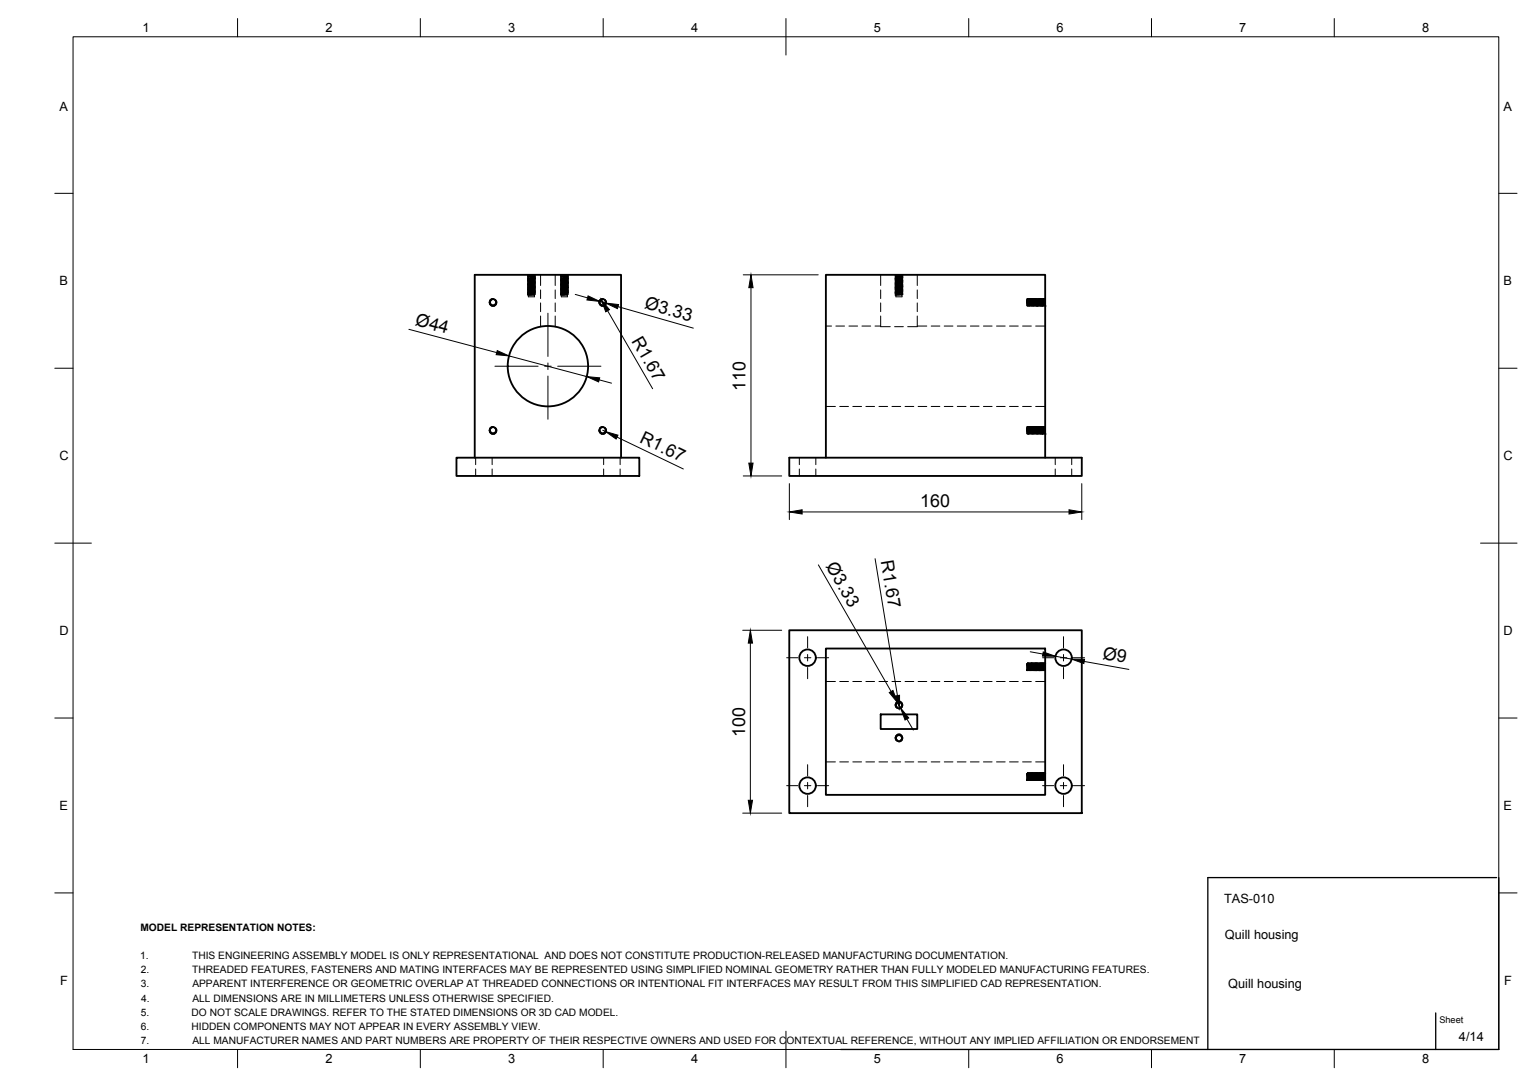
ISO-10303-21;
HEADER;
/* Generated by software containing ST-Developer
 * from STEP Tools, Inc. (www.steptools.com) 
 */

FILE_DESCRIPTION(
/* description */ (
'Independent keyed-quill tailstock, native coupled50mm slider andM16x2
 feed screw, conical dead center, bronze sleeves/thrust washers, cross
-pinned handwheel and bolted guide key. Custom center taper; no standa
rd taper compatibility, machine-bed compatibility or load rating assig
ned.'),
/* implementation_level */ '2;1');

FILE_NAME(
/* name */ 'Quill housing.step',
/* time_stamp */ '2026-11-14T07:17:36-08:00',
/* author */ (''),
/* organization */ (''),
/* preprocessor_version */ 'ST-DEVELOPER v20.2',
/* originating_system */ 'Autodesk Translation Framework v15.17.0.0',
/* authorisation */ '');

FILE_SCHEMA (('AUTOMOTIVE_DESIGN { 1 0 10303 214 3 1 1 }'));
ENDSEC;

DATA;
#10=MECHANICAL_DESIGN_GEOMETRIC_PRESENTATION_REPRESENTATION('',(#154),#289387);
#120=SHAPE_REPRESENTATION_RELATIONSHIP('SRR','None',#289455,#137);
#137=ADVANCED_BREP_SHAPE_REPRESENTATION('',(#171),#289371);
#154=STYLED_ITEM('',(#289549),#171);
#171=MANIFOLD_SOLID_BREP('Body1',#16842);
#199=FACE_BOUND('',#1414,.T.);
#200=FACE_BOUND('',#1416,.T.);
#201=FACE_BOUND('',#1417,.T.);
#202=FACE_BOUND('',#1418,.T.);
#203=FACE_BOUND('',#1419,.T.);
#204=FACE_BOUND('',#1420,.T.);
#205=FACE_BOUND('',#1426,.T.);
#206=FACE_BOUND('',#1427,.T.);
#207=FACE_BOUND('',#1428,.T.);
#208=FACE_BOUND('',#1429,.T.);
#209=FACE_BOUND('',#1432,.T.);
#210=FACE_BOUND('',#1435,.T.);
#211=FACE_BOUND('',#1436,.T.);
#212=FACE_BOUND('',#1437,.T.);
#213=FACE_BOUND('',#1438,.T.);
#214=FACE_BOUND('',#1439,.T.);
#215=FACE_BOUND('',#1441,.T.);
#216=FACE_BOUND('',#1442,.T.);
#217=FACE_BOUND('',#1443,.T.);
#281=B_SPLINE_SURFACE_WITH_KNOTS('',3,3,((#129776,#129777,#129778,#129779,
#129780,#129781,#129782,#129783,#129784,#129785,#129786,#129787,#129788,
#129789,#129790,#129791,#129792,#129793,#129794,#129795,#129796,#129797,
#129798,#129799,#129800,#129801,#129802,#129803,#129804,#129805,#129806,
#129807,#129808,#129809,#129810,#129811,#129812,#129813,#129814,#129815,
#129816,#129817,#129818,#129819,#129820,#129821,#129822,#129823,#129824,
#129825,#129826,#129827,#129828,#129829,#129830,#129831,#129832,#129833,
#129834,#129835,#129836,#129837,#129838,#129839,#129840,#129841,#129842,
#129843,#129844,#129845,#129846,#129847,#129848,#129849,#129850,#129851,
#129852,#129853,#129854,#129855,#129856,#129857,#129858,#129859,#129860,
#129861,#129862,#129863,#129864,#129865,#129866,#129867,#129868,#129869,
#129870,#129871,#129872,#129873,#129874,#129875,#129876,#129877,#129878,
#129879),(#129880,#129881,#129882,#129883,#129884,#129885,#129886,#129887,
#129888,#129889,#129890,#129891,#129892,#129893,#129894,#129895,#129896,
#129897,#129898,#129899,#129900,#129901,#129902,#129903,#129904,#129905,
#129906,#129907,#129908,#129909,#129910,#129911,#129912,#129913,#129914,
#129915,#129916,#129917,#129918,#129919,#129920,#129921,#129922,#129923,
#129924,#129925,#129926,#129927,#129928,#129929,#129930,#129931,#129932,
#129933,#129934,#129935,#129936,#129937,#129938,#129939,#129940,#129941,
#129942,#129943,#129944,#129945,#129946,#129947,#129948,#129949,#129950,
#129951,#129952,#129953,#129954,#129955,#129956,#129957,#129958,#129959,
#129960,#129961,#129962,#129963,#129964,#129965,#129966,#129967,#129968,
#129969,#129970,#129971,#129972,#129973,#129974,#129975,#129976,#129977,
#129978,#129979,#129980,#129981,#129982,#129983),(#129984,#129985,#129986,
#129987,#129988,#129989,#129990,#129991,#129992,#129993,#129994,#129995,
#129996,#129997,#129998,#129999,#130000,#130001,#130002,#130003,#130004,
#130005,#130006,#130007,#130008,#130009,#130010,#130011,#130012,#130013,
#130014,#130015,#130016,#130017,#130018,#130019,#130020,#130021,#130022,
#130023,#130024,#130025,#130026,#130027,#130028,#130029,#130030,#130031,
#130032,#130033,#130034,#130035,#130036,#130037,#130038,#130039,#130040,
#130041,#130042,#130043,#130044,#130045,#130046,#130047,#130048,#130049,
#130050,#130051,#130052,#130053,#130054,#130055,#130056,#130057,#130058,
#130059,#130060,#130061,#130062,#130063,#130064,#130065,#130066,#130067,
#130068,#130069,#130070,#130071,#130072,#130073,#130074,#130075,#130076,
#130077,#130078,#130079,#130080,#130081,#130082,#130083,#130084,#130085,
#130086,#130087),(#130088,#130089,#130090,#130091,#130092,#130093,#130094,
#130095,#130096,#130097,#130098,#130099,#130100,#130101,#130102,#130103,
#130104,#130105,#130106,#130107,#130108,#130109,#130110,#130111,#130112,
#130113,#130114,#130115,#130116,#130117,#130118,#130119,#130120,#130121,
#130122,#130123,#130124,#130125,#130126,#130127,#130128,#130129,#130130,
#130131,#130132,#130133,#130134,#130135,#130136,#130137,#130138,#130139,
#130140,#130141,#130142,#130143,#130144,#130145,#130146,#130147,#130148,
#130149,#130150,#130151,#130152,#130153,#130154,#130155,#130156,#130157,
#130158,#130159,#130160,#130161,#130162,#130163,#130164,#130165,#130166,
#130167,#130168,#130169,#130170,#130171,#130172,#130173,#130174,#130175,
#130176,#130177,#130178,#130179,#130180,#130181,#130182,#130183,#130184,
#130185,#130186,#130187,#130188,#130189,#130190,#130191)),.UNSPECIFIED.,
 .F.,.F.,.F.,(4,4),(4,1,1,1,1,1,1,1,1,1,1,1,1,1,1,1,1,1,1,1,1,1,1,1,1,1,
1,1,1,1,1,1,1,1,1,1,1,1,1,1,1,1,1,1,1,1,1,1,1,1,1,1,1,1,1,1,1,1,1,1,1,1,
1,1,1,1,1,1,1,1,1,1,1,1,1,1,1,1,1,1,1,1,1,1,1,1,1,1,1,1,1,1,1,1,1,1,1,1,
1,1,1,4),(-0.000353809570517248,0.0451882118607677),(11.8612261946863,12.8591085386934,
13.85663707313,14.8541656075666,15.8516941420032,16.8492226764398,17.8467512108764,
18.844279745313,19.8418082797496,20.8393368141862,21.8368653486228,22.8343938830594,
23.831922417496,24.8294509519326,25.8269794863692,26.8245080208058,27.8220365552424,
28.819565089679,29.8170936241156,30.8146221585522,31.8121506929888,32.8096792274254,
33.807207761862,34.8047362962986,35.8022648307352,36.7997933651718,37.7973218996084,
38.794850434045,39.7923789684816,40.7899075029182,41.7874360373548,42.7849645717913,
43.782493106228,44.7800216406646,45.7775501751012,46.7750787095378,47.7726072439743,
48.7701357784109,49.7676643128475,50.7651928472842,51.7627213817208,52.7602499161573,
53.7577784505939,54.7553069850305,55.7528355194671,56.7503640539037,57.7478925883403,
58.7454211227769,59.7429496572135,60.7404781916501,61.7380067260867,62.7355352605233,
63.7330637949599,64.7305923293965,65.7281208638331,66.7256493982697,67.7231779327063,
68.7207064671429,69.7182350015795,70.7157635360161,71.7132920704527,72.7108206048893,
73.7083491393259,74.7058776737625,75.7034062081991,76.7009347426357,77.6984632770723,
78.6959918115089,79.6935203459455,80.6910488803821,81.6885774148187,82.6861059492553,
83.6836344836919,84.6811630181285,85.6786915525651,86.6762200870017,87.6737486214383,
88.6712771558749,89.6688056903115,90.6663342247481,91.6638627591847,92.6613912936213,
93.6589198280579,94.6564483624945,95.6539768969311,96.6515054313677,97.6490339658043,
98.6465625002409,99.6440910346775,100.641619569114,101.639148103551,102.636676637987,
103.634205172424,104.631733706861,105.629262241297,106.626790775734,107.62431931017,
108.621847844607,109.619376379044,110.61690491348,111.614433447917,112.611961982353),
 .UNSPECIFIED.);
#282=B_SPLINE_SURFACE_WITH_KNOTS('',3,3,((#130274,#130275,#130276,#130277,
#130278,#130279,#130280,#130281,#130282,#130283,#130284,#130285,#130286,
#130287,#130288,#130289,#130290,#130291,#130292,#130293,#130294,#130295,
#130296,#130297,#130298,#130299,#130300,#130301,#130302,#130303,#130304,
#130305,#130306,#130307,#130308,#130309,#130310,#130311,#130312,#130313,
#130314,#130315,#130316,#130317,#130318,#130319,#130320,#130321,#130322,
#130323,#130324,#130325,#130326,#130327,#130328,#130329,#130330,#130331,
#130332,#130333,#130334,#130335,#130336,#130337,#130338,#130339,#130340,
#130341,#130342,#130343,#130344,#130345,#130346,#130347,#130348,#130349,
#130350,#130351,#130352,#130353,#130354,#130355,#130356,#130357,#130358,
#130359,#130360,#130361,#130362,#130363,#130364,#130365,#130366,#130367,
#130368,#130369,#130370,#130371,#130372,#130373,#130374,#130375,#130376,
#130377),(#130378,#130379,#130380,#130381,#130382,#130383,#130384,#130385,
#130386,#130387,#130388,#130389,#130390,#130391,#130392,#130393,#130394,
#130395,#130396,#130397,#130398,#130399,#130400,#130401,#130402,#130403,
#130404,#130405,#130406,#130407,#130408,#130409,#130410,#130411,#130412,
#130413,#130414,#130415,#130416,#130417,#130418,#130419,#130420,#130421,
#130422,#130423,#130424,#130425,#130426,#130427,#130428,#130429,#130430,
#130431,#130432,#130433,#130434,#130435,#130436,#130437,#130438,#130439,
#130440,#130441,#130442,#130443,#130444,#130445,#130446,#130447,#130448,
#130449,#130450,#130451,#130452,#130453,#130454,#130455,#130456,#130457,
#130458,#130459,#130460,#130461,#130462,#130463,#130464,#130465,#130466,
#130467,#130468,#130469,#130470,#130471,#130472,#130473,#130474,#130475,
#130476,#130477,#130478,#130479,#130480,#130481),(#130482,#130483,#130484,
#130485,#130486,#130487,#130488,#130489,#130490,#130491,#130492,#130493,
#130494,#130495,#130496,#130497,#130498,#130499,#130500,#130501,#130502,
#130503,#130504,#130505,#130506,#130507,#130508,#130509,#130510,#130511,
#130512,#130513,#130514,#130515,#130516,#130517,#130518,#130519,#130520,
#130521,#130522,#130523,#130524,#130525,#130526,#130527,#130528,#130529,
#130530,#130531,#130532,#130533,#130534,#130535,#130536,#130537,#130538,
#130539,#130540,#130541,#130542,#130543,#130544,#130545,#130546,#130547,
#130548,#130549,#130550,#130551,#130552,#130553,#130554,#130555,#130556,
#130557,#130558,#130559,#130560,#130561,#130562,#130563,#130564,#130565,
#130566,#130567,#130568,#130569,#130570,#130571,#130572,#130573,#130574,
#130575,#130576,#130577,#130578,#130579,#130580,#130581,#130582,#130583,
#130584,#130585),(#130586,#130587,#130588,#130589,#130590,#130591,#130592,
#130593,#130594,#130595,#130596,#130597,#130598,#130599,#130600,#130601,
#130602,#130603,#130604,#130605,#130606,#130607,#130608,#130609,#130610,
#130611,#130612,#130613,#130614,#130615,#130616,#130617,#130618,#130619,
#130620,#130621,#130622,#130623,#130624,#130625,#130626,#130627,#130628,
#130629,#130630,#130631,#130632,#130633,#130634,#130635,#130636,#130637,
#130638,#130639,#130640,#130641,#130642,#130643,#130644,#130645,#130646,
#130647,#130648,#130649,#130650,#130651,#130652,#130653,#130654,#130655,
#130656,#130657,#130658,#130659,#130660,#130661,#130662,#130663,#130664,
#130665,#130666,#130667,#130668,#130669,#130670,#130671,#130672,#130673,
#130674,#130675,#130676,#130677,#130678,#130679,#130680,#130681,#130682,
#130683,#130684,#130685,#130686,#130687,#130688,#130689)),.UNSPECIFIED.,
 .F.,.F.,.F.,(4,4),(4,1,1,1,1,1,1,1,1,1,1,1,1,1,1,1,1,1,1,1,1,1,1,1,1,1,
1,1,1,1,1,1,1,1,1,1,1,1,1,1,1,1,1,1,1,1,1,1,1,1,1,1,1,1,1,1,1,1,1,1,1,1,
1,1,1,1,1,1,1,1,1,1,1,1,1,1,1,1,1,1,1,1,1,1,1,1,1,1,1,1,1,1,1,1,1,1,1,1,
1,1,1,4),(-0.000311884246383574,0.0452427689821445),(14.398141012777,15.3956695472136,
16.3931980816502,17.3907266160868,18.3882551505234,19.38578368496,20.3833122193966,
21.3808407538332,22.3783692882698,23.3758978227064,24.373426357143,25.3709548915796,
26.3684834260162,27.3660119604528,28.3635404948894,29.361069029326,30.3585975637626,
31.3561260981992,32.3536546326358,33.3511831670724,34.348711701509,35.3462402359456,
36.3437687703822,37.3412973048188,38.3388258392554,39.336354373692,40.3338829081286,
41.3314114425652,42.3289399770018,43.3264685114384,44.323997045875,45.3215255803116,
46.3190541147482,47.3165826491848,48.3141111836214,49.311639718058,50.3091682524946,
51.3066967869312,52.3042253213678,53.3017538558044,54.299282390241,55.2968109246776,
56.2943394591142,57.2918679935508,58.2893965279874,59.286925062424,60.2844535968606,
61.2819821312972,62.2795106657338,63.2770392001704,64.274567734607,65.2720962690436,
66.2696248034802,67.2671533379168,68.2646818723534,69.26221040679,70.2597389412266,
71.2572674756632,72.2547960100998,73.2523245445364,74.249853078973,75.2473816134096,
76.2449101478462,77.2424386822828,78.2399672167194,79.237495751156,80.2350242855926,
81.2325528200292,82.2300813544658,83.2276098889024,84.225138423339,85.2226669577756,
86.2201954922122,87.2177240266488,88.2152525610854,89.212781095522,90.2103096299586,
91.2078381643952,92.2053666988318,93.2028952332684,94.2004237677049,95.1979523021416,
96.1954808365782,97.1930093710148,98.1905379054514,99.1880664398879,100.185594974325,
101.183123508761,102.180652043198,103.178180577634,104.175709112071,105.173237646508,
106.170766180944,107.168294715381,108.165823249817,109.163351784254,110.160880318691,
111.158408853127,112.155937387564,113.153465922,114.150994456437,115.148876776427),
 .UNSPECIFIED.);
#283=B_SPLINE_SURFACE_WITH_KNOTS('',3,3,((#130957,#130958,#130959,#130960,
#130961,#130962,#130963,#130964,#130965,#130966,#130967,#130968,#130969,
#130970,#130971,#130972,#130973,#130974,#130975,#130976,#130977,#130978,
#130979,#130980,#130981,#130982,#130983,#130984,#130985,#130986,#130987,
#130988,#130989,#130990,#130991,#130992,#130993,#130994,#130995,#130996,
#130997,#130998,#130999,#131000,#131001,#131002,#131003,#131004,#131005,
#131006,#131007,#131008,#131009,#131010,#131011,#131012,#131013,#131014,
#131015,#131016,#131017,#131018,#131019,#131020,#131021,#131022,#131023,
#131024,#131025,#131026,#131027,#131028,#131029,#131030,#131031,#131032,
#131033,#131034,#131035,#131036,#131037,#131038,#131039,#131040,#131041,
#131042,#131043,#131044,#131045,#131046,#131047,#131048,#131049,#131050,
#131051,#131052,#131053,#131054,#131055,#131056,#131057,#131058,#131059,
#131060),(#131061,#131062,#131063,#131064,#131065,#131066,#131067,#131068,
#131069,#131070,#131071,#131072,#131073,#131074,#131075,#131076,#131077,
#131078,#131079,#131080,#131081,#131082,#131083,#131084,#131085,#131086,
#131087,#131088,#131089,#131090,#131091,#131092,#131093,#131094,#131095,
#131096,#131097,#131098,#131099,#131100,#131101,#131102,#131103,#131104,
#131105,#131106,#131107,#131108,#131109,#131110,#131111,#131112,#131113,
#131114,#131115,#131116,#131117,#131118,#131119,#131120,#131121,#131122,
#131123,#131124,#131125,#131126,#131127,#131128,#131129,#131130,#131131,
#131132,#131133,#131134,#131135,#131136,#131137,#131138,#131139,#131140,
#131141,#131142,#131143,#131144,#131145,#131146,#131147,#131148,#131149,
#131150,#131151,#131152,#131153,#131154,#131155,#131156,#131157,#131158,
#131159,#131160,#131161,#131162,#131163,#131164),(#131165,#131166,#131167,
#131168,#131169,#131170,#131171,#131172,#131173,#131174,#131175,#131176,
#131177,#131178,#131179,#131180,#131181,#131182,#131183,#131184,#131185,
#131186,#131187,#131188,#131189,#131190,#131191,#131192,#131193,#131194,
#131195,#131196,#131197,#131198,#131199,#131200,#131201,#131202,#131203,
#131204,#131205,#131206,#131207,#131208,#131209,#131210,#131211,#131212,
#131213,#131214,#131215,#131216,#131217,#131218,#131219,#131220,#131221,
#131222,#131223,#131224,#131225,#131226,#131227,#131228,#131229,#131230,
#131231,#131232,#131233,#131234,#131235,#131236,#131237,#131238,#131239,
#131240,#131241,#131242,#131243,#131244,#131245,#131246,#131247,#131248,
#131249,#131250,#131251,#131252,#131253,#131254,#131255,#131256,#131257,
#131258,#131259,#131260,#131261,#131262,#131263,#131264,#131265,#131266,
#131267,#131268),(#131269,#131270,#131271,#131272,#131273,#131274,#131275,
#131276,#131277,#131278,#131279,#131280,#131281,#131282,#131283,#131284,
#131285,#131286,#131287,#131288,#131289,#131290,#131291,#131292,#131293,
#131294,#131295,#131296,#131297,#131298,#131299,#131300,#131301,#131302,
#131303,#131304,#131305,#131306,#131307,#131308,#131309,#131310,#131311,
#131312,#131313,#131314,#131315,#131316,#131317,#131318,#131319,#131320,
#131321,#131322,#131323,#131324,#131325,#131326,#131327,#131328,#131329,
#131330,#131331,#131332,#131333,#131334,#131335,#131336,#131337,#131338,
#131339,#131340,#131341,#131342,#131343,#131344,#131345,#131346,#131347,
#131348,#131349,#131350,#131351,#131352,#131353,#131354,#131355,#131356,
#131357,#131358,#131359,#131360,#131361,#131362,#131363,#131364,#131365,
#131366,#131367,#131368,#131369,#131370,#131371,#131372)),.UNSPECIFIED.,
 .F.,.F.,.F.,(4,4),(4,1,1,1,1,1,1,1,1,1,1,1,1,1,1,1,1,1,1,1,1,1,1,1,1,1,
1,1,1,1,1,1,1,1,1,1,1,1,1,1,1,1,1,1,1,1,1,1,1,1,1,1,1,1,1,1,1,1,1,1,1,1,
1,1,1,1,1,1,1,1,1,1,1,1,1,1,1,1,1,1,1,1,1,1,1,1,1,1,1,1,1,1,1,1,1,1,1,1,
1,1,1,4),(-0.000353803744797756,0.045188208347436),(11.8612262005118,12.8591085386932,
13.8566370731298,14.8541656075664,15.851694142003,16.8492226764396,17.8467512108762,
18.8442797453128,19.8418082797494,20.839336814186,21.8368653486226,22.8343938830592,
23.8319224174958,24.8294509519324,25.826979486369,26.8245080208056,27.8220365552422,
28.8195650896788,29.8170936241154,30.814622158552,31.8121506929886,32.8096792274252,
33.8072077618618,34.8047362962984,35.802264830735,36.7997933651716,37.7973218996082,
38.7948504340448,39.7923789684814,40.789907502918,41.7874360373546,42.7849645717912,
43.7824931062278,44.7800216406644,45.777550175101,46.7750787095376,47.7726072439742,
48.7701357784108,49.7676643128474,50.765192847284,51.7627213817206,52.7602499161572,
53.7577784505938,54.7553069850304,55.752835519467,56.7503640539036,57.7478925883402,
58.7454211227768,59.7429496572134,60.74047819165,61.7380067260866,62.7355352605232,
63.7330637949598,64.7305923293964,65.728120863833,66.7256493982696,67.7231779327062,
68.7207064671428,69.7182350015794,70.715763536016,71.7132920704526,72.7108206048892,
73.7083491393258,74.7058776737624,75.703406208199,76.7009347426356,77.6984632770722,
78.6959918115088,79.6935203459454,80.691048880382,81.6885774148186,82.6861059492552,
83.6836344836918,84.6811630181284,85.678691552565,86.6762200870016,87.6737486214382,
88.6712771558748,89.6688056903114,90.666334224748,91.6638627591846,92.6613912936212,
93.6589198280578,94.6564483624944,95.653976896931,96.6515054313676,97.6490339658042,
98.6465625002408,99.6440910346774,100.641619569114,101.639148103551,102.636676637987,
103.634205172424,104.63173370686,105.629262241297,106.626790775734,107.62431931017,
108.621847844607,109.619376379043,110.61690491348,111.614433447917,112.611961982353),
 .UNSPECIFIED.);
#284=B_SPLINE_SURFACE_WITH_KNOTS('',3,3,((#131455,#131456,#131457,#131458,
#131459,#131460,#131461,#131462,#131463,#131464,#131465,#131466,#131467,
#131468,#131469,#131470,#131471,#131472,#131473,#131474,#131475,#131476,
#131477,#131478,#131479,#131480,#131481,#131482,#131483,#131484,#131485,
#131486,#131487,#131488,#131489,#131490,#131491,#131492,#131493,#131494,
#131495,#131496,#131497,#131498,#131499,#131500,#131501,#131502,#131503,
#131504,#131505,#131506,#131507,#131508,#131509,#131510,#131511,#131512,
#131513,#131514,#131515,#131516,#131517,#131518,#131519,#131520,#131521,
#131522,#131523,#131524,#131525,#131526,#131527,#131528,#131529,#131530,
#131531,#131532,#131533,#131534,#131535,#131536,#131537,#131538,#131539,
#131540,#131541,#131542,#131543,#131544,#131545,#131546,#131547,#131548,
#131549,#131550,#131551,#131552,#131553,#131554,#131555,#131556,#131557,
#131558),(#131559,#131560,#131561,#131562,#131563,#131564,#131565,#131566,
#131567,#131568,#131569,#131570,#131571,#131572,#131573,#131574,#131575,
#131576,#131577,#131578,#131579,#131580,#131581,#131582,#131583,#131584,
#131585,#131586,#131587,#131588,#131589,#131590,#131591,#131592,#131593,
#131594,#131595,#131596,#131597,#131598,#131599,#131600,#131601,#131602,
#131603,#131604,#131605,#131606,#131607,#131608,#131609,#131610,#131611,
#131612,#131613,#131614,#131615,#131616,#131617,#131618,#131619,#131620,
#131621,#131622,#131623,#131624,#131625,#131626,#131627,#131628,#131629,
#131630,#131631,#131632,#131633,#131634,#131635,#131636,#131637,#131638,
#131639,#131640,#131641,#131642,#131643,#131644,#131645,#131646,#131647,
#131648,#131649,#131650,#131651,#131652,#131653,#131654,#131655,#131656,
#131657,#131658,#131659,#131660,#131661,#131662),(#131663,#131664,#131665,
#131666,#131667,#131668,#131669,#131670,#131671,#131672,#131673,#131674,
#131675,#131676,#131677,#131678,#131679,#131680,#131681,#131682,#131683,
#131684,#131685,#131686,#131687,#131688,#131689,#131690,#131691,#131692,
#131693,#131694,#131695,#131696,#131697,#131698,#131699,#131700,#131701,
#131702,#131703,#131704,#131705,#131706,#131707,#131708,#131709,#131710,
#131711,#131712,#131713,#131714,#131715,#131716,#131717,#131718,#131719,
#131720,#131721,#131722,#131723,#131724,#131725,#131726,#131727,#131728,
#131729,#131730,#131731,#131732,#131733,#131734,#131735,#131736,#131737,
#131738,#131739,#131740,#131741,#131742,#131743,#131744,#131745,#131746,
#131747,#131748,#131749,#131750,#131751,#131752,#131753,#131754,#131755,
#131756,#131757,#131758,#131759,#131760,#131761,#131762,#131763,#131764,
#131765,#131766),(#131767,#131768,#131769,#131770,#131771,#131772,#131773,
#131774,#131775,#131776,#131777,#131778,#131779,#131780,#131781,#131782,
#131783,#131784,#131785,#131786,#131787,#131788,#131789,#131790,#131791,
#131792,#131793,#131794,#131795,#131796,#131797,#131798,#131799,#131800,
#131801,#131802,#131803,#131804,#131805,#131806,#131807,#131808,#131809,
#131810,#131811,#131812,#131813,#131814,#131815,#131816,#131817,#131818,
#131819,#131820,#131821,#131822,#131823,#131824,#131825,#131826,#131827,
#131828,#131829,#131830,#131831,#131832,#131833,#131834,#131835,#131836,
#131837,#131838,#131839,#131840,#131841,#131842,#131843,#131844,#131845,
#131846,#131847,#131848,#131849,#131850,#131851,#131852,#131853,#131854,
#131855,#131856,#131857,#131858,#131859,#131860,#131861,#131862,#131863,
#131864,#131865,#131866,#131867,#131868,#131869,#131870)),.UNSPECIFIED.,
 .F.,.F.,.F.,(4,4),(4,1,1,1,1,1,1,1,1,1,1,1,1,1,1,1,1,1,1,1,1,1,1,1,1,1,
1,1,1,1,1,1,1,1,1,1,1,1,1,1,1,1,1,1,1,1,1,1,1,1,1,1,1,1,1,1,1,1,1,1,1,1,
1,1,1,1,1,1,1,1,1,1,1,1,1,1,1,1,1,1,1,1,1,1,1,1,1,1,1,1,1,1,1,1,1,1,1,1,
1,1,1,4),(-0.000311879380046352,0.0452427611100038),(14.3981410127768,15.3956695472134,
16.39319808165,17.3907266160866,18.3882551505232,19.3857836849598,20.3833122193964,
21.380840753833,22.3783692882696,23.3758978227062,24.3734263571428,25.3709548915794,
26.368483426016,27.3660119604526,28.3635404948892,29.3610690293258,30.3585975637624,
31.356126098199,32.3536546326356,33.3511831670722,34.3487117015088,35.3462402359454,
36.343768770382,37.3412973048186,38.3388258392552,39.3363543736918,40.3338829081284,
41.331411442565,42.3289399770016,43.3264685114382,44.3239970458748,45.3215255803114,
46.319054114748,47.3165826491846,48.3141111836212,49.3116397180578,50.3091682524944,
51.306696786931,52.3042253213676,53.3017538558042,54.2992823902408,55.2968109246774,
56.294339459114,57.2918679935506,58.2893965279872,59.2869250624238,60.2844535968604,
61.281982131297,62.2795106657336,63.2770392001702,64.2745677346068,65.2720962690434,
66.26962480348,67.2671533379166,68.2646818723532,69.2622104067898,70.2597389412264,
71.257267475663,72.2547960100996,73.2523245445362,74.2498530789728,75.2473816134094,
76.244910147846,77.2424386822826,78.2399672167192,79.2374957511558,80.2350242855924,
81.232552820029,82.2300813544656,83.2276098889022,84.2251384233388,85.2226669577754,
86.220195492212,87.2177240266486,88.2152525610852,89.2127810955218,90.2103096299584,
91.207838164395,92.2053666988316,93.2028952332682,94.2004237677048,95.1979523021414,
96.195480836578,97.1930093710146,98.1905379054512,99.1880664398878,100.185594974324,
101.183123508761,102.180652043198,103.178180577634,104.175709112071,105.173237646507,
106.170766180944,107.168294715381,108.165823249817,109.163351784254,110.16088031869,
111.158408853127,112.155937387564,113.153465922,114.150994456437,115.148876768553),
 .UNSPECIFIED.);
#285=B_SPLINE_SURFACE_WITH_KNOTS('',3,3,((#132011,#132012,#132013,#132014,
#132015,#132016,#132017,#132018,#132019,#132020,#132021,#132022,#132023,
#132024,#132025,#132026,#132027,#132028,#132029,#132030,#132031,#132032,
#132033,#132034,#132035,#132036,#132037,#132038,#132039,#132040,#132041,
#132042,#132043,#132044,#132045,#132046,#132047,#132048,#132049,#132050,
#132051,#132052,#132053,#132054,#132055,#132056,#132057,#132058,#132059,
#132060,#132061,#132062,#132063,#132064,#132065,#132066,#132067,#132068,
#132069,#132070,#132071,#132072,#132073,#132074,#132075,#132076,#132077,
#132078,#132079,#132080,#132081,#132082,#132083,#132084,#132085,#132086,
#132087,#132088,#132089,#132090,#132091,#132092,#132093,#132094,#132095,
#132096,#132097,#132098,#132099,#132100,#132101,#132102,#132103,#132104,
#132105),(#132106,#132107,#132108,#132109,#132110,#132111,#132112,#132113,
#132114,#132115,#132116,#132117,#132118,#132119,#132120,#132121,#132122,
#132123,#132124,#132125,#132126,#132127,#132128,#132129,#132130,#132131,
#132132,#132133,#132134,#132135,#132136,#132137,#132138,#132139,#132140,
#132141,#132142,#132143,#132144,#132145,#132146,#132147,#132148,#132149,
#132150,#132151,#132152,#132153,#132154,#132155,#132156,#132157,#132158,
#132159,#132160,#132161,#132162,#132163,#132164,#132165,#132166,#132167,
#132168,#132169,#132170,#132171,#132172,#132173,#132174,#132175,#132176,
#132177,#132178,#132179,#132180,#132181,#132182,#132183,#132184,#132185,
#132186,#132187,#132188,#132189,#132190,#132191,#132192,#132193,#132194,
#132195,#132196,#132197,#132198,#132199,#132200),(#132201,#132202,#132203,
#132204,#132205,#132206,#132207,#132208,#132209,#132210,#132211,#132212,
#132213,#132214,#132215,#132216,#132217,#132218,#132219,#132220,#132221,
#132222,#132223,#132224,#132225,#132226,#132227,#132228,#132229,#132230,
#132231,#132232,#132233,#132234,#132235,#132236,#132237,#132238,#132239,
#132240,#132241,#132242,#132243,#132244,#132245,#132246,#132247,#132248,
#132249,#132250,#132251,#132252,#132253,#132254,#132255,#132256,#132257,
#132258,#132259,#132260,#132261,#132262,#132263,#132264,#132265,#132266,
#132267,#132268,#132269,#132270,#132271,#132272,#132273,#132274,#132275,
#132276,#132277,#132278,#132279,#132280,#132281,#132282,#132283,#132284,
#132285,#132286,#132287,#132288,#132289,#132290,#132291,#132292,#132293,
#132294,#132295),(#132296,#132297,#132298,#132299,#132300,#132301,#132302,
#132303,#132304,#132305,#132306,#132307,#132308,#132309,#132310,#132311,
#132312,#132313,#132314,#132315,#132316,#132317,#132318,#132319,#132320,
#132321,#132322,#132323,#132324,#132325,#132326,#132327,#132328,#132329,
#132330,#132331,#132332,#132333,#132334,#132335,#132336,#132337,#132338,
#132339,#132340,#132341,#132342,#132343,#132344,#132345,#132346,#132347,
#132348,#132349,#132350,#132351,#132352,#132353,#132354,#132355,#132356,
#132357,#132358,#132359,#132360,#132361,#132362,#132363,#132364,#132365,
#132366,#132367,#132368,#132369,#132370,#132371,#132372,#132373,#132374,
#132375,#132376,#132377,#132378,#132379,#132380,#132381,#132382,#132383,
#132384,#132385,#132386,#132387,#132388,#132389,#132390)),.UNSPECIFIED.,
 .F.,.F.,.F.,(4,4),(4,1,1,1,1,1,1,1,1,1,1,1,1,1,1,1,1,1,1,1,1,1,1,1,1,1,
1,1,1,1,1,1,1,1,1,1,1,1,1,1,1,1,1,1,1,1,1,1,1,1,1,1,1,1,1,1,1,1,1,1,1,1,
1,1,1,1,1,1,1,1,1,1,1,1,1,1,1,1,1,1,1,1,1,1,1,1,1,1,1,1,1,1,4),(-0.000348318790885902,
0.0451835916777494),(11.8612316854658,12.8591278626027,13.8566757209488,
14.8542235792949,15.851771437641,16.8493192959871,17.8468671543332,18.8444150126793,
19.8419628710254,20.8395107293714,21.8370585877175,22.8346064460636,23.8321543044097,
24.8297021627558,25.8272500211019,26.824797879448,27.822345737794,28.8198935961401,
29.8174414544862,30.8149893128323,31.8125371711784,32.8100850295245,33.8076328878706,
34.8051807462166,35.8027286045627,36.8002764629088,37.7978243212549,38.795372179601,
39.7929200379471,40.7904678962932,41.7880157546393,42.7855636129853,43.7831114713314,
44.7806593296775,45.7782071880236,46.7757550463697,47.7733029047158,48.7708507630619,
49.768398621408,50.765946479754,51.7634943381001,52.7610421964462,53.7585900547923,
54.7561379131384,55.7536857714845,56.7512336298306,57.7487814881766,58.7463293465227,
59.7438772048688,60.7414250632149,61.738972921561,62.7365207799071,63.7340686382532,
64.7316164965993,65.7291643549453,66.7267122132914,67.7242600716375,68.7218079299836,
69.7193557883297,70.7169036466758,71.7144515050219,72.711999363368,73.709547221714,
74.7070950800601,75.7046429384062,76.7021907967523,77.6997386550984,78.6972865134445,
79.6948343717905,80.6923822301366,81.6899300884827,82.6874779468288,83.6850258051749,
84.682573663521,85.6801215218671,86.6776693802132,87.6752172385592,88.6727650969053,
89.6703129552514,90.6678608135975,91.6654086719436,92.6629565302897,93.6605043886358,
94.6580522469819,95.6556001053279,96.653147963674,97.6506958220201,98.6482436803662,
99.6457915387123,100.643339397058,101.640887255404,102.638435113751,103.635982972097),
 .UNSPECIFIED.);
#286=B_SPLINE_SURFACE_WITH_KNOTS('',3,3,((#132563,#132564,#132565,#132566,
#132567,#132568,#132569,#132570,#132571,#132572,#132573,#132574,#132575,
#132576,#132577,#132578,#132579,#132580,#132581,#132582,#132583,#132584,
#132585,#132586,#132587,#132588,#132589,#132590,#132591,#132592,#132593,
#132594,#132595,#132596,#132597,#132598,#132599,#132600,#132601,#132602,
#132603,#132604,#132605,#132606,#132607,#132608,#132609,#132610,#132611,
#132612,#132613,#132614,#132615,#132616,#132617,#132618,#132619,#132620,
#132621,#132622,#132623,#132624,#132625,#132626,#132627,#132628,#132629,
#132630,#132631,#132632,#132633,#132634,#132635,#132636,#132637,#132638,
#132639,#132640,#132641,#132642,#132643,#132644,#132645,#132646,#132647,
#132648,#132649,#132650,#132651,#132652,#132653,#132654,#132655,#132656,
#132657),(#132658,#132659,#132660,#132661,#132662,#132663,#132664,#132665,
#132666,#132667,#132668,#132669,#132670,#132671,#132672,#132673,#132674,
#132675,#132676,#132677,#132678,#132679,#132680,#132681,#132682,#132683,
#132684,#132685,#132686,#132687,#132688,#132689,#132690,#132691,#132692,
#132693,#132694,#132695,#132696,#132697,#132698,#132699,#132700,#132701,
#132702,#132703,#132704,#132705,#132706,#132707,#132708,#132709,#132710,
#132711,#132712,#132713,#132714,#132715,#132716,#132717,#132718,#132719,
#132720,#132721,#132722,#132723,#132724,#132725,#132726,#132727,#132728,
#132729,#132730,#132731,#132732,#132733,#132734,#132735,#132736,#132737,
#132738,#132739,#132740,#132741,#132742,#132743,#132744,#132745,#132746,
#132747,#132748,#132749,#132750,#132751,#132752),(#132753,#132754,#132755,
#132756,#132757,#132758,#132759,#132760,#132761,#132762,#132763,#132764,
#132765,#132766,#132767,#132768,#132769,#132770,#132771,#132772,#132773,
#132774,#132775,#132776,#132777,#132778,#132779,#132780,#132781,#132782,
#132783,#132784,#132785,#132786,#132787,#132788,#132789,#132790,#132791,
#132792,#132793,#132794,#132795,#132796,#132797,#132798,#132799,#132800,
#132801,#132802,#132803,#132804,#132805,#132806,#132807,#132808,#132809,
#132810,#132811,#132812,#132813,#132814,#132815,#132816,#132817,#132818,
#132819,#132820,#132821,#132822,#132823,#132824,#132825,#132826,#132827,
#132828,#132829,#132830,#132831,#132832,#132833,#132834,#132835,#132836,
#132837,#132838,#132839,#132840,#132841,#132842,#132843,#132844,#132845,
#132846,#132847),(#132848,#132849,#132850,#132851,#132852,#132853,#132854,
#132855,#132856,#132857,#132858,#132859,#132860,#132861,#132862,#132863,
#132864,#132865,#132866,#132867,#132868,#132869,#132870,#132871,#132872,
#132873,#132874,#132875,#132876,#132877,#132878,#132879,#132880,#132881,
#132882,#132883,#132884,#132885,#132886,#132887,#132888,#132889,#132890,
#132891,#132892,#132893,#132894,#132895,#132896,#132897,#132898,#132899,
#132900,#132901,#132902,#132903,#132904,#132905,#132906,#132907,#132908,
#132909,#132910,#132911,#132912,#132913,#132914,#132915,#132916,#132917,
#132918,#132919,#132920,#132921,#132922,#132923,#132924,#132925,#132926,
#132927,#132928,#132929,#132930,#132931,#132932,#132933,#132934,#132935,
#132936,#132937,#132938,#132939,#132940,#132941,#132942)),.UNSPECIFIED.,
 .F.,.F.,.F.,(4,4),(4,1,1,1,1,1,1,1,1,1,1,1,1,1,1,1,1,1,1,1,1,1,1,1,1,1,
1,1,1,1,1,1,1,1,1,1,1,1,1,1,1,1,1,1,1,1,1,1,1,1,1,1,1,1,1,1,1,1,1,1,1,1,
1,1,1,1,1,1,1,1,1,1,1,1,1,1,1,1,1,1,1,1,1,1,1,1,1,1,1,1,1,1,4),(-0.000309367040895943,
0.0452373400660471),(14.3981410127769,15.395688871123,16.3932367294691,
17.3907845878152,18.3883324461612,19.3858803045073,20.3834281628534,21.3809760211995,
22.3785238795456,23.3760717378917,24.3736195962378,25.3711674545839,26.3687153129299,
27.366263171276,28.3638110296221,29.3613588879682,30.3589067463143,31.3564546046604,
32.3540024630065,33.3515503213525,34.3490981796986,35.3466460380447,36.3441938963908,
37.3417417547369,38.339289613083,39.3368374714291,40.3343853297752,41.3319331881212,
42.3294810464673,43.3270289048134,44.3245767631595,45.3221246215056,46.3196724798517,
47.3172203381978,48.3147681965438,49.3123160548899,50.309863913236,51.3074117715821,
52.3049596299282,53.3025074882743,54.3000553466204,55.2976032049664,56.2951510633125,
57.2926989216586,58.2902467800047,59.2877946383508,60.2853424966969,61.282890355043,
62.2804382133891,63.2779860717351,64.2755339300812,65.2730817884273,66.2706296467734,
67.2681775051195,68.2657253634656,69.2632732218117,70.2608210801578,71.2583689385038,
72.2559167968499,73.253464655196,74.2510125135421,75.2485603718882,76.2461082302343,
77.2436560885804,78.2412039469264,79.2387518052725,80.2362996636186,81.2338475219647,
82.2313953803108,83.2289432386569,84.226491097003,85.2240389553491,86.2215868136952,
87.2191346720412,88.2166825303873,89.2142303887334,90.2117782470795,91.2093261054256,
92.2068739637717,93.2044218221178,94.2019696804638,95.1995175388099,96.197065397156,
97.1946132555021,98.1921611138482,99.1897089721943,100.18725683054,101.184804688886,
102.182352547233,103.179900405579,104.177448263925,105.174996122271,106.172892337254),
 .UNSPECIFIED.);
#287=B_SPLINE_SURFACE_WITH_KNOTS('',3,3,((#133121,#133122,#133123,#133124,
#133125,#133126,#133127,#133128,#133129,#133130,#133131,#133132,#133133,
#133134,#133135,#133136,#133137,#133138,#133139,#133140,#133141,#133142,
#133143,#133144,#133145,#133146,#133147,#133148,#133149,#133150,#133151,
#133152,#133153,#133154,#133155,#133156,#133157,#133158,#133159,#133160,
#133161,#133162,#133163,#133164,#133165,#133166,#133167,#133168,#133169,
#133170,#133171,#133172,#133173,#133174,#133175,#133176,#133177,#133178,
#133179,#133180,#133181,#133182,#133183,#133184,#133185,#133186,#133187,
#133188,#133189,#133190,#133191,#133192,#133193,#133194,#133195,#133196,
#133197,#133198,#133199,#133200,#133201,#133202,#133203,#133204,#133205,
#133206,#133207,#133208,#133209,#133210,#133211,#133212,#133213,#133214,
#133215),(#133216,#133217,#133218,#133219,#133220,#133221,#133222,#133223,
#133224,#133225,#133226,#133227,#133228,#133229,#133230,#133231,#133232,
#133233,#133234,#133235,#133236,#133237,#133238,#133239,#133240,#133241,
#133242,#133243,#133244,#133245,#133246,#133247,#133248,#133249,#133250,
#133251,#133252,#133253,#133254,#133255,#133256,#133257,#133258,#133259,
#133260,#133261,#133262,#133263,#133264,#133265,#133266,#133267,#133268,
#133269,#133270,#133271,#133272,#133273,#133274,#133275,#133276,#133277,
#133278,#133279,#133280,#133281,#133282,#133283,#133284,#133285,#133286,
#133287,#133288,#133289,#133290,#133291,#133292,#133293,#133294,#133295,
#133296,#133297,#133298,#133299,#133300,#133301,#133302,#133303,#133304,
#133305,#133306,#133307,#133308,#133309,#133310),(#133311,#133312,#133313,
#133314,#133315,#133316,#133317,#133318,#133319,#133320,#133321,#133322,
#133323,#133324,#133325,#133326,#133327,#133328,#133329,#133330,#133331,
#133332,#133333,#133334,#133335,#133336,#133337,#133338,#133339,#133340,
#133341,#133342,#133343,#133344,#133345,#133346,#133347,#133348,#133349,
#133350,#133351,#133352,#133353,#133354,#133355,#133356,#133357,#133358,
#133359,#133360,#133361,#133362,#133363,#133364,#133365,#133366,#133367,
#133368,#133369,#133370,#133371,#133372,#133373,#133374,#133375,#133376,
#133377,#133378,#133379,#133380,#133381,#133382,#133383,#133384,#133385,
#133386,#133387,#133388,#133389,#133390,#133391,#133392,#133393,#133394,
#133395,#133396,#133397,#133398,#133399,#133400,#133401,#133402,#133403,
#133404,#133405),(#133406,#133407,#133408,#133409,#133410,#133411,#133412,
#133413,#133414,#133415,#133416,#133417,#133418,#133419,#133420,#133421,
#133422,#133423,#133424,#133425,#133426,#133427,#133428,#133429,#133430,
#133431,#133432,#133433,#133434,#133435,#133436,#133437,#133438,#133439,
#133440,#133441,#133442,#133443,#133444,#133445,#133446,#133447,#133448,
#133449,#133450,#133451,#133452,#133453,#133454,#133455,#133456,#133457,
#133458,#133459,#133460,#133461,#133462,#133463,#133464,#133465,#133466,
#133467,#133468,#133469,#133470,#133471,#133472,#133473,#133474,#133475,
#133476,#133477,#133478,#133479,#133480,#133481,#133482,#133483,#133484,
#133485,#133486,#133487,#133488,#133489,#133490,#133491,#133492,#133493,
#133494,#133495,#133496,#133497,#133498,#133499,#133500)),.UNSPECIFIED.,
 .F.,.F.,.F.,(4,4),(4,1,1,1,1,1,1,1,1,1,1,1,1,1,1,1,1,1,1,1,1,1,1,1,1,1,
1,1,1,1,1,1,1,1,1,1,1,1,1,1,1,1,1,1,1,1,1,1,1,1,1,1,1,1,1,1,1,1,1,1,1,1,
1,1,1,1,1,1,1,1,1,1,1,1,1,1,1,1,1,1,1,1,1,1,1,1,1,1,1,1,1,1,4),(-0.000348309906186967,
0.0451835872598144),(11.8612316943504,12.8591278626027,13.8566757209488,
14.8542235792949,15.851771437641,16.8493192959871,17.8468671543332,18.8444150126793,
19.8419628710253,20.8395107293714,21.8370585877175,22.8346064460636,23.8321543044097,
24.8297021627558,25.8272500211019,26.8247978794479,27.822345737794,28.8198935961401,
29.8174414544862,30.8149893128323,31.8125371711784,32.8100850295245,33.8076328878706,
34.8051807462166,35.8027286045627,36.8002764629088,37.7978243212549,38.795372179601,
39.7929200379471,40.7904678962932,41.7880157546392,42.7855636129853,43.7831114713314,
44.7806593296775,45.7782071880236,46.7757550463697,47.7733029047158,48.7708507630619,
49.7683986214079,50.765946479754,51.7634943381001,52.7610421964462,53.7585900547923,
54.7561379131384,55.7536857714845,56.7512336298306,57.7487814881766,58.7463293465227,
59.7438772048688,60.7414250632149,61.738972921561,62.7365207799071,63.7340686382532,
64.7316164965992,65.7291643549453,66.7267122132914,67.7242600716375,68.7218079299836,
69.7193557883297,70.7169036466758,71.7144515050219,72.7119993633679,73.709547221714,
74.7070950800601,75.7046429384062,76.7021907967523,77.6997386550984,78.6972865134445,
79.6948343717906,80.6923822301366,81.6899300884827,82.6874779468288,83.6850258051749,
84.682573663521,85.6801215218671,86.6776693802132,87.6752172385592,88.6727650969053,
89.6703129552514,90.6678608135975,91.6654086719436,92.6629565302897,93.6605043886358,
94.6580522469818,95.6556001053279,96.653147963674,97.6506958220201,98.6482436803662,
99.6457915387123,100.643339397058,101.640887255404,102.638435113751,103.635982972097),
 .UNSPECIFIED.);
#288=B_SPLINE_SURFACE_WITH_KNOTS('',3,3,((#133673,#133674,#133675,#133676,
#133677,#133678,#133679,#133680,#133681,#133682,#133683,#133684,#133685,
#133686,#133687,#133688,#133689,#133690,#133691,#133692,#133693,#133694,
#133695,#133696,#133697,#133698,#133699,#133700,#133701,#133702,#133703,
#133704,#133705,#133706,#133707,#133708,#133709,#133710,#133711,#133712,
#133713,#133714,#133715,#133716,#133717,#133718,#133719,#133720,#133721,
#133722,#133723,#133724,#133725,#133726,#133727,#133728,#133729,#133730,
#133731,#133732,#133733,#133734,#133735,#133736,#133737,#133738,#133739,
#133740,#133741,#133742,#133743,#133744,#133745,#133746,#133747,#133748,
#133749,#133750,#133751,#133752,#133753,#133754,#133755,#133756,#133757,
#133758,#133759,#133760,#133761,#133762,#133763,#133764,#133765,#133766,
#133767),(#133768,#133769,#133770,#133771,#133772,#133773,#133774,#133775,
#133776,#133777,#133778,#133779,#133780,#133781,#133782,#133783,#133784,
#133785,#133786,#133787,#133788,#133789,#133790,#133791,#133792,#133793,
#133794,#133795,#133796,#133797,#133798,#133799,#133800,#133801,#133802,
#133803,#133804,#133805,#133806,#133807,#133808,#133809,#133810,#133811,
#133812,#133813,#133814,#133815,#133816,#133817,#133818,#133819,#133820,
#133821,#133822,#133823,#133824,#133825,#133826,#133827,#133828,#133829,
#133830,#133831,#133832,#133833,#133834,#133835,#133836,#133837,#133838,
#133839,#133840,#133841,#133842,#133843,#133844,#133845,#133846,#133847,
#133848,#133849,#133850,#133851,#133852,#133853,#133854,#133855,#133856,
#133857,#133858,#133859,#133860,#133861,#133862),(#133863,#133864,#133865,
#133866,#133867,#133868,#133869,#133870,#133871,#133872,#133873,#133874,
#133875,#133876,#133877,#133878,#133879,#133880,#133881,#133882,#133883,
#133884,#133885,#133886,#133887,#133888,#133889,#133890,#133891,#133892,
#133893,#133894,#133895,#133896,#133897,#133898,#133899,#133900,#133901,
#133902,#133903,#133904,#133905,#133906,#133907,#133908,#133909,#133910,
#133911,#133912,#133913,#133914,#133915,#133916,#133917,#133918,#133919,
#133920,#133921,#133922,#133923,#133924,#133925,#133926,#133927,#133928,
#133929,#133930,#133931,#133932,#133933,#133934,#133935,#133936,#133937,
#133938,#133939,#133940,#133941,#133942,#133943,#133944,#133945,#133946,
#133947,#133948,#133949,#133950,#133951,#133952,#133953,#133954,#133955,
#133956,#133957),(#133958,#133959,#133960,#133961,#133962,#133963,#133964,
#133965,#133966,#133967,#133968,#133969,#133970,#133971,#133972,#133973,
#133974,#133975,#133976,#133977,#133978,#133979,#133980,#133981,#133982,
#133983,#133984,#133985,#133986,#133987,#133988,#133989,#133990,#133991,
#133992,#133993,#133994,#133995,#133996,#133997,#133998,#133999,#134000,
#134001,#134002,#134003,#134004,#134005,#134006,#134007,#134008,#134009,
#134010,#134011,#134012,#134013,#134014,#134015,#134016,#134017,#134018,
#134019,#134020,#134021,#134022,#134023,#134024,#134025,#134026,#134027,
#134028,#134029,#134030,#134031,#134032,#134033,#134034,#134035,#134036,
#134037,#134038,#134039,#134040,#134041,#134042,#134043,#134044,#134045,
#134046,#134047,#134048,#134049,#134050,#134051,#134052)),.UNSPECIFIED.,
 .F.,.F.,.F.,(4,4),(4,1,1,1,1,1,1,1,1,1,1,1,1,1,1,1,1,1,1,1,1,1,1,1,1,1,
1,1,1,1,1,1,1,1,1,1,1,1,1,1,1,1,1,1,1,1,1,1,1,1,1,1,1,1,1,1,1,1,1,1,1,1,
1,1,1,1,1,1,1,1,1,1,1,1,1,1,1,1,1,1,1,1,1,1,1,1,1,1,1,1,1,1,4),(-0.000309363066806194,
0.0452373281646787),(14.3981410127769,15.395688871123,16.3932367294691,
17.3907845878152,18.3883324461612,19.3858803045073,20.3834281628534,21.3809760211995,
22.3785238795456,23.3760717378917,24.3736195962378,25.3711674545838,26.3687153129299,
27.366263171276,28.3638110296221,29.3613588879682,30.3589067463143,31.3564546046604,
32.3540024630065,33.3515503213525,34.3490981796986,35.3466460380447,36.3441938963908,
37.3417417547369,38.339289613083,39.3368374714291,40.3343853297751,41.3319331881212,
42.3294810464673,43.3270289048134,44.3245767631595,45.3221246215056,46.3196724798517,
47.3172203381977,48.3147681965438,49.3123160548899,50.309863913236,51.3074117715821,
52.3049596299282,53.3025074882743,54.3000553466204,55.2976032049664,56.2951510633125,
57.2926989216586,58.2902467800047,59.2877946383508,60.2853424966969,61.282890355043,
62.2804382133891,63.2779860717351,64.2755339300812,65.2730817884273,66.2706296467734,
67.2681775051195,68.2657253634656,69.2632732218117,70.2608210801577,71.2583689385038,
72.2559167968499,73.253464655196,74.2510125135421,75.2485603718882,76.2461082302343,
77.2436560885804,78.2412039469264,79.2387518052725,80.2362996636186,81.2338475219647,
82.2313953803108,83.2289432386569,84.226491097003,85.224038955349,86.2215868136951,
87.2191346720412,88.2166825303873,89.2142303887334,90.2117782470795,91.2093261054256,
92.2068739637717,93.2044218221177,94.2019696804638,95.1995175388099,96.197065397156,
97.1946132555021,98.1921611138482,99.1897089721943,100.18725683054,101.184804688886,
102.182352547233,103.179900405579,104.177448263925,105.174996122271,106.172892325352),
 .UNSPECIFIED.);
#289=B_SPLINE_SURFACE_WITH_KNOTS('',3,3,((#134231,#134232,#134233,#134234,
#134235,#134236,#134237,#134238,#134239,#134240,#134241,#134242,#134243,
#134244,#134245,#134246,#134247,#134248,#134249,#134250,#134251,#134252,
#134253,#134254,#134255,#134256,#134257,#134258,#134259,#134260,#134261,
#134262,#134263,#134264,#134265,#134266,#134267,#134268,#134269,#134270,
#134271,#134272,#134273,#134274,#134275,#134276,#134277,#134278,#134279,
#134280,#134281,#134282,#134283,#134284,#134285,#134286,#134287,#134288,
#134289,#134290,#134291,#134292,#134293,#134294,#134295,#134296,#134297,
#134298,#134299,#134300,#134301,#134302,#134303,#134304,#134305,#134306,
#134307,#134308,#134309,#134310,#134311,#134312,#134313,#134314,#134315,
#134316,#134317,#134318,#134319,#134320,#134321,#134322,#134323,#134324,
#134325),(#134326,#134327,#134328,#134329,#134330,#134331,#134332,#134333,
#134334,#134335,#134336,#134337,#134338,#134339,#134340,#134341,#134342,
#134343,#134344,#134345,#134346,#134347,#134348,#134349,#134350,#134351,
#134352,#134353,#134354,#134355,#134356,#134357,#134358,#134359,#134360,
#134361,#134362,#134363,#134364,#134365,#134366,#134367,#134368,#134369,
#134370,#134371,#134372,#134373,#134374,#134375,#134376,#134377,#134378,
#134379,#134380,#134381,#134382,#134383,#134384,#134385,#134386,#134387,
#134388,#134389,#134390,#134391,#134392,#134393,#134394,#134395,#134396,
#134397,#134398,#134399,#134400,#134401,#134402,#134403,#134404,#134405,
#134406,#134407,#134408,#134409,#134410,#134411,#134412,#134413,#134414,
#134415,#134416,#134417,#134418,#134419,#134420),(#134421,#134422,#134423,
#134424,#134425,#134426,#134427,#134428,#134429,#134430,#134431,#134432,
#134433,#134434,#134435,#134436,#134437,#134438,#134439,#134440,#134441,
#134442,#134443,#134444,#134445,#134446,#134447,#134448,#134449,#134450,
#134451,#134452,#134453,#134454,#134455,#134456,#134457,#134458,#134459,
#134460,#134461,#134462,#134463,#134464,#134465,#134466,#134467,#134468,
#134469,#134470,#134471,#134472,#134473,#134474,#134475,#134476,#134477,
#134478,#134479,#134480,#134481,#134482,#134483,#134484,#134485,#134486,
#134487,#134488,#134489,#134490,#134491,#134492,#134493,#134494,#134495,
#134496,#134497,#134498,#134499,#134500,#134501,#134502,#134503,#134504,
#134505,#134506,#134507,#134508,#134509,#134510,#134511,#134512,#134513,
#134514,#134515),(#134516,#134517,#134518,#134519,#134520,#134521,#134522,
#134523,#134524,#134525,#134526,#134527,#134528,#134529,#134530,#134531,
#134532,#134533,#134534,#134535,#134536,#134537,#134538,#134539,#134540,
#134541,#134542,#134543,#134544,#134545,#134546,#134547,#134548,#134549,
#134550,#134551,#134552,#134553,#134554,#134555,#134556,#134557,#134558,
#134559,#134560,#134561,#134562,#134563,#134564,#134565,#134566,#134567,
#134568,#134569,#134570,#134571,#134572,#134573,#134574,#134575,#134576,
#134577,#134578,#134579,#134580,#134581,#134582,#134583,#134584,#134585,
#134586,#134587,#134588,#134589,#134590,#134591,#134592,#134593,#134594,
#134595,#134596,#134597,#134598,#134599,#134600,#134601,#134602,#134603,
#134604,#134605,#134606,#134607,#134608,#134609,#134610)),.UNSPECIFIED.,
 .F.,.F.,.F.,(4,4),(4,1,1,1,1,1,1,1,1,1,1,1,1,1,1,1,1,1,1,1,1,1,1,1,1,1,
1,1,1,1,1,1,1,1,1,1,1,1,1,1,1,1,1,1,1,1,1,1,1,1,1,1,1,1,1,1,1,1,1,1,1,1,
1,1,1,1,1,1,1,1,1,1,1,1,1,1,1,1,1,1,1,1,1,1,1,1,1,1,1,1,1,1,4),(-0.000351924294538534,
0.0451855438310995),(11.8612280799621,12.8591278626027,13.8566757209488,
14.8542235792949,15.851771437641,16.8493192959871,17.8468671543332,18.8444150126793,
19.8419628710253,20.8395107293714,21.8370585877175,22.8346064460636,23.8321543044097,
24.8297021627558,25.8272500211019,26.8247978794479,27.822345737794,28.8198935961401,
29.8174414544862,30.8149893128323,31.8125371711784,32.8100850295245,33.8076328878706,
34.8051807462166,35.8027286045627,36.8002764629088,37.7978243212549,38.795372179601,
39.7929200379471,40.7904678962932,41.7880157546392,42.7855636129853,43.7831114713314,
44.7806593296775,45.7782071880236,46.7757550463697,47.7733029047158,48.7708507630618,
49.7683986214079,50.765946479754,51.7634943381001,52.7610421964462,53.7585900547923,
54.7561379131384,55.7536857714845,56.7512336298305,57.7487814881766,58.7463293465227,
59.7438772048688,60.7414250632149,61.738972921561,62.7365207799071,63.7340686382531,
64.7316164965992,65.7291643549453,66.7267122132914,67.7242600716375,68.7218079299836,
69.7193557883297,70.7169036466757,71.7144515050218,72.7119993633679,73.709547221714,
74.7070950800601,75.7046429384062,76.7021907967523,77.6997386550984,78.6972865134445,
79.6948343717905,80.6923822301366,81.6899300884827,82.6874779468288,83.6850258051749,
84.682573663521,85.6801215218671,86.6776693802131,87.6752172385592,88.6727650969053,
89.6703129552514,90.6678608135975,91.6654086719436,92.6629565302897,93.6605043886357,
94.6580522469818,95.6556001053279,96.653147963674,97.6506958220201,98.6482436803662,
99.6457915387123,100.643339397058,101.640887255404,102.638435113751,103.635982972097),
 .UNSPECIFIED.);
#290=B_SPLINE_SURFACE_WITH_KNOTS('',3,3,((#134783,#134784,#134785,#134786,
#134787,#134788,#134789,#134790,#134791,#134792,#134793,#134794,#134795,
#134796,#134797,#134798,#134799,#134800,#134801,#134802,#134803,#134804,
#134805,#134806,#134807,#134808,#134809,#134810,#134811,#134812,#134813,
#134814,#134815,#134816,#134817,#134818,#134819,#134820,#134821,#134822,
#134823,#134824,#134825,#134826,#134827,#134828,#134829,#134830,#134831,
#134832,#134833,#134834,#134835,#134836,#134837,#134838,#134839,#134840,
#134841,#134842,#134843,#134844,#134845,#134846,#134847,#134848,#134849,
#134850,#134851,#134852,#134853,#134854,#134855,#134856,#134857,#134858,
#134859,#134860,#134861,#134862,#134863,#134864,#134865,#134866,#134867,
#134868,#134869,#134870,#134871,#134872,#134873,#134874,#134875,#134876,
#134877),(#134878,#134879,#134880,#134881,#134882,#134883,#134884,#134885,
#134886,#134887,#134888,#134889,#134890,#134891,#134892,#134893,#134894,
#134895,#134896,#134897,#134898,#134899,#134900,#134901,#134902,#134903,
#134904,#134905,#134906,#134907,#134908,#134909,#134910,#134911,#134912,
#134913,#134914,#134915,#134916,#134917,#134918,#134919,#134920,#134921,
#134922,#134923,#134924,#134925,#134926,#134927,#134928,#134929,#134930,
#134931,#134932,#134933,#134934,#134935,#134936,#134937,#134938,#134939,
#134940,#134941,#134942,#134943,#134944,#134945,#134946,#134947,#134948,
#134949,#134950,#134951,#134952,#134953,#134954,#134955,#134956,#134957,
#134958,#134959,#134960,#134961,#134962,#134963,#134964,#134965,#134966,
#134967,#134968,#134969,#134970,#134971,#134972),(#134973,#134974,#134975,
#134976,#134977,#134978,#134979,#134980,#134981,#134982,#134983,#134984,
#134985,#134986,#134987,#134988,#134989,#134990,#134991,#134992,#134993,
#134994,#134995,#134996,#134997,#134998,#134999,#135000,#135001,#135002,
#135003,#135004,#135005,#135006,#135007,#135008,#135009,#135010,#135011,
#135012,#135013,#135014,#135015,#135016,#135017,#135018,#135019,#135020,
#135021,#135022,#135023,#135024,#135025,#135026,#135027,#135028,#135029,
#135030,#135031,#135032,#135033,#135034,#135035,#135036,#135037,#135038,
#135039,#135040,#135041,#135042,#135043,#135044,#135045,#135046,#135047,
#135048,#135049,#135050,#135051,#135052,#135053,#135054,#135055,#135056,
#135057,#135058,#135059,#135060,#135061,#135062,#135063,#135064,#135065,
#135066,#135067),(#135068,#135069,#135070,#135071,#135072,#135073,#135074,
#135075,#135076,#135077,#135078,#135079,#135080,#135081,#135082,#135083,
#135084,#135085,#135086,#135087,#135088,#135089,#135090,#135091,#135092,
#135093,#135094,#135095,#135096,#135097,#135098,#135099,#135100,#135101,
#135102,#135103,#135104,#135105,#135106,#135107,#135108,#135109,#135110,
#135111,#135112,#135113,#135114,#135115,#135116,#135117,#135118,#135119,
#135120,#135121,#135122,#135123,#135124,#135125,#135126,#135127,#135128,
#135129,#135130,#135131,#135132,#135133,#135134,#135135,#135136,#135137,
#135138,#135139,#135140,#135141,#135142,#135143,#135144,#135145,#135146,
#135147,#135148,#135149,#135150,#135151,#135152,#135153,#135154,#135155,
#135156,#135157,#135158,#135159,#135160,#135161,#135162)),.UNSPECIFIED.,
 .F.,.F.,.F.,(4,4),(4,1,1,1,1,1,1,1,1,1,1,1,1,1,1,1,1,1,1,1,1,1,1,1,1,1,
1,1,1,1,1,1,1,1,1,1,1,1,1,1,1,1,1,1,1,1,1,1,1,1,1,1,1,1,1,1,1,1,1,1,1,1,
1,1,1,1,1,1,1,1,1,1,1,1,1,1,1,1,1,1,1,1,1,1,1,1,1,1,1,1,1,1,4),(-0.000310865142038579,
0.0452409353936679),(14.3981410127769,15.395688871123,16.3932367294691,
17.3907845878152,18.3883324461612,19.3858803045073,20.3834281628534,21.3809760211995,
22.3785238795456,23.3760717378917,24.3736195962378,25.3711674545838,26.3687153129299,
27.366263171276,28.3638110296221,29.3613588879682,30.3589067463143,31.3564546046604,
32.3540024630065,33.3515503213525,34.3490981796986,35.3466460380447,36.3441938963908,
37.3417417547369,38.339289613083,39.3368374714291,40.3343853297751,41.3319331881212,
42.3294810464673,43.3270289048134,44.3245767631595,45.3221246215056,46.3196724798517,
47.3172203381978,48.3147681965438,49.3123160548899,50.309863913236,51.3074117715821,
52.3049596299282,53.3025074882743,54.3000553466204,55.2976032049664,56.2951510633125,
57.2926989216586,58.2902467800047,59.2877946383508,60.2853424966969,61.282890355043,
62.2804382133891,63.2779860717351,64.2755339300812,65.2730817884273,66.2706296467734,
67.2681775051195,68.2657253634656,69.2632732218117,70.2608210801578,71.2583689385038,
72.2559167968499,73.253464655196,74.2510125135421,75.2485603718882,76.2461082302343,
77.2436560885804,78.2412039469264,79.2387518052725,80.2362996636186,81.2338475219647,
82.2313953803108,83.2289432386569,84.226491097003,85.2240389553491,86.2215868136951,
87.2191346720412,88.2166825303873,89.2142303887334,90.2117782470795,91.2093261054256,
92.2068739637717,93.2044218221178,94.2019696804638,95.1995175388099,96.197065397156,
97.1946132555021,98.1921611138482,99.1897089721943,100.18725683054,101.184804688886,
102.182352547233,103.179900405579,104.177448263925,105.174996122271,106.172895932581),
 .UNSPECIFIED.);
#291=B_SPLINE_SURFACE_WITH_KNOTS('',3,3,((#135341,#135342,#135343,#135344,
#135345,#135346,#135347,#135348,#135349,#135350,#135351,#135352,#135353,
#135354,#135355,#135356,#135357,#135358,#135359,#135360,#135361,#135362,
#135363,#135364,#135365,#135366,#135367,#135368,#135369,#135370,#135371,
#135372,#135373,#135374,#135375,#135376,#135377,#135378,#135379,#135380,
#135381,#135382,#135383,#135384,#135385,#135386,#135387,#135388,#135389,
#135390,#135391,#135392,#135393,#135394,#135395,#135396,#135397,#135398,
#135399,#135400,#135401,#135402,#135403,#135404,#135405,#135406,#135407,
#135408,#135409,#135410,#135411,#135412,#135413,#135414,#135415,#135416,
#135417,#135418,#135419,#135420,#135421,#135422,#135423,#135424,#135425,
#135426,#135427,#135428,#135429,#135430,#135431,#135432,#135433,#135434,
#135435),(#135436,#135437,#135438,#135439,#135440,#135441,#135442,#135443,
#135444,#135445,#135446,#135447,#135448,#135449,#135450,#135451,#135452,
#135453,#135454,#135455,#135456,#135457,#135458,#135459,#135460,#135461,
#135462,#135463,#135464,#135465,#135466,#135467,#135468,#135469,#135470,
#135471,#135472,#135473,#135474,#135475,#135476,#135477,#135478,#135479,
#135480,#135481,#135482,#135483,#135484,#135485,#135486,#135487,#135488,
#135489,#135490,#135491,#135492,#135493,#135494,#135495,#135496,#135497,
#135498,#135499,#135500,#135501,#135502,#135503,#135504,#135505,#135506,
#135507,#135508,#135509,#135510,#135511,#135512,#135513,#135514,#135515,
#135516,#135517,#135518,#135519,#135520,#135521,#135522,#135523,#135524,
#135525,#135526,#135527,#135528,#135529,#135530),(#135531,#135532,#135533,
#135534,#135535,#135536,#135537,#135538,#135539,#135540,#135541,#135542,
#135543,#135544,#135545,#135546,#135547,#135548,#135549,#135550,#135551,
#135552,#135553,#135554,#135555,#135556,#135557,#135558,#135559,#135560,
#135561,#135562,#135563,#135564,#135565,#135566,#135567,#135568,#135569,
#135570,#135571,#135572,#135573,#135574,#135575,#135576,#135577,#135578,
#135579,#135580,#135581,#135582,#135583,#135584,#135585,#135586,#135587,
#135588,#135589,#135590,#135591,#135592,#135593,#135594,#135595,#135596,
#135597,#135598,#135599,#135600,#135601,#135602,#135603,#135604,#135605,
#135606,#135607,#135608,#135609,#135610,#135611,#135612,#135613,#135614,
#135615,#135616,#135617,#135618,#135619,#135620,#135621,#135622,#135623,
#135624,#135625),(#135626,#135627,#135628,#135629,#135630,#135631,#135632,
#135633,#135634,#135635,#135636,#135637,#135638,#135639,#135640,#135641,
#135642,#135643,#135644,#135645,#135646,#135647,#135648,#135649,#135650,
#135651,#135652,#135653,#135654,#135655,#135656,#135657,#135658,#135659,
#135660,#135661,#135662,#135663,#135664,#135665,#135666,#135667,#135668,
#135669,#135670,#135671,#135672,#135673,#135674,#135675,#135676,#135677,
#135678,#135679,#135680,#135681,#135682,#135683,#135684,#135685,#135686,
#135687,#135688,#135689,#135690,#135691,#135692,#135693,#135694,#135695,
#135696,#135697,#135698,#135699,#135700,#135701,#135702,#135703,#135704,
#135705,#135706,#135707,#135708,#135709,#135710,#135711,#135712,#135713,
#135714,#135715,#135716,#135717,#135718,#135719,#135720)),.UNSPECIFIED.,
 .F.,.F.,.F.,(4,4),(4,1,1,1,1,1,1,1,1,1,1,1,1,1,1,1,1,1,1,1,1,1,1,1,1,1,
1,1,1,1,1,1,1,1,1,1,1,1,1,1,1,1,1,1,1,1,1,1,1,1,1,1,1,1,1,1,1,1,1,1,1,1,
1,1,1,1,1,1,1,1,1,1,1,1,1,1,1,1,1,1,1,1,1,1,1,1,1,1,1,1,1,1,4),(-0.000351931351939438,
0.0451855479770649),(11.8612280729047,12.8591278626027,13.8566757209488,
14.8542235792949,15.851771437641,16.8493192959871,17.8468671543332,18.8444150126792,
19.8419628710253,20.8395107293714,21.8370585877175,22.8346064460636,23.8321543044097,
24.8297021627558,25.8272500211019,26.8247978794479,27.822345737794,28.8198935961401,
29.8174414544862,30.8149893128323,31.8125371711784,32.8100850295245,33.8076328878705,
34.8051807462166,35.8027286045627,36.8002764629088,37.7978243212549,38.795372179601,
39.7929200379471,40.7904678962932,41.7880157546392,42.7855636129853,43.7831114713314,
44.7806593296775,45.7782071880236,46.7757550463697,47.7733029047158,48.7708507630618,
49.7683986214079,50.765946479754,51.7634943381001,52.7610421964462,53.7585900547923,
54.7561379131384,55.7536857714844,56.7512336298305,57.7487814881766,58.7463293465227,
59.7438772048688,60.7414250632149,61.738972921561,62.7365207799071,63.7340686382531,
64.7316164965992,65.7291643549453,66.7267122132914,67.7242600716375,68.7218079299836,
69.7193557883297,70.7169036466757,71.7144515050218,72.7119993633679,73.709547221714,
74.7070950800601,75.7046429384062,76.7021907967523,77.6997386550983,78.6972865134445,
79.6948343717905,80.6923822301366,81.6899300884827,82.6874779468288,83.6850258051749,
84.682573663521,85.6801215218671,86.6776693802131,87.6752172385592,88.6727650969053,
89.6703129552514,90.6678608135975,91.6654086719436,92.6629565302896,93.6605043886357,
94.6580522469818,95.6556001053279,96.653147963674,97.6506958220201,98.6482436803662,
99.6457915387122,100.643339397058,101.640887255404,102.638435113751,103.635982972097),
 .UNSPECIFIED.);
#292=B_SPLINE_SURFACE_WITH_KNOTS('',3,3,((#135893,#135894,#135895,#135896,
#135897,#135898,#135899,#135900,#135901,#135902,#135903,#135904,#135905,
#135906,#135907,#135908,#135909,#135910,#135911,#135912,#135913,#135914,
#135915,#135916,#135917,#135918,#135919,#135920,#135921,#135922,#135923,
#135924,#135925,#135926,#135927,#135928,#135929,#135930,#135931,#135932,
#135933,#135934,#135935,#135936,#135937,#135938,#135939,#135940,#135941,
#135942,#135943,#135944,#135945,#135946,#135947,#135948,#135949,#135950,
#135951,#135952,#135953,#135954,#135955,#135956,#135957,#135958,#135959,
#135960,#135961,#135962,#135963,#135964,#135965,#135966,#135967,#135968,
#135969,#135970,#135971,#135972,#135973,#135974,#135975,#135976,#135977,
#135978,#135979,#135980,#135981,#135982,#135983,#135984,#135985,#135986,
#135987),(#135988,#135989,#135990,#135991,#135992,#135993,#135994,#135995,
#135996,#135997,#135998,#135999,#136000,#136001,#136002,#136003,#136004,
#136005,#136006,#136007,#136008,#136009,#136010,#136011,#136012,#136013,
#136014,#136015,#136016,#136017,#136018,#136019,#136020,#136021,#136022,
#136023,#136024,#136025,#136026,#136027,#136028,#136029,#136030,#136031,
#136032,#136033,#136034,#136035,#136036,#136037,#136038,#136039,#136040,
#136041,#136042,#136043,#136044,#136045,#136046,#136047,#136048,#136049,
#136050,#136051,#136052,#136053,#136054,#136055,#136056,#136057,#136058,
#136059,#136060,#136061,#136062,#136063,#136064,#136065,#136066,#136067,
#136068,#136069,#136070,#136071,#136072,#136073,#136074,#136075,#136076,
#136077,#136078,#136079,#136080,#136081,#136082),(#136083,#136084,#136085,
#136086,#136087,#136088,#136089,#136090,#136091,#136092,#136093,#136094,
#136095,#136096,#136097,#136098,#136099,#136100,#136101,#136102,#136103,
#136104,#136105,#136106,#136107,#136108,#136109,#136110,#136111,#136112,
#136113,#136114,#136115,#136116,#136117,#136118,#136119,#136120,#136121,
#136122,#136123,#136124,#136125,#136126,#136127,#136128,#136129,#136130,
#136131,#136132,#136133,#136134,#136135,#136136,#136137,#136138,#136139,
#136140,#136141,#136142,#136143,#136144,#136145,#136146,#136147,#136148,
#136149,#136150,#136151,#136152,#136153,#136154,#136155,#136156,#136157,
#136158,#136159,#136160,#136161,#136162,#136163,#136164,#136165,#136166,
#136167,#136168,#136169,#136170,#136171,#136172,#136173,#136174,#136175,
#136176,#136177),(#136178,#136179,#136180,#136181,#136182,#136183,#136184,
#136185,#136186,#136187,#136188,#136189,#136190,#136191,#136192,#136193,
#136194,#136195,#136196,#136197,#136198,#136199,#136200,#136201,#136202,
#136203,#136204,#136205,#136206,#136207,#136208,#136209,#136210,#136211,
#136212,#136213,#136214,#136215,#136216,#136217,#136218,#136219,#136220,
#136221,#136222,#136223,#136224,#136225,#136226,#136227,#136228,#136229,
#136230,#136231,#136232,#136233,#136234,#136235,#136236,#136237,#136238,
#136239,#136240,#136241,#136242,#136243,#136244,#136245,#136246,#136247,
#136248,#136249,#136250,#136251,#136252,#136253,#136254,#136255,#136256,
#136257,#136258,#136259,#136260,#136261,#136262,#136263,#136264,#136265,
#136266,#136267,#136268,#136269,#136270,#136271,#136272)),.UNSPECIFIED.,
 .F.,.F.,.F.,(4,4),(4,1,1,1,1,1,1,1,1,1,1,1,1,1,1,1,1,1,1,1,1,1,1,1,1,1,
1,1,1,1,1,1,1,1,1,1,1,1,1,1,1,1,1,1,1,1,1,1,1,1,1,1,1,1,1,1,1,1,1,1,1,1,
1,1,1,1,1,1,1,1,1,1,1,1,1,1,1,1,1,1,1,1,1,1,1,1,1,1,1,1,1,1,4),(-0.000310869945906298,
0.0452409448509825),(14.3981410127769,15.395688871123,16.3932367294691,
17.3907845878152,18.3883324461612,19.3858803045073,20.3834281628534,21.3809760211995,
22.3785238795456,23.3760717378917,24.3736195962378,25.3711674545838,26.3687153129299,
27.366263171276,28.3638110296221,29.3613588879682,30.3589067463143,31.3564546046604,
32.3540024630065,33.3515503213525,34.3490981796986,35.3466460380447,36.3441938963908,
37.3417417547369,38.339289613083,39.3368374714291,40.3343853297751,41.3319331881212,
42.3294810464673,43.3270289048134,44.3245767631595,45.3221246215056,46.3196724798517,
47.3172203381978,48.3147681965438,49.3123160548899,50.309863913236,51.3074117715821,
52.3049596299282,53.3025074882743,54.3000553466204,55.2976032049664,56.2951510633125,
57.2926989216586,58.2902467800047,59.2877946383508,60.2853424966969,61.282890355043,
62.2804382133891,63.2779860717351,64.2755339300812,65.2730817884273,66.2706296467734,
67.2681775051195,68.2657253634656,69.2632732218117,70.2608210801578,71.2583689385038,
72.2559167968499,73.253464655196,74.2510125135421,75.2485603718882,76.2461082302343,
77.2436560885804,78.2412039469264,79.2387518052725,80.2362996636186,81.2338475219647,
82.2313953803108,83.2289432386569,84.226491097003,85.2240389553491,86.2215868136951,
87.2191346720412,88.2166825303873,89.2142303887334,90.2117782470795,91.2093261054256,
92.2068739637717,93.2044218221178,94.2019696804638,95.1995175388099,96.197065397156,
97.1946132555021,98.1921611138482,99.1897089721943,100.18725683054,101.184804688886,
102.182352547233,103.179900405579,104.177448263925,105.174996122271,106.172895942038),
 .UNSPECIFIED.);
#317=PLANE('',#17399);
#318=PLANE('',#17400);
#319=PLANE('',#17401);
#320=PLANE('',#17402);
#321=PLANE('',#17403);
#322=PLANE('',#17404);
#323=PLANE('',#17406);
#324=PLANE('',#17407);
#325=PLANE('',#17421);
#326=PLANE('',#17422);
#327=PLANE('',#17423);
#328=PLANE('',#17424);
#329=PLANE('',#17428);
#330=PLANE('',#17429);
#331=PLANE('',#17430);
#332=PLANE('',#17431);
#333=PLANE('',#17432);
#334=PLANE('',#17433);
#335=PLANE('',#17434);
#336=PLANE('',#17435);
#337=PLANE('',#17436);
#338=PLANE('',#17437);
#339=PLANE('',#17438);
#537=FACE_OUTER_BOUND('',#1199,.T.);
#538=FACE_OUTER_BOUND('',#1200,.T.);
#539=FACE_OUTER_BOUND('',#1201,.T.);
#540=FACE_OUTER_BOUND('',#1202,.T.);
#541=FACE_OUTER_BOUND('',#1203,.T.);
#542=FACE_OUTER_BOUND('',#1204,.T.);
#543=FACE_OUTER_BOUND('',#1205,.T.);
#544=FACE_OUTER_BOUND('',#1206,.T.);
#545=FACE_OUTER_BOUND('',#1207,.T.);
#546=FACE_OUTER_BOUND('',#1208,.T.);
#547=FACE_OUTER_BOUND('',#1209,.T.);
#548=FACE_OUTER_BOUND('',#1210,.T.);
#549=FACE_OUTER_BOUND('',#1211,.T.);
#550=FACE_OUTER_BOUND('',#1212,.T.);
#551=FACE_OUTER_BOUND('',#1213,.T.);
#552=FACE_OUTER_BOUND('',#1214,.T.);
#553=FACE_OUTER_BOUND('',#1215,.T.);
#554=FACE_OUTER_BOUND('',#1216,.T.);
#555=FACE_OUTER_BOUND('',#1217,.T.);
#556=FACE_OUTER_BOUND('',#1218,.T.);
#557=FACE_OUTER_BOUND('',#1219,.T.);
#558=FACE_OUTER_BOUND('',#1220,.T.);
#559=FACE_OUTER_BOUND('',#1221,.T.);
#560=FACE_OUTER_BOUND('',#1222,.T.);
#561=FACE_OUTER_BOUND('',#1223,.T.);
#562=FACE_OUTER_BOUND('',#1224,.T.);
#563=FACE_OUTER_BOUND('',#1225,.T.);
#564=FACE_OUTER_BOUND('',#1226,.T.);
#565=FACE_OUTER_BOUND('',#1227,.T.);
#566=FACE_OUTER_BOUND('',#1228,.T.);
#567=FACE_OUTER_BOUND('',#1229,.T.);
#568=FACE_OUTER_BOUND('',#1230,.T.);
#569=FACE_OUTER_BOUND('',#1231,.T.);
#570=FACE_OUTER_BOUND('',#1232,.T.);
#571=FACE_OUTER_BOUND('',#1233,.T.);
#572=FACE_OUTER_BOUND('',#1234,.T.);
#573=FACE_OUTER_BOUND('',#1235,.T.);
#574=FACE_OUTER_BOUND('',#1236,.T.);
#575=FACE_OUTER_BOUND('',#1237,.T.);
#576=FACE_OUTER_BOUND('',#1238,.T.);
#577=FACE_OUTER_BOUND('',#1239,.T.);
#578=FACE_OUTER_BOUND('',#1240,.T.);
#579=FACE_OUTER_BOUND('',#1241,.T.);
#580=FACE_OUTER_BOUND('',#1242,.T.);
#581=FACE_OUTER_BOUND('',#1243,.T.);
#582=FACE_OUTER_BOUND('',#1244,.T.);
#583=FACE_OUTER_BOUND('',#1245,.T.);
#584=FACE_OUTER_BOUND('',#1246,.T.);
#585=FACE_OUTER_BOUND('',#1247,.T.);
#586=FACE_OUTER_BOUND('',#1248,.T.);
#587=FACE_OUTER_BOUND('',#1249,.T.);
#588=FACE_OUTER_BOUND('',#1250,.T.);
#589=FACE_OUTER_BOUND('',#1251,.T.);
#590=FACE_OUTER_BOUND('',#1252,.T.);
#591=FACE_OUTER_BOUND('',#1253,.T.);
#592=FACE_OUTER_BOUND('',#1254,.T.);
#593=FACE_OUTER_BOUND('',#1255,.T.);
#594=FACE_OUTER_BOUND('',#1256,.T.);
#595=FACE_OUTER_BOUND('',#1257,.T.);
#596=FACE_OUTER_BOUND('',#1258,.T.);
#597=FACE_OUTER_BOUND('',#1259,.T.);
#598=FACE_OUTER_BOUND('',#1260,.T.);
#599=FACE_OUTER_BOUND('',#1261,.T.);
#600=FACE_OUTER_BOUND('',#1262,.T.);
#601=FACE_OUTER_BOUND('',#1263,.T.);
#602=FACE_OUTER_BOUND('',#1264,.T.);
#603=FACE_OUTER_BOUND('',#1265,.T.);
#604=FACE_OUTER_BOUND('',#1266,.T.);
#605=FACE_OUTER_BOUND('',#1267,.T.);
#606=FACE_OUTER_BOUND('',#1268,.T.);
#607=FACE_OUTER_BOUND('',#1269,.T.);
#608=FACE_OUTER_BOUND('',#1270,.T.);
#609=FACE_OUTER_BOUND('',#1271,.T.);
#610=FACE_OUTER_BOUND('',#1272,.T.);
#611=FACE_OUTER_BOUND('',#1273,.T.);
#612=FACE_OUTER_BOUND('',#1274,.T.);
#613=FACE_OUTER_BOUND('',#1275,.T.);
#614=FACE_OUTER_BOUND('',#1276,.T.);
#615=FACE_OUTER_BOUND('',#1277,.T.);
#616=FACE_OUTER_BOUND('',#1278,.T.);
#617=FACE_OUTER_BOUND('',#1279,.T.);
#618=FACE_OUTER_BOUND('',#1280,.T.);
#619=FACE_OUTER_BOUND('',#1281,.T.);
#620=FACE_OUTER_BOUND('',#1282,.T.);
#621=FACE_OUTER_BOUND('',#1283,.T.);
#622=FACE_OUTER_BOUND('',#1284,.T.);
#623=FACE_OUTER_BOUND('',#1285,.T.);
#624=FACE_OUTER_BOUND('',#1286,.T.);
#625=FACE_OUTER_BOUND('',#1287,.T.);
#626=FACE_OUTER_BOUND('',#1288,.T.);
#627=FACE_OUTER_BOUND('',#1289,.T.);
#628=FACE_OUTER_BOUND('',#1290,.T.);
#629=FACE_OUTER_BOUND('',#1291,.T.);
#630=FACE_OUTER_BOUND('',#1292,.T.);
#631=FACE_OUTER_BOUND('',#1293,.T.);
#632=FACE_OUTER_BOUND('',#1294,.T.);
#633=FACE_OUTER_BOUND('',#1295,.T.);
#634=FACE_OUTER_BOUND('',#1296,.T.);
#635=FACE_OUTER_BOUND('',#1297,.T.);
#636=FACE_OUTER_BOUND('',#1298,.T.);
#637=FACE_OUTER_BOUND('',#1299,.T.);
#638=FACE_OUTER_BOUND('',#1300,.T.);
#639=FACE_OUTER_BOUND('',#1301,.T.);
#640=FACE_OUTER_BOUND('',#1302,.T.);
#641=FACE_OUTER_BOUND('',#1303,.T.);
#642=FACE_OUTER_BOUND('',#1304,.T.);
#643=FACE_OUTER_BOUND('',#1305,.T.);
#644=FACE_OUTER_BOUND('',#1306,.T.);
#645=FACE_OUTER_BOUND('',#1307,.T.);
#646=FACE_OUTER_BOUND('',#1308,.T.);
#647=FACE_OUTER_BOUND('',#1309,.T.);
#648=FACE_OUTER_BOUND('',#1310,.T.);
#649=FACE_OUTER_BOUND('',#1311,.T.);
#650=FACE_OUTER_BOUND('',#1312,.T.);
#651=FACE_OUTER_BOUND('',#1313,.T.);
#652=FACE_OUTER_BOUND('',#1314,.T.);
#653=FACE_OUTER_BOUND('',#1315,.T.);
#654=FACE_OUTER_BOUND('',#1316,.T.);
#655=FACE_OUTER_BOUND('',#1317,.T.);
#656=FACE_OUTER_BOUND('',#1318,.T.);
#657=FACE_OUTER_BOUND('',#1319,.T.);
#658=FACE_OUTER_BOUND('',#1320,.T.);
#659=FACE_OUTER_BOUND('',#1321,.T.);
#660=FACE_OUTER_BOUND('',#1322,.T.);
#661=FACE_OUTER_BOUND('',#1323,.T.);
#662=FACE_OUTER_BOUND('',#1324,.T.);
#663=FACE_OUTER_BOUND('',#1325,.T.);
#664=FACE_OUTER_BOUND('',#1326,.T.);
#665=FACE_OUTER_BOUND('',#1327,.T.);
#666=FACE_OUTER_BOUND('',#1328,.T.);
#667=FACE_OUTER_BOUND('',#1329,.T.);
#668=FACE_OUTER_BOUND('',#1330,.T.);
#669=FACE_OUTER_BOUND('',#1331,.T.);
#670=FACE_OUTER_BOUND('',#1332,.T.);
#671=FACE_OUTER_BOUND('',#1333,.T.);
#672=FACE_OUTER_BOUND('',#1334,.T.);
#673=FACE_OUTER_BOUND('',#1335,.T.);
#674=FACE_OUTER_BOUND('',#1336,.T.);
#675=FACE_OUTER_BOUND('',#1337,.T.);
#676=FACE_OUTER_BOUND('',#1338,.T.);
#677=FACE_OUTER_BOUND('',#1339,.T.);
#678=FACE_OUTER_BOUND('',#1340,.T.);
#679=FACE_OUTER_BOUND('',#1341,.T.);
#680=FACE_OUTER_BOUND('',#1342,.T.);
#681=FACE_OUTER_BOUND('',#1343,.T.);
#682=FACE_OUTER_BOUND('',#1344,.T.);
#683=FACE_OUTER_BOUND('',#1345,.T.);
#684=FACE_OUTER_BOUND('',#1346,.T.);
#685=FACE_OUTER_BOUND('',#1347,.T.);
#686=FACE_OUTER_BOUND('',#1348,.T.);
#687=FACE_OUTER_BOUND('',#1349,.T.);
#688=FACE_OUTER_BOUND('',#1350,.T.);
#689=FACE_OUTER_BOUND('',#1351,.T.);
#690=FACE_OUTER_BOUND('',#1352,.T.);
#691=FACE_OUTER_BOUND('',#1353,.T.);
#692=FACE_OUTER_BOUND('',#1354,.T.);
#693=FACE_OUTER_BOUND('',#1355,.T.);
#694=FACE_OUTER_BOUND('',#1356,.T.);
#695=FACE_OUTER_BOUND('',#1357,.T.);
#696=FACE_OUTER_BOUND('',#1358,.T.);
#697=FACE_OUTER_BOUND('',#1359,.T.);
#698=FACE_OUTER_BOUND('',#1360,.T.);
#699=FACE_OUTER_BOUND('',#1361,.T.);
#700=FACE_OUTER_BOUND('',#1362,.T.);
#701=FACE_OUTER_BOUND('',#1363,.T.);
#702=FACE_OUTER_BOUND('',#1364,.T.);
#703=FACE_OUTER_BOUND('',#1365,.T.);
#704=FACE_OUTER_BOUND('',#1366,.T.);
#705=FACE_OUTER_BOUND('',#1367,.T.);
#706=FACE_OUTER_BOUND('',#1368,.T.);
#707=FACE_OUTER_BOUND('',#1369,.T.);
#708=FACE_OUTER_BOUND('',#1370,.T.);
#709=FACE_OUTER_BOUND('',#1371,.T.);
#710=FACE_OUTER_BOUND('',#1372,.T.);
#711=FACE_OUTER_BOUND('',#1373,.T.);
#712=FACE_OUTER_BOUND('',#1374,.T.);
#713=FACE_OUTER_BOUND('',#1375,.T.);
#714=FACE_OUTER_BOUND('',#1376,.T.);
#715=FACE_OUTER_BOUND('',#1377,.T.);
#716=FACE_OUTER_BOUND('',#1378,.T.);
#717=FACE_OUTER_BOUND('',#1379,.T.);
#718=FACE_OUTER_BOUND('',#1380,.T.);
#719=FACE_OUTER_BOUND('',#1381,.T.);
#720=FACE_OUTER_BOUND('',#1382,.T.);
#721=FACE_OUTER_BOUND('',#1383,.T.);
#722=FACE_OUTER_BOUND('',#1384,.T.);
#723=FACE_OUTER_BOUND('',#1385,.T.);
#724=FACE_OUTER_BOUND('',#1386,.T.);
#725=FACE_OUTER_BOUND('',#1387,.T.);
#726=FACE_OUTER_BOUND('',#1388,.T.);
#727=FACE_OUTER_BOUND('',#1389,.T.);
#728=FACE_OUTER_BOUND('',#1390,.T.);
#729=FACE_OUTER_BOUND('',#1391,.T.);
#730=FACE_OUTER_BOUND('',#1392,.T.);
#731=FACE_OUTER_BOUND('',#1393,.T.);
#732=FACE_OUTER_BOUND('',#1394,.T.);
#733=FACE_OUTER_BOUND('',#1395,.T.);
#734=FACE_OUTER_BOUND('',#1396,.T.);
#735=FACE_OUTER_BOUND('',#1397,.T.);
#736=FACE_OUTER_BOUND('',#1398,.T.);
#737=FACE_OUTER_BOUND('',#1399,.T.);
#738=FACE_OUTER_BOUND('',#1400,.T.);
#739=FACE_OUTER_BOUND('',#1401,.T.);
#740=FACE_OUTER_BOUND('',#1402,.T.);
#741=FACE_OUTER_BOUND('',#1403,.T.);
#742=FACE_OUTER_BOUND('',#1404,.T.);
#743=FACE_OUTER_BOUND('',#1405,.T.);
#744=FACE_OUTER_BOUND('',#1406,.T.);
#745=FACE_OUTER_BOUND('',#1407,.T.);
#746=FACE_OUTER_BOUND('',#1408,.T.);
#747=FACE_OUTER_BOUND('',#1409,.T.);
#748=FACE_OUTER_BOUND('',#1410,.T.);
#749=FACE_OUTER_BOUND('',#1411,.T.);
#750=FACE_OUTER_BOUND('',#1412,.T.);
#751=FACE_OUTER_BOUND('',#1413,.T.);
#752=FACE_OUTER_BOUND('',#1415,.T.);
#753=FACE_OUTER_BOUND('',#1421,.T.);
#754=FACE_OUTER_BOUND('',#1422,.T.);
#755=FACE_OUTER_BOUND('',#1423,.T.);
#756=FACE_OUTER_BOUND('',#1424,.T.);
#757=FACE_OUTER_BOUND('',#1425,.T.);
#758=FACE_OUTER_BOUND('',#1430,.T.);
#759=FACE_OUTER_BOUND('',#1431,.T.);
#760=FACE_OUTER_BOUND('',#1433,.T.);
#761=FACE_OUTER_BOUND('',#1434,.T.);
#762=FACE_OUTER_BOUND('',#1440,.T.);
#1199=EDGE_LOOP('',(#11073,#11074,#11075,#11076));
#1200=EDGE_LOOP('',(#11077,#11078,#11079,#11080,#11081,#11082));
#1201=EDGE_LOOP('',(#11083,#11084,#11085,#11086,#11087,#11088));
#1202=EDGE_LOOP('',(#11089,#11090,#11091,#11092,#11093,#11094));
#1203=EDGE_LOOP('',(#11095,#11096,#11097,#11098,#11099,#11100));
#1204=EDGE_LOOP('',(#11101,#11102,#11103,#11104,#11105,#11106));
#1205=EDGE_LOOP('',(#11107,#11108,#11109,#11110,#11111,#11112));
#1206=EDGE_LOOP('',(#11113,#11114,#11115,#11116,#11117,#11118));
#1207=EDGE_LOOP('',(#11119,#11120,#11121,#11122,#11123,#11124));
#1208=EDGE_LOOP('',(#11125,#11126,#11127,#11128,#11129,#11130));
#1209=EDGE_LOOP('',(#11131,#11132,#11133,#11134,#11135,#11136));
#1210=EDGE_LOOP('',(#11137,#11138,#11139,#11140,#11141,#11142));
#1211=EDGE_LOOP('',(#11143,#11144,#11145,#11146,#11147,#11148));
#1212=EDGE_LOOP('',(#11149,#11150,#11151,#11152,#11153,#11154));
#1213=EDGE_LOOP('',(#11155,#11156,#11157,#11158,#11159,#11160));
#1214=EDGE_LOOP('',(#11161,#11162,#11163,#11164,#11165,#11166));
#1215=EDGE_LOOP('',(#11167,#11168,#11169,#11170,#11171,#11172,#11173,#11174));
#1216=EDGE_LOOP('',(#11175,#11176,#11177,#11178,#11179));
#1217=EDGE_LOOP('',(#11180,#11181,#11182,#11183,#11184,#11185));
#1218=EDGE_LOOP('',(#11186,#11187,#11188,#11189));
#1219=EDGE_LOOP('',(#11190,#11191,#11192,#11193,#11194,#11195));
#1220=EDGE_LOOP('',(#11196,#11197,#11198,#11199));
#1221=EDGE_LOOP('',(#11200,#11201,#11202,#11203,#11204,#11205));
#1222=EDGE_LOOP('',(#11206,#11207,#11208,#11209));
#1223=EDGE_LOOP('',(#11210,#11211,#11212,#11213,#11214,#11215));
#1224=EDGE_LOOP('',(#11216,#11217,#11218,#11219));
#1225=EDGE_LOOP('',(#11220,#11221,#11222,#11223,#11224,#11225));
#1226=EDGE_LOOP('',(#11226,#11227,#11228,#11229));
#1227=EDGE_LOOP('',(#11230,#11231,#11232,#11233,#11234,#11235));
#1228=EDGE_LOOP('',(#11236,#11237,#11238,#11239));
#1229=EDGE_LOOP('',(#11240,#11241,#11242,#11243));
#1230=EDGE_LOOP('',(#11244,#11245,#11246,#11247));
#1231=EDGE_LOOP('',(#11248,#11249,#11250,#11251,#11252,#11253));
#1232=EDGE_LOOP('',(#11254,#11255,#11256,#11257,#11258,#11259));
#1233=EDGE_LOOP('',(#11260,#11261,#11262,#11263,#11264,#11265));
#1234=EDGE_LOOP('',(#11266,#11267,#11268,#11269,#11270,#11271));
#1235=EDGE_LOOP('',(#11272,#11273,#11274,#11275,#11276,#11277));
#1236=EDGE_LOOP('',(#11278,#11279,#11280,#11281,#11282,#11283));
#1237=EDGE_LOOP('',(#11284,#11285,#11286,#11287,#11288,#11289));
#1238=EDGE_LOOP('',(#11290,#11291,#11292,#11293,#11294,#11295));
#1239=EDGE_LOOP('',(#11296,#11297,#11298,#11299,#11300,#11301));
#1240=EDGE_LOOP('',(#11302,#11303,#11304,#11305,#11306,#11307));
#1241=EDGE_LOOP('',(#11308,#11309,#11310,#11311,#11312,#11313));
#1242=EDGE_LOOP('',(#11314,#11315,#11316,#11317,#11318,#11319));
#1243=EDGE_LOOP('',(#11320,#11321,#11322,#11323,#11324,#11325));
#1244=EDGE_LOOP('',(#11326,#11327,#11328,#11329,#11330,#11331));
#1245=EDGE_LOOP('',(#11332,#11333,#11334,#11335,#11336,#11337));
#1246=EDGE_LOOP('',(#11338,#11339,#11340,#11341,#11342,#11343,#11344,#11345));
#1247=EDGE_LOOP('',(#11346,#11347,#11348,#11349,#11350));
#1248=EDGE_LOOP('',(#11351,#11352,#11353,#11354,#11355,#11356));
#1249=EDGE_LOOP('',(#11357,#11358,#11359,#11360));
#1250=EDGE_LOOP('',(#11361,#11362,#11363,#11364,#11365,#11366));
#1251=EDGE_LOOP('',(#11367,#11368,#11369,#11370));
#1252=EDGE_LOOP('',(#11371,#11372,#11373,#11374,#11375,#11376));
#1253=EDGE_LOOP('',(#11377,#11378,#11379,#11380));
#1254=EDGE_LOOP('',(#11381,#11382,#11383,#11384,#11385,#11386));
#1255=EDGE_LOOP('',(#11387,#11388,#11389,#11390));
#1256=EDGE_LOOP('',(#11391,#11392,#11393,#11394,#11395,#11396));
#1257=EDGE_LOOP('',(#11397,#11398,#11399,#11400));
#1258=EDGE_LOOP('',(#11401,#11402,#11403,#11404,#11405,#11406));
#1259=EDGE_LOOP('',(#11407,#11408,#11409,#11410));
#1260=EDGE_LOOP('',(#11411,#11412,#11413,#11414));
#1261=EDGE_LOOP('',(#11415,#11416,#11417,#11418,#11419));
#1262=EDGE_LOOP('',(#11420,#11421,#11422,#11423,#11424,#11425));
#1263=EDGE_LOOP('',(#11426,#11427,#11428,#11429,#11430,#11431));
#1264=EDGE_LOOP('',(#11432,#11433,#11434,#11435,#11436,#11437));
#1265=EDGE_LOOP('',(#11438,#11439,#11440,#11441,#11442,#11443));
#1266=EDGE_LOOP('',(#11444,#11445,#11446,#11447,#11448,#11449));
#1267=EDGE_LOOP('',(#11450,#11451,#11452,#11453,#11454,#11455));
#1268=EDGE_LOOP('',(#11456,#11457,#11458,#11459,#11460,#11461));
#1269=EDGE_LOOP('',(#11462,#11463,#11464,#11465,#11466,#11467));
#1270=EDGE_LOOP('',(#11468,#11469,#11470,#11471,#11472,#11473));
#1271=EDGE_LOOP('',(#11474,#11475,#11476,#11477,#11478,#11479));
#1272=EDGE_LOOP('',(#11480,#11481,#11482,#11483,#11484,#11485));
#1273=EDGE_LOOP('',(#11486,#11487,#11488,#11489,#11490,#11491));
#1274=EDGE_LOOP('',(#11492,#11493,#11494,#11495,#11496,#11497));
#1275=EDGE_LOOP('',(#11498,#11499,#11500,#11501,#11502));
#1276=EDGE_LOOP('',(#11503,#11504,#11505,#11506,#11507,#11508));
#1277=EDGE_LOOP('',(#11509,#11510,#11511,#11512,#11513,#11514));
#1278=EDGE_LOOP('',(#11515,#11516,#11517,#11518,#11519,#11520));
#1279=EDGE_LOOP('',(#11521,#11522,#11523,#11524,#11525,#11526));
#1280=EDGE_LOOP('',(#11527,#11528,#11529,#11530,#11531,#11532));
#1281=EDGE_LOOP('',(#11533,#11534,#11535,#11536,#11537,#11538));
#1282=EDGE_LOOP('',(#11539,#11540,#11541,#11542,#11543,#11544));
#1283=EDGE_LOOP('',(#11545,#11546,#11547,#11548,#11549,#11550));
#1284=EDGE_LOOP('',(#11551,#11552,#11553,#11554,#11555,#11556));
#1285=EDGE_LOOP('',(#11557,#11558,#11559,#11560,#11561,#11562));
#1286=EDGE_LOOP('',(#11563,#11564,#11565,#11566,#11567,#11568));
#1287=EDGE_LOOP('',(#11569,#11570,#11571,#11572,#11573,#11574));
#1288=EDGE_LOOP('',(#11575,#11576,#11577,#11578,#11579,#11580));
#1289=EDGE_LOOP('',(#11581,#11582,#11583,#11584,#11585));
#1290=EDGE_LOOP('',(#11586,#11587,#11588,#11589,#11590,#11591));
#1291=EDGE_LOOP('',(#11592,#11593,#11594,#11595,#11596,#11597));
#1292=EDGE_LOOP('',(#11598,#11599,#11600,#11601,#11602,#11603));
#1293=EDGE_LOOP('',(#11604,#11605,#11606,#11607,#11608,#11609));
#1294=EDGE_LOOP('',(#11610,#11611,#11612,#11613,#11614,#11615));
#1295=EDGE_LOOP('',(#11616,#11617,#11618,#11619,#11620,#11621));
#1296=EDGE_LOOP('',(#11622,#11623,#11624,#11625,#11626,#11627));
#1297=EDGE_LOOP('',(#11628,#11629,#11630,#11631,#11632,#11633));
#1298=EDGE_LOOP('',(#11634,#11635,#11636,#11637,#11638,#11639));
#1299=EDGE_LOOP('',(#11640,#11641,#11642,#11643,#11644,#11645));
#1300=EDGE_LOOP('',(#11646,#11647,#11648,#11649,#11650,#11651));
#1301=EDGE_LOOP('',(#11652,#11653,#11654,#11655,#11656,#11657));
#1302=EDGE_LOOP('',(#11658,#11659,#11660,#11661,#11662,#11663));
#1303=EDGE_LOOP('',(#11664,#11665,#11666,#11667,#11668));
#1304=EDGE_LOOP('',(#11669,#11670,#11671,#11672,#11673,#11674));
#1305=EDGE_LOOP('',(#11675,#11676,#11677,#11678,#11679,#11680));
#1306=EDGE_LOOP('',(#11681,#11682,#11683,#11684,#11685,#11686));
#1307=EDGE_LOOP('',(#11687,#11688,#11689,#11690,#11691,#11692));
#1308=EDGE_LOOP('',(#11693,#11694,#11695,#11696,#11697,#11698));
#1309=EDGE_LOOP('',(#11699,#11700,#11701,#11702,#11703,#11704));
#1310=EDGE_LOOP('',(#11705,#11706,#11707,#11708,#11709,#11710));
#1311=EDGE_LOOP('',(#11711,#11712,#11713,#11714,#11715,#11716));
#1312=EDGE_LOOP('',(#11717,#11718,#11719,#11720,#11721,#11722));
#1313=EDGE_LOOP('',(#11723,#11724,#11725,#11726,#11727,#11728));
#1314=EDGE_LOOP('',(#11729,#11730,#11731,#11732,#11733,#11734));
#1315=EDGE_LOOP('',(#11735,#11736,#11737,#11738,#11739,#11740));
#1316=EDGE_LOOP('',(#11741,#11742,#11743,#11744,#11745,#11746));
#1317=EDGE_LOOP('',(#11747,#11748,#11749,#11750));
#1318=EDGE_LOOP('',(#11751,#11752,#11753,#11754,#11755));
#1319=EDGE_LOOP('',(#11756,#11757,#11758,#11759,#11760));
#1320=EDGE_LOOP('',(#11761,#11762,#11763,#11764,#11765));
#1321=EDGE_LOOP('',(#11766,#11767,#11768,#11769,#11770));
#1322=EDGE_LOOP('',(#11771,#11772,#11773,#11774,#11775));
#1323=EDGE_LOOP('',(#11776,#11777,#11778,#11779,#11780));
#1324=EDGE_LOOP('',(#11781,#11782,#11783,#11784,#11785,#11786));
#1325=EDGE_LOOP('',(#11787,#11788,#11789,#11790,#11791));
#1326=EDGE_LOOP('',(#11792,#11793,#11794,#11795,#11796));
#1327=EDGE_LOOP('',(#11797,#11798,#11799,#11800,#11801));
#1328=EDGE_LOOP('',(#11802,#11803,#11804,#11805,#11806));
#1329=EDGE_LOOP('',(#11807,#11808,#11809,#11810,#11811));
#1330=EDGE_LOOP('',(#11812,#11813,#11814,#11815,#11816));
#1331=EDGE_LOOP('',(#11817,#11818,#11819,#11820));
#1332=EDGE_LOOP('',(#11821,#11822,#11823,#11824,#11825));
#1333=EDGE_LOOP('',(#11826,#11827,#11828,#11829,#11830));
#1334=EDGE_LOOP('',(#11831,#11832,#11833,#11834,#11835));
#1335=EDGE_LOOP('',(#11836,#11837,#11838,#11839,#11840));
#1336=EDGE_LOOP('',(#11841,#11842,#11843,#11844,#11845));
#1337=EDGE_LOOP('',(#11846,#11847,#11848,#11849,#11850));
#1338=EDGE_LOOP('',(#11851,#11852,#11853,#11854,#11855,#11856));
#1339=EDGE_LOOP('',(#11857,#11858,#11859,#11860,#11861));
#1340=EDGE_LOOP('',(#11862,#11863,#11864,#11865,#11866));
#1341=EDGE_LOOP('',(#11867,#11868,#11869,#11870,#11871));
#1342=EDGE_LOOP('',(#11872,#11873,#11874,#11875,#11876));
#1343=EDGE_LOOP('',(#11877,#11878,#11879,#11880,#11881));
#1344=EDGE_LOOP('',(#11882,#11883,#11884,#11885,#11886));
#1345=EDGE_LOOP('',(#11887,#11888,#11889,#11890));
#1346=EDGE_LOOP('',(#11891,#11892,#11893,#11894));
#1347=EDGE_LOOP('',(#11895,#11896,#11897,#11898,#11899));
#1348=EDGE_LOOP('',(#11900,#11901,#11902,#11903));
#1349=EDGE_LOOP('',(#11904,#11905,#11906,#11907,#11908));
#1350=EDGE_LOOP('',(#11909,#11910,#11911,#11912,#11913));
#1351=EDGE_LOOP('',(#11914,#11915,#11916,#11917,#11918));
#1352=EDGE_LOOP('',(#11919,#11920,#11921,#11922,#11923,#11924));
#1353=EDGE_LOOP('',(#11925,#11926,#11927,#11928,#11929));
#1354=EDGE_LOOP('',(#11930,#11931,#11932,#11933,#11934));
#1355=EDGE_LOOP('',(#11935,#11936,#11937,#11938,#11939));
#1356=EDGE_LOOP('',(#11940,#11941,#11942,#11943,#11944));
#1357=EDGE_LOOP('',(#11945,#11946,#11947,#11948));
#1358=EDGE_LOOP('',(#11949,#11950,#11951,#11952));
#1359=EDGE_LOOP('',(#11953,#11954,#11955,#11956));
#1360=EDGE_LOOP('',(#11957,#11958,#11959,#11960));
#1361=EDGE_LOOP('',(#11961,#11962,#11963,#11964,#11965));
#1362=EDGE_LOOP('',(#11966,#11967,#11968,#11969));
#1363=EDGE_LOOP('',(#11970,#11971,#11972,#11973,#11974));
#1364=EDGE_LOOP('',(#11975,#11976,#11977,#11978,#11979));
#1365=EDGE_LOOP('',(#11980,#11981,#11982,#11983,#11984));
#1366=EDGE_LOOP('',(#11985,#11986,#11987,#11988,#11989,#11990));
#1367=EDGE_LOOP('',(#11991,#11992,#11993,#11994,#11995));
#1368=EDGE_LOOP('',(#11996,#11997,#11998,#11999,#12000));
#1369=EDGE_LOOP('',(#12001,#12002,#12003,#12004,#12005));
#1370=EDGE_LOOP('',(#12006,#12007,#12008,#12009,#12010));
#1371=EDGE_LOOP('',(#12011,#12012,#12013,#12014));
#1372=EDGE_LOOP('',(#12015,#12016,#12017,#12018));
#1373=EDGE_LOOP('',(#12019,#12020,#12021,#12022,#12023));
#1374=EDGE_LOOP('',(#12024,#12025,#12026,#12027,#12028));
#1375=EDGE_LOOP('',(#12029,#12030,#12031,#12032,#12033));
#1376=EDGE_LOOP('',(#12034,#12035,#12036,#12037,#12038));
#1377=EDGE_LOOP('',(#12039,#12040,#12041,#12042,#12043,#12044));
#1378=EDGE_LOOP('',(#12045,#12046,#12047,#12048,#12049,#12050));
#1379=EDGE_LOOP('',(#12051,#12052,#12053,#12054,#12055,#12056));
#1380=EDGE_LOOP('',(#12057,#12058,#12059,#12060,#12061,#12062));
#1381=EDGE_LOOP('',(#12063,#12064,#12065,#12066,#12067));
#1382=EDGE_LOOP('',(#12068,#12069,#12070,#12071,#12072,#12073));
#1383=EDGE_LOOP('',(#12074,#12075,#12076,#12077,#12078));
#1384=EDGE_LOOP('',(#12079,#12080,#12081,#12082,#12083,#12084));
#1385=EDGE_LOOP('',(#12085,#12086,#12087,#12088));
#1386=EDGE_LOOP('',(#12089,#12090,#12091,#12092,#12093,#12094,#12095,#12096,
#12097,#12098,#12099,#12100,#12101,#12102,#12103,#12104,#12105,#12106,#12107,
#12108,#12109,#12110,#12111,#12112,#12113,#12114,#12115,#12116,#12117,#12118,
#12119,#12120,#12121,#12122,#12123,#12124,#12125,#12126,#12127,#12128,#12129,
#12130,#12131,#12132,#12133,#12134,#12135,#12136,#12137,#12138,#12139,#12140,
#12141,#12142,#12143,#12144,#12145,#12146,#12147));
#1387=EDGE_LOOP('',(#12148,#12149,#12150,#12151,#12152,#12153,#12154,#12155,
#12156,#12157,#12158,#12159,#12160,#12161,#12162,#12163,#12164,#12165,#12166,
#12167,#12168,#12169,#12170,#12171,#12172,#12173,#12174,#12175,#12176,#12177,
#12178,#12179,#12180,#12181,#12182,#12183,#12184,#12185,#12186,#12187,#12188,
#12189,#12190,#12191,#12192,#12193,#12194,#12195,#12196,#12197,#12198,#12199,
#12200,#12201,#12202,#12203,#12204,#12205,#12206));
#1388=EDGE_LOOP('',(#12207,#12208,#12209,#12210));
#1389=EDGE_LOOP('',(#12211,#12212,#12213,#12214,#12215,#12216,#12217,#12218,
#12219,#12220,#12221,#12222,#12223,#12224,#12225,#12226,#12227,#12228,#12229,
#12230,#12231,#12232,#12233,#12234,#12235,#12236,#12237,#12238,#12239,#12240,
#12241,#12242,#12243,#12244,#12245,#12246,#12247,#12248,#12249,#12250,#12251,
#12252,#12253,#12254,#12255,#12256,#12257,#12258,#12259,#12260,#12261,#12262,
#12263,#12264,#12265,#12266,#12267,#12268,#12269));
#1390=EDGE_LOOP('',(#12270,#12271,#12272,#12273,#12274,#12275,#12276,#12277,
#12278,#12279,#12280,#12281,#12282,#12283,#12284,#12285,#12286,#12287,#12288,
#12289,#12290,#12291,#12292,#12293,#12294,#12295,#12296,#12297,#12298,#12299,
#12300,#12301,#12302,#12303,#12304,#12305,#12306,#12307,#12308,#12309,#12310,
#12311,#12312,#12313,#12314,#12315,#12316,#12317,#12318,#12319,#12320,#12321,
#12322,#12323,#12324,#12325,#12326,#12327,#12328));
#1391=EDGE_LOOP('',(#12329));
#1392=EDGE_LOOP('',(#12330));
#1393=EDGE_LOOP('',(#12331,#12332,#12333,#12334));
#1394=EDGE_LOOP('',(#12335,#12336,#12337,#12338));
#1395=EDGE_LOOP('',(#12339,#12340,#12341,#12342));
#1396=EDGE_LOOP('',(#12343,#12344,#12345,#12346));
#1397=EDGE_LOOP('',(#12347,#12348,#12349,#12350));
#1398=EDGE_LOOP('',(#12351,#12352,#12353,#12354));
#1399=EDGE_LOOP('',(#12355,#12356,#12357,#12358));
#1400=EDGE_LOOP('',(#12359,#12360,#12361,#12362));
#1401=EDGE_LOOP('',(#12363,#12364,#12365,#12366,#12367,#12368,#12369,#12370,
#12371,#12372,#12373,#12374,#12375,#12376,#12377,#12378,#12379,#12380,#12381,
#12382,#12383,#12384,#12385,#12386,#12387,#12388,#12389,#12390,#12391,#12392,
#12393,#12394,#12395,#12396,#12397,#12398,#12399,#12400,#12401,#12402,#12403,
#12404,#12405,#12406,#12407,#12408,#12409,#12410,#12411,#12412,#12413,#12414,
#12415,#12416,#12417));
#1402=EDGE_LOOP('',(#12418,#12419,#12420,#12421,#12422,#12423,#12424,#12425,
#12426,#12427,#12428,#12429,#12430,#12431,#12432,#12433,#12434,#12435,#12436,
#12437,#12438,#12439,#12440,#12441,#12442,#12443,#12444,#12445,#12446,#12447,
#12448,#12449,#12450,#12451,#12452,#12453,#12454,#12455,#12456,#12457,#12458,
#12459,#12460,#12461,#12462,#12463,#12464,#12465,#12466,#12467,#12468,#12469,
#12470,#12471,#12472));
#1403=EDGE_LOOP('',(#12473,#12474,#12475,#12476,#12477,#12478,#12479,#12480,
#12481,#12482,#12483,#12484,#12485,#12486,#12487,#12488,#12489,#12490,#12491,
#12492,#12493,#12494,#12495,#12496,#12497,#12498,#12499,#12500,#12501,#12502,
#12503,#12504,#12505,#12506,#12507,#12508,#12509,#12510,#12511,#12512,#12513,
#12514,#12515,#12516,#12517,#12518,#12519,#12520,#12521,#12522,#12523,#12524,
#12525,#12526,#12527));
#1404=EDGE_LOOP('',(#12528,#12529,#12530,#12531,#12532,#12533,#12534,#12535,
#12536,#12537,#12538,#12539,#12540,#12541,#12542,#12543,#12544,#12545,#12546,
#12547,#12548,#12549,#12550,#12551,#12552,#12553,#12554,#12555,#12556,#12557,
#12558,#12559,#12560,#12561,#12562,#12563,#12564,#12565,#12566,#12567,#12568,
#12569,#12570,#12571,#12572,#12573,#12574,#12575,#12576,#12577,#12578,#12579,
#12580,#12581,#12582));
#1405=EDGE_LOOP('',(#12583,#12584,#12585,#12586,#12587,#12588,#12589,#12590,
#12591,#12592,#12593,#12594,#12595,#12596,#12597,#12598,#12599,#12600,#12601,
#12602,#12603,#12604,#12605,#12606,#12607,#12608,#12609,#12610,#12611,#12612,
#12613,#12614,#12615,#12616,#12617,#12618,#12619,#12620,#12621,#12622,#12623,
#12624,#12625,#12626,#12627,#12628,#12629,#12630,#12631,#12632,#12633,#12634,
#12635));
#1406=EDGE_LOOP('',(#12636,#12637,#12638,#12639,#12640,#12641,#12642,#12643,
#12644,#12645,#12646,#12647,#12648,#12649,#12650,#12651,#12652,#12653,#12654,
#12655,#12656,#12657,#12658,#12659,#12660,#12661,#12662,#12663,#12664,#12665,
#12666,#12667,#12668,#12669,#12670,#12671,#12672,#12673,#12674,#12675,#12676,
#12677,#12678,#12679,#12680,#12681,#12682,#12683,#12684,#12685,#12686,#12687,
#12688));
#1407=EDGE_LOOP('',(#12689,#12690,#12691,#12692,#12693,#12694,#12695,#12696,
#12697,#12698,#12699,#12700,#12701,#12702,#12703,#12704,#12705,#12706,#12707,
#12708,#12709,#12710,#12711,#12712,#12713,#12714,#12715,#12716,#12717,#12718,
#12719,#12720,#12721,#12722,#12723,#12724,#12725,#12726,#12727,#12728,#12729,
#12730,#12731,#12732,#12733,#12734,#12735,#12736,#12737,#12738,#12739,#12740,
#12741));
#1408=EDGE_LOOP('',(#12742,#12743,#12744,#12745,#12746,#12747,#12748,#12749,
#12750,#12751,#12752,#12753,#12754,#12755,#12756,#12757,#12758,#12759,#12760,
#12761,#12762,#12763,#12764,#12765,#12766,#12767,#12768,#12769,#12770,#12771,
#12772,#12773,#12774,#12775,#12776,#12777,#12778,#12779,#12780,#12781,#12782,
#12783,#12784,#12785,#12786,#12787,#12788,#12789,#12790,#12791,#12792,#12793,
#12794));
#1409=EDGE_LOOP('',(#12795,#12796,#12797,#12798,#12799));
#1410=EDGE_LOOP('',(#12800,#12801,#12802,#12803,#12804));
#1411=EDGE_LOOP('',(#12805,#12806,#12807,#12808,#12809));
#1412=EDGE_LOOP('',(#12810,#12811,#12812,#12813,#12814));
#1413=EDGE_LOOP('',(#12815,#12816,#12817,#12818));
#1414=EDGE_LOOP('',(#12819,#12820,#12821,#12822));
#1415=EDGE_LOOP('',(#12823,#12824,#12825,#12826));
#1416=EDGE_LOOP('',(#12827,#12828,#12829,#12830));
#1417=EDGE_LOOP('',(#12831));
#1418=EDGE_LOOP('',(#12832));
#1419=EDGE_LOOP('',(#12833));
#1420=EDGE_LOOP('',(#12834));
#1421=EDGE_LOOP('',(#12835,#12836,#12837,#12838));
#1422=EDGE_LOOP('',(#12839,#12840,#12841,#12842));
#1423=EDGE_LOOP('',(#12843,#12844,#12845,#12846));
#1424=EDGE_LOOP('',(#12847,#12848,#12849,#12850));
#1425=EDGE_LOOP('',(#12851,#12852,#12853,#12854));
#1426=EDGE_LOOP('',(#12855));
#1427=EDGE_LOOP('',(#12856));
#1428=EDGE_LOOP('',(#12857));
#1429=EDGE_LOOP('',(#12858));
#1430=EDGE_LOOP('',(#12859,#12860,#12861,#12862));
#1431=EDGE_LOOP('',(#12863,#12864,#12865,#12866));
#1432=EDGE_LOOP('',(#12867));
#1433=EDGE_LOOP('',(#12868,#12869,#12870,#12871));
#1434=EDGE_LOOP('',(#12872,#12873,#12874,#12875));
#1435=EDGE_LOOP('',(#12876,#12877,#12878,#12879,#12880));
#1436=EDGE_LOOP('',(#12881,#12882,#12883,#12884,#12885));
#1437=EDGE_LOOP('',(#12886,#12887,#12888,#12889,#12890));
#1438=EDGE_LOOP('',(#12891,#12892,#12893,#12894,#12895));
#1439=EDGE_LOOP('',(#12896));
#1440=EDGE_LOOP('',(#12897,#12898,#12899,#12900));
#1441=EDGE_LOOP('',(#12901,#12902,#12903,#12904,#12905));
#1442=EDGE_LOOP('',(#12906,#12907,#12908,#12909,#12910));
#1443=EDGE_LOOP('',(#12911,#12912,#12913,#12914));
#1841=CIRCLE('',#17188,2.05475);
#1842=CIRCLE('',#17204,2.05475);
#1843=CIRCLE('',#17206,1.666);
#1844=CIRCLE('',#17207,1.666);
#1845=CIRCLE('',#17222,1.666);
#1846=CIRCLE('',#17224,2.05475);
#1847=CIRCLE('',#17240,2.05475);
#1848=CIRCLE('',#17242,1.666);
#1849=CIRCLE('',#17243,1.666);
#1850=CIRCLE('',#17258,1.666);
#1851=CIRCLE('',#17260,2.05475);
#1852=CIRCLE('',#17274,2.05475);
#1853=CIRCLE('',#17276,2.05475);
#1854=CIRCLE('',#17290,2.05475);
#1855=CIRCLE('',#17292,2.05475);
#1856=CIRCLE('',#17306,2.05475);
#1857=CIRCLE('',#17308,2.05475);
#1858=CIRCLE('',#17322,2.05475);
#1859=CIRCLE('',#17324,1.666);
#1860=CIRCLE('',#17338,1.666);
#1861=CIRCLE('',#17340,1.666);
#1862=CIRCLE('',#17354,1.666);
#1863=CIRCLE('',#17356,1.666);
#1864=CIRCLE('',#17370,1.666);
#1865=CIRCLE('',#17372,1.666);
#1866=CIRCLE('',#17386,1.666);
#1867=CIRCLE('',#17405,22.);
#1868=CIRCLE('',#17408,22.);
#1869=CIRCLE('',#17410,4.5);
#1870=CIRCLE('',#17411,4.5);
#1871=CIRCLE('',#17413,4.5);
#1872=CIRCLE('',#17414,4.5);
#1873=CIRCLE('',#17416,4.5);
#1874=CIRCLE('',#17417,4.5);
#1875=CIRCLE('',#17419,4.5);
#1876=CIRCLE('',#17420,4.5);
#1877=CIRCLE('',#17426,22.);
#1878=CIRCLE('',#17427,22.);
#2313=B_SPLINE_CURVE_WITH_KNOTS('',3,(#59501,#59502,#59503,#59504),
 .UNSPECIFIED.,.F.,.F.,(4,4),(112.182489743597,112.611961982353),
 .UNSPECIFIED.);
#2314=B_SPLINE_CURVE_WITH_KNOTS('',3,(#59507,#59508,#59509,#59510,#59511,
#59512,#59513,#59514,#59515,#59516,#59517,#59518,#59519,#59520,#59521,#59522,
#59523,#59524,#59525,#59526,#59527,#59528,#59529,#59530,#59531,#59532,#59533,
#59534,#59535,#59536,#59537),.UNSPECIFIED.,.F.,.F.,(4,3,3,3,3,3,3,3,3,3,
4),(112.181968556931,112.285773472651,112.391790544659,112.495346156522,
112.59884907986,112.702334544286,112.810228420394,112.91385103149,113.017546973854,
113.121410915295,113.133910048719),.UNSPECIFIED.);
#2315=B_SPLINE_CURVE_WITH_KNOTS('',3,(#59543,#59544,#59545,#59546,#59547,
#59548,#59549,#59550,#59551,#59552,#59553,#59554,#59555,#59556,#59557,#59558,
#59559,#59560,#59561,#59562,#59563,#59564,#59565,#59566,#59567,#59568,#59569,
#59570,#59571,#59572,#59573,#59574,#59575,#59576,#59577,#59578,#59579,#59580,
#59581,#59582,#59583,#59584,#59585,#59586,#59587,#59588,#59589,#59590,#59591,
#59592,#59593,#59594,#59595,#59596,#59597,#59598,#59599,#59600,#59601,#59602,
#59603,#59604,#59605,#59606,#59607,#59608,#59609,#59610,#59611,#59612,#59613,
#59614,#59615,#59616,#59617,#59618,#59619,#59620,#59621,#59622,#59623,#59624,
#59625,#59626,#59627,#59628,#59629,#59630,#59631,#59632,#59633,#59634,#59635,
#59636,#59637,#59638,#59639,#59640,#59641,#59642,#59643,#59644,#59645,#59646,
#59647,#59648,#59649,#59650,#59651,#59652,#59653,#59654,#59655,#59656,#59657,
#59658,#59659,#59660,#59661,#59662,#59663),.UNSPECIFIED.,.F.,.F.,(4,3,3,
3,3,3,3,3,3,3,3,3,3,3,3,3,3,3,3,3,3,3,3,3,3,3,3,3,3,3,3,3,3,3,3,3,3,3,3,
3,4),(105.899140451686,106.003024815435,106.106864212787,106.210693366653,
106.314717718923,106.418692007997,106.522861281791,106.626790775734,106.730987263758,
106.835028766578,106.93894855402,107.042803073214,107.146627085189,107.250455307722,
107.354392349897,107.458388337965,107.562566286003,107.62431931017,107.728406127187,
107.832337435927,107.936146784475,108.039890771643,108.143604319905,108.24732230847,
108.351150224774,108.455037544721,108.55910873153,108.621847844607,108.726214065306,
108.830424643138,108.934511720786,109.038532332813,109.142520999285,109.246512195638,
109.350608540247,109.454761991411,109.559092813096,109.619376379044,109.740298293392,
109.860139275301,109.955742676499),.UNSPECIFIED.);
#2316=B_SPLINE_CURVE_WITH_KNOTS('',3,(#59664,#59665,#59666,#59667,#59668,
#59669),.UNSPECIFIED.,.F.,.F.,(4,1,1,4),(109.955742875643,110.61690491348,
111.614433447917,112.182489743597),.UNSPECIFIED.);
#2317=B_SPLINE_CURVE_WITH_KNOTS('',3,(#59671,#59672,#59673,#59674,#59675,
#59676,#59677,#59678,#59679,#59680,#59681,#59682,#59683,#59684,#59685,#59686,
#59687,#59688,#59689,#59690,#59691,#59692,#59693,#59694,#59695,#59696,#59697,
#59698,#59699,#59700,#59701,#59702,#59703,#59704,#59705,#59706,#59707,#59708,
#59709,#59710,#59711,#59712,#59713,#59714,#59715,#59716,#59717,#59718,#59719,
#59720,#59721,#59722,#59723,#59724,#59725,#59726,#59727,#59728,#59729,#59730,
#59731,#59732,#59733,#59734,#59735,#59736,#59737,#59738,#59739,#59740),
 .UNSPECIFIED.,.F.,.F.,(4,3,3,3,3,3,3,3,3,3,3,3,3,3,3,3,3,3,3,3,3,3,3,4),
(109.955742875643,110.103310972773,110.160880318691,110.264967062808,110.368898298551,
110.472707574298,110.576451488819,110.68016496469,110.783882881219,110.887710726514,
110.991597975919,111.095669093687,111.158408853127,111.262775109417,111.366985722483,
111.47107283468,111.575093480817,111.679082180912,111.783073410354,111.887169787029,
111.991323269728,112.095654121783,112.155937387564,112.181968556931),
 .UNSPECIFIED.);
#2318=B_SPLINE_CURVE_WITH_KNOTS('',3,(#59741,#59742,#59743,#59744,#59745,
#59746,#59747,#59748,#59749,#59750,#59751,#59752,#59753,#59754,#59755,#59756,
#59757,#59758,#59759,#59760,#59761,#59762,#59763,#59764,#59765,#59766,#59767,
#59768,#59769,#59770,#59771,#59772,#59773,#59774,#59775,#59776,#59777,#59778,
#59779,#59780,#59781,#59782,#59783,#59784,#59785,#59786,#59787,#59788,#59789,
#59790,#59791,#59792,#59793,#59794,#59795,#59796,#59797,#59798,#59799,#59800,
#59801,#59802,#59803,#59804,#59805,#59806,#59807,#59808,#59809,#59810,#59811,
#59812,#59813,#59814,#59815,#59816,#59817,#59818,#59819,#59820,#59821,#59822,
#59823,#59824,#59825,#59826,#59827,#59828,#59829,#59830,#59831,#59832,#59833,
#59834,#59835,#59836,#59837,#59838,#59839,#59840,#59841,#59842,#59843,#59844,
#59845,#59846,#59847,#59848,#59849,#59850,#59851,#59852,#59853,#59854,#59855,
#59856,#59857,#59858,#59859,#59860,#59861,#59862,#59863,#59864),
 .UNSPECIFIED.,.F.,.F.,(4,3,3,3,3,3,3,3,3,3,3,3,3,3,3,3,3,3,3,3,3,3,3,3,
3,3,3,3,3,3,3,3,3,3,3,3,3,3,3,3,3,4),(105.898025478301,106.00200980369,
106.106176851874,106.170766180944,106.274954662883,106.378987940918,106.482899222427,
106.586745067332,106.690560250991,106.794379505344,106.89830743079,107.002294204721,
107.106462887271,107.168294715381,107.27246889799,107.376487822855,107.480384740769,
107.584216223424,107.688017067289,107.791822025433,107.895735819492,107.999708533646,
108.10386342229,108.165823249817,108.270028204319,108.37407786237,108.478005309915,
108.581867180328,108.685698226556,108.78953315797,108.893476372029,108.997478238522,
109.101661542088,109.163351784254,109.266012649306,109.368536778223,109.470960989788,
109.57332195874,109.675698114947,109.778078147715,109.88056957456,109.955742875311),
 .UNSPECIFIED.);
#2319=B_SPLINE_CURVE_WITH_KNOTS('',3,(#59870,#59871,#59872,#59873,#59874,
#59875,#59876,#59877,#59878,#59879,#59880,#59881,#59882,#59883,#59884,#59885,
#59886,#59887,#59888,#59889,#59890,#59891,#59892,#59893,#59894,#59895,#59896,
#59897,#59898,#59899,#59900,#59901,#59902,#59903,#59904,#59905,#59906,#59907,
#59908,#59909,#59910,#59911,#59912,#59913,#59914,#59915,#59916,#59917,#59918,
#59919,#59920,#59921,#59922,#59923,#59924,#59925,#59926,#59927,#59928,#59929,
#59930,#59931,#59932,#59933,#59934,#59935,#59936,#59937,#59938,#59939,#59940,
#59941,#59942,#59943,#59944,#59945,#59946,#59947,#59948,#59949,#59950,#59951,
#59952,#59953,#59954,#59955,#59956,#59957,#59958,#59959,#59960,#59961,#59962,
#59963,#59964,#59965,#59966,#59967,#59968,#59969,#59970,#59971,#59972,#59973,
#59974,#59975,#59976,#59977,#59978,#59979,#59980,#59981,#59982,#59983,#59984,
#59985,#59986,#59987,#59988,#59989,#59990,#59991,#59992,#59993,#59994,#59995,
#59996),.UNSPECIFIED.,.F.,.F.,(4,3,3,3,3,3,3,3,3,3,3,3,3,3,3,3,3,3,3,3,
3,3,3,3,3,3,3,3,3,3,3,3,3,3,3,3,3,3,3,3,3,3,4),(99.6152316573692,99.6440910346775,
99.7482776242847,99.852308980079,99.9562183047007,100.060062172463,100.163875361819,
100.267692607789,100.371618517559,100.475603268673,100.579769939392,100.641619569114,
100.745806326648,100.849837854855,100.953747357642,101.057591407011,101.161404781119,
101.265222214687,101.369148315049,101.473133258728,101.577300122986,101.639148103551,
101.743333059736,101.847362781364,101.951270478531,102.055112723852,102.158924298124,
102.262739938717,102.366664268879,102.470647452536,102.574812591943,102.636676637987,
102.740864888504,102.8448978973,102.948808855441,103.052654343846,103.156469138697,
103.260287972727,103.36421543326,103.468201716448,103.572369873255,103.634205172424,
103.672557568463),.UNSPECIFIED.);
#2320=B_SPLINE_CURVE_WITH_KNOTS('',3,(#59997,#59998,#59999,#60000,#60001,
#60002,#60003,#60004,#60005,#60006,#60007,#60008,#60009,#60010,#60011,#60012,
#60013,#60014,#60015,#60016,#60017,#60018,#60019,#60020,#60021,#60022,#60023,
#60024,#60025,#60026,#60027,#60028,#60029,#60030,#60031,#60032,#60033,#60034,
#60035,#60036,#60037,#60038,#60039,#60040,#60041,#60042,#60043,#60044,#60045,
#60046,#60047,#60048,#60049,#60050,#60051,#60052,#60053,#60054,#60055,#60056,
#60057,#60058,#60059,#60060,#60061,#60062,#60063,#60064,#60065,#60066),
 .UNSPECIFIED.,.F.,.F.,(4,3,3,3,3,3,3,3,3,3,3,3,3,3,3,3,3,3,3,3,3,3,3,4),
(103.672557568736,103.776099131449,103.883053453376,103.986323984164,104.089534941353,
104.192721969991,104.295920677775,104.399231122839,104.502608908511,104.606156363019,
104.631733706861,104.735907902116,104.839926839642,104.943823770182,105.047655265435,
105.151456121852,105.255261092482,105.359174898845,105.463147625218,105.567302525815,
105.629262241297,105.73346168362,105.837495278037,105.899140451686),
 .UNSPECIFIED.);
#2321=B_SPLINE_CURVE_WITH_KNOTS('',3,(#60068,#60069,#60070,#60071,#60072,
#60073,#60074,#60075,#60076,#60077,#60078,#60079,#60080,#60081,#60082,#60083,
#60084,#60085,#60086,#60087,#60088,#60089,#60090,#60091,#60092,#60093,#60094,
#60095,#60096,#60097,#60098,#60099,#60100,#60101,#60102,#60103,#60104,#60105,
#60106,#60107,#60108,#60109,#60110,#60111,#60112,#60113,#60114,#60115,#60116,
#60117,#60118,#60119,#60120,#60121,#60122,#60123,#60124,#60125,#60126,#60127,
#60128,#60129,#60130,#60131,#60132,#60133,#60134),.UNSPECIFIED.,.F.,.F.,
(4,3,3,3,3,3,3,3,3,3,3,3,3,3,3,3,3,3,3,3,3,3,4),(103.672557568463,103.781092798507,
103.889920271511,103.998901190727,104.108175816525,104.175709112071,104.279894066294,
104.383923785958,104.487831481169,104.591673724538,104.695485296866,104.799300935527,
104.903225263787,105.007208445554,105.111373583115,105.173237646508,105.277400211582,
105.381419534253,105.485330617835,105.58918653948,105.69300465016,105.796876384297,
105.898025478301),.UNSPECIFIED.);
#2322=B_SPLINE_CURVE_WITH_KNOTS('',3,(#60135,#60136,#60137,#60138,#60139,
#60140,#60141,#60142,#60143,#60144,#60145,#60146,#60147,#60148,#60149,#60150,
#60151,#60152,#60153,#60154,#60155,#60156,#60157,#60158,#60159,#60160,#60161,
#60162,#60163,#60164,#60165,#60166,#60167,#60168,#60169,#60170,#60171,#60172,
#60173,#60174,#60175,#60176,#60177,#60178,#60179,#60180,#60181,#60182,#60183,
#60184,#60185,#60186,#60187,#60188,#60189,#60190,#60191,#60192,#60193,#60194,
#60195,#60196,#60197,#60198,#60199,#60200,#60201,#60202,#60203,#60204,#60205,
#60206,#60207,#60208,#60209,#60210,#60211,#60212,#60213,#60214,#60215,#60216,
#60217,#60218,#60219,#60220,#60221,#60222,#60223,#60224,#60225,#60226,#60227,
#60228,#60229,#60230,#60231,#60232,#60233,#60234,#60235,#60236,#60237,#60238,
#60239,#60240,#60241,#60242,#60243,#60244,#60245,#60246,#60247,#60248,#60249,
#60250,#60251,#60252,#60253,#60254,#60255,#60256,#60257,#60258),
 .UNSPECIFIED.,.F.,.F.,(4,3,3,3,3,3,3,3,3,3,3,3,3,3,3,3,3,3,3,3,3,3,3,3,
3,3,3,3,3,3,3,3,3,3,3,3,3,3,3,3,3,4),(99.6156110735334,99.7194228461579,
99.8232425484925,99.9271733249442,100.031166423026,100.135337924969,100.185594974325,
100.289781443786,100.393812681037,100.497721890031,100.601565644022,100.705378721615,
100.809195857982,100.913121662166,101.0171063098,101.121272881461,101.183123508761,
101.287309756554,101.391340771663,101.49524975888,101.599093291441,101.70290614827,
101.806723064866,101.910648652299,102.014633084558,102.118799445352,102.180652043198,
102.284838632953,102.388869988893,102.492779313656,102.596623181558,102.700436371051,
102.804253617154,102.908179527053,103.012164278294,103.116330949132,103.178180577634,
103.287930451885,103.397356063251,103.506584798371,103.615565394141,103.672557568099),
 .UNSPECIFIED.);
#2323=B_SPLINE_CURVE_WITH_KNOTS('',3,(#60264,#60265,#60266,#60267,#60268,
#60269,#60270,#60271,#60272,#60273,#60274,#60275,#60276,#60277,#60278,#60279,
#60280,#60281,#60282,#60283,#60284,#60285,#60286,#60287,#60288,#60289,#60290,
#60291,#60292,#60293,#60294,#60295,#60296,#60297,#60298,#60299,#60300,#60301,
#60302,#60303,#60304,#60305,#60306,#60307,#60308,#60309,#60310,#60311,#60312,
#60313,#60314,#60315,#60316,#60317,#60318,#60319,#60320,#60321,#60322,#60323,
#60324,#60325,#60326,#60327,#60328,#60329,#60330,#60331,#60332,#60333,#60334,
#60335,#60336,#60337,#60338,#60339,#60340,#60341,#60342,#60343,#60344,#60345,
#60346,#60347,#60348,#60349,#60350,#60351,#60352,#60353,#60354,#60355,#60356,
#60357,#60358,#60359,#60360,#60361,#60362,#60363,#60364,#60365,#60366,#60367,
#60368,#60369,#60370,#60371,#60372,#60373,#60374,#60375,#60376,#60377,#60378,
#60379,#60380,#60381,#60382,#60383,#60384,#60385,#60386,#60387,#60388,#60389,
#60390),.UNSPECIFIED.,.F.,.F.,(4,3,3,3,3,3,3,3,3,3,3,3,3,3,3,3,3,3,3,3,
3,3,3,3,3,3,3,3,3,3,3,3,3,3,3,3,3,3,3,3,3,3,4),(93.3317416570353,93.4356900182446,
93.5397112732845,93.6439007855695,93.6589198280579,93.7631062483201,93.867137435993,
93.9710465950891,94.0748902990129,94.1787033264439,94.2825204126295,94.3864461669513,
94.4904307648283,94.5945972874407,94.6564483624945,94.7606347887181,94.8646659824113,
94.9685751475859,95.0724188576205,95.1762318911854,95.2800489835188,95.3839747439665,
95.4879593479663,95.5921258766296,95.6539768969311,95.7581632966126,95.8621944637261,
95.9661036023919,96.069947285976,96.1737602931869,96.2775773593012,96.3815030939157,
96.4854876722607,96.589654175829,96.6515054313677,96.7545601138384,96.8574737137944,
96.960282655331,97.0675550568191,97.1702894267118,97.2730248740603,97.3758310709248,
97.3893722612835),.UNSPECIFIED.);
#2324=B_SPLINE_CURVE_WITH_KNOTS('',3,(#60391,#60392,#60393,#60394,#60395,
#60396,#60397,#60398,#60399,#60400,#60401,#60402,#60403,#60404,#60405,#60406,
#60407,#60408,#60409,#60410,#60411,#60412,#60413,#60414,#60415,#60416,#60417,
#60418,#60419,#60420,#60421,#60422,#60423,#60424,#60425,#60426,#60427,#60428,
#60429,#60430,#60431,#60432,#60433,#60434,#60435,#60436,#60437,#60438,#60439,
#60440,#60441,#60442,#60443,#60444,#60445,#60446,#60447,#60448,#60449,#60450,
#60451,#60452,#60453,#60454,#60455,#60456,#60457),.UNSPECIFIED.,.F.,.F.,
(4,3,3,3,3,3,3,3,3,3,3,3,3,3,3,3,3,3,3,3,3,3,4),(97.3893722615608,97.5221133461261,
97.6490339658043,97.7532204351495,97.8572516722844,97.961160881162,98.0650046350367,
98.1688177125131,98.2726348487633,98.3765606528317,98.4805453003508,98.5847118718985,
98.6465625002409,98.750750772808,98.8588108833781,98.9627158777204,99.0665559339843,
99.170365829249,99.274180297392,99.3780947560921,99.4820689269285,99.5862024311775,
99.6152316573692),.UNSPECIFIED.);
#2325=B_SPLINE_CURVE_WITH_KNOTS('',3,(#60459,#60460,#60461,#60462,#60463,
#60464,#60465,#60466,#60467,#60468,#60469,#60470,#60471,#60472,#60473,#60474,
#60475,#60476,#60477,#60478,#60479,#60480,#60481,#60482,#60483,#60484,#60485,
#60486,#60487,#60488,#60489,#60490,#60491,#60492,#60493,#60494,#60495,#60496,
#60497,#60498,#60499,#60500,#60501,#60502,#60503,#60504,#60505,#60506,#60507,
#60508,#60509,#60510,#60511,#60512,#60513,#60514,#60515,#60516,#60517,#60518,
#60519,#60520,#60521,#60522,#60523,#60524,#60525),.UNSPECIFIED.,.F.,.F.,
(4,3,3,3,3,3,3,3,3,3,3,3,3,3,3,3,3,3,3,3,3,3,4),(97.389372261676,97.4918503890655,
97.5942398116576,97.6965771922798,97.7988991181241,97.9013122938342,98.0037702233957,
98.1064116155926,98.1905379054514,98.2947243050946,98.3987554721697,98.5026646107974,
98.6065082943435,98.7103213015167,98.8141383675937,98.9180641021713,99.0220486804797,
99.1262151840124,99.1880664398879,99.2949525982993,99.3989655196461,99.5072882965898,
99.6156110735334),.UNSPECIFIED.);
#2326=B_SPLINE_CURVE_WITH_KNOTS('',3,(#60526,#60527,#60528,#60529,#60530,
#60531,#60532,#60533,#60534,#60535,#60536,#60537,#60538,#60539,#60540,#60541,
#60542,#60543,#60544,#60545,#60546,#60547,#60548,#60549,#60550,#60551,#60552,
#60553,#60554,#60555,#60556,#60557,#60558,#60559,#60560,#60561,#60562,#60563,
#60564,#60565,#60566,#60567,#60568,#60569,#60570,#60571,#60572,#60573,#60574,
#60575,#60576,#60577,#60578,#60579,#60580,#60581,#60582,#60583,#60584,#60585,
#60586,#60587,#60588,#60589,#60590,#60591,#60592,#60593,#60594,#60595,#60596,
#60597,#60598,#60599,#60600,#60601,#60602,#60603,#60604,#60605,#60606,#60607,
#60608,#60609,#60610,#60611,#60612,#60613,#60614,#60615,#60616,#60617,#60618,
#60619,#60620,#60621,#60622,#60623,#60624,#60625,#60626,#60627,#60628,#60629,
#60630,#60631,#60632,#60633,#60634,#60635,#60636,#60637,#60638,#60639,#60640,
#60641,#60642,#60643,#60644,#60645,#60646,#60647,#60648,#60649),
 .UNSPECIFIED.,.F.,.F.,(4,3,3,3,3,3,3,3,3,3,3,3,3,3,3,3,3,3,3,3,3,3,3,3,
3,3,3,3,3,3,3,3,3,3,3,3,3,3,3,3,3,4),(93.3327269072094,93.4411890147714,
93.545075652954,93.6489069061472,93.7527175368652,93.8565422742999,93.9604818343983,
94.0644892674887,94.1686696731495,94.2004237677049,94.3046101878998,94.40864137553,
94.5125505346197,94.6163942385596,94.7202072660287,94.8240243522744,94.9279501066888,
95.0319347046769,95.1361012274282,95.1979523021416,95.302138719216,95.4061699037234,
95.5100790597019,95.6139227605392,95.7177357849191,95.8215528680932,95.9254786194841,
96.0294632144714,96.1336297342899,96.1954808365782,96.2996672568408,96.403698444514,
96.5076076036104,96.6114513075345,96.7152643349658,96.8190814211517,96.9230071754736,
97.0269917733508,97.1311582959633,97.1930093710148,97.3433995555629,97.3893722612835),
 .UNSPECIFIED.);
#2327=B_SPLINE_CURVE_WITH_KNOTS('',3,(#60655,#60656,#60657,#60658,#60659,
#60660,#60661,#60662,#60663,#60664,#60665,#60666,#60667,#60668,#60669,#60670,
#60671,#60672,#60673,#60674,#60675,#60676,#60677,#60678,#60679,#60680,#60681,
#60682,#60683,#60684,#60685,#60686,#60687,#60688,#60689,#60690,#60691,#60692,
#60693,#60694,#60695,#60696,#60697,#60698,#60699,#60700,#60701,#60702,#60703,
#60704,#60705,#60706,#60707,#60708,#60709,#60710,#60711,#60712,#60713,#60714,
#60715,#60716,#60717,#60718,#60719,#60720,#60721,#60722,#60723,#60724,#60725,
#60726,#60727,#60728,#60729,#60730,#60731,#60732,#60733,#60734,#60735,#60736,
#60737,#60738,#60739,#60740,#60741,#60742,#60743,#60744,#60745,#60746,#60747,
#60748,#60749,#60750,#60751,#60752,#60753,#60754,#60755,#60756,#60757,#60758,
#60759,#60760,#60761,#60762,#60763,#60764,#60765,#60766,#60767,#60768,#60769,
#60770,#60771,#60772,#60773,#60774,#60775),.UNSPECIFIED.,.F.,.F.,(4,3,3,
3,3,3,3,3,3,3,3,3,3,3,3,3,3,3,3,3,3,3,3,3,3,3,3,3,3,3,3,3,3,3,3,3,3,3,3,
3,4),(87.0493885881288,87.1532100506506,87.2570212560048,87.3612030973632,
87.4651598347553,87.5694542280968,87.6737486214383,87.7779350407011,87.881966227395,
87.9858753855465,88.0897190885474,88.1935321150783,88.297349200388,88.4012749538761,
88.505259550942,88.6094260727875,88.6712771558749,88.775463575262,88.8794947620805,
88.9834039203575,89.0872476234842,89.1910606501409,89.2948777355758,89.3988034891882,
89.502788086378,89.6069546083453,89.6688056903115,89.7729921093415,89.8770232958033,
89.9809324537247,90.0847761564972,90.1885891828012,90.2924062678863,90.3963320211544,
90.5003166180026,90.6044831396363,90.6663342247481,90.7790776483305,90.8915379903017,
91.0035447872594,91.1061869538188),.UNSPECIFIED.);
#2328=B_SPLINE_CURVE_WITH_KNOTS('',3,(#60776,#60777,#60778,#60779,#60780,
#60781,#60782,#60783,#60784,#60785,#60786,#60787,#60788,#60789,#60790,#60791,
#60792,#60793,#60794,#60795,#60796,#60797,#60798,#60799,#60800,#60801,#60802,
#60803,#60804,#60805,#60806,#60807,#60808,#60809,#60810,#60811,#60812,#60813,
#60814,#60815,#60816,#60817,#60818,#60819,#60820,#60821,#60822,#60823,#60824,
#60825,#60826,#60827,#60828,#60829,#60830,#60831,#60832,#60833,#60834,#60835,
#60836,#60837,#60838,#60839,#60840,#60841,#60842,#60843,#60844,#60845),
 .UNSPECIFIED.,.F.,.F.,(4,3,3,3,3,3,3,3,3,3,3,3,3,3,3,3,3,3,3,3,3,3,3,4),
(91.106186954104,91.2126211265272,91.3191385231278,91.425852667608,91.5326811228738,
91.6397298025484,91.6638627591847,91.768049179377,91.8720803670044,91.9759895260916,
92.0798332300288,92.1836462574954,92.2874633437386,92.3913890981505,92.495373696136,
92.5995402188847,92.6613912936213,92.7655571769376,92.8695782420305,92.9734895025858,
93.0773351539117,93.1811423844798,93.28497571317,93.3317416570353),
 .UNSPECIFIED.);
#2329=B_SPLINE_CURVE_WITH_KNOTS('',3,(#60847,#60848,#60849,#60850,#60851,
#60852,#60853,#60854,#60855,#60856,#60857,#60858,#60859,#60860,#60861,#60862,
#60863,#60864,#60865,#60866,#60867,#60868,#60869,#60870,#60871,#60872,#60873,
#60874,#60875,#60876,#60877,#60878,#60879,#60880,#60881,#60882,#60883,#60884,
#60885,#60886,#60887,#60888,#60889,#60890,#60891,#60892,#60893,#60894,#60895,
#60896,#60897,#60898,#60899,#60900,#60901,#60902,#60903,#60904,#60905,#60906,
#60907,#60908,#60909,#60910,#60911,#60912,#60913,#60914,#60915,#60916),
 .UNSPECIFIED.,.F.,.F.,(4,3,3,3,3,3,3,3,3,3,3,3,3,3,3,3,3,3,3,3,3,3,3,4),
(91.106186954104,91.2078381643952,91.3120245837827,91.4160557706019,91.5199649288792,
91.6238086320062,91.7276216586632,91.8314387440987,91.9353644977115,92.0393490949017,
92.1435156168694,92.2053666988318,92.3095531178613,92.4135843043225,92.5174934622435,
92.6213371650153,92.725150191319,92.8289672764033,92.9328930296709,93.0368776265185,
93.1410441481518,93.2028952332684,93.3070788474263,93.3327269072094),
 .UNSPECIFIED.);
#2330=B_SPLINE_CURVE_WITH_KNOTS('',3,(#60917,#60918,#60919,#60920,#60921,
#60922,#60923,#60924,#60925,#60926,#60927,#60928,#60929,#60930,#60931,#60932,
#60933,#60934,#60935,#60936,#60937,#60938,#60939,#60940,#60941,#60942,#60943,
#60944,#60945,#60946,#60947,#60948,#60949,#60950,#60951,#60952,#60953,#60954,
#60955,#60956,#60957,#60958,#60959,#60960,#60961,#60962,#60963,#60964,#60965,
#60966,#60967,#60968,#60969,#60970,#60971,#60972,#60973,#60974,#60975,#60976,
#60977,#60978,#60979,#60980,#60981,#60982,#60983,#60984,#60985,#60986,#60987,
#60988,#60989,#60990,#60991,#60992,#60993,#60994,#60995,#60996,#60997,#60998,
#60999,#61000,#61001,#61002,#61003,#61004,#61005,#61006,#61007,#61008,#61009,
#61010,#61011,#61012,#61013,#61014,#61015,#61016,#61017,#61018,#61019,#61020,
#61021,#61022,#61023,#61024,#61025,#61026,#61027,#61028,#61029,#61030,#61031,
#61032,#61033,#61034,#61035,#61036,#61037,#61038,#61039,#61040),
 .UNSPECIFIED.,.F.,.F.,(4,3,3,3,3,3,3,3,3,3,3,3,3,3,3,3,3,3,3,3,3,3,3,3,
3,3,3,3,3,3,3,3,3,3,3,3,3,3,3,3,3,4),(87.0484498294534,87.1526150410913,
87.2177240266488,87.3219104459156,87.4259416326137,87.5298507907699,87.6336944937756,
87.7375075203117,87.8413246056266,87.9452503591202,88.0492349561918,88.1534014780432,
88.2152525610854,88.3194389803689,88.4234701670837,88.5273793252565,88.631223028279,
88.7350360548318,88.8388531401634,88.9427788936735,89.0467634907616,89.1509300126291,
89.212781095522,89.3169675147653,89.4209987014401,89.5249078595731,89.6287515625559,
89.7325645890692,89.8363816743616,89.9403074278333,90.0442920248832,90.1484585467135,
90.2103096299586,90.3131827203157,90.4158805807014,90.5184806860294,90.621019531032,
90.7235335248247,90.8261208448599,90.9287446854245,91.0315305435812,91.1061869536406),
 .UNSPECIFIED.);
#2331=B_SPLINE_CURVE_WITH_KNOTS('',3,(#61046,#61047,#61048,#61049,#61050,
#61051,#61052,#61053,#61054,#61055,#61056,#61057,#61058,#61059,#61060,#61061,
#61062,#61063,#61064,#61065,#61066,#61067,#61068,#61069,#61070,#61071,#61072,
#61073,#61074,#61075,#61076,#61077,#61078,#61079,#61080,#61081,#61082,#61083,
#61084,#61085,#61086,#61087,#61088,#61089,#61090,#61091,#61092,#61093,#61094,
#61095,#61096,#61097,#61098,#61099,#61100,#61101,#61102,#61103,#61104,#61105,
#61106,#61107,#61108,#61109,#61110,#61111,#61112,#61113,#61114,#61115,#61116,
#61117,#61118,#61119,#61120,#61121,#61122,#61123,#61124,#61125,#61126,#61127,
#61128,#61129,#61130,#61131,#61132,#61133,#61134,#61135,#61136,#61137,#61138,
#61139,#61140,#61141,#61142,#61143,#61144,#61145,#61146,#61147,#61148,#61149,
#61150,#61151,#61152,#61153,#61154,#61155,#61156,#61157,#61158,#61159,#61160,
#61161,#61162,#61163,#61164,#61165,#61166),.UNSPECIFIED.,.F.,.F.,(4,3,3,
3,3,3,3,3,3,3,3,3,3,3,3,3,3,3,3,3,3,3,3,3,3,3,3,3,3,3,3,3,3,3,3,3,3,3,3,
3,4),(80.7662045556485,80.8702751267713,80.9742087479646,81.0780672034999,
81.1818852904301,81.2856977526014,81.3896126700318,81.4935777329238,81.5977339187956,
81.6885774148187,81.792763834087,81.8967950207866,82.0007041789443,82.1045478819516,
82.2083609084893,82.3121779938057,82.416103747301,82.5200883443742,82.6242548662273,
82.6861059492553,82.7902923685257,82.8943235552275,82.9982327133873,83.1020764163968,
83.2058894429367,83.3097065282554,83.4136322817528,83.5176168788281,83.6217834006832,
83.6836344836919,83.787820902958,83.8918520896554,83.9957612478108,84.099604950816,
84.2034179773515,84.3072350626659,84.4111608161591,84.5151454132304,84.6193119350814,
84.6811630181285,84.8230016469244),.UNSPECIFIED.);
#2332=B_SPLINE_CURVE_WITH_KNOTS('',3,(#61167,#61168,#61169,#61170,#61171,
#61172,#61173,#61174,#61175,#61176,#61177,#61178,#61179,#61180,#61181,#61182,
#61183,#61184,#61185,#61186,#61187,#61188,#61189,#61190,#61191,#61192,#61193,
#61194,#61195,#61196,#61197,#61198,#61199,#61200,#61201,#61202,#61203,#61204,
#61205,#61206,#61207,#61208,#61209,#61210,#61211,#61212,#61213,#61214,#61215,
#61216,#61217,#61218,#61219,#61220,#61221,#61222,#61223,#61224,#61225,#61226,
#61227,#61228,#61229,#61230,#61231,#61232,#61233,#61234,#61235,#61236),
 .UNSPECIFIED.,.F.,.F.,(4,3,3,3,3,3,3,3,3,3,3,3,3,3,3,3,3,3,3,3,3,3,3,4),
(84.8230016473368,84.9299628854903,85.0323879596833,85.1347430254586,85.2370647046657,
85.3393895675522,85.4418181479453,85.544308232961,85.6469663801133,85.6786915525651,
85.7828779718485,85.8869091585633,85.9908183167361,86.0946620197585,86.1984750463114,
86.3022921316428,86.4062178851529,86.510202482241,86.6143690041085,86.6762200870017,
86.7803789666152,86.8844021488389,86.9883093146419,87.0493885881288),
 .UNSPECIFIED.);
#2333=B_SPLINE_CURVE_WITH_KNOTS('',3,(#61238,#61239,#61240,#61241,#61242,
#61243,#61244,#61245,#61246,#61247,#61248,#61249,#61250,#61251,#61252,#61253,
#61254,#61255,#61256,#61257,#61258,#61259,#61260,#61261,#61262,#61263,#61264,
#61265,#61266,#61267,#61268,#61269,#61270,#61271,#61272,#61273,#61274,#61275,
#61276,#61277,#61278,#61279,#61280,#61281,#61282,#61283,#61284,#61285,#61286,
#61287,#61288,#61289,#61290,#61291,#61292,#61293,#61294,#61295,#61296,#61297,
#61298,#61299,#61300,#61301,#61302,#61303,#61304),.UNSPECIFIED.,.F.,.F.,
(4,3,3,3,3,3,3,3,3,3,3,3,3,3,3,3,3,3,3,3,3,3,4),(84.8230016473359,84.9377580239963,
85.0529300598084,85.1686593350748,85.2226669577756,85.3268533770461,85.4308845637479,
85.5347937219076,85.6386374249172,85.742450451457,85.8462675367755,85.9501932902729,
86.0541778873482,86.1583444092033,86.2201954922122,86.3243482554789,86.4283607948039,
86.5322681022207,86.6361050469233,86.739945971975,86.8437814338426,86.947723902542,
87.0484498294534),.UNSPECIFIED.);
#2334=B_SPLINE_CURVE_WITH_KNOTS('',3,(#61305,#61306,#61307,#61308,#61309,
#61310,#61311,#61312,#61313,#61314,#61315,#61316,#61317,#61318,#61319,#61320,
#61321,#61322,#61323,#61324,#61325,#61326,#61327,#61328,#61329,#61330,#61331,
#61332,#61333,#61334,#61335,#61336,#61337,#61338,#61339,#61340,#61341,#61342,
#61343,#61344,#61345,#61346,#61347,#61348,#61349,#61350,#61351,#61352,#61353,
#61354,#61355,#61356,#61357,#61358,#61359,#61360,#61361,#61362,#61363,#61364,
#61365,#61366,#61367,#61368,#61369,#61370,#61371,#61372,#61373,#61374,#61375,
#61376,#61377,#61378,#61379,#61380,#61381,#61382,#61383,#61384,#61385,#61386,
#61387,#61388,#61389,#61390,#61391,#61392,#61393,#61394,#61395,#61396,#61397,
#61398,#61399,#61400,#61401,#61402,#61403,#61404,#61405,#61406,#61407,#61408,
#61409,#61410,#61411,#61412,#61413,#61414,#61415,#61416,#61417,#61418,#61419,
#61420,#61421,#61422,#61423,#61424,#61425,#61426,#61427,#61428),
 .UNSPECIFIED.,.F.,.F.,(4,3,3,3,3,3,3,3,3,3,3,3,3,3,3,3,3,3,3,3,3,3,3,3,
3,3,3,3,3,3,3,3,3,3,3,3,3,3,3,3,3,4),(80.76574074697,80.8695602808333,80.9734907573594,
81.0774833634171,81.1816545661312,81.2325528200292,81.3367392392979,81.4407704259977,
81.5446795841557,81.6485232871634,81.7523363137014,81.8561533990182,81.9600791525138,
82.0640637495873,82.1682302714407,82.2300813544658,82.3342677737346,82.438298960435,
82.5422081185932,82.6460518216011,82.7498648481394,82.8536819334565,82.9576076869522,
83.0615922840261,83.1657588058797,83.2276098889024,83.3317963081708,83.4358274948703,
83.539736653028,83.6435803560355,83.7473933825735,83.8512104678899,83.9551362213854,
84.0591208184588,84.1632873403121,84.225138423339,84.3308712802875,84.4364337114794,
84.5418329411289,84.6471360606506,84.7523779621414,84.8230016469245),
 .UNSPECIFIED.);
#2335=B_SPLINE_CURVE_WITH_KNOTS('',3,(#61434,#61435,#61436,#61437,#61438,
#61439,#61440,#61441,#61442,#61443,#61444,#61445,#61446,#61447,#61448,#61449,
#61450,#61451,#61452,#61453,#61454,#61455,#61456,#61457,#61458,#61459,#61460,
#61461,#61462,#61463,#61464,#61465,#61466,#61467,#61468,#61469,#61470,#61471,
#61472,#61473,#61474,#61475,#61476,#61477,#61478,#61479,#61480,#61481,#61482,
#61483,#61484,#61485,#61486,#61487,#61488,#61489,#61490,#61491,#61492,#61493,
#61494,#61495,#61496,#61497,#61498,#61499,#61500,#61501,#61502,#61503,#61504,
#61505,#61506,#61507,#61508,#61509,#61510,#61511,#61512,#61513,#61514,#61515,
#61516,#61517,#61518,#61519,#61520,#61521,#61522,#61523,#61524,#61525,#61526,
#61527,#61528,#61529,#61530,#61531,#61532,#61533,#61534,#61535,#61536,#61537,
#61538,#61539,#61540,#61541,#61542,#61543,#61544,#61545,#61546,#61547,#61548,
#61549,#61550,#61551,#61552,#61553,#61554,#61555,#61556,#61557,#61558,#61559,
#61560),.UNSPECIFIED.,.F.,.F.,(4,3,3,3,3,3,3,3,3,3,3,3,3,3,3,3,3,3,3,3,
3,3,3,3,3,3,3,3,3,3,3,3,3,3,3,3,3,3,3,3,3,3,4),(74.482061581652,74.5860823401427,
74.6902715180945,74.7058776737625,74.8100640930311,74.9140952797311,75.0180044378891,
75.1218481408968,75.2256611674348,75.3294782527516,75.4334040062472,75.5373886033208,
75.6415551251742,75.7034062081991,75.8075926274677,75.9116238141677,76.0155329723257,
76.1193766753334,76.2231897018714,76.3270067871883,76.4309325406839,76.5349171377575,
76.6390836596109,76.7009347426357,76.8051211619044,76.9091523486044,77.0130615067624,
77.1169052097702,77.2207182363082,77.3245353216251,77.4284610751208,77.5324456721944,
77.6366121940478,77.6984632770723,77.8036324098607,77.9060965907541,78.0084634414062,
78.1107696824821,78.2180313467064,78.3203753326912,78.4227592903787,78.5252692706971,
78.5398163393791),.UNSPECIFIED.);
#2336=B_SPLINE_CURVE_WITH_KNOTS('',3,(#61561,#61562,#61563,#61564,#61565,
#61566,#61567,#61568,#61569,#61570,#61571,#61572,#61573,#61574,#61575,#61576,
#61577,#61578,#61579,#61580,#61581,#61582,#61583,#61584,#61585,#61586,#61587,
#61588,#61589,#61590,#61591,#61592,#61593,#61594,#61595,#61596,#61597,#61598,
#61599,#61600,#61601,#61602,#61603,#61604,#61605,#61606,#61607,#61608,#61609,
#61610,#61611,#61612,#61613,#61614,#61615,#61616,#61617,#61618,#61619,#61620,
#61621,#61622,#61623,#61624,#61625,#61626,#61627),.UNSPECIFIED.,.F.,.F.,
(4,3,3,3,3,3,3,3,3,3,3,3,3,3,3,3,3,3,3,3,3,3,4),(78.5398163397449,78.6959918115089,
78.8001782307774,78.9042094174774,79.0081185756353,79.111962278643,79.2157753051809,
79.3195923904978,79.4235181439933,79.5275027410669,79.6316692629202,79.6935203459455,
79.7977067652144,79.9017379519145,80.0056471100728,80.1094908130807,80.2133038396189,
80.317120924936,80.4210466784318,80.5250312755056,80.6291977973592,80.6910488803821,
80.7662045556485),.UNSPECIFIED.);
#2337=B_SPLINE_CURVE_WITH_KNOTS('',3,(#61629,#61630,#61631,#61632,#61633,
#61634,#61635,#61636,#61637,#61638,#61639,#61640,#61641,#61642,#61643,#61644,
#61645,#61646,#61647,#61648,#61649,#61650,#61651,#61652,#61653,#61654,#61655,
#61656,#61657,#61658,#61659,#61660,#61661,#61662,#61663,#61664,#61665,#61666,
#61667,#61668,#61669,#61670,#61671,#61672,#61673,#61674,#61675,#61676,#61677,
#61678,#61679,#61680,#61681,#61682,#61683,#61684,#61685,#61686,#61687,#61688,
#61689,#61690,#61691,#61692,#61693,#61694,#61695),.UNSPECIFIED.,.F.,.F.,
(4,3,3,3,3,3,3,3,3,3,3,3,3,3,3,3,3,3,3,3,3,3,4),(78.5398163397448,78.6430648259428,
78.7462751676037,78.8494829022752,78.9527963206924,79.0561639752372,79.1597213368926,
79.237495751156,79.3416821704247,79.4457133571247,79.5496225152827,79.6534662182905,
79.7572792448284,79.8610963301453,79.9650220836409,80.0690066807144,80.1731732025678,
80.2350242855926,80.3392063862691,80.4458399764443,80.5497449585483,80.6577428527591,
80.76574074697),.UNSPECIFIED.);
#2338=B_SPLINE_CURVE_WITH_KNOTS('',3,(#61696,#61697,#61698,#61699,#61700,
#61701,#61702,#61703,#61704,#61705,#61706,#61707,#61708,#61709,#61710,#61711,
#61712,#61713,#61714,#61715,#61716,#61717,#61718,#61719,#61720,#61721,#61722,
#61723,#61724,#61725,#61726,#61727,#61728,#61729,#61730,#61731,#61732,#61733,
#61734,#61735,#61736,#61737,#61738,#61739,#61740,#61741,#61742,#61743,#61744,
#61745,#61746,#61747,#61748,#61749,#61750,#61751,#61752,#61753,#61754,#61755,
#61756,#61757,#61758,#61759,#61760,#61761,#61762,#61763,#61764,#61765,#61766,
#61767,#61768,#61769,#61770,#61771,#61772,#61773,#61774,#61775,#61776,#61777,
#61778,#61779,#61780,#61781,#61782,#61783,#61784,#61785,#61786,#61787,#61788,
#61789,#61790,#61791,#61792,#61793,#61794,#61795,#61796,#61797,#61798,#61799,
#61800,#61801,#61802,#61803,#61804,#61805,#61806,#61807,#61808,#61809,#61810,
#61811,#61812,#61813,#61814,#61815,#61816,#61817,#61818,#61819),
 .UNSPECIFIED.,.F.,.F.,(4,3,3,3,3,3,3,3,3,3,3,3,3,3,3,3,3,3,3,3,3,3,3,3,
3,3,3,3,3,3,3,3,3,3,3,3,3,3,3,3,3,4),(74.4832427137469,74.5871328253029,
74.6909659100892,74.7947767330557,74.898600024183,75.0025371546479,75.1065406853698,
75.2107186073821,75.2473816134096,75.3515680326783,75.4555992193782,75.5595083775362,
75.663352080544,75.7671651070821,75.8709821923987,75.9749079458944,76.0788925429681,
76.1830590648215,76.2449101478462,76.3490965671148,76.453127753815,76.557036911973,
76.6608806149807,76.7646936415184,76.8685107268352,76.9724364803309,77.0764210774044,
77.1805875992577,77.2424386822828,77.3466251015514,77.4506562882513,77.5545654464092,
77.658409149417,77.7622221759551,77.866039261272,77.9699650147675,78.0739496118412,
78.1781161336946,78.2399672167194,78.3667743014798,78.4918646575237,78.5398163394183),
 .UNSPECIFIED.);
#2339=B_SPLINE_CURVE_WITH_KNOTS('',3,(#61825,#61826,#61827,#61828,#61829,
#61830,#61831,#61832,#61833,#61834,#61835,#61836,#61837,#61838,#61839,#61840,
#61841,#61842,#61843,#61844,#61845,#61846,#61847,#61848,#61849,#61850,#61851,
#61852,#61853,#61854,#61855,#61856,#61857,#61858,#61859,#61860,#61861,#61862,
#61863,#61864,#61865,#61866,#61867,#61868,#61869,#61870,#61871,#61872,#61873,
#61874,#61875,#61876,#61877,#61878,#61879,#61880,#61881,#61882,#61883,#61884,
#61885,#61886,#61887,#61888,#61889,#61890,#61891,#61892,#61893,#61894,#61895,
#61896,#61897,#61898,#61899,#61900,#61901,#61902,#61903,#61904,#61905,#61906,
#61907,#61908,#61909,#61910,#61911,#61912,#61913,#61914,#61915,#61916,#61917,
#61918,#61919,#61920,#61921,#61922,#61923,#61924,#61925,#61926,#61927,#61928,
#61929,#61930,#61931,#61932,#61933,#61934,#61935,#61936,#61937,#61938,#61939,
#61940,#61941,#61942,#61943,#61944,#61945),.UNSPECIFIED.,.F.,.F.,(4,3,3,
3,3,3,3,3,3,3,3,3,3,3,3,3,3,3,3,3,3,3,3,3,3,3,3,3,3,3,3,3,3,3,3,3,3,3,3,
3,4),(68.1995378123589,68.303348975242,68.4076883482173,68.5116448055075,
68.6161756363252,68.7207064671429,68.8248928864116,68.9289240731113,69.0328332312694,
69.1366769342771,69.2404899608151,69.3443070461318,69.4482327996275,69.5522173967011,
69.6563839185545,69.7182350015795,69.8224214208481,69.9264526075479,70.0303617657059,
70.1342054687136,70.2380184952514,70.3418355805683,70.4457613340638,70.5497459311376,
70.653912452991,70.7157635360161,70.8199499552846,70.9239811419846,71.0278903001425,
71.1317340031501,71.2355470296882,71.339364115005,71.4432898685007,71.5472744655741,
71.6514409874275,71.7132920704527,71.8208733890792,71.9298127999507,72.0369795361949,
72.1468052843801,72.2566310325652),.UNSPECIFIED.);
#2340=B_SPLINE_CURVE_WITH_KNOTS('',3,(#61946,#61947,#61948,#61949,#61950,
#61951,#61952,#61953,#61954,#61955,#61956,#61957,#61958,#61959,#61960,#61961,
#61962,#61963,#61964,#61965,#61966,#61967,#61968,#61969,#61970,#61971,#61972,
#61973,#61974,#61975,#61976,#61977,#61978,#61979,#61980,#61981,#61982,#61983,
#61984,#61985,#61986,#61987,#61988,#61989,#61990,#61991,#61992,#61993,#61994,
#61995,#61996,#61997,#61998,#61999,#62000,#62001,#62002,#62003,#62004,#62005,
#62006,#62007,#62008,#62009,#62010,#62011,#62012),.UNSPECIFIED.,.F.,.F.,
(4,3,3,3,3,3,3,3,3,3,3,3,3,3,3,3,3,3,3,3,3,3,4),(72.2566310330111,72.3701784259807,
72.4815873942032,72.5962039995462,72.7108206048893,72.8150070241579,72.9190382108579,
73.022947369016,73.1267910720237,73.2306040985618,73.3344211838786,73.4383469373742,
73.5423315344479,73.6464980563013,73.7083491393259,73.8125058091446,73.9165206688818,
74.0204287176382,74.1242648292319,74.2280916123974,74.3319123054245,74.4358068055344,
74.482061581652),.UNSPECIFIED.);
#2341=B_SPLINE_CURVE_WITH_KNOTS('',3,(#62014,#62015,#62016,#62017,#62018,
#62019,#62020,#62021,#62022,#62023,#62024,#62025,#62026,#62027,#62028,#62029,
#62030,#62031,#62032,#62033,#62034,#62035,#62036,#62037,#62038,#62039,#62040,
#62041,#62042,#62043,#62044,#62045,#62046,#62047,#62048,#62049,#62050,#62051,
#62052,#62053,#62054,#62055,#62056,#62057,#62058,#62059,#62060,#62061,#62062,
#62063,#62064,#62065,#62066,#62067,#62068,#62069,#62070,#62071,#62072,#62073,
#62074,#62075,#62076,#62077,#62078,#62079,#62080,#62081,#62082,#62083),
 .UNSPECIFIED.,.F.,.F.,(4,3,3,3,3,3,3,3,3,3,3,3,3,3,3,3,3,3,3,3,3,3,3,4),
(72.2566310325652,72.3607828828408,72.4647795326403,72.5686542861375,72.6724637223968,
72.7762426721719,72.880025922937,72.9839179050169,73.0878690474532,73.1920015684937,
73.2523245445364,73.3565109638049,73.4605421505048,73.5644513086627,73.6682950116704,
73.7721080382084,73.8759251235251,73.9798508770207,74.0838354740943,74.1880019959476,
74.249853078973,74.3540440480012,74.4580688912286,74.4832427137469),
 .UNSPECIFIED.);
#2342=B_SPLINE_CURVE_WITH_KNOTS('',3,(#62084,#62085,#62086,#62087,#62088,
#62089,#62090,#62091,#62092,#62093,#62094,#62095,#62096,#62097,#62098,#62099,
#62100,#62101,#62102,#62103,#62104,#62105,#62106,#62107,#62108,#62109,#62110,
#62111,#62112,#62113,#62114,#62115,#62116,#62117,#62118,#62119,#62120,#62121,
#62122,#62123,#62124,#62125,#62126,#62127,#62128,#62129,#62130,#62131,#62132,
#62133,#62134,#62135,#62136,#62137,#62138,#62139,#62140,#62141,#62142,#62143,
#62144,#62145,#62146,#62147,#62148,#62149,#62150,#62151,#62152,#62153,#62154,
#62155,#62156,#62157,#62158,#62159,#62160,#62161,#62162,#62163,#62164,#62165,
#62166,#62167,#62168,#62169,#62170,#62171,#62172,#62173,#62174,#62175,#62176,
#62177,#62178,#62179,#62180,#62181,#62182,#62183,#62184,#62185,#62186,#62187,
#62188,#62189,#62190,#62191,#62192,#62193,#62194,#62195,#62196,#62197,#62198,
#62199,#62200,#62201,#62202,#62203,#62204,#62205,#62206,#62207,#62208,#62209,
#62210),.UNSPECIFIED.,.F.,.F.,(4,3,3,3,3,3,3,3,3,3,3,3,3,3,3,3,3,3,3,3,
3,3,3,3,3,3,3,3,3,3,3,3,3,3,3,3,3,3,3,3,3,3,4),(68.1991393899546,68.2646818723534,
68.368868291622,68.4728994783219,68.5768086364799,68.6806523394876,68.7844653660256,
68.8882824513424,68.992208204838,69.0961928019116,69.200359323765,69.26221040679,
69.3663968260586,69.4704280127586,69.5743371709166,69.6781808739243,69.7819939004623,
69.8858109857791,69.9897367392748,70.0937213363484,70.1978878582018,70.2597389412266,
70.3639253604953,70.4679565471953,70.5718657053533,70.675709408361,70.779522434899,
70.8833395202159,70.9872652737115,71.0912498707852,71.1954163926385,71.2572674756632,
71.3614538949318,71.4654850816318,71.5693942397898,71.6732379427976,71.7770509693356,
71.8808680546524,71.9847938081481,72.0887784052216,72.192944927075,72.2547960100998,
72.256631032138),.UNSPECIFIED.);
#2343=B_SPLINE_CURVE_WITH_KNOTS('',3,(#62216,#62217,#62218,#62219,#62220,
#62221,#62222,#62223,#62224,#62225,#62226,#62227,#62228,#62229,#62230,#62231,
#62232,#62233,#62234,#62235,#62236,#62237,#62238,#62239,#62240,#62241,#62242,
#62243,#62244,#62245,#62246,#62247,#62248,#62249,#62250,#62251,#62252,#62253,
#62254,#62255,#62256,#62257,#62258,#62259,#62260,#62261,#62262,#62263,#62264,
#62265,#62266,#62267,#62268,#62269,#62270,#62271,#62272,#62273,#62274,#62275,
#62276,#62277,#62278,#62279,#62280,#62281,#62282,#62283,#62284,#62285,#62286,
#62287,#62288,#62289,#62290,#62291,#62292,#62293,#62294,#62295,#62296,#62297,
#62298,#62299,#62300,#62301,#62302,#62303,#62304,#62305,#62306,#62307,#62308,
#62309,#62310,#62311,#62312,#62313,#62314,#62315,#62316,#62317,#62318,#62319,
#62320,#62321,#62322,#62323,#62324,#62325,#62326,#62327,#62328,#62329,#62330,
#62331,#62332,#62333,#62334,#62335,#62336),.UNSPECIFIED.,.F.,.F.,(4,3,3,
3,3,3,3,3,3,3,3,3,3,3,3,3,3,3,3,3,3,3,3,3,3,3,3,3,3,3,3,3,3,3,3,3,3,3,3,
3,4),(61.916866067234,62.0208000153523,62.1246586748948,62.2284768431646,
62.332289264134,62.436204059969,62.5401688912189,62.6443249654368,62.7355352605233,
62.8397216797919,62.9437528664919,63.0476620246499,63.1515057276576,63.2553187541956,
63.3591358395125,63.4630615930081,63.5670461900817,63.6712127119351,63.7330637949599,
63.8372502142285,63.9412814009285,64.0451905590865,64.1490342620942,64.2528472886322,
64.3566643739491,64.4605901274447,64.5645747245183,64.6687412463717,64.7305923293965,
64.8347787486651,64.9388099353651,65.0427190935231,65.1465627965308,65.2503758230689,
65.3541929083857,65.4581186618813,65.5621032589549,65.6662697808083,65.7281208638331,
65.8639211020862,65.9734457249235),.UNSPECIFIED.);
#2344=B_SPLINE_CURVE_WITH_KNOTS('',3,(#62337,#62338,#62339,#62340,#62341,
#62342,#62343,#62344,#62345,#62346,#62347,#62348,#62349,#62350,#62351,#62352,
#62353,#62354,#62355,#62356,#62357,#62358,#62359,#62360,#62361,#62362,#62363,
#62364,#62365,#62366,#62367,#62368,#62369,#62370,#62371,#62372,#62373,#62374,
#62375,#62376,#62377,#62378,#62379,#62380,#62381,#62382,#62383,#62384,#62385,
#62386,#62387,#62388,#62389,#62390,#62391,#62392,#62393,#62394,#62395,#62396,
#62397,#62398,#62399,#62400,#62401,#62402,#62403,#62404,#62405,#62406),
 .UNSPECIFIED.,.F.,.F.,(4,3,3,3,3,3,3,3,3,3,3,3,3,3,3,3,3,3,3,3,3,3,3,4),
(65.9734457253856,66.0761394376291,66.1787659097615,66.2813614741682,66.3839624163265,
66.4866699517349,66.5894404069822,66.6923813783738,66.7256493982697,66.8298358175384,
66.9338670042384,67.0377761623964,67.1416198654042,67.2454328919421,67.3492499772588,
67.4531757307544,67.557160327828,67.6613268496814,67.7231779327063,67.8273675151293,
67.9313793154479,68.0352880094723,68.1391301362491,68.1995378123589),
 .UNSPECIFIED.);
#2345=B_SPLINE_CURVE_WITH_KNOTS('',3,(#62408,#62409,#62410,#62411,#62412,
#62413,#62414,#62415,#62416,#62417,#62418,#62419,#62420,#62421,#62422,#62423,
#62424,#62425,#62426,#62427,#62428,#62429,#62430,#62431,#62432,#62433,#62434,
#62435,#62436,#62437,#62438,#62439,#62440,#62441,#62442,#62443,#62444,#62445,
#62446,#62447,#62448,#62449,#62450,#62451,#62452,#62453,#62454,#62455,#62456,
#62457,#62458,#62459,#62460,#62461,#62462,#62463,#62464,#62465,#62466,#62467,
#62468,#62469,#62470,#62471,#62472,#62473,#62474),.UNSPECIFIED.,.F.,.F.,
(4,3,3,3,3,3,3,3,3,3,3,3,3,3,3,3,3,3,3,3,3,3,4),(65.973445725698,66.0988776153497,
66.226129946551,66.2696248034802,66.3738112227488,66.4778424094487,66.5817515676067,
66.6855952706144,66.7894082971523,66.8932253824693,66.9971511359649,67.1011357330385,
67.2053022548918,67.2671533379168,67.3713444216424,67.4753543191426,67.5792620015281,
67.6831023303074,67.7869100855494,67.8907809267929,67.9946786620491,68.0987368470952,
68.1991393899546),.UNSPECIFIED.);
#2346=B_SPLINE_CURVE_WITH_KNOTS('',3,(#62475,#62476,#62477,#62478,#62479,
#62480,#62481,#62482,#62483,#62484,#62485,#62486,#62487,#62488,#62489,#62490,
#62491,#62492,#62493,#62494,#62495,#62496,#62497,#62498,#62499,#62500,#62501,
#62502,#62503,#62504,#62505,#62506,#62507,#62508,#62509,#62510,#62511,#62512,
#62513,#62514,#62515,#62516,#62517,#62518,#62519,#62520,#62521,#62522,#62523,
#62524,#62525,#62526,#62527,#62528,#62529,#62530,#62531,#62532,#62533,#62534,
#62535,#62536,#62537,#62538,#62539,#62540,#62541,#62542,#62543,#62544,#62545,
#62546,#62547,#62548,#62549,#62550,#62551,#62552,#62553,#62554,#62555,#62556,
#62557,#62558,#62559,#62560,#62561,#62562,#62563,#62564,#62565,#62566,#62567,
#62568,#62569,#62570,#62571,#62572,#62573,#62574,#62575,#62576,#62577,#62578,
#62579,#62580,#62581,#62582,#62583,#62584,#62585,#62586,#62587,#62588,#62589,
#62590,#62591,#62592,#62593,#62594,#62595,#62596,#62597,#62598),
 .UNSPECIFIED.,.F.,.F.,(4,3,3,3,3,3,3,3,3,3,3,3,3,3,3,3,3,3,3,3,3,3,3,3,
3,3,3,3,3,3,3,3,3,3,3,3,3,3,3,3,3,4),(61.9158957506032,62.0198259490519,
62.1238180900071,62.2279890148855,62.2795106657338,62.3836970850024,62.4877282717021,
62.5916374298601,62.6954811328678,62.7992941594057,62.9031112447225,63.0070369982182,
63.1110215952918,63.2151881171452,63.2770392001704,63.3812256194391,63.4852568061391,
63.5891659642971,63.6930096673048,63.7968226938427,63.9006397791598,64.0045655326555,
64.1085501297291,64.2127166515826,64.274567734607,64.3787541538756,64.4827853405758,
64.5866944987338,64.6905382017415,64.7943512282798,64.8981683135967,65.0020940670924,
65.1060786641661,65.2102451860196,65.2720962690436,65.3756018854378,65.4789620265338,
65.5822125841125,65.6854054642092,65.7885610860738,65.8917634870123,65.9734457253856),
 .UNSPECIFIED.);
#2347=B_SPLINE_CURVE_WITH_KNOTS('',3,(#62604,#62605,#62606,#62607,#62608,
#62609,#62610,#62611,#62612,#62613,#62614,#62615,#62616,#62617,#62618,#62619,
#62620,#62621,#62622,#62623,#62624,#62625,#62626,#62627,#62628,#62629,#62630,
#62631,#62632,#62633,#62634,#62635,#62636,#62637,#62638,#62639,#62640,#62641,
#62642,#62643,#62644,#62645,#62646,#62647,#62648,#62649,#62650,#62651,#62652,
#62653,#62654,#62655,#62656,#62657,#62658,#62659,#62660,#62661,#62662,#62663,
#62664,#62665,#62666,#62667,#62668,#62669,#62670,#62671,#62672,#62673,#62674,
#62675,#62676,#62677,#62678,#62679,#62680,#62681,#62682,#62683,#62684,#62685,
#62686,#62687,#62688,#62689,#62690,#62691,#62692,#62693,#62694,#62695,#62696,
#62697,#62698,#62699,#62700,#62701,#62702,#62703,#62704,#62705,#62706,#62707,
#62708,#62709,#62710,#62711,#62712,#62713,#62714,#62715,#62716,#62717,#62718,
#62719,#62720,#62721,#62722,#62723,#62724,#62725,#62726,#62727,#62728,#62729,
#62730),.UNSPECIFIED.,.F.,.F.,(4,3,3,3,3,3,3,3,3,3,3,3,3,3,3,3,3,3,3,3,
3,3,3,3,3,3,3,3,3,3,3,3,3,3,3,3,3,3,3,3,3,3,4),(55.6326012668771,55.7367901940337,
55.7528355194671,55.8570219387357,55.9610531254356,56.0649622835936,56.1688059866013,
56.2726190131393,56.3764360984561,56.4803618519517,56.5843464490253,56.6885129708787,
56.7503640539037,56.8545504731724,56.9585816598724,57.0624908180304,57.1663345210382,
57.2701475475762,57.3739646328931,57.4778903863887,57.5818749834624,57.6860415053158,
57.7478925883403,57.8520790076089,57.9561101943089,58.0600193524668,58.1638630554745,
58.2676760820125,58.3714931673293,58.4754189208249,58.5794035178985,58.6835700397519,
58.7454211227769,58.8487780338705,58.95396333187,59.0570447634803,59.160064366593,
59.2630580262836,59.3698586241792,59.4729706208884,59.5761501528113,59.679489744252,
59.6902604178662),.UNSPECIFIED.);
#2348=B_SPLINE_CURVE_WITH_KNOTS('',3,(#62731,#62732,#62733,#62734,#62735,
#62736,#62737,#62738,#62739,#62740,#62741,#62742,#62743,#62744,#62745,#62746,
#62747,#62748,#62749,#62750,#62751,#62752,#62753,#62754,#62755,#62756,#62757,
#62758,#62759,#62760,#62761,#62762,#62763,#62764,#62765,#62766,#62767,#62768,
#62769,#62770,#62771,#62772,#62773,#62774,#62775,#62776,#62777,#62778,#62779,
#62780,#62781,#62782,#62783,#62784,#62785,#62786,#62787,#62788,#62789,#62790,
#62791,#62792,#62793,#62794,#62795,#62796,#62797,#62798,#62799,#62800),
 .UNSPECIFIED.,.F.,.F.,(4,3,3,3,3,3,3,3,3,3,3,3,3,3,3,3,3,3,3,3,3,3,3,4),
(59.690260418206,59.7429496572135,59.8471360764822,59.9511672631822,60.0550764213402,
60.1589201243479,60.2627331508859,60.3665502362028,60.4704759896984,60.574460586772,
60.6786271086254,60.7404781916501,60.8446646109187,60.9486957976186,61.0526049557766,
61.1564486587843,61.2602616853224,61.3640787706392,61.4680045241348,61.5719891212084,
61.6761556430618,61.7380067260867,61.8421682999702,61.916866067234),
 .UNSPECIFIED.);
#2349=B_SPLINE_CURVE_WITH_KNOTS('',3,(#62802,#62803,#62804,#62805,#62806,
#62807,#62808,#62809,#62810,#62811,#62812,#62813,#62814,#62815,#62816,#62817,
#62818,#62819,#62820,#62821,#62822,#62823,#62824,#62825,#62826,#62827,#62828,
#62829,#62830,#62831,#62832,#62833,#62834,#62835,#62836,#62837,#62838,#62839,
#62840,#62841,#62842,#62843,#62844,#62845,#62846,#62847,#62848,#62849,#62850,
#62851,#62852,#62853,#62854,#62855,#62856,#62857,#62858,#62859,#62860,#62861,
#62862,#62863,#62864,#62865,#62866,#62867,#62868),.UNSPECIFIED.,.F.,.F.,
(4,3,3,3,3,3,3,3,3,3,3,3,3,3,3,3,3,3,3,3,3,3,4),(59.690260418206,59.7955870148004,
59.900955252961,60.0064809160437,60.1120913042759,60.2179183210518,60.2844535968606,
60.3886400161293,60.4926712028292,60.5965803609872,60.7004240639949,60.804237090533,
60.9080541758499,61.0119799293455,61.115964526419,61.2201310482724,61.2819821312972,
61.3861518308917,61.4901756511522,61.5966056760149,61.7004458108553,61.8081707807292,
61.9158957506032),.UNSPECIFIED.);
#2350=B_SPLINE_CURVE_WITH_KNOTS('',3,(#62869,#62870,#62871,#62872,#62873,
#62874,#62875,#62876,#62877,#62878,#62879,#62880,#62881,#62882,#62883,#62884,
#62885,#62886,#62887,#62888,#62889,#62890,#62891,#62892,#62893,#62894,#62895,
#62896,#62897,#62898,#62899,#62900,#62901,#62902,#62903,#62904,#62905,#62906,
#62907,#62908,#62909,#62910,#62911,#62912,#62913,#62914,#62915,#62916,#62917,
#62918,#62919,#62920,#62921,#62922,#62923,#62924,#62925,#62926,#62927,#62928,
#62929,#62930,#62931,#62932,#62933,#62934,#62935,#62936,#62937,#62938,#62939,
#62940,#62941,#62942,#62943,#62944,#62945,#62946,#62947,#62948,#62949,#62950,
#62951,#62952,#62953,#62954,#62955,#62956,#62957,#62958,#62959,#62960,#62961,
#62962,#62963,#62964,#62965,#62966,#62967,#62968,#62969,#62970,#62971,#62972,
#62973,#62974,#62975,#62976,#62977,#62978,#62979,#62980,#62981,#62982,#62983,
#62984,#62985,#62986,#62987,#62988,#62989,#62990,#62991,#62992),
 .UNSPECIFIED.,.F.,.F.,(4,3,3,3,3,3,3,3,3,3,3,3,3,3,3,3,3,3,3,3,3,3,3,3,
3,3,3,3,3,3,3,3,3,3,3,3,3,3,3,3,3,4),(55.6335465335838,55.7373798265119,
55.841190675596,55.9450138109094,56.0489506758914,56.1529537776165,56.2571314291437,
56.2943394591142,56.3985258783828,56.5025570650831,56.606466223241,56.7103099262487,
56.8141229527868,56.9179400381039,57.0218657915995,57.1258503886731,57.2300169105264,
57.2918679935508,57.3960544128195,57.5000855995193,57.6039947576773,57.7078384606851,
57.8116514872232,57.9154685725402,58.0193943260358,58.1233789231093,58.2275454449626,
58.2893965279874,58.3935829472562,58.4976141339562,58.6015232921141,58.7053669951219,
58.80918002166,58.9129971069773,59.0169228604729,59.1209074575463,59.2250739793998,
59.286925062424,59.4023023747485,59.517314278657,59.6317214277123,59.6902604178031),
 .UNSPECIFIED.);
#2351=B_SPLINE_CURVE_WITH_KNOTS('',3,(#62998,#62999,#63000,#63001,#63002,
#63003,#63004,#63005,#63006,#63007,#63008,#63009,#63010,#63011,#63012,#63013,
#63014,#63015,#63016,#63017,#63018,#63019,#63020,#63021,#63022,#63023,#63024,
#63025,#63026,#63027,#63028,#63029,#63030,#63031,#63032,#63033,#63034,#63035,
#63036,#63037,#63038,#63039,#63040,#63041,#63042,#63043,#63044,#63045,#63046,
#63047,#63048,#63049,#63050,#63051,#63052,#63053,#63054,#63055,#63056,#63057,
#63058,#63059,#63060,#63061,#63062,#63063,#63064,#63065,#63066,#63067,#63068,
#63069,#63070,#63071,#63072,#63073,#63074,#63075,#63076,#63077,#63078,#63079,
#63080,#63081,#63082,#63083,#63084,#63085,#63086,#63087,#63088,#63089,#63090,
#63091,#63092,#63093,#63094,#63095,#63096,#63097,#63098,#63099,#63100,#63101,
#63102,#63103,#63104,#63105,#63106,#63107,#63108,#63109,#63110,#63111,#63112,
#63113,#63114,#63115,#63116,#63117,#63118,#63119,#63120,#63121),
 .UNSPECIFIED.,.F.,.F.,(4,3,3,3,3,3,3,3,3,3,3,3,3,3,3,3,3,3,3,3,3,3,3,3,
3,3,3,3,3,3,3,3,3,3,3,3,3,3,3,3,3,4),(49.3496692790113,49.4541680374703,
49.5581242119948,49.6628942624211,49.7676643128475,49.8718507321162,49.975881918816,
50.079791076974,50.1836347799817,50.2874478065198,50.3912648918367,50.4951906453324,
50.5991752424061,50.7033417642595,50.7651928472842,50.8693792665528,50.9734104532528,
51.0773196114108,51.1811633144184,51.2849763409564,51.3887934262732,51.4927191797688,
51.5967037768424,51.7008702986958,51.7627213817208,51.8669078009894,51.9709389876895,
52.0748481458475,52.1786918488552,52.2825048753932,52.3863219607103,52.4902477142059,
52.5942323112796,52.6983988331331,52.7602499161573,52.8647413337414,52.9690770723351,
53.0785765820079,53.1827008676145,53.2867777522309,53.39085559745,53.4070751110264),
 .UNSPECIFIED.);
#2352=B_SPLINE_CURVE_WITH_KNOTS('',3,(#63122,#63123,#63124,#63125,#63126,
#63127,#63128,#63129,#63130,#63131,#63132,#63133,#63134,#63135,#63136,#63137,
#63138,#63139,#63140,#63141,#63142,#63143,#63144,#63145,#63146,#63147,#63148,
#63149,#63150,#63151,#63152,#63153,#63154,#63155,#63156,#63157,#63158,#63159,
#63160,#63161,#63162,#63163,#63164,#63165,#63166,#63167,#63168,#63169,#63170,
#63171,#63172,#63173,#63174,#63175,#63176,#63177,#63178,#63179,#63180,#63181,
#63182,#63183,#63184,#63185,#63186,#63187,#63188),.UNSPECIFIED.,.F.,.F.,
(4,3,3,3,3,3,3,3,3,3,3,3,3,3,3,3,3,3,3,3,3,3,4),(53.4070751114695,53.5260746317928,
53.646159585465,53.7577784505939,53.8619648698625,53.9659960565624,54.0699052147203,
54.173748917728,54.277561944266,54.3813790295827,54.4853047830783,54.5892893801519,
54.6934559020053,54.7553069850305,54.8649687702613,54.9689734123707,55.0728760912958,
55.1767116670854,55.2805149180024,55.3843665183207,55.4882460132565,55.592246094713,
55.6326012668771),.UNSPECIFIED.);
#2353=B_SPLINE_CURVE_WITH_KNOTS('',3,(#63190,#63191,#63192,#63193,#63194,
#63195,#63196,#63197,#63198,#63199,#63200,#63201,#63202,#63203,#63204,#63205,
#63206,#63207,#63208,#63209,#63210,#63211,#63212,#63213,#63214,#63215,#63216,
#63217,#63218,#63219,#63220,#63221,#63222,#63223,#63224,#63225,#63226,#63227,
#63228,#63229,#63230,#63231,#63232,#63233,#63234,#63235,#63236,#63237,#63238,
#63239,#63240,#63241,#63242,#63243,#63244,#63245,#63246,#63247,#63248,#63249,
#63250,#63251,#63252,#63253,#63254,#63255,#63256,#63257,#63258,#63259),
 .UNSPECIFIED.,.F.,.F.,(4,3,3,3,3,3,3,3,3,3,3,3,3,3,3,3,3,3,3,3,3,3,3,4),
(53.407075111485,53.5098558320716,53.6124863111895,53.7150344153237,53.8175366234483,
53.9200293486254,54.0226180274753,54.1252565130567,54.2280753277761,54.299282390241,
54.4034688095096,54.5074999962097,54.6114091543677,54.7152528573754,54.8190658839134,
54.9228829692301,55.0268087227257,55.1307933197994,55.2349598416528,55.2968109246776,
55.4009764972008,55.505005936927,55.6089152722148,55.6335465335838),
 .UNSPECIFIED.);
#2354=B_SPLINE_CURVE_WITH_KNOTS('',3,(#63260,#63261,#63262,#63263,#63264,
#63265,#63266,#63267,#63268,#63269,#63270,#63271,#63272,#63273,#63274,#63275,
#63276,#63277,#63278,#63279,#63280,#63281,#63282,#63283,#63284,#63285,#63286,
#63287,#63288,#63289,#63290,#63291,#63292,#63293,#63294,#63295,#63296,#63297,
#63298,#63299,#63300,#63301,#63302,#63303,#63304,#63305,#63306,#63307,#63308,
#63309,#63310,#63311,#63312,#63313,#63314,#63315,#63316,#63317,#63318,#63319,
#63320,#63321,#63322,#63323,#63324,#63325,#63326,#63327,#63328,#63329,#63330,
#63331,#63332,#63333,#63334,#63335,#63336,#63337,#63338,#63339,#63340,#63341,
#63342,#63343,#63344,#63345,#63346,#63347,#63348,#63349,#63350,#63351,#63352,
#63353,#63354,#63355,#63356,#63357,#63358,#63359,#63360,#63361,#63362,#63363,
#63364,#63365,#63366,#63367,#63368,#63369,#63370,#63371,#63372,#63373,#63374,
#63375,#63376,#63377,#63378,#63379,#63380,#63381,#63382,#63383),
 .UNSPECIFIED.,.F.,.F.,(4,3,3,3,3,3,3,3,3,3,3,3,3,3,3,3,3,3,3,3,3,3,3,3,
3,3,3,3,3,3,3,3,3,3,3,3,3,3,3,3,3,4),(49.350124038248,49.4542486334836,
49.56111358586,49.6649925950448,49.7688199617351,49.8726304431839,49.9817648955116,
50.0857131347655,50.1897342001324,50.2939235850304,50.3091682524946,50.4133546717632,
50.5173858584632,50.6212950166212,50.725138719629,50.828951746167,50.9327688314839,
51.0366945849795,51.1406791820532,51.2448457039066,51.3066967869312,51.4108832061998,
51.5149143928998,51.6188235510578,51.7226672540655,51.8264802806035,51.9302973659203,
52.0342231194159,52.1382077164896,52.2423742383429,52.3042253213678,52.4084117406365,
52.5124429273365,52.6163520854945,52.7201957885023,52.8240088150403,52.9278259003573,
53.0317516538529,53.1357362509266,53.23990277278,53.3017538558044,53.4070751110264),
 .UNSPECIFIED.);
#2355=B_SPLINE_CURVE_WITH_KNOTS('',3,(#63389,#63390,#63391,#63392,#63393,
#63394,#63395,#63396,#63397,#63398,#63399,#63400,#63401,#63402,#63403,#63404,
#63405,#63406,#63407,#63408,#63409,#63410,#63411,#63412,#63413,#63414,#63415,
#63416,#63417,#63418,#63419,#63420,#63421,#63422,#63423,#63424,#63425,#63426,
#63427,#63428,#63429,#63430,#63431,#63432,#63433,#63434,#63435,#63436,#63437,
#63438,#63439,#63440,#63441,#63442,#63443,#63444,#63445,#63446,#63447,#63448,
#63449,#63450,#63451,#63452,#63453,#63454,#63455,#63456,#63457,#63458,#63459,
#63460,#63461,#63462,#63463,#63464,#63465,#63466,#63467,#63468,#63469,#63470,
#63471,#63472,#63473,#63474,#63475,#63476,#63477,#63478,#63479,#63480,#63481,
#63482,#63483,#63484,#63485,#63486,#63487,#63488,#63489,#63490,#63491,#63492,
#63493,#63494,#63495,#63496,#63497,#63498,#63499,#63500,#63501,#63502,#63503,
#63504,#63505,#63506,#63507,#63508,#63509),.UNSPECIFIED.,.F.,.F.,(4,3,3,
3,3,3,3,3,3,3,3,3,3,3,3,3,3,3,3,3,3,3,3,3,3,3,3,3,3,3,3,3,3,3,3,3,3,3,3,
3,4),(43.0672711160795,43.171130047172,43.2749483241126,43.3787606910417,
43.4826753260211,43.5866398502954,43.6907957769975,43.782493106228,43.8866795254969,
43.9907107121971,44.0946198703554,44.1984635733632,44.3022765999014,44.4060936852183,
44.5100194387141,44.614004035788,44.7181705576416,44.7800216406646,44.8842080599332,
44.9882392466327,45.0921484047906,45.1959921077983,45.299805134336,45.4036222196529,
45.5075479731484,45.6115325702219,45.7156990920752,45.7775501751012,45.8817365943696,
45.9857677810696,46.0896769392276,46.1935206422352,46.2973336687731,46.4011507540897,
46.5050765075852,46.6090611046589,46.7132276265123,46.7750787095378,46.8955468165434,
47.0149579004648,47.1238898034052),.UNSPECIFIED.);
#2356=B_SPLINE_CURVE_WITH_KNOTS('',3,(#63510,#63511,#63512,#63513,#63514,
#63515,#63516,#63517,#63518,#63519,#63520,#63521,#63522,#63523,#63524,#63525,
#63526,#63527,#63528,#63529,#63530,#63531,#63532,#63533,#63534,#63535,#63536,
#63537,#63538,#63539,#63540,#63541,#63542,#63543,#63544,#63545,#63546,#63547,
#63548,#63549,#63550,#63551,#63552,#63553,#63554,#63555,#63556,#63557,#63558,
#63559,#63560,#63561,#63562,#63563,#63564,#63565,#63566,#63567,#63568,#63569,
#63570,#63571,#63572,#63573,#63574,#63575,#63576,#63577,#63578,#63579),
 .UNSPECIFIED.,.F.,.F.,(4,3,3,3,3,3,3,3,3,3,3,3,3,3,3,3,3,3,3,3,3,3,3,4),
(47.1238898038468,47.2279417400956,47.3319880830487,47.4360629830603,47.5402700680329,
47.6445565808272,47.749025499834,47.7726072439743,47.8767936632429,47.9808248499428,
48.0847340081008,48.1885777111084,48.2923907376463,48.396207822963,48.5001335764586,
48.6041181735321,48.7082846953855,48.7701357784109,48.8743117183295,48.9783401946021,
49.0822482051315,49.1860855662751,49.2899055677676,49.3496692790113),
 .UNSPECIFIED.);
#2357=B_SPLINE_CURVE_WITH_KNOTS('',3,(#63581,#63582,#63583,#63584,#63585,
#63586,#63587,#63588,#63589,#63590,#63591,#63592,#63593,#63594,#63595,#63596,
#63597,#63598,#63599,#63600,#63601,#63602,#63603,#63604,#63605,#63606,#63607,
#63608,#63609,#63610,#63611,#63612,#63613,#63614,#63615,#63616,#63617,#63618,
#63619,#63620,#63621,#63622,#63623,#63624,#63625,#63626,#63627,#63628,#63629,
#63630,#63631,#63632,#63633,#63634,#63635,#63636,#63637,#63638,#63639,#63640,
#63641,#63642,#63643,#63644,#63645,#63646,#63647,#63648,#63649,#63650),
 .UNSPECIFIED.,.F.,.F.,(4,3,3,3,3,3,3,3,3,3,3,3,3,3,3,3,3,3,3,3,3,3,3,4),
(47.1238898038468,47.2757519674211,47.3165826491848,47.4207690684534,47.5248002551535,
47.6287094133114,47.7325531163191,47.8363661428571,47.9401832281739,48.0441089816695,
48.1480935787431,48.2522601005964,48.3141111836214,48.41829760289,48.52232878959,
48.626237947748,48.7300816507557,48.8338946772937,48.9377117626105,49.0416375161061,
49.1456221131797,49.249788635033,49.311639718058,49.350124038248),
 .UNSPECIFIED.);
#2358=B_SPLINE_CURVE_WITH_KNOTS('',3,(#63651,#63652,#63653,#63654,#63655,
#63656,#63657,#63658,#63659,#63660,#63661,#63662,#63663,#63664,#63665,#63666,
#63667,#63668,#63669,#63670,#63671,#63672,#63673,#63674,#63675,#63676,#63677,
#63678,#63679,#63680,#63681,#63682,#63683,#63684,#63685,#63686,#63687,#63688,
#63689,#63690,#63691,#63692,#63693,#63694,#63695,#63696,#63697,#63698,#63699,
#63700,#63701,#63702,#63703,#63704,#63705,#63706,#63707,#63708,#63709,#63710,
#63711,#63712,#63713,#63714,#63715,#63716,#63717,#63718,#63719,#63720,#63721,
#63722,#63723,#63724,#63725,#63726,#63727,#63728,#63729,#63730,#63731,#63732,
#63733,#63734,#63735,#63736,#63737,#63738,#63739,#63740,#63741,#63742,#63743,
#63744,#63745,#63746,#63747,#63748,#63749,#63750,#63751,#63752,#63753,#63754,
#63755,#63756,#63757,#63758,#63759,#63760,#63761,#63762,#63763,#63764,#63765,
#63766,#63767,#63768,#63769,#63770,#63771,#63772,#63773,#63774),
 .UNSPECIFIED.,.F.,.F.,(4,3,3,3,3,3,3,3,3,3,3,3,3,3,3,3,3,3,3,3,3,3,3,3,
3,3,3,3,3,3,3,3,3,3,3,3,3,3,3,3,3,4),(43.0661580857027,43.1701497603984,
43.2743204074643,43.3264685114384,43.4306549307087,43.5346861174104,43.6385952755701,
43.7424389785796,43.8462520051194,43.950069090438,44.0539948439354,44.1579794410109,
44.262145962866,44.323997045875,44.4281834651433,44.5322146518429,44.6361238100006,
44.7399675130079,44.8437805395456,44.9475976248621,45.0515233783574,45.1555079754306,
45.2596744972837,45.3215255803116,45.42571199958,45.5297431862797,45.6336523444374,
45.7374960474449,45.8413090739826,45.9451261592993,46.0490519127946,46.153036509868,
46.2572030317211,46.3190541147482,46.4216814718161,46.5241724459798,46.6265638875465,
46.728892502623,46.831240038188,46.9335916782507,47.0360639088855,47.1238898034172),
 .UNSPECIFIED.);
#2359=B_SPLINE_CURVE_WITH_KNOTS('',3,(#63780,#63781,#63782,#63783,#63784,
#63785,#63786,#63787,#63788,#63789,#63790,#63791,#63792,#63793,#63794,#63795,
#63796,#63797,#63798,#63799,#63800,#63801,#63802,#63803,#63804,#63805,#63806,
#63807,#63808,#63809,#63810,#63811,#63812,#63813,#63814,#63815,#63816,#63817,
#63818,#63819,#63820,#63821,#63822,#63823,#63824,#63825,#63826,#63827,#63828,
#63829,#63830,#63831,#63832,#63833,#63834,#63835,#63836,#63837,#63838,#63839,
#63840,#63841,#63842,#63843,#63844,#63845,#63846,#63847,#63848,#63849,#63850,
#63851,#63852,#63853,#63854,#63855,#63856,#63857,#63858,#63859,#63860,#63861,
#63862,#63863,#63864,#63865,#63866,#63867,#63868,#63869,#63870,#63871,#63872,
#63873,#63874,#63875,#63876,#63877,#63878,#63879,#63880,#63881,#63882,#63883,
#63884,#63885,#63886,#63887,#63888,#63889,#63890,#63891,#63892,#63893,#63894,
#63895,#63896,#63897,#63898,#63899,#63900,#63901,#63902,#63903,#63904,#63905,
#63906),.UNSPECIFIED.,.F.,.F.,(4,3,3,3,3,3,3,3,3,3,3,3,3,3,3,3,3,3,3,3,
3,3,3,3,3,3,3,3,3,3,3,3,3,3,3,3,3,3,3,3,3,3,4),(36.78344581208,36.7997933651718,
36.9039797844176,37.0080109710943,37.1119201292284,37.2157638322118,37.3195768587253,
37.4233939440173,37.5273196974879,37.6313042945363,37.7354708163644,37.7973218996084,
37.9015083188911,38.0055395056052,38.1094486637777,38.2132923668,38.3171053933527,
38.4209224786844,38.5248482321949,38.6288328292834,38.7329993511516,38.794850434045,
38.8990368533117,39.0030680400096,39.1069771981657,39.2108209011714,39.3146339277075,
39.4184510130225,39.5223767665163,39.626361363588,39.7305278854396,39.7923789684816,
39.8965653877479,40.0005965744455,40.1045057326011,40.2083494356064,40.3121624621419,
40.4159795474563,40.5199053009494,40.6238898980205,40.7280564198712,40.7899075029182,
40.8407044966672),.UNSPECIFIED.);
#2360=B_SPLINE_CURVE_WITH_KNOTS('',3,(#63907,#63908,#63909,#63910,#63911,
#63912,#63913,#63914,#63915,#63916,#63917,#63918,#63919,#63920,#63921,#63922,
#63923,#63924,#63925,#63926,#63927,#63928,#63929,#63930,#63931,#63932,#63933,
#63934,#63935,#63936,#63937,#63938,#63939,#63940,#63941,#63942,#63943,#63944,
#63945,#63946,#63947,#63948,#63949,#63950,#63951,#63952,#63953,#63954,#63955,
#63956,#63957,#63958,#63959,#63960,#63961,#63962,#63963,#63964,#63965,#63966,
#63967,#63968,#63969,#63970,#63971,#63972,#63973,#63974,#63975,#63976),
 .UNSPECIFIED.,.F.,.F.,(4,3,3,3,3,3,3,3,3,3,3,3,3,3,3,3,3,3,3,3,3,3,3,4),
(40.8407044970057,40.9440672893056,41.0494883828117,41.152586115044,41.2556259852181,
41.3586438439567,41.4658418923063,41.5689883265361,41.672205701304,41.7755885097155,
41.7874360373548,41.8916224566231,41.9956536433224,42.09956280148,42.2034065044874,
42.3072195310251,42.4110366163415,42.5149623698368,42.61894696691,42.723113488763,
42.7849645717913,42.889142338587,42.993155286009,43.0672711160795),
 .UNSPECIFIED.);
#2361=B_SPLINE_CURVE_WITH_KNOTS('',3,(#63978,#63979,#63980,#63981,#63982,
#63983,#63984,#63985,#63986,#63987,#63988,#63989,#63990,#63991,#63992,#63993,
#63994,#63995,#63996,#63997,#63998,#63999,#64000,#64001,#64002,#64003,#64004,
#64005,#64006,#64007,#64008,#64009,#64010,#64011,#64012,#64013,#64014,#64015,
#64016,#64017,#64018,#64019,#64020,#64021,#64022,#64023,#64024,#64025,#64026,
#64027,#64028,#64029,#64030,#64031,#64032,#64033,#64034,#64035,#64036,#64037,
#64038,#64039,#64040,#64041,#64042,#64043,#64044),.UNSPECIFIED.,.F.,.F.,
(4,3,3,3,3,3,3,3,3,3,3,3,3,3,3,3,3,3,3,3,3,3,4),(40.8407044970049,40.9498036597885,
41.059225021957,41.1688181464335,41.2787131705263,41.3314114425652,41.4355978618318,
41.5396290485299,41.6435382066859,41.7473819096916,41.8511949362276,41.9550120215426,
42.0589377750363,42.162922372108,42.2670888939596,42.3289399770018,42.4330996296936,
42.537116410545,42.6410253236269,42.7473085141458,42.8511267993879,42.9586424425453,
43.0661580857027),.UNSPECIFIED.);
#2362=B_SPLINE_CURVE_WITH_KNOTS('',3,(#64045,#64046,#64047,#64048,#64049,
#64050,#64051,#64052,#64053,#64054,#64055,#64056,#64057,#64058,#64059,#64060,
#64061,#64062,#64063,#64064,#64065,#64066,#64067,#64068,#64069,#64070,#64071,
#64072,#64073,#64074,#64075,#64076,#64077,#64078,#64079,#64080,#64081,#64082,
#64083,#64084,#64085,#64086,#64087,#64088,#64089,#64090,#64091,#64092,#64093,
#64094,#64095,#64096,#64097,#64098,#64099,#64100,#64101,#64102,#64103,#64104,
#64105,#64106,#64107,#64108,#64109,#64110,#64111,#64112,#64113,#64114,#64115,
#64116,#64117,#64118,#64119,#64120,#64121,#64122,#64123,#64124,#64125,#64126,
#64127,#64128,#64129,#64130,#64131,#64132,#64133,#64134,#64135,#64136,#64137,
#64138,#64139,#64140,#64141,#64142,#64143,#64144,#64145,#64146,#64147,#64148,
#64149,#64150,#64151,#64152,#64153,#64154,#64155,#64156,#64157,#64158,#64159,
#64160,#64161,#64162,#64163,#64164,#64165,#64166,#64167,#64168),
 .UNSPECIFIED.,.F.,.F.,(4,3,3,3,3,3,3,3,3,3,3,3,3,3,3,3,3,3,3,3,3,3,3,3,
3,3,3,3,3,3,3,3,3,3,3,3,3,3,3,3,3,4),(36.7837215602892,36.8875324398736,
36.9913553996099,37.0952919646733,37.1992945812679,37.3034719274497,37.3412973048188,
37.4454837242011,37.5495149110163,37.6534240692914,37.7572677724171,37.861080799074,
37.9648978845105,38.068823638126,38.1728082353197,38.2769747572924,38.3388258392554,
38.443012258516,38.5470434452082,38.6509526033586,38.7547963063589,38.8586093328897,
38.9624264181996,39.0663521716886,39.170336768756,39.2745032906034,39.336354373692,
39.4405407929378,39.5445719796144,39.6484811377484,39.7523248407317,39.8561378672449,
39.9599549525368,40.0638807060072,40.1678653030555,40.2720318248834,40.3338829081286,
40.4430298277098,40.5518710894771,40.6605292198773,40.7689635848472,40.8407044966672),
 .UNSPECIFIED.);
#2363=B_SPLINE_CURVE_WITH_KNOTS('',3,(#64174,#64175,#64176,#64177,#64178,
#64179,#64180,#64181,#64182,#64183,#64184,#64185,#64186,#64187,#64188,#64189,
#64190,#64191,#64192,#64193,#64194,#64195,#64196,#64197,#64198,#64199,#64200,
#64201,#64202,#64203,#64204,#64205,#64206,#64207,#64208,#64209,#64210,#64211,
#64212,#64213,#64214,#64215,#64216,#64217,#64218,#64219,#64220,#64221,#64222,
#64223,#64224,#64225,#64226,#64227,#64228,#64229,#64230,#64231,#64232,#64233,
#64234,#64235,#64236,#64237,#64238,#64239,#64240,#64241,#64242,#64243,#64244,
#64245,#64246,#64247,#64248,#64249,#64250,#64251,#64252,#64253,#64254,#64255,
#64256,#64257,#64258,#64259,#64260,#64261,#64262,#64263,#64264,#64265,#64266,
#64267,#64268,#64269,#64270,#64271,#64272,#64273,#64274,#64275,#64276,#64277,
#64278,#64279,#64280,#64281,#64282,#64283,#64284,#64285,#64286,#64287,#64288,
#64289,#64290,#64291,#64292,#64293,#64294,#64295,#64296,#64297),
 .UNSPECIFIED.,.F.,.F.,(4,3,3,3,3,3,3,3,3,3,3,3,3,3,3,3,3,3,3,3,3,3,3,3,
3,3,3,3,3,3,3,3,3,3,3,3,3,3,3,3,3,4),(30.4998648058973,30.6038202387868,
30.7092211986695,30.8146221585522,30.9188085758045,31.0228397604511,31.1267489165103,
31.2305926173923,31.3344056417809,31.438222724928,31.5421484762373,31.6461330711119,
31.7502995907701,31.8121506929888,31.9163371131478,32.0203683007497,32.1242774598222,
32.2281211637518,32.3319341912178,32.4357512774668,32.5396770318953,32.6436616299036,
32.7478281526841,32.8096792274254,32.9138656467037,33.0178968334161,33.1218059915907,
33.2256496946177,33.3294627211775,33.4332798065179,33.5372055600414,33.6411901571448,
33.7453566790312,33.807207761862,33.9101447146387,34.0129417465494,34.1156354071316,
34.2182621038502,34.3208882127981,34.4235151981878,34.5262219085223,34.5575191894877),
 .UNSPECIFIED.);
#2364=B_SPLINE_CURVE_WITH_KNOTS('',3,(#64298,#64299,#64300,#64301,#64302,
#64303,#64304,#64305,#64306,#64307,#64308,#64309,#64310,#64311,#64312,#64313,
#64314,#64315,#64316,#64317,#64318,#64319,#64320,#64321,#64322,#64323,#64324,
#64325,#64326,#64327,#64328,#64329,#64330,#64331,#64332,#64333,#64334,#64335,
#64336,#64337,#64338,#64339,#64340,#64341,#64342,#64343,#64344,#64345,#64346,
#64347,#64348,#64349,#64350,#64351,#64352,#64353,#64354,#64355,#64356,#64357,
#64358,#64359,#64360,#64361,#64362,#64363,#64364),.UNSPECIFIED.,.F.,.F.,
(4,3,3,3,3,3,3,3,3,3,3,3,3,3,3,3,3,3,3,3,3,3,4),(34.5575191897626,34.6928922558157,
34.8047362962986,34.9089227156805,35.0129539024955,35.1168630607702,35.2207067638956,
35.3245197905522,35.4283368759883,35.5322626296034,35.6362472267968,35.7404137487692,
35.8022648307352,35.9064523911116,36.0104843860351,36.1143930817558,36.2182358509204,
36.3220474724968,36.4258626813829,36.5297810858963,36.6337581406846,36.7379046401028,
36.78344581208),.UNSPECIFIED.);
#2365=B_SPLINE_CURVE_WITH_KNOTS('',3,(#64366,#64367,#64368,#64369,#64370,
#64371,#64372,#64373,#64374,#64375,#64376,#64377,#64378,#64379,#64380,#64381,
#64382,#64383,#64384,#64385,#64386,#64387,#64388,#64389,#64390,#64391,#64392,
#64393,#64394,#64395,#64396,#64397,#64398,#64399,#64400,#64401,#64402,#64403,
#64404,#64405,#64406,#64407,#64408,#64409,#64410,#64411,#64412,#64413,#64414,
#64415,#64416,#64417,#64418,#64419,#64420,#64421,#64422,#64423,#64424,#64425,
#64426,#64427,#64428,#64429,#64430,#64431,#64432,#64433,#64434,#64435),
 .UNSPECIFIED.,.F.,.F.,(4,3,3,3,3,3,3,3,3,3,3,3,3,3,3,3,3,3,3,3,3,3,3,4),
(34.5575191897576,34.6600276231159,34.7624524447675,34.8648302599766,34.9671976054275,
35.0696598596247,35.1721712597452,35.2748625288751,35.3462402359456,35.4504266552239,
35.5544578419364,35.658367000111,35.7622107031378,35.8660237296973,35.9698408150383,
36.0737665685617,36.1777511656652,36.2819176875515,36.3437687703822,36.4479637300609,
36.5519784470328,36.6558896321121,36.7597264522879,36.7837215602892),
 .UNSPECIFIED.);
#2366=B_SPLINE_CURVE_WITH_KNOTS('',3,(#64436,#64437,#64438,#64439,#64440,
#64441,#64442,#64443,#64444,#64445,#64446,#64447,#64448,#64449,#64450,#64451,
#64452,#64453,#64454,#64455,#64456,#64457,#64458,#64459,#64460,#64461,#64462,
#64463,#64464,#64465,#64466,#64467,#64468,#64469,#64470,#64471,#64472,#64473,
#64474,#64475,#64476,#64477,#64478,#64479,#64480,#64481,#64482,#64483,#64484,
#64485,#64486,#64487,#64488,#64489,#64490,#64491,#64492,#64493,#64494,#64495,
#64496,#64497,#64498,#64499,#64500,#64501,#64502,#64503,#64504,#64505,#64506,
#64507,#64508,#64509,#64510,#64511,#64512,#64513,#64514,#64515,#64516,#64517,
#64518,#64519,#64520,#64521,#64522,#64523,#64524,#64525,#64526,#64527,#64528,
#64529,#64530,#64531,#64532,#64533,#64534,#64535,#64536,#64537,#64538,#64539,
#64540,#64541,#64542,#64543,#64544,#64545,#64546,#64547,#64548,#64549,#64550,
#64551,#64552,#64553,#64554,#64555,#64556,#64557,#64558,#64559),
 .UNSPECIFIED.,.F.,.F.,(4,3,3,3,3,3,3,3,3,3,3,3,3,3,3,3,3,3,3,3,3,3,3,3,
3,3,3,3,3,3,3,3,3,3,3,3,3,3,3,3,3,4),(30.5008964778001,30.60780018035,30.7116793508395,
30.8155067878367,30.9193172487462,31.0285194611095,31.1324675689032,31.2364884416467,
31.3406776902349,31.3561260981992,31.4603125242579,31.5643437178277,31.66825288294,
31.7720965929505,31.8759096265291,31.9797267189139,32.0836524794704,32.1876370836113,
32.2918036124655,32.3536546326358,32.4578410526536,32.5618722401372,32.6657813991263,
32.769625102994,32.8734381304197,32.9772552166506,33.0811809710948,33.1851655691379,
33.2893320919833,33.3511831670724,33.4553695843202,33.5594007689621,33.6633099250166,
33.7671536258938,33.8709666502777,33.9747837334197,34.078709484724,34.1826940795938,
34.2868605992471,34.348711701509,34.4945927534407,34.5575191894877),
 .UNSPECIFIED.);
#2367=B_SPLINE_CURVE_WITH_KNOTS('',3,(#64565,#64566,#64567,#64568,#64569,
#64570,#64571,#64572,#64573,#64574,#64575,#64576,#64577,#64578,#64579,#64580,
#64581,#64582,#64583,#64584,#64585,#64586,#64587,#64588,#64589,#64590,#64591,
#64592,#64593,#64594,#64595,#64596,#64597,#64598,#64599,#64600,#64601,#64602,
#64603,#64604,#64605,#64606,#64607,#64608,#64609,#64610,#64611,#64612,#64613,
#64614,#64615,#64616,#64617,#64618,#64619,#64620,#64621,#64622,#64623,#64624,
#64625,#64626,#64627,#64628,#64629,#64630,#64631,#64632,#64633,#64634,#64635,
#64636,#64637,#64638,#64639,#64640,#64641,#64642,#64643,#64644,#64645,#64646,
#64647,#64648,#64649,#64650,#64651,#64652,#64653,#64654,#64655,#64656,#64657,
#64658,#64659,#64660,#64661,#64662,#64663,#64664,#64665,#64666,#64667,#64668,
#64669,#64670,#64671,#64672,#64673,#64674,#64675,#64676,#64677,#64678,#64679,
#64680,#64681,#64682,#64683,#64684,#64685),.UNSPECIFIED.,.F.,.F.,(4,3,3,
3,3,3,3,3,3,3,3,3,3,3,3,3,3,3,3,3,3,3,3,3,3,3,3,3,3,3,3,3,3,3,3,3,3,3,3,
3,4),(24.217503635835,24.3213222059318,24.425134673036,24.5290492826193,
24.6330136077226,24.7371695283197,24.8294509519326,24.9336372114634,25.0376682357345,
25.1415772282558,25.2454207637364,25.3492336211072,25.4530505358651,25.5569761178482,
25.6609605426126,25.765126892764,25.8269794863692,25.9311659550804,26.0351971917238,
26.1391064003233,26.2429501540519,26.3467632315137,26.450580367881,26.554506172266,
26.6584908202149,26.7626573923662,26.8245080208058,26.9286944520351,27.0327256510729,
27.1366348220718,27.2404785382244,27.3442915781914,27.4481086772032,27.5520344447068,
27.6560190559863,27.7601855922066,27.8220365552424,27.935110886893,28.0468017146134,
28.1605677982292,28.274333881845),.UNSPECIFIED.);
#2368=B_SPLINE_CURVE_WITH_KNOTS('',3,(#64686,#64687,#64688,#64689,#64690,
#64691,#64692,#64693,#64694,#64695,#64696,#64697,#64698,#64699,#64700,#64701,
#64702,#64703,#64704,#64705,#64706,#64707,#64708,#64709,#64710,#64711,#64712,
#64713,#64714,#64715,#64716,#64717,#64718,#64719,#64720,#64721,#64722,#64723,
#64724,#64725,#64726,#64727,#64728,#64729,#64730,#64731,#64732,#64733,#64734,
#64735,#64736,#64737,#64738,#64739,#64740,#64741,#64742,#64743,#64744,#64745,
#64746,#64747,#64748,#64749,#64750,#64751,#64752),.UNSPECIFIED.,.F.,.F.,
(4,3,3,3,3,3,3,3,3,3,3,3,3,3,3,3,3,3,3,3,3,3,4),(28.2743338823081,28.3811973776,
28.4907893056198,28.5979678654125,28.7087664775457,28.819565089679,28.9237515157207,
29.0277827092731,29.131691874368,29.2355355843608,29.3393486179216,29.4431657102888,
29.5470914708273,29.6510760749505,29.755242603787,29.8170936241156,29.9212582775509,
30.0252784744297,30.1291892265987,30.23303658542,30.3368456659329,30.440686438367,
30.4998648058973),.UNSPECIFIED.);
#2369=B_SPLINE_CURVE_WITH_KNOTS('',3,(#64754,#64755,#64756,#64757,#64758,
#64759,#64760,#64761,#64762,#64763,#64764,#64765,#64766,#64767,#64768,#64769,
#64770,#64771,#64772,#64773,#64774,#64775,#64776,#64777,#64778,#64779,#64780,
#64781,#64782,#64783,#64784,#64785,#64786,#64787,#64788,#64789,#64790,#64791,
#64792,#64793,#64794,#64795,#64796,#64797,#64798,#64799,#64800,#64801,#64802,
#64803,#64804,#64805,#64806,#64807,#64808,#64809,#64810,#64811,#64812,#64813,
#64814,#64815,#64816,#64817,#64818,#64819,#64820,#64821,#64822,#64823),
 .UNSPECIFIED.,.F.,.F.,(4,3,3,3,3,3,3,3,3,3,3,3,3,3,3,3,3,3,3,3,3,3,3,4),
(28.2743338823081,28.3635404948894,28.4677269637131,28.5717582004703,28.6756674091851,
28.7795111630297,28.8833242406082,28.9871413770926,29.0910671815947,29.1950518296606,
29.299218401928,29.361069029326,29.4652554605646,29.5692866596124,29.6731958306218,
29.777039546785,29.8808525867634,29.9846696857866,30.0885954533024,30.1925800645945,
30.2967466008277,30.3585975637626,30.4627747459839,30.5008964778001),
 .UNSPECIFIED.);
#2370=B_SPLINE_CURVE_WITH_KNOTS('',3,(#64824,#64825,#64826,#64827,#64828,
#64829,#64830,#64831,#64832,#64833,#64834,#64835,#64836,#64837,#64838,#64839,
#64840,#64841,#64842,#64843,#64844,#64845,#64846,#64847,#64848,#64849,#64850,
#64851,#64852,#64853,#64854,#64855,#64856,#64857,#64858,#64859,#64860,#64861,
#64862,#64863,#64864,#64865,#64866,#64867,#64868,#64869,#64870,#64871,#64872,
#64873,#64874,#64875,#64876,#64877,#64878,#64879,#64880,#64881,#64882,#64883,
#64884,#64885,#64886,#64887,#64888,#64889,#64890,#64891,#64892,#64893,#64894,
#64895,#64896,#64897,#64898,#64899,#64900,#64901,#64902,#64903,#64904,#64905,
#64906,#64907,#64908,#64909,#64910,#64911,#64912,#64913,#64914,#64915,#64916,
#64917,#64918,#64919,#64920,#64921,#64922,#64923,#64924,#64925,#64926,#64927,
#64928,#64929,#64930,#64931,#64932,#64933,#64934,#64935,#64936,#64937,#64938,
#64939,#64940,#64941,#64942,#64943,#64944,#64945,#64946,#64947),
 .UNSPECIFIED.,.F.,.F.,(4,3,3,3,3,3,3,3,3,3,3,3,3,3,3,3,3,3,3,3,3,3,3,3,
3,3,3,3,3,3,3,3,3,3,3,3,3,3,3,3,3,4),(24.216610822454,24.3207830806826,
24.373426357143,24.4776114009861,24.5816411901214,24.6855489246265,24.7893911886519,
24.8932027630289,24.9970183851422,25.1009426686368,25.2049257896555,25.3090908418869,
25.3709548915796,25.4751416524088,25.5791731833385,25.683082687985,25.7869267386815,
25.8907401135825,25.9945575474114,26.0984836472173,26.2024685898807,26.3066354524068,
26.3684834260162,26.4726699929772,26.5767013312479,26.6806106460173,26.7844545086655,
26.8882676976377,26.9920849479502,27.0960108692345,27.1999956359264,27.3041623284679,
27.3660119604528,27.4689825722287,27.5717780278883,27.6744756345683,27.7771117866933,
27.8797227943392,27.9824096578291,28.0851324769858,28.1880251700446,28.2743338818544),
 .UNSPECIFIED.);
#2371=B_SPLINE_CURVE_WITH_KNOTS('',3,(#64953,#64954,#64955,#64956,#64957,
#64958,#64959,#64960,#64961,#64962,#64963,#64964,#64965,#64966,#64967,#64968,
#64969,#64970,#64971,#64972,#64973,#64974,#64975,#64976,#64977,#64978,#64979,
#64980,#64981,#64982,#64983,#64984,#64985,#64986,#64987,#64988,#64989,#64990,
#64991,#64992,#64993,#64994,#64995,#64996,#64997,#64998,#64999,#65000,#65001,
#65002,#65003,#65004,#65005,#65006,#65007,#65008,#65009,#65010,#65011,#65012,
#65013,#65014,#65015,#65016,#65017,#65018,#65019,#65020,#65021,#65022),
 .UNSPECIFIED.,.F.,.F.,(4,3,3,3,3,3,3,3,3,3,3,3,3,3,3,3,3,3,3,3,3,3,3,4),
(15.7079632679489,15.8108075207976,15.9136176294312,16.0164295592376,16.1193522355562,
16.2223337901453,16.3255055953843,16.3931980816502,16.4974234526802,16.601492102817,
16.7054363083021,16.8093135437171,16.913158532871,17.0170059545467,17.1209593297386,
17.2249700571636,17.3291600474277,17.3907266160868,17.4950704177087,17.5992688449958,
17.7033463481182,17.8073550286743,17.9113372683337,17.9338028151035),
 .UNSPECIFIED.);
#2372=B_SPLINE_CURVE_WITH_KNOTS('',3,(#65024,#65025,#65026,#65027,#65028),
 .UNSPECIFIED.,.F.,.F.,(4,1,4),(14.398141012777,15.3956695472136,15.7079548703062),
 .UNSPECIFIED.);
#2373=B_SPLINE_CURVE_WITH_KNOTS('',3,(#65032,#65033,#65034,#65035,#65036,
#65037,#65038,#65039,#65040,#65041,#65042,#65043,#65044,#65045,#65046,#65047,
#65048,#65049,#65050,#65051,#65052,#65053,#65054,#65055,#65056,#65057,#65058,
#65059,#65060,#65061,#65062,#65063,#65064,#65065,#65066,#65067,#65068,#65069,
#65070,#65071,#65072,#65073,#65074,#65075,#65076,#65077,#65078,#65079,#65080,
#65081,#65082,#65083,#65084,#65085,#65086,#65087,#65088,#65089),
 .UNSPECIFIED.,.F.,.F.,(4,3,3,3,3,3,3,3,3,3,3,3,3,3,3,3,3,3,3,4),(13.8761929464654,
13.9800533101315,14.0837576809506,14.1873395169571,14.2908561363859,14.3943427883844,
14.4978346788727,14.6014334411966,14.7050930721393,14.808926366747,14.8541656075666,
14.9608903150643,15.0635179860614,15.1660515649805,15.2685276082899,15.3709825899125,
15.4735044952598,15.5760669075167,15.6787650973359,15.7079632675479),
 .UNSPECIFIED.);
#2374=B_SPLINE_CURVE_WITH_KNOTS('',3,(#65090,#65091,#65092,#65093,#65094,
#65095,#65096,#65097,#65098,#65099,#65100,#65101,#65102,#65103,#65104,#65105,
#65106,#65107,#65108,#65109,#65110,#65111,#65112,#65113,#65114,#65115,#65116,
#65117,#65118,#65119,#65120,#65121,#65122,#65123,#65124,#65125,#65126,#65127,
#65128,#65129,#65130,#65131,#65132,#65133,#65134,#65135,#65136,#65137,#65138,
#65139,#65140,#65141,#65142,#65143,#65144,#65145,#65146,#65147,#65148,#65149,
#65150,#65151,#65152,#65153,#65154,#65155,#65156),.UNSPECIFIED.,.F.,.F.,
(4,3,3,3,3,3,3,3,3,3,3,3,3,3,3,3,3,3,3,3,3,3,4),(15.7079632679489,15.8516941420032,
15.9557858042368,16.0597208697947,16.1635323445499,16.2672774512289,16.3709911139846,
16.4747082126587,16.5785337136997,16.6824177550802,16.7864843330176,16.8492226764398,
16.9534205021522,17.0574630418792,17.1613834157788,17.2652382431943,17.3690622856147,
17.4728902609929,17.576826634821,17.6808217159442,17.7849983901856,17.8467512108764,
17.9343860548896),.UNSPECIFIED.);
#2375=B_SPLINE_CURVE_WITH_KNOTS('',3,(#65162,#65163,#65164,#65165,#65166,
#65167,#65168,#65169,#65170,#65171,#65172,#65173,#65174,#65175,#65176,#65177,
#65178,#65179,#65180,#65181,#65182,#65183,#65184,#65185,#65186,#65187,#65188,
#65189,#65190,#65191,#65192,#65193,#65194,#65195,#65196,#65197,#65198,#65199,
#65200,#65201,#65202,#65203,#65204,#65205,#65206,#65207,#65208,#65209,#65210,
#65211,#65212,#65213,#65214,#65215,#65216,#65217,#65218,#65219,#65220,#65221,
#65222,#65223,#65224,#65225,#65226,#65227,#65228,#65229,#65230,#65231,#65232,
#65233,#65234,#65235,#65236,#65237,#65238,#65239,#65240,#65241,#65242,#65243,
#65244,#65245,#65246,#65247,#65248,#65249,#65250,#65251,#65252,#65253,#65254,
#65255,#65256,#65257,#65258,#65259,#65260,#65261,#65262,#65263,#65264,#65265,
#65266,#65267,#65268,#65269,#65270,#65271,#65272,#65273,#65274,#65275,#65276,
#65277,#65278,#65279,#65280,#65281,#65282,#65283,#65284,#65285,#65286,#65287,
#65288,#65289,#65290,#65291,#65292,#65293,#65294,#65295,#65296,#65297,#65298,
#65299,#65300,#65301,#65302,#65303,#65304,#65305,#65306,#65307,#65308,#65309,
#65310,#65311,#65312,#65313,#65314,#65315,#65316,#65317,#65318,#65319,#65320,
#65321),.UNSPECIFIED.,.F.,.F.,(4,2,2,2,2,2,2,2,2,2,2,2,2,2,2,2,2,2,2,2,
2,2,2,2,2,2,2,2,2,2,2,2,2,2,2,2,2,2,2,2,2,2,2,2,2,2,2,2,2,2,2,2,2,2,2,2,
2,2,2,2,2,2,2,2,2,2,2,2,2,2,2,2,2,2,2,2,2,2,2,4),(-0.808582055129663,-0.803750614026372,
-0.763920330281699,-0.755667253465798,-0.75190245147688,-0.748972613107904,
-0.745765373766368,-0.740511450747678,-0.719053209338083,-0.69846875698509,
-0.691967490889064,-0.672374345367434,-0.668941281667516,-0.667023789605648,
-0.665537186039255,-0.663440027933879,-0.659063955571724,-0.641129598341453,
-0.609238275446381,-0.591965953341908,-0.586791614385876,-0.583578500081481,
-0.580606426328198,-0.576666530975811,-0.567786478554396,-0.555350320334861,
-0.532819209479985,-0.507841520573553,-0.503028370410831,-0.500866708614739,
-0.499194069315333,-0.497221158872559,-0.493559031526201,-0.488855239769308,
-0.477797381356973,-0.456889776921505,-0.42796240650032,-0.422295505956326,
-0.418967878059288,-0.41600699396248,-0.412244951825184,-0.404420493997271,
-0.393962716344978,-0.367392978153513,-0.342227285733235,-0.337519719142119,
-0.33535920705291,-0.333720165398493,-0.331917713334656,-0.328671763421213,
-0.310469465232343,-0.274328821835838,-0.257188434838968,-0.252160474892508,
-0.249075844823561,-0.246251013205195,-0.242552244870408,-0.234440828804303,
-0.215769155900156,-0.187732945517661,-0.171746381145023,-0.168478623810818,
-0.16662470038414,-0.164968853319369,-0.163325419308313,-0.159701628571505,
-0.154862417972763,-0.143393153682017,-0.108931284928433,-0.0861875646209558,
-0.0802886329468558,-0.0767063052521176,-0.0734367767388694,-0.0691524045541401,
-0.0595712385022908,-0.0329949355909643,-0.00749774509555919,-0.00328704030493268,
-0.00149795699922902,-5.90725362616208E-5),.UNSPECIFIED.);
#2376=B_SPLINE_CURVE_WITH_KNOTS('',3,(#65325,#65326,#65327,#65328,#65329,
#65330,#65331,#65332,#65333,#65334),.UNSPECIFIED.,.F.,.F.,(4,2,2,2,4),(-1.15749276218983,
-1.15572035722263,-1.15208331877872,-1.12811344528877,-1.10921379458959),
 .UNSPECIFIED.);
#2377=B_SPLINE_CURVE_WITH_KNOTS('',3,(#65338,#65339,#65340,#65341,#65342,
#65343,#65344,#65345,#65346,#65347,#65348,#65349,#65350,#65351,#65352,#65353,
#65354,#65355,#65356,#65357,#65358,#65359,#65360,#65361,#65362,#65363,#65364,
#65365,#65366,#65367,#65368,#65369,#65370,#65371,#65372,#65373,#65374,#65375,
#65376,#65377,#65378,#65379,#65380,#65381,#65382,#65383,#65384,#65385,#65386,
#65387,#65388,#65389,#65390,#65391,#65392,#65393,#65394,#65395,#65396,#65397,
#65398,#65399,#65400,#65401,#65402,#65403,#65404,#65405,#65406,#65407,#65408,
#65409,#65410,#65411,#65412,#65413,#65414,#65415,#65416,#65417,#65418,#65419,
#65420,#65421,#65422,#65423,#65424,#65425,#65426,#65427,#65428,#65429,#65430,
#65431,#65432,#65433,#65434,#65435,#65436,#65437,#65438,#65439,#65440,#65441,
#65442,#65443,#65444,#65445,#65446,#65447,#65448,#65449,#65450,#65451,#65452,
#65453,#65454,#65455,#65456,#65457,#65458,#65459,#65460,#65461,#65462,#65463,
#65464,#65465,#65466,#65467,#65468,#65469,#65470,#65471,#65472,#65473,#65474,
#65475,#65476,#65477,#65478,#65479,#65480,#65481,#65482,#65483,#65484,#65485,
#65486,#65487,#65488,#65489,#65490,#65491,#65492,#65493,#65494,#65495,#65496,
#65497,#65498,#65499,#65500,#65501,#65502,#65503,#65504,#65505,#65506,#65507,
#65508,#65509,#65510,#65511,#65512,#65513,#65514,#65515,#65516,#65517,#65518,
#65519,#65520,#65521,#65522,#65523,#65524,#65525,#65526,#65527,#65528,#65529,
#65530,#65531,#65532,#65533,#65534,#65535,#65536,#65537,#65538,#65539,#65540,
#65541,#65542,#65543,#65544,#65545,#65546,#65547,#65548,#65549,#65550,#65551,
#65552,#65553,#65554,#65555,#65556,#65557,#65558,#65559,#65560,#65561,#65562,
#65563,#65564,#65565,#65566,#65567,#65568,#65569,#65570,#65571,#65572,#65573,
#65574,#65575,#65576,#65577,#65578,#65579,#65580,#65581,#65582,#65583),
 .UNSPECIFIED.,.F.,.F.,(4,2,2,2,2,2,2,2,2,2,2,2,2,2,2,2,2,2,2,2,2,2,2,2,
2,2,2,2,2,2,2,2,2,2,2,2,2,2,2,2,2,2,2,2,2,2,2,2,2,2,2,2,2,2,2,2,2,2,2,2,
2,2,2,2,2,2,2,2,2,2,2,2,2,2,2,2,2,2,2,2,2,2,2,2,2,2,2,2,2,2,2,2,2,2,2,2,
2,2,2,2,2,2,2,2,2,2,2,2,2,2,2,2,2,2,2,2,2,2,2,2,2,2,4),(-1.10921379458959,
-1.1076622373938,-1.08543029392662,-1.08007660077131,-1.07681618900784,
-1.07384144573965,-1.07002200227276,-1.06362969737749,-1.03625654951167,
-1.01337557673973,-1.00413366587587,-0.998062465708908,-0.995654503029387,
-0.995584277422565,-0.995514581954951,-0.994634984079058,-0.992976116028102,
-0.990699970051695,-0.986534035181013,-0.95638691292609,-0.932673550488202,
-0.918981357511638,-0.914363492443028,-0.911268149014135,-0.908270632900765,
-0.903997613306416,-0.893720029061984,-0.856272923844288,-0.840725640414238,
-0.834891118125428,-0.830578552244249,-0.828493879803355,-0.827008934693503,
-0.825083117447351,-0.821611454849291,-0.800373373787523,-0.795878501794505,
-0.775697105914707,-0.75357378904031,-0.748280596185468,-0.745065450117817,
-0.742138744625703,-0.738392298060851,-0.732156623046581,-0.694465634680216,
-0.666738258049506,-0.663195678002921,-0.661278515404786,-0.65963265045503,
-0.657494032312746,-0.652918871567297,-0.623432265430871,-0.59912137250215,
-0.589806414114396,-0.582658273763377,-0.579044736771133,-0.576119956577928,
-0.572745584710808,-0.566772416941517,-0.53448537490031,-0.501621091196771,
-0.497196429139702,-0.49509160053332,-0.493444676853058,-0.491454876526423,
-0.487604356959964,-0.482567470634422,-0.470231421438504,-0.433118198255328,
-0.419075378204661,-0.414291071255023,-0.411172166491054,-0.408181866721782,
-0.40405128380816,-0.393914186715727,-0.378950192964909,-0.359038211076391,
-0.356823833118952,-0.333520724434363,-0.33002920063043,-0.32809416072214,
-0.32644584832746,-0.324277862816438,-0.319490470960679,-0.297575056806468,
-0.256724250613953,-0.24961066582482,-0.245962076794916,-0.243040707618046,
-0.239705129944953,-0.233893905956809,-0.226762494548428,-0.211069025012032,
-0.181557437977702,-0.16648146851152,-0.163191867885106,-0.161303248197036,
-0.159692646635295,-0.159675204713457,-0.159658113308516,-0.15964134997403,
-0.159624893753413,-0.159608725047098,-0.159592825484932,-0.159577177801894,
-0.159561765764004,-0.159546574017785,-0.159531588127396,-0.15951679434262,
-0.159502179667159,-0.159487731745921,-0.159473438765623,-0.157288660723066,
-0.154702145306918,-0.150102155419665,-0.106320137254155,-0.0867330356464405,
-0.0814335128342001,-0.0782058172347371,-0.0752616337348794,-0.0714195197704843,
-0.0630253608599946,-0.0594837367698858),.UNSPECIFIED.);
#2378=B_SPLINE_CURVE_WITH_KNOTS('',3,(#65588,#65589,#65590,#65591,#65592,
#65593,#65594,#65595,#65596,#65597,#65598,#65599,#65600,#65601,#65602,#65603,
#65604,#65605,#65606,#65607,#65608,#65609,#65610,#65611,#65612,#65613,#65614,
#65615,#65616,#65617,#65618,#65619,#65620,#65621,#65622,#65623,#65624,#65625,
#65626,#65627,#65628,#65629,#65630,#65631,#65632,#65633,#65634,#65635,#65636,
#65637,#65638,#65639,#65640,#65641,#65642,#65643,#65644,#65645,#65646,#65647,
#65648,#65649,#65650,#65651,#65652,#65653,#65654,#65655,#65656,#65657,#65658,
#65659,#65660,#65661,#65662,#65663,#65664,#65665,#65666,#65667,#65668,#65669,
#65670,#65671,#65672,#65673,#65674,#65675,#65676,#65677,#65678,#65679,#65680,
#65681,#65682,#65683,#65684,#65685,#65686,#65687,#65688,#65689,#65690,#65691,
#65692,#65693,#65694,#65695,#65696,#65697,#65698,#65699,#65700,#65701,#65702,
#65703,#65704,#65705,#65706,#65707,#65708,#65709,#65710,#65711,#65712,#65713,
#65714,#65715,#65716,#65717,#65718,#65719,#65720,#65721,#65722,#65723,#65724,
#65725,#65726,#65727,#65728,#65729,#65730,#65731,#65732,#65733,#65734,#65735,
#65736,#65737,#65738,#65739,#65740,#65741,#65742,#65743,#65744,#65745,#65746,
#65747,#65748,#65749,#65750,#65751,#65752,#65753,#65754,#65755,#65756,#65757,
#65758,#65759,#65760,#65761,#65762,#65763,#65764,#65765,#65766,#65767,#65768,
#65769,#65770,#65771,#65772,#65773,#65774,#65775,#65776,#65777,#65778,#65779,
#65780,#65781,#65782,#65783,#65784,#65785,#65786,#65787,#65788,#65789,#65790,
#65791,#65792,#65793),.UNSPECIFIED.,.F.,.F.,(4,2,2,2,2,2,2,2,2,2,2,2,2,
2,2,2,2,2,2,2,2,2,2,2,2,2,2,2,2,2,2,2,2,2,2,2,2,2,2,2,2,2,2,2,2,2,2,2,2,
2,2,2,2,2,2,2,2,2,2,2,2,2,2,2,2,2,2,2,2,2,2,2,2,2,2,2,2,2,2,2,2,2,2,2,2,
2,2,2,2,2,2,2,2,2,2,2,2,2,2,2,2,2,4),(-1.85846886095936,-1.83940746062439,
-1.83584410856664,-1.83391468281092,-1.83226448898463,-1.83012226369945,
-1.82535591730456,-1.80035676732322,-1.77297800175295,-1.76304851740448,
-1.75554658385211,-1.75259517608712,-1.74960920593114,-1.74648440515245,
-1.74166992480376,-1.72733708559932,-1.69375758835966,-1.67430341423461,
-1.6697663072851,-1.66764318548338,-1.66615436934787,-1.66425192801052,
-1.66090687750724,-1.64486336622851,-1.61437034361168,-1.59258605810712,
-1.58729403195599,-1.58406722219309,-1.58112146812251,-1.57733837612187,
-1.57101172952175,-1.53487894154682,-1.51483572827075,-1.50806052845142,
-1.50323563971223,-1.50105966179817,-1.49942416983499,-1.49749802835678,
-1.49404903860049,-1.47439651711881,-1.46756476285612,-1.44599525673569,
-1.42575798766076,-1.4205649458911,-1.41735896958992,-1.41440623622628,
-1.41057755467444,-1.40203015604819,-1.36270968135944,-1.34127876933968,
-1.33653713800039,-1.33437620702495,-1.33274284051056,-1.33080884318828,
-1.32731946098936,-1.30448740517577,-1.30173400770234,-1.28561352722048,
-1.25963283693165,-1.25413250054938,-1.25086226218927,-1.24792908125744,
-1.24417130761191,-1.23807099264858,-1.19226636828357,-1.1740287969165,
-1.1696260424052,-1.16752863401233,-1.16604278240289,-1.16412267488346,
-1.1607005570197,-1.14311944415211,-1.09804721401168,-1.08934483797966,
-1.08544687611174,-1.08249299916335,-1.07928692081737,-1.07409623560765,
-1.05598913768461,-1.02459976863163,-1.01174140477052,-1.00656771909017,
-1.00263635224312,-1.00062973789446,-0.998983142740153,-0.996896518036183,
-0.992569302577529,-0.958661620705056,-0.926714198535095,-0.921025586144166,
-0.9177109377958,-0.915071589931665,-0.911511887496554,-0.904639540027466,
-0.879761342924638,-0.862527715430148,-0.839367465758799,-0.835876498401726,
-0.833941437923539,-0.832298862120824,-0.830144346188354,-0.825392157409788,
-0.808582055129663),.UNSPECIFIED.);
#2379=B_SPLINE_CURVE_WITH_KNOTS('',3,(#65795,#65796,#65797,#65798,#65799,
#65800,#65801,#65802),.UNSPECIFIED.,.F.,.F.,(4,2,2,4),(-0.0594837367698858,
-0.0402893593164964,-0.00570478766600024,-0.000519914712907845),
 .UNSPECIFIED.);
#2380=B_SPLINE_CURVE_WITH_KNOTS('',3,(#65803,#65804,#65805,#65806,#65807,
#65808,#65809,#65810,#65811,#65812,#65813),.UNSPECIFIED.,.F.,.F.,(4,2,1,
1,1,1,1,4),(-91.8109775642064,-91.7726251681672,-90.7750966337306,-89.777568099294,
-88.7800395648573,-87.7825110304207,-86.7849824959842,-85.8810481711785),
 .UNSPECIFIED.);
#2381=B_SPLINE_CURVE_WITH_KNOTS('',3,(#65819,#65820,#65821,#65822,#65823,
#65824,#65825,#65826,#65827,#65828,#65829,#65830,#65831,#65832,#65833,#65834,
#65835,#65836,#65837,#65838,#65839,#65840,#65841,#65842,#65843,#65844,#65845,
#65846,#65847,#65848,#65849,#65850,#65851,#65852,#65853,#65854,#65855,#65856,
#65857,#65858,#65859,#65860,#65861,#65862,#65863,#65864,#65865,#65866,#65867,
#65868,#65869,#65870,#65871,#65872,#65873,#65874,#65875,#65876,#65877,#65878,
#65879,#65880,#65881,#65882,#65883,#65884,#65885,#65886,#65887,#65888,#65889,
#65890,#65891,#65892,#65893,#65894,#65895,#65896,#65897,#65898,#65899,#65900,
#65901,#65902,#65903,#65904,#65905,#65906,#65907,#65908,#65909,#65910,#65911,
#65912,#65913,#65914,#65915,#65916,#65917,#65918,#65919,#65920,#65921,#65922,
#65923,#65924,#65925,#65926,#65927,#65928,#65929,#65930,#65931,#65932,#65933,
#65934,#65935,#65936,#65937,#65938,#65939,#65940,#65941,#65942,#65943,#65944,
#65945,#65946,#65947,#65948,#65949,#65950,#65951,#65952,#65953,#65954,#65955,
#65956,#65957,#65958,#65959,#65960,#65961,#65962,#65963,#65964,#65965,#65966,
#65967,#65968,#65969,#65970,#65971,#65972,#65973,#65974,#65975,#65976,#65977,
#65978,#65979,#65980,#65981,#65982,#65983,#65984,#65985,#65986,#65987,#65988,
#65989,#65990,#65991,#65992,#65993,#65994,#65995,#65996,#65997,#65998,#65999,
#66000,#66001,#66002,#66003,#66004,#66005,#66006,#66007,#66008,#66009,#66010),
 .UNSPECIFIED.,.F.,.F.,(4,2,2,2,2,2,2,2,2,2,2,2,2,2,2,2,2,2,2,2,2,2,2,2,
2,2,2,2,2,2,2,2,2,2,2,2,2,2,2,2,2,2,2,2,2,2,2,2,2,2,2,2,2,2,2,2,2,2,2,2,
2,2,2,2,2,2,2,2,2,2,2,2,2,2,2,2,2,2,2,2,2,2,2,2,2,2,2,2,2,2,2,2,2,2,2,4),
(-0.991262637114908,-0.990030252789208,-0.964527390077046,-0.944362212569878,
-0.922374036844681,-0.918886818977652,-0.916952565365279,-0.91531878672021,
-0.913156466960908,-0.908406383444986,-0.886886962178832,-0.847304463235204,
-0.838984566926019,-0.835196135180223,-0.832249899261719,-0.829026281497939,
-0.823748072949235,-0.80217954981134,-0.781695306292921,-0.775418038969063,
-0.755652765737664,-0.752201922684275,-0.750275855961832,-0.74864097689561,
-0.746466720698178,-0.741650014618699,-0.734888983996405,-0.714919338689796,
-0.678641842268481,-0.672321416351242,-0.668540371424746,-0.665595239400699,
-0.662368125913504,-0.657073298748417,-0.635227958438309,-0.604487035879512,
-0.588763616771329,-0.585445145543287,-0.583548821242408,-0.581892680820745,
-0.579660050052783,-0.574510941017902,-0.567116707527369,-0.543611162637253,
-0.512259918175071,-0.505168607929871,-0.501522597149624,-0.498598920688561,
-0.495255888335385,-0.489418751926246,-0.454493428867502,-0.42414295424235,
-0.419520884632951,-0.417404696033666,-0.415757055510615,-0.413809412693716,
-0.410158687053075,-0.40545650268177,-0.394352189656478,-0.372833388782713,
-0.343029282271306,-0.337355579530089,-0.334047276832857,-0.331411905411525,
-0.327856286025243,-0.320987859283398,-0.296099589263666,-0.278896086712574,
-0.255762494913994,-0.252271942542737,-0.25033702846841,-0.248703473997468,
-0.246542473035566,-0.24179918967524,-0.220346644129287,-0.1809766917338,
-0.172464914557856,-0.168643181998464,-0.165692330929846,-0.162957682269341,
-0.158213118362014,-0.143229348464024,-0.115398714033831,-0.108393955572286,
-0.0890224012168137,-0.0855820925314036,-0.0836584253521946,-0.0821731792243276,
-0.0800811858767538,-0.0757086538011402,-0.0577400170824042,-0.020644334918703,
-0.00771115206037433,-0.00324887219255287,-0.00155419658315507,-0.000491736839017494),
 .UNSPECIFIED.);
#2382=B_SPLINE_CURVE_WITH_KNOTS('',3,(#66011,#66012,#66013,#66014,#66015,
#66016,#66017,#66018,#66019,#66020,#66021,#66022,#66023,#66024),
 .UNSPECIFIED.,.F.,.F.,(4,2,2,2,2,2,4),(-1.91741114141026,-1.91639157322029,
-1.91462258465228,-1.91113044186193,-1.90404850449963,-1.8694194204246,
-1.85846886095936),.UNSPECIFIED.);
#2383=B_SPLINE_CURVE_WITH_KNOTS('',3,(#66026,#66027,#66028,#66029,#66030),
 .UNSPECIFIED.,.F.,.F.,(4,1,4),(-85.8810481711785,-85.7874539615476,-85.5277944653042),
 .UNSPECIFIED.);
#2384=B_SPLINE_CURVE_WITH_KNOTS('',3,(#66031,#66032,#66033,#66034,#66035,
#66036,#66037,#66038,#66039,#66040,#66041,#66042,#66043,#66044,#66045,#66046,
#66047,#66048,#66049,#66050,#66051,#66052,#66053,#66054,#66055,#66056,#66057,
#66058,#66059,#66060,#66061,#66062,#66063,#66064,#66065,#66066,#66067,#66068,
#66069,#66070,#66071,#66072,#66073,#66074,#66075,#66076,#66077,#66078,#66079,
#66080,#66081,#66082,#66083,#66084,#66085,#66086,#66087,#66088,#66089,#66090,
#66091,#66092,#66093,#66094,#66095,#66096,#66097,#66098,#66099,#66100,#66101,
#66102,#66103,#66104,#66105,#66106,#66107,#66108,#66109,#66110,#66111,#66112,
#66113,#66114,#66115,#66116,#66117,#66118,#66119,#66120,#66121,#66122,#66123,
#66124,#66125,#66126,#66127,#66128,#66129,#66130,#66131,#66132,#66133,#66134,
#66135,#66136,#66137,#66138,#66139,#66140,#66141,#66142,#66143,#66144,#66145,
#66146,#66147,#66148,#66149,#66150,#66151,#66152,#66153,#66154,#66155,#66156,
#66157,#66158,#66159,#66160,#66161,#66162,#66163,#66164,#66165,#66166,#66167,
#66168,#66169,#66170,#66171,#66172,#66173,#66174,#66175,#66176,#66177,#66178,
#66179,#66180,#66181,#66182,#66183,#66184,#66185,#66186,#66187,#66188,#66189,
#66190,#66191,#66192,#66193,#66194,#66195,#66196,#66197,#66198,#66199,#66200,
#66201,#66202,#66203,#66204,#66205,#66206,#66207,#66208,#66209,#66210,#66211,
#66212,#66213,#66214,#66215,#66216,#66217,#66218,#66219,#66220,#66221,#66222,
#66223,#66224,#66225,#66226),.UNSPECIFIED.,.F.,.F.,(4,2,2,2,2,2,2,2,2,2,
2,2,2,2,2,2,2,2,2,2,2,2,2,2,2,2,2,2,2,2,2,2,2,2,2,2,2,2,2,2,2,2,2,2,2,2,
2,2,2,2,2,2,2,2,2,2,2,2,2,2,2,2,2,2,2,2,2,2,2,2,2,2,2,2,2,2,2,2,2,2,2,2,
2,2,2,2,2,2,2,2,2,2,2,2,2,2,2,4),(-2.10008743950006,-2.07854758539132,-2.06877862930352,
-2.06503838939257,-2.06216829021424,-2.05922429423112,-2.05599570021913,
-2.05069216043087,-2.03102510249862,-2.00168280493975,-1.98255848273885,
-1.9792220524613,-1.97728355240748,-1.97563519043276,-1.97350747600006,
-1.96898873895325,-1.93818697272705,-1.90358154539059,-1.8977555977107,
-1.89441544227115,-1.89149226372879,-1.88784424526438,-1.88074062426806,
-1.84985466702855,-1.82603089322516,-1.81858514856592,-1.81340927420629,
-1.81117240061264,-1.80951606479392,-1.80762300535485,-1.80431769066657,
-1.7888211309634,-1.75993741222275,-1.74412320851496,-1.73695564665984,
-1.73112123017635,-1.72777932196644,-1.72485640810646,-1.72121107940999,
-1.71412029633266,-1.68295169443865,-1.65933233966515,-1.65192035299934,
-1.64676189882025,-1.64452803392657,-1.64287210544079,-1.64097741210199,
-1.6376647637853,-1.62201995662916,-1.59123768309075,-1.56931402662564,
-1.56401518113037,-1.56078779532817,-1.5578438456884,-1.55406632578062,
-1.54775647857148,-1.51134486933854,-1.49148906085177,-1.48475078730921,
-1.47994609221674,-1.47777436960016,-1.47614015179838,-1.47421345641829,
-1.4707582897344,-1.45080620780897,-1.44422628400323,-1.42257348373837,
-1.40244782344601,-1.39726429089917,-1.39406159600309,-1.39111021501586,
-1.38728096677913,-1.3787223542671,-1.33942298786977,-1.31799890436937,
-1.31325885529179,-1.31109876033984,-1.30946563868309,-1.30753101246325,
-1.30404046854004,-1.2809101718976,-1.26371676454656,-1.23878206653153,
-1.2319085560276,-1.22835246299673,-1.22571764938885,-1.22241122638425,
-1.21674379980181,-1.1859481371649,-1.16109781882375,-1.15268110023202,
-1.14701778961442,-1.14470027386306,-1.14303250902419,-1.14118049436591,
-1.13797580709458,-1.12495134819297,-1.10916695937962),.UNSPECIFIED.);
#2385=B_SPLINE_CURVE_WITH_KNOTS('',3,(#66231,#66232,#66233,#66234,#66235,
#66236,#66237,#66238,#66239,#66240,#66241,#66242,#66243,#66244,#66245,#66246,
#66247,#66248,#66249,#66250,#66251,#66252,#66253,#66254,#66255,#66256,#66257,
#66258,#66259,#66260,#66261,#66262,#66263,#66264,#66265,#66266,#66267,#66268,
#66269,#66270,#66271,#66272,#66273,#66274,#66275,#66276,#66277,#66278,#66279,
#66280,#66281,#66282,#66283,#66284,#66285,#66286,#66287,#66288,#66289,#66290,
#66291,#66292,#66293,#66294,#66295,#66296,#66297,#66298,#66299,#66300,#66301,
#66302,#66303,#66304,#66305,#66306,#66307,#66308,#66309,#66310,#66311,#66312,
#66313,#66314,#66315,#66316,#66317,#66318,#66319,#66320,#66321,#66322,#66323,
#66324,#66325,#66326,#66327,#66328,#66329,#66330,#66331,#66332,#66333,#66334,
#66335,#66336,#66337,#66338,#66339,#66340,#66341,#66342,#66343,#66344,#66345,
#66346,#66347,#66348,#66349,#66350,#66351,#66352,#66353,#66354,#66355,#66356,
#66357,#66358,#66359,#66360,#66361,#66362,#66363,#66364,#66365,#66366,#66367,
#66368,#66369,#66370,#66371,#66372,#66373,#66374,#66375,#66376,#66377,#66378,
#66379,#66380,#66381,#66382,#66383,#66384,#66385,#66386,#66387,#66388,#66389,
#66390,#66391,#66392,#66393,#66394,#66395,#66396,#66397,#66398,#66399,#66400,
#66401,#66402,#66403,#66404,#66405,#66406,#66407,#66408,#66409,#66410,#66411,
#66412,#66413,#66414,#66415,#66416,#66417,#66418,#66419,#66420,#66421,#66422,
#66423,#66424,#66425,#66426,#66427,#66428,#66429,#66430,#66431,#66432,#66433,
#66434),.UNSPECIFIED.,.F.,.F.,(4,2,2,2,2,2,2,2,2,2,2,2,2,2,2,2,2,2,2,2,
2,2,2,2,2,2,2,2,2,2,2,2,2,2,2,2,2,2,2,2,2,2,2,2,2,2,2,2,2,2,2,2,2,2,2,2,
2,2,2,2,2,2,2,2,2,2,2,2,2,2,2,2,2,2,2,2,2,2,2,2,2,2,2,2,2,2,2,2,2,2,2,2,
2,2,2,2,2,2,2,2,2,4),(-2.04109563196961,-2.03715166773698,-2.01184485869293,
-2.00492313862756,-2.00135674269587,-1.99872014403853,-1.99541903998376,
-1.98977977271561,-1.9625587603051,-1.94281058529977,-1.92394171208846,
-1.91946817563695,-1.91735695221755,-1.91586952367419,-1.91395912560044,
-1.91057850924682,-1.89356466756653,-1.86496597641253,-1.84241737865986,
-1.83708119169235,-1.83384507126245,-1.8309021145354,-1.82713819870818,
-1.82087882015238,-1.78367129416691,-1.75594594539535,-1.75229721405626,
-1.75034989376827,-1.74870208936822,-1.74658510843154,-1.74195918188692,
-1.70306723415312,-1.68077297087022,-1.67238655265899,-1.66854520687439,
-1.66560053599183,-1.66237124360447,-1.65706660533259,-1.6373914453673,
-1.593689662428,-1.58911259941301,-1.5855370929312,-1.58360513725545,-1.58195527996346,
-1.57981668163954,-1.57507102486309,-1.54946079707402,-1.52714225126485,
-1.51476112371381,-1.50591628141653,-1.50199508401009,-1.49903907249871,
-1.49584558576601,-1.49070872035556,-1.47365075930622,-1.44171997951546,
-1.42375032635273,-1.41937730102091,-1.41728507992514,-1.41579964612381,
-1.41387572895629,-1.41043498620636,-1.39107237832122,-1.38403770584597,
-1.36305971324366,-1.34919519049433,-1.33959438691019,-1.33554818274283,
-1.33257256844589,-1.3294269142354,-1.32451446334915,-1.30929130373869,
-1.27648270213017,-1.25730678594088,-1.2527995987844,-1.25068199203506,
-1.24919377127372,-1.24728753521754,-1.24392567755249,-1.2274651145437,
-1.19771105536898,-1.17567014700486,-1.17036299720748,-1.16713301119125,
-1.16418825384889,-1.16041184023517,-1.15216101112613,-1.11252226898492,
-1.09098941404171,-1.08623779520677,-1.08407512288789,-1.08244121292983,
-1.08050699739299,-1.07702023269248,-1.05524045376991,-1.05036481417599,
-1.0116168663927,-1.00548338386893,-1.00171495280942,-0.998779155699581,
-0.995511802796277,-0.991262637114908),.UNSPECIFIED.);
#2386=B_SPLINE_CURVE_WITH_KNOTS('',3,(#66435,#66436,#66437,#66438,#66439,
#66440,#66441,#66442,#66443,#66444,#66445,#66446,#66447,#66448,#66449,#66450,
#66451,#66452,#66453,#66454,#66455,#66456,#66457,#66458,#66459,#66460,#66461,
#66462,#66463,#66464,#66465,#66466,#66467,#66468,#66469,#66470,#66471,#66472,
#66473,#66474,#66475,#66476,#66477,#66478,#66479,#66480,#66481,#66482,#66483,
#66484,#66485,#66486,#66487,#66488,#66489,#66490,#66491,#66492,#66493,#66494,
#66495,#66496,#66497,#66498,#66499,#66500,#66501,#66502,#66503,#66504,#66505,
#66506,#66507,#66508,#66509,#66510,#66511,#66512,#66513,#66514,#66515,#66516,
#66517,#66518,#66519,#66520,#66521,#66522,#66523,#66524,#66525,#66526,#66527,
#66528,#66529,#66530,#66531,#66532,#66533,#66534,#66535,#66536,#66537,#66538,
#66539,#66540,#66541,#66542,#66543,#66544,#66545,#66546,#66547,#66548,#66549,
#66550,#66551,#66552,#66553,#66554,#66555,#66556,#66557,#66558,#66559,#66560,
#66561,#66562,#66563,#66564,#66565,#66566,#66567,#66568,#66569,#66570,#66571,
#66572,#66573,#66574,#66575,#66576,#66577,#66578,#66579,#66580,#66581,#66582,
#66583,#66584,#66585,#66586,#66587,#66588,#66589,#66590,#66591,#66592,#66593,
#66594,#66595,#66596,#66597,#66598,#66599,#66600,#66601,#66602,#66603,#66604,
#66605,#66606,#66607,#66608,#66609,#66610,#66611,#66612,#66613,#66614,#66615,
#66616,#66617,#66618,#66619,#66620,#66621,#66622,#66623,#66624,#66625,#66626,
#66627,#66628,#66629,#66630,#66631,#66632,#66633,#66634,#66635,#66636,#66637,
#66638,#66639,#66640,#66641,#66642,#66643,#66644,#66645,#66646,#66647,#66648,
#66649,#66650,#66651,#66652,#66653,#66654,#66655,#66656,#66657,#66658,#66659,
#66660,#66661,#66662,#66663,#66664,#66665,#66666,#66667,#66668,#66669,#66670,
#66671,#66672),.UNSPECIFIED.,.F.,.F.,(4,2,2,2,2,2,2,2,2,2,2,2,2,2,2,2,2,
2,2,2,2,2,2,2,2,2,2,2,2,2,2,2,2,2,2,2,2,2,2,2,2,2,2,2,2,2,2,2,2,2,2,2,2,
2,2,2,2,2,2,2,2,2,2,2,2,2,2,2,2,2,2,2,2,2,2,2,2,2,2,2,2,2,2,2,2,2,2,2,2,
2,2,2,2,2,2,2,2,2,2,2,2,2,2,2,2,2,2,2,2,2,2,2,2,2,2,2,2,2,4),(-1.10916695937962,
-1.09785195841207,-1.07226864233564,-1.06531323034322,-1.06174092605676,
-1.05910454465279,-1.0558096438895,-1.05019595022401,-1.02083592305063,
-0.991387429212326,-0.981669540765042,-0.978749037959597,-0.97695925254149,
-0.975263122680412,-0.9727837578719,-0.966034814558207,-0.922226828297954,
-0.902675719034099,-0.897378507909132,-0.89415160224643,-0.891207758227922,
-0.887365563769124,-0.878969252877936,-0.85619628815039,-0.830091811939781,
-0.815697950286459,-0.812447122794245,-0.810566532129448,-0.808907449766328,
-0.806648381931185,-0.801340698496335,-0.79363595111145,-0.76818292718107,
-0.73937940400311,-0.732254783421282,-0.72860268913279,-0.725679490342722,
-0.722342831441816,-0.716532187548575,-0.682184275913402,-0.651090204741507,
-0.646551180600829,-0.6444281909992,-0.642783289586587,-0.640815528728321,
-0.637066012409968,-0.63219831607411,-0.620489823571801,-0.599279371849155,
-0.570182032143738,-0.564536252593569,-0.561202930568941,-0.558307094544375,
-0.554663791565358,-0.547344301304792,-0.537731571237426,-0.511962107665647,
-0.484744484464426,-0.480019022507963,-0.477884616107571,-0.476235812879305,
-0.474302546218574,-0.470718319451695,-0.442099374994455,-0.405754974018102,
-0.39943990984595,-0.395661162926829,-0.392717324841462,-0.38949114357372,
-0.384196767274576,-0.362335538446676,-0.331560175530213,-0.315888801721569,
-0.312575041309464,-0.31068023933258,-0.309024620880329,-0.306791669882353,
-0.301637556163642,-0.294232777094044,-0.270658540912069,-0.239402364645259,
-0.232311699916303,-0.228666690483956,-0.225744166606889,-0.222402851162856,
-0.216569825877009,-0.209404896987984,-0.193599036620314,-0.165317328395053,
-0.14932369071598,-0.145982141213971,-0.144081071524549,-0.142592923032059,
-0.142579128536054,-0.142565964393677,-0.142553393344733,-0.142541380979266,
-0.142529895482768,-0.142509885233177,-0.142490030749955,-0.142470325188627,
-0.14245076194988,-0.142431334553265,-0.142412036723164,-0.142392862367559,
-0.142373805566179,-0.142354860503376,-0.142336021523246,-0.142317283109273,
-0.142298639845394,-0.142280086458585,-0.140162043029368,-0.135247659671907,
-0.128141754728387,-0.106305341310492,-0.072704223676547,-0.0656632114127612,
-0.0620284846312131,-0.0595287291512849),.UNSPECIFIED.);
#2387=B_SPLINE_CURVE_WITH_KNOTS('',3,(#66678,#66679,#66680,#66681,#66682,
#66683,#66684,#66685,#66686,#66687,#66688,#66689,#66690,#66691,#66692,#66693,
#66694,#66695,#66696,#66697,#66698,#66699,#66700,#66701,#66702,#66703,#66704,
#66705,#66706,#66707,#66708,#66709,#66710,#66711,#66712,#66713,#66714,#66715,
#66716,#66717,#66718,#66719,#66720,#66721,#66722,#66723,#66724,#66725,#66726,
#66727,#66728,#66729,#66730,#66731,#66732,#66733,#66734,#66735,#66736,#66737,
#66738,#66739,#66740,#66741,#66742,#66743,#66744,#66745,#66746,#66747,#66748,
#66749,#66750,#66751,#66752,#66753,#66754,#66755,#66756,#66757,#66758,#66759,
#66760,#66761,#66762,#66763,#66764,#66765,#66766,#66767,#66768,#66769,#66770,
#66771,#66772,#66773,#66774,#66775,#66776,#66777,#66778,#66779,#66780,#66781,
#66782,#66783,#66784,#66785,#66786,#66787,#66788,#66789,#66790,#66791,#66792,
#66793,#66794,#66795,#66796,#66797,#66798,#66799,#66800,#66801,#66802,#66803,
#66804,#66805,#66806,#66807,#66808,#66809,#66810,#66811,#66812,#66813,#66814,
#66815,#66816,#66817,#66818,#66819,#66820,#66821,#66822,#66823,#66824,#66825,
#66826,#66827,#66828,#66829,#66830,#66831,#66832,#66833,#66834,#66835,#66836,
#66837,#66838,#66839,#66840,#66841,#66842,#66843,#66844,#66845,#66846,#66847,
#66848,#66849,#66850,#66851,#66852,#66853,#66854,#66855,#66856,#66857,#66858,
#66859,#66860,#66861,#66862,#66863,#66864,#66865,#66866,#66867,#66868,#66869,
#66870,#66871,#66872,#66873,#66874,#66875,#66876,#66877,#66878,#66879,#66880,
#66881,#66882,#66883,#66884,#66885,#66886,#66887,#66888,#66889,#66890,#66891,
#66892,#66893,#66894,#66895,#66896,#66897,#66898,#66899,#66900,#66901,#66902,
#66903),.UNSPECIFIED.,.F.,.F.,(4,2,2,2,2,2,2,2,2,2,2,2,2,2,2,2,2,2,2,2,
2,2,2,2,2,2,2,2,2,2,2,2,2,2,2,2,2,2,2,2,2,2,2,2,2,2,2,2,2,2,2,2,2,2,2,2,
2,2,2,2,2,2,2,2,2,2,2,2,2,2,2,2,2,2,2,2,2,2,2,2,2,2,2,2,2,2,2,2,2,2,2,2,
2,2,2,2,2,2,2,2,2,2,2,2,2,2,2,2,2,2,2,2,4),(-0.991194904658961,-0.989058491626383,
-0.985746034335273,-0.983851197030988,-0.982194965446795,-0.979960349182465,
-0.974798752808426,-0.967380016124243,-0.943724386415452,-0.912576510451123,
-0.90548403672454,-0.901838034646032,-0.89891465974563,-0.895572292867348,
-0.889737164279442,-0.882569425933697,-0.866755685093601,-0.837909878960278,
-0.822426100828139,-0.819121429452957,-0.817228355206994,-0.815571733408831,
-0.813334003219074,-0.808154192747193,-0.800700081459465,-0.77682948391001,
-0.745962654520282,-0.738867704777704,-0.735221196377737,-0.732297786767454,
-0.728955783804222,-0.72312235362758,-0.715957282228572,-0.700152639618032,
-0.671304545212078,-0.655809351069932,-0.652504140663196,-0.650610946596399,
-0.648954355676494,-0.64671684902612,-0.641538331851979,-0.634086729332441,
-0.610231397602398,-0.579344742099706,-0.57224998935752,-0.568603525612343,
-0.565680124390798,-0.562338101220941,-0.556504557299234,-0.549339303327267,
-0.533534020766918,-0.504686172267139,-0.489191833461697,-0.485886668598096,
-0.483993486958045,-0.482336897099563,-0.480099378739821,-0.47492077839181,
-0.467469009380936,-0.443612622131685,-0.412727460531904,-0.405632707781558,
-0.401986248085462,-0.399062852073509,-0.395720836993071,-0.389887312809662,
-0.382722086150404,-0.366916880819668,-0.338069072199305,-0.322574702883354,
-0.319269541326764,-0.317376362560824,-0.315719775922348,-0.313482262853182,
-0.308303678767825,-0.300851936514463,-0.27699567239423,-0.246110465049564,
-0.23901572641041,-0.235369273677834,-0.232445883108845,-0.229103874098857,
-0.223270360112144,-0.216105145760034,-0.200299966375875,-0.171802739950951,
-0.156005557003889,-0.152674181454946,-0.150775084015369,-0.149175409652698,
-0.149155773580123,-0.149136266281287,-0.149116881360587,-0.14909761257984,
-0.149078453872716,-0.149059399305514,-0.149040443054649,-0.14902157946385,
-0.14900280305385,-0.148984108405387,-0.14686707330857,-0.144354652225158,
-0.13994845932989,-0.129882787025892,-0.0914884568668121,-0.0755866350468697,
-0.07060407606162,-0.0674441109984219,-0.0644762356056652,-0.0604736220423971,
-0.0511374369443929,-0.0378016688393984,-0.000492023165766259),
 .UNSPECIFIED.);
#2388=B_SPLINE_CURVE_WITH_KNOTS('',3,(#66904,#66905,#66906,#66907,#66908,
#66909,#66910,#66911,#66912,#66913,#66914,#66915,#66916,#66917,#66918,#66919,
#66920,#66921,#66922,#66923),.UNSPECIFIED.,.F.,.F.,(4,2,2,2,2,2,2,2,2,4),
(-2.09991839469697,-2.0886857961363,-2.08627102604875,-2.08454940902833,
-2.08301335512356,-2.08147524148558,-2.07935219203929,-2.0739136789937,
-2.059231498808,-2.04109563196961),.UNSPECIFIED.);
#2389=B_SPLINE_CURVE_WITH_KNOTS('',3,(#66925,#66926,#66927,#66928,#66929,
#66930,#66931,#66932,#66933,#66934,#66935,#66936),.UNSPECIFIED.,.F.,.F.,
(4,2,2,2,2,4),(-0.0595287291512849,-0.059106780442287,-0.0557582976601512,
-0.0498913034740727,-0.016627889067852,-0.00049195452369095),
 .UNSPECIFIED.);
#2390=B_SPLINE_CURVE_WITH_KNOTS('',3,(#66937,#66938,#66939,#66940,#66941,
#66942,#66943,#66944,#66945,#66946,#66947,#66948,#66949,#66950,#66951,#66952,
#66953,#66954,#66955,#66956,#66957,#66958,#66959,#66960,#66961,#66962,#66963,
#66964,#66965,#66966,#66967,#66968,#66969,#66970,#66971,#66972,#66973,#66974,
#66975,#66976,#66977,#66978,#66979,#66980,#66981,#66982,#66983,#66984,#66985,
#66986,#66987,#66988,#66989,#66990,#66991,#66992,#66993,#66994,#66995,#66996,
#66997,#66998,#66999,#67000,#67001,#67002,#67003,#67004,#67005,#67006,#67007,
#67008,#67009,#67010,#67011,#67012,#67013,#67014,#67015,#67016,#67017,#67018,
#67019,#67020,#67021,#67022,#67023,#67024,#67025,#67026,#67027,#67028,#67029,
#67030,#67031,#67032,#67033,#67034,#67035,#67036,#67037,#67038,#67039,#67040,
#67041,#67042,#67043,#67044,#67045,#67046,#67047,#67048,#67049,#67050,#67051,
#67052,#67053,#67054,#67055,#67056,#67057,#67058,#67059,#67060,#67061,#67062,
#67063,#67064,#67065,#67066,#67067,#67068,#67069,#67070,#67071,#67072,#67073,
#67074,#67075,#67076,#67077,#67078,#67079,#67080,#67081,#67082,#67083,#67084,
#67085,#67086,#67087,#67088,#67089,#67090,#67091,#67092,#67093,#67094,#67095,
#67096,#67097,#67098,#67099,#67100,#67101,#67102,#67103,#67104,#67105,#67106,
#67107,#67108,#67109,#67110,#67111,#67112,#67113,#67114,#67115,#67116,#67117,
#67118,#67119,#67120,#67121,#67122,#67123,#67124,#67125,#67126,#67127,#67128),
 .UNSPECIFIED.,.F.,.F.,(4,2,2,2,2,2,2,2,2,2,2,2,2,2,2,2,2,2,2,2,2,2,2,2,
2,2,2,2,2,2,2,2,2,2,2,2,2,2,2,2,2,2,2,2,2,2,2,2,2,2,2,2,2,2,2,2,2,2,2,2,
2,2,2,2,2,2,2,2,2,2,2,2,2,2,2,2,2,2,2,2,2,2,2,2,2,2,2,2,2,2,2,2,2,2,2,4),
(-2.09972951695153,-2.08762494873157,-2.08160922163102,-2.07926464619698,
-2.07756995289858,-2.07588864726461,-2.07407041354946,-2.0710206138509,
-2.0599397817213,-2.04192034850692,-2.01035678597967,-1.99976485160584,
-1.99556694831247,-1.99256567514997,-1.98983237580441,-1.98544641751165,
-1.97436485107193,-1.93166229369477,-1.92046297263968,-1.91573442843177,
-1.91206766930225,-1.91011685239375,-1.90846990090058,-1.90635882692954,
-1.90176372976302,-1.86272928461758,-1.83584647360384,-1.83031075555954,
-1.82703240618409,-1.82409985914047,-1.82035378996897,-1.81429550014344,
-1.77483027179431,-1.74914995239231,-1.74540675712624,-1.74344009580529,
-1.74179479404348,-1.7396695685506,-1.73511973418902,-1.7040896211669,-1.66971564387023,
-1.66386534967124,-1.66051996650054,-1.65759726293833,-1.65395645029617,
-1.64688811049169,-1.6142995184733,-1.59174317797869,-1.58099321034783,
-1.57807440153557,-1.57628491885698,-1.57460818384061,-1.57253670508038,
-1.56841806937079,-1.53751669813052,-1.50300585905392,-1.49717290596144,
-1.49383125417834,-1.49090822736861,-1.48726231554419,-1.4801689744172,
-1.44927314347284,-1.42544383362372,-1.41799716422669,-1.41282080725194,
-1.41058384417993,-1.40892749041593,-1.4070344668602,-1.40372933182265,
-1.38823677207131,-1.35935394998613,-1.34353633706865,-1.336367767452,-1.3305327051611,
-1.32719065175309,-1.32426774116309,-1.32062258740339,-1.31353269480601,
-1.28226643076721,-1.25872134993977,-1.2513216573233,-1.24616953939659,
-1.24393675552747,-1.24228095677482,-1.24038563639913,-1.23707023673077,
-1.22138033464888,-1.19067429075411,-1.16872688871161,-1.16342661352892,
-1.16019891038352,-1.15725502804261,-1.15347808863828,-1.14717033205657,
-1.11072211711538,-1.10894444197162),.UNSPECIFIED.);
#2391=B_SPLINE_CURVE_WITH_KNOTS('',3,(#67133,#67134,#67135,#67136,#67137,
#67138,#67139,#67140,#67141,#67142,#67143,#67144,#67145,#67146,#67147,#67148,
#67149,#67150,#67151,#67152,#67153,#67154,#67155,#67156,#67157,#67158,#67159,
#67160,#67161,#67162,#67163,#67164,#67165,#67166,#67167,#67168,#67169,#67170,
#67171,#67172,#67173,#67174,#67175,#67176,#67177,#67178,#67179,#67180,#67181,
#67182,#67183,#67184,#67185,#67186,#67187,#67188,#67189,#67190,#67191,#67192,
#67193,#67194,#67195,#67196,#67197,#67198,#67199,#67200,#67201,#67202,#67203,
#67204,#67205,#67206,#67207,#67208,#67209,#67210,#67211,#67212,#67213,#67214,
#67215,#67216,#67217,#67218,#67219,#67220,#67221,#67222,#67223,#67224,#67225,
#67226,#67227,#67228,#67229,#67230,#67231,#67232,#67233,#67234,#67235,#67236,
#67237,#67238,#67239,#67240,#67241,#67242,#67243,#67244,#67245,#67246,#67247,
#67248,#67249,#67250,#67251,#67252,#67253,#67254,#67255,#67256,#67257,#67258,
#67259,#67260,#67261,#67262,#67263,#67264,#67265,#67266,#67267,#67268,#67269,
#67270,#67271,#67272,#67273,#67274,#67275,#67276,#67277,#67278,#67279,#67280,
#67281,#67282,#67283,#67284,#67285,#67286,#67287,#67288,#67289,#67290,#67291,
#67292,#67293,#67294,#67295,#67296,#67297,#67298,#67299,#67300,#67301,#67302,
#67303,#67304,#67305,#67306,#67307,#67308,#67309,#67310,#67311,#67312,#67313,
#67314,#67315,#67316,#67317,#67318,#67319,#67320,#67321,#67322,#67323,#67324,
#67325,#67326,#67327,#67328,#67329,#67330,#67331,#67332,#67333,#67334),
 .UNSPECIFIED.,.F.,.F.,(4,2,2,2,2,2,2,2,2,2,2,2,2,2,2,2,2,2,2,2,2,2,2,2,
2,2,2,2,2,2,2,2,2,2,2,2,2,2,2,2,2,2,2,2,2,2,2,2,2,2,2,2,2,2,2,2,2,2,2,2,
2,2,2,2,2,2,2,2,2,2,2,2,2,2,2,2,2,2,2,2,2,2,2,2,2,2,2,2,2,2,2,2,2,2,2,2,
2,2,2,2,4),(-2.04074305503047,-2.02176080152629,-1.99384987027655,-1.98710611557191,
-1.98462713436291,-1.98293077150667,-1.98114019282429,-1.97821731248195,
-1.96848114424382,-1.9329647641981,-1.91720136870814,-1.91004840441284,
-1.9042230673634,-1.90088266277738,-1.89795889794749,-1.89430964280617,
-1.88720188374861,-1.85636083673836,-1.83251384732456,-1.82506419838601,
-1.81988617265438,-1.81764869367751,-1.81599202616616,-1.81409867224156,
-1.81079296270405,-1.79529482930241,-1.7664215516926,-1.75060743488931,
-1.74343967161567,-1.73760494974324,-1.734262600938,-1.73133912750374,-1.72769285124944,
-1.72059932197814,-1.68974702487582,-1.66589205386159,-1.65844117369326,
-1.65326254347845,-1.65102499052903,-1.64936834343959,-1.64747509951189,
-1.64416976632013,-1.62867836833479,-1.59980717527062,-1.5839882391475,
-1.57681912105258,-1.5709835654804,-1.56764108564395,-1.56471769844216,
-1.56107179312776,-1.55397983344114,-1.5229640496197,-1.49923529656856,
-1.49180522827657,-1.48663734319411,-1.48440165718248,-1.4827452756282,
-1.48085104734367,-1.47754125304301,-1.46195639825263,-1.43191758295835,
-1.41687236308896,-1.40669916778648,-1.40256401223938,-1.39957377750021,
-1.39645793794689,-1.39168439733425,-1.37773034360203,-1.34383483598883,
-1.32426896056079,-1.31972036402197,-1.31759532801764,-1.31610652886066,
-1.31420602388915,-1.31086836948689,-1.29499934795618,-1.26456344967935,
-1.24258072683854,-1.23727798761749,-1.23404945875012,-1.23110523923404,
-1.22732842082489,-1.2210220479472,-1.18455963312416,-1.15609582848917,
-1.15250324513326,-1.15056793435959,-1.1489189499622,-1.14678618252229,
-1.14207156602555,-1.11468307184424,-1.08900037948016,-1.07466390661277,
-1.06998852261704,-1.0668931076755,-1.06392412876924,-1.05974129419506,
-1.05002072744021,-1.03548481317483,-1.00469839400656,-0.991194904658961),
 .UNSPECIFIED.);
#2392=B_SPLINE_CURVE_WITH_KNOTS('',3,(#67335,#67336,#67337,#67338,#67339,
#67340,#67341,#67342,#67343,#67344,#67345,#67346,#67347,#67348,#67349,#67350,
#67351,#67352,#67353,#67354,#67355,#67356,#67357,#67358,#67359,#67360,#67361,
#67362,#67363,#67364,#67365,#67366,#67367,#67368,#67369,#67370,#67371,#67372,
#67373,#67374,#67375,#67376,#67377,#67378,#67379,#67380,#67381,#67382,#67383,
#67384,#67385,#67386,#67387,#67388,#67389,#67390,#67391,#67392,#67393,#67394,
#67395,#67396,#67397,#67398,#67399,#67400,#67401,#67402,#67403,#67404,#67405,
#67406,#67407,#67408,#67409,#67410,#67411,#67412,#67413,#67414,#67415,#67416,
#67417,#67418,#67419,#67420,#67421,#67422,#67423,#67424,#67425,#67426,#67427,
#67428,#67429,#67430,#67431,#67432,#67433,#67434,#67435,#67436,#67437,#67438,
#67439,#67440,#67441,#67442,#67443,#67444,#67445,#67446,#67447,#67448,#67449,
#67450,#67451,#67452,#67453,#67454,#67455,#67456,#67457,#67458,#67459,#67460,
#67461,#67462,#67463,#67464,#67465,#67466,#67467,#67468,#67469,#67470,#67471,
#67472,#67473,#67474,#67475,#67476,#67477,#67478,#67479,#67480,#67481,#67482,
#67483,#67484,#67485,#67486,#67487,#67488,#67489,#67490,#67491,#67492,#67493,
#67494,#67495,#67496,#67497,#67498,#67499,#67500,#67501,#67502,#67503,#67504,
#67505,#67506,#67507,#67508,#67509,#67510,#67511,#67512,#67513,#67514,#67515,
#67516,#67517,#67518,#67519,#67520,#67521,#67522,#67523,#67524,#67525,#67526,
#67527,#67528,#67529,#67530,#67531,#67532,#67533,#67534,#67535,#67536,#67537,
#67538,#67539,#67540,#67541,#67542,#67543,#67544,#67545,#67546,#67547,#67548,
#67549,#67550,#67551,#67552,#67553,#67554,#67555,#67556,#67557,#67558,#67559,
#67560),.UNSPECIFIED.,.F.,.F.,(4,2,2,2,2,2,2,2,2,2,2,2,2,2,2,2,2,2,2,2,
2,2,2,2,2,2,2,2,2,2,2,2,2,2,2,2,2,2,2,2,2,2,2,2,2,2,2,2,2,2,2,2,2,2,2,2,
2,2,2,2,2,2,2,2,2,2,2,2,2,2,2,2,2,2,2,2,2,2,2,2,2,2,2,2,2,2,2,2,2,2,2,2,
2,2,2,2,2,2,2,2,2,2,2,2,2,2,2,2,2,2,2,2,4),(-1.10894444197162,-1.09089037655592,
-1.08415673956179,-1.07935451739902,-1.07718323275036,-1.0755490522122,
-1.07362205003105,-1.07016553621993,-1.05015894330672,-1.00482988921112,
-0.9986247928755,-0.994877149968059,-0.991937411299972,-0.988695082365399,
-0.98332570959186,-0.960135671977726,-0.928328678479021,-0.914931135687885,
-0.911703892112214,-0.909847096522318,-0.908181184114637,-0.90587463306034,
-0.900278591256796,-0.891997440140209,-0.862453253489691,-0.836016300195138,
-0.830390634826198,-0.827093385934435,-0.824457656189739,-0.82088957566476,
-0.813954305730896,-0.788529788800003,-0.761746855292337,-0.748309387119202,
-0.745079594319196,-0.743222243293156,-0.74155650652568,-0.739251122986672,
-0.733662316760718,-0.725395842303092,-0.695965248052592,-0.669394038897802,
-0.663766083718624,-0.660468342903045,-0.657832680934087,-0.654265296671087,
-0.647333552011604,-0.621937100275696,-0.595212690067308,-0.581701278464992,
-0.57846136206839,-0.576601810292879,-0.574936768258777,-0.572636000128682,
-0.56707569812071,-0.558866924475694,-0.52987746694275,-0.502782721339736,
-0.497146456614218,-0.493846937544746,-0.491211528055736,-0.487646677809804,
-0.480727720528842,-0.455432768920035,-0.428921743268478,-0.41509896592003,
-0.411845751260955,-0.409983311383686,-0.408319160044401,-0.406024373637239,
-0.400500848305203,-0.392366270165909,-0.363931998791517,-0.336176653628017,
-0.330529219537321,-0.327227312306831,-0.324592238284008,-0.321030774621129,
-0.314128881203692,-0.288968850040101,-0.262745703274513,-0.24852090429876,
-0.24524096413246,-0.243372730086959,-0.241710296067741,-0.239427261335879,
-0.233975446541185,-0.225984731803385,-0.198590728969246,-0.169517932224578,
-0.163887738783788,-0.160589509162061,-0.157732828173098,-0.157546413679192,
-0.157380327295911,-0.157228306947839,-0.157086037941978,-0.156950352757707,
-0.15681878652873,-0.156689310236186,-0.156560158753731,-0.156429711576455,
-0.152313747556579,-0.140655079980355,-0.122288555785325,-0.0959586558801422,
-0.0818862949928874,-0.0786145565632204,-0.0767481097014717,-0.075085175726414,
-0.0727986058168453,-0.0673252172130096,-0.0593761644650439),
 .UNSPECIFIED.);
#2393=B_SPLINE_CURVE_WITH_KNOTS('',3,(#67566,#67567,#67568,#67569,#67570,
#67571,#67572,#67573,#67574,#67575,#67576,#67577,#67578,#67579,#67580,#67581,
#67582,#67583,#67584,#67585,#67586,#67587,#67588,#67589,#67590,#67591,#67592,
#67593,#67594,#67595,#67596,#67597,#67598,#67599,#67600,#67601,#67602,#67603,
#67604,#67605,#67606,#67607,#67608,#67609,#67610,#67611,#67612,#67613,#67614,
#67615,#67616,#67617,#67618,#67619,#67620,#67621,#67622,#67623,#67624,#67625,
#67626,#67627,#67628,#67629,#67630,#67631,#67632,#67633,#67634,#67635,#67636,
#67637,#67638,#67639,#67640,#67641,#67642,#67643,#67644,#67645,#67646,#67647,
#67648,#67649,#67650,#67651,#67652,#67653,#67654,#67655,#67656,#67657,#67658,
#67659,#67660,#67661,#67662,#67663,#67664,#67665,#67666,#67667,#67668,#67669,
#67670,#67671,#67672,#67673,#67674,#67675,#67676,#67677,#67678,#67679,#67680,
#67681,#67682,#67683,#67684,#67685,#67686,#67687,#67688,#67689,#67690,#67691,
#67692,#67693,#67694,#67695,#67696,#67697,#67698,#67699,#67700,#67701,#67702,
#67703,#67704,#67705,#67706,#67707,#67708,#67709,#67710,#67711,#67712,#67713,
#67714,#67715,#67716,#67717,#67718,#67719,#67720,#67721,#67722,#67723,#67724,
#67725,#67726,#67727,#67728,#67729,#67730,#67731,#67732,#67733,#67734,#67735,
#67736,#67737,#67738,#67739,#67740,#67741,#67742,#67743,#67744,#67745,#67746,
#67747,#67748,#67749,#67750,#67751,#67752,#67753,#67754,#67755,#67756,#67757,
#67758,#67759,#67760,#67761,#67762,#67763,#67764,#67765,#67766,#67767,#67768,
#67769,#67770,#67771,#67772,#67773),.UNSPECIFIED.,.F.,.F.,(4,2,2,2,2,2,
2,2,2,2,2,2,2,2,2,2,2,2,2,2,2,2,2,2,2,2,2,2,2,2,2,2,2,2,2,2,2,2,2,2,2,2,
2,2,2,2,2,2,2,2,2,2,2,2,2,2,2,2,2,2,2,2,2,2,2,2,2,2,2,2,2,2,2,2,2,2,2,2,
2,2,2,2,2,2,2,2,2,2,2,2,2,2,2,2,2,2,2,2,2,2,2,2,2,4),(-0.991238213430677,
-0.976641098909451,-0.971230807864263,-0.967978531114308,-0.965039079154578,
-0.961241742758999,-0.953103229758448,-0.925083580910352,-0.891127935454698,
-0.886797858173586,-0.884713751144305,-0.883070102675632,-0.881068500737586,
-0.877156636841558,-0.872014680897714,-0.859274844728248,-0.828002733313391,
-0.809602906575744,-0.804375953569787,-0.801163009680009,-0.798213051105526,
-0.794335341475655,-0.785743700959912,-0.758090115601303,-0.72450349102752,
-0.720134861275554,-0.71804337759993,-0.716399431371068,-0.714404184847302,
-0.710523612973384,-0.705435001796337,-0.692899901914688,-0.654316896289965,
-0.641653679920653,-0.637036579568481,-0.634260816191678,-0.631290139889179,
-0.627274387086287,-0.617862219996585,-0.604377302909968,-0.582858406290926,
-0.576004895198285,-0.556406456687993,-0.552959641722108,-0.551034353252153,
-0.549399146856339,-0.54722316280081,-0.542397598994321,-0.535620209360751,
-0.51556697007537,-0.479407361604222,-0.473079687412401,-0.469296387173338,
-0.466350689785722,-0.463124164445328,-0.457833101308611,-0.436057485466618,
-0.405583031730287,-0.389553840963494,-0.386209695742535,-0.384307459223142,
-0.382818572822939,-0.380695026841,-0.376155991265821,-0.356683892684253,
-0.323061797240769,-0.308751121174757,-0.303938737272029,-0.300814288931752,
-0.297827927808991,-0.29371776307728,-0.283710276033602,-0.269014953284204,
-0.248834278459128,-0.244849051881725,-0.223158171046896,-0.219672848435838,
-0.217739029785914,-0.216105209456666,-0.213942302507689,-0.209188904993565,
-0.18763574474434,-0.147983885056826,-0.139736774480289,-0.135961189517189,
-0.133016750198675,-0.131759432379266,-0.131703476977391,-0.13157000340885,
-0.131441985762563,-0.131318625722611,-0.131199224891469,-0.13108316602606,
-0.127592372240812,-0.119051126452774,-0.107127561791166,-0.0807651978249793,
-0.0565214939093335,-0.0530212881142028,-0.0510842239026097,-0.0494352662233957,
-0.0472681091763347,-0.0424908150203636,-0.000491816551951527),
 .UNSPECIFIED.);
#2394=B_SPLINE_CURVE_WITH_KNOTS('',3,(#67774,#67775,#67776,#67777,#67778,
#67779,#67780,#67781,#67782,#67783,#67784,#67785,#67786,#67787,#67788,#67789,
#67790,#67791),.UNSPECIFIED.,.F.,.F.,(4,2,2,2,2,2,2,2,4),(-2.09980330258049,
-2.07619390304051,-2.07214372682003,-2.06916417689941,-2.06616224626754,
-2.06306409603706,-2.05837678839064,-2.04518472895466,-2.04074305503047),
 .UNSPECIFIED.);
#2395=B_SPLINE_CURVE_WITH_KNOTS('',3,(#67793,#67794,#67795,#67796,#67797,
#67798,#67799,#67800,#67801,#67802),.UNSPECIFIED.,.F.,.F.,(4,2,2,2,4),(-0.0593761644650439,
-0.0592913074490973,-0.0342070986254461,-0.00945211975966167,-0.00049169905348269),
 .UNSPECIFIED.);
#2396=B_SPLINE_CURVE_WITH_KNOTS('',3,(#67803,#67804,#67805,#67806,#67807,
#67808,#67809,#67810,#67811,#67812,#67813,#67814,#67815,#67816,#67817,#67818,
#67819,#67820,#67821,#67822,#67823,#67824,#67825,#67826,#67827,#67828,#67829,
#67830,#67831,#67832,#67833,#67834,#67835,#67836,#67837,#67838,#67839,#67840,
#67841,#67842,#67843,#67844,#67845,#67846,#67847,#67848,#67849,#67850,#67851,
#67852,#67853,#67854,#67855,#67856,#67857,#67858,#67859,#67860,#67861,#67862,
#67863,#67864,#67865,#67866,#67867,#67868,#67869,#67870,#67871,#67872,#67873,
#67874,#67875,#67876,#67877,#67878,#67879,#67880,#67881,#67882,#67883,#67884,
#67885,#67886,#67887,#67888,#67889,#67890,#67891,#67892,#67893,#67894,#67895,
#67896,#67897,#67898,#67899,#67900,#67901,#67902,#67903,#67904,#67905,#67906,
#67907,#67908,#67909,#67910,#67911,#67912,#67913,#67914,#67915,#67916,#67917,
#67918,#67919,#67920,#67921,#67922,#67923,#67924,#67925,#67926,#67927,#67928,
#67929,#67930,#67931,#67932,#67933,#67934,#67935,#67936,#67937,#67938,#67939,
#67940,#67941,#67942,#67943,#67944,#67945,#67946,#67947,#67948,#67949,#67950,
#67951,#67952,#67953,#67954,#67955,#67956,#67957,#67958,#67959,#67960,#67961,
#67962,#67963,#67964,#67965,#67966,#67967,#67968,#67969,#67970,#67971,#67972,
#67973,#67974,#67975,#67976,#67977,#67978,#67979,#67980,#67981,#67982,#67983,
#67984,#67985,#67986,#67987,#67988,#67989,#67990,#67991,#67992),
 .UNSPECIFIED.,.F.,.F.,(4,2,2,2,2,2,2,2,2,2,2,2,2,2,2,2,2,2,2,2,2,2,2,2,
2,2,2,2,2,2,2,2,2,2,2,2,2,2,2,2,2,2,2,2,2,2,2,2,2,2,2,2,2,2,2,2,2,2,2,2,
2,2,2,2,2,2,2,2,2,2,2,2,2,2,2,2,2,2,2,2,2,2,2,2,2,2,2,2,2,2,2,2,2,2,4),
(-2.10024504072334,-2.09787273841388,-2.09523860874424,-2.09246330528043,
-2.08935977733162,-2.08464641798153,-2.07112934357474,-2.04408003428377,
-2.01566772564429,-2.01200283565764,-2.01005224938009,-2.00840502045651,
-2.00629300155547,-2.00169366717601,-1.97108418808107,-1.93630774981785,
-1.93048139131627,-1.92714074190697,-1.92421698095752,-1.92056803847037,
-1.91346198160399,-1.88096440418894,-1.85837622794891,-1.84761720780912,
-1.8446972972018,-1.8429073874589,-1.84123046149147,-1.83915896107834,-1.83504093330713,
-1.80412213877854,-1.76961599056957,-1.76378213197677,-1.76043994885644,
-1.75751644997828,-1.75386993977086,-1.74677540363776,-1.71588047192911,
-1.6920428168382,-1.68459420820755,-1.67941663649243,-1.67717924779383,
-1.67552261877299,-1.67362932661174,-1.6703238203993,-1.65483216059785,
-1.62594546978692,-1.61012255769803,-1.60295202816064,-1.5971155138448,
-1.59377281327351,-1.59084944358724,-1.58720385745557,-1.58011357497684,
-1.54876799246582,-1.52527567895461,-1.51788419285912,-1.51273609566101,
-1.51050378408327,-1.50884782213758,-1.50695172217838,-1.5036336910992,
-1.48791320988004,-1.45713439125066,-1.43527278329857,-1.42997697129172,
-1.4267498888739,-1.42380521958709,-1.42002539514928,-1.41370856253163,
-1.37739504125981,-1.35746665629243,-1.35071390093406,-1.3459012665092,
-1.34372789953177,-1.34209327888696,-1.34016710917275,-1.33671515486238,
-1.31691095177069,-1.31065234924921,-1.29014526813032,-1.26856989282184,
-1.26329131237934,-1.26006788303582,-1.25712211529855,-1.25333472147441,
-1.24699120920666,-1.21118885186706,-1.18240397849715,-1.17863478312334,
-1.17666264847304,-1.17501765314872,-1.17289908874325,-1.16838552857327,
-1.13691431709602,-1.10919217566827),.UNSPECIFIED.);
#2397=B_SPLINE_CURVE_WITH_KNOTS('',3,(#67997,#67998,#67999,#68000,#68001,
#68002,#68003,#68004,#68005,#68006,#68007,#68008,#68009,#68010,#68011,#68012,
#68013,#68014,#68015,#68016,#68017,#68018,#68019,#68020,#68021,#68022,#68023,
#68024,#68025,#68026,#68027,#68028,#68029,#68030,#68031,#68032,#68033,#68034,
#68035,#68036,#68037,#68038,#68039,#68040,#68041,#68042,#68043,#68044,#68045,
#68046,#68047,#68048,#68049,#68050,#68051,#68052,#68053,#68054,#68055,#68056,
#68057,#68058,#68059,#68060,#68061,#68062,#68063,#68064,#68065,#68066,#68067,
#68068,#68069,#68070,#68071,#68072,#68073,#68074,#68075,#68076,#68077,#68078,
#68079,#68080,#68081,#68082,#68083,#68084,#68085,#68086,#68087,#68088,#68089,
#68090,#68091,#68092,#68093,#68094,#68095,#68096,#68097,#68098,#68099,#68100,
#68101,#68102,#68103,#68104,#68105,#68106,#68107,#68108,#68109,#68110,#68111,
#68112,#68113,#68114,#68115,#68116,#68117,#68118,#68119,#68120,#68121,#68122,
#68123,#68124,#68125,#68126,#68127,#68128,#68129,#68130,#68131,#68132,#68133,
#68134,#68135,#68136,#68137,#68138,#68139,#68140,#68141,#68142,#68143,#68144,
#68145,#68146,#68147,#68148,#68149,#68150,#68151,#68152,#68153,#68154,#68155,
#68156,#68157,#68158,#68159,#68160,#68161,#68162,#68163,#68164,#68165,#68166,
#68167,#68168,#68169,#68170,#68171,#68172,#68173,#68174,#68175,#68176,#68177,
#68178,#68179,#68180,#68181,#68182,#68183,#68184,#68185,#68186,#68187,#68188,
#68189,#68190,#68191,#68192),.UNSPECIFIED.,.F.,.F.,(4,2,2,2,2,2,2,2,2,2,
2,2,2,2,2,2,2,2,2,2,2,2,2,2,2,2,2,2,2,2,2,2,2,2,2,2,2,2,2,2,2,2,2,2,2,2,
2,2,2,2,2,2,2,2,2,2,2,2,2,2,2,2,2,2,2,2,2,2,2,2,2,2,2,2,2,2,2,2,2,2,2,2,
2,2,2,2,2,2,2,2,2,2,2,2,2,2,2,4),(-2.0412663643322,-2.01060717261452,-1.98828790130411,
-1.97511847098684,-1.97112742661626,-1.96803319828237,-1.96508135997042,
-1.9612574310206,-1.95273657878317,-1.91339267278809,-1.89194377310661,
-1.88720010779772,-1.8850386909596,-1.88340469790752,-1.88146914146686,
-1.87797709584422,-1.8548274488637,-1.83760928190919,-1.81269888917485,
-1.80582684315187,-1.80226992237025,-1.79963383762293,-1.79632494669173,
-1.79065101663131,-1.76084503878615,-1.73931689071548,-1.7282336780585,
-1.72353686181082,-1.71988887908675,-1.71794149996365,-1.71629336048578,
-1.71417559231816,-1.70954661352483,-1.67065837436693,-1.64367872984786,
-1.63813790037239,-1.63485759808724,-1.63192394379233,-1.62817732016164,
-1.6203166952437,-1.58023817567784,-1.5585658093168,-1.55380013103779,-1.55163477525613,
-1.55000045310844,-1.54806769301185,-1.54458801201727,-1.5234848008202,
-1.5187966136912,-1.4987575837135,-1.47655718878509,-1.47124012733842,-1.46800770745067,
-1.46506304478681,-1.46128994989667,-1.45499950750342,-1.41822384803917,
-1.39859794336622,-1.38865786258578,-1.38581134779563,-1.384037184282,-1.38234962929046,
-1.379830723386,-1.37332386187274,-1.34126769928369,-1.31543259691161,-1.3067129472373,
-1.30281286390363,-1.29985957088073,-1.29665627485738,-1.29147502602385,
-1.27349368529231,-1.24202474900111,-1.22910099098222,-1.22391134039225,
-1.21997121665099,-1.21796381967116,-1.21632029735965,-1.21424250100709,
-1.20994565330823,-1.17565638974526,-1.1487627648545,-1.14002778855009,
-1.13612517425918,-1.13317162651532,-1.12996966128824,-1.12479418140525,
-1.10689369033933,-1.06939817794942,-1.06025456089091,-1.05424110806619,
-1.05186817121142,-1.05019077942413,-1.04836130290588,-1.04526232091129,
-1.03215413643346,-0.998040183333568,-0.991238213430677),.UNSPECIFIED.);
#2398=B_SPLINE_CURVE_WITH_KNOTS('',3,(#68193,#68194,#68195,#68196,#68197,
#68198,#68199,#68200,#68201,#68202,#68203,#68204,#68205,#68206,#68207,#68208,
#68209,#68210,#68211,#68212,#68213,#68214,#68215,#68216,#68217,#68218,#68219,
#68220,#68221,#68222,#68223,#68224,#68225,#68226,#68227,#68228,#68229,#68230,
#68231,#68232,#68233,#68234,#68235,#68236,#68237,#68238,#68239,#68240,#68241,
#68242,#68243,#68244,#68245,#68246,#68247,#68248,#68249,#68250,#68251,#68252,
#68253,#68254,#68255,#68256,#68257,#68258,#68259,#68260,#68261,#68262,#68263,
#68264,#68265,#68266,#68267,#68268,#68269,#68270,#68271,#68272,#68273,#68274,
#68275,#68276,#68277,#68278,#68279,#68280,#68281,#68282,#68283,#68284,#68285,
#68286,#68287,#68288,#68289,#68290,#68291,#68292,#68293,#68294,#68295,#68296,
#68297,#68298,#68299,#68300,#68301,#68302,#68303,#68304,#68305,#68306,#68307,
#68308,#68309,#68310,#68311,#68312,#68313,#68314,#68315,#68316,#68317,#68318,
#68319,#68320,#68321,#68322,#68323,#68324,#68325,#68326,#68327,#68328,#68329,
#68330,#68331,#68332,#68333,#68334,#68335,#68336,#68337,#68338,#68339,#68340,
#68341,#68342,#68343,#68344,#68345,#68346,#68347,#68348,#68349,#68350,#68351,
#68352,#68353,#68354,#68355,#68356,#68357,#68358,#68359,#68360,#68361,#68362,
#68363,#68364,#68365,#68366,#68367,#68368,#68369,#68370,#68371,#68372,#68373,
#68374,#68375,#68376,#68377,#68378,#68379,#68380,#68381,#68382,#68383,#68384,
#68385,#68386,#68387,#68388,#68389,#68390,#68391,#68392),.UNSPECIFIED.,
 .F.,.F.,(4,2,2,2,2,2,2,2,2,2,2,2,2,2,2,2,2,2,2,2,2,2,2,2,2,2,2,2,2,2,2,
2,2,2,2,2,2,2,2,2,2,2,2,2,2,2,2,2,2,2,2,2,2,2,2,2,2,2,2,2,2,2,2,2,2,2,2,
2,2,2,2,2,2,2,2,2,2,2,2,2,2,2,2,2,2,2,2,2,2,2,2,2,2,2,2,2,2,2,2,4),(-1.10919217566827,
-1.10285109736999,-1.09703854338629,-1.09370097916952,-1.09077710882766,
-1.08712433418365,-1.0799988642058,-1.05011741528275,-1.016673667526,-1.01229135522323,
-1.01019762194584,-1.00855403458269,-1.00656186397993,-1.00269470075188,
-0.997628539458234,-0.985177693009459,-0.947242927744185,-0.933976867973413,
-0.929280727424155,-0.926181092711504,-0.923180991732553,-0.918990174932144,
-0.908446744395041,-0.892613381054371,-0.863756518159548,-0.848295087897,
-0.844991443623137,-0.84309864886408,-0.841442073412207,-0.839204199365472,
-0.834023256276718,-0.826567030450243,-0.802685929930445,-0.771815824415442,
-0.764719877234269,-0.761073243945101,-0.758149946739275,-0.75480832178638,
-0.748976269457675,-0.714573756006922,-0.683572745356013,-0.679022836427378,
-0.676897560246747,-0.675252201047247,-0.673285470285616,-0.669542102515961,
-0.642615199985557,-0.604620306015733,-0.598419830165685,-0.594632581617534,
-0.591695266433446,-0.588439619122877,-0.583010017818449,-0.558639141554511,
-0.547105513424786,-0.517020980839767,-0.512442047091056,-0.510302697376582,
-0.50865319759588,-0.506722874304056,-0.503153394592692,-0.498585490451799,
-0.454907512380181,-0.435164561979905,-0.429857209668909,-0.426628074085135,
-0.42368473772664,-0.419846870705144,-0.411475346106364,-0.389611885824379,
-0.350104274878984,-0.345668989673887,-0.343557720325191,-0.341910995435389,
-0.339960935820364,-0.336296810781593,-0.308459750706929,-0.271382650059542,
-0.265113250095761,-0.261347333872226,-0.258405141660985,-0.255172255417685,
-0.249847029937188,-0.227459982195111,-0.207626394063551,-0.183840506494559,
-0.17909860665286,-0.176961315837899,-0.175312293245642,-0.173381190221304,
-0.169806965046338,-0.14118435153848,-0.104828648157685,-0.0985146312613983,
-0.0947362774301334,-0.0917926116789703,-0.0885664833990601,-0.0832718787415284,
-0.0614035604514639,-0.0593668323253494),.UNSPECIFIED.);
#2399=B_SPLINE_CURVE_WITH_KNOTS('',3,(#68398,#68399,#68400,#68401,#68402,
#68403,#68404,#68405,#68406,#68407,#68408,#68409,#68410,#68411,#68412,#68413,
#68414,#68415,#68416,#68417,#68418,#68419,#68420,#68421,#68422,#68423,#68424,
#68425,#68426,#68427,#68428,#68429,#68430,#68431,#68432,#68433,#68434,#68435,
#68436,#68437,#68438,#68439,#68440,#68441,#68442,#68443,#68444,#68445,#68446,
#68447,#68448,#68449,#68450,#68451,#68452,#68453,#68454,#68455,#68456,#68457,
#68458,#68459,#68460,#68461,#68462,#68463,#68464,#68465,#68466,#68467,#68468,
#68469,#68470,#68471,#68472,#68473,#68474,#68475,#68476,#68477,#68478,#68479,
#68480,#68481,#68482,#68483,#68484,#68485,#68486,#68487,#68488,#68489,#68490,
#68491,#68492,#68493,#68494,#68495,#68496,#68497,#68498,#68499,#68500,#68501,
#68502,#68503,#68504,#68505,#68506,#68507,#68508,#68509,#68510,#68511,#68512,
#68513,#68514,#68515,#68516,#68517,#68518,#68519,#68520,#68521,#68522,#68523,
#68524,#68525,#68526,#68527,#68528,#68529,#68530,#68531,#68532,#68533,#68534,
#68535,#68536,#68537,#68538,#68539,#68540,#68541,#68542,#68543,#68544,#68545,
#68546,#68547,#68548,#68549,#68550,#68551,#68552,#68553,#68554,#68555,#68556,
#68557,#68558,#68559,#68560,#68561,#68562,#68563,#68564,#68565,#68566,#68567,
#68568,#68569,#68570,#68571,#68572,#68573,#68574,#68575,#68576,#68577,#68578,
#68579,#68580,#68581,#68582,#68583,#68584,#68585,#68586,#68587,#68588,#68589,
#68590,#68591,#68592,#68593,#68594,#68595),.UNSPECIFIED.,.F.,.F.,(4,2,2,
2,2,2,2,2,2,2,2,2,2,2,2,2,2,2,2,2,2,2,2,2,2,2,2,2,2,2,2,2,2,2,2,2,2,2,2,
2,2,2,2,2,2,2,2,2,2,2,2,2,2,2,2,2,2,2,2,2,2,2,2,2,2,2,2,2,2,2,2,2,2,2,2,
2,2,2,2,2,2,2,2,2,2,2,2,2,2,2,2,2,2,2,2,2,2,2,4),(-0.991317167272335,-0.971269366237599,
-0.956601880946314,-0.953336414956754,-0.951452096944215,-0.949793172520064,
-0.947538903310674,-0.942262563977142,-0.934620200965425,-0.909575086141311,
-0.8776750491207,-0.87204184857997,-0.868710676257753,-0.865813490371843,
-0.86216424209734,-0.854817562117453,-0.84515866654821,-0.81916330323871,
-0.81766818945004,-0.79230722832396,-0.787549888779139,-0.785409366960424,
-0.783759480653418,-0.781829275791654,-0.778261359027506,-0.749637794469464,
-0.713265210641895,-0.706950799053849,-0.703171613546739,-0.700226932995384,
-0.696999302507008,-0.691701278980093,-0.669796948385164,-0.639023568800072,
-0.623392855537778,-0.62008083009688,-0.618186055919584,-0.616529747807254,
-0.61429485201946,-0.609131861330975,-0.601710497585804,-0.578039612039028,
-0.546909828799278,-0.539816970239891,-0.536170823043493,-0.533247357323859,
-0.529904914376362,-0.524069726140404,-0.516901954488812,-0.501088361452861,
-0.472241543781939,-0.456756494487105,-0.453451685267782,-0.451558545332174,
-0.449901875585303,-0.44766409340259,-0.442484217105164,-0.435030056613093,
-0.411159810067018,-0.380290652944542,-0.373195502510553,-0.3695488869495,
-0.366625389483783,-0.363283283971826,-0.357449669232071,-0.350284368098833,
-0.334479201918933,-0.305630252231526,-0.290134649832783,-0.286829342649177,
-0.284936092182368,-0.283279451215878,-0.281041876037474,-0.275863196291234,
-0.268411356523578,-0.24455522826089,-0.213690410647705,-0.206581480733163,
-0.202932030775213,-0.20000831507877,-0.196668190564797,-0.190843899976307,
-0.157099963228134,-0.125363236630374,-0.120921297079108,-0.118808420797331,
-0.117161188585463,-0.11521138282097,-0.111549863208933,-0.0816363119513023,
-0.0570291304981712,-0.0427557720175263,-0.0379479202928798,-0.0348247944232061,
-0.0318385255683217,-0.028886410225576,-0.0249107123818784,-0.016294700971784,
-0.000491204019444046),.UNSPECIFIED.);
#2400=B_SPLINE_CURVE_WITH_KNOTS('',3,(#68596,#68597,#68598,#68599,#68600,
#68601,#68602,#68603,#68604,#68605,#68606,#68607,#68608,#68609,#68610,#68611,
#68612,#68613),.UNSPECIFIED.,.F.,.F.,(4,2,2,2,2,2,2,2,4),(-2.10008377485422,
-2.05932312996458,-2.05571269775278,-2.05274146765247,-2.05093995362208,
-2.04926853040962,-2.04722042808529,-2.04319839434716,-2.0412663643322),
 .UNSPECIFIED.);
#2401=B_SPLINE_CURVE_WITH_KNOTS('',3,(#68615,#68616,#68617,#68618,#68619,
#68620,#68621,#68622,#68623,#68624,#68625,#68626,#68627,#68628,#68629,#68630,
#68631,#68632),.UNSPECIFIED.,.F.,.F.,(4,2,2,2,2,2,2,2,4),(-0.0593668323253494,
-0.0244934904075403,-0.0142512542297031,-0.0112790705132887,-0.00947813354296127,
-0.00791635031254044,-0.00623769422981492,-0.00362381055065628,-0.000491106187273373),
 .UNSPECIFIED.);
#2402=B_SPLINE_CURVE_WITH_KNOTS('',3,(#68633,#68634,#68635,#68636,#68637,
#68638,#68639,#68640,#68641,#68642,#68643,#68644,#68645,#68646,#68647,#68648,
#68649,#68650,#68651,#68652,#68653,#68654,#68655,#68656,#68657,#68658,#68659,
#68660,#68661,#68662,#68663,#68664,#68665,#68666,#68667,#68668,#68669,#68670,
#68671,#68672,#68673,#68674,#68675,#68676,#68677,#68678,#68679,#68680,#68681,
#68682,#68683,#68684,#68685,#68686,#68687,#68688,#68689,#68690,#68691,#68692,
#68693,#68694,#68695,#68696,#68697,#68698,#68699,#68700,#68701,#68702,#68703,
#68704,#68705,#68706,#68707,#68708,#68709,#68710,#68711,#68712,#68713,#68714,
#68715,#68716,#68717,#68718,#68719,#68720,#68721,#68722,#68723,#68724,#68725,
#68726,#68727,#68728,#68729,#68730,#68731,#68732,#68733,#68734,#68735,#68736,
#68737,#68738,#68739,#68740,#68741,#68742,#68743,#68744,#68745,#68746,#68747,
#68748,#68749,#68750,#68751,#68752,#68753,#68754,#68755,#68756,#68757,#68758,
#68759,#68760,#68761,#68762,#68763,#68764,#68765,#68766,#68767,#68768,#68769,
#68770,#68771,#68772,#68773,#68774,#68775,#68776,#68777,#68778,#68779,#68780,
#68781,#68782,#68783,#68784,#68785,#68786,#68787,#68788,#68789,#68790,#68791,
#68792,#68793,#68794,#68795,#68796,#68797,#68798,#68799,#68800,#68801,#68802,
#68803,#68804,#68805,#68806,#68807,#68808,#68809,#68810,#68811,#68812,#68813,
#68814,#68815,#68816,#68817,#68818,#68819,#68820,#68821,#68822,#68823,#68824,
#68825,#68826,#68827,#68828,#68829,#68830,#68831,#68832,#68833,#68834,#68835,
#68836,#68837,#68838,#68839,#68840,#68841,#68842,#68843,#68844,#68845,#68846),
 .UNSPECIFIED.,.F.,.F.,(4,2,2,2,2,2,2,2,2,2,2,2,2,2,2,2,2,2,2,2,2,2,2,2,
2,2,2,2,2,2,2,2,2,2,2,2,2,2,2,2,2,2,2,2,2,2,2,2,2,2,2,2,2,2,2,2,2,2,2,2,
2,2,2,2,2,2,2,2,2,2,2,2,2,2,2,2,2,2,2,2,2,2,2,2,2,2,2,2,2,2,2,2,2,2,2,2,
2,2,2,2,2,2,2,2,2,2,4),(-2.10004855717667,-2.05968761413315,-2.03975706519315,
-2.03143220897157,-2.02760249894487,-2.0246601144664,-2.02142674536316,
-2.01610008933595,-1.99598846901806,-1.95258145943588,-1.94809650511923,
-1.9455538598408,-1.94340707952417,-1.9433868459708,-1.94336657917876,-1.94334627310399,
-1.94332592166687,-1.94330551860702,-1.94329463534735,-1.94328348333027,
-1.9432720490865,-1.94326031831007,-1.94324827571214,-1.94323590498146,
-1.94322318859647,-1.94321010778596,-1.94160157551812,-1.9397063782228,
-1.93639165246691,-1.92091182682553,-1.89202782939398,-1.87621349707516,
-1.86904587472698,-1.86321140840924,-1.85986947092063,-1.85694653106624,
-1.85330116949128,-1.84621032123755,-1.81504121816665,-1.79142177788148,
-1.78400974459386,-1.77885125434831,-1.77661737146842,-1.77496142847113,
-1.7730667168685,-1.7697540346938,-1.7541090257833,-1.72332658729998,-1.70140266668787,
-1.69610376797199,-1.69287635112243,-1.68993237403934,-1.68615482012498,
-1.67984491880162,-1.64343290472883,-1.62357696288477,-1.61683863647587,
-1.61203390181177,-1.60986215968526,-1.60822792651323,-1.60630121216711,
-1.60284600940396,-1.58289359533735,-1.57631373898952,-1.5546607004643,
-1.53453490564711,-1.52935132810845,-1.52614860385069,-1.5231971947656,
-1.51936790859076,-1.51080920467632,-1.47150948359011,-1.45008520417026,
-1.44534511109266,-1.44318499591757,-1.44155185895655,-1.43961721464028,
-1.43612663783686,-1.4129960351218,-1.39580234125571,-1.37086758946653,
-1.36399403779003,-1.36043791624384,-1.35780307860567,-1.35449662167666,
-1.34882912739601,-1.31805963838061,-1.29321564236277,-1.28477925339823,
-1.27910630227377,-1.27678723158176,-1.27511921296331,-1.27326788565249,
-1.27006640430231,-1.25709197869054,-1.22995706084433,-1.20196211208017,
-1.19638823425894,-1.19310183322284,-1.19017096081421,-1.1864392185505,
-1.18042976981119,-1.13421948993561,-1.11619276436942,-1.11181376051969,
-1.10972075181354,-1.10913504811783),.UNSPECIFIED.);
#2403=B_SPLINE_CURVE_WITH_KNOTS('',3,(#68851,#68852,#68853,#68854,#68855,
#68856,#68857,#68858,#68859,#68860,#68861,#68862,#68863,#68864,#68865,#68866,
#68867,#68868,#68869,#68870,#68871,#68872,#68873,#68874,#68875,#68876,#68877,
#68878,#68879,#68880,#68881,#68882,#68883,#68884,#68885,#68886,#68887,#68888,
#68889,#68890,#68891,#68892,#68893,#68894,#68895,#68896,#68897,#68898,#68899,
#68900,#68901,#68902,#68903,#68904,#68905,#68906,#68907,#68908,#68909,#68910,
#68911,#68912,#68913,#68914,#68915,#68916,#68917,#68918,#68919,#68920,#68921,
#68922,#68923,#68924,#68925,#68926,#68927,#68928,#68929,#68930,#68931,#68932,
#68933,#68934,#68935,#68936,#68937,#68938,#68939,#68940,#68941,#68942,#68943,
#68944,#68945,#68946,#68947,#68948,#68949,#68950,#68951,#68952,#68953,#68954,
#68955,#68956,#68957,#68958,#68959,#68960,#68961,#68962,#68963,#68964,#68965,
#68966,#68967,#68968,#68969,#68970,#68971,#68972,#68973,#68974,#68975,#68976,
#68977,#68978,#68979,#68980,#68981,#68982,#68983,#68984,#68985,#68986,#68987,
#68988,#68989,#68990,#68991,#68992,#68993,#68994,#68995,#68996,#68997,#68998,
#68999,#69000,#69001,#69002,#69003,#69004,#69005,#69006,#69007,#69008,#69009,
#69010,#69011,#69012,#69013,#69014,#69015,#69016,#69017,#69018,#69019,#69020,
#69021,#69022,#69023,#69024,#69025,#69026,#69027,#69028,#69029,#69030,#69031,
#69032,#69033,#69034,#69035,#69036,#69037,#69038,#69039,#69040,#69041,#69042,
#69043,#69044,#69045,#69046,#69047,#69048,#69049,#69050,#69051,#69052,#69053,
#69054,#69055,#69056,#69057,#69058,#69059,#69060,#69061,#69062,#69063,#69064,
#69065,#69066,#69067,#69068,#69069,#69070,#69071,#69072),.UNSPECIFIED.,
 .F.,.F.,(4,2,2,2,2,2,2,2,2,2,2,2,2,2,2,2,2,2,2,2,2,2,2,2,2,2,2,2,2,2,2,
2,2,2,2,2,2,2,2,2,2,2,2,2,2,2,2,2,2,2,2,2,2,2,2,2,2,2,2,2,2,2,2,2,2,2,2,
2,2,2,2,2,2,2,2,2,2,2,2,2,2,2,2,2,2,2,2,2,2,2,2,2,2,2,2,2,2,2,2,2,2,2,2,
2,2,2,2,2,2,2,4),(-2.04101140854792,-2.04046337870567,-2.03653625905841,
-2.03357960775552,-2.03038909176893,-2.02526514219354,-2.00834243620288,
-1.97136839202077,-1.9612482612546,-1.9568258979117,-1.95430708832056,-1.95218567019774,
-1.95216703017222,-1.95214830931894,-1.9521295023838,-1.95211060384299,
-1.95209160806915,-1.95207250935541,-1.95046480157463,-1.94859516110489,
-1.94531075704223,-1.93108870305978,-1.90488147509855,-1.87967340979029,
-1.87276446354262,-1.8692007754161,-1.8665646254764,-1.86326207227536,-1.85761525405566,
-1.82993192835102,-1.80146430773374,-1.79332570216422,-1.78779927473401,
-1.78550352819917,-1.78383873054021,-1.78197561983068,-1.77872121911457,
-1.76497882626153,-1.73366860665032,-1.71034598777799,-1.70496803706325,
-1.7017231267894,-1.69878268551681,-1.69503636317025,-1.68695308718502,
-1.64713531104907,-1.6255469237547,-1.62079014296674,-1.6186267004731,-1.6169928963441,
-1.61505963420629,-1.61157649017881,-1.59014769302804,-1.58584023140218,
-1.56599649612362,-1.54359177332018,-1.53826389971339,-1.53502964742402,
-1.53208635606883,-1.52831921112367,-1.52204815025309,-1.48501177542775,
-1.4573154741099,-1.45356216169409,-1.45159316073597,-1.44994766514024,
-1.44782439748652,-1.44328647981571,-1.4121377777625,-1.37785279325446,
-1.37201179059481,-1.36866793711337,-1.3657443598411,-1.36209954296318,
-1.35501396406215,-1.32333438623621,-1.30010544265524,-1.29275819707013,
-1.28763293603589,-1.2854044257926,-1.28374879282641,-1.28185013881087,
-1.27852129110098,-1.26271797510652,-1.23202119299304,-1.21019098936377,
-1.20489685657338,-1.2016699283642,-1.1987248198463,-1.19494360491054,-1.1886224959578,
-1.15240226435025,-1.13242106683317,-1.12565825687406,-1.12084021722084,
-1.11866575663189,-1.11703087675297,-1.11510502490475,-1.11165499438319,
-1.09192898410201,-1.08515634493058,-1.06398241637997,-1.05030761329503,
-1.04100698586047,-1.03730468635691,-1.03456653400743,-1.03156857619638,
-1.02739150479001,-1.01694276714278,-1.00131402756476,-0.991317167272335),
 .UNSPECIFIED.);
#2404=B_SPLINE_CURVE_WITH_KNOTS('',3,(#69073,#69074,#69075,#69076,#69077,
#69078,#69079,#69080,#69081,#69082,#69083,#69084,#69085,#69086,#69087,#69088,
#69089,#69090,#69091,#69092,#69093,#69094,#69095,#69096,#69097,#69098,#69099,
#69100,#69101,#69102,#69103,#69104,#69105,#69106,#69107,#69108,#69109,#69110,
#69111,#69112,#69113,#69114,#69115,#69116,#69117,#69118,#69119,#69120,#69121,
#69122,#69123,#69124,#69125,#69126,#69127,#69128,#69129,#69130,#69131,#69132,
#69133,#69134,#69135,#69136,#69137,#69138,#69139,#69140,#69141,#69142,#69143,
#69144,#69145,#69146,#69147,#69148,#69149,#69150,#69151,#69152,#69153,#69154,
#69155,#69156,#69157,#69158,#69159,#69160,#69161,#69162,#69163,#69164,#69165,
#69166,#69167,#69168,#69169,#69170,#69171,#69172,#69173,#69174,#69175,#69176,
#69177,#69178,#69179,#69180,#69181,#69182,#69183,#69184,#69185,#69186,#69187,
#69188,#69189,#69190,#69191,#69192,#69193,#69194,#69195,#69196,#69197,#69198,
#69199,#69200,#69201,#69202,#69203,#69204,#69205,#69206,#69207,#69208,#69209,
#69210,#69211,#69212,#69213,#69214,#69215,#69216,#69217,#69218,#69219,#69220,
#69221,#69222,#69223,#69224,#69225,#69226,#69227,#69228,#69229,#69230,#69231,
#69232,#69233,#69234,#69235,#69236,#69237,#69238,#69239,#69240,#69241,#69242,
#69243,#69244,#69245,#69246,#69247,#69248,#69249,#69250,#69251,#69252,#69253,
#69254,#69255,#69256,#69257,#69258,#69259,#69260,#69261,#69262,#69263,#69264,
#69265,#69266,#69267,#69268,#69269,#69270,#69271,#69272,#69273,#69274,#69275,
#69276,#69277,#69278,#69279,#69280,#69281,#69282),.UNSPECIFIED.,.F.,.F.,
(4,2,2,2,2,2,2,2,2,2,2,2,2,2,2,2,2,2,2,2,2,2,2,2,2,2,2,2,2,2,2,2,2,2,2,
2,2,2,2,2,2,2,2,2,2,2,2,2,2,2,2,2,2,2,2,2,2,2,2,2,2,2,2,2,2,2,2,2,2,2,2,
2,2,2,2,2,2,2,2,2,2,2,2,2,2,2,2,2,2,2,2,2,2,2,2,2,2,2,2,2,2,2,2,2,4),(-1.10913504811783,
-1.10823560503746,-1.10631330339019,-1.10287832932864,-1.08370403298245,
-1.05030685623411,-1.03416536900961,-1.02915549735935,-1.02598982139593,
-1.02302460379695,-1.01903794937058,-1.0097982501277,-0.996652896361306,
-0.974781043006941,-0.969710435674911,-0.948164892381695,-0.94468152465253,
-0.942748483825111,-0.941115138832031,-0.938952681783957,-0.934199661955977,
-0.912644467143313,-0.872950197330228,-0.864733254059146,-0.860963676975315,
-0.858020786486407,-0.854789336661378,-0.849471623255825,-0.827221407080959,
-0.807213264855721,-0.802961309911672,-0.781508944026267,-0.778026731674855,
-0.776094023368769,-0.774460754865315,-0.772298132842778,-0.76754373499156,
-0.74597288823947,-0.706227413696758,-0.698866794604389,-0.695167444018825,
-0.692430646405077,-0.689433383240041,-0.685255826313089,-0.674798033122222,
-0.659148240024944,-0.629313387590438,-0.614488009316962,-0.611215445706952,
-0.609329912615716,-0.607672042447271,-0.605422123259851,-0.600168787258228,
-0.592570798251011,-0.567803909265849,-0.538167540447757,-0.531018828690988,
-0.527361765927307,-0.524438140402175,-0.521104833478843,-0.515310066090627,
-0.508205327189741,-0.492604851163101,-0.462266997689265,-0.447827701524631,
-0.44453646012659,-0.442665759508467,-0.441003990244195,-0.438725754101463,
-0.433303165466993,-0.425370829025148,-0.398386656774325,-0.36888498189887,
-0.363210094915109,-0.3599022908539,-0.3572679728734,-0.353714645907345,
-0.346853825140484,-0.322016627510291,-0.304779644281041,-0.281622361172221,
-0.278132616732218,-0.27619829662491,-0.274549670659312,-0.272380386757878,
-0.267588715152776,-0.260873851115541,-0.241139611040287,-0.204522650875372,
-0.19821743862134,-0.194441404982222,-0.191497854760682,-0.188270134535489,
-0.182968924783193,-0.160995004480972,-0.130535732850021,-0.123177334826571,
-0.113800611199239,-0.110916416949167,-0.109134732495719,-0.107433892212634,
-0.104929514194292,-0.0979968478002638,-0.0868051149359963,-0.0595087853850942),
 .UNSPECIFIED.);
#2405=B_SPLINE_CURVE_WITH_KNOTS('',3,(#69288,#69289,#69290,#69291,#69292,
#69293,#69294,#69295,#69296,#69297,#69298,#69299,#69300,#69301,#69302,#69303,
#69304,#69305,#69306,#69307,#69308,#69309,#69310,#69311,#69312,#69313,#69314,
#69315,#69316,#69317,#69318,#69319,#69320,#69321,#69322,#69323,#69324,#69325,
#69326,#69327,#69328,#69329,#69330,#69331,#69332,#69333,#69334,#69335,#69336,
#69337,#69338,#69339,#69340,#69341,#69342,#69343,#69344,#69345,#69346,#69347,
#69348,#69349,#69350,#69351,#69352,#69353,#69354,#69355,#69356,#69357,#69358,
#69359,#69360,#69361,#69362,#69363,#69364,#69365,#69366,#69367,#69368,#69369,
#69370,#69371,#69372,#69373,#69374,#69375,#69376,#69377,#69378,#69379,#69380,
#69381,#69382,#69383,#69384,#69385,#69386,#69387,#69388,#69389,#69390,#69391,
#69392,#69393,#69394,#69395,#69396,#69397,#69398,#69399,#69400,#69401,#69402,
#69403,#69404,#69405,#69406,#69407,#69408,#69409,#69410,#69411,#69412,#69413,
#69414,#69415,#69416,#69417,#69418,#69419,#69420,#69421,#69422,#69423,#69424,
#69425,#69426,#69427,#69428,#69429,#69430,#69431,#69432,#69433,#69434,#69435,
#69436,#69437,#69438,#69439,#69440,#69441,#69442,#69443,#69444,#69445,#69446,
#69447,#69448,#69449,#69450,#69451,#69452,#69453,#69454,#69455,#69456,#69457,
#69458,#69459,#69460,#69461,#69462,#69463,#69464,#69465,#69466,#69467,#69468,
#69469,#69470,#69471,#69472,#69473,#69474,#69475,#69476,#69477,#69478,#69479),
 .UNSPECIFIED.,.F.,.F.,(4,2,2,2,2,2,2,2,2,2,2,2,2,2,2,2,2,2,2,2,2,2,2,2,
2,2,2,2,2,2,2,2,2,2,2,2,2,2,2,2,2,2,2,2,2,2,2,2,2,2,2,2,2,2,2,2,2,2,2,2,
2,2,2,2,2,2,2,2,2,2,2,2,2,2,2,2,2,2,2,2,2,2,2,2,2,2,2,2,2,2,2,2,2,2,2,4),
(-0.991163524485056,-0.983026878049841,-0.946840881123856,-0.940514739899372,
-0.936731902269777,-0.933786305147567,-0.930559626163103,-0.925267700523123,
-0.903476746194706,-0.872928633379073,-0.85698523250164,-0.853644440917111,
-0.851742977510495,-0.850253978123014,-0.848129332477108,-0.843584299672713,
-0.824055904383233,-0.790277106245328,-0.7761488197356,-0.771355848435598,
-0.768235512862652,-0.765246922322243,-0.761123713198903,-0.75103148423286,
-0.736159374155473,-0.716318227516734,-0.711906048239111,-0.690591657393007,
-0.687110183998657,-0.685177241068084,-0.683543325407487,-0.681379204472702,
-0.676618987639848,-0.654996410856421,-0.61508748628777,-0.607064295570715,
-0.603288286669525,-0.600351826229788,-0.597089090892841,-0.591628249201624,
-0.566591761526637,-0.545401491976722,-0.52393317807978,-0.520450148231912,
-0.518516925855081,-0.516883161525052,-0.514719745650531,-0.50996300585608,
-0.488374089218609,-0.448570204691978,-0.44045511065525,-0.43670314900139,
-0.433762050818472,-0.430520289160432,-0.425156685979125,-0.402095391058122,
-0.369991487142957,-0.356731237735257,-0.353512132287395,-0.351656734925377,
-0.349989612670611,-0.347677940578411,-0.342052879929887,-0.333713513013906,
-0.307620851035729,-0.277916229645545,-0.272241940121711,-0.268933628690639,
-0.266298428938596,-0.26274327309274,-0.255876562220893,-0.231000047624151,
-0.213789577352936,-0.190640688277787,-0.187157545067066,-0.185224344104027,
-0.183590653753023,-0.181427408603687,-0.176671321802497,-0.155087942023666,
-0.11530042288264,-0.107172335637809,-0.103418147571817,-0.100476855747706,
-0.0972364734954749,-0.0918789076298382,-0.0689263607924405,-0.0424639151764528,
-0.0276457662303507,-0.0218131531556057,-0.0194033301914297,-0.0177365551928999,
-0.0162021746202994,-0.0143991140069215,-0.0117759024763317,-0.000490981604578286),
 .UNSPECIFIED.);
#2406=B_SPLINE_CURVE_WITH_KNOTS('',3,(#69480,#69481,#69482,#69483,#69484,
#69485,#69486,#69487),.UNSPECIFIED.,.F.,.F.,(4,2,2,4),(-2.10006443375851,
-2.06179515910853,-2.04934439557115,-2.04101140854792),.UNSPECIFIED.);
#2407=B_SPLINE_CURVE_WITH_KNOTS('',3,(#69489,#69490,#69491,#69492,#69493,
#69494,#69495,#69496,#69497,#69498,#69499,#69500,#69501,#69502,#69503,#69504,
#69505,#69506,#69507,#69508),.UNSPECIFIED.,.F.,.F.,(4,2,2,2,2,2,2,2,2,4),
(-0.0595087853850942,-0.058697510888168,-0.0373425346330193,-0.0313459871363057,
-0.0276182118008791,-0.0246879939402665,-0.0219472169507867,-0.0187144205006066,
-0.0116643663455923,-0.000491076436926665),.UNSPECIFIED.);
#2408=B_SPLINE_CURVE_WITH_KNOTS('',3,(#69509,#69510,#69511,#69512,#69513,
#69514,#69515,#69516,#69517,#69518,#69519,#69520,#69521,#69522,#69523,#69524,
#69525,#69526,#69527,#69528,#69529,#69530,#69531,#69532,#69533,#69534,#69535,
#69536,#69537,#69538,#69539,#69540,#69541,#69542,#69543,#69544,#69545,#69546,
#69547,#69548,#69549,#69550,#69551,#69552,#69553,#69554,#69555,#69556,#69557,
#69558,#69559,#69560,#69561,#69562,#69563,#69564,#69565,#69566,#69567,#69568,
#69569,#69570,#69571,#69572,#69573,#69574,#69575,#69576,#69577,#69578,#69579,
#69580,#69581,#69582,#69583,#69584,#69585,#69586,#69587,#69588,#69589,#69590,
#69591,#69592,#69593,#69594,#69595,#69596,#69597,#69598,#69599,#69600,#69601,
#69602,#69603,#69604,#69605,#69606,#69607,#69608,#69609,#69610,#69611,#69612,
#69613,#69614,#69615,#69616,#69617,#69618,#69619,#69620,#69621,#69622,#69623,
#69624,#69625,#69626,#69627,#69628,#69629,#69630,#69631,#69632,#69633,#69634,
#69635,#69636,#69637,#69638,#69639,#69640,#69641,#69642,#69643,#69644,#69645,
#69646,#69647,#69648,#69649,#69650,#69651,#69652,#69653,#69654,#69655,#69656,
#69657,#69658,#69659,#69660,#69661,#69662,#69663,#69664,#69665,#69666,#69667,
#69668,#69669,#69670,#69671,#69672,#69673,#69674,#69675,#69676,#69677,#69678,
#69679,#69680,#69681,#69682,#69683,#69684,#69685,#69686,#69687,#69688,#69689,
#69690,#69691,#69692,#69693,#69694,#69695,#69696,#69697,#69698,#69699,#69700,
#69701,#69702,#69703,#69704,#69705,#69706,#69707,#69708,#69709,#69710),
 .UNSPECIFIED.,.F.,.F.,(4,2,2,2,2,2,2,2,2,2,2,2,2,2,2,2,2,2,2,2,2,2,2,2,
2,2,2,2,2,2,2,2,2,2,2,2,2,2,2,2,2,2,2,2,2,2,2,2,2,2,2,2,2,2,2,2,2,2,2,2,
2,2,2,2,2,2,2,2,2,2,2,2,2,2,2,2,2,2,2,2,2,2,2,2,2,2,2,2,2,2,2,2,2,2,2,2,
2,2,2,2,4),(-2.0999449091563,-2.07666843174284,-2.05663022798428,-2.04985598714527,
-2.04503172429198,-2.04285609986559,-2.04122106328592,-2.03929593936723,
-2.03584933571057,-2.0162658540418,-2.00970872068847,-1.98894044934525,
-1.97479736590467,-1.9681325953507,-1.96270191399168,-1.95952553435962,
-1.95660082664708,-1.95294252311187,-1.9457917166481,-1.91498654752645,
-1.89114436075095,-1.88369465537011,-1.87851638492341,-1.87627874169996,
-1.87462194326698,-1.87272847944043,-1.86942272020192,-1.85393113535256,
-1.82504191296418,-1.80921612105338,-1.80204449518046,-1.79620715621365,
-1.79286407052072,-1.78994041453539,-1.78629453759939,-1.77920390264542,
-1.74782168489845,-1.72435250645261,-1.71696452366693,-1.71181810224293,
-1.70958594355634,-1.70792986295426,-1.70603335916057,-1.70271404796654,
-1.68698096982917,-1.65632445893487,-1.63435970241686,-1.62905735206147,
-1.62582865660556,-1.62288404414013,-1.61910641025159,-1.61279804328298,
-1.57632257064629,-1.55649737904291,-1.5497642500766,-1.54496198523726,
-1.54279035075285,-1.54115576473028,-1.53922811379701,-1.53577004856255,
-1.51573153165179,-1.50922182889146,-1.48754394320841,-1.46744096082619,
-1.46225798541871,-1.4590548516825,-1.45610254825058,-1.45227136855492,
-1.44370518965421,-1.40440103426611,-1.3829730660501,-1.37823193432449,
-1.37607129600652,-1.3744377417672,-1.37250257691791,-1.36901100049347,
-1.34584796857757,-1.3286126925848,-1.30372432040562,-1.29685574863177,
-1.29330005676774,-1.29066467190686,-1.28735640231491,-1.28168294109517,
-1.2519057211615,-1.23044639716875,-1.21929854323627,-1.21458402175456,
-1.2109255560697,-1.20897628078701,-1.20732885317225,-1.20521494849235,
-1.20060545823935,-1.17008388438205,-1.1352766573348,-1.12942594440636,
-1.12608007836878,-1.12315681226014,-1.11951511480466,-1.11244446697478,
-1.10905562449139),.UNSPECIFIED.);
#2409=B_SPLINE_CURVE_WITH_KNOTS('',3,(#69715,#69716,#69717,#69718,#69719,
#69720,#69721,#69722,#69723,#69724,#69725,#69726,#69727,#69728,#69729,#69730,
#69731,#69732,#69733,#69734,#69735,#69736,#69737,#69738,#69739,#69740,#69741,
#69742,#69743,#69744,#69745,#69746,#69747,#69748,#69749,#69750,#69751,#69752,
#69753,#69754,#69755,#69756,#69757,#69758,#69759,#69760,#69761,#69762,#69763,
#69764,#69765,#69766,#69767,#69768,#69769,#69770,#69771,#69772,#69773,#69774,
#69775,#69776,#69777,#69778,#69779,#69780,#69781,#69782,#69783,#69784,#69785,
#69786,#69787,#69788,#69789,#69790,#69791,#69792,#69793,#69794,#69795,#69796,
#69797,#69798,#69799,#69800,#69801,#69802,#69803,#69804,#69805,#69806,#69807,
#69808,#69809,#69810,#69811,#69812,#69813,#69814,#69815,#69816,#69817,#69818,
#69819,#69820,#69821,#69822,#69823,#69824,#69825,#69826,#69827,#69828,#69829,
#69830,#69831,#69832,#69833,#69834,#69835,#69836,#69837,#69838,#69839,#69840,
#69841,#69842,#69843,#69844,#69845,#69846,#69847,#69848,#69849,#69850,#69851,
#69852,#69853,#69854,#69855,#69856,#69857,#69858,#69859,#69860,#69861,#69862,
#69863,#69864,#69865,#69866,#69867,#69868,#69869,#69870,#69871,#69872,#69873,
#69874,#69875,#69876,#69877,#69878,#69879,#69880,#69881,#69882,#69883,#69884,
#69885,#69886,#69887,#69888,#69889,#69890,#69891,#69892,#69893,#69894,#69895,
#69896,#69897,#69898,#69899,#69900,#69901,#69902,#69903,#69904,#69905,#69906,
#69907,#69908,#69909,#69910,#69911,#69912,#69913,#69914,#69915,#69916,#69917,
#69918,#69919,#69920,#69921,#69922),.UNSPECIFIED.,.F.,.F.,(4,2,2,2,2,2,
2,2,2,2,2,2,2,2,2,2,2,2,2,2,2,2,2,2,2,2,2,2,2,2,2,2,2,2,2,2,2,2,2,2,2,2,
2,2,2,2,2,2,2,2,2,2,2,2,2,2,2,2,2,2,2,2,2,2,2,2,2,2,2,2,2,2,2,2,2,2,2,2,
2,2,2,2,2,2,2,2,2,2,2,2,2,2,2,2,2,2,2,2,2,2,2,2,2,4),(-2.04100968074023,
-2.03439341721675,-2.02297208680151,-2.01999681466115,-2.01819454724547,
-2.01652381416569,-2.01409361028992,-2.00813160460378,-1.97558280665141,
-1.94549964499961,-1.93931383584393,-1.93648730330084,-1.93361592778463,
-1.93031666442807,-1.92468625636374,-1.89486258036765,-1.87346874408809,
-1.86226766895491,-1.85753836365978,-1.853870983418,-1.8519197458714,-1.85027236297233,
-1.84816058519643,-1.84356332864188,-1.81294426093334,-1.77816547431661,
-1.77235132864021,-1.76901303600551,-1.76608861529528,-1.76243524726692,
-1.7553088240529,-1.72544357404806,-1.70085180256665,-1.69328148741012,
-1.68804138603088,-1.68579317299043,-1.68413495334223,-1.68224716875178,
-1.67896667939265,-1.66400272486342,-1.63388848960519,-1.61069216619181,
-1.6053206322687,-1.60207697036066,-1.59913599462872,-1.59538671563614,
-1.58728770367076,-1.54748442042224,-1.52590005392727,-1.52114350990261,
-1.51898003055573,-1.51734613570246,-1.51541269050827,-1.51192904273728,
-1.49047240580192,-1.48619489444995,-1.46600864759744,-1.44390691087414,
-1.4385962932408,-1.43536561622489,-1.43242114244946,-1.42864635593185,
-1.42234871711739,-1.38571080260644,-1.36600217559981,-1.35929174677412,
-1.35450159301531,-1.35233201506896,-1.35068270295506,-1.3487470087112,
-1.34525335447357,-1.32166210329583,-1.31974023549024,-1.2997534085865,
-1.27728565163176,-1.27195389524837,-1.26871865536853,-1.26577534259461,
-1.26200937866661,-1.25574300697643,-1.21862978724824,-1.19081885319169,
-1.18717087943119,-1.18522367818891,-1.18357579699012,-1.1814584954005,
-1.17683103946109,-1.13794450673776,-1.11097149976371,-1.10543158939837,
-1.10215179506053,-1.09921857283084,-1.09547247037635,-1.08941581554992,
-1.04993129528466,-1.04347828010905,-1.02384316590393,-1.02039543059192,
-1.01846995372311,-1.0168348062201,-1.01465918681382,-1.00983554628724,
-1.00306172752569,-0.991163524485056),.UNSPECIFIED.);
#2410=B_SPLINE_CURVE_WITH_KNOTS('',3,(#69923,#69924,#69925,#69926,#69927,
#69928,#69929,#69930,#69931,#69932,#69933,#69934,#69935,#69936,#69937,#69938,
#69939,#69940,#69941,#69942,#69943,#69944,#69945,#69946,#69947,#69948,#69949,
#69950,#69951,#69952,#69953,#69954,#69955,#69956,#69957,#69958,#69959,#69960,
#69961,#69962,#69963,#69964,#69965,#69966,#69967,#69968,#69969,#69970,#69971,
#69972,#69973,#69974,#69975,#69976,#69977,#69978,#69979,#69980,#69981,#69982,
#69983,#69984,#69985,#69986,#69987,#69988,#69989,#69990,#69991,#69992,#69993,
#69994,#69995,#69996,#69997,#69998,#69999,#70000,#70001,#70002,#70003,#70004,
#70005,#70006,#70007,#70008,#70009,#70010,#70011,#70012,#70013,#70014,#70015,
#70016,#70017,#70018,#70019,#70020,#70021,#70022,#70023,#70024,#70025,#70026,
#70027,#70028,#70029,#70030,#70031,#70032,#70033,#70034,#70035,#70036,#70037,
#70038,#70039,#70040,#70041,#70042,#70043,#70044,#70045,#70046,#70047,#70048,
#70049,#70050,#70051,#70052,#70053,#70054,#70055,#70056,#70057,#70058,#70059,
#70060,#70061,#70062,#70063,#70064,#70065,#70066,#70067,#70068,#70069,#70070,
#70071,#70072,#70073,#70074,#70075,#70076,#70077,#70078,#70079,#70080,#70081,
#70082,#70083,#70084,#70085,#70086,#70087,#70088,#70089,#70090,#70091,#70092,
#70093,#70094,#70095,#70096,#70097,#70098,#70099,#70100,#70101,#70102,#70103,
#70104,#70105,#70106,#70107,#70108,#70109,#70110,#70111,#70112,#70113,#70114,
#70115,#70116,#70117,#70118,#70119,#70120,#70121,#70122),.UNSPECIFIED.,
 .F.,.F.,(4,2,2,2,2,2,2,2,2,2,2,2,2,2,2,2,2,2,2,2,2,2,2,2,2,2,2,2,2,2,2,
2,2,2,2,2,2,2,2,2,2,2,2,2,2,2,2,2,2,2,2,2,2,2,2,2,2,2,2,2,2,2,2,2,2,2,2,
2,2,2,2,2,2,2,2,2,2,2,2,2,2,2,2,2,2,2,2,2,2,2,2,2,2,2,2,2,2,2,2,4),(-1.10905562449139,
-1.07989244897315,-1.05730042595185,-1.05006129332725,-1.04499207021526,
-1.04279696482964,-1.04114070610046,-1.03924522530671,-1.03584062890829,
-1.0163425517279,-0.984420591344482,-0.967263607724238,-0.962117959284015,
-0.958922924628183,-0.955968117583588,-0.952052472653241,-0.943237867116354,
-0.930915726366584,-0.908812842023499,-0.882916425894852,-0.878169764964598,
-0.876031218996987,-0.874381621456611,-0.872450319227578,-0.868876896109351,
-0.864302653965787,-0.820600428693777,-0.800882681570439,-0.795576107638928,
-0.792346877254098,-0.789403088582272,-0.785564104439011,-0.777187939684759,
-0.755187724277675,-0.715881435606778,-0.711346817088701,-0.709224458103667,
-0.707579373329921,-0.705610585271609,-0.701856962634299,-0.69698258240651,
-0.685250360640255,-0.664060526454366,-0.634967456491648,-0.629321590846922,
-0.625987938810331,-0.623091647262524,-0.619447549811745,-0.612125676554942,
-0.602509287955301,-0.576724986844258,-0.549531944393667,-0.544796766739653,
-0.542660424558333,-0.541011212689661,-0.539078777207386,-0.535499337812354,
-0.50710062650664,-0.470489299967225,-0.464188636666517,-0.460413659685079,
-0.457469975402225,-0.454241134674979,-0.448935820559023,-0.426900089951852,
-0.39720995078659,-0.380724528236157,-0.377362509239088,-0.375456655652501,
-0.373969076554226,-0.371852839288409,-0.367350471909351,-0.348211383825908,
-0.315511320694204,-0.300136343144856,-0.295209195026829,-0.292061234930895,
-0.28908845702985,-0.285054003249958,-0.275520291811714,-0.261790984403908,
-0.240704888547187,-0.233880753958874,-0.214246581124304,-0.210799804236854,
-0.208874988957851,-0.207240509976586,-0.205065977117349,-0.200245586322434,
-0.193477133505267,-0.173466367316549,-0.137203133275546,-0.130905950455872,
-0.127132055051805,-0.124188637422674,-0.120959502684205,-0.116856108227694,
-0.10229688074443,-0.0758263288672487,-0.0592761367658359),
 .UNSPECIFIED.);
#2411=B_SPLINE_CURVE_WITH_KNOTS('',3,(#70128,#70129,#70130,#70131,#70132,
#70133,#70134,#70135,#70136,#70137,#70138,#70139,#70140,#70141,#70142,#70143,
#70144,#70145,#70146,#70147,#70148,#70149,#70150,#70151,#70152,#70153,#70154,
#70155,#70156,#70157,#70158,#70159,#70160,#70161,#70162,#70163,#70164,#70165,
#70166,#70167,#70168,#70169,#70170,#70171,#70172,#70173,#70174,#70175,#70176,
#70177,#70178,#70179,#70180,#70181,#70182,#70183,#70184,#70185,#70186,#70187,
#70188,#70189,#70190,#70191,#70192,#70193,#70194,#70195,#70196,#70197,#70198,
#70199,#70200,#70201,#70202,#70203,#70204,#70205,#70206,#70207,#70208,#70209,
#70210,#70211,#70212,#70213,#70214,#70215,#70216,#70217,#70218,#70219,#70220,
#70221,#70222,#70223,#70224,#70225,#70226,#70227,#70228,#70229,#70230,#70231,
#70232,#70233,#70234,#70235,#70236,#70237,#70238,#70239,#70240,#70241,#70242,
#70243,#70244,#70245,#70246,#70247,#70248,#70249,#70250,#70251,#70252,#70253,
#70254,#70255,#70256,#70257,#70258,#70259,#70260,#70261,#70262,#70263,#70264,
#70265,#70266,#70267,#70268,#70269,#70270,#70271,#70272,#70273,#70274,#70275,
#70276,#70277,#70278,#70279,#70280,#70281,#70282,#70283,#70284,#70285,#70286,
#70287,#70288,#70289,#70290,#70291,#70292,#70293,#70294,#70295,#70296,#70297,
#70298,#70299,#70300,#70301,#70302,#70303,#70304,#70305,#70306,#70307,#70308,
#70309,#70310,#70311,#70312,#70313,#70314,#70315,#70316,#70317,#70318,#70319,
#70320,#70321,#70322,#70323,#70324,#70325,#70326,#70327),.UNSPECIFIED.,
 .F.,.F.,(4,2,2,2,2,2,2,2,2,2,2,2,2,2,2,2,2,2,2,2,2,2,2,2,2,2,2,2,2,2,2,
2,2,2,2,2,2,2,2,2,2,2,2,2,2,2,2,2,2,2,2,2,2,2,2,2,2,2,2,2,2,2,2,2,2,2,2,
2,2,2,2,2,2,2,2,2,2,2,2,2,2,2,2,2,2,2,2,2,2,2,2,2,2,2,2,2,2,2,2,4),(-0.99120270234892,
-0.97052252555347,-0.939735350119543,-0.924083754505977,-0.920770361811558,
-0.9188751846278,-0.917218795782781,-0.914984154366355,-0.909823293709255,
-0.902406274798288,-0.878763406618566,-0.847591871469973,-0.840498787049143,
-0.836852414567577,-0.833928715320508,-0.830585947864055,-0.824750041580279,
-0.817581305133379,-0.801765125299225,-0.772916237343243,-0.757431589785655,
-0.754126589546358,-0.752233312669292,-0.75057650330905,-0.748338506059432,
-0.743158018947439,-0.735702885127382,-0.71182846794561,-0.680959680363722,
-0.673863922219174,-0.67021700265696,-0.667293265511549,-0.663950890391726,
-0.658116816619414,-0.650950957983923,-0.635144597049421,-0.606293257588039,
-0.590796265317911,-0.587490681830606,-0.585597275112588,-0.58394049885595,
-0.581702742875006,-0.576523652940169,-0.569071229829163,-0.54521331101059,
-0.514323087469682,-0.507227541313684,-0.503580669463235,-0.500656940906681,
-0.49731454335963,-0.491480345509626,-0.484314288078922,-0.468507231841814,
-0.439656154821301,-0.424160086011945,-0.420854551289094,-0.418961157710516,
-0.4173043823476,-0.415066613351608,-0.409887432561786,-0.402434828022451,
-0.378575762536819,-0.347687151906452,-0.340591604679309,-0.336944736677004,
-0.334021013336721,-0.330678624071017,-0.324844446784518,-0.317678417953824,
-0.301871443319617,-0.273020404257259,-0.257524299505362,-0.2542187678492,
-0.252325377102621,-0.250668604979746,-0.248430841390909,-0.243251677543792,
-0.235799101082807,-0.211940166784878,-0.181091284246506,-0.173971234913882,
-0.170319325609872,-0.167395208383418,-0.164646527632672,-0.159497944058016,
-0.139876590636164,-0.117778313715728,-0.112151457641064,-0.0911956300773815,
-0.0877194391207717,-0.0857877493419125,-0.0841537775195616,-0.0819881285101866,
-0.077218988696509,-0.0555040962299258,-0.0133614193897104,-0.00693652874026658,
-0.0034762226063785,-0.00170446823000911,-0.000491451950976528),
 .UNSPECIFIED.);
#2412=B_SPLINE_CURVE_WITH_KNOTS('',3,(#70328,#70329,#70330,#70331,#70332,
#70333,#70334,#70335,#70336,#70337,#70338,#70339),.UNSPECIFIED.,.F.,.F.,
(4,2,2,2,2,4),(-2.09993530652335,-2.09836798240351,-2.09573911449367,-2.0897004343036,
-2.05968687098578,-2.04100968074023),.UNSPECIFIED.);
#2413=B_SPLINE_CURVE_WITH_KNOTS('',3,(#70341,#70342,#70343,#70344,#70345,
#70346,#70347,#70348,#70349,#70350,#70351,#70352,#70353,#70354,#70355,#70356,
#70357,#70358),.UNSPECIFIED.,.F.,.F.,(4,2,2,2,2,2,2,2,4),(-0.0592761367658359,
-0.0496220222850414,-0.0448654569977602,-0.0427254520128323,-0.0410760525436666,
-0.0391465757575324,-0.0370769471246982,-0.0337915651063874,-0.000491569424012399),
 .UNSPECIFIED.);
#2414=B_SPLINE_CURVE_WITH_KNOTS('',3,(#70359,#70360,#70361,#70362,#70363,
#70364,#70365,#70366,#70367,#70368,#70369,#70370,#70371,#70372,#70373,#70374,
#70375,#70376,#70377,#70378,#70379,#70380,#70381,#70382,#70383,#70384,#70385,
#70386,#70387,#70388,#70389,#70390,#70391,#70392,#70393,#70394,#70395,#70396,
#70397,#70398,#70399,#70400,#70401,#70402,#70403,#70404,#70405,#70406,#70407,
#70408,#70409,#70410,#70411,#70412,#70413,#70414,#70415,#70416,#70417,#70418,
#70419,#70420,#70421,#70422,#70423,#70424,#70425,#70426,#70427,#70428,#70429,
#70430,#70431,#70432,#70433,#70434,#70435,#70436,#70437,#70438,#70439,#70440,
#70441,#70442,#70443,#70444,#70445,#70446,#70447,#70448,#70449,#70450,#70451,
#70452,#70453,#70454,#70455,#70456,#70457,#70458,#70459,#70460,#70461,#70462,
#70463,#70464,#70465,#70466,#70467,#70468,#70469,#70470,#70471,#70472,#70473,
#70474,#70475,#70476,#70477,#70478,#70479,#70480,#70481,#70482,#70483,#70484,
#70485,#70486,#70487,#70488,#70489,#70490,#70491,#70492,#70493,#70494,#70495,
#70496,#70497,#70498,#70499,#70500,#70501,#70502,#70503,#70504,#70505,#70506,
#70507,#70508,#70509,#70510,#70511,#70512,#70513,#70514,#70515,#70516,#70517,
#70518,#70519,#70520,#70521,#70522,#70523,#70524,#70525,#70526,#70527,#70528,
#70529,#70530,#70531,#70532,#70533,#70534,#70535,#70536,#70537,#70538,#70539,
#70540,#70541,#70542,#70543,#70544,#70545,#70546,#70547,#70548,#70549,#70550),
 .UNSPECIFIED.,.F.,.F.,(4,2,2,2,2,2,2,2,2,2,2,2,2,2,2,2,2,2,2,2,2,2,2,2,
2,2,2,2,2,2,2,2,2,2,2,2,2,2,2,2,2,2,2,2,2,2,2,2,2,2,2,2,2,2,2,2,2,2,2,2,
2,2,2,2,2,2,2,2,2,2,2,2,2,2,2,2,2,2,2,2,2,2,2,2,2,2,2,2,2,2,2,2,2,2,2,4),
(-3.79226700229728,-3.76869309243093,-3.75873057225281,-3.75503207360883,
-3.75217532363195,-3.74923690382806,-3.74598349774788,-3.7405659291042,
-3.71904230119387,-3.6861177964198,-3.67290152969814,-3.66940475781104,
-3.66743175262454,-3.66578672717982,-3.66366901637314,-3.65916039317879,
-3.62759765040527,-3.59368461298066,-3.58783286893347,-3.58448687771056,
-3.58156377063674,-3.57792262239557,-3.57085416670093,-3.54294319709848,
-3.51990632971899,-3.51017510517246,-3.50388851079092,-3.50147502727588,
-3.49979093442464,-3.4979780454196,-3.49495313928996,-3.48415790858637,
-3.45546593040333,-3.42655658270721,-3.42095409978053,-3.41766127227018,
-3.41473100106272,-3.41100867096407,-3.4032750674506,-3.36305414166583,
-3.34133723487464,-3.33656779911085,-3.33440216903122,-3.33275347136614,
-3.3308157274676,-3.32731200828443,-3.30286778409506,-3.29864108845374,
-3.28401949248064,-3.25954979435285,-3.25411463701085,-3.25085755282036,
-3.24792013742936,-3.24413443934036,-3.23794020488466,-3.19989419800612,
-3.17306207259627,-3.16930240833762,-3.16733219363184,-3.16568696971176,
-3.16356576112158,-3.15903832496542,-3.12775840538289,-3.09355822524701,
-3.08772545474756,-3.08438352009275,-3.08146002118793,-3.07781322579846,
-3.07071721640639,-3.03998361348104,-3.01602287067233,-3.00855415536765,
-3.00336625129351,-3.00112710906581,-2.99947026858237,-2.99757798606214,
-2.99427690186518,-2.9788781286353,-2.94974049468255,-2.93400996604774,
-2.92686653039648,-2.92104726342291,-2.91770824027695,-2.91478448473236,
-2.91113368530306,-2.90401799207782,-2.87398594511903,-2.8495040927997,
-2.84195134189891,-2.83672035646905,-2.83447391380086,-2.8328161651913,
-2.83092800895798,-2.82764501847077,-2.81262343738359,-2.8011229575537),
 .UNSPECIFIED.);
#2415=B_SPLINE_CURVE_WITH_KNOTS('',3,(#70555,#70556,#70557,#70558,#70559,
#70560,#70561,#70562,#70563,#70564,#70565,#70566,#70567,#70568,#70569,#70570,
#70571,#70572,#70573,#70574,#70575,#70576,#70577,#70578,#70579,#70580,#70581,
#70582,#70583,#70584,#70585,#70586,#70587,#70588,#70589,#70590,#70591,#70592,
#70593,#70594,#70595,#70596,#70597,#70598,#70599,#70600,#70601,#70602,#70603,
#70604,#70605,#70606,#70607,#70608,#70609,#70610,#70611,#70612,#70613,#70614,
#70615,#70616,#70617,#70618,#70619,#70620,#70621,#70622,#70623,#70624,#70625,
#70626,#70627,#70628,#70629,#70630,#70631,#70632,#70633,#70634,#70635,#70636,
#70637,#70638,#70639,#70640,#70641,#70642,#70643,#70644,#70645,#70646,#70647,
#70648,#70649,#70650,#70651,#70652,#70653,#70654,#70655,#70656,#70657,#70658,
#70659,#70660,#70661,#70662,#70663,#70664,#70665,#70666,#70667,#70668,#70669,
#70670,#70671,#70672,#70673,#70674,#70675,#70676,#70677,#70678,#70679,#70680,
#70681,#70682,#70683,#70684,#70685,#70686,#70687,#70688,#70689,#70690,#70691,
#70692,#70693,#70694,#70695,#70696,#70697,#70698,#70699,#70700,#70701,#70702,
#70703,#70704,#70705,#70706,#70707,#70708,#70709,#70710,#70711,#70712,#70713,
#70714,#70715,#70716,#70717,#70718,#70719,#70720,#70721,#70722,#70723,#70724,
#70725,#70726,#70727,#70728,#70729,#70730,#70731,#70732,#70733,#70734,#70735,
#70736,#70737,#70738,#70739,#70740,#70741,#70742,#70743,#70744,#70745,#70746,
#70747,#70748,#70749,#70750,#70751,#70752,#70753,#70754,#70755,#70756,#70757,
#70758,#70759,#70760,#70761,#70762),.UNSPECIFIED.,.F.,.F.,(4,2,2,2,2,2,
2,2,2,2,2,2,2,2,2,2,2,2,2,2,2,2,2,2,2,2,2,2,2,2,2,2,2,2,2,2,2,2,2,2,2,2,
2,2,2,2,2,2,2,2,2,2,2,2,2,2,2,2,2,2,2,2,2,2,2,2,2,2,2,2,2,2,2,2,2,2,2,2,
2,2,2,2,2,2,2,2,2,2,2,2,2,2,2,2,2,2,2,2,2,2,2,2,2,4),(-2.04091635741276,
-2.01188440141379,-2.00604604582115,-2.0027028119587,-1.99977925725802,
-1.99613378764944,-1.98904474763334,-1.95766446818376,-1.93421060428989,
-1.92682581712301,-1.92168118733302,-1.91944938286909,-1.91779338148413,
-1.9158967080275,-1.91257647188455,-1.8968382004011,-1.8662062219757,-1.84424795757977,
-1.83894632433521,-1.8357178542413,-1.83277329220927,-1.82899548590859,
-1.82268621963769,-1.78626073551712,-1.76641764465789,-1.75968154248347,
-1.75487781196599,-1.75270596542566,-1.75107139944688,-1.74914393610478,
-1.74568652200117,-1.72566178062299,-1.71914866046625,-1.6978608478062,
-1.67742568669057,-1.67222031391028,-1.66901245037617,-1.66606177377225,
-1.66224114435686,-1.65373551905202,-1.61438138215118,-1.592940603598,-1.58819848549181,
-1.58603771825878,-1.58440419154811,-1.58246915722536,-1.57897798674924,
-1.55580604680546,-1.53855216395096,-1.51370641022303,-1.50684367675923,
-1.50328923016203,-1.5006540324295,-1.49734502271663,-1.49166775627426,
-1.463070649468,-1.43539023864011,-1.42735975105312,-1.42188719356276,-1.41960028864593,
-1.41793681308113,-1.41606941644598,-1.41279514919074,-1.39869421968225,
-1.3723603288208,-1.3494621286389,-1.34105924791458,-1.33721511682368,-1.33427020961318,
-1.33104253967295,-1.32574493653194,-1.30619974878455,-1.26241174157648,
-1.25566851990902,-1.25318956160024,-1.25149316267505,-1.24970249091616,
-1.2467793601807,-1.2370413872218,-1.22916886224959,-1.19970539116409,-1.17765134840756,
-1.17234377523831,-1.16911388030224,-1.16616943053372,-1.16239372201584,
-1.15609238692101,-1.11952338704043,-1.09977209988514,-1.09305356543346,
-1.08825914618606,-1.08608888036663,-1.08445437127228,-1.08252561457446,
-1.07906278484435,-1.05881614755769,-1.05029467111737,-1.01396627163369,
-1.00764867838686,-1.003868430845,-1.00092340556157,-0.997695887130462,
-0.992399184576247,-0.99120270234892),.UNSPECIFIED.);
#2416=B_SPLINE_CURVE_WITH_KNOTS('',3,(#70763,#70764,#70765,#70766,#70767,
#70768,#70769,#70770,#70771,#70772,#70773,#70774,#70775,#70776,#70777,#70778,
#70779,#70780,#70781,#70782,#70783,#70784,#70785,#70786,#70787,#70788,#70789,
#70790,#70791,#70792,#70793,#70794,#70795,#70796,#70797,#70798,#70799,#70800,
#70801,#70802,#70803,#70804,#70805,#70806,#70807,#70808,#70809,#70810,#70811,
#70812,#70813,#70814,#70815,#70816,#70817,#70818,#70819,#70820,#70821,#70822,
#70823,#70824,#70825,#70826,#70827,#70828,#70829,#70830,#70831,#70832,#70833,
#70834,#70835,#70836,#70837,#70838,#70839,#70840,#70841,#70842,#70843,#70844,
#70845,#70846,#70847,#70848,#70849,#70850,#70851,#70852,#70853,#70854,#70855,
#70856,#70857,#70858,#70859,#70860,#70861,#70862,#70863,#70864,#70865,#70866,
#70867,#70868,#70869,#70870,#70871,#70872,#70873,#70874,#70875,#70876,#70877,
#70878,#70879,#70880,#70881,#70882,#70883,#70884,#70885,#70886,#70887,#70888,
#70889,#70890,#70891,#70892,#70893,#70894,#70895,#70896,#70897,#70898,#70899,
#70900,#70901,#70902,#70903,#70904,#70905,#70906,#70907,#70908,#70909,#70910,
#70911,#70912,#70913,#70914,#70915,#70916,#70917,#70918,#70919,#70920,#70921,
#70922,#70923,#70924,#70925,#70926,#70927,#70928,#70929,#70930,#70931,#70932,
#70933,#70934,#70935,#70936,#70937,#70938,#70939,#70940,#70941,#70942,#70943,
#70944,#70945,#70946,#70947,#70948,#70949,#70950,#70951,#70952,#70953,#70954,
#70955,#70956,#70957,#70958,#70959,#70960,#70961,#70962,#70963,#70964,#70965,
#70966),.UNSPECIFIED.,.F.,.F.,(4,2,2,2,2,2,2,2,2,2,2,2,2,2,2,2,2,2,2,2,
2,2,2,2,2,2,2,2,2,2,2,2,2,2,2,2,2,2,2,2,2,2,2,2,2,2,2,2,2,2,2,2,2,2,2,2,
2,2,2,2,2,2,2,2,2,2,2,2,2,2,2,2,2,2,2,2,2,2,2,2,2,2,2,2,2,2,2,2,2,2,2,2,
2,2,2,2,2,2,2,2,2,4),(-2.8011229575537,-2.78201200322399,-2.75931380357193,
-2.75396983018629,-2.7507324431721,-2.74779056166631,-2.74403110375789,
-2.73778613865376,-2.7003798056338,-2.67286380037986,-2.66918924645564,
-2.66723676339263,-2.66558993475131,-2.66348092555206,-2.65889735871189,
-2.62816051076856,-2.59350948324537,-2.58767554299368,-2.58433349504516,
-2.5814102199381,-2.57776412729436,-2.57067084939012,-2.53969193573025,
-2.5159220617994,-2.50848483988439,-2.50331322692069,-2.50107695364546,
-2.49942056148905,-2.4975268568489,-2.49421918710097,-2.47867860536094,
-2.44977528617931,-2.43399856307833,-2.42684173657609,-2.4210140261735,
-2.41767333674605,-2.41474996701798,-2.41110207207943,-2.40399985778457,
-2.37365955652556,-2.34940500599255,-2.34188894447155,-2.33667684138815,
-2.33443368952596,-2.33277645504829,-2.3308866901916,-2.32759625015505,
-2.31241645765007,-2.28346467734357,-2.26747742931689,-2.25686425335046,
-2.25266320235526,-2.24966134668931,-2.24692864066463,-2.24254611002863,
-2.23148686410769,-2.1949111663011,-2.17252573584712,-2.16904399777374,
-2.16713220022499,-2.16547953798074,-2.16331186084413,-2.15858497934311,
-2.13261461629105,-2.11057936863224,-2.09827401605867,-2.08946926238429,
-2.0855554898841,-2.08260116725428,-2.07940576609371,-2.07425752039094,
-2.05706600201563,-2.0252071235108,-2.00730754564543,-2.00294293579344,
-2.00085262050588,-1.99936767593071,-1.99744320189741,-1.99399889126439,
-1.9744865486143,-1.96754022107747,-1.94602522857578,-1.93251513734213,
-1.92309164822183,-1.91907459867671,-1.91610427769247,-1.91332981030916,
-1.90871713231743,-1.89608118171501,-1.87465946199703,-1.84057714992198,
-1.8362615595842,-1.83418062354002,-1.83253765966788,-1.83053475220116,
-1.82661407884321,-1.82145657163933,-1.80865474801016,-1.77730579185153,
-1.75902463604075,-1.75382443359162,-1.75130590682506),.UNSPECIFIED.);
#2417=B_SPLINE_CURVE_WITH_KNOTS('',3,(#70972,#70973,#70974,#70975,#70976,
#70977,#70978,#70979,#70980,#70981,#70982,#70983,#70984,#70985,#70986,#70987,
#70988,#70989,#70990,#70991,#70992,#70993,#70994,#70995,#70996,#70997,#70998,
#70999,#71000,#71001,#71002,#71003,#71004,#71005,#71006,#71007,#71008,#71009,
#71010,#71011,#71012,#71013,#71014,#71015,#71016,#71017,#71018,#71019,#71020,
#71021,#71022,#71023,#71024,#71025,#71026,#71027,#71028,#71029,#71030,#71031,
#71032,#71033,#71034,#71035,#71036,#71037,#71038,#71039,#71040,#71041,#71042,
#71043,#71044,#71045,#71046,#71047,#71048,#71049,#71050,#71051,#71052,#71053,
#71054,#71055,#71056,#71057,#71058,#71059,#71060,#71061,#71062,#71063,#71064,
#71065,#71066,#71067,#71068,#71069,#71070,#71071,#71072,#71073,#71074,#71075,
#71076,#71077,#71078,#71079,#71080,#71081,#71082,#71083,#71084,#71085,#71086,
#71087,#71088,#71089,#71090,#71091,#71092,#71093,#71094,#71095,#71096,#71097,
#71098,#71099,#71100,#71101,#71102,#71103,#71104,#71105),.UNSPECIFIED.,
 .F.,.F.,(4,2,2,2,2,2,2,2,2,2,2,2,2,2,2,2,2,2,2,2,2,2,2,2,2,2,2,2,2,2,2,
2,2,2,2,2,2,2,2,2,2,2,2,2,2,2,2,2,2,2,2,2,2,2,2,2,2,2,2,2,2,2,2,2,2,2,4),
(-0.70148998943205,-0.674345982124341,-0.669634945455482,-0.667508045624986,
-0.665860654918974,-0.66392105878315,-0.660327484968321,-0.631872921662852,
-0.595208727900692,-0.588883875984432,-0.585091036444246,-0.582131102575772,
-0.578881721765312,-0.573535203379432,-0.551080372117306,-0.522334388217699,
-0.507846378871563,-0.503479856208418,-0.501339156663809,-0.499631792915702,
-0.497824610182475,-0.494927290037092,-0.484780961145284,-0.464415855447431,
-0.43024241330435,-0.423924288357904,-0.42012594748679,-0.417154262742281,
-0.413883542885037,-0.408480900672828,-0.385371235409442,-0.353258122573531,
-0.339703210370992,-0.33650341488823,-0.334637737794428,-0.333038569022195,
-0.330913764757876,-0.325971684055829,-0.318891048670801,-0.296964711156488,
-0.260800289639285,-0.253654577622875,-0.250133257313443,-0.247329437297859,
-0.244147924441893,-0.238664866797341,-0.20809129696095,-0.176127965725983,
-0.169958056443735,-0.167532591865511,-0.165880672760035,-0.164092500729214,
-0.161545039821543,-0.153204821355754,-0.138616386182872,-0.106317607615673,
-0.0858385280892805,-0.080091366127395,-0.0765419995099983,-0.0732636428181496,
-0.0689097683989476,-0.0588996440771098,-0.0327532108786773,-0.00751310391364335,
-0.0032923198447157,-0.00149869915253042,-2.71738506628892E-6),
 .UNSPECIFIED.);
#2418=B_SPLINE_CURVE_WITH_KNOTS('',3,(#71108,#71109,#71110,#71111,#71112,
#71113,#71114,#71115,#71116,#71117,#71118,#71119,#71120,#71121,#71122,#71123,
#71124,#71125,#71126,#71127,#71128,#71129,#71130,#71131,#71132,#71133,#71134,
#71135,#71136,#71137,#71138,#71139,#71140,#71141,#71142,#71143,#71144,#71145,
#71146,#71147,#71148,#71149,#71150,#71151,#71152,#71153,#71154,#71155,#71156,
#71157,#71158,#71159,#71160,#71161,#71162,#71163,#71164,#71165,#71166,#71167,
#71168,#71169,#71170,#71171,#71172,#71173,#71174,#71175,#71176,#71177,#71178,
#71179,#71180,#71181,#71182,#71183,#71184,#71185,#71186,#71187,#71188,#71189,
#71190,#71191,#71192,#71193,#71194,#71195,#71196,#71197,#71198,#71199,#71200,
#71201,#71202,#71203,#71204,#71205,#71206,#71207,#71208,#71209,#71210,#71211,
#71212,#71213,#71214,#71215,#71216,#71217,#71218,#71219,#71220,#71221,#71222,
#71223,#71224,#71225,#71226,#71227,#71228,#71229,#71230,#71231,#71232,#71233,
#71234,#71235,#71236,#71237,#71238,#71239,#71240,#71241,#71242,#71243,#71244,
#71245,#71246,#71247,#71248,#71249,#71250,#71251,#71252,#71253,#71254,#71255,
#71256,#71257,#71258,#71259,#71260,#71261,#71262,#71263,#71264,#71265,#71266,
#71267,#71268,#71269,#71270,#71271,#71272,#71273,#71274,#71275,#71276,#71277,
#71278,#71279,#71280,#71281,#71282,#71283,#71284,#71285,#71286,#71287,#71288,
#71289,#71290,#71291,#71292,#71293,#71294,#71295,#71296,#71297,#71298,#71299,
#71300,#71301,#71302,#71303,#71304,#71305,#71306,#71307,#71308,#71309),
 .UNSPECIFIED.,.F.,.F.,(4,2,2,2,2,2,2,2,2,2,2,2,2,2,2,2,2,2,2,2,2,2,2,2,
2,2,2,2,2,2,2,2,2,2,2,2,2,2,2,2,2,2,2,2,2,2,2,2,2,2,2,2,2,2,2,2,2,2,2,2,
2,2,2,2,2,2,2,2,2,2,2,2,2,2,2,2,2,2,2,2,2,2,2,2,2,2,2,2,2,2,2,2,2,2,2,2,
2,2,2,2,4),(-1.97976470944902,-1.9789712957795,-1.97074210865653,-1.93649408360935,
-1.91058676406563,-1.90504851710588,-1.90174802558588,-1.89878194842719,
-1.89497249570069,-1.88876114646882,-1.84487804431934,-1.82653872045245,
-1.82209852679182,-1.82038768953402,-1.82033407244368,-1.82028049490831,
-1.8202261642487,-1.8201701514512,-1.82011129453788,-1.82004803697691,-1.8199781321918,
-1.8198980424709,-1.81980152783548,-1.81967551012305,-1.81957959146175,
-1.81797039159875,-1.81583786265784,-1.81107867663494,-1.78734873691932,
-1.76750359022668,-1.74521560180538,-1.73987704677321,-1.73662860265687,
-1.73366700024715,-1.72986851373612,-1.72352627521349,-1.68717785705456,
-1.65852384971955,-1.65489808386762,-1.65295131809612,-1.65130413467331,
-1.64918560379227,-1.64469069652582,-1.61372580922956,-1.57916926509896,
-1.57340079941526,-1.57008337888019,-1.56717457013396,-1.56353770564219,
-1.5564364795931,-1.52588130075209,-1.50157454603749,-1.49405384932749,
-1.48884432047777,-1.48660977662906,-1.48495885435688,-1.48307271734828,
-1.47979937055345,-1.46498187316288,-1.43913539251414,-1.41412704498556,
-1.40723837650883,-1.40367550035633,-1.40103594761735,-1.39772381672729,
-1.39204657758675,-1.36003638674829,-1.33522098697313,-1.32391346182469,
-1.32094309913931,-1.31913907659717,-1.31746480371394,-1.31541036793998,
-1.3113658157162,-1.27921958619855,-1.25664684563837,-1.24335503377768,
-1.23879707130675,-1.23572440008365,-1.23273601301409,-1.22845400895434,
-1.21805065760952,-1.18081533402403,-1.15817687343832,-1.15468855825223,
-1.15277487992886,-1.15112250965675,-1.14895719108698,-1.14424089400683,
-1.11903185060416,-1.09613103324159,-1.08387831592845,-1.0751019600958,
-1.07119397330868,-1.06824145213024,-1.06504555872083,-1.05989114519951,
-1.0423194907008,-1.01063738401214,-0.991343892686251,-0.991336294305795),
 .UNSPECIFIED.);
#2419=B_SPLINE_CURVE_WITH_KNOTS('',3,(#71315,#71316,#71317,#71318),
 .UNSPECIFIED.,.F.,.F.,(4,4),(112.182489717842,112.611961982353),
 .UNSPECIFIED.);
#2420=B_SPLINE_CURVE_WITH_KNOTS('',3,(#71321,#71322,#71323,#71324,#71325,
#71326,#71327,#71328,#71329,#71330,#71331,#71332,#71333,#71334,#71335,#71336,
#71337,#71338,#71339,#71340,#71341,#71342,#71343,#71344,#71345,#71346,#71347,
#71348,#71349,#71350,#71351),.UNSPECIFIED.,.F.,.F.,(4,3,3,3,3,3,3,3,3,3,
4),(112.181968561873,112.285773547054,112.391790609764,112.495346290868,
112.598849283204,112.70233481629,112.810228624402,112.913851302595,113.017547311481,
113.121411318193,113.133910048737),.UNSPECIFIED.);
#2421=B_SPLINE_CURVE_WITH_KNOTS('',3,(#71357,#71358,#71359,#71360,#71361,
#71362,#71363,#71364,#71365,#71366,#71367,#71368,#71369,#71370,#71371,#71372,
#71373,#71374,#71375,#71376,#71377,#71378,#71379,#71380,#71381,#71382,#71383,
#71384,#71385,#71386,#71387,#71388,#71389,#71390,#71391,#71392,#71393,#71394,
#71395,#71396,#71397,#71398,#71399,#71400,#71401,#71402,#71403,#71404,#71405,
#71406,#71407,#71408,#71409,#71410,#71411,#71412,#71413,#71414,#71415,#71416,
#71417,#71418,#71419,#71420,#71421,#71422,#71423,#71424,#71425,#71426,#71427,
#71428,#71429,#71430,#71431,#71432,#71433,#71434,#71435,#71436,#71437,#71438,
#71439,#71440,#71441,#71442,#71443,#71444,#71445,#71446,#71447,#71448,#71449,
#71450,#71451,#71452,#71453,#71454,#71455,#71456,#71457,#71458,#71459,#71460,
#71461,#71462,#71463,#71464,#71465,#71466,#71467,#71468,#71469,#71470,#71471,
#71472,#71473,#71474,#71475,#71476,#71477),.UNSPECIFIED.,.F.,.F.,(4,3,3,
3,3,3,3,3,3,3,3,3,3,3,3,3,3,3,3,3,3,3,3,3,3,3,3,3,3,3,3,3,3,3,3,3,3,3,3,
3,4),(105.89914045238,106.003024818123,106.106864217443,106.21069337325,
106.314717723871,106.4186920148,106.522861290385,106.626790775734,106.730987270237,
106.835028779578,106.938948573574,107.042803099337,107.146627117888,107.250455346994,
107.354392395691,107.458388390263,107.562566344703,107.62431931017,107.728406109515,
107.832337400558,107.936146731458,108.039890701015,108.143604231727,108.24732220283,
108.351150101919,108.455037404766,108.559108574838,108.621847844607,108.726214073937,
108.830424660313,108.934511746338,109.038532366638,109.142521041264,109.24651224564,
109.350608598025,109.454762056837,109.559092885886,109.619376379043,109.74029827114,
109.860139236864,109.955742676496),.UNSPECIFIED.);
#2422=B_SPLINE_CURVE_WITH_KNOTS('',3,(#71478,#71479,#71480,#71481,#71482,
#71483),.UNSPECIFIED.,.F.,.F.,(4,1,1,4),(109.955742875643,110.61690491348,
111.614433447917,112.182489717842),.UNSPECIFIED.);
#2423=B_SPLINE_CURVE_WITH_KNOTS('',3,(#71485,#71486,#71487,#71488,#71489,
#71490,#71491,#71492,#71493,#71494,#71495,#71496,#71497,#71498,#71499,#71500,
#71501,#71502,#71503,#71504,#71505,#71506,#71507,#71508,#71509,#71510,#71511,
#71512,#71513,#71514,#71515,#71516,#71517,#71518,#71519,#71520,#71521,#71522,
#71523,#71524,#71525,#71526,#71527,#71528,#71529,#71530,#71531,#71532,#71533,
#71534,#71535,#71536,#71537,#71538,#71539,#71540,#71541,#71542,#71543,#71544,
#71545,#71546,#71547,#71548,#71549,#71550,#71551,#71552,#71553,#71554),
 .UNSPECIFIED.,.F.,.F.,(4,3,3,3,3,3,3,3,3,3,3,3,3,3,3,3,3,3,3,3,3,3,3,4),
(109.955742875643,110.103311094288,110.16088031869,110.264967038889,110.368898250683,
110.472707502544,110.576451393231,110.680164845351,110.783882738247,110.887710560244,
110.991597786505,111.095668881621,111.158408853127,111.262775121087,111.366985745707,
111.471072869233,111.575093526554,111.679082237674,111.783073477966,111.887169865156,
111.991323358195,112.095654220209,112.155937387564,112.181968561873),
 .UNSPECIFIED.);
#2424=B_SPLINE_CURVE_WITH_KNOTS('',3,(#71555,#71556,#71557,#71558,#71559,
#71560,#71561,#71562,#71563,#71564,#71565,#71566,#71567,#71568,#71569,#71570,
#71571,#71572,#71573,#71574,#71575,#71576,#71577,#71578,#71579,#71580,#71581,
#71582,#71583,#71584,#71585,#71586,#71587,#71588,#71589,#71590,#71591,#71592,
#71593,#71594,#71595,#71596,#71597,#71598,#71599,#71600,#71601,#71602,#71603,
#71604,#71605,#71606,#71607,#71608,#71609,#71610,#71611,#71612,#71613,#71614,
#71615,#71616,#71617,#71618,#71619,#71620,#71621,#71622,#71623,#71624,#71625,
#71626,#71627,#71628,#71629,#71630,#71631,#71632,#71633,#71634,#71635,#71636,
#71637,#71638,#71639,#71640,#71641,#71642,#71643,#71644,#71645,#71646,#71647,
#71648,#71649,#71650,#71651,#71652,#71653,#71654,#71655,#71656,#71657,#71658,
#71659,#71660,#71661,#71662,#71663,#71664,#71665,#71666,#71667,#71668,#71669,
#71670,#71671,#71672,#71673,#71674,#71675,#71676,#71677,#71678),
 .UNSPECIFIED.,.F.,.F.,(4,3,3,3,3,3,3,3,3,3,3,3,3,3,3,3,3,3,3,3,3,3,3,3,
3,3,3,3,3,3,3,3,3,3,3,3,3,3,3,3,3,4),(105.898025479477,106.002009805234,
106.106176853772,106.170766180944,106.274954664328,106.378987943816,106.482899226787,
106.586745073159,106.690560258285,106.794379514107,106.89830744101,107.002294216394,
107.106462900374,107.168294715381,107.27246889384,107.37648781455,107.48038472832,
107.584216206841,107.688017046587,107.791822000632,107.895735790654,107.999708500798,
108.103863385519,108.165823249817,108.270028207098,108.374077867905,108.478005318162,
108.581867191257,108.685698240133,108.789533174159,108.893476390757,108.997478259752,
109.101661565735,109.163351784254,109.266012653708,109.368536787086,109.470961003165,
109.573321976682,109.675698137509,109.778078174934,109.88056960646,109.955742875311),
 .UNSPECIFIED.);
#2425=B_SPLINE_CURVE_WITH_KNOTS('',3,(#71684,#71685,#71686,#71687,#71688,
#71689,#71690,#71691,#71692,#71693,#71694,#71695,#71696,#71697,#71698,#71699,
#71700,#71701,#71702,#71703,#71704,#71705,#71706,#71707,#71708,#71709,#71710,
#71711,#71712,#71713,#71714,#71715,#71716,#71717,#71718,#71719,#71720,#71721,
#71722,#71723,#71724,#71725,#71726,#71727,#71728,#71729,#71730,#71731,#71732,
#71733,#71734,#71735,#71736,#71737,#71738,#71739,#71740,#71741,#71742,#71743,
#71744,#71745,#71746,#71747,#71748,#71749,#71750,#71751,#71752,#71753,#71754,
#71755,#71756,#71757,#71758,#71759,#71760,#71761,#71762,#71763,#71764,#71765,
#71766,#71767,#71768,#71769,#71770,#71771,#71772,#71773,#71774,#71775,#71776,
#71777,#71778,#71779,#71780,#71781,#71782,#71783,#71784,#71785,#71786,#71787,
#71788,#71789,#71790,#71791,#71792,#71793,#71794,#71795,#71796,#71797,#71798,
#71799,#71800,#71801,#71802,#71803,#71804,#71805,#71806,#71807,#71808,#71809,
#71810),.UNSPECIFIED.,.F.,.F.,(4,3,3,3,3,3,3,3,3,3,3,3,3,3,3,3,3,3,3,3,
3,3,3,3,3,3,3,3,3,3,3,3,3,3,3,3,3,3,3,3,3,3,4),(99.6152316583351,99.6440910346774,
99.7482776243203,99.8523089801499,99.956218304806,100.060062172602,100.163875361992,
100.267692607994,100.371618517795,100.47560326894,100.579769939687,100.641619569114,
100.745806326823,100.849837855208,100.953747358172,101.05759140772,101.161404782005,
101.265222215752,101.36914831629,101.473133260145,101.577300124576,101.639148103551,
101.743333059261,101.847362780412,101.951270477105,102.055112721953,102.158924295754,
102.262739935879,102.366664265581,102.470647448779,102.574812587739,102.636676637987,
102.740864888811,102.844897897912,102.948808856351,103.052654345051,103.156469140193,
103.260287974509,103.36421543532,103.46820171878,103.57236987585,103.634205172424,
103.672557568463),.UNSPECIFIED.);
#2426=B_SPLINE_CURVE_WITH_KNOTS('',3,(#71811,#71812,#71813,#71814,#71815,
#71816,#71817,#71818,#71819,#71820,#71821,#71822,#71823,#71824,#71825,#71826,
#71827,#71828,#71829,#71830,#71831,#71832,#71833,#71834,#71835,#71836,#71837,
#71838,#71839,#71840,#71841,#71842,#71843,#71844,#71845,#71846,#71847,#71848,
#71849,#71850,#71851,#71852,#71853,#71854,#71855,#71856,#71857,#71858,#71859,
#71860,#71861,#71862,#71863,#71864,#71865,#71866,#71867,#71868,#71869,#71870,
#71871,#71872,#71873,#71874,#71875,#71876,#71877,#71878,#71879,#71880),
 .UNSPECIFIED.,.F.,.F.,(4,3,3,3,3,3,3,3,3,3,3,3,3,3,3,3,3,3,3,3,3,3,3,4),
(103.672557568736,103.776099132589,103.883053454373,103.986323986313,104.089534944656,
104.192721974449,104.295920683386,104.399231129595,104.502608916411,104.606156372049,
104.63173370686,104.73590789905,104.839926833507,104.943823760987,105.047655253186,
105.151456106561,105.255261074165,105.359174877546,105.463147600957,105.567302498657,
105.629262241297,105.733461685671,105.837495282119,105.89914045238),
 .UNSPECIFIED.);
#2427=B_SPLINE_CURVE_WITH_KNOTS('',3,(#71882,#71883,#71884,#71885,#71886,
#71887,#71888,#71889,#71890,#71891,#71892,#71893,#71894,#71895,#71896,#71897,
#71898,#71899,#71900,#71901,#71902,#71903,#71904,#71905,#71906,#71907,#71908,
#71909,#71910,#71911,#71912,#71913,#71914,#71915,#71916,#71917,#71918,#71919,
#71920,#71921,#71922,#71923,#71924,#71925,#71926,#71927,#71928,#71929,#71930,
#71931,#71932,#71933,#71934,#71935,#71936,#71937,#71938,#71939,#71940,#71941,
#71942,#71943,#71944,#71945,#71946,#71947,#71948),.UNSPECIFIED.,.F.,.F.,
(4,3,3,3,3,3,3,3,3,3,3,3,3,3,3,3,3,3,3,3,3,3,4),(103.672557568463,103.781092799078,
103.889920272668,103.998901192476,104.108175818866,104.175709112071,104.27989406565,
104.38392378467,104.487831479238,104.591673721967,104.695485293658,104.799300931684,
104.903225259319,105.007208440466,105.111373577421,105.173237646507,105.277400211996,
105.381419535078,105.485330619066,105.589186541108,105.693004652181,105.796876386701,
105.898025479477),.UNSPECIFIED.);
#2428=B_SPLINE_CURVE_WITH_KNOTS('',3,(#71949,#71950,#71951,#71952,#71953,
#71954,#71955,#71956,#71957,#71958,#71959,#71960,#71961,#71962,#71963,#71964,
#71965,#71966,#71967,#71968,#71969,#71970,#71971,#71972,#71973,#71974,#71975,
#71976,#71977,#71978,#71979,#71980,#71981,#71982,#71983,#71984,#71985,#71986,
#71987,#71988,#71989,#71990,#71991,#71992,#71993,#71994,#71995,#71996,#71997,
#71998,#71999,#72000,#72001,#72002,#72003,#72004,#72005,#72006,#72007,#72008,
#72009,#72010,#72011,#72012,#72013,#72014,#72015,#72016,#72017,#72018,#72019,
#72020,#72021,#72022,#72023,#72024,#72025,#72026,#72027,#72028,#72029,#72030,
#72031,#72032,#72033,#72034,#72035,#72036,#72037,#72038,#72039,#72040,#72041,
#72042,#72043,#72044,#72045,#72046,#72047,#72048,#72049,#72050,#72051,#72052,
#72053,#72054,#72055,#72056,#72057,#72058,#72059,#72060,#72061,#72062,#72063,
#72064,#72065,#72066,#72067,#72068,#72069,#72070,#72071,#72072),
 .UNSPECIFIED.,.F.,.F.,(4,3,3,3,3,3,3,3,3,3,3,3,3,3,3,3,3,3,3,3,3,3,3,3,
3,3,3,3,3,3,3,3,3,3,3,3,3,3,3,3,3,4),(99.6156110745197,99.7194228471478,
99.8232425494864,99.9271733259419,100.031166424027,100.135337925974,100.185594974324,
100.289781443823,100.393812681112,100.497721890145,100.601565644175,100.705378721806,
100.809195858211,100.913121662433,101.017106310105,101.121272881802,101.183123508761,
101.287309756461,101.391340771478,101.495249758603,101.599093291071,101.70290614781,
101.806723064315,101.910648651658,102.014633083828,102.118799444536,102.180652043198,
102.284838633001,102.388869988989,102.492779313799,102.596623181746,102.700436371284,
102.804253617431,102.908179527372,103.012164278654,103.116330949532,103.178180577634,
103.287930451836,103.397356063165,103.506584798252,103.615565393999,103.672557568099),
 .UNSPECIFIED.);
#2429=B_SPLINE_CURVE_WITH_KNOTS('',3,(#72078,#72079,#72080,#72081,#72082,
#72083,#72084,#72085,#72086,#72087,#72088,#72089,#72090,#72091,#72092,#72093,
#72094,#72095,#72096,#72097,#72098,#72099,#72100,#72101,#72102,#72103,#72104,
#72105,#72106,#72107,#72108,#72109,#72110,#72111,#72112,#72113,#72114,#72115,
#72116,#72117,#72118,#72119,#72120,#72121,#72122,#72123,#72124,#72125,#72126,
#72127,#72128,#72129,#72130,#72131,#72132,#72133,#72134,#72135,#72136,#72137,
#72138,#72139,#72140,#72141,#72142,#72143,#72144,#72145,#72146,#72147,#72148,
#72149,#72150,#72151,#72152,#72153,#72154,#72155,#72156,#72157,#72158,#72159,
#72160,#72161,#72162,#72163,#72164,#72165,#72166,#72167,#72168,#72169,#72170,
#72171,#72172,#72173,#72174,#72175,#72176,#72177,#72178,#72179,#72180,#72181,
#72182,#72183,#72184,#72185,#72186,#72187,#72188,#72189,#72190,#72191,#72192,
#72193,#72194,#72195,#72196,#72197,#72198,#72199,#72200,#72201,#72202,#72203,
#72204),.UNSPECIFIED.,.F.,.F.,(4,3,3,3,3,3,3,3,3,3,3,3,3,3,3,3,3,3,3,3,
3,3,3,3,3,3,3,3,3,3,3,3,3,3,3,3,3,3,3,3,3,3,4),(93.3317416580215,93.4356900192302,
93.5397112742701,93.643900786555,93.6589198280578,93.7631062483201,93.867137435993,
93.9710465950891,94.0748902990131,94.1787033264443,94.2825204126297,94.3864461669516,
94.4904307648287,94.5945972874411,94.6564483624944,94.7606347887222,94.8646659824197,
94.9685751475987,95.0724188576377,95.1762318912073,95.2800489835447,95.3839747439967,
95.4879593480006,95.5921258766681,95.653976896931,95.7581632966032,95.862194463707,
95.9661036023635,96.0699472859383,96.1737602931401,96.2775773592453,96.3815030938508,
96.4854876721868,96.5896541757464,96.6515054313676,96.7545601138494,96.8574737138164,
96.9602826553637,97.0675550568436,97.1702894267471,97.2730248741062,97.3758310709812,
97.3893722612835),.UNSPECIFIED.);
#2430=B_SPLINE_CURVE_WITH_KNOTS('',3,(#72205,#72206,#72207,#72208,#72209,
#72210,#72211,#72212,#72213,#72214,#72215,#72216,#72217,#72218,#72219,#72220,
#72221,#72222,#72223,#72224,#72225,#72226,#72227,#72228,#72229,#72230,#72231,
#72232,#72233,#72234,#72235,#72236,#72237,#72238,#72239,#72240,#72241,#72242,
#72243,#72244,#72245,#72246,#72247,#72248,#72249,#72250,#72251,#72252,#72253,
#72254,#72255,#72256,#72257,#72258,#72259,#72260,#72261,#72262,#72263,#72264,
#72265,#72266,#72267,#72268,#72269,#72270,#72271),.UNSPECIFIED.,.F.,.F.,
(4,3,3,3,3,3,3,3,3,3,3,3,3,3,3,3,3,3,3,3,3,3,4),(97.3893722615608,97.5221133460531,
97.6490339658042,97.7532204351774,97.8572516723404,97.9611608812461,98.0650046351491,
98.1688177126537,98.2726348489321,98.3765606530284,98.4805453005753,98.5847118721504,
98.6465625002408,98.7507507727395,98.8588108834389,98.9627158777129,99.0665559339089,
99.170365829106,99.2741802971821,99.3780947558165,99.4820689265879,99.5862024307738,
99.6152316583351),.UNSPECIFIED.);
#2431=B_SPLINE_CURVE_WITH_KNOTS('',3,(#72273,#72274,#72275,#72276,#72277,
#72278,#72279,#72280,#72281,#72282,#72283,#72284,#72285,#72286,#72287,#72288,
#72289,#72290,#72291,#72292,#72293,#72294,#72295,#72296,#72297,#72298,#72299,
#72300,#72301,#72302,#72303,#72304,#72305,#72306,#72307,#72308,#72309,#72310,
#72311,#72312,#72313,#72314,#72315,#72316,#72317,#72318,#72319,#72320,#72321,
#72322,#72323,#72324,#72325,#72326,#72327,#72328,#72329,#72330,#72331,#72332,
#72333,#72334,#72335,#72336,#72337,#72338,#72339),.UNSPECIFIED.,.F.,.F.,
(4,3,3,3,3,3,3,3,3,3,3,3,3,3,3,3,3,3,3,3,3,3,4),(97.389372261676,97.4918503890726,
97.5942398116719,97.6965771923013,97.7988991181528,97.9013122938702,98.0037702234387,
98.1064116156427,98.1905379054512,98.2947243050817,98.3987554721441,98.5026646107592,
98.6065082942927,98.7103213014536,98.8141383675183,98.9180641020837,99.0220486803801,
99.1262151839011,99.1880664398878,99.2949525985458,99.3989655198962,99.507288297208,
99.6156110745197),.UNSPECIFIED.);
#2432=B_SPLINE_CURVE_WITH_KNOTS('',3,(#72340,#72341,#72342,#72343,#72344,
#72345,#72346,#72347,#72348,#72349,#72350,#72351,#72352,#72353,#72354,#72355,
#72356,#72357,#72358,#72359,#72360,#72361,#72362,#72363,#72364,#72365,#72366,
#72367,#72368,#72369,#72370,#72371,#72372,#72373,#72374,#72375,#72376,#72377,
#72378,#72379,#72380,#72381,#72382,#72383,#72384,#72385,#72386,#72387,#72388,
#72389,#72390,#72391,#72392,#72393,#72394,#72395,#72396,#72397,#72398,#72399,
#72400,#72401,#72402,#72403,#72404,#72405,#72406,#72407,#72408,#72409,#72410,
#72411,#72412,#72413,#72414,#72415,#72416,#72417,#72418,#72419,#72420,#72421,
#72422,#72423,#72424,#72425,#72426,#72427,#72428,#72429,#72430,#72431,#72432,
#72433,#72434,#72435,#72436,#72437,#72438,#72439,#72440,#72441,#72442,#72443,
#72444,#72445,#72446,#72447,#72448,#72449,#72450,#72451,#72452,#72453,#72454,
#72455,#72456,#72457,#72458,#72459,#72460,#72461,#72462,#72463),
 .UNSPECIFIED.,.F.,.F.,(4,3,3,3,3,3,3,3,3,3,3,3,3,3,3,3,3,3,3,3,3,3,3,3,
3,3,3,3,3,3,3,3,3,3,3,3,3,3,3,3,3,4),(93.3327269082001,93.4411890156382,
93.5450756538202,93.648906907013,93.7527175377309,93.8565422751658,93.9604818352646,
94.0644892683557,94.1686696740169,94.2004237677048,94.3046101879005,94.4086413755316,
94.5125505346222,94.6163942385629,94.7202072660329,94.8240243522793,94.9279501066946,
95.0319347046836,95.1361012274356,95.1979523021414,95.3021387192142,95.40616990372,
95.5100790596968,95.6139227605325,95.7177357849108,95.8215528680832,95.9254786194727,
96.0294632144584,96.1336297342753,96.195480836578,96.2996672568408,96.4036984445142,
96.5076076036108,96.6114513075351,96.7152643349665,96.8190814211525,96.9230071754745,
97.0269917733517,97.1311582959642,97.1930093710146,97.3433995555511,97.3893722612835),
 .UNSPECIFIED.);
#2433=B_SPLINE_CURVE_WITH_KNOTS('',3,(#72469,#72470,#72471,#72472,#72473,
#72474,#72475,#72476,#72477,#72478,#72479,#72480,#72481,#72482,#72483,#72484,
#72485,#72486,#72487,#72488,#72489,#72490,#72491,#72492,#72493,#72494,#72495,
#72496,#72497,#72498,#72499,#72500,#72501,#72502,#72503,#72504,#72505,#72506,
#72507,#72508,#72509,#72510,#72511,#72512,#72513,#72514,#72515,#72516,#72517,
#72518,#72519,#72520,#72521,#72522,#72523,#72524,#72525,#72526,#72527,#72528,
#72529,#72530,#72531,#72532,#72533,#72534,#72535,#72536,#72537,#72538,#72539,
#72540,#72541,#72542,#72543,#72544,#72545,#72546,#72547,#72548,#72549,#72550,
#72551,#72552,#72553,#72554,#72555,#72556,#72557,#72558,#72559,#72560,#72561,
#72562,#72563,#72564,#72565,#72566,#72567,#72568,#72569,#72570,#72571,#72572,
#72573,#72574,#72575,#72576,#72577,#72578,#72579,#72580,#72581,#72582,#72583,
#72584,#72585,#72586,#72587,#72588,#72589),.UNSPECIFIED.,.F.,.F.,(4,3,3,
3,3,3,3,3,3,3,3,3,3,3,3,3,3,3,3,3,3,3,3,3,3,3,3,3,3,3,3,3,3,3,3,3,3,3,3,
3,4),(87.0493885891151,87.1532100516366,87.2570212569905,87.3612030981024,
87.465159835495,87.5694542284666,87.6737486214382,87.777935040701,87.8819662273946,
87.985875385546,88.0897190885468,88.1935321150776,88.297349200387,88.401274953875,
88.505259550941,88.6094260727864,88.6712771558748,88.7754635752621,88.879494762081,
88.983403920358,89.0872476234846,89.1910606501414,89.2948777355764,89.3988034891889,
89.5027880863789,89.6069546083463,89.6688056903114,89.7729921093414,89.8770232958027,
89.9809324537241,90.0847761564964,90.1885891828006,90.2924062678855,90.3963320211534,
90.5003166180017,90.6044831396355,90.666334224748,90.7790776483314,90.8915379903038,
91.003544787262,91.1061869538187),.UNSPECIFIED.);
#2434=B_SPLINE_CURVE_WITH_KNOTS('',3,(#72590,#72591,#72592,#72593,#72594,
#72595,#72596,#72597,#72598,#72599,#72600,#72601,#72602,#72603,#72604,#72605,
#72606,#72607,#72608,#72609,#72610,#72611,#72612,#72613,#72614,#72615,#72616,
#72617,#72618,#72619,#72620,#72621,#72622,#72623,#72624,#72625,#72626,#72627,
#72628,#72629,#72630,#72631,#72632,#72633,#72634,#72635,#72636,#72637,#72638,
#72639,#72640,#72641,#72642,#72643,#72644,#72645,#72646,#72647,#72648,#72649,
#72650,#72651,#72652,#72653,#72654,#72655,#72656,#72657,#72658,#72659),
 .UNSPECIFIED.,.F.,.F.,(4,3,3,3,3,3,3,3,3,3,3,3,3,3,3,3,3,3,3,3,3,3,3,4),
(91.1061869541039,91.2126211265267,91.3191385231275,91.4258526676074,91.5326811228729,
91.639729802547,91.6638627591846,91.7680491793775,91.872080367006,91.9759895260938,
92.0798332300317,92.1836462574988,92.2874633437425,92.391389098155,92.4953736961413,
92.5995402188908,92.6613912936212,92.7655571769362,92.8695782420278,92.9734895025819,
93.0773351539067,93.1811423844738,93.2849757131635,93.3317416580215),
 .UNSPECIFIED.);
#2435=B_SPLINE_CURVE_WITH_KNOTS('',3,(#72661,#72662,#72663,#72664,#72665,
#72666,#72667,#72668,#72669,#72670,#72671,#72672,#72673,#72674,#72675,#72676,
#72677,#72678,#72679,#72680,#72681,#72682,#72683,#72684,#72685,#72686,#72687,
#72688,#72689,#72690,#72691,#72692,#72693,#72694,#72695,#72696,#72697,#72698,
#72699,#72700,#72701,#72702,#72703,#72704,#72705,#72706,#72707,#72708,#72709,
#72710,#72711,#72712,#72713,#72714,#72715,#72716,#72717,#72718,#72719,#72720,
#72721,#72722,#72723,#72724,#72725,#72726,#72727,#72728,#72729,#72730),
 .UNSPECIFIED.,.F.,.F.,(4,3,3,3,3,3,3,3,3,3,3,3,3,3,3,3,3,3,3,3,3,3,3,4),
(91.1061869541039,91.207838164395,91.3120245837827,91.4160557706021,91.5199649288795,
91.6238086320066,91.7276216586639,91.8314387440995,91.9353644977125,92.0393490949027,
92.1435156168706,92.2053666988316,92.3095531178609,92.4135843043219,92.5174934622426,
92.6213371650143,92.7251501913177,92.8289672764019,92.9328930296692,93.0368776265167,
93.1410441481497,93.2028952332682,93.3070788474255,93.3327269082001),
 .UNSPECIFIED.);
#2436=B_SPLINE_CURVE_WITH_KNOTS('',3,(#72731,#72732,#72733,#72734,#72735,
#72736,#72737,#72738,#72739,#72740,#72741,#72742,#72743,#72744,#72745,#72746,
#72747,#72748,#72749,#72750,#72751,#72752,#72753,#72754,#72755,#72756,#72757,
#72758,#72759,#72760,#72761,#72762,#72763,#72764,#72765,#72766,#72767,#72768,
#72769,#72770,#72771,#72772,#72773,#72774,#72775,#72776,#72777,#72778,#72779,
#72780,#72781,#72782,#72783,#72784,#72785,#72786,#72787,#72788,#72789,#72790,
#72791,#72792,#72793,#72794,#72795,#72796,#72797,#72798,#72799,#72800,#72801,
#72802,#72803,#72804,#72805,#72806,#72807,#72808,#72809,#72810,#72811,#72812,
#72813,#72814,#72815,#72816,#72817,#72818,#72819,#72820,#72821,#72822,#72823,
#72824,#72825,#72826,#72827,#72828,#72829,#72830,#72831,#72832,#72833,#72834,
#72835,#72836,#72837,#72838,#72839,#72840,#72841,#72842,#72843,#72844,#72845,
#72846,#72847,#72848,#72849,#72850,#72851,#72852,#72853,#72854),
 .UNSPECIFIED.,.F.,.F.,(4,3,3,3,3,3,3,3,3,3,3,3,3,3,3,3,3,3,3,3,3,3,3,3,
3,3,3,3,3,3,3,3,3,3,3,3,3,3,3,3,3,4),(87.048449830443,87.1526150420814,
87.2177240266486,87.3219104459154,87.4259416326135,87.5298507907696,87.6336944937754,
87.7375075203115,87.8413246056263,87.94525035912,88.0492349561916,88.153401478043,
88.2152525610852,88.3194389803687,88.4234701670835,88.5273793252564,88.631223028279,
88.7350360548318,88.8388531401634,88.9427788936735,89.0467634907616,89.1509300126291,
89.2127810955218,89.3169675147651,89.4209987014398,89.5249078595728,89.6287515625556,
89.7325645890689,89.8363816743613,89.9403074278329,90.0442920248827,90.148458546713,
90.2103096299584,90.3131827203155,90.4158805807012,90.5184806860292,90.6210195310318,
90.7235335248246,90.8261208448598,90.9287446854243,91.031530543581,91.1061869536405),
 .UNSPECIFIED.);
#2437=B_SPLINE_CURVE_WITH_KNOTS('',3,(#72860,#72861,#72862,#72863,#72864,
#72865,#72866,#72867,#72868,#72869,#72870,#72871,#72872,#72873,#72874,#72875,
#72876,#72877,#72878,#72879,#72880,#72881,#72882,#72883,#72884,#72885,#72886,
#72887,#72888,#72889,#72890,#72891,#72892,#72893,#72894,#72895,#72896,#72897,
#72898,#72899,#72900,#72901,#72902,#72903,#72904,#72905,#72906,#72907,#72908,
#72909,#72910,#72911,#72912,#72913,#72914,#72915,#72916,#72917,#72918,#72919,
#72920,#72921,#72922,#72923,#72924,#72925,#72926,#72927,#72928,#72929,#72930,
#72931,#72932,#72933,#72934,#72935,#72936,#72937,#72938,#72939,#72940,#72941,
#72942,#72943,#72944,#72945,#72946,#72947,#72948,#72949,#72950,#72951,#72952,
#72953,#72954,#72955,#72956,#72957,#72958,#72959,#72960,#72961,#72962,#72963,
#72964,#72965,#72966,#72967,#72968,#72969,#72970,#72971,#72972,#72973,#72974,
#72975,#72976,#72977,#72978,#72979,#72980),.UNSPECIFIED.,.F.,.F.,(4,3,3,
3,3,3,3,3,3,3,3,3,3,3,3,3,3,3,3,3,3,3,3,3,3,3,3,3,3,3,3,3,3,3,3,3,3,3,3,
3,4),(80.7662045566408,80.8702751277622,80.9742087489547,81.0780672044894,
81.1818852914194,81.2856977535908,81.3896126710214,81.4935777339141,81.5977339197861,
81.6885774148186,81.7927638340869,81.8967950207865,82.0007041789442,82.1045478819516,
82.2083609084892,82.3121779938057,82.416103747301,82.5200883443743,82.6242548662274,
82.6861059492552,82.7902923685257,82.8943235552275,82.9982327133873,83.1020764163968,
83.2058894429366,83.3097065282552,83.4136322817526,83.517616878828,83.6217834006831,
83.6836344836918,83.7878209029578,83.8918520896552,83.9957612478106,84.0996049508158,
84.2034179773513,84.3072350626658,84.4111608161589,84.5151454132301,84.6193119350812,
84.6811630181284,84.8230016469245),.UNSPECIFIED.);
#2438=B_SPLINE_CURVE_WITH_KNOTS('',3,(#72981,#72982,#72983,#72984,#72985,
#72986,#72987,#72988,#72989,#72990,#72991,#72992,#72993,#72994,#72995,#72996,
#72997,#72998,#72999,#73000,#73001,#73002,#73003,#73004,#73005,#73006,#73007,
#73008,#73009,#73010,#73011,#73012,#73013,#73014,#73015,#73016,#73017,#73018,
#73019,#73020,#73021,#73022,#73023,#73024,#73025,#73026,#73027,#73028,#73029,
#73030,#73031,#73032,#73033,#73034,#73035,#73036,#73037,#73038,#73039,#73040,
#73041,#73042,#73043,#73044,#73045,#73046,#73047,#73048,#73049,#73050),
 .UNSPECIFIED.,.F.,.F.,(4,3,3,3,3,3,3,3,3,3,3,3,3,3,3,3,3,3,3,3,3,3,3,4),
(84.8230016473369,84.9299628854904,85.0323879596834,85.1347430254586,85.2370647046656,
85.3393895675522,85.4418181479453,85.5443082329609,85.6469663801132,85.678691552565,
85.7828779718483,85.8869091585631,85.9908183167359,86.0946620197583,86.1984750463112,
86.3022921316428,86.4062178851529,86.5102024822409,86.6143690041083,86.6762200870016,
86.7803789666147,86.8844021488383,86.9883093146412,87.0493885891151),
 .UNSPECIFIED.);
#2439=B_SPLINE_CURVE_WITH_KNOTS('',3,(#73052,#73053,#73054,#73055,#73056,
#73057,#73058,#73059,#73060,#73061,#73062,#73063,#73064,#73065,#73066,#73067,
#73068,#73069,#73070,#73071,#73072,#73073,#73074,#73075,#73076,#73077,#73078,
#73079,#73080,#73081,#73082,#73083,#73084,#73085,#73086,#73087,#73088,#73089,
#73090,#73091,#73092,#73093,#73094,#73095,#73096,#73097,#73098,#73099,#73100,
#73101,#73102,#73103,#73104,#73105,#73106,#73107,#73108,#73109,#73110,#73111,
#73112,#73113,#73114,#73115,#73116,#73117,#73118),.UNSPECIFIED.,.F.,.F.,
(4,3,3,3,3,3,3,3,3,3,3,3,3,3,3,3,3,3,3,3,3,3,4),(84.8230016473359,84.9377580239967,
85.0529300598089,85.1686593350758,85.2226669577754,85.3268533770458,85.4308845637476,
85.5347937219074,85.6386374249169,85.7424504514566,85.8462675367751,85.9501932902725,
86.0541778873479,86.1583444092029,86.220195492212,86.3243482554787,86.4283607948036,
86.5322681022204,86.6361050469229,86.739945971975,86.8437814338429,86.9477239025433,
87.048449830443),.UNSPECIFIED.);
#2440=B_SPLINE_CURVE_WITH_KNOTS('',3,(#73119,#73120,#73121,#73122,#73123,
#73124,#73125,#73126,#73127,#73128,#73129,#73130,#73131,#73132,#73133,#73134,
#73135,#73136,#73137,#73138,#73139,#73140,#73141,#73142,#73143,#73144,#73145,
#73146,#73147,#73148,#73149,#73150,#73151,#73152,#73153,#73154,#73155,#73156,
#73157,#73158,#73159,#73160,#73161,#73162,#73163,#73164,#73165,#73166,#73167,
#73168,#73169,#73170,#73171,#73172,#73173,#73174,#73175,#73176,#73177,#73178,
#73179,#73180,#73181,#73182,#73183,#73184,#73185,#73186,#73187,#73188,#73189,
#73190,#73191,#73192,#73193,#73194,#73195,#73196,#73197,#73198,#73199,#73200,
#73201,#73202,#73203,#73204,#73205,#73206,#73207,#73208,#73209,#73210,#73211,
#73212,#73213,#73214,#73215,#73216,#73217,#73218,#73219,#73220,#73221,#73222,
#73223,#73224,#73225,#73226,#73227,#73228,#73229,#73230,#73231,#73232,#73233,
#73234,#73235,#73236,#73237,#73238,#73239,#73240,#73241,#73242),
 .UNSPECIFIED.,.F.,.F.,(4,3,3,3,3,3,3,3,3,3,3,3,3,3,3,3,3,3,3,3,3,3,3,3,
3,3,3,3,3,3,3,3,3,3,3,3,3,3,3,3,3,4),(80.7657407479557,80.8695602818193,
80.9734907583458,81.077483364404,81.1816545671184,81.232552820029,81.3367392392976,
81.4407704259972,81.5446795841552,81.6485232871629,81.7523363137008,81.8561533990176,
81.9600791525132,82.0640637495867,82.1682302714401,82.2300813544656,82.3342677737345,
82.4382989604349,82.5422081185931,82.646051821601,82.7498648481392,82.8536819334563,
82.9576076869522,83.061592284026,83.1657588058796,83.2276098889022,83.3317963081706,
83.4358274948705,83.5397366530282,83.6435803560358,83.7473933825737,83.8512104678904,
83.9551362213858,84.0591208184592,84.1632873403125,84.2251384233388,84.3308712802876,
84.43643371148,84.5418329411296,84.6471360606518,84.7523779621428,84.8230016469245),
 .UNSPECIFIED.);
#2441=B_SPLINE_CURVE_WITH_KNOTS('',3,(#73248,#73249,#73250,#73251,#73252,
#73253,#73254,#73255,#73256,#73257,#73258,#73259,#73260,#73261,#73262,#73263,
#73264,#73265,#73266,#73267,#73268,#73269,#73270,#73271,#73272,#73273,#73274,
#73275,#73276,#73277,#73278,#73279,#73280,#73281,#73282,#73283,#73284,#73285,
#73286,#73287,#73288,#73289,#73290,#73291,#73292,#73293,#73294,#73295,#73296,
#73297,#73298,#73299,#73300,#73301,#73302,#73303,#73304,#73305,#73306,#73307,
#73308,#73309,#73310,#73311,#73312,#73313,#73314,#73315,#73316,#73317,#73318,
#73319,#73320,#73321,#73322,#73323,#73324,#73325,#73326,#73327,#73328,#73329,
#73330,#73331,#73332,#73333,#73334,#73335,#73336,#73337,#73338,#73339,#73340,
#73341,#73342,#73343,#73344,#73345,#73346,#73347,#73348,#73349,#73350,#73351,
#73352,#73353,#73354,#73355,#73356,#73357,#73358,#73359,#73360,#73361,#73362,
#73363,#73364,#73365,#73366,#73367,#73368,#73369,#73370,#73371,#73372,#73373,
#73374),.UNSPECIFIED.,.F.,.F.,(4,3,3,3,3,3,3,3,3,3,3,3,3,3,3,3,3,3,3,3,
3,3,3,3,3,3,3,3,3,3,3,3,3,3,3,3,3,3,3,3,3,3,4),(74.4820615826405,74.586082341132,
74.6902715190842,74.7058776737624,74.810064093031,74.914095279731,75.018004437889,
75.1218481408967,75.2256611674347,75.3294782527516,75.4334040062472,75.5373886033208,
75.6415551251742,75.703406208199,75.8075926274676,75.9116238141675,76.0155329723255,
76.1193766753332,76.2231897018712,76.327006787188,76.4309325406836,76.5349171377572,
76.6390836596106,76.7009347426356,76.8051211619043,76.9091523486042,77.0130615067623,
77.11690520977,77.220718236308,77.3245353216249,77.4284610751206,77.5324456721942,
77.6366121940476,77.6984632770722,77.8036324098605,77.906096590754,78.008463441406,
78.1107696824819,78.2180313467062,78.320375332691,78.4227592903783,78.5252692706967,
78.539816339379),.UNSPECIFIED.);
#2442=B_SPLINE_CURVE_WITH_KNOTS('',3,(#73375,#73376,#73377,#73378,#73379,
#73380,#73381,#73382,#73383,#73384,#73385,#73386,#73387,#73388,#73389,#73390,
#73391,#73392,#73393,#73394,#73395,#73396,#73397,#73398,#73399,#73400,#73401,
#73402,#73403,#73404,#73405,#73406,#73407,#73408,#73409,#73410,#73411,#73412,
#73413,#73414,#73415,#73416,#73417,#73418,#73419,#73420,#73421,#73422,#73423,
#73424,#73425,#73426,#73427,#73428,#73429,#73430,#73431,#73432,#73433,#73434,
#73435,#73436,#73437,#73438,#73439,#73440,#73441),.UNSPECIFIED.,.F.,.F.,
(4,3,3,3,3,3,3,3,3,3,3,3,3,3,3,3,3,3,3,3,3,3,4),(78.5398163397448,78.6959918115088,
78.8001782307773,78.9042094174771,79.008118575635,79.1119622786427,79.2157753051806,
79.3195923904974,79.4235181439929,79.5275027410665,79.6316692629198,79.6935203459454,
79.7977067652143,79.9017379519144,80.0056471100727,80.1094908130806,80.2133038396189,
80.317120924936,80.4210466784319,80.5250312755058,80.6291977973594,80.691048880382,
80.7662045566408),.UNSPECIFIED.);
#2443=B_SPLINE_CURVE_WITH_KNOTS('',3,(#73443,#73444,#73445,#73446,#73447,
#73448,#73449,#73450,#73451,#73452,#73453,#73454,#73455,#73456,#73457,#73458,
#73459,#73460,#73461,#73462,#73463,#73464,#73465,#73466,#73467,#73468,#73469,
#73470,#73471,#73472,#73473,#73474,#73475,#73476,#73477,#73478,#73479,#73480,
#73481,#73482,#73483,#73484,#73485,#73486,#73487,#73488,#73489,#73490,#73491,
#73492,#73493,#73494,#73495,#73496,#73497,#73498,#73499,#73500,#73501,#73502,
#73503,#73504,#73505,#73506,#73507,#73508,#73509),.UNSPECIFIED.,.F.,.F.,
(4,3,3,3,3,3,3,3,3,3,3,3,3,3,3,3,3,3,3,3,3,3,4),(78.5398163397448,78.6430648259427,
78.7462751676035,78.849482902275,78.9527963206921,79.0561639752369,79.1597213368922,
79.2374957511558,79.3416821704245,79.4457133571245,79.5496225152826,79.6534662182904,
79.7572792448286,79.8610963301457,79.9650220836414,80.0690066807151,80.1731732025685,
80.2350242855924,80.3392063862685,80.4458399766903,80.5497449587941,80.6577428533749,
80.7657407479557),.UNSPECIFIED.);
#2444=B_SPLINE_CURVE_WITH_KNOTS('',3,(#73510,#73511,#73512,#73513,#73514,
#73515,#73516,#73517,#73518,#73519,#73520,#73521,#73522,#73523,#73524,#73525,
#73526,#73527,#73528,#73529,#73530,#73531,#73532,#73533,#73534,#73535,#73536,
#73537,#73538,#73539,#73540,#73541,#73542,#73543,#73544,#73545,#73546,#73547,
#73548,#73549,#73550,#73551,#73552,#73553,#73554,#73555,#73556,#73557,#73558,
#73559,#73560,#73561,#73562,#73563,#73564,#73565,#73566,#73567,#73568,#73569,
#73570,#73571,#73572,#73573,#73574,#73575,#73576,#73577,#73578,#73579,#73580,
#73581,#73582,#73583,#73584,#73585,#73586,#73587,#73588,#73589,#73590,#73591,
#73592,#73593,#73594,#73595,#73596,#73597,#73598,#73599,#73600,#73601,#73602,
#73603,#73604,#73605,#73606,#73607,#73608,#73609,#73610,#73611,#73612,#73613,
#73614,#73615,#73616,#73617,#73618,#73619,#73620,#73621,#73622,#73623,#73624,
#73625,#73626,#73627,#73628,#73629,#73630,#73631,#73632,#73633),
 .UNSPECIFIED.,.F.,.F.,(4,3,3,3,3,3,3,3,3,3,3,3,3,3,3,3,3,3,3,3,3,3,3,3,
3,3,3,3,3,3,3,3,3,3,3,3,3,3,3,3,3,4),(74.4832427147351,74.5871328262904,
74.6909659110764,74.7947767340429,74.8986000251703,75.0025371556357,75.1065406863584,
75.2107186083713,75.2473816134094,75.351568032678,75.4555992193779,75.5595083775359,
75.6633520805436,75.7671651070816,75.8709821923983,75.974907945894,76.0788925429675,
76.1830590648209,76.244910147846,76.3490965671146,76.4531277538149,76.5570369119729,
76.6608806149806,76.7646936415186,76.8685107268354,76.972436480331,77.0764210774045,
77.1805875992579,77.2424386822826,77.3466251015511,77.4506562882511,77.5545654464091,
77.6584091494169,77.7622221759549,77.8660392612711,77.9699650147667,78.0739496118403,
78.1781161336937,78.2399672167192,78.3667743014806,78.4918646575244,78.5398163394183),
 .UNSPECIFIED.);
#2445=B_SPLINE_CURVE_WITH_KNOTS('',3,(#73639,#73640,#73641,#73642,#73643,
#73644,#73645,#73646,#73647,#73648,#73649,#73650,#73651,#73652,#73653,#73654,
#73655,#73656,#73657,#73658,#73659,#73660,#73661,#73662,#73663,#73664,#73665,
#73666,#73667,#73668,#73669,#73670,#73671,#73672,#73673,#73674,#73675,#73676,
#73677,#73678,#73679,#73680,#73681,#73682,#73683,#73684,#73685,#73686,#73687,
#73688,#73689,#73690,#73691,#73692,#73693,#73694,#73695,#73696,#73697,#73698,
#73699,#73700,#73701,#73702,#73703,#73704,#73705,#73706,#73707,#73708,#73709,
#73710,#73711,#73712,#73713,#73714,#73715,#73716,#73717,#73718,#73719,#73720,
#73721,#73722,#73723,#73724,#73725,#73726,#73727,#73728,#73729,#73730,#73731,
#73732,#73733,#73734,#73735,#73736,#73737,#73738,#73739,#73740,#73741,#73742,
#73743,#73744,#73745,#73746,#73747,#73748,#73749,#73750,#73751,#73752,#73753,
#73754,#73755,#73756,#73757,#73758,#73759),.UNSPECIFIED.,.F.,.F.,(4,3,3,
3,3,3,3,3,3,3,3,3,3,3,3,3,3,3,3,3,3,3,3,3,3,3,3,3,3,3,3,3,3,3,3,3,3,3,3,
3,4),(68.1995378133446,68.3033489762282,68.4076883489568,68.5116448062476,
68.6161756366952,68.7207064671428,68.8248928864114,68.9289240731113,69.0328332312693,
69.1366769342769,69.240489960815,69.3443070461318,69.4482327996275,69.5522173967011,
69.6563839185545,69.7182350015794,69.822421420848,69.9264526075478,70.0303617657057,
70.1342054687134,70.2380184952513,70.341835580568,70.4457613340636,70.5497459311372,
70.6539124529906,70.715763536016,70.8199499552846,70.9239811419848,71.0278903001428,
71.1317340031507,71.2355470296887,71.3393641150054,71.4432898685011,71.5472744655748,
71.6514409874282,71.7132920704526,71.820873389079,71.9298127999506,72.0369795361944,
72.1468052843798,72.2566310325652),.UNSPECIFIED.);
#2446=B_SPLINE_CURVE_WITH_KNOTS('',3,(#73760,#73761,#73762,#73763,#73764,
#73765,#73766,#73767,#73768,#73769,#73770,#73771,#73772,#73773,#73774,#73775,
#73776,#73777,#73778,#73779,#73780,#73781,#73782,#73783,#73784,#73785,#73786,
#73787,#73788,#73789,#73790,#73791,#73792,#73793,#73794,#73795,#73796,#73797,
#73798,#73799,#73800,#73801,#73802,#73803,#73804,#73805,#73806,#73807,#73808,
#73809,#73810,#73811,#73812,#73813,#73814,#73815,#73816,#73817,#73818,#73819,
#73820,#73821,#73822,#73823,#73824,#73825,#73826),.UNSPECIFIED.,.F.,.F.,
(4,3,3,3,3,3,3,3,3,3,3,3,3,3,3,3,3,3,3,3,3,3,4),(72.2566310330111,72.3701784259806,
72.4815873942033,72.5962039995462,72.7108206048892,72.8150070241578,72.9190382108577,
73.0229473690157,73.1267910720234,73.2306040985614,73.3344211838782,73.4383469373738,
73.5423315344474,73.6464980563008,73.7083491393258,73.8125058091445,73.9165206688817,
74.020428717638,74.1242648292318,74.2280916123976,74.3319123054249,74.4358068055356,
74.4820615826405),.UNSPECIFIED.);
#2447=B_SPLINE_CURVE_WITH_KNOTS('',3,(#73828,#73829,#73830,#73831,#73832,
#73833,#73834,#73835,#73836,#73837,#73838,#73839,#73840,#73841,#73842,#73843,
#73844,#73845,#73846,#73847,#73848,#73849,#73850,#73851,#73852,#73853,#73854,
#73855,#73856,#73857,#73858,#73859,#73860,#73861,#73862,#73863,#73864,#73865,
#73866,#73867,#73868,#73869,#73870,#73871,#73872,#73873,#73874,#73875,#73876,
#73877,#73878,#73879,#73880,#73881,#73882,#73883,#73884,#73885,#73886,#73887,
#73888,#73889,#73890,#73891,#73892,#73893,#73894,#73895,#73896,#73897),
 .UNSPECIFIED.,.F.,.F.,(4,3,3,3,3,3,3,3,3,3,3,3,3,3,3,3,3,3,3,3,3,3,3,4),
(72.2566310325652,72.3607828828408,72.4647795326403,72.5686542861374,72.6724637223968,
72.7762426721719,72.880025922937,72.983917905017,73.0878690474532,73.1920015684936,
73.2523245445362,73.3565109638048,73.460542150505,73.5644513086631,73.6682950116708,
73.7721080382089,73.8759251235256,73.9798508770212,74.0838354740948,74.1880019959482,
74.2498530789728,74.3540440480005,74.4580688912275,74.4832427147351),
 .UNSPECIFIED.);
#2448=B_SPLINE_CURVE_WITH_KNOTS('',3,(#73898,#73899,#73900,#73901,#73902,
#73903,#73904,#73905,#73906,#73907,#73908,#73909,#73910,#73911,#73912,#73913,
#73914,#73915,#73916,#73917,#73918,#73919,#73920,#73921,#73922,#73923,#73924,
#73925,#73926,#73927,#73928,#73929,#73930,#73931,#73932,#73933,#73934,#73935,
#73936,#73937,#73938,#73939,#73940,#73941,#73942,#73943,#73944,#73945,#73946,
#73947,#73948,#73949,#73950,#73951,#73952,#73953,#73954,#73955,#73956,#73957,
#73958,#73959,#73960,#73961,#73962,#73963,#73964,#73965,#73966,#73967,#73968,
#73969,#73970,#73971,#73972,#73973,#73974,#73975,#73976,#73977,#73978,#73979,
#73980,#73981,#73982,#73983,#73984,#73985,#73986,#73987,#73988,#73989,#73990,
#73991,#73992,#73993,#73994,#73995,#73996,#73997,#73998,#73999,#74000,#74001,
#74002,#74003,#74004,#74005,#74006,#74007,#74008,#74009,#74010,#74011,#74012,
#74013,#74014,#74015,#74016,#74017,#74018,#74019,#74020,#74021,#74022,#74023,
#74024),.UNSPECIFIED.,.F.,.F.,(4,3,3,3,3,3,3,3,3,3,3,3,3,3,3,3,3,3,3,3,
3,3,3,3,3,3,3,3,3,3,3,3,3,3,3,3,3,3,3,3,3,3,4),(68.1991393909471,68.2646818723532,
68.3688682916219,68.4728994783218,68.5768086364799,68.6806523394876,68.7844653660257,
68.8882824513425,68.9922082048382,69.0961928019119,69.2003593237653,69.2622104067898,
69.3663968260585,69.4704280127584,69.5743371709164,69.6781808739241,69.7819939004622,
69.885810985779,69.9897367392746,70.0937213363482,70.1978878582016,70.2597389412264,
70.3639253604951,70.467956547195,70.571865705353,70.6757094083608,70.7795224348988,
70.8833395202156,70.9872652737112,71.0912498707849,71.1954163926383,71.257267475663,
71.3614538949317,71.4654850816316,71.5693942397896,71.6732379427972,71.7770509693352,
71.880868054652,71.9847938081477,72.0887784052212,72.1929449270746,72.2547960100996,
72.256631032138),.UNSPECIFIED.);
#2449=B_SPLINE_CURVE_WITH_KNOTS('',3,(#74030,#74031,#74032,#74033,#74034,
#74035,#74036,#74037,#74038,#74039,#74040,#74041,#74042,#74043,#74044,#74045,
#74046,#74047,#74048,#74049,#74050,#74051,#74052,#74053,#74054,#74055,#74056,
#74057,#74058,#74059,#74060,#74061,#74062,#74063,#74064,#74065,#74066,#74067,
#74068,#74069,#74070,#74071,#74072,#74073,#74074,#74075,#74076,#74077,#74078,
#74079,#74080,#74081,#74082,#74083,#74084,#74085,#74086,#74087,#74088,#74089,
#74090,#74091,#74092,#74093,#74094,#74095,#74096,#74097,#74098,#74099,#74100,
#74101,#74102,#74103,#74104,#74105,#74106,#74107,#74108,#74109,#74110,#74111,
#74112,#74113,#74114,#74115,#74116,#74117,#74118,#74119,#74120,#74121,#74122,
#74123,#74124,#74125,#74126,#74127,#74128,#74129,#74130,#74131,#74132,#74133,
#74134,#74135,#74136,#74137,#74138,#74139,#74140,#74141,#74142,#74143,#74144,
#74145,#74146,#74147,#74148,#74149,#74150),.UNSPECIFIED.,.F.,.F.,(4,3,3,
3,3,3,3,3,3,3,3,3,3,3,3,3,3,3,3,3,3,3,3,3,3,3,3,3,3,3,3,3,3,3,3,3,3,3,3,
3,4),(61.9168660682235,62.020800016341,62.1246586758828,62.2284768441524,
62.332289265122,62.4362040609573,62.5401688922078,62.644324966426,62.7355352605232,
62.8397216797919,62.9437528664918,63.0476620246499,63.1515057276576,63.2553187541956,
63.3591358395125,63.4630615930081,63.5670461900818,63.6712127119352,63.7330637949598,
63.8372502142284,63.9412814009284,64.0451905590864,64.149034262094,64.252847288632,
64.3566643739488,64.4605901274444,64.5645747245179,64.6687412463713,64.7305923293964,
64.8347787486651,64.9388099353651,65.0427190935232,65.1465627965309,65.250375823069,
65.354192908386,65.4581186618817,65.5621032589553,65.6662697808087,65.728120863833,
65.8639211020867,65.9734457249234),.UNSPECIFIED.);
#2450=B_SPLINE_CURVE_WITH_KNOTS('',3,(#74151,#74152,#74153,#74154,#74155,
#74156,#74157,#74158,#74159,#74160,#74161,#74162,#74163,#74164,#74165,#74166,
#74167,#74168,#74169,#74170,#74171,#74172,#74173,#74174,#74175,#74176,#74177,
#74178,#74179,#74180,#74181,#74182,#74183,#74184,#74185,#74186,#74187,#74188,
#74189,#74190,#74191,#74192,#74193,#74194,#74195,#74196,#74197,#74198,#74199,
#74200,#74201,#74202,#74203,#74204,#74205,#74206,#74207,#74208,#74209,#74210,
#74211,#74212,#74213,#74214,#74215,#74216,#74217,#74218,#74219,#74220),
 .UNSPECIFIED.,.F.,.F.,(4,3,3,3,3,3,3,3,3,3,3,3,3,3,3,3,3,3,3,3,3,3,3,4),
(65.9734457253856,66.0761394376291,66.1787659097615,66.2813614741681,66.3839624163262,
66.4866699517346,66.5894404069818,66.6923813783733,66.7256493982696,66.8298358175382,
66.9338670042381,67.0377761623961,67.1416198654038,67.2454328919417,67.3492499772587,
67.4531757307542,67.5571603278279,67.6613268496813,67.7231779327062,67.8273675151291,
67.9313793154477,68.035288009472,68.1391301362488,68.1995378133446),
 .UNSPECIFIED.);
#2451=B_SPLINE_CURVE_WITH_KNOTS('',3,(#74222,#74223,#74224,#74225,#74226,
#74227,#74228,#74229,#74230,#74231,#74232,#74233,#74234,#74235,#74236,#74237,
#74238,#74239,#74240,#74241,#74242,#74243,#74244,#74245,#74246,#74247,#74248,
#74249,#74250,#74251,#74252,#74253,#74254,#74255,#74256,#74257,#74258,#74259,
#74260,#74261,#74262,#74263,#74264,#74265,#74266,#74267,#74268,#74269,#74270,
#74271,#74272,#74273,#74274,#74275,#74276,#74277,#74278,#74279,#74280,#74281,
#74282,#74283,#74284,#74285,#74286,#74287,#74288),.UNSPECIFIED.,.F.,.F.,
(4,3,3,3,3,3,3,3,3,3,3,3,3,3,3,3,3,3,3,3,3,3,4),(65.973445725698,66.0988776153487,
66.2261299465501,66.26962480348,66.3738112227487,66.4778424094486,66.5817515676066,
66.6855952706143,66.7894082971523,66.8932253824692,66.9971511359649,67.1011357330385,
67.2053022548919,67.2671533379166,67.3713444216421,67.4753543191422,67.5792620015276,
67.683102330307,67.786910085549,67.8907809267929,67.9946786620494,68.0987368470966,
68.1991393909471),.UNSPECIFIED.);
#2452=B_SPLINE_CURVE_WITH_KNOTS('',3,(#74289,#74290,#74291,#74292,#74293,
#74294,#74295,#74296,#74297,#74298,#74299,#74300,#74301,#74302,#74303,#74304,
#74305,#74306,#74307,#74308,#74309,#74310,#74311,#74312,#74313,#74314,#74315,
#74316,#74317,#74318,#74319,#74320,#74321,#74322,#74323,#74324,#74325,#74326,
#74327,#74328,#74329,#74330,#74331,#74332,#74333,#74334,#74335,#74336,#74337,
#74338,#74339,#74340,#74341,#74342,#74343,#74344,#74345,#74346,#74347,#74348,
#74349,#74350,#74351,#74352,#74353,#74354,#74355,#74356,#74357,#74358,#74359,
#74360,#74361,#74362,#74363,#74364,#74365,#74366,#74367,#74368,#74369,#74370,
#74371,#74372,#74373,#74374,#74375,#74376,#74377,#74378,#74379,#74380,#74381,
#74382,#74383,#74384,#74385,#74386,#74387,#74388,#74389,#74390,#74391,#74392,
#74393,#74394,#74395,#74396,#74397,#74398,#74399,#74400,#74401,#74402,#74403,
#74404,#74405,#74406,#74407,#74408,#74409,#74410,#74411,#74412),
 .UNSPECIFIED.,.F.,.F.,(4,3,3,3,3,3,3,3,3,3,3,3,3,3,3,3,3,3,3,3,3,3,3,3,
3,3,3,3,3,3,3,3,3,3,3,3,3,3,3,3,3,4),(61.9158957515895,62.0198259500386,
62.1238180909945,62.2279890158734,62.2795106657336,62.3836970850022,62.4877282717022,
62.5916374298602,62.6954811328679,62.7992941594058,62.9031112447227,63.0070369982183,
63.1110215952918,63.2151881171452,63.2770392001702,63.3812256194389,63.4852568061389,
63.589165964297,63.6930096673046,63.7968226938427,63.9006397791592,64.0045655326549,
64.1085501297284,64.2127166515818,64.2745677346068,64.3787541538753,64.4827853405749,
64.5866944987329,64.6905382017405,64.7943512282787,64.8981683135958,65.0020940670913,
65.1060786641648,65.2102451860182,65.2720962690434,65.3756018854376,65.4789620265334,
65.5822125841115,65.6854054642083,65.7885610860729,65.8917634870112,65.9734457253856),
 .UNSPECIFIED.);
#2453=B_SPLINE_CURVE_WITH_KNOTS('',3,(#74418,#74419,#74420,#74421,#74422,
#74423,#74424,#74425,#74426,#74427,#74428,#74429,#74430,#74431,#74432,#74433,
#74434,#74435,#74436,#74437,#74438,#74439,#74440,#74441,#74442,#74443,#74444,
#74445,#74446,#74447,#74448,#74449,#74450,#74451,#74452,#74453,#74454,#74455,
#74456,#74457,#74458,#74459,#74460,#74461,#74462,#74463,#74464,#74465,#74466,
#74467,#74468,#74469,#74470,#74471,#74472,#74473,#74474,#74475,#74476,#74477,
#74478,#74479,#74480,#74481,#74482,#74483,#74484,#74485,#74486,#74487,#74488,
#74489,#74490,#74491,#74492,#74493,#74494,#74495,#74496,#74497,#74498,#74499,
#74500,#74501,#74502,#74503,#74504,#74505,#74506,#74507,#74508,#74509,#74510,
#74511,#74512,#74513,#74514,#74515,#74516,#74517,#74518,#74519,#74520,#74521,
#74522,#74523,#74524,#74525,#74526,#74527,#74528,#74529,#74530,#74531,#74532,
#74533,#74534,#74535,#74536,#74537,#74538,#74539,#74540,#74541,#74542,#74543,
#74544),.UNSPECIFIED.,.F.,.F.,(4,3,3,3,3,3,3,3,3,3,3,3,3,3,3,3,3,3,3,3,
3,3,3,3,3,3,3,3,3,3,3,3,3,3,3,3,3,3,3,3,3,3,4),(55.632601267868,55.7367901950251,
55.752835519467,55.8570219387357,55.9610531254356,56.0649622835936,56.1688059866013,
56.2726190131393,56.3764360984562,56.4803618519518,56.5843464490254,56.6885129708788,
56.7503640539036,56.8545504731722,56.9585816598722,57.0624908180302,57.1663345210379,
57.270147547576,57.3739646328928,57.4778903863884,57.581874983462,57.6860415053154,
57.7478925883402,57.8520790076088,57.9561101943088,58.0600193524668,58.1638630554745,
58.2676760820125,58.3714931673294,58.475418920825,58.5794035178986,58.683570039752,
58.7454211227768,58.8487780338704,58.9539633318698,59.0570447634801,59.1600643665929,
59.2630580262833,59.369858624179,59.4729706208883,59.5761501528112,59.6794897442517,
59.6902604178662),.UNSPECIFIED.);
#2454=B_SPLINE_CURVE_WITH_KNOTS('',3,(#74545,#74546,#74547,#74548,#74549,
#74550,#74551,#74552,#74553,#74554,#74555,#74556,#74557,#74558,#74559,#74560,
#74561,#74562,#74563,#74564,#74565,#74566,#74567,#74568,#74569,#74570,#74571,
#74572,#74573,#74574,#74575,#74576,#74577,#74578,#74579,#74580,#74581,#74582,
#74583,#74584,#74585,#74586,#74587,#74588,#74589,#74590,#74591,#74592,#74593,
#74594,#74595,#74596,#74597,#74598,#74599,#74600,#74601,#74602,#74603,#74604,
#74605,#74606,#74607,#74608,#74609,#74610,#74611,#74612,#74613,#74614),
 .UNSPECIFIED.,.F.,.F.,(4,3,3,3,3,3,3,3,3,3,3,3,3,3,3,3,3,3,3,3,3,3,3,4),
(59.690260418206,59.7429496572134,59.847136076482,59.9511672631821,60.0550764213401,
60.1589201243478,60.2627331508858,60.3665502362027,60.4704759896983,60.5744605867719,
60.6786271086253,60.74047819165,60.8446646109187,60.9486957976187,61.0526049557767,
61.1564486587844,61.2602616853225,61.3640787706394,61.468004524135,61.5719891212086,
61.676155643062,61.7380067260866,61.8421682999697,61.9168660682235),
 .UNSPECIFIED.);
#2455=B_SPLINE_CURVE_WITH_KNOTS('',3,(#74616,#74617,#74618,#74619,#74620,
#74621,#74622,#74623,#74624,#74625,#74626,#74627,#74628,#74629,#74630,#74631,
#74632,#74633,#74634,#74635,#74636,#74637,#74638,#74639,#74640,#74641,#74642,
#74643,#74644,#74645,#74646,#74647,#74648,#74649,#74650,#74651,#74652,#74653,
#74654,#74655,#74656,#74657,#74658,#74659,#74660,#74661,#74662,#74663,#74664,
#74665,#74666,#74667,#74668,#74669,#74670,#74671,#74672,#74673,#74674,#74675,
#74676,#74677,#74678,#74679,#74680,#74681,#74682),.UNSPECIFIED.,.F.,.F.,
(4,3,3,3,3,3,3,3,3,3,3,3,3,3,3,3,3,3,3,3,3,3,4),(59.690260418206,59.7955870148005,
59.9009552529612,60.0064809160439,60.1120913042762,60.2179183210521,60.2844535968604,
60.388640016129,60.492671202829,60.596580360987,60.7004240639947,60.8042370905327,
60.9080541758494,61.011979929345,61.1159645264186,61.220131048272,61.281982131297,
61.3861518308915,61.4901756511519,61.5966056762613,61.7004458111016,61.8081707813456,
61.9158957515895),.UNSPECIFIED.);
#2456=B_SPLINE_CURVE_WITH_KNOTS('',3,(#74683,#74684,#74685,#74686,#74687,
#74688,#74689,#74690,#74691,#74692,#74693,#74694,#74695,#74696,#74697,#74698,
#74699,#74700,#74701,#74702,#74703,#74704,#74705,#74706,#74707,#74708,#74709,
#74710,#74711,#74712,#74713,#74714,#74715,#74716,#74717,#74718,#74719,#74720,
#74721,#74722,#74723,#74724,#74725,#74726,#74727,#74728,#74729,#74730,#74731,
#74732,#74733,#74734,#74735,#74736,#74737,#74738,#74739,#74740,#74741,#74742,
#74743,#74744,#74745,#74746,#74747,#74748,#74749,#74750,#74751,#74752,#74753,
#74754,#74755,#74756,#74757,#74758,#74759,#74760,#74761,#74762,#74763,#74764,
#74765,#74766,#74767,#74768,#74769,#74770,#74771,#74772,#74773,#74774,#74775,
#74776,#74777,#74778,#74779,#74780,#74781,#74782,#74783,#74784,#74785,#74786,
#74787,#74788,#74789,#74790,#74791,#74792,#74793,#74794,#74795,#74796,#74797,
#74798,#74799,#74800,#74801,#74802,#74803,#74804,#74805,#74806),
 .UNSPECIFIED.,.F.,.F.,(4,3,3,3,3,3,3,3,3,3,3,3,3,3,3,3,3,3,3,3,3,3,3,3,
3,3,3,3,3,3,3,3,3,3,3,3,3,3,3,3,3,4),(55.6335465345705,55.7373798274981,
55.8411906765822,55.9450138118952,56.0489506768776,56.1529537786039,56.2571314301315,
56.294339459114,56.3985258783826,56.5025570650827,56.6064662232407,56.7103099262484,
56.8141229527865,56.9179400381034,57.021865791599,57.1258503886726,57.230016910526,
57.2918679935506,57.3960544128192,57.5000855995191,57.6039947576771,57.7078384606849,
57.8116514872229,57.9154685725399,58.0193943260355,58.1233789231092,58.2275454449625,
58.2893965279872,58.3935829472558,58.4976141339561,58.6015232921142,58.7053669951219,
58.8091800216597,58.9129971069763,59.0169228604719,59.1209074575456,59.2250739793991,
59.2869250624238,59.4023023747482,59.5173142786563,59.6317214277102,59.6902604178031),
 .UNSPECIFIED.);
#2457=B_SPLINE_CURVE_WITH_KNOTS('',3,(#74812,#74813,#74814,#74815,#74816,
#74817,#74818,#74819,#74820,#74821,#74822,#74823,#74824,#74825,#74826,#74827,
#74828,#74829,#74830,#74831,#74832,#74833,#74834,#74835,#74836,#74837,#74838,
#74839,#74840,#74841,#74842,#74843,#74844,#74845,#74846,#74847,#74848,#74849,
#74850,#74851,#74852,#74853,#74854,#74855,#74856,#74857,#74858,#74859,#74860,
#74861,#74862,#74863,#74864,#74865,#74866,#74867,#74868,#74869,#74870,#74871,
#74872,#74873,#74874,#74875,#74876,#74877,#74878,#74879,#74880,#74881,#74882,
#74883,#74884,#74885,#74886,#74887,#74888,#74889,#74890,#74891,#74892,#74893,
#74894,#74895,#74896,#74897,#74898,#74899,#74900,#74901,#74902,#74903,#74904,
#74905,#74906,#74907,#74908,#74909,#74910,#74911,#74912,#74913,#74914,#74915,
#74916,#74917,#74918,#74919,#74920,#74921,#74922,#74923,#74924,#74925,#74926,
#74927,#74928,#74929,#74930,#74931,#74932,#74933,#74934,#74935),
 .UNSPECIFIED.,.F.,.F.,(4,3,3,3,3,3,3,3,3,3,3,3,3,3,3,3,3,3,3,3,3,3,3,3,
3,3,3,3,3,3,3,3,3,3,3,3,3,3,3,3,3,4),(49.3496692799972,49.4541680382097,
49.5581242127346,49.662894262791,49.7676643128474,49.871850732116,49.9758819188161,
50.0797910769742,50.1836347799818,50.2874478065199,50.3912648918368,50.4951906453325,
50.5991752424062,50.7033417642596,50.765192847284,50.8693792665526,50.9734104532527,
51.0773196114107,51.1811633144184,51.2849763409564,51.3887934262736,51.4927191797692,
51.5967037768428,51.7008702986961,51.7627213817206,51.8669078009892,51.9709389876889,
52.0748481458469,52.1786918488547,52.2825048753927,52.3863219607096,52.4902477142051,
52.5942323112789,52.6983988331322,52.7602499161572,52.8647413337412,52.9690770723351,
53.0785765820079,53.1827008676143,53.2867777522301,53.3908555974491,53.4070751110264),
 .UNSPECIFIED.);
#2458=B_SPLINE_CURVE_WITH_KNOTS('',3,(#74936,#74937,#74938,#74939,#74940,
#74941,#74942,#74943,#74944,#74945,#74946,#74947,#74948,#74949,#74950,#74951,
#74952,#74953,#74954,#74955,#74956,#74957,#74958,#74959,#74960,#74961,#74962,
#74963,#74964,#74965,#74966,#74967,#74968,#74969,#74970,#74971,#74972,#74973,
#74974,#74975,#74976,#74977,#74978,#74979,#74980,#74981,#74982,#74983,#74984,
#74985,#74986,#74987,#74988,#74989,#74990,#74991,#74992,#74993,#74994,#74995,
#74996,#74997,#74998,#74999,#75000,#75001,#75002),.UNSPECIFIED.,.F.,.F.,
(4,3,3,3,3,3,3,3,3,3,3,3,3,3,3,3,3,3,3,3,3,3,4),(53.4070751114695,53.5260746317924,
53.6461595854636,53.7577784505938,53.8619648698624,53.9659960565624,54.0699052147205,
54.1737489177282,54.2775619442662,54.3813790295831,54.4853047830788,54.5892893801525,
54.6934559020058,54.7553069850304,54.8649687703851,54.9689734124943,55.0728760914193,
55.1767116672088,55.280514918126,55.3843665184446,55.4882460133807,55.5922460948382,
55.632601267868),.UNSPECIFIED.);
#2459=B_SPLINE_CURVE_WITH_KNOTS('',3,(#75004,#75005,#75006,#75007,#75008,
#75009,#75010,#75011,#75012,#75013,#75014,#75015,#75016,#75017,#75018,#75019,
#75020,#75021,#75022,#75023,#75024,#75025,#75026,#75027,#75028,#75029,#75030,
#75031,#75032,#75033,#75034,#75035,#75036,#75037,#75038,#75039,#75040,#75041,
#75042,#75043,#75044,#75045,#75046,#75047,#75048,#75049,#75050,#75051,#75052,
#75053,#75054,#75055,#75056,#75057,#75058,#75059,#75060,#75061,#75062,#75063,
#75064,#75065,#75066,#75067,#75068,#75069,#75070,#75071,#75072,#75073),
 .UNSPECIFIED.,.F.,.F.,(4,3,3,3,3,3,3,3,3,3,3,3,3,3,3,3,3,3,3,3,3,3,3,4),
(53.407075111485,53.5098558320716,53.6124863111895,53.7150344153237,53.8175366234483,
53.9200293486255,54.0226180274754,54.1252565130568,54.2280753277761,54.2992823902408,
54.4034688095096,54.5074999962094,54.6114091543675,54.7152528573751,54.8190658839131,
54.9228829692299,55.0268087227256,55.1307933197992,55.2349598416526,55.2968109246774,
55.4009764972003,55.5050059369267,55.6089152722145,55.6335465345705),
 .UNSPECIFIED.);
#2460=B_SPLINE_CURVE_WITH_KNOTS('',3,(#75074,#75075,#75076,#75077,#75078,
#75079,#75080,#75081,#75082,#75083,#75084,#75085,#75086,#75087,#75088,#75089,
#75090,#75091,#75092,#75093,#75094,#75095,#75096,#75097,#75098,#75099,#75100,
#75101,#75102,#75103,#75104,#75105,#75106,#75107,#75108,#75109,#75110,#75111,
#75112,#75113,#75114,#75115,#75116,#75117,#75118,#75119,#75120,#75121,#75122,
#75123,#75124,#75125,#75126,#75127,#75128,#75129,#75130,#75131,#75132,#75133,
#75134,#75135,#75136,#75137,#75138,#75139,#75140,#75141,#75142,#75143,#75144,
#75145,#75146,#75147,#75148,#75149,#75150,#75151,#75152,#75153,#75154,#75155,
#75156,#75157,#75158,#75159,#75160,#75161,#75162,#75163,#75164,#75165,#75166,
#75167,#75168,#75169,#75170,#75171,#75172,#75173,#75174,#75175,#75176,#75177,
#75178,#75179,#75180,#75181,#75182,#75183,#75184,#75185,#75186,#75187,#75188,
#75189,#75190,#75191,#75192,#75193,#75194,#75195,#75196,#75197),
 .UNSPECIFIED.,.F.,.F.,(4,3,3,3,3,3,3,3,3,3,3,3,3,3,3,3,3,3,3,3,3,3,3,3,
3,3,3,3,3,3,3,3,3,3,3,3,3,3,3,3,3,4),(49.3501240392415,49.4542486344756,
49.5611135867279,49.6649925959122,49.7688199626021,49.8726304440509,49.9817648961618,
50.0857131354161,50.1897342007835,50.2939235856819,50.3091682524944,50.413354671763,
50.517385858463,50.621295016621,50.7251387196287,50.8289517461667,50.9327688314835,
51.0366945849791,51.1406791820528,51.2448457039061,51.306696786931,51.4108832061996,
51.5149143928996,51.6188235510576,51.7226672540653,51.8264802806034,51.9302973659202,
52.0342231194158,52.1382077164894,52.2423742383427,52.3042253213676,52.4084117406363,
52.5124429273362,52.6163520854942,52.720195788502,52.82400881504,52.9278259003569,
53.0317516538525,53.1357362509261,53.2399027727795,53.3017538558042,53.4070751110264),
 .UNSPECIFIED.);
#2461=B_SPLINE_CURVE_WITH_KNOTS('',3,(#75203,#75204,#75205,#75206,#75207,
#75208,#75209,#75210,#75211,#75212,#75213,#75214,#75215,#75216,#75217,#75218,
#75219,#75220,#75221,#75222,#75223,#75224,#75225,#75226,#75227,#75228,#75229,
#75230,#75231,#75232,#75233,#75234,#75235,#75236,#75237,#75238,#75239,#75240,
#75241,#75242,#75243,#75244,#75245,#75246,#75247,#75248,#75249,#75250,#75251,
#75252,#75253,#75254,#75255,#75256,#75257,#75258,#75259,#75260,#75261,#75262,
#75263,#75264,#75265,#75266,#75267,#75268,#75269,#75270,#75271,#75272,#75273,
#75274,#75275,#75276,#75277,#75278,#75279,#75280,#75281,#75282,#75283,#75284,
#75285,#75286,#75287,#75288,#75289,#75290,#75291,#75292,#75293,#75294,#75295,
#75296,#75297,#75298,#75299,#75300,#75301,#75302,#75303,#75304,#75305,#75306,
#75307,#75308,#75309,#75310,#75311,#75312,#75313,#75314,#75315,#75316,#75317,
#75318,#75319,#75320,#75321,#75322,#75323),.UNSPECIFIED.,.F.,.F.,(4,3,3,
3,3,3,3,3,3,3,3,3,3,3,3,3,3,3,3,3,3,3,3,3,3,3,3,3,3,3,3,3,3,3,3,3,3,3,3,
3,4),(43.0672711170668,43.1711300481588,43.2749483250992,43.3787606920285,
43.4826753270082,43.5866398512832,43.6907957779855,43.7824931062278,43.8866795254967,
43.990710712197,44.0946198703552,44.1984635733631,44.3022765999014,44.4060936852184,
44.5100194387142,44.6140040357881,44.7181705576417,44.7800216406644,44.884208059933,
44.9882392466327,45.0921484047907,45.1959921077982,45.2998051343363,45.4036222196529,
45.5075479731485,45.6115325702221,45.7156990920753,45.777550175101,45.8817365943698,
45.9857677810699,46.0896769392279,46.1935206422355,46.2973336687735,46.4011507540907,
46.5050765075864,46.6090611046601,46.7132276265135,46.7750787095376,46.8955468165443,
47.0149579004655,47.1238898034052),.UNSPECIFIED.);
#2462=B_SPLINE_CURVE_WITH_KNOTS('',3,(#75324,#75325,#75326,#75327,#75328,
#75329,#75330,#75331,#75332,#75333,#75334,#75335,#75336,#75337,#75338,#75339,
#75340,#75341,#75342,#75343,#75344,#75345,#75346,#75347,#75348,#75349,#75350,
#75351,#75352,#75353,#75354,#75355,#75356,#75357,#75358,#75359,#75360,#75361,
#75362,#75363,#75364,#75365,#75366,#75367,#75368,#75369,#75370,#75371,#75372,
#75373,#75374,#75375,#75376,#75377,#75378,#75379,#75380,#75381,#75382,#75383,
#75384,#75385,#75386,#75387,#75388,#75389,#75390,#75391,#75392,#75393),
 .UNSPECIFIED.,.F.,.F.,(4,3,3,3,3,3,3,3,3,3,3,3,3,3,3,3,3,3,3,3,3,3,3,4),
(47.1238898038468,47.2279417400956,47.3319880830488,47.4360629830602,47.5402700680327,
47.6445565808268,47.7490254998337,47.7726072439742,47.8767936632428,47.9808248499427,
48.0847340081007,48.1885777111083,48.2923907376463,48.3962078229629,48.5001335764585,
48.6041181735321,48.7082846953854,48.7701357784108,48.8743117183293,48.9783401946018,
49.0822482051312,49.1860855662745,49.2899055677676,49.3496692799972),
 .UNSPECIFIED.);
#2463=B_SPLINE_CURVE_WITH_KNOTS('',3,(#75395,#75396,#75397,#75398,#75399,
#75400,#75401,#75402,#75403,#75404,#75405,#75406,#75407,#75408,#75409,#75410,
#75411,#75412,#75413,#75414,#75415,#75416,#75417,#75418,#75419,#75420,#75421,
#75422,#75423,#75424,#75425,#75426,#75427,#75428,#75429,#75430,#75431,#75432,
#75433,#75434,#75435,#75436,#75437,#75438,#75439,#75440,#75441,#75442,#75443,
#75444,#75445,#75446,#75447,#75448,#75449,#75450,#75451,#75452,#75453,#75454,
#75455,#75456,#75457,#75458,#75459,#75460,#75461,#75462,#75463,#75464),
 .UNSPECIFIED.,.F.,.F.,(4,3,3,3,3,3,3,3,3,3,3,3,3,3,3,3,3,3,3,3,3,3,3,4),
(47.1238898038468,47.2757519674259,47.3165826491846,47.4207690684532,47.5248002551532,
47.6287094133112,47.7325531163188,47.8363661428568,47.9401832281736,48.0441089816691,
48.1480935787427,48.252260100596,48.3141111836212,48.4182976028898,48.5223287895898,
48.6262379477478,48.7300816507555,48.8338946772934,48.9377117626103,49.0416375161059,
49.1456221131795,49.2497886350328,49.3116397180578,49.3501240392415),
 .UNSPECIFIED.);
#2464=B_SPLINE_CURVE_WITH_KNOTS('',3,(#75465,#75466,#75467,#75468,#75469,
#75470,#75471,#75472,#75473,#75474,#75475,#75476,#75477,#75478,#75479,#75480,
#75481,#75482,#75483,#75484,#75485,#75486,#75487,#75488,#75489,#75490,#75491,
#75492,#75493,#75494,#75495,#75496,#75497,#75498,#75499,#75500,#75501,#75502,
#75503,#75504,#75505,#75506,#75507,#75508,#75509,#75510,#75511,#75512,#75513,
#75514,#75515,#75516,#75517,#75518,#75519,#75520,#75521,#75522,#75523,#75524,
#75525,#75526,#75527,#75528,#75529,#75530,#75531,#75532,#75533,#75534,#75535,
#75536,#75537,#75538,#75539,#75540,#75541,#75542,#75543,#75544,#75545,#75546,
#75547,#75548,#75549,#75550,#75551,#75552,#75553,#75554,#75555,#75556,#75557,
#75558,#75559,#75560,#75561,#75562,#75563,#75564,#75565,#75566,#75567,#75568,
#75569,#75570,#75571,#75572,#75573,#75574,#75575,#75576,#75577,#75578,#75579,
#75580,#75581,#75582,#75583,#75584,#75585,#75586,#75587,#75588),
 .UNSPECIFIED.,.F.,.F.,(4,3,3,3,3,3,3,3,3,3,3,3,3,3,3,3,3,3,3,3,3,3,3,3,
3,3,3,3,3,3,3,3,3,3,3,3,3,3,3,3,3,4),(43.0661580866905,43.1701497613869,
43.2743204084533,43.3264685114382,43.4306549307085,43.5346861174102,43.63859527557,
43.7424389785794,43.8462520051192,43.9500690904379,44.0539948439353,44.1579794410107,
44.2621459628659,44.3239970458748,44.4281834651431,44.5322146518427,44.6361238100004,
44.7399675130077,44.8437805395454,44.9475976248619,45.0515233783572,45.1555079754305,
45.2596744972836,45.3215255803114,45.4257119995798,45.5297431862795,45.6336523444373,
45.7374960474447,45.8413090739825,45.9451261592991,46.0490519127945,46.1530365098678,
46.2572030317209,46.319054114748,46.4216814718159,46.5241724459795,46.6265638875462,
46.7288925026225,46.8312400381875,46.9335916782503,47.036063908885,47.1238898034172),
 .UNSPECIFIED.);
#2465=B_SPLINE_CURVE_WITH_KNOTS('',3,(#75594,#75595,#75596,#75597,#75598,
#75599,#75600,#75601,#75602,#75603,#75604,#75605,#75606,#75607,#75608,#75609,
#75610,#75611,#75612,#75613,#75614,#75615,#75616,#75617,#75618,#75619,#75620,
#75621,#75622,#75623,#75624,#75625,#75626,#75627,#75628,#75629,#75630,#75631,
#75632,#75633,#75634,#75635,#75636,#75637,#75638,#75639,#75640,#75641,#75642,
#75643,#75644,#75645,#75646,#75647,#75648,#75649,#75650,#75651,#75652,#75653,
#75654,#75655,#75656,#75657,#75658,#75659,#75660,#75661,#75662,#75663,#75664,
#75665,#75666,#75667,#75668,#75669,#75670,#75671,#75672,#75673,#75674,#75675,
#75676,#75677,#75678,#75679,#75680,#75681,#75682,#75683,#75684,#75685,#75686,
#75687,#75688,#75689,#75690,#75691,#75692,#75693,#75694,#75695,#75696,#75697,
#75698,#75699,#75700,#75701,#75702,#75703,#75704,#75705,#75706,#75707,#75708,
#75709,#75710,#75711,#75712,#75713,#75714,#75715,#75716,#75717,#75718,#75719,
#75720),.UNSPECIFIED.,.F.,.F.,(4,3,3,3,3,3,3,3,3,3,3,3,3,3,3,3,3,3,3,3,
3,3,3,3,3,3,3,3,3,3,3,3,3,3,3,3,3,3,3,3,3,3,4),(36.7834458130743,36.7997933651716,
36.9039797844174,37.008010971094,37.1119201292281,37.2157638322115,37.3195768587249,
37.4233939440169,37.5273196974874,37.6313042945357,37.7354708163638,37.7973218996082,
37.9015083188909,38.005539505605,38.1094486637775,38.2132923667998,38.3171053933525,
38.4209224786842,38.5248482321947,38.6288328292833,38.7329993511515,38.7948504340448,
38.8990368533114,39.0030680400094,39.1069771981654,39.2108209011712,39.3146339277072,
39.4184510130221,39.5223767665159,39.6263613635876,39.7305278854392,39.7923789684814,
39.8965653877477,40.0005965744453,40.1045057326009,40.2083494356062,40.3121624621417,
40.4159795474562,40.5199053009493,40.6238898980203,40.7280564198711,40.789907502918,
40.8407044966673),.UNSPECIFIED.);
#2466=B_SPLINE_CURVE_WITH_KNOTS('',3,(#75721,#75722,#75723,#75724,#75725,
#75726,#75727,#75728,#75729,#75730,#75731,#75732,#75733,#75734,#75735,#75736,
#75737,#75738,#75739,#75740,#75741,#75742,#75743,#75744,#75745,#75746,#75747,
#75748,#75749,#75750,#75751,#75752,#75753,#75754,#75755,#75756,#75757,#75758,
#75759,#75760,#75761,#75762,#75763,#75764,#75765,#75766,#75767,#75768,#75769,
#75770,#75771,#75772,#75773,#75774,#75775,#75776,#75777,#75778,#75779,#75780,
#75781,#75782,#75783,#75784,#75785,#75786,#75787,#75788,#75789,#75790),
 .UNSPECIFIED.,.F.,.F.,(4,3,3,3,3,3,3,3,3,3,3,3,3,3,3,3,3,3,3,3,3,3,3,4),
(40.8407044970058,40.9440672893056,41.0494883828118,41.1525861150441,41.2556259852182,
41.3586438439569,41.4658418923063,41.5689883265361,41.6722057013042,41.7755885097156,
41.7874360373546,41.8916224566229,41.9956536433225,42.0995628014801,42.2034065044874,
42.307219531025,42.4110366163413,42.5149623698365,42.6189469669099,42.7231134887628,
42.7849645717912,42.8891423385872,42.9931552860089,43.0672711170668),
 .UNSPECIFIED.);
#2467=B_SPLINE_CURVE_WITH_KNOTS('',3,(#75792,#75793,#75794,#75795,#75796,
#75797,#75798,#75799,#75800,#75801,#75802,#75803,#75804,#75805,#75806,#75807,
#75808,#75809,#75810,#75811,#75812,#75813,#75814,#75815,#75816,#75817,#75818,
#75819,#75820,#75821,#75822,#75823,#75824,#75825,#75826,#75827,#75828,#75829,
#75830,#75831,#75832,#75833,#75834,#75835,#75836,#75837,#75838,#75839,#75840,
#75841,#75842,#75843,#75844,#75845,#75846,#75847,#75848,#75849,#75850,#75851,
#75852,#75853,#75854,#75855,#75856,#75857,#75858),.UNSPECIFIED.,.F.,.F.,
(4,3,3,3,3,3,3,3,3,3,3,3,3,3,3,3,3,3,3,3,3,3,4),(40.8407044970049,40.9498036597887,
41.0592250219573,41.1688181464341,41.2787131705271,41.331411442565,41.4355978618316,
41.5396290485296,41.6435382066856,41.7473819096913,41.8511949362273,41.9550120215421,
42.0589377750358,42.1629223721075,42.2670888939591,42.3289399770016,42.4330996296933,
42.5371164105446,42.6410253236265,42.7473085143925,42.8511267996347,42.9586424431626,
43.0661580866905),.UNSPECIFIED.);
#2468=B_SPLINE_CURVE_WITH_KNOTS('',3,(#75859,#75860,#75861,#75862,#75863,
#75864,#75865,#75866,#75867,#75868,#75869,#75870,#75871,#75872,#75873,#75874,
#75875,#75876,#75877,#75878,#75879,#75880,#75881,#75882,#75883,#75884,#75885,
#75886,#75887,#75888,#75889,#75890,#75891,#75892,#75893,#75894,#75895,#75896,
#75897,#75898,#75899,#75900,#75901,#75902,#75903,#75904,#75905,#75906,#75907,
#75908,#75909,#75910,#75911,#75912,#75913,#75914,#75915,#75916,#75917,#75918,
#75919,#75920,#75921,#75922,#75923,#75924,#75925,#75926,#75927,#75928,#75929,
#75930,#75931,#75932,#75933,#75934,#75935,#75936,#75937,#75938,#75939,#75940,
#75941,#75942,#75943,#75944,#75945,#75946,#75947,#75948,#75949,#75950,#75951,
#75952,#75953,#75954,#75955,#75956,#75957,#75958,#75959,#75960,#75961,#75962,
#75963,#75964,#75965,#75966,#75967,#75968,#75969,#75970,#75971,#75972,#75973,
#75974,#75975,#75976,#75977,#75978,#75979,#75980,#75981,#75982),
 .UNSPECIFIED.,.F.,.F.,(4,3,3,3,3,3,3,3,3,3,3,3,3,3,3,3,3,3,3,3,3,3,3,3,
3,3,3,3,3,3,3,3,3,3,3,3,3,3,3,3,3,4),(36.783721561275,36.8875324408591,
36.991355400596,37.0952919656597,37.1992945822548,37.303471928437,37.3412973048186,
37.445483724201,37.5495149110165,37.6534240692916,37.7572677724174,37.8610807990743,
37.964897884511,38.0688236381266,38.1728082353203,38.2769747572932,38.3388258392552,
38.4430122585159,38.5470434452078,38.6509526033583,38.7547963063587,38.8586093328897,
38.9624264181998,39.0663521716889,39.1703367687562,39.2745032906037,39.3363543736918,
39.4405407929374,39.5445719796139,39.6484811377479,39.7523248407311,39.8561378672445,
39.9599549525365,40.0638807060069,40.1678653030551,40.2720318248831,40.3338829081284,
40.4430298277097,40.551871089477,40.6605292198771,40.7689635848466,40.8407044966672),
 .UNSPECIFIED.);
#2469=B_SPLINE_CURVE_WITH_KNOTS('',3,(#75988,#75989,#75990,#75991,#75992,
#75993,#75994,#75995,#75996,#75997,#75998,#75999,#76000,#76001,#76002,#76003,
#76004,#76005,#76006,#76007,#76008,#76009,#76010,#76011,#76012,#76013,#76014,
#76015,#76016,#76017,#76018,#76019,#76020,#76021,#76022,#76023,#76024,#76025,
#76026,#76027,#76028,#76029,#76030,#76031,#76032,#76033,#76034,#76035,#76036,
#76037,#76038,#76039,#76040,#76041,#76042,#76043,#76044,#76045,#76046,#76047,
#76048,#76049,#76050,#76051,#76052,#76053,#76054,#76055,#76056,#76057,#76058,
#76059,#76060,#76061,#76062,#76063,#76064,#76065,#76066,#76067,#76068,#76069,
#76070,#76071,#76072,#76073,#76074,#76075,#76076,#76077,#76078,#76079,#76080,
#76081,#76082,#76083,#76084,#76085,#76086,#76087,#76088,#76089,#76090,#76091,
#76092,#76093,#76094,#76095,#76096,#76097,#76098,#76099,#76100,#76101,#76102,
#76103,#76104,#76105,#76106,#76107,#76108,#76109,#76110,#76111),
 .UNSPECIFIED.,.F.,.F.,(4,3,3,3,3,3,3,3,3,3,3,3,3,3,3,3,3,3,3,3,3,3,3,3,
3,3,3,3,3,3,3,3,3,3,3,3,3,3,3,3,3,4),(30.4998648068842,30.6038202397747,
30.7092211991633,30.814622158552,30.9188085758033,31.0228397604486,31.1267489165067,
31.2305926173876,31.3344056417751,31.4382227249208,31.5421484762289,31.6461330711024,
31.7502995907594,31.8121506929886,31.9163371131481,32.0203683007503,32.1242774598234,
32.2281211637535,32.3319341912199,32.4357512774697,32.5396770318988,32.6436616299078,
32.747828152689,32.8096792274252,32.9138656467035,33.0178968334163,33.1218059915909,
33.2256496946177,33.3294627211775,33.4332798065188,33.5372055600422,33.6411901571455,
33.7453566790319,33.8072077618618,33.9101447146383,34.0129417465488,34.1156354071306,
34.2182621038491,34.320888212797,34.4235151981865,34.5262219085209,34.5575191894877),
 .UNSPECIFIED.);
#2470=B_SPLINE_CURVE_WITH_KNOTS('',3,(#76112,#76113,#76114,#76115,#76116,
#76117,#76118,#76119,#76120,#76121,#76122,#76123,#76124,#76125,#76126,#76127,
#76128,#76129,#76130,#76131,#76132,#76133,#76134,#76135,#76136,#76137,#76138,
#76139,#76140,#76141,#76142,#76143,#76144,#76145,#76146,#76147,#76148,#76149,
#76150,#76151,#76152,#76153,#76154,#76155,#76156,#76157,#76158,#76159,#76160,
#76161,#76162,#76163,#76164,#76165,#76166,#76167,#76168,#76169,#76170,#76171,
#76172,#76173,#76174,#76175,#76176,#76177,#76178),.UNSPECIFIED.,.F.,.F.,
(4,3,3,3,3,3,3,3,3,3,3,3,3,3,3,3,3,3,3,3,3,3,4),(34.5575191897626,34.6928922558173,
34.8047362962984,34.9089227156804,35.0129539024952,35.1168630607699,35.2207067638953,
35.324519790552,35.4283368759881,35.5322626296032,35.6362472267967,35.7404137487691,
35.802264830735,35.9064523911115,36.0104843860349,36.1143930817557,36.2182358509203,
36.3220474724968,36.4258626813831,36.529781085897,36.6337581406858,36.7379046401052,
36.7834458130743),.UNSPECIFIED.);
#2471=B_SPLINE_CURVE_WITH_KNOTS('',3,(#76180,#76181,#76182,#76183,#76184,
#76185,#76186,#76187,#76188,#76189,#76190,#76191,#76192,#76193,#76194,#76195,
#76196,#76197,#76198,#76199,#76200,#76201,#76202,#76203,#76204,#76205,#76206,
#76207,#76208,#76209,#76210,#76211,#76212,#76213,#76214,#76215,#76216,#76217,
#76218,#76219,#76220,#76221,#76222,#76223,#76224,#76225,#76226,#76227,#76228,
#76229,#76230,#76231,#76232,#76233,#76234,#76235,#76236,#76237,#76238,#76239,
#76240,#76241,#76242,#76243,#76244,#76245,#76246,#76247,#76248,#76249),
 .UNSPECIFIED.,.F.,.F.,(4,3,3,3,3,3,3,3,3,3,3,3,3,3,3,3,3,3,3,3,3,3,3,4),
(34.5575191897576,34.6600276231165,34.7624524447688,34.8648302599786,34.9671976054302,
35.0696598596281,35.1721712597493,35.2748625288798,35.3462402359454,35.4504266552236,
35.554457841936,35.6583670001104,35.7622107031371,35.8660237296966,35.9698408150375,
36.0737665685608,36.1777511656642,36.2819176875504,36.343768770382,36.4479637300599,
36.5519784470317,36.6558896321107,36.7597264522864,36.783721561275),
 .UNSPECIFIED.);
#2472=B_SPLINE_CURVE_WITH_KNOTS('',3,(#76250,#76251,#76252,#76253,#76254,
#76255,#76256,#76257,#76258,#76259,#76260,#76261,#76262,#76263,#76264,#76265,
#76266,#76267,#76268,#76269,#76270,#76271,#76272,#76273,#76274,#76275,#76276,
#76277,#76278,#76279,#76280,#76281,#76282,#76283,#76284,#76285,#76286,#76287,
#76288,#76289,#76290,#76291,#76292,#76293,#76294,#76295,#76296,#76297,#76298,
#76299,#76300,#76301,#76302,#76303,#76304,#76305,#76306,#76307,#76308,#76309,
#76310,#76311,#76312,#76313,#76314,#76315,#76316,#76317,#76318,#76319,#76320,
#76321,#76322,#76323,#76324,#76325,#76326,#76327,#76328,#76329,#76330,#76331,
#76332,#76333,#76334,#76335,#76336,#76337,#76338,#76339,#76340,#76341,#76342,
#76343,#76344,#76345,#76346,#76347,#76348,#76349,#76350,#76351,#76352,#76353,
#76354,#76355,#76356,#76357,#76358,#76359,#76360,#76361,#76362,#76363,#76364,
#76365,#76366,#76367,#76368,#76369,#76370,#76371,#76372,#76373),
 .UNSPECIFIED.,.F.,.F.,(4,3,3,3,3,3,3,3,3,3,3,3,3,3,3,3,3,3,3,3,3,3,3,3,
3,3,3,3,3,3,3,3,3,3,3,3,3,3,3,3,3,4),(30.5008964787964,30.6078001812217,
30.7116793516984,30.8155067886831,30.9193172495801,31.0285194617349,31.1324675695164,
31.2364884422478,31.3406776908237,31.356126098199,31.4603125242633,31.5643437178387,
31.6682528829569,31.7720965929731,31.8759096265576,31.9797267189483,32.0836524795105,
32.1876370836574,32.2918036125174,32.3536546326356,32.4578410526534,32.5618722401369,
32.6657813991261,32.7696251029939,32.8734381304197,32.9772552166507,33.0811809710951,
33.1851655691382,33.2893320919839,33.3511831670722,33.4553695843185,33.5594007689589,
33.6633099250119,33.7671536258876,33.8709666502698,33.9747837334102,34.0787094847129,
34.1826940795811,34.2868605992328,34.3487117015088,34.494592753444,34.5575191894877),
 .UNSPECIFIED.);
#2473=B_SPLINE_CURVE_WITH_KNOTS('',3,(#76379,#76380,#76381,#76382,#76383,
#76384,#76385,#76386,#76387,#76388,#76389,#76390,#76391,#76392,#76393,#76394,
#76395,#76396,#76397,#76398,#76399,#76400,#76401,#76402,#76403,#76404,#76405,
#76406,#76407,#76408,#76409,#76410,#76411,#76412,#76413,#76414,#76415,#76416,
#76417,#76418,#76419,#76420,#76421,#76422,#76423,#76424,#76425,#76426,#76427,
#76428,#76429,#76430,#76431,#76432,#76433,#76434,#76435,#76436,#76437,#76438,
#76439,#76440,#76441,#76442,#76443,#76444,#76445,#76446,#76447,#76448,#76449,
#76450,#76451,#76452,#76453,#76454,#76455,#76456,#76457,#76458,#76459,#76460,
#76461,#76462,#76463,#76464,#76465,#76466,#76467,#76468,#76469,#76470,#76471,
#76472,#76473,#76474,#76475,#76476,#76477,#76478,#76479,#76480,#76481,#76482,
#76483,#76484,#76485,#76486,#76487,#76488,#76489,#76490,#76491,#76492,#76493,
#76494,#76495,#76496,#76497,#76498,#76499),.UNSPECIFIED.,.F.,.F.,(4,3,3,
3,3,3,3,3,3,3,3,3,3,3,3,3,3,3,3,3,3,3,3,3,3,3,3,3,3,3,3,3,3,3,3,3,3,3,3,
3,4),(24.2175036368067,24.3213222069362,24.425134674074,24.5290492836921,
24.6330136088311,24.7371695294641,24.8294509519324,24.9336372113995,25.0376682356061,
25.1415772280614,25.2454207634752,25.3492336207785,25.4530505354683,25.556976117383,
25.6609605420786,25.7651268921614,25.826979486369,25.9311659551075,26.0351971917786,
26.1391064004061,26.2429501541627,26.346763231653,26.4505803680486,26.554506172462,
26.6584908204392,26.7626573926187,26.8245080208056,26.9286944520373,27.0327256510777,
27.1366348220792,27.2404785382343,27.3442915782043,27.448108677219,27.5520344447255,
27.6560190560083,27.7601855922317,27.8220365552422,27.9351108868929,28.0468017146056,
28.1605677982253,28.274333881845),.UNSPECIFIED.);
#2474=B_SPLINE_CURVE_WITH_KNOTS('',3,(#76500,#76501,#76502,#76503,#76504,
#76505,#76506,#76507,#76508,#76509,#76510,#76511,#76512,#76513,#76514,#76515,
#76516,#76517,#76518,#76519,#76520,#76521,#76522,#76523,#76524,#76525,#76526,
#76527,#76528,#76529,#76530,#76531,#76532,#76533,#76534,#76535,#76536,#76537,
#76538,#76539,#76540,#76541,#76542,#76543,#76544,#76545,#76546,#76547,#76548,
#76549,#76550,#76551,#76552,#76553,#76554,#76555,#76556,#76557,#76558,#76559,
#76560,#76561,#76562,#76563,#76564,#76565,#76566),.UNSPECIFIED.,.F.,.F.,
(4,3,3,3,3,3,3,3,3,3,3,3,3,3,3,3,3,3,3,3,3,3,4),(28.2743338823081,28.3811973775882,
28.4907893056108,28.5979678653913,28.7087664775351,28.8195650896788,28.9237515157247,
29.0277827092813,29.1316918743805,29.2355355843776,29.3393486179428,29.4431657103141,
29.5470914708569,29.6510760749844,29.7552426038252,29.8170936241154,29.9212582775505,
30.0252784744292,30.1291892265981,30.2330365854196,30.3368456659329,30.4406864383677,
30.4998648068842),.UNSPECIFIED.);
#2475=B_SPLINE_CURVE_WITH_KNOTS('',3,(#76568,#76569,#76570,#76571,#76572,
#76573,#76574,#76575,#76576,#76577,#76578,#76579,#76580,#76581,#76582,#76583,
#76584,#76585,#76586,#76587,#76588,#76589,#76590,#76591,#76592,#76593,#76594,
#76595,#76596,#76597,#76598,#76599,#76600,#76601,#76602,#76603,#76604,#76605,
#76606,#76607,#76608,#76609,#76610,#76611,#76612,#76613,#76614,#76615,#76616,
#76617,#76618,#76619,#76620,#76621,#76622,#76623,#76624,#76625,#76626,#76627,
#76628,#76629,#76630,#76631,#76632,#76633,#76634,#76635,#76636,#76637),
 .UNSPECIFIED.,.F.,.F.,(4,3,3,3,3,3,3,3,3,3,3,3,3,3,3,3,3,3,3,3,3,3,3,4),
(28.2743338823081,28.3635404948892,28.4677269637498,28.5717582005445,28.6756674092971,
28.7795111631798,28.8833242407966,28.9871413773194,29.0910671818599,29.1950518299642,
29.2992184022696,29.3610690293258,29.4652554605675,29.5692866596186,29.6731958306314,
29.7770395467982,29.8808525867803,29.9846696858073,30.0885954533271,30.1925800646233,
30.2967466008608,30.3585975637624,30.4627747459715,30.5008964787964),
 .UNSPECIFIED.);
#2476=B_SPLINE_CURVE_WITH_KNOTS('',3,(#76638,#76639,#76640,#76641,#76642,
#76643,#76644,#76645,#76646,#76647,#76648,#76649,#76650,#76651,#76652,#76653,
#76654,#76655,#76656,#76657,#76658,#76659,#76660,#76661,#76662,#76663,#76664,
#76665,#76666,#76667,#76668,#76669,#76670,#76671,#76672,#76673,#76674,#76675,
#76676,#76677,#76678,#76679,#76680,#76681,#76682,#76683,#76684,#76685,#76686,
#76687,#76688,#76689,#76690,#76691,#76692,#76693,#76694,#76695,#76696,#76697,
#76698,#76699,#76700,#76701,#76702,#76703,#76704,#76705,#76706,#76707,#76708,
#76709,#76710,#76711,#76712,#76713,#76714,#76715,#76716,#76717,#76718,#76719,
#76720,#76721,#76722,#76723,#76724,#76725,#76726,#76727,#76728,#76729,#76730,
#76731,#76732,#76733,#76734,#76735,#76736,#76737,#76738,#76739,#76740,#76741,
#76742,#76743,#76744,#76745,#76746,#76747,#76748,#76749,#76750,#76751,#76752,
#76753,#76754,#76755,#76756,#76757,#76758,#76759,#76760,#76761),
 .UNSPECIFIED.,.F.,.F.,(4,3,3,3,3,3,3,3,3,3,3,3,3,3,3,3,3,3,3,3,3,3,3,3,
3,3,3,3,3,3,3,3,3,3,3,3,3,3,3,3,3,4),(24.2166108235789,24.3207830822233,
24.3734263571428,24.4776114003836,24.5816411889067,24.6855489227878,24.7893911861822,
24.8932027599223,24.9970183813936,25.1009426642427,25.2049257846131,25.3090908361986,
25.3709548915794,25.4751416526421,25.5791731838078,25.683082688693,25.7869267396297,
25.890740114772,25.9945575488429,26.0984836488904,26.2024685917955,26.3066354545608,
26.368483426016,26.4726699930161,26.5767013313274,26.6806106461392,26.7844545088309,
26.8882676978477,26.9920849482059,27.0960108695371,27.1999956362766,27.3041623288664,
27.3660119604526,27.4689825721463,27.571778027722,27.6744756343169,27.7771117863559,
27.8797227939149,27.982409657317,28.0851324763853,28.1880251693553,28.2743338818544),
 .UNSPECIFIED.);
#2477=B_SPLINE_CURVE_WITH_KNOTS('',3,(#76767,#76768,#76769,#76770,#76771,
#76772,#76773,#76774,#76775,#76776,#76777,#76778,#76779,#76780,#76781,#76782,
#76783,#76784,#76785,#76786,#76787,#76788,#76789,#76790,#76791,#76792,#76793,
#76794,#76795,#76796,#76797,#76798,#76799,#76800,#76801,#76802,#76803,#76804,
#76805,#76806,#76807,#76808,#76809,#76810,#76811,#76812,#76813,#76814,#76815,
#76816,#76817,#76818,#76819,#76820,#76821,#76822,#76823,#76824,#76825,#76826,
#76827,#76828,#76829,#76830,#76831,#76832,#76833,#76834,#76835,#76836),
 .UNSPECIFIED.,.F.,.F.,(4,3,3,3,3,3,3,3,3,3,3,3,3,3,3,3,3,3,3,3,3,3,3,4),
(15.7079632679489,15.8108073354867,15.9136172573649,16.0164289991591,16.1193514864967,
16.2223328513092,16.3255044670683,16.39319808165,16.4974235198284,16.6014922383089,
16.7054365135598,16.8093138195759,16.9131588800528,17.0170063736613,17.1209598212046,
17.2249706213236,17.3291606840235,17.3907266160866,17.4950704275919,17.5992688650338,
17.7033463786647,17.8073550699353,17.9113373205562,17.9338028153519),
 .UNSPECIFIED.);
#2478=B_SPLINE_CURVE_WITH_KNOTS('',3,(#76838,#76839,#76840,#76841,#76842),
 .UNSPECIFIED.,.F.,.F.,(4,1,4),(14.3981410127768,15.3956695472134,15.7079548702164),
 .UNSPECIFIED.);
#2479=B_SPLINE_CURVE_WITH_KNOTS('',3,(#76846,#76847,#76848,#76849,#76850,
#76851,#76852,#76853,#76854,#76855,#76856,#76857,#76858,#76859,#76860,#76861,
#76862,#76863,#76864,#76865,#76866,#76867,#76868,#76869,#76870,#76871,#76872,
#76873,#76874,#76875,#76876,#76877,#76878,#76879,#76880,#76881,#76882,#76883,
#76884,#76885,#76886,#76887,#76888,#76889,#76890,#76891,#76892,#76893,#76894,
#76895,#76896,#76897,#76898,#76899,#76900,#76901,#76902,#76903),
 .UNSPECIFIED.,.F.,.F.,(4,3,3,3,3,3,3,3,3,3,3,3,3,3,3,3,3,3,3,4),(13.876192946452,
13.9800533582401,14.0837577779462,14.1873396637409,14.2908563334949,14.3943430362838,
14.4978349779569,14.6014337917251,14.7050934743387,14.808926820442,14.8541656075664,
14.9608903150641,15.0635179865448,15.1660515661335,15.2685276102982,15.3709825929619,
15.4735044996228,15.5760669133534,15.6787651048717,15.7079632675479),
 .UNSPECIFIED.);
#2480=B_SPLINE_CURVE_WITH_KNOTS('',3,(#76904,#76905,#76906,#76907,#76908,
#76909,#76910,#76911,#76912,#76913,#76914,#76915,#76916,#76917,#76918,#76919,
#76920,#76921,#76922,#76923,#76924,#76925,#76926,#76927,#76928,#76929,#76930,
#76931,#76932,#76933,#76934,#76935,#76936,#76937,#76938,#76939,#76940,#76941,
#76942,#76943,#76944,#76945,#76946,#76947,#76948,#76949,#76950,#76951,#76952,
#76953,#76954,#76955,#76956,#76957,#76958,#76959,#76960,#76961,#76962,#76963,
#76964,#76965,#76966,#76967,#76968,#76969,#76970),.UNSPECIFIED.,.F.,.F.,
(4,3,3,3,3,3,3,3,3,3,3,3,3,3,3,3,3,3,3,3,3,3,4),(15.7079632679489,15.851694142003,
15.9557857876061,16.0597208362763,16.1635322938407,16.2672773831501,16.3709910283821,
16.474708109403,16.5785335927115,16.6824176162874,16.7864841764974,16.8492226764396,
16.9534205085217,17.0574630546861,17.1613834350916,17.2652382690518,17.3690623180458,
17.4728903000167,17.5768266804211,17.6808217681209,17.7849984488684,17.8467512108762,
17.9343860550099),.UNSPECIFIED.);
#2481=B_SPLINE_CURVE_WITH_KNOTS('',3,(#76976,#76977,#76978,#76979,#76980,
#76981,#76982,#76983,#76984,#76985,#76986,#76987,#76988,#76989,#76990,#76991,
#76992,#76993,#76994,#76995,#76996,#76997,#76998,#76999,#77000,#77001,#77002,
#77003,#77004,#77005,#77006,#77007,#77008,#77009,#77010,#77011,#77012,#77013,
#77014,#77015,#77016,#77017,#77018,#77019,#77020,#77021,#77022,#77023,#77024,
#77025,#77026,#77027,#77028,#77029,#77030,#77031,#77032,#77033,#77034,#77035,
#77036,#77037,#77038,#77039,#77040,#77041,#77042,#77043,#77044,#77045,#77046,
#77047,#77048,#77049,#77050,#77051,#77052,#77053,#77054,#77055,#77056,#77057,
#77058,#77059,#77060,#77061,#77062,#77063,#77064,#77065,#77066,#77067,#77068,
#77069,#77070,#77071,#77072,#77073,#77074,#77075,#77076,#77077,#77078,#77079,
#77080,#77081,#77082,#77083,#77084,#77085,#77086,#77087,#77088,#77089,#77090,
#77091,#77092,#77093,#77094,#77095,#77096,#77097,#77098,#77099,#77100,#77101,
#77102,#77103,#77104,#77105,#77106,#77107,#77108,#77109,#77110,#77111,#77112,
#77113,#77114,#77115,#77116,#77117,#77118,#77119,#77120,#77121,#77122,#77123,
#77124,#77125,#77126,#77127,#77128,#77129,#77130,#77131,#77132,#77133,#77134,
#77135),.UNSPECIFIED.,.F.,.F.,(4,2,2,2,2,2,2,2,2,2,2,2,2,2,2,2,2,2,2,2,
2,2,2,2,2,2,2,2,2,2,2,2,2,2,2,2,2,2,2,2,2,2,2,2,2,2,2,2,2,2,2,2,2,2,2,2,
2,2,2,2,2,2,2,2,2,2,2,2,2,2,2,2,2,2,2,2,2,2,2,4),(-0.808582078280263,-0.80375073768972,
-0.763920677015728,-0.755667383612783,-0.751902546185843,-0.748972705871124,
-0.745765490437097,-0.740511666997364,-0.719054979581247,-0.698469123996048,
-0.691966489838367,-0.67237433173504,-0.668941290065012,-0.667023804346531,
-0.665537202421465,-0.663440042769142,-0.659063952645029,-0.64112942335304,
-0.609237968511569,-0.591965807738614,-0.586791483937901,-0.583578373841748,
-0.580606300588323,-0.576666400900211,-0.567786316437348,-0.555350092855608,
-0.532818709676239,-0.507841569834796,-0.503028355554244,-0.50086668124496,
-0.499194036422899,-0.497221122700889,-0.493559006971449,-0.488855239208183,
-0.477797482513651,-0.456889868740997,-0.42796259767417,-0.422295691517184,
-0.418968054825641,-0.416007159183182,-0.412245096918113,-0.404420574707277,
-0.393962693740305,-0.367392504352035,-0.342227416889973,-0.337519843331241,
-0.335359327113237,-0.333720281885442,-0.331917834124533,-0.328671895219693,
-0.310469648551046,-0.274329221166817,-0.257188758276896,-0.252160820829705,
-0.24907621421,-0.246251410997066,-0.242552690871855,-0.234441434443417,
-0.215777455632103,-0.187749031893301,-0.171748096241792,-0.168479233864655,
-0.166625078437752,-0.164969301318631,-0.163326004565586,-0.159703725776366,
-0.154866878239808,-0.143406084942028,-0.108936770040443,-0.0861876884502441,
-0.0802883743038012,-0.0767059478252727,-0.0734364140006466,-0.069152157193184,
-0.0595717908539198,-0.0329949830249145,-0.00749777013076311,-0.00328705758577433,
-0.00149796591859924,-5.90712218287499E-5),.UNSPECIFIED.);
#2482=B_SPLINE_CURVE_WITH_KNOTS('',3,(#77139,#77140,#77141,#77142,#77143,
#77144,#77145,#77146,#77147,#77148,#77149,#77150),.UNSPECIFIED.,.F.,.F.,
(4,2,2,2,2,4),(-1.15749903584995,-1.15636148542137,-1.15405073254735,-1.14499624866471,
-1.11159362809321,-1.10921304536313),.UNSPECIFIED.);
#2483=B_SPLINE_CURVE_WITH_KNOTS('',3,(#77154,#77155,#77156,#77157,#77158,
#77159,#77160,#77161,#77162,#77163,#77164,#77165,#77166,#77167,#77168,#77169,
#77170,#77171,#77172,#77173,#77174,#77175,#77176,#77177,#77178,#77179,#77180,
#77181,#77182,#77183,#77184,#77185,#77186,#77187,#77188,#77189,#77190,#77191,
#77192,#77193,#77194,#77195,#77196,#77197,#77198,#77199,#77200,#77201,#77202,
#77203,#77204,#77205,#77206,#77207,#77208,#77209,#77210,#77211,#77212,#77213,
#77214,#77215,#77216,#77217,#77218,#77219,#77220,#77221,#77222,#77223,#77224,
#77225,#77226,#77227,#77228,#77229,#77230,#77231,#77232,#77233,#77234,#77235,
#77236,#77237,#77238,#77239,#77240,#77241,#77242,#77243,#77244,#77245,#77246,
#77247,#77248,#77249,#77250,#77251,#77252,#77253,#77254,#77255,#77256,#77257,
#77258,#77259,#77260,#77261,#77262,#77263,#77264,#77265,#77266,#77267,#77268,
#77269,#77270,#77271,#77272,#77273,#77274,#77275,#77276,#77277,#77278,#77279,
#77280,#77281,#77282,#77283,#77284,#77285,#77286,#77287,#77288,#77289,#77290,
#77291,#77292,#77293,#77294,#77295,#77296,#77297,#77298,#77299,#77300,#77301,
#77302,#77303,#77304,#77305,#77306,#77307,#77308,#77309,#77310,#77311,#77312,
#77313,#77314,#77315,#77316,#77317,#77318,#77319,#77320,#77321,#77322,#77323,
#77324,#77325,#77326,#77327,#77328,#77329,#77330,#77331,#77332,#77333,#77334,
#77335,#77336,#77337,#77338,#77339,#77340,#77341,#77342,#77343,#77344,#77345,
#77346,#77347,#77348,#77349,#77350,#77351,#77352,#77353,#77354,#77355,#77356,
#77357,#77358,#77359,#77360,#77361,#77362,#77363,#77364,#77365,#77366,#77367,
#77368,#77369,#77370,#77371,#77372,#77373,#77374,#77375,#77376,#77377,#77378,
#77379,#77380,#77381,#77382,#77383,#77384,#77385,#77386,#77387,#77388,#77389,
#77390,#77391,#77392,#77393,#77394,#77395,#77396,#77397,#77398,#77399,#77400,
#77401,#77402,#77403,#77404,#77405,#77406,#77407,#77408,#77409,#77410,#77411,
#77412,#77413,#77414,#77415,#77416,#77417,#77418,#77419,#77420,#77421,#77422,
#77423,#77424,#77425,#77426,#77427,#77428,#77429,#77430,#77431,#77432,#77433,
#77434,#77435,#77436,#77437,#77438,#77439,#77440,#77441,#77442,#77443,#77444,
#77445),.UNSPECIFIED.,.F.,.F.,(4,2,2,2,2,2,2,2,2,2,2,2,2,2,2,2,2,2,2,2,
2,2,2,2,2,2,2,2,2,2,2,2,2,2,2,2,2,2,2,2,2,2,2,2,2,2,2,2,2,2,2,2,2,2,2,2,
2,2,2,2,2,2,2,2,2,2,2,2,2,2,2,2,2,2,2,2,2,2,2,2,2,2,2,2,2,2,2,2,2,2,2,2,
2,2,2,2,2,2,2,2,2,2,2,2,2,2,2,2,2,2,2,2,2,2,2,2,2,2,2,2,2,2,2,2,2,2,2,2,
2,2,2,2,2,2,2,2,2,2,2,2,2,2,2,2,2,4),(-1.10921304536313,-1.08577119322405,
-1.08023789382835,-1.07693925638659,-1.07397418658779,-1.07016513228311,
-1.06395257927994,-1.02008265239652,-1.00173885418572,-0.997298899019347,
-0.995588566735163,-0.995518644712131,-0.995448796458939,-0.995377673235652,
-0.995303608163833,-0.995224348210243,-0.995136529222863,-0.995034488957759,
-0.994906967059261,-0.994779717941947,-0.993170997624818,-0.991039059035374,
-0.986280553047312,-0.96227438564749,-0.941787766874852,-0.927527236686034,
-0.917726530430184,-0.913636099260019,-0.910640938109294,-0.907486036037498,
-0.902582190720856,-0.887581496086737,-0.851324751753463,-0.834868822453056,
-0.830557604876965,-0.828473231876027,-0.82698835841122,-0.825062426160662,
-0.821590084065918,-0.800290720371377,-0.795867224537264,-0.775684410828935,
-0.753556406652984,-0.748263067150557,-0.745047955270015,-0.742121360064723,
-0.738375163877525,-0.732140151813139,-0.694444213623796,-0.666722858872337,
-0.663180423026752,-0.661263327820058,-0.659617512803783,-0.6574789506901,
-0.652903880244482,-0.623419046990851,-0.599108331163135,-0.589793535635475,
-0.582645542039741,-0.579032101247776,-0.576107409243365,-0.572733150550537,
-0.566760214001137,-0.534475438739381,-0.501610642558943,-0.497186242311823,
-0.495081501618787,-0.49343462931103,-0.491444869845802,-0.487594369368031,
-0.482557469483099,-0.470221161640095,-0.433104684538486,-0.419066668075373,
-0.414282975853528,-0.411164265394002,-0.408174001606482,-0.404043224012585,
-0.393904338163363,-0.378936396887228,-0.359032533171688,-0.356815362649411,
-0.333515590386699,-0.330024186704325,-0.328089209449799,-0.326440947869545,
-0.324273025928824,-0.319485762091414,-0.297570820176915,-0.2567206097833,
-0.249607788516314,-0.245959424378439,-0.243038154814013,-0.239702603673773,
-0.233891197218771,-0.198245857868445,-0.168549564860159,-0.163927082024161,
-0.16181214618442,-0.160223079670209,-0.160199713943012,-0.160162681572964,
-0.160127591614206,-0.160094253908694,-0.16006250290469,-0.160032193600147,
-0.160003198416574,-0.159975404506412,-0.159948711611694,-0.159923030353875,
-0.159898280637115,-0.159874390473207,-0.159851294966483,-0.159828935373871,
-0.159807258363925,-0.159786215393173,-0.159765762141485,-0.159745858072496,
-0.159726465948691,-0.159707551462467,-0.159689083040975,-0.15967103147113,
-0.15965336966453,-0.159636072497843,-0.15961911659791,-0.159602480131411,
-0.159586142697773,-0.159570085204795,-0.159554289786106,-0.159538739575203,
-0.159523418664764,-0.159508312135062,-0.159493405771622,-0.159478686223586,
-0.15946414071833,-0.159449757148495,-0.15727084496776,-0.154692765577617,
-0.12620987529064,-0.0896910803513349,-0.0833849232407711,-0.0796082418622991,
-0.0766641226864439,-0.0734356955169596,-0.0681330712760033,-0.0594613373173496),
 .UNSPECIFIED.);
#2484=B_SPLINE_CURVE_WITH_KNOTS('',3,(#77450,#77451,#77452,#77453,#77454,
#77455,#77456,#77457,#77458,#77459,#77460,#77461,#77462,#77463,#77464,#77465,
#77466,#77467,#77468,#77469,#77470,#77471,#77472,#77473,#77474,#77475,#77476,
#77477,#77478,#77479,#77480,#77481,#77482,#77483,#77484,#77485,#77486,#77487,
#77488,#77489,#77490,#77491,#77492,#77493,#77494,#77495,#77496,#77497,#77498,
#77499,#77500,#77501,#77502,#77503,#77504,#77505,#77506,#77507,#77508,#77509,
#77510,#77511,#77512,#77513,#77514,#77515,#77516,#77517,#77518,#77519,#77520,
#77521,#77522,#77523,#77524,#77525,#77526,#77527,#77528,#77529,#77530,#77531,
#77532,#77533,#77534,#77535,#77536,#77537,#77538,#77539,#77540,#77541,#77542,
#77543,#77544,#77545,#77546,#77547,#77548,#77549,#77550,#77551,#77552,#77553,
#77554,#77555,#77556,#77557,#77558,#77559,#77560,#77561,#77562,#77563,#77564,
#77565,#77566,#77567,#77568,#77569,#77570,#77571,#77572,#77573,#77574,#77575,
#77576,#77577,#77578,#77579,#77580,#77581,#77582,#77583,#77584,#77585,#77586,
#77587,#77588,#77589,#77590,#77591,#77592,#77593,#77594,#77595,#77596,#77597,
#77598,#77599,#77600,#77601,#77602,#77603,#77604,#77605,#77606,#77607,#77608,
#77609,#77610,#77611,#77612,#77613,#77614,#77615,#77616,#77617,#77618,#77619,
#77620,#77621,#77622,#77623,#77624,#77625,#77626,#77627,#77628,#77629,#77630,
#77631,#77632,#77633,#77634,#77635,#77636,#77637,#77638,#77639,#77640,#77641,
#77642,#77643,#77644,#77645,#77646,#77647,#77648,#77649,#77650,#77651,#77652,
#77653,#77654,#77655,#77656,#77657),.UNSPECIFIED.,.F.,.F.,(4,2,2,2,2,2,
2,2,2,2,2,2,2,2,2,2,2,2,2,2,2,2,2,2,2,2,2,2,2,2,2,2,2,2,2,2,2,2,2,2,2,2,
2,2,2,2,2,2,2,2,2,2,2,2,2,2,2,2,2,2,2,2,2,2,2,2,2,2,2,2,2,2,2,2,2,2,2,2,
2,2,2,2,2,2,2,2,2,2,2,2,2,2,2,2,2,2,2,2,2,2,2,2,2,4),(-1.85845337396871,
-1.84131054128932,-1.83654050741002,-1.83437450613097,-1.83274032618178,
-1.8308085474797,-1.82733226476466,-1.80641330329208,-1.800721727262,-1.77859509583064,
-1.75897648724238,-1.75382760231245,-1.75107863399526,-1.74815434146029,
-1.74450217234471,-1.7373814774257,-1.70622943200099,-1.68262934433417,
-1.67521982763483,-1.67006229476785,-1.66782815892246,-1.66617172039623,
-1.66427600621078,-1.66096075542767,-1.64528537056015,-1.61447922017851,
-1.59259734538965,-1.58729948150606,-1.58407142410794,-1.58112602325968,
-1.57734545413148,-1.57102772809561,-1.53473165997819,-1.51479785309131,
-1.50804367998779,-1.50323002005008,-1.50105606062821,-1.49942077879233,
-1.49749331889511,-1.49403841837235,-1.47415479593914,-1.46751760455528,
-1.44626826366349,-1.42578977715592,-1.42058038169334,-1.41737090220697,
-1.41441928374303,-1.41059818004274,-1.40209463227193,-1.36272680903702,
-1.34128070722827,-1.33653756879021,-1.33437636584309,-1.33274297467705,
-1.3308091670142,-1.3273206300265,-1.30478747307554,-1.30170640644457,-1.28561597609658,
-1.25963304110213,-1.25413261511685,-1.25086235852088,-1.24792918292639,
-1.2441714462761,-1.23807125582121,-1.19226605905035,-1.17402877644563,
-1.16962605528447,-1.16752865379655,-1.16604280349328,-1.16412269273341,
-1.16070055814407,-1.14311916245153,-1.09804723870709,-1.08934485135883,
-1.08544688816033,-1.08249301169568,-1.07928693534511,-1.07409625673538,
-1.05598924312224,-1.02459983214061,-1.01174143731849,-1.006567743755,-1.00263637235194,
-1.00062975715949,-0.998983161499943,-0.996896536437269,-0.992569322989255,
-0.958661648316373,-0.926714267688992,-0.921025653446815,-0.917711004123216,
-0.915071655499159,-0.911511952038025,-0.904639602485034,-0.87976139783165,
-0.862527766013537,-0.839367510086651,-0.835876542736559,-0.83394148237466,
-0.832298907904304,-0.830144395165269,-0.825392215126631,-0.808582078280263),
 .UNSPECIFIED.);
#2485=B_SPLINE_CURVE_WITH_KNOTS('',3,(#77659,#77660,#77661,#77662,#77663,
#77664,#77665,#77666,#77667,#77668),.UNSPECIFIED.,.F.,.F.,(4,2,2,2,4),(-0.0594613373173496,
-0.0461429177535532,-0.0258669114392458,-0.00683129514723689,-0.000519912267460154),
 .UNSPECIFIED.);
#2486=B_SPLINE_CURVE_WITH_KNOTS('',3,(#77669,#77670,#77671,#77672,#77673,
#77674,#77675,#77676,#77677,#77678,#77679),.UNSPECIFIED.,.F.,.F.,(4,2,1,
1,1,1,1,4),(-91.8109775642065,-91.7726251681672,-90.7750966337306,-89.777568099294,
-88.7800395648574,-87.7825110304208,-86.7849824959842,-85.8810481731868),
 .UNSPECIFIED.);
#2487=B_SPLINE_CURVE_WITH_KNOTS('',3,(#77685,#77686,#77687,#77688,#77689,
#77690,#77691,#77692,#77693,#77694,#77695,#77696,#77697,#77698,#77699,#77700,
#77701,#77702,#77703,#77704,#77705,#77706,#77707,#77708,#77709,#77710,#77711,
#77712,#77713,#77714,#77715,#77716,#77717,#77718,#77719,#77720,#77721,#77722,
#77723,#77724,#77725,#77726,#77727,#77728,#77729,#77730,#77731,#77732,#77733,
#77734,#77735,#77736,#77737,#77738,#77739,#77740,#77741,#77742,#77743,#77744,
#77745,#77746,#77747,#77748,#77749,#77750,#77751,#77752,#77753,#77754,#77755,
#77756,#77757,#77758,#77759,#77760,#77761,#77762,#77763,#77764,#77765,#77766,
#77767,#77768,#77769,#77770,#77771,#77772,#77773,#77774,#77775,#77776,#77777,
#77778,#77779,#77780,#77781,#77782,#77783,#77784,#77785,#77786,#77787,#77788,
#77789,#77790,#77791,#77792,#77793,#77794,#77795,#77796,#77797,#77798,#77799,
#77800,#77801,#77802,#77803,#77804,#77805,#77806,#77807,#77808,#77809,#77810,
#77811,#77812,#77813,#77814,#77815,#77816,#77817,#77818,#77819,#77820,#77821,
#77822,#77823,#77824,#77825,#77826,#77827,#77828,#77829,#77830,#77831,#77832,
#77833,#77834,#77835,#77836,#77837,#77838,#77839,#77840,#77841,#77842,#77843,
#77844,#77845,#77846,#77847,#77848,#77849,#77850,#77851,#77852,#77853,#77854,
#77855,#77856,#77857,#77858,#77859,#77860,#77861,#77862,#77863,#77864,#77865,
#77866,#77867,#77868,#77869,#77870,#77871,#77872),.UNSPECIFIED.,.F.,.F.,
(4,2,2,2,2,2,2,2,2,2,2,2,2,2,2,2,2,2,2,2,2,2,2,2,2,2,2,2,2,2,2,2,2,2,2,
2,2,2,2,2,2,2,2,2,2,2,2,2,2,2,2,2,2,2,2,2,2,2,2,2,2,2,2,2,2,2,2,2,2,2,2,
2,2,2,2,2,2,2,2,2,2,2,2,2,2,2,2,2,2,2,2,2,2,4),(-0.991334733589914,-0.990102265102668,
-0.964597591785105,-0.944430702475018,-0.922441130210619,-0.918953660764064,
-0.917019267435139,-0.915385370687477,-0.913222894564673,-0.908472467431247,
-0.88695149042055,-0.847366140145738,-0.839045619107897,-0.835256909385074,
-0.832310459919263,-0.82908661118544,-0.823808030704901,-0.802238109082765,
-0.781752229472162,-0.775474297656371,-0.755707750683598,-0.752256661904654,
-0.750330456779003,-0.748695459417471,-0.746521044894084,-0.741703984253366,
-0.734942453136958,-0.714971305485189,-0.678691251199009,-0.672370362892898,
-0.668589043069049,-0.665643697933355,-0.662416351976517,-0.657121145870946,
-0.635274293929251,-0.604531306456788,-0.588806529328377,-0.58548779833751,
-0.583591332459823,-0.581935073317462,-0.579702289154817,-0.574552854601264,
-0.567158177300022,-0.543651482000971,-0.512297228346512,-0.505205411759204,
-0.501559138690346,-0.498635250985148,-0.495291976109734,-0.489454413729528,
-0.455740342694028,-0.423984861309953,-0.419542819874911,-0.417407110622622,
-0.415760662980193,-0.413800941799578,-0.410092643436106,-0.381161874569464,
-0.345381283411759,-0.339035085119007,-0.335246690997869,-0.332300445847088,
-0.329076779607281,-0.323798404474412,-0.302227641210784,-0.281744814060202,
-0.275469268701799,-0.255702403588537,-0.252251495373005,-0.250325406847744,
-0.248690516096501,-0.246516257422108,-0.241699609367859,-0.234938715713343,
-0.21497000995162,-0.178708160723568,-0.172377387379905,-0.168593392444139,
-0.165647817545095,-0.1629120783284,-0.158110450006515,-0.142566963737101,
-0.116188035330296,-0.0911116313795588,-0.086383436873767,-0.0842153247984322,
-0.0825623561530884,-0.0806501880045891,-0.0771677145706554,-0.0547810151635225,
-0.0157430710729671,-0.00643938555809663,-0.00281936615891565,-0.000491738252050606),
 .UNSPECIFIED.);
#2488=B_SPLINE_CURVE_WITH_KNOTS('',3,(#77873,#77874,#77875,#77876,#77877,
#77878,#77879,#77880,#77881,#77882,#77883,#77884,#77885,#77886),
 .UNSPECIFIED.,.F.,.F.,(4,2,2,2,2,2,4),(-1.91741621048356,-1.91647148486793,
-1.91479231205858,-1.91153539840836,-1.90506053883497,-1.8630301192281,
-1.85845337396871),.UNSPECIFIED.);
#2489=B_SPLINE_CURVE_WITH_KNOTS('',3,(#77888,#77889,#77890,#77891,#77892),
 .UNSPECIFIED.,.F.,.F.,(4,1,4),(-85.8810481731868,-85.7874539615476,-85.5277944654987),
 .UNSPECIFIED.);
#2490=B_SPLINE_CURVE_WITH_KNOTS('',3,(#77893,#77894,#77895,#77896,#77897,
#77898,#77899,#77900,#77901,#77902,#77903,#77904,#77905,#77906,#77907,#77908,
#77909,#77910,#77911,#77912,#77913,#77914,#77915,#77916,#77917,#77918,#77919,
#77920,#77921,#77922,#77923,#77924,#77925,#77926,#77927,#77928,#77929,#77930,
#77931,#77932,#77933,#77934,#77935,#77936,#77937,#77938,#77939,#77940,#77941,
#77942,#77943,#77944,#77945,#77946,#77947,#77948,#77949,#77950,#77951,#77952,
#77953,#77954,#77955,#77956,#77957,#77958,#77959,#77960,#77961,#77962,#77963,
#77964,#77965,#77966,#77967,#77968,#77969,#77970,#77971,#77972,#77973,#77974,
#77975,#77976,#77977,#77978,#77979,#77980,#77981,#77982,#77983,#77984,#77985,
#77986,#77987,#77988,#77989,#77990,#77991,#77992,#77993,#77994,#77995,#77996,
#77997,#77998,#77999,#78000,#78001,#78002,#78003,#78004,#78005,#78006,#78007,
#78008,#78009,#78010,#78011,#78012,#78013,#78014,#78015,#78016,#78017,#78018,
#78019,#78020,#78021,#78022,#78023,#78024,#78025,#78026,#78027,#78028,#78029,
#78030,#78031,#78032,#78033,#78034,#78035,#78036,#78037,#78038,#78039,#78040,
#78041,#78042,#78043,#78044,#78045,#78046,#78047,#78048,#78049,#78050,#78051,
#78052,#78053,#78054,#78055,#78056,#78057,#78058,#78059,#78060,#78061,#78062,
#78063,#78064,#78065,#78066,#78067,#78068,#78069,#78070,#78071,#78072,#78073,
#78074,#78075,#78076,#78077,#78078,#78079,#78080,#78081,#78082,#78083,#78084,
#78085,#78086,#78087,#78088,#78089,#78090),.UNSPECIFIED.,.F.,.F.,(4,2,2,
2,2,2,2,2,2,2,2,2,2,2,2,2,2,2,2,2,2,2,2,2,2,2,2,2,2,2,2,2,2,2,2,2,2,2,2,
2,2,2,2,2,2,2,2,2,2,2,2,2,2,2,2,2,2,2,2,2,2,2,2,2,2,2,2,2,2,2,2,2,2,2,2,
2,2,2,2,2,2,2,2,2,2,2,2,2,2,2,2,2,2,2,2,2,2,2,4),(-2.10003485435709,-2.07850560390307,
-2.06873850594009,-2.06499512105155,-2.06212405960105,-2.05917970464634,
-2.05595308752978,-2.0506582991449,-2.03115413057728,-2.00232285686385,
-1.98394654317753,-1.97972213189053,-1.9776034371064,-1.97611556214451,
-1.97421137067608,-1.9708566830803,-1.9545420992892,-1.92445096184892,-1.90257565119817,
-1.89727962506651,-1.89405281362857,-1.89110865072312,-1.88732983556868,
-1.88101550585438,-1.84455493658851,-1.82474049876445,-1.81801017899794,
-1.81320971901879,-1.81103873882641,-1.80940457509716,-1.80747733747423,
-1.8040198242005,-1.7839732054177,-1.77747686119903,-1.75580139364505,-1.73570783528188,
-1.73052646350142,-1.72732419823762,-1.72437261414037,-1.72054225281815,
-1.71197739413161,-1.67268402166767,-1.65126173154683,-1.64652181929395,
-1.64436172820778,-1.64272858427348,-1.64079390156835,-1.63730318445725,
-1.6141414406195,-1.59690412174929,-1.5720310402902,-1.56516535075129,-1.56161078295364,
-1.55897608281634,-1.55566847969271,-1.54999567083819,-1.52030823166117,
-1.49905667838791,-1.48772979684491,-1.48073863687029,-1.47822619213792,
-1.47652360855114,-1.47474404827802,-1.47187015349627,-1.46259104948464,
-1.45418552540459,-1.42469859942303,-1.40264392524141,-1.39733718731262,
-1.39410802915073,-1.39116441707891,-1.38739003477805,-1.38109155753135,
-1.3444838638238,-1.32475599329554,-1.31804238698899,-1.31325084264328,
-1.31108143716655,-1.30943262390914,-1.30749800166354,-1.30400746472248,
-1.28087720299464,-1.26368381722062,-1.23874917991307,-1.23187568466448,
-1.22831959923908,-1.225684791166,-1.22237837499058,-1.21671095986433,-1.18591530836976,
-1.16106502622968,-1.1526483558149,-1.14698507190639,-1.14466756337246,
-1.14299980239345,-1.14114779056651,-1.13794310521154,-1.12491860040256,
-1.10913431935646),.UNSPECIFIED.);
#2491=B_SPLINE_CURVE_WITH_KNOTS('',3,(#78095,#78096,#78097,#78098,#78099,
#78100,#78101,#78102,#78103,#78104,#78105,#78106,#78107,#78108,#78109,#78110,
#78111,#78112,#78113,#78114,#78115,#78116,#78117,#78118,#78119,#78120,#78121,
#78122,#78123,#78124,#78125,#78126,#78127,#78128,#78129,#78130,#78131,#78132,
#78133,#78134,#78135,#78136,#78137,#78138,#78139,#78140,#78141,#78142,#78143,
#78144,#78145,#78146,#78147,#78148,#78149,#78150,#78151,#78152,#78153,#78154,
#78155,#78156,#78157,#78158,#78159,#78160,#78161,#78162,#78163,#78164,#78165,
#78166,#78167,#78168,#78169,#78170,#78171,#78172,#78173,#78174,#78175,#78176,
#78177,#78178,#78179,#78180,#78181,#78182,#78183,#78184,#78185,#78186,#78187,
#78188,#78189,#78190,#78191,#78192,#78193,#78194,#78195,#78196,#78197,#78198,
#78199,#78200,#78201,#78202,#78203,#78204,#78205,#78206,#78207,#78208,#78209,
#78210,#78211,#78212,#78213,#78214,#78215,#78216,#78217,#78218,#78219,#78220,
#78221,#78222,#78223,#78224,#78225,#78226,#78227,#78228,#78229,#78230,#78231,
#78232,#78233,#78234,#78235,#78236,#78237,#78238,#78239,#78240,#78241,#78242,
#78243,#78244,#78245,#78246,#78247,#78248,#78249,#78250,#78251,#78252,#78253,
#78254,#78255,#78256,#78257,#78258,#78259,#78260,#78261,#78262,#78263,#78264,
#78265,#78266,#78267,#78268,#78269,#78270,#78271,#78272,#78273,#78274,#78275,
#78276,#78277,#78278,#78279,#78280,#78281,#78282,#78283,#78284,#78285,#78286,
#78287,#78288,#78289,#78290,#78291,#78292,#78293,#78294,#78295,#78296,#78297,
#78298,#78299,#78300,#78301,#78302,#78303,#78304),.UNSPECIFIED.,.F.,.F.,
(4,2,2,2,2,2,2,2,2,2,2,2,2,2,2,2,2,2,2,2,2,2,2,2,2,2,2,2,2,2,2,2,2,2,2,
2,2,2,2,2,2,2,2,2,2,2,2,2,2,2,2,2,2,2,2,2,2,2,2,2,2,2,2,2,2,2,2,2,2,2,2,
2,2,2,2,2,2,2,2,2,2,2,2,2,2,2,2,2,2,2,2,2,2,2,2,2,2,2,2,2,2,2,2,2,4),(-2.041194238912,
-2.03308372227273,-2.01726389886191,-2.0100937942116,-2.00425724602399,
-2.00091395364408,-1.99798971438316,-1.99434256101024,-1.98724757679346,
-1.95633935560485,-1.93251464995055,-1.92506779672676,-1.91989088397756,
-1.9176532671926,-1.91599624905273,-1.91410220792294,-1.91079468905737,
-1.89530638199369,-1.86642842142523,-1.85060179359057,-1.84342975318844,
-1.83759200180659,-1.83424849980843,-1.83132435512702,-1.82767768415656,
-1.82058481152324,-1.78944983567494,-1.76579967476789,-1.75838164414872,
-1.75321960883726,-1.75098456727759,-1.74932790299428,-1.74743247440499,
-1.74411871213512,-1.72847022164124,-1.69766006537984,-1.67575727173645,
-1.67045817199177,-1.66722984744401,-1.66428451698462,-1.66050447606793,
-1.6541886432,-1.61784983238833,-1.58922739944954,-1.58565204897448,-1.58372004111667,
-1.58207005196638,-1.57993117280608,-1.57518446704707,-1.54959169305137,
-1.52725906575456,-1.51487375200263,-1.50602654743202,-1.5021047729433,
-1.4991485047876,-1.49595491192632,-1.49081825693143,-1.47376538737418,
-1.44182880612635,-1.42385444566274,-1.41948071598479,-1.41738826965094,
-1.41590272101662,-1.41397871877751,-1.41053796856741,-1.39118285066854,
-1.38414460233122,-1.36318504073295,-1.34930407770668,-1.33969492554978,
-1.33564720283574,-1.33267117065915,-1.32952571297752,-1.32461490616774,
-1.30940992439892,-1.27658245477355,-1.25739919109829,-1.25289103087495,
-1.25077314971435,-1.24928480724988,-1.24737851483225,-1.24401677610271,
-1.22756277939691,-1.19779757004878,-1.17575557117689,-1.17044806709,-1.16721785387563,
-1.16427288196664,-1.16049618293017,-1.15224468715182,-1.11260314132832,
-1.09106874607068,-1.08631678512989,-1.08415395671605,-1.08251992867439,
-1.08058557322332,-1.07709855607751,-1.05531719734113,-1.05044120166454,
-1.01169043941936,-1.00555651234072,-1.00178780850829,-0.998851799137522,
-0.995584210270059,-0.991334733589914),.UNSPECIFIED.);
#2492=B_SPLINE_CURVE_WITH_KNOTS('',3,(#78305,#78306,#78307,#78308,#78309,
#78310,#78311,#78312,#78313,#78314,#78315,#78316,#78317,#78318,#78319,#78320,
#78321,#78322,#78323,#78324,#78325,#78326,#78327,#78328,#78329,#78330,#78331,
#78332,#78333,#78334,#78335,#78336,#78337,#78338,#78339,#78340,#78341,#78342,
#78343,#78344,#78345,#78346,#78347,#78348,#78349,#78350,#78351,#78352,#78353,
#78354,#78355,#78356,#78357,#78358,#78359,#78360,#78361,#78362,#78363,#78364,
#78365,#78366,#78367,#78368,#78369,#78370,#78371,#78372,#78373,#78374,#78375,
#78376,#78377,#78378,#78379,#78380,#78381,#78382,#78383,#78384,#78385,#78386,
#78387,#78388,#78389,#78390,#78391,#78392,#78393,#78394,#78395,#78396,#78397,
#78398,#78399,#78400,#78401,#78402,#78403,#78404,#78405,#78406,#78407,#78408,
#78409,#78410,#78411,#78412,#78413,#78414,#78415,#78416,#78417,#78418,#78419,
#78420,#78421,#78422,#78423,#78424,#78425,#78426,#78427,#78428,#78429,#78430,
#78431,#78432,#78433,#78434,#78435,#78436,#78437,#78438,#78439,#78440,#78441,
#78442,#78443,#78444,#78445,#78446,#78447,#78448,#78449,#78450,#78451,#78452,
#78453,#78454,#78455,#78456,#78457,#78458,#78459,#78460,#78461,#78462,#78463,
#78464,#78465,#78466,#78467,#78468,#78469,#78470,#78471,#78472,#78473,#78474,
#78475,#78476,#78477,#78478,#78479,#78480,#78481,#78482,#78483,#78484,#78485,
#78486,#78487,#78488,#78489,#78490,#78491,#78492,#78493,#78494,#78495,#78496,
#78497,#78498,#78499,#78500,#78501,#78502,#78503,#78504,#78505,#78506),
 .UNSPECIFIED.,.F.,.F.,(4,2,2,2,2,2,2,2,2,2,2,2,2,2,2,2,2,2,2,2,2,2,2,2,
2,2,2,2,2,2,2,2,2,2,2,2,2,2,2,2,2,2,2,2,2,2,2,2,2,2,2,2,2,2,2,2,2,2,2,2,
2,2,2,2,2,2,2,2,2,2,2,2,2,2,2,2,2,2,2,2,2,2,2,2,2,2,2,2,2,2,2,2,2,2,2,2,
2,2,2,2,4),(-1.10913431935646,-1.09781930985798,-1.07223606504576,-1.0652806695971,
-1.06170837316959,-1.05907199732737,-1.05577710322132,-1.05016342020783,
-1.02080342513179,-0.991354948502371,-0.981637127978031,-0.97871663617906,
-0.976926855580005,-0.975230728648835,-0.972751365795229,-0.966002413402223,
-0.922194469142564,-0.902643457043816,-0.897346259745326,-0.894119361422423,
-0.891175523416381,-0.887333335837165,-0.878937036052964,-0.856163927241126,
-0.830059152552783,-0.815665810777979,-0.812377000601324,-0.81050684523887,
-0.80884495821503,-0.806565742205296,-0.801137086709259,-0.793192609444553,
-0.766123429011453,-0.736730094066658,-0.731120955789178,-0.727795905742393,
-0.725163804162955,-0.721634021674743,-0.7148905967575,-0.690956391977639,
-0.677288939969948,-0.651397443677576,-0.646651577444513,-0.64451356645842,
-0.642864459728906,-0.640933826329793,-0.63736187328623,-0.608745836965906,
-0.572377866117934,-0.56606447896315,-0.562286287478029,-0.559342625252688,
-0.556116376073141,-0.550821283475333,-0.528945304044135,-0.498156258215985,
-0.482514710219044,-0.479202839900898,-0.477308512033124,-0.475652873695394,
-0.473419314974251,-0.468261334213619,-0.460848950628351,-0.43722796370488,
-0.4060355796341,-0.398944610029881,-0.395299626919058,-0.392377212841247,
-0.389036119376414,-0.383203735717486,-0.376039733824192,-0.360236687326912,
-0.331382629821045,-0.315892063539941,-0.312587772879159,-0.31069516145134,
-0.309039144172838,-0.306802556979367,-0.30162686658604,-0.294180097575663,
-0.270350460839101,-0.239430976621142,-0.232337603292078,-0.228692128934005,
-0.225769681483076,-0.222428941716038,-0.216598207433253,-0.182099864476957,
-0.151225305399553,-0.146669298363086,-0.144543254571615,-0.142898273871101,
-0.140936052663352,-0.137463837855134,-0.132881079484305,-0.122199874554399,
-0.0934396652852915,-0.0699637714697171,-0.0644321743130892,-0.0611551620833314,
-0.0595329710308153),.UNSPECIFIED.);
#2493=B_SPLINE_CURVE_WITH_KNOTS('',3,(#78512,#78513,#78514,#78515,#78516,
#78517,#78518,#78519,#78520,#78521,#78522,#78523,#78524,#78525,#78526,#78527,
#78528,#78529,#78530,#78531,#78532,#78533,#78534,#78535,#78536,#78537,#78538,
#78539,#78540,#78541,#78542,#78543,#78544,#78545,#78546,#78547,#78548,#78549,
#78550,#78551,#78552,#78553,#78554,#78555,#78556,#78557,#78558,#78559,#78560,
#78561,#78562,#78563,#78564,#78565,#78566,#78567,#78568,#78569,#78570,#78571,
#78572,#78573,#78574,#78575,#78576,#78577,#78578,#78579,#78580,#78581,#78582,
#78583,#78584,#78585,#78586,#78587,#78588,#78589,#78590,#78591,#78592,#78593,
#78594,#78595,#78596,#78597,#78598,#78599,#78600,#78601,#78602,#78603,#78604,
#78605,#78606,#78607,#78608,#78609,#78610,#78611,#78612,#78613,#78614,#78615,
#78616,#78617,#78618,#78619,#78620,#78621,#78622,#78623,#78624,#78625,#78626,
#78627,#78628,#78629,#78630,#78631,#78632,#78633,#78634,#78635,#78636,#78637,
#78638,#78639,#78640,#78641,#78642,#78643,#78644,#78645,#78646,#78647,#78648,
#78649,#78650,#78651,#78652,#78653,#78654,#78655,#78656,#78657,#78658,#78659,
#78660,#78661,#78662,#78663,#78664,#78665,#78666,#78667,#78668,#78669,#78670,
#78671,#78672,#78673,#78674,#78675,#78676,#78677,#78678,#78679,#78680,#78681,
#78682,#78683,#78684,#78685,#78686,#78687,#78688,#78689,#78690,#78691,#78692,
#78693,#78694,#78695,#78696,#78697,#78698,#78699,#78700,#78701,#78702,#78703,
#78704,#78705,#78706,#78707,#78708,#78709,#78710,#78711,#78712,#78713,#78714,
#78715,#78716,#78717,#78718,#78719,#78720,#78721,#78722,#78723,#78724,#78725,
#78726,#78727,#78728,#78729,#78730,#78731,#78732,#78733,#78734,#78735,#78736,
#78737),.UNSPECIFIED.,.F.,.F.,(4,2,2,2,2,2,2,2,2,2,2,2,2,2,2,2,2,2,2,2,
2,2,2,2,2,2,2,2,2,2,2,2,2,2,2,2,2,2,2,2,2,2,2,2,2,2,2,2,2,2,2,2,2,2,2,2,
2,2,2,2,2,2,2,2,2,2,2,2,2,2,2,2,2,2,2,2,2,2,2,2,2,2,2,2,2,2,2,2,2,2,2,2,
2,2,2,2,2,2,2,2,2,2,2,2,2,2,2,2,2,2,2,2,4),(-0.991195152289668,-0.989058737366125,
-0.985746280099643,-0.983851442811526,-0.982195211269073,-0.979960595162866,
-0.974798999678037,-0.96738026490964,-0.943724650164412,-0.912576733438614,
-0.905484258671559,-0.901838256388501,-0.898914881511217,-0.895572514883543,
-0.889737387391909,-0.882569650841099,-0.866755916923555,-0.837910091686941,
-0.822426299183513,-0.819121626992332,-0.817228552572286,-0.815571930858969,
-0.813334201167262,-0.80815439357529,-0.800700288077559,-0.776829729324303,
-0.745962828097812,-0.738867877613459,-0.73522136907014,-0.732297959487918,
-0.728955956732874,-0.72312252745063,-0.715957457528714,-0.700152820751079,
-0.671304706731191,-0.655809500323241,-0.65250428919936,-0.650611094981761,
-0.648954504142384,-0.646716997950348,-0.641538483424944,-0.634086886242263,
-0.610231590499407,-0.579344866883861,-0.572250113360556,-0.568603649466183,
-0.565680248275633,-0.562338225324299,-0.55650468233309,-0.549339429892438,
-0.533534153341871,-0.50468628527434,-0.489191933969395,-0.485886768380858,
-0.48399358658996,-0.482336996814266,-0.480099478917327,-0.474920881242815,
-0.467469117620409,-0.443612766683756,-0.412727536516204,-0.405632782987422,
-0.401986323141544,-0.399062927157852,-0.395720912291749,-0.389887389030682,
-0.382722163892274,-0.366916964541923,-0.3380691363239,-0.322574754519552,
-0.319269592236183,-0.317376413316051,-0.31571982675763,-0.313482314150901,
-0.308303732737519,-0.300851995868541,-0.276995768039286,-0.246110492151411,
-0.239015752732565,-0.235369299849701,-0.232445909308944,-0.229103900513498,
-0.223270387449267,-0.216105174617946,-0.200300001214167,-0.171802768170646,
-0.156005560667715,-0.152674183893643,-0.150775086188452,-0.149175411933742,
-0.149155775872824,-0.14913626859957,-0.149116883729205,-0.14909761504051,
-0.149078456409151,-0.149059401867339,-0.149040445661379,-0.149021582134666,
-0.149002805768776,-0.148984111130622,-0.146867077204812,-0.144354657772053,
-0.139948468617413,-0.129882808126354,-0.0914865226515943,-0.0755862809040869,
-0.070603894380746,-0.0674439666543175,-0.0644760764373484,-0.0604733657444209,
-0.0511365831183054,-0.0377996321450267,-0.000492023790732501),
 .UNSPECIFIED.);
#2494=B_SPLINE_CURVE_WITH_KNOTS('',3,(#78738,#78739,#78740,#78741,#78742,
#78743,#78744,#78745,#78746,#78747,#78748,#78749,#78750,#78751,#78752,#78753,
#78754,#78755,#78756,#78757),.UNSPECIFIED.,.F.,.F.,(4,2,2,2,2,2,2,2,2,4),
(-2.10002542706347,-2.08879172315445,-2.08637671723263,-2.08465493193565,
-2.08311872769319,-2.08158046349029,-2.07945720600073,-2.07401815885657,
-2.05933454423903,-2.041194238912),.UNSPECIFIED.);
#2495=B_SPLINE_CURVE_WITH_KNOTS('',3,(#78759,#78760,#78761,#78762,#78763,
#78764,#78765,#78766,#78767,#78768,#78769,#78770),.UNSPECIFIED.,.F.,.F.,
(4,2,2,2,2,4),(-0.0595329710308153,-0.0582231334989721,-0.0544767912751946,
-0.0466099706509627,-0.0360357102531513,-0.000491966010066645),
 .UNSPECIFIED.);
#2496=B_SPLINE_CURVE_WITH_KNOTS('',3,(#78771,#78772,#78773,#78774,#78775,
#78776,#78777,#78778,#78779,#78780,#78781,#78782,#78783,#78784,#78785,#78786,
#78787,#78788,#78789,#78790,#78791,#78792,#78793,#78794,#78795,#78796,#78797,
#78798,#78799,#78800,#78801,#78802,#78803,#78804,#78805,#78806,#78807,#78808,
#78809,#78810,#78811,#78812,#78813,#78814,#78815,#78816,#78817,#78818,#78819,
#78820,#78821,#78822,#78823,#78824,#78825,#78826,#78827,#78828,#78829,#78830,
#78831,#78832,#78833,#78834,#78835,#78836,#78837,#78838,#78839,#78840,#78841,
#78842,#78843,#78844,#78845,#78846,#78847,#78848,#78849,#78850,#78851,#78852,
#78853,#78854,#78855,#78856,#78857,#78858,#78859,#78860,#78861,#78862,#78863,
#78864,#78865,#78866,#78867,#78868,#78869,#78870,#78871,#78872,#78873,#78874,
#78875,#78876,#78877,#78878,#78879,#78880,#78881,#78882,#78883,#78884,#78885,
#78886,#78887,#78888,#78889,#78890,#78891,#78892,#78893,#78894,#78895,#78896,
#78897,#78898,#78899,#78900,#78901,#78902,#78903,#78904,#78905,#78906,#78907,
#78908,#78909,#78910,#78911,#78912,#78913,#78914,#78915,#78916,#78917,#78918,
#78919,#78920,#78921,#78922,#78923,#78924,#78925,#78926,#78927,#78928,#78929,
#78930,#78931,#78932,#78933,#78934,#78935,#78936,#78937,#78938,#78939,#78940,
#78941,#78942,#78943,#78944,#78945,#78946,#78947,#78948,#78949,#78950,#78951,
#78952,#78953,#78954,#78955,#78956,#78957,#78958,#78959,#78960,#78961,#78962,
#78963,#78964),.UNSPECIFIED.,.F.,.F.,(4,2,2,2,2,2,2,2,2,2,2,2,2,2,2,2,2,
2,2,2,2,2,2,2,2,2,2,2,2,2,2,2,2,2,2,2,2,2,2,2,2,2,2,2,2,2,2,2,2,2,2,2,2,
2,2,2,2,2,2,2,2,2,2,2,2,2,2,2,2,2,2,2,2,2,2,2,2,2,2,2,2,2,2,2,2,2,2,2,2,
2,2,2,2,2,2,2,4),(-2.10005280646433,-2.0877597629007,-2.08172244365619,
-2.07944716492984,-2.07777813107226,-2.07610982925215,-2.07425779309637,
-2.07105426528615,-2.05805651907365,-2.03137046923152,-2.00296064397461,
-1.9973726251449,-1.99408272127116,-1.99115166457165,-1.98742370918956,
-1.97966090812949,-1.93946926949472,-1.91776072920575,-1.91299190557234,
-1.91082628185997,-1.90917746883294,-1.90723944714018,-1.90373489576291,
-1.8805961089851,-1.86335972444155,-1.83847241728195,-1.83160406865398,
-1.8280484729552,-1.82541315158058,-1.82210495156465,-1.81643158399557,
-1.78665917735656,-1.76520973906637,-1.75405354523577,-1.74933674551142,
-1.74567692997824,-1.74372740094089,-1.74208004726036,-1.73996659763525,
-1.73535943661535,-1.70481855439636,-1.67003000907514,-1.66417877955591,
-1.66083285404909,-1.65790967236107,-1.65426825849505,-1.64719873351372,
-1.61460605219853,-1.59204510201406,-1.58129313707818,-1.57837383047155,
-1.57658405077925,-1.57490704437578,-1.57283523745277,-1.56871597092744,
-1.53780912361497,-1.50329298016392,-1.49745907442349,-1.49411687664774,
-1.49119337212889,-1.48754686431964,-1.48045236331481,-1.44955142963723,
-1.42571825408513,-1.41827037195165,-1.41309317112305,-1.41085584282117,
-1.40919921841139,-1.40730588533527,-1.40400020950129,-1.38850510678613,
-1.35961754925217,-1.34379735703839,-1.33662761736679,-1.33079160236652,
-1.32744900296032,-1.32452561467342,-1.32087986496728,-1.31378881264165,
-1.28251743255758,-1.25896849631792,-1.2515675927052,-1.24641463182871,
-1.24418148289032,-1.24252541351683,-1.24062978354035,-1.237313842706,-1.22162138737103,
-1.19091029750774,-1.16895930632299,-1.16365816462727,-1.16042993391906,
-1.1574855704957,-1.15370801401654,-1.14739922726299,-1.11094501937456,
-1.10916707781729),.UNSPECIFIED.);
#2497=B_SPLINE_CURVE_WITH_KNOTS('',3,(#78969,#78970,#78971,#78972,#78973,
#78974,#78975,#78976,#78977,#78978,#78979,#78980,#78981,#78982,#78983,#78984,
#78985,#78986,#78987,#78988,#78989,#78990,#78991,#78992,#78993,#78994,#78995,
#78996,#78997,#78998,#78999,#79000,#79001,#79002,#79003,#79004,#79005,#79006,
#79007,#79008,#79009,#79010,#79011,#79012,#79013,#79014,#79015,#79016,#79017,
#79018,#79019,#79020,#79021,#79022,#79023,#79024,#79025,#79026,#79027,#79028,
#79029,#79030,#79031,#79032,#79033,#79034,#79035,#79036,#79037,#79038,#79039,
#79040,#79041,#79042,#79043,#79044,#79045,#79046,#79047,#79048,#79049,#79050,
#79051,#79052,#79053,#79054,#79055,#79056,#79057,#79058,#79059,#79060,#79061,
#79062,#79063,#79064,#79065,#79066,#79067,#79068,#79069,#79070,#79071,#79072,
#79073,#79074,#79075,#79076,#79077,#79078,#79079,#79080,#79081,#79082,#79083,
#79084,#79085,#79086,#79087,#79088,#79089,#79090,#79091,#79092,#79093,#79094,
#79095,#79096,#79097,#79098,#79099,#79100,#79101,#79102,#79103,#79104,#79105,
#79106,#79107,#79108,#79109,#79110,#79111,#79112,#79113,#79114,#79115,#79116,
#79117,#79118,#79119,#79120,#79121,#79122,#79123,#79124,#79125,#79126,#79127,
#79128,#79129,#79130,#79131,#79132,#79133,#79134,#79135,#79136,#79137,#79138,
#79139,#79140,#79141,#79142,#79143,#79144,#79145,#79146,#79147,#79148,#79149,
#79150,#79151,#79152,#79153,#79154,#79155,#79156,#79157,#79158,#79159,#79160,
#79161,#79162,#79163,#79164,#79165,#79166),.UNSPECIFIED.,.F.,.F.,(4,2,2,
2,2,2,2,2,2,2,2,2,2,2,2,2,2,2,2,2,2,2,2,2,2,2,2,2,2,2,2,2,2,2,2,2,2,2,2,
2,2,2,2,2,2,2,2,2,2,2,2,2,2,2,2,2,2,2,2,2,2,2,2,2,2,2,2,2,2,2,2,2,2,2,2,
2,2,2,2,2,2,2,2,2,2,2,2,2,2,2,2,2,2,2,2,2,2,2,4),(-2.04073105386379,-2.01788573118281,
-1.99770242346565,-1.98788298098068,-1.98503652231967,-1.98326279792523,
-1.98157601515141,-1.9790587938368,-1.97255913313296,-1.93157182655116,
-1.91665091197269,-1.90653703053737,-1.90241108072283,-1.89942256326465,
-1.89630413499345,-1.8915177851908,-1.87744267553201,-1.8436541590879,-1.82412698116097,
-1.81958263756561,-1.81745845374037,-1.81596981437242,-1.81406890364664,
-1.81072921267484,-1.79480388389642,-1.76422447883087,-1.74242735628701,
-1.73713586443389,-1.73390984754384,-1.73096511971517,-1.72718376780104,
-1.72086100746439,-1.68469636504952,-1.66468520152603,-1.65791711877805,
-1.65309646339385,-1.65092174930524,-1.64928707586521,-1.64736194306839,
-1.64391427796677,-1.62426068280426,-1.61781278124661,-1.59714270782084,
-1.57576531612937,-1.57049941015663,-1.5672788397993,-1.56433249769137,
-1.56053990144258,-1.55250394374847,-1.51275489361259,-1.49118950094329,
-1.48643536924891,-1.48427259321251,-1.48263905806711,-1.48070583220232,
-1.47722210549815,-1.45569353991343,-1.45150361788558,-1.43156538227889,
-1.41673251373306,-1.40666057071851,-1.40254095316983,-1.39955343442379,
-1.39643286013491,-1.39163675686681,-1.3774714617082,-1.34375869992897,
-1.32425849193193,-1.31971692326121,-1.31759319794413,-1.31610455649027,
-1.31420319198498,-1.31086172334449,-1.29489352658803,-1.26457729768814,
-1.24258245085058,-1.23727899537566,-1.23405031296662,-1.23110613549109,
-1.22732962308369,-1.22102433277704,-1.18454356864269,-1.15609611901115,
-1.15250353815158,-1.15056822791244,-1.1489192434793,-1.14678647543737,
-1.14207185555499,-1.11468329984751,-1.08900063900744,-1.07466417491557,
-1.06998879182356,-1.06689337709286,-1.06392439812577,-1.05974156304932,
-1.05002099290182,-1.03548507247329,-1.00469863726224,-0.991195152289668),
 .UNSPECIFIED.);
#2498=B_SPLINE_CURVE_WITH_KNOTS('',3,(#79167,#79168,#79169,#79170,#79171,
#79172,#79173,#79174,#79175,#79176,#79177,#79178,#79179,#79180,#79181,#79182,
#79183,#79184,#79185,#79186,#79187,#79188,#79189,#79190,#79191,#79192,#79193,
#79194,#79195,#79196,#79197,#79198,#79199,#79200,#79201,#79202,#79203,#79204,
#79205,#79206,#79207,#79208,#79209,#79210,#79211,#79212,#79213,#79214,#79215,
#79216,#79217,#79218,#79219,#79220,#79221,#79222,#79223,#79224,#79225,#79226,
#79227,#79228,#79229,#79230,#79231,#79232,#79233,#79234,#79235,#79236,#79237,
#79238,#79239,#79240,#79241,#79242,#79243,#79244,#79245,#79246,#79247,#79248,
#79249,#79250,#79251,#79252,#79253,#79254,#79255,#79256,#79257,#79258,#79259,
#79260,#79261,#79262,#79263,#79264,#79265,#79266,#79267,#79268,#79269,#79270,
#79271,#79272,#79273,#79274,#79275,#79276,#79277,#79278,#79279,#79280,#79281,
#79282,#79283,#79284,#79285,#79286,#79287,#79288,#79289,#79290,#79291,#79292,
#79293,#79294,#79295,#79296,#79297,#79298,#79299,#79300,#79301,#79302,#79303,
#79304,#79305,#79306,#79307,#79308,#79309,#79310,#79311,#79312,#79313,#79314,
#79315,#79316,#79317,#79318,#79319,#79320,#79321,#79322,#79323,#79324,#79325,
#79326,#79327,#79328,#79329,#79330,#79331,#79332,#79333,#79334,#79335,#79336,
#79337,#79338,#79339,#79340,#79341,#79342,#79343,#79344,#79345,#79346,#79347,
#79348,#79349,#79350,#79351,#79352,#79353,#79354,#79355,#79356,#79357,#79358,
#79359,#79360,#79361,#79362,#79363,#79364,#79365,#79366,#79367,#79368,#79369,
#79370,#79371,#79372,#79373,#79374,#79375,#79376,#79377,#79378,#79379,#79380,
#79381,#79382,#79383,#79384,#79385,#79386,#79387,#79388,#79389,#79390,#79391,
#79392),.UNSPECIFIED.,.F.,.F.,(4,2,2,2,2,2,2,2,2,2,2,2,2,2,2,2,2,2,2,2,
2,2,2,2,2,2,2,2,2,2,2,2,2,2,2,2,2,2,2,2,2,2,2,2,2,2,2,2,2,2,2,2,2,2,2,2,
2,2,2,2,2,2,2,2,2,2,2,2,2,2,2,2,2,2,2,2,2,2,2,2,2,2,2,2,2,2,2,2,2,2,2,2,
2,2,2,2,2,2,2,2,2,2,2,2,2,2,2,2,2,2,2,2,4),(-1.10916707781729,-1.09111005051036,
-1.08437531519816,-1.07957230929726,-1.0774006699881,-1.07576622240333,
-1.07383890522614,-1.07038182622291,-1.05037195859777,-1.00503548555728,
-0.99882937402838,-0.995081118323409,-0.99214089918231,-0.988898040559397,
-0.983527791216712,-0.960333984789916,-0.930255836988196,-0.91528849065879,
-0.912008612459382,-0.910121261011901,-0.908463533073702,-0.906216147456696,
-0.900978895097846,-0.893412754136719,-0.868849967399443,-0.838903260267914,
-0.831779106211155,-0.828126783088954,-0.825203175430626,-0.821865805284968,
-0.816053281751308,-0.808920952252066,-0.793227918181996,-0.763827919844489,
-0.748658963323564,-0.745369347094501,-0.743479788226645,-0.741822579646835,
-0.739579198092381,-0.734365530458577,-0.726845447361443,-0.702570185551568,
-0.672223437673162,-0.665119151694647,-0.661470915525603,-0.658547631114411,
-0.655207430293604,-0.649381571504329,-0.615617569649209,-0.583892867035995,
-0.579449934977405,-0.577337011823108,-0.575689965108573,-0.573740701726336,
-0.570081090091581,-0.542248640752413,-0.505148187639104,-0.498879320270475,
-0.495113310376012,-0.492170806413761,-0.488937334145717,-0.483610574010584,
-0.461205328655347,-0.441388928167931,-0.436937911633644,-0.415658863703378,
-0.412178539154411,-0.410246206462,-0.40861280977731,-0.406449437731836,
-0.40169117591681,-0.380082259441481,-0.340217446042829,-0.33295252926446,
-0.329276223730558,-0.326544913199139,-0.323542361876597,-0.319336083541556,
-0.30868502953963,-0.292616303977421,-0.263539992876104,-0.260487630636203,
-0.248334354819878,-0.245189861020655,-0.243351038619057,-0.241678699999058,
-0.239331890452382,-0.233482786241947,-0.224681658745724,-0.190699845878194,
-0.169194737364665,-0.163766776555625,-0.160511769363704,-0.157646324101798,
-0.157475736519576,-0.157320586494377,-0.157176158205232,-0.157039043053849,
-0.156906627047732,-0.156776788899757,-0.156647708924034,-0.15651773901719,
-0.156385307023362,-0.153274062122428,-0.148877173631576,-0.115650479679955,
-0.0839169527816737,-0.0794751547393593,-0.0773626137672975,-0.0757157884155579,
-0.0737666939116656,-0.070107160882403,-0.0593894328077706),
 .UNSPECIFIED.);
#2499=B_SPLINE_CURVE_WITH_KNOTS('',3,(#79398,#79399,#79400,#79401,#79402,
#79403,#79404,#79405,#79406,#79407,#79408,#79409,#79410,#79411,#79412,#79413,
#79414,#79415,#79416,#79417,#79418,#79419,#79420,#79421,#79422,#79423,#79424,
#79425,#79426,#79427,#79428,#79429,#79430,#79431,#79432,#79433,#79434,#79435,
#79436,#79437,#79438,#79439,#79440,#79441,#79442,#79443,#79444,#79445,#79446,
#79447,#79448,#79449,#79450,#79451,#79452,#79453,#79454,#79455,#79456,#79457,
#79458,#79459,#79460,#79461,#79462,#79463,#79464,#79465,#79466,#79467,#79468,
#79469,#79470,#79471,#79472,#79473,#79474,#79475,#79476,#79477,#79478,#79479,
#79480,#79481,#79482,#79483,#79484,#79485,#79486,#79487,#79488,#79489,#79490,
#79491,#79492,#79493,#79494,#79495,#79496,#79497,#79498,#79499,#79500,#79501,
#79502,#79503,#79504,#79505,#79506,#79507,#79508,#79509,#79510,#79511,#79512,
#79513,#79514,#79515,#79516,#79517,#79518,#79519,#79520,#79521,#79522,#79523,
#79524,#79525,#79526,#79527,#79528,#79529,#79530,#79531,#79532,#79533,#79534,
#79535,#79536,#79537,#79538,#79539,#79540,#79541,#79542,#79543,#79544,#79545,
#79546,#79547,#79548,#79549,#79550,#79551,#79552,#79553,#79554,#79555,#79556,
#79557,#79558,#79559,#79560,#79561,#79562,#79563,#79564,#79565,#79566,#79567,
#79568,#79569,#79570,#79571,#79572,#79573,#79574,#79575,#79576,#79577,#79578,
#79579,#79580,#79581,#79582,#79583),.UNSPECIFIED.,.F.,.F.,(4,2,2,2,2,2,
2,2,2,2,2,2,2,2,2,2,2,2,2,2,2,2,2,2,2,2,2,2,2,2,2,2,2,2,2,2,2,2,2,2,2,2,
2,2,2,2,2,2,2,2,2,2,2,2,2,2,2,2,2,2,2,2,2,2,2,2,2,2,2,2,2,2,2,2,2,2,2,2,
2,2,2,2,2,2,2,2,2,2,2,2,2,2,4),(-0.991309629175169,-0.976712442897297,-0.971302120168656,
-0.968049826107873,-0.965110359617235,-0.961313006050606,-0.953174462853071,
-0.925021072452987,-0.891225409952512,-0.886878244931272,-0.884790856603695,
-0.883147072261764,-0.881148294324108,-0.877250383151033,-0.872132242708788,
-0.85948407060637,-0.828328745793215,-0.809705627784808,-0.80446223390786,
-0.801245753691646,-0.798296841362354,-0.794426783850327,-0.785879079445045,
-0.758917436432243,-0.724418734700649,-0.720149274913234,-0.718076841380421,
-0.716433571742665,-0.714421598709655,-0.710458417627441,-0.686991859704004,
-0.645122196010641,-0.639335331082444,-0.635668184529889,-0.632742487414995,
-0.629413253066882,-0.623642246159036,-0.58925948691401,-0.558106058843816,
-0.553570727268718,-0.551447826590666,-0.549802208635513,-0.547832592819959,
-0.54407682407163,-0.517791031746947,-0.479054908839158,-0.472920325757895,
-0.469151582002897,-0.466215756384377,-0.462948592225075,-0.457467894255967,
-0.431984730623042,-0.411714045452939,-0.389809541094334,-0.386322752234575,
-0.384388597228262,-0.38275480858553,-0.380592354762241,-0.375841519551348,
-0.354314463689881,-0.314707927377083,-0.306410089545184,-0.302625539800229,
-0.299679847136787,-0.29645431729276,-0.291167179866853,-0.26945181549805,
-0.239312824709431,-0.222912954694419,-0.219554343178574,-0.217648932795758,
-0.216160744505729,-0.214042343867601,-0.209530327769631,-0.190307154362733,
-0.157403488206974,-0.142277943590563,-0.137375828169927,-0.134232581601323,
-0.131256277672675,-0.131138659838767,-0.13102409447788,-0.127507537188148,
-0.118778756966979,-0.106504121992404,-0.0804932699024008,-0.0565150980680115,
-0.0530185413914019,-0.051082288915653,-0.0494332201491776,-0.0472648689814095,
-0.0424809567350256,-0.000491817198503198),.UNSPECIFIED.);
#2500=B_SPLINE_CURVE_WITH_KNOTS('',3,(#79584,#79585,#79586,#79587,#79588,
#79589,#79590,#79591,#79592,#79593,#79594,#79595,#79596,#79597,#79598,#79599,
#79600,#79601,#79602,#79603),.UNSPECIFIED.,.F.,.F.,(4,2,2,2,2,2,2,2,2,4),
(-2.09977849986764,-2.0844228726502,-2.07591358257984,-2.07195021108648,
-2.06900251719241,-2.06601878699063,-2.06289098508343,-2.05806093965961,
-2.04357697080365,-2.04073105386379),.UNSPECIFIED.);
#2501=B_SPLINE_CURVE_WITH_KNOTS('',3,(#79605,#79606,#79607,#79608,#79609,
#79610,#79611,#79612),.UNSPECIFIED.,.F.,.F.,(4,2,2,4),(-0.0593894328077706,
-0.0422597363646323,-0.00975713810380856,-0.000491699695232061),
 .UNSPECIFIED.);
#2502=B_SPLINE_CURVE_WITH_KNOTS('',3,(#79613,#79614,#79615,#79616,#79617,
#79618,#79619,#79620,#79621,#79622,#79623,#79624,#79625,#79626,#79627,#79628,
#79629,#79630,#79631,#79632,#79633,#79634,#79635,#79636,#79637,#79638,#79639,
#79640,#79641,#79642,#79643,#79644,#79645,#79646,#79647,#79648,#79649,#79650,
#79651,#79652,#79653,#79654,#79655,#79656,#79657,#79658,#79659,#79660,#79661,
#79662,#79663,#79664,#79665,#79666,#79667,#79668,#79669,#79670,#79671,#79672,
#79673,#79674,#79675,#79676,#79677,#79678,#79679,#79680,#79681,#79682,#79683,
#79684,#79685,#79686,#79687,#79688,#79689,#79690,#79691,#79692,#79693,#79694,
#79695,#79696,#79697,#79698,#79699,#79700,#79701,#79702,#79703,#79704,#79705,
#79706,#79707,#79708,#79709,#79710,#79711,#79712,#79713,#79714,#79715,#79716,
#79717,#79718,#79719,#79720,#79721,#79722,#79723,#79724,#79725,#79726,#79727,
#79728,#79729,#79730,#79731,#79732,#79733,#79734,#79735,#79736,#79737,#79738,
#79739,#79740,#79741,#79742,#79743,#79744,#79745,#79746,#79747,#79748,#79749,
#79750,#79751,#79752,#79753,#79754,#79755,#79756,#79757,#79758,#79759,#79760,
#79761,#79762,#79763,#79764,#79765,#79766,#79767,#79768,#79769,#79770,#79771,
#79772,#79773,#79774,#79775,#79776,#79777,#79778,#79779,#79780,#79781,#79782,
#79783,#79784,#79785,#79786,#79787,#79788,#79789,#79790,#79791,#79792,#79793,
#79794,#79795,#79796,#79797,#79798,#79799,#79800,#79801,#79802),
 .UNSPECIFIED.,.F.,.F.,(4,2,2,2,2,2,2,2,2,2,2,2,2,2,2,2,2,2,2,2,2,2,2,2,
2,2,2,2,2,2,2,2,2,2,2,2,2,2,2,2,2,2,2,2,2,2,2,2,2,2,2,2,2,2,2,2,2,2,2,2,
2,2,2,2,2,2,2,2,2,2,2,2,2,2,2,2,2,2,2,2,2,2,2,2,2,2,2,2,2,2,2,2,2,2,4),
(-2.09983941200445,-2.09746751631786,-2.0948338360985,-2.09205900815291,
-2.08895601197975,-2.08424346038491,-2.07072870422845,-2.04417007690264,
-2.01545120294433,-2.01168261622109,-2.00971072883515,-2.00806589739413,
-2.00594748975691,-2.00143407369735,-1.96997115631921,-1.93593070229513,
-1.93010550852794,-1.9267654771214,-1.92384222814522,-1.92019388666864,
-1.91308887786692,-1.88061006830047,-1.85801612226665,-1.84725646898209,
-1.84433685500827,-1.8425472129118,-1.84087060996899,-1.83879958263684,
-1.83468272029919,-1.80376504574054,-1.76926853712739,-1.76343571849032,
-1.7600941269723,-1.75717114317716,-1.75352527229697,-1.74643196998487,
-1.71554427387772,-1.69170943797669,-1.6842619151255,-1.67908513905351,
-1.67684812474515,-1.67519178522279,-1.6732988381194,-1.66999396460366,
-1.65450608953998,-1.62562470986355,-1.60980373877781,-1.60263422492724,
-1.59679858154048,-1.59345643673825,-1.59053358612691,-1.58688869062496,
-1.57979989082555,-1.54843769500868,-1.52496635054924,-1.51757896761954,
-1.51243322356617,-1.5102015535971,-1.50854591443657,-1.50665000725737,
-1.50333193524757,-1.48760685047761,-1.45683903482583,-1.4349838879438,
-1.42968916476265,-1.4264626843352,-1.42351852468058,-1.41973929942555,
-1.41342334332628,-1.37712041031413,-1.35719273061045,-1.35044062428245,
-1.34562854885656,-1.34345551289555,-1.34182117493535,-1.33989537880054,
-1.3364441858045,-1.31664949145988,-1.3103841727319,-1.28987487506093,-1.26830987181352,
-1.26303262378709,-1.25980984873576,-1.25686457570851,-1.25307767435187,
-1.24673465949466,-1.2109515999346,-1.18215998900108,-1.17839141487176,
-1.17641961891532,-1.1747749142392,-1.17265673463904,-1.16814403101848,
-1.13667735610574,-1.10896100326588),.UNSPECIFIED.);
#2503=B_SPLINE_CURVE_WITH_KNOTS('',3,(#79807,#79808,#79809,#79810,#79811,
#79812,#79813,#79814,#79815,#79816,#79817,#79818,#79819,#79820,#79821,#79822,
#79823,#79824,#79825,#79826,#79827,#79828,#79829,#79830,#79831,#79832,#79833,
#79834,#79835,#79836,#79837,#79838,#79839,#79840,#79841,#79842,#79843,#79844,
#79845,#79846,#79847,#79848,#79849,#79850,#79851,#79852,#79853,#79854,#79855,
#79856,#79857,#79858,#79859,#79860,#79861,#79862,#79863,#79864,#79865,#79866,
#79867,#79868,#79869,#79870,#79871,#79872,#79873,#79874,#79875,#79876,#79877,
#79878,#79879,#79880,#79881,#79882,#79883,#79884,#79885,#79886,#79887,#79888,
#79889,#79890,#79891,#79892,#79893,#79894,#79895,#79896,#79897,#79898,#79899,
#79900,#79901,#79902,#79903,#79904,#79905,#79906,#79907,#79908,#79909,#79910,
#79911,#79912,#79913,#79914,#79915,#79916,#79917,#79918,#79919,#79920,#79921,
#79922,#79923,#79924,#79925,#79926,#79927,#79928,#79929,#79930,#79931,#79932,
#79933,#79934,#79935,#79936,#79937,#79938,#79939,#79940,#79941,#79942,#79943,
#79944,#79945,#79946,#79947,#79948,#79949,#79950,#79951,#79952,#79953,#79954,
#79955,#79956,#79957,#79958,#79959,#79960,#79961,#79962,#79963,#79964,#79965,
#79966,#79967,#79968,#79969,#79970,#79971,#79972,#79973,#79974,#79975,#79976,
#79977,#79978,#79979,#79980,#79981,#79982,#79983,#79984,#79985,#79986,#79987,
#79988,#79989,#79990,#79991,#79992,#79993,#79994,#79995,#79996,#79997,#79998,
#79999,#80000,#80001,#80002,#80003,#80004,#80005,#80006,#80007,#80008,#80009,
#80010,#80011,#80012,#80013,#80014,#80015,#80016,#80017,#80018,#80019,#80020,
#80021,#80022,#80023,#80024),.UNSPECIFIED.,.F.,.F.,(4,2,2,2,2,2,2,2,2,2,
2,2,2,2,2,2,2,2,2,2,2,2,2,2,2,2,2,2,2,2,2,2,2,2,2,2,2,2,2,2,2,2,2,2,2,2,
2,2,2,2,2,2,2,2,2,2,2,2,2,2,2,2,2,2,2,2,2,2,2,2,2,2,2,2,2,2,2,2,2,2,2,2,
2,2,2,2,2,2,2,2,2,2,2,2,2,2,2,2,2,2,2,2,2,2,2,2,2,2,4),(-2.04129650139704,
-2.02050217143667,-1.99426655112003,-1.98221452337952,-1.97360583333227,
-1.97010352814216,-1.96998780013201,-1.9698688148636,-1.96974596659654,
-1.96961857114194,-1.96948584782904,-1.96943549110545,-1.96937038609358,
-1.9692853020307,-1.96917249655033,-1.96901997039242,-1.96638351810006,
-1.96307725609551,-1.95741566967795,-1.92990954666347,-1.90130402088819,
-1.89314571267282,-1.88760910985177,-1.88531133445469,-1.88364588390244,
-1.88178296643051,-1.87853087229507,-1.8647544620661,-1.83817666852669,
-1.81284218465127,-1.80591636255214,-1.80234879391527,-1.79971170487989,
-1.79641047388868,-1.79077221717103,-1.76366977906844,-1.73470132532085,
-1.72649480152456,-1.72093434154722,-1.71863272123562,-1.71696672914608,
-1.71510573723172,-1.71186238123998,-1.69827517011355,-1.66630217610909,
-1.64340450040082,-1.63804832203251,-1.63480758504775,-1.63186521873499,
-1.62810862968909,-1.61997095566159,-1.58020192101911,-1.55862677998297,
-1.55387068497824,-1.55170705715486,-1.55007289666676,-1.54813895240977,
-1.54465398097334,-1.52312554234726,-1.51892456839007,-1.49898714598307,
-1.47664707068934,-1.47132193213445,-1.46808777018811,-1.4651435540136,
-1.46137383687282,-1.45509536143535,-1.41813714279326,-1.39862980620633,
-1.3887247358984,-1.38588152843768,-1.38410808345957,-1.38242003202009,
-1.37989861330407,-1.37337562863872,-1.34133360627301,-1.3155059098064,
-1.30678609826977,-1.30288597496673,-1.29993266419096,-1.29672936104297,
-1.29154812806111,-1.27356731064997,-1.24209788214621,-1.22917380128435,
-1.22398405804918,-1.22004387557362,-1.21803646063817,-1.21639293036682,
-1.21431513251944,-1.21001830968317,-1.17572844148365,-1.1488350020391,
-1.14009999130656,-1.13619735900707,-1.13324379665879,-1.13004181467583,
-1.12486630568284,-1.10696568358054,-1.06947000405028,-1.06032634168688,
-1.05431285877752,-1.05193991000559,-1.05026250979406,-1.0484330241394,
-1.04533402683798,-1.03222578157483,-0.998111700818972,-0.991309629175169),
 .UNSPECIFIED.);
#2504=B_SPLINE_CURVE_WITH_KNOTS('',3,(#80025,#80026,#80027,#80028,#80029,
#80030,#80031,#80032,#80033,#80034,#80035,#80036,#80037,#80038,#80039,#80040,
#80041,#80042,#80043,#80044,#80045,#80046,#80047,#80048,#80049,#80050,#80051,
#80052,#80053,#80054,#80055,#80056,#80057,#80058,#80059,#80060,#80061,#80062,
#80063,#80064,#80065,#80066,#80067,#80068,#80069,#80070,#80071,#80072,#80073,
#80074,#80075,#80076,#80077,#80078,#80079,#80080,#80081,#80082,#80083,#80084,
#80085,#80086,#80087,#80088,#80089,#80090,#80091,#80092,#80093,#80094,#80095,
#80096,#80097,#80098,#80099,#80100,#80101,#80102,#80103,#80104,#80105,#80106,
#80107,#80108,#80109,#80110,#80111,#80112,#80113,#80114,#80115,#80116,#80117,
#80118,#80119,#80120,#80121,#80122,#80123,#80124,#80125,#80126,#80127,#80128,
#80129,#80130,#80131,#80132,#80133,#80134,#80135,#80136,#80137,#80138,#80139,
#80140,#80141,#80142,#80143,#80144,#80145,#80146,#80147,#80148,#80149,#80150,
#80151,#80152,#80153,#80154,#80155,#80156,#80157,#80158,#80159,#80160,#80161,
#80162,#80163,#80164,#80165,#80166,#80167,#80168,#80169,#80170,#80171,#80172,
#80173,#80174,#80175,#80176,#80177,#80178,#80179,#80180,#80181,#80182,#80183,
#80184,#80185,#80186,#80187,#80188,#80189,#80190,#80191,#80192,#80193,#80194,
#80195,#80196,#80197,#80198,#80199,#80200,#80201,#80202,#80203,#80204,#80205,
#80206,#80207,#80208,#80209,#80210,#80211,#80212,#80213,#80214,#80215,#80216,
#80217,#80218,#80219,#80220,#80221,#80222,#80223,#80224,#80225,#80226,#80227,
#80228,#80229,#80230),.UNSPECIFIED.,.F.,.F.,(4,2,2,2,2,2,2,2,2,2,2,2,2,
2,2,2,2,2,2,2,2,2,2,2,2,2,2,2,2,2,2,2,2,2,2,2,2,2,2,2,2,2,2,2,2,2,2,2,2,
2,2,2,2,2,2,2,2,2,2,2,2,2,2,2,2,2,2,2,2,2,2,2,2,2,2,2,2,2,2,2,2,2,2,2,2,
2,2,2,2,2,2,2,2,2,2,2,2,2,2,2,2,2,4),(-1.10896100326588,-1.10262103694887,
-1.09680950829537,-1.09347253248744,-1.09054917744227,-1.08689704633842,
-1.0797728310934,-1.04989664098759,-1.01645877921795,-1.01207723862595,
-1.00998387422742,-1.0083405765361,-1.00634875720638,-1.00248227637776,
-0.997417009453012,-0.984968363565762,-0.947040343215284,-0.933776552618257,
-0.929081231408675,-0.925982141253907,-0.922982570162637,-0.918792498268505,
-0.90825096870595,-0.892420489245415,-0.863568688361532,-0.848109848545278,
-0.844806780010933,-0.842914317368835,-0.841258034223744,-0.839020557297983,
-0.833840543231992,-0.826385662620472,-0.802508963608914,-0.771644030973076,
-0.764549335811273,-0.760903345492693,-0.757980563523399,-0.754639527340026,
-0.74880850210391,-0.714411980850648,-0.683416500478926,-0.678867385009774,
-0.676742481818722,-0.675097412500106,-0.673131029622788,-0.669388327723223,
-0.642520965989869,-0.604467894639204,-0.598274003720881,-0.594489006285154,
-0.591552398663583,-0.588296480525749,-0.582863895335284,-0.55841418540684,
-0.543849367171461,-0.542495082316909,-0.517075007846038,-0.512323397368113,
-0.510184367439247,-0.508535166710451,-0.506605256642582,-0.503036697028638,
-0.474375738926622,-0.438051858426659,-0.4317360382244,-0.427957173251727,
-0.425013434844205,-0.421787557268093,-0.416494130552386,-0.394645610858004,
-0.363891692130062,-0.348191822161565,-0.344876158178873,-0.342980980957539,
-0.341325544493112,-0.339093520889043,-0.333944436473672,-0.326549281630532,
-0.303031993480562,-0.271704051062899,-0.26461445842908,-0.260969774914935,
-0.258047403262549,-0.254706143252063,-0.248872902315979,-0.241707537936841,
-0.225899772874974,-0.197047311799649,-0.181568423389682,-0.17826133638004,
-0.176368100924025,-0.174712239129969,-0.17247680124674,-0.167307772205462,
-0.159873923085579,-0.13612272070742,-0.105101243386457,-0.0980088199640418,
-0.0943635576300295,-0.0914411464006612,-0.0881003026529644,-0.0822690040247909,
-0.0593466407402418),.UNSPECIFIED.);
#2505=B_SPLINE_CURVE_WITH_KNOTS('',3,(#80236,#80237,#80238,#80239,#80240,
#80241,#80242,#80243,#80244,#80245,#80246,#80247,#80248,#80249,#80250,#80251,
#80252,#80253,#80254,#80255,#80256,#80257,#80258,#80259,#80260,#80261,#80262,
#80263,#80264,#80265,#80266,#80267,#80268,#80269,#80270,#80271,#80272,#80273,
#80274,#80275,#80276,#80277,#80278,#80279,#80280,#80281,#80282,#80283,#80284,
#80285,#80286,#80287,#80288,#80289,#80290,#80291,#80292,#80293,#80294,#80295,
#80296,#80297,#80298,#80299,#80300,#80301,#80302,#80303,#80304,#80305,#80306,
#80307,#80308,#80309,#80310,#80311,#80312,#80313,#80314,#80315,#80316,#80317,
#80318,#80319,#80320,#80321,#80322,#80323,#80324,#80325,#80326,#80327,#80328,
#80329,#80330,#80331,#80332,#80333,#80334,#80335,#80336,#80337,#80338,#80339,
#80340,#80341,#80342,#80343,#80344,#80345,#80346,#80347,#80348,#80349,#80350,
#80351,#80352,#80353,#80354,#80355,#80356,#80357,#80358,#80359,#80360,#80361,
#80362,#80363,#80364,#80365,#80366,#80367,#80368,#80369,#80370,#80371,#80372,
#80373,#80374,#80375,#80376,#80377,#80378,#80379,#80380,#80381,#80382,#80383,
#80384,#80385,#80386,#80387,#80388,#80389,#80390,#80391,#80392,#80393,#80394,
#80395,#80396,#80397,#80398,#80399,#80400,#80401,#80402,#80403,#80404,#80405,
#80406,#80407,#80408,#80409,#80410,#80411,#80412,#80413,#80414,#80415,#80416,
#80417,#80418,#80419,#80420,#80421,#80422,#80423,#80424,#80425,#80426,#80427,
#80428,#80429,#80430,#80431),.UNSPECIFIED.,.F.,.F.,(4,2,2,2,2,2,2,2,2,2,
2,2,2,2,2,2,2,2,2,2,2,2,2,2,2,2,2,2,2,2,2,2,2,2,2,2,2,2,2,2,2,2,2,2,2,2,
2,2,2,2,2,2,2,2,2,2,2,2,2,2,2,2,2,2,2,2,2,2,2,2,2,2,2,2,2,2,2,2,2,2,2,2,
2,2,2,2,2,2,2,2,2,2,2,2,2,2,2,4),(-0.991375509315892,-0.971325647813708,
-0.956656946350987,-0.953391182320626,-0.951506689619944,-0.949847609452942,
-0.947593126047794,-0.942316274240613,-0.934673159706958,-0.909625473790717,
-0.877722768848919,-0.872089010915296,-0.868757519973074,-0.865860063663532,
-0.862210483579645,-0.854863167175326,-0.845203456380488,-0.819206108415393,
-0.813692841681796,-0.790404323367302,-0.786912860339961,-0.784977658463859,
-0.783344007246142,-0.781183064370636,-0.776440602213076,-0.754998072415802,
-0.715655928564857,-0.7071146577489,-0.703287680514103,-0.700335905265575,
-0.697130631576916,-0.691938003285569,-0.671690929813469,-0.65014110811581,
-0.643366909545774,-0.623672966677335,-0.620223945958354,-0.618298279848431,
-0.616663326782288,-0.614488430502789,-0.609668200140982,-0.602900579483171,
-0.582896724136379,-0.546670099216769,-0.540346852572707,-0.536565001517774,
-0.533619746346397,-0.530393009767133,-0.525099987881885,-0.503285136397791,
-0.47263504888351,-0.465714154600991,-0.455981719639317,-0.453059268566414,
-0.451268762047407,-0.44957232481929,-0.447092995787216,-0.440347040601106,
-0.396536034896136,-0.376986912031471,-0.371688981728305,-0.368461388271975,
-0.365516736840972,-0.361673205304913,-0.353272626051038,-0.33037475660221,
-0.304036260414623,-0.289977806463287,-0.286706271216534,-0.284839558690544,
-0.283176085859649,-0.280888303557429,-0.275409744945854,-0.267366027029317,
-0.239596839505482,-0.211024487297737,-0.205376326231097,-0.202073719706845,
-0.19943792172997,-0.195875244917472,-0.188970070985356,-0.163789678747696,
-0.137521325723465,-0.123362936621702,-0.1200860067375,-0.118218123681791,
-0.116554989982739,-0.114269556516894,-0.108805308367515,-0.0803572397899584,
-0.0564804299161656,-0.0426614192773625,-0.0379022588577338,-0.0347893747368273,
-0.0317972752601317,-0.0288347686752118,-0.0248304547526201,-0.000491209455975046),
 .UNSPECIFIED.);
#2506=B_SPLINE_CURVE_WITH_KNOTS('',3,(#80432,#80433,#80434,#80435,#80436,
#80437,#80438,#80439,#80440,#80441,#80442,#80443,#80444,#80445,#80446,#80447),
 .UNSPECIFIED.,.F.,.F.,(4,2,2,2,2,2,2,4),(-2.10011893460937,-2.05874039818313,
-2.0539606684199,-2.0517927065913,-2.0501432533371,-2.04820577425607,-2.0447051496043,
-2.04129650139704),.UNSPECIFIED.);
#2507=B_SPLINE_CURVE_WITH_KNOTS('',3,(#80449,#80450,#80451,#80452,#80453,
#80454,#80455,#80456,#80457,#80458,#80459,#80460,#80461,#80462,#80463,#80464,
#80465,#80466,#80467,#80468),.UNSPECIFIED.,.F.,.F.,(4,2,2,2,2,2,2,2,2,4),
(-0.0593466407402418,-0.0475921036961166,-0.0244934883160425,-0.0142512537367275,
-0.0112790705691864,-0.00947813397535948,-0.00791635107762846,-0.00623769541915255,
-0.00362381139487444,-0.000491106664933776),.UNSPECIFIED.);
#2508=B_SPLINE_CURVE_WITH_KNOTS('',3,(#80469,#80470,#80471,#80472,#80473,
#80474,#80475,#80476,#80477,#80478,#80479,#80480,#80481,#80482,#80483,#80484,
#80485,#80486,#80487,#80488,#80489,#80490,#80491,#80492,#80493,#80494,#80495,
#80496,#80497,#80498,#80499,#80500,#80501,#80502,#80503,#80504,#80505,#80506,
#80507,#80508,#80509,#80510,#80511,#80512,#80513,#80514,#80515,#80516,#80517,
#80518,#80519,#80520,#80521,#80522,#80523,#80524,#80525,#80526,#80527,#80528,
#80529,#80530,#80531,#80532,#80533,#80534,#80535,#80536,#80537,#80538,#80539,
#80540,#80541,#80542,#80543,#80544,#80545,#80546,#80547,#80548,#80549,#80550,
#80551,#80552,#80553,#80554,#80555,#80556,#80557,#80558,#80559,#80560,#80561,
#80562,#80563,#80564,#80565,#80566,#80567,#80568,#80569,#80570,#80571,#80572,
#80573,#80574,#80575,#80576,#80577,#80578,#80579,#80580,#80581,#80582,#80583,
#80584,#80585,#80586,#80587,#80588,#80589,#80590,#80591,#80592,#80593,#80594,
#80595,#80596,#80597,#80598,#80599,#80600,#80601,#80602,#80603,#80604,#80605,
#80606,#80607,#80608,#80609,#80610,#80611,#80612,#80613,#80614,#80615,#80616,
#80617,#80618,#80619,#80620,#80621,#80622,#80623,#80624,#80625,#80626,#80627,
#80628,#80629,#80630,#80631,#80632,#80633,#80634,#80635,#80636,#80637,#80638,
#80639,#80640,#80641,#80642,#80643,#80644,#80645,#80646,#80647,#80648,#80649,
#80650,#80651,#80652,#80653,#80654,#80655,#80656,#80657,#80658,#80659,#80660,
#80661,#80662,#80663,#80664,#80665,#80666,#80667,#80668,#80669,#80670,#80671,
#80672,#80673,#80674,#80675,#80676,#80677,#80678,#80679,#80680,#80681,#80682),
 .UNSPECIFIED.,.F.,.F.,(4,2,2,2,2,2,2,2,2,2,2,2,2,2,2,2,2,2,2,2,2,2,2,2,
2,2,2,2,2,2,2,2,2,2,2,2,2,2,2,2,2,2,2,2,2,2,2,2,2,2,2,2,2,2,2,2,2,2,2,2,
2,2,2,2,2,2,2,2,2,2,2,2,2,2,2,2,2,2,2,2,2,2,2,2,2,2,2,2,2,2,2,2,2,2,2,2,
2,2,2,2,2,2,2,2,2,2,4),(-2.10025436568081,-2.05988935967928,-2.03995709080465,
-2.03163144250381,-2.02780136713765,-2.02485870160554,-2.02162502330748,
-2.01629785714225,-1.99618429740599,-1.95277314195091,-1.94828775920848,
-1.94574487101294,-1.94359788555784,-1.94357765013498,-1.94355738141956,
-1.9435370734256,-1.94351672001049,-1.94349631496814,-1.94348543071906,
-1.94347427766195,-1.94346284237382,-1.94345111059155,-1.94343906694274,
-1.94342669509122,-1.9434139775649,-1.94340089554668,-1.94179220588074,
-1.93989682336244,-1.93658177415496,-1.92110045184647,-1.89221362083911,
-1.87639772330963,-1.86922939426582,-1.8633943536282,-1.86005208844235,
-1.85712886272789,-1.85348314564426,-1.84639160917657,-1.81521873512535,
-1.79159752295975,-1.78418485327014,-1.77902590403342,-1.77679181042879,
-1.77513570641277,-1.77324080506401,-1.76992777942584,-1.7542808926877,
-1.7234962075332,-1.70156978300996,-1.69627034437933,-1.69304260715778,
-1.69009834331992,-1.68632042906834,-1.68000994317976,-1.64359377630011,
-1.62373627241731,-1.61699735994837,-1.61219219426706,-1.61002024668369,
-1.60838585434544,-1.60645894691865,-1.6030033856196,-1.58304819400471,
-1.57646841529328,-1.55481305118713,-1.53468557648691,-1.52950151165228,
-1.52629847830387,-1.5233467791006,-1.51951710904556,-1.51095751424969,
-1.47165399466463,-1.45022763169339,-1.44548707594442,-1.44332674962259,
-1.44169345290579,-1.43975861923866,-1.43626770061208,-1.41313482149133,
-1.39593943117429,-1.37100224826789,-1.36412802496839,-1.36057155566827,
-1.35793646027117,-1.35462967976717,-1.34896163061532,-1.31818921891525,
-1.29334281292321,-1.28490552376879,-1.27923198092879,-1.27691267747497,
-1.2752444947542,-1.27339298905891,-1.27019120708184,-1.25721570791507,
-1.23007798867549,-1.20208021574403,-1.19650578957859,-1.1932190663698,
-1.19028790734917,-1.18655580114359,-1.18054576845566,-1.13433093390365,
-1.11630245151555,-1.11192301990235,-1.10982980654801,-1.1092440461416),
 .UNSPECIFIED.);
#2509=B_SPLINE_CURVE_WITH_KNOTS('',3,(#80687,#80688,#80689,#80690,#80691,
#80692,#80693,#80694,#80695,#80696,#80697,#80698,#80699,#80700,#80701,#80702,
#80703,#80704,#80705,#80706,#80707,#80708,#80709,#80710,#80711,#80712,#80713,
#80714,#80715,#80716,#80717,#80718,#80719,#80720,#80721,#80722,#80723,#80724,
#80725,#80726,#80727,#80728,#80729,#80730,#80731,#80732,#80733,#80734,#80735,
#80736,#80737,#80738,#80739,#80740,#80741,#80742,#80743,#80744,#80745,#80746,
#80747,#80748,#80749,#80750,#80751,#80752,#80753,#80754,#80755,#80756,#80757,
#80758,#80759,#80760,#80761,#80762,#80763,#80764,#80765,#80766,#80767,#80768,
#80769,#80770,#80771,#80772,#80773,#80774,#80775,#80776,#80777,#80778,#80779,
#80780,#80781,#80782,#80783,#80784,#80785,#80786,#80787,#80788,#80789,#80790,
#80791,#80792,#80793,#80794,#80795,#80796,#80797,#80798,#80799,#80800,#80801,
#80802,#80803,#80804,#80805,#80806,#80807,#80808,#80809,#80810,#80811,#80812,
#80813,#80814,#80815,#80816,#80817,#80818,#80819,#80820,#80821,#80822,#80823,
#80824,#80825,#80826,#80827,#80828,#80829,#80830,#80831,#80832,#80833,#80834,
#80835,#80836,#80837,#80838,#80839,#80840,#80841,#80842,#80843,#80844,#80845,
#80846,#80847,#80848,#80849,#80850,#80851,#80852,#80853,#80854,#80855,#80856,
#80857,#80858,#80859,#80860,#80861,#80862,#80863,#80864,#80865,#80866,#80867,
#80868,#80869,#80870,#80871,#80872,#80873,#80874,#80875,#80876,#80877,#80878,
#80879,#80880,#80881,#80882,#80883,#80884,#80885,#80886,#80887,#80888,#80889,
#80890,#80891,#80892,#80893,#80894,#80895,#80896,#80897,#80898,#80899,#80900,
#80901,#80902,#80903,#80904,#80905,#80906,#80907,#80908,#80909,#80910,#80911,
#80912,#80913,#80914,#80915,#80916,#80917,#80918),.UNSPECIFIED.,.F.,.F.,
(4,2,2,2,2,2,2,2,2,2,2,2,2,2,2,2,2,2,2,2,2,2,2,2,2,2,2,2,2,2,2,2,2,2,2,
2,2,2,2,2,2,2,2,2,2,2,2,2,2,2,2,2,2,2,2,2,2,2,2,2,2,2,2,2,2,2,2,2,2,2,2,
2,2,2,2,2,2,2,2,2,2,2,2,2,2,2,2,2,2,2,2,2,2,2,2,2,2,2,2,2,2,2,2,2,2,2,2,
2,2,2,2,2,2,2,2,4),(-2.04114771859458,-2.03955044215046,-2.0359873324451,
-2.03335094243348,-2.03004722296548,-2.02439622375842,-1.99426110152052,
-1.97146852859624,-1.96137220605286,-1.95695661231143,-1.95444032036714,
-1.95232057439764,-1.95230191979688,-1.95228318355207,-1.95226436027608,
-1.95224544449622,-1.95222643057772,-1.95220731278866,-1.95218808522726,
-1.95216874185421,-1.95214927649478,-1.95212968277069,-1.95052983024196,
-1.94863206629821,-1.94530782384571,-1.92968643462709,-1.89896211512878,
-1.87697689695211,-1.87167301735613,-1.86844372537231,-1.86549876562277,
-1.86172093631104,-1.8554127364574,-1.81894571801047,-1.79912306194497,
-1.79239043970653,-1.78758837442089,-1.78541661388233,-1.78378182562157,
-1.78185375549402,-1.77839446936323,-1.75831195675354,-1.75184651269745,
-1.73053971193123,-1.71697501531594,-1.70752370297998,-1.70350157902085,
-1.70052989019903,-1.69737570651913,-1.6924231617866,-1.67681314288446,
-1.64433457652749,-1.62527779231291,-1.62078354944626,-1.61866836142678,
-1.61718041098861,-1.61527252070741,-1.61190334846076,-1.59528796598961,
-1.56571231358035,-1.54366161884458,-1.53835386255701,-1.5351237303543,
-1.53217898328665,-1.52840278148661,-1.52210036933827,-1.48553581095097,
-1.45727936758489,-1.45360822980282,-1.45165617107427,-1.45000882202314,
-1.44789799477105,-1.44346777915029,-1.41139822010568,-1.37794745453774,
-1.37210589899874,-1.36876173115749,-1.3658378803048,-1.36219272404055,
-1.35510649089822,-1.32342317864337,-1.30019262299668,-1.29284478356411,
-1.28771909121993,-1.28549038067231,-1.28383459371998,-1.28193575719009,
-1.27860657681105,-1.26280177682535,-1.23210213589126,-1.21026988985006,
-1.20497526123325,-1.2017480308493,-1.19880264659717,-1.19502107774251,
-1.18869937743779,-1.15247571026872,-1.13249265593414,-1.12572921501757,
-1.12091072535199,-1.11873606135403,-1.11710102842371,-1.11517499620138,
-1.11172464242704,-1.09199678587012,-1.08522350290935,-1.06404758724812,
-1.05037149736466,-1.0410699957019,-1.03736734894764,-1.03462894007553,
-1.03163070170678,-1.02745323999756,-1.01700352970447,-1.00137333991101,
-0.991375509315892),.UNSPECIFIED.);
#2510=B_SPLINE_CURVE_WITH_KNOTS('',3,(#80919,#80920,#80921,#80922,#80923,
#80924,#80925,#80926,#80927,#80928,#80929,#80930,#80931,#80932,#80933,#80934,
#80935,#80936,#80937,#80938,#80939,#80940,#80941,#80942,#80943,#80944,#80945,
#80946,#80947,#80948,#80949,#80950,#80951,#80952,#80953,#80954,#80955,#80956,
#80957,#80958,#80959,#80960,#80961,#80962,#80963,#80964,#80965,#80966,#80967,
#80968,#80969,#80970,#80971,#80972,#80973,#80974,#80975,#80976,#80977,#80978,
#80979,#80980,#80981,#80982,#80983,#80984,#80985,#80986,#80987,#80988,#80989,
#80990,#80991,#80992,#80993,#80994,#80995,#80996,#80997,#80998,#80999,#81000,
#81001,#81002,#81003,#81004,#81005,#81006,#81007,#81008,#81009,#81010,#81011,
#81012,#81013,#81014,#81015,#81016,#81017,#81018,#81019,#81020,#81021,#81022,
#81023,#81024,#81025,#81026,#81027,#81028,#81029,#81030,#81031,#81032,#81033,
#81034,#81035,#81036,#81037,#81038,#81039,#81040,#81041,#81042,#81043,#81044,
#81045,#81046,#81047,#81048,#81049,#81050,#81051,#81052,#81053,#81054,#81055,
#81056,#81057,#81058,#81059,#81060,#81061,#81062,#81063,#81064,#81065,#81066,
#81067,#81068,#81069,#81070,#81071,#81072,#81073,#81074,#81075,#81076,#81077,
#81078,#81079,#81080,#81081,#81082,#81083,#81084,#81085,#81086,#81087,#81088,
#81089,#81090,#81091,#81092,#81093,#81094,#81095,#81096,#81097,#81098,#81099,
#81100,#81101,#81102,#81103,#81104,#81105,#81106,#81107,#81108,#81109,#81110,
#81111,#81112,#81113,#81114,#81115,#81116,#81117,#81118,#81119,#81120,#81121,
#81122,#81123,#81124,#81125,#81126),.UNSPECIFIED.,.F.,.F.,(4,2,2,2,2,2,
2,2,2,2,2,2,2,2,2,2,2,2,2,2,2,2,2,2,2,2,2,2,2,2,2,2,2,2,2,2,2,2,2,2,2,2,
2,2,2,2,2,2,2,2,2,2,2,2,2,2,2,2,2,2,2,2,2,2,2,2,2,2,2,2,2,2,2,2,2,2,2,2,
2,2,2,2,2,2,2,2,2,2,2,2,2,2,2,2,2,2,2,2,2,2,2,2,2,4),(-1.1092440461416,
-1.10834451449087,-1.10642202474537,-1.10298671449132,-1.08381054346351,
-1.0504100854777,-1.03426701466328,-1.02925665226071,-1.02609066645499,
-1.02312515882606,-1.01913811477839,-1.00989751419581,-0.996750879904674,
-0.974876872255874,-0.969805854640356,-0.94825810638846,-0.944774396692011,
-0.942841166484129,-0.941207661746437,-0.939044993609643,-0.934291511417377,
-0.91273423613294,-0.873036179927103,-0.864818334381091,-0.861048371066553,
-0.85810519030908,-0.854873433241854,-0.849555241083263,-0.827303569840712,
-0.807292604730401,-0.803040718692191,-0.781585822563856,-0.778103264704438,
-0.776170366235679,-0.774536938111132,-0.772374106185186,-0.767619252470507,
-0.746046390857894,-0.706297337120878,-0.698935735727955,-0.695235960067629,
-0.69249887939359,-0.689501336746625,-0.68532344758395,-0.674865143808652,
-0.659214923536852,-0.629365499275763,-0.614547677125586,-0.611275237441311,
-0.609389620513822,-0.607731563596552,-0.605481238897973,-0.600226293513572,
-0.592625416003843,-0.567842517002867,-0.53822360296346,-0.531072297611526,
-0.527414488088338,-0.524490544361041,-0.521157175903367,-0.515363088287735,
-0.508259610180924,-0.492664244006215,-0.462258486331871,-0.447867117307472,
-0.444578118847412,-0.44270778988695,-0.441045700710015,-0.438766142346748,
-0.43333637407794,-0.425390008211735,-0.398310902818856,-0.368922795369496,
-0.363246544866067,-0.359938244165254,-0.357303690848199,-0.353750254844742,
-0.346889962726889,-0.32205971132695,-0.304814407871312,-0.281650150469743,
-0.278160044115444,-0.276225529854654,-0.274592437922467,-0.272432264596464,
-0.267691676801547,-0.246261209468699,-0.206960920297067,-0.198384182370283,
-0.194551864359339,-0.191600104691203,-0.188398969347303,-0.183222381242241,
-0.163191711660756,-0.141495438283894,-0.135264345803247,-0.114955763361533,
-0.111492672353607,-0.109564250233118,-0.107930389284136,-0.105761481838837,
-0.10097214377063,-0.0942617145351005,-0.0595087977532423),
 .UNSPECIFIED.);
#2511=B_SPLINE_CURVE_WITH_KNOTS('',3,(#81132,#81133,#81134,#81135,#81136,
#81137,#81138,#81139,#81140,#81141,#81142,#81143,#81144,#81145,#81146,#81147,
#81148,#81149,#81150,#81151,#81152,#81153,#81154,#81155,#81156,#81157,#81158,
#81159,#81160,#81161,#81162,#81163,#81164,#81165,#81166,#81167,#81168,#81169,
#81170,#81171,#81172,#81173,#81174,#81175,#81176,#81177,#81178,#81179,#81180,
#81181,#81182,#81183,#81184,#81185,#81186,#81187,#81188,#81189,#81190,#81191,
#81192,#81193,#81194,#81195,#81196,#81197,#81198,#81199,#81200,#81201,#81202,
#81203,#81204,#81205,#81206,#81207,#81208,#81209,#81210,#81211,#81212,#81213,
#81214,#81215,#81216,#81217,#81218,#81219,#81220,#81221,#81222,#81223,#81224,
#81225,#81226,#81227,#81228,#81229,#81230,#81231,#81232,#81233,#81234,#81235,
#81236,#81237,#81238,#81239,#81240,#81241,#81242,#81243,#81244,#81245,#81246,
#81247,#81248,#81249,#81250,#81251,#81252,#81253,#81254,#81255,#81256,#81257,
#81258,#81259,#81260,#81261,#81262,#81263,#81264,#81265,#81266,#81267,#81268,
#81269,#81270,#81271,#81272,#81273,#81274,#81275,#81276,#81277,#81278,#81279,
#81280,#81281,#81282,#81283,#81284,#81285,#81286,#81287,#81288,#81289,#81290,
#81291,#81292,#81293,#81294,#81295,#81296,#81297,#81298,#81299,#81300,#81301,
#81302,#81303,#81304,#81305,#81306,#81307,#81308,#81309,#81310,#81311,#81312,
#81313,#81314,#81315,#81316,#81317,#81318,#81319,#81320,#81321,#81322,#81323),
 .UNSPECIFIED.,.F.,.F.,(4,2,2,2,2,2,2,2,2,2,2,2,2,2,2,2,2,2,2,2,2,2,2,2,
2,2,2,2,2,2,2,2,2,2,2,2,2,2,2,2,2,2,2,2,2,2,2,2,2,2,2,2,2,2,2,2,2,2,2,2,
2,2,2,2,2,2,2,2,2,2,2,2,2,2,2,2,2,2,2,2,2,2,2,2,2,2,2,2,2,2,2,2,2,2,2,4),
(-0.991163431562309,-0.983026812983697,-0.946840791955441,-0.940514654088063,
-0.93673181834429,-0.933786222648764,-0.930559545204441,-0.925267622091985,
-0.903476681762918,-0.872928619819918,-0.856985166116892,-0.853644373617409,
-0.851742910550934,-0.85025391199805,-0.848129268342275,-0.843584242970056,
-0.824055907907021,-0.790277275137965,-0.776148805171909,-0.771355815786866,
-0.768235477427027,-0.765246890764966,-0.761123697641,-0.751031564934833,
-0.736159654005757,-0.716318134095772,-0.711906387224396,-0.690591623746885,
-0.687110147030128,-0.685177203908985,-0.683543289207713,-0.681379171066148,
-0.676618966274426,-0.654996501094427,-0.615087927979628,-0.607064429282978,
-0.603288365301109,-0.600351899616149,-0.597089196853831,-0.591628502524685,
-0.566595277446982,-0.54540975777923,-0.523933315526696,-0.520450202276971,
-0.518516961887957,-0.516883201098184,-0.514719814405494,-0.50996323232123,
-0.488375900745767,-0.448577027546068,-0.440457420126384,-0.436704653655309,
-0.433763451149865,-0.43052211536294,-0.425160492711937,-0.402135965730442,
-0.370001367280284,-0.356732274298548,-0.353512600958904,-0.351657080526661,
-0.349989999528961,-0.347678593320234,-0.34205518155407,-0.333719168119961,
-0.307647687571344,-0.277915753685912,-0.272241716735928,-0.26893345999275,
-0.266298254058415,-0.262743025146357,-0.255875943489336,-0.230996521707243,
-0.213788097923434,-0.190640849959093,-0.187157610616563,-0.185224388704467,
-0.18359070214555,-0.181427490070131,-0.176671583085754,-0.155090014022952,
-0.115308219377761,-0.107174966849337,-0.103419858380921,-0.100478446324007,
-0.0972385481211124,-0.0918832347812257,-0.0689721053730947,-0.0424639122988463,
-0.0276457692725278,-0.0218131539447601,-0.0194033311085543,-0.0177365565132501,
-0.0162021764441248,-0.0143991166696238,-0.0117759066718596,-0.000490982254256552),
 .UNSPECIFIED.);
#2512=B_SPLINE_CURVE_WITH_KNOTS('',3,(#81324,#81325,#81326,#81327,#81328,
#81329,#81330,#81331),.UNSPECIFIED.,.F.,.F.,(4,2,2,4),(-2.10019346878139,
-2.07162495664198,-2.04645503985977,-2.04114771859458),.UNSPECIFIED.);
#2513=B_SPLINE_CURVE_WITH_KNOTS('',3,(#81333,#81334,#81335,#81336,#81337,
#81338,#81339,#81340,#81341,#81342,#81343,#81344,#81345,#81346,#81347,#81348,
#81349,#81350,#81351,#81352),.UNSPECIFIED.,.F.,.F.,(4,2,2,2,2,2,2,2,2,4),
(-0.0595087977532423,-0.0586975082944341,-0.0373425380828879,-0.0313459888537824,
-0.0276182134449585,-0.0246879961510923,-0.0219472198498188,-0.0187144246772699,
-0.0116643696517348,-0.00049107690068497),.UNSPECIFIED.);
#2514=B_SPLINE_CURVE_WITH_KNOTS('',3,(#81353,#81354,#81355,#81356,#81357,
#81358,#81359,#81360,#81361,#81362,#81363,#81364,#81365,#81366,#81367,#81368,
#81369,#81370,#81371,#81372,#81373,#81374,#81375,#81376,#81377,#81378,#81379,
#81380,#81381,#81382,#81383,#81384,#81385,#81386,#81387,#81388,#81389,#81390,
#81391,#81392,#81393,#81394,#81395,#81396,#81397,#81398,#81399,#81400,#81401,
#81402,#81403,#81404,#81405,#81406,#81407,#81408,#81409,#81410,#81411,#81412,
#81413,#81414,#81415,#81416,#81417,#81418,#81419,#81420,#81421,#81422,#81423,
#81424,#81425,#81426,#81427,#81428,#81429,#81430,#81431,#81432,#81433,#81434,
#81435,#81436,#81437,#81438,#81439,#81440,#81441,#81442,#81443,#81444,#81445,
#81446,#81447,#81448,#81449,#81450,#81451,#81452,#81453,#81454,#81455,#81456,
#81457,#81458,#81459,#81460,#81461,#81462,#81463,#81464,#81465,#81466,#81467,
#81468,#81469,#81470,#81471,#81472,#81473,#81474,#81475,#81476,#81477,#81478,
#81479,#81480,#81481,#81482,#81483,#81484,#81485,#81486,#81487,#81488,#81489,
#81490,#81491,#81492,#81493,#81494,#81495,#81496,#81497,#81498,#81499,#81500,
#81501,#81502,#81503,#81504,#81505,#81506,#81507,#81508,#81509,#81510,#81511,
#81512,#81513,#81514,#81515,#81516,#81517,#81518,#81519,#81520,#81521,#81522,
#81523,#81524,#81525,#81526,#81527,#81528,#81529,#81530,#81531,#81532,#81533,
#81534,#81535,#81536,#81537,#81538,#81539,#81540,#81541,#81542,#81543,#81544,
#81545,#81546,#81547,#81548,#81549,#81550,#81551,#81552,#81553,#81554),
 .UNSPECIFIED.,.F.,.F.,(4,2,2,2,2,2,2,2,2,2,2,2,2,2,2,2,2,2,2,2,2,2,2,2,
2,2,2,2,2,2,2,2,2,2,2,2,2,2,2,2,2,2,2,2,2,2,2,2,2,2,2,2,2,2,2,2,2,2,2,2,
2,2,2,2,2,2,2,2,2,2,2,2,2,2,2,2,2,2,2,2,2,2,2,2,2,2,2,2,2,2,2,2,2,2,2,2,
2,2,2,2,4),(-2.09985433564141,-2.07657965371477,-2.05654300630488,-2.04976929128882,
-2.04494540288815,-2.04276994739049,-2.04113503780234,-2.03921006349314,
-2.03576372793023,-2.01618178886459,-2.00962512910649,-1.98885844223598,
-1.97471647142805,-1.96805222276279,-1.962621965938,-1.95944583360317,-1.95652135298477,
-1.95286333271904,-1.94571307748359,-1.91491073286433,-1.89107005387601,
-1.88362087024361,-1.87844297263702,-1.87620549818488,-1.87454882780183,
-1.87265551391689,-1.86935002416176,-1.85385991267236,-1.82497297918086,
-1.80914819767212,-1.80197706462812,-1.7961401381916,-1.79279730349086,
-1.78987387556106,-1.78622829424746,-1.7791382704522,-1.74775279268874,
-1.72428975604382,-1.71690306601617,-1.71175741547485,-1.70952549386682,
-1.70786954981482,-1.7059731570057,-1.7026539429633,-1.68692030590257,-1.6562687506758,
-1.63430523221504,-1.62900326569337,-1.62577481493943,-1.62283043273642,
-1.61905310408836,-1.61274526921994,-1.57627188535292,-1.55644871384975,
-1.5497162003448,-1.54491435786216,-1.54274290088386,-1.54110844267879,
-1.5391809355745,-1.53572311271344,-1.51568507597026,-1.50917683223058,
-1.4875003775627,-1.46739930889587,-1.46221676020551,-1.45901388037046,
-1.45606180447947,-1.45223091089343,-1.44366533127775,-1.40436428711742,
-1.38293799933997,-1.37819723722115,-1.37603676692299,-1.37440333954468,
-1.37246832481659,-1.36897701892388,-1.34581571155995,-1.32858167438782,
-1.30369536362377,-1.29682734142661,-1.29327192886806,-1.29063674894047,
-1.28732873391396,-1.28165570246101,-1.25188183601931,-1.23042656095483,
-1.21927738019487,-1.21456261563906,-1.21090406784536,-1.20895486746383,
-1.20730757669922,-1.20519393951989,-1.20058537384566,-1.1700610192424,
-1.13526077399985,-1.12941051648516,-1.1260649105148,-1.12314187142691,
-1.11950045654299,-1.11243035665219,-1.1090417761794),.UNSPECIFIED.);
#2515=B_SPLINE_CURVE_WITH_KNOTS('',3,(#81559,#81560,#81561,#81562,#81563,
#81564,#81565,#81566,#81567,#81568,#81569,#81570,#81571,#81572,#81573,#81574,
#81575,#81576,#81577,#81578,#81579,#81580,#81581,#81582,#81583,#81584,#81585,
#81586,#81587,#81588,#81589,#81590,#81591,#81592,#81593,#81594,#81595,#81596,
#81597,#81598,#81599,#81600,#81601,#81602,#81603,#81604,#81605,#81606,#81607,
#81608,#81609,#81610,#81611,#81612,#81613,#81614,#81615,#81616,#81617,#81618,
#81619,#81620,#81621,#81622,#81623,#81624,#81625,#81626,#81627,#81628,#81629,
#81630,#81631,#81632,#81633,#81634,#81635,#81636,#81637,#81638,#81639,#81640,
#81641,#81642,#81643,#81644,#81645,#81646,#81647,#81648,#81649,#81650,#81651,
#81652,#81653,#81654,#81655,#81656,#81657,#81658,#81659,#81660,#81661,#81662,
#81663,#81664,#81665,#81666,#81667,#81668,#81669,#81670,#81671,#81672,#81673,
#81674,#81675,#81676,#81677,#81678,#81679,#81680,#81681,#81682,#81683,#81684,
#81685,#81686,#81687,#81688,#81689,#81690,#81691,#81692,#81693,#81694,#81695,
#81696,#81697,#81698,#81699,#81700,#81701,#81702,#81703,#81704,#81705,#81706,
#81707,#81708,#81709,#81710,#81711,#81712,#81713,#81714,#81715,#81716,#81717,
#81718,#81719,#81720,#81721,#81722,#81723,#81724,#81725,#81726,#81727,#81728,
#81729,#81730,#81731,#81732,#81733,#81734,#81735,#81736,#81737,#81738,#81739,
#81740,#81741,#81742,#81743,#81744,#81745,#81746,#81747,#81748,#81749,#81750,
#81751,#81752,#81753,#81754,#81755,#81756,#81757,#81758,#81759,#81760,#81761,
#81762,#81763,#81764,#81765,#81766,#81767,#81768,#81769,#81770,#81771,#81772),
 .UNSPECIFIED.,.F.,.F.,(4,2,2,2,2,2,2,2,2,2,2,2,2,2,2,2,2,2,2,2,2,2,2,2,
2,2,2,2,2,2,2,2,2,2,2,2,2,2,2,2,2,2,2,2,2,2,2,2,2,2,2,2,2,2,2,2,2,2,2,2,
2,2,2,2,2,2,2,2,2,2,2,2,2,2,2,2,2,2,2,2,2,2,2,2,2,2,2,2,2,2,2,2,2,2,2,2,
2,2,2,2,2,2,2,2,2,2,4),(-2.04098557160315,-2.03563970820405,-2.02721151915856,
-2.02154202375354,-2.01922288867902,-2.01755427494498,-2.01570162385464,
-2.01249641222889,-1.99947887565978,-1.96066340863327,-1.94321709398517,
-1.93823899648528,-1.93549755095925,-1.93273585369067,-1.92908317184212,
-1.92196074102959,-1.89115500174544,-1.86728847958394,-1.85983496990153,
-1.85465470693968,-1.85241659378497,-1.85075959027282,-1.84886600631082,
-1.84556022263514,-1.83007058311279,-1.8011943549787,-1.78536820180773,
-1.77819644395789,-1.7723589444424,-1.76901561486162,-1.76609163729158,
-1.76244519612132,-1.75535283932053,-1.72420677790114,-1.70056776856453,
-1.69315177983521,-1.68799087287038,-1.68575610094944,-1.68409954824832,
-1.68220414545671,-1.67889021088619,-1.66323617717807,-1.63246337766471,
-1.6105362474992,-1.60523592518145,-1.60200745612423,-1.59906238096588,
-1.59528320413929,-1.58897003262656,-1.55259277947306,-1.53271181706041,
-1.52596801241401,-1.52116000269857,-1.51898721050742,-1.51735235775532,
-1.51542506572358,-1.51196911578833,-1.49202070237809,-1.48543673595591,
-1.4641707523055,-1.44370011333476,-1.4384918382117,-1.43528307077011,-1.43233214484196,
-1.4285120140822,-1.42001109821947,-1.38064535966,-1.35919967996132,-1.35445672368895,
-1.3522956293284,-1.35066187982258,-1.34872661164412,-1.34523508561935,
-1.32208877616988,-1.30487302360003,-1.27996654209721,-1.27309554531736,
-1.26953915959961,-1.26690346818418,-1.26359506681647,-1.25792196573599,
-1.22812200957773,-1.20660055156191,-1.19551575715169,-1.19081873993744,
-1.18717075868413,-1.18522355643755,-1.18357567627554,-1.18145837843927,
-1.17683093982489,-1.13794433370012,-1.11097138129367,-1.10543147475197,
-1.10215168223015,-1.09921846137134,-1.09547236034357,-1.0894157072123,
-1.04993119268329,-1.0434781664719,-1.02384306614861,-1.02039533237019,
-1.01846985639277,-1.01683470969483,-1.01465909148722,-1.00983545419509,
-1.00306164058815,-0.991163431562309),.UNSPECIFIED.);
#2516=B_SPLINE_CURVE_WITH_KNOTS('',3,(#81773,#81774,#81775,#81776,#81777,
#81778,#81779,#81780,#81781,#81782,#81783,#81784,#81785,#81786,#81787,#81788,
#81789,#81790,#81791,#81792,#81793,#81794,#81795,#81796,#81797,#81798,#81799,
#81800,#81801,#81802,#81803,#81804,#81805,#81806,#81807,#81808,#81809,#81810,
#81811,#81812,#81813,#81814,#81815,#81816,#81817,#81818,#81819,#81820,#81821,
#81822,#81823,#81824,#81825,#81826,#81827,#81828,#81829,#81830,#81831,#81832,
#81833,#81834,#81835,#81836,#81837,#81838,#81839,#81840,#81841,#81842,#81843,
#81844,#81845,#81846,#81847,#81848,#81849,#81850,#81851,#81852,#81853,#81854,
#81855,#81856,#81857,#81858,#81859,#81860,#81861,#81862,#81863,#81864,#81865,
#81866,#81867,#81868,#81869,#81870,#81871,#81872,#81873,#81874,#81875,#81876,
#81877,#81878,#81879,#81880,#81881,#81882,#81883,#81884,#81885,#81886,#81887,
#81888,#81889,#81890,#81891,#81892,#81893,#81894,#81895,#81896,#81897,#81898,
#81899,#81900,#81901,#81902,#81903,#81904,#81905,#81906,#81907,#81908,#81909,
#81910,#81911,#81912,#81913,#81914,#81915,#81916,#81917,#81918,#81919,#81920,
#81921,#81922,#81923,#81924,#81925,#81926,#81927,#81928,#81929,#81930,#81931,
#81932,#81933,#81934,#81935,#81936,#81937,#81938,#81939,#81940,#81941,#81942,
#81943,#81944,#81945,#81946,#81947,#81948,#81949,#81950,#81951,#81952,#81953,
#81954,#81955,#81956,#81957,#81958,#81959,#81960,#81961,#81962,#81963,#81964,
#81965,#81966),.UNSPECIFIED.,.F.,.F.,(4,2,2,2,2,2,2,2,2,2,2,2,2,2,2,2,2,
2,2,2,2,2,2,2,2,2,2,2,2,2,2,2,2,2,2,2,2,2,2,2,2,2,2,2,2,2,2,2,2,2,2,2,2,
2,2,2,2,2,2,2,2,2,2,2,2,2,2,2,2,2,2,2,2,2,2,2,2,2,2,2,2,2,2,2,2,2,2,2,2,
2,2,2,2,2,2,2,4),(-1.1090417761794,-1.07988086625166,-1.05729058618643,
-1.05005201336957,-1.04498318261964,-1.04278824747931,-1.0411321173552,
-1.03923678396174,-1.03583245287252,-1.01633592113168,-0.984416466042156,
-0.967260749509081,-0.962115494665457,-0.958920706854573,-0.955966129746268,
-0.952050792004092,-0.943236889210629,-0.93091574040323,-0.908814707192146,
-0.882920137911538,-0.87817381196359,-0.876035426052958,-0.874385956020462,
-0.872454807990772,-0.86888168237218,-0.864307828480602,-0.820609106792188,
-0.800892714355112,-0.795586543110736,-0.792357561489918,-0.789414002000317,
-0.785575320221527,-0.777199829895772,-0.755202250859291,-0.715897573098805,
-0.711363607055685,-0.709241468934196,-0.707596515637242,-0.705627837219407,
-0.701874296690441,-0.674622394323279,-0.637038786295313,-0.630806184936431,
-0.627050603703619,-0.624109669725413,-0.620871185835822,-0.615520349037995,
-0.592678764357737,-0.560884677171424,-0.547125872121436,-0.543876284284986,
-0.542014563100982,-0.54035005960954,-0.538053428045315,-0.532519087268654,
-0.524362897063695,-0.495770183643399,-0.468199425752467,-0.462555140124699,
-0.459253781368635,-0.456618446620025,-0.453055717410229,-0.446148106701857,
-0.420944683457092,-0.394630088295682,-0.380532404007987,-0.37725912367687,
-0.375392263624808,-0.373729299752075,-0.371443149625252,-0.365972894134721,
-0.357945459765812,-0.330292062635853,-0.301627450836764,-0.295947942145964,
-0.292639065264374,-0.290004763357313,-0.286452589986169,-0.279598008689047,
-0.254810676685214,-0.216118799307858,-0.211914807871398,-0.209822563100135,
-0.208140569202345,-0.206360285111265,-0.203482890147348,-0.193199397885009,
-0.172371538738913,-0.137331708581453,-0.130962802562926,-0.127168680490406,
-0.12422246343744,-0.121003367345744,-0.116909623789973,-0.102586557738656,
-0.0768746775274151,-0.0592762986750658),.UNSPECIFIED.);
#2517=B_SPLINE_CURVE_WITH_KNOTS('',3,(#81972,#81973,#81974,#81975,#81976,
#81977,#81978,#81979,#81980,#81981,#81982,#81983,#81984,#81985,#81986,#81987,
#81988,#81989,#81990,#81991,#81992,#81993,#81994,#81995,#81996,#81997,#81998,
#81999,#82000,#82001,#82002,#82003,#82004,#82005,#82006,#82007,#82008,#82009,
#82010,#82011,#82012,#82013,#82014,#82015,#82016,#82017,#82018,#82019,#82020,
#82021,#82022,#82023,#82024,#82025,#82026,#82027,#82028,#82029,#82030,#82031,
#82032,#82033,#82034,#82035,#82036,#82037,#82038,#82039,#82040,#82041,#82042,
#82043,#82044,#82045,#82046,#82047,#82048,#82049,#82050,#82051,#82052,#82053,
#82054,#82055,#82056,#82057,#82058,#82059,#82060,#82061,#82062,#82063,#82064,
#82065,#82066,#82067,#82068,#82069,#82070,#82071,#82072,#82073,#82074,#82075,
#82076,#82077,#82078,#82079,#82080,#82081,#82082,#82083,#82084,#82085,#82086,
#82087,#82088,#82089,#82090,#82091,#82092,#82093,#82094,#82095,#82096,#82097,
#82098,#82099,#82100,#82101,#82102,#82103,#82104,#82105,#82106,#82107,#82108,
#82109,#82110,#82111,#82112,#82113,#82114,#82115,#82116,#82117,#82118,#82119,
#82120,#82121,#82122,#82123,#82124,#82125,#82126,#82127,#82128,#82129,#82130,
#82131,#82132,#82133,#82134,#82135,#82136,#82137,#82138,#82139,#82140,#82141,
#82142,#82143,#82144,#82145,#82146,#82147,#82148,#82149,#82150,#82151,#82152,
#82153,#82154,#82155,#82156,#82157,#82158,#82159,#82160,#82161,#82162,#82163,
#82164,#82165,#82166,#82167,#82168,#82169,#82170,#82171),.UNSPECIFIED.,
 .F.,.F.,(4,2,2,2,2,2,2,2,2,2,2,2,2,2,2,2,2,2,2,2,2,2,2,2,2,2,2,2,2,2,2,
2,2,2,2,2,2,2,2,2,2,2,2,2,2,2,2,2,2,2,2,2,2,2,2,2,2,2,2,2,2,2,2,2,2,2,2,
2,2,2,2,2,2,2,2,2,2,2,2,2,2,2,2,2,2,2,2,2,2,2,2,2,2,2,2,2,2,2,2,4),(-0.991202703725535,
-0.970522559222933,-0.939735394018657,-0.924083759353349,-0.920770364998682,
-0.918875187784806,-0.917218799597893,-0.914984160051106,-0.909823307970298,
-0.902406305126986,-0.878763531249245,-0.847591869623134,-0.840498787106726,
-0.836852415666169,-0.833928717311233,-0.830585950957878,-0.824750046886789,
-0.817581313403194,-0.801765141945526,-0.772916244083387,-0.757431590730897,
-0.754126590834429,-0.752233314380364,-0.750576505579371,-0.748338509404223,
-0.743158026232733,-0.735702899500169,-0.711828522715385,-0.680959679338312,
-0.673863922461446,-0.670217003808648,-0.667293267545249,-0.663950893619949,
-0.658116822490968,-0.650950967495996,-0.635144617249224,-0.606293266531227,
-0.590796266244502,-0.587490682993342,-0.585597276674732,-0.583940500982808,
-0.581702746118521,-0.576523660374982,-0.569071244836912,-0.545213369345774,
-0.514323086198759,-0.507227541336903,-0.503580670401441,-0.50065694272665,
-0.497314546370527,-0.491480351148642,-0.484314297334193,-0.468507251701242,
-0.439656163517481,-0.424160086739221,-0.420854552255572,-0.418961159077121,
-0.417304384280238,-0.415066616403597,-0.409887439804569,-0.402434842836434,
-0.378575820652435,-0.347687150498304,-0.340591604570006,-0.336944737486079,
-0.334021015030818,-0.330678626959087,-0.324844452304657,-0.317678427094565,
-0.301871463072638,-0.273020412866674,-0.257524300170147,-0.254218768756,
-0.252325378410742,-0.250668606854038,-0.248430844383581,-0.24325168472544,
-0.235799115831433,-0.211940224808054,-0.181091284162821,-0.173971235279214,
-0.170319326718561,-0.16739521036242,-0.164646530503026,-0.159497949413282,
-0.139876617129393,-0.117778325588309,-0.112151591383416,-0.0911956334541362,
-0.087719441072008,-0.0857877513251872,-0.0841537801009711,-0.0819881326914908,
-0.077218999577992,-0.0555041694092805,-0.0133613952491335,-0.00693651896192096,
-0.00347621653055332,-0.0017044654462795,-0.000491452588193953),
 .UNSPECIFIED.);
#2518=B_SPLINE_CURVE_WITH_KNOTS('',3,(#82172,#82173,#82174,#82175,#82176,
#82177,#82178,#82179,#82180,#82181),.UNSPECIFIED.,.F.,.F.,(4,2,2,2,4),(-2.09994892392206,
-2.09740773666934,-2.09305353736742,-2.08013651306197,-2.04098557160315),
 .UNSPECIFIED.);
#2519=B_SPLINE_CURVE_WITH_KNOTS('',3,(#82183,#82184,#82185,#82186,#82187,
#82188,#82189,#82190,#82191,#82192,#82193,#82194,#82195,#82196,#82197,#82198,
#82199,#82200),.UNSPECIFIED.,.F.,.F.,(4,2,2,2,2,2,2,2,4),(-0.0592762986750658,
-0.0495542205447057,-0.0448430910167832,-0.0427112328124616,-0.0410626509152269,
-0.0391275338177746,-0.0370497816162303,-0.0337442454856563,-0.000491569883824227),
 .UNSPECIFIED.);
#2520=B_SPLINE_CURVE_WITH_KNOTS('',3,(#82201,#82202,#82203,#82204,#82205,
#82206,#82207,#82208,#82209,#82210,#82211,#82212,#82213,#82214,#82215,#82216,
#82217,#82218,#82219,#82220,#82221,#82222,#82223,#82224,#82225,#82226,#82227,
#82228,#82229,#82230,#82231,#82232,#82233,#82234,#82235,#82236,#82237,#82238,
#82239,#82240,#82241,#82242,#82243,#82244,#82245,#82246,#82247,#82248,#82249,
#82250,#82251,#82252,#82253,#82254,#82255,#82256,#82257,#82258,#82259,#82260,
#82261,#82262,#82263,#82264,#82265,#82266,#82267,#82268,#82269,#82270,#82271,
#82272,#82273,#82274,#82275,#82276,#82277,#82278,#82279,#82280,#82281,#82282,
#82283,#82284,#82285,#82286,#82287,#82288,#82289,#82290,#82291,#82292,#82293,
#82294,#82295,#82296,#82297,#82298,#82299,#82300,#82301,#82302,#82303,#82304,
#82305,#82306,#82307,#82308,#82309,#82310,#82311,#82312,#82313,#82314,#82315,
#82316,#82317,#82318,#82319,#82320,#82321,#82322,#82323,#82324,#82325,#82326,
#82327,#82328,#82329,#82330,#82331,#82332,#82333,#82334,#82335,#82336,#82337,
#82338,#82339,#82340,#82341,#82342,#82343,#82344,#82345,#82346,#82347,#82348,
#82349,#82350,#82351,#82352,#82353,#82354,#82355,#82356,#82357,#82358,#82359,
#82360,#82361,#82362,#82363,#82364,#82365,#82366,#82367,#82368,#82369,#82370,
#82371,#82372,#82373,#82374,#82375,#82376,#82377,#82378,#82379,#82380,#82381,
#82382,#82383,#82384,#82385,#82386,#82387,#82388,#82389,#82390),
 .UNSPECIFIED.,.F.,.F.,(4,2,2,2,2,2,2,2,2,2,2,2,2,2,2,2,2,2,2,2,2,2,2,2,
2,2,2,2,2,2,2,2,2,2,2,2,2,2,2,2,2,2,2,2,2,2,2,2,2,2,2,2,2,2,2,2,2,2,2,2,
2,2,2,2,2,2,2,2,2,2,2,2,2,2,2,2,2,2,2,2,2,2,2,2,2,2,2,2,2,2,2,2,2,2,4),
(-3.79235008026687,-3.76879104347154,-3.75883026516241,-3.75512635641919,
-3.75226780474209,-3.74932856094105,-3.74607818361715,-3.74067505922862,
-3.71937735048599,-3.68731998843125,-3.67635882076812,-3.67058549835473,
-3.66820568956278,-3.66652741236532,-3.66470137813792,-3.66161693879173,
-3.65015300503789,-3.6219716319717,-3.5933140491505,-3.5877185302108,-3.58442701644351,
-3.58149622845065,-3.57777094090938,-3.57178518594219,-3.53165638983071,
-3.50653993698235,-3.50276659469806,-3.50079349474002,-3.4991484104026,
-3.49703064963911,-3.49252201064742,-3.46095531282508,-3.42698696341232,
-3.42116638000915,-3.4178269176096,-3.41490296122218,-3.41125215266787,
-3.40413722284319,-3.37511937734592,-3.34983534343432,-3.34215632841335,
-3.33686081537245,-3.33460336692293,-3.3329440564725,-3.33106162722549,
-3.32780427023879,-3.31330283380641,-3.28300653913868,-3.26738435055625,
-3.26027265974359,-3.25447355349318,-3.2511387167445,-3.24821432322312,
-3.24455705540249,-3.23741036201886,-3.20777528667571,-3.18301921430959,
-3.17542276176001,-3.17016937059013,-3.16791907195565,-3.16626075763165,
-3.16437457171243,-3.16110049826273,-3.14626360082182,-3.11546827062215,
-3.09275149299329,-3.0874063116763,-3.08416857478599,-3.08122661918422,
-3.07746740143087,-3.07122358693279,-3.03379680981587,-3.00627035238142,
-3.00261077882638,-3.00066136853779,-2.999014108332,-2.99690077018904,-2.99245653363706,
-2.9607122720554,-2.92693317192425,-2.9211019549393,-2.91776039548315,-2.91483692612768,
-2.91118977566164,-2.90409181244655,-2.87352577323981,-2.8494382911359,
-2.84194902811961,-2.83675059471398,-2.83450968654787,-2.83285265165939,
-2.83096142877433,-2.8276649057338,-2.81236115396795,-2.80116782631181),
 .UNSPECIFIED.);
#2521=B_SPLINE_CURVE_WITH_KNOTS('',3,(#82395,#82396,#82397,#82398,#82399,
#82400,#82401,#82402,#82403,#82404,#82405,#82406,#82407,#82408,#82409,#82410,
#82411,#82412,#82413,#82414,#82415,#82416,#82417,#82418,#82419,#82420,#82421,
#82422,#82423,#82424,#82425,#82426,#82427,#82428,#82429,#82430,#82431,#82432,
#82433,#82434,#82435,#82436,#82437,#82438,#82439,#82440,#82441,#82442,#82443,
#82444,#82445,#82446,#82447,#82448,#82449,#82450,#82451,#82452,#82453,#82454,
#82455,#82456,#82457,#82458,#82459,#82460,#82461,#82462,#82463,#82464,#82465,
#82466,#82467,#82468,#82469,#82470,#82471,#82472,#82473,#82474,#82475,#82476,
#82477,#82478,#82479,#82480,#82481,#82482,#82483,#82484,#82485,#82486,#82487,
#82488,#82489,#82490,#82491,#82492,#82493,#82494,#82495,#82496,#82497,#82498,
#82499,#82500,#82501,#82502,#82503,#82504,#82505,#82506,#82507,#82508,#82509,
#82510,#82511,#82512,#82513,#82514,#82515,#82516,#82517,#82518,#82519,#82520,
#82521,#82522,#82523,#82524,#82525,#82526,#82527,#82528,#82529,#82530,#82531,
#82532,#82533,#82534,#82535,#82536,#82537,#82538,#82539,#82540,#82541,#82542,
#82543,#82544,#82545,#82546,#82547,#82548,#82549,#82550,#82551,#82552,#82553,
#82554,#82555,#82556,#82557,#82558,#82559,#82560,#82561,#82562,#82563,#82564,
#82565,#82566,#82567,#82568,#82569,#82570,#82571,#82572,#82573,#82574,#82575,
#82576,#82577,#82578,#82579,#82580,#82581,#82582,#82583,#82584,#82585,#82586,
#82587,#82588,#82589,#82590,#82591,#82592,#82593,#82594,#82595,#82596,#82597,
#82598,#82599,#82600,#82601,#82602,#82603,#82604,#82605,#82606),
 .UNSPECIFIED.,.F.,.F.,(4,2,2,2,2,2,2,2,2,2,2,2,2,2,2,2,2,2,2,2,2,2,2,2,
2,2,2,2,2,2,2,2,2,2,2,2,2,2,2,2,2,2,2,2,2,2,2,2,2,2,2,2,2,2,2,2,2,2,2,2,
2,2,2,2,2,2,2,2,2,2,2,2,2,2,2,2,2,2,2,2,2,2,2,2,2,2,2,2,2,2,2,2,2,2,2,2,
2,2,2,2,2,2,2,2,2,4),(-2.04089325283701,-2.03488002345817,-2.01905373839352,
-2.01188227520751,-2.00604512953212,-2.00270214928738,-1.99977856191135,
-1.99613271797884,-1.98904187672968,-1.95783920246601,-1.93424999138621,
-1.92684271232618,-1.92168647215752,-1.91945267404391,-1.91779642241602,
-1.91590088077647,-1.91258565837322,-1.89694549843513,-1.86614272293891,
-1.84424133897509,-1.83894308347855,-1.83571533796038,-1.83277057751776,
-1.82899132605999,-1.82267694399171,-1.78634047600345,-1.76643820778235,
-1.75969068256678,-1.75488084600167,-1.75270790168013,-1.75107322378854,
-1.74914648520908,-1.74569231611137,-1.7257996322519,-1.7191700797636,-1.69792530801829,
-1.6774333267711,-1.67222413498434,-1.66901545280829,-1.66606503292354,
-1.66224616064027,-1.6537506877938,-1.61438555152277,-1.5929412425914,-1.58819877356428,
-1.58603794271696,-1.58440440997375,-1.58246941923715,-1.57897844440839,
-1.55585755676623,-1.53867538939302,-1.51372775712608,-1.50685199516778,
-1.50329495167688,-1.50065950146912,-1.49735235032511,-1.49168379841302,
-1.4632566528171,-1.4354259318336,-1.42737453362951,-1.42189153944527,-1.41960292161523,
-1.41793919682846,-1.41607264897645,-1.41280229794322,-1.39877347449417,
-1.37238893832772,-1.34946330208362,-1.34105963914633,-1.33721537056422,
-1.33427044600554,-1.33104284422303,-1.32574555533296,-1.30620631217469,
-1.26241419098538,-1.25566910647138,-1.25318988995585,-1.25149344190071,
-1.24970285388847,-1.24678010302129,-1.23704579310809,-1.2291690541304,
-1.1997053828338,-1.17765134794191,-1.17234377622827,-1.1691138822367,-1.16616943338814,
-1.16239372615637,-1.15609239353053,-1.1195233629592,-1.09977209401011,
-1.09305356353447,-1.08825914668566,-1.08608888168716,-1.08445437311293,
-1.08252561696834,-1.0790627881582,-1.05881616229235,-1.05029467310212,
-1.01396627191361,-1.00764867937674,-1.0038684326236,-1.00092340819177,
-0.997695890953684,-0.992399191014008,-0.991202703725535),.UNSPECIFIED.);
#2522=B_SPLINE_CURVE_WITH_KNOTS('',3,(#82607,#82608,#82609,#82610,#82611,
#82612,#82613,#82614,#82615,#82616,#82617,#82618,#82619,#82620,#82621,#82622,
#82623,#82624,#82625,#82626,#82627,#82628,#82629,#82630,#82631,#82632,#82633,
#82634,#82635,#82636,#82637,#82638,#82639,#82640,#82641,#82642,#82643,#82644,
#82645,#82646,#82647,#82648,#82649,#82650,#82651,#82652,#82653,#82654,#82655,
#82656,#82657,#82658,#82659,#82660,#82661,#82662,#82663,#82664,#82665,#82666,
#82667,#82668,#82669,#82670,#82671,#82672,#82673,#82674,#82675,#82676,#82677,
#82678,#82679,#82680,#82681,#82682,#82683,#82684,#82685,#82686,#82687,#82688,
#82689,#82690,#82691,#82692,#82693,#82694,#82695,#82696,#82697,#82698,#82699,
#82700,#82701,#82702,#82703,#82704,#82705,#82706,#82707,#82708,#82709,#82710,
#82711,#82712,#82713,#82714,#82715,#82716,#82717,#82718,#82719,#82720,#82721,
#82722,#82723,#82724,#82725,#82726,#82727,#82728,#82729,#82730,#82731,#82732,
#82733,#82734,#82735,#82736,#82737,#82738,#82739,#82740,#82741,#82742,#82743,
#82744,#82745,#82746,#82747,#82748,#82749,#82750,#82751,#82752,#82753,#82754,
#82755,#82756,#82757,#82758,#82759,#82760,#82761,#82762,#82763,#82764,#82765,
#82766,#82767,#82768,#82769,#82770,#82771,#82772,#82773,#82774,#82775,#82776,
#82777,#82778,#82779,#82780,#82781,#82782,#82783,#82784,#82785,#82786,#82787,
#82788,#82789,#82790,#82791,#82792,#82793,#82794,#82795,#82796,#82797,#82798,
#82799,#82800,#82801,#82802,#82803,#82804,#82805,#82806,#82807,#82808,#82809,
#82810,#82811,#82812,#82813,#82814,#82815,#82816),.UNSPECIFIED.,.F.,.F.,
(4,2,2,2,2,2,2,2,2,2,2,2,2,2,2,2,2,2,2,2,2,2,2,2,2,2,2,2,2,2,2,2,2,2,2,
2,2,2,2,2,2,2,2,2,2,2,2,2,2,2,2,2,2,2,2,2,2,2,2,2,2,2,2,2,2,2,2,2,2,2,2,
2,2,2,2,2,2,2,2,2,2,2,2,2,2,2,2,2,2,2,2,2,2,2,2,2,2,2,2,2,2,2,2,2,4),(-2.80116782631181,
-2.78345590479573,-2.76752029609109,-2.76031694495084,-2.75445961730744,
-2.75111257458051,-2.74818978514135,-2.74455064852746,-2.73749127432704,
-2.70985972968383,-2.68710773507315,-2.6770199676966,-2.67057130291734,
-2.66813428564755,-2.66644599107477,-2.66464174578481,-2.66165588854913,
-2.65128716642556,-2.64412803770998,-2.61526530905202,-2.60027008346914,
-2.59012040289523,-2.58598888338326,-2.58299935706053,-2.57988257312088,
-2.57510423029716,-2.56110563901031,-2.52723649010585,-2.50767777851583,
-2.50312984630463,-2.50100496403787,-2.49951622113102,-2.49761576272922,
-2.49427820286278,-2.47841408752629,-2.44776855049549,-2.42595142674195,
-2.42065845973856,-2.41743208075945,-2.41448738785635,-2.4107066097561,
-2.40438608446808,-2.36814603262279,-2.34817067278152,-2.34140901587174,
-2.33659168369742,-2.3344175340602,-2.33278290413906,-2.3308574243206,-2.32740826826218,
-2.30770686444933,-2.30131499788068,-2.2807009110262,-2.25924717837823,
-2.25397629975452,-2.25075463981858,-2.24780858690943,-2.24401817826321,
-2.23766357188359,-2.20211151093786,-2.17275056624929,-2.16918864667136,
-2.16725981503818,-2.16560993671905,-2.16346797894878,-2.15870199111724,
-2.13274418915726,-2.11067813679549,-2.09836429633697,-2.08955500120654,
-2.08564036330166,-2.08268582671481,-2.07949061657841,-2.07434362233748,
-2.05716749156462,-2.02529865620164,-2.0073898210671,-2.00302406836584,
-2.00093348852086,-1.99944847027742,-1.9975240620685,-1.99408023644856,
-1.97459008553509,-1.96762703131112,-1.94612239807934,-1.93260090140743,
-1.92317158612055,-1.91915349793937,-1.91618292336195,-1.91340858598037,
-1.90879699485854,-1.8961697534092,-1.87477223497412,-1.84064401704851,
-1.83633318782534,-1.83425312099807,-1.83261013002256,-1.83060631706391,
-1.82668138959702,-1.82151666665777,-1.80868719972153,-1.77730233395422,
-1.75908736583416,-1.75389141464338,-1.75137704512006),.UNSPECIFIED.);
#2523=B_SPLINE_CURVE_WITH_KNOTS('',3,(#82822,#82823,#82824,#82825,#82826,
#82827,#82828,#82829,#82830,#82831,#82832,#82833,#82834,#82835,#82836,#82837,
#82838,#82839,#82840,#82841,#82842,#82843,#82844,#82845,#82846,#82847,#82848,
#82849,#82850,#82851,#82852,#82853,#82854,#82855,#82856,#82857,#82858,#82859,
#82860,#82861,#82862,#82863,#82864,#82865,#82866,#82867,#82868,#82869,#82870,
#82871,#82872,#82873,#82874,#82875,#82876,#82877,#82878,#82879,#82880,#82881,
#82882,#82883,#82884,#82885,#82886,#82887,#82888,#82889,#82890,#82891,#82892,
#82893,#82894,#82895,#82896,#82897,#82898,#82899,#82900,#82901,#82902,#82903,
#82904,#82905,#82906,#82907,#82908,#82909,#82910,#82911,#82912,#82913,#82914,
#82915,#82916,#82917,#82918,#82919,#82920,#82921,#82922,#82923,#82924,#82925,
#82926,#82927,#82928,#82929,#82930,#82931,#82932,#82933,#82934,#82935,#82936,
#82937,#82938,#82939,#82940,#82941,#82942,#82943,#82944,#82945,#82946,#82947,
#82948,#82949,#82950,#82951,#82952,#82953,#82954,#82955,#82956,#82957,#82958,
#82959,#82960,#82961,#82962,#82963,#82964,#82965),.UNSPECIFIED.,.F.,.F.,
(4,2,2,2,2,2,2,2,2,2,2,2,2,2,2,2,2,2,2,2,2,2,2,2,2,2,2,2,2,2,2,2,2,2,2,
2,2,2,2,2,2,2,2,2,2,2,2,2,2,2,2,2,2,2,2,2,2,2,2,2,2,2,2,2,2,2,2,2,2,2,2,
4),(-0.701455818686197,-0.698653963592177,-0.691733645617641,-0.67233866922822,
-0.668909941523022,-0.666993636225862,-0.665507204284839,-0.663409406310534,
-0.659028751159122,-0.641051618920354,-0.609116173669334,-0.591917434080134,
-0.586750285374402,-0.58353911656745,-0.580567178226023,-0.576625002024718,
-0.567728957486467,-0.555261715585714,-0.532610357436752,-0.507747248261715,
-0.50296958310099,-0.500814510256348,-0.499142720004325,-0.497165956102399,
-0.493484291703485,-0.466294859234326,-0.430016946196202,-0.423807661692584,
-0.419999365597747,-0.417034130629177,-0.413734538725469,-0.408197743417828,
-0.382292138534256,-0.361569207108754,-0.340175889225034,-0.337002642524091,
-0.334978232915764,-0.333362195540539,-0.331436557804319,-0.327574485585619,
-0.322455936128793,-0.309597496131773,-0.269851509362339,-0.256289974976441,
-0.251669583775284,-0.248672768437047,-0.245813765045003,-0.241891739593872,
-0.232442279509338,-0.218698164151186,-0.197987678407573,-0.193654360067149,
-0.171938229712865,-0.168523693226541,-0.166637316892073,-0.164990049769026,
-0.162823727698003,-0.158373869897881,-0.152163018407613,-0.135220922452886,
-0.103808910639883,-0.0854968837232444,-0.0799212842823975,-0.0764082854379601,
-0.0731161486297614,-0.0686710206803845,-0.058080089679953,-0.0324939177520532,
-0.00750210209393403,-0.00328873696137956,-0.00149728998100912,-2.30206508348421E-6),
 .UNSPECIFIED.);
#2524=B_SPLINE_CURVE_WITH_KNOTS('',3,(#82968,#82969,#82970,#82971,#82972,
#82973,#82974,#82975,#82976,#82977,#82978,#82979,#82980,#82981,#82982,#82983,
#82984,#82985,#82986,#82987,#82988,#82989,#82990,#82991,#82992,#82993,#82994,
#82995,#82996,#82997,#82998,#82999,#83000,#83001,#83002,#83003,#83004,#83005,
#83006,#83007,#83008,#83009,#83010,#83011,#83012,#83013,#83014,#83015,#83016,
#83017,#83018,#83019,#83020,#83021,#83022,#83023,#83024,#83025,#83026,#83027,
#83028,#83029,#83030,#83031,#83032,#83033,#83034,#83035,#83036,#83037,#83038,
#83039,#83040,#83041,#83042,#83043,#83044,#83045,#83046,#83047,#83048,#83049,
#83050,#83051,#83052,#83053,#83054,#83055,#83056,#83057,#83058,#83059,#83060,
#83061,#83062,#83063,#83064,#83065,#83066,#83067,#83068,#83069,#83070,#83071,
#83072,#83073,#83074,#83075,#83076,#83077,#83078,#83079,#83080,#83081,#83082,
#83083,#83084,#83085,#83086,#83087,#83088,#83089,#83090,#83091,#83092,#83093,
#83094,#83095,#83096,#83097,#83098,#83099,#83100,#83101,#83102,#83103,#83104,
#83105,#83106,#83107,#83108,#83109,#83110,#83111,#83112,#83113,#83114,#83115,
#83116,#83117,#83118,#83119,#83120,#83121,#83122,#83123,#83124,#83125,#83126,
#83127,#83128,#83129,#83130,#83131,#83132,#83133,#83134,#83135,#83136,#83137,
#83138,#83139,#83140,#83141,#83142,#83143,#83144,#83145,#83146,#83147,#83148,
#83149,#83150,#83151,#83152,#83153,#83154,#83155,#83156,#83157,#83158,#83159,
#83160,#83161,#83162,#83163,#83164,#83165,#83166,#83167,#83168,#83169,#83170,
#83171,#83172,#83173),.UNSPECIFIED.,.F.,.F.,(4,2,2,2,2,2,2,2,2,2,2,2,2,
2,2,2,2,2,2,2,2,2,2,2,2,2,2,2,2,2,2,2,2,2,2,2,2,2,2,2,2,2,2,2,2,2,2,2,2,
2,2,2,2,2,2,2,2,2,2,2,2,2,2,2,2,2,2,2,2,2,2,2,2,2,2,2,2,2,2,2,2,2,2,2,2,
2,2,2,2,2,2,2,2,2,2,2,2,2,2,2,2,2,4),(-1.97983394230133,-1.97900451886366,
-1.97063146157784,-1.93648801128863,-1.91065213232886,-1.90511696257423,
-1.90181716899311,-1.89885101333463,-1.89504047381688,-1.88882522384161,
-1.84496296546329,-1.82661363535744,-1.82217236919534,-1.8204614449492,
-1.82040777467674,-1.82035415061966,-1.82029977953099,-1.82024373210191,
-1.82018484641563,-1.82012156651851,-1.82005164731877,-1.8199715544604,
-1.81987505596187,-1.81974909698431,-1.81965240054471,-1.81804302975405,
-1.81591017172596,-1.81114898786551,-1.78667034155205,-1.76371333245863,
-1.75116537602916,-1.7422277354903,-1.73827787479246,-1.735304195007,-1.73209500887285,
-1.72693958121286,-1.70956507108421,-1.67774153037674,-1.65983436156657,
-1.65546120451375,-1.65336455111082,-1.65187793303597,-1.64995992905371,
-1.646524764736,-1.62685214439612,-1.62043001027448,-1.59988466043694,-1.57835621247424,
-1.57309756788494,-1.56988924018687,-1.56695957608449,-1.56319662250912,
-1.55495434497435,-1.51513377921272,-1.49350021054638,-1.48874870441909,
-1.48659429026472,-1.48495168817658,-1.48301649259009,-1.47952499891444,
-1.4563828866039,-1.43917887815406,-1.4142276305881,-1.40734606897575,-1.40378450037163,
-1.40114496183966,-1.39783160731943,-1.39214911656198,-1.36018433952475,
-1.33533804670777,-1.32402299358437,-1.32105191789151,-1.31924768161973,
-1.31757339097878,-1.31551911809628,-1.31147543164471,-1.27930347712204,
-1.25674501813584,-1.24345805845707,-1.23890052791752,-1.23582783994372,
-1.23283920424316,-1.22855643497251,-1.21814946913638,-1.18091548599778,
-1.15827711380007,-1.15478865391077,-1.15287488798208,-1.15122243670024,
-1.14905700523686,-1.14434043776846,-1.11913052204263,-1.09622838271795,
-1.08397500647484,-1.07519819064596,-1.07129000843219,-1.0683373432556,
-1.06514129752539,-1.05998664636342,-1.04241427631523,-1.01073053722208,
-0.991436009503103,-0.991428410285835),.UNSPECIFIED.);
#2525=B_SPLINE_CURVE_WITH_KNOTS('',3,(#83179,#83180,#83181,#83182,#83183,
#83184,#83185,#83186),.UNSPECIFIED.,.F.,.F.,(4,1,1,1,1,4),(99.6151588638684,
99.6457915387123,100.643339397058,101.640887255404,102.638435113751,103.635982972097),
 .UNSPECIFIED.);
#2526=B_SPLINE_CURVE_WITH_KNOTS('',3,(#83190,#83191,#83192,#83193,#83194,
#83195,#83196,#83197,#83198,#83199,#83200,#83201,#83202,#83203,#83204,#83205),
 .UNSPECIFIED.,.F.,.F.,(4,3,3,3,3,4),(103.672557568922,103.780375531908,
103.888461548137,103.996693219235,104.105202005396,104.157845013106),
 .UNSPECIFIED.);
#2527=B_SPLINE_CURVE_WITH_KNOTS('',3,(#83206,#83207,#83208,#83209,#83210,
#83211,#83212,#83213,#83214,#83215,#83216,#83217,#83218,#83219,#83220,#83221,
#83222,#83223,#83224,#83225,#83226,#83227,#83228,#83229,#83230,#83231,#83232,
#83233,#83234,#83235,#83236,#83237,#83238,#83239,#83240,#83241,#83242,#83243,
#83244,#83245,#83246,#83247,#83248,#83249,#83250,#83251,#83252,#83253,#83254,
#83255,#83256,#83257,#83258,#83259,#83260,#83261,#83262,#83263,#83264,#83265,
#83266,#83267,#83268,#83269,#83270,#83271,#83272,#83273,#83274,#83275,#83276,
#83277,#83278,#83279,#83280,#83281,#83282,#83283,#83284,#83285,#83286,#83287,
#83288,#83289,#83290,#83291,#83292,#83293,#83294,#83295,#83296,#83297,#83298,
#83299,#83300,#83301,#83302,#83303,#83304,#83305,#83306,#83307,#83308,#83309,
#83310,#83311,#83312,#83313,#83314,#83315,#83316,#83317,#83318,#83319,#83320,
#83321,#83322,#83323,#83324,#83325,#83326,#83327,#83328,#83329),
 .UNSPECIFIED.,.F.,.F.,(4,3,3,3,3,3,3,3,3,3,3,3,3,3,3,3,3,3,3,3,3,3,3,3,
3,3,3,3,3,3,3,3,3,3,3,3,3,3,3,3,3,4),(99.615625602745,99.7194574215928,
99.823296387637,99.9272456323374,100.031256457386,100.135445667234,100.18725683054,
100.291460612789,100.395509455028,100.499436614079,100.603298520284,100.707129923664,
100.810965531,100.91490990262,101.018913196422,101.12309834819,101.184804688886,
101.288871403733,101.392782575209,101.496571828225,101.600295754678,101.703989304635,
101.807687384949,101.911495669506,102.01536347923,102.119415573608,102.182352547233,
102.286727524034,102.390946759316,102.495042311179,102.599071279357,102.703068173021,
102.807067456587,102.911171629233,103.015332769855,103.119670998472,103.179900405579,
103.28927700551,103.398344095977,103.507224113031,103.615874575054,103.672557568463),
 .UNSPECIFIED.);
#2528=B_SPLINE_CURVE_WITH_KNOTS('',3,(#83335,#83336,#83337,#83338,#83339,
#83340,#83341,#83342,#83343,#83344,#83345,#83346,#83347,#83348,#83349,#83350,
#83351,#83352,#83353,#83354,#83355,#83356,#83357,#83358,#83359,#83360,#83361,
#83362,#83363,#83364,#83365,#83366,#83367,#83368,#83369,#83370,#83371,#83372,
#83373,#83374,#83375,#83376,#83377,#83378,#83379,#83380,#83381,#83382,#83383,
#83384,#83385,#83386,#83387,#83388,#83389,#83390,#83391,#83392,#83393,#83394,
#83395,#83396,#83397,#83398,#83399,#83400,#83401,#83402,#83403,#83404,#83405,
#83406,#83407,#83408,#83409,#83410,#83411,#83412,#83413,#83414,#83415,#83416,
#83417,#83418,#83419,#83420,#83421,#83422,#83423,#83424,#83425,#83426,#83427,
#83428,#83429,#83430,#83431,#83432,#83433,#83434,#83435,#83436,#83437,#83438,
#83439,#83440,#83441,#83442,#83443,#83444,#83445,#83446,#83447,#83448,#83449,
#83450,#83451,#83452,#83453,#83454,#83455,#83456,#83457,#83458,#83459,#83460,
#83461),.UNSPECIFIED.,.F.,.F.,(4,3,3,3,3,3,3,3,3,3,3,3,3,3,3,3,3,3,3,3,
3,3,3,3,3,3,3,3,3,3,3,3,3,3,3,3,3,3,3,3,3,3,4),(93.3317490773308,93.4356943203675,
93.5397120063864,93.6438984303392,93.6605043886358,93.7646927373985,93.8687258349393,
93.9726368683761,94.0764824233719,94.1802972760791,94.284116159193,94.3880436609508,
94.492029977504,94.5961981698983,94.6580522469819,94.7622418063083,94.8662761651276,
94.9701885281509,95.0740354540436,95.1778517165687,95.2816720460736,95.3856010393288,
95.4895888750435,95.5937586132198,95.6556001053279,95.7597703830589,95.8637853923205,
95.967678398161,96.071505972573,96.1753029176117,96.2791039919371,96.3830139571369,
96.4869828641112,96.5911340358051,96.653147963674,96.7562487060057,96.8592080768891,
96.9620624522899,97.0688899045384,97.1716683414833,97.2744473203426,97.3772955171232,
97.3893722612836),.UNSPECIFIED.);
#2529=B_SPLINE_CURVE_WITH_KNOTS('',3,(#83462,#83463,#83464,#83465,#83466,
#83467),.UNSPECIFIED.,.F.,.F.,(4,1,1,4),(97.3893748526128,97.6506958220201,
98.6482436803662,99.6151588638684),.UNSPECIFIED.);
#2530=B_SPLINE_CURVE_WITH_KNOTS('',3,(#83469,#83470,#83471,#83472,#83473,
#83474,#83475,#83476,#83477,#83478,#83479,#83480,#83481,#83482,#83483,#83484,
#83485,#83486,#83487,#83488,#83489,#83490,#83491,#83492,#83493,#83494,#83495,
#83496,#83497,#83498,#83499,#83500,#83501,#83502,#83503,#83504,#83505,#83506,
#83507,#83508,#83509,#83510,#83511,#83512,#83513,#83514,#83515,#83516,#83517,
#83518,#83519,#83520,#83521,#83522,#83523,#83524,#83525,#83526,#83527,#83528,
#83529,#83530,#83531,#83532,#83533,#83534,#83535),.UNSPECIFIED.,.F.,.F.,
(4,3,3,3,3,3,3,3,3,3,3,3,3,3,3,3,3,3,3,3,3,3,4),(97.3893722616737,97.4918529892095,
97.5942444088535,97.6965831845408,97.7989059037925,97.9013194298888,98.0037771698216,
98.1064188388956,98.1921611138482,98.2963314227872,98.4003464633012,98.5042395003148,
98.6080671058345,98.7118640818712,98.8156651870409,98.9195751826418,99.0235441198136,
99.1276953210577,99.1897089721943,99.296188129832,99.4002221364742,99.5079238696096,
99.615625602745),.UNSPECIFIED.);
#2531=B_SPLINE_CURVE_WITH_KNOTS('',3,(#83536,#83537,#83538,#83539,#83540,
#83541,#83542,#83543,#83544,#83545,#83546,#83547,#83548,#83549,#83550,#83551,
#83552,#83553,#83554,#83555,#83556,#83557,#83558,#83559,#83560,#83561,#83562,
#83563,#83564,#83565,#83566,#83567,#83568,#83569,#83570,#83571,#83572,#83573,
#83574,#83575,#83576,#83577,#83578,#83579,#83580,#83581,#83582,#83583,#83584,
#83585,#83586,#83587,#83588,#83589,#83590,#83591,#83592,#83593,#83594,#83595,
#83596,#83597,#83598,#83599,#83600,#83601,#83602,#83603,#83604,#83605,#83606,
#83607,#83608,#83609,#83610,#83611,#83612,#83613,#83614,#83615,#83616,#83617,
#83618,#83619,#83620,#83621,#83622,#83623,#83624,#83625,#83626,#83627,#83628,
#83629,#83630,#83631,#83632,#83633,#83634,#83635,#83636,#83637,#83638,#83639,
#83640,#83641,#83642,#83643,#83644,#83645,#83646,#83647,#83648,#83649,#83650,
#83651,#83652,#83653,#83654,#83655,#83656,#83657,#83658,#83659),
 .UNSPECIFIED.,.F.,.F.,(4,3,3,3,3,3,3,3,3,3,3,3,3,3,3,3,3,3,3,3,3,3,3,3,
3,3,3,3,3,3,3,3,3,3,3,3,3,3,3,3,3,4),(93.3327290376809,93.4413841180287,
93.5452716275018,93.6491032997823,93.7529138981754,93.8567381522104,93.9606769597197,
94.0646832349844,94.1688628732916,94.2019696804638,94.3061564126513,94.4101879112232,
94.5140973791007,94.6179413899405,94.7217547219675,94.8255721099723,94.9294981655111,
95.0334830612258,95.1376498879826,95.1995175388099,95.3037016482382,95.4077305168747,
95.5116373568137,95.6154787423622,95.7192894555727,95.8231042350685,95.9270277156885,
96.0310100515411,96.135174369962,96.197065397156,96.3012537430123,96.4052868376805,
96.5091978683075,96.6130434205334,96.7168582705147,96.8206771509499,96.9246046501185,
97.0285909641294,97.1327591540816,97.1946132555021,97.3456022854055,97.3893722612836),
 .UNSPECIFIED.);
#2532=B_SPLINE_CURVE_WITH_KNOTS('',3,(#83665,#83666,#83667,#83668,#83669,
#83670,#83671,#83672,#83673,#83674,#83675,#83676,#83677,#83678,#83679,#83680,
#83681,#83682,#83683,#83684,#83685,#83686,#83687,#83688,#83689,#83690,#83691,
#83692,#83693,#83694,#83695,#83696,#83697,#83698,#83699,#83700,#83701,#83702,
#83703,#83704,#83705,#83706,#83707,#83708,#83709,#83710,#83711,#83712,#83713,
#83714,#83715,#83716,#83717,#83718,#83719,#83720,#83721,#83722,#83723,#83724,
#83725,#83726,#83727,#83728,#83729,#83730,#83731,#83732,#83733,#83734,#83735,
#83736,#83737,#83738,#83739,#83740,#83741,#83742,#83743,#83744,#83745,#83746,
#83747,#83748,#83749,#83750,#83751,#83752,#83753,#83754,#83755,#83756,#83757,
#83758,#83759,#83760,#83761,#83762,#83763,#83764,#83765,#83766,#83767,#83768,
#83769,#83770,#83771,#83772,#83773,#83774,#83775,#83776,#83777,#83778,#83779,
#83780,#83781,#83782,#83783,#83784,#83785),.UNSPECIFIED.,.F.,.F.,(4,3,3,
3,3,3,3,3,3,3,3,3,3,3,3,3,3,3,3,3,3,3,3,3,3,3,3,3,3,3,3,3,3,3,3,3,3,3,3,
3,4),(87.0493974330828,87.1532189759333,87.2570297769115,87.3615766423234,
87.4655324356433,87.5703748371013,87.6752172385592,87.7794034197749,87.8834343624418,
87.9873432698304,88.0911867176639,88.1949994850163,88.2988163075253,88.4027418002447,
88.5067261338019,88.6108924055833,88.6727650969053,88.7769513493665,88.8809823641162,
88.9848913444718,89.0887348657768,89.1925477069926,89.2963646036455,89.4002901704179,
89.5042745780882,89.6084409232665,89.6703129552514,89.7744988577207,89.8785295217727,
89.9824381520657,90.0862813238876,90.1900938167078,90.2939103665602,90.3978355913381,
90.5018196592078,90.60598567173,90.6678608135975,90.7807059010898,90.8932651225515,
91.0053652788941,91.106186953809),.UNSPECIFIED.);
#2533=B_SPLINE_CURVE_WITH_KNOTS('',3,(#83786,#83787,#83788,#83789,#83790,
#83791,#83792,#83793,#83794,#83795,#83796,#83797,#83798,#83799,#83800,#83801,
#83802,#83803,#83804,#83805,#83806,#83807,#83808,#83809,#83810,#83811,#83812,
#83813,#83814,#83815,#83816,#83817,#83818,#83819,#83820,#83821,#83822,#83823,
#83824,#83825,#83826,#83827,#83828,#83829,#83830,#83831,#83832,#83833,#83834,
#83835,#83836,#83837,#83838,#83839,#83840,#83841,#83842,#83843,#83844,#83845,
#83846,#83847,#83848,#83849,#83850,#83851,#83852,#83853,#83854,#83855),
 .UNSPECIFIED.,.F.,.F.,(4,3,3,3,3,3,3,3,3,3,3,3,3,3,3,3,3,3,3,3,3,3,3,4),
(91.106186954104,91.212569719702,91.3190337392315,91.4256926630366,91.5324645384253,
91.6394564162905,91.6654086719436,91.7695954062995,91.873626907053,91.977536377121,
92.0813803901557,92.1851937243787,92.2890111145775,92.3929371722919,92.4969220701752,
92.6010888990659,92.6629565302897,92.7671202580396,92.8711391143289,92.9750481164967,
93.0788912429734,93.1826959325472,93.2865260637055,93.3317490773308),
 .UNSPECIFIED.);
#2534=B_SPLINE_CURVE_WITH_KNOTS('',3,(#83857,#83858,#83859,#83860,#83861,
#83862,#83863,#83864,#83865,#83866,#83867,#83868,#83869,#83870,#83871,#83872,
#83873,#83874,#83875,#83876,#83877,#83878,#83879,#83880,#83881,#83882,#83883,
#83884,#83885,#83886,#83887,#83888,#83889,#83890,#83891,#83892,#83893,#83894,
#83895,#83896,#83897,#83898,#83899,#83900,#83901,#83902,#83903,#83904,#83905,
#83906,#83907,#83908,#83909,#83910,#83911,#83912,#83913,#83914,#83915,#83916,
#83917,#83918,#83919,#83920,#83921,#83922,#83923,#83924,#83925,#83926),
 .UNSPECIFIED.,.F.,.F.,(4,3,3,3,3,3,3,3,3,3,3,3,3,3,3,3,3,3,3,3,3,3,3,4),
(91.106186954104,91.2093261054256,91.3135123575092,91.4175433718793,91.5214523518541,
91.6252958727778,91.7291087136125,91.8329256098846,91.9368511762801,92.040835583575,
92.145001928384,92.2068739637717,92.3110598670734,92.4150905319584,92.5189991630805,
92.6228423357289,92.7266548293718,92.8304713800421,92.9343966056245,93.0383806742926,
93.1425466875947,93.2044218221178,93.3086062150329,93.3327290376809),
 .UNSPECIFIED.);
#2535=B_SPLINE_CURVE_WITH_KNOTS('',3,(#83927,#83928,#83929,#83930,#83931,
#83932,#83933,#83934,#83935,#83936,#83937,#83938,#83939,#83940,#83941,#83942,
#83943,#83944,#83945,#83946,#83947,#83948,#83949,#83950,#83951,#83952,#83953,
#83954,#83955,#83956,#83957,#83958,#83959,#83960,#83961,#83962,#83963,#83964,
#83965,#83966,#83967,#83968,#83969,#83970,#83971,#83972,#83973,#83974,#83975,
#83976,#83977,#83978,#83979,#83980,#83981,#83982,#83983,#83984,#83985,#83986,
#83987,#83988,#83989,#83990,#83991,#83992,#83993,#83994,#83995,#83996,#83997,
#83998,#83999,#84000,#84001,#84002,#84003,#84004,#84005,#84006,#84007,#84008,
#84009,#84010,#84011,#84012,#84013,#84014,#84015,#84016,#84017,#84018,#84019,
#84020,#84021,#84022,#84023,#84024,#84025,#84026,#84027,#84028,#84029,#84030,
#84031,#84032,#84033,#84034,#84035,#84036,#84037,#84038,#84039,#84040,#84041,
#84042,#84043,#84044,#84045,#84046,#84047,#84048,#84049,#84050),
 .UNSPECIFIED.,.F.,.F.,(4,3,3,3,3,3,3,3,3,3,3,3,3,3,3,3,3,3,3,3,3,3,3,3,
3,3,3,3,3,3,3,3,3,3,3,3,3,3,3,3,3,4),(87.0484536449252,87.1526180428666,
87.2191346720412,87.3233208365449,87.427351762735,87.5312606540702,87.6351040861194,
87.7389168379772,87.8427336453024,87.9466591234119,88.0506434426604,88.1548097007605,
88.2166825303873,88.3208687069942,88.4248996453911,88.5288085490268,88.6326519934275,
88.7364647576692,88.8402815773922,88.9442070678346,89.048191399398,89.1523576696502,
89.2142303887334,89.318416520009,89.4224474130143,89.5263562713859,89.6301996706254,
89.7340123898743,89.8378291648382,89.9417546111836,90.0457388989569,90.1499051263774,
90.2117782470795,90.3146405386459,90.4173275776686,90.519916863471,90.6224449017458,
90.7249481124086,90.8275243327546,90.9301371295155,91.0329110104793,91.1061869536468),
 .UNSPECIFIED.);
#2536=B_SPLINE_CURVE_WITH_KNOTS('',3,(#84056,#84057,#84058,#84059,#84060,
#84061,#84062,#84063,#84064,#84065,#84066,#84067,#84068,#84069,#84070,#84071,
#84072,#84073,#84074,#84075,#84076,#84077,#84078,#84079,#84080,#84081,#84082,
#84083,#84084,#84085,#84086,#84087,#84088,#84089,#84090,#84091,#84092,#84093,
#84094,#84095,#84096,#84097,#84098,#84099,#84100,#84101,#84102,#84103,#84104,
#84105,#84106,#84107,#84108,#84109,#84110,#84111,#84112,#84113,#84114,#84115,
#84116,#84117,#84118,#84119,#84120,#84121,#84122,#84123,#84124,#84125,#84126,
#84127,#84128,#84129,#84130,#84131,#84132,#84133,#84134,#84135,#84136,#84137,
#84138,#84139,#84140,#84141,#84142,#84143,#84144,#84145,#84146,#84147,#84148,
#84149,#84150,#84151,#84152,#84153,#84154,#84155,#84156,#84157,#84158,#84159,
#84160,#84161,#84162,#84163,#84164,#84165,#84166,#84167,#84168,#84169,#84170,
#84171,#84172,#84173,#84174,#84175,#84176),.UNSPECIFIED.,.F.,.F.,(4,3,3,
3,3,3,3,3,3,3,3,3,3,3,3,3,3,3,3,3,3,3,3,3,3,3,3,3,3,3,3,3,3,3,3,3,3,3,3,
3,4),(80.7662049517566,80.8702771424413,80.9742116846458,81.0780706111053,
81.1818887201993,81.2857007566465,81.3896149590624,81.4935789052622,81.5977344251198,
81.6899300884827,81.7941162519364,81.8981471771091,82.0020560674793,82.1058994985962,
82.2097122495556,82.3135290560174,82.4174545333221,82.5214388517977,82.6256051091832,
82.6874779468288,82.7916641121974,82.8956950392976,82.9996039316046,83.103447364663,
83.2072601175657,83.3110769259696,83.4150024052014,83.5189867255985,83.6231529848757,
83.6850258051749,83.7892119647545,83.8932428860618,83.997151772598,84.1009951999023,
84.2048079470758,84.3086247497839,84.4125502234095,84.5165345382425,84.6207007920821,
84.682573663521,84.8230016469244),.UNSPECIFIED.);
#2537=B_SPLINE_CURVE_WITH_KNOTS('',3,(#84177,#84178,#84179,#84180,#84181,
#84182,#84183,#84184,#84185,#84186,#84187,#84188,#84189,#84190,#84191,#84192,
#84193,#84194,#84195,#84196,#84197,#84198,#84199,#84200,#84201,#84202,#84203,
#84204,#84205,#84206,#84207,#84208,#84209,#84210,#84211,#84212,#84213,#84214,
#84215,#84216,#84217,#84218,#84219,#84220,#84221,#84222,#84223,#84224,#84225,
#84226,#84227,#84228,#84229,#84230,#84231,#84232,#84233,#84234,#84235,#84236,
#84237,#84238,#84239,#84240,#84241,#84242,#84243,#84244,#84245,#84246),
 .UNSPECIFIED.,.F.,.F.,(4,3,3,3,3,3,3,3,3,3,3,3,3,3,3,3,3,3,3,3,3,3,3,4),
(84.8230016473326,84.9301416316494,85.0325714156837,85.1349307967564,85.2372563939059,
85.3395847740871,85.4420166327826,85.5445096289189,85.647171050854,85.6801215218671,
85.7843076985368,85.8883386369968,85.9922475406958,86.0960909851597,86.1999037494645,
86.3037205692504,86.4076460597552,86.5116303913806,86.6157966616937,86.6776693802132,
86.7818282136128,86.8858513274357,86.9897581895972,87.0493974330828),
 .UNSPECIFIED.);
#2538=B_SPLINE_CURVE_WITH_KNOTS('',3,(#84248,#84249,#84250,#84251,#84252,
#84253,#84254,#84255,#84256,#84257,#84258,#84259,#84260,#84261,#84262,#84263,
#84264,#84265,#84266,#84267,#84268,#84269,#84270,#84271,#84272,#84273,#84274,
#84275,#84276,#84277,#84278,#84279,#84280,#84281,#84282,#84283,#84284,#84285,
#84286,#84287,#84288,#84289,#84290,#84291,#84292,#84293,#84294,#84295,#84296,
#84297,#84298,#84299,#84300,#84301,#84302,#84303,#84304,#84305,#84306,#84307,
#84308,#84309,#84310,#84311,#84312,#84313,#84314),.UNSPECIFIED.,.F.,.F.,
(4,3,3,3,3,3,3,3,3,3,3,3,3,3,3,3,3,3,3,3,3,3,4),(84.8230016473381,84.9376554433318,
85.0527190367478,85.1683359261974,85.2240389553491,85.3282251207077,85.4322560477978,
85.5361649400947,85.6400083731431,85.7438211260357,85.8476379344296,85.9515634136515,
86.0555477340388,86.1597139933064,86.2215868136952,86.3257394075668,86.4297517315697,
86.5336587783484,86.6374954176377,86.7413356684595,86.8451704367942,86.949111266428,
87.0484536449252),.UNSPECIFIED.);
#2539=B_SPLINE_CURVE_WITH_KNOTS('',3,(#84315,#84316,#84317,#84318,#84319,
#84320,#84321,#84322,#84323,#84324,#84325,#84326,#84327,#84328,#84329,#84330,
#84331,#84332,#84333,#84334,#84335,#84336,#84337,#84338,#84339,#84340,#84341,
#84342,#84343,#84344,#84345,#84346,#84347,#84348,#84349,#84350,#84351,#84352,
#84353,#84354,#84355,#84356,#84357,#84358,#84359,#84360,#84361,#84362,#84363,
#84364,#84365,#84366,#84367,#84368,#84369,#84370,#84371,#84372,#84373,#84374,
#84375,#84376,#84377,#84378,#84379,#84380,#84381,#84382,#84383,#84384,#84385,
#84386,#84387,#84388,#84389,#84390,#84391,#84392,#84393,#84394,#84395,#84396,
#84397,#84398,#84399,#84400,#84401,#84402,#84403,#84404,#84405,#84406,#84407,
#84408,#84409,#84410,#84411,#84412,#84413,#84414,#84415,#84416,#84417,#84418,
#84419,#84420,#84421,#84422,#84423,#84424,#84425,#84426,#84427,#84428,#84429,
#84430,#84431,#84432,#84433,#84434,#84435,#84436,#84437,#84438),
 .UNSPECIFIED.,.F.,.F.,(4,3,3,3,3,3,3,3,3,3,3,3,3,3,3,3,3,3,3,3,3,3,3,3,
3,3,3,3,3,3,3,3,3,3,3,3,3,3,3,3,3,4),(80.7657498360629,80.8695687878009,
80.9734984237827,81.0774898067219,81.1816601811464,81.2338475219647,81.3380336854277,
81.442064610614,81.5459735010043,81.6498169321452,81.7536296831326,81.8574464896258,
81.9613719669677,82.0653562854834,82.1695225429137,82.2313953803108,82.3355815440577,
82.4396124695294,82.5435213602058,82.6473647916331,82.7511775429067,82.8549943496858,
82.9589198273108,83.0629041461088,83.1670704038163,83.2289432386569,83.3331294016878,
83.4371603264439,83.541069216408,83.6449126471255,83.7487253976928,83.8525422037707,
83.9564676807057,84.060451998819,84.1646182558581,84.226491097003,84.3322636670966,
84.4378652907378,84.5433026053193,84.6486432054607,84.7539210457271,84.8230016469244),
 .UNSPECIFIED.);
#2540=B_SPLINE_CURVE_WITH_KNOTS('',3,(#84444,#84445,#84446,#84447,#84448,
#84449,#84450,#84451,#84452,#84453,#84454,#84455,#84456,#84457,#84458,#84459,
#84460,#84461,#84462,#84463,#84464,#84465,#84466,#84467,#84468,#84469,#84470,
#84471,#84472,#84473,#84474,#84475,#84476,#84477,#84478,#84479,#84480,#84481,
#84482,#84483,#84484,#84485,#84486,#84487,#84488,#84489,#84490,#84491,#84492,
#84493,#84494,#84495,#84496,#84497,#84498,#84499,#84500,#84501,#84502,#84503,
#84504,#84505,#84506,#84507,#84508,#84509,#84510,#84511,#84512,#84513,#84514,
#84515,#84516,#84517,#84518,#84519,#84520,#84521,#84522,#84523,#84524,#84525,
#84526,#84527,#84528,#84529,#84530,#84531,#84532,#84533,#84534,#84535,#84536,
#84537,#84538,#84539,#84540,#84541,#84542,#84543,#84544,#84545,#84546,#84547,
#84548,#84549,#84550,#84551,#84552,#84553,#84554,#84555,#84556,#84557,#84558,
#84559,#84560,#84561,#84562,#84563,#84564,#84565,#84566,#84567,#84568,#84569,
#84570),.UNSPECIFIED.,.F.,.F.,(4,3,3,3,3,3,3,3,3,3,3,3,3,3,3,3,3,3,3,3,
3,3,3,3,3,3,3,3,3,3,3,3,3,3,3,3,3,3,3,3,3,3,4),(74.4820670614279,74.586086530966,
74.6902747630355,74.7070950800601,74.8112812435426,74.9153121687491,75.0192210591604,
75.1230644903229,75.2268772413324,75.3306940478484,75.4346195252135,75.538603843753,
75.6427701012071,75.7046429384062,75.8088291018885,75.9128600270946,76.0167689175055,
76.1206123486675,76.2244250996763,76.3282419061915,76.4321673835557,76.5361517020942,
76.6403179595472,76.7021907967523,76.8063769602756,76.9104078855229,77.014316775975,
77.1181602071782,77.2219729582282,77.3257897647846,77.4297152421893,77.5336995607682,
77.637865818261,77.6997386550984,77.8047483656351,77.9072108121554,78.0095758369095,
78.11188016269,78.2188642068654,78.3212057259318,78.423587071241,78.5260937325055,
78.5398163393917),.UNSPECIFIED.);
#2541=B_SPLINE_CURVE_WITH_KNOTS('',3,(#84571,#84572,#84573,#84574,#84575,
#84576,#84577,#84578,#84579,#84580,#84581,#84582,#84583,#84584,#84585,#84586,
#84587,#84588,#84589,#84590,#84591,#84592,#84593,#84594,#84595,#84596,#84597,
#84598,#84599,#84600,#84601,#84602,#84603,#84604,#84605,#84606,#84607,#84608,
#84609,#84610,#84611,#84612,#84613,#84614,#84615,#84616,#84617,#84618,#84619,
#84620,#84621,#84622,#84623,#84624,#84625,#84626,#84627,#84628,#84629,#84630,
#84631,#84632,#84633,#84634,#84635,#84636,#84637),.UNSPECIFIED.,.F.,.F.,
(4,3,3,3,3,3,3,3,3,3,3,3,3,3,3,3,3,3,3,3,3,3,4),(78.5398163397448,78.6972865134445,
78.8014726769072,78.9055036020933,79.0094124924833,79.113255923624,79.217068674611,
79.3208854811044,79.4248109584459,79.5287952769616,79.6329615343917,79.6948343717905,
79.7990205355389,79.9030514610121,80.0069603516901,80.1108037831191,80.2146165343943,
80.3184333411751,80.4223588188016,80.5263431376011,80.6305093953101,80.6923822301366,
80.7662049517566),.UNSPECIFIED.);
#2542=B_SPLINE_CURVE_WITH_KNOTS('',3,(#84639,#84640,#84641,#84642,#84643,
#84644,#84645,#84646,#84647,#84648,#84649,#84650,#84651,#84652,#84653,#84654,
#84655,#84656,#84657,#84658,#84659,#84660,#84661,#84662,#84663,#84664,#84665,
#84666,#84667,#84668,#84669,#84670,#84671,#84672,#84673,#84674,#84675,#84676,
#84677,#84678,#84679,#84680,#84681,#84682,#84683,#84684,#84685,#84686,#84687,
#84688,#84689,#84690,#84691,#84692,#84693,#84694,#84695,#84696,#84697,#84698,
#84699,#84700,#84701,#84702,#84703,#84704,#84705),.UNSPECIFIED.,.F.,.F.,
(4,3,3,3,3,3,3,3,3,3,3,3,3,3,3,3,3,3,3,3,3,3,4),(78.5398163397448,78.6430480181452,
78.7462408135878,78.849430289094,78.9527248465251,79.0560730499682,79.1596112159241,
79.2387518052725,79.3429379687956,79.4469688940427,79.5508777844945,79.6547212156975,
79.7585339667471,79.8623507733033,79.9662762507078,80.0702605692864,80.174426826779,
80.2362996636186,80.3404816764164,80.446798716328,80.5507036981358,80.6582267670993,
80.7657498360629),.UNSPECIFIED.);
#2543=B_SPLINE_CURVE_WITH_KNOTS('',3,(#84706,#84707,#84708,#84709,#84710,
#84711,#84712,#84713,#84714,#84715,#84716,#84717,#84718,#84719,#84720,#84721,
#84722,#84723,#84724,#84725,#84726,#84727,#84728,#84729,#84730,#84731,#84732,
#84733,#84734,#84735,#84736,#84737,#84738,#84739,#84740,#84741,#84742,#84743,
#84744,#84745,#84746,#84747,#84748,#84749,#84750,#84751,#84752,#84753,#84754,
#84755,#84756,#84757,#84758,#84759,#84760,#84761,#84762,#84763,#84764,#84765,
#84766,#84767,#84768,#84769,#84770,#84771,#84772,#84773,#84774,#84775,#84776,
#84777,#84778,#84779,#84780,#84781,#84782,#84783,#84784,#84785,#84786,#84787,
#84788,#84789,#84790,#84791,#84792,#84793,#84794,#84795,#84796,#84797,#84798,
#84799,#84800,#84801,#84802,#84803,#84804,#84805,#84806,#84807,#84808,#84809,
#84810,#84811,#84812,#84813,#84814,#84815,#84816,#84817,#84818,#84819,#84820,
#84821,#84822,#84823,#84824,#84825,#84826,#84827,#84828,#84829),
 .UNSPECIFIED.,.F.,.F.,(4,3,3,3,3,3,3,3,3,3,3,3,3,3,3,3,3,3,3,3,3,3,3,3,
3,3,3,3,3,3,3,3,3,3,3,3,3,3,3,3,3,4),(74.4832484951464,74.5871391658907,
74.690972419831,74.7947830229148,74.8986057057301,75.0025419983178,75.1065443425921,
75.2107214275004,75.2485603718882,75.3527465353754,75.4567774605867,75.5606863510026,
75.6645297821697,75.7683425331835,75.8721593397041,75.9760848170733,76.080069135617,
76.1842353930752,76.2461082302343,76.350294393727,76.454325318944,76.5582342093655,
76.6620776405382,76.7658903915577,76.8697071980837,76.9736326754586,77.0776169940078,
77.1817832514714,77.2436560885804,77.3478422520627,77.451873177269,77.5557820676804,
77.6596254988429,77.7634382498522,77.8672550563685,77.9711805337336,78.0751648522732,
78.1793311097274,78.2412039469264,78.3682032552001,78.4934616304961,78.5398163394136),
 .UNSPECIFIED.);
#2544=B_SPLINE_CURVE_WITH_KNOTS('',3,(#84835,#84836,#84837,#84838,#84839,
#84840,#84841,#84842,#84843,#84844,#84845,#84846,#84847,#84848,#84849,#84850,
#84851,#84852,#84853,#84854,#84855,#84856,#84857,#84858,#84859,#84860,#84861,
#84862,#84863,#84864,#84865,#84866,#84867,#84868,#84869,#84870,#84871,#84872,
#84873,#84874,#84875,#84876,#84877,#84878,#84879,#84880,#84881,#84882,#84883,
#84884,#84885,#84886,#84887,#84888,#84889,#84890,#84891,#84892,#84893,#84894,
#84895,#84896,#84897,#84898,#84899,#84900,#84901,#84902,#84903,#84904,#84905,
#84906,#84907,#84908,#84909,#84910,#84911,#84912,#84913,#84914,#84915,#84916,
#84917,#84918,#84919,#84920,#84921,#84922,#84923,#84924,#84925,#84926,#84927,
#84928,#84929,#84930,#84931,#84932,#84933,#84934,#84935,#84936,#84937,#84938,
#84939,#84940,#84941,#84942,#84943,#84944,#84945,#84946,#84947,#84948,#84949,
#84950,#84951,#84952,#84953,#84954,#84955),.UNSPECIFIED.,.F.,.F.,(4,3,3,
3,3,3,3,3,3,3,3,3,3,3,3,3,3,3,3,3,3,3,3,3,3,3,3,3,3,3,3,3,3,3,3,3,3,3,3,
3,4),(68.1995463442873,68.303357160343,68.4079698527532,68.5119255604329,
68.6168667452082,68.7218079299836,68.8259940934717,68.9300250186839,69.0339339091008,
69.1377773402689,69.2415900912838,69.3454068978052,69.4493323751756,69.5533166937201,
69.6574829511793,69.7193557883297,69.8235419518176,69.9275728770298,70.0314817674466,
70.1353251986145,70.2391379496291,70.3429547561503,70.4468802335205,70.5508645520649,
70.655030809524,70.7169036466758,70.8210898101647,70.9251207353772,71.0290296257948,
71.1328730569634,71.2366858079789,71.3405026145003,71.4444280918713,71.5484124104167,
71.6525786678765,71.7144515050219,71.8220784528936,71.9307165978115,72.0379272940082,
72.1472791632867,72.2566310325652),.UNSPECIFIED.);
#2545=B_SPLINE_CURVE_WITH_KNOTS('',3,(#84956,#84957,#84958,#84959,#84960,
#84961,#84962,#84963,#84964,#84965,#84966,#84967,#84968,#84969,#84970,#84971,
#84972,#84973,#84974,#84975,#84976,#84977,#84978,#84979,#84980,#84981,#84982,
#84983,#84984,#84985,#84986,#84987,#84988,#84989,#84990,#84991,#84992,#84993,
#84994,#84995,#84996,#84997,#84998,#84999,#85000,#85001,#85002,#85003,#85004,
#85005,#85006,#85007,#85008,#85009,#85010,#85011,#85012,#85013,#85014,#85015,
#85016,#85017,#85018,#85019,#85020,#85021,#85022),.UNSPECIFIED.,.F.,.F.,
(4,3,3,3,3,3,3,3,3,3,3,3,3,3,3,3,3,3,3,3,3,3,4),(72.2566310330054,72.3704731155961,
72.4818133112498,72.5969063373089,72.711999363368,72.8161855268551,72.9202164520663,
73.0241253424822,73.1279687736492,73.231781524663,73.3355983311835,73.4395238085528,
73.5435081270964,73.6476743845545,73.709547221714,73.8137037279895,73.9177183838733,
74.021626189057,74.1254620178884,74.2292882438035,74.3331083624519,74.437001647525,
74.4820670614279),.UNSPECIFIED.);
#2546=B_SPLINE_CURVE_WITH_KNOTS('',3,(#85024,#85025,#85026,#85027,#85028,
#85029,#85030,#85031,#85032,#85033,#85034,#85035,#85036,#85037,#85038,#85039,
#85040,#85041,#85042,#85043,#85044,#85045,#85046,#85047,#85048,#85049,#85050,
#85051,#85052,#85053,#85054,#85055,#85056,#85057,#85058,#85059,#85060,#85061,
#85062,#85063,#85064,#85065,#85066,#85067,#85068,#85069,#85070,#85071,#85072,
#85073,#85074,#85075,#85076,#85077,#85078,#85079,#85080,#85081,#85082,#85083,
#85084,#85085,#85086,#85087,#85088,#85089,#85090,#85091,#85092,#85093),
 .UNSPECIFIED.,.F.,.F.,(4,3,3,3,3,3,3,3,3,3,3,3,3,3,3,3,3,3,3,3,3,3,3,4),
(72.2566310325652,72.3608036974115,72.4648211348936,72.5687165871306,72.6725466326848,
72.7763460710619,72.8801496583902,72.9840619405009,73.0880331866151,73.1921861589882,
73.253464655196,73.3576508186848,73.4616817438974,73.565590634315,73.6694340654837,
73.7732468164993,73.8770636230215,73.9809891003924,74.0849734189378,74.1891396763976,
74.2510125135421,74.3552035653643,74.4592285306948,74.4832484951464),
 .UNSPECIFIED.);
#2547=B_SPLINE_CURVE_WITH_KNOTS('',3,(#85094,#85095,#85096,#85097,#85098,
#85099,#85100,#85101,#85102,#85103,#85104,#85105,#85106,#85107,#85108,#85109,
#85110,#85111,#85112,#85113,#85114,#85115,#85116,#85117,#85118,#85119,#85120,
#85121,#85122,#85123,#85124,#85125,#85126,#85127,#85128,#85129,#85130,#85131,
#85132,#85133,#85134,#85135,#85136,#85137,#85138,#85139,#85140,#85141,#85142,
#85143,#85144,#85145,#85146,#85147,#85148,#85149,#85150,#85151,#85152,#85153,
#85154,#85155,#85156,#85157,#85158,#85159,#85160,#85161,#85162,#85163,#85164,
#85165,#85166,#85167,#85168,#85169,#85170,#85171,#85172,#85173,#85174,#85175,
#85176,#85177,#85178,#85179,#85180,#85181,#85182,#85183,#85184,#85185,#85186,
#85187,#85188,#85189,#85190,#85191,#85192,#85193,#85194,#85195,#85196,#85197,
#85198,#85199,#85200,#85201,#85202,#85203,#85204,#85205,#85206,#85207,#85208,
#85209,#85210,#85211,#85212,#85213,#85214,#85215,#85216,#85217,#85218,#85219,
#85220),.UNSPECIFIED.,.F.,.F.,(4,3,3,3,3,3,3,3,3,3,3,3,3,3,3,3,3,3,3,3,
3,3,3,3,3,3,3,3,3,3,3,3,3,3,3,3,3,3,3,3,3,3,4),(68.1991404978387,68.2657253634656,
68.3699115269538,68.473942452166,68.5778513425829,68.6816947737511,68.785507524766,
68.8893243312875,68.9932498086579,69.0972341272027,69.2014003846619,69.2632732218117,
69.3674593852998,69.4714903105119,69.5753992009289,69.6792426320969,69.7830553831118,
69.8868721896332,69.9907976670036,70.0947819855483,70.1989482430075,70.2608210801578,
70.365007243646,70.4690381688583,70.5729470592753,70.6767904904435,70.7806032414585,
70.8844200479801,70.9883455253506,71.0923298438955,71.1964961013548,71.2583689385038,
71.3625551019919,71.466586027204,71.5704949176209,71.674338348789,71.7781510998038,
71.8819679063252,71.9858933836955,72.0898777022403,72.1940439596994,72.2559167968499,
72.2566310325397),.UNSPECIFIED.);
#2548=B_SPLINE_CURVE_WITH_KNOTS('',3,(#85226,#85227,#85228,#85229,#85230,
#85231,#85232,#85233,#85234,#85235,#85236,#85237,#85238,#85239,#85240,#85241,
#85242,#85243,#85244,#85245,#85246,#85247,#85248,#85249,#85250,#85251,#85252,
#85253,#85254,#85255,#85256,#85257,#85258,#85259,#85260,#85261,#85262,#85263,
#85264,#85265,#85266,#85267,#85268,#85269,#85270,#85271,#85272,#85273,#85274,
#85275,#85276,#85277,#85278,#85279,#85280,#85281,#85282,#85283,#85284,#85285,
#85286,#85287,#85288,#85289,#85290,#85291,#85292,#85293,#85294,#85295,#85296,
#85297,#85298,#85299,#85300,#85301,#85302,#85303,#85304,#85305,#85306,#85307,
#85308,#85309,#85310,#85311,#85312,#85313,#85314,#85315,#85316,#85317,#85318,
#85319,#85320,#85321,#85322,#85323,#85324,#85325,#85326,#85327,#85328,#85329,
#85330,#85331,#85332,#85333,#85334,#85335,#85336,#85337,#85338,#85339,#85340,
#85341,#85342,#85343,#85344,#85345,#85346),.UNSPECIFIED.,.F.,.F.,(4,3,3,
3,3,3,3,3,3,3,3,3,3,3,3,3,3,3,3,3,3,3,3,3,3,3,3,3,3,3,3,3,3,3,3,3,3,3,3,
3,4),(61.9168706104259,62.0208051506025,62.1246640759619,62.2284821848811,
62.3322942220771,62.4362084258424,62.5401723742201,62.6443278953337,62.7365207799071,
62.8407069433953,62.9447378686075,63.0486467590245,63.1524901901926,63.2563029412075,
63.3601197477291,63.4640452250995,63.5680295436442,63.6721958011035,63.7340686382532,
63.8382548017414,63.9422857269535,64.0461946173705,64.1500380485386,64.2538507995536,
64.357667606075,64.4615930834454,64.5655774019902,64.6697436594494,64.7316164965993,
64.8358026600875,64.9398335852996,65.0437424757166,65.1475859068847,65.2513986578996,
65.3552154644213,65.4591409417916,65.5631252603364,65.6672915177956,65.7291643549453,
65.8652061647553,65.973445725137),.UNSPECIFIED.);
#2549=B_SPLINE_CURVE_WITH_KNOTS('',3,(#85347,#85348,#85349,#85350,#85351,
#85352,#85353,#85354,#85355,#85356,#85357,#85358,#85359,#85360,#85361,#85362,
#85363,#85364,#85365,#85366,#85367,#85368,#85369,#85370,#85371,#85372,#85373,
#85374,#85375,#85376,#85377,#85378,#85379,#85380,#85381,#85382,#85383,#85384,
#85385,#85386,#85387,#85388,#85389,#85390,#85391,#85392,#85393,#85394,#85395,
#85396,#85397,#85398,#85399,#85400,#85401,#85402,#85403,#85404,#85405,#85406,
#85407,#85408,#85409,#85410,#85411,#85412,#85413,#85414,#85415,#85416),
 .UNSPECIFIED.,.F.,.F.,(4,3,3,3,3,3,3,3,3,3,3,3,3,3,3,3,3,3,3,3,3,3,3,4),
(65.9734457253856,66.07613177282,66.1787500761625,66.2813369783484,66.3839287747715,
66.4866268116115,66.5893873525257,66.6923186639464,66.7267122132914,66.8308983767795,
66.9349293019917,67.0388381924086,67.1426816235766,67.2464943745915,67.3503111811129,
67.4542366584833,67.558220977028,67.6623872344871,67.7242600716375,67.8284495541671,
67.9324611612316,68.036369644885,68.1402112750346,68.1995463442873),
 .UNSPECIFIED.);
#2550=B_SPLINE_CURVE_WITH_KNOTS('',3,(#85418,#85419,#85420,#85421,#85422,
#85423,#85424,#85425,#85426,#85427,#85428,#85429,#85430,#85431,#85432,#85433,
#85434,#85435,#85436,#85437,#85438,#85439,#85440,#85441,#85442,#85443,#85444,
#85445,#85446,#85447,#85448,#85449,#85450,#85451,#85452,#85453,#85454,#85455,
#85456,#85457,#85458,#85459,#85460,#85461,#85462,#85463,#85464,#85465,#85466,
#85467,#85468,#85469,#85470,#85471,#85472,#85473,#85474,#85475,#85476,#85477,
#85478,#85479,#85480,#85481,#85482,#85483,#85484),.UNSPECIFIED.,.F.,.F.,
(4,3,3,3,3,3,3,3,3,3,3,3,3,3,3,3,3,3,3,3,3,3,4),(65.9734457257113,66.0987387056004,
66.225833092448,66.2706296467734,66.3748158102615,66.4788467354737,66.5827556258906,
66.6865990570587,66.7904118080736,66.8942286145952,66.9981540919656,67.1021384105103,
67.2063046679696,67.2681775051195,67.3723684093497,67.4763780578101,67.580285456456,
67.684125467286,67.7879328708108,67.8918030347045,67.995700077725,68.099756768058,
68.1991404978387),.UNSPECIFIED.);
#2551=B_SPLINE_CURVE_WITH_KNOTS('',3,(#85485,#85486,#85487,#85488,#85489,
#85490,#85491,#85492,#85493,#85494,#85495,#85496,#85497,#85498,#85499,#85500,
#85501,#85502,#85503,#85504,#85505,#85506,#85507,#85508,#85509,#85510,#85511,
#85512,#85513,#85514,#85515,#85516,#85517,#85518,#85519,#85520,#85521,#85522,
#85523,#85524,#85525,#85526,#85527,#85528,#85529,#85530,#85531,#85532,#85533,
#85534,#85535,#85536,#85537,#85538,#85539,#85540,#85541,#85542,#85543,#85544,
#85545,#85546,#85547,#85548,#85549,#85550,#85551,#85552,#85553,#85554,#85555,
#85556,#85557,#85558,#85559,#85560,#85561,#85562,#85563,#85564,#85565,#85566,
#85567,#85568,#85569,#85570,#85571,#85572,#85573,#85574,#85575,#85576,#85577,
#85578,#85579,#85580,#85581,#85582,#85583,#85584,#85585,#85586,#85587,#85588,
#85589,#85590,#85591,#85592,#85593,#85594,#85595,#85596,#85597,#85598,#85599,
#85600,#85601,#85602,#85603,#85604,#85605,#85606,#85607,#85608),
 .UNSPECIFIED.,.F.,.F.,(4,3,3,3,3,3,3,3,3,3,3,3,3,3,3,3,3,3,3,3,3,3,3,3,
3,3,3,3,3,3,3,3,3,3,3,3,3,3,3,3,3,4),(61.9159031139283,62.0198326362226,
62.1238238284354,62.2279940894635,62.2804382133891,62.3846243768772,62.4886553020894,
62.5925641925064,62.6964076236745,62.8002203746894,62.9040371812111,63.0079626585815,
63.1119469771264,63.2161132345856,63.2779860717351,63.3821722352233,63.4862031604358,
63.5901120508527,63.6939554820209,63.7977682330357,63.9015850395574,64.0055105169278,
64.1094948354724,64.2136610929316,64.2755339300812,64.3797200935694,64.4837510187815,
64.5876599091985,64.6915033403665,64.7953160913815,64.8991328979027,65.0030583752731,
65.1070426938177,65.2112089512769,65.2730817884273,65.376601737324,65.4799760620944,
65.583240636246,65.6864470474333,65.789616042058,65.8928309399417,65.9734457253856),
 .UNSPECIFIED.);
#2552=B_SPLINE_CURVE_WITH_KNOTS('',3,(#85614,#85615,#85616,#85617,#85618,
#85619,#85620,#85621,#85622,#85623,#85624,#85625,#85626,#85627,#85628,#85629,
#85630,#85631,#85632,#85633,#85634,#85635,#85636,#85637,#85638,#85639,#85640,
#85641,#85642,#85643,#85644,#85645,#85646,#85647,#85648,#85649,#85650,#85651,
#85652,#85653,#85654,#85655,#85656,#85657,#85658,#85659,#85660,#85661,#85662,
#85663,#85664,#85665,#85666,#85667,#85668,#85669,#85670,#85671,#85672,#85673,
#85674,#85675,#85676,#85677,#85678,#85679,#85680,#85681,#85682,#85683,#85684,
#85685,#85686,#85687,#85688,#85689,#85690,#85691,#85692,#85693,#85694,#85695,
#85696,#85697,#85698,#85699,#85700,#85701,#85702,#85703,#85704,#85705,#85706,
#85707,#85708,#85709,#85710,#85711,#85712,#85713,#85714,#85715,#85716,#85717,
#85718,#85719,#85720,#85721,#85722,#85723,#85724,#85725,#85726,#85727,#85728,
#85729,#85730,#85731,#85732,#85733,#85734,#85735,#85736,#85737),
 .UNSPECIFIED.,.F.,.F.,(4,3,3,3,3,3,3,3,3,3,3,3,3,3,3,3,3,3,3,3,3,3,3,3,
3,3,3,3,3,3,3,3,3,3,3,3,3,3,3,3,3,4),(55.6326045181743,55.7367927089603,
55.7536857714845,55.8578719349726,55.9619028601848,56.0658117506018,56.1696551817699,
56.2734679327848,56.3772847393064,56.4812102166767,56.5851945352215,56.6893607926807,
56.7512336298306,56.8554197933188,56.959450718531,57.0633596089479,57.1672030401161,
57.271015791131,57.3748325976526,57.478758075023,57.5827423935677,57.6869086510269,
57.7487814881766,57.8529676516647,57.9569985768769,58.0609074672939,58.1647508984619,
58.2685636494768,58.3723804559983,58.4763059333687,58.5802902519134,58.6844565093726,
58.7463293465227,58.8496743122095,58.9547475754165,59.0578171667581,59.1608249277454,
59.2638067574364,59.3704201725438,59.4735201525633,59.5818902852146,59.6902604178659),
 .UNSPECIFIED.);
#2553=B_SPLINE_CURVE_WITH_KNOTS('',3,(#85738,#85739,#85740,#85741,#85742,
#85743,#85744,#85745,#85746,#85747,#85748,#85749,#85750,#85751,#85752,#85753,
#85754,#85755,#85756,#85757,#85758,#85759,#85760,#85761,#85762,#85763,#85764,
#85765,#85766,#85767,#85768,#85769,#85770,#85771,#85772,#85773,#85774,#85775,
#85776,#85777,#85778,#85779,#85780,#85781,#85782,#85783,#85784,#85785,#85786,
#85787,#85788,#85789,#85790,#85791,#85792,#85793,#85794,#85795,#85796,#85797,
#85798,#85799,#85800,#85801,#85802,#85803,#85804,#85805,#85806,#85807),
 .UNSPECIFIED.,.F.,.F.,(4,3,3,3,3,3,3,3,3,3,3,3,3,3,3,3,3,3,3,3,3,3,3,4),
(59.690260418206,59.7438772048688,59.8480633683569,59.9520942935691,60.0560031839861,
60.1598466151541,60.2636593661691,60.3674761726906,60.471401650061,60.5753859686057,
60.679552226065,60.7414250632149,60.8456112267031,60.9496421519151,61.0535510423321,
61.1573944735002,61.2612072245151,61.3650240310367,61.468949508407,61.5729338269518,
61.677100084411,61.738972921561,61.8431345897348,61.9168706104259),
 .UNSPECIFIED.);
#2554=B_SPLINE_CURVE_WITH_KNOTS('',3,(#85809,#85810,#85811,#85812,#85813,
#85814,#85815,#85816,#85817,#85818,#85819,#85820,#85821,#85822,#85823,#85824,
#85825,#85826,#85827,#85828,#85829,#85830,#85831,#85832,#85833,#85834,#85835,
#85836,#85837,#85838,#85839,#85840,#85841,#85842,#85843,#85844,#85845,#85846,
#85847,#85848,#85849,#85850,#85851,#85852,#85853,#85854,#85855,#85856,#85857,
#85858,#85859,#85860,#85861,#85862,#85863,#85864,#85865,#85866,#85867,#85868,
#85869,#85870,#85871,#85872,#85873,#85874,#85875),.UNSPECIFIED.,.F.,.F.,
(4,3,3,3,3,3,3,3,3,3,3,3,3,3,3,3,3,3,3,3,3,3,4),(59.690260418206,59.7955628120766,
59.9009059652378,60.0064057077464,60.1119895277645,60.2177899509134,60.2853424966969,
60.3895286601851,60.4935595853974,60.5974684758143,60.7013119069825,60.8051246579974,
60.9089414645189,61.0128669418892,61.116851260434,61.2210175178932,61.282890355043,
61.3870598972607,61.4910835282165,61.5972884246445,61.701128313575,61.8085157137517,
61.9159031139283),.UNSPECIFIED.);
#2555=B_SPLINE_CURVE_WITH_KNOTS('',3,(#85876,#85877,#85878,#85879,#85880,
#85881,#85882,#85883,#85884,#85885,#85886,#85887,#85888,#85889,#85890,#85891,
#85892,#85893,#85894,#85895,#85896,#85897,#85898,#85899,#85900,#85901,#85902,
#85903,#85904,#85905,#85906,#85907,#85908,#85909,#85910,#85911,#85912,#85913,
#85914,#85915,#85916,#85917,#85918,#85919,#85920,#85921,#85922,#85923,#85924,
#85925,#85926,#85927,#85928,#85929,#85930,#85931,#85932,#85933,#85934,#85935,
#85936,#85937,#85938,#85939,#85940,#85941,#85942,#85943,#85944,#85945,#85946,
#85947,#85948,#85949,#85950,#85951,#85952,#85953,#85954,#85955,#85956,#85957,
#85958,#85959,#85960,#85961,#85962,#85963,#85964,#85965,#85966,#85967,#85968,
#85969,#85970,#85971,#85972,#85973,#85974,#85975,#85976,#85977,#85978,#85979,
#85980,#85981,#85982,#85983,#85984,#85985,#85986,#85987,#85988,#85989,#85990,
#85991,#85992,#85993,#85994,#85995,#85996,#85997,#85998,#85999),
 .UNSPECIFIED.,.F.,.F.,(4,3,3,3,3,3,3,3,3,3,3,3,3,3,3,3,3,3,3,3,3,3,3,3,
3,3,3,3,3,3,3,3,3,3,3,3,3,3,3,3,3,4),(55.6335534449754,55.7373867669536,
55.8411973790614,55.9450200119163,56.0489562189317,56.1529584246219,56.2571354224554,
56.2951510633125,56.3993372268006,56.5033681520127,56.6072770424296,56.7111204735977,
56.8149332246126,56.9187500311341,57.0226755085045,57.1266598270492,57.2308260845083,
57.2926989216586,57.3968850851468,57.5009160103587,57.6048249007757,57.7086683319439,
57.812481082959,57.9162978894803,58.0202233668508,58.1242076853956,58.2283739428548,
58.2902467800047,58.3944329434929,58.4984638687049,58.6023727591219,58.70621619029,
58.8100289413049,58.9138457478266,59.0177712251969,59.1217555437416,59.2259218012008,
59.2877946383508,59.4032420886154,59.5183215991948,59.6327919924172,59.6902604177957),
 .UNSPECIFIED.);
#2556=B_SPLINE_CURVE_WITH_KNOTS('',3,(#86005,#86006,#86007,#86008,#86009,
#86010,#86011,#86012,#86013,#86014,#86015,#86016,#86017,#86018,#86019,#86020,
#86021,#86022,#86023,#86024,#86025,#86026,#86027,#86028,#86029,#86030,#86031,
#86032,#86033,#86034,#86035,#86036,#86037,#86038,#86039,#86040,#86041,#86042,
#86043,#86044,#86045,#86046,#86047,#86048,#86049,#86050,#86051,#86052,#86053,
#86054,#86055,#86056,#86057,#86058,#86059,#86060,#86061,#86062,#86063,#86064,
#86065,#86066,#86067,#86068,#86069,#86070,#86071,#86072,#86073,#86074,#86075,
#86076,#86077,#86078,#86079,#86080,#86081,#86082,#86083,#86084,#86085,#86086,
#86087,#86088,#86089,#86090,#86091,#86092,#86093,#86094,#86095,#86096,#86097,
#86098,#86099,#86100,#86101,#86102,#86103,#86104,#86105,#86106,#86107,#86108,
#86109,#86110,#86111,#86112,#86113,#86114,#86115,#86116,#86117,#86118,#86119,
#86120,#86121,#86122,#86123,#86124,#86125,#86126,#86127,#86128),
 .UNSPECIFIED.,.F.,.F.,(4,3,3,3,3,3,3,3,3,3,3,3,3,3,3,3,3,3,3,3,3,3,3,3,
3,3,3,3,3,3,3,3,3,3,3,3,3,3,3,3,3,4),(49.3496765008647,49.4543570310005,
49.5583126187223,49.6633556200652,49.768398621408,49.8725847848962,49.9766157101085,
50.0805246005255,50.1843680316935,50.2881807827084,50.3919975892301,50.4959230666004,
50.5999073851451,50.7040736426044,50.765946479754,50.8701326432422,50.9741635684545,
51.0780724588715,51.1819158900396,51.2857286410545,51.3895454475762,51.4934709249466,
51.5974552434913,51.7016215009506,51.7634943381001,51.8676805015883,51.9717114268002,
52.0756203172172,52.1794637483851,52.2832764994002,52.3870933059214,52.4910187832919,
52.5950031018364,52.6991693592957,52.7610421964462,52.8655509126695,52.9699037514312,
53.07919659133,53.1833373805659,53.2874304651171,53.3915238347378,53.4070751110264),
 .UNSPECIFIED.);
#2557=B_SPLINE_CURVE_WITH_KNOTS('',3,(#86129,#86130,#86131,#86132,#86133,
#86134,#86135,#86136,#86137,#86138,#86139,#86140,#86141,#86142,#86143,#86144,
#86145,#86146,#86147,#86148,#86149,#86150,#86151,#86152,#86153,#86154,#86155,
#86156,#86157,#86158,#86159,#86160,#86161,#86162,#86163,#86164,#86165,#86166,
#86167,#86168,#86169,#86170,#86171,#86172,#86173,#86174,#86175,#86176,#86177,
#86178,#86179,#86180,#86181,#86182,#86183,#86184,#86185,#86186,#86187,#86188,
#86189,#86190,#86191,#86192,#86193,#86194,#86195),.UNSPECIFIED.,.F.,.F.,
(4,3,3,3,3,3,3,3,3,3,3,3,3,3,3,3,3,3,3,3,3,3,4),(53.4070751114777,53.5259953052185,
53.6459937542286,53.7585900547923,53.8627762182805,53.9668071434928,54.0707160339098,
54.1745594650779,54.2783722160929,54.3821890226143,54.4861144999848,54.5900988185296,
54.6942650759888,54.7561379131384,54.8656962387679,54.9697007565417,55.0736032474321,
55.1774385720688,55.28124150922,55.38509253526,55.4889714123817,55.5929703714219,
55.6326045181743),.UNSPECIFIED.);
#2558=B_SPLINE_CURVE_WITH_KNOTS('',3,(#86197,#86198,#86199,#86200,#86201,
#86202,#86203,#86204,#86205,#86206,#86207,#86208,#86209,#86210,#86211,#86212,
#86213,#86214,#86215,#86216,#86217,#86218,#86219,#86220,#86221,#86222,#86223,
#86224,#86225,#86226,#86227,#86228,#86229,#86230,#86231,#86232,#86233,#86234,
#86235,#86236,#86237,#86238,#86239,#86240,#86241,#86242,#86243,#86244,#86245,
#86246,#86247,#86248,#86249,#86250,#86251,#86252,#86253,#86254,#86255,#86256,
#86257,#86258,#86259,#86260,#86261,#86262,#86263,#86264,#86265,#86266),
 .UNSPECIFIED.,.F.,.F.,(4,3,3,3,3,3,3,3,3,3,3,3,3,3,3,3,3,3,3,3,3,3,3,4),
(53.4070751114785,53.5098614913148,53.6124973139475,53.7150505550742,53.8175576893134,
53.9200551251567,54.0226483900827,54.1252912590462,54.2281147116669,54.3000553466204,
54.4042415101085,54.5082724353207,54.6121813257377,54.7160247569058,54.8198375079206,
54.9236543144423,55.0275797918127,55.1315641103575,55.2357303678167,55.2976032049664,
55.401768679066,55.5057980059528,55.609707173043,55.6335534449754),
 .UNSPECIFIED.);
#2559=B_SPLINE_CURVE_WITH_KNOTS('',3,(#86267,#86268,#86269,#86270,#86271,
#86272,#86273,#86274,#86275,#86276,#86277,#86278,#86279,#86280,#86281,#86282,
#86283,#86284,#86285,#86286,#86287,#86288,#86289,#86290,#86291,#86292,#86293,
#86294,#86295,#86296,#86297,#86298,#86299,#86300,#86301,#86302,#86303,#86304,
#86305,#86306,#86307,#86308,#86309,#86310,#86311,#86312,#86313,#86314,#86315,
#86316,#86317,#86318,#86319,#86320,#86321,#86322,#86323,#86324,#86325,#86326,
#86327,#86328,#86329,#86330,#86331,#86332,#86333,#86334,#86335,#86336,#86337,
#86338,#86339,#86340,#86341,#86342,#86343,#86344,#86345,#86346,#86347,#86348,
#86349,#86350,#86351,#86352,#86353,#86354,#86355,#86356,#86357,#86358,#86359,
#86360,#86361,#86362,#86363,#86364,#86365,#86366,#86367,#86368,#86369,#86370,
#86371,#86372,#86373,#86374,#86375,#86376,#86377,#86378,#86379,#86380,#86381,
#86382,#86383,#86384,#86385,#86386,#86387,#86388,#86389,#86390),
 .UNSPECIFIED.,.F.,.F.,(4,3,3,3,3,3,3,3,3,3,3,3,3,3,3,3,3,3,3,3,3,3,3,3,
3,3,3,3,3,3,3,3,3,3,3,3,3,3,3,3,3,4),(49.3501259974606,49.4542513728051,
49.561202940359,49.6650820702675,49.7689093574742,49.8727195599115,49.9820056482427,
50.085953371695,50.1899737885933,50.2941626580275,50.309863913236,50.4140500767242,
50.5180810019363,50.6219898923532,50.7258333235213,50.8296460745363,50.9334628810578,
51.0373883584282,51.1413726769729,51.2455389344321,51.3074117715821,51.4115979350703,
51.5156288602825,51.6195377506995,51.7233811818676,51.8271939328825,51.9310107394041,
52.0349362167745,52.1389205353193,52.2430867927785,52.3049596299282,52.4091457934164,
52.5131767186286,52.6170856090455,52.7209290402137,52.8247417912286,52.9285585977501,
53.0324840751205,53.1364683936651,53.2406346511244,53.3025074882743,53.4070751110264),
 .UNSPECIFIED.);
#2560=B_SPLINE_CURVE_WITH_KNOTS('',3,(#86396,#86397,#86398,#86399,#86400,
#86401,#86402,#86403,#86404,#86405,#86406,#86407,#86408,#86409,#86410,#86411,
#86412,#86413,#86414,#86415,#86416,#86417,#86418,#86419,#86420,#86421,#86422,
#86423,#86424,#86425,#86426,#86427,#86428,#86429,#86430,#86431,#86432,#86433,
#86434,#86435,#86436,#86437,#86438,#86439,#86440,#86441,#86442,#86443,#86444,
#86445,#86446,#86447,#86448,#86449,#86450,#86451,#86452,#86453,#86454,#86455,
#86456,#86457,#86458,#86459,#86460,#86461,#86462,#86463,#86464,#86465,#86466,
#86467,#86468,#86469,#86470,#86471,#86472,#86473,#86474,#86475,#86476,#86477,
#86478,#86479,#86480,#86481,#86482,#86483,#86484,#86485,#86486,#86487,#86488,
#86489,#86490,#86491,#86492,#86493,#86494,#86495,#86496,#86497,#86498,#86499,
#86500,#86501,#86502,#86503,#86504,#86505,#86506,#86507,#86508,#86509,#86510,
#86511,#86512,#86513,#86514,#86515,#86516),.UNSPECIFIED.,.F.,.F.,(4,3,3,
3,3,3,3,3,3,3,3,3,3,3,3,3,3,3,3,3,3,3,3,3,3,3,3,3,3,3,3,3,3,3,3,3,3,3,3,
3,4),(43.0672771687041,43.171136160571,43.2749542962854,43.3787663206053,
43.482680485421,43.5866443592237,43.690799844705,43.7831114713314,43.8872976348201,
43.9913285600328,44.0952374504504,44.1990808816191,44.3028936326345,44.4067104391567,
44.5106359165277,44.614620235073,44.7187864925329,44.7806593296775,44.8848454931656,
44.9888764183777,45.0927853087945,45.1966287399624,45.3004414909772,45.4042582974987,
45.5081837748689,45.6121680934133,45.7163343508724,45.7782071880236,45.8823933515117,
45.9864242767239,46.0903331671409,46.1941765983088,46.2979893493237,46.401806155845,
46.5057316332152,46.6097159517598,46.713882209219,46.7757550463697,46.8962986192151,
47.0157785770634,47.123889803398),.UNSPECIFIED.);
#2561=B_SPLINE_CURVE_WITH_KNOTS('',3,(#86517,#86518,#86519,#86520,#86521,
#86522,#86523,#86524,#86525,#86526,#86527,#86528,#86529,#86530,#86531,#86532,
#86533,#86534,#86535,#86536,#86537,#86538,#86539,#86540,#86541,#86542,#86543,
#86544,#86545,#86546,#86547,#86548,#86549,#86550,#86551,#86552,#86553,#86554,
#86555,#86556,#86557,#86558,#86559,#86560,#86561,#86562,#86563,#86564,#86565,
#86566,#86567,#86568,#86569,#86570,#86571,#86572,#86573,#86574,#86575,#86576,
#86577,#86578,#86579,#86580,#86581,#86582,#86583,#86584,#86585,#86586),
 .UNSPECIFIED.,.F.,.F.,(4,3,3,3,3,3,3,3,3,3,3,3,3,3,3,3,3,3,3,3,3,3,3,4),
(47.1238898038468,47.2279281355325,47.3319603652862,47.4360206698574,47.5402127556636,
47.644483889522,47.7489375131547,47.7733029047158,47.877489068204,47.9815199934162,
48.0854288838331,48.1892723150013,48.2930850660162,48.3969018725376,48.500827349908,
48.6048116684528,48.7089779259121,48.7708507630619,48.8750265334989,48.9790548139493,
49.0829625287115,49.186799581749,49.2906190127585,49.3496765008647),
 .UNSPECIFIED.);
#2562=B_SPLINE_CURVE_WITH_KNOTS('',3,(#86588,#86589,#86590,#86591,#86592,
#86593,#86594,#86595,#86596,#86597,#86598,#86599,#86600,#86601,#86602,#86603,
#86604,#86605,#86606,#86607,#86608,#86609,#86610,#86611,#86612,#86613,#86614,
#86615,#86616,#86617,#86618,#86619,#86620,#86621,#86622,#86623,#86624,#86625,
#86626,#86627,#86628,#86629,#86630,#86631,#86632,#86633,#86634,#86635,#86636,
#86637,#86638,#86639,#86640,#86641,#86642,#86643,#86644,#86645,#86646,#86647,
#86648,#86649,#86650,#86651,#86652,#86653,#86654,#86655,#86656,#86657),
 .UNSPECIFIED.,.F.,.F.,(4,3,3,3,3,3,3,3,3,3,3,3,3,3,3,3,3,3,3,3,3,3,3,4),
(47.1238898038468,47.2754958859011,47.3172203381978,47.4214065016858,47.5254374268979,
47.6293463173146,47.7331897484826,47.8370024994973,47.9408193060187,48.0447447833889,
48.1487291019335,48.2528953593925,48.3147681965438,48.4189543600319,48.522985285244,
48.6268941756609,48.730737606829,48.8345503578439,48.9383671643653,49.0422926417356,
49.1462769602803,49.2504432177395,49.3123160548899,49.3501259974606),
 .UNSPECIFIED.);
#2563=B_SPLINE_CURVE_WITH_KNOTS('',3,(#86658,#86659,#86660,#86661,#86662,
#86663,#86664,#86665,#86666,#86667,#86668,#86669,#86670,#86671,#86672,#86673,
#86674,#86675,#86676,#86677,#86678,#86679,#86680,#86681,#86682,#86683,#86684,
#86685,#86686,#86687,#86688,#86689,#86690,#86691,#86692,#86693,#86694,#86695,
#86696,#86697,#86698,#86699,#86700,#86701,#86702,#86703,#86704,#86705,#86706,
#86707,#86708,#86709,#86710,#86711,#86712,#86713,#86714,#86715,#86716,#86717,
#86718,#86719,#86720,#86721,#86722,#86723,#86724,#86725,#86726,#86727,#86728,
#86729,#86730,#86731,#86732,#86733,#86734,#86735,#86736,#86737,#86738,#86739,
#86740,#86741,#86742,#86743,#86744,#86745,#86746,#86747,#86748,#86749,#86750,
#86751,#86752,#86753,#86754,#86755,#86756,#86757,#86758,#86759,#86760,#86761,
#86762,#86763,#86764,#86765,#86766,#86767,#86768,#86769,#86770,#86771,#86772,
#86773,#86774,#86775,#86776,#86777,#86778,#86779,#86780,#86781),
 .UNSPECIFIED.,.F.,.F.,(4,3,3,3,3,3,3,3,3,3,3,3,3,3,3,3,3,3,3,3,3,3,3,3,
3,3,3,3,3,3,3,3,3,3,3,3,3,3,3,3,3,4),(43.0661637600767,43.1701547594049,
43.2743249058554,43.3270289048134,43.431215068306,43.5352459935225,43.639154883944,
43.7429983151167,43.8468110661362,43.9506278726624,44.0545533500374,44.1585376685868,
44.2627039260507,44.3245767631595,44.4287629266466,44.5327938518577,44.6367027422735,
44.7405461734405,44.8443589244543,44.9481757309747,45.052101208344,45.1560855268876,
45.2602517843458,45.3221246215056,45.4263107849933,45.530341710205,45.6342506006214,
45.738094031789,45.8419067828034,45.9457235893243,46.0496490666941,46.1536333852383,
46.2577996426969,46.3196724798517,46.4223012412914,46.5247935864418,46.6271863644391,
46.729516280193,46.8318649061931,46.9342176129156,47.0366904241979,47.1238898034407),
 .UNSPECIFIED.);
#2564=B_SPLINE_CURVE_WITH_KNOTS('',3,(#86787,#86788,#86789,#86790,#86791,
#86792,#86793,#86794,#86795,#86796,#86797,#86798,#86799,#86800,#86801,#86802,
#86803,#86804,#86805,#86806,#86807,#86808,#86809,#86810,#86811,#86812,#86813,
#86814,#86815,#86816,#86817,#86818,#86819,#86820,#86821,#86822,#86823,#86824,
#86825,#86826,#86827,#86828,#86829,#86830,#86831,#86832,#86833,#86834,#86835,
#86836,#86837,#86838,#86839,#86840,#86841,#86842,#86843,#86844,#86845,#86846,
#86847,#86848,#86849,#86850,#86851,#86852,#86853,#86854,#86855,#86856,#86857,
#86858,#86859,#86860,#86861,#86862,#86863,#86864,#86865,#86866,#86867,#86868,
#86869,#86870,#86871,#86872,#86873,#86874,#86875,#86876,#86877,#86878,#86879,
#86880,#86881,#86882,#86883,#86884,#86885,#86886,#86887,#86888,#86889,#86890,
#86891,#86892,#86893,#86894,#86895,#86896,#86897,#86898,#86899,#86900,#86901,
#86902,#86903,#86904,#86905,#86906,#86907,#86908,#86909,#86910,#86911,#86912,
#86913),.UNSPECIFIED.,.F.,.F.,(4,3,3,3,3,3,3,3,3,3,3,3,3,3,3,3,3,3,3,3,
3,3,3,3,3,3,3,3,3,3,3,3,3,3,3,3,3,3,3,3,3,3,4),(36.7834483157109,36.8002764629088,
36.9044626263498,37.0084935515138,37.1124024418814,37.2162458729993,37.3200586239635,
37.4238754304336,37.527800907752,37.6317852262444,37.7359514836513,37.7978243212549,
37.9020104847763,38.0060414100222,38.1099503004735,38.2137937316762,38.3176064827261,
38.4214232892828,38.5253487666884,38.6293330852686,38.733499342763,38.795372179601,
38.899558343083,39.003589268289,39.1074981586998,39.2113415898617,39.3151543408705,
39.4189711473858,39.5228966247501,39.6268809432888,39.7310472007422,39.7929200379471,
39.8971062014302,40.0011371266371,40.1050460170487,40.2088894482114,40.3127021992209,
40.4165190057369,40.5204444831017,40.6244288016407,40.7285950590942,40.7904678962932,
40.8407044966673),.UNSPECIFIED.);
#2565=B_SPLINE_CURVE_WITH_KNOTS('',3,(#86914,#86915,#86916,#86917,#86918,
#86919,#86920,#86921,#86922,#86923,#86924,#86925,#86926,#86927,#86928,#86929,
#86930,#86931,#86932,#86933,#86934,#86935,#86936,#86937,#86938,#86939,#86940,
#86941,#86942,#86943,#86944,#86945,#86946,#86947,#86948,#86949,#86950,#86951,
#86952,#86953,#86954,#86955,#86956,#86957,#86958,#86959,#86960,#86961,#86962,
#86963,#86964,#86965,#86966,#86967,#86968,#86969,#86970,#86971,#86972,#86973,
#86974,#86975,#86976,#86977,#86978,#86979,#86980,#86981,#86982,#86983),
 .UNSPECIFIED.,.F.,.F.,(4,3,3,3,3,3,3,3,3,3,3,3,3,3,3,3,3,3,3,3,3,3,3,4),
(40.8407044969994,40.9440746115611,41.0495672544459,41.1526720053879,41.2557188072319,
41.3587435025164,41.4660615655471,41.5692147500897,41.6724388016654,41.7758284060395,
41.7880157546393,41.8922019181263,41.9962328433371,42.100141733753,42.20398516492,
42.3077979159338,42.4116147224541,42.5155401998234,42.6195245183671,42.7236907758253,
42.7855636129853,42.8897412721982,42.9937540506562,43.0672771687041),
 .UNSPECIFIED.);
#2566=B_SPLINE_CURVE_WITH_KNOTS('',3,(#86985,#86986,#86987,#86988,#86989,
#86990,#86991,#86992,#86993,#86994,#86995,#86996,#86997,#86998,#86999,#87000,
#87001,#87002,#87003,#87004,#87005,#87006,#87007,#87008,#87009,#87010,#87011,
#87012,#87013,#87014,#87015,#87016,#87017,#87018,#87019,#87020,#87021,#87022,
#87023,#87024,#87025,#87026,#87027,#87028,#87029,#87030,#87031,#87032,#87033,
#87034,#87035,#87036,#87037,#87038,#87039,#87040,#87041,#87042,#87043,#87044,
#87045,#87046,#87047,#87048,#87049,#87050,#87051),.UNSPECIFIED.,.F.,.F.,
(4,3,3,3,3,3,3,3,3,3,3,3,3,3,3,3,3,3,3,3,3,3,4),(40.8407044969871,40.9497796083699,
41.0591756422983,41.1687426604485,41.2786112447893,41.3319331881212,41.4361193516032,
41.5401502768092,41.64405916722,41.7479025983819,41.8517153493907,41.9555321559061,
42.0594576332705,42.1634419518092,42.2676082092626,42.3294810464673,42.4336404890036,
42.5376570384834,42.6415656994843,42.7477152146324,42.8515331414174,42.9588484507471,
43.0661637600767),.UNSPECIFIED.);
#2567=B_SPLINE_CURVE_WITH_KNOTS('',3,(#87052,#87053,#87054,#87055,#87056,
#87057,#87058,#87059,#87060,#87061,#87062,#87063,#87064,#87065,#87066,#87067,
#87068,#87069,#87070,#87071,#87072,#87073,#87074,#87075,#87076,#87077,#87078,
#87079,#87080,#87081,#87082,#87083,#87084,#87085,#87086,#87087,#87088,#87089,
#87090,#87091,#87092,#87093,#87094,#87095,#87096,#87097,#87098,#87099,#87100,
#87101,#87102,#87103,#87104,#87105,#87106,#87107,#87108,#87109,#87110,#87111,
#87112,#87113,#87114,#87115,#87116,#87117,#87118,#87119,#87120,#87121,#87122,
#87123,#87124,#87125,#87126,#87127,#87128,#87129,#87130,#87131,#87132,#87133,
#87134,#87135,#87136,#87137,#87138,#87139,#87140,#87141,#87142,#87143,#87144,
#87145,#87146,#87147,#87148,#87149,#87150,#87151,#87152,#87153,#87154,#87155,
#87156,#87157,#87158,#87159,#87160,#87161,#87162,#87163,#87164,#87165,#87166,
#87167,#87168,#87169,#87170,#87171,#87172,#87173,#87174,#87175),
 .UNSPECIFIED.,.F.,.F.,(4,3,3,3,3,3,3,3,3,3,3,3,3,3,3,3,3,3,3,3,3,3,3,3,
3,3,3,3,3,3,3,3,3,3,3,3,3,3,3,3,3,4),(36.7837280398568,36.8875386644498,
36.9913612263603,37.095297312041,37.1992993214154,37.3034761958223,37.3417417547369,
37.4459279184719,37.5499588439342,37.6538677346054,37.75771116603,37.8615239173034,
37.9653407240849,38.069266201716,38.1732505205219,38.2774167782407,38.339289613083,
38.4434757765423,38.5475067017258,38.6514155921144,38.7552590232545,38.8590717742416,
38.9628885807358,39.0668140580795,39.170798376598,39.2749646340317,39.3368374714291,
39.4410236348703,39.5450545600342,39.6489634504021,39.7528068815202,39.8566196324845,
39.9604364389551,40.0643619162737,40.1683462347665,40.2725124921736,40.3343853297752,
40.4435562695039,40.5524208008743,40.6611016633605,40.769557770341,40.8407044966673),
 .UNSPECIFIED.);
#2568=B_SPLINE_CURVE_WITH_KNOTS('',3,(#87181,#87182,#87183,#87184,#87185,
#87186,#87187,#87188),.UNSPECIFIED.,.F.,.F.,(4,1,1,1,1,4),(30.4995505102364,
30.8149893128323,31.8125371711784,32.8100850295245,33.8076328878706,34.5575191894876),
 .UNSPECIFIED.);
#2569=B_SPLINE_CURVE_WITH_KNOTS('',3,(#87189,#87190,#87191,#87192,#87193,
#87194,#87195,#87196,#87197,#87198,#87199,#87200,#87201,#87202,#87203,#87204,
#87205,#87206,#87207,#87208,#87209,#87210,#87211,#87212,#87213,#87214,#87215,
#87216,#87217,#87218,#87219,#87220,#87221,#87222,#87223,#87224,#87225,#87226,
#87227,#87228,#87229,#87230,#87231,#87232,#87233,#87234,#87235,#87236,#87237,
#87238,#87239,#87240,#87241,#87242,#87243,#87244,#87245,#87246,#87247,#87248,
#87249,#87250,#87251,#87252,#87253,#87254,#87255),.UNSPECIFIED.,.F.,.F.,
(4,3,3,3,3,3,3,3,3,3,3,3,3,3,3,3,3,3,3,3,3,3,4),(34.557519274484,34.6927957333214,
34.8051807462166,34.909366909953,35.0133978354169,35.1173067260896,35.2211501575158,
35.3249629087908,35.4287797155739,35.5327051932064,35.6366895120138,35.7408557697342,
35.8027286045627,35.9069159429535,36.0109477003919,36.1148561156626,36.2186985864117,
36.3225098920313,36.426324767821,36.5302426834859,36.6342192413344,36.73836490079,
36.7834483157109),.UNSPECIFIED.);
#2570=B_SPLINE_CURVE_WITH_KNOTS('',3,(#87257,#87258,#87259,#87260,#87261,
#87262,#87263,#87264,#87265,#87266,#87267,#87268,#87269,#87270,#87271,#87272,
#87273,#87274,#87275,#87276,#87277,#87278,#87279,#87280,#87281,#87282,#87283,
#87284,#87285,#87286,#87287,#87288,#87289,#87290,#87291,#87292,#87293,#87294,
#87295,#87296,#87297,#87298,#87299,#87300,#87301,#87302,#87303,#87304,#87305,
#87306,#87307,#87308,#87309,#87310,#87311,#87312,#87313,#87314,#87315,#87316,
#87317,#87318,#87319,#87320,#87321,#87322,#87323,#87324,#87325,#87326),
 .UNSPECIFIED.,.F.,.F.,(4,3,3,3,3,3,3,3,3,3,3,3,3,3,3,3,3,3,3,3,3,3,3,4),
(34.5575191897439,34.6600261058214,34.7624492437677,34.8648252112055,34.9671905469454,
35.0696506767749,35.1721598105506,35.2748489352923,35.3466460380447,35.4508322014595,
35.554863126602,35.6587720169556,35.7626154480643,35.8664281990237,35.970245005494,
36.0741704828196,36.1781548013232,36.2823210587477,36.3441938963908,36.4483886654221,
36.5524031605798,36.6563141143402,36.7601506285695,36.7837280398568),
 .UNSPECIFIED.);
#2571=B_SPLINE_CURVE_WITH_KNOTS('',3,(#87327,#87328,#87329,#87330,#87331,
#87332,#87333,#87334,#87335,#87336,#87337,#87338,#87339,#87340,#87341,#87342,
#87343,#87344,#87345,#87346,#87347,#87348,#87349,#87350,#87351,#87352,#87353,
#87354,#87355,#87356,#87357,#87358,#87359,#87360,#87361,#87362,#87363,#87364,
#87365,#87366,#87367,#87368,#87369,#87370,#87371,#87372,#87373,#87374,#87375,
#87376,#87377,#87378,#87379,#87380,#87381,#87382,#87383,#87384,#87385,#87386,
#87387,#87388,#87389,#87390,#87391,#87392,#87393,#87394,#87395,#87396,#87397,
#87398,#87399,#87400,#87401,#87402,#87403,#87404,#87405,#87406,#87407,#87408,
#87409,#87410,#87411,#87412,#87413,#87414,#87415,#87416,#87417,#87418,#87419,
#87420,#87421,#87422,#87423,#87424,#87425,#87426,#87427,#87428,#87429,#87430,
#87431,#87432,#87433,#87434,#87435,#87436,#87437,#87438,#87439,#87440,#87441,
#87442,#87443,#87444,#87445,#87446,#87447,#87448,#87449,#87450),
 .UNSPECIFIED.,.F.,.F.,(4,3,3,3,3,3,3,3,3,3,3,3,3,3,3,3,3,3,3,3,3,3,3,3,
3,3,3,3,3,3,3,3,3,3,3,3,3,3,3,3,3,4),(30.5009012256866,30.6078453980583,
30.7117244622742,30.8155517007811,30.9193618715342,31.0286350548158,31.1325827673511,
31.2366031848782,31.3407920442357,31.3564546046604,31.4606407808707,31.5646717189603,
31.6685806224221,31.7724240667314,31.8762368309641,31.9800536507603,32.0839791414007,
32.1879634732329,32.2921297438626,32.3540024630065,32.4581886271226,32.5622195530122,
32.6661284441775,32.7699718761373,32.8737846279862,32.9776014353829,33.081526913686,
33.1855112331973,33.2896774916665,33.3515503213525,33.455736481262,33.5597674028288,
33.6636762895192,33.7675197169125,33.8713324641099,33.975149266777,34.0790747402627,
34.1830590548998,34.2872253084573,34.3490981796986,34.4951131661248,34.5575191894876),
 .UNSPECIFIED.);
#2572=B_SPLINE_CURVE_WITH_KNOTS('',3,(#87456,#87457,#87458,#87459,#87460,
#87461,#87462,#87463,#87464,#87465,#87466,#87467,#87468,#87469,#87470,#87471,
#87472,#87473,#87474,#87475,#87476,#87477,#87478,#87479,#87480,#87481,#87482,
#87483,#87484,#87485,#87486,#87487,#87488,#87489,#87490,#87491,#87492,#87493,
#87494,#87495,#87496,#87497,#87498,#87499,#87500,#87501,#87502,#87503,#87504,
#87505,#87506,#87507,#87508,#87509,#87510,#87511,#87512,#87513,#87514,#87515,
#87516,#87517,#87518,#87519,#87520,#87521,#87522,#87523,#87524,#87525,#87526,
#87527,#87528,#87529,#87530,#87531,#87532,#87533,#87534,#87535,#87536,#87537,
#87538,#87539,#87540,#87541,#87542,#87543,#87544,#87545,#87546,#87547,#87548,
#87549,#87550,#87551,#87552,#87553,#87554,#87555,#87556,#87557,#87558,#87559,
#87560,#87561,#87562,#87563,#87564,#87565,#87566,#87567,#87568,#87569,#87570,
#87571,#87572,#87573,#87574,#87575,#87576),.UNSPECIFIED.,.F.,.F.,(4,3,3,
3,3,3,3,3,3,3,3,3,3,3,3,3,3,3,3,3,3,3,3,3,3,3,3,3,3,3,3,3,3,3,3,3,3,3,3,
3,4),(24.2175094594017,24.3213278434285,24.4251400466915,24.5290543466609,
24.633018292731,24.737173924033,24.8297021627558,24.9338880829223,25.0379187606929,
25.1418273987454,25.2456705746464,25.3494830678712,25.4532996144562,25.5572248303944,
25.6612088862683,25.7653748819406,25.8272500211019,25.9314362718495,26.0354672852708,
26.1393762648751,26.2432197857851,26.3470326269618,26.4508495239306,26.5547750915589,
26.6587595003909,26.7629258472006,26.824797879448,26.9289840570988,27.0330149970021,
27.1369239028275,27.2407673498393,27.3445801171099,27.4483969402773,27.5523224347774,
27.6563067707512,27.7604730459268,27.822345737794,27.9353427130054,28.0470527868882,
28.160693212764,28.2743336386397),.UNSPECIFIED.);
#2573=B_SPLINE_CURVE_WITH_KNOTS('',3,(#87577,#87578,#87579,#87580,#87581,
#87582),.UNSPECIFIED.,.F.,.F.,(4,1,1,4),(28.2743338823081,28.8198935961401,
29.8174414544862,30.4995505102364),.UNSPECIFIED.);
#2574=B_SPLINE_CURVE_WITH_KNOTS('',3,(#87584,#87585,#87586,#87587,#87588,
#87589,#87590,#87591,#87592,#87593,#87594,#87595,#87596,#87597,#87598,#87599,
#87600,#87601,#87602,#87603,#87604,#87605,#87606,#87607,#87608,#87609,#87610,
#87611,#87612,#87613,#87614,#87615,#87616,#87617,#87618,#87619,#87620,#87621,
#87622,#87623,#87624,#87625,#87626,#87627,#87628,#87629,#87630,#87631,#87632,
#87633,#87634,#87635,#87636,#87637,#87638,#87639,#87640,#87641,#87642,#87643,
#87644,#87645,#87646,#87647,#87648,#87649,#87650,#87651,#87652,#87653),
 .UNSPECIFIED.,.F.,.F.,(4,3,3,3,3,3,3,3,3,3,3,3,3,3,3,3,3,3,3,3,3,3,3,4),
(28.2743338823081,28.3638110296221,28.4679972800027,28.5720282930528,28.675937272281,
28.7797807928121,28.8835936336079,28.9874105301943,29.0913360974404,29.1953205058895,
29.29948685232,29.3613588879682,29.4655450656047,29.5695760054923,29.6734849113002,
29.7773283582932,29.881141125544,29.9849579486899,30.0888834431674,30.1928677791174,
30.2970340542683,30.3589067463143,30.4630838119772,30.5009012256866),
 .UNSPECIFIED.);
#2575=B_SPLINE_CURVE_WITH_KNOTS('',3,(#87654,#87655,#87656,#87657,#87658,
#87659,#87660,#87661,#87662,#87663,#87664,#87665,#87666,#87667,#87668,#87669,
#87670,#87671,#87672,#87673,#87674,#87675,#87676,#87677,#87678,#87679,#87680,
#87681,#87682,#87683,#87684,#87685,#87686,#87687,#87688,#87689,#87690,#87691,
#87692,#87693,#87694,#87695,#87696,#87697,#87698,#87699,#87700,#87701,#87702,
#87703,#87704,#87705,#87706,#87707,#87708,#87709,#87710,#87711,#87712,#87713,
#87714,#87715,#87716,#87717,#87718,#87719,#87720,#87721,#87722,#87723,#87724,
#87725,#87726,#87727,#87728,#87729,#87730,#87731,#87732,#87733,#87734,#87735,
#87736,#87737,#87738,#87739,#87740,#87741,#87742,#87743,#87744,#87745,#87746,
#87747,#87748,#87749,#87750,#87751,#87752,#87753,#87754,#87755,#87756,#87757,
#87758,#87759,#87760,#87761,#87762,#87763,#87764,#87765,#87766,#87767,#87768,
#87769,#87770,#87771,#87772,#87773,#87774,#87775,#87776,#87777),
 .UNSPECIFIED.,.F.,.F.,(4,3,3,3,3,3,3,3,3,3,3,3,3,3,3,3,3,3,3,3,3,3,3,3,
3,3,3,3,3,3,3,3,3,3,3,3,3,3,3,3,3,4),(24.2166158528785,24.3207881219797,
24.3736195962378,24.4778038331522,24.5818328006132,24.685739696451,24.7895811113854,
24.8933918275129,24.9972065834734,25.101130000418,25.2051122498594,25.3092764469012,
25.3711674545839,25.4753541846193,25.5793856815231,25.6832951484569,25.7871391588007,
25.8909524907785,25.9947698791806,26.0986959357944,26.2026808329677,26.3068476617735,
26.3687153129299,26.4729016564542,26.5769327668191,26.680841849117,26.7846854762195,
26.8884984269359,26.9923154366431,27.0962411211505,27.2002256493751,27.3043921182881,
27.366263171276,27.4692311191777,27.572023901783,27.6747188328349,27.7773523095505,
27.8799606447598,27.9826447839181,28.085364888699,28.1882547111826,28.27433388186),
 .UNSPECIFIED.);
#2576=B_SPLINE_CURVE_WITH_KNOTS('',3,(#87783,#87784,#87785,#87786,#87787,
#87788,#87789,#87790,#87791,#87792,#87793,#87794,#87795,#87796,#87797,#87798,
#87799,#87800,#87801,#87802,#87803,#87804,#87805,#87806,#87807,#87808,#87809,
#87810,#87811,#87812,#87813,#87814,#87815,#87816,#87817,#87818,#87819,#87820,
#87821,#87822,#87823,#87824,#87825,#87826,#87827,#87828,#87829,#87830,#87831,
#87832,#87833,#87834,#87835,#87836,#87837,#87838,#87839,#87840,#87841,#87842,
#87843,#87844,#87845,#87846,#87847,#87848,#87849,#87850,#87851,#87852),
 .UNSPECIFIED.,.F.,.F.,(4,3,3,3,3,3,3,3,3,3,3,3,3,3,3,3,3,3,3,3,3,3,3,4),
(15.7079632679489,15.8106738927763,15.9133494515527,16.0160260414383,16.1188128612619,
16.2216580789275,16.3246939332088,16.3932367294691,16.4975142314111,16.6016358337152,
16.7056339423556,16.8095656348978,16.9134655491479,17.0173682784092,17.1213771604187,
17.2254435848118,17.3296889783796,17.3907845878152,17.4951357241063,17.6048037953017,
17.7088847254726,17.8128986127177,17.9168871416275,17.9338080088879),
 .UNSPECIFIED.);
#2577=B_SPLINE_CURVE_WITH_KNOTS('',3,(#87854,#87855,#87856,#87857,#87858),
 .UNSPECIFIED.,.F.,.F.,(4,1,4),(14.3981410127769,15.395688871123,15.7079548164659),
 .UNSPECIFIED.);
#2578=B_SPLINE_CURVE_WITH_KNOTS('',3,(#87862,#87863,#87864,#87865,#87866,
#87867,#87868,#87869,#87870,#87871,#87872,#87873,#87874,#87875,#87876,#87877,
#87878,#87879,#87880,#87881,#87882,#87883,#87884,#87885,#87886,#87887,#87888,
#87889,#87890,#87891,#87892,#87893,#87894,#87895,#87896,#87897,#87898,#87899,
#87900,#87901,#87902,#87903,#87904,#87905,#87906,#87907,#87908,#87909,#87910,
#87911,#87912,#87913,#87914,#87915,#87916,#87917,#87918,#87919),
 .UNSPECIFIED.,.F.,.F.,(4,3,3,3,3,3,3,3,3,3,3,3,3,3,3,3,3,3,3,4),(13.8761929172068,
13.9801050066969,14.0838618081371,14.1874968767277,14.2910672014661,14.3946079563068,
14.4981542724688,14.6018076115749,14.7055219776147,14.8094097434174,14.8542235792949,
14.9609410403274,15.0635681569975,15.1661013730925,15.2685772460228,15.3710322508939,
15.4735544551065,15.5761173355011,15.6788162057539,15.7079632675546),
 .UNSPECIFIED.);
#2579=B_SPLINE_CURVE_WITH_KNOTS('',3,(#87920,#87921,#87922,#87923,#87924,
#87925,#87926,#87927,#87928,#87929,#87930,#87931,#87932,#87933,#87934,#87935,
#87936,#87937,#87938,#87939,#87940,#87941,#87942,#87943,#87944,#87945,#87946,
#87947,#87948,#87949,#87950,#87951,#87952,#87953,#87954,#87955,#87956,#87957,
#87958,#87959,#87960,#87961,#87962,#87963,#87964,#87965,#87966,#87967,#87968,
#87969,#87970,#87971,#87972,#87973,#87974,#87975,#87976,#87977,#87978,#87979,
#87980,#87981,#87982,#87983,#87984,#87985,#87986),.UNSPECIFIED.,.F.,.F.,
(4,3,3,3,3,3,3,3,3,3,3,3,3,3,3,3,3,3,3,3,3,3,4),(15.7079632679489,15.851771437641,
15.9558439816741,16.0597596364386,16.1635513569498,16.2672765065998,16.3709700377575,
16.4746668582794,16.5784719990463,16.6823355986529,16.7863818407608,16.8493192959871,
16.9535243585492,17.0575742080196,17.1615019650239,17.2653642163339,17.3691957122932,
17.4730311597456,17.5769749880005,17.6809775212887,17.785161578003,17.8468671543332,
17.9343899947098),.UNSPECIFIED.);
#2580=B_SPLINE_CURVE_WITH_KNOTS('',3,(#87992,#87993,#87994,#87995,#87996,
#87997,#87998,#87999),.UNSPECIFIED.,.F.,.F.,(4,1,1,1,1,4),(99.6151588600969,
99.6457915387123,100.643339397058,101.640887255404,102.638435113751,103.635982972097),
 .UNSPECIFIED.);
#2581=B_SPLINE_CURVE_WITH_KNOTS('',3,(#88003,#88004,#88005,#88006,#88007,
#88008,#88009,#88010,#88011,#88012,#88013,#88014,#88015,#88016,#88017,#88018),
 .UNSPECIFIED.,.F.,.F.,(4,3,3,3,3,4),(103.672557568922,103.78037580106,
103.888462090901,103.99669403761,104.105203098963,104.157845063177),
 .UNSPECIFIED.);
#2582=B_SPLINE_CURVE_WITH_KNOTS('',3,(#88019,#88020,#88021,#88022,#88023,
#88024,#88025,#88026,#88027,#88028,#88029,#88030,#88031,#88032,#88033,#88034,
#88035,#88036,#88037,#88038,#88039,#88040,#88041,#88042,#88043,#88044,#88045,
#88046,#88047,#88048,#88049,#88050,#88051,#88052,#88053,#88054,#88055,#88056,
#88057,#88058,#88059,#88060,#88061,#88062,#88063,#88064,#88065,#88066,#88067,
#88068,#88069,#88070,#88071,#88072,#88073,#88074,#88075,#88076,#88077,#88078,
#88079,#88080,#88081,#88082,#88083,#88084,#88085,#88086,#88087,#88088,#88089,
#88090,#88091,#88092,#88093,#88094,#88095,#88096,#88097,#88098,#88099,#88100,
#88101,#88102,#88103,#88104,#88105,#88106,#88107,#88108,#88109,#88110,#88111,
#88112,#88113,#88114,#88115,#88116,#88117,#88118,#88119,#88120,#88121,#88122,
#88123,#88124,#88125,#88126,#88127,#88128,#88129,#88130,#88131,#88132,#88133,
#88134,#88135,#88136,#88137,#88138,#88139,#88140,#88141,#88142),
 .UNSPECIFIED.,.F.,.F.,(4,3,3,3,3,3,3,3,3,3,3,3,3,3,3,3,3,3,3,3,3,3,3,3,
3,3,3,3,3,3,3,3,3,3,3,3,3,3,3,3,3,4),(99.6156256169323,99.7194574413302,
99.8232964128399,99.9272456628453,100.031256493114,100.135445708004,100.18725683054,
100.291460632875,100.395509495336,100.499436674714,100.603298601299,100.707130025082,
100.810965652815,100.914910044679,101.018913358671,101.123098530321,101.184804688886,
101.288871352726,101.392782473111,101.49657167515,101.600295550718,101.703989049953,
101.807687079777,101.911495314534,102.015363074771,102.119415120688,102.182352547233,
102.286727546173,102.39094680336,102.495042376685,102.59907136604,102.703068280569,
102.807067584658,102.911171777178,103.015332937334,103.11967118475,103.179900405579,
103.289277016351,103.398344121045,103.507224154213,103.615874635127,103.672557568463),
 .UNSPECIFIED.);
#2583=B_SPLINE_CURVE_WITH_KNOTS('',3,(#88148,#88149,#88150,#88151,#88152,
#88153,#88154,#88155,#88156,#88157,#88158,#88159,#88160,#88161,#88162,#88163,
#88164,#88165,#88166,#88167,#88168,#88169,#88170,#88171,#88172,#88173,#88174,
#88175,#88176,#88177,#88178,#88179,#88180,#88181,#88182,#88183,#88184,#88185,
#88186,#88187,#88188,#88189,#88190,#88191,#88192,#88193,#88194,#88195,#88196,
#88197,#88198,#88199,#88200,#88201,#88202,#88203,#88204,#88205,#88206,#88207,
#88208,#88209,#88210,#88211,#88212,#88213,#88214,#88215,#88216,#88217,#88218,
#88219,#88220,#88221,#88222,#88223,#88224,#88225,#88226,#88227,#88228,#88229,
#88230,#88231,#88232,#88233,#88234,#88235,#88236,#88237,#88238,#88239,#88240,
#88241,#88242,#88243,#88244,#88245,#88246,#88247,#88248,#88249,#88250,#88251,
#88252,#88253,#88254,#88255,#88256,#88257,#88258,#88259,#88260,#88261,#88262,
#88263,#88264,#88265,#88266,#88267,#88268,#88269,#88270,#88271,#88272,#88273,
#88274),.UNSPECIFIED.,.F.,.F.,(4,3,3,3,3,3,3,3,3,3,3,3,3,3,3,3,3,3,3,3,
3,3,3,3,3,3,3,3,3,3,3,3,3,3,3,3,3,3,3,3,3,3,4),(93.3317490905774,93.435694332417,
93.5397120172538,93.6438984400441,93.6605043886358,93.7646927380818,93.8687258362982,
93.9726368703958,94.0764824260428,94.180297279391,94.284116163135,94.3880436655015,
94.4920299826526,94.596198175621,94.6580522469818,94.7622418091092,94.8662761707485,
94.9701885366066,95.0740354653412,95.1778517307116,95.2816720630607,95.3856010591389,
95.489588897669,95.5937586386179,95.6556001053279,95.7597703757183,95.8637853776279,
95.9676783761358,96.0715059432305,96.1753028809778,96.2791039480478,96.3830139060965,
96.4869828059679,96.5911339707109,96.653147963674,96.7562487155586,96.8592080959374,
96.9620624807666,97.0688899258958,97.1716683720447,97.2744473600228,97.3772955657622,
97.3893722612836),.UNSPECIFIED.);
#2584=B_SPLINE_CURVE_WITH_KNOTS('',3,(#88275,#88276,#88277,#88278,#88279,
#88280),.UNSPECIFIED.,.F.,.F.,(4,1,1,4),(97.3893748528935,97.6506958220201,
98.6482436803662,99.6151588600969),.UNSPECIFIED.);
#2585=B_SPLINE_CURVE_WITH_KNOTS('',3,(#88282,#88283,#88284,#88285,#88286,
#88287,#88288,#88289,#88290,#88291,#88292,#88293,#88294,#88295,#88296,#88297,
#88298,#88299,#88300,#88301,#88302,#88303,#88304,#88305,#88306,#88307,#88308,
#88309,#88310,#88311,#88312,#88313,#88314,#88315,#88316,#88317,#88318,#88319,
#88320,#88321,#88322,#88323,#88324,#88325,#88326,#88327,#88328,#88329,#88330,
#88331,#88332,#88333,#88334,#88335,#88336,#88337,#88338,#88339,#88340,#88341,
#88342,#88343,#88344,#88345,#88346,#88347,#88348),.UNSPECIFIED.,.F.,.F.,
(4,3,3,3,3,3,3,3,3,3,3,3,3,3,3,3,3,3,3,3,3,3,4),(97.3893722616736,97.4918529942681,
97.5942444189893,97.6965831997679,97.7989059241202,97.9013194553043,98.0037772003265,
98.1064188744439,98.1921611138482,98.296331412984,98.4003464436805,98.5042394709017,
98.6080670666496,98.711864032949,98.8156651284298,98.9195751144808,99.0235440421667,
99.1276952341283,99.1897089721943,99.2961881333788,99.4002221458023,99.5079238813673,
99.6156256169323),.UNSPECIFIED.);
#2586=B_SPLINE_CURVE_WITH_KNOTS('',3,(#88349,#88350,#88351,#88352,#88353,
#88354,#88355,#88356,#88357,#88358,#88359,#88360,#88361,#88362,#88363,#88364,
#88365,#88366,#88367,#88368,#88369,#88370,#88371,#88372,#88373,#88374,#88375,
#88376,#88377,#88378,#88379,#88380,#88381,#88382,#88383,#88384,#88385,#88386,
#88387,#88388,#88389,#88390,#88391,#88392,#88393,#88394,#88395,#88396,#88397,
#88398,#88399,#88400,#88401,#88402,#88403,#88404,#88405,#88406,#88407,#88408,
#88409,#88410,#88411,#88412,#88413,#88414,#88415,#88416,#88417,#88418,#88419,
#88420,#88421,#88422,#88423,#88424,#88425,#88426,#88427,#88428,#88429,#88430,
#88431,#88432,#88433,#88434,#88435,#88436,#88437,#88438,#88439,#88440,#88441,
#88442,#88443,#88444,#88445,#88446,#88447,#88448,#88449,#88450,#88451,#88452,
#88453,#88454,#88455,#88456,#88457,#88458,#88459,#88460,#88461,#88462,#88463,
#88464,#88465,#88466,#88467,#88468,#88469,#88470,#88471,#88472),
 .UNSPECIFIED.,.F.,.F.,(4,3,3,3,3,3,3,3,3,3,3,3,3,3,3,3,3,3,3,3,3,3,3,3,
3,3,3,3,3,3,3,3,3,3,3,3,3,3,3,3,3,4),(93.3327290514497,93.4413841300764,
93.5452716396415,93.6491033120159,93.7529139105045,93.8567381646366,93.9606769722411,
94.0646832476024,94.1688628859985,94.2019696804638,94.3061564133321,94.410187912589,
94.5140973811542,94.6179413926832,94.7217547253996,94.8255721140933,94.9294981703152,
95.0334830667106,95.1376498941375,95.1995175388099,95.3037016465712,95.4077305135391,
95.5116373518152,95.615478735705,95.7192894472635,95.8231042251162,95.9270277041183,
96.0310100383646,96.1351743552147,96.197065397156,96.3012537439254,96.4052868394961,
96.509197871006,96.6130434241022,96.71685827494,96.8206771562169,96.9246046561991,
97.0285909710088,97.1327591617284,97.1946132555021,97.345602266741,97.3893722612836),
 .UNSPECIFIED.);
#2587=B_SPLINE_CURVE_WITH_KNOTS('',3,(#88478,#88479,#88480,#88481,#88482,
#88483,#88484,#88485,#88486,#88487,#88488,#88489,#88490,#88491,#88492,#88493,
#88494,#88495,#88496,#88497,#88498,#88499,#88500,#88501,#88502,#88503,#88504,
#88505,#88506,#88507,#88508,#88509,#88510,#88511,#88512,#88513,#88514,#88515,
#88516,#88517,#88518,#88519,#88520,#88521,#88522,#88523,#88524,#88525,#88526,
#88527,#88528,#88529,#88530,#88531,#88532,#88533,#88534,#88535,#88536,#88537,
#88538,#88539,#88540,#88541,#88542,#88543,#88544,#88545,#88546,#88547,#88548,
#88549,#88550,#88551,#88552,#88553,#88554,#88555,#88556,#88557,#88558,#88559,
#88560,#88561,#88562,#88563,#88564,#88565,#88566,#88567,#88568,#88569,#88570,
#88571,#88572,#88573,#88574,#88575,#88576,#88577,#88578,#88579,#88580,#88581,
#88582,#88583,#88584,#88585,#88586,#88587,#88588,#88589,#88590,#88591,#88592,
#88593,#88594,#88595,#88596,#88597,#88598),.UNSPECIFIED.,.F.,.F.,(4,3,3,
3,3,3,3,3,3,3,3,3,3,3,3,3,3,3,3,3,3,3,3,3,3,3,3,3,3,3,3,3,3,3,3,3,3,3,3,
3,4),(87.0493974468485,87.1532189896668,87.2570297906175,87.3615766526029,
87.4655324459015,87.5703748422304,87.6752172385592,87.7794034197809,87.8834343624533,
87.9873432698471,88.0911867176855,88.1949994850426,88.2988163075558,88.4027418002793,
88.5067261338403,88.6108924056251,88.6727650969053,88.7769513494554,88.8809823642944,
88.9848913447398,89.0887348661345,89.1925477074401,89.2963646041826,89.4002901710438,
89.5042745788026,89.6084409240676,89.6703129552514,89.7744988575247,89.8785295213807,
89.9824381514785,90.0862813231058,90.1900938157322,90.2939103653924,90.3978355899808,
90.5018196576624,90.6059856700009,90.6678608135975,90.7807059016893,90.8932651237372,
91.005365280633,91.106186953809),.UNSPECIFIED.);
#2588=B_SPLINE_CURVE_WITH_KNOTS('',3,(#88599,#88600,#88601,#88602,#88603,
#88604,#88605,#88606,#88607,#88608,#88609,#88610,#88611,#88612,#88613,#88614,
#88615,#88616,#88617,#88618,#88619,#88620,#88621,#88622,#88623,#88624,#88625,
#88626,#88627,#88628,#88629,#88630,#88631,#88632,#88633,#88634,#88635,#88636,
#88637,#88638,#88639,#88640,#88641,#88642,#88643,#88644,#88645,#88646,#88647,
#88648,#88649,#88650,#88651,#88652,#88653,#88654,#88655,#88656,#88657,#88658,
#88659,#88660,#88661,#88662,#88663,#88664,#88665,#88666,#88667,#88668),
 .UNSPECIFIED.,.F.,.F.,(4,3,3,3,3,3,3,3,3,3,3,3,3,3,3,3,3,3,3,3,3,3,3,4),
(91.106186954104,91.2125697194757,91.3190337387694,91.4256926623267,91.5324645374607,
91.6394564150643,91.6654086719436,91.76959540681,91.8736269080771,91.9775363786608,
92.0813803922122,92.1851937269521,92.2890111176673,92.3929371758939,92.4969220742875,
92.6010889036804,92.6629565302897,92.7671202567895,92.8711391118278,92.9750481127459,
93.078891237982,93.1826959263191,93.2865260562585,93.3317490905774),
 .UNSPECIFIED.);
#2589=B_SPLINE_CURVE_WITH_KNOTS('',3,(#88670,#88671,#88672,#88673,#88674,
#88675,#88676,#88677,#88678,#88679,#88680,#88681,#88682,#88683,#88684,#88685,
#88686,#88687,#88688,#88689,#88690,#88691,#88692,#88693,#88694,#88695,#88696,
#88697,#88698,#88699,#88700,#88701,#88702,#88703,#88704,#88705,#88706,#88707,
#88708,#88709,#88710,#88711,#88712,#88713,#88714,#88715,#88716,#88717,#88718,
#88719,#88720,#88721,#88722,#88723,#88724,#88725,#88726,#88727,#88728,#88729,
#88730,#88731,#88732,#88733,#88734,#88735,#88736,#88737,#88738,#88739),
 .UNSPECIFIED.,.F.,.F.,(4,3,3,3,3,3,3,3,3,3,3,3,3,3,3,3,3,3,3,3,3,3,3,4),
(91.106186954104,91.2093261054256,91.3135123576276,91.4175433721169,91.5214523522112,
91.6252958732545,91.7291087142088,91.8329256106003,91.9368511771141,92.0408355845268,
92.1450019294517,92.2068739637717,92.3110598668121,92.4150905314355,92.5189991622972,
92.6228423346862,92.7266548280707,92.8304713784842,92.9343966038141,93.0383806722314,
93.1425466852886,93.2044218221177,93.3086062151315,93.3327290514497),
 .UNSPECIFIED.);
#2590=B_SPLINE_CURVE_WITH_KNOTS('',3,(#88740,#88741,#88742,#88743,#88744,
#88745,#88746,#88747,#88748,#88749,#88750,#88751,#88752,#88753,#88754,#88755,
#88756,#88757,#88758,#88759,#88760,#88761,#88762,#88763,#88764,#88765,#88766,
#88767,#88768,#88769,#88770,#88771,#88772,#88773,#88774,#88775,#88776,#88777,
#88778,#88779,#88780,#88781,#88782,#88783,#88784,#88785,#88786,#88787,#88788,
#88789,#88790,#88791,#88792,#88793,#88794,#88795,#88796,#88797,#88798,#88799,
#88800,#88801,#88802,#88803,#88804,#88805,#88806,#88807,#88808,#88809,#88810,
#88811,#88812,#88813,#88814,#88815,#88816,#88817,#88818,#88819,#88820,#88821,
#88822,#88823,#88824,#88825,#88826,#88827,#88828,#88829,#88830,#88831,#88832,
#88833,#88834,#88835,#88836,#88837,#88838,#88839,#88840,#88841,#88842,#88843,
#88844,#88845,#88846,#88847,#88848,#88849,#88850,#88851,#88852,#88853,#88854,
#88855,#88856,#88857,#88858,#88859,#88860,#88861,#88862,#88863),
 .UNSPECIFIED.,.F.,.F.,(4,3,3,3,3,3,3,3,3,3,3,3,3,3,3,3,3,3,3,3,3,3,3,3,
3,3,3,3,3,3,3,3,3,3,3,3,3,3,3,3,3,4),(87.0484536587393,87.1526180566811,
87.2191346720412,87.3233208365446,87.4273517627344,87.5312606540692,87.6351040861179,
87.7389168379752,87.8427336452998,87.9466591234087,88.0506434426566,88.154809700756,
88.2166825303873,88.3208687070139,88.4248996454306,88.5288085490861,88.6326519935066,
88.7364647577682,88.840281577511,88.9442070679729,89.0481913995558,89.1523576698271,
89.2142303887334,89.3184165199705,89.4224474129372,89.5263562712705,89.6301996704719,
89.7340123896828,89.8378291646089,89.9417546109172,90.0457388986538,90.1499051260383,
90.2117782470795,90.3146405386673,90.4173275777108,90.5199168635336,90.6224449018284,
90.7249481125111,90.8275243328762,90.9301371296558,91.0329110106376,91.1061869536468),
 .UNSPECIFIED.);
#2591=B_SPLINE_CURVE_WITH_KNOTS('',3,(#88869,#88870,#88871,#88872,#88873,
#88874,#88875,#88876,#88877,#88878,#88879,#88880,#88881,#88882,#88883,#88884,
#88885,#88886,#88887,#88888,#88889,#88890,#88891,#88892,#88893,#88894,#88895,
#88896,#88897,#88898,#88899,#88900,#88901,#88902,#88903,#88904,#88905,#88906,
#88907,#88908,#88909,#88910,#88911,#88912,#88913,#88914,#88915,#88916,#88917,
#88918,#88919,#88920,#88921,#88922,#88923,#88924,#88925,#88926,#88927,#88928,
#88929,#88930,#88931,#88932,#88933,#88934,#88935,#88936,#88937,#88938,#88939,
#88940,#88941,#88942,#88943,#88944,#88945,#88946,#88947,#88948,#88949,#88950,
#88951,#88952,#88953,#88954,#88955,#88956,#88957,#88958,#88959,#88960,#88961,
#88962,#88963,#88964,#88965,#88966,#88967,#88968,#88969,#88970,#88971,#88972,
#88973,#88974,#88975,#88976,#88977,#88978,#88979,#88980,#88981,#88982,#88983,
#88984,#88985,#88986,#88987,#88988,#88989),.UNSPECIFIED.,.F.,.F.,(4,3,3,
3,3,3,3,3,3,3,3,3,3,3,3,3,3,3,3,3,3,3,3,3,3,3,3,3,3,3,3,3,3,3,3,3,3,3,3,
3,4),(80.7662049656111,80.8702771562758,80.9742116984674,81.0780706249186,
81.181888734009,81.2857007704572,81.3896149728771,81.4935789190852,81.5977344389464,
81.6899300884827,81.7941162519362,81.8981471771086,82.0020560674785,82.1058994985952,
82.2097122495543,82.3135290560159,82.4174545333203,82.5214388517957,82.6256051091809,
82.6874779468288,82.7916641121998,82.8956950393023,82.9996039316116,83.1034473646724,
83.2072601175775,83.3110769259838,83.4150024052179,83.5189867256173,83.6231529848968,
83.6850258051749,83.7892119647504,83.8932428860536,83.9971517725858,84.100995199886,
84.2048079470555,84.3086247497596,84.4125502233813,84.5165345382103,84.6207007920462,
84.682573663521,84.8230016469244),.UNSPECIFIED.);
#2592=B_SPLINE_CURVE_WITH_KNOTS('',3,(#88990,#88991,#88992,#88993,#88994,
#88995,#88996,#88997,#88998,#88999,#89000,#89001,#89002,#89003,#89004,#89005,
#89006,#89007,#89008,#89009,#89010,#89011,#89012,#89013,#89014,#89015,#89016,
#89017,#89018,#89019,#89020,#89021,#89022,#89023,#89024,#89025,#89026,#89027,
#89028,#89029,#89030,#89031,#89032,#89033,#89034,#89035,#89036,#89037,#89038,
#89039,#89040,#89041,#89042,#89043,#89044,#89045,#89046,#89047,#89048,#89049,
#89050,#89051,#89052,#89053,#89054,#89055,#89056,#89057,#89058,#89059),
 .UNSPECIFIED.,.F.,.F.,(4,3,3,3,3,3,3,3,3,3,3,3,3,3,3,3,3,3,3,3,3,3,3,4),
(84.8230016473325,84.9301416316494,85.0325714156815,85.1349307967517,85.2372563938986,
85.3395847740774,85.4420166327704,85.5445096289043,85.6471710508368,85.6801215218671,
85.7843076985516,85.8883386370265,85.9922475407404,86.0960909852193,86.1999037495391,
86.3037205693399,86.4076460598594,86.5116303914995,86.6157966618271,86.6776693802132,
86.7818282135815,86.8858513273734,86.9897581895063,87.0493974468485),
 .UNSPECIFIED.);
#2593=B_SPLINE_CURVE_WITH_KNOTS('',3,(#89061,#89062,#89063,#89064,#89065,
#89066,#89067,#89068,#89069,#89070,#89071,#89072,#89073,#89074,#89075,#89076,
#89077,#89078,#89079,#89080,#89081,#89082,#89083,#89084,#89085,#89086,#89087,
#89088,#89089,#89090,#89091,#89092,#89093,#89094,#89095,#89096,#89097,#89098,
#89099,#89100,#89101,#89102,#89103,#89104,#89105,#89106,#89107,#89108,#89109,
#89110,#89111,#89112,#89113,#89114,#89115,#89116,#89117,#89118,#89119,#89120,
#89121,#89122,#89123,#89124,#89125,#89126,#89127),.UNSPECIFIED.,.F.,.F.,
(4,3,3,3,3,3,3,3,3,3,3,3,3,3,3,3,3,3,3,3,3,3,4),(84.8230016473381,84.9376554433282,
85.0527190367408,85.1683359261865,85.224038955349,85.3282251207107,85.4322560478039,
85.536164940104,85.6400083731555,85.7438211260512,85.8476379344483,85.9515634136733,
86.0555477340635,86.1597139933341,86.2215868136951,86.3257394075604,86.4297517315574,
86.5336587783306,86.6374954176148,86.7413356684352,86.8451704367688,86.9491112664109,
87.0484536587393),.UNSPECIFIED.);
#2594=B_SPLINE_CURVE_WITH_KNOTS('',3,(#89128,#89129,#89130,#89131,#89132,
#89133,#89134,#89135,#89136,#89137,#89138,#89139,#89140,#89141,#89142,#89143,
#89144,#89145,#89146,#89147,#89148,#89149,#89150,#89151,#89152,#89153,#89154,
#89155,#89156,#89157,#89158,#89159,#89160,#89161,#89162,#89163,#89164,#89165,
#89166,#89167,#89168,#89169,#89170,#89171,#89172,#89173,#89174,#89175,#89176,
#89177,#89178,#89179,#89180,#89181,#89182,#89183,#89184,#89185,#89186,#89187,
#89188,#89189,#89190,#89191,#89192,#89193,#89194,#89195,#89196,#89197,#89198,
#89199,#89200,#89201,#89202,#89203,#89204,#89205,#89206,#89207,#89208,#89209,
#89210,#89211,#89212,#89213,#89214,#89215,#89216,#89217,#89218,#89219,#89220,
#89221,#89222,#89223,#89224,#89225,#89226,#89227,#89228,#89229,#89230,#89231,
#89232,#89233,#89234,#89235,#89236,#89237,#89238,#89239,#89240,#89241,#89242,
#89243,#89244,#89245,#89246,#89247,#89248,#89249,#89250,#89251),
 .UNSPECIFIED.,.F.,.F.,(4,3,3,3,3,3,3,3,3,3,3,3,3,3,3,3,3,3,3,3,3,3,3,3,
3,3,3,3,3,3,3,3,3,3,3,3,3,3,3,3,3,4),(80.7657498498246,80.8695688015658,
80.9734984375536,81.0774898205032,81.1816601949338,81.2338475219647,81.3380336854276,
81.4420646106138,81.545973501004,81.6498169321448,81.7536296831319,81.8574464896251,
81.9613719669668,82.0653562854825,82.1695225429127,82.2313953803108,82.3355815440582,
82.4396124695303,82.5435213602072,82.6473647916352,82.7511775429095,82.8549943496892,
82.9589198273146,83.0629041461133,83.1670704038213,83.2289432386569,83.3331294016869,
83.4371603264421,83.5410692164054,83.6449126471221,83.7487253976887,83.8525422037659,
83.9564676807001,84.0604519988128,84.1646182558513,84.226491097003,84.3322636670979,
84.4378652907398,84.5433026053224,84.6486432054657,84.7539210457329,84.8230016469244),
 .UNSPECIFIED.);
#2595=B_SPLINE_CURVE_WITH_KNOTS('',3,(#89257,#89258,#89259,#89260,#89261,
#89262,#89263,#89264,#89265,#89266,#89267,#89268,#89269,#89270,#89271,#89272,
#89273,#89274,#89275,#89276,#89277,#89278,#89279,#89280,#89281,#89282,#89283,
#89284,#89285,#89286,#89287,#89288,#89289,#89290,#89291,#89292,#89293,#89294,
#89295,#89296,#89297,#89298,#89299,#89300,#89301,#89302,#89303,#89304,#89305,
#89306,#89307,#89308,#89309,#89310,#89311,#89312,#89313,#89314,#89315,#89316,
#89317,#89318,#89319,#89320,#89321,#89322,#89323,#89324,#89325,#89326,#89327,
#89328,#89329,#89330,#89331,#89332,#89333,#89334,#89335,#89336,#89337,#89338,
#89339,#89340,#89341,#89342,#89343,#89344,#89345,#89346,#89347,#89348,#89349,
#89350,#89351,#89352,#89353,#89354,#89355,#89356,#89357,#89358,#89359,#89360,
#89361,#89362,#89363,#89364,#89365,#89366,#89367,#89368,#89369,#89370,#89371,
#89372,#89373,#89374,#89375,#89376,#89377,#89378,#89379,#89380,#89381,#89382,
#89383),.UNSPECIFIED.,.F.,.F.,(4,3,3,3,3,3,3,3,3,3,3,3,3,3,3,3,3,3,3,3,
3,3,3,3,3,3,3,3,3,3,3,3,3,3,3,3,3,3,3,3,3,3,4),(74.4820670752277,74.5860865447775,
74.6902747768549,74.7070950800601,74.8112812435426,74.9153121687491,75.0192210591604,
75.123064490323,75.2268772413324,75.3306940478485,75.4346195252135,75.538603843753,
75.6427701012072,75.7046429384062,75.8088291018885,75.9128600270946,76.0167689175055,
76.1206123486675,76.2244250996762,76.3282419061915,76.4321673835557,76.5361517020941,
76.6403179595472,76.7021907967523,76.8063769602756,76.9104078855229,77.0143167759751,
77.1181602071783,77.2219729582282,77.3257897647846,77.4297152421894,77.5336995607683,
77.6378658182611,77.6997386550984,77.8047483656351,77.9072108121553,78.0095758369094,
78.1118801626899,78.2188642068654,78.3212057259318,78.4235870712412,78.5260937325057,
78.5398163393917),.UNSPECIFIED.);
#2596=B_SPLINE_CURVE_WITH_KNOTS('',3,(#89384,#89385,#89386,#89387,#89388,
#89389,#89390,#89391,#89392,#89393,#89394,#89395,#89396,#89397,#89398,#89399,
#89400,#89401,#89402,#89403,#89404,#89405,#89406,#89407,#89408,#89409,#89410,
#89411,#89412,#89413,#89414,#89415,#89416,#89417,#89418,#89419,#89420,#89421,
#89422,#89423,#89424,#89425,#89426,#89427,#89428,#89429,#89430,#89431,#89432,
#89433,#89434,#89435,#89436,#89437,#89438,#89439,#89440,#89441,#89442,#89443,
#89444,#89445,#89446,#89447,#89448,#89449,#89450),.UNSPECIFIED.,.F.,.F.,
(4,3,3,3,3,3,3,3,3,3,3,3,3,3,3,3,3,3,3,3,3,3,4),(78.5398163397448,78.6972865134445,
78.8014726769072,78.9055036020932,79.0094124924832,79.1132559236238,79.2170686746107,
79.3208854811037,79.4248109584452,79.5287952769607,79.6329615343907,79.6948343717906,
79.7990205355393,79.9030514610129,80.0069603516911,80.1108037831204,80.214616534396,
80.3184333411772,80.4223588188041,80.5263431376039,80.6305093953132,80.6923822301366,
80.7662049656111),.UNSPECIFIED.);
#2597=B_SPLINE_CURVE_WITH_KNOTS('',3,(#89452,#89453,#89454,#89455,#89456,
#89457,#89458,#89459,#89460,#89461,#89462,#89463,#89464,#89465,#89466,#89467,
#89468,#89469,#89470,#89471,#89472,#89473,#89474,#89475,#89476,#89477,#89478,
#89479,#89480,#89481,#89482,#89483,#89484,#89485,#89486,#89487,#89488,#89489,
#89490,#89491,#89492,#89493,#89494,#89495,#89496,#89497,#89498,#89499,#89500,
#89501,#89502,#89503,#89504,#89505,#89506,#89507,#89508,#89509,#89510,#89511,
#89512,#89513,#89514,#89515,#89516,#89517,#89518),.UNSPECIFIED.,.F.,.F.,
(4,3,3,3,3,3,3,3,3,3,3,3,3,3,3,3,3,3,3,3,3,3,4),(78.5398163397448,78.6430480181452,
78.7462408135878,78.8494302890941,78.9527248465251,79.0560730499683,79.1596112159242,
79.2387518052725,79.3429379687955,79.4469688940425,79.5508777844944,79.6547212156974,
79.7585339667471,79.8623507733033,79.9662762507079,80.0702605692866,80.1744268267791,
80.2362996636186,80.3404816764144,80.4467987197669,80.5507037015718,80.6582267756982,
80.7657498498246),.UNSPECIFIED.);
#2598=B_SPLINE_CURVE_WITH_KNOTS('',3,(#89519,#89520,#89521,#89522,#89523,
#89524,#89525,#89526,#89527,#89528,#89529,#89530,#89531,#89532,#89533,#89534,
#89535,#89536,#89537,#89538,#89539,#89540,#89541,#89542,#89543,#89544,#89545,
#89546,#89547,#89548,#89549,#89550,#89551,#89552,#89553,#89554,#89555,#89556,
#89557,#89558,#89559,#89560,#89561,#89562,#89563,#89564,#89565,#89566,#89567,
#89568,#89569,#89570,#89571,#89572,#89573,#89574,#89575,#89576,#89577,#89578,
#89579,#89580,#89581,#89582,#89583,#89584,#89585,#89586,#89587,#89588,#89589,
#89590,#89591,#89592,#89593,#89594,#89595,#89596,#89597,#89598,#89599,#89600,
#89601,#89602,#89603,#89604,#89605,#89606,#89607,#89608,#89609,#89610,#89611,
#89612,#89613,#89614,#89615,#89616,#89617,#89618,#89619,#89620,#89621,#89622,
#89623,#89624,#89625,#89626,#89627,#89628,#89629,#89630,#89631,#89632,#89633,
#89634,#89635,#89636,#89637,#89638,#89639,#89640,#89641,#89642),
 .UNSPECIFIED.,.F.,.F.,(4,3,3,3,3,3,3,3,3,3,3,3,3,3,3,3,3,3,3,3,3,3,3,3,
3,3,3,3,3,3,3,3,3,3,3,3,3,3,3,3,3,4),(74.4832485089442,74.5871391796787,
74.6909724336135,74.7947830366967,74.8986057195159,75.0025420121103,75.1065443563955,
75.2107214413106,75.2485603718882,75.3527465353754,75.4567774605866,75.5606863510025,
75.6645297821696,75.7683425331833,75.8721593397041,75.9760848170734,76.0800691356172,
76.1842353930753,76.2461082302343,76.350294393727,76.4543253189437,76.5582342093654,
76.662077640538,76.7658903915576,76.8697071980835,76.9736326754583,77.0776169940075,
77.1817832514711,77.2436560885804,77.3478422520629,77.4518731772695,77.5557820676809,
77.6596254988434,77.7634382498528,77.867255056369,77.9711805337341,78.0751648522737,
78.1793311097278,78.2412039469264,78.3682032551961,78.4934616304905,78.5398163394136),
 .UNSPECIFIED.);
#2599=B_SPLINE_CURVE_WITH_KNOTS('',3,(#89648,#89649,#89650,#89651,#89652,
#89653,#89654,#89655,#89656,#89657,#89658,#89659,#89660,#89661,#89662,#89663,
#89664,#89665,#89666,#89667,#89668,#89669,#89670,#89671,#89672,#89673,#89674,
#89675,#89676,#89677,#89678,#89679,#89680,#89681,#89682,#89683,#89684,#89685,
#89686,#89687,#89688,#89689,#89690,#89691,#89692,#89693,#89694,#89695,#89696,
#89697,#89698,#89699,#89700,#89701,#89702,#89703,#89704,#89705,#89706,#89707,
#89708,#89709,#89710,#89711,#89712,#89713,#89714,#89715,#89716,#89717,#89718,
#89719,#89720,#89721,#89722,#89723,#89724,#89725,#89726,#89727,#89728,#89729,
#89730,#89731,#89732,#89733,#89734,#89735,#89736,#89737,#89738,#89739,#89740,
#89741,#89742,#89743,#89744,#89745,#89746,#89747,#89748,#89749,#89750,#89751,
#89752,#89753,#89754,#89755,#89756,#89757,#89758,#89759,#89760,#89761,#89762,
#89763,#89764,#89765,#89766,#89767,#89768),.UNSPECIFIED.,.F.,.F.,(4,3,3,
3,3,3,3,3,3,3,3,3,3,3,3,3,3,3,3,3,3,3,3,3,3,3,3,3,3,3,3,3,3,3,3,3,3,3,3,
3,4),(68.1995463580489,68.3033571741053,68.4079698630748,68.5119255707606,
68.6168667503721,68.7218079299836,68.8259940934717,68.930025018684,69.0339339091009,
69.1377773402689,69.2415900912839,69.3454068978052,69.4493323751755,69.5533166937202,
69.6574829511794,69.7193557883297,69.8235419518177,69.9275728770295,70.0314817674464,
70.1353251986144,70.239137949629,70.34295475615,70.4468802335202,70.550864552065,
70.6550308095241,70.7169036466758,70.8210898101646,70.9251207353769,71.0290296257945,
71.1328730569633,71.2366858079789,71.3405026145007,71.4444280918716,71.5484124104166,
71.6525786678764,71.7144515050219,71.8220784528937,71.9307165978116,72.0379272940085,
72.1472791632869,72.2566310325652),.UNSPECIFIED.);
#2600=B_SPLINE_CURVE_WITH_KNOTS('',3,(#89769,#89770,#89771,#89772,#89773,
#89774,#89775,#89776,#89777,#89778,#89779,#89780,#89781,#89782,#89783,#89784,
#89785,#89786,#89787,#89788,#89789,#89790,#89791,#89792,#89793,#89794,#89795,
#89796,#89797,#89798,#89799,#89800,#89801,#89802,#89803,#89804,#89805,#89806,
#89807,#89808,#89809,#89810,#89811,#89812,#89813,#89814,#89815,#89816,#89817,
#89818,#89819,#89820,#89821,#89822,#89823,#89824,#89825,#89826,#89827,#89828,
#89829,#89830,#89831,#89832,#89833,#89834,#89835),.UNSPECIFIED.,.F.,.F.,
(4,3,3,3,3,3,3,3,3,3,3,3,3,3,3,3,3,3,3,3,3,3,4),(72.2566310330055,72.3704731155961,
72.4818133112497,72.5969063373088,72.7119993633679,72.816185526855,72.9202164520661,
73.024125342482,73.127968773649,73.2317815246628,73.3355983311831,73.4395238085524,
73.543508127096,73.6476743845542,73.709547221714,73.8137037279885,73.9177183838715,
74.021626189055,74.1254620178865,74.2292882438049,74.3331083624566,74.4370016475404,
74.4820670752277),.UNSPECIFIED.);
#2601=B_SPLINE_CURVE_WITH_KNOTS('',3,(#89837,#89838,#89839,#89840,#89841,
#89842,#89843,#89844,#89845,#89846,#89847,#89848,#89849,#89850,#89851,#89852,
#89853,#89854,#89855,#89856,#89857,#89858,#89859,#89860,#89861,#89862,#89863,
#89864,#89865,#89866,#89867,#89868,#89869,#89870,#89871,#89872,#89873,#89874,
#89875,#89876,#89877,#89878,#89879,#89880,#89881,#89882,#89883,#89884,#89885,
#89886,#89887,#89888,#89889,#89890,#89891,#89892,#89893,#89894,#89895,#89896,
#89897,#89898,#89899,#89900,#89901,#89902,#89903,#89904,#89905,#89906),
 .UNSPECIFIED.,.F.,.F.,(4,3,3,3,3,3,3,3,3,3,3,3,3,3,3,3,3,3,3,3,3,3,3,4),
(72.2566310325652,72.3608036974116,72.4648211348936,72.5687165871306,72.6725466326848,
72.776346071062,72.8801496583905,72.9840619405011,73.0880331866153,73.1921861589884,
73.253464655196,73.3576508186849,73.4616817438977,73.5655906343152,73.6694340654839,
73.7732468164996,73.8770636230217,73.9809891003927,74.0849734189379,74.1891396763978,
74.2510125135421,74.3552035653614,74.459228530687,74.4832485089442),
 .UNSPECIFIED.);
#2602=B_SPLINE_CURVE_WITH_KNOTS('',3,(#89907,#89908,#89909,#89910,#89911,
#89912,#89913,#89914,#89915,#89916,#89917,#89918,#89919,#89920,#89921,#89922,
#89923,#89924,#89925,#89926,#89927,#89928,#89929,#89930,#89931,#89932,#89933,
#89934,#89935,#89936,#89937,#89938,#89939,#89940,#89941,#89942,#89943,#89944,
#89945,#89946,#89947,#89948,#89949,#89950,#89951,#89952,#89953,#89954,#89955,
#89956,#89957,#89958,#89959,#89960,#89961,#89962,#89963,#89964,#89965,#89966,
#89967,#89968,#89969,#89970,#89971,#89972,#89973,#89974,#89975,#89976,#89977,
#89978,#89979,#89980,#89981,#89982,#89983,#89984,#89985,#89986,#89987,#89988,
#89989,#89990,#89991,#89992,#89993,#89994,#89995,#89996,#89997,#89998,#89999,
#90000,#90001,#90002,#90003,#90004,#90005,#90006,#90007,#90008,#90009,#90010,
#90011,#90012,#90013,#90014,#90015,#90016,#90017,#90018,#90019,#90020,#90021,
#90022,#90023,#90024,#90025,#90026,#90027,#90028,#90029,#90030,#90031,#90032,
#90033),.UNSPECIFIED.,.F.,.F.,(4,3,3,3,3,3,3,3,3,3,3,3,3,3,3,3,3,3,3,3,
3,3,3,3,3,3,3,3,3,3,3,3,3,3,3,3,3,3,3,3,3,3,4),(68.1991405116964,68.2657253634656,
68.3699115269538,68.4739424521659,68.5778513425829,68.681694773751,68.785507524766,
68.8893243312875,68.9932498086579,69.0972341272026,69.2014003846619,69.2632732218117,
69.3674593852998,69.471490310512,69.5753992009289,69.679242632097,69.7830553831119,
69.8868721896334,69.9907976670037,70.0947819855484,70.1989482430077,70.2608210801577,
70.365007243646,70.4690381688582,70.5729470592752,70.6767904904434,70.7806032414584,
70.8844200479799,70.9883455253504,71.0923298438952,71.1964961013545,71.2583689385038,
71.3625551019919,71.4665860272041,71.570494917621,71.674338348789,71.7781510998039,
71.8819679063254,71.9858933836958,72.0898777022405,72.1940439596997,72.2559167968499,
72.2566310325397),.UNSPECIFIED.);
#2603=B_SPLINE_CURVE_WITH_KNOTS('',3,(#90039,#90040,#90041,#90042,#90043,
#90044,#90045,#90046,#90047,#90048,#90049,#90050,#90051,#90052,#90053,#90054,
#90055,#90056,#90057,#90058,#90059,#90060,#90061,#90062,#90063,#90064,#90065,
#90066,#90067,#90068,#90069,#90070,#90071,#90072,#90073,#90074,#90075,#90076,
#90077,#90078,#90079,#90080,#90081,#90082,#90083,#90084,#90085,#90086,#90087,
#90088,#90089,#90090,#90091,#90092,#90093,#90094,#90095,#90096,#90097,#90098,
#90099,#90100,#90101,#90102,#90103,#90104,#90105,#90106,#90107,#90108,#90109,
#90110,#90111,#90112,#90113,#90114,#90115,#90116,#90117,#90118,#90119,#90120,
#90121,#90122,#90123,#90124,#90125,#90126,#90127,#90128,#90129,#90130,#90131,
#90132,#90133,#90134,#90135,#90136,#90137,#90138,#90139,#90140,#90141,#90142,
#90143,#90144,#90145,#90146,#90147,#90148,#90149,#90150,#90151,#90152,#90153,
#90154,#90155,#90156,#90157,#90158,#90159),.UNSPECIFIED.,.F.,.F.,(4,3,3,
3,3,3,3,3,3,3,3,3,3,3,3,3,3,3,3,3,3,3,3,3,3,3,3,3,3,3,3,3,3,3,3,3,3,3,3,
3,4),(61.9168706242402,62.0208051644045,62.1246640897561,62.2284821986722,
62.3322942358697,62.4362084396395,62.540172388026,62.6443279091437,62.7365207799071,
62.8407069433953,62.9447378686074,63.0486467590244,63.1524901901925,63.2563029412074,
63.3601197477289,63.4640452250993,63.5680295436441,63.6721958011033,63.7340686382532,
63.8382548017414,63.9422857269536,64.0461946173705,64.1500380485386,64.2538507995535,
64.357667606075,64.4615930834454,64.5655774019901,64.6697436594494,64.7316164965992,
64.8358026600874,64.9398335852995,65.0437424757165,65.1475859068846,65.2513986578996,
65.3552154644212,65.4591409417916,65.5631252603363,65.6672915177955,65.7291643549453,
65.8652061647477,65.9734457251369),.UNSPECIFIED.);
#2604=B_SPLINE_CURVE_WITH_KNOTS('',3,(#90160,#90161,#90162,#90163,#90164,
#90165,#90166,#90167,#90168,#90169,#90170,#90171,#90172,#90173,#90174,#90175,
#90176,#90177,#90178,#90179,#90180,#90181,#90182,#90183,#90184,#90185,#90186,
#90187,#90188,#90189,#90190,#90191,#90192,#90193,#90194,#90195,#90196,#90197,
#90198,#90199,#90200,#90201,#90202,#90203,#90204,#90205,#90206,#90207,#90208,
#90209,#90210,#90211,#90212,#90213,#90214,#90215,#90216,#90217,#90218,#90219,
#90220,#90221,#90222,#90223,#90224,#90225,#90226,#90227,#90228,#90229),
 .UNSPECIFIED.,.F.,.F.,(4,3,3,3,3,3,3,3,3,3,3,3,3,3,3,3,3,3,3,3,3,3,3,4),
(65.9734457253856,66.0761317728201,66.1787500761627,66.2813369783486,66.3839287747718,
66.4866268116119,66.5893873525262,66.692318663947,66.7267122132914,66.8308983767796,
66.9349293019916,67.0388381924084,67.1426816235765,67.2464943745914,67.3503111811128,
67.4542366584832,67.5582209770279,67.6623872344871,67.7242600716375,67.8284495541652,
67.9324611612288,68.0363696448814,68.1402112750339,68.1995463580489),
 .UNSPECIFIED.);
#2605=B_SPLINE_CURVE_WITH_KNOTS('',3,(#90231,#90232,#90233,#90234,#90235,
#90236,#90237,#90238,#90239,#90240,#90241,#90242,#90243,#90244,#90245,#90246,
#90247,#90248,#90249,#90250,#90251,#90252,#90253,#90254,#90255,#90256,#90257,
#90258,#90259,#90260,#90261,#90262,#90263,#90264,#90265,#90266,#90267,#90268,
#90269,#90270,#90271,#90272,#90273,#90274,#90275,#90276,#90277,#90278,#90279,
#90280,#90281,#90282,#90283,#90284,#90285,#90286,#90287,#90288,#90289,#90290,
#90291,#90292,#90293,#90294,#90295,#90296,#90297),.UNSPECIFIED.,.F.,.F.,
(4,3,3,3,3,3,3,3,3,3,3,3,3,3,3,3,3,3,3,3,3,3,4),(65.9734457257113,66.0987387055991,
66.2258330924451,66.2706296467734,66.3748158102616,66.4788467354737,66.5827556258907,
66.6865990570588,66.7904118080738,66.8942286145953,66.9981540919657,67.1021384105105,
67.2063046679698,67.2681775051195,67.3723684093487,67.4763780578089,67.580285456455,
67.6841254672856,67.7879328708114,67.8918030347104,67.9957000777364,68.0997567680858,
68.1991405116964),.UNSPECIFIED.);
#2606=B_SPLINE_CURVE_WITH_KNOTS('',3,(#90298,#90299,#90300,#90301,#90302,
#90303,#90304,#90305,#90306,#90307,#90308,#90309,#90310,#90311,#90312,#90313,
#90314,#90315,#90316,#90317,#90318,#90319,#90320,#90321,#90322,#90323,#90324,
#90325,#90326,#90327,#90328,#90329,#90330,#90331,#90332,#90333,#90334,#90335,
#90336,#90337,#90338,#90339,#90340,#90341,#90342,#90343,#90344,#90345,#90346,
#90347,#90348,#90349,#90350,#90351,#90352,#90353,#90354,#90355,#90356,#90357,
#90358,#90359,#90360,#90361,#90362,#90363,#90364,#90365,#90366,#90367,#90368,
#90369,#90370,#90371,#90372,#90373,#90374,#90375,#90376,#90377,#90378,#90379,
#90380,#90381,#90382,#90383,#90384,#90385,#90386,#90387,#90388,#90389,#90390,
#90391,#90392,#90393,#90394,#90395,#90396,#90397,#90398,#90399,#90400,#90401,
#90402,#90403,#90404,#90405,#90406,#90407,#90408,#90409,#90410,#90411,#90412,
#90413,#90414,#90415,#90416,#90417,#90418,#90419,#90420,#90421),
 .UNSPECIFIED.,.F.,.F.,(4,3,3,3,3,3,3,3,3,3,3,3,3,3,3,3,3,3,3,3,3,3,3,3,
3,3,3,3,3,3,3,3,3,3,3,3,3,3,3,3,3,4),(61.9159031276989,62.0198326499991,
62.1238238422221,62.2279941032561,62.2804382133891,62.3846243768772,62.4886553020894,
62.5925641925064,62.6964076236745,62.8002203746894,62.9040371812107,63.0079626585811,
63.1119469771257,63.216113234585,63.2779860717351,63.3821722352232,63.4862031604353,
63.5901120508523,63.6939554820204,63.7977682330354,63.901585039557,64.0055105169275,
64.1094948354721,64.2136610929313,64.2755339300812,64.3797200935694,64.4837510187816,
64.5876599091986,64.6915033403668,64.7953160913818,64.8991328979035,65.0030583752739,
65.1070426938189,65.2112089512782,65.2730817884273,65.3766017373238,65.4799760620943,
65.5832406362457,65.6864470474328,65.7896160420576,65.8928309399411,65.9734457253856),
 .UNSPECIFIED.);
#2607=B_SPLINE_CURVE_WITH_KNOTS('',3,(#90427,#90428,#90429,#90430,#90431,
#90432,#90433,#90434,#90435,#90436,#90437,#90438,#90439,#90440,#90441,#90442,
#90443,#90444,#90445,#90446,#90447,#90448,#90449,#90450,#90451,#90452,#90453,
#90454,#90455,#90456,#90457,#90458,#90459,#90460,#90461,#90462,#90463,#90464,
#90465,#90466,#90467,#90468,#90469,#90470,#90471,#90472,#90473,#90474,#90475,
#90476,#90477,#90478,#90479,#90480,#90481,#90482,#90483,#90484,#90485,#90486,
#90487,#90488,#90489,#90490,#90491,#90492,#90493,#90494,#90495,#90496,#90497,
#90498,#90499,#90500,#90501,#90502,#90503,#90504,#90505,#90506,#90507,#90508,
#90509,#90510,#90511,#90512,#90513,#90514,#90515,#90516,#90517,#90518,#90519,
#90520,#90521,#90522,#90523,#90524,#90525,#90526,#90527,#90528,#90529,#90530,
#90531,#90532,#90533,#90534,#90535,#90536,#90537,#90538,#90539,#90540,#90541,
#90542,#90543,#90544,#90545,#90546,#90547,#90548,#90549,#90550),
 .UNSPECIFIED.,.F.,.F.,(4,3,3,3,3,3,3,3,3,3,3,3,3,3,3,3,3,3,3,3,3,3,3,3,
3,3,3,3,3,3,3,3,3,3,3,3,3,3,3,3,3,4),(55.6326045320091,55.736792722803,
55.7536857714845,55.8578719349727,55.9619028601848,56.0658117506018,56.1696551817699,
56.2734679327848,56.3772847393064,56.4812102166767,56.5851945352215,56.6893607926807,
56.7512336298306,56.8554197933188,56.959450718531,57.063359608948,57.1672030401161,
57.2710157911311,57.3748325976526,57.478758075023,57.5827423935677,57.686908651027,
57.7487814881766,57.8529676516648,57.9569985768769,58.0609074672938,58.1647508984619,
58.2685636494768,58.3723804559983,58.4763059333687,58.5802902519134,58.6844565093726,
58.7463293465227,58.8496743122095,58.9547475754165,59.0578171667581,59.1608249277454,
59.2638067574364,59.3704201725438,59.4735201525633,59.5818902852146,59.6902604178659),
 .UNSPECIFIED.);
#2608=B_SPLINE_CURVE_WITH_KNOTS('',3,(#90551,#90552,#90553,#90554,#90555,
#90556,#90557,#90558,#90559,#90560,#90561,#90562,#90563,#90564,#90565,#90566,
#90567,#90568,#90569,#90570,#90571,#90572,#90573,#90574,#90575,#90576,#90577,
#90578,#90579,#90580,#90581,#90582,#90583,#90584,#90585,#90586,#90587,#90588,
#90589,#90590,#90591,#90592,#90593,#90594,#90595,#90596,#90597,#90598,#90599,
#90600,#90601,#90602,#90603,#90604,#90605,#90606,#90607,#90608,#90609,#90610,
#90611,#90612,#90613,#90614,#90615,#90616,#90617,#90618,#90619,#90620),
 .UNSPECIFIED.,.F.,.F.,(4,3,3,3,3,3,3,3,3,3,3,3,3,3,3,3,3,3,3,3,3,3,3,4),
(59.690260418206,59.7438772048688,59.8480633683569,59.9520942935691,60.056003183986,
60.1598466151541,60.263659366169,60.3674761726906,60.4714016500609,60.5753859686056,
60.6795522260648,60.7414250632149,60.845611226703,60.9496421519152,61.0535510423322,
61.1573944735003,61.2612072245152,61.3650240310368,61.4689495084072,61.5729338269519,
61.6771000844111,61.738972921561,61.8431345897298,61.9168706242402),
 .UNSPECIFIED.);
#2609=B_SPLINE_CURVE_WITH_KNOTS('',3,(#90622,#90623,#90624,#90625,#90626,
#90627,#90628,#90629,#90630,#90631,#90632,#90633,#90634,#90635,#90636,#90637,
#90638,#90639,#90640,#90641,#90642,#90643,#90644,#90645,#90646,#90647,#90648,
#90649,#90650,#90651,#90652,#90653,#90654,#90655,#90656,#90657,#90658,#90659,
#90660,#90661,#90662,#90663,#90664,#90665,#90666,#90667,#90668,#90669,#90670,
#90671,#90672,#90673,#90674,#90675,#90676,#90677,#90678,#90679,#90680,#90681,
#90682,#90683,#90684,#90685,#90686,#90687,#90688),.UNSPECIFIED.,.F.,.F.,
(4,3,3,3,3,3,3,3,3,3,3,3,3,3,3,3,3,3,3,3,3,3,4),(59.690260418206,59.7955628120765,
59.9009059652381,60.0064057077468,60.1119895277649,60.2177899509138,60.2853424966969,
60.3895286601852,60.4935595853974,60.5974684758143,60.7013119069825,60.8051246579975,
60.9089414645191,61.0128669418895,61.1168512604342,61.2210175178934,61.282890355043,
61.3870598972592,61.4910835282141,61.5972884280853,61.7011283170153,61.8085157223571,
61.9159031276989),.UNSPECIFIED.);
#2610=B_SPLINE_CURVE_WITH_KNOTS('',3,(#90689,#90690,#90691,#90692,#90693,
#90694,#90695,#90696,#90697,#90698,#90699,#90700,#90701,#90702,#90703,#90704,
#90705,#90706,#90707,#90708,#90709,#90710,#90711,#90712,#90713,#90714,#90715,
#90716,#90717,#90718,#90719,#90720,#90721,#90722,#90723,#90724,#90725,#90726,
#90727,#90728,#90729,#90730,#90731,#90732,#90733,#90734,#90735,#90736,#90737,
#90738,#90739,#90740,#90741,#90742,#90743,#90744,#90745,#90746,#90747,#90748,
#90749,#90750,#90751,#90752,#90753,#90754,#90755,#90756,#90757,#90758,#90759,
#90760,#90761,#90762,#90763,#90764,#90765,#90766,#90767,#90768,#90769,#90770,
#90771,#90772,#90773,#90774,#90775,#90776,#90777,#90778,#90779,#90780,#90781,
#90782,#90783,#90784,#90785,#90786,#90787,#90788,#90789,#90790,#90791,#90792,
#90793,#90794,#90795,#90796,#90797,#90798,#90799,#90800,#90801,#90802,#90803,
#90804,#90805,#90806,#90807,#90808,#90809,#90810,#90811,#90812),
 .UNSPECIFIED.,.F.,.F.,(4,3,3,3,3,3,3,3,3,3,3,3,3,3,3,3,3,3,3,3,3,3,3,3,
3,3,3,3,3,3,3,3,3,3,3,3,3,3,3,3,3,4),(55.6335534587503,55.7373867807232,
55.8411973928298,55.9450200256885,56.0489562327104,56.1529584384112,56.2571354362515,
56.2951510633125,56.3993372268008,56.5033681520131,56.6072770424301,56.7111204735982,
56.8149332246131,56.9187500311349,57.0226755085053,57.12665982705,57.2308260845093,
57.2926989216586,57.3968850851468,57.5009160103588,57.6048249007758,57.7086683319439,
57.8124810829588,57.9162978894801,58.0202233668504,58.124207685395,58.2283739428542,
58.2902467800047,58.3944329434929,58.498463868705,58.6023727591219,58.7062161902901,
58.8100289413054,58.9138457478275,59.0177712251979,59.1217555437426,59.2259218012019,
59.2877946383508,59.4032420886161,59.5183215991953,59.6327919924175,59.6902604177957),
 .UNSPECIFIED.);
#2611=B_SPLINE_CURVE_WITH_KNOTS('',3,(#90818,#90819,#90820,#90821,#90822,
#90823,#90824,#90825,#90826,#90827,#90828,#90829,#90830,#90831,#90832,#90833,
#90834,#90835,#90836,#90837,#90838,#90839,#90840,#90841,#90842,#90843,#90844,
#90845,#90846,#90847,#90848,#90849,#90850,#90851,#90852,#90853,#90854,#90855,
#90856,#90857,#90858,#90859,#90860,#90861,#90862,#90863,#90864,#90865,#90866,
#90867,#90868,#90869,#90870,#90871,#90872,#90873,#90874,#90875,#90876,#90877,
#90878,#90879,#90880,#90881,#90882,#90883,#90884,#90885,#90886,#90887,#90888,
#90889,#90890,#90891,#90892,#90893,#90894,#90895,#90896,#90897,#90898,#90899,
#90900,#90901,#90902,#90903,#90904,#90905,#90906,#90907,#90908,#90909,#90910,
#90911,#90912,#90913,#90914,#90915,#90916,#90917,#90918,#90919,#90920,#90921,
#90922,#90923,#90924,#90925,#90926,#90927,#90928,#90929,#90930,#90931,#90932,
#90933,#90934,#90935,#90936,#90937,#90938,#90939,#90940,#90941),
 .UNSPECIFIED.,.F.,.F.,(4,3,3,3,3,3,3,3,3,3,3,3,3,3,3,3,3,3,3,3,3,3,3,3,
3,3,3,3,3,3,3,3,3,3,3,3,3,3,3,3,3,4),(49.3496765146293,49.4543570413239,
49.558312629052,49.6633556252299,49.7683986214079,49.872584784896,49.9766157101083,
50.0805246005252,50.1843680316934,50.2881807827085,50.3919975892302,50.4959230666005,
50.5999073851452,50.7040736426044,50.765946479754,50.8701326432422,50.9741635684541,
51.0780724588711,51.1819158900391,51.2857286410542,51.3895454475755,51.493470924946,
51.5974552434908,51.70162150095,51.7634943381001,51.8676805015882,51.9717114268003,
52.0756203172173,52.1794637483854,52.2832764994004,52.387093305922,52.4910187832924,
52.5950031018373,52.6991693592965,52.7610421964462,52.8655509126696,52.9699037514317,
53.0791965913304,53.1833373805663,53.2874304651177,53.3915238347385,53.4070751110264),
 .UNSPECIFIED.);
#2612=B_SPLINE_CURVE_WITH_KNOTS('',3,(#90942,#90943,#90944,#90945,#90946,
#90947,#90948,#90949,#90950,#90951,#90952,#90953,#90954,#90955,#90956,#90957,
#90958,#90959,#90960,#90961,#90962,#90963,#90964,#90965,#90966,#90967,#90968,
#90969,#90970,#90971,#90972,#90973,#90974,#90975,#90976,#90977,#90978,#90979,
#90980,#90981,#90982,#90983,#90984,#90985,#90986,#90987,#90988,#90989,#90990,
#90991,#90992,#90993,#90994,#90995,#90996,#90997,#90998,#90999,#91000,#91001,
#91002,#91003,#91004,#91005,#91006,#91007,#91008),.UNSPECIFIED.,.F.,.F.,
(4,3,3,3,3,3,3,3,3,3,3,3,3,3,3,3,3,3,3,3,3,3,4),(53.4070751114778,53.5259953052186,
53.6459937542289,53.7585900547923,53.8627762182805,53.9668071434927,54.0707160339097,
54.1745594650778,54.2783722160927,54.3821890226141,54.4861144999845,54.5900988185292,
54.6942650759884,54.7561379131384,54.8656962404972,54.9697007582687,55.0736032491578,
55.1774385737942,55.281241510946,55.385092536991,55.4889714141182,55.5929703731723,
55.6326045320091),.UNSPECIFIED.);
#2613=B_SPLINE_CURVE_WITH_KNOTS('',3,(#91010,#91011,#91012,#91013,#91014,
#91015,#91016,#91017,#91018,#91019,#91020,#91021,#91022,#91023,#91024,#91025,
#91026,#91027,#91028,#91029,#91030,#91031,#91032,#91033,#91034,#91035,#91036,
#91037,#91038,#91039,#91040,#91041,#91042,#91043,#91044,#91045,#91046,#91047,
#91048,#91049,#91050,#91051,#91052,#91053,#91054,#91055,#91056,#91057,#91058,
#91059,#91060,#91061,#91062,#91063,#91064,#91065,#91066,#91067,#91068,#91069,
#91070,#91071,#91072,#91073,#91074,#91075,#91076,#91077,#91078,#91079),
 .UNSPECIFIED.,.F.,.F.,(4,3,3,3,3,3,3,3,3,3,3,3,3,3,3,3,3,3,3,3,3,3,3,4),
(53.4070751114786,53.5098614913149,53.6124973139476,53.7150505550743,53.8175576893134,
53.9200551251567,54.0226483900827,54.1252912590462,54.2281147116669,54.3000553466204,
54.4042415101086,54.5082724353209,54.6121813257378,54.7160247569059,54.8198375079208,
54.9236543144422,55.0275797918125,55.1315641103571,55.2357303678164,55.2976032049664,
55.4017686790633,55.5057980059472,55.6097071730358,55.6335534587503),
 .UNSPECIFIED.);
#2614=B_SPLINE_CURVE_WITH_KNOTS('',3,(#91080,#91081,#91082,#91083,#91084,
#91085,#91086,#91087,#91088,#91089,#91090,#91091,#91092,#91093,#91094,#91095,
#91096,#91097,#91098,#91099,#91100,#91101,#91102,#91103,#91104,#91105,#91106,
#91107,#91108,#91109,#91110,#91111,#91112,#91113,#91114,#91115,#91116,#91117,
#91118,#91119,#91120,#91121,#91122,#91123,#91124,#91125,#91126,#91127,#91128,
#91129,#91130,#91131,#91132,#91133,#91134,#91135,#91136,#91137,#91138,#91139,
#91140,#91141,#91142,#91143,#91144,#91145,#91146,#91147,#91148,#91149,#91150,
#91151,#91152,#91153,#91154,#91155,#91156,#91157,#91158,#91159,#91160,#91161,
#91162,#91163,#91164,#91165,#91166,#91167,#91168,#91169,#91170,#91171,#91172,
#91173,#91174,#91175,#91176,#91177,#91178,#91179,#91180,#91181,#91182,#91183,
#91184,#91185,#91186,#91187,#91188,#91189,#91190,#91191,#91192,#91193,#91194,
#91195,#91196,#91197,#91198,#91199,#91200,#91201,#91202,#91203),
 .UNSPECIFIED.,.F.,.F.,(4,3,3,3,3,3,3,3,3,3,3,3,3,3,3,3,3,3,3,3,3,3,3,3,
3,3,3,3,3,3,3,3,3,3,3,3,3,3,3,3,3,4),(49.3501260113316,49.4542513866548,
49.5612029524774,49.6650820823779,49.7689093695806,49.872719572018,49.9820056573225,
50.0859533807799,50.1899737976859,50.2941626671254,50.309863913236,50.4140500767241,
50.5180810019363,50.6219898923532,50.7258333235213,50.8296460745361,50.9334628810576,
51.0373883584279,51.1413726769726,51.2455389344318,51.3074117715821,51.4115979350703,
51.5156288602825,51.6195377506995,51.7233811818676,51.8271939328825,51.9310107394041,
52.0349362167745,52.1389205353193,52.2430867927785,52.3049596299282,52.4091457934164,
52.5131767186285,52.6170856090454,52.7209290402135,52.8247417912284,52.92855859775,
53.0324840751203,53.136468393665,53.2406346511242,53.3025074882743,53.4070751110265),
 .UNSPECIFIED.);
#2615=B_SPLINE_CURVE_WITH_KNOTS('',3,(#91209,#91210,#91211,#91212,#91213,
#91214,#91215,#91216,#91217,#91218,#91219,#91220,#91221,#91222,#91223,#91224,
#91225,#91226,#91227,#91228,#91229,#91230,#91231,#91232,#91233,#91234,#91235,
#91236,#91237,#91238,#91239,#91240,#91241,#91242,#91243,#91244,#91245,#91246,
#91247,#91248,#91249,#91250,#91251,#91252,#91253,#91254,#91255,#91256,#91257,
#91258,#91259,#91260,#91261,#91262,#91263,#91264,#91265,#91266,#91267,#91268,
#91269,#91270,#91271,#91272,#91273,#91274,#91275,#91276,#91277,#91278,#91279,
#91280,#91281,#91282,#91283,#91284,#91285,#91286,#91287,#91288,#91289,#91290,
#91291,#91292,#91293,#91294,#91295,#91296,#91297,#91298,#91299,#91300,#91301,
#91302,#91303,#91304,#91305,#91306,#91307,#91308,#91309,#91310,#91311,#91312,
#91313,#91314,#91315,#91316,#91317,#91318,#91319,#91320,#91321,#91322,#91323,
#91324,#91325,#91326,#91327,#91328,#91329),.UNSPECIFIED.,.F.,.F.,(4,3,3,
3,3,3,3,3,3,3,3,3,3,3,3,3,3,3,3,3,3,3,3,3,3,3,3,3,3,3,3,3,3,3,3,3,3,3,3,
3,4),(43.0672771824896,43.1711361743488,43.2749543100599,43.3787663343812,
43.4826804992014,43.5866443730128,43.6907998584982,43.7831114713314,43.8872976348202,
43.991328560033,44.0952374504505,44.1990808816192,44.3028936326347,44.4067104391569,
44.5106359165279,44.6146202350732,44.718786492533,44.7806593296775,44.8848454931655,
44.9888764183773,45.0927853087942,45.1966287399621,45.3004414909768,45.4042582974981,
45.5081837748683,45.6121680934129,45.7163343508719,45.7782071880236,45.8823933515116,
45.9864242767236,46.0903331671405,46.1941765983085,46.2979893493234,46.4018061558448,
46.5057316332153,46.60971595176,46.7138822092192,46.7757550463697,46.8962986192144,
47.0157785770619,47.123889803398),.UNSPECIFIED.);
#2616=B_SPLINE_CURVE_WITH_KNOTS('',3,(#91330,#91331,#91332,#91333,#91334,
#91335,#91336,#91337,#91338,#91339,#91340,#91341,#91342,#91343,#91344,#91345,
#91346,#91347,#91348,#91349,#91350,#91351,#91352,#91353,#91354,#91355,#91356,
#91357,#91358,#91359,#91360,#91361,#91362,#91363,#91364,#91365,#91366,#91367,
#91368,#91369,#91370,#91371,#91372,#91373,#91374,#91375,#91376,#91377,#91378,
#91379,#91380,#91381,#91382,#91383,#91384,#91385,#91386,#91387,#91388,#91389,
#91390,#91391,#91392,#91393,#91394,#91395,#91396,#91397,#91398,#91399),
 .UNSPECIFIED.,.F.,.F.,(4,3,3,3,3,3,3,3,3,3,3,3,3,3,3,3,3,3,3,3,3,3,3,4),
(47.1238898038468,47.2279281355327,47.3319603652865,47.4360206698572,47.5402127556636,
47.6444838895222,47.7489375131551,47.7733029047158,47.8774890682039,47.981519993416,
48.0854288838329,48.189272315001,48.2930850660159,48.3969018725375,48.5008273499079,
48.6048116684526,48.7089779259118,48.7708507630619,48.8750265334971,48.9790548139466,
49.0829625287093,49.1867995817475,49.2906190127626,49.3496765146293),
 .UNSPECIFIED.);
#2617=B_SPLINE_CURVE_WITH_KNOTS('',3,(#91401,#91402,#91403,#91404,#91405,
#91406,#91407,#91408,#91409,#91410,#91411,#91412,#91413,#91414,#91415,#91416,
#91417,#91418,#91419,#91420,#91421,#91422,#91423,#91424,#91425,#91426,#91427,
#91428,#91429,#91430,#91431,#91432,#91433,#91434,#91435,#91436,#91437,#91438,
#91439,#91440,#91441,#91442,#91443,#91444,#91445,#91446,#91447,#91448,#91449,
#91450,#91451,#91452,#91453,#91454,#91455,#91456,#91457,#91458,#91459,#91460,
#91461,#91462,#91463,#91464,#91465,#91466,#91467,#91468,#91469,#91470),
 .UNSPECIFIED.,.F.,.F.,(4,3,3,3,3,3,3,3,3,3,3,3,3,3,3,3,3,3,3,3,3,3,3,4),
(47.1238898038469,47.2754958859209,47.3172203381977,47.4214065016857,47.5254374268976,
47.6293463173144,47.7331897484823,47.837002499497,47.9408193060184,48.0447447833886,
48.1487291019331,48.2528953593921,48.3147681965438,48.4189543600319,48.522985285244,
48.626894175661,48.730737606829,48.8345503578439,48.9383671643654,49.0422926417358,
49.1462769602805,49.2504432177397,49.3123160548899,49.3501260113316),
 .UNSPECIFIED.);
#2618=B_SPLINE_CURVE_WITH_KNOTS('',3,(#91471,#91472,#91473,#91474,#91475,
#91476,#91477,#91478,#91479,#91480,#91481,#91482,#91483,#91484,#91485,#91486,
#91487,#91488,#91489,#91490,#91491,#91492,#91493,#91494,#91495,#91496,#91497,
#91498,#91499,#91500,#91501,#91502,#91503,#91504,#91505,#91506,#91507,#91508,
#91509,#91510,#91511,#91512,#91513,#91514,#91515,#91516,#91517,#91518,#91519,
#91520,#91521,#91522,#91523,#91524,#91525,#91526,#91527,#91528,#91529,#91530,
#91531,#91532,#91533,#91534,#91535,#91536,#91537,#91538,#91539,#91540,#91541,
#91542,#91543,#91544,#91545,#91546,#91547,#91548,#91549,#91550,#91551,#91552,
#91553,#91554,#91555,#91556,#91557,#91558,#91559,#91560,#91561,#91562,#91563,
#91564,#91565,#91566,#91567,#91568,#91569,#91570,#91571,#91572,#91573,#91574,
#91575,#91576,#91577,#91578,#91579,#91580,#91581,#91582,#91583,#91584,#91585,
#91586,#91587,#91588,#91589,#91590,#91591,#91592,#91593,#91594),
 .UNSPECIFIED.,.F.,.F.,(4,3,3,3,3,3,3,3,3,3,3,3,3,3,3,3,3,3,3,3,3,3,3,3,
3,3,3,3,3,3,3,3,3,3,3,3,3,3,3,3,3,4),(43.0661637738671,43.1701547732055,
43.2743249196621,43.3270289048134,43.431215068306,43.5352459935225,43.639154883944,
43.7429983151167,43.8468110661362,43.9506278726623,44.0545533500374,44.1585376685868,
44.2627039260507,44.3245767631595,44.4287629266466,44.5327938518577,44.6367027422736,
44.7405461734406,44.8443589244544,44.9481757309749,45.0521012083441,45.1560855268878,
45.260251784346,45.3221246215056,45.4263107849932,45.5303417102049,45.6342506006213,
45.7380940317888,45.8419067828031,45.9457235893239,46.0496490666937,46.1536333852379,
46.2577996426965,46.3196724798517,46.4223012412915,46.524793586442,46.6271863644393,
46.7295162801934,46.8318649061936,46.9342176129162,47.0366904241986,47.1238898034408),
 .UNSPECIFIED.);
#2619=B_SPLINE_CURVE_WITH_KNOTS('',3,(#91600,#91601,#91602,#91603,#91604,
#91605,#91606,#91607,#91608,#91609,#91610,#91611,#91612,#91613,#91614,#91615,
#91616,#91617,#91618,#91619,#91620,#91621,#91622,#91623,#91624,#91625,#91626,
#91627,#91628,#91629,#91630,#91631,#91632,#91633,#91634,#91635,#91636,#91637,
#91638,#91639,#91640,#91641,#91642,#91643,#91644,#91645,#91646,#91647,#91648,
#91649,#91650,#91651,#91652,#91653,#91654,#91655,#91656,#91657,#91658,#91659,
#91660,#91661,#91662,#91663,#91664,#91665,#91666,#91667,#91668,#91669,#91670,
#91671,#91672,#91673,#91674,#91675,#91676,#91677,#91678,#91679,#91680,#91681,
#91682,#91683,#91684,#91685,#91686,#91687,#91688,#91689,#91690,#91691,#91692,
#91693,#91694,#91695,#91696,#91697,#91698,#91699,#91700,#91701,#91702,#91703,
#91704,#91705,#91706,#91707,#91708,#91709,#91710,#91711,#91712,#91713,#91714,
#91715,#91716,#91717,#91718,#91719,#91720,#91721,#91722,#91723,#91724,#91725,
#91726),.UNSPECIFIED.,.F.,.F.,(4,3,3,3,3,3,3,3,3,3,3,3,3,3,3,3,3,3,3,3,
3,3,3,3,3,3,3,3,3,3,3,3,3,3,3,3,3,3,3,3,3,3,4),(36.7834483295922,36.8002764629088,
36.9044626263497,37.0084935515136,37.1124024418811,37.216245872999,37.3200586239631,
37.4238754304332,37.5278009077515,37.6317852262439,37.7359514836507,37.7978243212549,
37.9020104847764,38.0060414100223,38.1099503004736,38.2137937316764,38.3176064827263,
38.4214232892831,38.5253487666888,38.629333085269,38.7334993427635,38.795372179601,
38.899558343083,39.0035892682889,39.1074981586996,39.2113415898615,39.3151543408703,
39.4189711473856,39.5228966247499,39.6268809432886,39.7310472007419,39.7929200379471,
39.8971062014302,40.0011371266371,40.1050460170488,40.2088894482115,40.3127021992209,
40.4165190057368,40.5204444831015,40.6244288016405,40.7285950590941,40.7904678962932,
40.8407044966673),.UNSPECIFIED.);
#2620=B_SPLINE_CURVE_WITH_KNOTS('',3,(#91727,#91728,#91729,#91730,#91731,
#91732,#91733,#91734,#91735,#91736,#91737,#91738,#91739,#91740,#91741,#91742,
#91743,#91744,#91745,#91746,#91747,#91748,#91749,#91750,#91751,#91752,#91753,
#91754,#91755,#91756,#91757,#91758,#91759,#91760,#91761,#91762,#91763,#91764,
#91765,#91766,#91767,#91768,#91769,#91770,#91771,#91772,#91773,#91774,#91775,
#91776,#91777,#91778,#91779,#91780,#91781,#91782,#91783,#91784,#91785,#91786,
#91787,#91788,#91789,#91790,#91791,#91792,#91793,#91794,#91795,#91796),
 .UNSPECIFIED.,.F.,.F.,(4,3,3,3,3,3,3,3,3,3,3,3,3,3,3,3,3,3,3,3,3,3,3,4),
(40.8407044969994,40.9440746115612,41.0495672544459,41.152672005388,41.2557188072321,
41.3587435025167,41.4660615655473,41.56921475009,41.6724388016659,41.7758284060399,
41.7880157546392,41.8922019181263,41.9962328433373,42.1001417337531,42.2039851649202,
42.3077979159341,42.4116147224543,42.5155401998236,42.6195245183673,42.7236907758254,
42.7855636129853,42.8897412721946,42.9937540506505,43.0672771824896),
 .UNSPECIFIED.);
#2621=B_SPLINE_CURVE_WITH_KNOTS('',3,(#91798,#91799,#91800,#91801,#91802,
#91803,#91804,#91805,#91806,#91807,#91808,#91809,#91810,#91811,#91812,#91813,
#91814,#91815,#91816,#91817,#91818,#91819,#91820,#91821,#91822,#91823,#91824,
#91825,#91826,#91827,#91828,#91829,#91830,#91831,#91832,#91833,#91834,#91835,
#91836,#91837,#91838,#91839,#91840,#91841,#91842,#91843,#91844,#91845,#91846,
#91847,#91848,#91849,#91850,#91851,#91852,#91853,#91854,#91855,#91856,#91857,
#91858,#91859,#91860,#91861,#91862,#91863,#91864),.UNSPECIFIED.,.F.,.F.,
(4,3,3,3,3,3,3,3,3,3,3,3,3,3,3,3,3,3,3,3,3,3,4),(40.8407044969871,40.9497796083695,
41.0591756422976,41.1687426604475,41.278611244788,41.3319331881212,41.4361193516033,
41.5401502768092,41.64405916722,41.747902598382,41.8517153493908,41.9555321559062,
42.0594576332706,42.1634419518094,42.2676082092628,42.3294810464673,42.4336404890024,
42.5376570384814,42.6415656994819,42.7477152180782,42.8515331448653,42.9588484593662,
43.0661637738671),.UNSPECIFIED.);
#2622=B_SPLINE_CURVE_WITH_KNOTS('',3,(#91865,#91866,#91867,#91868,#91869,
#91870,#91871,#91872,#91873,#91874,#91875,#91876,#91877,#91878,#91879,#91880,
#91881,#91882,#91883,#91884,#91885,#91886,#91887,#91888,#91889,#91890,#91891,
#91892,#91893,#91894,#91895,#91896,#91897,#91898,#91899,#91900,#91901,#91902,
#91903,#91904,#91905,#91906,#91907,#91908,#91909,#91910,#91911,#91912,#91913,
#91914,#91915,#91916,#91917,#91918,#91919,#91920,#91921,#91922,#91923,#91924,
#91925,#91926,#91927,#91928,#91929,#91930,#91931,#91932,#91933,#91934,#91935,
#91936,#91937,#91938,#91939,#91940,#91941,#91942,#91943,#91944,#91945,#91946,
#91947,#91948,#91949,#91950,#91951,#91952,#91953,#91954,#91955,#91956,#91957,
#91958,#91959,#91960,#91961,#91962,#91963,#91964,#91965,#91966,#91967,#91968,
#91969,#91970,#91971,#91972,#91973,#91974,#91975,#91976,#91977,#91978,#91979,
#91980,#91981,#91982,#91983,#91984,#91985,#91986,#91987,#91988),
 .UNSPECIFIED.,.F.,.F.,(4,3,3,3,3,3,3,3,3,3,3,3,3,3,3,3,3,3,3,3,3,3,3,3,
3,3,3,3,3,3,3,3,3,3,3,3,3,3,3,3,3,4),(36.7837280536202,36.8875386782118,
36.9913612401259,37.0952973258126,37.199299335197,37.30347620961,37.3417417547369,
37.4459279184724,37.5499588439353,37.6538677346069,37.7577111660321,37.861523917306,
37.9653407240879,38.0692662017194,38.173250520526,38.2774167782453,38.339289613083,
38.443475776542,38.547506701725,38.6514155921136,38.7552590232534,38.8590717742405,
38.9628885807346,39.0668140580781,39.1707983765966,39.2749646340303,39.3368374714291,
39.4410236348703,39.5450545600343,39.6489634504021,39.7528068815202,39.8566196324846,
39.9604364389555,40.0643619162741,40.1683462347668,40.272512492174,40.3343853297751,
40.4435562695043,40.5524208008746,40.6611016633604,40.769557770341,40.8407044966673),
 .UNSPECIFIED.);
#2623=B_SPLINE_CURVE_WITH_KNOTS('',3,(#91994,#91995,#91996,#91997,#91998,
#91999,#92000,#92001),.UNSPECIFIED.,.F.,.F.,(4,1,1,1,1,4),(30.4995505242199,
30.8149893128323,31.8125371711784,32.8100850295245,33.8076328878706,34.5575191894876),
 .UNSPECIFIED.);
#2624=B_SPLINE_CURVE_WITH_KNOTS('',3,(#92002,#92003,#92004,#92005,#92006,
#92007,#92008,#92009,#92010,#92011,#92012,#92013,#92014,#92015,#92016,#92017,
#92018,#92019,#92020,#92021,#92022,#92023,#92024,#92025,#92026,#92027,#92028,
#92029,#92030,#92031,#92032,#92033,#92034,#92035,#92036,#92037,#92038,#92039,
#92040,#92041,#92042,#92043,#92044,#92045,#92046,#92047,#92048,#92049,#92050,
#92051,#92052,#92053,#92054,#92055,#92056,#92057,#92058,#92059,#92060,#92061,
#92062,#92063,#92064,#92065,#92066,#92067,#92068),.UNSPECIFIED.,.F.,.F.,
(4,3,3,3,3,3,3,3,3,3,3,3,3,3,3,3,3,3,3,3,3,3,4),(34.5575192744995,34.6927957333311,
34.8051807462166,34.9093669099533,35.0133978354175,35.1173067260906,35.2211501575171,
35.3249629087925,35.4287797155758,35.5327051932087,35.6366895120167,35.7408557697374,
35.8027286045627,35.9069159429525,36.0109477003902,36.1148561156612,36.218698586411,
36.3225098920317,36.4263247678229,36.5302426834939,36.6342192413487,36.7383649008209,
36.7834483295922),.UNSPECIFIED.);
#2625=B_SPLINE_CURVE_WITH_KNOTS('',3,(#92070,#92071,#92072,#92073,#92074,
#92075,#92076,#92077,#92078,#92079,#92080,#92081,#92082,#92083,#92084,#92085,
#92086,#92087,#92088,#92089,#92090,#92091,#92092,#92093,#92094,#92095,#92096,
#92097,#92098,#92099,#92100,#92101,#92102,#92103,#92104,#92105,#92106,#92107,
#92108,#92109,#92110,#92111,#92112,#92113,#92114,#92115,#92116,#92117,#92118,
#92119,#92120,#92121,#92122,#92123,#92124,#92125,#92126,#92127,#92128,#92129,
#92130,#92131,#92132,#92133,#92134,#92135,#92136,#92137,#92138,#92139),
 .UNSPECIFIED.,.F.,.F.,(4,3,3,3,3,3,3,3,3,3,3,3,3,3,3,3,3,3,3,3,3,3,3,4),
(34.5575191897439,34.6600261058238,34.7624492437726,34.8648252112128,34.9671905469551,
35.0696506767871,35.1721598105652,35.2748489353093,35.3466460380447,35.4508322014592,
35.5548631266016,35.6587720169549,35.7626154480633,35.8664281990224,35.9702450054921,
36.0741704828175,36.1781548013209,36.2823210587452,36.3441938963908,36.4483886654195,
36.5524031605752,36.6563141143339,36.7601506285633,36.7837280536202),
 .UNSPECIFIED.);
#2626=B_SPLINE_CURVE_WITH_KNOTS('',3,(#92140,#92141,#92142,#92143,#92144,
#92145,#92146,#92147,#92148,#92149,#92150,#92151,#92152,#92153,#92154,#92155,
#92156,#92157,#92158,#92159,#92160,#92161,#92162,#92163,#92164,#92165,#92166,
#92167,#92168,#92169,#92170,#92171,#92172,#92173,#92174,#92175,#92176,#92177,
#92178,#92179,#92180,#92181,#92182,#92183,#92184,#92185,#92186,#92187,#92188,
#92189,#92190,#92191,#92192,#92193,#92194,#92195,#92196,#92197,#92198,#92199,
#92200,#92201,#92202,#92203,#92204,#92205,#92206,#92207,#92208,#92209,#92210,
#92211,#92212,#92213,#92214,#92215,#92216,#92217,#92218,#92219,#92220,#92221,
#92222,#92223,#92224,#92225,#92226,#92227,#92228,#92229,#92230,#92231,#92232,
#92233,#92234,#92235,#92236,#92237,#92238,#92239,#92240,#92241,#92242,#92243,
#92244,#92245,#92246,#92247,#92248,#92249,#92250,#92251,#92252,#92253,#92254,
#92255,#92256,#92257,#92258,#92259,#92260,#92261,#92262,#92263),
 .UNSPECIFIED.,.F.,.F.,(4,3,3,3,3,3,3,3,3,3,3,3,3,3,3,3,3,3,3,3,3,3,3,3,
3,3,3,3,3,3,3,3,3,3,3,3,3,3,3,3,3,4),(30.5009012395315,30.6078454101726,
30.7117244743431,30.8155517128082,30.9193618835234,31.0286350638077,31.1325827763094,
31.2366031938056,31.3407920531297,31.3564546046604,31.4606407808898,31.5646717189986,
31.6685806224799,31.7724240668089,31.8762368310614,31.9800536508775,32.0839791415378,
32.18796347339,32.2921297440395,32.3540024630065,32.4581886271218,32.5622195530108,
32.6661284441755,32.7699718761347,32.873784627983,32.9776014353793,33.0815269136819,
33.1855112331928,33.2896774916617,33.3515503213525,33.4557364812571,33.5597674028189,
33.6636762895042,33.7675197168922,33.8713324640845,33.9751492667464,34.0790747402267,
34.1830590548584,34.2872253084106,34.3490981796986,34.4951131661409,34.5575191894877),
 .UNSPECIFIED.);
#2627=B_SPLINE_CURVE_WITH_KNOTS('',3,(#92269,#92270,#92271,#92272,#92273,
#92274,#92275,#92276,#92277,#92278,#92279,#92280,#92281,#92282,#92283,#92284,
#92285,#92286,#92287,#92288,#92289,#92290,#92291,#92292,#92293,#92294,#92295,
#92296,#92297,#92298,#92299,#92300,#92301,#92302,#92303,#92304,#92305,#92306,
#92307,#92308,#92309,#92310,#92311,#92312,#92313,#92314,#92315,#92316,#92317,
#92318,#92319,#92320,#92321,#92322,#92323,#92324,#92325,#92326,#92327,#92328,
#92329,#92330,#92331,#92332,#92333,#92334,#92335,#92336,#92337,#92338,#92339,
#92340,#92341,#92342,#92343,#92344,#92345,#92346,#92347,#92348,#92349,#92350,
#92351,#92352,#92353,#92354,#92355,#92356,#92357,#92358,#92359,#92360,#92361,
#92362,#92363,#92364,#92365,#92366,#92367,#92368,#92369,#92370,#92371,#92372,
#92373,#92374,#92375,#92376,#92377,#92378,#92379,#92380,#92381,#92382,#92383,
#92384,#92385,#92386,#92387,#92388,#92389),.UNSPECIFIED.,.F.,.F.,(4,3,3,
3,3,3,3,3,3,3,3,3,3,3,3,3,3,3,3,3,3,3,3,3,3,3,3,3,3,3,3,3,3,3,3,3,3,3,3,
3,4),(24.2175094731414,24.3213278572364,24.4251400605738,24.5290543606235,
24.6330183067792,24.7371739381643,24.8297021627558,24.93388808274,25.037918760325,
25.1418273981882,25.2456705738977,25.3494830669292,25.4532996133197,25.5572248290617,
25.6612088847385,25.7653748802143,25.8272500211019,25.931436271936,26.0354672854447,
26.1393762651375,26.2432197861367,26.347032627403,26.450849524462,26.5547750921803,
26.6587595011022,26.7629258480012,26.8247978794479,26.928984057102,27.0330149970091,
27.1369239028387,27.2407673498547,27.34458011713,27.4483969403018,27.5523224348072,
27.6563067707863,27.7604730459679,27.822345737794,27.9353427130044,28.0470527868677,
28.1606932127517,28.2743336386358),.UNSPECIFIED.);
#2628=B_SPLINE_CURVE_WITH_KNOTS('',3,(#92390,#92391,#92392,#92393,#92394,
#92395),.UNSPECIFIED.,.F.,.F.,(4,1,1,4),(28.2743338823081,28.8198935961401,
29.8174414544862,30.4995505242199),.UNSPECIFIED.);
#2629=B_SPLINE_CURVE_WITH_KNOTS('',3,(#92397,#92398,#92399,#92400,#92401,
#92402,#92403,#92404,#92405,#92406,#92407,#92408,#92409,#92410,#92411,#92412,
#92413,#92414,#92415,#92416,#92417,#92418,#92419,#92420,#92421,#92422,#92423,
#92424,#92425,#92426,#92427,#92428,#92429,#92430,#92431,#92432,#92433,#92434,
#92435,#92436,#92437,#92438,#92439,#92440,#92441,#92442,#92443,#92444,#92445,
#92446,#92447,#92448,#92449,#92450,#92451,#92452,#92453,#92454,#92455,#92456,
#92457,#92458,#92459,#92460,#92461,#92462,#92463,#92464,#92465,#92466),
 .UNSPECIFIED.,.F.,.F.,(4,3,3,3,3,3,3,3,3,3,3,3,3,3,3,3,3,3,3,3,3,3,3,4),
(28.2743338823081,28.3638110296221,28.4679972801179,28.5720282932844,28.6759372726305,
28.7797807932806,28.8835936341959,28.9874105309025,29.0913360982685,29.1953205068379,
29.2994868533873,29.3613588879682,29.4655450656092,29.5695760055018,29.6734849113152,
29.7773283583141,29.8811411255711,29.9849579487237,30.0888834432082,30.1928677791657,
30.2970340543243,30.3589067463143,30.4630838119347,30.5009012395315),
 .UNSPECIFIED.);
#2630=B_SPLINE_CURVE_WITH_KNOTS('',3,(#92467,#92468,#92469,#92470,#92471,
#92472,#92473,#92474,#92475,#92476,#92477,#92478,#92479,#92480,#92481,#92482,
#92483,#92484,#92485,#92486,#92487,#92488,#92489,#92490,#92491,#92492,#92493,
#92494,#92495,#92496,#92497,#92498,#92499,#92500,#92501,#92502,#92503,#92504,
#92505,#92506,#92507,#92508,#92509,#92510,#92511,#92512,#92513,#92514,#92515,
#92516,#92517,#92518,#92519,#92520,#92521,#92522,#92523,#92524,#92525,#92526,
#92527,#92528,#92529,#92530,#92531,#92532,#92533,#92534,#92535,#92536,#92537,
#92538,#92539,#92540,#92541,#92542,#92543,#92544,#92545,#92546,#92547,#92548,
#92549,#92550,#92551,#92552,#92553,#92554,#92555,#92556,#92557,#92558,#92559,
#92560,#92561,#92562,#92563,#92564,#92565,#92566,#92567,#92568,#92569,#92570,
#92571,#92572,#92573,#92574,#92575,#92576,#92577,#92578,#92579,#92580,#92581,
#92582,#92583,#92584,#92585,#92586,#92587,#92588,#92589,#92590),
 .UNSPECIFIED.,.F.,.F.,(4,3,3,3,3,3,3,3,3,3,3,3,3,3,3,3,3,3,3,3,3,3,3,3,
3,3,3,3,3,3,3,3,3,3,3,3,3,3,3,3,3,4),(24.2166158670722,24.3207881370909,
24.3736195962378,24.4778038315917,24.5818327974666,24.6857396916881,24.7895811049884,
24.8933918194664,24.9972065737642,25.1011299890377,25.2051122368004,25.3092764321701,
25.3711674545838,25.4753541852857,25.5793856828633,25.6832951504786,25.7871391615083,
25.8909524941752,25.9947698832689,26.098695940573,26.2026808384369,26.3068476679265,
26.3687153129299,26.4729016565365,26.576932766987,26.6808418493753,26.7846854765711,
26.8884984273835,26.9923154371893,27.0962411217986,27.2002256501272,27.3043921191463,
27.366263171276,27.4692311189486,27.5720239013197,27.6747188321344,27.77735230861,
27.8799606435766,27.9826447824898,28.0853648870236,28.1882547092596,28.27433388186),
 .UNSPECIFIED.);
#2631=B_SPLINE_CURVE_WITH_KNOTS('',3,(#92596,#92597,#92598,#92599,#92600,
#92601,#92602,#92603,#92604,#92605,#92606,#92607,#92608,#92609,#92610,#92611,
#92612,#92613,#92614,#92615,#92616,#92617,#92618,#92619,#92620,#92621,#92622,
#92623,#92624,#92625,#92626,#92627,#92628,#92629,#92630,#92631,#92632,#92633,
#92634,#92635,#92636,#92637,#92638,#92639,#92640,#92641,#92642,#92643,#92644,
#92645,#92646,#92647,#92648,#92649,#92650,#92651,#92652,#92653,#92654,#92655,
#92656,#92657,#92658,#92659,#92660,#92661,#92662,#92663,#92664,#92665),
 .UNSPECIFIED.,.F.,.F.,(4,3,3,3,3,3,3,3,3,3,3,3,3,3,3,3,3,3,3,3,3,3,3,4),
(15.7079632679489,15.8106735934767,15.91334885119,16.0160251385365,16.1188116550667,
16.2216565686017,16.3246921199071,16.3932367294691,16.4975143581255,16.6016360889328,
16.7056343280856,16.8095661523013,16.9134661991799,17.0173690618201,17.1213780774191,
17.2254446357146,17.329690162223,17.3907845878152,17.495135742761,17.6048038128368,
17.7088847629099,17.8128986704477,17.916887220124,17.9338080230641),
 .UNSPECIFIED.);
#2632=B_SPLINE_CURVE_WITH_KNOTS('',3,(#92667,#92668,#92669,#92670,#92671),
 .UNSPECIFIED.,.F.,.F.,(4,1,4),(14.3981410127769,15.395688871123,15.7079548163673),
 .UNSPECIFIED.);
#2633=B_SPLINE_CURVE_WITH_KNOTS('',3,(#92675,#92676,#92677,#92678,#92679,
#92680,#92681,#92682,#92683,#92684,#92685,#92686,#92687,#92688,#92689,#92690,
#92691,#92692,#92693,#92694,#92695,#92696,#92697,#92698,#92699,#92700,#92701,
#92702,#92703,#92704,#92705,#92706,#92707,#92708,#92709,#92710,#92711,#92712,
#92713,#92714,#92715,#92716,#92717,#92718,#92719,#92720,#92721,#92722,#92723,
#92724,#92725,#92726,#92727,#92728,#92729,#92730,#92731,#92732),
 .UNSPECIFIED.,.F.,.F.,(4,3,3,3,3,3,3,3,3,3,3,3,3,3,3,3,3,3,3,4),(13.8761929171444,
13.9801050982006,14.0838619923275,14.1874971548373,14.2910675742173,14.394608424291,
14.4981548361472,14.6018082710274,14.7055227330307,14.809410594129,14.8542235792949,
14.9609410403274,15.0635681563456,15.1661013721572,15.2685772451739,15.3710322505032,
15.473554455726,15.5761173374535,15.6788162095048,15.7079632675546),
 .UNSPECIFIED.);
#2634=B_SPLINE_CURVE_WITH_KNOTS('',3,(#92733,#92734,#92735,#92736,#92737,
#92738,#92739,#92740,#92741,#92742,#92743,#92744,#92745,#92746,#92747,#92748,
#92749,#92750,#92751,#92752,#92753,#92754,#92755,#92756,#92757,#92758,#92759,
#92760,#92761,#92762,#92763,#92764,#92765,#92766,#92767,#92768,#92769,#92770,
#92771,#92772,#92773,#92774,#92775,#92776,#92777,#92778,#92779,#92780,#92781,
#92782,#92783,#92784,#92785,#92786,#92787,#92788,#92789,#92790,#92791,#92792,
#92793,#92794,#92795,#92796,#92797,#92798,#92799),.UNSPECIFIED.,.F.,.F.,
(4,3,3,3,3,3,3,3,3,3,3,3,3,3,3,3,3,3,3,3,3,3,4),(15.7079632679489,15.851771437641,
15.9558439456397,16.0597595638296,16.1635512471327,16.2672763592019,16.3709698524584,
16.4746666348114,16.5784717372559,16.6823352983937,16.7863815022145,16.8493192959871,
16.9535243733574,17.0575742377897,17.1615020099112,17.2653642764257,17.3691957876541,
17.4730312504175,17.5769750939415,17.6809776424981,17.7851617143139,17.8468671543332,
17.9343900068785),.UNSPECIFIED.);
#2635=B_SPLINE_CURVE_WITH_KNOTS('',3,(#92805,#92806,#92807,#92808,#92809,
#92810,#92811,#92812),.UNSPECIFIED.,.F.,.F.,(4,1,1,1,1,4),(99.6151611513019,
99.6457915387123,100.643339397058,101.640887255404,102.638435113751,103.635982972097),
 .UNSPECIFIED.);
#2636=B_SPLINE_CURVE_WITH_KNOTS('',3,(#92816,#92817,#92818,#92819,#92820,
#92821,#92822,#92823,#92824,#92825,#92826,#92827,#92828,#92829,#92830,#92831),
 .UNSPECIFIED.,.F.,.F.,(4,3,3,3,3,4),(103.672557568829,103.780299930425,
103.88830919533,103.996463610122,104.104895341938,104.157833394917),
 .UNSPECIFIED.);
#2637=B_SPLINE_CURVE_WITH_KNOTS('',3,(#92832,#92833,#92834,#92835,#92836,
#92837,#92838,#92839,#92840,#92841,#92842,#92843,#92844,#92845,#92846,#92847,
#92848,#92849,#92850,#92851,#92852,#92853,#92854,#92855,#92856,#92857,#92858,
#92859,#92860,#92861,#92862,#92863,#92864,#92865,#92866,#92867,#92868,#92869,
#92870,#92871,#92872,#92873,#92874,#92875,#92876,#92877,#92878,#92879,#92880,
#92881,#92882,#92883,#92884,#92885,#92886,#92887,#92888,#92889,#92890,#92891,
#92892,#92893,#92894,#92895,#92896,#92897,#92898,#92899,#92900,#92901,#92902,
#92903,#92904,#92905,#92906,#92907,#92908,#92909,#92910,#92911,#92912,#92913,
#92914,#92915,#92916,#92917,#92918,#92919,#92920,#92921,#92922,#92923,#92924,
#92925,#92926,#92927,#92928,#92929,#92930,#92931,#92932,#92933,#92934,#92935,
#92936,#92937,#92938,#92939,#92940,#92941,#92942,#92943,#92944,#92945,#92946,
#92947,#92948,#92949,#92950,#92951,#92952,#92953,#92954,#92955),
 .UNSPECIFIED.,.F.,.F.,(4,3,3,3,3,3,3,3,3,3,3,3,3,3,3,3,3,3,3,3,3,3,3,3,
3,3,3,3,3,3,3,3,3,3,3,3,3,3,3,3,3,4),(99.6156213899676,99.719451702261,
99.8232891842525,99.9272369878061,100.03124639439,100.135434233686,100.18725683054,
100.291455310788,100.395498815188,100.499420609254,100.603277136689,100.707103155531,
100.810933380572,100.914872410489,101.018870377466,101.123050283818,101.184804688886,
101.288885178202,101.392810145172,101.496613161362,101.600350824598,101.704058066099,
101.807769773832,101.911591496786,102.015472659481,102.119537827642,102.182352547233,
102.286721401994,102.390934579093,102.495024194029,102.599047303358,102.703038423928,
102.807032027915,102.911130699731,103.015286432589,103.119619455548,103.179900405579,
103.289272719893,103.398334669506,103.507209075267,103.615853248157,103.672557568463),
 .UNSPECIFIED.);
#2638=B_SPLINE_CURVE_WITH_KNOTS('',3,(#92961,#92962,#92963,#92964,#92965,
#92966,#92967,#92968,#92969,#92970,#92971,#92972,#92973,#92974,#92975,#92976,
#92977,#92978,#92979,#92980,#92981,#92982,#92983,#92984,#92985,#92986,#92987,
#92988,#92989,#92990,#92991,#92992,#92993,#92994,#92995,#92996,#92997,#92998,
#92999,#93000,#93001,#93002,#93003,#93004,#93005,#93006,#93007,#93008,#93009,
#93010,#93011,#93012,#93013,#93014,#93015,#93016,#93017,#93018,#93019,#93020,
#93021,#93022,#93023,#93024,#93025,#93026,#93027,#93028,#93029,#93030,#93031,
#93032,#93033,#93034,#93035,#93036,#93037,#93038,#93039,#93040,#93041,#93042,
#93043,#93044,#93045,#93046,#93047,#93048,#93049,#93050,#93051,#93052,#93053,
#93054,#93055,#93056,#93057,#93058,#93059,#93060,#93061,#93062,#93063,#93064,
#93065,#93066,#93067,#93068,#93069,#93070,#93071,#93072,#93073,#93074,#93075,
#93076,#93077,#93078,#93079,#93080,#93081,#93082,#93083,#93084,#93085,#93086,
#93087),.UNSPECIFIED.,.F.,.F.,(4,3,3,3,3,3,3,3,3,3,3,3,3,3,3,3,3,3,3,3,
3,3,3,3,3,3,3,3,3,3,3,3,3,3,3,3,3,3,3,3,3,3,4),(93.3317451830118,93.4356908335088,
93.539708921792,93.6438957414934,93.6605043886357,93.7646924917536,93.868725346352,
93.9726361419404,94.076481462347,94.1802960840316,94.28411474,94.3880420220064,
94.4920281226445,94.5961961074607,94.6580522469818,94.7622408524121,94.8662742508428,
94.9701856485116,95.0740316065126,95.1778469000452,95.2816662608905,95.3855942926708,
95.489581169514,95.5937499633514,95.6556001053279,95.7597729568001,95.8637905433978,
95.9676861197645,96.071516259166,96.1753157600107,96.279119377306,96.3830318486896,
96.4870032449124,96.5911568522755,96.653147963674,96.7562452951427,96.8592012753662,
96.9620522837591,97.0688822781402,97.1716574277158,97.2744331495273,97.3772781459456,
97.3893722612836),.UNSPECIFIED.);
#2639=B_SPLINE_CURVE_WITH_KNOTS('',3,(#93088,#93089,#93090,#93091,#93092,
#93093),.UNSPECIFIED.,.F.,.F.,(4,1,1,4),(97.3893747333975,97.6506958220201,
98.6482436803662,99.6151611513019),.UNSPECIFIED.);
#2640=B_SPLINE_CURVE_WITH_KNOTS('',3,(#93095,#93096,#93097,#93098,#93099,
#93100,#93101,#93102,#93103,#93104,#93105,#93106,#93107,#93108,#93109,#93110,
#93111,#93112,#93113,#93114,#93115,#93116,#93117,#93118,#93119,#93120,#93121,
#93122,#93123,#93124,#93125,#93126,#93127,#93128,#93129,#93130,#93131,#93132,
#93133,#93134,#93135,#93136,#93137,#93138,#93139,#93140,#93141,#93142,#93143,
#93144,#93145,#93146,#93147,#93148,#93149,#93150,#93151,#93152,#93153,#93154,
#93155,#93156,#93157,#93158,#93159,#93160,#93161),.UNSPECIFIED.,.F.,.F.,
(4,3,3,3,3,3,3,3,3,3,3,3,3,3,3,3,3,3,3,3,3,3,4),(97.3893722616848,97.4918516969082,
97.5942418193773,97.6965792942248,97.7989007101473,97.901312936064,98.0037693753309,
98.1064097553564,98.1921611138482,98.2963339822745,98.4003515858491,98.5042471791462,
98.6080773354404,98.7118768531167,98.8156804871574,98.9195929750428,99.0235643876549,
99.1277180110528,99.1897089721943,99.2961870766376,99.4002195153588,99.5079204526632,
99.6156213899676),.UNSPECIFIED.);
#2641=B_SPLINE_CURVE_WITH_KNOTS('',3,(#93162,#93163,#93164,#93165,#93166,
#93167,#93168,#93169,#93170,#93171,#93172,#93173,#93174,#93175,#93176,#93177,
#93178,#93179,#93180,#93181,#93182,#93183,#93184,#93185,#93186,#93187,#93188,
#93189,#93190,#93191,#93192,#93193,#93194,#93195,#93196,#93197,#93198,#93199,
#93200,#93201,#93202,#93203,#93204,#93205,#93206,#93207,#93208,#93209,#93210,
#93211,#93212,#93213,#93214,#93215,#93216,#93217,#93218,#93219,#93220,#93221,
#93222,#93223,#93224,#93225,#93226,#93227,#93228,#93229,#93230,#93231,#93232,
#93233,#93234,#93235,#93236,#93237,#93238,#93239,#93240,#93241,#93242,#93243,
#93244,#93245,#93246,#93247,#93248,#93249,#93250,#93251,#93252,#93253,#93254,
#93255,#93256,#93257,#93258,#93259,#93260,#93261,#93262,#93263,#93264,#93265,
#93266,#93267,#93268,#93269,#93270,#93271,#93272,#93273,#93274,#93275,#93276,
#93277,#93278,#93279,#93280,#93281,#93282,#93283,#93284,#93285),
 .UNSPECIFIED.,.F.,.F.,(4,3,3,3,3,3,3,3,3,3,3,3,3,3,3,3,3,3,3,3,3,3,3,3,
3,3,3,3,3,3,3,3,3,3,3,3,3,3,3,3,3,4),(93.3327249610222,93.4413805509524,
93.5452680358632,93.6490996829472,93.7529102555451,93.8567344832209,93.9606732647267,
94.0646795135131,94.1688591274354,94.2019696804638,94.3061562454964,94.4101875758906,
94.5140968748872,94.6179407165043,94.7217538792165,94.8255710980645,94.9294969858512,
95.033481714353,95.1376483765647,95.1995175388099,95.303702070536,95.4077313618506,
95.511638623033,95.6154804287179,95.7192915603578,95.8231067559746,95.9270306463741,
96.0310133890498,96.1351781052391,96.197065397156,96.3012534986124,96.4052863515668,
96.5091971455439,96.6130424643603,96.716857084478,96.8206757389046,96.9246030194181,
97.0285891185885,97.1327571019925,97.1946132555021,97.345607244739,97.3893722612836),
 .UNSPECIFIED.);
#2642=B_SPLINE_CURVE_WITH_KNOTS('',3,(#93291,#93292,#93293,#93294,#93295,
#93296,#93297,#93298,#93299,#93300,#93301,#93302,#93303,#93304,#93305,#93306,
#93307,#93308,#93309,#93310,#93311,#93312,#93313,#93314,#93315,#93316,#93317,
#93318,#93319,#93320,#93321,#93322,#93323,#93324,#93325,#93326,#93327,#93328,
#93329,#93330,#93331,#93332,#93333,#93334,#93335,#93336,#93337,#93338,#93339,
#93340,#93341,#93342,#93343,#93344,#93345,#93346,#93347,#93348,#93349,#93350,
#93351,#93352,#93353,#93354,#93355,#93356,#93357,#93358,#93359,#93360,#93361,
#93362,#93363,#93364,#93365,#93366,#93367,#93368,#93369,#93370,#93371,#93372,
#93373,#93374,#93375,#93376,#93377,#93378,#93379,#93380,#93381,#93382,#93383,
#93384,#93385,#93386,#93387,#93388,#93389,#93390,#93391,#93392,#93393,#93394,
#93395,#93396,#93397,#93398,#93399,#93400,#93401,#93402,#93403,#93404,#93405,
#93406,#93407,#93408,#93409,#93410,#93411),.UNSPECIFIED.,.F.,.F.,(4,3,3,
3,3,3,3,3,3,3,3,3,3,3,3,3,3,3,3,3,3,3,3,3,3,3,3,3,3,3,3,3,3,3,3,3,3,3,3,
3,4),(87.0493933608437,87.1532149139967,87.2570257238478,87.3615736025257,
87.4655294029247,87.5703733207419,87.6752172385592,87.7794034175018,87.8834343579763,
87.9873432633011,88.091186709151,88.194999474602,88.2988162952939,88.4027417863365,
88.5067261182931,88.6108923886106,88.6727650969053,88.7769513208729,88.8809823069786,
88.9848912586063,89.0887347511468,89.1925475636041,89.2963644315469,89.4002899698799,
89.5042743492206,89.6084406665499,89.6703129552514,89.7744989225328,89.8785296514156,
89.9824383462603,90.0862815824279,90.1900941392956,90.293910752806,90.3978360402153,
90.5018201702324,90.6059862434675,90.6678608135975,90.7807057008014,90.8932647263971,
91.0053646978595,91.1061869538111),.UNSPECIFIED.);
#2643=B_SPLINE_CURVE_WITH_KNOTS('',3,(#93412,#93413,#93414,#93415,#93416,
#93417,#93418,#93419,#93420,#93421,#93422,#93423,#93424,#93425,#93426,#93427,
#93428,#93429,#93430,#93431,#93432,#93433,#93434,#93435,#93436,#93437,#93438,
#93439,#93440,#93441,#93442,#93443,#93444,#93445,#93446,#93447,#93448,#93449,
#93450,#93451,#93452,#93453,#93454,#93455,#93456,#93457,#93458,#93459,#93460,
#93461,#93462,#93463,#93464,#93465,#93466,#93467,#93468,#93469,#93470,#93471,
#93472,#93473,#93474,#93475,#93476,#93477,#93478,#93479,#93480,#93481),
 .UNSPECIFIED.,.F.,.F.,(4,3,3,3,3,3,3,3,3,3,3,3,3,3,3,3,3,3,3,3,3,3,3,4),
(91.106186954104,91.2125697915894,91.3190338862199,91.4256928890665,91.5324648457377,
91.6394568072871,91.6654086719436,91.7695952380118,91.8736265694479,91.977535869491,
92.0813797121567,92.1851928759182,92.2890100958143,92.3929359846407,92.4969207141789,
92.6010873774105,92.6629565302897,92.7671206832539,92.8711399649714,92.9750493921735,
93.0788929406494,93.1826980509479,93.2865285969047,93.3317451830118),
 .UNSPECIFIED.);
#2644=B_SPLINE_CURVE_WITH_KNOTS('',3,(#93483,#93484,#93485,#93486,#93487,
#93488,#93489,#93490,#93491,#93492,#93493,#93494,#93495,#93496,#93497,#93498,
#93499,#93500,#93501,#93502,#93503,#93504,#93505,#93506,#93507,#93508,#93509,
#93510,#93511,#93512,#93513,#93514,#93515,#93516,#93517,#93518,#93519,#93520,
#93521,#93522,#93523,#93524,#93525,#93526,#93527,#93528,#93529,#93530,#93531,
#93532,#93533,#93534,#93535,#93536,#93537,#93538,#93539,#93540,#93541,#93542,
#93543,#93544,#93545,#93546,#93547,#93548,#93549,#93550,#93551,#93552),
 .UNSPECIFIED.,.F.,.F.,(4,3,3,3,3,3,3,3,3,3,3,3,3,3,3,3,3,3,3,3,3,3,3,4),
(91.106186954104,91.2093261054256,91.3135123292234,91.4175433151588,91.5214522666154,
91.6252957589846,91.7291085712708,91.8329254390422,91.9368509772058,92.0408353563778,
92.1450016735413,92.2068739637717,92.3110599314537,92.4150906607374,92.5189993559811,
92.6228425925464,92.7266551498102,92.830471763714,92.9343970515104,93.0383811819116,
93.1425472555219,93.2044218221178,93.3086061887592,93.3327249610222),
 .UNSPECIFIED.);
#2645=B_SPLINE_CURVE_WITH_KNOTS('',3,(#93553,#93554,#93555,#93556,#93557,
#93558,#93559,#93560,#93561,#93562,#93563,#93564,#93565,#93566,#93567,#93568,
#93569,#93570,#93571,#93572,#93573,#93574,#93575,#93576,#93577,#93578,#93579,
#93580,#93581,#93582,#93583,#93584,#93585,#93586,#93587,#93588,#93589,#93590,
#93591,#93592,#93593,#93594,#93595,#93596,#93597,#93598,#93599,#93600,#93601,
#93602,#93603,#93604,#93605,#93606,#93607,#93608,#93609,#93610,#93611,#93612,
#93613,#93614,#93615,#93616,#93617,#93618,#93619,#93620,#93621,#93622,#93623,
#93624,#93625,#93626,#93627,#93628,#93629,#93630,#93631,#93632,#93633,#93634,
#93635,#93636,#93637,#93638,#93639,#93640,#93641,#93642,#93643,#93644,#93645,
#93646,#93647,#93648,#93649,#93650,#93651,#93652,#93653,#93654,#93655,#93656,
#93657,#93658,#93659,#93660,#93661,#93662,#93663,#93664,#93665,#93666,#93667,
#93668,#93669,#93670,#93671,#93672,#93673,#93674,#93675,#93676),
 .UNSPECIFIED.,.F.,.F.,(4,3,3,3,3,3,3,3,3,3,3,3,3,3,3,3,3,3,3,3,3,3,3,3,
3,3,3,3,3,3,3,3,3,3,3,3,3,3,3,3,3,4),(87.0484495580493,87.1526139555506,
87.2191346720412,87.323320836556,87.4273517627698,87.5312606541471,87.6351040862496,
87.7389168381718,87.8427336455723,87.946659123773,88.0506434431219,88.1548097013355,
88.2166825303873,88.3208687024162,88.4248996362149,88.5288085352445,88.6326519750365,
88.736464734674,88.8402815498039,88.9442070357016,89.0481913627408,89.1523576285501,
89.2142303887334,89.3184165292485,89.4224474314894,89.5263562990473,89.6301997074378,
89.7340124357895,89.8378292197948,89.9417546750267,90.0457389716127,90.1499052076343,
90.2117782470795,90.3146405331901,90.4173275668862,90.5199168474419,90.6224448805545,
90.7249480861439,90.8275243015791,90.9301370935116,91.0329109698248,91.1061869536426),
 .UNSPECIFIED.);
#2646=B_SPLINE_CURVE_WITH_KNOTS('',3,(#93682,#93683,#93684,#93685,#93686,
#93687,#93688,#93689,#93690,#93691,#93692,#93693,#93694,#93695,#93696,#93697,
#93698,#93699,#93700,#93701,#93702,#93703,#93704,#93705,#93706,#93707,#93708,
#93709,#93710,#93711,#93712,#93713,#93714,#93715,#93716,#93717,#93718,#93719,
#93720,#93721,#93722,#93723,#93724,#93725,#93726,#93727,#93728,#93729,#93730,
#93731,#93732,#93733,#93734,#93735,#93736,#93737,#93738,#93739,#93740,#93741,
#93742,#93743,#93744,#93745,#93746,#93747,#93748,#93749,#93750,#93751,#93752,
#93753,#93754,#93755,#93756,#93757,#93758,#93759,#93760,#93761,#93762,#93763,
#93764,#93765,#93766,#93767,#93768,#93769,#93770,#93771,#93772,#93773,#93774,
#93775,#93776,#93777,#93778,#93779,#93780,#93781,#93782,#93783,#93784,#93785,
#93786,#93787,#93788,#93789,#93790,#93791,#93792,#93793,#93794,#93795,#93796,
#93797,#93798,#93799,#93800,#93801,#93802),.UNSPECIFIED.,.F.,.F.,(4,3,3,
3,3,3,3,3,3,3,3,3,3,3,3,3,3,3,3,3,3,3,3,3,3,3,3,3,3,3,3,3,3,3,3,3,3,3,3,
3,4),(80.7662008530864,80.8702730497271,80.9742075957574,81.0780665246705,
81.1818846348487,81.2856966710118,81.389610872242,81.4935748160271,81.5977303348073,
81.6899300884827,81.7941162519913,81.8981471772207,82.0020560676502,82.1058994988279,
82.2097122498495,82.3135290563748,82.4174545337446,82.5214388522863,82.6256051097386,
82.6874779468288,82.7916641114806,82.8956950378613,82.9996039294484,83.103447361787,
83.2072601139711,83.3110769216587,83.4150024001824,83.518986719875,83.6231529784611,
83.6850258051749,83.7892119660234,83.893242888598,83.9971517763933,84.1009952049509,
84.2048079533701,84.3086247573145,84.4125502321539,84.5165345481899,84.6207008032023,
84.682573663521,84.8230016469244),.UNSPECIFIED.);
#2647=B_SPLINE_CURVE_WITH_KNOTS('',3,(#93803,#93804,#93805,#93806,#93807,
#93808,#93809,#93810,#93811,#93812,#93813,#93814,#93815,#93816,#93817,#93818,
#93819,#93820,#93821,#93822,#93823,#93824,#93825,#93826,#93827,#93828,#93829,
#93830,#93831,#93832,#93833,#93834,#93835,#93836,#93837,#93838,#93839,#93840,
#93841,#93842,#93843,#93844,#93845,#93846,#93847,#93848,#93849,#93850,#93851,
#93852,#93853,#93854,#93855,#93856,#93857,#93858,#93859,#93860,#93861,#93862,
#93863,#93864,#93865,#93866,#93867,#93868,#93869,#93870,#93871,#93872),
 .UNSPECIFIED.,.F.,.F.,(4,3,3,3,3,3,3,3,3,3,3,3,3,3,3,3,3,3,3,3,3,3,3,4),
(84.8230016473375,84.9301416316537,85.0325714163376,85.1349307980759,85.2372563959065,
85.3395847767837,85.4420166361939,85.5445096330566,85.6471710557298,85.6801215218671,
85.7843076939228,85.8883386277482,85.9922475268047,86.0960909666236,86.199903726288,
86.3037205414444,86.4076460273685,86.5116303544343,86.6157966202695,86.6776693802131,
86.7818282235991,86.8858513473607,86.9897582187876,87.0493933608437),
 .UNSPECIFIED.);
#2648=B_SPLINE_CURVE_WITH_KNOTS('',3,(#93874,#93875,#93876,#93877,#93878,
#93879,#93880,#93881,#93882,#93883,#93884,#93885,#93886,#93887,#93888,#93889,
#93890,#93891,#93892,#93893,#93894,#93895,#93896,#93897,#93898,#93899,#93900,
#93901,#93902,#93903,#93904,#93905,#93906,#93907,#93908,#93909,#93910,#93911,
#93912,#93913,#93914,#93915,#93916,#93917,#93918,#93919,#93920,#93921,#93922,
#93923,#93924,#93925,#93926,#93927,#93928,#93929,#93930,#93931,#93932,#93933,
#93934,#93935,#93936,#93937,#93938,#93939,#93940),.UNSPECIFIED.,.F.,.F.,
(4,3,3,3,3,3,3,3,3,3,3,3,3,3,3,3,3,3,3,3,3,3,4),(84.8230016473347,84.9376554440836,
85.0527190382934,85.1683359285703,85.2240389553491,85.3282251199969,85.4322560463736,
85.5361649379567,85.6400083702913,85.7438211224714,85.847637930155,85.9515634086748,
86.0555477283636,86.1597139869458,86.2215868136951,86.3257394090933,86.4297517345021,
86.5336587825648,86.6374954230147,86.7413356739134,86.8451704422707,86.9491112691339,
87.0484495580493),.UNSPECIFIED.);
#2649=B_SPLINE_CURVE_WITH_KNOTS('',3,(#93941,#93942,#93943,#93944,#93945,
#93946,#93947,#93948,#93949,#93950,#93951,#93952,#93953,#93954,#93955,#93956,
#93957,#93958,#93959,#93960,#93961,#93962,#93963,#93964,#93965,#93966,#93967,
#93968,#93969,#93970,#93971,#93972,#93973,#93974,#93975,#93976,#93977,#93978,
#93979,#93980,#93981,#93982,#93983,#93984,#93985,#93986,#93987,#93988,#93989,
#93990,#93991,#93992,#93993,#93994,#93995,#93996,#93997,#93998,#93999,#94000,
#94001,#94002,#94003,#94004,#94005,#94006,#94007,#94008,#94009,#94010,#94011,
#94012,#94013,#94014,#94015,#94016,#94017,#94018,#94019,#94020,#94021,#94022,
#94023,#94024,#94025,#94026,#94027,#94028,#94029,#94030,#94031,#94032,#94033,
#94034,#94035,#94036,#94037,#94038,#94039,#94040,#94041,#94042,#94043,#94044,
#94045,#94046,#94047,#94048,#94049,#94050,#94051,#94052,#94053,#94054,#94055,
#94056,#94057,#94058,#94059,#94060,#94061,#94062,#94063,#94064),
 .UNSPECIFIED.,.F.,.F.,(4,3,3,3,3,3,3,3,3,3,3,3,3,3,3,3,3,3,3,3,3,3,3,3,
3,3,3,3,3,3,3,3,3,3,3,3,3,3,3,3,3,4),(80.7657457648301,80.8695647156208,
80.9734943498133,81.0774857297398,81.1816561023789,81.2338475219647,81.3380336854432,
81.4420646106447,81.5459735010509,81.6498169322079,81.7536296832115,81.8574464897212,
81.9613719670797,82.0653562856124,82.1695225430592,82.2313953803108,82.3355815439513,
82.4396124693163,82.5435213598861,82.6473647912069,82.7511775423742,82.8549943490479,
82.9589198265682,83.0629041452623,83.1670704028679,83.2289432386569,83.3331294018511,
83.4371603267697,83.5410692168954,83.6449126477737,83.7487253985006,83.8525422047368,
83.956467681827,84.0604520000942,84.1646182572832,84.226491097003,84.3322636668447,
84.4378652902381,84.5433026045803,84.6486432044876,84.7539210445285,84.8230016469244),
 .UNSPECIFIED.);
#2650=B_SPLINE_CURVE_WITH_KNOTS('',3,(#94070,#94071,#94072,#94073,#94074,
#94075,#94076,#94077,#94078,#94079,#94080,#94081,#94082,#94083,#94084,#94085,
#94086,#94087,#94088,#94089,#94090,#94091,#94092,#94093,#94094,#94095,#94096,
#94097,#94098,#94099,#94100,#94101,#94102,#94103,#94104,#94105,#94106,#94107,
#94108,#94109,#94110,#94111,#94112,#94113,#94114,#94115,#94116,#94117,#94118,
#94119,#94120,#94121,#94122,#94123,#94124,#94125,#94126,#94127,#94128,#94129,
#94130,#94131,#94132,#94133,#94134,#94135,#94136,#94137,#94138,#94139,#94140,
#94141,#94142,#94143,#94144,#94145,#94146,#94147,#94148,#94149,#94150,#94151,
#94152,#94153,#94154,#94155,#94156,#94157,#94158,#94159,#94160,#94161,#94162,
#94163,#94164,#94165,#94166,#94167,#94168,#94169,#94170,#94171,#94172,#94173,
#94174,#94175,#94176,#94177,#94178,#94179,#94180,#94181,#94182,#94183,#94184,
#94185,#94186,#94187,#94188,#94189,#94190,#94191,#94192,#94193,#94194,#94195,
#94196),.UNSPECIFIED.,.F.,.F.,(4,3,3,3,3,3,3,3,3,3,3,3,3,3,3,3,3,3,3,3,
3,3,3,3,3,3,3,3,3,3,3,3,3,3,3,3,3,3,3,3,3,3,4),(74.4820629789471,74.5860824450287,
74.6902706747757,74.7070950800601,74.811281243545,74.9153121687539,75.0192210591676,
75.1230644903326,75.2268772413443,75.3306940478627,75.43461952523,75.5386038437718,
75.6427701012281,75.7046429384062,75.8088291018917,75.9128600271012,76.0167689175154,
76.1206123486807,76.2244250996928,76.3282419062114,76.4321673835789,76.5361517021208,
76.6403179595772,76.7021907967523,76.80637696026,76.9104078854918,77.0143167759283,
77.1181602071159,77.2219729581504,77.3257897646913,77.4297152420809,77.5336995606446,
77.6378658181225,77.6997386550984,77.8047483656344,77.9072108121793,78.0095758369578,
78.1118801627626,78.2188642069186,78.3212057260089,78.4235870713419,78.5260937326297,
78.5398163393865),.UNSPECIFIED.);
#2651=B_SPLINE_CURVE_WITH_KNOTS('',3,(#94197,#94198,#94199,#94200,#94201,
#94202,#94203,#94204,#94205,#94206,#94207,#94208,#94209,#94210,#94211,#94212,
#94213,#94214,#94215,#94216,#94217,#94218,#94219,#94220,#94221,#94222,#94223,
#94224,#94225,#94226,#94227,#94228,#94229,#94230,#94231,#94232,#94233,#94234,
#94235,#94236,#94237,#94238,#94239,#94240,#94241,#94242,#94243,#94244,#94245,
#94246,#94247,#94248,#94249,#94250,#94251,#94252,#94253,#94254,#94255,#94256,
#94257,#94258,#94259,#94260,#94261,#94262,#94263),.UNSPECIFIED.,.F.,.F.,
(4,3,3,3,3,3,3,3,3,3,3,3,3,3,3,3,3,3,3,3,3,3,4),(78.5398163397448,78.6972865134445,
78.8014726769225,78.905503602124,79.0094124925299,79.1132559236866,79.2170686746898,
79.3208854811994,79.4248109585574,79.5287952770896,79.6329615345361,79.6948343717905,
79.7990205354316,79.9030514607972,80.0069603513676,80.1108037826891,80.2146165338571,
80.3184333405311,80.4223588180522,80.5263431367468,80.630509394353,80.6923822301366,
80.7662008530864),.UNSPECIFIED.);
#2652=B_SPLINE_CURVE_WITH_KNOTS('',3,(#94265,#94266,#94267,#94268,#94269,
#94270,#94271,#94272,#94273,#94274,#94275,#94276,#94277,#94278,#94279,#94280,
#94281,#94282,#94283,#94284,#94285,#94286,#94287,#94288,#94289,#94290,#94291,
#94292,#94293,#94294,#94295,#94296,#94297,#94298,#94299,#94300,#94301,#94302,
#94303,#94304,#94305,#94306,#94307,#94308,#94309,#94310,#94311,#94312,#94313,
#94314,#94315,#94316,#94317,#94318,#94319,#94320,#94321,#94322,#94323,#94324,
#94325,#94326,#94327,#94328,#94329,#94330,#94331),.UNSPECIFIED.,.F.,.F.,
(4,3,3,3,3,3,3,3,3,3,3,3,3,3,3,3,3,3,3,3,3,3,4),(78.5398163397448,78.6430480181522,
78.7462408136019,78.8494302891154,78.9527248465537,79.056073050004,79.159611215967,
79.2387518052725,79.3429379687801,79.4469688940118,79.5508777844482,79.6547212156358,
79.7585339666699,79.8623507732107,79.9662762506001,80.0702605691636,80.1744268266413,
80.2362996636186,80.3404816769733,80.4467976989375,80.550702681629,80.6582242232296,
80.7657457648301),.UNSPECIFIED.);
#2653=B_SPLINE_CURVE_WITH_KNOTS('',3,(#94332,#94333,#94334,#94335,#94336,
#94337,#94338,#94339,#94340,#94341,#94342,#94343,#94344,#94345,#94346,#94347,
#94348,#94349,#94350,#94351,#94352,#94353,#94354,#94355,#94356,#94357,#94358,
#94359,#94360,#94361,#94362,#94363,#94364,#94365,#94366,#94367,#94368,#94369,
#94370,#94371,#94372,#94373,#94374,#94375,#94376,#94377,#94378,#94379,#94380,
#94381,#94382,#94383,#94384,#94385,#94386,#94387,#94388,#94389,#94390,#94391,
#94392,#94393,#94394,#94395,#94396,#94397,#94398,#94399,#94400,#94401,#94402,
#94403,#94404,#94405,#94406,#94407,#94408,#94409,#94410,#94411,#94412,#94413,
#94414,#94415,#94416,#94417,#94418,#94419,#94420,#94421,#94422,#94423,#94424,
#94425,#94426,#94427,#94428,#94429,#94430,#94431,#94432,#94433,#94434,#94435,
#94436,#94437,#94438,#94439,#94440,#94441,#94442,#94443,#94444,#94445,#94446,
#94447,#94448,#94449,#94450,#94451,#94452,#94453,#94454,#94455),
 .UNSPECIFIED.,.F.,.F.,(4,3,3,3,3,3,3,3,3,3,3,3,3,3,3,3,3,3,3,3,3,3,3,3,
3,3,3,3,3,3,3,3,3,3,3,3,3,3,3,3,3,4),(74.4832444132594,74.5871350869426,
74.6909683424548,74.7947789457462,74.8986016274051,75.0025379180133,75.1065402590823,
75.210717341976,75.2485603718882,75.3527465353761,75.4567774605879,75.5606863510045,
75.6645297821723,75.7683425331867,75.8721593397079,75.9760848170779,76.0800691356223,
76.1842353930812,76.2461082302343,76.3502943937249,76.4543253189398,76.5582342093591,
76.6620776405297,76.7658903915471,76.8697071980708,76.9736326754436,77.0776169939906,
77.1817832514521,77.2436560885804,77.3478422520653,77.4518731772742,77.5557820676879,
77.6596254988527,77.7634382498646,77.8672550563835,77.9711805337506,78.0751648522923,
78.1793311097485,78.2412039469264,78.3682032551823,78.4934616304658,78.5398163394195),
 .UNSPECIFIED.);
#2654=B_SPLINE_CURVE_WITH_KNOTS('',3,(#94461,#94462,#94463,#94464,#94465,
#94466,#94467,#94468,#94469,#94470,#94471,#94472,#94473,#94474,#94475,#94476,
#94477,#94478,#94479,#94480,#94481,#94482,#94483,#94484,#94485,#94486,#94487,
#94488,#94489,#94490,#94491,#94492,#94493,#94494,#94495,#94496,#94497,#94498,
#94499,#94500,#94501,#94502,#94503,#94504,#94505,#94506,#94507,#94508,#94509,
#94510,#94511,#94512,#94513,#94514,#94515,#94516,#94517,#94518,#94519,#94520,
#94521,#94522,#94523,#94524,#94525,#94526,#94527,#94528,#94529,#94530,#94531,
#94532,#94533,#94534,#94535,#94536,#94537,#94538,#94539,#94540,#94541,#94542,
#94543,#94544,#94545,#94546,#94547,#94548,#94549,#94550,#94551,#94552,#94553,
#94554,#94555,#94556,#94557,#94558,#94559,#94560,#94561,#94562,#94563,#94564,
#94565,#94566,#94567,#94568,#94569,#94570,#94571,#94572,#94573,#94574,#94575,
#94576,#94577,#94578,#94579,#94580,#94581),.UNSPECIFIED.,.F.,.F.,(4,3,3,
3,3,3,3,3,3,3,3,3,3,3,3,3,3,3,3,3,3,3,3,3,3,3,3,3,3,3,3,3,3,3,3,3,3,3,3,
3,4),(68.199542273107,68.3033530889066,68.4079667991759,68.5119225050548,
68.6168652175192,68.7218079299836,68.8259940934717,68.9300250186838,69.0339339091007,
69.1377773402688,69.2415900912837,69.3454068978053,69.4493323751756,69.5533166937204,
69.6574829511797,69.7193557883297,69.8235419518178,69.9275728770296,70.0314817674465,
70.1353251986146,70.2391379496294,70.342954756151,70.4468802335214,70.5508645520662,
70.6550308095254,70.7169036466757,70.8210898101641,70.9251207353764,71.0290296257936,
71.1328730569619,71.2366858079772,71.340502614499,71.4444280918697,71.5484124104147,
71.6525786678742,71.7144515050218,71.8220784528947,71.9307165978123,72.0379272940099,
72.1472791632875,72.2566310325652),.UNSPECIFIED.);
#2655=B_SPLINE_CURVE_WITH_KNOTS('',3,(#94582,#94583,#94584,#94585,#94586,
#94587,#94588,#94589,#94590,#94591,#94592,#94593,#94594,#94595,#94596,#94597,
#94598,#94599,#94600,#94601,#94602,#94603,#94604,#94605,#94606,#94607,#94608,
#94609,#94610,#94611,#94612,#94613,#94614,#94615,#94616,#94617,#94618,#94619,
#94620,#94621,#94622,#94623,#94624,#94625,#94626,#94627,#94628,#94629,#94630,
#94631,#94632,#94633,#94634,#94635,#94636,#94637,#94638,#94639,#94640,#94641,
#94642,#94643,#94644,#94645,#94646,#94647,#94648),.UNSPECIFIED.,.F.,.F.,
(4,3,3,3,3,3,3,3,3,3,3,3,3,3,3,3,3,3,3,3,3,3,4),(72.2566310330023,72.3704731155937,
72.481813311248,72.5969063373079,72.7119993633679,72.8161855268555,72.920216452067,
73.0241253424834,73.127968773651,73.2317815246655,73.3355983311864,73.4395238085563,
73.5435081271006,73.6476743845593,73.709547221714,73.8137037283056,73.9177183843865,
74.0216261896493,74.125462018442,74.2292882433997,74.3331083610436,74.4370016429364,
74.4820629789471),.UNSPECIFIED.);
#2656=B_SPLINE_CURVE_WITH_KNOTS('',3,(#94650,#94651,#94652,#94653,#94654,
#94655,#94656,#94657,#94658,#94659,#94660,#94661,#94662,#94663,#94664,#94665,
#94666,#94667,#94668,#94669,#94670,#94671,#94672,#94673,#94674,#94675,#94676,
#94677,#94678,#94679,#94680,#94681,#94682,#94683,#94684,#94685,#94686,#94687,
#94688,#94689,#94690,#94691,#94692,#94693,#94694,#94695,#94696,#94697,#94698,
#94699,#94700,#94701,#94702,#94703,#94704,#94705,#94706,#94707,#94708,#94709,
#94710,#94711,#94712,#94713,#94714,#94715,#94716,#94717,#94718,#94719),
 .UNSPECIFIED.,.F.,.F.,(4,3,3,3,3,3,3,3,3,3,3,3,3,3,3,3,3,3,3,3,3,3,3,4),
(72.2566310325652,72.3608036974116,72.4648211348936,72.5687165871306,72.6725466326848,
72.7763460710619,72.8801496583902,72.9840619405008,73.088033186615,73.1921861589881,
73.253464655196,73.3576508186845,73.4616817438972,73.5655906343145,73.669434065483,
73.7732468164982,73.8770636230202,73.980989100391,74.0849734189361,74.1891396763956,
74.2510125135421,74.3552035665589,74.4592285332535,74.4832444132594),
 .UNSPECIFIED.);
#2657=B_SPLINE_CURVE_WITH_KNOTS('',3,(#94720,#94721,#94722,#94723,#94724,
#94725,#94726,#94727,#94728,#94729,#94730,#94731,#94732,#94733,#94734,#94735,
#94736,#94737,#94738,#94739,#94740,#94741,#94742,#94743,#94744,#94745,#94746,
#94747,#94748,#94749,#94750,#94751,#94752,#94753,#94754,#94755,#94756,#94757,
#94758,#94759,#94760,#94761,#94762,#94763,#94764,#94765,#94766,#94767,#94768,
#94769,#94770,#94771,#94772,#94773,#94774,#94775,#94776,#94777,#94778,#94779,
#94780,#94781,#94782,#94783,#94784,#94785,#94786,#94787,#94788,#94789,#94790,
#94791,#94792,#94793,#94794,#94795,#94796,#94797,#94798,#94799,#94800,#94801,
#94802,#94803,#94804,#94805,#94806,#94807,#94808,#94809,#94810,#94811,#94812,
#94813,#94814,#94815,#94816,#94817,#94818,#94819,#94820,#94821,#94822,#94823,
#94824,#94825,#94826,#94827,#94828,#94829,#94830,#94831,#94832,#94833,#94834,
#94835,#94836,#94837,#94838,#94839,#94840,#94841,#94842,#94843,#94844,#94845,
#94846),.UNSPECIFIED.,.F.,.F.,(4,3,3,3,3,3,3,3,3,3,3,3,3,3,3,3,3,3,3,3,
3,3,3,3,3,3,3,3,3,3,3,3,3,3,3,3,3,3,3,3,3,3,4),(68.1991363982496,68.2657253634656,
68.3699115269536,68.4739424521657,68.5778513425825,68.6816947737505,68.7855075247653,
68.8893243312867,68.993249808657,69.0972341272016,69.2014003846607,69.2632732218117,
69.3674593852999,69.4714903105121,69.5753992009292,69.6792426320973,69.7830553831123,
69.8868721896339,69.9907976670044,70.0947819855492,70.1989482430085,70.2608210801578,
70.365007243646,70.4690381688582,70.5729470592753,70.6767904904434,70.7806032414585,
70.88442004798,70.9883455253505,71.0923298438953,71.1964961013546,71.2583689385038,
71.3625551019918,71.4665860272038,71.5704949176206,71.6743383487885,71.7781510998033,
71.8819679063248,71.985893383695,72.0898777022396,72.1940439596986,72.2559167968499,
72.2566310325399),.UNSPECIFIED.);
#2658=B_SPLINE_CURVE_WITH_KNOTS('',3,(#94852,#94853,#94854,#94855,#94856,
#94857,#94858,#94859,#94860,#94861,#94862,#94863,#94864,#94865,#94866,#94867,
#94868,#94869,#94870,#94871,#94872,#94873,#94874,#94875,#94876,#94877,#94878,
#94879,#94880,#94881,#94882,#94883,#94884,#94885,#94886,#94887,#94888,#94889,
#94890,#94891,#94892,#94893,#94894,#94895,#94896,#94897,#94898,#94899,#94900,
#94901,#94902,#94903,#94904,#94905,#94906,#94907,#94908,#94909,#94910,#94911,
#94912,#94913,#94914,#94915,#94916,#94917,#94918,#94919,#94920,#94921,#94922,
#94923,#94924,#94925,#94926,#94927,#94928,#94929,#94930,#94931,#94932,#94933,
#94934,#94935,#94936,#94937,#94938,#94939,#94940,#94941,#94942,#94943,#94944,
#94945,#94946,#94947,#94948,#94949,#94950,#94951,#94952,#94953,#94954,#94955,
#94956,#94957,#94958,#94959,#94960,#94961,#94962,#94963,#94964,#94965,#94966,
#94967,#94968,#94969,#94970,#94971,#94972),.UNSPECIFIED.,.F.,.F.,(4,3,3,
3,3,3,3,3,3,3,3,3,3,3,3,3,3,3,3,3,3,3,3,3,3,3,3,3,3,3,3,3,3,3,3,3,3,3,3,
3,4),(61.9168665236723,62.0208010675058,62.1246599951528,62.2284781049933,
62.3322901417457,62.4362043441703,62.5401682899817,62.6443238098686,62.7365207799071,
62.8407069433952,62.9447378686072,63.048646759024,63.152490190192,63.2563029412068,
63.3601197477283,63.4640452250985,63.5680295436432,63.6721958011023,63.7340686382531,
63.8382548017413,63.9422857269535,64.0461946173705,64.1500380485387,64.2538507995537,
64.3576676060754,64.4615930834458,64.5655774019906,64.6697436594499,64.7316164965992,
64.8358026600872,64.9398335852992,65.043742475716,65.147585906884,65.2513986578987,
65.3552154644202,65.4591409417905,65.5631252603351,65.6672915177941,65.7291643549453,
65.8652061647349,65.9734457249408),.UNSPECIFIED.);
#2659=B_SPLINE_CURVE_WITH_KNOTS('',3,(#94973,#94974,#94975,#94976,#94977,
#94978,#94979,#94980,#94981,#94982,#94983,#94984,#94985,#94986,#94987,#94988,
#94989,#94990,#94991,#94992,#94993,#94994,#94995,#94996,#94997,#94998,#94999,
#95000,#95001,#95002,#95003,#95004,#95005,#95006,#95007,#95008,#95009,#95010,
#95011,#95012,#95013,#95014,#95015,#95016,#95017,#95018,#95019,#95020,#95021,
#95022,#95023,#95024,#95025,#95026,#95027,#95028,#95029,#95030,#95031,#95032,
#95033,#95034,#95035,#95036,#95037,#95038,#95039,#95040,#95041,#95042),
 .UNSPECIFIED.,.F.,.F.,(4,3,3,3,3,3,3,3,3,3,3,3,3,3,3,3,3,3,3,3,3,3,3,4),
(65.9734457253856,66.0761317728206,66.1787500761636,66.2813369783501,66.3839287747738,
66.4866268116144,66.5893873525292,66.6923186639505,66.7267122132914,66.8308983767795,
66.9349293019916,67.0388381924084,67.1426816235763,67.2464943745912,67.3503111811127,
67.454236658483,67.5582209770277,67.6623872344868,67.7242600716375,67.828449554753,
67.9324611620818,68.0363696459519,68.1402112752601,68.199542273107),
 .UNSPECIFIED.);
#2660=B_SPLINE_CURVE_WITH_KNOTS('',3,(#95044,#95045,#95046,#95047,#95048,
#95049,#95050,#95051,#95052,#95053,#95054,#95055,#95056,#95057,#95058,#95059,
#95060,#95061,#95062,#95063,#95064,#95065,#95066,#95067,#95068,#95069,#95070,
#95071,#95072,#95073,#95074,#95075,#95076,#95077,#95078,#95079,#95080,#95081,
#95082,#95083,#95084,#95085,#95086,#95087,#95088,#95089,#95090,#95091,#95092,
#95093,#95094,#95095,#95096,#95097,#95098,#95099,#95100,#95101,#95102,#95103,
#95104,#95105,#95106,#95107,#95108,#95109,#95110),.UNSPECIFIED.,.F.,.F.,
(4,3,3,3,3,3,3,3,3,3,3,3,3,3,3,3,3,3,3,3,3,3,4),(65.9734457257054,66.0987387056024,
66.2258330924599,66.2706296467734,66.3748158102617,66.4788467354739,66.582755625891,
66.6865990570591,66.7904118080742,66.8942286145957,66.9981540919662,67.102138410511,
67.2063046679703,67.2681775051195,67.3723684096492,67.4763780581656,67.580285456749,
67.6841254673981,67.7879328706238,67.8918030329342,67.9957000743238,68.0997567598233,
68.1991363982496),.UNSPECIFIED.);
#2661=B_SPLINE_CURVE_WITH_KNOTS('',3,(#95111,#95112,#95113,#95114,#95115,
#95116,#95117,#95118,#95119,#95120,#95121,#95122,#95123,#95124,#95125,#95126,
#95127,#95128,#95129,#95130,#95131,#95132,#95133,#95134,#95135,#95136,#95137,
#95138,#95139,#95140,#95141,#95142,#95143,#95144,#95145,#95146,#95147,#95148,
#95149,#95150,#95151,#95152,#95153,#95154,#95155,#95156,#95157,#95158,#95159,
#95160,#95161,#95162,#95163,#95164,#95165,#95166,#95167,#95168,#95169,#95170,
#95171,#95172,#95173,#95174,#95175,#95176,#95177,#95178,#95179,#95180,#95181,
#95182,#95183,#95184,#95185,#95186,#95187,#95188,#95189,#95190,#95191,#95192,
#95193,#95194,#95195,#95196,#95197,#95198,#95199,#95200,#95201,#95202,#95203,
#95204,#95205,#95206,#95207,#95208,#95209,#95210,#95211,#95212,#95213,#95214,
#95215,#95216,#95217,#95218,#95219,#95220,#95221,#95222,#95223,#95224,#95225,
#95226,#95227,#95228,#95229,#95230,#95231,#95232,#95233,#95234),
 .UNSPECIFIED.,.F.,.F.,(4,3,3,3,3,3,3,3,3,3,3,3,3,3,3,3,3,3,3,3,3,3,3,3,
3,3,3,3,3,3,3,3,3,3,3,3,3,3,3,3,3,4),(61.9158990401002,62.0198285605887,
62.1238197497715,62.2279900089989,62.2804382133891,62.3846243768772,62.4886553020892,
62.5925641925062,62.6964076236741,62.800220374689,62.9040371812104,63.0079626585807,
63.1119469771253,63.2161132345845,63.2779860717351,63.3821722352234,63.4862031604355,
63.5901120508525,63.6939554820206,63.7977682330355,63.9015850395571,64.0055105169275,
64.1094948354722,64.2136610929316,64.2755339300812,64.3797200935693,64.4837510187814,
64.5876599091983,64.6915033403663,64.795316091381,64.8991328979023,65.0030583752726,
65.107042693817,65.2112089512763,65.2730817884273,65.3766017373238,65.4799760620941,
65.5832406362455,65.6864470474328,65.7896160420574,65.892830939941,65.9734457253856),
 .UNSPECIFIED.);
#2662=B_SPLINE_CURVE_WITH_KNOTS('',3,(#95240,#95241,#95242,#95243,#95244,
#95245,#95246,#95247,#95248,#95249,#95250,#95251,#95252,#95253,#95254,#95255,
#95256,#95257,#95258,#95259,#95260,#95261,#95262,#95263,#95264,#95265,#95266,
#95267,#95268,#95269,#95270,#95271,#95272,#95273,#95274,#95275,#95276,#95277,
#95278,#95279,#95280,#95281,#95282,#95283,#95284,#95285,#95286,#95287,#95288,
#95289,#95290,#95291,#95292,#95293,#95294,#95295,#95296,#95297,#95298,#95299,
#95300,#95301,#95302,#95303,#95304,#95305,#95306,#95307,#95308,#95309,#95310,
#95311,#95312,#95313,#95314,#95315,#95316,#95317,#95318,#95319,#95320,#95321,
#95322,#95323,#95324,#95325,#95326,#95327,#95328,#95329,#95330,#95331,#95332,
#95333,#95334,#95335,#95336,#95337,#95338,#95339,#95340,#95341,#95342,#95343,
#95344,#95345,#95346,#95347,#95348,#95349,#95350,#95351,#95352,#95353,#95354,
#95355,#95356,#95357,#95358,#95359,#95360,#95361,#95362,#95363),
 .UNSPECIFIED.,.F.,.F.,(4,3,3,3,3,3,3,3,3,3,3,3,3,3,3,3,3,3,3,3,3,3,3,3,
3,3,3,3,3,3,3,3,3,3,3,3,3,3,3,3,3,4),(55.6326004253535,55.7367886138164,
55.7536857714845,55.8578719349726,55.9619028601848,56.0658117506017,56.1696551817698,
56.2734679327847,56.3772847393062,56.4812102166765,56.5851945352213,56.6893607926805,
56.7512336298305,56.8554197933186,56.9594507185307,57.0633596089476,57.1672030401157,
57.2710157911306,57.3748325976521,57.4787580750224,57.5827423935671,57.6869086510263,
57.7487814881766,57.8529676516648,57.9569985768771,58.0609074672941,58.1647508984623,
58.2685636494773,58.3723804559989,58.4763059333693,58.5802902519141,58.6844565093734,
58.7463293465227,58.8496743122095,58.9547475754163,59.057817166758,59.1608249277454,
59.2638067574365,59.3704201725432,59.4735201525628,59.5818902852131,59.6902604178635),
 .UNSPECIFIED.);
#2663=B_SPLINE_CURVE_WITH_KNOTS('',3,(#95364,#95365,#95366,#95367,#95368,
#95369,#95370,#95371,#95372,#95373,#95374,#95375,#95376,#95377,#95378,#95379,
#95380,#95381,#95382,#95383,#95384,#95385,#95386,#95387,#95388,#95389,#95390,
#95391,#95392,#95393,#95394,#95395,#95396,#95397,#95398,#95399,#95400,#95401,
#95402,#95403,#95404,#95405,#95406,#95407,#95408,#95409,#95410,#95411,#95412,
#95413,#95414,#95415,#95416,#95417,#95418,#95419,#95420,#95421,#95422,#95423,
#95424,#95425,#95426,#95427,#95428,#95429,#95430,#95431,#95432,#95433),
 .UNSPECIFIED.,.F.,.F.,(4,3,3,3,3,3,3,3,3,3,3,3,3,3,3,3,3,3,3,3,3,3,3,4),
(59.690260418206,59.7438772048688,59.8480633683568,59.9520942935688,60.0560031839856,
60.1598466151536,60.2636593661684,60.3674761726897,60.4714016500599,60.5753859686045,
60.6795522260636,60.7414250632149,60.8456112267031,60.9496421519152,61.0535510423322,
61.1573944735003,61.2612072245152,61.3650240310366,61.468949508407,61.5729338269518,
61.677100084411,61.738972921561,61.8431345912304,61.9168665236723),
 .UNSPECIFIED.);
#2664=B_SPLINE_CURVE_WITH_KNOTS('',3,(#95435,#95436,#95437,#95438,#95439,
#95440,#95441,#95442,#95443,#95444,#95445,#95446,#95447,#95448,#95449,#95450,
#95451,#95452,#95453,#95454,#95455,#95456,#95457,#95458,#95459,#95460,#95461,
#95462,#95463,#95464,#95465,#95466,#95467,#95468,#95469,#95470,#95471,#95472,
#95473,#95474,#95475,#95476,#95477,#95478,#95479,#95480,#95481,#95482,#95483,
#95484,#95485,#95486,#95487,#95488,#95489,#95490,#95491,#95492,#95493,#95494,
#95495,#95496,#95497,#95498,#95499,#95500,#95501),.UNSPECIFIED.,.F.,.F.,
(4,3,3,3,3,3,3,3,3,3,3,3,3,3,3,3,3,3,3,3,3,3,4),(59.690260418206,59.7955628120771,
59.9009059652391,60.0064057077483,60.1119895277669,60.2177899509164,60.2853424966969,
60.3895286601851,60.4935595853973,60.5974684758143,60.7013119069824,60.8051246579973,
60.9089414645188,61.0128669418892,61.116851260434,61.2210175178933,61.282890355043,
61.3870598977045,61.4910835289854,61.5972874067641,61.7011272958194,61.8085131679598,
61.9158990401002),.UNSPECIFIED.);
#2665=B_SPLINE_CURVE_WITH_KNOTS('',3,(#95502,#95503,#95504,#95505,#95506,
#95507,#95508,#95509,#95510,#95511,#95512,#95513,#95514,#95515,#95516,#95517,
#95518,#95519,#95520,#95521,#95522,#95523,#95524,#95525,#95526,#95527,#95528,
#95529,#95530,#95531,#95532,#95533,#95534,#95535,#95536,#95537,#95538,#95539,
#95540,#95541,#95542,#95543,#95544,#95545,#95546,#95547,#95548,#95549,#95550,
#95551,#95552,#95553,#95554,#95555,#95556,#95557,#95558,#95559,#95560,#95561,
#95562,#95563,#95564,#95565,#95566,#95567,#95568,#95569,#95570,#95571,#95572,
#95573,#95574,#95575,#95576,#95577,#95578,#95579,#95580,#95581,#95582,#95583,
#95584,#95585,#95586,#95587,#95588,#95589,#95590,#95591,#95592,#95593,#95594,
#95595,#95596,#95597,#95598,#95599,#95600,#95601,#95602,#95603,#95604,#95605,
#95606,#95607,#95608,#95609,#95610,#95611,#95612,#95613,#95614,#95615,#95616,
#95617,#95618,#95619,#95620,#95621,#95622,#95623,#95624,#95625),
 .UNSPECIFIED.,.F.,.F.,(4,3,3,3,3,3,3,3,3,3,3,3,3,3,3,3,3,3,3,3,3,3,3,3,
3,3,3,3,3,3,3,3,3,3,3,3,3,3,3,3,3,4),(55.6335493698586,55.7373826934096,
55.8411933057268,55.9450159374289,56.0489521424687,56.1529543449585,56.2571313407819,
56.2951510633125,56.3993372268007,56.503368152013,56.6072770424299,56.7111204735982,
56.8149332246131,56.9187500311345,57.0226755085049,57.1266598270495,57.2308260845087,
57.2926989216586,57.3968850851467,57.5009160103588,57.6048249007758,57.7086683319438,
57.8124810829587,57.9162978894804,58.0202233668507,58.1242076853955,58.2283739428547,
58.2902467800047,58.3944329434928,58.498463868705,58.602372759122,58.70621619029,
58.810028941305,58.9138457478263,59.0177712251967,59.1217555437414,59.2259218012006,
59.2877946383508,59.403242088617,59.5183215991976,59.6327919924206,59.690260417799),
 .UNSPECIFIED.);
#2666=B_SPLINE_CURVE_WITH_KNOTS('',3,(#95631,#95632,#95633,#95634,#95635,
#95636,#95637,#95638,#95639,#95640,#95641,#95642,#95643,#95644,#95645,#95646,
#95647,#95648,#95649,#95650,#95651,#95652,#95653,#95654,#95655,#95656,#95657,
#95658,#95659,#95660,#95661,#95662,#95663,#95664,#95665,#95666,#95667,#95668,
#95669,#95670,#95671,#95672,#95673,#95674,#95675,#95676,#95677,#95678,#95679,
#95680,#95681,#95682,#95683,#95684,#95685,#95686,#95687,#95688,#95689,#95690,
#95691,#95692,#95693,#95694,#95695,#95696,#95697,#95698,#95699,#95700,#95701,
#95702,#95703,#95704,#95705,#95706,#95707,#95708,#95709,#95710,#95711,#95712,
#95713,#95714,#95715,#95716,#95717,#95718,#95719,#95720,#95721,#95722,#95723,
#95724,#95725,#95726,#95727,#95728,#95729,#95730,#95731,#95732,#95733,#95734,
#95735,#95736,#95737,#95738,#95739,#95740,#95741,#95742,#95743,#95744,#95745,
#95746,#95747,#95748,#95749,#95750,#95751,#95752,#95753,#95754),
 .UNSPECIFIED.,.F.,.F.,(4,3,3,3,3,3,3,3,3,3,3,3,3,3,3,3,3,3,3,3,3,3,3,3,
3,3,3,3,3,3,3,3,3,3,3,3,3,3,3,3,3,4),(49.349672428797,49.4543539769497,
49.5583095628721,49.66335409214,49.7683986214079,49.872584784896,49.976615710108,
50.0805246005249,50.184368031693,50.2881807827079,50.3919975892296,50.4959230665999,
50.5999073851446,50.7040736426038,50.765946479754,50.8701326432423,50.9741635684547,
51.0780724588717,51.1819158900398,51.2857286410548,51.3895454475765,51.4934709249469,
51.5974552434917,51.701621500951,51.7634943381001,51.8676805015885,51.9717114268005,
52.0756203172177,52.1794637483859,52.283276499401,52.3870933059224,52.491018783293,
52.595003101838,52.6991693592974,52.7610421964462,52.8655509126688,52.9699037514302,
53.0791965913293,53.1833373805645,53.2874304651154,53.3915238347356,53.4070751110264),
 .UNSPECIFIED.);
#2667=B_SPLINE_CURVE_WITH_KNOTS('',3,(#95755,#95756,#95757,#95758,#95759,
#95760,#95761,#95762,#95763,#95764,#95765,#95766,#95767,#95768,#95769,#95770,
#95771,#95772,#95773,#95774,#95775,#95776,#95777,#95778,#95779,#95780,#95781,
#95782,#95783,#95784,#95785,#95786,#95787,#95788,#95789,#95790,#95791,#95792,
#95793,#95794,#95795,#95796,#95797,#95798,#95799,#95800,#95801,#95802,#95803,
#95804,#95805,#95806,#95807,#95808,#95809,#95810,#95811,#95812,#95813,#95814,
#95815,#95816,#95817,#95818,#95819,#95820,#95821),.UNSPECIFIED.,.F.,.F.,
(4,3,3,3,3,3,3,3,3,3,3,3,3,3,3,3,3,3,3,3,3,3,4),(53.407075111473,53.5259953052154,
53.6459937542275,53.7585900547923,53.8627762182805,53.9668071434925,54.0707160339095,
54.1745594650776,54.2783722160926,54.3821890226141,54.4861144999845,54.5900988185293,
54.6942650759886,54.7561379131384,54.8656957271653,54.9697002456262,55.0736027369136,
55.177438061658,55.2812409986278,55.3850920232226,55.4889708986981,55.5929698536114,
55.6326004253535),.UNSPECIFIED.);
#2668=B_SPLINE_CURVE_WITH_KNOTS('',3,(#95823,#95824,#95825,#95826,#95827,
#95828,#95829,#95830,#95831,#95832,#95833,#95834,#95835,#95836,#95837,#95838,
#95839,#95840,#95841,#95842,#95843,#95844,#95845,#95846,#95847,#95848,#95849,
#95850,#95851,#95852,#95853,#95854,#95855,#95856,#95857,#95858,#95859,#95860,
#95861,#95862,#95863,#95864,#95865,#95866,#95867,#95868,#95869,#95870,#95871,
#95872,#95873,#95874,#95875,#95876,#95877,#95878,#95879,#95880,#95881,#95882,
#95883,#95884,#95885,#95886,#95887,#95888,#95889,#95890,#95891,#95892),
 .UNSPECIFIED.,.F.,.F.,(4,3,3,3,3,3,3,3,3,3,3,3,3,3,3,3,3,3,3,3,3,3,3,4),
(53.4070751114826,53.5098614913189,53.6124973139516,53.7150505550782,53.8175576893174,
53.9200551251608,54.0226483900868,54.1252912590503,54.2281147116709,54.3000553466204,
54.4042415101085,54.5082724353208,54.6121813257378,54.7160247569059,54.8198375079209,
54.9236543144423,55.0275797918127,55.1315641103574,55.2357303678167,55.2976032049664,
55.4017686798836,55.5057980075389,55.6097071751473,55.6335493698586),
 .UNSPECIFIED.);
#2669=B_SPLINE_CURVE_WITH_KNOTS('',3,(#95893,#95894,#95895,#95896,#95897,
#95898,#95899,#95900,#95901,#95902,#95903,#95904,#95905,#95906,#95907,#95908,
#95909,#95910,#95911,#95912,#95913,#95914,#95915,#95916,#95917,#95918,#95919,
#95920,#95921,#95922,#95923,#95924,#95925,#95926,#95927,#95928,#95929,#95930,
#95931,#95932,#95933,#95934,#95935,#95936,#95937,#95938,#95939,#95940,#95941,
#95942,#95943,#95944,#95945,#95946,#95947,#95948,#95949,#95950,#95951,#95952,
#95953,#95954,#95955,#95956,#95957,#95958,#95959,#95960,#95961,#95962,#95963,
#95964,#95965,#95966,#95967,#95968,#95969,#95970,#95971,#95972,#95973,#95974,
#95975,#95976,#95977,#95978,#95979,#95980,#95981,#95982,#95983,#95984,#95985,
#95986,#95987,#95988,#95989,#95990,#95991,#95992,#95993,#95994,#95995,#95996,
#95997,#95998,#95999,#96000,#96001,#96002,#96003,#96004,#96005,#96006,#96007,
#96008,#96009,#96010,#96011,#96012,#96013,#96014,#96015,#96016),
 .UNSPECIFIED.,.F.,.F.,(4,3,3,3,3,3,3,3,3,3,3,3,3,3,3,3,3,3,3,3,3,3,3,3,
3,3,3,3,3,3,3,3,3,3,3,3,3,3,3,3,3,4),(49.3501218939192,49.4542472755859,
49.5611993552922,49.6650784875894,49.7689057759847,49.8727159784123,49.9820029621182,
50.0859506840952,50.1899710987106,50.2941599666065,50.309863913236,50.4140500767242,
50.5180810019365,50.6219898923535,50.7258333235217,50.8296460745367,50.9334628810583,
51.0373883584288,51.1413726769736,51.2455389344329,51.3074117715821,51.4115979350702,
51.5156288602824,51.6195377506993,51.7233811818674,51.8271939328822,51.9310107394038,
52.0349362167741,52.1389205353188,52.2430867927781,52.3049596299282,52.4091457934165,
52.5131767186288,52.6170856090459,52.7209290402142,52.8247417912293,52.928558597751,
53.0324840751215,53.1364683936664,53.2406346511258,53.3025074882743,53.4070751110264),
 .UNSPECIFIED.);
#2670=B_SPLINE_CURVE_WITH_KNOTS('',3,(#96022,#96023,#96024,#96025,#96026,
#96027,#96028,#96029,#96030,#96031,#96032,#96033,#96034,#96035,#96036,#96037,
#96038,#96039,#96040,#96041,#96042,#96043,#96044,#96045,#96046,#96047,#96048,
#96049,#96050,#96051,#96052,#96053,#96054,#96055,#96056,#96057,#96058,#96059,
#96060,#96061,#96062,#96063,#96064,#96065,#96066,#96067,#96068,#96069,#96070,
#96071,#96072,#96073,#96074,#96075,#96076,#96077,#96078,#96079,#96080,#96081,
#96082,#96083,#96084,#96085,#96086,#96087,#96088,#96089,#96090,#96091,#96092,
#96093,#96094,#96095,#96096,#96097,#96098,#96099,#96100,#96101,#96102,#96103,
#96104,#96105,#96106,#96107,#96108,#96109,#96110,#96111,#96112,#96113,#96114,
#96115,#96116,#96117,#96118,#96119,#96120,#96121,#96122,#96123,#96124,#96125,
#96126,#96127,#96128,#96129,#96130,#96131,#96132,#96133,#96134,#96135,#96136,
#96137,#96138,#96139,#96140,#96141,#96142),.UNSPECIFIED.,.F.,.F.,(4,3,3,
3,3,3,3,3,3,3,3,3,3,3,3,3,3,3,3,3,3,3,3,3,3,3,3,3,3,3,3,3,3,3,3,3,3,3,3,
3,4),(43.0672730904575,43.1711320846111,43.2749502212473,43.3787622451258,
43.482676408604,43.586640279845,43.6907957641029,43.7831114713314,43.8872976348199,
43.9913285600324,44.0952374504496,44.199080881618,44.3028936326331,44.4067104391551,
44.5106359165258,44.6146202350706,44.7187864925301,44.7806593296775,44.8848454931656,
44.9888764183775,45.0927853087944,45.1966287399624,45.3004414909772,45.4042582974986,
45.5081837748688,45.6121680934134,45.7163343508724,45.7782071880236,45.882393351512,
45.986424276724,46.090333167141,46.1941765983091,46.2979893493239,46.4018061558458,
46.5057316332163,46.6097159517613,46.7138822092206,46.7757550463697,46.8962986192127,
47.0157785770585,47.1238898034029),.UNSPECIFIED.);
#2671=B_SPLINE_CURVE_WITH_KNOTS('',3,(#96143,#96144,#96145,#96146,#96147,
#96148,#96149,#96150,#96151,#96152,#96153,#96154,#96155,#96156,#96157,#96158,
#96159,#96160,#96161,#96162,#96163,#96164,#96165,#96166,#96167,#96168,#96169,
#96170,#96171,#96172,#96173,#96174,#96175,#96176,#96177,#96178,#96179,#96180,
#96181,#96182,#96183,#96184,#96185,#96186,#96187,#96188,#96189,#96190,#96191,
#96192,#96193,#96194,#96195,#96196,#96197,#96198,#96199,#96200,#96201,#96202,
#96203,#96204,#96205,#96206,#96207,#96208,#96209,#96210,#96211,#96212),
 .UNSPECIFIED.,.F.,.F.,(4,3,3,3,3,3,3,3,3,3,3,3,3,3,3,3,3,3,3,3,3,3,3,4),
(47.1238898038468,47.227928135532,47.3319603652853,47.4360206698557,47.5402127556614,
47.6444838895193,47.7489375131514,47.7733029047158,47.8774890682039,47.981519993416,
48.0854288838329,48.189272315001,48.2930850660161,48.3969018725377,48.5008273499081,
48.6048116684528,48.7089779259121,48.7708507630618,48.8750265339913,48.9790548148158,
49.0829625294199,49.1867995822523,49.2906190115793,49.349672428797),
 .UNSPECIFIED.);
#2672=B_SPLINE_CURVE_WITH_KNOTS('',3,(#96214,#96215,#96216,#96217,#96218,
#96219,#96220,#96221,#96222,#96223,#96224,#96225,#96226,#96227,#96228,#96229,
#96230,#96231,#96232,#96233,#96234,#96235,#96236,#96237,#96238,#96239,#96240,
#96241,#96242,#96243,#96244,#96245,#96246,#96247,#96248,#96249,#96250,#96251,
#96252,#96253,#96254,#96255,#96256,#96257,#96258,#96259,#96260,#96261,#96262,
#96263,#96264,#96265,#96266,#96267,#96268,#96269,#96270,#96271,#96272,#96273,
#96274,#96275,#96276,#96277,#96278,#96279,#96280,#96281,#96282,#96283),
 .UNSPECIFIED.,.F.,.F.,(4,3,3,3,3,3,3,3,3,3,3,3,3,3,3,3,3,3,3,3,3,3,3,4),
(47.1238898038468,47.2754958859059,47.3172203381978,47.4214065016861,47.5254374268983,
47.6293463173154,47.7331897484836,47.8370024994987,47.9408193060204,48.0447447833909,
48.1487291019357,48.2528953593951,48.3147681965438,48.4189543600319,48.5229852852439,
48.6268941756608,48.7307376068289,48.8345503578437,48.9383671643652,49.0422926417355,
49.1462769602802,49.2504432177394,49.3123160548899,49.3501218939192),
 .UNSPECIFIED.);
#2673=B_SPLINE_CURVE_WITH_KNOTS('',3,(#96284,#96285,#96286,#96287,#96288,
#96289,#96290,#96291,#96292,#96293,#96294,#96295,#96296,#96297,#96298,#96299,
#96300,#96301,#96302,#96303,#96304,#96305,#96306,#96307,#96308,#96309,#96310,
#96311,#96312,#96313,#96314,#96315,#96316,#96317,#96318,#96319,#96320,#96321,
#96322,#96323,#96324,#96325,#96326,#96327,#96328,#96329,#96330,#96331,#96332,
#96333,#96334,#96335,#96336,#96337,#96338,#96339,#96340,#96341,#96342,#96343,
#96344,#96345,#96346,#96347,#96348,#96349,#96350,#96351,#96352,#96353,#96354,
#96355,#96356,#96357,#96358,#96359,#96360,#96361,#96362,#96363,#96364,#96365,
#96366,#96367,#96368,#96369,#96370,#96371,#96372,#96373,#96374,#96375,#96376,
#96377,#96378,#96379,#96380,#96381,#96382,#96383,#96384,#96385,#96386,#96387,
#96388,#96389,#96390,#96391,#96392,#96393,#96394,#96395,#96396,#96397,#96398,
#96399,#96400,#96401,#96402,#96403,#96404,#96405,#96406,#96407),
 .UNSPECIFIED.,.F.,.F.,(4,3,3,3,3,3,3,3,3,3,3,3,3,3,3,3,3,3,3,3,3,3,3,3,
3,3,3,3,3,3,3,3,3,3,3,3,3,3,3,3,3,4),(43.0661596803882,43.1701506766889,
43.274320821343,43.3270289048134,43.4312150683039,43.5352459935185,43.6391548839378,
43.7429983151084,43.8468110661257,43.9506278726497,44.0545533500226,44.1585376685698,
44.2627039260315,44.3245767631595,44.4287629266471,44.5327938518588,44.6367027422752,
44.7405461734428,44.8443589244572,44.9481757309782,45.0521012083481,45.1560855268923,
45.2602517843511,45.3221246215056,45.4263107849935,45.5303417102054,45.6342506006221,
45.7380940317899,45.8419067828045,45.9457235893257,46.0496490666958,46.1536333852403,
46.2577996426992,46.3196724798517,46.4223012412912,46.5247935864413,46.6271863644384,
46.729516280192,46.8318649061918,46.934217612914,47.0366904241961,47.1238898034296),
 .UNSPECIFIED.);
#2674=B_SPLINE_CURVE_WITH_KNOTS('',3,(#96413,#96414,#96415,#96416,#96417,
#96418,#96419,#96420,#96421,#96422,#96423,#96424,#96425,#96426,#96427,#96428,
#96429,#96430,#96431,#96432,#96433,#96434,#96435,#96436,#96437,#96438,#96439,
#96440,#96441,#96442,#96443,#96444,#96445,#96446,#96447,#96448,#96449,#96450,
#96451,#96452,#96453,#96454,#96455,#96456,#96457,#96458,#96459,#96460,#96461,
#96462,#96463,#96464,#96465,#96466,#96467,#96468,#96469,#96470,#96471,#96472,
#96473,#96474,#96475,#96476,#96477,#96478,#96479,#96480,#96481,#96482,#96483,
#96484,#96485,#96486,#96487,#96488,#96489,#96490,#96491,#96492,#96493,#96494,
#96495,#96496,#96497,#96498,#96499,#96500,#96501,#96502,#96503,#96504,#96505,
#96506,#96507,#96508,#96509,#96510,#96511,#96512,#96513,#96514,#96515,#96516,
#96517,#96518,#96519,#96520,#96521,#96522,#96523,#96524,#96525,#96526,#96527,
#96528,#96529,#96530,#96531,#96532,#96533,#96534,#96535,#96536,#96537,#96538,
#96539),.UNSPECIFIED.,.F.,.F.,(4,3,3,3,3,3,3,3,3,3,3,3,3,3,3,3,3,3,3,3,
3,3,3,3,3,3,3,3,3,3,3,3,3,3,3,3,3,3,3,3,3,3,4),(36.7834442091166,36.8002764629088,
36.904462626368,37.0084935515507,37.1124024419373,37.2162458730747,37.3200586240585,
37.4238754305486,37.5278009078871,37.6317852263998,37.735951483827,37.7978243212549,
37.9020104847617,38.0060414099927,38.1099503004289,38.2137937316164,38.3176064826509,
38.4214232891921,38.5253487665822,38.6293330851467,38.7334993426256,38.795372179601,
38.8995583430862,39.0035892682954,39.1074981587095,39.2113415898746,39.3151543408867,
39.4189711474052,39.5228966247727,39.6268809433146,39.7310472007711,39.7929200379471,
39.8971062014326,40.0011371266419,40.105046017056,40.2088894482213,40.3127021992333,
40.4165190057517,40.520444483119,40.6244288016607,40.7285950591169,40.7904678962932,
40.8407044966672),.UNSPECIFIED.);
#2675=B_SPLINE_CURVE_WITH_KNOTS('',3,(#96540,#96541,#96542,#96543,#96544,
#96545,#96546,#96547,#96548,#96549,#96550,#96551,#96552,#96553,#96554,#96555,
#96556,#96557,#96558,#96559,#96560,#96561,#96562,#96563,#96564,#96565,#96566,
#96567,#96568,#96569,#96570,#96571,#96572,#96573,#96574,#96575,#96576,#96577,
#96578,#96579,#96580,#96581,#96582,#96583,#96584,#96585,#96586,#96587,#96588,
#96589,#96590,#96591,#96592,#96593,#96594,#96595,#96596,#96597,#96598,#96599,
#96600,#96601,#96602,#96603,#96604,#96605,#96606,#96607,#96608,#96609),
 .UNSPECIFIED.,.F.,.F.,(4,3,3,3,3,3,3,3,3,3,3,3,3,3,3,3,3,3,3,3,3,3,3,4),
(40.8407044970017,40.9440746115611,41.0495672544458,41.1526720053855,41.2557188072273,
41.3587435025094,41.4660615655418,41.569214750082,41.6724388016555,41.7758284060269,
41.7880157546392,41.8922019181268,41.9962328433386,42.1001417337551,42.2039851649227,
42.3077979159372,42.4116147224583,42.5155401998282,42.6195245183725,42.7236907758313,
42.7855636129853,42.8897412732124,42.9937540523167,43.0672730904575),
 .UNSPECIFIED.);
#2676=B_SPLINE_CURVE_WITH_KNOTS('',3,(#96611,#96612,#96613,#96614,#96615,
#96616,#96617,#96618,#96619,#96620,#96621,#96622,#96623,#96624,#96625,#96626,
#96627,#96628,#96629,#96630,#96631,#96632,#96633,#96634,#96635,#96636,#96637,
#96638,#96639,#96640,#96641,#96642,#96643,#96644,#96645,#96646,#96647,#96648,
#96649,#96650,#96651,#96652,#96653,#96654,#96655,#96656,#96657,#96658,#96659,
#96660,#96661,#96662,#96663,#96664,#96665,#96666,#96667,#96668,#96669,#96670,
#96671,#96672,#96673,#96674,#96675,#96676,#96677),.UNSPECIFIED.,.F.,.F.,
(4,3,3,3,3,3,3,3,3,3,3,3,3,3,3,3,3,3,3,3,3,3,4),(40.8407044969848,40.9497796083564,
41.0591756422735,41.1687426604124,41.2786112447421,41.3319331881212,41.4361193516064,
41.5401502768156,41.6440591672297,41.7479025983948,41.8517153494069,41.9555321559254,
42.059457633293,42.1634419518348,42.2676082092913,42.3294810464673,42.4336404893563,
42.53765703907,42.6415657001868,42.7477141952371,42.851532121409,42.9588459008986,
43.0661596803882),.UNSPECIFIED.);
#2677=B_SPLINE_CURVE_WITH_KNOTS('',3,(#96678,#96679,#96680,#96681,#96682,
#96683,#96684,#96685,#96686,#96687,#96688,#96689,#96690,#96691,#96692,#96693,
#96694,#96695,#96696,#96697,#96698,#96699,#96700,#96701,#96702,#96703,#96704,
#96705,#96706,#96707,#96708,#96709,#96710,#96711,#96712,#96713,#96714,#96715,
#96716,#96717,#96718,#96719,#96720,#96721,#96722,#96723,#96724,#96725,#96726,
#96727,#96728,#96729,#96730,#96731,#96732,#96733,#96734,#96735,#96736,#96737,
#96738,#96739,#96740,#96741,#96742,#96743,#96744,#96745,#96746,#96747,#96748,
#96749,#96750,#96751,#96752,#96753,#96754,#96755,#96756,#96757,#96758,#96759,
#96760,#96761,#96762,#96763,#96764,#96765,#96766,#96767,#96768,#96769,#96770,
#96771,#96772,#96773,#96774,#96775,#96776,#96777,#96778,#96779,#96780,#96781,
#96782,#96783,#96784,#96785,#96786,#96787,#96788,#96789,#96790,#96791,#96792,
#96793,#96794,#96795,#96796,#96797,#96798,#96799,#96800,#96801),
 .UNSPECIFIED.,.F.,.F.,(4,3,3,3,3,3,3,3,3,3,3,3,3,3,3,3,3,3,3,3,3,3,3,3,
3,3,3,3,3,3,3,3,3,3,3,3,3,3,3,3,3,4),(36.783723968172,36.8875345931376,
36.9913571540606,37.0952932379323,37.1992952442744,37.3034721168394,37.3417417547369,
37.4459279183704,37.5499588437298,37.6538677342965,37.7577111656157,37.8615239167828,
37.965340723457,38.0692662009808,38.1732505196793,38.2774167772914,38.339289613083,
38.4434757765587,38.5475067017588,38.6514155921638,38.7552590233201,38.8590717743237,
38.9628885808336,39.0668140581933,39.1707983767274,39.2749646341767,39.3368374714291,
39.4410236348884,39.5450545600711,39.6489634504579,39.7528068815956,39.8566196325795,
39.9604364390695,40.0643619164082,40.168346234921,40.2725124923483,40.3343853297751,
40.443556269481,40.5524208008283,40.6611016632913,40.7695577702486,40.8407044966672),
 .UNSPECIFIED.);
#2678=B_SPLINE_CURVE_WITH_KNOTS('',3,(#96807,#96808,#96809,#96810,#96811,
#96812,#96813,#96814,#96815,#96816,#96817,#96818,#96819,#96820,#96821,#96822,
#96823,#96824,#96825,#96826,#96827,#96828,#96829,#96830,#96831,#96832,#96833,
#96834,#96835,#96836,#96837,#96838,#96839,#96840,#96841,#96842,#96843,#96844,
#96845,#96846,#96847,#96848,#96849,#96850,#96851,#96852,#96853,#96854,#96855,
#96856,#96857,#96858,#96859,#96860,#96861,#96862,#96863,#96864,#96865,#96866,
#96867,#96868,#96869,#96870,#96871,#96872,#96873,#96874,#96875,#96876,#96877,
#96878,#96879,#96880,#96881,#96882,#96883,#96884,#96885,#96886,#96887,#96888,
#96889,#96890,#96891,#96892,#96893,#96894,#96895,#96896,#96897,#96898,#96899,
#96900,#96901,#96902,#96903,#96904,#96905,#96906,#96907,#96908,#96909,#96910,
#96911,#96912,#96913,#96914,#96915,#96916,#96917,#96918,#96919,#96920,#96921,
#96922,#96923,#96924,#96925,#96926,#96927,#96928,#96929,#96930),
 .UNSPECIFIED.,.F.,.F.,(4,3,3,3,3,3,3,3,3,3,3,3,3,3,3,3,3,3,3,3,3,3,3,3,
3,3,3,3,3,3,3,3,3,3,3,3,3,3,3,3,3,4),(30.4998665259952,30.6038214794107,
30.7094053961215,30.8149893128323,30.9191754738907,31.0232063966284,31.1271152845158,
31.230958713122,31.3347714615463,31.4385882654523,31.5425137401869,31.6464980560807,
31.7506643108935,31.8125371711784,31.9167233357869,32.0207542621341,32.1246631537022,
32.2285065860308,32.3323193382138,32.4361361459094,32.5400616244546,32.6440459441764,
32.7482122028035,32.8100850295245,32.9142711930052,33.0183021182129,33.1222110086302,
33.2260544398017,33.3298671908226,33.4336839973534,33.5376094747372,33.6415937932978,
33.7457600507769,33.8076328878706,33.9105733956083,34.0133739392442,34.1160710646397,
34.2187011756055,34.3213305265982,34.4239607110243,34.5266703118432,34.5575191894876),
 .UNSPECIFIED.);
#2679=B_SPLINE_CURVE_WITH_KNOTS('',3,(#96931,#96932,#96933,#96934,#96935,
#96936,#96937,#96938,#96939,#96940,#96941,#96942,#96943,#96944,#96945,#96946,
#96947,#96948,#96949,#96950,#96951,#96952,#96953,#96954,#96955,#96956,#96957,
#96958,#96959,#96960,#96961,#96962,#96963,#96964,#96965,#96966,#96967,#96968,
#96969,#96970,#96971,#96972,#96973,#96974,#96975,#96976,#96977,#96978,#96979,
#96980,#96981,#96982,#96983,#96984,#96985,#96986,#96987,#96988,#96989,#96990,
#96991,#96992,#96993,#96994,#96995,#96996,#96997),.UNSPECIFIED.,.F.,.F.,
(4,3,3,3,3,3,3,3,3,3,3,3,3,3,3,3,3,3,3,3,3,3,4),(34.5575191897883,34.6927956482481,
34.8051807462166,34.909366909851,35.0133978352114,35.1173067257789,35.2211501570989,
35.3249629082669,35.4287797149424,35.532705192467,35.6366895111664,35.7408557687793,
35.8027286045627,35.9069159432588,36.0109477009189,36.1148561160979,36.2186985866368,
36.3225098919278,36.4263247672704,36.5302426811368,36.6342192371381,36.738364891705,
36.7834442091166),.UNSPECIFIED.);
#2680=B_SPLINE_CURVE_WITH_KNOTS('',3,(#96999,#97000,#97001,#97002,#97003,
#97004,#97005,#97006,#97007,#97008,#97009,#97010,#97011,#97012,#97013,#97014,
#97015,#97016,#97017,#97018,#97019,#97020,#97021,#97022,#97023,#97024,#97025,
#97026,#97027,#97028,#97029,#97030,#97031,#97032,#97033,#97034,#97035,#97036,
#97037,#97038,#97039,#97040,#97041,#97042,#97043,#97044,#97045,#97046,#97047,
#97048,#97049,#97050,#97051,#97052,#97053,#97054,#97055,#97056,#97057,#97058,
#97059,#97060,#97061,#97062,#97063,#97064,#97065,#97066,#97067,#97068),
 .UNSPECIFIED.,.F.,.F.,(4,3,3,3,3,3,3,3,3,3,3,3,3,3,3,3,3,3,3,3,3,3,3,4),
(34.557519189755,34.6600261052929,34.7624492426979,34.8648252095929,34.9671905447891,
35.0696506740761,35.1721598073091,35.2748489315128,35.3466460380447,35.4508322015257,
35.5548631267337,35.6587720171512,35.7626154483228,35.8664281993442,35.9702450058752,
36.0741704832593,36.1781548018204,36.2823210592997,36.3441938963908,36.4483886661888,
36.5524031618926,36.6563141161534,36.7601506302161,36.783723968172),
 .UNSPECIFIED.);
#2681=B_SPLINE_CURVE_WITH_KNOTS('',3,(#97069,#97070,#97071,#97072,#97073,
#97074,#97075,#97076,#97077,#97078,#97079,#97080,#97081,#97082,#97083,#97084,
#97085,#97086,#97087,#97088,#97089,#97090,#97091,#97092,#97093,#97094,#97095,
#97096,#97097,#97098,#97099,#97100,#97101,#97102,#97103,#97104,#97105,#97106,
#97107,#97108,#97109,#97110,#97111,#97112,#97113,#97114,#97115,#97116,#97117,
#97118,#97119,#97120,#97121,#97122,#97123,#97124,#97125,#97126,#97127,#97128,
#97129,#97130,#97131,#97132,#97133,#97134,#97135,#97136,#97137,#97138,#97139,
#97140,#97141,#97142,#97143,#97144,#97145,#97146,#97147,#97148,#97149,#97150,
#97151,#97152,#97153,#97154,#97155,#97156,#97157,#97158,#97159,#97160,#97161,
#97162,#97163,#97164,#97165,#97166,#97167,#97168,#97169,#97170,#97171,#97172,
#97173,#97174,#97175,#97176,#97177,#97178,#97179,#97180,#97181,#97182,#97183,
#97184,#97185,#97186,#97187,#97188,#97189,#97190,#97191,#97192),
 .UNSPECIFIED.,.F.,.F.,(4,3,3,3,3,3,3,3,3,3,3,3,3,3,3,3,3,3,3,3,3,3,3,3,
3,3,3,3,3,3,3,3,3,3,3,3,3,3,3,3,3,4),(30.5008971308904,30.6078418151117,
30.7117208906534,30.8155481393843,30.9193583192481,31.0286323906012,31.1325801108998,
31.2366005354176,31.3407894024993,31.3564546046604,31.4606407764529,31.5646717100683,
31.6685806089942,31.7724240487317,31.8762368083637,31.980053623537,32.0839791095526,
32.1879634367518,32.2921297027861,32.3540024630065,32.4581886272382,32.5622195532326,
32.6661284444858,32.7699718765231,32.8737846284388,32.9776014358916,33.0815269142338,
33.1855112337746,33.2896774922579,33.3515503213525,33.4557364824179,33.5597674051624,
33.663676293057,33.7675197216704,33.871332470102,33.9751492740155,34.0790747487577,
34.183059064659,34.2872253194792,34.3490981796986,34.4951131604683,34.5575191894876),
 .UNSPECIFIED.);
#2682=B_SPLINE_CURVE_WITH_KNOTS('',3,(#97198,#97199,#97200,#97201,#97202,
#97203,#97204,#97205,#97206,#97207,#97208,#97209,#97210,#97211,#97212,#97213,
#97214,#97215,#97216,#97217,#97218,#97219,#97220,#97221,#97222,#97223,#97224,
#97225,#97226,#97227,#97228,#97229,#97230,#97231,#97232,#97233,#97234,#97235,
#97236,#97237,#97238,#97239,#97240,#97241,#97242,#97243,#97244,#97245,#97246,
#97247,#97248,#97249,#97250,#97251,#97252,#97253,#97254,#97255,#97256,#97257,
#97258,#97259,#97260,#97261,#97262,#97263,#97264,#97265,#97266,#97267,#97268,
#97269,#97270,#97271,#97272,#97273,#97274,#97275,#97276,#97277,#97278,#97279,
#97280,#97281,#97282,#97283,#97284,#97285,#97286,#97287,#97288,#97289,#97290,
#97291,#97292,#97293,#97294,#97295,#97296,#97297,#97298,#97299,#97300,#97301,
#97302,#97303,#97304,#97305,#97306,#97307,#97308,#97309,#97310,#97311,#97312,
#97313,#97314,#97315,#97316,#97317,#97318),.UNSPECIFIED.,.F.,.F.,(4,3,3,
3,3,3,3,3,3,3,3,3,3,3,3,3,3,3,3,3,3,3,3,3,3,3,3,3,3,3,3,3,3,3,3,3,3,3,3,
3,4),(24.2175053970322,24.321323756092,24.4251359323839,24.5290502036337,
24.6330141192664,24.7371697208814,24.8297021627558,24.9338881432323,25.0379188823439,
25.1418275829741,25.2456708221829,25.3494833793523,25.4532999904265,25.5572252712448,
25.6612093923175,25.7653754529891,25.8272500211019,25.931436244153,26.035467229549,
26.1393761807748,26.2432196731041,26.3470324855408,26.4508493536522,26.5547748924429,
26.6587592724048,26.7629255906066,26.8247978794479,26.9289840556633,27.0330149940236,
27.1369238981528,27.2407673433741,27.3445801087626,27.4483969299582,27.5523224223632,
27.6563067561686,27.760473029083,27.822345737794,27.9353427738055,28.0470528540681,
28.1606933679541,28.27433388184),.UNSPECIFIED.);
#2683=B_SPLINE_CURVE_WITH_KNOTS('',3,(#97319,#97320,#97321,#97322,#97323,
#97324,#97325,#97326,#97327,#97328,#97329,#97330,#97331,#97332,#97333,#97334,
#97335,#97336,#97337,#97338,#97339,#97340,#97341,#97342,#97343,#97344,#97345,
#97346,#97347,#97348,#97349,#97350,#97351,#97352,#97353,#97354,#97355,#97356,
#97357,#97358,#97359,#97360,#97361,#97362,#97363,#97364,#97365,#97366,#97367,
#97368,#97369,#97370,#97371,#97372,#97373,#97374,#97375,#97376,#97377,#97378,
#97379,#97380,#97381,#97382,#97383,#97384,#97385),.UNSPECIFIED.,.F.,.F.,
(4,3,3,3,3,3,3,3,3,3,3,3,3,3,3,3,3,3,3,3,3,3,4),(28.2743338823081,28.381185874661,
28.4908628050308,28.5980291137702,28.7089613549551,28.8198935961401,28.9240797679585,
29.0281107016001,29.1320196005526,29.2358630403168,29.3396757999759,29.4434926151765,
29.5474181012193,29.6514024284455,29.7555686945067,29.8174414544862,29.9216058860559,
30.025625845333,30.1295363446483,30.2333833809726,30.3371921312322,30.4410324079646,
30.4998665259952),.UNSPECIFIED.);
#2684=B_SPLINE_CURVE_WITH_KNOTS('',3,(#97387,#97388,#97389,#97390,#97391,
#97392,#97393,#97394,#97395,#97396,#97397,#97398,#97399,#97400,#97401,#97402,
#97403,#97404,#97405,#97406,#97407,#97408,#97409,#97410,#97411,#97412,#97413,
#97414,#97415,#97416,#97417,#97418,#97419,#97420,#97421,#97422,#97423,#97424,
#97425,#97426,#97427,#97428,#97429,#97430,#97431,#97432,#97433,#97434,#97435,
#97436,#97437,#97438,#97439,#97440,#97441,#97442,#97443,#97444,#97445,#97446,
#97447,#97448,#97449,#97450,#97451,#97452,#97453,#97454,#97455,#97456),
 .UNSPECIFIED.,.F.,.F.,(4,3,3,3,3,3,3,3,3,3,3,3,3,3,3,3,3,3,3,3,3,3,3,4),
(28.2743338823081,28.3638110296221,28.4679972525077,28.5720282377358,28.6759371887921,
28.7797806809506,28.8835934932153,28.9874103611545,29.0913358997729,29.1953202795622,
29.2994865975932,29.3613588879682,29.4655450641724,29.569576002521,29.6734849066373,
29.7773283518453,29.8811411172201,29.9849579384014,30.0888834307912,30.1928677645809,
30.297034037479,30.3589067463143,30.4630838225526,30.5008971308904),
 .UNSPECIFIED.);
#2685=B_SPLINE_CURVE_WITH_KNOTS('',3,(#97457,#97458,#97459,#97460,#97461,
#97462,#97463,#97464,#97465,#97466,#97467,#97468,#97469,#97470,#97471,#97472,
#97473,#97474,#97475,#97476,#97477,#97478,#97479,#97480,#97481,#97482,#97483,
#97484,#97485,#97486,#97487,#97488,#97489,#97490,#97491,#97492,#97493,#97494,
#97495,#97496,#97497,#97498,#97499,#97500,#97501,#97502,#97503,#97504,#97505,
#97506,#97507,#97508,#97509,#97510,#97511,#97512,#97513,#97514,#97515,#97516,
#97517,#97518,#97519,#97520,#97521,#97522,#97523,#97524,#97525,#97526,#97527,
#97528,#97529,#97530,#97531,#97532,#97533,#97534,#97535,#97536,#97537,#97538,
#97539,#97540,#97541,#97542,#97543,#97544,#97545,#97546,#97547,#97548,#97549,
#97550,#97551,#97552,#97553,#97554,#97555,#97556,#97557,#97558,#97559,#97560,
#97561,#97562,#97563,#97564,#97565,#97566,#97567,#97568,#97569,#97570,#97571,
#97572,#97573,#97574,#97575,#97576,#97577,#97578,#97579,#97580),
 .UNSPECIFIED.,.F.,.F.,(4,3,3,3,3,3,3,3,3,3,3,3,3,3,3,3,3,3,3,3,3,3,3,3,
3,3,3,3,3,3,3,3,3,3,3,3,3,3,3,3,3,4),(24.2166116715314,24.3207836948893,
24.3736195962378,24.4778042283434,24.5818335974701,24.6857409026657,24.789582731488,
24.8933938654244,24.9972090425095,25.101132882772,25.2051155574088,25.3092801780267,
25.3711674545838,25.4753540209415,25.5793853523628,25.6832946519404,25.7871384938629,
25.8909516566054,25.9947688752086,26.0986947623334,26.2026794899368,26.3068461508868,
26.3687153129299,26.4729016340226,26.5769327210748,26.6808417788562,26.7846853807111,
26.8884983054843,26.9923152885876,27.096240945657,27.2002254459312,27.304391886379,
27.366263171276,27.4692311758098,27.5720240162915,27.674719005969,27.7773525419992,
27.8799609371538,27.9826451368982,28.0853653027244,28.1882551863936,28.2743338818562),
 .UNSPECIFIED.);
#2686=B_SPLINE_CURVE_WITH_KNOTS('',3,(#97586,#97587,#97588,#97589,#97590,
#97591,#97592,#97593,#97594,#97595,#97596,#97597,#97598,#97599,#97600,#97601,
#97602,#97603,#97604,#97605,#97606,#97607,#97608,#97609,#97610,#97611,#97612,
#97613,#97614,#97615,#97616,#97617,#97618,#97619,#97620,#97621,#97622,#97623,
#97624,#97625,#97626,#97627,#97628,#97629,#97630,#97631,#97632,#97633,#97634,
#97635,#97636,#97637,#97638,#97639,#97640,#97641,#97642,#97643,#97644,#97645,
#97646,#97647,#97648,#97649,#97650,#97651,#97652,#97653,#97654,#97655),
 .UNSPECIFIED.,.F.,.F.,(4,3,3,3,3,3,3,3,3,3,3,3,3,3,3,3,3,3,3,3,3,3,3,4),
(15.7079632679489,15.810762470857,15.9135271820867,16.0162934123199,16.1191701702764,
16.2221056149525,16.325231416605,16.3932367294691,16.4974784029602,16.6015636324797,
16.7055247443385,16.8094190773204,16.9132813279835,17.0171461480443,17.1211170127319,
17.2251453032834,17.3293527949952,17.3907845878152,17.495130558486,17.6047989097489,
17.7088743312222,17.8128826024111,17.9168653850884,17.9338039635375),
 .UNSPECIFIED.);
#2687=B_SPLINE_CURVE_WITH_KNOTS('',3,(#97657,#97658,#97659,#97660,#97661),
 .UNSPECIFIED.,.F.,.F.,(4,1,4),(14.3981410127769,15.395688871123,15.7079548497411),
 .UNSPECIFIED.);
#2688=B_SPLINE_CURVE_WITH_KNOTS('',3,(#97665,#97666,#97667,#97668,#97669,
#97670,#97671,#97672,#97673,#97674,#97675,#97676,#97677,#97678,#97679,#97680,
#97681,#97682,#97683,#97684,#97685,#97686,#97687,#97688,#97689,#97690,#97691,
#97692,#97693,#97694,#97695,#97696,#97697,#97698,#97699,#97700,#97701,#97702,
#97703,#97704,#97705,#97706,#97707,#97708,#97709,#97710,#97711,#97712,#97713,
#97714,#97715,#97716,#97717,#97718,#97719,#97720,#97721,#97722),
 .UNSPECIFIED.,.F.,.F.,(4,3,3,3,3,3,3,3,3,3,3,3,3,3,3,3,3,3,3,4),(13.8761929392347,
13.9800702154537,14.0837917405706,14.1873910108393,14.2909252293335,14.3944296203396,
14.4979393650901,14.6015560560448,14.7052336748237,14.809084909705,14.8542235792949,
14.9609410403269,15.0635682984915,15.1661015202186,15.2685772625233,15.3710319999417,
15.473553733857,15.5761160252208,15.6788141359347,15.7079632675506),
 .UNSPECIFIED.);
#2689=B_SPLINE_CURVE_WITH_KNOTS('',3,(#97723,#97724,#97725,#97726,#97727,
#97728,#97729,#97730,#97731,#97732,#97733,#97734,#97735,#97736,#97737,#97738,
#97739,#97740,#97741,#97742,#97743,#97744,#97745,#97746,#97747,#97748,#97749,
#97750,#97751,#97752,#97753,#97754,#97755,#97756,#97757,#97758,#97759,#97760,
#97761,#97762,#97763,#97764,#97765,#97766,#97767,#97768,#97769,#97770,#97771,
#97772,#97773,#97774,#97775,#97776,#97777,#97778,#97779,#97780,#97781,#97782,
#97783,#97784,#97785,#97786,#97787,#97788,#97789),.UNSPECIFIED.,.F.,.F.,
(4,3,3,3,3,3,3,3,3,3,3,3,3,3,3,3,3,3,3,3,3,3,4),(15.7079632679489,15.851771437641,
15.9558570373361,16.0597859454429,16.1635911514287,16.2673299233138,16.3710371942513,
16.4747478530179,16.5785668897293,16.682444439463,16.7865045674077,16.8493192959871,
16.9535191120831,17.0575636601841,17.1614860602557,17.2653429233163,17.3691690078,
17.4729990286134,17.5769374445946,17.6809345655956,17.7851132688137,17.8468671543332,
17.9343865323097),.UNSPECIFIED.);
#2690=B_SPLINE_CURVE_WITH_KNOTS('',3,(#97795,#97796,#97797,#97798,#97799,
#97800,#97801,#97802),.UNSPECIFIED.,.F.,.F.,(4,1,1,1,1,4),(99.6151611575392,
99.6457915387122,100.643339397058,101.640887255404,102.638435113751,103.635982972097),
 .UNSPECIFIED.);
#2691=B_SPLINE_CURVE_WITH_KNOTS('',3,(#97806,#97807,#97808,#97809,#97810,
#97811,#97812,#97813,#97814,#97815,#97816,#97817,#97818,#97819,#97820,#97821),
 .UNSPECIFIED.,.F.,.F.,(4,3,3,3,3,4),(103.672557568828,103.780299746495,
103.888308824944,103.996463052203,104.104894597203,104.157833373966),
 .UNSPECIFIED.);
#2692=B_SPLINE_CURVE_WITH_KNOTS('',3,(#97822,#97823,#97824,#97825,#97826,
#97827,#97828,#97829,#97830,#97831,#97832,#97833,#97834,#97835,#97836,#97837,
#97838,#97839,#97840,#97841,#97842,#97843,#97844,#97845,#97846,#97847,#97848,
#97849,#97850,#97851,#97852,#97853,#97854,#97855,#97856,#97857,#97858,#97859,
#97860,#97861,#97862,#97863,#97864,#97865,#97866,#97867,#97868,#97869,#97870,
#97871,#97872,#97873,#97874,#97875,#97876,#97877,#97878,#97879,#97880,#97881,
#97882,#97883,#97884,#97885,#97886,#97887,#97888,#97889,#97890,#97891,#97892,
#97893,#97894,#97895,#97896,#97897,#97898,#97899,#97900,#97901,#97902,#97903,
#97904,#97905,#97906,#97907,#97908,#97909,#97910,#97911,#97912,#97913,#97914,
#97915,#97916,#97917,#97918,#97919,#97920,#97921,#97922,#97923,#97924,#97925,
#97926,#97927,#97928,#97929,#97930,#97931,#97932,#97933,#97934,#97935,#97936,
#97937,#97938,#97939,#97940,#97941,#97942,#97943,#97944,#97945),
 .UNSPECIFIED.,.F.,.F.,(4,3,3,3,3,3,3,3,3,3,3,3,3,3,3,3,3,3,3,3,3,3,3,3,
3,3,3,3,3,3,3,3,3,3,3,3,3,3,3,3,3,4),(99.615621384741,99.7194516934841,
99.823289171979,99.9272369721367,100.031246375379,100.135434211443,100.18725683054,
100.291455298671,100.395498790872,100.499420572679,100.603277087823,100.707103094362,
100.810933307106,100.91487232482,101.018870279629,101.123050173999,101.184804688886,
101.28888521047,101.392810209752,101.496613258174,101.600350953578,101.704058227136,
101.807769966774,101.911591721183,102.015472915131,102.119538113885,102.182352547233,
102.286721387124,102.390934549507,102.495024150017,102.599047245106,102.703038351641,
102.807031941819,102.911130600256,103.015286319959,103.119619330251,103.179900405579,
103.289272706435,103.398334640765,103.507209030259,103.615853185506,103.672557568463),
 .UNSPECIFIED.);
#2693=B_SPLINE_CURVE_WITH_KNOTS('',3,(#97951,#97952,#97953,#97954,#97955,
#97956,#97957,#97958,#97959,#97960,#97961,#97962,#97963,#97964,#97965,#97966,
#97967,#97968,#97969,#97970,#97971,#97972,#97973,#97974,#97975,#97976,#97977,
#97978,#97979,#97980,#97981,#97982,#97983,#97984,#97985,#97986,#97987,#97988,
#97989,#97990,#97991,#97992,#97993,#97994,#97995,#97996,#97997,#97998,#97999,
#98000,#98001,#98002,#98003,#98004,#98005,#98006,#98007,#98008,#98009,#98010,
#98011,#98012,#98013,#98014,#98015,#98016,#98017,#98018,#98019,#98020,#98021,
#98022,#98023,#98024,#98025,#98026,#98027,#98028,#98029,#98030,#98031,#98032,
#98033,#98034,#98035,#98036,#98037,#98038,#98039,#98040,#98041,#98042,#98043,
#98044,#98045,#98046,#98047,#98048,#98049,#98050,#98051,#98052,#98053,#98054,
#98055,#98056,#98057,#98058,#98059,#98060,#98061,#98062,#98063,#98064,#98065,
#98066,#98067,#98068,#98069,#98070,#98071,#98072,#98073,#98074,#98075,#98076,
#98077),.UNSPECIFIED.,.F.,.F.,(4,3,3,3,3,3,3,3,3,3,3,3,3,3,3,3,3,3,3,3,
3,3,3,3,3,3,3,3,3,3,3,3,3,3,3,3,3,3,3,3,3,3,4),(93.3317451784711,93.4356908296324,
93.5397089185721,93.6438957389185,93.6605043886357,93.7646924913296,93.8687253455085,
93.9726361406856,94.0764814606864,94.1802960819711,94.2841147375458,94.388042019171,
94.4920281194343,94.5961961038901,94.6580522469818,94.7622408508587,94.8662742477253,
94.970185643822,95.0740316002466,95.1778468922007,95.2816662514685,95.3855942816827,
95.4895811569642,95.5937499492636,95.6556001053279,95.759772961128,95.8637905520596,
95.9676861327482,96.0715162764619,96.1753157816034,96.2791194031735,96.3830318787696,
96.4870032791763,96.5911568906327,96.653147963674,96.7562452892943,96.8592012637035,
96.9620522663221,97.0688822650625,97.1716574089993,97.2744331252244,97.3772781161521,
97.3893722612836),.UNSPECIFIED.);
#2694=B_SPLINE_CURVE_WITH_KNOTS('',3,(#98078,#98079,#98080,#98081,#98082,
#98083),.UNSPECIFIED.,.F.,.F.,(4,1,1,4),(97.3893747331526,97.6506958220201,
98.6482436803662,99.6151611575392),.UNSPECIFIED.);
#2695=B_SPLINE_CURVE_WITH_KNOTS('',3,(#98085,#98086,#98087,#98088,#98089,
#98090,#98091,#98092,#98093,#98094,#98095,#98096,#98097,#98098,#98099,#98100,
#98101,#98102,#98103,#98104,#98105,#98106,#98107,#98108,#98109,#98110,#98111,
#98112,#98113,#98114,#98115,#98116,#98117,#98118,#98119,#98120,#98121,#98122,
#98123,#98124,#98125,#98126,#98127,#98128,#98129,#98130,#98131,#98132,#98133,
#98134,#98135,#98136,#98137,#98138,#98139,#98140,#98141,#98142,#98143,#98144,
#98145,#98146,#98147,#98148,#98149,#98150,#98151),.UNSPECIFIED.,.F.,.F.,
(4,3,3,3,3,3,3,3,3,3,3,3,3,3,3,3,3,3,3,3,3,3,4),(97.3893722616848,97.4918516940551,
97.5942418136602,97.6965792856351,97.7989006986796,97.9013129217246,98.0037693581187,
98.1064097352967,98.1921611138482,98.2963339880605,98.400351597429,98.504247196504,
98.6080773585636,98.7118768819842,98.8156805217399,98.9195930152571,99.0235644334626,
99.1277180623331,99.1897089721943,99.296187075331,99.4002195103592,99.5079204475501,
99.615621384741),.UNSPECIFIED.);
#2696=B_SPLINE_CURVE_WITH_KNOTS('',3,(#98152,#98153,#98154,#98155,#98156,
#98157,#98158,#98159,#98160,#98161,#98162,#98163,#98164,#98165,#98166,#98167,
#98168,#98169,#98170,#98171,#98172,#98173,#98174,#98175,#98176,#98177,#98178,
#98179,#98180,#98181,#98182,#98183,#98184,#98185,#98186,#98187,#98188,#98189,
#98190,#98191,#98192,#98193,#98194,#98195,#98196,#98197,#98198,#98199,#98200,
#98201,#98202,#98203,#98204,#98205,#98206,#98207,#98208,#98209,#98210,#98211,
#98212,#98213,#98214,#98215,#98216,#98217,#98218,#98219,#98220,#98221,#98222,
#98223,#98224,#98225,#98226,#98227,#98228,#98229,#98230,#98231,#98232,#98233,
#98234,#98235,#98236,#98237,#98238,#98239,#98240,#98241,#98242,#98243,#98244,
#98245,#98246,#98247,#98248,#98249,#98250,#98251,#98252,#98253,#98254,#98255,
#98256,#98257,#98258,#98259,#98260,#98261,#98262,#98263,#98264,#98265,#98266,
#98267,#98268,#98269,#98270,#98271,#98272,#98273,#98274,#98275),
 .UNSPECIFIED.,.F.,.F.,(4,3,3,3,3,3,3,3,3,3,3,3,3,3,3,3,3,3,3,3,3,3,3,3,
3,3,3,3,3,3,3,3,3,3,3,3,3,3,3,3,3,4),(93.3327249561973,93.4413805467306,
93.5452680315814,93.6490996786052,93.7529102511427,93.8567344787581,93.960673260205,
94.0646795089325,94.1688591227995,94.2019696804638,94.3061562451431,94.4101875751818,
94.5140968738215,94.6179407150807,94.721753877435,94.8255710959254,94.9294969833574,
95.0334817115056,95.1376483733693,95.1995175388099,95.3037020714602,95.4077313636999,
95.5116386258043,95.6154804324086,95.7192915649643,95.8231067614917,95.9270306527879,
96.0310133963537,96.1351781134134,96.197065397156,96.3012534980456,96.405286350439,
96.5091971438664,96.6130424621404,96.7168570817235,96.8206757356245,96.9246030156287,
97.0285891142985,97.1327570972207,97.1946132555021,97.3456072562199,97.3893722612836),
 .UNSPECIFIED.);
#2697=B_SPLINE_CURVE_WITH_KNOTS('',3,(#98281,#98282,#98283,#98284,#98285,
#98286,#98287,#98288,#98289,#98290,#98291,#98292,#98293,#98294,#98295,#98296,
#98297,#98298,#98299,#98300,#98301,#98302,#98303,#98304,#98305,#98306,#98307,
#98308,#98309,#98310,#98311,#98312,#98313,#98314,#98315,#98316,#98317,#98318,
#98319,#98320,#98321,#98322,#98323,#98324,#98325,#98326,#98327,#98328,#98329,
#98330,#98331,#98332,#98333,#98334,#98335,#98336,#98337,#98338,#98339,#98340,
#98341,#98342,#98343,#98344,#98345,#98346,#98347,#98348,#98349,#98350,#98351,
#98352,#98353,#98354,#98355,#98356,#98357,#98358,#98359,#98360,#98361,#98362,
#98363,#98364,#98365,#98366,#98367,#98368,#98369,#98370,#98371,#98372,#98373,
#98374,#98375,#98376,#98377,#98378,#98379,#98380,#98381,#98382,#98383,#98384,
#98385,#98386,#98387,#98388,#98389,#98390,#98391,#98392,#98393,#98394,#98395,
#98396,#98397,#98398,#98399,#98400,#98401),.UNSPECIFIED.,.F.,.F.,(4,3,3,
3,3,3,3,3,3,3,3,3,3,3,3,3,3,3,3,3,3,3,3,3,3,3,3,3,3,3,3,3,3,3,3,3,3,3,3,
3,4),(87.0493933560106,87.1532149091787,87.2570257190436,87.3615735989225,
87.4655293993329,87.570373318946,87.6752172385592,87.7794034174978,87.8834343579682,
87.9873432632894,88.0911867091357,88.1949994745833,88.2988162952719,88.4027417863115,
88.5067261182652,88.6108923885799,88.6727650969053,88.7769513208292,88.8809823068916,
88.9848912584753,89.088734750972,89.1925475633854,89.2963644312838,89.4002899695733,
89.5042743488706,89.6084406661575,89.6703129552514,89.7744989226349,89.8785296516199,
89.9824383465664,90.0862815828356,90.1900941398043,90.2939107534151,90.3978360409233,
90.5018201710385,90.6059862443694,90.6678608135975,90.7807057004803,90.8932647257622,
91.0053646969276,91.1061869538112),.UNSPECIFIED.);
#2698=B_SPLINE_CURVE_WITH_KNOTS('',3,(#98402,#98403,#98404,#98405,#98406,
#98407,#98408,#98409,#98410,#98411,#98412,#98413,#98414,#98415,#98416,#98417,
#98418,#98419,#98420,#98421,#98422,#98423,#98424,#98425,#98426,#98427,#98428,
#98429,#98430,#98431,#98432,#98433,#98434,#98435,#98436,#98437,#98438,#98439,
#98440,#98441,#98442,#98443,#98444,#98445,#98446,#98447,#98448,#98449,#98450,
#98451,#98452,#98453,#98454,#98455,#98456,#98457,#98458,#98459,#98460,#98461,
#98462,#98463,#98464,#98465,#98466,#98467,#98468,#98469,#98470,#98471),
 .UNSPECIFIED.,.F.,.F.,(4,3,3,3,3,3,3,3,3,3,3,3,3,3,3,3,3,3,3,3,3,3,3,4),
(91.106186954104,91.2125697916978,91.319033886442,91.4256928894083,91.5324648462027,
91.6394568078794,91.6654086719436,91.7695952377474,91.8736265689175,91.9775358686934,
92.0813797110913,92.1851928745849,92.2890100942136,92.3929359827745,92.496920712048,
92.6010873750192,92.6629565302896,92.7671206839459,92.8711399663559,92.9750493942499,
93.078892943413,93.1826980543968,93.2865286010299,93.3317451784711),
 .UNSPECIFIED.);
#2699=B_SPLINE_CURVE_WITH_KNOTS('',3,(#98473,#98474,#98475,#98476,#98477,
#98478,#98479,#98480,#98481,#98482,#98483,#98484,#98485,#98486,#98487,#98488,
#98489,#98490,#98491,#98492,#98493,#98494,#98495,#98496,#98497,#98498,#98499,
#98500,#98501,#98502,#98503,#98504,#98505,#98506,#98507,#98508,#98509,#98510,
#98511,#98512,#98513,#98514,#98515,#98516,#98517,#98518,#98519,#98520,#98521,
#98522,#98523,#98524,#98525,#98526,#98527,#98528,#98529,#98530,#98531,#98532,
#98533,#98534,#98535,#98536,#98537,#98538,#98539,#98540,#98541,#98542),
 .UNSPECIFIED.,.F.,.F.,(4,3,3,3,3,3,3,3,3,3,3,3,3,3,3,3,3,3,3,3,3,3,3,4),
(91.106186954104,91.2093261054256,91.3135123291656,91.4175433150428,91.5214522664409,
91.6252957587517,91.7291085709795,91.8329254386925,91.9368509767983,92.0408353559126,
92.1450016730195,92.2068739637717,92.3110599315904,92.4150906610108,92.5189993563906,
92.6228425930916,92.7266551504905,92.8304717645285,92.934397052457,93.0383811829892,
93.1425472567276,93.2044218221178,93.3086061886958,93.3327249561973),
 .UNSPECIFIED.);
#2700=B_SPLINE_CURVE_WITH_KNOTS('',3,(#98543,#98544,#98545,#98546,#98547,
#98548,#98549,#98550,#98551,#98552,#98553,#98554,#98555,#98556,#98557,#98558,
#98559,#98560,#98561,#98562,#98563,#98564,#98565,#98566,#98567,#98568,#98569,
#98570,#98571,#98572,#98573,#98574,#98575,#98576,#98577,#98578,#98579,#98580,
#98581,#98582,#98583,#98584,#98585,#98586,#98587,#98588,#98589,#98590,#98591,
#98592,#98593,#98594,#98595,#98596,#98597,#98598,#98599,#98600,#98601,#98602,
#98603,#98604,#98605,#98606,#98607,#98608,#98609,#98610,#98611,#98612,#98613,
#98614,#98615,#98616,#98617,#98618,#98619,#98620,#98621,#98622,#98623,#98624,
#98625,#98626,#98627,#98628,#98629,#98630,#98631,#98632,#98633,#98634,#98635,
#98636,#98637,#98638,#98639,#98640,#98641,#98642,#98643,#98644,#98645,#98646,
#98647,#98648,#98649,#98650,#98651,#98652,#98653,#98654,#98655,#98656,#98657,
#98658,#98659,#98660,#98661,#98662,#98663,#98664,#98665,#98666),
 .UNSPECIFIED.,.F.,.F.,(4,3,3,3,3,3,3,3,3,3,3,3,3,3,3,3,3,3,3,3,3,3,3,3,
3,3,3,3,3,3,3,3,3,3,3,3,3,3,3,3,3,4),(87.0484495531988,87.1526139507006,
87.2191346720412,87.3233208365559,87.4273517627696,87.5312606541469,87.6351040862493,
87.7389168381715,87.8427336455721,87.9466591237729,88.0506434431218,88.1548097013355,
88.2166825303873,88.3208687024072,88.4248996361967,88.5288085352171,88.632651975,
88.7364647346284,88.8402815497491,88.9442070356378,89.048191362668,89.1523576284685,
89.2142303887334,89.3184165292674,89.4224474315273,89.5263562991041,89.6301997075135,
89.7340124358838,89.8378292199076,89.9417546751579,90.0457389717619,90.1499052078012,
90.2117782470795,90.3146405331782,90.4173275668627,90.519916847407,90.6224448805082,
90.7249480860865,90.8275243015109,90.9301370934329,91.0329109697359,91.1061869536426),
 .UNSPECIFIED.);
#2701=B_SPLINE_CURVE_WITH_KNOTS('',3,(#98672,#98673,#98674,#98675,#98676,
#98677,#98678,#98679,#98680,#98681,#98682,#98683,#98684,#98685,#98686,#98687,
#98688,#98689,#98690,#98691,#98692,#98693,#98694,#98695,#98696,#98697,#98698,
#98699,#98700,#98701,#98702,#98703,#98704,#98705,#98706,#98707,#98708,#98709,
#98710,#98711,#98712,#98713,#98714,#98715,#98716,#98717,#98718,#98719,#98720,
#98721,#98722,#98723,#98724,#98725,#98726,#98727,#98728,#98729,#98730,#98731,
#98732,#98733,#98734,#98735,#98736,#98737,#98738,#98739,#98740,#98741,#98742,
#98743,#98744,#98745,#98746,#98747,#98748,#98749,#98750,#98751,#98752,#98753,
#98754,#98755,#98756,#98757,#98758,#98759,#98760,#98761,#98762,#98763,#98764,
#98765,#98766,#98767,#98768,#98769,#98770,#98771,#98772,#98773,#98774,#98775,
#98776,#98777,#98778,#98779,#98780,#98781,#98782,#98783,#98784,#98785,#98786,
#98787,#98788,#98789,#98790,#98791,#98792),.UNSPECIFIED.,.F.,.F.,(4,3,3,
3,3,3,3,3,3,3,3,3,3,3,3,3,3,3,3,3,3,3,3,3,3,3,3,3,3,3,3,3,3,3,3,3,3,3,3,
3,4),(80.7662008482215,80.8702730448693,80.974207590904,81.0780665198201,
81.1818846299995,81.2856966661622,81.389610867391,81.4935748111732,81.5977303299521,
81.6899300884827,81.7941162519914,81.8981471772209,82.0020560676505,82.1058994988283,
82.2097122498501,82.3135290563755,82.4174545337454,82.5214388522872,82.6256051097397,
82.6874779468288,82.7916641114795,82.8956950378591,82.9996039294452,83.1034473617827,
83.2072601139657,83.3110769216523,83.4150024001749,83.5189867198666,83.6231529784516,
83.6850258051749,83.7892119660255,83.8932428886023,83.9971517763997,84.1009952049595,
84.2048079533809,84.3086247573275,84.412550232169,84.5165345482068,84.6207008032212,
84.682573663521,84.8230016469244),.UNSPECIFIED.);
#2702=B_SPLINE_CURVE_WITH_KNOTS('',3,(#98793,#98794,#98795,#98796,#98797,
#98798,#98799,#98800,#98801,#98802,#98803,#98804,#98805,#98806,#98807,#98808,
#98809,#98810,#98811,#98812,#98813,#98814,#98815,#98816,#98817,#98818,#98819,
#98820,#98821,#98822,#98823,#98824,#98825,#98826,#98827,#98828,#98829,#98830,
#98831,#98832,#98833,#98834,#98835,#98836,#98837,#98838,#98839,#98840,#98841,
#98842,#98843,#98844,#98845,#98846,#98847,#98848,#98849,#98850,#98851,#98852,
#98853,#98854,#98855,#98856,#98857,#98858,#98859,#98860,#98861,#98862),
 .UNSPECIFIED.,.F.,.F.,(4,3,3,3,3,3,3,3,3,3,3,3,3,3,3,3,3,3,3,3,3,3,3,4),
(84.8230016473375,84.9301416316537,85.0325714163389,85.1349307980786,85.2372563959105,
85.3395847767895,85.4420166362011,85.5445096330654,85.64717105574,85.6801215218671,
85.7843076939159,85.8883386277345,85.9922475267839,86.096090966596,86.1999037262534,
86.3037205414031,86.4076460273204,86.5116303543791,86.6157966202077,86.6776693802131,
86.7818282236142,86.8858513473907,86.9897582188318,87.0493933560106),
 .UNSPECIFIED.);
#2703=B_SPLINE_CURVE_WITH_KNOTS('',3,(#98864,#98865,#98866,#98867,#98868,
#98869,#98870,#98871,#98872,#98873,#98874,#98875,#98876,#98877,#98878,#98879,
#98880,#98881,#98882,#98883,#98884,#98885,#98886,#98887,#98888,#98889,#98890,
#98891,#98892,#98893,#98894,#98895,#98896,#98897,#98898,#98899,#98900,#98901,
#98902,#98903,#98904,#98905,#98906,#98907,#98908,#98909,#98910,#98911,#98912,
#98913,#98914,#98915,#98916,#98917,#98918,#98919,#98920,#98921,#98922,#98923,
#98924,#98925,#98926,#98927,#98928,#98929,#98930),.UNSPECIFIED.,.F.,.F.,
(4,3,3,3,3,3,3,3,3,3,3,3,3,3,3,3,3,3,3,3,3,3,4),(84.8230016473347,84.9376554440844,
85.0527190382953,85.1683359285729,85.2240389553491,85.3282251199953,85.4322560463704,
85.5361649379519,85.640008370285,85.7438211224634,85.8476379301455,85.9515634086638,
86.0555477283509,86.1597139869317,86.2215868136951,86.3257394090962,86.4297517345076,
86.5336587825729,86.6374954230253,86.741335673925,86.8451704422834,86.9491112691442,
87.0484495531988),.UNSPECIFIED.);
#2704=B_SPLINE_CURVE_WITH_KNOTS('',3,(#98931,#98932,#98933,#98934,#98935,
#98936,#98937,#98938,#98939,#98940,#98941,#98942,#98943,#98944,#98945,#98946,
#98947,#98948,#98949,#98950,#98951,#98952,#98953,#98954,#98955,#98956,#98957,
#98958,#98959,#98960,#98961,#98962,#98963,#98964,#98965,#98966,#98967,#98968,
#98969,#98970,#98971,#98972,#98973,#98974,#98975,#98976,#98977,#98978,#98979,
#98980,#98981,#98982,#98983,#98984,#98985,#98986,#98987,#98988,#98989,#98990,
#98991,#98992,#98993,#98994,#98995,#98996,#98997,#98998,#98999,#99000,#99001,
#99002,#99003,#99004,#99005,#99006,#99007,#99008,#99009,#99010,#99011,#99012,
#99013,#99014,#99015,#99016,#99017,#99018,#99019,#99020,#99021,#99022,#99023,
#99024,#99025,#99026,#99027,#99028,#99029,#99030,#99031,#99032,#99033,#99034,
#99035,#99036,#99037,#99038,#99039,#99040,#99041,#99042,#99043,#99044,#99045,
#99046,#99047,#99048,#99049,#99050,#99051,#99052,#99053,#99054),
 .UNSPECIFIED.,.F.,.F.,(4,3,3,3,3,3,3,3,3,3,3,3,3,3,3,3,3,3,3,3,3,3,3,3,
3,3,3,3,3,3,3,3,3,3,3,3,3,3,3,3,3,4),(80.7657457599978,80.8695647107879,
80.9734943449784,81.0774857249014,81.1816560975386,81.2338475219647,81.3380336854428,
81.4420646106446,81.5459735010506,81.6498169322074,81.7536296832108,81.8574464897206,
81.9613719670788,82.065356285611,82.1695225430577,82.2313953803108,82.335581543951,
82.439612469316,82.5435213598856,82.6473647912064,82.7511775423736,82.8549943490468,
82.9589198265672,83.0629041452611,83.1670704028666,83.2289432386569,83.3331294018515,
83.4371603267706,83.5410692168966,83.6449126477754,83.748725398503,83.8525422047394,
83.95646768183,84.0604520000977,84.1646182572869,84.226491097003,84.3322636668441,
84.437865290237,84.5433026045784,84.6486432044847,84.7539210445246,84.8230016469244),
 .UNSPECIFIED.);
#2705=B_SPLINE_CURVE_WITH_KNOTS('',3,(#99060,#99061,#99062,#99063,#99064,
#99065,#99066,#99067,#99068,#99069,#99070,#99071,#99072,#99073,#99074,#99075,
#99076,#99077,#99078,#99079,#99080,#99081,#99082,#99083,#99084,#99085,#99086,
#99087,#99088,#99089,#99090,#99091,#99092,#99093,#99094,#99095,#99096,#99097,
#99098,#99099,#99100,#99101,#99102,#99103,#99104,#99105,#99106,#99107,#99108,
#99109,#99110,#99111,#99112,#99113,#99114,#99115,#99116,#99117,#99118,#99119,
#99120,#99121,#99122,#99123,#99124,#99125,#99126,#99127,#99128,#99129,#99130,
#99131,#99132,#99133,#99134,#99135,#99136,#99137,#99138,#99139,#99140,#99141,
#99142,#99143,#99144,#99145,#99146,#99147,#99148,#99149,#99150,#99151,#99152,
#99153,#99154,#99155,#99156,#99157,#99158,#99159,#99160,#99161,#99162,#99163,
#99164,#99165,#99166,#99167,#99168,#99169,#99170,#99171,#99172,#99173,#99174,
#99175,#99176,#99177,#99178,#99179,#99180,#99181,#99182,#99183,#99184,#99185,
#99186),.UNSPECIFIED.,.F.,.F.,(4,3,3,3,3,3,3,3,3,3,3,3,3,3,3,3,3,3,3,3,
3,3,3,3,3,3,3,3,3,3,3,3,3,3,3,3,3,3,3,3,3,3,4),(74.4820629741015,74.5860824401791,
74.6902706699235,74.7070950800601,74.8112812435448,74.9153121687535,75.0192210591671,
75.1230644903318,75.2268772413434,75.3306940478616,75.4346195252287,75.5386038437702,
75.6427701012263,75.7046429384062,75.8088291018918,75.9128600271013,76.0167689175156,
76.120612348681,76.2244250996931,76.3282419062119,76.4321673835794,76.5361517021214,
76.6403179595778,76.7021907967523,76.8063769602599,76.9104078854914,77.0143167759279,
77.1181602071154,77.2219729581496,77.3257897646905,77.4297152420799,77.5336995606436,
77.6378658181213,77.6997386550983,77.8047483656343,77.9072108121797,78.0095758369587,
78.111880162764,78.2188642069196,78.3212057260103,78.4235870713438,78.526093732632,
78.5398163393865),.UNSPECIFIED.);
#2706=B_SPLINE_CURVE_WITH_KNOTS('',3,(#99187,#99188,#99189,#99190,#99191,
#99192,#99193,#99194,#99195,#99196,#99197,#99198,#99199,#99200,#99201,#99202,
#99203,#99204,#99205,#99206,#99207,#99208,#99209,#99210,#99211,#99212,#99213,
#99214,#99215,#99216,#99217,#99218,#99219,#99220,#99221,#99222,#99223,#99224,
#99225,#99226,#99227,#99228,#99229,#99230,#99231,#99232,#99233,#99234,#99235,
#99236,#99237,#99238,#99239,#99240,#99241,#99242,#99243,#99244,#99245,#99246,
#99247,#99248,#99249,#99250,#99251,#99252,#99253),.UNSPECIFIED.,.F.,.F.,
(4,3,3,3,3,3,3,3,3,3,3,3,3,3,3,3,3,3,3,3,3,3,4),(78.5398163397448,78.6972865134445,
78.8014726769226,78.9055036021242,79.0094124925302,79.1132559236869,79.2170686746902,
79.3208854811998,79.4248109585579,79.5287952770901,79.6329615345367,79.6948343717905,
79.7990205354315,79.9030514607969,80.0069603513672,80.1108037826886,80.2146165338564,
80.3184333405304,80.4223588180514,80.5263431367459,80.630509394352,80.6923822301366,
80.7662008482215),.UNSPECIFIED.);
#2707=B_SPLINE_CURVE_WITH_KNOTS('',3,(#99255,#99256,#99257,#99258,#99259,
#99260,#99261,#99262,#99263,#99264,#99265,#99266,#99267,#99268,#99269,#99270,
#99271,#99272,#99273,#99274,#99275,#99276,#99277,#99278,#99279,#99280,#99281,
#99282,#99283,#99284,#99285,#99286,#99287,#99288,#99289,#99290,#99291,#99292,
#99293,#99294,#99295,#99296,#99297,#99298,#99299,#99300,#99301,#99302,#99303,
#99304,#99305,#99306,#99307,#99308,#99309,#99310,#99311,#99312,#99313,#99314,
#99315,#99316,#99317,#99318,#99319,#99320,#99321),.UNSPECIFIED.,.F.,.F.,
(4,3,3,3,3,3,3,3,3,3,3,3,3,3,3,3,3,3,3,3,3,3,4),(78.5398163397448,78.6430480181532,
78.7462408136039,78.8494302891181,78.9527248465574,79.0560730500088,79.159611215973,
79.2387518052725,79.3429379687799,79.4469688940115,79.5508777844477,79.6547212156351,
79.7585339666693,79.8623507732101,79.9662762505993,80.0702605691627,80.1744268266403,
80.2362996636186,80.3404816769743,80.4467976977302,80.5507026804229,80.6582242202103,
80.7657457599978),.UNSPECIFIED.);
#2708=B_SPLINE_CURVE_WITH_KNOTS('',3,(#99322,#99323,#99324,#99325,#99326,
#99327,#99328,#99329,#99330,#99331,#99332,#99333,#99334,#99335,#99336,#99337,
#99338,#99339,#99340,#99341,#99342,#99343,#99344,#99345,#99346,#99347,#99348,
#99349,#99350,#99351,#99352,#99353,#99354,#99355,#99356,#99357,#99358,#99359,
#99360,#99361,#99362,#99363,#99364,#99365,#99366,#99367,#99368,#99369,#99370,
#99371,#99372,#99373,#99374,#99375,#99376,#99377,#99378,#99379,#99380,#99381,
#99382,#99383,#99384,#99385,#99386,#99387,#99388,#99389,#99390,#99391,#99392,
#99393,#99394,#99395,#99396,#99397,#99398,#99399,#99400,#99401,#99402,#99403,
#99404,#99405,#99406,#99407,#99408,#99409,#99410,#99411,#99412,#99413,#99414,
#99415,#99416,#99417,#99418,#99419,#99420,#99421,#99422,#99423,#99424,#99425,
#99426,#99427,#99428,#99429,#99430,#99431,#99432,#99433,#99434,#99435,#99436,
#99437,#99438,#99439,#99440,#99441,#99442,#99443,#99444,#99445),
 .UNSPECIFIED.,.F.,.F.,(4,3,3,3,3,3,3,3,3,3,3,3,3,3,3,3,3,3,3,3,3,3,3,3,
3,3,3,3,3,3,3,3,3,3,3,3,3,3,3,3,3,4),(74.4832444084144,74.5871350821012,
74.6909683376155,74.7947789409073,74.8986016225652,75.0025379131712,75.1065402542367,
75.2107173371283,75.2485603718882,75.3527465353759,75.4567774605873,75.5606863510037,
75.6645297821712,75.7683425331857,75.8721593397066,75.9760848170764,76.0800691356207,
76.1842353930795,76.2461082302343,76.3502943937249,76.4543253189395,76.5582342093588,
76.6620776405292,76.7658903915466,76.8697071980705,76.9736326754433,77.0776169939903,
77.1817832514518,77.2436560885804,77.3478422520654,77.4518731772744,77.5557820676882,
77.6596254988533,77.7634382498651,77.8672550563838,77.9711805337513,78.0751648522932,
78.1793311097497,78.2412039469264,78.3682032551631,78.4934616304309,78.5398163394195),
 .UNSPECIFIED.);
#2709=B_SPLINE_CURVE_WITH_KNOTS('',3,(#99451,#99452,#99453,#99454,#99455,
#99456,#99457,#99458,#99459,#99460,#99461,#99462,#99463,#99464,#99465,#99466,
#99467,#99468,#99469,#99470,#99471,#99472,#99473,#99474,#99475,#99476,#99477,
#99478,#99479,#99480,#99481,#99482,#99483,#99484,#99485,#99486,#99487,#99488,
#99489,#99490,#99491,#99492,#99493,#99494,#99495,#99496,#99497,#99498,#99499,
#99500,#99501,#99502,#99503,#99504,#99505,#99506,#99507,#99508,#99509,#99510,
#99511,#99512,#99513,#99514,#99515,#99516,#99517,#99518,#99519,#99520,#99521,
#99522,#99523,#99524,#99525,#99526,#99527,#99528,#99529,#99530,#99531,#99532,
#99533,#99534,#99535,#99536,#99537,#99538,#99539,#99540,#99541,#99542,#99543,
#99544,#99545,#99546,#99547,#99548,#99549,#99550,#99551,#99552,#99553,#99554,
#99555,#99556,#99557,#99558,#99559,#99560,#99561,#99562,#99563,#99564,#99565,
#99566,#99567,#99568,#99569,#99570,#99571),.UNSPECIFIED.,.F.,.F.,(4,3,3,
3,3,3,3,3,3,3,3,3,3,3,3,3,3,3,3,3,3,3,3,3,3,3,3,3,3,3,3,3,3,3,3,3,3,3,3,
3,4),(68.1995422682746,68.3033530840735,68.407966795551,68.5119225014276,
68.6168652157056,68.7218079299836,68.8259940934719,68.9300250186842,69.0339339091014,
69.1377773402697,69.2415900912848,69.3454068978068,69.4493323751773,69.5533166937223,
69.6574829511817,69.7193557883297,69.8235419518177,69.9275728770298,70.0314817674467,
70.1353251986146,70.2391379496294,70.3429547561507,70.4468802335209,70.5508645520653,
70.6550308095243,70.7169036466757,70.821089810164,70.9251207353765,71.0290296257937,
71.132873056962,71.2366858079771,71.3405026144985,71.4444280918692,71.5484124104144,
71.6525786678739,71.7144515050218,71.8220784528942,71.930716597812,72.0379272940092,
72.1472791632872,72.2566310325652),.UNSPECIFIED.);
#2710=B_SPLINE_CURVE_WITH_KNOTS('',3,(#99572,#99573,#99574,#99575,#99576,
#99577,#99578,#99579,#99580,#99581,#99582,#99583,#99584,#99585,#99586,#99587,
#99588,#99589,#99590,#99591,#99592,#99593,#99594,#99595,#99596,#99597,#99598,
#99599,#99600,#99601,#99602,#99603,#99604,#99605,#99606,#99607,#99608,#99609,
#99610,#99611,#99612,#99613,#99614,#99615,#99616,#99617,#99618,#99619,#99620,
#99621,#99622,#99623,#99624,#99625,#99626,#99627,#99628,#99629,#99630,#99631,
#99632,#99633,#99634,#99635,#99636,#99637,#99638),.UNSPECIFIED.,.F.,.F.,
(4,3,3,3,3,3,3,3,3,3,3,3,3,3,3,3,3,3,3,3,3,3,4),(72.2566310330023,72.3704731155937,
72.4818133112494,72.5969063373086,72.7119993633679,72.8161855268553,72.9202164520667,
73.0241253424829,73.1279687736503,73.2317815246645,73.3355983311853,73.439523808555,
73.5435081270989,73.6476743845574,73.709547221714,73.8137037283061,73.9177183843876,
74.0216261896506,74.1254620184434,74.2292882434002,74.3331083610432,74.4370016429324,
74.4820629741015),.UNSPECIFIED.);
#2711=B_SPLINE_CURVE_WITH_KNOTS('',3,(#99640,#99641,#99642,#99643,#99644,
#99645,#99646,#99647,#99648,#99649,#99650,#99651,#99652,#99653,#99654,#99655,
#99656,#99657,#99658,#99659,#99660,#99661,#99662,#99663,#99664,#99665,#99666,
#99667,#99668,#99669,#99670,#99671,#99672,#99673,#99674,#99675,#99676,#99677,
#99678,#99679,#99680,#99681,#99682,#99683,#99684,#99685,#99686,#99687,#99688,
#99689,#99690,#99691,#99692,#99693,#99694,#99695,#99696,#99697,#99698,#99699,
#99700,#99701,#99702,#99703,#99704,#99705,#99706,#99707,#99708,#99709),
 .UNSPECIFIED.,.F.,.F.,(4,3,3,3,3,3,3,3,3,3,3,3,3,3,3,3,3,3,3,3,3,3,3,4),
(72.256631032763,72.3608036976092,72.4648211350913,72.5687165873283,72.6725466328826,
72.7763460712598,72.8801496585883,72.9840619406992,73.0880331868138,73.1921861591871,
73.253464655196,73.3576508186844,73.4616817438966,73.5655906343139,73.6694340654822,
73.7732468164974,73.8770636230193,73.9809891003899,74.084973418935,74.1891396763946,
74.2510125135421,74.3552035665601,74.4592285332565,74.4832444084144),
 .UNSPECIFIED.);
#2712=B_SPLINE_CURVE_WITH_KNOTS('',3,(#99710,#99711,#99712,#99713,#99714,
#99715,#99716,#99717,#99718,#99719,#99720,#99721,#99722,#99723,#99724,#99725,
#99726,#99727,#99728,#99729,#99730,#99731,#99732,#99733,#99734,#99735,#99736,
#99737,#99738,#99739,#99740,#99741,#99742,#99743,#99744,#99745,#99746,#99747,
#99748,#99749,#99750,#99751,#99752,#99753,#99754,#99755,#99756,#99757,#99758,
#99759,#99760,#99761,#99762,#99763,#99764,#99765,#99766,#99767,#99768,#99769,
#99770,#99771,#99772,#99773,#99774,#99775,#99776,#99777,#99778,#99779,#99780,
#99781,#99782,#99783,#99784,#99785,#99786,#99787,#99788,#99789,#99790,#99791,
#99792,#99793,#99794,#99795,#99796,#99797,#99798,#99799,#99800,#99801,#99802,
#99803,#99804,#99805,#99806,#99807,#99808,#99809,#99810,#99811,#99812,#99813,
#99814,#99815,#99816,#99817,#99818,#99819,#99820,#99821,#99822,#99823,#99824,
#99825,#99826,#99827,#99828,#99829,#99830,#99831,#99832,#99833,#99834,#99835,
#99836),.UNSPECIFIED.,.F.,.F.,(4,3,3,3,3,3,3,3,3,3,3,3,3,3,3,3,3,3,3,3,
3,3,3,3,3,3,3,3,3,3,3,3,3,3,3,3,3,3,3,3,3,3,4),(68.1991363933835,68.2657253634656,
68.3699115269538,68.4739424521661,68.5778513425831,68.6816947737513,68.7855075247663,
68.8893243312879,68.9932498086583,69.0972341272032,69.2014003846625,69.2632732218117,
69.3674593852998,69.4714903105119,69.5753992009287,69.6792426320967,69.7830553831116,
69.886872189633,69.9907976670033,70.094781985548,70.1989482430071,70.2608210801578,
70.3650072436461,70.4690381688584,70.5729470592755,70.6767904904437,70.7806032414588,
70.8844200479804,70.988345525351,71.0923298438958,71.1964961013552,71.2583689385038,
71.3625551019916,71.4665860272034,71.57049491762,71.6743383487877,71.7781510998022,
71.8819679063233,71.9858933836933,72.0898777022377,72.1940439596966,72.2559167968499,
72.2566310325399),.UNSPECIFIED.);
#2713=B_SPLINE_CURVE_WITH_KNOTS('',3,(#99842,#99843,#99844,#99845,#99846,
#99847,#99848,#99849,#99850,#99851,#99852,#99853,#99854,#99855,#99856,#99857,
#99858,#99859,#99860,#99861,#99862,#99863,#99864,#99865,#99866,#99867,#99868,
#99869,#99870,#99871,#99872,#99873,#99874,#99875,#99876,#99877,#99878,#99879,
#99880,#99881,#99882,#99883,#99884,#99885,#99886,#99887,#99888,#99889,#99890,
#99891,#99892,#99893,#99894,#99895,#99896,#99897,#99898,#99899,#99900,#99901,
#99902,#99903,#99904,#99905,#99906,#99907,#99908,#99909,#99910,#99911,#99912,
#99913,#99914,#99915,#99916,#99917,#99918,#99919,#99920,#99921,#99922,#99923,
#99924,#99925,#99926,#99927,#99928,#99929,#99930,#99931,#99932,#99933,#99934,
#99935,#99936,#99937,#99938,#99939,#99940,#99941,#99942,#99943,#99944,#99945,
#99946,#99947,#99948,#99949,#99950,#99951,#99952,#99953,#99954,#99955,#99956,
#99957,#99958,#99959,#99960,#99961,#99962),.UNSPECIFIED.,.F.,.F.,(4,3,3,
3,3,3,3,3,3,3,3,3,3,3,3,3,3,3,3,3,3,3,3,3,3,3,3,3,3,3,3,3,3,3,3,3,3,3,3,
3,4),(61.9168665188216,62.0208010626594,62.1246599903092,62.2284781001507,
62.3322901369026,62.4362043393257,62.540168285134,62.6443238050195,62.7365207799071,
62.8407069433951,62.944737868607,63.0486467590238,63.1524901901917,63.2563029412064,
63.3601197477278,63.464045225098,63.5680295436425,63.6721958011016,63.7340686382531,
63.8382548017414,63.9422857269537,64.0461946173708,64.1500380485391,64.2538507995541,
64.3576676060758,64.4615930834463,64.5655774019912,64.6697436594505,64.7316164965992,
64.8358026600872,64.9398335852992,65.043742475716,65.147585906884,65.2513986578988,
65.3552154644202,65.4591409417905,65.5631252603351,65.6672915177942,65.7291643549453,
65.8652061647753,65.9734457249409),.UNSPECIFIED.);
#2714=B_SPLINE_CURVE_WITH_KNOTS('',3,(#99963,#99964,#99965,#99966,#99967,
#99968,#99969,#99970,#99971,#99972,#99973,#99974,#99975,#99976,#99977,#99978,
#99979,#99980,#99981,#99982,#99983,#99984,#99985,#99986,#99987,#99988,#99989,
#99990,#99991,#99992,#99993,#99994,#99995,#99996,#99997,#99998,#99999,#100000,
#100001,#100002,#100003,#100004,#100005,#100006,#100007,#100008,#100009,
#100010,#100011,#100012,#100013,#100014,#100015,#100016,#100017,#100018,
#100019,#100020,#100021,#100022,#100023,#100024,#100025,#100026,#100027,
#100028,#100029,#100030,#100031,#100032),.UNSPECIFIED.,.F.,.F.,(4,3,3,3,
3,3,3,3,3,3,3,3,3,3,3,3,3,3,3,3,3,3,3,4),(65.9734457253856,66.07613177282,
66.1787500761624,66.2813369783481,66.3839287747712,66.4866268116111,66.5893873525251,
66.6923186639457,66.7267122132914,66.8308983767795,66.9349293019917,67.0388381924087,
67.1426816235768,67.2464943745917,67.3503111811132,67.4542366584835,67.5582209770282,
67.6623872344874,67.7242600716375,67.8284495547535,67.9324611620825,68.0363696459528,
68.14021127526,68.1995422682746),.UNSPECIFIED.);
#2715=B_SPLINE_CURVE_WITH_KNOTS('',3,(#100034,#100035,#100036,#100037,#100038,
#100039,#100040,#100041,#100042,#100043,#100044,#100045,#100046,#100047,
#100048,#100049,#100050,#100051,#100052,#100053,#100054,#100055,#100056,
#100057,#100058,#100059,#100060,#100061,#100062,#100063,#100064,#100065,
#100066,#100067,#100068,#100069,#100070,#100071,#100072,#100073,#100074,
#100075,#100076,#100077,#100078,#100079,#100080,#100081,#100082,#100083,
#100084,#100085,#100086,#100087,#100088,#100089,#100090,#100091,#100092,
#100093,#100094,#100095,#100096,#100097,#100098,#100099,#100100),
 .UNSPECIFIED.,.F.,.F.,(4,3,3,3,3,3,3,3,3,3,3,3,3,3,3,3,3,3,3,3,3,3,4),
(65.9734457257054,66.0987387055914,66.2258330924359,66.2706296467734,66.3748158102617,
66.4788467354739,66.582755625891,66.6865990570592,66.7904118080743,66.8942286145959,
66.9981540919664,67.1021384105113,67.2063046679707,67.2681775051195,67.3723684096495,
67.4763780581658,67.580285456749,67.6841254673978,67.7879328706231,67.8918030329315,
67.995700074319,68.0997567598127,68.1991363933835),.UNSPECIFIED.);
#2716=B_SPLINE_CURVE_WITH_KNOTS('',3,(#100101,#100102,#100103,#100104,#100105,
#100106,#100107,#100108,#100109,#100110,#100111,#100112,#100113,#100114,
#100115,#100116,#100117,#100118,#100119,#100120,#100121,#100122,#100123,
#100124,#100125,#100126,#100127,#100128,#100129,#100130,#100131,#100132,
#100133,#100134,#100135,#100136,#100137,#100138,#100139,#100140,#100141,
#100142,#100143,#100144,#100145,#100146,#100147,#100148,#100149,#100150,
#100151,#100152,#100153,#100154,#100155,#100156,#100157,#100158,#100159,
#100160,#100161,#100162,#100163,#100164,#100165,#100166,#100167,#100168,
#100169,#100170,#100171,#100172,#100173,#100174,#100175,#100176,#100177,
#100178,#100179,#100180,#100181,#100182,#100183,#100184,#100185,#100186,
#100187,#100188,#100189,#100190,#100191,#100192,#100193,#100194,#100195,
#100196,#100197,#100198,#100199,#100200,#100201,#100202,#100203,#100204,
#100205,#100206,#100207,#100208,#100209,#100210,#100211,#100212,#100213,
#100214,#100215,#100216,#100217,#100218,#100219,#100220,#100221,#100222,
#100223,#100224),.UNSPECIFIED.,.F.,.F.,(4,3,3,3,3,3,3,3,3,3,3,3,3,3,3,3,
3,3,3,3,3,3,3,3,3,3,3,3,3,3,3,3,3,3,3,3,3,3,3,3,3,4),(61.9158990352648,
62.0198285557511,62.1238197449305,62.2279900041556,62.2804382133891,62.3846243768772,
62.4886553020892,62.5925641925061,62.6964076236741,62.8002203746889,62.9040371812104,
63.0079626585807,63.1119469771254,63.2161132345845,63.2779860717351,63.3821722352233,
63.4862031604357,63.5901120508526,63.6939554820208,63.7977682330357,63.9015850395572,
64.0055105169275,64.1094948354721,64.2136610929314,64.2755339300812,64.3797200935694,
64.4837510187817,64.5876599091986,64.6915033403668,64.7953160913816,64.899132897903,
65.0030583752734,65.1070426938181,65.2112089512772,65.2730817884273,65.3766017373241,
65.4799760620947,65.583240636247,65.6864470474344,65.7896160420592,65.8928309399432,
65.9734457253856),.UNSPECIFIED.);
#2717=B_SPLINE_CURVE_WITH_KNOTS('',3,(#100230,#100231,#100232,#100233,#100234,
#100235,#100236,#100237,#100238,#100239,#100240,#100241,#100242,#100243,
#100244,#100245,#100246,#100247,#100248,#100249,#100250,#100251,#100252,
#100253,#100254,#100255,#100256,#100257,#100258,#100259,#100260,#100261,
#100262,#100263,#100264,#100265,#100266,#100267,#100268,#100269,#100270,
#100271,#100272,#100273,#100274,#100275,#100276,#100277,#100278,#100279,
#100280,#100281,#100282,#100283,#100284,#100285,#100286,#100287,#100288,
#100289,#100290,#100291,#100292,#100293,#100294,#100295,#100296,#100297,
#100298,#100299,#100300,#100301,#100302,#100303,#100304,#100305,#100306,
#100307,#100308,#100309,#100310,#100311,#100312,#100313,#100314,#100315,
#100316,#100317,#100318,#100319,#100320,#100321,#100322,#100323,#100324,
#100325,#100326,#100327,#100328,#100329,#100330,#100331,#100332,#100333,
#100334,#100335,#100336,#100337,#100338,#100339,#100340,#100341,#100342,
#100343,#100344,#100345,#100346,#100347,#100348,#100349,#100350,#100351,
#100352,#100353),.UNSPECIFIED.,.F.,.F.,(4,3,3,3,3,3,3,3,3,3,3,3,3,3,3,3,
3,3,3,3,3,3,3,3,3,3,3,3,3,3,3,3,3,3,3,3,3,3,3,3,3,4),(55.6326004204955,
55.7367886089557,55.7536857714844,55.8578719349727,55.961902860185,56.065811750602,
56.1696551817703,56.2734679327853,56.3772847393069,56.4812102166774,56.5851945352223,
56.6893607926816,56.7512336298305,56.8554197933186,56.9594507185306,57.0633596089474,
57.1672030401154,57.2710157911302,57.3748325976516,57.4787580750219,57.5827423935665,
57.6869086510257,57.7487814881766,57.8529676516648,57.956998576877,58.060907467294,
58.1647508984621,58.2685636494771,58.3723804559986,58.4763059333691,58.5802902519139,
58.6844565093732,58.7463293465227,58.8496743122095,58.9547475754162,59.0578171667579,
59.1608249277453,59.2638067574362,59.370420172543,59.4735201525627,59.5818902852131,
59.6902604178635),.UNSPECIFIED.);
#2718=B_SPLINE_CURVE_WITH_KNOTS('',3,(#100354,#100355,#100356,#100357,#100358,
#100359,#100360,#100361,#100362,#100363,#100364,#100365,#100366,#100367,
#100368,#100369,#100370,#100371,#100372,#100373,#100374,#100375,#100376,
#100377,#100378,#100379,#100380,#100381,#100382,#100383,#100384,#100385,
#100386,#100387,#100388,#100389,#100390,#100391,#100392,#100393,#100394,
#100395,#100396,#100397,#100398,#100399,#100400,#100401,#100402,#100403,
#100404,#100405,#100406,#100407,#100408,#100409,#100410,#100411,#100412,
#100413,#100414,#100415,#100416,#100417,#100418,#100419,#100420,#100421,
#100422,#100423),.UNSPECIFIED.,.F.,.F.,(4,3,3,3,3,3,3,3,3,3,3,3,3,3,3,3,
3,3,3,3,3,3,3,4),(59.690260418206,59.7438772048688,59.8480633683569,59.952094293569,
60.0560031839859,60.1598466151539,60.2636593661687,60.36747617269,60.4714016500603,
60.5753859686049,60.6795522260641,60.7414250632149,60.8456112267031,60.9496421519152,
61.0535510423322,61.1573944735003,61.2612072245153,61.3650240310368,61.4689495084072,
61.5729338269519,61.6771000844112,61.738972921561,61.8431345912322,61.9168665188216),
 .UNSPECIFIED.);
#2719=B_SPLINE_CURVE_WITH_KNOTS('',3,(#100425,#100426,#100427,#100428,#100429,
#100430,#100431,#100432,#100433,#100434,#100435,#100436,#100437,#100438,
#100439,#100440,#100441,#100442,#100443,#100444,#100445,#100446,#100447,
#100448,#100449,#100450,#100451,#100452,#100453,#100454,#100455,#100456,
#100457,#100458,#100459,#100460,#100461,#100462,#100463,#100464,#100465,
#100466,#100467,#100468,#100469,#100470,#100471,#100472,#100473,#100474,
#100475,#100476,#100477,#100478,#100479,#100480,#100481,#100482,#100483,
#100484,#100485,#100486,#100487,#100488,#100489,#100490,#100491),
 .UNSPECIFIED.,.F.,.F.,(4,3,3,3,3,3,3,3,3,3,3,3,3,3,3,3,3,3,3,3,3,3,4),
(59.690260418206,59.7955628120765,59.9009059652381,60.0064057077467,60.1119895277649,
60.2177899509138,60.2853424966969,60.3895286601851,60.4935595853973,60.5974684758143,
60.7013119069824,60.8051246579975,60.9089414645192,61.0128669418897,61.1168512604345,
61.2210175178938,61.282890355043,61.3870598977049,61.4910835289864,61.597287405556,
61.7011272946116,61.8085131649381,61.9158990352648),.UNSPECIFIED.);
#2720=B_SPLINE_CURVE_WITH_KNOTS('',3,(#100492,#100493,#100494,#100495,#100496,
#100497,#100498,#100499,#100500,#100501,#100502,#100503,#100504,#100505,
#100506,#100507,#100508,#100509,#100510,#100511,#100512,#100513,#100514,
#100515,#100516,#100517,#100518,#100519,#100520,#100521,#100522,#100523,
#100524,#100525,#100526,#100527,#100528,#100529,#100530,#100531,#100532,
#100533,#100534,#100535,#100536,#100537,#100538,#100539,#100540,#100541,
#100542,#100543,#100544,#100545,#100546,#100547,#100548,#100549,#100550,
#100551,#100552,#100553,#100554,#100555,#100556,#100557,#100558,#100559,
#100560,#100561,#100562,#100563,#100564,#100565,#100566,#100567,#100568,
#100569,#100570,#100571,#100572,#100573,#100574,#100575,#100576,#100577,
#100578,#100579,#100580,#100581,#100582,#100583,#100584,#100585,#100586,
#100587,#100588,#100589,#100590,#100591,#100592,#100593,#100594,#100595,
#100596,#100597,#100598,#100599,#100600,#100601,#100602,#100603,#100604,
#100605,#100606,#100607,#100608,#100609,#100610,#100611,#100612,#100613,
#100614,#100615),.UNSPECIFIED.,.F.,.F.,(4,3,3,3,3,3,3,3,3,3,3,3,3,3,3,3,
3,3,3,3,3,3,3,3,3,3,3,3,3,3,3,3,3,3,3,3,3,3,3,3,3,4),(55.6335493650217,
55.7373826885747,55.8411933008923,55.945015932593,56.0489521376303,56.1529543401164,
56.2571313359375,56.2951510633125,56.3993372268005,56.5033681520124,56.6072770424293,
56.7111204735973,56.8149332246122,56.9187500311337,57.022675508504,57.1266598270485,
57.2308260845077,57.2926989216586,57.3968850851468,57.500916010359,57.604824900776,
57.7086683319441,57.812481082959,57.9162978894807,58.0202233668511,58.124207685396,
58.2283739428553,58.2902467800047,58.3944329434927,58.4984638687049,58.6023727591218,
58.7062161902899,58.8100289413047,58.9138457478264,59.0177712251967,59.1217555437412,
59.2259218012003,59.2877946383508,59.4032420886146,59.5183215991923,59.6327919924132,
59.690260417799),.UNSPECIFIED.);
#2721=B_SPLINE_CURVE_WITH_KNOTS('',3,(#100621,#100622,#100623,#100624,#100625,
#100626,#100627,#100628,#100629,#100630,#100631,#100632,#100633,#100634,
#100635,#100636,#100637,#100638,#100639,#100640,#100641,#100642,#100643,
#100644,#100645,#100646,#100647,#100648,#100649,#100650,#100651,#100652,
#100653,#100654,#100655,#100656,#100657,#100658,#100659,#100660,#100661,
#100662,#100663,#100664,#100665,#100666,#100667,#100668,#100669,#100670,
#100671,#100672,#100673,#100674,#100675,#100676,#100677,#100678,#100679,
#100680,#100681,#100682,#100683,#100684,#100685,#100686,#100687,#100688,
#100689,#100690,#100691,#100692,#100693,#100694,#100695,#100696,#100697,
#100698,#100699,#100700,#100701,#100702,#100703,#100704,#100705,#100706,
#100707,#100708,#100709,#100710,#100711,#100712,#100713,#100714,#100715,
#100716,#100717,#100718,#100719,#100720,#100721,#100722,#100723,#100724,
#100725,#100726,#100727,#100728,#100729,#100730,#100731,#100732,#100733,
#100734,#100735,#100736,#100737,#100738,#100739,#100740,#100741,#100742,
#100743,#100744),.UNSPECIFIED.,.F.,.F.,(4,3,3,3,3,3,3,3,3,3,3,3,3,3,3,3,
3,3,3,3,3,3,3,3,3,3,3,3,3,3,3,3,3,3,3,3,3,3,3,3,3,4),(49.3496724239637,
49.4543539733247,49.5583095592452,49.6633540903265,49.7683986214079,49.8725847848961,
49.9766157101083,50.0805246005253,50.1843680316935,50.2881807827085,50.3919975892302,
50.4959230666006,50.5999073851454,50.7040736426047,50.765946479754,50.8701326432421,
50.9741635684544,51.0780724588712,51.1819158900393,51.2857286410541,51.3895454475756,
51.493470924946,51.5974552434907,51.7016215009499,51.7634943381001,51.8676805015883,
51.9717114268001,52.0756203172171,52.1794637483852,52.2832764994001,52.387093305922,
52.4910187832923,52.5950031018368,52.699169359296,52.7610421964462,52.86555091267,
52.9699037514327,53.0791965913311,53.1833373805671,53.2874304651186,53.3915238347397,
53.4070751110264),.UNSPECIFIED.);
#2722=B_SPLINE_CURVE_WITH_KNOTS('',3,(#100745,#100746,#100747,#100748,#100749,
#100750,#100751,#100752,#100753,#100754,#100755,#100756,#100757,#100758,
#100759,#100760,#100761,#100762,#100763,#100764,#100765,#100766,#100767,
#100768,#100769,#100770,#100771,#100772,#100773,#100774,#100775,#100776,
#100777,#100778,#100779,#100780,#100781,#100782,#100783,#100784,#100785,
#100786,#100787,#100788,#100789,#100790,#100791,#100792,#100793,#100794,
#100795,#100796,#100797,#100798,#100799,#100800,#100801,#100802,#100803,
#100804,#100805,#100806,#100807,#100808,#100809,#100810,#100811),
 .UNSPECIFIED.,.F.,.F.,(4,3,3,3,3,3,3,3,3,3,3,3,3,3,3,3,3,3,3,3,3,3,4),
(53.407075111473,53.5259953052066,53.6459937542086,53.7585900547923,53.8627762182803,
53.9668071434923,54.070716033909,54.174559465077,54.2783722160917,54.3821890226131,
54.4861144999833,54.5900988185279,54.6942650759869,54.7561379131384,54.865695726558,
54.9697002450198,55.0736027363077,55.1774380610522,55.2812409980219,55.3850920226149,
55.4889708980885,55.5929698529969,55.6326004204955),.UNSPECIFIED.);
#2723=B_SPLINE_CURVE_WITH_KNOTS('',3,(#100813,#100814,#100815,#100816,#100817,
#100818,#100819,#100820,#100821,#100822,#100823,#100824,#100825,#100826,
#100827,#100828,#100829,#100830,#100831,#100832,#100833,#100834,#100835,
#100836,#100837,#100838,#100839,#100840,#100841,#100842,#100843,#100844,
#100845,#100846,#100847,#100848,#100849,#100850,#100851,#100852,#100853,
#100854,#100855,#100856,#100857,#100858,#100859,#100860,#100861,#100862,
#100863,#100864,#100865,#100866,#100867,#100868,#100869,#100870,#100871,
#100872,#100873,#100874,#100875,#100876,#100877,#100878,#100879,#100880,
#100881,#100882),.UNSPECIFIED.,.F.,.F.,(4,3,3,3,3,3,3,3,3,3,3,3,3,3,3,3,
3,3,3,3,3,3,3,4),(53.4070751114826,53.509861491319,53.6124973139519,53.7150505550788,
53.8175576893182,53.9200551251618,54.0226483900881,54.1252912590518,54.2281147116727,
54.3000553466204,54.4042415101085,54.5082724353208,54.6121813257378,54.7160247569059,
54.8198375079208,54.9236543144423,55.0275797918127,55.1315641103575,55.2357303678167,
55.2976032049664,55.4017686798842,55.5057980075404,55.609707175149,55.6335493650217),
 .UNSPECIFIED.);
#2724=B_SPLINE_CURVE_WITH_KNOTS('',3,(#100883,#100884,#100885,#100886,#100887,
#100888,#100889,#100890,#100891,#100892,#100893,#100894,#100895,#100896,
#100897,#100898,#100899,#100900,#100901,#100902,#100903,#100904,#100905,
#100906,#100907,#100908,#100909,#100910,#100911,#100912,#100913,#100914,
#100915,#100916,#100917,#100918,#100919,#100920,#100921,#100922,#100923,
#100924,#100925,#100926,#100927,#100928,#100929,#100930,#100931,#100932,
#100933,#100934,#100935,#100936,#100937,#100938,#100939,#100940,#100941,
#100942,#100943,#100944,#100945,#100946,#100947,#100948,#100949,#100950,
#100951,#100952,#100953,#100954,#100955,#100956,#100957,#100958,#100959,
#100960,#100961,#100962,#100963,#100964,#100965,#100966,#100967,#100968,
#100969,#100970,#100971,#100972,#100973,#100974,#100975,#100976,#100977,
#100978,#100979,#100980,#100981,#100982,#100983,#100984,#100985,#100986,
#100987,#100988,#100989,#100990,#100991,#100992,#100993,#100994,#100995,
#100996,#100997,#100998,#100999,#101000,#101001,#101002,#101003,#101004,
#101005,#101006),.UNSPECIFIED.,.F.,.F.,(4,3,3,3,3,3,3,3,3,3,3,3,3,3,3,3,
3,3,3,3,3,3,3,3,3,3,3,3,3,3,3,3,3,3,3,3,3,3,3,3,3,4),(49.3501218890484,
49.4542472707228,49.5611993510369,49.6650784833371,49.7689057717339,49.8727159741616,
49.9820029589302,50.0859506809055,50.1899710955183,50.2941599634125,50.309863913236,
50.4140500767242,50.5180810019363,50.6219898923533,50.7258333235213,50.8296460745363,
50.9334628810577,51.0373883584281,51.1413726769728,51.2455389344321,51.3074117715821,
51.4115979350702,51.5156288602823,51.6195377506992,51.7233811818673,51.8271939328822,
51.9310107394036,52.0349362167739,52.1389205353186,52.2430867927778,52.3049596299282,
52.4091457934165,52.5131767186289,52.6170856090461,52.7209290402144,52.8247417912295,
52.9285585977512,53.0324840751217,53.1364683936667,53.2406346511261,53.3025074882743,
53.4070751110264),.UNSPECIFIED.);
#2725=B_SPLINE_CURVE_WITH_KNOTS('',3,(#101012,#101013,#101014,#101015,#101016,
#101017,#101018,#101019,#101020,#101021,#101022,#101023,#101024,#101025,
#101026,#101027,#101028,#101029,#101030,#101031,#101032,#101033,#101034,
#101035,#101036,#101037,#101038,#101039,#101040,#101041,#101042,#101043,
#101044,#101045,#101046,#101047,#101048,#101049,#101050,#101051,#101052,
#101053,#101054,#101055,#101056,#101057,#101058,#101059,#101060,#101061,
#101062,#101063,#101064,#101065,#101066,#101067,#101068,#101069,#101070,
#101071,#101072,#101073,#101074,#101075,#101076,#101077,#101078,#101079,
#101080,#101081,#101082,#101083,#101084,#101085,#101086,#101087,#101088,
#101089,#101090,#101091,#101092,#101093,#101094,#101095,#101096,#101097,
#101098,#101099,#101100,#101101,#101102,#101103,#101104,#101105,#101106,
#101107,#101108,#101109,#101110,#101111,#101112,#101113,#101114,#101115,
#101116,#101117,#101118,#101119,#101120,#101121,#101122,#101123,#101124,
#101125,#101126,#101127,#101128,#101129,#101130,#101131,#101132),
 .UNSPECIFIED.,.F.,.F.,(4,3,3,3,3,3,3,3,3,3,3,3,3,3,3,3,3,3,3,3,3,3,3,3,
3,3,3,3,3,3,3,3,3,3,3,3,3,3,3,3,4),(43.0672730856169,43.1711320797731,43.2749502164102,
43.3787622402884,43.4826764037649,43.5866402750026,43.6907957592589,43.7831114713314,
43.8872976348198,43.991328560032,44.0952374504493,44.1990808816178,44.3028936326331,
44.406710439155,44.5106359165257,44.6146202350708,44.7187864925303,44.7806593296775,
44.8848454931656,44.9888764183774,45.0927853087944,45.1966287399625,45.3004414909774,
45.4042582974991,45.5081837748694,45.6121680934142,45.7163343508734,45.7782071880236,
45.8823933515121,45.9864242767244,46.0903331671415,46.1941765983097,46.2979893493246,
46.401806155846,46.5057316332165,46.6097159517615,46.7138822092208,46.7757550463697,
46.8962986192121,47.0157785770578,47.123889803403),.UNSPECIFIED.);
#2726=B_SPLINE_CURVE_WITH_KNOTS('',3,(#101133,#101134,#101135,#101136,#101137,
#101138,#101139,#101140,#101141,#101142,#101143,#101144,#101145,#101146,
#101147,#101148,#101149,#101150,#101151,#101152,#101153,#101154,#101155,
#101156,#101157,#101158,#101159,#101160,#101161,#101162,#101163,#101164,
#101165,#101166,#101167,#101168,#101169,#101170,#101171,#101172,#101173,
#101174,#101175,#101176,#101177,#101178,#101179,#101180,#101181,#101182,
#101183,#101184,#101185,#101186,#101187,#101188,#101189,#101190,#101191,
#101192,#101193,#101194,#101195,#101196,#101197,#101198,#101199,#101200,
#101201,#101202),.UNSPECIFIED.,.F.,.F.,(4,3,3,3,3,3,3,3,3,3,3,3,3,3,3,3,
3,3,3,3,3,3,3,4),(47.1238898038469,47.227928135533,47.3319603652871,47.4360206698583,
47.540212755665,47.6444838895238,47.7489375131569,47.7733029047158,47.8774890682039,
47.981519993416,48.0854288838329,48.1892723150009,48.2930850660158,48.3969018725371,
48.5008273499074,48.604811668452,48.7089779259112,48.7708507630618,48.8750265339919,
48.9790548148166,49.0829625294207,49.1867995822529,49.290619011578,49.3496724239637),
 .UNSPECIFIED.);
#2727=B_SPLINE_CURVE_WITH_KNOTS('',3,(#101204,#101205,#101206,#101207,#101208,
#101209,#101210,#101211,#101212,#101213,#101214,#101215,#101216,#101217,
#101218,#101219,#101220,#101221,#101222,#101223,#101224,#101225,#101226,
#101227,#101228,#101229,#101230,#101231,#101232,#101233,#101234,#101235,
#101236,#101237,#101238,#101239,#101240,#101241,#101242,#101243,#101244,
#101245,#101246,#101247,#101248,#101249,#101250,#101251,#101252,#101253,
#101254,#101255,#101256,#101257,#101258,#101259,#101260,#101261,#101262,
#101263,#101264,#101265,#101266,#101267,#101268,#101269,#101270,#101271,
#101272,#101273),.UNSPECIFIED.,.F.,.F.,(4,3,3,3,3,3,3,3,3,3,3,3,3,3,3,3,
3,3,3,3,3,3,3,4),(47.1238898038468,47.2754958858741,47.3172203381978,47.4214065016859,
47.5254374268981,47.629346317315,47.7331897484832,47.8370024994981,47.9408193060197,
48.0447447833901,48.1487291019349,48.2528953593942,48.3147681965438,48.4189543600319,
48.5229852852439,48.6268941756608,48.7307376068288,48.8345503578437,48.9383671643651,
49.0422926417354,49.14627696028,49.2504432177392,49.3123160548899,49.3501218890484),
 .UNSPECIFIED.);
#2728=B_SPLINE_CURVE_WITH_KNOTS('',3,(#101274,#101275,#101276,#101277,#101278,
#101279,#101280,#101281,#101282,#101283,#101284,#101285,#101286,#101287,
#101288,#101289,#101290,#101291,#101292,#101293,#101294,#101295,#101296,
#101297,#101298,#101299,#101300,#101301,#101302,#101303,#101304,#101305,
#101306,#101307,#101308,#101309,#101310,#101311,#101312,#101313,#101314,
#101315,#101316,#101317,#101318,#101319,#101320,#101321,#101322,#101323,
#101324,#101325,#101326,#101327,#101328,#101329,#101330,#101331,#101332,
#101333,#101334,#101335,#101336,#101337,#101338,#101339,#101340,#101341,
#101342,#101343,#101344,#101345,#101346,#101347,#101348,#101349,#101350,
#101351,#101352,#101353,#101354,#101355,#101356,#101357,#101358,#101359,
#101360,#101361,#101362,#101363,#101364,#101365,#101366,#101367,#101368,
#101369,#101370,#101371,#101372,#101373,#101374,#101375,#101376,#101377,
#101378,#101379,#101380,#101381,#101382,#101383,#101384,#101385,#101386,
#101387,#101388,#101389,#101390,#101391,#101392,#101393,#101394,#101395,
#101396,#101397),.UNSPECIFIED.,.F.,.F.,(4,3,3,3,3,3,3,3,3,3,3,3,3,3,3,3,
3,3,3,3,3,3,3,3,3,3,3,3,3,3,3,3,3,3,3,3,3,3,3,3,3,4),(43.0661596755458,
43.1701506718428,43.2743208164948,43.3270289048134,43.4312150683038,43.5352459935183,
43.6391548839376,43.7429983151081,43.8468110661254,43.9506278726493,44.0545533500222,
44.1585376685693,44.262703926031,44.3245767631595,44.4287629266472,44.5327938518589,
44.6367027422754,44.740546173443,44.8443589244575,44.9481757309785,45.0521012083484,
45.1560855268927,45.2602517843515,45.3221246215056,45.4263107849935,45.5303417102053,
45.6342506006219,45.7380940317896,45.8419067828042,45.9457235893253,46.0496490666953,
46.1536333852397,46.2577996426985,46.3196724798517,46.4223012412911,46.5247935864412,
46.6271863644381,46.7295162801918,46.8318649061915,46.9342176129136,47.0366904241956,
47.1238898034296),.UNSPECIFIED.);
#2729=B_SPLINE_CURVE_WITH_KNOTS('',3,(#101403,#101404,#101405,#101406,#101407,
#101408,#101409,#101410,#101411,#101412,#101413,#101414,#101415,#101416,
#101417,#101418,#101419,#101420,#101421,#101422,#101423,#101424,#101425,
#101426,#101427,#101428,#101429,#101430,#101431,#101432,#101433,#101434,
#101435,#101436,#101437,#101438,#101439,#101440,#101441,#101442,#101443,
#101444,#101445,#101446,#101447,#101448,#101449,#101450,#101451,#101452,
#101453,#101454,#101455,#101456,#101457,#101458,#101459,#101460,#101461,
#101462,#101463,#101464,#101465,#101466,#101467,#101468,#101469,#101470,
#101471,#101472,#101473,#101474,#101475,#101476,#101477,#101478,#101479,
#101480,#101481,#101482,#101483,#101484,#101485,#101486,#101487,#101488,
#101489,#101490,#101491,#101492,#101493,#101494,#101495,#101496,#101497,
#101498,#101499,#101500,#101501,#101502,#101503,#101504,#101505,#101506,
#101507,#101508,#101509,#101510,#101511,#101512,#101513,#101514,#101515,
#101516,#101517,#101518,#101519,#101520,#101521,#101522,#101523,#101524,
#101525,#101526,#101527,#101528,#101529),.UNSPECIFIED.,.F.,.F.,(4,3,3,3,
3,3,3,3,3,3,3,3,3,3,3,3,3,3,3,3,3,3,3,3,3,3,3,3,3,3,3,3,3,3,3,3,3,3,3,3,
3,3,4),(36.7834442042422,36.8002764629088,36.904462626368,37.0084935515507,
37.1124024419373,37.2162458730747,37.3200586240585,37.4238754305485,37.5278009078871,
37.6317852263998,37.735951483827,37.7978243212549,37.9020104847617,38.0060414099928,
38.1099503004289,38.2137937316164,38.317606482651,38.4214232891922,38.5253487665823,
38.6293330851469,38.7334993426258,38.795372179601,38.8995583430862,39.0035892682954,
39.1074981587095,39.2113415898747,39.3151543408867,39.4189711474052,39.5228966247728,
39.6268809433147,39.7310472007711,39.7929200379471,39.8971062014322,40.0011371266412,
40.1050460170549,40.2088894482198,40.3127021992315,40.4165190057495,40.5204444831166,
40.624428801658,40.7285950591138,40.7904678962932,40.8407044966673),
 .UNSPECIFIED.);
#2730=B_SPLINE_CURVE_WITH_KNOTS('',3,(#101530,#101531,#101532,#101533,#101534,
#101535,#101536,#101537,#101538,#101539,#101540,#101541,#101542,#101543,
#101544,#101545,#101546,#101547,#101548,#101549,#101550,#101551,#101552,
#101553,#101554,#101555,#101556,#101557,#101558,#101559,#101560,#101561,
#101562,#101563,#101564,#101565,#101566,#101567,#101568,#101569,#101570,
#101571,#101572,#101573,#101574,#101575,#101576,#101577,#101578,#101579,
#101580,#101581,#101582,#101583,#101584,#101585,#101586,#101587,#101588,
#101589,#101590,#101591,#101592,#101593,#101594,#101595,#101596,#101597,
#101598,#101599),.UNSPECIFIED.,.F.,.F.,(4,3,3,3,3,3,3,3,3,3,3,3,3,3,3,3,
3,3,3,3,3,3,3,4),(40.8407044970018,40.9440746115614,41.0495672544461,41.1526720053859,
41.2557188072278,41.3587435025102,41.4660615655424,41.5692147500828,41.6724388016563,
41.7758284060282,41.7880157546392,41.8922019181269,41.9962328433386,42.1001417337551,
42.2039851649228,42.3077979159374,42.4116147224584,42.5155401998284,42.6195245183727,
42.7236907758316,42.7855636129853,42.8897412732137,42.9937540523187,43.0672730856169),
 .UNSPECIFIED.);
#2731=B_SPLINE_CURVE_WITH_KNOTS('',3,(#101601,#101602,#101603,#101604,#101605,
#101606,#101607,#101608,#101609,#101610,#101611,#101612,#101613,#101614,
#101615,#101616,#101617,#101618,#101619,#101620,#101621,#101622,#101623,
#101624,#101625,#101626,#101627,#101628,#101629,#101630,#101631,#101632,
#101633,#101634,#101635,#101636,#101637,#101638,#101639,#101640,#101641,
#101642,#101643,#101644,#101645,#101646,#101647,#101648,#101649,#101650,
#101651,#101652,#101653,#101654,#101655,#101656,#101657,#101658,#101659,
#101660,#101661,#101662,#101663,#101664,#101665,#101666,#101667),
 .UNSPECIFIED.,.F.,.F.,(4,3,3,3,3,3,3,3,3,3,3,3,3,3,3,3,3,3,3,3,3,3,4),
(40.8407044969849,40.9497796083558,41.0591756422725,41.1687426604111,41.2786112447405,
41.3319331881212,41.4361193516065,41.5401502768156,41.6440591672296,41.7479025983948,
41.8517153494068,41.9555321559254,42.059457633293,42.1634419518349,42.2676082092914,
42.3294810464673,42.4336404893567,42.5376570390707,42.6415657001877,42.7477141940272,
42.8515321201983,42.9588458978721,43.0661596755458),.UNSPECIFIED.);
#2732=B_SPLINE_CURVE_WITH_KNOTS('',3,(#101668,#101669,#101670,#101671,#101672,
#101673,#101674,#101675,#101676,#101677,#101678,#101679,#101680,#101681,
#101682,#101683,#101684,#101685,#101686,#101687,#101688,#101689,#101690,
#101691,#101692,#101693,#101694,#101695,#101696,#101697,#101698,#101699,
#101700,#101701,#101702,#101703,#101704,#101705,#101706,#101707,#101708,
#101709,#101710,#101711,#101712,#101713,#101714,#101715,#101716,#101717,
#101718,#101719,#101720,#101721,#101722,#101723,#101724,#101725,#101726,
#101727,#101728,#101729,#101730,#101731,#101732,#101733,#101734,#101735,
#101736,#101737,#101738,#101739,#101740,#101741,#101742,#101743,#101744,
#101745,#101746,#101747,#101748,#101749,#101750,#101751,#101752,#101753,
#101754,#101755,#101756,#101757,#101758,#101759,#101760,#101761,#101762,
#101763,#101764,#101765,#101766,#101767,#101768,#101769,#101770,#101771,
#101772,#101773,#101774,#101775,#101776,#101777,#101778,#101779,#101780,
#101781,#101782,#101783,#101784,#101785,#101786,#101787,#101788,#101789,
#101790,#101791),.UNSPECIFIED.,.F.,.F.,(4,3,3,3,3,3,3,3,3,3,3,3,3,3,3,3,
3,3,3,3,3,3,3,3,3,3,3,3,3,3,3,3,3,3,3,3,3,3,3,3,3,4),(36.7837239633391,
36.8875345883055,36.9913571492279,37.0952932330975,37.1992952394363,37.3034721119993,
37.3417417547369,37.4459279183704,37.5499588437299,37.6538677342964,37.7577111656155,
37.8615239167826,37.9653407234571,38.0692662009808,38.1732505196793,38.2774167772912,
38.339289613083,38.4434757765587,38.5475067017587,38.6514155921638,38.7552590233201,
38.8590717743235,38.9628885808337,39.0668140581934,39.1707983767275,39.2749646341767,
39.3368374714291,39.4410236348886,39.5450545600716,39.6489634504586,39.7528068815964,
39.8566196325803,39.960436439071,40.0643619164099,40.1683462349231,40.2725124923507,
40.3343853297751,40.4435562694802,40.5524208008269,40.6611016632894,40.7695577702461,
40.8407044966673),.UNSPECIFIED.);
#2733=B_SPLINE_CURVE_WITH_KNOTS('',3,(#101797,#101798,#101799,#101800,#101801,
#101802,#101803,#101804,#101805,#101806,#101807,#101808,#101809,#101810,
#101811,#101812,#101813,#101814,#101815,#101816,#101817,#101818,#101819,
#101820,#101821,#101822,#101823,#101824,#101825,#101826,#101827,#101828,
#101829,#101830,#101831,#101832,#101833,#101834,#101835,#101836,#101837,
#101838,#101839,#101840,#101841,#101842,#101843,#101844,#101845,#101846,
#101847,#101848,#101849,#101850,#101851,#101852,#101853,#101854,#101855,
#101856,#101857,#101858,#101859,#101860,#101861,#101862,#101863,#101864,
#101865,#101866,#101867,#101868,#101869,#101870,#101871,#101872,#101873,
#101874,#101875,#101876,#101877,#101878,#101879,#101880,#101881,#101882,
#101883,#101884,#101885,#101886,#101887,#101888,#101889,#101890,#101891,
#101892,#101893,#101894,#101895,#101896,#101897,#101898,#101899,#101900,
#101901,#101902,#101903,#101904,#101905,#101906,#101907,#101908,#101909,
#101910,#101911,#101912,#101913,#101914,#101915,#101916,#101917,#101918,
#101919,#101920),.UNSPECIFIED.,.F.,.F.,(4,3,3,3,3,3,3,3,3,3,3,3,3,3,3,3,
3,3,3,3,3,3,3,3,3,3,3,3,3,3,3,3,3,3,3,3,3,3,3,3,3,4),(30.4998665211569,
30.6038214745698,30.7094053937011,30.8149893128323,30.9191754738923,31.0232063966314,
31.1271152845205,31.2309587131284,31.3347714615544,31.4385882654618,31.5425137401983,
31.6464980560938,31.7506643109082,31.8125371711784,31.916723335786,32.0207542621321,
32.1246631536991,32.2285065860268,32.3323193382088,32.4361361459029,32.5400616244471,
32.6440459441679,32.7482122027941,32.8100850295245,32.9142711930052,33.0183021182129,
33.1222110086303,33.2260544398016,33.3298671908228,33.4336839973533,33.5376094747372,
33.641593793298,33.7457600507772,33.8076328878705,33.9105733956088,34.0133739392451,
34.1160710646413,34.2187011756074,34.3213305266006,34.4239607110272,34.5266703118465,
34.5575191894877),.UNSPECIFIED.);
#2734=B_SPLINE_CURVE_WITH_KNOTS('',3,(#101921,#101922,#101923,#101924,#101925,
#101926,#101927,#101928,#101929,#101930,#101931,#101932,#101933,#101934,
#101935,#101936,#101937,#101938,#101939,#101940,#101941,#101942,#101943,
#101944,#101945,#101946,#101947,#101948,#101949,#101950,#101951,#101952,
#101953,#101954,#101955,#101956,#101957,#101958,#101959,#101960,#101961,
#101962,#101963,#101964,#101965,#101966,#101967,#101968,#101969,#101970,
#101971,#101972,#101973,#101974,#101975,#101976,#101977,#101978,#101979,
#101980,#101981,#101982,#101983,#101984,#101985,#101986,#101987),
 .UNSPECIFIED.,.F.,.F.,(4,3,3,3,3,3,3,3,3,3,3,3,3,3,3,3,3,3,3,3,3,3,4),
(34.5575191897883,34.6927956482503,34.8051807462166,34.9093669098508,35.0133978352109,
35.1173067257782,35.221150157098,35.3249629082657,35.4287797149408,35.5327051924652,
35.6366895111642,35.7408557687768,35.8027286045627,35.9069159432592,36.0109477009195,
36.1148561160984,36.2186985866371,36.3225098919277,36.4263247672698,36.5302426811341,
36.6342192371332,36.7383648916943,36.7834442042422),.UNSPECIFIED.);
#2735=B_SPLINE_CURVE_WITH_KNOTS('',3,(#101989,#101990,#101991,#101992,#101993,
#101994,#101995,#101996,#101997,#101998,#101999,#102000,#102001,#102002,
#102003,#102004,#102005,#102006,#102007,#102008,#102009,#102010,#102011,
#102012,#102013,#102014,#102015,#102016,#102017,#102018,#102019,#102020,
#102021,#102022,#102023,#102024,#102025,#102026,#102027,#102028,#102029,
#102030,#102031,#102032,#102033,#102034,#102035,#102036,#102037,#102038,
#102039,#102040,#102041,#102042,#102043,#102044,#102045,#102046,#102047,
#102048,#102049,#102050,#102051,#102052,#102053,#102054,#102055,#102056,
#102057,#102058),.UNSPECIFIED.,.F.,.F.,(4,3,3,3,3,3,3,3,3,3,3,3,3,3,3,3,
3,3,3,3,3,3,3,4),(34.557519189755,34.6600261052919,34.7624492426958,34.8648252095896,
34.9671905447845,35.0696506740705,35.1721598073025,35.274848931505,35.3466460380447,
35.4508322015257,35.5548631267338,35.6587720171514,35.7626154483231,35.8664281993446,
35.9702450058755,36.0741704832597,36.1781548018206,36.2823210593,36.3441938963908,
36.44838866619,36.5524031618947,36.6563141161565,36.7601506302188,36.7837239633391),
 .UNSPECIFIED.);
#2736=B_SPLINE_CURVE_WITH_KNOTS('',3,(#102059,#102060,#102061,#102062,#102063,
#102064,#102065,#102066,#102067,#102068,#102069,#102070,#102071,#102072,
#102073,#102074,#102075,#102076,#102077,#102078,#102079,#102080,#102081,
#102082,#102083,#102084,#102085,#102086,#102087,#102088,#102089,#102090,
#102091,#102092,#102093,#102094,#102095,#102096,#102097,#102098,#102099,
#102100,#102101,#102102,#102103,#102104,#102105,#102106,#102107,#102108,
#102109,#102110,#102111,#102112,#102113,#102114,#102115,#102116,#102117,
#102118,#102119,#102120,#102121,#102122,#102123,#102124,#102125,#102126,
#102127,#102128,#102129,#102130,#102131,#102132,#102133,#102134,#102135,
#102136,#102137,#102138,#102139,#102140,#102141,#102142,#102143,#102144,
#102145,#102146,#102147,#102148,#102149,#102150,#102151,#102152,#102153,
#102154,#102155,#102156,#102157,#102158,#102159,#102160,#102161,#102162,
#102163,#102164,#102165,#102166,#102167,#102168,#102169,#102170,#102171,
#102172,#102173,#102174,#102175,#102176,#102177,#102178,#102179,#102180,
#102181,#102182),.UNSPECIFIED.,.F.,.F.,(4,3,3,3,3,3,3,3,3,3,3,3,3,3,3,3,
3,3,3,3,3,3,3,3,3,3,3,3,3,3,3,3,3,3,3,3,3,3,3,3,3,4),(30.5008971260263,
30.6078418108556,30.7117208864184,30.8155481351692,30.9193583150517,31.0286323874539,
31.1325801077697,31.2366005323038,31.3407893994026,31.3564546046604,31.4606407764442,
31.5646717100508,31.6685806089678,31.7724240486963,31.8762368083192,31.9800536234836,
32.0839791094901,32.1879634366803,32.2921297027055,32.3540024630065,32.4581886272383,
32.5622195532328,32.6661284444861,32.7699718765233,32.8737846284391,32.977601435892,
33.0815269142341,33.1855112337748,33.2896774922579,33.3515503213525,33.45573648242,
33.5597674051667,33.6636762930636,33.7675197216792,33.8713324701132,33.9751492740289,
34.0790747487735,34.1830590646772,34.2872253194997,34.3490981796986,34.4951131604689,
34.5575191894876),.UNSPECIFIED.);
#2737=B_SPLINE_CURVE_WITH_KNOTS('',3,(#102188,#102189,#102190,#102191,#102192,
#102193,#102194,#102195,#102196,#102197,#102198,#102199,#102200,#102201,
#102202,#102203,#102204,#102205,#102206,#102207,#102208,#102209,#102210,
#102211,#102212,#102213,#102214,#102215,#102216,#102217,#102218,#102219,
#102220,#102221,#102222,#102223,#102224,#102225,#102226,#102227,#102228,
#102229,#102230,#102231,#102232,#102233,#102234,#102235,#102236,#102237,
#102238,#102239,#102240,#102241,#102242,#102243,#102244,#102245,#102246,
#102247,#102248,#102249,#102250,#102251,#102252,#102253,#102254,#102255,
#102256,#102257,#102258,#102259,#102260,#102261,#102262,#102263,#102264,
#102265,#102266,#102267,#102268,#102269,#102270,#102271,#102272,#102273,
#102274,#102275,#102276,#102277,#102278,#102279,#102280,#102281,#102282,
#102283,#102284,#102285,#102286,#102287,#102288,#102289,#102290,#102291,
#102292,#102293,#102294,#102295,#102296,#102297,#102298,#102299,#102300,
#102301,#102302,#102303,#102304,#102305,#102306,#102307,#102308),
 .UNSPECIFIED.,.F.,.F.,(4,3,3,3,3,3,3,3,3,3,3,3,3,3,3,3,3,3,3,3,3,3,3,3,
3,3,3,3,3,3,3,3,3,3,3,3,3,3,3,3,4),(24.2175053922168,24.3213237512326,24.4251359274773,
24.529050198678,24.6330141142592,24.7371697158236,24.8297021627558,24.9338881433276,
25.0379188825363,25.1418275832654,25.2456708225743,25.3494833798447,25.4532999910205,
25.5572252719414,25.6612093931172,25.7653754538915,25.8272500211019,25.9314362441109,
26.0354672294637,26.1393761806463,26.2432196729321,26.3470324853247,26.4508493533922,
26.5547748921389,26.6587592720567,26.762925590215,26.8247978794479,26.9289840556603,
27.0330149940174,27.1369238981433,27.2407673433612,27.3445801087465,27.4483969299387,
27.5523224223397,27.6563067561414,27.7604730290516,27.822345737794,27.9353427738055,
28.0470528540771,28.1606933679585,28.27433388184),.UNSPECIFIED.);
#2738=B_SPLINE_CURVE_WITH_KNOTS('',3,(#102309,#102310,#102311,#102312,#102313,
#102314,#102315,#102316,#102317,#102318,#102319,#102320,#102321,#102322,
#102323,#102324,#102325,#102326,#102327,#102328,#102329,#102330,#102331,
#102332,#102333,#102334,#102335,#102336,#102337,#102338,#102339,#102340,
#102341,#102342,#102343,#102344,#102345,#102346,#102347,#102348,#102349,
#102350,#102351,#102352,#102353,#102354,#102355,#102356,#102357,#102358,
#102359,#102360,#102361,#102362,#102363,#102364,#102365,#102366,#102367,
#102368,#102369,#102370,#102371,#102372,#102373,#102374,#102375),
 .UNSPECIFIED.,.F.,.F.,(4,3,3,3,3,3,3,3,3,3,3,3,3,3,3,3,3,3,3,3,3,3,4),
(28.2743338823081,28.3811858746811,28.4908628050458,28.598029113806,28.7089613549731,
28.8198935961401,28.9240797679517,29.0281107015868,29.1320196005323,29.2358630402896,
29.3396757999416,29.4434926151352,29.5474181011709,29.6514024283902,29.7555686944444,
29.8174414544862,29.9216058860566,30.0256258453343,30.1295363446499,30.2333833809737,
30.3371921312327,30.4410324079623,30.4998665211569),.UNSPECIFIED.);
#2739=B_SPLINE_CURVE_WITH_KNOTS('',3,(#102377,#102378,#102379,#102380,#102381,
#102382,#102383,#102384,#102385,#102386,#102387,#102388,#102389,#102390,
#102391,#102392,#102393,#102394,#102395,#102396,#102397,#102398,#102399,
#102400,#102401,#102402,#102403,#102404,#102405,#102406,#102407,#102408,
#102409,#102410,#102411,#102412,#102413,#102414,#102415,#102416,#102417,
#102418,#102419,#102420,#102421,#102422,#102423,#102424,#102425,#102426,
#102427,#102428,#102429,#102430,#102431,#102432,#102433,#102434,#102435,
#102436,#102437,#102438,#102439,#102440,#102441,#102442,#102443,#102444,
#102445,#102446),.UNSPECIFIED.,.F.,.F.,(4,3,3,3,3,3,3,3,3,3,3,3,3,3,3,3,
3,3,3,3,3,3,3,4),(28.2743338823081,28.3638110296221,28.4679972524518,28.5720282376233,
28.6759371886222,28.779780680723,28.8835934929296,28.9874103608106,29.0913358993708,
29.1953202791018,29.2994865970749,29.3613588879682,29.4655450641685,29.569576002513,
29.6734849066249,29.7773283518282,29.8811411171982,29.9849579383745,30.0888834307589,
30.1928677645433,30.2970340374357,30.3589067463143,30.4630838225724,30.5008971260263),
 .UNSPECIFIED.);
#2740=B_SPLINE_CURVE_WITH_KNOTS('',3,(#102447,#102448,#102449,#102450,#102451,
#102452,#102453,#102454,#102455,#102456,#102457,#102458,#102459,#102460,
#102461,#102462,#102463,#102464,#102465,#102466,#102467,#102468,#102469,
#102470,#102471,#102472,#102473,#102474,#102475,#102476,#102477,#102478,
#102479,#102480,#102481,#102482,#102483,#102484,#102485,#102486,#102487,
#102488,#102489,#102490,#102491,#102492,#102493,#102494,#102495,#102496,
#102497,#102498,#102499,#102500,#102501,#102502,#102503,#102504,#102505,
#102506,#102507,#102508,#102509,#102510,#102511,#102512,#102513,#102514,
#102515,#102516,#102517,#102518,#102519,#102520,#102521,#102522,#102523,
#102524,#102525,#102526,#102527,#102528,#102529,#102530,#102531,#102532,
#102533,#102534,#102535,#102536,#102537,#102538,#102539,#102540,#102541,
#102542,#102543,#102544,#102545,#102546,#102547,#102548,#102549,#102550,
#102551,#102552,#102553,#102554,#102555,#102556,#102557,#102558,#102559,
#102560,#102561,#102562,#102563,#102564,#102565,#102566,#102567,#102568,
#102569,#102570),.UNSPECIFIED.,.F.,.F.,(4,3,3,3,3,3,3,3,3,3,3,3,3,3,3,3,
3,3,3,3,3,3,3,3,3,3,3,3,3,3,3,3,3,3,3,3,3,3,3,3,3,4),(24.2166116664802,
24.3207836892698,24.3736195962378,24.4778042292082,24.5818335992139,24.6857409053055,
24.7895827350337,24.8933938698845,24.9972090478915,25.1011328890806,25.2051155646482,
25.3092801861933,25.3711674545838,25.4753540205954,25.5793853516668,25.6832946508906,
25.787138492457,25.8909516548417,25.994768873086,26.0986947598526,26.2026794870977,
26.3068461476929,26.3687153129299,26.4729016339696,26.5769327209669,26.6808417786907,
26.7846853804865,26.8884983051989,26.9923152882402,27.0962409452456,27.2002254454547,
27.3043918858362,27.366263171276,27.4692311759306,27.5720240165358,27.6747190063384,
27.7773525424952,27.8799609377777,27.9826451376514,28.0853653036078,28.1882551874075,
28.2743338818562),.UNSPECIFIED.);
#2741=B_SPLINE_CURVE_WITH_KNOTS('',3,(#102576,#102577,#102578,#102579,#102580,
#102581,#102582,#102583,#102584,#102585,#102586,#102587,#102588,#102589,
#102590,#102591,#102592,#102593,#102594,#102595,#102596,#102597,#102598,
#102599,#102600,#102601,#102602,#102603,#102604,#102605,#102606,#102607,
#102608,#102609,#102610,#102611,#102612,#102613,#102614,#102615,#102616,
#102617,#102618,#102619,#102620,#102621,#102622,#102623,#102624,#102625,
#102626,#102627,#102628,#102629,#102630,#102631,#102632,#102633,#102634,
#102635,#102636,#102637,#102638,#102639,#102640,#102641,#102642,#102643,
#102644,#102645),.UNSPECIFIED.,.F.,.F.,(4,3,3,3,3,3,3,3,3,3,3,3,3,3,3,3,
3,3,3,3,3,3,3,4),(15.7079632679489,15.8107626988751,15.9135276397438,16.0162941010105,
16.1191710909696,16.2221067685037,16.3252328024632,16.3932367294691,16.4974783152938,
16.601563455709,16.7055244767834,16.8094187179986,16.9132808760585,17.0171456028236,
17.1211163738189,17.2251445703169,17.3293519684345,17.3907845878152,17.4951305459153,
17.6047988992279,17.7088743073029,17.8128825648351,17.9168653335439,17.9338039591658),
 .UNSPECIFIED.);
#2742=B_SPLINE_CURVE_WITH_KNOTS('',3,(#102647,#102648,#102649,#102650,#102651),
 .UNSPECIFIED.,.F.,.F.,(4,1,4),(14.3981410127769,15.395688871123,15.7079548498383),
 .UNSPECIFIED.);
#2743=B_SPLINE_CURVE_WITH_KNOTS('',3,(#102655,#102656,#102657,#102658,#102659,
#102660,#102661,#102662,#102663,#102664,#102665,#102666,#102667,#102668,
#102669,#102670,#102671,#102672,#102673,#102674,#102675,#102676,#102677,
#102678,#102679,#102680,#102681,#102682,#102683,#102684,#102685,#102686,
#102687,#102688,#102689,#102690,#102691,#102692,#102693,#102694,#102695,
#102696,#102697,#102698,#102699,#102700,#102701,#102702,#102703,#102704,
#102705,#102706,#102707,#102708,#102709,#102710,#102711,#102712),
 .UNSPECIFIED.,.F.,.F.,(4,3,3,3,3,3,3,3,3,3,3,3,3,3,3,3,3,3,3,4),(13.8761929392676,
13.9800701520378,14.0837916127864,14.1873908176266,14.2909249700636,14.3944292944766,
14.4979389721904,14.6015555958747,14.7052331471479,14.8090843148421,14.8542235792949,
14.9609410403269,15.0635682984263,15.1661015198455,15.2685772615991,15.3710319982226,
15.473553730983,15.5761160209808,15.6788141300276,15.7079632675506),
 .UNSPECIFIED.);
#2744=B_SPLINE_CURVE_WITH_KNOTS('',3,(#102713,#102714,#102715,#102716,#102717,
#102718,#102719,#102720,#102721,#102722,#102723,#102724,#102725,#102726,
#102727,#102728,#102729,#102730,#102731,#102732,#102733,#102734,#102735,
#102736,#102737,#102738,#102739,#102740,#102741,#102742,#102743,#102744,
#102745,#102746,#102747,#102748,#102749,#102750,#102751,#102752,#102753,
#102754,#102755,#102756,#102757,#102758,#102759,#102760,#102761,#102762,
#102763,#102764,#102765,#102766,#102767,#102768,#102769,#102770,#102771,
#102772,#102773,#102774,#102775,#102776,#102777,#102778,#102779),
 .UNSPECIFIED.,.F.,.F.,(4,3,3,3,3,3,3,3,3,3,3,3,3,3,3,3,3,3,3,3,3,3,4),
(15.7079632679489,15.851771437641,15.9558570600629,16.0597859912443,16.1635912207135,
16.2673300163232,16.3710373111926,16.4747479940652,16.578567054987,16.6824446290273,
16.7865047811698,16.8493192959871,16.9535191031687,17.0575636422614,17.1614860332293,
17.2653428871325,17.3691689624188,17.4729989740083,17.5769373807894,17.6809344925897,
17.7851131867065,17.8468671543332,17.9343865285971),.UNSPECIFIED.);
#2745=B_SPLINE_CURVE_WITH_KNOTS('',3,(#102785,#102786,#102787,#102788,#102789,
#102790,#102791,#102792,#102793,#102794,#102795,#102796,#102797,#102798,
#102799,#102800,#102801,#102802,#102803,#102804,#102805,#102806,#102807,
#102808,#102809,#102810,#102811,#102812,#102813,#102814,#102815,#102816,
#102817,#102818,#102819,#102820,#102821,#102822,#102823,#102824,#102825,
#102826,#102827,#102828,#102829,#102830,#102831,#102832,#102833,#102834,
#102835,#102836,#102837,#102838,#102839,#102840,#102841,#102842,#102843,
#102844,#102845,#102846,#102847,#102848),.UNSPECIFIED.,.F.,.F.,(4,3,3,3,
3,3,3,3,3,3,3,3,3,3,3,3,3,3,3,3,3,4),(89.6265204900684,89.7423240812235,
89.7793072511478,89.8880546694006,89.9991547244123,90.1076029303331,90.2159879164032,
90.324351856268,90.4374776695745,90.5460056337737,90.6546213577008,90.7634384533039,
90.7768551094939,90.8896161868303,91.0021364331478,91.1145147206211,91.2267846088042,
91.3389795079967,91.4511679814058,91.5633431986276,91.675606607642,91.7744029678399),
 .UNSPECIFIED.);
#2746=B_SPLINE_CURVE_WITH_KNOTS('',3,(#102851,#102852,#102853,#102854,#102855,
#102856,#102857,#102858,#102859,#102860,#102861,#102862,#102863,#102864,
#102865,#102866,#102867,#102868,#102869,#102870,#102871,#102872,#102873,
#102874,#102875,#102876,#102877,#102878,#102879,#102880,#102881,#102882,
#102883,#102884,#102885,#102886,#102887,#102888,#102889,#102890,#102891,
#102892,#102893,#102894,#102895,#102896,#102897,#102898,#102899,#102900,
#102901,#102902,#102903,#102904,#102905,#102906,#102907,#102908,#102909,
#102910,#102911,#102912,#102913,#102914,#102915,#102916,#102917,#102918,
#102919,#102920,#102921,#102922,#102923,#102924,#102925,#102926,#102927,
#102928,#102929,#102930,#102931,#102932,#102933,#102934,#102935,#102936,
#102937,#102938,#102939,#102940,#102941,#102942,#102943,#102944,#102945,
#102946,#102947,#102948,#102949,#102950,#102951,#102952,#102953,#102954,
#102955,#102956,#102957,#102958,#102959,#102960,#102961,#102962,#102963,
#102964,#102965,#102966,#102967,#102968,#102969,#102970),.UNSPECIFIED.,
 .F.,.F.,(4,2,2,2,2,2,2,2,2,2,2,2,2,2,2,2,2,2,2,2,2,2,2,2,2,2,2,2,2,2,2,
2,2,2,2,2,2,2,2,2,2,2,2,2,2,2,2,2,2,2,2,2,2,2,2,2,2,2,2,4),(-1.75478141683255,
-1.75474714622055,-1.75154566303739,-1.71244934856324,-1.69483238573248,
-1.68695596995421,-1.68054846350455,-1.67685394387567,-1.67359857524207,
-1.66949553212815,-1.66293957404403,-1.62998536351094,-1.60154438751122,
-1.59714207279607,-1.59489598236586,-1.59305759514252,-1.59070389455029,
-1.58582216073164,-1.56157050494364,-1.53947860741533,-1.5267269204622,
-1.51753715024743,-1.51332270787878,-1.51007730786042,-1.50649576904019,
-1.50053816651313,-1.47409251915458,-1.44517675981777,-1.4368177153129,
-1.43108068460839,-1.42861752332292,-1.42679807750872,-1.42471145136723,
-1.42100639265604,-1.39657501271319,-1.36801382302935,-1.352634645584,-1.34759671952704,
-1.34423546772831,-1.34098617056533,-1.33635431768738,-1.32511563116455,
-1.28876527539643,-1.27368221212848,-1.26508274154723,-1.26223065867346,
-1.26035249587754,-1.25841798138827,-1.25534160276798,-1.24569846165095,
-1.21643969142406,-1.19706671198549,-1.18479961744929,-1.18011648208558,
-1.1768052418789,-1.17380872819427,-1.16903000431917,-1.15701838544427,
-1.11837736041743,-1.10915475680411),.UNSPECIFIED.);
#2747=B_SPLINE_CURVE_WITH_KNOTS('',3,(#102976,#102977,#102978,#102979,#102980,
#102981,#102982,#102983,#102984,#102985,#102986,#102987,#102988,#102989,
#102990,#102991,#102992,#102993,#102994,#102995,#102996,#102997,#102998,
#102999,#103000,#103001,#103002,#103003,#103004,#103005,#103006,#103007,
#103008,#103009,#103010,#103011,#103012,#103013,#103014,#103015,#103016,
#103017,#103018,#103019,#103020,#103021,#103022,#103023,#103024,#103025,
#103026,#103027,#103028,#103029,#103030,#103031,#103032,#103033,#103034,
#103035,#103036,#103037,#103038,#103039,#103040,#103041,#103042,#103043,
#103044,#103045,#103046,#103047,#103048,#103049,#103050,#103051,#103052,
#103053,#103054,#103055,#103056,#103057,#103058,#103059,#103060,#103061,
#103062,#103063,#103064,#103065,#103066,#103067,#103068,#103069,#103070,
#103071,#103072,#103073,#103074,#103075,#103076,#103077,#103078,#103079,
#103080,#103081,#103082,#103083,#103084,#103085,#103086,#103087,#103088,
#103089,#103090,#103091,#103092,#103093,#103094,#103095,#103096,#103097,
#103098,#103099,#103100,#103101,#103102,#103103,#103104,#103105,#103106,
#103107,#103108,#103109,#103110,#103111,#103112,#103113,#103114,#103115,
#103116,#103117,#103118,#103119,#103120,#103121,#103122,#103123,#103124,
#103125,#103126,#103127,#103128,#103129,#103130,#103131,#103132,#103133,
#103134,#103135,#103136,#103137,#103138,#103139,#103140,#103141,#103142,
#103143,#103144,#103145,#103146,#103147,#103148,#103149,#103150,#103151,
#103152,#103153,#103154,#103155,#103156,#103157,#103158,#103159,#103160,
#103161,#103162,#103163,#103164,#103165,#103166,#103167,#103168,#103169,
#103170,#103171),.UNSPECIFIED.,.F.,.F.,(4,2,2,2,2,2,2,2,2,2,2,2,2,2,2,2,
2,2,2,2,2,2,2,2,2,2,2,2,2,2,2,2,2,2,2,2,2,2,2,2,2,2,2,2,2,2,2,2,2,2,2,2,
2,2,2,2,2,2,2,2,2,2,2,2,2,2,2,2,2,2,2,2,2,2,2,2,2,2,2,2,2,2,2,2,2,2,2,2,
2,2,2,2,2,2,2,2,2,4),(-0.991222240709418,-0.988027886510137,-0.950886399888337,
-0.924345861055636,-0.91939272677848,-0.917071588897676,-0.915265403854227,
-0.913074670459631,-0.908788938176693,-0.903122234160721,-0.888766291940011,
-0.854914221798932,-0.841198188334745,-0.836187351597118,-0.833155052601022,
-0.829888975005128,-0.825426509686339,-0.81463091207118,-0.798615464231531,
-0.781977473278559,-0.777830949901933,-0.755715088919002,-0.752024837541532,
-0.749936119343352,-0.74811598639392,-0.745645412251508,-0.739842832637144,
-0.731343456422572,-0.701271273382964,-0.676328173391544,-0.670426337811458,
-0.666867761715694,-0.663636852275534,-0.659432704790222,-0.650233601775503,
-0.637457774523331,-0.61531379424856,-0.611209132472771,-0.589073143637183,
-0.585379077426616,-0.583287273735827,-0.581461429124973,-0.57897943684902,
-0.573136104128642,-0.564558346736028,-0.533822637681052,-0.509893132988251,
-0.50402697404592,-0.500472737586186,-0.497234545897751,-0.493004471675793,
-0.483676907308556,-0.43930484978909,-0.42235425926687,-0.418771555600446,
-0.416705924315107,-0.41488881339156,-0.412392684417977,-0.406370448494366,
-0.397410028659741,-0.363340767616483,-0.342468561364955,-0.336809871273662,
-0.333317967621712,-0.33009612876436,-0.325828838066538,-0.31616398715047,
-0.302460908956749,-0.281564485489673,-0.277755910692359,-0.255644113267809,
-0.251963257435088,-0.24988178959726,-0.248060682024771,-0.245587143236691,
-0.239789998047193,-0.231309788374238,-0.201479588045942,-0.176111312588489,
-0.170162170914639,-0.166582013185077,-0.163335511683964,-0.159116231810544,
-0.149901036997746,-0.137102693271951,-0.115168965334172,-0.111682021691364,
-0.0889718063890053,-0.0852573968865036,-0.0831502676931111,-0.0812886601938547,
-0.0787377028270211,-0.0726542678425233,-0.0363620134325881,-0.0113176275066724,
-0.00552567108098689,-0.00256674334763014,-0.000511608811820447),
 .UNSPECIFIED.);
#2748=B_SPLINE_CURVE_WITH_KNOTS('',3,(#103172,#103173,#103174,#103175,#103176,
#103177,#103178,#103179,#103180,#103181),.UNSPECIFIED.,.F.,.F.,(4,3,3,4),
(89.2744165561713,89.3894329271381,89.5079767086033,89.6265204900684),
 .UNSPECIFIED.);
#2749=B_SPLINE_CURVE_WITH_KNOTS('',3,(#103182,#103183,#103184,#103185,#103186,
#103187,#103188,#103189,#103190,#103191,#103192,#103193,#103194,#103195,
#103196,#103197,#103198,#103199,#103200,#103201,#103202,#103203,#103204,
#103205,#103206,#103207,#103208,#103209,#103210,#103211,#103212,#103213,
#103214,#103215,#103216,#103217,#103218,#103219,#103220,#103221,#103222,
#103223,#103224,#103225,#103226,#103227,#103228,#103229,#103230,#103231,
#103232,#103233,#103234,#103235,#103236,#103237,#103238,#103239,#103240,
#103241,#103242,#103243,#103244,#103245,#103246,#103247,#103248,#103249,
#103250,#103251,#103252,#103253,#103254,#103255,#103256,#103257,#103258,
#103259,#103260,#103261,#103262,#103263,#103264,#103265,#103266,#103267,
#103268,#103269,#103270,#103271,#103272,#103273,#103274,#103275,#103276,
#103277,#103278,#103279,#103280,#103281,#103282,#103283,#103284,#103285,
#103286,#103287,#103288,#103289,#103290,#103291,#103292,#103293,#103294,
#103295,#103296,#103297,#103298,#103299,#103300,#103301,#103302,#103303,
#103304,#103305,#103306,#103307,#103308,#103309,#103310,#103311,#103312,
#103313,#103314,#103315,#103316,#103317,#103318,#103319,#103320,#103321,
#103322,#103323,#103324,#103325,#103326,#103327,#103328,#103329,#103330,
#103331,#103332,#103333,#103334,#103335,#103336,#103337,#103338,#103339,
#103340,#103341,#103342,#103343,#103344,#103345,#103346,#103347,#103348,
#103349,#103350,#103351,#103352,#103353,#103354,#103355,#103356,#103357,
#103358,#103359,#103360,#103361,#103362,#103363,#103364,#103365,#103366,
#103367,#103368,#103369,#103370,#103371,#103372,#103373,#103374,#103375,
#103376,#103377,#103378,#103379,#103380,#103381,#103382,#103383,#103384,
#103385,#103386,#103387,#103388,#103389,#103390,#103391,#103392,#103393,
#103394,#103395,#103396,#103397,#103398,#103399),.UNSPECIFIED.,.F.,.F.,
(4,2,2,2,2,2,2,2,2,2,2,2,2,2,2,2,2,2,2,2,2,2,2,2,2,2,2,2,2,2,2,2,2,2,2,
2,2,2,2,2,2,2,2,2,2,2,2,2,2,2,2,2,2,2,2,2,2,2,2,2,2,2,2,2,2,2,2,2,2,2,2,
2,2,2,2,2,2,2,2,2,2,2,2,2,2,2,2,2,2,2,2,2,2,2,2,2,2,2,2,2,2,2,2,2,2,2,2,
2,4),(-1.10915475680411,-1.10590829758048,-1.09831161527419,-1.0955682913694,
-1.09369941402947,-1.09172085515654,-1.08844853815534,-1.07683204011244,
-1.04904897643187,-1.02093801199038,-1.01503665165844,-1.01147865015438,
-1.00824844491306,-1.00411566609876,-0.995066094606954,-0.952417953911051,
-0.939448552235861,-0.931650082640437,-0.928885238508515,-0.927016294348523,
-0.925051909309595,-0.921834195894843,-0.910795265200498,-0.878917578122148,
-0.854166835149102,-0.848276575307823,-0.844723781974713,-0.841497499285981,
-0.837298670188879,-0.828109782162662,-0.81535121284868,-0.79317009368756,
-0.789184196923743,-0.766857343376418,-0.763166659664749,-0.761078350117616,
-0.759258782181685,-0.756789566808509,-0.750993529741101,-0.742506521548799,
-0.712520275057755,-0.687505554106076,-0.681603733744546,-0.678046098167778,
-0.674816651296248,-0.670615317425667,-0.661426604830529,-0.648670055245723,
-0.626513207218797,-0.622406915862476,-0.600236593914423,-0.596544406651792,
-0.594454130792412,-0.592633539121673,-0.590162332514379,-0.584354649314002,
-0.575844183719526,-0.545670575765058,-0.520882316207129,-0.514988473781557,
-0.511433178795329,-0.50820432315119,-0.504001605406358,-0.494801135016941,
-0.482022284355135,-0.459859124408289,-0.455687901260009,-0.43359084300555,
-0.42989958696087,-0.427810164081731,-0.425990265862755,-0.423520359822213,
-0.417718389337441,-0.409218909876642,-0.379129533244734,-0.354240080201269,
-0.348343609205929,-0.34478809507672,-0.341559918258493,-0.337359357241499,
-0.328169097342547,-0.315409057612669,-0.293241579517659,-0.289168801363912,
-0.266951351589867,-0.263259953184448,-0.261170607434454,-0.259350666912133,
-0.256880707718876,-0.251079153859075,-0.242580682598317,-0.2124999395904,
-0.187582914355486,-0.181696072390992,-0.178142339924079,-0.174913216716446,
-0.170707721102072,-0.161490724083596,-0.148679746909174,-0.126536571672967,
-0.122249600366427,-0.100319329977102,-0.0966288118337607,-0.094539486612291,
-0.0927194160660713,-0.0902488910351242,-0.0844437354937957,-0.0759379299276961,
-0.0594803408397951),.UNSPECIFIED.);
#2750=B_SPLINE_CURVE_WITH_KNOTS('',3,(#103404,#103405,#103406,#103407,#103408,
#103409,#103410,#103411,#103412,#103413,#103414,#103415,#103416,#103417,
#103418,#103419,#103420,#103421,#103422,#103423,#103424,#103425,#103426,
#103427,#103428,#103429,#103430,#103431,#103432,#103433,#103434,#103435,
#103436,#103437,#103438,#103439,#103440,#103441,#103442,#103443,#103444,
#103445,#103446,#103447,#103448,#103449,#103450,#103451,#103452,#103453,
#103454,#103455,#103456,#103457,#103458,#103459,#103460,#103461,#103462,
#103463,#103464,#103465,#103466,#103467,#103468,#103469,#103470,#103471,
#103472,#103473,#103474,#103475,#103476,#103477,#103478,#103479,#103480,
#103481,#103482,#103483,#103484,#103485,#103486,#103487,#103488,#103489,
#103490,#103491,#103492,#103493,#103494,#103495,#103496,#103497,#103498,
#103499,#103500,#103501,#103502,#103503,#103504,#103505,#103506,#103507,
#103508,#103509,#103510,#103511,#103512,#103513,#103514,#103515,#103516,
#103517,#103518,#103519,#103520,#103521,#103522,#103523,#103524,#103525,
#103526,#103527,#103528,#103529,#103530,#103531,#103532,#103533,#103534,
#103535,#103536,#103537,#103538,#103539,#103540,#103541,#103542,#103543,
#103544,#103545,#103546,#103547,#103548,#103549,#103550,#103551,#103552,
#103553,#103554,#103555,#103556,#103557,#103558,#103559,#103560,#103561,
#103562,#103563,#103564,#103565,#103566,#103567,#103568,#103569,#103570,
#103571,#103572,#103573,#103574,#103575,#103576,#103577,#103578,#103579,
#103580,#103581,#103582,#103583,#103584,#103585,#103586,#103587,#103588,
#103589,#103590,#103591,#103592,#103593,#103594,#103595,#103596,#103597,
#103598,#103599,#103600,#103601,#103602,#103603,#103604,#103605,#103606,
#103607,#103608,#103609,#103610,#103611,#103612,#103613,#103614,#103615,
#103616,#103617,#103618,#103619),.UNSPECIFIED.,.F.,.F.,(4,2,2,2,2,2,2,2,
2,2,2,2,2,2,2,2,2,2,2,2,2,2,2,2,2,2,2,2,2,2,2,2,2,2,2,2,2,2,2,2,2,2,2,2,
2,2,2,2,2,2,2,2,2,2,2,2,2,2,2,2,2,2,2,2,2,2,2,2,2,2,2,2,2,2,2,2,2,2,2,2,
2,2,2,2,2,2,2,2,2,2,2,2,2,2,2,2,2,2,2,2,2,2,2,2,2,2,2,4),(-2.040887232292,
-2.03666953291386,-2.0185720126827,-2.01059751838255,-2.00414950872928,
-2.00047651251808,-1.99726744017411,-1.99326106182471,-1.98694722344255,
-1.94834691626407,-1.92309843911034,-1.91886514099533,-1.91668379939785,
-1.91487611940143,-1.91254070485979,-1.90768712736404,-1.88333166076441,
-1.86116015524922,-1.84836589844149,-1.83915786005575,-1.83495306334523,
-1.83172313944319,-1.82816717314162,-1.82227332125794,-1.79749633400461,
-1.76734066126651,-1.75883371237663,-1.75302706307418,-1.75055576875164,
-1.7487350547587,-1.74664493382882,-1.74295259629403,-1.7209534966772,-1.71668992074694,
-1.69451921602787,-1.68172257591819,-1.67251327119726,-1.66830824174573,
-1.66507827484309,-1.66152239593185,-1.65562900606932,-1.63086664042829,
-1.60069923242269,-1.59219081053239,-1.58638341468938,-1.58391196909029,
-1.58209118032001,-1.58000095951105,-1.57630853701169,-1.55430482274811,
-1.55004567236767,-1.52787603274915,-1.51508209200769,-1.50587422114435,
-1.50166935980776,-1.49843931856505,-1.49488314919549,-1.4889887699192,
-1.46419883956259,-1.43405487367914,-1.42554940409071,-1.41974347875045,
-1.41727228543911,-1.41545162873656,-1.41336166106002,-1.40966942642515,
-1.38763559713052,-1.38339728456899,-1.36122341224976,-1.34843346352139,
-1.33922783408728,-1.33502371350972,-1.33179415647721,-1.32823845050265,
-1.32234471172692,-1.2975590206639,-1.2674111639463,-1.25890541597281,-1.25309947941384,
-1.25062844768177,-1.24880788817346,-1.24671787694427,-1.24302578039765,
-1.22108241257199,-1.21677978374381,-1.19461377713962,-1.18180182076469,
-1.17258438924115,-1.16837790792402,-1.16514771916264,-1.1615924861753,
-1.15570227338321,-1.13103844638362,-1.10078946033223,-1.09227077558248,
-1.08645820359103,-1.0839857597272,-1.0821645353642,-1.08007383292645,-1.07638136684009,
-1.05448561699236,-1.05031828120701,-1.01168417378539,-1.00537323267675,
-1.0013672146156,-0.998157426840153,-0.994482483610981,-0.991222240709418),
 .UNSPECIFIED.);
#2751=B_SPLINE_CURVE_WITH_KNOTS('',3,(#103621,#103622,#103623,#103624,#103625,
#103626,#103627,#103628,#103629,#103630,#103631,#103632,#103633,#103634,
#103635,#103636),.UNSPECIFIED.,.F.,.F.,(4,2,2,2,2,2,2,4),(-0.0594803408397951,
-0.0341317359818735,-0.0193897131176647,-0.0142713275473659,-0.0108796444644127,
-0.00784109551082508,-0.0042585004903553,-0.000493910869673254),
 .UNSPECIFIED.);
#2752=B_SPLINE_CURVE_WITH_KNOTS('',3,(#103637,#103638,#103639,#103640,#103641,
#103642,#103643,#103644,#103645,#103646,#103647,#103648,#103649,#103650,
#103651,#103652,#103653,#103654,#103655,#103656,#103657,#103658,#103659,
#103660,#103661,#103662,#103663,#103664,#103665,#103666,#103667,#103668,
#103669,#103670,#103671,#103672,#103673,#103674,#103675,#103676,#103677,
#103678,#103679,#103680,#103681,#103682,#103683,#103684,#103685,#103686,
#103687,#103688,#103689,#103690,#103691,#103692,#103693,#103694,#103695,
#103696,#103697,#103698,#103699,#103700,#103701,#103702,#103703,#103704,
#103705,#103706,#103707,#103708,#103709,#103710,#103711,#103712,#103713,
#103714,#103715,#103716,#103717,#103718,#103719,#103720,#103721,#103722,
#103723,#103724,#103725,#103726,#103727,#103728,#103729,#103730,#103731,
#103732,#103733,#103734,#103735,#103736,#103737,#103738,#103739,#103740,
#103741,#103742,#103743,#103744,#103745,#103746,#103747,#103748,#103749,
#103750,#103751,#103752,#103753,#103754,#103755,#103756,#103757,#103758,
#103759,#103760,#103761,#103762,#103763,#103764,#103765,#103766,#103767,
#103768,#103769,#103770,#103771,#103772,#103773,#103774,#103775,#103776,
#103777,#103778,#103779,#103780,#103781,#103782,#103783,#103784,#103785,
#103786,#103787,#103788,#103789,#103790,#103791,#103792,#103793,#103794,
#103795,#103796,#103797,#103798,#103799,#103800,#103801,#103802,#103803,
#103804,#103805,#103806,#103807,#103808,#103809,#103810,#103811,#103812,
#103813,#103814,#103815,#103816,#103817,#103818,#103819,#103820,#103821,
#103822,#103823,#103824,#103825,#103826,#103827,#103828,#103829,#103830,
#103831,#103832),.UNSPECIFIED.,.F.,.F.,(4,2,2,2,2,2,2,2,2,2,2,2,2,2,2,2,
2,2,2,2,2,2,2,2,2,2,2,2,2,2,2,2,2,2,2,2,2,2,2,2,2,2,2,2,2,2,2,2,2,2,2,2,
2,2,2,2,2,2,2,2,2,2,2,2,2,2,2,2,2,2,2,2,2,2,2,2,2,2,2,2,2,2,2,2,2,2,2,2,
2,2,2,2,2,2,2,2,2,4),(-2.09955737348478,-2.09249363804168,-2.05186478690352,
-2.03400314306285,-2.02947537347083,-2.0272357297974,-2.02543105400486,
-2.02316384751153,-2.01849400394995,-1.9873709083723,-1.9541141692392,-1.94952711601161,
-1.9453345446043,-1.94210703370573,-1.93854676517244,-1.93262924894321,
-1.90781234846578,-1.87772525631266,-1.86922745320003,-1.86342568254911,
-1.86095566271704,-1.85913558857435,-1.85704591490962,-1.853353868358,-1.83124248110219,
-1.82705931735847,-1.80487911738487,-1.79210538553673,-1.78290858945313,
-1.77870651816563,-1.77547777925015,-1.77192223645062,-1.76602706289011,
-1.74117144173959,-1.71108225543972,-1.70258421325185,-1.69678231830782,
-1.69431226066999,-1.69249217443838,-1.69040251932229,-1.68671050682692,
-1.66460000893884,-1.66041651063186,-1.6382365892748,-1.62546275382996,
-1.61626593658586,-1.61206389636168,-1.60883519830179,-1.60527971819416,
-1.59938469322923,-1.57453249944831,-1.54444016056601,-1.53594174913135,
-1.53013968954824,-1.52766962982034,-1.52584956587825,-1.52375996058633,
-1.52006811355725,-1.49799401422789,-1.49378267950112,-1.47160508382937,
-1.45882522618436,-1.44962527419592,-1.44542270858241,-1.44219396510963,
-1.43863879273166,-1.43274512905879,-1.40793663212211,-1.37780676136823,
-1.36930365386673,-1.36349927471159,-1.36102883831851,-1.35920873596894,
-1.35711936331163,-1.35342852653399,-1.33159286973978,-1.32723609446333,
-1.30470510220014,-1.29207102500343,-1.2829475836689,-1.2787583958394,-1.27553135379609,
-1.27196945817642,-1.26604409931025,-1.23992280513,-1.21091816593292,-1.19851546132101,
-1.19528414826038,-1.19331603493944,-1.19147054838449,-1.18917264054935,
-1.18337493725435,-1.15093572219253,-1.12524601824734,-1.11623303387197,
-1.11206331586998,-1.10883870340174,-1.10882130641878),.UNSPECIFIED.);
#2753=B_SPLINE_CURVE_WITH_KNOTS('',3,(#103838,#103839,#103840,#103841,#103842,
#103843,#103844,#103845,#103846,#103847,#103848,#103849,#103850,#103851,
#103852,#103853,#103854,#103855,#103856,#103857,#103858,#103859,#103860,
#103861,#103862,#103863,#103864,#103865,#103866,#103867,#103868,#103869,
#103870,#103871,#103872,#103873,#103874,#103875,#103876,#103877,#103878,
#103879,#103880,#103881,#103882,#103883,#103884,#103885,#103886,#103887,
#103888,#103889,#103890,#103891,#103892,#103893,#103894,#103895,#103896,
#103897,#103898,#103899,#103900,#103901,#103902,#103903,#103904,#103905,
#103906,#103907,#103908,#103909,#103910,#103911,#103912,#103913,#103914,
#103915,#103916,#103917,#103918,#103919,#103920,#103921,#103922,#103923,
#103924,#103925,#103926,#103927,#103928,#103929,#103930,#103931,#103932,
#103933,#103934,#103935,#103936,#103937,#103938,#103939,#103940,#103941,
#103942,#103943,#103944,#103945,#103946,#103947,#103948,#103949,#103950,
#103951,#103952,#103953,#103954,#103955,#103956,#103957,#103958,#103959,
#103960,#103961,#103962,#103963,#103964,#103965,#103966,#103967,#103968,
#103969,#103970,#103971,#103972,#103973,#103974,#103975,#103976,#103977,
#103978,#103979,#103980,#103981,#103982,#103983,#103984,#103985,#103986,
#103987,#103988,#103989,#103990,#103991,#103992,#103993,#103994,#103995,
#103996,#103997,#103998,#103999,#104000,#104001,#104002,#104003,#104004,
#104005,#104006,#104007,#104008,#104009,#104010,#104011,#104012,#104013,
#104014,#104015,#104016,#104017,#104018,#104019,#104020,#104021,#104022,
#104023,#104024,#104025,#104026,#104027,#104028,#104029,#104030,#104031,
#104032,#104033,#104034,#104035,#104036,#104037,#104038,#104039,#104040,
#104041),.UNSPECIFIED.,.F.,.F.,(4,2,2,2,2,2,2,2,2,2,2,2,2,2,2,2,2,2,2,2,
2,2,2,2,2,2,2,2,2,2,2,2,2,2,2,2,2,2,2,2,2,2,2,2,2,2,2,2,2,2,2,2,2,2,2,2,
2,2,2,2,2,2,2,2,2,2,2,2,2,2,2,2,2,2,2,2,2,2,2,2,2,2,2,2,2,2,2,2,2,2,2,2,
2,2,2,2,2,2,2,2,2,4),(-0.991134658234024,-0.989393770439243,-0.985702139618141,
-0.983612358447809,-0.981791924665051,-0.979320930487852,-0.973514818048519,
-0.96500746119274,-0.934855935054433,-0.9100501113684,-0.90415544427592,
-0.900599670820795,-0.89737036637796,-0.89316700846563,-0.883964624168734,
-0.871182009641986,-0.849028683931204,-0.844834803383067,-0.82277855198614,
-0.819087319716109,-0.816997653907286,-0.815177242189328,-0.812706172704248,
-0.806899418659536,-0.798390701952386,-0.768227605827526,-0.743436286898861,
-0.737542171952347,-0.73398656428089,-0.73075730455012,-0.726553852890641,
-0.717350616097084,-0.704566271854376,-0.682414222128694,-0.678212664596025,
-0.656167297778629,-0.652476182179802,-0.650386569088503,-0.648566193710558,
-0.64609516089619,-0.640288437683084,-0.631779716589814,-0.601615813029859,
-0.576826631096773,-0.570932687960036,-0.567377164647168,-0.564147969337476,
-0.55994458402742,-0.550741417839805,-0.53795710810973,-0.515805619963614,
-0.511603297382461,-0.489559558032337,-0.485868523031835,-0.483778953869424,
-0.481958614062506,-0.479487626576206,-0.473680999501288,-0.465172407768735,
-0.435008749362983,-0.410220601814559,-0.40432679571375,-0.400771347344671,
-0.397542215077954,-0.393338904482458,-0.384135869830907,-0.371351715421386,
-0.34920072853768,-0.344998000516914,-0.322955350331874,-0.319264393601979,
-0.317174867834826,-0.315354568567354,-0.312883637679022,-0.307077143138314,
-0.298568747939646,-0.268405860680431,-0.243617990564167,-0.237724305658577,
-0.234168935720165,-0.230939878292876,-0.226736670573006,-0.217533886255367,
-0.204750103840634,-0.182599525294963,-0.158267438071558,-0.153413460110191,
-0.151078328699636,-0.149271108133408,-0.147179669269353,-0.143468184043144,
-0.138511203216898,-0.126878925379223,-0.105635912780473,-0.0772181914200325,
-0.0712212824659521,-0.0676440420580335,-0.0644202985524751,-0.0602596924002813,
-0.0512989624219987,-0.00636760239601622,-0.000492473137004156),
 .UNSPECIFIED.);
#2754=B_SPLINE_CURVE_WITH_KNOTS('',3,(#104042,#104043,#104044,#104045,#104046,
#104047,#104048,#104049,#104050,#104051,#104052,#104053,#104054,#104055,
#104056,#104057,#104058,#104059,#104060,#104061),.UNSPECIFIED.,.F.,.F.,
(4,2,2,2,2,2,2,2,2,4),(-2.09970265449674,-2.09186541748599,-2.08704536647685,
-2.08492637274696,-2.08321642563898,-2.08140245998211,-2.07903034634331,
-2.07385587384966,-2.057152820964,-2.040887232292),.UNSPECIFIED.);
#2755=B_SPLINE_CURVE_WITH_KNOTS('',3,(#104062,#104063,#104064,#104065,#104066,
#104067,#104068,#104069,#104070,#104071,#104072,#104073,#104074,#104075,
#104076,#104077,#104078,#104079,#104080,#104081,#104082,#104083,#104084,
#104085,#104086,#104087,#104088,#104089,#104090,#104091,#104092,#104093,
#104094,#104095,#104096,#104097,#104098,#104099,#104100,#104101,#104102,
#104103,#104104,#104105,#104106,#104107,#104108,#104109,#104110,#104111,
#104112,#104113,#104114,#104115,#104116,#104117,#104118,#104119,#104120,
#104121,#104122,#104123,#104124,#104125,#104126,#104127,#104128,#104129,
#104130,#104131,#104132,#104133,#104134,#104135,#104136,#104137,#104138,
#104139,#104140,#104141,#104142,#104143,#104144,#104145,#104146,#104147,
#104148,#104149,#104150,#104151,#104152,#104153,#104154,#104155,#104156,
#104157,#104158,#104159,#104160,#104161,#104162,#104163,#104164,#104165,
#104166,#104167,#104168,#104169,#104170,#104171,#104172,#104173,#104174,
#104175,#104176,#104177,#104178,#104179,#104180,#104181,#104182,#104183,
#104184,#104185,#104186,#104187,#104188,#104189,#104190,#104191,#104192,
#104193,#104194,#104195,#104196,#104197,#104198,#104199,#104200,#104201,
#104202,#104203,#104204,#104205,#104206,#104207,#104208,#104209,#104210,
#104211,#104212,#104213,#104214,#104215,#104216,#104217,#104218,#104219,
#104220,#104221,#104222,#104223,#104224,#104225,#104226,#104227,#104228,
#104229,#104230,#104231,#104232,#104233,#104234,#104235,#104236,#104237,
#104238,#104239,#104240,#104241,#104242,#104243,#104244,#104245,#104246,
#104247,#104248,#104249,#104250,#104251,#104252,#104253,#104254,#104255,
#104256,#104257,#104258,#104259,#104260,#104261,#104262,#104263,#104264,
#104265,#104266,#104267,#104268,#104269),.UNSPECIFIED.,.F.,.F.,(4,2,2,2,
2,2,2,2,2,2,2,2,2,2,2,2,2,2,2,2,2,2,2,2,2,2,2,2,2,2,2,2,2,2,2,2,2,2,2,2,
2,2,2,2,2,2,2,2,2,2,2,2,2,2,2,2,2,2,2,2,2,2,2,2,2,2,2,2,2,2,2,2,2,2,2,2,
2,2,2,2,2,2,2,2,2,2,2,2,2,2,2,2,2,2,2,2,2,2,2,2,2,2,2,4),(-1.10882130641878,
-1.10526679940843,-1.09929416858599,-1.07124182863778,-1.04978224507737,
-1.03261309916525,-1.02901859513812,-1.0269508692399,-1.02512549235125,
-1.02261513154994,-1.01656742080071,-1.0075668423812,-0.97311244338185,
-0.952936247658493,-0.947296301784389,-0.943795119647905,-0.940550174283224,
-0.936229606484671,-0.926332766823546,-0.912188999288603,-0.891751518712453,
-0.890602302139632,-0.866184405812538,-0.862471273019752,-0.860376962533257,
-0.858558048943376,-0.856096500177943,-0.850344966230737,-0.841946911634021,
-0.812645844209904,-0.786842140877459,-0.780922528658991,-0.777361961893787,
-0.774134797989161,-0.769943554181892,-0.760807455057905,-0.748150693251636,
-0.725521450964616,-0.721449714601169,-0.6995129487726,-0.695822543273843,
-0.69373333814469,-0.691913357886711,-0.689442999862523,-0.683638606677296,
-0.675134267439443,-0.645005466786183,-0.620165728542786,-0.614270716983036,
-0.610715424066274,-0.607487021297597,-0.603285541068394,-0.594090516808393,
-0.581321345463812,-0.559159715171629,-0.555024203999076,-0.532886515600972,
-0.52919542362308,-0.527106091103647,-0.52528618644532,-0.522816180975426,
-0.517013717335917,-0.508513200005048,-0.478413903667141,-0.453541477754723,
-0.447645590053882,-0.444090158226479,-0.440861875705518,-0.436660905531994,
-0.427468502450932,-0.414704238642015,-0.392541428554948,-0.388430977889081,
-0.366262337160064,-0.362571204701923,-0.360481888980159,-0.358662027335582,
-0.356192118217168,-0.350390048069933,-0.341890258147388,-0.311795956979986,
-0.286919007150828,-0.281023090080332,-0.277467699139969,-0.274239490806532,
-0.270038670350879,-0.260846821164539,-0.248083517011967,-0.225920921886999,
-0.201545888528755,-0.196697066266929,-0.194363217222348,-0.192556416795263,
-0.19037583703054,-0.186143204541015,-0.160916035860181,-0.122261374434154,
-0.11595196999513,-0.111947958382465,-0.108740517883322,-0.105069133520523,
-0.0986233217537091,-0.0777398511691188,-0.059270596115177),
 .UNSPECIFIED.);
#2756=B_SPLINE_CURVE_WITH_KNOTS('',3,(#104274,#104275,#104276,#104277,#104278,
#104279,#104280,#104281,#104282,#104283,#104284,#104285,#104286,#104287,
#104288,#104289,#104290,#104291,#104292,#104293,#104294,#104295,#104296,
#104297,#104298,#104299,#104300,#104301,#104302,#104303,#104304,#104305,
#104306,#104307,#104308,#104309,#104310,#104311,#104312,#104313,#104314,
#104315,#104316,#104317,#104318,#104319,#104320,#104321,#104322,#104323,
#104324,#104325,#104326,#104327,#104328,#104329,#104330,#104331,#104332,
#104333,#104334,#104335,#104336,#104337,#104338,#104339,#104340,#104341,
#104342,#104343,#104344,#104345,#104346,#104347,#104348,#104349,#104350,
#104351,#104352,#104353,#104354,#104355,#104356,#104357,#104358,#104359,
#104360,#104361,#104362,#104363,#104364,#104365,#104366,#104367,#104368,
#104369,#104370,#104371,#104372,#104373,#104374,#104375,#104376,#104377,
#104378,#104379,#104380,#104381,#104382,#104383,#104384,#104385,#104386,
#104387,#104388,#104389,#104390,#104391,#104392,#104393,#104394,#104395,
#104396,#104397,#104398,#104399,#104400,#104401,#104402,#104403,#104404,
#104405,#104406,#104407,#104408,#104409,#104410,#104411,#104412,#104413,
#104414,#104415,#104416,#104417,#104418,#104419,#104420,#104421,#104422,
#104423,#104424,#104425,#104426,#104427,#104428,#104429,#104430,#104431,
#104432,#104433,#104434,#104435,#104436,#104437,#104438,#104439,#104440,
#104441,#104442,#104443,#104444,#104445,#104446,#104447,#104448,#104449,
#104450,#104451,#104452,#104453,#104454,#104455,#104456,#104457,#104458,
#104459,#104460,#104461,#104462,#104463,#104464,#104465,#104466,#104467,
#104468,#104469,#104470,#104471,#104472,#104473),.UNSPECIFIED.,.F.,.F.,
(4,2,2,2,2,2,2,2,2,2,2,2,2,2,2,2,2,2,2,2,2,2,2,2,2,2,2,2,2,2,2,2,2,2,2,
2,2,2,2,2,2,2,2,2,2,2,2,2,2,2,2,2,2,2,2,2,2,2,2,2,2,2,2,2,2,2,2,2,2,2,2,
2,2,2,2,2,2,2,2,2,2,2,2,2,2,2,2,2,2,2,2,2,2,2,2,2,2,2,2,4),(-2.04071874618918,
-2.01961546049806,-1.99508613993201,-1.98732410099392,-1.98456387022839,
-1.98269551899839,-1.98072776909657,-1.9774994004954,-1.96635980234788,
-1.93822854429145,-1.91932946004213,-1.90726512582464,-1.9026149791725,
-1.89931415047375,-1.89592079794045,-1.89079831020504,-1.87611539979841,
-1.84315966082654,-1.82906442346955,-1.82082638711687,-1.81800560900694,
-1.81612529129228,-1.81441340890215,-1.81149639993504,-1.80316570486508,
-1.76971950645519,-1.75201166396843,-1.74045465128701,-1.73587666863379,
-1.73258894838706,-1.72917596183277,-1.72395779314342,-1.70837145446095,
-1.66922697733333,-1.65979372110739,-1.65353803863191,-1.65099419516361,
-1.64916361240751,-1.64711177126416,-1.6434964357234,-1.62670620419294,
-1.59208048384329,-1.57521728519362,-1.57000985238046,-1.56659913551912,
-1.56334728386305,-1.55878770901516,-1.5481986355223,-1.51142267142515,
-1.49626443202158,-1.48763084957389,-1.48476232305994,-1.48287230012894,
-1.48093546872148,-1.47784842443634,-1.46810946931968,-1.43894936540656,
-1.41963182371838,-1.40739501512038,-1.40272119391912,-1.39941615380399,
-1.39642515253182,-1.39241496618285,-1.38245951795514,-1.34503893597047,
-1.32970696593158,-1.32380454627599,-1.31938266977623,-1.31716371042709,
-1.31535829981061,-1.31306805182323,-1.30827846743112,-1.2782909051088,
-1.26674571982802,-1.2509211652044,-1.24021410642035,-1.23576340877781,
-1.23249747474174,-1.22945930711066,-1.22442441322099,-1.21052708360301,
-1.17090754868407,-1.16048900064823,-1.15377736382872,-1.15116374621136,
-1.14932207539876,-1.14730143844741,-1.14383046949961,-1.1296720110462,
-1.09931376619849,-1.07624189647906,-1.07056686680982,-1.06705771578794,
-1.0638145043765,-1.05958375829601,-1.04995277931304,-1.03633858779808,
-1.01533355633792,-1.01153671361318,-0.991134658234024),.UNSPECIFIED.);
#2757=B_SPLINE_CURVE_WITH_KNOTS('',3,(#104475,#104476,#104477,#104478,#104479,
#104480,#104481,#104482,#104483,#104484,#104485,#104486,#104487,#104488,
#104489,#104490,#104491,#104492,#104493,#104494),.UNSPECIFIED.,.F.,.F.,
(4,2,2,2,2,2,2,2,2,4),(-0.059270596115177,-0.0463606215788353,-0.0324747524269931,
-0.0290287076097999,-0.0270139937505328,-0.0251710223838709,-0.0233127838313809,
-0.0207405458901744,-0.0142423388580124,-0.000491547373460261),
 .UNSPECIFIED.);
#2758=B_SPLINE_CURVE_WITH_KNOTS('',3,(#104495,#104496,#104497,#104498,#104499,
#104500,#104501,#104502,#104503,#104504,#104505,#104506,#104507,#104508,
#104509,#104510,#104511,#104512,#104513,#104514,#104515,#104516,#104517,
#104518,#104519,#104520,#104521,#104522,#104523,#104524,#104525,#104526,
#104527,#104528,#104529,#104530,#104531,#104532,#104533,#104534,#104535,
#104536,#104537,#104538,#104539,#104540,#104541,#104542,#104543,#104544,
#104545,#104546,#104547,#104548,#104549,#104550,#104551,#104552,#104553,
#104554,#104555,#104556,#104557,#104558,#104559,#104560,#104561,#104562,
#104563,#104564,#104565,#104566,#104567,#104568,#104569,#104570,#104571,
#104572,#104573,#104574,#104575,#104576,#104577,#104578,#104579,#104580,
#104581,#104582,#104583,#104584,#104585,#104586,#104587,#104588,#104589,
#104590,#104591,#104592,#104593,#104594,#104595,#104596,#104597,#104598,
#104599,#104600,#104601,#104602,#104603,#104604,#104605,#104606,#104607,
#104608,#104609,#104610,#104611,#104612,#104613,#104614,#104615,#104616,
#104617,#104618,#104619,#104620,#104621,#104622,#104623,#104624,#104625,
#104626,#104627,#104628,#104629,#104630,#104631,#104632,#104633,#104634,
#104635,#104636,#104637,#104638,#104639,#104640,#104641,#104642,#104643,
#104644,#104645,#104646,#104647,#104648,#104649,#104650,#104651,#104652,
#104653,#104654,#104655,#104656,#104657,#104658,#104659,#104660,#104661,
#104662,#104663,#104664,#104665,#104666,#104667,#104668,#104669,#104670,
#104671,#104672,#104673,#104674,#104675,#104676,#104677,#104678,#104679,
#104680,#104681,#104682,#104683,#104684,#104685,#104686,#104687,#104688,
#104689,#104690,#104691,#104692,#104693,#104694,#104695,#104696,#104697,
#104698,#104699,#104700,#104701,#104702,#104703,#104704,#104705,#104706,
#104707,#104708,#104709,#104710,#104711,#104712,#104713,#104714,#104715,
#104716,#104717,#104718,#104719,#104720,#104721,#104722,#104723,#104724,
#104725,#104726,#104727,#104728,#104729,#104730,#104731,#104732,#104733,
#104734,#104735,#104736,#104737,#104738,#104739,#104740,#104741,#104742,
#104743,#104744,#104745,#104746,#104747,#104748,#104749,#104750,#104751,
#104752,#104753,#104754),.UNSPECIFIED.,.F.,.F.,(4,2,2,2,2,2,2,2,2,2,2,2,
2,2,2,2,2,2,2,2,2,2,2,2,2,2,2,2,2,2,2,2,2,2,2,2,2,2,2,2,2,2,2,2,2,2,2,2,
2,2,2,2,2,2,2,2,2,2,2,2,2,2,2,2,2,2,2,2,2,2,2,2,2,2,2,2,2,2,2,2,2,2,2,2,
2,2,2,2,2,2,2,2,2,2,2,2,2,2,2,2,2,2,2,2,2,2,2,2,2,2,2,2,2,2,2,2,2,2,2,2,
2,2,2,2,2,2,2,2,2,4),(-2.09991236431288,-2.05890814058238,-2.04942205507822,
-2.04517041685067,-2.04193540108864,-2.03840424310071,-2.03262268862309,
-2.01022431038967,-1.97796231366217,-1.96917168160048,-1.96331605603006,
-1.96094125373947,-1.96092453242584,-1.96090748382121,-1.96089009076418,
-1.96087233502679,-1.96085419725018,-1.96083565682671,-1.96081669174899,
-1.9607972786029,-1.96077739238786,-1.96075700641465,-1.96073609197738,
-1.96071461834799,-1.96069255255636,-1.96066985907439,-1.96064649965018,
-1.96062243302663,-1.96059761458855,-1.96057199603318,-1.96054552493718,
-1.96051814433738,-1.96048979225843,-1.960460401058,-1.96042989675817,-1.96039819832757,
-1.96036521684046,-1.9603308543533,-1.96029500277823,-1.96025754263415,
-1.96021834137281,-1.96017725155573,-1.95837029312953,-1.95603585834615,
-1.95118461416921,-1.92679835442126,-1.90461953487397,-1.89184728047984,
-1.88265144690322,-1.87844974116405,-1.87522125468098,-1.87166596212373,
-1.86577113961512,-1.84091474816518,-1.81082947983554,-1.80233226152457,
-1.79653089347695,-1.79406104145929,-1.79224109639157,-1.79015158736273,
-1.78645982225327,-1.76434674591972,-1.76016667379764,-1.73798804520478,
-1.72521579651358,-1.71601998411648,-1.71181830091257,-1.70858983682433,
-1.70503457400087,-1.6991398128623,-1.67428422602823,-1.64419863240782,
-1.63570140706375,-1.62990004699466,-1.62743020720255,-1.62561027461307,
-1.62352078394823,-1.61982905998773,-1.59772008498846,-1.59353698491781,
-1.57135873861843,-1.55858594727366,-1.54938986898487,-1.5451881582712,
-1.54195971016492,-1.53840450200631,-1.53250991970523,-1.50765906946368,
-1.47756972979603,-1.46907206543475,-1.46327049884719,-1.46080063550284,
-1.45898071086584,-1.4568912587972,-1.45319966646328,-1.43111947532519,
-1.4269144080036,-1.40473803983379,-1.3919605448457,-1.38276202263598,-1.37855990482942,
-1.37533142411474,-1.37177645978604,-1.36588294731705,-1.34106641469367,
-1.31094757684405,-1.30244622415752,-1.2966428378658,-1.29417268199262,
-1.29235273130574,-1.29026346994139,-1.2865726894119,-1.26469242852159,
-1.26050792417017,-1.23789272794201,-1.22523750836744,-1.21610314271166,
-1.21191224626731,-1.20868520387774,-1.20512462787616,-1.19920462500042,
-1.17333065400964,-1.14412056857565,-1.13573616760502,-1.12999101849191,
-1.12753061443486,-1.12571188575448,-1.1236170637095,-1.11990136925088,
-1.10912241679603),.UNSPECIFIED.);
#2759=B_SPLINE_CURVE_WITH_KNOTS('',3,(#104760,#104761,#104762,#104763,#104764,
#104765,#104766,#104767,#104768,#104769,#104770,#104771,#104772,#104773,
#104774,#104775,#104776,#104777,#104778,#104779,#104780,#104781,#104782,
#104783,#104784,#104785,#104786,#104787,#104788,#104789,#104790,#104791,
#104792,#104793,#104794,#104795,#104796,#104797,#104798,#104799,#104800,
#104801,#104802,#104803,#104804,#104805,#104806,#104807,#104808,#104809,
#104810,#104811,#104812,#104813,#104814,#104815,#104816,#104817,#104818,
#104819,#104820,#104821,#104822,#104823,#104824,#104825,#104826,#104827,
#104828,#104829,#104830,#104831,#104832,#104833,#104834,#104835,#104836,
#104837,#104838,#104839,#104840,#104841,#104842,#104843,#104844,#104845,
#104846,#104847,#104848,#104849,#104850,#104851,#104852,#104853,#104854,
#104855,#104856,#104857,#104858,#104859,#104860,#104861,#104862,#104863,
#104864,#104865,#104866,#104867,#104868,#104869,#104870,#104871,#104872,
#104873,#104874,#104875,#104876,#104877,#104878,#104879,#104880,#104881,
#104882,#104883,#104884,#104885,#104886,#104887,#104888,#104889,#104890,
#104891,#104892,#104893,#104894,#104895,#104896,#104897,#104898,#104899,
#104900,#104901,#104902,#104903,#104904,#104905,#104906,#104907,#104908,
#104909,#104910,#104911,#104912,#104913,#104914,#104915,#104916,#104917,
#104918,#104919,#104920,#104921,#104922,#104923,#104924,#104925,#104926,
#104927,#104928,#104929,#104930,#104931,#104932,#104933,#104934,#104935,
#104936,#104937,#104938,#104939,#104940,#104941,#104942,#104943,#104944,
#104945,#104946,#104947,#104948,#104949,#104950,#104951,#104952,#104953,
#104954,#104955,#104956,#104957,#104958,#104959,#104960,#104961,#104962,
#104963,#104964,#104965,#104966,#104967,#104968,#104969,#104970,#104971,
#104972,#104973,#104974,#104975,#104976,#104977,#104978,#104979,#104980,
#104981),.UNSPECIFIED.,.F.,.F.,(4,2,2,2,2,2,2,2,2,2,2,2,2,2,2,2,2,2,2,2,
2,2,2,2,2,2,2,2,2,2,2,2,2,2,2,2,2,2,2,2,2,2,2,2,2,2,2,2,2,2,2,2,2,2,2,2,
2,2,2,2,2,2,2,2,2,2,2,2,2,2,2,2,2,2,2,2,2,2,2,2,2,2,2,2,2,2,2,2,2,2,2,2,
2,2,2,2,2,2,2,2,2,2,2,2,2,2,2,2,2,2,4),(-0.991205554037858,-0.979929488239522,
-0.973239680348427,-0.969124100324602,-0.96590456768069,-0.962300386779387,
-0.956179932514309,-0.921052257246141,-0.891628407896895,-0.886845712937254,
-0.884556476683887,-0.882750718757385,-0.88052993113071,-0.876100275497577,
-0.870183962523765,-0.854795534377931,-0.817182797173947,-0.807377773103285,
-0.803391583271509,-0.8001073485437,-0.796741462203431,-0.791755968593157,
-0.777027038131106,-0.750739733210124,-0.725140728152079,-0.7202978832177,
-0.71796453677848,-0.716156915981696,-0.713973798356414,-0.70973188745755,
-0.704142062956238,-0.690100988823647,-0.657347521488646,-0.642394121064468,
-0.637243019677451,-0.633843521538133,-0.630546274055562,-0.625917293356997,
-0.614005991356797,-0.595475186460841,-0.568243261838846,-0.555883599898062,
-0.552541068481579,-0.550548245130541,-0.548693674369856,-0.546007268064864,
-0.538792364667649,-0.527228811182223,-0.506007000557386,-0.477461266304887,
-0.471451539889824,-0.467870895582047,-0.464646712316049,-0.460489238715048,
-0.451550443978713,-0.425068681636558,-0.391103554260244,-0.386665001386152,
-0.384442506470657,-0.38263688140735,-0.380349724468751,-0.375577694724279,
-0.355540891292406,-0.31978169523648,-0.308117911232646,-0.303394216420157,
-0.30011249911231,-0.296743747198049,-0.291743575231823,-0.276883187416715,
-0.250164442692066,-0.225260701749933,-0.220294179723399,-0.217970593637933,
-0.216163578025005,-0.213972707013279,-0.209692181873003,-0.185106378317987,
-0.145694351108715,-0.139480476804126,-0.135503536322483,-0.132296684993092,
-0.131787137618101,-0.131527804925709,-0.13132014286362,-0.131149430904764,
-0.131006168900059,-0.13088392131668,-0.130778157724808,-0.130685587416395,
-0.130603757150829,-0.130530797308936,-0.130465255932637,-0.130405986857194,
-0.130352072267633,-0.130302767846003,-0.130257463110954,-0.130215652326327,
-0.130057786506376,-0.129899898005545,-0.124976252442725,-0.10988205423827,
-0.0822694396196656,-0.0804589308759995,-0.0566193668578111,-0.0529166787477501,
-0.0508243112860018,-0.0490042430694455,-0.0465372457426665,-0.0407558851820747,
-0.000492258923205386),.UNSPECIFIED.);
#2760=B_SPLINE_CURVE_WITH_KNOTS('',3,(#104982,#104983,#104984,#104985,#104986,
#104987,#104988,#104989,#104990,#104991,#104992,#104993,#104994,#104995,
#104996,#104997,#104998,#104999),.UNSPECIFIED.,.F.,.F.,(4,2,2,2,2,2,2,2,
4),(-2.09977792447378,-2.07701759521765,-2.07253004579203,-2.06924681052091,
-2.06594529428715,-2.06295025244637,-2.05815818445511,-2.04603073547732,
-2.04071874618918),.UNSPECIFIED.);
#2761=B_SPLINE_CURVE_WITH_KNOTS('',3,(#105000,#105001,#105002,#105003,#105004,
#105005,#105006,#105007,#105008,#105009,#105010,#105011,#105012,#105013,
#105014,#105015,#105016,#105017,#105018,#105019,#105020,#105021,#105022,
#105023,#105024,#105025,#105026,#105027,#105028,#105029,#105030,#105031,
#105032,#105033,#105034,#105035,#105036,#105037,#105038,#105039,#105040,
#105041,#105042,#105043,#105044,#105045,#105046,#105047,#105048,#105049,
#105050,#105051,#105052,#105053,#105054,#105055,#105056,#105057,#105058,
#105059,#105060,#105061,#105062,#105063,#105064,#105065,#105066,#105067,
#105068,#105069,#105070,#105071,#105072,#105073,#105074,#105075,#105076,
#105077,#105078,#105079,#105080,#105081,#105082,#105083,#105084,#105085,
#105086,#105087,#105088,#105089,#105090,#105091,#105092,#105093,#105094,
#105095,#105096,#105097,#105098,#105099,#105100,#105101,#105102,#105103,
#105104,#105105,#105106,#105107,#105108,#105109,#105110,#105111,#105112,
#105113,#105114,#105115,#105116,#105117,#105118,#105119,#105120,#105121,
#105122,#105123,#105124,#105125,#105126,#105127,#105128,#105129,#105130,
#105131,#105132,#105133,#105134,#105135,#105136,#105137,#105138,#105139,
#105140,#105141,#105142,#105143,#105144,#105145,#105146,#105147,#105148,
#105149,#105150,#105151,#105152,#105153,#105154,#105155,#105156,#105157,
#105158,#105159,#105160,#105161,#105162,#105163,#105164,#105165,#105166,
#105167,#105168,#105169,#105170,#105171,#105172,#105173,#105174,#105175,
#105176,#105177,#105178,#105179,#105180,#105181,#105182,#105183,#105184,
#105185,#105186,#105187,#105188,#105189,#105190,#105191,#105192,#105193,
#105194,#105195,#105196,#105197),.UNSPECIFIED.,.F.,.F.,(4,2,2,2,2,2,2,2,
2,2,2,2,2,2,2,2,2,2,2,2,2,2,2,2,2,2,2,2,2,2,2,2,2,2,2,2,2,2,2,2,2,2,2,2,
2,2,2,2,2,2,2,2,2,2,2,2,2,2,2,2,2,2,2,2,2,2,2,2,2,2,2,2,2,2,2,2,2,2,2,2,
2,2,2,2,2,2,2,2,2,2,2,2,2,2,2,2,2,2,4),(-1.10912241679603,-1.09537616038099,
-1.07747396274481,-1.06117113868342,-1.05024299434426,-1.04620603905425,
-1.04320923530063,-1.03991167869396,-1.03527510639529,-1.02330113889305,
-1.00461877832252,-0.977009612586079,-0.965169028350568,-0.961879849746099,
-0.959899223268496,-0.958039491207421,-0.955321984160442,-0.947876355979257,
-0.935765227971143,-0.900051965429733,-0.885129537697124,-0.879983103809995,
-0.876585638973385,-0.873289611476752,-0.868661120861592,-0.856744178551556,
-0.838197160155459,-0.810923613877317,-0.798628264142535,-0.795291796493434,
-0.793300872978823,-0.791446689910993,-0.788758967192956,-0.781529311498818,
-0.769929524591374,-0.748753934919004,-0.720223032384794,-0.714216426599012,
-0.710637494906361,-0.707414793028382,-0.703259179597336,-0.694324410716642,
-0.667815224220001,-0.633886307497032,-0.629445156774992,-0.627222756755551,
-0.625418003697579,-0.623133036513319,-0.618369249228712,-0.598400130521092,
-0.562835222525317,-0.550973114514668,-0.54622232076107,-0.542936663406515,
-0.539576175286326,-0.534611778118246,-0.520054724256004,-0.494312875574829,
-0.467968686324046,-0.463123628792559,-0.46079051256424,-0.458983741420501,
-0.456802543264675,-0.452566915501582,-0.42679727919605,-0.388813513831111,
-0.38243847116907,-0.378415241075314,-0.375206226601998,-0.371547978758963,
-0.365164920259045,-0.357293913441052,-0.339569945749232,-0.30613493905344,
-0.297849302311913,-0.294938933959659,-0.293228785125839,-0.291348251526259,
-0.288523707660054,-0.280249850114902,-0.26605718374843,-0.232768512616576,
-0.218444422325762,-0.213361428469145,-0.210315254278324,-0.207056460603241,
-0.202643586668177,-0.192171767052842,-0.176846014280266,-0.146551191965447,
-0.132329082941721,-0.128859438601076,-0.126839594476986,-0.124998726569516,
-0.12238641645134,-0.11606002628771,-0.0944046175112616,-0.0678885621054014,
-0.0595555566481069),.UNSPECIFIED.);
#2762=B_SPLINE_CURVE_WITH_KNOTS('',3,(#105202,#105203,#105204,#105205,#105206,
#105207,#105208,#105209,#105210,#105211,#105212,#105213,#105214,#105215,
#105216,#105217,#105218,#105219,#105220,#105221,#105222,#105223,#105224,
#105225,#105226,#105227,#105228,#105229,#105230,#105231,#105232,#105233,
#105234,#105235,#105236,#105237,#105238,#105239,#105240,#105241,#105242,
#105243,#105244,#105245,#105246,#105247,#105248,#105249,#105250,#105251,
#105252,#105253,#105254,#105255,#105256,#105257,#105258,#105259,#105260,
#105261,#105262,#105263,#105264,#105265,#105266,#105267,#105268,#105269,
#105270,#105271,#105272,#105273,#105274,#105275,#105276,#105277,#105278,
#105279,#105280,#105281,#105282,#105283,#105284,#105285,#105286,#105287,
#105288,#105289,#105290,#105291,#105292,#105293,#105294,#105295,#105296,
#105297,#105298,#105299,#105300,#105301,#105302,#105303,#105304,#105305,
#105306,#105307,#105308,#105309,#105310,#105311,#105312,#105313,#105314,
#105315,#105316,#105317,#105318,#105319,#105320,#105321,#105322,#105323,
#105324,#105325,#105326,#105327,#105328,#105329,#105330,#105331,#105332,
#105333,#105334,#105335,#105336,#105337,#105338,#105339,#105340,#105341,
#105342,#105343,#105344,#105345,#105346,#105347,#105348,#105349,#105350,
#105351,#105352,#105353,#105354,#105355,#105356,#105357,#105358,#105359,
#105360,#105361,#105362,#105363,#105364,#105365,#105366,#105367,#105368,
#105369,#105370,#105371,#105372,#105373,#105374,#105375,#105376,#105377,
#105378,#105379,#105380,#105381,#105382,#105383,#105384,#105385,#105386,
#105387,#105388,#105389,#105390,#105391,#105392,#105393,#105394,#105395,
#105396,#105397,#105398,#105399,#105400,#105401,#105402,#105403,#105404,
#105405,#105406,#105407,#105408,#105409,#105410,#105411,#105412,#105413,
#105414,#105415,#105416,#105417,#105418,#105419,#105420,#105421,#105422,
#105423,#105424,#105425,#105426,#105427,#105428,#105429,#105430,#105431,
#105432,#105433,#105434,#105435,#105436,#105437),.UNSPECIFIED.,.F.,.F.,
(4,2,2,2,2,2,2,2,2,2,2,2,2,2,2,2,2,2,2,2,2,2,2,2,2,2,2,2,2,2,2,2,2,2,2,
2,2,2,2,2,2,2,2,2,2,2,2,2,2,2,2,2,2,2,2,2,2,2,2,2,2,2,2,2,2,2,2,2,2,2,2,
2,2,2,2,2,2,2,2,2,2,2,2,2,2,2,2,2,2,2,2,2,2,2,2,2,2,2,2,2,2,2,2,2,2,2,2,
2,2,2,2,2,2,2,2,2,2,4),(-2.04099839520778,-2.01939573360936,-2.01831944035928,
-1.9906444489668,-1.9755310051931,-1.97060527853868,-1.97044735083837,-1.97028944353156,
-1.97024760888034,-1.97020227361801,-1.97015293101081,-1.97009896938324,
-1.97003964291678,-1.96997403196382,-1.96990098801235,-1.96981905616593,
-1.96972636299089,-1.96962045018923,-1.96949802030445,-1.96935453368078,
-1.96918354181598,-1.96897552594511,-1.96871573814881,-1.96806955035828,
-1.96485695328726,-1.9608084691524,-1.9524682042581,-1.91308143183545,-1.89722023380667,
-1.88833466357603,-1.88543653049693,-1.88354015844704,-1.8816103879941,
-1.87855663265051,-1.86911353166549,-1.83634965688227,-1.81908433252053,
-1.80772124937577,-1.80317125991983,-1.79988820011862,-1.7968724903244,
-1.7919632564458,-1.7790259856766,-1.74450215625132,-1.72996454631121,-1.72425243998551,
-1.7199395222239,-1.71774215112674,-1.71593556301261,-1.71361988816888,
-1.70869584268628,-1.68530494250538,-1.66523433708602,-1.65068347229347,
-1.64058578819142,-1.63623137082558,-1.63298039200552,-1.62949100537016,
-1.62391058415889,-1.60471680059066,-1.56121982196668,-1.55440303719899,
-1.55177363457131,-1.54992907673756,-1.54791442729921,-1.54447190894558,
-1.53066901158982,-1.50442861802324,-1.48627728381298,-1.47452804242991,
-1.46992189534187,-1.46662870195648,-1.46362423583537,-1.45955919989408,
-1.44926613205415,-1.40847253598747,-1.39572105892504,-1.38801067860277,
-1.38525694464806,-1.38338963129241,-1.38141936946125,-1.37818045677944,
-1.36692740607782,-1.33516254934427,-1.31862416523762,-1.3075871883527,
-1.30308554780868,-1.29981062285941,-1.29678386394173,-1.2918139878612,
-1.27843362866053,-1.24431536573725,-1.22989107396882,-1.22420650605244,
-1.21990938860676,-1.21771508652841,-1.21590816366619,-1.21358840858768,
-1.20864304259139,-1.18220319675944,-1.16749602490232,-1.15157547130906,
-1.14082292105715,-1.13636460945623,-1.13309689095308,-1.13005973846244,
-1.12503283608603,-1.11120709438071,-1.07749135416292,-1.06318025572464,
-1.05485981693471,-1.05202857007244,-1.0501459009344,-1.04819854897539,
-1.04506450603386,-1.03384432349115,-1.01015486702639,-0.991205554037858),
 .UNSPECIFIED.);
#2763=B_SPLINE_CURVE_WITH_KNOTS('',3,(#105439,#105440,#105441,#105442,#105443,
#105444,#105445,#105446,#105447,#105448,#105449,#105450,#105451,#105452,
#105453,#105454),.UNSPECIFIED.,.F.,.F.,(4,2,2,2,2,2,2,4),(-0.0595555566481069,
-0.052158634671153,-0.0469231542530946,-0.0435074117017776,-0.0402233239291963,
-0.0369694877437875,-0.0325599867995973,-0.000491890560030468),
 .UNSPECIFIED.);
#2764=B_SPLINE_CURVE_WITH_KNOTS('',3,(#105455,#105456,#105457,#105458,#105459,
#105460,#105461,#105462,#105463,#105464,#105465,#105466,#105467,#105468,
#105469,#105470,#105471,#105472,#105473,#105474,#105475,#105476,#105477,
#105478,#105479,#105480,#105481,#105482,#105483,#105484,#105485,#105486,
#105487,#105488,#105489,#105490,#105491,#105492,#105493,#105494,#105495,
#105496,#105497,#105498,#105499,#105500,#105501,#105502,#105503,#105504,
#105505,#105506,#105507,#105508,#105509,#105510,#105511,#105512,#105513,
#105514,#105515,#105516,#105517,#105518,#105519,#105520,#105521,#105522,
#105523,#105524,#105525,#105526,#105527,#105528,#105529,#105530,#105531,
#105532,#105533,#105534,#105535,#105536,#105537,#105538,#105539,#105540,
#105541,#105542,#105543,#105544,#105545,#105546,#105547,#105548,#105549,
#105550,#105551,#105552,#105553,#105554,#105555,#105556,#105557,#105558,
#105559,#105560,#105561,#105562,#105563,#105564,#105565,#105566,#105567,
#105568,#105569,#105570,#105571,#105572,#105573,#105574,#105575,#105576,
#105577,#105578,#105579,#105580,#105581,#105582,#105583,#105584,#105585,
#105586,#105587,#105588,#105589,#105590,#105591,#105592,#105593,#105594,
#105595,#105596,#105597,#105598,#105599,#105600,#105601,#105602,#105603,
#105604,#105605,#105606,#105607,#105608,#105609,#105610,#105611,#105612,
#105613,#105614,#105615,#105616,#105617),.UNSPECIFIED.,.F.,.F.,(4,3,3,3,
3,3,3,3,3,3,3,3,3,3,3,3,3,3,3,3,3,3,3,3,3,3,3,3,3,3,3,3,3,3,3,3,3,3,3,3,
3,3,3,3,3,3,3,3,3,3,3,3,3,3,4),(-54.1118657207119,-53.968500634934,-53.8675843506887,
-53.7577897347117,-53.6468205794156,-53.5373284361958,-53.4279032844601,
-53.3185044306203,-53.2063874460508,-53.0968489113658,-52.9834427018542,
-52.8700364923426,-52.7602418763654,-52.6492727210693,-52.5397805778494,
-52.4303554261136,-52.3209565722737,-52.2088395877044,-52.0993010530191,
-51.9858948435078,-51.8724886339965,-51.7626940180194,-51.6517248627233,
-51.5422327195034,-51.4328075677676,-51.3234087139278,-51.2112917293584,
-51.1017531946732,-50.9883469851618,-50.8749407756504,-50.7651461596733,
-50.6541770043772,-50.5446848611574,-50.4352597094216,-50.3258608555818,
-50.2137438710124,-50.1042053363273,-49.9907991268158,-49.8773929173043,
-49.7675983013272,-49.6566291460311,-49.5471370028112,-49.4377118510754,
-49.3283129972355,-49.2161960126662,-49.1066574779811,-48.9932512684696,
-48.8798450589582,-48.7700749181095,-48.6604636787918,-48.5509703718656,
-48.4415394130409,-48.3321442536605,-48.2227090186297,-48.1819144221909),
 .UNSPECIFIED.);
#2765=B_SPLINE_CURVE_WITH_KNOTS('',3,(#105623,#105624,#105625,#105626,#105627,
#105628,#105629,#105630,#105631,#105632,#105633,#105634,#105635,#105636,
#105637,#105638,#105639,#105640,#105641,#105642,#105643,#105644,#105645,
#105646,#105647,#105648,#105649,#105650,#105651,#105652,#105653,#105654,
#105655,#105656,#105657,#105658,#105659,#105660,#105661,#105662,#105663,
#105664,#105665,#105666,#105667,#105668,#105669,#105670,#105671,#105672,
#105673,#105674,#105675,#105676,#105677,#105678,#105679,#105680,#105681,
#105682,#105683,#105684,#105685,#105686,#105687,#105688,#105689,#105690,
#105691,#105692,#105693,#105694,#105695,#105696,#105697,#105698,#105699,
#105700,#105701,#105702,#105703,#105704,#105705,#105706,#105707,#105708,
#105709,#105710,#105711,#105712,#105713,#105714,#105715,#105716,#105717,
#105718,#105719,#105720,#105721,#105722,#105723,#105724,#105725,#105726,
#105727,#105728,#105729,#105730,#105731,#105732,#105733,#105734,#105735,
#105736,#105737,#105738,#105739,#105740,#105741,#105742,#105743,#105744,
#105745,#105746,#105747,#105748,#105749,#105750,#105751,#105752,#105753,
#105754,#105755,#105756,#105757,#105758,#105759,#105760,#105761,#105762,
#105763,#105764,#105765,#105766,#105767,#105768,#105769,#105770,#105771,
#105772,#105773,#105774,#105775,#105776,#105777,#105778,#105779,#105780,
#105781,#105782,#105783,#105784,#105785,#105786,#105787,#105788,#105789,
#105790,#105791,#105792,#105793,#105794,#105795,#105796,#105797,#105798,
#105799,#105800,#105801,#105802,#105803,#105804,#105805,#105806,#105807,
#105808,#105809,#105810,#105811,#105812,#105813,#105814,#105815,#105816,
#105817,#105818,#105819,#105820,#105821,#105822,#105823,#105824,#105825,
#105826,#105827,#105828),.UNSPECIFIED.,.F.,.F.,(4,2,2,2,2,2,2,2,2,2,2,2,
2,2,2,2,2,2,2,2,2,2,2,2,2,2,2,2,2,2,2,2,2,2,2,2,2,2,2,2,2,2,2,2,2,2,2,2,
2,2,2,2,2,2,2,2,2,2,2,2,2,2,2,2,2,2,2,2,2,2,2,2,2,2,2,2,2,2,2,2,2,2,2,2,
2,2,2,2,2,2,2,2,2,2,2,2,2,2,2,2,2,2,4),(-0.991228980721755,-0.983399078957842,
-0.979460113584548,-0.957084565640262,-0.953391691373635,-0.951301495530232,
-0.949480907430011,-0.947009980657939,-0.941205245558575,-0.932701008487992,
-0.902578244436011,-0.877732967343426,-0.871836546988952,-0.868280152433777,
-0.865050560141928,-0.860847224092474,-0.851646576915701,-0.83886779977462,
-0.816710006188954,-0.812537405379585,-0.790450018785875,-0.786758279881265,
-0.784668364252601,-0.782847761123251,-0.780376467081482,-0.774569341318892,
-0.766060220822828,-0.735897959636949,-0.711099264715003,-0.705204368136027,
-0.701648345184216,-0.698418743869457,-0.694214898646253,-0.685011017654734,
-0.672225961689675,-0.650071244330366,-0.645871809402301,-0.623820593470023,
-0.620129065532894,-0.618039223390797,-0.616218651426804,-0.613747355708804,
-0.607940032226353,-0.599430446836377,-0.569263718166024,-0.544471384435351,
-0.538576790007748,-0.535020879171879,-0.531791335278851,-0.527587501045188,
-0.518383372429963,-0.505597743317259,-0.483443832258745,-0.479241265067081,
-0.457194845703296,-0.453503410940628,-0.451413615940351,-0.449593081035736,
-0.447121830257443,-0.441314588734614,-0.432805102066618,-0.40263837927036,
-0.377847274631405,-0.371952824777447,-0.368396992584879,-0.365167514691985,
-0.360963758579918,-0.35175976781384,-0.338974302188154,-0.316820894417893,
-0.312618024795321,-0.290572590485879,-0.286881234515208,-0.284791483440623,
-0.282970986315148,-0.280499786167051,-0.274692660752007,-0.26618334162358,
-0.236017170985046,-0.211219097846803,-0.205328748067624,-0.201773835172136,
-0.198544207948106,-0.194338843513685,-0.185125300529055,-0.172321473124871,
-0.149944659398351,-0.145934749141311,-0.123953037556204,-0.120261997744582,
-0.118172343197543,-0.116351871197342,-0.113880626212398,-0.108073047562501,
-0.0818761565133594,-0.0549676500763384,-0.0424561977089353,-0.0376077067301623,
-0.0346029870465107,-0.0313111572356573,-0.0280446275150207,-0.0236019623783744,
-0.000491634459526482),.UNSPECIFIED.);
#2766=B_SPLINE_CURVE_WITH_KNOTS('',3,(#105829,#105830,#105831,#105832,#105833,
#105834,#105835,#105836,#105837,#105838,#105839,#105840,#105841,#105842,
#105843,#105844),.UNSPECIFIED.,.F.,.F.,(4,2,2,2,2,2,2,4),(-2.09980207912905,
-2.05974703936122,-2.05399628535234,-2.05153435059402,-2.04971481350122,
-2.04761936391674,-2.04390312850233,-2.04099839520778),.UNSPECIFIED.);
#2767=B_SPLINE_CURVE_WITH_KNOTS('',3,(#105846,#105847,#105848,#105849,#105850,
#105851,#105852,#105853,#105854,#105855,#105856,#105857,#105858),
 .UNSPECIFIED.,.F.,.F.,(4,3,3,3,4),(-48.1819144221909,-48.0723535220419,
-47.9625891320687,-47.8822972006122,-47.8286804139494),.UNSPECIFIED.);
#2768=B_SPLINE_CURVE_WITH_KNOTS('',3,(#105859,#105860,#105861,#105862,#105863,
#105864,#105865,#105866,#105867),.UNSPECIFIED.,.F.,.F.,(4,1,1,1,1,1,4),
(-47.8286738934412,-46.8847493422661,-45.88720148392,-44.8896536255739,
-43.8921057672278,-42.8945579088817,-41.8982186577127),.UNSPECIFIED.);
#2769=B_SPLINE_CURVE_WITH_KNOTS('',3,(#105872,#105873,#105874,#105875,#105876,
#105877,#105878,#105879,#105880,#105881,#105882,#105883,#105884,#105885,
#105886,#105887,#105888,#105889,#105890,#105891,#105892,#105893,#105894,
#105895,#105896,#105897,#105898,#105899,#105900,#105901,#105902,#105903,
#105904,#105905,#105906,#105907,#105908,#105909,#105910,#105911,#105912,
#105913,#105914,#105915,#105916,#105917,#105918,#105919,#105920,#105921,
#105922,#105923,#105924,#105925,#105926,#105927,#105928,#105929,#105930,
#105931,#105932,#105933,#105934,#105935,#105936,#105937,#105938,#105939,
#105940,#105941,#105942,#105943,#105944,#105945,#105946,#105947,#105948,
#105949,#105950,#105951,#105952,#105953,#105954,#105955,#105956,#105957,
#105958,#105959,#105960,#105961,#105962,#105963,#105964,#105965,#105966,
#105967,#105968,#105969,#105970,#105971,#105972,#105973,#105974,#105975,
#105976,#105977,#105978,#105979,#105980,#105981,#105982,#105983,#105984,
#105985,#105986,#105987,#105988,#105989,#105990,#105991,#105992,#105993,
#105994,#105995,#105996,#105997,#105998,#105999,#106000,#106001,#106002,
#106003,#106004,#106005,#106006,#106007,#106008,#106009,#106010,#106011,
#106012,#106013,#106014,#106015,#106016,#106017,#106018,#106019,#106020,
#106021,#106022,#106023,#106024,#106025,#106026,#106027,#106028,#106029,
#106030,#106031,#106032,#106033,#106034,#106035,#106036,#106037,#106038,
#106039,#106040,#106041,#106042,#106043,#106044,#106045,#106046,#106047,
#106048,#106049,#106050,#106051,#106052,#106053,#106054,#106055,#106056,
#106057,#106058,#106059,#106060,#106061,#106062,#106063,#106064,#106065,
#106066,#106067,#106068,#106069,#106070,#106071,#106072,#106073,#106074,
#106075,#106076,#106077),.UNSPECIFIED.,.F.,.F.,(4,2,2,2,2,2,2,2,2,2,2,2,
2,2,2,2,2,2,2,2,2,2,2,2,2,2,2,2,2,2,2,2,2,2,2,2,2,2,2,2,2,2,2,2,2,2,2,2,
2,2,2,2,2,2,2,2,2,2,2,2,2,2,2,2,2,2,2,2,2,2,2,2,2,2,2,2,2,2,2,2,2,2,2,2,
2,2,2,2,2,2,2,2,2,2,2,2,2,2,2,2,2,2,4),(-2.04104007014271,-2.0387525359055,
-2.03514317100133,-2.03192444057663,-2.0278173682406,-2.02115754469679,
-1.98880506671721,-1.96672848881058,-1.95943883257924,-1.95580738612716,
-1.95292532574864,-1.95103268219419,-1.94919305726299,-1.94692052220931,
-1.94119266427461,-1.90869784896389,-1.8829003498935,-1.87389715730153,
-1.86972808226165,-1.86650235363778,-1.86292755179802,-1.85694596726494,
-1.82754916128068,-1.80533947904071,-1.79492278112375,-1.78821162585083,
-1.78559779403393,-1.7837558389576,-1.78173474119667,-1.77826268249817,
-1.76402689582707,-1.73369326423287,-1.71836584183501,-1.70789277115906,
-1.70347813427133,-1.70021760141858,-1.69716948850042,-1.69208239359735,
-1.67773598291939,-1.64145865182086,-1.62927324680306,-1.62179529747193,
-1.61907264261978,-1.617211282177,-1.6154769339966,-1.61244502578709,-1.60319029021224,
-1.57031221478931,-1.5529701490403,-1.54157292972686,-1.53701777282535,
-1.53373367625438,-1.53071885529284,-1.52581525223006,-1.51291955083575,
-1.47835452282733,-1.46380512849904,-1.45809003230311,-1.4537753371727,
-1.4515775381009,-1.44977087104003,-1.44745544311587,-1.44253312301147,
-1.41924099168559,-1.39126246543584,-1.37603081688486,-1.37098945439346,
-1.36761232917214,-1.36433695078348,-1.35964795279919,-1.34818367976645,
-1.30873945363392,-1.29614993194195,-1.28850546335625,-1.28576047473732,
-1.28389486636067,-1.28192185865187,-1.27867028479885,-1.26727401006814,
-1.23932112787998,-1.22049431678454,-1.20845948096966,-1.20381300759226,
-1.20051248893365,-1.19711749130626,-1.19198866924457,-1.17725004030893,
-1.13717557409296,-1.12766615899306,-1.12137410103298,-1.11882424158117,
-1.11699247244179,-1.11494287637059,-1.11133911737094,-1.09484515789665,
-1.05022618693345,-1.04074433881468,-1.0365382240233,-1.03329840976035,
-1.02977758489838,-1.02404866411753,-0.999989180191607,-0.991228980721755),
 .UNSPECIFIED.);
#2770=B_SPLINE_CURVE_WITH_KNOTS('',3,(#106079,#106080,#106081,#106082,#106083),
 .UNSPECIFIED.,.F.,.F.,(4,1,4),(-41.8982186577127,-41.8970100505357,-41.5455025263571),
 .UNSPECIFIED.);
#2771=B_SPLINE_CURVE_WITH_KNOTS('',3,(#106084,#106085,#106086,#106087,#106088,
#106089,#106090,#106091,#106092,#106093,#106094,#106095,#106096,#106097,
#106098,#106099,#106100,#106101,#106102,#106103,#106104,#106105,#106106,
#106107,#106108,#106109,#106110,#106111,#106112,#106113,#106114,#106115,
#106116,#106117,#106118,#106119,#106120,#106121,#106122,#106123,#106124,
#106125,#106126,#106127,#106128,#106129,#106130,#106131,#106132,#106133,
#106134,#106135,#106136,#106137,#106138,#106139,#106140,#106141,#106142,
#106143,#106144,#106145,#106146,#106147,#106148,#106149,#106150,#106151,
#106152,#106153,#106154,#106155,#106156,#106157,#106158,#106159,#106160,
#106161,#106162,#106163,#106164,#106165,#106166,#106167,#106168,#106169,
#106170,#106171,#106172,#106173,#106174,#106175,#106176,#106177,#106178,
#106179,#106180,#106181,#106182,#106183,#106184,#106185,#106186,#106187,
#106188,#106189,#106190,#106191,#106192,#106193,#106194,#106195,#106196,
#106197,#106198,#106199,#106200,#106201,#106202,#106203,#106204,#106205,
#106206,#106207,#106208,#106209,#106210,#106211,#106212,#106213,#106214,
#106215,#106216,#106217,#106218,#106219,#106220,#106221,#106222,#106223,
#106224,#106225,#106226,#106227,#106228,#106229,#106230,#106231,#106232,
#106233,#106234,#106235,#106236,#106237,#106238,#106239,#106240,#106241,
#106242,#106243,#106244,#106245,#106246,#106247,#106248,#106249,#106250,
#106251,#106252,#106253,#106254,#106255,#106256,#106257,#106258,#106259,
#106260,#106261,#106262,#106263,#106264,#106265,#106266,#106267,#106268,
#106269,#106270,#106271),.UNSPECIFIED.,.F.,.F.,(4,2,2,2,2,2,2,2,2,2,2,2,
2,2,2,2,2,2,2,2,2,2,2,2,2,2,2,2,2,2,2,2,2,2,2,2,2,2,2,2,2,2,2,2,2,2,2,2,
2,2,2,2,2,2,2,2,2,2,2,2,2,2,2,2,2,2,2,2,2,2,2,2,2,2,2,2,2,2,2,2,2,2,2,2,
2,2,2,2,2,2,2,2,2,4),(-2.0999861052273,-2.08479811344361,-2.08072130504199,
-2.07758229687025,-2.07447976083113,-2.07095046814617,-2.06517836607562,
-2.04122384415751,-2.01745915487528,-1.99960623806886,-1.99507973234757,
-1.99284046335875,-1.99103595124351,-1.98876877237535,-1.98409842203353,
-1.95299505284556,-1.91972780320091,-1.91339999589749,-1.90975309020251,
-1.90654219000092,-1.90250081158415,-1.89606440827894,-1.85879803922154,
-1.8324595733498,-1.82822129934136,-1.82603943778134,-1.8242325383008,-1.82189977284635,
-1.8170571352358,-1.79135334870695,-1.76511595349078,-1.75040359007509,
-1.74542112761741,-1.74205683803193,-1.73877385721018,-1.73478886659469,
-1.72488166282933,-1.68737042139817,-1.67201284469986,-1.66610457837662,
-1.6616795163636,-1.65946020386398,-1.65765522167537,-1.65536650363912,
-1.65058348758094,-1.6205343449857,-1.58619676800124,-1.57997261724512,
-1.57634752311013,-1.57313334449525,-1.56905744179811,-1.56250213901544,
-1.51862602993176,-1.50465899356999,-1.49647018029549,-1.49365587960851,
-1.49177716149441,-1.48982624360926,-1.48667353911659,-1.47632350257792,
-1.44407866758827,-1.42717771362486,-1.41953697949825,-1.41329945485087,
-1.40967146361122,-1.40645762206397,-1.40238608746289,-1.39584612765182,
-1.35189016674987,-1.33795594904815,-1.32977963593475,-1.32696683364986,
-1.32508837421632,-1.32313694257043,-1.31998207182596,-1.3096118970306,
-1.2773769983291,-1.2604835037349,-1.2492867578625,-1.24476216742133,-1.24148425132606,
-1.23846421036066,-1.23352724709438,-1.22038282572925,-1.18604888771317,
-1.17156359541554,-1.16317837008891,-1.16033989869803,-1.15845627809937,
-1.15651204009753,-1.15338998818168,-1.14332915741797,-1.11092203612512,
-1.1089889728157),.UNSPECIFIED.);
#2772=B_SPLINE_CURVE_WITH_KNOTS('',3,(#106277,#106278,#106279,#106280,#106281,
#106282,#106283,#106284,#106285,#106286,#106287,#106288,#106289,#106290,
#106291,#106292,#106293,#106294,#106295,#106296,#106297,#106298,#106299,
#106300,#106301,#106302,#106303,#106304,#106305,#106306,#106307,#106308,
#106309,#106310,#106311,#106312,#106313,#106314,#106315,#106316,#106317,
#106318,#106319,#106320,#106321,#106322,#106323,#106324,#106325,#106326,
#106327,#106328,#106329,#106330,#106331,#106332,#106333,#106334,#106335,
#106336,#106337,#106338,#106339,#106340,#106341,#106342,#106343,#106344,
#106345,#106346,#106347,#106348,#106349,#106350,#106351,#106352,#106353,
#106354,#106355,#106356,#106357,#106358,#106359,#106360,#106361,#106362,
#106363,#106364,#106365,#106366,#106367,#106368,#106369,#106370,#106371,
#106372,#106373,#106374,#106375,#106376,#106377,#106378,#106379,#106380,
#106381,#106382,#106383,#106384,#106385,#106386,#106387,#106388,#106389,
#106390,#106391,#106392,#106393,#106394,#106395,#106396,#106397,#106398,
#106399,#106400,#106401,#106402,#106403,#106404,#106405,#106406,#106407,
#106408,#106409,#106410,#106411,#106412,#106413,#106414,#106415,#106416,
#106417,#106418,#106419,#106420,#106421,#106422,#106423,#106424,#106425,
#106426,#106427,#106428,#106429,#106430,#106431,#106432,#106433,#106434,
#106435,#106436,#106437,#106438,#106439,#106440,#106441,#106442,#106443,
#106444,#106445,#106446,#106447,#106448,#106449,#106450,#106451,#106452,
#106453,#106454,#106455,#106456,#106457,#106458,#106459,#106460,#106461,
#106462,#106463,#106464,#106465,#106466,#106467,#106468,#106469,#106470,
#106471,#106472,#106473,#106474,#106475,#106476,#106477,#106478,#106479,
#106480),.UNSPECIFIED.,.F.,.F.,(4,2,2,2,2,2,2,2,2,2,2,2,2,2,2,2,2,2,2,2,
2,2,2,2,2,2,2,2,2,2,2,2,2,2,2,2,2,2,2,2,2,2,2,2,2,2,2,2,2,2,2,2,2,2,2,2,
2,2,2,2,2,2,2,2,2,2,2,2,2,2,2,2,2,2,2,2,2,2,2,2,2,2,2,2,2,2,2,2,2,2,2,2,
2,2,2,2,2,2,2,2,2,4),(-0.991072635368184,-0.969596543045493,-0.944678719631752,
-0.938779709992405,-0.935222573374277,-0.931992825682933,-0.927790031406633,
-0.918593737599609,-0.905823675865204,-0.883660390886621,-0.879534039801498,
-0.857384842615779,-0.853692572712348,-0.851602432914164,-0.849781689150038,
-0.847310277367632,-0.841503197222112,-0.832994434878307,-0.802838130039271,
-0.778027646791767,-0.772131961052143,-0.768575578377908,-0.765345723986346,
-0.761141655047993,-0.751937734662634,-0.739153003863647,-0.716995871741904,
-0.712801538341332,-0.690741174039202,-0.687049310762138,-0.684959288211624,
-0.683138565829683,-0.680667074960377,-0.674859332681809,-0.666349169592394,
-0.636180971994663,-0.61138537080215,-0.605490247999528,-0.601934032840117,
-0.598704221680831,-0.594500052655769,-0.58529524686925,-0.572508724189121,
-0.550352894801331,-0.546150634773762,-0.524101489984738,-0.520409744085937,
-0.518319774092841,-0.51649908756241,-0.514027632059696,-0.508219914290156,
-0.499709734140254,-0.46954062331062,-0.444747305679363,-0.438852359866513,
-0.435296230240233,-0.432066483322266,-0.427862378619087,-0.418657631417134,
-0.405871120740144,-0.383715857180284,-0.379512716851832,-0.357465336771777,
-0.353773672614241,-0.351683747207611,-0.349863098311555,-0.347391692278746,
-0.341584083637129,-0.333074056956888,-0.302905386541787,-0.278112799595176,
-0.272217983039022,-0.268661928804817,-0.265432248724814,-0.261228228676944,
-0.252023656825121,-0.239237381295077,-0.217082591459106,-0.19274122279055,
-0.187889351840766,-0.185554371677818,-0.183746838367228,-0.181565469863344,
-0.177331470787363,-0.15204128050393,-0.113463271695869,-0.107144754786843,
-0.103137247646399,-0.0999283891798736,-0.0962568557303748,-0.0898146312481536,
-0.0818500030684211,-0.0637876457998723,-0.0434746717486012,-0.0267336435729644,
-0.0214005665803968,-0.0190362204664168,-0.0172232234894831,-0.0155121948018241,
-0.0133884108843324,-0.00853636427515829,-0.000491426210657643),
 .UNSPECIFIED.);
#2773=B_SPLINE_CURVE_WITH_KNOTS('',3,(#106481,#106482,#106483,#106484,#106485,
#106486,#106487,#106488,#106489,#106490),.UNSPECIFIED.,.F.,.F.,(4,2,2,2,
4),(-2.10008367110316,-2.06877505387508,-2.05239041309396,-2.04489701650639,
-2.04104007014271),.UNSPECIFIED.);
#2774=B_SPLINE_CURVE_WITH_KNOTS('',3,(#106491,#106492,#106493,#106494,#106495,
#106496,#106497,#106498,#106499,#106500,#106501,#106502,#106503,#106504,
#106505,#106506,#106507,#106508,#106509,#106510,#106511,#106512,#106513,
#106514,#106515,#106516,#106517,#106518,#106519,#106520,#106521,#106522,
#106523,#106524,#106525,#106526,#106527,#106528,#106529,#106530,#106531,
#106532,#106533,#106534,#106535,#106536,#106537,#106538,#106539,#106540,
#106541,#106542,#106543,#106544,#106545,#106546,#106547,#106548,#106549,
#106550,#106551,#106552,#106553,#106554,#106555,#106556,#106557,#106558,
#106559,#106560,#106561,#106562,#106563,#106564,#106565,#106566,#106567,
#106568,#106569,#106570,#106571,#106572,#106573,#106574,#106575,#106576,
#106577,#106578,#106579,#106580,#106581,#106582,#106583,#106584,#106585,
#106586,#106587,#106588,#106589,#106590,#106591,#106592,#106593,#106594,
#106595,#106596,#106597,#106598,#106599,#106600,#106601,#106602,#106603,
#106604,#106605,#106606,#106607,#106608,#106609,#106610,#106611,#106612,
#106613,#106614,#106615,#106616,#106617,#106618,#106619,#106620,#106621,
#106622,#106623,#106624,#106625,#106626,#106627,#106628,#106629,#106630,
#106631,#106632,#106633,#106634,#106635,#106636,#106637,#106638,#106639,
#106640,#106641,#106642,#106643,#106644,#106645,#106646,#106647,#106648,
#106649,#106650,#106651,#106652,#106653,#106654,#106655,#106656,#106657,
#106658,#106659,#106660,#106661,#106662,#106663,#106664,#106665,#106666,
#106667,#106668,#106669,#106670,#106671,#106672,#106673,#106674,#106675,
#106676,#106677,#106678,#106679,#106680,#106681,#106682,#106683,#106684,
#106685,#106686,#106687,#106688,#106689,#106690,#106691,#106692,#106693,
#106694,#106695,#106696,#106697,#106698,#106699,#106700,#106701,#106702,
#106703,#106704,#106705,#106706),.UNSPECIFIED.,.F.,.F.,(4,2,2,2,2,2,2,2,
2,2,2,2,2,2,2,2,2,2,2,2,2,2,2,2,2,2,2,2,2,2,2,2,2,2,2,2,2,2,2,2,2,2,2,2,
2,2,2,2,2,2,2,2,2,2,2,2,2,2,2,2,2,2,2,2,2,2,2,2,2,2,2,2,2,2,2,2,2,2,2,2,
2,2,2,2,2,2,2,2,2,2,2,2,2,2,2,2,2,2,2,2,2,2,2,2,2,2,2,4),(-1.1089889728157,
-1.09390413199034,-1.08265173652397,-1.07811894729916,-1.07483967776895,
-1.07141429716938,-1.06613416749878,-1.04996520560814,-1.02124021050552,
-0.998263004278718,-0.994568306427569,-0.992478075489208,-0.990658204302517,
-0.988189336114603,-0.982394345455833,-0.973909108028063,-0.943933102140492,
-0.918914312155114,-0.913013794878952,-0.909457211950628,-0.906228921420988,
-0.902029428305775,-0.892846582087099,-0.880100909907931,-0.857930445448674,
-0.853947569498232,-0.831621684569698,-0.827929712876744,-0.825840117333333,
-0.824020151489138,-0.821550287698292,-0.815749145962188,-0.807251458413545,
-0.777176491751801,-0.752272965702892,-0.74637588459982,-0.742820078557052,
-0.739591674739637,-0.735390860198296,-0.726200131530252,-0.713439315930764,
-0.6912739573022,-0.687187080682848,-0.66498773275848,-0.661296298047347,
-0.659206848475852,-0.657386896882586,-0.654916901325263,-0.649114784964344,
-0.640615069012252,-0.610523300550814,-0.585640320492522,-0.579743953767783,
-0.576188346635443,-0.572959976771102,-0.568758996004514,-0.559567008353891,
-0.546803690778839,-0.52463971049363,-0.520536775452562,-0.498357893186431,
-0.494666607719804,-0.492577217418344,-0.490757299434606,-0.488287325375634,
-0.482485153348242,-0.473985259954077,-0.443891326351587,-0.419012054787095,
-0.41311590403831,-0.40956038996555,-0.406332081080179,-0.402131145921418,
-0.392939114469771,-0.380175615144535,-0.358012239679808,-0.35390686628024,
-0.331731579184435,-0.328040380915067,-0.325951036008301,-0.324131154733593,
-0.321661226706775,-0.31585914612673,-0.307359371626219,-0.277265617386782,
-0.252387358302804,-0.246491343327156,-0.242935905281727,-0.239707661728668,
-0.235506806278244,-0.226314926651039,-0.213551619119762,-0.191388721522952,
-0.167084329966978,-0.162128643290664,-0.159807694581368,-0.158001596142522,
-0.155810531906684,-0.151526082090662,-0.145862056975638,-0.131518121766425,
-0.0976949918441955,-0.0839718529526503,-0.0789592205958121,-0.0759258305504556,
-0.0726585305873539,-0.0681942348434812,-0.0594454739927945),
 .UNSPECIFIED.);
#2775=B_SPLINE_CURVE_WITH_KNOTS('',3,(#106711,#106712,#106713,#106714,#106715,
#106716,#106717,#106718,#106719,#106720,#106721,#106722,#106723,#106724,
#106725,#106726,#106727,#106728,#106729,#106730,#106731,#106732,#106733,
#106734,#106735,#106736,#106737,#106738,#106739,#106740,#106741,#106742,
#106743,#106744,#106745,#106746,#106747,#106748,#106749,#106750,#106751,
#106752,#106753,#106754,#106755,#106756,#106757,#106758,#106759,#106760,
#106761,#106762,#106763,#106764,#106765,#106766,#106767,#106768,#106769,
#106770,#106771,#106772,#106773,#106774,#106775,#106776,#106777,#106778,
#106779,#106780,#106781,#106782,#106783,#106784,#106785,#106786,#106787,
#106788,#106789,#106790,#106791,#106792,#106793,#106794,#106795,#106796,
#106797,#106798,#106799,#106800,#106801,#106802,#106803,#106804,#106805,
#106806,#106807,#106808,#106809,#106810,#106811,#106812,#106813,#106814,
#106815,#106816,#106817,#106818,#106819,#106820,#106821,#106822,#106823,
#106824,#106825,#106826,#106827,#106828,#106829,#106830,#106831,#106832,
#106833,#106834,#106835,#106836,#106837,#106838,#106839,#106840,#106841,
#106842,#106843,#106844,#106845,#106846,#106847,#106848,#106849,#106850,
#106851,#106852,#106853,#106854,#106855,#106856,#106857,#106858,#106859,
#106860,#106861,#106862,#106863,#106864,#106865,#106866,#106867,#106868,
#106869,#106870,#106871,#106872,#106873,#106874,#106875,#106876,#106877,
#106878,#106879,#106880,#106881,#106882,#106883,#106884,#106885,#106886,
#106887,#106888,#106889,#106890,#106891,#106892,#106893,#106894,#106895,
#106896,#106897,#106898,#106899,#106900,#106901,#106902,#106903,#106904,
#106905,#106906,#106907,#106908),.UNSPECIFIED.,.F.,.F.,(4,2,2,2,2,2,2,2,
2,2,2,2,2,2,2,2,2,2,2,2,2,2,2,2,2,2,2,2,2,2,2,2,2,2,2,2,2,2,2,2,2,2,2,2,
2,2,2,2,2,2,2,2,2,2,2,2,2,2,2,2,2,2,2,2,2,2,2,2,2,2,2,2,2,2,2,2,2,2,2,2,
2,2,2,2,2,2,2,2,2,2,2,2,2,2,2,2,2,2,4),(-2.04093771886338,-2.02934880549598,
-2.02208728420423,-2.01939460153838,-2.01753903188509,-2.01554880266114,
-2.01221744650086,-1.99999639770519,-1.97264867053721,-1.95406888501436,
-1.94596437990255,-1.93943534866577,-1.93574559522477,-1.93253853150594,
-1.92855634836747,-1.92232435336443,-1.87687277414369,-1.858814724624,-1.85426367841449,
-1.852019179815,-1.85021411053806,-1.8479507327422,-1.84330238579878,-1.8117269651815,
-1.77921103001925,-1.77270841521009,-1.76902409775747,-1.76581637920758,
-1.76182637916616,-1.75379651199526,-1.70985147132532,-1.692063355684,-1.6875437850885,
-1.68530540896126,-1.68350022696993,-1.68123038059221,-1.67654859845027,
-1.64560421939891,-1.61181826504183,-1.60569498564409,-1.60209046598481,
-1.59887144737075,-1.59475764912396,-1.58807322779605,-1.54327776624413,
-1.52537337940295,-1.52084010980807,-1.51859901171743,-1.51679381025957,
-1.51452666899179,-1.50985916867113,-1.47869032466852,-1.44518440640319,
-1.43901777186325,-1.43540400857167,-1.43218654237743,-1.42808820227649,
-1.42145778039966,-1.3879596731307,-1.36671281712231,-1.35957386728726,
-1.35447057091157,-1.35212188061865,-1.3504853011976,-1.348389114066,-1.34466952444868,
-1.32003753521421,-1.30210209767399,-1.28588654130804,-1.27499766230629,
-1.27051871073989,-1.26724780750002,-1.26380366587999,-1.25843743789684,
-1.24145938424182,-1.20379992283226,-1.18998986735269,-1.18665622691549,
-1.18466533684014,-1.18283105292315,-1.1801557120098,-1.17350603734251,
-1.14182623222866,-1.11243487352282,-1.10595171469238,-1.10227130429957,
-1.09906293989677,-1.09506685072939,-1.08878828639482,-1.04984422968113,
-1.04683086993838,-1.0240357954697,-1.0203409895536,-1.01825025635086,-1.01642959739132,
-1.01395910600654,-1.0081577327812,-0.999660533259873,-0.991072635368184),
 .UNSPECIFIED.);
#2776=B_SPLINE_CURVE_WITH_KNOTS('',3,(#106910,#106911,#106912,#106913,#106914,
#106915,#106916,#106917,#106918,#106919),.UNSPECIFIED.,.F.,.F.,(4,2,2,2,
4),(-0.0594454739927945,-0.0573927227399692,-0.0413658239800665,-0.0230003290355216,
-0.000492308750634391),.UNSPECIFIED.);
#2777=B_SPLINE_CURVE_WITH_KNOTS('',3,(#106920,#106921,#106922,#106923,#106924,
#106925,#106926,#106927,#106928,#106929,#106930,#106931,#106932,#106933,
#106934,#106935,#106936,#106937,#106938,#106939,#106940,#106941,#106942,
#106943,#106944,#106945,#106946,#106947,#106948,#106949,#106950,#106951,
#106952,#106953,#106954,#106955,#106956,#106957,#106958,#106959,#106960,
#106961,#106962,#106963,#106964,#106965,#106966,#106967,#106968,#106969,
#106970,#106971,#106972,#106973,#106974,#106975,#106976,#106977,#106978,
#106979,#106980,#106981,#106982,#106983,#106984,#106985,#106986,#106987,
#106988,#106989,#106990,#106991,#106992,#106993,#106994,#106995,#106996,
#106997,#106998,#106999,#107000,#107001,#107002,#107003,#107004,#107005,
#107006,#107007,#107008,#107009,#107010,#107011,#107012,#107013,#107014,
#107015,#107016,#107017,#107018,#107019,#107020,#107021,#107022,#107023,
#107024,#107025,#107026,#107027,#107028,#107029,#107030,#107031,#107032,
#107033,#107034,#107035,#107036,#107037,#107038,#107039,#107040,#107041,
#107042,#107043,#107044,#107045,#107046,#107047,#107048,#107049,#107050,
#107051,#107052,#107053,#107054,#107055,#107056,#107057,#107058,#107059,
#107060,#107061,#107062,#107063,#107064,#107065,#107066,#107067,#107068,
#107069,#107070,#107071,#107072,#107073,#107074,#107075,#107076,#107077,
#107078,#107079,#107080,#107081,#107082,#107083,#107084,#107085,#107086,
#107087,#107088,#107089,#107090,#107091,#107092,#107093,#107094,#107095,
#107096,#107097,#107098,#107099,#107100,#107101,#107102,#107103,#107104,
#107105,#107106,#107107,#107108,#107109,#107110,#107111,#107112,#107113,
#107114,#107115),.UNSPECIFIED.,.F.,.F.,(4,2,2,2,2,2,2,2,2,2,2,2,2,2,2,2,
2,2,2,2,2,2,2,2,2,2,2,2,2,2,2,2,2,2,2,2,2,2,2,2,2,2,2,2,2,2,2,2,2,2,2,2,
2,2,2,2,2,2,2,2,2,2,2,2,2,2,2,2,2,2,2,2,2,2,2,2,2,2,2,2,2,2,2,2,2,2,2,2,
2,2,2,2,2,2,2,2,2,4),(-2.0999332011157,-2.09739257213916,-2.09498989078277,
-2.09312545477489,-2.09142054753589,-2.08945798611463,-2.08625190489876,
-2.07532885103696,-2.05324117035067,-2.01909304476526,-2.01291996774835,
-2.00930561995666,-2.00608958104554,-2.00199576136644,-1.9953785284513,
-1.96145632974956,-1.9322235428279,-1.92791495351409,-1.92571887553611,
-1.92391285774309,-1.92159736719967,-1.91667193680883,-1.89231320551945,
-1.87013520243629,-1.8573569327959,-1.84815782576031,-1.84395542035515,
-1.84072671060947,-1.83717148603319,-1.8312775229547,-1.8064582405382,-1.77633810170779,
-1.76783624896193,-1.76203250133046,-1.75956217786685,-1.7577420982829,
-1.7556526826346,-1.75196161597438,-1.73007499878915,-1.7258976861844,-1.70327904647239,
-1.6906224535315,-1.68148718866209,-1.67729594969833,-1.67406867142039,
-1.6705078630853,-1.6645875407792,-1.63871671453179,-1.60950030599841,-1.60111475018943,
-1.59536891312331,-1.59290828673919,-1.59108942246822,-1.58899447782239,
-1.58527863890755,-1.56075626580516,-1.54281501020186,-1.52653120562676,
-1.51561153054425,-1.51112874037027,-1.5078580121975,-1.50482851831038,
-1.49983880987619,-1.48629841320236,-1.45232893461133,-1.43794613501771,
-1.43227234129906,-1.42798177683983,-1.42578931697462,-1.42398307511072,
-1.4216632082487,-1.41671428804292,-1.39165550396451,-1.36500095017407,
-1.35016065053659,-1.34516366344477,-1.34179638079056,-1.3385156210613,
-1.3345396637354,-1.32676441568341,-1.28361005229642,-1.27058873479754,
-1.26277026407991,-1.26000299063039,-1.25813353583669,-1.25641064298414,
-1.2534354337856,-1.24464497765278,-1.21148405375483,-1.19395537315626,
-1.18247674363694,-1.17791061589915,-1.17462545041544,-1.17161433286871,
-1.1667274068165,-1.15394354632791,-1.11927429955175,-1.10920668715445),
 .UNSPECIFIED.);
#2778=B_SPLINE_CURVE_WITH_KNOTS('',3,(#107121,#107122,#107123,#107124,#107125,
#107126,#107127,#107128,#107129,#107130,#107131,#107132,#107133,#107134,
#107135,#107136,#107137,#107138,#107139,#107140,#107141,#107142,#107143,
#107144,#107145,#107146,#107147,#107148,#107149,#107150,#107151,#107152,
#107153,#107154,#107155,#107156,#107157,#107158,#107159,#107160,#107161,
#107162,#107163,#107164,#107165,#107166,#107167,#107168,#107169,#107170,
#107171,#107172,#107173,#107174,#107175,#107176,#107177,#107178,#107179,
#107180,#107181,#107182,#107183,#107184,#107185,#107186,#107187,#107188,
#107189,#107190,#107191,#107192,#107193,#107194,#107195,#107196,#107197,
#107198,#107199,#107200,#107201,#107202,#107203,#107204,#107205,#107206,
#107207,#107208,#107209,#107210,#107211,#107212,#107213,#107214,#107215,
#107216,#107217,#107218,#107219,#107220,#107221,#107222,#107223,#107224,
#107225,#107226,#107227,#107228,#107229,#107230,#107231,#107232,#107233,
#107234,#107235,#107236,#107237,#107238,#107239,#107240,#107241,#107242,
#107243,#107244,#107245,#107246,#107247,#107248,#107249,#107250,#107251,
#107252,#107253,#107254,#107255,#107256,#107257,#107258,#107259,#107260,
#107261,#107262,#107263,#107264,#107265,#107266,#107267,#107268,#107269,
#107270,#107271,#107272,#107273,#107274,#107275,#107276,#107277,#107278,
#107279,#107280,#107281,#107282,#107283,#107284,#107285,#107286,#107287,
#107288,#107289,#107290,#107291,#107292,#107293,#107294,#107295,#107296,
#107297,#107298,#107299,#107300,#107301,#107302,#107303,#107304),
 .UNSPECIFIED.,.F.,.F.,(4,2,2,2,2,2,2,2,2,2,2,2,2,2,2,2,2,2,2,2,2,2,2,2,
2,2,2,2,2,2,2,2,2,2,2,2,2,2,2,2,2,2,2,2,2,2,2,2,2,2,2,2,2,2,2,2,2,2,2,2,
2,2,2,2,2,2,2,2,2,2,2,2,2,2,2,2,2,2,2,2,2,2,2,2,2,2,2,2,2,2,2,4),(-0.991330164355917,
-0.990766673158264,-0.959591636185856,-0.925979033127857,-0.921500948499669,
-0.919270680392501,-0.917465297118865,-0.915186703690311,-0.910459471075429,
-0.890836516252776,-0.856260979658556,-0.843351122288363,-0.83844554343868,
-0.835430412585874,-0.832146711864749,-0.827593431388309,-0.816208070289606,
-0.798894632841549,-0.766094469815978,-0.756774845606066,-0.753735485512362,
-0.751999734313239,-0.750139600382626,-0.747423060730761,-0.739989739037843,
-0.727909772889895,-0.692422293359357,-0.677270997051221,-0.672099599596438,
-0.66869598311718,-0.665401620099456,-0.66078822864453,-0.648986548240062,
-0.630713966697872,-0.604142184920789,-0.590846857313886,-0.587436936983213,
-0.585429456181567,-0.58358195392054,-0.580934936181083,-0.573996687579575,
-0.534763104895739,-0.511901266438737,-0.506090472113298,-0.50255235059563,
-0.499317956599565,-0.495077316434386,-0.485660193901215,-0.441152234568637,
-0.424501457388614,-0.420892603736543,-0.418841993136153,-0.417010739822306,
-0.414463475561524,-0.408187368209675,-0.39871031712467,-0.359075980765575,
-0.343908557072825,-0.33873560008038,-0.335331731704337,-0.332037698399195,
-0.327425728979654,-0.315633435910989,-0.297382590401466,-0.270867039032409,
-0.25749308392221,-0.254078082402757,-0.252069533138092,-0.250222590701594,
-0.247578545543798,-0.240660485235741,-0.196897818160312,-0.178027596320046,
-0.172473276582961,-0.168989755030561,-0.165737165851204,-0.161369754541182,
-0.151189044584545,-0.136469210954872,-0.106935850396378,-0.0910898619089166,
-0.0875346131291738,-0.0854957609543481,-0.0836610100241452,-0.0810895833329044,
-0.0746565105184794,-0.064844202217108,-0.0421401538965219,-0.0122237431867097,
-0.00636347452454314,-0.00292195652754838,-0.000491893798650521),
 .UNSPECIFIED.);
#2779=B_SPLINE_CURVE_WITH_KNOTS('',3,(#107305,#107306,#107307,#107308,#107309,
#107310,#107311,#107312,#107313,#107314,#107315,#107316),.UNSPECIFIED.,
 .F.,.F.,(4,2,2,2,2,4),(-2.09986416909328,-2.09704942948014,-2.09234257063096,
-2.07828695470315,-2.04102086288901,-2.04093771886338),.UNSPECIFIED.);
#2780=B_SPLINE_CURVE_WITH_KNOTS('',3,(#107317,#107318,#107319,#107320,#107321,
#107322,#107323,#107324,#107325,#107326,#107327,#107328,#107329,#107330,
#107331,#107332,#107333,#107334,#107335,#107336,#107337,#107338,#107339,
#107340,#107341,#107342,#107343,#107344,#107345,#107346,#107347,#107348,
#107349,#107350,#107351,#107352,#107353,#107354,#107355,#107356,#107357,
#107358,#107359,#107360,#107361,#107362,#107363,#107364,#107365,#107366,
#107367,#107368,#107369,#107370,#107371,#107372,#107373,#107374,#107375,
#107376,#107377,#107378,#107379,#107380,#107381,#107382,#107383,#107384,
#107385,#107386,#107387,#107388,#107389,#107390,#107391,#107392,#107393,
#107394,#107395,#107396,#107397,#107398,#107399,#107400,#107401,#107402,
#107403,#107404,#107405,#107406,#107407,#107408,#107409,#107410,#107411,
#107412,#107413,#107414,#107415,#107416,#107417,#107418,#107419,#107420,
#107421,#107422,#107423,#107424,#107425,#107426,#107427,#107428,#107429,
#107430,#107431,#107432,#107433,#107434,#107435,#107436,#107437,#107438,
#107439,#107440,#107441,#107442,#107443,#107444,#107445,#107446,#107447,
#107448,#107449,#107450,#107451,#107452,#107453,#107454,#107455,#107456,
#107457,#107458,#107459,#107460,#107461,#107462,#107463,#107464,#107465,
#107466,#107467,#107468,#107469,#107470,#107471,#107472,#107473,#107474,
#107475,#107476,#107477,#107478,#107479,#107480,#107481,#107482,#107483,
#107484,#107485,#107486,#107487,#107488,#107489,#107490,#107491,#107492,
#107493,#107494,#107495,#107496,#107497,#107498,#107499,#107500,#107501,
#107502,#107503,#107504,#107505,#107506,#107507,#107508,#107509,#107510,
#107511,#107512,#107513,#107514,#107515,#107516),.UNSPECIFIED.,.F.,.F.,
(4,2,2,2,2,2,2,2,2,2,2,2,2,2,2,2,2,2,2,2,2,2,2,2,2,2,2,2,2,2,2,2,2,2,2,
2,2,2,2,2,2,2,2,2,2,2,2,2,2,2,2,2,2,2,2,2,2,2,2,2,2,2,2,2,2,2,2,2,2,2,2,
2,2,2,2,2,2,2,2,2,2,2,2,2,2,2,2,2,2,2,2,2,2,2,2,2,2,2,2,4),(-1.10920668715445,
-1.0996208901351,-1.09489094482217,-1.09261228347598,-1.09080749542534,
-1.08857885286122,-1.08410677844814,-1.05041616918713,-1.02139402565753,
-1.01465732244867,-1.01052920981668,-1.00730947983556,-1.00371501157452,
-0.997635836565699,-0.963375204078934,-0.93293484609209,-0.928205233836145,
-0.925926673263352,-0.92412193484134,-0.921893316214902,-0.91742117838395,
-0.911429462598563,-0.895715643008634,-0.856865639577424,-0.848010232232837,
-0.843868615178909,-0.840647407737652,-0.837060572532154,-0.831017203768369,
-0.823681911626312,-0.807834520690982,-0.79509607326041,-0.766424290357316,
-0.761603593758634,-0.7593078388466,-0.757502742922307,-0.755289986964268,
-0.750897506396175,-0.721124777032205,-0.687884599740569,-0.681246898014919,
-0.677147393987621,-0.673931008264072,-0.670320567965648,-0.664164974236288,
-0.630349770704053,-0.599552372370897,-0.594862189026562,-0.592591300529295,
-0.590786864391447,-0.588551451550751,-0.584044123259823,-0.548497466815328,
-0.521257443239317,-0.514596958620304,-0.51049097885111,-0.507274007092641,
-0.503667582783319,-0.497530589476048,-0.463714253489563,-0.432881191133514,
-0.428194387216505,-0.425924194315586,-0.424119829481707,-0.421883907545715,
-0.417373747266782,-0.411314614179666,-0.395307361004748,-0.355298314354327,
-0.347564513551573,-0.343582449680913,-0.340376568042505,-0.336689399422382,
-0.330168327408791,-0.322076682893815,-0.303541812768545,-0.276297384622105,
-0.263964430063889,-0.260625139999804,-0.258633686713554,-0.256779967352318,
-0.254094280815001,-0.246878396123331,-0.235310453118137,-0.214100216860016,
-0.185482989472097,-0.179517064827112,-0.175946926720627,-0.172722520394608,
-0.168551098522937,-0.159526083262268,-0.114639209580094,-0.0978078882512786,
-0.0941910559951095,-0.0921392492594382,-0.0903094205536025,-0.0877676294695378,
-0.0815223303886219,-0.0721091902688607,-0.0594666017457383),
 .UNSPECIFIED.);
#2781=B_SPLINE_CURVE_WITH_KNOTS('',3,(#107521,#107522,#107523,#107524,#107525,
#107526,#107527,#107528,#107529,#107530,#107531,#107532,#107533,#107534,
#107535,#107536,#107537,#107538,#107539,#107540,#107541,#107542,#107543,
#107544,#107545,#107546,#107547,#107548,#107549,#107550,#107551,#107552,
#107553,#107554,#107555,#107556,#107557,#107558,#107559,#107560,#107561,
#107562,#107563,#107564,#107565,#107566,#107567,#107568,#107569,#107570,
#107571,#107572,#107573,#107574,#107575,#107576,#107577,#107578,#107579,
#107580,#107581,#107582,#107583,#107584,#107585,#107586,#107587,#107588,
#107589,#107590,#107591,#107592,#107593,#107594,#107595,#107596,#107597,
#107598,#107599,#107600,#107601,#107602,#107603,#107604,#107605,#107606,
#107607,#107608,#107609,#107610,#107611,#107612,#107613,#107614,#107615,
#107616,#107617,#107618,#107619,#107620,#107621,#107622,#107623,#107624,
#107625,#107626,#107627,#107628,#107629,#107630,#107631,#107632,#107633,
#107634,#107635,#107636,#107637,#107638,#107639,#107640,#107641,#107642,
#107643,#107644,#107645,#107646,#107647,#107648,#107649,#107650,#107651,
#107652,#107653,#107654,#107655,#107656,#107657,#107658,#107659,#107660,
#107661,#107662,#107663,#107664,#107665,#107666,#107667,#107668,#107669,
#107670,#107671,#107672,#107673,#107674,#107675,#107676,#107677,#107678,
#107679,#107680,#107681,#107682,#107683,#107684,#107685,#107686,#107687,
#107688,#107689,#107690,#107691,#107692,#107693,#107694,#107695,#107696,
#107697,#107698,#107699,#107700,#107701,#107702,#107703,#107704,#107705,
#107706,#107707,#107708,#107709,#107710,#107711,#107712,#107713,#107714,
#107715,#107716,#107717,#107718),.UNSPECIFIED.,.F.,.F.,(4,2,2,2,2,2,2,2,
2,2,2,2,2,2,2,2,2,2,2,2,2,2,2,2,2,2,2,2,2,2,2,2,2,2,2,2,2,2,2,2,2,2,2,2,
2,2,2,2,2,2,2,2,2,2,2,2,2,2,2,2,2,2,2,2,2,2,2,2,2,2,2,2,2,2,2,2,2,2,2,2,
2,2,2,2,2,2,2,2,2,2,2,2,2,2,2,2,2,2,4),(-2.0412420799731,-2.04034028984006,
-2.02158199735914,-2.00957594468979,-2.00493359672236,-2.00163391631721,
-1.99863650512635,-1.99460071303198,-1.98448875220065,-1.94722404217195,
-1.93193304781641,-1.9260399202716,-1.92162316274255,-1.91940498657613,
-1.91759923076491,-1.91530729835558,-1.91051003425248,-1.88146752229286,
-1.84673917232611,-1.84018223804752,-1.83648641450168,-1.83327953241321,
-1.82930464138898,-1.82309820286662,-1.77751834262795,-1.7595199556566,
-1.75497558586645,-1.75273224635372,-1.75092697206141,-1.74866191211158,
-1.74400559751323,-1.71259623433521,-1.67981225399705,-1.67336865881302,
-1.66969644353272,-1.66648706129433,-1.66247899304551,-1.65435520769229,
-1.61470143687081,-1.59878745547793,-1.59274894142858,-1.58824956964224,
-1.58601505429387,-1.5842096706824,-1.58193540040753,-1.5772311046547,-1.54652905447861,
-1.51275274146498,-1.50650813211005,-1.50287778022188,-1.49966286065376,
-1.49559129860902,-1.487127133432,-1.44786181710417,-1.43204628652902,-1.42317663268646,
-1.42028021952343,-1.41838413325667,-1.41645378952942,-1.41339772770353,
-1.40393557935066,-1.37118077950192,-1.35392191498966,-1.34256148238213,
-1.33801171939212,-1.33472855794252,-1.33171257327552,-1.32680247897091,
-1.31386029331505,-1.27933837199892,-1.26480101608667,-1.25639572777873,
-1.25355421855214,-1.25166952241778,-1.24996145219351,-1.24706530673577,
-1.23889475695405,-1.20533945783425,-1.18756518601257,-1.1796791906009,
-1.17328659578504,-1.16962515881791,-1.1664146460508,-1.16239122297399,
-1.15601930283333,-1.11801032093176,-1.09228266080915,-1.08804663163659,
-1.0858647006441,-1.08405699639688,-1.0817221501291,-1.07687173054787,-1.05042524709968,
-1.01446375046852,-1.0079305684096,-1.00386026813836,-1.000645543293,-0.997014566849272,
-0.991330164355917),.UNSPECIFIED.);
#2782=B_SPLINE_CURVE_WITH_KNOTS('',3,(#107720,#107721,#107722,#107723,#107724,
#107725,#107726,#107727,#107728,#107729,#107730,#107731,#107732,#107733,
#107734,#107735),.UNSPECIFIED.,.F.,.F.,(4,2,2,2,2,2,2,4),(-0.0594666017457383,
-0.032621887068177,-0.0172456592650443,-0.012157102551331,-0.008731466438282,
-0.0056783971083446,-0.00301214739693347,-0.000491717955116048),
 .UNSPECIFIED.);
#2783=B_SPLINE_CURVE_WITH_KNOTS('',3,(#107736,#107737,#107738,#107739,#107740,
#107741,#107742,#107743,#107744,#107745,#107746,#107747,#107748,#107749,
#107750,#107751,#107752,#107753,#107754,#107755,#107756,#107757,#107758,
#107759,#107760,#107761,#107762,#107763,#107764,#107765,#107766,#107767,
#107768,#107769,#107770,#107771,#107772,#107773,#107774,#107775,#107776,
#107777,#107778,#107779,#107780,#107781,#107782,#107783,#107784,#107785,
#107786,#107787,#107788,#107789,#107790,#107791,#107792,#107793,#107794,
#107795,#107796,#107797,#107798,#107799,#107800,#107801,#107802,#107803,
#107804,#107805,#107806,#107807,#107808,#107809,#107810,#107811,#107812,
#107813,#107814,#107815,#107816,#107817,#107818,#107819,#107820,#107821,
#107822,#107823,#107824,#107825,#107826,#107827,#107828,#107829,#107830,
#107831,#107832,#107833,#107834,#107835,#107836,#107837,#107838,#107839,
#107840,#107841,#107842,#107843,#107844,#107845,#107846,#107847,#107848,
#107849,#107850,#107851,#107852,#107853,#107854,#107855,#107856,#107857,
#107858,#107859,#107860,#107861,#107862,#107863,#107864,#107865,#107866,
#107867,#107868,#107869,#107870,#107871,#107872,#107873,#107874,#107875,
#107876,#107877,#107878,#107879,#107880,#107881,#107882,#107883,#107884,
#107885,#107886,#107887,#107888,#107889,#107890,#107891,#107892,#107893,
#107894,#107895,#107896,#107897,#107898,#107899,#107900,#107901,#107902,
#107903,#107904,#107905,#107906,#107907,#107908,#107909,#107910,#107911,
#107912,#107913,#107914,#107915,#107916,#107917,#107918,#107919,#107920,
#107921,#107922,#107923,#107924,#107925,#107926,#107927,#107928,#107929,
#107930,#107931,#107932,#107933),.UNSPECIFIED.,.F.,.F.,(4,2,2,2,2,2,2,2,
2,2,2,2,2,2,2,2,2,2,2,2,2,2,2,2,2,2,2,2,2,2,2,2,2,2,2,2,2,2,2,2,2,2,2,2,
2,2,2,2,2,2,2,2,2,2,2,2,2,2,2,2,2,2,2,2,2,2,2,2,2,2,2,2,2,2,2,2,2,2,2,2,
2,2,2,2,2,2,2,2,2,2,2,2,2,2,2,2,2,2,4),(-2.09987818931514,-2.09265685916745,
-2.04920876173439,-2.03648785482216,-2.02879046050777,-2.02603905676681,
-2.02417269259838,-2.02244616551281,-2.019452239282,-2.01050935080262,-1.9774428436789,
-1.95997517026093,-1.95217475319003,-1.94758124349242,-1.94338415960361,
-1.94015612592297,-1.9365982335642,-1.93069171455341,-1.90585709216354,
-1.87576930286984,-1.86727153065022,-1.86146980714479,-1.85899981872863,
-1.85717977494456,-1.85509014713664,-1.85139817990397,-1.82928256869064,
-1.82510347560292,-1.80292379079051,-1.79015128634646,-1.78095521137088,
-1.77675333815717,-1.77352469905287,-1.76996921381308,-1.76407401157867,
-1.73921302722891,-1.7091295051988,-1.70063230028604,-1.69483086794757,
-1.69236093685382,-1.69054092080869,-1.68845132825768,-1.68475936950186,
-1.66262952579751,-1.65846163420306,-1.63628113390123,-1.62351070725589,
-1.61431575741793,-1.61011414106341,-1.60688560092258,-1.60333012823298,
-1.59743472210822,-1.57256366448291,-1.54248915881248,-1.53399315068875,
-1.5281923400351,-1.52572254473798,-1.52390257009703,-1.52181294613885,
-1.5181208168879,-1.49594210025623,-1.49181276074532,-1.4696297562061,-1.45686643453461,
-1.44767518629898,-1.44347420405053,-1.44024573278455,-1.43668991729546,
-1.43079294299026,-1.40586805919897,-1.37584136231047,-1.36735140769438,
-1.36155358860689,-1.35908426598509,-1.35726429563889,-1.35517421925982,
-1.35148042744211,-1.32885913541171,-1.31192821630655,-1.29380910736794,
-1.2820746357516,-1.27747158899413,-1.27417983369694,-1.27117617106732,
-1.26711146923517,-1.2568150911615,-1.21602760324243,-1.20327728745127,
-1.19556800697994,-1.19281505441106,-1.19094842809758,-1.18897931324107,
-1.18574278720833,-1.17450551448091,-1.14643858817064,-1.12756418754894,
-1.11938163011068,-1.11280441351441,-1.10915669663231),.UNSPECIFIED.);
#2784=B_SPLINE_CURVE_WITH_KNOTS('',3,(#107939,#107940,#107941,#107942,#107943,
#107944,#107945,#107946,#107947,#107948,#107949,#107950,#107951,#107952,
#107953,#107954,#107955,#107956,#107957,#107958),.UNSPECIFIED.,.F.,.F.,
(4,2,2,2,2,2,2,2,2,4),(-0.0592977063510342,-0.0406565713569759,-0.0296459142995207,
-0.0264393932675981,-0.0244829701643915,-0.0227840180597207,-0.0209206230480024,
-0.0183407941751122,-0.012273668438799,-0.000511201039480913),
 .UNSPECIFIED.);
#2785=B_SPLINE_CURVE_WITH_KNOTS('',3,(#107960,#107961,#107962,#107963,#107964,
#107965,#107966,#107967,#107968,#107969,#107970,#107971,#107972,#107973,
#107974,#107975,#107976,#107977,#107978,#107979,#107980,#107981,#107982,
#107983,#107984,#107985,#107986,#107987,#107988,#107989,#107990,#107991,
#107992,#107993,#107994,#107995,#107996,#107997,#107998,#107999,#108000,
#108001,#108002,#108003,#108004,#108005,#108006,#108007,#108008,#108009,
#108010,#108011,#108012,#108013,#108014,#108015,#108016,#108017,#108018,
#108019,#108020,#108021,#108022,#108023,#108024,#108025,#108026,#108027,
#108028,#108029,#108030,#108031,#108032,#108033,#108034,#108035,#108036,
#108037,#108038,#108039,#108040,#108041,#108042,#108043,#108044,#108045,
#108046,#108047,#108048,#108049,#108050,#108051,#108052,#108053,#108054,
#108055,#108056,#108057,#108058,#108059,#108060,#108061,#108062,#108063,
#108064,#108065,#108066,#108067,#108068),.UNSPECIFIED.,.F.,.F.,(4,3,3,3,
3,3,3,3,3,3,3,3,3,3,3,3,3,3,3,3,3,3,3,3,3,3,3,3,3,3,3,3,3,3,3,3,4),(-3.84638326322104,
-3.73817304644031,-3.63008307635761,-3.52207051640325,-3.41409265085555,
-3.30603153247512,-3.19793262975346,-3.08963570929982,-2.99264357503826,
-2.88276576904152,-2.77180701249785,-2.6622259577447,-2.55271003115832,
-2.44321871026559,-2.33118796187223,-2.22155393901983,-2.108324827856,-1.99509571669217,
-1.88634917197483,-1.77524900777124,-1.66680167782881,-1.55841756692922,
-1.45005450048505,-1.33692783995031,-1.22840073648774,-1.11978586886727,
-1.01096961743765,-0.997547858346085,-0.884786118899249,-0.772265208178043,
-0.659886256614288,-0.547615706777961,-0.43542015049968,-0.323231033746395,
-0.211055181000669,-0.0987911575872374,0.),.UNSPECIFIED.);
#2786=B_SPLINE_CURVE_WITH_KNOTS('',3,(#108071,#108072,#108073,#108074,#108075,
#108076,#108077,#108078,#108079,#108080,#108081,#108082,#108083,#108084,
#108085,#108086,#108087,#108088,#108089,#108090,#108091,#108092,#108093,
#108094,#108095,#108096,#108097,#108098,#108099,#108100,#108101,#108102,
#108103,#108104,#108105,#108106,#108107,#108108,#108109,#108110,#108111,
#108112,#108113,#108114,#108115,#108116,#108117,#108118,#108119,#108120,
#108121,#108122,#108123,#108124,#108125,#108126,#108127,#108128,#108129,
#108130,#108131,#108132,#108133,#108134,#108135,#108136,#108137,#108138,
#108139,#108140,#108141,#108142,#108143,#108144,#108145,#108146,#108147,
#108148,#108149,#108150,#108151,#108152,#108153,#108154,#108155,#108156,
#108157,#108158,#108159,#108160,#108161,#108162,#108163,#108164,#108165,
#108166,#108167,#108168,#108169,#108170,#108171,#108172,#108173,#108174,
#108175,#108176,#108177,#108178,#108179,#108180,#108181,#108182,#108183,
#108184,#108185,#108186,#108187,#108188,#108189,#108190,#108191,#108192,
#108193,#108194,#108195,#108196,#108197,#108198,#108199,#108200,#108201,
#108202,#108203,#108204,#108205,#108206,#108207,#108208,#108209,#108210,
#108211,#108212,#108213,#108214,#108215,#108216,#108217,#108218,#108219,
#108220,#108221,#108222,#108223,#108224,#108225,#108226,#108227,#108228,
#108229,#108230,#108231,#108232,#108233,#108234,#108235,#108236,#108237,
#108238,#108239,#108240,#108241,#108242,#108243,#108244,#108245,#108246,
#108247,#108248,#108249,#108250),.UNSPECIFIED.,.F.,.F.,(4,2,2,2,2,2,2,2,
2,2,2,2,2,2,2,2,2,2,2,2,2,2,2,2,2,2,2,2,2,2,2,2,2,2,2,2,2,2,2,2,2,2,2,2,
2,2,2,2,2,2,2,2,2,2,2,2,2,2,2,2,2,2,2,2,2,2,2,2,2,2,2,2,2,2,2,2,2,2,2,2,
2,2,2,2,2,2,2,2,2,4),(-1.9798082478801,-1.97972857885761,-1.97636370684344,
-1.93875794853755,-1.92034230820633,-1.90842989899881,-1.90376413773363,
-1.900427415003,-1.89697415830706,-1.89171126908936,-1.8759895379423,-1.84031468570726,
-1.82499010409875,-1.82151830834034,-1.81946738308023,-1.81761159279483,
-1.8153496532383,-1.81090414679126,-1.78707124954771,-1.76439509235973,
-1.75172599216021,-1.74257924009979,-1.7383717667015,-1.73512660116134,
-1.73154013228812,-1.72556177893816,-1.69808723799443,-1.67004433406912,
-1.65781653480299,-1.65459244300484,-1.6526222427315,-1.65078120674275,
-1.64804459181953,-1.64097352945887,-1.60966033578755,-1.58067315828821,
-1.57409363647062,-1.57040718173468,-1.56722144981701,-1.56329026534161,
-1.55718906344407,-1.51650588498505,-1.49271417254024,-1.48844567288275,
-1.48626659336839,-1.48446520562592,-1.48214832529626,-1.47721925534661,
-1.45363371065508,-1.43337047940566,-1.41901690938295,-1.40901067535155,
-1.40466598470465,-1.40141121869766,-1.3979070732372,-1.39227857560915,
-1.3724240621606,-1.33789274299452,-1.32453323833562,-1.32122410181192,
-1.31923432254535,-1.31739280198788,-1.31512089888867,-1.30949427575413,
-1.27689820567008,-1.25112716224158,-1.24212609660851,-1.23795630698055,
-1.23472924745761,-1.23115214436295,-1.22516464537184,-1.19608432621958,
-1.16951459537087,-1.15761641614849,-1.15442448805689,-1.15246445640105,
-1.15061397541791,-1.1478474270415,-1.14061619101804,-1.10944393232432,
-1.08438063722298,-1.0753951491831,-1.07123121727475,-1.06800835004163,
-1.06443566654792,-1.05845531946044,-1.02913335488853,-1.00714774457551,
-0.991411872917561,-0.991403523612787),.UNSPECIFIED.);
#2787=B_SPLINE_CURVE_WITH_KNOTS('',3,(#108256,#108257,#108258,#108259,#108260,
#108261,#108262,#108263,#108264,#108265,#108266,#108267,#108268,#108269,
#108270,#108271,#108272,#108273,#108274,#108275,#108276,#108277,#108278,
#108279,#108280,#108281,#108282,#108283,#108284,#108285,#108286,#108287,
#108288,#108289,#108290,#108291,#108292,#108293,#108294,#108295,#108296,
#108297,#108298,#108299,#108300,#108301,#108302,#108303,#108304,#108305,
#108306,#108307,#108308,#108309,#108310,#108311,#108312,#108313,#108314,
#108315,#108316,#108317,#108318,#108319),.UNSPECIFIED.,.F.,.F.,(4,3,3,3,
3,3,3,3,3,3,3,3,3,3,3,3,3,3,3,3,3,4),(89.6265204120243,89.7423236955964,
89.7793072511478,89.8880549678023,89.9991549855138,90.1076034906654,90.2159887756881,
90.3243530139057,90.4374785378027,90.5460067960164,90.6546228124427,90.7634401963979,
90.7768551094939,90.8896159606061,91.0021359799181,91.1145140404942,91.2267837026141,
91.3389783773049,91.4511666309088,91.5633416309981,91.6756048300988,91.77440296784),
 .UNSPECIFIED.);
#2788=B_SPLINE_CURVE_WITH_KNOTS('',3,(#108322,#108323,#108324,#108325,#108326,
#108327,#108328,#108329,#108330,#108331,#108332,#108333,#108334,#108335,
#108336,#108337,#108338,#108339,#108340,#108341,#108342,#108343,#108344,
#108345,#108346,#108347,#108348,#108349,#108350,#108351,#108352,#108353,
#108354,#108355,#108356,#108357,#108358,#108359,#108360,#108361,#108362,
#108363,#108364,#108365,#108366,#108367,#108368,#108369,#108370,#108371,
#108372,#108373,#108374,#108375,#108376,#108377,#108378,#108379,#108380,
#108381,#108382,#108383,#108384,#108385,#108386,#108387,#108388,#108389,
#108390,#108391,#108392,#108393,#108394,#108395,#108396,#108397,#108398,
#108399,#108400,#108401,#108402,#108403,#108404,#108405,#108406,#108407,
#108408,#108409,#108410,#108411,#108412,#108413,#108414,#108415,#108416,
#108417,#108418,#108419,#108420,#108421,#108422,#108423,#108424,#108425,
#108426,#108427,#108428,#108429,#108430,#108431,#108432,#108433,#108434,
#108435,#108436,#108437,#108438,#108439),.UNSPECIFIED.,.F.,.F.,(4,2,2,2,
2,2,2,2,2,2,2,2,2,2,2,2,2,2,2,2,2,2,2,2,2,2,2,2,2,2,2,2,2,2,2,2,2,2,2,2,
2,2,2,2,2,2,2,2,2,2,2,2,2,2,2,2,2,2,4),(-1.75481728510969,-1.75477181337264,
-1.75153187178093,-1.71275849427788,-1.69497582072548,-1.683337395363,-1.67871180999002,
-1.67538295114897,-1.67191960250538,-1.66660456046912,-1.65037913960663,
-1.60504731770615,-1.59826860042396,-1.59560949386773,-1.59373031824308,
-1.59167630480205,-1.58810673052832,-1.57241518926486,-1.54292081107085,
-1.52819502118948,-1.51800868340683,-1.51362687471493,-1.51035825589616,
-1.50685212820087,-1.50124890871277,-1.48201218035526,-1.4384075977429,
-1.43151370044267,-1.42886927969711,-1.42702102419335,-1.4250209951348,
-1.42161605848922,-1.40824164098538,-1.38168743495141,-1.36341339699232,
-1.35162601713303,-1.34703193709419,-1.34375687734004,-1.34037859829957,
-1.33525779623736,-1.32041932433269,-1.28441371753311,-1.27223733355736,
-1.26477052417365,-1.26206143967995,-1.26021071906368,-1.2584793794237,
-1.25546173708441,-1.2463249096779,-1.21667700630301,-1.19715006646039,
-1.18482019530896,-1.1801284704705,-1.17681564299213,-1.17382065619317,
-1.16905081057468,-1.15709755632943,-1.11839002684626,-1.10915476758989),
 .UNSPECIFIED.);
#2789=B_SPLINE_CURVE_WITH_KNOTS('',3,(#108445,#108446,#108447,#108448,#108449,
#108450,#108451,#108452,#108453,#108454,#108455,#108456,#108457,#108458,
#108459,#108460,#108461,#108462,#108463,#108464,#108465,#108466,#108467,
#108468,#108469,#108470,#108471,#108472,#108473,#108474,#108475,#108476,
#108477,#108478,#108479,#108480,#108481,#108482,#108483,#108484,#108485,
#108486,#108487,#108488,#108489,#108490,#108491,#108492,#108493,#108494,
#108495,#108496,#108497,#108498,#108499,#108500,#108501,#108502,#108503,
#108504,#108505,#108506,#108507,#108508,#108509,#108510,#108511,#108512,
#108513,#108514,#108515,#108516,#108517,#108518,#108519,#108520,#108521,
#108522,#108523,#108524,#108525,#108526,#108527,#108528,#108529,#108530,
#108531,#108532,#108533,#108534,#108535,#108536,#108537,#108538,#108539,
#108540,#108541,#108542,#108543,#108544,#108545,#108546,#108547,#108548,
#108549,#108550,#108551,#108552,#108553,#108554,#108555,#108556,#108557,
#108558,#108559,#108560,#108561,#108562,#108563,#108564,#108565,#108566,
#108567,#108568,#108569,#108570,#108571,#108572,#108573,#108574,#108575,
#108576,#108577,#108578,#108579,#108580,#108581,#108582,#108583,#108584,
#108585,#108586,#108587,#108588,#108589,#108590,#108591,#108592,#108593,
#108594,#108595,#108596,#108597,#108598,#108599,#108600,#108601,#108602,
#108603,#108604,#108605,#108606,#108607,#108608,#108609,#108610,#108611,
#108612,#108613,#108614,#108615,#108616,#108617,#108618,#108619,#108620,
#108621,#108622,#108623,#108624,#108625,#108626,#108627,#108628),
 .UNSPECIFIED.,.F.,.F.,(4,2,2,2,2,2,2,2,2,2,2,2,2,2,2,2,2,2,2,2,2,2,2,2,
2,2,2,2,2,2,2,2,2,2,2,2,2,2,2,2,2,2,2,2,2,2,2,2,2,2,2,2,2,2,2,2,2,2,2,2,
2,2,2,2,2,2,2,2,2,2,2,2,2,2,2,2,2,2,2,2,2,2,2,2,2,2,2,2,2,2,2,4),(-0.991365966097619,
-0.988171403346623,-0.951027708418659,-0.924485213621447,-0.919532060449943,
-0.917210835975265,-0.91540454613298,-0.913213639481231,-0.908927440911297,
-0.877285678772001,-0.84577788527823,-0.839101439246275,-0.834991520611357,
-0.83177503323073,-0.828172910207905,-0.822052804129883,-0.788117655616523,
-0.757375988151864,-0.752680411982564,-0.750408822704871,-0.748604220264088,
-0.746369106028614,-0.741866430389762,-0.735821578711076,-0.71988238002869,
-0.680158740793254,-0.672049915076576,-0.668043654999549,-0.66483322181507,
-0.661157052101005,-0.654698917509413,-0.621093460965964,-0.590739757177692,
-0.585998485575938,-0.58371576167084,-0.581906308604257,-0.579668955140634,
-0.575176607633632,-0.569153334899086,-0.553314308664931,-0.513867326472703,
-0.505674317180689,-0.501648920062505,-0.498432738193541,-0.494760148481005,
-0.488334920949002,-0.480402422841681,-0.462476277896191,-0.428742094787966,
-0.42089209671108,-0.418039325772129,-0.416339634829174,-0.414459619557906,
-0.411599685015836,-0.402936981831098,-0.387679147675741,-0.350697237862635,
-0.340099791172841,-0.335556591542221,-0.332322551037855,-0.328936500753204,
-0.323780105104325,-0.307248622439695,-0.274080309521543,-0.255531550411014,
-0.251924635015031,-0.24985975941104,-0.248034397591261,-0.245530546972807,
-0.239549921144152,-0.230697456376526,-0.206475386124692,-0.1787310156925,
-0.172040192323377,-0.167912677850742,-0.164676766789898,-0.161046485613818,
-0.154860499093797,-0.14730965957079,-0.130746118999874,-0.0988550790677954,
-0.0879914983010599,-0.0847701619770891,-0.0827915461032264,-0.0808695332414206,
-0.0779944094387794,-0.0696293301742921,-0.0552214154328846,-0.0133076718806713,
-0.00643057283658562,-0.00291508547563278,-0.0005116043560236),
 .UNSPECIFIED.);
#2790=B_SPLINE_CURVE_WITH_KNOTS('',3,(#108629,#108630,#108631,#108632,#108633,
#108634,#108635,#108636,#108637,#108638),.UNSPECIFIED.,.F.,.F.,(4,3,3,4),
(89.2744165561707,89.38943262493,89.5079765184772,89.6265204120243),
 .UNSPECIFIED.);
#2791=B_SPLINE_CURVE_WITH_KNOTS('',3,(#108639,#108640,#108641,#108642,#108643,
#108644,#108645,#108646,#108647,#108648,#108649,#108650,#108651,#108652,
#108653,#108654,#108655,#108656,#108657,#108658,#108659,#108660,#108661,
#108662,#108663,#108664,#108665,#108666,#108667,#108668,#108669,#108670,
#108671,#108672,#108673,#108674,#108675,#108676,#108677,#108678,#108679,
#108680,#108681,#108682,#108683,#108684,#108685,#108686,#108687,#108688,
#108689,#108690,#108691,#108692,#108693,#108694,#108695,#108696,#108697,
#108698,#108699,#108700,#108701,#108702,#108703,#108704,#108705,#108706,
#108707,#108708,#108709,#108710,#108711,#108712,#108713,#108714,#108715,
#108716,#108717,#108718,#108719,#108720,#108721,#108722,#108723,#108724,
#108725,#108726,#108727,#108728,#108729,#108730,#108731,#108732,#108733,
#108734,#108735,#108736,#108737,#108738,#108739,#108740,#108741,#108742,
#108743,#108744,#108745,#108746,#108747,#108748,#108749,#108750,#108751,
#108752,#108753,#108754,#108755,#108756,#108757,#108758,#108759,#108760,
#108761,#108762,#108763,#108764,#108765,#108766,#108767,#108768,#108769,
#108770,#108771,#108772,#108773,#108774,#108775,#108776,#108777,#108778,
#108779,#108780,#108781,#108782,#108783,#108784,#108785,#108786,#108787,
#108788,#108789,#108790,#108791,#108792,#108793,#108794,#108795,#108796,
#108797,#108798,#108799,#108800,#108801,#108802,#108803,#108804,#108805,
#108806,#108807,#108808,#108809,#108810,#108811,#108812,#108813,#108814,
#108815,#108816,#108817,#108818,#108819,#108820,#108821,#108822,#108823,
#108824,#108825,#108826,#108827,#108828,#108829,#108830,#108831,#108832,
#108833,#108834,#108835,#108836,#108837,#108838,#108839,#108840,#108841,
#108842,#108843,#108844,#108845,#108846,#108847,#108848,#108849,#108850,
#108851,#108852,#108853,#108854,#108855,#108856),.UNSPECIFIED.,.F.,.F.,
(4,2,2,2,2,2,2,2,2,2,2,2,2,2,2,2,2,2,2,2,2,2,2,2,2,2,2,2,2,2,2,2,2,2,2,
2,2,2,2,2,2,2,2,2,2,2,2,2,2,2,2,2,2,2,2,2,2,2,2,2,2,2,2,2,2,2,2,2,2,2,2,
2,2,2,2,2,2,2,2,2,2,2,2,2,2,2,2,2,2,2,2,2,2,2,2,2,2,2,2,2,2,2,2,2,2,2,2,
2,4),(-1.10915476758989,-1.10591269887554,-1.09831262663028,-1.09556885125491,
-1.09369988839749,-1.09172147898789,-1.08844984566113,-1.07684122676752,
-1.04905253340296,-1.02093818842599,-1.01503671458796,-1.011478688229,-1.00824848794993,
-1.00411575334142,-0.995066440372814,-0.95241799962058,-0.939448567678061,
-0.931650085503435,-0.928885238733866,-0.927016293223566,-0.925051907038574,
-0.921834192030397,-0.910795257199551,-0.878917573244537,-0.854166838220865,
-0.848276576579817,-0.844723781452716,-0.841497496625485,-0.837298663939667,
-0.828109764114612,-0.815351174088964,-0.793170065098792,-0.78918399667406,
-0.76685734926639,-0.763166664998647,-0.761078354558164,-0.759258785846163,
-0.756789568927929,-0.75099352474985,-0.742506502740908,-0.712520149688132,
-0.687505557982705,-0.681603740934655,-0.678046105746995,-0.674816658201571,
-0.670615321973303,-0.661426597907566,-0.648670027263927,-0.626513181060461,
-0.622406803408179,-0.600236589277191,-0.596544402090522,-0.594454126190604,
-0.592633534159041,-0.590162326809779,-0.584354641376705,-0.57584417185639,
-0.545670536684166,-0.520882308009663,-0.514988465362761,-0.511433169593473,
-0.508204312797849,-0.504001592882966,-0.494801114593605,-0.482022249631789,
-0.459859098790976,-0.455687809651332,-0.433590842226422,-0.429899585768213,
-0.427810162328844,-0.425990263346943,-0.423520355790637,-0.41771837945405,
-0.409218889008852,-0.379129430160548,-0.354240075731908,-0.348343606438635,
-0.344788091837284,-0.341559913607819,-0.337359349303703,-0.328169075750749,
-0.315409011071738,-0.293241542476824,-0.289168613256107,-0.266951351457106,
-0.263259952931647,-0.261170606702629,-0.259350665511173,-0.256880704924071,
-0.251079145312153,-0.242580663107586,-0.212499837262792,-0.187582909402351,
-0.181696070158885,-0.178142337625143,-0.174913213247982,-0.170707714485491,
-0.161490703421122,-0.148679700319745,-0.126536537743213,-0.122249519500312,
-0.10031932867716,-0.0966288102038732,-0.0945394845739377,-0.0927194134372372,
-0.0902488872540718,-0.0844437274590148,-0.0759379139851325,-0.0594803364103627),
 .UNSPECIFIED.);
#2792=B_SPLINE_CURVE_WITH_KNOTS('',3,(#108861,#108862,#108863,#108864,#108865,
#108866,#108867,#108868,#108869,#108870,#108871,#108872,#108873,#108874,
#108875,#108876,#108877,#108878,#108879,#108880,#108881,#108882,#108883,
#108884,#108885,#108886,#108887,#108888,#108889,#108890,#108891,#108892,
#108893,#108894,#108895,#108896,#108897,#108898,#108899,#108900,#108901,
#108902,#108903,#108904,#108905,#108906,#108907,#108908,#108909,#108910,
#108911,#108912,#108913,#108914,#108915,#108916,#108917,#108918,#108919,
#108920,#108921,#108922,#108923,#108924,#108925,#108926,#108927,#108928,
#108929,#108930,#108931,#108932,#108933,#108934,#108935,#108936,#108937,
#108938,#108939,#108940,#108941,#108942,#108943,#108944,#108945,#108946,
#108947,#108948,#108949,#108950,#108951,#108952,#108953,#108954,#108955,
#108956,#108957,#108958,#108959,#108960,#108961,#108962,#108963,#108964,
#108965,#108966,#108967,#108968,#108969,#108970,#108971,#108972,#108973,
#108974,#108975,#108976,#108977,#108978,#108979,#108980,#108981,#108982,
#108983,#108984,#108985,#108986,#108987,#108988,#108989,#108990,#108991,
#108992,#108993,#108994,#108995,#108996,#108997,#108998,#108999,#109000,
#109001,#109002,#109003,#109004,#109005,#109006,#109007,#109008,#109009,
#109010,#109011,#109012,#109013,#109014,#109015,#109016,#109017,#109018,
#109019,#109020,#109021,#109022,#109023,#109024,#109025,#109026,#109027,
#109028,#109029,#109030,#109031,#109032,#109033,#109034,#109035,#109036,
#109037,#109038,#109039,#109040,#109041,#109042,#109043,#109044,#109045,
#109046,#109047,#109048,#109049,#109050,#109051,#109052,#109053,#109054,
#109055,#109056,#109057,#109058,#109059,#109060,#109061,#109062,#109063,
#109064,#109065,#109066,#109067,#109068,#109069,#109070,#109071,#109072,
#109073,#109074,#109075,#109076),.UNSPECIFIED.,.F.,.F.,(4,2,2,2,2,2,2,2,
2,2,2,2,2,2,2,2,2,2,2,2,2,2,2,2,2,2,2,2,2,2,2,2,2,2,2,2,2,2,2,2,2,2,2,2,
2,2,2,2,2,2,2,2,2,2,2,2,2,2,2,2,2,2,2,2,2,2,2,2,2,2,2,2,2,2,2,2,2,2,2,2,
2,2,2,2,2,2,2,2,2,2,2,2,2,2,2,2,2,2,2,2,2,2,2,2,2,2,2,4),(-2.04109288767521,
-2.03687409690353,-2.01877604215181,-2.01080122194488,-2.00435292186267,
-2.00067972693583,-1.99747046188616,-1.99346381783989,-1.98714950953611,
-1.94854787787447,-1.92329715138688,-1.91906359849201,-1.91688212668974,
-1.91507433937708,-1.91273878684722,-1.90788492461484,-1.88352805463694,
-1.86135525310743,-1.84856021519006,-1.83935161916744,-1.83514657090432,
-1.83191645493625,-1.82836027830888,-1.82246608040773,-1.79768773004298,
-1.76753019545428,-1.75902273361361,-1.75321573581784,-1.75074429413677,
-1.74892347192538,-1.74683322707306,-1.74314067118672,-1.72114037231852,
-1.71687648042423,-1.69470447950986,-1.68190706046456,-1.67269719927741,
-1.66849191849167,-1.66526175956431,-1.66170567024749,-1.6558119339385,
-1.63104819090398,-1.60087893266394,-1.59236999930377,-1.58656225572344,
-1.58409066292257,-1.58226976601499,-1.58017942139659,-1.57648678065388,
-1.55448186952836,-1.55022240019711,-1.52805146305322,-1.51525674181924,
-1.50604831367855,-1.50184320097003,-1.49861296781623,-1.49505658831395,
-1.4891618634075,-1.46437057717612,-1.43422474338118,-1.42571876013822,
-1.41991248598996,-1.41744114531021,-1.41562038039269,-1.41353028875066,
-1.40983783581059,-1.38780284910498,-1.38356418636957,-1.3613890194487,
-1.34859828616354,-1.33939209720686,-1.33518772461819,-1.33195797531807,
-1.32840205894175,-1.32250797435515,-1.29772093261388,-1.26757120412798,
-1.25906494186905,-1.25325865609181,-1.25078747679406,-1.2489668089471,
-1.24687667366901,-1.24318435855359,-1.22123974221259,-1.21693683767769,
-1.19476953421665,-1.18195680853648,-1.17273882568845,-1.16853209392249,
-1.16530171323064,-1.16174626935345,-1.15585570791226,-1.13119043522373,
-1.10093965540801,-1.09242046631484,-1.0866075501802,-1.08413495980609,
-1.08231362761373,-1.08022280171974,-1.07653011743228,-1.05463307154296,
-1.05046548987067,-1.01182908984538,-1.00551777533215,-1.00151152028973,
-0.998301542668516,-0.994626382112296,-0.991365966097619),.UNSPECIFIED.);
#2793=B_SPLINE_CURVE_WITH_KNOTS('',3,(#109078,#109079,#109080,#109081,#109082,
#109083,#109084,#109085,#109086,#109087,#109088,#109089,#109090,#109091,
#109092,#109093),.UNSPECIFIED.,.F.,.F.,(4,2,2,2,2,2,2,4),(-0.0594803364103627,
-0.034131742218652,-0.0193897135688908,-0.014271326393632,-0.0108796422400385,
-0.0078410923203492,-0.0042584985369012,-0.000493909690971492),
 .UNSPECIFIED.);
#2794=B_SPLINE_CURVE_WITH_KNOTS('',3,(#109094,#109095,#109096,#109097,#109098,
#109099,#109100,#109101,#109102,#109103,#109104,#109105,#109106,#109107,
#109108,#109109,#109110,#109111,#109112,#109113,#109114,#109115,#109116,
#109117,#109118,#109119,#109120,#109121,#109122,#109123,#109124,#109125,
#109126,#109127,#109128,#109129,#109130,#109131,#109132,#109133,#109134,
#109135,#109136,#109137,#109138,#109139,#109140,#109141,#109142,#109143,
#109144,#109145,#109146,#109147,#109148,#109149,#109150,#109151,#109152,
#109153,#109154,#109155,#109156,#109157,#109158,#109159,#109160,#109161,
#109162,#109163,#109164,#109165,#109166,#109167,#109168,#109169,#109170,
#109171,#109172,#109173,#109174,#109175,#109176,#109177,#109178,#109179,
#109180,#109181,#109182,#109183,#109184,#109185,#109186,#109187,#109188,
#109189,#109190,#109191,#109192,#109193,#109194,#109195,#109196,#109197,
#109198,#109199,#109200,#109201,#109202,#109203,#109204,#109205,#109206,
#109207,#109208,#109209,#109210,#109211,#109212,#109213,#109214,#109215,
#109216,#109217,#109218,#109219,#109220,#109221,#109222,#109223,#109224,
#109225,#109226,#109227,#109228,#109229,#109230,#109231,#109232,#109233,
#109234,#109235,#109236,#109237,#109238,#109239,#109240,#109241,#109242,
#109243,#109244,#109245,#109246,#109247,#109248,#109249,#109250,#109251,
#109252,#109253,#109254,#109255,#109256,#109257,#109258,#109259,#109260,
#109261,#109262,#109263,#109264,#109265,#109266,#109267,#109268,#109269,
#109270,#109271,#109272,#109273,#109274,#109275,#109276,#109277,#109278,
#109279,#109280,#109281,#109282,#109283,#109284,#109285,#109286,#109287,
#109288,#109289),.UNSPECIFIED.,.F.,.F.,(4,2,2,2,2,2,2,2,2,2,2,2,2,2,2,2,
2,2,2,2,2,2,2,2,2,2,2,2,2,2,2,2,2,2,2,2,2,2,2,2,2,2,2,2,2,2,2,2,2,2,2,2,
2,2,2,2,2,2,2,2,2,2,2,2,2,2,2,2,2,2,2,2,2,2,2,2,2,2,2,2,2,2,2,2,2,2,2,2,
2,2,2,2,2,2,2,2,2,4),(-2.0995573720879,-2.09249387521299,-2.05186434588951,
-2.03400307225783,-2.02947534543108,-2.02723570969831,-2.02543103320115,
-2.02316381682362,-2.01849392411303,-1.98737166433328,-1.95411421456467,
-1.94952714451913,-1.94533456101474,-1.94210704772032,-1.9385467834496,
-1.93262929074251,-1.9078124325039,-1.87772526984883,-1.86922745731235,
-1.86342568163711,-1.86095566050007,-1.85913558570642,-1.85704591159258,
-1.85335386477429,-1.83124259739022,-1.82705934336081,-1.80487915151732,
-1.79210539935868,-1.78290859214452,-1.77870651814824,-1.77547777804642,
-1.7719222348084,-1.76602706251188,-1.7411715190181,-1.71108226749418,-1.70258421655863,
-1.69678231693862,-1.69431225807351,-1.69249217121317,-1.69040251562105,
-1.68671050274879,-1.66460009727419,-1.66041652985141,-1.63823661501789,
-1.62546276368338,-1.61626593760668,-1.61206389505721,-1.60883519584189,
-1.60527971506497,-1.59938469034904,-1.57453254064439,-1.54444016618074,
-1.53594174974159,-1.53013968733281,-1.52766962667202,-1.52584956212675,
-1.52375995616905,-1.52006810793253,-1.49799387613972,-1.49378264450325,
-1.47160504151074,-1.45882520625341,-1.44962526546874,-1.44542270101988,
-1.44219395683686,-1.43863878204683,-1.43274511042184,-1.40793638725411,
-1.37780671616153,-1.36930363331068,-1.36349926605032,-1.36102883117992,
-1.35920872853993,-1.35711935383474,-1.35342850965987,-1.33159158669275,
-1.32723501167766,-1.30470476004276,-1.29207087331815,-1.28294753169795,
-1.2787583605621,-1.27553131974899,-1.27196941378826,-1.26604400961055,
-1.23992041729621,-1.21091772203325,-1.19851540047147,-1.19528411658948,
-1.19331600925641,-1.1914705182135,-1.18917259443,-1.18337479633972,-1.15093567368114,
-1.12524602335481,-1.11623303348141,-1.1120633137374,-1.10883870020187,
-1.10882129953008),.UNSPECIFIED.);
#2795=B_SPLINE_CURVE_WITH_KNOTS('',3,(#109295,#109296,#109297,#109298,#109299,
#109300,#109301,#109302,#109303,#109304,#109305,#109306,#109307,#109308,
#109309,#109310,#109311,#109312,#109313,#109314,#109315,#109316,#109317,
#109318,#109319,#109320,#109321,#109322,#109323,#109324,#109325,#109326,
#109327,#109328,#109329,#109330,#109331,#109332,#109333,#109334,#109335,
#109336,#109337,#109338,#109339,#109340,#109341,#109342,#109343,#109344,
#109345,#109346,#109347,#109348,#109349,#109350,#109351,#109352,#109353,
#109354,#109355,#109356,#109357,#109358,#109359,#109360,#109361,#109362,
#109363,#109364,#109365,#109366,#109367,#109368,#109369,#109370,#109371,
#109372,#109373,#109374,#109375,#109376,#109377,#109378,#109379,#109380,
#109381,#109382,#109383,#109384,#109385,#109386,#109387,#109388,#109389,
#109390,#109391,#109392,#109393,#109394,#109395,#109396,#109397,#109398,
#109399,#109400,#109401,#109402,#109403,#109404,#109405,#109406,#109407,
#109408,#109409,#109410,#109411,#109412,#109413,#109414,#109415,#109416,
#109417,#109418,#109419,#109420,#109421,#109422,#109423,#109424,#109425,
#109426,#109427,#109428,#109429,#109430,#109431,#109432,#109433,#109434,
#109435,#109436,#109437,#109438,#109439,#109440,#109441,#109442,#109443,
#109444,#109445,#109446,#109447,#109448,#109449,#109450,#109451,#109452,
#109453,#109454,#109455,#109456,#109457,#109458,#109459,#109460,#109461,
#109462,#109463,#109464,#109465,#109466,#109467,#109468,#109469,#109470,
#109471,#109472,#109473,#109474,#109475,#109476,#109477,#109478,#109479,
#109480,#109481,#109482,#109483,#109484,#109485,#109486,#109487,#109488,
#109489,#109490,#109491,#109492,#109493,#109494,#109495,#109496,#109497,
#109498),.UNSPECIFIED.,.F.,.F.,(4,2,2,2,2,2,2,2,2,2,2,2,2,2,2,2,2,2,2,2,
2,2,2,2,2,2,2,2,2,2,2,2,2,2,2,2,2,2,2,2,2,2,2,2,2,2,2,2,2,2,2,2,2,2,2,2,
2,2,2,2,2,2,2,2,2,2,2,2,2,2,2,2,2,2,2,2,2,2,2,2,2,2,2,2,2,2,2,2,2,2,2,2,
2,2,2,2,2,2,2,2,2,4),(-0.991134662338154,-0.989393772578213,-0.985702140833392,
-0.983612358980175,-0.981791924446668,-0.97932092894059,-0.973514811855033,
-0.965007446467625,-0.934855857628895,-0.910050109404556,-0.904155443320496,
-0.900599669208326,-0.897370363333034,-0.893167002313335,-0.883964605623374,
-0.871181968600566,-0.849028653124806,-0.844834692257524,-0.822778552785723,
-0.819087320069484,-0.816997653685516,-0.815177241193076,-0.812706170189455,
-0.806899410365834,-0.798390682843575,-0.768227505857458,-0.743436283209991,
-0.737542169922906,-0.733986561731969,-0.730757300532083,-0.72655384548527,
-0.717350594695106,-0.704566224891441,-0.682414186805858,-0.678212540654213,
-0.656167298020162,-0.652476182021449,-0.650386568364238,-0.648566192208087,
-0.646095157854975,-0.64028842874351,-0.631779696595099,-0.601615710259276,
-0.576826626836023,-0.5709326854297,-0.567377161612114,-0.564147964829037,
-0.559944576101074,-0.550741395741389,-0.537957060115449,-0.515805583759316,
-0.5116031716918,-0.489559557810953,-0.485868522416741,-0.483778952690514,
-0.481958612108759,-0.479487623089475,-0.473680990127681,-0.465172387358052,
-0.435008646302392,-0.410220597040677,-0.404326792668917,-0.400771343799169,
-0.397542210066243,-0.393338896067229,-0.384135847296285,-0.371351667082328,
-0.349200691987352,-0.344997875086687,-0.322955349682106,-0.319264392560079,
-0.317174866231494,-0.31535456618774,-0.312883633761692,-0.307077133325061,
-0.298568727074793,-0.268405757051954,-0.24361798544822,-0.237724302272828,
-0.23416893182949,-0.230939872928728,-0.226736661790037,-0.217533863293973,
-0.204750054967559,-0.182599488272133,-0.158267438953356,-0.153413459536601,
-0.151078327325675,-0.149271106059955,-0.14717966677521,-0.143468180324395,
-0.138511197619789,-0.126878914663252,-0.105635883196703,-0.0772181880988006,
-0.0712212799721465,-0.0676440388692883,-0.0644202939646342,-0.0602596848747935,
-0.0512989436365756,-0.00636782713373653,-0.000492472357443245),
 .UNSPECIFIED.);
#2796=B_SPLINE_CURVE_WITH_KNOTS('',3,(#109499,#109500,#109501,#109502,#109503,
#109504,#109505,#109506,#109507,#109508,#109509,#109510,#109511,#109512,
#109513,#109514,#109515,#109516,#109517,#109518),.UNSPECIFIED.,.F.,.F.,
(4,2,2,2,2,2,2,2,2,4),(-2.09991177729522,-2.09207408138876,-2.08725374609279,
-2.08513462603622,-2.08342457726091,-2.08161050394509,-2.07923825003836,
-2.07406347330844,-2.05735942596725,-2.04109288767521),.UNSPECIFIED.);
#2797=B_SPLINE_CURVE_WITH_KNOTS('',3,(#109519,#109520,#109521,#109522,#109523,
#109524,#109525,#109526,#109527,#109528,#109529,#109530,#109531,#109532,
#109533,#109534,#109535,#109536,#109537,#109538,#109539,#109540,#109541,
#109542,#109543,#109544,#109545,#109546,#109547,#109548,#109549,#109550,
#109551,#109552,#109553,#109554,#109555,#109556,#109557,#109558,#109559,
#109560,#109561,#109562,#109563,#109564,#109565,#109566,#109567,#109568,
#109569,#109570,#109571,#109572,#109573,#109574,#109575,#109576,#109577,
#109578,#109579,#109580,#109581,#109582,#109583,#109584,#109585,#109586,
#109587,#109588,#109589,#109590,#109591,#109592,#109593,#109594,#109595,
#109596,#109597,#109598,#109599,#109600,#109601,#109602,#109603,#109604,
#109605,#109606,#109607,#109608,#109609,#109610,#109611,#109612,#109613,
#109614,#109615,#109616,#109617,#109618,#109619,#109620,#109621,#109622,
#109623,#109624,#109625,#109626,#109627,#109628,#109629,#109630,#109631,
#109632,#109633,#109634,#109635,#109636,#109637,#109638,#109639,#109640,
#109641,#109642,#109643,#109644,#109645,#109646,#109647,#109648,#109649,
#109650,#109651,#109652,#109653,#109654,#109655,#109656,#109657,#109658,
#109659,#109660,#109661,#109662,#109663,#109664,#109665,#109666,#109667,
#109668,#109669,#109670,#109671,#109672,#109673,#109674,#109675,#109676,
#109677,#109678,#109679,#109680,#109681,#109682,#109683,#109684,#109685,
#109686,#109687,#109688,#109689,#109690,#109691,#109692,#109693,#109694,
#109695,#109696,#109697,#109698,#109699,#109700,#109701,#109702,#109703,
#109704,#109705,#109706,#109707,#109708,#109709,#109710,#109711,#109712,
#109713,#109714,#109715,#109716,#109717,#109718,#109719,#109720,#109721,
#109722,#109723,#109724,#109725,#109726),.UNSPECIFIED.,.F.,.F.,(4,2,2,2,
2,2,2,2,2,2,2,2,2,2,2,2,2,2,2,2,2,2,2,2,2,2,2,2,2,2,2,2,2,2,2,2,2,2,2,2,
2,2,2,2,2,2,2,2,2,2,2,2,2,2,2,2,2,2,2,2,2,2,2,2,2,2,2,2,2,2,2,2,2,2,2,2,
2,2,2,2,2,2,2,2,2,2,2,2,2,2,2,2,2,2,2,2,2,2,2,2,2,2,2,4),(-1.10882129953008,
-1.10526679528211,-1.09929416345195,-1.07124182550192,-1.04978224149019,
-1.03261309667385,-1.0290185920319,-1.02695086560713,-1.02512548808884,
-1.02261512611383,-1.01656741095832,-1.00756682415849,-0.973112349166505,
-0.952936237953287,-0.947296295079374,-0.943795112865223,-0.940550166108246,
-0.936229594429629,-0.926332736062728,-0.91218893201069,-0.891751501520659,
-0.890602460875589,-0.866184410411082,-0.86247127304989,-0.860376961154501,
-0.858558047134264,-0.856096498761252,-0.850344969839385,-0.841946925977698,
-0.812645944373628,-0.786842143338621,-0.780922527996549,-0.777361959856718,
-0.774134794994737,-0.769943550320701,-0.760807450656747,-0.748150688772646,
-0.725521448732133,-0.721449722606859,-0.699512946972071,-0.695822540733412,
-0.693733335049984,-0.691913354177291,-0.689442995058895,-0.683638598029587,
-0.675134251720369,-0.645005398979941,-0.620165723773691,-0.61427071306575,
-0.610715419617843,-0.607487015676931,-0.603285532896211,-0.594090498440146,
-0.581321308581274,-0.559159686034164,-0.555024085602284,-0.53288651341158,
-0.529195421161299,-0.527106088192019,-0.52528618289593,-0.522816176147932,
-0.517013707557131,-0.50851318092388,-0.47841381489131,-0.453541472344877,
-0.447645586081739,-0.444090153848873,-0.440861870125438,-0.43666089715462,
-0.427468482464292,-0.414704197444107,-0.392541395749679,-0.388430832861548,
-0.366262335317689,-0.362571202686006,-0.360481886536925,-0.358662024250052,
-0.356192113814487,-0.350390038484483,-0.341890238794491,-0.311795864278021,
-0.286919002007577,-0.281023086493249,-0.277467695171247,-0.274239485627579,
-0.270038662322151,-0.260846801230966,-0.248083475305109,-0.225920888704558,
-0.20154588699152,-0.196697064740808,-0.194363215280882,-0.192556414298842,
-0.190375833504921,-0.1861431979326,-0.160915595012162,-0.122261479818827,
-0.115952019129516,-0.111947990382275,-0.108740547642508,-0.105069173181969,
-0.0986234121112929,-0.0777398413434496,-0.059270592353646),
 .UNSPECIFIED.);
#2798=B_SPLINE_CURVE_WITH_KNOTS('',3,(#109731,#109732,#109733,#109734,#109735,
#109736,#109737,#109738,#109739,#109740,#109741,#109742,#109743,#109744,
#109745,#109746,#109747,#109748,#109749,#109750,#109751,#109752,#109753,
#109754,#109755,#109756,#109757,#109758,#109759,#109760,#109761,#109762,
#109763,#109764,#109765,#109766,#109767,#109768,#109769,#109770,#109771,
#109772,#109773,#109774,#109775,#109776,#109777,#109778,#109779,#109780,
#109781,#109782,#109783,#109784,#109785,#109786,#109787,#109788,#109789,
#109790,#109791,#109792,#109793,#109794,#109795,#109796,#109797,#109798,
#109799,#109800,#109801,#109802,#109803,#109804,#109805,#109806,#109807,
#109808,#109809,#109810,#109811,#109812,#109813,#109814,#109815,#109816,
#109817,#109818,#109819,#109820,#109821,#109822,#109823,#109824,#109825,
#109826,#109827,#109828,#109829,#109830,#109831,#109832,#109833,#109834,
#109835,#109836,#109837,#109838,#109839,#109840,#109841,#109842,#109843,
#109844,#109845,#109846,#109847,#109848,#109849,#109850,#109851,#109852,
#109853,#109854,#109855,#109856,#109857,#109858,#109859,#109860,#109861,
#109862,#109863,#109864,#109865,#109866,#109867,#109868,#109869,#109870,
#109871,#109872,#109873,#109874,#109875,#109876,#109877,#109878,#109879,
#109880,#109881,#109882,#109883,#109884,#109885,#109886,#109887,#109888,
#109889,#109890,#109891,#109892,#109893,#109894,#109895,#109896,#109897,
#109898,#109899,#109900,#109901,#109902,#109903,#109904,#109905,#109906,
#109907,#109908,#109909,#109910,#109911,#109912,#109913,#109914,#109915,
#109916,#109917,#109918,#109919,#109920,#109921,#109922,#109923,#109924,
#109925,#109926,#109927,#109928,#109929,#109930,#109931,#109932,#109933,
#109934,#109935,#109936,#109937,#109938),.UNSPECIFIED.,.F.,.F.,(4,2,2,2,
2,2,2,2,2,2,2,2,2,2,2,2,2,2,2,2,2,2,2,2,2,2,2,2,2,2,2,2,2,2,2,2,2,2,2,2,
2,2,2,2,2,2,2,2,2,2,2,2,2,2,2,2,2,2,2,2,2,2,2,2,2,2,2,2,2,2,2,2,2,2,2,2,
2,2,2,2,2,2,2,2,2,2,2,2,2,2,2,2,2,2,2,2,2,2,2,2,2,2,2,4),(-2.0406532363113,
-2.01879651888547,-1.99238066791252,-1.98657417046703,-1.98410307949025,
-1.98228257015237,-1.98019274581841,-1.97650105154882,-1.95454871727625,
-1.95046807602693,-1.92810477819024,-1.9152929004022,-1.90607597756734,
-1.90186996389921,-1.89864022294136,-1.89508557179966,-1.88919654334807,
-1.86441758445059,-1.8342642856284,-1.82575826484962,-1.81995228083814,
-1.81748128633533,-1.81566080012792,-1.81357094653259,-1.80987908044253,
-1.78787432395361,-1.78361778033117,-1.76144966868946,-1.74865705504362,
-1.73945022254613,-1.73524598260645,-1.7320164868859,-1.72846099132732,
-1.72256791491311,-1.69779327829074,-1.66764318319486,-1.65913759824842,
-1.65333184146872,-1.65086089519909,-1.64904042548142,-1.64695056864638,
-1.64325864911555,-1.62123294175447,-1.61699149170688,-1.59482168700347,
-1.58203367703209,-1.57282927028346,-1.56862547074867,-1.56539604996123,
-1.56184037403629,-1.5559463735015,-1.53114033476139,-1.50101796151513,
-1.49251590193294,-1.48671190598062,-1.48424126358828,-1.48242084262927,
-1.48033083784776,-1.47663821803773,-1.4544137137572,-1.45069200970983,
-1.42326105907623,-1.40818941285548,-1.40316621558188,-1.39979321671459,
-1.39651582226178,-1.39255487107151,-1.38289952391565,-1.34516178337439,
-1.3297452207056,-1.32382287957242,-1.31938965239073,-1.31716844311672,
-1.31536310200235,-1.31307534335792,-1.30829889124567,-1.27819911735721,
-1.26674243556599,-1.25091986982357,-1.24021374006788,-1.23576318522774,
-1.23249727370469,-1.22945906902001,-1.22442397663453,-1.21052500807858,
-1.17090762880138,-1.16048903259338,-1.15377737352765,-1.1511637520117,
-1.14932208000624,-1.14730144340032,-1.14383047825102,-1.12967209877461,
-1.09931381951288,-1.07624190458356,-1.07056687101835,-1.06705771829471,
-1.06381450574458,-1.05958375875845,-1.04995278007793,-1.03633859043345,
-1.0153335574178,-1.01153673043049,-0.991134662338154),.UNSPECIFIED.);
#2799=B_SPLINE_CURVE_WITH_KNOTS('',3,(#109940,#109941,#109942,#109943,#109944,
#109945,#109946,#109947,#109948,#109949,#109950,#109951,#109952,#109953,
#109954,#109955,#109956,#109957,#109958,#109959),.UNSPECIFIED.,.F.,.F.,
(4,2,2,2,2,2,2,2,2,4),(-0.059270592353646,-0.0463606160273744,-0.0324747523360294,
-0.0290287071869147,-0.0270139928621692,-0.0251710208137734,-0.023312781478327,
-0.0207405421945336,-0.0142423352689885,-0.000491546785663075),
 .UNSPECIFIED.);
#2800=B_SPLINE_CURVE_WITH_KNOTS('',3,(#109960,#109961,#109962,#109963,#109964,
#109965,#109966,#109967,#109968,#109969,#109970,#109971,#109972,#109973,
#109974,#109975,#109976,#109977,#109978,#109979,#109980,#109981,#109982,
#109983,#109984,#109985,#109986,#109987,#109988,#109989,#109990,#109991,
#109992,#109993,#109994,#109995,#109996,#109997,#109998,#109999,#110000,
#110001,#110002,#110003,#110004,#110005,#110006,#110007,#110008,#110009,
#110010,#110011,#110012,#110013,#110014,#110015,#110016,#110017,#110018,
#110019,#110020,#110021,#110022,#110023,#110024,#110025,#110026,#110027,
#110028,#110029,#110030,#110031,#110032,#110033,#110034,#110035,#110036,
#110037,#110038,#110039,#110040,#110041,#110042,#110043,#110044,#110045,
#110046,#110047,#110048,#110049,#110050,#110051,#110052,#110053,#110054,
#110055,#110056,#110057,#110058,#110059,#110060,#110061,#110062,#110063,
#110064,#110065,#110066,#110067,#110068,#110069,#110070,#110071,#110072,
#110073,#110074,#110075,#110076,#110077,#110078,#110079,#110080,#110081,
#110082,#110083,#110084,#110085,#110086,#110087,#110088,#110089,#110090,
#110091,#110092,#110093,#110094,#110095,#110096,#110097,#110098,#110099,
#110100,#110101,#110102,#110103,#110104,#110105,#110106,#110107,#110108,
#110109,#110110,#110111,#110112,#110113,#110114,#110115,#110116,#110117,
#110118,#110119,#110120,#110121,#110122,#110123,#110124,#110125,#110126,
#110127,#110128,#110129,#110130,#110131,#110132,#110133,#110134,#110135,
#110136,#110137,#110138,#110139,#110140,#110141,#110142,#110143,#110144,
#110145,#110146,#110147,#110148,#110149,#110150,#110151,#110152,#110153,
#110154,#110155,#110156,#110157,#110158,#110159,#110160,#110161,#110162,
#110163,#110164,#110165,#110166,#110167,#110168,#110169,#110170,#110171,
#110172,#110173,#110174,#110175,#110176,#110177,#110178,#110179,#110180,
#110181,#110182,#110183,#110184,#110185,#110186,#110187,#110188,#110189,
#110190,#110191,#110192,#110193,#110194,#110195,#110196,#110197,#110198,
#110199,#110200,#110201,#110202,#110203,#110204,#110205,#110206,#110207,
#110208,#110209,#110210,#110211,#110212,#110213,#110214,#110215,#110216,
#110217,#110218,#110219),.UNSPECIFIED.,.F.,.F.,(4,2,2,2,2,2,2,2,2,2,2,2,
2,2,2,2,2,2,2,2,2,2,2,2,2,2,2,2,2,2,2,2,2,2,2,2,2,2,2,2,2,2,2,2,2,2,2,2,
2,2,2,2,2,2,2,2,2,2,2,2,2,2,2,2,2,2,2,2,2,2,2,2,2,2,2,2,2,2,2,2,2,2,2,2,
2,2,2,2,2,2,2,2,2,2,2,2,2,2,2,2,2,2,2,2,2,2,2,2,2,2,2,2,2,2,2,2,2,2,2,2,
2,2,2,2,2,2,2,2,2,4),(-2.10016655421883,-2.05915717791619,-2.04966988750992,
-2.04541771109872,-2.04218228650197,-2.03865068287498,-2.03286840012186,
-2.01046722110432,-1.97820115934944,-1.96940940620449,-1.96355303580982,
-1.9611779328342,-1.96116120944313,-1.96114415872831,-1.96112676351043,
-1.96110900550471,-1.961090865398,-1.9610723226097,-1.96105335515769,-1.96103393962189,
-1.96101405095407,-1.96099366237524,-1.9609727452907,-1.96095126897391,
-1.96092920041967,-1.96090650411634,-1.96088314179674,-1.96085907218092,
-1.96083425064338,-1.96080862887707,-1.9607821544609,-1.96075477045221,
-1.96072641487644,-1.96069702003232,-1.96066651196783,-1.96063480962126,
-1.96060182401781,-1.96056745725225,-1.9605316012524,-1.96049413645845,
-1.9604549303156,-1.96041383539265,-1.95860665287326,-1.95627192877903,
-1.95142008391805,-1.92703083938438,-1.90484928473807,-1.89207542889865,
-1.8828784460171,-1.8786762176849,-1.87544733061379,-1.87189159784961,-1.86599604759875,
-1.84113666609858,-1.81104760506436,-1.80254932613724,-1.79674723539548,
-1.79427707655157,-1.79245690570709,-1.79036713775207,-1.78667491571159,
-1.76455923127716,-1.7603785457002,-1.73819718197419,-1.72542333198084,
-1.71622637035485,-1.7120241645721,-1.70879529989845,-1.70523959686264,
-1.69934410795363,-1.67448553005861,-1.64439614462895,-1.63589785878363,
-1.63009577607805,-1.62762562946949,-1.62580547110471,-1.62371572150919,
-1.6200235405967,-1.59791195105464,-1.59372824276747,-1.57154726109244,
-1.55877286929777,-1.54957564222735,-1.5453734090141,-1.54214456033358,
-1.53858891192559,-1.53269360167488,-1.50783975415642,-1.47774662810177,
-1.46924790392769,-1.46344561504617,-1.46097544494368,-1.45915529453949,
-1.45706558350824,-1.45337353408022,-1.43129068858072,-1.42708504511212,
-1.40490593989988,-1.39212684990688,-1.38292718176827,-1.3787245419601,
-1.37549566073552,-1.37194025591082,-1.3660460143265,-1.34122644492246,
-1.31110385504905,-1.30260144689542,-1.29679734046845,-1.29432687819739,
-1.29250670178993,-1.29041718126206,-1.28672594272973,-1.26484282150886,
-1.26065803570967,-1.23803998838052,-1.22538318888839,-1.21624768519038,
-1.21205626812063,-1.20882882540122,-1.20526780822604,-1.19934707303047,
-1.173469953063,-1.14425621295001,-1.13587076886993,-1.13012490576551,-1.12766419633862,
-1.12584524206693,-1.12375016027356,-1.1200340051944,-1.10925371751591),
 .UNSPECIFIED.);
#2801=B_SPLINE_CURVE_WITH_KNOTS('',3,(#110225,#110226,#110227,#110228,#110229,
#110230,#110231,#110232,#110233,#110234,#110235,#110236,#110237,#110238,
#110239,#110240,#110241,#110242,#110243,#110244,#110245,#110246,#110247,
#110248,#110249,#110250,#110251,#110252,#110253,#110254,#110255,#110256,
#110257,#110258,#110259,#110260,#110261,#110262,#110263,#110264,#110265,
#110266,#110267,#110268,#110269,#110270,#110271,#110272,#110273,#110274,
#110275,#110276,#110277,#110278,#110279,#110280,#110281,#110282,#110283,
#110284,#110285,#110286,#110287,#110288,#110289,#110290,#110291,#110292,
#110293,#110294,#110295,#110296,#110297,#110298,#110299,#110300,#110301,
#110302,#110303,#110304,#110305,#110306,#110307,#110308,#110309,#110310,
#110311,#110312,#110313,#110314,#110315,#110316,#110317,#110318,#110319,
#110320,#110321,#110322,#110323,#110324,#110325,#110326,#110327,#110328,
#110329,#110330,#110331,#110332,#110333,#110334,#110335,#110336,#110337,
#110338,#110339,#110340,#110341,#110342,#110343,#110344,#110345,#110346,
#110347,#110348,#110349,#110350,#110351,#110352,#110353,#110354,#110355,
#110356,#110357,#110358,#110359,#110360,#110361,#110362,#110363,#110364,
#110365,#110366,#110367,#110368,#110369,#110370,#110371,#110372,#110373,
#110374,#110375,#110376,#110377,#110378,#110379,#110380,#110381,#110382,
#110383,#110384,#110385,#110386,#110387,#110388,#110389,#110390,#110391,
#110392,#110393,#110394,#110395,#110396,#110397,#110398,#110399,#110400,
#110401,#110402,#110403,#110404,#110405,#110406,#110407,#110408,#110409,
#110410,#110411,#110412,#110413,#110414,#110415,#110416,#110417,#110418,
#110419,#110420,#110421,#110422,#110423,#110424,#110425,#110426,#110427,
#110428,#110429,#110430,#110431,#110432,#110433,#110434,#110435,#110436,
#110437,#110438,#110439,#110440,#110441,#110442,#110443,#110444,#110445,
#110446,#110447,#110448),.UNSPECIFIED.,.F.,.F.,(4,2,2,2,2,2,2,2,2,2,2,2,
2,2,2,2,2,2,2,2,2,2,2,2,2,2,2,2,2,2,2,2,2,2,2,2,2,2,2,2,2,2,2,2,2,2,2,2,
2,2,2,2,2,2,2,2,2,2,2,2,2,2,2,2,2,2,2,2,2,2,2,2,2,2,2,2,2,2,2,2,2,2,2,2,
2,2,2,2,2,2,2,2,2,2,2,2,2,2,2,2,2,2,2,2,2,2,2,2,2,2,2,4),(-0.991198145747101,
-0.979922139387548,-0.973232366071378,-0.969116806922089,-0.965897290328937,
-0.962293127073538,-0.9561727018672,-0.921045055981403,-0.891621506969829,
-0.886838852062437,-0.88454963029269,-0.882743881421336,-0.880523101915277,
-0.876093453497073,-0.870177143769939,-0.854788679461095,-0.817175695968832,
-0.807371148699922,-0.803385048987159,-0.800100848466217,-0.796734956829209,
-0.791749378218907,-0.777019549346137,-0.750729215994269,-0.725134844432903,
-0.720291958278169,-0.717958610530376,-0.716150997953339,-0.713967901386552,
-0.709726061906691,-0.704136351782836,-0.690095693703073,-0.657343598080886,
-0.64238888567584,-0.637237667375068,-0.633838156814175,-0.63054094544253,
-0.625912096471104,-0.614001624710468,-0.595472736993051,-0.568245519300723,
-0.555879485407219,-0.552536464519145,-0.550543540630084,-0.548689034921384,
-0.546002948478418,-0.538790272453764,-0.527231894476751,-0.506004313869084,
-0.477456941445017,-0.471447069061,-0.467866405285966,-0.46464224625417,
-0.460484862635421,-0.451546501851753,-0.425059047755777,-0.391100545075304,
-0.386661277976547,-0.384438648506088,-0.382633036795257,-0.380346051650563,
-0.37557488977765,-0.355546054752669,-0.319809736554227,-0.308122495890007,
-0.303395286082738,-0.300112929251811,-0.296745016497769,-0.291748957244756,
-0.27692509249976,-0.250326697406234,-0.22521380130329,-0.220276037671602,
-0.217957798506011,-0.216151063702564,-0.213955796125457,-0.20965339983341,
-0.184256259388925,-0.14589091042111,-0.13957251014971,-0.135564879815861,
-0.13235580040956,-0.132069740304737,-0.131797747524467,-0.131536018698235,
-0.131326680520065,-0.131154744544695,-0.13101055825957,-0.130887593749863,
-0.130781261702504,-0.130688232298338,-0.130606025406809,-0.130532752426627,
-0.130466947644139,-0.130407454724,-0.130353348164902,-0.130303877767377,
-0.130258428498361,-0.130216490986225,-0.130058621965028,-0.129900736399659,
-0.124978408329008,-0.109896163487368,-0.0823246596791248,-0.0799968337057307,
-0.0566107160938009,-0.0529128640661709,-0.0508215781362848,-0.0490012733873011,
-0.04653238028064,-0.040739670100114,-0.00049225813125148),
 .UNSPECIFIED.);
#2802=B_SPLINE_CURVE_WITH_KNOTS('',3,(#110449,#110450,#110451,#110452,#110453,
#110454,#110455,#110456,#110457,#110458,#110459,#110460,#110461,#110462,
#110463,#110464,#110465,#110466),.UNSPECIFIED.,.F.,.F.,(4,2,2,2,2,2,2,2,
4),(-2.09971007316713,-2.07686154414363,-2.07240379950036,-2.0691316260327,
-2.06583659076626,-2.06283508760716,-2.05800539344515,-2.04562339467567,
-2.0406532363113),.UNSPECIFIED.);
#2803=B_SPLINE_CURVE_WITH_KNOTS('',3,(#110467,#110468,#110469,#110470,#110471,
#110472,#110473,#110474,#110475,#110476,#110477,#110478,#110479,#110480,
#110481,#110482,#110483,#110484,#110485,#110486,#110487,#110488,#110489,
#110490,#110491,#110492,#110493,#110494,#110495,#110496,#110497,#110498,
#110499,#110500,#110501,#110502,#110503,#110504,#110505,#110506,#110507,
#110508,#110509,#110510,#110511,#110512,#110513,#110514,#110515,#110516,
#110517,#110518,#110519,#110520,#110521,#110522,#110523,#110524,#110525,
#110526,#110527,#110528,#110529,#110530,#110531,#110532,#110533,#110534,
#110535,#110536,#110537,#110538,#110539,#110540,#110541,#110542,#110543,
#110544,#110545,#110546,#110547,#110548,#110549,#110550,#110551,#110552,
#110553,#110554,#110555,#110556,#110557,#110558,#110559,#110560,#110561,
#110562,#110563,#110564,#110565,#110566,#110567,#110568,#110569,#110570,
#110571,#110572,#110573,#110574,#110575,#110576,#110577,#110578,#110579,
#110580,#110581,#110582,#110583,#110584,#110585,#110586,#110587,#110588,
#110589,#110590,#110591,#110592,#110593,#110594,#110595,#110596,#110597,
#110598,#110599,#110600,#110601,#110602,#110603,#110604,#110605,#110606,
#110607,#110608,#110609,#110610,#110611,#110612,#110613,#110614,#110615,
#110616,#110617,#110618,#110619,#110620,#110621,#110622,#110623,#110624,
#110625,#110626,#110627,#110628,#110629,#110630,#110631,#110632,#110633,
#110634,#110635,#110636,#110637,#110638,#110639,#110640,#110641,#110642,
#110643,#110644,#110645,#110646,#110647,#110648,#110649,#110650,#110651,
#110652,#110653,#110654,#110655,#110656,#110657,#110658,#110659,#110660,
#110661,#110662),.UNSPECIFIED.,.F.,.F.,(4,2,2,2,2,2,2,2,2,2,2,2,2,2,2,2,
2,2,2,2,2,2,2,2,2,2,2,2,2,2,2,2,2,2,2,2,2,2,2,2,2,2,2,2,2,2,2,2,2,2,2,2,
2,2,2,2,2,2,2,2,2,2,2,2,2,2,2,2,2,2,2,2,2,2,2,2,2,2,2,2,2,2,2,2,2,2,2,2,
2,2,2,2,2,2,2,2,2,4),(-1.10925371751591,-1.09550575347277,-1.07760134236261,
-1.06129650828734,-1.0503670145866,-1.0463295595019,-1.04333238429216,-1.04003441850288,
-1.03539726996905,-1.02342180831539,-1.00473710734787,-0.977124452427724,
-0.965282507648974,-0.961992930843178,-0.960012060857267,-0.958152096937334,
-0.955434246388055,-0.947987646926929,-0.935874901400657,-0.900156364718153,
-0.885232944651148,-0.880085961122931,-0.87668809317706,-0.873391644591205,
-0.868762512047352,-0.856843608831029,-0.838293143269312,-0.811013335325888,
-0.798720539667249,-0.795383983253299,-0.793392883780173,-0.791538434537175,
-0.788850180178022,-0.78161820620513,-0.770013652602038,-0.748839355675297,
-0.720306026606756,-0.714298783809371,-0.710719431158664,-0.707496324550867,
-0.703340153062685,-0.694404035854607,-0.66789503648395,-0.633958123959357,
-0.629516857310411,-0.62729426764726,-0.625489288238946,-0.623203943024099,
-0.618439067109707,-0.598462838181849,-0.562880173529267,-0.55103040634141,
-0.546281146697222,-0.542995478854425,-0.539634097367556,-0.534666702572268,
-0.520087043393112,-0.494275953501948,-0.468025303824664,-0.463176653256218,
-0.460842655797137,-0.459035625313025,-0.456854627929886,-0.452620800670174,
-0.427274460800672,-0.388759280375416,-0.38243442669773,-0.378425603973951,
-0.375217403096375,-0.371548509222647,-0.365116058244221,-0.357166576372186,
-0.339158256166385,-0.305244122311836,-0.297669328822782,-0.29485592966468,
-0.293163719407085,-0.291262116354979,-0.288336762155728,-0.279205017395535,
-0.262630674196795,-0.221534827622289,-0.214918434208845,-0.211172390744529,
-0.208001126639539,-0.20410778017653,-0.196572793331421,-0.186801821689084,
-0.161111208546359,-0.134697968926734,-0.129851213757669,-0.127517758502845,
-0.12571096330473,-0.123530025758696,-0.119668349808246,-0.095716333480646,
-0.0686383347465613,-0.059539451546452),.UNSPECIFIED.);
#2804=B_SPLINE_CURVE_WITH_KNOTS('',3,(#110667,#110668,#110669,#110670,#110671,
#110672,#110673,#110674,#110675,#110676,#110677,#110678,#110679,#110680,
#110681,#110682,#110683,#110684,#110685,#110686,#110687,#110688,#110689,
#110690,#110691,#110692,#110693,#110694,#110695,#110696,#110697,#110698,
#110699,#110700,#110701,#110702,#110703,#110704,#110705,#110706,#110707,
#110708,#110709,#110710,#110711,#110712,#110713,#110714,#110715,#110716,
#110717,#110718,#110719,#110720,#110721,#110722,#110723,#110724,#110725,
#110726,#110727,#110728,#110729,#110730,#110731,#110732,#110733,#110734,
#110735,#110736,#110737,#110738,#110739,#110740,#110741,#110742,#110743,
#110744,#110745,#110746,#110747,#110748,#110749,#110750,#110751,#110752,
#110753,#110754,#110755,#110756,#110757,#110758,#110759,#110760,#110761,
#110762,#110763,#110764,#110765,#110766,#110767,#110768,#110769,#110770,
#110771,#110772,#110773,#110774,#110775,#110776,#110777,#110778,#110779,
#110780,#110781,#110782,#110783,#110784,#110785,#110786,#110787,#110788,
#110789,#110790,#110791,#110792,#110793,#110794,#110795,#110796,#110797,
#110798,#110799,#110800,#110801,#110802,#110803,#110804,#110805,#110806,
#110807,#110808,#110809,#110810,#110811,#110812,#110813,#110814,#110815,
#110816,#110817,#110818,#110819,#110820,#110821,#110822,#110823,#110824,
#110825,#110826,#110827,#110828,#110829,#110830,#110831,#110832,#110833,
#110834,#110835,#110836,#110837,#110838,#110839,#110840,#110841,#110842,
#110843,#110844,#110845,#110846,#110847,#110848,#110849,#110850,#110851,
#110852,#110853,#110854,#110855,#110856,#110857,#110858,#110859,#110860,
#110861,#110862,#110863,#110864,#110865,#110866,#110867,#110868,#110869,
#110870,#110871,#110872,#110873,#110874,#110875,#110876,#110877,#110878,
#110879,#110880,#110881,#110882,#110883,#110884,#110885,#110886,#110887,
#110888,#110889,#110890,#110891,#110892,#110893,#110894,#110895,#110896,
#110897,#110898,#110899,#110900,#110901,#110902),.UNSPECIFIED.,.F.,.F.,
(4,2,2,2,2,2,2,2,2,2,2,2,2,2,2,2,2,2,2,2,2,2,2,2,2,2,2,2,2,2,2,2,2,2,2,
2,2,2,2,2,2,2,2,2,2,2,2,2,2,2,2,2,2,2,2,2,2,2,2,2,2,2,2,2,2,2,2,2,2,2,2,
2,2,2,2,2,2,2,2,2,2,2,2,2,2,2,2,2,2,2,2,2,2,2,2,2,2,2,2,2,2,2,2,2,2,2,2,
2,2,2,2,2,2,2,2,2,2,4),(-2.040918156169,-2.02175067309694,-2.01788165223792,
-1.99046735632266,-1.97542931270169,-1.97051160677594,-1.97035368350289,
-1.97019574120493,-1.97015308637871,-1.97010681483818,-1.97005639631913,
-1.9700011892782,-1.96994040937482,-1.96987308657721,-1.96979800545037,
-1.96971362041797,-1.9696179325652,-1.96950830560969,-1.96938118221942,
-1.96923162994881,-1.9659999595357,-1.96244981971617,-1.95658396976085,
-1.93175403352981,-1.90159550124659,-1.89308797260048,-1.88728095462328,
-1.88480951680331,-1.88298870270076,-1.88089847119671,-1.87720593428999,
-1.85519579285069,-1.85093948269398,-1.82876724466515,-1.81597263871272,
-1.80676431068209,-1.80255934145753,-1.79932926724188,-1.79577311653556,
-1.78987891082858,-1.76509762745267,-1.73494399884569,-1.72643712010952,
-1.72063043561765,-1.71815906373745,-1.7163382683564,-1.71424802358168,
-1.71055538841534,-1.68851223904125,-1.68427982208249,-1.6621049388479,
-1.64931735030738,-1.64011271100341,-1.63590840219731,-1.63267843107337,
-1.62912199039068,-1.62322634437522,-1.59839657334952,-1.56828554296313,
-1.55978406623875,-1.5539800742714,-1.55150916162431,-1.54968843463254,
-1.54759795403942,-1.54390422553654,-1.52155174540561,-1.51756637299942,
-1.4953777226605,-1.48263425390937,-1.47345273724259,-1.46925247885318,
-1.46602304387734,-1.46246461936437,-1.456559552413,-1.43139637668425,-1.40157465600602,
-1.39310994954888,-1.38732424137398,-1.3848563916168,-1.38303606022093,
-1.38094386444565,-1.37724242397059,-1.35355262152704,-1.35154159802529,
-1.33516457613535,-1.31862774103887,-1.31109053263891,-1.30491825651194,
-1.30130316409646,-1.29808570272378,-1.29398899693472,-1.28736469788042,
-1.25363524697903,-1.224200131285,-1.21990163021065,-1.21770705640311,-1.21590015950091,
-1.21358075658974,-1.20863724765885,-1.18219637948464,-1.16748776792177,
-1.15156724093908,-1.1408147202471,-1.13635642719867,-1.13308872434762,
-1.13005158782473,-1.12502471516559,-1.11119907948001,-1.07748349221746,
-1.06317246346268,-1.05485206601686,-1.05202083327608,-1.05013817351247,
-1.04819083116008,-1.04505680342147,-1.03383667143882,-1.01014730675737,
-0.991198145747101),.UNSPECIFIED.);
#2805=B_SPLINE_CURVE_WITH_KNOTS('',3,(#110904,#110905,#110906,#110907,#110908,
#110909,#110910,#110911,#110912,#110913,#110914,#110915,#110916,#110917,
#110918,#110919,#110920,#110921),.UNSPECIFIED.,.F.,.F.,(4,2,2,2,2,2,2,2,
4),(-0.059539451546452,-0.0522753828638611,-0.0469759703147907,-0.0435468468193094,
-0.0402703039018171,-0.0370299854246382,-0.0326579013504971,-0.0227235598706649,
-0.000491884265946706),.UNSPECIFIED.);
#2806=B_SPLINE_CURVE_WITH_KNOTS('',3,(#110922,#110923,#110924,#110925,#110926,
#110927,#110928,#110929,#110930,#110931,#110932,#110933,#110934,#110935,
#110936,#110937,#110938,#110939,#110940,#110941,#110942,#110943,#110944,
#110945,#110946,#110947,#110948,#110949,#110950,#110951,#110952,#110953,
#110954,#110955,#110956,#110957,#110958,#110959,#110960,#110961,#110962,
#110963,#110964,#110965,#110966,#110967,#110968,#110969,#110970,#110971,
#110972,#110973,#110974,#110975,#110976,#110977,#110978,#110979,#110980,
#110981,#110982,#110983,#110984,#110985,#110986,#110987,#110988,#110989,
#110990,#110991,#110992,#110993,#110994,#110995,#110996,#110997,#110998,
#110999,#111000,#111001,#111002,#111003,#111004,#111005,#111006,#111007,
#111008,#111009,#111010,#111011,#111012,#111013,#111014,#111015,#111016,
#111017,#111018,#111019,#111020,#111021,#111022,#111023,#111024,#111025,
#111026,#111027,#111028,#111029,#111030,#111031,#111032,#111033,#111034,
#111035,#111036,#111037,#111038,#111039,#111040,#111041,#111042,#111043,
#111044,#111045,#111046,#111047,#111048,#111049,#111050,#111051,#111052,
#111053,#111054,#111055,#111056,#111057,#111058,#111059,#111060,#111061,
#111062,#111063,#111064,#111065,#111066,#111067,#111068,#111069,#111070,
#111071,#111072,#111073,#111074,#111075,#111076,#111077,#111078,#111079,
#111080,#111081,#111082,#111083,#111084),.UNSPECIFIED.,.F.,.F.,(4,3,3,3,
3,3,3,3,3,3,3,3,3,3,3,3,3,3,3,3,3,3,3,3,3,3,3,3,3,3,3,3,3,3,3,3,3,3,3,3,
3,3,3,3,3,3,3,3,3,3,3,3,3,3,4),(-54.111865720712,-53.9685006349437,-53.8675843506887,
-53.7577897347117,-53.6468205794155,-53.5373284361958,-53.42790328446,-53.3185044306203,
-53.2063874460508,-53.0968489113657,-52.9834427018542,-52.8700364923426,
-52.7602418763655,-52.6492727210694,-52.5397805778495,-52.4303554261137,
-52.3209565722739,-52.2088395877045,-52.0993010530194,-51.9858948435079,
-51.8724886339965,-51.7626940180194,-51.6517248627233,-51.5422327195034,
-51.4328075677676,-51.3234087139277,-51.2112917293584,-51.1017531946732,
-50.9883469851618,-50.8749407756504,-50.7651461596733,-50.6541770043772,
-50.5446848611574,-50.4352597094216,-50.3258608555818,-50.2137438710124,
-50.1042053363273,-49.9907991268158,-49.8773929173043,-49.7675983013272,
-49.6566291460311,-49.5471370028112,-49.4377118510755,-49.3283129972356,
-49.2161960126663,-49.1066574779811,-48.9932512684697,-48.8798450589583,
-48.7700749181116,-48.6604636787953,-48.5509703718697,-48.4415394130417,
-48.3321442536577,-48.2227090186136,-48.1819144021787),.UNSPECIFIED.);
#2807=B_SPLINE_CURVE_WITH_KNOTS('',3,(#111090,#111091,#111092,#111093,#111094,
#111095,#111096,#111097,#111098,#111099,#111100,#111101,#111102,#111103,
#111104,#111105,#111106,#111107,#111108,#111109,#111110,#111111,#111112,
#111113,#111114,#111115,#111116,#111117,#111118,#111119,#111120,#111121,
#111122,#111123,#111124,#111125,#111126,#111127,#111128,#111129,#111130,
#111131,#111132,#111133,#111134,#111135,#111136,#111137,#111138,#111139,
#111140,#111141,#111142,#111143,#111144,#111145,#111146,#111147,#111148,
#111149,#111150,#111151,#111152,#111153,#111154,#111155,#111156,#111157,
#111158,#111159,#111160,#111161,#111162,#111163,#111164,#111165,#111166,
#111167,#111168,#111169,#111170,#111171,#111172,#111173,#111174,#111175,
#111176,#111177,#111178,#111179,#111180,#111181,#111182,#111183,#111184,
#111185,#111186,#111187,#111188,#111189,#111190,#111191,#111192,#111193,
#111194,#111195,#111196,#111197,#111198,#111199,#111200,#111201,#111202,
#111203,#111204,#111205,#111206,#111207,#111208,#111209,#111210,#111211,
#111212,#111213,#111214,#111215,#111216,#111217,#111218,#111219,#111220,
#111221,#111222,#111223,#111224,#111225,#111226,#111227,#111228,#111229,
#111230,#111231,#111232,#111233,#111234,#111235,#111236,#111237,#111238,
#111239,#111240,#111241,#111242,#111243,#111244,#111245,#111246,#111247,
#111248,#111249,#111250,#111251,#111252,#111253,#111254,#111255,#111256,
#111257,#111258,#111259,#111260,#111261,#111262,#111263,#111264,#111265,
#111266,#111267,#111268,#111269,#111270,#111271,#111272,#111273,#111274,
#111275,#111276,#111277,#111278,#111279,#111280,#111281,#111282,#111283,
#111284,#111285,#111286,#111287,#111288,#111289,#111290,#111291,#111292,
#111293,#111294,#111295),.UNSPECIFIED.,.F.,.F.,(4,2,2,2,2,2,2,2,2,2,2,2,
2,2,2,2,2,2,2,2,2,2,2,2,2,2,2,2,2,2,2,2,2,2,2,2,2,2,2,2,2,2,2,2,2,2,2,2,
2,2,2,2,2,2,2,2,2,2,2,2,2,2,2,2,2,2,2,2,2,2,2,2,2,2,2,2,2,2,2,2,2,2,2,2,
2,2,2,2,2,2,2,2,2,2,2,2,2,2,2,2,2,2,4),(-0.991228979995648,-0.983398525141886,
-0.979456642710194,-0.957084543893986,-0.953391681410358,-0.951301487728045,
-0.949480898246093,-0.947009965128886,-0.941205195284152,-0.932700889037199,
-0.902577581866334,-0.877732932348373,-0.871836529632574,-0.868280137956607,
-0.865050543334509,-0.860847197111809,-0.851646496958872,-0.838867619783047,
-0.816709866285661,-0.812536837742524,-0.790450015766714,-0.786758278114422,
-0.784668362291761,-0.782847758306616,-0.780376462084198,-0.774569326542554,
-0.766060187161313,-0.735897780977709,-0.711099256102759,-0.70520436345605,
-0.701648340474268,-0.698418737576984,-0.694214888018101,-0.685010987541685,
-0.67222589551464,-0.650071194126225,-0.645871628579444,-0.623820593002631,
-0.620129064887983,-0.618039222233125,-0.616218649486103,-0.613747352154976,
-0.607940022297441,-0.59943042488059,-0.569263605607128,-0.544471379517814,
-0.538576787116965,-0.535020875847633,-0.531791330477299,-0.527587492722427,
-0.518383349291159,-0.50559769303497,-0.483443794371823,-0.479241132714011,
-0.457194845616134,-0.45350341049653,-0.451413614944705,-0.449593079267466,
-0.447121826948301,-0.441314579481198,-0.432805081653765,-0.402638275129165,
-0.377847270257112,-0.371952822190027,-0.368396989513062,-0.365167510156696,
-0.360963750627403,-0.35175974563816,-0.338974254000734,-0.316820858173598,
-0.312617898578013,-0.290572590536178,-0.286881234186267,-0.28479148255478,
-0.28297098465775,-0.28049978297823,-0.274692651672097,-0.266183321492254,
-0.236017067984694,-0.21121909433528,-0.205328745936947,-0.201773832470939,
-0.198544203804684,-0.194338836121906,-0.185125279874042,-0.172321428276487,
-0.149944620177697,-0.145934869022723,-0.123953039086726,-0.120261997965209,
-0.118172342653606,-0.11635186992887,-0.113880623781306,-0.108073041451337,
-0.0818761625613097,-0.0549676433734573,-0.0424561965430678,-0.037607705320321,
-0.0346029847776142,-0.0313111534385748,-0.0280446219939228,-0.0236019538334248,
-0.000491633709745548),.UNSPECIFIED.);
#2808=B_SPLINE_CURVE_WITH_KNOTS('',3,(#111296,#111297,#111298,#111299,#111300,
#111301,#111302,#111303,#111304,#111305,#111306,#111307,#111308,#111309,
#111310,#111311),.UNSPECIFIED.,.F.,.F.,(4,2,2,2,2,2,2,4),(-2.09972660864104,
-2.05974670160645,-2.05394046144309,-2.05146911933196,-2.04964828326592,
-2.04755791888203,-2.04386491549341,-2.040918156169),.UNSPECIFIED.);
#2809=B_SPLINE_CURVE_WITH_KNOTS('',3,(#111313,#111314,#111315,#111316,#111317,
#111318,#111319,#111320,#111321,#111322,#111323,#111324,#111325),
 .UNSPECIFIED.,.F.,.F.,(4,3,3,3,4),(-48.1819144021787,-48.0723535020162,
-47.9625891120362,-47.8822972006122,-47.8286804139494),.UNSPECIFIED.);
#2810=B_SPLINE_CURVE_WITH_KNOTS('',3,(#111326,#111327,#111328,#111329,#111330,
#111331,#111332,#111333,#111334),.UNSPECIFIED.,.F.,.F.,(4,1,1,1,1,1,4),
(-47.8286738933328,-46.8847493422661,-45.88720148392,-44.8896536255739,
-43.8921057672278,-42.8945579088817,-41.8982186375431),.UNSPECIFIED.);
#2811=B_SPLINE_CURVE_WITH_KNOTS('',3,(#111339,#111340,#111341,#111342,#111343,
#111344,#111345,#111346,#111347,#111348,#111349,#111350,#111351,#111352,
#111353,#111354,#111355,#111356,#111357,#111358,#111359,#111360,#111361,
#111362,#111363,#111364,#111365,#111366,#111367,#111368,#111369,#111370,
#111371,#111372,#111373,#111374,#111375,#111376,#111377,#111378,#111379,
#111380,#111381,#111382,#111383,#111384,#111385,#111386,#111387,#111388,
#111389,#111390,#111391,#111392,#111393,#111394,#111395,#111396,#111397,
#111398,#111399,#111400,#111401,#111402,#111403,#111404,#111405,#111406,
#111407,#111408,#111409,#111410,#111411,#111412,#111413,#111414,#111415,
#111416,#111417,#111418,#111419,#111420,#111421,#111422,#111423,#111424,
#111425,#111426,#111427,#111428,#111429,#111430,#111431,#111432,#111433,
#111434,#111435,#111436,#111437,#111438,#111439,#111440,#111441,#111442,
#111443,#111444,#111445,#111446,#111447,#111448,#111449,#111450,#111451,
#111452,#111453,#111454,#111455,#111456,#111457,#111458,#111459,#111460,
#111461,#111462,#111463,#111464,#111465,#111466,#111467,#111468,#111469,
#111470,#111471,#111472,#111473,#111474,#111475,#111476,#111477,#111478,
#111479,#111480,#111481,#111482,#111483,#111484,#111485,#111486,#111487,
#111488,#111489,#111490,#111491,#111492,#111493,#111494,#111495,#111496,
#111497,#111498,#111499,#111500,#111501,#111502,#111503,#111504,#111505,
#111506,#111507,#111508,#111509,#111510,#111511,#111512,#111513,#111514,
#111515,#111516,#111517,#111518,#111519,#111520,#111521,#111522,#111523,
#111524,#111525,#111526,#111527,#111528,#111529,#111530,#111531,#111532,
#111533,#111534,#111535,#111536,#111537,#111538,#111539,#111540,#111541,
#111542,#111543,#111544),.UNSPECIFIED.,.F.,.F.,(4,2,2,2,2,2,2,2,2,2,2,2,
2,2,2,2,2,2,2,2,2,2,2,2,2,2,2,2,2,2,2,2,2,2,2,2,2,2,2,2,2,2,2,2,2,2,2,2,
2,2,2,2,2,2,2,2,2,2,2,2,2,2,2,2,2,2,2,2,2,2,2,2,2,2,2,2,2,2,2,2,2,2,2,2,
2,2,2,2,2,2,2,2,2,2,2,2,2,2,2,2,2,2,4),(-2.04103609068276,-2.04054941593494,
-2.03638930931414,-2.0331647411395,-2.02958535692507,-2.02358182574604,
-1.99511926535833,-1.97392481751964,-1.96230843101843,-1.95735522553996,
-1.95364416819374,-1.95155528640585,-1.94974748440359,-1.94741148929928,
-1.94255537899236,-1.91820227759977,-1.89602978402057,-1.88323506906757,
-1.87402665648728,-1.86982164406692,-1.86659153486022,-1.86303534382467,
-1.8571410669784,-1.83235929653687,-1.80220552606283,-1.7936985779156,-1.78789184163143,
-1.78542044466259,-1.78359962960099,-1.78150936084036,-1.77781668030054,
-1.75577195471019,-1.75154046932956,-1.72936523983956,-1.71657777544251,
-1.70737317358789,-1.7031688428402,-1.6999388394456,-1.69638234784322,-1.69048658081274,
-1.66565466455493,-1.6355449355966,-1.62704357161517,-1.62123961829485,
-1.61876869564025,-1.61694795087102,-1.6148574377532,-1.61116362569786,
-1.58879882328383,-1.58524470974868,-1.54571246651399,-1.53912333351665,
-1.53542081779393,-1.53221454242607,-1.52824867188314,-1.52207278698063,
-1.48219759365406,-1.4579488398525,-1.45372092376101,-1.4515406349014,-1.44973280232156,
-1.44739587751078,-1.44253495436364,-1.41929935626618,-1.39127773326232,
-1.37603376065766,-1.37099105646683,-1.36761365849837,-1.36433848231425,
-1.359650594565,-1.34819225379622,-1.30874080178992,-1.29615039921359,-1.28850557048288,
-1.28576053342001,-1.28389491523809,-1.28192192195282,-1.27867041630235,
-1.26727492418798,-1.23932148366182,-1.22049444413354,-1.20845951221053,
-1.20381302436367,-1.2005125021138,-1.19711750647856,-1.19198869851601,
-1.17725021657295,-1.13717559364277,-1.12766616554681,-1.12137410099424,
-1.11882423992933,-1.1169924699832,-1.11494287332612,-1.11133911386276,
-1.09484516582397,-1.05022618321615,-1.04074433564576,-1.03653821998532,
-1.03329840457556,-1.02977757796083,-1.02404865308315,-0.999989116222332,
-0.991228979995648),.UNSPECIFIED.);
#2812=B_SPLINE_CURVE_WITH_KNOTS('',3,(#111546,#111547,#111548,#111549,#111550),
 .UNSPECIFIED.,.F.,.F.,(4,1,4),(-41.8982186375431,-41.8970100505357,-41.5455025261802),
 .UNSPECIFIED.);
#2813=B_SPLINE_CURVE_WITH_KNOTS('',3,(#111551,#111552,#111553,#111554,#111555,
#111556,#111557,#111558,#111559,#111560,#111561,#111562,#111563,#111564,
#111565,#111566,#111567,#111568,#111569,#111570,#111571,#111572,#111573,
#111574,#111575,#111576,#111577,#111578,#111579,#111580,#111581,#111582,
#111583,#111584,#111585,#111586,#111587,#111588,#111589,#111590,#111591,
#111592,#111593,#111594,#111595,#111596,#111597,#111598,#111599,#111600,
#111601,#111602,#111603,#111604,#111605,#111606,#111607,#111608,#111609,
#111610,#111611,#111612,#111613,#111614,#111615,#111616,#111617,#111618,
#111619,#111620,#111621,#111622,#111623,#111624,#111625,#111626,#111627,
#111628,#111629,#111630,#111631,#111632,#111633,#111634,#111635,#111636,
#111637,#111638,#111639,#111640,#111641,#111642,#111643,#111644,#111645,
#111646,#111647,#111648,#111649,#111650,#111651,#111652,#111653,#111654,
#111655,#111656,#111657,#111658,#111659,#111660,#111661,#111662,#111663,
#111664,#111665,#111666,#111667,#111668,#111669,#111670,#111671,#111672,
#111673,#111674,#111675,#111676,#111677,#111678,#111679,#111680,#111681,
#111682,#111683,#111684,#111685,#111686,#111687,#111688,#111689,#111690,
#111691,#111692,#111693,#111694,#111695,#111696,#111697,#111698,#111699,
#111700,#111701,#111702,#111703,#111704,#111705,#111706,#111707,#111708,
#111709,#111710,#111711,#111712,#111713,#111714,#111715,#111716,#111717,
#111718,#111719,#111720,#111721,#111722,#111723,#111724,#111725,#111726,
#111727,#111728,#111729,#111730,#111731,#111732),.UNSPECIFIED.,.F.,.F.,
(4,2,2,2,2,2,2,2,2,2,2,2,2,2,2,2,2,2,2,2,2,2,2,2,2,2,2,2,2,2,2,2,2,2,2,
2,2,2,2,2,2,2,2,2,2,2,2,2,2,2,2,2,2,2,2,2,2,2,2,2,2,2,2,2,2,2,2,2,2,2,2,
2,2,2,2,2,2,2,2,2,2,2,2,2,2,2,2,2,2,2,4),(-2.10002519268564,-2.08483697761129,
-2.08076010466194,-2.07762104738156,-2.07451846365738,-2.07098911710212,
-2.06521692955025,-2.0412620342241,-2.01777849298488,-1.99968771820987,
-1.99513344827512,-1.99288873432114,-1.99108424964152,-1.98882263458331,
-1.98418126591821,-1.952465126248,-1.92007509049889,-1.91357429925143,-1.90989107678948,
-1.90668437857483,-1.90269576781476,-1.89643994721236,-1.85729541493937,
-1.8325934643758,-1.82829243893082,-1.82609788722754,-1.82429178973132,
-1.82197449252604,-1.81703932319838,-1.79232357174609,-1.76540498367543,
-1.75048509424041,-1.7454792391055,-1.74211019255397,-1.73883088408269,
-1.73411547576099,-1.72249744487282,-1.68671915254156,-1.66667894727015,
-1.66190728080995,-1.6596207041872,-1.65781576035324,-1.65559446835355,
-1.65115947511068,-1.61714294401893,-1.58677871070461,-1.58024841123671,
-1.5765590208519,-1.57335291429377,-1.56937278509163,-1.56314583015784,
-1.51766815206114,-1.49962009538053,-1.49507069463302,-1.49282688068273,
-1.49102232151892,-1.48875961312834,-1.48411283977927,-1.45250755888057,
-1.41953482703475,-1.41329846734298,-1.40967072118342,-1.40645683990408,
-1.40238490678399,-1.39584357224068,-1.35189453119925,-1.33795738379518,
-1.3297799453804,-1.32696700235239,-1.3250885142317,-1.32313712161813,-1.31998243146455,
-1.3096139964638,-1.27737813414181,-1.26048393738696,-1.24928687557285,
-1.24476223722666,-1.24148431207925,-1.23846428044022,-1.23352737292429,
-1.22038336666716,-1.18604904588521,-1.17156364698001,-1.16317838123143,
-1.160339904387,-1.15845628226542,-1.15651204482705,-1.15338999731221,-1.14332921274324,
-1.110922065625,-1.10898896929382),.UNSPECIFIED.);
#2814=B_SPLINE_CURVE_WITH_KNOTS('',3,(#111738,#111739,#111740,#111741,#111742,
#111743,#111744,#111745,#111746,#111747,#111748,#111749,#111750,#111751,
#111752,#111753,#111754,#111755,#111756,#111757,#111758,#111759,#111760,
#111761,#111762,#111763,#111764,#111765,#111766,#111767,#111768,#111769,
#111770,#111771,#111772,#111773,#111774,#111775,#111776,#111777,#111778,
#111779,#111780,#111781,#111782,#111783,#111784,#111785,#111786,#111787,
#111788,#111789,#111790,#111791,#111792,#111793,#111794,#111795,#111796,
#111797,#111798,#111799,#111800,#111801,#111802,#111803,#111804,#111805,
#111806,#111807,#111808,#111809,#111810,#111811,#111812,#111813,#111814,
#111815,#111816,#111817,#111818,#111819,#111820,#111821,#111822,#111823,
#111824,#111825,#111826,#111827,#111828,#111829,#111830,#111831,#111832,
#111833,#111834,#111835,#111836,#111837,#111838,#111839,#111840,#111841,
#111842,#111843,#111844,#111845,#111846,#111847,#111848,#111849,#111850,
#111851,#111852,#111853,#111854,#111855,#111856,#111857,#111858,#111859,
#111860,#111861,#111862,#111863,#111864,#111865,#111866,#111867,#111868,
#111869,#111870,#111871,#111872,#111873,#111874,#111875,#111876,#111877,
#111878,#111879,#111880,#111881,#111882,#111883,#111884,#111885,#111886,
#111887,#111888,#111889,#111890,#111891,#111892,#111893,#111894,#111895,
#111896,#111897,#111898,#111899,#111900,#111901,#111902,#111903,#111904,
#111905,#111906,#111907,#111908,#111909,#111910,#111911,#111912,#111913,
#111914,#111915,#111916,#111917,#111918,#111919,#111920,#111921,#111922,
#111923,#111924,#111925,#111926,#111927,#111928,#111929,#111930,#111931,
#111932,#111933,#111934,#111935,#111936,#111937,#111938,#111939,#111940,
#111941),.UNSPECIFIED.,.F.,.F.,(4,2,2,2,2,2,2,2,2,2,2,2,2,2,2,2,2,2,2,2,
2,2,2,2,2,2,2,2,2,2,2,2,2,2,2,2,2,2,2,2,2,2,2,2,2,2,2,2,2,2,2,2,2,2,2,2,
2,2,2,2,2,2,2,2,2,2,2,2,2,2,2,2,2,2,2,2,2,2,2,2,2,2,2,2,2,2,2,2,2,2,2,2,
2,2,2,2,2,2,2,2,2,4),(-0.991072633050833,-0.96959646129034,-0.944678711933136,
-0.938779703203733,-0.935222565921512,-0.931992816825189,-0.927790019527473,
-0.918593713735521,-0.905823630266165,-0.883660354338812,-0.879533898535787,
-0.857384837860035,-0.853692567617605,-0.851602427275458,-0.849781682743783,
-0.847310269425852,-0.841503183341829,-0.83299440984175,-0.802838021238123,
-0.778027638027302,-0.772131954079662,-0.768575570929295,-0.765345715084556,
-0.761141642746596,-0.751937708198761,-0.739152951492851,-0.716995831160663,
-0.712801403497338,-0.690741169910172,-0.687049306280662,-0.684959283183059,
-0.683138560034392,-0.680667067635752,-0.674859319450391,-0.66634914526616,
-0.636180864331508,-0.611385362667729,-0.605490241659954,-0.601934026026214,
-0.598704213415621,-0.594500040993152,-0.585295221045302,-0.57250867245532,
-0.550352855042596,-0.546150504741942,-0.524101486558228,-0.520409740294744,
-0.518319769752558,-0.5164990824572,-0.514027625432059,-0.50821990179108,
-0.499709710617032,-0.469540516995256,-0.444747298279119,-0.438852354245613,
-0.435296224142,-0.4320664757741,-0.427862367681426,-0.418657606361045,
-0.405871069855022,-0.383715818262087,-0.379512588450659,-0.357465334068013,
-0.353773669542994,-0.351683743586794,-0.349863093926034,-0.347391686372291,
-0.341584071870001,-0.333074034185266,-0.302905281117464,-0.2781127929516,
-0.272217978172867,-0.268661923461474,-0.265432241932784,-0.261228218498917,
-0.252023632543302,-0.239237331210165,-0.217082553343851,-0.192741218097675,
-0.187889348685176,-0.185554368323922,-0.183746834363978,-0.181565464383872,
-0.177331460424884,-0.152040531888699,-0.113463448222951,-0.107144837200523,
-0.103137301711613,-0.09992843993598,-0.0962569237434189,-0.0898147857437402,
-0.081850296451155,-0.0637884509081943,-0.0434746763101988,-0.0267336396863527,
-0.0214005651163529,-0.0190362188986482,-0.0172232213069115,-0.0155121918094399,
-0.0133884064464265,-0.0085363605493341,-0.000491425429689316),
 .UNSPECIFIED.);
#2815=B_SPLINE_CURVE_WITH_KNOTS('',3,(#111942,#111943,#111944,#111945,#111946,
#111947,#111948,#111949),.UNSPECIFIED.,.F.,.F.,(4,2,2,4),(-2.10007518485579,
-2.07578500626469,-2.04950247907538,-2.04103609068276),.UNSPECIFIED.);
#2816=B_SPLINE_CURVE_WITH_KNOTS('',3,(#111950,#111951,#111952,#111953,#111954,
#111955,#111956,#111957,#111958,#111959,#111960,#111961,#111962,#111963,
#111964,#111965,#111966,#111967,#111968,#111969,#111970,#111971,#111972,
#111973,#111974,#111975,#111976,#111977,#111978,#111979,#111980,#111981,
#111982,#111983,#111984,#111985,#111986,#111987,#111988,#111989,#111990,
#111991,#111992,#111993,#111994,#111995,#111996,#111997,#111998,#111999,
#112000,#112001,#112002,#112003,#112004,#112005,#112006,#112007,#112008,
#112009,#112010,#112011,#112012,#112013,#112014,#112015,#112016,#112017,
#112018,#112019,#112020,#112021,#112022,#112023,#112024,#112025,#112026,
#112027,#112028,#112029,#112030,#112031,#112032,#112033,#112034,#112035,
#112036,#112037,#112038,#112039,#112040,#112041,#112042,#112043,#112044,
#112045,#112046,#112047,#112048,#112049,#112050,#112051,#112052,#112053,
#112054,#112055,#112056,#112057,#112058,#112059,#112060,#112061,#112062,
#112063,#112064,#112065,#112066,#112067,#112068,#112069,#112070,#112071,
#112072,#112073,#112074,#112075,#112076,#112077,#112078,#112079,#112080,
#112081,#112082,#112083,#112084,#112085,#112086,#112087,#112088,#112089,
#112090,#112091,#112092,#112093,#112094,#112095,#112096,#112097,#112098,
#112099,#112100,#112101,#112102,#112103,#112104,#112105,#112106,#112107,
#112108,#112109,#112110,#112111,#112112,#112113,#112114,#112115,#112116,
#112117,#112118,#112119,#112120,#112121,#112122,#112123,#112124,#112125,
#112126,#112127,#112128,#112129,#112130,#112131,#112132,#112133,#112134,
#112135,#112136,#112137,#112138,#112139,#112140,#112141,#112142,#112143,
#112144,#112145,#112146,#112147,#112148,#112149,#112150,#112151,#112152,
#112153,#112154,#112155,#112156,#112157,#112158,#112159,#112160,#112161,
#112162,#112163,#112164,#112165),.UNSPECIFIED.,.F.,.F.,(4,2,2,2,2,2,2,2,
2,2,2,2,2,2,2,2,2,2,2,2,2,2,2,2,2,2,2,2,2,2,2,2,2,2,2,2,2,2,2,2,2,2,2,2,
2,2,2,2,2,2,2,2,2,2,2,2,2,2,2,2,2,2,2,2,2,2,2,2,2,2,2,2,2,2,2,2,2,2,2,2,
2,2,2,2,2,2,2,2,2,2,2,2,2,2,2,2,2,2,2,2,2,2,2,2,2,2,2,4),(-1.10898896929382,
-1.09390414405012,-1.08265174018518,-1.07811894887099,-1.07483967818805,
-1.07141429667589,-1.06613416613628,-1.04996520517984,-1.0212402150986,
-0.998263005053497,-0.994568306464459,-0.992478074967628,-0.990658203159696,
-0.988189333864909,-0.982394339314872,-0.97390909473674,-0.943933036608764,
-0.918914309952309,-0.913013793398772,-0.909457209904748,-0.906228918199669,
-0.902029422570637,-0.892846566427281,-0.88010087628242,-0.857930417791147,
-0.853947411233765,-0.831621684243135,-0.827929712412916,-0.825840116445942,
-0.824020149951253,-0.821550284817142,-0.815749137769432,-0.807251440203605,
-0.777176398388081,-0.752272961871932,-0.746375882345796,-0.742820075919541,
-0.739591670881674,-0.735390853465189,-0.726200112785101,-0.713439275221727,
-0.691273924862846,-0.687186923354377,-0.66498773247137,-0.661296297625461,
-0.659206847631488,-0.657386895388385,-0.654916898488686,-0.649114776814038,
-0.640615050839285,-0.610523207114743,-0.585640316679858,-0.579743951555371,
-0.576188344045373,-0.572959972959557,-0.568758989307938,-0.559566989587237,
-0.546803649935171,-0.524639678165284,-0.52053662343781,-0.498357892991948,
-0.494666607373074,-0.492577216645518,-0.490757298013267,-0.488287322619683,
-0.482485145323523,-0.473985241995247,-0.443891233805176,-0.419012051104974,
-0.413115901939393,-0.409560387486356,-0.406332077382064,-0.40213113934847,
-0.392939095878337,-0.380175574572132,-0.358012207634889,-0.353906715989856,
-0.331731579130073,-0.328040380704382,-0.325951035371735,-0.324131153449181,
-0.321661224087886,-0.315859138247062,-0.307359353831219,-0.27726552517987,
-0.252387354711478,-0.246491341308215,-0.242935902878609,-0.239707658104643,
-0.235506799779487,-0.226314908143842,-0.213551578653512,-0.191388689565356,
-0.167084324828378,-0.162128641449716,-0.159807692922468,-0.158001593951376,
-0.155810528171104,-0.151526072728155,-0.145862038301895,-0.131518066937979,
-0.0976948063532052,-0.0839718135821706,-0.0789591985615271,-0.0759258110012352,
-0.0726585076248189,-0.0681941961652964,-0.0594454700439993),
 .UNSPECIFIED.);
#2817=B_SPLINE_CURVE_WITH_KNOTS('',3,(#112170,#112171,#112172,#112173,#112174,
#112175,#112176,#112177,#112178,#112179,#112180,#112181,#112182,#112183,
#112184,#112185,#112186,#112187,#112188,#112189,#112190,#112191,#112192,
#112193,#112194,#112195,#112196,#112197,#112198,#112199,#112200,#112201,
#112202,#112203,#112204,#112205,#112206,#112207,#112208,#112209,#112210,
#112211,#112212,#112213,#112214,#112215,#112216,#112217,#112218,#112219,
#112220,#112221,#112222,#112223,#112224,#112225,#112226,#112227,#112228,
#112229,#112230,#112231,#112232,#112233,#112234,#112235,#112236,#112237,
#112238,#112239,#112240,#112241,#112242,#112243,#112244,#112245,#112246,
#112247,#112248,#112249,#112250,#112251,#112252,#112253,#112254,#112255,
#112256,#112257,#112258,#112259,#112260,#112261,#112262,#112263,#112264,
#112265,#112266,#112267,#112268,#112269,#112270,#112271,#112272,#112273,
#112274,#112275,#112276,#112277,#112278,#112279,#112280,#112281,#112282,
#112283,#112284,#112285,#112286,#112287,#112288,#112289,#112290,#112291,
#112292,#112293,#112294,#112295,#112296,#112297,#112298,#112299,#112300,
#112301,#112302,#112303,#112304,#112305,#112306,#112307,#112308,#112309,
#112310,#112311,#112312,#112313,#112314,#112315,#112316,#112317,#112318,
#112319,#112320,#112321,#112322,#112323,#112324,#112325,#112326,#112327,
#112328,#112329,#112330,#112331,#112332,#112333,#112334,#112335,#112336,
#112337,#112338,#112339,#112340,#112341,#112342,#112343,#112344,#112345,
#112346,#112347,#112348,#112349,#112350,#112351,#112352,#112353,#112354,
#112355,#112356,#112357,#112358,#112359,#112360,#112361,#112362,#112363,
#112364,#112365,#112366,#112367,#112368,#112369,#112370,#112371,#112372,
#112373,#112374,#112375,#112376,#112377,#112378,#112379,#112380,#112381,
#112382,#112383,#112384,#112385,#112386,#112387),.UNSPECIFIED.,.F.,.F.,
(4,2,2,2,2,2,2,2,2,2,2,2,2,2,2,2,2,2,2,2,2,2,2,2,2,2,2,2,2,2,2,2,2,2,2,
2,2,2,2,2,2,2,2,2,2,2,2,2,2,2,2,2,2,2,2,2,2,2,2,2,2,2,2,2,2,2,2,2,2,2,2,
2,2,2,2,2,2,2,2,2,2,2,2,2,2,2,2,2,2,2,2,2,2,2,2,2,2,2,2,2,2,2,2,2,2,2,2,
2,4),(-2.04074275515961,-2.03567152604733,-2.02716445779139,-2.02135773787919,
-2.01888641574544,-2.01706568248613,-2.01497553868023,-2.01128314570221,
-1.98926911488306,-1.9850164310383,-1.96284472739362,-1.95005174554692,
-1.94084437755,-1.93663968972439,-1.9334097697126,-1.92985372694521,-1.92395955310253,
-1.89918605886234,-1.86902859243381,-1.86052143735779,-1.85471468531573,
-1.85224336822928,-1.85042264604395,-1.84833252351285,-1.84464018655162,
-1.82263444372556,-1.81837603816447,-1.79620522974131,-1.78341054614093,
-1.77420230531716,-1.76999748347622,-1.76676756491554,-1.76321162793297,
-1.75731787718544,-1.73254290960076,-1.70238640492463,-1.69387940337996,
-1.68807273845119,-1.68560144623766,-1.68378073758281,-1.68169062500232,
-1.67799829360566,-1.65598740217461,-1.65173276604165,-1.62956162348202,
-1.6167681999837,-1.60756063565841,-1.60335594954367,-1.60012606690004,
-1.59657010125634,-1.59067614081617,-1.56589319683425,-1.53574400245634,
-1.52723795392019,-1.52143177291809,-1.51896057172024,-1.51713988495493,
-1.51504974491978,-1.51135725184818,-1.48929621441268,-1.48536041100123,
-1.4626987670826,-1.45003044035949,-1.4408884844046,-1.43669526989925,-1.4334668605366,
-1.42990516749844,-1.42398416471475,-1.39813346218269,-1.36890257175063,
-1.36051458655116,-1.3547671903463,-1.35230583284256,-1.35048638025678,
-1.34839062841658,-1.34467298790539,-1.32011159936551,-1.3021563694808,
-1.2859076860515,-1.27500355436319,-1.2705222754074,-1.26725098092633,-1.26380760725131,
-1.25844504228341,-1.24149757322114,-1.20380483139539,-1.18999041672601,
-1.18665648394224,-1.18466552957027,-1.18283127595654,-1.18015610877049,
-1.17350749935577,-1.14182673800396,-1.11243487519151,-1.10595171198221,
-1.10227129981328,-1.09906293422879,-1.0950668440296,-1.08878827885696,
-1.04984422365689,-1.04683088503486,-1.02403579115356,-1.02034098430461,
-1.01825025042474,-1.01642959072702,-1.01395909804104,-1.0081577202863,
-0.999660512452531,-0.991072633050833),.UNSPECIFIED.);
#2818=B_SPLINE_CURVE_WITH_KNOTS('',3,(#112389,#112390,#112391,#112392,#112393,
#112394,#112395,#112396,#112397,#112398),.UNSPECIFIED.,.F.,.F.,(4,2,2,2,
4),(-0.0594454700439993,-0.0573925871556223,-0.0413654807553726,-0.0230001708345523,
-0.000492308184977265),.UNSPECIFIED.);
#2819=B_SPLINE_CURVE_WITH_KNOTS('',3,(#112399,#112400,#112401,#112402,#112403,
#112404,#112405,#112406,#112407,#112408,#112409,#112410,#112411,#112412,
#112413,#112414,#112415,#112416,#112417,#112418,#112419,#112420,#112421,
#112422,#112423,#112424,#112425,#112426,#112427,#112428,#112429,#112430,
#112431,#112432,#112433,#112434,#112435,#112436,#112437,#112438,#112439,
#112440,#112441,#112442,#112443,#112444,#112445,#112446,#112447,#112448,
#112449,#112450,#112451,#112452,#112453,#112454,#112455,#112456,#112457,
#112458,#112459,#112460,#112461,#112462,#112463,#112464,#112465,#112466,
#112467,#112468,#112469,#112470,#112471,#112472,#112473,#112474,#112475,
#112476,#112477,#112478,#112479,#112480,#112481,#112482,#112483,#112484,
#112485,#112486,#112487,#112488,#112489,#112490,#112491,#112492,#112493,
#112494,#112495,#112496,#112497,#112498,#112499,#112500,#112501,#112502,
#112503,#112504,#112505,#112506,#112507,#112508,#112509,#112510,#112511,
#112512,#112513,#112514,#112515,#112516,#112517,#112518,#112519,#112520,
#112521,#112522,#112523,#112524,#112525,#112526,#112527,#112528,#112529,
#112530,#112531,#112532,#112533,#112534,#112535,#112536,#112537,#112538,
#112539,#112540,#112541,#112542,#112543,#112544,#112545,#112546,#112547,
#112548,#112549,#112550,#112551,#112552,#112553,#112554,#112555,#112556,
#112557,#112558,#112559,#112560,#112561,#112562,#112563,#112564,#112565,
#112566,#112567,#112568,#112569,#112570,#112571,#112572,#112573,#112574,
#112575,#112576,#112577,#112578),.UNSPECIFIED.,.F.,.F.,(4,2,2,2,2,2,2,2,
2,2,2,2,2,2,2,2,2,2,2,2,2,2,2,2,2,2,2,2,2,2,2,2,2,2,2,2,2,2,2,2,2,2,2,2,
2,2,2,2,2,2,2,2,2,2,2,2,2,2,2,2,2,2,2,2,2,2,2,2,2,2,2,2,2,2,2,2,2,2,2,2,
2,2,2,2,2,2,2,2,2,4),(-2.10013203330852,-2.09759133984381,-2.09518859571947,
-2.09332411054461,-2.09161915840831,-2.08965654530031,-2.08645037965014,
-2.0755270373007,-2.05064612886903,-2.01943176311094,-2.01318289201795,
-2.00955246284213,-2.0063389283563,-2.00227112178533,-1.99574418275092,
-1.95172132127184,-1.9329171861995,-1.92828117442073,-1.92602048956945,
-1.92421587321082,-1.9219699096027,-1.91740976479451,-1.88478270033251,
-1.85269560506489,-1.84645767066889,-1.84282950840846,-1.83961555528948,
-1.83554393342112,-1.82900394740178,-1.79321394901279,-1.7657959211102,
-1.76142857768398,-1.75922066872306,-1.75741515094544,-1.75511328725454,
-1.75026105181688,-1.72215353043311,-1.68631970579769,-1.67990532972719,
-1.67624006501671,-1.67303120972583,-1.66901651982944,-1.66267215261942,
-1.61774987856709,-1.59941743577169,-1.59483504998088,-1.59258473951846,
-1.59078012093854,-1.58852379390723,-1.58391040438392,-1.5517110974274,
-1.51966212114605,-1.51321232924929,-1.50953957456019,-1.50633146505512,
-1.50232730979013,-1.49601914469461,-1.45736350723146,-1.43223071045562,
-1.42795099687785,-1.42576062150971,-1.42395410072611,-1.42163132223635,
-1.41666728715779,-1.39171226642141,-1.36499522660805,-1.35013547676979,
-1.34513605508485,-1.34176810199038,-1.33848742013393,-1.3345124571801,
-1.32674197855803,-1.28357657343487,-1.27055340575811,-1.26273399565356,
-1.25996646627421,-1.25809685991349,-1.25637384538573,-1.25339846029372,
-1.2446077475669,-1.21144404316211,-1.19391386449296,-1.18243428876635,
-1.17786780202552,-1.17458238365523,-1.17157103797963,-1.16668374991637,
-1.15389899343611,-1.11922703591869,-1.10915862425753),.UNSPECIFIED.);
#2820=B_SPLINE_CURVE_WITH_KNOTS('',3,(#112584,#112585,#112586,#112587,#112588,
#112589,#112590,#112591,#112592,#112593,#112594,#112595,#112596,#112597,
#112598,#112599,#112600,#112601,#112602,#112603,#112604,#112605,#112606,
#112607,#112608,#112609,#112610,#112611,#112612,#112613,#112614,#112615,
#112616,#112617,#112618,#112619,#112620,#112621,#112622,#112623,#112624,
#112625,#112626,#112627,#112628,#112629,#112630,#112631,#112632,#112633,
#112634,#112635,#112636,#112637,#112638,#112639,#112640,#112641,#112642,
#112643,#112644,#112645,#112646,#112647,#112648,#112649,#112650,#112651,
#112652,#112653,#112654,#112655,#112656,#112657,#112658,#112659,#112660,
#112661,#112662,#112663,#112664,#112665,#112666,#112667,#112668,#112669,
#112670,#112671,#112672,#112673,#112674,#112675,#112676,#112677,#112678,
#112679,#112680,#112681,#112682,#112683,#112684,#112685,#112686,#112687,
#112688,#112689,#112690,#112691,#112692,#112693,#112694,#112695,#112696,
#112697,#112698,#112699,#112700,#112701,#112702,#112703,#112704,#112705,
#112706,#112707,#112708,#112709,#112710,#112711,#112712,#112713,#112714,
#112715,#112716,#112717,#112718,#112719,#112720,#112721,#112722,#112723,
#112724,#112725,#112726,#112727,#112728,#112729,#112730,#112731,#112732,
#112733,#112734,#112735,#112736,#112737,#112738,#112739,#112740,#112741,
#112742,#112743,#112744,#112745,#112746,#112747,#112748,#112749,#112750,
#112751,#112752,#112753,#112754,#112755,#112756,#112757,#112758,#112759,
#112760,#112761,#112762,#112763,#112764,#112765,#112766,#112767,#112768,
#112769),.UNSPECIFIED.,.F.,.F.,(4,2,2,2,2,2,2,2,2,2,2,2,2,2,2,2,2,2,2,2,
2,2,2,2,2,2,2,2,2,2,2,2,2,2,2,2,2,2,2,2,2,2,2,2,2,2,2,2,2,2,2,2,2,2,2,2,
2,2,2,2,2,2,2,2,2,2,2,2,2,2,2,2,2,2,2,2,2,2,2,2,2,2,2,2,2,2,2,2,2,2,2,2,
4),(-0.991436796285106,-0.990873237000083,-0.959694946413161,-0.926078997117896,
-0.921600444224151,-0.919369945546251,-0.917564377032642,-0.915285551485311,
-0.910557842618623,-0.890932952857412,-0.856354081040102,-0.843442690479383,
-0.838536579266132,-0.835521133852138,-0.832237100385693,-0.827683376769096,
-0.816297010993809,-0.79898216555433,-0.766179185054227,-0.756857710136171,
-0.753817933684952,-0.752081983920873,-0.750221674330721,-0.747504937187699,
-0.740071449256155,-0.727991669949014,-0.692510586278405,-0.677347736849901,
-0.672174775334541,-0.668770596327473,-0.665476034563454,-0.660862943687471,
-0.64906549850864,-0.630803816212285,-0.604262694454322,-0.59091843245324,
-0.587505034000453,-0.585496666053101,-0.583649279181806,-0.58100373777366,
-0.574076853981764,-0.534863724499452,-0.511962982677311,-0.506149512588472,
-0.502610585636146,-0.499375985242109,-0.495135846774915,-0.485723229113441,
-0.441218178082258,-0.424551201922221,-0.420941449638163,-0.418890514763205,
-0.417059109091292,-0.41451182058211,-0.408236580046016,-0.398761750883128,
-0.359162915599921,-0.343957269007202,-0.338779983990421,-0.335374982044542,
-0.332081120105781,-0.32747151259717,-0.315697938945907,-0.297491903760072,
-0.271096452551978,-0.257545955725953,-0.254119349432689,-0.252108144248591,
-0.250262091054276,-0.247623996452157,-0.240748029607144,-0.197089898625644,
-0.178075038189032,-0.172508447131054,-0.169022087870296,-0.165770138875317,
-0.161408622714191,-0.151266142330518,-0.136625311781776,-0.116709169310579,
-0.0933595528039877,-0.0884373357017265,-0.0861220891024877,-0.0843156172162147,
-0.0821181388438962,-0.0778042765599675,-0.0720898137195765,-0.0575422230559856,
-0.0173414858727192,-0.0084227495550825,-0.00426260359061961,-0.00206331470985932,
-0.000491892551814876),.UNSPECIFIED.);
#2821=B_SPLINE_CURVE_WITH_KNOTS('',3,(#112770,#112771,#112772,#112773,#112774,
#112775,#112776,#112777,#112778,#112779,#112780,#112781),.UNSPECIFIED.,
 .F.,.F.,(4,2,2,2,2,4),(-2.09967868133144,-2.09854857464352,-2.09658609675878,
-2.09129232863807,-2.07408596053682,-2.04074275515961),.UNSPECIFIED.);
#2822=B_SPLINE_CURVE_WITH_KNOTS('',3,(#112782,#112783,#112784,#112785,#112786,
#112787,#112788,#112789,#112790,#112791,#112792,#112793,#112794,#112795,
#112796,#112797,#112798,#112799,#112800,#112801,#112802,#112803,#112804,
#112805,#112806,#112807,#112808,#112809,#112810,#112811,#112812,#112813,
#112814,#112815,#112816,#112817,#112818,#112819,#112820,#112821,#112822,
#112823,#112824,#112825,#112826,#112827,#112828,#112829,#112830,#112831,
#112832,#112833,#112834,#112835,#112836,#112837,#112838,#112839,#112840,
#112841,#112842,#112843,#112844,#112845,#112846,#112847,#112848,#112849,
#112850,#112851,#112852,#112853,#112854,#112855,#112856,#112857,#112858,
#112859,#112860,#112861,#112862,#112863,#112864,#112865,#112866,#112867,
#112868,#112869,#112870,#112871,#112872,#112873,#112874,#112875,#112876,
#112877,#112878,#112879,#112880,#112881,#112882,#112883,#112884,#112885,
#112886,#112887,#112888,#112889,#112890,#112891,#112892,#112893,#112894,
#112895,#112896,#112897,#112898,#112899,#112900,#112901,#112902,#112903,
#112904,#112905,#112906,#112907,#112908,#112909,#112910,#112911,#112912,
#112913,#112914,#112915,#112916,#112917,#112918,#112919,#112920,#112921,
#112922,#112923,#112924,#112925,#112926,#112927,#112928,#112929,#112930,
#112931,#112932,#112933,#112934,#112935,#112936,#112937,#112938,#112939,
#112940,#112941,#112942,#112943,#112944,#112945,#112946,#112947,#112948,
#112949,#112950,#112951,#112952,#112953,#112954,#112955,#112956,#112957,
#112958,#112959,#112960,#112961,#112962,#112963,#112964,#112965,#112966,
#112967,#112968,#112969,#112970,#112971,#112972,#112973,#112974,#112975,
#112976,#112977,#112978,#112979,#112980,#112981,#112982,#112983,#112984,
#112985,#112986,#112987,#112988,#112989,#112990,#112991,#112992,#112993,
#112994,#112995),.UNSPECIFIED.,.F.,.F.,(4,2,2,2,2,2,2,2,2,2,2,2,2,2,2,2,
2,2,2,2,2,2,2,2,2,2,2,2,2,2,2,2,2,2,2,2,2,2,2,2,2,2,2,2,2,2,2,2,2,2,2,2,
2,2,2,2,2,2,2,2,2,2,2,2,2,2,2,2,2,2,2,2,2,2,2,2,2,2,2,2,2,2,2,2,2,2,2,2,
2,2,2,2,2,2,2,2,2,2,2,2,2,2,2,2,2,2,4),(-1.10915862425753,-1.09957210592967,
-1.09484179727824,-1.09256296141637,-1.09075803538217,-1.08852922264832,
-1.08405680732055,-1.05036363381549,-1.02133928243396,-1.01460206567239,
-1.01047363790624,-1.00725366183995,-1.00365891852038,-0.997579277411207,
-0.963305891606409,-0.932875775063358,-0.928144245981082,-0.925865214356625,
-0.924060331650434,-0.921831817932682,-0.91736073514768,-0.911371024271775,
-0.895666606520307,-0.856854632074688,-0.848073379039098,-0.843929396786707,
-0.840699048998021,-0.837149698070751,-0.831283659047388,-0.804123490951329,
-0.787193995873125,-0.764574926695985,-0.760881652399191,-0.758791692521814,
-0.756971675552142,-0.754502098642413,-0.748703198242827,-0.740210208396916,
-0.71017447799593,-0.685222364066652,-0.679323562997927,-0.675767258293627,
-0.672538742150467,-0.668338269719849,-0.659150365976129,-0.64639521976583,
-0.624226550142749,-0.62017969728572,-0.597929761116141,-0.594237932509529,
-0.592148321706141,-0.590328273987628,-0.587858207029735,-0.582056182221982,
-0.57355683436559,-0.543470115374455,-0.518577910446857,-0.512680972733161,
-0.509125111514382,-0.505896568002824,-0.501695443119888,-0.4925034882971,
-0.479740509337504,-0.457574892404385,-0.45347790684298,-0.431290064530191,
-0.427598538235355,-0.425509021254347,-0.423688999964353,-0.421218895037618,
-0.415416456431553,-0.406916209673484,-0.376821623946476,-0.351939660087849,
-0.346043131569558,-0.342487404384609,-0.3392589112882,-0.335057749733842,
-0.325865279395831,-0.31310121748992,-0.290936514004643,-0.286831906161462,
-0.264654111038677,-0.260962695081183,-0.258873228272477,-0.257053240419455,
-0.254583167787781,-0.248780750098684,-0.240280482221082,-0.210184964095294,
-0.185286677485233,-0.17940013856418,-0.175846579580633,-0.172617612476978,
-0.168412324610933,-0.159195857633063,-0.14638583744142,-0.124240829247567,
-0.119957852905529,-0.0980203369861578,-0.0943299017410368,-0.0922406803234062,
-0.0904206881795931,-0.0879503157389445,-0.0821458916829303,-0.0736415108296685,
-0.0594688639043352),.UNSPECIFIED.);
#2823=B_SPLINE_CURVE_WITH_KNOTS('',3,(#113000,#113001,#113002,#113003,#113004,
#113005,#113006,#113007,#113008,#113009,#113010,#113011,#113012,#113013,
#113014,#113015,#113016,#113017,#113018,#113019,#113020,#113021,#113022,
#113023,#113024,#113025,#113026,#113027,#113028,#113029,#113030,#113031,
#113032,#113033,#113034,#113035,#113036,#113037,#113038,#113039,#113040,
#113041,#113042,#113043,#113044,#113045,#113046,#113047,#113048,#113049,
#113050,#113051,#113052,#113053,#113054,#113055,#113056,#113057,#113058,
#113059,#113060,#113061,#113062,#113063,#113064,#113065,#113066,#113067,
#113068,#113069,#113070,#113071,#113072,#113073,#113074,#113075,#113076,
#113077,#113078,#113079,#113080,#113081,#113082,#113083,#113084,#113085,
#113086,#113087,#113088,#113089,#113090,#113091,#113092,#113093,#113094,
#113095,#113096,#113097,#113098,#113099,#113100,#113101,#113102,#113103,
#113104,#113105,#113106,#113107,#113108,#113109,#113110,#113111,#113112,
#113113,#113114,#113115,#113116,#113117,#113118,#113119,#113120,#113121,
#113122,#113123,#113124,#113125,#113126,#113127,#113128,#113129,#113130,
#113131,#113132,#113133,#113134,#113135,#113136,#113137,#113138,#113139,
#113140,#113141,#113142,#113143,#113144,#113145,#113146,#113147,#113148,
#113149,#113150,#113151,#113152,#113153,#113154,#113155,#113156,#113157,
#113158,#113159,#113160,#113161,#113162,#113163,#113164,#113165,#113166,
#113167,#113168,#113169,#113170,#113171,#113172,#113173,#113174,#113175,
#113176,#113177,#113178,#113179,#113180,#113181,#113182,#113183,#113184,
#113185,#113186,#113187,#113188,#113189,#113190,#113191,#113192,#113193,
#113194,#113195,#113196,#113197,#113198,#113199,#113200,#113201),
 .UNSPECIFIED.,.F.,.F.,(4,2,2,2,2,2,2,2,2,2,2,2,2,2,2,2,2,2,2,2,2,2,2,2,
2,2,2,2,2,2,2,2,2,2,2,2,2,2,2,2,2,2,2,2,2,2,2,2,2,2,2,2,2,2,2,2,2,2,2,2,
2,2,2,2,2,2,2,2,2,2,2,2,2,2,2,2,2,2,2,2,2,2,2,2,2,2,2,2,2,2,2,2,2,2,2,2,
2,2,2,2,4),(-2.04139270538101,-2.03966297411823,-2.02143180415736,-2.00964813248972,
-2.00503685889942,-2.00174255800547,-1.99873880357734,-1.99467736075789,
-1.98440851892978,-1.94730249018665,-1.93205365570485,-1.92338634940782,
-1.92051332622025,-1.91862200772741,-1.91691962021657,-1.91405434050606,
-1.90611416035622,-1.87553438979116,-1.84674360174858,-1.8402635075626,
-1.83658349869667,-1.83337472229398,-1.82937712371914,-1.8230941722876,
-1.77786825265898,-1.7596877588869,-1.75512201921192,-1.75287437799442,
-1.75106895911633,-1.74880786954449,-1.74417282306118,-1.71230093028663,
-1.67943786113303,-1.67326966219273,-1.66965522303164,-1.66643730007494,
-1.662338577063,-1.6557079612845,-1.6221760222767,-1.60094644885751,-1.59381020216466,
-1.58870815112307,-1.5863594754392,-1.58472269424159,-1.58262594992414,
-1.57890472223976,-1.55423117001562,-1.53631271472844,-1.52010697864088,
-1.51266553036367,-1.50655413693591,-1.5029517122836,-1.49973158725669,
-1.49561225750841,-1.48688771423292,-1.44790822996209,-1.4321652724848,
-1.42332094406712,-1.42042725510494,-1.4185316067398,-1.41660032053548,
-1.41354051948908,-1.40404758720192,-1.37130702441355,-1.35405837832461,
-1.3427020929498,-1.33815264483204,-1.33486928295805,-1.33185282123776,
-1.32694128349747,-1.31399101295887,-1.27947185340709,-1.26493477226171,
-1.25652928216197,-1.2536875615668,-1.25180268839609,-1.25009442727391,
-1.24719790207228,-1.23902589273424,-1.20546757144143,-1.18769173174651,
-1.17980499814139,-1.17341179203,-1.16974998873271,-1.16653914534787,-1.16251529544889,
-1.15614267358652,-1.11813033375047,-1.09239961558534,-1.08816315014852,
-1.08598099494507,-1.08417310520198,-1.08183801958286,-1.07698710341559,
-1.05053791714071,-1.01457274599916,-1.00803889506752,-1.0039681775919,
-1.00075312290307,-0.997121773519071,-0.991436796285106),.UNSPECIFIED.);
#2824=B_SPLINE_CURVE_WITH_KNOTS('',3,(#113203,#113204,#113205,#113206,#113207,
#113208,#113209,#113210,#113211,#113212,#113213,#113214,#113215,#113216,
#113217,#113218),.UNSPECIFIED.,.F.,.F.,(4,2,2,2,2,2,2,4),(-0.0594688639043352,
-0.0326218974226338,-0.0172456618715315,-0.0121571034009043,-0.00873146617640893,
-0.0056783958676778,-0.00301214665044019,-0.000491717384029574),
 .UNSPECIFIED.);
#2825=B_SPLINE_CURVE_WITH_KNOTS('',3,(#113219,#113220,#113221,#113222,#113223,
#113224,#113225,#113226,#113227,#113228,#113229,#113230,#113231,#113232,
#113233,#113234,#113235,#113236,#113237,#113238,#113239,#113240,#113241,
#113242,#113243,#113244,#113245,#113246,#113247,#113248,#113249,#113250,
#113251,#113252,#113253,#113254,#113255,#113256,#113257,#113258,#113259,
#113260,#113261,#113262,#113263,#113264,#113265,#113266,#113267,#113268,
#113269,#113270,#113271,#113272,#113273,#113274,#113275,#113276,#113277,
#113278,#113279,#113280,#113281,#113282,#113283,#113284,#113285,#113286,
#113287,#113288,#113289,#113290,#113291,#113292,#113293,#113294,#113295,
#113296,#113297,#113298,#113299,#113300,#113301,#113302,#113303,#113304,
#113305,#113306,#113307,#113308,#113309,#113310,#113311,#113312,#113313,
#113314,#113315,#113316,#113317,#113318,#113319,#113320,#113321,#113322,
#113323,#113324,#113325,#113326,#113327,#113328,#113329,#113330,#113331,
#113332,#113333,#113334,#113335,#113336,#113337,#113338,#113339,#113340,
#113341,#113342,#113343,#113344,#113345,#113346,#113347,#113348,#113349,
#113350,#113351,#113352,#113353,#113354,#113355,#113356,#113357,#113358,
#113359,#113360,#113361,#113362,#113363,#113364,#113365,#113366,#113367,
#113368,#113369,#113370,#113371,#113372,#113373,#113374,#113375,#113376,
#113377,#113378,#113379,#113380,#113381,#113382,#113383,#113384,#113385,
#113386,#113387,#113388,#113389,#113390,#113391,#113392,#113393,#113394,
#113395,#113396,#113397,#113398,#113399,#113400,#113401,#113402,#113403,
#113404,#113405,#113406,#113407,#113408,#113409,#113410,#113411,#113412,
#113413,#113414,#113415,#113416),.UNSPECIFIED.,.F.,.F.,(4,2,2,2,2,2,2,2,
2,2,2,2,2,2,2,2,2,2,2,2,2,2,2,2,2,2,2,2,2,2,2,2,2,2,2,2,2,2,2,2,2,2,2,2,
2,2,2,2,2,2,2,2,2,2,2,2,2,2,2,2,2,2,2,2,2,2,2,2,2,2,2,2,2,2,2,2,2,2,2,2,
2,2,2,2,2,2,2,2,2,2,2,2,2,2,2,2,2,2,4),(-2.09998383653095,-2.09276187432922,
-2.04931092824687,-2.03658895661001,-2.02889094500792,-2.02613933279381,
-2.02427283064363,-2.02254617878129,-2.01955204162526,-2.01060856563066,
-1.97753960942744,-1.96007063848493,-1.95226964552112,-1.94767579772682,
-1.94347840532854,-1.94025013518944,-1.93669198300295,-1.9307850344639,
-1.90594868743843,-1.8758586343696,-1.86736023334257,-1.86155808195318,
-1.8590879122204,-1.85726773514597,-1.85517795460678,-1.8514857180737,-1.82936862835452,
-1.82518912950081,-1.80300783675231,-1.79023437904749,-1.78103762161853,
-1.77683543925848,-1.77360656362741,-1.77005081890408,-1.76415518870671,
-1.73929248468774,-1.70920669243844,-1.70070885790683,-1.69490699728263,
-1.69243688480716,-1.69061673545728,-1.6885269901847,-1.6848347622449,-1.66270347852578,
-1.65853515017027,-1.63635304366883,-1.62358165866505,-1.61438602368991,
-1.61018409769296,-1.60695532093096,-1.60339958893912,-1.59750375582772,
-1.57263101302232,-1.54255420729113,-1.5340575657574,-1.52825632492363,
-1.52578634791339,-1.52396623991239,-1.52187646339001,-1.51818406568841,
-1.49600411278805,-1.49187417032022,-1.46968956732065,-1.45692526173437,
-1.44773331499792,-1.44353202078688,-1.44030331261454,-1.43674723900525,
-1.43084984323837,-1.40592346679972,-1.37589430228139,-1.36740369301914,
-1.36160543321638,-1.35913592714686,-1.35731582326821,-1.35522559545671,
-1.35153153995683,-1.3289102431425,-1.31198036598065,-1.29385744310058,
-1.28212104668599,-1.27751751088763,-1.27422548739567,-1.27122163501549,
-1.26715676047054,-1.25686043765124,-1.21606900355127,-1.20331764375839,
-1.19560775446792,-1.19285459455618,-1.19098783047074,-1.1890185731371,
-1.18578181812122,-1.174543811827,-1.14647477958792,-1.12759897919872,-1.11941581829126,
-1.11283811745965,-1.10919012835353),.UNSPECIFIED.);
#2826=B_SPLINE_CURVE_WITH_KNOTS('',3,(#113422,#113423,#113424,#113425,#113426,
#113427,#113428,#113429,#113430,#113431,#113432,#113433,#113434,#113435,
#113436,#113437,#113438,#113439,#113440,#113441),.UNSPECIFIED.,.F.,.F.,
(4,2,2,2,2,2,2,2,2,4),(-0.0593009426660634,-0.0417078351293523,-0.0297985383297815,
-0.0265125915388237,-0.0245388090859083,-0.0228313209054354,-0.020979224624226,
-0.0184296819045016,-0.0123504048007048,-0.000511197579002299),
 .UNSPECIFIED.);
#2827=B_SPLINE_CURVE_WITH_KNOTS('',3,(#113443,#113444,#113445,#113446,#113447,
#113448,#113449,#113450,#113451,#113452,#113453,#113454,#113455,#113456,
#113457,#113458,#113459,#113460,#113461,#113462,#113463,#113464,#113465,
#113466,#113467,#113468,#113469,#113470,#113471,#113472,#113473,#113474,
#113475,#113476,#113477,#113478,#113479,#113480,#113481,#113482,#113483,
#113484,#113485,#113486,#113487,#113488,#113489,#113490,#113491,#113492,
#113493,#113494,#113495,#113496,#113497,#113498,#113499,#113500,#113501,
#113502,#113503,#113504,#113505,#113506,#113507,#113508,#113509,#113510,
#113511,#113512,#113513,#113514,#113515,#113516,#113517,#113518,#113519,
#113520,#113521,#113522,#113523,#113524,#113525,#113526,#113527,#113528,
#113529,#113530,#113531,#113532,#113533,#113534,#113535,#113536,#113537,
#113538,#113539,#113540,#113541,#113542,#113543,#113544,#113545,#113546,
#113547,#113548,#113549,#113550,#113551),.UNSPECIFIED.,.F.,.F.,(4,3,3,3,
3,3,3,3,3,3,3,3,3,3,3,3,3,3,3,3,3,3,3,3,3,3,3,3,3,3,3,3,3,3,3,3,4),(-3.84638326322101,
-3.73817304815445,-3.63008307936253,-3.5220705202799,-3.41409265518859,
-3.30603153662545,-3.1979326333689,-3.08963571181038,-2.99264357503826,
-2.88276587336857,-2.77180710378402,-2.66222615391215,-2.55271033211294,
-2.44321911573495,-2.33118826597426,-2.22155434572583,-2.108325031209,-1.99509571669217,
-1.88634894910193,-1.77524881275745,-1.6668012593166,-1.55841692512387,
-1.45005363583211,-1.3369271914606,-1.22839986838443,-1.11978478227982,
-1.01096831546058,-0.997547858346086,-0.884786287810336,-0.772265546586226,
-0.659886764440191,-0.547616383400315,-0.435420994753685,-0.323232042127002,
-0.211056351513135,-0.0987924848427668,0.),.UNSPECIFIED.);
#2828=B_SPLINE_CURVE_WITH_KNOTS('',3,(#113554,#113555,#113556,#113557,#113558,
#113559,#113560,#113561,#113562,#113563,#113564,#113565,#113566,#113567,
#113568,#113569,#113570,#113571,#113572,#113573,#113574,#113575,#113576,
#113577,#113578,#113579,#113580,#113581,#113582,#113583,#113584,#113585,
#113586,#113587,#113588,#113589,#113590,#113591,#113592,#113593,#113594,
#113595,#113596,#113597,#113598,#113599,#113600,#113601,#113602,#113603,
#113604,#113605,#113606,#113607,#113608,#113609,#113610,#113611,#113612,
#113613,#113614,#113615,#113616,#113617,#113618,#113619,#113620,#113621,
#113622,#113623,#113624,#113625,#113626,#113627,#113628,#113629,#113630,
#113631,#113632,#113633,#113634,#113635,#113636,#113637,#113638,#113639,
#113640,#113641,#113642,#113643,#113644,#113645,#113646,#113647,#113648,
#113649,#113650,#113651,#113652,#113653,#113654,#113655,#113656,#113657,
#113658,#113659,#113660,#113661,#113662,#113663,#113664,#113665,#113666,
#113667,#113668,#113669,#113670,#113671,#113672,#113673,#113674,#113675,
#113676,#113677,#113678,#113679,#113680,#113681,#113682,#113683,#113684,
#113685,#113686,#113687,#113688,#113689,#113690,#113691,#113692,#113693,
#113694,#113695,#113696,#113697,#113698,#113699,#113700,#113701,#113702,
#113703,#113704,#113705,#113706,#113707,#113708,#113709,#113710,#113711,
#113712,#113713,#113714,#113715,#113716,#113717,#113718,#113719,#113720,
#113721,#113722,#113723,#113724,#113725,#113726,#113727),.UNSPECIFIED.,
 .F.,.F.,(4,2,2,2,2,2,2,2,2,2,2,2,2,2,2,2,2,2,2,2,2,2,2,2,2,2,2,2,2,2,2,
2,2,2,2,2,2,2,2,2,2,2,2,2,2,2,2,2,2,2,2,2,2,2,2,2,2,2,2,2,2,2,2,2,2,2,2,
2,2,2,2,2,2,2,2,2,2,2,2,2,2,2,2,2,2,2,4),(-1.97974873256733,-1.97958676484942,
-1.97600317519578,-1.94100267198266,-1.91218505529882,-1.90564031731873,
-1.9019167803576,-1.89866458475273,-1.8946035001476,-1.88819277658925,-1.84516230481906,
-1.8268530631516,-1.8222403185383,-1.81995237340242,-1.81811430865174,-1.81580717439324,
-1.8109982706693,-1.78203085302772,-1.74742922907714,-1.74088809205394,
-1.73718328526767,-1.73395784525245,-1.72994542773198,-1.72365032994016,
-1.67819898302672,-1.66000371616132,-1.65543013307975,-1.65317771385458,
-1.65137444696111,-1.64912511855927,-1.64451610078777,-1.61236237640466,
-1.58034694595528,-1.57386903681223,-1.57020392136783,-1.5670165564695,
-1.56305737434019,-1.55537141625159,-1.50598651336961,-1.49589568419349,
-1.48933969801489,-1.48676018964219,-1.48493100819737,-1.48290460177259,
-1.47940855239251,-1.46481199898505,-1.43463085145165,-1.41942457669491,
-1.40900371157641,-1.40459236030265,-1.40132744991803,-1.39784947166614,
-1.39234398857133,-1.37407308225253,-1.33797363397781,-1.32438480726431,
-1.32105986807721,-1.3190667047929,-1.31722705114186,-1.31496256381588,
-1.30937921898769,-1.27674225740609,-1.25095248133566,-1.24195152052659,
-1.23778188066505,-1.23455497790459,-1.23097808993293,-1.22499105122535,
-1.19589143082964,-1.1693394209813,-1.15744545711871,-1.15425398771316,
-1.15229412002961,-1.1504436913603,-1.14767706816644,-1.14044464862549,
-1.10927529676266,-1.08421404337261,-1.07522899956281,-1.07106527631507,
-1.06784257160284,-1.06427006922935,-1.058290027436,-1.02896945181402,-1.00698497526331,
-0.991250018193274,-0.991241672647406),.UNSPECIFIED.);
#2829=B_SPLINE_CURVE_WITH_KNOTS('',3,(#113733,#113734,#113735,#113736,#113737,
#113738,#113739,#113740,#113741,#113742,#113743,#113744,#113745,#113746,
#113747,#113748,#113749,#113750,#113751,#113752,#113753,#113754,#113755,
#113756,#113757,#113758,#113759,#113760,#113761,#113762,#113763,#113764,
#113765,#113766,#113767,#113768,#113769,#113770,#113771,#113772,#113773,
#113774,#113775,#113776,#113777,#113778,#113779,#113780,#113781,#113782,
#113783,#113784,#113785,#113786,#113787,#113788,#113789,#113790,#113791,
#113792,#113793,#113794,#113795,#113796,#113797,#113798,#113799,#113800,
#113801,#113802,#113803,#113804),.UNSPECIFIED.,.F.,.F.,(4,2,2,2,2,2,2,2,
2,2,2,2,2,2,2,2,2,2,2,2,2,2,2,2,2,2,2,2,2,2,2,2,2,2,2,4),(-0.358760731569834,
-0.357588714416537,-0.340406456573176,-0.336834571924863,-0.334774389493125,
-0.333018019472239,-0.330672679582775,-0.325139584554118,-0.317082275139463,
-0.290068178055794,-0.258861954651025,-0.252959280030101,-0.249499198163838,
-0.246422960364231,-0.242515505307593,-0.234373396072529,-0.201704582837242,
-0.174054602645336,-0.16974968847418,-0.167567493002712,-0.165748347082853,
-0.163743231260215,-0.160392353643154,-0.146811877258289,-0.113203671548509,
-0.086995627305843,-0.0805483037650247,-0.0766221547171091,-0.0730213521738901,
-0.0682621214379093,-0.0572868734598832,-0.0321802295361602,-0.00778597364073482,
-0.0034563959859211,-0.00158264500599872,-5.87679558657036E-5),
 .UNSPECIFIED.);
#2830=B_SPLINE_CURVE_WITH_KNOTS('',3,(#113807,#113808,#113809,#113810,#113811,
#113812,#113813,#113814,#113815,#113816,#113817,#113818,#113819,#113820,
#113821,#113822,#113823,#113824,#113825,#113826,#113827,#113828,#113829,
#113830,#113831,#113832,#113833,#113834,#113835,#113836,#113837,#113838,
#113839,#113840,#113841,#113842,#113843,#113844,#113845,#113846,#113847,
#113848,#113849,#113850,#113851,#113852,#113853,#113854,#113855,#113856,
#113857,#113858,#113859,#113860,#113861,#113862,#113863,#113864,#113865,
#113866,#113867,#113868,#113869,#113870,#113871,#113872,#113873,#113874,
#113875,#113876,#113877,#113878,#113879,#113880,#113881,#113882,#113883,
#113884,#113885,#113886,#113887,#113888,#113889,#113890,#113891,#113892,
#113893,#113894,#113895,#113896,#113897,#113898,#113899,#113900,#113901,
#113902,#113903,#113904,#113905,#113906,#113907,#113908,#113909,#113910,
#113911,#113912,#113913,#113914,#113915,#113916,#113917,#113918,#113919,
#113920,#113921,#113922,#113923,#113924,#113925,#113926),.UNSPECIFIED.,
 .F.,.F.,(4,2,2,2,2,2,2,2,2,2,2,2,2,2,2,2,2,2,2,2,2,2,2,2,2,2,2,2,2,2,2,
2,2,2,2,2,2,2,2,2,2,2,2,2,2,2,2,2,2,2,2,2,2,2,2,2,2,2,2,4),(-1.75478037324913,
-1.75157699880387,-1.72680890478214,-1.70436781523072,-1.69162498350517,
-1.68241391197646,-1.67818088615358,-1.67491705814343,-1.67131004331383,
-1.66529325591384,-1.63706718497493,-1.61632460687294,-1.60530876936184,
-1.59831925399475,-1.59563330166604,-1.59375272143998,-1.59171445466058,
-1.58821527004706,-1.57390064920759,-1.54363468613963,-1.52844718498748,
-1.51803625632712,-1.51361751510249,-1.51034227165868,-1.50684850913675,
-1.50130739417962,-1.4828116871778,-1.44660558241407,-1.43297165383395,
-1.4296425648391,-1.42764863798456,-1.42581830637429,-1.42314642011918,
-1.41647814742639,-1.38016276823827,-1.36286107158849,-1.35149411852575,
-1.34695871618315,-1.34369238877248,-1.34069673237757,-1.33583180407813,
-1.32310319370023,-1.28487643314327,-1.27240852083981,-1.26482026775864,
-1.26209371528085,-1.2602390155936,-1.25826751071241,-1.25502208329052,
-1.24369353186293,-1.21196073855142,-1.19542895810817,-1.1843900026814,
-1.17988418445069,-1.17660488891761,-1.17357302530719,-1.16859195814515,
-1.15515324807121,-1.12121414778627,-1.10916128661629),.UNSPECIFIED.);
#2831=B_SPLINE_CURVE_WITH_KNOTS('',3,(#113931,#113932,#113933,#113934,#113935,
#113936,#113937,#113938,#113939,#113940,#113941,#113942,#113943,#113944,
#113945,#113946,#113947,#113948,#113949,#113950,#113951,#113952,#113953,
#113954,#113955,#113956,#113957,#113958,#113959,#113960,#113961,#113962,
#113963,#113964,#113965,#113966,#113967,#113968,#113969,#113970,#113971,
#113972,#113973,#113974,#113975,#113976,#113977,#113978,#113979,#113980,
#113981,#113982,#113983,#113984,#113985,#113986,#113987,#113988,#113989,
#113990,#113991,#113992,#113993,#113994,#113995,#113996,#113997,#113998,
#113999,#114000,#114001,#114002,#114003,#114004,#114005,#114006,#114007,
#114008,#114009,#114010,#114011,#114012,#114013,#114014,#114015,#114016,
#114017,#114018,#114019,#114020,#114021,#114022,#114023,#114024,#114025,
#114026,#114027,#114028,#114029,#114030,#114031,#114032,#114033,#114034,
#114035,#114036,#114037,#114038,#114039,#114040,#114041,#114042,#114043,
#114044,#114045,#114046,#114047,#114048,#114049,#114050,#114051,#114052,
#114053,#114054,#114055,#114056,#114057,#114058,#114059,#114060,#114061,
#114062,#114063,#114064,#114065,#114066,#114067,#114068,#114069,#114070,
#114071,#114072,#114073,#114074,#114075,#114076,#114077,#114078,#114079,
#114080,#114081,#114082,#114083,#114084,#114085,#114086,#114087,#114088,
#114089,#114090,#114091,#114092,#114093,#114094,#114095,#114096,#114097,
#114098,#114099,#114100,#114101,#114102,#114103,#114104,#114105,#114106,
#114107,#114108,#114109,#114110,#114111,#114112,#114113,#114114,#114115,
#114116,#114117,#114118,#114119,#114120,#114121,#114122,#114123,#114124,
#114125,#114126,#114127,#114128,#114129,#114130,#114131,#114132,#114133,
#114134),.UNSPECIFIED.,.F.,.F.,(4,2,2,2,2,2,2,2,2,2,2,2,2,2,2,2,2,2,2,2,
2,2,2,2,2,2,2,2,2,2,2,2,2,2,2,2,2,2,2,2,2,2,2,2,2,2,2,2,2,2,2,2,2,2,2,2,
2,2,2,2,2,2,2,2,2,2,2,2,2,2,2,2,2,2,2,2,2,2,2,2,2,2,2,2,2,2,2,2,2,2,2,2,
2,2,2,2,2,2,2,2,2,4),(-1.40833512650497,-1.40069098176856,-1.38787474148805,
-1.36573398785996,-1.36142474486855,-1.33952291888054,-1.33583168467958,
-1.33374174701002,-1.33192195928846,-1.3294522385009,-1.32364851669501,
-1.31514499277648,-1.28502396579597,-1.26015341685752,-1.25425797890798,
-1.2507032120157,-1.24747582068171,-1.2432764626835,-1.23408973699226,-1.22133535388231,
-1.19916987032535,-1.19515532407055,-1.17287860500929,-1.1691874323788,
-1.16709828604177,-1.16527782164968,-1.16280676494455,-1.15700274439171,
-1.14850063352328,-1.11840425844881,-1.09350544645594,-1.08760505451081,
-1.08404663296064,-1.08081539307692,-1.07661012370494,-1.06740554943454,
-1.05461967175103,-1.03247886802765,-1.02833096610872,-1.00625015383823,
-1.002556444386,-1.00046480350253,-0.998639633790782,-0.996158960985884,
-0.990319553033095,-0.981749001120184,-0.951072859652514,-0.927051797544536,
-0.921182418045694,-0.917628104023132,-0.91439107207908,-0.910164325254045,
-0.900852081647703,-0.856495923805341,-0.839524843366962,-0.835941140859538,
-0.833875333054979,-0.832057501469606,-0.829560052009865,-0.82353535656955,
-0.814571150674254,-0.780470453505149,-0.759646769933166,-0.753989719912425,
-0.750496765690896,-0.747272530583065,-0.742999853831133,-0.733312013273571,
-0.719565278171568,-0.698733462106393,-0.695051892923753,-0.672835017627635,
-0.669152369497,-0.667069703583026,-0.665247106699071,-0.662770814571849,
-0.656963692222392,-0.648464165926929,-0.61847180994102,-0.593341832579235,
-0.587413589620244,-0.583837432304097,-0.580589073195544,-0.576359462345094,
-0.567087876225144,-0.554183574582817,-0.532300339159159,-0.528708008494463,
-0.506205857281313,-0.502493257712591,-0.500387207557482,-0.498530469081444,
-0.495988404157892,-0.489933486740911,-0.45408616114669,-0.428439332762879,
-0.422521926965401,-0.418935970626578,-0.415666728570026,-0.411391351813892,
-0.401935764996784,-0.358760731569834),.UNSPECIFIED.);
#2832=B_SPLINE_CURVE_WITH_KNOTS('',3,(#114135,#114136,#114137,#114138,#114139,
#114140,#114141,#114142,#114143,#114144,#114145,#114146,#114147,#114148,
#114149,#114150,#114151,#114152,#114153,#114154,#114155,#114156,#114157,
#114158,#114159,#114160,#114161,#114162,#114163,#114164,#114165,#114166,
#114167,#114168,#114169,#114170,#114171,#114172,#114173,#114174,#114175,
#114176,#114177,#114178,#114179,#114180,#114181,#114182,#114183,#114184,
#114185,#114186,#114187,#114188,#114189,#114190,#114191,#114192,#114193,
#114194,#114195,#114196,#114197,#114198,#114199,#114200,#114201,#114202,
#114203,#114204,#114205,#114206,#114207,#114208,#114209,#114210,#114211,
#114212,#114213,#114214,#114215,#114216,#114217,#114218,#114219,#114220,
#114221,#114222,#114223,#114224,#114225,#114226,#114227,#114228,#114229,
#114230,#114231,#114232,#114233,#114234,#114235,#114236,#114237,#114238,
#114239,#114240,#114241,#114242,#114243,#114244,#114245,#114246,#114247,
#114248,#114249,#114250,#114251,#114252,#114253,#114254,#114255,#114256,
#114257,#114258,#114259,#114260,#114261,#114262,#114263,#114264,#114265,
#114266,#114267,#114268,#114269,#114270,#114271,#114272,#114273,#114274,
#114275,#114276,#114277,#114278,#114279,#114280,#114281,#114282,#114283,
#114284,#114285,#114286,#114287,#114288,#114289,#114290,#114291,#114292,
#114293,#114294,#114295,#114296,#114297,#114298,#114299,#114300,#114301,
#114302,#114303,#114304,#114305,#114306,#114307,#114308,#114309,#114310,
#114311,#114312,#114313,#114314,#114315,#114316,#114317,#114318,#114319,
#114320,#114321,#114322,#114323,#114324,#114325,#114326,#114327,#114328,
#114329,#114330,#114331,#114332,#114333,#114334,#114335,#114336,#114337,
#114338,#114339,#114340,#114341,#114342,#114343,#114344,#114345,#114346,
#114347,#114348,#114349,#114350,#114351,#114352),.UNSPECIFIED.,.F.,.F.,
(4,2,2,2,2,2,2,2,2,2,2,2,2,2,2,2,2,2,2,2,2,2,2,2,2,2,2,2,2,2,2,2,2,2,2,
2,2,2,2,2,2,2,2,2,2,2,2,2,2,2,2,2,2,2,2,2,2,2,2,2,2,2,2,2,2,2,2,2,2,2,2,
2,2,2,2,2,2,2,2,2,2,2,2,2,2,2,2,2,2,2,2,2,2,2,2,2,2,2,2,2,2,2,2,2,2,2,2,
2,4),(-1.10916128661629,-1.1068588965783,-1.09852086339214,-1.09568326149892,
-1.09379611024995,-1.09208378124754,-1.08917097179547,-1.08088503629987,
-1.05059279909283,-1.02100922286385,-1.01506309006501,-1.01149527084022,
-1.00826692931509,-1.00415127566961,-0.995201602349336,-0.952436159590886,
-0.939454819477996,-0.931651380621814,-0.928885506458069,-0.927016041622359,
-0.925051224025353,-0.921832934565604,-0.910792820809623,-0.878916105003638,
-0.854168053021811,-0.848277080273857,-0.844723588494016,-0.841496478241594,
-0.837296265876073,-0.828102846067531,-0.81533632466192,-0.793159236903368,
-0.789112411061338,-0.76685967816142,-0.763168754363048,-0.761080091243742,
-0.759260204867692,-0.756790362652809,-0.750991517565072,-0.742499079037655,
-0.712471105207643,-0.68750691684465,-0.681606342784592,-0.678048810090404,
-0.674819040719495,-0.67061668530613,-0.66142315451214,-0.648657768073693,
-0.626502235929794,-0.622360398120677,-0.600235247130315,-0.596543063041667,
-0.594452738884643,-0.592631974565978,-0.590160416588509,-0.584351596258526,
-0.575839087038066,-0.54565089345244,-0.520879544049048,-0.514985742609532,
-0.511430149464382,-0.50820080629351,-0.503997126759067,-0.494793038202192,
-0.482007620330627,-0.459848371053637,-0.455649576826883,-0.433590902091073,
-0.429899478776002,-0.427809829004612,-0.425989620877812,-0.423519099229366,
-0.417714756101117,-0.409210824442457,-0.379088111536539,-0.354238613563417,
-0.348342834854102,-0.344787126252018,-0.341558371680152,-0.337356466024755,
-0.328160622381927,-0.31539037793302,-0.293226968063353,-0.289097820187359,
-0.266951706979895,-0.26326023877772,-0.261170691826645,-0.259350472016111,
-0.256879936560673,-0.251076035023471,-0.24257310800339,-0.212458684830971,
-0.187581296624008,-0.181695527966676,-0.178141746162406,-0.174912124997448,
-0.170705316048839,-0.161482509779152,-0.148660816668445,-0.126636332986425,
-0.122694017829648,-0.100322083409943,-0.0966296442692932,-0.0945397429891191,
-0.092719507624359,-0.0902491906182205,-0.0844464131731029,-0.0759456808677562,
-0.0594792545525924),.UNSPECIFIED.);
#2833=B_SPLINE_CURVE_WITH_KNOTS('',3,(#114357,#114358,#114359,#114360,#114361,
#114362,#114363,#114364,#114365,#114366,#114367,#114368,#114369,#114370,
#114371,#114372,#114373,#114374,#114375,#114376,#114377,#114378,#114379,
#114380,#114381,#114382,#114383,#114384,#114385,#114386,#114387,#114388,
#114389,#114390,#114391,#114392,#114393,#114394,#114395,#114396,#114397,
#114398,#114399,#114400,#114401,#114402,#114403,#114404,#114405,#114406,
#114407,#114408,#114409,#114410,#114411,#114412,#114413,#114414,#114415,
#114416,#114417,#114418,#114419,#114420,#114421,#114422,#114423,#114424,
#114425,#114426,#114427,#114428,#114429,#114430,#114431,#114432,#114433,
#114434,#114435,#114436,#114437,#114438,#114439,#114440,#114441,#114442,
#114443,#114444,#114445,#114446,#114447,#114448,#114449,#114450,#114451,
#114452,#114453,#114454,#114455,#114456,#114457,#114458,#114459,#114460,
#114461,#114462,#114463,#114464,#114465,#114466,#114467,#114468,#114469,
#114470,#114471,#114472,#114473,#114474,#114475,#114476,#114477,#114478,
#114479,#114480,#114481,#114482,#114483,#114484,#114485,#114486,#114487,
#114488,#114489,#114490,#114491,#114492,#114493,#114494,#114495,#114496,
#114497,#114498,#114499,#114500,#114501,#114502,#114503,#114504,#114505,
#114506,#114507,#114508,#114509,#114510,#114511,#114512,#114513,#114514,
#114515,#114516,#114517,#114518,#114519,#114520,#114521,#114522,#114523,
#114524,#114525,#114526,#114527,#114528,#114529,#114530,#114531,#114532,
#114533,#114534,#114535,#114536,#114537,#114538,#114539,#114540,#114541,
#114542,#114543,#114544,#114545,#114546,#114547,#114548,#114549,#114550,
#114551,#114552,#114553,#114554,#114555,#114556,#114557,#114558,#114559,
#114560,#114561,#114562,#114563,#114564,#114565,#114566,#114567,#114568,
#114569,#114570),.UNSPECIFIED.,.F.,.F.,(4,2,2,2,2,2,2,2,2,2,2,2,2,2,2,2,
2,2,2,2,2,2,2,2,2,2,2,2,2,2,2,2,2,2,2,2,2,2,2,2,2,2,2,2,2,2,2,2,2,2,2,2,
2,2,2,2,2,2,2,2,2,2,2,2,2,2,2,2,2,2,2,2,2,2,2,2,2,2,2,2,2,2,2,2,2,2,2,2,
2,2,2,2,2,2,2,2,2,2,2,2,2,2,2,2,2,2,4),(-2.45793897795708,-2.45615588549777,
-2.43177484350015,-2.422770787873,-2.41860144465758,-2.41537554387078,-2.4118005758735,
-2.40581874108697,-2.3757599172176,-2.35166693513045,-2.34279824546252,
-2.33681354770945,-2.33431273065983,-2.33248795396218,-2.33041355500885,
-2.32679191692295,-2.30813529131414,-2.26748366486948,-2.25705557726181,
-2.25297054985888,-2.24996125765374,-2.24667237344482,-2.24209027298485,
-2.23050772719489,-2.21274425295155,-2.17924202763386,-2.17105341531066,
-2.16815489995836,-2.16644635967471,-2.164562085245,-2.16172271163067,-2.15333558004233,
-2.13884522533033,-2.10449960657346,-2.09134549528806,-2.08640611142508,
-2.08338484027012,-2.08010577929559,-2.07557986682592,-2.06438030184675,
-2.0474837375862,-2.0152778102446,-2.00492997510858,-2.00177688807338,-1.99982539359666,
-1.99794570017531,-1.9951292220909,-1.98692889493808,-1.97293182164206,
-1.95227316982027,-1.92671054005153,-1.92079468807121,-1.91723381909934,
-1.91400471938894,-1.9098085300844,-1.90065100469766,-1.88795498508286,
-1.86517631931624,-1.86233811018274,-1.8393949897911,-1.83569957863761,
-1.83360867524846,-1.83178810163029,-1.8293179304999,-1.82351788735836,
-1.81502314868086,-1.78497591757588,-1.76004335518708,-1.7541442494569,
-1.75058722713463,-1.74735768969231,-1.74315531823811,-1.73396055598287,
-1.72119305852158,-1.69903174454589,-1.69491721654909,-1.6727573919502,
-1.66906533783053,-1.66697531287706,-1.6651545875148,-1.662683134092,-1.65687582763822,
-1.64836658292982,-1.6182055819652,-1.59340262799116,-1.58750704379221,
-1.58395055907596,-1.58072049703089,-1.57651597597271,-1.56731015486083,
-1.55452164405268,-1.53237067567287,-1.52816814108077,-1.50612815974973,
-1.50243625349907,-1.50034606538026,-1.49852471174085,-1.49605182893906,
-1.49023903029735,-1.48171913363843,-1.45146950699641,-1.42679775646766,
-1.42090631466174,-1.41735031433094,-1.41411938081594,-1.40991180845125,
-1.40833512650497),.UNSPECIFIED.);
#2834=B_SPLINE_CURVE_WITH_KNOTS('',3,(#114572,#114573,#114574,#114575,#114576,
#114577,#114578,#114579,#114580,#114581,#114582,#114583,#114584,#114585,
#114586,#114587),.UNSPECIFIED.,.F.,.F.,(4,2,2,2,2,2,2,4),(-0.0594792545525924,
-0.0341344864849067,-0.019390033663532,-0.0142709737956861,-0.010878840635614,
-0.00783988566160054,-0.00425775618985681,-0.000493435409444853),
 .UNSPECIFIED.);
#2835=B_SPLINE_CURVE_WITH_KNOTS('',3,(#114588,#114589,#114590,#114591,#114592,
#114593,#114594,#114595,#114596,#114597,#114598,#114599,#114600,#114601,
#114602,#114603,#114604,#114605,#114606,#114607,#114608,#114609,#114610,
#114611,#114612,#114613,#114614,#114615,#114616,#114617,#114618,#114619,
#114620,#114621,#114622,#114623,#114624,#114625,#114626,#114627,#114628,
#114629,#114630,#114631,#114632,#114633,#114634,#114635,#114636,#114637,
#114638,#114639,#114640,#114641,#114642,#114643,#114644,#114645,#114646,
#114647,#114648,#114649,#114650,#114651,#114652,#114653,#114654,#114655,
#114656,#114657,#114658,#114659,#114660,#114661,#114662,#114663,#114664,
#114665,#114666,#114667,#114668,#114669,#114670,#114671,#114672,#114673,
#114674,#114675,#114676,#114677,#114678,#114679,#114680,#114681,#114682,
#114683,#114684,#114685,#114686,#114687,#114688,#114689,#114690,#114691,
#114692,#114693,#114694,#114695,#114696,#114697,#114698,#114699,#114700,
#114701,#114702,#114703,#114704,#114705,#114706,#114707,#114708,#114709,
#114710,#114711,#114712,#114713,#114714,#114715,#114716,#114717,#114718,
#114719,#114720,#114721,#114722,#114723,#114724,#114725,#114726,#114727,
#114728,#114729,#114730,#114731,#114732,#114733,#114734,#114735,#114736,
#114737,#114738,#114739,#114740,#114741,#114742,#114743,#114744,#114745,
#114746,#114747,#114748,#114749,#114750,#114751,#114752,#114753,#114754,
#114755,#114756,#114757,#114758,#114759,#114760,#114761,#114762,#114763,
#114764,#114765,#114766,#114767,#114768,#114769,#114770,#114771,#114772,
#114773,#114774,#114775,#114776,#114777),.UNSPECIFIED.,.F.,.F.,(4,2,2,2,
2,2,2,2,2,2,2,2,2,2,2,2,2,2,2,2,2,2,2,2,2,2,2,2,2,2,2,2,2,2,2,2,2,2,2,2,
2,2,2,2,2,2,2,2,2,2,2,2,2,2,2,2,2,2,2,2,2,2,2,2,2,2,2,2,2,2,2,2,2,2,2,2,
2,2,2,2,2,2,2,2,2,2,2,2,2,2,2,2,2,2,4),(-2.09963543973955,-2.09246016825572,
-2.05214587400277,-2.03411221550204,-2.0295640431354,-2.02732018798611,
-2.02551524420154,-2.02325158294973,-2.01860131270733,-1.98705841801055,
-1.9541653926891,-1.94958605950917,-1.94539874969976,-1.94217144551413,
-1.93860753350505,-1.93267464846004,-1.90794177813569,-1.87780813839569,
-1.86930410252211,-1.86349904491058,-1.86102823590822,-1.85920781240094,
-1.85711798013648,-1.85342612918277,-1.83147633674116,-1.8010425187358,
-1.78514656111749,-1.78003536689141,-1.77664449778827,-1.77338010703456,
-1.76874907804524,-1.75760008563841,-1.71777425874744,-1.70513848736707,
-1.6974754699745,-1.69472835409607,-1.6928626086916,-1.69089090727048,-1.68764412572019,
-1.6762975315996,-1.64458222116772,-1.62808152417664,-1.6205551223639,-1.61438996085163,
-1.61077684469602,-1.60755984276245,-1.60346196095107,-1.59683205799805,
-1.56331925309136,-1.54207957645314,-1.53494210168959,-1.52983971505768,
-1.52749139392588,-1.52585506336916,-1.52375922601036,-1.52004037660899,
-1.4954233957183,-1.49447237304159,-1.47404277590453,-1.4598737595407,-1.4499648701824,
-1.44564178967674,-1.44239598064091,-1.43889483500637,-1.43325706269018,
-1.41312913216072,-1.37865819240984,-1.36965775011106,-1.36360937822551,
-1.36109867339561,-1.35927297595365,-1.35720482846713,-1.35360935419312,
-1.33576538698223,-1.30453320706305,-1.2919951550504,-1.28292211503648,
-1.27874144678629,-1.27551509896906,-1.2719480514783,-1.26599986233491,
-1.23868978064015,-1.21068491649701,-1.19848378036798,-1.195268059158,-1.19330318875485,
-1.19145535674275,-1.18914899894471,-1.18330057417155,-1.15091055774667,
-1.12524857048015,-1.11623326674394,-1.11206281319984,-1.10883774977028,
-1.10881952756263),.UNSPECIFIED.);
#2836=B_SPLINE_CURVE_WITH_KNOTS('',3,(#114782,#114783,#114784,#114785,#114786,
#114787,#114788,#114789,#114790,#114791,#114792,#114793,#114794,#114795,
#114796,#114797,#114798,#114799,#114800,#114801,#114802,#114803,#114804,
#114805,#114806,#114807,#114808,#114809,#114810,#114811,#114812,#114813,
#114814,#114815,#114816,#114817,#114818,#114819,#114820,#114821,#114822,
#114823,#114824,#114825,#114826,#114827,#114828,#114829,#114830,#114831,
#114832,#114833,#114834,#114835,#114836,#114837,#114838,#114839,#114840,
#114841,#114842,#114843,#114844,#114845,#114846,#114847,#114848,#114849,
#114850,#114851,#114852,#114853,#114854,#114855,#114856,#114857,#114858,
#114859,#114860,#114861,#114862,#114863,#114864,#114865,#114866,#114867,
#114868,#114869,#114870,#114871,#114872,#114873,#114874,#114875,#114876,
#114877,#114878,#114879,#114880,#114881,#114882,#114883,#114884,#114885,
#114886,#114887,#114888,#114889,#114890,#114891,#114892,#114893,#114894,
#114895,#114896,#114897,#114898,#114899,#114900,#114901,#114902,#114903,
#114904,#114905,#114906,#114907,#114908,#114909,#114910,#114911,#114912,
#114913,#114914,#114915,#114916,#114917,#114918,#114919,#114920,#114921,
#114922,#114923,#114924,#114925,#114926,#114927,#114928,#114929,#114930,
#114931,#114932,#114933,#114934,#114935,#114936,#114937,#114938,#114939,
#114940,#114941,#114942,#114943,#114944,#114945,#114946,#114947,#114948,
#114949,#114950,#114951,#114952,#114953,#114954,#114955,#114956,#114957,
#114958,#114959,#114960,#114961,#114962,#114963,#114964,#114965,#114966,
#114967,#114968,#114969,#114970,#114971,#114972,#114973,#114974,#114975,
#114976,#114977,#114978,#114979,#114980,#114981),.UNSPECIFIED.,.F.,.F.,
(4,2,2,2,2,2,2,2,2,2,2,2,2,2,2,2,2,2,2,2,2,2,2,2,2,2,2,2,2,2,2,2,2,2,2,
2,2,2,2,2,2,2,2,2,2,2,2,2,2,2,2,2,2,2,2,2,2,2,2,2,2,2,2,2,2,2,2,2,2,2,2,
2,2,2,2,2,2,2,2,2,2,2,2,2,2,2,2,2,2,2,2,2,2,2,2,2,2,2,2,4),(-3.50773961833004,
-3.50421851324702,-3.50140422409568,-3.49952512581685,-3.49781174931706,
-3.49488732096498,-3.48650041962016,-3.45309269569678,-3.43540885820288,
-3.42754817280637,-3.42117159836907,-3.41751368105993,-3.41430296631894,
-3.4102749156194,-3.4038866306081,-3.359189777365,-3.34075014175589,-3.33615510086918,
-3.33390199359663,-3.33209689304258,-3.32984205206654,-3.32523807673874,
-3.2929181834735,-3.2610020422903,-3.25454568610755,-3.25087097401481,-3.24766212901855,
-3.24365828861399,-3.23735299799631,-3.19867971531989,-3.1734976500103,
-3.16926497027186,-3.1670837683819,-3.16527607312614,-3.16294044288485,
-3.1580857852602,-3.13510956096479,-3.1077653779617,-3.091761871451,-3.08663914360522,
-3.08324551126884,-3.07998200934138,-3.07535831287171,-3.06426076892656,
-3.02795873720578,-3.01292965956498,-3.00434285530471,-3.00147959659049,
-2.99959045940212,-2.9976518215459,-2.99455738830669,-2.98475461330809,
-2.95564198409292,-2.93634341310926,-2.92411398166636,-2.91944073329676,
-2.91613541498287,-2.9131437018507,-2.90913185905408,-2.89916841868622,
-2.85339010162891,-2.84349418300337,-2.83702142701227,-2.83444358813303,
-2.83260750499024,-2.83057082863891,-2.82702687572773,-2.81144639395432,
-2.7817423009744,-2.76692582871821,-2.75669858123361,-2.75232310330469,
-2.74906874623193,-2.74558729376446,-2.74004489986829,-2.72107097154034,
-2.67738520586696,-2.67049253016324,-2.6678519606445,-2.66600540600267,
-2.66399501833808,-2.66057239144719,-2.64708876071342,-2.62062747577998,
-2.60239359734701,-2.59438178236599,-2.58791028038803,-2.58423206844143,
-2.58102308927683,-2.57702290942623,-2.57073114778078,-2.52555606454651,
-2.51212497284043,-2.50414335298965,-2.50135431986496,-2.49947999037183,
-2.49776079997681,-2.49480737267149,-2.4861971077323,-2.45793897795708),
 .UNSPECIFIED.);
#2837=B_SPLINE_CURVE_WITH_KNOTS('',3,(#114982,#114983,#114984,#114985,#114986,
#114987,#114988,#114989,#114990,#114991,#114992,#114993,#114994,#114995,
#114996,#114997,#114998,#114999,#115000,#115001,#115002,#115003,#115004,
#115005,#115006,#115007,#115008,#115009,#115010,#115011,#115012,#115013,
#115014,#115015,#115016,#115017,#115018,#115019,#115020,#115021,#115022,
#115023,#115024,#115025,#115026,#115027,#115028,#115029,#115030,#115031,
#115032,#115033,#115034,#115035,#115036,#115037,#115038,#115039,#115040,
#115041,#115042,#115043,#115044,#115045,#115046,#115047,#115048,#115049,
#115050,#115051,#115052,#115053,#115054,#115055,#115056,#115057,#115058,
#115059,#115060,#115061,#115062,#115063,#115064,#115065,#115066,#115067,
#115068,#115069,#115070,#115071,#115072,#115073,#115074,#115075,#115076,
#115077,#115078,#115079,#115080,#115081,#115082,#115083,#115084,#115085,
#115086,#115087,#115088,#115089,#115090,#115091,#115092,#115093,#115094,
#115095,#115096,#115097,#115098,#115099,#115100,#115101,#115102,#115103,
#115104,#115105,#115106,#115107,#115108,#115109,#115110,#115111,#115112,
#115113,#115114,#115115,#115116,#115117,#115118,#115119,#115120,#115121,
#115122,#115123,#115124,#115125,#115126,#115127,#115128,#115129,#115130,
#115131,#115132,#115133,#115134,#115135,#115136,#115137,#115138,#115139,
#115140,#115141,#115142,#115143,#115144,#115145,#115146,#115147,#115148,
#115149,#115150,#115151,#115152,#115153,#115154,#115155,#115156,#115157,
#115158,#115159,#115160,#115161,#115162,#115163,#115164,#115165,#115166,
#115167,#115168,#115169,#115170,#115171,#115172,#115173,#115174,#115175,
#115176,#115177,#115178,#115179,#115180,#115181,#115182,#115183,#115184,
#115185,#115186,#115187,#115188,#115189),.UNSPECIFIED.,.F.,.F.,(4,2,2,2,
2,2,2,2,2,2,2,2,2,2,2,2,2,2,2,2,2,2,2,2,2,2,2,2,2,2,2,2,2,2,2,2,2,2,2,2,
2,2,2,2,2,2,2,2,2,2,2,2,2,2,2,2,2,2,2,2,2,2,2,2,2,2,2,2,2,2,2,2,2,2,2,2,
2,2,2,2,2,2,2,2,2,2,2,2,2,2,2,2,2,2,2,2,2,2,2,2,2,2,2,4),(-1.10881952756263,
-1.10526545399088,-1.09929239582824,-1.07124087827899,-1.04978109997219,
-1.03261241192772,-1.02901764768895,-1.02694969915861,-1.02512405626675,
-1.02261320002931,-1.01656362981476,-1.00755951542083,-0.973073045011544,
-0.952932463075774,-0.94729379316776,-0.943792579956133,-0.940547045415271,
-0.936224833044692,-0.926320057601762,-0.912160792999993,-0.891744393308104,
-0.890671867433004,-0.866186808478679,-0.862471651204054,-0.860376723898788,
-0.858557632186536,-0.856096284592217,-0.850347086728083,-0.841953994196577,
-0.812692423777212,-0.786843576578137,-0.780922568284288,-0.777361404005235,
-0.774133838775332,-0.769942259306126,-0.760806110455771,-0.748149656686722,
-0.725522705128143,-0.721448598660605,-0.6995123715649,-0.695821670641751,
-0.693732235042527,-0.691911994143761,-0.689441167079172,-0.683635108764058,
-0.675127699342708,-0.644976234310481,-0.620163851146711,-0.614269224860633,
-0.610713712917142,-0.607484813396225,-0.603282244222032,-0.59408284925815,
-0.581305735078787,-0.559147509791194,-0.554976486444893,-0.532885759700978,
-0.529194545150015,-0.52710502090039,-0.52528484718224,-0.52281430474735,
-0.517009767680641,-0.50850535761216,-0.478376903370673,-0.453539325064248,
-0.447644039466366,-0.444088434989167,-0.440859644516826,-0.43665749441707,
-0.427460197067178,-0.414686990999679,-0.392527839470723,-0.38837380375174,
-0.366261674775286,-0.362570454821976,-0.360480955412108,-0.358660823271831,
-0.356190363955751,-0.350386139688619,-0.34188229407636,-0.311757544241278,
-0.286916937434843,-0.281021666409002,-0.277466112498312,-0.274237394376277,
-0.270035376372078,-0.260838529656829,-0.248066085519974,-0.225907205357697,
-0.201545621156838,-0.196696607247021,-0.194362544109177,-0.192555507068455,
-0.190374523689871,-0.186140743347986,-0.160758199549301,-0.12229858435053,
-0.11596928382334,-0.111959169966519,-0.108750866326691,-0.10508285304095,
-0.0986545714332097,-0.0777366651724035,-0.0592697367048556),
 .UNSPECIFIED.);
#2838=B_SPLINE_CURVE_WITH_KNOTS('',3,(#115194,#115195,#115196,#115197,#115198,
#115199,#115200,#115201,#115202,#115203,#115204,#115205,#115206,#115207,
#115208,#115209,#115210,#115211,#115212,#115213,#115214,#115215,#115216,
#115217,#115218,#115219,#115220,#115221,#115222,#115223,#115224,#115225,
#115226,#115227,#115228,#115229,#115230,#115231,#115232,#115233,#115234,
#115235,#115236,#115237,#115238,#115239,#115240,#115241,#115242,#115243,
#115244,#115245,#115246,#115247,#115248,#115249,#115250,#115251,#115252,
#115253,#115254,#115255,#115256,#115257,#115258,#115259,#115260,#115261,
#115262,#115263,#115264,#115265,#115266,#115267,#115268,#115269,#115270,
#115271,#115272,#115273,#115274,#115275,#115276,#115277,#115278,#115279,
#115280,#115281,#115282,#115283,#115284,#115285,#115286,#115287,#115288,
#115289,#115290,#115291,#115292,#115293,#115294,#115295,#115296,#115297,
#115298,#115299,#115300,#115301,#115302,#115303,#115304,#115305,#115306,
#115307,#115308,#115309,#115310,#115311,#115312,#115313,#115314,#115315,
#115316,#115317,#115318,#115319,#115320,#115321,#115322,#115323,#115324,
#115325,#115326,#115327,#115328,#115329,#115330,#115331,#115332,#115333,
#115334,#115335,#115336,#115337,#115338,#115339,#115340,#115341,#115342,
#115343,#115344,#115345,#115346,#115347,#115348,#115349,#115350,#115351,
#115352,#115353,#115354,#115355,#115356,#115357,#115358,#115359,#115360,
#115361,#115362,#115363,#115364,#115365,#115366,#115367,#115368,#115369,
#115370,#115371,#115372,#115373,#115374,#115375,#115376,#115377,#115378,
#115379,#115380,#115381,#115382,#115383,#115384,#115385,#115386,#115387,
#115388,#115389,#115390,#115391,#115392,#115393,#115394,#115395,#115396,
#115397),.UNSPECIFIED.,.F.,.F.,(4,2,2,2,2,2,2,2,2,2,2,2,2,2,2,2,2,2,2,2,
2,2,2,2,2,2,2,2,2,2,2,2,2,2,2,2,2,2,2,2,2,2,2,2,2,2,2,2,2,2,2,2,2,2,2,2,
2,2,2,2,2,2,2,2,2,2,2,2,2,2,2,2,2,2,2,2,2,2,2,2,2,2,2,2,2,2,2,2,2,2,2,2,
2,2,2,2,2,2,2,2,2,4),(-4.55723119340549,-4.53542832434012,-4.50896448142615,
-4.50315716589731,-4.50068590262253,-4.49886532687413,-4.49677546896773,
-4.49308377390169,-4.47111463237268,-4.46705960011841,-4.44470686225495,
-4.43188840544058,-4.4226680833791,-4.41846141968583,-4.41523151747225,
-4.41167701522777,-4.40578897923254,-4.38104299002909,-4.35086699346539,
-4.34235836236679,-4.33655110072032,-4.33407985738933,-4.33225929516264,
-4.33016945141772,-4.3264777784293,-4.30450751493001,-4.30023042820911,
-4.27806833262354,-4.26526862974408,-4.25605812824239,-4.2518531905726,
-4.24862352737678,-4.24506820457166,-4.23917623405573,-4.21443515666992,
-4.18426169514232,-4.17575341482362,-4.16994633799681,-4.1674751356603,
-4.16565458884208,-4.16356474556491,-4.15987303635166,-4.13788669860107,
-4.13362061826904,-4.11145693602026,-4.09866131259351,-4.08945296167763,
-4.08524841607183,-4.08201882134212,-4.07846334174193,-4.07257055938531,
-4.04780211202449,-4.01765287466579,-4.00914767472118,-4.00334213740832,
-4.00087120183978,-3.9990506989405,-3.99696072838722,-3.99326841192948,
-3.9711107381612,-3.96730661424229,-3.94463125680002,-3.93196069340678,
-3.92281792141579,-3.91862484134117,-3.915396720625,-3.91183552108742,-3.90591572765924,
-3.88008502814496,-3.85084962367526,-3.84246186834696,-3.83671480575467,
-3.83425366226978,-3.83243438760605,-3.83033883582133,-3.82662150615858,
-3.8020569584203,-3.78411049970614,-3.76786872080134,-3.76041756915105,
-3.75430035560356,-3.75069728500477,-3.74747826158471,-3.74336264926896,
-3.73667133881025,-3.69189773896525,-3.67399856592375,-3.66946614775791,
-3.66722531440779,-3.66542023230273,-3.66315309239069,-3.65848508199062,
-3.6273443310578,-3.59394615017214,-3.58771472518229,-3.58408743406314,
-3.58087247761976,-3.57679712967696,-3.57024583531637,-3.52635959716301,
-3.51240340853765,-3.50773961833004),.UNSPECIFIED.);
#2839=B_SPLINE_CURVE_WITH_KNOTS('',3,(#115399,#115400,#115401,#115402,#115403,
#115404,#115405,#115406,#115407,#115408,#115409,#115410,#115411,#115412,
#115413,#115414,#115415,#115416,#115417,#115418),.UNSPECIFIED.,.F.,.F.,
(4,2,2,2,2,2,2,2,2,4),(-0.0592697367048556,-0.0463583666809266,-0.0324747160269597,
-0.0290285262924044,-0.027013615035921,-0.0251703567530109,-0.0233117892002817,
-0.0207389877446909,-0.0142408263042859,-0.000491288661123149),
 .UNSPECIFIED.);
#2840=B_SPLINE_CURVE_WITH_KNOTS('',3,(#115419,#115420,#115421,#115422,#115423,
#115424,#115425,#115426,#115427,#115428,#115429,#115430,#115431,#115432,
#115433,#115434,#115435,#115436,#115437,#115438,#115439,#115440,#115441,
#115442,#115443,#115444,#115445,#115446,#115447,#115448,#115449,#115450,
#115451,#115452,#115453,#115454,#115455,#115456,#115457,#115458,#115459,
#115460,#115461,#115462,#115463,#115464,#115465,#115466,#115467,#115468,
#115469,#115470,#115471,#115472,#115473,#115474,#115475,#115476,#115477,
#115478,#115479,#115480,#115481,#115482,#115483,#115484,#115485,#115486,
#115487,#115488,#115489,#115490,#115491,#115492,#115493,#115494,#115495,
#115496,#115497,#115498,#115499,#115500,#115501,#115502,#115503,#115504,
#115505,#115506,#115507,#115508,#115509,#115510,#115511,#115512,#115513,
#115514,#115515,#115516,#115517,#115518,#115519,#115520,#115521,#115522,
#115523,#115524,#115525,#115526,#115527,#115528,#115529,#115530,#115531,
#115532,#115533,#115534,#115535,#115536,#115537,#115538,#115539,#115540,
#115541,#115542,#115543,#115544,#115545,#115546,#115547,#115548,#115549,
#115550,#115551,#115552,#115553,#115554,#115555,#115556,#115557,#115558,
#115559,#115560,#115561,#115562,#115563,#115564,#115565,#115566,#115567,
#115568,#115569,#115570,#115571,#115572,#115573,#115574,#115575,#115576,
#115577,#115578,#115579,#115580,#115581,#115582,#115583,#115584,#115585,
#115586,#115587,#115588,#115589,#115590,#115591,#115592,#115593,#115594,
#115595,#115596,#115597,#115598,#115599,#115600,#115601,#115602,#115603,
#115604,#115605,#115606,#115607,#115608,#115609,#115610,#115611,#115612,
#115613,#115614,#115615,#115616,#115617,#115618,#115619,#115620,#115621,
#115622,#115623,#115624,#115625,#115626,#115627,#115628,#115629,#115630,
#115631,#115632,#115633,#115634,#115635,#115636,#115637,#115638,#115639,
#115640,#115641,#115642,#115643,#115644,#115645,#115646,#115647,#115648,
#115649,#115650,#115651,#115652,#115653,#115654,#115655,#115656,#115657,
#115658,#115659,#115660,#115661,#115662,#115663,#115664,#115665,#115666,
#115667,#115668,#115669,#115670,#115671,#115672,#115673,#115674,#115675,
#115676,#115677,#115678),.UNSPECIFIED.,.F.,.F.,(4,2,2,2,2,2,2,2,2,2,2,2,
2,2,2,2,2,2,2,2,2,2,2,2,2,2,2,2,2,2,2,2,2,2,2,2,2,2,2,2,2,2,2,2,2,2,2,2,
2,2,2,2,2,2,2,2,2,2,2,2,2,2,2,2,2,2,2,2,2,2,2,2,2,2,2,2,2,2,2,2,2,2,2,2,
2,2,2,2,2,2,2,2,2,2,2,2,2,2,2,2,2,2,2,2,2,2,2,2,2,2,2,2,2,2,2,2,2,2,2,2,
2,2,2,2,2,2,2,2,2,4),(-2.09994048470851,-2.05894043935947,-2.04944988533331,
-2.04519702509862,-2.04196135890193,-2.03842975304143,-2.03264804227002,
-2.01025775568754,-1.97799440335339,-1.9691977268642,-1.96333889887151,
-1.96096338195135,-1.9609466439916,-1.96092957897279,-1.96091216966876,
-1.96089439783931,-1.96087624407058,-1.9608576877646,-1.96083870708189,
-1.96081927849993,-1.96079937700362,-1.9607789758323,-1.96075804639954,
-1.96073655794338,-1.96071447746922,-1.96069176947358,-1.96066839572713,
-1.96064431499208,-1.96061948256786,-1.96059385023083,-1.96056736555582,
-1.96053997163244,-1.96051160648292,-1.96048220244113,-1.96045168554925,
-1.96041997482767,-1.96038698133963,-1.96035260718332,-1.96031674436325,
-1.96027927338378,-1.96024006176422,-1.96019896214376,-1.95839169712927,
-1.95605694997279,-1.95120528464012,-1.92683135224008,-1.90465539517672,
-1.89187364807633,-1.88267253745642,-1.87846948558848,-1.87524036669506,
-1.87168476754328,-1.86579033211436,-1.84096818824147,-1.81085229888347,
-1.8023508250377,-1.79654714241649,-1.79407665569003,-1.79225637149713,
-1.79016659264472,-1.78647457203492,-1.76441056172453,-1.76019334415021,
-1.73801755634917,-1.72523586766422,-1.71603480541696,-1.71183178040185,
-1.70860268401789,-1.70504711152692,-1.69915272475734,-1.67433098467606,
-1.64421511017746,-1.6357136715291,-1.62991001760038,-1.62743954630897,
-1.62561927475397,-1.62352951188227,-1.61983752268174,-1.59777509026306,
-1.59355683706387,-1.57138130495276,-1.5585994458685,-1.54939831224275,
-1.54519529321184,-1.5419662166612,-1.53841068121885,-1.53251639205084,
-1.50769667405415,-1.47757940530244,-1.46907782412491,-1.46327411065517,
-1.46080364008518,-1.45898337930664,-1.45689364073358,-1.45320172013757,
-1.43115092236588,-1.42692413980631,-1.40474958360488,-1.39196566997983,
-1.3827634789852,-1.37856029415126,-1.37533121543923,-1.37177580261758,
-1.36588201407026,-1.34107759647615,-1.31094736749012,-1.30244418553558,
-1.29663968862182,-1.29416909808649,-1.29234883283046,-1.29025918681035,
-1.28656764000556,-1.2646097013561,-1.26053672195974,-1.23789810131862,
-1.22523632756718,-1.21609820982578,-1.21190623038655,-1.20867858948283,
-1.2051175777133,-1.19919735541953,-1.17334413446036,-1.14411561858126,
-1.13572841400601,-1.12998166527577,-1.12752074458941,-1.12570169168781,
-1.12360653326024,-1.11989028656003,-1.10911089706055),.UNSPECIFIED.);
#2841=B_SPLINE_CURVE_WITH_KNOTS('',3,(#115684,#115685,#115686,#115687,#115688,
#115689,#115690,#115691,#115692,#115693,#115694,#115695,#115696,#115697,
#115698,#115699,#115700,#115701,#115702,#115703,#115704,#115705,#115706,
#115707,#115708,#115709,#115710,#115711,#115712,#115713,#115714,#115715,
#115716,#115717,#115718,#115719,#115720,#115721,#115722,#115723,#115724,
#115725,#115726,#115727,#115728,#115729,#115730,#115731,#115732,#115733,
#115734,#115735,#115736,#115737,#115738,#115739,#115740,#115741,#115742,
#115743,#115744,#115745,#115746,#115747,#115748,#115749,#115750,#115751,
#115752,#115753,#115754,#115755,#115756,#115757,#115758,#115759,#115760,
#115761,#115762,#115763,#115764,#115765,#115766,#115767,#115768,#115769,
#115770,#115771,#115772,#115773,#115774,#115775,#115776,#115777,#115778,
#115779,#115780,#115781,#115782,#115783,#115784,#115785,#115786,#115787,
#115788,#115789,#115790,#115791,#115792,#115793,#115794,#115795,#115796,
#115797,#115798,#115799,#115800,#115801,#115802,#115803,#115804,#115805,
#115806,#115807,#115808,#115809,#115810,#115811,#115812,#115813,#115814,
#115815,#115816,#115817,#115818,#115819,#115820,#115821,#115822,#115823,
#115824,#115825,#115826,#115827,#115828,#115829,#115830,#115831,#115832,
#115833,#115834,#115835,#115836,#115837,#115838,#115839,#115840,#115841,
#115842,#115843,#115844,#115845,#115846,#115847,#115848,#115849,#115850,
#115851,#115852,#115853,#115854,#115855,#115856,#115857,#115858,#115859,
#115860,#115861,#115862,#115863,#115864,#115865,#115866,#115867,#115868,
#115869,#115870,#115871,#115872,#115873,#115874,#115875,#115876,#115877,
#115878,#115879,#115880,#115881,#115882,#115883,#115884,#115885,#115886,
#115887,#115888,#115889),.UNSPECIFIED.,.F.,.F.,(4,2,2,2,2,2,2,2,2,2,2,2,
2,2,2,2,2,2,2,2,2,2,2,2,2,2,2,2,2,2,2,2,2,2,2,2,2,2,2,2,2,2,2,2,2,2,2,2,
2,2,2,2,2,2,2,2,2,2,2,2,2,2,2,2,2,2,2,2,2,2,2,2,2,2,2,2,2,2,2,2,2,2,2,2,
2,2,2,2,2,2,2,2,2,2,2,2,2,2,2,2,2,2,4),(-0.991117350869854,-0.97984114832981,
-0.97315088018324,-0.969034875902649,-0.965814913416383,-0.96221013912214,
-0.956088364065775,-0.922212018621459,-0.89139638286004,-0.886705650402648,
-0.884433775824448,-0.882628151356282,-0.880390653797248,-0.875877129508642,
-0.869813159247332,-0.853790017647763,-0.813718357180651,-0.806027118561792,
-0.802052141548575,-0.798844714949337,-0.795147729252929,-0.788587180245253,
-0.780433524141206,-0.761672250318317,-0.733869798740763,-0.722294141832624,
-0.719026802650053,-0.717050204070622,-0.71518636533546,-0.712451356666229,
-0.704883288898493,-0.692479135787954,-0.654558944539558,-0.641728001349262,
-0.636833076423305,-0.633819537974329,-0.630533689629472,-0.625970175679782,
-0.614517540205833,-0.597052167100155,-0.564022075176314,-0.555081553385852,
-0.552087202000881,-0.550360083667683,-0.54849269948845,-0.545739031266206,
-0.538030256209511,-0.525281516417833,-0.484547396888387,-0.474186772710357,
-0.47011130745134,-0.467104206214309,-0.463813027832059,-0.459218900211225,
-0.44755411924597,-0.429601229977824,-0.395780606180549,-0.388066975755315,
-0.385233144566462,-0.383536612427477,-0.381638432420609,-0.378732291569356,
-0.369778809938577,-0.353723321308674,-0.31351842856002,-0.306607384464841,
-0.302473506591906,-0.299243524743061,-0.295686865876557,-0.289790337620561,
-0.261804282803683,-0.234243515820459,-0.222334976743252,-0.219038586989944,
-0.217055762409074,-0.215195723081021,-0.212480165594264,-0.205054796833161,
-0.192993933742022,-0.157614396084684,-0.142354688441775,-0.137171881433024,
-0.133765755930204,-0.130472649978809,-0.130401637889918,-0.130337722882927,
-0.130279824211306,-0.130227073492749,-0.130178764235331,-0.130134315424739,
-0.12997631229673,-0.12981840149605,-0.124918477348795,-0.110040017949518,
-0.0831589239800696,-0.0584362202721239,-0.0535016838739476,-0.0511839823228503,
-0.0493771883808169,-0.0471812350995658,-0.0428757301979037,-0.0371759277505071,
-0.00039473036140113),.UNSPECIFIED.);
#2842=B_SPLINE_CURVE_WITH_KNOTS('',3,(#115890,#115891,#115892,#115893,#115894,
#115895,#115896,#115897,#115898,#115899,#115900,#115901,#115902,#115903,
#115904,#115905,#115906,#115907),.UNSPECIFIED.,.F.,.F.,(4,2,2,2,2,2,2,2,
4),(-4.61628182467573,-4.59344808068452,-4.58898643506661,-4.58571278198089,
-4.58241685164426,-4.57941610975834,-4.57459111966926,-4.56224152719433,
-4.55723119340549),.UNSPECIFIED.);
#2843=B_SPLINE_CURVE_WITH_KNOTS('',3,(#115908,#115909,#115910,#115911,#115912,
#115913,#115914,#115915,#115916,#115917,#115918,#115919,#115920,#115921,
#115922,#115923,#115924,#115925,#115926,#115927,#115928,#115929,#115930,
#115931,#115932,#115933,#115934,#115935,#115936,#115937,#115938,#115939,
#115940,#115941,#115942,#115943,#115944,#115945,#115946,#115947,#115948,
#115949,#115950,#115951,#115952,#115953,#115954,#115955,#115956,#115957,
#115958,#115959,#115960,#115961,#115962,#115963,#115964,#115965,#115966,
#115967,#115968,#115969,#115970,#115971,#115972,#115973,#115974,#115975,
#115976,#115977,#115978,#115979,#115980,#115981,#115982,#115983,#115984,
#115985,#115986,#115987,#115988,#115989,#115990,#115991,#115992,#115993,
#115994,#115995,#115996,#115997,#115998,#115999,#116000,#116001,#116002,
#116003,#116004,#116005,#116006,#116007,#116008,#116009,#116010,#116011,
#116012,#116013,#116014,#116015,#116016,#116017,#116018,#116019,#116020,
#116021,#116022,#116023,#116024,#116025,#116026,#116027,#116028,#116029,
#116030,#116031,#116032,#116033,#116034,#116035,#116036,#116037,#116038,
#116039,#116040,#116041,#116042,#116043,#116044,#116045,#116046,#116047,
#116048,#116049,#116050,#116051,#116052,#116053,#116054,#116055,#116056,
#116057,#116058,#116059,#116060,#116061,#116062,#116063,#116064,#116065,
#116066,#116067,#116068,#116069,#116070,#116071,#116072,#116073,#116074,
#116075,#116076,#116077,#116078,#116079,#116080,#116081,#116082,#116083,
#116084,#116085,#116086,#116087,#116088,#116089,#116090,#116091,#116092,
#116093,#116094,#116095,#116096,#116097,#116098,#116099,#116100,#116101,
#116102,#116103,#116104,#116105,#116106,#116107),.UNSPECIFIED.,.F.,.F.,
(4,2,2,2,2,2,2,2,2,2,2,2,2,2,2,2,2,2,2,2,2,2,2,2,2,2,2,2,2,2,2,2,2,2,2,
2,2,2,2,2,2,2,2,2,2,2,2,2,2,2,2,2,2,2,2,2,2,2,2,2,2,2,2,2,2,2,2,2,2,2,2,
2,2,2,2,2,2,2,2,2,2,2,2,2,2,2,2,2,2,2,2,2,2,2,2,2,2,2,2,4),(-1.10911089706055,
-1.09536029552188,-1.07745793675764,-1.06115734615668,-1.05022985049061,
-1.04619257319148,-1.04319534546673,-1.03989713287019,-1.03525925835878,
-1.02327938236834,-1.0045839344241,-0.976942564988807,-0.965145595450497,
-0.96185992353093,-0.959879849791299,-0.958019289807807,-0.955298600738319,
-0.94783158868073,-0.935669812887117,-0.899590940595222,-0.885029401543547,
-0.879920000095205,-0.876868450620587,-0.873611642311612,-0.869215130994038,
-0.858850743905504,-0.84375085594157,-0.824247732367925,-0.801248771186571,
-0.796394867994558,-0.794059799098971,-0.792252654269116,-0.790072355452397,
-0.785842137889164,-0.761130010121192,-0.721824007066994,-0.715582876189345,
-0.711598568957438,-0.708392120598604,-0.704705650115049,-0.698189441331689,
-0.690105872516136,-0.671602084187366,-0.644435189368545,-0.631992992293171,
-0.628644872050281,-0.62665131852,-0.624798248140955,-0.622117165970806,
-0.614935723784745,-0.603448560816518,-0.582547219523575,-0.553527797774557,
-0.547543880083569,-0.543969608259826,-0.54074558535044,-0.53658046698623,
-0.527593033377261,-0.502797192499772,-0.472074461225718,-0.464339701664443,
-0.461503676613933,-0.45980727868709,-0.457910810065908,-0.455010014635448,
-0.446096154750107,-0.430150965791991,-0.390388305733253,-0.382348520519313,
-0.378357379187259,-0.375150507862693,-0.371469115056092,-0.36497695357909,
-0.333679093611474,-0.300758822563763,-0.296210472234194,-0.293966957403228,
-0.292162511143119,-0.289899751249717,-0.285252218322695,-0.266342011292558,
-0.245695073367644,-0.220114961852737,-0.21420045061068,-0.210640929160301,
-0.207413425676202,-0.203219885717632,-0.194070840020895,-0.181389305457178,
-0.158661196553583,-0.155314707243115,-0.132807718545252,-0.129115302201541,
-0.127025625334977,-0.125205695777603,-0.122735989446099,-0.11733032510801,
-0.0949096646472632,-0.0681866851383444,-0.0595548159224536),
 .UNSPECIFIED.);
#2844=B_SPLINE_CURVE_WITH_KNOTS('',3,(#116112,#116113,#116114,#116115,#116116,
#116117,#116118,#116119,#116120,#116121,#116122,#116123,#116124,#116125,
#116126,#116127,#116128,#116129,#116130,#116131,#116132,#116133,#116134,
#116135,#116136,#116137,#116138,#116139,#116140,#116141,#116142,#116143,
#116144,#116145,#116146,#116147,#116148,#116149,#116150,#116151,#116152,
#116153,#116154,#116155,#116156,#116157,#116158,#116159,#116160,#116161,
#116162,#116163,#116164,#116165,#116166,#116167,#116168,#116169,#116170,
#116171,#116172,#116173,#116174,#116175,#116176,#116177,#116178,#116179,
#116180,#116181,#116182,#116183,#116184,#116185,#116186,#116187,#116188,
#116189,#116190,#116191,#116192,#116193,#116194,#116195,#116196,#116197,
#116198,#116199,#116200,#116201,#116202,#116203,#116204,#116205,#116206,
#116207,#116208,#116209,#116210,#116211,#116212,#116213,#116214,#116215,
#116216,#116217,#116218,#116219,#116220,#116221,#116222,#116223,#116224,
#116225,#116226,#116227,#116228,#116229,#116230,#116231,#116232,#116233,
#116234,#116235,#116236,#116237,#116238,#116239,#116240,#116241,#116242,
#116243,#116244,#116245,#116246,#116247,#116248,#116249,#116250,#116251,
#116252,#116253,#116254,#116255,#116256,#116257,#116258,#116259,#116260,
#116261,#116262,#116263,#116264,#116265,#116266,#116267,#116268,#116269,
#116270,#116271,#116272,#116273,#116274,#116275,#116276,#116277,#116278,
#116279,#116280,#116281,#116282,#116283,#116284,#116285,#116286,#116287,
#116288,#116289,#116290,#116291,#116292,#116293,#116294,#116295,#116296,
#116297,#116298,#116299,#116300,#116301,#116302,#116303,#116304,#116305,
#116306,#116307,#116308,#116309,#116310,#116311,#116312,#116313,#116314,
#116315,#116316,#116317,#116318,#116319,#116320,#116321,#116322,#116323,
#116324,#116325,#116326,#116327,#116328,#116329,#116330,#116331,#116332,
#116333,#116334,#116335,#116336,#116337,#116338,#116339,#116340,#116341),
 .UNSPECIFIED.,.F.,.F.,(4,2,2,2,2,2,2,2,2,2,2,2,2,2,2,2,2,2,2,2,2,2,2,2,
2,2,2,2,2,2,2,2,2,2,2,2,2,2,2,2,2,2,2,2,2,2,2,2,2,2,2,2,2,2,2,2,2,2,2,2,
2,2,2,2,2,2,2,2,2,2,2,2,2,2,2,2,2,2,2,2,2,2,2,2,2,2,2,2,2,2,2,2,2,2,2,2,
2,2,2,2,2,2,2,2,2,2,2,2,2,2,2,2,2,2,4),(-2.04091987557192,-2.0214364672295,
-2.01795486345245,-1.99048502414608,-1.97542996731522,-1.97050981628791,
-1.97035181158444,-1.97019379604683,-1.97015105764711,-1.97010470448076,
-1.97005420664619,-1.96999892305641,-1.96993806999392,-1.96987067832227,
-1.96979553378446,-1.96971109244413,-1.96961535776459,-1.96950569690538,
-1.96937855768623,-1.96922901564825,-1.9659966455919,-1.96244616112557,
-1.95658071392048,-1.93177799622883,-1.90159286333757,-1.89308148004259,
-1.88727231358038,-1.88480024145603,-1.88297906150313,-1.8808885003324,
-1.87719554210386,-1.85520996783483,-1.85093669278227,-1.82876619989233,
-1.81596410538435,-1.80675149718162,-1.80254530794657,-1.79931456915889,
-1.79575794824884,-1.78986355531596,-1.76510057004488,-1.73492861745318,
-1.72641892425985,-1.72061060729511,-1.71813868693701,-1.71631753638898,
-1.71422691303833,-1.71053363851319,-1.68845667774375,-1.68424910428063,
-1.66207096420474,-1.64928823997298,-1.64008578306475,-1.63588137965813,
-1.63265088769092,-1.62909341550034,-1.62319494011144,-1.59829546438007,
-1.56824268921601,-1.55974806512833,-1.55394724049454,-1.5514765796572,
-1.5496555982326,-1.54756428526641,-1.54386788877696,-1.52095915663146,
-1.51804887530415,-1.4952644517905,-1.48256373641869,-1.4734042903589,-1.46920741993812,
-1.46597791203902,-1.46241671581398,-1.45650059382646,-1.43092008409314,
-1.41028446701765,-1.39138437548358,-1.38673666997502,-1.3844730986558,
-1.38266760104559,-1.38042220123916,-1.37586815433095,-1.34295204710857,
-1.31160807899895,-1.30511190262722,-1.30142839889663,-1.29821976723592,
-1.29422650381571,-1.28795872529718,-1.24890691838106,-1.22401413920869,
-1.21978223072504,-1.21760092102095,-1.21579283991067,-1.2134563302972,
-1.20859861389451,-1.18281016658834,-1.1674554137225,-1.15150727932758,
-1.14074161219738,-1.13628091436378,-1.13301245193946,-1.1299753068327,
-1.12495004358513,-1.11114100498908,-1.07740997159974,-1.06309475938427,
-1.05477253568418,-1.05194083493369,-1.05005789433015,-1.04811026978677,
-1.04497576778931,-1.03375343852834,-1.01005667358214,-0.991117350869854),
 .UNSPECIFIED.);
#2845=B_SPLINE_CURVE_WITH_KNOTS('',3,(#116343,#116344,#116345,#116346,#116347,
#116348,#116349,#116350,#116351,#116352,#116353,#116354,#116355,#116356,
#116357,#116358),.UNSPECIFIED.,.F.,.F.,(4,2,2,2,2,2,2,4),(-0.0595548159224536,
-0.0522110906588228,-0.0469503809994493,-0.0435290859888312,-0.0402475629379682,
-0.0369986128403095,-0.0326031491967441,-0.000491644909933951),
 .UNSPECIFIED.);
#2846=B_SPLINE_CURVE_WITH_KNOTS('',3,(#116359,#116360,#116361,#116362,#116363,
#116364,#116365,#116366,#116367,#116368,#116369,#116370,#116371,#116372,
#116373,#116374,#116375,#116376,#116377,#116378,#116379,#116380,#116381,
#116382,#116383,#116384,#116385,#116386,#116387,#116388,#116389,#116390,
#116391,#116392,#116393,#116394,#116395,#116396,#116397,#116398,#116399,
#116400,#116401,#116402,#116403,#116404,#116405,#116406,#116407,#116408,
#116409,#116410,#116411,#116412,#116413,#116414,#116415,#116416,#116417,
#116418,#116419,#116420,#116421,#116422,#116423,#116424,#116425,#116426,
#116427,#116428,#116429,#116430,#116431,#116432,#116433,#116434,#116435,
#116436,#116437,#116438,#116439,#116440,#116441,#116442,#116443,#116444,
#116445,#116446,#116447,#116448,#116449,#116450,#116451,#116452,#116453,
#116454,#116455,#116456,#116457,#116458,#116459,#116460,#116461,#116462,
#116463,#116464,#116465,#116466,#116467,#116468,#116469,#116470,#116471,
#116472,#116473,#116474,#116475,#116476,#116477,#116478,#116479,#116480,
#116481,#116482,#116483,#116484,#116485,#116486,#116487,#116488,#116489,
#116490,#116491,#116492,#116493,#116494,#116495,#116496,#116497,#116498,
#116499,#116500,#116501,#116502,#116503,#116504,#116505,#116506,#116507,
#116508,#116509,#116510,#116511,#116512,#116513,#116514,#116515,#116516,
#116517,#116518,#116519,#116520,#116521),.UNSPECIFIED.,.F.,.F.,(4,3,3,3,
3,3,3,3,3,3,3,3,3,3,3,3,3,3,3,3,3,3,3,3,3,3,3,3,3,3,3,3,3,3,3,3,3,3,3,3,
3,3,3,3,3,3,3,3,3,3,3,3,3,3,4),(-54.111865720756,-53.9685006350433,-53.8675843506887,
-53.7577897347099,-53.646820579414,-53.5373284361922,-53.4279032844545,
-53.3185044306127,-53.2063874460452,-53.0968489113581,-52.9834427018503,
-52.8700364923426,-52.7602418763656,-52.6492727210695,-52.5397805778498,
-52.4303554261141,-52.3209565722744,-52.208839587705,-52.0993010530199,
-51.9858948435082,-51.8724886339965,-51.76269401802,-51.6517248627238,-51.5422327195046,
-51.4328075677695,-51.3234087139303,-51.2112917293603,-51.1017531946758,
-50.9883469851631,-50.8749407756504,-50.7651461596728,-50.6541770043767,
-50.5446848611563,-50.43525970942,-50.3258608555796,-50.2137438710108,-50.1042053363251,
-49.9907991268147,-49.8773929173043,-49.7675983013272,-49.6566291460311,
-49.5471370028112,-49.4377118510754,-49.3283129972356,-49.2161960126663,
-49.1066574779811,-48.9932512684696,-48.8798450589582,-48.770074918514,
-48.6604636794697,-48.5509703726863,-48.4415394131865,-48.3321442530794,
-48.22270901535,-48.1819103663467),.UNSPECIFIED.);
#2847=B_SPLINE_CURVE_WITH_KNOTS('',3,(#116527,#116528,#116529,#116530,#116531,
#116532,#116533,#116534,#116535,#116536,#116537,#116538,#116539,#116540,
#116541,#116542,#116543,#116544,#116545,#116546,#116547,#116548,#116549,
#116550,#116551,#116552,#116553,#116554,#116555,#116556,#116557,#116558,
#116559,#116560,#116561,#116562,#116563,#116564,#116565,#116566,#116567,
#116568,#116569,#116570,#116571,#116572,#116573,#116574,#116575,#116576,
#116577,#116578,#116579,#116580,#116581,#116582,#116583,#116584,#116585,
#116586,#116587,#116588,#116589,#116590,#116591,#116592,#116593,#116594,
#116595,#116596,#116597,#116598,#116599,#116600,#116601,#116602,#116603,
#116604,#116605,#116606,#116607,#116608,#116609,#116610,#116611,#116612,
#116613,#116614,#116615,#116616,#116617,#116618,#116619,#116620,#116621,
#116622,#116623,#116624,#116625,#116626,#116627,#116628,#116629,#116630,
#116631,#116632,#116633,#116634,#116635,#116636,#116637,#116638,#116639,
#116640,#116641,#116642,#116643,#116644,#116645,#116646,#116647,#116648,
#116649,#116650,#116651,#116652,#116653,#116654,#116655,#116656,#116657,
#116658,#116659,#116660,#116661,#116662,#116663,#116664,#116665,#116666,
#116667,#116668,#116669,#116670,#116671,#116672,#116673,#116674,#116675,
#116676,#116677,#116678,#116679,#116680,#116681,#116682,#116683,#116684,
#116685,#116686,#116687,#116688,#116689,#116690,#116691,#116692,#116693,
#116694,#116695,#116696,#116697,#116698,#116699,#116700,#116701,#116702,
#116703,#116704,#116705,#116706,#116707,#116708,#116709,#116710,#116711,
#116712,#116713,#116714,#116715,#116716,#116717,#116718,#116719,#116720,
#116721,#116722,#116723,#116724,#116725,#116726,#116727,#116728,#116729,
#116730,#116731,#116732),.UNSPECIFIED.,.F.,.F.,(4,2,2,2,2,2,2,2,2,2,2,2,
2,2,2,2,2,2,2,2,2,2,2,2,2,2,2,2,2,2,2,2,2,2,2,2,2,2,2,2,2,2,2,2,2,2,2,2,
2,2,2,2,2,2,2,2,2,2,2,2,2,2,2,2,2,2,2,2,2,2,2,2,2,2,2,2,2,2,2,2,2,2,2,2,
2,2,2,2,2,2,2,2,2,2,2,2,2,2,2,2,2,2,4),(-0.991229013558196,-0.983226807241693,
-0.978905720506465,-0.957081037524643,-0.953390024519641,-0.951300091834927,
-0.949479154193232,-0.947006945545792,-0.941195589161653,-0.932678274344057,
-0.902453257244407,-0.877726437790873,-0.871833252991677,-0.868277265642927,
-0.865047054071154,-0.860841477772183,-0.851629717019773,-0.838830079244984,
-0.816681461932387,-0.8124367997064,-0.790449607248132,-0.786757969855074,
-0.784667923948854,-0.782847059550454,-0.780375180480012,-0.774565613368112,
-0.766051838499369,-0.735854191130525,-0.71109726075852,-0.705203239670551,
-0.701647122844623,-0.698417031180796,-0.694211952144567,-0.685002735411832,
-0.672207860662359,-0.650057696043303,-0.645826704446605,-0.623820542642875,
-0.620128908148945,-0.618038889331176,-0.616218066731327,-0.613746268767549,
-0.607936999666053,-0.599423758636789,-0.569229570716515,-0.544469917019493,
-0.538575918279128,-0.535019854380151,-0.53178983576337,-0.527584887688922,
-0.518376110689972,-0.505581975967506,-0.483432066825163,-0.479202667774492,
-0.457194844287983,-0.453503278898882,-0.451413301976146,-0.449592517856909,
-0.447120774783903,-0.441311646381643,-0.432798622115862,-0.402605373502923,
-0.377845884641074,-0.371951998169329,-0.368396006298207,-0.365166055822773,
-0.36096120035973,-0.351752642818699,-0.338958827043643,-0.316809358516629,
-0.312580212461516,-0.290572617361072,-0.286881128281577,-0.284791194864381,
-0.282970448863579,-0.280498757826556,-0.274689752997988,-0.266176910979542,
-0.235984327366617,-0.211217976131495,-0.205328065501688,-0.201772966766826,
-0.198542873748514,-0.194336462231084,-0.185118648564916,-0.172307031514681,
-0.149932020347275,-0.14597502588274,-0.123953541227381,-0.120262072847819,
-0.118172169834451,-0.116351463683811,-0.11387984463443,-0.108071087843485,
-0.0818781132822752,-0.0549654806149681,-0.0424558181115558,-0.0376072481790382,
-0.0346022506871433,-0.0313099267277518,-0.0280428395245619,-0.0235991964975932,
-0.000491388196465075),.UNSPECIFIED.);
#2848=B_SPLINE_CURVE_WITH_KNOTS('',3,(#116733,#116734,#116735,#116736,#116737,
#116738,#116739,#116740,#116741,#116742,#116743,#116744,#116745,#116746,
#116747,#116748),.UNSPECIFIED.,.F.,.F.,(4,2,2,2,2,2,2,4),(-2.0997315227576,
-2.05974751902068,-2.05394201031784,-2.05147051231299,-2.04964936915767,
-2.0475584005859,-2.04386375467915,-2.04091987557192),.UNSPECIFIED.);
#2849=B_SPLINE_CURVE_WITH_KNOTS('',3,(#116750,#116751,#116752,#116753,#116754,
#116755,#116756,#116757,#116758,#116759,#116760,#116761,#116762),
 .UNSPECIFIED.,.F.,.F.,(4,3,3,3,4),(-48.1819103663467,-48.072349463502,
-47.9625850721489,-47.8822972006122,-47.8286804139494),.UNSPECIFIED.);
#2850=B_SPLINE_CURVE_WITH_KNOTS('',3,(#116763,#116764,#116765,#116766,#116767,
#116768,#116769,#116770,#116771),.UNSPECIFIED.,.F.,.F.,(4,1,1,1,1,1,4),
(-47.8286738455222,-46.8847493422661,-45.88720148392,-44.8896536255739,
-43.8921057672278,-42.8945579088817,-41.8982145706828),.UNSPECIFIED.);
#2851=B_SPLINE_CURVE_WITH_KNOTS('',3,(#116776,#116777,#116778,#116779,#116780,
#116781,#116782,#116783,#116784,#116785,#116786,#116787,#116788,#116789,
#116790,#116791,#116792,#116793,#116794,#116795,#116796,#116797,#116798,
#116799,#116800,#116801,#116802,#116803,#116804,#116805,#116806,#116807,
#116808,#116809,#116810,#116811,#116812,#116813,#116814,#116815,#116816,
#116817,#116818,#116819,#116820,#116821,#116822,#116823,#116824,#116825,
#116826,#116827,#116828,#116829,#116830,#116831,#116832,#116833,#116834,
#116835,#116836,#116837,#116838,#116839,#116840,#116841,#116842,#116843,
#116844,#116845,#116846,#116847,#116848,#116849,#116850,#116851,#116852,
#116853,#116854,#116855,#116856,#116857,#116858,#116859,#116860,#116861,
#116862,#116863,#116864,#116865,#116866,#116867,#116868,#116869,#116870,
#116871,#116872,#116873,#116874,#116875,#116876,#116877,#116878,#116879,
#116880,#116881,#116882,#116883,#116884,#116885,#116886,#116887,#116888,
#116889,#116890,#116891,#116892,#116893,#116894,#116895,#116896,#116897,
#116898,#116899,#116900,#116901,#116902,#116903,#116904,#116905,#116906,
#116907,#116908,#116909,#116910,#116911,#116912,#116913,#116914,#116915,
#116916,#116917,#116918,#116919,#116920,#116921,#116922,#116923,#116924,
#116925,#116926,#116927,#116928,#116929,#116930,#116931,#116932,#116933,
#116934,#116935,#116936,#116937,#116938,#116939,#116940,#116941,#116942,
#116943,#116944,#116945,#116946,#116947,#116948,#116949,#116950,#116951,
#116952,#116953,#116954,#116955,#116956,#116957,#116958,#116959,#116960,
#116961,#116962,#116963,#116964,#116965,#116966,#116967,#116968,#116969,
#116970,#116971,#116972,#116973,#116974,#116975,#116976,#116977,#116978,
#116979,#116980,#116981,#116982,#116983,#116984,#116985,#116986,#116987),
 .UNSPECIFIED.,.F.,.F.,(4,2,2,2,2,2,2,2,2,2,2,2,2,2,2,2,2,2,2,2,2,2,2,2,
2,2,2,2,2,2,2,2,2,2,2,2,2,2,2,2,2,2,2,2,2,2,2,2,2,2,2,2,2,2,2,2,2,2,2,2,
2,2,2,2,2,2,2,2,2,2,2,2,2,2,2,2,2,2,2,2,2,2,2,2,2,2,2,2,2,2,2,2,2,2,2,2,
2,2,2,2,2,2,2,2,2,4),(-2.04102384583476,-2.03717390456845,-2.03386856318245,
-2.03087609430279,-2.02610132939005,-2.01409214424512,-1.97527843971127,
-1.96276676574619,-1.95757056645696,-1.95468374034383,-1.95229856898726,
-1.9522812677756,-1.95226367370402,-1.95224577013204,-1.9504566851066,-1.94845249689006,
-1.9450585732234,-1.93200836201607,-1.90526296711851,-1.88689799636911,
-1.87505751891548,-1.87043815277717,-1.86714234946013,-1.86414009400134,
-1.8593090550742,-1.84692258743775,-1.80853471522224,-1.79607605977328,
-1.78848507236628,-1.78574705589783,-1.78388265434416,-1.78190709148508,
-1.77864436332611,-1.76712279750479,-1.73926078485881,-1.72047168354213,
-1.70845247017219,-1.70380792676097,-1.70050752884884,-1.69711157551711,
-1.69197916848967,-1.67720862078734,-1.64136463985673,-1.62923867236717,
-1.62178538057471,-1.61906592455901,-1.61720504149698,-1.61546965723968,
-1.61243298547157,-1.60313903830861,-1.57028576242051,-1.55296054728561,
-1.54157065124103,-1.53701632864956,-1.53373214880123,-1.53071677533512,
-1.52581117415722,-1.51290293781228,-1.47835134793742,-1.46380613887436,
-1.45809196666741,-1.45377773840045,-1.45157991397355,-1.4497730646489,
-1.44745716595493,-1.44253298524169,-1.41915283243522,-1.39915608757709,
-1.37721353684339,-1.37160533272437,-1.36810973120506,-1.36486045710184,
-1.36059487808944,-1.35115454588705,-1.30919352609576,-1.29630658157641,
-1.28854134334157,-1.28578023304681,-1.28391134998825,-1.28194308352469,
-1.2787139104237,-1.26757167050972,-1.23943731070387,-1.22053611421464,
-1.20847003305595,-1.20381886605605,-1.20051718586692,-1.19712283901868,
-1.19199859608921,-1.17730755383502,-1.13718238987883,-1.12766878359463,
-1.1213746016566,-1.11882422358746,-1.11699219571001,-1.11494241266772,
-1.11133850798002,-1.09484826360241,-1.05022558244646,-1.04074392397264,
-1.03653753341718,-1.03329735228271,-1.02977596482141,-1.02404572578345,
-0.99996913194226,-0.991229013558196),.UNSPECIFIED.);
#2852=B_SPLINE_CURVE_WITH_KNOTS('',3,(#116989,#116990,#116991,#116992,#116993),
 .UNSPECIFIED.,.F.,.F.,(4,1,4),(-41.8982145706828,-41.8970100505356,-41.5455022209794),
 .UNSPECIFIED.);
#2853=B_SPLINE_CURVE_WITH_KNOTS('',3,(#116994,#116995,#116996,#116997,#116998,
#116999,#117000,#117001,#117002,#117003,#117004,#117005,#117006,#117007,
#117008,#117009,#117010,#117011,#117012,#117013,#117014,#117015,#117016,
#117017,#117018,#117019,#117020,#117021,#117022,#117023,#117024,#117025,
#117026,#117027,#117028,#117029,#117030,#117031,#117032,#117033,#117034,
#117035,#117036,#117037,#117038,#117039,#117040,#117041,#117042,#117043,
#117044,#117045,#117046,#117047,#117048,#117049,#117050,#117051,#117052,
#117053,#117054,#117055,#117056,#117057,#117058,#117059,#117060,#117061,
#117062,#117063,#117064,#117065,#117066,#117067,#117068,#117069,#117070,
#117071,#117072,#117073,#117074,#117075,#117076,#117077,#117078,#117079,
#117080,#117081,#117082,#117083,#117084,#117085,#117086,#117087,#117088,
#117089,#117090,#117091,#117092,#117093,#117094,#117095,#117096,#117097,
#117098,#117099,#117100,#117101,#117102,#117103,#117104,#117105,#117106,
#117107,#117108,#117109,#117110,#117111,#117112,#117113,#117114,#117115,
#117116,#117117,#117118,#117119,#117120,#117121,#117122,#117123,#117124,
#117125,#117126,#117127,#117128,#117129,#117130,#117131,#117132,#117133,
#117134,#117135,#117136,#117137,#117138,#117139,#117140,#117141,#117142,
#117143,#117144,#117145,#117146,#117147,#117148,#117149,#117150,#117151,
#117152,#117153,#117154,#117155,#117156,#117157,#117158,#117159,#117160,
#117161,#117162,#117163,#117164,#117165,#117166,#117167,#117168,#117169,
#117170,#117171,#117172,#117173,#117174,#117175,#117176,#117177,#117178,
#117179,#117180,#117181,#117182,#117183,#117184,#117185),.UNSPECIFIED.,
 .F.,.F.,(4,2,2,2,2,2,2,2,2,2,2,2,2,2,2,2,2,2,2,2,2,2,2,2,2,2,2,2,2,2,2,
2,2,2,2,2,2,2,2,2,2,2,2,2,2,2,2,2,2,2,2,2,2,2,2,2,2,2,2,2,2,2,2,2,2,2,2,
2,2,2,2,2,2,2,2,2,2,2,2,2,2,2,2,2,2,2,2,2,2,2,2,2,2,2,2,4),(-2.10009212962413,
-2.08490754922681,-2.08082970724367,-2.07769015352275,-2.07458743933971,
-2.07105810229777,-2.06528703791036,-2.04132892984664,-2.01676155463722,
-2.00413300982311,-1.99647320851046,-1.99372671244327,-1.99186123545881,
-1.98988964740601,-1.98664276414969,-1.97529230046428,-1.94358297681593,
-1.9270860547046,-1.91956103523844,-1.91339689896894,-1.90978424484896,
-1.90656757076755,-1.90246999196441,-1.89584033369671,-1.8617643040054,
-1.83271131688535,-1.82840298143906,-1.82620684143748,-1.82440065117089,
-1.82208475070102,-1.81715775098882,-1.79356838485433,-1.77357042685395,
-1.75909779056585,-1.7490389808044,-1.74469150256002,-1.74144219680918,
-1.7379513106206,-1.7323612416949,-1.71302518102365,-1.66963618258593,-1.66286242183498,
-1.66023972487545,-1.65839664295815,-1.65638005092924,-1.65292722128992,
-1.63894650536415,-1.63524495756845,-1.60109049047854,-1.58432538648303,
-1.57912754172571,-1.57571896554424,-1.57246620255507,-1.56790039549497,
-1.55726104784524,-1.5123446410461,-1.50249967742783,-1.49605079062568,
-1.49347696546924,-1.49164184000464,-1.48960418084608,-1.48605432980396,
-1.47033536664883,-1.44099831528898,-1.4185312217029,-1.41289174465181,
-1.4093902567661,-1.40614461851851,-1.40189702317331,-1.39216355071117,
-1.35427493631468,-1.33881700675578,-1.33007499052363,-1.3271937448826,
-1.3253011060979,-1.32336759872777,-1.32029572815181,-1.31069170443886,
-1.27802107309806,-1.26081908534582,-1.24948433851868,-1.24493894381946,
-1.24165708611289,-1.23864104407536,-1.23372802603151,-1.2207603576303,
-1.18626292302198,-1.17173212778256,-1.16332966745509,-1.16048887435627,
-1.15860460638206,-1.15666060994102,-1.15354043430082,-1.14349926014873,
-1.11108111999421,-1.10913474690605),.UNSPECIFIED.);
#2854=B_SPLINE_CURVE_WITH_KNOTS('',3,(#117191,#117192,#117193,#117194,#117195,
#117196,#117197,#117198,#117199,#117200,#117201,#117202,#117203,#117204,
#117205,#117206,#117207,#117208,#117209,#117210,#117211,#117212,#117213,
#117214,#117215,#117216,#117217,#117218,#117219,#117220,#117221,#117222,
#117223,#117224,#117225,#117226,#117227,#117228,#117229,#117230,#117231,
#117232,#117233,#117234,#117235,#117236,#117237,#117238,#117239,#117240,
#117241,#117242,#117243,#117244,#117245,#117246,#117247,#117248,#117249,
#117250,#117251,#117252,#117253,#117254,#117255,#117256,#117257,#117258,
#117259,#117260,#117261,#117262,#117263,#117264,#117265,#117266,#117267,
#117268,#117269,#117270,#117271,#117272,#117273,#117274,#117275,#117276,
#117277,#117278,#117279,#117280,#117281,#117282,#117283,#117284,#117285,
#117286,#117287,#117288,#117289,#117290,#117291,#117292,#117293,#117294,
#117295,#117296,#117297,#117298,#117299,#117300,#117301,#117302,#117303,
#117304,#117305,#117306,#117307,#117308,#117309,#117310,#117311,#117312,
#117313,#117314,#117315,#117316,#117317,#117318,#117319,#117320,#117321,
#117322,#117323,#117324,#117325,#117326,#117327,#117328,#117329,#117330,
#117331,#117332,#117333,#117334,#117335,#117336,#117337,#117338,#117339,
#117340,#117341,#117342,#117343,#117344,#117345,#117346,#117347,#117348,
#117349,#117350,#117351,#117352,#117353,#117354,#117355,#117356,#117357,
#117358,#117359,#117360,#117361,#117362,#117363,#117364,#117365,#117366,
#117367,#117368,#117369,#117370,#117371,#117372,#117373,#117374,#117375,
#117376,#117377,#117378,#117379,#117380,#117381,#117382,#117383,#117384,
#117385,#117386,#117387,#117388,#117389,#117390,#117391,#117392),
 .UNSPECIFIED.,.F.,.F.,(4,2,2,2,2,2,2,2,2,2,2,2,2,2,2,2,2,2,2,2,2,2,2,2,
2,2,2,2,2,2,2,2,2,2,2,2,2,2,2,2,2,2,2,2,2,2,2,2,2,2,2,2,2,2,2,2,2,2,2,2,
2,2,2,2,2,2,2,2,2,2,2,2,2,2,2,2,2,2,2,2,2,2,2,2,2,2,2,2,2,2,2,2,2,2,2,2,
2,2,2,2,4),(-0.991067550591075,-0.969566444920773,-0.944672893744101,-0.938774257899021,
-0.93521695335431,-0.931986793055493,-0.927783074758645,-0.918583015696578,
-0.905806073276034,-0.883646087270495,-0.879488069453632,-0.857381114331676,
-0.853688774908553,-0.851598484581849,-0.849777516680721,-0.847305643612251,
-0.841496736283739,-0.832984512122551,-0.80280177488619,-0.778023648310773,
-0.772128614964703,-0.768572123824428,-0.765341841835967,-0.761136729971568,
-0.751928357736591,-0.739135429703427,-0.716982499516558,-0.712760451921669,
-0.690739821070485,-0.687047882069024,-0.684957707740074,-0.683136761734768,
-0.680664812413146,-0.674855258847695,-0.666341665386737,-0.636147266425527,
-0.611383750563235,-0.605489277480675,-0.601932953539672,-0.598702715276033,
-0.594497505030695,-0.585288255243221,-0.572493549211428,-0.550341971535362,
-0.546113285198583,-0.524102525380969,-0.520410699398215,-0.518320576787415,
-0.516499667065637,-0.514027755253209,-0.508218238072402,-0.499704651117111,
-0.469509520453648,-0.4447480847128,-0.438853783472498,-0.435297544217477,
-0.432067370851557,-0.42786222782289,-0.418653051607689,-0.405858385644574,
-0.383707370871188,-0.379478042220937,-0.357468771112168,-0.353777026247587,
-0.351686948219359,-0.349866076378106,-0.347394214704811,-0.341584809696551,
-0.333071382001998,-0.302876733591189,-0.278115986605916,-0.272221813941492,
-0.268665650181972,-0.265435544072389,-0.261230486709362,-0.25202149004021,
-0.239227066724125,-0.21707652607314,-0.192746236712413,-0.187894860924606,
-0.185559834444997,-0.183752114101933,-0.181570306669531,-0.177334833101406,
-0.151815053196087,-0.113524426206123,-0.107177305066877,-0.103161200548965,
-0.0999513432637862,-0.0962850354621321,-0.0898689258003784,-0.0672497308052082,
-0.0434761411833771,-0.0267323817985043,-0.0214000897555977,-0.0190357103558771,
-0.0172225145287875,-0.0155112239908774,-0.0133869725079222,-0.00853515704896566,
-0.00049116967053566),.UNSPECIFIED.);
#2855=B_SPLINE_CURVE_WITH_KNOTS('',3,(#117393,#117394,#117395,#117396,#117397,
#117398,#117399,#117400,#117401,#117402),.UNSPECIFIED.,.F.,.F.,(4,2,2,2,
4),(-2.10005510352121,-2.07332448423479,-2.05406114578682,-2.04184561685977,
-2.04102384583476),.UNSPECIFIED.);
#2856=B_SPLINE_CURVE_WITH_KNOTS('',3,(#117403,#117404,#117405,#117406,#117407,
#117408,#117409,#117410,#117411,#117412,#117413,#117414,#117415,#117416,
#117417,#117418,#117419,#117420,#117421,#117422,#117423,#117424,#117425,
#117426,#117427,#117428,#117429,#117430,#117431,#117432,#117433,#117434,
#117435,#117436,#117437,#117438,#117439,#117440,#117441,#117442,#117443,
#117444,#117445,#117446,#117447,#117448,#117449,#117450,#117451,#117452,
#117453,#117454,#117455,#117456,#117457,#117458,#117459,#117460,#117461,
#117462,#117463,#117464,#117465,#117466,#117467,#117468,#117469,#117470,
#117471,#117472,#117473,#117474,#117475,#117476,#117477,#117478,#117479,
#117480,#117481,#117482,#117483,#117484,#117485,#117486,#117487,#117488,
#117489,#117490,#117491,#117492,#117493,#117494,#117495,#117496,#117497,
#117498,#117499,#117500,#117501,#117502,#117503,#117504,#117505,#117506,
#117507,#117508,#117509,#117510,#117511,#117512,#117513,#117514,#117515,
#117516,#117517,#117518,#117519,#117520,#117521,#117522,#117523,#117524,
#117525,#117526,#117527,#117528,#117529,#117530,#117531,#117532,#117533,
#117534,#117535,#117536,#117537,#117538,#117539,#117540,#117541,#117542,
#117543,#117544,#117545,#117546,#117547,#117548,#117549,#117550,#117551,
#117552,#117553,#117554,#117555,#117556,#117557,#117558,#117559,#117560,
#117561,#117562,#117563,#117564,#117565,#117566,#117567,#117568,#117569,
#117570,#117571,#117572,#117573,#117574,#117575,#117576,#117577,#117578,
#117579,#117580,#117581,#117582,#117583,#117584,#117585,#117586,#117587,
#117588,#117589,#117590,#117591,#117592,#117593,#117594,#117595,#117596,
#117597,#117598,#117599,#117600,#117601,#117602,#117603,#117604,#117605,
#117606,#117607,#117608,#117609,#117610,#117611,#117612,#117613,#117614,
#117615,#117616,#117617,#117618),.UNSPECIFIED.,.F.,.F.,(4,2,2,2,2,2,2,2,
2,2,2,2,2,2,2,2,2,2,2,2,2,2,2,2,2,2,2,2,2,2,2,2,2,2,2,2,2,2,2,2,2,2,2,2,
2,2,2,2,2,2,2,2,2,2,2,2,2,2,2,2,2,2,2,2,2,2,2,2,2,2,2,2,2,2,2,2,2,2,2,2,
2,2,2,2,2,2,2,2,2,2,2,2,2,2,2,2,2,2,2,2,2,2,2,2,2,2,2,4),(-1.10913474690605,
-1.09405577864177,-1.08279980310246,-1.07826612582831,-1.07498636782013,
-1.07156060223005,-1.06628011075756,-1.05011160751438,-1.02138896784798,
-0.998409798010556,-0.994714785429516,-0.992624317599637,-0.990804183579028,
-0.988334847959111,-0.982538217590795,-0.97404996881074,-0.944051974893915,
-0.919059796258301,-0.913159581922442,-0.909602758784431,-0.906373970703262,
-0.902173414618555,-0.892986374032505,-0.880233109938923,-0.858065249111541,
-0.854030551272188,-0.831767927548374,-0.82807588384919,-0.82598610590262,
-0.824165865359523,-0.821695438568383,-0.815892081749962,-0.807390221684309,
-0.77728397436924,-0.752417670586788,-0.746521243032921,-0.742965271631544,
-0.7397363515573,-0.735534324979346,-0.726338542003137,-0.713568487318554,
-0.691406728957578,-0.687271479146896,-0.665133878532598,-0.661442369110651,
-0.659352736718786,-0.657532510829956,-0.655061953827518,-0.649257630184002,
-0.640753756560917,-0.610630795677304,-0.585784924543672,-0.579889216925326,
-0.576333445951882,-0.573104559985799,-0.568902365546806,-0.559705311546098,
-0.546932730299792,-0.524772448679891,-0.520623351499045,-0.498503970857649,
-0.494812603522999,-0.492723028981166,-0.490902837341678,-0.488432305215404,
-0.48262794484907,-0.474123931434673,-0.443999094661869,-0.419156604762584,
-0.413261105285596,-0.409705426035708,-0.406476601970075,-0.402274457388477,
-0.393077381776438,-0.380304660344582,-0.358144985515712,-0.353994012833381,
-0.331877601814207,-0.328186319967777,-0.326096790617799,-0.324276636055914,
-0.321806151191492,-0.316001888372612,-0.307498005686736,-0.277373436276523,
-0.252531865444521,-0.246636499845286,-0.243080896543273,-0.239852138409481,
-0.235650075280472,-0.226453159398117,-0.213680644168415,-0.191521447692658,
-0.167222930703103,-0.162272064729742,-0.159951829229269,-0.158145538600874,
-0.1559532972431,-0.151663863205703,-0.14599139004664,-0.131613805531639,
-0.09767025037255,-0.0840808012901606,-0.0790847074119322,-0.0760540389961014,
-0.072784119565897,-0.0683061592401258,-0.0595903483156433),
 .UNSPECIFIED.);
#2857=B_SPLINE_CURVE_WITH_KNOTS('',3,(#117623,#117624,#117625,#117626,#117627,
#117628,#117629,#117630,#117631,#117632,#117633,#117634,#117635,#117636,
#117637,#117638,#117639,#117640,#117641,#117642,#117643,#117644,#117645,
#117646,#117647,#117648,#117649,#117650,#117651,#117652,#117653,#117654,
#117655,#117656,#117657,#117658,#117659,#117660,#117661,#117662,#117663,
#117664,#117665,#117666,#117667,#117668,#117669,#117670,#117671,#117672,
#117673,#117674,#117675,#117676,#117677,#117678,#117679,#117680,#117681,
#117682,#117683,#117684,#117685,#117686,#117687,#117688,#117689,#117690,
#117691,#117692,#117693,#117694,#117695,#117696,#117697,#117698,#117699,
#117700,#117701,#117702,#117703,#117704,#117705,#117706,#117707,#117708,
#117709,#117710,#117711,#117712,#117713,#117714,#117715,#117716,#117717,
#117718,#117719,#117720,#117721,#117722,#117723,#117724,#117725,#117726,
#117727,#117728,#117729,#117730,#117731,#117732,#117733,#117734,#117735,
#117736,#117737,#117738,#117739,#117740,#117741,#117742,#117743,#117744,
#117745,#117746,#117747,#117748,#117749,#117750,#117751,#117752,#117753,
#117754,#117755,#117756,#117757,#117758,#117759,#117760,#117761,#117762,
#117763,#117764,#117765,#117766,#117767,#117768,#117769,#117770,#117771,
#117772,#117773,#117774,#117775,#117776,#117777,#117778,#117779,#117780,
#117781,#117782,#117783,#117784,#117785,#117786,#117787,#117788,#117789,
#117790,#117791,#117792,#117793,#117794,#117795,#117796,#117797,#117798,
#117799,#117800,#117801,#117802,#117803,#117804,#117805,#117806,#117807,
#117808,#117809,#117810,#117811,#117812,#117813,#117814),.UNSPECIFIED.,
 .F.,.F.,(4,2,2,2,2,2,2,2,2,2,2,2,2,2,2,2,2,2,2,2,2,2,2,2,2,2,2,2,2,2,2,
2,2,2,2,2,2,2,2,2,2,2,2,2,2,2,2,2,2,2,2,2,2,2,2,2,2,2,2,2,2,2,2,2,2,2,2,
2,2,2,2,2,2,2,2,2,2,2,2,2,2,2,2,2,2,2,2,2,2,2,2,2,2,2,2,4),(-2.04098006789499,
-2.02522521486599,-2.02086040667168,-2.01865248161769,-2.01684618147899,
-2.01454223012355,-2.00968175907203,-1.9817750950153,-1.94576838995064,
-1.93934734843213,-1.93567977524879,-1.93246971838089,-1.92845456020461,
-1.92211144006445,-1.87718498781505,-1.85885824647768,-1.8542757962952,
-1.85202494365312,-1.85021958394375,-1.84796183626162,-1.8433438518936,
-1.81120632585006,-1.77924205456829,-1.77271612362426,-1.76902653269481,
-1.76581869982293,-1.76183436658643,-1.75559657229383,-1.71016533658795,
-1.69209394211437,-1.68754090276748,-1.6852957337116,-1.68349028122673,
-1.68122658768647,-1.67657807347583,-1.64499021822129,-1.61190735517013,
-1.60572096682812,-1.60210267046644,-1.59888538161607,-1.59479301900264,
-1.58818449594299,-1.55394305729052,-1.525010106732,-1.52070087857754,-1.51850402153859,
-1.51669706348198,-1.51437987167012,-1.50944895745569,-1.48349956513394,
-1.45746841759021,-1.44281857824617,-1.4378416429685,-1.43447722624759,
-1.43119115960431,-1.42644584581865,-1.41462968076956,-1.37903874842166,
-1.35906409526328,-1.35429846704416,-1.35201236213213,-1.35020654161012,
-1.34798251871097,-1.34353705634913,-1.30960304018494,-1.28296758976692,
-1.27409376101385,-1.26994761831544,-1.26672450789409,-1.26313716876311,
-1.25709680652037,-1.22771236752431,-1.20603640852029,-1.19020915967174,
-1.18675406011428,-1.18473657007402,-1.18289298590798,-1.18026990277285,
-1.17397661585752,-1.14198363602638,-1.11242990987644,-1.10594541898531,
-1.10226448200625,-1.09905577707768,-1.09505940613091,-1.08878065242618,
-1.04983758824488,-1.04683110841985,-1.0240300419919,-1.02033498226642,
-1.01824405716327,-1.016423183105,-1.01395230309862,-1.00814954041404,-0.999649762948563,
-0.991067550591075),.UNSPECIFIED.);
#2858=B_SPLINE_CURVE_WITH_KNOTS('',3,(#117816,#117817,#117818,#117819,#117820,
#117821,#117822,#117823,#117824,#117825),.UNSPECIFIED.,.F.,.F.,(4,2,2,2,
4),(-0.0595903483156433,-0.0574176870545041,-0.0412032104811654,-0.0229709702128129,
-0.000637632363922989),.UNSPECIFIED.);
#2859=B_SPLINE_CURVE_WITH_KNOTS('',3,(#117826,#117827,#117828,#117829,#117830,
#117831,#117832,#117833,#117834,#117835,#117836,#117837,#117838,#117839,
#117840,#117841,#117842,#117843,#117844,#117845,#117846,#117847,#117848,
#117849,#117850,#117851,#117852,#117853,#117854,#117855,#117856,#117857,
#117858,#117859,#117860,#117861,#117862,#117863,#117864,#117865,#117866,
#117867,#117868,#117869,#117870,#117871,#117872,#117873,#117874,#117875,
#117876,#117877,#117878,#117879,#117880,#117881,#117882,#117883,#117884,
#117885,#117886,#117887,#117888,#117889,#117890,#117891,#117892,#117893,
#117894,#117895,#117896,#117897,#117898,#117899,#117900,#117901,#117902,
#117903,#117904,#117905,#117906,#117907,#117908,#117909,#117910,#117911,
#117912,#117913,#117914,#117915,#117916,#117917,#117918,#117919,#117920,
#117921,#117922,#117923,#117924,#117925,#117926,#117927,#117928,#117929,
#117930,#117931,#117932,#117933,#117934,#117935,#117936,#117937,#117938,
#117939,#117940,#117941,#117942,#117943,#117944,#117945,#117946,#117947,
#117948,#117949,#117950,#117951,#117952,#117953,#117954,#117955,#117956,
#117957,#117958,#117959,#117960,#117961,#117962,#117963,#117964,#117965,
#117966,#117967,#117968,#117969,#117970,#117971,#117972,#117973,#117974,
#117975,#117976,#117977,#117978,#117979,#117980,#117981,#117982,#117983,
#117984,#117985,#117986,#117987,#117988,#117989,#117990,#117991,#117992,
#117993,#117994,#117995,#117996,#117997,#117998,#117999,#118000,#118001,
#118002,#118003,#118004,#118005,#118006,#118007,#118008,#118009,#118010,
#118011,#118012,#118013,#118014,#118015,#118016,#118017),.UNSPECIFIED.,
 .F.,.F.,(4,2,2,2,2,2,2,2,2,2,2,2,2,2,2,2,2,2,2,2,2,2,2,2,2,2,2,2,2,2,2,
2,2,2,2,2,2,2,2,2,2,2,2,2,2,2,2,2,2,2,2,2,2,2,2,2,2,2,2,2,2,2,2,2,2,2,2,
2,2,2,2,2,2,2,2,2,2,2,2,2,2,2,2,2,2,2,2,2,2,2,2,2,2,2,2,4),(-4.84271254774332,
-4.84012768829738,-4.83777417014381,-4.83590804710275,-4.83420334357131,
-4.83224168845127,-4.8290415726128,-4.81818716236885,-4.79064993423761,
-4.77113401652686,-4.76278265360574,-4.75610047150057,-4.75237866273415,
-4.7491739283282,-4.74523326551119,-4.73914256559883,-4.69853163718669,
-4.68170896766004,-4.67249140236879,-4.66955583113591,-4.66765153314793,
-4.66596008167783,-4.66315345728532,-4.65563211266913,-4.62163345122425,
-4.60359803047165,-4.59189843136318,-4.58729954245183,-4.58400782125478,
-4.58060026889897,-4.575409625978,-4.56007206107721,-4.52478866764198,-4.51274045237939,
-4.50531974472201,-4.5026049912957,-4.500745224134,-4.4987624799809,-4.4954658740778,
-4.48355459791503,-4.45596543489156,-4.43728588230758,-4.42915421528554,
-4.42260810879727,-4.41891459717433,-4.41570760574005,-4.41172985926363,
-4.40551357025942,-4.35996858521503,-4.34194556880708,-4.33739828460921,
-4.33515440472622,-4.33334919027422,-4.33108487220036,-4.3264322554881,
-4.29492302645612,-4.2616947666015,-4.25553988143409,-4.2519285365293,-4.24871055012987,
-4.24460789708212,-4.23796274221672,-4.2049774005901,-4.17498073713445,
-4.17058515702043,-4.16837120942027,-4.16656534220687,-4.16426881425934,
-4.15944717647472,-4.13071733800393,-4.11960641266917,-4.10276015417838,
-4.09513405656174,-4.08890530508023,-4.0852782862359,-4.08206283742387,
-4.0779859024176,-4.07143012023272,-4.02753425890174,-4.01356689740275,
-4.00537696017486,-4.00256179019265,-4.00068235366973,-3.9989689219708,
-3.99604494820572,-3.98766363502708,-3.95423511197276,-3.9365387416129,
-3.92867386204842,-3.92229439490861,-3.91863557603538,-3.91542453955849,
-3.91139674080356,-3.90316849788938,-3.8636243306166,-3.85165705040524),
 .UNSPECIFIED.);
#2860=B_SPLINE_CURVE_WITH_KNOTS('',3,(#118023,#118024,#118025,#118026,#118027,
#118028,#118029,#118030,#118031,#118032,#118033,#118034,#118035,#118036,
#118037,#118038,#118039,#118040,#118041,#118042,#118043,#118044,#118045,
#118046,#118047,#118048,#118049,#118050,#118051,#118052,#118053,#118054,
#118055,#118056,#118057,#118058,#118059,#118060,#118061,#118062,#118063,
#118064,#118065,#118066,#118067,#118068,#118069,#118070,#118071,#118072,
#118073,#118074,#118075,#118076,#118077,#118078,#118079,#118080,#118081,
#118082,#118083,#118084,#118085,#118086,#118087,#118088,#118089,#118090,
#118091,#118092,#118093,#118094,#118095,#118096,#118097,#118098,#118099,
#118100,#118101,#118102,#118103,#118104,#118105,#118106,#118107,#118108,
#118109,#118110,#118111,#118112,#118113,#118114,#118115,#118116,#118117,
#118118,#118119,#118120,#118121,#118122,#118123,#118124,#118125,#118126,
#118127,#118128,#118129,#118130,#118131,#118132,#118133,#118134,#118135,
#118136,#118137,#118138,#118139,#118140,#118141,#118142,#118143,#118144,
#118145,#118146,#118147,#118148,#118149,#118150,#118151,#118152,#118153,
#118154,#118155,#118156,#118157,#118158,#118159,#118160,#118161,#118162,
#118163,#118164,#118165,#118166,#118167,#118168,#118169,#118170,#118171,
#118172,#118173,#118174,#118175,#118176,#118177,#118178,#118179,#118180,
#118181,#118182,#118183,#118184,#118185,#118186,#118187,#118188,#118189,
#118190,#118191,#118192,#118193,#118194,#118195,#118196,#118197,#118198,
#118199,#118200,#118201,#118202,#118203,#118204),.UNSPECIFIED.,.F.,.F.,
(4,2,2,2,2,2,2,2,2,2,2,2,2,2,2,2,2,2,2,2,2,2,2,2,2,2,2,2,2,2,2,2,2,2,2,
2,2,2,2,2,2,2,2,2,2,2,2,2,2,2,2,2,2,2,2,2,2,2,2,2,2,2,2,2,2,2,2,2,2,2,2,
2,2,2,2,2,2,2,2,2,2,2,2,2,2,2,2,2,2,2,4),(-0.991352361073962,-0.990785819095057,
-0.959585665065777,-0.925998326718025,-0.921516348606512,-0.919284995238621,
-0.917479186863969,-0.915200597113129,-0.910475083406357,-0.890872791533548,
-0.856357510059553,-0.843377392364806,-0.838461333403668,-0.835443822219316,
-0.832160681069746,-0.827614016808728,-0.8162781471615,-0.799077934258794,
-0.766442539955367,-0.756836394738463,-0.75376361475442,-0.751829392196886,
-0.749935898574271,-0.747052981652967,-0.738303174683399,-0.722824525338107,
-0.684872011772322,-0.675173622661728,-0.67093078325403,-0.667684848926292,
-0.66417916475887,-0.658524129209144,-0.635813856385057,-0.616312219791162,
-0.593318764350412,-0.58846360436213,-0.586127622592189,-0.584319593906533,
-0.58213793803104,-0.577904195217436,-0.552813301292244,-0.513977098190511,
-0.507683421879438,-0.5036826457543,-0.500473551250248,-0.49679560475275,
-0.490325592592735,-0.460876725520823,-0.429121763263375,-0.42258002933251,
-0.419921706549396,-0.418090261206941,-0.416092750127235,-0.412729337964036,
-0.398469412503287,-0.357073354133918,-0.343504508377478,-0.338509941723328,
-0.335478742611898,-0.332207118541547,-0.327724727981747,-0.316813858900941,
-0.300552487738364,-0.28264373837956,-0.25810368914916,-0.254386489001736,
-0.252290780158785,-0.250471238260137,-0.24800950370595,-0.242260237354865,
-0.233867514389904,-0.204610844989118,-0.178869962029906,-0.172891292784176,
-0.169317285617291,-0.166091685045245,-0.161921924948362,-0.152913474476151,
-0.127226133212799,-0.0947870245274841,-0.0889866339693035,-0.0867034225230636,
-0.0848612479928007,-0.0828855227919735,-0.0796212086708388,-0.066794844031369,
-0.0427074182221363,-0.0122260965999769,-0.00636443773219676,-0.00292236187236719,
-0.000491642045001233),.UNSPECIFIED.);
#2861=B_SPLINE_CURVE_WITH_KNOTS('',3,(#118205,#118206,#118207,#118208,#118209,
#118210,#118211,#118212,#118213,#118214,#118215,#118216),.UNSPECIFIED.,
 .F.,.F.,(4,2,2,2,2,4),(-2.09991228399511,-2.0981766975392,-2.09536860074707,
-2.08896114076016,-2.05232170099698,-2.04098006789499),.UNSPECIFIED.);
#2862=B_SPLINE_CURVE_WITH_KNOTS('',3,(#118217,#118218,#118219,#118220,#118221,
#118222,#118223,#118224,#118225,#118226,#118227,#118228,#118229,#118230,
#118231,#118232,#118233,#118234,#118235,#118236,#118237,#118238,#118239,
#118240,#118241,#118242,#118243,#118244,#118245,#118246,#118247,#118248,
#118249,#118250,#118251,#118252,#118253,#118254,#118255,#118256,#118257,
#118258,#118259,#118260,#118261,#118262,#118263,#118264,#118265,#118266,
#118267,#118268,#118269,#118270,#118271,#118272,#118273,#118274,#118275,
#118276,#118277,#118278,#118279,#118280,#118281,#118282,#118283,#118284,
#118285,#118286,#118287,#118288,#118289,#118290,#118291,#118292,#118293,
#118294,#118295,#118296,#118297,#118298,#118299,#118300,#118301,#118302,
#118303,#118304,#118305,#118306,#118307,#118308,#118309,#118310,#118311,
#118312,#118313,#118314,#118315,#118316,#118317,#118318,#118319,#118320,
#118321,#118322,#118323,#118324,#118325,#118326,#118327,#118328,#118329,
#118330,#118331,#118332,#118333,#118334,#118335,#118336,#118337,#118338,
#118339,#118340,#118341,#118342,#118343,#118344,#118345,#118346,#118347,
#118348,#118349,#118350,#118351,#118352,#118353,#118354,#118355,#118356,
#118357,#118358,#118359,#118360,#118361,#118362,#118363,#118364,#118365,
#118366,#118367,#118368,#118369,#118370,#118371,#118372,#118373,#118374,
#118375,#118376,#118377,#118378,#118379,#118380,#118381,#118382,#118383,
#118384,#118385,#118386,#118387,#118388,#118389,#118390,#118391,#118392,
#118393,#118394,#118395,#118396,#118397,#118398,#118399,#118400,#118401,
#118402,#118403,#118404,#118405,#118406,#118407,#118408,#118409,#118410),
 .UNSPECIFIED.,.F.,.F.,(4,2,2,2,2,2,2,2,2,2,2,2,2,2,2,2,2,2,2,2,2,2,2,2,
2,2,2,2,2,2,2,2,2,2,2,2,2,2,2,2,2,2,2,2,2,2,2,2,2,2,2,2,2,2,2,2,2,2,2,2,
2,2,2,2,2,2,2,2,2,2,2,2,2,2,2,2,2,2,2,2,2,2,2,2,2,2,2,2,2,2,2,2,2,2,2,2,
4),(-3.85165705040524,-3.84773626708953,-3.84170348636172,-3.83720728714827,
-3.83497336099093,-3.83316793769921,-3.83089301598045,-3.82618549112559,
-3.79550069641113,-3.76200603729926,-3.75558970629686,-3.75192316520475,
-3.74871308777263,-3.74469671700828,-3.73834934471633,-3.69342273925938,
-3.67508294657127,-3.6704988670315,-3.66824772085402,-3.66644241898978,
-3.66418518826562,-3.65956975372796,-3.62737305006666,-3.59502640566234,
-3.58873073175417,-3.58508949428779,-3.5818760268942,-3.57782126255208,
-3.57134233279209,-3.52705805416671,-3.50838183381107,-3.50375932557205,
-3.50150069562743,-3.49969534882156,-3.49744548676033,-3.49286816583341,
-3.46018889526995,-3.42823556803621,-3.42195506515446,-3.41831697775172,
-3.41510297692661,-3.41104307937502,-3.4045466152527,-3.36034805304638,
-3.3416255366469,-3.33699773965129,-3.33473805978999,-3.33293267330861,
-3.33068375835262,-3.32611143923264,-3.29337438452813,-3.26191577247669,
-3.25538698090293,-3.25169674423949,-3.24848892995598,-3.24450540488065,
-3.23827053909956,-3.19889354396288,-3.17423895585541,-3.17000794674697,
-3.16782686271051,-3.16601885794631,-3.16368238497483,-3.15882464407283,
-3.13577803230431,-3.10759604463177,-3.09230455359476,-3.08725619975889,
-3.08387736472069,-3.08060255860486,-3.0759183254839,-3.06448126138436,
-3.02850150745686,-3.01355765144878,-3.00500111239543,-3.00214113029365,
-3.00025246372277,-2.99831260667428,-2.99521349854256,-2.9853718913831,
-2.95627064920763,-2.93697235825231,-2.92474164431994,-2.92006767763124,
-2.9167618460622,-2.91376968455636,-2.90899709029393,-2.89700330787531,
-2.85815267040784,-2.84563357950202,-2.83801740928312,-2.83527596055657,
-2.83341087066797,-2.83143641886148,-2.82817892831593,-2.81671901668128,
-2.80139424742162),.UNSPECIFIED.);
#2863=B_SPLINE_CURVE_WITH_KNOTS('',3,(#118415,#118416,#118417,#118418,#118419,
#118420,#118421,#118422,#118423,#118424,#118425,#118426,#118427,#118428,
#118429,#118430,#118431,#118432,#118433,#118434,#118435,#118436,#118437,
#118438,#118439,#118440,#118441,#118442,#118443,#118444,#118445,#118446,
#118447,#118448,#118449,#118450,#118451,#118452,#118453,#118454,#118455,
#118456,#118457,#118458,#118459,#118460,#118461,#118462,#118463,#118464,
#118465,#118466,#118467,#118468,#118469,#118470,#118471,#118472,#118473,
#118474,#118475,#118476,#118477,#118478,#118479,#118480,#118481,#118482,
#118483,#118484,#118485,#118486,#118487,#118488,#118489,#118490,#118491,
#118492,#118493,#118494,#118495,#118496,#118497,#118498,#118499,#118500,
#118501,#118502,#118503,#118504,#118505,#118506,#118507,#118508,#118509,
#118510,#118511,#118512,#118513,#118514,#118515,#118516,#118517,#118518,
#118519,#118520,#118521,#118522,#118523,#118524,#118525,#118526,#118527,
#118528,#118529,#118530,#118531,#118532,#118533,#118534,#118535,#118536,
#118537,#118538,#118539,#118540,#118541,#118542,#118543,#118544,#118545,
#118546,#118547,#118548,#118549,#118550,#118551,#118552,#118553,#118554,
#118555,#118556,#118557,#118558,#118559,#118560,#118561,#118562,#118563,
#118564,#118565,#118566,#118567,#118568,#118569,#118570,#118571,#118572,
#118573,#118574,#118575,#118576,#118577,#118578,#118579,#118580,#118581,
#118582,#118583,#118584,#118585,#118586,#118587,#118588,#118589,#118590,
#118591,#118592,#118593,#118594,#118595,#118596,#118597,#118598,#118599,
#118600,#118601,#118602,#118603,#118604,#118605,#118606,#118607,#118608,
#118609,#118610,#118611,#118612,#118613,#118614,#118615,#118616,#118617,
#118618,#118619,#118620,#118621,#118622),.UNSPECIFIED.,.F.,.F.,(4,2,2,2,
2,2,2,2,2,2,2,2,2,2,2,2,2,2,2,2,2,2,2,2,2,2,2,2,2,2,2,2,2,2,2,2,2,2,2,2,
2,2,2,2,2,2,2,2,2,2,2,2,2,2,2,2,2,2,2,2,2,2,2,2,2,2,2,2,2,2,2,2,2,2,2,2,
2,2,2,2,2,2,2,2,2,2,2,2,2,2,2,2,2,2,2,2,2,2,2,2,2,2,2,4),(-2.04123955694236,
-2.01327501084785,-2.00679074355191,-2.00310945529361,-1.99990017148169,
-1.99590272256132,-1.98962155099611,-1.9506852467667,-1.92569508725374,
-1.92146217165324,-1.91928049978993,-1.91747221512462,-1.91513556324801,
-1.91027792484376,-1.88593457720521,-1.86376311785202,-1.85095801790333,
-1.84174363074351,-1.83753691654822,-1.83430588785183,-1.83074906089007,
-1.82485459557057,-1.80010304267298,-1.76991672286717,-1.76140482883313,
-1.75559528866267,-1.75312304129038,-1.75130172600092,-1.74921100262007,
-1.74551774366588,-1.72352468874556,-1.71925502626877,-1.69708222718193,
-1.68428057181914,-1.67506800306226,-1.67086162494451,-1.66763065960917,
-1.66407370809877,-1.65817857445507,-1.63340415052541,-1.6032382173864,
-1.5947289241423,-1.58892068591823,-1.58644866549858,-1.5846273881578,-1.5825365565741,
-1.57884278307905,-1.55670484848467,-1.55254233311288,-1.53035892953634,
-1.51758528106422,-1.50838738289188,-1.5041835748061,-1.50095295246795,
-1.49739474956413,-1.49149366469679,-1.46651784237616,-1.43652744124927,
-1.42804036269385,-1.4222431656361,-1.41977299473349,-1.41795195925015,
-1.41586010095475,-1.41216169650971,-1.38892565404076,-1.38639127722076,
-1.36357218520573,-1.35086214106202,-1.34169761278491,-1.33749966044732,
-1.33426981455549,-1.33070874082922,-1.32479400527926,-1.29929036373455,
-1.27861601125049,-1.26460256702155,-1.25639487085693,-1.25357719866206,
-1.25169701972495,-1.24998363870439,-1.24706102653929,-1.23869241426644,
-1.20526110597922,-1.18756357370876,-1.17969819538669,-1.17331823412724,
-1.16965889852808,-1.16644724285562,-1.16241841512708,-1.15602972836495,
-1.11818667978574,-1.09231760570813,-1.08808005212805,-1.08589749888602,
-1.08408936332077,-1.08175403657471,-1.07690282671219,-1.05045357632628,
-1.0144885612206,-1.007954313239,-1.0038831925696,-1.00066771132886,-0.997035755158936,
-0.991352361073962),.UNSPECIFIED.);
#2864=B_SPLINE_CURVE_WITH_KNOTS('',3,(#118623,#118624,#118625,#118626,#118627,
#118628,#118629,#118630,#118631,#118632,#118633,#118634,#118635,#118636,
#118637,#118638,#118639,#118640,#118641,#118642,#118643,#118644,#118645,
#118646,#118647,#118648,#118649,#118650,#118651,#118652,#118653,#118654,
#118655,#118656,#118657,#118658,#118659,#118660,#118661,#118662,#118663,
#118664,#118665,#118666,#118667,#118668,#118669,#118670,#118671,#118672,
#118673,#118674,#118675,#118676,#118677,#118678,#118679,#118680,#118681,
#118682,#118683,#118684,#118685,#118686,#118687,#118688,#118689,#118690,
#118691,#118692,#118693,#118694,#118695,#118696,#118697,#118698,#118699,
#118700,#118701,#118702,#118703,#118704,#118705,#118706,#118707,#118708,
#118709,#118710,#118711,#118712,#118713,#118714,#118715,#118716,#118717,
#118718,#118719,#118720,#118721,#118722,#118723,#118724,#118725,#118726,
#118727,#118728,#118729,#118730,#118731,#118732,#118733,#118734,#118735,
#118736,#118737,#118738,#118739,#118740,#118741,#118742,#118743,#118744,
#118745,#118746,#118747,#118748,#118749,#118750,#118751,#118752,#118753,
#118754,#118755,#118756,#118757,#118758,#118759,#118760,#118761,#118762,
#118763,#118764,#118765,#118766,#118767,#118768,#118769,#118770,#118771,
#118772,#118773,#118774,#118775,#118776,#118777,#118778,#118779,#118780,
#118781,#118782,#118783,#118784,#118785,#118786,#118787,#118788,#118789,
#118790,#118791,#118792,#118793,#118794,#118795,#118796,#118797,#118798,
#118799,#118800,#118801,#118802,#118803,#118804,#118805,#118806,#118807,
#118808,#118809,#118810,#118811,#118812,#118813,#118814,#118815,#118816,
#118817,#118818,#118819,#118820,#118821,#118822,#118823,#118824,#118825,
#118826,#118827,#118828,#118829,#118830),.UNSPECIFIED.,.F.,.F.,(4,2,2,2,
2,2,2,2,2,2,2,2,2,2,2,2,2,2,2,2,2,2,2,2,2,2,2,2,2,2,2,2,2,2,2,2,2,2,2,2,
2,2,2,2,2,2,2,2,2,2,2,2,2,2,2,2,2,2,2,2,2,2,2,2,2,2,2,2,2,2,2,2,2,2,2,2,
2,2,2,2,2,2,2,2,2,2,2,2,2,2,2,2,2,2,2,2,2,2,2,2,2,2,2,4),(-2.80139424742162,
-2.78879988481108,-2.76059118451529,-2.75468573714338,-2.75112695351419,
-2.7478971404036,-2.74376640214512,-2.73472788769955,-2.69208714102528,
-2.67912025544343,-2.67132247751412,-2.66855705497056,-2.66668731004663,
-2.66496282540459,-2.66198230834239,-2.65315624447851,-2.62327143071968,
-2.59897543857137,-2.58997243766197,-2.58580315645675,-2.58257717533914,
-2.57900201601199,-2.57301969250743,-2.54358894258563,-2.52138064730654,
-2.51097123635177,-2.50426305974586,-2.5016495181741,-2.49980749003473,
-2.49778603533429,-2.49431287701566,-2.48006188648858,-2.44972465011842,
-2.42668927079624,-2.42101499953902,-2.41750539194453,-2.41426116266904,
-2.40995431598043,-2.40014826329148,-2.38618880427075,-2.36563868474424,
-2.3625331492555,-2.33981071641887,-2.33611569806529,-2.33402482029518,
-2.33220405294256,-2.32973347922363,-2.32393224533036,-2.31543573385929,
-2.28538439452081,-2.26043431254946,-2.25453367291383,-2.25097603889298,
-2.24774616505472,-2.24354369600926,-2.23435035092273,-2.22158656367306,
-2.19941354038118,-2.19533658760213,-2.17311683009265,-2.16942380250306,
-2.1673334092204,-2.16551258808853,-2.1630413201258,-2.15723576975335,-2.14873051427573,
-2.11860951176809,-2.09374024754866,-2.08784205241695,-2.08428496192231,
-2.08105499242064,-2.07685155247179,-2.06765247109752,-2.05487764317136,
-2.03270916866623,-2.02857009567257,-2.00642906012432,-2.00273635625956,
-2.00064603668727,-1.99882515297661,-1.99635364640066,-1.99054693353229,
-1.98203934201765,-1.95189874177632,-1.92705684519228,-1.92115955207053,
-1.91760263146637,-1.9143725745099,-1.91016866896318,-1.90096704712059,
-1.88818741556761,-1.86602095158355,-1.86185377720641,-1.83974773467214,
-1.83605522742889,-1.83396497793084,-1.83214430146993,-1.82967317323945,
-1.82386741517223,-1.815361459849,-1.78523282504622,-1.76037274810103,-1.75447527727419,
-1.75139041054252),.UNSPECIFIED.);
#2865=B_SPLINE_CURVE_WITH_KNOTS('',3,(#118836,#118837,#118838,#118839,#118840,
#118841,#118842,#118843,#118844,#118845,#118846,#118847,#118848,#118849,
#118850,#118851,#118852,#118853,#118854,#118855,#118856,#118857,#118858,
#118859,#118860,#118861,#118862,#118863,#118864,#118865,#118866,#118867,
#118868,#118869,#118870,#118871,#118872,#118873,#118874,#118875,#118876,
#118877,#118878,#118879,#118880,#118881,#118882,#118883,#118884,#118885,
#118886,#118887,#118888,#118889,#118890,#118891,#118892,#118893,#118894,
#118895,#118896,#118897,#118898,#118899,#118900,#118901,#118902,#118903,
#118904,#118905,#118906,#118907,#118908,#118909,#118910,#118911,#118912,
#118913,#118914,#118915,#118916,#118917,#118918,#118919,#118920,#118921,
#118922,#118923,#118924,#118925,#118926,#118927,#118928,#118929,#118930,
#118931,#118932,#118933,#118934,#118935,#118936,#118937,#118938,#118939,
#118940,#118941,#118942,#118943,#118944,#118945,#118946,#118947,#118948,
#118949,#118950,#118951,#118952,#118953,#118954,#118955,#118956,#118957,
#118958,#118959,#118960,#118961,#118962,#118963,#118964,#118965),
 .UNSPECIFIED.,.F.,.F.,(4,2,2,2,2,2,2,2,2,2,2,2,2,2,2,2,2,2,2,2,2,2,2,2,
2,2,2,2,2,2,2,2,2,2,2,2,2,2,2,2,2,2,2,2,2,2,2,2,2,2,2,2,2,2,2,2,2,2,2,2,
2,2,2,2,4),(-0.701622587363262,-0.69782520809542,-0.674829255171103,-0.669922846048609,
-0.667616398149043,-0.665811282498163,-0.663608201244988,-0.659287945074347,
-0.630959998494923,-0.595874548539514,-0.589266617774786,-0.585162989422959,
-0.581929453747833,-0.578284673240364,-0.572030341479378,-0.538732930775711,
-0.507736833265961,-0.503053466152945,-0.500771249654345,-0.498936855248173,
-0.496634187412443,-0.491925021622171,-0.47271714137948,-0.438767709036483,
-0.426269118459773,-0.421396439902457,-0.41836328394742,-0.415028341171548,
-0.410341821925662,-0.398238653475179,-0.379359681618992,-0.35152676465907,
-0.339810678256997,-0.336535629198157,-0.33456067082642,-0.332769732602333,
-0.330225049012681,-0.323393145686127,-0.286831973998349,-0.258805743436394,
-0.252937601621296,-0.249485437965486,-0.246408799842315,-0.242490682540656,
-0.234287538356714,-0.210701559508584,-0.183370211347027,-0.171493461538258,
-0.168263425178072,-0.166329600535944,-0.164466454136752,-0.161776174892017,
-0.154649964298831,-0.116968940589261,-0.0871764818775304,-0.0806335737492376,
-0.0766880313159956,-0.073094175717419,-0.068380569947616,-0.0576891236866487,
-0.0323137982564055,-0.00779173997406027,-0.00345811667600707,-0.00158327751243333,
-5.87629350645707E-5),.UNSPECIFIED.);
#2866=B_SPLINE_CURVE_WITH_KNOTS('',3,(#118968,#118969,#118970,#118971,#118972,
#118973,#118974,#118975,#118976,#118977,#118978,#118979,#118980,#118981,
#118982,#118983,#118984,#118985,#118986,#118987,#118988,#118989,#118990,
#118991,#118992,#118993,#118994,#118995,#118996,#118997,#118998,#118999,
#119000,#119001,#119002,#119003,#119004,#119005,#119006,#119007,#119008,
#119009,#119010,#119011,#119012,#119013,#119014,#119015,#119016,#119017,
#119018,#119019,#119020,#119021,#119022,#119023,#119024,#119025,#119026,
#119027,#119028,#119029,#119030,#119031,#119032,#119033,#119034,#119035,
#119036,#119037,#119038,#119039,#119040,#119041,#119042,#119043,#119044,
#119045,#119046,#119047,#119048,#119049,#119050,#119051,#119052,#119053,
#119054,#119055,#119056,#119057,#119058,#119059,#119060,#119061,#119062,
#119063,#119064,#119065,#119066,#119067,#119068,#119069,#119070,#119071,
#119072,#119073,#119074,#119075,#119076,#119077,#119078,#119079,#119080,
#119081,#119082,#119083,#119084,#119085,#119086,#119087,#119088,#119089,
#119090,#119091,#119092,#119093,#119094,#119095,#119096,#119097,#119098,
#119099,#119100,#119101,#119102,#119103,#119104,#119105,#119106,#119107,
#119108,#119109,#119110,#119111,#119112,#119113,#119114,#119115,#119116,
#119117,#119118,#119119,#119120,#119121,#119122,#119123,#119124,#119125,
#119126,#119127,#119128,#119129,#119130,#119131,#119132,#119133,#119134,
#119135,#119136,#119137,#119138,#119139,#119140,#119141,#119142,#119143,
#119144,#119145,#119146,#119147,#119148,#119149,#119150,#119151,#119152,
#119153,#119154,#119155),.UNSPECIFIED.,.F.,.F.,(4,2,2,2,2,2,2,2,2,2,2,2,
2,2,2,2,2,2,2,2,2,2,2,2,2,2,2,2,2,2,2,2,2,2,2,2,2,2,2,2,2,2,2,2,2,2,2,2,
2,2,2,2,2,2,2,2,2,2,2,2,2,2,2,2,2,2,2,2,2,2,2,2,2,2,2,2,2,2,2,2,2,2,2,2,
2,2,2,2,2,2,2,2,2,4),(-1.97963597789807,-1.97911067462062,-1.97224667709571,
-1.93765234953483,-1.91989061416732,-1.91197821045077,-1.9055506793358,
-1.9018562152793,-1.8986078498892,-1.89452319207106,-1.88801757096771,-1.85356143477461,
-1.8263655964811,-1.82198065731588,-1.81974157734617,-1.81790619020366,
-1.8155529425272,-1.81067156433301,-1.78639735018608,-1.76444854551698,
-1.75161386122014,-1.74237922748276,-1.73815580252188,-1.73490801345122,
-1.73132830795588,-1.7253841935851,-1.699589449833,-1.67019323447981,-1.66177185612889,
-1.65600305061343,-1.65353308438504,-1.65171121529384,-1.6496247175336,
-1.64592526592048,-1.62182019415646,-1.62032066973509,-1.59985864135478,
-1.58571524772036,-1.57582953022289,-1.57152386326298,-1.56829467044939,
-1.56481536620152,-1.55922304091608,-1.53963040587853,-1.49637493856359,
-1.48949938211316,-1.48687155964858,-1.48503396364113,-1.4830266243612,
-1.47961824512937,-1.46635505603671,-1.43972422161585,-1.42141361064092,
-1.40959049038942,-1.40496920547385,-1.40166911105502,-1.39866083063639,
-1.39381505113879,-1.38135377026963,-1.34650958156531,-1.3319022443993,
-1.32617103933515,-1.32184531493975,-1.31964157356574,-1.31783128421811,
-1.31551153706946,-1.31057397859131,-1.28586393467364,-1.25896291674913,
-1.24895028845789,-1.24127410510196,-1.23735060493909,-1.23414477678659,
-1.23040459988526,-1.22382601853695,-1.1824229670469,-1.16601160169481,
-1.15693324864388,-1.15401263966414,-1.15211117226386,-1.15041776427746,
-1.1475982143147,-1.13998043185423,-1.10913161968521,-1.08425772901165,
-1.07526848621783,-1.07110341817376,-1.06787988252065,-1.06430665059646,
-1.05832579086072,-1.02900642671826,-1.00699144824307,-0.991285459946718,
-0.991277804245244),.UNSPECIFIED.);
#2867=B_SPLINE_CURVE_WITH_KNOTS('',3,(#119161,#119162,#119163,#119164,#119165,
#119166,#119167,#119168,#119169,#119170,#119171,#119172,#119173,#119174,
#119175,#119176,#119177,#119178,#119179,#119180,#119181,#119182,#119183,
#119184,#119185,#119186,#119187,#119188,#119189,#119190,#119191,#119192,
#119193,#119194,#119195,#119196,#119197,#119198,#119199,#119200,#119201,
#119202,#119203,#119204,#119205,#119206,#119207,#119208,#119209,#119210,
#119211,#119212,#119213,#119214,#119215,#119216,#119217,#119218,#119219,
#119220,#119221,#119222,#119223,#119224,#119225,#119226,#119227,#119228,
#119229,#119230,#119231,#119232,#119233,#119234),.UNSPECIFIED.,.F.,.F.,
(4,2,2,2,2,2,2,2,2,2,2,2,2,2,2,2,2,2,2,2,2,2,2,2,2,2,2,2,2,2,2,2,2,2,2,
2,4),(-0.358752339019158,-0.35758003104028,-0.340398688796483,-0.336826897283715,
-0.33476676533837,-0.333010439188268,-0.330665170257151,-0.325132231676164,
-0.31707514359999,-0.290061737059928,-0.258856486316567,-0.25295401397713,
-0.249494058015947,-0.246417937613128,-0.242510640506838,-0.234368903731933,
-0.199769648266984,-0.174157594760246,-0.169316644024535,-0.167058190656923,
-0.165265662645593,-0.163073803167974,-0.158845281495978,-0.153310662188677,
-0.139694106829365,-0.103511073302855,-0.0857756328518154,-0.0799370029750358,
-0.0761379594961528,-0.0724812087849253,-0.0673685912890846,-0.0538912888095538,
-0.030966518726725,-0.00771475696196283,-0.00343253357673936,-0.00157316844153016,
-5.8766376665821E-5),.UNSPECIFIED.);
#2868=B_SPLINE_CURVE_WITH_KNOTS('',3,(#119237,#119238,#119239,#119240,#119241,
#119242,#119243,#119244,#119245,#119246,#119247,#119248,#119249,#119250,
#119251,#119252,#119253,#119254,#119255,#119256,#119257,#119258,#119259,
#119260,#119261,#119262,#119263,#119264,#119265,#119266,#119267,#119268,
#119269,#119270,#119271,#119272,#119273,#119274,#119275,#119276,#119277,
#119278,#119279,#119280,#119281,#119282,#119283,#119284,#119285,#119286,
#119287,#119288,#119289,#119290,#119291,#119292,#119293,#119294,#119295,
#119296,#119297,#119298,#119299,#119300,#119301,#119302,#119303,#119304,
#119305,#119306,#119307,#119308,#119309,#119310,#119311,#119312,#119313,
#119314,#119315,#119316,#119317,#119318,#119319,#119320,#119321,#119322,
#119323,#119324,#119325,#119326,#119327,#119328,#119329,#119330,#119331,
#119332,#119333,#119334,#119335,#119336,#119337,#119338,#119339,#119340,
#119341,#119342,#119343,#119344,#119345,#119346,#119347,#119348,#119349,
#119350,#119351,#119352,#119353,#119354,#119355,#119356,#119357,#119358),
 .UNSPECIFIED.,.F.,.F.,(4,2,2,2,2,2,2,2,2,2,2,2,2,2,2,2,2,2,2,2,2,2,2,2,
2,2,2,2,2,2,2,2,2,2,2,2,2,2,2,2,2,2,2,2,2,2,2,2,2,2,2,2,2,2,2,2,2,2,2,2,
4),(-1.75473859914493,-1.75154088040687,-1.72689079662622,-1.70467625101938,
-1.69173746421963,-1.68242362321274,-1.67817272951846,-1.67490672226881,
-1.67130890727376,-1.66533530028674,-1.63676084184676,-1.61487708686701,
-1.5998560152629,-1.59640767418699,-1.59436566649252,-1.59251150052433,
-1.59024704870894,-1.58578837015164,-1.56116797072278,-1.53901736556639,
-1.52648093052477,-1.51740303061522,-1.51320745070685,-1.50996354794196,
-1.50637047787112,-1.50036170283648,-1.47112902592979,-1.44979535915428,
-1.43862692122266,-1.43157598618139,-1.42890757062421,-1.42705372906987,
-1.42506024854931,-1.42168964849452,-1.40884212253478,-1.38191893140923,
-1.36350388087488,-1.35165518326397,-1.34705047948789,-1.34377172622376,
-1.34039291048129,-1.33527761912014,-1.32051306287125,-1.2844406463443,
-1.27225590916121,-1.26478465725884,-1.26207378716518,-1.26022197076231,
-1.25824532632989,-1.25497638312579,-1.24337961458778,-1.21178438857809,
-1.19536079393811,-1.18437122843983,-1.17987288167479,-1.1765948503032,
-1.17356125046985,-1.16857057843087,-1.15505860396329,-1.12118637585851,
-1.10916127312679),.UNSPECIFIED.);
#2869=B_SPLINE_CURVE_WITH_KNOTS('',3,(#119363,#119364,#119365,#119366,#119367,
#119368,#119369,#119370,#119371,#119372,#119373,#119374,#119375,#119376,
#119377,#119378,#119379,#119380,#119381,#119382,#119383,#119384,#119385,
#119386,#119387,#119388,#119389,#119390,#119391,#119392,#119393,#119394,
#119395,#119396,#119397,#119398,#119399,#119400,#119401,#119402,#119403,
#119404,#119405,#119406,#119407,#119408,#119409,#119410,#119411,#119412,
#119413,#119414,#119415,#119416,#119417,#119418,#119419,#119420,#119421,
#119422,#119423,#119424,#119425,#119426,#119427,#119428,#119429,#119430,
#119431,#119432,#119433,#119434,#119435,#119436,#119437,#119438,#119439,
#119440,#119441,#119442,#119443,#119444,#119445,#119446,#119447,#119448,
#119449,#119450,#119451,#119452,#119453,#119454,#119455,#119456,#119457,
#119458,#119459,#119460,#119461,#119462,#119463,#119464,#119465,#119466,
#119467,#119468,#119469,#119470,#119471,#119472,#119473,#119474,#119475,
#119476,#119477,#119478,#119479,#119480,#119481,#119482,#119483,#119484,
#119485,#119486,#119487,#119488,#119489,#119490,#119491,#119492,#119493,
#119494,#119495,#119496,#119497,#119498,#119499,#119500,#119501,#119502,
#119503,#119504,#119505,#119506,#119507,#119508,#119509,#119510,#119511,
#119512,#119513,#119514,#119515,#119516,#119517,#119518,#119519,#119520,
#119521,#119522,#119523,#119524,#119525,#119526,#119527,#119528,#119529,
#119530,#119531,#119532,#119533,#119534,#119535,#119536,#119537,#119538,
#119539,#119540,#119541,#119542,#119543,#119544,#119545,#119546,#119547,
#119548,#119549,#119550,#119551,#119552,#119553,#119554,#119555,#119556,
#119557,#119558,#119559,#119560,#119561,#119562,#119563,#119564,#119565,
#119566),.UNSPECIFIED.,.F.,.F.,(4,2,2,2,2,2,2,2,2,2,2,2,2,2,2,2,2,2,2,2,
2,2,2,2,2,2,2,2,2,2,2,2,2,2,2,2,2,2,2,2,2,2,2,2,2,2,2,2,2,2,2,2,2,2,2,2,
2,2,2,2,2,2,2,2,2,2,2,2,2,2,2,2,2,2,2,2,2,2,2,2,2,2,2,2,2,2,2,2,2,2,2,2,
2,2,2,2,2,2,2,2,2,4),(-1.4082992289097,-1.4006552888223,-1.3878393759836,
-1.36569920472157,-1.36139004195681,-1.33948882989881,-1.33579769323099,
-1.33370781087495,-1.33188807180438,-1.32941841755152,-1.32361485359034,
-1.31511156287969,-1.28499140100962,-1.26012140732392,-1.25422612287674,
-1.25067145026165,-1.24744414566674,-1.24324490224264,-1.23405843495863,
-1.22130441803123,-1.1991395030373,-1.1951252761621,-1.17284887851717,-1.16915780297844,
-1.16706871220799,-1.16524829673333,-1.162777307309,-1.15697344907893,-1.14847158070023,
-1.11837615034095,-1.09347778154855,-1.08757753858206,-1.08401920986116,
-1.08078805620498,-1.07658290187221,-1.0673785916205,-1.05459309089071,
-1.03245285482807,-1.02830520677559,-1.00622478069049,-1.00253116757083,
-1.00043958145166,-0.99861445840005,-0.996133848230994,-0.990294586525929,
-0.981724246627302,-0.951048798860375,-0.927028553861187,-0.921159335391849,
-0.917605115086725,-0.914368165997088,-0.910141523679551,-0.900829494129505,
-0.85647447470958,-0.839503876800746,-0.835920270476699,-0.833854517442367,
-0.832036735584689,-0.829539355501921,-0.823514827105592,-0.814550871432306,
-0.780451195333079,-0.759627894309259,-0.753970985735232,-0.750478125285507,
-0.747253981141342,-0.742981431706823,-0.733293912473096,-0.719547665976067,
-0.698716209736333,-0.695034411371129,-0.672818392628126,-0.66913584587516,
-0.667053237701345,-0.665230692390564,-0.662754472044112,-0.656947526264486,
-0.648448269514703,-0.618457088136563,-0.593327152240948,-0.587399045923802,
-0.583822979777057,-0.580574709162931,-0.576345221812675,-0.567073941984854,
-0.554170094308864,-0.53228738943782,-0.528695248397369,-0.506193517731935,
-0.502481013139736,-0.500375016286649,-0.498518315441251,-0.495976296299316,
-0.489921469046412,-0.454074013905421,-0.428429311324733,-0.422512079111116,
-0.418926209619868,-0.415657034357046,-0.411381726273356,-0.401926205740997,
-0.358752339019158),.UNSPECIFIED.);
#2870=B_SPLINE_CURVE_WITH_KNOTS('',3,(#119567,#119568,#119569,#119570,#119571,
#119572,#119573,#119574,#119575,#119576,#119577,#119578,#119579,#119580,
#119581,#119582,#119583,#119584,#119585,#119586,#119587,#119588,#119589,
#119590,#119591,#119592,#119593,#119594,#119595,#119596,#119597,#119598,
#119599,#119600,#119601,#119602,#119603,#119604,#119605,#119606,#119607,
#119608,#119609,#119610,#119611,#119612,#119613,#119614,#119615,#119616,
#119617,#119618,#119619,#119620,#119621,#119622,#119623,#119624,#119625,
#119626,#119627,#119628,#119629,#119630,#119631,#119632,#119633,#119634,
#119635,#119636,#119637,#119638,#119639,#119640,#119641,#119642,#119643,
#119644,#119645,#119646,#119647,#119648,#119649,#119650,#119651,#119652,
#119653,#119654,#119655,#119656,#119657,#119658,#119659,#119660,#119661,
#119662,#119663,#119664,#119665,#119666,#119667,#119668,#119669,#119670,
#119671,#119672,#119673,#119674,#119675,#119676,#119677,#119678,#119679,
#119680,#119681,#119682,#119683,#119684,#119685,#119686,#119687,#119688,
#119689,#119690,#119691,#119692,#119693,#119694,#119695,#119696,#119697,
#119698,#119699,#119700,#119701,#119702,#119703,#119704,#119705,#119706,
#119707,#119708,#119709,#119710,#119711,#119712,#119713,#119714,#119715,
#119716,#119717,#119718,#119719,#119720,#119721,#119722,#119723,#119724,
#119725,#119726,#119727,#119728,#119729,#119730,#119731,#119732,#119733,
#119734,#119735,#119736,#119737,#119738,#119739,#119740,#119741,#119742,
#119743,#119744,#119745,#119746,#119747,#119748,#119749,#119750,#119751,
#119752,#119753,#119754,#119755,#119756,#119757,#119758,#119759,#119760,
#119761,#119762,#119763,#119764,#119765,#119766,#119767,#119768,#119769,
#119770,#119771,#119772,#119773,#119774,#119775,#119776,#119777,#119778,
#119779,#119780,#119781,#119782,#119783,#119784),.UNSPECIFIED.,.F.,.F.,
(4,2,2,2,2,2,2,2,2,2,2,2,2,2,2,2,2,2,2,2,2,2,2,2,2,2,2,2,2,2,2,2,2,2,2,
2,2,2,2,2,2,2,2,2,2,2,2,2,2,2,2,2,2,2,2,2,2,2,2,2,2,2,2,2,2,2,2,2,2,2,2,
2,2,2,2,2,2,2,2,2,2,2,2,2,2,2,2,2,2,2,2,2,2,2,2,2,2,2,2,2,2,2,2,2,2,2,2,
2,4),(-1.10916127312679,-1.10684992829868,-1.09851897869292,-1.09568224371337,
-1.09379526882295,-1.09208276821439,-1.08916905046944,-1.08087619471203,
-1.05058953079179,-1.02100908595183,-1.01506303853347,-1.01149523805187,
-1.00826689314242,-1.00415120741369,-0.995201347428553,-0.952436126518047,
-0.93945480919547,-0.931651379837895,-0.928885507616449,-0.927016043747836,
-0.925051226932677,-0.921832938457102,-0.910792826002045,-0.878916108873371,
-0.854168052641419,-0.848277081248516,-0.84472359077435,-0.841496482060365,
-0.837296272257313,-0.828102860813718,-0.81533635407929,-0.793159258660976,
-0.789112536219431,-0.766859675684666,-0.763168752377515,-0.761080089928424,
-0.759260204177435,-0.756790363183674,-0.750991523428633,-0.742499095167402,
-0.71247119994093,-0.68750691652322,-0.681606340209787,-0.678048807414275,
-0.67481903875931,-0.670616685451146,-0.661423164336513,-0.64865779563753,
-0.626502259855582,-0.622360491332471,-0.60023525072509,-0.596543066681321,
-0.594452742674484,-0.592631978737739,-0.590160421532918,-0.584351603822365,
-0.575839099370099,-0.545650940385055,-0.520879550394758,-0.514985748646116,
-0.51143015604782,-0.508200813862756,-0.503997136345933,-0.494793055567726,
-0.482007651843694,-0.459848394515748,-0.455649654479213,-0.433590903204346,
-0.429899480218252,-0.42780983088922,-0.425989623366819,-0.423519102918438,
-0.417714764405128,-0.409210841403266,-0.379088193343223,-0.354238617680801,
-0.348342837619647,-0.34478712940166,-0.341558375964348,-0.337356472947442,
-0.328160640260706,-0.315390415839926,-0.293226997624212,-0.289097950171124,
-0.266951707406135,-0.263260239378087,-0.261170692832636,-0.25935047358136,
-0.256879939267643,-0.251076042327961,-0.2425731240137,-0.212458766561942,
-0.18758130092732,-0.181695530236592,-0.178141748568729,-0.174912128415632,
-0.17070532208897,-0.16148252732833,-0.148660855434975,-0.126636360293058,
-0.122694179406678,-0.100322084771383,-0.0966296456084877,-0.0945397446247031,
-0.0927195097909353,-0.0902491939164962,-0.0844464209777026,-0.0759456971816959,
-0.059479256607861),.UNSPECIFIED.);
#2871=B_SPLINE_CURVE_WITH_KNOTS('',3,(#119789,#119790,#119791,#119792,#119793,
#119794,#119795,#119796,#119797,#119798,#119799,#119800,#119801,#119802,
#119803,#119804,#119805,#119806,#119807,#119808,#119809,#119810,#119811,
#119812,#119813,#119814,#119815,#119816,#119817,#119818,#119819,#119820,
#119821,#119822,#119823,#119824,#119825,#119826,#119827,#119828,#119829,
#119830,#119831,#119832,#119833,#119834,#119835,#119836,#119837,#119838,
#119839,#119840,#119841,#119842,#119843,#119844,#119845,#119846,#119847,
#119848,#119849,#119850,#119851,#119852,#119853,#119854,#119855,#119856,
#119857,#119858,#119859,#119860,#119861,#119862,#119863,#119864,#119865,
#119866,#119867,#119868,#119869,#119870,#119871,#119872,#119873,#119874,
#119875,#119876,#119877,#119878,#119879,#119880,#119881,#119882,#119883,
#119884,#119885,#119886,#119887,#119888,#119889,#119890,#119891,#119892,
#119893,#119894,#119895,#119896,#119897,#119898,#119899,#119900,#119901,
#119902,#119903,#119904,#119905,#119906,#119907,#119908,#119909,#119910,
#119911,#119912,#119913,#119914,#119915,#119916,#119917,#119918,#119919,
#119920,#119921,#119922,#119923,#119924,#119925,#119926,#119927,#119928,
#119929,#119930,#119931,#119932,#119933,#119934,#119935,#119936,#119937,
#119938,#119939,#119940,#119941,#119942,#119943,#119944,#119945,#119946,
#119947,#119948,#119949,#119950,#119951,#119952,#119953,#119954,#119955,
#119956,#119957,#119958,#119959,#119960,#119961,#119962,#119963,#119964,
#119965,#119966,#119967,#119968,#119969,#119970,#119971,#119972,#119973,
#119974,#119975,#119976,#119977,#119978,#119979,#119980,#119981,#119982,
#119983,#119984,#119985,#119986,#119987,#119988,#119989,#119990,#119991,
#119992,#119993,#119994,#119995,#119996,#119997,#119998,#119999,#120000,
#120001,#120002),.UNSPECIFIED.,.F.,.F.,(4,2,2,2,2,2,2,2,2,2,2,2,2,2,2,2,
2,2,2,2,2,2,2,2,2,2,2,2,2,2,2,2,2,2,2,2,2,2,2,2,2,2,2,2,2,2,2,2,2,2,2,2,
2,2,2,2,2,2,2,2,2,2,2,2,2,2,2,2,2,2,2,2,2,2,2,2,2,2,2,2,2,2,2,2,2,2,2,2,
2,2,2,2,2,2,2,2,2,2,2,2,2,2,2,2,2,2,4),(-2.45787557075319,-2.4560892806585,
-2.43171211345447,-2.42270830022384,-2.41853906802341,-2.41531325268146,
-2.41173837894919,-2.40575670094468,-2.37569865246704,-2.35160629332699,
-2.34273784398871,-2.33675330716433,-2.33425255668742,-2.33242782833755,
-2.33035348416521,-2.32673194141415,-2.30807580213373,-2.26742523312263,
-2.25699742029425,-2.25291250078726,-2.24990328817644,-2.2466144910873,
-2.24203251229508,-2.23045027627985,-2.21268728113272,-2.17918595748121,
-2.17099751766033,-2.16809907310687,-2.16639057692035,-2.16450635358482,
-2.1616670611253,-2.15328020122357,-2.13879036408145,-2.10444614120628,
-2.09129183178161,-2.08635250401723,-2.08333129942591,-2.08005233564363,
-2.07552660338358,-2.06432774102652,-2.04743252989996,-2.01522869464926,
-2.00487887289385,-2.00172563327065,-1.99977413889167,-1.99789453183547,
-1.9950783105745,-1.98687966763053,-1.97288679736377,-1.95223340085464,
-1.92666144498823,-1.92074551811907,-1.91718469412539,-1.91395569200765,
-1.90975971082744,-1.90060298394815,-1.88790836033308,-1.8651344733792,
-1.8622507540964,-1.8393474606752,-1.83565233377208,-1.83356152749511,-1.83174099303775,
-1.82927081431317,-1.82347048632978,-1.81497508977261,-1.784921688362,-1.75999778692551,
-1.75409907118345,-1.75054219294227,-1.7473127287515,-1.74311037006333,
-1.73391528472747,-1.72114704352049,-1.6989866899069,-1.69486658782451,
-1.6727145166617,-1.66902258671762,-1.66693262314929,-1.66511194493657,
-1.6626405471572,-1.6568333348081,-1.64832419526621,-1.61816304597322,-1.59336181147711,
-1.58746641563755,-1.58391003210748,-1.58068005412256,-1.57647563126804,
-1.56726997763091,-1.55448165977799,-1.532331331972,-1.52812840508173,-1.50608969203846,
-1.50239788585388,-1.5003077536233,-1.49848644795217,-1.49601362949135,
-1.49020097915688,-1.48168129722469,-1.45143239026524,-1.42676137799863,
-1.42087009445924,-1.41731418862032,-1.41408334031537,-1.40987587801174,
-1.4082992289097),.UNSPECIFIED.);
#2872=B_SPLINE_CURVE_WITH_KNOTS('',3,(#120004,#120005,#120006,#120007,#120008,
#120009,#120010,#120011,#120012,#120013,#120014,#120015,#120016,#120017,
#120018,#120019),.UNSPECIFIED.,.F.,.F.,(4,2,2,2,2,2,2,4),(-0.059479256607861,
-0.0341344807334151,-0.0193900327960261,-0.0142709742838432,-0.0108788420291215,
-0.00783988787161742,-0.00425775755582772,-0.000493436327504615),
 .UNSPECIFIED.);
#2873=B_SPLINE_CURVE_WITH_KNOTS('',3,(#120020,#120021,#120022,#120023,#120024,
#120025,#120026,#120027,#120028,#120029,#120030,#120031,#120032,#120033,
#120034,#120035,#120036,#120037,#120038,#120039,#120040,#120041,#120042,
#120043,#120044,#120045,#120046,#120047,#120048,#120049,#120050,#120051,
#120052,#120053,#120054,#120055,#120056,#120057,#120058,#120059,#120060,
#120061,#120062,#120063,#120064,#120065,#120066,#120067,#120068,#120069,
#120070,#120071,#120072,#120073,#120074,#120075,#120076,#120077,#120078,
#120079,#120080,#120081,#120082,#120083,#120084,#120085,#120086,#120087,
#120088,#120089,#120090,#120091,#120092,#120093,#120094,#120095,#120096,
#120097,#120098,#120099,#120100,#120101,#120102,#120103,#120104,#120105,
#120106,#120107,#120108,#120109,#120110,#120111,#120112,#120113,#120114,
#120115,#120116,#120117,#120118,#120119,#120120,#120121,#120122,#120123,
#120124,#120125,#120126,#120127,#120128,#120129,#120130,#120131,#120132,
#120133,#120134,#120135,#120136,#120137,#120138,#120139,#120140,#120141,
#120142,#120143,#120144,#120145,#120146,#120147,#120148,#120149,#120150,
#120151,#120152,#120153,#120154,#120155,#120156,#120157,#120158,#120159,
#120160,#120161,#120162,#120163,#120164,#120165,#120166,#120167,#120168,
#120169,#120170,#120171,#120172,#120173,#120174,#120175,#120176,#120177,
#120178,#120179,#120180,#120181,#120182,#120183,#120184,#120185,#120186,
#120187,#120188,#120189,#120190,#120191,#120192,#120193,#120194,#120195,
#120196,#120197,#120198,#120199,#120200,#120201,#120202,#120203,#120204,
#120205,#120206,#120207),.UNSPECIFIED.,.F.,.F.,(4,2,2,2,2,2,2,2,2,2,2,2,
2,2,2,2,2,2,2,2,2,2,2,2,2,2,2,2,2,2,2,2,2,2,2,2,2,2,2,2,2,2,2,2,2,2,2,2,
2,2,2,2,2,2,2,2,2,2,2,2,2,2,2,2,2,2,2,2,2,2,2,2,2,2,2,2,2,2,2,2,2,2,2,2,
2,2,2,2,2,2,2,2,2,4),(-2.09996244461801,-2.08157373924918,-2.03783073252861,
-2.0309126457687,-2.02826864878956,-2.02642174480607,-2.02441331549537,
-2.02099866755253,-2.00763364657633,-1.98108316517676,-1.95595416763879,
-1.95085521205658,-1.94630520621802,-1.94302229887663,-1.94000685411733,
-1.93509836541476,-1.92216551037023,-1.8876305583691,-1.87308870326431,
-1.86737552789088,-1.86306201100004,-1.86086459686778,-1.85905813002354,
-1.85674286313071,-1.85182065890753,-1.82853418279768,-1.8271798322326,
-1.80018667625805,-1.78524312797341,-1.7802337337003,-1.77686330084659,
-1.77358338025717,-1.76886838053297,-1.75725745698622,-1.72146557792443,
-1.70657460017759,-1.69803818204913,-1.6951810089968,-1.69329320835359,
-1.69135321857799,-1.68825218632507,-1.67838899428806,-1.64931233365744,
-1.62041385138224,-1.61448801535696,-1.61092545065065,-1.60769756211002,
-1.60357663525929,-1.59459088120873,-1.55189552818646,-1.53892445554888,
-1.5311256175077,-1.52836047569698,-1.52649110442872,-1.52476712008828,
-1.52178776512585,-1.51296744161078,-1.47982063791151,-1.4623018971236,
-1.45448665277853,-1.44813857207455,-1.44448663536194,-1.44127517035593,
-1.4372382229071,-1.43081948515339,-1.39332078934756,-1.36727035981716,
-1.36296726884326,-1.36077189181912,-1.3589652331119,-1.35664733329347,
-1.35171124610737,-1.32692131061649,-1.30475451107767,-1.29221393423136,
-1.28313913358878,-1.27895770538371,-1.27573079167078,-1.27216313928785,
-1.26621399152472,-1.23890265707268,-1.21088995053926,-1.19868607597286,
-1.19546974578855,-1.19350452244951,-1.19165637504518,-1.18934964051302,
-1.18350035104981,-1.15110453375573,-1.12543798825827,-1.11642111640819,
-1.11224993677954,-1.10902431162195,-1.10900608777772),.UNSPECIFIED.);
#2874=B_SPLINE_CURVE_WITH_KNOTS('',3,(#120212,#120213,#120214,#120215,#120216,
#120217,#120218,#120219,#120220,#120221,#120222,#120223,#120224,#120225,
#120226,#120227,#120228,#120229,#120230,#120231,#120232,#120233,#120234,
#120235,#120236,#120237,#120238,#120239,#120240,#120241,#120242,#120243,
#120244,#120245,#120246,#120247,#120248,#120249,#120250,#120251,#120252,
#120253,#120254,#120255,#120256,#120257,#120258,#120259,#120260,#120261,
#120262,#120263,#120264,#120265,#120266,#120267,#120268,#120269,#120270,
#120271,#120272,#120273,#120274,#120275,#120276,#120277,#120278,#120279,
#120280,#120281,#120282,#120283,#120284,#120285,#120286,#120287,#120288,
#120289,#120290,#120291,#120292,#120293,#120294,#120295,#120296,#120297,
#120298,#120299,#120300,#120301,#120302,#120303,#120304,#120305,#120306,
#120307,#120308,#120309,#120310,#120311,#120312,#120313,#120314,#120315,
#120316,#120317,#120318,#120319,#120320,#120321,#120322,#120323,#120324,
#120325,#120326,#120327,#120328,#120329,#120330,#120331,#120332,#120333,
#120334,#120335,#120336,#120337,#120338,#120339,#120340,#120341,#120342,
#120343,#120344,#120345,#120346,#120347,#120348,#120349,#120350,#120351,
#120352,#120353,#120354,#120355,#120356,#120357,#120358,#120359,#120360,
#120361,#120362,#120363,#120364,#120365,#120366,#120367,#120368,#120369,
#120370,#120371,#120372,#120373,#120374,#120375,#120376,#120377,#120378,
#120379,#120380,#120381,#120382,#120383,#120384,#120385,#120386,#120387,
#120388,#120389,#120390,#120391,#120392,#120393,#120394,#120395,#120396,
#120397,#120398,#120399,#120400,#120401,#120402,#120403,#120404,#120405,
#120406,#120407,#120408,#120409,#120410,#120411,#120412,#120413,#120414,
#120415,#120416,#120417,#120418,#120419,#120420,#120421,#120422,#120423),
 .UNSPECIFIED.,.F.,.F.,(4,2,2,2,2,2,2,2,2,2,2,2,2,2,2,2,2,2,2,2,2,2,2,2,
2,2,2,2,2,2,2,2,2,2,2,2,2,2,2,2,2,2,2,2,2,2,2,2,2,2,2,2,2,2,2,2,2,2,2,2,
2,2,2,2,2,2,2,2,2,2,2,2,2,2,2,2,2,2,2,2,2,2,2,2,2,2,2,2,2,2,2,2,2,2,2,2,
2,2,2,2,2,2,2,2,2,4),(-3.50758932112955,-3.50326607780528,-3.50079423187189,
-3.49897322688236,-3.49688287624308,-3.49319031109068,-3.47121619820863,
-3.46693706942608,-3.44476974818732,-3.43196655138824,-3.4227536106868,
-3.4185476159197,-3.41531716311827,-3.41176099337353,-3.40586767232834,
-3.38112322683398,-3.35094010361961,-3.34242946150377,-3.3366208272391,
-3.3341489998827,-3.33232800752881,-3.33023767036684,-3.32654512618697,
-3.30457000327504,-3.30029167548298,-3.27812437271735,-3.26532155636205,
-3.25610883190379,-3.25190289283497,-3.24867246587322,-3.24511630768812,
-3.239222965705,-3.21447671298175,-3.18429551574369,-3.17578514806509,-3.16997666091744,
-3.16750486851562,-3.16568389102516,-3.16359355824415,-3.15990099480974,
-3.13791430816717,-3.1336438955831,-3.11147546561411,-3.09867564466832,
-3.08946450349017,-3.08525885760357,-3.08202848634971,-3.07847222038706,
-3.07257829774191,-3.04781217963822,-3.017648669765,-3.00914055926497,-3.00333320283615,
-3.00086160875178,-2.99904066581063,-2.99695024202945,-2.99325723855445,
-2.97114570015141,-2.96696672690247,-2.94478871182247,-2.93201385004535,
-2.9228157857984,-2.91861243426604,-2.91538237316369,-2.91182499855187,
-2.90592578776943,-2.88098154639055,-2.85097333805115,-2.84248487425747,
-2.83668728408946,-2.83421732872331,-2.8323966033404,-2.83030527815063,
-2.8266081963218,-2.80348296664562,-2.77484417510541,-2.75845207107761,
-2.75328979462628,-2.74988782298085,-2.74662925781049,-2.74203469914272,
-2.73115917144329,-2.69464288990083,-2.67955486592204,-2.6709462566399,
-2.66808024234911,-2.66619041807537,-2.66448679822252,-2.66161475329431,
-2.65362442408945,-2.62308648845793,-2.59432929986754,-2.58784992150024,
-2.58417012355828,-2.5809614076584,-2.57696371053926,-2.57068021708651,
-2.52546769247341,-2.51205237661471,-2.50407702746396,-2.50128884125485,
-2.49941471422187,-2.49769540121728,-2.49474118218841,-2.48612426776342,
-2.45787557075319),.UNSPECIFIED.);
#2875=B_SPLINE_CURVE_WITH_KNOTS('',3,(#120424,#120425,#120426,#120427,#120428,
#120429,#120430,#120431,#120432,#120433,#120434,#120435,#120436,#120437,
#120438,#120439,#120440,#120441,#120442,#120443,#120444,#120445,#120446,
#120447,#120448,#120449,#120450,#120451,#120452,#120453,#120454,#120455,
#120456,#120457,#120458,#120459,#120460,#120461,#120462,#120463,#120464,
#120465,#120466,#120467,#120468,#120469,#120470,#120471,#120472,#120473,
#120474,#120475,#120476,#120477,#120478,#120479,#120480,#120481,#120482,
#120483,#120484,#120485,#120486,#120487,#120488,#120489,#120490,#120491,
#120492,#120493,#120494,#120495,#120496,#120497,#120498,#120499,#120500,
#120501,#120502,#120503,#120504,#120505,#120506,#120507,#120508,#120509,
#120510,#120511,#120512,#120513,#120514,#120515,#120516,#120517,#120518,
#120519,#120520,#120521,#120522,#120523,#120524,#120525,#120526,#120527,
#120528,#120529,#120530,#120531,#120532,#120533,#120534,#120535,#120536,
#120537,#120538,#120539,#120540,#120541,#120542,#120543,#120544,#120545,
#120546,#120547,#120548,#120549,#120550,#120551,#120552,#120553,#120554,
#120555,#120556,#120557,#120558,#120559,#120560,#120561,#120562,#120563,
#120564,#120565,#120566,#120567,#120568,#120569,#120570,#120571,#120572,
#120573,#120574,#120575,#120576,#120577,#120578,#120579,#120580,#120581,
#120582,#120583,#120584,#120585,#120586,#120587,#120588,#120589,#120590,
#120591,#120592,#120593,#120594,#120595,#120596,#120597,#120598,#120599,
#120600,#120601,#120602,#120603,#120604,#120605,#120606,#120607,#120608,
#120609,#120610,#120611,#120612,#120613,#120614,#120615,#120616,#120617,
#120618,#120619,#120620,#120621,#120622,#120623),.UNSPECIFIED.,.F.,.F.,
(4,2,2,2,2,2,2,2,2,2,2,2,2,2,2,2,2,2,2,2,2,2,2,2,2,2,2,2,2,2,2,2,2,2,2,
2,2,2,2,2,2,2,2,2,2,2,2,2,2,2,2,2,2,2,2,2,2,2,2,2,2,2,2,2,2,2,2,2,2,2,2,
2,2,2,2,2,2,2,2,2,2,2,2,2,2,2,2,2,2,2,2,2,2,2,2,2,2,2,2,4),(-1.10900608777772,
-1.10545139341803,-1.09947729407191,-1.07142088108024,-1.04995735933683,
-1.03278567515519,-1.02914828651982,-1.02709159286259,-1.02526233148902,
-1.02272801005496,-1.01653354013363,-1.00722847017117,-0.969627029959607,
-0.952560546317377,-0.947183262997452,-0.943736907974779,-0.940467375339906,
-0.935995856459047,-0.925154559814216,-0.909044306241189,-0.891499869558333,
-0.868213455465457,-0.863292167320898,-0.860977130563375,-0.859170727773056,
-0.856973263964287,-0.852659293234556,-0.846944663378402,-0.83239676275621,
-0.797850516980509,-0.784905556412788,-0.779995426927117,-0.776979759363738,
-0.773697247989051,-0.769148938770557,-0.757795148543991,-0.740552733335049,
-0.707857661685441,-0.698356281477206,-0.695296102610414,-0.693365081899662,
-0.691470245806252,-0.688578626646476,-0.679748272137217,-0.664041823595915,
-0.625220852497486,-0.616447547972186,-0.61230472294534,-0.609074158238372,
-0.605523418072018,-0.599652329166598,-0.572369311100458,-0.546032573426438,
-0.532398526305794,-0.528967111313501,-0.526955124571645,-0.525110004392858,
-0.522475610176029,-0.515622730908919,-0.472028954160963,-0.452891447081516,
-0.447339572300788,-0.443856812389304,-0.440604427478022,-0.436236536103075,
-0.42605122199956,-0.411321761042372,-0.38175362970548,-0.365947927471022,
-0.362394686034681,-0.360356400595963,-0.35852174247136,-0.355949922001723,
-0.349513273134975,-0.339693122008154,-0.295231615598122,-0.284190392509096,
-0.279575593646994,-0.276314497194065,-0.272920078327508,-0.267789652890676,
-0.251699059252475,-0.22406652340404,-0.201534498859147,-0.196613723098055,
-0.194299124529777,-0.192493158599055,-0.190296342329874,-0.185983970152466,
-0.180271679975482,-0.16573119296879,-0.13120715471522,-0.118250598598311,
-0.113339620552802,-0.110324326612007,-0.107042918372219,-0.102497431494663,
-0.0911580184665465,-0.0666476919421411,-0.0592664597001961),
 .UNSPECIFIED.);
#2876=B_SPLINE_CURVE_WITH_KNOTS('',3,(#120628,#120629,#120630,#120631,#120632,
#120633,#120634,#120635,#120636,#120637,#120638,#120639,#120640,#120641,
#120642,#120643,#120644,#120645,#120646,#120647,#120648,#120649,#120650,
#120651,#120652,#120653,#120654,#120655,#120656,#120657,#120658,#120659,
#120660,#120661,#120662,#120663,#120664,#120665,#120666,#120667,#120668,
#120669,#120670,#120671,#120672,#120673,#120674,#120675,#120676,#120677,
#120678,#120679,#120680,#120681,#120682,#120683,#120684,#120685,#120686,
#120687,#120688,#120689,#120690,#120691,#120692,#120693,#120694,#120695,
#120696,#120697,#120698,#120699,#120700,#120701,#120702,#120703,#120704,
#120705,#120706,#120707,#120708,#120709,#120710,#120711,#120712,#120713,
#120714,#120715,#120716,#120717,#120718,#120719,#120720,#120721,#120722,
#120723,#120724,#120725,#120726,#120727,#120728,#120729,#120730,#120731,
#120732,#120733,#120734,#120735,#120736,#120737,#120738,#120739,#120740,
#120741,#120742,#120743,#120744,#120745,#120746,#120747,#120748,#120749,
#120750,#120751,#120752,#120753,#120754,#120755,#120756,#120757,#120758,
#120759,#120760,#120761,#120762,#120763,#120764,#120765,#120766,#120767,
#120768,#120769,#120770,#120771,#120772,#120773,#120774,#120775,#120776,
#120777,#120778,#120779,#120780,#120781,#120782,#120783,#120784,#120785,
#120786,#120787,#120788,#120789,#120790,#120791,#120792,#120793,#120794,
#120795,#120796,#120797,#120798,#120799,#120800,#120801,#120802,#120803,
#120804,#120805,#120806,#120807,#120808,#120809,#120810,#120811,#120812,
#120813,#120814,#120815,#120816,#120817,#120818,#120819,#120820,#120821,
#120822,#120823,#120824,#120825,#120826,#120827,#120828,#120829,#120830,
#120831,#120832,#120833,#120834,#120835,#120836,#120837,#120838,#120839),
 .UNSPECIFIED.,.F.,.F.,(4,2,2,2,2,2,2,2,2,2,2,2,2,2,2,2,2,2,2,2,2,2,2,2,
2,2,2,2,2,2,2,2,2,2,2,2,2,2,2,2,2,2,2,2,2,2,2,2,2,2,2,2,2,2,2,2,2,2,2,2,
2,2,2,2,2,2,2,2,2,2,2,2,2,2,2,2,2,2,2,2,2,2,2,2,2,2,2,2,2,2,2,2,2,2,2,2,
2,2,2,2,2,2,2,2,2,4),(-4.55725054622971,-4.53544163392311,-4.50897044576888,
-4.50316152446864,-4.50068957721346,-4.49886849734356,-4.49677806055521,
-4.49308534258128,-4.47111009193486,-4.46705396399047,-4.44469504134589,
-4.43187301532949,-4.4226501294377,-4.41844229892793,-4.4152115020168,-4.41165601637588,
-4.40576635435688,-4.38101369904171,-4.35082916311207,-4.34231815166661,
-4.33650926970097,-4.33403733996817,-4.3322162733169,-4.33012585206608,
-4.32643316231025,-4.30445841021736,-4.30017906553463,-4.2780110038721,
-4.26520734459116,-4.25599407676876,-4.25178793703333,-4.24855737462706,
-4.24500108597025,-4.23910757202739,-4.21436249943664,-4.18417816870753,
-4.1756672150268,-4.16985837247322,-4.16738645950494,-4.16556540520201,
-4.16347499812535,-4.15978233340483,-4.13780773121874,-4.13352841481556,
-4.11136050343049,-4.09855693060044,-4.08934372504939,-4.08513761379573,
-4.08190707328687,-4.07835080875626,-4.07245733484652,-4.04771243253357,
-4.01752830426367,-4.00901740800195,-4.00320860468576,-4.00073670844734,
-3.99891566647474,-3.99682527354528,-3.99313263383623,-3.97115818149917,
-3.9668788936373,-3.94471113281501,-3.93190764680303,-3.92269450371204,
-3.91848842094588,-3.91525790230331,-3.91170166182919,-3.90580822774859,
-3.88106349057684,-3.8508795691259,-3.84236873082204,-3.83655996700689,
-3.83408808753619,-3.83226705791252,-3.83017667917522,-3.82648406450324,
-3.80450975403519,-3.80023049993793,-3.77806288850072,-3.76525949086604,
-3.75604641108258,-3.7518403570185,-3.7486098603463,-3.74505364398424,-3.7391602496926,
-3.71441567341441,-3.68423196219169,-3.67572118231075,-3.66991245825377,
-3.66744059563131,-3.66561957839373,-3.66352921385181,-3.65983662421744,
-3.63786246229042,-3.63358323679476,-3.61141577488531,-3.59861246352816,
-3.58939944589447,-3.58519342029235,-3.58196294551784,-3.5784067533001,
-3.57251339911424,-3.54776899467422,-3.51758548525494,-3.50907476269372,
-3.50758932112955),.UNSPECIFIED.);
#2877=B_SPLINE_CURVE_WITH_KNOTS('',3,(#120841,#120842,#120843,#120844,#120845,
#120846,#120847,#120848,#120849,#120850,#120851,#120852,#120853,#120854,
#120855,#120856,#120857,#120858,#120859,#120860),.UNSPECIFIED.,.F.,.F.,
(4,2,2,2,2,2,2,2,2,4),(-0.0592664597001961,-0.044487464262689,-0.0322596332417712,
-0.0289284677612067,-0.0269386209323888,-0.0250836837176406,-0.0232035109203273,
-0.0205734943312831,-0.0140923816516964,-0.000491289129905891),
 .UNSPECIFIED.);
#2878=B_SPLINE_CURVE_WITH_KNOTS('',3,(#120861,#120862,#120863,#120864,#120865,
#120866,#120867,#120868,#120869,#120870,#120871,#120872,#120873,#120874,
#120875,#120876,#120877,#120878,#120879,#120880,#120881,#120882,#120883,
#120884,#120885,#120886,#120887,#120888,#120889,#120890,#120891,#120892,
#120893,#120894,#120895,#120896,#120897,#120898,#120899,#120900,#120901,
#120902,#120903,#120904,#120905,#120906,#120907,#120908,#120909,#120910,
#120911,#120912,#120913,#120914,#120915,#120916,#120917,#120918,#120919,
#120920,#120921,#120922,#120923,#120924,#120925,#120926,#120927,#120928,
#120929,#120930,#120931,#120932,#120933,#120934,#120935,#120936,#120937,
#120938,#120939,#120940,#120941,#120942,#120943,#120944,#120945,#120946,
#120947,#120948,#120949,#120950,#120951,#120952,#120953,#120954,#120955,
#120956,#120957,#120958,#120959,#120960,#120961,#120962,#120963,#120964,
#120965,#120966,#120967,#120968,#120969,#120970,#120971,#120972,#120973,
#120974,#120975,#120976,#120977,#120978,#120979,#120980,#120981,#120982,
#120983,#120984,#120985,#120986,#120987,#120988,#120989,#120990,#120991,
#120992,#120993,#120994,#120995,#120996,#120997,#120998,#120999,#121000,
#121001,#121002,#121003,#121004,#121005,#121006,#121007,#121008,#121009,
#121010,#121011,#121012,#121013,#121014,#121015,#121016,#121017,#121018,
#121019,#121020,#121021,#121022,#121023,#121024,#121025,#121026,#121027,
#121028,#121029,#121030,#121031,#121032,#121033,#121034,#121035,#121036,
#121037,#121038,#121039,#121040,#121041,#121042,#121043,#121044,#121045,
#121046,#121047,#121048,#121049,#121050,#121051,#121052,#121053,#121054,
#121055,#121056,#121057,#121058,#121059,#121060,#121061,#121062,#121063,
#121064,#121065,#121066,#121067,#121068,#121069,#121070,#121071,#121072,
#121073,#121074,#121075,#121076,#121077,#121078,#121079,#121080,#121081,
#121082,#121083,#121084,#121085,#121086,#121087,#121088,#121089,#121090,
#121091,#121092,#121093,#121094,#121095,#121096,#121097,#121098,#121099,
#121100,#121101,#121102,#121103,#121104,#121105,#121106,#121107,#121108,
#121109,#121110,#121111,#121112,#121113,#121114,#121115,#121116,#121117,
#121118,#121119,#121120),.UNSPECIFIED.,.F.,.F.,(4,2,2,2,2,2,2,2,2,2,2,2,
2,2,2,2,2,2,2,2,2,2,2,2,2,2,2,2,2,2,2,2,2,2,2,2,2,2,2,2,2,2,2,2,2,2,2,2,
2,2,2,2,2,2,2,2,2,2,2,2,2,2,2,2,2,2,2,2,2,2,2,2,2,2,2,2,2,2,2,2,2,2,2,2,
2,2,2,2,2,2,2,2,2,2,2,2,2,2,2,2,2,2,2,2,2,2,2,2,2,2,2,2,2,2,2,2,2,2,2,2,
2,2,2,2,2,2,2,2,2,4),(-2.10010132658151,-2.05909871254268,-2.04960757489194,
-2.04535445155139,-2.04211858461491,-2.03858675912585,-2.03280468762879,
-2.010412986564,-1.97814762227775,-1.96935040867242,-1.96349122128359,-1.9611155574656,
-1.96109881849124,-1.9610817523395,-1.96106434189489,-1.96104656894127,
-1.96102841406951,-1.96100985661037,-1.96099087460414,-1.96097144472476,
-1.96095154193326,-1.96093113946981,-1.96091020873649,-1.96088871894084,
-1.96086663698487,-1.96084392747736,-1.96082055216478,-1.9607964698133,
-1.96077163577537,-1.9607460017532,-1.96071951530737,-1.96069211955835,
-1.96066375252865,-1.9606343465167,-1.96060382759794,-1.9605721147809,-1.96053911910075,
-1.96050474266919,-1.9604688774505,-1.96043140393448,-1.96039218966669,
-1.96035108723155,-1.95854369721215,-1.95620878839875,-1.9513567866793,
-1.92698113559443,-1.90480363110378,-1.89202101462245,-1.88281927504242,
-1.87861593373155,-1.87538659166102,-1.87183074598661,-1.8659359000808,
-1.84111196286137,-1.81099404103307,-1.80249198472382,-1.79668790330436,
-1.79421724612741,-1.79239683609119,-1.79030691253007,-1.78661463583356,
-1.76454900029655,-1.76033155745025,-1.73815422228204,-1.72537166413491,
-1.71616997288781,-1.71196665842624,-1.70873733886666,-1.70518151986088,
-1.69928672264213,-1.67446318993796,-1.64434528239983,-1.63584326122125,
-1.63003920846295,-1.62756856671766,-1.6257481693208,-1.62365826174634,
-1.61996601647707,-1.59790196319905,-1.59368348138443,-1.57150640217843,
-1.55872367291172,-1.54952190991072,-1.54531860136918,-1.54208930163608,
-1.53853351971351,-1.53263882025434,-1.50781731482975,-1.47769800854007,
-1.46919584426651,-1.46339173168703,-1.46092109061689,-1.45910070399122,
-1.45701082074339,-1.45331864420221,-1.43126625813019,-1.42703922213361,
-1.40486312089635,-1.39207833149864,-1.38287550820517,-1.37867203335387,
-1.37544273139674,-1.37188707235244,-1.36599287471854,-1.34118670951267,
-1.31105440836896,-1.30255063895464,-1.2967457407654,-1.29427497937038,
-1.29245458822376,-1.29036479773676,-1.28667299590718,-1.26471371171253,
-1.26064020020926,-1.23800005326314,-1.22533741263083,-1.21619866728069,
-1.21200639864797,-1.20877853460267,-1.20521727619113,-1.1992966428348,
-1.17344158319503,-1.14421107271519,-1.13582329079243,-1.13007614583047,
-1.12761505512968,-1.12579587644223,-1.12370057306247,-1.11998406916987,
-1.10920393116059),.UNSPECIFIED.);
#2879=B_SPLINE_CURVE_WITH_KNOTS('',3,(#121126,#121127,#121128,#121129,#121130,
#121131,#121132,#121133,#121134,#121135,#121136,#121137,#121138,#121139,
#121140,#121141,#121142,#121143,#121144,#121145,#121146,#121147,#121148,
#121149,#121150,#121151,#121152,#121153,#121154,#121155,#121156,#121157,
#121158,#121159,#121160,#121161,#121162,#121163,#121164,#121165,#121166,
#121167,#121168,#121169,#121170,#121171,#121172,#121173,#121174,#121175,
#121176,#121177,#121178,#121179,#121180,#121181,#121182,#121183,#121184,
#121185,#121186,#121187,#121188,#121189,#121190,#121191,#121192,#121193,
#121194,#121195,#121196,#121197,#121198,#121199,#121200,#121201,#121202,
#121203,#121204,#121205,#121206,#121207,#121208,#121209,#121210,#121211,
#121212,#121213,#121214,#121215,#121216,#121217,#121218,#121219,#121220,
#121221,#121222,#121223,#121224,#121225,#121226,#121227,#121228,#121229,
#121230,#121231,#121232,#121233,#121234,#121235,#121236,#121237,#121238,
#121239,#121240,#121241,#121242,#121243,#121244,#121245,#121246,#121247,
#121248,#121249,#121250,#121251,#121252,#121253,#121254,#121255,#121256,
#121257,#121258,#121259,#121260,#121261,#121262,#121263,#121264,#121265,
#121266,#121267,#121268,#121269,#121270,#121271,#121272,#121273,#121274,
#121275,#121276,#121277,#121278,#121279,#121280,#121281,#121282,#121283,
#121284,#121285,#121286,#121287,#121288,#121289,#121290,#121291,#121292,
#121293,#121294,#121295,#121296,#121297,#121298,#121299,#121300,#121301,
#121302,#121303,#121304,#121305,#121306,#121307,#121308,#121309,#121310,
#121311,#121312,#121313,#121314,#121315,#121316,#121317,#121318,#121319,
#121320,#121321,#121322,#121323,#121324,#121325,#121326,#121327,#121328,
#121329,#121330,#121331,#121332,#121333,#121334,#121335,#121336,#121337,
#121338,#121339,#121340,#121341,#121342,#121343,#121344,#121345,#121346,
#121347,#121348,#121349,#121350,#121351,#121352,#121353,#121354,#121355),
 .UNSPECIFIED.,.F.,.F.,(4,2,2,2,2,2,2,2,2,2,2,2,2,2,2,2,2,2,2,2,2,2,2,2,
2,2,2,2,2,2,2,2,2,2,2,2,2,2,2,2,2,2,2,2,2,2,2,2,2,2,2,2,2,2,2,2,2,2,2,2,
2,2,2,2,2,2,2,2,2,2,2,2,2,2,2,2,2,2,2,2,2,2,2,2,2,2,2,2,2,2,2,2,2,2,2,2,
2,2,2,2,2,2,2,2,2,2,2,2,2,2,2,2,2,2,4),(-0.990948248867995,-0.979672455295316,
-0.9729824314885,-0.968866577885365,-0.965646733523735,-0.962042091760025,
-0.955920542585719,-0.948463977709807,-0.932206608285816,-0.914289696023135,
-0.889742600356832,-0.886024818384269,-0.883928817823629,-0.882109048395981,
-0.879647040461974,-0.873897285336823,-0.86550398302534,-0.836247344745194,
-0.810391097282374,-0.804468465538512,-0.800906067000483,-0.79767719191891,
-0.79348360323458,-0.784341535802918,-0.771675142627436,-0.749014066464878,
-0.745144139235457,-0.72305312630508,-0.719360850125708,-0.717270575387693,
-0.715449606649019,-0.712977713232605,-0.707168673574408,-0.698656179402299,
-0.668471262965041,-0.64369567950319,-0.63780073013176,-0.634244259464411,
-0.63101397699056,-0.626808837131111,-0.617600287210655,-0.604807014617657,
-0.582654254540736,-0.578431014816997,-0.556412062067877,-0.552720133122025,
-0.550629962485371,-0.548809018303582,-0.546337069682407,-0.540527510083862,
-0.532013901151589,-0.501819344713932,-0.477056053765409,-0.471161592954264,
-0.467605274252917,-0.46437503941024,-0.460169831734166,-0.450960579806937,
-0.438165864759744,-0.416014312308193,-0.411785558904403,-0.389774911020015,
-0.386083089138364,-0.383992968887352,-0.382172061286059,-0.379700152530363,
-0.373890643459777,-0.365377069540588,-0.335182007953019,-0.310420537464163,
-0.304526240420762,-0.300970004689545,-0.297739835183687,-0.293534698165558,
-0.284325539581565,-0.271530902397935,-0.249379896282433,-0.245150621965675,
-0.22314129192691,-0.219449550512143,-0.21735947469704,-0.215538605008919,
-0.213066746651598,-0.207257351302723,-0.198743939766618,-0.168549385239458,
-0.143733525969834,-0.137868207155276,-0.134318178656801,-0.131086476558862,
-0.130937166136611,-0.130810214512794,-0.130700707519312,-0.130605100312627,
-0.130520765388843,-0.130445710163882,-0.13037839377642,-0.130317604294817,
-0.130262374402493,-0.130211921922581,-0.130165606914334,-0.130122900457604,
-0.129964945395609,-0.129806999613464,-0.124889320967317,-0.10985157029812,
-0.0824337556331517,-0.0786938298884941,-0.0565031873151528,-0.0528107881770321,
-0.0507205723091913,-0.0488997467220234,-0.0464281706108214,-0.0406204185046636,
-0.000394732259851559),.UNSPECIFIED.);
#2880=B_SPLINE_CURVE_WITH_KNOTS('',3,(#121356,#121357,#121358,#121359,#121360,
#121361,#121362,#121363,#121364,#121365,#121366,#121367,#121368,#121369,
#121370,#121371,#121372,#121373),.UNSPECIFIED.,.F.,.F.,(4,2,2,2,2,2,2,2,
4),(-4.61631755219529,-4.59347746858498,-4.58901458892267,-4.58574002981368,
-4.58244318705041,-4.57944161384394,-4.57461528573861,-4.56226226150011,
-4.55725054622971),.UNSPECIFIED.);
#2881=B_SPLINE_CURVE_WITH_KNOTS('',3,(#121374,#121375,#121376,#121377,#121378,
#121379,#121380,#121381,#121382,#121383,#121384,#121385,#121386,#121387,
#121388,#121389,#121390,#121391,#121392,#121393,#121394,#121395,#121396,
#121397,#121398,#121399,#121400,#121401,#121402,#121403,#121404,#121405,
#121406,#121407,#121408,#121409,#121410,#121411,#121412,#121413,#121414,
#121415,#121416,#121417,#121418,#121419,#121420,#121421,#121422,#121423,
#121424,#121425,#121426,#121427,#121428,#121429,#121430,#121431,#121432,
#121433,#121434,#121435,#121436,#121437,#121438,#121439,#121440,#121441,
#121442,#121443,#121444,#121445,#121446,#121447,#121448,#121449,#121450,
#121451,#121452,#121453,#121454,#121455,#121456,#121457,#121458,#121459,
#121460,#121461,#121462,#121463,#121464,#121465,#121466,#121467,#121468,
#121469,#121470,#121471,#121472,#121473,#121474,#121475,#121476,#121477,
#121478,#121479,#121480,#121481,#121482,#121483,#121484,#121485,#121486,
#121487,#121488,#121489,#121490,#121491,#121492,#121493,#121494,#121495,
#121496,#121497,#121498,#121499,#121500,#121501,#121502,#121503,#121504,
#121505,#121506,#121507,#121508,#121509,#121510,#121511,#121512,#121513,
#121514,#121515,#121516,#121517,#121518,#121519,#121520,#121521,#121522,
#121523,#121524,#121525,#121526,#121527,#121528,#121529,#121530,#121531,
#121532,#121533,#121534,#121535,#121536,#121537,#121538,#121539,#121540,
#121541,#121542,#121543,#121544,#121545,#121546,#121547,#121548,#121549,
#121550,#121551,#121552,#121553,#121554,#121555,#121556,#121557,#121558,
#121559,#121560,#121561,#121562,#121563,#121564,#121565,#121566,#121567,
#121568,#121569),.UNSPECIFIED.,.F.,.F.,(4,2,2,2,2,2,2,2,2,2,2,2,2,2,2,2,
2,2,2,2,2,2,2,2,2,2,2,2,2,2,2,2,2,2,2,2,2,2,2,2,2,2,2,2,2,2,2,2,2,2,2,2,
2,2,2,2,2,2,2,2,2,2,2,2,2,2,2,2,2,2,2,2,2,2,2,2,2,2,2,2,2,2,2,2,2,2,2,2,
2,2,2,2,2,2,2,2,2,4),(-1.10920393116059,-1.09545238288575,-1.07754877998225,
-1.06124705181696,-1.05031879527491,-1.04628123799819,-1.04328380279532,
-1.03998536226846,-1.03534716801461,-1.02336647125924,-1.00466975027437,
-0.977026524576556,-0.965228646836615,-0.96194273950729,-0.959962527031071,
-0.958101839391524,-0.955380967614092,-0.94791347960185,-0.935750960576131,
-0.899670325468565,-0.88510704318887,-0.879997210234699,-0.876945435282821,
-0.873688410207201,-0.869291648473138,-0.858926882346821,-0.843826654134602,
-0.824321712371313,-0.801320453629943,-0.796466197493382,-0.794130963671087,
-0.792323693643512,-0.790143246806896,-0.785912750439751,-0.761201507267572,
-0.72188945679387,-0.715648255304336,-0.71166377864048,-0.708457116007543,
-0.704770313589069,-0.698253285582592,-0.690168566300328,-0.671661295578562,
-0.644486982967404,-0.632051739530787,-0.62870399332545,-0.626710434067188,
-0.624857169476173,-0.622175537833955,-0.614991004919582,-0.603497008081052,
-0.58260144584094,-0.553582276257446,-0.547597928525964,-0.544023406016454,
-0.540799160857263,-0.536633760867165,-0.527645742479134,-0.502845970348658,
-0.472117369601396,-0.464386583012527,-0.461550992195022,-0.459854593020427,
-0.457957850420898,-0.455056174332297,-0.446135751111089,-0.430172511085007,
-0.390339533374479,-0.382455664197478,-0.378442682477746,-0.375233945566496,
-0.371567454837926,-0.365147222348091,-0.332841176353624,-0.300920563530067,
-0.296292264495551,-0.294033125964616,-0.292228581255045,-0.289981224950562,
-0.285413647684281,-0.260909675478603,-0.222021586841373,-0.215735631499108,
-0.211738131613172,-0.208530683930541,-0.204853581918325,-0.198382343042951,
-0.170477631411324,-0.141387560819282,-0.131593262330374,-0.128500501728611,
-0.12656267104444,-0.12467417677269,-0.121811716440772,-0.113580981861986,
-0.0993097405969179,-0.0703226089993763,-0.0595389284169461),
 .UNSPECIFIED.);
#2882=B_SPLINE_CURVE_WITH_KNOTS('',3,(#121574,#121575,#121576,#121577,#121578,
#121579,#121580,#121581,#121582,#121583,#121584,#121585,#121586,#121587,
#121588,#121589,#121590,#121591,#121592,#121593,#121594,#121595,#121596,
#121597,#121598,#121599,#121600,#121601,#121602,#121603,#121604,#121605,
#121606,#121607,#121608,#121609,#121610,#121611,#121612,#121613,#121614,
#121615,#121616,#121617,#121618,#121619,#121620,#121621,#121622,#121623,
#121624,#121625,#121626,#121627,#121628,#121629,#121630,#121631,#121632,
#121633,#121634,#121635,#121636,#121637,#121638,#121639,#121640,#121641,
#121642,#121643,#121644,#121645,#121646,#121647,#121648,#121649,#121650,
#121651,#121652,#121653,#121654,#121655,#121656,#121657,#121658,#121659,
#121660,#121661,#121662,#121663,#121664,#121665,#121666,#121667,#121668,
#121669,#121670,#121671,#121672,#121673,#121674,#121675,#121676,#121677,
#121678,#121679,#121680,#121681,#121682,#121683,#121684,#121685,#121686,
#121687,#121688,#121689,#121690,#121691,#121692,#121693,#121694,#121695,
#121696,#121697,#121698,#121699,#121700,#121701,#121702,#121703,#121704,
#121705,#121706,#121707,#121708,#121709,#121710,#121711,#121712,#121713,
#121714,#121715,#121716,#121717,#121718,#121719,#121720,#121721,#121722,
#121723,#121724,#121725,#121726,#121727,#121728,#121729,#121730,#121731,
#121732,#121733,#121734,#121735,#121736,#121737,#121738,#121739,#121740,
#121741,#121742,#121743,#121744,#121745,#121746,#121747,#121748,#121749,
#121750,#121751,#121752,#121753,#121754,#121755,#121756,#121757,#121758,
#121759,#121760,#121761,#121762,#121763,#121764,#121765,#121766,#121767,
#121768,#121769,#121770,#121771,#121772,#121773,#121774,#121775,#121776,
#121777,#121778,#121779,#121780,#121781,#121782,#121783,#121784,#121785,
#121786,#121787,#121788,#121789,#121790,#121791,#121792,#121793),
 .UNSPECIFIED.,.F.,.F.,(4,2,2,2,2,2,2,2,2,2,2,2,2,2,2,2,2,2,2,2,2,2,2,2,
2,2,2,2,2,2,2,2,2,2,2,2,2,2,2,2,2,2,2,2,2,2,2,2,2,2,2,2,2,2,2,2,2,2,2,2,
2,2,2,2,2,2,2,2,2,2,2,2,2,2,2,2,2,2,2,2,2,2,2,2,2,2,2,2,2,2,2,2,2,2,2,2,
2,2,2,2,2,2,2,2,2,2,2,2,2,4),(-2.04079439360869,-2.01832232010227,-1.99049537877606,
-1.97533771893915,-1.9704067674467,-1.97024875981206,-1.97009079499496,
-1.97004916905279,-1.97000408540807,-1.96995504583547,-1.96990144953348,
-1.96984256472043,-1.9697774900404,-1.96970510125454,-1.96962397628702,
-1.96953228694736,-1.96942763891705,-1.96930682773932,-1.96916545357647,
-1.96899728677888,-1.96879316848958,-1.96778835158514,-1.9645712676515,
-1.96047979810822,-1.95387406447519,-1.91929814144932,-1.89069615561188,
-1.88638777793846,-1.8841911447973,-1.8823842508756,-1.88006698821341,-1.87513539421651,
-1.84993687316705,-1.823366335713,-1.80855054804381,-1.80355496652656,-1.80018689839258,
-1.79690402950124,-1.7921754059665,-1.78047978243619,-1.74131194830112,
-1.72875667254374,-1.72112613377165,-1.71838287379085,-1.71651749291244,
-1.71454368155929,-1.71128887113857,-1.69985734884655,-1.67193163462875,
-1.65311654936921,-1.64108655176165,-1.63644055183092,-1.6331399291254,
-1.62974443757469,-1.62461408894545,-1.60986279884279,-1.57696170163996,
-1.55793792431243,-1.55327655566788,-1.55101045008676,-1.54920505897758,
-1.54696243768545,-1.54242211451408,-1.50937094860917,-1.47822566960969,
-1.47168486444353,-1.46799220879308,-1.46478472601858,-1.46080473830769,
-1.45458159127082,-1.40908262477423,-1.39104586784176,-1.38649689377451,
-1.38425254071481,-1.38244711150284,-1.38018265392315,-1.37553006031856,
-1.34403633925316,-1.31144178087576,-1.30493780235371,-1.30125275389038,
-1.2980444103757,-1.2940536354481,-1.28779405904147,-1.24866916810283,-1.22383604239752,
-1.21960461170361,-1.21742344740542,-1.21561542766506,-1.21327892147486,
-1.20842096692003,-1.18263287407177,-1.16727981523855,-1.15133231258097,
-1.1405670616318,-1.13610653068114,-1.13283818872568,-1.12980115431093,
-1.12477607132239,-1.11096750683819,-1.07723772368443,-1.06292303788748,
-1.05460111952307,-1.05176952263733,-1.04988665111793,-1.047939098118,-1.04480471150353,
-1.03358279893802,-1.00988692766837,-0.990948248867995),.UNSPECIFIED.);
#2883=B_SPLINE_CURVE_WITH_KNOTS('',3,(#121795,#121796,#121797,#121798,#121799,
#121800,#121801,#121802,#121803,#121804,#121805,#121806,#121807,#121808,
#121809,#121810,#121811,#121812),.UNSPECIFIED.,.F.,.F.,(4,2,2,2,2,2,2,2,
4),(-0.0595389284169461,-0.0526460477562469,-0.0471652681643023,-0.0436977380443621,
-0.0404394032049224,-0.0372330969659463,-0.032957136393493,-0.0229767669222253,
-0.000491639810663164),.UNSPECIFIED.);
#2884=B_SPLINE_CURVE_WITH_KNOTS('',3,(#121813,#121814,#121815,#121816,#121817,
#121818,#121819,#121820,#121821,#121822,#121823,#121824,#121825,#121826,
#121827,#121828,#121829,#121830,#121831,#121832,#121833,#121834,#121835,
#121836,#121837,#121838,#121839,#121840,#121841,#121842,#121843,#121844,
#121845,#121846,#121847,#121848,#121849,#121850,#121851,#121852,#121853,
#121854,#121855,#121856,#121857,#121858,#121859,#121860,#121861,#121862,
#121863,#121864,#121865,#121866,#121867,#121868,#121869,#121870,#121871,
#121872,#121873,#121874,#121875,#121876,#121877,#121878,#121879,#121880,
#121881,#121882,#121883,#121884,#121885,#121886,#121887,#121888,#121889,
#121890,#121891,#121892,#121893,#121894,#121895,#121896,#121897,#121898,
#121899,#121900,#121901,#121902,#121903,#121904,#121905,#121906,#121907,
#121908,#121909,#121910,#121911,#121912,#121913,#121914,#121915,#121916,
#121917,#121918,#121919,#121920,#121921,#121922,#121923,#121924,#121925,
#121926,#121927,#121928,#121929,#121930,#121931,#121932,#121933,#121934,
#121935,#121936,#121937,#121938,#121939,#121940,#121941,#121942,#121943,
#121944,#121945,#121946,#121947,#121948,#121949,#121950,#121951,#121952,
#121953,#121954,#121955,#121956,#121957,#121958,#121959,#121960,#121961,
#121962,#121963,#121964,#121965,#121966,#121967,#121968,#121969,#121970,
#121971,#121972,#121973,#121974,#121975),.UNSPECIFIED.,.F.,.F.,(4,3,3,3,
3,3,3,3,3,3,3,3,3,3,3,3,3,3,3,3,3,3,3,3,3,3,3,3,3,3,3,3,3,3,3,3,3,3,3,3,
3,3,3,3,3,3,3,3,3,3,3,3,3,3,4),(-54.1118657207559,-53.9685006349923,-53.8675843506887,
-53.7577897347119,-53.6468205794158,-53.5373284361963,-53.4279032844608,
-53.3185044306213,-53.2063874460516,-53.0968489113668,-52.9834427018547,
-52.8700364923426,-52.7602418763654,-52.6492727210693,-52.5397805778494,
-52.4303554261136,-52.3209565722737,-52.2088395877044,-52.0993010530192,
-51.9858948435079,-51.8724886339965,-51.7626940180193,-51.6517248627232,
-51.5422327195032,-51.4328075677673,-51.3234087139274,-51.2112917293581,
-51.1017531946728,-50.9883469851616,-50.8749407756504,-50.7651461596733,
-50.6541770043772,-50.5446848611573,-50.4352597094216,-50.3258608555817,
-50.2137438710124,-50.1042053363272,-49.9907991268158,-49.8773929173043,
-49.7675983013271,-49.656629146031,-49.5471370028111,-49.4377118510753,
-49.3283129972354,-49.2161960126661,-49.1066574779808,-48.9932512684695,
-48.8798450589582,-48.7700749185132,-48.6604636794684,-48.5509703726848,
-48.4415394131861,-48.3321442530804,-48.2227090153558,-48.1819103737702),
 .UNSPECIFIED.);
#2885=B_SPLINE_CURVE_WITH_KNOTS('',3,(#121981,#121982,#121983,#121984,#121985,
#121986,#121987,#121988,#121989,#121990,#121991,#121992,#121993,#121994,
#121995,#121996,#121997,#121998,#121999,#122000,#122001,#122002,#122003,
#122004,#122005,#122006,#122007,#122008,#122009,#122010,#122011,#122012,
#122013,#122014,#122015,#122016,#122017,#122018,#122019,#122020,#122021,
#122022,#122023,#122024,#122025,#122026,#122027,#122028,#122029,#122030,
#122031,#122032,#122033,#122034,#122035,#122036,#122037,#122038,#122039,
#122040,#122041,#122042,#122043,#122044,#122045,#122046,#122047,#122048,
#122049,#122050,#122051,#122052,#122053,#122054,#122055,#122056,#122057,
#122058,#122059,#122060,#122061,#122062,#122063,#122064,#122065,#122066,
#122067,#122068,#122069,#122070,#122071,#122072,#122073,#122074,#122075,
#122076,#122077,#122078,#122079,#122080,#122081,#122082,#122083,#122084,
#122085,#122086,#122087,#122088,#122089,#122090,#122091,#122092,#122093,
#122094,#122095,#122096,#122097,#122098,#122099,#122100,#122101,#122102,
#122103,#122104,#122105,#122106,#122107,#122108,#122109,#122110,#122111,
#122112,#122113,#122114,#122115,#122116,#122117,#122118,#122119,#122120,
#122121,#122122,#122123,#122124,#122125,#122126,#122127,#122128,#122129,
#122130,#122131,#122132,#122133,#122134,#122135,#122136,#122137,#122138,
#122139,#122140,#122141,#122142,#122143,#122144,#122145,#122146,#122147,
#122148,#122149,#122150,#122151,#122152,#122153,#122154,#122155,#122156,
#122157,#122158,#122159,#122160,#122161,#122162,#122163,#122164,#122165,
#122166,#122167,#122168,#122169,#122170,#122171,#122172,#122173,#122174,
#122175,#122176,#122177,#122178,#122179,#122180,#122181,#122182,#122183,
#122184,#122185,#122186),.UNSPECIFIED.,.F.,.F.,(4,2,2,2,2,2,2,2,2,2,2,2,
2,2,2,2,2,2,2,2,2,2,2,2,2,2,2,2,2,2,2,2,2,2,2,2,2,2,2,2,2,2,2,2,2,2,2,2,
2,2,2,2,2,2,2,2,2,2,2,2,2,2,2,2,2,2,2,2,2,2,2,2,2,2,2,2,2,2,2,2,2,2,2,2,
2,2,2,2,2,2,2,2,2,2,2,2,2,2,2,2,2,2,4),(-0.99122901227168,-0.983227268753514,
-0.978906015803561,-0.957081038950441,-0.953390025194915,-0.951300092768376,
-0.949479155878613,-0.947006949049697,-0.941195600594014,-0.932678301015368,
-0.902453400744925,-0.877726444255291,-0.871833256301421,-0.868277269064003,
-0.865047058902015,-0.860841486355785,-0.851629742266183,-0.838830135286176,
-0.816681502993497,-0.812436920807133,-0.790449606973926,-0.786757969892135,
-0.784667924485216,-0.782847060789057,-0.780375183117481,-0.774565621412512,
-0.76605185669774,-0.735854285600317,-0.711097264555212,-0.705203241805246,
-0.701647125408222,-0.69841703507173,-0.694211959148986,-0.685002755409117,
-0.672207904435414,-0.650057728330045,-0.64582680367583,-0.62382054238759,
-0.620128908290396,-0.618038889988993,-0.61621806808448,-0.61374627148331,
-0.607937007578999,-0.59942377628223,-0.569229661290363,-0.544469920718849,
-0.538575920435688,-0.535019856989821,-0.531789839691983,-0.527584894676421,
-0.5183761303656,-0.505582018838782,-0.483432098484161,-0.479202765304772,
-0.457194844110276,-0.453503279123129,-0.451413302716797,-0.4495925192915,
-0.447120777577551,-0.441311654353651,-0.432798639784977,-0.402605463838678,
-0.377845888367626,-0.371952000358812,-0.368396008940593,-0.365166059781741,
-0.360961207371143,-0.351752662490332,-0.338958869860906,-0.316809390129865,
-0.312580309891305,-0.290572617179392,-0.286881128500756,-0.284791195598822,
-0.282970450291284,-0.280498760613538,-0.274689760959446,-0.266176928631103,
-0.235984417645231,-0.211217979187828,-0.205328067355939,-0.201772969145187,
-0.198542877425826,-0.19433646882046,-0.185118667016619,-0.172307071600673,
-0.149932055461014,-0.145974909398137,-0.123953539802761,-0.120262072634282,
-0.11817217031765,-0.116351464819597,-0.113879846807658,-0.108071093268383,
-0.0818781078266959,-0.0549654866670009,-0.0424558191754459,-0.0376072494629689,
-0.0346022527455657,-0.0313099301635705,-0.0280428445143505,-0.0235992042135266,
-0.000491388890533752),.UNSPECIFIED.);
#2886=B_SPLINE_CURVE_WITH_KNOTS('',3,(#122187,#122188,#122189,#122190,#122191,
#122192,#122193,#122194,#122195,#122196,#122197,#122198,#122199,#122200,
#122201,#122202,#122203,#122204),.UNSPECIFIED.,.F.,.F.,(4,2,2,2,2,2,2,2,
4),(-2.0995834550408,-2.06307905068172,-2.05736778314294,-2.05305526557987,
-2.05085783283395,-2.04905103120409,-2.04673484375579,-2.04180884207193,
-2.04079439360869),.UNSPECIFIED.);
#2887=B_SPLINE_CURVE_WITH_KNOTS('',3,(#122206,#122207,#122208,#122209,#122210,
#122211,#122212,#122213,#122214,#122215,#122216,#122217,#122218),
 .UNSPECIFIED.,.F.,.F.,(4,3,3,3,4),(-48.1819103737702,-48.0723494709303,
-47.9625850795796,-47.8822972006122,-47.8286804139494),.UNSPECIFIED.);
#2888=B_SPLINE_CURVE_WITH_KNOTS('',3,(#122219,#122220,#122221,#122222,#122223,
#122224,#122225,#122226,#122227),.UNSPECIFIED.,.F.,.F.,(4,1,1,1,1,1,4),
(-47.8286738456232,-46.8847493422661,-45.88720148392,-44.8896536255739,
-43.8921057672278,-42.8945579088817,-41.8982145781629),.UNSPECIFIED.);
#2889=B_SPLINE_CURVE_WITH_KNOTS('',3,(#122232,#122233,#122234,#122235,#122236,
#122237,#122238,#122239,#122240,#122241,#122242,#122243,#122244,#122245,
#122246,#122247,#122248,#122249,#122250,#122251,#122252,#122253,#122254,
#122255,#122256,#122257,#122258,#122259,#122260,#122261,#122262,#122263,
#122264,#122265,#122266,#122267,#122268,#122269,#122270,#122271,#122272,
#122273,#122274,#122275,#122276,#122277,#122278,#122279,#122280,#122281,
#122282,#122283,#122284,#122285,#122286,#122287,#122288,#122289,#122290,
#122291,#122292,#122293,#122294,#122295,#122296,#122297,#122298,#122299,
#122300,#122301,#122302,#122303,#122304,#122305,#122306,#122307,#122308,
#122309,#122310,#122311,#122312,#122313,#122314,#122315,#122316,#122317,
#122318,#122319,#122320,#122321,#122322,#122323,#122324,#122325,#122326,
#122327,#122328,#122329,#122330,#122331,#122332,#122333,#122334,#122335,
#122336,#122337,#122338,#122339,#122340,#122341,#122342,#122343,#122344,
#122345,#122346,#122347,#122348,#122349,#122350,#122351,#122352,#122353,
#122354,#122355,#122356,#122357,#122358,#122359,#122360,#122361,#122362,
#122363,#122364,#122365,#122366,#122367,#122368,#122369,#122370,#122371,
#122372,#122373,#122374,#122375,#122376,#122377,#122378,#122379,#122380,
#122381,#122382,#122383,#122384,#122385,#122386,#122387,#122388,#122389,
#122390,#122391,#122392,#122393,#122394,#122395,#122396,#122397,#122398,
#122399,#122400,#122401,#122402,#122403,#122404,#122405,#122406,#122407,
#122408,#122409,#122410,#122411,#122412,#122413,#122414,#122415,#122416,
#122417,#122418,#122419,#122420,#122421,#122422,#122423,#122424,#122425,
#122426,#122427,#122428,#122429,#122430,#122431,#122432,#122433,#122434,
#122435,#122436,#122437),.UNSPECIFIED.,.F.,.F.,(4,2,2,2,2,2,2,2,2,2,2,2,
2,2,2,2,2,2,2,2,2,2,2,2,2,2,2,2,2,2,2,2,2,2,2,2,2,2,2,2,2,2,2,2,2,2,2,2,
2,2,2,2,2,2,2,2,2,2,2,2,2,2,2,2,2,2,2,2,2,2,2,2,2,2,2,2,2,2,2,2,2,2,2,2,
2,2,2,2,2,2,2,2,2,2,2,2,2,2,2,2,2,2,4),(-2.04104836935547,-2.03714760643148,
-2.03384845018572,-2.03084882225062,-2.02603457887804,-2.0137649795725,
-1.97860410490939,-1.96388825609362,-1.95813225930661,-1.95503846348167,
-1.95251440409047,-1.95066795756041,-1.94895862152159,-1.94605733496182,
-1.93785136604741,-1.89539815447764,-1.88293084620018,-1.87389455395044,
-1.86971942006444,-1.86649271851588,-1.86292058366996,-1.85695249516301,
-1.82903629522694,-1.80749470991633,-1.79570851325417,-1.78839802852381,
-1.78569813276929,-1.7838408838656,-1.78185241498258,-1.77853061208035,
-1.76643333284362,-1.73899316752314,-1.72037545542265,-1.70842810153789,
-1.70379362613964,-1.70049506138052,-1.69709643016222,-1.69195099152614,
-1.67705435586687,-1.64133739110251,-1.62922903399014,-1.62178308966165,
-1.61906463265654,-1.61720393742357,-1.61546830423004,-1.61243035898823,
-1.60312554052276,-1.57027875748764,-1.55295790183522,-1.54156993263592,
-1.53701589354917,-1.53373176397268,-1.53071633122226,-1.52581039405415,
-1.51289974496388,-1.4783503978887,-1.46380581493756,-1.45809179571037,
-1.45377765578006,-1.45157984942926,-1.44977299960447,-1.44745708076006,
-1.44253279004588,-1.41914693007446,-1.39911833192168,-1.37720930719193,
-1.37160322612921,-1.36810807540033,-1.36485863475455,-1.36059198584682,
-1.35114565726767,-1.3091922065552,-1.2963061283585,-1.28854123950048,-1.28578017549339,
-1.28391130187087,-1.281943021965,-1.27871378539896,-1.26757083438192,-1.2394369833839,
-1.22053599577561,-1.20847000221757,-1.20381884834996,-1.20051717140189,
-1.19712282272305,-1.19199856697369,-1.17730739190922,-1.13718236939856,
-1.1276687747763,-1.1213745987438,-1.11882422211446,-1.11699219495391,-1.11494241242747,
-1.11133850813704,-1.09484825336649,-1.05022558243909,-1.04074392341031,
-1.03653753361252,-1.03329735349281,-1.02977596759147,-1.02404573221537,
-0.999969186069353,-0.99122901227168),.UNSPECIFIED.);
#2890=B_SPLINE_CURVE_WITH_KNOTS('',3,(#122439,#122440,#122441,#122442,#122443),
 .UNSPECIFIED.,.F.,.F.,(4,1,4),(-41.8982145781629,-41.8970100505356,-41.5455022211392),
 .UNSPECIFIED.);
#2891=B_SPLINE_CURVE_WITH_KNOTS('',3,(#122444,#122445,#122446,#122447,#122448,
#122449,#122450,#122451,#122452,#122453,#122454,#122455,#122456,#122457,
#122458,#122459,#122460,#122461,#122462,#122463,#122464,#122465,#122466,
#122467,#122468,#122469,#122470,#122471,#122472,#122473,#122474,#122475,
#122476,#122477,#122478,#122479,#122480,#122481,#122482,#122483,#122484,
#122485,#122486,#122487,#122488,#122489,#122490,#122491,#122492,#122493,
#122494,#122495,#122496,#122497,#122498,#122499,#122500,#122501,#122502,
#122503,#122504,#122505,#122506,#122507,#122508,#122509,#122510,#122511,
#122512,#122513,#122514,#122515,#122516,#122517,#122518,#122519,#122520,
#122521,#122522,#122523,#122524,#122525,#122526,#122527,#122528,#122529,
#122530,#122531,#122532,#122533,#122534,#122535,#122536,#122537,#122538,
#122539,#122540,#122541,#122542,#122543,#122544,#122545,#122546,#122547,
#122548,#122549,#122550,#122551,#122552,#122553,#122554,#122555,#122556,
#122557,#122558,#122559,#122560,#122561,#122562,#122563,#122564,#122565,
#122566,#122567,#122568,#122569,#122570,#122571,#122572,#122573,#122574,
#122575,#122576,#122577,#122578,#122579,#122580,#122581,#122582,#122583,
#122584,#122585,#122586,#122587,#122588,#122589,#122590,#122591,#122592,
#122593,#122594,#122595,#122596,#122597,#122598,#122599,#122600,#122601,
#122602,#122603,#122604,#122605,#122606,#122607,#122608,#122609,#122610,
#122611,#122612,#122613,#122614,#122615,#122616,#122617,#122618,#122619,
#122620,#122621,#122622,#122623,#122624,#122625,#122626,#122627,#122628,
#122629,#122630,#122631,#122632,#122633,#122634,#122635,#122636,#122637,
#122638,#122639,#122640,#122641,#122642,#122643),.UNSPECIFIED.,.F.,.F.,
(4,2,2,2,2,2,2,2,2,2,2,2,2,2,2,2,2,2,2,2,2,2,2,2,2,2,2,2,2,2,2,2,2,2,2,
2,2,2,2,2,2,2,2,2,2,2,2,2,2,2,2,2,2,2,2,2,2,2,2,2,2,2,2,2,2,2,2,2,2,2,2,
2,2,2,2,2,2,2,2,2,2,2,2,2,2,2,2,2,2,2,2,2,2,2,2,2,2,2,2,4),(-2.1000414668587,
-2.08485542041858,-2.08077718866876,-2.07763733435763,-2.07453432238086,
-2.07100464627802,-2.06523302522097,-2.04127262215763,-2.01005811635457,
-2.00155299813749,-1.99574737751126,-1.99327644547223,-1.99145598237474,
-1.98936617189274,-1.98567446947417,-1.96376871100479,-1.95944263777065,
-1.93728236085358,-1.92446023275039,-1.91523781786169,-1.91103086424852,
-1.90780104534508,-1.90424696669279,-1.89836049584397,-1.87352015997578,
-1.8434022656422,-1.83490018635286,-1.82909608462182,-1.82662541561,-1.82480499559872,
-1.82271505912222,-1.81902275646713,-1.79695558933515,-1.79273917895481,
-1.77056162210722,-1.75777924941491,-1.74857764109656,-1.74437432646234,
-1.7411449917458,-1.73758914105032,-1.73169425561274,-1.70686876120012,
-1.6767522709345,-1.66825040207843,-1.66244641603708,-1.6599757769634,-1.65815537142206,
-1.65606544272256,-1.65237313478429,-1.63029759444262,-1.62608763847407,
-1.60390966358946,-1.59112892038175,-1.58192818266925,-1.57772503815865,
-1.57449574428734,-1.57093984885771,-1.56504467583315,-1.54020843369436,
-1.51010166697522,-1.50160105823871,-1.49579770902668,-1.49332718678545,
-1.49150680669156,-1.48941683660854,-1.4857243035667,-1.46358018107037,
-1.4332958309038,-1.41743831176737,-1.4123311420795,-1.40894112918672,-1.40567623321714,
-1.401765487456,-1.39214405565269,-1.35426952809928,-1.33881532900511,-1.33007465122383,
-1.32719356222227,-1.32530095638157,-1.32336741030808,-1.32029536025266,
-1.31068974797531,-1.27802004463933,-1.26081869484812,-1.24948423174351,
-1.24493887957704,-1.24165702995712,-1.23864097985865,-1.2337279134282,
-1.22075989088108,-1.18626278481832,-1.1717320809302,-1.16332965516964,
-1.16048886672462,-1.15860460005043,-1.15666060313107,-1.15354042374703,
-1.14349921037197,-1.11108109221267,-1.10913474556486),.UNSPECIFIED.);
#2892=B_SPLINE_CURVE_WITH_KNOTS('',3,(#122649,#122650,#122651,#122652,#122653,
#122654,#122655,#122656,#122657,#122658,#122659,#122660,#122661,#122662,
#122663,#122664,#122665,#122666,#122667,#122668,#122669,#122670,#122671,
#122672,#122673,#122674,#122675,#122676,#122677,#122678,#122679,#122680,
#122681,#122682,#122683,#122684,#122685,#122686,#122687,#122688,#122689,
#122690,#122691,#122692,#122693,#122694,#122695,#122696,#122697,#122698,
#122699,#122700,#122701,#122702,#122703,#122704,#122705,#122706,#122707,
#122708,#122709,#122710,#122711,#122712,#122713,#122714,#122715,#122716,
#122717,#122718,#122719,#122720,#122721,#122722,#122723,#122724,#122725,
#122726,#122727,#122728,#122729,#122730,#122731,#122732,#122733,#122734,
#122735,#122736,#122737,#122738,#122739,#122740,#122741,#122742,#122743,
#122744,#122745,#122746,#122747,#122748,#122749,#122750,#122751,#122752,
#122753,#122754,#122755,#122756,#122757,#122758,#122759,#122760,#122761,
#122762,#122763,#122764,#122765,#122766,#122767,#122768,#122769,#122770,
#122771,#122772,#122773,#122774,#122775,#122776,#122777,#122778,#122779,
#122780,#122781,#122782,#122783,#122784,#122785,#122786,#122787,#122788,
#122789,#122790,#122791,#122792,#122793,#122794,#122795,#122796,#122797,
#122798,#122799,#122800,#122801,#122802,#122803,#122804,#122805,#122806,
#122807,#122808,#122809,#122810,#122811,#122812,#122813,#122814,#122815,
#122816,#122817,#122818,#122819,#122820,#122821,#122822,#122823,#122824,
#122825,#122826,#122827,#122828,#122829,#122830,#122831,#122832,#122833,
#122834,#122835,#122836,#122837,#122838,#122839,#122840,#122841,#122842,
#122843,#122844,#122845,#122846,#122847,#122848,#122849,#122850),
 .UNSPECIFIED.,.F.,.F.,(4,2,2,2,2,2,2,2,2,2,2,2,2,2,2,2,2,2,2,2,2,2,2,2,
2,2,2,2,2,2,2,2,2,2,2,2,2,2,2,2,2,2,2,2,2,2,2,2,2,2,2,2,2,2,2,2,2,2,2,2,
2,2,2,2,2,2,2,2,2,2,2,2,2,2,2,2,2,2,2,2,2,2,2,2,2,2,2,2,2,2,2,2,2,2,2,2,
2,2,2,2,4),(-0.991067510703159,-0.969566476182921,-0.944672859721234,-0.938774223388853,
-0.935216919650418,-0.931986760811124,-0.927783045495996,-0.91858299783399,
-0.905806075864837,-0.883646082544692,-0.879488147545464,-0.857381082759265,
-0.853688743904557,-0.851598454201426,-0.84977748709762,-0.847305615543153,
-0.841496713817424,-0.832984500027537,-0.802801838660546,-0.778023625108033,
-0.772128590518732,-0.768572100025024,-0.765341819538381,-0.761136710980887,
-0.751928352019178,-0.73913544802847,-0.716982507979576,-0.712760530712895,
-0.690739798845815,-0.687047860436213,-0.68495768673693,-0.683136741528078,
-0.680664793709547,-0.67485524568444,-0.666341662471877,-0.636147338465189,
-0.611383736675271,-0.605489262364102,-0.601932939070134,-0.59870270230495,
-0.594497495356017,-0.585288258792793,-0.572493576715306,-0.550341989050687,
-0.546113369480386,-0.52410251242266,-0.520410687042745,-0.518320565062926,
-0.516499656135749,-0.514027745820546,-0.508218234146404,-0.499704657372448,
-0.469509601148857,-0.444748080051911,-0.438853777598179,-0.435297538992551,
-0.432067367121868,-0.427862227380027,-0.418653064344215,-0.405858422252137,
-0.383707397496495,-0.379478134999086,-0.357468767370291,-0.353777023110643,
-0.351686945712757,-0.349866074664626,-0.347394214486147,-0.341584814974732,
-0.333071397443817,-0.302876823348433,-0.278115991124243,-0.272221817247314,
-0.26866565413597,-0.265435549521099,-0.26123049544298,-0.252021511942407,
-0.239227112477597,-0.217076561846425,-0.192746244043969,-0.187894867516914,
-0.185559841425146,-0.183752121778224,-0.181570315748068,-0.177334846557921,
-0.151815685007491,-0.113524293960377,-0.107177248464375,-0.103161166903685,
-0.0999513126258957,-0.0962849916768693,-0.0898688149715362,-0.0673539059889128,
-0.043476137094742,-0.026732385323984,-0.0214000910904637,-0.0190357117834795,
-0.0172225165109289,-0.0155112267029777,-0.0133869765241974,-0.00853516041908881,
-0.000491170393658215),.UNSPECIFIED.);
#2893=B_SPLINE_CURVE_WITH_KNOTS('',3,(#122851,#122852,#122853,#122854,#122855,
#122856,#122857,#122858,#122859,#122860),.UNSPECIFIED.,.F.,.F.,(4,2,2,2,
4),(-2.10008953608574,-2.07237373101306,-2.05373873006262,-2.04178356612171,
-2.04104836935547),.UNSPECIFIED.);
#2894=B_SPLINE_CURVE_WITH_KNOTS('',3,(#122861,#122862,#122863,#122864,#122865,
#122866,#122867,#122868,#122869,#122870,#122871,#122872,#122873,#122874,
#122875,#122876,#122877,#122878,#122879,#122880,#122881,#122882,#122883,
#122884,#122885,#122886,#122887,#122888,#122889,#122890,#122891,#122892,
#122893,#122894,#122895,#122896,#122897,#122898,#122899,#122900,#122901,
#122902,#122903,#122904,#122905,#122906,#122907,#122908,#122909,#122910,
#122911,#122912,#122913,#122914,#122915,#122916,#122917,#122918,#122919,
#122920,#122921,#122922,#122923,#122924,#122925,#122926,#122927,#122928,
#122929,#122930,#122931,#122932,#122933,#122934,#122935,#122936,#122937,
#122938,#122939,#122940,#122941,#122942,#122943,#122944,#122945,#122946,
#122947,#122948,#122949,#122950,#122951,#122952,#122953,#122954,#122955,
#122956,#122957,#122958,#122959,#122960,#122961,#122962,#122963,#122964,
#122965,#122966,#122967,#122968,#122969,#122970,#122971,#122972,#122973,
#122974,#122975,#122976,#122977,#122978,#122979,#122980,#122981,#122982,
#122983,#122984,#122985,#122986,#122987,#122988,#122989,#122990,#122991,
#122992,#122993,#122994,#122995,#122996,#122997,#122998,#122999,#123000,
#123001,#123002,#123003,#123004,#123005,#123006,#123007,#123008,#123009,
#123010,#123011,#123012,#123013,#123014,#123015,#123016,#123017,#123018,
#123019,#123020,#123021,#123022,#123023,#123024,#123025,#123026,#123027,
#123028,#123029,#123030,#123031,#123032,#123033,#123034,#123035,#123036,
#123037,#123038,#123039,#123040,#123041,#123042,#123043,#123044,#123045,
#123046,#123047,#123048,#123049,#123050,#123051,#123052,#123053,#123054,
#123055,#123056,#123057,#123058,#123059,#123060,#123061,#123062,#123063,
#123064,#123065,#123066,#123067,#123068,#123069,#123070,#123071,#123072,
#123073,#123074,#123075,#123076),.UNSPECIFIED.,.F.,.F.,(4,2,2,2,2,2,2,2,
2,2,2,2,2,2,2,2,2,2,2,2,2,2,2,2,2,2,2,2,2,2,2,2,2,2,2,2,2,2,2,2,2,2,2,2,
2,2,2,2,2,2,2,2,2,2,2,2,2,2,2,2,2,2,2,2,2,2,2,2,2,2,2,2,2,2,2,2,2,2,2,2,
2,2,2,2,2,2,2,2,2,2,2,2,2,2,2,2,2,2,2,2,2,2,2,2,2,2,2,4),(-1.10913474556486,
-1.09405576568703,-1.08279979728913,-1.07826612179371,-1.0749863647678,
-1.07156059995665,-1.06628010922902,-1.05011160521927,-1.0213889613544,
-0.998409794735737,-0.994714782785097,-0.992624315431684,-0.990804181940742,
-0.988334847264225,-0.982538220210314,-0.974049977518646,-0.944052028088183,
-0.919059795644637,-0.913159580686374,-0.909602758030787,-0.906373970953528,
-0.902173417017199,-0.892986384919195,-0.880233136193736,-0.858065269904299,
-0.854030670440583,-0.831767925363533,-0.828075881831663,-0.825986104259027,
-0.824165864269339,-0.821695438602947,-0.815892086195546,-0.807390234433797,
-0.77728404937972,-0.752417671497103,-0.746521242636705,-0.742965271570152,
-0.739736352535635,-0.735534328395455,-0.726338555578801,-0.713568519466804,
-0.691406753585429,-0.687271593018449,-0.665133876505458,-0.66144236726291,
-0.659352735245371,-0.657532509906766,-0.655061954021645,-0.649257634751549,
-0.640753769360755,-0.610630870260464,-0.585784925552515,-0.579889216621454,
-0.576333445978787,-0.573104561047988,-0.568902369041317,-0.559705325191687,
-0.546932762510047,-0.524772473165564,-0.520623460756081,-0.498503968793178,
-0.494812601649143,-0.492723027482836,-0.490902836391282,-0.488432305375315,
-0.482627949343261,-0.474123944083238,-0.443999168495455,-0.419156605698403,
-0.41326110492502,-0.409705426009209,-0.406476602977054,-0.402274460818685,
-0.393077395310913,-0.380304692356088,-0.358145009801013,-0.353994120845126,
-0.331877599673955,-0.328186318020879,-0.326096789046958,-0.324276635032258,
-0.321806151275039,-0.316001892778133,-0.307498018223077,-0.277373509828933,
-0.252531866268621,-0.246636499375252,-0.243080896407582,-0.239852139307401,
-0.235650078599824,-0.226453172809721,-0.213680676034172,-0.191521471838072,
-0.167222933306922,-0.162272064254352,-0.1599518285471,-0.158145538368494,
-0.155953298366559,-0.151663869331122,-0.14599140447005,-0.131613852291793,
-0.0976704140317422,-0.0840808351867522,-0.0790847254395175,-0.0760540547136202,
-0.0727841383799814,-0.0683061924789343,-0.0595903478899269),
 .UNSPECIFIED.);
#2895=B_SPLINE_CURVE_WITH_KNOTS('',3,(#123081,#123082,#123083,#123084,#123085,
#123086,#123087,#123088,#123089,#123090,#123091,#123092,#123093,#123094,
#123095,#123096,#123097,#123098,#123099,#123100,#123101,#123102,#123103,
#123104,#123105,#123106,#123107,#123108,#123109,#123110,#123111,#123112,
#123113,#123114,#123115,#123116,#123117,#123118,#123119,#123120,#123121,
#123122,#123123,#123124,#123125,#123126,#123127,#123128,#123129,#123130,
#123131,#123132,#123133,#123134,#123135,#123136,#123137,#123138,#123139,
#123140,#123141,#123142,#123143,#123144,#123145,#123146,#123147,#123148,
#123149,#123150,#123151,#123152,#123153,#123154,#123155,#123156,#123157,
#123158,#123159,#123160,#123161,#123162,#123163,#123164,#123165,#123166,
#123167,#123168,#123169,#123170,#123171,#123172,#123173,#123174,#123175,
#123176,#123177,#123178,#123179,#123180,#123181,#123182,#123183,#123184,
#123185,#123186,#123187,#123188,#123189,#123190,#123191,#123192,#123193,
#123194,#123195,#123196,#123197,#123198,#123199,#123200,#123201,#123202,
#123203,#123204,#123205,#123206,#123207,#123208,#123209,#123210,#123211,
#123212,#123213,#123214,#123215,#123216,#123217,#123218,#123219,#123220,
#123221,#123222,#123223,#123224,#123225,#123226,#123227,#123228,#123229,
#123230,#123231,#123232,#123233,#123234,#123235,#123236,#123237,#123238,
#123239,#123240,#123241,#123242,#123243,#123244,#123245,#123246,#123247,
#123248,#123249,#123250,#123251,#123252,#123253,#123254,#123255,#123256,
#123257,#123258,#123259,#123260,#123261,#123262,#123263,#123264,#123265,
#123266,#123267,#123268,#123269,#123270,#123271,#123272,#123273,#123274,
#123275,#123276,#123277,#123278,#123279,#123280,#123281,#123282,#123283,
#123284,#123285,#123286),.UNSPECIFIED.,.F.,.F.,(4,2,2,2,2,2,2,2,2,2,2,2,
2,2,2,2,2,2,2,2,2,2,2,2,2,2,2,2,2,2,2,2,2,2,2,2,2,2,2,2,2,2,2,2,2,2,2,2,
2,2,2,2,2,2,2,2,2,2,2,2,2,2,2,2,2,2,2,2,2,2,2,2,2,2,2,2,2,2,2,2,2,2,2,2,
2,2,2,2,2,2,2,2,2,2,2,2,2,2,2,2,2,2,4),(-2.04084412535128,-2.03783344299161,
-2.02809527437528,-2.02169589036857,-2.01912933929048,-2.01729501143891,
-2.01525320173045,-2.01168551557941,-1.99558471766472,-1.9662330821357,
-1.9515417756892,-1.94137540720377,-1.93700972669471,-1.93375687175612,
-1.93027160010572,-1.92471122137928,-1.9057732633403,-1.86208714680868,
-1.85519439216568,-1.85255380240412,-1.85070723674901,-1.84869684021687,
-1.8452742039963,-1.83179062892292,-1.80532919468405,-1.78709524173683,
-1.77908339465956,-1.77261186671085,-1.76893363887402,-1.76572464513885,
-1.76172444617817,-1.75543265269942,-1.71661397467131,-1.69153946808137,
-1.68730677657481,-1.6851253779524,-1.68331740777108,-1.68098127868356,
-1.67612512020677,-1.65311220368238,-1.63359347797964,-1.61848303859685,
-1.60811353163126,-1.60371499750885,-1.6004567341046,-1.59740385141958,
-1.59229217527738,-1.57772052372698,-1.5416740848356,-1.52952015345061,
-1.52205515309274,-1.51933406933972,-1.51747285027636,-1.51573781778083,
-1.51270307408575,-1.50342592679449,-1.47390592434904,-1.4544444405685,
-1.44214780051682,-1.43746488447436,-1.43415740784466,-1.43116683353677,
-1.42640341801443,-1.41446931791054,-1.37899245107612,-1.35905741507545,
-1.35429604918236,-1.35201075564647,-1.35020495714318,-1.34798019687965,
-1.34353099980867,-1.30962977344053,-1.28297203494131,-1.27409521596028,
-1.26994854026439,-1.26672536961805,-1.26313832552059,-1.25709934955502,
-1.22770826950123,-1.20603167292204,-1.19020868362467,-1.18675381386956,
-1.18473637427786,-1.18289277029456,-1.18026956689495,-1.17397521987442,
-1.14198312886049,-1.11242985742344,-1.10594537086438,-1.10226443570444,
-1.09905573203107,-1.09505936225061,-1.08878060967185,-1.04983754644215,
-1.04683104770034,-1.02403000017116,-1.02033494150564,-1.01824401713651,
-1.01642314385123,-1.01395226516392,-1.00814950690654,-0.999649737438738,
-0.991067510703159),.UNSPECIFIED.);
#2896=B_SPLINE_CURVE_WITH_KNOTS('',3,(#123288,#123289,#123290,#123291,#123292,
#123293,#123294,#123295,#123296,#123297),.UNSPECIFIED.,.F.,.F.,(4,2,2,2,
4),(-0.0595903478899269,-0.0574178101975677,-0.0412035277078622,-0.0229711166027303,
-0.000637630673692526),.UNSPECIFIED.);
#2897=B_SPLINE_CURVE_WITH_KNOTS('',3,(#123298,#123299,#123300,#123301,#123302,
#123303,#123304,#123305,#123306,#123307,#123308,#123309,#123310,#123311,
#123312,#123313,#123314,#123315,#123316,#123317,#123318,#123319,#123320,
#123321,#123322,#123323,#123324,#123325,#123326,#123327,#123328,#123329,
#123330,#123331,#123332,#123333,#123334,#123335,#123336,#123337,#123338,
#123339,#123340,#123341,#123342,#123343,#123344,#123345,#123346,#123347,
#123348,#123349,#123350,#123351,#123352,#123353,#123354,#123355,#123356,
#123357,#123358,#123359,#123360,#123361,#123362,#123363,#123364,#123365,
#123366,#123367,#123368,#123369,#123370,#123371,#123372,#123373,#123374,
#123375,#123376,#123377,#123378,#123379,#123380,#123381,#123382,#123383,
#123384,#123385,#123386,#123387,#123388,#123389,#123390,#123391,#123392,
#123393,#123394,#123395,#123396,#123397,#123398,#123399,#123400,#123401,
#123402,#123403,#123404,#123405,#123406,#123407,#123408,#123409,#123410,
#123411,#123412,#123413,#123414,#123415,#123416,#123417,#123418,#123419,
#123420,#123421,#123422,#123423,#123424,#123425,#123426,#123427,#123428,
#123429,#123430,#123431,#123432,#123433,#123434,#123435,#123436,#123437,
#123438,#123439,#123440,#123441,#123442,#123443,#123444,#123445,#123446,
#123447,#123448,#123449,#123450,#123451,#123452,#123453,#123454,#123455,
#123456,#123457,#123458,#123459,#123460,#123461,#123462,#123463,#123464,
#123465,#123466,#123467,#123468,#123469,#123470,#123471,#123472,#123473,
#123474,#123475,#123476,#123477,#123478,#123479,#123480,#123481,#123482,
#123483,#123484,#123485,#123486,#123487,#123488,#123489,#123490,#123491,
#123492,#123493,#123494,#123495),.UNSPECIFIED.,.F.,.F.,(4,2,2,2,2,2,2,2,
2,2,2,2,2,2,2,2,2,2,2,2,2,2,2,2,2,2,2,2,2,2,2,2,2,2,2,2,2,2,2,2,2,2,2,2,
2,2,2,2,2,2,2,2,2,2,2,2,2,2,2,2,2,2,2,2,2,2,2,2,2,2,2,2,2,2,2,2,2,2,2,2,
2,2,2,2,2,2,2,2,2,2,2,2,2,2,2,2,2,2,4),(-4.84275027886607,-4.84016473224924,
-4.83781058688713,-4.8359439682687,-4.83423881191794,-4.83227663570649,
-4.82907566964572,-4.81821837465505,-4.78590128633185,-4.76939626374703,
-4.76186754653844,-4.75570038046285,-4.75208594971086,-4.74886769319487,
-4.74476809788961,-4.7381351756049,-4.70462640946889,-4.67497749940669,
-4.67066585404631,-4.66846839615449,-4.66666133332427,-4.66434458374319,
-4.65941670883551,-4.63505226931717,-4.61286602466617,-4.60007876296943,
-4.59087361610647,-4.58666867067668,-4.58343807736947,-4.57988083516064,
-4.57398362939074,-4.54914776203764,-4.5190201234511,-4.51051501377239,
-4.50470880122425,-4.50223720464507,-4.50041608977555,-4.49832534227604,
-4.49463157816885,-4.47254312207794,-4.46833478111313,-4.44614787245157,
-4.43336290723675,-4.4241589800867,-4.41995426562249,-4.41672372095439,
-4.41316640370285,-4.40726876756833,-4.38241739881447,-4.3523036213571,
-4.34380029404838,-4.33799497763074,-4.33552354112721,-4.3337024571724,
-4.3316116438335,-4.32791754524114,-4.30573021130639,-4.3019450688493,-4.27924799478739,
-4.26656801350084,-4.25741915716489,-4.25322407723578,-4.24999477459079,
-4.24643265670455,-4.24051233517303,-4.21477341083528,-4.18542359623272,
-4.17701837068339,-4.17126189229053,-4.16879863404778,-4.16697857985096,
-4.16488311622511,-4.16116817101942,-4.13674691676291,-4.11776137357766,
-4.09412199189254,-4.08841367945736,-4.08489665642377,-4.08165455002852,
-4.0774372352923,-4.06789238573397,-4.02978623754438,-4.01426865956622,
-4.00550399190194,-4.00261936019934,-4.00072549845072,-3.99879177759986,
-3.99572125639844,-3.98613613015403,-3.95343909709813,-3.93622106346518,
-3.92487771208003,-3.92032989752612,-3.91704662057629,-3.91362310414737,
-3.90835816025227,-3.89235947550556,-3.85363058724457,-3.85161562629314),
 .UNSPECIFIED.);
#2898=B_SPLINE_CURVE_WITH_KNOTS('',3,(#123501,#123502,#123503,#123504,#123505,
#123506,#123507,#123508,#123509,#123510,#123511,#123512,#123513,#123514,
#123515,#123516,#123517,#123518,#123519,#123520,#123521,#123522,#123523,
#123524,#123525,#123526,#123527,#123528,#123529,#123530,#123531,#123532,
#123533,#123534,#123535,#123536,#123537,#123538,#123539,#123540,#123541,
#123542,#123543,#123544,#123545,#123546,#123547,#123548,#123549,#123550,
#123551,#123552,#123553,#123554,#123555,#123556,#123557,#123558,#123559,
#123560,#123561,#123562,#123563,#123564,#123565,#123566,#123567,#123568,
#123569,#123570,#123571,#123572,#123573,#123574,#123575,#123576,#123577,
#123578,#123579,#123580,#123581,#123582,#123583,#123584,#123585,#123586,
#123587,#123588,#123589,#123590,#123591,#123592,#123593,#123594,#123595,
#123596,#123597,#123598,#123599,#123600,#123601,#123602,#123603,#123604,
#123605,#123606,#123607,#123608,#123609,#123610,#123611,#123612,#123613,
#123614,#123615,#123616,#123617,#123618,#123619,#123620,#123621,#123622,
#123623,#123624,#123625,#123626,#123627,#123628,#123629,#123630,#123631,
#123632,#123633,#123634,#123635,#123636,#123637,#123638,#123639,#123640,
#123641,#123642,#123643,#123644,#123645,#123646,#123647,#123648,#123649,
#123650,#123651,#123652,#123653,#123654,#123655,#123656,#123657,#123658,
#123659,#123660,#123661,#123662,#123663,#123664,#123665,#123666,#123667,
#123668,#123669,#123670,#123671,#123672,#123673,#123674,#123675,#123676,
#123677,#123678,#123679,#123680,#123681,#123682,#123683,#123684,#123685,
#123686,#123687,#123688),.UNSPECIFIED.,.F.,.F.,(4,2,2,2,2,2,2,2,2,2,2,2,
2,2,2,2,2,2,2,2,2,2,2,2,2,2,2,2,2,2,2,2,2,2,2,2,2,2,2,2,2,2,2,2,2,2,2,2,
2,2,2,2,2,2,2,2,2,2,2,2,2,2,2,2,2,2,2,2,2,2,2,2,2,2,2,2,2,2,2,2,2,2,2,2,
2,2,2,2,2,2,2,2,2,4),(-0.991269537285924,-0.990703049540231,-0.95950551951661,
-0.925920860047596,-0.921439259655927,-0.919208091960617,-0.917402432588172,
-0.915124029349346,-0.910398897690839,-0.89079815305279,-0.856285529713042,
-0.843306669751067,-0.838391042245147,-0.835373784673303,-0.832090910761312,
-0.827544600475137,-0.816209522722367,-0.799010407219534,-0.766377237774403,
-0.756772664097815,-0.753700225855695,-0.751766182089873,-0.749872828918714,
-0.746990073976569,-0.738240338359172,-0.722761152276517,-0.684804927974626,
-0.675113854394691,-0.670872442820286,-0.667626940805385,-0.664121076440339,
-0.658464295085302,-0.635718332442822,-0.616234319537125,-0.5932677177682,
-0.588413548878501,-0.586077876644514,-0.584270004264512,-0.582088435938074,
-0.577854585990412,-0.552682616179897,-0.513954012550315,-0.507650058425638,
-0.503646446615236,-0.500437376027691,-0.496761961955253,-0.490303135060156,
-0.456188255095197,-0.426416994098503,-0.421610575446495,-0.419316885964097,
-0.417511034148025,-0.415294311147537,-0.410884957570827,-0.405004152691311,
-0.38976535247827,-0.352705900857596,-0.342377724326619,-0.338307306313728,
-0.335301571860482,-0.332009608003629,-0.327410077377925,-0.315706132234414,
-0.297661638587813,-0.280686460663491,-0.258037466083515,-0.25434354042531,
-0.252253047272971,-0.250432399530354,-0.247961626157025,-0.242158231868365,
-0.233656732839965,-0.203554561739876,-0.178684499340552,-0.172790928289895,
-0.169235024933393,-0.166005090441219,-0.161800163308476,-0.152591054755118,
-0.139796141315294,-0.117647405365759,-0.113414453814164,-0.0914124834427105,
-0.0877210490486593,-0.0856311396626544,-0.0838104096785013,-0.0813387338904072,
-0.07552973642375,-0.0670168797564971,-0.0429024945777408,-0.0122258448422594,
-0.00636431777156412,-0.00292231655515231,-0.000491642754462011),
 .UNSPECIFIED.);
#2899=B_SPLINE_CURVE_WITH_KNOTS('',3,(#123689,#123690,#123691,#123692,#123693,
#123694,#123695,#123696,#123697,#123698,#123699,#123700),.UNSPECIFIED.,
 .F.,.F.,(4,2,2,2,2,4),(-2.09975934511255,-2.09808945502736,-2.09537980374138,
-2.08928500501059,-2.06056864970726,-2.04084412535128),.UNSPECIFIED.);
#2900=B_SPLINE_CURVE_WITH_KNOTS('',3,(#123701,#123702,#123703,#123704,#123705,
#123706,#123707,#123708,#123709,#123710,#123711,#123712,#123713,#123714,
#123715,#123716,#123717,#123718,#123719,#123720,#123721,#123722,#123723,
#123724,#123725,#123726,#123727,#123728,#123729,#123730,#123731,#123732,
#123733,#123734,#123735,#123736,#123737,#123738,#123739,#123740,#123741,
#123742,#123743,#123744,#123745,#123746,#123747,#123748,#123749,#123750,
#123751,#123752,#123753,#123754,#123755,#123756,#123757,#123758,#123759,
#123760,#123761,#123762,#123763,#123764,#123765,#123766,#123767,#123768,
#123769,#123770,#123771,#123772,#123773,#123774,#123775,#123776,#123777,
#123778,#123779,#123780,#123781,#123782,#123783,#123784,#123785,#123786,
#123787,#123788,#123789,#123790,#123791,#123792,#123793,#123794,#123795,
#123796,#123797,#123798,#123799,#123800,#123801,#123802,#123803,#123804,
#123805,#123806,#123807,#123808,#123809,#123810,#123811,#123812,#123813,
#123814,#123815,#123816,#123817,#123818,#123819,#123820,#123821,#123822,
#123823,#123824,#123825,#123826,#123827,#123828,#123829,#123830,#123831,
#123832,#123833,#123834,#123835,#123836,#123837,#123838,#123839,#123840,
#123841,#123842,#123843,#123844,#123845,#123846,#123847,#123848,#123849,
#123850,#123851,#123852,#123853,#123854,#123855,#123856,#123857,#123858,
#123859,#123860,#123861,#123862,#123863,#123864,#123865,#123866,#123867,
#123868,#123869,#123870,#123871,#123872,#123873,#123874,#123875,#123876,
#123877,#123878,#123879,#123880,#123881,#123882,#123883,#123884,#123885,
#123886,#123887,#123888,#123889,#123890,#123891,#123892,#123893,#123894,
#123895,#123896,#123897,#123898,#123899,#123900,#123901,#123902),
 .UNSPECIFIED.,.F.,.F.,(4,2,2,2,2,2,2,2,2,2,2,2,2,2,2,2,2,2,2,2,2,2,2,2,
2,2,2,2,2,2,2,2,2,2,2,2,2,2,2,2,2,2,2,2,2,2,2,2,2,2,2,2,2,2,2,2,2,2,2,2,
2,2,2,2,2,2,2,2,2,2,2,2,2,2,2,2,2,2,2,2,2,2,2,2,2,2,2,2,2,2,2,2,2,2,2,2,
2,2,2,2,4),(-3.85161562629314,-3.84422898914919,-3.83798758874284,-3.83544544478692,
-3.83361461612228,-3.83156086629186,-3.82793872235395,-3.81104232570972,
-3.76661694324815,-3.75728141288532,-3.75305420445616,-3.74982106203738,
-3.74627544532569,-3.74043157114328,-3.71695604383362,-3.68562584202229,
-3.67278495216338,-3.66951931682024,-3.66754312803081,-3.66570087304714,
-3.66341793431746,-3.65762050424875,-3.6251407403044,-3.59942500517989,
-3.59041095938543,-3.58623988922321,-3.58301386561286,-3.57944001720798,
-3.5734631783833,-3.54361456492192,-3.51766322693072,-3.50590426735176,
-3.50272387945276,-3.50076633606268,-3.49891296446719,-3.49613569747234,
-3.48883454057117,-3.45771289498189,-3.4326781868821,-3.42368807467503,
-3.41952125061821,-3.41629575074859,-3.41271968558842,-3.40673235307988,
-3.37846980362368,-3.35711780516387,-3.34544249729264,-3.33817898138171,
-3.33548568813289,-3.3336297504521,-3.33163922331026,-3.32830760265149,
-3.31608955147722,-3.28872548937564,-3.27013588463974,-3.25819998694201,
-3.25356726072747,-3.25026918906866,-3.24726975266234,-3.24322596209173,
-3.23306607732978,-3.18752384558539,-3.1776393815424,-3.17117158652448,
-3.16859437418031,-3.16675829128008,-3.16472117835881,-3.16117565342831,
-3.14556988072911,-3.11584778519816,-3.10104078083207,-3.09081751466479,
-3.08644243092351,-3.08318795252335,-3.0797060088438,-3.07416210705314,
-3.05517421163516,-3.0114791587665,-3.0045824383886,-3.0019411378807,-3.00009435699782,
-2.99808410321265,-2.99466253744258,-2.98120061049044,-2.95470942306851,
-2.93646039638031,-2.92466850831725,-2.92005587535993,-2.9167612068738,
-2.91375753592395,-2.90969686342703,-2.89943386723997,-2.85858612601351,
-2.84582565906082,-2.83811110538271,-2.8353565848152,-2.83348895174086,
-2.83151862172262,-2.82828012678467,-2.81703552151411,-2.80145779137746),
 .UNSPECIFIED.);
#2901=B_SPLINE_CURVE_WITH_KNOTS('',3,(#123907,#123908,#123909,#123910,#123911,
#123912,#123913,#123914,#123915,#123916,#123917,#123918,#123919,#123920,
#123921,#123922,#123923,#123924,#123925,#123926,#123927,#123928,#123929,
#123930,#123931,#123932,#123933,#123934,#123935,#123936,#123937,#123938,
#123939,#123940,#123941,#123942,#123943,#123944,#123945,#123946,#123947,
#123948,#123949,#123950,#123951,#123952,#123953,#123954,#123955,#123956,
#123957,#123958,#123959,#123960,#123961,#123962,#123963,#123964,#123965,
#123966,#123967,#123968,#123969,#123970,#123971,#123972,#123973,#123974,
#123975,#123976,#123977,#123978,#123979,#123980,#123981,#123982,#123983,
#123984,#123985,#123986,#123987,#123988,#123989,#123990,#123991,#123992,
#123993,#123994,#123995,#123996,#123997,#123998,#123999,#124000,#124001,
#124002,#124003,#124004,#124005,#124006,#124007,#124008,#124009,#124010,
#124011,#124012,#124013,#124014,#124015,#124016,#124017,#124018,#124019,
#124020,#124021,#124022,#124023,#124024,#124025,#124026,#124027,#124028,
#124029,#124030,#124031,#124032,#124033,#124034,#124035,#124036,#124037,
#124038,#124039,#124040,#124041,#124042,#124043,#124044,#124045,#124046,
#124047,#124048,#124049,#124050,#124051,#124052,#124053,#124054,#124055,
#124056,#124057,#124058,#124059,#124060,#124061,#124062,#124063,#124064,
#124065,#124066,#124067,#124068,#124069,#124070,#124071,#124072,#124073,
#124074,#124075,#124076,#124077,#124078,#124079,#124080,#124081,#124082,
#124083,#124084,#124085,#124086,#124087,#124088,#124089,#124090,#124091,
#124092,#124093,#124094,#124095,#124096,#124097,#124098,#124099,#124100,
#124101,#124102,#124103,#124104,#124105,#124106,#124107,#124108,#124109,
#124110,#124111,#124112,#124113,#124114),.UNSPECIFIED.,.F.,.F.,(4,2,2,2,
2,2,2,2,2,2,2,2,2,2,2,2,2,2,2,2,2,2,2,2,2,2,2,2,2,2,2,2,2,2,2,2,2,2,2,2,
2,2,2,2,2,2,2,2,2,2,2,2,2,2,2,2,2,2,2,2,2,2,2,2,2,2,2,2,2,2,2,2,2,2,2,2,
2,2,2,2,2,2,2,2,2,2,2,2,2,2,2,2,2,2,2,2,2,2,2,2,2,2,2,4),(-2.04107054618519,
-2.01310847198346,-2.00662462122167,-2.00294361178816,-1.99973459518817,
-1.99573751068811,-1.98945697572702,-1.95052272761901,-1.92553552185573,
-1.92130295956127,-1.91912146844143,-1.91731333282856,-1.9149768726701,
-1.91011963004885,-1.88577824426209,-1.86360859074923,-1.85080457342558,
-1.84159095974072,-1.83738459475986,-1.83415383279138,-1.83059729799196,
-1.8247033134626,-1.79995365193905,-1.76976993096714,-1.76125875153898,
-1.75544969655322,-1.75297765404215,-1.75115648906623,-1.74906593760263,
-1.74537298107917,-1.72338130415929,-1.71911228084971,-1.69694125636454,
-1.68414075681005,-1.67492899980363,-1.67072297756311,-1.66749227980551,
-1.66393561713663,-1.65804094865667,-1.63326790790759,-1.60310501672582,
-1.59459649388533,-1.58878876853925,-1.58631695759483,-1.5844958311485,
-1.58240516886669,-1.57871168611666,-1.55657190302086,-1.55241258667971,
-1.53023080902313,-1.51745878609539,-1.50826194567617,-1.50405853636767,
-1.50082818708284,-1.4972702515797,-1.49136953088272,-1.46639150666275,
-1.43640725307171,-1.42792133953288,-1.42212485147269,-1.41965492279101,
-1.4178340423157,-1.41574233471353,-1.41204413776501,-1.38879472627267,
-1.38627809892863,-1.36345942603214,-1.3507500573391,-1.34158608909442,
-1.33738844886172,-1.33415886518938,-1.33059810271997,-1.3246839371242,
-1.29918590247435,-1.27851159046928,-1.26449794602418,-1.25629040763044,
-1.25347290339832,-1.25159286662889,-1.24987964025549,-1.24695733860765,
-1.238589950454,-1.20516104438669,-1.18746475181874,-1.17959996114186,-1.17322048769713,
-1.16956144594394,-1.16635005634423,-1.16232157327202,-1.15593345555153,
-1.11809304305186,-1.09222648107476,-1.08798927861505,-1.08580690576362,
-1.0839989194083,-1.0816637851635,-1.07681297460773,-1.05036589697884,-1.0144038356493,
-1.00787012551006,-1.00379934037544,-1.00058412445147,-0.996952468312172,
-0.991269537285924),.UNSPECIFIED.);
#2902=B_SPLINE_CURVE_WITH_KNOTS('',3,(#124115,#124116,#124117,#124118,#124119,
#124120,#124121,#124122,#124123,#124124,#124125,#124126,#124127,#124128,
#124129,#124130,#124131,#124132,#124133,#124134,#124135,#124136,#124137,
#124138,#124139,#124140,#124141,#124142,#124143,#124144,#124145,#124146,
#124147,#124148,#124149,#124150,#124151,#124152,#124153,#124154,#124155,
#124156,#124157,#124158,#124159,#124160,#124161,#124162,#124163,#124164,
#124165,#124166,#124167,#124168,#124169,#124170,#124171,#124172,#124173,
#124174,#124175,#124176,#124177,#124178,#124179,#124180,#124181,#124182,
#124183,#124184,#124185,#124186,#124187,#124188,#124189,#124190,#124191,
#124192,#124193,#124194,#124195,#124196,#124197,#124198,#124199,#124200,
#124201,#124202,#124203,#124204,#124205,#124206,#124207,#124208,#124209,
#124210,#124211,#124212,#124213,#124214,#124215,#124216,#124217,#124218,
#124219,#124220,#124221,#124222,#124223,#124224,#124225,#124226,#124227,
#124228,#124229,#124230,#124231,#124232,#124233,#124234,#124235,#124236,
#124237,#124238,#124239,#124240,#124241,#124242,#124243,#124244,#124245,
#124246,#124247,#124248,#124249,#124250,#124251,#124252,#124253,#124254,
#124255,#124256,#124257,#124258,#124259,#124260,#124261,#124262,#124263,
#124264,#124265,#124266,#124267,#124268,#124269,#124270,#124271,#124272,
#124273,#124274,#124275,#124276,#124277,#124278,#124279,#124280,#124281,
#124282,#124283,#124284,#124285,#124286,#124287,#124288,#124289,#124290,
#124291,#124292,#124293,#124294,#124295,#124296,#124297,#124298,#124299,
#124300,#124301,#124302,#124303,#124304,#124305,#124306,#124307,#124308,
#124309,#124310,#124311,#124312,#124313,#124314,#124315,#124316,#124317,
#124318,#124319,#124320,#124321,#124322),.UNSPECIFIED.,.F.,.F.,(4,2,2,2,
2,2,2,2,2,2,2,2,2,2,2,2,2,2,2,2,2,2,2,2,2,2,2,2,2,2,2,2,2,2,2,2,2,2,2,2,
2,2,2,2,2,2,2,2,2,2,2,2,2,2,2,2,2,2,2,2,2,2,2,2,2,2,2,2,2,2,2,2,2,2,2,2,
2,2,2,2,2,2,2,2,2,2,2,2,2,2,2,2,2,2,2,2,2,2,2,2,2,2,2,4),(-2.80145779137746,
-2.78896159018484,-2.76065937660977,-2.75475076405021,-2.75119125405688,
-2.74796152760446,-2.74383192612798,-2.73480028451152,-2.69214947388333,
-2.67918126361283,-2.67138289311765,-2.66861735239108,-2.66674755332195,
-2.66502304060338,-2.66204251681594,-2.65321675681465,-2.62333083237893,
-2.59903401702736,-2.59003080747544,-2.58586142906437,-2.58263537253487,
-2.57906012945557,-2.57307766544307,-2.54364620796484,-2.5214373896112,
-2.51102773651572,-2.50431940340741,-2.50170580074452,-2.49986372952664,
-2.4978422275805,-2.49436898823024,-2.48011767320355,-2.44977971349942,
-2.42674378021518,-2.42106937511479,-2.41755968518172,-2.41431538011272,
-2.41000843331411,-2.40020215529185,-2.38624237839934,-2.36569175343155,
-2.36258610885424,-2.33986316981788,-2.33616806478412,-2.33407713804524,
-2.33225632814433,-2.32978569688586,-2.32398432882326,-2.31548762194585,
-2.28543561237568,-2.26048489065247,-2.25458411090553,-2.25102639323188,
-2.24779644399342,-2.24359387765608,-2.23440032340412,-2.22163624925089,
-2.19946269564246,-2.19538573290667,-2.1731653409063,-2.16947222616816,
-2.16738178382152,-2.16556092017402,-2.16308959487641,-2.15728391154746,
-2.14877846310981,-2.11865680998143,-2.09378688310051,-2.08788854710639,
-2.08433137279343,-2.08110132792379,-2.07689779098648,-2.06769850222521,
-2.05492339079155,-2.03275438431432,-2.02861530251389,-2.00647362740441,
-2.00278083635211,-2.00069046769594,-1.99886954142242,-1.99639797741833,
-1.99059113130804,-1.98208334630553,-1.95194209120561,-1.92709953879681,
-1.92120210497237,-1.91764510054041,-1.91441496813857,-1.91021096540058,
-1.90100913527937,-1.88822921860791,-1.86606222275285,-1.86189502278057,
-1.83978835955354,-1.83609576517553,-1.8340054666012,-1.83218474764661,
-1.82971356212138,-1.82390767112326,-1.81540152283688,-1.78527223705395,
-1.7604114978068,-1.75451388622684,-1.75142894609207),.UNSPECIFIED.);
#2903=B_SPLINE_CURVE_WITH_KNOTS('',3,(#124328,#124329,#124330,#124331,#124332,
#124333,#124334,#124335,#124336,#124337,#124338,#124339,#124340,#124341,
#124342,#124343,#124344,#124345,#124346,#124347,#124348,#124349,#124350,
#124351,#124352,#124353,#124354,#124355,#124356,#124357,#124358,#124359,
#124360,#124361,#124362,#124363,#124364,#124365,#124366,#124367,#124368,
#124369,#124370,#124371,#124372,#124373,#124374,#124375,#124376,#124377,
#124378,#124379,#124380,#124381,#124382,#124383,#124384,#124385,#124386,
#124387,#124388,#124389,#124390,#124391,#124392,#124393,#124394,#124395,
#124396,#124397,#124398,#124399,#124400,#124401,#124402,#124403,#124404,
#124405,#124406,#124407,#124408,#124409,#124410,#124411,#124412,#124413,
#124414,#124415,#124416,#124417,#124418,#124419,#124420,#124421,#124422,
#124423,#124424,#124425,#124426,#124427,#124428,#124429,#124430,#124431,
#124432,#124433,#124434,#124435,#124436,#124437,#124438,#124439,#124440,
#124441,#124442,#124443,#124444,#124445,#124446,#124447,#124448,#124449,
#124450,#124451,#124452,#124453,#124454,#124455,#124456,#124457,#124458,
#124459),.UNSPECIFIED.,.F.,.F.,(4,2,2,2,2,2,2,2,2,2,2,2,2,2,2,2,2,2,2,2,
2,2,2,2,2,2,2,2,2,2,2,2,2,2,2,2,2,2,2,2,2,2,2,2,2,2,2,2,2,2,2,2,2,2,2,2,
2,2,2,2,2,2,2,2,2,4),(-0.701636287487779,-0.697839022662261,-0.674842325607004,
-0.669935798104173,-0.667629296920877,-0.665824141089188,-0.663621013114632,
-0.659300671945522,-0.630980069288784,-0.59588492751791,-0.589277207730714,
-0.585173589306852,-0.581939989173495,-0.578295060076084,-0.57204027932623,
-0.538649314979816,-0.507757634175514,-0.503066608646091,-0.500782882059722,
-0.498948465648512,-0.496647185185076,-0.491945406013739,-0.472805016475768,
-0.439048031476098,-0.426344007398241,-0.421441693617695,-0.418403301137768,
-0.415073076198448,-0.410413078920198,-0.398498664926513,-0.380066513848475,
-0.353359115340523,-0.340063944669906,-0.336658492707012,-0.334655043329414,
-0.332872377637875,-0.330400026083402,-0.324064296950665,-0.314351289671585,
-0.272080613631591,-0.257154727894049,-0.252128682248939,-0.248855833352114,
-0.245718104367162,-0.241379608577404,-0.230653790706167,-0.214561853511444,
-0.183199278226535,-0.17147019173188,-0.16825229308572,-0.166320947747948,
-0.164456275517811,-0.161758386229062,-0.154578958792954,-0.116805722640352,
-0.0871659769434536,-0.0806283029311778,-0.0766838441689992,-0.0730896597176575,
-0.0683736923888758,-0.0576675656256708,-0.0323065871038856,-0.00779140283112945,
-0.00345801209014825,-0.00158323791527608,-5.8761756664911E-5),
 .UNSPECIFIED.);
#2904=B_SPLINE_CURVE_WITH_KNOTS('',3,(#124462,#124463,#124464,#124465,#124466,
#124467,#124468,#124469,#124470,#124471,#124472,#124473,#124474,#124475,
#124476,#124477,#124478,#124479,#124480,#124481,#124482,#124483,#124484,
#124485,#124486,#124487,#124488,#124489,#124490,#124491,#124492,#124493,
#124494,#124495,#124496,#124497,#124498,#124499,#124500,#124501,#124502,
#124503,#124504,#124505,#124506,#124507,#124508,#124509,#124510,#124511,
#124512,#124513,#124514,#124515,#124516,#124517,#124518,#124519,#124520,
#124521,#124522,#124523,#124524,#124525,#124526,#124527,#124528,#124529,
#124530,#124531,#124532,#124533,#124534,#124535,#124536,#124537,#124538,
#124539,#124540,#124541,#124542,#124543,#124544,#124545,#124546,#124547,
#124548,#124549,#124550,#124551,#124552,#124553,#124554,#124555,#124556,
#124557,#124558,#124559,#124560,#124561,#124562,#124563,#124564,#124565,
#124566,#124567,#124568,#124569,#124570,#124571,#124572,#124573,#124574,
#124575,#124576,#124577,#124578,#124579,#124580,#124581,#124582,#124583,
#124584,#124585,#124586,#124587,#124588,#124589,#124590,#124591,#124592,
#124593,#124594,#124595,#124596,#124597,#124598,#124599,#124600,#124601,
#124602,#124603,#124604,#124605,#124606,#124607,#124608,#124609,#124610,
#124611,#124612,#124613,#124614,#124615,#124616,#124617,#124618,#124619,
#124620,#124621,#124622,#124623,#124624,#124625,#124626,#124627,#124628,
#124629,#124630,#124631,#124632,#124633,#124634,#124635,#124636,#124637,
#124638,#124639,#124640,#124641,#124642,#124643,#124644,#124645,#124646,
#124647,#124648,#124649),.UNSPECIFIED.,.F.,.F.,(4,2,2,2,2,2,2,2,2,2,2,2,
2,2,2,2,2,2,2,2,2,2,2,2,2,2,2,2,2,2,2,2,2,2,2,2,2,2,2,2,2,2,2,2,2,2,2,2,
2,2,2,2,2,2,2,2,2,2,2,2,2,2,2,2,2,2,2,2,2,2,2,2,2,2,2,2,2,2,2,2,2,2,2,2,
2,2,2,2,2,2,2,2,2,4),(-1.97964531136435,-1.97911906260677,-1.97225183621543,
-1.93766010376271,-1.91989896127257,-1.91198669364148,-1.90555923283692,
-1.90186475831735,-1.8986163535856,-1.89453160537323,-1.88802575250684,
-1.85357382618518,-1.82637417573715,-1.82198916105945,-1.81975004909482,
-1.81791464338252,-1.81556138103437,-1.81067997802214,-1.78640428098552,
-1.76445474780961,-1.75162112186658,-1.74238702862777,-1.73816368383357,
-1.73491589042239,-1.73133611421782,-1.72539172543349,-1.69958592330072,
-1.67019866891438,-1.66177843083949,-1.65601018612154,-1.65354030782054,
-1.65171844439193,-1.64963188226422,-1.64593216701741,-1.62181468261427,
-1.62032922398492,-1.59987229126258,-1.58572494923463,-1.57583725480986,
-1.57153125059668,-1.56830199632932,-1.56482280808428,-1.55923107601898,
-1.539648107259,-1.49638525171747,-1.48950671320994,-1.48687845082069,-1.48504077470034,
-1.48303359177249,-1.47962596458339,-1.46637430092727,-1.43973515849324,
-1.4214213025529,-1.40959677425905,-1.40497527064041,-1.40167512107569,
-1.39866685832657,-1.39382125836553,-1.38136134147017,-1.34651562821764,
-1.3319078439555,-1.32617651666678,-1.32185071527014,-1.31964694934694,
-1.31783664899341,-1.31551689909332,-1.31057937031736,-1.2858478321638,
-1.25896213776951,-1.24895244016569,-1.24127794540381,-1.23735476108039,
-1.23414893049417,-1.23040845522217,-1.22382856709703,-1.18243440748928,
-1.16601811569556,-1.15693804872218,-1.15401723704396,-1.15211571981282,
-1.15042233358238,-1.14760293755012,-1.13998630650627,-1.1091363132709,
-1.08426168631806,-1.07527240257569,-1.0711073135409,-1.06788376091033,
-1.0643105094788,-1.0583296155778,-1.02901015493119,-1.00699503835577,-0.99128888870559,
-0.991281231630979),.UNSPECIFIED.);
#2905=B_SPLINE_CURVE_WITH_KNOTS('',3,(#124652,#124653,#124654,#124655,#124656,
#124657,#124658,#124659,#124660,#124661,#124662,#124663,#124664,#124665,
#124666,#124667,#124668,#124669,#124670,#124671,#124672,#124673,#124674,
#124675,#124676,#124677,#124678,#124679,#124680,#124681,#124682,#124683,
#124684,#124685,#124686,#124687,#124688,#124689,#124690,#124691,#124692,
#124693,#124694,#124695,#124696,#124697,#124698,#124699,#124700,#124701,
#124702,#124703,#124704,#124705,#124706,#124707,#124708,#124709,#124710,
#124711,#124712,#124713,#124714,#124715,#124716,#124717,#124718,#124719,
#124720,#124721,#124722,#124723,#124724,#124725,#124726,#124727,#124728,
#124729,#124730,#124731,#124732,#124733,#124734,#124735,#124736,#124737,
#124738,#124739,#124740,#124741,#124742,#124743,#124744,#124745,#124746,
#124747,#124748,#124749,#124750,#124751,#124752,#124753,#124754,#124755,
#124756,#124757,#124758,#124759,#124760,#124761,#124762,#124763,#124764,
#124765,#124766,#124767,#124768,#124769,#124770,#124771,#124772,#124773,
#124774,#124775,#124776,#124777,#124778,#124779,#124780,#124781,#124782,
#124783,#124784,#124785,#124786,#124787,#124788,#124789,#124790,#124791,
#124792,#124793,#124794,#124795,#124796,#124797,#124798,#124799,#124800,
#124801,#124802,#124803,#124804,#124805,#124806,#124807,#124808,#124809,
#124810,#124811,#124812,#124813,#124814,#124815,#124816,#124817,#124818,
#124819,#124820,#124821,#124822,#124823,#124824,#124825,#124826,#124827,
#124828,#124829,#124830,#124831,#124832,#124833,#124834,#124835,#124836,
#124837,#124838,#124839,#124840,#124841,#124842,#124843,#124844,#124845,
#124846,#124847,#124848,#124849,#124850,#124851,#124852,#124853,#124854,
#124855,#124856,#124857,#124858,#124859,#124860,#124861,#124862,#124863,
#124864,#124865,#124866,#124867,#124868,#124869,#124870,#124871,#124872,
#124873,#124874,#124875,#124876,#124877,#124878,#124879,#124880,#124881,
#124882,#124883,#124884,#124885,#124886,#124887,#124888,#124889,#124890,
#124891,#124892,#124893,#124894,#124895,#124896,#124897,#124898,#124899,
#124900,#124901,#124902,#124903,#124904,#124905,#124906,#124907),
 .UNSPECIFIED.,.F.,.F.,(4,2,2,2,2,2,2,2,2,2,2,2,2,2,2,2,2,2,2,2,2,2,2,2,
2,2,2,2,2,2,2,2,2,2,2,2,2,2,2,2,2,2,2,2,2,2,2,2,2,2,2,2,2,2,2,2,2,2,2,2,
2,2,2,2,2,2,2,2,2,2,2,2,2,2,2,2,2,2,2,2,2,2,2,2,2,2,2,2,2,2,2,2,2,2,2,2,
2,2,2,2,2,2,2,2,2,2,2,2,2,2,2,2,2,2,2,2,2,2,2,2,2,2,2,2,2,2,2,4),(-0.991281231630979,
-0.987841854375976,-0.985827044042622,-0.983983179222014,-0.98135732077623,
-0.974566319623724,-0.931108639327705,-0.911819953225727,-0.906231241791206,
-0.902739454556782,-0.899488089452126,-0.895135911242685,-0.8850558789029,
-0.870542721323148,-0.850460109323952,-0.82708850730907,-0.822165749574291,
-0.819849781275316,-0.818042680006527,-0.815844301721315,-0.811527240667509,
-0.80580748114327,-0.791239087038924,-0.75661318667677,-0.743766727958745,
-0.738869990459187,-0.735856370801476,-0.732571241315397,-0.728010229665721,
-0.716572520714517,-0.699140392147666,-0.666165381766055,-0.657142292836879,
-0.654138218993048,-0.652409390323099,-0.650544039211167,-0.64779948203039,
-0.640156770976696,-0.627569281044651,-0.588167522956102,-0.5766552017642,
-0.571957755024135,-0.568681194006056,-0.565306807515165,-0.560277176713261,
-0.545146916752413,-0.517514277810206,-0.516002232605101,-0.491903183835174,
-0.488196457495654,-0.486103263408001,-0.484283385877947,-0.481817932880979,
-0.476046074904421,-0.467607887531038,-0.438000026011006,-0.412566265076903,
-0.406653986717998,-0.40309413949198,-0.39986525522998,-0.395668327792562,
-0.386504863542936,-0.373796875944327,-0.351624831145559,-0.347995439706742,
-0.32526916214332,-0.321575095137334,-0.319484593450501,-0.31766403004118,
-0.315193446071637,-0.309390695753284,-0.300890308539575,-0.270794594335009,
-0.245927954475505,-0.240031187576714,-0.236474752157447,-0.233245217746195,
-0.229042079835067,-0.219842298474118,-0.20706492889809,-0.184910337920613,
-0.160592686606324,-0.155661279801007,-0.153344353186599,-0.151609418164389,
-0.151583300442266,-0.151541932247801,-0.1515024327774,-0.151464648530632,
-0.151428442165346,-0.151393690519353,-0.151360282819415,-0.151328119031109,
-0.151297108611142,-0.151267169372692,-0.151238226498512,-0.151210211768088,
-0.151183062866975,-0.151156722613911,-0.151131138490097,-0.151106262085664,
-0.151082048741073,-0.151058457392603,-0.151035449836252,-0.151012990563013,
-0.15099104666073,-0.150969587475618,-0.150948584314081,-0.150928010558224,
-0.1509078410711,-0.150888052474096,-0.150868622766498,-0.150849531147258,
-0.150830758147573,-0.15081228521397,-0.150794094974534,-0.148405459333805,
-0.145516080973216,-0.140312230792917,-0.127769787531509,-0.0887276269360894,
-0.0769078943937671,-0.0721628819432224,-0.0688776120374353,-0.0655145066124617,
-0.0605404380655912,-0.0459057461101224,-0.000494228016458911),
 .UNSPECIFIED.);
#2906=B_SPLINE_CURVE_WITH_KNOTS('',3,(#124908,#124909,#124910,#124911,#124912,
#124913,#124914,#124915,#124916,#124917,#124918,#124919,#124920,#124921,
#124922,#124923,#124924,#124925,#124926,#124927),.UNSPECIFIED.,.F.,.F.,
(4,2,2,2,2,2,2,2,2,4),(-2.09990490037868,-2.09043166092189,-2.08804132421848,
-2.08624835223061,-2.08446713995306,-2.0823589812838,-2.07858689204649,
-2.0625197928987,-2.04247110725939,-2.04107054618519),.UNSPECIFIED.);
#2907=B_SPLINE_CURVE_WITH_KNOTS('',3,(#124928,#124929,#124930,#124931,#124932,
#124933,#124934,#124935,#124936,#124937,#124938,#124939,#124940,#124941,
#124942,#124943,#124944,#124945,#124946,#124947,#124948,#124949,#124950,
#124951,#124952,#124953,#124954,#124955,#124956,#124957,#124958,#124959,
#124960,#124961,#124962,#124963,#124964,#124965,#124966,#124967,#124968,
#124969,#124970,#124971,#124972,#124973,#124974,#124975,#124976,#124977,
#124978,#124979,#124980,#124981,#124982,#124983,#124984,#124985,#124986,
#124987,#124988,#124989,#124990,#124991,#124992,#124993,#124994,#124995,
#124996,#124997,#124998,#124999,#125000,#125001,#125002,#125003,#125004,
#125005,#125006,#125007,#125008,#125009,#125010,#125011,#125012,#125013,
#125014,#125015,#125016,#125017,#125018,#125019,#125020,#125021,#125022,
#125023,#125024,#125025,#125026,#125027,#125028,#125029,#125030,#125031,
#125032,#125033,#125034,#125035,#125036,#125037,#125038,#125039,#125040,
#125041,#125042,#125043,#125044,#125045,#125046,#125047,#125048,#125049,
#125050,#125051,#125052,#125053,#125054,#125055,#125056,#125057,#125058,
#125059,#125060,#125061,#125062,#125063,#125064,#125065,#125066,#125067,
#125068,#125069,#125070,#125071,#125072,#125073,#125074,#125075,#125076,
#125077,#125078,#125079,#125080,#125081,#125082,#125083,#125084,#125085,
#125086,#125087,#125088,#125089,#125090,#125091,#125092,#125093,#125094,
#125095,#125096,#125097,#125098,#125099,#125100,#125101,#125102,#125103,
#125104,#125105,#125106,#125107,#125108,#125109,#125110,#125111,#125112,
#125113,#125114,#125115,#125116,#125117,#125118,#125119,#125120,#125121,
#125122,#125123,#125124,#125125,#125126,#125127,#125128,#125129,#125130,
#125131,#125132,#125133,#125134,#125135,#125136,#125137,#125138,#125139,
#125140,#125141,#125142,#125143,#125144,#125145,#125146,#125147),
 .UNSPECIFIED.,.F.,.F.,(4,2,2,2,2,2,2,2,2,2,2,2,2,2,2,2,2,2,2,2,2,2,2,2,
2,2,2,2,2,2,2,2,2,2,2,2,2,2,2,2,2,2,2,2,2,2,2,2,2,2,2,2,2,2,2,2,2,2,2,2,
2,2,2,2,2,2,2,2,2,2,2,2,2,2,2,2,2,2,2,2,2,2,2,2,2,2,2,2,2,2,2,2,2,2,2,2,
2,2,2,2,2,2,2,2,2,2,2,2,2,4),(-1.75142894609207,-1.75095713874224,-1.74772748361246,
-1.74352446718888,-1.73432644337936,-1.72155332420707,-1.69938424111941,
-1.69525426652509,-1.67310192840444,-1.66940942498326,-1.66731927438308,
-1.66549856604467,-1.66302738794025,-1.65722197012572,-1.64871690159625,
-1.61859723219913,-1.59372423678049,-1.58782589978092,-1.58426878683924,
-1.58103883626336,-1.57683547439035,-1.56763675368805,-1.55486241908422,
-1.53269596525806,-1.52856245150482,-1.50641870843793,-1.50272593505734,
-1.50063552704098,-1.49881420938223,-1.49634176309703,-1.49053183263272,
-1.48201809215829,-1.45182576528587,-1.42706593931722,-1.42117109341108,
-1.41761432461896,-1.41438353616731,-1.41017739928,-1.40096528114554,-1.38816631177653,
-1.36600722716564,-1.36174248910034,-1.3397586580243,-1.33606662227047,
-1.33397647904982,-1.3321567252544,-1.32968741846762,-1.32388641432743,
-1.31538873480248,-1.28532212280671,-1.2603663198895,-1.25446772902036,
-1.25091224982781,-1.24768499218589,-1.24348696239449,-1.23430829110508,
-1.22156988424774,-1.19939047269532,-1.19552891957004,-1.17306010274023,
-1.16936774074632,-1.16727830310697,-1.16545789277088,-1.16298740348159,
-1.15718702352554,-1.14869261632144,-1.11866528213641,-1.09366419091909,
-1.08776016999212,-1.08420093187642,-1.0809698469739,-1.07676610057186,
-1.06757072604844,-1.05480303659534,-1.03264531143523,-1.02857602498704,
-1.00637624614241,-1.00268161094015,-1.00058973459417,-0.99876459702422,
-0.996284369391697,-0.990447932930247,-0.981883776358615,-0.951268355677309,
-0.927157000105235,-0.921283515208742,-0.917728276059511,-0.914491424142104,
-0.910266424699868,-0.90096480605169,-0.888000799238241,-0.866041260337691,
-0.861497363765283,-0.839845667046236,-0.836155330683252,-0.834065657641216,
-0.832435350289788,-0.830094796724561,-0.82498563971461,-0.817825118097722,
-0.796437579356522,-0.762792692199946,-0.756158679111235,-0.752070995436364,
-0.748870480093518,-0.745285310224462,-0.739193186305052,-0.731771727027432,
-0.715598489243652,-0.701636287487779),.UNSPECIFIED.);
#2908=B_SPLINE_CURVE_WITH_KNOTS('',3,(#125150,#125151,#125152,#125153,#125154,
#125155,#125156,#125157,#125158,#125159,#125160,#125161,#125162,#125163,
#125164,#125165,#125166,#125167,#125168,#125169,#125170,#125171,#125172,
#125173,#125174,#125175,#125176,#125177,#125178,#125179,#125180,#125181,
#125182,#125183,#125184,#125185,#125186,#125187,#125188,#125189,#125190,
#125191,#125192,#125193,#125194,#125195,#125196,#125197,#125198,#125199,
#125200,#125201,#125202,#125203,#125204,#125205,#125206,#125207,#125208,
#125209,#125210,#125211,#125212,#125213,#125214,#125215,#125216,#125217,
#125218,#125219,#125220,#125221,#125222,#125223,#125224,#125225,#125226,
#125227,#125228,#125229,#125230,#125231,#125232,#125233,#125234,#125235,
#125236,#125237,#125238,#125239,#125240,#125241,#125242,#125243,#125244,
#125245,#125246,#125247,#125248,#125249,#125250,#125251,#125252,#125253,
#125254,#125255,#125256,#125257,#125258,#125259,#125260,#125261,#125262,
#125263,#125264,#125265,#125266,#125267,#125268,#125269,#125270,#125271,
#125272,#125273,#125274,#125275,#125276,#125277,#125278,#125279,#125280,
#125281,#125282,#125283,#125284,#125285,#125286,#125287,#125288,#125289,
#125290,#125291,#125292,#125293,#125294,#125295,#125296,#125297,#125298,
#125299,#125300,#125301,#125302,#125303,#125304,#125305,#125306,#125307,
#125308,#125309,#125310,#125311,#125312,#125313,#125314,#125315,#125316,
#125317,#125318,#125319,#125320,#125321,#125322,#125323,#125324,#125325,
#125326,#125327,#125328,#125329,#125330,#125331,#125332,#125333,#125334,
#125335,#125336,#125337,#125338,#125339,#125340,#125341,#125342,#125343,
#125344,#125345,#125346,#125347,#125348,#125349,#125350,#125351,#125352,
#125353,#125354,#125355,#125356,#125357,#125358,#125359,#125360,#125361,
#125362,#125363,#125364,#125365,#125366,#125367,#125368,#125369,#125370,
#125371,#125372,#125373,#125374,#125375,#125376,#125377,#125378,#125379,
#125380,#125381,#125382,#125383,#125384,#125385,#125386,#125387,#125388,
#125389,#125390,#125391,#125392,#125393,#125394,#125395,#125396,#125397,
#125398,#125399,#125400,#125401,#125402,#125403,#125404,#125405),
 .UNSPECIFIED.,.F.,.F.,(4,2,2,2,2,2,2,2,2,2,2,2,2,2,2,2,2,2,2,2,2,2,2,2,
2,2,2,2,2,2,2,2,2,2,2,2,2,2,2,2,2,2,2,2,2,2,2,2,2,2,2,2,2,2,2,2,2,2,2,2,
2,2,2,2,2,2,2,2,2,2,2,2,2,2,2,2,2,2,2,2,2,2,2,2,2,2,2,2,2,2,2,2,2,2,2,2,
2,2,2,2,2,2,2,2,2,2,2,2,2,2,2,2,2,2,2,2,2,2,2,2,2,2,2,2,2,2,2,4),(-0.991277804245244,
-0.987838448409618,-0.985823649756141,-0.983979794703957,-0.98135394827412,
-0.974562966697378,-0.931105483638177,-0.911816991114433,-0.906228317826688,
-0.902736551807322,-0.899485204675701,-0.895133047792989,-0.885053051592897,
-0.870539933308402,-0.850457508069912,-0.827086044899166,-0.822163315600623,
-0.819847360658439,-0.81804026966992,-0.815841903638442,-0.811524866438444,
-0.805805138274295,-0.791236822040495,-0.756611094699905,-0.743764744147221,
-0.738868039097699,-0.735854437103005,-0.732569325042841,-0.728008334130301,
-0.71657065681125,-0.699138550843459,-0.666163608442,-0.657140782212213,
-0.654136750727445,-0.652407936626109,-0.650542591683229,-0.647798028158866,
-0.640155197245282,-0.627567378870247,-0.588162555419262,-0.576653032048378,
-0.571956112453222,-0.568679661538219,-0.565305172825671,-0.560274972272466,
-0.545139343808745,-0.517488068241534,-0.516247630991732,-0.491911198802518,
-0.488199484486295,-0.48610518199033,-0.484285553773042,-0.481822057758018,
-0.476061839671524,-0.467646997273333,-0.4382190656533,-0.412575153260324,
-0.406658005106013,-0.40309713426503,-0.39986852461374,-0.395673675123066,
-0.386522030649031,-0.373836535048676,-0.35109515600548,-0.347920538781888,
-0.325267942885641,-0.321574187066173,-0.319483759665895,-0.317663188142843,
-0.315192495640078,-0.30938906116643,-0.300887283669319,-0.270780418733576,
-0.245926838186652,-0.240030481959969,-0.236474142258809,-0.233244598582025,
-0.229041310507891,-0.219840611989913,-0.207061471873289,-0.184907685339927,
-0.160592809930546,-0.15566131976479,-0.153344382769017,-0.15160945433713,
-0.151583329528716,-0.151541959998941,-0.151502459357567,-0.151464673950257,
-0.151428466513842,-0.151393713866275,-0.151360305234534,-0.15132814056872,
-0.151297129297126,-0.151267189253574,-0.151238245600769,-0.151210230223545,
-0.151183080707512,-0.151156739847435,-0.151131155108219,-0.151106278201253,
-0.151082064444723,-0.151058472662611,-0.151035464570663,-0.151013004791237,
-0.15099106048062,-0.150969600899822,-0.15094859739742,-0.150928023288037,
-0.150907853609781,-0.150888064783097,-0.150868634772398,-0.150849542917034,
-0.150830769580642,-0.150812296239459,-0.150794105727963,-0.148405476337537,
-0.145516107341229,-0.140312282915775,-0.127769938121448,-0.0887285733398078,
-0.0769081481431902,-0.0721630279763587,-0.0688777371691399,-0.0655146546045517,
-0.0605407041033007,-0.0459070567405313,-0.000494226792898512),
 .UNSPECIFIED.);
#2909=B_SPLINE_CURVE_WITH_KNOTS('',3,(#125406,#125407,#125408,#125409,#125410,
#125411,#125412,#125413,#125414,#125415,#125416,#125417,#125418,#125419,
#125420,#125421,#125422,#125423,#125424,#125425),.UNSPECIFIED.,.F.,.F.,
(4,2,2,2,2,2,2,2,2,4),(-2.1000787529661,-2.09060473924815,-2.08821420497033,
-2.08642108497951,-2.08463972604253,-2.08253139390499,-2.0787589951723,
-2.0626905691525,-2.04262123048289,-2.04123955694236),.UNSPECIFIED.);
#2910=B_SPLINE_CURVE_WITH_KNOTS('',3,(#125426,#125427,#125428,#125429,#125430,
#125431,#125432,#125433,#125434,#125435,#125436,#125437,#125438,#125439,
#125440,#125441,#125442,#125443,#125444,#125445,#125446,#125447,#125448,
#125449,#125450,#125451,#125452,#125453,#125454,#125455,#125456,#125457,
#125458,#125459,#125460,#125461,#125462,#125463,#125464,#125465,#125466,
#125467,#125468,#125469,#125470,#125471,#125472,#125473,#125474,#125475,
#125476,#125477,#125478,#125479,#125480,#125481,#125482,#125483,#125484,
#125485,#125486,#125487,#125488,#125489,#125490,#125491,#125492,#125493,
#125494,#125495,#125496,#125497,#125498,#125499,#125500,#125501,#125502,
#125503,#125504,#125505,#125506,#125507,#125508,#125509,#125510,#125511,
#125512,#125513,#125514,#125515,#125516,#125517,#125518,#125519,#125520,
#125521,#125522,#125523,#125524,#125525,#125526,#125527,#125528,#125529,
#125530,#125531,#125532,#125533,#125534,#125535,#125536,#125537,#125538,
#125539,#125540,#125541,#125542,#125543,#125544,#125545,#125546,#125547,
#125548,#125549,#125550,#125551,#125552,#125553,#125554,#125555,#125556,
#125557,#125558,#125559,#125560,#125561,#125562,#125563,#125564,#125565,
#125566,#125567,#125568,#125569,#125570,#125571,#125572,#125573,#125574,
#125575,#125576,#125577,#125578,#125579,#125580,#125581,#125582,#125583,
#125584,#125585,#125586,#125587,#125588,#125589,#125590,#125591,#125592,
#125593,#125594,#125595,#125596,#125597,#125598,#125599,#125600,#125601,
#125602,#125603,#125604,#125605,#125606,#125607,#125608,#125609,#125610,
#125611,#125612,#125613,#125614,#125615,#125616,#125617,#125618,#125619,
#125620,#125621,#125622,#125623,#125624,#125625,#125626,#125627,#125628,
#125629,#125630,#125631,#125632,#125633,#125634,#125635,#125636,#125637,
#125638,#125639,#125640,#125641,#125642,#125643,#125644,#125645),
 .UNSPECIFIED.,.F.,.F.,(4,2,2,2,2,2,2,2,2,2,2,2,2,2,2,2,2,2,2,2,2,2,2,2,
2,2,2,2,2,2,2,2,2,2,2,2,2,2,2,2,2,2,2,2,2,2,2,2,2,2,2,2,2,2,2,2,2,2,2,2,
2,2,2,2,2,2,2,2,2,2,2,2,2,2,2,2,2,2,2,2,2,2,2,2,2,2,2,2,2,2,2,2,2,2,2,2,
2,2,2,2,2,2,2,2,2,2,2,2,2,4),(-1.75139041054252,-1.75091861351771,-1.74768903365539,
-1.74348611405865,-1.734288297127,-1.72151546056368,-1.69934690996806,-1.69521693622104,
-1.67306524734637,-1.6693728310676,-1.6672827294943,-1.6654620636133,-1.66299094271596,
-1.65718565731196,-1.64868078066227,-1.61856175284192,-1.5936894333588,
-1.58779123767793,-1.58423420864993,-1.58100433341346,-1.57680106832482,
-1.56760255385934,-1.55482850063813,-1.53266257892508,-1.52852906289671,
-1.50638597233275,-1.50269328624427,-1.50060292737515,-1.49878165248302,
-1.49630926403521,-1.49049946810993,-1.48198592353092,-1.45179427085578,
-1.4270350706234,-1.42114036468366,-1.41758367976233,-1.41435296711625,
-1.41014692835945,-1.400935022627,-1.38813634586288,-1.36597779158899,-1.36171313379183,
-1.33972985928813,-1.33603791052661,-1.33394781638972,-1.33212810489372,
-1.329658855026,-1.32385798305222,-1.31536049528632,-1.28529452616742,-1.26033939970604,
-1.25444094943778,-1.2508855535634,-1.24765837059915,-1.2434604365347,-1.23428196817663,
-1.22154383691827,-1.19936495812372,-1.19550325868213,-1.17303525131699,
-1.1693429767004,-1.16725358793298,-1.16543321972153,-1.16296278682649,
-1.15716253556433,-1.14866831284602,-1.11864155909669,-1.09364123173764,
-1.08773735497822,-1.08417820141472,-1.08094719174171,-1.07674354099047,
-1.06754836606575,-1.05478094569836,-1.03262375266717,-1.02855439687768,
-1.00635534843598,-1.00266080118208,-1.00056897439197,-0.99874388084189,
-0.996263713532163,-0.990427419550083,-0.981863473668625,-0.95124884871039,
-0.927137935427773,-0.921264584662462,-0.917709429289234,-0.914472655349134,
-0.91024776020222,-0.900946382214685,-0.887982719896956,-0.866023680170908,
-0.861479939346711,-0.839828679330764,-0.836138429701869,-0.834048805862784,
-0.832418535713938,-0.830078034263107,-0.82496898973213,-0.817808623856327,
-0.796421525510616,-0.762777552759297,-0.756143691609615,-0.752056100635309,
-0.748855657166228,-0.745270566959701,-0.739178575936893,-0.731757276806803,
-0.715584375973475,-0.701622587363262),.UNSPECIFIED.);
#2911=B_SPLINE_CURVE_WITH_KNOTS('',3,(#125648,#125649,#125650,#125651,#125652,
#125653,#125654,#125655,#125656,#125657,#125658,#125659,#125660,#125661,
#125662,#125663,#125664,#125665,#125666,#125667,#125668,#125669,#125670,
#125671,#125672,#125673,#125674,#125675,#125676,#125677,#125678,#125679,
#125680,#125681,#125682,#125683,#125684,#125685,#125686,#125687,#125688,
#125689,#125690,#125691,#125692,#125693,#125694,#125695,#125696,#125697,
#125698,#125699,#125700,#125701,#125702,#125703,#125704,#125705,#125706,
#125707,#125708,#125709,#125710,#125711,#125712,#125713,#125714,#125715,
#125716,#125717,#125718,#125719,#125720,#125721,#125722,#125723,#125724,
#125725,#125726,#125727,#125728,#125729,#125730,#125731,#125732,#125733,
#125734,#125735,#125736,#125737,#125738,#125739,#125740,#125741,#125742,
#125743,#125744,#125745,#125746,#125747,#125748,#125749,#125750,#125751,
#125752,#125753,#125754,#125755,#125756,#125757,#125758,#125759,#125760,
#125761,#125762,#125763,#125764,#125765,#125766,#125767,#125768,#125769,
#125770,#125771,#125772,#125773,#125774,#125775,#125776,#125777,#125778,
#125779,#125780,#125781,#125782,#125783,#125784,#125785,#125786,#125787,
#125788,#125789,#125790,#125791,#125792,#125793,#125794,#125795,#125796,
#125797,#125798,#125799,#125800,#125801,#125802,#125803,#125804,#125805,
#125806,#125807,#125808,#125809,#125810,#125811,#125812,#125813,#125814,
#125815,#125816,#125817,#125818,#125819,#125820,#125821,#125822,#125823,
#125824,#125825,#125826,#125827,#125828,#125829,#125830,#125831,#125832,
#125833,#125834,#125835,#125836,#125837,#125838,#125839,#125840,#125841),
 .UNSPECIFIED.,.F.,.F.,(4,2,2,2,2,2,2,2,2,2,2,2,2,2,2,2,2,2,2,2,2,2,2,2,
2,2,2,2,2,2,2,2,2,2,2,2,2,2,2,2,2,2,2,2,2,2,2,2,2,2,2,2,2,2,2,2,2,2,2,2,
2,2,2,2,2,2,2,2,2,2,2,2,2,2,2,2,2,2,2,2,2,2,2,2,2,2,2,2,2,2,2,2,2,2,2,2,
4),(-0.991241672647406,-0.987801969057869,-0.985787251833555,-0.983943844576314,
-0.98131941668712,-0.974536850515025,-0.931103314466294,-0.911783187657511,
-0.906192464811081,-0.902700439670065,-0.899449543974688,-0.895099050706998,
-0.885028019935898,-0.870532653808531,-0.850424789455911,-0.827053982341092,
-0.822131543385535,-0.819815705223421,-0.818008752444826,-0.815810639713148,
-0.811494104550115,-0.805775079343375,-0.791208931698783,-0.756591530319789,
-0.743737556131094,-0.738840178503933,-0.735826755702091,-0.732542311574434,
-0.727983146023538,-0.716555396200904,-0.699145320780396,-0.666205792614875,
-0.65712477184505,-0.654114006252745,-0.652384056219475,-0.650520149227365,
-0.647782007792058,-0.640185482990252,-0.62771022543606,-0.589215949700183,
-0.576908372559458,-0.572090036841543,-0.569090867154059,-0.565794660217369,
-0.56116750046865,-0.549263264734076,-0.530747045972717,-0.503549298549489,
-0.491149133524473,-0.487804077729745,-0.485811074377502,-0.483957262456012,
-0.48127350053131,-0.474075338245919,-0.462549890183645,-0.441694548303605,
-0.41269008695447,-0.406705223403245,-0.403130210426581,-0.399905387081769,
-0.395739020600716,-0.386747818274057,-0.362152876872644,-0.331764774982016,
-0.323623983186662,-0.3207320817232,-0.319024957349219,-0.317139807864442,
-0.314294952251012,-0.305859814869978,-0.291239717000893,-0.256429593668564,
-0.243779394345411,-0.238911013336089,-0.235902840794419,-0.232614223483765,
-0.228030711621876,-0.216434369678132,-0.198637853958558,-0.165082934194895,
-0.156979916535476,-0.154093190700569,-0.152387132188572,-0.150557471433941,
-0.148033041673921,-0.14494182417323,-0.139191493718343,-0.124495614464095,
-0.0894136332252241,-0.0770511115725383,-0.0722244674544098,-0.069223671106362,
-0.0659284937116466,-0.061308128069644,-0.0494535380316552,-0.0310548575729361,
-0.000494688380018427),.UNSPECIFIED.);
#2912=B_SPLINE_CURVE_WITH_KNOTS('',3,(#125842,#125843,#125844,#125845,#125846,
#125847,#125848,#125849,#125850,#125851,#125852,#125853,#125854,#125855,
#125856,#125857,#125858,#125859),.UNSPECIFIED.,.F.,.F.,(4,2,2,2,2,2,2,2,
4),(-2.1002328439837,-2.09075795692932,-2.08836800179074,-2.0865752450318,
-2.08479410976863,-2.0826860017187,-2.07891367771575,-2.06284869790601,
-2.04139270538101),.UNSPECIFIED.);
#2913=B_SPLINE_CURVE_WITH_KNOTS('',3,(#125860,#125861,#125862,#125863,#125864,
#125865,#125866,#125867,#125868,#125869,#125870,#125871,#125872,#125873,
#125874,#125875,#125876,#125877,#125878,#125879,#125880,#125881,#125882,
#125883,#125884,#125885,#125886,#125887,#125888,#125889,#125890,#125891,
#125892,#125893,#125894,#125895,#125896,#125897,#125898,#125899,#125900,
#125901,#125902,#125903,#125904,#125905,#125906,#125907,#125908,#125909,
#125910,#125911,#125912,#125913,#125914,#125915,#125916,#125917,#125918,
#125919,#125920,#125921,#125922,#125923,#125924,#125925,#125926,#125927,
#125928,#125929,#125930,#125931,#125932,#125933,#125934,#125935,#125936,
#125937,#125938,#125939,#125940,#125941,#125942,#125943,#125944,#125945,
#125946,#125947,#125948,#125949,#125950,#125951,#125952,#125953,#125954,
#125955,#125956,#125957,#125958,#125959,#125960,#125961,#125962,#125963,
#125964,#125965,#125966,#125967,#125968,#125969,#125970,#125971,#125972,
#125973,#125974,#125975,#125976,#125977,#125978,#125979,#125980,#125981,
#125982,#125983,#125984,#125985,#125986,#125987,#125988,#125989,#125990,
#125991,#125992,#125993,#125994,#125995,#125996,#125997,#125998,#125999,
#126000,#126001,#126002,#126003,#126004,#126005,#126006,#126007,#126008,
#126009,#126010,#126011,#126012,#126013,#126014,#126015,#126016,#126017,
#126018,#126019,#126020,#126021,#126022,#126023,#126024,#126025,#126026,
#126027,#126028,#126029,#126030,#126031,#126032,#126033,#126034,#126035,
#126036,#126037,#126038,#126039,#126040,#126041,#126042,#126043,#126044,
#126045,#126046,#126047,#126048,#126049,#126050,#126051,#126052,#126053,
#126054,#126055,#126056,#126057),.UNSPECIFIED.,.F.,.F.,(4,2,2,2,2,2,2,2,
2,2,2,2,2,2,2,2,2,2,2,2,2,2,2,2,2,2,2,2,2,2,2,2,2,2,2,2,2,2,2,2,2,2,2,2,
2,2,2,2,2,2,2,2,2,2,2,2,2,2,2,2,2,2,2,2,2,2,2,2,2,2,2,2,2,2,2,2,2,2,2,2,
2,2,2,2,2,2,2,2,2,2,2,2,2,2,2,2,2,2,4),(-1.10919012835353,-1.10913875417106,
-1.10593342114521,-1.10196645615564,-1.09578448318376,-1.0500864642212,
-1.03072304953975,-1.0270802212056,-1.02500150158327,-1.02317867498968,
-1.02068840394978,-1.01476547192955,-1.00602163637137,-0.981814942237135,
-0.951595900714783,-0.945614220704339,-0.942039871157921,-0.938814911385374,
-0.93464736987415,-0.925649751212604,-0.901338062431275,-0.871421105147256,
-0.862674342874921,-0.859704134962655,-0.85798190232104,-0.856110348158008,
-0.85333607858205,-0.845471552122435,-0.832335192846778,-0.788160082136583,
-0.780385814105817,-0.776394129439986,-0.773185836631225,-0.76950170701144,
-0.763001666553775,-0.730914529150247,-0.698881751937265,-0.694258618415944,
-0.692000232246089,-0.690196236265524,-0.687949721338137,-0.683381333738985,
-0.658877518901604,-0.619939582641716,-0.613655103108357,-0.609659392014902,
-0.606454040653568,-0.60278015979646,-0.59631710004486,-0.588317513035871,
-0.570121671574884,-0.543757980180209,-0.530156781362266,-0.52672900048763,
-0.524718769931408,-0.522874002160885,-0.520239705715888,-0.513387030987529,
-0.469825673898867,-0.450655181612665,-0.445075319115728,-0.441585726434461,
-0.438334197254077,-0.433978473811924,-0.423874383380412,-0.409310896292576,
-0.389308092099506,-0.365945659924148,-0.36108235132119,-0.358743999396581,
-0.356933054192068,-0.354745094212323,-0.350497797610437,-0.344901582146626,
-0.330842171519697,-0.2979484331142,-0.283332375685576,-0.278212655171611,
-0.275155343231835,-0.271892483482143,-0.267487649245627,-0.257101019259404,
-0.241966369841405,-0.211896127282767,-0.197129491172343,-0.193625802333691,
-0.191598252214357,-0.189770593270479,-0.187196905370401,-0.180675249612337,
-0.170656664963624,-0.122908095629107,-0.113977499342045,-0.109881990866413,
-0.106675228360909,-0.103137900339826,-0.0972603476961556,-0.0691137077990027,
-0.0593009426660634),.UNSPECIFIED.);
#2914=B_SPLINE_CURVE_WITH_KNOTS('',3,(#126060,#126061,#126062,#126063,#126064,
#126065,#126066,#126067,#126068,#126069,#126070,#126071,#126072,#126073,
#126074,#126075,#126076,#126077,#126078,#126079,#126080,#126081,#126082,
#126083,#126084,#126085,#126086,#126087,#126088,#126089,#126090,#126091,
#126092,#126093,#126094,#126095,#126096,#126097,#126098,#126099,#126100,
#126101,#126102,#126103,#126104,#126105,#126106,#126107,#126108,#126109,
#126110,#126111,#126112,#126113,#126114,#126115,#126116,#126117,#126118,
#126119,#126120,#126121,#126122,#126123,#126124,#126125,#126126,#126127,
#126128,#126129,#126130,#126131,#126132,#126133,#126134,#126135,#126136,
#126137,#126138,#126139,#126140,#126141,#126142,#126143,#126144,#126145,
#126146,#126147,#126148,#126149,#126150,#126151,#126152,#126153,#126154,
#126155,#126156,#126157,#126158,#126159,#126160,#126161,#126162,#126163,
#126164,#126165,#126166,#126167,#126168,#126169,#126170,#126171,#126172,
#126173,#126174,#126175,#126176,#126177,#126178,#126179,#126180,#126181,
#126182,#126183,#126184,#126185,#126186,#126187,#126188,#126189,#126190,
#126191,#126192,#126193,#126194,#126195,#126196,#126197,#126198,#126199,
#126200,#126201,#126202,#126203,#126204,#126205,#126206,#126207,#126208,
#126209,#126210,#126211,#126212,#126213,#126214,#126215,#126216,#126217,
#126218,#126219,#126220,#126221,#126222,#126223,#126224,#126225,#126226,
#126227,#126228,#126229,#126230,#126231,#126232,#126233,#126234,#126235,
#126236,#126237,#126238,#126239,#126240,#126241,#126242,#126243,#126244,
#126245,#126246,#126247),.UNSPECIFIED.,.F.,.F.,(4,2,2,2,2,2,2,2,2,2,2,2,
2,2,2,2,2,2,2,2,2,2,2,2,2,2,2,2,2,2,2,2,2,2,2,2,2,2,2,2,2,2,2,2,2,2,2,2,
2,2,2,2,2,2,2,2,2,2,2,2,2,2,2,2,2,2,2,2,2,2,2,2,2,2,2,2,2,2,2,2,2,2,2,2,
2,2,2,2,2,2,2,2,2,4),(-0.991403523612787,-0.987963642821703,-0.985948822364639,
-0.984105321973104,-0.981480764294791,-0.974697879765066,-0.931262196775588,
-0.911940967777414,-0.906349950602837,-0.902857745100171,-0.899606683850455,
-0.895255972618923,-0.885184454504479,-0.870688403025017,-0.850579423167714,
-0.827207420967211,-0.822344972442386,-0.820007291415794,-0.818199058221792,
-0.816018537885941,-0.811789534988751,-0.787448795578598,-0.747669641655126,
-0.741481014250267,-0.737511615470875,-0.734305398334489,-0.730606174008498,
-0.724031722976422,-0.68939917349318,-0.660331441517993,-0.655535125391971,
-0.653243639221105,-0.651438286732821,-0.649220721612908,-0.644805316034479,
-0.638913490495356,-0.623626330875805,-0.586388315789502,-0.576234872873496,
-0.572192897897606,-0.569194552209554,-0.565897428171752,-0.561265503200992,
-0.54932785567536,-0.530732586900761,-0.503337572388864,-0.491214431464943,
-0.487891523741086,-0.485903328305085,-0.484046987026729,-0.48134957160757,
-0.474053624903393,-0.46229902588501,-0.440810893855001,-0.412772996888117,
-0.406800605632133,-0.403228189056408,-0.400002682827013,-0.395831152665152,
-0.386811070180518,-0.374374706742553,-0.327302348459393,-0.322323206557624,
-0.319997287952923,-0.31819018476347,-0.316001311014742,-0.311730357115074,
-0.283243699264422,-0.248428409195011,-0.241840072325533,-0.237754078483996,
-0.23453812620516,-0.230917498814929,-0.224717376189783,-0.217136823783367,
-0.200448139197663,-0.168523618213428,-0.15765772047135,-0.154454553250421,
-0.152492343536114,-0.150677171307585,-0.148216037619876,-0.145218916596553,
-0.139725312086273,-0.126066129584397,-0.0814235618930086,-0.0750182323098244,
-0.0709854884195602,-0.0677747342105745,-0.0641207645063932,-0.0577615849681248,
-0.0499291798106559,-0.0323468223698187,-0.000494690693803759),
 .UNSPECIFIED.);
#2915=B_SPLINE_CURVE_WITH_KNOTS('',3,(#126248,#126249,#126250,#126251,#126252,
#126253,#126254,#126255,#126256,#126257,#126258,#126259,#126260,#126261,
#126262,#126263,#126264,#126265),.UNSPECIFIED.,.F.,.F.,(4,2,2,2,2,2,2,2,
4),(-2.10007532875945,-2.0906014191503,-2.08821171307978,-2.08641914292706,
-2.08463819261998,-2.08253030334906,-2.07875836979288,-2.06269506268221,
-2.0412420799731),.UNSPECIFIED.);
#2916=B_SPLINE_CURVE_WITH_KNOTS('',3,(#126266,#126267,#126268,#126269,#126270,
#126271,#126272,#126273,#126274,#126275,#126276,#126277,#126278,#126279,
#126280,#126281,#126282,#126283,#126284,#126285,#126286,#126287,#126288,
#126289,#126290,#126291,#126292,#126293,#126294,#126295,#126296,#126297,
#126298,#126299,#126300,#126301,#126302,#126303,#126304,#126305,#126306,
#126307,#126308,#126309,#126310,#126311,#126312,#126313,#126314,#126315,
#126316,#126317,#126318,#126319,#126320,#126321,#126322,#126323,#126324,
#126325,#126326,#126327,#126328,#126329,#126330,#126331,#126332,#126333,
#126334,#126335,#126336,#126337,#126338,#126339,#126340,#126341,#126342,
#126343,#126344,#126345,#126346,#126347,#126348,#126349,#126350,#126351,
#126352,#126353,#126354,#126355,#126356,#126357,#126358,#126359,#126360,
#126361,#126362,#126363,#126364,#126365,#126366,#126367,#126368,#126369,
#126370,#126371,#126372,#126373,#126374,#126375,#126376,#126377,#126378,
#126379,#126380,#126381,#126382,#126383,#126384,#126385,#126386,#126387,
#126388,#126389,#126390,#126391,#126392,#126393,#126394,#126395,#126396,
#126397,#126398,#126399,#126400,#126401,#126402,#126403,#126404,#126405,
#126406,#126407,#126408,#126409,#126410,#126411,#126412,#126413,#126414,
#126415,#126416,#126417,#126418,#126419,#126420,#126421,#126422,#126423,
#126424,#126425,#126426,#126427,#126428,#126429,#126430,#126431,#126432,
#126433,#126434,#126435,#126436,#126437,#126438,#126439,#126440,#126441,
#126442,#126443,#126444,#126445,#126446,#126447,#126448,#126449,#126450,
#126451,#126452,#126453,#126454,#126455,#126456,#126457,#126458,#126459),
 .UNSPECIFIED.,.F.,.F.,(4,2,2,2,2,2,2,2,2,2,2,2,2,2,2,2,2,2,2,2,2,2,2,2,
2,2,2,2,2,2,2,2,2,2,2,2,2,2,2,2,2,2,2,2,2,2,2,2,2,2,2,2,2,2,2,2,2,2,2,2,
2,2,2,2,2,2,2,2,2,2,2,2,2,2,2,2,2,2,2,2,2,2,2,2,2,2,2,2,2,2,2,2,2,2,2,2,
4),(-1.10915669663231,-1.10910532171049,-1.10590022347286,-1.10193354852953,
-1.09575202659879,-1.05005733740566,-1.03069533293189,-1.02705277091948,
-1.02497420345805,-1.02315151048225,-1.02066142234617,-1.01473892716117,
-1.00599573860429,-0.981790799667696,-0.951573944185358,-0.945592701348895,
-0.942018613321529,-0.938793889716136,-0.934626653734317,-0.925629696316969,
-0.901319497113162,-0.871404258772762,-0.862658720247753,-0.859688802304535,
-0.857966709744681,-0.856095279788858,-0.853321149648226,-0.845456710341012,
-0.832320086986627,-0.788136837005273,-0.780371288386305,-0.776381555805368,
-0.773173617037327,-0.769488561997317,-0.762983280400771,-0.754918204531033,
-0.736487450828257,-0.709514301513081,-0.696783567833986,-0.693413309283975,
-0.691414733393968,-0.689565230657145,-0.686899534787704,-0.679818508622548,
-0.668562553195977,-0.6473706194628,-0.618227667962999,-0.612245495167454,
-0.608673157429048,-0.605451537953733,-0.601290572072463,-0.59231714259212,
-0.566855992752182,-0.534969172607089,-0.528571081335433,-0.525936210195109,
-0.524110051136577,-0.522105620554195,-0.518708344248468,-0.503891324519974,
-0.456498464670831,-0.447464401826884,-0.443334614889865,-0.440105146715298,
-0.436546315642099,-0.430639634673135,-0.402327357768225,-0.374202936201015,
-0.363100614784437,-0.359874221289477,-0.357905864330772,-0.356031190392509,
-0.353257075600444,-0.345425355063952,-0.332373552100607,-0.288782401483648,
-0.280604428910652,-0.276582820453261,-0.273368099744482,-0.269695511161125,
-0.263265941294114,-0.232755830952575,-0.19928539238687,-0.194466407168421,
-0.192170852235826,-0.190371466264548,-0.18817642497511,-0.183824932519784,
-0.156777231243627,-0.120224568449024,-0.113721030701917,-0.109673133659428,
-0.106479523132496,-0.102876701450989,-0.0966903149974414,-0.0631983996702185,
-0.0592977063510342),.UNSPECIFIED.);
#2917=B_SPLINE_CURVE_WITH_KNOTS('',3,(#126462,#126463,#126464,#126465,#126466,
#126467,#126468,#126469,#126470,#126471,#126472,#126473,#126474,#126475,
#126476,#126477,#126478,#126479,#126480,#126481,#126482,#126483,#126484,
#126485,#126486,#126487,#126488,#126489,#126490,#126491,#126492,#126493,
#126494,#126495,#126496,#126497,#126498,#126499,#126500,#126501,#126502,
#126503,#126504,#126505,#126506,#126507,#126508,#126509,#126510,#126511,
#126512,#126513,#126514,#126515,#126516,#126517,#126518,#126519,#126520,
#126521,#126522,#126523,#126524,#126525,#126526,#126527,#126528,#126529,
#126530,#126531,#126532,#126533,#126534,#126535,#126536,#126537,#126538,
#126539,#126540,#126541,#126542,#126543,#126544,#126545,#126546,#126547,
#126548,#126549,#126550,#126551,#126552,#126553,#126554,#126555,#126556,
#126557,#126558,#126559,#126560,#126561,#126562,#126563,#126564,#126565,
#126566,#126567,#126568,#126569,#126570,#126571,#126572,#126573,#126574,
#126575,#126576,#126577,#126578,#126579,#126580,#126581,#126582),
 .UNSPECIFIED.,.F.,.F.,(4,3,3,3,3,3,3,3,3,3,3,3,3,3,3,3,3,3,3,3,3,3,3,3,
3,3,3,3,3,3,3,3,3,3,3,3,3,3,3,3,4),(17.9343865285971,18.0384572998024,18.1423979804763,
18.2462679090633,18.3501018475111,18.4539345090056,18.5578725321006,18.6618645536724,
18.7660437678494,18.8444150126792,18.9485886091815,19.0526067743066,19.1565026798016,
19.2603329942975,19.3641325164526,19.4679360013634,19.5718481070875,19.6758190055391,
19.7799719118523,19.8419628710253,19.9461515595277,20.0501850219937,20.1540964551946,
20.2579424311235,20.3617577250111,20.4655770686522,20.5695050565948,20.6734918745117,
20.7776605862359,20.8395107293714,20.9436986058482,21.0477312846702,21.1516419806614,
21.2554872485236,21.3593018646391,21.4631205619848,21.5670479566075,21.6710342102137,
21.7752024100578,21.8370585877175,21.9911485751285),.UNSPECIFIED.);
#2918=B_SPLINE_CURVE_WITH_KNOTS('',3,(#126583,#126584,#126585,#126586,#126587,
#126588,#126589,#126590,#126591,#126592,#126593,#126594,#126595,#126596,
#126597,#126598,#126599,#126600,#126601,#126602,#126603,#126604,#126605,
#126606,#126607,#126608,#126609,#126610,#126611,#126612,#126613,#126614,
#126615,#126616,#126617,#126618,#126619,#126620,#126621,#126622,#126623,
#126624,#126625,#126626,#126627,#126628,#126629,#126630,#126631,#126632,
#126633,#126634,#126635,#126636,#126637,#126638,#126639,#126640,#126641,
#126642,#126643,#126644,#126645,#126646,#126647,#126648,#126649,#126650,
#126651,#126652),.UNSPECIFIED.,.F.,.F.,(4,3,3,3,3,3,3,3,3,3,3,3,3,3,3,3,
3,3,3,3,3,3,3,4),(21.9911485755009,22.0965808093213,22.1989692644131,22.3012912063502,
22.4035832768669,22.505882070425,22.6082867494055,22.7107561649705,22.8133906742477,
22.8346064460636,22.9387930131769,23.0428243453621,23.1467336457121,23.2505774884119,
23.3543906519354,23.4582078713222,23.5621337592291,23.666118487615,23.7702851493394,
23.8321543044097,23.9363111118011,24.0403323654621,24.1442397578549,24.2175053922168),
 .UNSPECIFIED.);
#2919=B_SPLINE_CURVE_WITH_KNOTS('',3,(#126654,#126655,#126656,#126657,#126658,
#126659,#126660,#126661,#126662,#126663,#126664,#126665,#126666,#126667,
#126668,#126669,#126670,#126671,#126672,#126673,#126674,#126675,#126676,
#126677,#126678,#126679,#126680,#126681,#126682,#126683,#126684,#126685,
#126686,#126687,#126688,#126689,#126690,#126691,#126692,#126693,#126694,
#126695,#126696,#126697,#126698,#126699,#126700,#126701,#126702,#126703,
#126704,#126705,#126706,#126707,#126708,#126709,#126710,#126711,#126712,
#126713,#126714,#126715,#126716,#126717,#126718,#126719,#126720),
 .UNSPECIFIED.,.F.,.F.,(4,3,3,3,3,3,3,3,3,3,3,3,3,3,3,3,3,3,3,3,3,3,4),
(21.9911485755661,22.1068555809328,22.2230357332073,22.3398118814748,22.3785238795456,
22.4827125615403,22.5867460174313,22.6906574439895,22.7945034132374,22.8983187004159,
23.0021380373295,23.1060660185635,23.2100528297722,23.3142215348618,23.3760717378917,
23.4811392289653,23.5851517657021,23.6890597620316,23.7928980829185,23.8988264788089,
24.0026675510491,24.1096396087646,24.2166116664802),.UNSPECIFIED.);
#2920=B_SPLINE_CURVE_WITH_KNOTS('',3,(#126721,#126722,#126723,#126724,#126725,
#126726,#126727,#126728,#126729,#126730,#126731,#126732,#126733,#126734,
#126735,#126736,#126737,#126738,#126739,#126740,#126741,#126742,#126743,
#126744,#126745,#126746,#126747,#126748,#126749,#126750,#126751,#126752,
#126753,#126754,#126755,#126756,#126757,#126758,#126759,#126760,#126761,
#126762,#126763,#126764,#126765,#126766,#126767,#126768,#126769,#126770,
#126771,#126772,#126773,#126774,#126775,#126776,#126777,#126778,#126779,
#126780,#126781,#126782,#126783,#126784,#126785,#126786,#126787,#126788,
#126789,#126790,#126791,#126792,#126793,#126794,#126795,#126796,#126797,
#126798,#126799,#126800,#126801,#126802,#126803,#126804,#126805,#126806,
#126807,#126808,#126809,#126810,#126811,#126812,#126813,#126814,#126815,
#126816,#126817,#126818,#126819,#126820,#126821,#126822,#126823,#126824,
#126825,#126826,#126827,#126828,#126829,#126830,#126831,#126832,#126833,
#126834,#126835,#126836,#126837,#126838,#126839,#126840,#126841,#126842,
#126843,#126844),.UNSPECIFIED.,.F.,.F.,(4,3,3,3,3,3,3,3,3,3,3,3,3,3,3,3,
3,3,3,3,3,3,3,3,3,3,3,3,3,3,3,3,3,3,3,3,3,3,3,3,3,4),(17.9338039591658,
18.0378065512601,18.1419241164839,18.2461084709875,18.3504680705561,18.3883324461612,
18.4924181653028,18.5963471946834,18.7001525240931,18.8038914206691,18.9075988173882,
19.0113096028515,19.1151287668075,19.2190064442924,19.3230666994159,19.3858803045073,
19.4900800737608,19.5941245745256,19.6980469267599,19.8019037417006,19.905729777854,
20.0095597501986,20.1134981178355,20.2174951904896,20.3216738458828,20.3834281628534,
20.4876315786543,20.591680131366,20.6956071218429,20.7994689350635,20.9033003228197,
21.0071359937425,21.1110805544,21.2150841085133,21.3192696347798,21.3809760211995,
21.4863458581892,21.5915494442598,21.6965991972893,21.8015577704351,21.9064689038258,
21.9911485751285),.UNSPECIFIED.);
#2921=B_SPLINE_CURVE_WITH_KNOTS('',3,(#126847,#126848,#126849,#126850,#126851,
#126852,#126853,#126854,#126855,#126856,#126857,#126858,#126859,#126860,
#126861,#126862,#126863,#126864,#126865,#126866,#126867,#126868,#126869,
#126870,#126871,#126872,#126873,#126874,#126875,#126876,#126877,#126878,
#126879,#126880,#126881,#126882,#126883,#126884,#126885,#126886,#126887,
#126888,#126889,#126890,#126891,#126892,#126893,#126894,#126895,#126896,
#126897,#126898,#126899,#126900,#126901,#126902,#126903,#126904,#126905,
#126906,#126907,#126908,#126909,#126910,#126911,#126912,#126913,#126914,
#126915,#126916,#126917,#126918,#126919,#126920,#126921,#126922,#126923,
#126924,#126925,#126926,#126927,#126928,#126929,#126930,#126931,#126932,
#126933,#126934,#126935,#126936,#126937,#126938,#126939,#126940,#126941,
#126942,#126943,#126944,#126945,#126946,#126947,#126948,#126949,#126950,
#126951,#126952,#126953,#126954,#126955,#126956,#126957,#126958,#126959,
#126960,#126961,#126962,#126963,#126964,#126965,#126966,#126967),
 .UNSPECIFIED.,.F.,.F.,(4,3,3,3,3,3,3,3,3,3,3,3,3,3,3,3,3,3,3,3,3,3,3,3,
3,3,3,3,3,3,3,3,3,3,3,3,3,3,3,3,4),(17.9343865323097,18.0384573059669,18.1423979891803,
18.2462679203589,18.350101861447,18.4539345256267,18.5578725514576,18.6618645757981,
18.7660437927651,18.8444150126793,18.9485886051143,19.0526067661076,19.156502667395,
19.2603329776386,19.3641324955029,19.4679359760908,19.5718480774722,19.6758189715633,
19.779971873535,19.8419628710253,19.9461515610579,20.0501850250699,20.1540964598329,
20.2579424373327,20.3617577327979,20.4655770780209,20.5695050675409,20.6734918870352,
20.7776606003195,20.8395107293714,20.9436986062052,21.0477312853947,21.1516419817676,
21.2554872500202,21.359301866534,21.4631205642854,21.5670479593226,21.6710342133488,
21.7752024136171,21.8370585877175,21.9911485751285),.UNSPECIFIED.);
#2922=B_SPLINE_CURVE_WITH_KNOTS('',3,(#126968,#126969,#126970,#126971,#126972,
#126973,#126974,#126975,#126976,#126977,#126978,#126979,#126980,#126981,
#126982,#126983,#126984,#126985,#126986,#126987,#126988,#126989,#126990,
#126991,#126992,#126993,#126994,#126995,#126996,#126997,#126998,#126999,
#127000,#127001,#127002,#127003,#127004,#127005,#127006,#127007,#127008,
#127009,#127010,#127011,#127012,#127013,#127014,#127015,#127016,#127017,
#127018,#127019,#127020,#127021,#127022,#127023,#127024,#127025,#127026,
#127027,#127028,#127029,#127030,#127031,#127032,#127033,#127034,#127035,
#127036,#127037),.UNSPECIFIED.,.F.,.F.,(4,3,3,3,3,3,3,3,3,3,3,3,3,3,3,3,
3,3,3,3,3,3,3,4),(21.9911485755009,22.0965808093213,22.1989692637443,22.3012912050081,
22.4035832748472,22.5058820677243,22.6082867460218,22.7107561609016,22.8133906694953,
22.8346064460636,22.9387930134359,23.042824345883,23.1467336464979,23.250577489464,
23.3543906532553,23.4582078729108,23.5621337610859,23.66611848974,23.77028515173,
23.8321543044097,23.9363111118405,24.0403323655425,24.1442397579785,24.2175053970322),
 .UNSPECIFIED.);
#2923=B_SPLINE_CURVE_WITH_KNOTS('',3,(#127039,#127040,#127041,#127042,#127043,
#127044,#127045,#127046,#127047,#127048,#127049,#127050,#127051,#127052,
#127053,#127054,#127055,#127056,#127057,#127058,#127059,#127060,#127061,
#127062,#127063,#127064,#127065,#127066,#127067,#127068,#127069,#127070,
#127071,#127072,#127073,#127074,#127075,#127076,#127077,#127078,#127079,
#127080,#127081,#127082,#127083,#127084,#127085,#127086,#127087,#127088,
#127089,#127090,#127091,#127092,#127093,#127094,#127095,#127096,#127097,
#127098,#127099,#127100,#127101,#127102,#127103,#127104,#127105),
 .UNSPECIFIED.,.F.,.F.,(4,3,3,3,3,3,3,3,3,3,3,3,3,3,3,3,3,3,3,3,3,3,4),
(21.9911485755662,22.1068555730249,22.2230357171705,22.3398118572522,22.3785238795456,
22.4827125635847,22.5867460215413,22.6906574501864,22.7945034215332,22.8983187108193,
23.0021380498465,23.1060660331879,23.210052846504,23.3142215536779,23.3760717378917,
23.4811392295967,23.5851517668296,23.6890597636676,23.7928980850748,23.898826481689,
24.0026675544749,24.1096396130032,24.2166116715314),.UNSPECIFIED.);
#2924=B_SPLINE_CURVE_WITH_KNOTS('',3,(#127106,#127107,#127108,#127109,#127110,
#127111,#127112,#127113,#127114,#127115,#127116,#127117,#127118,#127119,
#127120,#127121,#127122,#127123,#127124,#127125,#127126,#127127,#127128,
#127129,#127130,#127131,#127132,#127133,#127134,#127135,#127136,#127137,
#127138,#127139,#127140,#127141,#127142,#127143,#127144,#127145,#127146,
#127147,#127148,#127149,#127150,#127151,#127152,#127153,#127154,#127155,
#127156,#127157,#127158,#127159,#127160,#127161,#127162,#127163,#127164,
#127165,#127166,#127167,#127168,#127169,#127170,#127171,#127172,#127173,
#127174,#127175,#127176,#127177,#127178,#127179,#127180,#127181,#127182,
#127183,#127184,#127185,#127186,#127187,#127188,#127189,#127190,#127191,
#127192,#127193,#127194,#127195,#127196,#127197,#127198,#127199,#127200,
#127201,#127202,#127203,#127204,#127205,#127206,#127207,#127208,#127209,
#127210,#127211,#127212,#127213,#127214,#127215,#127216,#127217,#127218,
#127219,#127220,#127221,#127222,#127223,#127224,#127225,#127226,#127227,
#127228,#127229),.UNSPECIFIED.,.F.,.F.,(4,3,3,3,3,3,3,3,3,3,3,3,3,3,3,3,
3,3,3,3,3,3,3,3,3,3,3,3,3,3,3,3,3,3,3,3,3,3,3,3,3,4),(17.9338039635375,
18.0378065699095,18.141924149687,18.2461085189123,18.3504681333591,18.3883324461612,
18.4924181349029,18.5963471334187,18.7001524314161,18.8038912962574,18.907598660964,
19.0113094141818,19.115128545753,19.2190061907243,19.3230664134798,19.3858803045073,
19.4900800856805,19.5941245984907,19.6980469628977,19.8019037900831,19.9057298385346,
20.0095598232127,20.1134982031513,20.2174952881079,20.3216739556707,20.3834281628534,
20.4876315818645,20.5916801378724,20.6956071317597,20.7994689484591,20.9033003397573,
21.0071360142814,21.1110805786052,21.2150841364274,21.3192696664305,21.3809760211995,
21.4863458526797,21.5915494331531,21.6965991804852,21.8015577478801,21.9064688754743,
21.9911485751285),.UNSPECIFIED.);
#2925=B_SPLINE_CURVE_WITH_KNOTS('',3,(#127232,#127233,#127234,#127235,#127236,
#127237,#127238,#127239,#127240,#127241,#127242,#127243,#127244,#127245,
#127246,#127247,#127248,#127249,#127250,#127251,#127252,#127253,#127254,
#127255,#127256,#127257,#127258,#127259,#127260,#127261,#127262,#127263,
#127264,#127265,#127266,#127267,#127268,#127269,#127270,#127271,#127272,
#127273,#127274,#127275,#127276,#127277,#127278,#127279,#127280,#127281,
#127282,#127283,#127284,#127285,#127286,#127287,#127288,#127289,#127290,
#127291,#127292,#127293,#127294,#127295,#127296,#127297,#127298,#127299,
#127300,#127301,#127302,#127303,#127304,#127305,#127306,#127307,#127308,
#127309,#127310,#127311,#127312,#127313,#127314,#127315,#127316,#127317,
#127318,#127319,#127320,#127321,#127322,#127323,#127324,#127325,#127326,
#127327,#127328,#127329,#127330,#127331,#127332,#127333,#127334,#127335,
#127336,#127337,#127338,#127339,#127340,#127341,#127342,#127343,#127344,
#127345,#127346,#127347,#127348,#127349,#127350,#127351,#127352),
 .UNSPECIFIED.,.F.,.F.,(4,3,3,3,3,3,3,3,3,3,3,3,3,3,3,3,3,3,3,3,3,3,3,3,
3,3,3,3,3,3,3,3,3,3,3,3,3,3,3,3,4),(17.9343900068785,18.0384621797793,18.1424043135119,
18.2462757259662,18.3501111769658,18.4539453776036,18.5578849698345,18.6618785800864,
18.766059395221,18.8444150126793,18.9485861780031,19.0526018736708,19.1564952646259,
19.2603230380769,19.3641199963983,19.4679208983768,19.5718304095614,19.6757987029868,
19.7799490157806,19.8419628710253,19.9461525033199,20.0501869193504,20.1540993159731,
20.2579462608792,20.361762527852,20.4655828472436,20.5695118082714,20.6734995992369,
20.7776692733765,20.8395107293714,20.9436988123426,21.0477317039952,21.1516426212559,
21.2554881154862,21.3593029627459,21.4631218956947,21.5670495311687,21.6710360289524,
21.7752044756406,21.8370585877175,21.9911485751285),.UNSPECIFIED.);
#2926=B_SPLINE_CURVE_WITH_KNOTS('',3,(#127353,#127354,#127355,#127356,#127357,
#127358,#127359,#127360,#127361,#127362,#127363,#127364,#127365,#127366,
#127367,#127368,#127369,#127370,#127371,#127372,#127373,#127374,#127375,
#127376,#127377,#127378,#127379,#127380,#127381,#127382,#127383,#127384,
#127385,#127386,#127387,#127388,#127389,#127390,#127391,#127392,#127393,
#127394,#127395,#127396,#127397,#127398,#127399,#127400,#127401,#127402,
#127403,#127404,#127405,#127406,#127407,#127408,#127409,#127410,#127411,
#127412,#127413,#127414,#127415,#127416,#127417,#127418,#127419,#127420,
#127421,#127422),.UNSPECIFIED.,.F.,.F.,(4,3,3,3,3,3,3,3,3,3,3,3,3,3,3,3,
3,3,3,3,3,3,3,4),(21.9911485754958,22.0965808093167,22.1989688491809,22.301290373003,
22.4035820228761,22.5058803936157,22.6082846484721,22.7107536385604,22.8133877234273,
22.8346064460636,22.9387931787213,23.0428246782763,23.1467341478916,23.2505781609339,
23.3543914956235,23.4582088867465,23.5621349460763,23.6661198459672,23.7702866774631,
23.8321543044097,23.9363111340917,24.0403324108138,24.1442398280771,24.2175094731414),
 .UNSPECIFIED.);
#2927=B_SPLINE_CURVE_WITH_KNOTS('',3,(#127424,#127425,#127426,#127427,#127428,
#127429,#127430,#127431,#127432,#127433,#127434,#127435,#127436,#127437,
#127438,#127439,#127440,#127441,#127442,#127443,#127444,#127445,#127446,
#127447,#127448,#127449,#127450,#127451,#127452,#127453,#127454,#127455,
#127456,#127457,#127458,#127459,#127460,#127461,#127462,#127463,#127464,
#127465,#127466,#127467,#127468,#127469,#127470,#127471,#127472,#127473,
#127474,#127475,#127476,#127477,#127478,#127479,#127480,#127481,#127482,
#127483,#127484,#127485,#127486,#127487,#127488,#127489,#127490),
 .UNSPECIFIED.,.F.,.F.,(4,3,3,3,3,3,3,3,3,3,3,3,3,3,3,3,3,3,3,3,3,3,4),
(21.99114857557,22.1068519865695,22.2230284424145,22.3398008663504,22.3785238795456,
22.4827135010409,22.5867479061601,22.6906602917587,22.7945072255769,22.8983234814147,
23.0021437896405,23.1060727395329,23.2100605193632,23.3142301824888,23.3760717378917,
23.4811397540393,23.5851525044163,23.6890607200774,23.7928992656579,23.8988284160114,
24.0026697250665,24.1096427960693,24.2166158670722),.UNSPECIFIED.);
#2928=B_SPLINE_CURVE_WITH_KNOTS('',3,(#127491,#127492,#127493,#127494,#127495,
#127496,#127497,#127498,#127499,#127500,#127501,#127502,#127503,#127504,
#127505,#127506,#127507,#127508,#127509,#127510,#127511,#127512,#127513,
#127514,#127515,#127516,#127517,#127518,#127519,#127520,#127521,#127522,
#127523,#127524,#127525,#127526,#127527,#127528,#127529,#127530,#127531,
#127532,#127533,#127534,#127535,#127536,#127537,#127538,#127539,#127540,
#127541,#127542,#127543,#127544,#127545,#127546,#127547,#127548,#127549,
#127550,#127551,#127552,#127553,#127554,#127555,#127556,#127557,#127558,
#127559,#127560,#127561,#127562,#127563,#127564,#127565,#127566,#127567,
#127568,#127569,#127570,#127571,#127572,#127573,#127574,#127575,#127576,
#127577,#127578,#127579,#127580,#127581,#127582,#127583,#127584,#127585,
#127586,#127587,#127588,#127589,#127590,#127591,#127592,#127593,#127594,
#127595,#127596,#127597,#127598,#127599,#127600,#127601,#127602,#127603,
#127604,#127605,#127606,#127607,#127608,#127609,#127610,#127611,#127612,
#127613,#127614),.UNSPECIFIED.,.F.,.F.,(4,3,3,3,3,3,3,3,3,3,3,3,3,3,3,3,
3,3,3,3,3,3,3,3,3,3,3,3,3,3,3,3,3,3,3,3,3,3,3,3,3,4),(17.9338080230641,
18.037816525777,18.1419401180095,18.2461305705873,18.3504963338971,18.3883324461612,
18.4924050953013,18.5963208567489,18.7001126857905,18.803837945059,18.9075315867694,
19.0112285186248,19.1150337711737,19.2188974829894,19.3229438367761,19.3858803045073,
19.4900853238861,19.5941351297246,19.6980628426444,19.801925049615,19.9057565010466,
20.0095919038493,20.1135356875764,20.2175381763388,20.3217221890141,20.3834281628534,
20.4876329473777,20.5916829062076,20.6956113519136,20.799474649947,20.9033075499886,
21.0071447585888,21.1110908855051,21.2150960243741,21.3192831478159,21.3809760211995,
21.4863434371408,21.5915445630699,21.6965918110537,21.8015478551884,21.9064564387841,
21.9911485751285),.UNSPECIFIED.);
#2929=B_SPLINE_CURVE_WITH_KNOTS('',3,(#127617,#127618,#127619,#127620,#127621,
#127622,#127623,#127624,#127625,#127626,#127627,#127628,#127629,#127630,
#127631,#127632,#127633,#127634,#127635,#127636,#127637,#127638,#127639,
#127640,#127641,#127642,#127643,#127644,#127645,#127646,#127647,#127648,
#127649,#127650,#127651,#127652,#127653,#127654,#127655,#127656,#127657,
#127658,#127659,#127660,#127661,#127662,#127663,#127664,#127665,#127666,
#127667,#127668,#127669,#127670,#127671,#127672,#127673,#127674,#127675,
#127676,#127677,#127678,#127679,#127680,#127681,#127682,#127683,#127684,
#127685,#127686,#127687,#127688,#127689,#127690,#127691,#127692,#127693,
#127694,#127695,#127696,#127697,#127698,#127699,#127700,#127701,#127702,
#127703,#127704,#127705,#127706,#127707,#127708,#127709,#127710,#127711,
#127712,#127713,#127714,#127715,#127716,#127717,#127718,#127719,#127720,
#127721,#127722,#127723,#127724,#127725,#127726,#127727,#127728,#127729,
#127730,#127731,#127732,#127733,#127734,#127735,#127736,#127737),
 .UNSPECIFIED.,.F.,.F.,(4,3,3,3,3,3,3,3,3,3,3,3,3,3,3,3,3,3,3,3,3,3,3,3,
3,3,3,3,3,3,3,3,3,3,3,3,3,3,3,3,4),(17.9343899947098,18.0384621637907,18.1424042935601,
18.2462757019651,18.3501111488352,18.4539453452689,18.5578849332116,18.6618785391202,
18.7660593498775,18.8444150126793,18.9485861849099,19.0526018875928,19.1564952856901,
19.2603230663583,19.3641200319611,19.4679209412748,19.5718304598269,19.6757987606494,
19.779949080807,19.8419628710254,19.9461525005616,20.050186913805,20.1540993076118,
20.2579462496858,20.3617625138143,20.4655828303539,20.5695117885374,20.6734995766586,
20.7776692479848,20.8395107293714,20.9436988117741,21.0477317028403,21.1516426194906,
21.2554881130961,21.3593029597174,21.4631218920152,21.567049526823,21.6710360239309,
21.7752044699356,21.8370585877175,21.9911485751285),.UNSPECIFIED.);
#2930=B_SPLINE_CURVE_WITH_KNOTS('',3,(#127738,#127739,#127740,#127741,#127742,
#127743,#127744,#127745,#127746,#127747,#127748,#127749,#127750,#127751,
#127752,#127753,#127754,#127755,#127756,#127757,#127758,#127759,#127760,
#127761,#127762,#127763,#127764,#127765,#127766,#127767,#127768,#127769,
#127770,#127771,#127772,#127773,#127774,#127775,#127776,#127777,#127778,
#127779,#127780,#127781,#127782,#127783,#127784,#127785,#127786,#127787,
#127788,#127789,#127790,#127791,#127792,#127793,#127794,#127795,#127796,
#127797,#127798,#127799,#127800,#127801,#127802,#127803,#127804,#127805,
#127806,#127807),.UNSPECIFIED.,.F.,.F.,(4,3,3,3,3,3,3,3,3,3,3,3,3,3,3,3,
3,3,3,3,3,3,3,4),(21.9911485754958,22.0965808093167,22.1989688504026,22.3012903754547,
22.4035820265653,22.5058803985488,22.6082846546529,22.7107536459929,22.8133877321084,
22.8346064460636,22.9387931782215,23.0428246772713,23.1467341463756,23.2505781589037,
23.3543914930764,23.458208883681,23.5621349424933,23.6661198418661,23.7702866728494,
23.8321543044097,23.9363111340315,24.0403324106909,24.1442398278863,24.2175094594017),
 .UNSPECIFIED.);
#2931=B_SPLINE_CURVE_WITH_KNOTS('',3,(#127809,#127810,#127811,#127812,#127813,
#127814,#127815,#127816,#127817,#127818,#127819,#127820,#127821,#127822,
#127823,#127824,#127825,#127826,#127827,#127828,#127829,#127830,#127831,
#127832,#127833,#127834,#127835,#127836,#127837,#127838,#127839,#127840,
#127841,#127842,#127843,#127844,#127845,#127846,#127847,#127848,#127849,
#127850,#127851,#127852,#127853,#127854,#127855,#127856,#127857,#127858,
#127859,#127860,#127861,#127862,#127863,#127864,#127865,#127866,#127867,
#127868,#127869,#127870,#127871,#127872,#127873,#127874,#127875),
 .UNSPECIFIED.,.F.,.F.,(4,3,3,3,3,3,3,3,3,3,3,3,3,3,3,3,3,3,3,3,3,3,4),
(21.99114857557,22.1068520005075,22.2230284706919,22.3398009090817,22.3785238795456,
22.4827134973594,22.5867478987589,22.6906602805993,22.7945072106377,22.8983234626795,
23.0021437670992,23.1060727131954,23.2100604892296,23.3142301486006,23.3760717378917,
23.481139752265,23.5851525018523,23.6890607167021,23.7928992614511,23.8988284093079,
24.0026697174858,24.1096427851821,24.2166158528785),.UNSPECIFIED.);
#2932=B_SPLINE_CURVE_WITH_KNOTS('',3,(#127876,#127877,#127878,#127879,#127880,
#127881,#127882,#127883,#127884,#127885,#127886,#127887,#127888,#127889,
#127890,#127891,#127892,#127893,#127894,#127895,#127896,#127897,#127898,
#127899,#127900,#127901,#127902,#127903,#127904,#127905,#127906,#127907,
#127908,#127909,#127910,#127911,#127912,#127913,#127914,#127915,#127916,
#127917,#127918,#127919,#127920,#127921,#127922,#127923,#127924,#127925,
#127926,#127927,#127928,#127929,#127930,#127931,#127932,#127933,#127934,
#127935,#127936,#127937,#127938,#127939,#127940,#127941,#127942,#127943,
#127944,#127945,#127946,#127947,#127948,#127949,#127950,#127951,#127952,
#127953,#127954,#127955,#127956,#127957,#127958,#127959,#127960,#127961,
#127962,#127963,#127964,#127965,#127966,#127967,#127968,#127969,#127970,
#127971,#127972,#127973,#127974,#127975,#127976,#127977,#127978,#127979,
#127980,#127981,#127982,#127983,#127984,#127985,#127986,#127987,#127988,
#127989,#127990,#127991,#127992,#127993,#127994,#127995,#127996,#127997,
#127998,#127999),.UNSPECIFIED.,.F.,.F.,(4,3,3,3,3,3,3,3,3,3,3,3,3,3,3,3,
3,3,3,3,3,3,3,3,3,3,3,3,3,3,3,3,3,3,3,3,3,3,3,3,3,4),(17.9338080088879,
18.0378164903648,18.1419400609392,18.2461304916012,18.3504962327555,18.3883324461612,
18.4924051434582,18.5963209537852,18.7001128325525,18.8038381420455,18.9075318344083,
19.0112288172744,19.115034121039,19.2188978842661,19.3229442892214,19.3858803045073,
19.4900853041056,19.5941350899583,19.6980627826847,19.8019249693451,19.9057564003801,
20.0095917827304,20.113535546061,20.2175380144279,20.3217220069307,20.3834281628534,
20.4876329423721,20.5916828960584,20.6956113364386,20.7994746290363,20.9033075235404,
21.0071447265092,21.1110908476868,21.2150959807482,21.3192830983351,21.3809760211995,
21.4863434462503,21.5915445814378,21.6965918388519,21.8015478925087,21.9064564857074,
21.9911485751285),.UNSPECIFIED.);
#2933=B_SPLINE_CURVE_WITH_KNOTS('',3,(#128002,#128003,#128004,#128005,#128006,
#128007,#128008,#128009,#128010,#128011,#128012,#128013,#128014,#128015,
#128016,#128017,#128018,#128019,#128020,#128021,#128022,#128023,#128024,
#128025,#128026,#128027,#128028,#128029,#128030,#128031,#128032,#128033,
#128034,#128035,#128036,#128037,#128038,#128039,#128040,#128041,#128042,
#128043,#128044,#128045,#128046,#128047,#128048,#128049,#128050,#128051,
#128052,#128053,#128054,#128055,#128056,#128057,#128058,#128059,#128060,
#128061,#128062,#128063,#128064,#128065,#128066,#128067,#128068,#128069,
#128070,#128071,#128072,#128073,#128074,#128075,#128076,#128077,#128078,
#128079,#128080,#128081,#128082,#128083,#128084,#128085,#128086,#128087,
#128088,#128089,#128090,#128091,#128092,#128093,#128094,#128095,#128096,
#128097,#128098,#128099,#128100,#128101,#128102,#128103,#128104,#128105,
#128106,#128107,#128108,#128109,#128110,#128111,#128112,#128113,#128114,
#128115,#128116,#128117,#128118,#128119,#128120,#128121,#128122,#128123,
#128124,#128125,#128126,#128127,#128128,#128129,#128130,#128131,#128132,
#128133,#128134,#128135,#128136,#128137,#128138,#128139,#128140,#128141,
#128142,#128143,#128144,#128145,#128146,#128147,#128148,#128149,#128150,
#128151,#128152,#128153,#128154,#128155,#128156,#128157,#128158,#128159,
#128160,#128161,#128162,#128163,#128164,#128165,#128166,#128167,#128168,
#128169,#128170,#128171,#128172,#128173,#128174,#128175,#128176,#128177,
#128178,#128179,#128180,#128181,#128182,#128183,#128184,#128185,#128186,
#128187,#128188,#128189,#128190,#128191,#128192,#128193),.UNSPECIFIED.,
 .F.,.F.,(4,2,2,2,2,2,2,2,2,2,2,2,2,2,2,2,2,2,2,2,2,2,2,2,2,2,2,2,2,2,2,
2,2,2,2,2,2,2,2,2,2,2,2,2,2,2,2,2,2,2,2,2,2,2,2,2,2,2,2,2,2,2,2,2,2,2,2,
2,2,2,2,2,2,2,2,2,2,2,2,2,2,2,2,2,2,2,2,2,2,2,2,2,2,2,2,4),(-0.991428410285835,
-0.988079051914102,-0.986174702512279,-0.984686720637925,-0.982568327636504,
-0.978057342726682,-0.958846858953674,-0.925949063822915,-0.910796371618096,
-0.905890468462402,-0.90274575578572,-0.89976872626918,-0.895716929755394,
-0.886083974166438,-0.872156372916892,-0.851296795768739,-0.844281720716043,
-0.824951803310466,-0.821511726513893,-0.819587581485021,-0.818101821779044,
-0.816008744738817,-0.811631822475302,-0.793628448958833,-0.761621483382622,
-0.744632225717325,-0.739501522247694,-0.736309326998721,-0.733352816301539,
-0.729428417369128,-0.720564804316846,-0.708149564548891,-0.675417687548301,
-0.658218517705773,-0.654819631418646,-0.652905103656635,-0.65141838021344,
-0.649313192190328,-0.644871404736423,-0.626288555738524,-0.581124760367325,
-0.574882839187131,-0.571124120715254,-0.568182147552947,-0.56494395926655,
-0.559596962681835,-0.536841489904728,-0.505575230366341,-0.491254572171557,
-0.487968880243975,-0.48609905153233,-0.484436286563665,-0.482154321579273,
-0.476712199079443,-0.468741731538051,-0.441496748860293,-0.412387717576688,
-0.406739585552727,-0.403404967233731,-0.400508038898117,-0.396863382055824,
-0.389541116597339,-0.379924474232353,-0.354139622884094,-0.326964804441683,
-0.322224587258243,-0.320087043524696,-0.318437380115702,-0.316504946503874,
-0.312926655053968,-0.308344436582049,-0.26461115235902,-0.244951083691612,
-0.239647439108722,-0.236418664904477,-0.233474418659642,-0.229633554968816,
-0.221247768178535,-0.198872379938102,-0.160140751580241,-0.1559475005551,
-0.153857693129254,-0.152176139033525,-0.150430206099431,-0.14781516987963,
-0.144570044779037,-0.138158827217404,-0.119941501135129,-0.0808892449979691,
-0.0747875341691031,-0.0710287905266305,-0.068094704374682,-0.0648232573106013,
-0.0593202236501849,-0.0332727463327188,-0.000493937522251609),
 .UNSPECIFIED.);
#2934=B_SPLINE_CURVE_WITH_KNOTS('',3,(#128194,#128195,#128196,#128197,#128198,
#128199,#128200,#128201,#128202,#128203,#128204,#128205,#128206,#128207,
#128208,#128209,#128210,#128211,#128212,#128213),.UNSPECIFIED.,.F.,.F.,
(4,2,2,2,2,2,2,2,2,4),(-2.09972702821217,-2.09332876904563,-2.08914070274811,
-2.08717690472677,-2.08561029790526,-2.08408096225861,-2.08202773782795,
-2.07785554176778,-2.06362842930142,-2.04089325283701),.UNSPECIFIED.);
#2935=B_SPLINE_CURVE_WITH_KNOTS('',3,(#128214,#128215,#128216,#128217,#128218,
#128219,#128220,#128221,#128222,#128223,#128224,#128225,#128226,#128227,
#128228,#128229,#128230,#128231,#128232,#128233,#128234,#128235,#128236,
#128237,#128238,#128239,#128240,#128241,#128242,#128243,#128244,#128245,
#128246,#128247,#128248,#128249,#128250,#128251,#128252,#128253,#128254,
#128255,#128256,#128257,#128258,#128259,#128260,#128261,#128262,#128263,
#128264,#128265,#128266,#128267,#128268,#128269,#128270,#128271,#128272,
#128273,#128274,#128275,#128276,#128277,#128278,#128279,#128280,#128281,
#128282,#128283,#128284,#128285,#128286,#128287,#128288,#128289,#128290,
#128291,#128292,#128293,#128294,#128295,#128296,#128297,#128298,#128299,
#128300,#128301,#128302,#128303,#128304,#128305,#128306,#128307,#128308,
#128309,#128310,#128311,#128312,#128313,#128314,#128315,#128316,#128317,
#128318,#128319,#128320,#128321,#128322,#128323,#128324,#128325,#128326,
#128327,#128328,#128329,#128330,#128331,#128332,#128333,#128334,#128335,
#128336,#128337,#128338,#128339,#128340,#128341,#128342,#128343,#128344,
#128345,#128346,#128347,#128348,#128349,#128350,#128351,#128352,#128353,
#128354,#128355,#128356,#128357,#128358,#128359,#128360,#128361,#128362,
#128363,#128364,#128365,#128366,#128367,#128368,#128369,#128370,#128371,
#128372,#128373,#128374,#128375,#128376,#128377,#128378,#128379,#128380,
#128381,#128382,#128383,#128384,#128385,#128386,#128387,#128388,#128389,
#128390,#128391,#128392,#128393,#128394,#128395,#128396,#128397,#128398,
#128399,#128400,#128401,#128402,#128403,#128404,#128405,#128406,#128407,
#128408,#128409,#128410,#128411,#128412,#128413),.UNSPECIFIED.,.F.,.F.,
(4,2,2,2,2,2,2,2,2,2,2,2,2,2,2,2,2,2,2,2,2,2,2,2,2,2,2,2,2,2,2,2,2,2,2,
2,2,2,2,2,2,2,2,2,2,2,2,2,2,2,2,2,2,2,2,2,2,2,2,2,2,2,2,2,2,2,2,2,2,2,2,
2,2,2,2,2,2,2,2,2,2,2,2,2,2,2,2,2,2,2,2,2,2,2,2,2,2,2,2,4),(-1.75137704512006,
-1.75068586141549,-1.74773502972146,-1.74384492978998,-1.73517717150812,
-1.70756333847727,-1.67406144166101,-1.6696848637827,-1.66759229681557,
-1.6659488161001,-1.66395579085683,-1.66008441585536,-1.65501110865308,
-1.64253315520674,-1.60439630157427,-1.59131627393385,-1.58664387665479,
-1.58385831735353,-1.58089453160312,-1.5769185418947,-1.56774476698758,
-1.52303114913358,-1.50580683490755,-1.50240662273871,-1.50049185289282,
-1.4990049665169,-1.49689969713169,-1.49245905629593,-1.47388979843424,
-1.42871407639495,-1.42247706030726,-1.41871950393603,-1.41577738265347,
-1.41253793923695,-1.40718629000793,-1.38435578994611,-1.352638704996,-1.33878463943771,
-1.33552894718525,-1.33366566185352,-1.33200215173781,-1.32970942554851,
-1.32419459703652,-1.31607697962534,-1.28777223434872,-1.25982060941732,
-1.25416928215468,-1.25086734937448,-1.24823352273214,-1.24467544776299,
-1.23778643396667,-1.21272093777518,-1.18670930496516,-1.17216906670648,
-1.16891123022386,-1.16702936965349,-1.16537041375951,-1.16311396155721,
-1.15782516983446,-1.15015885150216,-1.12496725237433,-1.09577693192094,
-1.08865718470918,-1.08500453074326,-1.08207938288981,-1.0787388427316,
-1.07291697071022,-1.03935143486294,-1.00742403873065,-1.00298861170436,
-1.0008532998799,-0.999204598484219,-0.997238008388753,-0.993510036178509,
-0.988681208620626,-0.977124402256908,-0.955825141315264,-0.926759379615489,
-0.921110912166493,-0.917773525313023,-0.914872458758619,-0.911220183221169,
-0.903873501595287,-0.894219283714354,-0.868273613820256,-0.841255103291184,
-0.836525628966603,-0.834390221870311,-0.832744582165012,-0.830824946150585,
-0.827271074801043,-0.798463059903333,-0.761980772425169,-0.755661402129203,
-0.751891185075146,-0.748961058139669,-0.745757486285535,-0.740518802882096,
-0.719296593176995,-0.701455818686197),.UNSPECIFIED.);
#2936=B_SPLINE_CURVE_WITH_KNOTS('',3,(#128416,#128417,#128418,#128419,#128420,
#128421,#128422,#128423,#128424,#128425,#128426,#128427,#128428,#128429,
#128430,#128431,#128432,#128433,#128434,#128435,#128436,#128437,#128438,
#128439,#128440,#128441,#128442,#128443,#128444,#128445,#128446,#128447,
#128448,#128449,#128450,#128451,#128452,#128453,#128454,#128455,#128456,
#128457,#128458,#128459,#128460,#128461,#128462,#128463,#128464,#128465,
#128466,#128467,#128468,#128469,#128470,#128471,#128472,#128473,#128474,
#128475,#128476,#128477,#128478,#128479,#128480,#128481,#128482,#128483,
#128484,#128485,#128486,#128487,#128488,#128489,#128490,#128491,#128492,
#128493,#128494,#128495,#128496,#128497,#128498,#128499,#128500,#128501,
#128502,#128503,#128504,#128505,#128506,#128507,#128508,#128509,#128510,
#128511,#128512,#128513,#128514,#128515,#128516,#128517,#128518,#128519,
#128520,#128521,#128522,#128523,#128524,#128525,#128526,#128527,#128528,
#128529,#128530,#128531,#128532,#128533,#128534,#128535,#128536),
 .UNSPECIFIED.,.F.,.F.,(4,3,3,3,3,3,3,3,3,3,3,3,3,3,3,3,3,3,3,3,3,3,3,3,
3,3,3,3,3,3,3,3,3,3,3,3,3,3,3,3,4),(17.9343860550099,18.0384563012467,18.1423965009774,
18.2462659783595,18.3500994957989,18.4539317669694,18.5578694092301,18.6618610789189,
18.7660398843486,18.8442797453128,18.9484546129248,19.0524740709654,19.1563712946165,
19.2602029425331,19.3640038114039,19.4678086543699,19.5717221204532,19.675694386121,
19.779848640803,19.8418082797494,19.9459968485137,20.0500301930795,20.1539415107437,
20.2577873730439,20.3616025553732,20.46542178969,20.5693496667369,20.6733363761974,
20.7775049695994,20.839336814186,20.9435248555288,21.0475577022467,21.1514685688393,
21.2553140092606,21.3591287996192,21.4629476726207,21.5668752380743,21.6708616635392,
21.7750300200673,21.8368653486226,21.9911485751285),.UNSPECIFIED.);
#2937=B_SPLINE_CURVE_WITH_KNOTS('',3,(#128537,#128538,#128539,#128540,#128541,
#128542,#128543,#128544,#128545,#128546,#128547,#128548,#128549,#128550,
#128551,#128552,#128553,#128554,#128555,#128556,#128557,#128558,#128559,
#128560,#128561,#128562,#128563,#128564,#128565,#128566,#128567,#128568,
#128569,#128570,#128571,#128572,#128573,#128574,#128575,#128576,#128577,
#128578,#128579,#128580,#128581,#128582,#128583,#128584,#128585,#128586,
#128587,#128588,#128589,#128590,#128591,#128592,#128593,#128594,#128595,
#128596,#128597,#128598,#128599,#128600,#128601,#128602,#128603,#128604,
#128605,#128606),.UNSPECIFIED.,.F.,.F.,(4,3,3,3,3,3,3,3,3,3,3,3,3,3,3,3,
3,3,3,3,3,3,3,4),(21.9911485755033,22.0965542389478,22.1989427477135,22.3012648047145,
22.4035570514261,22.5058560821305,22.6082610316386,22.7107307725331,22.8133655493976,
22.8343938830592,22.9385806433496,23.0426121737347,23.1465216778305,23.2503657279729,
23.3541791023172,23.4579965355874,23.5619226348359,23.6659075769415,23.7700744389157,
23.8319224174958,23.9360794349529,24.0401009061163,24.1440085667296,24.2175036368067),
 .UNSPECIFIED.);
#2938=B_SPLINE_CURVE_WITH_KNOTS('',3,(#128608,#128609,#128610,#128611,#128612,
#128613,#128614,#128615,#128616,#128617,#128618,#128619,#128620,#128621,
#128622,#128623,#128624,#128625,#128626,#128627,#128628,#128629,#128630,
#128631,#128632,#128633,#128634,#128635,#128636,#128637,#128638,#128639,
#128640,#128641,#128642,#128643,#128644,#128645,#128646,#128647,#128648,
#128649,#128650,#128651,#128652,#128653,#128654,#128655,#128656,#128657,
#128658,#128659,#128660,#128661,#128662,#128663,#128664,#128665,#128666,
#128667,#128668,#128669,#128670,#128671,#128672,#128673,#128674),
 .UNSPECIFIED.,.F.,.F.,(4,3,3,3,3,3,3,3,3,3,3,3,3,3,3,3,3,3,3,3,3,3,4),
(21.9911485755641,22.1068686936971,22.2230626932475,22.3398531219692,22.3783692882696,
22.4825578617427,22.5865912110659,22.6905025335363,22.7943484006702,22.8981635878534,
23.0019828270372,23.1059107089372,23.2098974232505,23.3140660214517,23.3758978227062,
23.4809869478153,23.5849996243381,23.6889077755763,23.7927462661774,23.8987124055277,
24.0025537182315,24.1095822709052,24.2166108235789),.UNSPECIFIED.);
#2939=B_SPLINE_CURVE_WITH_KNOTS('',3,(#128675,#128676,#128677,#128678,#128679,
#128680,#128681,#128682,#128683,#128684,#128685,#128686,#128687,#128688,
#128689,#128690,#128691,#128692,#128693,#128694,#128695,#128696,#128697,
#128698,#128699,#128700,#128701,#128702,#128703,#128704,#128705,#128706,
#128707,#128708,#128709,#128710,#128711,#128712,#128713,#128714,#128715,
#128716,#128717,#128718,#128719,#128720,#128721,#128722,#128723,#128724,
#128725,#128726,#128727,#128728,#128729,#128730,#128731,#128732,#128733,
#128734,#128735,#128736,#128737,#128738,#128739,#128740,#128741,#128742,
#128743,#128744,#128745,#128746,#128747,#128748,#128749,#128750,#128751,
#128752,#128753,#128754,#128755,#128756,#128757,#128758,#128759,#128760,
#128761,#128762,#128763,#128764,#128765,#128766,#128767,#128768,#128769,
#128770,#128771,#128772,#128773,#128774,#128775,#128776,#128777,#128778,
#128779,#128780,#128781,#128782,#128783,#128784,#128785,#128786,#128787,
#128788,#128789,#128790,#128791,#128792,#128793,#128794,#128795,#128796,
#128797,#128798),.UNSPECIFIED.,.F.,.F.,(4,3,3,3,3,3,3,3,3,3,3,3,3,3,3,3,
3,3,3,3,3,3,3,3,3,3,3,3,3,3,3,3,3,3,3,3,3,3,3,3,3,4),(17.9338028153519,
18.037802986915,18.1419180880466,18.2460999659707,18.3504570297057,18.3882551505232,
18.4923467216465,18.5962816946849,18.7000930752598,18.8038380867795,18.9075516535319,
19.0112686554929,19.1150940593869,19.2189780032249,19.3230444840438,19.3857836849598,
19.4899815455746,19.5940241205743,19.6979445301226,19.8017993933992,19.905623471839,
20.0094514833414,20.113387893203,20.2173830103628,20.3215597202534,20.3833122193964,
20.4875152949366,20.5915634971424,20.6954901224722,20.7993515620656,20.9031825682167,
21.0070178500512,21.1109620069549,21.2149651519192,21.319150249886,21.380840753833,
21.4862078208751,21.5914087085921,21.6964558994253,21.8014119807972,21.9063207971622,
21.9911485751285),.UNSPECIFIED.);
#2940=B_SPLINE_CURVE_WITH_KNOTS('',3,(#128801,#128802,#128803,#128804,#128805,
#128806,#128807,#128808,#128809,#128810,#128811,#128812,#128813,#128814,
#128815,#128816,#128817,#128818,#128819,#128820,#128821,#128822,#128823,
#128824,#128825,#128826,#128827,#128828,#128829,#128830,#128831,#128832,
#128833,#128834,#128835,#128836,#128837,#128838,#128839,#128840,#128841,
#128842,#128843,#128844,#128845,#128846,#128847,#128848,#128849,#128850,
#128851,#128852,#128853,#128854,#128855,#128856,#128857,#128858,#128859,
#128860,#128861,#128862,#128863,#128864,#128865,#128866,#128867,#128868,
#128869,#128870,#128871,#128872,#128873,#128874,#128875,#128876,#128877,
#128878,#128879,#128880,#128881,#128882,#128883,#128884,#128885,#128886,
#128887,#128888,#128889,#128890,#128891,#128892,#128893,#128894,#128895,
#128896,#128897,#128898,#128899,#128900,#128901,#128902,#128903,#128904,
#128905,#128906,#128907,#128908,#128909,#128910,#128911,#128912,#128913,
#128914,#128915,#128916,#128917,#128918,#128919,#128920,#128921,#128922,
#128923,#128924,#128925,#128926,#128927,#128928,#128929,#128930,#128931,
#128932,#128933,#128934,#128935,#128936,#128937,#128938,#128939,#128940,
#128941,#128942,#128943,#128944,#128945,#128946,#128947,#128948,#128949,
#128950,#128951,#128952,#128953,#128954,#128955,#128956,#128957,#128958,
#128959,#128960,#128961,#128962,#128963,#128964,#128965,#128966,#128967,
#128968,#128969,#128970,#128971,#128972,#128973,#128974,#128975,#128976,
#128977,#128978,#128979,#128980,#128981,#128982,#128983,#128984,#128985,
#128986,#128987,#128988,#128989,#128990,#128991,#128992),.UNSPECIFIED.,
 .F.,.F.,(4,2,2,2,2,2,2,2,2,2,2,2,2,2,2,2,2,2,2,2,2,2,2,2,2,2,2,2,2,2,2,
2,2,2,2,2,2,2,2,2,2,2,2,2,2,2,2,2,2,2,2,2,2,2,2,2,2,2,2,2,2,2,2,2,2,2,2,
2,2,2,2,2,2,2,2,2,2,2,2,2,2,2,2,2,2,2,2,2,2,2,2,2,2,2,2,4),(-0.991336294305795,
-0.987987101398143,-0.986082845117753,-0.984594935419473,-0.982476644211697,
-0.97796587170094,-0.958756254912108,-0.925859865691171,-0.910708157934416,
-0.905802519572545,-0.902657965632366,-0.899681078608121,-0.895629463748385,
-0.885996878357646,-0.872069755009444,-0.851211466103253,-0.844196737899769,
-0.824867832965056,-0.821427925970876,-0.819503875272155,-0.818018187896217,
-0.815925212111296,-0.811548499507635,-0.793545971044919,-0.761540534867801,
-0.744552177334396,-0.739421730477923,-0.736229692036535,-0.733273324640428,
-0.729349113007491,-0.720485909664926,-0.708071232202234,-0.67534783706546,
-0.658143341132571,-0.654744275577906,-0.652829763641028,-0.651343124631843,
-0.649238149828613,-0.644797164492093,-0.626220490021437,-0.581048922266406,
-0.57480940999282,-0.571051471845711,-0.568109721197564,-0.56487138004869,
-0.559523195959956,-0.536742575705524,-0.505289792168805,-0.491167620015925,
-0.487892604346136,-0.486025143280338,-0.484361799559493,-0.482075384822308,
-0.476605830689058,-0.468580378857207,-0.440944363429201,-0.412262885621592,
-0.406581292007913,-0.403271345951693,-0.400636251064664,-0.397083063475046,
-0.390226616239235,-0.365430809386113,-0.348165274326103,-0.324988850227267,
-0.321498237784412,-0.31956331640413,-0.317929805578128,-0.315768895589642,
-0.311025822745156,-0.289574163504058,-0.250200258349139,-0.241694054567859,
-0.237873414071076,-0.234922852552908,-0.231715236094792,-0.226510522016004,
-0.206078785196696,-0.184811426749428,-0.160274311105911,-0.155528860473532,
-0.153390586163907,-0.151808624763331,-0.1499682351261,-0.146859212096279,
-0.142857193929927,-0.134136398320465,-0.100900011079064,-0.0785973214288766,
-0.0731311387372958,-0.0698675843457679,-0.0669318734674677,-0.0631589053512889,
-0.0551502767508302,-0.019766497034221,-0.000493928755314768),
 .UNSPECIFIED.);
#2941=B_SPLINE_CURVE_WITH_KNOTS('',3,(#128993,#128994,#128995,#128996,#128997,
#128998,#128999,#129000,#129001,#129002,#129003,#129004,#129005,#129006,
#129007,#129008,#129009,#129010,#129011,#129012,#129013,#129014),
 .UNSPECIFIED.,.F.,.F.,(4,2,2,2,2,2,2,2,2,2,4),(-2.09974145399818,-2.09334315366096,
-2.08915505855463,-2.0871912462299,-2.08562462813712,-2.08409528173233,
-2.08204204294441,-2.0778698186273,-2.06364260288612,-2.04644554779855,
-2.04091635741276),.UNSPECIFIED.);
#2942=B_SPLINE_CURVE_WITH_KNOTS('',3,(#129015,#129016,#129017,#129018,#129019,
#129020,#129021,#129022,#129023,#129024,#129025,#129026,#129027,#129028,
#129029,#129030,#129031,#129032,#129033,#129034,#129035,#129036,#129037,
#129038,#129039,#129040,#129041,#129042,#129043,#129044,#129045,#129046,
#129047,#129048,#129049,#129050,#129051,#129052,#129053,#129054,#129055,
#129056,#129057,#129058,#129059,#129060,#129061,#129062,#129063,#129064,
#129065,#129066,#129067,#129068,#129069,#129070,#129071,#129072,#129073,
#129074,#129075,#129076,#129077,#129078,#129079,#129080,#129081,#129082,
#129083,#129084,#129085,#129086,#129087,#129088,#129089,#129090,#129091,
#129092,#129093,#129094,#129095,#129096,#129097,#129098,#129099,#129100,
#129101,#129102,#129103,#129104,#129105,#129106,#129107,#129108,#129109,
#129110,#129111,#129112,#129113,#129114,#129115,#129116,#129117,#129118,
#129119,#129120,#129121,#129122,#129123,#129124,#129125,#129126,#129127,
#129128,#129129,#129130,#129131,#129132,#129133,#129134,#129135,#129136,
#129137,#129138,#129139,#129140,#129141,#129142,#129143,#129144,#129145,
#129146,#129147,#129148,#129149,#129150,#129151,#129152,#129153,#129154,
#129155,#129156,#129157,#129158,#129159,#129160,#129161,#129162,#129163,
#129164,#129165,#129166,#129167,#129168,#129169,#129170,#129171,#129172,
#129173,#129174,#129175,#129176,#129177,#129178,#129179,#129180,#129181,
#129182,#129183,#129184,#129185,#129186,#129187,#129188,#129189,#129190,
#129191,#129192,#129193,#129194,#129195,#129196,#129197,#129198,#129199,
#129200,#129201,#129202,#129203,#129204,#129205,#129206,#129207,#129208,
#129209,#129210,#129211,#129212,#129213,#129214,#129215,#129216),
 .UNSPECIFIED.,.F.,.F.,(4,2,2,2,2,2,2,2,2,2,2,2,2,2,2,2,2,2,2,2,2,2,2,2,
2,2,2,2,2,2,2,2,2,2,2,2,2,2,2,2,2,2,2,2,2,2,2,2,2,2,2,2,2,2,2,2,2,2,2,2,
2,2,2,2,2,2,2,2,2,2,2,2,2,2,2,2,2,2,2,2,2,2,2,2,2,2,2,2,2,2,2,2,2,2,2,2,
2,2,2,2,4),(-1.75130590682506,-1.75061804629367,-1.74766762561627,-1.74377980457627,
-1.73512470195656,-1.70734178850423,-1.67401985750049,-1.66962622496779,
-1.66753045685401,-1.66588688574552,-1.66389669415773,-1.66003900346778,
-1.65498889582004,-1.64259896704644,-1.60511275082854,-1.59141072418469,
-1.5866644495711,-1.58355435656397,-1.58056081662683,-1.5764066612657,-1.56610809015788,
-1.5507999490363,-1.51866019675941,-1.50539963831284,-1.50218052644649,
-1.50032516243598,-1.49865779364918,-1.49634566606401,-1.49071948012675,
-1.48237815950512,-1.45627308193678,-1.42659499878978,-1.42092049689232,
-1.41761197985444,-1.41497656647377,-1.41142105868874,-1.40455345080713,
-1.37967351499626,-1.36245840759542,-1.33931437673376,-1.33582399778277,
-1.3338892891024,-1.33224112786826,-1.33007316787738,-1.32528507609731,
-1.30336304724814,-1.26250389254157,-1.255379422689,-1.25172840870059,-1.24880663367437,
-1.24547225710487,-1.23966746663796,-1.20514407131681,-1.17423617344591,
-1.17012218360522,-1.16805239224227,-1.16637654611349,-1.16458659938468,
-1.16166646043304,-1.15090593393718,-1.12831455185246,-1.0957114459424,
-1.08863811929518,-1.0849952741147,-1.08207118331994,-1.07872445072472,
-1.07287227130779,-1.03970996496604,-1.00741513181906,-1.00337939226342,
-1.0013274128128,-0.999654052427862,-0.997849692926993,-0.99487632835588,
-0.983526600014533,-0.958531015489666,-0.926759634757129,-0.921055737384536,
-0.917738503173626,-0.915100499254351,-0.911547044420506,-0.904702531898288,
-0.880033831251204,-0.841083278609066,-0.836470880983687,-0.834356776632777,
-0.832713508390733,-0.830779098882874,-0.827154299592165,-0.822488474943991,
-0.811491760080047,-0.789736134853379,-0.759698371655822,-0.754103557698703,
-0.750792344359605,-0.747911395839402,-0.744281645528209,-0.736973319207148,
-0.727366827344797,-0.701574795806025,-0.70148998943205),.UNSPECIFIED.);
#2943=B_SPLINE_CURVE_WITH_KNOTS('',3,(#129219,#129220,#129221,#129222,#129223,
#129224,#129225,#129226,#129227,#129228,#129229,#129230,#129231,#129232,
#129233,#129234,#129235,#129236,#129237,#129238,#129239,#129240,#129241,
#129242,#129243,#129244,#129245,#129246,#129247,#129248,#129249,#129250,
#129251,#129252,#129253,#129254,#129255,#129256,#129257,#129258,#129259,
#129260,#129261,#129262,#129263,#129264,#129265,#129266,#129267,#129268,
#129269,#129270,#129271,#129272,#129273,#129274,#129275,#129276,#129277,
#129278,#129279,#129280,#129281,#129282,#129283,#129284,#129285,#129286,
#129287,#129288,#129289,#129290,#129291,#129292,#129293,#129294,#129295,
#129296,#129297,#129298,#129299,#129300,#129301,#129302,#129303,#129304,
#129305,#129306,#129307,#129308,#129309,#129310,#129311,#129312,#129313,
#129314,#129315,#129316,#129317,#129318,#129319,#129320,#129321,#129322,
#129323,#129324,#129325,#129326,#129327,#129328,#129329,#129330,#129331,
#129332,#129333,#129334,#129335,#129336,#129337,#129338,#129339),
 .UNSPECIFIED.,.F.,.F.,(4,3,3,3,3,3,3,3,3,3,3,3,3,3,3,3,3,3,3,3,3,3,3,3,
3,3,3,3,3,3,3,3,3,3,3,3,3,3,3,3,4),(17.9343860548896,18.0384562993147,18.1423964971713,
18.2462659726421,18.3500994881357,18.4539317573288,18.5578693975759,18.6618610652281,
18.7660398686056,18.844279745313,18.9484546158039,19.0524740767691,19.1563713033989,
19.2602029543261,19.3640038262347,19.4678086722615,19.5717221414199,19.6756944101755,
19.7798486679322,19.8418082797496,19.945996847463,20.0500301909672,20.1539415075587,
20.2577873687803,20.3616025500263,20.465421783257,20.5693496592209,20.6733363675984,
20.7775049599295,20.8393368141862,20.9435248552688,21.0475577017188,21.1514685680337,
21.255314008171,21.3591287982401,21.4629476709467,21.5668752360994,21.6708616612596,
21.7750300174801,21.8368653486228,21.9911485751285),.UNSPECIFIED.);
#2944=B_SPLINE_CURVE_WITH_KNOTS('',3,(#129340,#129341,#129342,#129343,#129344,
#129345,#129346,#129347,#129348,#129349,#129350,#129351,#129352,#129353,
#129354,#129355,#129356,#129357,#129358,#129359,#129360,#129361,#129362,
#129363,#129364,#129365,#129366,#129367,#129368,#129369,#129370,#129371,
#129372,#129373,#129374,#129375,#129376,#129377,#129378,#129379,#129380,
#129381,#129382,#129383,#129384,#129385,#129386,#129387,#129388,#129389,
#129390,#129391,#129392,#129393,#129394,#129395,#129396,#129397,#129398,
#129399,#129400,#129401,#129402,#129403,#129404,#129405,#129406,#129407,
#129408,#129409),.UNSPECIFIED.,.F.,.F.,(4,3,3,3,3,3,3,3,3,3,3,3,3,3,3,3,
3,3,3,3,3,3,3,4),(21.9911485755033,22.0965542389478,22.1989427481708,22.3012648056322,
22.4035570528071,22.5058560839769,22.6082610339522,22.7107307753153,22.8133655526472,
22.8343938830594,22.9385806431776,23.0426121733884,23.1465216773082,23.2503657272733,
23.3541791014396,23.4579965345313,23.5619226336016,23.6659075755289,23.7700744373266,
23.831922417496,23.9360794349241,24.0401009060572,24.1440085666394,24.217503635835),
 .UNSPECIFIED.);
#2945=B_SPLINE_CURVE_WITH_KNOTS('',3,(#129411,#129412,#129413,#129414,#129415,
#129416,#129417,#129418,#129419,#129420,#129421,#129422,#129423,#129424,
#129425,#129426,#129427,#129428,#129429,#129430,#129431,#129432,#129433,
#129434,#129435,#129436,#129437,#129438,#129439,#129440,#129441,#129442,
#129443,#129444,#129445,#129446,#129447,#129448,#129449,#129450,#129451,
#129452,#129453,#129454,#129455,#129456,#129457,#129458,#129459,#129460,
#129461,#129462,#129463,#129464,#129465,#129466,#129467,#129468,#129469,
#129470,#129471,#129472,#129473,#129474,#129475,#129476,#129477),
 .UNSPECIFIED.,.F.,.F.,(4,3,3,3,3,3,3,3,3,3,3,3,3,3,3,3,3,3,3,3,3,3,4),
(21.9911485755641,22.1068686992636,22.2230627045344,22.3398531390132,22.3783692882698,
22.4825578603194,22.5865912082046,22.6905025292221,22.7943483948948,22.8981635806107,
23.0019828183231,23.1059106987561,23.2098974116023,23.3140660083528,23.3758978227064,
23.4809869476749,23.5849996238318,23.6889077746951,23.7927462649133,23.8987124042985,
24.0025537166019,24.109582269528,24.216610822454),.UNSPECIFIED.);
#2946=B_SPLINE_CURVE_WITH_KNOTS('',3,(#129478,#129479,#129480,#129481,#129482,
#129483,#129484,#129485,#129486,#129487,#129488,#129489,#129490,#129491,
#129492,#129493,#129494,#129495,#129496,#129497,#129498,#129499,#129500,
#129501,#129502,#129503,#129504,#129505,#129506,#129507,#129508,#129509,
#129510,#129511,#129512,#129513,#129514,#129515,#129516,#129517,#129518,
#129519,#129520,#129521,#129522,#129523,#129524,#129525,#129526,#129527,
#129528,#129529,#129530,#129531,#129532,#129533,#129534,#129535,#129536,
#129537,#129538,#129539,#129540,#129541,#129542,#129543,#129544,#129545,
#129546,#129547,#129548,#129549,#129550,#129551,#129552,#129553,#129554,
#129555,#129556,#129557,#129558,#129559,#129560,#129561,#129562,#129563,
#129564,#129565,#129566,#129567,#129568,#129569,#129570,#129571,#129572,
#129573,#129574,#129575,#129576,#129577,#129578,#129579,#129580,#129581,
#129582,#129583,#129584,#129585,#129586,#129587,#129588,#129589,#129590,
#129591,#129592,#129593,#129594,#129595,#129596,#129597,#129598,#129599,
#129600,#129601),.UNSPECIFIED.,.F.,.F.,(4,3,3,3,3,3,3,3,3,3,3,3,3,3,3,3,
3,3,3,3,3,3,3,3,3,3,3,3,3,3,3,3,3,3,3,3,3,3,3,3,3,4),(17.9338028151035,
18.0378029754529,18.1419180651585,18.2460999315279,18.350456983587,18.3882551505234,
18.4923467441545,18.5962817400488,18.70009314389,18.8038381789175,18.9075517693863,
19.0112687952391,19.115094223132,19.2189781910668,19.3230446958775,19.38578368496,
19.4899815369513,19.5940241032359,19.6979445039763,19.8017993583924,19.9056234279328,
20.00945143051,20.1133878314687,20.2173829397245,20.321559640807,20.3833122193966,
20.4875152925416,20.5915634922881,20.695490115075,20.7993515520751,20.903182555586,
21.0070178347373,21.1109619889101,21.2149651311122,21.3191502262971,21.3808407538332,
21.4862078248736,21.5914087166519,21.6964559116178,21.8014119971609,21.9063208177285,
21.9911485751285),.UNSPECIFIED.);
#2947=B_SPLINE_CURVE_WITH_KNOTS('',3,(#129603,#129604,#129605,#129606,#129607,
#129608,#129609,#129610,#129611,#129612,#129613,#129614,#129615,#129616,
#129617,#129618,#129619,#129620,#129621,#129622,#129623,#129624,#129625,
#129626,#129627,#129628,#129629,#129630,#129631,#129632,#129633,#129634,
#129635,#129636,#129637,#129638,#129639,#129640,#129641,#129642,#129643,
#129644,#129645,#129646,#129647,#129648,#129649,#129650,#129651,#129652,
#129653,#129654,#129655,#129656,#129657,#129658,#129659,#129660,#129661,
#129662,#129663,#129664,#129665,#129666,#129667,#129668,#129669,#129670,
#129671,#129672,#129673,#129674,#129675,#129676,#129677,#129678,#129679,
#129680,#129681,#129682,#129683,#129684,#129685,#129686,#129687,#129688,
#129689,#129690),.UNSPECIFIED.,.F.,.F.,(4,3,3,3,3,3,3,3,3,3,3,3,3,3,3,3,
3,3,3,3,3,3,3,3,3,3,3,3,3,4),(-0.378621596831377,-0.359800574898229,-0.347867415310614,
-0.339791008828829,-0.335413943756389,-0.315538205554487,-0.301206604784367,
-0.297325827080498,-0.293234930684288,-0.272788407631258,-0.252085100561485,
-0.239312075104769,-0.228816208612987,-0.224508526527948,-0.203203874900672,
-0.200837552551317,-0.179573256408454,-0.15830896026559,-0.154318299386255,
-0.150807254524542,-0.129197322625765,-0.107587390726988,-0.0856207534556525,
-0.0801950788551404,-0.0759413631771757,-0.0534076236452386,-0.0309843347957576,
-0.00876238345449811,-0.0040342792039191,-4.65033222477994E-5),
 .UNSPECIFIED.);
#2948=B_SPLINE_CURVE_WITH_KNOTS('',3,(#129691,#129692,#129693,#129694,#129695,
#129696,#129697,#129698,#129699,#129700,#129701,#129702,#129703,#129704,
#129705,#129706,#129707,#129708,#129709,#129710,#129711,#129712,#129713,
#129714,#129715,#129716,#129717,#129718,#129719,#129720,#129721,#129722,
#129723,#129724,#129725,#129726,#129727,#129728,#129729,#129730,#129731,
#129732,#129733,#129734,#129735,#129736,#129737,#129738,#129739,#129740,
#129741,#129742,#129743,#129744,#129745,#129746,#129747,#129748,#129749,
#129750,#129751,#129752,#129753,#129754,#129755,#129756,#129757,#129758,
#129759,#129760,#129761,#129762,#129763,#129764,#129765,#129766,#129767,
#129768,#129769,#129770,#129771,#129772,#129773,#129774,#129775),
 .UNSPECIFIED.,.F.,.F.,(4,3,3,3,3,3,3,3,3,3,3,3,3,3,3,3,3,3,3,3,3,3,3,3,
3,3,3,3,4),(-0.376940817211572,-0.354434745142103,-0.332914589324204,-0.328066558023255,
-0.30581833788643,-0.290198565614503,-0.28426487902006,-0.278600185330508,
-0.256937232807856,-0.235771146027844,-0.214945582624746,-0.208198463847886,
-0.20440189481038,-0.183824971878735,-0.180862865680233,-0.159776402420874,
-0.140305786244226,-0.136020080940874,-0.132586895718958,-0.112127717435514,
-0.0917629328401109,-0.071833700248866,-0.0676158682049212,-0.0636581831340513,
-0.0440997736349179,-0.0251751445195747,-0.0063477261176011,-0.00328482218945227,
0.),.UNSPECIFIED.);
#2949=B_SPLINE_CURVE_WITH_KNOTS('',3,(#130192,#130193,#130194,#130195,#130196,
#130197,#130198,#130199,#130200,#130201,#130202,#130203,#130204,#130205,
#130206,#130207,#130208,#130209,#130210,#130211,#130212,#130213,#130214,
#130215,#130216,#130217,#130218,#130219,#130220,#130221,#130222,#130223,
#130224,#130225,#130226,#130227,#130228,#130229,#130230,#130231,#130232,
#130233,#130234,#130235,#130236,#130237,#130238,#130239,#130240,#130241,
#130242,#130243,#130244,#130245,#130246,#130247,#130248,#130249,#130250,
#130251,#130252,#130253,#130254,#130255,#130256,#130257,#130258,#130259,
#130260,#130261,#130262,#130263,#130264,#130265,#130266,#130267,#130268,
#130269,#130270,#130271,#130272,#130273),.UNSPECIFIED.,.F.,.F.,(4,3,3,3,
3,3,3,3,3,3,3,3,3,3,3,3,3,3,3,3,3,3,3,3,3,3,3,4),(0.,0.0185942586373532,
0.0384196304941899,0.055766830868922,0.0644671558767212,0.0684494988071322,
0.0886798835323776,0.108910268257623,0.129281600569207,0.133842973757118,
0.137281880988472,0.158357027632817,0.177197233492047,0.197726581113147,
0.205650448408311,0.209125900862407,0.230376280882011,0.251626660901614,
0.273336565247494,0.278315660173636,0.284045110735794,0.306314217788196,
0.322966455755941,0.328173582351109,0.333184502846979,0.355705889915315,
0.372923169659177,0.376894494387216),.UNSPECIFIED.);
#2950=B_SPLINE_CURVE_WITH_KNOTS('',3,(#130691,#130692,#130693,#130694),
 .UNSPECIFIED.,.F.,.F.,(4,4),(-0.015320457083931,0.),.UNSPECIFIED.);
#2951=B_SPLINE_CURVE_WITH_KNOTS('',3,(#130695,#130696,#130697,#130698,#130699,
#130700,#130701,#130702,#130703,#130704,#130705,#130706,#130707,#130708,
#130709,#130710,#130711,#130712,#130713,#130714,#130715,#130716,#130717,
#130718,#130719,#130720,#130721,#130722,#130723,#130724,#130725,#130726,
#130727,#130728,#130729,#130730,#130731,#130732,#130733,#130734,#130735,
#130736,#130737,#130738,#130739,#130740,#130741,#130742,#130743,#130744,
#130745,#130746,#130747,#130748,#130749,#130750,#130751,#130752,#130753,
#130754,#130755,#130756,#130757,#130758,#130759,#130760,#130761,#130762,
#130763,#130764,#130765,#130766,#130767,#130768,#130769,#130770,#130771,
#130772,#130773,#130774,#130775,#130776,#130777,#130778,#130779,#130780,
#130781,#130782),.UNSPECIFIED.,.F.,.F.,(4,3,3,3,3,3,3,3,3,3,3,3,3,3,3,3,
3,3,3,3,3,3,3,3,3,3,3,3,3,4),(0.,0.022076465099833,0.0446500161040329,0.0636175020481042,
0.0720961742632357,0.0767527781954435,0.0810480993262889,0.102995208587912,
0.12460210360104,0.142867742472728,0.150422572110747,0.153916820895177,
0.157566347805364,0.178337891460959,0.197155519647459,0.219426672701599,
0.224328424195588,0.229401239967913,0.250066209825086,0.270727085266657,
0.285675668497039,0.294182634390874,0.299799559450732,0.300624251727421,
0.320446372412837,0.334305514499652,0.338771695116765,0.357798190520139,
0.375324744080579,0.378621596831434),.UNSPECIFIED.);
#2952=B_SPLINE_CURVE_WITH_KNOTS('',3,(#130784,#130785,#130786,#130787,#130788,
#130789,#130790,#130791,#130792,#130793,#130794,#130795,#130796,#130797,
#130798,#130799,#130800,#130801,#130802,#130803,#130804,#130805,#130806,
#130807,#130808,#130809,#130810,#130811,#130812,#130813,#130814,#130815,
#130816,#130817,#130818,#130819,#130820,#130821,#130822,#130823,#130824,
#130825,#130826,#130827,#130828,#130829,#130830,#130831,#130832,#130833,
#130834,#130835,#130836,#130837,#130838,#130839,#130840,#130841,#130842,
#130843,#130844,#130845,#130846,#130847,#130848,#130849,#130850,#130851,
#130852,#130853,#130854,#130855,#130856,#130857,#130858,#130859,#130860,
#130861,#130862,#130863,#130864,#130865,#130866,#130867,#130868,#130869,
#130870,#130871),.UNSPECIFIED.,.F.,.F.,(4,3,3,3,3,3,3,3,3,3,3,3,3,3,3,3,
3,3,3,3,3,3,3,3,3,3,3,3,3,4),(-0.37862159683151,-0.359800569631031,-0.347867401893819,
-0.33979089123365,-0.335413899311082,-0.315538156337577,-0.301206561819263,
-0.297325731230975,-0.293234920420453,-0.272730298566073,-0.252027833031437,
-0.231534606194204,-0.22881619359477,-0.224508521722788,-0.203203870189045,
-0.200837552551386,-0.17957325789842,-0.158308963245454,-0.154318319294633,
-0.15080725817,-0.129484179150672,-0.107552470160347,-0.0856207611700218,
-0.0801950922726167,-0.075941367905241,-0.0534076290690578,-0.0309843400776861,
-0.0087623891159908,-0.0040342792039104,-4.65028613182856E-5),
 .UNSPECIFIED.);
#2953=B_SPLINE_CURVE_WITH_KNOTS('',3,(#130872,#130873,#130874,#130875,#130876,
#130877,#130878,#130879,#130880,#130881,#130882,#130883,#130884,#130885,
#130886,#130887,#130888,#130889,#130890,#130891,#130892,#130893,#130894,
#130895,#130896,#130897,#130898,#130899,#130900,#130901,#130902,#130903,
#130904,#130905,#130906,#130907,#130908,#130909,#130910,#130911,#130912,
#130913,#130914,#130915,#130916,#130917,#130918,#130919,#130920,#130921,
#130922,#130923,#130924,#130925,#130926,#130927,#130928,#130929,#130930,
#130931,#130932,#130933,#130934,#130935,#130936,#130937,#130938,#130939,
#130940,#130941,#130942,#130943,#130944,#130945,#130946,#130947,#130948,
#130949,#130950,#130951,#130952,#130953,#130954,#130955,#130956),
 .UNSPECIFIED.,.F.,.F.,(4,3,3,3,3,3,3,3,3,3,3,3,3,3,3,3,3,3,3,3,3,3,3,3,
3,3,3,3,4),(-0.37694081721158,-0.354434743621784,-0.332914587130445,-0.328066555497701,
-0.305817948776869,-0.290198563389788,-0.284264874081428,-0.278600185634699,
-0.256937233660704,-0.235771147852844,-0.214945584943483,-0.208198462262405,
-0.204401894988106,-0.183824973032507,-0.180862865680225,-0.159776402234228,
-0.14030578623386,-0.136020082340253,-0.132586896844658,-0.11213480581913,
-0.0918985800495415,-0.0718337025226597,-0.0676158747446753,-0.0636581853937461,
-0.0440844999903763,-0.0251601150180132,-0.00634773272082092,-0.00328482218946405,
0.),.UNSPECIFIED.);
#2954=B_SPLINE_CURVE_WITH_KNOTS('',3,(#131373,#131374,#131375,#131376,#131377,
#131378,#131379,#131380,#131381,#131382,#131383,#131384,#131385,#131386,
#131387,#131388,#131389,#131390,#131391,#131392,#131393,#131394,#131395,
#131396,#131397,#131398,#131399,#131400,#131401,#131402,#131403,#131404,
#131405,#131406,#131407,#131408,#131409,#131410,#131411,#131412,#131413,
#131414,#131415,#131416,#131417,#131418,#131419,#131420,#131421,#131422,
#131423,#131424,#131425,#131426,#131427,#131428,#131429,#131430,#131431,
#131432,#131433,#131434,#131435,#131436,#131437,#131438,#131439,#131440,
#131441,#131442,#131443,#131444,#131445,#131446,#131447,#131448,#131449,
#131450,#131451,#131452,#131453,#131454),.UNSPECIFIED.,.F.,.F.,(4,3,3,3,
3,3,3,3,3,3,3,3,3,3,3,3,3,3,3,3,3,3,3,3,3,3,3,4),(0.,0.0185942627018445,
0.0384196340506189,0.0557668339807965,0.0644671612702412,0.0684495001941655,
0.0885013648033302,0.108965744896479,0.125982013797114,0.1338429804339,
0.137281884411352,0.158357030774089,0.17719723349204,0.197726579166287,
0.205650447451187,0.20912590019485,0.230033568486251,0.25139264958201,0.273102086639384,
0.278315662662554,0.284045110154865,0.30631421705641,0.322966455207104,
0.328173581206648,0.33318450226615,0.355705889383306,0.372923169659185,
0.376894494728837),.UNSPECIFIED.);
#2955=B_SPLINE_CURVE_WITH_KNOTS('',3,(#131872,#131873,#131874,#131875),
 .UNSPECIFIED.,.F.,.F.,(4,4),(-0.0153203085855325,0.),.UNSPECIFIED.);
#2956=B_SPLINE_CURVE_WITH_KNOTS('',3,(#131876,#131877,#131878,#131879,#131880,
#131881,#131882,#131883,#131884,#131885,#131886,#131887,#131888,#131889,
#131890,#131891,#131892,#131893,#131894,#131895,#131896,#131897,#131898,
#131899,#131900,#131901,#131902,#131903,#131904,#131905,#131906,#131907,
#131908,#131909,#131910,#131911,#131912,#131913,#131914,#131915,#131916,
#131917,#131918,#131919,#131920,#131921,#131922,#131923,#131924,#131925,
#131926,#131927,#131928,#131929,#131930,#131931,#131932,#131933,#131934,
#131935,#131936,#131937,#131938,#131939,#131940,#131941,#131942,#131943,
#131944,#131945,#131946,#131947,#131948,#131949,#131950,#131951,#131952,
#131953,#131954,#131955,#131956,#131957,#131958,#131959,#131960),
 .UNSPECIFIED.,.F.,.F.,(4,3,3,3,3,3,3,3,3,3,3,3,3,3,3,3,3,3,3,3,3,3,3,3,
3,3,3,3,4),(0.,0.0220764692885148,0.0446500209087305,0.0636175065071147,
0.0720961755907872,0.0767527810215644,0.0810481000867341,0.102973125105672,
0.124771816179149,0.142867742046223,0.150422572478512,0.153916822796493,
0.157566348353921,0.178337890695287,0.197155519647444,0.21942667270158,
0.224328423930133,0.229401239955034,0.25009123940773,0.270727085421763,
0.285678464935528,0.296896068115054,0.300624249977848,0.320446369477332,
0.334305509215125,0.338771690168848,0.357798183302138,0.375324744080529,
0.378621596831382),.UNSPECIFIED.);
#2957=B_SPLINE_CURVE_WITH_KNOTS('',3,(#132392,#132393,#132394,#132395,#132396,
#132397,#132398,#132399,#132400,#132401,#132402,#132403,#132404,#132405,
#132406,#132407,#132408,#132409,#132410,#132411,#132412,#132413,#132414,
#132415,#132416,#132417,#132418,#132419,#132420,#132421,#132422,#132423,
#132424,#132425,#132426,#132427,#132428,#132429,#132430,#132431,#132432,
#132433,#132434,#132435,#132436,#132437,#132438,#132439,#132440,#132441,
#132442,#132443,#132444,#132445,#132446,#132447,#132448,#132449,#132450,
#132451,#132452,#132453,#132454,#132455,#132456,#132457,#132458,#132459,
#132460,#132461,#132462,#132463,#132464,#132465,#132466,#132467,#132468,
#132469,#132470,#132471,#132472,#132473,#132474,#132475,#132476),
 .UNSPECIFIED.,.F.,.F.,(4,3,3,3,3,3,3,3,3,3,3,3,3,3,3,3,3,3,3,3,3,3,3,3,
3,3,3,3,4),(-0.37694081721164,-0.354433306894873,-0.332912068438051,-0.328063707750488,
-0.305815531960939,-0.290195622062823,-0.284258173761416,-0.278600680525688,
-0.256917565609304,-0.235752667545141,-0.214948063833036,-0.208200328709319,
-0.204401454487156,-0.183825513702696,-0.180859240376696,-0.159772587659609,
-0.140301766015443,-0.136001540232934,-0.132615023040107,-0.112155832609778,
-0.0919195811109376,-0.0718621010890796,-0.0660721542666673,-0.0628432174816503,
-0.0432905316599473,-0.0240214811309868,-0.0047524306020263,-0.00327832057784897,
0.),.UNSPECIFIED.);
#2958=B_SPLINE_CURVE_WITH_KNOTS('',3,(#132477,#132478,#132479,#132480,#132481,
#132482,#132483,#132484,#132485,#132486,#132487,#132488,#132489,#132490,
#132491,#132492,#132493,#132494,#132495,#132496,#132497,#132498,#132499,
#132500,#132501,#132502,#132503,#132504,#132505,#132506,#132507,#132508,
#132509,#132510,#132511,#132512,#132513,#132514,#132515,#132516,#132517,
#132518,#132519,#132520,#132521,#132522,#132523,#132524,#132525,#132526,
#132527,#132528,#132529,#132530,#132531,#132532,#132533,#132534,#132535,
#132536,#132537,#132538,#132539,#132540,#132541,#132542,#132543,#132544,
#132545,#132546,#132547,#132548,#132549,#132550,#132551,#132552,#132553,
#132554,#132555,#132556,#132557,#132558),.UNSPECIFIED.,.F.,.F.,(4,3,3,3,
3,3,3,3,3,3,3,3,3,3,3,3,3,3,3,3,3,3,3,3,3,3,3,4),(0.,0.0186893861989584,
0.0380628975178282,0.0557706344050115,0.0644740455004294,0.0684512583734907,
0.0885273404451008,0.108992143028824,0.125987244216384,0.133851910987726,
0.138086378825073,0.158361294974393,0.177200852458616,0.197728340288859,
0.205651029746871,0.209126190448893,0.229948761197729,0.251461698426111,
0.268072642545509,0.278312078768208,0.284045428971702,0.306303003925287,
0.32296858048919,0.328170230546098,0.333183543693291,0.355704946189745,
0.372931104637556,0.376894629385132),.UNSPECIFIED.);
#2959=B_SPLINE_CURVE_WITH_KNOTS('',3,(#132559,#132560,#132561,#132562),
 .UNSPECIFIED.,.F.,.F.,(4,4),(0.,0.0152331259156648),.UNSPECIFIED.);
#2960=B_SPLINE_CURVE_WITH_KNOTS('',3,(#132943,#132944,#132945,#132946,#132947,
#132948,#132949,#132950,#132951,#132952,#132953,#132954,#132955,#132956,
#132957,#132958,#132959,#132960,#132961,#132962,#132963,#132964,#132965,
#132966,#132967,#132968,#132969,#132970,#132971,#132972,#132973,#132974,
#132975,#132976,#132977,#132978,#132979,#132980,#132981,#132982,#132983,
#132984,#132985,#132986,#132987,#132988,#132989,#132990,#132991,#132992,
#132993,#132994,#132995,#132996,#132997,#132998,#132999,#133000,#133001,
#133002,#133003,#133004,#133005,#133006,#133007,#133008,#133009,#133010,
#133011,#133012,#133013,#133014,#133015,#133016,#133017,#133018,#133019,
#133020,#133021,#133022,#133023,#133024,#133025,#133026,#133027,#133028,
#133029,#133030),.UNSPECIFIED.,.F.,.F.,(4,3,3,3,3,3,3,3,3,3,3,3,3,3,3,3,
3,3,3,3,3,3,3,3,3,3,3,3,3,4),(-0.378621596831385,-0.359796914683931,-0.347856916184549,
-0.339696030242093,-0.335370733333621,-0.315491445945434,-0.301165295210856,
-0.29723257379588,-0.293223461848749,-0.272774488137517,-0.252071366520374,
-0.239300846331472,-0.228798122014357,-0.224502765173222,-0.203198222803892,
-0.200833918205808,-0.180346956049432,-0.158306875253142,-0.154304247957037,
-0.150804929022692,-0.129421873498757,-0.107501185980079,-0.0856211676534625,
-0.079697906231664,-0.0759421505311957,-0.0534088813988902,-0.0309855250275342,
-0.00876395290387212,-0.00402630967910949,-3.65615898988344E-5),
 .UNSPECIFIED.);
#2961=B_SPLINE_CURVE_WITH_KNOTS('',3,(#133032,#133033,#133034,#133035),
 .UNSPECIFIED.,.F.,.F.,(4,4),(-0.0152759716381044,0.),.UNSPECIFIED.);
#2962=B_SPLINE_CURVE_WITH_KNOTS('',3,(#133036,#133037,#133038,#133039,#133040,
#133041,#133042,#133043,#133044,#133045,#133046,#133047,#133048,#133049,
#133050,#133051,#133052,#133053,#133054,#133055,#133056,#133057,#133058,
#133059,#133060,#133061,#133062,#133063,#133064,#133065,#133066,#133067,
#133068,#133069,#133070,#133071,#133072,#133073,#133074,#133075,#133076,
#133077,#133078,#133079,#133080,#133081,#133082,#133083,#133084,#133085,
#133086,#133087,#133088,#133089,#133090,#133091,#133092,#133093,#133094,
#133095,#133096,#133097,#133098,#133099,#133100,#133101,#133102,#133103,
#133104,#133105,#133106,#133107,#133108,#133109,#133110,#133111,#133112,
#133113,#133114,#133115,#133116,#133117,#133118,#133119,#133120),
 .UNSPECIFIED.,.F.,.F.,(4,3,3,3,3,3,3,3,3,3,3,3,3,3,3,3,3,3,3,3,3,3,3,3,
3,3,3,3,4),(0.,0.0220793683187804,0.0446533402441453,0.0636210331214285,
0.0720970319424637,0.0767544326890563,0.0810485639074834,0.102973109377672,
0.124771319639633,0.142868280227078,0.150423140460159,0.153919004023562,
0.157566869486277,0.17833745054201,0.197159161989412,0.21943067529714,0.224333068719436,
0.229400005005982,0.250090151731939,0.270725926661941,0.285677006128735,
0.29689344012605,0.300623371473114,0.320444582327625,0.334304749326293,
0.338770888038792,0.357795589733676,0.375331268451236,0.378621596831424),
 .UNSPECIFIED.);
#2963=B_SPLINE_CURVE_WITH_KNOTS('',3,(#133502,#133503,#133504,#133505,#133506,
#133507,#133508,#133509,#133510,#133511,#133512,#133513,#133514,#133515,
#133516,#133517,#133518,#133519,#133520,#133521,#133522,#133523,#133524,
#133525,#133526,#133527,#133528,#133529,#133530,#133531,#133532,#133533,
#133534,#133535,#133536,#133537,#133538,#133539,#133540,#133541,#133542,
#133543,#133544,#133545,#133546,#133547,#133548,#133549,#133550,#133551,
#133552,#133553,#133554,#133555,#133556,#133557,#133558,#133559,#133560,
#133561,#133562,#133563,#133564,#133565,#133566,#133567,#133568,#133569,
#133570,#133571,#133572,#133573,#133574,#133575,#133576,#133577,#133578,
#133579,#133580,#133581,#133582,#133583,#133584,#133585,#133586),
 .UNSPECIFIED.,.F.,.F.,(4,3,3,3,3,3,3,3,3,3,3,3,3,3,3,3,3,3,3,3,3,3,3,3,
3,3,3,3,4),(-0.376940817211642,-0.35463389721075,-0.332912065106493,-0.328063703915442,
-0.305815101391439,-0.290195618764596,-0.284258166436133,-0.278600681034138,
-0.256938276420847,-0.235773098280606,-0.214948067698175,-0.208200326246104,
-0.204401454712377,-0.183825515521996,-0.180859240376695,-0.159772587429043,
-0.140301766028677,-0.136001542949448,-0.132615024954702,-0.112162993959112,
-0.0919266612212684,-0.0718621053887858,-0.066072166338472,-0.0628432204529464,
-0.0432905357930386,-0.0240214863956556,-0.00475243699827259,-0.00327832057784904,
0.),.UNSPECIFIED.);
#2964=B_SPLINE_CURVE_WITH_KNOTS('',3,(#133587,#133588,#133589,#133590,#133591,
#133592,#133593,#133594,#133595,#133596,#133597,#133598,#133599,#133600,
#133601,#133602,#133603,#133604,#133605,#133606,#133607,#133608,#133609,
#133610,#133611,#133612,#133613,#133614,#133615,#133616,#133617,#133618,
#133619,#133620,#133621,#133622,#133623,#133624,#133625,#133626,#133627,
#133628,#133629,#133630,#133631,#133632,#133633,#133634,#133635,#133636,
#133637,#133638,#133639,#133640,#133641,#133642,#133643,#133644,#133645,
#133646,#133647,#133648,#133649,#133650,#133651,#133652,#133653,#133654,
#133655,#133656,#133657,#133658,#133659,#133660,#133661,#133662,#133663,
#133664,#133665,#133666,#133667,#133668),.UNSPECIFIED.,.F.,.F.,(4,3,3,3,
3,3,3,3,3,3,3,3,3,3,3,3,3,3,3,3,3,3,3,3,3,3,3,4),(0.,0.0186893924207011,
0.0380629085124009,0.0557706391965121,0.064474053792627,0.0684512605343887,
0.0885059134327574,0.108970690515085,0.125987250609254,0.133851921051149,
0.137286474827157,0.158361299681457,0.177200852458622,0.197728337128931,
0.20565102804809,0.209126189226868,0.230374857434889,0.25162352564291,0.268072644125497,
0.278312082409732,0.284045428046126,0.306314404619063,0.322968579623693,
0.328170228633061,0.33318354273328,0.355704945255065,0.372931104637582,
0.376894629338845),.UNSPECIFIED.);
#2965=B_SPLINE_CURVE_WITH_KNOTS('',3,(#133669,#133670,#133671,#133672),
 .UNSPECIFIED.,.F.,.F.,(4,4),(0.,0.015233203817751),.UNSPECIFIED.);
#2966=B_SPLINE_CURVE_WITH_KNOTS('',3,(#134053,#134054,#134055,#134056,#134057,
#134058,#134059,#134060,#134061,#134062,#134063,#134064,#134065,#134066,
#134067,#134068,#134069,#134070,#134071,#134072,#134073,#134074,#134075,
#134076,#134077,#134078,#134079,#134080,#134081,#134082,#134083,#134084,
#134085,#134086,#134087,#134088,#134089,#134090,#134091,#134092,#134093,
#134094,#134095,#134096,#134097,#134098,#134099,#134100,#134101,#134102,
#134103,#134104,#134105,#134106,#134107,#134108,#134109,#134110,#134111,
#134112,#134113,#134114,#134115,#134116,#134117,#134118,#134119,#134120,
#134121,#134122,#134123,#134124,#134125,#134126,#134127,#134128,#134129,
#134130,#134131,#134132,#134133,#134134,#134135,#134136,#134137,#134138,
#134139,#134140),.UNSPECIFIED.,.F.,.F.,(4,3,3,3,3,3,3,3,3,3,3,3,3,3,3,3,
3,3,3,3,3,3,3,3,3,3,3,3,3,4),(-0.378621596831399,-0.359796906651946,-0.347856895762323,
-0.339695845366797,-0.335370634830925,-0.315498242912406,-0.301165202324081,
-0.29723236113593,-0.293223432251235,-0.272820719782585,-0.252123121204613,
-0.239300820454911,-0.228798083868718,-0.224502752790907,-0.20319821077641,
-0.200833918205805,-0.18034696156604,-0.158306880080173,-0.154304280740517,
-0.150804935247414,-0.12948390702316,-0.107552543701982,-0.0856211803808043,
-0.0801967363324338,-0.0759421583469307,-0.0533545697894654,-0.0308224381853329,
-0.00876396243776301,-0.00402630967910655,-3.65718562400641E-5),
 .UNSPECIFIED.);
#2967=B_SPLINE_CURVE_WITH_KNOTS('',3,(#134142,#134143,#134144,#134145),
 .UNSPECIFIED.,.F.,.F.,(4,4),(-0.0152760659177977,0.),.UNSPECIFIED.);
#2968=B_SPLINE_CURVE_WITH_KNOTS('',3,(#134146,#134147,#134148,#134149,#134150,
#134151,#134152,#134153,#134154,#134155,#134156,#134157,#134158,#134159,
#134160,#134161,#134162,#134163,#134164,#134165,#134166,#134167,#134168,
#134169,#134170,#134171,#134172,#134173,#134174,#134175,#134176,#134177,
#134178,#134179,#134180,#134181,#134182,#134183,#134184,#134185,#134186,
#134187,#134188,#134189,#134190,#134191,#134192,#134193,#134194,#134195,
#134196,#134197,#134198,#134199,#134200,#134201,#134202,#134203,#134204,
#134205,#134206,#134207,#134208,#134209,#134210,#134211,#134212,#134213,
#134214,#134215,#134216,#134217,#134218,#134219,#134220,#134221,#134222,
#134223,#134224,#134225,#134226,#134227,#134228,#134229,#134230),
 .UNSPECIFIED.,.F.,.F.,(4,3,3,3,3,3,3,3,3,3,3,3,3,3,3,3,3,3,3,3,3,3,3,3,
3,3,3,3,4),(0.,0.0220793746690922,0.0446533474471028,0.0636210397963064,
0.0720970339368394,0.0767544369062487,0.0810485650370603,0.102995575329966,
0.124601454003273,0.14286827936694,0.150423140796222,0.153919006124083,
0.157566870163833,0.178337449110706,0.197159161989394,0.219430675297117,
0.224333068139837,0.229400004999726,0.25009015204505,0.270725926647151,
0.285676999682712,0.296893429032277,0.300623368319006,0.320395536074228,
0.334304739895041,0.338770879251483,0.357795576917732,0.375331268451179,
0.378621596831367),.UNSPECIFIED.);
#2969=B_SPLINE_CURVE_WITH_KNOTS('',3,(#134612,#134613,#134614,#134615,#134616,
#134617,#134618,#134619,#134620,#134621,#134622,#134623,#134624,#134625,
#134626,#134627,#134628,#134629,#134630,#134631,#134632,#134633,#134634,
#134635,#134636,#134637,#134638,#134639,#134640,#134641,#134642,#134643,
#134644,#134645,#134646,#134647,#134648,#134649,#134650,#134651,#134652,
#134653,#134654,#134655,#134656,#134657,#134658,#134659,#134660,#134661,
#134662,#134663,#134664,#134665,#134666,#134667,#134668,#134669,#134670,
#134671,#134672,#134673,#134674,#134675,#134676,#134677,#134678,#134679,
#134680,#134681,#134682,#134683,#134684,#134685,#134686,#134687,#134688,
#134689,#134690,#134691,#134692,#134693,#134694,#134695,#134696),
 .UNSPECIFIED.,.F.,.F.,(4,3,3,3,3,3,3,3,3,3,3,3,3,3,3,3,3,3,3,3,3,3,3,3,
3,3,3,3,4),(-0.376940817211701,-0.35463544655944,-0.332913420786601,-0.328065270514049,
-0.305816652822842,-0.290196976267078,-0.284261180291901,-0.278600481960197,
-0.25691711770642,-0.235699073322327,-0.214946538919852,-0.208201321496629,
-0.204401317171364,-0.183824744173427,-0.180859240376724,-0.159876540755593,
-0.140301763233375,-0.136000503582363,-0.132614278284648,-0.11215519219308,
-0.0917900641439051,-0.0718604732108804,-0.066067545564457,-0.0628420724025775,
-0.0432965324819232,-0.0232874265298861,-0.00474996033762646,-0.00327832057784897,
0.),.UNSPECIFIED.);
#2970=B_SPLINE_CURVE_WITH_KNOTS('',3,(#134697,#134698,#134699,#134700,#134701,
#134702,#134703,#134704,#134705,#134706,#134707,#134708,#134709,#134710,
#134711,#134712,#134713,#134714,#134715,#134716,#134717,#134718,#134719,
#134720,#134721,#134722,#134723,#134724,#134725,#134726,#134727,#134728,
#134729,#134730,#134731,#134732,#134733,#134734,#134735,#134736,#134737,
#134738,#134739,#134740,#134741,#134742,#134743,#134744,#134745,#134746,
#134747,#134748,#134749,#134750,#134751,#134752,#134753,#134754,#134755,
#134756,#134757,#134758,#134759,#134760,#134761,#134762,#134763,#134764,
#134765,#134766,#134767,#134768,#134769,#134770,#134771,#134772,#134773,
#134774,#134775,#134776,#134777,#134778),.UNSPECIFIED.,.F.,.F.,(4,3,3,3,
3,3,3,3,3,3,3,3,3,3,3,3,3,3,3,3,3,3,3,3,3,3,3,4),(0.,0.0185955873360213,
0.0384212454763452,0.0557686963491286,0.0644706897478566,0.0684503846967035,
0.088503222386054,0.108967755523642,0.1259846405568,0.133847808883134,0.137284316290468,
0.158359366945259,0.177200852458612,0.197729598395159,0.205651689526663,
0.20912665907553,0.230133427396579,0.251626259267865,0.268071993510044,
0.278310573550478,0.284045805095789,0.306314875310516,0.322968932642282,
0.328170988094391,0.333183924524744,0.355705311564313,0.372931104637579,
0.376894576726578),.UNSPECIFIED.);
#2971=B_SPLINE_CURVE_WITH_KNOTS('',3,(#134779,#134780,#134781,#134782),
 .UNSPECIFIED.,.F.,.F.,(4,4),(0.,0.0152452198817276),.UNSPECIFIED.);
#2972=B_SPLINE_CURVE_WITH_KNOTS('',3,(#135163,#135164,#135165,#135166,#135167,
#135168,#135169,#135170,#135171,#135172,#135173,#135174,#135175,#135176,
#135177,#135178,#135179,#135180,#135181,#135182,#135183,#135184,#135185,
#135186,#135187,#135188,#135189,#135190,#135191,#135192,#135193,#135194,
#135195,#135196,#135197,#135198,#135199,#135200,#135201,#135202,#135203,
#135204,#135205,#135206,#135207,#135208,#135209,#135210,#135211,#135212,
#135213,#135214,#135215,#135216,#135217,#135218,#135219,#135220,#135221,
#135222,#135223,#135224,#135225,#135226,#135227,#135228,#135229,#135230,
#135231,#135232,#135233,#135234,#135235,#135236,#135237,#135238,#135239,
#135240,#135241,#135242,#135243,#135244,#135245,#135246,#135247,#135248,
#135249,#135250),.UNSPECIFIED.,.F.,.F.,(4,3,3,3,3,3,3,3,3,3,3,3,3,3,3,3,
3,3,3,3,3,3,3,3,3,3,3,3,3,4),(-0.378621596831381,-0.359799334642644,-0.347863072493078,
-0.339751236649128,-0.335397642749941,-0.315527515100311,-0.3011908154885,
-0.297290501565233,-0.293230948264074,-0.27282995282436,-0.252132128052805,
-0.23930757559106,-0.228808049628064,-0.224505962571255,-0.203201329216816,
-0.200833918205823,-0.17956968323802,-0.158305448270218,-0.154294547940623,
-0.150803075770128,-0.129418690026976,-0.10758400477419,-0.0856173806055649,
-0.0801901203801154,-0.0759398217123878,-0.0533520823575455,-0.0308198729383457,
-0.00876113397239242,-0.00402630967911263,-3.42586534900411E-5),
 .UNSPECIFIED.);
#2973=B_SPLINE_CURVE_WITH_KNOTS('',3,(#135252,#135253,#135254,#135255),
 .UNSPECIFIED.,.F.,.F.,(4,4),(-0.015294280875507,0.),.UNSPECIFIED.);
#2974=B_SPLINE_CURVE_WITH_KNOTS('',3,(#135256,#135257,#135258,#135259,#135260,
#135261,#135262,#135263,#135264,#135265,#135266,#135267,#135268,#135269,
#135270,#135271,#135272,#135273,#135274,#135275,#135276,#135277,#135278,
#135279,#135280,#135281,#135282,#135283,#135284,#135285,#135286,#135287,
#135288,#135289,#135290,#135291,#135292,#135293,#135294,#135295,#135296,
#135297,#135298,#135299,#135300,#135301,#135302,#135303,#135304,#135305,
#135306,#135307,#135308,#135309,#135310,#135311,#135312,#135313,#135314,
#135315,#135316,#135317,#135318,#135319,#135320,#135321,#135322,#135323,
#135324,#135325,#135326,#135327,#135328,#135329,#135330,#135331,#135332,
#135333,#135334,#135335,#135336,#135337,#135338,#135339,#135340),
 .UNSPECIFIED.,.F.,.F.,(4,3,3,3,3,3,3,3,3,3,3,3,3,3,3,3,3,3,3,3,3,3,3,3,
3,3,3,3,4),(0.,0.0219645252128417,0.044541845696888,0.0636190102334506,
0.0720964280805716,0.076753153335081,0.0810482200245811,0.102994855000476,
0.124771637962689,0.142868518969364,0.150423017612877,0.153918288000301,
0.157566649003441,0.178337855554218,0.197159161989389,0.219430675297114,
0.224333226672903,0.229400011405901,0.250090054224483,0.270725909831617,
0.285678847355051,0.296896590893469,0.300624275912145,0.320397170032721,
0.334307458733279,0.338773433419682,0.357799291046648,0.375331268451191,
0.378621596831382),.UNSPECIFIED.);
#2975=B_SPLINE_CURVE_WITH_KNOTS('',3,(#135722,#135723,#135724,#135725,#135726,
#135727,#135728,#135729,#135730,#135731,#135732,#135733,#135734,#135735,
#135736,#135737,#135738,#135739,#135740,#135741,#135742,#135743,#135744,
#135745,#135746,#135747,#135748,#135749,#135750,#135751,#135752,#135753,
#135754,#135755,#135756,#135757,#135758,#135759,#135760,#135761,#135762,
#135763,#135764,#135765,#135766,#135767,#135768,#135769,#135770,#135771,
#135772,#135773,#135774,#135775,#135776,#135777,#135778,#135779,#135780,
#135781,#135782,#135783,#135784,#135785,#135786,#135787,#135788,#135789,
#135790,#135791,#135792,#135793,#135794,#135795,#135796,#135797,#135798,
#135799,#135800,#135801,#135802,#135803,#135804,#135805,#135806),
 .UNSPECIFIED.,.F.,.F.,(4,3,3,3,3,3,3,3,3,3,3,3,3,3,3,3,3,3,3,3,3,3,3,3,
3,3,3,3,4),(-0.376940817211664,-0.354635449587131,-0.33291342343583,-0.328065273459223,
-0.305816655761636,-0.290196978838522,-0.28426118601974,-0.278600481540187,
-0.256993860807461,-0.235699071189167,-0.214946535975349,-0.208201323450052,
-0.204401316925529,-0.183824742722166,-0.180859240376722,-0.159876540758328,
-0.140301763235768,-0.136000501696498,-0.132614276957988,-0.112155191085992,
-0.0917900627476849,-0.0718604703137309,-0.0660675372545504,-0.0628420703116484,
-0.0432965295468417,-0.0232874250623442,-0.00474995575000378,-0.00327832057784658,
0.),.UNSPECIFIED.);
#2976=B_SPLINE_CURVE_WITH_KNOTS('',3,(#135807,#135808,#135809,#135810,#135811,
#135812,#135813,#135814,#135815,#135816,#135817,#135818,#135819,#135820,
#135821,#135822,#135823,#135824,#135825,#135826,#135827,#135828,#135829,
#135830,#135831,#135832,#135833,#135834,#135835,#135836,#135837,#135838,
#135839,#135840,#135841,#135842,#135843,#135844,#135845,#135846,#135847,
#135848,#135849,#135850,#135851,#135852,#135853,#135854,#135855,#135856,
#135857,#135858,#135859,#135860,#135861,#135862,#135863,#135864,#135865,
#135866,#135867,#135868,#135869,#135870,#135871,#135872,#135873,#135874,
#135875,#135876,#135877,#135878,#135879,#135880,#135881,#135882,#135883,
#135884,#135885,#135886,#135887,#135888),.UNSPECIFIED.,.F.,.F.,(4,3,3,3,
3,3,3,3,3,3,3,3,3,3,3,3,3,3,3,3,3,3,3,3,3,3,3,4),(0.,0.0185955823964664,
0.038421241154236,0.0557686925672843,0.0644706831960225,0.0684503830038135,
0.0885032171437632,0.108912563113654,0.125984635449896,0.1338478008296,
0.137284312079196,0.158359363131109,0.177200852458623,0.197729600808643,
0.205651690758548,0.209126659942652,0.2301334310946,0.251648890514138,0.268071992223651,
0.278310570548695,0.284045805818415,0.306303539327454,0.322968933321467,
0.328170989556339,0.333183925255598,0.355705312250232,0.372931104637538,
0.376894576477768),.UNSPECIFIED.);
#2977=B_SPLINE_CURVE_WITH_KNOTS('',3,(#135889,#135890,#135891,#135892),
 .UNSPECIFIED.,.F.,.F.,(4,4),(0.,0.0152452936035568),.UNSPECIFIED.);
#2978=B_SPLINE_CURVE_WITH_KNOTS('',3,(#136273,#136274,#136275,#136276,#136277,
#136278,#136279,#136280,#136281,#136282,#136283,#136284,#136285,#136286,
#136287,#136288,#136289,#136290,#136291,#136292,#136293,#136294,#136295,
#136296,#136297,#136298,#136299,#136300,#136301,#136302,#136303,#136304,
#136305,#136306,#136307,#136308,#136309,#136310,#136311,#136312,#136313,
#136314,#136315,#136316,#136317,#136318,#136319,#136320,#136321,#136322,
#136323,#136324,#136325,#136326,#136327,#136328,#136329,#136330,#136331,
#136332,#136333,#136334,#136335,#136336,#136337,#136338,#136339,#136340,
#136341,#136342,#136343,#136344,#136345,#136346,#136347,#136348,#136349,
#136350,#136351,#136352,#136353,#136354,#136355,#136356,#136357,#136358,
#136359,#136360),.UNSPECIFIED.,.F.,.F.,(4,3,3,3,3,3,3,3,3,3,3,3,3,3,3,3,
3,3,3,3,3,3,3,3,3,3,3,3,3,4),(-0.378621596831333,-0.359799340993963,-0.347863088648493,
-0.339751380172106,-0.335397706196632,-0.315527584340703,-0.301190876073838,
-0.297290637950947,-0.29323096453051,-0.272829973526033,-0.252132148232715,
-0.239307590725982,-0.228808071982614,-0.224505969731213,-0.203201336186886,
-0.200833918205781,-0.180345321018525,-0.158305444601098,-0.154294522931056,
-0.150803070963683,-0.129418681789645,-0.107583994998281,-0.0856173707996288,
-0.0801901033259043,-0.0759398156227559,-0.0533919939915826,-0.0308198662669975,
-0.00876112667829501,-0.00402630967910949,-3.42547819880877E-5),
 .UNSPECIFIED.);
#2979=B_SPLINE_CURVE_WITH_KNOTS('',3,(#136362,#136363,#136364,#136365),
 .UNSPECIFIED.,.F.,.F.,(4,4),(-0.0152943911553443,0.),.UNSPECIFIED.);
#2980=B_SPLINE_CURVE_WITH_KNOTS('',3,(#136366,#136367,#136368,#136369,#136370,
#136371,#136372,#136373,#136374,#136375,#136376,#136377,#136378,#136379,
#136380,#136381,#136382,#136383,#136384,#136385,#136386,#136387,#136388,
#136389,#136390,#136391,#136392,#136393,#136394,#136395,#136396,#136397,
#136398,#136399,#136400,#136401,#136402,#136403,#136404,#136405,#136406,
#136407,#136408,#136409,#136410,#136411,#136412,#136413,#136414,#136415,
#136416,#136417,#136418,#136419,#136420,#136421,#136422,#136423,#136424,
#136425,#136426,#136427,#136428,#136429,#136430,#136431,#136432,#136433,
#136434,#136435,#136436,#136437,#136438,#136439,#136440,#136441,#136442,
#136443,#136444,#136445,#136446,#136447,#136448,#136449,#136450),
 .UNSPECIFIED.,.F.,.F.,(4,3,3,3,3,3,3,3,3,3,3,3,3,3,3,3,3,3,3,3,3,3,3,3,
3,3,3,3,4),(0.,0.0219645196906565,0.0445418395961537,0.0636190048953165,
0.0720964264886179,0.0767531499549516,0.0810482191086478,0.102973098393797,
0.124771638719259,0.142868519536808,0.150423017229364,0.153918285920911,
0.15756664838456,0.178337856551124,0.197159161989456,0.219430675297187,
0.224333227042281,0.229400011424028,0.250065016189275,0.270725909719807,
0.285678851884929,0.296896598603033,0.30062427815181,0.320397174054837,
0.334307465475236,0.338773439815346,0.357799300327208,0.375331268451302,
0.378621596831489),.UNSPECIFIED.);
#4041=LINE('',#59499,#4678);
#4042=LINE('',#59541,#4679);
#4043=LINE('',#59868,#4680);
#4044=LINE('',#60262,#4681);
#4045=LINE('',#60653,#4682);
#4046=LINE('',#61044,#4683);
#4047=LINE('',#61432,#4684);
#4048=LINE('',#61823,#4685);
#4049=LINE('',#62214,#4686);
#4050=LINE('',#62602,#4687);
#4051=LINE('',#62996,#4688);
#4052=LINE('',#63387,#4689);
#4053=LINE('',#63778,#4690);
#4054=LINE('',#64172,#4691);
#4055=LINE('',#64563,#4692);
#4056=LINE('',#64951,#4693);
#4057=LINE('',#65160,#4694);
#4058=LINE('',#65336,#4695);
#4059=LINE('',#65587,#4696);
#4060=LINE('',#65817,#4697);
#4061=LINE('',#66230,#4698);
#4062=LINE('',#66676,#4699);
#4063=LINE('',#67132,#4700);
#4064=LINE('',#67564,#4701);
#4065=LINE('',#67996,#4702);
#4066=LINE('',#68396,#4703);
#4067=LINE('',#68850,#4704);
#4068=LINE('',#69286,#4705);
#4069=LINE('',#69714,#4706);
#4070=LINE('',#70126,#4707);
#4071=LINE('',#70554,#4708);
#4072=LINE('',#70970,#4709);
#4073=LINE('',#71313,#4710);
#4074=LINE('',#71355,#4711);
#4075=LINE('',#71682,#4712);
#4076=LINE('',#72076,#4713);
#4077=LINE('',#72467,#4714);
#4078=LINE('',#72858,#4715);
#4079=LINE('',#73246,#4716);
#4080=LINE('',#73637,#4717);
#4081=LINE('',#74028,#4718);
#4082=LINE('',#74416,#4719);
#4083=LINE('',#74810,#4720);
#4084=LINE('',#75201,#4721);
#4085=LINE('',#75592,#4722);
#4086=LINE('',#75986,#4723);
#4087=LINE('',#76377,#4724);
#4088=LINE('',#76765,#4725);
#4089=LINE('',#76974,#4726);
#4090=LINE('',#77152,#4727);
#4091=LINE('',#77449,#4728);
#4092=LINE('',#77683,#4729);
#4093=LINE('',#78094,#4730);
#4094=LINE('',#78510,#4731);
#4095=LINE('',#78968,#4732);
#4096=LINE('',#79396,#4733);
#4097=LINE('',#79806,#4734);
#4098=LINE('',#80234,#4735);
#4099=LINE('',#80686,#4736);
#4100=LINE('',#81130,#4737);
#4101=LINE('',#81558,#4738);
#4102=LINE('',#81970,#4739);
#4103=LINE('',#82394,#4740);
#4104=LINE('',#82820,#4741);
#4105=LINE('',#83177,#4742);
#4106=LINE('',#83333,#4743);
#4107=LINE('',#83663,#4744);
#4108=LINE('',#84054,#4745);
#4109=LINE('',#84442,#4746);
#4110=LINE('',#84833,#4747);
#4111=LINE('',#85224,#4748);
#4112=LINE('',#85612,#4749);
#4113=LINE('',#86003,#4750);
#4114=LINE('',#86394,#4751);
#4115=LINE('',#86785,#4752);
#4116=LINE('',#87179,#4753);
#4117=LINE('',#87454,#4754);
#4118=LINE('',#87781,#4755);
#4119=LINE('',#87990,#4756);
#4120=LINE('',#88146,#4757);
#4121=LINE('',#88476,#4758);
#4122=LINE('',#88867,#4759);
#4123=LINE('',#89255,#4760);
#4124=LINE('',#89646,#4761);
#4125=LINE('',#90037,#4762);
#4126=LINE('',#90425,#4763);
#4127=LINE('',#90816,#4764);
#4128=LINE('',#91207,#4765);
#4129=LINE('',#91598,#4766);
#4130=LINE('',#91992,#4767);
#4131=LINE('',#92267,#4768);
#4132=LINE('',#92594,#4769);
#4133=LINE('',#92803,#4770);
#4134=LINE('',#92959,#4771);
#4135=LINE('',#93289,#4772);
#4136=LINE('',#93680,#4773);
#4137=LINE('',#94068,#4774);
#4138=LINE('',#94459,#4775);
#4139=LINE('',#94850,#4776);
#4140=LINE('',#95238,#4777);
#4141=LINE('',#95629,#4778);
#4142=LINE('',#96020,#4779);
#4143=LINE('',#96411,#4780);
#4144=LINE('',#96805,#4781);
#4145=LINE('',#97196,#4782);
#4146=LINE('',#97584,#4783);
#4147=LINE('',#97793,#4784);
#4148=LINE('',#97949,#4785);
#4149=LINE('',#98279,#4786);
#4150=LINE('',#98670,#4787);
#4151=LINE('',#99058,#4788);
#4152=LINE('',#99449,#4789);
#4153=LINE('',#99840,#4790);
#4154=LINE('',#100228,#4791);
#4155=LINE('',#100619,#4792);
#4156=LINE('',#101010,#4793);
#4157=LINE('',#101401,#4794);
#4158=LINE('',#101795,#4795);
#4159=LINE('',#102186,#4796);
#4160=LINE('',#102574,#4797);
#4161=LINE('',#102783,#4798);
#4162=LINE('',#102974,#4799);
#4163=LINE('',#103403,#4800);
#4164=LINE('',#103836,#4801);
#4165=LINE('',#104273,#4802);
#4166=LINE('',#104758,#4803);
#4167=LINE('',#105201,#4804);
#4168=LINE('',#105621,#4805);
#4169=LINE('',#105871,#4806);
#4170=LINE('',#106275,#4807);
#4171=LINE('',#106710,#4808);
#4172=LINE('',#107119,#4809);
#4173=LINE('',#107520,#4810);
#4174=LINE('',#107937,#4811);
#4175=LINE('',#108254,#4812);
#4176=LINE('',#108443,#4813);
#4177=LINE('',#108860,#4814);
#4178=LINE('',#109293,#4815);
#4179=LINE('',#109730,#4816);
#4180=LINE('',#110223,#4817);
#4181=LINE('',#110666,#4818);
#4182=LINE('',#111088,#4819);
#4183=LINE('',#111338,#4820);
#4184=LINE('',#111736,#4821);
#4185=LINE('',#112169,#4822);
#4186=LINE('',#112582,#4823);
#4187=LINE('',#112999,#4824);
#4188=LINE('',#113420,#4825);
#4189=LINE('',#113731,#4826);
#4190=LINE('',#113930,#4827);
#4191=LINE('',#114356,#4828);
#4192=LINE('',#114781,#4829);
#4193=LINE('',#115193,#4830);
#4194=LINE('',#115682,#4831);
#4195=LINE('',#116111,#4832);
#4196=LINE('',#116525,#4833);
#4197=LINE('',#116775,#4834);
#4198=LINE('',#117189,#4835);
#4199=LINE('',#117622,#4836);
#4200=LINE('',#118021,#4837);
#4201=LINE('',#118414,#4838);
#4202=LINE('',#118834,#4839);
#4203=LINE('',#119159,#4840);
#4204=LINE('',#119362,#4841);
#4205=LINE('',#119788,#4842);
#4206=LINE('',#120211,#4843);
#4207=LINE('',#120627,#4844);
#4208=LINE('',#121124,#4845);
#4209=LINE('',#121573,#4846);
#4210=LINE('',#121979,#4847);
#4211=LINE('',#122231,#4848);
#4212=LINE('',#122647,#4849);
#4213=LINE('',#123080,#4850);
#4214=LINE('',#123499,#4851);
#4215=LINE('',#123906,#4852);
#4216=LINE('',#124326,#4853);
#4217=LINE('',#131966,#4854);
#4218=LINE('',#131968,#4855);
#4219=LINE('',#131970,#4856);
#4220=LINE('',#131971,#4857);
#4221=LINE('',#131976,#4858);
#4222=LINE('',#131977,#4859);
#4223=LINE('',#131980,#4860);
#4224=LINE('',#131982,#4861);
#4225=LINE('',#131983,#4862);
#4226=LINE('',#131986,#4863);
#4227=LINE('',#131991,#4864);
#4228=LINE('',#131997,#4865);
#4229=LINE('',#132003,#4866);
#4230=LINE('',#132009,#4867);
#4231=LINE('',#136459,#4868);
#4232=LINE('',#136464,#4869);
#4233=LINE('',#136466,#4870);
#4234=LINE('',#136468,#4871);
#4235=LINE('',#136469,#4872);
#4236=LINE('',#136472,#4873);
#4237=LINE('',#136474,#4874);
#4238=LINE('',#136476,#4875);
#4239=LINE('',#136477,#4876);
#4240=LINE('',#136481,#4877);
#4241=LINE('',#136482,#4878);
#4242=LINE('',#136483,#4879);
#4243=LINE('',#136486,#4880);
#4244=LINE('',#136487,#4881);
#4245=LINE('',#136490,#4882);
#4246=LINE('',#136491,#4883);
#4247=LINE('',#136493,#4884);
#4248=LINE('',#136497,#4885);
#4249=LINE('',#136499,#4886);
#4250=LINE('',#136500,#4887);
#4251=LINE('',#136503,#4888);
#4252=LINE('',#136504,#4889);
#4253=LINE('',#136507,#4890);
#4254=LINE('',#136508,#4891);
#4255=LINE('',#136510,#4892);
#4678=VECTOR('',#18273,2.05475);
#4679=VECTOR('',#18278,2.05475);
#4680=VECTOR('',#18281,2.05475);
#4681=VECTOR('',#18284,2.05475);
#4682=VECTOR('',#18287,2.05475);
#4683=VECTOR('',#18290,2.05475);
#4684=VECTOR('',#18293,2.05475);
#4685=VECTOR('',#18296,2.05475);
#4686=VECTOR('',#18299,2.05475);
#4687=VECTOR('',#18302,2.05475);
#4688=VECTOR('',#18305,2.05475);
#4689=VECTOR('',#18308,2.05475);
#4690=VECTOR('',#18311,2.05475);
#4691=VECTOR('',#18314,2.05475);
#4692=VECTOR('',#18317,2.05475);
#4693=VECTOR('',#18320,2.05475);
#4694=VECTOR('',#18325,1.666);
#4695=VECTOR('',#18328,1.666);
#4696=VECTOR('',#18333,1.666);
#4697=VECTOR('',#18336,1.666);
#4698=VECTOR('',#18339,1.666);
#4699=VECTOR('',#18342,1.666);
#4700=VECTOR('',#18345,1.666);
#4701=VECTOR('',#18348,1.666);
#4702=VECTOR('',#18351,1.666);
#4703=VECTOR('',#18354,1.666);
#4704=VECTOR('',#18357,1.666);
#4705=VECTOR('',#18360,1.666);
#4706=VECTOR('',#18363,1.666);
#4707=VECTOR('',#18366,1.666);
#4708=VECTOR('',#18369,1.666);
#4709=VECTOR('',#18372,1.666);
#4710=VECTOR('',#18377,2.05475);
#4711=VECTOR('',#18382,2.05475);
#4712=VECTOR('',#18385,2.05475);
#4713=VECTOR('',#18388,2.05475);
#4714=VECTOR('',#18391,2.05475);
#4715=VECTOR('',#18394,2.05475);
#4716=VECTOR('',#18397,2.05475);
#4717=VECTOR('',#18400,2.05475);
#4718=VECTOR('',#18403,2.05475);
#4719=VECTOR('',#18406,2.05475);
#4720=VECTOR('',#18409,2.05475);
#4721=VECTOR('',#18412,2.05475);
#4722=VECTOR('',#18415,2.05475);
#4723=VECTOR('',#18418,2.05475);
#4724=VECTOR('',#18421,2.05475);
#4725=VECTOR('',#18424,2.05475);
#4726=VECTOR('',#18429,1.666);
#4727=VECTOR('',#18432,1.666);
#4728=VECTOR('',#18437,1.666);
#4729=VECTOR('',#18440,1.666);
#4730=VECTOR('',#18443,1.666);
#4731=VECTOR('',#18446,1.666);
#4732=VECTOR('',#18449,1.666);
#4733=VECTOR('',#18452,1.666);
#4734=VECTOR('',#18455,1.666);
#4735=VECTOR('',#18458,1.666);
#4736=VECTOR('',#18461,1.666);
#4737=VECTOR('',#18464,1.666);
#4738=VECTOR('',#18467,1.666);
#4739=VECTOR('',#18470,1.666);
#4740=VECTOR('',#18473,1.666);
#4741=VECTOR('',#18476,1.666);
#4742=VECTOR('',#18481,2.05475);
#4743=VECTOR('',#18486,2.05475);
#4744=VECTOR('',#18489,2.05475);
#4745=VECTOR('',#18492,2.05475);
#4746=VECTOR('',#18495,2.05475);
#4747=VECTOR('',#18498,2.05475);
#4748=VECTOR('',#18501,2.05475);
#4749=VECTOR('',#18504,2.05475);
#4750=VECTOR('',#18507,2.05475);
#4751=VECTOR('',#18510,2.05475);
#4752=VECTOR('',#18513,2.05475);
#4753=VECTOR('',#18516,2.05475);
#4754=VECTOR('',#18519,2.05475);
#4755=VECTOR('',#18522,2.05475);
#4756=VECTOR('',#18527,2.05475);
#4757=VECTOR('',#18532,2.05475);
#4758=VECTOR('',#18535,2.05475);
#4759=VECTOR('',#18538,2.05475);
#4760=VECTOR('',#18541,2.05475);
#4761=VECTOR('',#18544,2.05475);
#4762=VECTOR('',#18547,2.05475);
#4763=VECTOR('',#18550,2.05475);
#4764=VECTOR('',#18553,2.05475);
#4765=VECTOR('',#18556,2.05475);
#4766=VECTOR('',#18559,2.05475);
#4767=VECTOR('',#18562,2.05475);
#4768=VECTOR('',#18565,2.05475);
#4769=VECTOR('',#18568,2.05475);
#4770=VECTOR('',#18573,2.05475);
#4771=VECTOR('',#18578,2.05475);
#4772=VECTOR('',#18581,2.05475);
#4773=VECTOR('',#18584,2.05475);
#4774=VECTOR('',#18587,2.05475);
#4775=VECTOR('',#18590,2.05475);
#4776=VECTOR('',#18593,2.05475);
#4777=VECTOR('',#18596,2.05475);
#4778=VECTOR('',#18599,2.05475);
#4779=VECTOR('',#18602,2.05475);
#4780=VECTOR('',#18605,2.05475);
#4781=VECTOR('',#18608,2.05475);
#4782=VECTOR('',#18611,2.05475);
#4783=VECTOR('',#18614,2.05475);
#4784=VECTOR('',#18619,2.05475);
#4785=VECTOR('',#18624,2.05475);
#4786=VECTOR('',#18627,2.05475);
#4787=VECTOR('',#18630,2.05475);
#4788=VECTOR('',#18633,2.05475);
#4789=VECTOR('',#18636,2.05475);
#4790=VECTOR('',#18639,2.05475);
#4791=VECTOR('',#18642,2.05475);
#4792=VECTOR('',#18645,2.05475);
#4793=VECTOR('',#18648,2.05475);
#4794=VECTOR('',#18651,2.05475);
#4795=VECTOR('',#18654,2.05475);
#4796=VECTOR('',#18657,2.05475);
#4797=VECTOR('',#18660,2.05475);
#4798=VECTOR('',#18665,1.666);
#4799=VECTOR('',#18670,1.666);
#4800=VECTOR('',#18673,1.666);
#4801=VECTOR('',#18676,1.666);
#4802=VECTOR('',#18679,1.666);
#4803=VECTOR('',#18682,1.666);
#4804=VECTOR('',#18685,1.666);
#4805=VECTOR('',#18688,1.666);
#4806=VECTOR('',#18691,1.666);
#4807=VECTOR('',#18694,1.666);
#4808=VECTOR('',#18697,1.666);
#4809=VECTOR('',#18700,1.666);
#4810=VECTOR('',#18703,1.666);
#4811=VECTOR('',#18706,1.666);
#4812=VECTOR('',#18711,1.666);
#4813=VECTOR('',#18716,1.666);
#4814=VECTOR('',#18719,1.666);
#4815=VECTOR('',#18722,1.666);
#4816=VECTOR('',#18725,1.666);
#4817=VECTOR('',#18728,1.666);
#4818=VECTOR('',#18731,1.666);
#4819=VECTOR('',#18734,1.666);
#4820=VECTOR('',#18737,1.666);
#4821=VECTOR('',#18740,1.666);
#4822=VECTOR('',#18743,1.666);
#4823=VECTOR('',#18746,1.666);
#4824=VECTOR('',#18749,1.666);
#4825=VECTOR('',#18752,1.666);
#4826=VECTOR('',#18757,1.666);
#4827=VECTOR('',#18762,1.666);
#4828=VECTOR('',#18765,1.666);
#4829=VECTOR('',#18768,1.666);
#4830=VECTOR('',#18771,1.666);
#4831=VECTOR('',#18774,1.666);
#4832=VECTOR('',#18777,1.666);
#4833=VECTOR('',#18780,1.666);
#4834=VECTOR('',#18783,1.666);
#4835=VECTOR('',#18786,1.666);
#4836=VECTOR('',#18789,1.666);
#4837=VECTOR('',#18792,1.666);
#4838=VECTOR('',#18795,1.666);
#4839=VECTOR('',#18798,1.666);
#4840=VECTOR('',#18803,1.666);
#4841=VECTOR('',#18808,1.666);
#4842=VECTOR('',#18811,1.666);
#4843=VECTOR('',#18814,1.666);
#4844=VECTOR('',#18817,1.666);
#4845=VECTOR('',#18820,1.666);
#4846=VECTOR('',#18823,1.666);
#4847=VECTOR('',#18826,1.666);
#4848=VECTOR('',#18829,1.666);
#4849=VECTOR('',#18832,1.666);
#4850=VECTOR('',#18835,1.666);
#4851=VECTOR('',#18838,1.666);
#4852=VECTOR('',#18841,1.666);
#4853=VECTOR('',#18844,1.666);
#4854=VECTOR('',#18881,10.);
#4855=VECTOR('',#18882,10.);
#4856=VECTOR('',#18883,10.);
#4857=VECTOR('',#18884,10.);
#4858=VECTOR('',#18889,10.);
#4859=VECTOR('',#18890,10.);
#4860=VECTOR('',#18893,10.);
#4861=VECTOR('',#18894,10.);
#4862=VECTOR('',#18895,10.);
#4863=VECTOR('',#18900,10.);
#4864=VECTOR('',#18905,4.5);
#4865=VECTOR('',#18912,4.5);
#4866=VECTOR('',#18919,4.5);
#4867=VECTOR('',#18926,4.5);
#4868=VECTOR('',#18941,22.);
#4869=VECTOR('',#18946,10.);
#4870=VECTOR('',#18947,10.);
#4871=VECTOR('',#18948,10.);
#4872=VECTOR('',#18949,10.);
#4873=VECTOR('',#18950,10.);
#4874=VECTOR('',#18951,10.);
#4875=VECTOR('',#18952,10.);
#4876=VECTOR('',#18953,10.);
#4877=VECTOR('',#18956,10.);
#4878=VECTOR('',#18957,10.);
#4879=VECTOR('',#18958,10.);
#4880=VECTOR('',#18961,10.);
#4881=VECTOR('',#18962,10.);
#4882=VECTOR('',#18965,10.);
#4883=VECTOR('',#18966,10.);
#4884=VECTOR('',#18969,10.);
#4885=VECTOR('',#18974,10.);
#4886=VECTOR('',#18975,10.);
#4887=VECTOR('',#18976,10.);
#4888=VECTOR('',#18979,10.);
#4889=VECTOR('',#18980,10.);
#4890=VECTOR('',#18983,10.);
#4891=VECTOR('',#18984,10.);
#4892=VECTOR('',#18987,10.);
#5563=VERTEX_POINT('',#59497);
#5564=VERTEX_POINT('',#59498);
#5565=VERTEX_POINT('',#59500);
#5566=VERTEX_POINT('',#59505);
#5567=VERTEX_POINT('',#59539);
#5568=VERTEX_POINT('',#59540);
#5569=VERTEX_POINT('',#59542);
#5570=VERTEX_POINT('',#59670);
#5571=VERTEX_POINT('',#59866);
#5572=VERTEX_POINT('',#59867);
#5573=VERTEX_POINT('',#59869);
#5574=VERTEX_POINT('',#60067);
#5575=VERTEX_POINT('',#60260);
#5576=VERTEX_POINT('',#60261);
#5577=VERTEX_POINT('',#60263);
#5578=VERTEX_POINT('',#60458);
#5579=VERTEX_POINT('',#60651);
#5580=VERTEX_POINT('',#60652);
#5581=VERTEX_POINT('',#60654);
#5582=VERTEX_POINT('',#60846);
#5583=VERTEX_POINT('',#61042);
#5584=VERTEX_POINT('',#61043);
#5585=VERTEX_POINT('',#61045);
#5586=VERTEX_POINT('',#61237);
#5587=VERTEX_POINT('',#61430);
#5588=VERTEX_POINT('',#61431);
#5589=VERTEX_POINT('',#61433);
#5590=VERTEX_POINT('',#61628);
#5591=VERTEX_POINT('',#61821);
#5592=VERTEX_POINT('',#61822);
#5593=VERTEX_POINT('',#61824);
#5594=VERTEX_POINT('',#62013);
#5595=VERTEX_POINT('',#62212);
#5596=VERTEX_POINT('',#62213);
#5597=VERTEX_POINT('',#62215);
#5598=VERTEX_POINT('',#62407);
#5599=VERTEX_POINT('',#62600);
#5600=VERTEX_POINT('',#62601);
#5601=VERTEX_POINT('',#62603);
#5602=VERTEX_POINT('',#62801);
#5603=VERTEX_POINT('',#62994);
#5604=VERTEX_POINT('',#62995);
#5605=VERTEX_POINT('',#62997);
#5606=VERTEX_POINT('',#63189);
#5607=VERTEX_POINT('',#63385);
#5608=VERTEX_POINT('',#63386);
#5609=VERTEX_POINT('',#63388);
#5610=VERTEX_POINT('',#63580);
#5611=VERTEX_POINT('',#63776);
#5612=VERTEX_POINT('',#63777);
#5613=VERTEX_POINT('',#63779);
#5614=VERTEX_POINT('',#63977);
#5615=VERTEX_POINT('',#64170);
#5616=VERTEX_POINT('',#64171);
#5617=VERTEX_POINT('',#64173);
#5618=VERTEX_POINT('',#64365);
#5619=VERTEX_POINT('',#64561);
#5620=VERTEX_POINT('',#64562);
#5621=VERTEX_POINT('',#64564);
#5622=VERTEX_POINT('',#64753);
#5623=VERTEX_POINT('',#64949);
#5624=VERTEX_POINT('',#64950);
#5625=VERTEX_POINT('',#64952);
#5626=VERTEX_POINT('',#65023);
#5627=VERTEX_POINT('',#65029);
#5628=VERTEX_POINT('',#65031);
#5629=VERTEX_POINT('',#65158);
#5630=VERTEX_POINT('',#65159);
#5631=VERTEX_POINT('',#65161);
#5632=VERTEX_POINT('',#65322);
#5633=VERTEX_POINT('',#65324);
#5634=VERTEX_POINT('',#65335);
#5635=VERTEX_POINT('',#65585);
#5636=VERTEX_POINT('',#65586);
#5637=VERTEX_POINT('',#65794);
#5638=VERTEX_POINT('',#65815);
#5639=VERTEX_POINT('',#65816);
#5640=VERTEX_POINT('',#65818);
#5641=VERTEX_POINT('',#66025);
#5642=VERTEX_POINT('',#66228);
#5643=VERTEX_POINT('',#66229);
#5644=VERTEX_POINT('',#66674);
#5645=VERTEX_POINT('',#66675);
#5646=VERTEX_POINT('',#66677);
#5647=VERTEX_POINT('',#66924);
#5648=VERTEX_POINT('',#67130);
#5649=VERTEX_POINT('',#67131);
#5650=VERTEX_POINT('',#67562);
#5651=VERTEX_POINT('',#67563);
#5652=VERTEX_POINT('',#67565);
#5653=VERTEX_POINT('',#67792);
#5654=VERTEX_POINT('',#67994);
#5655=VERTEX_POINT('',#67995);
#5656=VERTEX_POINT('',#68394);
#5657=VERTEX_POINT('',#68395);
#5658=VERTEX_POINT('',#68397);
#5659=VERTEX_POINT('',#68614);
#5660=VERTEX_POINT('',#68848);
#5661=VERTEX_POINT('',#68849);
#5662=VERTEX_POINT('',#69284);
#5663=VERTEX_POINT('',#69285);
#5664=VERTEX_POINT('',#69287);
#5665=VERTEX_POINT('',#69488);
#5666=VERTEX_POINT('',#69712);
#5667=VERTEX_POINT('',#69713);
#5668=VERTEX_POINT('',#70124);
#5669=VERTEX_POINT('',#70125);
#5670=VERTEX_POINT('',#70127);
#5671=VERTEX_POINT('',#70340);
#5672=VERTEX_POINT('',#70552);
#5673=VERTEX_POINT('',#70553);
#5674=VERTEX_POINT('',#70968);
#5675=VERTEX_POINT('',#70969);
#5676=VERTEX_POINT('',#70971);
#5677=VERTEX_POINT('',#71106);
#5678=VERTEX_POINT('',#71311);
#5679=VERTEX_POINT('',#71312);
#5680=VERTEX_POINT('',#71314);
#5681=VERTEX_POINT('',#71319);
#5682=VERTEX_POINT('',#71353);
#5683=VERTEX_POINT('',#71354);
#5684=VERTEX_POINT('',#71356);
#5685=VERTEX_POINT('',#71484);
#5686=VERTEX_POINT('',#71680);
#5687=VERTEX_POINT('',#71681);
#5688=VERTEX_POINT('',#71683);
#5689=VERTEX_POINT('',#71881);
#5690=VERTEX_POINT('',#72074);
#5691=VERTEX_POINT('',#72075);
#5692=VERTEX_POINT('',#72077);
#5693=VERTEX_POINT('',#72272);
#5694=VERTEX_POINT('',#72465);
#5695=VERTEX_POINT('',#72466);
#5696=VERTEX_POINT('',#72468);
#5697=VERTEX_POINT('',#72660);
#5698=VERTEX_POINT('',#72856);
#5699=VERTEX_POINT('',#72857);
#5700=VERTEX_POINT('',#72859);
#5701=VERTEX_POINT('',#73051);
#5702=VERTEX_POINT('',#73244);
#5703=VERTEX_POINT('',#73245);
#5704=VERTEX_POINT('',#73247);
#5705=VERTEX_POINT('',#73442);
#5706=VERTEX_POINT('',#73635);
#5707=VERTEX_POINT('',#73636);
#5708=VERTEX_POINT('',#73638);
#5709=VERTEX_POINT('',#73827);
#5710=VERTEX_POINT('',#74026);
#5711=VERTEX_POINT('',#74027);
#5712=VERTEX_POINT('',#74029);
#5713=VERTEX_POINT('',#74221);
#5714=VERTEX_POINT('',#74414);
#5715=VERTEX_POINT('',#74415);
#5716=VERTEX_POINT('',#74417);
#5717=VERTEX_POINT('',#74615);
#5718=VERTEX_POINT('',#74808);
#5719=VERTEX_POINT('',#74809);
#5720=VERTEX_POINT('',#74811);
#5721=VERTEX_POINT('',#75003);
#5722=VERTEX_POINT('',#75199);
#5723=VERTEX_POINT('',#75200);
#5724=VERTEX_POINT('',#75202);
#5725=VERTEX_POINT('',#75394);
#5726=VERTEX_POINT('',#75590);
#5727=VERTEX_POINT('',#75591);
#5728=VERTEX_POINT('',#75593);
#5729=VERTEX_POINT('',#75791);
#5730=VERTEX_POINT('',#75984);
#5731=VERTEX_POINT('',#75985);
#5732=VERTEX_POINT('',#75987);
#5733=VERTEX_POINT('',#76179);
#5734=VERTEX_POINT('',#76375);
#5735=VERTEX_POINT('',#76376);
#5736=VERTEX_POINT('',#76378);
#5737=VERTEX_POINT('',#76567);
#5738=VERTEX_POINT('',#76763);
#5739=VERTEX_POINT('',#76764);
#5740=VERTEX_POINT('',#76766);
#5741=VERTEX_POINT('',#76837);
#5742=VERTEX_POINT('',#76843);
#5743=VERTEX_POINT('',#76845);
#5744=VERTEX_POINT('',#76972);
#5745=VERTEX_POINT('',#76973);
#5746=VERTEX_POINT('',#76975);
#5747=VERTEX_POINT('',#77136);
#5748=VERTEX_POINT('',#77138);
#5749=VERTEX_POINT('',#77151);
#5750=VERTEX_POINT('',#77447);
#5751=VERTEX_POINT('',#77448);
#5752=VERTEX_POINT('',#77658);
#5753=VERTEX_POINT('',#77681);
#5754=VERTEX_POINT('',#77682);
#5755=VERTEX_POINT('',#77684);
#5756=VERTEX_POINT('',#77887);
#5757=VERTEX_POINT('',#78092);
#5758=VERTEX_POINT('',#78093);
#5759=VERTEX_POINT('',#78508);
#5760=VERTEX_POINT('',#78509);
#5761=VERTEX_POINT('',#78511);
#5762=VERTEX_POINT('',#78758);
#5763=VERTEX_POINT('',#78966);
#5764=VERTEX_POINT('',#78967);
#5765=VERTEX_POINT('',#79394);
#5766=VERTEX_POINT('',#79395);
#5767=VERTEX_POINT('',#79397);
#5768=VERTEX_POINT('',#79604);
#5769=VERTEX_POINT('',#79804);
#5770=VERTEX_POINT('',#79805);
#5771=VERTEX_POINT('',#80232);
#5772=VERTEX_POINT('',#80233);
#5773=VERTEX_POINT('',#80235);
#5774=VERTEX_POINT('',#80448);
#5775=VERTEX_POINT('',#80684);
#5776=VERTEX_POINT('',#80685);
#5777=VERTEX_POINT('',#81128);
#5778=VERTEX_POINT('',#81129);
#5779=VERTEX_POINT('',#81131);
#5780=VERTEX_POINT('',#81332);
#5781=VERTEX_POINT('',#81556);
#5782=VERTEX_POINT('',#81557);
#5783=VERTEX_POINT('',#81968);
#5784=VERTEX_POINT('',#81969);
#5785=VERTEX_POINT('',#81971);
#5786=VERTEX_POINT('',#82182);
#5787=VERTEX_POINT('',#82392);
#5788=VERTEX_POINT('',#82393);
#5789=VERTEX_POINT('',#82818);
#5790=VERTEX_POINT('',#82819);
#5791=VERTEX_POINT('',#82821);
#5792=VERTEX_POINT('',#82966);
#5793=VERTEX_POINT('',#83175);
#5794=VERTEX_POINT('',#83176);
#5795=VERTEX_POINT('',#83178);
#5796=VERTEX_POINT('',#83187);
#5797=VERTEX_POINT('',#83189);
#5798=VERTEX_POINT('',#83331);
#5799=VERTEX_POINT('',#83332);
#5800=VERTEX_POINT('',#83334);
#5801=VERTEX_POINT('',#83468);
#5802=VERTEX_POINT('',#83661);
#5803=VERTEX_POINT('',#83662);
#5804=VERTEX_POINT('',#83664);
#5805=VERTEX_POINT('',#83856);
#5806=VERTEX_POINT('',#84052);
#5807=VERTEX_POINT('',#84053);
#5808=VERTEX_POINT('',#84055);
#5809=VERTEX_POINT('',#84247);
#5810=VERTEX_POINT('',#84440);
#5811=VERTEX_POINT('',#84441);
#5812=VERTEX_POINT('',#84443);
#5813=VERTEX_POINT('',#84638);
#5814=VERTEX_POINT('',#84831);
#5815=VERTEX_POINT('',#84832);
#5816=VERTEX_POINT('',#84834);
#5817=VERTEX_POINT('',#85023);
#5818=VERTEX_POINT('',#85222);
#5819=VERTEX_POINT('',#85223);
#5820=VERTEX_POINT('',#85225);
#5821=VERTEX_POINT('',#85417);
#5822=VERTEX_POINT('',#85610);
#5823=VERTEX_POINT('',#85611);
#5824=VERTEX_POINT('',#85613);
#5825=VERTEX_POINT('',#85808);
#5826=VERTEX_POINT('',#86001);
#5827=VERTEX_POINT('',#86002);
#5828=VERTEX_POINT('',#86004);
#5829=VERTEX_POINT('',#86196);
#5830=VERTEX_POINT('',#86392);
#5831=VERTEX_POINT('',#86393);
#5832=VERTEX_POINT('',#86395);
#5833=VERTEX_POINT('',#86587);
#5834=VERTEX_POINT('',#86783);
#5835=VERTEX_POINT('',#86784);
#5836=VERTEX_POINT('',#86786);
#5837=VERTEX_POINT('',#86984);
#5838=VERTEX_POINT('',#87177);
#5839=VERTEX_POINT('',#87178);
#5840=VERTEX_POINT('',#87180);
#5841=VERTEX_POINT('',#87256);
#5842=VERTEX_POINT('',#87452);
#5843=VERTEX_POINT('',#87453);
#5844=VERTEX_POINT('',#87455);
#5845=VERTEX_POINT('',#87583);
#5846=VERTEX_POINT('',#87779);
#5847=VERTEX_POINT('',#87780);
#5848=VERTEX_POINT('',#87782);
#5849=VERTEX_POINT('',#87853);
#5850=VERTEX_POINT('',#87859);
#5851=VERTEX_POINT('',#87861);
#5852=VERTEX_POINT('',#87988);
#5853=VERTEX_POINT('',#87989);
#5854=VERTEX_POINT('',#87991);
#5855=VERTEX_POINT('',#88000);
#5856=VERTEX_POINT('',#88002);
#5857=VERTEX_POINT('',#88144);
#5858=VERTEX_POINT('',#88145);
#5859=VERTEX_POINT('',#88147);
#5860=VERTEX_POINT('',#88281);
#5861=VERTEX_POINT('',#88474);
#5862=VERTEX_POINT('',#88475);
#5863=VERTEX_POINT('',#88477);
#5864=VERTEX_POINT('',#88669);
#5865=VERTEX_POINT('',#88865);
#5866=VERTEX_POINT('',#88866);
#5867=VERTEX_POINT('',#88868);
#5868=VERTEX_POINT('',#89060);
#5869=VERTEX_POINT('',#89253);
#5870=VERTEX_POINT('',#89254);
#5871=VERTEX_POINT('',#89256);
#5872=VERTEX_POINT('',#89451);
#5873=VERTEX_POINT('',#89644);
#5874=VERTEX_POINT('',#89645);
#5875=VERTEX_POINT('',#89647);
#5876=VERTEX_POINT('',#89836);
#5877=VERTEX_POINT('',#90035);
#5878=VERTEX_POINT('',#90036);
#5879=VERTEX_POINT('',#90038);
#5880=VERTEX_POINT('',#90230);
#5881=VERTEX_POINT('',#90423);
#5882=VERTEX_POINT('',#90424);
#5883=VERTEX_POINT('',#90426);
#5884=VERTEX_POINT('',#90621);
#5885=VERTEX_POINT('',#90814);
#5886=VERTEX_POINT('',#90815);
#5887=VERTEX_POINT('',#90817);
#5888=VERTEX_POINT('',#91009);
#5889=VERTEX_POINT('',#91205);
#5890=VERTEX_POINT('',#91206);
#5891=VERTEX_POINT('',#91208);
#5892=VERTEX_POINT('',#91400);
#5893=VERTEX_POINT('',#91596);
#5894=VERTEX_POINT('',#91597);
#5895=VERTEX_POINT('',#91599);
#5896=VERTEX_POINT('',#91797);
#5897=VERTEX_POINT('',#91990);
#5898=VERTEX_POINT('',#91991);
#5899=VERTEX_POINT('',#91993);
#5900=VERTEX_POINT('',#92069);
#5901=VERTEX_POINT('',#92265);
#5902=VERTEX_POINT('',#92266);
#5903=VERTEX_POINT('',#92268);
#5904=VERTEX_POINT('',#92396);
#5905=VERTEX_POINT('',#92592);
#5906=VERTEX_POINT('',#92593);
#5907=VERTEX_POINT('',#92595);
#5908=VERTEX_POINT('',#92666);
#5909=VERTEX_POINT('',#92672);
#5910=VERTEX_POINT('',#92674);
#5911=VERTEX_POINT('',#92801);
#5912=VERTEX_POINT('',#92802);
#5913=VERTEX_POINT('',#92804);
#5914=VERTEX_POINT('',#92813);
#5915=VERTEX_POINT('',#92815);
#5916=VERTEX_POINT('',#92957);
#5917=VERTEX_POINT('',#92958);
#5918=VERTEX_POINT('',#92960);
#5919=VERTEX_POINT('',#93094);
#5920=VERTEX_POINT('',#93287);
#5921=VERTEX_POINT('',#93288);
#5922=VERTEX_POINT('',#93290);
#5923=VERTEX_POINT('',#93482);
#5924=VERTEX_POINT('',#93678);
#5925=VERTEX_POINT('',#93679);
#5926=VERTEX_POINT('',#93681);
#5927=VERTEX_POINT('',#93873);
#5928=VERTEX_POINT('',#94066);
#5929=VERTEX_POINT('',#94067);
#5930=VERTEX_POINT('',#94069);
#5931=VERTEX_POINT('',#94264);
#5932=VERTEX_POINT('',#94457);
#5933=VERTEX_POINT('',#94458);
#5934=VERTEX_POINT('',#94460);
#5935=VERTEX_POINT('',#94649);
#5936=VERTEX_POINT('',#94848);
#5937=VERTEX_POINT('',#94849);
#5938=VERTEX_POINT('',#94851);
#5939=VERTEX_POINT('',#95043);
#5940=VERTEX_POINT('',#95236);
#5941=VERTEX_POINT('',#95237);
#5942=VERTEX_POINT('',#95239);
#5943=VERTEX_POINT('',#95434);
#5944=VERTEX_POINT('',#95627);
#5945=VERTEX_POINT('',#95628);
#5946=VERTEX_POINT('',#95630);
#5947=VERTEX_POINT('',#95822);
#5948=VERTEX_POINT('',#96018);
#5949=VERTEX_POINT('',#96019);
#5950=VERTEX_POINT('',#96021);
#5951=VERTEX_POINT('',#96213);
#5952=VERTEX_POINT('',#96409);
#5953=VERTEX_POINT('',#96410);
#5954=VERTEX_POINT('',#96412);
#5955=VERTEX_POINT('',#96610);
#5956=VERTEX_POINT('',#96803);
#5957=VERTEX_POINT('',#96804);
#5958=VERTEX_POINT('',#96806);
#5959=VERTEX_POINT('',#96998);
#5960=VERTEX_POINT('',#97194);
#5961=VERTEX_POINT('',#97195);
#5962=VERTEX_POINT('',#97197);
#5963=VERTEX_POINT('',#97386);
#5964=VERTEX_POINT('',#97582);
#5965=VERTEX_POINT('',#97583);
#5966=VERTEX_POINT('',#97585);
#5967=VERTEX_POINT('',#97656);
#5968=VERTEX_POINT('',#97662);
#5969=VERTEX_POINT('',#97664);
#5970=VERTEX_POINT('',#97791);
#5971=VERTEX_POINT('',#97792);
#5972=VERTEX_POINT('',#97794);
#5973=VERTEX_POINT('',#97803);
#5974=VERTEX_POINT('',#97805);
#5975=VERTEX_POINT('',#97947);
#5976=VERTEX_POINT('',#97948);
#5977=VERTEX_POINT('',#97950);
#5978=VERTEX_POINT('',#98084);
#5979=VERTEX_POINT('',#98277);
#5980=VERTEX_POINT('',#98278);
#5981=VERTEX_POINT('',#98280);
#5982=VERTEX_POINT('',#98472);
#5983=VERTEX_POINT('',#98668);
#5984=VERTEX_POINT('',#98669);
#5985=VERTEX_POINT('',#98671);
#5986=VERTEX_POINT('',#98863);
#5987=VERTEX_POINT('',#99056);
#5988=VERTEX_POINT('',#99057);
#5989=VERTEX_POINT('',#99059);
#5990=VERTEX_POINT('',#99254);
#5991=VERTEX_POINT('',#99447);
#5992=VERTEX_POINT('',#99448);
#5993=VERTEX_POINT('',#99450);
#5994=VERTEX_POINT('',#99639);
#5995=VERTEX_POINT('',#99838);
#5996=VERTEX_POINT('',#99839);
#5997=VERTEX_POINT('',#99841);
#5998=VERTEX_POINT('',#100033);
#5999=VERTEX_POINT('',#100226);
#6000=VERTEX_POINT('',#100227);
#6001=VERTEX_POINT('',#100229);
#6002=VERTEX_POINT('',#100424);
#6003=VERTEX_POINT('',#100617);
#6004=VERTEX_POINT('',#100618);
#6005=VERTEX_POINT('',#100620);
#6006=VERTEX_POINT('',#100812);
#6007=VERTEX_POINT('',#101008);
#6008=VERTEX_POINT('',#101009);
#6009=VERTEX_POINT('',#101011);
#6010=VERTEX_POINT('',#101203);
#6011=VERTEX_POINT('',#101399);
#6012=VERTEX_POINT('',#101400);
#6013=VERTEX_POINT('',#101402);
#6014=VERTEX_POINT('',#101600);
#6015=VERTEX_POINT('',#101793);
#6016=VERTEX_POINT('',#101794);
#6017=VERTEX_POINT('',#101796);
#6018=VERTEX_POINT('',#101988);
#6019=VERTEX_POINT('',#102184);
#6020=VERTEX_POINT('',#102185);
#6021=VERTEX_POINT('',#102187);
#6022=VERTEX_POINT('',#102376);
#6023=VERTEX_POINT('',#102572);
#6024=VERTEX_POINT('',#102573);
#6025=VERTEX_POINT('',#102575);
#6026=VERTEX_POINT('',#102646);
#6027=VERTEX_POINT('',#102652);
#6028=VERTEX_POINT('',#102654);
#6029=VERTEX_POINT('',#102781);
#6030=VERTEX_POINT('',#102782);
#6031=VERTEX_POINT('',#102784);
#6032=VERTEX_POINT('',#102849);
#6033=VERTEX_POINT('',#102972);
#6034=VERTEX_POINT('',#102973);
#6035=VERTEX_POINT('',#102975);
#6036=VERTEX_POINT('',#103401);
#6037=VERTEX_POINT('',#103402);
#6038=VERTEX_POINT('',#103620);
#6039=VERTEX_POINT('',#103834);
#6040=VERTEX_POINT('',#103835);
#6041=VERTEX_POINT('',#103837);
#6042=VERTEX_POINT('',#104271);
#6043=VERTEX_POINT('',#104272);
#6044=VERTEX_POINT('',#104474);
#6045=VERTEX_POINT('',#104756);
#6046=VERTEX_POINT('',#104757);
#6047=VERTEX_POINT('',#104759);
#6048=VERTEX_POINT('',#105199);
#6049=VERTEX_POINT('',#105200);
#6050=VERTEX_POINT('',#105438);
#6051=VERTEX_POINT('',#105619);
#6052=VERTEX_POINT('',#105620);
#6053=VERTEX_POINT('',#105622);
#6054=VERTEX_POINT('',#105845);
#6055=VERTEX_POINT('',#105869);
#6056=VERTEX_POINT('',#105870);
#6057=VERTEX_POINT('',#106078);
#6058=VERTEX_POINT('',#106273);
#6059=VERTEX_POINT('',#106274);
#6060=VERTEX_POINT('',#106276);
#6061=VERTEX_POINT('',#106708);
#6062=VERTEX_POINT('',#106709);
#6063=VERTEX_POINT('',#106909);
#6064=VERTEX_POINT('',#107117);
#6065=VERTEX_POINT('',#107118);
#6066=VERTEX_POINT('',#107120);
#6067=VERTEX_POINT('',#107518);
#6068=VERTEX_POINT('',#107519);
#6069=VERTEX_POINT('',#107719);
#6070=VERTEX_POINT('',#107935);
#6071=VERTEX_POINT('',#107936);
#6072=VERTEX_POINT('',#107938);
#6073=VERTEX_POINT('',#107959);
#6074=VERTEX_POINT('',#108069);
#6075=VERTEX_POINT('',#108252);
#6076=VERTEX_POINT('',#108253);
#6077=VERTEX_POINT('',#108255);
#6078=VERTEX_POINT('',#108320);
#6079=VERTEX_POINT('',#108441);
#6080=VERTEX_POINT('',#108442);
#6081=VERTEX_POINT('',#108444);
#6082=VERTEX_POINT('',#108858);
#6083=VERTEX_POINT('',#108859);
#6084=VERTEX_POINT('',#109077);
#6085=VERTEX_POINT('',#109291);
#6086=VERTEX_POINT('',#109292);
#6087=VERTEX_POINT('',#109294);
#6088=VERTEX_POINT('',#109728);
#6089=VERTEX_POINT('',#109729);
#6090=VERTEX_POINT('',#109939);
#6091=VERTEX_POINT('',#110221);
#6092=VERTEX_POINT('',#110222);
#6093=VERTEX_POINT('',#110224);
#6094=VERTEX_POINT('',#110664);
#6095=VERTEX_POINT('',#110665);
#6096=VERTEX_POINT('',#110903);
#6097=VERTEX_POINT('',#111086);
#6098=VERTEX_POINT('',#111087);
#6099=VERTEX_POINT('',#111089);
#6100=VERTEX_POINT('',#111312);
#6101=VERTEX_POINT('',#111336);
#6102=VERTEX_POINT('',#111337);
#6103=VERTEX_POINT('',#111545);
#6104=VERTEX_POINT('',#111734);
#6105=VERTEX_POINT('',#111735);
#6106=VERTEX_POINT('',#111737);
#6107=VERTEX_POINT('',#112167);
#6108=VERTEX_POINT('',#112168);
#6109=VERTEX_POINT('',#112388);
#6110=VERTEX_POINT('',#112580);
#6111=VERTEX_POINT('',#112581);
#6112=VERTEX_POINT('',#112583);
#6113=VERTEX_POINT('',#112997);
#6114=VERTEX_POINT('',#112998);
#6115=VERTEX_POINT('',#113202);
#6116=VERTEX_POINT('',#113418);
#6117=VERTEX_POINT('',#113419);
#6118=VERTEX_POINT('',#113421);
#6119=VERTEX_POINT('',#113442);
#6120=VERTEX_POINT('',#113552);
#6121=VERTEX_POINT('',#113729);
#6122=VERTEX_POINT('',#113730);
#6123=VERTEX_POINT('',#113732);
#6124=VERTEX_POINT('',#113805);
#6125=VERTEX_POINT('',#113928);
#6126=VERTEX_POINT('',#113929);
#6127=VERTEX_POINT('',#114354);
#6128=VERTEX_POINT('',#114355);
#6129=VERTEX_POINT('',#114571);
#6130=VERTEX_POINT('',#114779);
#6131=VERTEX_POINT('',#114780);
#6132=VERTEX_POINT('',#115191);
#6133=VERTEX_POINT('',#115192);
#6134=VERTEX_POINT('',#115398);
#6135=VERTEX_POINT('',#115680);
#6136=VERTEX_POINT('',#115681);
#6137=VERTEX_POINT('',#115683);
#6138=VERTEX_POINT('',#116109);
#6139=VERTEX_POINT('',#116110);
#6140=VERTEX_POINT('',#116342);
#6141=VERTEX_POINT('',#116523);
#6142=VERTEX_POINT('',#116524);
#6143=VERTEX_POINT('',#116526);
#6144=VERTEX_POINT('',#116749);
#6145=VERTEX_POINT('',#116773);
#6146=VERTEX_POINT('',#116774);
#6147=VERTEX_POINT('',#116988);
#6148=VERTEX_POINT('',#117187);
#6149=VERTEX_POINT('',#117188);
#6150=VERTEX_POINT('',#117190);
#6151=VERTEX_POINT('',#117620);
#6152=VERTEX_POINT('',#117621);
#6153=VERTEX_POINT('',#117815);
#6154=VERTEX_POINT('',#118019);
#6155=VERTEX_POINT('',#118020);
#6156=VERTEX_POINT('',#118022);
#6157=VERTEX_POINT('',#118412);
#6158=VERTEX_POINT('',#118413);
#6159=VERTEX_POINT('',#118832);
#6160=VERTEX_POINT('',#118833);
#6161=VERTEX_POINT('',#118835);
#6162=VERTEX_POINT('',#118966);
#6163=VERTEX_POINT('',#119157);
#6164=VERTEX_POINT('',#119158);
#6165=VERTEX_POINT('',#119160);
#6166=VERTEX_POINT('',#119235);
#6167=VERTEX_POINT('',#119360);
#6168=VERTEX_POINT('',#119361);
#6169=VERTEX_POINT('',#119786);
#6170=VERTEX_POINT('',#119787);
#6171=VERTEX_POINT('',#120003);
#6172=VERTEX_POINT('',#120209);
#6173=VERTEX_POINT('',#120210);
#6174=VERTEX_POINT('',#120625);
#6175=VERTEX_POINT('',#120626);
#6176=VERTEX_POINT('',#120840);
#6177=VERTEX_POINT('',#121122);
#6178=VERTEX_POINT('',#121123);
#6179=VERTEX_POINT('',#121125);
#6180=VERTEX_POINT('',#121571);
#6181=VERTEX_POINT('',#121572);
#6182=VERTEX_POINT('',#121794);
#6183=VERTEX_POINT('',#121977);
#6184=VERTEX_POINT('',#121978);
#6185=VERTEX_POINT('',#121980);
#6186=VERTEX_POINT('',#122205);
#6187=VERTEX_POINT('',#122229);
#6188=VERTEX_POINT('',#122230);
#6189=VERTEX_POINT('',#122438);
#6190=VERTEX_POINT('',#122645);
#6191=VERTEX_POINT('',#122646);
#6192=VERTEX_POINT('',#122648);
#6193=VERTEX_POINT('',#123078);
#6194=VERTEX_POINT('',#123079);
#6195=VERTEX_POINT('',#123287);
#6196=VERTEX_POINT('',#123497);
#6197=VERTEX_POINT('',#123498);
#6198=VERTEX_POINT('',#123500);
#6199=VERTEX_POINT('',#123904);
#6200=VERTEX_POINT('',#123905);
#6201=VERTEX_POINT('',#124324);
#6202=VERTEX_POINT('',#124325);
#6203=VERTEX_POINT('',#124327);
#6204=VERTEX_POINT('',#124460);
#6205=VERTEX_POINT('',#124651);
#6206=VERTEX_POINT('',#125149);
#6207=VERTEX_POINT('',#125647);
#6208=VERTEX_POINT('',#126059);
#6209=VERTEX_POINT('',#126461);
#6210=VERTEX_POINT('',#126653);
#6211=VERTEX_POINT('',#126846);
#6212=VERTEX_POINT('',#127038);
#6213=VERTEX_POINT('',#127231);
#6214=VERTEX_POINT('',#127423);
#6215=VERTEX_POINT('',#127616);
#6216=VERTEX_POINT('',#127808);
#6217=VERTEX_POINT('',#128001);
#6218=VERTEX_POINT('',#128415);
#6219=VERTEX_POINT('',#128607);
#6220=VERTEX_POINT('',#128800);
#6221=VERTEX_POINT('',#129218);
#6222=VERTEX_POINT('',#129410);
#6223=VERTEX_POINT('',#130690);
#6224=VERTEX_POINT('',#131871);
#6225=VERTEX_POINT('',#131964);
#6226=VERTEX_POINT('',#131965);
#6227=VERTEX_POINT('',#131967);
#6228=VERTEX_POINT('',#131969);
#6229=VERTEX_POINT('',#131973);
#6230=VERTEX_POINT('',#131975);
#6231=VERTEX_POINT('',#131979);
#6232=VERTEX_POINT('',#131981);
#6233=VERTEX_POINT('',#131988);
#6234=VERTEX_POINT('',#131990);
#6235=VERTEX_POINT('',#131994);
#6236=VERTEX_POINT('',#131996);
#6237=VERTEX_POINT('',#132000);
#6238=VERTEX_POINT('',#132002);
#6239=VERTEX_POINT('',#132006);
#6240=VERTEX_POINT('',#132008);
#6241=VERTEX_POINT('',#132391);
#6242=VERTEX_POINT('',#133031);
#6243=VERTEX_POINT('',#133501);
#6244=VERTEX_POINT('',#134141);
#6245=VERTEX_POINT('',#134611);
#6246=VERTEX_POINT('',#135251);
#6247=VERTEX_POINT('',#135721);
#6248=VERTEX_POINT('',#136361);
#6249=VERTEX_POINT('',#136456);
#6250=VERTEX_POINT('',#136458);
#6251=VERTEX_POINT('',#136462);
#6252=VERTEX_POINT('',#136463);
#6253=VERTEX_POINT('',#136465);
#6254=VERTEX_POINT('',#136467);
#6255=VERTEX_POINT('',#136470);
#6256=VERTEX_POINT('',#136471);
#6257=VERTEX_POINT('',#136473);
#6258=VERTEX_POINT('',#136475);
#6259=VERTEX_POINT('',#136479);
#6260=VERTEX_POINT('',#136480);
#6261=VERTEX_POINT('',#136485);
#6262=VERTEX_POINT('',#136489);
#6263=VERTEX_POINT('',#136496);
#6264=VERTEX_POINT('',#136498);
#6265=VERTEX_POINT('',#136502);
#6266=VERTEX_POINT('',#136506);
#7848=EDGE_CURVE('',#5563,#5564,#4041,.T.);
#7849=EDGE_CURVE('',#5564,#5565,#2313,.T.);
#7850=EDGE_CURVE('',#5566,#5565,#1841,.T.);
#7851=EDGE_CURVE('',#5563,#5566,#2314,.T.);
#7852=EDGE_CURVE('',#5567,#5568,#4042,.T.);
#7853=EDGE_CURVE('',#5568,#5569,#2315,.T.);
#7854=EDGE_CURVE('',#5569,#5564,#2316,.T.);
#7855=EDGE_CURVE('',#5570,#5563,#2317,.T.);
#7856=EDGE_CURVE('',#5567,#5570,#2318,.T.);
#7857=EDGE_CURVE('',#5571,#5572,#4043,.T.);
#7858=EDGE_CURVE('',#5572,#5573,#2319,.T.);
#7859=EDGE_CURVE('',#5573,#5568,#2320,.T.);
#7860=EDGE_CURVE('',#5574,#5567,#2321,.T.);
#7861=EDGE_CURVE('',#5571,#5574,#2322,.T.);
#7862=EDGE_CURVE('',#5575,#5576,#4044,.T.);
#7863=EDGE_CURVE('',#5576,#5577,#2323,.T.);
#7864=EDGE_CURVE('',#5577,#5572,#2324,.T.);
#7865=EDGE_CURVE('',#5578,#5571,#2325,.T.);
#7866=EDGE_CURVE('',#5575,#5578,#2326,.T.);
#7867=EDGE_CURVE('',#5579,#5580,#4045,.T.);
#7868=EDGE_CURVE('',#5580,#5581,#2327,.T.);
#7869=EDGE_CURVE('',#5581,#5576,#2328,.T.);
#7870=EDGE_CURVE('',#5582,#5575,#2329,.T.);
#7871=EDGE_CURVE('',#5579,#5582,#2330,.T.);
#7872=EDGE_CURVE('',#5583,#5584,#4046,.T.);
#7873=EDGE_CURVE('',#5584,#5585,#2331,.T.);
#7874=EDGE_CURVE('',#5585,#5580,#2332,.T.);
#7875=EDGE_CURVE('',#5586,#5579,#2333,.T.);
#7876=EDGE_CURVE('',#5583,#5586,#2334,.T.);
#7877=EDGE_CURVE('',#5587,#5588,#4047,.T.);
#7878=EDGE_CURVE('',#5588,#5589,#2335,.T.);
#7879=EDGE_CURVE('',#5589,#5584,#2336,.T.);
#7880=EDGE_CURVE('',#5590,#5583,#2337,.T.);
#7881=EDGE_CURVE('',#5587,#5590,#2338,.T.);
#7882=EDGE_CURVE('',#5591,#5592,#4048,.T.);
#7883=EDGE_CURVE('',#5592,#5593,#2339,.T.);
#7884=EDGE_CURVE('',#5593,#5588,#2340,.T.);
#7885=EDGE_CURVE('',#5594,#5587,#2341,.T.);
#7886=EDGE_CURVE('',#5591,#5594,#2342,.T.);
#7887=EDGE_CURVE('',#5595,#5596,#4049,.T.);
#7888=EDGE_CURVE('',#5596,#5597,#2343,.T.);
#7889=EDGE_CURVE('',#5597,#5592,#2344,.T.);
#7890=EDGE_CURVE('',#5598,#5591,#2345,.T.);
#7891=EDGE_CURVE('',#5595,#5598,#2346,.T.);
#7892=EDGE_CURVE('',#5599,#5600,#4050,.T.);
#7893=EDGE_CURVE('',#5600,#5601,#2347,.T.);
#7894=EDGE_CURVE('',#5601,#5596,#2348,.T.);
#7895=EDGE_CURVE('',#5602,#5595,#2349,.T.);
#7896=EDGE_CURVE('',#5599,#5602,#2350,.T.);
#7897=EDGE_CURVE('',#5603,#5604,#4051,.T.);
#7898=EDGE_CURVE('',#5604,#5605,#2351,.T.);
#7899=EDGE_CURVE('',#5605,#5600,#2352,.T.);
#7900=EDGE_CURVE('',#5606,#5599,#2353,.T.);
#7901=EDGE_CURVE('',#5603,#5606,#2354,.T.);
#7902=EDGE_CURVE('',#5607,#5608,#4052,.T.);
#7903=EDGE_CURVE('',#5608,#5609,#2355,.T.);
#7904=EDGE_CURVE('',#5609,#5604,#2356,.T.);
#7905=EDGE_CURVE('',#5610,#5603,#2357,.T.);
#7906=EDGE_CURVE('',#5607,#5610,#2358,.T.);
#7907=EDGE_CURVE('',#5611,#5612,#4053,.T.);
#7908=EDGE_CURVE('',#5612,#5613,#2359,.T.);
#7909=EDGE_CURVE('',#5613,#5608,#2360,.T.);
#7910=EDGE_CURVE('',#5614,#5607,#2361,.T.);
#7911=EDGE_CURVE('',#5611,#5614,#2362,.T.);
#7912=EDGE_CURVE('',#5615,#5616,#4054,.T.);
#7913=EDGE_CURVE('',#5616,#5617,#2363,.T.);
#7914=EDGE_CURVE('',#5617,#5612,#2364,.T.);
#7915=EDGE_CURVE('',#5618,#5611,#2365,.T.);
#7916=EDGE_CURVE('',#5615,#5618,#2366,.T.);
#7917=EDGE_CURVE('',#5619,#5620,#4055,.T.);
#7918=EDGE_CURVE('',#5620,#5621,#2367,.T.);
#7919=EDGE_CURVE('',#5621,#5616,#2368,.T.);
#7920=EDGE_CURVE('',#5622,#5615,#2369,.T.);
#7921=EDGE_CURVE('',#5619,#5622,#2370,.T.);
#7922=EDGE_CURVE('',#5623,#5624,#4056,.T.);
#7923=EDGE_CURVE('',#5625,#5623,#2371,.T.);
#7924=EDGE_CURVE('',#5626,#5625,#2372,.T.);
#7925=EDGE_CURVE('',#5627,#5626,#1842,.T.);
#7926=EDGE_CURVE('',#5627,#5628,#2373,.T.);
#7927=EDGE_CURVE('',#5628,#5624,#2374,.T.);
#7928=EDGE_CURVE('',#5629,#5630,#4057,.T.);
#7929=EDGE_CURVE('',#5630,#5631,#2375,.T.);
#7930=EDGE_CURVE('',#5631,#5632,#1843,.T.);
#7931=EDGE_CURVE('',#5632,#5633,#2376,.T.);
#7932=EDGE_CURVE('',#5633,#5634,#4058,.T.);
#7933=EDGE_CURVE('',#5634,#5634,#1844,.F.);
#7934=EDGE_CURVE('',#5633,#5629,#2377,.T.);
#7935=EDGE_CURVE('',#5635,#5636,#4059,.T.);
#7936=EDGE_CURVE('',#5636,#5630,#2378,.T.);
#7937=EDGE_CURVE('',#5629,#5637,#2379,.T.);
#7938=EDGE_CURVE('',#5637,#5635,#2380,.T.);
#7939=EDGE_CURVE('',#5638,#5639,#4060,.T.);
#7940=EDGE_CURVE('',#5639,#5640,#2381,.T.);
#7941=EDGE_CURVE('',#5640,#5636,#2382,.T.);
#7942=EDGE_CURVE('',#5635,#5641,#2383,.T.);
#7943=EDGE_CURVE('',#5641,#5638,#2384,.T.);
#7944=EDGE_CURVE('',#5642,#5643,#4061,.T.);
#7945=EDGE_CURVE('',#5643,#5639,#2385,.T.);
#7946=EDGE_CURVE('',#5638,#5642,#2386,.T.);
#7947=EDGE_CURVE('',#5644,#5645,#4062,.T.);
#7948=EDGE_CURVE('',#5645,#5646,#2387,.T.);
#7949=EDGE_CURVE('',#5646,#5643,#2388,.T.);
#7950=EDGE_CURVE('',#5642,#5647,#2389,.T.);
#7951=EDGE_CURVE('',#5647,#5644,#2390,.T.);
#7952=EDGE_CURVE('',#5648,#5649,#4063,.T.);
#7953=EDGE_CURVE('',#5649,#5645,#2391,.T.);
#7954=EDGE_CURVE('',#5644,#5648,#2392,.T.);
#7955=EDGE_CURVE('',#5650,#5651,#4064,.T.);
#7956=EDGE_CURVE('',#5651,#5652,#2393,.T.);
#7957=EDGE_CURVE('',#5652,#5649,#2394,.T.);
#7958=EDGE_CURVE('',#5648,#5653,#2395,.T.);
#7959=EDGE_CURVE('',#5653,#5650,#2396,.T.);
#7960=EDGE_CURVE('',#5654,#5655,#4065,.T.);
#7961=EDGE_CURVE('',#5655,#5651,#2397,.T.);
#7962=EDGE_CURVE('',#5650,#5654,#2398,.T.);
#7963=EDGE_CURVE('',#5656,#5657,#4066,.T.);
#7964=EDGE_CURVE('',#5657,#5658,#2399,.T.);
#7965=EDGE_CURVE('',#5658,#5655,#2400,.T.);
#7966=EDGE_CURVE('',#5654,#5659,#2401,.T.);
#7967=EDGE_CURVE('',#5659,#5656,#2402,.T.);
#7968=EDGE_CURVE('',#5660,#5661,#4067,.T.);
#7969=EDGE_CURVE('',#5661,#5657,#2403,.T.);
#7970=EDGE_CURVE('',#5656,#5660,#2404,.T.);
#7971=EDGE_CURVE('',#5662,#5663,#4068,.T.);
#7972=EDGE_CURVE('',#5663,#5664,#2405,.T.);
#7973=EDGE_CURVE('',#5664,#5661,#2406,.T.);
#7974=EDGE_CURVE('',#5660,#5665,#2407,.T.);
#7975=EDGE_CURVE('',#5665,#5662,#2408,.T.);
#7976=EDGE_CURVE('',#5666,#5667,#4069,.T.);
#7977=EDGE_CURVE('',#5667,#5663,#2409,.T.);
#7978=EDGE_CURVE('',#5662,#5666,#2410,.T.);
#7979=EDGE_CURVE('',#5668,#5669,#4070,.T.);
#7980=EDGE_CURVE('',#5669,#5670,#2411,.T.);
#7981=EDGE_CURVE('',#5670,#5667,#2412,.T.);
#7982=EDGE_CURVE('',#5666,#5671,#2413,.T.);
#7983=EDGE_CURVE('',#5671,#5668,#2414,.T.);
#7984=EDGE_CURVE('',#5672,#5673,#4071,.T.);
#7985=EDGE_CURVE('',#5673,#5669,#2415,.T.);
#7986=EDGE_CURVE('',#5668,#5672,#2416,.T.);
#7987=EDGE_CURVE('',#5674,#5675,#4072,.T.);
#7988=EDGE_CURVE('',#5674,#5676,#2417,.T.);
#7989=EDGE_CURVE('',#5677,#5676,#1845,.T.);
#7990=EDGE_CURVE('',#5677,#5675,#2418,.T.);
#7991=EDGE_CURVE('',#5678,#5679,#4073,.T.);
#7992=EDGE_CURVE('',#5679,#5680,#2419,.T.);
#7993=EDGE_CURVE('',#5681,#5680,#1846,.T.);
#7994=EDGE_CURVE('',#5678,#5681,#2420,.T.);
#7995=EDGE_CURVE('',#5682,#5683,#4074,.T.);
#7996=EDGE_CURVE('',#5683,#5684,#2421,.T.);
#7997=EDGE_CURVE('',#5684,#5679,#2422,.T.);
#7998=EDGE_CURVE('',#5685,#5678,#2423,.T.);
#7999=EDGE_CURVE('',#5682,#5685,#2424,.T.);
#8000=EDGE_CURVE('',#5686,#5687,#4075,.T.);
#8001=EDGE_CURVE('',#5687,#5688,#2425,.T.);
#8002=EDGE_CURVE('',#5688,#5683,#2426,.T.);
#8003=EDGE_CURVE('',#5689,#5682,#2427,.T.);
#8004=EDGE_CURVE('',#5686,#5689,#2428,.T.);
#8005=EDGE_CURVE('',#5690,#5691,#4076,.T.);
#8006=EDGE_CURVE('',#5691,#5692,#2429,.T.);
#8007=EDGE_CURVE('',#5692,#5687,#2430,.T.);
#8008=EDGE_CURVE('',#5693,#5686,#2431,.T.);
#8009=EDGE_CURVE('',#5690,#5693,#2432,.T.);
#8010=EDGE_CURVE('',#5694,#5695,#4077,.T.);
#8011=EDGE_CURVE('',#5695,#5696,#2433,.T.);
#8012=EDGE_CURVE('',#5696,#5691,#2434,.T.);
#8013=EDGE_CURVE('',#5697,#5690,#2435,.T.);
#8014=EDGE_CURVE('',#5694,#5697,#2436,.T.);
#8015=EDGE_CURVE('',#5698,#5699,#4078,.T.);
#8016=EDGE_CURVE('',#5699,#5700,#2437,.T.);
#8017=EDGE_CURVE('',#5700,#5695,#2438,.T.);
#8018=EDGE_CURVE('',#5701,#5694,#2439,.T.);
#8019=EDGE_CURVE('',#5698,#5701,#2440,.T.);
#8020=EDGE_CURVE('',#5702,#5703,#4079,.T.);
#8021=EDGE_CURVE('',#5703,#5704,#2441,.T.);
#8022=EDGE_CURVE('',#5704,#5699,#2442,.T.);
#8023=EDGE_CURVE('',#5705,#5698,#2443,.T.);
#8024=EDGE_CURVE('',#5702,#5705,#2444,.T.);
#8025=EDGE_CURVE('',#5706,#5707,#4080,.T.);
#8026=EDGE_CURVE('',#5707,#5708,#2445,.T.);
#8027=EDGE_CURVE('',#5708,#5703,#2446,.T.);
#8028=EDGE_CURVE('',#5709,#5702,#2447,.T.);
#8029=EDGE_CURVE('',#5706,#5709,#2448,.T.);
#8030=EDGE_CURVE('',#5710,#5711,#4081,.T.);
#8031=EDGE_CURVE('',#5711,#5712,#2449,.T.);
#8032=EDGE_CURVE('',#5712,#5707,#2450,.T.);
#8033=EDGE_CURVE('',#5713,#5706,#2451,.T.);
#8034=EDGE_CURVE('',#5710,#5713,#2452,.T.);
#8035=EDGE_CURVE('',#5714,#5715,#4082,.T.);
#8036=EDGE_CURVE('',#5715,#5716,#2453,.T.);
#8037=EDGE_CURVE('',#5716,#5711,#2454,.T.);
#8038=EDGE_CURVE('',#5717,#5710,#2455,.T.);
#8039=EDGE_CURVE('',#5714,#5717,#2456,.T.);
#8040=EDGE_CURVE('',#5718,#5719,#4083,.T.);
#8041=EDGE_CURVE('',#5719,#5720,#2457,.T.);
#8042=EDGE_CURVE('',#5720,#5715,#2458,.T.);
#8043=EDGE_CURVE('',#5721,#5714,#2459,.T.);
#8044=EDGE_CURVE('',#5718,#5721,#2460,.T.);
#8045=EDGE_CURVE('',#5722,#5723,#4084,.T.);
#8046=EDGE_CURVE('',#5723,#5724,#2461,.T.);
#8047=EDGE_CURVE('',#5724,#5719,#2462,.T.);
#8048=EDGE_CURVE('',#5725,#5718,#2463,.T.);
#8049=EDGE_CURVE('',#5722,#5725,#2464,.T.);
#8050=EDGE_CURVE('',#5726,#5727,#4085,.T.);
#8051=EDGE_CURVE('',#5727,#5728,#2465,.T.);
#8052=EDGE_CURVE('',#5728,#5723,#2466,.T.);
#8053=EDGE_CURVE('',#5729,#5722,#2467,.T.);
#8054=EDGE_CURVE('',#5726,#5729,#2468,.T.);
#8055=EDGE_CURVE('',#5730,#5731,#4086,.T.);
#8056=EDGE_CURVE('',#5731,#5732,#2469,.T.);
#8057=EDGE_CURVE('',#5732,#5727,#2470,.T.);
#8058=EDGE_CURVE('',#5733,#5726,#2471,.T.);
#8059=EDGE_CURVE('',#5730,#5733,#2472,.T.);
#8060=EDGE_CURVE('',#5734,#5735,#4087,.T.);
#8061=EDGE_CURVE('',#5735,#5736,#2473,.T.);
#8062=EDGE_CURVE('',#5736,#5731,#2474,.T.);
#8063=EDGE_CURVE('',#5737,#5730,#2475,.T.);
#8064=EDGE_CURVE('',#5734,#5737,#2476,.T.);
#8065=EDGE_CURVE('',#5738,#5739,#4088,.T.);
#8066=EDGE_CURVE('',#5740,#5738,#2477,.T.);
#8067=EDGE_CURVE('',#5741,#5740,#2478,.T.);
#8068=EDGE_CURVE('',#5742,#5741,#1847,.T.);
#8069=EDGE_CURVE('',#5742,#5743,#2479,.T.);
#8070=EDGE_CURVE('',#5743,#5739,#2480,.T.);
#8071=EDGE_CURVE('',#5744,#5745,#4089,.T.);
#8072=EDGE_CURVE('',#5745,#5746,#2481,.T.);
#8073=EDGE_CURVE('',#5746,#5747,#1848,.T.);
#8074=EDGE_CURVE('',#5747,#5748,#2482,.T.);
#8075=EDGE_CURVE('',#5748,#5749,#4090,.T.);
#8076=EDGE_CURVE('',#5749,#5749,#1849,.F.);
#8077=EDGE_CURVE('',#5748,#5744,#2483,.T.);
#8078=EDGE_CURVE('',#5750,#5751,#4091,.T.);
#8079=EDGE_CURVE('',#5751,#5745,#2484,.T.);
#8080=EDGE_CURVE('',#5744,#5752,#2485,.T.);
#8081=EDGE_CURVE('',#5752,#5750,#2486,.T.);
#8082=EDGE_CURVE('',#5753,#5754,#4092,.T.);
#8083=EDGE_CURVE('',#5754,#5755,#2487,.T.);
#8084=EDGE_CURVE('',#5755,#5751,#2488,.T.);
#8085=EDGE_CURVE('',#5750,#5756,#2489,.T.);
#8086=EDGE_CURVE('',#5756,#5753,#2490,.T.);
#8087=EDGE_CURVE('',#5757,#5758,#4093,.T.);
#8088=EDGE_CURVE('',#5758,#5754,#2491,.T.);
#8089=EDGE_CURVE('',#5753,#5757,#2492,.T.);
#8090=EDGE_CURVE('',#5759,#5760,#4094,.T.);
#8091=EDGE_CURVE('',#5760,#5761,#2493,.T.);
#8092=EDGE_CURVE('',#5761,#5758,#2494,.T.);
#8093=EDGE_CURVE('',#5757,#5762,#2495,.T.);
#8094=EDGE_CURVE('',#5762,#5759,#2496,.T.);
#8095=EDGE_CURVE('',#5763,#5764,#4095,.T.);
#8096=EDGE_CURVE('',#5764,#5760,#2497,.T.);
#8097=EDGE_CURVE('',#5759,#5763,#2498,.T.);
#8098=EDGE_CURVE('',#5765,#5766,#4096,.T.);
#8099=EDGE_CURVE('',#5766,#5767,#2499,.T.);
#8100=EDGE_CURVE('',#5767,#5764,#2500,.T.);
#8101=EDGE_CURVE('',#5763,#5768,#2501,.T.);
#8102=EDGE_CURVE('',#5768,#5765,#2502,.T.);
#8103=EDGE_CURVE('',#5769,#5770,#4097,.T.);
#8104=EDGE_CURVE('',#5770,#5766,#2503,.T.);
#8105=EDGE_CURVE('',#5765,#5769,#2504,.T.);
#8106=EDGE_CURVE('',#5771,#5772,#4098,.T.);
#8107=EDGE_CURVE('',#5772,#5773,#2505,.T.);
#8108=EDGE_CURVE('',#5773,#5770,#2506,.T.);
#8109=EDGE_CURVE('',#5769,#5774,#2507,.T.);
#8110=EDGE_CURVE('',#5774,#5771,#2508,.T.);
#8111=EDGE_CURVE('',#5775,#5776,#4099,.T.);
#8112=EDGE_CURVE('',#5776,#5772,#2509,.T.);
#8113=EDGE_CURVE('',#5771,#5775,#2510,.T.);
#8114=EDGE_CURVE('',#5777,#5778,#4100,.T.);
#8115=EDGE_CURVE('',#5778,#5779,#2511,.T.);
#8116=EDGE_CURVE('',#5779,#5776,#2512,.T.);
#8117=EDGE_CURVE('',#5775,#5780,#2513,.T.);
#8118=EDGE_CURVE('',#5780,#5777,#2514,.T.);
#8119=EDGE_CURVE('',#5781,#5782,#4101,.T.);
#8120=EDGE_CURVE('',#5782,#5778,#2515,.T.);
#8121=EDGE_CURVE('',#5777,#5781,#2516,.T.);
#8122=EDGE_CURVE('',#5783,#5784,#4102,.T.);
#8123=EDGE_CURVE('',#5784,#5785,#2517,.T.);
#8124=EDGE_CURVE('',#5785,#5782,#2518,.T.);
#8125=EDGE_CURVE('',#5781,#5786,#2519,.T.);
#8126=EDGE_CURVE('',#5786,#5783,#2520,.T.);
#8127=EDGE_CURVE('',#5787,#5788,#4103,.T.);
#8128=EDGE_CURVE('',#5788,#5784,#2521,.T.);
#8129=EDGE_CURVE('',#5783,#5787,#2522,.T.);
#8130=EDGE_CURVE('',#5789,#5790,#4104,.T.);
#8131=EDGE_CURVE('',#5789,#5791,#2523,.T.);
#8132=EDGE_CURVE('',#5792,#5791,#1850,.T.);
#8133=EDGE_CURVE('',#5792,#5790,#2524,.T.);
#8134=EDGE_CURVE('',#5793,#5794,#4105,.T.);
#8135=EDGE_CURVE('',#5794,#5795,#2525,.T.);
#8136=EDGE_CURVE('',#5796,#5795,#1851,.T.);
#8137=EDGE_CURVE('',#5797,#5796,#2526,.T.);
#8138=EDGE_CURVE('',#5793,#5797,#2527,.T.);
#8139=EDGE_CURVE('',#5798,#5799,#4106,.T.);
#8140=EDGE_CURVE('',#5799,#5800,#2528,.T.);
#8141=EDGE_CURVE('',#5800,#5794,#2529,.T.);
#8142=EDGE_CURVE('',#5801,#5793,#2530,.T.);
#8143=EDGE_CURVE('',#5798,#5801,#2531,.T.);
#8144=EDGE_CURVE('',#5802,#5803,#4107,.T.);
#8145=EDGE_CURVE('',#5803,#5804,#2532,.T.);
#8146=EDGE_CURVE('',#5804,#5799,#2533,.T.);
#8147=EDGE_CURVE('',#5805,#5798,#2534,.T.);
#8148=EDGE_CURVE('',#5802,#5805,#2535,.T.);
#8149=EDGE_CURVE('',#5806,#5807,#4108,.T.);
#8150=EDGE_CURVE('',#5807,#5808,#2536,.T.);
#8151=EDGE_CURVE('',#5808,#5803,#2537,.T.);
#8152=EDGE_CURVE('',#5809,#5802,#2538,.T.);
#8153=EDGE_CURVE('',#5806,#5809,#2539,.T.);
#8154=EDGE_CURVE('',#5810,#5811,#4109,.T.);
#8155=EDGE_CURVE('',#5811,#5812,#2540,.T.);
#8156=EDGE_CURVE('',#5812,#5807,#2541,.T.);
#8157=EDGE_CURVE('',#5813,#5806,#2542,.T.);
#8158=EDGE_CURVE('',#5810,#5813,#2543,.T.);
#8159=EDGE_CURVE('',#5814,#5815,#4110,.T.);
#8160=EDGE_CURVE('',#5815,#5816,#2544,.T.);
#8161=EDGE_CURVE('',#5816,#5811,#2545,.T.);
#8162=EDGE_CURVE('',#5817,#5810,#2546,.T.);
#8163=EDGE_CURVE('',#5814,#5817,#2547,.T.);
#8164=EDGE_CURVE('',#5818,#5819,#4111,.T.);
#8165=EDGE_CURVE('',#5819,#5820,#2548,.T.);
#8166=EDGE_CURVE('',#5820,#5815,#2549,.T.);
#8167=EDGE_CURVE('',#5821,#5814,#2550,.T.);
#8168=EDGE_CURVE('',#5818,#5821,#2551,.T.);
#8169=EDGE_CURVE('',#5822,#5823,#4112,.T.);
#8170=EDGE_CURVE('',#5823,#5824,#2552,.T.);
#8171=EDGE_CURVE('',#5824,#5819,#2553,.T.);
#8172=EDGE_CURVE('',#5825,#5818,#2554,.T.);
#8173=EDGE_CURVE('',#5822,#5825,#2555,.T.);
#8174=EDGE_CURVE('',#5826,#5827,#4113,.T.);
#8175=EDGE_CURVE('',#5827,#5828,#2556,.T.);
#8176=EDGE_CURVE('',#5828,#5823,#2557,.T.);
#8177=EDGE_CURVE('',#5829,#5822,#2558,.T.);
#8178=EDGE_CURVE('',#5826,#5829,#2559,.T.);
#8179=EDGE_CURVE('',#5830,#5831,#4114,.T.);
#8180=EDGE_CURVE('',#5831,#5832,#2560,.T.);
#8181=EDGE_CURVE('',#5832,#5827,#2561,.T.);
#8182=EDGE_CURVE('',#5833,#5826,#2562,.T.);
#8183=EDGE_CURVE('',#5830,#5833,#2563,.T.);
#8184=EDGE_CURVE('',#5834,#5835,#4115,.T.);
#8185=EDGE_CURVE('',#5835,#5836,#2564,.T.);
#8186=EDGE_CURVE('',#5836,#5831,#2565,.T.);
#8187=EDGE_CURVE('',#5837,#5830,#2566,.T.);
#8188=EDGE_CURVE('',#5834,#5837,#2567,.T.);
#8189=EDGE_CURVE('',#5838,#5839,#4116,.T.);
#8190=EDGE_CURVE('',#5839,#5840,#2568,.T.);
#8191=EDGE_CURVE('',#5840,#5835,#2569,.T.);
#8192=EDGE_CURVE('',#5841,#5834,#2570,.T.);
#8193=EDGE_CURVE('',#5838,#5841,#2571,.T.);
#8194=EDGE_CURVE('',#5842,#5843,#4117,.T.);
#8195=EDGE_CURVE('',#5843,#5844,#2572,.T.);
#8196=EDGE_CURVE('',#5844,#5839,#2573,.T.);
#8197=EDGE_CURVE('',#5845,#5838,#2574,.T.);
#8198=EDGE_CURVE('',#5842,#5845,#2575,.T.);
#8199=EDGE_CURVE('',#5846,#5847,#4118,.T.);
#8200=EDGE_CURVE('',#5848,#5846,#2576,.T.);
#8201=EDGE_CURVE('',#5849,#5848,#2577,.T.);
#8202=EDGE_CURVE('',#5850,#5849,#1852,.T.);
#8203=EDGE_CURVE('',#5850,#5851,#2578,.T.);
#8204=EDGE_CURVE('',#5851,#5847,#2579,.T.);
#8205=EDGE_CURVE('',#5852,#5853,#4119,.T.);
#8206=EDGE_CURVE('',#5853,#5854,#2580,.T.);
#8207=EDGE_CURVE('',#5855,#5854,#1853,.T.);
#8208=EDGE_CURVE('',#5856,#5855,#2581,.T.);
#8209=EDGE_CURVE('',#5852,#5856,#2582,.T.);
#8210=EDGE_CURVE('',#5857,#5858,#4120,.T.);
#8211=EDGE_CURVE('',#5858,#5859,#2583,.T.);
#8212=EDGE_CURVE('',#5859,#5853,#2584,.T.);
#8213=EDGE_CURVE('',#5860,#5852,#2585,.T.);
#8214=EDGE_CURVE('',#5857,#5860,#2586,.T.);
#8215=EDGE_CURVE('',#5861,#5862,#4121,.T.);
#8216=EDGE_CURVE('',#5862,#5863,#2587,.T.);
#8217=EDGE_CURVE('',#5863,#5858,#2588,.T.);
#8218=EDGE_CURVE('',#5864,#5857,#2589,.T.);
#8219=EDGE_CURVE('',#5861,#5864,#2590,.T.);
#8220=EDGE_CURVE('',#5865,#5866,#4122,.T.);
#8221=EDGE_CURVE('',#5866,#5867,#2591,.T.);
#8222=EDGE_CURVE('',#5867,#5862,#2592,.T.);
#8223=EDGE_CURVE('',#5868,#5861,#2593,.T.);
#8224=EDGE_CURVE('',#5865,#5868,#2594,.T.);
#8225=EDGE_CURVE('',#5869,#5870,#4123,.T.);
#8226=EDGE_CURVE('',#5870,#5871,#2595,.T.);
#8227=EDGE_CURVE('',#5871,#5866,#2596,.T.);
#8228=EDGE_CURVE('',#5872,#5865,#2597,.T.);
#8229=EDGE_CURVE('',#5869,#5872,#2598,.T.);
#8230=EDGE_CURVE('',#5873,#5874,#4124,.T.);
#8231=EDGE_CURVE('',#5874,#5875,#2599,.T.);
#8232=EDGE_CURVE('',#5875,#5870,#2600,.T.);
#8233=EDGE_CURVE('',#5876,#5869,#2601,.T.);
#8234=EDGE_CURVE('',#5873,#5876,#2602,.T.);
#8235=EDGE_CURVE('',#5877,#5878,#4125,.T.);
#8236=EDGE_CURVE('',#5878,#5879,#2603,.T.);
#8237=EDGE_CURVE('',#5879,#5874,#2604,.T.);
#8238=EDGE_CURVE('',#5880,#5873,#2605,.T.);
#8239=EDGE_CURVE('',#5877,#5880,#2606,.T.);
#8240=EDGE_CURVE('',#5881,#5882,#4126,.T.);
#8241=EDGE_CURVE('',#5882,#5883,#2607,.T.);
#8242=EDGE_CURVE('',#5883,#5878,#2608,.T.);
#8243=EDGE_CURVE('',#5884,#5877,#2609,.T.);
#8244=EDGE_CURVE('',#5881,#5884,#2610,.T.);
#8245=EDGE_CURVE('',#5885,#5886,#4127,.T.);
#8246=EDGE_CURVE('',#5886,#5887,#2611,.T.);
#8247=EDGE_CURVE('',#5887,#5882,#2612,.T.);
#8248=EDGE_CURVE('',#5888,#5881,#2613,.T.);
#8249=EDGE_CURVE('',#5885,#5888,#2614,.T.);
#8250=EDGE_CURVE('',#5889,#5890,#4128,.T.);
#8251=EDGE_CURVE('',#5890,#5891,#2615,.T.);
#8252=EDGE_CURVE('',#5891,#5886,#2616,.T.);
#8253=EDGE_CURVE('',#5892,#5885,#2617,.T.);
#8254=EDGE_CURVE('',#5889,#5892,#2618,.T.);
#8255=EDGE_CURVE('',#5893,#5894,#4129,.T.);
#8256=EDGE_CURVE('',#5894,#5895,#2619,.T.);
#8257=EDGE_CURVE('',#5895,#5890,#2620,.T.);
#8258=EDGE_CURVE('',#5896,#5889,#2621,.T.);
#8259=EDGE_CURVE('',#5893,#5896,#2622,.T.);
#8260=EDGE_CURVE('',#5897,#5898,#4130,.T.);
#8261=EDGE_CURVE('',#5898,#5899,#2623,.T.);
#8262=EDGE_CURVE('',#5899,#5894,#2624,.T.);
#8263=EDGE_CURVE('',#5900,#5893,#2625,.T.);
#8264=EDGE_CURVE('',#5897,#5900,#2626,.T.);
#8265=EDGE_CURVE('',#5901,#5902,#4131,.T.);
#8266=EDGE_CURVE('',#5902,#5903,#2627,.T.);
#8267=EDGE_CURVE('',#5903,#5898,#2628,.T.);
#8268=EDGE_CURVE('',#5904,#5897,#2629,.T.);
#8269=EDGE_CURVE('',#5901,#5904,#2630,.T.);
#8270=EDGE_CURVE('',#5905,#5906,#4132,.T.);
#8271=EDGE_CURVE('',#5907,#5905,#2631,.T.);
#8272=EDGE_CURVE('',#5908,#5907,#2632,.T.);
#8273=EDGE_CURVE('',#5909,#5908,#1854,.T.);
#8274=EDGE_CURVE('',#5909,#5910,#2633,.T.);
#8275=EDGE_CURVE('',#5910,#5906,#2634,.T.);
#8276=EDGE_CURVE('',#5911,#5912,#4133,.T.);
#8277=EDGE_CURVE('',#5912,#5913,#2635,.T.);
#8278=EDGE_CURVE('',#5914,#5913,#1855,.T.);
#8279=EDGE_CURVE('',#5915,#5914,#2636,.T.);
#8280=EDGE_CURVE('',#5911,#5915,#2637,.T.);
#8281=EDGE_CURVE('',#5916,#5917,#4134,.T.);
#8282=EDGE_CURVE('',#5917,#5918,#2638,.T.);
#8283=EDGE_CURVE('',#5918,#5912,#2639,.T.);
#8284=EDGE_CURVE('',#5919,#5911,#2640,.T.);
#8285=EDGE_CURVE('',#5916,#5919,#2641,.T.);
#8286=EDGE_CURVE('',#5920,#5921,#4135,.T.);
#8287=EDGE_CURVE('',#5921,#5922,#2642,.T.);
#8288=EDGE_CURVE('',#5922,#5917,#2643,.T.);
#8289=EDGE_CURVE('',#5923,#5916,#2644,.T.);
#8290=EDGE_CURVE('',#5920,#5923,#2645,.T.);
#8291=EDGE_CURVE('',#5924,#5925,#4136,.T.);
#8292=EDGE_CURVE('',#5925,#5926,#2646,.T.);
#8293=EDGE_CURVE('',#5926,#5921,#2647,.T.);
#8294=EDGE_CURVE('',#5927,#5920,#2648,.T.);
#8295=EDGE_CURVE('',#5924,#5927,#2649,.T.);
#8296=EDGE_CURVE('',#5928,#5929,#4137,.T.);
#8297=EDGE_CURVE('',#5929,#5930,#2650,.T.);
#8298=EDGE_CURVE('',#5930,#5925,#2651,.T.);
#8299=EDGE_CURVE('',#5931,#5924,#2652,.T.);
#8300=EDGE_CURVE('',#5928,#5931,#2653,.T.);
#8301=EDGE_CURVE('',#5932,#5933,#4138,.T.);
#8302=EDGE_CURVE('',#5933,#5934,#2654,.T.);
#8303=EDGE_CURVE('',#5934,#5929,#2655,.T.);
#8304=EDGE_CURVE('',#5935,#5928,#2656,.T.);
#8305=EDGE_CURVE('',#5932,#5935,#2657,.T.);
#8306=EDGE_CURVE('',#5936,#5937,#4139,.T.);
#8307=EDGE_CURVE('',#5937,#5938,#2658,.T.);
#8308=EDGE_CURVE('',#5938,#5933,#2659,.T.);
#8309=EDGE_CURVE('',#5939,#5932,#2660,.T.);
#8310=EDGE_CURVE('',#5936,#5939,#2661,.T.);
#8311=EDGE_CURVE('',#5940,#5941,#4140,.T.);
#8312=EDGE_CURVE('',#5941,#5942,#2662,.T.);
#8313=EDGE_CURVE('',#5942,#5937,#2663,.T.);
#8314=EDGE_CURVE('',#5943,#5936,#2664,.T.);
#8315=EDGE_CURVE('',#5940,#5943,#2665,.T.);
#8316=EDGE_CURVE('',#5944,#5945,#4141,.T.);
#8317=EDGE_CURVE('',#5945,#5946,#2666,.T.);
#8318=EDGE_CURVE('',#5946,#5941,#2667,.T.);
#8319=EDGE_CURVE('',#5947,#5940,#2668,.T.);
#8320=EDGE_CURVE('',#5944,#5947,#2669,.T.);
#8321=EDGE_CURVE('',#5948,#5949,#4142,.T.);
#8322=EDGE_CURVE('',#5949,#5950,#2670,.T.);
#8323=EDGE_CURVE('',#5950,#5945,#2671,.T.);
#8324=EDGE_CURVE('',#5951,#5944,#2672,.T.);
#8325=EDGE_CURVE('',#5948,#5951,#2673,.T.);
#8326=EDGE_CURVE('',#5952,#5953,#4143,.T.);
#8327=EDGE_CURVE('',#5953,#5954,#2674,.T.);
#8328=EDGE_CURVE('',#5954,#5949,#2675,.T.);
#8329=EDGE_CURVE('',#5955,#5948,#2676,.T.);
#8330=EDGE_CURVE('',#5952,#5955,#2677,.T.);
#8331=EDGE_CURVE('',#5956,#5957,#4144,.T.);
#8332=EDGE_CURVE('',#5957,#5958,#2678,.T.);
#8333=EDGE_CURVE('',#5958,#5953,#2679,.T.);
#8334=EDGE_CURVE('',#5959,#5952,#2680,.T.);
#8335=EDGE_CURVE('',#5956,#5959,#2681,.T.);
#8336=EDGE_CURVE('',#5960,#5961,#4145,.T.);
#8337=EDGE_CURVE('',#5961,#5962,#2682,.T.);
#8338=EDGE_CURVE('',#5962,#5957,#2683,.T.);
#8339=EDGE_CURVE('',#5963,#5956,#2684,.T.);
#8340=EDGE_CURVE('',#5960,#5963,#2685,.T.);
#8341=EDGE_CURVE('',#5964,#5965,#4146,.T.);
#8342=EDGE_CURVE('',#5966,#5964,#2686,.T.);
#8343=EDGE_CURVE('',#5967,#5966,#2687,.T.);
#8344=EDGE_CURVE('',#5968,#5967,#1856,.T.);
#8345=EDGE_CURVE('',#5968,#5969,#2688,.T.);
#8346=EDGE_CURVE('',#5969,#5965,#2689,.T.);
#8347=EDGE_CURVE('',#5970,#5971,#4147,.T.);
#8348=EDGE_CURVE('',#5971,#5972,#2690,.T.);
#8349=EDGE_CURVE('',#5973,#5972,#1857,.T.);
#8350=EDGE_CURVE('',#5974,#5973,#2691,.T.);
#8351=EDGE_CURVE('',#5970,#5974,#2692,.T.);
#8352=EDGE_CURVE('',#5975,#5976,#4148,.T.);
#8353=EDGE_CURVE('',#5976,#5977,#2693,.T.);
#8354=EDGE_CURVE('',#5977,#5971,#2694,.T.);
#8355=EDGE_CURVE('',#5978,#5970,#2695,.T.);
#8356=EDGE_CURVE('',#5975,#5978,#2696,.T.);
#8357=EDGE_CURVE('',#5979,#5980,#4149,.T.);
#8358=EDGE_CURVE('',#5980,#5981,#2697,.T.);
#8359=EDGE_CURVE('',#5981,#5976,#2698,.T.);
#8360=EDGE_CURVE('',#5982,#5975,#2699,.T.);
#8361=EDGE_CURVE('',#5979,#5982,#2700,.T.);
#8362=EDGE_CURVE('',#5983,#5984,#4150,.T.);
#8363=EDGE_CURVE('',#5984,#5985,#2701,.T.);
#8364=EDGE_CURVE('',#5985,#5980,#2702,.T.);
#8365=EDGE_CURVE('',#5986,#5979,#2703,.T.);
#8366=EDGE_CURVE('',#5983,#5986,#2704,.T.);
#8367=EDGE_CURVE('',#5987,#5988,#4151,.T.);
#8368=EDGE_CURVE('',#5988,#5989,#2705,.T.);
#8369=EDGE_CURVE('',#5989,#5984,#2706,.T.);
#8370=EDGE_CURVE('',#5990,#5983,#2707,.T.);
#8371=EDGE_CURVE('',#5987,#5990,#2708,.T.);
#8372=EDGE_CURVE('',#5991,#5992,#4152,.T.);
#8373=EDGE_CURVE('',#5992,#5993,#2709,.T.);
#8374=EDGE_CURVE('',#5993,#5988,#2710,.T.);
#8375=EDGE_CURVE('',#5994,#5987,#2711,.T.);
#8376=EDGE_CURVE('',#5991,#5994,#2712,.T.);
#8377=EDGE_CURVE('',#5995,#5996,#4153,.T.);
#8378=EDGE_CURVE('',#5996,#5997,#2713,.T.);
#8379=EDGE_CURVE('',#5997,#5992,#2714,.T.);
#8380=EDGE_CURVE('',#5998,#5991,#2715,.T.);
#8381=EDGE_CURVE('',#5995,#5998,#2716,.T.);
#8382=EDGE_CURVE('',#5999,#6000,#4154,.T.);
#8383=EDGE_CURVE('',#6000,#6001,#2717,.T.);
#8384=EDGE_CURVE('',#6001,#5996,#2718,.T.);
#8385=EDGE_CURVE('',#6002,#5995,#2719,.T.);
#8386=EDGE_CURVE('',#5999,#6002,#2720,.T.);
#8387=EDGE_CURVE('',#6003,#6004,#4155,.T.);
#8388=EDGE_CURVE('',#6004,#6005,#2721,.T.);
#8389=EDGE_CURVE('',#6005,#6000,#2722,.T.);
#8390=EDGE_CURVE('',#6006,#5999,#2723,.T.);
#8391=EDGE_CURVE('',#6003,#6006,#2724,.T.);
#8392=EDGE_CURVE('',#6007,#6008,#4156,.T.);
#8393=EDGE_CURVE('',#6008,#6009,#2725,.T.);
#8394=EDGE_CURVE('',#6009,#6004,#2726,.T.);
#8395=EDGE_CURVE('',#6010,#6003,#2727,.T.);
#8396=EDGE_CURVE('',#6007,#6010,#2728,.T.);
#8397=EDGE_CURVE('',#6011,#6012,#4157,.T.);
#8398=EDGE_CURVE('',#6012,#6013,#2729,.T.);
#8399=EDGE_CURVE('',#6013,#6008,#2730,.T.);
#8400=EDGE_CURVE('',#6014,#6007,#2731,.T.);
#8401=EDGE_CURVE('',#6011,#6014,#2732,.T.);
#8402=EDGE_CURVE('',#6015,#6016,#4158,.T.);
#8403=EDGE_CURVE('',#6016,#6017,#2733,.T.);
#8404=EDGE_CURVE('',#6017,#6012,#2734,.T.);
#8405=EDGE_CURVE('',#6018,#6011,#2735,.T.);
#8406=EDGE_CURVE('',#6015,#6018,#2736,.T.);
#8407=EDGE_CURVE('',#6019,#6020,#4159,.T.);
#8408=EDGE_CURVE('',#6020,#6021,#2737,.T.);
#8409=EDGE_CURVE('',#6021,#6016,#2738,.T.);
#8410=EDGE_CURVE('',#6022,#6015,#2739,.T.);
#8411=EDGE_CURVE('',#6019,#6022,#2740,.T.);
#8412=EDGE_CURVE('',#6023,#6024,#4160,.T.);
#8413=EDGE_CURVE('',#6025,#6023,#2741,.T.);
#8414=EDGE_CURVE('',#6026,#6025,#2742,.T.);
#8415=EDGE_CURVE('',#6027,#6026,#1858,.T.);
#8416=EDGE_CURVE('',#6027,#6028,#2743,.T.);
#8417=EDGE_CURVE('',#6028,#6024,#2744,.T.);
#8418=EDGE_CURVE('',#6029,#6030,#4161,.T.);
#8419=EDGE_CURVE('',#6030,#6031,#2745,.T.);
#8420=EDGE_CURVE('',#6031,#6032,#1859,.F.);
#8421=EDGE_CURVE('',#6032,#6029,#2746,.T.);
#8422=EDGE_CURVE('',#6033,#6034,#4162,.T.);
#8423=EDGE_CURVE('',#6034,#6035,#2747,.T.);
#8424=EDGE_CURVE('',#6035,#6030,#2748,.T.);
#8425=EDGE_CURVE('',#6029,#6033,#2749,.T.);
#8426=EDGE_CURVE('',#6036,#6037,#4163,.T.);
#8427=EDGE_CURVE('',#6037,#6034,#2750,.T.);
#8428=EDGE_CURVE('',#6033,#6038,#2751,.T.);
#8429=EDGE_CURVE('',#6038,#6036,#2752,.T.);
#8430=EDGE_CURVE('',#6039,#6040,#4164,.T.);
#8431=EDGE_CURVE('',#6040,#6041,#2753,.T.);
#8432=EDGE_CURVE('',#6041,#6037,#2754,.T.);
#8433=EDGE_CURVE('',#6036,#6039,#2755,.T.);
#8434=EDGE_CURVE('',#6042,#6043,#4165,.T.);
#8435=EDGE_CURVE('',#6043,#6040,#2756,.T.);
#8436=EDGE_CURVE('',#6039,#6044,#2757,.T.);
#8437=EDGE_CURVE('',#6044,#6042,#2758,.T.);
#8438=EDGE_CURVE('',#6045,#6046,#4166,.T.);
#8439=EDGE_CURVE('',#6046,#6047,#2759,.T.);
#8440=EDGE_CURVE('',#6047,#6043,#2760,.T.);
#8441=EDGE_CURVE('',#6042,#6045,#2761,.T.);
#8442=EDGE_CURVE('',#6048,#6049,#4167,.T.);
#8443=EDGE_CURVE('',#6049,#6046,#2762,.T.);
#8444=EDGE_CURVE('',#6045,#6050,#2763,.T.);
#8445=EDGE_CURVE('',#6050,#6048,#2764,.T.);
#8446=EDGE_CURVE('',#6051,#6052,#4168,.T.);
#8447=EDGE_CURVE('',#6052,#6053,#2765,.T.);
#8448=EDGE_CURVE('',#6053,#6049,#2766,.T.);
#8449=EDGE_CURVE('',#6048,#6054,#2767,.T.);
#8450=EDGE_CURVE('',#6054,#6051,#2768,.T.);
#8451=EDGE_CURVE('',#6055,#6056,#4169,.T.);
#8452=EDGE_CURVE('',#6056,#6052,#2769,.T.);
#8453=EDGE_CURVE('',#6051,#6057,#2770,.T.);
#8454=EDGE_CURVE('',#6057,#6055,#2771,.T.);
#8455=EDGE_CURVE('',#6058,#6059,#4170,.T.);
#8456=EDGE_CURVE('',#6059,#6060,#2772,.T.);
#8457=EDGE_CURVE('',#6060,#6056,#2773,.T.);
#8458=EDGE_CURVE('',#6055,#6058,#2774,.T.);
#8459=EDGE_CURVE('',#6061,#6062,#4171,.T.);
#8460=EDGE_CURVE('',#6062,#6059,#2775,.T.);
#8461=EDGE_CURVE('',#6058,#6063,#2776,.T.);
#8462=EDGE_CURVE('',#6063,#6061,#2777,.T.);
#8463=EDGE_CURVE('',#6064,#6065,#4172,.T.);
#8464=EDGE_CURVE('',#6065,#6066,#2778,.T.);
#8465=EDGE_CURVE('',#6066,#6062,#2779,.T.);
#8466=EDGE_CURVE('',#6061,#6064,#2780,.T.);
#8467=EDGE_CURVE('',#6067,#6068,#4173,.T.);
#8468=EDGE_CURVE('',#6068,#6065,#2781,.T.);
#8469=EDGE_CURVE('',#6064,#6069,#2782,.T.);
#8470=EDGE_CURVE('',#6069,#6067,#2783,.T.);
#8471=EDGE_CURVE('',#6070,#6071,#4174,.T.);
#8472=EDGE_CURVE('',#6070,#6072,#2784,.T.);
#8473=EDGE_CURVE('',#6072,#6073,#2785,.T.);
#8474=EDGE_CURVE('',#6074,#6073,#1860,.T.);
#8475=EDGE_CURVE('',#6074,#6071,#2786,.T.);
#8476=EDGE_CURVE('',#6075,#6076,#4175,.T.);
#8477=EDGE_CURVE('',#6076,#6077,#2787,.T.);
#8478=EDGE_CURVE('',#6077,#6078,#1861,.F.);
#8479=EDGE_CURVE('',#6078,#6075,#2788,.T.);
#8480=EDGE_CURVE('',#6079,#6080,#4176,.T.);
#8481=EDGE_CURVE('',#6080,#6081,#2789,.T.);
#8482=EDGE_CURVE('',#6081,#6076,#2790,.T.);
#8483=EDGE_CURVE('',#6075,#6079,#2791,.T.);
#8484=EDGE_CURVE('',#6082,#6083,#4177,.T.);
#8485=EDGE_CURVE('',#6083,#6080,#2792,.T.);
#8486=EDGE_CURVE('',#6079,#6084,#2793,.T.);
#8487=EDGE_CURVE('',#6084,#6082,#2794,.T.);
#8488=EDGE_CURVE('',#6085,#6086,#4178,.T.);
#8489=EDGE_CURVE('',#6086,#6087,#2795,.T.);
#8490=EDGE_CURVE('',#6087,#6083,#2796,.T.);
#8491=EDGE_CURVE('',#6082,#6085,#2797,.T.);
#8492=EDGE_CURVE('',#6088,#6089,#4179,.T.);
#8493=EDGE_CURVE('',#6089,#6086,#2798,.T.);
#8494=EDGE_CURVE('',#6085,#6090,#2799,.T.);
#8495=EDGE_CURVE('',#6090,#6088,#2800,.T.);
#8496=EDGE_CURVE('',#6091,#6092,#4180,.T.);
#8497=EDGE_CURVE('',#6092,#6093,#2801,.T.);
#8498=EDGE_CURVE('',#6093,#6089,#2802,.T.);
#8499=EDGE_CURVE('',#6088,#6091,#2803,.T.);
#8500=EDGE_CURVE('',#6094,#6095,#4181,.T.);
#8501=EDGE_CURVE('',#6095,#6092,#2804,.T.);
#8502=EDGE_CURVE('',#6091,#6096,#2805,.T.);
#8503=EDGE_CURVE('',#6096,#6094,#2806,.T.);
#8504=EDGE_CURVE('',#6097,#6098,#4182,.T.);
#8505=EDGE_CURVE('',#6098,#6099,#2807,.T.);
#8506=EDGE_CURVE('',#6099,#6095,#2808,.T.);
#8507=EDGE_CURVE('',#6094,#6100,#2809,.T.);
#8508=EDGE_CURVE('',#6100,#6097,#2810,.T.);
#8509=EDGE_CURVE('',#6101,#6102,#4183,.T.);
#8510=EDGE_CURVE('',#6102,#6098,#2811,.T.);
#8511=EDGE_CURVE('',#6097,#6103,#2812,.T.);
#8512=EDGE_CURVE('',#6103,#6101,#2813,.T.);
#8513=EDGE_CURVE('',#6104,#6105,#4184,.T.);
#8514=EDGE_CURVE('',#6105,#6106,#2814,.T.);
#8515=EDGE_CURVE('',#6106,#6102,#2815,.T.);
#8516=EDGE_CURVE('',#6101,#6104,#2816,.T.);
#8517=EDGE_CURVE('',#6107,#6108,#4185,.T.);
#8518=EDGE_CURVE('',#6108,#6105,#2817,.T.);
#8519=EDGE_CURVE('',#6104,#6109,#2818,.T.);
#8520=EDGE_CURVE('',#6109,#6107,#2819,.T.);
#8521=EDGE_CURVE('',#6110,#6111,#4186,.T.);
#8522=EDGE_CURVE('',#6111,#6112,#2820,.T.);
#8523=EDGE_CURVE('',#6112,#6108,#2821,.T.);
#8524=EDGE_CURVE('',#6107,#6110,#2822,.T.);
#8525=EDGE_CURVE('',#6113,#6114,#4187,.T.);
#8526=EDGE_CURVE('',#6114,#6111,#2823,.T.);
#8527=EDGE_CURVE('',#6110,#6115,#2824,.T.);
#8528=EDGE_CURVE('',#6115,#6113,#2825,.T.);
#8529=EDGE_CURVE('',#6116,#6117,#4188,.T.);
#8530=EDGE_CURVE('',#6116,#6118,#2826,.T.);
#8531=EDGE_CURVE('',#6118,#6119,#2827,.T.);
#8532=EDGE_CURVE('',#6120,#6119,#1862,.T.);
#8533=EDGE_CURVE('',#6120,#6117,#2828,.T.);
#8534=EDGE_CURVE('',#6121,#6122,#4189,.T.);
#8535=EDGE_CURVE('',#6122,#6123,#2829,.T.);
#8536=EDGE_CURVE('',#6123,#6124,#1863,.F.);
#8537=EDGE_CURVE('',#6124,#6121,#2830,.T.);
#8538=EDGE_CURVE('',#6125,#6126,#4190,.T.);
#8539=EDGE_CURVE('',#6126,#6122,#2831,.T.);
#8540=EDGE_CURVE('',#6121,#6125,#2832,.T.);
#8541=EDGE_CURVE('',#6127,#6128,#4191,.T.);
#8542=EDGE_CURVE('',#6128,#6126,#2833,.T.);
#8543=EDGE_CURVE('',#6125,#6129,#2834,.T.);
#8544=EDGE_CURVE('',#6129,#6127,#2835,.T.);
#8545=EDGE_CURVE('',#6130,#6131,#4192,.T.);
#8546=EDGE_CURVE('',#6131,#6128,#2836,.T.);
#8547=EDGE_CURVE('',#6127,#6130,#2837,.T.);
#8548=EDGE_CURVE('',#6132,#6133,#4193,.T.);
#8549=EDGE_CURVE('',#6133,#6131,#2838,.T.);
#8550=EDGE_CURVE('',#6130,#6134,#2839,.T.);
#8551=EDGE_CURVE('',#6134,#6132,#2840,.T.);
#8552=EDGE_CURVE('',#6135,#6136,#4194,.T.);
#8553=EDGE_CURVE('',#6136,#6137,#2841,.T.);
#8554=EDGE_CURVE('',#6137,#6133,#2842,.T.);
#8555=EDGE_CURVE('',#6132,#6135,#2843,.T.);
#8556=EDGE_CURVE('',#6138,#6139,#4195,.T.);
#8557=EDGE_CURVE('',#6139,#6136,#2844,.T.);
#8558=EDGE_CURVE('',#6135,#6140,#2845,.T.);
#8559=EDGE_CURVE('',#6140,#6138,#2846,.T.);
#8560=EDGE_CURVE('',#6141,#6142,#4196,.T.);
#8561=EDGE_CURVE('',#6142,#6143,#2847,.T.);
#8562=EDGE_CURVE('',#6143,#6139,#2848,.T.);
#8563=EDGE_CURVE('',#6138,#6144,#2849,.T.);
#8564=EDGE_CURVE('',#6144,#6141,#2850,.T.);
#8565=EDGE_CURVE('',#6145,#6146,#4197,.T.);
#8566=EDGE_CURVE('',#6146,#6142,#2851,.T.);
#8567=EDGE_CURVE('',#6141,#6147,#2852,.T.);
#8568=EDGE_CURVE('',#6147,#6145,#2853,.T.);
#8569=EDGE_CURVE('',#6148,#6149,#4198,.T.);
#8570=EDGE_CURVE('',#6149,#6150,#2854,.T.);
#8571=EDGE_CURVE('',#6150,#6146,#2855,.T.);
#8572=EDGE_CURVE('',#6145,#6148,#2856,.T.);
#8573=EDGE_CURVE('',#6151,#6152,#4199,.T.);
#8574=EDGE_CURVE('',#6152,#6149,#2857,.T.);
#8575=EDGE_CURVE('',#6148,#6153,#2858,.T.);
#8576=EDGE_CURVE('',#6153,#6151,#2859,.T.);
#8577=EDGE_CURVE('',#6154,#6155,#4200,.T.);
#8578=EDGE_CURVE('',#6155,#6156,#2860,.T.);
#8579=EDGE_CURVE('',#6156,#6152,#2861,.T.);
#8580=EDGE_CURVE('',#6151,#6154,#2862,.T.);
#8581=EDGE_CURVE('',#6157,#6158,#4201,.T.);
#8582=EDGE_CURVE('',#6158,#6155,#2863,.T.);
#8583=EDGE_CURVE('',#6154,#6157,#2864,.T.);
#8584=EDGE_CURVE('',#6159,#6160,#4202,.T.);
#8585=EDGE_CURVE('',#6159,#6161,#2865,.T.);
#8586=EDGE_CURVE('',#6162,#6161,#1864,.T.);
#8587=EDGE_CURVE('',#6162,#6160,#2866,.T.);
#8588=EDGE_CURVE('',#6163,#6164,#4203,.T.);
#8589=EDGE_CURVE('',#6164,#6165,#2867,.T.);
#8590=EDGE_CURVE('',#6165,#6166,#1865,.F.);
#8591=EDGE_CURVE('',#6166,#6163,#2868,.T.);
#8592=EDGE_CURVE('',#6167,#6168,#4204,.T.);
#8593=EDGE_CURVE('',#6168,#6164,#2869,.T.);
#8594=EDGE_CURVE('',#6163,#6167,#2870,.T.);
#8595=EDGE_CURVE('',#6169,#6170,#4205,.T.);
#8596=EDGE_CURVE('',#6170,#6168,#2871,.T.);
#8597=EDGE_CURVE('',#6167,#6171,#2872,.T.);
#8598=EDGE_CURVE('',#6171,#6169,#2873,.T.);
#8599=EDGE_CURVE('',#6172,#6173,#4206,.T.);
#8600=EDGE_CURVE('',#6173,#6170,#2874,.T.);
#8601=EDGE_CURVE('',#6169,#6172,#2875,.T.);
#8602=EDGE_CURVE('',#6174,#6175,#4207,.T.);
#8603=EDGE_CURVE('',#6175,#6173,#2876,.T.);
#8604=EDGE_CURVE('',#6172,#6176,#2877,.T.);
#8605=EDGE_CURVE('',#6176,#6174,#2878,.T.);
#8606=EDGE_CURVE('',#6177,#6178,#4208,.T.);
#8607=EDGE_CURVE('',#6178,#6179,#2879,.T.);
#8608=EDGE_CURVE('',#6179,#6175,#2880,.T.);
#8609=EDGE_CURVE('',#6174,#6177,#2881,.T.);
#8610=EDGE_CURVE('',#6180,#6181,#4209,.T.);
#8611=EDGE_CURVE('',#6181,#6178,#2882,.T.);
#8612=EDGE_CURVE('',#6177,#6182,#2883,.T.);
#8613=EDGE_CURVE('',#6182,#6180,#2884,.T.);
#8614=EDGE_CURVE('',#6183,#6184,#4210,.T.);
#8615=EDGE_CURVE('',#6184,#6185,#2885,.T.);
#8616=EDGE_CURVE('',#6185,#6181,#2886,.T.);
#8617=EDGE_CURVE('',#6180,#6186,#2887,.T.);
#8618=EDGE_CURVE('',#6186,#6183,#2888,.T.);
#8619=EDGE_CURVE('',#6187,#6188,#4211,.T.);
#8620=EDGE_CURVE('',#6188,#6184,#2889,.T.);
#8621=EDGE_CURVE('',#6183,#6189,#2890,.T.);
#8622=EDGE_CURVE('',#6189,#6187,#2891,.T.);
#8623=EDGE_CURVE('',#6190,#6191,#4212,.T.);
#8624=EDGE_CURVE('',#6191,#6192,#2892,.T.);
#8625=EDGE_CURVE('',#6192,#6188,#2893,.T.);
#8626=EDGE_CURVE('',#6187,#6190,#2894,.T.);
#8627=EDGE_CURVE('',#6193,#6194,#4213,.T.);
#8628=EDGE_CURVE('',#6194,#6191,#2895,.T.);
#8629=EDGE_CURVE('',#6190,#6195,#2896,.T.);
#8630=EDGE_CURVE('',#6195,#6193,#2897,.T.);
#8631=EDGE_CURVE('',#6196,#6197,#4214,.T.);
#8632=EDGE_CURVE('',#6197,#6198,#2898,.T.);
#8633=EDGE_CURVE('',#6198,#6194,#2899,.T.);
#8634=EDGE_CURVE('',#6193,#6196,#2900,.T.);
#8635=EDGE_CURVE('',#6199,#6200,#4215,.T.);
#8636=EDGE_CURVE('',#6200,#6197,#2901,.T.);
#8637=EDGE_CURVE('',#6196,#6199,#2902,.T.);
#8638=EDGE_CURVE('',#6201,#6202,#4216,.T.);
#8639=EDGE_CURVE('',#6201,#6203,#2903,.T.);
#8640=EDGE_CURVE('',#6204,#6203,#1866,.T.);
#8641=EDGE_CURVE('',#6204,#6202,#2904,.T.);
#8642=EDGE_CURVE('',#6202,#6205,#2905,.T.);
#8643=EDGE_CURVE('',#6205,#6200,#2906,.T.);
#8644=EDGE_CURVE('',#6199,#6201,#2907,.T.);
#8645=EDGE_CURVE('',#6160,#6206,#2908,.T.);
#8646=EDGE_CURVE('',#6206,#6158,#2909,.T.);
#8647=EDGE_CURVE('',#6157,#6159,#2910,.T.);
#8648=EDGE_CURVE('',#6117,#6207,#2911,.T.);
#8649=EDGE_CURVE('',#6207,#6114,#2912,.T.);
#8650=EDGE_CURVE('',#6113,#6116,#2913,.T.);
#8651=EDGE_CURVE('',#6071,#6208,#2914,.T.);
#8652=EDGE_CURVE('',#6208,#6068,#2915,.T.);
#8653=EDGE_CURVE('',#6067,#6070,#2916,.T.);
#8654=EDGE_CURVE('',#6024,#6209,#2917,.T.);
#8655=EDGE_CURVE('',#6209,#6020,#2918,.T.);
#8656=EDGE_CURVE('',#6210,#6019,#2919,.T.);
#8657=EDGE_CURVE('',#6023,#6210,#2920,.T.);
#8658=EDGE_CURVE('',#5965,#6211,#2921,.T.);
#8659=EDGE_CURVE('',#6211,#5961,#2922,.T.);
#8660=EDGE_CURVE('',#6212,#5960,#2923,.T.);
#8661=EDGE_CURVE('',#5964,#6212,#2924,.T.);
#8662=EDGE_CURVE('',#5906,#6213,#2925,.T.);
#8663=EDGE_CURVE('',#6213,#5902,#2926,.T.);
#8664=EDGE_CURVE('',#6214,#5901,#2927,.T.);
#8665=EDGE_CURVE('',#5905,#6214,#2928,.T.);
#8666=EDGE_CURVE('',#5847,#6215,#2929,.T.);
#8667=EDGE_CURVE('',#6215,#5843,#2930,.T.);
#8668=EDGE_CURVE('',#6216,#5842,#2931,.T.);
#8669=EDGE_CURVE('',#5846,#6216,#2932,.T.);
#8670=EDGE_CURVE('',#5790,#6217,#2933,.T.);
#8671=EDGE_CURVE('',#6217,#5788,#2934,.T.);
#8672=EDGE_CURVE('',#5787,#5789,#2935,.T.);
#8673=EDGE_CURVE('',#5739,#6218,#2936,.T.);
#8674=EDGE_CURVE('',#6218,#5735,#2937,.T.);
#8675=EDGE_CURVE('',#6219,#5734,#2938,.T.);
#8676=EDGE_CURVE('',#5738,#6219,#2939,.T.);
#8677=EDGE_CURVE('',#5675,#6220,#2940,.T.);
#8678=EDGE_CURVE('',#6220,#5673,#2941,.T.);
#8679=EDGE_CURVE('',#5672,#5674,#2942,.T.);
#8680=EDGE_CURVE('',#5624,#6221,#2943,.T.);
#8681=EDGE_CURVE('',#6221,#5620,#2944,.T.);
#8682=EDGE_CURVE('',#6222,#5619,#2945,.T.);
#8683=EDGE_CURVE('',#5623,#6222,#2946,.T.);
#8684=EDGE_CURVE('',#5631,#5566,#2947,.T.);
#8685=EDGE_CURVE('',#5565,#5632,#2948,.T.);
#8686=EDGE_CURVE('',#5676,#5627,#2949,.T.);
#8687=EDGE_CURVE('',#6223,#5677,#2950,.T.);
#8688=EDGE_CURVE('',#5626,#6223,#2951,.T.);
#8689=EDGE_CURVE('',#5746,#5681,#2952,.T.);
#8690=EDGE_CURVE('',#5680,#5747,#2953,.T.);
#8691=EDGE_CURVE('',#5791,#5742,#2954,.T.);
#8692=EDGE_CURVE('',#6224,#5792,#2955,.T.);
#8693=EDGE_CURVE('',#5741,#6224,#2956,.T.);
#8694=EDGE_CURVE('',#6225,#6226,#4217,.T.);
#8695=EDGE_CURVE('',#6227,#6225,#4218,.T.);
#8696=EDGE_CURVE('',#6228,#6227,#4219,.T.);
#8697=EDGE_CURVE('',#6228,#6226,#4220,.T.);
#8698=EDGE_CURVE('',#6226,#6229,#1867,.T.);
#8699=EDGE_CURVE('',#6230,#6228,#4221,.T.);
#8700=EDGE_CURVE('',#6230,#6229,#4222,.T.);
#8701=EDGE_CURVE('',#6229,#6231,#4223,.T.);
#8702=EDGE_CURVE('',#6232,#6230,#4224,.T.);
#8703=EDGE_CURVE('',#6232,#6231,#4225,.T.);
#8704=EDGE_CURVE('',#6231,#6225,#1868,.T.);
#8705=EDGE_CURVE('',#6227,#6232,#4226,.T.);
#8706=EDGE_CURVE('',#6233,#6233,#1869,.T.);
#8707=EDGE_CURVE('',#6233,#6234,#4227,.T.);
#8708=EDGE_CURVE('',#6234,#6234,#1870,.T.);
#8709=EDGE_CURVE('',#6235,#6235,#1871,.T.);
#8710=EDGE_CURVE('',#6235,#6236,#4228,.T.);
#8711=EDGE_CURVE('',#6236,#6236,#1872,.T.);
#8712=EDGE_CURVE('',#6237,#6237,#1873,.T.);
#8713=EDGE_CURVE('',#6237,#6238,#4229,.T.);
#8714=EDGE_CURVE('',#6238,#6238,#1874,.T.);
#8715=EDGE_CURVE('',#6239,#6239,#1875,.T.);
#8716=EDGE_CURVE('',#6239,#6240,#4230,.T.);
#8717=EDGE_CURVE('',#6240,#6240,#1876,.T.);
#8718=EDGE_CURVE('',#5795,#6241,#2957,.T.);
#8719=EDGE_CURVE('',#6119,#5850,#2958,.T.);
#8720=EDGE_CURVE('',#6078,#6241,#2959,.T.);
#8721=EDGE_CURVE('',#6077,#5796,#2960,.T.);
#8722=EDGE_CURVE('',#6242,#6120,#2961,.T.);
#8723=EDGE_CURVE('',#5849,#6242,#2962,.T.);
#8724=EDGE_CURVE('',#5854,#6243,#2963,.T.);
#8725=EDGE_CURVE('',#6073,#5909,#2964,.T.);
#8726=EDGE_CURVE('',#6032,#6243,#2965,.T.);
#8727=EDGE_CURVE('',#6031,#5855,#2966,.T.);
#8728=EDGE_CURVE('',#6244,#6074,#2967,.T.);
#8729=EDGE_CURVE('',#5908,#6244,#2968,.T.);
#8730=EDGE_CURVE('',#5913,#6245,#2969,.T.);
#8731=EDGE_CURVE('',#6203,#5968,#2970,.T.);
#8732=EDGE_CURVE('',#6166,#6245,#2971,.T.);
#8733=EDGE_CURVE('',#6165,#5914,#2972,.T.);
#8734=EDGE_CURVE('',#6246,#6204,#2973,.T.);
#8735=EDGE_CURVE('',#5967,#6246,#2974,.T.);
#8736=EDGE_CURVE('',#5972,#6247,#2975,.T.);
#8737=EDGE_CURVE('',#6161,#6027,#2976,.T.);
#8738=EDGE_CURVE('',#6124,#6247,#2977,.T.);
#8739=EDGE_CURVE('',#6123,#5973,#2978,.T.);
#8740=EDGE_CURVE('',#6248,#6162,#2979,.T.);
#8741=EDGE_CURVE('',#6026,#6248,#2980,.T.);
#8742=EDGE_CURVE('',#6249,#6249,#1877,.T.);
#8743=EDGE_CURVE('',#6249,#6250,#4231,.T.);
#8744=EDGE_CURVE('',#6250,#6250,#1878,.T.);
#8745=EDGE_CURVE('',#6251,#6252,#4232,.T.);
#8746=EDGE_CURVE('',#6252,#6253,#4233,.T.);
#8747=EDGE_CURVE('',#6253,#6254,#4234,.T.);
#8748=EDGE_CURVE('',#6254,#6251,#4235,.T.);
#8749=EDGE_CURVE('',#6255,#6256,#4236,.T.);
#8750=EDGE_CURVE('',#6257,#6255,#4237,.T.);
#8751=EDGE_CURVE('',#6258,#6257,#4238,.T.);
#8752=EDGE_CURVE('',#6256,#6258,#4239,.T.);
#8753=EDGE_CURVE('',#6259,#6260,#4240,.T.);
#8754=EDGE_CURVE('',#6260,#6251,#4241,.T.);
#8755=EDGE_CURVE('',#6259,#6254,#4242,.T.);
#8756=EDGE_CURVE('',#6261,#6259,#4243,.T.);
#8757=EDGE_CURVE('',#6261,#6253,#4244,.T.);
#8758=EDGE_CURVE('',#6262,#6261,#4245,.T.);
#8759=EDGE_CURVE('',#6262,#6252,#4246,.T.);
#8760=EDGE_CURVE('',#6260,#6262,#4247,.T.);
#8761=EDGE_CURVE('',#6256,#6263,#4248,.T.);
#8762=EDGE_CURVE('',#6264,#6263,#4249,.T.);
#8763=EDGE_CURVE('',#6255,#6264,#4250,.T.);
#8764=EDGE_CURVE('',#6265,#6264,#4251,.T.);
#8765=EDGE_CURVE('',#6257,#6265,#4252,.T.);
#8766=EDGE_CURVE('',#6266,#6265,#4253,.T.);
#8767=EDGE_CURVE('',#6258,#6266,#4254,.T.);
#8768=EDGE_CURVE('',#6263,#6266,#4255,.T.);
#11073=ORIENTED_EDGE('',*,*,#7848,.T.);
#11074=ORIENTED_EDGE('',*,*,#7849,.T.);
#11075=ORIENTED_EDGE('',*,*,#7850,.F.);
#11076=ORIENTED_EDGE('',*,*,#7851,.F.);
#11077=ORIENTED_EDGE('',*,*,#7852,.T.);
#11078=ORIENTED_EDGE('',*,*,#7853,.T.);
#11079=ORIENTED_EDGE('',*,*,#7854,.T.);
#11080=ORIENTED_EDGE('',*,*,#7848,.F.);
#11081=ORIENTED_EDGE('',*,*,#7855,.F.);
#11082=ORIENTED_EDGE('',*,*,#7856,.F.);
#11083=ORIENTED_EDGE('',*,*,#7857,.T.);
#11084=ORIENTED_EDGE('',*,*,#7858,.T.);
#11085=ORIENTED_EDGE('',*,*,#7859,.T.);
#11086=ORIENTED_EDGE('',*,*,#7852,.F.);
#11087=ORIENTED_EDGE('',*,*,#7860,.F.);
#11088=ORIENTED_EDGE('',*,*,#7861,.F.);
#11089=ORIENTED_EDGE('',*,*,#7862,.T.);
#11090=ORIENTED_EDGE('',*,*,#7863,.T.);
#11091=ORIENTED_EDGE('',*,*,#7864,.T.);
#11092=ORIENTED_EDGE('',*,*,#7857,.F.);
#11093=ORIENTED_EDGE('',*,*,#7865,.F.);
#11094=ORIENTED_EDGE('',*,*,#7866,.F.);
#11095=ORIENTED_EDGE('',*,*,#7867,.T.);
#11096=ORIENTED_EDGE('',*,*,#7868,.T.);
#11097=ORIENTED_EDGE('',*,*,#7869,.T.);
#11098=ORIENTED_EDGE('',*,*,#7862,.F.);
#11099=ORIENTED_EDGE('',*,*,#7870,.F.);
#11100=ORIENTED_EDGE('',*,*,#7871,.F.);
#11101=ORIENTED_EDGE('',*,*,#7872,.T.);
#11102=ORIENTED_EDGE('',*,*,#7873,.T.);
#11103=ORIENTED_EDGE('',*,*,#7874,.T.);
#11104=ORIENTED_EDGE('',*,*,#7867,.F.);
#11105=ORIENTED_EDGE('',*,*,#7875,.F.);
#11106=ORIENTED_EDGE('',*,*,#7876,.F.);
#11107=ORIENTED_EDGE('',*,*,#7877,.T.);
#11108=ORIENTED_EDGE('',*,*,#7878,.T.);
#11109=ORIENTED_EDGE('',*,*,#7879,.T.);
#11110=ORIENTED_EDGE('',*,*,#7872,.F.);
#11111=ORIENTED_EDGE('',*,*,#7880,.F.);
#11112=ORIENTED_EDGE('',*,*,#7881,.F.);
#11113=ORIENTED_EDGE('',*,*,#7882,.T.);
#11114=ORIENTED_EDGE('',*,*,#7883,.T.);
#11115=ORIENTED_EDGE('',*,*,#7884,.T.);
#11116=ORIENTED_EDGE('',*,*,#7877,.F.);
#11117=ORIENTED_EDGE('',*,*,#7885,.F.);
#11118=ORIENTED_EDGE('',*,*,#7886,.F.);
#11119=ORIENTED_EDGE('',*,*,#7887,.T.);
#11120=ORIENTED_EDGE('',*,*,#7888,.T.);
#11121=ORIENTED_EDGE('',*,*,#7889,.T.);
#11122=ORIENTED_EDGE('',*,*,#7882,.F.);
#11123=ORIENTED_EDGE('',*,*,#7890,.F.);
#11124=ORIENTED_EDGE('',*,*,#7891,.F.);
#11125=ORIENTED_EDGE('',*,*,#7892,.T.);
#11126=ORIENTED_EDGE('',*,*,#7893,.T.);
#11127=ORIENTED_EDGE('',*,*,#7894,.T.);
#11128=ORIENTED_EDGE('',*,*,#7887,.F.);
#11129=ORIENTED_EDGE('',*,*,#7895,.F.);
#11130=ORIENTED_EDGE('',*,*,#7896,.F.);
#11131=ORIENTED_EDGE('',*,*,#7897,.T.);
#11132=ORIENTED_EDGE('',*,*,#7898,.T.);
#11133=ORIENTED_EDGE('',*,*,#7899,.T.);
#11134=ORIENTED_EDGE('',*,*,#7892,.F.);
#11135=ORIENTED_EDGE('',*,*,#7900,.F.);
#11136=ORIENTED_EDGE('',*,*,#7901,.F.);
#11137=ORIENTED_EDGE('',*,*,#7902,.T.);
#11138=ORIENTED_EDGE('',*,*,#7903,.T.);
#11139=ORIENTED_EDGE('',*,*,#7904,.T.);
#11140=ORIENTED_EDGE('',*,*,#7897,.F.);
#11141=ORIENTED_EDGE('',*,*,#7905,.F.);
#11142=ORIENTED_EDGE('',*,*,#7906,.F.);
#11143=ORIENTED_EDGE('',*,*,#7907,.T.);
#11144=ORIENTED_EDGE('',*,*,#7908,.T.);
#11145=ORIENTED_EDGE('',*,*,#7909,.T.);
#11146=ORIENTED_EDGE('',*,*,#7902,.F.);
#11147=ORIENTED_EDGE('',*,*,#7910,.F.);
#11148=ORIENTED_EDGE('',*,*,#7911,.F.);
#11149=ORIENTED_EDGE('',*,*,#7912,.T.);
#11150=ORIENTED_EDGE('',*,*,#7913,.T.);
#11151=ORIENTED_EDGE('',*,*,#7914,.T.);
#11152=ORIENTED_EDGE('',*,*,#7907,.F.);
#11153=ORIENTED_EDGE('',*,*,#7915,.F.);
#11154=ORIENTED_EDGE('',*,*,#7916,.F.);
#11155=ORIENTED_EDGE('',*,*,#7917,.T.);
#11156=ORIENTED_EDGE('',*,*,#7918,.T.);
#11157=ORIENTED_EDGE('',*,*,#7919,.T.);
#11158=ORIENTED_EDGE('',*,*,#7912,.F.);
#11159=ORIENTED_EDGE('',*,*,#7920,.F.);
#11160=ORIENTED_EDGE('',*,*,#7921,.F.);
#11161=ORIENTED_EDGE('',*,*,#7922,.F.);
#11162=ORIENTED_EDGE('',*,*,#7923,.F.);
#11163=ORIENTED_EDGE('',*,*,#7924,.F.);
#11164=ORIENTED_EDGE('',*,*,#7925,.F.);
#11165=ORIENTED_EDGE('',*,*,#7926,.T.);
#11166=ORIENTED_EDGE('',*,*,#7927,.T.);
#11167=ORIENTED_EDGE('',*,*,#7928,.T.);
#11168=ORIENTED_EDGE('',*,*,#7929,.T.);
#11169=ORIENTED_EDGE('',*,*,#7930,.T.);
#11170=ORIENTED_EDGE('',*,*,#7931,.T.);
#11171=ORIENTED_EDGE('',*,*,#7932,.T.);
#11172=ORIENTED_EDGE('',*,*,#7933,.T.);
#11173=ORIENTED_EDGE('',*,*,#7932,.F.);
#11174=ORIENTED_EDGE('',*,*,#7934,.T.);
#11175=ORIENTED_EDGE('',*,*,#7935,.T.);
#11176=ORIENTED_EDGE('',*,*,#7936,.T.);
#11177=ORIENTED_EDGE('',*,*,#7928,.F.);
#11178=ORIENTED_EDGE('',*,*,#7937,.T.);
#11179=ORIENTED_EDGE('',*,*,#7938,.T.);
#11180=ORIENTED_EDGE('',*,*,#7939,.T.);
#11181=ORIENTED_EDGE('',*,*,#7940,.T.);
#11182=ORIENTED_EDGE('',*,*,#7941,.T.);
#11183=ORIENTED_EDGE('',*,*,#7935,.F.);
#11184=ORIENTED_EDGE('',*,*,#7942,.T.);
#11185=ORIENTED_EDGE('',*,*,#7943,.T.);
#11186=ORIENTED_EDGE('',*,*,#7944,.T.);
#11187=ORIENTED_EDGE('',*,*,#7945,.T.);
#11188=ORIENTED_EDGE('',*,*,#7939,.F.);
#11189=ORIENTED_EDGE('',*,*,#7946,.T.);
#11190=ORIENTED_EDGE('',*,*,#7947,.T.);
#11191=ORIENTED_EDGE('',*,*,#7948,.T.);
#11192=ORIENTED_EDGE('',*,*,#7949,.T.);
#11193=ORIENTED_EDGE('',*,*,#7944,.F.);
#11194=ORIENTED_EDGE('',*,*,#7950,.T.);
#11195=ORIENTED_EDGE('',*,*,#7951,.T.);
#11196=ORIENTED_EDGE('',*,*,#7952,.T.);
#11197=ORIENTED_EDGE('',*,*,#7953,.T.);
#11198=ORIENTED_EDGE('',*,*,#7947,.F.);
#11199=ORIENTED_EDGE('',*,*,#7954,.T.);
#11200=ORIENTED_EDGE('',*,*,#7955,.T.);
#11201=ORIENTED_EDGE('',*,*,#7956,.T.);
#11202=ORIENTED_EDGE('',*,*,#7957,.T.);
#11203=ORIENTED_EDGE('',*,*,#7952,.F.);
#11204=ORIENTED_EDGE('',*,*,#7958,.T.);
#11205=ORIENTED_EDGE('',*,*,#7959,.T.);
#11206=ORIENTED_EDGE('',*,*,#7960,.T.);
#11207=ORIENTED_EDGE('',*,*,#7961,.T.);
#11208=ORIENTED_EDGE('',*,*,#7955,.F.);
#11209=ORIENTED_EDGE('',*,*,#7962,.T.);
#11210=ORIENTED_EDGE('',*,*,#7963,.T.);
#11211=ORIENTED_EDGE('',*,*,#7964,.T.);
#11212=ORIENTED_EDGE('',*,*,#7965,.T.);
#11213=ORIENTED_EDGE('',*,*,#7960,.F.);
#11214=ORIENTED_EDGE('',*,*,#7966,.T.);
#11215=ORIENTED_EDGE('',*,*,#7967,.T.);
#11216=ORIENTED_EDGE('',*,*,#7968,.T.);
#11217=ORIENTED_EDGE('',*,*,#7969,.T.);
#11218=ORIENTED_EDGE('',*,*,#7963,.F.);
#11219=ORIENTED_EDGE('',*,*,#7970,.T.);
#11220=ORIENTED_EDGE('',*,*,#7971,.T.);
#11221=ORIENTED_EDGE('',*,*,#7972,.T.);
#11222=ORIENTED_EDGE('',*,*,#7973,.T.);
#11223=ORIENTED_EDGE('',*,*,#7968,.F.);
#11224=ORIENTED_EDGE('',*,*,#7974,.T.);
#11225=ORIENTED_EDGE('',*,*,#7975,.T.);
#11226=ORIENTED_EDGE('',*,*,#7976,.T.);
#11227=ORIENTED_EDGE('',*,*,#7977,.T.);
#11228=ORIENTED_EDGE('',*,*,#7971,.F.);
#11229=ORIENTED_EDGE('',*,*,#7978,.T.);
#11230=ORIENTED_EDGE('',*,*,#7979,.T.);
#11231=ORIENTED_EDGE('',*,*,#7980,.T.);
#11232=ORIENTED_EDGE('',*,*,#7981,.T.);
#11233=ORIENTED_EDGE('',*,*,#7976,.F.);
#11234=ORIENTED_EDGE('',*,*,#7982,.T.);
#11235=ORIENTED_EDGE('',*,*,#7983,.T.);
#11236=ORIENTED_EDGE('',*,*,#7984,.T.);
#11237=ORIENTED_EDGE('',*,*,#7985,.T.);
#11238=ORIENTED_EDGE('',*,*,#7979,.F.);
#11239=ORIENTED_EDGE('',*,*,#7986,.T.);
#11240=ORIENTED_EDGE('',*,*,#7987,.F.);
#11241=ORIENTED_EDGE('',*,*,#7988,.T.);
#11242=ORIENTED_EDGE('',*,*,#7989,.F.);
#11243=ORIENTED_EDGE('',*,*,#7990,.T.);
#11244=ORIENTED_EDGE('',*,*,#7991,.T.);
#11245=ORIENTED_EDGE('',*,*,#7992,.T.);
#11246=ORIENTED_EDGE('',*,*,#7993,.F.);
#11247=ORIENTED_EDGE('',*,*,#7994,.F.);
#11248=ORIENTED_EDGE('',*,*,#7995,.T.);
#11249=ORIENTED_EDGE('',*,*,#7996,.T.);
#11250=ORIENTED_EDGE('',*,*,#7997,.T.);
#11251=ORIENTED_EDGE('',*,*,#7991,.F.);
#11252=ORIENTED_EDGE('',*,*,#7998,.F.);
#11253=ORIENTED_EDGE('',*,*,#7999,.F.);
#11254=ORIENTED_EDGE('',*,*,#8000,.T.);
#11255=ORIENTED_EDGE('',*,*,#8001,.T.);
#11256=ORIENTED_EDGE('',*,*,#8002,.T.);
#11257=ORIENTED_EDGE('',*,*,#7995,.F.);
#11258=ORIENTED_EDGE('',*,*,#8003,.F.);
#11259=ORIENTED_EDGE('',*,*,#8004,.F.);
#11260=ORIENTED_EDGE('',*,*,#8005,.T.);
#11261=ORIENTED_EDGE('',*,*,#8006,.T.);
#11262=ORIENTED_EDGE('',*,*,#8007,.T.);
#11263=ORIENTED_EDGE('',*,*,#8000,.F.);
#11264=ORIENTED_EDGE('',*,*,#8008,.F.);
#11265=ORIENTED_EDGE('',*,*,#8009,.F.);
#11266=ORIENTED_EDGE('',*,*,#8010,.T.);
#11267=ORIENTED_EDGE('',*,*,#8011,.T.);
#11268=ORIENTED_EDGE('',*,*,#8012,.T.);
#11269=ORIENTED_EDGE('',*,*,#8005,.F.);
#11270=ORIENTED_EDGE('',*,*,#8013,.F.);
#11271=ORIENTED_EDGE('',*,*,#8014,.F.);
#11272=ORIENTED_EDGE('',*,*,#8015,.T.);
#11273=ORIENTED_EDGE('',*,*,#8016,.T.);
#11274=ORIENTED_EDGE('',*,*,#8017,.T.);
#11275=ORIENTED_EDGE('',*,*,#8010,.F.);
#11276=ORIENTED_EDGE('',*,*,#8018,.F.);
#11277=ORIENTED_EDGE('',*,*,#8019,.F.);
#11278=ORIENTED_EDGE('',*,*,#8020,.T.);
#11279=ORIENTED_EDGE('',*,*,#8021,.T.);
#11280=ORIENTED_EDGE('',*,*,#8022,.T.);
#11281=ORIENTED_EDGE('',*,*,#8015,.F.);
#11282=ORIENTED_EDGE('',*,*,#8023,.F.);
#11283=ORIENTED_EDGE('',*,*,#8024,.F.);
#11284=ORIENTED_EDGE('',*,*,#8025,.T.);
#11285=ORIENTED_EDGE('',*,*,#8026,.T.);
#11286=ORIENTED_EDGE('',*,*,#8027,.T.);
#11287=ORIENTED_EDGE('',*,*,#8020,.F.);
#11288=ORIENTED_EDGE('',*,*,#8028,.F.);
#11289=ORIENTED_EDGE('',*,*,#8029,.F.);
#11290=ORIENTED_EDGE('',*,*,#8030,.T.);
#11291=ORIENTED_EDGE('',*,*,#8031,.T.);
#11292=ORIENTED_EDGE('',*,*,#8032,.T.);
#11293=ORIENTED_EDGE('',*,*,#8025,.F.);
#11294=ORIENTED_EDGE('',*,*,#8033,.F.);
#11295=ORIENTED_EDGE('',*,*,#8034,.F.);
#11296=ORIENTED_EDGE('',*,*,#8035,.T.);
#11297=ORIENTED_EDGE('',*,*,#8036,.T.);
#11298=ORIENTED_EDGE('',*,*,#8037,.T.);
#11299=ORIENTED_EDGE('',*,*,#8030,.F.);
#11300=ORIENTED_EDGE('',*,*,#8038,.F.);
#11301=ORIENTED_EDGE('',*,*,#8039,.F.);
#11302=ORIENTED_EDGE('',*,*,#8040,.T.);
#11303=ORIENTED_EDGE('',*,*,#8041,.T.);
#11304=ORIENTED_EDGE('',*,*,#8042,.T.);
#11305=ORIENTED_EDGE('',*,*,#8035,.F.);
#11306=ORIENTED_EDGE('',*,*,#8043,.F.);
#11307=ORIENTED_EDGE('',*,*,#8044,.F.);
#11308=ORIENTED_EDGE('',*,*,#8045,.T.);
#11309=ORIENTED_EDGE('',*,*,#8046,.T.);
#11310=ORIENTED_EDGE('',*,*,#8047,.T.);
#11311=ORIENTED_EDGE('',*,*,#8040,.F.);
#11312=ORIENTED_EDGE('',*,*,#8048,.F.);
#11313=ORIENTED_EDGE('',*,*,#8049,.F.);
#11314=ORIENTED_EDGE('',*,*,#8050,.T.);
#11315=ORIENTED_EDGE('',*,*,#8051,.T.);
#11316=ORIENTED_EDGE('',*,*,#8052,.T.);
#11317=ORIENTED_EDGE('',*,*,#8045,.F.);
#11318=ORIENTED_EDGE('',*,*,#8053,.F.);
#11319=ORIENTED_EDGE('',*,*,#8054,.F.);
#11320=ORIENTED_EDGE('',*,*,#8055,.T.);
#11321=ORIENTED_EDGE('',*,*,#8056,.T.);
#11322=ORIENTED_EDGE('',*,*,#8057,.T.);
#11323=ORIENTED_EDGE('',*,*,#8050,.F.);
#11324=ORIENTED_EDGE('',*,*,#8058,.F.);
#11325=ORIENTED_EDGE('',*,*,#8059,.F.);
#11326=ORIENTED_EDGE('',*,*,#8060,.T.);
#11327=ORIENTED_EDGE('',*,*,#8061,.T.);
#11328=ORIENTED_EDGE('',*,*,#8062,.T.);
#11329=ORIENTED_EDGE('',*,*,#8055,.F.);
#11330=ORIENTED_EDGE('',*,*,#8063,.F.);
#11331=ORIENTED_EDGE('',*,*,#8064,.F.);
#11332=ORIENTED_EDGE('',*,*,#8065,.F.);
#11333=ORIENTED_EDGE('',*,*,#8066,.F.);
#11334=ORIENTED_EDGE('',*,*,#8067,.F.);
#11335=ORIENTED_EDGE('',*,*,#8068,.F.);
#11336=ORIENTED_EDGE('',*,*,#8069,.T.);
#11337=ORIENTED_EDGE('',*,*,#8070,.T.);
#11338=ORIENTED_EDGE('',*,*,#8071,.T.);
#11339=ORIENTED_EDGE('',*,*,#8072,.T.);
#11340=ORIENTED_EDGE('',*,*,#8073,.T.);
#11341=ORIENTED_EDGE('',*,*,#8074,.T.);
#11342=ORIENTED_EDGE('',*,*,#8075,.T.);
#11343=ORIENTED_EDGE('',*,*,#8076,.T.);
#11344=ORIENTED_EDGE('',*,*,#8075,.F.);
#11345=ORIENTED_EDGE('',*,*,#8077,.T.);
#11346=ORIENTED_EDGE('',*,*,#8078,.T.);
#11347=ORIENTED_EDGE('',*,*,#8079,.T.);
#11348=ORIENTED_EDGE('',*,*,#8071,.F.);
#11349=ORIENTED_EDGE('',*,*,#8080,.T.);
#11350=ORIENTED_EDGE('',*,*,#8081,.T.);
#11351=ORIENTED_EDGE('',*,*,#8082,.T.);
#11352=ORIENTED_EDGE('',*,*,#8083,.T.);
#11353=ORIENTED_EDGE('',*,*,#8084,.T.);
#11354=ORIENTED_EDGE('',*,*,#8078,.F.);
#11355=ORIENTED_EDGE('',*,*,#8085,.T.);
#11356=ORIENTED_EDGE('',*,*,#8086,.T.);
#11357=ORIENTED_EDGE('',*,*,#8087,.T.);
#11358=ORIENTED_EDGE('',*,*,#8088,.T.);
#11359=ORIENTED_EDGE('',*,*,#8082,.F.);
#11360=ORIENTED_EDGE('',*,*,#8089,.T.);
#11361=ORIENTED_EDGE('',*,*,#8090,.T.);
#11362=ORIENTED_EDGE('',*,*,#8091,.T.);
#11363=ORIENTED_EDGE('',*,*,#8092,.T.);
#11364=ORIENTED_EDGE('',*,*,#8087,.F.);
#11365=ORIENTED_EDGE('',*,*,#8093,.T.);
#11366=ORIENTED_EDGE('',*,*,#8094,.T.);
#11367=ORIENTED_EDGE('',*,*,#8095,.T.);
#11368=ORIENTED_EDGE('',*,*,#8096,.T.);
#11369=ORIENTED_EDGE('',*,*,#8090,.F.);
#11370=ORIENTED_EDGE('',*,*,#8097,.T.);
#11371=ORIENTED_EDGE('',*,*,#8098,.T.);
#11372=ORIENTED_EDGE('',*,*,#8099,.T.);
#11373=ORIENTED_EDGE('',*,*,#8100,.T.);
#11374=ORIENTED_EDGE('',*,*,#8095,.F.);
#11375=ORIENTED_EDGE('',*,*,#8101,.T.);
#11376=ORIENTED_EDGE('',*,*,#8102,.T.);
#11377=ORIENTED_EDGE('',*,*,#8103,.T.);
#11378=ORIENTED_EDGE('',*,*,#8104,.T.);
#11379=ORIENTED_EDGE('',*,*,#8098,.F.);
#11380=ORIENTED_EDGE('',*,*,#8105,.T.);
#11381=ORIENTED_EDGE('',*,*,#8106,.T.);
#11382=ORIENTED_EDGE('',*,*,#8107,.T.);
#11383=ORIENTED_EDGE('',*,*,#8108,.T.);
#11384=ORIENTED_EDGE('',*,*,#8103,.F.);
#11385=ORIENTED_EDGE('',*,*,#8109,.T.);
#11386=ORIENTED_EDGE('',*,*,#8110,.T.);
#11387=ORIENTED_EDGE('',*,*,#8111,.T.);
#11388=ORIENTED_EDGE('',*,*,#8112,.T.);
#11389=ORIENTED_EDGE('',*,*,#8106,.F.);
#11390=ORIENTED_EDGE('',*,*,#8113,.T.);
#11391=ORIENTED_EDGE('',*,*,#8114,.T.);
#11392=ORIENTED_EDGE('',*,*,#8115,.T.);
#11393=ORIENTED_EDGE('',*,*,#8116,.T.);
#11394=ORIENTED_EDGE('',*,*,#8111,.F.);
#11395=ORIENTED_EDGE('',*,*,#8117,.T.);
#11396=ORIENTED_EDGE('',*,*,#8118,.T.);
#11397=ORIENTED_EDGE('',*,*,#8119,.T.);
#11398=ORIENTED_EDGE('',*,*,#8120,.T.);
#11399=ORIENTED_EDGE('',*,*,#8114,.F.);
#11400=ORIENTED_EDGE('',*,*,#8121,.T.);
#11401=ORIENTED_EDGE('',*,*,#8122,.T.);
#11402=ORIENTED_EDGE('',*,*,#8123,.T.);
#11403=ORIENTED_EDGE('',*,*,#8124,.T.);
#11404=ORIENTED_EDGE('',*,*,#8119,.F.);
#11405=ORIENTED_EDGE('',*,*,#8125,.T.);
#11406=ORIENTED_EDGE('',*,*,#8126,.T.);
#11407=ORIENTED_EDGE('',*,*,#8127,.T.);
#11408=ORIENTED_EDGE('',*,*,#8128,.T.);
#11409=ORIENTED_EDGE('',*,*,#8122,.F.);
#11410=ORIENTED_EDGE('',*,*,#8129,.T.);
#11411=ORIENTED_EDGE('',*,*,#8130,.F.);
#11412=ORIENTED_EDGE('',*,*,#8131,.T.);
#11413=ORIENTED_EDGE('',*,*,#8132,.F.);
#11414=ORIENTED_EDGE('',*,*,#8133,.T.);
#11415=ORIENTED_EDGE('',*,*,#8134,.T.);
#11416=ORIENTED_EDGE('',*,*,#8135,.T.);
#11417=ORIENTED_EDGE('',*,*,#8136,.F.);
#11418=ORIENTED_EDGE('',*,*,#8137,.F.);
#11419=ORIENTED_EDGE('',*,*,#8138,.F.);
#11420=ORIENTED_EDGE('',*,*,#8139,.T.);
#11421=ORIENTED_EDGE('',*,*,#8140,.T.);
#11422=ORIENTED_EDGE('',*,*,#8141,.T.);
#11423=ORIENTED_EDGE('',*,*,#8134,.F.);
#11424=ORIENTED_EDGE('',*,*,#8142,.F.);
#11425=ORIENTED_EDGE('',*,*,#8143,.F.);
#11426=ORIENTED_EDGE('',*,*,#8144,.T.);
#11427=ORIENTED_EDGE('',*,*,#8145,.T.);
#11428=ORIENTED_EDGE('',*,*,#8146,.T.);
#11429=ORIENTED_EDGE('',*,*,#8139,.F.);
#11430=ORIENTED_EDGE('',*,*,#8147,.F.);
#11431=ORIENTED_EDGE('',*,*,#8148,.F.);
#11432=ORIENTED_EDGE('',*,*,#8149,.T.);
#11433=ORIENTED_EDGE('',*,*,#8150,.T.);
#11434=ORIENTED_EDGE('',*,*,#8151,.T.);
#11435=ORIENTED_EDGE('',*,*,#8144,.F.);
#11436=ORIENTED_EDGE('',*,*,#8152,.F.);
#11437=ORIENTED_EDGE('',*,*,#8153,.F.);
#11438=ORIENTED_EDGE('',*,*,#8154,.T.);
#11439=ORIENTED_EDGE('',*,*,#8155,.T.);
#11440=ORIENTED_EDGE('',*,*,#8156,.T.);
#11441=ORIENTED_EDGE('',*,*,#8149,.F.);
#11442=ORIENTED_EDGE('',*,*,#8157,.F.);
#11443=ORIENTED_EDGE('',*,*,#8158,.F.);
#11444=ORIENTED_EDGE('',*,*,#8159,.T.);
#11445=ORIENTED_EDGE('',*,*,#8160,.T.);
#11446=ORIENTED_EDGE('',*,*,#8161,.T.);
#11447=ORIENTED_EDGE('',*,*,#8154,.F.);
#11448=ORIENTED_EDGE('',*,*,#8162,.F.);
#11449=ORIENTED_EDGE('',*,*,#8163,.F.);
#11450=ORIENTED_EDGE('',*,*,#8164,.T.);
#11451=ORIENTED_EDGE('',*,*,#8165,.T.);
#11452=ORIENTED_EDGE('',*,*,#8166,.T.);
#11453=ORIENTED_EDGE('',*,*,#8159,.F.);
#11454=ORIENTED_EDGE('',*,*,#8167,.F.);
#11455=ORIENTED_EDGE('',*,*,#8168,.F.);
#11456=ORIENTED_EDGE('',*,*,#8169,.T.);
#11457=ORIENTED_EDGE('',*,*,#8170,.T.);
#11458=ORIENTED_EDGE('',*,*,#8171,.T.);
#11459=ORIENTED_EDGE('',*,*,#8164,.F.);
#11460=ORIENTED_EDGE('',*,*,#8172,.F.);
#11461=ORIENTED_EDGE('',*,*,#8173,.F.);
#11462=ORIENTED_EDGE('',*,*,#8174,.T.);
#11463=ORIENTED_EDGE('',*,*,#8175,.T.);
#11464=ORIENTED_EDGE('',*,*,#8176,.T.);
#11465=ORIENTED_EDGE('',*,*,#8169,.F.);
#11466=ORIENTED_EDGE('',*,*,#8177,.F.);
#11467=ORIENTED_EDGE('',*,*,#8178,.F.);
#11468=ORIENTED_EDGE('',*,*,#8179,.T.);
#11469=ORIENTED_EDGE('',*,*,#8180,.T.);
#11470=ORIENTED_EDGE('',*,*,#8181,.T.);
#11471=ORIENTED_EDGE('',*,*,#8174,.F.);
#11472=ORIENTED_EDGE('',*,*,#8182,.F.);
#11473=ORIENTED_EDGE('',*,*,#8183,.F.);
#11474=ORIENTED_EDGE('',*,*,#8184,.T.);
#11475=ORIENTED_EDGE('',*,*,#8185,.T.);
#11476=ORIENTED_EDGE('',*,*,#8186,.T.);
#11477=ORIENTED_EDGE('',*,*,#8179,.F.);
#11478=ORIENTED_EDGE('',*,*,#8187,.F.);
#11479=ORIENTED_EDGE('',*,*,#8188,.F.);
#11480=ORIENTED_EDGE('',*,*,#8189,.T.);
#11481=ORIENTED_EDGE('',*,*,#8190,.T.);
#11482=ORIENTED_EDGE('',*,*,#8191,.T.);
#11483=ORIENTED_EDGE('',*,*,#8184,.F.);
#11484=ORIENTED_EDGE('',*,*,#8192,.F.);
#11485=ORIENTED_EDGE('',*,*,#8193,.F.);
#11486=ORIENTED_EDGE('',*,*,#8194,.T.);
#11487=ORIENTED_EDGE('',*,*,#8195,.T.);
#11488=ORIENTED_EDGE('',*,*,#8196,.T.);
#11489=ORIENTED_EDGE('',*,*,#8189,.F.);
#11490=ORIENTED_EDGE('',*,*,#8197,.F.);
#11491=ORIENTED_EDGE('',*,*,#8198,.F.);
#11492=ORIENTED_EDGE('',*,*,#8199,.F.);
#11493=ORIENTED_EDGE('',*,*,#8200,.F.);
#11494=ORIENTED_EDGE('',*,*,#8201,.F.);
#11495=ORIENTED_EDGE('',*,*,#8202,.F.);
#11496=ORIENTED_EDGE('',*,*,#8203,.T.);
#11497=ORIENTED_EDGE('',*,*,#8204,.T.);
#11498=ORIENTED_EDGE('',*,*,#8205,.T.);
#11499=ORIENTED_EDGE('',*,*,#8206,.T.);
#11500=ORIENTED_EDGE('',*,*,#8207,.F.);
#11501=ORIENTED_EDGE('',*,*,#8208,.F.);
#11502=ORIENTED_EDGE('',*,*,#8209,.F.);
#11503=ORIENTED_EDGE('',*,*,#8210,.T.);
#11504=ORIENTED_EDGE('',*,*,#8211,.T.);
#11505=ORIENTED_EDGE('',*,*,#8212,.T.);
#11506=ORIENTED_EDGE('',*,*,#8205,.F.);
#11507=ORIENTED_EDGE('',*,*,#8213,.F.);
#11508=ORIENTED_EDGE('',*,*,#8214,.F.);
#11509=ORIENTED_EDGE('',*,*,#8215,.T.);
#11510=ORIENTED_EDGE('',*,*,#8216,.T.);
#11511=ORIENTED_EDGE('',*,*,#8217,.T.);
#11512=ORIENTED_EDGE('',*,*,#8210,.F.);
#11513=ORIENTED_EDGE('',*,*,#8218,.F.);
#11514=ORIENTED_EDGE('',*,*,#8219,.F.);
#11515=ORIENTED_EDGE('',*,*,#8220,.T.);
#11516=ORIENTED_EDGE('',*,*,#8221,.T.);
#11517=ORIENTED_EDGE('',*,*,#8222,.T.);
#11518=ORIENTED_EDGE('',*,*,#8215,.F.);
#11519=ORIENTED_EDGE('',*,*,#8223,.F.);
#11520=ORIENTED_EDGE('',*,*,#8224,.F.);
#11521=ORIENTED_EDGE('',*,*,#8225,.T.);
#11522=ORIENTED_EDGE('',*,*,#8226,.T.);
#11523=ORIENTED_EDGE('',*,*,#8227,.T.);
#11524=ORIENTED_EDGE('',*,*,#8220,.F.);
#11525=ORIENTED_EDGE('',*,*,#8228,.F.);
#11526=ORIENTED_EDGE('',*,*,#8229,.F.);
#11527=ORIENTED_EDGE('',*,*,#8230,.T.);
#11528=ORIENTED_EDGE('',*,*,#8231,.T.);
#11529=ORIENTED_EDGE('',*,*,#8232,.T.);
#11530=ORIENTED_EDGE('',*,*,#8225,.F.);
#11531=ORIENTED_EDGE('',*,*,#8233,.F.);
#11532=ORIENTED_EDGE('',*,*,#8234,.F.);
#11533=ORIENTED_EDGE('',*,*,#8235,.T.);
#11534=ORIENTED_EDGE('',*,*,#8236,.T.);
#11535=ORIENTED_EDGE('',*,*,#8237,.T.);
#11536=ORIENTED_EDGE('',*,*,#8230,.F.);
#11537=ORIENTED_EDGE('',*,*,#8238,.F.);
#11538=ORIENTED_EDGE('',*,*,#8239,.F.);
#11539=ORIENTED_EDGE('',*,*,#8240,.T.);
#11540=ORIENTED_EDGE('',*,*,#8241,.T.);
#11541=ORIENTED_EDGE('',*,*,#8242,.T.);
#11542=ORIENTED_EDGE('',*,*,#8235,.F.);
#11543=ORIENTED_EDGE('',*,*,#8243,.F.);
#11544=ORIENTED_EDGE('',*,*,#8244,.F.);
#11545=ORIENTED_EDGE('',*,*,#8245,.T.);
#11546=ORIENTED_EDGE('',*,*,#8246,.T.);
#11547=ORIENTED_EDGE('',*,*,#8247,.T.);
#11548=ORIENTED_EDGE('',*,*,#8240,.F.);
#11549=ORIENTED_EDGE('',*,*,#8248,.F.);
#11550=ORIENTED_EDGE('',*,*,#8249,.F.);
#11551=ORIENTED_EDGE('',*,*,#8250,.T.);
#11552=ORIENTED_EDGE('',*,*,#8251,.T.);
#11553=ORIENTED_EDGE('',*,*,#8252,.T.);
#11554=ORIENTED_EDGE('',*,*,#8245,.F.);
#11555=ORIENTED_EDGE('',*,*,#8253,.F.);
#11556=ORIENTED_EDGE('',*,*,#8254,.F.);
#11557=ORIENTED_EDGE('',*,*,#8255,.T.);
#11558=ORIENTED_EDGE('',*,*,#8256,.T.);
#11559=ORIENTED_EDGE('',*,*,#8257,.T.);
#11560=ORIENTED_EDGE('',*,*,#8250,.F.);
#11561=ORIENTED_EDGE('',*,*,#8258,.F.);
#11562=ORIENTED_EDGE('',*,*,#8259,.F.);
#11563=ORIENTED_EDGE('',*,*,#8260,.T.);
#11564=ORIENTED_EDGE('',*,*,#8261,.T.);
#11565=ORIENTED_EDGE('',*,*,#8262,.T.);
#11566=ORIENTED_EDGE('',*,*,#8255,.F.);
#11567=ORIENTED_EDGE('',*,*,#8263,.F.);
#11568=ORIENTED_EDGE('',*,*,#8264,.F.);
#11569=ORIENTED_EDGE('',*,*,#8265,.T.);
#11570=ORIENTED_EDGE('',*,*,#8266,.T.);
#11571=ORIENTED_EDGE('',*,*,#8267,.T.);
#11572=ORIENTED_EDGE('',*,*,#8260,.F.);
#11573=ORIENTED_EDGE('',*,*,#8268,.F.);
#11574=ORIENTED_EDGE('',*,*,#8269,.F.);
#11575=ORIENTED_EDGE('',*,*,#8270,.F.);
#11576=ORIENTED_EDGE('',*,*,#8271,.F.);
#11577=ORIENTED_EDGE('',*,*,#8272,.F.);
#11578=ORIENTED_EDGE('',*,*,#8273,.F.);
#11579=ORIENTED_EDGE('',*,*,#8274,.T.);
#11580=ORIENTED_EDGE('',*,*,#8275,.T.);
#11581=ORIENTED_EDGE('',*,*,#8276,.T.);
#11582=ORIENTED_EDGE('',*,*,#8277,.T.);
#11583=ORIENTED_EDGE('',*,*,#8278,.F.);
#11584=ORIENTED_EDGE('',*,*,#8279,.F.);
#11585=ORIENTED_EDGE('',*,*,#8280,.F.);
#11586=ORIENTED_EDGE('',*,*,#8281,.T.);
#11587=ORIENTED_EDGE('',*,*,#8282,.T.);
#11588=ORIENTED_EDGE('',*,*,#8283,.T.);
#11589=ORIENTED_EDGE('',*,*,#8276,.F.);
#11590=ORIENTED_EDGE('',*,*,#8284,.F.);
#11591=ORIENTED_EDGE('',*,*,#8285,.F.);
#11592=ORIENTED_EDGE('',*,*,#8286,.T.);
#11593=ORIENTED_EDGE('',*,*,#8287,.T.);
#11594=ORIENTED_EDGE('',*,*,#8288,.T.);
#11595=ORIENTED_EDGE('',*,*,#8281,.F.);
#11596=ORIENTED_EDGE('',*,*,#8289,.F.);
#11597=ORIENTED_EDGE('',*,*,#8290,.F.);
#11598=ORIENTED_EDGE('',*,*,#8291,.T.);
#11599=ORIENTED_EDGE('',*,*,#8292,.T.);
#11600=ORIENTED_EDGE('',*,*,#8293,.T.);
#11601=ORIENTED_EDGE('',*,*,#8286,.F.);
#11602=ORIENTED_EDGE('',*,*,#8294,.F.);
#11603=ORIENTED_EDGE('',*,*,#8295,.F.);
#11604=ORIENTED_EDGE('',*,*,#8296,.T.);
#11605=ORIENTED_EDGE('',*,*,#8297,.T.);
#11606=ORIENTED_EDGE('',*,*,#8298,.T.);
#11607=ORIENTED_EDGE('',*,*,#8291,.F.);
#11608=ORIENTED_EDGE('',*,*,#8299,.F.);
#11609=ORIENTED_EDGE('',*,*,#8300,.F.);
#11610=ORIENTED_EDGE('',*,*,#8301,.T.);
#11611=ORIENTED_EDGE('',*,*,#8302,.T.);
#11612=ORIENTED_EDGE('',*,*,#8303,.T.);
#11613=ORIENTED_EDGE('',*,*,#8296,.F.);
#11614=ORIENTED_EDGE('',*,*,#8304,.F.);
#11615=ORIENTED_EDGE('',*,*,#8305,.F.);
#11616=ORIENTED_EDGE('',*,*,#8306,.T.);
#11617=ORIENTED_EDGE('',*,*,#8307,.T.);
#11618=ORIENTED_EDGE('',*,*,#8308,.T.);
#11619=ORIENTED_EDGE('',*,*,#8301,.F.);
#11620=ORIENTED_EDGE('',*,*,#8309,.F.);
#11621=ORIENTED_EDGE('',*,*,#8310,.F.);
#11622=ORIENTED_EDGE('',*,*,#8311,.T.);
#11623=ORIENTED_EDGE('',*,*,#8312,.T.);
#11624=ORIENTED_EDGE('',*,*,#8313,.T.);
#11625=ORIENTED_EDGE('',*,*,#8306,.F.);
#11626=ORIENTED_EDGE('',*,*,#8314,.F.);
#11627=ORIENTED_EDGE('',*,*,#8315,.F.);
#11628=ORIENTED_EDGE('',*,*,#8316,.T.);
#11629=ORIENTED_EDGE('',*,*,#8317,.T.);
#11630=ORIENTED_EDGE('',*,*,#8318,.T.);
#11631=ORIENTED_EDGE('',*,*,#8311,.F.);
#11632=ORIENTED_EDGE('',*,*,#8319,.F.);
#11633=ORIENTED_EDGE('',*,*,#8320,.F.);
#11634=ORIENTED_EDGE('',*,*,#8321,.T.);
#11635=ORIENTED_EDGE('',*,*,#8322,.T.);
#11636=ORIENTED_EDGE('',*,*,#8323,.T.);
#11637=ORIENTED_EDGE('',*,*,#8316,.F.);
#11638=ORIENTED_EDGE('',*,*,#8324,.F.);
#11639=ORIENTED_EDGE('',*,*,#8325,.F.);
#11640=ORIENTED_EDGE('',*,*,#8326,.T.);
#11641=ORIENTED_EDGE('',*,*,#8327,.T.);
#11642=ORIENTED_EDGE('',*,*,#8328,.T.);
#11643=ORIENTED_EDGE('',*,*,#8321,.F.);
#11644=ORIENTED_EDGE('',*,*,#8329,.F.);
#11645=ORIENTED_EDGE('',*,*,#8330,.F.);
#11646=ORIENTED_EDGE('',*,*,#8331,.T.);
#11647=ORIENTED_EDGE('',*,*,#8332,.T.);
#11648=ORIENTED_EDGE('',*,*,#8333,.T.);
#11649=ORIENTED_EDGE('',*,*,#8326,.F.);
#11650=ORIENTED_EDGE('',*,*,#8334,.F.);
#11651=ORIENTED_EDGE('',*,*,#8335,.F.);
#11652=ORIENTED_EDGE('',*,*,#8336,.T.);
#11653=ORIENTED_EDGE('',*,*,#8337,.T.);
#11654=ORIENTED_EDGE('',*,*,#8338,.T.);
#11655=ORIENTED_EDGE('',*,*,#8331,.F.);
#11656=ORIENTED_EDGE('',*,*,#8339,.F.);
#11657=ORIENTED_EDGE('',*,*,#8340,.F.);
#11658=ORIENTED_EDGE('',*,*,#8341,.F.);
#11659=ORIENTED_EDGE('',*,*,#8342,.F.);
#11660=ORIENTED_EDGE('',*,*,#8343,.F.);
#11661=ORIENTED_EDGE('',*,*,#8344,.F.);
#11662=ORIENTED_EDGE('',*,*,#8345,.T.);
#11663=ORIENTED_EDGE('',*,*,#8346,.T.);
#11664=ORIENTED_EDGE('',*,*,#8347,.T.);
#11665=ORIENTED_EDGE('',*,*,#8348,.T.);
#11666=ORIENTED_EDGE('',*,*,#8349,.F.);
#11667=ORIENTED_EDGE('',*,*,#8350,.F.);
#11668=ORIENTED_EDGE('',*,*,#8351,.F.);
#11669=ORIENTED_EDGE('',*,*,#8352,.T.);
#11670=ORIENTED_EDGE('',*,*,#8353,.T.);
#11671=ORIENTED_EDGE('',*,*,#8354,.T.);
#11672=ORIENTED_EDGE('',*,*,#8347,.F.);
#11673=ORIENTED_EDGE('',*,*,#8355,.F.);
#11674=ORIENTED_EDGE('',*,*,#8356,.F.);
#11675=ORIENTED_EDGE('',*,*,#8357,.T.);
#11676=ORIENTED_EDGE('',*,*,#8358,.T.);
#11677=ORIENTED_EDGE('',*,*,#8359,.T.);
#11678=ORIENTED_EDGE('',*,*,#8352,.F.);
#11679=ORIENTED_EDGE('',*,*,#8360,.F.);
#11680=ORIENTED_EDGE('',*,*,#8361,.F.);
#11681=ORIENTED_EDGE('',*,*,#8362,.T.);
#11682=ORIENTED_EDGE('',*,*,#8363,.T.);
#11683=ORIENTED_EDGE('',*,*,#8364,.T.);
#11684=ORIENTED_EDGE('',*,*,#8357,.F.);
#11685=ORIENTED_EDGE('',*,*,#8365,.F.);
#11686=ORIENTED_EDGE('',*,*,#8366,.F.);
#11687=ORIENTED_EDGE('',*,*,#8367,.T.);
#11688=ORIENTED_EDGE('',*,*,#8368,.T.);
#11689=ORIENTED_EDGE('',*,*,#8369,.T.);
#11690=ORIENTED_EDGE('',*,*,#8362,.F.);
#11691=ORIENTED_EDGE('',*,*,#8370,.F.);
#11692=ORIENTED_EDGE('',*,*,#8371,.F.);
#11693=ORIENTED_EDGE('',*,*,#8372,.T.);
#11694=ORIENTED_EDGE('',*,*,#8373,.T.);
#11695=ORIENTED_EDGE('',*,*,#8374,.T.);
#11696=ORIENTED_EDGE('',*,*,#8367,.F.);
#11697=ORIENTED_EDGE('',*,*,#8375,.F.);
#11698=ORIENTED_EDGE('',*,*,#8376,.F.);
#11699=ORIENTED_EDGE('',*,*,#8377,.T.);
#11700=ORIENTED_EDGE('',*,*,#8378,.T.);
#11701=ORIENTED_EDGE('',*,*,#8379,.T.);
#11702=ORIENTED_EDGE('',*,*,#8372,.F.);
#11703=ORIENTED_EDGE('',*,*,#8380,.F.);
#11704=ORIENTED_EDGE('',*,*,#8381,.F.);
#11705=ORIENTED_EDGE('',*,*,#8382,.T.);
#11706=ORIENTED_EDGE('',*,*,#8383,.T.);
#11707=ORIENTED_EDGE('',*,*,#8384,.T.);
#11708=ORIENTED_EDGE('',*,*,#8377,.F.);
#11709=ORIENTED_EDGE('',*,*,#8385,.F.);
#11710=ORIENTED_EDGE('',*,*,#8386,.F.);
#11711=ORIENTED_EDGE('',*,*,#8387,.T.);
#11712=ORIENTED_EDGE('',*,*,#8388,.T.);
#11713=ORIENTED_EDGE('',*,*,#8389,.T.);
#11714=ORIENTED_EDGE('',*,*,#8382,.F.);
#11715=ORIENTED_EDGE('',*,*,#8390,.F.);
#11716=ORIENTED_EDGE('',*,*,#8391,.F.);
#11717=ORIENTED_EDGE('',*,*,#8392,.T.);
#11718=ORIENTED_EDGE('',*,*,#8393,.T.);
#11719=ORIENTED_EDGE('',*,*,#8394,.T.);
#11720=ORIENTED_EDGE('',*,*,#8387,.F.);
#11721=ORIENTED_EDGE('',*,*,#8395,.F.);
#11722=ORIENTED_EDGE('',*,*,#8396,.F.);
#11723=ORIENTED_EDGE('',*,*,#8397,.T.);
#11724=ORIENTED_EDGE('',*,*,#8398,.T.);
#11725=ORIENTED_EDGE('',*,*,#8399,.T.);
#11726=ORIENTED_EDGE('',*,*,#8392,.F.);
#11727=ORIENTED_EDGE('',*,*,#8400,.F.);
#11728=ORIENTED_EDGE('',*,*,#8401,.F.);
#11729=ORIENTED_EDGE('',*,*,#8402,.T.);
#11730=ORIENTED_EDGE('',*,*,#8403,.T.);
#11731=ORIENTED_EDGE('',*,*,#8404,.T.);
#11732=ORIENTED_EDGE('',*,*,#8397,.F.);
#11733=ORIENTED_EDGE('',*,*,#8405,.F.);
#11734=ORIENTED_EDGE('',*,*,#8406,.F.);
#11735=ORIENTED_EDGE('',*,*,#8407,.T.);
#11736=ORIENTED_EDGE('',*,*,#8408,.T.);
#11737=ORIENTED_EDGE('',*,*,#8409,.T.);
#11738=ORIENTED_EDGE('',*,*,#8402,.F.);
#11739=ORIENTED_EDGE('',*,*,#8410,.F.);
#11740=ORIENTED_EDGE('',*,*,#8411,.F.);
#11741=ORIENTED_EDGE('',*,*,#8412,.F.);
#11742=ORIENTED_EDGE('',*,*,#8413,.F.);
#11743=ORIENTED_EDGE('',*,*,#8414,.F.);
#11744=ORIENTED_EDGE('',*,*,#8415,.F.);
#11745=ORIENTED_EDGE('',*,*,#8416,.T.);
#11746=ORIENTED_EDGE('',*,*,#8417,.T.);
#11747=ORIENTED_EDGE('',*,*,#8418,.T.);
#11748=ORIENTED_EDGE('',*,*,#8419,.T.);
#11749=ORIENTED_EDGE('',*,*,#8420,.T.);
#11750=ORIENTED_EDGE('',*,*,#8421,.T.);
#11751=ORIENTED_EDGE('',*,*,#8422,.T.);
#11752=ORIENTED_EDGE('',*,*,#8423,.T.);
#11753=ORIENTED_EDGE('',*,*,#8424,.T.);
#11754=ORIENTED_EDGE('',*,*,#8418,.F.);
#11755=ORIENTED_EDGE('',*,*,#8425,.T.);
#11756=ORIENTED_EDGE('',*,*,#8426,.T.);
#11757=ORIENTED_EDGE('',*,*,#8427,.T.);
#11758=ORIENTED_EDGE('',*,*,#8422,.F.);
#11759=ORIENTED_EDGE('',*,*,#8428,.T.);
#11760=ORIENTED_EDGE('',*,*,#8429,.T.);
#11761=ORIENTED_EDGE('',*,*,#8430,.T.);
#11762=ORIENTED_EDGE('',*,*,#8431,.T.);
#11763=ORIENTED_EDGE('',*,*,#8432,.T.);
#11764=ORIENTED_EDGE('',*,*,#8426,.F.);
#11765=ORIENTED_EDGE('',*,*,#8433,.T.);
#11766=ORIENTED_EDGE('',*,*,#8434,.T.);
#11767=ORIENTED_EDGE('',*,*,#8435,.T.);
#11768=ORIENTED_EDGE('',*,*,#8430,.F.);
#11769=ORIENTED_EDGE('',*,*,#8436,.T.);
#11770=ORIENTED_EDGE('',*,*,#8437,.T.);
#11771=ORIENTED_EDGE('',*,*,#8438,.T.);
#11772=ORIENTED_EDGE('',*,*,#8439,.T.);
#11773=ORIENTED_EDGE('',*,*,#8440,.T.);
#11774=ORIENTED_EDGE('',*,*,#8434,.F.);
#11775=ORIENTED_EDGE('',*,*,#8441,.T.);
#11776=ORIENTED_EDGE('',*,*,#8442,.T.);
#11777=ORIENTED_EDGE('',*,*,#8443,.T.);
#11778=ORIENTED_EDGE('',*,*,#8438,.F.);
#11779=ORIENTED_EDGE('',*,*,#8444,.T.);
#11780=ORIENTED_EDGE('',*,*,#8445,.T.);
#11781=ORIENTED_EDGE('',*,*,#8446,.T.);
#11782=ORIENTED_EDGE('',*,*,#8447,.T.);
#11783=ORIENTED_EDGE('',*,*,#8448,.T.);
#11784=ORIENTED_EDGE('',*,*,#8442,.F.);
#11785=ORIENTED_EDGE('',*,*,#8449,.T.);
#11786=ORIENTED_EDGE('',*,*,#8450,.T.);
#11787=ORIENTED_EDGE('',*,*,#8451,.T.);
#11788=ORIENTED_EDGE('',*,*,#8452,.T.);
#11789=ORIENTED_EDGE('',*,*,#8446,.F.);
#11790=ORIENTED_EDGE('',*,*,#8453,.T.);
#11791=ORIENTED_EDGE('',*,*,#8454,.T.);
#11792=ORIENTED_EDGE('',*,*,#8455,.T.);
#11793=ORIENTED_EDGE('',*,*,#8456,.T.);
#11794=ORIENTED_EDGE('',*,*,#8457,.T.);
#11795=ORIENTED_EDGE('',*,*,#8451,.F.);
#11796=ORIENTED_EDGE('',*,*,#8458,.T.);
#11797=ORIENTED_EDGE('',*,*,#8459,.T.);
#11798=ORIENTED_EDGE('',*,*,#8460,.T.);
#11799=ORIENTED_EDGE('',*,*,#8455,.F.);
#11800=ORIENTED_EDGE('',*,*,#8461,.T.);
#11801=ORIENTED_EDGE('',*,*,#8462,.T.);
#11802=ORIENTED_EDGE('',*,*,#8463,.T.);
#11803=ORIENTED_EDGE('',*,*,#8464,.T.);
#11804=ORIENTED_EDGE('',*,*,#8465,.T.);
#11805=ORIENTED_EDGE('',*,*,#8459,.F.);
#11806=ORIENTED_EDGE('',*,*,#8466,.T.);
#11807=ORIENTED_EDGE('',*,*,#8467,.T.);
#11808=ORIENTED_EDGE('',*,*,#8468,.T.);
#11809=ORIENTED_EDGE('',*,*,#8463,.F.);
#11810=ORIENTED_EDGE('',*,*,#8469,.T.);
#11811=ORIENTED_EDGE('',*,*,#8470,.T.);
#11812=ORIENTED_EDGE('',*,*,#8471,.F.);
#11813=ORIENTED_EDGE('',*,*,#8472,.T.);
#11814=ORIENTED_EDGE('',*,*,#8473,.T.);
#11815=ORIENTED_EDGE('',*,*,#8474,.F.);
#11816=ORIENTED_EDGE('',*,*,#8475,.T.);
#11817=ORIENTED_EDGE('',*,*,#8476,.T.);
#11818=ORIENTED_EDGE('',*,*,#8477,.T.);
#11819=ORIENTED_EDGE('',*,*,#8478,.T.);
#11820=ORIENTED_EDGE('',*,*,#8479,.T.);
#11821=ORIENTED_EDGE('',*,*,#8480,.T.);
#11822=ORIENTED_EDGE('',*,*,#8481,.T.);
#11823=ORIENTED_EDGE('',*,*,#8482,.T.);
#11824=ORIENTED_EDGE('',*,*,#8476,.F.);
#11825=ORIENTED_EDGE('',*,*,#8483,.T.);
#11826=ORIENTED_EDGE('',*,*,#8484,.T.);
#11827=ORIENTED_EDGE('',*,*,#8485,.T.);
#11828=ORIENTED_EDGE('',*,*,#8480,.F.);
#11829=ORIENTED_EDGE('',*,*,#8486,.T.);
#11830=ORIENTED_EDGE('',*,*,#8487,.T.);
#11831=ORIENTED_EDGE('',*,*,#8488,.T.);
#11832=ORIENTED_EDGE('',*,*,#8489,.T.);
#11833=ORIENTED_EDGE('',*,*,#8490,.T.);
#11834=ORIENTED_EDGE('',*,*,#8484,.F.);
#11835=ORIENTED_EDGE('',*,*,#8491,.T.);
#11836=ORIENTED_EDGE('',*,*,#8492,.T.);
#11837=ORIENTED_EDGE('',*,*,#8493,.T.);
#11838=ORIENTED_EDGE('',*,*,#8488,.F.);
#11839=ORIENTED_EDGE('',*,*,#8494,.T.);
#11840=ORIENTED_EDGE('',*,*,#8495,.T.);
#11841=ORIENTED_EDGE('',*,*,#8496,.T.);
#11842=ORIENTED_EDGE('',*,*,#8497,.T.);
#11843=ORIENTED_EDGE('',*,*,#8498,.T.);
#11844=ORIENTED_EDGE('',*,*,#8492,.F.);
#11845=ORIENTED_EDGE('',*,*,#8499,.T.);
#11846=ORIENTED_EDGE('',*,*,#8500,.T.);
#11847=ORIENTED_EDGE('',*,*,#8501,.T.);
#11848=ORIENTED_EDGE('',*,*,#8496,.F.);
#11849=ORIENTED_EDGE('',*,*,#8502,.T.);
#11850=ORIENTED_EDGE('',*,*,#8503,.T.);
#11851=ORIENTED_EDGE('',*,*,#8504,.T.);
#11852=ORIENTED_EDGE('',*,*,#8505,.T.);
#11853=ORIENTED_EDGE('',*,*,#8506,.T.);
#11854=ORIENTED_EDGE('',*,*,#8500,.F.);
#11855=ORIENTED_EDGE('',*,*,#8507,.T.);
#11856=ORIENTED_EDGE('',*,*,#8508,.T.);
#11857=ORIENTED_EDGE('',*,*,#8509,.T.);
#11858=ORIENTED_EDGE('',*,*,#8510,.T.);
#11859=ORIENTED_EDGE('',*,*,#8504,.F.);
#11860=ORIENTED_EDGE('',*,*,#8511,.T.);
#11861=ORIENTED_EDGE('',*,*,#8512,.T.);
#11862=ORIENTED_EDGE('',*,*,#8513,.T.);
#11863=ORIENTED_EDGE('',*,*,#8514,.T.);
#11864=ORIENTED_EDGE('',*,*,#8515,.T.);
#11865=ORIENTED_EDGE('',*,*,#8509,.F.);
#11866=ORIENTED_EDGE('',*,*,#8516,.T.);
#11867=ORIENTED_EDGE('',*,*,#8517,.T.);
#11868=ORIENTED_EDGE('',*,*,#8518,.T.);
#11869=ORIENTED_EDGE('',*,*,#8513,.F.);
#11870=ORIENTED_EDGE('',*,*,#8519,.T.);
#11871=ORIENTED_EDGE('',*,*,#8520,.T.);
#11872=ORIENTED_EDGE('',*,*,#8521,.T.);
#11873=ORIENTED_EDGE('',*,*,#8522,.T.);
#11874=ORIENTED_EDGE('',*,*,#8523,.T.);
#11875=ORIENTED_EDGE('',*,*,#8517,.F.);
#11876=ORIENTED_EDGE('',*,*,#8524,.T.);
#11877=ORIENTED_EDGE('',*,*,#8525,.T.);
#11878=ORIENTED_EDGE('',*,*,#8526,.T.);
#11879=ORIENTED_EDGE('',*,*,#8521,.F.);
#11880=ORIENTED_EDGE('',*,*,#8527,.T.);
#11881=ORIENTED_EDGE('',*,*,#8528,.T.);
#11882=ORIENTED_EDGE('',*,*,#8529,.F.);
#11883=ORIENTED_EDGE('',*,*,#8530,.T.);
#11884=ORIENTED_EDGE('',*,*,#8531,.T.);
#11885=ORIENTED_EDGE('',*,*,#8532,.F.);
#11886=ORIENTED_EDGE('',*,*,#8533,.T.);
#11887=ORIENTED_EDGE('',*,*,#8534,.T.);
#11888=ORIENTED_EDGE('',*,*,#8535,.T.);
#11889=ORIENTED_EDGE('',*,*,#8536,.T.);
#11890=ORIENTED_EDGE('',*,*,#8537,.T.);
#11891=ORIENTED_EDGE('',*,*,#8538,.T.);
#11892=ORIENTED_EDGE('',*,*,#8539,.T.);
#11893=ORIENTED_EDGE('',*,*,#8534,.F.);
#11894=ORIENTED_EDGE('',*,*,#8540,.T.);
#11895=ORIENTED_EDGE('',*,*,#8541,.T.);
#11896=ORIENTED_EDGE('',*,*,#8542,.T.);
#11897=ORIENTED_EDGE('',*,*,#8538,.F.);
#11898=ORIENTED_EDGE('',*,*,#8543,.T.);
#11899=ORIENTED_EDGE('',*,*,#8544,.T.);
#11900=ORIENTED_EDGE('',*,*,#8545,.T.);
#11901=ORIENTED_EDGE('',*,*,#8546,.T.);
#11902=ORIENTED_EDGE('',*,*,#8541,.F.);
#11903=ORIENTED_EDGE('',*,*,#8547,.T.);
#11904=ORIENTED_EDGE('',*,*,#8548,.T.);
#11905=ORIENTED_EDGE('',*,*,#8549,.T.);
#11906=ORIENTED_EDGE('',*,*,#8545,.F.);
#11907=ORIENTED_EDGE('',*,*,#8550,.T.);
#11908=ORIENTED_EDGE('',*,*,#8551,.T.);
#11909=ORIENTED_EDGE('',*,*,#8552,.T.);
#11910=ORIENTED_EDGE('',*,*,#8553,.T.);
#11911=ORIENTED_EDGE('',*,*,#8554,.T.);
#11912=ORIENTED_EDGE('',*,*,#8548,.F.);
#11913=ORIENTED_EDGE('',*,*,#8555,.T.);
#11914=ORIENTED_EDGE('',*,*,#8556,.T.);
#11915=ORIENTED_EDGE('',*,*,#8557,.T.);
#11916=ORIENTED_EDGE('',*,*,#8552,.F.);
#11917=ORIENTED_EDGE('',*,*,#8558,.T.);
#11918=ORIENTED_EDGE('',*,*,#8559,.T.);
#11919=ORIENTED_EDGE('',*,*,#8560,.T.);
#11920=ORIENTED_EDGE('',*,*,#8561,.T.);
#11921=ORIENTED_EDGE('',*,*,#8562,.T.);
#11922=ORIENTED_EDGE('',*,*,#8556,.F.);
#11923=ORIENTED_EDGE('',*,*,#8563,.T.);
#11924=ORIENTED_EDGE('',*,*,#8564,.T.);
#11925=ORIENTED_EDGE('',*,*,#8565,.T.);
#11926=ORIENTED_EDGE('',*,*,#8566,.T.);
#11927=ORIENTED_EDGE('',*,*,#8560,.F.);
#11928=ORIENTED_EDGE('',*,*,#8567,.T.);
#11929=ORIENTED_EDGE('',*,*,#8568,.T.);
#11930=ORIENTED_EDGE('',*,*,#8569,.T.);
#11931=ORIENTED_EDGE('',*,*,#8570,.T.);
#11932=ORIENTED_EDGE('',*,*,#8571,.T.);
#11933=ORIENTED_EDGE('',*,*,#8565,.F.);
#11934=ORIENTED_EDGE('',*,*,#8572,.T.);
#11935=ORIENTED_EDGE('',*,*,#8573,.T.);
#11936=ORIENTED_EDGE('',*,*,#8574,.T.);
#11937=ORIENTED_EDGE('',*,*,#8569,.F.);
#11938=ORIENTED_EDGE('',*,*,#8575,.T.);
#11939=ORIENTED_EDGE('',*,*,#8576,.T.);
#11940=ORIENTED_EDGE('',*,*,#8577,.T.);
#11941=ORIENTED_EDGE('',*,*,#8578,.T.);
#11942=ORIENTED_EDGE('',*,*,#8579,.T.);
#11943=ORIENTED_EDGE('',*,*,#8573,.F.);
#11944=ORIENTED_EDGE('',*,*,#8580,.T.);
#11945=ORIENTED_EDGE('',*,*,#8581,.T.);
#11946=ORIENTED_EDGE('',*,*,#8582,.T.);
#11947=ORIENTED_EDGE('',*,*,#8577,.F.);
#11948=ORIENTED_EDGE('',*,*,#8583,.T.);
#11949=ORIENTED_EDGE('',*,*,#8584,.F.);
#11950=ORIENTED_EDGE('',*,*,#8585,.T.);
#11951=ORIENTED_EDGE('',*,*,#8586,.F.);
#11952=ORIENTED_EDGE('',*,*,#8587,.T.);
#11953=ORIENTED_EDGE('',*,*,#8588,.T.);
#11954=ORIENTED_EDGE('',*,*,#8589,.T.);
#11955=ORIENTED_EDGE('',*,*,#8590,.T.);
#11956=ORIENTED_EDGE('',*,*,#8591,.T.);
#11957=ORIENTED_EDGE('',*,*,#8592,.T.);
#11958=ORIENTED_EDGE('',*,*,#8593,.T.);
#11959=ORIENTED_EDGE('',*,*,#8588,.F.);
#11960=ORIENTED_EDGE('',*,*,#8594,.T.);
#11961=ORIENTED_EDGE('',*,*,#8595,.T.);
#11962=ORIENTED_EDGE('',*,*,#8596,.T.);
#11963=ORIENTED_EDGE('',*,*,#8592,.F.);
#11964=ORIENTED_EDGE('',*,*,#8597,.T.);
#11965=ORIENTED_EDGE('',*,*,#8598,.T.);
#11966=ORIENTED_EDGE('',*,*,#8599,.T.);
#11967=ORIENTED_EDGE('',*,*,#8600,.T.);
#11968=ORIENTED_EDGE('',*,*,#8595,.F.);
#11969=ORIENTED_EDGE('',*,*,#8601,.T.);
#11970=ORIENTED_EDGE('',*,*,#8602,.T.);
#11971=ORIENTED_EDGE('',*,*,#8603,.T.);
#11972=ORIENTED_EDGE('',*,*,#8599,.F.);
#11973=ORIENTED_EDGE('',*,*,#8604,.T.);
#11974=ORIENTED_EDGE('',*,*,#8605,.T.);
#11975=ORIENTED_EDGE('',*,*,#8606,.T.);
#11976=ORIENTED_EDGE('',*,*,#8607,.T.);
#11977=ORIENTED_EDGE('',*,*,#8608,.T.);
#11978=ORIENTED_EDGE('',*,*,#8602,.F.);
#11979=ORIENTED_EDGE('',*,*,#8609,.T.);
#11980=ORIENTED_EDGE('',*,*,#8610,.T.);
#11981=ORIENTED_EDGE('',*,*,#8611,.T.);
#11982=ORIENTED_EDGE('',*,*,#8606,.F.);
#11983=ORIENTED_EDGE('',*,*,#8612,.T.);
#11984=ORIENTED_EDGE('',*,*,#8613,.T.);
#11985=ORIENTED_EDGE('',*,*,#8614,.T.);
#11986=ORIENTED_EDGE('',*,*,#8615,.T.);
#11987=ORIENTED_EDGE('',*,*,#8616,.T.);
#11988=ORIENTED_EDGE('',*,*,#8610,.F.);
#11989=ORIENTED_EDGE('',*,*,#8617,.T.);
#11990=ORIENTED_EDGE('',*,*,#8618,.T.);
#11991=ORIENTED_EDGE('',*,*,#8619,.T.);
#11992=ORIENTED_EDGE('',*,*,#8620,.T.);
#11993=ORIENTED_EDGE('',*,*,#8614,.F.);
#11994=ORIENTED_EDGE('',*,*,#8621,.T.);
#11995=ORIENTED_EDGE('',*,*,#8622,.T.);
#11996=ORIENTED_EDGE('',*,*,#8623,.T.);
#11997=ORIENTED_EDGE('',*,*,#8624,.T.);
#11998=ORIENTED_EDGE('',*,*,#8625,.T.);
#11999=ORIENTED_EDGE('',*,*,#8619,.F.);
#12000=ORIENTED_EDGE('',*,*,#8626,.T.);
#12001=ORIENTED_EDGE('',*,*,#8627,.T.);
#12002=ORIENTED_EDGE('',*,*,#8628,.T.);
#12003=ORIENTED_EDGE('',*,*,#8623,.F.);
#12004=ORIENTED_EDGE('',*,*,#8629,.T.);
#12005=ORIENTED_EDGE('',*,*,#8630,.T.);
#12006=ORIENTED_EDGE('',*,*,#8631,.T.);
#12007=ORIENTED_EDGE('',*,*,#8632,.T.);
#12008=ORIENTED_EDGE('',*,*,#8633,.T.);
#12009=ORIENTED_EDGE('',*,*,#8627,.F.);
#12010=ORIENTED_EDGE('',*,*,#8634,.T.);
#12011=ORIENTED_EDGE('',*,*,#8635,.T.);
#12012=ORIENTED_EDGE('',*,*,#8636,.T.);
#12013=ORIENTED_EDGE('',*,*,#8631,.F.);
#12014=ORIENTED_EDGE('',*,*,#8637,.T.);
#12015=ORIENTED_EDGE('',*,*,#8638,.F.);
#12016=ORIENTED_EDGE('',*,*,#8639,.T.);
#12017=ORIENTED_EDGE('',*,*,#8640,.F.);
#12018=ORIENTED_EDGE('',*,*,#8641,.T.);
#12019=ORIENTED_EDGE('',*,*,#8638,.T.);
#12020=ORIENTED_EDGE('',*,*,#8642,.T.);
#12021=ORIENTED_EDGE('',*,*,#8643,.T.);
#12022=ORIENTED_EDGE('',*,*,#8635,.F.);
#12023=ORIENTED_EDGE('',*,*,#8644,.T.);
#12024=ORIENTED_EDGE('',*,*,#8584,.T.);
#12025=ORIENTED_EDGE('',*,*,#8645,.T.);
#12026=ORIENTED_EDGE('',*,*,#8646,.T.);
#12027=ORIENTED_EDGE('',*,*,#8581,.F.);
#12028=ORIENTED_EDGE('',*,*,#8647,.T.);
#12029=ORIENTED_EDGE('',*,*,#8529,.T.);
#12030=ORIENTED_EDGE('',*,*,#8648,.T.);
#12031=ORIENTED_EDGE('',*,*,#8649,.T.);
#12032=ORIENTED_EDGE('',*,*,#8525,.F.);
#12033=ORIENTED_EDGE('',*,*,#8650,.T.);
#12034=ORIENTED_EDGE('',*,*,#8471,.T.);
#12035=ORIENTED_EDGE('',*,*,#8651,.T.);
#12036=ORIENTED_EDGE('',*,*,#8652,.T.);
#12037=ORIENTED_EDGE('',*,*,#8467,.F.);
#12038=ORIENTED_EDGE('',*,*,#8653,.T.);
#12039=ORIENTED_EDGE('',*,*,#8412,.T.);
#12040=ORIENTED_EDGE('',*,*,#8654,.T.);
#12041=ORIENTED_EDGE('',*,*,#8655,.T.);
#12042=ORIENTED_EDGE('',*,*,#8407,.F.);
#12043=ORIENTED_EDGE('',*,*,#8656,.F.);
#12044=ORIENTED_EDGE('',*,*,#8657,.F.);
#12045=ORIENTED_EDGE('',*,*,#8341,.T.);
#12046=ORIENTED_EDGE('',*,*,#8658,.T.);
#12047=ORIENTED_EDGE('',*,*,#8659,.T.);
#12048=ORIENTED_EDGE('',*,*,#8336,.F.);
#12049=ORIENTED_EDGE('',*,*,#8660,.F.);
#12050=ORIENTED_EDGE('',*,*,#8661,.F.);
#12051=ORIENTED_EDGE('',*,*,#8270,.T.);
#12052=ORIENTED_EDGE('',*,*,#8662,.T.);
#12053=ORIENTED_EDGE('',*,*,#8663,.T.);
#12054=ORIENTED_EDGE('',*,*,#8265,.F.);
#12055=ORIENTED_EDGE('',*,*,#8664,.F.);
#12056=ORIENTED_EDGE('',*,*,#8665,.F.);
#12057=ORIENTED_EDGE('',*,*,#8199,.T.);
#12058=ORIENTED_EDGE('',*,*,#8666,.T.);
#12059=ORIENTED_EDGE('',*,*,#8667,.T.);
#12060=ORIENTED_EDGE('',*,*,#8194,.F.);
#12061=ORIENTED_EDGE('',*,*,#8668,.F.);
#12062=ORIENTED_EDGE('',*,*,#8669,.F.);
#12063=ORIENTED_EDGE('',*,*,#8130,.T.);
#12064=ORIENTED_EDGE('',*,*,#8670,.T.);
#12065=ORIENTED_EDGE('',*,*,#8671,.T.);
#12066=ORIENTED_EDGE('',*,*,#8127,.F.);
#12067=ORIENTED_EDGE('',*,*,#8672,.T.);
#12068=ORIENTED_EDGE('',*,*,#8065,.T.);
#12069=ORIENTED_EDGE('',*,*,#8673,.T.);
#12070=ORIENTED_EDGE('',*,*,#8674,.T.);
#12071=ORIENTED_EDGE('',*,*,#8060,.F.);
#12072=ORIENTED_EDGE('',*,*,#8675,.F.);
#12073=ORIENTED_EDGE('',*,*,#8676,.F.);
#12074=ORIENTED_EDGE('',*,*,#7987,.T.);
#12075=ORIENTED_EDGE('',*,*,#8677,.T.);
#12076=ORIENTED_EDGE('',*,*,#8678,.T.);
#12077=ORIENTED_EDGE('',*,*,#7984,.F.);
#12078=ORIENTED_EDGE('',*,*,#8679,.T.);
#12079=ORIENTED_EDGE('',*,*,#7922,.T.);
#12080=ORIENTED_EDGE('',*,*,#8680,.T.);
#12081=ORIENTED_EDGE('',*,*,#8681,.T.);
#12082=ORIENTED_EDGE('',*,*,#7917,.F.);
#12083=ORIENTED_EDGE('',*,*,#8682,.F.);
#12084=ORIENTED_EDGE('',*,*,#8683,.F.);
#12085=ORIENTED_EDGE('',*,*,#7930,.F.);
#12086=ORIENTED_EDGE('',*,*,#8684,.T.);
#12087=ORIENTED_EDGE('',*,*,#7850,.T.);
#12088=ORIENTED_EDGE('',*,*,#8685,.T.);
#12089=ORIENTED_EDGE('',*,*,#8685,.F.);
#12090=ORIENTED_EDGE('',*,*,#7849,.F.);
#12091=ORIENTED_EDGE('',*,*,#7854,.F.);
#12092=ORIENTED_EDGE('',*,*,#7853,.F.);
#12093=ORIENTED_EDGE('',*,*,#7859,.F.);
#12094=ORIENTED_EDGE('',*,*,#7858,.F.);
#12095=ORIENTED_EDGE('',*,*,#7864,.F.);
#12096=ORIENTED_EDGE('',*,*,#7863,.F.);
#12097=ORIENTED_EDGE('',*,*,#7869,.F.);
#12098=ORIENTED_EDGE('',*,*,#7868,.F.);
#12099=ORIENTED_EDGE('',*,*,#7874,.F.);
#12100=ORIENTED_EDGE('',*,*,#7873,.F.);
#12101=ORIENTED_EDGE('',*,*,#7879,.F.);
#12102=ORIENTED_EDGE('',*,*,#7878,.F.);
#12103=ORIENTED_EDGE('',*,*,#7884,.F.);
#12104=ORIENTED_EDGE('',*,*,#7883,.F.);
#12105=ORIENTED_EDGE('',*,*,#7889,.F.);
#12106=ORIENTED_EDGE('',*,*,#7888,.F.);
#12107=ORIENTED_EDGE('',*,*,#7894,.F.);
#12108=ORIENTED_EDGE('',*,*,#7893,.F.);
#12109=ORIENTED_EDGE('',*,*,#7899,.F.);
#12110=ORIENTED_EDGE('',*,*,#7898,.F.);
#12111=ORIENTED_EDGE('',*,*,#7904,.F.);
#12112=ORIENTED_EDGE('',*,*,#7903,.F.);
#12113=ORIENTED_EDGE('',*,*,#7909,.F.);
#12114=ORIENTED_EDGE('',*,*,#7908,.F.);
#12115=ORIENTED_EDGE('',*,*,#7914,.F.);
#12116=ORIENTED_EDGE('',*,*,#7913,.F.);
#12117=ORIENTED_EDGE('',*,*,#7919,.F.);
#12118=ORIENTED_EDGE('',*,*,#7918,.F.);
#12119=ORIENTED_EDGE('',*,*,#8681,.F.);
#12120=ORIENTED_EDGE('',*,*,#8680,.F.);
#12121=ORIENTED_EDGE('',*,*,#7927,.F.);
#12122=ORIENTED_EDGE('',*,*,#7926,.F.);
#12123=ORIENTED_EDGE('',*,*,#8686,.F.);
#12124=ORIENTED_EDGE('',*,*,#7988,.F.);
#12125=ORIENTED_EDGE('',*,*,#8679,.F.);
#12126=ORIENTED_EDGE('',*,*,#7986,.F.);
#12127=ORIENTED_EDGE('',*,*,#7983,.F.);
#12128=ORIENTED_EDGE('',*,*,#7982,.F.);
#12129=ORIENTED_EDGE('',*,*,#7978,.F.);
#12130=ORIENTED_EDGE('',*,*,#7975,.F.);
#12131=ORIENTED_EDGE('',*,*,#7974,.F.);
#12132=ORIENTED_EDGE('',*,*,#7970,.F.);
#12133=ORIENTED_EDGE('',*,*,#7967,.F.);
#12134=ORIENTED_EDGE('',*,*,#7966,.F.);
#12135=ORIENTED_EDGE('',*,*,#7962,.F.);
#12136=ORIENTED_EDGE('',*,*,#7959,.F.);
#12137=ORIENTED_EDGE('',*,*,#7958,.F.);
#12138=ORIENTED_EDGE('',*,*,#7954,.F.);
#12139=ORIENTED_EDGE('',*,*,#7951,.F.);
#12140=ORIENTED_EDGE('',*,*,#7950,.F.);
#12141=ORIENTED_EDGE('',*,*,#7946,.F.);
#12142=ORIENTED_EDGE('',*,*,#7943,.F.);
#12143=ORIENTED_EDGE('',*,*,#7942,.F.);
#12144=ORIENTED_EDGE('',*,*,#7938,.F.);
#12145=ORIENTED_EDGE('',*,*,#7937,.F.);
#12146=ORIENTED_EDGE('',*,*,#7934,.F.);
#12147=ORIENTED_EDGE('',*,*,#7931,.F.);
#12148=ORIENTED_EDGE('',*,*,#8684,.F.);
#12149=ORIENTED_EDGE('',*,*,#7929,.F.);
#12150=ORIENTED_EDGE('',*,*,#7936,.F.);
#12151=ORIENTED_EDGE('',*,*,#7941,.F.);
#12152=ORIENTED_EDGE('',*,*,#7940,.F.);
#12153=ORIENTED_EDGE('',*,*,#7945,.F.);
#12154=ORIENTED_EDGE('',*,*,#7949,.F.);
#12155=ORIENTED_EDGE('',*,*,#7948,.F.);
#12156=ORIENTED_EDGE('',*,*,#7953,.F.);
#12157=ORIENTED_EDGE('',*,*,#7957,.F.);
#12158=ORIENTED_EDGE('',*,*,#7956,.F.);
#12159=ORIENTED_EDGE('',*,*,#7961,.F.);
#12160=ORIENTED_EDGE('',*,*,#7965,.F.);
#12161=ORIENTED_EDGE('',*,*,#7964,.F.);
#12162=ORIENTED_EDGE('',*,*,#7969,.F.);
#12163=ORIENTED_EDGE('',*,*,#7973,.F.);
#12164=ORIENTED_EDGE('',*,*,#7972,.F.);
#12165=ORIENTED_EDGE('',*,*,#7977,.F.);
#12166=ORIENTED_EDGE('',*,*,#7981,.F.);
#12167=ORIENTED_EDGE('',*,*,#7980,.F.);
#12168=ORIENTED_EDGE('',*,*,#7985,.F.);
#12169=ORIENTED_EDGE('',*,*,#8678,.F.);
#12170=ORIENTED_EDGE('',*,*,#8677,.F.);
#12171=ORIENTED_EDGE('',*,*,#7990,.F.);
#12172=ORIENTED_EDGE('',*,*,#8687,.F.);
#12173=ORIENTED_EDGE('',*,*,#8688,.F.);
#12174=ORIENTED_EDGE('',*,*,#7924,.T.);
#12175=ORIENTED_EDGE('',*,*,#7923,.T.);
#12176=ORIENTED_EDGE('',*,*,#8683,.T.);
#12177=ORIENTED_EDGE('',*,*,#8682,.T.);
#12178=ORIENTED_EDGE('',*,*,#7921,.T.);
#12179=ORIENTED_EDGE('',*,*,#7920,.T.);
#12180=ORIENTED_EDGE('',*,*,#7916,.T.);
#12181=ORIENTED_EDGE('',*,*,#7915,.T.);
#12182=ORIENTED_EDGE('',*,*,#7911,.T.);
#12183=ORIENTED_EDGE('',*,*,#7910,.T.);
#12184=ORIENTED_EDGE('',*,*,#7906,.T.);
#12185=ORIENTED_EDGE('',*,*,#7905,.T.);
#12186=ORIENTED_EDGE('',*,*,#7901,.T.);
#12187=ORIENTED_EDGE('',*,*,#7900,.T.);
#12188=ORIENTED_EDGE('',*,*,#7896,.T.);
#12189=ORIENTED_EDGE('',*,*,#7895,.T.);
#12190=ORIENTED_EDGE('',*,*,#7891,.T.);
#12191=ORIENTED_EDGE('',*,*,#7890,.T.);
#12192=ORIENTED_EDGE('',*,*,#7886,.T.);
#12193=ORIENTED_EDGE('',*,*,#7885,.T.);
#12194=ORIENTED_EDGE('',*,*,#7881,.T.);
#12195=ORIENTED_EDGE('',*,*,#7880,.T.);
#12196=ORIENTED_EDGE('',*,*,#7876,.T.);
#12197=ORIENTED_EDGE('',*,*,#7875,.T.);
#12198=ORIENTED_EDGE('',*,*,#7871,.T.);
#12199=ORIENTED_EDGE('',*,*,#7870,.T.);
#12200=ORIENTED_EDGE('',*,*,#7866,.T.);
#12201=ORIENTED_EDGE('',*,*,#7865,.T.);
#12202=ORIENTED_EDGE('',*,*,#7861,.T.);
#12203=ORIENTED_EDGE('',*,*,#7860,.T.);
#12204=ORIENTED_EDGE('',*,*,#7856,.T.);
#12205=ORIENTED_EDGE('',*,*,#7855,.T.);
#12206=ORIENTED_EDGE('',*,*,#7851,.T.);
#12207=ORIENTED_EDGE('',*,*,#8073,.F.);
#12208=ORIENTED_EDGE('',*,*,#8689,.T.);
#12209=ORIENTED_EDGE('',*,*,#7993,.T.);
#12210=ORIENTED_EDGE('',*,*,#8690,.T.);
#12211=ORIENTED_EDGE('',*,*,#8690,.F.);
#12212=ORIENTED_EDGE('',*,*,#7992,.F.);
#12213=ORIENTED_EDGE('',*,*,#7997,.F.);
#12214=ORIENTED_EDGE('',*,*,#7996,.F.);
#12215=ORIENTED_EDGE('',*,*,#8002,.F.);
#12216=ORIENTED_EDGE('',*,*,#8001,.F.);
#12217=ORIENTED_EDGE('',*,*,#8007,.F.);
#12218=ORIENTED_EDGE('',*,*,#8006,.F.);
#12219=ORIENTED_EDGE('',*,*,#8012,.F.);
#12220=ORIENTED_EDGE('',*,*,#8011,.F.);
#12221=ORIENTED_EDGE('',*,*,#8017,.F.);
#12222=ORIENTED_EDGE('',*,*,#8016,.F.);
#12223=ORIENTED_EDGE('',*,*,#8022,.F.);
#12224=ORIENTED_EDGE('',*,*,#8021,.F.);
#12225=ORIENTED_EDGE('',*,*,#8027,.F.);
#12226=ORIENTED_EDGE('',*,*,#8026,.F.);
#12227=ORIENTED_EDGE('',*,*,#8032,.F.);
#12228=ORIENTED_EDGE('',*,*,#8031,.F.);
#12229=ORIENTED_EDGE('',*,*,#8037,.F.);
#12230=ORIENTED_EDGE('',*,*,#8036,.F.);
#12231=ORIENTED_EDGE('',*,*,#8042,.F.);
#12232=ORIENTED_EDGE('',*,*,#8041,.F.);
#12233=ORIENTED_EDGE('',*,*,#8047,.F.);
#12234=ORIENTED_EDGE('',*,*,#8046,.F.);
#12235=ORIENTED_EDGE('',*,*,#8052,.F.);
#12236=ORIENTED_EDGE('',*,*,#8051,.F.);
#12237=ORIENTED_EDGE('',*,*,#8057,.F.);
#12238=ORIENTED_EDGE('',*,*,#8056,.F.);
#12239=ORIENTED_EDGE('',*,*,#8062,.F.);
#12240=ORIENTED_EDGE('',*,*,#8061,.F.);
#12241=ORIENTED_EDGE('',*,*,#8674,.F.);
#12242=ORIENTED_EDGE('',*,*,#8673,.F.);
#12243=ORIENTED_EDGE('',*,*,#8070,.F.);
#12244=ORIENTED_EDGE('',*,*,#8069,.F.);
#12245=ORIENTED_EDGE('',*,*,#8691,.F.);
#12246=ORIENTED_EDGE('',*,*,#8131,.F.);
#12247=ORIENTED_EDGE('',*,*,#8672,.F.);
#12248=ORIENTED_EDGE('',*,*,#8129,.F.);
#12249=ORIENTED_EDGE('',*,*,#8126,.F.);
#12250=ORIENTED_EDGE('',*,*,#8125,.F.);
#12251=ORIENTED_EDGE('',*,*,#8121,.F.);
#12252=ORIENTED_EDGE('',*,*,#8118,.F.);
#12253=ORIENTED_EDGE('',*,*,#8117,.F.);
#12254=ORIENTED_EDGE('',*,*,#8113,.F.);
#12255=ORIENTED_EDGE('',*,*,#8110,.F.);
#12256=ORIENTED_EDGE('',*,*,#8109,.F.);
#12257=ORIENTED_EDGE('',*,*,#8105,.F.);
#12258=ORIENTED_EDGE('',*,*,#8102,.F.);
#12259=ORIENTED_EDGE('',*,*,#8101,.F.);
#12260=ORIENTED_EDGE('',*,*,#8097,.F.);
#12261=ORIENTED_EDGE('',*,*,#8094,.F.);
#12262=ORIENTED_EDGE('',*,*,#8093,.F.);
#12263=ORIENTED_EDGE('',*,*,#8089,.F.);
#12264=ORIENTED_EDGE('',*,*,#8086,.F.);
#12265=ORIENTED_EDGE('',*,*,#8085,.F.);
#12266=ORIENTED_EDGE('',*,*,#8081,.F.);
#12267=ORIENTED_EDGE('',*,*,#8080,.F.);
#12268=ORIENTED_EDGE('',*,*,#8077,.F.);
#12269=ORIENTED_EDGE('',*,*,#8074,.F.);
#12270=ORIENTED_EDGE('',*,*,#8689,.F.);
#12271=ORIENTED_EDGE('',*,*,#8072,.F.);
#12272=ORIENTED_EDGE('',*,*,#8079,.F.);
#12273=ORIENTED_EDGE('',*,*,#8084,.F.);
#12274=ORIENTED_EDGE('',*,*,#8083,.F.);
#12275=ORIENTED_EDGE('',*,*,#8088,.F.);
#12276=ORIENTED_EDGE('',*,*,#8092,.F.);
#12277=ORIENTED_EDGE('',*,*,#8091,.F.);
#12278=ORIENTED_EDGE('',*,*,#8096,.F.);
#12279=ORIENTED_EDGE('',*,*,#8100,.F.);
#12280=ORIENTED_EDGE('',*,*,#8099,.F.);
#12281=ORIENTED_EDGE('',*,*,#8104,.F.);
#12282=ORIENTED_EDGE('',*,*,#8108,.F.);
#12283=ORIENTED_EDGE('',*,*,#8107,.F.);
#12284=ORIENTED_EDGE('',*,*,#8112,.F.);
#12285=ORIENTED_EDGE('',*,*,#8116,.F.);
#12286=ORIENTED_EDGE('',*,*,#8115,.F.);
#12287=ORIENTED_EDGE('',*,*,#8120,.F.);
#12288=ORIENTED_EDGE('',*,*,#8124,.F.);
#12289=ORIENTED_EDGE('',*,*,#8123,.F.);
#12290=ORIENTED_EDGE('',*,*,#8128,.F.);
#12291=ORIENTED_EDGE('',*,*,#8671,.F.);
#12292=ORIENTED_EDGE('',*,*,#8670,.F.);
#12293=ORIENTED_EDGE('',*,*,#8133,.F.);
#12294=ORIENTED_EDGE('',*,*,#8692,.F.);
#12295=ORIENTED_EDGE('',*,*,#8693,.F.);
#12296=ORIENTED_EDGE('',*,*,#8067,.T.);
#12297=ORIENTED_EDGE('',*,*,#8066,.T.);
#12298=ORIENTED_EDGE('',*,*,#8676,.T.);
#12299=ORIENTED_EDGE('',*,*,#8675,.T.);
#12300=ORIENTED_EDGE('',*,*,#8064,.T.);
#12301=ORIENTED_EDGE('',*,*,#8063,.T.);
#12302=ORIENTED_EDGE('',*,*,#8059,.T.);
#12303=ORIENTED_EDGE('',*,*,#8058,.T.);
#12304=ORIENTED_EDGE('',*,*,#8054,.T.);
#12305=ORIENTED_EDGE('',*,*,#8053,.T.);
#12306=ORIENTED_EDGE('',*,*,#8049,.T.);
#12307=ORIENTED_EDGE('',*,*,#8048,.T.);
#12308=ORIENTED_EDGE('',*,*,#8044,.T.);
#12309=ORIENTED_EDGE('',*,*,#8043,.T.);
#12310=ORIENTED_EDGE('',*,*,#8039,.T.);
#12311=ORIENTED_EDGE('',*,*,#8038,.T.);
#12312=ORIENTED_EDGE('',*,*,#8034,.T.);
#12313=ORIENTED_EDGE('',*,*,#8033,.T.);
#12314=ORIENTED_EDGE('',*,*,#8029,.T.);
#12315=ORIENTED_EDGE('',*,*,#8028,.T.);
#12316=ORIENTED_EDGE('',*,*,#8024,.T.);
#12317=ORIENTED_EDGE('',*,*,#8023,.T.);
#12318=ORIENTED_EDGE('',*,*,#8019,.T.);
#12319=ORIENTED_EDGE('',*,*,#8018,.T.);
#12320=ORIENTED_EDGE('',*,*,#8014,.T.);
#12321=ORIENTED_EDGE('',*,*,#8013,.T.);
#12322=ORIENTED_EDGE('',*,*,#8009,.T.);
#12323=ORIENTED_EDGE('',*,*,#8008,.T.);
#12324=ORIENTED_EDGE('',*,*,#8004,.T.);
#12325=ORIENTED_EDGE('',*,*,#8003,.T.);
#12326=ORIENTED_EDGE('',*,*,#7999,.T.);
#12327=ORIENTED_EDGE('',*,*,#7998,.T.);
#12328=ORIENTED_EDGE('',*,*,#7994,.T.);
#12329=ORIENTED_EDGE('',*,*,#8076,.F.);
#12330=ORIENTED_EDGE('',*,*,#7933,.F.);
#12331=ORIENTED_EDGE('',*,*,#8694,.F.);
#12332=ORIENTED_EDGE('',*,*,#8695,.F.);
#12333=ORIENTED_EDGE('',*,*,#8696,.F.);
#12334=ORIENTED_EDGE('',*,*,#8697,.T.);
#12335=ORIENTED_EDGE('',*,*,#8698,.F.);
#12336=ORIENTED_EDGE('',*,*,#8697,.F.);
#12337=ORIENTED_EDGE('',*,*,#8699,.F.);
#12338=ORIENTED_EDGE('',*,*,#8700,.T.);
#12339=ORIENTED_EDGE('',*,*,#8701,.F.);
#12340=ORIENTED_EDGE('',*,*,#8700,.F.);
#12341=ORIENTED_EDGE('',*,*,#8702,.F.);
#12342=ORIENTED_EDGE('',*,*,#8703,.T.);
#12343=ORIENTED_EDGE('',*,*,#8704,.F.);
#12344=ORIENTED_EDGE('',*,*,#8703,.F.);
#12345=ORIENTED_EDGE('',*,*,#8705,.F.);
#12346=ORIENTED_EDGE('',*,*,#8695,.T.);
#12347=ORIENTED_EDGE('',*,*,#8706,.F.);
#12348=ORIENTED_EDGE('',*,*,#8707,.T.);
#12349=ORIENTED_EDGE('',*,*,#8708,.F.);
#12350=ORIENTED_EDGE('',*,*,#8707,.F.);
#12351=ORIENTED_EDGE('',*,*,#8709,.F.);
#12352=ORIENTED_EDGE('',*,*,#8710,.T.);
#12353=ORIENTED_EDGE('',*,*,#8711,.F.);
#12354=ORIENTED_EDGE('',*,*,#8710,.F.);
#12355=ORIENTED_EDGE('',*,*,#8712,.F.);
#12356=ORIENTED_EDGE('',*,*,#8713,.T.);
#12357=ORIENTED_EDGE('',*,*,#8714,.F.);
#12358=ORIENTED_EDGE('',*,*,#8713,.F.);
#12359=ORIENTED_EDGE('',*,*,#8715,.F.);
#12360=ORIENTED_EDGE('',*,*,#8716,.T.);
#12361=ORIENTED_EDGE('',*,*,#8717,.F.);
#12362=ORIENTED_EDGE('',*,*,#8716,.F.);
#12363=ORIENTED_EDGE('',*,*,#8718,.F.);
#12364=ORIENTED_EDGE('',*,*,#8135,.F.);
#12365=ORIENTED_EDGE('',*,*,#8141,.F.);
#12366=ORIENTED_EDGE('',*,*,#8140,.F.);
#12367=ORIENTED_EDGE('',*,*,#8146,.F.);
#12368=ORIENTED_EDGE('',*,*,#8145,.F.);
#12369=ORIENTED_EDGE('',*,*,#8151,.F.);
#12370=ORIENTED_EDGE('',*,*,#8150,.F.);
#12371=ORIENTED_EDGE('',*,*,#8156,.F.);
#12372=ORIENTED_EDGE('',*,*,#8155,.F.);
#12373=ORIENTED_EDGE('',*,*,#8161,.F.);
#12374=ORIENTED_EDGE('',*,*,#8160,.F.);
#12375=ORIENTED_EDGE('',*,*,#8166,.F.);
#12376=ORIENTED_EDGE('',*,*,#8165,.F.);
#12377=ORIENTED_EDGE('',*,*,#8171,.F.);
#12378=ORIENTED_EDGE('',*,*,#8170,.F.);
#12379=ORIENTED_EDGE('',*,*,#8176,.F.);
#12380=ORIENTED_EDGE('',*,*,#8175,.F.);
#12381=ORIENTED_EDGE('',*,*,#8181,.F.);
#12382=ORIENTED_EDGE('',*,*,#8180,.F.);
#12383=ORIENTED_EDGE('',*,*,#8186,.F.);
#12384=ORIENTED_EDGE('',*,*,#8185,.F.);
#12385=ORIENTED_EDGE('',*,*,#8191,.F.);
#12386=ORIENTED_EDGE('',*,*,#8190,.F.);
#12387=ORIENTED_EDGE('',*,*,#8196,.F.);
#12388=ORIENTED_EDGE('',*,*,#8195,.F.);
#12389=ORIENTED_EDGE('',*,*,#8667,.F.);
#12390=ORIENTED_EDGE('',*,*,#8666,.F.);
#12391=ORIENTED_EDGE('',*,*,#8204,.F.);
#12392=ORIENTED_EDGE('',*,*,#8203,.F.);
#12393=ORIENTED_EDGE('',*,*,#8719,.F.);
#12394=ORIENTED_EDGE('',*,*,#8531,.F.);
#12395=ORIENTED_EDGE('',*,*,#8530,.F.);
#12396=ORIENTED_EDGE('',*,*,#8650,.F.);
#12397=ORIENTED_EDGE('',*,*,#8528,.F.);
#12398=ORIENTED_EDGE('',*,*,#8527,.F.);
#12399=ORIENTED_EDGE('',*,*,#8524,.F.);
#12400=ORIENTED_EDGE('',*,*,#8520,.F.);
#12401=ORIENTED_EDGE('',*,*,#8519,.F.);
#12402=ORIENTED_EDGE('',*,*,#8516,.F.);
#12403=ORIENTED_EDGE('',*,*,#8512,.F.);
#12404=ORIENTED_EDGE('',*,*,#8511,.F.);
#12405=ORIENTED_EDGE('',*,*,#8508,.F.);
#12406=ORIENTED_EDGE('',*,*,#8507,.F.);
#12407=ORIENTED_EDGE('',*,*,#8503,.F.);
#12408=ORIENTED_EDGE('',*,*,#8502,.F.);
#12409=ORIENTED_EDGE('',*,*,#8499,.F.);
#12410=ORIENTED_EDGE('',*,*,#8495,.F.);
#12411=ORIENTED_EDGE('',*,*,#8494,.F.);
#12412=ORIENTED_EDGE('',*,*,#8491,.F.);
#12413=ORIENTED_EDGE('',*,*,#8487,.F.);
#12414=ORIENTED_EDGE('',*,*,#8486,.F.);
#12415=ORIENTED_EDGE('',*,*,#8483,.F.);
#12416=ORIENTED_EDGE('',*,*,#8479,.F.);
#12417=ORIENTED_EDGE('',*,*,#8720,.T.);
#12418=ORIENTED_EDGE('',*,*,#8721,.F.);
#12419=ORIENTED_EDGE('',*,*,#8477,.F.);
#12420=ORIENTED_EDGE('',*,*,#8482,.F.);
#12421=ORIENTED_EDGE('',*,*,#8481,.F.);
#12422=ORIENTED_EDGE('',*,*,#8485,.F.);
#12423=ORIENTED_EDGE('',*,*,#8490,.F.);
#12424=ORIENTED_EDGE('',*,*,#8489,.F.);
#12425=ORIENTED_EDGE('',*,*,#8493,.F.);
#12426=ORIENTED_EDGE('',*,*,#8498,.F.);
#12427=ORIENTED_EDGE('',*,*,#8497,.F.);
#12428=ORIENTED_EDGE('',*,*,#8501,.F.);
#12429=ORIENTED_EDGE('',*,*,#8506,.F.);
#12430=ORIENTED_EDGE('',*,*,#8505,.F.);
#12431=ORIENTED_EDGE('',*,*,#8510,.F.);
#12432=ORIENTED_EDGE('',*,*,#8515,.F.);
#12433=ORIENTED_EDGE('',*,*,#8514,.F.);
#12434=ORIENTED_EDGE('',*,*,#8518,.F.);
#12435=ORIENTED_EDGE('',*,*,#8523,.F.);
#12436=ORIENTED_EDGE('',*,*,#8522,.F.);
#12437=ORIENTED_EDGE('',*,*,#8526,.F.);
#12438=ORIENTED_EDGE('',*,*,#8649,.F.);
#12439=ORIENTED_EDGE('',*,*,#8648,.F.);
#12440=ORIENTED_EDGE('',*,*,#8533,.F.);
#12441=ORIENTED_EDGE('',*,*,#8722,.F.);
#12442=ORIENTED_EDGE('',*,*,#8723,.F.);
#12443=ORIENTED_EDGE('',*,*,#8201,.T.);
#12444=ORIENTED_EDGE('',*,*,#8200,.T.);
#12445=ORIENTED_EDGE('',*,*,#8669,.T.);
#12446=ORIENTED_EDGE('',*,*,#8668,.T.);
#12447=ORIENTED_EDGE('',*,*,#8198,.T.);
#12448=ORIENTED_EDGE('',*,*,#8197,.T.);
#12449=ORIENTED_EDGE('',*,*,#8193,.T.);
#12450=ORIENTED_EDGE('',*,*,#8192,.T.);
#12451=ORIENTED_EDGE('',*,*,#8188,.T.);
#12452=ORIENTED_EDGE('',*,*,#8187,.T.);
#12453=ORIENTED_EDGE('',*,*,#8183,.T.);
#12454=ORIENTED_EDGE('',*,*,#8182,.T.);
#12455=ORIENTED_EDGE('',*,*,#8178,.T.);
#12456=ORIENTED_EDGE('',*,*,#8177,.T.);
#12457=ORIENTED_EDGE('',*,*,#8173,.T.);
#12458=ORIENTED_EDGE('',*,*,#8172,.T.);
#12459=ORIENTED_EDGE('',*,*,#8168,.T.);
#12460=ORIENTED_EDGE('',*,*,#8167,.T.);
#12461=ORIENTED_EDGE('',*,*,#8163,.T.);
#12462=ORIENTED_EDGE('',*,*,#8162,.T.);
#12463=ORIENTED_EDGE('',*,*,#8158,.T.);
#12464=ORIENTED_EDGE('',*,*,#8157,.T.);
#12465=ORIENTED_EDGE('',*,*,#8153,.T.);
#12466=ORIENTED_EDGE('',*,*,#8152,.T.);
#12467=ORIENTED_EDGE('',*,*,#8148,.T.);
#12468=ORIENTED_EDGE('',*,*,#8147,.T.);
#12469=ORIENTED_EDGE('',*,*,#8143,.T.);
#12470=ORIENTED_EDGE('',*,*,#8142,.T.);
#12471=ORIENTED_EDGE('',*,*,#8138,.T.);
#12472=ORIENTED_EDGE('',*,*,#8137,.T.);
#12473=ORIENTED_EDGE('',*,*,#8724,.F.);
#12474=ORIENTED_EDGE('',*,*,#8206,.F.);
#12475=ORIENTED_EDGE('',*,*,#8212,.F.);
#12476=ORIENTED_EDGE('',*,*,#8211,.F.);
#12477=ORIENTED_EDGE('',*,*,#8217,.F.);
#12478=ORIENTED_EDGE('',*,*,#8216,.F.);
#12479=ORIENTED_EDGE('',*,*,#8222,.F.);
#12480=ORIENTED_EDGE('',*,*,#8221,.F.);
#12481=ORIENTED_EDGE('',*,*,#8227,.F.);
#12482=ORIENTED_EDGE('',*,*,#8226,.F.);
#12483=ORIENTED_EDGE('',*,*,#8232,.F.);
#12484=ORIENTED_EDGE('',*,*,#8231,.F.);
#12485=ORIENTED_EDGE('',*,*,#8237,.F.);
#12486=ORIENTED_EDGE('',*,*,#8236,.F.);
#12487=ORIENTED_EDGE('',*,*,#8242,.F.);
#12488=ORIENTED_EDGE('',*,*,#8241,.F.);
#12489=ORIENTED_EDGE('',*,*,#8247,.F.);
#12490=ORIENTED_EDGE('',*,*,#8246,.F.);
#12491=ORIENTED_EDGE('',*,*,#8252,.F.);
#12492=ORIENTED_EDGE('',*,*,#8251,.F.);
#12493=ORIENTED_EDGE('',*,*,#8257,.F.);
#12494=ORIENTED_EDGE('',*,*,#8256,.F.);
#12495=ORIENTED_EDGE('',*,*,#8262,.F.);
#12496=ORIENTED_EDGE('',*,*,#8261,.F.);
#12497=ORIENTED_EDGE('',*,*,#8267,.F.);
#12498=ORIENTED_EDGE('',*,*,#8266,.F.);
#12499=ORIENTED_EDGE('',*,*,#8663,.F.);
#12500=ORIENTED_EDGE('',*,*,#8662,.F.);
#12501=ORIENTED_EDGE('',*,*,#8275,.F.);
#12502=ORIENTED_EDGE('',*,*,#8274,.F.);
#12503=ORIENTED_EDGE('',*,*,#8725,.F.);
#12504=ORIENTED_EDGE('',*,*,#8473,.F.);
#12505=ORIENTED_EDGE('',*,*,#8472,.F.);
#12506=ORIENTED_EDGE('',*,*,#8653,.F.);
#12507=ORIENTED_EDGE('',*,*,#8470,.F.);
#12508=ORIENTED_EDGE('',*,*,#8469,.F.);
#12509=ORIENTED_EDGE('',*,*,#8466,.F.);
#12510=ORIENTED_EDGE('',*,*,#8462,.F.);
#12511=ORIENTED_EDGE('',*,*,#8461,.F.);
#12512=ORIENTED_EDGE('',*,*,#8458,.F.);
#12513=ORIENTED_EDGE('',*,*,#8454,.F.);
#12514=ORIENTED_EDGE('',*,*,#8453,.F.);
#12515=ORIENTED_EDGE('',*,*,#8450,.F.);
#12516=ORIENTED_EDGE('',*,*,#8449,.F.);
#12517=ORIENTED_EDGE('',*,*,#8445,.F.);
#12518=ORIENTED_EDGE('',*,*,#8444,.F.);
#12519=ORIENTED_EDGE('',*,*,#8441,.F.);
#12520=ORIENTED_EDGE('',*,*,#8437,.F.);
#12521=ORIENTED_EDGE('',*,*,#8436,.F.);
#12522=ORIENTED_EDGE('',*,*,#8433,.F.);
#12523=ORIENTED_EDGE('',*,*,#8429,.F.);
#12524=ORIENTED_EDGE('',*,*,#8428,.F.);
#12525=ORIENTED_EDGE('',*,*,#8425,.F.);
#12526=ORIENTED_EDGE('',*,*,#8421,.F.);
#12527=ORIENTED_EDGE('',*,*,#8726,.T.);
#12528=ORIENTED_EDGE('',*,*,#8727,.F.);
#12529=ORIENTED_EDGE('',*,*,#8419,.F.);
#12530=ORIENTED_EDGE('',*,*,#8424,.F.);
#12531=ORIENTED_EDGE('',*,*,#8423,.F.);
#12532=ORIENTED_EDGE('',*,*,#8427,.F.);
#12533=ORIENTED_EDGE('',*,*,#8432,.F.);
#12534=ORIENTED_EDGE('',*,*,#8431,.F.);
#12535=ORIENTED_EDGE('',*,*,#8435,.F.);
#12536=ORIENTED_EDGE('',*,*,#8440,.F.);
#12537=ORIENTED_EDGE('',*,*,#8439,.F.);
#12538=ORIENTED_EDGE('',*,*,#8443,.F.);
#12539=ORIENTED_EDGE('',*,*,#8448,.F.);
#12540=ORIENTED_EDGE('',*,*,#8447,.F.);
#12541=ORIENTED_EDGE('',*,*,#8452,.F.);
#12542=ORIENTED_EDGE('',*,*,#8457,.F.);
#12543=ORIENTED_EDGE('',*,*,#8456,.F.);
#12544=ORIENTED_EDGE('',*,*,#8460,.F.);
#12545=ORIENTED_EDGE('',*,*,#8465,.F.);
#12546=ORIENTED_EDGE('',*,*,#8464,.F.);
#12547=ORIENTED_EDGE('',*,*,#8468,.F.);
#12548=ORIENTED_EDGE('',*,*,#8652,.F.);
#12549=ORIENTED_EDGE('',*,*,#8651,.F.);
#12550=ORIENTED_EDGE('',*,*,#8475,.F.);
#12551=ORIENTED_EDGE('',*,*,#8728,.F.);
#12552=ORIENTED_EDGE('',*,*,#8729,.F.);
#12553=ORIENTED_EDGE('',*,*,#8272,.T.);
#12554=ORIENTED_EDGE('',*,*,#8271,.T.);
#12555=ORIENTED_EDGE('',*,*,#8665,.T.);
#12556=ORIENTED_EDGE('',*,*,#8664,.T.);
#12557=ORIENTED_EDGE('',*,*,#8269,.T.);
#12558=ORIENTED_EDGE('',*,*,#8268,.T.);
#12559=ORIENTED_EDGE('',*,*,#8264,.T.);
#12560=ORIENTED_EDGE('',*,*,#8263,.T.);
#12561=ORIENTED_EDGE('',*,*,#8259,.T.);
#12562=ORIENTED_EDGE('',*,*,#8258,.T.);
#12563=ORIENTED_EDGE('',*,*,#8254,.T.);
#12564=ORIENTED_EDGE('',*,*,#8253,.T.);
#12565=ORIENTED_EDGE('',*,*,#8249,.T.);
#12566=ORIENTED_EDGE('',*,*,#8248,.T.);
#12567=ORIENTED_EDGE('',*,*,#8244,.T.);
#12568=ORIENTED_EDGE('',*,*,#8243,.T.);
#12569=ORIENTED_EDGE('',*,*,#8239,.T.);
#12570=ORIENTED_EDGE('',*,*,#8238,.T.);
#12571=ORIENTED_EDGE('',*,*,#8234,.T.);
#12572=ORIENTED_EDGE('',*,*,#8233,.T.);
#12573=ORIENTED_EDGE('',*,*,#8229,.T.);
#12574=ORIENTED_EDGE('',*,*,#8228,.T.);
#12575=ORIENTED_EDGE('',*,*,#8224,.T.);
#12576=ORIENTED_EDGE('',*,*,#8223,.T.);
#12577=ORIENTED_EDGE('',*,*,#8219,.T.);
#12578=ORIENTED_EDGE('',*,*,#8218,.T.);
#12579=ORIENTED_EDGE('',*,*,#8214,.T.);
#12580=ORIENTED_EDGE('',*,*,#8213,.T.);
#12581=ORIENTED_EDGE('',*,*,#8209,.T.);
#12582=ORIENTED_EDGE('',*,*,#8208,.T.);
#12583=ORIENTED_EDGE('',*,*,#8730,.F.);
#12584=ORIENTED_EDGE('',*,*,#8277,.F.);
#12585=ORIENTED_EDGE('',*,*,#8283,.F.);
#12586=ORIENTED_EDGE('',*,*,#8282,.F.);
#12587=ORIENTED_EDGE('',*,*,#8288,.F.);
#12588=ORIENTED_EDGE('',*,*,#8287,.F.);
#12589=ORIENTED_EDGE('',*,*,#8293,.F.);
#12590=ORIENTED_EDGE('',*,*,#8292,.F.);
#12591=ORIENTED_EDGE('',*,*,#8298,.F.);
#12592=ORIENTED_EDGE('',*,*,#8297,.F.);
#12593=ORIENTED_EDGE('',*,*,#8303,.F.);
#12594=ORIENTED_EDGE('',*,*,#8302,.F.);
#12595=ORIENTED_EDGE('',*,*,#8308,.F.);
#12596=ORIENTED_EDGE('',*,*,#8307,.F.);
#12597=ORIENTED_EDGE('',*,*,#8313,.F.);
#12598=ORIENTED_EDGE('',*,*,#8312,.F.);
#12599=ORIENTED_EDGE('',*,*,#8318,.F.);
#12600=ORIENTED_EDGE('',*,*,#8317,.F.);
#12601=ORIENTED_EDGE('',*,*,#8323,.F.);
#12602=ORIENTED_EDGE('',*,*,#8322,.F.);
#12603=ORIENTED_EDGE('',*,*,#8328,.F.);
#12604=ORIENTED_EDGE('',*,*,#8327,.F.);
#12605=ORIENTED_EDGE('',*,*,#8333,.F.);
#12606=ORIENTED_EDGE('',*,*,#8332,.F.);
#12607=ORIENTED_EDGE('',*,*,#8338,.F.);
#12608=ORIENTED_EDGE('',*,*,#8337,.F.);
#12609=ORIENTED_EDGE('',*,*,#8659,.F.);
#12610=ORIENTED_EDGE('',*,*,#8658,.F.);
#12611=ORIENTED_EDGE('',*,*,#8346,.F.);
#12612=ORIENTED_EDGE('',*,*,#8345,.F.);
#12613=ORIENTED_EDGE('',*,*,#8731,.F.);
#12614=ORIENTED_EDGE('',*,*,#8639,.F.);
#12615=ORIENTED_EDGE('',*,*,#8644,.F.);
#12616=ORIENTED_EDGE('',*,*,#8637,.F.);
#12617=ORIENTED_EDGE('',*,*,#8634,.F.);
#12618=ORIENTED_EDGE('',*,*,#8630,.F.);
#12619=ORIENTED_EDGE('',*,*,#8629,.F.);
#12620=ORIENTED_EDGE('',*,*,#8626,.F.);
#12621=ORIENTED_EDGE('',*,*,#8622,.F.);
#12622=ORIENTED_EDGE('',*,*,#8621,.F.);
#12623=ORIENTED_EDGE('',*,*,#8618,.F.);
#12624=ORIENTED_EDGE('',*,*,#8617,.F.);
#12625=ORIENTED_EDGE('',*,*,#8613,.F.);
#12626=ORIENTED_EDGE('',*,*,#8612,.F.);
#12627=ORIENTED_EDGE('',*,*,#8609,.F.);
#12628=ORIENTED_EDGE('',*,*,#8605,.F.);
#12629=ORIENTED_EDGE('',*,*,#8604,.F.);
#12630=ORIENTED_EDGE('',*,*,#8601,.F.);
#12631=ORIENTED_EDGE('',*,*,#8598,.F.);
#12632=ORIENTED_EDGE('',*,*,#8597,.F.);
#12633=ORIENTED_EDGE('',*,*,#8594,.F.);
#12634=ORIENTED_EDGE('',*,*,#8591,.F.);
#12635=ORIENTED_EDGE('',*,*,#8732,.T.);
#12636=ORIENTED_EDGE('',*,*,#8733,.F.);
#12637=ORIENTED_EDGE('',*,*,#8589,.F.);
#12638=ORIENTED_EDGE('',*,*,#8593,.F.);
#12639=ORIENTED_EDGE('',*,*,#8596,.F.);
#12640=ORIENTED_EDGE('',*,*,#8600,.F.);
#12641=ORIENTED_EDGE('',*,*,#8603,.F.);
#12642=ORIENTED_EDGE('',*,*,#8608,.F.);
#12643=ORIENTED_EDGE('',*,*,#8607,.F.);
#12644=ORIENTED_EDGE('',*,*,#8611,.F.);
#12645=ORIENTED_EDGE('',*,*,#8616,.F.);
#12646=ORIENTED_EDGE('',*,*,#8615,.F.);
#12647=ORIENTED_EDGE('',*,*,#8620,.F.);
#12648=ORIENTED_EDGE('',*,*,#8625,.F.);
#12649=ORIENTED_EDGE('',*,*,#8624,.F.);
#12650=ORIENTED_EDGE('',*,*,#8628,.F.);
#12651=ORIENTED_EDGE('',*,*,#8633,.F.);
#12652=ORIENTED_EDGE('',*,*,#8632,.F.);
#12653=ORIENTED_EDGE('',*,*,#8636,.F.);
#12654=ORIENTED_EDGE('',*,*,#8643,.F.);
#12655=ORIENTED_EDGE('',*,*,#8642,.F.);
#12656=ORIENTED_EDGE('',*,*,#8641,.F.);
#12657=ORIENTED_EDGE('',*,*,#8734,.F.);
#12658=ORIENTED_EDGE('',*,*,#8735,.F.);
#12659=ORIENTED_EDGE('',*,*,#8343,.T.);
#12660=ORIENTED_EDGE('',*,*,#8342,.T.);
#12661=ORIENTED_EDGE('',*,*,#8661,.T.);
#12662=ORIENTED_EDGE('',*,*,#8660,.T.);
#12663=ORIENTED_EDGE('',*,*,#8340,.T.);
#12664=ORIENTED_EDGE('',*,*,#8339,.T.);
#12665=ORIENTED_EDGE('',*,*,#8335,.T.);
#12666=ORIENTED_EDGE('',*,*,#8334,.T.);
#12667=ORIENTED_EDGE('',*,*,#8330,.T.);
#12668=ORIENTED_EDGE('',*,*,#8329,.T.);
#12669=ORIENTED_EDGE('',*,*,#8325,.T.);
#12670=ORIENTED_EDGE('',*,*,#8324,.T.);
#12671=ORIENTED_EDGE('',*,*,#8320,.T.);
#12672=ORIENTED_EDGE('',*,*,#8319,.T.);
#12673=ORIENTED_EDGE('',*,*,#8315,.T.);
#12674=ORIENTED_EDGE('',*,*,#8314,.T.);
#12675=ORIENTED_EDGE('',*,*,#8310,.T.);
#12676=ORIENTED_EDGE('',*,*,#8309,.T.);
#12677=ORIENTED_EDGE('',*,*,#8305,.T.);
#12678=ORIENTED_EDGE('',*,*,#8304,.T.);
#12679=ORIENTED_EDGE('',*,*,#8300,.T.);
#12680=ORIENTED_EDGE('',*,*,#8299,.T.);
#12681=ORIENTED_EDGE('',*,*,#8295,.T.);
#12682=ORIENTED_EDGE('',*,*,#8294,.T.);
#12683=ORIENTED_EDGE('',*,*,#8290,.T.);
#12684=ORIENTED_EDGE('',*,*,#8289,.T.);
#12685=ORIENTED_EDGE('',*,*,#8285,.T.);
#12686=ORIENTED_EDGE('',*,*,#8284,.T.);
#12687=ORIENTED_EDGE('',*,*,#8280,.T.);
#12688=ORIENTED_EDGE('',*,*,#8279,.T.);
#12689=ORIENTED_EDGE('',*,*,#8736,.F.);
#12690=ORIENTED_EDGE('',*,*,#8348,.F.);
#12691=ORIENTED_EDGE('',*,*,#8354,.F.);
#12692=ORIENTED_EDGE('',*,*,#8353,.F.);
#12693=ORIENTED_EDGE('',*,*,#8359,.F.);
#12694=ORIENTED_EDGE('',*,*,#8358,.F.);
#12695=ORIENTED_EDGE('',*,*,#8364,.F.);
#12696=ORIENTED_EDGE('',*,*,#8363,.F.);
#12697=ORIENTED_EDGE('',*,*,#8369,.F.);
#12698=ORIENTED_EDGE('',*,*,#8368,.F.);
#12699=ORIENTED_EDGE('',*,*,#8374,.F.);
#12700=ORIENTED_EDGE('',*,*,#8373,.F.);
#12701=ORIENTED_EDGE('',*,*,#8379,.F.);
#12702=ORIENTED_EDGE('',*,*,#8378,.F.);
#12703=ORIENTED_EDGE('',*,*,#8384,.F.);
#12704=ORIENTED_EDGE('',*,*,#8383,.F.);
#12705=ORIENTED_EDGE('',*,*,#8389,.F.);
#12706=ORIENTED_EDGE('',*,*,#8388,.F.);
#12707=ORIENTED_EDGE('',*,*,#8394,.F.);
#12708=ORIENTED_EDGE('',*,*,#8393,.F.);
#12709=ORIENTED_EDGE('',*,*,#8399,.F.);
#12710=ORIENTED_EDGE('',*,*,#8398,.F.);
#12711=ORIENTED_EDGE('',*,*,#8404,.F.);
#12712=ORIENTED_EDGE('',*,*,#8403,.F.);
#12713=ORIENTED_EDGE('',*,*,#8409,.F.);
#12714=ORIENTED_EDGE('',*,*,#8408,.F.);
#12715=ORIENTED_EDGE('',*,*,#8655,.F.);
#12716=ORIENTED_EDGE('',*,*,#8654,.F.);
#12717=ORIENTED_EDGE('',*,*,#8417,.F.);
#12718=ORIENTED_EDGE('',*,*,#8416,.F.);
#12719=ORIENTED_EDGE('',*,*,#8737,.F.);
#12720=ORIENTED_EDGE('',*,*,#8585,.F.);
#12721=ORIENTED_EDGE('',*,*,#8647,.F.);
#12722=ORIENTED_EDGE('',*,*,#8583,.F.);
#12723=ORIENTED_EDGE('',*,*,#8580,.F.);
#12724=ORIENTED_EDGE('',*,*,#8576,.F.);
#12725=ORIENTED_EDGE('',*,*,#8575,.F.);
#12726=ORIENTED_EDGE('',*,*,#8572,.F.);
#12727=ORIENTED_EDGE('',*,*,#8568,.F.);
#12728=ORIENTED_EDGE('',*,*,#8567,.F.);
#12729=ORIENTED_EDGE('',*,*,#8564,.F.);
#12730=ORIENTED_EDGE('',*,*,#8563,.F.);
#12731=ORIENTED_EDGE('',*,*,#8559,.F.);
#12732=ORIENTED_EDGE('',*,*,#8558,.F.);
#12733=ORIENTED_EDGE('',*,*,#8555,.F.);
#12734=ORIENTED_EDGE('',*,*,#8551,.F.);
#12735=ORIENTED_EDGE('',*,*,#8550,.F.);
#12736=ORIENTED_EDGE('',*,*,#8547,.F.);
#12737=ORIENTED_EDGE('',*,*,#8544,.F.);
#12738=ORIENTED_EDGE('',*,*,#8543,.F.);
#12739=ORIENTED_EDGE('',*,*,#8540,.F.);
#12740=ORIENTED_EDGE('',*,*,#8537,.F.);
#12741=ORIENTED_EDGE('',*,*,#8738,.T.);
#12742=ORIENTED_EDGE('',*,*,#8739,.F.);
#12743=ORIENTED_EDGE('',*,*,#8535,.F.);
#12744=ORIENTED_EDGE('',*,*,#8539,.F.);
#12745=ORIENTED_EDGE('',*,*,#8542,.F.);
#12746=ORIENTED_EDGE('',*,*,#8546,.F.);
#12747=ORIENTED_EDGE('',*,*,#8549,.F.);
#12748=ORIENTED_EDGE('',*,*,#8554,.F.);
#12749=ORIENTED_EDGE('',*,*,#8553,.F.);
#12750=ORIENTED_EDGE('',*,*,#8557,.F.);
#12751=ORIENTED_EDGE('',*,*,#8562,.F.);
#12752=ORIENTED_EDGE('',*,*,#8561,.F.);
#12753=ORIENTED_EDGE('',*,*,#8566,.F.);
#12754=ORIENTED_EDGE('',*,*,#8571,.F.);
#12755=ORIENTED_EDGE('',*,*,#8570,.F.);
#12756=ORIENTED_EDGE('',*,*,#8574,.F.);
#12757=ORIENTED_EDGE('',*,*,#8579,.F.);
#12758=ORIENTED_EDGE('',*,*,#8578,.F.);
#12759=ORIENTED_EDGE('',*,*,#8582,.F.);
#12760=ORIENTED_EDGE('',*,*,#8646,.F.);
#12761=ORIENTED_EDGE('',*,*,#8645,.F.);
#12762=ORIENTED_EDGE('',*,*,#8587,.F.);
#12763=ORIENTED_EDGE('',*,*,#8740,.F.);
#12764=ORIENTED_EDGE('',*,*,#8741,.F.);
#12765=ORIENTED_EDGE('',*,*,#8414,.T.);
#12766=ORIENTED_EDGE('',*,*,#8413,.T.);
#12767=ORIENTED_EDGE('',*,*,#8657,.T.);
#12768=ORIENTED_EDGE('',*,*,#8656,.T.);
#12769=ORIENTED_EDGE('',*,*,#8411,.T.);
#12770=ORIENTED_EDGE('',*,*,#8410,.T.);
#12771=ORIENTED_EDGE('',*,*,#8406,.T.);
#12772=ORIENTED_EDGE('',*,*,#8405,.T.);
#12773=ORIENTED_EDGE('',*,*,#8401,.T.);
#12774=ORIENTED_EDGE('',*,*,#8400,.T.);
#12775=ORIENTED_EDGE('',*,*,#8396,.T.);
#12776=ORIENTED_EDGE('',*,*,#8395,.T.);
#12777=ORIENTED_EDGE('',*,*,#8391,.T.);
#12778=ORIENTED_EDGE('',*,*,#8390,.T.);
#12779=ORIENTED_EDGE('',*,*,#8386,.T.);
#12780=ORIENTED_EDGE('',*,*,#8385,.T.);
#12781=ORIENTED_EDGE('',*,*,#8381,.T.);
#12782=ORIENTED_EDGE('',*,*,#8380,.T.);
#12783=ORIENTED_EDGE('',*,*,#8376,.T.);
#12784=ORIENTED_EDGE('',*,*,#8375,.T.);
#12785=ORIENTED_EDGE('',*,*,#8371,.T.);
#12786=ORIENTED_EDGE('',*,*,#8370,.T.);
#12787=ORIENTED_EDGE('',*,*,#8366,.T.);
#12788=ORIENTED_EDGE('',*,*,#8365,.T.);
#12789=ORIENTED_EDGE('',*,*,#8361,.T.);
#12790=ORIENTED_EDGE('',*,*,#8360,.T.);
#12791=ORIENTED_EDGE('',*,*,#8356,.T.);
#12792=ORIENTED_EDGE('',*,*,#8355,.T.);
#12793=ORIENTED_EDGE('',*,*,#8351,.T.);
#12794=ORIENTED_EDGE('',*,*,#8350,.T.);
#12795=ORIENTED_EDGE('',*,*,#8727,.T.);
#12796=ORIENTED_EDGE('',*,*,#8207,.T.);
#12797=ORIENTED_EDGE('',*,*,#8724,.T.);
#12798=ORIENTED_EDGE('',*,*,#8726,.F.);
#12799=ORIENTED_EDGE('',*,*,#8420,.F.);
#12800=ORIENTED_EDGE('',*,*,#8721,.T.);
#12801=ORIENTED_EDGE('',*,*,#8136,.T.);
#12802=ORIENTED_EDGE('',*,*,#8718,.T.);
#12803=ORIENTED_EDGE('',*,*,#8720,.F.);
#12804=ORIENTED_EDGE('',*,*,#8478,.F.);
#12805=ORIENTED_EDGE('',*,*,#8739,.T.);
#12806=ORIENTED_EDGE('',*,*,#8349,.T.);
#12807=ORIENTED_EDGE('',*,*,#8736,.T.);
#12808=ORIENTED_EDGE('',*,*,#8738,.F.);
#12809=ORIENTED_EDGE('',*,*,#8536,.F.);
#12810=ORIENTED_EDGE('',*,*,#8733,.T.);
#12811=ORIENTED_EDGE('',*,*,#8278,.T.);
#12812=ORIENTED_EDGE('',*,*,#8730,.T.);
#12813=ORIENTED_EDGE('',*,*,#8732,.F.);
#12814=ORIENTED_EDGE('',*,*,#8590,.F.);
#12815=ORIENTED_EDGE('',*,*,#8742,.F.);
#12816=ORIENTED_EDGE('',*,*,#8743,.T.);
#12817=ORIENTED_EDGE('',*,*,#8744,.F.);
#12818=ORIENTED_EDGE('',*,*,#8743,.F.);
#12819=ORIENTED_EDGE('',*,*,#8701,.T.);
#12820=ORIENTED_EDGE('',*,*,#8704,.T.);
#12821=ORIENTED_EDGE('',*,*,#8694,.T.);
#12822=ORIENTED_EDGE('',*,*,#8698,.T.);
#12823=ORIENTED_EDGE('',*,*,#8745,.T.);
#12824=ORIENTED_EDGE('',*,*,#8746,.T.);
#12825=ORIENTED_EDGE('',*,*,#8747,.T.);
#12826=ORIENTED_EDGE('',*,*,#8748,.T.);
#12827=ORIENTED_EDGE('',*,*,#8749,.F.);
#12828=ORIENTED_EDGE('',*,*,#8750,.F.);
#12829=ORIENTED_EDGE('',*,*,#8751,.F.);
#12830=ORIENTED_EDGE('',*,*,#8752,.F.);
#12831=ORIENTED_EDGE('',*,*,#8715,.T.);
#12832=ORIENTED_EDGE('',*,*,#8712,.T.);
#12833=ORIENTED_EDGE('',*,*,#8709,.T.);
#12834=ORIENTED_EDGE('',*,*,#8706,.T.);
#12835=ORIENTED_EDGE('',*,*,#8753,.T.);
#12836=ORIENTED_EDGE('',*,*,#8754,.T.);
#12837=ORIENTED_EDGE('',*,*,#8748,.F.);
#12838=ORIENTED_EDGE('',*,*,#8755,.F.);
#12839=ORIENTED_EDGE('',*,*,#8756,.T.);
#12840=ORIENTED_EDGE('',*,*,#8755,.T.);
#12841=ORIENTED_EDGE('',*,*,#8747,.F.);
#12842=ORIENTED_EDGE('',*,*,#8757,.F.);
#12843=ORIENTED_EDGE('',*,*,#8758,.T.);
#12844=ORIENTED_EDGE('',*,*,#8757,.T.);
#12845=ORIENTED_EDGE('',*,*,#8746,.F.);
#12846=ORIENTED_EDGE('',*,*,#8759,.F.);
#12847=ORIENTED_EDGE('',*,*,#8760,.T.);
#12848=ORIENTED_EDGE('',*,*,#8759,.T.);
#12849=ORIENTED_EDGE('',*,*,#8745,.F.);
#12850=ORIENTED_EDGE('',*,*,#8754,.F.);
#12851=ORIENTED_EDGE('',*,*,#8760,.F.);
#12852=ORIENTED_EDGE('',*,*,#8753,.F.);
#12853=ORIENTED_EDGE('',*,*,#8756,.F.);
#12854=ORIENTED_EDGE('',*,*,#8758,.F.);
#12855=ORIENTED_EDGE('',*,*,#8708,.T.);
#12856=ORIENTED_EDGE('',*,*,#8711,.T.);
#12857=ORIENTED_EDGE('',*,*,#8714,.T.);
#12858=ORIENTED_EDGE('',*,*,#8717,.T.);
#12859=ORIENTED_EDGE('',*,*,#8749,.T.);
#12860=ORIENTED_EDGE('',*,*,#8761,.T.);
#12861=ORIENTED_EDGE('',*,*,#8762,.F.);
#12862=ORIENTED_EDGE('',*,*,#8763,.F.);
#12863=ORIENTED_EDGE('',*,*,#8750,.T.);
#12864=ORIENTED_EDGE('',*,*,#8763,.T.);
#12865=ORIENTED_EDGE('',*,*,#8764,.F.);
#12866=ORIENTED_EDGE('',*,*,#8765,.F.);
#12867=ORIENTED_EDGE('',*,*,#8742,.T.);
#12868=ORIENTED_EDGE('',*,*,#8751,.T.);
#12869=ORIENTED_EDGE('',*,*,#8765,.T.);
#12870=ORIENTED_EDGE('',*,*,#8766,.F.);
#12871=ORIENTED_EDGE('',*,*,#8767,.F.);
#12872=ORIENTED_EDGE('',*,*,#8752,.T.);
#12873=ORIENTED_EDGE('',*,*,#8767,.T.);
#12874=ORIENTED_EDGE('',*,*,#8768,.F.);
#12875=ORIENTED_EDGE('',*,*,#8761,.F.);
#12876=ORIENTED_EDGE('',*,*,#8723,.T.);
#12877=ORIENTED_EDGE('',*,*,#8722,.T.);
#12878=ORIENTED_EDGE('',*,*,#8532,.T.);
#12879=ORIENTED_EDGE('',*,*,#8719,.T.);
#12880=ORIENTED_EDGE('',*,*,#8202,.T.);
#12881=ORIENTED_EDGE('',*,*,#8729,.T.);
#12882=ORIENTED_EDGE('',*,*,#8728,.T.);
#12883=ORIENTED_EDGE('',*,*,#8474,.T.);
#12884=ORIENTED_EDGE('',*,*,#8725,.T.);
#12885=ORIENTED_EDGE('',*,*,#8273,.T.);
#12886=ORIENTED_EDGE('',*,*,#8735,.T.);
#12887=ORIENTED_EDGE('',*,*,#8734,.T.);
#12888=ORIENTED_EDGE('',*,*,#8640,.T.);
#12889=ORIENTED_EDGE('',*,*,#8731,.T.);
#12890=ORIENTED_EDGE('',*,*,#8344,.T.);
#12891=ORIENTED_EDGE('',*,*,#8741,.T.);
#12892=ORIENTED_EDGE('',*,*,#8740,.T.);
#12893=ORIENTED_EDGE('',*,*,#8586,.T.);
#12894=ORIENTED_EDGE('',*,*,#8737,.T.);
#12895=ORIENTED_EDGE('',*,*,#8415,.T.);
#12896=ORIENTED_EDGE('',*,*,#8744,.T.);
#12897=ORIENTED_EDGE('',*,*,#8768,.T.);
#12898=ORIENTED_EDGE('',*,*,#8766,.T.);
#12899=ORIENTED_EDGE('',*,*,#8764,.T.);
#12900=ORIENTED_EDGE('',*,*,#8762,.T.);
#12901=ORIENTED_EDGE('',*,*,#8688,.T.);
#12902=ORIENTED_EDGE('',*,*,#8687,.T.);
#12903=ORIENTED_EDGE('',*,*,#7989,.T.);
#12904=ORIENTED_EDGE('',*,*,#8686,.T.);
#12905=ORIENTED_EDGE('',*,*,#7925,.T.);
#12906=ORIENTED_EDGE('',*,*,#8693,.T.);
#12907=ORIENTED_EDGE('',*,*,#8692,.T.);
#12908=ORIENTED_EDGE('',*,*,#8132,.T.);
#12909=ORIENTED_EDGE('',*,*,#8691,.T.);
#12910=ORIENTED_EDGE('',*,*,#8068,.T.);
#12911=ORIENTED_EDGE('',*,*,#8702,.T.);
#12912=ORIENTED_EDGE('',*,*,#8699,.T.);
#12913=ORIENTED_EDGE('',*,*,#8696,.T.);
#12914=ORIENTED_EDGE('',*,*,#8705,.T.);
#15791=CYLINDRICAL_SURFACE('',#17187,2.05475);
#15792=CYLINDRICAL_SURFACE('',#17189,2.05475);
#15793=CYLINDRICAL_SURFACE('',#17190,2.05475);
#15794=CYLINDRICAL_SURFACE('',#17191,2.05475);
#15795=CYLINDRICAL_SURFACE('',#17192,2.05475);
#15796=CYLINDRICAL_SURFACE('',#17193,2.05475);
#15797=CYLINDRICAL_SURFACE('',#17194,2.05475);
#15798=CYLINDRICAL_SURFACE('',#17195,2.05475);
#15799=CYLINDRICAL_SURFACE('',#17196,2.05475);
#15800=CYLINDRICAL_SURFACE('',#17197,2.05475);
#15801=CYLINDRICAL_SURFACE('',#17198,2.05475);
#15802=CYLINDRICAL_SURFACE('',#17199,2.05475);
#15803=CYLINDRICAL_SURFACE('',#17200,2.05475);
#15804=CYLINDRICAL_SURFACE('',#17201,2.05475);
#15805=CYLINDRICAL_SURFACE('',#17202,2.05475);
#15806=CYLINDRICAL_SURFACE('',#17203,2.05475);
#15807=CYLINDRICAL_SURFACE('',#17205,1.666);
#15808=CYLINDRICAL_SURFACE('',#17208,1.666);
#15809=CYLINDRICAL_SURFACE('',#17209,1.666);
#15810=CYLINDRICAL_SURFACE('',#17210,1.666);
#15811=CYLINDRICAL_SURFACE('',#17211,1.666);
#15812=CYLINDRICAL_SURFACE('',#17212,1.666);
#15813=CYLINDRICAL_SURFACE('',#17213,1.666);
#15814=CYLINDRICAL_SURFACE('',#17214,1.666);
#15815=CYLINDRICAL_SURFACE('',#17215,1.666);
#15816=CYLINDRICAL_SURFACE('',#17216,1.666);
#15817=CYLINDRICAL_SURFACE('',#17217,1.666);
#15818=CYLINDRICAL_SURFACE('',#17218,1.666);
#15819=CYLINDRICAL_SURFACE('',#17219,1.666);
#15820=CYLINDRICAL_SURFACE('',#17220,1.666);
#15821=CYLINDRICAL_SURFACE('',#17221,1.666);
#15822=CYLINDRICAL_SURFACE('',#17223,2.05475);
#15823=CYLINDRICAL_SURFACE('',#17225,2.05475);
#15824=CYLINDRICAL_SURFACE('',#17226,2.05475);
#15825=CYLINDRICAL_SURFACE('',#17227,2.05475);
#15826=CYLINDRICAL_SURFACE('',#17228,2.05475);
#15827=CYLINDRICAL_SURFACE('',#17229,2.05475);
#15828=CYLINDRICAL_SURFACE('',#17230,2.05475);
#15829=CYLINDRICAL_SURFACE('',#17231,2.05475);
#15830=CYLINDRICAL_SURFACE('',#17232,2.05475);
#15831=CYLINDRICAL_SURFACE('',#17233,2.05475);
#15832=CYLINDRICAL_SURFACE('',#17234,2.05475);
#15833=CYLINDRICAL_SURFACE('',#17235,2.05475);
#15834=CYLINDRICAL_SURFACE('',#17236,2.05475);
#15835=CYLINDRICAL_SURFACE('',#17237,2.05475);
#15836=CYLINDRICAL_SURFACE('',#17238,2.05475);
#15837=CYLINDRICAL_SURFACE('',#17239,2.05475);
#15838=CYLINDRICAL_SURFACE('',#17241,1.666);
#15839=CYLINDRICAL_SURFACE('',#17244,1.666);
#15840=CYLINDRICAL_SURFACE('',#17245,1.666);
#15841=CYLINDRICAL_SURFACE('',#17246,1.666);
#15842=CYLINDRICAL_SURFACE('',#17247,1.666);
#15843=CYLINDRICAL_SURFACE('',#17248,1.666);
#15844=CYLINDRICAL_SURFACE('',#17249,1.666);
#15845=CYLINDRICAL_SURFACE('',#17250,1.666);
#15846=CYLINDRICAL_SURFACE('',#17251,1.666);
#15847=CYLINDRICAL_SURFACE('',#17252,1.666);
#15848=CYLINDRICAL_SURFACE('',#17253,1.666);
#15849=CYLINDRICAL_SURFACE('',#17254,1.666);
#15850=CYLINDRICAL_SURFACE('',#17255,1.666);
#15851=CYLINDRICAL_SURFACE('',#17256,1.666);
#15852=CYLINDRICAL_SURFACE('',#17257,1.666);
#15853=CYLINDRICAL_SURFACE('',#17259,2.05475);
#15854=CYLINDRICAL_SURFACE('',#17261,2.05475);
#15855=CYLINDRICAL_SURFACE('',#17262,2.05475);
#15856=CYLINDRICAL_SURFACE('',#17263,2.05475);
#15857=CYLINDRICAL_SURFACE('',#17264,2.05475);
#15858=CYLINDRICAL_SURFACE('',#17265,2.05475);
#15859=CYLINDRICAL_SURFACE('',#17266,2.05475);
#15860=CYLINDRICAL_SURFACE('',#17267,2.05475);
#15861=CYLINDRICAL_SURFACE('',#17268,2.05475);
#15862=CYLINDRICAL_SURFACE('',#17269,2.05475);
#15863=CYLINDRICAL_SURFACE('',#17270,2.05475);
#15864=CYLINDRICAL_SURFACE('',#17271,2.05475);
#15865=CYLINDRICAL_SURFACE('',#17272,2.05475);
#15866=CYLINDRICAL_SURFACE('',#17273,2.05475);
#15867=CYLINDRICAL_SURFACE('',#17275,2.05475);
#15868=CYLINDRICAL_SURFACE('',#17277,2.05475);
#15869=CYLINDRICAL_SURFACE('',#17278,2.05475);
#15870=CYLINDRICAL_SURFACE('',#17279,2.05475);
#15871=CYLINDRICAL_SURFACE('',#17280,2.05475);
#15872=CYLINDRICAL_SURFACE('',#17281,2.05475);
#15873=CYLINDRICAL_SURFACE('',#17282,2.05475);
#15874=CYLINDRICAL_SURFACE('',#17283,2.05475);
#15875=CYLINDRICAL_SURFACE('',#17284,2.05475);
#15876=CYLINDRICAL_SURFACE('',#17285,2.05475);
#15877=CYLINDRICAL_SURFACE('',#17286,2.05475);
#15878=CYLINDRICAL_SURFACE('',#17287,2.05475);
#15879=CYLINDRICAL_SURFACE('',#17288,2.05475);
#15880=CYLINDRICAL_SURFACE('',#17289,2.05475);
#15881=CYLINDRICAL_SURFACE('',#17291,2.05475);
#15882=CYLINDRICAL_SURFACE('',#17293,2.05475);
#15883=CYLINDRICAL_SURFACE('',#17294,2.05475);
#15884=CYLINDRICAL_SURFACE('',#17295,2.05475);
#15885=CYLINDRICAL_SURFACE('',#17296,2.05475);
#15886=CYLINDRICAL_SURFACE('',#17297,2.05475);
#15887=CYLINDRICAL_SURFACE('',#17298,2.05475);
#15888=CYLINDRICAL_SURFACE('',#17299,2.05475);
#15889=CYLINDRICAL_SURFACE('',#17300,2.05475);
#15890=CYLINDRICAL_SURFACE('',#17301,2.05475);
#15891=CYLINDRICAL_SURFACE('',#17302,2.05475);
#15892=CYLINDRICAL_SURFACE('',#17303,2.05475);
#15893=CYLINDRICAL_SURFACE('',#17304,2.05475);
#15894=CYLINDRICAL_SURFACE('',#17305,2.05475);
#15895=CYLINDRICAL_SURFACE('',#17307,2.05475);
#15896=CYLINDRICAL_SURFACE('',#17309,2.05475);
#15897=CYLINDRICAL_SURFACE('',#17310,2.05475);
#15898=CYLINDRICAL_SURFACE('',#17311,2.05475);
#15899=CYLINDRICAL_SURFACE('',#17312,2.05475);
#15900=CYLINDRICAL_SURFACE('',#17313,2.05475);
#15901=CYLINDRICAL_SURFACE('',#17314,2.05475);
#15902=CYLINDRICAL_SURFACE('',#17315,2.05475);
#15903=CYLINDRICAL_SURFACE('',#17316,2.05475);
#15904=CYLINDRICAL_SURFACE('',#17317,2.05475);
#15905=CYLINDRICAL_SURFACE('',#17318,2.05475);
#15906=CYLINDRICAL_SURFACE('',#17319,2.05475);
#15907=CYLINDRICAL_SURFACE('',#17320,2.05475);
#15908=CYLINDRICAL_SURFACE('',#17321,2.05475);
#15909=CYLINDRICAL_SURFACE('',#17323,1.666);
#15910=CYLINDRICAL_SURFACE('',#17325,1.666);
#15911=CYLINDRICAL_SURFACE('',#17326,1.666);
#15912=CYLINDRICAL_SURFACE('',#17327,1.666);
#15913=CYLINDRICAL_SURFACE('',#17328,1.666);
#15914=CYLINDRICAL_SURFACE('',#17329,1.666);
#15915=CYLINDRICAL_SURFACE('',#17330,1.666);
#15916=CYLINDRICAL_SURFACE('',#17331,1.666);
#15917=CYLINDRICAL_SURFACE('',#17332,1.666);
#15918=CYLINDRICAL_SURFACE('',#17333,1.666);
#15919=CYLINDRICAL_SURFACE('',#17334,1.666);
#15920=CYLINDRICAL_SURFACE('',#17335,1.666);
#15921=CYLINDRICAL_SURFACE('',#17336,1.666);
#15922=CYLINDRICAL_SURFACE('',#17337,1.666);
#15923=CYLINDRICAL_SURFACE('',#17339,1.666);
#15924=CYLINDRICAL_SURFACE('',#17341,1.666);
#15925=CYLINDRICAL_SURFACE('',#17342,1.666);
#15926=CYLINDRICAL_SURFACE('',#17343,1.666);
#15927=CYLINDRICAL_SURFACE('',#17344,1.666);
#15928=CYLINDRICAL_SURFACE('',#17345,1.666);
#15929=CYLINDRICAL_SURFACE('',#17346,1.666);
#15930=CYLINDRICAL_SURFACE('',#17347,1.666);
#15931=CYLINDRICAL_SURFACE('',#17348,1.666);
#15932=CYLINDRICAL_SURFACE('',#17349,1.666);
#15933=CYLINDRICAL_SURFACE('',#17350,1.666);
#15934=CYLINDRICAL_SURFACE('',#17351,1.666);
#15935=CYLINDRICAL_SURFACE('',#17352,1.666);
#15936=CYLINDRICAL_SURFACE('',#17353,1.666);
#15937=CYLINDRICAL_SURFACE('',#17355,1.666);
#15938=CYLINDRICAL_SURFACE('',#17357,1.666);
#15939=CYLINDRICAL_SURFACE('',#17358,1.666);
#15940=CYLINDRICAL_SURFACE('',#17359,1.666);
#15941=CYLINDRICAL_SURFACE('',#17360,1.666);
#15942=CYLINDRICAL_SURFACE('',#17361,1.666);
#15943=CYLINDRICAL_SURFACE('',#17362,1.666);
#15944=CYLINDRICAL_SURFACE('',#17363,1.666);
#15945=CYLINDRICAL_SURFACE('',#17364,1.666);
#15946=CYLINDRICAL_SURFACE('',#17365,1.666);
#15947=CYLINDRICAL_SURFACE('',#17366,1.666);
#15948=CYLINDRICAL_SURFACE('',#17367,1.666);
#15949=CYLINDRICAL_SURFACE('',#17368,1.666);
#15950=CYLINDRICAL_SURFACE('',#17369,1.666);
#15951=CYLINDRICAL_SURFACE('',#17371,1.666);
#15952=CYLINDRICAL_SURFACE('',#17373,1.666);
#15953=CYLINDRICAL_SURFACE('',#17374,1.666);
#15954=CYLINDRICAL_SURFACE('',#17375,1.666);
#15955=CYLINDRICAL_SURFACE('',#17376,1.666);
#15956=CYLINDRICAL_SURFACE('',#17377,1.666);
#15957=CYLINDRICAL_SURFACE('',#17378,1.666);
#15958=CYLINDRICAL_SURFACE('',#17379,1.666);
#15959=CYLINDRICAL_SURFACE('',#17380,1.666);
#15960=CYLINDRICAL_SURFACE('',#17381,1.666);
#15961=CYLINDRICAL_SURFACE('',#17382,1.666);
#15962=CYLINDRICAL_SURFACE('',#17383,1.666);
#15963=CYLINDRICAL_SURFACE('',#17384,1.666);
#15964=CYLINDRICAL_SURFACE('',#17385,1.666);
#15965=CYLINDRICAL_SURFACE('',#17387,1.666);
#15966=CYLINDRICAL_SURFACE('',#17388,1.666);
#15967=CYLINDRICAL_SURFACE('',#17389,1.666);
#15968=CYLINDRICAL_SURFACE('',#17390,1.666);
#15969=CYLINDRICAL_SURFACE('',#17391,2.05475);
#15970=CYLINDRICAL_SURFACE('',#17392,2.05475);
#15971=CYLINDRICAL_SURFACE('',#17393,2.05475);
#15972=CYLINDRICAL_SURFACE('',#17394,2.05475);
#15973=CYLINDRICAL_SURFACE('',#17395,1.666);
#15974=CYLINDRICAL_SURFACE('',#17396,2.05475);
#15975=CYLINDRICAL_SURFACE('',#17397,1.666);
#15976=CYLINDRICAL_SURFACE('',#17398,2.05475);
#15977=CYLINDRICAL_SURFACE('',#17409,4.5);
#15978=CYLINDRICAL_SURFACE('',#17412,4.5);
#15979=CYLINDRICAL_SURFACE('',#17415,4.5);
#15980=CYLINDRICAL_SURFACE('',#17418,4.5);
#15981=CYLINDRICAL_SURFACE('',#17425,22.);
#16305=ADVANCED_FACE('',(#537),#15791,.F.);
#16306=ADVANCED_FACE('',(#538),#15792,.F.);
#16307=ADVANCED_FACE('',(#539),#15793,.F.);
#16308=ADVANCED_FACE('',(#540),#15794,.F.);
#16309=ADVANCED_FACE('',(#541),#15795,.F.);
#16310=ADVANCED_FACE('',(#542),#15796,.F.);
#16311=ADVANCED_FACE('',(#543),#15797,.F.);
#16312=ADVANCED_FACE('',(#544),#15798,.F.);
#16313=ADVANCED_FACE('',(#545),#15799,.F.);
#16314=ADVANCED_FACE('',(#546),#15800,.F.);
#16315=ADVANCED_FACE('',(#547),#15801,.F.);
#16316=ADVANCED_FACE('',(#548),#15802,.F.);
#16317=ADVANCED_FACE('',(#549),#15803,.F.);
#16318=ADVANCED_FACE('',(#550),#15804,.F.);
#16319=ADVANCED_FACE('',(#551),#15805,.F.);
#16320=ADVANCED_FACE('',(#552),#15806,.F.);
#16321=ADVANCED_FACE('',(#553),#15807,.F.);
#16322=ADVANCED_FACE('',(#554),#15808,.F.);
#16323=ADVANCED_FACE('',(#555),#15809,.F.);
#16324=ADVANCED_FACE('',(#556),#15810,.F.);
#16325=ADVANCED_FACE('',(#557),#15811,.F.);
#16326=ADVANCED_FACE('',(#558),#15812,.F.);
#16327=ADVANCED_FACE('',(#559),#15813,.F.);
#16328=ADVANCED_FACE('',(#560),#15814,.F.);
#16329=ADVANCED_FACE('',(#561),#15815,.F.);
#16330=ADVANCED_FACE('',(#562),#15816,.F.);
#16331=ADVANCED_FACE('',(#563),#15817,.F.);
#16332=ADVANCED_FACE('',(#564),#15818,.F.);
#16333=ADVANCED_FACE('',(#565),#15819,.F.);
#16334=ADVANCED_FACE('',(#566),#15820,.F.);
#16335=ADVANCED_FACE('',(#567),#15821,.F.);
#16336=ADVANCED_FACE('',(#568),#15822,.F.);
#16337=ADVANCED_FACE('',(#569),#15823,.F.);
#16338=ADVANCED_FACE('',(#570),#15824,.F.);
#16339=ADVANCED_FACE('',(#571),#15825,.F.);
#16340=ADVANCED_FACE('',(#572),#15826,.F.);
#16341=ADVANCED_FACE('',(#573),#15827,.F.);
#16342=ADVANCED_FACE('',(#574),#15828,.F.);
#16343=ADVANCED_FACE('',(#575),#15829,.F.);
#16344=ADVANCED_FACE('',(#576),#15830,.F.);
#16345=ADVANCED_FACE('',(#577),#15831,.F.);
#16346=ADVANCED_FACE('',(#578),#15832,.F.);
#16347=ADVANCED_FACE('',(#579),#15833,.F.);
#16348=ADVANCED_FACE('',(#580),#15834,.F.);
#16349=ADVANCED_FACE('',(#581),#15835,.F.);
#16350=ADVANCED_FACE('',(#582),#15836,.F.);
#16351=ADVANCED_FACE('',(#583),#15837,.F.);
#16352=ADVANCED_FACE('',(#584),#15838,.F.);
#16353=ADVANCED_FACE('',(#585),#15839,.F.);
#16354=ADVANCED_FACE('',(#586),#15840,.F.);
#16355=ADVANCED_FACE('',(#587),#15841,.F.);
#16356=ADVANCED_FACE('',(#588),#15842,.F.);
#16357=ADVANCED_FACE('',(#589),#15843,.F.);
#16358=ADVANCED_FACE('',(#590),#15844,.F.);
#16359=ADVANCED_FACE('',(#591),#15845,.F.);
#16360=ADVANCED_FACE('',(#592),#15846,.F.);
#16361=ADVANCED_FACE('',(#593),#15847,.F.);
#16362=ADVANCED_FACE('',(#594),#15848,.F.);
#16363=ADVANCED_FACE('',(#595),#15849,.F.);
#16364=ADVANCED_FACE('',(#596),#15850,.F.);
#16365=ADVANCED_FACE('',(#597),#15851,.F.);
#16366=ADVANCED_FACE('',(#598),#15852,.F.);
#16367=ADVANCED_FACE('',(#599),#15853,.F.);
#16368=ADVANCED_FACE('',(#600),#15854,.F.);
#16369=ADVANCED_FACE('',(#601),#15855,.F.);
#16370=ADVANCED_FACE('',(#602),#15856,.F.);
#16371=ADVANCED_FACE('',(#603),#15857,.F.);
#16372=ADVANCED_FACE('',(#604),#15858,.F.);
#16373=ADVANCED_FACE('',(#605),#15859,.F.);
#16374=ADVANCED_FACE('',(#606),#15860,.F.);
#16375=ADVANCED_FACE('',(#607),#15861,.F.);
#16376=ADVANCED_FACE('',(#608),#15862,.F.);
#16377=ADVANCED_FACE('',(#609),#15863,.F.);
#16378=ADVANCED_FACE('',(#610),#15864,.F.);
#16379=ADVANCED_FACE('',(#611),#15865,.F.);
#16380=ADVANCED_FACE('',(#612),#15866,.F.);
#16381=ADVANCED_FACE('',(#613),#15867,.F.);
#16382=ADVANCED_FACE('',(#614),#15868,.F.);
#16383=ADVANCED_FACE('',(#615),#15869,.F.);
#16384=ADVANCED_FACE('',(#616),#15870,.F.);
#16385=ADVANCED_FACE('',(#617),#15871,.F.);
#16386=ADVANCED_FACE('',(#618),#15872,.F.);
#16387=ADVANCED_FACE('',(#619),#15873,.F.);
#16388=ADVANCED_FACE('',(#620),#15874,.F.);
#16389=ADVANCED_FACE('',(#621),#15875,.F.);
#16390=ADVANCED_FACE('',(#622),#15876,.F.);
#16391=ADVANCED_FACE('',(#623),#15877,.F.);
#16392=ADVANCED_FACE('',(#624),#15878,.F.);
#16393=ADVANCED_FACE('',(#625),#15879,.F.);
#16394=ADVANCED_FACE('',(#626),#15880,.F.);
#16395=ADVANCED_FACE('',(#627),#15881,.F.);
#16396=ADVANCED_FACE('',(#628),#15882,.F.);
#16397=ADVANCED_FACE('',(#629),#15883,.F.);
#16398=ADVANCED_FACE('',(#630),#15884,.F.);
#16399=ADVANCED_FACE('',(#631),#15885,.F.);
#16400=ADVANCED_FACE('',(#632),#15886,.F.);
#16401=ADVANCED_FACE('',(#633),#15887,.F.);
#16402=ADVANCED_FACE('',(#634),#15888,.F.);
#16403=ADVANCED_FACE('',(#635),#15889,.F.);
#16404=ADVANCED_FACE('',(#636),#15890,.F.);
#16405=ADVANCED_FACE('',(#637),#15891,.F.);
#16406=ADVANCED_FACE('',(#638),#15892,.F.);
#16407=ADVANCED_FACE('',(#639),#15893,.F.);
#16408=ADVANCED_FACE('',(#640),#15894,.F.);
#16409=ADVANCED_FACE('',(#641),#15895,.F.);
#16410=ADVANCED_FACE('',(#642),#15896,.F.);
#16411=ADVANCED_FACE('',(#643),#15897,.F.);
#16412=ADVANCED_FACE('',(#644),#15898,.F.);
#16413=ADVANCED_FACE('',(#645),#15899,.F.);
#16414=ADVANCED_FACE('',(#646),#15900,.F.);
#16415=ADVANCED_FACE('',(#647),#15901,.F.);
#16416=ADVANCED_FACE('',(#648),#15902,.F.);
#16417=ADVANCED_FACE('',(#649),#15903,.F.);
#16418=ADVANCED_FACE('',(#650),#15904,.F.);
#16419=ADVANCED_FACE('',(#651),#15905,.F.);
#16420=ADVANCED_FACE('',(#652),#15906,.F.);
#16421=ADVANCED_FACE('',(#653),#15907,.F.);
#16422=ADVANCED_FACE('',(#654),#15908,.F.);
#16423=ADVANCED_FACE('',(#655),#15909,.F.);
#16424=ADVANCED_FACE('',(#656),#15910,.F.);
#16425=ADVANCED_FACE('',(#657),#15911,.F.);
#16426=ADVANCED_FACE('',(#658),#15912,.F.);
#16427=ADVANCED_FACE('',(#659),#15913,.F.);
#16428=ADVANCED_FACE('',(#660),#15914,.F.);
#16429=ADVANCED_FACE('',(#661),#15915,.F.);
#16430=ADVANCED_FACE('',(#662),#15916,.F.);
#16431=ADVANCED_FACE('',(#663),#15917,.F.);
#16432=ADVANCED_FACE('',(#664),#15918,.F.);
#16433=ADVANCED_FACE('',(#665),#15919,.F.);
#16434=ADVANCED_FACE('',(#666),#15920,.F.);
#16435=ADVANCED_FACE('',(#667),#15921,.F.);
#16436=ADVANCED_FACE('',(#668),#15922,.F.);
#16437=ADVANCED_FACE('',(#669),#15923,.F.);
#16438=ADVANCED_FACE('',(#670),#15924,.F.);
#16439=ADVANCED_FACE('',(#671),#15925,.F.);
#16440=ADVANCED_FACE('',(#672),#15926,.F.);
#16441=ADVANCED_FACE('',(#673),#15927,.F.);
#16442=ADVANCED_FACE('',(#674),#15928,.F.);
#16443=ADVANCED_FACE('',(#675),#15929,.F.);
#16444=ADVANCED_FACE('',(#676),#15930,.F.);
#16445=ADVANCED_FACE('',(#677),#15931,.F.);
#16446=ADVANCED_FACE('',(#678),#15932,.F.);
#16447=ADVANCED_FACE('',(#679),#15933,.F.);
#16448=ADVANCED_FACE('',(#680),#15934,.F.);
#16449=ADVANCED_FACE('',(#681),#15935,.F.);
#16450=ADVANCED_FACE('',(#682),#15936,.F.);
#16451=ADVANCED_FACE('',(#683),#15937,.F.);
#16452=ADVANCED_FACE('',(#684),#15938,.F.);
#16453=ADVANCED_FACE('',(#685),#15939,.F.);
#16454=ADVANCED_FACE('',(#686),#15940,.F.);
#16455=ADVANCED_FACE('',(#687),#15941,.F.);
#16456=ADVANCED_FACE('',(#688),#15942,.F.);
#16457=ADVANCED_FACE('',(#689),#15943,.F.);
#16458=ADVANCED_FACE('',(#690),#15944,.F.);
#16459=ADVANCED_FACE('',(#691),#15945,.F.);
#16460=ADVANCED_FACE('',(#692),#15946,.F.);
#16461=ADVANCED_FACE('',(#693),#15947,.F.);
#16462=ADVANCED_FACE('',(#694),#15948,.F.);
#16463=ADVANCED_FACE('',(#695),#15949,.F.);
#16464=ADVANCED_FACE('',(#696),#15950,.F.);
#16465=ADVANCED_FACE('',(#697),#15951,.F.);
#16466=ADVANCED_FACE('',(#698),#15952,.F.);
#16467=ADVANCED_FACE('',(#699),#15953,.F.);
#16468=ADVANCED_FACE('',(#700),#15954,.F.);
#16469=ADVANCED_FACE('',(#701),#15955,.F.);
#16470=ADVANCED_FACE('',(#702),#15956,.F.);
#16471=ADVANCED_FACE('',(#703),#15957,.F.);
#16472=ADVANCED_FACE('',(#704),#15958,.F.);
#16473=ADVANCED_FACE('',(#705),#15959,.F.);
#16474=ADVANCED_FACE('',(#706),#15960,.F.);
#16475=ADVANCED_FACE('',(#707),#15961,.F.);
#16476=ADVANCED_FACE('',(#708),#15962,.F.);
#16477=ADVANCED_FACE('',(#709),#15963,.F.);
#16478=ADVANCED_FACE('',(#710),#15964,.F.);
#16479=ADVANCED_FACE('',(#711),#15965,.F.);
#16480=ADVANCED_FACE('',(#712),#15966,.F.);
#16481=ADVANCED_FACE('',(#713),#15967,.F.);
#16482=ADVANCED_FACE('',(#714),#15968,.F.);
#16483=ADVANCED_FACE('',(#715),#15969,.F.);
#16484=ADVANCED_FACE('',(#716),#15970,.F.);
#16485=ADVANCED_FACE('',(#717),#15971,.F.);
#16486=ADVANCED_FACE('',(#718),#15972,.F.);
#16487=ADVANCED_FACE('',(#719),#15973,.F.);
#16488=ADVANCED_FACE('',(#720),#15974,.F.);
#16489=ADVANCED_FACE('',(#721),#15975,.F.);
#16490=ADVANCED_FACE('',(#722),#15976,.F.);
#16491=ADVANCED_FACE('',(#723),#317,.T.);
#16492=ADVANCED_FACE('',(#724),#281,.F.);
#16493=ADVANCED_FACE('',(#725),#282,.F.);
#16494=ADVANCED_FACE('',(#726),#318,.T.);
#16495=ADVANCED_FACE('',(#727),#283,.F.);
#16496=ADVANCED_FACE('',(#728),#284,.F.);
#16497=ADVANCED_FACE('',(#729),#319,.F.);
#16498=ADVANCED_FACE('',(#730),#320,.F.);
#16499=ADVANCED_FACE('',(#731),#321,.F.);
#16500=ADVANCED_FACE('',(#732),#322,.F.);
#16501=ADVANCED_FACE('',(#733),#323,.F.);
#16502=ADVANCED_FACE('',(#734),#324,.F.);
#16503=ADVANCED_FACE('',(#735),#15977,.F.);
#16504=ADVANCED_FACE('',(#736),#15978,.F.);
#16505=ADVANCED_FACE('',(#737),#15979,.F.);
#16506=ADVANCED_FACE('',(#738),#15980,.F.);
#16507=ADVANCED_FACE('',(#739),#285,.F.);
#16508=ADVANCED_FACE('',(#740),#286,.F.);
#16509=ADVANCED_FACE('',(#741),#287,.F.);
#16510=ADVANCED_FACE('',(#742),#288,.F.);
#16511=ADVANCED_FACE('',(#743),#289,.F.);
#16512=ADVANCED_FACE('',(#744),#290,.F.);
#16513=ADVANCED_FACE('',(#745),#291,.F.);
#16514=ADVANCED_FACE('',(#746),#292,.F.);
#16515=ADVANCED_FACE('',(#747),#325,.F.);
#16516=ADVANCED_FACE('',(#748),#326,.F.);
#16517=ADVANCED_FACE('',(#749),#327,.F.);
#16518=ADVANCED_FACE('',(#750),#328,.F.);
#16519=ADVANCED_FACE('',(#751,#199),#15981,.F.);
#16520=ADVANCED_FACE('',(#752,#200,#201,#202,#203,#204),#329,.T.);
#16521=ADVANCED_FACE('',(#753),#330,.T.);
#16522=ADVANCED_FACE('',(#754),#331,.T.);
#16523=ADVANCED_FACE('',(#755),#332,.T.);
#16524=ADVANCED_FACE('',(#756),#333,.T.);
#16525=ADVANCED_FACE('',(#757,#205,#206,#207,#208),#334,.F.);
#16526=ADVANCED_FACE('',(#758),#335,.T.);
#16527=ADVANCED_FACE('',(#759,#209),#336,.T.);
#16528=ADVANCED_FACE('',(#760),#337,.T.);
#16529=ADVANCED_FACE('',(#761,#210,#211,#212,#213,#214),#338,.T.);
#16530=ADVANCED_FACE('',(#762,#215,#216,#217),#339,.T.);
#16842=CLOSED_SHELL('',(#16305,#16306,#16307,#16308,#16309,#16310,#16311,
#16312,#16313,#16314,#16315,#16316,#16317,#16318,#16319,#16320,#16321,#16322,
#16323,#16324,#16325,#16326,#16327,#16328,#16329,#16330,#16331,#16332,#16333,
#16334,#16335,#16336,#16337,#16338,#16339,#16340,#16341,#16342,#16343,#16344,
#16345,#16346,#16347,#16348,#16349,#16350,#16351,#16352,#16353,#16354,#16355,
#16356,#16357,#16358,#16359,#16360,#16361,#16362,#16363,#16364,#16365,#16366,
#16367,#16368,#16369,#16370,#16371,#16372,#16373,#16374,#16375,#16376,#16377,
#16378,#16379,#16380,#16381,#16382,#16383,#16384,#16385,#16386,#16387,#16388,
#16389,#16390,#16391,#16392,#16393,#16394,#16395,#16396,#16397,#16398,#16399,
#16400,#16401,#16402,#16403,#16404,#16405,#16406,#16407,#16408,#16409,#16410,
#16411,#16412,#16413,#16414,#16415,#16416,#16417,#16418,#16419,#16420,#16421,
#16422,#16423,#16424,#16425,#16426,#16427,#16428,#16429,#16430,#16431,#16432,
#16433,#16434,#16435,#16436,#16437,#16438,#16439,#16440,#16441,#16442,#16443,
#16444,#16445,#16446,#16447,#16448,#16449,#16450,#16451,#16452,#16453,#16454,
#16455,#16456,#16457,#16458,#16459,#16460,#16461,#16462,#16463,#16464,#16465,
#16466,#16467,#16468,#16469,#16470,#16471,#16472,#16473,#16474,#16475,#16476,
#16477,#16478,#16479,#16480,#16481,#16482,#16483,#16484,#16485,#16486,#16487,
#16488,#16489,#16490,#16491,#16492,#16493,#16494,#16495,#16496,#16497,#16498,
#16499,#16500,#16501,#16502,#16503,#16504,#16505,#16506,#16507,#16508,#16509,
#16510,#16511,#16512,#16513,#16514,#16515,#16516,#16517,#16518,#16519,#16520,
#16521,#16522,#16523,#16524,#16525,#16526,#16527,#16528,#16529,#16530));
#17186=AXIS2_PLACEMENT_3D('',#59495,#18269,#18270);
#17187=AXIS2_PLACEMENT_3D('',#59496,#18271,#18272);
#17188=AXIS2_PLACEMENT_3D('',#59506,#18274,#18275);
#17189=AXIS2_PLACEMENT_3D('',#59538,#18276,#18277);
#17190=AXIS2_PLACEMENT_3D('',#59865,#18279,#18280);
#17191=AXIS2_PLACEMENT_3D('',#60259,#18282,#18283);
#17192=AXIS2_PLACEMENT_3D('',#60650,#18285,#18286);
#17193=AXIS2_PLACEMENT_3D('',#61041,#18288,#18289);
#17194=AXIS2_PLACEMENT_3D('',#61429,#18291,#18292);
#17195=AXIS2_PLACEMENT_3D('',#61820,#18294,#18295);
#17196=AXIS2_PLACEMENT_3D('',#62211,#18297,#18298);
#17197=AXIS2_PLACEMENT_3D('',#62599,#18300,#18301);
#17198=AXIS2_PLACEMENT_3D('',#62993,#18303,#18304);
#17199=AXIS2_PLACEMENT_3D('',#63384,#18306,#18307);
#17200=AXIS2_PLACEMENT_3D('',#63775,#18309,#18310);
#17201=AXIS2_PLACEMENT_3D('',#64169,#18312,#18313);
#17202=AXIS2_PLACEMENT_3D('',#64560,#18315,#18316);
#17203=AXIS2_PLACEMENT_3D('',#64948,#18318,#18319);
#17204=AXIS2_PLACEMENT_3D('',#65030,#18321,#18322);
#17205=AXIS2_PLACEMENT_3D('',#65157,#18323,#18324);
#17206=AXIS2_PLACEMENT_3D('',#65323,#18326,#18327);
#17207=AXIS2_PLACEMENT_3D('',#65337,#18329,#18330);
#17208=AXIS2_PLACEMENT_3D('',#65584,#18331,#18332);
#17209=AXIS2_PLACEMENT_3D('',#65814,#18334,#18335);
#17210=AXIS2_PLACEMENT_3D('',#66227,#18337,#18338);
#17211=AXIS2_PLACEMENT_3D('',#66673,#18340,#18341);
#17212=AXIS2_PLACEMENT_3D('',#67129,#18343,#18344);
#17213=AXIS2_PLACEMENT_3D('',#67561,#18346,#18347);
#17214=AXIS2_PLACEMENT_3D('',#67993,#18349,#18350);
#17215=AXIS2_PLACEMENT_3D('',#68393,#18352,#18353);
#17216=AXIS2_PLACEMENT_3D('',#68847,#18355,#18356);
#17217=AXIS2_PLACEMENT_3D('',#69283,#18358,#18359);
#17218=AXIS2_PLACEMENT_3D('',#69711,#18361,#18362);
#17219=AXIS2_PLACEMENT_3D('',#70123,#18364,#18365);
#17220=AXIS2_PLACEMENT_3D('',#70551,#18367,#18368);
#17221=AXIS2_PLACEMENT_3D('',#70967,#18370,#18371);
#17222=AXIS2_PLACEMENT_3D('',#71107,#18373,#18374);
#17223=AXIS2_PLACEMENT_3D('',#71310,#18375,#18376);
#17224=AXIS2_PLACEMENT_3D('',#71320,#18378,#18379);
#17225=AXIS2_PLACEMENT_3D('',#71352,#18380,#18381);
#17226=AXIS2_PLACEMENT_3D('',#71679,#18383,#18384);
#17227=AXIS2_PLACEMENT_3D('',#72073,#18386,#18387);
#17228=AXIS2_PLACEMENT_3D('',#72464,#18389,#18390);
#17229=AXIS2_PLACEMENT_3D('',#72855,#18392,#18393);
#17230=AXIS2_PLACEMENT_3D('',#73243,#18395,#18396);
#17231=AXIS2_PLACEMENT_3D('',#73634,#18398,#18399);
#17232=AXIS2_PLACEMENT_3D('',#74025,#18401,#18402);
#17233=AXIS2_PLACEMENT_3D('',#74413,#18404,#18405);
#17234=AXIS2_PLACEMENT_3D('',#74807,#18407,#18408);
#17235=AXIS2_PLACEMENT_3D('',#75198,#18410,#18411);
#17236=AXIS2_PLACEMENT_3D('',#75589,#18413,#18414);
#17237=AXIS2_PLACEMENT_3D('',#75983,#18416,#18417);
#17238=AXIS2_PLACEMENT_3D('',#76374,#18419,#18420);
#17239=AXIS2_PLACEMENT_3D('',#76762,#18422,#18423);
#17240=AXIS2_PLACEMENT_3D('',#76844,#18425,#18426);
#17241=AXIS2_PLACEMENT_3D('',#76971,#18427,#18428);
#17242=AXIS2_PLACEMENT_3D('',#77137,#18430,#18431);
#17243=AXIS2_PLACEMENT_3D('',#77153,#18433,#18434);
#17244=AXIS2_PLACEMENT_3D('',#77446,#18435,#18436);
#17245=AXIS2_PLACEMENT_3D('',#77680,#18438,#18439);
#17246=AXIS2_PLACEMENT_3D('',#78091,#18441,#18442);
#17247=AXIS2_PLACEMENT_3D('',#78507,#18444,#18445);
#17248=AXIS2_PLACEMENT_3D('',#78965,#18447,#18448);
#17249=AXIS2_PLACEMENT_3D('',#79393,#18450,#18451);
#17250=AXIS2_PLACEMENT_3D('',#79803,#18453,#18454);
#17251=AXIS2_PLACEMENT_3D('',#80231,#18456,#18457);
#17252=AXIS2_PLACEMENT_3D('',#80683,#18459,#18460);
#17253=AXIS2_PLACEMENT_3D('',#81127,#18462,#18463);
#17254=AXIS2_PLACEMENT_3D('',#81555,#18465,#18466);
#17255=AXIS2_PLACEMENT_3D('',#81967,#18468,#18469);
#17256=AXIS2_PLACEMENT_3D('',#82391,#18471,#18472);
#17257=AXIS2_PLACEMENT_3D('',#82817,#18474,#18475);
#17258=AXIS2_PLACEMENT_3D('',#82967,#18477,#18478);
#17259=AXIS2_PLACEMENT_3D('',#83174,#18479,#18480);
#17260=AXIS2_PLACEMENT_3D('',#83188,#18482,#18483);
#17261=AXIS2_PLACEMENT_3D('',#83330,#18484,#18485);
#17262=AXIS2_PLACEMENT_3D('',#83660,#18487,#18488);
#17263=AXIS2_PLACEMENT_3D('',#84051,#18490,#18491);
#17264=AXIS2_PLACEMENT_3D('',#84439,#18493,#18494);
#17265=AXIS2_PLACEMENT_3D('',#84830,#18496,#18497);
#17266=AXIS2_PLACEMENT_3D('',#85221,#18499,#18500);
#17267=AXIS2_PLACEMENT_3D('',#85609,#18502,#18503);
#17268=AXIS2_PLACEMENT_3D('',#86000,#18505,#18506);
#17269=AXIS2_PLACEMENT_3D('',#86391,#18508,#18509);
#17270=AXIS2_PLACEMENT_3D('',#86782,#18511,#18512);
#17271=AXIS2_PLACEMENT_3D('',#87176,#18514,#18515);
#17272=AXIS2_PLACEMENT_3D('',#87451,#18517,#18518);
#17273=AXIS2_PLACEMENT_3D('',#87778,#18520,#18521);
#17274=AXIS2_PLACEMENT_3D('',#87860,#18523,#18524);
#17275=AXIS2_PLACEMENT_3D('',#87987,#18525,#18526);
#17276=AXIS2_PLACEMENT_3D('',#88001,#18528,#18529);
#17277=AXIS2_PLACEMENT_3D('',#88143,#18530,#18531);
#17278=AXIS2_PLACEMENT_3D('',#88473,#18533,#18534);
#17279=AXIS2_PLACEMENT_3D('',#88864,#18536,#18537);
#17280=AXIS2_PLACEMENT_3D('',#89252,#18539,#18540);
#17281=AXIS2_PLACEMENT_3D('',#89643,#18542,#18543);
#17282=AXIS2_PLACEMENT_3D('',#90034,#18545,#18546);
#17283=AXIS2_PLACEMENT_3D('',#90422,#18548,#18549);
#17284=AXIS2_PLACEMENT_3D('',#90813,#18551,#18552);
#17285=AXIS2_PLACEMENT_3D('',#91204,#18554,#18555);
#17286=AXIS2_PLACEMENT_3D('',#91595,#18557,#18558);
#17287=AXIS2_PLACEMENT_3D('',#91989,#18560,#18561);
#17288=AXIS2_PLACEMENT_3D('',#92264,#18563,#18564);
#17289=AXIS2_PLACEMENT_3D('',#92591,#18566,#18567);
#17290=AXIS2_PLACEMENT_3D('',#92673,#18569,#18570);
#17291=AXIS2_PLACEMENT_3D('',#92800,#18571,#18572);
#17292=AXIS2_PLACEMENT_3D('',#92814,#18574,#18575);
#17293=AXIS2_PLACEMENT_3D('',#92956,#18576,#18577);
#17294=AXIS2_PLACEMENT_3D('',#93286,#18579,#18580);
#17295=AXIS2_PLACEMENT_3D('',#93677,#18582,#18583);
#17296=AXIS2_PLACEMENT_3D('',#94065,#18585,#18586);
#17297=AXIS2_PLACEMENT_3D('',#94456,#18588,#18589);
#17298=AXIS2_PLACEMENT_3D('',#94847,#18591,#18592);
#17299=AXIS2_PLACEMENT_3D('',#95235,#18594,#18595);
#17300=AXIS2_PLACEMENT_3D('',#95626,#18597,#18598);
#17301=AXIS2_PLACEMENT_3D('',#96017,#18600,#18601);
#17302=AXIS2_PLACEMENT_3D('',#96408,#18603,#18604);
#17303=AXIS2_PLACEMENT_3D('',#96802,#18606,#18607);
#17304=AXIS2_PLACEMENT_3D('',#97193,#18609,#18610);
#17305=AXIS2_PLACEMENT_3D('',#97581,#18612,#18613);
#17306=AXIS2_PLACEMENT_3D('',#97663,#18615,#18616);
#17307=AXIS2_PLACEMENT_3D('',#97790,#18617,#18618);
#17308=AXIS2_PLACEMENT_3D('',#97804,#18620,#18621);
#17309=AXIS2_PLACEMENT_3D('',#97946,#18622,#18623);
#17310=AXIS2_PLACEMENT_3D('',#98276,#18625,#18626);
#17311=AXIS2_PLACEMENT_3D('',#98667,#18628,#18629);
#17312=AXIS2_PLACEMENT_3D('',#99055,#18631,#18632);
#17313=AXIS2_PLACEMENT_3D('',#99446,#18634,#18635);
#17314=AXIS2_PLACEMENT_3D('',#99837,#18637,#18638);
#17315=AXIS2_PLACEMENT_3D('',#100225,#18640,#18641);
#17316=AXIS2_PLACEMENT_3D('',#100616,#18643,#18644);
#17317=AXIS2_PLACEMENT_3D('',#101007,#18646,#18647);
#17318=AXIS2_PLACEMENT_3D('',#101398,#18649,#18650);
#17319=AXIS2_PLACEMENT_3D('',#101792,#18652,#18653);
#17320=AXIS2_PLACEMENT_3D('',#102183,#18655,#18656);
#17321=AXIS2_PLACEMENT_3D('',#102571,#18658,#18659);
#17322=AXIS2_PLACEMENT_3D('',#102653,#18661,#18662);
#17323=AXIS2_PLACEMENT_3D('',#102780,#18663,#18664);
#17324=AXIS2_PLACEMENT_3D('',#102850,#18666,#18667);
#17325=AXIS2_PLACEMENT_3D('',#102971,#18668,#18669);
#17326=AXIS2_PLACEMENT_3D('',#103400,#18671,#18672);
#17327=AXIS2_PLACEMENT_3D('',#103833,#18674,#18675);
#17328=AXIS2_PLACEMENT_3D('',#104270,#18677,#18678);
#17329=AXIS2_PLACEMENT_3D('',#104755,#18680,#18681);
#17330=AXIS2_PLACEMENT_3D('',#105198,#18683,#18684);
#17331=AXIS2_PLACEMENT_3D('',#105618,#18686,#18687);
#17332=AXIS2_PLACEMENT_3D('',#105868,#18689,#18690);
#17333=AXIS2_PLACEMENT_3D('',#106272,#18692,#18693);
#17334=AXIS2_PLACEMENT_3D('',#106707,#18695,#18696);
#17335=AXIS2_PLACEMENT_3D('',#107116,#18698,#18699);
#17336=AXIS2_PLACEMENT_3D('',#107517,#18701,#18702);
#17337=AXIS2_PLACEMENT_3D('',#107934,#18704,#18705);
#17338=AXIS2_PLACEMENT_3D('',#108070,#18707,#18708);
#17339=AXIS2_PLACEMENT_3D('',#108251,#18709,#18710);
#17340=AXIS2_PLACEMENT_3D('',#108321,#18712,#18713);
#17341=AXIS2_PLACEMENT_3D('',#108440,#18714,#18715);
#17342=AXIS2_PLACEMENT_3D('',#108857,#18717,#18718);
#17343=AXIS2_PLACEMENT_3D('',#109290,#18720,#18721);
#17344=AXIS2_PLACEMENT_3D('',#109727,#18723,#18724);
#17345=AXIS2_PLACEMENT_3D('',#110220,#18726,#18727);
#17346=AXIS2_PLACEMENT_3D('',#110663,#18729,#18730);
#17347=AXIS2_PLACEMENT_3D('',#111085,#18732,#18733);
#17348=AXIS2_PLACEMENT_3D('',#111335,#18735,#18736);
#17349=AXIS2_PLACEMENT_3D('',#111733,#18738,#18739);
#17350=AXIS2_PLACEMENT_3D('',#112166,#18741,#18742);
#17351=AXIS2_PLACEMENT_3D('',#112579,#18744,#18745);
#17352=AXIS2_PLACEMENT_3D('',#112996,#18747,#18748);
#17353=AXIS2_PLACEMENT_3D('',#113417,#18750,#18751);
#17354=AXIS2_PLACEMENT_3D('',#113553,#18753,#18754);
#17355=AXIS2_PLACEMENT_3D('',#113728,#18755,#18756);
#17356=AXIS2_PLACEMENT_3D('',#113806,#18758,#18759);
#17357=AXIS2_PLACEMENT_3D('',#113927,#18760,#18761);
#17358=AXIS2_PLACEMENT_3D('',#114353,#18763,#18764);
#17359=AXIS2_PLACEMENT_3D('',#114778,#18766,#18767);
#17360=AXIS2_PLACEMENT_3D('',#115190,#18769,#18770);
#17361=AXIS2_PLACEMENT_3D('',#115679,#18772,#18773);
#17362=AXIS2_PLACEMENT_3D('',#116108,#18775,#18776);
#17363=AXIS2_PLACEMENT_3D('',#116522,#18778,#18779);
#17364=AXIS2_PLACEMENT_3D('',#116772,#18781,#18782);
#17365=AXIS2_PLACEMENT_3D('',#117186,#18784,#18785);
#17366=AXIS2_PLACEMENT_3D('',#117619,#18787,#18788);
#17367=AXIS2_PLACEMENT_3D('',#118018,#18790,#18791);
#17368=AXIS2_PLACEMENT_3D('',#118411,#18793,#18794);
#17369=AXIS2_PLACEMENT_3D('',#118831,#18796,#18797);
#17370=AXIS2_PLACEMENT_3D('',#118967,#18799,#18800);
#17371=AXIS2_PLACEMENT_3D('',#119156,#18801,#18802);
#17372=AXIS2_PLACEMENT_3D('',#119236,#18804,#18805);
#17373=AXIS2_PLACEMENT_3D('',#119359,#18806,#18807);
#17374=AXIS2_PLACEMENT_3D('',#119785,#18809,#18810);
#17375=AXIS2_PLACEMENT_3D('',#120208,#18812,#18813);
#17376=AXIS2_PLACEMENT_3D('',#120624,#18815,#18816);
#17377=AXIS2_PLACEMENT_3D('',#121121,#18818,#18819);
#17378=AXIS2_PLACEMENT_3D('',#121570,#18821,#18822);
#17379=AXIS2_PLACEMENT_3D('',#121976,#18824,#18825);
#17380=AXIS2_PLACEMENT_3D('',#122228,#18827,#18828);
#17381=AXIS2_PLACEMENT_3D('',#122644,#18830,#18831);
#17382=AXIS2_PLACEMENT_3D('',#123077,#18833,#18834);
#17383=AXIS2_PLACEMENT_3D('',#123496,#18836,#18837);
#17384=AXIS2_PLACEMENT_3D('',#123903,#18839,#18840);
#17385=AXIS2_PLACEMENT_3D('',#124323,#18842,#18843);
#17386=AXIS2_PLACEMENT_3D('',#124461,#18845,#18846);
#17387=AXIS2_PLACEMENT_3D('',#124650,#18847,#18848);
#17388=AXIS2_PLACEMENT_3D('',#125148,#18849,#18850);
#17389=AXIS2_PLACEMENT_3D('',#125646,#18851,#18852);
#17390=AXIS2_PLACEMENT_3D('',#126058,#18853,#18854);
#17391=AXIS2_PLACEMENT_3D('',#126460,#18855,#18856);
#17392=AXIS2_PLACEMENT_3D('',#126845,#18857,#18858);
#17393=AXIS2_PLACEMENT_3D('',#127230,#18859,#18860);
#17394=AXIS2_PLACEMENT_3D('',#127615,#18861,#18862);
#17395=AXIS2_PLACEMENT_3D('',#128000,#18863,#18864);
#17396=AXIS2_PLACEMENT_3D('',#128414,#18865,#18866);
#17397=AXIS2_PLACEMENT_3D('',#128799,#18867,#18868);
#17398=AXIS2_PLACEMENT_3D('',#129217,#18869,#18870);
#17399=AXIS2_PLACEMENT_3D('',#129602,#18871,#18872);
#17400=AXIS2_PLACEMENT_3D('',#130783,#18873,#18874);
#17401=AXIS2_PLACEMENT_3D('',#131961,#18875,#18876);
#17402=AXIS2_PLACEMENT_3D('',#131962,#18877,#18878);
#17403=AXIS2_PLACEMENT_3D('',#131963,#18879,#18880);
#17404=AXIS2_PLACEMENT_3D('',#131972,#18885,#18886);
#17405=AXIS2_PLACEMENT_3D('',#131974,#18887,#18888);
#17406=AXIS2_PLACEMENT_3D('',#131978,#18891,#18892);
#17407=AXIS2_PLACEMENT_3D('',#131984,#18896,#18897);
#17408=AXIS2_PLACEMENT_3D('',#131985,#18898,#18899);
#17409=AXIS2_PLACEMENT_3D('',#131987,#18901,#18902);
#17410=AXIS2_PLACEMENT_3D('',#131989,#18903,#18904);
#17411=AXIS2_PLACEMENT_3D('',#131992,#18906,#18907);
#17412=AXIS2_PLACEMENT_3D('',#131993,#18908,#18909);
#17413=AXIS2_PLACEMENT_3D('',#131995,#18910,#18911);
#17414=AXIS2_PLACEMENT_3D('',#131998,#18913,#18914);
#17415=AXIS2_PLACEMENT_3D('',#131999,#18915,#18916);
#17416=AXIS2_PLACEMENT_3D('',#132001,#18917,#18918);
#17417=AXIS2_PLACEMENT_3D('',#132004,#18920,#18921);
#17418=AXIS2_PLACEMENT_3D('',#132005,#18922,#18923);
#17419=AXIS2_PLACEMENT_3D('',#132007,#18924,#18925);
#17420=AXIS2_PLACEMENT_3D('',#132010,#18927,#18928);
#17421=AXIS2_PLACEMENT_3D('',#136451,#18929,#18930);
#17422=AXIS2_PLACEMENT_3D('',#136452,#18931,#18932);
#17423=AXIS2_PLACEMENT_3D('',#136453,#18933,#18934);
#17424=AXIS2_PLACEMENT_3D('',#136454,#18935,#18936);
#17425=AXIS2_PLACEMENT_3D('',#136455,#18937,#18938);
#17426=AXIS2_PLACEMENT_3D('',#136457,#18939,#18940);
#17427=AXIS2_PLACEMENT_3D('',#136460,#18942,#18943);
#17428=AXIS2_PLACEMENT_3D('',#136461,#18944,#18945);
#17429=AXIS2_PLACEMENT_3D('',#136478,#18954,#18955);
#17430=AXIS2_PLACEMENT_3D('',#136484,#18959,#18960);
#17431=AXIS2_PLACEMENT_3D('',#136488,#18963,#18964);
#17432=AXIS2_PLACEMENT_3D('',#136492,#18967,#18968);
#17433=AXIS2_PLACEMENT_3D('',#136494,#18970,#18971);
#17434=AXIS2_PLACEMENT_3D('',#136495,#18972,#18973);
#17435=AXIS2_PLACEMENT_3D('',#136501,#18977,#18978);
#17436=AXIS2_PLACEMENT_3D('',#136505,#18981,#18982);
#17437=AXIS2_PLACEMENT_3D('',#136509,#18985,#18986);
#17438=AXIS2_PLACEMENT_3D('',#136511,#18988,#18989);
#18269=DIRECTION('axis',(0.,0.,1.));
#18270=DIRECTION('refdir',(1.,0.,0.));
#18271=DIRECTION('center_axis',(0.,0.,-1.));
#18272=DIRECTION('ref_axis',(-0.609338902105852,-0.792909895499126,0.));
#18273=DIRECTION('',(0.,0.,-1.));
#18274=DIRECTION('center_axis',(0.,0.,1.));
#18275=DIRECTION('ref_axis',(1.,-8.10480368384347E-14,0.));
#18276=DIRECTION('center_axis',(0.,0.,-1.));
#18277=DIRECTION('ref_axis',(-0.609338902105852,-0.792909895499126,0.));
#18278=DIRECTION('',(0.,0.,-1.));
#18279=DIRECTION('center_axis',(0.,0.,-1.));
#18280=DIRECTION('ref_axis',(-0.609338902105852,-0.792909895499126,0.));
#18281=DIRECTION('',(0.,0.,-1.));
#18282=DIRECTION('center_axis',(0.,0.,-1.));
#18283=DIRECTION('ref_axis',(-0.609338902105852,-0.792909895499126,0.));
#18284=DIRECTION('',(0.,0.,-1.));
#18285=DIRECTION('center_axis',(0.,0.,-1.));
#18286=DIRECTION('ref_axis',(-0.609338902105852,-0.792909895499126,0.));
#18287=DIRECTION('',(0.,0.,-1.));
#18288=DIRECTION('center_axis',(0.,0.,-1.));
#18289=DIRECTION('ref_axis',(-0.609338902105852,-0.792909895499126,0.));
#18290=DIRECTION('',(0.,0.,-1.));
#18291=DIRECTION('center_axis',(0.,0.,-1.));
#18292=DIRECTION('ref_axis',(-0.609338902105852,-0.792909895499126,0.));
#18293=DIRECTION('',(0.,0.,-1.));
#18294=DIRECTION('center_axis',(0.,0.,-1.));
#18295=DIRECTION('ref_axis',(-0.609338902105852,-0.792909895499126,0.));
#18296=DIRECTION('',(0.,0.,-1.));
#18297=DIRECTION('center_axis',(0.,0.,-1.));
#18298=DIRECTION('ref_axis',(-0.609338902105852,-0.792909895499126,0.));
#18299=DIRECTION('',(0.,0.,-1.));
#18300=DIRECTION('center_axis',(0.,0.,-1.));
#18301=DIRECTION('ref_axis',(-0.609338902105852,-0.792909895499126,0.));
#18302=DIRECTION('',(0.,0.,-1.));
#18303=DIRECTION('center_axis',(0.,0.,-1.));
#18304=DIRECTION('ref_axis',(-0.609338902105852,-0.792909895499126,0.));
#18305=DIRECTION('',(0.,0.,-1.));
#18306=DIRECTION('center_axis',(0.,0.,-1.));
#18307=DIRECTION('ref_axis',(-0.609338902105852,-0.792909895499126,0.));
#18308=DIRECTION('',(0.,0.,-1.));
#18309=DIRECTION('center_axis',(0.,0.,-1.));
#18310=DIRECTION('ref_axis',(-0.609338902105852,-0.792909895499126,0.));
#18311=DIRECTION('',(0.,0.,-1.));
#18312=DIRECTION('center_axis',(0.,0.,-1.));
#18313=DIRECTION('ref_axis',(-0.609338902105852,-0.792909895499126,0.));
#18314=DIRECTION('',(0.,0.,-1.));
#18315=DIRECTION('center_axis',(0.,0.,-1.));
#18316=DIRECTION('ref_axis',(-0.609338902105852,-0.792909895499126,0.));
#18317=DIRECTION('',(0.,0.,-1.));
#18318=DIRECTION('center_axis',(0.,0.,-1.));
#18319=DIRECTION('ref_axis',(-0.609338902105852,-0.792909895499126,0.));
#18320=DIRECTION('',(0.,0.,-1.));
#18321=DIRECTION('center_axis',(0.,0.,-1.));
#18322=DIRECTION('ref_axis',(1.,-8.10480368384347E-14,0.));
#18323=DIRECTION('center_axis',(0.,0.,-1.));
#18324=DIRECTION('ref_axis',(0.938439751642368,-0.345442951205277,0.));
#18325=DIRECTION('',(0.,0.,-1.));
#18326=DIRECTION('center_axis',(0.,0.,1.));
#18327=DIRECTION('ref_axis',(1.,0.,0.));
#18328=DIRECTION('',(0.,0.,-1.));
#18329=DIRECTION('center_axis',(0.,0.,1.));
#18330=DIRECTION('ref_axis',(1.,0.,0.));
#18331=DIRECTION('center_axis',(0.,0.,-1.));
#18332=DIRECTION('ref_axis',(0.938439751642368,-0.345442951205277,0.));
#18333=DIRECTION('',(0.,0.,-1.));
#18334=DIRECTION('center_axis',(0.,0.,-1.));
#18335=DIRECTION('ref_axis',(0.938439751642368,-0.345442951205277,0.));
#18336=DIRECTION('',(0.,0.,-1.));
#18337=DIRECTION('center_axis',(0.,0.,-1.));
#18338=DIRECTION('ref_axis',(0.938439751642368,-0.345442951205277,0.));
#18339=DIRECTION('',(0.,0.,-1.));
#18340=DIRECTION('center_axis',(0.,0.,-1.));
#18341=DIRECTION('ref_axis',(0.938439751642368,-0.345442951205277,0.));
#18342=DIRECTION('',(0.,0.,-1.));
#18343=DIRECTION('center_axis',(0.,0.,-1.));
#18344=DIRECTION('ref_axis',(0.938439751642368,-0.345442951205277,0.));
#18345=DIRECTION('',(0.,0.,-1.));
#18346=DIRECTION('center_axis',(0.,0.,-1.));
#18347=DIRECTION('ref_axis',(0.938439751642368,-0.345442951205277,0.));
#18348=DIRECTION('',(0.,0.,-1.));
#18349=DIRECTION('center_axis',(0.,0.,-1.));
#18350=DIRECTION('ref_axis',(0.938439751642368,-0.345442951205277,0.));
#18351=DIRECTION('',(0.,0.,-1.));
#18352=DIRECTION('center_axis',(0.,0.,-1.));
#18353=DIRECTION('ref_axis',(0.938439751642368,-0.345442951205277,0.));
#18354=DIRECTION('',(0.,0.,-1.));
#18355=DIRECTION('center_axis',(0.,0.,-1.));
#18356=DIRECTION('ref_axis',(0.938439751642368,-0.345442951205277,0.));
#18357=DIRECTION('',(0.,0.,-1.));
#18358=DIRECTION('center_axis',(0.,0.,-1.));
#18359=DIRECTION('ref_axis',(0.938439751642368,-0.345442951205277,0.));
#18360=DIRECTION('',(0.,0.,-1.));
#18361=DIRECTION('center_axis',(0.,0.,-1.));
#18362=DIRECTION('ref_axis',(0.938439751642368,-0.345442951205277,0.));
#18363=DIRECTION('',(0.,0.,-1.));
#18364=DIRECTION('center_axis',(0.,0.,-1.));
#18365=DIRECTION('ref_axis',(0.938439751642368,-0.345442951205277,0.));
#18366=DIRECTION('',(0.,0.,-1.));
#18367=DIRECTION('center_axis',(0.,0.,-1.));
#18368=DIRECTION('ref_axis',(0.938439751642368,-0.345442951205277,0.));
#18369=DIRECTION('',(0.,0.,-1.));
#18370=DIRECTION('center_axis',(0.,0.,-1.));
#18371=DIRECTION('ref_axis',(0.938439751642368,-0.345442951205277,0.));
#18372=DIRECTION('',(0.,0.,-1.));
#18373=DIRECTION('center_axis',(0.,0.,-1.));
#18374=DIRECTION('ref_axis',(1.,0.,0.));
#18375=DIRECTION('center_axis',(0.,0.,-1.));
#18376=DIRECTION('ref_axis',(-0.609338902889834,-0.792909894896648,0.));
#18377=DIRECTION('',(0.,0.,-1.));
#18378=DIRECTION('center_axis',(0.,0.,1.));
#18379=DIRECTION('ref_axis',(1.,-8.10480368384347E-14,0.));
#18380=DIRECTION('center_axis',(0.,0.,-1.));
#18381=DIRECTION('ref_axis',(-0.609338902889834,-0.792909894896648,0.));
#18382=DIRECTION('',(0.,0.,-1.));
#18383=DIRECTION('center_axis',(0.,0.,-1.));
#18384=DIRECTION('ref_axis',(-0.609338902889834,-0.792909894896648,0.));
#18385=DIRECTION('',(0.,0.,-1.));
#18386=DIRECTION('center_axis',(0.,0.,-1.));
#18387=DIRECTION('ref_axis',(-0.609338902889834,-0.792909894896648,0.));
#18388=DIRECTION('',(0.,0.,-1.));
#18389=DIRECTION('center_axis',(0.,0.,-1.));
#18390=DIRECTION('ref_axis',(-0.609338902889834,-0.792909894896648,0.));
#18391=DIRECTION('',(0.,0.,-1.));
#18392=DIRECTION('center_axis',(0.,0.,-1.));
#18393=DIRECTION('ref_axis',(-0.609338902889834,-0.792909894896648,0.));
#18394=DIRECTION('',(0.,0.,-1.));
#18395=DIRECTION('center_axis',(0.,0.,-1.));
#18396=DIRECTION('ref_axis',(-0.609338902889834,-0.792909894896648,0.));
#18397=DIRECTION('',(0.,0.,-1.));
#18398=DIRECTION('center_axis',(0.,0.,-1.));
#18399=DIRECTION('ref_axis',(-0.609338902889834,-0.792909894896648,0.));
#18400=DIRECTION('',(0.,0.,-1.));
#18401=DIRECTION('center_axis',(0.,0.,-1.));
#18402=DIRECTION('ref_axis',(-0.609338902889834,-0.792909894896648,0.));
#18403=DIRECTION('',(0.,0.,-1.));
#18404=DIRECTION('center_axis',(0.,0.,-1.));
#18405=DIRECTION('ref_axis',(-0.609338902889834,-0.792909894896648,0.));
#18406=DIRECTION('',(0.,0.,-1.));
#18407=DIRECTION('center_axis',(0.,0.,-1.));
#18408=DIRECTION('ref_axis',(-0.609338902889834,-0.792909894896648,0.));
#18409=DIRECTION('',(0.,0.,-1.));
#18410=DIRECTION('center_axis',(0.,0.,-1.));
#18411=DIRECTION('ref_axis',(-0.609338902889834,-0.792909894896648,0.));
#18412=DIRECTION('',(0.,0.,-1.));
#18413=DIRECTION('center_axis',(0.,0.,-1.));
#18414=DIRECTION('ref_axis',(-0.609338902889834,-0.792909894896648,0.));
#18415=DIRECTION('',(0.,0.,-1.));
#18416=DIRECTION('center_axis',(0.,0.,-1.));
#18417=DIRECTION('ref_axis',(-0.609338902889834,-0.792909894896648,0.));
#18418=DIRECTION('',(0.,0.,-1.));
#18419=DIRECTION('center_axis',(0.,0.,-1.));
#18420=DIRECTION('ref_axis',(-0.609338902889834,-0.792909894896648,0.));
#18421=DIRECTION('',(0.,0.,-1.));
#18422=DIRECTION('center_axis',(0.,0.,-1.));
#18423=DIRECTION('ref_axis',(-0.609338902889834,-0.792909894896648,0.));
#18424=DIRECTION('',(0.,0.,-1.));
#18425=DIRECTION('center_axis',(0.,0.,-1.));
#18426=DIRECTION('ref_axis',(1.,-8.10480368384347E-14,0.));
#18427=DIRECTION('center_axis',(0.,0.,-1.));
#18428=DIRECTION('ref_axis',(0.938439750900799,-0.345442953219843,0.));
#18429=DIRECTION('',(0.,0.,-1.));
#18430=DIRECTION('center_axis',(0.,0.,1.));
#18431=DIRECTION('ref_axis',(1.,0.,0.));
#18432=DIRECTION('',(0.,0.,-1.));
#18433=DIRECTION('center_axis',(0.,0.,1.));
#18434=DIRECTION('ref_axis',(1.,0.,0.));
#18435=DIRECTION('center_axis',(0.,0.,-1.));
#18436=DIRECTION('ref_axis',(0.938439750900799,-0.345442953219843,0.));
#18437=DIRECTION('',(0.,0.,-1.));
#18438=DIRECTION('center_axis',(0.,0.,-1.));
#18439=DIRECTION('ref_axis',(0.938439750900799,-0.345442953219843,0.));
#18440=DIRECTION('',(0.,0.,-1.));
#18441=DIRECTION('center_axis',(0.,0.,-1.));
#18442=DIRECTION('ref_axis',(0.938439750900799,-0.345442953219843,0.));
#18443=DIRECTION('',(0.,0.,-1.));
#18444=DIRECTION('center_axis',(0.,0.,-1.));
#18445=DIRECTION('ref_axis',(0.938439750900799,-0.345442953219843,0.));
#18446=DIRECTION('',(0.,0.,-1.));
#18447=DIRECTION('center_axis',(0.,0.,-1.));
#18448=DIRECTION('ref_axis',(0.938439750900799,-0.345442953219843,0.));
#18449=DIRECTION('',(0.,0.,-1.));
#18450=DIRECTION('center_axis',(0.,0.,-1.));
#18451=DIRECTION('ref_axis',(0.938439750900799,-0.345442953219843,0.));
#18452=DIRECTION('',(0.,0.,-1.));
#18453=DIRECTION('center_axis',(0.,0.,-1.));
#18454=DIRECTION('ref_axis',(0.938439750900799,-0.345442953219843,0.));
#18455=DIRECTION('',(0.,0.,-1.));
#18456=DIRECTION('center_axis',(0.,0.,-1.));
#18457=DIRECTION('ref_axis',(0.938439750900799,-0.345442953219843,0.));
#18458=DIRECTION('',(0.,0.,-1.));
#18459=DIRECTION('center_axis',(0.,0.,-1.));
#18460=DIRECTION('ref_axis',(0.938439750900799,-0.345442953219843,0.));
#18461=DIRECTION('',(0.,0.,-1.));
#18462=DIRECTION('center_axis',(0.,0.,-1.));
#18463=DIRECTION('ref_axis',(0.938439750900799,-0.345442953219843,0.));
#18464=DIRECTION('',(0.,0.,-1.));
#18465=DIRECTION('center_axis',(0.,0.,-1.));
#18466=DIRECTION('ref_axis',(0.938439750900799,-0.345442953219843,0.));
#18467=DIRECTION('',(0.,0.,-1.));
#18468=DIRECTION('center_axis',(0.,0.,-1.));
#18469=DIRECTION('ref_axis',(0.938439750900799,-0.345442953219843,0.));
#18470=DIRECTION('',(0.,0.,-1.));
#18471=DIRECTION('center_axis',(0.,0.,-1.));
#18472=DIRECTION('ref_axis',(0.938439750900799,-0.345442953219843,0.));
#18473=DIRECTION('',(0.,0.,-1.));
#18474=DIRECTION('center_axis',(0.,0.,-1.));
#18475=DIRECTION('ref_axis',(0.859566642449979,-0.511023665975726,0.));
#18476=DIRECTION('',(0.,0.,-1.));
#18477=DIRECTION('center_axis',(0.,0.,-1.));
#18478=DIRECTION('ref_axis',(1.,0.,0.));
#18479=DIRECTION('center_axis',(1.,0.,0.));
#18480=DIRECTION('ref_axis',(0.,0.609343021033316,-0.792906730150521));
#18481=DIRECTION('',(1.,0.,0.));
#18482=DIRECTION('center_axis',(-1.,0.,0.));
#18483=DIRECTION('ref_axis',(0.,-1.,-7.34835534001807E-14));
#18484=DIRECTION('center_axis',(1.,0.,0.));
#18485=DIRECTION('ref_axis',(0.,0.609343021033316,-0.792906730150521));
#18486=DIRECTION('',(1.,0.,0.));
#18487=DIRECTION('center_axis',(1.,0.,0.));
#18488=DIRECTION('ref_axis',(0.,0.609343021033316,-0.792906730150521));
#18489=DIRECTION('',(1.,0.,0.));
#18490=DIRECTION('center_axis',(1.,0.,0.));
#18491=DIRECTION('ref_axis',(0.,0.609343021033316,-0.792906730150521));
#18492=DIRECTION('',(1.,0.,0.));
#18493=DIRECTION('center_axis',(1.,0.,0.));
#18494=DIRECTION('ref_axis',(0.,0.609343021033316,-0.792906730150521));
#18495=DIRECTION('',(1.,0.,0.));
#18496=DIRECTION('center_axis',(1.,0.,0.));
#18497=DIRECTION('ref_axis',(0.,0.609343021033316,-0.792906730150521));
#18498=DIRECTION('',(1.,0.,0.));
#18499=DIRECTION('center_axis',(1.,0.,0.));
#18500=DIRECTION('ref_axis',(0.,0.609343021033316,-0.792906730150521));
#18501=DIRECTION('',(1.,0.,0.));
#18502=DIRECTION('center_axis',(1.,0.,0.));
#18503=DIRECTION('ref_axis',(0.,0.609343021033316,-0.792906730150521));
#18504=DIRECTION('',(1.,0.,0.));
#18505=DIRECTION('center_axis',(1.,0.,0.));
#18506=DIRECTION('ref_axis',(0.,0.609343021033316,-0.792906730150521));
#18507=DIRECTION('',(1.,0.,0.));
#18508=DIRECTION('center_axis',(1.,0.,0.));
#18509=DIRECTION('ref_axis',(0.,0.609343021033316,-0.792906730150521));
#18510=DIRECTION('',(1.,0.,0.));
#18511=DIRECTION('center_axis',(1.,0.,0.));
#18512=DIRECTION('ref_axis',(0.,0.609343021033316,-0.792906730150521));
#18513=DIRECTION('',(1.,0.,0.));
#18514=DIRECTION('center_axis',(1.,0.,0.));
#18515=DIRECTION('ref_axis',(0.,0.609343021033316,-0.792906730150521));
#18516=DIRECTION('',(1.,0.,0.));
#18517=DIRECTION('center_axis',(1.,0.,0.));
#18518=DIRECTION('ref_axis',(0.,0.609343021033316,-0.792906730150521));
#18519=DIRECTION('',(1.,0.,0.));
#18520=DIRECTION('center_axis',(1.,0.,0.));
#18521=DIRECTION('ref_axis',(0.,0.609343021033316,-0.792906730150521));
#18522=DIRECTION('',(1.,0.,0.));
#18523=DIRECTION('center_axis',(1.,0.,0.));
#18524=DIRECTION('ref_axis',(0.,-1.,-7.34835534001808E-14));
#18525=DIRECTION('center_axis',(1.,0.,0.));
#18526=DIRECTION('ref_axis',(0.,0.609343031978545,-0.792906721739193));
#18527=DIRECTION('',(1.,0.,0.));
#18528=DIRECTION('center_axis',(-1.,0.,0.));
#18529=DIRECTION('ref_axis',(0.,-1.,-7.78061153648973E-14));
#18530=DIRECTION('center_axis',(1.,0.,0.));
#18531=DIRECTION('ref_axis',(0.,0.609343031978545,-0.792906721739193));
#18532=DIRECTION('',(1.,0.,0.));
#18533=DIRECTION('center_axis',(1.,0.,0.));
#18534=DIRECTION('ref_axis',(0.,0.609343031978545,-0.792906721739193));
#18535=DIRECTION('',(1.,0.,0.));
#18536=DIRECTION('center_axis',(1.,0.,0.));
#18537=DIRECTION('ref_axis',(0.,0.609343031978545,-0.792906721739193));
#18538=DIRECTION('',(1.,0.,0.));
#18539=DIRECTION('center_axis',(1.,0.,0.));
#18540=DIRECTION('ref_axis',(0.,0.609343031978545,-0.792906721739193));
#18541=DIRECTION('',(1.,0.,0.));
#18542=DIRECTION('center_axis',(1.,0.,0.));
#18543=DIRECTION('ref_axis',(0.,0.609343031978545,-0.792906721739193));
#18544=DIRECTION('',(1.,0.,0.));
#18545=DIRECTION('center_axis',(1.,0.,0.));
#18546=DIRECTION('ref_axis',(0.,0.609343031978545,-0.792906721739193));
#18547=DIRECTION('',(1.,0.,0.));
#18548=DIRECTION('center_axis',(1.,0.,0.));
#18549=DIRECTION('ref_axis',(0.,0.609343031978545,-0.792906721739193));
#18550=DIRECTION('',(1.,0.,0.));
#18551=DIRECTION('center_axis',(1.,0.,0.));
#18552=DIRECTION('ref_axis',(0.,0.609343031978545,-0.792906721739193));
#18553=DIRECTION('',(1.,0.,0.));
#18554=DIRECTION('center_axis',(1.,0.,0.));
#18555=DIRECTION('ref_axis',(0.,0.609343031978545,-0.792906721739193));
#18556=DIRECTION('',(1.,0.,0.));
#18557=DIRECTION('center_axis',(1.,0.,0.));
#18558=DIRECTION('ref_axis',(0.,0.609343031978545,-0.792906721739193));
#18559=DIRECTION('',(1.,0.,0.));
#18560=DIRECTION('center_axis',(1.,0.,0.));
#18561=DIRECTION('ref_axis',(0.,0.609343031978545,-0.792906721739193));
#18562=DIRECTION('',(1.,0.,0.));
#18563=DIRECTION('center_axis',(1.,0.,0.));
#18564=DIRECTION('ref_axis',(0.,0.609343031978545,-0.792906721739193));
#18565=DIRECTION('',(1.,0.,0.));
#18566=DIRECTION('center_axis',(1.,0.,0.));
#18567=DIRECTION('ref_axis',(0.,0.609343031978545,-0.792906721739193));
#18568=DIRECTION('',(1.,0.,0.));
#18569=DIRECTION('center_axis',(1.,0.,0.));
#18570=DIRECTION('ref_axis',(0.,-1.,-7.78061153648973E-14));
#18571=DIRECTION('center_axis',(1.,0.,0.));
#18572=DIRECTION('ref_axis',(0.,0.609339783037272,-0.792909218516275));
#18573=DIRECTION('',(1.,0.,0.));
#18574=DIRECTION('center_axis',(-1.,0.,0.));
#18575=DIRECTION('ref_axis',(0.,-1.,-7.78061153648971E-14));
#18576=DIRECTION('center_axis',(1.,0.,0.));
#18577=DIRECTION('ref_axis',(0.,0.609339783037272,-0.792909218516275));
#18578=DIRECTION('',(1.,0.,0.));
#18579=DIRECTION('center_axis',(1.,0.,0.));
#18580=DIRECTION('ref_axis',(0.,0.609339783037272,-0.792909218516275));
#18581=DIRECTION('',(1.,0.,0.));
#18582=DIRECTION('center_axis',(1.,0.,0.));
#18583=DIRECTION('ref_axis',(0.,0.609339783037272,-0.792909218516275));
#18584=DIRECTION('',(1.,0.,0.));
#18585=DIRECTION('center_axis',(1.,0.,0.));
#18586=DIRECTION('ref_axis',(0.,0.609339783037272,-0.792909218516275));
#18587=DIRECTION('',(1.,0.,0.));
#18588=DIRECTION('center_axis',(1.,0.,0.));
#18589=DIRECTION('ref_axis',(0.,0.609339783037272,-0.792909218516275));
#18590=DIRECTION('',(1.,0.,0.));
#18591=DIRECTION('center_axis',(1.,0.,0.));
#18592=DIRECTION('ref_axis',(0.,0.609339783037272,-0.792909218516275));
#18593=DIRECTION('',(1.,0.,0.));
#18594=DIRECTION('center_axis',(1.,0.,0.));
#18595=DIRECTION('ref_axis',(0.,0.609339783037272,-0.792909218516275));
#18596=DIRECTION('',(1.,0.,0.));
#18597=DIRECTION('center_axis',(1.,0.,0.));
#18598=DIRECTION('ref_axis',(0.,0.609339783037272,-0.792909218516275));
#18599=DIRECTION('',(1.,0.,0.));
#18600=DIRECTION('center_axis',(1.,0.,0.));
#18601=DIRECTION('ref_axis',(0.,0.609339783037272,-0.792909218516275));
#18602=DIRECTION('',(1.,0.,0.));
#18603=DIRECTION('center_axis',(1.,0.,0.));
#18604=DIRECTION('ref_axis',(0.,0.609339783037272,-0.792909218516275));
#18605=DIRECTION('',(1.,0.,0.));
#18606=DIRECTION('center_axis',(1.,0.,0.));
#18607=DIRECTION('ref_axis',(0.,0.609339783037272,-0.792909218516275));
#18608=DIRECTION('',(1.,0.,0.));
#18609=DIRECTION('center_axis',(1.,0.,0.));
#18610=DIRECTION('ref_axis',(0.,0.609339783037272,-0.792909218516275));
#18611=DIRECTION('',(1.,0.,0.));
#18612=DIRECTION('center_axis',(1.,0.,0.));
#18613=DIRECTION('ref_axis',(0.,0.609339783037272,-0.792909218516275));
#18614=DIRECTION('',(1.,0.,0.));
#18615=DIRECTION('center_axis',(1.,0.,0.));
#18616=DIRECTION('ref_axis',(0.,-1.,-7.78061153648971E-14));
#18617=DIRECTION('center_axis',(1.,0.,0.));
#18618=DIRECTION('ref_axis',(0.,0.609339779193897,-0.792909221469856));
#18619=DIRECTION('',(1.,0.,0.));
#18620=DIRECTION('center_axis',(-1.,0.,0.));
#18621=DIRECTION('ref_axis',(0.,-1.,-6.91609914354641E-14));
#18622=DIRECTION('center_axis',(1.,0.,0.));
#18623=DIRECTION('ref_axis',(0.,0.609339779193897,-0.792909221469856));
#18624=DIRECTION('',(1.,0.,0.));
#18625=DIRECTION('center_axis',(1.,0.,0.));
#18626=DIRECTION('ref_axis',(0.,0.609339779193897,-0.792909221469856));
#18627=DIRECTION('',(1.,0.,0.));
#18628=DIRECTION('center_axis',(1.,0.,0.));
#18629=DIRECTION('ref_axis',(0.,0.609339779193897,-0.792909221469856));
#18630=DIRECTION('',(1.,0.,0.));
#18631=DIRECTION('center_axis',(1.,0.,0.));
#18632=DIRECTION('ref_axis',(0.,0.609339779193897,-0.792909221469856));
#18633=DIRECTION('',(1.,0.,0.));
#18634=DIRECTION('center_axis',(1.,0.,0.));
#18635=DIRECTION('ref_axis',(0.,0.609339779193897,-0.792909221469856));
#18636=DIRECTION('',(1.,0.,0.));
#18637=DIRECTION('center_axis',(1.,0.,0.));
#18638=DIRECTION('ref_axis',(0.,0.609339779193897,-0.792909221469856));
#18639=DIRECTION('',(1.,0.,0.));
#18640=DIRECTION('center_axis',(1.,0.,0.));
#18641=DIRECTION('ref_axis',(0.,0.609339779193897,-0.792909221469856));
#18642=DIRECTION('',(1.,0.,0.));
#18643=DIRECTION('center_axis',(1.,0.,0.));
#18644=DIRECTION('ref_axis',(0.,0.609339779193897,-0.792909221469856));
#18645=DIRECTION('',(1.,0.,0.));
#18646=DIRECTION('center_axis',(1.,0.,0.));
#18647=DIRECTION('ref_axis',(0.,0.609339779193897,-0.792909221469856));
#18648=DIRECTION('',(1.,0.,0.));
#18649=DIRECTION('center_axis',(1.,0.,0.));
#18650=DIRECTION('ref_axis',(0.,0.609339779193897,-0.792909221469856));
#18651=DIRECTION('',(1.,0.,0.));
#18652=DIRECTION('center_axis',(1.,0.,0.));
#18653=DIRECTION('ref_axis',(0.,0.609339779193897,-0.792909221469856));
#18654=DIRECTION('',(1.,0.,0.));
#18655=DIRECTION('center_axis',(1.,0.,0.));
#18656=DIRECTION('ref_axis',(0.,0.609339779193897,-0.792909221469856));
#18657=DIRECTION('',(1.,0.,0.));
#18658=DIRECTION('center_axis',(1.,0.,0.));
#18659=DIRECTION('ref_axis',(0.,0.609339779193897,-0.792909221469856));
#18660=DIRECTION('',(1.,0.,0.));
#18661=DIRECTION('center_axis',(1.,0.,0.));
#18662=DIRECTION('ref_axis',(0.,-1.,-6.91609914354641E-14));
#18663=DIRECTION('center_axis',(1.,0.,0.));
#18664=DIRECTION('ref_axis',(0.,-0.938437982150219,-0.345447758217975));
#18665=DIRECTION('',(1.,0.,0.));
#18666=DIRECTION('center_axis',(-1.,0.,0.));
#18667=DIRECTION('ref_axis',(0.,-1.,0.));
#18668=DIRECTION('center_axis',(1.,0.,0.));
#18669=DIRECTION('ref_axis',(0.,-0.938437982150219,-0.345447758217975));
#18670=DIRECTION('',(1.,0.,0.));
#18671=DIRECTION('center_axis',(1.,0.,0.));
#18672=DIRECTION('ref_axis',(0.,-0.938437982150219,-0.345447758217975));
#18673=DIRECTION('',(1.,0.,0.));
#18674=DIRECTION('center_axis',(1.,0.,0.));
#18675=DIRECTION('ref_axis',(0.,-0.938437982150219,-0.345447758217975));
#18676=DIRECTION('',(1.,0.,0.));
#18677=DIRECTION('center_axis',(1.,0.,0.));
#18678=DIRECTION('ref_axis',(0.,-0.938437982150219,-0.345447758217975));
#18679=DIRECTION('',(1.,0.,0.));
#18680=DIRECTION('center_axis',(1.,0.,0.));
#18681=DIRECTION('ref_axis',(0.,-0.938437982150219,-0.345447758217975));
#18682=DIRECTION('',(1.,0.,0.));
#18683=DIRECTION('center_axis',(1.,0.,0.));
#18684=DIRECTION('ref_axis',(0.,-0.938437982150219,-0.345447758217975));
#18685=DIRECTION('',(1.,0.,0.));
#18686=DIRECTION('center_axis',(1.,0.,0.));
#18687=DIRECTION('ref_axis',(0.,-0.938437982150219,-0.345447758217975));
#18688=DIRECTION('',(1.,0.,0.));
#18689=DIRECTION('center_axis',(1.,0.,0.));
#18690=DIRECTION('ref_axis',(0.,-0.938437982150219,-0.345447758217975));
#18691=DIRECTION('',(1.,0.,0.));
#18692=DIRECTION('center_axis',(1.,0.,0.));
#18693=DIRECTION('ref_axis',(0.,-0.938437982150219,-0.345447758217975));
#18694=DIRECTION('',(1.,0.,0.));
#18695=DIRECTION('center_axis',(1.,0.,0.));
#18696=DIRECTION('ref_axis',(0.,-0.938437982150219,-0.345447758217975));
#18697=DIRECTION('',(1.,0.,0.));
#18698=DIRECTION('center_axis',(1.,0.,0.));
#18699=DIRECTION('ref_axis',(0.,-0.938437982150219,-0.345447758217975));
#18700=DIRECTION('',(1.,0.,0.));
#18701=DIRECTION('center_axis',(1.,0.,0.));
#18702=DIRECTION('ref_axis',(0.,-0.938437982150219,-0.345447758217975));
#18703=DIRECTION('',(1.,0.,0.));
#18704=DIRECTION('center_axis',(1.,0.,0.));
#18705=DIRECTION('ref_axis',(0.,-0.938437982150219,-0.345447758217975));
#18706=DIRECTION('',(1.,0.,0.));
#18707=DIRECTION('center_axis',(1.,0.,0.));
#18708=DIRECTION('ref_axis',(0.,-1.,0.));
#18709=DIRECTION('center_axis',(1.,0.,0.));
#18710=DIRECTION('ref_axis',(0.,-0.938437989074542,-0.345447739407467));
#18711=DIRECTION('',(1.,0.,0.));
#18712=DIRECTION('center_axis',(-1.,0.,0.));
#18713=DIRECTION('ref_axis',(0.,-1.,0.));
#18714=DIRECTION('center_axis',(1.,0.,0.));
#18715=DIRECTION('ref_axis',(0.,-0.938437989074542,-0.345447739407467));
#18716=DIRECTION('',(1.,0.,0.));
#18717=DIRECTION('center_axis',(1.,0.,0.));
#18718=DIRECTION('ref_axis',(0.,-0.938437989074542,-0.345447739407467));
#18719=DIRECTION('',(1.,0.,0.));
#18720=DIRECTION('center_axis',(1.,0.,0.));
#18721=DIRECTION('ref_axis',(0.,-0.938437989074542,-0.345447739407467));
#18722=DIRECTION('',(1.,0.,0.));
#18723=DIRECTION('center_axis',(1.,0.,0.));
#18724=DIRECTION('ref_axis',(0.,-0.938437989074542,-0.345447739407467));
#18725=DIRECTION('',(1.,0.,0.));
#18726=DIRECTION('center_axis',(1.,0.,0.));
#18727=DIRECTION('ref_axis',(0.,-0.938437989074542,-0.345447739407467));
#18728=DIRECTION('',(1.,0.,0.));
#18729=DIRECTION('center_axis',(1.,0.,0.));
#18730=DIRECTION('ref_axis',(0.,-0.938437989074542,-0.345447739407467));
#18731=DIRECTION('',(1.,0.,0.));
#18732=DIRECTION('center_axis',(1.,0.,0.));
#18733=DIRECTION('ref_axis',(0.,-0.938437989074542,-0.345447739407467));
#18734=DIRECTION('',(1.,0.,0.));
#18735=DIRECTION('center_axis',(1.,0.,0.));
#18736=DIRECTION('ref_axis',(0.,-0.938437989074542,-0.345447739407467));
#18737=DIRECTION('',(1.,0.,0.));
#18738=DIRECTION('center_axis',(1.,0.,0.));
#18739=DIRECTION('ref_axis',(0.,-0.938437989074542,-0.345447739407467));
#18740=DIRECTION('',(1.,0.,0.));
#18741=DIRECTION('center_axis',(1.,0.,0.));
#18742=DIRECTION('ref_axis',(0.,-0.938437989074542,-0.345447739407467));
#18743=DIRECTION('',(1.,0.,0.));
#18744=DIRECTION('center_axis',(1.,0.,0.));
#18745=DIRECTION('ref_axis',(0.,-0.938437989074542,-0.345447739407467));
#18746=DIRECTION('',(1.,0.,0.));
#18747=DIRECTION('center_axis',(1.,0.,0.));
#18748=DIRECTION('ref_axis',(0.,-0.938437989074542,-0.345447739407467));
#18749=DIRECTION('',(1.,0.,0.));
#18750=DIRECTION('center_axis',(1.,0.,0.));
#18751=DIRECTION('ref_axis',(0.,-0.938437989074542,-0.345447739407467));
#18752=DIRECTION('',(1.,0.,0.));
#18753=DIRECTION('center_axis',(1.,0.,0.));
#18754=DIRECTION('ref_axis',(0.,-1.,0.));
#18755=DIRECTION('center_axis',(1.,0.,0.));
#18756=DIRECTION('ref_axis',(0.,-0.938439385487086,-0.345443945911084));
#18757=DIRECTION('',(1.,0.,0.));
#18758=DIRECTION('center_axis',(-1.,0.,0.));
#18759=DIRECTION('ref_axis',(0.,-1.,0.));
#18760=DIRECTION('center_axis',(1.,0.,0.));
#18761=DIRECTION('ref_axis',(0.,-0.938439385487086,-0.345443945911084));
#18762=DIRECTION('',(1.,0.,0.));
#18763=DIRECTION('center_axis',(1.,0.,0.));
#18764=DIRECTION('ref_axis',(0.,-0.938439385487086,-0.345443945911084));
#18765=DIRECTION('',(1.,0.,0.));
#18766=DIRECTION('center_axis',(1.,0.,0.));
#18767=DIRECTION('ref_axis',(0.,-0.938439385487086,-0.345443945911084));
#18768=DIRECTION('',(1.,0.,0.));
#18769=DIRECTION('center_axis',(1.,0.,0.));
#18770=DIRECTION('ref_axis',(0.,-0.938439385487086,-0.345443945911084));
#18771=DIRECTION('',(1.,0.,0.));
#18772=DIRECTION('center_axis',(1.,0.,0.));
#18773=DIRECTION('ref_axis',(0.,-0.938439385487086,-0.345443945911084));
#18774=DIRECTION('',(1.,0.,0.));
#18775=DIRECTION('center_axis',(1.,0.,0.));
#18776=DIRECTION('ref_axis',(0.,-0.938439385487086,-0.345443945911084));
#18777=DIRECTION('',(1.,0.,0.));
#18778=DIRECTION('center_axis',(1.,0.,0.));
#18779=DIRECTION('ref_axis',(0.,-0.938439385487086,-0.345443945911084));
#18780=DIRECTION('',(1.,0.,0.));
#18781=DIRECTION('center_axis',(1.,0.,0.));
#18782=DIRECTION('ref_axis',(0.,-0.938439385487086,-0.345443945911084));
#18783=DIRECTION('',(1.,0.,0.));
#18784=DIRECTION('center_axis',(1.,0.,0.));
#18785=DIRECTION('ref_axis',(0.,-0.938439385487086,-0.345443945911084));
#18786=DIRECTION('',(1.,0.,0.));
#18787=DIRECTION('center_axis',(1.,0.,0.));
#18788=DIRECTION('ref_axis',(0.,-0.938439385487086,-0.345443945911084));
#18789=DIRECTION('',(1.,0.,0.));
#18790=DIRECTION('center_axis',(1.,0.,0.));
#18791=DIRECTION('ref_axis',(0.,-0.938439385487086,-0.345443945911084));
#18792=DIRECTION('',(1.,0.,0.));
#18793=DIRECTION('center_axis',(1.,0.,0.));
#18794=DIRECTION('ref_axis',(0.,-0.938439385487086,-0.345443945911084));
#18795=DIRECTION('',(1.,0.,0.));
#18796=DIRECTION('center_axis',(1.,0.,0.));
#18797=DIRECTION('ref_axis',(0.,-0.859572185905443,-0.511014341499081));
#18798=DIRECTION('',(1.,0.,0.));
#18799=DIRECTION('center_axis',(1.,0.,0.));
#18800=DIRECTION('ref_axis',(0.,-1.,0.));
#18801=DIRECTION('center_axis',(1.,0.,0.));
#18802=DIRECTION('ref_axis',(0.,-0.938439382918495,-0.345443952888967));
#18803=DIRECTION('',(1.,0.,0.));
#18804=DIRECTION('center_axis',(-1.,0.,0.));
#18805=DIRECTION('ref_axis',(0.,-1.,0.));
#18806=DIRECTION('center_axis',(1.,0.,0.));
#18807=DIRECTION('ref_axis',(0.,-0.938439382918495,-0.345443952888967));
#18808=DIRECTION('',(1.,0.,0.));
#18809=DIRECTION('center_axis',(1.,0.,0.));
#18810=DIRECTION('ref_axis',(0.,-0.938439382918495,-0.345443952888967));
#18811=DIRECTION('',(1.,0.,0.));
#18812=DIRECTION('center_axis',(1.,0.,0.));
#18813=DIRECTION('ref_axis',(0.,-0.938439382918495,-0.345443952888967));
#18814=DIRECTION('',(1.,0.,0.));
#18815=DIRECTION('center_axis',(1.,0.,0.));
#18816=DIRECTION('ref_axis',(0.,-0.938439382918495,-0.345443952888967));
#18817=DIRECTION('',(1.,0.,0.));
#18818=DIRECTION('center_axis',(1.,0.,0.));
#18819=DIRECTION('ref_axis',(0.,-0.938439382918495,-0.345443952888967));
#18820=DIRECTION('',(1.,0.,0.));
#18821=DIRECTION('center_axis',(1.,0.,0.));
#18822=DIRECTION('ref_axis',(0.,-0.938439382918495,-0.345443952888967));
#18823=DIRECTION('',(1.,0.,0.));
#18824=DIRECTION('center_axis',(1.,0.,0.));
#18825=DIRECTION('ref_axis',(0.,-0.938439382918495,-0.345443952888967));
#18826=DIRECTION('',(1.,0.,0.));
#18827=DIRECTION('center_axis',(1.,0.,0.));
#18828=DIRECTION('ref_axis',(0.,-0.938439382918495,-0.345443952888967));
#18829=DIRECTION('',(1.,0.,0.));
#18830=DIRECTION('center_axis',(1.,0.,0.));
#18831=DIRECTION('ref_axis',(0.,-0.938439382918495,-0.345443952888967));
#18832=DIRECTION('',(1.,0.,0.));
#18833=DIRECTION('center_axis',(1.,0.,0.));
#18834=DIRECTION('ref_axis',(0.,-0.938439382918495,-0.345443952888967));
#18835=DIRECTION('',(1.,0.,0.));
#18836=DIRECTION('center_axis',(1.,0.,0.));
#18837=DIRECTION('ref_axis',(0.,-0.938439382918495,-0.345443952888967));
#18838=DIRECTION('',(1.,0.,0.));
#18839=DIRECTION('center_axis',(1.,0.,0.));
#18840=DIRECTION('ref_axis',(0.,-0.938439382918495,-0.345443952888967));
#18841=DIRECTION('',(1.,0.,0.));
#18842=DIRECTION('center_axis',(1.,0.,0.));
#18843=DIRECTION('ref_axis',(0.,-0.859572206969555,-0.511014306067344));
#18844=DIRECTION('',(1.,0.,0.));
#18845=DIRECTION('center_axis',(1.,0.,0.));
#18846=DIRECTION('ref_axis',(0.,-1.,0.));
#18847=DIRECTION('center_axis',(1.,0.,0.));
#18848=DIRECTION('ref_axis',(0.,-0.938439382918495,-0.345443952888967));
#18849=DIRECTION('center_axis',(1.,0.,0.));
#18850=DIRECTION('ref_axis',(0.,-0.938439385487086,-0.345443945911084));
#18851=DIRECTION('center_axis',(1.,0.,0.));
#18852=DIRECTION('ref_axis',(0.,-0.938437989074542,-0.345447739407467));
#18853=DIRECTION('center_axis',(1.,0.,0.));
#18854=DIRECTION('ref_axis',(0.,-0.938437982150219,-0.345447758217975));
#18855=DIRECTION('center_axis',(1.,0.,0.));
#18856=DIRECTION('ref_axis',(0.,0.609339779193897,-0.792909221469856));
#18857=DIRECTION('center_axis',(1.,0.,0.));
#18858=DIRECTION('ref_axis',(0.,0.609339783037272,-0.792909218516275));
#18859=DIRECTION('center_axis',(1.,0.,0.));
#18860=DIRECTION('ref_axis',(0.,0.609343031978545,-0.792906721739193));
#18861=DIRECTION('center_axis',(1.,0.,0.));
#18862=DIRECTION('ref_axis',(0.,0.609343021033316,-0.792906730150521));
#18863=DIRECTION('center_axis',(0.,0.,-1.));
#18864=DIRECTION('ref_axis',(0.938439750900799,-0.345442953219843,0.));
#18865=DIRECTION('center_axis',(0.,0.,-1.));
#18866=DIRECTION('ref_axis',(-0.609338902889834,-0.792909894896648,0.));
#18867=DIRECTION('center_axis',(0.,0.,-1.));
#18868=DIRECTION('ref_axis',(0.938439751642368,-0.345442951205277,0.));
#18869=DIRECTION('center_axis',(0.,0.,-1.));
#18870=DIRECTION('ref_axis',(-0.609338902105852,-0.792909895499126,0.));
#18871=DIRECTION('center_axis',(0.,0.,1.));
#18872=DIRECTION('ref_axis',(1.,0.,0.));
#18873=DIRECTION('center_axis',(0.,0.,1.));
#18874=DIRECTION('ref_axis',(1.,0.,0.));
#18875=DIRECTION('center_axis',(0.,0.,-1.));
#18876=DIRECTION('ref_axis',(1.,0.,0.));
#18877=DIRECTION('center_axis',(0.,0.,-1.));
#18878=DIRECTION('ref_axis',(1.,0.,0.));
#18879=DIRECTION('center_axis',(0.,1.,0.));
#18880=DIRECTION('ref_axis',(1.,0.,0.));
#18881=DIRECTION('',(-1.,0.,0.));
#18882=DIRECTION('',(0.,0.,-1.));
#18883=DIRECTION('',(1.,0.,0.));
#18884=DIRECTION('',(0.,0.,-1.));
#18885=DIRECTION('center_axis',(-1.,0.,0.));
#18886=DIRECTION('ref_axis',(0.,1.,0.));
#18887=DIRECTION('center_axis',(1.,0.,0.));
#18888=DIRECTION('ref_axis',(0.,1.,0.));
#18889=DIRECTION('',(0.,1.,0.));
#18890=DIRECTION('',(0.,0.,-1.));
#18891=DIRECTION('center_axis',(0.,-1.,0.));
#18892=DIRECTION('ref_axis',(-1.,0.,0.));
#18893=DIRECTION('',(1.,0.,0.));
#18894=DIRECTION('',(-1.,0.,0.));
#18895=DIRECTION('',(0.,0.,-1.));
#18896=DIRECTION('center_axis',(1.,0.,0.));
#18897=DIRECTION('ref_axis',(0.,-1.,0.));
#18898=DIRECTION('center_axis',(-1.,0.,0.));
#18899=DIRECTION('ref_axis',(0.,1.,0.));
#18900=DIRECTION('',(0.,-1.,0.));
#18901=DIRECTION('center_axis',(0.,0.,-1.));
#18902=DIRECTION('ref_axis',(1.,0.,0.));
#18903=DIRECTION('center_axis',(0.,0.,-1.));
#18904=DIRECTION('ref_axis',(1.,0.,0.));
#18905=DIRECTION('',(0.,0.,-1.));
#18906=DIRECTION('center_axis',(0.,0.,1.));
#18907=DIRECTION('ref_axis',(1.,0.,0.));
#18908=DIRECTION('center_axis',(0.,0.,-1.));
#18909=DIRECTION('ref_axis',(1.,0.,0.));
#18910=DIRECTION('center_axis',(0.,0.,-1.));
#18911=DIRECTION('ref_axis',(1.,0.,0.));
#18912=DIRECTION('',(0.,0.,-1.));
#18913=DIRECTION('center_axis',(0.,0.,1.));
#18914=DIRECTION('ref_axis',(1.,0.,0.));
#18915=DIRECTION('center_axis',(0.,0.,-1.));
#18916=DIRECTION('ref_axis',(1.,0.,0.));
#18917=DIRECTION('center_axis',(0.,0.,-1.));
#18918=DIRECTION('ref_axis',(1.,0.,0.));
#18919=DIRECTION('',(0.,0.,-1.));
#18920=DIRECTION('center_axis',(0.,0.,1.));
#18921=DIRECTION('ref_axis',(1.,0.,0.));
#18922=DIRECTION('center_axis',(0.,0.,-1.));
#18923=DIRECTION('ref_axis',(1.,0.,0.));
#18924=DIRECTION('center_axis',(0.,0.,-1.));
#18925=DIRECTION('ref_axis',(1.,0.,0.));
#18926=DIRECTION('',(0.,0.,-1.));
#18927=DIRECTION('center_axis',(0.,0.,1.));
#18928=DIRECTION('ref_axis',(1.,0.,0.));
#18929=DIRECTION('center_axis',(1.,0.,0.));
#18930=DIRECTION('ref_axis',(0.,-1.,0.));
#18931=DIRECTION('center_axis',(1.,0.,0.));
#18932=DIRECTION('ref_axis',(0.,-1.,0.));
#18933=DIRECTION('center_axis',(1.,0.,0.));
#18934=DIRECTION('ref_axis',(0.,-1.,0.));
#18935=DIRECTION('center_axis',(1.,0.,0.));
#18936=DIRECTION('ref_axis',(0.,-1.,0.));
#18937=DIRECTION('center_axis',(-1.,0.,0.));
#18938=DIRECTION('ref_axis',(0.,1.,0.));
#18939=DIRECTION('center_axis',(-1.,0.,0.));
#18940=DIRECTION('ref_axis',(0.,1.,0.));
#18941=DIRECTION('',(-1.,0.,0.));
#18942=DIRECTION('center_axis',(1.,0.,0.));
#18943=DIRECTION('ref_axis',(0.,1.,0.));
#18944=DIRECTION('center_axis',(0.,0.,1.));
#18945=DIRECTION('ref_axis',(1.,0.,0.));
#18946=DIRECTION('',(0.,-1.,0.));
#18947=DIRECTION('',(1.,0.,0.));
#18948=DIRECTION('',(0.,1.,0.));
#18949=DIRECTION('',(-1.,0.,0.));
#18950=DIRECTION('',(-1.,0.,0.));
#18951=DIRECTION('',(0.,1.,0.));
#18952=DIRECTION('',(1.,0.,0.));
#18953=DIRECTION('',(0.,-1.,0.));
#18954=DIRECTION('center_axis',(0.,1.,0.));
#18955=DIRECTION('ref_axis',(-1.,0.,0.));
#18956=DIRECTION('',(-1.,0.,0.));
#18957=DIRECTION('',(0.,0.,1.));
#18958=DIRECTION('',(0.,0.,1.));
#18959=DIRECTION('center_axis',(1.,0.,0.));
#18960=DIRECTION('ref_axis',(0.,1.,0.));
#18961=DIRECTION('',(0.,1.,0.));
#18962=DIRECTION('',(0.,0.,1.));
#18963=DIRECTION('center_axis',(0.,-1.,0.));
#18964=DIRECTION('ref_axis',(1.,0.,0.));
#18965=DIRECTION('',(1.,0.,0.));
#18966=DIRECTION('',(0.,0.,1.));
#18967=DIRECTION('center_axis',(-1.,0.,0.));
#18968=DIRECTION('ref_axis',(0.,-1.,0.));
#18969=DIRECTION('',(0.,-1.,0.));
#18970=DIRECTION('center_axis',(0.,0.,1.));
#18971=DIRECTION('ref_axis',(1.,0.,0.));
#18972=DIRECTION('center_axis',(0.,1.,0.));
#18973=DIRECTION('ref_axis',(-1.,0.,0.));
#18974=DIRECTION('',(0.,0.,1.));
#18975=DIRECTION('',(-1.,0.,0.));
#18976=DIRECTION('',(0.,0.,1.));
#18977=DIRECTION('center_axis',(1.,0.,0.));
#18978=DIRECTION('ref_axis',(0.,1.,0.));
#18979=DIRECTION('',(0.,1.,0.));
#18980=DIRECTION('',(0.,0.,1.));
#18981=DIRECTION('center_axis',(0.,-1.,0.));
#18982=DIRECTION('ref_axis',(1.,0.,0.));
#18983=DIRECTION('',(1.,0.,0.));
#18984=DIRECTION('',(0.,0.,1.));
#18985=DIRECTION('center_axis',(-1.,0.,0.));
#18986=DIRECTION('ref_axis',(0.,-1.,0.));
#18987=DIRECTION('',(0.,-1.,0.));
#18988=DIRECTION('center_axis',(0.,0.,1.));
#18989=DIRECTION('ref_axis',(1.,0.,0.));
#59495=CARTESIAN_POINT('',(0.,0.,0.));
#59496=CARTESIAN_POINT('Origin',(80.,9.,141.545925280538));
#59497=CARTESIAN_POINT('',(81.252039109102,10.6292316077768,129.106054344332));
#59498=CARTESIAN_POINT('',(81.2492121323183,10.6255440252465,129.047846840803));
#59499=CARTESIAN_POINT('',(81.252039109102,10.6292316077768,141.545925280538));
#59500=CARTESIAN_POINT('',(81.8174278887596,9.95862058795898,129.));
#59501=CARTESIAN_POINT('Ctrl Pts',(81.2492121323183,10.6255440252465,129.047846840803));
#59502=CARTESIAN_POINT('Ctrl Pts',(81.4831295089877,10.4461916147052,129.031897893869));
#59503=CARTESIAN_POINT('Ctrl Pts',(81.6801942454166,10.2187988626804,129.015948946934));
#59504=CARTESIAN_POINT('Ctrl Pts',(81.8174278887596,9.95862058795898,129.));
#59505=CARTESIAN_POINT('',(82.0533682613732,8.92465847303635,129.000000008565));
#59506=CARTESIAN_POINT('Origin',(80.,9.,129.));
#59507=CARTESIAN_POINT('Ctrl Pts',(81.252039109102,10.6292316077768,129.106054344332));
#59508=CARTESIAN_POINT('Ctrl Pts',(81.3081324428432,10.5861247546636,129.102199429059));
#59509=CARTESIAN_POINT('Ctrl Pts',(81.3621028162874,10.5400362316538,129.098344513787));
#59510=CARTESIAN_POINT('Ctrl Pts',(81.4136152532126,10.49120403647,129.094489598514));
#59511=CARTESIAN_POINT('Ctrl Pts',(81.4662254566598,10.4413311926145,129.090552532266));
#59512=CARTESIAN_POINT('Ctrl Pts',(81.5162712916801,10.3885966287696,129.086615466018));
#59513=CARTESIAN_POINT('Ctrl Pts',(81.5634291489626,10.3332992382335,129.08267839977));
#59514=CARTESIAN_POINT('Ctrl Pts',(81.6094921147899,10.2792857194398,129.078832742684));
#59515=CARTESIAN_POINT('Ctrl Pts',(81.6527994239459,10.2228274898001,129.074987085598));
#59516=CARTESIAN_POINT('Ctrl Pts',(81.6930862822707,10.164240698175,129.071141428511));
#59517=CARTESIAN_POINT('Ctrl Pts',(81.7333526428636,10.1056837151871,129.067297728074));
#59518=CARTESIAN_POINT('Ctrl Pts',(81.7706013247367,10.0450007212822,129.063454027637));
#59519=CARTESIAN_POINT('Ctrl Pts',(81.8046092461277,9.98253907367099,129.0596103272));
#59520=CARTESIAN_POINT('Ctrl Pts',(81.83861143105,9.92008796211362,129.055767275119));
#59521=CARTESIAN_POINT('Ctrl Pts',(81.8693737075422,9.85585922244642,129.051924223039));
#59522=CARTESIAN_POINT('Ctrl Pts',(81.896718484156,9.79022563509474,129.048081170959));
#59523=CARTESIAN_POINT('Ctrl Pts',(81.9252281299942,9.72179610074859,129.044074407426));
#59524=CARTESIAN_POINT('Ctrl Pts',(81.9500223238438,9.65183985848909,129.040067643893));
#59525=CARTESIAN_POINT('Ctrl Pts',(81.9709559793998,9.58080124807728,129.03606088036));
#59526=CARTESIAN_POINT('Ctrl Pts',(81.9910609207249,9.51257488931614,129.03221273518));
#59527=CARTESIAN_POINT('Ctrl Pts',(82.0076051816575,9.44335075661424,129.02836459));
#59528=CARTESIAN_POINT('Ctrl Pts',(82.0205121917149,9.37353453070845,129.02451644482));
#59529=CARTESIAN_POINT('Ctrl Pts',(82.0334283357576,9.30366889751318,129.020665576398));
#59530=CARTESIAN_POINT('Ctrl Pts',(82.0427020466773,9.23321082209362,129.016814707977));
#59531=CARTESIAN_POINT('Ctrl Pts',(82.0483086039853,9.16257129309895,129.012963839556));
#59532=CARTESIAN_POINT('Ctrl Pts',(82.053924244546,9.09181732013021,129.009106732295));
#59533=CARTESIAN_POINT('Ctrl Pts',(82.0558608740505,9.02088179457733,129.005249625034));
#59534=CARTESIAN_POINT('Ctrl Pts',(82.054145810819,8.95017480160856,129.001392517773));
#59535=CARTESIAN_POINT('Ctrl Pts',(82.0539394176871,8.94166582219882,129.000928348037));
#59536=CARTESIAN_POINT('Ctrl Pts',(82.0536802019389,8.93316014380039,129.000464178301));
#59537=CARTESIAN_POINT('Ctrl Pts',(82.0533682613732,8.92465847303635,129.000000008565));
#59538=CARTESIAN_POINT('Origin',(80.,9.,141.545925280538));
#59539=CARTESIAN_POINT('',(81.252039109102,10.6292316077768,129.806138766482));
#59540=CARTESIAN_POINT('',(81.252039109102,10.6292316077768,129.74786511009));
#59541=CARTESIAN_POINT('',(81.252039109102,10.6292316077768,141.545925280538));
#59542=CARTESIAN_POINT('',(77.945443344794,8.99850140731331,129.295925300345));
#59543=CARTESIAN_POINT('Ctrl Pts',(81.252039109102,10.6292316077768,129.74786511009));
#59544=CARTESIAN_POINT('Ctrl Pts',(81.3085193333677,10.5858274353228,129.744007244423));
#59545=CARTESIAN_POINT('Ctrl Pts',(81.3627900115786,10.5394443174509,129.740149378756));
#59546=CARTESIAN_POINT('Ctrl Pts',(81.4145261411931,10.4903400143529,129.736291513089));
#59547=CARTESIAN_POINT('Ctrl Pts',(81.4662398767985,10.4412569660766,129.732435317301));
#59548=CARTESIAN_POINT('Ctrl Pts',(81.515420889261,10.3894554040803,129.728579121513));
#59549=CARTESIAN_POINT('Ctrl Pts',(81.5617787889323,10.3352320311246,129.724722925726));
#59550=CARTESIAN_POINT('Ctrl Pts',(81.6081321155176,10.2810140071633,129.720867110342));
#59551=CARTESIAN_POINT('Ctrl Pts',(81.6516625677301,10.2243750165204,129.717011294957));
#59552=CARTESIAN_POINT('Ctrl Pts',(81.692119193999,10.1656458277711,129.713155479573));
#59553=CARTESIAN_POINT('Ctrl Pts',(81.7326518785676,10.1068062283758,129.709292415271));
#59554=CARTESIAN_POINT('Ctrl Pts',(81.7700988932371,10.0458689678327,129.705429350969));
#59555=CARTESIAN_POINT('Ctrl Pts',(81.8042518602189,9.98319519292799,129.701566286667));
#59556=CARTESIAN_POINT('Ctrl Pts',(81.8383883906004,9.92055158066739,129.69770508152));
#59557=CARTESIAN_POINT('Ctrl Pts',(81.8692338507331,9.85617357356739,129.693843876372));
#59558=CARTESIAN_POINT('Ctrl Pts',(81.8966275623393,9.79044383246044,129.689982671225));
#59559=CARTESIAN_POINT('Ctrl Pts',(81.9240726458304,9.72459082727232,129.686114225095));
#59560=CARTESIAN_POINT('Ctrl Pts',(81.9480528801327,9.6573814808109,129.682245778965));
#59561=CARTESIAN_POINT('Ctrl Pts',(81.9684568154499,9.58921585875539,129.678377332835));
#59562=CARTESIAN_POINT('Ctrl Pts',(81.9888137843977,9.52120714230307,129.674517791206));
#59563=CARTESIAN_POINT('Ctrl Pts',(82.0056108658398,9.45224703112079,129.670658249578));
#59564=CARTESIAN_POINT('Ctrl Pts',(82.0187884999237,9.3827408458422,129.666798707949));
#59565=CARTESIAN_POINT('Ctrl Pts',(82.0319999872495,9.313056099701,129.662929251187));
#59566=CARTESIAN_POINT('Ctrl Pts',(82.0416249737109,9.24255035252164,129.659059794426));
#59567=CARTESIAN_POINT('Ctrl Pts',(82.0475698214487,9.17162572299227,129.655190337664));
#59568=CARTESIAN_POINT('Ctrl Pts',(82.0535058266289,9.10080658903576,129.651326636456));
#59569=CARTESIAN_POINT('Ctrl Pts',(82.0557725185925,9.02957028953356,129.647462935249));
#59570=CARTESIAN_POINT('Ctrl Pts',(82.054327394704,8.95832845252654,129.643599234042));
#59571=CARTESIAN_POINT('Ctrl Pts',(82.0528839614273,8.88716995944365,129.639740052875));
#59572=CARTESIAN_POINT('Ctrl Pts',(82.0477373475193,8.81600642494071,129.635880871709));
#59573=CARTESIAN_POINT('Ctrl Pts',(82.0388970300604,8.74525215739669,129.632021690542));
#59574=CARTESIAN_POINT('Ctrl Pts',(82.0300622648841,8.67454232804085,129.628164933187));
#59575=CARTESIAN_POINT('Ctrl Pts',(82.0175384588747,8.60424173644822,129.624308175832));
#59576=CARTESIAN_POINT('Ctrl Pts',(82.0013870241082,8.53476076881736,129.620451418478));
#59577=CARTESIAN_POINT('Ctrl Pts',(81.9852403338186,8.46530021119049,129.616595794043));
#59578=CARTESIAN_POINT('Ctrl Pts',(81.9654682402386,8.3966592723316,129.612740169609));
#59579=CARTESIAN_POINT('Ctrl Pts',(81.9421831510885,8.3292376202201,129.608884545175));
#59580=CARTESIAN_POINT('Ctrl Pts',(81.9188971176168,8.26181323383866,129.605028764377));
#59581=CARTESIAN_POINT('Ctrl Pts',(81.8920979663439,8.1956086907147,129.601172983579));
#59582=CARTESIAN_POINT('Ctrl Pts',(81.8619472520006,8.13100633301075,129.597317202781));
#59583=CARTESIAN_POINT('Ctrl Pts',(81.8317649374834,8.06633626726792,129.59345738084));
#59584=CARTESIAN_POINT('Ctrl Pts',(81.7982242536195,8.00327218000733,129.5895975589));
#59585=CARTESIAN_POINT('Ctrl Pts',(81.7615336137239,7.94217350656126,129.585737736959));
#59586=CARTESIAN_POINT('Ctrl Pts',(81.7248221654374,7.8810401821776,129.581875725994));
#59587=CARTESIAN_POINT('Ctrl Pts',(81.6849574763693,7.82187489349001,129.578013715029));
#59588=CARTESIAN_POINT('Ctrl Pts',(81.6421908386299,7.76500736357659,129.574151704065));
#59589=CARTESIAN_POINT('Ctrl Pts',(81.5993493728494,7.70804033353673,129.570282935807));
#59590=CARTESIAN_POINT('Ctrl Pts',(81.5535961328667,7.65337946154818,129.566414167549));
#59591=CARTESIAN_POINT('Ctrl Pts',(81.5052216848136,7.60132017885905,129.562545399291));
#59592=CARTESIAN_POINT('Ctrl Pts',(81.4765470131007,7.57046126675146,129.560252129513));
#59593=CARTESIAN_POINT('Ctrl Pts',(81.4469520253758,7.54051576286219,129.557958859736));
#59594=CARTESIAN_POINT('Ctrl Pts',(81.416502734468,7.51153852392995,129.555665589958));
#59595=CARTESIAN_POINT('Ctrl Pts',(81.3651794217435,7.46269640474508,129.551800205955));
#59596=CARTESIAN_POINT('Ctrl Pts',(81.3112252599378,7.41641511917265,129.547934821953));
#59597=CARTESIAN_POINT('Ctrl Pts',(81.2549263703187,7.37299128226715,129.544069437951));
#59598=CARTESIAN_POINT('Ctrl Pts',(81.1987115926323,7.32963232164728,129.540209828927));
#59599=CARTESIAN_POINT('Ctrl Pts',(81.1401594225051,7.28912263103086,129.536350219904));
#59600=CARTESIAN_POINT('Ctrl Pts',(81.0795917608502,7.25172107705769,129.532490610881));
#59601=CARTESIAN_POINT('Ctrl Pts',(81.019095173482,7.21436341265691,129.52863553099));
#59602=CARTESIAN_POINT('Ctrl Pts',(80.9565882043631,7.18010689512892,129.524780451099));
#59603=CARTESIAN_POINT('Ctrl Pts',(80.8924232503983,7.14916821276258,129.520925371209));
#59604=CARTESIAN_POINT('Ctrl Pts',(80.8282986965517,7.118249010289,129.517072718588));
#59605=CARTESIAN_POINT('Ctrl Pts',(80.7625186662802,7.09064370965583,129.513220065967));
#59606=CARTESIAN_POINT('Ctrl Pts',(80.6954604719183,7.06652326248824,129.509367413347));
#59607=CARTESIAN_POINT('Ctrl Pts',(80.6284219527023,7.04240989235757,129.50551589111));
#59608=CARTESIAN_POINT('Ctrl Pts',(80.5601064716975,7.02177951062841,129.501664368873));
#59609=CARTESIAN_POINT('Ctrl Pts',(80.4909100257795,7.00475442386427,129.497812846637));
#59610=CARTESIAN_POINT('Ctrl Pts',(80.421710617344,6.98772860820264,129.493961159504));
#59611=CARTESIAN_POINT('Ctrl Pts',(80.3516306423667,6.97430850810218,129.490109472372));
#59612=CARTESIAN_POINT('Ctrl Pts',(80.2810782143665,6.96456574660134,129.486257785239));
#59613=CARTESIAN_POINT('Ctrl Pts',(80.2104510098597,6.9548126590254,129.482402015814));
#59614=CARTESIAN_POINT('Ctrl Pts',(80.139350835998,6.9487447569335,129.478546246388));
#59615=CARTESIAN_POINT('Ctrl Pts',(80.068191985698,6.9463818720155,129.474690476962));
#59616=CARTESIAN_POINT('Ctrl Pts',(79.9969924228888,6.944017635207,129.470832501513));
#59617=CARTESIAN_POINT('Ctrl Pts',(79.9257346037539,6.94536262570084,129.466974526065));
#59618=CARTESIAN_POINT('Ctrl Pts',(79.8548310998208,6.95038453535285,129.463116550616));
#59619=CARTESIAN_POINT('Ctrl Pts',(79.7838021060318,6.95541533312298,129.459251747059));
#59620=CARTESIAN_POINT('Ctrl Pts',(79.7131291626912,6.96413598279352,129.455386943503));
#59621=CARTESIAN_POINT('Ctrl Pts',(79.6432173161427,6.97646258275278,129.451522139946));
#59622=CARTESIAN_POINT('Ctrl Pts',(79.6010710950756,6.98389364962538,129.449192250619));
#59623=CARTESIAN_POINT('Ctrl Pts',(79.5592012548522,6.99263422302007,129.446862361293));
#59624=CARTESIAN_POINT('Ctrl Pts',(79.5176937420075,7.00265720618587,129.444532471966));
#59625=CARTESIAN_POINT('Ctrl Pts',(79.4486461888338,7.01933039172912,129.440656711986));
#59626=CARTESIAN_POINT('Ctrl Pts',(79.3803311134737,7.03962034190895,129.436780952005));
#59627=CARTESIAN_POINT('Ctrl Pts',(79.3131544745362,7.06344615704848,129.432905192025));
#59628=CARTESIAN_POINT('Ctrl Pts',(79.2460780170999,7.08723644040247,129.429035212022));
#59629=CARTESIAN_POINT('Ctrl Pts',(79.1801370782105,7.11455196023636,129.425165232019));
#59630=CARTESIAN_POINT('Ctrl Pts',(79.115725168422,7.14526131632033,129.421295252016));
#59631=CARTESIAN_POINT('Ctrl Pts',(79.0513895933296,7.17593427867882,129.417429858334));
#59632=CARTESIAN_POINT('Ctrl Pts',(78.9885798822686,7.20999287981601,129.413564464653));
#59633=CARTESIAN_POINT('Ctrl Pts',(78.9276705405346,7.24725726563691,129.409699070972));
#59634=CARTESIAN_POINT('Ctrl Pts',(78.8668000929382,7.28449785599208,129.405836145568));
#59635=CARTESIAN_POINT('Ctrl Pts',(78.8078280186592,7.32493991718004,129.401973220164));
#59636=CARTESIAN_POINT('Ctrl Pts',(78.7511038510315,7.36835789108281,129.398110294761));
#59637=CARTESIAN_POINT('Ctrl Pts',(78.6943971038458,7.41176253098132,129.394248555692));
#59638=CARTESIAN_POINT('Ctrl Pts',(78.6399372767077,7.45814097500666,129.390386816623));
#59639=CARTESIAN_POINT('Ctrl Pts',(78.5880431440327,7.50722560331881,129.386525077554));
#59640=CARTESIAN_POINT('Ctrl Pts',(78.5361477488554,7.55631142578241,129.382663244536));
#59641=CARTESIAN_POINT('Ctrl Pts',(78.4868185221684,7.60810322910186,129.378801411517));
#59642=CARTESIAN_POINT('Ctrl Pts',(78.4403382347849,7.66229572003898,129.374939578498));
#59643=CARTESIAN_POINT('Ctrl Pts',(78.39381094995,7.71654300644102,129.371073840678));
#59644=CARTESIAN_POINT('Ctrl Pts',(78.3501386708224,7.77319545824749,129.367208102857));
#59645=CARTESIAN_POINT('Ctrl Pts',(78.3095640209211,7.8319144880893,129.363342365037));
#59646=CARTESIAN_POINT('Ctrl Pts',(78.2689671120395,7.89066573079638,129.359474506498));
#59647=CARTESIAN_POINT('Ctrl Pts',(78.2314714702368,7.95148539676405,129.35560664796));
#59648=CARTESIAN_POINT('Ctrl Pts',(78.1972750294098,8.01400799044285,129.351738789422));
#59649=CARTESIAN_POINT('Ctrl Pts',(78.1630203529657,8.07663705841363,129.347864344024));
#59650=CARTESIAN_POINT('Ctrl Pts',(78.132076305444,8.14097440811675,129.343989898627));
#59651=CARTESIAN_POINT('Ctrl Pts',(78.1045934316036,8.20663280696784,129.34011545323));
#59652=CARTESIAN_POINT('Ctrl Pts',(78.0887135064689,8.24457099582957,129.337876753478));
#59653=CARTESIAN_POINT('Ctrl Pts',(78.0739882366105,8.28294990542073,129.335638053726));
#59654=CARTESIAN_POINT('Ctrl Pts',(78.0604390140864,8.32169273598019,129.333399353975));
#59655=CARTESIAN_POINT('Ctrl Pts',(78.033260828792,8.39940640744042,129.328908779215));
#59656=CARTESIAN_POINT('Ctrl Pts',(78.010731418976,8.47882922479276,129.324418204456));
#59657=CARTESIAN_POINT('Ctrl Pts',(77.993036431149,8.55943809083774,129.319927629697));
#59658=CARTESIAN_POINT('Ctrl Pts',(77.9754996204933,8.63932638659772,129.315477196611));
#59659=CARTESIAN_POINT('Ctrl Pts',(77.9627112748633,8.72037946475493,129.311026763524));
#59660=CARTESIAN_POINT('Ctrl Pts',(77.9548055650093,8.80206747214528,129.306576330438));
#59661=CARTESIAN_POINT('Ctrl Pts',(77.9484987679612,8.86723425582204,129.303025987867));
#59662=CARTESIAN_POINT('Ctrl Pts',(77.9452984670482,8.93280468883457,129.299475645296));
#59663=CARTESIAN_POINT('Ctrl Pts',(77.9452505466197,8.99850122269098,129.295925302724));
#59664=CARTESIAN_POINT('Ctrl Pts',(77.9470482356371,8.99850294414681,129.295925280538));
#59665=CARTESIAN_POINT('Ctrl Pts',(77.9500644391936,9.45244375993743,129.271372265686));
#59666=CARTESIAN_POINT('Ctrl Pts',(78.321762223559,10.5960398895428,129.209774878171));
#59667=CARTESIAN_POINT('Ctrl Pts',(79.9094066588576,11.2849415874619,129.127082064926));
#59668=CARTESIAN_POINT('Ctrl Pts',(80.939813231773,10.8627706880183,129.068942266533));
#59669=CARTESIAN_POINT('Ctrl Pts',(81.2492121323183,10.6255440252465,129.047846840803));
#59670=CARTESIAN_POINT('',(77.9452508134379,9.00182833865366,129.354074719499));
#59671=CARTESIAN_POINT('Ctrl Pts',(77.9452508134385,9.00182833933565,129.354074719462));
#59672=CARTESIAN_POINT('Ctrl Pts',(77.9453406304354,9.10276769878956,129.348594607972));
#59673=CARTESIAN_POINT('Ctrl Pts',(77.9528718856253,9.2033869237755,129.343114496482));
#59674=CARTESIAN_POINT('Ctrl Pts',(77.9676835434894,9.3027992455346,129.337634384992));
#59675=CARTESIAN_POINT('Ctrl Pts',(77.9734618754717,9.34158203430287,129.335496480932));
#59676=CARTESIAN_POINT('Ctrl Pts',(77.9803477636373,9.38018147547678,129.333358576871));
#59677=CARTESIAN_POINT('Ctrl Pts',(77.9883298389047,9.41854596576566,129.331220672811));
#59678=CARTESIAN_POINT('Ctrl Pts',(78.0027616204826,9.48790987498085,129.327355291515));
#59679=CARTESIAN_POINT('Ctrl Pts',(78.0208138006321,9.556663936971,129.32348991022));
#59680=CARTESIAN_POINT('Ctrl Pts',(78.0424197606568,9.62440144861534,129.319624528925));
#59681=CARTESIAN_POINT('Ctrl Pts',(78.0639934408006,9.69203775860952,129.315764922612));
#59682=CARTESIAN_POINT('Ctrl Pts',(78.0891102156646,9.75866007280167,129.3119053163));
#59683=CARTESIAN_POINT('Ctrl Pts',(78.1176525675056,9.82387238446372,129.308045709988));
#59684=CARTESIAN_POINT('Ctrl Pts',(78.1461614258055,9.88900817155401,129.3041906328));
#59685=CARTESIAN_POINT('Ctrl Pts',(78.1780876826902,9.95273679869852,129.300335555613));
#59686=CARTESIAN_POINT('Ctrl Pts',(78.2132647473922,10.0146796044016,129.296480478426));
#59687=CARTESIAN_POINT('Ctrl Pts',(78.2484196636299,10.0765834091808,129.292627828503));
#59688=CARTESIAN_POINT('Ctrl Pts',(78.2868210873334,10.1367032008444,129.28877517858));
#59689=CARTESIAN_POINT('Ctrl Pts',(78.3282559207096,10.1946837639549,129.284922528658));
#59690=CARTESIAN_POINT('Ctrl Pts',(78.3696785970312,10.2526473154639,129.281071009109));
#59691=CARTESIAN_POINT('Ctrl Pts',(78.4141326333405,10.3084724885383,129.277219489561));
#59692=CARTESIAN_POINT('Ctrl Pts',(78.4613618953665,10.3618334499747,129.273367970013));
#59693=CARTESIAN_POINT('Ctrl Pts',(78.5085931795893,10.4151966961464,129.269516285555));
#59694=CARTESIAN_POINT('Ctrl Pts',(78.5585996011231,10.4660951581404,129.265664601098));
#59695=CARTESIAN_POINT('Ctrl Pts',(78.6110862317618,10.5142377973418,129.261812916641));
#59696=CARTESIAN_POINT('Ctrl Pts',(78.6636284920416,10.5624314620654,129.257957149852));
#59697=CARTESIAN_POINT('Ctrl Pts',(78.7186558493627,10.607863143692,129.254101383063));
#59698=CARTESIAN_POINT('Ctrl Pts',(78.7758388347598,10.6502808864002,129.250245616274));
#59699=CARTESIAN_POINT('Ctrl Pts',(78.8330545368563,10.6927228980151,129.246387643445));
#59700=CARTESIAN_POINT('Ctrl Pts',(78.8924279161816,10.7321472689681,129.242529670616));
#59701=CARTESIAN_POINT('Ctrl Pts',(78.9536012630827,10.7683459067382,129.238671697787));
#59702=CARTESIAN_POINT('Ctrl Pts',(79.0148828797013,10.804608611892,129.234806896795));
#59703=CARTESIAN_POINT('Ctrl Pts',(79.0779703927226,10.8376339598158,129.230942095802));
#59704=CARTESIAN_POINT('Ctrl Pts',(79.1424829361018,10.8672605730383,129.227077294809));
#59705=CARTESIAN_POINT('Ctrl Pts',(79.1813746242017,10.8851211151989,129.224747381479));
#59706=CARTESIAN_POINT('Ctrl Pts',(79.2207838360795,10.9017473816217,129.222417468149));
#59707=CARTESIAN_POINT('Ctrl Pts',(79.2606244670148,10.9171127728235,129.220087554819));
#59708=CARTESIAN_POINT('Ctrl Pts',(79.3268985097602,10.942672774495,129.216211793517));
#59709=CARTESIAN_POINT('Ctrl Pts',(79.3946272743244,10.9648414181532,129.212336032215));
#59710=CARTESIAN_POINT('Ctrl Pts',(79.4634308512325,10.9834543380403,129.208460270913));
#59711=CARTESIAN_POINT('Ctrl Pts',(79.5321318201631,11.0020395001545,129.204590289601));
#59712=CARTESIAN_POINT('Ctrl Pts',(79.6019039559843,11.017079339933,129.20072030829));
#59713=CARTESIAN_POINT('Ctrl Pts',(79.6723488634407,11.0284581078276,129.196850326978));
#59714=CARTESIAN_POINT('Ctrl Pts',(79.7427102860479,11.0398233906491,129.192984932014));
#59715=CARTESIAN_POINT('Ctrl Pts',(79.8137424208771,11.0475361441803,129.189119537049));
#59716=CARTESIAN_POINT('Ctrl Pts',(79.8850349442187,11.0515312813723,129.185254142085));
#59717=CARTESIAN_POINT('Ctrl Pts',(79.9562819428734,11.0555238674221,129.181391215415));
#59718=CARTESIAN_POINT('Ctrl Pts',(80.027788518058,11.0558035205452,129.177528288744));
#59719=CARTESIAN_POINT('Ctrl Pts',(80.0991388891969,11.0523569482789,129.173665362074));
#59720=CARTESIAN_POINT('Ctrl Pts',(80.1704673477443,11.0489114344981,129.169803621756));
#59721=CARTESIAN_POINT('Ctrl Pts',(80.2416392143741,11.0417419908114,129.165941881439));
#59722=CARTESIAN_POINT('Ctrl Pts',(80.3122400830185,11.0308874151603,129.162080141122));
#59723=CARTESIAN_POINT('Ctrl Pts',(80.3828426689081,11.0200325754903,129.158218306874));
#59724=CARTESIAN_POINT('Ctrl Pts',(80.4528737512294,11.0054925015909,129.154356472627));
#59725=CARTESIAN_POINT('Ctrl Pts',(80.5219271081132,10.9873574555969,129.150494638379));
#59726=CARTESIAN_POINT('Ctrl Pts',(80.5910502859759,10.9692040729612,129.146628899368));
#59727=CARTESIAN_POINT('Ctrl Pts',(80.6591932958107,10.9474485848929,129.142763160356));
#59728=CARTESIAN_POINT('Ctrl Pts',(80.7259639989441,10.9222314727257,129.138897421345));
#59729=CARTESIAN_POINT('Ctrl Pts',(80.7927713316841,10.8970005267533,129.135029561635));
#59730=CARTESIAN_POINT('Ctrl Pts',(80.8582044152026,10.8683043698804,129.131161701926));
#59731=CARTESIAN_POINT('Ctrl Pts',(80.9218925622573,10.8363310339246,129.127293842217));
#59732=CARTESIAN_POINT('Ctrl Pts',(80.9856891677658,10.804303248613,129.123419395692));
#59733=CARTESIAN_POINT('Ctrl Pts',(81.0477344828468,10.7689873806112,129.119544949167));
#59734=CARTESIAN_POINT('Ctrl Pts',(81.1076844332874,10.7306162944896,129.115670502641));
#59735=CARTESIAN_POINT('Ctrl Pts',(81.1423240314956,10.7084451501216,129.113431814037));
#59736=CARTESIAN_POINT('Ctrl Pts',(81.1762646277231,10.6852547759275,129.111193125432));
#59737=CARTESIAN_POINT('Ctrl Pts',(81.2094449454566,10.6610961701266,129.108954436827));
#59738=CARTESIAN_POINT('Ctrl Pts',(81.2237726773633,10.6506641414181,129.107987739329));
#59739=CARTESIAN_POINT('Ctrl Pts',(81.2379725780439,10.6400415177553,129.10702104183));
#59740=CARTESIAN_POINT('Ctrl Pts',(81.252039109102,10.6292316077768,129.106054344332));
#59741=CARTESIAN_POINT('Ctrl Pts',(81.252039109102,10.6292316077768,129.806138766482));
#59742=CARTESIAN_POINT('Ctrl Pts',(81.3085776991369,10.5857825821384,129.802277188624));
#59743=CARTESIAN_POINT('Ctrl Pts',(81.3628020004145,10.5394254826911,129.798415610767));
#59744=CARTESIAN_POINT('Ctrl Pts',(81.4144129894673,10.490447401865,129.794554032909));
#59745=CARTESIAN_POINT('Ctrl Pts',(81.4661146701134,10.441383256031,129.79068566943));
#59746=CARTESIAN_POINT('Ctrl Pts',(81.5151935348951,10.3896892853797,129.78681730595));
#59747=CARTESIAN_POINT('Ctrl Pts',(81.5613890748026,10.335687732813,129.782948942471));
#59748=CARTESIAN_POINT('Ctrl Pts',(81.5900328636082,10.3022037845792,129.780550343239));
#59749=CARTESIAN_POINT('Ctrl Pts',(81.6175689177519,10.2678332878201,129.778151744008));
#59750=CARTESIAN_POINT('Ctrl Pts',(81.6439435865611,10.2326585280217,129.775753144776));
#59751=CARTESIAN_POINT('Ctrl Pts',(81.6864883341909,10.1759184305673,129.77188398533));
#59752=CARTESIAN_POINT('Ctrl Pts',(81.7261753858345,10.1168620335078,129.768014825883));
#59753=CARTESIAN_POINT('Ctrl Pts',(81.7627435644833,10.0558090207858,129.764145666437));
#59754=CARTESIAN_POINT('Ctrl Pts',(81.7992572695089,9.99484695541022,129.760282270666));
#59755=CARTESIAN_POINT('Ctrl Pts',(81.8326610761952,9.93189459151865,129.756418874895));
#59756=CARTESIAN_POINT('Ctrl Pts',(81.8627355219774,9.86730267938221,129.752555479125));
#59757=CARTESIAN_POINT('Ctrl Pts',(81.8927747004109,9.80278651213253,129.748696613836));
#59758=CARTESIAN_POINT('Ctrl Pts',(81.9194920690401,9.73663505389883,129.744837748547));
#59759=CARTESIAN_POINT('Ctrl Pts',(81.9427136477607,9.66922436096161,129.740978883258));
#59760=CARTESIAN_POINT('Ctrl Pts',(81.965920603033,9.60185611891828,129.737122448033));
#59761=CARTESIAN_POINT('Ctrl Pts',(81.9856359781547,9.53323067363172,129.733266012808));
#59762=CARTESIAN_POINT('Ctrl Pts',(82.0017341442023,9.46374344031431,129.729409577583));
#59763=CARTESIAN_POINT('Ctrl Pts',(82.0178275571484,9.39427672361183,129.725554280999));
#59764=CARTESIAN_POINT('Ctrl Pts',(82.0303057717423,9.32394919700083,129.721698984414));
#59765=CARTESIAN_POINT('Ctrl Pts',(82.039093661386,9.25316911856549,129.71784368783));
#59766=CARTESIAN_POINT('Ctrl Pts',(82.0478818956115,9.18238626477412,129.713988240076));
#59767=CARTESIAN_POINT('Ctrl Pts',(82.0529794599358,9.11115130625805,129.710132792321));
#59768=CARTESIAN_POINT('Ctrl Pts',(82.0543629815708,9.03987859640918,129.706277344567));
#59769=CARTESIAN_POINT('Ctrl Pts',(82.0557479513842,8.96853128302626,129.702417861186));
#59770=CARTESIAN_POINT('Ctrl Pts',(82.0534111085149,8.89714662609191,129.698558377806));
#59771=CARTESIAN_POINT('Ctrl Pts',(82.0473812380801,8.8261390542485,129.694698894425));
#59772=CARTESIAN_POINT('Ctrl Pts',(82.041347953272,8.75509127484793,129.690837225638));
#59773=CARTESIAN_POINT('Ctrl Pts',(82.0316175443434,8.68442148704298,129.686975556851));
#59774=CARTESIAN_POINT('Ctrl Pts',(82.0182703789565,8.61453633124921,129.683113888064));
#59775=CARTESIAN_POINT('Ctrl Pts',(82.0048998647885,8.54452892229111,129.67924546389));
#59776=CARTESIAN_POINT('Ctrl Pts',(81.9879000781151,8.47530935765307,129.675377039717));
#59777=CARTESIAN_POINT('Ctrl Pts',(81.9674017498609,8.40727078936132,129.671508615544));
#59778=CARTESIAN_POINT('Ctrl Pts',(81.9552344738799,8.36688485995832,129.669212419291));
#59779=CARTESIAN_POINT('Ctrl Pts',(81.9418354981883,8.32691469877441,129.666916223038));
#59780=CARTESIAN_POINT('Ctrl Pts',(81.9272400716739,8.28743893690832,129.664620026785));
#59781=CARTESIAN_POINT('Ctrl Pts',(81.9026497162947,8.2209302252788,129.66075139836));
#59782=CARTESIAN_POINT('Ctrl Pts',(81.8745642826625,8.15556547524259,129.656882769936));
#59783=CARTESIAN_POINT('Ctrl Pts',(81.8431105948871,8.09173742920077,129.653014141511));
#59784=CARTESIAN_POINT('Ctrl Pts',(81.8117037846444,8.02800451036091,129.649151278762));
#59785=CARTESIAN_POINT('Ctrl Pts',(81.7769388976484,7.96580418176457,129.645288416013));
#59786=CARTESIAN_POINT('Ctrl Pts',(81.7389914861927,7.90551099893629,129.641425553264));
#59787=CARTESIAN_POINT('Ctrl Pts',(81.7010885844062,7.84528853581008,129.637567221384));
#59788=CARTESIAN_POINT('Ctrl Pts',(81.6600108304285,7.78696918439063,129.633708889504));
#59789=CARTESIAN_POINT('Ctrl Pts',(81.6159797094141,7.73090302133297,129.629850557624));
#59790=CARTESIAN_POINT('Ctrl Pts',(81.5719763196151,7.67487216927354,129.625994655757));
#59791=CARTESIAN_POINT('Ctrl Pts',(81.5250235524811,7.62109207141463,129.622138753891));
#59792=CARTESIAN_POINT('Ctrl Pts',(81.475385385291,7.56988268754986,129.618282852024));
#59793=CARTESIAN_POINT('Ctrl Pts',(81.4257618654248,7.51868841464652,129.614428087965));
#59794=CARTESIAN_POINT('Ctrl Pts',(81.3734548566607,7.47006369848698,129.610573323905));
#59795=CARTESIAN_POINT('Ctrl Pts',(81.3187665200082,7.42429303859968,129.606718559846));
#59796=CARTESIAN_POINT('Ctrl Pts',(81.2640760157143,7.37852056453442,129.602863642998));
#59797=CARTESIAN_POINT('Ctrl Pts',(81.20700437018,7.33560268150686,129.599008726149));
#59798=CARTESIAN_POINT('Ctrl Pts',(81.1478869368393,7.29578371597568,129.595153809301));
#59799=CARTESIAN_POINT('Ctrl Pts',(81.08870752091,7.25592300163336,129.591294850706));
#59800=CARTESIAN_POINT('Ctrl Pts',(81.0274784392499,7.21916796272987,129.587435892111));
#59801=CARTESIAN_POINT('Ctrl Pts',(80.9645633986281,7.18571914728537,129.583576933515));
#59802=CARTESIAN_POINT('Ctrl Pts',(80.901612684589,7.15225136604917,129.579715786854));
#59803=CARTESIAN_POINT('Ctrl Pts',(80.8369745491523,7.12209374562773,129.575854640193));
#59804=CARTESIAN_POINT('Ctrl Pts',(80.7710341310293,7.09539927247522,129.571993493532));
#59805=CARTESIAN_POINT('Ctrl Pts',(80.7049781762283,7.0686580269358,129.568125581612));
#59806=CARTESIAN_POINT('Ctrl Pts',(80.637615842551,7.04539220205611,129.564257669691));
#59807=CARTESIAN_POINT('Ctrl Pts',(80.569348250249,7.02570515564711,129.56038975777));
#59808=CARTESIAN_POINT('Ctrl Pts',(80.5287371152381,7.01399369384332,129.558088808111));
#59809=CARTESIAN_POINT('Ctrl Pts',(80.4878058559495,7.00354773124927,129.555787858452));
#59810=CARTESIAN_POINT('Ctrl Pts',(80.4466401967145,6.99438037076347,129.553486908793));
#59811=CARTESIAN_POINT('Ctrl Pts',(80.3774071820531,6.9789625682865,129.549617137619));
#59812=CARTESIAN_POINT('Ctrl Pts',(80.307239509545,6.96710365544103,129.545747366445));
#59813=CARTESIAN_POINT('Ctrl Pts',(80.2365361422388,6.95891004217972,129.541877595271));
#59814=CARTESIAN_POINT('Ctrl Pts',(80.16593814403,6.95072863984509,129.538013591209));
#59815=CARTESIAN_POINT('Ctrl Pts',(80.0948065141796,6.94620174973747,129.534149587148));
#59816=CARTESIAN_POINT('Ctrl Pts',(80.0235513509058,6.94538497611584,129.530285583086));
#59817=CARTESIAN_POINT('Ctrl Pts',(79.9523798796856,6.94456916182766,129.526426117453));
#59818=CARTESIAN_POINT('Ctrl Pts',(79.8810856464657,6.94745481361333,129.52256665182));
#59819=CARTESIAN_POINT('Ctrl Pts',(79.810083084742,6.954045668203,129.518707186187));
#59820=CARTESIAN_POINT('Ctrl Pts',(79.7391253248915,6.96063236403242,129.514850155836));
#59821=CARTESIAN_POINT('Ctrl Pts',(79.6684593537717,6.97091957938468,129.510993125485));
#59822=CARTESIAN_POINT('Ctrl Pts',(79.5984973427476,6.98485901765677,129.507136095134));
#59823=CARTESIAN_POINT('Ctrl Pts',(79.5285560950896,6.99879431897429,129.503280209475));
#59824=CARTESIAN_POINT('Ctrl Pts',(79.4593188687309,7.01637959649254,129.499424323816));
#59825=CARTESIAN_POINT('Ctrl Pts',(79.3911887511958,7.03751524188606,129.495568438157));
#59826=CARTESIAN_POINT('Ctrl Pts',(79.3230560843437,7.05865167814072,129.491712408217));
#59827=CARTESIAN_POINT('Ctrl Pts',(79.2560310717025,7.08333860004452,129.487856378277));
#59828=CARTESIAN_POINT('Ctrl Pts',(79.1905010544802,7.11142672376675,129.484000348336));
#59829=CARTESIAN_POINT('Ctrl Pts',(79.1249027002981,7.1395441387522,129.480140297196));
#59830=CARTESIAN_POINT('Ctrl Pts',(79.0608029009693,7.17106964428378,129.476280246055));
#59831=CARTESIAN_POINT('Ctrl Pts',(78.9985675987183,7.20580639055781,129.472420194914));
#59832=CARTESIAN_POINT('Ctrl Pts',(78.9362971787157,7.2405627378683,129.468557965647));
#59833=CARTESIAN_POINT('Ctrl Pts',(78.8758937615436,7.27853367462545,129.46469573638));
#59834=CARTESIAN_POINT('Ctrl Pts',(78.8176949647001,7.31947854342635,129.460833507114));
#59835=CARTESIAN_POINT('Ctrl Pts',(78.7593946368001,7.36049484284114,129.456964539972));
#59836=CARTESIAN_POINT('Ctrl Pts',(78.7033069902807,7.40449513291138,129.45309557283));
#59837=CARTESIAN_POINT('Ctrl Pts',(78.6497366239544,7.45119840592477,129.449226605688));
#59838=CARTESIAN_POINT('Ctrl Pts',(78.6180159090372,7.47885289684122,129.446935667393));
#59839=CARTESIAN_POINT('Ctrl Pts',(78.587177113685,7.5074543877569,129.444644729097));
#59840=CARTESIAN_POINT('Ctrl Pts',(78.5572770043333,7.53693885285868,129.442353790802));
#59841=CARTESIAN_POINT('Ctrl Pts',(78.507519198505,7.58600497071898,129.43854136117));
#59842=CARTESIAN_POINT('Ctrl Pts',(78.4601566137214,7.63772181533481,129.434728931539));
#59843=CARTESIAN_POINT('Ctrl Pts',(78.4154907258652,7.69182267154611,129.430916501907));
#59844=CARTESIAN_POINT('Ctrl Pts',(78.3708843294308,7.74585146970567,129.42710915013));
#59845=CARTESIAN_POINT('Ctrl Pts',(78.3289678286292,7.80225760548264,129.423301798352));
#59846=CARTESIAN_POINT('Ctrl Pts',(78.2900066810319,7.86073689975305,129.419494446575));
#59847=CARTESIAN_POINT('Ctrl Pts',(78.2510835039569,7.91915920162234,129.415690805344));
#59848=CARTESIAN_POINT('Ctrl Pts',(78.2151102469513,7.97965024231591,129.411887164112));
#59849=CARTESIAN_POINT('Ctrl Pts',(78.1823115521101,8.04187356319355,129.408083522881));
#59850=CARTESIAN_POINT('Ctrl Pts',(78.1495331090737,8.10405846380596,129.404282230237));
#59851=CARTESIAN_POINT('Ctrl Pts',(78.1199255730656,8.16797308076684,129.400480937593));
#59852=CARTESIAN_POINT('Ctrl Pts',(78.0936687399069,8.23325448205287,129.396679644949));
#59853=CARTESIAN_POINT('Ctrl Pts',(78.0674080110329,8.29854556911333,129.392877788309));
#59854=CARTESIAN_POINT('Ctrl Pts',(78.0444991802892,8.36520338671441,129.389075931669));
#59855=CARTESIAN_POINT('Ctrl Pts',(78.0250741653868,8.43284436855716,129.385274075029));
#59856=CARTESIAN_POINT('Ctrl Pts',(78.0056484149394,8.50048791168432,129.381472074428));
#59857=CARTESIAN_POINT('Ctrl Pts',(77.9897068701602,8.56911420800702,129.377670073827));
#59858=CARTESIAN_POINT('Ctrl Pts',(77.9773310505391,8.63832627495641,129.373868073226));
#59859=CARTESIAN_POINT('Ctrl Pts',(77.9649417654702,8.70761364774499,129.370061935878));
#59860=CARTESIAN_POINT('Ctrl Pts',(77.9561260270523,8.77748756743294,129.36625579853));
#59861=CARTESIAN_POINT('Ctrl Pts',(77.9509137023551,8.84754375282076,129.362449661181));
#59862=CARTESIAN_POINT('Ctrl Pts',(77.9470906737942,8.89892712073455,129.359658013954));
#59863=CARTESIAN_POINT('Ctrl Pts',(77.9452050593912,8.9504083842497,129.356866366726));
#59864=CARTESIAN_POINT('Ctrl Pts',(77.9452508134379,9.00182833865365,129.354074719499));
#59865=CARTESIAN_POINT('Origin',(80.,9.,141.545925280538));
#59866=CARTESIAN_POINT('',(81.252039109102,10.6292316077768,130.506052881431));
#59867=CARTESIAN_POINT('',(81.252039109102,10.6292316077768,130.447945712677));
#59868=CARTESIAN_POINT('',(81.252039109102,10.6292316077768,141.545925280538));
#59869=CARTESIAN_POINT('',(77.9452500565798,8.99951780232932,129.995925280508));
#59870=CARTESIAN_POINT('Ctrl Pts',(81.252039109102,10.6292316077768,130.447945712677));
#59871=CARTESIAN_POINT('Ctrl Pts',(81.2676313183556,10.6172492378733,130.446873986415));
#59872=CARTESIAN_POINT('Ctrl Pts',(81.283043563841,10.6050491142855,130.445802260153));
#59873=CARTESIAN_POINT('Ctrl Pts',(81.2982695699005,10.5926373367375,130.44473053389));
#59874=CARTESIAN_POINT('Ctrl Pts',(81.3532376874634,10.5478289973244,130.440861444718));
#59875=CARTESIAN_POINT('Ctrl Pts',(81.4059909767705,10.5000838098986,130.436992355545));
#59876=CARTESIAN_POINT('Ctrl Pts',(81.4561988948284,10.4496490406993,130.433123266372));
#59877=CARTESIAN_POINT('Ctrl Pts',(81.5063320051152,10.3992894172703,130.429259941986));
#59878=CARTESIAN_POINT('Ctrl Pts',(81.5539269322296,10.3462485080518,130.4253966176));
#59879=CARTESIAN_POINT('Ctrl Pts',(81.5986861256879,10.2908137875127,130.421533293214));
#59880=CARTESIAN_POINT('Ctrl Pts',(81.643392815583,10.2354440931756,130.417674500597));
#59881=CARTESIAN_POINT('Ctrl Pts',(81.6852700754498,10.177686541274,130.413815707979));
#59882=CARTESIAN_POINT('Ctrl Pts',(81.7240583933976,10.1178641324666,130.409956915362));
#59883=CARTESIAN_POINT('Ctrl Pts',(81.7628222769504,10.0580794083137,130.40610055356));
#59884=CARTESIAN_POINT('Ctrl Pts',(81.7985008154704,9.99623281453984,130.402244191758));
#59885=CARTESIAN_POINT('Ctrl Pts',(81.830876753814,9.93267779797929,130.398387829957));
#59886=CARTESIAN_POINT('Ctrl Pts',(81.8632431273927,9.86914155736234,130.394532607433));
#59887=CARTESIAN_POINT('Ctrl Pts',(81.8923086174108,9.80389832857846,130.39067738491));
#59888=CARTESIAN_POINT('Ctrl Pts',(81.9179018844489,9.73732619926814,130.386822162386));
#59889=CARTESIAN_POINT('Ctrl Pts',(81.9434961515718,9.67075146857944,130.382966789215));
#59890=CARTESIAN_POINT('Ctrl Pts',(81.9656177540764,9.60284818848602,130.379111416045));
#59891=CARTESIAN_POINT('Ctrl Pts',(81.9841441098762,9.53401284042958,130.375256042874));
#59892=CARTESIAN_POINT('Ctrl Pts',(82.0026898569072,9.46510544354896,130.371396634348));
#59893=CARTESIAN_POINT('Ctrl Pts',(82.0176327187617,9.39526450127846,130.367537225822));
#59894=CARTESIAN_POINT('Ctrl Pts',(82.0289007144248,9.32489914359176,130.363677817295));
#59895=CARTESIAN_POINT('Ctrl Pts',(82.0401750898638,9.25449394605857,130.359816223628));
#59896=CARTESIAN_POINT('Ctrl Pts',(82.0477704054185,9.18356422528882,130.35595462996));
#59897=CARTESIAN_POINT('Ctrl Pts',(82.0516666187131,9.11252398925642,130.352093036293));
#59898=CARTESIAN_POINT('Ctrl Pts',(82.0555696483686,9.04135946950529,130.348224686831));
#59899=CARTESIAN_POINT('Ctrl Pts',(82.0557606538919,8.97008453440691,130.34435633737));
#59900=CARTESIAN_POINT('Ctrl Pts',(82.0522717225443,8.89911224383035,130.340487987908));
#59901=CARTESIAN_POINT('Ctrl Pts',(82.05020014715,8.85697199049934,130.338191130572));
#59902=CARTESIAN_POINT('Ctrl Pts',(82.0468322168767,8.81493833801628,130.335894273235));
#59903=CARTESIAN_POINT('Ctrl Pts',(82.0421831982151,8.7730961714123,130.333597415899));
#59904=CARTESIAN_POINT('Ctrl Pts',(82.0343518468839,8.70261232718845,130.32972832049));
#59905=CARTESIAN_POINT('Ctrl Pts',(82.0228518584094,8.63239635192647,130.325859225081));
#59906=CARTESIAN_POINT('Ctrl Pts',(82.0077116911561,8.56286005936857,130.321990129672));
#59907=CARTESIAN_POINT('Ctrl Pts',(81.9925940814525,8.49342736991812,130.318126798884));
#59908=CARTESIAN_POINT('Ctrl Pts',(81.973847161083,8.4246728238438,130.314263468095));
#59909=CARTESIAN_POINT('Ctrl Pts',(81.9515510631405,8.35700232468914,130.310400137306));
#59910=CARTESIAN_POINT('Ctrl Pts',(81.9292811177576,8.28941120071327,130.306541338072));
#59911=CARTESIAN_POINT('Ctrl Pts',(81.9034704153359,8.22290205707025,130.302682538838));
#59912=CARTESIAN_POINT('Ctrl Pts',(81.8742495670342,8.15786810832739,130.298823739604));
#59913=CARTESIAN_POINT('Ctrl Pts',(81.8450471251758,8.09287512498284,130.294967371059));
#59914=CARTESIAN_POINT('Ctrl Pts',(81.8124389978158,8.02935593500499,130.291111002513));
#59915=CARTESIAN_POINT('Ctrl Pts',(81.7766042941104,7.96768476488599,130.287254633967));
#59916=CARTESIAN_POINT('Ctrl Pts',(81.7407801758834,7.90603181227041,130.283399404582));
#59917=CARTESIAN_POINT('Ctrl Pts',(81.7017316174486,7.84622621554188,130.279544175198));
#59918=CARTESIAN_POINT('Ctrl Pts',(81.6596833332211,7.78861699040805,130.275688945813));
#59919=CARTESIAN_POINT('Ctrl Pts',(81.6176334047604,7.7310055125544,130.271833565676));
#59920=CARTESIAN_POINT('Ctrl Pts',(81.5725838057957,7.67559096789019,130.267978185538));
#59921=CARTESIAN_POINT('Ctrl Pts',(81.5248011489136,7.62269138579189,130.264122805401));
#59922=CARTESIAN_POINT('Ctrl Pts',(81.4769684774253,7.56973643314834,130.260263389797));
#59923=CARTESIAN_POINT('Ctrl Pts',(81.426397363668,7.51930205923476,130.256403974193));
#59924=CARTESIAN_POINT('Ctrl Pts',(81.3733924916258,7.4716706420258,130.252544558589));
#59925=CARTESIAN_POINT('Ctrl Pts',(81.3203576080414,7.42401225574343,130.24868295777));
#59926=CARTESIAN_POINT('Ctrl Pts',(81.2648866009189,7.37916029105891,130.244821356952));
#59927=CARTESIAN_POINT('Ctrl Pts',(81.2073164228308,7.33735613625078,130.240959756133));
#59928=CARTESIAN_POINT('Ctrl Pts',(81.1496455263141,7.29547884550793,130.237091399484));
#59929=CARTESIAN_POINT('Ctrl Pts',(81.0898685341668,7.25666027500702,130.233223042835));
#59930=CARTESIAN_POINT('Ctrl Pts',(81.0283498764503,7.22109750292359,130.229354686186));
#59931=CARTESIAN_POINT('Ctrl Pts',(80.9918238201664,7.19998248086451,130.227057890093));
#59932=CARTESIAN_POINT('Ctrl Pts',(80.9546842397429,7.1800143268547,130.224761094));
#59933=CARTESIAN_POINT('Ctrl Pts',(80.9170107235692,7.16122625226509,130.222464297907));
#59934=CARTESIAN_POINT('Ctrl Pts',(80.8535484472579,7.12957712306075,130.218595269394));
#59935=CARTESIAN_POINT('Ctrl Pts',(80.7883214520981,7.10115529781342,130.21472624088));
#59936=CARTESIAN_POINT('Ctrl Pts',(80.7216911370353,7.07616022880679,130.210857212366));
#59937=CARTESIAN_POINT('Ctrl Pts',(80.6551601004848,7.05120240220646,130.206993948667));
#59938=CARTESIAN_POINT('Ctrl Pts',(80.5872303456127,7.02966136615534,130.203130684968));
#59939=CARTESIAN_POINT('Ctrl Pts',(80.5182863343939,7.01168995423737,130.199267421268));
#59940=CARTESIAN_POINT('Ctrl Pts',(80.4494231929077,6.99373962237048,130.195408689088));
#59941=CARTESIAN_POINT('Ctrl Pts',(80.379548626026,6.97935071961538,130.191549956908));
#59942=CARTESIAN_POINT('Ctrl Pts',(80.3090638144979,6.96862678932009,130.187691224728));
#59943=CARTESIAN_POINT('Ctrl Pts',(80.2386234016157,6.95790961406854,130.183834923177));
#59944=CARTESIAN_POINT('Ctrl Pts',(80.1675739858566,6.9508529039936,130.179978621627));
#59945=CARTESIAN_POINT('Ctrl Pts',(80.0963271004719,6.94750915904244,130.176122320077));
#59946=CARTESIAN_POINT('Ctrl Pts',(80.0251012587066,6.94416640170632,130.172267157531));
#59947=CARTESIAN_POINT('Ctrl Pts',(79.9536785481068,6.94453445506637,130.168411994985));
#59948=CARTESIAN_POINT('Ctrl Pts',(79.8824740573168,6.94861383077285,130.16455683244));
#59949=CARTESIAN_POINT('Ctrl Pts',(79.8112667774319,6.95269336626935,130.160701518887));
#59950=CARTESIAN_POINT('Ctrl Pts',(79.740278219204,6.96048448274595,130.156846205334));
#59951=CARTESIAN_POINT('Ctrl Pts',(79.6699201635377,6.97193568542291,130.15299089178));
#59952=CARTESIAN_POINT('Ctrl Pts',(79.5994884466511,6.98339887691275,130.149131541915));
#59953=CARTESIAN_POINT('Ctrl Pts',(79.5296890305112,6.99852972577124,130.145272192049));
#59954=CARTESIAN_POINT('Ctrl Pts',(79.4609243933277,7.01722541553738,130.141412842183));
#59955=CARTESIAN_POINT('Ctrl Pts',(79.3921208139723,7.03593169287869,130.137551306725));
#59956=CARTESIAN_POINT('Ctrl Pts',(79.3243536418541,7.05820667817763,130.133689771267));
#59957=CARTESIAN_POINT('Ctrl Pts',(79.2580084198717,7.08389821316334,130.129828235809));
#59958=CARTESIAN_POINT('Ctrl Pts',(79.1915471032066,7.1096347046736,130.125959943215));
#59959=CARTESIAN_POINT('Ctrl Pts',(79.1265131478625,7.13879948321254,130.12209165062));
#59960=CARTESIAN_POINT('Ctrl Pts',(79.0632697732558,7.17119327297723,130.118223358025));
#59961=CARTESIAN_POINT('Ctrl Pts',(79.025709308585,7.1904320597051,130.115925965322));
#59962=CARTESIAN_POINT('Ctrl Pts',(78.9887799235412,7.21080892047137,130.113628572619));
#59963=CARTESIAN_POINT('Ctrl Pts',(78.9525527429518,7.23227496306631,130.111331179916));
#59964=CARTESIAN_POINT('Ctrl Pts',(78.8915407851485,7.26842697003174,130.107462029063));
#59965=CARTESIAN_POINT('Ctrl Pts',(78.8322831878937,7.30781216979145,130.103592878211));
#59966=CARTESIAN_POINT('Ctrl Pts',(78.7751435465107,7.3502350983108,130.099723727359));
#59967=CARTESIAN_POINT('Ctrl Pts',(78.7180890438663,7.392594816167,130.095860341587));
#59968=CARTESIAN_POINT('Ctrl Pts',(78.6631466197984,7.43798299107895,130.091996955814));
#59969=CARTESIAN_POINT('Ctrl Pts',(78.6106532113617,7.48615949869204,130.088133570042));
#59970=CARTESIAN_POINT('Ctrl Pts',(78.5582213877529,7.53427948602916,130.084274716762));
#59971=CARTESIAN_POINT('Ctrl Pts',(78.5082332288406,7.58518098138821,130.080415863482));
#59972=CARTESIAN_POINT('Ctrl Pts',(78.4609933282997,7.63858308113869,130.076557010202));
#59973=CARTESIAN_POINT('Ctrl Pts',(78.4137831915473,7.69195153456925,130.072700588216));
#59974=CARTESIAN_POINT('Ctrl Pts',(78.3693181988724,7.74781710360056,130.06884416623));
#59975=CARTESIAN_POINT('Ctrl Pts',(78.3278656752727,7.80586250265354,130.064987744243));
#59976=CARTESIAN_POINT('Ctrl Pts',(78.2864254037727,7.8638907452598,130.061132462098));
#59977=CARTESIAN_POINT('Ctrl Pts',(78.24799611582,7.9240971436945,130.057277179952));
#59978=CARTESIAN_POINT('Ctrl Pts',(78.2128033876072,7.98613322810559,130.053421897807));
#59979=CARTESIAN_POINT('Ctrl Pts',(78.1776092901316,8.04817172618856,130.049566465662));
#59980=CARTESIAN_POINT('Ctrl Pts',(78.1456522401799,8.11203962798427,130.045711033517));
#59981=CARTESIAN_POINT('Ctrl Pts',(78.1171123277082,8.17736303509301,130.041855601371));
#59982=CARTESIAN_POINT('Ctrl Pts',(78.0885425536903,8.24275479062207,130.037996135256));
#59983=CARTESIAN_POINT('Ctrl Pts',(78.0633972492933,8.30960464548333,130.03413666914));
#59984=CARTESIAN_POINT('Ctrl Pts',(78.0418083419939,8.37751868058912,130.030277203025));
#59985=CARTESIAN_POINT('Ctrl Pts',(78.0202072154328,8.44547115485051,130.026415552462));
#59986=CARTESIAN_POINT('Ctrl Pts',(78.0021666159711,8.5144885382013,130.022553901899));
#59987=CARTESIAN_POINT('Ctrl Pts',(77.9877678323499,8.58416437625648,130.018692251336));
#59988=CARTESIAN_POINT('Ctrl Pts',(77.9733438650333,8.65396207843101,130.014823846687));
#59989=CARTESIAN_POINT('Ctrl Pts',(77.9625745040558,8.72442005426722,130.010955442038));
#59990=CARTESIAN_POINT('Ctrl Pts',(77.9554893455248,8.79512504731584,130.007087037388));
#59991=CARTESIAN_POINT('Ctrl Pts',(77.9512835218753,8.83709626512267,130.004790712234));
#59992=CARTESIAN_POINT('Ctrl Pts',(77.9483749151369,8.87915447197554,130.002494387079));
#59993=CARTESIAN_POINT('Ctrl Pts',(77.9467610336869,8.92121351820568,130.000198061924));
#59994=CARTESIAN_POINT('Ctrl Pts',(77.9457600484671,8.94729999663671,129.998773801462));
#59995=CARTESIAN_POINT('Ctrl Pts',(77.9452561844405,8.97340567540233,129.997349541));
#59996=CARTESIAN_POINT('Ctrl Pts',(77.9452500565799,8.99951780177073,129.995925280538));
#59997=CARTESIAN_POINT('Ctrl Pts',(77.9452500565798,8.99951780232931,129.995925280508));
#59998=CARTESIAN_POINT('Ctrl Pts',(77.9452335129583,9.07001379864739,129.992080145153));
#59999=CARTESIAN_POINT('Ctrl Pts',(77.9488491930074,9.14065511061305,129.988235009798));
#60000=CARTESIAN_POINT('Ctrl Pts',(77.9561158549005,9.2110335611009,129.984389874443));
#60001=CARTESIAN_POINT('Ctrl Pts',(77.9636220280264,9.28373170523678,129.980418002338));
#60002=CARTESIAN_POINT('Ctrl Pts',(77.975024177992,9.35614883199943,129.976446130233));
#60003=CARTESIAN_POINT('Ctrl Pts',(77.9902844919774,9.4278330741228,129.972474258129));
#60004=CARTESIAN_POINT('Ctrl Pts',(78.0050192001863,9.49704832040622,129.968639187857));
#60005=CARTESIAN_POINT('Ctrl Pts',(78.02335052537,9.56557981566392,129.964804117585));
#60006=CARTESIAN_POINT('Ctrl Pts',(78.0451918512736,9.63302659041542,129.960969047313));
#60007=CARTESIAN_POINT('Ctrl Pts',(78.0670205775869,9.70043445719311,129.957136189376));
#60008=CARTESIAN_POINT('Ctrl Pts',(78.0923551372306,9.76675837705386,129.953303331438));
#60009=CARTESIAN_POINT('Ctrl Pts',(78.1210586664692,9.83161110361127,129.949470473501));
#60010=CARTESIAN_POINT('Ctrl Pts',(78.1497555410476,9.89644879463568,129.945638504178));
#60011=CARTESIAN_POINT('Ctrl Pts',(78.1818196352711,9.95981551941986,129.941806534854));
#60012=CARTESIAN_POINT('Ctrl Pts',(78.2170660925413,10.0213443318167,129.937974565531));
#60013=CARTESIAN_POINT('Ctrl Pts',(78.2523165391549,10.0828801083052,129.934142162489));
#60014=CARTESIAN_POINT('Ctrl Pts',(78.2907498162761,10.1425771338496,129.930309759448));
#60015=CARTESIAN_POINT('Ctrl Pts',(78.3321362084666,10.200094969322,129.926477356406));
#60016=CARTESIAN_POINT('Ctrl Pts',(78.373567411324,10.2576750816064,129.922640803871));
#60017=CARTESIAN_POINT('Ctrl Pts',(78.4179578187722,10.3130708973975,129.918804251337));
#60018=CARTESIAN_POINT('Ctrl Pts',(78.4650362908378,10.3659736359297,129.914967698802));
#60019=CARTESIAN_POINT('Ctrl Pts',(78.5121454499549,10.4189108579316,129.911128645497));
#60020=CARTESIAN_POINT('Ctrl Pts',(78.5619458123617,10.4693514211948,129.907289592191));
#60021=CARTESIAN_POINT('Ctrl Pts',(78.6141300837946,10.5170241058919,129.903450538885));
#60022=CARTESIAN_POINT('Ctrl Pts',(78.6664000026858,10.5647750334034,129.899605184732));
#60023=CARTESIAN_POINT('Ctrl Pts',(78.7210612535677,10.6097487117794,129.895759830578));
#60024=CARTESIAN_POINT('Ctrl Pts',(78.7777751229153,10.6517154453281,129.891914476425));
#60025=CARTESIAN_POINT('Ctrl Pts',(78.7917840634903,10.6620816834842,129.890964632261));
#60026=CARTESIAN_POINT('Ctrl Pts',(78.8059181176275,10.6722646699556,129.890014788096));
#60027=CARTESIAN_POINT('Ctrl Pts',(78.820171946148,10.6822613726303,129.889064943932));
#60028=CARTESIAN_POINT('Ctrl Pts',(78.8782264933528,10.7229770334427,129.885196315038));
#60029=CARTESIAN_POINT('Ctrl Pts',(78.938505015448,10.7607638442889,129.881327686144));
#60030=CARTESIAN_POINT('Ctrl Pts',(79.0006798143163,10.7953709168261,129.87745905725));
#60031=CARTESIAN_POINT('Ctrl Pts',(79.0627619499484,10.8299264121425,129.873596194031));
#60032=CARTESIAN_POINT('Ctrl Pts',(79.1267343314652,10.8613113414234,129.869733330812));
#60033=CARTESIAN_POINT('Ctrl Pts',(79.192239527078,10.8893174907582,129.865870467592));
#60034=CARTESIAN_POINT('Ctrl Pts',(79.2576678896478,10.9172907908258,129.862012135243));
#60035=CARTESIAN_POINT('Ctrl Pts',(79.32462505052,10.9418929927971,129.858153802894));
#60036=CARTESIAN_POINT('Ctrl Pts',(79.3927297221528,10.9629621423103,129.854295470545));
#60037=CARTESIAN_POINT('Ctrl Pts',(79.4607915008078,10.9840180222703,129.850439568211));
#60038=CARTESIAN_POINT('Ctrl Pts',(79.5299988932787,11.0015451211287,129.846583665877));
#60039=CARTESIAN_POINT('Ctrl Pts',(79.599952793044,11.0154304241791,129.842727763542));
#60040=CARTESIAN_POINT('Ctrl Pts',(79.6698860506518,11.0293116299224,129.838872999017));
#60041=CARTESIAN_POINT('Ctrl Pts',(79.7405649018862,11.0395530787255,129.835018234491));
#60042=CARTESIAN_POINT('Ctrl Pts',(79.8115790040935,11.0460926398386,129.831163469965));
#60043=CARTESIAN_POINT('Ctrl Pts',(79.8825959209901,11.0526324601514,129.827308552654));
#60044=CARTESIAN_POINT('Ctrl Pts',(79.9539476311761,11.0554700591059,129.823453635342));
#60045=CARTESIAN_POINT('Ctrl Pts',(80.0252193417206,11.0545952271197,129.81959871803));
#60046=CARTESIAN_POINT('Ctrl Pts',(80.0965657780592,11.0537194779041,129.815739758978));
#60047=CARTESIAN_POINT('Ctrl Pts',(80.1678315604504,11.0491235337427,129.811880799926));
#60048=CARTESIAN_POINT('Ctrl Pts',(80.2386034764512,11.0408493191623,129.808021840873));
#60049=CARTESIAN_POINT('Ctrl Pts',(80.3094155207289,11.0325704130321,129.804160693759));
#60050=CARTESIAN_POINT('Ctrl Pts',(80.3797326619261,11.0206091662598,129.800299546644));
#60051=CARTESIAN_POINT('Ctrl Pts',(80.4491511126179,11.0050588122382,129.796438399529));
#60052=CARTESIAN_POINT('Ctrl Pts',(80.5186911937878,10.9894812119013,129.792570487164));
#60053=CARTESIAN_POINT('Ctrl Pts',(80.5873289725487,10.9703020797991,129.7887025748));
#60054=CARTESIAN_POINT('Ctrl Pts',(80.6546757450919,10.9476645582051,129.784834662435));
#60055=CARTESIAN_POINT('Ctrl Pts',(80.6947390243179,10.9341979388801,129.782533716937));
#60056=CARTESIAN_POINT('Ctrl Pts',(80.7343458013838,10.9195083881302,129.780232771439));
#60057=CARTESIAN_POINT('Ctrl Pts',(80.7734181170445,10.903633887786,129.777931825941));
#60058=CARTESIAN_POINT('Ctrl Pts',(80.8391271583217,10.8769372822551,129.774062259468));
#60059=CARTESIAN_POINT('Ctrl Pts',(80.903580819736,10.8467822905527,129.770192692995));
#60060=CARTESIAN_POINT('Ctrl Pts',(80.9663904970254,10.8133082941847,129.766323126522));
#60061=CARTESIAN_POINT('Ctrl Pts',(81.0291002039768,10.779887576338,129.762459719002));
#60062=CARTESIAN_POINT('Ctrl Pts',(81.0901706983107,10.74315857112,129.758596311482));
#60063=CARTESIAN_POINT('Ctrl Pts',(81.1492332216771,10.7033087109193,129.754732903962));
#60064=CARTESIAN_POINT('Ctrl Pts',(81.1842307580926,10.6796956504872,129.752443639338));
#60065=CARTESIAN_POINT('Ctrl Pts',(81.218523639527,10.6549877240144,129.750154374714));
#60066=CARTESIAN_POINT('Ctrl Pts',(81.252039109102,10.6292316077768,129.74786511009));
#60067=CARTESIAN_POINT('',(77.9452500005989,8.99995038927704,130.054074719503));
#60068=CARTESIAN_POINT('Ctrl Pts',(77.9452500005989,8.99995039003008,130.054074719462));
#60069=CARTESIAN_POINT('Ctrl Pts',(77.9452481959203,9.07469672239711,130.050044138511));
#60070=CARTESIAN_POINT('Ctrl Pts',(77.9493293030444,9.14936770606286,130.04601355756));
#60071=CARTESIAN_POINT('Ctrl Pts',(77.9574429752524,9.22351367554211,130.041982976609));
#60072=CARTESIAN_POINT('Ctrl Pts',(77.965578494409,9.2978592911421,130.037941542879));
#60073=CARTESIAN_POINT('Ctrl Pts',(77.9777682288688,9.37167665110889,130.033900109149));
#60074=CARTESIAN_POINT('Ctrl Pts',(77.9939102839952,9.44452403066627,130.029858675418));
#60075=CARTESIAN_POINT('Ctrl Pts',(78.0100750993415,9.51747412467749,130.025811543286));
#60076=CARTESIAN_POINT('Ctrl Pts',(78.0302032317879,9.58945110973448,130.021764411154));
#60077=CARTESIAN_POINT('Ctrl Pts',(78.0541430533931,9.66002901893903,130.017717279021));
#60078=CARTESIAN_POINT('Ctrl Pts',(78.0781473934775,9.73079713755454,130.013659239756));
#60079=CARTESIAN_POINT('Ctrl Pts',(78.1059837999931,9.80015825502306,130.009601200491));
#60080=CARTESIAN_POINT('Ctrl Pts',(78.1374525208473,9.8677064310018,130.005543161226));
#60081=CARTESIAN_POINT('Ctrl Pts',(78.1569006444202,9.90945217845837,130.003035234404));
#60082=CARTESIAN_POINT('Ctrl Pts',(78.1777351870459,9.95050597400759,130.000527307582));
#60083=CARTESIAN_POINT('Ctrl Pts',(78.1999006273473,9.99077737715166,129.99801938076));
#60084=CARTESIAN_POINT('Ctrl Pts',(78.2340956916408,10.0529048693632,129.994150352319));
#60085=CARTESIAN_POINT('Ctrl Pts',(78.2715778611207,10.1133817065652,129.990281323878));
#60086=CARTESIAN_POINT('Ctrl Pts',(78.3121633370003,10.1718382830126,129.986412295437));
#60087=CARTESIAN_POINT('Ctrl Pts',(78.3526883409194,10.2302077597351,129.982549031811));
#60088=CARTESIAN_POINT('Ctrl Pts',(78.3963071981439,10.2865625550009,129.978685768185));
#60089=CARTESIAN_POINT('Ctrl Pts',(78.4427906247499,10.3405582882267,129.974822504558));
#60090=CARTESIAN_POINT('Ctrl Pts',(78.4892195273723,10.394490685707,129.970963772451));
#60091=CARTESIAN_POINT('Ctrl Pts',(78.5385060097335,10.44606915121,129.967105040343));
#60092=CARTESIAN_POINT('Ctrl Pts',(78.5903790012833,10.4949803351472,129.963246308236));
#60093=CARTESIAN_POINT('Ctrl Pts',(78.642219317844,10.5438607097489,129.959390006758));
#60094=CARTESIAN_POINT('Ctrl Pts',(78.6966425585689,10.5900768036493,129.95553370528));
#60095=CARTESIAN_POINT('Ctrl Pts',(78.7533401052594,10.6333513612647,129.951677403802));
#60096=CARTESIAN_POINT('Ctrl Pts',(78.8100209056556,10.6766131372252,129.947822241329));
#60097=CARTESIAN_POINT('Ctrl Pts',(78.8689742924639,10.7169348071598,129.943967078855));
#60098=CARTESIAN_POINT('Ctrl Pts',(78.9298591529066,10.7540798527668,129.940111916382));
#60099=CARTESIAN_POINT('Ctrl Pts',(78.9907463982287,10.791226353357,129.9362566029));
#60100=CARTESIAN_POINT('Ctrl Pts',(79.0535648515318,10.8251957314521,129.932401289419));
#60101=CARTESIAN_POINT('Ctrl Pts',(79.1179465399631,10.8557961246152,129.928545975937));
#60102=CARTESIAN_POINT('Ctrl Pts',(79.182395632689,10.8864285548058,129.924686626142));
#60103=CARTESIAN_POINT('Ctrl Pts',(79.2484107879555,10.9136847501106,129.920827276347));
#60104=CARTESIAN_POINT('Ctrl Pts',(79.3156024930666,10.9374203506218,129.916967926552));
#60105=CARTESIAN_POINT('Ctrl Pts',(79.3828322495905,10.9611693928685,129.913106391164));
#60106=CARTESIAN_POINT('Ctrl Pts',(79.451239416256,10.9813937335869,129.909244855777));
#60107=CARTESIAN_POINT('Ctrl Pts',(79.520420344357,10.9979992283265,129.905383320389));
#60108=CARTESIAN_POINT('Ctrl Pts',(79.5897223292526,11.0146337803225,129.901515027863));
#60109=CARTESIAN_POINT('Ctrl Pts',(79.6598003010311,11.0276367547423,129.897646735336));
#60110=CARTESIAN_POINT('Ctrl Pts',(79.7302421718041,11.0369654578876,129.89377844281));
#60111=CARTESIAN_POINT('Ctrl Pts',(79.7720778613746,11.0425058094512,129.891481049463));
#60112=CARTESIAN_POINT('Ctrl Pts',(79.8140418210399,11.0467511619059,129.889183656115));
#60113=CARTESIAN_POINT('Ctrl Pts',(79.8560477423787,11.049701273363,129.886886262768));
#60114=CARTESIAN_POINT('Ctrl Pts',(79.9267744983491,11.0546684733781,129.883018065774));
#60115=CARTESIAN_POINT('Ctrl Pts',(79.9978971266534,11.0559803693969,129.87914986878));
#60116=CARTESIAN_POINT('Ctrl Pts',(80.0690057026482,11.0535909464891,129.875281671786));
#60117=CARTESIAN_POINT('Ctrl Pts',(80.1400164914646,11.0512048094708,129.871418794264));
#60118=CARTESIAN_POINT('Ctrl Pts',(80.2110127852759,11.0451274670466,129.867555916742));
#60119=CARTESIAN_POINT('Ctrl Pts',(80.2815810425782,11.0353647532962,129.86369303922));
#60120=CARTESIAN_POINT('Ctrl Pts',(80.3520758688713,11.0256121983049,129.859834181281));
#60121=CARTESIAN_POINT('Ctrl Pts',(80.422143063926,11.0121819488409,129.855975323343));
#60122=CARTESIAN_POINT('Ctrl Pts',(80.4913723260528,10.9951317750188,129.852116465404));
#60123=CARTESIAN_POINT('Ctrl Pts',(80.5605648373335,10.9780906524026,129.848259655968));
#60124=CARTESIAN_POINT('Ctrl Pts',(80.6289198260969,10.9574335277133,129.844402846531));
#60125=CARTESIAN_POINT('Ctrl Pts',(80.6960368287023,10.9332693282598,129.840546037095));
#60126=CARTESIAN_POINT('Ctrl Pts',(80.7631293959301,10.9091139262989,129.836690631812));
#60127=CARTESIAN_POINT('Ctrl Pts',(80.8289844162549,10.881454152868,129.832835226529));
#60128=CARTESIAN_POINT('Ctrl Pts',(80.8932181094343,10.850448316349,129.828979821247));
#60129=CARTESIAN_POINT('Ctrl Pts',(80.9574849801847,10.8194264648961,129.825122424595));
#60130=CARTESIAN_POINT('Ctrl Pts',(81.0201284102717,10.7850553046203,129.821265027943));
#60131=CARTESIAN_POINT('Ctrl Pts',(81.0807870582173,10.7475402419659,129.817407631292));
#60132=CARTESIAN_POINT('Ctrl Pts',(81.1398557484067,10.711008507606,129.813651343022));
#60133=CARTESIAN_POINT('Ctrl Pts',(81.1970420974188,10.6714959544679,129.809895054752));
#60134=CARTESIAN_POINT('Ctrl Pts',(81.252039109102,10.6292316077768,129.806138766482));
#60135=CARTESIAN_POINT('Ctrl Pts',(81.252039109102,10.6292316077768,130.506052881431));
#60136=CARTESIAN_POINT('Ctrl Pts',(81.3085807231097,10.5857802582625,130.50219771152));
#60137=CARTESIAN_POINT('Ctrl Pts',(81.3628732049477,10.5393702223445,130.498342541608));
#60138=CARTESIAN_POINT('Ctrl Pts',(81.4145999473004,10.4902699593019,130.494487371696));
#60139=CARTESIAN_POINT('Ctrl Pts',(81.4663306408243,10.441165945713,130.490631907306));
#60140=CARTESIAN_POINT('Ctrl Pts',(81.5154948550975,10.3893716331966,130.486776442915));
#60141=CARTESIAN_POINT('Ctrl Pts',(81.561812210644,10.3351929378121,130.482920978525));
#60142=CARTESIAN_POINT('Ctrl Pts',(81.6081791199772,10.280956277989,130.479061389268));
#60143=CARTESIAN_POINT('Ctrl Pts',(81.6516927756994,10.2243305140825,130.475201800012));
#60144=CARTESIAN_POINT('Ctrl Pts',(81.6921131545386,10.1656545949541,130.471342210756));
#60145=CARTESIAN_POINT('Ctrl Pts',(81.7325577712789,10.1069434910705,130.467480307115));
#60146=CARTESIAN_POINT('Ctrl Pts',(81.7699051651171,10.0461801991002,130.463618403473));
#60147=CARTESIAN_POINT('Ctrl Pts',(81.803960185088,9.98373025424512,130.459756499831));
#60148=CARTESIAN_POINT('Ctrl Pts',(81.8380736276579,9.9211731742867,130.455887970957));
#60149=CARTESIAN_POINT('Ctrl Pts',(81.8688832130284,9.85692410394344,130.452019442082));
#60150=CARTESIAN_POINT('Ctrl Pts',(81.896241347074,9.79136989843372,130.448150913207));
#60151=CARTESIAN_POINT('Ctrl Pts',(81.9094401496965,9.75974358144321,130.446284559713));
#60152=CARTESIAN_POINT('Ctrl Pts',(81.921836354179,9.72781373601789,130.44441820622));
#60153=CARTESIAN_POINT('Ctrl Pts',(81.9334175758377,9.69562492763128,130.442551852726));
#60154=CARTESIAN_POINT('Ctrl Pts',(81.9574262793351,9.62889521816968,130.438682768015));
#60155=CARTESIAN_POINT('Ctrl Pts',(81.9780233007368,9.56079040286018,130.434813683304));
#60156=CARTESIAN_POINT('Ctrl Pts',(81.9950528338149,9.49169274225609,130.430944598593));
#60157=CARTESIAN_POINT('Ctrl Pts',(82.0120569938088,9.4226980334326,130.42708127861));
#60158=CARTESIAN_POINT('Ctrl Pts',(82.025504101033,9.35271388348272,130.423217958626));
#60159=CARTESIAN_POINT('Ctrl Pts',(82.0352873460187,9.28214000360805,130.419354638642));
#60160=CARTESIAN_POINT('Ctrl Pts',(82.0450591152943,9.21164890663373,130.415495850318));
#60161=CARTESIAN_POINT('Ctrl Pts',(82.0511754926331,9.14056993263242,130.411637061995));
#60162=CARTESIAN_POINT('Ctrl Pts',(82.0535805762484,9.06931363037274,130.407778273671));
#60163=CARTESIAN_POINT('Ctrl Pts',(82.0559841448415,8.99810221423524,130.403921916095));
#60164=CARTESIAN_POINT('Ctrl Pts',(82.0546810415938,8.92671417581581,130.400065558518));
#60165=CARTESIAN_POINT('Ctrl Pts',(82.0496672687178,8.85556437403794,130.396209200941));
#60166=CARTESIAN_POINT('Ctrl Pts',(82.0446549769562,8.78443559056478,130.392353982568));
#60167=CARTESIAN_POINT('Ctrl Pts',(82.0359342258887,8.71354538833167,130.388498764195));
#60168=CARTESIAN_POINT('Ctrl Pts',(82.0235530649906,8.64330607565128,130.384643545822));
#60169=CARTESIAN_POINT('Ctrl Pts',(82.0111714200269,8.57306401682869,130.380788176721));
#60170=CARTESIAN_POINT('Ctrl Pts',(81.9951291676038,8.50347337610662,130.376932807621));
#60171=CARTESIAN_POINT('Ctrl Pts',(81.9755256196588,8.43493709326139,130.37307743852));
#60172=CARTESIAN_POINT('Ctrl Pts',(81.9559015522231,8.36632907189102,130.369218033915));
#60173=CARTESIAN_POINT('Ctrl Pts',(81.9327088818243,8.2987780794815,130.36535862931));
#60174=CARTESIAN_POINT('Ctrl Pts',(81.9060968015639,8.23267181364955,130.361499224705));
#60175=CARTESIAN_POINT('Ctrl Pts',(81.8794696533747,8.16652811803004,130.35763763488));
#60176=CARTESIAN_POINT('Ctrl Pts',(81.8494194458972,8.10183121818607,130.353776045056));
#60177=CARTESIAN_POINT('Ctrl Pts',(81.8161423944517,8.03894622128876,130.349914455231));
#60178=CARTESIAN_POINT('Ctrl Pts',(81.7828071238814,7.97595120534435,130.346046109448));
#60179=CARTESIAN_POINT('Ctrl Pts',(81.746233987383,7.91477483837574,130.342177763665));
#60180=CARTESIAN_POINT('Ctrl Pts',(81.7066633832417,7.85575454608636,130.338309417882));
#60181=CARTESIAN_POINT('Ctrl Pts',(81.6831676816,7.82071026994933,130.336012523499));
#60182=CARTESIAN_POINT('Ctrl Pts',(81.6586159997449,7.78642554225776,130.333715629117));
#60183=CARTESIAN_POINT('Ctrl Pts',(81.6330651749068,7.75296523825247,130.331418734734));
#60184=CARTESIAN_POINT('Ctrl Pts',(81.5900252788846,7.6966019695759,130.327549658255));
#60185=CARTESIAN_POINT('Ctrl Pts',(81.5439796920784,7.64235912550215,130.323680581776));
#60186=CARTESIAN_POINT('Ctrl Pts',(81.495165056335,7.59057493394831,130.319811505297));
#60187=CARTESIAN_POINT('Ctrl Pts',(81.4464231521381,7.53886789844155,130.315948193563));
#60188=CARTESIAN_POINT('Ctrl Pts',(81.3949207190144,7.48961259455697,130.312084881829));
#60189=CARTESIAN_POINT('Ctrl Pts',(81.3409356346372,7.44311555141037,130.308221570095));
#60190=CARTESIAN_POINT('Ctrl Pts',(81.2870138745101,7.39667304907682,130.304362790007));
#60191=CARTESIAN_POINT('Ctrl Pts',(81.2306156139143,7.35298269631473,130.300504009919));
#60192=CARTESIAN_POINT('Ctrl Pts',(81.1720554469248,7.3123141311743,130.296645229832));
#60193=CARTESIAN_POINT('Ctrl Pts',(81.1135321683292,7.27167118409694,130.292788880478));
#60194=CARTESIAN_POINT('Ctrl Pts',(81.052850083258,7.23404652458339,130.288932531125));
#60195=CARTESIAN_POINT('Ctrl Pts',(80.9903555586582,7.19966852220633,130.285076181771));
#60196=CARTESIAN_POINT('Ctrl Pts',(80.9278794951522,7.16530067520734,130.281220971596));
#60197=CARTESIAN_POINT('Ctrl Pts',(80.8635924804399,7.1341778153307,130.277365761421));
#60198=CARTESIAN_POINT('Ctrl Pts',(80.7978669680663,7.10648320214244,130.273510551246));
#60199=CARTESIAN_POINT('Ctrl Pts',(80.7321388853924,7.07878750591246,130.269655190307));
#60200=CARTESIAN_POINT('Ctrl Pts',(80.6649726418922,7.05452050914529,130.265799829368));
#60201=CARTESIAN_POINT('Ctrl Pts',(80.5967606240574,7.03381732281188,130.261944468429));
#60202=CARTESIAN_POINT('Ctrl Pts',(80.528477204978,7.01309246532262,130.258085071874));
#60203=CARTESIAN_POINT('Ctrl Pts',(80.4591462921572,6.99593900642655,130.254225675318));
#60204=CARTESIAN_POINT('Ctrl Pts',(80.389174521208,6.98244188323049,130.250366278762));
#60205=CARTESIAN_POINT('Ctrl Pts',(80.3191631307887,6.96893711768293,130.246504696936));
#60206=CARTESIAN_POINT('Ctrl Pts',(80.2485106412491,6.95909287621989,130.242643115109));
#60207=CARTESIAN_POINT('Ctrl Pts',(80.177630213097,6.95294233840492,130.238781533283));
#60208=CARTESIAN_POINT('Ctrl Pts',(80.1066257743388,6.9467810397644,130.234913195331));
#60209=CARTESIAN_POINT('Ctrl Pts',(80.0353930864115,6.94432636389211,130.231044857378));
#60210=CARTESIAN_POINT('Ctrl Pts',(79.9643460176259,6.9455593568952,130.227176519426));
#60211=CARTESIAN_POINT('Ctrl Pts',(79.9221592143221,6.94629149172054,130.224879551865));
#60212=CARTESIAN_POINT('Ctrl Pts',(79.8800377932647,6.94832283725827,130.222582584304));
#60213=CARTESIAN_POINT('Ctrl Pts',(79.8380670940032,6.95164082825901,130.220285616743));
#60214=CARTESIAN_POINT('Ctrl Pts',(79.7673702408721,6.95722976355429,130.216416527565));
#60215=CARTESIAN_POINT('Ctrl Pts',(79.6968246045509,6.96649397761275,130.212547438387));
#60216=CARTESIAN_POINT('Ctrl Pts',(79.6268426934916,6.97941810680701,130.208678349209));
#60217=CARTESIAN_POINT('Ctrl Pts',(79.5569650526557,6.9923229795703,130.204815024817));
#60218=CARTESIAN_POINT('Ctrl Pts',(79.4876499436599,7.0088768556617,130.200951700426));
#60219=CARTESIAN_POINT('Ctrl Pts',(79.4193056091046,7.02901253507726,130.197088376034));
#60220=CARTESIAN_POINT('Ctrl Pts',(79.3510414440278,7.04912459487707,130.193229583412));
#60221=CARTESIAN_POINT('Ctrl Pts',(79.2837462551835,7.07280997570245,130.189370790789));
#60222=CARTESIAN_POINT('Ctrl Pts',(79.217817205908,7.09995062192413,130.185511998166));
#60223=CARTESIAN_POINT('Ctrl Pts',(79.1519296881186,7.12707417110922,130.181655636359));
#60224=CARTESIAN_POINT('Ctrl Pts',(79.0874070506485,7.15764848282999,130.177799274552));
#60225=CARTESIAN_POINT('Ctrl Pts',(79.0246290187541,7.19150642482661,130.173942912745));
#60226=CARTESIAN_POINT('Ctrl Pts',(78.9618695332617,7.22535436423186,130.170087690217));
#60227=CARTESIAN_POINT('Ctrl Pts',(78.9008540574504,7.2624837775702,130.166232467688));
#60228=CARTESIAN_POINT('Ctrl Pts',(78.8419385670213,7.30268114959286,130.162377245159));
#60229=CARTESIAN_POINT('Ctrl Pts',(78.783020774407,7.3428800923705,130.158521871984));
#60230=CARTESIAN_POINT('Ctrl Pts',(78.726203530129,7.3861469562388,130.154666498808));
#60231=CARTESIAN_POINT('Ctrl Pts',(78.6718131699329,7.43222536474902,130.150811125632));
#60232=CARTESIAN_POINT('Ctrl Pts',(78.6173658802461,7.47835200276759,130.146951717101));
#60233=CARTESIAN_POINT('Ctrl Pts',(78.5653509168195,7.52729574525971,130.14309230857));
#60234=CARTESIAN_POINT('Ctrl Pts',(78.5160601911565,7.57876103127255,130.139232900039));
#60235=CARTESIAN_POINT('Ctrl Pts',(78.4667415577998,7.63025545618356,130.135371306367));
#60236=CARTESIAN_POINT('Ctrl Pts',(78.4201505501253,7.68427389861833,130.131509712695));
#60237=CARTESIAN_POINT('Ctrl Pts',(78.3765391354799,7.74048724346613,130.127648119023));
#60238=CARTESIAN_POINT('Ctrl Pts',(78.3328514233877,7.79679893262852,130.123779769557));
#60239=CARTESIAN_POINT('Ctrl Pts',(78.2921539891894,7.85531279183206,130.11991142009));
#60240=CARTESIAN_POINT('Ctrl Pts',(78.2546553851637,7.91567083504972,130.116043070624));
#60241=CARTESIAN_POINT('Ctrl Pts',(78.2323903486635,7.95150881009529,130.113746213333));
#60242=CARTESIAN_POINT('Ctrl Pts',(78.2112521766875,7.98799645884686,130.111449356042));
#60243=CARTESIAN_POINT('Ctrl Pts',(78.1912765943839,8.02505528132276,130.109152498751));
#60244=CARTESIAN_POINT('Ctrl Pts',(78.1558306636805,8.09081478877886,130.105076810587));
#60245=CARTESIAN_POINT('Ctrl Pts',(78.1239212018672,8.15860872697479,130.101001122422));
#60246=CARTESIAN_POINT('Ctrl Pts',(78.0957732939045,8.22804260849929,130.096925434258));
#60247=CARTESIAN_POINT('Ctrl Pts',(78.0677085507005,8.29727134326781,130.092861787969));
#60248=CARTESIAN_POINT('Ctrl Pts',(78.0433833815485,8.36812999422939,130.088798141681));
#60249=CARTESIAN_POINT('Ctrl Pts',(78.0229762169732,8.4402013541938,130.084734495393));
#60250=CARTESIAN_POINT('Ctrl Pts',(78.0026057685371,8.5121430448907,130.080678160331));
#60251=CARTESIAN_POINT('Ctrl Pts',(77.9861394179251,8.58529271403991,130.076621825269));
#60252=CARTESIAN_POINT('Ctrl Pts',(77.9737071027707,8.65921464653235,130.072565490207));
#60253=CARTESIAN_POINT('Ctrl Pts',(77.9613030306111,8.73296864757114,130.068518370086));
#60254=CARTESIAN_POINT('Ctrl Pts',(77.9529148138812,8.80749101628244,130.064471249965));
#60255=CARTESIAN_POINT('Ctrl Pts',(77.9486218581135,8.88233402577495,130.060424129845));
#60256=CARTESIAN_POINT('Ctrl Pts',(77.9463768265079,8.92147370735203,130.058307659731));
#60257=CARTESIAN_POINT('Ctrl Pts',(77.9452509482554,8.96070086656248,130.056191189617));
#60258=CARTESIAN_POINT('Ctrl Pts',(77.9452500005989,8.99995038927706,130.054074719503));
#60259=CARTESIAN_POINT('Origin',(80.,9.,141.545925280538));
#60260=CARTESIAN_POINT('',(81.252039109102,10.6292316077768,131.206019331793));
#60261=CARTESIAN_POINT('',(81.252039109102,10.6292316077768,131.147979658073));
#60262=CARTESIAN_POINT('',(81.252039109102,10.6292316077768,141.545925280538));
#60263=CARTESIAN_POINT('',(77.9452508472645,9.00186596700246,130.695925280507));
#60264=CARTESIAN_POINT('Ctrl Pts',(81.252039109102,10.6292316077768,131.147979658073));
#60265=CARTESIAN_POINT('Ctrl Pts',(81.3086037731427,10.5857625446712,131.144119415786));
#60266=CARTESIAN_POINT('Ctrl Pts',(81.3628640477792,10.5393734651264,131.1402591735));
#60267=CARTESIAN_POINT('Ctrl Pts',(81.4145173023013,10.4903484035588,131.136398931214));
#60268=CARTESIAN_POINT('Ctrl Pts',(81.4662067786891,10.4412889631469,131.132535981931));
#60269=CARTESIAN_POINT('Ctrl Pts',(81.5152852644682,10.3895902156041,131.128673032648));
#60270=CARTESIAN_POINT('Ctrl Pts',(81.5614888507507,10.3355710881422,131.124810083366));
#60271=CARTESIAN_POINT('Ctrl Pts',(81.6077671726066,10.2814645832537,131.120940885656));
#60272=CARTESIAN_POINT('Ctrl Pts',(81.65116102721,10.2250305980703,131.117071687946));
#60273=CARTESIAN_POINT('Ctrl Pts',(81.6914490135609,10.1666181024756,131.113202490237));
#60274=CARTESIAN_POINT('Ctrl Pts',(81.6972565748548,10.1581978715527,131.112644740771));
#60275=CARTESIAN_POINT('Ctrl Pts',(81.7029996753843,10.1497365699715,131.112086991305));
#60276=CARTESIAN_POINT('Ctrl Pts',(81.7086777314092,10.1412352836669,131.11152924184));
#60277=CARTESIAN_POINT('Ctrl Pts',(81.7480661499276,10.0822622440483,131.107660158956));
#60278=CARTESIAN_POINT('Ctrl Pts',(81.7844750515846,10.0211321362282,131.103791076072));
#60279=CARTESIAN_POINT('Ctrl Pts',(81.8176610664462,9.95817838110956,131.099921993188));
#60280=CARTESIAN_POINT('Ctrl Pts',(81.8507976357946,9.89531842395793,131.096058675046));
#60281=CARTESIAN_POINT('Ctrl Pts',(81.8807206253813,9.83064063919304,131.092195356903));
#60282=CARTESIAN_POINT('Ctrl Pts',(81.9072300095337,9.76450719632596,131.088332038761));
#60283=CARTESIAN_POINT('Ctrl Pts',(81.9337082981801,9.69845132798336,131.08447325229));
#60284=CARTESIAN_POINT('Ctrl Pts',(81.9567807551403,9.63094364190379,131.080614465819));
#60285=CARTESIAN_POINT('Ctrl Pts',(81.9762941479208,9.56236909889694,131.076755679349));
#60286=CARTESIAN_POINT('Ctrl Pts',(81.9957952486906,9.49383775283796,131.072899323631));
#60287=CARTESIAN_POINT('Ctrl Pts',(82.0117416006339,9.42424134930235,131.069042967914));
#60288=CARTESIAN_POINT('Ctrl Pts',(82.0240293050706,9.35398154572728,131.065186612197));
#60289=CARTESIAN_POINT('Ctrl Pts',(82.0363133795937,9.2837424976172,131.061331395686));
#60290=CARTESIAN_POINT('Ctrl Pts',(82.0449408686595,9.21284091679222,131.057476179176));
#60291=CARTESIAN_POINT('Ctrl Pts',(82.0498590005134,9.14168853346027,131.053620962666));
#60292=CARTESIAN_POINT('Ctrl Pts',(82.0547773246505,9.07053336829956,131.049765595429));
#60293=CARTESIAN_POINT('Ctrl Pts',(82.0559859723494,8.99912786594283,131.045910228192));
#60294=CARTESIAN_POINT('Ctrl Pts',(82.0534841808734,8.92788702333957,131.042054860955));
#60295=CARTESIAN_POINT('Ctrl Pts',(82.0509797707049,8.85657161103036,131.038195458202));
#60296=CARTESIAN_POINT('Ctrl Pts',(82.0447571854772,8.78542168900987,131.034336055448));
#60297=CARTESIAN_POINT('Ctrl Pts',(82.0348677469965,8.71484948758009,131.030476652695));
#60298=CARTESIAN_POINT('Ctrl Pts',(82.0249727090403,8.64423732763135,131.026615064718));
#60299=CARTESIAN_POINT('Ctrl Pts',(82.0114067771825,8.5742040165918,131.022753476741));
#60300=CARTESIAN_POINT('Ctrl Pts',(81.994272354764,8.50515119730975,131.018891888764));
#60301=CARTESIAN_POINT('Ctrl Pts',(81.9771079550668,8.43597756767561,131.015023544803));
#60302=CARTESIAN_POINT('Ctrl Pts',(81.9563627415185,8.36778831955185,131.011155200841));
#60303=CARTESIAN_POINT('Ctrl Pts',(81.9321886708897,8.30096888296347,131.007286856879));
#60304=CARTESIAN_POINT('Ctrl Pts',(81.9178348053741,8.26129342981564,131.004989945869));
#60305=CARTESIAN_POINT('Ctrl Pts',(81.902272970537,8.22210053979701,131.002693034859));
#60306=CARTESIAN_POINT('Ctrl Pts',(81.8855426871364,8.18346687912466,131.000396123848));
#60307=CARTESIAN_POINT('Ctrl Pts',(81.8573609872113,8.11838954564444,130.996527040743));
#60308=CARTESIAN_POINT('Ctrl Pts',(81.8257510312571,8.0546454517863,130.992657957638));
#60309=CARTESIAN_POINT('Ctrl Pts',(81.7908609381909,7.99261990164489,130.988788874533));
#60310=CARTESIAN_POINT('Ctrl Pts',(81.7560228296071,7.93068676645084,130.984925556166));
#60311=CARTESIAN_POINT('Ctrl Pts',(81.7179145211702,7.87046751231053,130.9810622378));
#60312=CARTESIAN_POINT('Ctrl Pts',(81.6767317935264,7.81232662104522,130.977198919434));
#60313=CARTESIAN_POINT('Ctrl Pts',(81.6355973731938,7.75425392900539,130.973340132738));
#60314=CARTESIAN_POINT('Ctrl Pts',(81.591395976397,7.69825515179778,130.969481346042));
#60315=CARTESIAN_POINT('Ctrl Pts',(81.5443679112032,7.6446678202943,130.965622559345));
#60316=CARTESIAN_POINT('Ctrl Pts',(81.4973694702354,7.59111424487264,130.961766203401));
#60317=CARTESIAN_POINT('Ctrl Pts',(81.4475482132096,7.53996946567178,130.957909847457));
#60318=CARTESIAN_POINT('Ctrl Pts',(81.3951852332696,7.49153862251418,130.954053491512));
#60319=CARTESIAN_POINT('Ctrl Pts',(81.3428377218772,7.44312208631166,130.950198274774));
#60320=CARTESIAN_POINT('Ctrl Pts',(81.2879503346523,7.39741822417739,130.946343058036));
#60321=CARTESIAN_POINT('Ctrl Pts',(81.2308403574428,7.3546946857832,130.942487841298));
#60322=CARTESIAN_POINT('Ctrl Pts',(81.1737281474099,7.31196947703082,130.938632473833));
#60323=CARTESIAN_POINT('Ctrl Pts',(81.1143935651727,7.27222511258728,130.934777106368));
#60324=CARTESIAN_POINT('Ctrl Pts',(81.0531848497429,7.23568731944361,130.930921738902));
#60325=CARTESIAN_POINT('Ctrl Pts',(80.991912065521,7.19911128121911,130.927062335922));
#60326=CARTESIAN_POINT('Ctrl Pts',(80.9287616500761,7.1657487639317,130.923202932941));
#60327=CARTESIAN_POINT('Ctrl Pts',(80.8641077676973,7.1357802360491,130.91934352996));
#60328=CARTESIAN_POINT('Ctrl Pts',(80.7994172778011,7.10579473975922,130.915481941755));
#60329=CARTESIAN_POINT('Ctrl Pts',(80.7332220773407,7.07920723953435,130.911620353551));
#60330=CARTESIAN_POINT('Ctrl Pts',(80.6659151413543,7.05614954612885,130.907758765347));
#60331=CARTESIAN_POINT('Ctrl Pts',(80.598490449554,7.03305151249074,130.903890421161));
#60332=CARTESIAN_POINT('Ctrl Pts',(80.5299506062292,7.01349574859718,130.900022076975));
#60333=CARTESIAN_POINT('Ctrl Pts',(80.4607018422944,6.99756364021062,130.896153732788));
#60334=CARTESIAN_POINT('Ctrl Pts',(80.4195839634618,6.98810362294875,130.893856823811));
#60335=CARTESIAN_POINT('Ctrl Pts',(80.3782163235637,6.97992019115943,130.891559914834));
#60336=CARTESIAN_POINT('Ctrl Pts',(80.3366847674717,6.97302172437578,130.889263005857));
#60337=CARTESIAN_POINT('Ctrl Pts',(80.2667259651543,6.96140144044177,130.885393923737));
#60338=CARTESIAN_POINT('Ctrl Pts',(80.1960278428692,6.95338446885016,130.881524841618));
#60339=CARTESIAN_POINT('Ctrl Pts',(80.1249944439213,6.94905535143223,130.877655759498));
#60340=CARTESIAN_POINT('Ctrl Pts',(80.0540668812148,6.94473268418453,130.873792442119));
#60341=CARTESIAN_POINT('Ctrl Pts',(79.9828055143632,6.94408699355418,130.86992912474));
#60342=CARTESIAN_POINT('Ctrl Pts',(79.9116227439901,6.94715148558883,130.866065807361));
#60343=CARTESIAN_POINT('Ctrl Pts',(79.8405234709305,6.9502123829776,130.862207021649));
#60344=CARTESIAN_POINT('Ctrl Pts',(79.7695030942002,6.95697479761317,130.858348235937));
#60345=CARTESIAN_POINT('Ctrl Pts',(79.6989755228482,6.96741990891982,130.854489450225));
#60346=CARTESIAN_POINT('Ctrl Pts',(79.6284923786564,6.97785844057792,130.850633095263));
#60347=CARTESIAN_POINT('Ctrl Pts',(79.5585019033587,6.99197499540708,130.846776740301));
#60348=CARTESIAN_POINT('Ctrl Pts',(79.4894129142435,7.00969891967103,130.842920385339));
#60349=CARTESIAN_POINT('Ctrl Pts',(79.4203443346471,7.02741760812577,130.83906516958));
#60350=CARTESIAN_POINT('Ctrl Pts',(79.3521771828293,7.04874142975738,130.83520995382));
#60351=CARTESIAN_POINT('Ctrl Pts',(79.2853084095778,7.07354899022068,130.831354738061));
#60352=CARTESIAN_POINT('Ctrl Pts',(79.2184370218765,7.09835752061536,130.827499371569));
#60353=CARTESIAN_POINT('Ctrl Pts',(79.152864568212,7.12664988923231,130.823644005078));
#60354=CARTESIAN_POINT('Ctrl Pts',(79.0889695671289,7.15825595891212,130.819788638586));
#60355=CARTESIAN_POINT('Ctrl Pts',(79.0250076851929,7.18989511163228,130.815929236565));
#60356=CARTESIAN_POINT('Ctrl Pts',(78.9627271972069,7.22485467359619,130.812069834543));
#60357=CARTESIAN_POINT('Ctrl Pts',(78.9024826598933,7.26291817962851,130.808210432521));
#60358=CARTESIAN_POINT('Ctrl Pts',(78.8422040115549,7.3010032375767,130.80434884527));
#60359=CARTESIAN_POINT('Ctrl Pts',(78.7839640055023,7.34219545755186,130.800487258018));
#60360=CARTESIAN_POINT('Ctrl Pts',(78.7280865220779,7.38623617986394,130.796625670767));
#60361=CARTESIAN_POINT('Ctrl Pts',(78.6721112787374,7.43035395320006,130.792757327513));
#60362=CARTESIAN_POINT('Ctrl Pts',(78.6185071757931,7.4773298584405,130.788888984258));
#60363=CARTESIAN_POINT('Ctrl Pts',(78.5675629196051,7.52686674967611,130.785020641004));
#60364=CARTESIAN_POINT('Ctrl Pts',(78.5373135966484,7.55628041734706,130.782723723291));
#60365=CARTESIAN_POINT('Ctrl Pts',(78.5080013169371,7.58659631930302,130.780426805578));
#60366=CARTESIAN_POINT('Ctrl Pts',(78.4796796815665,7.61774687851383,130.778129887865));
#60367=CARTESIAN_POINT('Ctrl Pts',(78.432491033337,7.66964899368187,130.774302833369));
#60368=CARTESIAN_POINT('Ctrl Pts',(78.3878608320637,7.72408325904773,130.770475778874));
#60369=CARTESIAN_POINT('Ctrl Pts',(78.3460767383815,7.78076441686718,130.766648724378));
#60370=CARTESIAN_POINT('Ctrl Pts',(78.3043498473889,7.83736797782163,130.762826909144));
#60371=CARTESIAN_POINT('Ctrl Pts',(78.2654616325524,7.89621193790445,130.759005093911));
#60372=CARTESIAN_POINT('Ctrl Pts',(78.2296616569897,7.95697568879366,130.755183278677));
#60373=CARTESIAN_POINT('Ctrl Pts',(78.1938980883631,8.01767764573017,130.751365350054));
#60374=CARTESIAN_POINT('Ctrl Pts',(78.1612167818413,8.08029509593303,130.747547421432));
#60375=CARTESIAN_POINT('Ctrl Pts',(78.131824742173,8.14447748799764,130.743729492809));
#60376=CARTESIAN_POINT('Ctrl Pts',(78.1011566443136,8.21144636470353,130.739745808453));
#60377=CARTESIAN_POINT('Ctrl Pts',(78.0740702736719,8.28011871133061,130.735762124097));
#60378=CARTESIAN_POINT('Ctrl Pts',(78.0507474289291,8.35006771377833,130.731778439741));
#60379=CARTESIAN_POINT('Ctrl Pts',(78.0284112294451,8.41705760671818,130.727963280423));
#60380=CARTESIAN_POINT('Ctrl Pts',(78.0095266831971,8.48521779437095,130.724148121104));
#60381=CARTESIAN_POINT('Ctrl Pts',(77.9942033860812,8.55415528926336,130.720332961786));
#60382=CARTESIAN_POINT('Ctrl Pts',(77.9788799282579,8.62309350715724,130.716517762455));
#60383=CARTESIAN_POINT('Ctrl Pts',(77.9671178912865,8.69280856095067,130.712702563123));
#60384=CARTESIAN_POINT('Ctrl Pts',(77.9589758110982,8.76289702064792,130.708887363792));
#60385=CARTESIAN_POINT('Ctrl Pts',(77.9508281238068,8.83303374727478,130.705069537096));
#60386=CARTESIAN_POINT('Ctrl Pts',(77.9463054071717,8.90354389752152,130.701251710401));
#60387=CARTESIAN_POINT('Ctrl Pts',(77.945414248457,8.97402016057328,130.697433883705));
#60388=CARTESIAN_POINT('Ctrl Pts',(77.9452968688616,8.98330299101405,130.696931015982));
#60389=CARTESIAN_POINT('Ctrl Pts',(77.9452424192121,8.99258523549095,130.69642814826));
#60390=CARTESIAN_POINT('Ctrl Pts',(77.945250847264,9.00186596643237,130.695925280538));
#60391=CARTESIAN_POINT('Ctrl Pts',(77.9452508472645,9.00186596700247,130.695925280507));
#60392=CARTESIAN_POINT('Ctrl Pts',(77.9453334654876,9.09284277613626,130.69099578723));
#60393=CARTESIAN_POINT('Ctrl Pts',(77.9514620741529,9.1835503686496,130.686066293953));
#60394=CARTESIAN_POINT('Ctrl Pts',(77.9635073127509,9.27330403817156,130.681136800675));
#60395=CARTESIAN_POINT('Ctrl Pts',(77.9750243886588,9.35912216593073,130.676423457075));
#60396=CARTESIAN_POINT('Ctrl Pts',(77.9919501516287,9.4440686242144,130.671710113474));
#60397=CARTESIAN_POINT('Ctrl Pts',(78.0141316039583,9.52756447577781,130.666996769874));
#60398=CARTESIAN_POINT('Ctrl Pts',(78.0323398920129,9.59610446558729,130.663127685167));
#60399=CARTESIAN_POINT('Ctrl Pts',(78.0541363781817,9.66383493390369,130.659258600461));
#60400=CARTESIAN_POINT('Ctrl Pts',(78.0794317853549,9.73035285677203,130.655389515754));
#60401=CARTESIAN_POINT('Ctrl Pts',(78.1046895037382,9.79677167152922,130.651526195775));
#60402=CARTESIAN_POINT('Ctrl Pts',(78.1334356237984,9.86198107658305,130.647662875795));
#60403=CARTESIAN_POINT('Ctrl Pts',(78.1655306436492,9.92559156387147,130.643799555816));
#60404=CARTESIAN_POINT('Ctrl Pts',(78.1975880161602,9.98912743629294,130.639940767497));
#60405=CARTESIAN_POINT('Ctrl Pts',(78.2329862678671,10.0510676847769,130.636081979177));
#60406=CARTESIAN_POINT('Ctrl Pts',(78.2715378618458,10.1110428432186,130.632223190858));
#60407=CARTESIAN_POINT('Ctrl Pts',(78.3100651712137,10.1709802218119,130.628366833286));
#60408=CARTESIAN_POINT('Ctrl Pts',(78.3517416198771,10.2289545585805,130.624510475713));
#60409=CARTESIAN_POINT('Ctrl Pts',(78.396334529133,10.2846223647629,130.620654118141));
#60410=CARTESIAN_POINT('Ctrl Pts',(78.4409142652341,10.3402737261642,130.616798899772));
#60411=CARTESIAN_POINT('Ctrl Pts',(78.4884084479691,10.3936195307578,130.612943681403));
#60412=CARTESIAN_POINT('Ctrl Pts',(78.5385430413457,10.444347991483,130.609088463034));
#60413=CARTESIAN_POINT('Ctrl Pts',(78.5886795948317,10.495078435536,130.605233093938));
#60414=CARTESIAN_POINT('Ctrl Pts',(78.6414564208742,10.5431909885896,130.601377724842));
#60415=CARTESIAN_POINT('Ctrl Pts',(78.6965626496331,10.5884107265341,130.597522355746));
#60416=CARTESIAN_POINT('Ctrl Pts',(78.7517265593669,10.6336777970331,130.593662951145));
#60417=CARTESIAN_POINT('Ctrl Pts',(78.8092243627905,10.6760456991132,130.589803546544));
#60418=CARTESIAN_POINT('Ctrl Pts',(78.8687128331584,10.7152804169113,130.585944141943));
#60419=CARTESIAN_POINT('Ctrl Pts',(78.9282349862763,10.7545373496561,130.582082552123));
#60420=CARTESIAN_POINT('Ctrl Pts',(78.9897496309988,10.7906573204859,130.578220962303));
#60421=CARTESIAN_POINT('Ctrl Pts',(79.0528877147299,10.8234516394987,130.574359372483));
#60422=CARTESIAN_POINT('Ctrl Pts',(79.116136260292,10.8563033330834,130.570491026704));
#60423=CARTESIAN_POINT('Ctrl Pts',(79.1810134731886,10.8858175571895,130.566622680925));
#60424=CARTESIAN_POINT('Ctrl Pts',(79.2471297059274,10.9118535202267,130.562754335146));
#60425=CARTESIAN_POINT('Ctrl Pts',(79.2863873149451,10.9273128048073,130.560457440725));
#60426=CARTESIAN_POINT('Ctrl Pts',(79.3260814287917,10.9415467438447,130.558160546303));
#60427=CARTESIAN_POINT('Ctrl Pts',(79.3661283994795,10.9545343068244,130.555863651882));
#60428=CARTESIAN_POINT('Ctrl Pts',(79.4335880972922,10.9764120433645,130.551994500211));
#60429=CARTESIAN_POINT('Ctrl Pts',(79.5023139049624,10.9948360288297,130.548125348539));
#60430=CARTESIAN_POINT('Ctrl Pts',(79.5719187855566,11.0096626673003,130.544256196868));
#60431=CARTESIAN_POINT('Ctrl Pts',(79.6441103183262,11.0250402923731,130.540243260027));
#60432=CARTESIAN_POINT('Ctrl Pts',(79.7172470800184,11.0365476894604,130.536230323185));
#60433=CARTESIAN_POINT('Ctrl Pts',(79.790877229805,11.044080534002,130.532217386344));
#60434=CARTESIAN_POINT('Ctrl Pts',(79.8616761606652,11.0513237263822,130.528358754536));
#60435=CARTESIAN_POINT('Ctrl Pts',(79.9329306946829,11.0548923739865,130.524500122729));
#60436=CARTESIAN_POINT('Ctrl Pts',(80.0042284951781,11.0547456490594,130.520641490921));
#60437=CARTESIAN_POINT('Ctrl Pts',(80.075481736293,11.0545990158318,130.516785270664));
#60438=CARTESIAN_POINT('Ctrl Pts',(80.1467777055784,11.0507416184974,130.512929050407));
#60439=CARTESIAN_POINT('Ctrl Pts',(80.2177016825888,11.0431846563387,130.509072830149));
#60440=CARTESIAN_POINT('Ctrl Pts',(80.2886050592828,11.0356298891474,130.505217729956));
#60441=CARTESIAN_POINT('Ctrl Pts',(80.3591361755064,11.0243777424631,130.501362629762));
#60442=CARTESIAN_POINT('Ctrl Pts',(80.4288847878984,11.0094913289709,130.497507529568));
#60443=CARTESIAN_POINT('Ctrl Pts',(80.498636472752,10.9946042597248,130.493652259555));
#60444=CARTESIAN_POINT('Ctrl Pts',(80.567605110909,10.9760827099337,130.489796989542));
#60445=CARTESIAN_POINT('Ctrl Pts',(80.6353917190606,10.9540406663755,130.485941719529));
#60446=CARTESIAN_POINT('Ctrl Pts',(80.7032436169625,10.9319773926723,130.482082736252));
#60447=CARTESIAN_POINT('Ctrl Pts',(80.7699107506148,10.906387010034,130.478223752974));
#60448=CARTESIAN_POINT('Ctrl Pts',(80.8350113136356,10.8774327334423,130.474364769697));
#60449=CARTESIAN_POINT('Ctrl Pts',(80.9001492852494,10.8484618189184,130.47050356894));
#60450=CARTESIAN_POINT('Ctrl Pts',(80.9637184615834,10.8161233831014,130.466642368184));
#60451=CARTESIAN_POINT('Ctrl Pts',(81.0253613348939,10.780626770383,130.462781167427));
#60452=CARTESIAN_POINT('Ctrl Pts',(81.0870986717551,10.7450757614968,130.45891404964));
#60453=CARTESIAN_POINT('Ctrl Pts',(81.1469034091337,10.7063571836609,130.455046931854));
#60454=CARTESIAN_POINT('Ctrl Pts',(81.2044475334767,10.6647233108244,130.451179814067));
#60455=CARTESIAN_POINT('Ctrl Pts',(81.2204890699024,10.6531170643956,130.450101780271));
#60456=CARTESIAN_POINT('Ctrl Pts',(81.2363551335118,10.6412844986803,130.449023746474));
#60457=CARTESIAN_POINT('Ctrl Pts',(81.252039109102,10.6292316077768,130.447945712677));
#60458=CARTESIAN_POINT('',(77.9452507933687,8.99819435662442,130.754074719418));
#60459=CARTESIAN_POINT('Ctrl Pts',(77.9452507933687,8.99819435662443,130.754074719418));
#60460=CARTESIAN_POINT('Ctrl Pts',(77.9451892124666,9.06827093509326,130.750269075961));
#60461=CARTESIAN_POINT('Ctrl Pts',(77.9487167666399,9.13846487636557,130.746463432503));
#60462=CARTESIAN_POINT('Ctrl Pts',(77.955842851978,9.20837254303459,130.742657789045));
#60463=CARTESIAN_POINT('Ctrl Pts',(77.9629627689955,9.27821969781131,130.738855439743));
#60464=CARTESIAN_POINT('Ctrl Pts',(77.9736749941454,9.34778057278129,130.73505309044));
#60465=CARTESIAN_POINT('Ctrl Pts',(77.9879368904968,9.41665286015621,130.731250741137));
#60466=CARTESIAN_POINT('Ctrl Pts',(78.0021915378848,9.48549014147856,130.727450324473));
#60467=CARTESIAN_POINT('Ctrl Pts',(78.019992177926,9.55363903911737,130.723649907809));
#60468=CARTESIAN_POINT('Ctrl Pts',(78.0412447589067,9.62070562103915,130.719849491145));
#60469=CARTESIAN_POINT('Ctrl Pts',(78.0624941303669,9.6877620747055,130.716049648412));
#60470=CARTESIAN_POINT('Ctrl Pts',(78.0871942556541,9.75373605967473,130.712249805679));
#60471=CARTESIAN_POINT('Ctrl Pts',(78.1152012631751,9.81824891332844,130.708449962946));
#60472=CARTESIAN_POINT('Ctrl Pts',(78.1432332471189,9.88281929902329,130.704646731543));
#60473=CARTESIAN_POINT('Ctrl Pts',(78.17457780405,9.94592548974653,130.700843500141));
#60474=CARTESIAN_POINT('Ctrl Pts',(78.2090433737487,10.0072099708535,130.697040268739));
#60475=CARTESIAN_POINT('Ctrl Pts',(78.2435240046636,10.0685212328558,130.693235375351));
#60476=CARTESIAN_POINT('Ctrl Pts',(78.2811280946731,10.12800877667,130.689430481963));
#60477=CARTESIAN_POINT('Ctrl Pts',(78.3216202127085,10.1853433477737,130.685625588575));
#60478=CARTESIAN_POINT('Ctrl Pts',(78.3621848365102,10.2427805829813,130.68181388209));
#60479=CARTESIAN_POINT('Ctrl Pts',(78.4056475047835,10.2980567525532,130.678002175606));
#60480=CARTESIAN_POINT('Ctrl Pts',(78.4517323843278,10.3508756244602,130.674190469121));
#60481=CARTESIAN_POINT('Ctrl Pts',(78.4895041823488,10.3941666947873,130.671066342317));
#60482=CARTESIAN_POINT('Ctrl Pts',(78.5290366712771,10.4358076062443,130.667942215513));
#60483=CARTESIAN_POINT('Ctrl Pts',(78.5701610020028,10.4756551095383,130.664818088709));
#60484=CARTESIAN_POINT('Ctrl Pts',(78.621091525187,10.5250043428154,130.660949006591));
#60485=CARTESIAN_POINT('Ctrl Pts',(78.6746796484828,10.5718104253932,130.657079924472));
#60486=CARTESIAN_POINT('Ctrl Pts',(78.730641139085,10.6157740079344,130.653210842354));
#60487=CARTESIAN_POINT('Ctrl Pts',(78.7865192498416,10.6596720869182,130.649347524977));
#60488=CARTESIAN_POINT('Ctrl Pts',(78.8447633297575,10.7007357749319,130.645484207599));
#60489=CARTESIAN_POINT('Ctrl Pts',(78.9050530730826,10.7387031919606,130.641620890221));
#60490=CARTESIAN_POINT('Ctrl Pts',(78.9652720966034,10.77662607325,130.637762104511));
#60491=CARTESIAN_POINT('Ctrl Pts',(79.0275316081242,10.8114596401715,130.6339033188));
#60492=CARTESIAN_POINT('Ctrl Pts',(79.0914804691145,10.8429839458063,130.63004453309));
#60493=CARTESIAN_POINT('Ctrl Pts',(79.1553890470463,10.8744883934572,130.626188178129));
#60494=CARTESIAN_POINT('Ctrl Pts',(79.2209844284724,10.9026875013314,130.622331823169));
#60495=CARTESIAN_POINT('Ctrl Pts',(79.2878901806696,10.9274068505931,130.618475468208));
#60496=CARTESIAN_POINT('Ctrl Pts',(79.3547761682962,10.9521188975332,130.61462025245));
#60497=CARTESIAN_POINT('Ctrl Pts',(79.4229713027732,10.9733530583668,130.610765036692));
#60498=CARTESIAN_POINT('Ctrl Pts',(79.4920800507304,10.9909833971266,130.606909820934));
#60499=CARTESIAN_POINT('Ctrl Pts',(79.5611915007165,11.0086144252013,130.603054454444));
#60500=CARTESIAN_POINT('Ctrl Pts',(79.6312161638495,11.02264123351,130.599199087954));
#60501=CARTESIAN_POINT('Ctrl Pts',(79.7017459426531,11.0329884603155,130.595343721464));
#60502=CARTESIAN_POINT('Ctrl Pts',(79.7723495471349,11.0433465178801,130.591484319443));
#60503=CARTESIAN_POINT('Ctrl Pts',(79.8434588411079,11.0500172347658,130.587624917423));
#60504=CARTESIAN_POINT('Ctrl Pts',(79.9146590844894,11.0529769824915,130.583765515403));
#60505=CARTESIAN_POINT('Ctrl Pts',(79.98589964212,11.0559384060542,130.579903928153));
#60506=CARTESIAN_POINT('Ctrl Pts',(80.0572307656864,11.0551846827794,130.576042340903));
#60507=CARTESIAN_POINT('Ctrl Pts',(80.1282389462027,11.0507443368633,130.572180753653));
#60508=CARTESIAN_POINT('Ctrl Pts',(80.1993713584019,11.0462962223825,130.5683124104));
#60509=CARTESIAN_POINT('Ctrl Pts',(80.2701792167571,11.0381486634102,130.564444067147));
#60510=CARTESIAN_POINT('Ctrl Pts',(80.34025605182,11.0263818449887,130.560575723893));
#60511=CARTESIAN_POINT('Ctrl Pts',(80.3818657834461,11.0193950260753,130.558278806168));
#60512=CARTESIAN_POINT('Ctrl Pts',(80.4232179920287,11.0111331547442,130.555981888443));
#60513=CARTESIAN_POINT('Ctrl Pts',(80.4642301545072,11.0016213243634,130.553684970717));
#60514=CARTESIAN_POINT('Ctrl Pts',(80.5351039376409,10.9851837760149,130.549715629943));
#60515=CARTESIAN_POINT('Ctrl Pts',(80.6052460381132,10.9649442735024,130.54574628917));
#60516=CARTESIAN_POINT('Ctrl Pts',(80.6742185437271,10.9409860684185,130.541776948396));
#60517=CARTESIAN_POINT('Ctrl Pts',(80.7413369799038,10.9176718906237,130.537914308594));
#60518=CARTESIAN_POINT('Ctrl Pts',(80.8073474054342,10.8908365645804,130.534051668793));
#60519=CARTESIAN_POINT('Ctrl Pts',(80.8718566420438,10.860608383896,130.530189028991));
#60520=CARTESIAN_POINT('Ctrl Pts',(80.9390388686133,10.829127675237,130.526166337731));
#60521=CARTESIAN_POINT('Ctrl Pts',(81.0045922542099,10.793966910179,130.522143646471));
#60522=CARTESIAN_POINT('Ctrl Pts',(81.0680928093577,10.7553276939359,130.518120955211));
#60523=CARTESIAN_POINT('Ctrl Pts',(81.1315933645054,10.7166884776928,130.514098263951));
#60524=CARTESIAN_POINT('Ctrl Pts',(81.1930405534724,10.6745710786514,130.510075572691));
#60525=CARTESIAN_POINT('Ctrl Pts',(81.252039109102,10.6292316077768,130.506052881431));
#60526=CARTESIAN_POINT('Ctrl Pts',(81.252039109102,10.6292316077768,131.206019331793));
#60527=CARTESIAN_POINT('Ctrl Pts',(81.3108254747807,10.5840552015738,131.201991466329));
#60528=CARTESIAN_POINT('Ctrl Pts',(81.3672518669379,10.5356251954291,131.197963600866));
#60529=CARTESIAN_POINT('Ctrl Pts',(81.4209427311286,10.4842234728479,131.193935735403));
#60530=CARTESIAN_POINT('Ctrl Pts',(81.4723686485046,10.4349901297404,131.190077785272));
#60531=CARTESIAN_POINT('Ctrl Pts',(81.52128479453,10.3830311202787,131.186219835142));
#60532=CARTESIAN_POINT('Ctrl Pts',(81.5673942489599,10.3286357028274,131.182361885011));
#60533=CARTESIAN_POINT('Ctrl Pts',(81.613479121098,10.2742692851558,131.178505991666));
#60534=CARTESIAN_POINT('Ctrl Pts',(81.6567599571315,10.217469406789,131.174650098321));
#60535=CARTESIAN_POINT('Ctrl Pts',(81.6969781573811,10.1585606138099,131.170794204976));
#60536=CARTESIAN_POINT('Ctrl Pts',(81.7371883696808,10.0996635210183,131.16693907747));
#60537=CARTESIAN_POINT('Ctrl Pts',(81.7743368805687,10.0386587466771,131.163083949965));
#60538=CARTESIAN_POINT('Ctrl Pts',(81.8082077324642,9.97590079350147,131.159228822459));
#60539=CARTESIAN_POINT('Ctrl Pts',(81.8420831870339,9.91313431221403,131.155373171084));
#60540=CARTESIAN_POINT('Ctrl Pts',(81.8726798700234,9.84861460785023,131.151517519709));
#60541=CARTESIAN_POINT('Ctrl Pts',(81.8998280279057,9.78272027371457,131.147661868334));
#60542=CARTESIAN_POINT('Ctrl Pts',(81.9270062096907,9.71675306520279,131.143801952888));
#60543=CARTESIAN_POINT('Ctrl Pts',(81.9507280723322,9.64940864383426,131.139942037441));
#60544=CARTESIAN_POINT('Ctrl Pts',(81.9708725883272,9.58108416178778,131.136082121994));
#60545=CARTESIAN_POINT('Ctrl Pts',(81.9910302587801,9.51271506355261,131.132219686005));
#60546=CARTESIAN_POINT('Ctrl Pts',(82.0076058219315,9.44336510344808,131.128357250016));
#60547=CARTESIAN_POINT('Ctrl Pts',(82.02052920906,9.37344246924429,131.124494814027));
#60548=CARTESIAN_POINT('Ctrl Pts',(82.0334740888014,9.30340354818092,131.120625954503));
#60549=CARTESIAN_POINT('Ctrl Pts',(82.0427546122951,9.23279053365593,131.116757094978));
#60550=CARTESIAN_POINT('Ctrl Pts',(82.0483525477548,9.16201667385336,131.112888235454));
#60551=CARTESIAN_POINT('Ctrl Pts',(82.0500587934809,9.14044486462523,131.111709010527));
#60552=CARTESIAN_POINT('Ctrl Pts',(82.0514232841471,9.11885810558639,131.110529785601));
#60553=CARTESIAN_POINT('Ctrl Pts',(82.0524464644487,9.09726804753776,131.109350560675));
#60554=CARTESIAN_POINT('Ctrl Pts',(82.0558035588435,9.02643022673454,131.105481477794));
#60555=CARTESIAN_POINT('Ctrl Pts',(82.055495594845,8.95527965835121,131.101612394913));
#60556=CARTESIAN_POINT('Ctrl Pts',(82.0514858739565,8.88422750129229,131.097743312031));
#60557=CARTESIAN_POINT('Ctrl Pts',(82.0474821273519,8.81328120840016,131.09387999389));
#60558=CARTESIAN_POINT('Ctrl Pts',(82.0397875989872,8.74243351684024,131.090016675749));
#60559=CARTESIAN_POINT('Ctrl Pts',(82.0284175513193,8.67209788045864,131.086153357608));
#60560=CARTESIAN_POINT('Ctrl Pts',(82.0170608407127,8.60184474774972,131.082294571138));
#60561=CARTESIAN_POINT('Ctrl Pts',(82.002037251815,8.53210295437389,131.078435784668));
#60562=CARTESIAN_POINT('Ctrl Pts',(81.9834138929847,8.46328136643552,131.074576998197));
#60563=CARTESIAN_POINT('Ctrl Pts',(81.9648022655047,8.39450313105044,131.070720642479));
#60564=CARTESIAN_POINT('Ctrl Pts',(81.9425954935482,8.32664441887198,131.066864286761));
#60565=CARTESIAN_POINT('Ctrl Pts',(81.9169115671849,8.26010297602124,131.063007931044));
#60566=CARTESIAN_POINT('Ctrl Pts',(81.8912352281108,8.19358119017946,131.059152714532));
#60567=CARTESIAN_POINT('Ctrl Pts',(81.8620839487106,8.1283763540738,131.05529749802));
#60568=CARTESIAN_POINT('Ctrl Pts',(81.8296247232406,8.06486849341557,131.051442281508));
#60569=CARTESIAN_POINT('Ctrl Pts',(81.7971642287126,8.00135814979139,131.047586914269));
#60570=CARTESIAN_POINT('Ctrl Pts',(81.7613957543905,7.93954534489364,131.04373154703));
#60571=CARTESIAN_POINT('Ctrl Pts',(81.7225325466121,7.87978609705021,131.039876179791));
#60572=CARTESIAN_POINT('Ctrl Pts',(81.6836286596568,7.81996429757617,131.036016777034));
#60573=CARTESIAN_POINT('Ctrl Pts',(81.6416238381762,7.76220075414289,131.032157374277));
#60574=CARTESIAN_POINT('Ctrl Pts',(81.5967745355487,7.7068222685481,131.02829797152));
#60575=CARTESIAN_POINT('Ctrl Pts',(81.5518998388958,7.65141242722229,131.024436383539));
#60576=CARTESIAN_POINT('Ctrl Pts',(81.5041777800879,7.5983906932835,131.020574795558));
#60577=CARTESIAN_POINT('Ctrl Pts',(81.453903128989,7.54804846705679,131.016713207578));
#60578=CARTESIAN_POINT('Ctrl Pts',(81.4035405205947,7.4976181653097,131.012844863611));
#60579=CARTESIAN_POINT('Ctrl Pts',(81.3506167645328,7.44987705627581,131.008976519644));
#60580=CARTESIAN_POINT('Ctrl Pts',(81.2954607382095,7.40507710585823,131.005108175677));
#60581=CARTESIAN_POINT('Ctrl Pts',(81.2627106817143,7.37847618833455,131.002811264679));
#60582=CARTESIAN_POINT('Ctrl Pts',(81.22917419994,7.35291141379814,131.000514353682));
#60583=CARTESIAN_POINT('Ctrl Pts',(81.1949246752979,7.32842811017166,130.998217442684));
#60584=CARTESIAN_POINT('Ctrl Pts',(81.1372323025217,7.28718666538178,130.994348359918));
#60585=CARTESIAN_POINT('Ctrl Pts',(81.0772893247036,7.24885472904751,130.990479277153));
#60586=CARTESIAN_POINT('Ctrl Pts',(81.0154212654727,7.21368613728555,130.986610194388));
#60587=CARTESIAN_POINT('Ctrl Pts',(80.9536453865656,7.17856994497192,130.982746876363));
#60588=CARTESIAN_POINT('Ctrl Pts',(80.8899505385721,7.14660797971772,130.978883558338));
#60589=CARTESIAN_POINT('Ctrl Pts',(80.8246923557782,7.11801166825588,130.975020240312));
#60590=CARTESIAN_POINT('Ctrl Pts',(80.7595107208011,7.08944890025352,130.971161453958));
#60591=CARTESIAN_POINT('Ctrl Pts',(80.6927698363328,7.06424413818421,130.967302667603));
#60592=CARTESIAN_POINT('Ctrl Pts',(80.6248496025437,7.04256276302381,130.963443881248));
#60593=CARTESIAN_POINT('Ctrl Pts',(80.5569721535164,7.02089504553831,130.959587525645));
#60594=CARTESIAN_POINT('Ctrl Pts',(80.4879172907597,7.00274645893529,130.955731170043));
#60595=CARTESIAN_POINT('Ctrl Pts',(80.4180831694177,6.98823360552234,130.95187481444));
#60596=CARTESIAN_POINT('Ctrl Pts',(80.3482696777666,6.97372503934997,130.948019598043));
#60597=CARTESIAN_POINT('Ctrl Pts',(80.2776778599043,6.96285017290605,130.944164381646));
#60598=CARTESIAN_POINT('Ctrl Pts',(80.2067175623795,6.95567482725867,130.940309165249));
#60599=CARTESIAN_POINT('Ctrl Pts',(80.1357544905088,6.94849920107567,130.936453798124));
#60600=CARTESIAN_POINT('Ctrl Pts',(80.0644233939133,6.94502342953479,130.932598430999));
#60601=CARTESIAN_POINT('Ctrl Pts',(79.9931390359637,6.94526145466814,130.928743063873));
#60602=CARTESIAN_POINT('Ctrl Pts',(79.9217800627019,6.94549972894899,130.924883661229));
#60603=CARTESIAN_POINT('Ctrl Pts',(79.8504684125221,6.94945955826817,130.921024258584));
#60604=CARTESIAN_POINT('Ctrl Pts',(79.7796177376698,6.95710273852301,130.91716485594));
#60605=CARTESIAN_POINT('Ctrl Pts',(79.7087269465955,6.96475024640798,130.91330326807));
#60606=CARTESIAN_POINT('Ctrl Pts',(79.6382981302733,6.97608517967534,130.909441680201));
#60607=CARTESIAN_POINT('Ctrl Pts',(79.5687359811075,6.99101794221335,130.905580092331));
#60608=CARTESIAN_POINT('Ctrl Pts',(79.4990521304315,7.00597683016258,130.901711748473));
#60609=CARTESIAN_POINT('Ctrl Pts',(79.4302384433347,7.02454598799566,130.897843404615));
#60610=CARTESIAN_POINT('Ctrl Pts',(79.3626849813179,7.04658577627215,130.893975060758));
#60611=CARTESIAN_POINT('Ctrl Pts',(79.3225736663156,7.05967237263228,130.891678148736));
#60612=CARTESIAN_POINT('Ctrl Pts',(79.2829063081009,7.07398165553897,130.889381236714));
#60613=CARTESIAN_POINT('Ctrl Pts',(79.2437607894417,7.08947655892053,130.887084324692));
#60614=CARTESIAN_POINT('Ctrl Pts',(79.177821278139,7.11557728236622,130.883215241808));
#60615=CARTESIAN_POINT('Ctrl Pts',(79.1131054573439,7.14514687385421,130.879346158925));
#60616=CARTESIAN_POINT('Ctrl Pts',(79.0500031408005,7.17804952591704,130.875477076041));
#60617=CARTESIAN_POINT('Ctrl Pts',(78.9869948435733,7.21090315466317,130.871613757898));
#60618=CARTESIAN_POINT('Ctrl Pts',(78.9255957058782,7.24707976365544,130.867750439756));
#60619=CARTESIAN_POINT('Ctrl Pts',(78.8661762433599,7.28639524645307,130.863887121613));
#60620=CARTESIAN_POINT('Ctrl Pts',(78.8068264798676,7.32566461219179,130.860028335142));
#60621=CARTESIAN_POINT('Ctrl Pts',(78.7494521821217,7.36806527148104,130.856169548672));
#60622=CARTESIAN_POINT('Ctrl Pts',(78.694398342541,7.41336775699586,130.852310762201));
#60623=CARTESIAN_POINT('Ctrl Pts',(78.6393791828537,7.45864170525735,130.848454406484));
#60624=CARTESIAN_POINT('Ctrl Pts',(78.5866779555281,7.50681354520323,130.844598050767));
#60625=CARTESIAN_POINT('Ctrl Pts',(78.5366085735487,7.55761201631153,130.840741695049));
#60626=CARTESIAN_POINT('Ctrl Pts',(78.4865539825771,7.60839548103162,130.836886478539));
#60627=CARTESIAN_POINT('Ctrl Pts',(78.4391300342729,7.66180369068438,130.833031262028));
#60628=CARTESIAN_POINT('Ctrl Pts',(78.3946143198094,7.71752801966709,130.829176045518));
#60629=CARTESIAN_POINT('Ctrl Pts',(78.350096864925,7.77325452729132,130.825320678281));
#60630=CARTESIAN_POINT('Ctrl Pts',(78.3084881711032,7.8312969531067,130.821465311044));
#60631=CARTESIAN_POINT('Ctrl Pts',(78.270024911011,7.89131440255697,130.817609943807));
#60632=CARTESIAN_POINT('Ctrl Pts',(78.2315213903901,7.95139467388565,130.813750541054));
#60633=CARTESIAN_POINT('Ctrl Pts',(78.1961701385391,8.01345368582609,130.8098911383));
#60634=CARTESIAN_POINT('Ctrl Pts',(78.1641634157805,8.07712319427703,130.806031735547));
#60635=CARTESIAN_POINT('Ctrl Pts',(78.1321385705713,8.14082875288952,130.80217014757));
#60636=CARTESIAN_POINT('Ctrl Pts',(78.1034622195977,8.20614617826129,130.798308559593));
#60637=CARTESIAN_POINT('Ctrl Pts',(78.0782785874146,8.27268687973425,130.794446971617));
#60638=CARTESIAN_POINT('Ctrl Pts',(78.0530508955754,8.3393439965202,130.790578627655));
#60639=CARTESIAN_POINT('Ctrl Pts',(78.0313282706822,8.40722819948842,130.786710283693));
#60640=CARTESIAN_POINT('Ctrl Pts',(78.0132049587206,8.47593604736861,130.782841939732));
#60641=CARTESIAN_POINT('Ctrl Pts',(78.002443859087,8.51673278464356,130.780545028721));
#60642=CARTESIAN_POINT('Ctrl Pts',(77.9929507711793,8.55781969999827,130.778248117711));
#60643=CARTESIAN_POINT('Ctrl Pts',(77.9847367966347,8.5991112577513,130.775951206701));
#60644=CARTESIAN_POINT('Ctrl Pts',(77.9647646110808,8.69951121014636,130.770366293739));
#60645=CARTESIAN_POINT('Ctrl Pts',(77.9522903129537,8.80144853340686,130.764781380778));
#60646=CARTESIAN_POINT('Ctrl Pts',(77.9474937711074,8.90400133929624,130.759196467816));
#60647=CARTESIAN_POINT('Ctrl Pts',(77.9460275184564,8.93535065893526,130.757489218365));
#60648=CARTESIAN_POINT('Ctrl Pts',(77.945278419186,8.96675730674471,130.755781968913));
#60649=CARTESIAN_POINT('Ctrl Pts',(77.9452507933694,8.99819435581925,130.754074719462));
#60650=CARTESIAN_POINT('Origin',(80.,9.,141.545925280538));
#60651=CARTESIAN_POINT('',(81.252039109102,10.6292316077769,131.906140964271));
#60652=CARTESIAN_POINT('',(81.252039109102,10.6292316077768,131.847886939688));
#60653=CARTESIAN_POINT('',(81.252039109102,10.6292316077768,141.545925280538));
#60654=CARTESIAN_POINT('',(77.9452501035681,8.99934760960447,131.39592528057));
#60655=CARTESIAN_POINT('Ctrl Pts',(81.252039109102,10.6292316077768,131.847886939688));
#60656=CARTESIAN_POINT('Ctrl Pts',(81.3085634809923,10.585793508561,131.844031409931));
#60657=CARTESIAN_POINT('Ctrl Pts',(81.3628520463242,10.5393893355674,131.840175880174));
#60658=CARTESIAN_POINT('Ctrl Pts',(81.4145852345703,10.4902839248397,131.836320350417));
#60659=CARTESIAN_POINT('Ctrl Pts',(81.4663133117732,10.4411833655407,131.832465201571));
#60660=CARTESIAN_POINT('Ctrl Pts',(81.5154861617407,10.3893824337431,131.828610052726));
#60661=CARTESIAN_POINT('Ctrl Pts',(81.5618198975157,10.3351839462127,131.82475490388));
#60662=CARTESIAN_POINT('Ctrl Pts',(81.6083190581177,10.2807919544186,131.82088599104));
#60663=CARTESIAN_POINT('Ctrl Pts',(81.65195846601,10.2239856221613,131.817017078199));
#60664=CARTESIAN_POINT('Ctrl Pts',(81.6924922182366,10.1651041385681,131.813148165358));
#60665=CARTESIAN_POINT('Ctrl Pts',(81.7329383898611,10.106349879214,131.809287612012));
#60666=CARTESIAN_POINT('Ctrl Pts',(81.7702920860257,10.0455298612198,131.805427058667));
#60667=CARTESIAN_POINT('Ctrl Pts',(81.8043538914048,9.98300793337198,131.801566505321));
#60668=CARTESIAN_POINT('Ctrl Pts',(81.8385263309912,9.92028293161642,131.797693412732));
#60669=CARTESIAN_POINT('Ctrl Pts',(81.8693852587684,9.85584539410209,131.793820320144));
#60670=CARTESIAN_POINT('Ctrl Pts',(81.8967778289509,9.79008317922887,131.789947227555));
#60671=CARTESIAN_POINT('Ctrl Pts',(81.9241703991334,9.72432096435564,131.786074134966));
#60672=CARTESIAN_POINT('Ctrl Pts',(81.9480965075822,9.65723455181734,131.782201042378));
#60673=CARTESIAN_POINT('Ctrl Pts',(81.9684540117227,9.58922522538739,131.778327949789));
#60674=CARTESIAN_POINT('Ctrl Pts',(81.9887904401114,9.52128630776972,131.774458866942));
#60675=CARTESIAN_POINT('Ctrl Pts',(82.0056453207932,9.45216025530351,131.770589784096));
#60676=CARTESIAN_POINT('Ctrl Pts',(82.0188839110768,9.38223725105644,131.766720701249));
#60677=CARTESIAN_POINT('Ctrl Pts',(82.0321027765212,9.31241842859865,131.762857383143));
#60678=CARTESIAN_POINT('Ctrl Pts',(82.0417159571495,9.24180548476804,131.758994065037));
#60679=CARTESIAN_POINT('Ctrl Pts',(82.0476385852172,9.17080335719701,131.75513074693));
#60680=CARTESIAN_POINT('Ctrl Pts',(82.0535542660444,9.0998845150946,131.751271960495));
#60681=CARTESIAN_POINT('Ctrl Pts',(82.0557879530187,9.02857787779235,131.747413174059));
#60682=CARTESIAN_POINT('Ctrl Pts',(82.0543062010364,8.9572964300878,131.743554387624));
#60683=CARTESIAN_POINT('Ctrl Pts',(82.0528253824493,8.88605988446865,131.739698031941));
#60684=CARTESIAN_POINT('Ctrl Pts',(82.0476337784021,8.81484898149624,131.735841676258));
#60685=CARTESIAN_POINT('Ctrl Pts',(82.0387500055476,8.74407818111861,131.731985320575));
#60686=CARTESIAN_POINT('Ctrl Pts',(82.0298688570486,8.67332828714428,131.728130104098));
#60687=CARTESIAN_POINT('Ctrl Pts',(82.0172977655639,8.60301871939521,131.724274887621));
#60688=CARTESIAN_POINT('Ctrl Pts',(82.0011071786636,8.53355855458501,131.720419671144));
#60689=CARTESIAN_POINT('Ctrl Pts',(81.9849159587599,8.46409567409016,131.71656430394));
#60690=CARTESIAN_POINT('Ctrl Pts',(81.9651050749096,8.3954827350673,131.712708936735));
#60691=CARTESIAN_POINT('Ctrl Pts',(81.9417956504084,8.32811666596407,131.708853569531));
#60692=CARTESIAN_POINT('Ctrl Pts',(81.918461827296,8.26068008295663,131.704994166808));
#60693=CARTESIAN_POINT('Ctrl Pts',(81.8916223124959,8.19449343522535,131.701134764086));
#60694=CARTESIAN_POINT('Ctrl Pts',(81.8614472056873,8.1299357133298,131.697275361363));
#60695=CARTESIAN_POINT('Ctrl Pts',(81.8312550134963,8.06534143834507,131.693413773417));
#60696=CARTESIAN_POINT('Ctrl Pts',(81.7977236980523,8.00237835420563,131.68955218547));
#60697=CARTESIAN_POINT('Ctrl Pts',(81.7610690802565,7.94140033201186,131.685690597524));
#60698=CARTESIAN_POINT('Ctrl Pts',(81.724350333893,7.88031562658267,131.68182225359));
#60699=CARTESIAN_POINT('Ctrl Pts',(81.6844976471958,7.82122331979352,131.677953909657));
#60700=CARTESIAN_POINT('Ctrl Pts',(81.641769449805,7.7644472345598,131.674085565724));
#60701=CARTESIAN_POINT('Ctrl Pts',(81.6163986757773,7.73073522898493,131.671788654415));
#60702=CARTESIAN_POINT('Ctrl Pts',(81.5900148690261,7.69783920296017,131.669491743107));
#60703=CARTESIAN_POINT('Ctrl Pts',(81.5626783192383,7.66582083921145,131.667194831798));
#60704=CARTESIAN_POINT('Ctrl Pts',(81.5166306657679,7.61188680108156,131.663325748947));
#60705=CARTESIAN_POINT('Ctrl Pts',(81.4676973380779,7.56023384777018,131.659456666095));
#60706=CARTESIAN_POINT('Ctrl Pts',(81.4161330600869,7.51118680868661,131.655587583244));
#60707=CARTESIAN_POINT('Ctrl Pts',(81.3646456102985,7.46221284724508,131.651724265133));
#60708=CARTESIAN_POINT('Ctrl Pts',(81.3105353403875,7.41583742508861,131.647860947022));
#60709=CARTESIAN_POINT('Ctrl Pts',(81.2540964212598,7.37235147261969,131.643997628911));
#60710=CARTESIAN_POINT('Ctrl Pts',(81.1977237049623,7.32891652915604,131.640138842471));
#60711=CARTESIAN_POINT('Ctrl Pts',(81.1390281480815,7.28836461804355,131.636280056031));
#60712=CARTESIAN_POINT('Ctrl Pts',(81.0783385728415,7.25094783244693,131.632421269591));
#60713=CARTESIAN_POINT('Ctrl Pts',(81.0176872275837,7.21355461668153,131.628564913903));
#60714=CARTESIAN_POINT('Ctrl Pts',(80.955044768553,7.1792928626006,131.624708558215));
#60715=CARTESIAN_POINT('Ctrl Pts',(80.8907694945681,7.14837172465776,131.620852202528));
#60716=CARTESIAN_POINT('Ctrl Pts',(80.826513208143,7.11745972112878,131.616996986046));
#60717=CARTESIAN_POINT('Ctrl Pts',(80.7606255018848,7.08988658504439,131.613141769564));
#60718=CARTESIAN_POINT('Ctrl Pts',(80.6934882640487,7.06581500622956,131.609286553083));
#60719=CARTESIAN_POINT('Ctrl Pts',(80.6263484013477,7.04174248628813,131.605431185874));
#60720=CARTESIAN_POINT('Ctrl Pts',(80.5579593681003,7.02117195729456,131.601575818665));
#60721=CARTESIAN_POINT('Ctrl Pts',(80.4887203319175,7.00421694574024,131.597720451456));
#60722=CARTESIAN_POINT('Ctrl Pts',(80.4194088213454,6.98724418691246,131.593861048729));
#60723=CARTESIAN_POINT('Ctrl Pts',(80.3492460045637,6.97389461593553,131.590001646001));
#60724=CARTESIAN_POINT('Ctrl Pts',(80.278642542797,6.96423088346354,131.586142243274));
#60725=CARTESIAN_POINT('Ctrl Pts',(80.207999104796,6.95456167931038,131.582280655323));
#60726=CARTESIAN_POINT('Ctrl Pts',(80.1369150094421,6.948582508874,131.578419067372));
#60727=CARTESIAN_POINT('Ctrl Pts',(80.0658046125619,6.94630398659744,131.574557479421));
#60728=CARTESIAN_POINT('Ctrl Pts',(79.9945698054951,6.94402147796453,131.570689135483));
#60729=CARTESIAN_POINT('Ctrl Pts',(79.9233090908698,6.94545253409038,131.566820791545));
#60730=CARTESIAN_POINT('Ctrl Pts',(79.8524346901804,6.95055567486261,131.562952447607));
#60731=CARTESIAN_POINT('Ctrl Pts',(79.8103515114051,6.95358577294237,131.56065553634));
#60732=CARTESIAN_POINT('Ctrl Pts',(79.7684044150234,6.95790952452471,131.558358625073));
#60733=CARTESIAN_POINT('Ctrl Pts',(79.7266779226685,6.96350973374701,131.556061713806));
#60734=CARTESIAN_POINT('Ctrl Pts',(79.65639081242,6.97294312967386,131.552192630968));
#60735=CARTESIAN_POINT('Ctrl Pts',(79.5864549840656,6.98603809145479,131.54832354813));
#60736=CARTESIAN_POINT('Ctrl Pts',(79.5172814947748,7.00275679818075,131.544454465292));
#60737=CARTESIAN_POINT('Ctrl Pts',(79.4482110705333,7.01945059486749,131.540591147194));
#60738=CARTESIAN_POINT('Ctrl Pts',(79.3799011990709,7.03975730604368,131.536727829097));
#60739=CARTESIAN_POINT('Ctrl Pts',(79.3127558531502,7.06358758392726,131.532864510999));
#60740=CARTESIAN_POINT('Ctrl Pts',(79.2456892686935,7.08738990890437,131.529005724572));
#60741=CARTESIAN_POINT('Ctrl Pts',(79.1797849520477,7.11470742907931,131.525146938145));
#60742=CARTESIAN_POINT('Ctrl Pts',(79.1154330417206,7.14540062039794,131.521288151718));
#60743=CARTESIAN_POINT('Ctrl Pts',(79.0511216683776,7.176074477257,131.517431796044));
#60744=CARTESIAN_POINT('Ctrl Pts',(78.9883611986377,7.21011957783073,131.513575440369));
#60745=CARTESIAN_POINT('Ctrl Pts',(78.9275216843021,7.24734834469085,131.509719084695));
#60746=CARTESIAN_POINT('Ctrl Pts',(78.8667001425676,7.2845661138009,131.505863868226));
#60747=CARTESIAN_POINT('Ctrl Pts',(78.8077988437883,7.32496542865309,131.502008651758));
#60748=CARTESIAN_POINT('Ctrl Pts',(78.7511615977401,7.36831369205322,131.498153435289));
#60749=CARTESIAN_POINT('Ctrl Pts',(78.6945221373438,7.41166365024171,131.494298068093));
#60750=CARTESIAN_POINT('Ctrl Pts',(78.6401472898425,7.45796248888234,131.490442700897));
#60751=CARTESIAN_POINT('Ctrl Pts',(78.5883489332518,7.50693642859771,131.486587333701));
#60752=CARTESIAN_POINT('Ctrl Pts',(78.5364963579042,7.55596163067553,131.482727930987));
#60753=CARTESIAN_POINT('Ctrl Pts',(78.4872260107637,7.60766718903243,131.478868528272));
#60754=CARTESIAN_POINT('Ctrl Pts',(78.4408132612819,7.66174207407326,131.475009125558));
#60755=CARTESIAN_POINT('Ctrl Pts',(78.3943742325358,7.71584757673993,131.471147537619));
#60756=CARTESIAN_POINT('Ctrl Pts',(78.3507963192765,7.77232469188178,131.467285949681));
#60757=CARTESIAN_POINT('Ctrl Pts',(78.310313177493,7.8308310625293,131.463424361742));
#60758=CARTESIAN_POINT('Ctrl Pts',(78.2697592089995,7.88943979217287,131.459556017817));
#60759=CARTESIAN_POINT('Ctrl Pts',(78.2323110773245,7.95008445204625,131.455687673892));
#60760=CARTESIAN_POINT('Ctrl Pts',(78.1981575144778,8.01239622324165,131.451819329966));
#60761=CARTESIAN_POINT('Ctrl Pts',(78.1778781109865,8.04939516112711,131.449522418582));
#60762=CARTESIAN_POINT('Ctrl Pts',(78.1587593571232,8.08698142395406,131.447225507198));
#60763=CARTESIAN_POINT('Ctrl Pts',(78.1408326489501,8.12507467559231,131.444928595814));
#60764=CARTESIAN_POINT('Ctrl Pts',(78.108155478463,8.19451183416958,131.440741738743));
#60765=CARTESIAN_POINT('Ctrl Pts',(78.0793295383059,8.26587225791199,131.436554881671));
#60766=CARTESIAN_POINT('Ctrl Pts',(78.0545656017949,8.33872655823763,131.432368024599));
#60767=CARTESIAN_POINT('Ctrl Pts',(78.0298638437669,8.41139793248148,131.42819168009));
#60768=CARTESIAN_POINT('Ctrl Pts',(78.0092039024862,8.48555538334085,131.42401533558));
#60769=CARTESIAN_POINT('Ctrl Pts',(77.9927491649578,8.56074876468895,131.419838991071));
#60770=CARTESIAN_POINT('Ctrl Pts',(77.9763607882817,8.63563889617533,131.415679489478));
#60771=CARTESIAN_POINT('Ctrl Pts',(77.9641439076397,8.7115562901603,131.411519987886));
#60772=CARTESIAN_POINT('Ctrl Pts',(77.9562120164597,8.7880371710974,131.407360486294));
#60773=CARTESIAN_POINT('Ctrl Pts',(77.9489432924382,8.8581236616763,131.403548751052));
#60774=CARTESIAN_POINT('Ctrl Pts',(77.9452725398498,8.92868294650349,131.399737015811));
#60775=CARTESIAN_POINT('Ctrl Pts',(77.9452501035681,8.99934760960448,131.39592528057));
#60776=CARTESIAN_POINT('Ctrl Pts',(77.9452501035679,8.99934761019358,131.395925280538));
#60777=CARTESIAN_POINT('Ctrl Pts',(77.9452268384226,9.07262290424563,131.391972724785));
#60778=CARTESIAN_POINT('Ctrl Pts',(77.9491275646018,9.14586509410072,131.388020169032));
#60779=CARTESIAN_POINT('Ctrl Pts',(77.956915517632,9.21863979602808,131.384067613279));
#60780=CARTESIAN_POINT('Ctrl Pts',(77.964709560304,9.29147140274994,131.3801119669));
#60781=CARTESIAN_POINT('Ctrl Pts',(77.9763968270618,9.36383434707673,131.376156320522));
#60782=CARTESIAN_POINT('Ctrl Pts',(77.9918890690414,9.4353022529972,131.372200674143));
#60783=CARTESIAN_POINT('Ctrl Pts',(78.0074099266823,9.5069021670158,131.368237721305));
#60784=CARTESIAN_POINT('Ctrl Pts',(78.0267496922357,9.57760330200735,131.364274768467));
#60785=CARTESIAN_POINT('Ctrl Pts',(78.0497697059516,9.64699255225699,131.360311815629));
#60786=CARTESIAN_POINT('Ctrl Pts',(78.072814378403,9.71645613135731,131.356344617728));
#60787=CARTESIAN_POINT('Ctrl Pts',(78.0995469862578,9.78460460843077,131.352377419827));
#60788=CARTESIAN_POINT('Ctrl Pts',(78.1297809942066,9.85104549400674,131.348410221926));
#60789=CARTESIAN_POINT('Ctrl Pts',(78.160077328869,9.91762334594345,131.344434845737));
#60790=CARTESIAN_POINT('Ctrl Pts',(78.1938892656041,9.98248618042066,131.340459469549));
#60791=CARTESIAN_POINT('Ctrl Pts',(78.2309848912312,10.045267002946,131.336484093361));
#60792=CARTESIAN_POINT('Ctrl Pts',(78.2393476952132,10.0594202542724,131.335587888181));
#60793=CARTESIAN_POINT('Ctrl Pts',(78.2478772169349,10.0734678168532,131.334691683002));
#60794=CARTESIAN_POINT('Ctrl Pts',(78.2565705111979,10.0874057108896,131.333795477822));
#60795=CARTESIAN_POINT('Ctrl Pts',(78.2941010642334,10.1475781674418,131.329926394941));
#60796=CARTESIAN_POINT('Ctrl Pts',(78.3348239566212,10.2059232122907,131.32605731206));
#60797=CARTESIAN_POINT('Ctrl Pts',(78.3785355099976,10.2620818001069,131.322188229179));
#60798=CARTESIAN_POINT('Ctrl Pts',(78.4221819353415,10.3181567144309,131.318324911038));
#60799=CARTESIAN_POINT('Ctrl Pts',(78.4688078867301,10.372051257967,131.314461592897));
#60800=CARTESIAN_POINT('Ctrl Pts',(78.5181656434058,10.4234340526055,131.310598274756));
#60801=CARTESIAN_POINT('Ctrl Pts',(78.5674655034532,10.474756575247,131.306739488286));
#60802=CARTESIAN_POINT('Ctrl Pts',(78.6194904688571,10.523572852667,131.302880701816));
#60803=CARTESIAN_POINT('Ctrl Pts',(78.6739527858832,10.569584769432,131.299021915345));
#60804=CARTESIAN_POINT('Ctrl Pts',(78.7283807956436,10.6155677020639,131.295165559628));
#60805=CARTESIAN_POINT('Ctrl Pts',(78.7852427407071,10.6587494660693,131.29130920391));
#60806=CARTESIAN_POINT('Ctrl Pts',(78.8442153428553,10.6988700329363,131.287452848192));
#60807=CARTESIAN_POINT('Ctrl Pts',(78.903170523906,10.7389787477859,131.28359763168));
#60808=CARTESIAN_POINT('Ctrl Pts',(78.9642347227752,10.7760277876989,131.279742415169));
#60809=CARTESIAN_POINT('Ctrl Pts',(79.0270544352387,10.8097995719171,131.275887198657));
#60810=CARTESIAN_POINT('Ctrl Pts',(79.0898766037636,10.8435726765103,131.272031831418));
#60811=CARTESIAN_POINT('Ctrl Pts',(79.1544539932342,10.8740680429386,131.268176464179));
#60812=CARTESIAN_POINT('Ctrl Pts',(79.2204087129387,10.9011141437689,131.26432109694));
#60813=CARTESIAN_POINT('Ctrl Pts',(79.2864324692427,10.9281885544887,131.260461694183));
#60814=CARTESIAN_POINT('Ctrl Pts',(79.3538359833336,10.9518063076746,131.256602291426));
#60815=CARTESIAN_POINT('Ctrl Pts',(79.4222224454108,10.9718444816752,131.252742888669));
#60816=CARTESIAN_POINT('Ctrl Pts',(79.4906476284368,10.9918940014464,131.248881300689));
#60817=CARTESIAN_POINT('Ctrl Pts',(79.5600563944854,11.0083597951441,131.245019712708));
#60818=CARTESIAN_POINT('Ctrl Pts',(79.6300405549925,11.0211698522266,131.241158124727));
#60819=CARTESIAN_POINT('Ctrl Pts',(79.7001471552846,11.0340023209609,131.23728978076));
#60820=CARTESIAN_POINT('Ctrl Pts',(79.7708306779828,11.0431662211242,131.233421436794));
#60821=CARTESIAN_POINT('Ctrl Pts',(79.8416773114418,11.0486413763242,131.229553092827));
#60822=CARTESIAN_POINT('Ctrl Pts',(79.8837439976024,11.0518923654572,131.227256181828));
#60823=CARTESIAN_POINT('Ctrl Pts',(79.9258681602445,11.0538438341146,131.22495927083));
#60824=CARTESIAN_POINT('Ctrl Pts',(79.9679636615187,11.0545002398434,131.222662359831));
#60825=CARTESIAN_POINT('Ctrl Pts',(80.0388583887734,11.0556057191395,131.21879403961));
#60826=CARTESIAN_POINT('Ctrl Pts',(80.1099492315853,11.0530395060358,131.21492571939));
#60827=CARTESIAN_POINT('Ctrl Pts',(80.1808243171346,11.0467779871869,131.211057399169));
#60828=CARTESIAN_POINT('Ctrl Pts',(80.2516008675047,11.040525173511,131.20719445694));
#60829=CARTESIAN_POINT('Ctrl Pts',(80.3221617761546,11.0305872888518,131.203331514711));
#60830=CARTESIAN_POINT('Ctrl Pts',(80.3920944026495,11.0169926975354,131.199468572483));
#60831=CARTESIAN_POINT('Ctrl Pts',(80.4619532083301,11.0034124566566,131.195609707972));
#60832=CARTESIAN_POINT('Ctrl Pts',(80.5311845737788,10.9861832627287,131.191750843461));
#60833=CARTESIAN_POINT('Ctrl Pts',(80.5993819433257,10.9653851654358,131.18789197895));
#60834=CARTESIAN_POINT('Ctrl Pts',(80.6675362532769,10.9446001999934,131.184035550914));
#60835=CARTESIAN_POINT('Ctrl Pts',(80.7346573990156,10.92025094335,131.180179122878));
#60836=CARTESIAN_POINT('Ctrl Pts',(80.8003515559622,10.8924679520058,131.176322694841));
#60837=CARTESIAN_POINT('Ctrl Pts',(80.86602140742,10.8646952397977,131.172467693604));
#60838=CARTESIAN_POINT('Ctrl Pts',(80.9302648728577,10.8334915082904,131.168612692367));
#60839=CARTESIAN_POINT('Ctrl Pts',(80.9927074781201,10.7990356931935,131.16475769113));
#60840=CARTESIAN_POINT('Ctrl Pts',(81.0551657820457,10.764571215578,131.160901720709));
#60841=CARTESIAN_POINT('Ctrl Pts',(81.1158218958457,10.7268532559481,131.157045750288));
#60842=CARTESIAN_POINT('Ctrl Pts',(81.174326582638,10.6861063548335,131.153189779867));
#60843=CARTESIAN_POINT('Ctrl Pts',(81.2006767626129,10.6677541810734,131.151453072602));
#60844=CARTESIAN_POINT('Ctrl Pts',(81.2265908973889,10.6487881620257,131.149716365337));
#60845=CARTESIAN_POINT('Ctrl Pts',(81.252039109102,10.6292316077768,131.147979658073));
#60846=CARTESIAN_POINT('',(77.9452503396332,9.00118140704016,131.454074719514));
#60847=CARTESIAN_POINT('Ctrl Pts',(77.9452503396338,9.00118140798793,131.454074719462));
#60848=CARTESIAN_POINT('Ctrl Pts',(77.9452901831621,9.07047878642176,131.450299784525));
#60849=CARTESIAN_POINT('Ctrl Pts',(77.9488353855608,9.13967381098879,131.446524849588));
#60850=CARTESIAN_POINT('Ctrl Pts',(77.955856695627,9.20850830603872,131.44274991465));
#60851=CARTESIAN_POINT('Ctrl Pts',(77.9630531190943,9.27905955229594,131.438880831799));
#60852=CARTESIAN_POINT('Ctrl Pts',(77.9739204176304,9.34937597973054,131.435011748947));
#60853=CARTESIAN_POINT('Ctrl Pts',(77.9884338439667,9.41904553738384,131.431142666096));
#60854=CARTESIAN_POINT('Ctrl Pts',(78.0029256460216,9.48861129087124,131.427279347985));
#60855=CARTESIAN_POINT('Ctrl Pts',(78.0210526941545,9.5575316160017,131.423416029874));
#60856=CARTESIAN_POINT('Ctrl Pts',(78.0427385152251,9.62539990623353,131.419552711764));
#60857=CARTESIAN_POINT('Ctrl Pts',(78.064398898836,9.69318858698713,131.415693925323));
#60858=CARTESIAN_POINT('Ctrl Pts',(78.0896096163955,9.7599272235673,131.411835138883));
#60859=CARTESIAN_POINT('Ctrl Pts',(78.1182436044463,9.82522144318533,131.407976352443));
#60860=CARTESIAN_POINT('Ctrl Pts',(78.1468595551843,9.89047453223283,131.404119996755));
#60861=CARTESIAN_POINT('Ctrl Pts',(78.1788943034939,9.95428456566709,131.400263641067));
#60862=CARTESIAN_POINT('Ctrl Pts',(78.2141721188591,10.01627572117,131.39640728538));
#60863=CARTESIAN_POINT('Ctrl Pts',(78.2494395128043,10.0782485638648,131.392552068898));
#60864=CARTESIAN_POINT('Ctrl Pts',(78.2879478317042,10.1384031733724,131.388696852417));
#60865=CARTESIAN_POINT('Ctrl Pts',(78.3294755145786,10.1963885264025,131.384841635935));
#60866=CARTESIAN_POINT('Ctrl Pts',(78.371004821061,10.2543761464861,131.380986268726));
#60867=CARTESIAN_POINT('Ctrl Pts',(78.4155534412464,10.3101939480482,131.377130901517));
#60868=CARTESIAN_POINT('Ctrl Pts',(78.4628576386396,10.3635215155659,131.373275534308));
#60869=CARTESIAN_POINT('Ctrl Pts',(78.5102113506275,10.4169049025044,131.369416131581));
#60870=CARTESIAN_POINT('Ctrl Pts',(78.5603260745845,10.4677924878938,131.365556728853));
#60871=CARTESIAN_POINT('Ctrl Pts',(78.6128996831301,10.5158991633481,131.361697326126));
#60872=CARTESIAN_POINT('Ctrl Pts',(78.6655030592655,10.5640330771796,131.357835738175));
#60873=CARTESIAN_POINT('Ctrl Pts',(78.7205677163487,10.6093826376158,131.353974150224));
#60874=CARTESIAN_POINT('Ctrl Pts',(78.7777588906698,10.6517034337808,131.350112562272));
#60875=CARTESIAN_POINT('Ctrl Pts',(78.8350501229989,10.6940982716946,131.346244218335));
#60876=CARTESIAN_POINT('Ctrl Pts',(78.8944748953416,10.7334534975559,131.342375874397));
#60877=CARTESIAN_POINT('Ctrl Pts',(78.9556705686791,10.7695687614153,131.338507530459));
#60878=CARTESIAN_POINT('Ctrl Pts',(78.9920067977846,10.7910129653963,131.336210619192));
#60879=CARTESIAN_POINT('Ctrl Pts',(79.0289669160085,10.8113157578957,131.333913707925));
#60880=CARTESIAN_POINT('Ctrl Pts',(79.066471624849,10.8304432073375,131.331616796658));
#60881=CARTESIAN_POINT('Ctrl Pts',(79.1296472587565,10.8626628613723,131.32774771382));
#60882=CARTESIAN_POINT('Ctrl Pts',(79.1946166239922,10.8916711307533,131.323878630982));
#60883=CARTESIAN_POINT('Ctrl Pts',(79.2610201204873,10.9172653181486,131.320009548144));
#60884=CARTESIAN_POINT('Ctrl Pts',(79.3273246790844,10.9428213714811,131.316146230047));
#60885=CARTESIAN_POINT('Ctrl Pts',(79.3950586778971,10.9649732667228,131.312282911949));
#60886=CARTESIAN_POINT('Ctrl Pts',(79.4638390357964,10.9835647161019,131.308419593851));
#60887=CARTESIAN_POINT('Ctrl Pts',(79.5325387143634,11.0021343577183,131.304560807424));
#60888=CARTESIAN_POINT('Ctrl Pts',(79.6022818473495,11.017151723076,131.300702020997));
#60889=CARTESIAN_POINT('Ctrl Pts',(79.6726681924137,11.0285096623488,131.296843234571));
#60890=CARTESIAN_POINT('Ctrl Pts',(79.7430101992425,11.0398604469528,131.292986878896));
#60891=CARTESIAN_POINT('Ctrl Pts',(79.81399413584,11.0475563016886,131.289130523221));
#60892=CARTESIAN_POINT('Ctrl Pts',(79.8852089486743,11.0515410249458,131.285274167547));
#60893=CARTESIAN_POINT('Ctrl Pts',(79.9564027239408,11.0555245710759,131.281418951078));
#60894=CARTESIAN_POINT('Ctrl Pts',(80.0278267552817,11.0557991350738,131.27756373461));
#60895=CARTESIAN_POINT('Ctrl Pts',(80.0990659661064,11.0523604695227,131.273708518141));
#60896=CARTESIAN_POINT('Ctrl Pts',(80.1703079621725,11.04892166953,131.269853150945));
#60897=CARTESIAN_POINT('Ctrl Pts',(80.2413646382644,11.0417693773813,131.265997783749));
#60898=CARTESIAN_POINT('Ctrl Pts',(80.3118237572204,11.030951379756,131.262142416554));
#60899=CARTESIAN_POINT('Ctrl Pts',(80.3823566276638,11.0201220586367,131.258283013839));
#60900=CARTESIAN_POINT('Ctrl Pts',(80.452290211234,11.0056194464126,131.254423611125));
#60901=CARTESIAN_POINT('Ctrl Pts',(80.521221111002,10.9875427331119,131.250564208411));
#60902=CARTESIAN_POINT('Ctrl Pts',(80.5901910399885,10.9694557846337,131.246702620472));
#60903=CARTESIAN_POINT('Ctrl Pts',(80.6581566919459,10.9477908541529,131.242841032534));
#60904=CARTESIAN_POINT('Ctrl Pts',(80.7247311599672,10.9226966240862,131.238979444595));
#60905=CARTESIAN_POINT('Ctrl Pts',(80.7914221024105,10.8975584907631,131.23511110067));
#60906=CARTESIAN_POINT('Ctrl Pts',(80.856716556353,10.8689792741642,131.231242756744));
#60907=CARTESIAN_POINT('Ctrl Pts',(80.9202495129103,10.8371549734544,131.227374412819));
#60908=CARTESIAN_POINT('Ctrl Pts',(80.9579735555502,10.8182586188377,131.225077501435));
#60909=CARTESIAN_POINT('Ctrl Pts',(80.9950770457667,10.7982190350941,131.222780590051));
#60910=CARTESIAN_POINT('Ctrl Pts',(81.0314884665628,10.7770844397068,131.220483678667));
#60911=CARTESIAN_POINT('Ctrl Pts',(81.0928208329716,10.7414847646637,131.216614699991));
#60912=CARTESIAN_POINT('Ctrl Pts',(81.1524281864628,10.7026364999002,131.212745721315));
#60913=CARTESIAN_POINT('Ctrl Pts',(81.2099452235117,10.6607318021286,131.208876742639));
#60914=CARTESIAN_POINT('Ctrl Pts',(81.2241048436853,10.6504156482657,131.207924272357));
#60915=CARTESIAN_POINT('Ctrl Pts',(81.2381378835472,10.6399144830512,131.206971802075));
#60916=CARTESIAN_POINT('Ctrl Pts',(81.252039109102,10.6292316077768,131.206019331793));
#60917=CARTESIAN_POINT('Ctrl Pts',(81.252039109102,10.6292316077769,131.906140964271));
#60918=CARTESIAN_POINT('Ctrl Pts',(81.3085547227941,10.5858002390999,131.902272668994));
#60919=CARTESIAN_POINT('Ctrl Pts',(81.3627348175322,10.539480934796,131.898404373717));
#60920=CARTESIAN_POINT('Ctrl Pts',(81.4142868161189,10.4905671283952,131.89453607844));
#60921=CARTESIAN_POINT('Ctrl Pts',(81.4465096501982,10.4599933095123,131.892118181165));
#60922=CARTESIAN_POINT('Ctrl Pts',(81.4777064486786,10.4284065658194,131.889700283891));
#60923=CARTESIAN_POINT('Ctrl Pts',(81.5078138187366,10.395885042017,131.887282386616));
#60924=CARTESIAN_POINT('Ctrl Pts',(81.555991179404,10.3438445888436,131.883413303769));
#60925=CARTESIAN_POINT('Ctrl Pts',(81.6015655640656,10.28920510133,131.879544220922));
#60926=CARTESIAN_POINT('Ctrl Pts',(81.6442441695773,10.2322575515334,131.875675138076));
#60927=CARTESIAN_POINT('Ctrl Pts',(81.6868591860952,10.1753948507458,131.871811819969));
#60928=CARTESIAN_POINT('Ctrl Pts',(81.726586698802,10.1162312993567,131.867948501863));
#60929=CARTESIAN_POINT('Ctrl Pts',(81.7631721851422,10.0550930802734,131.864085183757));
#60930=CARTESIAN_POINT('Ctrl Pts',(81.799714756721,9.99402657629762,131.860226397321));
#60931=CARTESIAN_POINT('Ctrl Pts',(81.8331223745403,9.93099042037825,131.856367610885));
#60932=CARTESIAN_POINT('Ctrl Pts',(81.8631831399907,9.86634066587836,131.852508824449));
#60933=CARTESIAN_POINT('Ctrl Pts',(81.893224969363,9.80173163598326,131.848652468766));
#60934=CARTESIAN_POINT('Ctrl Pts',(81.9199239248086,9.73551146357781,131.844796113083));
#60935=CARTESIAN_POINT('Ctrl Pts',(81.943114199668,9.66806045351347,131.8409397574));
#60936=CARTESIAN_POINT('Ctrl Pts',(81.966297623888,9.60062936915292,131.837084540923));
#60937=CARTESIAN_POINT('Ctrl Pts',(81.9859742674043,9.53196862812393,131.833229324446));
#60938=CARTESIAN_POINT('Ctrl Pts',(82.0020272285704,9.46247652758042,131.829374107968));
#60939=CARTESIAN_POINT('Ctrl Pts',(82.0180808173592,9.39298171010365,131.825518740764));
#60940=CARTESIAN_POINT('Ctrl Pts',(82.0305103353282,9.32265594239479,131.821663373559));
#60941=CARTESIAN_POINT('Ctrl Pts',(82.0392497279014,9.25190893146906,131.817808006355));
#60942=CARTESIAN_POINT('Ctrl Pts',(82.0479982682356,9.18108786771468,131.813948603632));
#60943=CARTESIAN_POINT('Ctrl Pts',(82.0530489129702,9.10984516366102,131.810089200909));
#60944=CARTESIAN_POINT('Ctrl Pts',(82.054387478561,9.03859598984201,131.806229798187));
#60945=CARTESIAN_POINT('Ctrl Pts',(82.0557268020581,8.96730647418111,131.80236821024));
#60946=CARTESIAN_POINT('Ctrl Pts',(82.0533498785534,8.89601096720569,131.798506622293));
#60947=CARTESIAN_POINT('Ctrl Pts',(82.0472946356544,8.82512222176385,131.794645034346));
#60948=CARTESIAN_POINT('Ctrl Pts',(82.0412287988908,8.75410945392093,131.790776690413));
#60949=CARTESIAN_POINT('Ctrl Pts',(82.0314718608921,8.68350534979087,131.786908346479));
#60950=CARTESIAN_POINT('Ctrl Pts',(82.0181132365228,8.61371444879264,131.783040002546));
#60951=CARTESIAN_POINT('Ctrl Pts',(82.0101812697977,8.57227462017489,131.780743091239));
#60952=CARTESIAN_POINT('Ctrl Pts',(82.0009804488128,8.53112126457092,131.778446179932));
#60953=CARTESIAN_POINT('Ctrl Pts',(81.9905377382802,8.49033631188563,131.776149268625));
#60954=CARTESIAN_POINT('Ctrl Pts',(81.9729472844919,8.42163519992567,131.772280185777));
#60955=CARTESIAN_POINT('Ctrl Pts',(81.9517614930238,8.35371126913166,131.76841110293));
#60956=CARTESIAN_POINT('Ctrl Pts',(81.9270660084627,8.28696833062777,131.764542020082));
#60957=CARTESIAN_POINT('Ctrl Pts',(81.9024073189419,8.22032483577358,131.760678701975));
#60958=CARTESIAN_POINT('Ctrl Pts',(81.8742494834812,8.15485929229784,131.756815383868));
#60959=CARTESIAN_POINT('Ctrl Pts',(81.8427284911056,8.09096244820819,131.752952065761));
#60960=CARTESIAN_POINT('Ctrl Pts',(81.8112444728419,8.02714055509204,131.749093279325));
#60961=CARTESIAN_POINT('Ctrl Pts',(81.776405347604,7.96488413987531,131.745234492889));
#60962=CARTESIAN_POINT('Ctrl Pts',(81.7383953179642,7.90456434192598,131.741375706452));
#60963=CARTESIAN_POINT('Ctrl Pts',(81.700409231856,7.84428254102631,131.737519350769));
#60964=CARTESIAN_POINT('Ctrl Pts',(81.6592564626002,7.78593534709736,131.733662995085));
#60965=CARTESIAN_POINT('Ctrl Pts',(81.6151665866135,7.72986832966531,131.729806639401));
#60966=CARTESIAN_POINT('Ctrl Pts',(81.5710897352177,7.67381787499165,131.725951422923));
#60967=CARTESIAN_POINT('Ctrl Pts',(81.5240777997389,7.62004664120675,131.722096206445));
#60968=CARTESIAN_POINT('Ctrl Pts',(81.4744019976384,7.5688688697887,131.718240989968));
#60969=CARTESIAN_POINT('Ctrl Pts',(81.4247242533627,7.5176890974729,131.714385622762));
#60970=CARTESIAN_POINT('Ctrl Pts',(81.3723827756188,7.46910333587675,131.710530255557));
#60971=CARTESIAN_POINT('Ctrl Pts',(81.3176859461205,7.42338929665673,131.706674888352));
#60972=CARTESIAN_POINT('Ctrl Pts',(81.2629318639569,7.37762740730336,131.702815485629));
#60973=CARTESIAN_POINT('Ctrl Pts',(81.2058178820311,7.33474355296152,131.698956082905));
#60974=CARTESIAN_POINT('Ctrl Pts',(81.1466851059665,7.29497483002314,131.695096680182));
#60975=CARTESIAN_POINT('Ctrl Pts',(81.0875188484596,7.25518358972147,131.691235092235));
#60976=CARTESIAN_POINT('Ctrl Pts',(81.026331938212,7.21851124188097,131.687373504287));
#60977=CARTESIAN_POINT('Ctrl Pts',(80.9634917137323,7.18514979128601,131.68351191634));
#60978=CARTESIAN_POINT('Ctrl Pts',(80.9005415480276,7.15172997363754,131.679643572406));
#60979=CARTESIAN_POINT('Ctrl Pts',(80.8359327335557,7.12163282338651,131.675775228472));
#60980=CARTESIAN_POINT('Ctrl Pts',(80.7700536341266,7.09500263436707,131.671906884538));
#60981=CARTESIAN_POINT('Ctrl Pts',(80.7309365208099,7.07919039451337,131.669609973236));
#60982=CARTESIAN_POINT('Ctrl Pts',(80.6913718813705,7.06459953841317,131.667313061935));
#60983=CARTESIAN_POINT('Ctrl Pts',(80.6514431729601,7.05125184928793,131.665016150633));
#60984=CARTESIAN_POINT('Ctrl Pts',(80.5841843803937,7.02876804027297,131.661147067787));
#60985=CARTESIAN_POINT('Ctrl Pts',(80.5156284830307,7.00972632113528,131.657277984941));
#60986=CARTESIAN_POINT('Ctrl Pts',(80.4461611878916,6.99427375823141,131.653408902095));
#60987=CARTESIAN_POINT('Ctrl Pts',(80.3767973955577,6.9788442188756,131.64954558399));
#60988=CARTESIAN_POINT('Ctrl Pts',(80.3065253712456,6.96699332541082,131.645682265884));
#60989=CARTESIAN_POINT('Ctrl Pts',(80.2357471530522,6.9588187629885,131.641818947779));
#60990=CARTESIAN_POINT('Ctrl Pts',(80.1650519576813,6.95065378932474,131.637960161344));
#60991=CARTESIAN_POINT('Ctrl Pts',(80.093852228081,6.94615663641099,131.634101374909));
#60992=CARTESIAN_POINT('Ctrl Pts',(80.0225596785607,6.9453738482626,131.630242588474));
#60993=CARTESIAN_POINT('Ctrl Pts',(79.9513120381188,6.94459155321334,131.626386232792));
#60994=CARTESIAN_POINT('Ctrl Pts',(79.8799721783654,6.94751898616858,131.622529877109));
#60995=CARTESIAN_POINT('Ctrl Pts',(79.8089549414203,6.95415070249731,131.618673521427));
#60996=CARTESIAN_POINT('Ctrl Pts',(79.7379586836779,6.96078045975063,131.614818304951));
#60997=CARTESIAN_POINT('Ctrl Pts',(79.6672853429502,6.97111228278093,131.610963088474));
#60998=CARTESIAN_POINT('Ctrl Pts',(79.5973460269105,6.98508875122122,131.607107871998));
#60999=CARTESIAN_POINT('Ctrl Pts',(79.5274039764526,6.99906576609965,131.603252504794));
#61000=CARTESIAN_POINT('Ctrl Pts',(79.458196483592,7.01668761193721,131.599397137591));
#61001=CARTESIAN_POINT('Ctrl Pts',(79.3901241232495,7.03784583239292,131.595541770387));
#61002=CARTESIAN_POINT('Ctrl Pts',(79.3219805097079,7.05902619973599,131.591682367665));
#61003=CARTESIAN_POINT('Ctrl Pts',(79.2549748653884,7.08375018647811,131.587822964943));
#61004=CARTESIAN_POINT('Ctrl Pts',(79.1894913917896,7.11185981491924,131.583963562221));
#61005=CARTESIAN_POINT('Ctrl Pts',(79.1239708409334,7.13998535925287,131.580101974275));
#61006=CARTESIAN_POINT('Ctrl Pts',(79.0599746125178,7.17150014668207,131.576240386329));
#61007=CARTESIAN_POINT('Ctrl Pts',(78.9978632532908,7.20619970359154,131.572378798383));
#61008=CARTESIAN_POINT('Ctrl Pts',(78.9356432280141,7.24095996861979,131.568510454451));
#61009=CARTESIAN_POINT('Ctrl Pts',(78.8753150670732,7.27891586874659,131.564642110518));
#61010=CARTESIAN_POINT('Ctrl Pts',(78.8172106373783,7.31981938882486,131.560773766585));
#61011=CARTESIAN_POINT('Ctrl Pts',(78.7827098989949,7.34410672203832,131.558476855271));
#61012=CARTESIAN_POINT('Ctrl Pts',(78.7489925561506,7.36943249127378,131.556179943956));
#61013=CARTESIAN_POINT('Ctrl Pts',(78.7161221751678,7.39573839620713,131.553883032642));
#61014=CARTESIAN_POINT('Ctrl Pts',(78.661450898684,7.43949138472648,131.550062721779));
#61015=CARTESIAN_POINT('Ctrl Pts',(78.6088985784268,7.48613870942767,131.546242410916));
#61016=CARTESIAN_POINT('Ctrl Pts',(78.5587935921189,7.53544489609219,131.542422100053));
#61017=CARTESIAN_POINT('Ctrl Pts',(78.5087739526717,7.58466709653985,131.538608296557));
#61018=CARTESIAN_POINT('Ctrl Pts',(78.4611937228877,7.63653881976069,131.534794493061));
#61019=CARTESIAN_POINT('Ctrl Pts',(78.4163489115398,7.69078390152009,131.530980689565));
#61020=CARTESIAN_POINT('Ctrl Pts',(78.3715467866424,7.7449773489896,131.527170516316));
#61021=CARTESIAN_POINT('Ctrl Pts',(78.3294752360328,7.80153929492881,131.523360343067));
#61022=CARTESIAN_POINT('Ctrl Pts',(78.2903930042301,7.86015725535729,131.519550169818));
#61023=CARTESIAN_POINT('Ctrl Pts',(78.251334107591,7.91874021625701,131.515742271541));
#61024=CARTESIAN_POINT('Ctrl Pts',(78.215261266858,7.97937634294027,131.511934373265));
#61025=CARTESIAN_POINT('Ctrl Pts',(78.1823913627715,8.04172216744194,131.508126474989));
#61026=CARTESIAN_POINT('Ctrl Pts',(78.1495294250013,8.10405288187323,131.504319499591));
#61027=CARTESIAN_POINT('Ctrl Pts',(78.1198691151503,8.16809202988376,131.500512524193));
#61028=CARTESIAN_POINT('Ctrl Pts',(78.0935816345596,8.23347108442563,131.496705548795));
#61029=CARTESIAN_POINT('Ctrl Pts',(78.0672753510514,8.29889690331867,131.492895850343));
#61030=CARTESIAN_POINT('Ctrl Pts',(78.0443469047301,8.36566407997194,131.48908615189));
#61031=CARTESIAN_POINT('Ctrl Pts',(78.0249190681297,8.43338472041204,131.485276453437));
#61032=CARTESIAN_POINT('Ctrl Pts',(78.005484315325,8.50112946903271,131.481465398753));
#61033=CARTESIAN_POINT('Ctrl Pts',(77.9895527685954,8.56982787082582,131.477654344068));
#61034=CARTESIAN_POINT('Ctrl Pts',(77.9771963820947,8.63908022236322,131.473843289384));
#61035=CARTESIAN_POINT('Ctrl Pts',(77.9648204879244,8.7084419061882,131.470026217989));
#61036=CARTESIAN_POINT('Ctrl Pts',(77.95603108832,8.77835879022988,131.466209146595));
#61037=CARTESIAN_POINT('Ctrl Pts',(77.9508483050221,8.84842528750064,131.4623920752));
#61038=CARTESIAN_POINT('Ctrl Pts',(77.947083896162,8.89931665763151,131.459619623304));
#61039=CARTESIAN_POINT('Ctrl Pts',(77.9452210770952,8.95028684822795,131.456847171409));
#61040=CARTESIAN_POINT('Ctrl Pts',(77.9452503396332,9.00118140704017,131.454074719514));
#61041=CARTESIAN_POINT('Origin',(80.,9.,141.545925280538));
#61042=CARTESIAN_POINT('',(81.252039109102,10.6292316077768,132.606087908811));
#61043=CARTESIAN_POINT('',(81.252039109102,10.6292316077768,132.547886797676));
#61044=CARTESIAN_POINT('',(81.252039109102,10.6292316077768,141.545925280538));
#61045=CARTESIAN_POINT('',(77.9452505617457,8.99848062725763,132.095925280492));
#61046=CARTESIAN_POINT('Ctrl Pts',(81.252039109102,10.6292316077768,132.547886797676));
#61047=CARTESIAN_POINT('Ctrl Pts',(81.3083538591921,10.5859545996489,132.544022016983));
#61048=CARTESIAN_POINT('Ctrl Pts',(81.3625154590115,10.5396826637711,132.540157236291));
#61049=CARTESIAN_POINT('Ctrl Pts',(81.4141896908426,10.4906592772376,132.536292455599));
#61050=CARTESIAN_POINT('Ctrl Pts',(81.4657959228315,10.4417004022107,132.5324327607));
#61051=CARTESIAN_POINT('Ctrl Pts',(81.5149209386215,10.3899976014555,132.528573065801));
#61052=CARTESIAN_POINT('Ctrl Pts',(81.5612632568425,10.3358347971713,132.524713370902));
#61053=CARTESIAN_POINT('Ctrl Pts',(81.607572059914,10.281711163877,132.520856467367));
#61054=CARTESIAN_POINT('Ctrl Pts',(81.6511018428738,10.2251314243555,132.516999563831));
#61055=CARTESIAN_POINT('Ctrl Pts',(81.6915887013729,10.1664155468304,132.513142660296));
#61056=CARTESIAN_POINT('Ctrl Pts',(81.7320598230887,10.1077224915017,132.509287255895));
#61057=CARTESIAN_POINT('Ctrl Pts',(81.769490092302,10.0468953456498,132.505431851494));
#61058=CARTESIAN_POINT('Ctrl Pts',(81.8036576212695,9.98428489155141,132.501576447094));
#61059=CARTESIAN_POINT('Ctrl Pts',(81.8378232990749,9.92167782962407,132.497721251575));
#61060=CARTESIAN_POINT('Ctrl Pts',(81.8687263563342,9.8572880784718,132.493866056056));
#61061=CARTESIAN_POINT('Ctrl Pts',(81.8961906147685,9.79149144970981,132.490010860537));
#61062=CARTESIAN_POINT('Ctrl Pts',(81.9236819784045,9.72562988451821,132.486151860224));
#61063=CARTESIAN_POINT('Ctrl Pts',(81.947727576468,9.65835911760964,132.482292859911));
#61064=CARTESIAN_POINT('Ctrl Pts',(81.9681995647198,9.5900746020095,132.478433859598));
#61065=CARTESIAN_POINT('Ctrl Pts',(81.9886814319893,9.52175713485006,132.474572997076));
#61066=CARTESIAN_POINT('Ctrl Pts',(82.0055861388274,9.4524254171311,132.470712134553));
#61067=CARTESIAN_POINT('Ctrl Pts',(82.0188366080988,9.38248700932207,132.466851272031));
#61068=CARTESIAN_POINT('Ctrl Pts',(82.0321114362183,9.31242003104405,132.462983311936));
#61069=CARTESIAN_POINT('Ctrl Pts',(82.0417185395784,9.24174461693172,132.459115351841));
#61070=CARTESIAN_POINT('Ctrl Pts',(82.0476326157001,9.17087490635356,132.455247391746));
#61071=CARTESIAN_POINT('Ctrl Pts',(82.0527907860587,9.10906338534611,132.451873813743));
#61072=CARTESIAN_POINT('Ctrl Pts',(82.0551404635228,9.04710432326967,132.448500235741));
#61073=CARTESIAN_POINT('Ctrl Pts',(82.0546972072604,8.98527081210231,132.445126657738));
#61074=CARTESIAN_POINT('Ctrl Pts',(82.0541888463451,8.91435531015297,132.441257574891));
#61075=CARTESIAN_POINT('Ctrl Pts',(82.0500038297876,8.84332726097794,132.437388492044));
#61076=CARTESIAN_POINT('Ctrl Pts',(82.0421279206532,8.77259921242762,132.433519409197));
#61077=CARTESIAN_POINT('Ctrl Pts',(82.0342637462307,8.70197654514227,132.429656091091));
#61078=CARTESIAN_POINT('Ctrl Pts',(82.0227196484063,8.63165347009274,132.425792772985));
#61079=CARTESIAN_POINT('Ctrl Pts',(82.0075333990489,8.56204199493211,132.421929454878));
#61080=CARTESIAN_POINT('Ctrl Pts',(81.9923649631562,8.49251217400505,132.418070668442));
#61081=CARTESIAN_POINT('Ctrl Pts',(81.9735629648897,8.42369276727413,132.414211882007));
#61082=CARTESIAN_POINT('Ctrl Pts',(81.9512166949536,8.35598837600995,132.410353095571));
#61083=CARTESIAN_POINT('Ctrl Pts',(81.928884501529,8.28832663354772,132.406496739888));
#61084=CARTESIAN_POINT('Ctrl Pts',(81.9030126178372,8.22177897326064,132.402640384204));
#61085=CARTESIAN_POINT('Ctrl Pts',(81.8737405346709,8.15673612004825,132.398784028521));
#61086=CARTESIAN_POINT('Ctrl Pts',(81.844477098771,8.091712481146,132.394928812044));
#61087=CARTESIAN_POINT('Ctrl Pts',(81.8118156567701,8.02819320954054,132.391073595567));
#61088=CARTESIAN_POINT('Ctrl Pts',(81.7759436651095,7.96654866546242,132.38721837909));
#61089=CARTESIAN_POINT('Ctrl Pts',(81.7400702709613,7.90490171126702,132.383363011885));
#61090=CARTESIAN_POINT('Ctrl Pts',(81.7009863241764,7.84513004887886,132.37950764468));
#61091=CARTESIAN_POINT('Ctrl Pts',(81.6589241562072,7.78757754621083,132.375652277476));
#61092=CARTESIAN_POINT('Ctrl Pts',(81.616817960618,7.72996480176631,132.371792874753));
#61093=CARTESIAN_POINT('Ctrl Pts',(81.5717276080722,7.67457624698685,132.36793347203));
#61094=CARTESIAN_POINT('Ctrl Pts',(81.5239269806332,7.62172422200847,132.364074069307));
#61095=CARTESIAN_POINT('Ctrl Pts',(81.4760992881035,7.56884227179838,132.360212481361));
#61096=CARTESIAN_POINT('Ctrl Pts',(81.4255586101456,7.51850005341321,132.356350893414));
#61097=CARTESIAN_POINT('Ctrl Pts',(81.3726151590845,7.47097246998247,132.352489305467));
#61098=CARTESIAN_POINT('Ctrl Pts',(81.319579081558,7.42336173534094,132.348620961533));
#61099=CARTESIAN_POINT('Ctrl Pts',(81.2641322160707,7.37857577250758,132.3447526176));
#61100=CARTESIAN_POINT('Ctrl Pts',(81.2066166827356,7.33684825002526,132.340884273666));
#61101=CARTESIAN_POINT('Ctrl Pts',(81.1724656141924,7.31207164798752,132.33858736236));
#61102=CARTESIAN_POINT('Ctrl Pts',(81.1375857558046,7.28837250744841,132.336290451053));
#61103=CARTESIAN_POINT('Ctrl Pts',(81.1020528512102,7.26579208984635,132.333993539747));
#61104=CARTESIAN_POINT('Ctrl Pts',(81.0421986673426,7.22775600801214,132.3301244569));
#61105=CARTESIAN_POINT('Ctrl Pts',(80.9802557831634,7.19274776279809,132.326255374053));
#61106=CARTESIAN_POINT('Ctrl Pts',(80.9165630719347,7.16100307295918,132.322386291206));
#61107=CARTESIAN_POINT('Ctrl Pts',(80.8529652596692,7.12930568112495,132.318522973099));
#61108=CARTESIAN_POINT('Ctrl Pts',(80.7876232267179,7.100862407597,132.314659654993));
#61109=CARTESIAN_POINT('Ctrl Pts',(80.7209036010567,7.07586498382168,132.310796336886));
#61110=CARTESIAN_POINT('Ctrl Pts',(80.6542622374906,7.05089688201483,132.306937550451));
#61111=CARTESIAN_POINT('Ctrl Pts',(80.5862469436659,7.02936677082744,132.303078764015));
#61112=CARTESIAN_POINT('Ctrl Pts',(80.517246068014,7.01141908195213,132.299219977579));
#61113=CARTESIAN_POINT('Ctrl Pts',(80.448288657854,6.99348269880476,132.295363621895));
#61114=CARTESIAN_POINT('Ctrl Pts',(80.3783473666403,6.97912438278268,132.291507266212));
#61115=CARTESIAN_POINT('Ctrl Pts',(80.3078261123458,6.96843886455315,132.287650910529));
#61116=CARTESIAN_POINT('Ctrl Pts',(80.237325690736,6.95775650293271,132.283795694051));
#61117=CARTESIAN_POINT('Ctrl Pts',(80.1662461262162,6.95074485785234,132.279940477574));
#61118=CARTESIAN_POINT('Ctrl Pts',(80.0950002433514,6.94744731705537,132.276085261097));
#61119=CARTESIAN_POINT('Ctrl Pts',(80.0237515749856,6.94414964733442,132.272229893892));
#61120=CARTESIAN_POINT('Ctrl Pts',(79.9523370607304,6.94456639045237,132.268374526687));
#61121=CARTESIAN_POINT('Ctrl Pts',(79.8811716074013,6.94868886425964,132.264519159483));
#61122=CARTESIAN_POINT('Ctrl Pts',(79.8099316632486,6.95281565317284,132.26065975676));
#61123=CARTESIAN_POINT('Ctrl Pts',(79.738941786399,6.96065588775716,132.256800354037));
#61124=CARTESIAN_POINT('Ctrl Pts',(79.6686129323736,6.97214887777481,132.252940951314));
#61125=CARTESIAN_POINT('Ctrl Pts',(79.5982442575986,6.98364837521368,132.249079363367));
#61126=CARTESIAN_POINT('Ctrl Pts',(79.5285378256331,6.99880464201056,132.24521777542));
#61127=CARTESIAN_POINT('Ctrl Pts',(79.4598928447495,7.01750616057775,132.241356187473));
#61128=CARTESIAN_POINT('Ctrl Pts',(79.3911277670113,7.036240398122,132.23748784354));
#61129=CARTESIAN_POINT('Ctrl Pts',(79.3234283095602,7.05853211901331,132.233619499606));
#61130=CARTESIAN_POINT('Ctrl Pts',(79.2571763442846,7.08422063404745,132.229751155673));
#61131=CARTESIAN_POINT('Ctrl Pts',(79.2178378338805,7.09947373501935,132.227454244367));
#61132=CARTESIAN_POINT('Ctrl Pts',(79.1790092532518,7.11592351035826,132.225157333061));
#61133=CARTESIAN_POINT('Ctrl Pts',(79.1407663493563,7.13352870472071,132.222860421755));
#61134=CARTESIAN_POINT('Ctrl Pts',(79.0763472474524,7.16318416218213,132.218991338908));
#61135=CARTESIAN_POINT('Ctrl Pts',(79.013339061303,7.19623664486004,132.215122256061));
#61136=CARTESIAN_POINT('Ctrl Pts',(78.9521236242196,7.23252930333163,132.211253173215));
#61137=CARTESIAN_POINT('Ctrl Pts',(78.8909993950846,7.26876788755209,132.207389855108));
#61138=CARTESIAN_POINT('Ctrl Pts',(78.8316630274031,7.30823681899428,132.203526537002));
#61139=CARTESIAN_POINT('Ctrl Pts',(78.7744744529044,7.35073207273163,132.199663218896));
#61140=CARTESIAN_POINT('Ctrl Pts',(78.7173529605816,7.39317747955271,132.19580443246));
#61141=CARTESIAN_POINT('Ctrl Pts',(78.6623746451652,7.4386418690834,132.191945646024));
#61142=CARTESIAN_POINT('Ctrl Pts',(78.6098714810442,7.48687731386848,132.188086859588));
#61143=CARTESIAN_POINT('Ctrl Pts',(78.5574013900668,7.53508237386029,132.184230503905));
#61144=CARTESIAN_POINT('Ctrl Pts',(78.5074037139143,7.58605469806288,132.180374148222));
#61145=CARTESIAN_POINT('Ctrl Pts',(78.4601771161135,7.63950632167599,132.176517792539));
#61146=CARTESIAN_POINT('Ctrl Pts',(78.4129644695226,7.69294215514429,132.172662576062));
#61147=CARTESIAN_POINT('Ctrl Pts',(78.3685215975986,7.74885547014025,132.168807359585));
#61148=CARTESIAN_POINT('Ctrl Pts',(78.3271088597398,7.80692297174955,132.164952143108));
#61149=CARTESIAN_POINT('Ctrl Pts',(78.2856945027668,7.86499274362452,132.161096775903));
#61150=CARTESIAN_POINT('Ctrl Pts',(78.2473107953371,7.9252164725418,132.157241408699));
#61151=CARTESIAN_POINT('Ctrl Pts',(78.2121754805812,7.98724087253438,132.153386041494));
#61152=CARTESIAN_POINT('Ctrl Pts',(78.1770033887317,8.04933019516052,132.149526638771));
#61153=CARTESIAN_POINT('Ctrl Pts',(78.1450867170065,8.11322352782564,132.145667236049));
#61154=CARTESIAN_POINT('Ctrl Pts',(78.1165973717164,8.17854269601251,132.141807833326));
#61155=CARTESIAN_POINT('Ctrl Pts',(78.0880918955352,8.24389884842555,132.137946245379));
#61156=CARTESIAN_POINT('Ctrl Pts',(78.063017779716,8.310681988484,132.134084657432));
#61157=CARTESIAN_POINT('Ctrl Pts',(78.0414978573552,8.37849624316854,132.130223069485));
#61158=CARTESIAN_POINT('Ctrl Pts',(78.0199402851188,8.44642914132239,132.126354725552));
#61159=CARTESIAN_POINT('Ctrl Pts',(78.001949443788,8.51539628558163,132.122486381619));
#61160=CARTESIAN_POINT('Ctrl Pts',(77.9875974528441,8.58498969807929,132.118618037685));
#61161=CARTESIAN_POINT('Ctrl Pts',(77.9790756536327,8.626312263712,132.116321126378));
#61162=CARTESIAN_POINT('Ctrl Pts',(77.9718357960167,8.66785547309974,132.114024215071));
#61163=CARTESIAN_POINT('Ctrl Pts',(77.9658843036767,8.70953331263113,132.111727303764));
#61164=CARTESIAN_POINT('Ctrl Pts',(77.9522361754433,8.80511009672412,132.106459962688));
#61165=CARTESIAN_POINT('Ctrl Pts',(77.9453221472454,8.90167081914922,132.101192621613));
#61166=CARTESIAN_POINT('Ctrl Pts',(77.9452505617463,8.99848062641328,132.095925280538));
#61167=CARTESIAN_POINT('Ctrl Pts',(77.9452505617457,8.99848062725764,132.095925280492));
#61168=CARTESIAN_POINT('Ctrl Pts',(77.9451965787833,9.07148539992385,132.091953151545));
#61169=CARTESIAN_POINT('Ctrl Pts',(77.9490383631329,9.14463767470539,132.087981022599));
#61170=CARTESIAN_POINT('Ctrl Pts',(77.9567917436018,9.21748007606708,132.084008893652));
#61171=CARTESIAN_POINT('Ctrl Pts',(77.9642163077101,9.28723327351193,132.080205220386));
#61172=CARTESIAN_POINT('Ctrl Pts',(77.9752273595376,9.35670178529796,132.07640154712));
#61173=CARTESIAN_POINT('Ctrl Pts',(77.989785708765,9.42548333200558,132.072597873854));
#61174=CARTESIAN_POINT('Ctrl Pts',(78.0043341072357,9.49421786593538,132.068796800431));
#61175=CARTESIAN_POINT('Ctrl Pts',(78.0224248939572,9.56226587652216,132.064995727008));
#61176=CARTESIAN_POINT('Ctrl Pts',(78.0439673846338,9.62923284253429,132.061194653586));
#61177=CARTESIAN_POINT('Ctrl Pts',(78.0655028484982,9.69617796500439,132.057394820012));
#61178=CARTESIAN_POINT('Ctrl Pts',(78.0904876294811,9.76204226555299,132.053594986438));
#61179=CARTESIAN_POINT('Ctrl Pts',(78.1187810484405,9.82644589586581,132.049795152864));
#61180=CARTESIAN_POINT('Ctrl Pts',(78.1470753477332,9.8908515300601,132.04599520106));
#61181=CARTESIAN_POINT('Ctrl Pts',(78.1786782846807,9.95379594626292,132.042195249257));
#61182=CARTESIAN_POINT('Ctrl Pts',(78.2134016340244,10.0149206083204,132.038395297453));
#61183=CARTESIAN_POINT('Ctrl Pts',(78.2481601793031,10.076107226948,132.03459149398));
#61184=CARTESIAN_POINT('Ctrl Pts',(78.2860451976125,10.1354699758928,132.030787690508));
#61185=CARTESIAN_POINT('Ctrl Pts',(78.3268238180268,10.1926772516391,132.026983887035));
#61186=CARTESIAN_POINT('Ctrl Pts',(78.3676269245136,10.2499188782657,132.023177799517));
#61187=CARTESIAN_POINT('Ctrl Pts',(78.4113267751392,10.3050020670922,132.019371711999));
#61188=CARTESIAN_POINT('Ctrl Pts',(78.4576505098364,10.3576286726097,132.015565624481));
#61189=CARTESIAN_POINT('Ctrl Pts',(78.5040502056944,10.4103415746677,132.011753295782));
#61190=CARTESIAN_POINT('Ctrl Pts',(78.5530820149242,10.4605895045058,132.007940967083));
#61191=CARTESIAN_POINT('Ctrl Pts',(78.6044374301093,10.5081122889294,132.004128638384));
#61192=CARTESIAN_POINT('Ctrl Pts',(78.6203081568687,10.5227985907287,132.002950487513));
#61193=CARTESIAN_POINT('Ctrl Pts',(78.6364005734968,10.5372249326002,132.001772336643));
#61194=CARTESIAN_POINT('Ctrl Pts',(78.6527050052885,10.5513844654777,132.000594185772));
#61195=CARTESIAN_POINT('Ctrl Pts',(78.7062492490403,10.5978847967674,131.996725102925));
#61196=CARTESIAN_POINT('Ctrl Pts',(78.7623085494613,10.6417009236037,131.992856020077));
#61197=CARTESIAN_POINT('Ctrl Pts',(78.820582782277,10.6825494313804,131.98898693723));
#61198=CARTESIAN_POINT('Ctrl Pts',(78.8787701893921,10.7233370769178,131.985123619123));
#61199=CARTESIAN_POINT('Ctrl Pts',(78.9391655836706,10.7611656035921,131.981260301016));
#61200=CARTESIAN_POINT('Ctrl Pts',(79.0014348634834,10.7957909763203,131.977396982909));
#61201=CARTESIAN_POINT('Ctrl Pts',(79.0636311014549,10.8303757334996,131.973538196473));
#61202=CARTESIAN_POINT('Ctrl Pts',(79.1276964363556,10.8617645650649,131.969679410036));
#61203=CARTESIAN_POINT('Ctrl Pts',(79.1932682648415,10.8897569870193,131.9658206236));
#61204=CARTESIAN_POINT('Ctrl Pts',(79.2587987878836,10.9177317758004,131.961964267916));
#61205=CARTESIAN_POINT('Ctrl Pts',(79.325833476029,10.9423142094072,131.958107912232));
#61206=CARTESIAN_POINT('Ctrl Pts',(79.3939869504902,10.963350642734,131.954251556549));
#61207=CARTESIAN_POINT('Ctrl Pts',(79.4621202917326,10.9843808616877,131.950396340071));
#61208=CARTESIAN_POINT('Ctrl Pts',(79.5313712992336,11.001867016792,131.946541123593));
#61209=CARTESIAN_POINT('Ctrl Pts',(79.6013381641291,11.0157049146936,131.942685907115));
#61210=CARTESIAN_POINT('Ctrl Pts',(79.6713077645197,11.0295433536157,131.93883053991));
#61211=CARTESIAN_POINT('Ctrl Pts',(79.7419928008916,11.0397331600597,131.934975172705));
#61212=CARTESIAN_POINT('Ctrl Pts',(79.8129816751027,11.0462213244546,131.9311198055));
#61213=CARTESIAN_POINT('Ctrl Pts',(79.8840448553073,11.0527162801883,131.927260402777));
#61214=CARTESIAN_POINT('Ctrl Pts',(79.9554120234629,11.0555018149779,131.923401000053));
#61215=CARTESIAN_POINT('Ctrl Pts',(80.0266677680113,11.054576937632,131.91954159733));
#61216=CARTESIAN_POINT('Ctrl Pts',(80.097963858122,11.0536515366133,131.915680009382));
#61217=CARTESIAN_POINT('Ctrl Pts',(80.169147914051,11.0490115728982,131.911818421435));
#61218=CARTESIAN_POINT('Ctrl Pts',(80.2398085956789,11.0407080633786,131.907956833487));
#61219=CARTESIAN_POINT('Ctrl Pts',(80.3105929007018,11.0323900265716,131.904088489553));
#61220=CARTESIAN_POINT('Ctrl Pts',(80.3808515242716,11.0203957289771,131.90022014562));
#61221=CARTESIAN_POINT('Ctrl Pts',(80.4501829707135,11.0048273879263,131.896351801686));
#61222=CARTESIAN_POINT('Ctrl Pts',(80.491349988332,10.9955833550492,131.894054890384));
#61223=CARTESIAN_POINT('Ctrl Pts',(80.5321903805207,10.9850802059216,131.891757979082));
#61224=CARTESIAN_POINT('Ctrl Pts',(80.5726231150621,10.9733474936251,131.889461067781));
#61225=CARTESIAN_POINT('Ctrl Pts',(80.6407129225893,10.9535892919824,131.885593007651));
#61226=CARTESIAN_POINT('Ctrl Pts',(80.7079122298131,10.9302641370807,131.881724947521));
#61227=CARTESIAN_POINT('Ctrl Pts',(80.7738204657355,10.9034703699582,131.877856887391));
#61228=CARTESIAN_POINT('Ctrl Pts',(80.8396428369133,10.8767115095501,131.87399386654));
#61229=CARTESIAN_POINT('Ctrl Pts',(80.9041770261002,10.8464931786054,131.870130845689));
#61230=CARTESIAN_POINT('Ctrl Pts',(80.96703688535,10.8129636579018,131.866267824838));
#61231=CARTESIAN_POINT('Ctrl Pts',(81.0298266373822,10.7794715324681,131.86240911239));
#61232=CARTESIAN_POINT('Ctrl Pts',(81.0909453409541,10.7426757775587,131.858550399943));
#61233=CARTESIAN_POINT('Ctrl Pts',(81.1500279067695,10.702772261975,131.854691687496));
#61234=CARTESIAN_POINT('Ctrl Pts',(81.1847581408959,10.6793159611261,131.852423438227));
#61235=CARTESIAN_POINT('Ctrl Pts',(81.2187852183793,10.6547867047415,131.850155188957));
#61236=CARTESIAN_POINT('Ctrl Pts',(81.252039109102,10.6292316077768,131.847886939688));
#61237=CARTESIAN_POINT('',(77.945250271645,9.00105656286654,132.154074719416));
#61238=CARTESIAN_POINT('Ctrl Pts',(77.945250271645,9.00105656286652,132.154074719416));
#61239=CARTESIAN_POINT('Ctrl Pts',(77.945290872253,9.08001456044151,132.14981310901));
#61240=CARTESIAN_POINT('Ctrl Pts',(77.9498868100455,9.15881521208162,132.145551498605));
#61241=CARTESIAN_POINT('Ctrl Pts',(77.9589591217713,9.23695927054993,132.141289888199));
#61242=CARTESIAN_POINT('Ctrl Pts',(77.9680642943238,9.31538637466667,132.137012841811));
#61243=CARTESIAN_POINT('Ctrl Pts',(77.9816781914328,9.39315183738754,132.132735795423));
#61244=CARTESIAN_POINT('Ctrl Pts',(77.9996710506677,9.46976766274754,132.128458749035));
#61245=CARTESIAN_POINT('Ctrl Pts',(78.0177509651587,9.5467541801807,132.124161008917));
#61246=CARTESIAN_POINT('Ctrl Pts',(78.0402521766353,9.62257963403658,132.1198632688));
#61247=CARTESIAN_POINT('Ctrl Pts',(78.0669947748148,9.69676994905539,132.115565528682));
#61248=CARTESIAN_POINT('Ctrl Pts',(78.0794747989849,9.73139249838321,132.113559893321));
#61249=CARTESIAN_POINT('Ctrl Pts',(78.092877854504,9.76565926600136,132.11155425796));
#61250=CARTESIAN_POINT('Ctrl Pts',(78.1071822245978,9.79952387808082,132.109548622599));
#61251=CARTESIAN_POINT('Ctrl Pts',(78.1347768681956,9.86485229833167,132.105679539752));
#61252=CARTESIAN_POINT('Ctrl Pts',(78.1658116320374,9.92887839899923,132.101810456905));
#61253=CARTESIAN_POINT('Ctrl Pts',(78.2001418722774,9.9912155580755,132.097941374058));
#61254=CARTESIAN_POINT('Ctrl Pts',(78.2344209621716,10.0534598378936,132.094078055952));
#61255=CARTESIAN_POINT('Ctrl Pts',(78.2719855496265,10.1140197491266,132.090214737845));
#61256=CARTESIAN_POINT('Ctrl Pts',(78.3126431435276,10.1725290620772,132.086351419739));
#61257=CARTESIAN_POINT('Ctrl Pts',(78.3532530460867,10.2309697436262,132.082492633303));
#61258=CARTESIAN_POINT('Ctrl Pts',(78.3969484726027,10.2873642077462,132.078633846867));
#61259=CARTESIAN_POINT('Ctrl Pts',(78.4434921636946,10.3413727736987,132.074775060431));
#61260=CARTESIAN_POINT('Ctrl Pts',(78.4900065356741,10.3953473182149,132.070918704748));
#61261=CARTESIAN_POINT('Ctrl Pts',(78.5393652961919,10.4469385792557,132.067062349065));
#61262=CARTESIAN_POINT('Ctrl Pts',(78.5912901108146,10.4958388986155,132.063205993381));
#61263=CARTESIAN_POINT('Ctrl Pts',(78.6431995863272,10.5447247723314,132.059350776904));
#61264=CARTESIAN_POINT('Ctrl Pts',(78.6976732575757,10.59092094966,132.055495560427));
#61265=CARTESIAN_POINT('Ctrl Pts',(78.754396261352,10.6341569351706,132.051640343949));
#61266=CARTESIAN_POINT('Ctrl Pts',(78.8111214828281,10.6773946110789,132.047784976745));
#61267=CARTESIAN_POINT('Ctrl Pts',(78.8700958237476,10.7176715726603,132.04392960954));
#61268=CARTESIAN_POINT('Ctrl Pts',(78.9309730915489,10.7547589667836,132.040074242335));
#61269=CARTESIAN_POINT('Ctrl Pts',(78.9919140812491,10.7918851812953,132.036214839613));
#61270=CARTESIAN_POINT('Ctrl Pts',(79.0547615582919,10.8258149104839,132.03235543689));
#61271=CARTESIAN_POINT('Ctrl Pts',(79.1191429984107,10.8563643244932,132.028496034167));
#61272=CARTESIAN_POINT('Ctrl Pts',(79.1835608918065,10.8869310358206,132.02463444622));
#61273=CARTESIAN_POINT('Ctrl Pts',(79.2495140279323,10.9141134366664,132.020772858273));
#61274=CARTESIAN_POINT('Ctrl Pts',(79.3166106344549,10.9377761835568,132.016911270326));
#61275=CARTESIAN_POINT('Ctrl Pts',(79.3838246288955,10.961480329271,132.013042926392));
#61276=CARTESIAN_POINT('Ctrl Pts',(79.4521856218031,10.981652389358,132.009174582459));
#61277=CARTESIAN_POINT('Ctrl Pts',(79.5212881315139,10.9982073239458,132.005306238525));
#61278=CARTESIAN_POINT('Ctrl Pts',(79.5623192131717,11.0080371676917,132.00300932722));
#61279=CARTESIAN_POINT('Ctrl Pts',(79.6036115398423,11.0165927238093,132.000712415914));
#61280=CARTESIAN_POINT('Ctrl Pts',(79.6450793453087,11.023864840194,131.998415504608));
#61281=CARTESIAN_POINT('Ctrl Pts',(79.7149081391765,11.0361105597419,131.994547671615));
#61282=CARTESIAN_POINT('Ctrl Pts',(79.7855081655636,11.0447620939113,131.990679838623));
#61283=CARTESIAN_POINT('Ctrl Pts',(79.8564765514179,11.04973134391,131.98681200563));
#61284=CARTESIAN_POINT('Ctrl Pts',(79.9273493904378,11.0546939036607,131.982949380016));
#61285=CARTESIAN_POINT('Ctrl Pts',(79.9985891252934,11.0559839786253,131.979086754401));
#61286=CARTESIAN_POINT('Ctrl Pts',(80.069783895318,11.0535646496895,131.975224128786));
#61287=CARTESIAN_POINT('Ctrl Pts',(80.1409066359359,11.0511477684451,131.97136541108));
#61288=CARTESIAN_POINT('Ctrl Pts',(80.2119840191092,11.0450289459532,131.967506693374));
#61289=CARTESIAN_POINT('Ctrl Pts',(80.2826020050072,11.0352232480163,131.963647975667));
#61290=CARTESIAN_POINT('Ctrl Pts',(80.3531721706576,11.0254241901852,131.959791870961));
#61291=CARTESIAN_POINT('Ctrl Pts',(80.4232830766721,11.011943279796,131.955935766256));
#61292=CARTESIAN_POINT('Ctrl Pts',(80.4925253618703,10.9948474453989,131.95207966155));
#61293=CARTESIAN_POINT('Ctrl Pts',(80.5617703013114,10.9777509556725,131.948223409029));
#61294=CARTESIAN_POINT('Ctrl Pts',(80.6301460772591,10.9570393630094,131.944367156508));
#61295=CARTESIAN_POINT('Ctrl Pts',(80.6972543344538,10.9328305553217,131.940510903988));
#61296=CARTESIAN_POINT('Ctrl Pts',(80.7643590610101,10.9086230212858,131.936654854349));
#61297=CARTESIAN_POINT('Ctrl Pts',(80.830195946503,10.8809188100334,131.93279880471));
#61298=CARTESIAN_POINT('Ctrl Pts',(80.8943847491103,10.8498847215594,131.928942755071));
#61299=CARTESIAN_POINT('Ctrl Pts',(80.9586397009917,10.8188186511455,131.925082731609));
#61300=CARTESIAN_POINT('Ctrl Pts',(81.0212427411801,10.7844160658132,131.921222708148));
#61301=CARTESIAN_POINT('Ctrl Pts',(81.0818372046246,10.7468903300408,131.917362684687));
#61302=CARTESIAN_POINT('Ctrl Pts',(81.1405565478585,10.7105258433588,131.913622111215));
#61303=CARTESIAN_POINT('Ctrl Pts',(81.1973895050298,10.671228977131,131.909881537743));
#61304=CARTESIAN_POINT('Ctrl Pts',(81.252039109102,10.6292316077769,131.906140964271));
#61305=CARTESIAN_POINT('Ctrl Pts',(81.252039109102,10.6292316077768,132.606087908811));
#61306=CARTESIAN_POINT('Ctrl Pts',(81.3085934766705,10.5857704573497,132.602232450677));
#61307=CARTESIAN_POINT('Ctrl Pts',(81.3628750366858,10.5393667122732,132.598376992543));
#61308=CARTESIAN_POINT('Ctrl Pts',(81.4145730936508,10.4902954489695,132.594521534409));
#61309=CARTESIAN_POINT('Ctrl Pts',(81.4663263957117,10.4411717475896,132.590661956291));
#61310=CARTESIAN_POINT('Ctrl Pts',(81.5154903318637,10.389375174002,132.586802378173));
#61311=CARTESIAN_POINT('Ctrl Pts',(81.5617909040319,10.3352178603446,132.582942800055));
#61312=CARTESIAN_POINT('Ctrl Pts',(81.6081191546343,10.281028171501,132.579080914685));
#61313=CARTESIAN_POINT('Ctrl Pts',(81.651580338457,10.2244753190296,132.575219029315));
#61314=CARTESIAN_POINT('Ctrl Pts',(81.6919423182945,10.1659025491285,132.571357143945));
#61315=CARTESIAN_POINT('Ctrl Pts',(81.732373615701,10.1072291864904,132.567488626183));
#61316=CARTESIAN_POINT('Ctrl Pts',(81.7696948311514,10.0465293960011,132.56362010842));
#61317=CARTESIAN_POINT('Ctrl Pts',(81.8037189047984,9.98417258393685,132.559751590658));
#61318=CARTESIAN_POINT('Ctrl Pts',(81.8203431338944,9.95370492329718,132.557861425294));
#61319=CARTESIAN_POINT('Ctrl Pts',(81.8361809518681,9.92284200712804,132.55597125993));
#61320=CARTESIAN_POINT('Ctrl Pts',(81.8512147628781,9.89162854608986,132.554081094566));
#61321=CARTESIAN_POINT('Ctrl Pts',(81.8819882927564,9.82773600578652,132.550212011719));
#61322=CARTESIAN_POINT('Ctrl Pts',(81.9095104472027,9.76212328485629,132.546342928872));
#61323=CARTESIAN_POINT('Ctrl Pts',(81.933586765323,9.6951545033067,132.542473846025));
#61324=CARTESIAN_POINT('Ctrl Pts',(81.9576272109301,9.62828550190184,132.538610527919));
#61325=CARTESIAN_POINT('Ctrl Pts',(81.9782318482965,9.5600649038539,132.534747209812));
#61326=CARTESIAN_POINT('Ctrl Pts',(81.9952531484607,9.49087924793937,132.530883891706));
#61327=CARTESIAN_POINT('Ctrl Pts',(82.0122544826464,9.42177474677252,132.52702510527));
#61328=CARTESIAN_POINT('Ctrl Pts',(82.0256807132235,9.35170790572679,132.523166318834));
#61329=CARTESIAN_POINT('Ctrl Pts',(82.0354338270114,9.28108130204246,132.519307532398));
#61330=CARTESIAN_POINT('Ctrl Pts',(82.0451807970527,9.2104991879396,132.515451176715));
#61331=CARTESIAN_POINT('Ctrl Pts',(82.0512591745402,9.13935849084858,132.511594821032));
#61332=CARTESIAN_POINT('Ctrl Pts',(82.053622127359,9.06807143689828,132.507738465349));
#61333=CARTESIAN_POINT('Ctrl Pts',(82.0559843821379,8.99680544185754,132.503883248871));
#61334=CARTESIAN_POINT('Ctrl Pts',(82.0546333751518,8.92539366104356,132.500028032394));
#61335=CARTESIAN_POINT('Ctrl Pts',(82.0495743065814,8.85425116020526,132.496172815917));
#61336=CARTESIAN_POINT('Ctrl Pts',(82.0445150402164,8.78310587790798,132.492317448712));
#61337=CARTESIAN_POINT('Ctrl Pts',(82.0357474610953,8.7122303808916,132.488462081508));
#61338=CARTESIAN_POINT('Ctrl Pts',(82.0233287253964,8.6420357119965,132.484606714303));
#61339=CARTESIAN_POINT('Ctrl Pts',(82.0108969906676,8.57176756842425,132.48074731158));
#61340=CARTESIAN_POINT('Ctrl Pts',(81.9948065550643,8.50218215489968,132.476887908857));
#61341=CARTESIAN_POINT('Ctrl Pts',(81.9751657636099,8.43368050646001,132.473028506135));
#61342=CARTESIAN_POINT('Ctrl Pts',(81.955513851385,8.36514007184891,132.469166918188));
#61343=CARTESIAN_POINT('Ctrl Pts',(81.932307739648,8.29768508346071,132.465305330241));
#61344=CARTESIAN_POINT('Ctrl Pts',(81.9057048777047,8.23169896421214,132.461443742294));
#61345=CARTESIAN_POINT('Ctrl Pts',(81.8790554731008,8.16559739988277,132.45757539836));
#61346=CARTESIAN_POINT('Ctrl Pts',(81.848997658377,8.10097027606216,132.453707054427));
#61347=CARTESIAN_POINT('Ctrl Pts',(81.8157356889673,8.0381780464605,132.449838710493));
#61348=CARTESIAN_POINT('Ctrl Pts',(81.7959856887279,8.00089382752599,132.447541799187));
#61349=CARTESIAN_POINT('Ctrl Pts',(81.7751068783498,7.96425601836013,132.44524488788));
#61350=CARTESIAN_POINT('Ctrl Pts',(81.7531490904374,7.92833502007459,132.442947976574));
#61351=CARTESIAN_POINT('Ctrl Pts',(81.7161618108982,7.86782710323811,132.439078893727));
#61352=CARTESIAN_POINT('Ctrl Pts',(81.6759658686668,7.80911778233093,132.43520981088));
#61353=CARTESIAN_POINT('Ctrl Pts',(81.6327617012439,7.75256792190871,132.431340728033));
#61354=CARTESIAN_POINT('Ctrl Pts',(81.5896219058757,7.69610231795813,132.427477409927));
#61355=CARTESIAN_POINT('Ctrl Pts',(81.5434830746862,7.64179017073909,132.42361409182));
#61356=CARTESIAN_POINT('Ctrl Pts',(81.4945899348819,7.58996507523763,132.419750773714));
#61357=CARTESIAN_POINT('Ctrl Pts',(81.4457541467119,7.53820077055332,132.415891987278));
#61358=CARTESIAN_POINT('Ctrl Pts',(81.3941707991377,7.48891807445518,132.412033200842));
#61359=CARTESIAN_POINT('Ctrl Pts',(81.3401249501949,7.44241768103089,132.408174414406));
#61360=CARTESIAN_POINT('Ctrl Pts',(81.2861131461738,7.39594657944474,132.404318058723));
#61361=CARTESIAN_POINT('Ctrl Pts',(81.2296422857038,7.3522546193917,132.40046170304));
#61362=CARTESIAN_POINT('Ctrl Pts',(81.1710332927737,7.31160472942042,132.396605347356));
#61363=CARTESIAN_POINT('Ctrl Pts',(81.112441613527,7.27096684783369,132.392750130879));
#61364=CARTESIAN_POINT('Ctrl Pts',(81.0517134547249,7.23336952894758,132.388894914402));
#61365=CARTESIAN_POINT('Ctrl Pts',(80.9892003473081,7.19903352741216,132.385039697925));
#61366=CARTESIAN_POINT('Ctrl Pts',(80.9266847958158,7.16469618344176,132.38118433072));
#61367=CARTESIAN_POINT('Ctrl Pts',(80.8623845840016,7.13362064190744,132.377328963515));
#61368=CARTESIAN_POINT('Ctrl Pts',(80.7966760429388,7.10598182556042,132.373473596311));
#61369=CARTESIAN_POINT('Ctrl Pts',(80.7308987229513,7.07831407890945,132.369614193588));
#61370=CARTESIAN_POINT('Ctrl Pts',(80.6637105797082,7.05409042722656,132.365754790865));
#61371=CARTESIAN_POINT('Ctrl Pts',(80.5955073002181,7.03343735978563,132.361895388142));
#61372=CARTESIAN_POINT('Ctrl Pts',(80.5272654034953,7.01277259841565,132.358033800195));
#61373=CARTESIAN_POINT('Ctrl Pts',(80.458007698179,6.99568256229063,132.354172212249));
#61374=CARTESIAN_POINT('Ctrl Pts',(80.3881417079493,6.98224293408492,132.350310624302));
#61375=CARTESIAN_POINT('Ctrl Pts',(80.3181534846654,6.96877979276795,132.346442280368));
#61376=CARTESIAN_POINT('Ctrl Pts',(80.2475553330518,6.95897987705045,132.342573936435));
#61377=CARTESIAN_POINT('Ctrl Pts',(80.1767608663212,6.95286708818471,132.338705592501));
#61378=CARTESIAN_POINT('Ctrl Pts',(80.1347251492656,6.94923749006711,132.336408681195));
#61379=CARTESIAN_POINT('Ctrl Pts',(80.0926202580339,6.94690684262272,132.334111769889));
#61380=CARTESIAN_POINT('Ctrl Pts',(80.0505323671528,6.94587146400963,132.331814858582));
#61381=CARTESIAN_POINT('Ctrl Pts',(79.9796364922357,6.94412739769725,132.327945775735));
#61382=CARTESIAN_POINT('Ctrl Pts',(79.9085113617539,6.9460545580838,132.324076692888));
#61383=CARTESIAN_POINT('Ctrl Pts',(79.8375688633129,6.95168027682821,132.320207610042));
#61384=CARTESIAN_POINT('Ctrl Pts',(79.7667320656567,6.95729761353225,132.316344291935));
#61385=CARTESIAN_POINT('Ctrl Pts',(79.696077840223,6.96660253198248,132.312480973829));
#61386=CARTESIAN_POINT('Ctrl Pts',(79.6260191864149,6.97957036411307,132.308617655722));
#61387=CARTESIAN_POINT('Ctrl Pts',(79.5560427113805,6.99252298498158,132.304758869287));
#61388=CARTESIAN_POINT('Ctrl Pts',(79.486660895656,7.00912989704807,132.300900082851));
#61389=CARTESIAN_POINT('Ctrl Pts',(79.4182809721592,7.02931470418336,132.297041296415));
#61390=CARTESIAN_POINT('Ctrl Pts',(79.349944123,7.04948679637026,132.293184940732));
#61391=CARTESIAN_POINT('Ctrl Pts',(79.2826083787462,7.07323217489448,132.289328585049));
#61392=CARTESIAN_POINT('Ctrl Pts',(79.2166686972246,7.10042382816793,132.285472229365));
#61393=CARTESIAN_POINT('Ctrl Pts',(79.150748494945,7.12760744875476,132.281617012888));
#61394=CARTESIAN_POINT('Ctrl Pts',(79.0862239854998,7.15823513785706,132.277761796411));
#61395=CARTESIAN_POINT('Ctrl Pts',(79.0234712956366,7.19213129568149,132.273906579934));
#61396=CARTESIAN_POINT('Ctrl Pts',(78.9607161523311,7.22602877874419,132.270051212729));
#61397=CARTESIAN_POINT('Ctrl Pts',(78.8997333925084,7.26319475142531,132.266195845525));
#61398=CARTESIAN_POINT('Ctrl Pts',(78.8408740891257,7.30340792020011,132.26234047832));
#61399=CARTESIAN_POINT('Ctrl Pts',(78.7819531761023,7.34366318119709,132.258481075597));
#61400=CARTESIAN_POINT('Ctrl Pts',(78.7251605584152,7.38697173080948,132.254621672874));
#61401=CARTESIAN_POINT('Ctrl Pts',(78.6708171167339,7.43306974458579,132.250762270152));
#61402=CARTESIAN_POINT('Ctrl Pts',(78.616442905369,7.47919385941963,132.246900682205));
#61403=CARTESIAN_POINT('Ctrl Pts',(78.5645209843359,7.52811024927646,132.243039094258));
#61404=CARTESIAN_POINT('Ctrl Pts',(78.5153359699768,7.57951758882584,132.239177506311));
#61405=CARTESIAN_POINT('Ctrl Pts',(78.4660649046721,7.6310148673584,132.235309162378));
#61406=CARTESIAN_POINT('Ctrl Pts',(78.4195406232418,7.68501142832933,132.231440818444));
#61407=CARTESIAN_POINT('Ctrl Pts',(78.3760075415854,7.74117274516616,132.227572474511));
#61408=CARTESIAN_POINT('Ctrl Pts',(78.35015885047,7.77451971892297,132.225275563204));
#61409=CARTESIAN_POINT('Ctrl Pts',(78.3253639320698,7.80862933347536,132.222978651898));
#61410=CARTESIAN_POINT('Ctrl Pts',(78.3016664325151,7.84342719379448,132.220681740591));
#61411=CARTESIAN_POINT('Ctrl Pts',(78.2611561583561,7.90291325300599,132.216755228997));
#61412=CARTESIAN_POINT('Ctrl Pts',(78.22369963522,7.96464047795975,132.212828717404));
#61413=CARTESIAN_POINT('Ctrl Pts',(78.1895485268499,8.02826802776241,132.20890220581));
#61414=CARTESIAN_POINT('Ctrl Pts',(78.155452465025,8.09179301934779,132.204982023173));
#61415=CARTESIAN_POINT('Ctrl Pts',(78.124651456215,8.15721184504486,132.201061840536));
#61416=CARTESIAN_POINT('Ctrl Pts',(78.0973541022693,8.22415455769291,132.1971416579));
#61417=CARTESIAN_POINT('Ctrl Pts',(78.0700989505562,8.29099377562381,132.19322753594));
#61418=CARTESIAN_POINT('Ctrl Pts',(78.0463368576601,8.3593517657761,132.189313413981));
#61419=CARTESIAN_POINT('Ctrl Pts',(78.0262298521907,8.4288354299182,132.185399292022));
#61420=CARTESIAN_POINT('Ctrl Pts',(78.0061411816452,8.49825573416795,132.181488739223));
#61421=CARTESIAN_POINT('Ctrl Pts',(77.9897011084489,8.56879922704156,132.177578186424));
#61422=CARTESIAN_POINT('Ctrl Pts',(77.9770226384295,8.64005534165216,132.173667633625));
#61423=CARTESIAN_POINT('Ctrl Pts',(77.9643515390461,8.71127003147841,132.169759354229));
#61424=CARTESIAN_POINT('Ctrl Pts',(77.9554377814962,8.78319606135745,132.165851074832));
#61425=CARTESIAN_POINT('Ctrl Pts',(77.950343495397,8.85541170296763,132.161942795435));
#61426=CARTESIAN_POINT('Ctrl Pts',(77.9469249211356,8.9038727687336,132.159320103444));
#61427=CARTESIAN_POINT('Ctrl Pts',(77.9452252851269,8.9524640140981,132.156697411453));
#61428=CARTESIAN_POINT('Ctrl Pts',(77.9452502716446,9.00105656201739,132.154074719462));
#61429=CARTESIAN_POINT('Origin',(80.,9.,141.545925280538));
#61430=CARTESIAN_POINT('',(81.252039109102,10.6292316077768,133.306011340678));
#61431=CARTESIAN_POINT('',(81.252039109102,10.6292316077768,133.247993489861));
#61432=CARTESIAN_POINT('',(81.252039109102,10.6292316077768,141.545925280538));
#61433=CARTESIAN_POINT('',(77.9452506345969,9.00161489178516,132.795925280579));
#61434=CARTESIAN_POINT('Ctrl Pts',(81.252039109102,10.6292316077768,133.247993489861));
#61435=CARTESIAN_POINT('Ctrl Pts',(81.3085458565354,10.5858070526816,133.244130559018));
#61436=CARTESIAN_POINT('Ctrl Pts',(81.3627300216765,10.5394860857007,133.240267628176));
#61437=CARTESIAN_POINT('Ctrl Pts',(81.4142959510654,10.4905584608797,133.236404697333));
#61438=CARTESIAN_POINT('Ctrl Pts',(81.4659453705785,10.4415516175995,133.232535512039));
#61439=CARTESIAN_POINT('Ctrl Pts',(81.5149677678158,10.3899300517469,133.228666326745));
#61440=CARTESIAN_POINT('Ctrl Pts',(81.5611066388145,10.3360178235148,133.224797141451));
#61441=CARTESIAN_POINT('Ctrl Pts',(81.5680176291622,10.3279424874507,133.224217588861));
#61442=CARTESIAN_POINT('Ctrl Pts',(81.5748640032644,10.3198158116359,133.22363803627));
#61443=CARTESIAN_POINT('Ctrl Pts',(81.5816449834367,10.3116389399791,133.223058483679));
#61444=CARTESIAN_POINT('Ctrl Pts',(81.6269146871559,10.2570502893934,133.219189400832));
#61445=CARTESIAN_POINT('Ctrl Pts',(81.6694436428746,10.200008321872,133.215320317985));
#61446=CARTESIAN_POINT('Ctrl Pts',(81.7089553397542,10.1408195340305,133.211451235138));
#61447=CARTESIAN_POINT('Ctrl Pts',(81.7484081661761,10.0817189345309,133.207587917032));
#61448=CARTESIAN_POINT('Ctrl Pts',(81.7848523898166,10.0204782646923,133.203724598926));
#61449=CARTESIAN_POINT('Ctrl Pts',(81.8180516424326,9.95743709346783,133.199861280819));
#61450=CARTESIAN_POINT('Ctrl Pts',(81.851211952338,9.8944698695129,133.196002494383));
#61451=CARTESIAN_POINT('Ctrl Pts',(81.88113462666,9.82970676703115,133.192143707948));
#61452=CARTESIAN_POINT('Ctrl Pts',(81.9076274856163,9.76351485815351,133.188284921512));
#61453=CARTESIAN_POINT('Ctrl Pts',(81.9341036560141,9.69736464532483,133.184428565829));
#61454=CARTESIAN_POINT('Ctrl Pts',(81.9571541174251,9.62978786170638,133.180572210145));
#61455=CARTESIAN_POINT('Ctrl Pts',(81.9766340351604,9.56117328299337,133.176715854462));
#61456=CARTESIAN_POINT('Ctrl Pts',(81.9961081983329,9.49257897371396,133.172860637985));
#61457=CARTESIAN_POINT('Ctrl Pts',(82.0120137792494,9.422947945037,133.169005421508));
#61458=CARTESIAN_POINT('Ctrl Pts',(82.0242557560879,9.35268427303351,133.16515020503));
#61459=CARTESIAN_POINT('Ctrl Pts',(82.036498211551,9.28241785393061,133.161294837826));
#61460=CARTESIAN_POINT('Ctrl Pts',(82.0450766973487,9.21151922134589,133.157439470621));
#61461=CARTESIAN_POINT('Ctrl Pts',(82.0499475849728,9.1404010732302,133.153584103417));
#61462=CARTESIAN_POINT('Ctrl Pts',(82.054823571088,9.06920848380641,133.149724700694));
#61463=CARTESIAN_POINT('Ctrl Pts',(82.055984178733,8.99779640581406,133.145865297971));
#61464=CARTESIAN_POINT('Ctrl Pts',(82.0534378710938,8.92658016577487,133.142005895248));
#61465=CARTESIAN_POINT('Ctrl Pts',(82.0508901217152,8.85532360254116,133.138144307301));
#61466=CARTESIAN_POINT('Ctrl Pts',(82.0446313214623,8.78426358213725,133.134282719354));
#61467=CARTESIAN_POINT('Ctrl Pts',(82.0347218354742,8.71381017707747,133.130421131407));
#61468=CARTESIAN_POINT('Ctrl Pts',(82.0247950124852,8.64323351126023,133.126552787474));
#61469=CARTESIAN_POINT('Ctrl Pts',(82.0112048445784,8.57326605671479,133.122684443541));
#61470=CARTESIAN_POINT('Ctrl Pts',(81.9940626600268,8.50430687881827,133.118816099607));
#61471=CARTESIAN_POINT('Ctrl Pts',(81.9838841241492,8.46336090345577,133.116519188301));
#61472=CARTESIAN_POINT('Ctrl Pts',(81.972454231622,8.42277012445263,133.114222276994));
#61473=CARTESIAN_POINT('Ctrl Pts',(81.9598043720399,8.38261488045671,133.111925365688));
#61474=CARTESIAN_POINT('Ctrl Pts',(81.9384960374133,8.31497449516047,133.108056282841));
#61475=CARTESIAN_POINT('Ctrl Pts',(81.9136400623008,8.24830607209196,133.104187199994));
#61476=CARTESIAN_POINT('Ctrl Pts',(81.8853439706103,8.1830081548855,133.100318117147));
#61477=CARTESIAN_POINT('Ctrl Pts',(81.8570900386851,8.1178075283191,133.096454799041));
#61478=CARTESIAN_POINT('Ctrl Pts',(81.8254063559397,8.05397379643129,133.092591480934));
#61479=CARTESIAN_POINT('Ctrl Pts',(81.7904500040001,7.99188971551923,133.088728162828));
#61480=CARTESIAN_POINT('Ctrl Pts',(81.755534655848,7.92987845921018,133.084869376392));
#61481=CARTESIAN_POINT('Ctrl Pts',(81.7173545009174,7.86961319847797,133.081010589956));
#61482=CARTESIAN_POINT('Ctrl Pts',(81.6761136941158,7.81145448261441,133.07715180352));
#61483=CARTESIAN_POINT('Ctrl Pts',(81.6348988659985,7.75333240247726,133.073295447837));
#61484=CARTESIAN_POINT('Ctrl Pts',(81.5906274914358,7.69731462985278,133.069439092154));
#61485=CARTESIAN_POINT('Ctrl Pts',(81.5435476382642,7.64373370944009,133.065582736471));
#61486=CARTESIAN_POINT('Ctrl Pts',(81.4964816929526,7.59016861736779,133.061727519993));
#61487=CARTESIAN_POINT('Ctrl Pts',(81.4466092365961,7.5390393130905,133.057872303516));
#61488=CARTESIAN_POINT('Ctrl Pts',(81.3942182089018,7.49064479049277,133.054017087039));
#61489=CARTESIAN_POINT('Ctrl Pts',(81.341825132875,7.44224837581396,133.050161719834));
#61490=CARTESIAN_POINT('Ctrl Pts',(81.2869136483497,7.39658728309613,133.04630635263));
#61491=CARTESIAN_POINT('Ctrl Pts',(81.229806813281,7.35392200533889,133.042450985425));
#61492=CARTESIAN_POINT('Ctrl Pts',(81.1726402029284,7.31121206867012,133.038591582702));
#61493=CARTESIAN_POINT('Ctrl Pts',(81.1132740448049,7.27150449807019,133.034732179979));
#61494=CARTESIAN_POINT('Ctrl Pts',(81.052061858725,7.23501744826862,133.030872777257));
#61495=CARTESIAN_POINT('Ctrl Pts',(80.9908150138244,7.19850973921284,133.02701118931));
#61496=CARTESIAN_POINT('Ctrl Pts',(80.9277204900948,7.16522640771259,133.023149601363));
#61497=CARTESIAN_POINT('Ctrl Pts',(80.8631555438834,7.13533915427942,133.019288013416));
#61498=CARTESIAN_POINT('Ctrl Pts',(80.7984776389843,7.1053996120251,133.015419669482));
#61499=CARTESIAN_POINT('Ctrl Pts',(80.7323246264365,7.07886819121591,133.011551325549));
#61500=CARTESIAN_POINT('Ctrl Pts',(80.6650921565278,7.05586780649431,133.007682981615));
#61501=CARTESIAN_POINT('Ctrl Pts',(80.6251714506782,7.04221083994012,133.005386070309));
#61502=CARTESIAN_POINT('Ctrl Pts',(80.5848704458188,7.02979783101441,133.003089159003));
#61503=CARTESIAN_POINT('Ctrl Pts',(80.5442736622037,7.0186459823819,133.000792247696));
#61504=CARTESIAN_POINT('Ctrl Pts',(80.4758895157695,6.99986100529781,132.996923164849));
#61505=CARTESIAN_POINT('Ctrl Pts',(80.4063977765704,6.98458369151803,132.993054082002));
#61506=CARTESIAN_POINT('Ctrl Pts',(80.3361915931481,6.97293986887499,132.989184999155));
#61507=CARTESIAN_POINT('Ctrl Pts',(80.2660900134378,6.96131339494699,132.985321681049));
#61508=CARTESIAN_POINT('Ctrl Pts',(80.1952765778126,6.95330974490485,132.981458362943));
#61509=CARTESIAN_POINT('Ctrl Pts',(80.1241580504811,6.94900454876157,132.977595044836));
#61510=CARTESIAN_POINT('Ctrl Pts',(80.0531229451549,6.94470440261171,132.9737362584));
#61511=CARTESIAN_POINT('Ctrl Pts',(79.9817839415205,6.94409412226872,132.969877471965));
#61512=CARTESIAN_POINT('Ctrl Pts',(79.9105546785681,6.94719774528233,132.966018685529));
#61513=CARTESIAN_POINT('Ctrl Pts',(79.8393702848284,6.95029941324102,132.962162329846));
#61514=CARTESIAN_POINT('Ctrl Pts',(79.7682959787961,6.95711032195449,132.958305974162));
#61515=CARTESIAN_POINT('Ctrl Pts',(79.6977456893852,6.96760242712831,132.954449618479));
#61516=CARTESIAN_POINT('Ctrl Pts',(79.6272162412362,6.97809143282919,132.950594402002));
#61517=CARTESIAN_POINT('Ctrl Pts',(79.557210982625,6.99225940465597,132.946739185525));
#61518=CARTESIAN_POINT('Ctrl Pts',(79.4881372810345,7.01002660333531,132.942883969047));
#61519=CARTESIAN_POINT('Ctrl Pts',(79.4190608788688,7.02779449665898,132.939028601843));
#61520=CARTESIAN_POINT('Ctrl Pts',(79.3509165759529,7.04916177306653,132.935173234638));
#61521=CARTESIAN_POINT('Ctrl Pts',(79.2840984413495,7.07399830716018,132.931317867434));
#61522=CARTESIAN_POINT('Ctrl Pts',(79.2172103663797,7.09886083833244,132.927458464711));
#61523=CARTESIAN_POINT('Ctrl Pts',(79.1516516870314,7.12719970661276,132.923599061988));
#61524=CARTESIAN_POINT('Ctrl Pts',(79.0877974244993,7.15883623114352,132.919739659265));
#61525=CARTESIAN_POINT('Ctrl Pts',(79.023907007182,7.19049066852297,132.915878071318));
#61526=CARTESIAN_POINT('Ctrl Pts',(78.9617233514694,7.2254462409346,132.912016483371));
#61527=CARTESIAN_POINT('Ctrl Pts',(78.9015953250588,7.26347912982095,132.908154895425));
#61528=CARTESIAN_POINT('Ctrl Pts',(78.8413621025109,7.30157855860964,132.904286551491));
#61529=CARTESIAN_POINT('Ctrl Pts',(78.783192086163,7.34276577212785,132.900418207558));
#61530=CARTESIAN_POINT('Ctrl Pts',(78.7274031336019,7.38677503796476,132.896549863624));
#61531=CARTESIAN_POINT('Ctrl Pts',(78.6942772590376,7.41290647354205,132.894252952318));
#61532=CARTESIAN_POINT('Ctrl Pts',(78.6619902077257,7.44003210903366,132.891956041011));
#61533=CARTESIAN_POINT('Ctrl Pts',(78.6306022743162,7.46809026656532,132.889659129705));
#61534=CARTESIAN_POINT('Ctrl Pts',(78.5772314750466,7.51579924676339,132.885753552658));
#61535=CARTESIAN_POINT('Ctrl Pts',(78.5262345230156,7.56641041597008,132.881847975611));
#61536=CARTESIAN_POINT('Ctrl Pts',(78.477949149806,7.6196526625796,132.877942398564));
#61537=CARTESIAN_POINT('Ctrl Pts',(78.4309056772215,7.67152551769528,132.874137273026));
#61538=CARTESIAN_POINT('Ctrl Pts',(78.3864363620088,7.72589535691467,132.870332147487));
#61539=CARTESIAN_POINT('Ctrl Pts',(78.3448201620119,7.78247083549608,132.866527021949));
#61540=CARTESIAN_POINT('Ctrl Pts',(78.3032434930467,7.83899257329763,132.862725510881));
#61541=CARTESIAN_POINT('Ctrl Pts',(78.2645148635039,7.89771539628927,132.858923999814));
#61542=CARTESIAN_POINT('Ctrl Pts',(78.2288739527535,7.95831382496211,132.855122488746));
#61543=CARTESIAN_POINT('Ctrl Pts',(78.1932541443471,8.0188763743923,132.851323228485));
#61544=CARTESIAN_POINT('Ctrl Pts',(78.1607186828807,8.08131189584067,132.847523968224));
#61545=CARTESIAN_POINT('Ctrl Pts',(78.1314636677262,8.14526639385559,132.843724707962));
#61546=CARTESIAN_POINT('Ctrl Pts',(78.100791622899,8.21231866573619,132.839741422347));
#61547=CARTESIAN_POINT('Ctrl Pts',(78.0737261978919,8.28104029941798,132.835758136732));
#61548=CARTESIAN_POINT('Ctrl Pts',(78.0504379098928,8.35099674937886,132.831774851116));
#61549=CARTESIAN_POINT('Ctrl Pts',(78.0282173314799,8.4177458715944,132.827974189155));
#61550=CARTESIAN_POINT('Ctrl Pts',(78.009435232024,8.48561853618905,132.824173527193));
#61551=CARTESIAN_POINT('Ctrl Pts',(77.9941886715372,8.55422149321622,132.820372865231));
#61552=CARTESIAN_POINT('Ctrl Pts',(77.9789361563187,8.6228512439721,132.816570718874));
#61553=CARTESIAN_POINT('Ctrl Pts',(77.9672220126629,8.69221136049643,132.812768572516));
#61554=CARTESIAN_POINT('Ctrl Pts',(77.9590918603005,8.76190017259942,132.808966426159));
#61555=CARTESIAN_POINT('Ctrl Pts',(77.950951700675,8.83167476344796,132.805159599806));
#61556=CARTESIAN_POINT('Ctrl Pts',(77.9464043599199,8.9017783571423,132.801352773453));
#61557=CARTESIAN_POINT('Ctrl Pts',(77.9454434209989,8.97180733812918,132.797545947101));
#61558=CARTESIAN_POINT('Ctrl Pts',(77.9453070553061,8.98174506705064,132.797005724927));
#61559=CARTESIAN_POINT('Ctrl Pts',(77.9452428274764,8.99168129996617,132.796465502753));
#61560=CARTESIAN_POINT('Ctrl Pts',(77.9452506345969,9.00161489178516,132.795925280579));
#61561=CARTESIAN_POINT('Ctrl Pts',(77.9452506345975,9.0016148925345,132.795925280538));
#61562=CARTESIAN_POINT('Ctrl Pts',(77.9453344508848,9.1082606658194,132.790125524263));
#61563=CARTESIAN_POINT('Ctrl Pts',(77.9537227446016,9.21458734448351,132.784325767988));
#61564=CARTESIAN_POINT('Ctrl Pts',(77.9702575839437,9.3195986341677,132.778526011713));
#61565=CARTESIAN_POINT('Ctrl Pts',(77.9812881618236,9.38965285030926,132.774656928866));
#61566=CARTESIAN_POINT('Ctrl Pts',(77.9959713625728,9.45927254399561,132.770787846019));
#61567=CARTESIAN_POINT('Ctrl Pts',(78.0142600200556,9.52804762526732,132.766918763172));
#61568=CARTESIAN_POINT('Ctrl Pts',(78.0325214283509,9.59672023509799,132.763055445066));
#61569=CARTESIAN_POINT('Ctrl Pts',(78.0543775063823,9.66455026482023,132.759192126959));
#61570=CARTESIAN_POINT('Ctrl Pts',(78.0797297357173,9.73113587971839,132.755328808853));
#61571=CARTESIAN_POINT('Ctrl Pts',(78.105052226897,9.79764338971588,132.751470022417));
#61572=CARTESIAN_POINT('Ctrl Pts',(78.1338625514211,9.86290893255779,132.747611235981));
#61573=CARTESIAN_POINT('Ctrl Pts',(78.1660123424271,9.92654564613423,132.743752449546));
#61574=CARTESIAN_POINT('Ctrl Pts',(78.1981418814222,9.9901422732474,132.739896093862));
#61575=CARTESIAN_POINT('Ctrl Pts',(78.2336064948162,10.0521116741827,132.736039738179));
#61576=CARTESIAN_POINT('Ctrl Pts',(78.2722102319607,10.1120881619543,132.732183382496));
#61577=CARTESIAN_POINT('Ctrl Pts',(78.3108025651747,10.1720469320708,132.728328166018));
#61578=CARTESIAN_POINT('Ctrl Pts',(78.3525319183583,10.2300135495482,132.724472949541));
#61579=CARTESIAN_POINT('Ctrl Pts',(78.3971579299853,10.2856495872091,132.720617733064));
#61580=CARTESIAN_POINT('Ctrl Pts',(78.4417856863558,10.3412878000726,132.716762365859));
#61581=CARTESIAN_POINT('Ctrl Pts',(78.4893100203429,10.3945948746504,132.712906998655));
#61582=CARTESIAN_POINT('Ctrl Pts',(78.5394501256207,10.4452652444969,132.70905163145));
#61583=CARTESIAN_POINT('Ctrl Pts',(78.5896427139162,10.4959886524034,132.705192228727));
#61584=CARTESIAN_POINT('Ctrl Pts',(78.6424561967735,10.5440695001681,132.701332826004));
#61585=CARTESIAN_POINT('Ctrl Pts',(78.6975733581752,10.5892395682102,132.697473423282));
#61586=CARTESIAN_POINT('Ctrl Pts',(78.7527217273466,10.6344352118997,132.693611835335));
#61587=CARTESIAN_POINT('Ctrl Pts',(78.8101759802012,10.6767165069286,132.689750247388));
#61588=CARTESIAN_POINT('Ctrl Pts',(78.8695885307946,10.7158576493371,132.685888659441));
#61589=CARTESIAN_POINT('Ctrl Pts',(78.9291050257748,10.7550672705773,132.682020315507));
#61590=CARTESIAN_POINT('Ctrl Pts',(78.990586239659,10.7911255248144,132.678151971574));
#61591=CARTESIAN_POINT('Ctrl Pts',(79.0536591538181,10.8238521226645,132.674283627641));
#61592=CARTESIAN_POINT('Ctrl Pts',(79.0911100351655,10.8432842346785,132.671986716334));
#61593=CARTESIAN_POINT('Ctrl Pts',(79.1291216747157,10.8615426311578,132.669689805028));
#61594=CARTESIAN_POINT('Ctrl Pts',(79.1676130426291,10.8785977525002,132.667392893721));
#61595=CARTESIAN_POINT('Ctrl Pts',(79.2324506752055,10.9073266273387,132.663523810874));
#61596=CARTESIAN_POINT('Ctrl Pts',(79.2989043618557,10.9327511364559,132.659654728027));
#61597=CARTESIAN_POINT('Ctrl Pts',(79.3666039904561,10.954688480959,132.65578564518));
#61598=CARTESIAN_POINT('Ctrl Pts',(79.4342027499863,10.9765931399129,132.651922327074));
#61599=CARTESIAN_POINT('Ctrl Pts',(79.5030433082192,10.995020799049,132.648059008968));
#61600=CARTESIAN_POINT('Ctrl Pts',(79.5727346360594,11.0098362797195,132.644195690861));
#61601=CARTESIAN_POINT('Ctrl Pts',(79.642344215999,11.0246343818369,132.640336904425));
#61602=CARTESIAN_POINT('Ctrl Pts',(79.7128021104158,11.0358286212486,132.63647811799));
#61603=CARTESIAN_POINT('Ctrl Pts',(79.7837028323885,11.0433338194684,132.632619331554));
#61604=CARTESIAN_POINT('Ctrl Pts',(79.8545588921052,11.0508342899636,132.628762975871));
#61605=CARTESIAN_POINT('Ctrl Pts',(79.9258567440054,11.0546502786843,132.624906620187));
#61606=CARTESIAN_POINT('Ctrl Pts',(79.9971828825806,11.0547480688273,132.621050264504));
#61607=CARTESIAN_POINT('Ctrl Pts',(80.0684879507002,11.0548458300821,132.617195048027));
#61608=CARTESIAN_POINT('Ctrl Pts',(80.1398208033875,11.0512275727087,132.61333983155));
#61609=CARTESIAN_POINT('Ctrl Pts',(80.2107667494145,11.0439116761351,132.609484615072));
#61610=CARTESIAN_POINT('Ctrl Pts',(80.2817154692159,11.0365954935317,132.605629247868));
#61611=CARTESIAN_POINT('Ctrl Pts',(80.3522767693298,11.0255814367308,132.601773880663));
#61612=CARTESIAN_POINT('Ctrl Pts',(80.4220416294529,11.0109396871882,132.597918513458));
#61613=CARTESIAN_POINT('Ctrl Pts',(80.4918795143607,10.9962826117265,132.594059110736));
#61614=CARTESIAN_POINT('Ctrl Pts',(80.560918818715,10.9779903634344,132.590199708013));
#61615=CARTESIAN_POINT('Ctrl Pts',(80.628762150649,10.9561839689588,132.58634030529));
#61616=CARTESIAN_POINT('Ctrl Pts',(80.6966438960105,10.9343652275313,132.582478717343));
#61617=CARTESIAN_POINT('Ctrl Pts',(80.7633278665926,10.9090285515885,132.578617129396));
#61618=CARTESIAN_POINT('Ctrl Pts',(80.8284358332439,10.8803434879557,132.574755541449));
#61619=CARTESIAN_POINT('Ctrl Pts',(80.8936577086166,10.8516082387759,132.570887197516));
#61620=CARTESIAN_POINT('Ctrl Pts',(80.9572976411981,10.8195131248122,132.567018853582));
#61621=CARTESIAN_POINT('Ctrl Pts',(81.0190018459501,10.7842737459399,132.563150509649));
#61622=CARTESIAN_POINT('Ctrl Pts',(81.0556400270381,10.7633496168672,132.560853598343));
#61623=CARTESIAN_POINT('Ctrl Pts',(81.0915962750952,10.7413177760724,132.558556687036));
#61624=CARTESIAN_POINT('Ctrl Pts',(81.1268018071315,10.7182302668575,132.55625977573));
#61625=CARTESIAN_POINT('Ctrl Pts',(81.1695802906112,10.690176476035,132.553468783045));
#61626=CARTESIAN_POINT('Ctrl Pts',(81.2113708104195,10.660484561751,132.55067779036));
#61627=CARTESIAN_POINT('Ctrl Pts',(81.252039109102,10.6292316077768,132.547886797676));
#61628=CARTESIAN_POINT('',(77.9452507493435,8.99824517046231,132.854074719498));
#61629=CARTESIAN_POINT('Ctrl Pts',(77.945250749343,8.99824517113454,132.854074719462));
#61630=CARTESIAN_POINT('Ctrl Pts',(77.9451902335234,9.0691038384727,132.850240467841));
#61631=CARTESIAN_POINT('Ctrl Pts',(77.9487993838056,9.14002687651476,132.846406216221));
#61632=CARTESIAN_POINT('Ctrl Pts',(77.9560714877068,9.21060341672155,132.8425719646));
#61633=CARTESIAN_POINT('Ctrl Pts',(77.9633409049725,9.28115388284672,132.838739129521));
#61634=CARTESIAN_POINT('Ctrl Pts',(77.9742705404255,9.35135761627535,132.834906294442));
#61635=CARTESIAN_POINT('Ctrl Pts',(77.988801718831,9.42080760012499,132.831073459363));
#61636=CARTESIAN_POINT('Ctrl Pts',(78.0033325301936,9.4902558297379,132.827240721097));
#61637=CARTESIAN_POINT('Ctrl Pts',(78.0214646012843,9.5589498665225,132.823407982832));
#61638=CARTESIAN_POINT('Ctrl Pts',(78.0430882613477,9.62649342344899,132.819575244566));
#61639=CARTESIAN_POINT('Ctrl Pts',(78.0647340638349,9.69410614433997,132.815738581613));
#61640=CARTESIAN_POINT('Ctrl Pts',(78.0898784440369,9.76056556353255,132.811901918659));
#61641=CARTESIAN_POINT('Ctrl Pts',(78.1183622815559,9.82549201027531,132.808065255706));
#61642=CARTESIAN_POINT('Ctrl Pts',(78.1468610721474,9.89045254125519,132.804226578632));
#61643=CARTESIAN_POINT('Ctrl Pts',(78.1787025884923,9.95387805807839,132.800387901557));
#61644=CARTESIAN_POINT('Ctrl Pts',(78.2136813665789,10.0154128728713,132.796549224483));
#61645=CARTESIAN_POINT('Ctrl Pts',(78.2487243400171,10.0770606203989,132.792703502416));
#61646=CARTESIAN_POINT('Ctrl Pts',(78.2869158076442,10.1368103218298,132.788857780349));
#61647=CARTESIAN_POINT('Ctrl Pts',(78.3280069113271,10.1943352435268,132.785012058282));
#61648=CARTESIAN_POINT('Ctrl Pts',(78.3588674553705,10.2375380348978,132.782123815704));
#61649=CARTESIAN_POINT('Ctrl Pts',(78.3913626087631,10.2794865660436,132.779235573126));
#61650=CARTESIAN_POINT('Ctrl Pts',(78.4253729722414,10.3200557889544,132.776347330549));
#61651=CARTESIAN_POINT('Ctrl Pts',(78.4709331737856,10.3744022229021,132.772478247702));
#61652=CARTESIAN_POINT('Ctrl Pts',(78.5193994699275,10.4264936451473,132.768609164855));
#61653=CARTESIAN_POINT('Ctrl Pts',(78.5705200716174,10.4760029460849,132.764740082008));
#61654=CARTESIAN_POINT('Ctrl Pts',(78.6215645061603,10.5254384806333,132.760876763902));
#61655=CARTESIAN_POINT('Ctrl Pts',(78.6752550500033,10.5722991953193,132.757013445795));
#61656=CARTESIAN_POINT('Ctrl Pts',(78.7313001635045,10.6162915230169,132.753150127689));
#61657=CARTESIAN_POINT('Ctrl Pts',(78.7872795361092,10.6602322477311,132.749291341253));
#61658=CARTESIAN_POINT('Ctrl Pts',(78.8456076120167,10.7013109702352,132.745432554817));
#61659=CARTESIAN_POINT('Ctrl Pts',(78.9059578520073,10.73927264709,132.741573768381));
#61660=CARTESIAN_POINT('Ctrl Pts',(78.966270075772,10.777210410872,132.737717412698));
#61661=CARTESIAN_POINT('Ctrl Pts',(79.0286015261645,10.8120347665365,132.733861057015));
#61662=CARTESIAN_POINT('Ctrl Pts',(79.0925958019739,10.8435333422275,132.730004701331));
#61663=CARTESIAN_POINT('Ctrl Pts',(79.1565711732334,10.8750226129239,132.726149484854));
#61664=CARTESIAN_POINT('Ctrl Pts',(79.2222079591012,10.9031878397086,132.722294268377));
#61665=CARTESIAN_POINT('Ctrl Pts',(79.2891257515502,10.9278629010879,132.7184390519));
#61666=CARTESIAN_POINT('Ctrl Pts',(79.3560461602849,10.9525389271883,132.714583684695));
#61667=CARTESIAN_POINT('Ctrl Pts',(79.4242472184884,10.9737243509719,132.710728317491));
#61668=CARTESIAN_POINT('Ctrl Pts',(79.4933307968446,10.9913020567141,132.706872950286));
#61669=CARTESIAN_POINT('Ctrl Pts',(79.5624866868691,11.0088981615211,132.703013547563));
#61670=CARTESIAN_POINT('Ctrl Pts',(79.6325264693269,11.0228788899197,132.69915414484));
#61671=CARTESIAN_POINT('Ctrl Pts',(79.7030400637026,11.0331778964799,132.695294742118));
#61672=CARTESIAN_POINT('Ctrl Pts',(79.7735935834293,11.0434827344185,132.691433154171));
#61673=CARTESIAN_POINT('Ctrl Pts',(79.8446209652123,11.0501016555882,132.687571566224));
#61674=CARTESIAN_POINT('Ctrl Pts',(79.9157079655849,11.0530203153973,132.683709978277));
#61675=CARTESIAN_POINT('Ctrl Pts',(79.9869193352128,11.0559440815064,132.679841634343));
#61676=CARTESIAN_POINT('Ctrl Pts',(80.0581900457709,11.0551546666323,132.67597329041));
#61677=CARTESIAN_POINT('Ctrl Pts',(80.1291075190145,11.0506898378433,132.672104946476));
#61678=CARTESIAN_POINT('Ctrl Pts',(80.1712162737992,11.048038750995,132.66980803517));
#61679=CARTESIAN_POINT('Ctrl Pts',(80.2132005988816,11.0440928378389,132.667511123864));
#61680=CARTESIAN_POINT('Ctrl Pts',(80.2549758212296,11.0388685325661,132.665214212557));
#61681=CARTESIAN_POINT('Ctrl Pts',(80.3253420978994,11.030068701241,132.661345290086));
#61682=CARTESIAN_POINT('Ctrl Pts',(80.3953900995657,11.0176045939,132.657476367615));
#61683=CARTESIAN_POINT('Ctrl Pts',(80.4647084963187,11.0015103237179,132.653607445144));
#61684=CARTESIAN_POINT('Ctrl Pts',(80.5356580112831,10.9850373422783,132.649647483783));
#61685=CARTESIAN_POINT('Ctrl Pts',(80.6058426316095,10.9647611560803,132.645687522422));
#61686=CARTESIAN_POINT('Ctrl Pts',(80.6748265776872,10.9407747557475,132.641727561061));
#61687=CARTESIAN_POINT('Ctrl Pts',(80.7420453187134,10.9174021346699,132.637868929708));
#61688=CARTESIAN_POINT('Ctrl Pts',(80.8081236063342,10.890507073603,132.634010298355));
#61689=CARTESIAN_POINT('Ctrl Pts',(80.8726704982589,10.8602268044431,132.630151667001));
#61690=CARTESIAN_POINT('Ctrl Pts',(80.9397599511857,10.8287537678361,132.626141040636));
#61691=CARTESIAN_POINT('Ctrl Pts',(81.0051943248821,10.793623421345,132.622130414271));
#61692=CARTESIAN_POINT('Ctrl Pts',(81.0685566242506,10.7550453849602,132.618119787906));
#61693=CARTESIAN_POINT('Ctrl Pts',(81.1319189236191,10.7164673485754,132.614109161541));
#61694=CARTESIAN_POINT('Ctrl Pts',(81.1932086330005,10.6744419121526,132.610098535176));
#61695=CARTESIAN_POINT('Ctrl Pts',(81.252039109102,10.6292316077768,132.606087908811));
#61696=CARTESIAN_POINT('Ctrl Pts',(81.252039109102,10.6292316077768,133.306011340678));
#61697=CARTESIAN_POINT('Ctrl Pts',(81.3084857783771,10.5858532218103,133.30215326156));
#61698=CARTESIAN_POINT('Ctrl Pts',(81.362733635988,10.539493193464,133.298295182442));
#61699=CARTESIAN_POINT('Ctrl Pts',(81.4144559732381,10.4904066097113,133.294437103324));
#61700=CARTESIAN_POINT('Ctrl Pts',(81.4661499193566,10.4413469702873,133.29058114196));
#61701=CARTESIAN_POINT('Ctrl Pts',(81.5153207440633,10.3895640788887,133.286725180597));
#61702=CARTESIAN_POINT('Ctrl Pts',(81.5616759642891,10.3353522924913,133.282869219233));
#61703=CARTESIAN_POINT('Ctrl Pts',(81.6080212459527,10.2811521291042,133.279014084588));
#61704=CARTESIAN_POINT('Ctrl Pts',(81.651551806428,10.2245244740596,133.275158949943));
#61705=CARTESIAN_POINT('Ctrl Pts',(81.6920142683062,10.1657981293296,133.271303815298));
#61706=CARTESIAN_POINT('Ctrl Pts',(81.7324815899134,10.1070647312935,133.267448217634));
#61707=CARTESIAN_POINT('Ctrl Pts',(81.7698798079035,10.04623254463,133.263592619969));
#61708=CARTESIAN_POINT('Ctrl Pts',(81.8039988342832,9.98365937620945,133.259737022305));
#61709=CARTESIAN_POINT('Ctrl Pts',(81.838155271222,9.92101759805821,133.255877197085));
#61710=CARTESIAN_POINT('Ctrl Pts',(81.8690251097147,9.85663145659424,133.252017371865));
#61711=CARTESIAN_POINT('Ctrl Pts',(81.896444661964,9.79088254918685,133.248157546646));
#61712=CARTESIAN_POINT('Ctrl Pts',(81.9238817311998,9.72509163807652,133.244295255576));
#61713=CARTESIAN_POINT('Ctrl Pts',(81.9478639650014,9.65793668596684,133.240432964506));
#61714=CARTESIAN_POINT('Ctrl Pts',(81.9682771234689,9.58981584221602,133.236570673436));
#61715=CARTESIAN_POINT('Ctrl Pts',(81.9887245103614,9.521580774633,133.232701906145));
#61716=CARTESIAN_POINT('Ctrl Pts',(82.0055907665823,9.45237705514605,133.228833138853));
#61717=CARTESIAN_POINT('Ctrl Pts',(82.018812624733,9.38261357623391,133.224964371562));
#61718=CARTESIAN_POINT('Ctrl Pts',(82.0234657513813,9.35806193613155,133.223602848546));
#61719=CARTESIAN_POINT('Ctrl Pts',(82.0276679804636,9.33344101299941,133.222241325531));
#61720=CARTESIAN_POINT('Ctrl Pts',(82.0314180869268,9.30876871377533,133.220879802515));
#61721=CARTESIAN_POINT('Ctrl Pts',(82.0420748826077,9.23865666378814,133.217010719668));
#61722=CARTESIAN_POINT('Ctrl Pts',(82.0491185350753,9.16785493292545,133.213141636821));
#61723=CARTESIAN_POINT('Ctrl Pts',(82.0524700687833,9.09676868940202,133.209272553974));
#61724=CARTESIAN_POINT('Ctrl Pts',(82.0558166088733,9.02578836083628,133.205409235868));
#61725=CARTESIAN_POINT('Ctrl Pts',(82.0554819269895,8.95452484234985,133.201545917761));
#61726=CARTESIAN_POINT('Ctrl Pts',(82.0514384934808,8.88339095247258,133.197682599655));
#61727=CARTESIAN_POINT('Ctrl Pts',(82.0473998029181,8.81234050262067,133.193823813219));
#61728=CARTESIAN_POINT('Ctrl Pts',(82.0396610294617,8.74141986199301,133.189965026783));
#61729=CARTESIAN_POINT('Ctrl Pts',(82.0282466859118,8.67104264168789,133.186106240347));
#61730=CARTESIAN_POINT('Ctrl Pts',(82.0168395325614,8.600709753871,133.182249884664));
#61731=CARTESIAN_POINT('Ctrl Pts',(82.0017614803032,8.53092008561283,133.178393528981));
#61732=CARTESIAN_POINT('Ctrl Pts',(81.9830888001473,8.46208144368299,133.174537173298));
#61733=CARTESIAN_POINT('Ctrl Pts',(81.9644216360882,8.3932631373773,133.17068195682));
#61734=CARTESIAN_POINT('Ctrl Pts',(81.9421620793813,8.3253957682363,133.166826740343));
#61735=CARTESIAN_POINT('Ctrl Pts',(81.9164369736019,8.25887457963469,133.162971523866));
#61736=CARTESIAN_POINT('Ctrl Pts',(81.8907108620478,8.19235079025377,133.159116156661));
#61737=CARTESIAN_POINT('Ctrl Pts',(81.8615191096896,8.12717373819403,133.155260789457));
#61738=CARTESIAN_POINT('Ctrl Pts',(81.8290370447406,8.06371956579946,133.151405422252));
#61739=CARTESIAN_POINT('Ctrl Pts',(81.7965209799269,8.00019897418937,133.147546019529));
#61740=CARTESIAN_POINT('Ctrl Pts',(81.7607079492153,7.9384052955115,133.143686616806));
#61741=CARTESIAN_POINT('Ctrl Pts',(81.72181927482,7.87869007524317,133.139827214084));
#61742=CARTESIAN_POINT('Ctrl Pts',(81.6829085813518,7.81894104374798,133.135965626137));
#61743=CARTESIAN_POINT('Ctrl Pts',(81.6409190635816,7.76127320628335,133.13210403819));
#61744=CARTESIAN_POINT('Ctrl Pts',(81.5961138122485,7.70600685440395,133.128242450243));
#61745=CARTESIAN_POINT('Ctrl Pts',(81.5512301725223,7.65064381206106,133.124374106309));
#61746=CARTESIAN_POINT('Ctrl Pts',(81.5035212891501,7.59769100470694,133.120505762376));
#61747=CARTESIAN_POINT('Ctrl Pts',(81.4532882515802,7.54743302380963,133.116637418442));
#61748=CARTESIAN_POINT('Ctrl Pts',(81.4234613194524,7.51759128105174,133.114340507136));
#61749=CARTESIAN_POINT('Ctrl Pts',(81.3927451338705,7.48869889924349,133.11204359583));
#61750=CARTESIAN_POINT('Ctrl Pts',(81.3612080022365,7.46080854434957,133.109746684523));
#61751=CARTESIAN_POINT('Ctrl Pts',(81.3080845861496,7.41382802167435,133.105877601676));
#61752=CARTESIAN_POINT('Ctrl Pts',(81.2524220485732,7.36950895079296,133.102008518829));
#61753=CARTESIAN_POINT('Ctrl Pts',(81.1945179499444,7.32813743694031,133.098139435982));
#61754=CARTESIAN_POINT('Ctrl Pts',(81.1367001255347,7.28682756457992,133.094276117876));
#61755=CARTESIAN_POINT('Ctrl Pts',(81.0766477615526,7.24845681192626,133.09041279977));
#61756=CARTESIAN_POINT('Ctrl Pts',(81.0146927489589,7.21327221219623,133.086549481663));
#61757=CARTESIAN_POINT('Ctrl Pts',(80.9528104095714,7.17812888398821,133.082690695227));
#61758=CARTESIAN_POINT('Ctrl Pts',(80.8890302750623,7.14616452377802,133.078831908792));
#61759=CARTESIAN_POINT('Ctrl Pts',(80.8237131290571,7.1175828720714,133.074973122356));
#61760=CARTESIAN_POINT('Ctrl Pts',(80.7584371280644,7.08901922470956,133.071116766673));
#61761=CARTESIAN_POINT('Ctrl Pts',(80.6916264804664,7.0638342525433,133.067260410989));
#61762=CARTESIAN_POINT('Ctrl Pts',(80.6236651661146,7.04218506414032,133.063404055306));
#61763=CARTESIAN_POINT('Ctrl Pts',(80.5557239282157,7.02054227112442,133.059548838829));
#61764=CARTESIAN_POINT('Ctrl Pts',(80.4866331610091,7.0024333356039,133.055693622352));
#61765=CARTESIAN_POINT('Ctrl Pts',(80.4167937189867,6.98796606432365,133.051838405874));
#61766=CARTESIAN_POINT('Ctrl Pts',(80.3469515464508,6.97349822741634,133.04798303867));
#61767=CARTESIAN_POINT('Ctrl Pts',(80.2763611171164,6.96267243380358,133.044127671465));
#61768=CARTESIAN_POINT('Ctrl Pts',(80.2054335351811,6.95554539665881,133.040272304261));
#61769=CARTESIAN_POINT('Ctrl Pts',(80.1344317114086,6.94841089944959,133.036412901538));
#61770=CARTESIAN_POINT('Ctrl Pts',(80.0630925148932,6.94498293593645,133.032553498815));
#61771=CARTESIAN_POINT('Ctrl Pts',(79.9918313314325,6.94526623735486,133.028694096092));
#61772=CARTESIAN_POINT('Ctrl Pts',(79.92052979933,6.94554969918076,133.024832508145));
#61773=CARTESIAN_POINT('Ctrl Pts',(79.849306853463,6.94954858182793,133.020970920198));
#61774=CARTESIAN_POINT('Ctrl Pts',(79.7785742766004,6.95721557389994,133.017109332251));
#61775=CARTESIAN_POINT('Ctrl Pts',(79.7077179505592,6.96489597964939,133.013240988318));
#61776=CARTESIAN_POINT('Ctrl Pts',(79.6373541861038,6.97625723006333,133.009372644385));
#61777=CARTESIAN_POINT('Ctrl Pts',(79.5678853829316,6.99120072674848,133.005504300451));
#61778=CARTESIAN_POINT('Ctrl Pts',(79.526636806746,7.00007374504374,133.003207389145));
#61779=CARTESIAN_POINT('Ctrl Pts',(79.4857035065237,7.01020876927607,133.000910477838));
#61780=CARTESIAN_POINT('Ctrl Pts',(79.4451667772744,7.02157697712044,132.998613566532));
#61781=CARTESIAN_POINT('Ctrl Pts',(79.3768837907397,7.04072640524487,132.994744483685));
#61782=CARTESIAN_POINT('Ctrl Pts',(79.3094596083654,7.06345255239703,132.990875400838));
#61783=CARTESIAN_POINT('Ctrl Pts',(79.243295987548,7.08966060606,132.987006317991));
#61784=CARTESIAN_POINT('Ctrl Pts',(79.177230947226,7.11582961103004,132.983142999885));
#61785=CARTESIAN_POINT('Ctrl Pts',(79.1124231883001,7.145470047296,132.979279681778));
#61786=CARTESIAN_POINT('Ctrl Pts',(79.049260262673,7.17843706823856,132.975416363672));
#61787=CARTESIAN_POINT('Ctrl Pts',(78.9861714271333,7.21136541887825,132.971557577236));
#61788=CARTESIAN_POINT('Ctrl Pts',(78.9247240210359,7.24761237965476,132.9676987908));
#61789=CARTESIAN_POINT('Ctrl Pts',(78.8652848954572,7.28698534915129,132.963840004364));
#61790=CARTESIAN_POINT('Ctrl Pts',(78.805883212169,7.32633351656419,132.959983648681));
#61791=CARTESIAN_POINT('Ctrl Pts',(78.7484877035544,7.36880351828716,132.956127292998));
#61792=CARTESIAN_POINT('Ctrl Pts',(78.6934386248325,7.41415797274114,132.952270937315));
#61793=CARTESIAN_POINT('Ctrl Pts',(78.6384058081597,7.45949902903517,132.948415720837));
#61794=CARTESIAN_POINT('Ctrl Pts',(78.5857184199867,7.50772253768425,132.94456050436));
#61795=CARTESIAN_POINT('Ctrl Pts',(78.5356844479136,7.55855019982731,132.940705287883));
#61796=CARTESIAN_POINT('Ctrl Pts',(78.4856485196619,7.60937984917983,132.936849920678));
#61797=CARTESIAN_POINT('Ctrl Pts',(78.4382665526904,7.66281350642767,132.932994553474));
#61798=CARTESIAN_POINT('Ctrl Pts',(78.3938091684385,7.71853654944516,132.929139186269));
#61799=CARTESIAN_POINT('Ctrl Pts',(78.3493052494283,7.77431791929373,132.925279783546));
#61800=CARTESIAN_POINT('Ctrl Pts',(78.3077323276436,7.83239307807583,132.921420380823));
#61801=CARTESIAN_POINT('Ctrl Pts',(78.2693196750335,7.89241561257217,132.917560978101));
#61802=CARTESIAN_POINT('Ctrl Pts',(78.2308852728778,7.95247213229911,132.913699390154));
#61803=CARTESIAN_POINT('Ctrl Pts',(78.1956149422791,8.01447780026488,132.909837802207));
#61804=CARTESIAN_POINT('Ctrl Pts',(78.1636922782386,8.07806100337411,132.90597621426));
#61805=CARTESIAN_POINT('Ctrl Pts',(78.1317137643532,8.14175544757624,132.902107870326));
#61806=CARTESIAN_POINT('Ctrl Pts',(78.1030948055349,8.20703249220501,132.898239526393));
#61807=CARTESIAN_POINT('Ctrl Pts',(78.0779708196889,8.27350059013615,132.894371182459));
#61808=CARTESIAN_POINT('Ctrl Pts',(78.063052919899,8.31296743390215,132.892074271153));
#61809=CARTESIAN_POINT('Ctrl Pts',(78.049366272519,8.35285389108696,132.889777359846));
#61810=CARTESIAN_POINT('Ctrl Pts',(78.0369307557736,8.39307603040213,132.88748044854));
#61811=CARTESIAN_POINT('Ctrl Pts',(78.0114354604796,8.47553945674731,132.88277132119));
#61812=CARTESIAN_POINT('Ctrl Pts',(77.9911203973394,8.55967521235693,132.878062193839));
#61813=CARTESIAN_POINT('Ctrl Pts',(77.9761678835397,8.64489279522422,132.873353066489));
#61814=CARTESIAN_POINT('Ctrl Pts',(77.9614177985701,8.7289566927755,132.868707691839));
#61815=CARTESIAN_POINT('Ctrl Pts',(77.9518860944981,8.81407332549794,132.86406231719));
#61816=CARTESIAN_POINT('Ctrl Pts',(77.9477016670827,8.89965501903518,132.859416942541));
#61817=CARTESIAN_POINT('Ctrl Pts',(77.946097623904,8.93246159401252,132.857636201526));
#61818=CARTESIAN_POINT('Ctrl Pts',(77.945278854709,8.96533628820413,132.855855460512));
#61819=CARTESIAN_POINT('Ctrl Pts',(77.9452507493435,8.99824517046232,132.854074719498));
#61820=CARTESIAN_POINT('Origin',(80.,9.,141.545925280538));
#61821=CARTESIAN_POINT('',(81.252039109102,10.6292316077768,134.006113615495));
#61822=CARTESIAN_POINT('',(81.252039109102,10.6292316077769,133.947919788944));
#61823=CARTESIAN_POINT('',(81.252039109102,10.6292316077768,141.545925280538));
#61824=CARTESIAN_POINT('',(77.94525006034,9.00049796301154,133.495925280488));
#61825=CARTESIAN_POINT('Ctrl Pts',(81.252039109102,10.6292316077769,133.947919788944));
#61826=CARTESIAN_POINT('Ctrl Pts',(81.3085900087084,10.5857731224245,133.944064641676));
#61827=CARTESIAN_POINT('Ctrl Pts',(81.3628803139282,10.539363224955,133.940209494408));
#61828=CARTESIAN_POINT('Ctrl Pts',(81.414596167302,10.4902735473578,133.936354347139));
#61829=CARTESIAN_POINT('Ctrl Pts',(81.466575160351,10.4409340925459,133.93247958418));
#61830=CARTESIAN_POINT('Ctrl Pts',(81.5159530592672,10.3888878396507,133.928604821221));
#61831=CARTESIAN_POINT('Ctrl Pts',(81.5624487554031,10.3344479942055,133.924730058262));
#61832=CARTESIAN_POINT('Ctrl Pts',(81.6087738167075,10.2802079378727,133.920869515318));
#61833=CARTESIAN_POINT('Ctrl Pts',(81.6522375312,10.2235922431463,133.917008972375));
#61834=CARTESIAN_POINT('Ctrl Pts',(81.6926037665952,10.1649420808812,133.913148429431));
#61835=CARTESIAN_POINT('Ctrl Pts',(81.7331930309163,10.1059678685141,133.909266556464));
#61836=CARTESIAN_POINT('Ctrl Pts',(81.7706502268193,10.0449370632542,133.905384683497));
#61837=CARTESIAN_POINT('Ctrl Pts',(81.8047817870842,9.9822221049789,133.90150281053));
#61838=CARTESIAN_POINT('Ctrl Pts',(81.8389133473491,9.91950714670365,133.897620937563));
#61839=CARTESIAN_POINT('Ctrl Pts',(81.8697191169326,9.85510850704433,133.893739064596));
#61840=CARTESIAN_POINT('Ctrl Pts',(81.897055014379,9.78941740221469,133.889857191629));
#61841=CARTESIAN_POINT('Ctrl Pts',(81.9243008446298,9.72394273855361,133.885988108782));
#61842=CARTESIAN_POINT('Ctrl Pts',(81.9482063861373,9.65692764160921,133.882119025935));
#61843=CARTESIAN_POINT('Ctrl Pts',(81.9685973105308,9.58874628786168,133.878249943088));
#61844=CARTESIAN_POINT('Ctrl Pts',(81.9889578534638,9.52066652093102,133.874386624982));
#61845=CARTESIAN_POINT('Ctrl Pts',(82.0058140357402,9.45142440803659,133.870523306875));
#61846=CARTESIAN_POINT('Ctrl Pts',(82.0190396129381,9.3814139534503,133.866659988769));
#61847=CARTESIAN_POINT('Ctrl Pts',(82.0322496765392,9.31148562110013,133.862801202333));
#61848=CARTESIAN_POINT('Ctrl Pts',(82.0418375045425,9.24079121229842,133.858942415897));
#61849=CARTESIAN_POINT('Ctrl Pts',(82.0477271687752,9.16973804747254,133.855083629461));
#61850=CARTESIAN_POINT('Ctrl Pts',(82.0536131229513,9.09872964093042,133.851227273778));
#61851=CARTESIAN_POINT('Ctrl Pts',(82.0558054951567,9.0273634097031,133.847370918095));
#61852=CARTESIAN_POINT('Ctrl Pts',(82.0542799880628,8.95605351954021,133.843514562412));
#61853=CARTESIAN_POINT('Ctrl Pts',(82.0527549316189,8.88476469503292,133.839659345934));
#61854=CARTESIAN_POINT('Ctrl Pts',(82.047514186688,8.8135326639551,133.835804129457));
#61855=CARTESIAN_POINT('Ctrl Pts',(82.0385855656644,8.74277159183953,133.83194891298));
#61856=CARTESIAN_POINT('Ctrl Pts',(82.0296565955584,8.67200775317777,133.828093545775));
#61857=CARTESIAN_POINT('Ctrl Pts',(82.0170395260989,8.60171539172073,133.824238178571));
#61858=CARTESIAN_POINT('Ctrl Pts',(82.0008138292302,8.53230182461196,133.820382811366));
#61859=CARTESIAN_POINT('Ctrl Pts',(81.9845711484813,8.46281560042647,133.816523408643));
#61860=CARTESIAN_POINT('Ctrl Pts',(81.9647124108874,8.3942104808327,133.81266400592));
#61861=CARTESIAN_POINT('Ctrl Pts',(81.9413676557692,8.32688100039217,133.808804603198));
#61862=CARTESIAN_POINT('Ctrl Pts',(81.9180096826674,8.25951339747097,133.804943015251));
#61863=CARTESIAN_POINT('Ctrl Pts',(81.8911619457095,8.19342332181168,133.801081427304));
#61864=CARTESIAN_POINT('Ctrl Pts',(81.8610025557139,8.12898504598001,133.797219839357));
#61865=CARTESIAN_POINT('Ctrl Pts',(81.8307904007844,8.06443403307509,133.793351495423));
#61866=CARTESIAN_POINT('Ctrl Pts',(81.7972552538553,8.00154101852065,133.78948315149));
#61867=CARTESIAN_POINT('Ctrl Pts',(81.7606207105567,7.9406547890047,133.785614807556));
#61868=CARTESIAN_POINT('Ctrl Pts',(81.7388681729964,7.90450229807125,133.78331789625));
#61869=CARTESIAN_POINT('Ctrl Pts',(81.7160237303533,7.8690567733382,133.781020984944));
#61870=CARTESIAN_POINT('Ctrl Pts',(81.6921409778437,7.83438579555573,133.778724073637));
#61871=CARTESIAN_POINT('Ctrl Pts',(81.6519111492852,7.77598350329134,133.77485499079));
#61872=CARTESIAN_POINT('Ctrl Pts',(81.6085754448932,7.71955199739188,133.770985907943));
#61873=CARTESIAN_POINT('Ctrl Pts',(81.5623536704282,7.66544068284709,133.767116825096));
#61874=CARTESIAN_POINT('Ctrl Pts',(81.516200764102,7.61140999146239,133.76325350699));
#61875=CARTESIAN_POINT('Ctrl Pts',(81.4671706362288,7.55969299580559,133.759390188884));
#61876=CARTESIAN_POINT('Ctrl Pts',(81.4155258303404,7.51060945815445,133.755526870777));
#61877=CARTESIAN_POINT('Ctrl Pts',(81.3639416037894,7.46158349547399,133.751668084341));
#61878=CARTESIAN_POINT('Ctrl Pts',(81.3097491417681,7.41518518794331,133.747809297906));
#61879=CARTESIAN_POINT('Ctrl Pts',(81.253249465694,7.37169924791589,133.74395051147));
#61880=CARTESIAN_POINT('Ctrl Pts',(81.1967853802729,7.328240700842,133.740094155787));
#61881=CARTESIAN_POINT('Ctrl Pts',(81.1380173483258,7.28769117708969,133.736237800103));
#61882=CARTESIAN_POINT('Ctrl Pts',(81.0772801458058,7.25029572500016,133.73238144442));
#61883=CARTESIAN_POINT('Ctrl Pts',(81.0165608856637,7.21291131990172,133.728526227943));
#61884=CARTESIAN_POINT('Ctrl Pts',(80.953874023249,7.17867939124625,133.724671011466));
#61885=CARTESIAN_POINT('Ctrl Pts',(80.8895825976207,7.14780120815545,133.720815794988));
#61886=CARTESIAN_POINT('Ctrl Pts',(80.8252886583898,7.11692181781997,133.716960427784));
#61887=CARTESIAN_POINT('Ctrl Pts',(80.7593904702457,7.08939664170252,133.713105060579));
#61888=CARTESIAN_POINT('Ctrl Pts',(80.6922733378124,7.06537983359678,133.709249693375));
#61889=CARTESIAN_POINT('Ctrl Pts',(80.6250859520435,7.04133788644204,133.705390290652));
#61890=CARTESIAN_POINT('Ctrl Pts',(80.5566775333176,7.02081180204424,133.701530887929));
#61891=CARTESIAN_POINT('Ctrl Pts',(80.4874500739385,7.00390631785045,133.697671485206));
#61892=CARTESIAN_POINT('Ctrl Pts',(80.418183417428,6.98699126163868,133.693809897259));
#61893=CARTESIAN_POINT('Ctrl Pts',(80.3480972745903,6.97370097712113,133.689948309312));
#61894=CARTESIAN_POINT('Ctrl Pts',(80.2776026879906,6.96408882558192,133.686086721365));
#61895=CARTESIAN_POINT('Ctrl Pts',(80.2069847685848,6.95445985723907,133.682218377432));
#61896=CARTESIAN_POINT('Ctrl Pts',(80.1359574629714,6.94852191006832,133.678350033499));
#61897=CARTESIAN_POINT('Ctrl Pts',(80.0649350722534,6.94627630902026,133.674481689565));
#61898=CARTESIAN_POINT('Ctrl Pts',(80.0227640204915,6.94494293574069,133.672184778259));
#61899=CARTESIAN_POINT('Ctrl Pts',(79.9805946865909,6.94491035259303,133.669887866952));
#61900=CARTESIAN_POINT('Ctrl Pts',(79.938512916366,6.94617018693218,133.667590955646));
#61901=CARTESIAN_POINT('Ctrl Pts',(79.8676273515256,6.94829234263664,133.663721872799));
#61902=CARTESIAN_POINT('Ctrl Pts',(79.7967129435705,6.9540927631037,133.659852789952));
#61903=CARTESIAN_POINT('Ctrl Pts',(79.7261824575087,6.96357629263357,133.655983707105));
#61904=CARTESIAN_POINT('Ctrl Pts',(79.6557570583536,6.97304569217743,133.652120388999));
#61905=CARTESIAN_POINT('Ctrl Pts',(79.5857149231673,6.98618724374451,133.648257070892));
#61906=CARTESIAN_POINT('Ctrl Pts',(79.5164670932613,7.00295380859611,133.644393752786));
#61907=CARTESIAN_POINT('Ctrl Pts',(79.4473004910331,7.01970070627358,133.64053496635));
#61908=CARTESIAN_POINT('Ctrl Pts',(79.3789268132236,7.04006405728557,133.636676179914));
#61909=CARTESIAN_POINT('Ctrl Pts',(79.3117485241913,7.0639453859596,133.632817393478));
#61910=CARTESIAN_POINT('Ctrl Pts',(79.2446125525552,7.08781167114769,133.628961037795));
#61911=CARTESIAN_POINT('Ctrl Pts',(79.1786709323809,7.11519137502217,133.625104682112));
#61912=CARTESIAN_POINT('Ctrl Pts',(79.1143111127741,7.14593615062896,133.621248326428));
#61913=CARTESIAN_POINT('Ctrl Pts',(79.0499703057024,7.17667184392122,133.617393109951));
#61914=CARTESIAN_POINT('Ctrl Pts',(78.9872108096165,7.21077042614907,133.613537893474));
#61915=CARTESIAN_POINT('Ctrl Pts',(78.9263986226043,7.24803606060112,133.609682676997));
#61916=CARTESIAN_POINT('Ctrl Pts',(78.8655840580174,7.28530315202802,133.605827309792));
#61917=CARTESIAN_POINT('Ctrl Pts',(78.8067173667056,7.32573728581333,133.601971942588));
#61918=CARTESIAN_POINT('Ctrl Pts',(78.7501370400154,7.36909836478144,133.598116575383));
#61919=CARTESIAN_POINT('Ctrl Pts',(78.6934974891518,7.41250483097526,133.59425717266));
#61920=CARTESIAN_POINT('Ctrl Pts',(78.6391494666409,7.45884406211309,133.590397769937));
#61921=CARTESIAN_POINT('Ctrl Pts',(78.5873989985908,7.50783513869356,133.586538367214));
#61922=CARTESIAN_POINT('Ctrl Pts',(78.5356192290193,7.55685395440631,133.582676779267));
#61923=CARTESIAN_POINT('Ctrl Pts',(78.4864402767907,7.6085272525214,133.578815191321));
#61924=CARTESIAN_POINT('Ctrl Pts',(78.440129913883,7.66253864469385,133.574953603374));
#61925=CARTESIAN_POINT('Ctrl Pts',(78.3937385293354,7.71664453173299,133.57108525944));
#61926=CARTESIAN_POINT('Ctrl Pts',(78.3502260507425,7.77309629491194,133.567216915507));
#61927=CARTESIAN_POINT('Ctrl Pts',(78.3098183000043,7.83154658479699,133.563348571573));
#61928=CARTESIAN_POINT('Ctrl Pts',(78.2858253404497,7.86625268487792,133.561051660267));
#61929=CARTESIAN_POINT('Ctrl Pts',(78.2629261494462,7.90166286469492,133.55875474896));
#61930=CARTESIAN_POINT('Ctrl Pts',(78.2411602539381,7.93770046118201,133.556457837654));
#61931=CARTESIAN_POINT('Ctrl Pts',(78.2033015192916,8.00038282599411,133.552462681304));
#61932=CARTESIAN_POINT('Ctrl Pts',(78.1687336620035,8.06519667391206,133.548467524953));
#61933=CARTESIAN_POINT('Ctrl Pts',(78.1376942678544,8.13177484342032,133.544472368603));
#61934=CARTESIAN_POINT('Ctrl Pts',(78.1062630365256,8.19919348687753,133.540426777931));
#61935=CARTESIAN_POINT('Ctrl Pts',(78.078450290962,8.26842096575299,133.536381187259));
#61936=CARTESIAN_POINT('Ctrl Pts',(78.0544569760338,8.33904621614173,133.532335596587));
#61937=CARTESIAN_POINT('Ctrl Pts',(78.0308540830866,8.40852224433065,133.528355836231));
#61938=CARTESIAN_POINT('Ctrl Pts',(78.0109474205576,8.47935046530343,133.524376075876));
#61939=CARTESIAN_POINT('Ctrl Pts',(77.9948811787214,8.55111685813086,133.520396315521));
#61940=CARTESIAN_POINT('Ctrl Pts',(77.9784163026598,8.62466391259056,133.51631780969));
#61941=CARTESIAN_POINT('Ctrl Pts',(77.9659851790174,8.69919589123697,133.51223930386));
#61942=CARTESIAN_POINT('Ctrl Pts',(77.9576890084772,8.77424930475158,133.508160798029));
#61943=CARTESIAN_POINT('Ctrl Pts',(77.9493928379371,8.84930271826618,133.504082292199));
#61944=CARTESIAN_POINT('Ctrl Pts',(77.9452317338588,8.92487707367048,133.500003786368));
#61945=CARTESIAN_POINT('Ctrl Pts',(77.9452500603398,9.00049796209039,133.495925280538));
#61946=CARTESIAN_POINT('Ctrl Pts',(77.94525006034,9.00049796301154,133.495925280488));
#61947=CARTESIAN_POINT('Ctrl Pts',(77.9452690078821,9.07868140246824,133.491708567086));
#61948=CARTESIAN_POINT('Ctrl Pts',(77.9497549266111,9.15674554238997,133.487491853684));
#61949=CARTESIAN_POINT('Ctrl Pts',(77.9586394355346,9.23418925753617,133.483275140282));
#61950=CARTESIAN_POINT('Ctrl Pts',(77.9673566235425,9.31017448426939,133.479137839749));
#61951=CARTESIAN_POINT('Ctrl Pts',(77.9803079746392,9.38556211302273,133.475000539217));
#61952=CARTESIAN_POINT('Ctrl Pts',(77.9973777224886,9.45989300507289,133.470863238684));
#61953=CARTESIAN_POINT('Ctrl Pts',(78.0149389348737,9.5363639988792,133.466606818847));
#61954=CARTESIAN_POINT('Ctrl Pts',(78.0368591598541,9.61171606121349,133.46235039901));
#61955=CARTESIAN_POINT('Ctrl Pts',(78.0629590532119,9.68547059234245,133.458093979173));
#61956=CARTESIAN_POINT('Ctrl Pts',(78.0890589465697,9.7592251234714,133.453837559336));
#61957=CARTESIAN_POINT('Ctrl Pts',(78.119338266365,9.8313817685356,133.4495811395));
#61958=CARTESIAN_POINT('Ctrl Pts',(78.153566954364,9.90148908506049,133.445324719663));
#61959=CARTESIAN_POINT('Ctrl Pts',(78.1846808093608,9.96521658991371,133.441455636816));
#61960=CARTESIAN_POINT('Ctrl Pts',(78.2191586994745,10.0274562334421,133.437586553969));
#61961=CARTESIAN_POINT('Ctrl Pts',(78.2568351259753,10.0878298508804,133.433717471122));
#61962=CARTESIAN_POINT('Ctrl Pts',(78.2944554164797,10.1481135146398,133.429854153016));
#61963=CARTESIAN_POINT('Ctrl Pts',(78.3352645285795,10.2065362623385,133.425990834909));
#61964=CARTESIAN_POINT('Ctrl Pts',(78.3790502987058,10.2627428987622,133.422127516803));
#61965=CARTESIAN_POINT('Ctrl Pts',(78.4227847081407,10.318883604823,133.418268730367));
#61966=CARTESIAN_POINT('Ctrl Pts',(78.4694885429769,10.3728129817268,133.414409943931));
#61967=CARTESIAN_POINT('Ctrl Pts',(78.5189063847538,10.4242047835114,133.410551157495));
#61968=CARTESIAN_POINT('Ctrl Pts',(78.5682930969139,10.4755642122293,133.406694801812));
#61969=CARTESIAN_POINT('Ctrl Pts',(78.6203900882308,10.5243888878679,133.402838446129));
#61970=CARTESIAN_POINT('Ctrl Pts',(78.6749026713719,10.5703867778871,133.398982090445));
#61971=CARTESIAN_POINT('Ctrl Pts',(78.7293991509501,10.6163710796691,133.395126873968));
#61972=CARTESIAN_POINT('Ctrl Pts',(78.7863094346104,10.6595299405508,133.391271657491));
#61973=CARTESIAN_POINT('Ctrl Pts',(78.8453043857994,10.6996104262583,133.387416441014));
#61974=CARTESIAN_POINT('Ctrl Pts',(78.9043016435144,10.7396924789928,133.383561073809));
#61975=CARTESIAN_POINT('Ctrl Pts',(78.9653833275151,10.776695646433,133.379705706604));
#61976=CARTESIAN_POINT('Ctrl Pts',(79.0281912878431,10.8104102820841,133.3758503394));
#61977=CARTESIAN_POINT('Ctrl Pts',(79.0910649909787,10.8441602077653,133.371990936677));
#61978=CARTESIAN_POINT('Ctrl Pts',(79.1556681486066,10.8746145000374,133.368131533954));
#61979=CARTESIAN_POINT('Ctrl Pts',(79.2216187718393,10.9016099037781,133.364272131231));
#61980=CARTESIAN_POINT('Ctrl Pts',(79.287606736833,10.9286205925285,133.360410543285));
#61981=CARTESIAN_POINT('Ctrl Pts',(79.3549432274509,10.9521683336448,133.356548955338));
#61982=CARTESIAN_POINT('Ctrl Pts',(79.4232296777173,10.9721393352991,133.352687367391));
#61983=CARTESIAN_POINT('Ctrl Pts',(79.4916355975762,10.9921452769366,133.348819023457));
#61984=CARTESIAN_POINT('Ctrl Pts',(79.560994322419,11.0085618736447,133.344950679524));
#61985=CARTESIAN_POINT('Ctrl Pts',(79.6308963387208,11.0213263095627,133.34108233559));
#61986=CARTESIAN_POINT('Ctrl Pts',(79.6724021443957,11.0289054642823,133.338785424284));
#61987=CARTESIAN_POINT('Ctrl Pts',(79.7140993616816,11.0351979879306,133.336488512977));
#61988=CARTESIAN_POINT('Ctrl Pts',(79.7559018530524,11.040199416027,133.334191601671));
#61989=CARTESIAN_POINT('Ctrl Pts',(79.8262968740995,11.0486217761438,133.330323623604));
#61990=CARTESIAN_POINT('Ctrl Pts',(79.897266151478,11.0534129893788,133.326455645537));
#61991=CARTESIAN_POINT('Ctrl Pts',(79.9684025636869,11.0545070368627,133.322587667471));
#61992=CARTESIAN_POINT('Ctrl Pts',(80.0394421231409,11.0555995947928,133.318724955685));
#61993=CARTESIAN_POINT('Ctrl Pts',(80.110647884865,11.0530049645083,133.314862243899));
#61994=CARTESIAN_POINT('Ctrl Pts',(80.1816065604028,11.0467087285979,133.310999532113));
#61995=CARTESIAN_POINT('Ctrl Pts',(80.2524923697582,11.0404189581784,133.307140786876));
#61996=CARTESIAN_POINT('Ctrl Pts',(80.323131115117,11.0304351676684,133.303282041639));
#61997=CARTESIAN_POINT('Ctrl Pts',(80.3931101843538,11.0167949686216,133.299423296402));
#61998=CARTESIAN_POINT('Ctrl Pts',(80.4630408059897,11.0031642128973,133.295567222635));
#61999=CARTESIAN_POINT('Ctrl Pts',(80.5323121827189,10.9858821674517,133.291711148868));
#62000=CARTESIAN_POINT('Ctrl Pts',(80.6005192195217,10.9650379715123,133.2878550751));
#62001=CARTESIAN_POINT('Ctrl Pts',(80.6687201287411,10.9441956481736,133.283999347755));
#62002=CARTESIAN_POINT('Ctrl Pts',(80.7358564197638,10.9197919393744,133.280143620409));
#62003=CARTESIAN_POINT('Ctrl Pts',(80.8015369135473,10.8919662097197,133.276287893064));
#62004=CARTESIAN_POINT('Ctrl Pts',(80.8672135547284,10.864142112231,133.272432391883));
#62005=CARTESIAN_POINT('Ctrl Pts',(80.9314341240358,10.8328965896448,133.268576890702));
#62006=CARTESIAN_POINT('Ctrl Pts',(80.9938281893631,10.7984168294718,133.264721389521));
#62007=CARTESIAN_POINT('Ctrl Pts',(81.0562666112036,10.7639125573211,133.260863147428));
#62008=CARTESIAN_POINT('Ctrl Pts',(81.1168755162782,10.7261697014419,133.257004905336));
#62009=CARTESIAN_POINT('Ctrl Pts',(81.1753108603474,10.6854204057295,133.253146663244));
#62010=CARTESIAN_POINT('Ctrl Pts',(81.2013268068549,10.6672784487623,133.251428938783));
#62011=CARTESIAN_POINT('Ctrl Pts',(81.2269123268175,10.6485411485174,133.249711214322));
#62012=CARTESIAN_POINT('Ctrl Pts',(81.252039109102,10.6292316077768,133.247993489861));
#62013=CARTESIAN_POINT('',(77.9452500001325,8.99997666224458,133.554074719471));
#62014=CARTESIAN_POINT('Ctrl Pts',(77.9452500001325,8.99997666241271,133.554074719462));
#62015=CARTESIAN_POINT('Ctrl Pts',(77.9452491949294,9.07087049904514,133.550206920375));
#62016=CARTESIAN_POINT('Ctrl Pts',(77.948921710863,9.14190368830042,133.546339121287));
#62017=CARTESIAN_POINT('Ctrl Pts',(77.9562848605137,9.21266403347663,133.5424713222));
#62018=CARTESIAN_POINT('Ctrl Pts',(77.9636370380662,9.28331893607806,133.538609286661));
#62019=CARTESIAN_POINT('Ctrl Pts',(77.97466888319,9.35370132203602,133.534747251122));
#62020=CARTESIAN_POINT('Ctrl Pts',(77.9893456969756,9.42339914528644,133.530885215583));
#62021=CARTESIAN_POINT('Ctrl Pts',(78.0040053078095,9.49301527449238,133.527027706804));
#62022=CARTESIAN_POINT('Ctrl Pts',(78.0223013014783,9.56194796136903,133.523170198025));
#62023=CARTESIAN_POINT('Ctrl Pts',(78.0441474066621,9.62979218448103,133.519312689246));
#62024=CARTESIAN_POINT('Ctrl Pts',(78.0659797748482,9.69759374662769,133.515457606098));
#62025=CARTESIAN_POINT('Ctrl Pts',(78.0913576770541,9.7643077412314,133.51160252295));
#62026=CARTESIAN_POINT('Ctrl Pts',(78.1201445418238,9.82954265644696,133.507747439802));
#62027=CARTESIAN_POINT('Ctrl Pts',(78.1489229525421,9.89475841364288,133.503893488805));
#62028=CARTESIAN_POINT('Ctrl Pts',(78.1811081421473,9.95849550926161,133.500039537807));
#62029=CARTESIAN_POINT('Ctrl Pts',(78.2165154281123,10.0203824500346,133.49618558681));
#62030=CARTESIAN_POINT('Ctrl Pts',(78.2519241814885,10.0822719556352,133.492331476091));
#62031=CARTESIAN_POINT('Ctrl Pts',(78.2905550529744,10.1423107333029,133.488477365371));
#62032=CARTESIAN_POINT('Ctrl Pts',(78.3321782980711,10.2001534623018,133.484623254651));
#62033=CARTESIAN_POINT('Ctrl Pts',(78.3738451508804,10.258056791792,133.480765106069));
#62034=CARTESIAN_POINT('Ctrl Pts',(78.4185103508028,10.3137590845539,133.476906957487));
#62035=CARTESIAN_POINT('Ctrl Pts',(78.4659023851082,10.3669462573501,133.473048808905));
#62036=CARTESIAN_POINT('Ctrl Pts',(78.513321406382,10.4201637171042,133.469188463334));
#62037=CARTESIAN_POINT('Ctrl Pts',(78.5634700109467,10.4708628601754,133.465328117764));
#62038=CARTESIAN_POINT('Ctrl Pts',(78.6160400988868,10.5187667874334,133.461467772193));
#62039=CARTESIAN_POINT('Ctrl Pts',(78.6687019134685,10.566754299607,133.457600690919));
#62040=CARTESIAN_POINT('Ctrl Pts',(78.7237932705989,10.6119365506021,133.453733609645));
#62041=CARTESIAN_POINT('Ctrl Pts',(78.7809738927825,10.6540776621496,133.449866528371));
#62042=CARTESIAN_POINT('Ctrl Pts',(78.8140980817258,10.6784896060542,133.44762636508));
#62043=CARTESIAN_POINT('Ctrl Pts',(78.8479228431126,10.7018818260453,133.445386201789));
#62044=CARTESIAN_POINT('Ctrl Pts',(78.882378183025,10.7242154844222,133.443146038498));
#62045=CARTESIAN_POINT('Ctrl Pts',(78.9418874898537,10.7627889111347,133.439276955651));
#62046=CARTESIAN_POINT('Ctrl Pts',(79.0035126729263,10.7983534291896,133.435407872804));
#62047=CARTESIAN_POINT('Ctrl Pts',(79.0669169949676,10.8306702784007,133.431538789957));
#62048=CARTESIAN_POINT('Ctrl Pts',(79.1302268477313,10.8629389771182,133.427675471851));
#62049=CARTESIAN_POINT('Ctrl Pts',(79.1953101483621,10.8919693932024,133.423812153744));
#62050=CARTESIAN_POINT('Ctrl Pts',(79.261802009964,10.917566502108,133.419948835638));
#62051=CARTESIAN_POINT('Ctrl Pts',(79.3282158766378,10.9431335856148,133.416090049202));
#62052=CARTESIAN_POINT('Ctrl Pts',(79.3960345712215,10.9652751877834,133.412231262766));
#62053=CARTESIAN_POINT('Ctrl Pts',(79.4648710613889,10.9838433863491,133.408372476331));
#62054=CARTESIAN_POINT('Ctrl Pts',(79.5336641896151,11.0023998883112,133.404516120647));
#62055=CARTESIAN_POINT('Ctrl Pts',(79.6034733735092,11.0173873263681,133.400659764964));
#62056=CARTESIAN_POINT('Ctrl Pts',(79.67389556436,11.0287073370883,133.396803409281));
#62057=CARTESIAN_POINT('Ctrl Pts',(79.7442969517905,11.040024003764,133.392948192804));
#62058=CARTESIAN_POINT('Ctrl Pts',(79.815310507302,11.0476753168868,133.389092976327));
#62059=CARTESIAN_POINT('Ctrl Pts',(79.8865238136955,11.0516141736793,133.385237759849));
#62060=CARTESIAN_POINT('Ctrl Pts',(79.9577399043162,11.0555531844694,133.381382392645));
#62061=CARTESIAN_POINT('Ctrl Pts',(80.0291552761605,11.0557794261325,133.37752702544));
#62062=CARTESIAN_POINT('Ctrl Pts',(80.1003549610611,11.0522978449266,133.373671658236));
#62063=CARTESIAN_POINT('Ctrl Pts',(80.1716291726167,11.0488126194546,133.369812255513));
#62064=CARTESIAN_POINT('Ctrl Pts',(80.2426867603528,11.0416118473837,133.36595285279));
#62065=CARTESIAN_POINT('Ctrl Pts',(80.313116238991,11.0307525165268,133.362093450067));
#62066=CARTESIAN_POINT('Ctrl Pts',(80.3835855953533,11.0198870370316,133.35823186212));
#62067=CARTESIAN_POINT('Ctrl Pts',(80.4534256588204,11.0053589740045,133.354370274173));
#62068=CARTESIAN_POINT('Ctrl Pts',(80.5222362332715,10.9872762463126,133.350508686226));
#62069=CARTESIAN_POINT('Ctrl Pts',(80.591167194289,10.9691618822405,133.346640342293));
#62070=CARTESIAN_POINT('Ctrl Pts',(80.6590646073791,10.9474805848859,133.34277199836));
#62071=CARTESIAN_POINT('Ctrl Pts',(80.7255451693941,10.9223895988246,133.338903654426));
#62072=CARTESIAN_POINT('Ctrl Pts',(80.7650194139748,10.907491293357,133.33660674312));
#62073=CARTESIAN_POINT('Ctrl Pts',(80.8039945234928,10.8913917709617,133.334309831813));
#62074=CARTESIAN_POINT('Ctrl Pts',(80.842394382625,10.8741316033358,133.332012920507));
#62075=CARTESIAN_POINT('Ctrl Pts',(80.9070806959089,10.8450560641121,133.328143668699));
#62076=CARTESIAN_POINT('Ctrl Pts',(80.9703866144579,10.8125706362717,133.324274416892));
#62077=CARTESIAN_POINT('Ctrl Pts',(81.0319288584356,10.7768287462859,133.320405165084));
#62078=CARTESIAN_POINT('Ctrl Pts',(81.0933729772624,10.7411438444454,133.31654208255));
#62079=CARTESIAN_POINT('Ctrl Pts',(81.1530585893509,10.702213033733,133.312679000016));
#62080=CARTESIAN_POINT('Ctrl Pts',(81.2106240071159,10.6602370541265,133.308815917482));
#62081=CARTESIAN_POINT('Ctrl Pts',(81.2245547333255,10.6500789435458,133.307881058547));
#62082=CARTESIAN_POINT('Ctrl Pts',(81.2383614027949,10.6397427119916,133.306946199613));
#62083=CARTESIAN_POINT('Ctrl Pts',(81.252039109102,10.6292316077768,133.306011340678));
#62084=CARTESIAN_POINT('Ctrl Pts',(81.252039109102,10.6292316077768,134.006113615495));
#62085=CARTESIAN_POINT('Ctrl Pts',(81.2874945667089,10.6019846409595,134.003679619815));
#62086=CARTESIAN_POINT('Ctrl Pts',(81.3220223711118,10.5736088323219,134.001245624136));
#62087=CARTESIAN_POINT('Ctrl Pts',(81.3555499459168,10.5441767731141,133.998811628456));
#62088=CARTESIAN_POINT('Ctrl Pts',(81.4088454244804,10.4973915317205,133.994942545609));
#62089=CARTESIAN_POINT('Ctrl Pts',(81.4598203372149,10.4477522689847,133.991073462762));
#62090=CARTESIAN_POINT('Ctrl Pts',(81.5081533895657,10.3955181532469,133.987204379915));
#62091=CARTESIAN_POINT('Ctrl Pts',(81.556414428079,10.3433618637364,133.983341061809));
#62092=CARTESIAN_POINT('Ctrl Pts',(81.6020410922966,10.2886187491794,133.979477743702));
#62093=CARTESIAN_POINT('Ctrl Pts',(81.6447465261169,10.2315869548377,133.975614425596));
#62094=CARTESIAN_POINT('Ctrl Pts',(81.6874018664798,10.1746220587688,133.97175563916));
#62095=CARTESIAN_POINT('Ctrl Pts',(81.7271424930792,10.1153742024436,133.967896852724));
#62096=CARTESIAN_POINT('Ctrl Pts',(81.7637208600582,10.0541756448978,133.964038066288));
#62097=CARTESIAN_POINT('Ctrl Pts',(81.8002761853481,9.9930156379557,133.960181710605));
#62098=CARTESIAN_POINT('Ctrl Pts',(81.8336729544594,9.92990778370281,133.956325354922));
#62099=CARTESIAN_POINT('Ctrl Pts',(81.8637069616786,9.86521322429253,133.952468999239));
#62100=CARTESIAN_POINT('Ctrl Pts',(81.8937320965514,9.8005377763029,133.948613782761));
#62101=CARTESIAN_POINT('Ctrl Pts',(81.9203962372521,9.73427699408904,133.944758566284));
#62102=CARTESIAN_POINT('Ctrl Pts',(81.9435419628081,9.6668149678164,133.940903349807));
#62103=CARTESIAN_POINT('Ctrl Pts',(81.9666885932928,9.59935030398031,133.937047982602));
#62104=CARTESIAN_POINT('Ctrl Pts',(81.9863163799621,9.5306847630487,133.933192615398));
#62105=CARTESIAN_POINT('Ctrl Pts',(82.0023172982287,9.46121903659115,133.929337248193));
#62106=CARTESIAN_POINT('Ctrl Pts',(82.0183349650936,9.39168059846039,133.92547784547));
#62107=CARTESIAN_POINT('Ctrl Pts',(82.0307180759414,9.32134077717102,133.921618442747));
#62108=CARTESIAN_POINT('Ctrl Pts',(82.0394096353204,9.25061105694344,133.917759040025));
#62109=CARTESIAN_POINT('Ctrl Pts',(82.0481061159286,9.17984128899266,133.913897452078));
#62110=CARTESIAN_POINT('Ctrl Pts',(82.053106850083,9.10868166744837,133.910035864131));
#62111=CARTESIAN_POINT('Ctrl Pts',(82.0544069244437,9.03754665494593,133.906174276184));
#62112=CARTESIAN_POINT('Ctrl Pts',(82.0557092733312,8.96628718918938,133.90230593225));
#62113=CARTESIAN_POINT('Ctrl Pts',(82.0532980524678,8.89505290409261,133.898437588317));
#62114=CARTESIAN_POINT('Ctrl Pts',(82.0472204087787,8.82425541152011,133.894569244383));
#62115=CARTESIAN_POINT('Ctrl Pts',(82.0436116788555,8.78221789780502,133.892272333077));
#62116=CARTESIAN_POINT('Ctrl Pts',(82.0387112898198,8.74033424979566,133.889975421771));
#62117=CARTESIAN_POINT('Ctrl Pts',(82.0325375986326,8.6986887445766,133.887678510464));
#62118=CARTESIAN_POINT('Ctrl Pts',(82.0221381885171,8.6285380559354,133.883809427617));
#62119=CARTESIAN_POINT('Ctrl Pts',(82.0080823914301,8.55878898639692,133.87994034477));
#62120=CARTESIAN_POINT('Ctrl Pts',(81.9904136794235,8.48985203395129,133.876071261923));
#62121=CARTESIAN_POINT('Ctrl Pts',(81.9727712929166,8.42101779412675,133.872207943817));
#62122=CARTESIAN_POINT('Ctrl Pts',(81.9515267963478,8.35299373629002,133.868344625711));
#62123=CARTESIAN_POINT('Ctrl Pts',(81.9267750863094,8.2861825658633,133.864481307604));
#62124=CARTESIAN_POINT('Ctrl Pts',(81.9020524100172,8.21944976491376,133.860622521168));
#62125=CARTESIAN_POINT('Ctrl Pts',(81.8738308599145,8.15392747869419,133.856763734733));
#62126=CARTESIAN_POINT('Ctrl Pts',(81.842255313806,8.09000388942938,133.852904948297));
#62127=CARTESIAN_POINT('Ctrl Pts',(81.8106996579762,8.0261205673385,133.849048592614));
#62128=CARTESIAN_POINT('Ctrl Pts',(81.7757944124787,7.96383437872305,133.84519223693));
#62129=CARTESIAN_POINT('Ctrl Pts',(81.7377322276222,7.90351275995428,133.841335881247));
#62130=CARTESIAN_POINT('Ctrl Pts',(81.6996812867163,7.8432089607957,133.83748066477));
#62131=CARTESIAN_POINT('Ctrl Pts',(81.6584755169941,7.7848689899309,133.833625448293));
#62132=CARTESIAN_POINT('Ctrl Pts',(81.614352223271,7.72883342487303,133.829770231815));
#62133=CARTESIAN_POINT('Ctrl Pts',(81.5702272044591,7.6727956689922,133.825914864611));
#62134=CARTESIAN_POINT('Ctrl Pts',(81.5231847374417,7.61906287809244,133.822059497406));
#62135=CARTESIAN_POINT('Ctrl Pts',(81.4735028660501,7.56794313442445,133.818204130202));
#62136=CARTESIAN_POINT('Ctrl Pts',(81.4237689912868,7.51676988232451,133.814344727479));
#62137=CARTESIAN_POINT('Ctrl Pts',(81.3713905363677,7.46821548650309,133.810485324756));
#62138=CARTESIAN_POINT('Ctrl Pts',(81.316682289586,7.42255101166775,133.806625922033));
#62139=CARTESIAN_POINT('Ctrl Pts',(81.2619430665653,7.37686068124805,133.802764334086));
#62140=CARTESIAN_POINT('Ctrl Pts',(81.2048718145002,7.33406382075419,133.798902746139));
#62141=CARTESIAN_POINT('Ctrl Pts',(81.1458140722613,7.29438935442232,133.795041158192));
#62142=CARTESIAN_POINT('Ctrl Pts',(81.0866530063856,7.25464547618953,133.791172814259));
#62143=CARTESIAN_POINT('Ctrl Pts',(81.0254989284646,7.21803514823513,133.787304470326));
#62144=CARTESIAN_POINT('Ctrl Pts',(80.9627232188051,7.18474201104264,133.783436126392));
#62145=CARTESIAN_POINT('Ctrl Pts',(80.9254488089371,7.16497350427086,133.781139215086));
#62146=CARTESIAN_POINT('Ctrl Pts',(80.8876030962549,7.14637361677536,133.778842303779));
#62147=CARTESIAN_POINT('Ctrl Pts',(80.8492668411795,7.12897263649808,133.776545392473));
#62148=CARTESIAN_POINT('Ctrl Pts',(80.7846904918394,7.09966117195791,133.772676309626));
#62149=CARTESIAN_POINT('Ctrl Pts',(80.7184684036558,7.07363938935495,133.768807226779));
#62150=CARTESIAN_POINT('Ctrl Pts',(80.6509690279539,7.05109341241178,133.764938143932));
#62151=CARTESIAN_POINT('Ctrl Pts',(80.5835702229554,7.02858102784983,133.761074825826));
#62152=CARTESIAN_POINT('Ctrl Pts',(80.5148983650352,7.00953432186643,133.757211507719));
#62153=CARTESIAN_POINT('Ctrl Pts',(80.4453432503829,6.99409198819128,133.753348189613));
#62154=CARTESIAN_POINT('Ctrl Pts',(80.3758697238534,6.97866776836761,133.749489403177));
#62155=CARTESIAN_POINT('Ctrl Pts',(80.3055154704918,6.96683962753385,133.745630616741));
#62156=CARTESIAN_POINT('Ctrl Pts',(80.2346851938957,6.95869639145322,133.741771830305));
#62157=CARTESIAN_POINT('Ctrl Pts',(80.1638995351801,6.9505582850142,133.737915474622));
#62158=CARTESIAN_POINT('Ctrl Pts',(80.0926389296103,6.94610053341757,133.734059118939));
#62159=CARTESIAN_POINT('Ctrl Pts',(80.0213165623717,6.94536057502328,133.730202763256));
#62160=CARTESIAN_POINT('Ctrl Pts',(79.9500152644746,6.94462083522012,133.726347546778));
#62161=CARTESIAN_POINT('Ctrl Pts',(79.8786527266226,6.94759671327875,133.722492330301));
#62162=CARTESIAN_POINT('Ctrl Pts',(79.8076437887117,6.95427356411498,133.718637113824));
#62163=CARTESIAN_POINT('Ctrl Pts',(79.7366320745637,6.96095067599612,133.714781746619));
#62164=CARTESIAN_POINT('Ctrl Pts',(79.6659744712473,6.97132900026171,133.710926379415));
#62165=CARTESIAN_POINT('Ctrl Pts',(79.5960806143545,6.98534204084173,133.70707101221));
#62166=CARTESIAN_POINT('Ctrl Pts',(79.5261135976526,6.99936974925407,133.703211609487));
#62167=CARTESIAN_POINT('Ctrl Pts',(79.4569124005045,7.0170396730388,133.699352206764));
#62168=CARTESIAN_POINT('Ctrl Pts',(79.3888754883123,7.03823436830124,133.695492804042));
#62169=CARTESIAN_POINT('Ctrl Pts',(79.3208000530859,7.05944106416663,133.691631216095));
#62170=CARTESIAN_POINT('Ctrl Pts',(79.2538906709939,7.08417633591524,133.687769628148));
#62171=CARTESIAN_POINT('Ctrl Pts',(79.1885270823425,7.11227404891269,133.683908040201));
#62172=CARTESIAN_POINT('Ctrl Pts',(79.12304913775,7.14042091986613,133.680039696267));
#62173=CARTESIAN_POINT('Ctrl Pts',(79.0591228218857,7.17194176216646,133.676171352334));
#62174=CARTESIAN_POINT('Ctrl Pts',(78.9971038465641,7.20662416991768,133.6723030084));
#62175=CARTESIAN_POINT('Ctrl Pts',(78.9602787637691,7.22721758556743,133.670006097094));
#62176=CARTESIAN_POINT('Ctrl Pts',(78.92412561328,7.24892480770593,133.667709185788));
#62177=CARTESIAN_POINT('Ctrl Pts',(78.8887136438618,7.27169441441594,133.665412274481));
#62178=CARTESIAN_POINT('Ctrl Pts',(78.8290631719135,7.31004918001196,133.661543191634));
#62179=CARTESIAN_POINT('Ctrl Pts',(78.7712838542149,7.35157084399013,133.657674108787));
#62180=CARTESIAN_POINT('Ctrl Pts',(78.7157319002096,7.39605080804882,133.65380502594));
#62181=CARTESIAN_POINT('Ctrl Pts',(78.6602627158453,7.44046449917939,133.649941707834));
#62182=CARTESIAN_POINT('Ctrl Pts',(78.6070146838403,7.48782744003637,133.646078389728));
#62183=CARTESIAN_POINT('Ctrl Pts',(78.5563157431666,7.53788737469662,133.642215071621));
#62184=CARTESIAN_POINT('Ctrl Pts',(78.5056762723309,7.58788858907282,133.638356285185));
#62185=CARTESIAN_POINT('Ctrl Pts',(78.4575802975035,7.64058017366701,133.63449749875));
#62186=CARTESIAN_POINT('Ctrl Pts',(78.4123219474131,7.69567030094621,133.630638712314));
#62187=CARTESIAN_POINT('Ctrl Pts',(78.3670921067645,7.75072572548481,133.626782356631));
#62188=CARTESIAN_POINT('Ctrl Pts',(78.3246966521299,7.80817632062366,133.622926000947));
#62189=CARTESIAN_POINT('Ctrl Pts',(78.285391140227,7.86769526165083,133.619069645264));
#62190=CARTESIAN_POINT('Ctrl Pts',(78.246097239566,7.9271966201868,133.615214428787));
#62191=CARTESIAN_POINT('Ctrl Pts',(78.2098917370284,7.98876470644017,133.61135921231));
#62192=CARTESIAN_POINT('Ctrl Pts',(78.1769873297903,8.05204305648689,133.607503995832));
#62193=CARTESIAN_POINT('Ctrl Pts',(78.1440816360882,8.11532388052786,133.603648628628));
#62194=CARTESIAN_POINT('Ctrl Pts',(78.1144775160843,8.18031466910409,133.599793261423));
#62195=CARTESIAN_POINT('Ctrl Pts',(78.0883412825139,8.24663520764542,133.595937894219));
#62196=CARTESIAN_POINT('Ctrl Pts',(78.062177691434,8.31302516570584,133.592078491496));
#62197=CARTESIAN_POINT('Ctrl Pts',(78.0394894114194,8.38074719936749,133.588219088773));
#62198=CARTESIAN_POINT('Ctrl Pts',(78.0203938937618,8.44940284540844,133.58435968605));
#62199=CARTESIAN_POINT('Ctrl Pts',(78.0012875640721,8.51809736481545,133.580498098103));
#62200=CARTESIAN_POINT('Ctrl Pts',(77.9857781519714,8.58772607453131,133.576636510156));
#62201=CARTESIAN_POINT('Ctrl Pts',(77.9739320459271,8.65787983400754,133.572774922209));
#62202=CARTESIAN_POINT('Ctrl Pts',(77.9620652146956,8.72815633000059,133.568906578276));
#62203=CARTESIAN_POINT('Ctrl Pts',(77.9538745412823,8.79895922703413,133.565038234342));
#62204=CARTESIAN_POINT('Ctrl Pts',(77.9493745075559,8.86987447506888,133.561169890409));
#62205=CARTESIAN_POINT('Ctrl Pts',(77.9467025170289,8.9119819085886,133.558872979102));
#62206=CARTESIAN_POINT('Ctrl Pts',(77.9453307150346,8.95412893627204,133.556576067796));
#62207=CARTESIAN_POINT('Ctrl Pts',(77.9452534594865,8.99622948970539,133.554279156489));
#62208=CARTESIAN_POINT('Ctrl Pts',(77.9452511674388,8.99747854533371,133.55421101083));
#62209=CARTESIAN_POINT('Ctrl Pts',(77.9452500143197,8.99872760305263,133.55414286517));
#62210=CARTESIAN_POINT('Ctrl Pts',(77.9452500001325,8.99997666154031,133.55407471951));
#62211=CARTESIAN_POINT('Origin',(80.,9.,141.545925280538));
#62212=CARTESIAN_POINT('',(81.252039109102,10.6292316077768,134.706120114193));
#62213=CARTESIAN_POINT('',(81.252039109102,10.6292316077768,134.647862573787));
#62214=CARTESIAN_POINT('',(81.252039109102,10.6292316077768,141.545925280538));
#62215=CARTESIAN_POINT('',(77.9452508583196,8.99812189887428,134.19592528059));
#62216=CARTESIAN_POINT('Ctrl Pts',(81.252039109102,10.6292316077768,134.647862573787));
#62217=CARTESIAN_POINT('Ctrl Pts',(81.3084423618865,10.585886586707,134.644002866747));
#62218=CARTESIAN_POINT('Ctrl Pts',(81.3626623260567,10.5395551758588,134.640143159707));
#62219=CARTESIAN_POINT('Ctrl Pts',(81.4143696942849,10.4904884871707,134.636283452668));
#62220=CARTESIAN_POINT('Ctrl Pts',(81.4660396062807,10.4414573418367,134.632426541556));
#62221=CARTESIAN_POINT('Ctrl Pts',(81.5152001817136,10.3896951826727,134.628569630445));
#62222=CARTESIAN_POINT('Ctrl Pts',(81.5615557470333,10.3354928720915,134.624712719334));
#62223=CARTESIAN_POINT('Ctrl Pts',(81.6078932397547,10.2813116933115,134.620857311912));
#62224=CARTESIAN_POINT('Ctrl Pts',(81.6514275774129,10.2246926201218,134.617001904491));
#62225=CARTESIAN_POINT('Ctrl Pts',(81.6919016788026,10.1659615224204,134.613146497069));
#62226=CARTESIAN_POINT('Ctrl Pts',(81.7323735395747,10.1072336760311,134.609291303081));
#62227=CARTESIAN_POINT('Ctrl Pts',(81.7697852261202,10.0463944381793,134.605436109092));
#62228=CARTESIAN_POINT('Ctrl Pts',(81.8039225228185,9.983799316003,134.601580915103));
#62229=CARTESIAN_POINT('Ctrl Pts',(81.8380934840931,9.92114246549826,134.597721919306));
#62230=CARTESIAN_POINT('Ctrl Pts',(81.8689833723166,9.85672669935811,134.593862923508));
#62231=CARTESIAN_POINT('Ctrl Pts',(81.8964240068341,9.7909320759731,134.590003927711));
#62232=CARTESIAN_POINT('Ctrl Pts',(81.9238778541335,9.72510577219794,134.586143073791));
#62233=CARTESIAN_POINT('Ctrl Pts',(81.9478789755098,9.6578997467298,134.58228221987));
#62234=CARTESIAN_POINT('Ctrl Pts',(81.9683084272647,9.5897113680935,134.57842136595));
#62235=CARTESIAN_POINT('Ctrl Pts',(81.9887754589296,9.52139755715708,134.574553410002));
#62236=CARTESIAN_POINT('Ctrl Pts',(82.0056575789907,9.45209825584912,134.570685454053));
#62237=CARTESIAN_POINT('Ctrl Pts',(82.0188866562537,9.38222275141696,134.566817498105));
#62238=CARTESIAN_POINT('Ctrl Pts',(82.0304714634763,9.32103222147011,134.563430298596));
#62239=CARTESIAN_POINT('Ctrl Pts',(82.0392556565754,9.25940017058367,134.560043099087));
#62240=CARTESIAN_POINT('Ctrl Pts',(82.045226284189,9.19760316030519,134.556655899578));
#62241=CARTESIAN_POINT('Ctrl Pts',(82.052046329133,9.12701453633118,134.552786816731));
#62242=CARTESIAN_POINT('Ctrl Pts',(82.0552210145704,9.05593416276994,134.548917733884));
#62243=CARTESIAN_POINT('Ctrl Pts',(82.054693562872,8.98477090967419,134.545048651037));
#62244=CARTESIAN_POINT('Ctrl Pts',(82.0541668970505,8.91371368627649,134.541185332931));
#62245=CARTESIAN_POINT('Ctrl Pts',(82.0499490467711,8.84257431027376,134.537322014824));
#62246=CARTESIAN_POINT('Ctrl Pts',(82.0420350207687,8.77176648700508,134.533458696718));
#62247=CARTESIAN_POINT('Ctrl Pts',(82.0341302779158,8.70104172128582,134.529599910282));
#62248=CARTESIAN_POINT('Ctrl Pts',(82.0225380250317,8.63064821622525,134.525741123846));
#62249=CARTESIAN_POINT('Ctrl Pts',(82.0073052791557,8.5609976323826,134.52188233741));
#62250=CARTESIAN_POINT('Ctrl Pts',(81.9920821287927,8.49139092330051,134.518025981727));
#62251=CARTESIAN_POINT('Ctrl Pts',(81.9732231387407,8.42252668040407,134.514169626044));
#62252=CARTESIAN_POINT('Ctrl Pts',(81.9508266910127,8.35480794786941,134.510313270361));
#62253=CARTESIAN_POINT('Ctrl Pts',(81.9284368594196,8.28710922012641,134.506458053883));
#62254=CARTESIAN_POINT('Ctrl Pts',(81.9025117972192,8.22055579189908,134.502602837406));
#62255=CARTESIAN_POINT('Ctrl Pts',(81.8731996991641,8.15553540657313,134.498747620929));
#62256=CARTESIAN_POINT('Ctrl Pts',(81.8438864550936,8.09051247914459,134.494892253724));
#62257=CARTESIAN_POINT('Ctrl Pts',(81.8111861139161,8.02702315557092,134.49103688652));
#62258=CARTESIAN_POINT('Ctrl Pts',(81.7752942420166,7.96543346431333,134.487181519315));
#62259=CARTESIAN_POINT('Ctrl Pts',(81.7393648011145,7.90377930544371,134.483322116592));
#62260=CARTESIAN_POINT('Ctrl Pts',(81.7002374058725,7.8440291687504,134.479462713869));
#62261=CARTESIAN_POINT('Ctrl Pts',(81.6581522078642,7.78652201583427,134.475603311147));
#62262=CARTESIAN_POINT('Ctrl Pts',(81.6160431808863,7.72898230191644,134.4717417232));
#62263=CARTESIAN_POINT('Ctrl Pts',(81.5709733243342,7.67368847666641,134.467880135253));
#62264=CARTESIAN_POINT('Ctrl Pts',(81.5232227929822,7.62094601793851,134.464018547306));
#62265=CARTESIAN_POINT('Ctrl Pts',(81.475388720364,7.56811128438857,134.460150203372));
#62266=CARTESIAN_POINT('Ctrl Pts',(81.424864953814,7.51783717203536,134.456281859439));
#62267=CARTESIAN_POINT('Ctrl Pts',(81.3719676447899,7.47039144087459,134.452413515505));
#62268=CARTESIAN_POINT('Ctrl Pts',(81.3405587449435,7.44221953108068,134.450116604199));
#62269=CARTESIAN_POINT('Ctrl Pts',(81.308313650705,7.41504403327825,134.447819692893));
#62270=CARTESIAN_POINT('Ctrl Pts',(81.2753034381162,7.38891381260064,134.445522781586));
#62271=CARTESIAN_POINT('Ctrl Pts',(81.2196986583658,7.34489818677875,134.441653698739));
#62272=CARTESIAN_POINT('Ctrl Pts',(81.1617035722648,7.30367843275997,134.437784615892));
#62273=CARTESIAN_POINT('Ctrl Pts',(81.1016308900003,7.26552401437867,134.433915533045));
#62274=CARTESIAN_POINT('Ctrl Pts',(81.0416477130365,7.22742644417791,134.430052214939));
#62275=CARTESIAN_POINT('Ctrl Pts',(80.9795934911436,7.19238540217982,134.426188896833));
#62276=CARTESIAN_POINT('Ctrl Pts',(80.9158130846975,7.16062946734575,134.422325578726));
#62277=CARTESIAN_POINT('Ctrl Pts',(80.8521074926436,7.12891078221101,134.41846679229));
#62278=CARTESIAN_POINT('Ctrl Pts',(80.786680170755,7.10046976549005,134.414608005855));
#62279=CARTESIAN_POINT('Ctrl Pts',(80.7199024698011,7.07549019319872,134.410749219419));
#62280=CARTESIAN_POINT('Ctrl Pts',(80.6531668339022,7.05052635620628,134.406892863736));
#62281=CARTESIAN_POINT('Ctrl Pts',(80.5850829605103,7.02901980744925,134.403036508052));
#62282=CARTESIAN_POINT('Ctrl Pts',(80.5160428208372,7.01110649617373,134.399180152369));
#62283=CARTESIAN_POINT('Ctrl Pts',(80.4470230763127,6.99319847666972,134.395324935892));
#62284=CARTESIAN_POINT('Ctrl Pts',(80.3770480962865,6.97888170925424,134.391469719415));
#62285=CARTESIAN_POINT('Ctrl Pts',(80.3065240147198,6.96824199499546,134.387614502937));
#62286=CARTESIAN_POINT('Ctrl Pts',(80.2359971758725,6.95760186475567,134.383759135733));
#62287=CARTESIAN_POINT('Ctrl Pts',(80.1649216735383,6.95063914338275,134.379903768528));
#62288=CARTESIAN_POINT('Ctrl Pts',(80.0937110916935,6.94738805572178,134.376048401324));
#62289=CARTESIAN_POINT('Ctrl Pts',(80.0224259717877,6.94413356505856,134.372188998601));
#62290=CARTESIAN_POINT('Ctrl Pts',(79.9510059763941,6.9445984857749,134.368329595878));
#62291=CARTESIAN_POINT('Ctrl Pts',(79.8798661318531,6.94876490469179,134.364470193155));
#62292=CARTESIAN_POINT('Ctrl Pts',(79.8086860073733,6.9529336826678,134.360608605208));
#62293=CARTESIAN_POINT('Ctrl Pts',(79.7377868325597,6.96080807732131,134.356747017261));
#62294=CARTESIAN_POINT('Ctrl Pts',(79.6675771998984,6.97231840653602,134.352885429315));
#62295=CARTESIAN_POINT('Ctrl Pts',(79.5972447329682,6.98384887348426,134.349017085381));
#62296=CARTESIAN_POINT('Ctrl Pts',(79.5276046915489,6.99902787181811,134.345148741448));
#62297=CARTESIAN_POINT('Ctrl Pts',(79.4590535039986,7.01773501999257,134.341280397514));
#62298=CARTESIAN_POINT('Ctrl Pts',(79.4183497815629,7.02884278623367,134.338983486208));
#62299=CARTESIAN_POINT('Ctrl Pts',(79.378029642418,7.04119350129801,134.336686574901));
#62300=CARTESIAN_POINT('Ctrl Pts',(79.3381726900253,7.05475395533839,134.334389663595));
#62301=CARTESIAN_POINT('Ctrl Pts',(79.2710347685908,7.07759616085897,134.330520580748));
#62302=CARTESIAN_POINT('Ctrl Pts',(79.2049492964154,7.10396296765435,134.326651497901));
#62303=CARTESIAN_POINT('Ctrl Pts',(79.140312266831,7.13373780943334,134.322782415054));
#62304=CARTESIAN_POINT('Ctrl Pts',(79.075771543197,7.16346828818303,134.318919096948));
#62305=CARTESIAN_POINT('Ctrl Pts',(79.0126754159973,7.19659652102821,134.315055778841));
#62306=CARTESIAN_POINT('Ctrl Pts',(78.9514029674593,7.23295675609033,134.311192460735));
#62307=CARTESIAN_POINT('Ctrl Pts',(78.8902023914798,7.26927434061071,134.307333674299));
#62308=CARTESIAN_POINT('Ctrl Pts',(78.8308216607735,7.30881615015988,134.303474887863));
#62309=CARTESIAN_POINT('Ctrl Pts',(78.7736165849994,7.3513698771673,134.299616101428));
#62310=CARTESIAN_POINT('Ctrl Pts',(78.7164475442283,7.39389679844704,134.295759745744));
#62311=CARTESIAN_POINT('Ctrl Pts',(78.6614518281799,7.43943158374137,134.291903390061));
#62312=CARTESIAN_POINT('Ctrl Pts',(78.6089562497839,7.48771866126542,134.288047034378));
#62313=CARTESIAN_POINT('Ctrl Pts',(78.5564761791075,7.53599147430328,134.284191817901));
#62314=CARTESIAN_POINT('Ctrl Pts',(78.5064951371637,7.58701463674079,134.280336601423));
#62315=CARTESIAN_POINT('Ctrl Pts',(78.4593054873361,7.64049347881392,134.276481384946));
#62316=CARTESIAN_POINT('Ctrl Pts',(78.4121139925344,7.69397441174974,134.272626017742));
#62317=CARTESIAN_POINT('Ctrl Pts',(78.3677144262844,7.74991084922807,134.268770650537));
#62318=CARTESIAN_POINT('Ctrl Pts',(78.3263598618199,7.80797388855254,134.264915283332));
#62319=CARTESIAN_POINT('Ctrl Pts',(78.2849620104032,7.86609770404621,134.261055880609));
#62320=CARTESIAN_POINT('Ctrl Pts',(78.2466158057059,7.92635216843353,134.257196477887));
#62321=CARTESIAN_POINT('Ctrl Pts',(78.211531300393,7.98837888860206,134.253337075164));
#62322=CARTESIAN_POINT('Ctrl Pts',(78.1764269299576,8.05044072878677,134.249475487217));
#62323=CARTESIAN_POINT('Ctrl Pts',(78.1445881522363,8.11427638742378,134.24561389927));
#62324=CARTESIAN_POINT('Ctrl Pts',(78.1161780375015,8.17950479824165,134.241752311323));
#62325=CARTESIAN_POINT('Ctrl Pts',(78.0877182182528,8.24484732850228,134.23788396739));
#62326=CARTESIAN_POINT('Ctrl Pts',(78.0626992088764,8.31158702080849,134.234015623456));
#62327=CARTESIAN_POINT('Ctrl Pts',(78.0412348877945,8.37932553000272,134.230147279523));
#62328=CARTESIAN_POINT('Ctrl Pts',(78.0284899916254,8.41954670741753,134.227850368216));
#62329=CARTESIAN_POINT('Ctrl Pts',(78.0169973859048,8.46011977480232,134.22555345691));
#62330=CARTESIAN_POINT('Ctrl Pts',(78.0067723452923,8.50095984228864,134.223256545603));
#62331=CARTESIAN_POINT('Ctrl Pts',(77.9843222460634,8.59062829470186,134.218213447125));
#62332=CARTESIAN_POINT('Ctrl Pts',(77.9679136797141,8.68186550115405,134.213170348647));
#62333=CARTESIAN_POINT('Ctrl Pts',(77.9577201042086,8.77396816651993,134.208127250169));
#62334=CARTESIAN_POINT('Ctrl Pts',(77.9494988556529,8.84825013992636,134.204059926976));
#62335=CARTESIAN_POINT('Ctrl Pts',(77.9453194352602,8.92309483675305,134.199992603783));
#62336=CARTESIAN_POINT('Ctrl Pts',(77.9452508583196,8.99812189887429,134.195925280589));
#62337=CARTESIAN_POINT('Ctrl Pts',(77.9452508583188,8.99812189982399,134.195925280538));
#62338=CARTESIAN_POINT('Ctrl Pts',(77.9451865584667,9.06846962007642,134.192111631088));
#62339=CARTESIAN_POINT('Ctrl Pts',(77.9487392155753,9.13891228886075,134.188297981638));
#62340=CARTESIAN_POINT('Ctrl Pts',(77.9559113871452,9.20904378798979,134.184484332188));
#62341=CARTESIAN_POINT('Ctrl Pts',(77.9630788626377,9.27912936756171,134.180673179777));
#62342=CARTESIAN_POINT('Ctrl Pts',(77.9738611037572,9.34890368688671,134.176862027366));
#62343=CARTESIAN_POINT('Ctrl Pts',(77.9882086454291,9.41796304642114,134.173050874956));
#62344=CARTESIAN_POINT('Ctrl Pts',(78.0025518660922,9.48700160754263,134.169240870339));
#62345=CARTESIAN_POINT('Ctrl Pts',(78.0204581554944,9.55532514838178,134.165430865722));
#62346=CARTESIAN_POINT('Ctrl Pts',(78.0418267999906,9.62253938129632,134.161620861105));
#62347=CARTESIAN_POINT('Ctrl Pts',(78.0631965645669,9.6897571373792,134.157810656779));
#62348=CARTESIAN_POINT('Ctrl Pts',(78.0880288903438,9.75586499614043,134.154000452454));
#62349=CARTESIAN_POINT('Ctrl Pts',(78.1161735511141,9.82048490112727,134.150190248128));
#62350=CARTESIAN_POINT('Ctrl Pts',(78.1443474516828,9.88517194044597,134.146376085339));
#62351=CARTESIAN_POINT('Ctrl Pts',(78.1758403520865,9.94836748481235,134.14256192255));
#62352=CARTESIAN_POINT('Ctrl Pts',(78.2104547888993,10.0097155539689,134.138747759761));
#62353=CARTESIAN_POINT('Ctrl Pts',(78.2450904309215,10.0711012056709,134.134931260371));
#62354=CARTESIAN_POINT('Ctrl Pts',(78.2828511440641,10.1306367118239,134.131114760981));
#62355=CARTESIAN_POINT('Ctrl Pts',(78.3234961567954,10.1879951288705,134.127298261591));
#62356=CARTESIAN_POINT('Ctrl Pts',(78.3642086074964,10.2454487146705,134.123475429888));
#62357=CARTESIAN_POINT('Ctrl Pts',(78.4078145926627,10.3007176182968,134.119652598184));
#62358=CARTESIAN_POINT('Ctrl Pts',(78.4540338348359,10.3535088395233,134.115829766481));
#62359=CARTESIAN_POINT('Ctrl Pts',(78.4689707705128,10.3705696790934,134.114594320191));
#62360=CARTESIAN_POINT('Ctrl Pts',(78.4841803654166,10.3873720424415,134.113358873901));
#62361=CARTESIAN_POINT('Ctrl Pts',(78.4996524028238,10.4039069236055,134.112123427611));
#62362=CARTESIAN_POINT('Ctrl Pts',(78.548106629474,10.4556896887627,134.108254344765));
#62363=CARTESIAN_POINT('Ctrl Pts',(78.5993397400989,10.5050624191808,134.104385261918));
#62364=CARTESIAN_POINT('Ctrl Pts',(78.6530824932537,10.5517122131762,134.100516179071));
#62365=CARTESIAN_POINT('Ctrl Pts',(78.7067451723865,10.5982925013052,134.096652860964));
#62366=CARTESIAN_POINT('Ctrl Pts',(78.7629097078902,10.6421575902791,134.092789542858));
#62367=CARTESIAN_POINT('Ctrl Pts',(78.821268994773,10.6830302373447,134.088926224751));
#62368=CARTESIAN_POINT('Ctrl Pts',(78.8795598262348,10.723854940811,134.085067438316));
#62369=CARTESIAN_POINT('Ctrl Pts',(78.9400398993909,10.7616938973594,134.08120865188));
#62370=CARTESIAN_POINT('Ctrl Pts',(79.0023692611189,10.7963102380545,134.077349865444));
#62371=CARTESIAN_POINT('Ctrl Pts',(79.0646593599195,10.8309047729934,134.073493509761));
#62372=CARTESIAN_POINT('Ctrl Pts',(79.1287960124374,10.8622804842886,134.069637154078));
#62373=CARTESIAN_POINT('Ctrl Pts',(79.1944117734203,10.8902447385712,134.065780798394));
#62374=CARTESIAN_POINT('Ctrl Pts',(79.2600081508502,10.9182007319331,134.061925581917));
#62375=CARTESIAN_POINT('Ctrl Pts',(79.3270823226435,10.9427470786496,134.05807036544));
#62376=CARTESIAN_POINT('Ctrl Pts',(79.3952453929252,10.9637386352878,134.054215148963));
#62377=CARTESIAN_POINT('Ctrl Pts',(79.463411128179,10.984731012633,134.050359781758));
#62378=CARTESIAN_POINT('Ctrl Pts',(79.5326653815291,11.0021681830996,134.046504414553));
#62379=CARTESIAN_POINT('Ctrl Pts',(79.602604232826,11.0159549019589,134.042649047349));
#62380=CARTESIAN_POINT('Ctrl Pts',(79.6726162910289,11.0297560517535,134.038789644626));
#62381=CARTESIAN_POINT('Ctrl Pts',(79.7433139000601,11.0398990281692,134.034930241903));
#62382=CARTESIAN_POINT('Ctrl Pts',(79.8142839731728,11.0463399326308,134.03107083918));
#62383=CARTESIAN_POINT('Ctrl Pts',(79.8852942300985,11.0527844839832,134.027209251234));
#62384=CARTESIAN_POINT('Ctrl Pts',(79.9565767725574,11.0555227719526,134.023347663287));
#62385=CARTESIAN_POINT('Ctrl Pts',(80.0277171909408,11.0545630483941,134.01948607534));
#62386=CARTESIAN_POINT('Ctrl Pts',(80.098982072036,11.0536016457648,134.015617731406));
#62387=CARTESIAN_POINT('Ctrl Pts',(80.170103847725,11.0489293463164,134.011749387473));
#62388=CARTESIAN_POINT('Ctrl Pts',(80.2406726110885,11.0406063453719,134.007881043539));
#62389=CARTESIAN_POINT('Ctrl Pts',(80.2825743119814,11.0356643869261,134.005584132233));
#62390=CARTESIAN_POINT('Ctrl Pts',(80.3242812036119,11.0294363074637,134.003287220927));
#62391=CARTESIAN_POINT('Ctrl Pts',(80.3657096343969,11.0219431312006,134.00099030962));
#62392=CARTESIAN_POINT('Ctrl Pts',(80.4354967859363,11.0093207021712,133.997121109306));
#62393=CARTESIAN_POINT('Ctrl Pts',(80.504766368103,10.9930562639826,133.993251908992));
#62394=CARTESIAN_POINT('Ctrl Pts',(80.5731094334081,10.973206309497,133.989382708677));
#62395=CARTESIAN_POINT('Ctrl Pts',(80.6413358826976,10.9533902256402,133.985520110506));
#62396=CARTESIAN_POINT('Ctrl Pts',(80.7086384934946,10.9300009151042,133.981657512336));
#62397=CARTESIAN_POINT('Ctrl Pts',(80.7746179998123,10.9031459525919,133.977794914165));
#62398=CARTESIAN_POINT('Ctrl Pts',(80.8405321010282,10.876317611248,133.973936144965));
#62399=CARTESIAN_POINT('Ctrl Pts',(80.9051252521823,10.846030615393,133.970077375766));
#62400=CARTESIAN_POINT('Ctrl Pts',(80.9680140702191,10.8124420880011,133.966218606566));
#62401=CARTESIAN_POINT('Ctrl Pts',(81.0308625996586,10.778875078499,133.962362309418));
#62402=CARTESIAN_POINT('Ctrl Pts',(81.0920085350437,10.7420109626267,133.95850601227));
#62403=CARTESIAN_POINT('Ctrl Pts',(81.151090755897,10.702053945734,133.954649715122));
#62404=CARTESIAN_POINT('Ctrl Pts',(81.1854604262026,10.678809905866,133.952406406396));
#62405=CARTESIAN_POINT('Ctrl Pts',(81.2191321621777,10.6545200838374,133.95016309767));
#62406=CARTESIAN_POINT('Ctrl Pts',(81.252039109102,10.6292316077769,133.947919788944));
#62407=CARTESIAN_POINT('',(77.9452507619582,9.00176953857242,134.254074719427));
#62408=CARTESIAN_POINT('Ctrl Pts',(77.9452507619582,9.00176953857242,134.254074719427));
#62409=CARTESIAN_POINT('Ctrl Pts',(77.9453248874363,9.08784241202325,134.249416661534));
#62410=CARTESIAN_POINT('Ctrl Pts',(77.950811182931,9.17367901479838,134.24475860364));
#62411=CARTESIAN_POINT('Ctrl Pts',(77.961598209329,9.25868069562512,134.240100545746));
#62412=CARTESIAN_POINT('Ctrl Pts',(77.972541792015,9.34491603873662,134.235374883655));
#62413=CARTESIAN_POINT('Ctrl Pts',(77.9889410126126,9.43029206338749,134.230649221565));
#62414=CARTESIAN_POINT('Ctrl Pts',(78.0106307458962,9.51420573054619,134.225923559474));
#62415=CARTESIAN_POINT('Ctrl Pts',(78.0180442984582,9.54288742865743,134.224308327796));
#62416=CARTESIAN_POINT('Ctrl Pts',(78.0260755171321,9.57139846976164,134.222693096117));
#62417=CARTESIAN_POINT('Ctrl Pts',(78.0347165430365,9.59971534604805,134.221077864439));
#62418=CARTESIAN_POINT('Ctrl Pts',(78.0554150258307,9.66754483563481,134.217208781592));
#62419=CARTESIAN_POINT('Ctrl Pts',(78.0796697562116,9.73443434293891,134.213339698745));
#62420=CARTESIAN_POINT('Ctrl Pts',(78.1073768028462,9.79998437240689,134.209470615898));
#62421=CARTESIAN_POINT('Ctrl Pts',(78.135042567363,9.86543673560005,134.205607297791));
#62422=CARTESIAN_POINT('Ctrl Pts',(78.1661502502832,9.92955313866793,134.201743979685));
#62423=CARTESIAN_POINT('Ctrl Pts',(78.2005462224256,9.99194942657027,134.197880661579));
#62424=CARTESIAN_POINT('Ctrl Pts',(78.2349018481058,10.054272523651,134.194021875143));
#62425=CARTESIAN_POINT('Ctrl Pts',(78.2725378680004,10.114879090029,134.190163088707));
#62426=CARTESIAN_POINT('Ctrl Pts',(78.313253381618,10.1734067529535,134.186304302271));
#62427=CARTESIAN_POINT('Ctrl Pts',(78.3539432474475,10.2318975477419,134.182447946588));
#62428=CARTESIAN_POINT('Ctrl Pts',(78.3977084815971,10.2883116393796,134.178591590905));
#62429=CARTESIAN_POINT('Ctrl Pts',(78.4443040202919,10.3423142632111,134.174735235221));
#62430=CARTESIAN_POINT('Ctrl Pts',(78.4908857941979,10.3963009341267,134.170880018744));
#62431=CARTESIAN_POINT('Ctrl Pts',(78.5402958955814,10.4478771838951,134.167024802267));
#62432=CARTESIAN_POINT('Ctrl Pts',(78.5922490883442,10.4967414383361,134.16316958579));
#62433=CARTESIAN_POINT('Ctrl Pts',(78.6442043123215,10.5456076032234,134.159314218585));
#62434=CARTESIAN_POINT('Ctrl Pts',(78.6987024697097,10.5917612310576,134.15545885138));
#62435=CARTESIAN_POINT('Ctrl Pts',(78.7554228609497,10.6349389308024,134.151603484176));
#62436=CARTESIAN_POINT('Ctrl Pts',(78.8122026229723,10.6781618258248,134.147744081453));
#62437=CARTESIAN_POINT('Ctrl Pts',(78.8712088748859,10.7184022797039,134.14388467873));
#62438=CARTESIAN_POINT('Ctrl Pts',(78.9320900753219,10.7554389636994,134.140025276007));
#62439=CARTESIAN_POINT('Ctrl Pts',(78.9930057471718,10.7924966181563,134.136163688061));
#62440=CARTESIAN_POINT('Ctrl Pts',(79.0557980530733,10.8263466609921,134.132302100114));
#62441=CARTESIAN_POINT('Ctrl Pts',(79.1200912978449,10.8568140020938,134.128440512167));
#62442=CARTESIAN_POINT('Ctrl Pts',(79.1844970259526,10.8873346469009,134.124572168233));
#62443=CARTESIAN_POINT('Ctrl Pts',(79.2504084863378,10.9144605892661,134.1207038243));
#62444=CARTESIAN_POINT('Ctrl Pts',(79.3174311513886,10.9380653573616,134.116835480366));
#62445=CARTESIAN_POINT('Ctrl Pts',(79.3572272811514,10.9520811893707,134.11453856906));
#62446=CARTESIAN_POINT('Ctrl Pts',(79.3974148942616,10.9648565381244,134.112241657753));
#62447=CARTESIAN_POINT('Ctrl Pts',(79.437909628772,10.976373440692,134.109944746447));
#62448=CARTESIAN_POINT('Ctrl Pts',(79.5061249302263,10.9957742094579,134.10607549038));
#62449=CARTESIAN_POINT('Ctrl Pts',(79.5754794623167,11.0116771155591,134.102206234313));
#62450=CARTESIAN_POINT('Ctrl Pts',(79.6455811722356,11.0239527803351,134.098336978246));
#62451=CARTESIAN_POINT('Ctrl Pts',(79.715560976673,11.0362070979737,134.094474450739));
#62452=CARTESIAN_POINT('Ctrl Pts',(79.786284902651,11.0448466246093,134.090611923232));
#62453=CARTESIAN_POINT('Ctrl Pts',(79.8573471332515,11.0497921168032,134.086749395724));
#62454=CARTESIAN_POINT('Ctrl Pts',(79.9283395278631,11.0547327488437,134.082890664093));
#62455=CARTESIAN_POINT('Ctrl Pts',(79.9996690856373,11.055986514164,134.079031932462));
#62456=CARTESIAN_POINT('Ctrl Pts',(80.0709224192409,11.0535256445803,134.07517320083));
#62457=CARTESIAN_POINT('Ctrl Pts',(80.1421295659905,11.0510663701476,134.071316970453));
#62458=CARTESIAN_POINT('Ctrl Pts',(80.2132601023318,11.0448972558307,134.067460740076));
#62459=CARTESIAN_POINT('Ctrl Pts',(80.2838999035955,11.0350426057551,134.063604509698));
#62460=CARTESIAN_POINT('Ctrl Pts',(80.3545175459519,11.0251910469718,134.059749488977));
#62461=CARTESIAN_POINT('Ctrl Pts',(80.4246442782314,11.0116563158045,134.055894468255));
#62462=CARTESIAN_POINT('Ctrl Pts',(80.4938720915145,10.9945144571356,134.052039447534));
#62463=CARTESIAN_POINT('Ctrl Pts',(80.5631419758927,10.9773621810243,134.048182084041));
#62464=CARTESIAN_POINT('Ctrl Pts',(80.631511375826,10.956598508231,134.044324720548));
#62465=CARTESIAN_POINT('Ctrl Pts',(80.6985844526089,10.9323502076676,134.040467357055));
#62466=CARTESIAN_POINT('Ctrl Pts',(80.7656748958071,10.908095628787,134.036608994822));
#62467=CARTESIAN_POINT('Ctrl Pts',(80.8314678959154,10.8803548068018,134.032750632588));
#62468=CARTESIAN_POINT('Ctrl Pts',(80.8955871455509,10.8493029030486,134.028892270355));
#62469=CARTESIAN_POINT('Ctrl Pts',(80.9598054148628,10.8182030456859,134.025027949634));
#62470=CARTESIAN_POINT('Ctrl Pts',(81.0223443385665,10.7837821180665,134.021163628913));
#62471=CARTESIAN_POINT('Ctrl Pts',(81.0828523129216,10.7462612722329,134.017299308192));
#62472=CARTESIAN_POINT('Ctrl Pts',(81.1412345966972,10.7100585618909,134.01357074396));
#62473=CARTESIAN_POINT('Ctrl Pts',(81.1977259678891,10.6709704106653,134.009842179727));
#62474=CARTESIAN_POINT('Ctrl Pts',(81.252039109102,10.6292316077768,134.006113615495));
#62475=CARTESIAN_POINT('Ctrl Pts',(81.252039109102,10.6292316077768,134.706120114193));
#62476=CARTESIAN_POINT('Ctrl Pts',(81.3086174334394,10.585752046946,134.702260546401));
#62477=CARTESIAN_POINT('Ctrl Pts',(81.3628983035071,10.539344867176,134.69840097861));
#62478=CARTESIAN_POINT('Ctrl Pts',(81.4145767274719,10.4902919997755,134.694541410819));
#62479=CARTESIAN_POINT('Ctrl Pts',(81.4662859518312,10.4412098968149,134.690679542721));
#62480=CARTESIAN_POINT('Ctrl Pts',(81.5153893085673,10.3894793202318,134.686817674624));
#62481=CARTESIAN_POINT('Ctrl Pts',(81.5616202009819,10.3354175041481,134.682955806526));
#62482=CARTESIAN_POINT('Ctrl Pts',(81.6079305738289,10.2812627446604,134.679087299081));
#62483=CARTESIAN_POINT('Ctrl Pts',(81.6513583294713,10.2247691308874,134.675218791636));
#62484=CARTESIAN_POINT('Ctrl Pts',(81.6916789789069,10.1662846114155,134.671350284191));
#62485=CARTESIAN_POINT('Ctrl Pts',(81.7116210733504,10.1373588915395,134.669436968263));
#62486=CARTESIAN_POINT('Ctrl Pts',(81.7308038117887,10.1079465715868,134.667523652334));
#62487=CARTESIAN_POINT('Ctrl Pts',(81.7492042338688,10.0780918841711,134.665610336405));
#62488=CARTESIAN_POINT('Ctrl Pts',(81.786413330588,10.0177201195048,134.661741253558));
#62489=CARTESIAN_POINT('Ctrl Pts',(81.8205661439276,9.95530150469948,134.657872170711));
#62490=CARTESIAN_POINT('Ctrl Pts',(81.851431639158,9.89117812362332,134.654003087864));
#62491=CARTESIAN_POINT('Ctrl Pts',(81.8822511463398,9.82715028318705,134.650139769758));
#62492=CARTESIAN_POINT('Ctrl Pts',(81.9097928487124,9.76142315249177,134.646276451652));
#62493=CARTESIAN_POINT('Ctrl Pts',(81.9338700765013,9.69436596238065,134.642413133545));
#62494=CARTESIAN_POINT('Ctrl Pts',(81.9579190617113,9.6273874303276,134.638554347109));
#62495=CARTESIAN_POINT('Ctrl Pts',(81.9785114811097,9.55908239284894,134.634695560674));
#62496=CARTESIAN_POINT('Ctrl Pts',(81.9955082589979,9.48984114850744,134.630836774238));
#62497=CARTESIAN_POINT('Ctrl Pts',(82.0124943301624,9.42064352107262,134.626980418555));
#62498=CARTESIAN_POINT('Ctrl Pts',(82.0258891379882,9.35051132747519,134.623124062871));
#62499=CARTESIAN_POINT('Ctrl Pts',(82.035603517282,9.27984975063267,134.619267707188));
#62500=CARTESIAN_POINT('Ctrl Pts',(82.0453150268509,9.20920904792752,134.615412490711));
#62501=CARTESIAN_POINT('Ctrl Pts',(82.0513482002261,9.13803975343951,134.611557274234));
#62502=CARTESIAN_POINT('Ctrl Pts',(82.0536653328037,9.06675524953479,134.607702057756));
#62503=CARTESIAN_POINT('Ctrl Pts',(82.0559825559742,8.9954679586192,134.603846690552));
#62504=CARTESIAN_POINT('Ctrl Pts',(82.0545834363202,8.92406593494232,134.599991323347));
#62505=CARTESIAN_POINT('Ctrl Pts',(82.0494823628482,8.85296392662273,134.596135956143));
#62506=CARTESIAN_POINT('Ctrl Pts',(82.0443759499432,8.78178749388894,134.59227655342));
#62507=CARTESIAN_POINT('Ctrl Pts',(82.0355598828126,8.71091218892561,134.588417150697));
#62508=CARTESIAN_POINT('Ctrl Pts',(82.0231004992737,8.64074809347968,134.584557747974));
#62509=CARTESIAN_POINT('Ctrl Pts',(82.010634061134,8.57054427057179,134.580696160027));
#62510=CARTESIAN_POINT('Ctrl Pts',(81.9945203098238,8.50105293226893,134.57683457208));
#62511=CARTESIAN_POINT('Ctrl Pts',(81.9748762440994,8.43267171497294,134.572972984134));
#62512=CARTESIAN_POINT('Ctrl Pts',(81.9551978103779,8.36417086228623,134.5691046402));
#62513=CARTESIAN_POINT('Ctrl Pts',(81.9319768891767,8.29678446768117,134.565236296267));
#62514=CARTESIAN_POINT('Ctrl Pts',(81.9053794077271,8.23089215638534,134.561367952333));
#62515=CARTESIAN_POINT('Ctrl Pts',(81.8895865886511,8.19176719815339,134.559071041027));
#62516=CARTESIAN_POINT('Ctrl Pts',(81.8726042233082,8.15316858353259,134.55677412972));
#62517=CARTESIAN_POINT('Ctrl Pts',(81.8544746051533,8.11517148478284,134.554477218414));
#62518=CARTESIAN_POINT('Ctrl Pts',(81.8239357704899,8.05116643478686,134.550608135567));
#62519=CARTESIAN_POINT('Ctrl Pts',(81.7900196413613,7.9886188983192,134.54673905272));
#62520=CARTESIAN_POINT('Ctrl Pts',(81.7528883050503,7.9279085148562,134.542869969873));
#62521=CARTESIAN_POINT('Ctrl Pts',(81.7158122925786,7.8672885868368,134.539006651767));
#62522=CARTESIAN_POINT('Ctrl Pts',(81.6755308333296,7.8085007894651,134.53514333366));
#62523=CARTESIAN_POINT('Ctrl Pts',(81.6322528843361,7.75190221373627,134.531280015554));
#62524=CARTESIAN_POINT('Ctrl Pts',(81.5890257003601,7.69537002811496,134.527421229118));
#62525=CARTESIAN_POINT('Ctrl Pts',(81.5428093020265,7.64102234732982,134.523562442682));
#62526=CARTESIAN_POINT('Ctrl Pts',(81.4938561601464,7.58918770373492,134.519703656246));
#62527=CARTESIAN_POINT('Ctrl Pts',(81.4449338551561,7.53738571216467,134.515847300563));
#62528=CARTESIAN_POINT('Ctrl Pts',(81.3932785596597,7.48809396942154,134.51199094488));
#62529=CARTESIAN_POINT('Ctrl Pts',(81.3391823197827,7.44160714937429,134.508134589197));
#62530=CARTESIAN_POINT('Ctrl Pts',(81.2851020604767,7.39513406199919,134.504279372719));
#62531=CARTESIAN_POINT('Ctrl Pts',(81.2285826565668,7.35146456875093,134.500424156242));
#62532=CARTESIAN_POINT('Ctrl Pts',(81.1699509540174,7.31085455697452,134.496568939765));
#62533=CARTESIAN_POINT('Ctrl Pts',(81.1113169591437,7.270242957468,134.49271357256));
#62534=CARTESIAN_POINT('Ctrl Pts',(81.0505709022709,7.2326913517047,134.488858205356));
#62535=CARTESIAN_POINT('Ctrl Pts',(80.9880690313265,7.1984126022217,134.485002838151));
#62536=CARTESIAN_POINT('Ctrl Pts',(80.9255017379667,7.1640979722354,134.481143435428));
#62537=CARTESIAN_POINT('Ctrl Pts',(80.8611753885608,7.13306327124748,134.477284032705));
#62538=CARTESIAN_POINT('Ctrl Pts',(80.7954704866755,7.10547518693255,134.473424629983));
#62539=CARTESIAN_POINT('Ctrl Pts',(80.7297283821587,7.07787148202758,134.469563042036));
#62540=CARTESIAN_POINT('Ctrl Pts',(80.6626066286407,7.05371844319009,134.465701454089));
#62541=CARTESIAN_POINT('Ctrl Pts',(80.5945027514386,7.03313344605386,134.461839866142));
#62542=CARTESIAN_POINT('Ctrl Pts',(80.5262797240621,7.01251243472729,134.457971522208));
#62543=CARTESIAN_POINT('Ctrl Pts',(80.4570716142902,6.995472044441,134.454103178275));
#62544=CARTESIAN_POINT('Ctrl Pts',(80.3872873534986,6.98207877549195,134.450234834341));
#62545=CARTESIAN_POINT('Ctrl Pts',(80.3458514676571,6.97412623781481,134.447937923035));
#62546=CARTESIAN_POINT('Ctrl Pts',(80.3042125940085,6.96745855572034,134.445641011728));
#62547=CARTESIAN_POINT('Ctrl Pts',(80.2624568263924,6.96208096903237,134.443344100422));
#62548=CARTESIAN_POINT('Ctrl Pts',(80.192120403827,6.95302257467726,134.439475017575));
#62549=CARTESIAN_POINT('Ctrl Pts',(80.1211767085347,6.94759208376961,134.435605934728));
#62550=CARTESIAN_POINT('Ctrl Pts',(80.0500326011492,6.94585923040259,134.431736851881));
#62551=CARTESIAN_POINT('Ctrl Pts',(79.9789944949355,6.94412895890066,134.427873533775));
#62552=CARTESIAN_POINT('Ctrl Pts',(79.9077570510322,6.94608540087243,134.424010215668));
#62553=CARTESIAN_POINT('Ctrl Pts',(79.8367336075784,6.95174668373132,134.420146897562));
#62554=CARTESIAN_POINT('Ctrl Pts',(79.7657934745967,6.95740132590758,134.416288111126));
#62555=CARTESIAN_POINT('Ctrl Pts',(79.6950673253459,6.96675213837446,134.41242932469));
#62556=CARTESIAN_POINT('Ctrl Pts',(79.624968105923,6.97976520153597,134.408570538255));
#62557=CARTESIAN_POINT('Ctrl Pts',(79.5549130438682,6.99277006742189,134.404714182571));
#62558=CARTESIAN_POINT('Ctrl Pts',(79.4854846046205,7.00943251859566,134.400857826888));
#62559=CARTESIAN_POINT('Ctrl Pts',(79.4170887535154,7.02966702275434,134.397001471205));
#62560=CARTESIAN_POINT('Ctrl Pts',(79.3487131072294,7.04989554943792,134.393146254728));
#62561=CARTESIAN_POINT('Ctrl Pts',(79.2813699090746,7.07369389646482,134.38929103825));
#62562=CARTESIAN_POINT('Ctrl Pts',(79.2154514132926,7.10092625798908,134.385435821773));
#62563=CARTESIAN_POINT('Ctrl Pts',(79.1495303402946,7.12815968421718,134.381580454569));
#62564=CARTESIAN_POINT('Ctrl Pts',(79.0850345283947,7.15882720397901,134.377725087364));
#62565=CARTESIAN_POINT('Ctrl Pts',(79.022336032316,7.19274497405804,134.373869720159));
#62566=CARTESIAN_POINT('Ctrl Pts',(78.9595719080091,7.22669824679341,134.370010317436));
#62567=CARTESIAN_POINT('Ctrl Pts',(78.8986092831646,7.26390832963901,134.366150914714));
#62568=CARTESIAN_POINT('Ctrl Pts',(78.8397945752582,7.30414595707656,134.362291511991));
#62569=CARTESIAN_POINT('Ctrl Pts',(78.7809465660022,7.34440636737485,134.358429924044));
#62570=CARTESIAN_POINT('Ctrl Pts',(78.7242492809826,7.38769743980121,134.354568336097));
#62571=CARTESIAN_POINT('Ctrl Pts',(78.6700169412605,7.43374886242149,134.35070674815));
#62572=CARTESIAN_POINT('Ctrl Pts',(78.6156897201163,7.47988085365626,134.346838404217));
#62573=CARTESIAN_POINT('Ctrl Pts',(78.5638364078417,7.52878250358203,134.342970060283));
#62574=CARTESIAN_POINT('Ctrl Pts',(78.5147346698664,7.58014632387587,134.33910171635));
#62575=CARTESIAN_POINT('Ctrl Pts',(78.4855794708822,7.6106446822438,134.336804805043));
#62576=CARTESIAN_POINT('Ctrl Pts',(78.4573936249812,7.64201045776524,134.334507893737));
#62577=CARTESIAN_POINT('Ctrl Pts',(78.430228229917,7.67417416213494,134.332210982431));
#62578=CARTESIAN_POINT('Ctrl Pts',(78.3847678948149,7.72799899241335,134.328367181984));
#62579=CARTESIAN_POINT('Ctrl Pts',(78.3419831696139,7.78427842280377,134.324523381537));
#62580=CARTESIAN_POINT('Ctrl Pts',(78.3021523840385,7.84271393533238,134.32067958109));
#62581=CARTESIAN_POINT('Ctrl Pts',(78.262377579922,7.90106731779013,134.316841183036));
#62582=CARTESIAN_POINT('Ctrl Pts',(78.2255487573432,7.96157037052464,134.313002784982));
#62583=CARTESIAN_POINT('Ctrl Pts',(78.1919047913615,8.02389074433322,134.309164386928));
#62584=CARTESIAN_POINT('Ctrl Pts',(78.1582964950691,8.08614504542086,134.305330058384));
#62585=CARTESIAN_POINT('Ctrl Pts',(78.1278665893404,8.15021241435526,134.301495729841));
#62586=CARTESIAN_POINT('Ctrl Pts',(78.10081028452,8.21573219681344,134.297661401297));
#62587=CARTESIAN_POINT('Ctrl Pts',(78.0737690938024,8.2812153788293,134.293829214673));
#62588=CARTESIAN_POINT('Ctrl Pts',(78.0500979587481,8.34814891320326,134.289997028049));
#62589=CARTESIAN_POINT('Ctrl Pts',(78.0299450759375,8.41614971210322,134.286164841425));
#62590=CARTESIAN_POINT('Ctrl Pts',(78.0097994694118,8.48412595902305,134.282334038429));
#62591=CARTESIAN_POINT('Ctrl Pts',(77.9931697296337,8.55316823242713,134.278503235433));
#62592=CARTESIAN_POINT('Ctrl Pts',(77.9801543906814,8.62287763654694,134.274672432436));
#62593=CARTESIAN_POINT('Ctrl Pts',(77.9671331495253,8.69261865252947,134.270839892245));
#62594=CARTESIAN_POINT('Ctrl Pts',(77.9577296763162,8.76302691922407,134.267007352053));
#62595=CARTESIAN_POINT('Ctrl Pts',(77.9519912481153,8.83369391260768,134.263174811862));
#62596=CARTESIAN_POINT('Ctrl Pts',(77.9474494190888,8.88962515205753,134.260141447729));
#62597=CARTESIAN_POINT('Ctrl Pts',(77.9452024908778,8.9457182021302,134.257108083595));
#62598=CARTESIAN_POINT('Ctrl Pts',(77.9452507619577,9.00176953792933,134.254074719462));
#62599=CARTESIAN_POINT('Origin',(80.,9.,141.545925280538));
#62600=CARTESIAN_POINT('',(81.252039109102,10.6292316077768,135.406026966675));
#62601=CARTESIAN_POINT('',(81.252039109102,10.6292316077768,135.347982838459));
#62602=CARTESIAN_POINT('',(81.252039109102,10.6292316077768,141.545925280538));
#62603=CARTESIAN_POINT('',(77.9452501039006,9.00065343667963,134.895925280576));
#62604=CARTESIAN_POINT('Ctrl Pts',(81.252039109102,10.6292316077768,135.347982838459));
#62605=CARTESIAN_POINT('Ctrl Pts',(81.3084942653525,10.585846699702,135.344113662479));
#62606=CARTESIAN_POINT('Ctrl Pts',(81.3626078688897,10.5395885223021,135.340244486498));
#62607=CARTESIAN_POINT('Ctrl Pts',(81.4140911481656,10.4907527585686,135.336375310518));
#62608=CARTESIAN_POINT('Ctrl Pts',(81.4220196871467,10.483231942842,135.335779448852));
#62609=CARTESIAN_POINT('Ctrl Pts',(81.4298859203367,10.4756500603419,135.335183587185));
#62610=CARTESIAN_POINT('Ctrl Pts',(81.4376888783052,10.4680082600917,135.334587725519));
#62611=CARTESIAN_POINT('Ctrl Pts',(81.4883554885788,10.4183880882766,135.330718642672));
#62612=CARTESIAN_POINT('Ctrl Pts',(81.5365494452545,10.3660446008768,135.326849559825));
#62613=CARTESIAN_POINT('Ctrl Pts',(81.5819640552088,10.3112540907572,135.322980476978));
#62614=CARTESIAN_POINT('Ctrl Pts',(81.6273109996591,10.2565452157652,135.319117158872));
#62615=CARTESIAN_POINT('Ctrl Pts',(81.6698865098526,10.1993969261075,135.315253840765));
#62616=CARTESIAN_POINT('Ctrl Pts',(81.7094204040751,10.1401225568471,135.311390522659));
#62617=CARTESIAN_POINT('Ctrl Pts',(81.748907925055,10.0809177163991,135.307531736223));
#62618=CARTESIAN_POINT('Ctrl Pts',(81.7853606487122,10.0195921522385,135.303672949787));
#62619=CARTESIAN_POINT('Ctrl Pts',(81.8185495042662,9.95649112020606,135.299814163351));
#62620=CARTESIAN_POINT('Ctrl Pts',(81.8517174532748,9.89342983719681,135.295957807668));
#62621=CARTESIAN_POINT('Ctrl Pts',(81.8816253876486,9.82859573415704,135.292101451985));
#62622=CARTESIAN_POINT('Ctrl Pts',(81.9080890863941,9.76236054520402,135.288245096302));
#62623=CARTESIAN_POINT('Ctrl Pts',(81.934544967498,9.69614492278905,135.284389879824));
#62624=CARTESIAN_POINT('Ctrl Pts',(81.9575584527788,9.6285294870208,135.280534663347));
#62625=CARTESIAN_POINT('Ctrl Pts',(81.9769932870615,9.55990633628632,135.27667944687));
#62626=CARTESIAN_POINT('Ctrl Pts',(81.9964288811882,9.49128050259189,135.272824079665));
#62627=CARTESIAN_POINT('Ctrl Pts',(82.0122854162816,9.42164734371053,135.268968712461));
#62628=CARTESIAN_POINT('Ctrl Pts',(82.0244768648761,9.35141284279525,135.265113345256));
#62629=CARTESIAN_POINT('Ctrl Pts',(82.0366810745928,9.28110482550954,135.261253942533));
#62630=CARTESIAN_POINT('Ctrl Pts',(82.0452124563531,9.21019468929086,135.25739453981));
#62631=CARTESIAN_POINT('Ctrl Pts',(82.0500365241631,9.13909641295679,135.253535137088));
#62632=CARTESIAN_POINT('Ctrl Pts',(82.0548633233981,9.06795788022017,135.249673549141));
#62633=CARTESIAN_POINT('Ctrl Pts',(82.0559786224031,8.99663148126061,135.245811961194));
#62634=CARTESIAN_POINT('Ctrl Pts',(82.0534001022136,8.92553133055263,135.241950373247));
#62635=CARTESIAN_POINT('Ctrl Pts',(82.0508170708106,8.85430678758249,135.238082029313));
#62636=CARTESIAN_POINT('Ctrl Pts',(82.0445273605926,8.78330976718955,135.23421368538));
#62637=CARTESIAN_POINT('Ctrl Pts',(82.0346004801355,8.71294870017266,135.230345341446));
#62638=CARTESIAN_POINT('Ctrl Pts',(82.0287061841907,8.67117032339324,135.22804843014));
#62639=CARTESIAN_POINT('Ctrl Pts',(82.0215305338992,8.62961597553206,135.225751518834));
#62640=CARTESIAN_POINT('Ctrl Pts',(82.0130964518113,8.58836880802734,135.223454607527));
#62641=CARTESIAN_POINT('Ctrl Pts',(81.9988894764508,8.51888910812375,135.21958552468));
#62642=CARTESIAN_POINT('Ctrl Pts',(81.9810534349363,8.45000969351871,135.215716441833));
#62643=CARTESIAN_POINT('Ctrl Pts',(81.9596541057284,8.3821380830625,135.211847358986));
#62644=CARTESIAN_POINT('Ctrl Pts',(81.9382866604538,8.31436759792095,135.20798404088));
#62645=CARTESIAN_POINT('Ctrl Pts',(81.9133666108286,8.2476023958639,135.204120722774));
#62646=CARTESIAN_POINT('Ctrl Pts',(81.8850106587592,8.18223941225805,135.200257404667));
#62647=CARTESIAN_POINT('Ctrl Pts',(81.8566879682107,8.11695309940681,135.196398618231));
#62648=CARTESIAN_POINT('Ctrl Pts',(81.824937573179,8.05306618136426,135.192539831796));
#62649=CARTESIAN_POINT('Ctrl Pts',(81.7899252910328,7.99095836804368,135.18868104536));
#62650=CARTESIAN_POINT('Ctrl Pts',(81.754935064057,7.92888967809133,135.184824689677));
#62651=CARTESIAN_POINT('Ctrl Pts',(81.7166872645513,7.86859829157177,135.180968333993));
#62652=CARTESIAN_POINT('Ctrl Pts',(81.6753942808023,7.8104405999047,135.17711197831));
#62653=CARTESIAN_POINT('Ctrl Pts',(81.6341134954141,7.75230008860211,135.173256761833));
#62654=CARTESIAN_POINT('Ctrl Pts',(81.5897895927765,7.69629241668233,135.169401545356));
#62655=CARTESIAN_POINT('Ctrl Pts',(81.5426780855886,7.64274472307355,135.165546328878));
#62656=CARTESIAN_POINT('Ctrl Pts',(81.4955647364817,7.58919493591011,135.161690961674));
#62657=CARTESIAN_POINT('Ctrl Pts',(81.4456638889808,7.53810568127019,135.157835594469));
#62658=CARTESIAN_POINT('Ctrl Pts',(81.3932699633574,7.48976943094574,135.153980227265));
#62659=CARTESIAN_POINT('Ctrl Pts',(81.3408211955811,7.44138258574787,135.150120824542));
#62660=CARTESIAN_POINT('Ctrl Pts',(81.2858744981693,7.39575482734537,135.146261421819));
#62661=CARTESIAN_POINT('Ctrl Pts',(81.228758963896,7.35313966252593,135.142402019096));
#62662=CARTESIAN_POINT('Ctrl Pts',(81.1716110903585,7.31050036866542,135.138540431149));
#62663=CARTESIAN_POINT('Ctrl Pts',(81.1122923395098,7.27087733397399,135.134678843202));
#62664=CARTESIAN_POINT('Ctrl Pts',(81.0511602124635,7.2344803115701,135.130817255255));
#62665=CARTESIAN_POINT('Ctrl Pts',(80.9899211325698,7.19801961127091,135.126948911322));
#62666=CARTESIAN_POINT('Ctrl Pts',(80.9268627722766,7.16479641822085,135.123080567389));
#62667=CARTESIAN_POINT('Ctrl Pts',(80.8623659678916,7.1349738607938,135.119212223455));
#62668=CARTESIAN_POINT('Ctrl Pts',(80.8240696215045,7.11726608441226,135.116915312149));
#62669=CARTESIAN_POINT('Ctrl Pts',(80.7852665078412,7.10075632507813,135.114618400842));
#62670=CARTESIAN_POINT('Ctrl Pts',(80.7460389179154,7.08547042450225,135.112321489536));
#62671=CARTESIAN_POINT('Ctrl Pts',(80.6799611399519,7.05972175255636,135.108452406689));
#62672=CARTESIAN_POINT('Ctrl Pts',(80.6124193474611,7.03734756206001,135.104583323842));
#62673=CARTESIAN_POINT('Ctrl Pts',(80.5437915874515,7.0185136205573,135.100714240995));
#62674=CARTESIAN_POINT('Ctrl Pts',(80.4752660793817,6.99970774068812,135.096850922889));
#62675=CARTESIAN_POINT('Ctrl Pts',(80.4056582801984,6.98443176700711,135.092987604782));
#62676=CARTESIAN_POINT('Ctrl Pts',(80.3353649652504,6.97280294431385,135.089124286676));
#62677=CARTESIAN_POINT('Ctrl Pts',(80.2651541043337,6.96118776222513,135.08526550024));
#62678=CARTESIAN_POINT('Ctrl Pts',(80.1942598018295,6.95321131225774,135.081406713804));
#62679=CARTESIAN_POINT('Ctrl Pts',(80.1230910006734,6.94894023293976,135.077547927368));
#62680=CARTESIAN_POINT('Ctrl Pts',(80.0519670306434,6.94467184408856,135.073691571685));
#62681=CARTESIAN_POINT('Ctrl Pts',(79.9805693887846,6.9441042240778,135.069835216002));
#62682=CARTESIAN_POINT('Ctrl Pts',(79.9093126865442,6.94725223817485,135.065978860319));
#62683=CARTESIAN_POINT('Ctrl Pts',(79.8380770342471,6.95039932231701,135.062123643841));
#62684=CARTESIAN_POINT('Ctrl Pts',(79.7669827239569,6.95725984002718,135.058268427364));
#62685=CARTESIAN_POINT('Ctrl Pts',(79.6964431809676,6.96779656035156,135.054413210887));
#62686=CARTESIAN_POINT('Ctrl Pts',(79.6259008800932,6.97833369263019,135.050557843682));
#62687=CARTESIAN_POINT('Ctrl Pts',(79.5559138697091,6.99254723893165,135.046702476478));
#62688=CARTESIAN_POINT('Ctrl Pts',(79.4868875528032,7.01034847799125,135.042847109273));
#62689=CARTESIAN_POINT('Ctrl Pts',(79.4177889841661,7.02816835009397,135.03898770655));
#62690=CARTESIAN_POINT('Ctrl Pts',(79.3496535877346,7.04958328988869,135.035128303828));
#62691=CARTESIAN_POINT('Ctrl Pts',(79.2828728363905,7.07445431274316,135.031268901105));
#62692=CARTESIAN_POINT('Ctrl Pts',(79.2160542732604,7.09933941776615,135.027407313158));
#62693=CARTESIAN_POINT('Ctrl Pts',(79.150592328098,7.12768430823989,135.023545725211));
#62694=CARTESIAN_POINT('Ctrl Pts',(79.0868571230049,7.15930240161697,135.019684137264));
#62695=CARTESIAN_POINT('Ctrl Pts',(79.0230104108859,7.1909758119817,135.015815793331));
#62696=CARTESIAN_POINT('Ctrl Pts',(78.9608968938108,7.22593362020604,135.011947449397));
#62697=CARTESIAN_POINT('Ctrl Pts',(78.9008601794406,7.26394435073046,135.008079105464));
#62698=CARTESIAN_POINT('Ctrl Pts',(78.8652121061538,7.28651402866228,135.005782194157));
#62699=CARTESIAN_POINT('Ctrl Pts',(78.8302956660187,7.31015923941541,135.003485282851));
#62700=CARTESIAN_POINT('Ctrl Pts',(78.7961772025377,7.33482486362246,135.001188371544));
#62701=CARTESIAN_POINT('Ctrl Pts',(78.7391631807262,7.37604261767866,134.99735009344));
#62702=CARTESIAN_POINT('Ctrl Pts',(78.6841480871174,7.42027912081088,134.993511815336));
#62703=CARTESIAN_POINT('Ctrl Pts',(78.6314732100562,7.46731216886606,134.989673537232));
#62704=CARTESIAN_POINT('Ctrl Pts',(78.5778665128151,7.51517723297413,134.985767359871));
#62705=CARTESIAN_POINT('Ctrl Pts',(78.5266841028894,7.56593851962773,134.981861182511));
#62706=CARTESIAN_POINT('Ctrl Pts',(78.4782549032977,7.6193155961037,134.97795500515));
#62707=CARTESIAN_POINT('Ctrl Pts',(78.4307943615623,7.67162504963916,134.974126957294));
#62708=CARTESIAN_POINT('Ctrl Pts',(78.3859782647129,7.72644623971398,134.970298909439));
#62709=CARTESIAN_POINT('Ctrl Pts',(78.3440811368766,7.78347614850676,134.966470861583));
#62710=CARTESIAN_POINT('Ctrl Pts',(78.3022091390411,7.84047185061926,134.9626451098));
#62711=CARTESIAN_POINT('Ctrl Pts',(78.2632529300739,7.89967324655135,134.958819358016));
#62712=CARTESIAN_POINT('Ctrl Pts',(78.2274466135476,7.96074447094278,134.954993606233));
#62713=CARTESIAN_POINT('Ctrl Pts',(78.1916493141244,8.0218003157704,134.951168817889));
#62714=CARTESIAN_POINT('Ctrl Pts',(78.1590005823019,8.08472462791576,134.947344029545));
#62715=CARTESIAN_POINT('Ctrl Pts',(78.1296900536076,8.14915438126208,134.9435192412));
#62716=CARTESIAN_POINT('Ctrl Pts',(78.0992961245191,8.2159656412982,134.939553077815));
#62717=CARTESIAN_POINT('Ctrl Pts',(78.0724922819993,8.28439531441747,134.93558691443));
#62718=CARTESIAN_POINT('Ctrl Pts',(78.0494357340078,8.35401501044195,134.931620751044));
#62719=CARTESIAN_POINT('Ctrl Pts',(78.0271754962613,8.42123023216181,134.927791568118));
#62720=CARTESIAN_POINT('Ctrl Pts',(78.0084080033321,8.48955410547027,134.923962385192));
#62721=CARTESIAN_POINT('Ctrl Pts',(77.9932234204897,8.55858712928934,134.920133202266));
#62722=CARTESIAN_POINT('Ctrl Pts',(77.9780288922086,8.62766536763404,134.916301511342));
#62723=CARTESIAN_POINT('Ctrl Pts',(77.9664220204801,8.69745319300213,134.912469820418));
#62724=CARTESIAN_POINT('Ctrl Pts',(77.9584413426124,8.76754395911139,134.908638129495));
#62725=CARTESIAN_POINT('Ctrl Pts',(77.9504482845426,8.83774345506282,134.904800494576));
#62726=CARTESIAN_POINT('Ctrl Pts',(77.9460926623442,8.90824633703059,134.900962859657));
#62727=CARTESIAN_POINT('Ctrl Pts',(77.9453609729324,8.97864511880522,134.897125224738));
#62728=CARTESIAN_POINT('Ctrl Pts',(77.9452847118622,8.98598250315872,134.896725243351));
#62729=CARTESIAN_POINT('Ctrl Pts',(77.9452477713803,8.9933187615579,134.896325261963));
#62730=CARTESIAN_POINT('Ctrl Pts',(77.9452501039006,9.00065343667963,134.895925280576));
#62731=CARTESIAN_POINT('Ctrl Pts',(77.9452501039008,9.00065343737377,134.895925280538));
#62732=CARTESIAN_POINT('Ctrl Pts',(77.9452615144079,9.03653405769225,134.893968604876));
#62733=CARTESIAN_POINT('Ctrl Pts',(77.9462127014812,9.07239853358728,134.892011929214));
#62734=CARTESIAN_POINT('Ctrl Pts',(77.9481014934011,9.10821312821006,134.890055253553));
#62735=CARTESIAN_POINT('Ctrl Pts',(77.9518363445886,9.17903203623747,134.886186170706));
#62736=CARTESIAN_POINT('Ctrl Pts',(77.9592491642671,9.24979606832758,134.882317087859));
#62737=CARTESIAN_POINT('Ctrl Pts',(77.9703354015929,9.32009245613253,134.878448005012));
#62738=CARTESIAN_POINT('Ctrl Pts',(77.981405120978,9.39028410582552,134.874584686905));
#62739=CARTESIAN_POINT('Ctrl Pts',(77.9961373187821,9.46000901835258,134.870721368799));
#62740=CARTESIAN_POINT('Ctrl Pts',(78.0144755138151,9.52885733166927,134.866858050692));
#62741=CARTESIAN_POINT('Ctrl Pts',(78.0327921981525,9.5976248859409,134.862999264257));
#62742=CARTESIAN_POINT('Ctrl Pts',(78.0547063534122,9.66551741631721,134.859140477821));
#62743=CARTESIAN_POINT('Ctrl Pts',(78.0801103699651,9.73213480383369,134.855281691385));
#62744=CARTESIAN_POINT('Ctrl Pts',(78.1054983838505,9.79871022728089,134.851425335702));
#62745=CARTESIAN_POINT('Ctrl Pts',(78.134371724842,9.86401164867024,134.847568980018));
#62746=CARTESIAN_POINT('Ctrl Pts',(78.1665732666698,9.92765509539378,134.843712624335));
#62747=CARTESIAN_POINT('Ctrl Pts',(78.1987652958396,9.99127974120586,134.839857407858));
#62748=CARTESIAN_POINT('Ctrl Pts',(78.2342833547566,10.0532469514842,134.836002191381));
#62749=CARTESIAN_POINT('Ctrl Pts',(78.2729233278854,10.1131952798756,134.832146974903));
#62750=CARTESIAN_POINT('Ctrl Pts',(78.3115648117215,10.1731459520675,134.828291607699));
#62751=CARTESIAN_POINT('Ctrl Pts',(78.353328187066,10.2310771785417,134.824436240494));
#62752=CARTESIAN_POINT('Ctrl Pts',(78.3979657153936,10.2866560198615,134.82058087329));
#62753=CARTESIAN_POINT('Ctrl Pts',(78.4426499670414,10.3422930370725,134.816721470567));
#62754=CARTESIAN_POINT('Ctrl Pts',(78.4902140724078,10.3955723742868,134.812862067844));
#62755=CARTESIAN_POINT('Ctrl Pts',(78.5403702200735,10.4461944779496,134.809002665121));
#62756=CARTESIAN_POINT('Ctrl Pts',(78.5905547665441,10.4968452442451,134.805141077174));
#62757=CARTESIAN_POINT('Ctrl Pts',(78.6433339173326,10.5448354549391,134.801279489227));
#62758=CARTESIAN_POINT('Ctrl Pts',(78.6983852719673,10.5899046079147,134.797417901281));
#62759=CARTESIAN_POINT('Ctrl Pts',(78.7535329409203,10.6350526109889,134.793549557347));
#62760=CARTESIAN_POINT('Ctrl Pts',(78.8109603589959,10.6772690652749,134.789681213414));
#62761=CARTESIAN_POINT('Ctrl Pts',(78.8703151273712,10.7163361124948,134.78581286948));
#62762=CARTESIAN_POINT('Ctrl Pts',(78.9055582807508,10.7395330008821,134.783515958174));
#62763=CARTESIAN_POINT('Ctrl Pts',(78.9414804390348,10.7616203802528,134.781219046867));
#62764=CARTESIAN_POINT('Ctrl Pts',(78.978004059442,10.7825604786326,134.778922135561));
#62765=CARTESIAN_POINT('Ctrl Pts',(79.0395270763863,10.8178334886212,134.775053052714));
#62766=CARTESIAN_POINT('Ctrl Pts',(79.1029988479684,10.8499867519932,134.771183969867));
#62767=CARTESIAN_POINT('Ctrl Pts',(79.1680701255576,10.8788002146344,134.76731488702));
#62768=CARTESIAN_POINT('Ctrl Pts',(79.2330444501884,10.9075707466532,134.763451568914));
#62769=CARTESIAN_POINT('Ctrl Pts',(79.2996131097051,10.9330111603523,134.759588250807));
#62770=CARTESIAN_POINT('Ctrl Pts',(79.3674011311609,10.9549466063408,134.755724932701));
#62771=CARTESIAN_POINT('Ctrl Pts',(79.4351096372937,10.9768563220596,134.751866146265));
#62772=CARTESIAN_POINT('Ctrl Pts',(79.504034204339,10.99526908772,134.74800735983));
#62773=CARTESIAN_POINT('Ctrl Pts',(79.5737803137746,11.0100582930786,134.744148573394));
#62774=CARTESIAN_POINT('Ctrl Pts',(79.6434824882756,11.0248381823222,134.740292217711));
#62775=CARTESIAN_POINT('Ctrl Pts',(79.7140047043384,11.0359989393333,134.736435862027));
#62776=CARTESIAN_POINT('Ctrl Pts',(79.7849391516778,11.0434643119024,134.732579506344));
#62777=CARTESIAN_POINT('Ctrl Pts',(79.8558526442711,11.0509274791258,134.728724289867));
#62778=CARTESIAN_POINT('Ctrl Pts',(79.9271776435275,11.0546973783256,134.72486907339));
#62779=CARTESIAN_POINT('Ctrl Pts',(79.9984997781607,11.0547494523261,134.721013856912));
#62780=CARTESIAN_POINT('Ctrl Pts',(80.0698247012759,11.0548015283625,134.717158489708));
#62781=CARTESIAN_POINT('Ctrl Pts',(80.1411462737611,11.0511354924629,134.713303122503));
#62782=CARTESIAN_POINT('Ctrl Pts',(80.2120504136818,11.0437788981584,134.709447755299));
#62783=CARTESIAN_POINT('Ctrl Pts',(80.2830287709023,11.0364146035056,134.705588352576));
#62784=CARTESIAN_POINT('Ctrl Pts',(80.3535883391529,11.0253520892534,134.701728949853));
#62785=CARTESIAN_POINT('Ctrl Pts',(80.423321350334,11.0106706833421,134.69786954713));
#62786=CARTESIAN_POINT('Ctrl Pts',(80.4930938448937,10.9959809647035,134.694007959183));
#62787=CARTESIAN_POINT('Ctrl Pts',(80.5620383810083,10.9776684001547,134.690146371236));
#62788=CARTESIAN_POINT('Ctrl Pts',(80.6297612385615,10.9558625577748,134.686284783289));
#62789=CARTESIAN_POINT('Ctrl Pts',(80.6976025796814,10.9340185652921,134.682416439356));
#62790=CARTESIAN_POINT('Ctrl Pts',(80.7642175207544,10.9086692657921,134.678548095423));
#62791=CARTESIAN_POINT('Ctrl Pts',(80.8292318976487,10.87999255914,134.674679751489));
#62792=CARTESIAN_POINT('Ctrl Pts',(80.8678355636976,10.8629651559738,134.672382840183));
#62793=CARTESIAN_POINT('Ctrl Pts',(80.9058753734192,10.8447655224717,134.670085928876));
#62794=CARTESIAN_POINT('Ctrl Pts',(80.9432775356499,10.8254383181138,134.66778901757));
#62795=CARTESIAN_POINT('Ctrl Pts',(81.0062654073906,10.7928899466669,134.663920857385));
#62796=CARTESIAN_POINT('Ctrl Pts',(81.0676899896179,10.757013862428,134.6600526972));
#62797=CARTESIAN_POINT('Ctrl Pts',(81.1271772473677,10.7179839974565,134.656184537015));
#62798=CARTESIAN_POINT('Ctrl Pts',(81.1698375602728,10.6899943688316,134.653410549272));
#62799=CARTESIAN_POINT('Ctrl Pts',(81.2115018532227,10.6603838573982,134.650636561529));
#62800=CARTESIAN_POINT('Ctrl Pts',(81.252039109102,10.6292316077768,134.647862573787));
#62801=CARTESIAN_POINT('',(77.9452502540764,8.99897817482853,134.954074719507));
#62802=CARTESIAN_POINT('Ctrl Pts',(77.9452502540759,8.99897817566031,134.954074719462));
#62803=CARTESIAN_POINT('Ctrl Pts',(77.9452142125462,9.07145278908982,134.950163294815));
#62804=CARTESIAN_POINT('Ctrl Pts',(77.9490169737962,9.14392164400065,134.946251870168));
#62805=CARTESIAN_POINT('Ctrl Pts',(77.9566303437358,9.21595835329659,134.942340445521));
#62806=CARTESIAN_POINT('Ctrl Pts',(77.9642467236715,9.28802354278169,134.938427474467));
#62807=CARTESIAN_POINT('Ctrl Pts',(77.9756766562268,9.35965578405013,134.934514503412));
#62808=CARTESIAN_POINT('Ctrl Pts',(77.9908402897156,9.43043561779875,134.930601532358));
#62809=CARTESIAN_POINT('Ctrl Pts',(78.0060265783599,9.50132119982606,134.926682715147));
#62810=CARTESIAN_POINT('Ctrl Pts',(78.0249576060861,9.57135137549333,134.922763897937));
#62811=CARTESIAN_POINT('Ctrl Pts',(78.0475028581238,9.64011910881129,134.918845080726));
#62812=CARTESIAN_POINT('Ctrl Pts',(78.0700662114441,9.7089420548265,134.914923117149));
#62813=CARTESIAN_POINT('Ctrl Pts',(78.0962493989038,9.77650010586642,134.911001153572));
#62814=CARTESIAN_POINT('Ctrl Pts',(78.125873680429,9.84240613767435,134.907079189996));
#62815=CARTESIAN_POINT('Ctrl Pts',(78.1555587274251,9.90844735625634,134.903149181668));
#62816=CARTESIAN_POINT('Ctrl Pts',(78.1886987529191,9.97282937301543,134.89921917334));
#62817=CARTESIAN_POINT('Ctrl Pts',(78.2250691444902,10.0351898476412,134.895289165013));
#62818=CARTESIAN_POINT('Ctrl Pts',(78.2479358387257,10.0743969566121,134.892818300805));
#62819=CARTESIAN_POINT('Ctrl Pts',(78.2720785667059,10.1128055448757,134.890347436597));
#62820=CARTESIAN_POINT('Ctrl Pts',(78.2974332054892,10.150332070634,134.887876572388));
#62821=CARTESIAN_POINT('Ctrl Pts',(78.3371355888425,10.209094197924,134.884007489541));
#62822=CARTESIAN_POINT('Ctrl Pts',(78.3799614657708,10.2659135819277,134.880138406695));
#62823=CARTESIAN_POINT('Ctrl Pts',(78.4256941852282,10.3204388528348,134.876269323848));
#62824=CARTESIAN_POINT('Ctrl Pts',(78.4713587652144,10.3748828838076,134.872406005741));
#62825=CARTESIAN_POINT('Ctrl Pts',(78.5199212810801,10.4270392173812,134.868542687635));
#62826=CARTESIAN_POINT('Ctrl Pts',(78.5711220788574,10.476585740474,134.864679369528));
#62827=CARTESIAN_POINT('Ctrl Pts',(78.6222628181186,10.5260741455143,134.860820583093));
#62828=CARTESIAN_POINT('Ctrl Pts',(78.6760353447626,10.5729584846901,134.856961796657));
#62829=CARTESIAN_POINT('Ctrl Pts',(78.7321412129297,10.6169513469949,134.853103010221));
#62830=CARTESIAN_POINT('Ctrl Pts',(78.7882117385139,10.6609164970222,134.849246654538));
#62831=CARTESIAN_POINT('Ctrl Pts',(78.846612308118,10.701993484806,134.845390298854));
#62832=CARTESIAN_POINT('Ctrl Pts',(78.9070103656069,10.7399342578412,134.841533943171));
#62833=CARTESIAN_POINT('Ctrl Pts',(78.9673905809049,10.7778638227921,134.837678726694));
#62834=CARTESIAN_POINT('Ctrl Pts',(79.0297667014886,10.8126587540296,134.833823510217));
#62835=CARTESIAN_POINT('Ctrl Pts',(79.0937775151041,10.8441145220319,134.82996829374));
#62836=CARTESIAN_POINT('Ctrl Pts',(79.1577908313509,10.8755715198607,134.826112926535));
#62837=CARTESIAN_POINT('Ctrl Pts',(79.2234385305612,10.9036888829903,134.82225755933));
#62838=CARTESIAN_POINT('Ctrl Pts',(79.2903367116241,10.9283089948531,134.818402192126));
#62839=CARTESIAN_POINT('Ctrl Pts',(79.3573049168402,10.9529548772595,134.814542789403));
#62840=CARTESIAN_POINT('Ctrl Pts',(79.4255257599696,10.9740960327627,134.81068338668));
#62841=CARTESIAN_POINT('Ctrl Pts',(79.4945982079864,10.9916241088944,134.806823983957));
#62842=CARTESIAN_POINT('Ctrl Pts',(79.5637097653658,11.0091621095605,134.80296239601));
#62843=CARTESIAN_POINT('Ctrl Pts',(79.6336734108459,11.0230828635466,134.799100808063));
#62844=CARTESIAN_POINT('Ctrl Pts',(79.7040785989502,11.0333293109825,134.795239220117));
#62845=CARTESIAN_POINT('Ctrl Pts',(79.7746069634547,11.0435936849456,134.791370876183));
#62846=CARTESIAN_POINT('Ctrl Pts',(79.8455779290275,11.0501708731723,134.78750253225));
#62847=CARTESIAN_POINT('Ctrl Pts',(79.9165772232863,11.0530558206794,134.783634188316));
#62848=CARTESIAN_POINT('Ctrl Pts',(79.9587345610352,11.0547688194875,134.78133727701));
#62849=CARTESIAN_POINT('Ctrl Pts',(80.0009018924252,11.0551810654193,134.779040365703));
#62850=CARTESIAN_POINT('Ctrl Pts',(80.0429932997398,11.0543001578828,134.776743454397));
#62851=CARTESIAN_POINT('Ctrl Pts',(80.1138837197785,11.0528165319065,134.772874992454));
#62852=CARTESIAN_POINT('Ctrl Pts',(80.1848360783879,11.0476562316637,134.769006530512));
#62853=CARTESIAN_POINT('Ctrl Pts',(80.2554378698445,11.0388106967419,134.765138068569));
#62854=CARTESIAN_POINT('Ctrl Pts',(80.3259407904934,11.0299775491147,134.761275024024));
#62855=CARTESIAN_POINT('Ctrl Pts',(80.3960936402557,11.0174694659644,134.757411979479));
#62856=CARTESIAN_POINT('Ctrl Pts',(80.4654850568478,11.0013298639533,134.753548934934));
#62857=CARTESIAN_POINT('Ctrl Pts',(80.5364815860529,10.9848169322131,134.749596533205));
#62858=CARTESIAN_POINT('Ctrl Pts',(80.6066804956812,10.9645023747784,134.745644131477));
#62859=CARTESIAN_POINT('Ctrl Pts',(80.675648519535,10.9404887633146,134.741691729748));
#62860=CARTESIAN_POINT('Ctrl Pts',(80.7429382613713,10.9170595039903,134.737835506573));
#62861=CARTESIAN_POINT('Ctrl Pts',(80.8090558645679,10.89010936257,134.733979283398));
#62862=CARTESIAN_POINT('Ctrl Pts',(80.8736130179299,10.8597843577693,134.730123060223));
#62863=CARTESIAN_POINT('Ctrl Pts',(80.9405853635626,10.8283248432607,134.726122569218));
#62864=CARTESIAN_POINT('Ctrl Pts',(81.0058776655747,10.793233114247,134.722122078213));
#62865=CARTESIAN_POINT('Ctrl Pts',(81.069080187921,10.754726506979,134.718121587208));
#62866=CARTESIAN_POINT('Ctrl Pts',(81.1322827102672,10.716219899711,134.714121096203));
#62867=CARTESIAN_POINT('Ctrl Pts',(81.1933949577799,10.6742987244623,134.710120605198));
#62868=CARTESIAN_POINT('Ctrl Pts',(81.252039109102,10.6292316077768,134.706120114193));
#62869=CARTESIAN_POINT('Ctrl Pts',(81.252039109102,10.6292316077768,135.406026966675));
#62870=CARTESIAN_POINT('Ctrl Pts',(81.3085478678901,10.5858055069868,135.402170997582));
#62871=CARTESIAN_POINT('Ctrl Pts',(81.3628300798522,10.5394088010384,135.398315028489));
#62872=CARTESIAN_POINT('Ctrl Pts',(81.4145642475669,10.4903038455313,135.394459059396));
#62873=CARTESIAN_POINT('Ctrl Pts',(81.466287232803,10.4412095041917,135.390603923781));
#62874=CARTESIAN_POINT('Ctrl Pts',(81.5154629153913,10.3894084102282,135.386748788166));
#62875=CARTESIAN_POINT('Ctrl Pts',(81.5618051096492,10.335201243998,135.382893652551));
#62876=CARTESIAN_POINT('Ctrl Pts',(81.6081527886018,10.2809876622372,135.379038060673));
#62877=CARTESIAN_POINT('Ctrl Pts',(81.6516659997839,10.2243678137742,135.375182468795));
#62878=CARTESIAN_POINT('Ctrl Pts',(81.6920985961299,10.1656757282689,135.371326876917));
#62879=CARTESIAN_POINT('Ctrl Pts',(81.7325754830453,10.1069193504322,135.367467061556));
#62880=CARTESIAN_POINT('Ctrl Pts',(81.7699647460227,10.0460866071276,135.363607246195));
#62881=CARTESIAN_POINT('Ctrl Pts',(81.8040639124926,9.98354001552652,135.359747430835));
#62882=CARTESIAN_POINT('Ctrl Pts',(81.8381848096327,9.9209535643191,135.355885155696));
#62883=CARTESIAN_POINT('Ctrl Pts',(81.8690112283502,9.85665152939536,135.352022880558));
#62884=CARTESIAN_POINT('Ctrl Pts',(81.8963881550408,9.79101803261434,135.348160605419));
#62885=CARTESIAN_POINT('Ctrl Pts',(81.923811028795,9.72527438225437,135.344291848172));
#62886=CARTESIAN_POINT('Ctrl Pts',(81.9477726962357,9.6581952681585,135.340423090926));
#62887=CARTESIAN_POINT('Ctrl Pts',(81.9681677224467,9.59018080180495,135.336554333679));
#62888=CARTESIAN_POINT('Ctrl Pts',(81.9754519982523,9.5658887942063,135.335172570571));
#62889=CARTESIAN_POINT('Ctrl Pts',(81.9822817780071,9.54147756623832,135.333790807462));
#62890=CARTESIAN_POINT('Ctrl Pts',(81.9886538483546,9.51696560226421,135.332409044354));
#62891=CARTESIAN_POINT('Ctrl Pts',(82.0064963192772,9.44832951059983,135.328539961507));
#62892=CARTESIAN_POINT('Ctrl Pts',(82.0208162221759,9.37863418425578,135.32467087866));
#62893=CARTESIAN_POINT('Ctrl Pts',(82.031493149485,9.30827446552624,135.320801795813));
#62894=CARTESIAN_POINT('Ctrl Pts',(82.0421541687049,9.23801957926842,135.316938477707));
#62895=CARTESIAN_POINT('Ctrl Pts',(82.0491829141827,9.16710274194419,135.313075159601));
#62896=CARTESIAN_POINT('Ctrl Pts',(82.0525093587264,9.09593171967852,135.309211841494));
#62897=CARTESIAN_POINT('Ctrl Pts',(82.0558319013519,9.02484418099479,135.305353055058));
#62898=CARTESIAN_POINT('Ctrl Pts',(82.0554607467397,8.95350353251239,135.301494268623));
#62899=CARTESIAN_POINT('Ctrl Pts',(82.0513775498521,8.88232370475398,135.297635482187));
#62900=CARTESIAN_POINT('Ctrl Pts',(82.0472969250791,8.81118871506761,135.293779126504));
#62901=CARTESIAN_POINT('Ctrl Pts',(82.0395089249652,8.74021482895654,135.28992277082));
#62902=CARTESIAN_POINT('Ctrl Pts',(82.0280472853771,8.66981555037436,135.286066415137));
#62903=CARTESIAN_POINT('Ctrl Pts',(82.0165890316721,8.599437068444,135.28221119866));
#62904=CARTESIAN_POINT('Ctrl Pts',(82.0014593709949,8.52963333626083,135.278355982183));
#62905=CARTESIAN_POINT('Ctrl Pts',(81.9827436390369,8.4608105858246,135.274500765705));
#62906=CARTESIAN_POINT('Ctrl Pts',(81.9640271753497,8.39198514462455,135.270645398501));
#62907=CARTESIAN_POINT('Ctrl Pts',(81.9417244916244,8.32414122949848,135.266790031296));
#62908=CARTESIAN_POINT('Ctrl Pts',(81.9159711219687,8.25767108214607,135.262934664091));
#62909=CARTESIAN_POINT('Ctrl Pts',(81.8901907955576,8.19113135867504,135.259075261369));
#62910=CARTESIAN_POINT('Ctrl Pts',(81.8609527488607,8.12596872736965,135.255215858646));
#62911=CARTESIAN_POINT('Ctrl Pts',(81.8284408048184,8.062555715909,135.251356455923));
#62912=CARTESIAN_POINT('Ctrl Pts',(81.7959104522581,7.99910679950317,135.247494867976));
#62913=CARTESIAN_POINT('Ctrl Pts',(81.7601027561561,7.93740989536472,135.243633280029));
#62914=CARTESIAN_POINT('Ctrl Pts',(81.7212463131001,7.87781075921244,135.239771692082));
#62915=CARTESIAN_POINT('Ctrl Pts',(81.6823218893042,7.81810735223518,135.235903348149));
#62916=CARTESIAN_POINT('Ctrl Pts',(81.6403383555219,7.76050943343201,135.232035004216));
#62917=CARTESIAN_POINT('Ctrl Pts',(81.5955657916367,7.70533117475602,135.228166660282));
#62918=CARTESIAN_POINT('Ctrl Pts',(81.5689811316442,7.6725679126466,135.225869748976));
#62919=CARTESIAN_POINT('Ctrl Pts',(81.5414139051121,7.6406570711572,135.223572837669));
#62920=CARTESIAN_POINT('Ctrl Pts',(81.5129266135235,7.60965809075886,135.221275926363));
#62921=CARTESIAN_POINT('Ctrl Pts',(81.4649405676832,7.55744117537499,135.217406843516));
#62922=CARTESIAN_POINT('Ctrl Pts',(81.4141540521789,7.50760917786172,135.213537760669));
#62923=CARTESIAN_POINT('Ctrl Pts',(81.3608334803881,7.46047741128786,135.209668677822));
#62924=CARTESIAN_POINT('Ctrl Pts',(81.3075923535901,7.41341586869575,135.205805359716));
#62925=CARTESIAN_POINT('Ctrl Pts',(81.2518250260103,7.36904689019028,135.201942041609));
#62926=CARTESIAN_POINT('Ctrl Pts',(81.1938360940872,7.32765047225327,135.198078723503));
#62927=CARTESIAN_POINT('Ctrl Pts',(81.1359151831588,7.28630261229848,135.194219937067));
#62928=CARTESIAN_POINT('Ctrl Pts',(81.0757782376257,7.24792066779854,135.190361150631));
#62929=CARTESIAN_POINT('Ctrl Pts',(81.0137630642245,7.21274455879579,135.186502364195));
#62930=CARTESIAN_POINT('Ctrl Pts',(80.9517869558352,7.17759060816235,135.182646008512));
#62931=CARTESIAN_POINT('Ctrl Pts',(80.887935388464,7.14563872559304,135.178789652829));
#62932=CARTESIAN_POINT('Ctrl Pts',(80.8225740581302,7.11708484487717,135.174933297146));
#62933=CARTESIAN_POINT('Ctrl Pts',(80.7572320361878,7.08853939926357,135.171078080668));
#62934=CARTESIAN_POINT('Ctrl Pts',(80.6903815816303,7.06339015704093,135.167222864191));
#62935=CARTESIAN_POINT('Ctrl Pts',(80.6224102677975,7.04178575711436,135.163367647714));
#62936=CARTESIAN_POINT('Ctrl Pts',(80.5544362964897,7.02018051252036,135.159512280509));
#62937=CARTESIAN_POINT('Ctrl Pts',(80.4853418425306,7.00212053043067,135.155656913305));
#62938=CARTESIAN_POINT('Ctrl Pts',(80.4155299521795,6.98770468833681,135.1518015461));
#62939=CARTESIAN_POINT('Ctrl Pts',(80.3456449878162,6.97327375678731,135.147942143377));
#62940=CARTESIAN_POINT('Ctrl Pts',(80.2750415646964,6.96249467811315,135.144082740654));
#62941=CARTESIAN_POINT('Ctrl Pts',(80.2041323575912,6.95541506826343,135.140223337932));
#62942=CARTESIAN_POINT('Ctrl Pts',(80.133183001136,6.948331449883,135.136361749985));
#62943=CARTESIAN_POINT('Ctrl Pts',(80.0619280014996,6.94495149319357,135.132500162038));
#62944=CARTESIAN_POINT('Ctrl Pts',(79.9907818257887,6.94527067773777,135.128638574091));
#62945=CARTESIAN_POINT('Ctrl Pts',(79.9195111772933,6.94559042070676,135.124770230157));
#62946=CARTESIAN_POINT('Ctrl Pts',(79.8483502180037,6.94962219851369,135.120901886224));
#62947=CARTESIAN_POINT('Ctrl Pts',(79.7777093801836,6.95730950879933,135.117033542291));
#62948=CARTESIAN_POINT('Ctrl Pts',(79.7357648835524,6.9618740124254,135.114736630984));
#62949=CARTESIAN_POINT('Ctrl Pts',(79.694003608926,6.96772633887129,135.112439719678));
#62950=CARTESIAN_POINT('Ctrl Pts',(79.6525093937844,6.97484621791531,135.110142808371));
#62951=CARTESIAN_POINT('Ctrl Pts',(79.5826135490466,6.98683945500908,135.106273725524));
#62952=CARTESIAN_POINT('Ctrl Pts',(79.5132024330664,7.00247899181911,135.102404642677));
#62953=CARTESIAN_POINT('Ctrl Pts',(79.4446854481558,7.02171202525768,135.098535559831));
#62954=CARTESIAN_POINT('Ctrl Pts',(79.3762705501358,7.04091640243557,135.094672241724));
#62955=CARTESIAN_POINT('Ctrl Pts',(79.3087476026799,7.06370351822278,135.090808923618));
#62956=CARTESIAN_POINT('Ctrl Pts',(79.242517047208,7.08996933565726,135.086945605511));
#62957=CARTESIAN_POINT('Ctrl Pts',(79.1763641801522,7.116204343298,135.083086819076));
#62958=CARTESIAN_POINT('Ctrl Pts',(79.1115011432173,7.14590976908554,135.07922803264));
#62959=CARTESIAN_POINT('Ctrl Pts',(79.0483127208929,7.17893193831597,135.075369246204));
#62960=CARTESIAN_POINT('Ctrl Pts',(78.985164102641,7.21193330600122,135.071512890521));
#62961=CARTESIAN_POINT('Ctrl Pts',(78.9236884356438,7.24824704751499,135.067656534837));
#62962=CARTESIAN_POINT('Ctrl Pts',(78.8642486766827,7.28767220016641,135.063800179154));
#62963=CARTESIAN_POINT('Ctrl Pts',(78.8048264768215,7.32708570623301,135.059944962677));
#62964=CARTESIAN_POINT('Ctrl Pts',(78.747439395603,7.36960853031767,135.0560897462));
#62965=CARTESIAN_POINT('Ctrl Pts',(78.69242252164,7.41499567805454,135.052234529723));
#62966=CARTESIAN_POINT('Ctrl Pts',(78.6374034966817,7.46038460029324,135.048379162518));
#62967=CARTESIAN_POINT('Ctrl Pts',(78.5847552362834,7.50863775768248,135.044523795313));
#62968=CARTESIAN_POINT('Ctrl Pts',(78.5347794150553,7.5594701669336,135.040668428109));
#62969=CARTESIAN_POINT('Ctrl Pts',(78.4847512827704,7.61035578385566,135.036809025386));
#62970=CARTESIAN_POINT('Ctrl Pts',(78.4374015149906,7.66382569487572,135.032949622663));
#62971=CARTESIAN_POINT('Ctrl Pts',(78.3929939421244,7.71955902422212,135.029090219941));
#62972=CARTESIAN_POINT('Ctrl Pts',(78.3485612253415,7.77532391021734,135.025228631994));
#62973=CARTESIAN_POINT('Ctrl Pts',(78.3070743024075,7.83335437037287,135.021367044047));
#62974=CARTESIAN_POINT('Ctrl Pts',(78.2687541743386,7.89329974535568,135.0175054561));
#62975=CARTESIAN_POINT('Ctrl Pts',(78.2303670038319,7.95334999692082,135.013637112166));
#62976=CARTESIAN_POINT('Ctrl Pts',(78.1951579298448,8.01532142959978,135.009768768233));
#62977=CARTESIAN_POINT('Ctrl Pts',(78.1633020932589,8.07883857990415,135.005900424299));
#62978=CARTESIAN_POINT('Ctrl Pts',(78.1443870142257,8.11655323588991,135.003603512993));
#62979=CARTESIAN_POINT('Ctrl Pts',(78.1266532537511,8.15481245076237,135.001306601687));
#62980=CARTESIAN_POINT('Ctrl Pts',(78.1101292539508,8.19353479571181,134.99900969038));
#62981=CARTESIAN_POINT('Ctrl Pts',(78.0793053040282,8.26576764708191,134.994725020812));
#62982=CARTESIAN_POINT('Ctrl Pts',(78.0525904917818,8.33985380574526,134.990440351244));
#62983=CARTESIAN_POINT('Ctrl Pts',(78.0301869119697,8.41533431713122,134.986155681676));
#62984=CARTESIAN_POINT('Ctrl Pts',(78.007854285939,8.49057577619793,134.981884581971));
#62985=CARTESIAN_POINT('Ctrl Pts',(77.9898057879733,8.56720250551917,134.977613482266));
#62986=CARTESIAN_POINT('Ctrl Pts',(77.9761951891261,8.64473720996497,134.973342382561));
#62987=CARTESIAN_POINT('Ctrl Pts',(77.9626561574421,8.72186422192664,134.969093741125));
#62988=CARTESIAN_POINT('Ctrl Pts',(77.9535086041256,8.79988940239672,134.964845099689));
#62989=CARTESIAN_POINT('Ctrl Pts',(77.9488557708438,8.87832455589048,134.960596458253));
#62990=CARTESIAN_POINT('Ctrl Pts',(77.9464750440831,8.9184576656747,134.958422545337));
#62991=CARTESIAN_POINT('Ctrl Pts',(77.9452702854505,8.95869783904917,134.956248632422));
#62992=CARTESIAN_POINT('Ctrl Pts',(77.9452502540763,8.99897817482853,134.954074719507));
#62993=CARTESIAN_POINT('Origin',(80.,9.,141.545925280538));
#62994=CARTESIAN_POINT('',(81.252039109102,10.6292316077768,136.106053391442));
#62995=CARTESIAN_POINT('',(81.252039109102,10.6292316077768,136.047954616544));
#62996=CARTESIAN_POINT('',(81.252039109102,10.6292316077768,141.545925280538));
#62997=CARTESIAN_POINT('',(77.9452505223076,9.00146506745653,135.595925280489));
#62998=CARTESIAN_POINT('Ctrl Pts',(81.252039109102,10.6292316077768,136.047954616544));
#62999=CARTESIAN_POINT('Ctrl Pts',(81.3089518203792,10.5854950757921,136.044073934621));
#63000=CARTESIAN_POINT('Ctrl Pts',(81.3635519286423,10.5387868553141,136.040193252698));
#63001=CARTESIAN_POINT('Ctrl Pts',(81.4155258477759,10.4893905252748,136.036312570775));
#63002=CARTESIAN_POINT('Ctrl Pts',(81.4672299052006,10.4402506734511,136.032452038332));
#63003=CARTESIAN_POINT('Ctrl Pts',(81.5163346813592,10.3884509528018,136.02859150589));
#63004=CARTESIAN_POINT('Ctrl Pts',(81.5625698786793,10.3343061630466,136.024730973447));
#63005=CARTESIAN_POINT('Ctrl Pts',(81.6091670526988,10.2797374721637,136.020840216784));
#63006=CARTESIAN_POINT('Ctrl Pts',(81.6528492120465,10.2227872289702,136.016949460121));
#63007=CARTESIAN_POINT('Ctrl Pts',(81.6933836043985,10.1638082019192,136.013058703458));
#63008=CARTESIAN_POINT('Ctrl Pts',(81.7339179967505,10.1048291748683,136.009167946794));
#63009=CARTESIAN_POINT('Ctrl Pts',(81.771304416678,10.043821822193,136.005277190131));
#63010=CARTESIAN_POINT('Ctrl Pts',(81.8053578201978,9.98116293425242,136.001386433468));
#63011=CARTESIAN_POINT('Ctrl Pts',(81.8392215261156,9.91885309338356,135.997517350621));
#63012=CARTESIAN_POINT('Ctrl Pts',(81.8699219428302,9.85466600319565,135.993648267774));
#63013=CARTESIAN_POINT('Ctrl Pts',(81.8972470215781,9.78895582995059,135.989779184927));
#63014=CARTESIAN_POINT('Ctrl Pts',(81.9245313873213,9.7233435615867,135.985915866821));
#63015=CARTESIAN_POINT('Ctrl Pts',(81.9484502126878,9.65621315959098,135.982052548715));
#63016=CARTESIAN_POINT('Ctrl Pts',(81.9688372273746,9.58794347908959,135.978189230608));
#63017=CARTESIAN_POINT('Ctrl Pts',(81.989200328101,9.51975387889703,135.974330444172));
#63018=CARTESIAN_POINT('Ctrl Pts',(82.0060397088494,9.4504281179012,135.970471657737));
#63019=CARTESIAN_POINT('Ctrl Pts',(82.019237770797,9.38036349389328,135.966612871301));
#63020=CARTESIAN_POINT('Ctrl Pts',(82.0324275189334,9.31034300546086,135.962756515618));
#63021=CARTESIAN_POINT('Ctrl Pts',(82.0419804093478,9.23958505368009,135.958900159934));
#63022=CARTESIAN_POINT('Ctrl Pts',(82.047829490708,9.16849907859232,135.955043804251));
#63023=CARTESIAN_POINT('Ctrl Pts',(82.0536768441911,9.09743410301335,135.951188587774));
#63024=CARTESIAN_POINT('Ctrl Pts',(82.0558225209815,9.02604178038674,135.947333371297));
#63025=CARTESIAN_POINT('Ctrl Pts',(82.0542514007093,8.9547369335569,135.943478154819));
#63026=CARTESIAN_POINT('Ctrl Pts',(82.052680219011,8.88342929892084,135.939622787615));
#63027=CARTESIAN_POINT('Ctrl Pts',(82.0473919646486,8.81220963248827,135.93576742041));
#63028=CARTESIAN_POINT('Ctrl Pts',(82.0384236078769,8.74149128186784,135.931912053206));
#63029=CARTESIAN_POINT('Ctrl Pts',(82.0294458636812,8.67069890841833,135.928052650483));
#63030=CARTESIAN_POINT('Ctrl Pts',(82.0167803887356,8.60040938119204,135.92419324776));
#63031=CARTESIAN_POINT('Ctrl Pts',(82.0005157706016,8.53102855729332,135.920333845037));
#63032=CARTESIAN_POINT('Ctrl Pts',(81.984241943313,8.46160844942698,135.91647225709));
#63033=CARTESIAN_POINT('Ctrl Pts',(81.964365051502,8.39309853589352,135.912610669143));
#63034=CARTESIAN_POINT('Ctrl Pts',(81.9410235901458,8.32588948606509,135.908749081196));
#63035=CARTESIAN_POINT('Ctrl Pts',(81.9176412920663,8.25856285159507,135.904880737263));
#63036=CARTESIAN_POINT('Ctrl Pts',(81.8907825058248,8.19254207485823,135.90101239333));
#63037=CARTESIAN_POINT('Ctrl Pts',(81.8606336006024,8.12819717435119,135.897144049396));
#63038=CARTESIAN_POINT('Ctrl Pts',(81.8427320482914,8.08999102411536,135.89484713809));
#63039=CARTESIAN_POINT('Ctrl Pts',(81.8236714017528,8.05237526230223,135.892550226783));
#63040=CARTESIAN_POINT('Ctrl Pts',(81.8034979882716,8.01542264458276,135.890253315477));
#63041=CARTESIAN_POINT('Ctrl Pts',(81.7695164375492,7.95317699366571,135.88638423263));
#63042=CARTESIAN_POINT('Ctrl Pts',(81.7322420417679,7.89257074355593,135.882515149783));
#63043=CARTESIAN_POINT('Ctrl Pts',(81.691857336643,7.83397413624427,135.878646066936));
#63044=CARTESIAN_POINT('Ctrl Pts',(81.6515328027146,7.77546483495515,135.87478274883));
#63045=CARTESIAN_POINT('Ctrl Pts',(81.6081074316386,7.71895962965557,135.870919430723));
#63046=CARTESIAN_POINT('Ctrl Pts',(81.5618093303979,7.66480369309158,135.867056112617));
#63047=CARTESIAN_POINT('Ctrl Pts',(81.5155655368122,7.61071128142028,135.863197326181));
#63048=CARTESIAN_POINT('Ctrl Pts',(81.466456020584,7.55896303219886,135.859338539745));
#63049=CARTESIAN_POINT('Ctrl Pts',(81.4147507814424,7.50987323059139,135.855479753309));
#63050=CARTESIAN_POINT('Ctrl Pts',(81.3630781128102,7.46081435195943,135.851623397626));
#63051=CARTESIAN_POINT('Ctrl Pts',(81.3088133167696,7.41441093219164,135.847767041943));
#63052=CARTESIAN_POINT('Ctrl Pts',(81.252264064358,7.37094129153745,135.84391068626));
#63053=CARTESIAN_POINT('Ctrl Pts',(81.1957315171616,7.32748449225032,135.840055469782));
#63054=CARTESIAN_POINT('Ctrl Pts',(81.1369162382928,7.28696004739923,135.836200253305));
#63055=CARTESIAN_POINT('Ctrl Pts',(81.0761585331535,7.24960565185417,135.832345036828));
#63056=CARTESIAN_POINT('Ctrl Pts',(81.0153984525697,7.212249795864,135.828489669623));
#63057=CARTESIAN_POINT('Ctrl Pts',(80.9526962099217,7.17806448779367,135.824634302419));
#63058=CARTESIAN_POINT('Ctrl Pts',(80.8884191241467,7.14724285931739,135.820778935214));
#63059=CARTESIAN_POINT('Ctrl Pts',(80.8240747577905,7.11638896900076,135.816919532491));
#63060=CARTESIAN_POINT('Ctrl Pts',(80.7581526965945,7.08890599716434,135.813060129768));
#63061=CARTESIAN_POINT('Ctrl Pts',(80.6910419626868,7.06493964737377,135.809200727046));
#63062=CARTESIAN_POINT('Ctrl Pts',(80.6238932301544,7.04095972764768,135.805339139099));
#63063=CARTESIAN_POINT('Ctrl Pts',(80.5555549506989,7.02050053310161,135.801477551152));
#63064=CARTESIAN_POINT('Ctrl Pts',(80.4864304555323,7.00365760090344,135.797615963205));
#63065=CARTESIAN_POINT('Ctrl Pts',(80.4171850245838,6.98678520139167,135.793747619271));
#63066=CARTESIAN_POINT('Ctrl Pts',(80.3471511091492,6.97354178611454,135.789879275338));
#63067=CARTESIAN_POINT('Ctrl Pts',(80.2767406569831,6.96397147090897,135.786010931404));
#63068=CARTESIAN_POINT('Ctrl Pts',(80.2349329567233,6.95828889314961,135.783714020098));
#63069=CARTESIAN_POINT('Ctrl Pts',(80.1929925914078,6.95390032385284,135.781417108791));
#63070=CARTESIAN_POINT('Ctrl Pts',(80.15100581249,6.95080630317819,135.779120197485));
#63071=CARTESIAN_POINT('Ctrl Pts',(80.0802802578494,6.94559451189713,135.775251114638));
#63072=CARTESIAN_POINT('Ctrl Pts',(80.0091460436972,6.94403832740463,135.771382031791));
#63073=CARTESIAN_POINT('Ctrl Pts',(79.9380132263564,6.94618520737792,135.767512948944));
#63074=CARTESIAN_POINT('Ctrl Pts',(79.8669863933657,6.94832888860713,135.763649630838));
#63075=CARTESIAN_POINT('Ctrl Pts',(79.7959614346618,6.9541646679172,135.759786312731));
#63076=CARTESIAN_POINT('Ctrl Pts',(79.7253520620245,6.963688119991,135.755922994625));
#63077=CARTESIAN_POINT('Ctrl Pts',(79.6548255141543,6.97320040105916,135.752064208189));
#63078=CARTESIAN_POINT('Ctrl Pts',(79.5847140631333,6.98639169809088,135.748205421753));
#63079=CARTESIAN_POINT('Ctrl Pts',(79.5154281928634,7.00320563747082,135.744346635317));
#63080=CARTESIAN_POINT('Ctrl Pts',(79.4461859676111,7.02000898530186,135.740490279634));
#63081=CARTESIAN_POINT('Ctrl Pts',(79.3777687622934,7.04043033373929,135.736633923951));
#63082=CARTESIAN_POINT('Ctrl Pts',(79.3105772776738,7.06436215359373,135.732777568268));
#63083=CARTESIAN_POINT('Ctrl Pts',(79.2434056420915,7.08828690374894,135.72892235179));
#63084=CARTESIAN_POINT('Ctrl Pts',(79.1774594657311,7.11571990362766,135.725067135313));
#63085=CARTESIAN_POINT('Ctrl Pts',(79.1131230188681,7.14650417242486,135.721211918836));
#63086=CARTESIAN_POINT('Ctrl Pts',(79.0487840566424,7.17728964479496,135.717356551631));
#63087=CARTESIAN_POINT('Ctrl Pts',(78.9860553861163,7.2114264345535,135.713501184427));
#63088=CARTESIAN_POINT('Ctrl Pts',(78.9252984901607,7.2487106957304,135.709645817222));
#63089=CARTESIAN_POINT('Ctrl Pts',(78.8644779983027,7.28603398336174,135.705786414499));
#63090=CARTESIAN_POINT('Ctrl Pts',(78.8056338159299,7.32651106445915,135.701927011776));
#63091=CARTESIAN_POINT('Ctrl Pts',(78.7490993513736,7.36989413541142,135.698067609054));
#63092=CARTESIAN_POINT('Ctrl Pts',(78.6925328765594,7.41330177019929,135.694206021107));
#63093=CARTESIAN_POINT('Ctrl Pts',(78.6382790925854,7.4596183547552,135.69034443316));
#63094=CARTESIAN_POINT('Ctrl Pts',(78.5866370222985,7.50855685466637,135.686482845213));
#63095=CARTESIAN_POINT('Ctrl Pts',(78.5349046023586,7.55758097423724,135.682614501279));
#63096=CARTESIAN_POINT('Ctrl Pts',(78.4857933536446,7.60923581533726,135.678746157346));
#63097=CARTESIAN_POINT('Ctrl Pts',(78.4395637716856,7.6631992145933,135.674877813413));
#63098=CARTESIAN_POINT('Ctrl Pts',(78.4121139762903,7.69524112813968,135.672580902106));
#63099=CARTESIAN_POINT('Ctrl Pts',(78.3856793652917,7.72809634271189,135.6702839908));
#63100=CARTESIAN_POINT('Ctrl Pts',(78.3603071735869,7.76169268858276,135.667987079493));
#63101=CARTESIAN_POINT('Ctrl Pts',(78.3174433117299,7.81845046280503,135.664106670182));
#63102=CARTESIAN_POINT('Ctrl Pts',(78.2774445565978,7.87754940196065,135.660226260871));
#63103=CARTESIAN_POINT('Ctrl Pts',(78.240575222393,7.93866969588037,135.65634585156));
#63104=CARTESIAN_POINT('Ctrl Pts',(78.203760818831,7.99969892829601,135.652471223568));
#63105=CARTESIAN_POINT('Ctrl Pts',(78.1700668305628,8.06274313086389,135.648596595576));
#63106=CARTESIAN_POINT('Ctrl Pts',(78.1397161676285,8.12745107557382,135.644721967583));
#63107=CARTESIAN_POINT('Ctrl Pts',(78.1078633935518,8.19536153763767,135.640655576996));
#63108=CARTESIAN_POINT('Ctrl Pts',(78.07969379902,8.26510427275798,135.636589186409));
#63109=CARTESIAN_POINT('Ctrl Pts',(78.055412144488,8.3362412827726,135.632522795822));
#63110=CARTESIAN_POINT('Ctrl Pts',(78.0323224526798,8.40388624639017,135.62865602038));
#63111=CARTESIAN_POINT('Ctrl Pts',(78.0127481522003,8.4727913054781,135.624789244939));
#63112=CARTESIAN_POINT('Ctrl Pts',(77.9968162204211,8.54255895709712,135.620922469497));
#63113=CARTESIAN_POINT('Ctrl Pts',(77.9808915414104,8.61229484805866,135.617057454346));
#63114=CARTESIAN_POINT('Ctrl Pts',(77.9686060422558,8.68289208198892,135.613192439195));
#63115=CARTESIAN_POINT('Ctrl Pts',(77.9600362376921,8.75394022886587,135.609327424043));
#63116=CARTESIAN_POINT('Ctrl Pts',(77.9514663540313,8.82498903149886,135.605462373219));
#63117=CARTESIAN_POINT('Ctrl Pts',(77.9466122932739,8.89648827757465,135.601597322395));
#63118=CARTESIAN_POINT('Ctrl Pts',(77.945498864882,8.96802112730593,135.59773227157));
#63119=CARTESIAN_POINT('Ctrl Pts',(77.9453253479641,8.97916882185064,135.597129941226));
#63120=CARTESIAN_POINT('Ctrl Pts',(77.9452425738058,8.99031732822184,135.596527610882));
#63121=CARTESIAN_POINT('Ctrl Pts',(77.9452505223069,9.00146506654286,135.595925280538));
#63122=CARTESIAN_POINT('Ctrl Pts',(77.9452505223076,9.00146506745653,135.595925280489));
#63123=CARTESIAN_POINT('Ctrl Pts',(77.9453088390013,9.08325392669816,135.591506096049));
#63124=CARTESIAN_POINT('Ctrl Pts',(77.9502545524832,9.1648475422697,135.587086911609));
#63125=CARTESIAN_POINT('Ctrl Pts',(77.9599940449638,9.24570971880849,135.582667727169));
#63126=CARTESIAN_POINT('Ctrl Pts',(77.9698223745248,9.32730946557315,135.57820823391));
#63127=CARTESIAN_POINT('Ctrl Pts',(77.9845322237858,9.40816418156723,135.573748740651));
#63128=CARTESIAN_POINT('Ctrl Pts',(78.0039776882024,9.48774224064146,135.569289247391));
#63129=CARTESIAN_POINT('Ctrl Pts',(78.0220522312963,9.56170998074051,135.565144152095));
#63130=CARTESIAN_POINT('Ctrl Pts',(78.0442176079849,9.63457482938802,135.560999056799));
#63131=CARTESIAN_POINT('Ctrl Pts',(78.0703199470976,9.70592666469722,135.556853961502));
#63132=CARTESIAN_POINT('Ctrl Pts',(78.0946841909335,9.77252734389711,135.552984878655));
#63133=CARTESIAN_POINT('Ctrl Pts',(78.1225481710408,9.83799563198995,135.549115795808));
#63134=CARTESIAN_POINT('Ctrl Pts',(78.153786339128,9.9019382910762,135.545246712961));
#63135=CARTESIAN_POINT('Ctrl Pts',(78.1849779639026,9.96578567878933,135.541383394855));
#63136=CARTESIAN_POINT('Ctrl Pts',(78.2195335859642,10.0281115166334,135.537520076748));
#63137=CARTESIAN_POINT('Ctrl Pts',(78.2572788690437,10.0885405928207,135.533656758642));
#63138=CARTESIAN_POINT('Ctrl Pts',(78.2949798769207,10.148898785725,135.529797972206));
#63139=CARTESIAN_POINT('Ctrl Pts',(78.3358628578837,10.2073642263649,135.52593918577));
#63140=CARTESIAN_POINT('Ctrl Pts',(78.3797074616772,10.2635860290283,135.522080399335));
#63141=CARTESIAN_POINT('Ctrl Pts',(78.4235244465854,10.3197724160787,135.518224043651));
#63142=CARTESIAN_POINT('Ctrl Pts',(78.4702990549621,10.3737175870088,135.514367687968));
#63143=CARTESIAN_POINT('Ctrl Pts',(78.5197683434639,10.4251006299516,135.510511332285));
#63144=CARTESIAN_POINT('Ctrl Pts',(78.5692230182425,10.476468493829,135.506656115807));
#63145=CARTESIAN_POINT('Ctrl Pts',(78.6213704560565,10.5252753825675,135.50280089933));
#63146=CARTESIAN_POINT('Ctrl Pts',(78.6759094097278,10.571235714733,135.498945682853));
#63147=CARTESIAN_POINT('Ctrl Pts',(78.7304504957091,10.6171978438101,135.495090315648));
#63148=CARTESIAN_POINT('Ctrl Pts',(78.7873829102914,10.6603128840023,135.491234948444));
#63149=CARTESIAN_POINT('Ctrl Pts',(78.8463720764135,10.7003353129373,135.487379581239));
#63150=CARTESIAN_POINT('Ctrl Pts',(78.9054229881071,10.7403996344418,135.483520178516));
#63151=CARTESIAN_POINT('Ctrl Pts',(78.9665345461115,10.7773646093717,135.479660775793));
#63152=CARTESIAN_POINT('Ctrl Pts',(79.0293436696688,10.8110283959364,135.475801373071));
#63153=CARTESIAN_POINT('Ctrl Pts',(79.0921883562452,10.8447112432015,135.471939785124));
#63154=CARTESIAN_POINT('Ctrl Pts',(79.1567320820348,10.8750889742164,135.468078197177));
#63155=CARTESIAN_POINT('Ctrl Pts',(79.2225901682393,10.90200723342,135.46421660923));
#63156=CARTESIAN_POINT('Ctrl Pts',(79.2885634755262,10.9289725870829,135.460348265296));
#63157=CARTESIAN_POINT('Ctrl Pts',(79.3558552755063,10.9524662248332,135.456479921363));
#63158=CARTESIAN_POINT('Ctrl Pts',(79.4240647345005,10.9723833634601,135.45261157743));
#63159=CARTESIAN_POINT('Ctrl Pts',(79.464565548354,10.9842095872114,135.450314666123));
#63160=CARTESIAN_POINT('Ctrl Pts',(79.505389660854,10.9947758363981,135.448017754817));
#63161=CARTESIAN_POINT('Ctrl Pts',(79.5464518564914,11.004068772278,135.44572084351));
#63162=CARTESIAN_POINT('Ctrl Pts',(79.6192550065553,11.0205451198015,135.441648426633));
#63163=CARTESIAN_POINT('Ctrl Pts',(79.6931072766589,11.0330831288442,135.437576009756));
#63164=CARTESIAN_POINT('Ctrl Pts',(79.7675435324096,11.0415586088025,135.433503592879));
#63165=CARTESIAN_POINT('Ctrl Pts',(79.8381398310474,11.0495968625834,135.429641260536));
#63166=CARTESIAN_POINT('Ctrl Pts',(79.909260795605,11.053981240602,135.425778928194));
#63167=CARTESIAN_POINT('Ctrl Pts',(79.9804964623781,11.0546574348344,135.421916595851));
#63168=CARTESIAN_POINT('Ctrl Pts',(80.0516622917356,11.0553329661452,135.418058050029));
#63169=CARTESIAN_POINT('Ctrl Pts',(80.1229421170099,11.0523075215454,135.414199504207));
#63170=CARTESIAN_POINT('Ctrl Pts',(80.1939215984958,11.0455786409075,135.410340958385));
#63171=CARTESIAN_POINT('Ctrl Pts',(80.2648552395298,11.038854105961,135.406484904516));
#63172=CARTESIAN_POINT('Ctrl Pts',(80.3354884393489,11.0284309281795,135.402628850646));
#63173=CARTESIAN_POINT('Ctrl Pts',(80.4054093391821,11.0143586647377,135.398772796776));
#63174=CARTESIAN_POINT('Ctrl Pts',(80.4753084720615,11.0002907821078,135.394917943328));
#63175=CARTESIAN_POINT('Ctrl Pts',(80.544495269775,10.9825761669819,135.39106308988));
#63176=CARTESIAN_POINT('Ctrl Pts',(80.6125671728234,10.9613156353018,135.387208236432));
#63177=CARTESIAN_POINT('Ctrl Pts',(80.6806707823523,10.940045200907,135.383351587473));
#63178=CARTESIAN_POINT('Ctrl Pts',(80.7476579947613,10.9152256926984,135.379494938514));
#63179=CARTESIAN_POINT('Ctrl Pts',(80.8131416936283,10.8870077235092,135.375638289555));
#63180=CARTESIAN_POINT('Ctrl Pts',(80.8786429814658,10.8587821749523,135.371780604697));
#63181=CARTESIAN_POINT('Ctrl Pts',(80.9426395124891,10.8271565562098,135.367922919839));
#63182=CARTESIAN_POINT('Ctrl Pts',(81.0047666250961,10.7923285389663,135.364065234981));
#63183=CARTESIAN_POINT('Ctrl Pts',(81.066965856771,10.7574600922865,135.360203072004));
#63184=CARTESIAN_POINT('Ctrl Pts',(81.12729092478,10.7193820818662,135.356340909027));
#63185=CARTESIAN_POINT('Ctrl Pts',(81.1854050201064,10.678336229963,135.352478746049));
#63186=CARTESIAN_POINT('Ctrl Pts',(81.2079550440027,10.6624091999359,135.350980110186));
#63187=CARTESIAN_POINT('Ctrl Pts',(81.2301725095293,10.646035748893,135.349481474322));
#63188=CARTESIAN_POINT('Ctrl Pts',(81.252039109102,10.6292316077768,135.347982838459));
#63189=CARTESIAN_POINT('',(77.945250359968,8.99878374008951,135.654074719411));
#63190=CARTESIAN_POINT('Ctrl Pts',(77.945250359968,8.99878374008951,135.654074719411));
#63191=CARTESIAN_POINT('Ctrl Pts',(77.9452088811236,9.068858104785,135.650257838806));
#63192=CARTESIAN_POINT('Ctrl Pts',(77.9487563144495,9.13907557315805,135.646440958201));
#63193=CARTESIAN_POINT('Ctrl Pts',(77.9559102037764,9.20903221635555,135.642624077596));
#63194=CARTESIAN_POINT('Ctrl Pts',(77.9630536357837,9.27888659923843,135.638812776381));
#63195=CARTESIAN_POINT('Ctrl Pts',(77.9737930081513,9.34848042062324,135.635001475166));
#63196=CARTESIAN_POINT('Ctrl Pts',(77.9880938466836,9.41741010139615,135.631190173951));
#63197=CARTESIAN_POINT('Ctrl Pts',(78.0023832068387,9.48628445668118,135.627381931827));
#63198=CARTESIAN_POINT('Ctrl Pts',(78.0202282665398,9.55449524075859,135.623573689702));
#63199=CARTESIAN_POINT('Ctrl Pts',(78.0415429670004,9.62164588987172,135.619765447577));
#63200=CARTESIAN_POINT('Ctrl Pts',(78.062848127941,9.68876648531526,135.615958909853));
#63201=CARTESIAN_POINT('Ctrl Pts',(78.0876196992428,9.75482741121009,135.61215237213));
#63202=CARTESIAN_POINT('Ctrl Pts',(78.1157214210871,9.81944603211567,135.608345834406));
#63203=CARTESIAN_POINT('Ctrl Pts',(78.1438205431129,9.8840586748575,135.604539648843));
#63204=CARTESIAN_POINT('Ctrl Pts',(78.1752490033443,9.94722882012437,135.60073346328));
#63205=CARTESIAN_POINT('Ctrl Pts',(78.2098226719939,10.0085944163998,135.596927277716));
#63206=CARTESIAN_POINT('Ctrl Pts',(78.2444287085065,10.0700174631367,135.593117528803));
#63207=CARTESIAN_POINT('Ctrl Pts',(78.2821855870685,10.1296321514811,135.589307779889));
#63208=CARTESIAN_POINT('Ctrl Pts',(78.3228640638332,10.1871026131374,135.585498030976));
#63209=CARTESIAN_POINT('Ctrl Pts',(78.3635622899696,10.2446009766625,135.581686432432));
#63210=CARTESIAN_POINT('Ctrl Pts',(78.4071846270008,10.2999526497124,135.577874833887));
#63211=CARTESIAN_POINT('Ctrl Pts',(78.4534612670306,10.3528545782624,135.574063235343));
#63212=CARTESIAN_POINT('Ctrl Pts',(78.4998192121046,10.4058494520572,135.570244940069));
#63213=CARTESIAN_POINT('Ctrl Pts',(78.5488404216444,10.4563856306972,135.566426644794));
#63214=CARTESIAN_POINT('Ctrl Pts',(78.6002185439981,10.5041972736092,135.56260834952));
#63215=CARTESIAN_POINT('Ctrl Pts',(78.6358004088325,10.5373091768409,135.559963993126));
#63216=CARTESIAN_POINT('Ctrl Pts',(78.6725119658445,10.5691151417946,135.557319636732));
#63217=CARTESIAN_POINT('Ctrl Pts',(78.710243122645,10.5995389210067,135.554675280338));
#63218=CARTESIAN_POINT('Ctrl Pts',(78.7654493618272,10.6440533905974,135.550806197491));
#63219=CARTESIAN_POINT('Ctrl Pts',(78.8230709826141,10.6857936224021,135.546937114644));
#63220=CARTESIAN_POINT('Ctrl Pts',(78.8827977135628,10.7244873480775,135.543068031797));
#63221=CARTESIAN_POINT('Ctrl Pts',(78.9424354546612,10.7631234220315,135.539204713691));
#63222=CARTESIAN_POINT('Ctrl Pts',(79.0041716756562,10.7987217379512,135.535341395584));
#63223=CARTESIAN_POINT('Ctrl Pts',(79.0676635881195,10.8310506212505,135.531478077478));
#63224=CARTESIAN_POINT('Ctrl Pts',(79.1310810245939,10.8633415827821,135.527619291042));
#63225=CARTESIAN_POINT('Ctrl Pts',(79.1962496310252,10.8923705100348,135.523760504606));
#63226=CARTESIAN_POINT('Ctrl Pts',(79.2627997262898,10.9179502910507,135.51990171817));
#63227=CARTESIAN_POINT('Ctrl Pts',(79.3293078998742,10.9435139586803,135.516045362487));
#63228=CARTESIAN_POINT('Ctrl Pts',(79.3971953833868,10.9656326168175,135.512189006804));
#63229=CARTESIAN_POINT('Ctrl Pts',(79.4660714454977,10.9841667926833,135.50833265112));
#63230=CARTESIAN_POINT('Ctrl Pts',(79.5349271609302,11.002695493368,135.504477434643));
#63231=CARTESIAN_POINT('Ctrl Pts',(79.6047704063481,11.0176416878133,135.500622218166));
#63232=CARTESIAN_POINT('Ctrl Pts',(79.6751958367456,11.0289159218737,135.496767001689));
#63233=CARTESIAN_POINT('Ctrl Pts',(79.7456240205668,11.0401905967229,135.492911634484));
#63234=CARTESIAN_POINT('Ctrl Pts',(79.8166339545343,11.0477929515476,135.48905626728));
#63235=CARTESIAN_POINT('Ctrl Pts',(79.8878123795722,11.0516850392599,135.485200900075));
#63236=CARTESIAN_POINT('Ctrl Pts',(79.9590653090118,11.0555812009267,135.481341497352));
#63237=CARTESIAN_POINT('Ctrl Pts',(80.0304865955321,11.0557593162919,135.477482094629));
#63238=CARTESIAN_POINT('Ctrl Pts',(80.1016610683358,11.0522335611925,135.473622691907));
#63239=CARTESIAN_POINT('Ctrl Pts',(80.1728758406852,11.0487058097829,135.46976110396));
#63240=CARTESIAN_POINT('Ctrl Pts',(80.2438430376168,11.0414700624067,135.465899516013));
#63241=CARTESIAN_POINT('Ctrl Pts',(80.3141534558345,11.0305923196662,135.462037928066));
#63242=CARTESIAN_POINT('Ctrl Pts',(80.384586884649,11.0196955459248,135.458169584132));
#63243=CARTESIAN_POINT('Ctrl Pts',(80.4543607649211,11.0051441545454,135.454301240199));
#63244=CARTESIAN_POINT('Ctrl Pts',(80.5230776005263,10.9870549530216,135.450432896265));
#63245=CARTESIAN_POINT('Ctrl Pts',(80.5638796800102,10.9763141057187,135.448135984959));
#63246=CARTESIAN_POINT('Ctrl Pts',(80.604309382419,10.9643269064461,135.445839073652));
#63247=CARTESIAN_POINT('Ctrl Pts',(80.6442868085188,10.9511258470095,135.443542162346));
#63248=CARTESIAN_POINT('Ctrl Pts',(80.7116141902564,10.9288934810286,135.439673853667));
#63249=CARTESIAN_POINT('Ctrl Pts',(80.777921307324,10.9031285968536,135.435805544988));
#63250=CARTESIAN_POINT('Ctrl Pts',(80.8428113700402,10.873944117905,135.431937236309));
#63251=CARTESIAN_POINT('Ctrl Pts',(80.9076166286747,10.8447977798186,135.428073983078));
#63252=CARTESIAN_POINT('Ctrl Pts',(80.9710080660991,10.8122409062393,135.424210729848));
#63253=CARTESIAN_POINT('Ctrl Pts',(81.0326051384999,10.7764358109551,135.420347476617));
#63254=CARTESIAN_POINT('Ctrl Pts',(81.0941310956297,10.7406720534967,135.416488683604));
#63255=CARTESIAN_POINT('Ctrl Pts',(81.153866384326,10.7016677655053,135.41262989059));
#63256=CARTESIAN_POINT('Ctrl Pts',(81.2114532906714,10.6596320336211,135.408771097576));
#63257=CARTESIAN_POINT('Ctrl Pts',(81.225104019335,10.6496676440308,135.407856387276));
#63258=CARTESIAN_POINT('Ctrl Pts',(81.238634140733,10.6395331171351,135.406941676975));
#63259=CARTESIAN_POINT('Ctrl Pts',(81.252039109102,10.6292316077768,135.406026966675));
#63260=CARTESIAN_POINT('Ctrl Pts',(81.252039109102,10.6292316077768,136.106053391442));
#63261=CARTESIAN_POINT('Ctrl Pts',(81.3083146843325,10.5859847049182,136.102186604502));
#63262=CARTESIAN_POINT('Ctrl Pts',(81.3624484325911,10.5397406392775,136.098319817562));
#63263=CARTESIAN_POINT('Ctrl Pts',(81.4141045122279,10.4907400816362,136.094453030622));
#63264=CARTESIAN_POINT('Ctrl Pts',(81.4671200795666,10.440449924475,136.090484477359));
#63265=CARTESIAN_POINT('Ctrl Pts',(81.5175252596536,10.3872563791613,136.086515924095));
#63266=CARTESIAN_POINT('Ctrl Pts',(81.5649910392335,10.3314655870952,136.082547370832));
#63267=CARTESIAN_POINT('Ctrl Pts',(81.6111305643379,10.277233660981,136.078689704013));
#63268=CARTESIAN_POINT('Ctrl Pts',(81.6544924626276,10.2205481259674,136.074832037194));
#63269=CARTESIAN_POINT('Ctrl Pts',(81.6948115861983,10.1617277003618,136.070974370375));
#63270=CARTESIAN_POINT('Ctrl Pts',(81.7351106654874,10.1029365167901,136.06711862136));
#63271=CARTESIAN_POINT('Ctrl Pts',(81.7723696975057,10.0420129487833,136.063262872345));
#63272=CARTESIAN_POINT('Ctrl Pts',(81.8063653518934,9.97930678440356,136.05940712333));
#63273=CARTESIAN_POINT('Ctrl Pts',(81.8403554776345,9.91661081780456,136.055552001367));
#63274=CARTESIAN_POINT('Ctrl Pts',(81.8710830487273,9.85213325781443,136.051696879405));
#63275=CARTESIAN_POINT('Ctrl Pts',(81.8983702878578,9.78624920520071,136.047841757443));
#63276=CARTESIAN_POINT('Ctrl Pts',(81.9270569662787,9.71698625700147,136.043788923681));
#63277=CARTESIAN_POINT('Ctrl Pts',(81.9519407103413,9.64616921090295,136.039736089919));
#63278=CARTESIAN_POINT('Ctrl Pts',(81.9728728497112,9.57425628544433,136.035683256158));
#63279=CARTESIAN_POINT('Ctrl Pts',(81.9928102662182,9.50576075702419,136.031823018401));
#63280=CARTESIAN_POINT('Ctrl Pts',(82.0091630510908,9.43627164366354,136.027962780643));
#63281=CARTESIAN_POINT('Ctrl Pts',(82.0218549345478,9.36619692263136,136.024102542886));
#63282=CARTESIAN_POINT('Ctrl Pts',(82.0345557099355,9.29607310726548,136.020239600647));
#63283=CARTESIAN_POINT('Ctrl Pts',(82.0435904205792,9.22536334930288,136.016376658408));
#63284=CARTESIAN_POINT('Ctrl Pts',(82.0489346541452,9.1544808905425,136.012513716169));
#63285=CARTESIAN_POINT('Ctrl Pts',(82.054287535372,9.08348373480052,136.00864452319));
#63286=CARTESIAN_POINT('Ctrl Pts',(82.0559380205628,9.01231380499041,136.004775330211));
#63287=CARTESIAN_POINT('Ctrl Pts',(82.0539137429832,8.94138345894926,136.000906137232));
#63288=CARTESIAN_POINT('Ctrl Pts',(82.0536175569697,8.9310051508368,136.000340008922));
#63289=CARTESIAN_POINT('Ctrl Pts',(82.0532427894648,8.92063195935964,135.999773880613));
#63290=CARTESIAN_POINT('Ctrl Pts',(82.0527896193309,8.91026516135016,135.999207752304));
#63291=CARTESIAN_POINT('Ctrl Pts',(82.0496925249742,8.83941549759563,135.995338669457));
#63292=CARTESIAN_POINT('Ctrl Pts',(82.0429171171316,8.76858759361845,135.99146958661));
#63293=CARTESIAN_POINT('Ctrl Pts',(82.0324642301757,8.69819424200943,135.987600503763));
#63294=CARTESIAN_POINT('Ctrl Pts',(82.0220269175001,8.6279057729836,135.983737185657));
#63295=CARTESIAN_POINT('Ctrl Pts',(82.0079230726633,8.55805104773285,135.97987386755));
#63296=CARTESIAN_POINT('Ctrl Pts',(81.990205484446,8.48904042020795,135.976010549444));
#63297=CARTESIAN_POINT('Ctrl Pts',(81.9725086789528,8.42011074212258,135.972151763008));
#63298=CARTESIAN_POINT('Ctrl Pts',(81.9512066702232,8.35202366327697,135.968292976572));
#63299=CARTESIAN_POINT('Ctrl Pts',(81.9264034611248,8.28518025526267,135.964434190136));
#63300=CARTESIAN_POINT('Ctrl Pts',(81.9016158762294,8.218378953694,135.960577834453));
#63301=CARTESIAN_POINT('Ctrl Pts',(81.8733316352396,8.15282022302366,135.95672147877));
#63302=CARTESIAN_POINT('Ctrl Pts',(81.8417044010275,8.08888943495536,135.952865123087));
#63303=CARTESIAN_POINT('Ctrl Pts',(81.8100865098171,8.024977532682,135.949009906609));
#63304=CARTESIAN_POINT('Ctrl Pts',(81.7751278012398,7.96269305344755,135.945154690132));
#63305=CARTESIAN_POINT('Ctrl Pts',(81.7370291283397,7.90239926667326,135.941299473655));
#63306=CARTESIAN_POINT('Ctrl Pts',(81.6989289658955,7.84210312259222,135.93744410645));
#63307=CARTESIAN_POINT('Ctrl Pts',(81.6576888567548,7.78379823498375,135.933588739246));
#63308=CARTESIAN_POINT('Ctrl Pts',(81.6135535318407,7.72781976026015,135.929733372041));
#63309=CARTESIAN_POINT('Ctrl Pts',(81.5693720092765,7.67178269133812,135.925873969318));
#63310=CARTESIAN_POINT('Ctrl Pts',(81.5222895227633,7.61807727860314,135.922014566595));
#63311=CARTESIAN_POINT('Ctrl Pts',(81.4725911750781,7.56700565472777,135.918155163873));
#63312=CARTESIAN_POINT('Ctrl Pts',(81.4228646877979,7.51590511369777,135.914293575926));
#63313=CARTESIAN_POINT('Ctrl Pts',(81.3705197475215,7.46744166037609,135.910431987979));
#63314=CARTESIAN_POINT('Ctrl Pts',(81.3158763962686,7.42187868899659,135.906570400032));
#63315=CARTESIAN_POINT('Ctrl Pts',(81.2611374445141,7.37623600356553,135.902702056098));
#63316=CARTESIAN_POINT('Ctrl Pts',(81.2040924423584,7.33350422278879,135.898833712165));
#63317=CARTESIAN_POINT('Ctrl Pts',(81.1450918128928,7.29390436887442,135.894965368231));
#63318=CARTESIAN_POINT('Ctrl Pts',(81.1100589370067,7.2703911152048,135.892668456925));
#63319=CARTESIAN_POINT('Ctrl Pts',(81.0743370944693,7.24798121228253,135.890371545619));
#63320=CARTESIAN_POINT('Ctrl Pts',(81.038003484846,7.22671312869363,135.888074634312));
#63321=CARTESIAN_POINT('Ctrl Pts',(80.9768005357521,7.19088763679479,135.884205551465));
#63322=CARTESIAN_POINT('Ctrl Pts',(80.9136208229207,7.15816421980074,135.880336468618));
#63323=CARTESIAN_POINT('Ctrl Pts',(80.8488115996088,7.12876606730488,135.876467385771));
#63324=CARTESIAN_POINT('Ctrl Pts',(80.7840989388074,7.09941171659008,135.872604067665));
#63325=CARTESIAN_POINT('Ctrl Pts',(80.7177620256111,7.07337299491202,135.868740749559));
#63326=CARTESIAN_POINT('Ctrl Pts',(80.6501742435433,7.05082812057713,135.864877431452));
#63327=CARTESIAN_POINT('Ctrl Pts',(80.5826657419179,7.02830969137116,135.861018645016));
#63328=CARTESIAN_POINT('Ctrl Pts',(80.5139097444993,7.0092771219014,135.857159858581));
#63329=CARTESIAN_POINT('Ctrl Pts',(80.4442996139068,6.9938605692569,135.853301072145));
#63330=CARTESIAN_POINT('Ctrl Pts',(80.3747333325923,6.97845372791013,135.849444716462));
#63331=CARTESIAN_POINT('Ctrl Pts',(80.3043144587388,6.96665848901139,135.845588360778));
#63332=CARTESIAN_POINT('Ctrl Pts',(80.2334500995796,6.95855477332693,135.841732005095));
#63333=CARTESIAN_POINT('Ctrl Pts',(80.1626066744617,6.95045345156123,135.837876788618));
#63334=CARTESIAN_POINT('Ctrl Pts',(80.091318507677,6.94604154320104,135.834021572141));
#63335=CARTESIAN_POINT('Ctrl Pts',(80.0199997326209,6.94534733514516,135.830166355663));
#63336=CARTESIAN_POINT('Ctrl Pts',(79.948678169214,6.94465309994782,135.826310988459));
#63337=CARTESIAN_POINT('Ctrl Pts',(79.8773264809413,6.94767685615559,135.822455621254));
#63338=CARTESIAN_POINT('Ctrl Pts',(79.8063589810274,6.95439477946715,135.81860025405));
#63339=CARTESIAN_POINT('Ctrl Pts',(79.735317197493,6.96111973461253,135.814740851327));
#63340=CARTESIAN_POINT('Ctrl Pts',(79.6646608896917,6.97154652995798,135.810881448604));
#63341=CARTESIAN_POINT('Ctrl Pts',(79.5947985234109,6.98559951204583,135.807022045881));
#63342=CARTESIAN_POINT('Ctrl Pts',(79.5248966005095,6.99966045104253,135.803160457934));
#63343=CARTESIAN_POINT('Ctrl Pts',(79.4557899848462,7.01735154348953,135.799298869987));
#63344=CARTESIAN_POINT('Ctrl Pts',(79.3878735471225,7.03854677134845,135.79543728204));
#63345=CARTESIAN_POINT('Ctrl Pts',(79.3198382871566,7.05977908101822,135.791568938107));
#63346=CARTESIAN_POINT('Ctrl Pts',(79.2529978181219,7.08452759730746,135.787700594174));
#63347=CARTESIAN_POINT('Ctrl Pts',(79.1877278906748,7.11261779628174,135.78383225024));
#63348=CARTESIAN_POINT('Ctrl Pts',(79.1489724860618,7.12929694806709,135.781535338934));
#63349=CARTESIAN_POINT('Ctrl Pts',(79.110770360955,7.14715335925725,135.779238427627));
#63350=CARTESIAN_POINT('Ctrl Pts',(79.073195705611,7.1661430365478,135.776941516321));
#63351=CARTESIAN_POINT('Ctrl Pts',(79.0099022497152,7.1981306167681,135.773072433474));
#63352=CARTESIAN_POINT('Ctrl Pts',(78.9481427918075,7.23346144597127,135.769203350627));
#63353=CARTESIAN_POINT('Ctrl Pts',(78.8882931841807,7.27196483885281,135.76533426778));
#63354=CARTESIAN_POINT('Ctrl Pts',(78.8285327494845,7.31041086359923,135.761470949674));
#63355=CARTESIAN_POINT('Ctrl Pts',(78.7706769218814,7.35201980844774,135.757607631567));
#63356=CARTESIAN_POINT('Ctrl Pts',(78.7150779443408,7.39657464365177,135.753744313461));
#63357=CARTESIAN_POINT('Ctrl Pts',(78.6595441843794,7.44107721605125,135.749885527025));
#63358=CARTESIAN_POINT('Ctrl Pts',(78.606262393319,7.48851851265072,135.746026740589));
#63359=CARTESIAN_POINT('Ctrl Pts',(78.5555552725787,7.53863865114589,135.742167954153));
#63360=CARTESIAN_POINT('Ctrl Pts',(78.5048800936062,7.58872721762896,135.73831159847));
#63361=CARTESIAN_POINT('Ctrl Pts',(78.4567767118996,7.64149093739805,135.734455242787));
#63362=CARTESIAN_POINT('Ctrl Pts',(78.4115330784898,7.69663113365102,135.730598887103));
#63363=CARTESIAN_POINT('Ctrl Pts',(78.3663028105023,7.75175504093786,135.726743670626));
#63364=CARTESIAN_POINT('Ctrl Pts',(78.3239309216265,7.80925365563422,135.722888454149));
#63365=CARTESIAN_POINT('Ctrl Pts',(78.2846657944253,7.86879439283327,135.719033237672));
#63366=CARTESIAN_POINT('Ctrl Pts',(78.2453991320751,7.92833745789711,135.715177870467));
#63367=CARTESIAN_POINT('Ctrl Pts',(78.2092397381526,7.98992239722593,135.711322503263));
#63368=CARTESIAN_POINT('Ctrl Pts',(78.1763923124136,8.0531882107431,135.707467136058));
#63369=CARTESIAN_POINT('Ctrl Pts',(78.143510504377,8.1165202463152,135.703607733335));
#63370=CARTESIAN_POINT('Ctrl Pts',(78.1139478091924,8.18153623624629,135.699748330612));
#63371=CARTESIAN_POINT('Ctrl Pts',(78.0878622116923,8.24785198197061,135.695888927889));
#63372=CARTESIAN_POINT('Ctrl Pts',(78.0617618443218,8.31420527619113,135.692027339943));
#63373=CARTESIAN_POINT('Ctrl Pts',(78.0391426479366,8.38185933028476,135.688165751996));
#63374=CARTESIAN_POINT('Ctrl Pts',(78.0201129207117,8.45041405060964,135.684304164049));
#63375=CARTESIAN_POINT('Ctrl Pts',(78.001049900297,8.51908870987492,135.680435820115));
#63376=CARTESIAN_POINT('Ctrl Pts',(77.9855889924591,8.58866670703014,135.676567476182));
#63377=CARTESIAN_POINT('Ctrl Pts',(77.9737873736293,8.65873770317237,135.672699132248));
#63378=CARTESIAN_POINT('Ctrl Pts',(77.9667799119893,8.70034384421349,135.670402220942));
#63379=CARTESIAN_POINT('Ctrl Pts',(77.9610615928321,8.74212367917311,135.668105309635));
#63380=CARTESIAN_POINT('Ctrl Pts',(77.9566356952624,8.78399101726015,135.665808398329));
#63381=CARTESIAN_POINT('Ctrl Pts',(77.9490991887904,8.85528355385796,135.66189717204));
#63382=CARTESIAN_POINT('Ctrl Pts',(77.94529286412,8.92697727577637,135.657985945751));
#63383=CARTESIAN_POINT('Ctrl Pts',(77.9452503599685,8.99878373915154,135.654074719462));
#63384=CARTESIAN_POINT('Origin',(80.,9.,141.545925280538));
#63385=CARTESIAN_POINT('',(81.252039109102,10.6292316077768,136.806140361941));
#63386=CARTESIAN_POINT('',(81.252039109102,10.6292316077768,136.747866922016));
#63387=CARTESIAN_POINT('',(81.252039109102,10.6292316077768,141.545925280538));
#63388=CARTESIAN_POINT('',(77.9452505319477,8.99852147413462,136.295925280587));
#63389=CARTESIAN_POINT('Ctrl Pts',(81.252039109102,10.6292316077768,136.747866922016));
#63390=CARTESIAN_POINT('Ctrl Pts',(81.3085184540973,10.5858281110284,136.74401000082));
#63391=CARTESIAN_POINT('Ctrl Pts',(81.3627855868937,10.5394478623079,136.740153079624));
#63392=CARTESIAN_POINT('Ctrl Pts',(81.4145162186297,10.4903494320908,136.736296158428));
#63393=CARTESIAN_POINT('Ctrl Pts',(81.4662266011205,10.4412702207799,136.732440746972));
#63394=CARTESIAN_POINT('Ctrl Pts',(81.5154021011393,10.3894752738317,136.728585335515));
#63395=CARTESIAN_POINT('Ctrl Pts',(81.5617531753342,10.3352619899605,136.724729924058));
#63396=CARTESIAN_POINT('Ctrl Pts',(81.6081016109247,10.281051792262,136.720874732076));
#63397=CARTESIAN_POINT('Ctrl Pts',(81.6516256254678,10.2244239012393,136.717019540094));
#63398=CARTESIAN_POINT('Ctrl Pts',(81.6920752293629,10.1657096468146,136.713164348112));
#63399=CARTESIAN_POINT('Ctrl Pts',(81.732564681132,10.106937551571,136.709305358288));
#63400=CARTESIAN_POINT('Ctrl Pts',(81.7699733961127,10.0460753883556,136.705446368464));
#63401=CARTESIAN_POINT('Ctrl Pts',(81.8040946189889,9.98348368986742,136.701587378641));
#63402=CARTESIAN_POINT('Ctrl Pts',(81.8382322234244,9.92086194117785,136.69772653612));
#63403=CARTESIAN_POINT('Ctrl Pts',(81.86907898119,9.85650944175953,136.6938656936));
#63404=CARTESIAN_POINT('Ctrl Pts',(81.8964753088183,9.79080905757488,136.690004851079));
#63405=CARTESIAN_POINT('Ctrl Pts',(81.923922074071,9.72498771662032,136.686136900609));
#63406=CARTESIAN_POINT('Ctrl Pts',(81.9479055535397,9.65781399157883,136.682268950139));
#63407=CARTESIAN_POINT('Ctrl Pts',(81.9683154621906,9.58968788676836,136.678400999669));
#63408=CARTESIAN_POINT('Ctrl Pts',(81.986284042303,9.52971067702336,136.674995713585));
#63409=CARTESIAN_POINT('Ctrl Pts',(82.0014835402419,9.46899572838118,136.671590427501));
#63410=CARTESIAN_POINT('Ctrl Pts',(82.0138717544802,9.40782118508842,136.668185141418));
#63411=CARTESIAN_POINT('Ctrl Pts',(82.0279472318518,9.33831472650817,136.664316058571));
#63412=CARTESIAN_POINT('Ctrl Pts',(82.0384476506383,9.26794257762408,136.660446975724));
#63413=CARTESIAN_POINT('Ctrl Pts',(82.045274300028,9.19710555584454,136.656577892877));
#63414=CARTESIAN_POINT('Ctrl Pts',(82.0520907780507,9.12637407769456,136.652714574771));
#63415=CARTESIAN_POINT('Ctrl Pts',(82.0552443056657,9.05517958111897,136.648851256664));
#63416=CARTESIAN_POINT('Ctrl Pts',(82.0546871818792,8.98393304255929,136.644987938558));
#63417=CARTESIAN_POINT('Ctrl Pts',(82.0541307115987,8.91277007616198,136.641129152122));
#63418=CARTESIAN_POINT('Ctrl Pts',(82.0498722394196,8.84155567244782,136.637270365686));
#63419=CARTESIAN_POINT('Ctrl Pts',(82.0419160056416,8.77070414655999,136.63341157925));
#63420=CARTESIAN_POINT('Ctrl Pts',(82.0339647837074,8.69989725193819,136.629555223567));
#63421=CARTESIAN_POINT('Ctrl Pts',(82.022320475588,8.62945326323857,136.625698867884));
#63422=CARTESIAN_POINT('Ctrl Pts',(82.0070393018439,8.55978323140311,136.6218425122));
#63423=CARTESIAN_POINT('Ctrl Pts',(81.9917626423116,8.49013378079267,136.617987295723));
#63424=CARTESIAN_POINT('Ctrl Pts',(81.9728513540896,8.42125830738812,136.614132079246));
#63425=CARTESIAN_POINT('Ctrl Pts',(81.9504127845803,8.35355778893574,136.610276862769));
#63426=CARTESIAN_POINT('Ctrl Pts',(81.9279733377901,8.28585462359568,136.606421495564));
#63427=CARTESIAN_POINT('Ctrl Pts',(81.9020064908408,8.21932696483277,136.602566128359));
#63428=CARTESIAN_POINT('Ctrl Pts',(81.8726689525194,8.15435908520832,136.598710761155));
#63429=CARTESIAN_POINT('Ctrl Pts',(81.8433007057954,8.08932320192966,136.594851358432));
#63430=CARTESIAN_POINT('Ctrl Pts',(81.8105549249677,8.02585080059414,136.590991955709));
#63431=CARTESIAN_POINT('Ctrl Pts',(81.7746354615354,7.96430383743053,136.587132552986));
#63432=CARTESIAN_POINT('Ctrl Pts',(81.7386956602207,7.90272202589287,136.583270965039));
#63433=CARTESIAN_POINT('Ctrl Pts',(81.6995788656066,7.84306822920265,136.579409377092));
#63434=CARTESIAN_POINT('Ctrl Pts',(81.6575321773042,7.7856752313729,136.575547789146));
#63435=CARTESIAN_POINT('Ctrl Pts',(81.6154119268134,7.7281818224363,136.571679445212));
#63436=CARTESIAN_POINT('Ctrl Pts',(81.5703518557311,7.67295748583205,136.567811101279));
#63437=CARTESIAN_POINT('Ctrl Pts',(81.5226387640879,7.62030120801794,136.563942757345));
#63438=CARTESIAN_POINT('Ctrl Pts',(81.4943081033344,7.58903542556877,136.561645846039));
#63439=CARTESIAN_POINT('Ctrl Pts',(81.4650427907926,7.55867434414894,136.559348934732));
#63440=CARTESIAN_POINT('Ctrl Pts',(81.4349084744055,7.52927390973731,136.557052023426));
#63441=CARTESIAN_POINT('Ctrl Pts',(81.3841480613612,7.47974970035277,136.553182940579));
#63442=CARTESIAN_POINT('Ctrl Pts',(81.3307213118376,7.43275948255617,136.549313857732));
#63443=CARTESIAN_POINT('Ctrl Pts',(81.2749114269959,7.38860358203972,136.545444774885));
#63444=CARTESIAN_POINT('Ctrl Pts',(81.2191846960995,7.34451347161309,136.541581456779));
#63445=CARTESIAN_POINT('Ctrl Pts',(81.1610822558932,7.30324959490401,136.537718138672));
#63446=CARTESIAN_POINT('Ctrl Pts',(81.1009235091995,7.2650749326291,136.533854820566));
#63447=CARTESIAN_POINT('Ctrl Pts',(81.0408353286922,7.22694504921818,136.52999603413));
#63448=CARTESIAN_POINT('Ctrl Pts',(80.9786960410184,7.1918974414676,136.526137247694));
#63449=CARTESIAN_POINT('Ctrl Pts',(80.9148560258897,7.16015326334141,136.522278461259));
#63450=CARTESIAN_POINT('Ctrl Pts',(80.8510562252894,7.12842908171974,136.518422105575));
#63451=CARTESIAN_POINT('Ctrl Pts',(80.7855582566907,7.10000441699144,136.514565749892));
#63452=CARTESIAN_POINT('Ctrl Pts',(80.7187379505123,7.07505498234537,136.510709394209));
#63453=CARTESIAN_POINT('Ctrl Pts',(80.6519373837216,7.05011291801217,136.506854177731));
#63454=CARTESIAN_POINT('Ctrl Pts',(80.5838157097105,7.0286442154711,136.502998961254));
#63455=CARTESIAN_POINT('Ctrl Pts',(80.5147680262655,7.01077617105698,136.499143744777));
#63456=CARTESIAN_POINT('Ctrl Pts',(80.4457176432624,6.99290742805571,136.495288377572));
#63457=CARTESIAN_POINT('Ctrl Pts',(80.3757416497901,6.97863974224021,136.491433010368));
#63458=CARTESIAN_POINT('Ctrl Pts',(80.3052478817002,6.96804987924961,136.487577643163));
#63459=CARTESIAN_POINT('Ctrl Pts',(80.2346803258581,6.9574489315602,136.48371824044));
#63460=CARTESIAN_POINT('Ctrl Pts',(80.1635943948842,6.95053356382926,136.479858837718));
#63461=CARTESIAN_POINT('Ctrl Pts',(80.0924047452203,6.94732883160483,136.475999434995));
#63462=CARTESIAN_POINT('Ctrl Pts',(80.0211747874175,6.94412228483584,136.472137847048));
#63463=CARTESIAN_POINT('Ctrl Pts',(79.9498414800195,6.94463055253553,136.468276259101));
#63464=CARTESIAN_POINT('Ctrl Pts',(79.8788184278493,6.94882653364688,136.464414671154));
#63465=CARTESIAN_POINT('Ctrl Pts',(79.8076711183036,6.95302985577759,136.46054632722));
#63466=CARTESIAN_POINT('Ctrl Pts',(79.7368356306462,6.96093371860795,136.456677983287));
#63467=CARTESIAN_POINT('Ctrl Pts',(79.6667187079827,6.97245933631621,136.452809639354));
#63468=CARTESIAN_POINT('Ctrl Pts',(79.6250852970938,6.97930291643309,136.450512728047));
#63469=CARTESIAN_POINT('Ctrl Pts',(79.5837050187288,6.98742242046764,136.448215816741));
#63470=CARTESIAN_POINT('Ctrl Pts',(79.5426604811077,6.99679303940922,136.445918905434));
#63471=CARTESIAN_POINT('Ctrl Pts',(79.4735221055763,7.01257758490282,136.442049822587));
#63472=CARTESIAN_POINT('Ctrl Pts',(79.4050664517631,7.03197659503789,136.43818073974));
#63473=CARTESIAN_POINT('Ctrl Pts',(79.3376994359528,7.05491503389628,136.434311656893));
#63474=CARTESIAN_POINT('Ctrl Pts',(79.2704327936362,7.0778192956248,136.430448338787));
#63475=CARTESIAN_POINT('Ctrl Pts',(79.2042520257748,7.10425236287628,136.426585020681));
#63476=CARTESIAN_POINT('Ctrl Pts',(79.1395513089728,7.13408853033979,136.422721702574));
#63477=CARTESIAN_POINT('Ctrl Pts',(79.0749264860866,7.16388969999036,136.418862916138));
#63478=CARTESIAN_POINT('Ctrl Pts',(79.0117787047756,7.19708583827694,136.415004129703));
#63479=CARTESIAN_POINT('Ctrl Pts',(78.9504838028604,7.23350252917202,136.411145343267));
#63480=CARTESIAN_POINT('Ctrl Pts',(78.8892275122389,7.26989628022215,136.407288987584));
#63481=CARTESIAN_POINT('Ctrl Pts',(78.8298222019973,7.3095063114083,136.4034326319));
#63482=CARTESIAN_POINT('Ctrl Pts',(78.7726193376205,7.35211217853979,136.399576276217));
#63483=CARTESIAN_POINT('Ctrl Pts',(78.7154333715427,7.39470545947148,136.39572105974));
#63484=CARTESIAN_POINT('Ctrl Pts',(78.6604489490401,7.44029252935922,136.391865843263));
#63485=CARTESIAN_POINT('Ctrl Pts',(78.6079873092383,7.48861049651041,136.388010626785));
#63486=CARTESIAN_POINT('Ctrl Pts',(78.5555236183434,7.53693035274952,136.384155259581));
#63487=CARTESIAN_POINT('Ctrl Pts',(78.5055832618023,7.58798098751036,136.380299892376));
#63488=CARTESIAN_POINT('Ctrl Pts',(78.4584519351075,7.64146140057548,136.376444525172));
#63489=CARTESIAN_POINT('Ctrl Pts',(78.4112712747657,7.6949977930498,136.372585122449));
#63490=CARTESIAN_POINT('Ctrl Pts',(78.3669058355876,7.75096867565695,136.368725719726));
#63491=CARTESIAN_POINT('Ctrl Pts',(78.3256015690616,7.80903927144048,136.364866317003));
#63492=CARTESIAN_POINT('Ctrl Pts',(78.2842739157354,7.86714274725158,136.361004729056));
#63493=CARTESIAN_POINT('Ctrl Pts',(78.2460111461352,7.92734789273723,136.357143141109));
#63494=CARTESIAN_POINT('Ctrl Pts',(78.2110148228832,7.98929252572442,136.353281553162));
#63495=CARTESIAN_POINT('Ctrl Pts',(78.1759572723093,8.05134553306729,136.349413209229));
#63496=CARTESIAN_POINT('Ctrl Pts',(78.1441777944383,8.11514366897695,136.345544865295));
#63497=CARTESIAN_POINT('Ctrl Pts',(78.115830808151,8.18030248323716,136.341676521362));
#63498=CARTESIAN_POINT('Ctrl Pts',(78.0989991834487,8.21899191203774,136.339379610056));
#63499=CARTESIAN_POINT('Ctrl Pts',(78.0833767987337,8.25816071185491,136.337082698749));
#63500=CARTESIAN_POINT('Ctrl Pts',(78.0689876162082,8.29772602487152,136.334785787443));
#63501=CARTESIAN_POINT('Ctrl Pts',(78.0409616303174,8.37478786646014,136.330312065342));
#63502=CARTESIAN_POINT('Ctrl Pts',(78.0175257042648,8.45360303856632,136.325838343242));
#63503=CARTESIAN_POINT('Ctrl Pts',(77.9988702448825,8.53365542172823,136.321364621142));
#63504=CARTESIAN_POINT('Ctrl Pts',(77.9803784740623,8.61300540141546,136.316930152813));
#63505=CARTESIAN_POINT('Ctrl Pts',(77.9665837380257,8.69357080831013,136.312495684485));
#63506=CARTESIAN_POINT('Ctrl Pts',(77.9576251286371,8.77482796060499,136.308061216156));
#63507=CARTESIAN_POINT('Ctrl Pts',(77.9494527016198,8.84895421368233,136.3040159043));
#63508=CARTESIAN_POINT('Ctrl Pts',(77.9453044026692,8.92365579951472,136.299970592443));
#63509=CARTESIAN_POINT('Ctrl Pts',(77.9452505319477,8.99852147413461,136.295925280587));
#63510=CARTESIAN_POINT('Ctrl Pts',(77.945250531947,8.9985214750451,136.295925280538));
#63511=CARTESIAN_POINT('Ctrl Pts',(77.9451990745752,9.07003329291146,136.292061191873));
#63512=CARTESIAN_POINT('Ctrl Pts',(77.9488851993071,9.14157794387393,136.288197103208));
#63513=CARTESIAN_POINT('Ctrl Pts',(77.9562925982608,9.21273838059117,136.284333014543));
#63514=CARTESIAN_POINT('Ctrl Pts',(77.963699599031,9.2838949920902,136.280469133592));
#63515=CARTESIAN_POINT('Ctrl Pts',(77.9748274258944,9.35466695085,136.276605252641));
#63516=CARTESIAN_POINT('Ctrl Pts',(77.9896079183788,9.42464248569205,136.272741371689));
#63517=CARTESIAN_POINT('Ctrl Pts',(78.004392467588,9.4946372263551,136.268876430239));
#63518=CARTESIAN_POINT('Ctrl Pts',(78.0228315710416,9.56383463791113,136.265011488788));
#63519=CARTESIAN_POINT('Ctrl Pts',(78.0448063606778,9.63183494304609,136.261146547337));
#63520=CARTESIAN_POINT('Ctrl Pts',(78.066809060374,9.69992161499648,136.257276697046));
#63521=CARTESIAN_POINT('Ctrl Pts',(78.0923562553077,9.76680768829056,136.253406846754));
#63522=CARTESIAN_POINT('Ctrl Pts',(78.1212800534335,9.83211112531514,136.249536996462));
#63523=CARTESIAN_POINT('Ctrl Pts',(78.1502258976062,9.89746433735987,136.245664196527));
#63524=CARTESIAN_POINT('Ctrl Pts',(78.1825532470504,9.96123208405092,136.241791396591));
#63525=CARTESIAN_POINT('Ctrl Pts',(78.2180484155873,10.0230572385303,136.237918596656));
#63526=CARTESIAN_POINT('Ctrl Pts',(78.2536056682719,10.0849905306007,136.234039022855));
#63527=CARTESIAN_POINT('Ctrl Pts',(78.2923415309165,10.1449740495301,136.230159449055));
#63528=CARTESIAN_POINT('Ctrl Pts',(78.3339997518961,10.2026806458148,136.226279875254));
#63529=CARTESIAN_POINT('Ctrl Pts',(78.3434032521698,10.2157067420139,136.225404139987));
#63530=CARTESIAN_POINT('Ctrl Pts',(78.3529555021341,10.228616961064,136.224528404719));
#63531=CARTESIAN_POINT('Ctrl Pts',(78.3626532888618,10.2414077936056,136.223652669452));
#63532=CARTESIAN_POINT('Ctrl Pts',(78.4054990456461,10.2979189250149,136.219783586605));
#63533=CARTESIAN_POINT('Ctrl Pts',(78.4513577800801,10.3523199783994,136.215914503758));
#63534=CARTESIAN_POINT('Ctrl Pts',(78.4999940143905,10.4042719129982,136.212045420911));
#63535=CARTESIAN_POINT('Ctrl Pts',(78.5485577831374,10.4561464418055,136.208182102804));
#63536=CARTESIAN_POINT('Ctrl Pts',(78.5998905079848,10.5055787433783,136.204318784698));
#63537=CARTESIAN_POINT('Ctrl Pts',(78.6537153665542,10.5522613337476,136.200455466592));
#63538=CARTESIAN_POINT('Ctrl Pts',(78.7074770885853,10.5988891654564,136.196596680156));
#63539=CARTESIAN_POINT('Ctrl Pts',(78.7637247725268,10.6427733759751,136.19273789372));
#63540=CARTESIAN_POINT('Ctrl Pts',(78.8221447529238,10.6836432458912,136.188879107284));
#63541=CARTESIAN_POINT('Ctrl Pts',(78.8805279330169,10.7244873707861,136.185022751601));
#63542=CARTESIAN_POINT('Ctrl Pts',(78.9410802976008,10.7623206444849,136.181166395918));
#63543=CARTESIAN_POINT('Ctrl Pts',(79.0034562665658,10.796913506503,136.177310040234));
#63544=CARTESIAN_POINT('Ctrl Pts',(79.065813809045,10.8314961494433,136.173454823757));
#63545=CARTESIAN_POINT('Ctrl Pts',(79.1299934618203,10.8628400456359,136.16959960728));
#63546=CARTESIAN_POINT('Ctrl Pts',(79.1956234031313,10.8907606545805,136.165744390803));
#63547=CARTESIAN_POINT('Ctrl Pts',(79.2612559103766,10.9186823551374,136.161889023598));
#63548=CARTESIAN_POINT('Ctrl Pts',(79.3283383708567,10.9431803145808,136.158033656394));
#63549=CARTESIAN_POINT('Ctrl Pts',(79.3964788642986,10.9641180721285,136.154178289189));
#63550=CARTESIAN_POINT('Ctrl Pts',(79.4646906822562,10.9850777457989,136.150318886466));
#63551=CARTESIAN_POINT('Ctrl Pts',(79.5339622786307,11.0024696355473,136.146459483743));
#63552=CARTESIAN_POINT('Ctrl Pts',(79.6038873114516,11.0162074051225,136.142600081021));
#63553=CARTESIAN_POINT('Ctrl Pts',(79.6738519363753,11.0299529531309,136.138738493074));
#63554=CARTESIAN_POINT('Ctrl Pts',(79.7444702531338,11.0400401935167,136.134876905127));
#63555=CARTESIAN_POINT('Ctrl Pts',(79.8153292167478,11.0464345248048,136.13101531718));
#63556=CARTESIAN_POINT('Ctrl Pts',(79.8863121506584,11.0528400432047,136.127146973246));
#63557=CARTESIAN_POINT('Ctrl Pts',(79.9575360864153,11.0555397347778,136.123278629313));
#63558=CARTESIAN_POINT('Ctrl Pts',(80.0285870917953,11.0545511287585,136.119410285379));
#63559=CARTESIAN_POINT('Ctrl Pts',(80.0707751341203,11.0539641229538,136.117113374073));
#63560=CARTESIAN_POINT('Ctrl Pts',(80.1129022677807,11.0520777526687,136.114816462766));
#63561=CARTESIAN_POINT('Ctrl Pts',(80.1548831168876,11.0489042882973,136.11251955146));
#63562=CARTESIAN_POINT('Ctrl Pts',(80.2255915701654,11.0435592140074,136.108650857776));
#63563=CARTESIAN_POINT('Ctrl Pts',(80.2961614847426,11.0345391130104,136.104782164092));
#63564=CARTESIAN_POINT('Ctrl Pts',(80.3661804272609,11.021857922108,136.100913470407));
#63565=CARTESIAN_POINT('Ctrl Pts',(80.4361002562164,11.0091946817483,136.097050252956));
#63566=CARTESIAN_POINT('Ctrl Pts',(80.5054701866998,10.992880720234,136.093187035504));
#63567=CARTESIAN_POINT('Ctrl Pts',(80.5738817794949,10.9729818209157,136.089323818053));
#63568=CARTESIAN_POINT('Ctrl Pts',(80.6422141511607,10.9531059646696,136.085465074235));
#63569=CARTESIAN_POINT('Ctrl Pts',(80.7095899251634,10.9296535509445,136.081606330418));
#63570=CARTESIAN_POINT('Ctrl Pts',(80.7756115466406,10.9027412570336,136.077747586601));
#63571=CARTESIAN_POINT('Ctrl Pts',(80.8415882785372,10.8758472613947,136.07389146643));
#63572=CARTESIAN_POINT('Ctrl Pts',(80.9062122370559,10.8454982386467,136.070035346259));
#63573=CARTESIAN_POINT('Ctrl Pts',(80.9691031912758,10.81185997449,136.066179226088));
#63574=CARTESIAN_POINT('Ctrl Pts',(81.0319836313127,10.7782273340175,136.062323750588));
#63575=CARTESIAN_POINT('Ctrl Pts',(81.0931312103808,10.7413067658456,136.058468275088));
#63576=CARTESIAN_POINT('Ctrl Pts',(81.1521891448271,10.7013105939371,136.054612799588));
#63577=CARTESIAN_POINT('Ctrl Pts',(81.1861856897139,10.6782869026018,136.05239340524));
#63578=CARTESIAN_POINT('Ctrl Pts',(81.2194902550006,10.6542448950816,136.050174010892));
#63579=CARTESIAN_POINT('Ctrl Pts',(81.252039109102,10.6292316077768,136.047954616544));
#63580=CARTESIAN_POINT('',(77.9452507823625,9.00179307496101,136.35407471951));
#63581=CARTESIAN_POINT('Ctrl Pts',(77.9452507823632,9.00179307584224,136.354074719462));
#63582=CARTESIAN_POINT('Ctrl Pts',(77.9453413919223,9.10562578405504,136.348435142862));
#63583=CARTESIAN_POINT('Ctrl Pts',(77.9533058453993,9.20912640739788,136.342795566262));
#63584=CARTESIAN_POINT('Ctrl Pts',(77.968974501846,9.31134063073801,136.337155989661));
#63585=CARTESIAN_POINT('Ctrl Pts',(77.9731872821066,9.3388226336721,136.3356396952));
#63586=CARTESIAN_POINT('Ctrl Pts',(77.9779567533559,9.36621181729645,136.334123400739));
#63587=CARTESIAN_POINT('Ctrl Pts',(77.9832790921584,9.39348995206298,136.332607106279));
#63588=CARTESIAN_POINT('Ctrl Pts',(77.9968599435676,9.46309474588194,136.328738023432));
#63589=CARTESIAN_POINT('Ctrl Pts',(78.014075118604,9.53213195238462,136.324868940585));
#63590=CARTESIAN_POINT('Ctrl Pts',(78.0348625104968,9.6001934770131,136.320999857738));
#63591=CARTESIAN_POINT('Ctrl Pts',(78.0556189302125,9.66815359336439,136.317136539631));
#63592=CARTESIAN_POINT('Ctrl Pts',(78.0799368611766,9.73514045261806,136.313273221525));
#63593=CARTESIAN_POINT('Ctrl Pts',(78.1077031799501,9.80075608479058,136.309409903418));
#63594=CARTESIAN_POINT('Ctrl Pts',(78.1354369288423,9.86629474985172,136.305551116983));
#63595=CARTESIAN_POINT('Ctrl Pts',(78.1666108424928,9.93046493755091,136.301692330547));
#63596=CARTESIAN_POINT('Ctrl Pts',(78.2010625289044,9.99288546045757,136.297833544111));
#63597=CARTESIAN_POINT('Ctrl Pts',(78.2354925132797,10.0552666630119,136.293977188428));
#63598=CARTESIAN_POINT('Ctrl Pts',(78.2731959397889,10.1158999631443,136.290120832745));
#63599=CARTESIAN_POINT('Ctrl Pts',(78.3139636374603,10.1744270716796,136.286264477061));
#63600=CARTESIAN_POINT('Ctrl Pts',(78.3547192919456,10.232936890721,136.282409260584));
#63601=CARTESIAN_POINT('Ctrl Pts',(78.398537142981,10.2893413549905,136.278554044107));
#63602=CARTESIAN_POINT('Ctrl Pts',(78.4451646335606,10.343311038356,136.27469882763));
#63603=CARTESIAN_POINT('Ctrl Pts',(78.4917939471356,10.3972828317747,136.270843460425));
#63604=CARTESIAN_POINT('Ctrl Pts',(78.5412327990926,10.4488192891436,136.26698809322));
#63605=CARTESIAN_POINT('Ctrl Pts',(78.5931894143111,10.4976252997641,136.263132726016));
#63606=CARTESIAN_POINT('Ctrl Pts',(78.6452004139378,10.546482396969,136.259273323293));
#63607=CARTESIAN_POINT('Ctrl Pts',(78.6997340829046,10.592603008872,136.25541392057));
#63608=CARTESIAN_POINT('Ctrl Pts',(78.7564636241796,10.6357306760318,136.251554517847));
#63609=CARTESIAN_POINT('Ctrl Pts',(78.8132252861664,10.6788827624155,136.2476929299));
#63610=CARTESIAN_POINT('Ctrl Pts',(78.8721848938307,10.7190382569895,136.243831341954));
#63611=CARTESIAN_POINT('Ctrl Pts',(78.9329868490235,10.7559841964389,136.239969754007));
#63612=CARTESIAN_POINT('Ctrl Pts',(78.9938951794163,10.7929947741337,136.236101410073));
#63613=CARTESIAN_POINT('Ctrl Pts',(79.056651864793,10.8267843553657,136.23223306614));
#63614=CARTESIAN_POINT('Ctrl Pts',(79.1208775529789,10.8571863895806,136.228364722206));
#63615=CARTESIAN_POINT('Ctrl Pts',(79.1590129183693,10.8752382426031,136.2260678109));
#63616=CARTESIAN_POINT('Ctrl Pts',(79.1976658166299,10.8920966897238,136.223770899593));
#63617=CARTESIAN_POINT('Ctrl Pts',(79.2367541927435,10.9077351493867,136.221473988287));
#63618=CARTESIAN_POINT('Ctrl Pts',(79.3025974689341,10.9340776972527,136.21760490544));
#63619=CARTESIAN_POINT('Ctrl Pts',(79.3699350818583,10.9570590814341,136.213735822593));
#63620=CARTESIAN_POINT('Ctrl Pts',(79.4383904922891,10.9765101374263,136.209866739746));
#63621=CARTESIAN_POINT('Ctrl Pts',(79.5067439075725,10.9959322123151,136.20600342164));
#63622=CARTESIAN_POINT('Ctrl Pts',(79.5762113509863,11.0118342683011,136.202140103533));
#63623=CARTESIAN_POINT('Ctrl Pts',(79.6463971188564,11.0240954930405,136.198276785427));
#63624=CARTESIAN_POINT('Ctrl Pts',(79.7165005588477,11.036342335368,136.194417998991));
#63625=CARTESIAN_POINT('Ctrl Pts',(79.7873201734043,11.0449567462995,136.190559212555));
#63626=CARTESIAN_POINT('Ctrl Pts',(79.8584476361334,11.0498684081628,136.186700426119));
#63627=CARTESIAN_POINT('Ctrl Pts',(79.9295302937766,11.0547769760392,136.182844070436));
#63628=CARTESIAN_POINT('Ctrl Pts',(80.0009199313711,11.0559873890258,136.178987714753));
#63629=CARTESIAN_POINT('Ctrl Pts',(80.0722020881111,11.0534810495771,136.17513135907));
#63630=CARTESIAN_POINT('Ctrl Pts',(80.1434631873882,11.0509754505262,136.171276142592));
#63631=CARTESIAN_POINT('Ctrl Pts',(80.2146163836265,11.0447552958678,136.167420926115));
#63632=CARTESIAN_POINT('Ctrl Pts',(80.285247933086,11.0348540928455,136.163565709638));
#63633=CARTESIAN_POINT('Ctrl Pts',(80.3558822440277,11.0249525027158,136.159710342433));
#63634=CARTESIAN_POINT('Ctrl Pts',(80.4259943869258,11.0113696481118,136.155854975229));
#63635=CARTESIAN_POINT('Ctrl Pts',(80.4951781764376,10.9941905967284,136.151999608024));
#63636=CARTESIAN_POINT('Ctrl Pts',(80.5644343825115,10.9769935635627,136.148140205301));
#63637=CARTESIAN_POINT('Ctrl Pts',(80.6327598229711,10.9561929366659,136.144280802578));
#63638=CARTESIAN_POINT('Ctrl Pts',(80.6997617894777,10.9319241704806,136.140421399856));
#63639=CARTESIAN_POINT('Ctrl Pts',(80.7668016930241,10.9076416631292,136.136559811909));
#63640=CARTESIAN_POINT('Ctrl Pts',(80.832516183151,10.8798872964858,136.132698223962));
#63641=CARTESIAN_POINT('Ctrl Pts',(80.8965334728954,10.8488443132071,136.128836636015));
#63642=CARTESIAN_POINT('Ctrl Pts',(80.9606627631828,10.8177470191164,136.124968292081));
#63643=CARTESIAN_POINT('Ctrl Pts',(81.0230884991667,10.7833498557715,136.121099948148));
#63644=CARTESIAN_POINT('Ctrl Pts',(81.0834650030633,10.7458811957396,136.117231604214));
#63645=CARTESIAN_POINT('Ctrl Pts',(81.1193148335926,10.7236333836668,136.114934692908));
#63646=CARTESIAN_POINT('Ctrl Pts',(81.1544427439925,10.7003034952357,136.112637781602));
#63647=CARTESIAN_POINT('Ctrl Pts',(81.188781897192,10.6759460502679,136.110340870295));
#63648=CARTESIAN_POINT('Ctrl Pts',(81.210148038287,10.6607906210448,136.108911710678));
#63649=CARTESIAN_POINT('Ctrl Pts',(81.2312397268701,10.6452156089926,136.10748255106));
#63650=CARTESIAN_POINT('Ctrl Pts',(81.252039109102,10.6292316077768,136.106053391442));
#63651=CARTESIAN_POINT('Ctrl Pts',(81.252039109102,10.6292316077768,136.806140361941));
#63652=CARTESIAN_POINT('Ctrl Pts',(81.3085695498613,10.5857888447297,136.802278511158));
#63653=CARTESIAN_POINT('Ctrl Pts',(81.3627835829033,10.5394409897777,136.798416660376));
#63654=CARTESIAN_POINT('Ctrl Pts',(81.4143830440724,10.4904758190391,136.794554809593));
#63655=CARTESIAN_POINT('Ctrl Pts',(81.466071309253,10.4414263779713,136.790686312465));
#63656=CARTESIAN_POINT('Ctrl Pts',(81.5151356865827,10.3897509821785,136.786817815337));
#63657=CARTESIAN_POINT('Ctrl Pts',(81.5613166914088,10.3357723427396,136.782949318209));
#63658=CARTESIAN_POINT('Ctrl Pts',(81.5844350256915,10.3087504917564,136.781012738221));
#63659=CARTESIAN_POINT('Ctrl Pts',(81.6068314366704,10.2811519287676,136.779076158233));
#63660=CARTESIAN_POINT('Ctrl Pts',(81.6284774886263,10.2530198049262,136.777139578245));
#63661=CARTESIAN_POINT('Ctrl Pts',(81.671724020576,10.1968147844913,136.773270495398));
#63662=CARTESIAN_POINT('Ctrl Pts',(81.7121420629603,10.1382581453866,136.769401412551));
#63663=CARTESIAN_POINT('Ctrl Pts',(81.7494664792501,10.0776662750964,136.765532329704));
#63664=CARTESIAN_POINT('Ctrl Pts',(81.7867352840212,10.0171646836711,136.761669011597));
#63665=CARTESIAN_POINT('Ctrl Pts',(81.8209193594216,9.95463429051528,136.757805693491));
#63666=CARTESIAN_POINT('Ctrl Pts',(81.8517948922017,9.89042306782545,136.753942375384));
#63667=CARTESIAN_POINT('Ctrl Pts',(81.8826342079938,9.82628716487507,136.750083588949));
#63668=CARTESIAN_POINT('Ctrl Pts',(81.9101724804935,9.76047478435637,136.746224802513));
#63669=CARTESIAN_POINT('Ctrl Pts',(81.9342310595732,9.69335977001998,136.742366016077));
#63670=CARTESIAN_POINT('Ctrl Pts',(81.9582744835123,9.62628703322128,136.738509660393));
#63671=CARTESIAN_POINT('Ctrl Pts',(81.9788423992928,9.55791374679973,136.73465330471));
#63672=CARTESIAN_POINT('Ctrl Pts',(81.9958042626972,9.48863371506656,136.730796949027));
#63673=CARTESIAN_POINT('Ctrl Pts',(82.0127611153972,9.41937414934849,136.72694173255));
#63674=CARTESIAN_POINT('Ctrl Pts',(82.0261139151062,9.34920884168869,136.723086516072));
#63675=CARTESIAN_POINT('Ctrl Pts',(82.0357824558692,9.27854506794288,136.719231299595));
#63676=CARTESIAN_POINT('Ctrl Pts',(82.0454513746432,9.20787853145486,136.71537593239));
#63677=CARTESIAN_POINT('Ctrl Pts',(82.0514356848208,9.13671397178629,136.711520565186));
#63678=CARTESIAN_POINT('Ctrl Pts',(82.0537068542763,9.06546540459287,136.707665197981));
#63679=CARTESIAN_POINT('Ctrl Pts',(82.0559804010269,8.99414225957815,136.703805795258));
#63680=CARTESIAN_POINT('Ctrl Pts',(82.0545330329303,8.92273541803588,136.699946392535));
#63681=CARTESIAN_POINT('Ctrl Pts',(82.0493883707933,8.85165962061112,136.696086989812));
#63682=CARTESIAN_POINT('Ctrl Pts',(82.0442407957081,8.78054357951155,136.692225401865));
#63683=CARTESIAN_POINT('Ctrl Pts',(82.0353918194841,8.7097594379235,136.688363813918));
#63684=CARTESIAN_POINT('Ctrl Pts',(82.022916738459,8.63971479108562,136.684502225971));
#63685=CARTESIAN_POINT('Ctrl Pts',(82.0104198318325,8.56954759862744,136.680633882038));
#63686=CARTESIAN_POINT('Ctrl Pts',(81.9942842644375,8.5001229572938,136.676765538104));
#63687=CARTESIAN_POINT('Ctrl Pts',(81.9746358599067,8.43183560189818,136.672897194171));
#63688=CARTESIAN_POINT('Ctrl Pts',(81.9629692027315,8.39128853541449,136.670600282865));
#63689=CARTESIAN_POINT('Ctrl Pts',(81.9500649911237,8.35114211458861,136.668303371559));
#63690=CARTESIAN_POINT('Ctrl Pts',(81.9359575268556,8.31147547849692,136.666006460253));
#63691=CARTESIAN_POINT('Ctrl Pts',(81.9121938979013,8.24465813953113,136.662137377406));
#63692=CARTESIAN_POINT('Ctrl Pts',(81.8849204792403,8.17894163652207,136.658268294559));
#63693=CARTESIAN_POINT('Ctrl Pts',(81.8542592736281,8.11472032178283,136.654399211712));
#63694=CARTESIAN_POINT('Ctrl Pts',(81.8236437516831,8.05059469359969,136.650535893606));
#63695=CARTESIAN_POINT('Ctrl Pts',(81.7896506697925,7.9879602664643,136.6466725755));
#63696=CARTESIAN_POINT('Ctrl Pts',(81.7524509790067,7.92719380656225,136.642809257393));
#63697=CARTESIAN_POINT('Ctrl Pts',(81.7152949234439,7.86649862569425,136.638950470957));
#63698=CARTESIAN_POINT('Ctrl Pts',(81.6749399827042,7.80766747204671,136.635091684522));
#63699=CARTESIAN_POINT('Ctrl Pts',(81.6316033389748,7.75105320099439,136.631232898086));
#63700=CARTESIAN_POINT('Ctrl Pts',(81.5882939941532,7.69447459278149,136.627376542403));
#63701=CARTESIAN_POINT('Ctrl Pts',(81.5420069673465,7.6401104814134,136.623520186719));
#63702=CARTESIAN_POINT('Ctrl Pts',(81.4930023019681,7.58828413311394,136.619663831036));
#63703=CARTESIAN_POINT('Ctrl Pts',(81.4440121130586,7.53647309483671,136.615808614559));
#63704=CARTESIAN_POINT('Ctrl Pts',(81.3923062129687,7.48719868408667,136.611953398082));
#63705=CARTESIAN_POINT('Ctrl Pts',(81.3381832654851,7.44074918294852,136.608098181605));
#63706=CARTESIAN_POINT('Ctrl Pts',(81.2840582019561,7.39429786577382,136.6042428144));
#63707=CARTESIAN_POINT('Ctrl Pts',(81.2275162734895,7.35067199218708,136.600387447195));
#63708=CARTESIAN_POINT('Ctrl Pts',(81.1688898330687,7.31012008691486,136.596532079991));
#63709=CARTESIAN_POINT('Ctrl Pts',(81.1102020267514,7.26952573485577,136.592672677268));
#63710=CARTESIAN_POINT('Ctrl Pts',(81.0494257532267,7.23201205108959,136.588813274545));
#63711=CARTESIAN_POINT('Ctrl Pts',(80.9869222612898,7.19778413815918,136.584953871822));
#63712=CARTESIAN_POINT('Ctrl Pts',(80.9243833793848,7.1635368451156,136.581092283876));
#63713=CARTESIAN_POINT('Ctrl Pts',(80.860115770103,7.13257923736585,136.577230695929));
#63714=CARTESIAN_POINT('Ctrl Pts',(80.7945027069386,7.10506912760196,136.573369107982));
#63715=CARTESIAN_POINT('Ctrl Pts',(80.7287748513684,7.07751088791499,136.569500764048));
#63716=CARTESIAN_POINT('Ctrl Pts',(80.6616972995672,7.05341235261474,136.565632420115));
#63717=CARTESIAN_POINT('Ctrl Pts',(80.5936699255708,7.0328819094999,136.561764076181));
#63718=CARTESIAN_POINT('Ctrl Pts',(80.5532772285471,7.0206915231924,136.559467164875));
#63719=CARTESIAN_POINT('Ctrl Pts',(80.5125499020234,7.00975814962006,136.557170253568));
#63720=CARTESIAN_POINT('Ctrl Pts',(80.4715730379618,7.00009589420705,136.554873342262));
#63721=CARTESIAN_POINT('Ctrl Pts',(80.4025486566506,6.98382009523546,136.551004259415));
#63722=CARTESIAN_POINT('Ctrl Pts',(80.3325454831749,6.97109005845098,136.547135176568));
#63723=CARTESIAN_POINT('Ctrl Pts',(80.2619609978507,6.96201717423697,136.543266093721));
#63724=CARTESIAN_POINT('Ctrl Pts',(80.1914816798895,6.95295780816795,136.539402775615));
#63725=CARTESIAN_POINT('Ctrl Pts',(80.1204232472092,6.947544840033,136.535539457508));
#63726=CARTESIAN_POINT('Ctrl Pts',(80.0491949540305,6.94583899876423,136.531676139402));
#63727=CARTESIAN_POINT('Ctrl Pts',(79.9780502116122,6.94413515844662,136.527817352966));
#63728=CARTESIAN_POINT('Ctrl Pts',(79.906736487753,6.94612981905869,136.52395856653));
#63729=CARTESIAN_POINT('Ctrl Pts',(79.8356680232693,6.95183190047209,136.520099780094));
#63730=CARTESIAN_POINT('Ctrl Pts',(79.7646443267069,6.95753038999231,136.516243424411));
#63731=CARTESIAN_POINT('Ctrl Pts',(79.6938660660859,6.96693162815089,136.512387068728));
#63732=CARTESIAN_POINT('Ctrl Pts',(79.6237458704835,6.97999247711257,136.508530713045));
#63733=CARTESIAN_POINT('Ctrl Pts',(79.5536463890891,6.99304946776869,136.504675496567));
#63734=CARTESIAN_POINT('Ctrl Pts',(79.4842050640865,7.00976383406735,136.50082028009));
#63735=CARTESIAN_POINT('Ctrl Pts',(79.4158260801511,7.03004101721169,136.496965063613));
#63736=CARTESIAN_POINT('Ctrl Pts',(79.3474444228019,7.05031899313324,136.493109696408));
#63737=CARTESIAN_POINT('Ctrl Pts',(79.2801256540914,7.07415992223124,136.489254329204));
#63738=CARTESIAN_POINT('Ctrl Pts',(79.2142588295807,7.10141937869151,136.485398961999));
#63739=CARTESIAN_POINT('Ctrl Pts',(79.1483230604658,7.12870736836938,136.481539559276));
#63740=CARTESIAN_POINT('Ctrl Pts',(79.0838427191725,7.15942084228506,136.477680156553));
#63741=CARTESIAN_POINT('Ctrl Pts',(79.0211860533687,7.19336754695926,136.473820753831));
#63742=CARTESIAN_POINT('Ctrl Pts',(78.9584939108685,7.22733347252431,136.469959165884));
#63743=CARTESIAN_POINT('Ctrl Pts',(78.8976279140908,7.26453601970387,136.466097577937));
#63744=CARTESIAN_POINT('Ctrl Pts',(78.8389285266988,7.30473878225623,136.46223598999));
#63745=CARTESIAN_POINT('Ctrl Pts',(78.7801264426245,7.34501188098269,136.458367646056));
#63746=CARTESIAN_POINT('Ctrl Pts',(78.7234989219706,7.38829537973079,136.454499302123));
#63747=CARTESIAN_POINT('Ctrl Pts',(78.6693539087197,7.43431211850494,136.45063095819));
#63748=CARTESIAN_POINT('Ctrl Pts',(78.637204158008,7.46163553374357,136.448334046883));
#63749=CARTESIAN_POINT('Ctrl Pts',(78.6059289688188,7.48992186126369,136.446037135576));
#63750=CARTESIAN_POINT('Ctrl Pts',(78.5755863437912,7.51910726299782,136.44374022427));
#63751=CARTESIAN_POINT('Ctrl Pts',(78.5252398783668,7.5675335879439,136.439929038996));
#63752=CARTESIAN_POINT('Ctrl Pts',(78.4772533655963,7.61863876644744,136.436117853722));
#63753=CARTESIAN_POINT('Ctrl Pts',(78.4319314969755,7.67216012549613,136.432306668448));
#63754=CARTESIAN_POINT('Ctrl Pts',(78.3866698572083,7.72561035927573,136.428500547911));
#63755=CARTESIAN_POINT('Ctrl Pts',(78.3440661660634,7.78147003319481,136.424694427373));
#63756=CARTESIAN_POINT('Ctrl Pts',(78.3043895848261,7.83943854860947,136.420888306836));
#63757=CARTESIAN_POINT('Ctrl Pts',(78.264751534915,7.8973507687559,136.417085882556));
#63758=CARTESIAN_POINT('Ctrl Pts',(78.2280352419786,7.95736735964087,136.413283458277));
#63759=CARTESIAN_POINT('Ctrl Pts',(78.1944694698458,8.0191549219264,136.409481033997));
#63760=CARTESIAN_POINT('Ctrl Pts',(78.1609242933764,8.08090457190576,136.405680942852));
#63761=CARTESIAN_POINT('Ctrl Pts',(78.1305260421692,8.14442259847235,136.401880851706));
#63762=CARTESIAN_POINT('Ctrl Pts',(78.1034589744871,8.20934855906894,136.398080760561));
#63763=CARTESIAN_POINT('Ctrl Pts',(78.0763869021232,8.27428652442972,136.394279966781));
#63764=CARTESIAN_POINT('Ctrl Pts',(78.0526474523865,8.34063248743644,136.390479173001));
#63765=CARTESIAN_POINT('Ctrl Pts',(78.0323772815507,8.40800472945968,136.386678379222));
#63766=CARTESIAN_POINT('Ctrl Pts',(78.0121062978094,8.47537967334783,136.382877433017));
#63767=CARTESIAN_POINT('Ctrl Pts',(77.9953050033774,8.5437804942492,136.379076486812));
#63768=CARTESIAN_POINT('Ctrl Pts',(77.9820598198688,8.61281142590203,136.375275540607));
#63769=CARTESIAN_POINT('Ctrl Pts',(77.9687990309018,8.68192368971067,136.371470116132));
#63770=CARTESIAN_POINT('Ctrl Pts',(77.9591028023244,8.75166705108641,136.367664691657));
#63771=CARTESIAN_POINT('Ctrl Pts',(77.9530059961544,8.82163769815253,136.363859267182));
#63772=CARTESIAN_POINT('Ctrl Pts',(77.9477806053111,8.88160745416809,136.360597751291));
#63773=CARTESIAN_POINT('Ctrl Pts',(77.9451983804903,8.9417438812321,136.357336235401));
#63774=CARTESIAN_POINT('Ctrl Pts',(77.9452507823624,9.00179307496101,136.35407471951));
#63775=CARTESIAN_POINT('Origin',(80.,9.,141.545925280538));
#63776=CARTESIAN_POINT('',(81.252039109102,10.6292316077768,137.506056941317));
#63777=CARTESIAN_POINT('',(81.252039109102,10.6292316077768,137.447938223076));
#63778=CARTESIAN_POINT('',(81.252039109102,10.6292316077768,141.545925280538));
#63779=CARTESIAN_POINT('',(77.9452500969073,8.99936893701588,136.9959252805));
#63780=CARTESIAN_POINT('Ctrl Pts',(81.252039109102,10.6292316077768,137.447938223076));
#63781=CARTESIAN_POINT('Ctrl Pts',(81.2608674552356,10.6224471613082,137.447331137836));
#63782=CARTESIAN_POINT('Ctrl Pts',(81.2696380418088,10.6155929637395,137.446724052597));
#63783=CARTESIAN_POINT('Ctrl Pts',(81.2783497233123,10.608670117646,137.446116967358));
#63784=CARTESIAN_POINT('Ctrl Pts',(81.3338711151904,10.5645493528188,137.442247884512));
#63785=CARTESIAN_POINT('Ctrl Pts',(81.387214404888,10.5174644128168,137.438378801666));
#63786=CARTESIAN_POINT('Ctrl Pts',(81.4380459985658,10.4676584304629,137.43450971882));
#63787=CARTESIAN_POINT('Ctrl Pts',(81.488801855704,10.417926656539,137.430646400714));
#63788=CARTESIAN_POINT('Ctrl Pts',(81.5370531010316,10.3654822249852,137.426783082609));
#63789=CARTESIAN_POINT('Ctrl Pts',(81.5824986302668,10.3106088843373,137.422919764503));
#63790=CARTESIAN_POINT('Ctrl Pts',(81.6278908519133,10.2557999100972,137.419060978068));
#63791=CARTESIAN_POINT('Ctrl Pts',(81.6704835863644,10.1985680583769,137.415202191633));
#63792=CARTESIAN_POINT('Ctrl Pts',(81.710013322863,10.1392330745423,137.411343405199));
#63793=CARTESIAN_POINT('Ctrl Pts',(81.7495181585261,10.0799354673968,137.407487049516));
#63794=CARTESIAN_POINT('Ctrl Pts',(81.785963555563,10.018537759882,137.403630693834));
#63795=CARTESIAN_POINT('Ctrl Pts',(81.8191278778125,9.95539066703914,137.399774338151));
#63796=CARTESIAN_POINT('Ctrl Pts',(81.8522824029889,9.89226222848004,137.395919121675));
#63797=CARTESIAN_POINT('Ctrl Pts',(81.8821575518827,9.82738586039962,137.392063905199));
#63798=CARTESIAN_POINT('Ctrl Pts',(81.9085772938752,9.76113748810835,137.388208688723));
#63799=CARTESIAN_POINT('Ctrl Pts',(81.9349980688006,9.69488652570406,137.384353321519));
#63800=CARTESIAN_POINT('Ctrl Pts',(81.9579629907077,9.62726390463224,137.380497954315));
#63801=CARTESIAN_POINT('Ctrl Pts',(81.9773445536542,9.55866454929059,137.376642587112));
#63802=CARTESIAN_POINT('Ctrl Pts',(81.996746403812,9.48999338913019,137.37278318439));
#63803=CARTESIAN_POINT('Ctrl Pts',(82.0125572752226,9.42034392225216,137.368923781668));
#63804=CARTESIAN_POINT('Ctrl Pts',(82.0247001017077,9.35012435026009,137.365064378946));
#63805=CARTESIAN_POINT('Ctrl Pts',(82.0368498035564,9.27986501939488,137.361202791));
#63806=CARTESIAN_POINT('Ctrl Pts',(82.0453272683025,9.2090354233933,137.357341203054));
#63807=CARTESIAN_POINT('Ctrl Pts',(82.0501073036935,9.13804928772871,137.353479615108));
#63808=CARTESIAN_POINT('Ctrl Pts',(82.0548957019278,9.06693895927535,137.349611271176));
#63809=CARTESIAN_POINT('Ctrl Pts',(82.0559737483448,8.99567203024745,137.345742927243));
#63810=CARTESIAN_POINT('Ctrl Pts',(82.0533683880917,8.92466192671876,137.341874583311));
#63811=CARTESIAN_POINT('Ctrl Pts',(82.0518214001433,8.88249817057678,137.339577671996));
#63812=CARTESIAN_POINT('Ctrl Pts',(82.048976770436,8.84042487883738,137.337280760681));
#63813=CARTESIAN_POINT('Ctrl Pts',(82.0448487092084,8.7985271260225,137.334983849367));
#63814=CARTESIAN_POINT('Ctrl Pts',(82.0378951055635,8.72795153360239,137.331114766519));
#63815=CARTESIAN_POINT('Ctrl Pts',(82.0272698405453,8.65759812659177,137.327245683672));
#63816=CARTESIAN_POINT('Ctrl Pts',(82.0129962433474,8.58787903866796,137.323376600825));
#63817=CARTESIAN_POINT('Ctrl Pts',(81.9987439130975,8.51826382870794,137.319513282718));
#63818=CARTESIAN_POINT('Ctrl Pts',(81.9808541372858,8.44928153386452,137.315649964611));
#63819=CARTESIAN_POINT('Ctrl Pts',(81.9594019894066,8.38133902142668,137.311786646504));
#63820=CARTESIAN_POINT('Ctrl Pts',(81.9379750048886,8.3134762055296,137.307927860067));
#63821=CARTESIAN_POINT('Ctrl Pts',(81.9129940940925,8.24665121036451,137.304069073631));
#63822=CARTESIAN_POINT('Ctrl Pts',(81.884584962628,8.18125884362858,137.300210287195));
#63823=CARTESIAN_POINT('Ctrl Pts',(81.8561937268332,8.11590766928859,137.296353931511));
#63824=CARTESIAN_POINT('Ctrl Pts',(81.8243787479479,8.05198777742893,137.292497575827));
#63825=CARTESIAN_POINT('Ctrl Pts',(81.7893144621874,7.98987559285651,137.288641220143));
#63826=CARTESIAN_POINT('Ctrl Pts',(81.754260534768,7.9277817568453,137.284786003665));
#63827=CARTESIAN_POINT('Ctrl Pts',(81.7159594447802,7.86749499075219,137.280930787188));
#63828=CARTESIAN_POINT('Ctrl Pts',(81.6746315439692,7.80936707821282,137.27707557071));
#63829=CARTESIAN_POINT('Ctrl Pts',(81.6333020273608,7.75123689304586,137.273220203505));
#63830=CARTESIAN_POINT('Ctrl Pts',(81.5889457482664,7.6952661236463,137.269364836299));
#63831=CARTESIAN_POINT('Ctrl Pts',(81.5418253390223,7.64177609119524,137.265509469094));
#63832=CARTESIAN_POINT('Ctrl Pts',(81.4946556075587,7.58823006926622,137.261650066371));
#63833=CARTESIAN_POINT('Ctrl Pts',(81.4447162920577,7.5371703330557,137.257790663648));
#63834=CARTESIAN_POINT('Ctrl Pts',(81.3923085370104,7.48888302892592,137.253931260924));
#63835=CARTESIAN_POINT('Ctrl Pts',(81.3398711082804,7.44056838414523,137.250069672977));
#63836=CARTESIAN_POINT('Ctrl Pts',(81.2849628318099,7.39502960663895,137.246208085029));
#63837=CARTESIAN_POINT('Ctrl Pts',(81.2279176282723,7.35251225780639,137.242346497082));
#63838=CARTESIAN_POINT('Ctrl Pts',(81.1707726221064,7.30992052334813,137.238478153148));
#63839=CARTESIAN_POINT('Ctrl Pts',(81.1114836288105,7.27036104111439,137.234609809214));
#63840=CARTESIAN_POINT('Ctrl Pts',(81.0504125958221,7.23403540776204,137.23074146528));
#63841=CARTESIAN_POINT('Ctrl Pts',(81.0141503739873,7.2124662920871,137.228444553978));
#63842=CARTESIAN_POINT('Ctrl Pts',(80.9772603389442,7.19203643427558,137.226147642677));
#63843=CARTESIAN_POINT('Ctrl Pts',(80.9398216719651,7.17278003858192,137.223850731375));
#63844=CARTESIAN_POINT('Ctrl Pts',(80.8767572845332,7.14034317860384,137.219981648528));
#63845=CARTESIAN_POINT('Ctrl Pts',(80.8118881255422,7.11111151178797,137.216112565681));
#63846=CARTESIAN_POINT('Ctrl Pts',(80.745573095422,7.08528897170284,137.212243482835));
#63847=CARTESIAN_POINT('Ctrl Pts',(80.6793568713896,7.05950490591462,137.208380164728));
#63848=CARTESIAN_POINT('Ctrl Pts',(80.6116995013936,7.03712005916351,137.204516846622));
#63849=CARTESIAN_POINT('Ctrl Pts',(80.5429835264874,7.01829203653433,137.200653528516));
#63850=CARTESIAN_POINT('Ctrl Pts',(80.4743481553933,6.99948609916842,137.19679474208));
#63851=CARTESIAN_POINT('Ctrl Pts',(80.4046571121522,6.98422882636421,137.192935955644));
#63852=CARTESIAN_POINT('Ctrl Pts',(80.3343102680185,6.97262874460611,137.189077169208));
#63853=CARTESIAN_POINT('Ctrl Pts',(80.2640077372383,6.96103597004892,137.185220813525));
#63854=CARTESIAN_POINT('Ctrl Pts',(80.1930507033395,6.95309589476036,137.181364457842));
#63855=CARTESIAN_POINT('Ctrl Pts',(80.1218500240238,6.94886613451355,137.177508102159));
#63856=CARTESIAN_POINT('Ctrl Pts',(80.0506703781018,6.94463762378026,137.173652885682));
#63857=CARTESIAN_POINT('Ctrl Pts',(79.9792477143178,6.94411728088903,137.169797669205));
#63858=CARTESIAN_POINT('Ctrl Pts',(79.9079970921904,6.94731078157102,137.165942452728));
#63859=CARTESIAN_POINT('Ctrl Pts',(79.8367436843767,6.95050440710934,137.162087085523));
#63860=CARTESIAN_POINT('Ctrl Pts',(79.7656628167711,6.9574121405448,137.158231718318));
#63861=CARTESIAN_POINT('Ctrl Pts',(79.6951668885367,6.96798761404966,137.154376351114));
#63862=CARTESIAN_POINT('Ctrl Pts',(79.6245971702888,6.97857415719149,137.150516948391));
#63863=CARTESIAN_POINT('Ctrl Pts',(79.5546140950361,6.9928360319378,137.146657545668));
#63864=CARTESIAN_POINT('Ctrl Pts',(79.485621398648,7.01067543699598,137.142798142946));
#63865=CARTESIAN_POINT('Ctrl Pts',(79.4165896380533,7.02852494286543,137.138936554999));
#63866=CARTESIAN_POINT('Ctrl Pts',(79.3485498361858,7.04995586543194,137.135074967052));
#63867=CARTESIAN_POINT('Ctrl Pts',(79.2818894093015,7.07482085456273,137.131213379105));
#63868=CARTESIAN_POINT('Ctrl Pts',(79.2151123576109,7.09972934588327,137.127345035172));
#63869=CARTESIAN_POINT('Ctrl Pts',(79.1497199448873,7.12808370564152,137.123476691238));
#63870=CARTESIAN_POINT('Ctrl Pts',(79.0860778523175,7.15968919188213,137.119608347305));
#63871=CARTESIAN_POINT('Ctrl Pts',(79.0482890091985,7.17845562009058,137.117311435998));
#63872=CARTESIAN_POINT('Ctrl Pts',(79.0111167807685,7.19836740599221,137.115014524691));
#63873=CARTESIAN_POINT('Ctrl Pts',(78.9746328495175,7.21937657849519,137.112717613384));
#63874=CARTESIAN_POINT('Ctrl Pts',(78.9131766878652,7.25476594190127,137.108848530537));
#63875=CARTESIAN_POINT('Ctrl Pts',(78.8534344424327,7.29340998728555,137.10497944769));
#63876=CARTESIAN_POINT('Ctrl Pts',(78.7957721050869,7.3351178000792,137.101110364844));
#63877=CARTESIAN_POINT('Ctrl Pts',(78.7381956817479,7.37676347031184,137.097247046737));
#63878=CARTESIAN_POINT('Ctrl Pts',(78.6826934055512,7.42146356444802,137.093383728631));
#63879=CARTESIAN_POINT('Ctrl Pts',(78.6296051684808,7.46898217899156,137.089520410524));
#63880=CARTESIAN_POINT('Ctrl Pts',(78.576579203892,7.51644505421851,137.085661624089));
#63881=CARTESIAN_POINT('Ctrl Pts',(78.5259620139861,7.56671956035663,137.081802837653));
#63882=CARTESIAN_POINT('Ctrl Pts',(78.4780616577513,7.61952861496759,137.077944051217));
#63883=CARTESIAN_POINT('Ctrl Pts',(78.4301914752286,7.67230440374645,137.074087695534));
#63884=CARTESIAN_POINT('Ctrl Pts',(78.3850350565734,7.72761121444358,137.070231339851));
#63885=CARTESIAN_POINT('Ctrl Pts',(78.3428636478342,7.78513512157504,137.066374984168));
#63886=CARTESIAN_POINT('Ctrl Pts',(78.3007046969514,7.8426420355683,137.062519767691));
#63887=CARTESIAN_POINT('Ctrl Pts',(78.2615292924246,7.90236435416734,137.058664551214));
#63888=CARTESIAN_POINT('Ctrl Pts',(78.2255673227379,7.96395645054636,137.054809334737));
#63889=CARTESIAN_POINT('Ctrl Pts',(78.1896039470457,8.02555095499218,137.050953967532));
#63890=CARTESIAN_POINT('Ctrl Pts',(78.1568544986653,8.08901496173253,137.047098600327));
#63891=CARTESIAN_POINT('Ctrl Pts',(78.1275036996412,8.15397685159183,137.043243233123));
#63892=CARTESIAN_POINT('Ctrl Pts',(78.098122178334,8.21900673883551,137.0393838304));
#63893=CARTESIAN_POINT('Ctrl Pts',(78.0721466082949,8.28553719542662,137.035524427677));
#63894=CARTESIAN_POINT('Ctrl Pts',(78.049713801813,8.35317598401014,137.031665024955));
#63895=CARTESIAN_POINT('Ctrl Pts',(78.0272682936998,8.42085307020704,137.027803437008));
#63896=CARTESIAN_POINT('Ctrl Pts',(78.008369671111,8.48963926900039,137.023941849061));
#63897=CARTESIAN_POINT('Ctrl Pts',(77.993104267279,8.55912917936653,137.020080261114));
#63898=CARTESIAN_POINT('Ctrl Pts',(77.9778121560757,8.62874066482163,137.016211917181));
#63899=CARTESIAN_POINT('Ctrl Pts',(77.9661660338546,8.6990578405065,137.012343573247));
#63900=CARTESIAN_POINT('Ctrl Pts',(77.9582006297367,8.76966786135613,137.008475229314));
#63901=CARTESIAN_POINT('Ctrl Pts',(77.953471001994,8.81159405977307,137.006178318007));
#63902=CARTESIAN_POINT('Ctrl Pts',(77.9500380668079,8.85362343926592,137.003881406699));
#63903=CARTESIAN_POINT('Ctrl Pts',(77.9479004012491,8.89566975842765,137.001584495392));
#63904=CARTESIAN_POINT('Ctrl Pts',(77.9461447814819,8.93020151610125,136.999698090441));
#63905=CARTESIAN_POINT('Ctrl Pts',(77.9452607206379,8.96477795933226,136.997811685489));
#63906=CARTESIAN_POINT('Ctrl Pts',(77.9452500969075,8.99936893632434,136.995925280538));
#63907=CARTESIAN_POINT('Ctrl Pts',(77.9452500969073,8.99936893701588,136.9959252805));
#63908=CARTESIAN_POINT('Ctrl Pts',(77.9452284795406,9.06975538523751,136.992086783991));
#63909=CARTESIAN_POINT('Ctrl Pts',(77.9488278088239,9.14028801803307,136.988248287481));
#63910=CARTESIAN_POINT('Ctrl Pts',(77.956066989778,9.2105597592725,136.984409790972));
#63911=CARTESIAN_POINT('Ctrl Pts',(77.9634503271985,9.28223084747754,136.980494857073));
#63912=CARTESIAN_POINT('Ctrl Pts',(77.9746201460017,9.3536300259173,136.976579923174));
#63913=CARTESIAN_POINT('Ctrl Pts',(77.9895405666956,9.42432349632931,136.972664989275));
#63914=CARTESIAN_POINT('Ctrl Pts',(78.0041321582483,9.49345896287313,136.968836336077));
#63915=CARTESIAN_POINT('Ctrl Pts',(78.0223106191684,9.56191899783839,136.965007682879));
#63916=CARTESIAN_POINT('Ctrl Pts',(78.0439901438108,9.62930358730175,136.961179029681));
#63917=CARTESIAN_POINT('Ctrl Pts',(78.0656575011448,9.69665035817348,136.957352525257));
#63918=CARTESIAN_POINT('Ctrl Pts',(78.0908218742363,9.76292241108565,136.953526020833));
#63919=CARTESIAN_POINT('Ctrl Pts',(78.1193471946889,9.82773340416793,136.949699516409));
#63920=CARTESIAN_POINT('Ctrl Pts',(78.1478664215463,9.89253055228909,136.945873829405));
#63921=CARTESIAN_POINT('Ctrl Pts',(78.1797449711962,9.95586680813673,136.942048142401));
#63922=CARTESIAN_POINT('Ctrl Pts',(78.2147987712682,10.0173761032354,136.938222455397));
#63923=CARTESIAN_POINT('Ctrl Pts',(78.2512749609402,10.0813812812762,136.934241532231));
#63924=CARTESIAN_POINT('Ctrl Pts',(78.2911893552542,10.1434075386599,136.930260609065));
#63925=CARTESIAN_POINT('Ctrl Pts',(78.3342831480841,10.2030731198657,136.926279685898));
#63926=CARTESIAN_POINT('Ctrl Pts',(78.3757481853333,10.2604836048734,136.922449224095));
#63927=CARTESIAN_POINT('Ctrl Pts',(78.4201562185496,10.3157083061125,136.918618762292));
#63928=CARTESIAN_POINT('Ctrl Pts',(78.467235362494,10.3684407654374,136.914788300489));
#63929=CARTESIAN_POINT('Ctrl Pts',(78.5143468858398,10.421209492318,136.910955204227));
#63930=CARTESIAN_POINT('Ctrl Pts',(78.5641328247557,10.4714822194488,136.907122107966));
#63931=CARTESIAN_POINT('Ctrl Pts',(78.6162853882316,10.5189902684608,136.903289011704));
#63932=CARTESIAN_POINT('Ctrl Pts',(78.6685215402371,10.566574461917,136.899449771873));
#63933=CARTESIAN_POINT('Ctrl Pts',(78.7231314966093,10.6113848335142,136.895610532042));
#63934=CARTESIAN_POINT('Ctrl Pts',(78.7797764230505,10.6531944788066,136.891771292212));
#63935=CARTESIAN_POINT('Ctrl Pts',(78.7862678537046,10.6579858066472,136.891331320608));
#63936=CARTESIAN_POINT('Ctrl Pts',(78.7927859814813,10.6627377753602,136.890891349004));
#63937=CARTESIAN_POINT('Ctrl Pts',(78.799330275612,10.6674500818429,136.8904513774));
#63938=CARTESIAN_POINT('Ctrl Pts',(78.8568803901065,10.7088898112004,136.886582294554));
#63939=CARTESIAN_POINT('Ctrl Pts',(78.9166911084278,10.747427793855,136.882713211707));
#63940=CARTESIAN_POINT('Ctrl Pts',(78.9784377823449,10.782809075016,136.87884412886));
#63941=CARTESIAN_POINT('Ctrl Pts',(79.0400924567972,10.8181376398326,136.874980810753));
#63942=CARTESIAN_POINT('Ctrl Pts',(79.1036769431804,10.8503185995815,136.871117492647));
#63943=CARTESIAN_POINT('Ctrl Pts',(79.1688363368494,10.8791393049899,136.867254174541));
#63944=CARTESIAN_POINT('Ctrl Pts',(79.2339192985749,10.9079262037222,136.863395388105));
#63945=CARTESIAN_POINT('Ctrl Pts',(79.3005730559833,10.9333604818709,136.859536601669));
#63946=CARTESIAN_POINT('Ctrl Pts',(79.3684182802395,10.9552754521459,136.855677815233));
#63947=CARTESIAN_POINT('Ctrl Pts',(79.4362207669791,10.9771766175966,136.85182145955));
#63948=CARTESIAN_POINT('Ctrl Pts',(79.5052127703407,10.9955627245148,136.847965103867));
#63949=CARTESIAN_POINT('Ctrl Pts',(79.574996538769,11.010315801172,136.844108748183));
#63950=CARTESIAN_POINT('Ctrl Pts',(79.6447596923733,11.0250645196225,136.840253531706));
#63951=CARTESIAN_POINT('Ctrl Pts',(79.7153136716781,11.0361822380541,136.836398315229));
#63952=CARTESIAN_POINT('Ctrl Pts',(79.7862488590477,11.043601725445,136.832543098752));
#63953=CARTESIAN_POINT('Ctrl Pts',(79.8571868197708,11.0510215029156,136.828687731547));
#63954=CARTESIAN_POINT('Ctrl Pts',(79.9285055347723,11.0547427139375,136.824832364343));
#63955=CARTESIAN_POINT('Ctrl Pts',(79.9997902910998,11.0547499892985,136.820976997138));
#63956=CARTESIAN_POINT('Ctrl Pts',(80.071149663129,11.0547572722748,136.817117594415));
#63957=CARTESIAN_POINT('Ctrl Pts',(80.1424745187492,11.0510428592633,136.813258191693));
#63958=CARTESIAN_POINT('Ctrl Pts',(80.2133510766842,11.0436435307014,136.80939878897));
#63959=CARTESIAN_POINT('Ctrl Pts',(80.284267765483,11.0362400125815,136.805537201023));
#63960=CARTESIAN_POINT('Ctrl Pts',(80.3547351711987,11.0251475010506,136.801675613076));
#63961=CARTESIAN_POINT('Ctrl Pts',(80.4243482954951,11.010454199083,136.797814025129));
#63962=CARTESIAN_POINT('Ctrl Pts',(80.4940832104478,10.9957351906568,136.793945681196));
#63963=CARTESIAN_POINT('Ctrl Pts',(80.5629603903896,10.977402939226,136.790077337262));
#63964=CARTESIAN_POINT('Ctrl Pts',(80.6305892955942,10.9555957411444,136.786208993329));
#63965=CARTESIAN_POINT('Ctrl Pts',(80.6707453933164,10.9426472544793,136.783912082022));
#63966=CARTESIAN_POINT('Ctrl Pts',(80.7104617445909,10.9284745615488,136.781615170716));
#63967=CARTESIAN_POINT('Ctrl Pts',(80.7496603396344,10.9131144601615,136.779318259409));
#63968=CARTESIAN_POINT('Ctrl Pts',(80.8156837929553,10.8872429477816,136.775449497882));
#63969=CARTESIAN_POINT('Ctrl Pts',(80.8804957013763,10.8578989545749,136.771580736354));
#63970=CARTESIAN_POINT('Ctrl Pts',(80.9437058827513,10.825216910222,136.767711974827));
#63971=CARTESIAN_POINT('Ctrl Pts',(81.0068160594629,10.7925865720466,136.763849334057));
#63972=CARTESIAN_POINT('Ctrl Pts',(81.0683291135876,10.7566288912025,136.759986693287));
#63973=CARTESIAN_POINT('Ctrl Pts',(81.1278740897059,10.7175265937592,136.756124052518));
#63974=CARTESIAN_POINT('Ctrl Pts',(81.1703036664166,10.6896637237559,136.753371675684));
#63975=CARTESIAN_POINT('Ctrl Pts',(81.2117343082329,10.6602052193443,136.75061929885));
#63976=CARTESIAN_POINT('Ctrl Pts',(81.252039109102,10.6292316077768,136.747866922016));
#63977=CARTESIAN_POINT('',(77.9452500020166,9.0000910330137,137.054074719424));
#63978=CARTESIAN_POINT('Ctrl Pts',(77.9452500020166,9.00009103301371,137.054074719424));
#63979=CARTESIAN_POINT('Ctrl Pts',(77.9452533307477,9.07522542642048,137.050023196181));
#63980=CARTESIAN_POINT('Ctrl Pts',(77.9493820167298,9.15027470161127,137.045971672937));
#63981=CARTESIAN_POINT('Ctrl Pts',(77.9575824977975,9.22478502885367,137.041920149694));
#63982=CARTESIAN_POINT('Ctrl Pts',(77.9658071971074,9.29951540527881,137.037856661204));
#63983=CARTESIAN_POINT('Ctrl Pts',(77.9781276780619,9.37370324566178,137.033793172715));
#63984=CARTESIAN_POINT('Ctrl Pts',(77.9944388833352,9.44690286396755,137.029729684225));
#63985=CARTESIAN_POINT('Ctrl Pts',(78.0107756928435,9.52021738611964,137.025659817145));
#63986=CARTESIAN_POINT('Ctrl Pts',(78.0311156065381,9.59254020057874,137.021589950064));
#63987=CARTESIAN_POINT('Ctrl Pts',(78.0553039258147,9.66344158864827,137.017520082983));
#63988=CARTESIAN_POINT('Ctrl Pts',(78.0795588774128,9.73453829099468,137.013439004512));
#63989=CARTESIAN_POINT('Ctrl Pts',(78.1076832711743,9.80420536132707,137.00935792604));
#63990=CARTESIAN_POINT('Ctrl Pts',(78.1394743984716,9.87203328408803,137.005276847569));
#63991=CARTESIAN_POINT('Ctrl Pts',(78.1547192877517,9.90455899992451,137.003319836455));
#63992=CARTESIAN_POINT('Ctrl Pts',(78.1708066784997,9.93666218503223,137.001362825341));
#63993=CARTESIAN_POINT('Ctrl Pts',(78.1877106415429,9.96829997610412,136.999405814228));
#63994=CARTESIAN_POINT('Ctrl Pts',(78.22113039731,10.0308490510122,136.995536731381));
#63995=CARTESIAN_POINT('Ctrl Pts',(78.2578576247283,10.0917884381047,136.991667648534));
#63996=CARTESIAN_POINT('Ctrl Pts',(78.2977131288889,10.1507462669689,136.987798565687));
#63997=CARTESIAN_POINT('Ctrl Pts',(78.337509250336,10.2096162516085,136.983935247581));
#63998=CARTESIAN_POINT('Ctrl Pts',(78.3804241267736,10.2665101393224,136.980071929474));
#63999=CARTESIAN_POINT('Ctrl Pts',(78.4262327681656,10.321080717634,136.976208611368));
#64000=CARTESIAN_POINT('Ctrl Pts',(78.4719876760388,10.3755872846782,136.972349824932));
#64001=CARTESIAN_POINT('Ctrl Pts',(78.5206292956546,10.4277755853078,136.968491038496));
#64002=CARTESIAN_POINT('Ctrl Pts',(78.571890467838,10.4773289162025,136.964632252061));
#64003=CARTESIAN_POINT('Ctrl Pts',(78.6231193492416,10.5268510321322,136.960775896378));
#64004=CARTESIAN_POINT('Ctrl Pts',(78.6769641609447,10.5737411345841,136.956919540694));
#64005=CARTESIAN_POINT('Ctrl Pts',(78.7331197501872,10.6177181445278,136.953063185011));
#64006=CARTESIAN_POINT('Ctrl Pts',(78.7892587505064,10.6616821632223,136.949207968534));
#64007=CARTESIAN_POINT('Ctrl Pts',(78.8477067909092,10.7027344985004,136.945352752057));
#64008=CARTESIAN_POINT('Ctrl Pts',(78.9081257198302,10.7406344012468,136.94149753558));
#64009=CARTESIAN_POINT('Ctrl Pts',(78.9685470109507,10.778535785766,136.937642168375));
#64010=CARTESIAN_POINT('Ctrl Pts',(79.0309389308829,10.8132842367812,136.933786801171));
#64011=CARTESIAN_POINT('Ctrl Pts',(79.094935914404,10.8446833233551,136.929931433966));
#64012=CARTESIAN_POINT('Ctrl Pts',(79.1589998853157,10.8761152762105,136.926072031243));
#64013=CARTESIAN_POINT('Ctrl Pts',(79.2246718365875,10.9041906517067,136.922212628521));
#64014=CARTESIAN_POINT('Ctrl Pts',(79.291564073675,10.928760249692,136.918353225798));
#64015=CARTESIAN_POINT('Ctrl Pts',(79.3584941856725,10.9533437591767,136.914491637851));
#64016=CARTESIAN_POINT('Ctrl Pts',(79.4266454946035,10.9744173960534,136.910630049904));
#64017=CARTESIAN_POINT('Ctrl Pts',(79.4956155457552,10.9918819957056,136.906768461957));
#64018=CARTESIAN_POINT('Ctrl Pts',(79.5647062624835,11.0093771503009,136.902900118024));
#64019=CARTESIAN_POINT('Ctrl Pts',(79.6346181046547,11.023250566727,136.899031774091));
#64020=CARTESIAN_POINT('Ctrl Pts',(79.7049395383999,11.0334544220366,136.895163430157));
#64021=CARTESIAN_POINT('Ctrl Pts',(79.7466943820955,11.0395131776799,136.89286651885));
#64022=CARTESIAN_POINT('Ctrl Pts',(79.7885935358452,11.0442791717332,136.890569607543));
#64023=CARTESIAN_POINT('Ctrl Pts',(79.8305507565544,11.0477510875093,136.888272696236));
#64024=CARTESIAN_POINT('Ctrl Pts',(79.9012083638594,11.053597930016,136.884404607397));
#64025=CARTESIAN_POINT('Ctrl Pts',(79.9723072994884,11.05579487151,136.880536518558));
#64026=CARTESIAN_POINT('Ctrl Pts',(80.0434382677727,11.0542907971835,136.876668429718));
#64027=CARTESIAN_POINT('Ctrl Pts',(80.1144716684088,11.0527887859386,136.87280564659));
#64028=CARTESIAN_POINT('Ctrl Pts',(80.1855365333495,11.0475958395282,136.868942863461));
#64029=CARTESIAN_POINT('Ctrl Pts',(80.2562193003067,11.0387126410189,136.865080080333));
#64030=CARTESIAN_POINT('Ctrl Pts',(80.3268287676256,11.0298386545887,136.861221302998));
#64031=CARTESIAN_POINT('Ctrl Pts',(80.3970564438634,11.0172820708638,136.857362525663));
#64032=CARTESIAN_POINT('Ctrl Pts',(80.4664913551483,11.0010955444636,136.853503748329));
#64033=CARTESIAN_POINT('Ctrl Pts',(80.5375128266071,10.9845391623572,136.849556799463));
#64034=CARTESIAN_POINT('Ctrl Pts',(80.6077043345164,10.964184925508,136.845609850597));
#64035=CARTESIAN_POINT('Ctrl Pts',(80.6766354064323,10.940144862958,136.841662901732));
#64036=CARTESIAN_POINT('Ctrl Pts',(80.7439678383179,10.916662334264,136.837807489967));
#64037=CARTESIAN_POINT('Ctrl Pts',(80.8100972020252,10.8896633060689,136.833952078201));
#64038=CARTESIAN_POINT('Ctrl Pts',(80.8746382140914,10.8593024382685,136.830096666436));
#64039=CARTESIAN_POINT('Ctrl Pts',(80.9414777732899,10.8278603062706,136.82610394902));
#64040=CARTESIAN_POINT('Ctrl Pts',(81.0066131911813,10.792812551216,136.822111231604));
#64041=CARTESIAN_POINT('Ctrl Pts',(81.0696421214655,10.7543840213838,136.818118514188));
#64042=CARTESIAN_POINT('Ctrl Pts',(81.1326710517497,10.7159554915516,136.814125796773));
#64043=CARTESIAN_POINT('Ctrl Pts',(81.1935930198934,10.6741465168137,136.810133079357));
#64044=CARTESIAN_POINT('Ctrl Pts',(81.252039109102,10.6292316077768,136.806140361941));
#64045=CARTESIAN_POINT('Ctrl Pts',(81.252039109102,10.6292316077768,137.506056941317));
#64046=CARTESIAN_POINT('Ctrl Pts',(81.3085836328015,10.5857780222097,137.502201804569));
#64047=CARTESIAN_POINT('Ctrl Pts',(81.3628760664577,10.5393675421866,137.498346667822));
#64048=CARTESIAN_POINT('Ctrl Pts',(81.4146004937637,10.4902694405856,137.494491531074));
#64049=CARTESIAN_POINT('Ctrl Pts',(81.4663309400818,10.44116562559,137.490635945716));
#64050=CARTESIAN_POINT('Ctrl Pts',(81.5154924362568,10.3893739044095,137.486780360358));
#64051=CARTESIAN_POINT('Ctrl Pts',(81.5618054162374,10.335200885377,137.482924775));
#64052=CARTESIAN_POINT('Ctrl Pts',(81.6081690728818,10.280968589056,137.479064970777));
#64053=CARTESIAN_POINT('Ctrl Pts',(81.6516776780836,10.2243501657366,137.475205166554));
#64054=CARTESIAN_POINT('Ctrl Pts',(81.6920921377846,10.1656851031679,137.471345362332));
#64055=CARTESIAN_POINT('Ctrl Pts',(81.7325322808141,10.1069827590399,137.467483105209));
#64056=CARTESIAN_POINT('Ctrl Pts',(81.7698741114574,10.0462316012982,137.463620848086));
#64057=CARTESIAN_POINT('Ctrl Pts',(81.8039234886228,9.9837975450746,137.459758590964));
#64058=CARTESIAN_POINT('Ctrl Pts',(81.8380300704416,9.92125859652008,137.455889845057));
#64059=CARTESIAN_POINT('Ctrl Pts',(81.868832952186,9.85703154543904,137.452021099149));
#64060=CARTESIAN_POINT('Ctrl Pts',(81.8961856371569,9.79150337456002,137.448152353242));
#64061=CARTESIAN_POINT('Ctrl Pts',(81.9061170250162,9.7677109870339,137.446747664226));
#64062=CARTESIAN_POINT('Ctrl Pts',(81.9155940428794,9.74374721974154,137.44534297521));
#64063=CARTESIAN_POINT('Ctrl Pts',(81.9246113195382,9.71963103824482,137.443938286194));
#64064=CARTESIAN_POINT('Ctrl Pts',(81.9494485540355,9.65320530044445,137.440069203343));
#64065=CARTESIAN_POINT('Ctrl Pts',(81.9708914866249,9.58536210780795,137.436200120492));
#64066=CARTESIAN_POINT('Ctrl Pts',(81.9887795660641,9.51648175195817,137.432331037641));
#64067=CARTESIAN_POINT('Ctrl Pts',(82.0066409931574,9.44770402440215,137.42846771953));
#64068=CARTESIAN_POINT('Ctrl Pts',(82.0209579595017,9.37789266740923,137.424604401419));
#64069=CARTESIAN_POINT('Ctrl Pts',(82.0316186896446,9.30744603166563,137.420741083309));
#64070=CARTESIAN_POINT('Ctrl Pts',(82.0422669147553,9.23708202979736,137.416882296868));
#64071=CARTESIAN_POINT('Ctrl Pts',(82.0492673502678,9.16608470734499,137.413023510428));
#64072=CARTESIAN_POINT('Ctrl Pts',(82.0525589895963,9.09486388526352,137.409164723988));
#64073=CARTESIAN_POINT('Ctrl Pts',(82.0558485554335,9.02368792707688,137.405308368301));
#64074=CARTESIAN_POINT('Ctrl Pts',(82.0554339378344,8.95228923270109,137.401452012613));
#64075=CARTESIAN_POINT('Ctrl Pts',(82.051305976554,8.88108257884583,137.397595656925));
#64076=CARTESIAN_POINT('Ctrl Pts',(82.0471792347146,8.80989696014851,137.393740440444));
#64077=CARTESIAN_POINT('Ctrl Pts',(82.0393413550609,8.73890375405027,137.389885223962));
#64078=CARTESIAN_POINT('Ctrl Pts',(82.0278352523221,8.66851583455668,137.38603000748));
#64079=CARTESIAN_POINT('Ctrl Pts',(82.016328699729,8.59812516310539,137.382174640271));
#64080=CARTESIAN_POINT('Ctrl Pts',(82.0011537198593,8.52834030430681,137.378319273062));
#64081=CARTESIAN_POINT('Ctrl Pts',(81.9824046025217,8.45956540229117,137.374463905853));
#64082=CARTESIAN_POINT('Ctrl Pts',(81.9636358599709,8.39071851170714,137.370604503126));
#64083=CARTESIAN_POINT('Ctrl Pts',(81.9412856398149,8.32288415785246,137.366745100399));
#64084=CARTESIAN_POINT('Ctrl Pts',(81.9154982988436,8.25645186461982,137.362885697672));
#64085=CARTESIAN_POINT('Ctrl Pts',(81.8896963568773,8.18998195690079,137.35902410972));
#64086=CARTESIAN_POINT('Ctrl Pts',(81.860453619195,8.12491613342951,137.355162521769));
#64087=CARTESIAN_POINT('Ctrl Pts',(81.8279617422855,8.0616219145565,137.351300933817));
#64088=CARTESIAN_POINT('Ctrl Pts',(81.795413019673,7.9982169601795,137.34743258988));
#64089=CARTESIAN_POINT('Ctrl Pts',(81.7596040527343,7.93659021876824,137.343564245942));
#64090=CARTESIAN_POINT('Ctrl Pts',(81.7207710219754,7.87708208116986,137.339695902004));
#64091=CARTESIAN_POINT('Ctrl Pts',(81.6977130862504,7.84174786220621,137.337398990737));
#64092=CARTESIAN_POINT('Ctrl Pts',(81.6735897842482,7.80716000273841,137.33510207947));
#64093=CARTESIAN_POINT('Ctrl Pts',(81.648457142774,7.77338408173651,137.332805168203));
#64094=CARTESIAN_POINT('Ctrl Pts',(81.6061219104926,7.71648948661011,137.328936085356));
#64095=CARTESIAN_POINT('Ctrl Pts',(81.5607548249675,7.66167775717641,137.32506700251));
#64096=CARTESIAN_POINT('Ctrl Pts',(81.5125883019347,7.60929004053679,137.321197919663));
#64097=CARTESIAN_POINT('Ctrl Pts',(81.464493544619,7.55698037898212,137.317334601557));
#64098=CARTESIAN_POINT('Ctrl Pts',(81.4136079552719,7.50708791587218,137.313471283451));
#64099=CARTESIAN_POINT('Ctrl Pts',(81.3602055766749,7.45992261503438,137.309607965345));
#64100=CARTESIAN_POINT('Ctrl Pts',(81.3068658390473,7.4128126390762,137.305749178909));
#64101=CARTESIAN_POINT('Ctrl Pts',(81.2510155385615,7.36842379119041,137.301890392473));
#64102=CARTESIAN_POINT('Ctrl Pts',(81.1929658905854,7.32702960384834,137.298031606038));
#64103=CARTESIAN_POINT('Ctrl Pts',(81.1349528096308,7.28566149180894,137.294175250355));
#64104=CARTESIAN_POINT('Ctrl Pts',(81.0747435244405,7.24728457906612,137.290318894672));
#64105=CARTESIAN_POINT('Ctrl Pts',(81.0126815343106,7.21213152816929,137.286462538989));
#64106=CARTESIAN_POINT('Ctrl Pts',(80.950637877914,7.17698886183566,137.282607322512));
#64107=CARTESIAN_POINT('Ctrl Pts',(80.8867430255922,7.14506840593426,137.278752106035));
#64108=CARTESIAN_POINT('Ctrl Pts',(80.8213671225576,7.11655804111691,137.274896889558));
#64109=CARTESIAN_POINT('Ctrl Pts',(80.7559886635206,7.08804656162947,137.271041522354));
#64110=CARTESIAN_POINT('Ctrl Pts',(80.689129484972,7.06294563009214,137.267186155149));
#64111=CARTESIAN_POINT('Ctrl Pts',(80.6211802626994,7.04139523034056,137.263330787945));
#64112=CARTESIAN_POINT('Ctrl Pts',(80.5531599161197,7.01982227319688,137.259471385222));
#64113=CARTESIAN_POINT('Ctrl Pts',(80.4840477121684,7.00180741384327,137.2556119825));
#64114=CARTESIAN_POINT('Ctrl Pts',(80.4142491990333,6.98744064345911,137.251752579777));
#64115=CARTESIAN_POINT('Ctrl Pts',(80.3444111654316,6.97306573849666,137.247890991831));
#64116=CARTESIAN_POINT('Ctrl Pts',(80.2738865295672,6.96234310748402,137.244029403884));
#64117=CARTESIAN_POINT('Ctrl Pts',(80.2030880081502,6.95531106927103,137.240167815937));
#64118=CARTESIAN_POINT('Ctrl Pts',(80.1321656221821,6.94826672825512,137.236299472004));
#64119=CARTESIAN_POINT('Ctrl Pts',(80.0609688793824,6.94492589404826,137.232431128071));
#64120=CARTESIAN_POINT('Ctrl Pts',(79.9899118530188,6.94527476489179,137.228562784137));
#64121=CARTESIAN_POINT('Ctrl Pts',(79.9477202355614,6.94548191435928,137.226265872829));
#64122=CARTESIAN_POINT('Ctrl Pts',(79.9055778257029,6.9469889240259,137.22396896152));
#64123=CARTESIAN_POINT('Ctrl Pts',(79.8635701063463,6.94978429266147,137.221672050211));
#64124=CARTESIAN_POINT('Ctrl Pts',(79.7928092782107,6.95449301293067,137.217802967365));
#64125=CARTESIAN_POINT('Ctrl Pts',(79.722153916906,6.96287859875673,137.213933884519));
#64126=CARTESIAN_POINT('Ctrl Pts',(79.6520166891177,6.97493082146625,137.210064801673));
#64127=CARTESIAN_POINT('Ctrl Pts',(79.5819839623012,6.98696508696495,137.206201483567));
#64128=CARTESIAN_POINT('Ctrl Pts',(79.5124683114819,7.00265506363271,137.202338165462));
#64129=CARTESIAN_POINT('Ctrl Pts',(79.4438787829355,7.02193863734446,137.198474847356));
#64130=CARTESIAN_POINT('Ctrl Pts',(79.3753697098801,7.04119959143154,137.194616060921));
#64131=CARTESIAN_POINT('Ctrl Pts',(79.3077850666392,7.06404563873356,137.190757274486));
#64132=CARTESIAN_POINT('Ctrl Pts',(79.2415234539804,7.09036367555543,137.186898488051));
#64133=CARTESIAN_POINT('Ctrl Pts',(79.1753035812791,7.11666513394383,137.183042132369));
#64134=CARTESIAN_POINT('Ctrl Pts',(79.1104055360912,7.14643406378743,137.179185776687));
#64135=CARTESIAN_POINT('Ctrl Pts',(79.0472110931786,7.1795080715537,137.175329421004));
#64136=CARTESIAN_POINT('Ctrl Pts',(78.9840353185376,7.21257230892673,137.171474204528));
#64137=CARTESIAN_POINT('Ctrl Pts',(78.9225625772242,7.24893946075519,137.167618988052));
#64138=CARTESIAN_POINT('Ctrl Pts',(78.8631514734676,7.28840045857067,137.163763771576));
#64139=CARTESIAN_POINT('Ctrl Pts',(78.8037380469146,7.32786299919311,137.159908404372));
#64140=CARTESIAN_POINT('Ctrl Pts',(78.7463868213836,7.37041935534479,137.156053037168));
#64141=CARTESIAN_POINT('Ctrl Pts',(78.6914272967841,7.41581723185161,137.152197669964));
#64142=CARTESIAN_POINT('Ctrl Pts',(78.6364102445493,7.46126262755558,137.148338267243));
#64143=CARTESIAN_POINT('Ctrl Pts',(78.5837902660095,7.50955517097194,137.144478864521));
#64144=CARTESIAN_POINT('Ctrl Pts',(78.5338629270875,7.5604029570982,137.140619461799));
#64145=CARTESIAN_POINT('Ctrl Pts',(78.483907318914,7.61127953364038,137.136757873853));
#64146=CARTESIAN_POINT('Ctrl Pts',(78.4366477073383,7.66471386896874,137.132896285907));
#64147=CARTESIAN_POINT('Ctrl Pts',(78.3923401347151,7.72038000951368,137.129034697961));
#64148=CARTESIAN_POINT('Ctrl Pts',(78.3479550444055,7.77614353996672,137.125166354028));
#64149=CARTESIAN_POINT('Ctrl Pts',(78.3065325869224,7.83414627587793,137.121298010096));
#64150=CARTESIAN_POINT('Ctrl Pts',(78.2682857521432,7.89403285479645,137.117429666163));
#64151=CARTESIAN_POINT('Ctrl Pts',(78.245575882213,7.9295917821078,137.115132754849));
#64152=CARTESIAN_POINT('Ctrl Pts',(78.2239847570714,7.96581438708238,137.112835843534));
#64153=CARTESIAN_POINT('Ctrl Pts',(78.2035490783992,8.00262261466407,137.11053893222));
#64154=CARTESIAN_POINT('Ctrl Pts',(78.1674867936404,8.0675770899133,137.106485635472));
#64155=CARTESIAN_POINT('Ctrl Pts',(78.1348950465756,8.1345905325921,137.102432338725));
#64156=CARTESIAN_POINT('Ctrl Pts',(78.1060020779534,8.20327581072033,137.098379041977));
#64157=CARTESIAN_POINT('Ctrl Pts',(78.0771900219366,8.27176874084605,137.094337096186));
#64158=CARTESIAN_POINT('Ctrl Pts',(78.0520562805303,8.34192379971445,137.090295150394));
#64159=CARTESIAN_POINT('Ctrl Pts',(78.0307828211536,8.41333036124561,137.086253204602));
#64160=CARTESIAN_POINT('Ctrl Pts',(78.0095451555341,8.48461677733726,137.082218059604));
#64161=CARTESIAN_POINT('Ctrl Pts',(77.9921549775742,8.55715011048446,137.078182914607));
#64162=CARTESIAN_POINT('Ctrl Pts',(77.9787459929169,8.63050060710388,137.074147769609));
#64163=CARTESIAN_POINT('Ctrl Pts',(77.9653646220904,8.70370004916919,137.070120934399));
#64164=CARTESIAN_POINT('Ctrl Pts',(77.9559481961506,8.7777128936758,137.066094099189));
#64165=CARTESIAN_POINT('Ctrl Pts',(77.950580037019,8.85209672811253,137.062067263979));
#64166=CARTESIAN_POINT('Ctrl Pts',(77.9470284265033,8.90130957782711,137.059403082473));
#64167=CARTESIAN_POINT('Ctrl Pts',(77.945247813142,8.95068451301232,137.056738900968));
#64168=CARTESIAN_POINT('Ctrl Pts',(77.9452500020165,9.00009103231601,137.054074719462));
#64169=CARTESIAN_POINT('Origin',(80.,9.,141.545925280538));
#64170=CARTESIAN_POINT('',(81.252039109102,10.6292316077768,138.206016809239));
#64171=CARTESIAN_POINT('',(81.252039109102,10.6292316077768,138.147982307292));
#64172=CARTESIAN_POINT('',(81.252039109102,10.6292316077768,141.545925280538));
#64173=CARTESIAN_POINT('',(77.9452508576385,9.00187735576022,137.695925280507));
#64174=CARTESIAN_POINT('Ctrl Pts',(81.252039109102,10.6292316077768,138.147982307292));
#64175=CARTESIAN_POINT('Ctrl Pts',(81.3085983146724,10.5857667394206,138.144121802391));
#64176=CARTESIAN_POINT('Ctrl Pts',(81.3628508290673,10.5393845312925,138.14026129749));
#64177=CARTESIAN_POINT('Ctrl Pts',(81.414494838156,10.4903697243738,138.136400792589));
#64178=CARTESIAN_POINT('Ctrl Pts',(81.4668569704548,10.4406733539764,138.132486606375));
#64179=CARTESIAN_POINT('Ctrl Pts',(81.516537134486,10.3882709770766,138.128572420162));
#64180=CARTESIAN_POINT('Ctrl Pts',(81.563262117768,10.3334950744759,138.124658233948));
#64181=CARTESIAN_POINT('Ctrl Pts',(81.60998710105,10.2787191718752,138.120744047735));
#64182=CARTESIAN_POINT('Ctrl Pts',(81.6537566438285,10.2215701911493,138.116829861521));
#64183=CARTESIAN_POINT('Ctrl Pts',(81.6943435741606,10.1624101751107,138.112915675308));
#64184=CARTESIAN_POINT('Ctrl Pts',(81.7344628184565,10.1039318640733,138.109046592536));
#64185=CARTESIAN_POINT('Ctrl Pts',(81.7716296199641,10.0432595740049,138.105177509764));
#64186=CARTESIAN_POINT('Ctrl Pts',(81.8055964784114,9.98072367140205,138.101308426992));
#64187=CARTESIAN_POINT('Ctrl Pts',(81.8395127279206,9.91828094419922,138.097445108962));
#64188=CARTESIAN_POINT('Ctrl Pts',(81.8702382682615,9.85398053951649,138.093581790931));
#64189=CARTESIAN_POINT('Ctrl Pts',(81.8975685823103,9.78818210962237,138.089718472901));
#64190=CARTESIAN_POINT('Ctrl Pts',(81.9248668378987,9.7224608612915,138.085859686543));
#64191=CARTESIAN_POINT('Ctrl Pts',(81.9487775925512,9.65524552455614,138.082000900185));
#64192=CARTESIAN_POINT('Ctrl Pts',(81.9691428350777,9.5869191235275,138.078142113828));
#64193=CARTESIAN_POINT('Ctrl Pts',(81.9894952489891,9.51863576313988,138.074285758223));
#64194=CARTESIAN_POINT('Ctrl Pts',(82.0063064434009,9.44924319147191,138.070429402619));
#64195=CARTESIAN_POINT('Ctrl Pts',(82.0194675293387,9.37914174189442,138.066573047015));
#64196=CARTESIAN_POINT('Ctrl Pts',(82.0326247273568,9.30906100100354,138.062717830617));
#64197=CARTESIAN_POINT('Ctrl Pts',(82.0421338679971,9.23827227512134,138.05886261422));
#64198=CARTESIAN_POINT('Ctrl Pts',(82.0479370599032,9.16718660584799,138.055007397822));
#64199=CARTESIAN_POINT('Ctrl Pts',(82.0537404786956,9.09609815735139,138.051152030698));
#64200=CARTESIAN_POINT('Ctrl Pts',(82.0558376237616,9.02471322676606,138.047296663574));
#64201=CARTESIAN_POINT('Ctrl Pts',(82.0542225680827,8.95344676939605,138.04344129645));
#64202=CARTESIAN_POINT('Ctrl Pts',(82.0526058218812,8.88210571548853,138.039581893809));
#64203=CARTESIAN_POINT('Ctrl Pts',(82.0472691293125,8.81088386899975,138.035722491167));
#64204=CARTESIAN_POINT('Ctrl Pts',(82.0382586782974,8.74019406695541,138.031863088525));
#64205=CARTESIAN_POINT('Ctrl Pts',(82.0292431254952,8.66946423979759,138.02800150066));
#64206=CARTESIAN_POINT('Ctrl Pts',(82.0165497598692,8.59926753503242,138.024139912795));
#64207=CARTESIAN_POINT('Ctrl Pts',(82.0002759786724,8.53000683872418,138.02027832493));
#64208=CARTESIAN_POINT('Ctrl Pts',(81.9839737259109,8.46062496834006,138.016409981078));
#64209=CARTESIAN_POINT('Ctrl Pts',(81.9640786868343,8.39218284251079,138.012541637226));
#64210=CARTESIAN_POINT('Ctrl Pts',(81.9407380100454,8.32506775238905,138.008673293374));
#64211=CARTESIAN_POINT('Ctrl Pts',(81.9268789832615,8.28521673007253,138.006376381355));
#64212=CARTESIAN_POINT('Ctrl Pts',(81.91180607447,8.24583320161199,138.004079469335));
#64213=CARTESIAN_POINT('Ctrl Pts',(81.8955578473675,8.20699431919846,138.001782557316));
#64214=CARTESIAN_POINT('Ctrl Pts',(81.8681881715652,8.14157132790987,137.997913474436));
#64215=CARTESIAN_POINT('Ctrl Pts',(81.8373739143585,8.07743881058132,137.994044391556));
#64216=CARTESIAN_POINT('Ctrl Pts',(81.8032583883217,8.01498388467632,137.990175308676));
#64217=CARTESIAN_POINT('Ctrl Pts',(81.7691936927131,7.95262201348841,137.986311990536));
#64218=CARTESIAN_POINT('Ctrl Pts',(81.7318377227886,7.89193319508389,137.982448672396));
#64219=CARTESIAN_POINT('Ctrl Pts',(81.6913817082807,7.83328431938484,137.978585354256));
#64220=CARTESIAN_POINT('Ctrl Pts',(81.650973148657,7.77470423878668,137.974726567787));
#64221=CARTESIAN_POINT('Ctrl Pts',(81.6074720419694,7.71815974581528,137.970867781317));
#64222=CARTESIAN_POINT('Ctrl Pts',(81.5611144773103,7.66399133564481,137.967008994847));
#64223=CARTESIAN_POINT('Ctrl Pts',(81.5147861145142,7.60985704759662,137.96315263913));
#64224=CARTESIAN_POINT('Ctrl Pts',(81.4656051787584,7.55809624101094,137.959296283412));
#64225=CARTESIAN_POINT('Ctrl Pts',(81.4138489441385,7.50901753006334,137.955439927695));
#64226=CARTESIAN_POINT('Ctrl Pts',(81.3621079988254,7.4599533174554,137.951584711183));
#64227=CARTESIAN_POINT('Ctrl Pts',(81.3077936172911,7.41356996159437,137.947729494671));
#64228=CARTESIAN_POINT('Ctrl Pts',(81.2512197300716,7.37013903980138,137.94387427816));
#64229=CARTESIAN_POINT('Ctrl Pts',(81.1946436309801,7.32670641998749,137.940018910921));
#64230=CARTESIAN_POINT('Ctrl Pts',(81.1358082374883,7.28622675748109,137.936163543681));
#64231=CARTESIAN_POINT('Ctrl Pts',(81.0750589525976,7.24893009535893,137.932308176442));
#64232=CARTESIAN_POINT('Ctrl Pts',(81.0142460797713,7.21159439380193,137.928448773685));
#64233=CARTESIAN_POINT('Ctrl Pts',(80.9515157313008,7.17744859820139,137.924589370927));
#64234=CARTESIAN_POINT('Ctrl Pts',(80.8872397966678,7.1466778192368,137.92072996817));
#64235=CARTESIAN_POINT('Ctrl Pts',(80.8229274684949,7.11588961761509,137.916868380188));
#64236=CARTESIAN_POINT('Ctrl Pts',(80.7570682607646,7.08848042350474,137.913006792207));
#64237=CARTESIAN_POINT('Ctrl Pts',(80.6900534777598,7.06458692772534,137.909145204225));
#64238=CARTESIAN_POINT('Ctrl Pts',(80.6229214499959,7.04065162942075,137.905276860257));
#64239=CARTESIAN_POINT('Ctrl Pts',(80.5546302761291,7.0202444489042,137.901408516289));
#64240=CARTESIAN_POINT('Ctrl Pts',(80.4855851427937,7.00345182086732,137.897540172321));
#64241=CARTESIAN_POINT('Ctrl Pts',(80.4445881354207,6.99348084301294,137.895243261322));
#64242=CARTESIAN_POINT('Ctrl Pts',(80.4033254996481,6.98478324591936,137.892946350324));
#64243=CARTESIAN_POINT('Ctrl Pts',(80.3618829696559,6.9773684767677,137.890649439325));
#64244=CARTESIAN_POINT('Ctrl Pts',(80.2920741777508,6.96487850386233,137.886780356478));
#64245=CARTESIAN_POINT('Ctrl Pts',(80.2214812825329,6.95598236534361,137.88291127363));
#64246=CARTESIAN_POINT('Ctrl Pts',(80.1505072441009,6.95076962447529,137.879042190783));
#64247=CARTESIAN_POINT('Ctrl Pts',(80.0796389534446,6.94556465033074,137.875178872676));
#64248=CARTESIAN_POINT('Ctrl Pts',(80.0083911273403,6.94403221544512,137.871315554569));
#64249=CARTESIAN_POINT('Ctrl Pts',(79.9371757213845,6.94621065527244,137.867452236462));
#64250=CARTESIAN_POINT('Ctrl Pts',(79.8660438510696,6.94838653979077,137.863593450026));
#64251=CARTESIAN_POINT('Ctrl Pts',(79.7949448085646,6.95426463799844,137.85973466359));
#64252=CARTESIAN_POINT('Ctrl Pts',(79.7242927051995,6.96383128152558,137.855875877153));
#64253=CARTESIAN_POINT('Ctrl Pts',(79.6536851074769,6.97339189876904,137.852019521469));
#64254=CARTESIAN_POINT('Ctrl Pts',(79.5835243705778,6.98663638649006,137.848163165785));
#64255=CARTESIAN_POINT('Ctrl Pts',(79.5142201594867,7.00349918380912,137.844306810101));
#64256=CARTESIAN_POINT('Ctrl Pts',(79.4449364215518,7.02035699968939,137.840451593623));
#64257=CARTESIAN_POINT('Ctrl Pts',(79.3765091788523,7.04083088834935,137.836596377145));
#64258=CARTESIAN_POINT('Ctrl Pts',(79.3093368622184,7.06480440456019,137.832741160667));
#64259=CARTESIAN_POINT('Ctrl Pts',(79.2421619193466,7.08877885806425,137.828885793462));
#64260=CARTESIAN_POINT('Ctrl Pts',(79.176242456728,7.11625304540635,137.825030426256));
#64261=CARTESIAN_POINT('Ctrl Pts',(79.1119590809463,7.14706155294187,137.821175059051));
#64262=CARTESIAN_POINT('Ctrl Pts',(79.0476084179968,7.17790230858494,137.817315656327));
#64263=CARTESIAN_POINT('Ctrl Pts',(78.9848976994599,7.21208414111098,137.813456253603));
#64264=CARTESIAN_POINT('Ctrl Pts',(78.9241841484722,7.24939501425894,137.809596850879));
#64265=CARTESIAN_POINT('Ctrl Pts',(78.8634362209937,7.28672701311709,137.805735262931));
#64266=CARTESIAN_POINT('Ctrl Pts',(78.8046881124189,7.32719130379329,137.801873674983));
#64267=CARTESIAN_POINT('Ctrl Pts',(78.7482668969645,7.37053327703049,137.798012087035));
#64268=CARTESIAN_POINT('Ctrl Pts',(78.6917469705695,7.41395107860471,137.7941437431));
#64269=CARTESIAN_POINT('Ctrl Pts',(78.637562434545,7.46025629878071,137.790275399166));
#64270=CARTESIAN_POINT('Ctrl Pts',(78.5860056707863,7.50915540734408,137.786407055231));
#64271=CARTESIAN_POINT('Ctrl Pts',(78.5553927482467,7.53819029071482,137.784110143932));
#64272=CARTESIAN_POINT('Ctrl Pts',(78.5257055636269,7.56813899419849,137.781813232633));
#64273=CARTESIAN_POINT('Ctrl Pts',(78.4969985543698,7.59893461361234,137.779516321333));
#64274=CARTESIAN_POINT('Ctrl Pts',(78.4492223163315,7.6501868646037,137.775693638866));
#64275=CARTESIAN_POINT('Ctrl Pts',(78.4039661357278,7.70399804441434,137.771870956398));
#64276=CARTESIAN_POINT('Ctrl Pts',(78.3615208436958,7.76008725433738,137.76804827393));
#64277=CARTESIAN_POINT('Ctrl Pts',(78.3191332469992,7.81610022292423,137.764230787586));
#64278=CARTESIAN_POINT('Ctrl Pts',(78.2795492636144,7.87438469113794,137.760413301241));
#64279=CARTESIAN_POINT('Ctrl Pts',(78.2430220975302,7.93462391019277,137.756595814896));
#64280=CARTESIAN_POINT('Ctrl Pts',(78.2065316626786,7.99480255348986,137.752782167364));
#64281=CARTESIAN_POINT('Ctrl Pts',(78.1730922068975,8.05693162628516,137.748968519833));
#64282=CARTESIAN_POINT('Ctrl Pts',(78.1429147652304,8.12066389059655,137.745154872302));
#64283=CARTESIAN_POINT('Ctrl Pts',(78.1127570014877,8.18435459675692,137.741343711551));
#64284=CARTESIAN_POINT('Ctrl Pts',(78.0858572438908,8.24964597086899,137.7375325508));
#64285=CARTESIAN_POINT('Ctrl Pts',(78.062380601309,8.31616622756962,137.733721390049));
#64286=CARTESIAN_POINT('Ctrl Pts',(78.0389040931843,8.38268610329087,137.729910251125));
#64287=CARTESIAN_POINT('Ctrl Pts',(78.0188508409774,8.45043438279459,137.726099112202));
#64288=CARTESIAN_POINT('Ctrl Pts',(78.0023372240668,8.51902079447142,137.722287973278));
#64289=CARTESIAN_POINT('Ctrl Pts',(77.9858234661275,8.58760779188607,137.718476801807));
#64290=CARTESIAN_POINT('Ctrl Pts',(77.9728495099846,8.65703244869873,137.714665630336));
#64291=CARTESIAN_POINT('Ctrl Pts',(77.9634808603815,8.72689314093621,137.710854458865));
#64292=CARTESIAN_POINT('Ctrl Pts',(77.9541049328187,8.79680810388833,137.707040326716));
#64293=CARTESIAN_POINT('Ctrl Pts',(77.9483399514157,8.86715928237804,137.703226194567));
#64294=CARTESIAN_POINT('Ctrl Pts',(77.946199539787,8.9375401558698,137.699412062418));
#64295=CARTESIAN_POINT('Ctrl Pts',(77.9455473032982,8.95898695292022,137.698249801791));
#64296=CARTESIAN_POINT('Ctrl Pts',(77.9452312678571,8.98043650827389,137.697087541165));
#64297=CARTESIAN_POINT('Ctrl Pts',(77.945250857638,9.00187735519529,137.695925280538));
#64298=CARTESIAN_POINT('Ctrl Pts',(77.9452508576385,9.00187735576021,137.695925280507));
#64299=CARTESIAN_POINT('Ctrl Pts',(77.9453355911812,9.09461746279061,137.690898045562));
#64300=CARTESIAN_POINT('Ctrl Pts',(77.9517027473501,9.18707803688478,137.685870810616));
#64301=CARTESIAN_POINT('Ctrl Pts',(77.9642171232008,9.27854199150456,137.68084357567));
#64302=CARTESIAN_POINT('Ctrl Pts',(77.9745563908267,9.35410870903171,137.676690118228));
#64303=CARTESIAN_POINT('Ctrl Pts',(77.9890907794787,9.42899580347728,137.672536660785));
#64304=CARTESIAN_POINT('Ctrl Pts',(78.0077202195898,9.50281093769801,137.668383203342));
#64305=CARTESIAN_POINT('Ctrl Pts',(78.0250741586275,9.57157217430436,137.664514120491));
#64306=CARTESIAN_POINT('Ctrl Pts',(78.0460260884595,9.63956860642717,137.66064503764));
#64307=CARTESIAN_POINT('Ctrl Pts',(78.0704917545785,9.70639613061694,137.656775954788));
#64308=CARTESIAN_POINT('Ctrl Pts',(78.0949209680756,9.77312408512974,137.652912636678));
#64309=CARTESIAN_POINT('Ctrl Pts',(78.122853360305,9.83868613630884,137.649049318567));
#64310=CARTESIAN_POINT('Ctrl Pts',(78.1541542876673,9.90269107050148,137.645186000456));
#64311=CARTESIAN_POINT('Ctrl Pts',(78.1854184990544,9.96662092693204,137.641327214016));
#64312=CARTESIAN_POINT('Ctrl Pts',(78.2200431845958,10.0289968601426,137.637468427576));
#64313=CARTESIAN_POINT('Ctrl Pts',(78.2578454199541,10.0894470990943,137.633609641136));
#64314=CARTESIAN_POINT('Ctrl Pts',(78.2956238426764,10.1498592588286,137.629753285448));
#64315=CARTESIAN_POINT('Ctrl Pts',(78.3365755870685,10.2083477200628,137.625896929761));
#64316=CARTESIAN_POINT('Ctrl Pts',(78.3804722672278,10.2645661253101,137.622040574073));
#64317=CARTESIAN_POINT('Ctrl Pts',(78.4243559798687,10.3207679230781,137.618185357591));
#64318=CARTESIAN_POINT('Ctrl Pts',(78.4711826023525,10.3747006135015,137.61433014111));
#64319=CARTESIAN_POINT('Ctrl Pts',(78.5206820001741,10.4260490236633,137.610474924628));
#64320=CARTESIAN_POINT('Ctrl Pts',(78.5701833332744,10.4773994413948,137.606619557419));
#64321=CARTESIAN_POINT('Ctrl Pts',(78.6223573104468,10.5261650300569,137.60276419021));
#64322=CARTESIAN_POINT('Ctrl Pts',(78.6768965074492,10.5720670184505,137.598908823001));
#64323=CARTESIAN_POINT('Ctrl Pts',(78.7314927921189,10.6180170537092,137.595049420274));
#64324=CARTESIAN_POINT('Ctrl Pts',(78.7884588663221,10.6610971917516,137.591190017547));
#64325=CARTESIAN_POINT('Ctrl Pts',(78.847454442338,10.7010691637948,137.587330614819));
#64326=CARTESIAN_POINT('Ctrl Pts',(78.9064834221127,10.7410637682828,137.583469026868));
#64327=CARTESIAN_POINT('Ctrl Pts',(78.9675437752333,10.7779464521318,137.579607438917));
#64328=CARTESIAN_POINT('Ctrl Pts',(79.0302688260821,10.8115239476286,137.575745850965));
#64329=CARTESIAN_POINT('Ctrl Pts',(79.0931036166551,10.8451601881569,137.571877507027));
#64330=CARTESIAN_POINT('Ctrl Pts',(79.1576084799627,10.8754794886075,137.568009163089));
#64331=CARTESIAN_POINT('Ctrl Pts',(79.2233955510299,10.9023362195837,137.564140819151));
#64332=CARTESIAN_POINT('Ctrl Pts',(79.2624580199291,10.9182829732766,137.561843907884));
#64333=CARTESIAN_POINT('Ctrl Pts',(79.3019722152479,10.9330098904872,137.559546996617));
#64334=CARTESIAN_POINT('Ctrl Pts',(79.3418547552921,10.9464949009356,137.55725008535));
#64335=CARTESIAN_POINT('Ctrl Pts',(79.4090365153638,10.9692102730134,137.553380960127));
#64336=CARTESIAN_POINT('Ctrl Pts',(79.4775272460009,10.9884879637316,137.549511834903));
#64337=CARTESIAN_POINT('Ctrl Pts',(79.5469417357711,11.0041795757152,137.54564270968));
#64338=CARTESIAN_POINT('Ctrl Pts',(79.6162525807636,11.0198477581002,137.541779361559));
#64339=CARTESIAN_POINT('Ctrl Pts',(79.6864839770015,11.0319403841584,137.537916013439));
#64340=CARTESIAN_POINT('Ctrl Pts',(79.757234215337,11.0403583842788,137.534052665318));
#64341=CARTESIAN_POINT('Ctrl Pts',(79.827900600162,11.0487664073465,137.530193896055));
#64342=CARTESIAN_POINT('Ctrl Pts',(79.899084125485,11.0535083988416,137.526335126793));
#64343=CARTESIAN_POINT('Ctrl Pts',(79.9703732449644,11.0545363997472,137.52247635753));
#64344=CARTESIAN_POINT('Ctrl Pts',(80.0416171339066,11.0555637484209,137.518620036526));
#64345=CARTESIAN_POINT('Ctrl Pts',(80.1129659995103,11.0528817748708,137.514763715522));
#64346=CARTESIAN_POINT('Ctrl Pts',(80.1840049945603,11.0464944965665,137.510907394518));
#64347=CARTESIAN_POINT('Ctrl Pts',(80.2550226814983,11.0401091341232,137.507052230216));
#64348=CARTESIAN_POINT('Ctrl Pts',(80.3257301988894,11.0300207171257,137.503197065913));
#64349=CARTESIAN_POINT('Ctrl Pts',(80.3957162605863,11.0162852485716,137.499341901611));
#64350=CARTESIAN_POINT('Ctrl Pts',(80.4657047407185,11.0025493053753,137.49548660409));
#64351=CARTESIAN_POINT('Ctrl Pts',(80.5349712394909,10.985166156402,137.491631306569));
#64352=CARTESIAN_POINT('Ctrl Pts',(80.6031148326331,10.9642428722431,137.487776009047));
#64353=CARTESIAN_POINT('Ctrl Pts',(80.6713261626792,10.9432987896728,137.483916879237));
#64354=CARTESIAN_POINT('Ctrl Pts',(80.7384118941879,10.9188076915413,137.480057749428));
#64355=CARTESIAN_POINT('Ctrl Pts',(80.8039873646162,10.8909261963486,137.476198619618));
#64356=CARTESIAN_POINT('Ctrl Pts',(80.869599845037,10.8630289651815,137.472337311762));
#64357=CARTESIAN_POINT('Ctrl Pts',(80.9336999310049,10.8317377409704,137.468476003907));
#64358=CARTESIAN_POINT('Ctrl Pts',(80.9959264492264,10.7972557052994,137.464614696051));
#64359=CARTESIAN_POINT('Ctrl Pts',(81.0582543739492,10.7627174765022,137.460747095674));
#64360=CARTESIAN_POINT('Ctrl Pts',(81.1187022253178,10.7249783151754,137.456879495297));
#64361=CARTESIAN_POINT('Ctrl Pts',(81.1769374678752,10.6842849400299,137.45301189492));
#64362=CARTESIAN_POINT('Ctrl Pts',(81.2024025695469,10.6664905445756,137.451320670972));
#64363=CARTESIAN_POINT('Ctrl Pts',(81.2274450168065,10.6481317845595,137.449629447024));
#64364=CARTESIAN_POINT('Ctrl Pts',(81.252039109102,10.6292316077768,137.447938223076));
#64365=CARTESIAN_POINT('',(77.9452508246239,8.99815913298199,137.754074719432));
#64366=CARTESIAN_POINT('Ctrl Pts',(77.9452508246239,8.998159132982,137.754074719432));
#64367=CARTESIAN_POINT('Ctrl Pts',(77.9451879957237,9.06828784391594,137.750267950527));
#64368=CARTESIAN_POINT('Ctrl Pts',(77.948719643209,9.1385287266768,137.746461181623));
#64369=CARTESIAN_POINT('Ctrl Pts',(77.955853571024,9.20847767123739,137.742654412718));
#64370=CARTESIAN_POINT('Ctrl Pts',(77.9629816800018,9.27836956146164,137.73885074883));
#64371=CARTESIAN_POINT('Ctrl Pts',(77.9737061958358,9.34796948932302,137.735047084943));
#64372=CARTESIAN_POINT('Ctrl Pts',(77.9879828890358,9.41687493050971,137.731243421055));
#64373=CARTESIAN_POINT('Ctrl Pts',(78.0022530301468,9.48574874850582,137.727441502806));
#64374=CARTESIAN_POINT('Ctrl Pts',(78.0200720145925,9.55392822213815,137.723639584557));
#64375=CARTESIAN_POINT('Ctrl Pts',(78.0413442350491,9.62101944971517,137.719837666308));
#64376=CARTESIAN_POINT('Ctrl Pts',(78.0626142800831,9.68810381614818,137.716036136865));
#64377=CARTESIAN_POINT('Ctrl Pts',(78.0873367072412,9.75409968062593,137.712234607423));
#64378=CARTESIAN_POINT('Ctrl Pts',(78.1153661610104,9.81862864318035,137.70843307798));
#64379=CARTESIAN_POINT('Ctrl Pts',(78.143421601976,9.88321743304506,137.704628023992));
#64380=CARTESIAN_POINT('Ctrl Pts',(78.1747899917167,9.94633614509237,137.700822970003));
#64381=CARTESIAN_POINT('Ctrl Pts',(78.2092783941031,10.0076277550137,137.697017916015));
#64382=CARTESIAN_POINT('Ctrl Pts',(78.243783338819,10.0689487633976,137.693211036936));
#64383=CARTESIAN_POINT('Ctrl Pts',(78.2814110055482,10.1284405026701,137.689404157857));
#64384=CARTESIAN_POINT('Ctrl Pts',(78.3219247244603,10.1857744018667,137.685597278778));
#64385=CARTESIAN_POINT('Ctrl Pts',(78.3625095297344,10.2432089005249,137.681783720056));
#64386=CARTESIAN_POINT('Ctrl Pts',(78.4059901860523,10.2984776074081,137.677970161334));
#64387=CARTESIAN_POINT('Ctrl Pts',(78.4520898455625,10.351285209084,137.674156602612));
#64388=CARTESIAN_POINT('Ctrl Pts',(78.4841323747905,10.3879902333325,137.671505909134));
#64389=CARTESIAN_POINT('Ctrl Pts',(78.5174393844088,10.423506973414,137.668855215655));
#64390=CARTESIAN_POINT('Ctrl Pts',(78.5519082624529,10.4577475371778,137.666204522177));
#64391=CARTESIAN_POINT('Ctrl Pts',(78.6022207357355,10.5077267516837,137.66233543933));
#64392=CARTESIAN_POINT('Ctrl Pts',(78.6552222517718,10.5551960831898,137.658466356483));
#64393=CARTESIAN_POINT('Ctrl Pts',(78.7106323248073,10.5998526684255,137.654597273635));
#64394=CARTESIAN_POINT('Ctrl Pts',(78.7659598395989,10.6444427175775,137.650733955528));
#64395=CARTESIAN_POINT('Ctrl Pts',(78.8236884129037,10.6862280368351,137.646870637421));
#64396=CARTESIAN_POINT('Ctrl Pts',(78.8835010225446,10.7249427804542,137.643007319315));
#64397=CARTESIAN_POINT('Ctrl Pts',(78.9432434720197,10.7636121116955,137.639148532878));
#64398=CARTESIAN_POINT('Ctrl Pts',(79.0050646962487,10.7992177589796,137.635289746442));
#64399=CARTESIAN_POINT('Ctrl Pts',(79.0686163208411,10.831535422725,137.631430960005));
#64400=CARTESIAN_POINT('Ctrl Pts',(79.1321279125715,10.8638327287127,137.627574604321));
#64401=CARTESIAN_POINT('Ctrl Pts',(79.1973673100851,10.8928459406904,137.623718248637));
#64402=CARTESIAN_POINT('Ctrl Pts',(79.2639602801978,10.9183959688692,137.619861892953));
#64403=CARTESIAN_POINT('Ctrl Pts',(79.3305335780819,10.9439384493143,137.616006676475));
#64404=CARTESIAN_POINT('Ctrl Pts',(79.3984592014349,10.9660196030974,137.612151459997));
#64405=CARTESIAN_POINT('Ctrl Pts',(79.4673432145737,10.9845085818508,137.608296243519));
#64406=CARTESIAN_POINT('Ctrl Pts',(79.5362299208732,11.0029982834684,137.604440876314));
#64407=CARTESIAN_POINT('Ctrl Pts',(79.6060746216028,11.0178954074216,137.600585509108));
#64408=CARTESIAN_POINT('Ctrl Pts',(79.6764701885863,11.0291195193055,137.596730141903));
#64409=CARTESIAN_POINT('Ctrl Pts',(79.7469394405348,11.0403553797743,137.592870739179));
#64410=CARTESIAN_POINT('Ctrl Pts',(79.8179602290672,11.047910476761,137.589011336455));
#64411=CARTESIAN_POINT('Ctrl Pts',(79.889118140131,11.0517560224481,137.585151933731));
#64412=CARTESIAN_POINT('Ctrl Pts',(79.9603163413645,11.0556037455135,137.581290345783));
#64413=CARTESIAN_POINT('Ctrl Pts',(80.0316513336741,11.0557377351632,137.577428757835));
#64414=CARTESIAN_POINT('Ctrl Pts',(80.102709285001,11.0521813675391,137.573567169887));
#64415=CARTESIAN_POINT('Ctrl Pts',(80.1738915547628,11.0486187779222,137.569698825952));
#64416=CARTESIAN_POINT('Ctrl Pts',(80.2447953324329,11.0413529901579,137.565830482018));
#64417=CARTESIAN_POINT('Ctrl Pts',(80.3150131820574,11.0304591248361,137.561962138083));
#64418=CARTESIAN_POINT('Ctrl Pts',(80.3567065203266,11.0239906611285,137.559665226784));
#64419=CARTESIAN_POINT('Ctrl Pts',(80.3981582238866,11.0162440461926,137.557368315484));
#64420=CARTESIAN_POINT('Ctrl Pts',(80.4392854645031,11.007243344285,137.555071404185));
#64421=CARTESIAN_POINT('Ctrl Pts',(80.5085688299935,10.9920806708212,137.55120200418));
#64422=CARTESIAN_POINT('Ctrl Pts',(80.5772019369505,10.9732969381624,137.547332604175));
#64423=CARTESIAN_POINT('Ctrl Pts',(80.6447781102469,10.9509635442638,137.543463204171));
#64424=CARTESIAN_POINT('Ctrl Pts',(80.7122373862153,10.928668784013,137.539600497686));
#64425=CARTESIAN_POINT('Ctrl Pts',(80.7786429038363,10.902836714354,137.535737791202));
#64426=CARTESIAN_POINT('Ctrl Pts',(80.84359955841,10.8735894287571,137.531875084718));
#64427=CARTESIAN_POINT('Ctrl Pts',(80.9084915578505,10.8443712546833,137.52801622301));
#64428=CARTESIAN_POINT('Ctrl Pts',(80.9719371146386,10.8117448069602,137.524157361303));
#64429=CARTESIAN_POINT('Ctrl Pts',(81.0335588124541,10.7758811175578,137.520298499595));
#64430=CARTESIAN_POINT('Ctrl Pts',(81.0951364101892,10.740043094303,137.516442399513));
#64431=CARTESIAN_POINT('Ctrl Pts',(81.1548923224202,10.7009726742508,137.512586299432));
#64432=CARTESIAN_POINT('Ctrl Pts',(81.2124731810451,10.6588870810717,137.508730199351));
#64433=CARTESIAN_POINT('Ctrl Pts',(81.2257792406795,10.6491617413326,137.507839113339));
#64434=CARTESIAN_POINT('Ctrl Pts',(81.2389692655704,10.6392755789184,137.506948027328));
#64435=CARTESIAN_POINT('Ctrl Pts',(81.252039109102,10.6292316077768,137.506056941317));
#64436=CARTESIAN_POINT('Ctrl Pts',(81.252039109102,10.6292316077768,138.206016809239));
#64437=CARTESIAN_POINT('Ctrl Pts',(81.3100004164792,10.5846892460251,138.202046816943));
#64438=CARTESIAN_POINT('Ctrl Pts',(81.365664648856,10.5369863629426,138.198076824648));
#64439=CARTESIAN_POINT('Ctrl Pts',(81.4186724477197,10.4863936385026,138.194106832352));
#64440=CARTESIAN_POINT('Ctrl Pts',(81.4701805437359,10.4372322893419,138.190249159543));
#64441=CARTESIAN_POINT('Ctrl Pts',(81.519180147956,10.3853428098416,138.186391486734));
#64442=CARTESIAN_POINT('Ctrl Pts',(81.5653745129687,10.3310147244295,138.182533813925));
#64443=CARTESIAN_POINT('Ctrl Pts',(81.611545872447,10.2767136952748,138.178678062298));
#64444=CARTESIAN_POINT('Ctrl Pts',(81.6549144507438,10.2199768396543,138.174822310672));
#64445=CARTESIAN_POINT('Ctrl Pts',(81.6952218725276,10.1611289185116,138.170966559046));
#64446=CARTESIAN_POINT('Ctrl Pts',(81.7355227039307,10.1022906191751,138.167111437846));
#64447=CARTESIAN_POINT('Ctrl Pts',(81.7727630987943,10.0413423408248,138.163256316647));
#64448=CARTESIAN_POINT('Ctrl Pts',(81.8067273659854,9.97863874207973,138.159401195447));
#64449=CARTESIAN_POINT('Ctrl Pts',(81.8424556835949,9.91267841740622,138.155345845338));
#64450=CARTESIAN_POINT('Ctrl Pts',(81.8745580059818,9.84477598534579,138.15129049523));
#64451=CARTESIAN_POINT('Ctrl Pts',(81.9028386321676,9.77537262166675,138.147235145121));
#64452=CARTESIAN_POINT('Ctrl Pts',(81.929758577429,9.70930849922059,138.143374912246));
#64453=CARTESIAN_POINT('Ctrl Pts',(81.9532159962972,9.64188504771407,138.13951467937));
#64454=CARTESIAN_POINT('Ctrl Pts',(81.9730927839647,9.57350015550693,138.135654446495));
#64455=CARTESIAN_POINT('Ctrl Pts',(81.9929834856272,9.50506739303689,138.131791511409));
#64456=CARTESIAN_POINT('Ctrl Pts',(82.0092884593221,9.4356723233551,138.127928576323));
#64457=CARTESIAN_POINT('Ctrl Pts',(82.0219406338674,9.36572344143639,138.124065641237));
#64458=CARTESIAN_POINT('Ctrl Pts',(82.0346132881541,9.29566133510642,138.12019645332));
#64459=CARTESIAN_POINT('Ctrl Pts',(82.0436212918391,9.22504410920679,138.116327265403));
#64460=CARTESIAN_POINT('Ctrl Pts',(82.0489494312964,9.15428477076475,138.112458077486));
#64461=CARTESIAN_POINT('Ctrl Pts',(82.0497394482429,9.1437931015921,138.111884383039));
#64462=CARTESIAN_POINT('Ctrl Pts',(82.0504486576402,9.13329830491125,138.111310688591));
#64463=CARTESIAN_POINT('Ctrl Pts',(82.0510771071998,9.12280172157117,138.110736994143));
#64464=CARTESIAN_POINT('Ctrl Pts',(82.0553154671478,9.05201115813191,138.106867911044));
#64465=CARTESIAN_POINT('Ctrl Pts',(82.0558929439494,8.98086226244677,138.102998827945));
#64466=CARTESIAN_POINT('Ctrl Pts',(82.0527677254126,8.90976570494383,138.099129744846));
#64467=CARTESIAN_POINT('Ctrl Pts',(82.0496471632929,8.83877507770455,138.095266426484));
#64468=CARTESIAN_POINT('Ctrl Pts',(82.0428348777455,8.76783711521766,138.091403108123));
#64469=CARTESIAN_POINT('Ctrl Pts',(82.0323409849502,8.69736542928556,138.087539789761));
#64470=CARTESIAN_POINT('Ctrl Pts',(82.0218594014778,8.62697640655115,138.083681003067));
#64471=CARTESIAN_POINT('Ctrl Pts',(82.007704860003,8.55705305211314,138.079822216373));
#64472=CARTESIAN_POINT('Ctrl Pts',(81.9899393756834,8.48800503556719,138.075963429679));
#64473=CARTESIAN_POINT('Ctrl Pts',(81.9721850823073,8.41900051417354,138.072107073736));
#64474=CARTESIAN_POINT('Ctrl Pts',(81.950824479671,8.35087070605488,138.068250717793));
#64475=CARTESIAN_POINT('Ctrl Pts',(81.9259705990824,8.28401479486638,138.064394361849));
#64476=CARTESIAN_POINT('Ctrl Pts',(81.9011240605695,8.2171786335578,138.060539145111));
#64477=CARTESIAN_POINT('Ctrl Pts',(81.8727864619881,8.15161607716593,138.056683928372));
#64478=CARTESIAN_POINT('Ctrl Pts',(81.8411200555549,8.08770920012657,138.052828711633));
#64479=CARTESIAN_POINT('Ctrl Pts',(81.8094524110515,8.02379982450278,138.048973344166));
#64480=CARTESIAN_POINT('Ctrl Pts',(81.7744559179631,7.96154669104812,138.045117976699));
#64481=CARTESIAN_POINT('Ctrl Pts',(81.7363393757596,7.90130844424522,138.041262609232));
#64482=CARTESIAN_POINT('Ctrl Pts',(81.6981829359356,7.84100714443256,138.037403206247));
#64483=CARTESIAN_POINT('Ctrl Pts',(81.6569001879319,7.78272535272691,138.033543803262));
#64484=CARTESIAN_POINT('Ctrl Pts',(81.6127434984906,7.72679303702179,138.029684400277));
#64485=CARTESIAN_POINT('Ctrl Pts',(81.5685618071839,7.67082905199876,138.025822812068));
#64486=CARTESIAN_POINT('Ctrl Pts',(81.5215032557044,7.61721755643728,138.021961223858));
#64487=CARTESIAN_POINT('Ctrl Pts',(81.4718589648583,7.56625359631968,138.018099635649));
#64488=CARTESIAN_POINT('Ctrl Pts',(81.4221278195836,7.51520047296578,138.014231291455));
#64489=CARTESIAN_POINT('Ctrl Pts',(81.3698022597075,7.46680446283967,138.010362947262));
#64490=CARTESIAN_POINT('Ctrl Pts',(81.3152080016696,7.42132160499855,138.006494603069));
#64491=CARTESIAN_POINT('Ctrl Pts',(81.2827915374538,7.39431522215488,138.004197694096));
#64492=CARTESIAN_POINT('Ctrl Pts',(81.2495758162514,7.36833511378297,138.001900785124));
#64493=CARTESIAN_POINT('Ctrl Pts',(81.2156336505183,7.34342751736379,137.999603876152));
#64494=CARTESIAN_POINT('Ctrl Pts',(81.1584589632513,7.30147132496761,137.995734793277));
#64495=CARTESIAN_POINT('Ctrl Pts',(81.0989976384081,7.26239640879816,137.991865710402));
#64496=CARTESIAN_POINT('Ctrl Pts',(81.0375720156332,7.22646063622065,137.987996627528));
#64497=CARTESIAN_POINT('Ctrl Pts',(80.9762379139519,7.19057840613981,137.984133309392));
#64498=CARTESIAN_POINT('Ctrl Pts',(80.9129457396515,7.15782627890905,137.980269991257));
#64499=CARTESIAN_POINT('Ctrl Pts',(80.8480484684533,7.12842009049735,137.976406673121));
#64500=CARTESIAN_POINT('Ctrl Pts',(80.7832273216991,7.09904839551966,137.972547886654));
#64501=CARTESIAN_POINT('Ctrl Pts',(80.716805258211,7.07301504293452,137.968689100188));
#64502=CARTESIAN_POINT('Ctrl Pts',(80.6491600907199,7.05049012848959,137.964830313721));
#64503=CARTESIAN_POINT('Ctrl Pts',(80.5815575347049,7.02797940308269,137.960973958006));
#64504=CARTESIAN_POINT('Ctrl Pts',(80.512733863091,7.00897288420731,137.957117602291));
#64505=CARTESIAN_POINT('Ctrl Pts',(80.4430857491829,6.99359211988912,137.953261246575));
#64506=CARTESIAN_POINT('Ctrl Pts',(80.3734582100062,6.97821589919857,137.949406030065));
#64507=CARTESIAN_POINT('Ctrl Pts',(80.303007186142,6.96646341136475,137.945550813555));
#64508=CARTESIAN_POINT('Ctrl Pts',(80.232141673328,6.95840557259664,137.941695597045));
#64509=CARTESIAN_POINT('Ctrl Pts',(80.1612733898665,6.95034741878909,137.937840229806));
#64510=CARTESIAN_POINT('Ctrl Pts',(80.0899910682033,6.94598425352913,137.933984862568));
#64511=CARTESIAN_POINT('Ctrl Pts',(80.0187092661136,6.94533517919309,137.930129495329));
#64512=CARTESIAN_POINT('Ctrl Pts',(79.9473528513918,6.944685425453,137.926270092571));
#64513=CARTESIAN_POINT('Ctrl Pts',(79.8759974440872,6.94775752767298,137.922410689813));
#64514=CARTESIAN_POINT('Ctrl Pts',(79.8050571398562,6.95451843230525,137.918551287055));
#64515=CARTESIAN_POINT('Ctrl Pts',(79.7340766686538,6.96128316501617,137.914689699072));
#64516=CARTESIAN_POINT('Ctrl Pts',(79.6635122491687,6.97174078670801,137.910828111089));
#64517=CARTESIAN_POINT('Ctrl Pts',(79.5937696574457,6.98580674430475,137.906966523106));
#64518=CARTESIAN_POINT('Ctrl Pts',(79.5239050485447,6.99989731080131,137.903098179136));
#64519=CARTESIAN_POINT('Ctrl Pts',(79.4548656087432,7.01760869636137,137.899229835166));
#64520=CARTESIAN_POINT('Ctrl Pts',(79.3870431070686,7.03880612638427,137.895361491195));
#64521=CARTESIAN_POINT('Ctrl Pts',(79.3467720628865,7.05139254858813,137.893064580184));
#64522=CARTESIAN_POINT('Ctrl Pts',(79.3069297253038,7.06520708629177,137.890767669172));
#64523=CARTESIAN_POINT('Ctrl Pts',(79.2675944322128,7.08021364553911,137.88847075816));
#64524=CARTESIAN_POINT('Ctrl Pts',(79.201335224064,7.10549177758364,137.884601675388));
#64525=CARTESIAN_POINT('Ctrl Pts',(79.1362564439872,7.13425373682997,137.880732592616));
#64526=CARTESIAN_POINT('Ctrl Pts',(79.0727495655537,7.1663685772983,137.876863509844));
#64527=CARTESIAN_POINT('Ctrl Pts',(79.0093373092264,7.19843556824356,137.873000191814));
#64528=CARTESIAN_POINT('Ctrl Pts',(78.9474927356015,7.2338453067949,137.869136873784));
#64529=CARTESIAN_POINT('Ctrl Pts',(78.8875886226931,7.27241831158752,137.865273555754));
#64530=CARTESIAN_POINT('Ctrl Pts',(78.8277547773136,7.31094607024263,137.861414769397));
#64531=CARTESIAN_POINT('Ctrl Pts',(78.769857277877,7.35262946308729,137.857555983039));
#64532=CARTESIAN_POINT('Ctrl Pts',(78.7142439456327,7.39724333376594,137.853697196681));
#64533=CARTESIAN_POINT('Ctrl Pts',(78.6586656457248,7.44182910096534,137.849840841077));
#64534=CARTESIAN_POINT('Ctrl Pts',(78.6053690363638,7.48934138033019,137.845984485473));
#64535=CARTESIAN_POINT('Ctrl Pts',(78.5546713818588,7.53951283878216,137.842128129869));
#64536=CARTESIAN_POINT('Ctrl Pts',(78.5039887039606,7.58966947607113,137.838272913472));
#64537=CARTESIAN_POINT('Ctrl Pts',(78.4559038018054,7.64248339139704,137.834417697074));
#64538=CARTESIAN_POINT('Ctrl Pts',(78.410698085686,7.69764943749475,137.830562480677));
#64539=CARTESIAN_POINT('Ctrl Pts',(78.3654906021672,7.75281764040895,137.826707113553));
#64540=CARTESIAN_POINT('Ctrl Pts',(78.3231628343684,7.81033777953276,137.82285174643));
#64541=CARTESIAN_POINT('Ctrl Pts',(78.2839556788086,7.86987193194451,137.818996379306));
#64542=CARTESIAN_POINT('Ctrl Pts',(78.2447074840536,7.92946840037153,137.815136976664));
#64543=CARTESIAN_POINT('Ctrl Pts',(78.2085866897949,7.99108268383364,137.811277574023));
#64544=CARTESIAN_POINT('Ctrl Pts',(78.1757901239915,8.05434895930209,137.807418171382));
#64545=CARTESIAN_POINT('Ctrl Pts',(78.1429749885184,8.11765105662577,137.803556583517));
#64546=CARTESIAN_POINT('Ctrl Pts',(78.1134880292856,8.18260656544209,137.799694995651));
#64547=CARTESIAN_POINT('Ctrl Pts',(78.0874782954018,8.24882871997077,137.795833407786));
#64548=CARTESIAN_POINT('Ctrl Pts',(78.0614230565543,8.31516673253733,137.791965063935));
#64549=CARTESIAN_POINT('Ctrl Pts',(78.0388573428445,8.38277535426736,137.788096720083));
#64550=CARTESIAN_POINT('Ctrl Pts',(78.0198804134868,8.45125234797139,137.784228376231));
#64551=CARTESIAN_POINT('Ctrl Pts',(78.0086124552002,8.49191202974123,137.781931464211));
#64552=CARTESIAN_POINT('Ctrl Pts',(77.9986088005083,8.53287764689449,137.77963455219));
#64553=CARTESIAN_POINT('Ctrl Pts',(77.9898816146324,8.57406380840876,137.777337640169));
#64554=CARTESIAN_POINT('Ctrl Pts',(77.96929780918,8.67120485112274,137.771920179048));
#64555=CARTESIAN_POINT('Ctrl Pts',(77.9557497500285,8.76988496615924,137.766502717927));
#64556=CARTESIAN_POINT('Ctrl Pts',(77.9494139417945,8.86925452056241,137.761085256806));
#64557=CARTESIAN_POINT('Ctrl Pts',(77.9466809629302,8.91211801672847,137.758748411025));
#64558=CARTESIAN_POINT('Ctrl Pts',(77.9452893931581,8.95510950520192,137.756411565243));
#64559=CARTESIAN_POINT('Ctrl Pts',(77.9452508246244,8.99815913242806,137.754074719462));
#64560=CARTESIAN_POINT('Origin',(80.,9.,141.545925280538));
#64561=CARTESIAN_POINT('',(81.252039109102,10.6292316077768,138.906139397334));
#64562=CARTESIAN_POINT('',(81.252039109102,10.6292316077768,138.847890491445));
#64563=CARTESIAN_POINT('',(81.252039109102,10.6292316077768,141.545925280538));
#64564=CARTESIAN_POINT('',(77.9452500654425,8.99948140989303,138.39592528059));
#64565=CARTESIAN_POINT('Ctrl Pts',(81.252039109102,10.6292316077768,138.847890491445));
#64566=CARTESIAN_POINT('Ctrl Pts',(81.3085681361867,10.5857899311167,138.844035069102));
#64567=CARTESIAN_POINT('Ctrl Pts',(81.3628582544148,10.539383794229,138.840179646758));
#64568=CARTESIAN_POINT('Ctrl Pts',(81.4145905601348,10.4902788697682,138.836324224414));
#64569=CARTESIAN_POINT('Ctrl Pts',(81.4663198247622,10.4411768319489,138.832469028712));
#64570=CARTESIAN_POINT('Ctrl Pts',(81.5154912241929,10.3893766571317,138.82861383301));
#64571=CARTESIAN_POINT('Ctrl Pts',(81.5618216637909,10.3351818801247,138.824758637308));
#64572=CARTESIAN_POINT('Ctrl Pts',(81.6081976885301,10.2809337801495,138.820899648428));
#64573=CARTESIAN_POINT('Ctrl Pts',(81.6517268533141,10.224286741716,138.817040659547));
#64574=CARTESIAN_POINT('Ctrl Pts',(81.69216602467,10.1655778427255,138.813181670666));
#64575=CARTESIAN_POINT('Ctrl Pts',(81.7326245432036,10.1068408558323,138.809320835542));
#64576=CARTESIAN_POINT('Ctrl Pts',(81.7699898684382,10.0460404577005,138.805460000418));
#64577=CARTESIAN_POINT('Ctrl Pts',(81.804063459511,9.9835408464101,138.801599165294));
#64578=CARTESIAN_POINT('Ctrl Pts',(81.8381998446866,9.92092605480304,138.797731215051));
#64579=CARTESIAN_POINT('Ctrl Pts',(81.8690321646211,9.85660623253018,138.793863264807));
#64580=CARTESIAN_POINT('Ctrl Pts',(81.8964091252976,9.79096775660459,138.789995314564));
#64581=CARTESIAN_POINT('Ctrl Pts',(81.9206649226727,9.73281252195765,138.786568337462));
#64582=CARTESIAN_POINT('Ctrl Pts',(81.9422089599303,9.6736226676844,138.783141360359));
#64583=CARTESIAN_POINT('Ctrl Pts',(81.9609690692891,9.61367570572054,138.779714383257));
#64584=CARTESIAN_POINT('Ctrl Pts',(81.9821493409619,9.54599523989408,138.775845306342));
#64585=CARTESIAN_POINT('Ctrl Pts',(81.9998631210447,9.47708440544685,138.771976229427));
#64586=CARTESIAN_POINT('Ctrl Pts',(82.0139708209142,9.40733167690024,138.768107152513));
#64587=CARTESIAN_POINT('Ctrl Pts',(82.0280575006178,9.33768287840135,138.764243840438));
#64588=CARTESIAN_POINT('Ctrl Pts',(82.0385486698086,9.26719514802455,138.760380528364));
#64589=CARTESIAN_POINT('Ctrl Pts',(82.0453544272793,9.19627233454816,138.756517216289));
#64590=CARTESIAN_POINT('Ctrl Pts',(82.0521522013768,9.12543271582156,138.752658436005));
#64591=CARTESIAN_POINT('Ctrl Pts',(82.0552731047301,9.05415950897263,138.74879965572));
#64592=CARTESIAN_POINT('Ctrl Pts',(82.0546785546215,8.98286524939013,138.744940875435));
#64593=CARTESIAN_POINT('Ctrl Pts',(82.0540843790473,8.91161590133201,138.741084525973));
#64594=CARTESIAN_POINT('Ctrl Pts',(82.0497793976358,8.84034601147169,138.737228176511));
#64595=CARTESIAN_POINT('Ctrl Pts',(82.0417770670292,8.76947023824714,138.733371827049));
#64596=CARTESIAN_POINT('Ctrl Pts',(82.0337771005213,8.69861540358891,138.729516616854));
#64597=CARTESIAN_POINT('Ctrl Pts',(82.0220820077972,8.62815493687063,138.725661406659));
#64598=CARTESIAN_POINT('Ctrl Pts',(82.0067571394029,8.5584987588291,138.721806196464));
#64599=CARTESIAN_POINT('Ctrl Pts',(81.9914316720566,8.48883985836872,138.717950835594));
#64600=CARTESIAN_POINT('Ctrl Pts',(81.9724762539173,8.41998578295924,138.714095474723));
#64601=CARTESIAN_POINT('Ctrl Pts',(81.9500070585298,8.35233493672745,138.710240113852));
#64602=CARTESIAN_POINT('Ctrl Pts',(81.9275143441895,8.28461327901221,138.706380717499));
#64603=CARTESIAN_POINT('Ctrl Pts',(81.9015006640426,8.21809782657285,138.702521321145));
#64604=CARTESIAN_POINT('Ctrl Pts',(81.8721313874739,8.15316965658103,138.698661924792));
#64605=CARTESIAN_POINT('Ctrl Pts',(81.8427454819877,8.0882047241864,138.694800343244));
#64606=CARTESIAN_POINT('Ctrl Pts',(81.8100004209771,8.02482929510083,138.690938761696));
#64607=CARTESIAN_POINT('Ctrl Pts',(81.7741076041258,7.96339989799194,138.687077180148));
#64608=CARTESIAN_POINT('Ctrl Pts',(81.7381519911912,7.90186302741413,138.683208842591));
#64609=CARTESIAN_POINT('Ctrl Pts',(81.6990378939293,7.84227939256143,138.679340505034));
#64610=CARTESIAN_POINT('Ctrl Pts',(81.6570196914156,7.78497600650816,138.675472167477));
#64611=CARTESIAN_POINT('Ctrl Pts',(81.632069841485,7.75095001784094,138.673175200073));
#64612=CARTESIAN_POINT('Ctrl Pts',(81.6060968319195,7.7177273775482,138.670878232669));
#64613=CARTESIAN_POINT('Ctrl Pts',(81.5791601846843,7.68537051850804,138.668581265266));
#64614=CARTESIAN_POINT('Ctrl Pts',(81.5337872424878,7.63086759978652,138.664712180583));
#64615=CARTESIAN_POINT('Ctrl Pts',(81.4855004608702,7.57860968239259,138.6608430959));
#64616=CARTESIAN_POINT('Ctrl Pts',(81.4345505022327,7.52892474052351,138.656974011217));
#64617=CARTESIAN_POINT('Ctrl Pts',(81.3836764562117,7.47931382646594,138.653110691256));
#64618=CARTESIAN_POINT('Ctrl Pts',(81.3301474544714,7.43226861475334,138.649247371294));
#64619=CARTESIAN_POINT('Ctrl Pts',(81.2742540251656,7.38808367405459,138.645384051333));
#64620=CARTESIAN_POINT('Ctrl Pts',(81.2184261585317,7.34395056203783,138.641525263024));
#64621=CARTESIAN_POINT('Ctrl Pts',(81.1602397526017,7.3026713565031,138.637666474715));
#64622=CARTESIAN_POINT('Ctrl Pts',(81.1000204674381,7.26450222307339,138.633807686406));
#64623=CARTESIAN_POINT('Ctrl Pts',(81.0398391158282,7.22635713328464,138.629951328839));
#64624=CARTESIAN_POINT('Ctrl Pts',(80.9776278349285,7.19131848821236,138.626094971273));
#64625=CARTESIAN_POINT('Ctrl Pts',(80.913742293429,7.15959988488941,138.622238613706));
#64626=CARTESIAN_POINT('Ctrl Pts',(80.8498756242241,7.12789065149294,138.618383395337));
#64627=CARTESIAN_POINT('Ctrl Pts',(80.7843361111867,7.09949972866039,138.614528176969));
#64628=CARTESIAN_POINT('Ctrl Pts',(80.7175035888128,7.07459454593566,138.610672958601));
#64629=CARTESIAN_POINT('Ctrl Pts',(80.6506684534069,7.04968838946285,138.6068175895));
#64630=CARTESIAN_POINT('Ctrl Pts',(80.5825406642678,7.02826841124369,138.6029622204));
#64631=CARTESIAN_POINT('Ctrl Pts',(80.5135179456951,7.0104530963184,138.599106851299));
#64632=CARTESIAN_POINT('Ctrl Pts',(80.4444229793004,6.9926191336532,138.595247446687));
#64633=CARTESIAN_POINT('Ctrl Pts',(80.3744316848496,6.97839748787347,138.591388042074));
#64634=CARTESIAN_POINT('Ctrl Pts',(80.3039539124666,6.96785591514867,138.587528637461));
#64635=CARTESIAN_POINT('Ctrl Pts',(80.2334362350443,6.95730837370693,138.583667047625));
#64636=CARTESIAN_POINT('Ctrl Pts',(80.1624320151168,6.95044510005407,138.579805457789));
#64637=CARTESIAN_POINT('Ctrl Pts',(80.0913554446739,6.94728186415464,138.575943867953));
#64638=CARTESIAN_POINT('Ctrl Pts',(80.0201545236788,6.9441130940809,138.572075522151));
#64639=CARTESIAN_POINT('Ctrl Pts',(79.9488814853711,6.9446572822268,138.56820717635));
#64640=CARTESIAN_POINT('Ctrl Pts',(79.8779490358511,6.94887808147582,138.564338830549));
#64641=CARTESIAN_POINT('Ctrl Pts',(79.8358317184722,6.95138425097605,138.562041936124));
#64642=CARTESIAN_POINT('Ctrl Pts',(79.7938343729143,6.955185648202,138.559745041699));
#64643=CARTESIAN_POINT('Ctrl Pts',(79.7520417263487,6.96026613083279,138.557448147274));
#64644=CARTESIAN_POINT('Ctrl Pts',(79.6816426567328,6.96882412559498,138.553579063983));
#64645=CARTESIAN_POINT('Ctrl Pts',(79.6115492768566,6.98104777513134,138.549709980692));
#64646=CARTESIAN_POINT('Ctrl Pts',(79.5421730827995,6.99690437662436,138.545840897401));
#64647=CARTESIAN_POINT('Ctrl Pts',(79.4729002555485,7.01273735263207,138.541977578836));
#64648=CARTESIAN_POINT('Ctrl Pts',(79.4043429627509,7.03219242877522,138.538114260271));
#64649=CARTESIAN_POINT('Ctrl Pts',(79.3369062578221,7.05518529119493,138.534250941707));
#64650=CARTESIAN_POINT('Ctrl Pts',(79.2695486557868,7.07815118311026,138.530392154794));
#64651=CARTESIAN_POINT('Ctrl Pts',(79.2033094882509,7.10464646237816,138.526533367881));
#64652=CARTESIAN_POINT('Ctrl Pts',(79.1385805998373,7.13453647059951,138.522674580969));
#64653=CARTESIAN_POINT('Ctrl Pts',(79.0738924856827,7.16440765039717,138.518818224797));
#64654=CARTESIAN_POINT('Ctrl Pts',(79.0107132031554,7.19766911338125,138.514961868626));
#64655=CARTESIAN_POINT('Ctrl Pts',(78.9494151097006,7.23413790154083,138.511105512455));
#64656=CARTESIAN_POINT('Ctrl Pts',(78.8881351241464,7.27059591655638,138.507250295479));
#64657=CARTESIAN_POINT('Ctrl Pts',(78.8287356416693,7.31025912751879,138.503395078503));
#64658=CARTESIAN_POINT('Ctrl Pts',(78.7715633399465,7.35289923358147,138.499539861527));
#64659=CARTESIAN_POINT('Ctrl Pts',(78.7143888028114,7.39554100685382,138.495684493814));
#64660=CARTESIAN_POINT('Ctrl Pts',(78.6594420074097,7.44115961412183,138.4918291261));
#64661=CARTESIAN_POINT('Ctrl Pts',(78.6070382146028,7.48948517818491,138.487973758387));
#64662=CARTESIAN_POINT('Ctrl Pts',(78.554579569164,7.5378613260748,138.484114355144));
#64663=CARTESIAN_POINT('Ctrl Pts',(78.504669597791,7.58894975696965,138.480254951901));
#64664=CARTESIAN_POINT('Ctrl Pts',(78.4575875191527,7.64244289202017,138.476395548658));
#64665=CARTESIAN_POINT('Ctrl Pts',(78.4104787821856,7.69596631540177,138.472533960184));
#64666=CARTESIAN_POINT('Ctrl Pts',(78.3662014270749,7.75189677233906,138.468672371709));
#64667=CARTESIAN_POINT('Ctrl Pts',(78.3249933520973,7.8098948399483,138.464810783235));
#64668=CARTESIAN_POINT('Ctrl Pts',(78.2837131820615,7.86799437733164,138.460942438768));
#64669=CARTESIAN_POINT('Ctrl Pts',(78.2455132735932,7.92816833730001,138.457074094301));
#64670=CARTESIAN_POINT('Ctrl Pts',(78.2105869337642,7.99005027804126,138.453205749834));
#64671=CARTESIAN_POINT('Ctrl Pts',(78.1898487213581,8.02679391729671,138.450908842983));
#64672=CARTESIAN_POINT('Ctrl Pts',(78.170263755318,8.06413927692115,138.448611936133));
#64673=CARTESIAN_POINT('Ctrl Pts',(78.1518644287987,8.10200641819649,138.446315029283));
#64674=CARTESIAN_POINT('Ctrl Pts',(78.1182272557155,8.17123414693458,138.442115883558));
#64675=CARTESIAN_POINT('Ctrl Pts',(78.0884378127231,8.24244848245112,138.437916737834));
#64676=CARTESIAN_POINT('Ctrl Pts',(78.0627161720013,8.3152161419288,138.433717592109));
#64677=CARTESIAN_POINT('Ctrl Pts',(78.0373092445351,8.38709346368423,138.429569824399));
#64678=CARTESIAN_POINT('Ctrl Pts',(78.0158713067275,8.46048596644007,138.425422056689));
#64679=CARTESIAN_POINT('Ctrl Pts',(77.9985686429253,8.53495152358244,138.421274288979));
#64680=CARTESIAN_POINT('Ctrl Pts',(77.980944489384,8.61080067765593,138.417049454247));
#64681=CARTESIAN_POINT('Ctrl Pts',(77.9676110562608,8.68776283901531,138.412824619516));
#64682=CARTESIAN_POINT('Ctrl Pts',(77.958692352975,8.76534993565489,138.408599784784));
#64683=CARTESIAN_POINT('Ctrl Pts',(77.9497736496892,8.84293703229448,138.404374950053));
#64684=CARTESIAN_POINT('Ctrl Pts',(77.9452698355283,8.92114867256129,138.400150115321));
#64685=CARTESIAN_POINT('Ctrl Pts',(77.9452500654424,8.99948140989304,138.39592528059));
#64686=CARTESIAN_POINT('Ctrl Pts',(77.9452500654422,8.99948141084969,138.395925280538));
#64687=CARTESIAN_POINT('Ctrl Pts',(77.9452314949112,9.07306142557031,138.391956781385));
#64688=CARTESIAN_POINT('Ctrl Pts',(77.949169578864,9.14659881544574,138.387988282232));
#64689=CARTESIAN_POINT('Ctrl Pts',(77.9570245321472,9.21965609541188,138.38401978308));
#64690=CARTESIAN_POINT('Ctrl Pts',(77.9650800376541,9.29457866972499,138.379949960431));
#64691=CARTESIAN_POINT('Ctrl Pts',(77.9772551019451,9.36899578842017,138.375880137782));
#64692=CARTESIAN_POINT('Ctrl Pts',(77.9934509662062,9.44244608426484,138.371810315133));
#64693=CARTESIAN_POINT('Ctrl Pts',(78.0092901747818,9.51427890140046,138.367830115696));
#64694=CARTESIAN_POINT('Ctrl Pts',(78.0289746941144,9.58518663635699,138.36384991626));
#64695=CARTESIAN_POINT('Ctrl Pts',(78.052361793148,9.65475413531354,138.359869716823));
#64696=CARTESIAN_POINT('Ctrl Pts',(78.0765388125048,9.72667133917291,138.355755082568));
#64697=CARTESIAN_POINT('Ctrl Pts',(78.1046727995203,9.79715566665106,138.351640448313));
#64698=CARTESIAN_POINT('Ctrl Pts',(78.1365533044659,9.86577362826731,138.347525814057));
#64699=CARTESIAN_POINT('Ctrl Pts',(78.1684338094115,9.93439158988357,138.343411179802));
#64700=CARTESIAN_POINT('Ctrl Pts',(78.2040605214235,10.0011427673637,138.339296545546));
#64701=CARTESIAN_POINT('Ctrl Pts',(78.2431735357086,10.0656257958895,138.335181911291));
#64702=CARTESIAN_POINT('Ctrl Pts',(78.2799523824072,10.1262606373654,138.331312828193));
#64703=CARTESIAN_POINT('Ctrl Pts',(78.3199460623988,10.1851079346325,138.327443745094));
#64704=CARTESIAN_POINT('Ctrl Pts',(78.3629553810925,10.2418061355163,138.323574661996));
#64705=CARTESIAN_POINT('Ctrl Pts',(78.4059006180832,10.2984198589572,138.319711343635));
#64706=CARTESIAN_POINT('Ctrl Pts',(78.4518522838045,10.3528904581085,138.315848025274));
#64707=CARTESIAN_POINT('Ctrl Pts',(78.5005668003867,10.4048834978024,138.311984706913));
#64708=CARTESIAN_POINT('Ctrl Pts',(78.5492241749031,10.456815549727,138.308125920219));
#64709=CARTESIAN_POINT('Ctrl Pts',(78.6006376323835,10.506275462065,138.304267133526));
#64710=CARTESIAN_POINT('Ctrl Pts',(78.6545231511545,10.5529615615722,138.300408346833));
#64711=CARTESIAN_POINT('Ctrl Pts',(78.7083747260272,10.5996182522837,138.29655199089));
#64712=CARTESIAN_POINT('Ctrl Pts',(78.7646949064156,10.6435042794298,138.292695634947));
#64713=CARTESIAN_POINT('Ctrl Pts',(78.823163674952,10.6843556116651,138.288839279005));
#64714=CARTESIAN_POINT('Ctrl Pts',(78.8816151712512,10.7251948760234,138.284984062267));
#64715=CARTESIAN_POINT('Ctrl Pts',(78.9422135976179,10.7630009471533,138.281128845529));
#64716=CARTESIAN_POINT('Ctrl Pts',(79.0046081847904,10.7975518620373,138.277273628791));
#64717=CARTESIAN_POINT('Ctrl Pts',(79.0670052114209,10.8321041277678,138.273418261324));
#64718=CARTESIAN_POINT('Ctrl Pts',(79.1311981122362,10.8634007511762,138.269562893858));
#64719=CARTESIAN_POINT('Ctrl Pts',(79.1968111602771,10.8912655155331,138.265707526391));
#64720=CARTESIAN_POINT('Ctrl Pts',(79.2624928872782,10.9191594466959,138.261848123407));
#64721=CARTESIAN_POINT('Ctrl Pts',(79.3295972808572,10.9436141576524,138.257988720422));
#64722=CARTESIAN_POINT('Ctrl Pts',(79.3977290915692,10.9645017982578,138.254129317438));
#64723=CARTESIAN_POINT('Ctrl Pts',(79.4658994790494,10.9854012656098,138.250267729229));
#64724=CARTESIAN_POINT('Ctrl Pts',(79.5350979702551,11.0027295239452,138.246406141021));
#64725=CARTESIAN_POINT('Ctrl Pts',(79.6049173043078,11.0164094886864,138.242544552812));
#64726=CARTESIAN_POINT('Ctrl Pts',(79.6748587897351,11.0301133870059,138.238676208619));
#64727=CARTESIAN_POINT('Ctrl Pts',(79.7454228055223,11.0401561797858,138.234807864426));
#64728=CARTESIAN_POINT('Ctrl Pts',(79.8161958231075,11.0465125426092,138.230939520234));
#64729=CARTESIAN_POINT('Ctrl Pts',(79.8582187588651,11.0502867638547,138.228642611255));
#64730=CARTESIAN_POINT('Ctrl Pts',(79.9003153380743,11.0527622827936,138.226345702277));
#64731=CARTESIAN_POINT('Ctrl Pts',(79.9423993743182,11.0539424846916,138.224048793299));
#64732=CARTESIAN_POINT('Ctrl Pts',(80.0132740183776,11.0559300884698,138.220180518752));
#64733=CARTESIAN_POINT('Ctrl Pts',(80.0843904485706,11.0542488114017,138.216312244204));
#64734=CARTESIAN_POINT('Ctrl Pts',(80.1553371324466,11.048869917243,138.212443969656));
#64735=CARTESIAN_POINT('Ctrl Pts',(80.2261854267701,11.0434984825871,138.20858105967));
#64736=CARTESIAN_POINT('Ctrl Pts',(80.2968639617745,11.0344396404561,138.204718149683));
#64737=CARTESIAN_POINT('Ctrl Pts',(80.3669597863491,11.0217166165669,138.200855239696));
#64738=CARTESIAN_POINT('Ctrl Pts',(80.4369818596963,11.0090069791901,138.196996394065));
#64739=CARTESIAN_POINT('Ctrl Pts',(80.5064219639407,10.9926408981213,138.193137548434));
#64740=CARTESIAN_POINT('Ctrl Pts',(80.5748725845545,10.9726933552956,138.189278702803));
#64741=CARTESIAN_POINT('Ctrl Pts',(80.643281445159,10.9527579819663,138.185422211356));
#64742=CARTESIAN_POINT('Ctrl Pts',(80.7107015541047,10.9292456161871,138.18156571991));
#64743=CARTESIAN_POINT('Ctrl Pts',(80.7767374728931,10.902281908841,138.177709228464));
#64744=CARTESIAN_POINT('Ctrl Pts',(80.8427490507325,10.875328140362,138.173854158527));
#64745=CARTESIAN_POINT('Ctrl Pts',(80.907377003523,10.8449257435894,138.16999908859));
#64746=CARTESIAN_POINT('Ctrl Pts',(80.970244639271,10.8112489896384,138.166144018653));
#64747=CARTESIAN_POINT('Ctrl Pts',(81.0331314679079,10.7775619544959,138.1622877718));
#64748=CARTESIAN_POINT('Ctrl Pts',(81.0942564769342,10.7405987939562,138.158431524947));
#64749=CARTESIAN_POINT('Ctrl Pts',(81.1532675878569,10.7005797344726,138.154575278094));
#64750=CARTESIAN_POINT('Ctrl Pts',(81.1868977422625,10.6777730608045,138.15237762116));
#64751=CARTESIAN_POINT('Ctrl Pts',(81.2198418360838,10.6539747104964,138.150179964226));
#64752=CARTESIAN_POINT('Ctrl Pts',(81.252039109102,10.6292316077768,138.147982307292));
#64753=CARTESIAN_POINT('',(77.9452502723122,9.00105785954894,138.454074719513));
#64754=CARTESIAN_POINT('Ctrl Pts',(77.9452502723127,9.00105786047649,138.454074719462));
#64755=CARTESIAN_POINT('Ctrl Pts',(77.9452815714097,9.06185208850311,138.450761929014));
#64756=CARTESIAN_POINT('Ctrl Pts',(77.9480107215796,9.12257484666211,138.447449138566));
#64757=CARTESIAN_POINT('Ctrl Pts',(77.9534202484127,9.18305431678253,138.444136348118));
#64758=CARTESIAN_POINT('Ctrl Pts',(77.9597381600835,9.25368969061685,138.440267263431));
#64759=CARTESIAN_POINT('Ctrl Pts',(77.9697295884017,9.32413594375426,138.436398178743));
#64760=CARTESIAN_POINT('Ctrl Pts',(77.983374915349,9.39398074883996,138.432529094056));
#64761=CARTESIAN_POINT('Ctrl Pts',(77.9969999115152,9.46372148903559,138.428665774091));
#64762=CARTESIAN_POINT('Ctrl Pts',(78.0142679075233,9.53286208707632,138.424802454126));
#64763=CARTESIAN_POINT('Ctrl Pts',(78.0351074957408,9.60099501595759,138.42093913416));
#64764=CARTESIAN_POINT('Ctrl Pts',(78.055922639241,9.6690480253051,138.417080345847));
#64765=CARTESIAN_POINT('Ctrl Pts',(78.0803009118727,9.73609525104177,138.413221557534));
#64766=CARTESIAN_POINT('Ctrl Pts',(78.108120167371,9.80174076944595,138.40936276922));
#64767=CARTESIAN_POINT('Ctrl Pts',(78.1359218988618,9.86734493618424,138.405506411649));
#64768=CARTESIAN_POINT('Ctrl Pts',(78.1671601237219,9.93154870116641,138.401650054078));
#64769=CARTESIAN_POINT('Ctrl Pts',(78.2016638015601,9.99397408410912,138.397793696507));
#64770=CARTESIAN_POINT('Ctrl Pts',(78.2361572867389,10.0563810261,138.393938478134));
#64771=CARTESIAN_POINT('Ctrl Pts',(78.2739140749496,10.1170102040835,138.390083259762));
#64772=CARTESIAN_POINT('Ctrl Pts',(78.3147169902911,10.1755078645787,138.386228041389));
#64773=CARTESIAN_POINT('Ctrl Pts',(78.3555215009537,10.234007812228,138.382372672284));
#64774=CARTESIAN_POINT('Ctrl Pts',(78.3993720954813,10.2903756797582,138.37851730318));
#64775=CARTESIAN_POINT('Ctrl Pts',(78.4460090448423,10.3442877942569,138.374661934075));
#64776=CARTESIAN_POINT('Ctrl Pts',(78.4926948102755,10.3982563399268,138.370802529458));
#64777=CARTESIAN_POINT('Ctrl Pts',(78.5421724341588,10.4497636331277,138.366943124841));
#64778=CARTESIAN_POINT('Ctrl Pts',(78.5941433601851,10.4985208276124,138.363083720224));
#64779=CARTESIAN_POINT('Ctrl Pts',(78.6461437125364,10.5473056287835,138.359222130383));
#64780=CARTESIAN_POINT('Ctrl Pts',(78.7006398060556,10.5933369178648,138.355360540543));
#64781=CARTESIAN_POINT('Ctrl Pts',(78.757299944185,10.6363661368341,138.351498950702));
#64782=CARTESIAN_POINT('Ctrl Pts',(78.8140592108931,10.679470636688,138.347630604897));
#64783=CARTESIAN_POINT('Ctrl Pts',(78.8729896794131,10.7195623069091,138.343762259091));
#64784=CARTESIAN_POINT('Ctrl Pts',(78.9337312317319,10.756436300102,138.339893913285));
#64785=CARTESIAN_POINT('Ctrl Pts',(78.9697975343688,10.7783308442346,138.337597018899));
#64786=CARTESIAN_POINT('Ctrl Pts',(79.0065018721909,10.7990918456519,138.335300124513));
#64787=CARTESIAN_POINT('Ctrl Pts',(79.0437653768912,10.8186843893507,138.333003230127));
#64788=CARTESIAN_POINT('Ctrl Pts',(79.1065351778374,10.8516877280838,138.329134146835));
#64789=CARTESIAN_POINT('Ctrl Pts',(79.1711385346629,10.8815022513654,138.325265063544));
#64790=CARTESIAN_POINT('Ctrl Pts',(79.2372183974119,10.907920802668,138.321395980252));
#64791=CARTESIAN_POINT('Ctrl Pts',(79.303199804712,10.934299991747,138.317532661687));
#64792=CARTESIAN_POINT('Ctrl Pts',(79.370652903771,10.9572930735746,138.313669343123));
#64793=CARTESIAN_POINT('Ctrl Pts',(79.4391965878754,10.9767390053948,138.309806024558));
#64794=CARTESIAN_POINT('Ctrl Pts',(79.507659870606,10.9961621272414,138.305947237644));
#64795=CARTESIAN_POINT('Ctrl Pts',(79.577210732286,11.0120462318728,138.302088450731));
#64796=CARTESIAN_POINT('Ctrl Pts',(79.6474502948483,11.0242791971212,138.298229663818));
#64797=CARTESIAN_POINT('Ctrl Pts',(79.7176456118477,11.0365044565352,138.294373307647));
#64798=CARTESIAN_POINT('Ctrl Pts',(79.7885282915718,11.0450830564567,138.290516951475));
#64799=CARTESIAN_POINT('Ctrl Pts',(79.8596880116023,11.0499536844553,138.286660595303));
#64800=CARTESIAN_POINT('Ctrl Pts',(79.9308267105368,11.0548228736352,138.282805378327));
#64801=CARTESIAN_POINT('Ctrl Pts',(80.0022418029183,11.0559862323347,138.27895016135));
#64802=CARTESIAN_POINT('Ctrl Pts',(80.0735182970643,11.0534343482315,138.275094944374));
#64803=CARTESIAN_POINT('Ctrl Pts',(80.1447975780902,11.0508823643506,138.27123957666));
#64804=CARTESIAN_POINT('Ctrl Pts',(80.2159377647285,11.0446148688463,138.267384208947));
#64805=CARTESIAN_POINT('Ctrl Pts',(80.2865260569924,11.034674514797,138.263528841233));
#64806=CARTESIAN_POINT('Ctrl Pts',(80.3571882361534,11.0247237558789,138.25966943799));
#64807=CARTESIAN_POINT('Ctrl Pts',(80.4272968857301,11.0110925318276,138.255810034746));
#64808=CARTESIAN_POINT('Ctrl Pts',(80.4964474056167,10.9938750050985,138.251950631503));
#64809=CARTESIAN_POINT('Ctrl Pts',(80.5656370791975,10.976647729639,138.248089043028));
#64810=CARTESIAN_POINT('Ctrl Pts',(80.633867078276,10.9558302510362,138.244227454553));
#64811=CARTESIAN_POINT('Ctrl Pts',(80.7007486756041,10.9315664255052,138.240365866078));
#64812=CARTESIAN_POINT('Ctrl Pts',(80.7677472847718,10.9072601495099,138.23649752161));
#64813=CARTESIAN_POINT('Ctrl Pts',(80.8333923346689,10.8794956777869,138.232629177143));
#64814=CARTESIAN_POINT('Ctrl Pts',(80.8973164055592,10.848464452137,138.228760832675));
#64815=CARTESIAN_POINT('Ctrl Pts',(80.9352726003437,10.8300390416655,138.226463925829));
#64816=CARTESIAN_POINT('Ctrl Pts',(80.97262251972,10.8104627729485,138.224167018982));
#64817=CARTESIAN_POINT('Ctrl Pts',(81.009294052642,10.7897829694691,138.221870112135));
#64818=CARTESIAN_POINT('Ctrl Pts',(81.0710608673569,10.7549514397217,138.218001372316));
#64819=CARTESIAN_POINT('Ctrl Pts',(81.1311434378446,10.7168505093526,138.214132632498));
#64820=CARTESIAN_POINT('Ctrl Pts',(81.1891741649048,10.6756677379549,138.210263892679));
#64821=CARTESIAN_POINT('Ctrl Pts',(81.2104094466327,10.6605976570294,138.208848198199));
#64822=CARTESIAN_POINT('Ctrl Pts',(81.2313701765688,10.6451153604314,138.207432503719));
#64823=CARTESIAN_POINT('Ctrl Pts',(81.252039109102,10.6292316077768,138.206016809239));
#64824=CARTESIAN_POINT('Ctrl Pts',(81.252039109102,10.6292316077768,138.906139397334));
#64825=CARTESIAN_POINT('Ctrl Pts',(81.3085407521982,10.5858109752852,138.902270840373));
#64826=CARTESIAN_POINT('Ctrl Pts',(81.3627052394123,10.5395059841607,138.898402283413));
#64827=CARTESIAN_POINT('Ctrl Pts',(81.4142409434871,10.4906106521371,138.894533726453));
#64828=CARTESIAN_POINT('Ctrl Pts',(81.4402844253443,10.4659014778799,138.892578757663));
#64829=CARTESIAN_POINT('Ctrl Pts',(81.4656571881398,10.4405313514877,138.890623788874));
#64830=CARTESIAN_POINT('Ctrl Pts',(81.4903255365783,10.4145413947717,138.888668820084));
#64831=CARTESIAN_POINT('Ctrl Pts',(81.5391460723885,10.3631052957673,138.884799788315));
#64832=CARTESIAN_POINT('Ctrl Pts',(81.5853962816342,10.3090380201616,138.880930756546));
#64833=CARTESIAN_POINT('Ctrl Pts',(81.6287797626174,10.2526268588004,138.877061724777));
#64834=CARTESIAN_POINT('Ctrl Pts',(81.6720985943052,10.1962997603531,138.873198458571));
#64835=CARTESIAN_POINT('Ctrl Pts',(81.712558883679,10.1376360912374,138.869335192365));
#64836=CARTESIAN_POINT('Ctrl Pts',(81.7499020673934,10.0769588279188,138.865471926159));
#64837=CARTESIAN_POINT('Ctrl Pts',(81.7872014376145,10.0163527551793,138.861613192592));
#64838=CARTESIAN_POINT('Ctrl Pts',(81.8213907132125,9.95373819263796,138.857754459025));
#64839=CARTESIAN_POINT('Ctrl Pts',(81.8522535789957,9.88946851636106,138.853895725458));
#64840=CARTESIAN_POINT('Ctrl Pts',(81.883096998617,9.82523933530386,138.850039423213));
#64841=CARTESIAN_POINT('Ctrl Pts',(81.9106179568823,9.75935754641112,138.846183120968));
#64842=CARTESIAN_POINT('Ctrl Pts',(81.9346459246051,9.69220134997619,138.842326818723));
#64843=CARTESIAN_POINT('Ctrl Pts',(81.9586667910779,9.62506500095187,138.838471656174));
#64844=CARTESIAN_POINT('Ctrl Pts',(81.9791965528858,9.55665544927177,138.834616493624));
#64845=CARTESIAN_POINT('Ctrl Pts',(81.9961133578074,9.48736949564268,138.830761331075));
#64846=CARTESIAN_POINT('Ctrl Pts',(82.0130308223352,9.41808084047218,138.826906018208));
#64847=CARTESIAN_POINT('Ctrl Pts',(82.0263349372039,9.34791618796618,138.823050705341));
#64848=CARTESIAN_POINT('Ctrl Pts',(82.0359545511563,9.27728438132338,138.819195392474));
#64849=CARTESIAN_POINT('Ctrl Pts',(82.0455842337334,9.20657864602208,138.815336044342));
#64850=CARTESIAN_POINT('Ctrl Pts',(82.0515216513016,9.1354052628522,138.811476696209));
#64851=CARTESIAN_POINT('Ctrl Pts',(82.0537474515665,9.06417918419796,138.807617348076));
#64852=CARTESIAN_POINT('Ctrl Pts',(82.0559745119851,8.99291278035721,138.803755814944));
#64853=CARTESIAN_POINT('Ctrl Pts',(82.0544857820866,8.92159410756425,138.799894281813));
#64854=CARTESIAN_POINT('Ctrl Pts',(82.0493140468048,8.85063634957434,138.796032748681));
#64855=CARTESIAN_POINT('Ctrl Pts',(82.0441332629383,8.77955444229137,138.792164459323));
#64856=CARTESIAN_POINT('Ctrl Pts',(82.0352566688447,8.70883519271668,138.788296169966));
#64857=CARTESIAN_POINT('Ctrl Pts',(82.022768635003,8.63888421282376,138.784427880609));
#64858=CARTESIAN_POINT('Ctrl Pts',(82.0153519407318,8.59734004034512,138.78213048777));
#64859=CARTESIAN_POINT('Ctrl Pts',(82.0066623866894,8.55606663228185,138.779833094931));
#64860=CARTESIAN_POINT('Ctrl Pts',(81.9967259333571,8.51514630087099,138.777535702093));
#64861=CARTESIAN_POINT('Ctrl Pts',(81.9799917090061,8.44623136880734,138.773666606562));
#64862=CARTESIAN_POINT('Ctrl Pts',(81.9596527305356,8.37804882930313,138.769797511031));
#64863=CARTESIAN_POINT('Ctrl Pts',(81.9357896132602,8.31100352998452,138.765928415499));
#64864=CARTESIAN_POINT('Ctrl Pts',(81.9119620501116,8.24405812277302,138.76206508461));
#64865=CARTESIAN_POINT('Ctrl Pts',(81.8846209321863,8.17824704634329,138.75820175372));
#64866=CARTESIAN_POINT('Ctrl Pts',(81.8538973778349,8.11396271243415,138.75433842283));
#64867=CARTESIAN_POINT('Ctrl Pts',(81.8232098614146,8.04975378237869,138.750479623527));
#64868=CARTESIAN_POINT('Ctrl Pts',(81.7891479978466,7.98706847381701,138.746620824224));
#64869=CARTESIAN_POINT('Ctrl Pts',(81.7518913592263,7.92628019112604,138.742762024921));
#64870=CARTESIAN_POINT('Ctrl Pts',(81.7146581890478,7.86553019976588,138.738905656326));
#64871=CARTESIAN_POINT('Ctrl Pts',(81.6742344896948,7.80667527669055,138.735049287731));
#64872=CARTESIAN_POINT('Ctrl Pts',(81.6308455216996,7.75006382288835,138.731192919135));
#64873=CARTESIAN_POINT('Ctrl Pts',(81.5874693709153,7.69346909225297,138.727337689721));
#64874=CARTESIAN_POINT('Ctrl Pts',(81.541129985835,7.63911690054514,138.723482460307));
#64875=CARTESIAN_POINT('Ctrl Pts',(81.4920946545808,7.58732484120678,138.719627230893));
#64876=CARTESIAN_POINT('Ctrl Pts',(81.4430574061278,7.53553075688624,138.715771850746));
#64877=CARTESIAN_POINT('Ctrl Pts',(81.3913243378103,7.48629735490751,138.711916470599));
#64878=CARTESIAN_POINT('Ctrl Pts',(81.3372003536463,7.43990616413363,138.708061090452));
#64879=CARTESIAN_POINT('Ctrl Pts',(81.2830197177678,7.39346641558012,138.704201674869));
#64880=CARTESIAN_POINT('Ctrl Pts',(81.226443539926,7.34987513368378,138.700342259285));
#64881=CARTESIAN_POINT('Ctrl Pts',(81.1678099508912,7.30937364237406,138.696482843702));
#64882=CARTESIAN_POINT('Ctrl Pts',(81.1091431635748,7.26884921915905,138.692621242921));
#64883=CARTESIAN_POINT('Ctrl Pts',(81.0484170598279,7.23141832413785,138.68875964214));
#64884=CARTESIAN_POINT('Ctrl Pts',(80.9859965624117,7.19727751957983,138.684898041359));
#64885=CARTESIAN_POINT('Ctrl Pts',(80.9234668614125,7.16307698627339,138.681029684775));
#64886=CARTESIAN_POINT('Ctrl Pts',(80.8592372863073,7.1321782460189,138.67716132819));
#64887=CARTESIAN_POINT('Ctrl Pts',(80.7936943772722,7.10473041548533,138.673292971605));
#64888=CARTESIAN_POINT('Ctrl Pts',(80.7547789678034,7.08843355622214,138.670996175771));
#64889=CARTESIAN_POINT('Ctrl Pts',(80.7154009159473,7.07335229548095,138.668699379936));
#64890=CARTESIAN_POINT('Ctrl Pts',(80.6756433883754,7.0595094501017,138.666402584101));
#64891=CARTESIAN_POINT('Ctrl Pts',(80.6086694833816,7.03619035890327,138.66253349577));
#64892=CARTESIAN_POINT('Ctrl Pts',(80.5403557403813,7.01629696299707,138.658664407438));
#64893=CARTESIAN_POINT('Ctrl Pts',(80.4710860080223,6.99998111620275,138.654795319106));
#64894=CARTESIAN_POINT('Ctrl Pts',(80.401919481385,6.98368957856462,138.650931995371));
#64895=CARTESIAN_POINT('Ctrl Pts',(80.3318002616527,6.97096512014625,138.647068671636));
#64896=CARTESIAN_POINT('Ctrl Pts',(80.2611291415901,6.9619104205378,138.643205347901));
#64897=CARTESIAN_POINT('Ctrl Pts',(80.1905409151791,6.9528663416343,138.639346555649));
#64898=CARTESIAN_POINT('Ctrl Pts',(80.119402553801,6.94748353289814,138.635487763397));
#64899=CARTESIAN_POINT('Ctrl Pts',(80.04812516192,6.94581365711624,138.631628971146));
#64900=CARTESIAN_POINT('Ctrl Pts',(79.9768926674239,6.94414483318336,138.627772609534));
#64901=CARTESIAN_POINT('Ctrl Pts',(79.9055218006725,6.94618431348433,138.623916247922));
#64902=CARTESIAN_POINT('Ctrl Pts',(79.8344274404792,6.95193181509166,138.62005988631));
#64903=CARTESIAN_POINT('Ctrl Pts',(79.7633540803268,6.95767761898671,138.616204663801));
#64904=CARTESIAN_POINT('Ctrl Pts',(79.6925575485226,6.96712923061955,138.612349441292));
#64905=CARTESIAN_POINT('Ctrl Pts',(79.622449636365,6.98023434888622,138.608494218782));
#64906=CARTESIAN_POINT('Ctrl Pts',(79.5523389814721,6.99333997984638,138.60463884545));
#64907=CARTESIAN_POINT('Ctrl Pts',(79.4829174768171,7.01009930978598,138.600783472118));
#64908=CARTESIAN_POINT('Ctrl Pts',(79.4145870167333,7.03040887453188,138.596928098786));
#64909=CARTESIAN_POINT('Ctrl Pts',(79.3461850315659,7.05073969836654,138.593068689833));
#64910=CARTESIAN_POINT('Ctrl Pts',(79.278876837367,7.07462803672365,138.589209280879));
#64911=CARTESIAN_POINT('Ctrl Pts',(79.2130485724695,7.10192070418339,138.585349871925));
#64912=CARTESIAN_POINT('Ctrl Pts',(79.1471830339926,7.12922882542137,138.581488277679));
#64913=CARTESIAN_POINT('Ctrl Pts',(79.0827995316105,7.15994490377779,138.577626683433));
#64914=CARTESIAN_POINT('Ctrl Pts',(79.0202611292601,7.193868967195,138.573765089187));
#64915=CARTESIAN_POINT('Ctrl Pts',(78.9576133132683,7.2278523822293,138.569896738915));
#64916=CARTESIAN_POINT('Ctrl Pts',(78.8968174567556,7.26505473422092,138.566028388643));
#64917=CARTESIAN_POINT('Ctrl Pts',(78.8382084878197,7.30523215609752,138.562160038371));
#64918=CARTESIAN_POINT('Ctrl Pts',(78.8034090421307,7.32908775424069,138.559863180951));
#64919=CARTESIAN_POINT('Ctrl Pts',(78.7693799733918,7.35399140607145,138.55756632353));
#64920=CARTESIAN_POINT('Ctrl Pts',(78.7361855638254,7.37988561100871,138.55526946611));
#64921=CARTESIAN_POINT('Ctrl Pts',(78.6809217158299,7.42299568358746,138.551445533676));
#64922=CARTESIAN_POINT('Ctrl Pts',(78.6277456591824,7.4690309331306,138.547621601243));
#64923=CARTESIAN_POINT('Ctrl Pts',(78.5769890146386,7.51775936567617,138.54379766881));
#64924=CARTESIAN_POINT('Ctrl Pts',(78.526318708678,7.5664049096883,138.539980241001));
#64925=CARTESIAN_POINT('Ctrl Pts',(78.4780599994551,7.61773419861886,138.536162813192));
#64926=CARTESIAN_POINT('Ctrl Pts',(78.432512620332,7.67147417146613,138.532345385383));
#64927=CARTESIAN_POINT('Ctrl Pts',(78.3870085968665,7.72516299028648,138.528531591308));
#64928=CARTESIAN_POINT('Ctrl Pts',(78.3442111085944,7.78125756695914,138.524717797234));
#64929=CARTESIAN_POINT('Ctrl Pts',(78.3043830638176,7.8394480760296,138.52090400316));
#64930=CARTESIAN_POINT('Ctrl Pts',(78.2645788522619,7.8976037637254,138.517092491271));
#64931=CARTESIAN_POINT('Ctrl Pts',(78.2277408414614,7.9578524865062,138.513280979383));
#64932=CARTESIAN_POINT('Ctrl Pts',(78.1940904589338,8.01985292328849,138.509469467494));
#64933=CARTESIAN_POINT('Ctrl Pts',(78.1604483202982,8.08183817079624,138.505658889375));
#64934=CARTESIAN_POINT('Ctrl Pts',(78.1299924969411,8.14557384247176,138.501848311256));
#64935=CARTESIAN_POINT('Ctrl Pts',(78.1028990533745,8.2106929869736,138.498037733137));
#64936=CARTESIAN_POINT('Ctrl Pts',(78.0757855808063,8.27586027121978,138.494224338023));
#64937=CARTESIAN_POINT('Ctrl Pts',(78.0520396483184,8.34241261158696,138.49041094291));
#64938=CARTESIAN_POINT('Ctrl Pts',(78.0317891512923,8.40996303714985,138.486597547796));
#64939=CARTESIAN_POINT('Ctrl Pts',(78.0115315635821,8.47753711540316,138.482782817427));
#64940=CARTESIAN_POINT('Ctrl Pts',(77.9947719694412,8.54610949060837,138.478968087059));
#64941=CARTESIAN_POINT('Ctrl Pts',(77.9815875948563,8.61528071888466,138.47515335669));
#64942=CARTESIAN_POINT('Ctrl Pts',(77.9683814171201,8.68456633641301,138.471332317858));
#64943=CARTESIAN_POINT('Ctrl Pts',(77.9587623377827,8.75445229062171,138.467511279026));
#64944=CARTESIAN_POINT('Ctrl Pts',(77.9527558264947,8.82453246297826,138.463690240194));
#64945=CARTESIAN_POINT('Ctrl Pts',(77.947717429342,8.88331729229607,138.460485066634));
#64946=CARTESIAN_POINT('Ctrl Pts',(77.9452199900013,8.94223854834861,138.457279893073));
#64947=CARTESIAN_POINT('Ctrl Pts',(77.9452502723122,9.00105785954894,138.454074719513));
#64948=CARTESIAN_POINT('Origin',(80.,9.,141.545925280538));
#64949=CARTESIAN_POINT('',(81.252039109102,10.6292316077768,139.606097362941));
#64950=CARTESIAN_POINT('',(81.252039109102,10.6292316077768,139.54788294617));
#64951=CARTESIAN_POINT('',(81.252039109102,10.6292316077768,141.545925280538));
#64952=CARTESIAN_POINT('',(77.9455904459809,8.99784754164576,139.854074871274));
#64953=CARTESIAN_POINT('Ctrl Pts',(77.9452511248424,8.99784999107146,139.854074719462));
#64954=CARTESIAN_POINT('Ctrl Pts',(77.9451772245318,9.06847601408026,139.850255479513));
#64955=CARTESIAN_POINT('Ctrl Pts',(77.948748952018,9.13916590444103,139.846436239564));
#64956=CARTESIAN_POINT('Ctrl Pts',(77.9559592417713,9.20951119588218,139.842616999616));
#64957=CARTESIAN_POINT('Ctrl Pts',(77.9631671377139,9.27983313273904,139.838799027652));
#64958=CARTESIAN_POINT('Ctrl Pts',(77.9740111489395,9.34981020491898,139.834981055688));
#64959=CARTESIAN_POINT('Ctrl Pts',(77.9884322523696,9.41903789708474,139.831163083724));
#64960=CARTESIAN_POINT('Ctrl Pts',(78.0028536112544,9.48826681554625,139.827345044128));
#64961=CARTESIAN_POINT('Ctrl Pts',(78.0208520847495,9.55674584287351,139.823527004533));
#64962=CARTESIAN_POINT('Ctrl Pts',(78.0423176863816,9.6240813420106,139.819708964937));
#64963=CARTESIAN_POINT('Ctrl Pts',(78.0638064102382,9.6914893733109,139.815886812643));
#64964=CARTESIAN_POINT('Ctrl Pts',(78.0887695660473,9.75775094445758,139.812064660348));
#64965=CARTESIAN_POINT('Ctrl Pts',(78.1170477875132,9.82248922667171,139.808242508053));
#64966=CARTESIAN_POINT('Ctrl Pts',(78.1453421859075,9.88726454327152,139.804418169246));
#64967=CARTESIAN_POINT('Ctrl Pts',(78.1769552003258,9.9505143942472,139.800593830438));
#64968=CARTESIAN_POINT('Ctrl Pts',(78.2116812500701,10.0118861651139,139.796769491631));
#64969=CARTESIAN_POINT('Ctrl Pts',(78.2464714535704,10.0733713156956,139.792938087646));
#64970=CARTESIAN_POINT('Ctrl Pts',(78.2843859059249,10.1329710424756,139.789106683661));
#64971=CARTESIAN_POINT('Ctrl Pts',(78.3251758574949,10.1903619845165,139.785275279677));
#64972=CARTESIAN_POINT('Ctrl Pts',(78.3519387238618,10.2280169964347,139.782761441124));
#64973=CARTESIAN_POINT('Ctrl Pts',(78.3799385966649,10.2647218133961,139.78024760257));
#64974=CARTESIAN_POINT('Ctrl Pts',(78.4090964374419,10.3003935624033,139.777733764017));
#64975=CARTESIAN_POINT('Ctrl Pts',(78.4539904417997,10.3553169590851,139.773863234652));
#64976=CARTESIAN_POINT('Ctrl Pts',(78.5018202761645,10.4080207897608,139.769992705286));
#64977=CARTESIAN_POINT('Ctrl Pts',(78.5523382569853,10.4581745575587,139.766122175921));
#64978=CARTESIAN_POINT('Ctrl Pts',(78.6027802752742,10.5082529104821,139.762257466566));
#64979=CARTESIAN_POINT('Ctrl Pts',(78.6559020748355,10.5557884727724,139.758392757212));
#64980=CARTESIAN_POINT('Ctrl Pts',(78.711415789056,10.6004837686793,139.754528047858));
#64981=CARTESIAN_POINT('Ctrl Pts',(78.7668631203186,10.6451256182264,139.750667959899));
#64982=CARTESIAN_POINT('Ctrl Pts',(78.8246963083252,10.6869336452058,139.74680787194));
#64983=CARTESIAN_POINT('Ctrl Pts',(78.8845919934093,10.7256484408284,139.742947783981));
#64984=CARTESIAN_POINT('Ctrl Pts',(78.9444490883844,10.7643382929482,139.739090183033));
#64985=CARTESIAN_POINT('Ctrl Pts',(79.0063656373174,10.7999386049239,139.735232582086));
#64986=CARTESIAN_POINT('Ctrl Pts',(79.069987857513,10.832232238917,139.731374981138));
#64987=CARTESIAN_POINT('Ctrl Pts',(79.1335903276766,10.8645158481058,139.727518577692));
#64988=CARTESIAN_POINT('Ctrl Pts',(79.198896985352,10.8934945976222,139.723662174246));
#64989=CARTESIAN_POINT('Ctrl Pts',(79.2655294269345,10.9189972745684,139.7198057708));
#64990=CARTESIAN_POINT('Ctrl Pts',(79.3321634293518,10.9445005489032,139.71594927702));
#64991=CARTESIAN_POINT('Ctrl Pts',(79.4001228232358,10.9665274175566,139.712092783239));
#64992=CARTESIAN_POINT('Ctrl Pts',(79.4690108268965,10.9849554303679,139.708236289459));
#64993=CARTESIAN_POINT('Ctrl Pts',(79.5379691156553,11.0034022449242,139.704375860973));
#64994=CARTESIAN_POINT('Ctrl Pts',(79.6078574357236,11.0182427478266,139.700515432486));
#64995=CARTESIAN_POINT('Ctrl Pts',(79.6782663795838,11.0294050950941,139.696655004));
#64996=CARTESIAN_POINT('Ctrl Pts',(79.7487141688414,11.0405736007527,139.692792445672));
#64997=CARTESIAN_POINT('Ctrl Pts',(79.8196826707769,11.0480598596463,139.688929887345));
#64998=CARTESIAN_POINT('Ctrl Pts',(79.8907576027215,11.0518439660795,139.685067329017));
#64999=CARTESIAN_POINT('Ctrl Pts',(79.9619550325507,11.0556345944329,139.681198113557));
#65000=CARTESIAN_POINT('Ctrl Pts',(80.0332587730399,11.0557103301937,139.677328898097));
#65001=CARTESIAN_POINT('Ctrl Pts',(80.104255499616,11.0521033973218,139.673459682637));
#65002=CARTESIAN_POINT('Ctrl Pts',(80.1462079446659,11.0499720363366,139.6711733371));
#65003=CARTESIAN_POINT('Ctrl Pts',(80.188053284814,11.0465557851209,139.668886991563));
#65004=CARTESIAN_POINT('Ctrl Pts',(80.2297077887632,11.0418697055105,139.666600646025));
#65005=CARTESIAN_POINT('Ctrl Pts',(80.3003043705021,11.0339276783372,139.662725718603));
#65006=CARTESIAN_POINT('Ctrl Pts',(80.3706219865153,11.0223050986904,139.658850791181));
#65007=CARTESIAN_POINT('Ctrl Pts',(80.4402478017776,11.0070324948864,139.654975863759));
#65008=CARTESIAN_POINT('Ctrl Pts',(80.5097766126523,10.9917811692473,139.65110633498));
#65009=CARTESIAN_POINT('Ctrl Pts',(80.5786150665536,10.972890014512,139.647236806202));
#65010=CARTESIAN_POINT('Ctrl Pts',(80.6463564374629,10.9504412111751,139.643367277423));
#65011=CARTESIAN_POINT('Ctrl Pts',(80.7140191932826,10.9280184600817,139.639502239303));
#65012=CARTESIAN_POINT('Ctrl Pts',(80.7805869383724,10.902046414884,139.635637201183));
#65013=CARTESIAN_POINT('Ctrl Pts',(80.8456659041088,10.8726576678955,139.631772163063));
#65014=CARTESIAN_POINT('Ctrl Pts',(80.9107018355553,10.8432883545879,139.627909680748));
#65015=CARTESIAN_POINT('Ctrl Pts',(80.9742505024658,10.8105070244793,139.624047198433));
#65016=CARTESIAN_POINT('Ctrl Pts',(81.0359374021744,10.7744946495485,139.620184716118));
#65017=CARTESIAN_POINT('Ctrl Pts',(81.097608619952,10.7384914296178,139.616323215717));
#65018=CARTESIAN_POINT('Ctrl Pts',(81.1574185920664,10.6992590385842,139.612461715315));
#65019=CARTESIAN_POINT('Ctrl Pts',(81.2150181804927,10.6570239538318,139.608600214913));
#65020=CARTESIAN_POINT('Ctrl Pts',(81.2274626734363,10.6478989890788,139.607765930923));
#65021=CARTESIAN_POINT('Ctrl Pts',(81.2398040956947,10.6386340249735,139.606931646932));
#65022=CARTESIAN_POINT('Ctrl Pts',(81.252039109102,10.6292316077768,139.606097362941));
#65023=CARTESIAN_POINT('',(79.4698297828112,7.01482567432834,140.));
#65024=CARTESIAN_POINT('Ctrl Pts',(79.4698297828112,7.01482567432834,140.));
#65025=CARTESIAN_POINT('Ctrl Pts',(78.8097404375817,7.19111231424644,139.962955627336));
#65026=CARTESIAN_POINT('Ctrl Pts',(78.0751152861664,7.88746878509532,139.914314179013));
#65027=CARTESIAN_POINT('Ctrl Pts',(77.9457329218076,8.78359621258651,139.86567273069));
#65028=CARTESIAN_POINT('Ctrl Pts',(77.9473422520121,8.99783489604774,139.85407565503));
#65029=CARTESIAN_POINT('',(80.5303700321158,7.01487904863873,139.999999991429));
#65030=CARTESIAN_POINT('Origin',(80.,9.,140.));
#65031=CARTESIAN_POINT('',(77.94525054989,9.00150325402769,139.795925280583));
#65032=CARTESIAN_POINT('Ctrl Pts',(80.5303700321158,7.01487904863873,139.999999991429));
#65033=CARTESIAN_POINT('Ctrl Pts',(80.4620742005438,6.99663227009389,139.996143017033));
#65034=CARTESIAN_POINT('Ctrl Pts',(80.3926969237085,6.98187705917305,139.992286042637));
#65035=CARTESIAN_POINT('Ctrl Pts',(80.3226296813442,6.97073716556584,139.988429068241));
#65036=CARTESIAN_POINT('Ctrl Pts',(80.2526676763219,6.95961400349758,139.984577886819));
#65037=CARTESIAN_POINT('Ctrl Pts',(80.1820182414636,6.95209545848432,139.980726705397));
#65038=CARTESIAN_POINT('Ctrl Pts',(80.1110863019471,6.94825503631184,139.976875523975));
#65039=CARTESIAN_POINT('Ctrl Pts',(80.0402381740564,6.94441915189807,139.973028893025));
#65040=CARTESIAN_POINT('Ctrl Pts',(79.9691086905236,6.94425278531202,139.969182262075));
#65041=CARTESIAN_POINT('Ctrl Pts',(79.8981094276751,6.94777782056345,139.965335631125));
#65042=CARTESIAN_POINT('Ctrl Pts',(79.8271548669589,6.95130063640322,139.961491422068));
#65043=CARTESIAN_POINT('Ctrl Pts',(79.7563308517412,6.95851021955747,139.95764721301));
#65044=CARTESIAN_POINT('Ctrl Pts',(79.6860489785746,6.96937637198669,139.953803003953));
#65045=CARTESIAN_POINT('Ctrl Pts',(79.6157874515818,6.98023937873102,139.949959907771));
#65046=CARTESIAN_POINT('Ctrl Pts',(79.5460682382953,6.99475677865711,139.946116811588));
#65047=CARTESIAN_POINT('Ctrl Pts',(79.4772960600091,7.01284672115663,139.942273715406));
#65048=CARTESIAN_POINT('Ctrl Pts',(79.4085204004781,7.03093757936825,139.938430424687));
#65049=CARTESIAN_POINT('Ctrl Pts',(79.3406923435553,7.05260121217767,139.934587133967));
#65050=CARTESIAN_POINT('Ctrl Pts',(79.2742029617191,7.07770547997382,139.930743843247));
#65051=CARTESIAN_POINT('Ctrl Pts',(79.2076449190222,7.10283567191889,139.926896583719));
#65052=CARTESIAN_POINT('Ctrl Pts',(79.1424287685514,7.13141341594115,139.92304932419));
#65053=CARTESIAN_POINT('Ctrl Pts',(79.078926116778,7.16325819339072,139.919202064662));
#65054=CARTESIAN_POINT('Ctrl Pts',(79.0153861545328,7.19512168098292,139.915352544707));
#65055=CARTESIAN_POINT('Ctrl Pts',(78.953562119514,7.23025577981269,139.911503024752));
#65056=CARTESIAN_POINT('Ctrl Pts',(78.8937990765748,7.26843507788096,139.907653504797));
#65057=CARTESIAN_POINT('Ctrl Pts',(78.8339359110614,7.30667833871634,139.903797535642));
#65058=CARTESIAN_POINT('Ctrl Pts',(78.7761410253502,7.34797669509396,139.899941566487));
#65059=CARTESIAN_POINT('Ctrl Pts',(78.7207279840538,7.39206322521163,139.896085597331));
#65060=CARTESIAN_POINT('Ctrl Pts',(78.6965850159507,7.41127133336641,139.894405585945));
#65061=CARTESIAN_POINT('Ctrl Pts',(78.6728937264846,7.43100822304824,139.892725574559));
#65062=CARTESIAN_POINT('Ctrl Pts',(78.6496778175411,7.4512496760099,139.891045563173));
#65063=CARTESIAN_POINT('Ctrl Pts',(78.5949087487768,7.4990016521157,139.887082218065));
#65064=CARTESIAN_POINT('Ctrl Pts',(78.5425524775813,7.54977030605766,139.883118872957));
#65065=CARTESIAN_POINT('Ctrl Pts',(78.4929635885723,7.60327568320336,139.879155527849));
#65066=CARTESIAN_POINT('Ctrl Pts',(78.4452783589226,7.65472705159813,139.875344330917));
#65067=CARTESIAN_POINT('Ctrl Pts',(78.4001523191138,7.70870846833804,139.871533133985));
#65068=CARTESIAN_POINT('Ctrl Pts',(78.3578674318731,7.76492988409682,139.867721937053));
#65069=CARTESIAN_POINT('Ctrl Pts',(78.3156213126652,7.82109975440216,139.863914234339));
#65070=CARTESIAN_POINT('Ctrl Pts',(78.2762114818338,7.87950515554645,139.860106531624));
#65071=CARTESIAN_POINT('Ctrl Pts',(78.2398808669802,7.93982161874629,139.85629882891));
#65072=CARTESIAN_POINT('Ctrl Pts',(78.2035706386586,8.00010423601464,139.852493262847));
#65073=CARTESIAN_POINT('Ctrl Pts',(78.1703364568118,8.06229536107818,139.848687696784));
#65074=CARTESIAN_POINT('Ctrl Pts',(78.1403778852329,8.12604167561079,139.844882130721));
#65075=CARTESIAN_POINT('Ctrl Pts',(78.1104254709766,8.18977488849674,139.841077346809));
#65076=CARTESIAN_POINT('Ctrl Pts',(78.0837475415326,8.25506220336587,139.837272562896));
#65077=CARTESIAN_POINT('Ctrl Pts',(78.0604967835646,8.32152757171954,139.833467778983));
#65078=CARTESIAN_POINT('Ctrl Pts',(78.0372308381719,8.38803635533663,139.82966050978));
#65079=CARTESIAN_POINT('Ctrl Pts',(78.0173966988217,8.45572425618672,139.825853240578));
#65080=CARTESIAN_POINT('Ctrl Pts',(78.0010976898141,8.52419844805488,139.822045971375));
#65081=CARTESIAN_POINT('Ctrl Pts',(77.9847922409877,8.59269969441341,139.818237197902));
#65082=CARTESIAN_POINT('Ctrl Pts',(77.9720247942908,8.66198735860674,139.814428424428));
#65083=CARTESIAN_POINT('Ctrl Pts',(77.9628473589046,8.73165939670294,139.810619650955));
#65084=CARTESIAN_POINT('Ctrl Pts',(77.9536577739424,8.80142367033923,139.806805835225));
#65085=CARTESIAN_POINT('Ctrl Pts',(77.9480677197906,8.87157283521784,139.802992019495));
#65086=CARTESIAN_POINT('Ctrl Pts',(77.9460771919704,8.94170196267724,139.799178203766));
#65087=CARTESIAN_POINT('Ctrl Pts',(77.9455112640781,8.96164040759028,139.798093896038));
#65088=CARTESIAN_POINT('Ctrl Pts',(77.9452359720325,8.98157725069431,139.79700958831));
#65089=CARTESIAN_POINT('Ctrl Pts',(77.94525054989,9.00150325402769,139.795925280583));
#65090=CARTESIAN_POINT('Ctrl Pts',(77.9452505498906,9.0015032548487,139.795925280538));
#65091=CARTESIAN_POINT('Ctrl Pts',(77.945322310872,9.0995909724926,139.790587668752));
#65092=CARTESIAN_POINT('Ctrl Pts',(77.9524183464193,9.19742452109931,139.785250056967));
#65093=CARTESIAN_POINT('Ctrl Pts',(77.9664267220482,9.29424018369419,139.779912445181));
#65094=CARTESIAN_POINT('Ctrl Pts',(77.9765717595288,9.36435527424839,139.776046881246));
#65095=CARTESIAN_POINT('Ctrl Pts',(77.990367502887,9.43408480533988,139.772181317311));
#65096=CARTESIAN_POINT('Ctrl Pts',(78.0077726792506,9.50301875209562,139.768315753376));
#65097=CARTESIAN_POINT('Ctrl Pts',(78.0251516710698,9.57184899384097,139.764456004839));
#65098=CARTESIAN_POINT('Ctrl Pts',(78.0461291999042,9.63988555882835,139.760596256302));
#65099=CARTESIAN_POINT('Ctrl Pts',(78.0706125287104,9.70672593565721,139.756736507765));
#65100=CARTESIAN_POINT('Ctrl Pts',(78.0950667440095,9.7734868315547,139.752881348915));
#65101=CARTESIAN_POINT('Ctrl Pts',(78.1230183124154,9.83905390971274,139.749026190065));
#65102=CARTESIAN_POINT('Ctrl Pts',(78.1543244441948,9.90303892784481,139.745171031215));
#65103=CARTESIAN_POINT('Ctrl Pts',(78.1856105615418,9.9669830394916,139.74131833702));
#65104=CARTESIAN_POINT('Ctrl Pts',(78.2202467742583,10.0293466614236,139.737465642825));
#65105=CARTESIAN_POINT('Ctrl Pts',(78.2580424198006,10.0897620617758,139.733612948631));
#65106=CARTESIAN_POINT('Ctrl Pts',(78.2958266099266,10.1501591509297,139.729761422142));
#65107=CARTESIAN_POINT('Ctrl Pts',(78.336768073914,10.2086087782143,139.725909895653));
#65108=CARTESIAN_POINT('Ctrl Pts',(78.3806313708818,10.2647698626737,139.722058369165));
#65109=CARTESIAN_POINT('Ctrl Pts',(78.4244961209918,10.3209328076874,139.71820671508));
#65110=CARTESIAN_POINT('Ctrl Pts',(78.4712825948598,10.3748066770552,139.714355060994));
#65111=CARTESIAN_POINT('Ctrl Pts',(78.5207144708289,10.4260827064673,139.710503406909));
#65112=CARTESIAN_POINT('Ctrl Pts',(78.5701980116868,10.4774123282285,139.706647727177));
#65113=CARTESIAN_POINT('Ctrl Pts',(78.6223321354694,10.5261383386816,139.702792047444));
#65114=CARTESIAN_POINT('Ctrl Pts',(78.676803622504,10.5719888387267,139.698936367712));
#65115=CARTESIAN_POINT('Ctrl Pts',(78.7313058224108,10.6178651908392,139.695078514017));
#65116=CARTESIAN_POINT('Ctrl Pts',(78.7881476204764,10.6608625113955,139.691220660322));
#65117=CARTESIAN_POINT('Ctrl Pts',(78.8469848839622,10.7007509237653,139.687362806626));
#65118=CARTESIAN_POINT('Ctrl Pts',(78.9059255314841,10.7407094247969,139.683498174226));
#65119=CARTESIAN_POINT('Ctrl Pts',(78.9668682279573,10.7775478593986,139.679633541825));
#65120=CARTESIAN_POINT('Ctrl Pts',(79.0294428290257,10.811081538852,139.675768909424));
#65121=CARTESIAN_POINT('Ctrl Pts',(79.0671670137654,10.8312978997572,139.673439048679));
#65122=CARTESIAN_POINT('Ctrl Pts',(79.105483874496,10.8503140641317,139.671109187935));
#65123=CARTESIAN_POINT('Ctrl Pts',(79.1443091091393,10.8680981403015,139.66877932719));
#65124=CARTESIAN_POINT('Ctrl Pts',(79.2087912872131,10.8976344966686,139.664909820751));
#65125=CARTESIAN_POINT('Ctrl Pts',(79.2749307245336,10.9238860812921,139.661040314313));
#65126=CARTESIAN_POINT('Ctrl Pts',(79.342359528159,10.9466655008749,139.657170807875));
#65127=CARTESIAN_POINT('Ctrl Pts',(79.4096878426605,10.9694109722963,139.653307068161));
#65128=CARTESIAN_POINT('Ctrl Pts',(79.4783012528629,10.9886943959418,139.649443328446));
#65129=CARTESIAN_POINT('Ctrl Pts',(79.5478103620977,11.0043757367005,139.645579588732));
#65130=CARTESIAN_POINT('Ctrl Pts',(79.6172378543529,11.0200386645681,139.641720385787));
#65131=CARTESIAN_POINT('Ctrl Pts',(79.6875584850885,11.032107804553,139.637861182842));
#65132=CARTESIAN_POINT('Ctrl Pts',(79.7583677824048,11.0404929389537,139.634001979896));
#65133=CARTESIAN_POINT('Ctrl Pts',(79.829132417637,11.0488727845352,139.630145211095));
#65134=CARTESIAN_POINT('Ctrl Pts',(79.9003846267903,11.0535731776611,139.626288442294));
#65135=CARTESIAN_POINT('Ctrl Pts',(79.9717112810358,11.054555258658,139.622431673493));
#65136=CARTESIAN_POINT('Ctrl Pts',(80.0430167923961,11.0555370485432,139.618576047929));
#65137=CARTESIAN_POINT('Ctrl Pts',(80.1143962196894,11.0528027077946,139.614720422364));
#65138=CARTESIAN_POINT('Ctrl Pts',(80.1854345999683,11.0463654540757,139.610864796799));
#65139=CARTESIAN_POINT('Ctrl Pts',(80.2564756712516,11.0399279565073,139.60700902518));
#65140=CARTESIAN_POINT('Ctrl Pts',(80.3271751863906,11.0297873135014,139.60315325356));
#65141=CARTESIAN_POINT('Ctrl Pts',(80.3971232064518,11.0160086114393,139.59929748194));
#65142=CARTESIAN_POINT('Ctrl Pts',(80.4671442536227,11.002215524141,139.595437684819));
#65143=CARTESIAN_POINT('Ctrl Pts',(80.5364117620413,10.9847768897435,139.591577887698));
#65144=CARTESIAN_POINT('Ctrl Pts',(80.6045267855586,10.963808780926,139.587718090577));
#65145=CARTESIAN_POINT('Ctrl Pts',(80.672680283083,10.9428288285075,139.583856113293));
#65146=CARTESIAN_POINT('Ctrl Pts',(80.7396795434922,10.9183155999389,139.579994136009));
#65147=CARTESIAN_POINT('Ctrl Pts',(80.8051441729494,10.8904339245966,139.576132158724));
#65148=CARTESIAN_POINT('Ctrl Pts',(80.8707231147958,10.8625035631019,139.57226343777));
#65149=CARTESIAN_POINT('Ctrl Pts',(80.9347616390688,10.8311932248292,139.568394716816));
#65150=CARTESIAN_POINT('Ctrl Pts',(80.9969032165026,10.796714095071,139.564525995862));
#65151=CARTESIAN_POINT('Ctrl Pts',(81.0337388874113,10.7762758968559,139.562232733641));
#65152=CARTESIAN_POINT('Ctrl Pts',(81.0699085400531,10.7547251089265,139.559939471419));
#65153=CARTESIAN_POINT('Ctrl Pts',(81.1053430762912,10.7321126540139,139.557646209198));
#65154=CARTESIAN_POINT('Ctrl Pts',(81.1556290392832,10.7000228006784,139.554391788189));
#65155=CARTESIAN_POINT('Ctrl Pts',(81.2045988673975,10.6656886944647,139.551137367179));
#65156=CARTESIAN_POINT('Ctrl Pts',(81.252039109102,10.6292316077768,139.54788294617));
#65157=CARTESIAN_POINT('Origin',(80.,9.,134.));
#65158=CARTESIAN_POINT('',(78.4365593800808,9.57550797386886,129.733376810833));
#65159=CARTESIAN_POINT('',(78.4365593657201,9.57550793485619,129.539973235759));
#65160=CARTESIAN_POINT('',(78.4365593737638,9.57550795670799,134.));
#65161=CARTESIAN_POINT('',(79.2300979593294,7.52256748114468,129.));
#65162=CARTESIAN_POINT('Ctrl Pts',(78.4365593657201,9.57550793485619,129.539973235759));
#65163=CARTESIAN_POINT('Ctrl Pts',(78.4421052637371,9.59057407345864,129.538809962392));
#65164=CARTESIAN_POINT('Ctrl Pts',(78.4478695319474,9.60556165591258,129.537643358189));
#65165=CARTESIAN_POINT('Ctrl Pts',(78.5031580487101,9.74333604487815,129.526842861615));
#65166=CARTESIAN_POINT('Ctrl Pts',(78.5669464972497,9.85991522303598,129.517194278958));
#65167=CARTESIAN_POINT('Ctrl Pts',(78.6598171209095,9.99006006994452,129.506139719031));
#65168=CARTESIAN_POINT('Ctrl Pts',(78.6763077958987,10.0120020731591,129.50426270079));
#65169=CARTESIAN_POINT('Ctrl Pts',(78.7011007282667,10.0433472219657,129.501560088528));
#65170=CARTESIAN_POINT('Ctrl Pts',(78.7089781487769,10.0530789800813,129.500717898703));
#65171=CARTESIAN_POINT('Ctrl Pts',(78.7231800079559,10.0702250439487,129.499228154612));
#65172=CARTESIAN_POINT('Ctrl Pts',(78.7294611210524,10.0776743018317,129.498578886966));
#65173=CARTESIAN_POINT('Ctrl Pts',(78.7427544320876,10.0931620902856,129.497224457056));
#65174=CARTESIAN_POINT('Ctrl Pts',(78.7497792260504,10.1011892657614,129.496519855671));
#65175=CARTESIAN_POINT('Ctrl Pts',(78.7685141268927,10.1221870976884,129.494669306634));
#65176=CARTESIAN_POINT('Ctrl Pts',(78.7803522397377,10.1350421651102,129.493528779948));
#65177=CARTESIAN_POINT('Ctrl Pts',(78.8415590012961,10.1994433750242,129.487770910074));
#65178=CARTESIAN_POINT('Ctrl Pts',(78.8940041737191,10.2479683608845,129.483290074258));
#65179=CARTESIAN_POINT('Ctrl Pts',(79.0025519003157,10.3361671038191,129.474652016076));
#65180=CARTESIAN_POINT('Ctrl Pts',(79.058309757714,10.3760323161562,129.470496763705));
#65181=CARTESIAN_POINT('Ctrl Pts',(79.1346986627444,10.4238249094655,129.464983961084));
#65182=CARTESIAN_POINT('Ctrl Pts',(79.1532553342286,10.4349380544061,129.463657588021));
#65183=CARTESIAN_POINT('Ctrl Pts',(79.2285831123431,10.478079965539,129.458304650354));
#65184=CARTESIAN_POINT('Ctrl Pts',(79.2869891060929,10.5071223578696,129.454225168522));
#65185=CARTESIAN_POINT('Ctrl Pts',(79.3574418761431,10.5371419664763,129.449214067501));
#65186=CARTESIAN_POINT('Ctrl Pts',(79.3679913198908,10.541509447957,129.448461390351));
#65187=CARTESIAN_POINT('Ctrl Pts',(79.384501113993,10.5481465646681,129.447278582831));
#65188=CARTESIAN_POINT('Ctrl Pts',(79.3904312540788,10.5504910850961,129.446852759523));
#65189=CARTESIAN_POINT('Ctrl Pts',(79.400982359402,10.5545926496143,129.446093148331));
#65190=CARTESIAN_POINT('Ctrl Pts',(79.4055979035018,10.5563632561535,129.445760176098));
#65191=CARTESIAN_POINT('Ctrl Pts',(79.4167433048174,10.5605820260795,129.444954544452));
#65192=CARTESIAN_POINT('Ctrl Pts',(79.423280699858,10.5630097495067,129.444480704337));
#65193=CARTESIAN_POINT('Ctrl Pts',(79.4435054582284,10.5703762482551,129.443011220069));
#65194=CARTESIAN_POINT('Ctrl Pts',(79.457242008678,10.575176645065,129.442008141136));
#65195=CARTESIAN_POINT('Ctrl Pts',(79.5275832894102,10.5987289149312,129.436852303154));
#65196=CARTESIAN_POINT('Ctrl Pts',(79.5850978491061,10.6146103213682,129.432574634257));
#65197=CARTESIAN_POINT('Ctrl Pts',(79.7468893872503,10.6500696849958,129.420573238285));
#65198=CARTESIAN_POINT('Ctrl Pts',(79.8523860621301,10.6628315071718,129.412800258245));
#65199=CARTESIAN_POINT('Ctrl Pts',(80.0157918246257,10.6669146285504,129.401185248619));
#65200=CARTESIAN_POINT('Ctrl Pts',(80.0732409160692,10.6653800937205,129.397177609033));
#65201=CARTESIAN_POINT('Ctrl Pts',(80.1476560853385,10.6595329932857,129.39208658213));
#65202=CARTESIAN_POINT('Ctrl Pts',(80.1647886741462,10.6579194210251,129.390921244584));
#65203=CARTESIAN_POINT('Ctrl Pts',(80.1925155230282,10.6548740001333,129.389045625889));
#65204=CARTESIAN_POINT('Ctrl Pts',(80.2031260221025,10.6536051557802,129.388330321576));
#65205=CARTESIAN_POINT('Ctrl Pts',(80.223526547605,10.6509662577916,129.386959496613));
#65206=CARTESIAN_POINT('Ctrl Pts',(80.2333179953775,10.6496109911206,129.386303544279));
#65207=CARTESIAN_POINT('Ctrl Pts',(80.2560603864477,10.6462565973157,129.384784306296));
#65208=CARTESIAN_POINT('Ctrl Pts',(80.2690010749719,10.6441916383344,129.383923119468));
#65209=CARTESIAN_POINT('Ctrl Pts',(80.3110258832341,10.6369762500305,129.381135923457));
#65210=CARTESIAN_POINT('Ctrl Pts',(80.3399986476222,10.6312049020792,129.37922935071));
#65211=CARTESIAN_POINT('Ctrl Pts',(80.4091450361678,10.615508461367,129.374702342521));
#65212=CARTESIAN_POINT('Ctrl Pts',(80.4491327278415,10.6048512079816,129.372103669431));
#65213=CARTESIAN_POINT('Ctrl Pts',(80.560341944949,10.5707294800036,129.364874693538));
#65214=CARTESIAN_POINT('Ctrl Pts',(80.6304358066673,10.5439317786606,129.360319236208));
#65215=CARTESIAN_POINT('Ctrl Pts',(80.7739282488995,10.4776657870666,129.350644234482));
#65216=CARTESIAN_POINT('Ctrl Pts',(80.8466481112711,10.4372351042523,129.345529949491));
#65217=CARTESIAN_POINT('Ctrl Pts',(80.9294111313012,10.3827534953977,129.33910314609));
#65218=CARTESIAN_POINT('Ctrl Pts',(80.9426545581567,10.3737593014519,129.338054850521));
#65219=CARTESIAN_POINT('Ctrl Pts',(80.9616541606417,10.360451748159,129.336518608309));
#65220=CARTESIAN_POINT('Ctrl Pts',(80.9675157024037,10.3562894398521,129.336040121293));
#65221=CARTESIAN_POINT('Ctrl Pts',(80.9778644109002,10.3488395514504,129.335186890215));
#65222=CARTESIAN_POINT('Ctrl Pts',(80.9823623132901,10.3455672502953,129.334813162941));
#65223=CARTESIAN_POINT('Ctrl Pts',(80.9921298270897,10.3383861369073,129.333995234183));
#65224=CARTESIAN_POINT('Ctrl Pts',(80.9973927282431,10.3344687284806,129.333550479961));
#65225=CARTESIAN_POINT('Ctrl Pts',(81.0123578563145,10.3231915472474,129.332274548498));
#65226=CARTESIAN_POINT('Ctrl Pts',(81.0220024797696,10.3157565163065,129.331438593885));
#65227=CARTESIAN_POINT('Ctrl Pts',(81.0438460953933,10.2985322323532,129.329515457863));
#65228=CARTESIAN_POINT('Ctrl Pts',(81.0559903525255,10.2886756638844,129.328424541292));
#65229=CARTESIAN_POINT('Ctrl Pts',(81.0962111605375,10.2550811973876,129.324742745478));
#65230=CARTESIAN_POINT('Ctrl Pts',(81.1236392228932,10.2305861584681,129.322117436049));
#65231=CARTESIAN_POINT('Ctrl Pts',(81.2005146447394,10.1572172330857,129.314467595596));
#65232=CARTESIAN_POINT('Ctrl Pts',(81.2477436994239,10.1061296456846,129.309398850474));
#65233=CARTESIAN_POINT('Ctrl Pts',(81.3523830233236,9.97768317039373,129.297428658333));
#65234=CARTESIAN_POINT('Ctrl Pts',(81.40656099785,9.89799550323873,129.290600319234));
#65235=CARTESIAN_POINT('Ctrl Pts',(81.4627742385456,9.79762313193904,129.282738186384));
#65236=CARTESIAN_POINT('Ctrl Pts',(81.4717032196639,9.78102549042416,129.281459998393));
#65237=CARTESIAN_POINT('Ctrl Pts',(81.4854258159986,9.754445899681,129.279446813918));
#65238=CARTESIAN_POINT('Ctrl Pts',(81.4904046423317,9.74456194007761,129.278705439598));
#65239=CARTESIAN_POINT('Ctrl Pts',(81.4996269501798,9.72579059027314,129.277310818001));
#65240=CARTESIAN_POINT('Ctrl Pts',(81.5038908127876,9.71691380297453,129.276656891018));
#65241=CARTESIAN_POINT('Ctrl Pts',(81.513393158668,9.69667331344693,129.275178164977));
#65242=CARTESIAN_POINT('Ctrl Pts',(81.5185828699014,9.68528726804384,129.274355058024));
#65243=CARTESIAN_POINT('Ctrl Pts',(81.5341701538642,9.65004248487715,129.271833019883));
#65244=CARTESIAN_POINT('Ctrl Pts',(81.5441376573839,9.62599705010563,129.270148554315));
#65245=CARTESIAN_POINT('Ctrl Pts',(81.566102383168,9.56928852987476,129.266251535939));
#65246=CARTESIAN_POINT('Ctrl Pts',(81.5776481006429,9.53646324109283,129.264053157243));
#65247=CARTESIAN_POINT('Ctrl Pts',(81.6148606590356,9.41903911259476,129.256350713396));
#65248=CARTESIAN_POINT('Ctrl Pts',(81.6348156733792,9.33278723538462,129.250992605335));
#65249=CARTESIAN_POINT('Ctrl Pts',(81.6601640139988,9.16254566183368,129.240471142832));
#65250=CARTESIAN_POINT('Ctrl Pts',(81.6662327894088,9.07893320225307,129.235324504706));
#65251=CARTESIAN_POINT('Ctrl Pts',(81.6659483502786,8.9795731222314,129.228879113168));
#65252=CARTESIAN_POINT('Ctrl Pts',(81.6656827969888,8.96391760074245,129.227853728557));
#65253=CARTESIAN_POINT('Ctrl Pts',(81.664973537675,8.9410869417171,129.226341018184));
#65254=CARTESIAN_POINT('Ctrl Pts',(81.6647039685041,8.93390671677452,129.225862761744));
#65255=CARTESIAN_POINT('Ctrl Pts',(81.6641482375454,8.92128307028129,129.225017162389));
#65256=CARTESIAN_POINT('Ctrl Pts',(81.6638817884667,8.91583882519387,129.224650916077));
#65257=CARTESIAN_POINT('Ctrl Pts',(81.6632662496597,8.9044107152855,129.223878657379));
#65258=CARTESIAN_POINT('Ctrl Pts',(81.6629115816535,8.89842738921801,129.223472308653));
#65259=CARTESIAN_POINT('Ctrl Pts',(81.6618278269037,8.88167512252505,129.222329119015));
#65260=CARTESIAN_POINT('Ctrl Pts',(81.6610263744618,8.87091138731775,129.221588264218));
#65261=CARTESIAN_POINT('Ctrl Pts',(81.6550401224703,8.79984691148014,129.21665855689));
#65262=CARTESIAN_POINT('Ctrl Pts',(81.6466777194428,8.73986584875166,129.212316118882));
#65263=CARTESIAN_POINT('Ctrl Pts',(81.6120314710883,8.5625710469104,129.199179394477));
#65264=CARTESIAN_POINT('Ctrl Pts',(81.5762996584439,8.44748338016553,129.190280313369));
#65265=CARTESIAN_POINT('Ctrl Pts',(81.5058252377969,8.28495162080501,129.177662769845));
#65266=CARTESIAN_POINT('Ctrl Pts',(81.4804837657359,8.23385834426226,129.173681908576));
#65267=CARTESIAN_POINT('Ctrl Pts',(81.4443816512748,8.16958008505786,129.168654392649));
#65268=CARTESIAN_POINT('Ctrl Pts',(81.4359741238892,8.15512489551793,129.167522293067));
#65269=CARTESIAN_POINT('Ctrl Pts',(81.4220593176879,8.13200890448575,129.165708807347));
#65270=CARTESIAN_POINT('Ctrl Pts',(81.4166873503246,8.123268453397,129.165022374217));
#65271=CARTESIAN_POINT('Ctrl Pts',(81.4062416354628,8.10661949144168,129.163713187218));
#65272=CARTESIAN_POINT('Ctrl Pts',(81.4011810706918,8.09870322095879,129.163089963262));
#65273=CARTESIAN_POINT('Ctrl Pts',(81.3893400792669,8.08052107595637,129.161656568709));
#65274=CARTESIAN_POINT('Ctrl Pts',(81.3825123108633,8.07028656464253,129.160848259831));
#65275=CARTESIAN_POINT('Ctrl Pts',(81.3603507215971,8.03785143932297,129.158280849402));
#65276=CARTESIAN_POINT('Ctrl Pts',(81.3445902443944,8.01594657222786,129.156538356072));
#65277=CARTESIAN_POINT('Ctrl Pts',(81.2908143401557,7.9449112745238,129.150844862917));
#65278=CARTESIAN_POINT('Ctrl Pts',(81.2505826803052,7.89752191058231,129.146978849729));
#65279=CARTESIAN_POINT('Ctrl Pts',(81.1435476543303,7.78486409520348,129.137424732861));
#65280=CARTESIAN_POINT('Ctrl Pts',(81.0737378659551,7.72275990899696,129.131817797626));
#65281=CARTESIAN_POINT('Ctrl Pts',(80.9565423541843,7.63493179343378,129.122726203493));
#65282=CARTESIAN_POINT('Ctrl Pts',(80.9124853750812,7.60509725697729,129.119367998485));
#65283=CARTESIAN_POINT('Ctrl Pts',(80.85780221054,7.57176700268609,129.115169872359));
#65284=CARTESIAN_POINT('Ctrl Pts',(80.8484668084741,7.566201483465,129.114452150317));
#65285=CARTESIAN_POINT('Ctrl Pts',(80.8337512761374,7.55762250909674,129.113318058977));
#65286=CARTESIAN_POINT('Ctrl Pts',(80.828407505868,7.55454677752086,129.112905668379));
#65287=CARTESIAN_POINT('Ctrl Pts',(80.8182589828174,7.5487803191333,129.11212117998));
#65288=CARTESIAN_POINT('Ctrl Pts',(80.8134577215516,7.54608361380095,129.111749496323));
#65289=CARTESIAN_POINT('Ctrl Pts',(80.8038649102653,7.54075804750255,129.111005926905));
#65290=CARTESIAN_POINT('Ctrl Pts',(80.7990736107777,7.53812885919815,129.110634067701));
#65291=CARTESIAN_POINT('Ctrl Pts',(80.7836765336083,7.52977814261942,129.109437770323));
#65292=CARTESIAN_POINT('Ctrl Pts',(80.7730218780729,7.52414825469413,129.108607961825));
#65293=CARTESIAN_POINT('Ctrl Pts',(80.7479994785996,7.51127178073218,129.106656052089));
#65294=CARTESIAN_POINT('Ctrl Pts',(80.7335861425987,7.50411689668719,129.105529360302));
#65295=CARTESIAN_POINT('Ctrl Pts',(80.6846726700445,7.48071281040507,129.101702845179));
#65296=CARTESIAN_POINT('Ctrl Pts',(80.6497205286664,7.46544043065128,129.098963851328));
#65297=CARTESIAN_POINT('Ctrl Pts',(80.5077824575865,7.40913901578415,129.087893673856));
#65298=CARTESIAN_POINT('Ctrl Pts',(80.3972036766103,7.37799080291186,129.0794112534));
#65299=CARTESIAN_POINT('Ctrl Pts',(80.2097943597768,7.34553314225501,129.065735328632));
#65300=CARTESIAN_POINT('Ctrl Pts',(80.1344841321471,7.33771508262403,129.060413112386));
#65301=CARTESIAN_POINT('Ctrl Pts',(80.0392876188853,7.33434777179128,129.053897753106));
#65302=CARTESIAN_POINT('Ctrl Pts',(80.0196706028896,7.33400060528584,129.052566066229));
#65303=CARTESIAN_POINT('Ctrl Pts',(79.9881368591672,7.33399963369054,129.050441638302));
#65304=CARTESIAN_POINT('Ctrl Pts',(79.9762224867312,7.33412707680401,129.049642681699));
#65305=CARTESIAN_POINT('Ctrl Pts',(79.9534381704869,7.33461528391728,129.048121448116));
#65306=CARTESIAN_POINT('Ctrl Pts',(79.9425684321,7.33495469124979,129.047398604261));
#65307=CARTESIAN_POINT('Ctrl Pts',(79.9174640604423,7.33598470685588,129.045735338325));
#65308=CARTESIAN_POINT('Ctrl Pts',(79.9032332937088,7.33675158191233,129.044797097068));
#65309=CARTESIAN_POINT('Ctrl Pts',(79.8572146220244,7.33982409655593,129.041776170394));
#65310=CARTESIAN_POINT('Ctrl Pts',(79.8254816201813,7.34285932669461,129.039713439047));
#65311=CARTESIAN_POINT('Ctrl Pts',(79.7061241588802,7.35774266817347,129.032002917664));
#65312=CARTESIAN_POINT('Ctrl Pts',(79.6194021641204,7.37564818230039,129.026506098934));
#65313=CARTESIAN_POINT('Ctrl Pts',(79.4530584097834,7.42405378440747,129.015705166427));
#65314=CARTESIAN_POINT('Ctrl Pts',(79.3735465083349,7.45393889046513,129.01041518196));
#65315=CARTESIAN_POINT('Ctrl Pts',(79.2839670996566,7.49565660341621,129.003983010553));
#65316=CARTESIAN_POINT('Ctrl Pts',(79.2713458564728,7.50172923543078,129.003065239095));
#65317=CARTESIAN_POINT('Ctrl Pts',(79.2534737802052,7.51060750191127,129.001747280436));
#65318=CARTESIAN_POINT('Ctrl Pts',(79.2481587877413,7.51328341649854,129.001352990102));
#65319=CARTESIAN_POINT('Ctrl Pts',(79.238595383939,7.51816265612658,129.000639116768));
#65320=CARTESIAN_POINT('Ctrl Pts',(79.2343418898436,7.52035593461265,129.000320021224));
#65321=CARTESIAN_POINT('Ctrl Pts',(79.2300979593294,7.52256748114467,129.));
#65322=CARTESIAN_POINT('',(78.6641544560541,9.99806607121007,128.999128940953));
#65323=CARTESIAN_POINT('Origin',(80.,9.,129.));
#65324=CARTESIAN_POINT('',(78.4365593751704,9.57550796052904,129.032769692033));
#65325=CARTESIAN_POINT('Ctrl Pts',(78.6653336530456,9.99710668551929,128.998257881905));
#65326=CARTESIAN_POINT('Ctrl Pts',(78.6618063509199,9.99238525348894,128.998659033531));
#65327=CARTESIAN_POINT('Ctrl Pts',(78.6583041843105,9.98764521447221,128.999061823807));
#65328=CARTESIAN_POINT('Ctrl Pts',(78.6476926070415,9.97312227605533,129.000295854233));
#65329=CARTESIAN_POINT('Ctrl Pts',(78.6406646880971,9.96328071655673,129.001132000887));
#65330=CARTESIAN_POINT('Ctrl Pts',(78.5881391515514,9.8880069505415,129.007521328091));
#65331=CARTESIAN_POINT('Ctrl Pts',(78.5472863866272,9.81946814375683,129.013299876743));
#65332=CARTESIAN_POINT('Ctrl Pts',(78.4832806040723,9.69214545423395,129.023673465825));
#65333=CARTESIAN_POINT('Ctrl Pts',(78.4582610564981,9.63446334002325,129.028253032547));
#65334=CARTESIAN_POINT('Ctrl Pts',(78.4365593751704,9.57550796052904,129.032769692033));
#65335=CARTESIAN_POINT('',(78.4365593737638,9.57550795670799,128.));
#65336=CARTESIAN_POINT('',(78.4365593737638,9.57550795670799,134.));
#65337=CARTESIAN_POINT('Origin',(80.,9.,128.));
#65338=CARTESIAN_POINT('Ctrl Pts',(78.4365593751704,9.57550796052904,129.032769692033));
#65339=CARTESIAN_POINT('Ctrl Pts',(78.4347777866976,9.57066804868406,129.033140484892));
#65340=CARTESIAN_POINT('Ctrl Pts',(78.4330185594245,9.56581955693993,129.033510872514));
#65341=CARTESIAN_POINT('Ctrl Pts',(78.4063955140418,9.49136886452314,129.039181825837));
#65342=CARTESIAN_POINT('Ctrl Pts',(78.3861651481576,9.4201885652767,129.044377203584));
#65343=CARTESIAN_POINT('Ctrl Pts',(78.3670101448335,9.33048005745388,129.050637648145));
#65344=CARTESIAN_POINT('Ctrl Pts',(78.3635718150495,9.31301081984255,129.051843862163));
#65345=CARTESIAN_POINT('Ctrl Pts',(78.3584909485671,9.28481853175811,129.053770529289));
#65346=CARTESIAN_POINT('Ctrl Pts',(78.3566720343398,9.27412910966829,129.054496466218));
#65347=CARTESIAN_POINT('Ctrl Pts',(78.3533933195721,9.25365392060171,129.05587850655));
#65348=CARTESIAN_POINT('Ctrl Pts',(78.3519160849664,9.24387145710935,129.056535127821));
#65349=CARTESIAN_POINT('Ctrl Pts',(78.3487413011671,9.22149958673453,129.058028695935));
#65350=CARTESIAN_POINT('Ctrl Pts',(78.3471004114896,9.20890266237401,129.058863850537));
#65351=CARTESIAN_POINT('Ctrl Pts',(78.343098820237,9.17517558433679,129.061085240416));
#65352=CARTESIAN_POINT('Ctrl Pts',(78.3409981990532,9.15401653667092,129.062463494616));
#65353=CARTESIAN_POINT('Ctrl Pts',(78.3320442728569,9.04206426885929,129.069685148554));
#65354=CARTESIAN_POINT('Ctrl Pts',(78.3322369658389,8.95085951131381,129.075312514644));
#65355=CARTESIAN_POINT('Ctrl Pts',(78.3462738045227,8.78426953166294,129.085567496954));
#65356=CARTESIAN_POINT('Ctrl Pts',(78.3578552328199,8.70895117483196,129.090198764656));
#65357=CARTESIAN_POINT('Ctrl Pts',(78.3812850995571,8.60469866154225,129.096890537881));
#65358=CARTESIAN_POINT('Ctrl Pts',(78.3888545189105,8.57489872039203,129.098837056392));
#65359=CARTESIAN_POINT('Ctrl Pts',(78.4027543438487,8.52590078818045,129.10211916224));
#65360=CARTESIAN_POINT('Ctrl Pts',(78.4086176559482,8.5065773645729,129.103434963398));
#65361=CARTESIAN_POINT('Ctrl Pts',(78.4172944788986,8.47974682900903,129.105298251857));
#65362=CARTESIAN_POINT('Ctrl Pts',(78.4198134187382,8.47214538884944,129.105830259008));
#65363=CARTESIAN_POINT('Ctrl Pts',(78.4224620540941,8.46434144852794,129.106380968942));
#65364=CARTESIAN_POINT('Ctrl Pts',(78.4225371561925,8.46412032045925,129.106396577302));
#65365=CARTESIAN_POINT('Ctrl Pts',(78.4226868859589,8.46367976544649,129.106427681441));
#65366=CARTESIAN_POINT('Ctrl Pts',(78.422761512932,8.46346033825167,129.106443177181));
#65367=CARTESIAN_POINT('Ctrl Pts',(78.4237785991695,8.46047182498789,129.106654273693));
#65368=CARTESIAN_POINT('Ctrl Pts',(78.4247282947769,8.45770523655226,129.106850285473));
#65369=CARTESIAN_POINT('Ctrl Pts',(78.4274900444015,8.44972836679543,129.107417190554));
#65370=CARTESIAN_POINT('Ctrl Pts',(78.4293206265183,8.44452476828116,129.107789181213));
#65371=CARTESIAN_POINT('Ctrl Pts',(78.4337241304446,8.43220321823269,129.108675118552));
#65372=CARTESIAN_POINT('Ctrl Pts',(78.4363197452551,8.42509362469957,129.109190346749));
#65373=CARTESIAN_POINT('Ctrl Pts',(78.4438026778957,8.40502288117145,129.110655833664));
#65374=CARTESIAN_POINT('Ctrl Pts',(78.4488032042892,8.39210498601955,129.111612064394));
#65375=CARTESIAN_POINT('Ctrl Pts',(78.4913106689426,8.28623591671504,129.119548155318));
#65376=CARTESIAN_POINT('Ctrl Pts',(78.5369720372605,8.19678864365701,129.126874362315));
#65377=CARTESIAN_POINT('Ctrl Pts',(78.6324060131299,8.04529759346339,129.139888978404));
#65378=CARTESIAN_POINT('Ctrl Pts',(78.6791076919509,7.98166026180064,129.145579759877));
#65379=CARTESIAN_POINT('Ctrl Pts',(78.7596137649616,7.88686457320794,129.154328737659));
#65380=CARTESIAN_POINT('Ctrl Pts',(78.7904948318971,7.85338479962445,129.157481101567));
#65381=CARTESIAN_POINT('Ctrl Pts',(78.833576827254,7.81035770208752,129.161620762236));
#65382=CARTESIAN_POINT('Ctrl Pts',(78.8445920853445,7.79965655210509,129.162658228661));
#65383=CARTESIAN_POINT('Ctrl Pts',(78.8632358937586,7.78203886336869,129.164380146634));
#65384=CARTESIAN_POINT('Ctrl Pts',(78.8707832394547,7.77503817224922,129.165068176284));
#65385=CARTESIAN_POINT('Ctrl Pts',(78.8857664572206,7.76139635422207,129.166416689183));
#65386=CARTESIAN_POINT('Ctrl Pts',(78.893198002534,7.75475113937178,129.167077327917));
#65387=CARTESIAN_POINT('Ctrl Pts',(78.9113672907195,7.7387955009853,129.168673085497));
#65388=CARTESIAN_POINT('Ctrl Pts',(78.9221655068856,7.72955488507779,129.169605309563));
#65389=CARTESIAN_POINT('Ctrl Pts',(78.9593349770426,7.69856202035065,129.172761403095));
#65390=CARTESIAN_POINT('Ctrl Pts',(78.9862578662103,7.67748283673119,129.174958513971));
#65391=CARTESIAN_POINT('Ctrl Pts',(79.114206734068,7.58351057113798,129.185037705792));
#65392=CARTESIAN_POINT('Ctrl Pts',(79.2225521275357,7.52126796767256,129.192526099914));
#65393=CARTESIAN_POINT('Ctrl Pts',(79.3842718805351,7.45109402431918,129.203355546841));
#65394=CARTESIAN_POINT('Ctrl Pts',(79.4326462624453,7.43272854468055,129.206560163478));
#65395=CARTESIAN_POINT('Ctrl Pts',(79.5002359686298,7.41060750318749,129.2110873664));
#65396=CARTESIAN_POINT('Ctrl Pts',(79.5187826226719,7.40489424692561,129.212334709194));
#65397=CARTESIAN_POINT('Ctrl Pts',(79.5512026615698,7.39552417899927,129.214530668929));
#65398=CARTESIAN_POINT('Ctrl Pts',(79.5650316368868,7.39172011126247,129.215472238595));
#65399=CARTESIAN_POINT('Ctrl Pts',(79.5856149125803,7.38634295462076,129.216883244935));
#65400=CARTESIAN_POINT('Ctrl Pts',(79.5923331215503,7.38463261989123,129.21734528632));
#65401=CARTESIAN_POINT('Ctrl Pts',(79.6038545031768,7.38177593364863,129.21814053735));
#65402=CARTESIAN_POINT('Ctrl Pts',(79.6086524149382,7.38060892602714,129.218472566003));
#65403=CARTESIAN_POINT('Ctrl Pts',(79.6196847313583,7.37797740252185,129.219238089481));
#65404=CARTESIAN_POINT('Ctrl Pts',(79.6259222878408,7.37652752653623,129.219672384669));
#65405=CARTESIAN_POINT('Ctrl Pts',(79.64342688159,7.37256494089247,129.220894991332));
#65406=CARTESIAN_POINT('Ctrl Pts',(79.6547116459802,7.37013338141764,129.221687613858));
#65407=CARTESIAN_POINT('Ctrl Pts',(79.7352020638562,7.35366329236513,129.22736830653));
#65408=CARTESIAN_POINT('Ctrl Pts',(79.8052063281276,7.34392159934582,129.23244867565));
#65409=CARTESIAN_POINT('Ctrl Pts',(79.8905084908212,7.33753470245526,129.238659942851));
#65410=CARTESIAN_POINT('Ctrl Pts',(79.9054227819681,7.33661958643051,129.239746823039));
#65411=CARTESIAN_POINT('Ctrl Pts',(79.9873562521137,7.33269779944641,129.24571766886));
#65412=CARTESIAN_POINT('Ctrl Pts',(80.0545010602895,7.33354059475028,129.250607147323));
#65413=CARTESIAN_POINT('Ctrl Pts',(80.1947665608827,7.34379009724053,129.260694913019));
#65414=CARTESIAN_POINT('Ctrl Pts',(80.2676912775604,7.35400201812732,129.265865668435));
#65415=CARTESIAN_POINT('Ctrl Pts',(80.3569433059803,7.37259185111791,129.272087507702));
#65416=CARTESIAN_POINT('Ctrl Pts',(80.3741174191915,7.37645387965648,129.273280049958));
#65417=CARTESIAN_POINT('Ctrl Pts',(80.4016206721994,7.38309828568305,129.275182953486));
#65418=CARTESIAN_POINT('Ctrl Pts',(80.4119894431973,7.38570912594357,129.275898771115));
#65419=CARTESIAN_POINT('Ctrl Pts',(80.4317477931971,7.39088702159278,129.277260036902));
#65420=CARTESIAN_POINT('Ctrl Pts',(80.4411413750809,7.39343688941268,129.277906010332));
#65421=CARTESIAN_POINT('Ctrl Pts',(80.4625078028249,7.39943829297402,129.279372854245));
#65422=CARTESIAN_POINT('Ctrl Pts',(80.4744654486544,7.40294214324621,129.280191985236));
#65423=CARTESIAN_POINT('Ctrl Pts',(80.5062186926012,7.41263465059423,129.282363217799));
#65424=CARTESIAN_POINT('Ctrl Pts',(80.5259403251162,7.41905947203715,129.283707606306));
#65425=CARTESIAN_POINT('Ctrl Pts',(80.6639914423166,7.46690251416941,129.29310124537));
#65426=CARTESIAN_POINT('Ctrl Pts',(80.7774346730707,7.52119243848336,129.300691901771));
#65427=CARTESIAN_POINT('Ctrl Pts',(80.9619136228956,7.63662704888598,129.313983320184));
#65428=CARTESIAN_POINT('Ctrl Pts',(81.0358953665722,7.69195585105125,129.319643762182));
#65429=CARTESIAN_POINT('Ctrl Pts',(81.1137259044816,7.76092397072454,129.326443676871));
#65430=CARTESIAN_POINT('Ctrl Pts',(81.1224599058962,7.76883041915964,129.327219942902));
#65431=CARTESIAN_POINT('Ctrl Pts',(81.1357897107494,7.78115695146703,129.328426571261));
#65432=CARTESIAN_POINT('Ctrl Pts',(81.140445426345,7.78551209552131,129.328852213041));
#65433=CARTESIAN_POINT('Ctrl Pts',(81.1490511772298,7.79365537907541,129.329647092406));
#65434=CARTESIAN_POINT('Ctrl Pts',(81.1530076900014,7.79743639851791,129.3300157968));
#65435=CARTESIAN_POINT('Ctrl Pts',(81.1620621088825,7.8061749621513,129.330867013768));
#65436=CARTESIAN_POINT('Ctrl Pts',(81.1671469916541,7.8111457359596,129.331350525344));
#65437=CARTESIAN_POINT('Ctrl Pts',(81.1830092431168,7.82685187163933,129.332875679245));
#65438=CARTESIAN_POINT('Ctrl Pts',(81.1936711422671,7.83770203307569,129.333925527378));
#65439=CARTESIAN_POINT('Ctrl Pts',(81.2719275150088,7.91955267277769,129.341807448212));
#65440=CARTESIAN_POINT('Ctrl Pts',(81.3332803237026,7.9962439060047,129.348972027664));
#65441=CARTESIAN_POINT('Ctrl Pts',(81.4322585482761,8.14517740855901,129.361983553953));
#65442=CARTESIAN_POINT('Ctrl Pts',(81.4720345507428,8.21565124300376,129.367826121522));
#65443=CARTESIAN_POINT('Ctrl Pts',(81.5197623801728,8.31674500962452,129.37569629884));
#65444=CARTESIAN_POINT('Ctrl Pts',(81.5322010794933,8.34511441011223,129.377853571202));
#65445=CARTESIAN_POINT('Ctrl Pts',(81.5527756795281,8.39584059315205,129.381621210999));
#65446=CARTESIAN_POINT('Ctrl Pts',(81.5612370336259,8.41805504932632,129.383241673076));
#65447=CARTESIAN_POINT('Ctrl Pts',(81.5732563561312,8.45176207278793,129.385657655368));
#65448=CARTESIAN_POINT('Ctrl Pts',(81.5771697052544,8.46312373783989,129.386464813307));
#65449=CARTESIAN_POINT('Ctrl Pts',(81.5840276272669,8.48375676707399,129.387917969608));
#65450=CARTESIAN_POINT('Ctrl Pts',(81.5870145455663,8.49301337441842,129.388565333821));
#65451=CARTESIAN_POINT('Ctrl Pts',(81.5932726866105,8.51300505818161,129.389953904057));
#65452=CARTESIAN_POINT('Ctrl Pts',(81.5965168684075,8.52374814805455,129.390694201176));
#65453=CARTESIAN_POINT('Ctrl Pts',(81.6052025699393,8.5535973462121,129.392735407041));
#65454=CARTESIAN_POINT('Ctrl Pts',(81.6104114046925,8.57276963825767,129.394028784438));
#65455=CARTESIAN_POINT('Ctrl Pts',(81.6415725961252,8.69614655347753,129.402248398149));
#65456=CARTESIAN_POINT('Ctrl Pts',(81.6577427127657,8.80256493602061,129.408846579788));
#65457=CARTESIAN_POINT('Ctrl Pts',(81.6694752598998,9.01897428520423,129.422090543117));
#65458=CARTESIAN_POINT('Ctrl Pts',(81.6646333286551,9.12843991030868,129.428709345097));
#65459=CARTESIAN_POINT('Ctrl Pts',(81.6470203446566,9.25119017299837,129.43677153411));
#65460=CARTESIAN_POINT('Ctrl Pts',(81.6447376193638,9.26572663750609,129.437736843581));
#65461=CARTESIAN_POINT('Ctrl Pts',(81.6410854518559,9.28712981107423,129.439176306087));
#65462=CARTESIAN_POINT('Ctrl Pts',(81.6398647082845,9.29402163666587,129.439642604748));
#65463=CARTESIAN_POINT('Ctrl Pts',(81.6376115023218,9.30629162092016,129.440478100688));
#65464=CARTESIAN_POINT('Ctrl Pts',(81.6365958990972,9.31167266643159,129.440846353045));
#65465=CARTESIAN_POINT('Ctrl Pts',(81.6342946628625,9.32354401430019,129.441662910215));
#65466=CARTESIAN_POINT('Ctrl Pts',(81.6329969083748,9.33003161621972,129.442111859903));
#65467=CARTESIAN_POINT('Ctrl Pts',(81.6290745956412,9.34904995358731,129.443435565807));
#65468=CARTESIAN_POINT('Ctrl Pts',(81.6263442653778,9.36155803657349,129.444315873255));
#65469=CARTESIAN_POINT('Ctrl Pts',(81.6197105334249,9.39035139977126,129.446362921784));
#65470=CARTESIAN_POINT('Ctrl Pts',(81.6157052318908,9.40661158858356,129.44753423841));
#65471=CARTESIAN_POINT('Ctrl Pts',(81.6010479660502,9.4624750961828,129.451605284335));
#65472=CARTESIAN_POINT('Ctrl Pts',(81.5891797667841,9.50174200902299,129.454548382122));
#65473=CARTESIAN_POINT('Ctrl Pts',(81.5358512393681,9.65721792035685,129.4664382622));
#65474=CARTESIAN_POINT('Ctrl Pts',(81.4829829089807,9.7691182369275,129.475500162609));
#65475=CARTESIAN_POINT('Ctrl Pts',(81.3937418889939,9.91390334882249,129.487486178465));
#65476=CARTESIAN_POINT('Ctrl Pts',(81.3675826585501,9.95260389991338,129.490723965499));
#65477=CARTESIAN_POINT('Ctrl Pts',(81.3303744326982,10.0029521260012,129.494984464727));
#65478=CARTESIAN_POINT('Ctrl Pts',(81.3207361097378,10.0156107803398,129.496060046533));
#65479=CARTESIAN_POINT('Ctrl Pts',(81.3045169540851,10.0362910259982,129.497825106386));
#65480=CARTESIAN_POINT('Ctrl Pts',(81.298040070851,10.0443924343476,129.498518619685));
#65481=CARTESIAN_POINT('Ctrl Pts',(81.2852057545574,10.0601420007298,129.499871155293));
#65482=CARTESIAN_POINT('Ctrl Pts',(81.2788546736406,10.0677947481888,129.50053039288));
#65483=CARTESIAN_POINT('Ctrl Pts',(81.2635681200239,10.0858822748211,129.50209373222));
#65484=CARTESIAN_POINT('Ctrl Pts',(81.2545712675656,10.0962644124401,129.502995282206));
#65485=CARTESIAN_POINT('Ctrl Pts',(81.2230539405644,10.1317383715663,129.506091858278));
#65486=CARTESIAN_POINT('Ctrl Pts',(81.199900057064,10.1562580960445,129.508260468486));
#65487=CARTESIAN_POINT('Ctrl Pts',(81.140760899942,10.215194636087,129.513565495721));
#65488=CARTESIAN_POINT('Ctrl Pts',(81.1039466648126,10.2487336585203,129.516667718456));
#65489=CARTESIAN_POINT('Ctrl Pts',(81.014768441482,10.3229469653433,129.523823324164));
#65490=CARTESIAN_POINT('Ctrl Pts',(80.9613716284186,10.3622438804543,129.52784437241));
#65491=CARTESIAN_POINT('Ctrl Pts',(80.8995940312351,10.4022627585908,129.532351109272));
#65492=CARTESIAN_POINT('Ctrl Pts',(80.8933849373708,10.4062267306376,129.532802546915));
#65493=CARTESIAN_POINT('Ctrl Pts',(80.8215338585801,10.4514295085387,129.538011258822));
#65494=CARTESIAN_POINT('Ctrl Pts',(80.7531250159643,10.488074270534,129.542821431468));
#65495=CARTESIAN_POINT('Ctrl Pts',(80.6718315826542,10.5245763877766,129.548650184149));
#65496=CARTESIAN_POINT('Ctrl Pts',(80.6611894169383,10.5292218197511,129.54941540588));
#65497=CARTESIAN_POINT('Ctrl Pts',(80.6445757042174,10.5362680661741,129.550614697985));
#65498=CARTESIAN_POINT('Ctrl Pts',(80.6386370933414,10.538746265356,129.551044310206));
#65499=CARTESIAN_POINT('Ctrl Pts',(80.6276137554963,10.5432715309818,129.55184373476));
#65500=CARTESIAN_POINT('Ctrl Pts',(80.6225331045855,10.5453279829771,129.552212982888));
#65501=CARTESIAN_POINT('Ctrl Pts',(80.6107467876728,10.5500310742925,129.553071371104));
#65502=CARTESIAN_POINT('Ctrl Pts',(80.6040340294598,10.5526592853368,129.553561567881));
#65503=CARTESIAN_POINT('Ctrl Pts',(80.5824444773069,10.5609509361831,129.555141853933));
#65504=CARTESIAN_POINT('Ctrl Pts',(80.5675040059945,10.5664445573315,129.556241079376));
#65505=CARTESIAN_POINT('Ctrl Pts',(80.4837476663599,10.5958863590341,129.562425804127));
#65506=CARTESIAN_POINT('Ctrl Pts',(80.4135028499004,10.6155118040121,129.567693364414));
#65507=CARTESIAN_POINT('Ctrl Pts',(80.2093102768779,10.6583681050053,129.58286567028));
#65508=CARTESIAN_POINT('Ctrl Pts',(80.0734733888392,10.6699134390871,129.592743073796));
#65509=CARTESIAN_POINT('Ctrl Pts',(79.9140871152084,10.663951483139,129.603723895439));
#65510=CARTESIAN_POINT('Ctrl Pts',(79.8904691072906,10.6625638770361,129.605337181268));
#65511=CARTESIAN_POINT('Ctrl Pts',(79.8547924971121,10.6597041940744,129.607754341897));
#65512=CARTESIAN_POINT('Ctrl Pts',(79.8427081067325,10.6586025758322,129.608569643622));
#65513=CARTESIAN_POINT('Ctrl Pts',(79.8209710349715,10.6563813049417,129.61003030904));
#65514=CARTESIAN_POINT('Ctrl Pts',(79.8113141765709,10.6553090540994,129.610677127022));
#65515=CARTESIAN_POINT('Ctrl Pts',(79.790652146366,10.6528316759417,129.612056830998));
#65516=CARTESIAN_POINT('Ctrl Pts',(79.7796504691827,10.651400971026,129.612788880886));
#65517=CARTESIAN_POINT('Ctrl Pts',(79.7495225479429,10.6471765637074,129.614787047563));
#65518=CARTESIAN_POINT('Ctrl Pts',(79.7304289630211,10.6441596919199,129.616046119965));
#65519=CARTESIAN_POINT('Ctrl Pts',(79.6880292075684,10.6367018388551,129.618828776504));
#65520=CARTESIAN_POINT('Ctrl Pts',(79.6647564931687,10.6320939187829,129.620347121593));
#65521=CARTESIAN_POINT('Ctrl Pts',(79.5906070408004,10.6157594872455,129.62516562559));
#65522=CARTESIAN_POINT('Ctrl Pts',(79.5401785324455,10.602137993007,129.628412610739));
#65523=CARTESIAN_POINT('Ctrl Pts',(79.3969926614764,10.5561419652216,129.63767205075));
#65524=CARTESIAN_POINT('Ctrl Pts',(79.3063576440549,10.517911196502,129.64357512185));
#65525=CARTESIAN_POINT('Ctrl Pts',(79.1753103881707,10.4484330408034,129.652810886703));
#65526=CARTESIAN_POINT('Ctrl Pts',(79.1320884604503,10.4229545831172,129.65598605807));
#65527=CARTESIAN_POINT('Ctrl Pts',(79.0809209660061,10.3895932622691,129.659987470087));
#65528=CARTESIAN_POINT('Ctrl Pts',(79.0718153432976,10.383527713008,129.660709318309));
#65529=CARTESIAN_POINT('Ctrl Pts',(79.0575775671282,10.3738396591732,129.661854612215));
#65530=CARTESIAN_POINT('Ctrl Pts',(79.0524048435202,10.3702769308661,129.66227420681));
#65531=CARTESIAN_POINT('Ctrl Pts',(79.0428586108828,10.3636220333786,129.663055321648));
#65532=CARTESIAN_POINT('Ctrl Pts',(79.0384797087742,10.3605379138305,129.663416306065));
#65533=CARTESIAN_POINT('Ctrl Pts',(79.0340685596031,10.357399151251,129.663782637891));
#65534=CARTESIAN_POINT('Ctrl Pts',(79.0340213028523,10.357365521892,129.663786562725));
#65535=CARTESIAN_POINT('Ctrl Pts',(79.0339277424457,10.3572989340651,129.663794333853));
#65536=CARTESIAN_POINT('Ctrl Pts',(79.0338814387615,10.357265975725,129.663798180137));
#65537=CARTESIAN_POINT('Ctrl Pts',(79.0337897235461,10.357200686996,129.66380579919));
#65538=CARTESIAN_POINT('Ctrl Pts',(79.033744311954,10.3571683566994,129.663809571953));
#65539=CARTESIAN_POINT('Ctrl Pts',(79.0336543239906,10.3571042839268,129.663817048659));
#65540=CARTESIAN_POINT('Ctrl Pts',(79.033609747549,10.3570725415254,129.663820752599));
#65541=CARTESIAN_POINT('Ctrl Pts',(79.0335213766921,10.3570096070329,129.663828096048));
#65542=CARTESIAN_POINT('Ctrl Pts',(79.0334775821751,10.3569784149841,129.663831735556));
#65543=CARTESIAN_POINT('Ctrl Pts',(79.0333907250902,10.3569165458693,129.663838954277));
#65544=CARTESIAN_POINT('Ctrl Pts',(79.0333476625048,10.3568858688963,129.663842533481));
#65545=CARTESIAN_POINT('Ctrl Pts',(79.0332622225816,10.3568249969763,129.663849635449));
#65546=CARTESIAN_POINT('Ctrl Pts',(79.033219845126,10.3567948020424,129.663853158213));
#65547=CARTESIAN_POINT('Ctrl Pts',(79.0331357309802,10.3567348627936,129.663860150975));
#65548=CARTESIAN_POINT('Ctrl Pts',(79.0330939943671,10.356705118623,129.663863620958));
#65549=CARTESIAN_POINT('Ctrl Pts',(79.0330111206988,10.3566460517983,129.66387051156));
#65550=CARTESIAN_POINT('Ctrl Pts',(79.0329699834751,10.3566167291066,129.663873932185));
#65551=CARTESIAN_POINT('Ctrl Pts',(79.032888268857,10.3565584771652,129.663880727356));
#65552=CARTESIAN_POINT('Ctrl Pts',(79.0328476915594,10.3565295480606,129.663884101886));
#65553=CARTESIAN_POINT('Ctrl Pts',(79.0327670597441,10.356472057104,129.663890807928));
#65554=CARTESIAN_POINT('Ctrl Pts',(79.0327270051818,10.3564434952904,129.663894139437));
#65555=CARTESIAN_POINT('Ctrl Pts',(79.032647383606,10.3563867140007,129.663900762349));
#65556=CARTESIAN_POINT('Ctrl Pts',(79.0326078165229,10.3563584945395,129.663904053753));
#65557=CARTESIAN_POINT('Ctrl Pts',(79.0325291360862,10.3563023740251,129.663910599251));
#65558=CARTESIAN_POINT('Ctrl Pts',(79.0324900228057,10.3562744730835,129.663913853335));
#65559=CARTESIAN_POINT('Ctrl Pts',(79.0324122183353,10.3562189672145,129.66392032681));
#65560=CARTESIAN_POINT('Ctrl Pts',(79.0323735270077,10.3561913622434,129.663923546209));
#65561=CARTESIAN_POINT('Ctrl Pts',(79.0264207909083,10.3519438992621,129.664418889186));
#65562=CARTESIAN_POINT('Ctrl Pts',(79.0205345479884,10.3476854998635,129.664913583756));
#65563=CARTESIAN_POINT('Ctrl Pts',(79.0077412375502,10.3383021037272,129.665999147917));
#65564=CARTESIAN_POINT('Ctrl Pts',(79.0008456604322,10.3331618696556,129.66659096064));
#65565=CARTESIAN_POINT('Ctrl Pts',(78.9817985734491,10.3187326483449,129.668243689541));
#65566=CARTESIAN_POINT('Ctrl Pts',(78.969735017926,10.3093295890135,129.669311074949));
#65567=CARTESIAN_POINT('Ctrl Pts',(78.8442370938526,10.2087007591404,129.680620020114));
#65568=CARTESIAN_POINT('Ctrl Pts',(78.7430949105268,10.1031494354936,129.691449345628));
#65569=CARTESIAN_POINT('Ctrl Pts',(78.6184171537561,9.93328804114736,129.706494452053));
#65570=CARTESIAN_POINT('Ctrl Pts',(78.5829878783349,9.87856490149784,129.711056760906));
#65571=CARTESIAN_POINT('Ctrl Pts',(78.5421550483921,9.80656974110068,129.716705271632));
#65572=CARTESIAN_POINT('Ctrl Pts',(78.5337033961841,9.7911011068514,129.717899442309));
#65573=CARTESIAN_POINT('Ctrl Pts',(78.5205013086131,9.76599926386559,129.719806951901));
#65574=CARTESIAN_POINT('Ctrl Pts',(78.5155959539046,9.75644952728044,129.720525713145));
#65575=CARTESIAN_POINT('Ctrl Pts',(78.5063930892301,9.73809911028932,129.721893930794));
#65576=CARTESIAN_POINT('Ctrl Pts',(78.5020802189354,9.72930668239751,129.722543902177));
#65577=CARTESIAN_POINT('Ctrl Pts',(78.4923182109651,9.70895342019374,129.724035940363));
#65578=CARTESIAN_POINT('Ctrl Pts',(78.4869240276894,9.69736679454486,129.724876082676));
#65579=CARTESIAN_POINT('Ctrl Pts',(78.470170671262,9.66027108577868,129.727537672019));
#65580=CARTESIAN_POINT('Ctrl Pts',(78.4593188578045,9.63453718989222,129.729341916015));
#65581=CARTESIAN_POINT('Ctrl Pts',(78.4448148482087,9.59757339521375,129.731880578999));
#65582=CARTESIAN_POINT('Ctrl Pts',(78.4406282675188,9.58656162418711,129.732630321618));
#65583=CARTESIAN_POINT('Ctrl Pts',(78.4365593800808,9.57550797386886,129.733376810833));
#65584=CARTESIAN_POINT('Origin',(80.,9.,134.));
#65585=CARTESIAN_POINT('',(78.4345148001033,9.5762760062711,130.432124665951));
#65586=CARTESIAN_POINT('',(78.4365593450135,9.57550787860402,130.240113160697));
#65587=CARTESIAN_POINT('',(78.4365593737638,9.57550795670799,134.));
#65588=CARTESIAN_POINT('Ctrl Pts',(78.4365593450135,9.57550787860402,130.240113160697));
#65589=CARTESIAN_POINT('Ctrl Pts',(78.4584396377415,9.63494848830862,130.236203505864));
#65590=CARTESIAN_POINT('Ctrl Pts',(78.48370025951,9.69311543856741,130.232233234758));
#65591=CARTESIAN_POINT('Ctrl Pts',(78.5175577135617,9.76030341362332,130.227313276936));
#65592=CARTESIAN_POINT('Ctrl Pts',(78.5230027528047,9.77082781830187,130.226532472749));
#65593=CARTESIAN_POINT('Ctrl Pts',(78.5315681194996,9.78695932128886,130.225318578752));
#65594=CARTESIAN_POINT('Ctrl Pts',(78.5346094847926,9.79260822322694,130.224890228581));
#65595=CARTESIAN_POINT('Ctrl Pts',(78.5403123336663,9.80305542989845,130.224091675299));
#65596=CARTESIAN_POINT('Ctrl Pts',(78.5429649853485,9.80785832270995,130.223722020747));
#65597=CARTESIAN_POINT('Ctrl Pts',(78.5491155823773,9.81886576320299,130.222869041378));
#65598=CARTESIAN_POINT('Ctrl Pts',(78.552629631519,9.82506105424188,130.222384723356));
#65599=CARTESIAN_POINT('Ctrl Pts',(78.5640897687712,9.84496681951748,130.220815338122));
#65600=CARTESIAN_POINT('Ctrl Pts',(78.5721915086987,9.85858603803132,130.219721181053));
#65601=CARTESIAN_POINT('Ctrl Pts',(78.6239893833583,9.94289851439503,130.212828785794));
#65602=CARTESIAN_POINT('Ctrl Pts',(78.6727263845778,10.0103489176001,130.206792932316));
#65603=CARTESIAN_POINT('Ctrl Pts',(78.7849432153425,10.1434483555392,130.194121185347));
#65604=CARTESIAN_POINT('Ctrl Pts',(78.8492083490042,10.2081054845086,130.187507124277));
#65605=CARTESIAN_POINT('Ctrl Pts',(78.9435463543594,10.2886238119911,130.178753033757));
#65606=CARTESIAN_POINT('Ctrl Pts',(78.9692868373261,10.30930373172,130.176448576161));
#65607=CARTESIAN_POINT('Ctrl Pts',(79.0155264189662,10.3442432398726,130.17245368182));
#65608=CARTESIAN_POINT('Ctrl Pts',(79.0357625266469,10.3588319731765,130.170751319968));
#65609=CARTESIAN_POINT('Ctrl Pts',(79.0644071402272,10.3785203334929,130.168403343902));
#65610=CARTESIAN_POINT('Ctrl Pts',(79.0725437973101,10.3840076980862,130.167743130963));
#65611=CARTESIAN_POINT('Ctrl Pts',(79.0890092917068,10.3949016147028,130.16642041019));
#65612=CARTESIAN_POINT('Ctrl Pts',(79.0973389253431,10.4003062439859,130.165757993237));
#65613=CARTESIAN_POINT('Ctrl Pts',(79.1144836587366,10.4112139395308,130.164407999066));
#65614=CARTESIAN_POINT('Ctrl Pts',(79.1233029362681,10.4167096528558,130.163720714678));
#65615=CARTESIAN_POINT('Ctrl Pts',(79.1458399657848,10.4304625020145,130.161982073889));
#65616=CARTESIAN_POINT('Ctrl Pts',(79.1596265880928,10.438605189575,130.160934908638));
#65617=CARTESIAN_POINT('Ctrl Pts',(79.2149162649246,10.4701944069642,130.156797282838));
#65618=CARTESIAN_POINT('Ctrl Pts',(79.2573019386848,10.4920550588343,130.153762979926));
#65619=CARTESIAN_POINT('Ctrl Pts',(79.4019403855505,10.5589596945325,130.143770081131));
#65620=CARTESIAN_POINT('Ctrl Pts',(79.507766621818,10.5955366874004,130.137058399044));
#65621=CARTESIAN_POINT('Ctrl Pts',(79.679428206345,10.636146959915,130.126203662879));
#65622=CARTESIAN_POINT('Ctrl Pts',(79.7432060297944,10.6473609673009,130.12217143354));
#65623=CARTESIAN_POINT('Ctrl Pts',(79.8224532895596,10.6565810608224,130.11698855349));
#65624=CARTESIAN_POINT('Ctrl Pts',(79.8374624756375,10.6581209725366,130.115999317393));
#65625=CARTESIAN_POINT('Ctrl Pts',(79.8595218555694,10.6600818445882,130.114531517717));
#65626=CARTESIAN_POINT('Ctrl Pts',(79.8665576017127,10.6606622057536,130.114061298943));
#65627=CARTESIAN_POINT('Ctrl Pts',(79.8785327299134,10.6615734133995,130.113257122165));
#65628=CARTESIAN_POINT('Ctrl Pts',(79.8834702415549,10.6619269900686,130.112924429056));
#65629=CARTESIAN_POINT('Ctrl Pts',(79.8947206927008,10.6626822546039,130.112163737765));
#65630=CARTESIAN_POINT('Ctrl Pts',(79.9010342473554,10.6630699891434,130.111734995978));
#65631=CARTESIAN_POINT('Ctrl Pts',(79.9184541870998,10.6640402555346,130.110547205473));
#65632=CARTESIAN_POINT('Ctrl Pts',(79.929564194952,10.6645475278126,130.109784245536));
#65633=CARTESIAN_POINT('Ctrl Pts',(79.9939823596229,10.6668427468095,130.105332213628));
#65634=CARTESIAN_POINT('Ctrl Pts',(80.0473418230552,10.6661808194633,130.101533324885));
#65635=CARTESIAN_POINT('Ctrl Pts',(80.2017424916781,10.656843068918,130.090375726615));
#65636=CARTESIAN_POINT('Ctrl Pts',(80.3021513344009,10.641503993704,130.082927733981));
#65637=CARTESIAN_POINT('Ctrl Pts',(80.4708338847551,10.5997235399595,130.070473194759));
#65638=CARTESIAN_POINT('Ctrl Pts',(80.5399226803025,10.5777471410824,130.065385513374));
#65639=CARTESIAN_POINT('Ctrl Pts',(80.6237556504052,10.5449254058465,130.059241761507));
#65640=CARTESIAN_POINT('Ctrl Pts',(80.6400385455896,10.5382510596255,130.058049607999));
#65641=CARTESIAN_POINT('Ctrl Pts',(80.6660756878975,10.5270934184494,130.056144477513));
#65642=CARTESIAN_POINT('Ctrl Pts',(80.6758973084406,10.5227718044534,130.055426102522));
#65643=CARTESIAN_POINT('Ctrl Pts',(80.6946042937851,10.5143238858072,130.054058091017));
#65644=CARTESIAN_POINT('Ctrl Pts',(80.7034963204906,10.5102135246776,130.053407944338));
#65645=CARTESIAN_POINT('Ctrl Pts',(80.7237243376113,10.5006456461992,130.051928930369));
#65646=CARTESIAN_POINT('Ctrl Pts',(80.7350358883612,10.4951376289706,130.051101843743));
#65647=CARTESIAN_POINT('Ctrl Pts',(80.7650953607622,10.4800769497162,130.048903034176));
#65648=CARTESIAN_POINT('Ctrl Pts',(80.7837269008944,10.4702961934403,130.047539240461));
#65649=CARTESIAN_POINT('Ctrl Pts',(80.9074946751918,10.4023020488292,130.038461107788));
#65650=CARTESIAN_POINT('Ctrl Pts',(81.0062529326323,10.3332128475217,130.031159541367));
#65651=CARTESIAN_POINT('Ctrl Pts',(81.1469125988658,10.2102034550111,130.019742157113));
#65652=CARTESIAN_POINT('Ctrl Pts',(81.1944157119895,10.1633446339648,130.01565827716));
#65653=CARTESIAN_POINT('Ctrl Pts',(81.2540444014471,10.09701248229,130.010013830069));
#65654=CARTESIAN_POINT('Ctrl Pts',(81.2687662662898,10.0799517614735,130.0085729031));
#65655=CARTESIAN_POINT('Ctrl Pts',(81.2933707213458,10.0502407467067,130.006071280877));
#65656=CARTESIAN_POINT('Ctrl Pts',(81.3034250661465,10.0377362378484,130.005020667906));
#65657=CARTESIAN_POINT('Ctrl Pts',(81.3177488380146,10.0193852821972,130.003478815302));
#65658=CARTESIAN_POINT('Ctrl Pts',(81.3221635803626,10.0136527095466,130.00299715874));
#65659=CARTESIAN_POINT('Ctrl Pts',(81.3298306653722,10.0035616445375,130.002148929247));
#65660=CARTESIAN_POINT('Ctrl Pts',(81.3330992226438,9.99921570960611,130.00178349062));
#65661=CARTESIAN_POINT('Ctrl Pts',(81.3401709167182,9.98971659088475,130.000984354978));
#65662=CARTESIAN_POINT('Ctrl Pts',(81.3439655749581,9.9845575382707,130.000550128481));
#65663=CARTESIAN_POINT('Ctrl Pts',(81.3544715323461,9.97010018478609,129.999332996871));
#65664=CARTESIAN_POINT('Ctrl Pts',(81.361116562477,9.96075448769974,129.998545876653));
#65665=CARTESIAN_POINT('Ctrl Pts',(81.4049740195483,9.89770426300165,129.993237415687));
#65666=CARTESIAN_POINT('Ctrl Pts',(81.4390920973017,9.84192456583974,129.988551816221));
#65667=CARTESIAN_POINT('Ctrl Pts',(81.4805337001838,9.76425886454824,129.982171680867));
#65668=CARTESIAN_POINT('Ctrl Pts',(81.490812938907,9.74400833928629,129.980520381267));
#65669=CARTESIAN_POINT('Ctrl Pts',(81.5318115955084,9.65897580128198,129.973650239493));
#65670=CARTESIAN_POINT('Ctrl Pts',(81.5587491220857,9.59245101053975,129.968430948267));
#65671=CARTESIAN_POINT('Ctrl Pts',(81.6024927256106,9.46054167359784,129.958500401865));
#65672=CARTESIAN_POINT('Ctrl Pts',(81.6197828134281,9.39545835218695,129.953786265238));
#65673=CARTESIAN_POINT('Ctrl Pts',(81.6365059221305,9.312573996056,129.948019147026));
#65674=CARTESIAN_POINT('Ctrl Pts',(81.6396576674137,9.2955958538804,129.946849781926));
#65675=CARTESIAN_POINT('Ctrl Pts',(81.6443275251638,9.26806087832203,129.94497198196));
#65676=CARTESIAN_POINT('Ctrl Pts',(81.6460091627837,9.25753347289706,129.944258427745));
#65677=CARTESIAN_POINT('Ctrl Pts',(81.6490453337277,9.23728020331689,129.942893796032));
#65678=CARTESIAN_POINT('Ctrl Pts',(81.6504151514682,9.22755711901948,129.942242262867));
#65679=CARTESIAN_POINT('Ctrl Pts',(81.6533636090416,9.20519961009279,129.940752058773));
#65680=CARTESIAN_POINT('Ctrl Pts',(81.6548835460823,9.19255795890532,129.939915263133));
#65681=CARTESIAN_POINT('Ctrl Pts',(81.6593278738961,9.15164099102099,129.937224523326));
#65682=CARTESIAN_POINT('Ctrl Pts',(81.6616737109153,9.12330699418316,129.93538860175));
#65683=CARTESIAN_POINT('Ctrl Pts',(81.6707448141518,8.96436217257609,129.925215961396));
#65684=CARTESIAN_POINT('Ctrl Pts',(81.6627981750819,8.8333778861654,129.917353388849));
#65685=CARTESIAN_POINT('Ctrl Pts',(81.626977310635,8.63451135661191,129.904955328123));
#65686=CARTESIAN_POINT('Ctrl Pts',(81.6098530056037,8.5652493924233,129.900536182257));
#65687=CARTESIAN_POINT('Ctrl Pts',(81.5835917996731,8.48227262855247,129.894889332106));
#65688=CARTESIAN_POINT('Ctrl Pts',(81.578621142618,8.46730884841996,129.893856503465));
#65689=CARTESIAN_POINT('Ctrl Pts',(81.571077433808,8.44563250026466,129.892336075947));
#65690=CARTESIAN_POINT('Ctrl Pts',(81.5686719621035,8.43886196141422,129.891857693171));
#65691=CARTESIAN_POINT('Ctrl Pts',(81.5643716149956,8.42700179417144,129.891013213612));
#65692=CARTESIAN_POINT('Ctrl Pts',(81.5624955366561,8.4219055523686,129.890648219713));
#65693=CARTESIAN_POINT('Ctrl Pts',(81.5583436261761,8.41079503495413,129.889847736274));
#65694=CARTESIAN_POINT('Ctrl Pts',(81.5560579182983,8.40478482925533,129.889411696266));
#65695=CARTESIAN_POINT('Ctrl Pts',(81.5495509905438,8.38796869772132,129.888183498437));
#65696=CARTESIAN_POINT('Ctrl Pts',(81.5452517046582,8.37719365954709,129.887386997125));
#65697=CARTESIAN_POINT('Ctrl Pts',(81.5119759071059,8.29626257375875,129.881336992445));
#65698=CARTESIAN_POINT('Ctrl Pts',(81.4783505602131,8.2281227339408,129.875862336352));
#65699=CARTESIAN_POINT('Ctrl Pts',(81.4356024673256,8.15460937656808,129.869681905552));
#65700=CARTESIAN_POINT('Ctrl Pts',(81.4309370072611,8.14673624797593,129.869016237437));
#65701=CARTESIAN_POINT('Ctrl Pts',(81.3985134747587,8.09303426970591,129.864451292215));
#65702=CARTESIAN_POINT('Ctrl Pts',(81.3686226565074,8.04852792971969,129.860546414805));
#65703=CARTESIAN_POINT('Ctrl Pts',(81.2850909161257,7.93625436121085,129.850449641161));
#65704=CARTESIAN_POINT('Ctrl Pts',(81.2282280395239,7.871074149271,129.844341359641));
#65705=CARTESIAN_POINT('Ctrl Pts',(81.1535016636901,7.7977835681413,129.837190913773));
#65706=CARTESIAN_POINT('Ctrl Pts',(81.1402351497289,7.78519372458252,129.835950907164));
#65707=CARTESIAN_POINT('Ctrl Pts',(81.1187539842749,7.76547022713178,129.833988567409));
#65708=CARTESIAN_POINT('Ctrl Pts',(81.1106724473106,7.75819447500012,129.833260229961));
#65709=CARTESIAN_POINT('Ctrl Pts',(81.0952079750569,7.74454366080545,129.831884909927));
#65710=CARTESIAN_POINT('Ctrl Pts',(81.0878391939669,7.73815332816009,129.831237306303));
#65711=CARTESIAN_POINT('Ctrl Pts',(81.0709027222248,7.7237243623422,129.829766073322));
#65712=CARTESIAN_POINT('Ctrl Pts',(81.0612997831911,7.71572786056812,129.828944189754));
#65713=CARTESIAN_POINT('Ctrl Pts',(81.0358733514287,7.6950348911552,129.826799188378));
#65714=CARTESIAN_POINT('Ctrl Pts',(81.0199060525578,7.68251784199807,129.825483205459));
#65715=CARTESIAN_POINT('Ctrl Pts',(80.8821310171022,7.57851982758275,129.814374571546));
#65716=CARTESIAN_POINT('Ctrl Pts',(80.7485436306297,7.50385666001635,129.805297286916));
#65717=CARTESIAN_POINT('Ctrl Pts',(80.5501760935155,7.42629697231077,129.792162776031));
#65718=CARTESIAN_POINT('Ctrl Pts',(80.4925279210409,7.40731371028175,129.788370911648));
#65719=CARTESIAN_POINT('Ctrl Pts',(80.419846098496,7.38770363504316,129.783476291972));
#65720=CARTESIAN_POINT('Ctrl Pts',(80.4056629557903,7.38407678236913,129.782515844207));
#65721=CARTESIAN_POINT('Ctrl Pts',(80.3846562163795,7.37899900544596,129.781082992177));
#65722=CARTESIAN_POINT('Ctrl Pts',(80.3778679007759,7.37740316950115,129.780618384398));
#65723=CARTESIAN_POINT('Ctrl Pts',(80.3662540756319,7.37474975617759,129.779820493409));
#65724=CARTESIAN_POINT('Ctrl Pts',(80.3614335655779,7.37367094977928,129.779488421072));
#65725=CARTESIAN_POINT('Ctrl Pts',(80.3503726349639,7.37124717456981,129.778724349434));
#65726=CARTESIAN_POINT('Ctrl Pts',(80.3441293699365,7.36991665151617,129.778291564562));
#65727=CARTESIAN_POINT('Ctrl Pts',(80.3267385481417,7.36631479511656,129.777082122721));
#65728=CARTESIAN_POINT('Ctrl Pts',(80.315575388386,7.36412176982262,129.776301330267));
#65729=CARTESIAN_POINT('Ctrl Pts',(80.2469314789489,7.35136527212779,129.771476416119));
#65730=CARTESIAN_POINT('Ctrl Pts',(80.1889557303079,7.34371926179262,129.767300871583));
#65731=CARTESIAN_POINT('Ctrl Pts',(79.9813694698386,7.32738284537932,129.75224532073));
#65732=CARTESIAN_POINT('Ctrl Pts',(79.8310939293539,7.33582386691991,129.741233678064));
#65733=CARTESIAN_POINT('Ctrl Pts',(79.655555976692,7.36973884939697,129.728852717221));
#65734=CARTESIAN_POINT('Ctrl Pts',(79.6272949355791,7.37596668127421,129.726871477612));
#65735=CARTESIAN_POINT('Ctrl Pts',(79.5866285560327,7.38604583854641,129.724036443155));
#65736=CARTESIAN_POINT('Ctrl Pts',(79.5740847748836,7.38931063719569,129.723164152799));
#65737=CARTESIAN_POINT('Ctrl Pts',(79.5521039765462,7.3953063751952,129.721639113229));
#65738=CARTESIAN_POINT('Ctrl Pts',(79.5426507708356,7.39797497928408,129.720984389695));
#65739=CARTESIAN_POINT('Ctrl Pts',(79.5229872476007,7.40371415546975,129.71962465741));
#65740=CARTESIAN_POINT('Ctrl Pts',(79.5127816669158,7.4067994576257,129.718920160765));
#65741=CARTESIAN_POINT('Ctrl Pts',(79.4861319848341,7.41513608738089,129.717083258668));
#65742=CARTESIAN_POINT('Ctrl Pts',(79.4697383768697,7.42054547204248,129.715956044717));
#65743=CARTESIAN_POINT('Ctrl Pts',(79.3965459086622,7.44596479959832,129.710931736298));
#65744=CARTESIAN_POINT('Ctrl Pts',(79.3407696868641,7.4687917096451,129.707127905632));
#65745=CARTESIAN_POINT('Ctrl Pts',(79.1920033861133,7.53931574632667,129.69689562568));
#65746=CARTESIAN_POINT('Ctrl Pts',(79.1020757738566,7.59280825793535,129.690622686182));
#65747=CARTESIAN_POINT('Ctrl Pts',(78.9832024540604,7.67958040109962,129.681531268652));
#65748=CARTESIAN_POINT('Ctrl Pts',(78.9496440237056,7.70611554138256,129.678860849499));
#65749=CARTESIAN_POINT('Ctrl Pts',(78.9040700977414,7.74509374912829,129.67502762809));
#65750=CARTESIAN_POINT('Ctrl Pts',(78.8911687822314,7.75647865717337,129.673917828306));
#65751=CARTESIAN_POINT('Ctrl Pts',(78.8687793946973,7.77686188174313,129.671943025247));
#65752=CARTESIAN_POINT('Ctrl Pts',(78.8592164332387,7.7857760741961,129.671083302788));
#65753=CARTESIAN_POINT('Ctrl Pts',(78.8449329266381,7.79940823933097,129.669772569093));
#65754=CARTESIAN_POINT('Ctrl Pts',(78.8401339421055,7.80404379526237,129.669327543101));
#65755=CARTESIAN_POINT('Ctrl Pts',(78.8314481082018,7.81253528418582,129.668513278921));
#65756=CARTESIAN_POINT('Ctrl Pts',(78.8275522570026,7.81638170748038,129.668144763176));
#65757=CARTESIAN_POINT('Ctrl Pts',(78.8187625615994,7.82514586161174,129.667305831887));
#65758=CARTESIAN_POINT('Ctrl Pts',(78.8138804556329,7.83007497910539,129.666834549982));
#65759=CARTESIAN_POINT('Ctrl Pts',(78.7989693094706,7.84531897930945,129.665379127904));
#65760=CARTESIAN_POINT('Ctrl Pts',(78.7890432867686,7.85573308044749,129.664387742278));
#65761=CARTESIAN_POINT('Ctrl Pts',(78.7025442093338,7.94887147343087,129.655556885467));
#65762=CARTESIAN_POINT('Ctrl Pts',(78.6344217207973,8.03903429878547,129.647274372975));
#65763=CARTESIAN_POINT('Ctrl Pts',(78.5208163116355,8.22614703515834,129.631386156901));
#65764=CARTESIAN_POINT('Ctrl Pts',(78.4745007280648,8.32199392122424,129.623806061303));
#65765=CARTESIAN_POINT('Ctrl Pts',(78.4310549688759,8.43935281318309,129.615249420679));
#65766=CARTESIAN_POINT('Ctrl Pts',(78.4247905745595,8.45720252776885,129.613966017212));
#65767=CARTESIAN_POINT('Ctrl Pts',(78.4153589338174,8.48561669847658,129.611950593604));
#65768=CARTESIAN_POINT('Ctrl Pts',(78.411990402685,8.49611209734192,129.611212027168));
#65769=CARTESIAN_POINT('Ctrl Pts',(78.4061270348181,8.5150237049355,129.609891468943));
#65770=CARTESIAN_POINT('Ctrl Pts',(78.4035941096849,8.52342757705197,129.609308253963));
#65771=CARTESIAN_POINT('Ctrl Pts',(78.3978011802359,8.54321221569553,129.607943484687));
#65772=CARTESIAN_POINT('Ctrl Pts',(78.394595801618,8.55460858803986,129.607163726408));
#65773=CARTESIAN_POINT('Ctrl Pts',(78.385558706467,8.58810477414046,129.604889751872));
#65774=CARTESIAN_POINT('Ctrl Pts',(78.3800598098539,8.61029212278691,129.603406228698));
#65775=CARTESIAN_POINT('Ctrl Pts',(78.3567709503096,8.71329311408802,129.596613030725));
#65776=CARTESIAN_POINT('Ctrl Pts',(78.344559571524,8.7952517264195,129.591479869621));
#65777=CARTESIAN_POINT('Ctrl Pts',(78.3342832370164,8.93496023441837,129.582891629397));
#65778=CARTESIAN_POINT('Ctrl Pts',(78.3330316953672,8.99231227401811,129.579409299768));
#65779=CARTESIAN_POINT('Ctrl Pts',(78.3370332831663,9.12662227422245,129.571163214109));
#65780=CARTESIAN_POINT('Ctrl Pts',(78.3446663326461,9.20336869120854,129.566381276082));
#65781=CARTESIAN_POINT('Ctrl Pts',(78.3595251703247,9.29074579232956,129.560584057839));
#65782=CARTESIAN_POINT('Ctrl Pts',(78.3615910027081,9.3021700210342,129.559819002062));
#65783=CARTESIAN_POINT('Ctrl Pts',(78.3649871346774,9.3198911330595,129.558619896541));
#65784=CARTESIAN_POINT('Ctrl Pts',(78.3662348614166,9.32620373274114,129.558190303674));
#65785=CARTESIAN_POINT('Ctrl Pts',(78.368609225478,9.337860879347,129.557392197737));
#65786=CARTESIAN_POINT('Ctrl Pts',(78.3697256115303,9.34320729673908,129.557024261282));
#65787=CARTESIAN_POINT('Ctrl Pts',(78.3723670577676,9.35555355090209,129.556170231338));
#65788=CARTESIAN_POINT('Ctrl Pts',(78.3739109820356,9.36254906299039,129.55568310139));
#65789=CARTESIAN_POINT('Ctrl Pts',(78.3790046809061,9.38494134313742,129.554113935181));
#65790=CARTESIAN_POINT('Ctrl Pts',(78.3827282745611,9.4002971179156,129.553022836315));
#65791=CARTESIAN_POINT('Ctrl Pts',(78.4006110602173,9.46971737512293,129.548028830699));
#65792=CARTESIAN_POINT('Ctrl Pts',(78.4172634432597,9.52308810287248,129.544020629459));
#65793=CARTESIAN_POINT('Ctrl Pts',(78.4365593657201,9.57550793485619,129.539973235759));
#65794=CARTESIAN_POINT('',(78.3314564671933,8.99960363844182,129.771406544454));
#65795=CARTESIAN_POINT('Ctrl Pts',(78.4365593800808,9.57550797386886,129.733376810833));
#65796=CARTESIAN_POINT('Ctrl Pts',(78.414507417672,9.51560101281142,129.737422524153));
#65797=CARTESIAN_POINT('Ctrl Pts',(78.3959123009134,9.45446380635038,129.741369971414));
#65798=CARTESIAN_POINT('Ctrl Pts',(78.3537670691965,9.28056134816839,129.752338051858));
#65799=CARTESIAN_POINT('Ctrl Pts',(78.3383266317708,9.16623277136057,129.759240425368));
#65800=CARTESIAN_POINT('Ctrl Pts',(78.334257702077,9.0340011424429,129.767706247489));
#65801=CARTESIAN_POINT('Ctrl Pts',(78.3339949934347,9.01675531302839,129.768820136022));
#65802=CARTESIAN_POINT('Ctrl Pts',(78.3340000722429,8.9995093746836,129.769946555234));
#65803=CARTESIAN_POINT('Ctrl Pts',(78.3313278592448,8.99960840453889,129.77148036339));
#65804=CARTESIAN_POINT('Ctrl Pts',(78.3312607575407,8.97840260638213,129.772904623852));
#65805=CARTESIAN_POINT('Ctrl Pts',(78.3316300830525,8.9571992057451,129.774328884314));
#65806=CARTESIAN_POINT('Ctrl Pts',(78.3535890732394,8.38496486156091,129.81279751744));
#65807=CARTESIAN_POINT('Ctrl Pts',(78.9961810022836,7.30590926040735,129.886886262768));
#65808=CARTESIAN_POINT('Ctrl Pts',(80.8788147478848,7.23781766213866,129.99801938076));
#65809=CARTESIAN_POINT('Ctrl Pts',(81.9571171728831,8.78254798385477,130.10915249875));
#65810=CARTESIAN_POINT('Ctrl Pts',(81.2441916059336,10.5262973432389,130.220285616743));
#65811=CARTESIAN_POINT('Ctrl Pts',(79.4504429460659,10.8622730768263,130.327943005808));
#65812=CARTESIAN_POINT('Ctrl Pts',(78.6106061858031,10.0444575566693,130.398556022212));
#65813=CARTESIAN_POINT('Ctrl Pts',(78.4345148001033,9.5762760062711,130.432124665951));
#65814=CARTESIAN_POINT('Origin',(80.,9.,134.));
#65815=CARTESIAN_POINT('',(78.4365594215428,9.57550808650568,131.131996250734));
#65816=CARTESIAN_POINT('',(78.4365593737218,9.57550795659375,130.937771496081));
#65817=CARTESIAN_POINT('',(78.4365593737638,9.57550795670799,134.));
#65818=CARTESIAN_POINT('',(78.3340004596976,8.99985719244809,130.276978875517));
#65819=CARTESIAN_POINT('Ctrl Pts',(78.4365593737218,9.57550795659375,130.937771496081));
#65820=CARTESIAN_POINT('Ctrl Pts',(78.4379751834906,9.57935418406338,130.937505244088));
#65821=CARTESIAN_POINT('Ctrl Pts',(78.4394052087154,9.58319524748535,130.937239436776));
#65822=CARTESIAN_POINT('Ctrl Pts',(78.4707358569938,9.66640923904976,130.931482506129));
#65823=CARTESIAN_POINT('Ctrl Pts',(78.5066422199259,9.7433944779014,130.926197199358));
#65824=CARTESIAN_POINT('Ctrl Pts',(78.5811685246371,9.87576981268402,130.916866755145));
#65825=CARTESIAN_POINT('Ctrl Pts',(78.6175760510482,9.93217992512712,130.912799799818));
#65826=CARTESIAN_POINT('Ctrl Pts',(78.7005830826991,10.0451896256856,130.904182177699));
#65827=CARTESIAN_POINT('Ctrl Pts',(78.747711173067,10.1012155235608,130.899629886433));
#65828=CARTESIAN_POINT('Ctrl Pts',(78.8063923458778,10.1623214944161,130.894088379128));
#65829=CARTESIAN_POINT('Ctrl Pts',(78.8145118041003,10.1706016432865,130.893324142678));
#65830=CARTESIAN_POINT('Ctrl Pts',(78.8272677976328,10.1833412662076,130.89212605099));
#65831=CARTESIAN_POINT('Ctrl Pts',(78.8318450244955,10.1878599751282,130.891696640511));
#65832=CARTESIAN_POINT('Ctrl Pts',(78.8403363103109,10.19614616166,130.890900684722));
#65833=CARTESIAN_POINT('Ctrl Pts',(78.8442427714225,10.1999211385471,130.890534728785));
#65834=CARTESIAN_POINT('Ctrl Pts',(78.8533621412183,10.2086477207897,130.889681001054));
#65835=CARTESIAN_POINT('Ctrl Pts',(78.8585886869604,10.2135847320351,130.889192159077));
#65836=CARTESIAN_POINT('Ctrl Pts',(78.8753979035261,10.2292581314186,130.887621891715));
#65837=CARTESIAN_POINT('Ctrl Pts',(78.8871009585734,10.2398633422209,130.886531495123));
#65838=CARTESIAN_POINT('Ctrl Pts',(78.952643611711,10.2975819471989,130.880448895773));
#65839=CARTESIAN_POINT('Ctrl Pts',(79.0093195498349,10.3413517606602,130.875280771577));
#65840=CARTESIAN_POINT('Ctrl Pts',(79.1777139782204,10.4548923896384,130.86051579327));
#65841=CARTESIAN_POINT('Ctrl Pts',(79.2951524804599,10.5152781903522,130.850933440117));
#65842=CARTESIAN_POINT('Ctrl Pts',(79.4444118699137,10.5708733631537,130.839919217809));
#65843=CARTESIAN_POINT('Ctrl Pts',(79.4705736242051,10.5798826426471,130.838026795321));
#65844=CARTESIAN_POINT('Ctrl Pts',(79.5089589691052,10.592040644828,130.835303612249));
#65845=CARTESIAN_POINT('Ctrl Pts',(79.5210119441027,10.5957083587699,130.834456067366));
#65846=CARTESIAN_POINT('Ctrl Pts',(79.5425108481101,10.6019849166262,130.832957301368));
#65847=CARTESIAN_POINT('Ctrl Pts',(79.5519402478758,10.6046477690668,130.832304350989));
#65848=CARTESIAN_POINT('Ctrl Pts',(79.5717352190971,10.6100497538394,130.830942588391));
#65849=CARTESIAN_POINT('Ctrl Pts',(79.5821048723999,10.612772334768,130.830234337694));
#65850=CARTESIAN_POINT('Ctrl Pts',(79.6095212898809,10.6196884043995,130.828374762362));
#65851=CARTESIAN_POINT('Ctrl Pts',(79.626609589312,10.6237129640936,130.827228880746));
#65852=CARTESIAN_POINT('Ctrl Pts',(79.7138364572567,10.6428063178926,130.821441573491));
#65853=CARTESIAN_POINT('Ctrl Pts',(79.7848364561503,10.6536047522235,130.816937519547));
#65854=CARTESIAN_POINT('Ctrl Pts',(79.9242077807574,10.6656695290136,130.808296220132));
#65855=CARTESIAN_POINT('Ctrl Pts',(79.9923934714281,10.6673757167706,130.8041594857));
#65856=CARTESIAN_POINT('Ctrl Pts',(80.081361403172,10.6641431416272,130.798710716352));
#65857=CARTESIAN_POINT('Ctrl Pts',(80.1022136202209,10.6629926111476,130.79742969099));
#65858=CARTESIAN_POINT('Ctrl Pts',(80.1886094363188,10.6565945862949,130.792087569456));
#65859=CARTESIAN_POINT('Ctrl Pts',(80.2538278840491,10.6478617817643,130.787973383496));
#65860=CARTESIAN_POINT('Ctrl Pts',(80.3296164783878,10.6331076791544,130.78292160702));
#65861=CARTESIAN_POINT('Ctrl Pts',(80.3408583486454,10.6307983574793,130.782165132843));
#65862=CARTESIAN_POINT('Ctrl Pts',(80.3583356251815,10.6270195470387,130.780976656589));
#65863=CARTESIAN_POINT('Ctrl Pts',(80.3645881837285,10.625629871642,130.780548986807));
#65864=CARTESIAN_POINT('Ctrl Pts',(80.3761326778587,10.6229940744072,130.779754483507));
#65865=CARTESIAN_POINT('Ctrl Pts',(80.38142671777,10.6217580623257,130.779388219889));
#65866=CARTESIAN_POINT('Ctrl Pts',(80.3937469828435,10.6188179591084,130.778531419909));
#65867=CARTESIAN_POINT('Ctrl Pts',(80.4007682341566,10.6170940259757,130.778039786706));
#65868=CARTESIAN_POINT('Ctrl Pts',(80.4233065847499,10.6114043699215,130.776451341093));
#65869=CARTESIAN_POINT('Ctrl Pts',(80.4387772555274,10.6072607072406,130.775345274263));
#65870=CARTESIAN_POINT('Ctrl Pts',(80.4758124162859,10.5967666835419,130.772663361832));
#65871=CARTESIAN_POINT('Ctrl Pts',(80.4973124638019,10.5902017193229,130.771078375536));
#65872=CARTESIAN_POINT('Ctrl Pts',(80.5817602739066,10.5625358540965,130.764757841005));
#65873=CARTESIAN_POINT('Ctrl Pts',(80.6435535133111,10.5381161465364,130.759924364264));
#65874=CARTESIAN_POINT('Ctrl Pts',(80.8130248808979,10.4591395914823,130.746314219354));
#65875=CARTESIAN_POINT('Ctrl Pts',(80.9164940894801,10.396476432135,130.737608136743));
#65876=CARTESIAN_POINT('Ctrl Pts',(81.0289943146054,10.3104077263546,130.727863912798));
#65877=CARTESIAN_POINT('Ctrl Pts',(81.0454439082223,10.29732217024,130.726430182854));
#65878=CARTESIAN_POINT('Ctrl Pts',(81.071332379409,10.2759157629804,130.724158394585));
#65879=CARTESIAN_POINT('Ctrl Pts',(81.08093180173,10.2677935780116,130.723312512529));
#65880=CARTESIAN_POINT('Ctrl Pts',(81.0978436067285,10.2531525633496,130.721815639502));
#65881=CARTESIAN_POINT('Ctrl Pts',(81.1051920852422,10.2466765392935,130.721162934409));
#65882=CARTESIAN_POINT('Ctrl Pts',(81.1204723230433,10.232969165474,130.719800643321));
#65883=CARTESIAN_POINT('Ctrl Pts',(81.1283921959165,10.2257251939178,130.71909162793));
#65884=CARTESIAN_POINT('Ctrl Pts',(81.1491205565637,10.2063946542118,130.717227670653));
#65885=CARTESIAN_POINT('Ctrl Pts',(81.161808582558,10.1941804600788,130.716078219406));
#65886=CARTESIAN_POINT('Ctrl Pts',(81.225841915318,10.1305516696461,130.710227969528));
#65887=CARTESIAN_POINT('Ctrl Pts',(81.273980786006,10.0760159614782,130.705668397266));
#65888=CARTESIAN_POINT('Ctrl Pts',(81.3809295934146,9.9375755129988,130.694867246262));
#65889=CARTESIAN_POINT('Ctrl Pts',(81.4358624136164,9.85106525470375,130.688726261868));
#65890=CARTESIAN_POINT('Ctrl Pts',(81.5063776286733,9.71352513366368,130.679116690121));
#65891=CARTESIAN_POINT('Ctrl Pts',(81.5280322765162,9.66588878563137,130.675810654387));
#65892=CARTESIAN_POINT('Ctrl Pts',(81.5514981865764,9.60706769079477,130.671662921655));
#65893=CARTESIAN_POINT('Ctrl Pts',(81.5554855446139,9.59677676613751,130.670934886726));
#65894=CARTESIAN_POINT('Ctrl Pts',(81.5615901230528,9.58054462139988,130.669781670562));
#65895=CARTESIAN_POINT('Ctrl Pts',(81.5637764315996,9.57462947935327,130.669360420274));
#65896=CARTESIAN_POINT('Ctrl Pts',(81.5678090406744,9.56352563651781,130.668567514503));
#65897=CARTESIAN_POINT('Ctrl Pts',(81.5696632596676,9.55834002074372,130.668196326457));
#65898=CARTESIAN_POINT('Ctrl Pts',(81.573956625873,9.54614252324408,130.667321211606));
#65899=CARTESIAN_POINT('Ctrl Pts',(81.5763746487272,9.53912343430509,130.666816086222));
#65900=CARTESIAN_POINT('Ctrl Pts',(81.5842137849916,9.51586414568231,130.665137711104));
#65901=CARTESIAN_POINT('Ctrl Pts',(81.5894312608824,9.4995571473227,130.663953740887));
#65902=CARTESIAN_POINT('Ctrl Pts',(81.6015260909296,9.45964611434461,130.661043135637));
#65903=CARTESIAN_POINT('Ctrl Pts',(81.6081339217301,9.43596505755872,130.659305325025));
#65904=CARTESIAN_POINT('Ctrl Pts',(81.633546312065,9.33643507725013,130.65197913931));
#65905=CARTESIAN_POINT('Ctrl Pts',(81.647526082088,9.25945914963048,130.646264701835));
#65906=CARTESIAN_POINT('Ctrl Pts',(81.667423910441,9.07819559960313,130.633008930474));
#65907=CARTESIAN_POINT('Ctrl Pts',(81.669052001544,8.97374774645698,130.625533904966));
#65908=CARTESIAN_POINT('Ctrl Pts',(81.6590634216884,8.84631013655199,130.616734301889));
#65909=CARTESIAN_POINT('Ctrl Pts',(81.6567219299989,8.82284312982841,130.615126257091));
#65910=CARTESIAN_POINT('Ctrl Pts',(81.652423251002,8.78739612316469,130.612714875513));
#65911=CARTESIAN_POINT('Ctrl Pts',(81.6508321860757,8.77537561175177,130.611900211062));
#65912=CARTESIAN_POINT('Ctrl Pts',(81.6477290037477,8.75374877024306,130.610439705239));
#65913=CARTESIAN_POINT('Ctrl Pts',(81.64626375615,8.74413638396045,130.609792420744));
#65914=CARTESIAN_POINT('Ctrl Pts',(81.6429428411197,8.72356115916944,130.608410659103));
#65915=CARTESIAN_POINT('Ctrl Pts',(81.6410614052011,8.71260291173512,130.60767702883));
#65916=CARTESIAN_POINT('Ctrl Pts',(81.6355939092437,8.68256425262057,130.605671737902));
#65917=CARTESIAN_POINT('Ctrl Pts',(81.6317837493595,8.66352602462411,130.604407193925));
#65918=CARTESIAN_POINT('Ctrl Pts',(81.6028575915234,8.53106720762236,130.595644496151));
#65919=CARTESIAN_POINT('Ctrl Pts',(81.5662715114293,8.42047566357502,130.588540312815));
#65920=CARTESIAN_POINT('Ctrl Pts',(81.476932078692,8.22255435650235,130.575280547878));
#65921=CARTESIAN_POINT('Ctrl Pts',(81.4271189293108,8.13450814711946,130.569139348136));
#65922=CARTESIAN_POINT('Ctrl Pts',(81.3609018802561,8.03888691193086,130.561587454789));
#65923=CARTESIAN_POINT('Ctrl Pts',(81.3519763410698,8.02637161722389,130.560579999477));
#65924=CARTESIAN_POINT('Ctrl Pts',(81.3387142794975,8.00830972481361,130.5590951707));
#65925=CARTESIAN_POINT('Ctrl Pts',(81.3345134474343,8.00266385898142,130.558626550384));
#65926=CARTESIAN_POINT('Ctrl Pts',(81.3269786699658,7.99267004996689,130.557788688147));
#65927=CARTESIAN_POINT('Ctrl Pts',(81.3236588661302,7.98831169647088,130.55742041788));
#65928=CARTESIAN_POINT('Ctrl Pts',(81.3163678386827,7.97883710556991,130.556613457213));
#65929=CARTESIAN_POINT('Ctrl Pts',(81.3123883197203,7.97372769774461,130.556174214063));
#65930=CARTESIAN_POINT('Ctrl Pts',(81.3008643653609,7.95910843049711,130.554905995547));
#65931=CARTESIAN_POINT('Ctrl Pts',(81.2932458339906,7.9496578900392,130.554072120965));
#65932=CARTESIAN_POINT('Ctrl Pts',(81.2755804531359,7.92822813368963,130.552150459386));
#65933=CARTESIAN_POINT('Ctrl Pts',(81.2654669809685,7.91630552886297,130.551058802804));
#65934=CARTESIAN_POINT('Ctrl Pts',(81.2309127485646,7.87671343903414,130.547361946567));
#65935=CARTESIAN_POINT('Ctrl Pts',(81.2057215142613,7.84971560884039,130.544720794932));
#65936=CARTESIAN_POINT('Ctrl Pts',(81.1291445831258,7.77292812281802,130.53689579221));
#65937=CARTESIAN_POINT('Ctrl Pts',(81.0754238043893,7.72558386155537,130.531661241336));
#65938=CARTESIAN_POINT('Ctrl Pts',(80.9404379982862,7.62125128455429,130.519296313703));
#65939=CARTESIAN_POINT('Ctrl Pts',(80.8567899206597,7.56776786926971,130.512245523886));
#65940=CARTESIAN_POINT('Ctrl Pts',(80.7521330391565,7.51332322641634,130.504179360152));
#65941=CARTESIAN_POINT('Ctrl Pts',(80.7352487806133,7.50490093334936,130.502899285896));
#65942=CARTESIAN_POINT('Ctrl Pts',(80.7082977092897,7.49202407490775,130.500888553128));
#65943=CARTESIAN_POINT('Ctrl Pts',(80.6983240025823,7.48737954756951,130.500151375384));
#65944=CARTESIAN_POINT('Ctrl Pts',(80.680323587927,7.47921315545119,130.498833058953));
#65945=CARTESIAN_POINT('Ctrl Pts',(80.6723137912849,7.4756552286603,130.498250701579));
#65946=CARTESIAN_POINT('Ctrl Pts',(80.6534318567758,7.46744571459277,130.496887656463));
#65947=CARTESIAN_POINT('Ctrl Pts',(80.6425374378173,7.46284630494088,130.496108764508));
#65948=CARTESIAN_POINT('Ctrl Pts',(80.6104565959959,7.44970307275177,130.493836452397));
#65949=CARTESIAN_POINT('Ctrl Pts',(80.5891418046517,7.44147831774979,130.492353729362));
#65950=CARTESIAN_POINT('Ctrl Pts',(80.4898363110133,7.40548781878745,130.485559013421));
#65951=CARTESIAN_POINT('Ctrl Pts',(80.4100103511362,7.38311950339621,130.480423833744));
#65952=CARTESIAN_POINT('Ctrl Pts',(80.2727397187093,7.35548050643793,130.471839427105));
#65953=CARTESIAN_POINT('Ctrl Pts',(80.2160909649248,7.34708259823131,130.468362901742));
#65954=CARTESIAN_POINT('Ctrl Pts',(80.0825177367668,7.3342661686926,130.460127696746));
#65955=CARTESIAN_POINT('Ctrl Pts',(80.0055050252363,7.33223354426396,130.45535075556));
#65956=CARTESIAN_POINT('Ctrl Pts',(79.9170408600521,7.33602627915006,130.449559160304));
#65957=CARTESIAN_POINT('Ctrl Pts',(79.9054486979025,7.33664471765062,130.448794160939));
#65958=CARTESIAN_POINT('Ctrl Pts',(79.8874428068185,7.33779415159064,130.447595126332));
#65959=CARTESIAN_POINT('Ctrl Pts',(79.8810238300042,7.33824127150751,130.447165547032));
#65960=CARTESIAN_POINT('Ctrl Pts',(79.8691909442959,7.33913441248831,130.446369451352));
#65961=CARTESIAN_POINT('Ctrl Pts',(79.8637764292165,7.33956974114881,130.446003526252));
#65962=CARTESIAN_POINT('Ctrl Pts',(79.8512043989583,7.34064244217347,130.445150100061));
#65963=CARTESIAN_POINT('Ctrl Pts',(79.8440488146847,7.3412996477322,130.444661531375));
#65964=CARTESIAN_POINT('Ctrl Pts',(79.8212019341303,7.34354716388725,130.443093031704));
#65965=CARTESIAN_POINT('Ctrl Pts',(79.8055294121196,7.34531395969264,130.442004156747));
#65966=CARTESIAN_POINT('Ctrl Pts',(79.719130041258,7.35629830664496,130.435938445662));
#65967=CARTESIAN_POINT('Ctrl Pts',(79.6490324121429,7.36982732819119,130.430786673978));
#65968=CARTESIAN_POINT('Ctrl Pts',(79.4533815193548,7.4207941395087,130.416088888591));
#65969=CARTESIAN_POINT('Ctrl Pts',(79.3310418462584,7.46859885380323,130.406555418746));
#65970=CARTESIAN_POINT('Ctrl Pts',(79.1905787409609,7.54356794918062,130.395537323088));
#65971=CARTESIAN_POINT('Ctrl Pts',(79.1659515198911,7.55752975915162,130.393600151537));
#65972=CARTESIAN_POINT('Ctrl Pts',(79.130797679826,7.57866089291665,130.390825443182));
#65973=CARTESIAN_POINT('Ctrl Pts',(79.1199797385251,7.58533329520533,130.389970214342));
#65974=CARTESIAN_POINT('Ctrl Pts',(79.1009457236331,7.59737613094564,130.388462666514));
#65975=CARTESIAN_POINT('Ctrl Pts',(79.0926988775666,7.60269652894867,130.387808548181));
#65976=CARTESIAN_POINT('Ctrl Pts',(79.0769006243771,7.61308750712869,130.386553418377));
#65977=CARTESIAN_POINT('Ctrl Pts',(79.0693428079217,7.61814765023938,130.385952048806));
#65978=CARTESIAN_POINT('Ctrl Pts',(79.0487863392184,7.63215586080771,130.384313557993));
#65979=CARTESIAN_POINT('Ctrl Pts',(79.0358725624422,7.64122727076419,130.383281119173));
#65980=CARTESIAN_POINT('Ctrl Pts',(78.9827183725594,7.67970535188176,130.379015587948));
#65981=CARTESIAN_POINT('Ctrl Pts',(78.9436766476088,7.71072827803331,130.375844971515));
#65982=CARTESIAN_POINT('Ctrl Pts',(78.836253223589,7.80424876936312,130.366923470229));
#65983=CARTESIAN_POINT('Ctrl Pts',(78.7716131032048,7.8707550438073,130.361314970597));
#65984=CARTESIAN_POINT('Ctrl Pts',(78.6980357500565,7.96029419829377,130.354223638092));
#65985=CARTESIAN_POINT('Ctrl Pts',(78.6836203236812,7.97860704175427,130.352794267241));
#65986=CARTESIAN_POINT('Ctrl Pts',(78.6308044802056,8.04867847097712,130.347379744998));
#65987=CARTESIAN_POINT('Ctrl Pts',(78.5950381104905,8.10234242618471,130.343343423165));
#65988=CARTESIAN_POINT('Ctrl Pts',(78.5566899316897,8.16780833247951,130.338378968576));
#65989=CARTESIAN_POINT('Ctrl Pts',(78.5510086192705,8.17774037824937,130.337624719736));
#65990=CARTESIAN_POINT('Ctrl Pts',(78.5423110812292,8.19331546141852,130.336438998139));
#65991=CARTESIAN_POINT('Ctrl Pts',(78.5392241732181,8.19891891224169,130.336011825583));
#65992=CARTESIAN_POINT('Ctrl Pts',(78.5338113326874,8.20887978890448,130.335251183753));
#65993=CARTESIAN_POINT('Ctrl Pts',(78.5314723965651,8.21322997498409,130.334918542861));
#65994=CARTESIAN_POINT('Ctrl Pts',(78.5258857265647,8.22373232375973,130.334114423012));
#65995=CARTESIAN_POINT('Ctrl Pts',(78.522657180175,8.22989443277911,130.333641775742));
#65996=CARTESIAN_POINT('Ctrl Pts',(78.512800337365,8.24899762312796,130.332174345595));
#65997=CARTESIAN_POINT('Ctrl Pts',(78.50630299643,8.26200499166559,130.331172111793));
#65998=CARTESIAN_POINT('Ctrl Pts',(78.4739807616227,8.32888838532927,130.326009272974));
#65999=CARTESIAN_POINT('Ctrl Pts',(78.4508994752541,8.38403598699598,130.321722937486));
#66000=CARTESIAN_POINT('Ctrl Pts',(78.3894022111586,8.55644829478213,130.30845887476));
#66001=CARTESIAN_POINT('Ctrl Pts',(78.3609911265938,8.67685813804039,130.299415487429));
#66002=CARTESIAN_POINT('Ctrl Pts',(78.3409517216926,8.84199936052571,130.287727994914));
#66003=CARTESIAN_POINT('Ctrl Pts',(78.3374257995158,8.88487833286846,130.284752268311));
#66004=CARTESIAN_POINT('Ctrl Pts',(78.3349203898872,8.9426753329174,130.28081837542));
#66005=CARTESIAN_POINT('Ctrl Pts',(78.3344758100571,8.95750973122619,130.279815428835));
#66006=CARTESIAN_POINT('Ctrl Pts',(78.3341359416264,8.97798396044864,130.278440093409));
#66007=CARTESIAN_POINT('Ctrl Pts',(78.3340709916946,8.98361990179935,130.278062435538));
#66008=CARTESIAN_POINT('Ctrl Pts',(78.3340118553245,8.99278969776598,130.277449460922));
#66009=CARTESIAN_POINT('Ctrl Pts',(78.3340003093644,8.99632335331074,130.277213604314));
#66010=CARTESIAN_POINT('Ctrl Pts',(78.3340000061339,8.99985703818127,130.276978098673));
#66011=CARTESIAN_POINT('Ctrl Pts',(78.3340000061251,8.99985714018325,130.276978091875));
#66012=CARTESIAN_POINT('Ctrl Pts',(78.3339997153914,9.00324761329807,130.276752130718));
#66013=CARTESIAN_POINT('Ctrl Pts',(78.3340097745725,9.00663810598721,130.27652649315));
#66014=CARTESIAN_POINT('Ctrl Pts',(78.3340655951653,9.01591115401808,130.275910246183));
#66015=CARTESIAN_POINT('Ctrl Pts',(78.3341321637657,9.02179357117993,130.27552028939));
#66016=CARTESIAN_POINT('Ctrl Pts',(78.3344228076602,9.03928718690984,130.274363386318));
#66017=CARTESIAN_POINT('Ctrl Pts',(78.3347371366475,9.05089669954057,130.273599264679));
#66018=CARTESIAN_POINT('Ctrl Pts',(78.3360564312599,9.08603780792438,130.271296633948));
#66019=CARTESIAN_POINT('Ctrl Pts',(78.3374390364098,9.1095528901347,130.269769849068));
#66020=CARTESIAN_POINT('Ctrl Pts',(78.3485166095364,9.24783798778132,130.260858993039));
#66021=CARTESIAN_POINT('Ctrl Pts',(78.3695931772456,9.36138392066019,130.253845393381));
#66022=CARTESIAN_POINT('Ctrl Pts',(78.4125350010222,9.50679159710878,130.244585066166));
#66023=CARTESIAN_POINT('Ctrl Pts',(78.4239893636677,9.54135991886436,130.242359213294));
#66024=CARTESIAN_POINT('Ctrl Pts',(78.4365593450135,9.57550787860402,130.240113160697));
#66025=CARTESIAN_POINT('',(78.33440142911,9.00151625010545,130.471480117369));
#66026=CARTESIAN_POINT('Ctrl Pts',(78.4345148001033,9.5762760062711,130.432124665951));
#66027=CARTESIAN_POINT('Ctrl Pts',(78.4162821325133,9.5278000484821,130.435600394876));
#66028=CARTESIAN_POINT('Ctrl Pts',(78.356496074576,9.34162384460564,130.448718878682));
#66029=CARTESIAN_POINT('Ctrl Pts',(78.3331165140057,9.14577591746124,130.461837362488));
#66030=CARTESIAN_POINT('Ctrl Pts',(78.33440142911,9.00151625010545,130.471480117369));
#66031=CARTESIAN_POINT('Ctrl Pts',(78.3340007022066,9.00152962470499,130.471710596613));
#66032=CARTESIAN_POINT('Ctrl Pts',(78.3339349670933,8.92993385869101,130.476901080138));
#66033=CARTESIAN_POINT('Ctrl Pts',(78.3384844518672,8.85840001862447,130.482032138836));
#66034=CARTESIAN_POINT('Ctrl Pts',(78.3517694833915,8.75515916674562,130.489305905419));
#66035=CARTESIAN_POINT('Ctrl Pts',(78.3568560013911,8.72307235552932,130.491548616382));
#66036=CARTESIAN_POINT('Ctrl Pts',(78.3651832410862,8.67893172959673,130.494610001404));
#66037=CARTESIAN_POINT('Ctrl Pts',(78.367625596883,8.66673660252718,130.495453285581));
#66038=CARTESIAN_POINT('Ctrl Pts',(78.3721831580371,8.6452332982515,130.496936029329));
#66039=CARTESIAN_POINT('Ctrl Pts',(78.3742421993977,8.63591393324561,130.497577239465));
#66040=CARTESIAN_POINT('Ctrl Pts',(78.3785753698302,8.61707179535778,130.498870991796));
#66041=CARTESIAN_POINT('Ctrl Pts',(78.3808535852037,8.6075503398954,130.49952337475));
#66042=CARTESIAN_POINT('Ctrl Pts',(78.3858060350955,8.58762987610369,130.50088559758));
#66043=CARTESIAN_POINT('Ctrl Pts',(78.3884971431201,8.57723549488165,130.501594861914));
#66044=CARTESIAN_POINT('Ctrl Pts',(78.3958740677599,8.54983661170472,130.503460844982));
#66045=CARTESIAN_POINT('Ctrl Pts',(78.4007298354169,8.53287896428565,130.504612048516));
#66046=CARTESIAN_POINT('Ctrl Pts',(78.4248565060553,8.45341301743886,130.509993928854));
#66047=CARTESIAN_POINT('Ctrl Pts',(78.4475295088691,8.39199408089226,130.51411291791));
#66048=CARTESIAN_POINT('Ctrl Pts',(78.5128897814093,8.24264556511574,130.524212896189));
#66049=CARTESIAN_POINT('Ctrl Pts',(78.559802257106,8.15684370752952,130.530086677449));
#66050=CARTESIAN_POINT('Ctrl Pts',(78.6492501745467,8.02271929388212,130.540039760952));
#66051=CARTESIAN_POINT('Ctrl Pts',(78.6875434077936,7.97186653027002,130.544027023178));
#66052=CARTESIAN_POINT('Ctrl Pts',(78.7358147800287,7.91486644300933,130.548915602511));
#66053=CARTESIAN_POINT('Ctrl Pts',(78.7430694160422,7.90647149200695,130.549647003246));
#66054=CARTESIAN_POINT('Ctrl Pts',(78.7546703987577,7.89331497871181,130.550812618005));
#66055=CARTESIAN_POINT('Ctrl Pts',(78.7589616143101,7.88850493756123,130.551242940473));
#66056=CARTESIAN_POINT('Ctrl Pts',(78.7669530552219,7.87965127123934,130.552043047157));
#66057=CARTESIAN_POINT('Ctrl Pts',(78.7706454515475,7.87560085685648,130.552412259912));
#66058=CARTESIAN_POINT('Ctrl Pts',(78.7791495899779,7.86636411201824,130.553261493479));
#66059=CARTESIAN_POINT('Ctrl Pts',(78.7839744310211,7.86119015582598,130.553742476706));
#66060=CARTESIAN_POINT('Ctrl Pts',(78.7991481678409,7.84512485570245,130.555252109593));
#66061=CARTESIAN_POINT('Ctrl Pts',(78.8096112027599,7.83434302046208,130.556288740022));
#66062=CARTESIAN_POINT('Ctrl Pts',(78.8925199174556,7.75118856805887,130.564459220716));
#66063=CARTESIAN_POINT('Ctrl Pts',(78.9713472063525,7.68549929084553,130.571956412736));
#66064=CARTESIAN_POINT('Ctrl Pts',(79.1504630765912,7.56226757199929,130.587768204633));
#66065=CARTESIAN_POINT('Ctrl Pts',(79.2517428498069,7.50704720212146,130.596016806403));
#66066=CARTESIAN_POINT('Ctrl Pts',(79.3757981899376,7.45523355036414,130.605215866465));
#66067=CARTESIAN_POINT('Ctrl Pts',(79.3938033944958,7.44807957225725,130.606530994378));
#66068=CARTESIAN_POINT('Ctrl Pts',(79.4223223577848,7.43732027734014,130.608583623627));
#66069=CARTESIAN_POINT('Ctrl Pts',(79.4327539147653,7.43350350684733,130.609328115552));
#66070=CARTESIAN_POINT('Ctrl Pts',(79.4523853109874,7.42654245257867,130.610717676921));
#66071=CARTESIAN_POINT('Ctrl Pts',(79.4615759577565,7.42337383671914,130.611363528665));
#66072=CARTESIAN_POINT('Ctrl Pts',(79.4822977338793,7.41643201866503,130.612809471937));
#66073=CARTESIAN_POINT('Ctrl Pts',(79.4938434842861,7.41270393988582,130.613608052565));
#66074=CARTESIAN_POINT('Ctrl Pts',(79.5279895054301,7.40208878553154,130.615949876095));
#66075=CARTESIAN_POINT('Ctrl Pts',(79.5506973044518,7.39555575540211,130.617481626438));
#66076=CARTESIAN_POINT('Ctrl Pts',(79.6728438715802,7.36321101846698,130.625598729195));
#66077=CARTESIAN_POINT('Ctrl Pts',(79.7743737672135,7.34615435164159,130.631898403886));
#66078=CARTESIAN_POINT('Ctrl Pts',(79.9558735343654,7.33269985091961,130.643013764065));
#66079=CARTESIAN_POINT('Ctrl Pts',(80.0352208257703,7.33248847788776,130.647830824273));
#66080=CARTESIAN_POINT('Ctrl Pts',(80.1389827755485,7.33962259595009,130.654388862713));
#66081=CARTESIAN_POINT('Ctrl Pts',(80.163647825943,7.34187196059625,130.655967458107));
#66082=CARTESIAN_POINT('Ctrl Pts',(80.205355856979,7.3466152021734,130.658683995238));
#66083=CARTESIAN_POINT('Ctrl Pts',(80.2224275011186,7.34882518558433,130.659809395225));
#66084=CARTESIAN_POINT('Ctrl Pts',(80.2468224335836,7.35236836033992,130.661440867223));
#66085=CARTESIAN_POINT('Ctrl Pts',(80.2541764399192,7.353486815758,130.661935731058));
#66086=CARTESIAN_POINT('Ctrl Pts',(80.2669620914676,7.35551905513369,130.662801795851));
#66087=CARTESIAN_POINT('Ctrl Pts',(80.2723970889858,7.3564105861812,130.663171753714));
#66088=CARTESIAN_POINT('Ctrl Pts',(80.2840344827063,7.35837883827611,130.663967901826));
#66089=CARTESIAN_POINT('Ctrl Pts',(80.2902351244666,7.35946374766563,130.664394513261));
#66090=CARTESIAN_POINT('Ctrl Pts',(80.307244545841,7.36253928844591,130.665571122954));
#66091=CARTESIAN_POINT('Ctrl Pts',(80.3180397798927,7.36460173806758,130.666324919242));
#66092=CARTESIAN_POINT('Ctrl Pts',(80.3793244857265,7.37694001572888,130.670641404663));
#66093=CARTESIAN_POINT('Ctrl Pts',(80.4293316251349,7.38944604413835,130.674306765041));
#66094=CARTESIAN_POINT('Ctrl Pts',(80.5706408205097,7.43183416271274,130.684938125982));
#66095=CARTESIAN_POINT('Ctrl Pts',(80.6600520111634,7.46732017385028,130.691990508206));
#66096=CARTESIAN_POINT('Ctrl Pts',(80.7929207132847,7.5338497158724,130.702676501373));
#66097=CARTESIAN_POINT('Ctrl Pts',(80.8387928166537,7.55960164785768,130.706410243536));
#66098=CARTESIAN_POINT('Ctrl Pts',(80.9035796892431,7.60011868429707,130.711735689284));
#66099=CARTESIAN_POINT('Ctrl Pts',(80.9235128048892,7.61318777367779,130.713382003522));
#66100=CARTESIAN_POINT('Ctrl Pts',(80.9591520528946,7.63766387001872,130.716340436158));
#66101=CARTESIAN_POINT('Ctrl Pts',(80.9749520443428,7.64892599830254,130.717657544614));
#66102=CARTESIAN_POINT('Ctrl Pts',(80.9994880135385,7.66706968690371,130.719712546723));
#66103=CARTESIAN_POINT('Ctrl Pts',(81.0083575622236,7.67376678301002,130.720457457919));
#66104=CARTESIAN_POINT('Ctrl Pts',(81.0248581170491,7.6864870278332,130.721847399327));
#66105=CARTESIAN_POINT('Ctrl Pts',(81.0325046596709,7.69248915005022,130.722493215984));
#66106=CARTESIAN_POINT('Ctrl Pts',(81.0495689159257,7.70612671873863,130.723938561877));
#66107=CARTESIAN_POINT('Ctrl Pts',(81.0589567626536,7.71379878516604,130.724736585766));
#66108=CARTESIAN_POINT('Ctrl Pts',(81.0863570763557,7.73669462624715,130.727075129104));
#66109=CARTESIAN_POINT('Ctrl Pts',(81.1041314703856,7.75219955510301,130.728604205435));
#66110=CARTESIAN_POINT('Ctrl Pts',(81.1982313123699,7.83787026496663,130.736779573197));
#66111=CARTESIAN_POINT('Ctrl Pts',(81.2682127008343,7.91466884671018,130.743134056571));
#66112=CARTESIAN_POINT('Ctrl Pts',(81.3778889258898,8.06023834334087,130.754264965202));
#66113=CARTESIAN_POINT('Ctrl Pts',(81.4206687124359,8.12625601637327,130.759042643378));
#66114=CARTESIAN_POINT('Ctrl Pts',(81.47053989672,8.21662510655833,130.765551998821));
#66115=CARTESIAN_POINT('Ctrl Pts',(81.4819706529042,8.23847083629505,130.767123714949));
#66116=CARTESIAN_POINT('Ctrl Pts',(81.5005265475841,8.27593479675374,130.769829562372));
#66117=CARTESIAN_POINT('Ctrl Pts',(81.5079029221145,8.29142462652006,130.770951281153));
#66118=CARTESIAN_POINT('Ctrl Pts',(81.5181284550755,8.31378051531,130.772578348521));
#66119=CARTESIAN_POINT('Ctrl Pts',(81.5211731876138,8.32055661358258,130.773072571699));
#66120=CARTESIAN_POINT('Ctrl Pts',(81.5263957183504,8.33239050811154,130.773937914446));
#66121=CARTESIAN_POINT('Ctrl Pts',(81.5285939207964,8.33743909944149,130.774307797431));
#66122=CARTESIAN_POINT('Ctrl Pts',(81.5332536521584,8.3482876906121,130.775104254059));
#66123=CARTESIAN_POINT('Ctrl Pts',(81.5357072808463,8.35409068722947,130.775531253031));
#66124=CARTESIAN_POINT('Ctrl Pts',(81.5423600229295,8.37007707285946,130.776709949134));
#66125=CARTESIAN_POINT('Ctrl Pts',(81.5464910584003,8.38028819234525,130.777465465534));
#66126=CARTESIAN_POINT('Ctrl Pts',(81.5695499588197,8.43895200483574,130.781817991473));
#66127=CARTESIAN_POINT('Ctrl Pts',(81.5862997607267,8.48822477531962,130.785519633376));
#66128=CARTESIAN_POINT('Ctrl Pts',(81.6290810310146,8.63651378204172,130.796644393227));
#66129=CARTESIAN_POINT('Ctrl Pts',(81.6483290203995,8.73724451009196,130.804166432138));
#66130=CARTESIAN_POINT('Ctrl Pts',(81.6652515442867,8.91164979887429,130.816727648109));
#66131=CARTESIAN_POINT('Ctrl Pts',(81.6675231792014,8.98458737357917,130.821849624644));
#66132=CARTESIAN_POINT('Ctrl Pts',(81.6644015842552,9.07505902154765,130.828027487396));
#66133=CARTESIAN_POINT('Ctrl Pts',(81.6635146000215,9.0926590919079,130.829221347458));
#66134=CARTESIAN_POINT('Ctrl Pts',(81.6616382991473,9.12095189503007,130.831128384632));
#66135=CARTESIAN_POINT('Ctrl Pts',(81.6608245839014,9.13165450595382,130.831846982175));
#66136=CARTESIAN_POINT('Ctrl Pts',(81.6590709170206,9.15210375652171,130.833214899008));
#66137=CARTESIAN_POINT('Ctrl Pts',(81.6581483628256,9.16185139570663,130.833864733082));
#66138=CARTESIAN_POINT('Ctrl Pts',(81.6558459261604,9.18408723825744,130.835342323088));
#66139=CARTESIAN_POINT('Ctrl Pts',(81.6544105920383,9.19656919850586,130.8361683077));
#66140=CARTESIAN_POINT('Ctrl Pts',(81.650200954025,9.2298548502577,130.838362574281));
#66141=CARTESIAN_POINT('Ctrl Pts',(81.6471744681804,9.25062476983929,130.839722976738));
#66142=CARTESIAN_POINT('Ctrl Pts',(81.6240309562504,9.39083008971631,130.848858832549));
#66143=CARTESIAN_POINT('Ctrl Pts',(81.5913343822639,9.50782225275512,130.856213892762));
#66144=CARTESIAN_POINT('Ctrl Pts',(81.5216463352326,9.68155087194645,130.867652201914));
#66145=CARTESIAN_POINT('Ctrl Pts',(81.4934320765618,9.74133564189957,130.871699999128));
#66146=CARTESIAN_POINT('Ctrl Pts',(81.4509934796962,9.81894826582743,130.877298986023));
#66147=CARTESIAN_POINT('Ctrl Pts',(81.4398453905923,9.83839339888407,130.878732475706));
#66148=CARTESIAN_POINT('Ctrl Pts',(81.420083078219,9.87130672371198,130.881222352099));
#66149=CARTESIAN_POINT('Ctrl Pts',(81.4116608121343,9.88488703310924,130.882268778605));
#66150=CARTESIAN_POINT('Ctrl Pts',(81.3991505077208,9.9044257944107,130.883805490688));
#66151=CARTESIAN_POINT('Ctrl Pts',(81.3952166949713,9.91048258089235,130.884286278145));
#66152=CARTESIAN_POINT('Ctrl Pts',(81.3882540577914,9.92105168399021,130.885133398084));
#66153=CARTESIAN_POINT('Ctrl Pts',(81.3852423477297,9.92557504849522,130.885498603588));
#66154=CARTESIAN_POINT('Ctrl Pts',(81.3786316481288,9.93539928796301,130.886297688812));
#66155=CARTESIAN_POINT('Ctrl Pts',(81.3750242529463,9.94069407859132,130.886732101832));
#66156=CARTESIAN_POINT('Ctrl Pts',(81.3648628274479,9.95542527908854,130.887950933577));
#66157=CARTESIAN_POINT('Ctrl Pts',(81.3582417370053,9.96481468026115,130.888739590056));
#66158=CARTESIAN_POINT('Ctrl Pts',(81.3127340311825,10.0279525415454,130.894119235841));
#66159=CARTESIAN_POINT('Ctrl Pts',(81.2707679350355,10.0793998113737,130.898879573392));
#66160=CARTESIAN_POINT('Ctrl Pts',(81.2110402372178,10.1442971578128,130.90527418687));
#66161=CARTESIAN_POINT('Ctrl Pts',(81.1959124148381,10.1600982367291,130.906864971188));
#66162=CARTESIAN_POINT('Ctrl Pts',(81.1296875273683,10.2265981037423,130.913695526737));
#66163=CARTESIAN_POINT('Ctrl Pts',(81.075642173953,10.2742573957305,130.918935484296));
#66164=CARTESIAN_POINT('Ctrl Pts',(80.9657371687861,10.3591852475982,130.92885848432));
#66165=CARTESIAN_POINT('Ctrl Pts',(80.9103715097435,10.3968745834076,130.933546328581));
#66166=CARTESIAN_POINT('Ctrl Pts',(80.8380747238104,10.4399596765993,130.939286400286));
#66167=CARTESIAN_POINT('Ctrl Pts',(80.8231312263737,10.4485538084109,130.940453720669));
#66168=CARTESIAN_POINT('Ctrl Pts',(80.798742503525,10.4620806581149,130.942328835508));
#66169=CARTESIAN_POINT('Ctrl Pts',(80.7893789600739,10.4671572186624,130.943041727857));
#66170=CARTESIAN_POINT('Ctrl Pts',(80.7712939490611,10.4767389699349,130.944405468081));
#66171=CARTESIAN_POINT('Ctrl Pts',(80.7625801178148,10.4812575441587,130.945056767822));
#66172=CARTESIAN_POINT('Ctrl Pts',(80.742469640984,10.4914613708557,130.946546948994));
#66173=CARTESIAN_POINT('Ctrl Pts',(80.7310466278264,10.4970935279538,130.947383950616));
#66174=CARTESIAN_POINT('Ctrl Pts',(80.6938862915828,10.5148888088814,130.950077510568));
#66175=CARTESIAN_POINT('Ctrl Pts',(80.6679006936046,10.5265238636066,130.951915982009));
#66176=CARTESIAN_POINT('Ctrl Pts',(80.5209915438054,10.5878323688928,130.96208716754));
#66177=CARTESIAN_POINT('Ctrl Pts',(80.3948510712179,10.6238038232796,130.969946361092));
#66178=CARTESIAN_POINT('Ctrl Pts',(80.1954414673756,10.6560306964566,130.982340185736));
#66179=CARTESIAN_POINT('Ctrl Pts',(80.1244376110809,10.6628734135012,130.986758475592));
#66180=CARTESIAN_POINT('Ctrl Pts',(80.0374668105584,10.6656532495786,130.992404188399));
#66181=CARTESIAN_POINT('Ctrl Pts',(80.0217050097537,10.6659331793492,130.993436795096));
#66182=CARTESIAN_POINT('Ctrl Pts',(79.998759082803,10.6660150238512,130.994956867852));
#66183=CARTESIAN_POINT('Ctrl Pts',(79.9915759186875,10.66599418657,130.995435121023));
#66184=CARTESIAN_POINT('Ctrl Pts',(79.9789629057277,10.6658760254634,130.99627945692));
#66185=CARTESIAN_POINT('Ctrl Pts',(79.9735330617507,10.6657986047097,130.996644438308));
#66186=CARTESIAN_POINT('Ctrl Pts',(79.9616716766522,10.6655714706829,130.997445097487));
#66187=CARTESIAN_POINT('Ctrl Pts',(79.9552406934064,10.6654110559558,130.997881327482));
#66188=CARTESIAN_POINT('Ctrl Pts',(79.9372100686732,10.6648567901944,130.999110064727));
#66189=CARTESIAN_POINT('Ctrl Pts',(79.9256136436994,10.6643789708214,130.999906915947));
#66190=CARTESIAN_POINT('Ctrl Pts',(79.837221257765,10.6598112626147,131.006026370728));
#66191=CARTESIAN_POINT('Ctrl Pts',(79.7607942880031,10.6505297004094,131.01157572479));
#66192=CARTESIAN_POINT('Ctrl Pts',(79.629167615956,10.6252094503092,131.021318545275));
#66193=CARTESIAN_POINT('Ctrl Pts',(79.5736354253558,10.6115321672092,131.025489188911));
#66194=CARTESIAN_POINT('Ctrl Pts',(79.4395578060655,10.571092320798,131.035609598302));
#66195=CARTESIAN_POINT('Ctrl Pts',(79.3620877741717,10.5412651095284,131.041496315316));
#66196=CARTESIAN_POINT('Ctrl Pts',(79.2664931051318,10.4960100242077,131.048767716817));
#66197=CARTESIAN_POINT('Ctrl Pts',(79.2460384139042,10.485806304336,131.050324696564));
#66198=CARTESIAN_POINT('Ctrl Pts',(79.2153282749773,10.4696891249464,131.052665109169));
#66199=CARTESIAN_POINT('Ctrl Pts',(79.204915880094,10.4640823388088,131.053459145629));
#66200=CARTESIAN_POINT('Ctrl Pts',(79.1868936901026,10.4541289160625,131.054834683528));
#66201=CARTESIAN_POINT('Ctrl Pts',(79.1792569673692,10.4498322851782,131.055417931629));
#66202=CARTESIAN_POINT('Ctrl Pts',(79.1621138857072,10.4400082539625,131.056728266123));
#66203=CARTESIAN_POINT('Ctrl Pts',(79.1526275755255,10.4344465469314,131.057454087016));
#66204=CARTESIAN_POINT('Ctrl Pts',(79.1270319126599,10.4190975967963,131.059415011104));
#66205=CARTESIAN_POINT('Ctrl Pts',(79.1110321582611,10.4091300486523,131.060643524565));
#66206=CARTESIAN_POINT('Ctrl Pts',(79.0091998969472,10.3432655470614,131.068488248232));
#66207=CARTESIAN_POINT('Ctrl Pts',(78.9285037580023,10.279822976562,131.074805775984));
#66208=CARTESIAN_POINT('Ctrl Pts',(78.7941289886919,10.1525038020543,131.086122604903));
#66209=CARTESIAN_POINT('Ctrl Pts',(78.7384389752836,10.0912616765704,131.091130794565));
#66210=CARTESIAN_POINT('Ctrl Pts',(78.6702839415317,10.0040891244896,131.098074834778));
#66211=CARTESIAN_POINT('Ctrl Pts',(78.6536000200431,9.98160413731893,131.099851611055));
#66212=CARTESIAN_POINT('Ctrl Pts',(78.6266525871325,9.94330676374587,131.102873844687));
#66213=CARTESIAN_POINT('Ctrl Pts',(78.6160762759367,9.9277207661565,131.104102747688));
#66214=CARTESIAN_POINT('Ctrl Pts',(78.6015483033417,9.90550993825809,131.10585761507));
#66215=CARTESIAN_POINT('Ctrl Pts',(78.5973744996113,9.89903119859064,131.106369922964));
#66216=CARTESIAN_POINT('Ctrl Pts',(78.5902748140422,9.88784100875058,131.107255946476));
#66217=CARTESIAN_POINT('Ctrl Pts',(78.5873272494154,9.88314350795715,131.107628241312));
#66218=CARTESIAN_POINT('Ctrl Pts',(78.5811559362732,9.87319840227937,131.108417322133));
#66219=CARTESIAN_POINT('Ctrl Pts',(78.577937861096,9.86794769250251,131.108834425622));
#66220=CARTESIAN_POINT('Ctrl Pts',(78.5692311644274,9.85356317347049,131.109978181863));
#66221=CARTESIAN_POINT('Ctrl Pts',(78.5638010595987,9.84439454093521,131.110708392939));
#66222=CARTESIAN_POINT('Ctrl Pts',(78.5367501787327,9.79770378399011,131.114430501027));
#66223=CARTESIAN_POINT('Ctrl Pts',(78.5165121254638,9.75940396939928,131.117494858768));
#66224=CARTESIAN_POINT('Ctrl Pts',(78.4751022088955,9.6730498221801,131.124362681666));
#66225=CARTESIAN_POINT('Ctrl Pts',(78.4546709720977,9.62471040657779,131.128179664619));
#66226=CARTESIAN_POINT('Ctrl Pts',(78.4365594215428,9.57550808650568,131.131996250734));
#66227=CARTESIAN_POINT('Origin',(80.,9.,134.));
#66228=CARTESIAN_POINT('',(78.4365593737656,9.57550795671282,131.83373138687));
#66229=CARTESIAN_POINT('',(78.4365593658221,9.57550793513344,131.638964603241));
#66230=CARTESIAN_POINT('',(78.4365593737638,9.57550795670799,134.));
#66231=CARTESIAN_POINT('Ctrl Pts',(78.4365593658221,9.57550793513344,131.638964603241));
#66232=CARTESIAN_POINT('Ctrl Pts',(78.4410865932633,9.58780672531445,131.638013474793));
#66233=CARTESIAN_POINT('Ctrl Pts',(78.4457595240313,9.60005367347163,131.637063674998));
#66234=CARTESIAN_POINT('Ctrl Pts',(78.4814911855288,9.690480448225,131.630033607877));
#66235=CARTESIAN_POINT('Ctrl Pts',(78.518289588667,9.7662703727031,131.624055371267));
#66236=CARTESIAN_POINT('Ctrl Pts',(78.5722517890723,9.85884847048592,131.616686802588));
#66237=CARTESIAN_POINT('Ctrl Pts',(78.5842524715201,9.87848999795307,131.615118761154));
#66238=CARTESIAN_POINT('Ctrl Pts',(78.6030481180432,9.90786677153953,131.612765155056));
#66239=CARTESIAN_POINT('Ctrl Pts',(78.609546036157,9.91778778724255,131.611968807391));
#66240=CARTESIAN_POINT('Ctrl Pts',(78.6210313403621,9.93492155110456,131.610590584195));
#66241=CARTESIAN_POINT('Ctrl Pts',(78.6259706903703,9.9421657668927,131.610006942427));
#66242=CARTESIAN_POINT('Ctrl Pts',(78.6372227168631,9.9583916663193,131.608697393663));
#66243=CARTESIAN_POINT('Ctrl Pts',(78.6435674842272,9.96735068582696,131.607972738205));
#66244=CARTESIAN_POINT('Ctrl Pts',(78.6609899248764,9.99144325481061,131.606019109763));
#66245=CARTESIAN_POINT('Ctrl Pts',(78.6722355385141,10.00645381903,131.60479663852));
#66246=CARTESIAN_POINT('Ctrl Pts',(78.7392294105224,10.092798952227,131.597726433202));
#66247=CARTESIAN_POINT('Ctrl Pts',(78.8004673337255,10.1596881025449,131.592105785667));
#66248=CARTESIAN_POINT('Ctrl Pts',(78.9150004674912,10.2659570793858,131.582529114542));
#66249=CARTESIAN_POINT('Ctrl Pts',(78.9657554679509,10.3077497090344,131.578545029437));
#66250=CARTESIAN_POINT('Ctrl Pts',(79.0695694592559,10.3833995646239,131.570632669384));
#66251=CARTESIAN_POINT('Ctrl Pts',(79.122337536334,10.4174633074637,131.566715485063));
#66252=CARTESIAN_POINT('Ctrl Pts',(79.1898292327841,10.4558161491801,131.561670528063));
#66253=CARTESIAN_POINT('Ctrl Pts',(79.202861240022,10.4629925126462,131.560694814238));
#66254=CARTESIAN_POINT('Ctrl Pts',(79.2221815807616,10.4732969131412,131.559243350765));
#66255=CARTESIAN_POINT('Ctrl Pts',(79.2283968022564,10.4765614746314,131.558775682831));
#66256=CARTESIAN_POINT('Ctrl Pts',(79.2390254716282,10.4820587807989,131.557974341266));
#66257=CARTESIAN_POINT('Ctrl Pts',(79.2434285260009,10.4843113104594,131.557641907458));
#66258=CARTESIAN_POINT('Ctrl Pts',(79.2535096884958,10.4894121546568,131.556879631707));
#66259=CARTESIAN_POINT('Ctrl Pts',(79.2591939716037,10.492247558727,131.556449027186));
#66260=CARTESIAN_POINT('Ctrl Pts',(79.2749812824152,10.5000100690363,131.555251175446));
#66261=CARTESIAN_POINT('Ctrl Pts',(79.2851179514816,10.5048674318992,131.554479912925));
#66262=CARTESIAN_POINT('Ctrl Pts',(79.3465597866294,10.533548722851,131.54979550102));
#66263=CARTESIAN_POINT('Ctrl Pts',(79.3989970903866,10.5548472392851,131.545758910591));
#66264=CARTESIAN_POINT('Ctrl Pts',(79.5421910286139,10.6046818880271,131.534806034923));
#66265=CARTESIAN_POINT('Ctrl Pts',(79.6344878401091,10.628187736783,131.52782898108));
#66266=CARTESIAN_POINT('Ctrl Pts',(79.8022403726075,10.6559184430193,131.51562674881));
#66267=CARTESIAN_POINT('Ctrl Pts',(79.8769440943925,10.6631400600698,131.510353790725));
#66268=CARTESIAN_POINT('Ctrl Pts',(79.9696264712868,10.6658176024287,131.504024885058));
#66269=CARTESIAN_POINT('Ctrl Pts',(79.9873703067059,10.6660466286799,131.502822526215));
#66270=CARTESIAN_POINT('Ctrl Pts',(80.0158762798348,10.6659591079554,131.500905141759));
#66271=CARTESIAN_POINT('Ctrl Pts',(80.0266371715041,10.6658218020348,131.500184591987));
#66272=CARTESIAN_POINT('Ctrl Pts',(80.0471805556072,10.6653605546711,131.498814961023));
#66273=CARTESIAN_POINT('Ctrl Pts',(80.0569629593501,10.6650546567961,131.498165345811));
#66274=CARTESIAN_POINT('Ctrl Pts',(80.079249614272,10.6641611050317,131.496690961775));
#66275=CARTESIAN_POINT('Ctrl Pts',(80.091751173574,10.6635186867707,131.495867934007));
#66276=CARTESIAN_POINT('Ctrl Pts',(80.1250211097009,10.6614328401725,131.493687518938));
#66277=CARTESIAN_POINT('Ctrl Pts',(80.145772081453,10.6597409201807,131.492337847951));
#66278=CARTESIAN_POINT('Ctrl Pts',(80.289619965818,10.6452935990251,131.483041029028));
#66279=CARTESIAN_POINT('Ctrl Pts',(80.4109935310661,10.6192464106593,131.475536083806));
#66280=CARTESIAN_POINT('Ctrl Pts',(80.6158378379316,10.5507435306029,131.462332877392));
#66281=CARTESIAN_POINT('Ctrl Pts',(80.7007114433986,10.5142854378087,131.456671525805));
#66282=CARTESIAN_POINT('Ctrl Pts',(80.7928337453661,10.4653047061575,131.449853061736));
#66283=CARTESIAN_POINT('Ctrl Pts',(80.8034844174734,10.4594916921608,131.449053913532));
#66284=CARTESIAN_POINT('Ctrl Pts',(80.8197199042674,10.4503989825166,131.447817521257));
#66285=CARTESIAN_POINT('Ctrl Pts',(80.8253509327864,10.4472020467607,131.44738529673));
#66286=CARTESIAN_POINT('Ctrl Pts',(80.8357119944896,10.441239564817,131.446583434735));
#66287=CARTESIAN_POINT('Ctrl Pts',(80.8404471949042,10.4384834133275,131.446214388775));
#66288=CARTESIAN_POINT('Ctrl Pts',(80.8512345304339,10.4321331360761,131.445367786591));
#66289=CARTESIAN_POINT('Ctrl Pts',(80.8572775417827,10.4285239784817,131.444889292235));
#66290=CARTESIAN_POINT('Ctrl Pts',(80.8764515893997,10.4169068999556,131.443357978796));
#66291=CARTESIAN_POINT('Ctrl Pts',(80.8894942466889,10.4087556547604,131.442296654562));
#66292=CARTESIAN_POINT('Ctrl Pts',(81.0111068004752,10.3303896126583,131.432227243793));
#66293=CARTESIAN_POINT('Ctrl Pts',(81.1112635131095,10.2479441466168,131.422659533723));
#66294=CARTESIAN_POINT('Ctrl Pts',(81.2522453839789,10.1013310585399,131.407965590616));
#66295=CARTESIAN_POINT('Ctrl Pts',(81.2999980282605,10.0445363745583,131.402693473354));
#66296=CARTESIAN_POINT('Ctrl Pts',(81.3602967435253,9.96225066708802,131.395637288046));
#66297=CARTESIAN_POINT('Ctrl Pts',(81.3762126076897,9.9393468994684,131.393729399413));
#66298=CARTESIAN_POINT('Ctrl Pts',(81.3985706186698,9.90538356367474,131.390979111804));
#66299=CARTESIAN_POINT('Ctrl Pts',(81.4054715963334,9.89463332178909,131.390119716124));
#66300=CARTESIAN_POINT('Ctrl Pts',(81.4174433447792,9.87550343199851,131.388609610631));
#66301=CARTESIAN_POINT('Ctrl Pts',(81.4225650738873,9.86715656757827,131.387957043791));
#66302=CARTESIAN_POINT('Ctrl Pts',(81.4331488513412,9.84956206784787,131.386594447773));
#66303=CARTESIAN_POINT('Ctrl Pts',(81.4385956886187,9.84030577233851,131.385884994388));
#66304=CARTESIAN_POINT('Ctrl Pts',(81.4527525912494,9.81570653568241,131.384018526801));
#66305=CARTESIAN_POINT('Ctrl Pts',(81.4613092581451,9.80027653627426,131.382867030597));
#66306=CARTESIAN_POINT('Ctrl Pts',(81.5004425464562,9.72698726940665,131.377482922703));
#66307=CARTESIAN_POINT('Ctrl Pts',(81.5278398522601,9.6674917078628,131.373362107518));
#66308=CARTESIAN_POINT('Ctrl Pts',(81.6045948230536,9.47113254555161,131.360300791297));
#66309=CARTESIAN_POINT('Ctrl Pts',(81.6395640625237,9.32940782173374,131.351719711866));
#66310=CARTESIAN_POINT('Ctrl Pts',(81.657390348583,9.16983799396937,131.341412464653));
#66311=CARTESIAN_POINT('Ctrl Pts',(81.6588728865297,9.1546881458148,131.340427062463));
#66312=CARTESIAN_POINT('Ctrl Pts',(81.6611433363872,9.12767221402564,131.338654338946));
#66313=CARTESIAN_POINT('Ctrl Pts',(81.662012189372,9.11581381932494,131.33787091085));
#66314=CARTESIAN_POINT('Ctrl Pts',(81.663154841474,9.09753585942371,131.336653799124));
#66315=CARTESIAN_POINT('Ctrl Pts',(81.6635185732042,9.09112202662904,131.336224894794));
#66316=CARTESIAN_POINT('Ctrl Pts',(81.6641241218618,9.07922753699883,131.335425861555));
#66317=CARTESIAN_POINT('Ctrl Pts',(81.6643759744755,9.07374759619245,131.335056287257));
#66318=CARTESIAN_POINT('Ctrl Pts',(81.6648921256197,9.06116184899341,131.334204209956));
#66319=CARTESIAN_POINT('Ctrl Pts',(81.6651379998377,9.0540555138625,131.33372072167));
#66320=CARTESIAN_POINT('Ctrl Pts',(81.6657830013253,9.03117602980832,131.332156901905));
#66321=CARTESIAN_POINT('Ctrl Pts',(81.666003532449,9.01539925543115,131.331067568332));
#66322=CARTESIAN_POINT('Ctrl Pts',(81.6659806632938,8.91448203356335,131.324039125622));
#66323=CARTESIAN_POINT('Ctrl Pts',(81.659434788834,8.82947631811198,131.317850294563));
#66324=CARTESIAN_POINT('Ctrl Pts',(81.6350846663098,8.67204071762693,131.306254004232));
#66325=CARTESIAN_POINT('Ctrl Pts',(81.6188610592164,8.59956339385728,131.300860253684));
#66326=CARTESIAN_POINT('Ctrl Pts',(81.5862085306613,8.48893004154032,131.292645014825));
#66327=CARTESIAN_POINT('Ctrl Pts',(81.5730982939475,8.44989798560129,131.289749120723));
#66328=CARTESIAN_POINT('Ctrl Pts',(81.5481651176254,8.38387864501267,131.284859533391));
#66329=CARTESIAN_POINT('Ctrl Pts',(81.5370484041738,8.3566469486293,131.282845120287));
#66330=CARTESIAN_POINT('Ctrl Pts',(81.519970276162,8.31778569464955,131.279972299204));
#66331=CARTESIAN_POINT('Ctrl Pts',(81.5145845141784,8.30591083783706,131.27909468369));
#66332=CARTESIAN_POINT('Ctrl Pts',(81.5048949101959,8.28519658050985,131.277563830432));
#66333=CARTESIAN_POINT('Ctrl Pts',(81.5006512643181,8.27632990301453,131.276908565233));
#66334=CARTESIAN_POINT('Ctrl Pts',(81.4916601534637,8.25796309944716,131.275551006098));
#66335=CARTESIAN_POINT('Ctrl Pts',(81.48689981391,8.2484697428402,131.274849195456));
#66336=CARTESIAN_POINT('Ctrl Pts',(81.4742460726599,8.22382583373515,131.273026586034));
#66337=CARTESIAN_POINT('Ctrl Pts',(81.4662097188689,8.20874977745495,131.271910834853));
#66338=CARTESIAN_POINT('Ctrl Pts',(81.4304902716076,8.14415429852324,131.267123130825));
#66339=CARTESIAN_POINT('Ctrl Pts',(81.4005183103492,8.09594039852424,131.26353298698));
#66340=CARTESIAN_POINT('Ctrl Pts',(81.3075365922007,7.96212500363168,131.253384620198));
#66341=CARTESIAN_POINT('Ctrl Pts',(81.2387315878149,7.88090205860205,131.247004433365));
#66342=CARTESIAN_POINT('Ctrl Pts',(81.1198548023238,7.76506933558316,131.236763365018));
#66343=CARTESIAN_POINT('Ctrl Pts',(81.0748367092265,7.72569507313518,131.233023959831));
#66344=CARTESIAN_POINT('Ctrl Pts',(81.0163610927935,7.67985697310843,131.228192162456));
#66345=CARTESIAN_POINT('Ctrl Pts',(81.0047994363253,7.67103591472545,131.227237948238));
#66346=CARTESIAN_POINT('Ctrl Pts',(80.9875384424815,7.65822050042419,131.225812519137));
#66347=CARTESIAN_POINT('Ctrl Pts',(80.9819268073224,7.65410842130923,131.225348977124));
#66348=CARTESIAN_POINT('Ctrl Pts',(80.9722874839488,7.64713731523539,131.22455220226));
#66349=CARTESIAN_POINT('Ctrl Pts',(80.9682725777707,7.64426086234522,131.224220168922));
#66350=CARTESIAN_POINT('Ctrl Pts',(80.9590281959238,7.63769979773673,131.22345521242));
#66351=CARTESIAN_POINT('Ctrl Pts',(80.9537903636151,7.63402750375541,131.223021494924));
#66352=CARTESIAN_POINT('Ctrl Pts',(80.9391268672623,7.62387224441488,131.221806758452));
#66353=CARTESIAN_POINT('Ctrl Pts',(80.9296555938553,7.61745621000202,131.221021546651));
#66354=CARTESIAN_POINT('Ctrl Pts',(80.8664544895885,7.57558554433474,131.215781824065));
#66355=CARTESIAN_POINT('Ctrl Pts',(80.8107798027646,7.54317667659819,131.211167713057));
#66356=CARTESIAN_POINT('Ctrl Pts',(80.7325220715034,7.50349936437941,131.204810285286));
#66357=CARTESIAN_POINT('Ctrl Pts',(80.7114469254506,7.49336600819205,131.203110009697));
#66358=CARTESIAN_POINT('Ctrl Pts',(80.6267034638844,7.45479431941971,131.196333694296));
#66359=CARTESIAN_POINT('Ctrl Pts',(80.5614868708045,7.42991995744521,131.191256414685));
#66360=CARTESIAN_POINT('Ctrl Pts',(80.4508932414423,7.39551398482469,131.182969789702));
#66361=CARTESIAN_POINT('Ctrl Pts',(80.4063337447617,7.38365424340168,131.179713294615));
#66362=CARTESIAN_POINT('Ctrl Pts',(80.3301768179263,7.36673391331792,131.174293407551));
#66363=CARTESIAN_POINT('Ctrl Pts',(80.2988230980426,7.36070751875075,131.172102740033));
#66364=CARTESIAN_POINT('Ctrl Pts',(80.2540341395632,7.35342669137153,131.169028972613));
#66365=CARTESIAN_POINT('Ctrl Pts',(80.2407286640204,7.35142888127001,131.168122732515));
#66366=CARTESIAN_POINT('Ctrl Pts',(80.2175981583668,7.34824186287692,131.166558838441));
#66367=CARTESIAN_POINT('Ctrl Pts',(80.2077842011987,7.34697863441529,131.165898885599));
#66368=CARTESIAN_POINT('Ctrl Pts',(80.1875731393064,7.34455995685847,131.164546894072));
#66369=CARTESIAN_POINT('Ctrl Pts',(80.1771752210296,7.34341484718729,131.163855208107));
#66370=CARTESIAN_POINT('Ctrl Pts',(80.15051287771,7.34073246753245,131.162091065625));
#66371=CARTESIAN_POINT('Ctrl Pts',(80.1342351287995,7.33933632790771,131.161023053958));
#66372=CARTESIAN_POINT('Ctrl Pts',(80.0674390118767,7.33459582304453,131.156674269505));
#66373=CARTESIAN_POINT('Ctrl Pts',(80.0167987504378,7.33331537134916,131.153457538602));
#66374=CARTESIAN_POINT('Ctrl Pts',(79.8570709782273,7.33655903920439,131.143462544086));
#66375=CARTESIAN_POINT('Ctrl Pts',(79.7484513633614,7.34948855735244,131.136903845277));
#66376=CARTESIAN_POINT('Ctrl Pts',(79.5795838957457,7.38665735135284,131.126258808066));
#66377=CARTESIAN_POINT('Ctrl Pts',(79.5181378420725,7.40393255876608,131.122281318358));
#66378=CARTESIAN_POINT('Ctrl Pts',(79.4436679096794,7.42956208097032,131.117164059071));
#66379=CARTESIAN_POINT('Ctrl Pts',(79.4295624329273,7.43463052413377,131.116181209754));
#66380=CARTESIAN_POINT('Ctrl Pts',(79.40893402193,7.44235864504746,131.114721115307));
#66381=CARTESIAN_POINT('Ctrl Pts',(79.4023560535668,7.44487065171404,131.114252089801));
#66382=CARTESIAN_POINT('Ctrl Pts',(79.3911828978629,7.44921883480678,131.113449235571));
#66383=CARTESIAN_POINT('Ctrl Pts',(79.3865796490973,7.4510339066486,131.11311665993));
#66384=CARTESIAN_POINT('Ctrl Pts',(79.3760985413356,7.45522068182605,131.112355217867));
#66385=CARTESIAN_POINT('Ctrl Pts',(79.3702262192284,7.45760538328177,131.111925598969));
#66386=CARTESIAN_POINT('Ctrl Pts',(79.3540357507133,7.46428807193745,131.110733076775));
#66387=CARTESIAN_POINT('Ctrl Pts',(79.3437472558831,7.46865638856319,131.109966213512));
#66388=CARTESIAN_POINT('Ctrl Pts',(79.2833493555423,7.49502072132314,131.105414030899));
#66389=CARTESIAN_POINT('Ctrl Pts',(79.2343090593134,7.5193694249011,131.101513148835));
#66390=CARTESIAN_POINT('Ctrl Pts',(79.1002519005994,7.59437188738399,131.090425460632));
#66391=CARTESIAN_POINT('Ctrl Pts',(79.0184081695503,7.65025329293981,131.08316172444));
#66392=CARTESIAN_POINT('Ctrl Pts',(78.8854079538635,7.75959332249958,131.070816527248));
#66393=CARTESIAN_POINT('Ctrl Pts',(78.8319356076494,7.80980992791756,131.065666786494));
#66394=CARTESIAN_POINT('Ctrl Pts',(78.769898191039,7.87629321882591,131.059460923687));
#66395=CARTESIAN_POINT('Ctrl Pts',(78.7580646006197,7.88938580243971,131.058265299305));
#66396=CARTESIAN_POINT('Ctrl Pts',(78.7393665219918,7.91074585583485,131.056356013149));
#66397=CARTESIAN_POINT('Ctrl Pts',(78.7323703660262,7.91889571415527,131.055636910379));
#66398=CARTESIAN_POINT('Ctrl Pts',(78.7191471873315,7.93460431641017,131.054268382645));
#66399=CARTESIAN_POINT('Ctrl Pts',(78.7129070663044,7.94215139204652,131.053618439313));
#66400=CARTESIAN_POINT('Ctrl Pts',(78.6988169351788,7.95950187675413,131.05214107284));
#66401=CARTESIAN_POINT('Ctrl Pts',(78.6910104434207,7.96933998438703,131.051315416562));
#66402=CARTESIAN_POINT('Ctrl Pts',(78.6665041686598,8.00095156461892,131.048699444944));
#66403=CARTESIAN_POINT('Ctrl Pts',(78.650230180274,8.02305042062074,131.046925747146));
#66404=CARTESIAN_POINT('Ctrl Pts',(78.5589795075367,8.1535978424108,131.036737001547));
#66405=CARTESIAN_POINT('Ctrl Pts',(78.4965435930344,8.27023424013042,131.02880988654));
#66406=CARTESIAN_POINT('Ctrl Pts',(78.4224132107557,8.4597170679087,131.01632754284));
#66407=CARTESIAN_POINT('Ctrl Pts',(78.4006499718142,8.52802239663518,131.011888479251));
#66408=CARTESIAN_POINT('Ctrl Pts',(78.3795331560638,8.61283997819181,131.006217747639));
#66409=CARTESIAN_POINT('Ctrl Pts',(78.3759342300766,8.62822586798793,131.005182776081));
#66410=CARTESIAN_POINT('Ctrl Pts',(78.3710167301025,8.65068464263671,131.003659777954));
#66411=CARTESIAN_POINT('Ctrl Pts',(78.3695241538756,8.6577190876727,131.003181011982));
#66412=CARTESIAN_POINT('Ctrl Pts',(78.3669840173551,8.67008438263633,131.002336024379));
#66413=CARTESIAN_POINT('Ctrl Pts',(78.3659169208175,8.67541102419258,131.001970908544));
#66414=CARTESIAN_POINT('Ctrl Pts',(78.3636434814016,8.68705479300864,131.001170254383));
#66415=CARTESIAN_POINT('Ctrl Pts',(78.3624476751794,8.69337361737917,131.000734166319));
#66416=CARTESIAN_POINT('Ctrl Pts',(78.359198905829,8.7111018199006,130.999506517904));
#66417=CARTESIAN_POINT('Ctrl Pts',(78.3572284489884,8.72252567410388,130.998710626697));
#66418=CARTESIAN_POINT('Ctrl Pts',(78.3438152440272,8.80544698478327,130.992903234864));
#66419=CARTESIAN_POINT('Ctrl Pts',(78.3369264836571,8.8775952243093,130.987690507324));
#66420=CARTESIAN_POINT('Ctrl Pts',(78.3342650540324,8.96615169152368,130.981256628272));
#66421=CARTESIAN_POINT('Ctrl Pts',(78.3340146151872,8.98235602539027,130.980077712919));
#66422=CARTESIAN_POINT('Ctrl Pts',(78.3338894071065,9.12734903413172,130.969524624792));
#66423=CARTESIAN_POINT('Ctrl Pts',(78.3487122805385,9.25574058191219,130.960198832495));
#66424=CARTESIAN_POINT('Ctrl Pts',(78.3828536558729,9.40101071746689,130.949942245357));
#66425=CARTESIAN_POINT('Ctrl Pts',(78.3878837037746,9.42077666899251,130.948551968283));
#66426=CARTESIAN_POINT('Ctrl Pts',(78.3965884142704,9.45253100131099,130.946326188072));
#66427=CARTESIAN_POINT('Ctrl Pts',(78.4000375337431,9.46457845608474,130.945483543669));
#66428=CARTESIAN_POINT('Ctrl Pts',(78.4064150746454,9.48594073036294,130.943992266882));
#66429=CARTESIAN_POINT('Ctrl Pts',(78.4092900356052,9.49527075815947,130.943341932972));
#66430=CARTESIAN_POINT('Ctrl Pts',(78.4155376911458,9.51493033611623,130.94197343865));
#66431=CARTESIAN_POINT('Ctrl Pts',(78.4189297746091,9.52525328275073,130.941255947176));
#66432=CARTESIAN_POINT('Ctrl Pts',(78.4269651646265,9.54892357731872,130.939612821827));
#66433=CARTESIAN_POINT('Ctrl Pts',(78.4316777713226,9.56224646224829,130.938689512326));
#66434=CARTESIAN_POINT('Ctrl Pts',(78.4365593737218,9.57550795659375,130.937771496081));
#66435=CARTESIAN_POINT('Ctrl Pts',(78.4365594215428,9.57550808650568,131.131996250734));
#66436=CARTESIAN_POINT('Ctrl Pts',(78.4235762003059,9.5402375222916,131.134732161266));
#66437=CARTESIAN_POINT('Ctrl Pts',(78.4117850163223,9.50452355026856,131.13746812972));
#66438=CARTESIAN_POINT('Ctrl Pts',(78.3772966037958,9.38681082419089,131.146340195646));
#66439=CARTESIAN_POINT('Ctrl Pts',(78.359665808306,9.30347410969482,131.152387267124));
#66440=CARTESIAN_POINT('Ctrl Pts',(78.345433631865,9.19621682020707,131.159828461515));
#66441=CARTESIAN_POINT('Ctrl Pts',(78.3428690187422,9.17322791705642,131.161404432355));
#66442=CARTESIAN_POINT('Ctrl Pts',(78.3397128500697,9.13836077904294,131.163767262995));
#66443=CARTESIAN_POINT('Ctrl Pts',(78.3387684405541,9.12651815671475,131.164565037516));
#66444=CARTESIAN_POINT('Ctrl Pts',(78.3373473110502,9.10591934266505,131.165944699593));
#66445=CARTESIAN_POINT('Ctrl Pts',(78.3368129071141,9.09716774322538,131.166528367109));
#66446=CARTESIAN_POINT('Ctrl Pts',(78.3357660832314,9.07746965506702,131.167836665302));
#66447=CARTESIAN_POINT('Ctrl Pts',(78.3352925226641,9.06652143821342,131.168560056616));
#66448=CARTESIAN_POINT('Ctrl Pts',(78.3343042583983,9.03690909074114,131.170507019118));
#66449=CARTESIAN_POINT('Ctrl Pts',(78.3339952102391,9.01823930776351,131.171724165173));
#66450=CARTESIAN_POINT('Ctrl Pts',(78.3340253996539,8.90191346801314,131.179250673094));
#66451=CARTESIAN_POINT('Ctrl Pts',(78.3426363780776,8.80444502640658,131.185291027661));
#66452=CARTESIAN_POINT('Ctrl Pts',(78.3768930542379,8.61182820431648,131.197262526315));
#66453=CARTESIAN_POINT('Ctrl Pts',(78.4025198774541,8.51708428296653,131.203173278665));
#66454=CARTESIAN_POINT('Ctrl Pts',(78.447470718423,8.39481108078381,131.211423044028));
#66455=CARTESIAN_POINT('Ctrl Pts',(78.4595035481729,8.36480620504668,131.213500902847));
#66456=CARTESIAN_POINT('Ctrl Pts',(78.476276242608,8.32626693308885,131.216263602511));
#66457=CARTESIAN_POINT('Ctrl Pts',(78.4802297979179,8.31739553475856,131.21690615221));
#66458=CARTESIAN_POINT('Ctrl Pts',(78.4867307764065,8.3031444328207,131.217949838884));
#66459=CARTESIAN_POINT('Ctrl Pts',(78.4892299286579,8.297742772678,131.218348118143));
#66460=CARTESIAN_POINT('Ctrl Pts',(78.4941536302193,8.28724862517868,131.219127347401));
#66461=CARTESIAN_POINT('Ctrl Pts',(78.496575177531,8.28215488355518,131.219508118904));
#66462=CARTESIAN_POINT('Ctrl Pts',(78.5025998881814,8.26964606367031,131.220449298143));
#66463=CARTESIAN_POINT('Ctrl Pts',(78.5062322894477,8.26224530702715,131.221011452269));
#66464=CARTESIAN_POINT('Ctrl Pts',(78.5199557776886,8.23480156012626,131.223115061736));
#66465=CARTESIAN_POINT('Ctrl Pts',(78.5303960739844,8.21493711603471,131.224675669072));
#66466=CARTESIAN_POINT('Ctrl Pts',(78.61158165603,8.06776495263437,131.236492723373));
#66467=CARTESIAN_POINT('Ctrl Pts',(78.6983468654732,7.95001404882297,131.247327947995));
#66468=CARTESIAN_POINT('Ctrl Pts',(78.8443871142556,7.7981928418889,131.262368632087));
#66469=CARTESIAN_POINT('Ctrl Pts',(78.892159349527,7.7540174237506,131.266921998763));
#66470=CARTESIAN_POINT('Ctrl Pts',(78.956008819376,7.70155910718446,131.272561377032));
#66471=CARTESIAN_POINT('Ctrl Pts',(78.9697973217676,7.6905921870938,131.2737549367));
#66472=CARTESIAN_POINT('Ctrl Pts',(78.9922618757992,7.67329918552118,131.275661612631));
#66473=CARTESIAN_POINT('Ctrl Pts',(79.000829325183,7.66683491269287,131.276380145632));
#66474=CARTESIAN_POINT('Ctrl Pts',(79.0173313379767,7.6546323305015,131.277748013801));
#66475=CARTESIAN_POINT('Ctrl Pts',(79.0252551635601,7.64888032496345,131.278397863051));
#66476=CARTESIAN_POINT('Ctrl Pts',(79.0436370363312,7.63578257029402,131.27988973555));
#66477=CARTESIAN_POINT('Ctrl Pts',(79.0541299041157,7.62848656928552,131.280729833309));
#66478=CARTESIAN_POINT('Ctrl Pts',(79.0878176248686,7.60563301429186,131.28339170792));
#66479=CARTESIAN_POINT('Ctrl Pts',(79.111320906235,7.59053712703901,131.285196268376));
#66480=CARTESIAN_POINT('Ctrl Pts',(79.1999431372831,7.53671470207934,131.291825193935));
#66481=CARTESIAN_POINT('Ctrl Pts',(79.2673026571117,7.50185075437514,131.296516656739));
#66482=CARTESIAN_POINT('Ctrl Pts',(79.4164798422585,7.43711701002357,131.306483645639));
#66483=CARTESIAN_POINT('Ctrl Pts',(79.4987298045304,7.40882879141641,131.311728152343));
#66484=CARTESIAN_POINT('Ctrl Pts',(79.6291641476374,7.37509086591643,131.320132710838));
#66485=CARTESIAN_POINT('Ctrl Pts',(79.6760138195103,7.36510521604603,131.323169988916));
#66486=CARTESIAN_POINT('Ctrl Pts',(79.7338855472494,7.35535535540694,131.327015757329));
#66487=CARTESIAN_POINT('Ctrl Pts',(79.7445646255032,7.3536629557517,131.327729307688));
#66488=CARTESIAN_POINT('Ctrl Pts',(79.7614457653593,7.35115586044723,131.328864478885));
#66489=CARTESIAN_POINT('Ctrl Pts',(79.7676374575457,7.35027191178136,131.329282366114));
#66490=CARTESIAN_POINT('Ctrl Pts',(79.7793003961619,7.34867382718593,131.330072638895));
#66491=CARTESIAN_POINT('Ctrl Pts',(79.7847703925035,7.3479519811486,131.330444595255));
#66492=CARTESIAN_POINT('Ctrl Pts',(79.7976965519505,7.34631147027733,131.331326575419));
#66493=CARTESIAN_POINT('Ctrl Pts',(79.8051554558104,7.34541605332656,131.331837857318));
#66494=CARTESIAN_POINT('Ctrl Pts',(79.8301578871399,7.34258599749483,131.333558965552));
#66495=CARTESIAN_POINT('Ctrl Pts',(79.8477253783501,7.34087978233342,131.334780249793));
#66496=CARTESIAN_POINT('Ctrl Pts',(79.8908503356319,7.33738198775142,131.337802362622));
#66497=CARTESIAN_POINT('Ctrl Pts',(79.9164279372204,7.33590028203161,131.339615436418));
#66498=CARTESIAN_POINT('Ctrl Pts',(80.0265993838604,7.33206431430459,131.347487411208));
#66499=CARTESIAN_POINT('Ctrl Pts',(80.1112693931006,7.33556754715333,131.353688194992));
#66500=CARTESIAN_POINT('Ctrl Pts',(80.290401117718,7.35671286504456,131.366779069647));
#66501=CARTESIAN_POINT('Ctrl Pts',(80.3843658708892,7.37611773348157,131.373623880965));
#66502=CARTESIAN_POINT('Ctrl Pts',(80.4988595815248,7.41026528695757,131.381849781459));
#66503=CARTESIAN_POINT('Ctrl Pts',(80.5214178253391,7.41752065055162,131.383465679649));
#66504=CARTESIAN_POINT('Ctrl Pts',(80.5552953409186,7.42921974523854,131.385886249113));
#66505=CARTESIAN_POINT('Ctrl Pts',(80.5667325638681,7.43330994162865,131.386702380894));
#66506=CARTESIAN_POINT('Ctrl Pts',(80.5872424428761,7.44089870885088,131.388164313768));
#66507=CARTESIAN_POINT('Ctrl Pts',(80.596331038977,7.44435228229296,131.388811572854));
#66508=CARTESIAN_POINT('Ctrl Pts',(80.6157282354767,7.45191799262971,131.390191995608));
#66509=CARTESIAN_POINT('Ctrl Pts',(80.6260270718441,7.45605399160166,131.390924324673));
#66510=CARTESIAN_POINT('Ctrl Pts',(80.6541460536771,7.46767416035524,131.392922718365));
#66511=CARTESIAN_POINT('Ctrl Pts',(80.6718788542828,7.47536614428118,131.394181747104));
#66512=CARTESIAN_POINT('Ctrl Pts',(80.7934853518374,7.53064943951328,131.402816423442));
#66513=CARTESIAN_POINT('Ctrl Pts',(80.892360480221,7.58850884789987,131.40981223985));
#66514=CARTESIAN_POINT('Ctrl Pts',(81.0679966421746,7.71717470052997,131.423107252336));
#66515=CARTESIAN_POINT('Ctrl Pts',(81.1455616145988,7.7859405755097,131.429390685733));
#66516=CARTESIAN_POINT('Ctrl Pts',(81.2265571595683,7.87246221681966,131.437089803609));
#66517=CARTESIAN_POINT('Ctrl Pts',(81.2367238273314,7.88362279942544,131.438079620097));
#66518=CARTESIAN_POINT('Ctrl Pts',(81.2514203350729,7.90020320235381,131.439548061852));
#66519=CARTESIAN_POINT('Ctrl Pts',(81.2560699417644,7.9055164925745,131.440018331003));
#66520=CARTESIAN_POINT('Ctrl Pts',(81.2642617062196,7.91499849668367,131.440857372002));
#66521=CARTESIAN_POINT('Ctrl Pts',(81.2678173055301,7.9191553292739,131.441225150972));
#66522=CARTESIAN_POINT('Ctrl Pts',(81.2755814521041,7.92832337874343,131.442036264536));
#66523=CARTESIAN_POINT('Ctrl Pts',(81.2797809131637,7.93334183913899,131.442480200937));
#66524=CARTESIAN_POINT('Ctrl Pts',(81.2918958564495,7.9479940302786,131.443775856325));
#66525=CARTESIAN_POINT('Ctrl Pts',(81.2997326858398,7.95769179871589,131.444632797467));
#66526=CARTESIAN_POINT('Ctrl Pts',(81.3174909108477,7.98017860567078,131.446616705633));
#66527=CARTESIAN_POINT('Ctrl Pts',(81.3273361401949,7.99302596634875,131.447747888699));
#66528=CARTESIAN_POINT('Ctrl Pts',(81.3602184211425,8.03725532337097,131.451629052493));
#66529=CARTESIAN_POINT('Ctrl Pts',(81.3823410662821,8.06929905044129,131.454418594285));
#66530=CARTESIAN_POINT('Ctrl Pts',(81.4413234942914,8.16148070103518,131.462325693619));
#66531=CARTESIAN_POINT('Ctrl Pts',(81.4755180261119,8.22322805971814,131.467484899157));
#66532=CARTESIAN_POINT('Ctrl Pts',(81.5470987445032,8.3743813658722,131.479599038857));
#66533=CARTESIAN_POINT('Ctrl Pts',(81.5808131634194,8.46525825756831,131.486477450796));
#66534=CARTESIAN_POINT('Ctrl Pts',(81.6114269662395,8.57666605409916,131.494378719636));
#66535=CARTESIAN_POINT('Ctrl Pts',(81.6160955118886,8.59485330585436,131.495652894904));
#66536=CARTESIAN_POINT('Ctrl Pts',(81.6230301398396,8.62389887354653,131.497663692752));
#66537=CARTESIAN_POINT('Ctrl Pts',(81.6254968554871,8.63470713771841,131.498406684726));
#66538=CARTESIAN_POINT('Ctrl Pts',(81.6299046894759,8.65495005903992,131.499788719347));
#66539=CARTESIAN_POINT('Ctrl Pts',(81.6318722144995,8.66437842629522,131.500428580265));
#66540=CARTESIAN_POINT('Ctrl Pts',(81.6361303237541,8.68570650969085,131.501867636462));
#66541=CARTESIAN_POINT('Ctrl Pts',(81.6383730783219,8.69761530537912,131.50266528239));
#66542=CARTESIAN_POINT('Ctrl Pts',(81.6447301724061,8.73352042679518,131.505053403141));
#66543=CARTESIAN_POINT('Ctrl Pts',(81.6484487741186,8.7575841582587,131.506631405808));
#66544=CARTESIAN_POINT('Ctrl Pts',(81.655828207381,8.81342187993793,131.51024766948));
#66545=CARTESIAN_POINT('Ctrl Pts',(81.6591043222183,8.84523733393254,131.512274375918));
#66546=CARTESIAN_POINT('Ctrl Pts',(81.6677853875625,8.96262269049376,131.519659214281));
#66547=CARTESIAN_POINT('Ctrl Pts',(81.6674999585984,9.04847849197426,131.524872500957));
#66548=CARTESIAN_POINT('Ctrl Pts',(81.6533278410382,9.22419335818003,131.535642664903));
#66549=CARTESIAN_POINT('Ctrl Pts',(81.6387024059977,9.31369703704057,131.541186384887));
#66550=CARTESIAN_POINT('Ctrl Pts',(81.6130939379413,9.41681048747162,131.548080407421));
#66551=CARTESIAN_POINT('Ctrl Pts',(81.6090900740642,9.43200940358648,131.549110011833));
#66552=CARTESIAN_POINT('Ctrl Pts',(81.6029667213484,9.45398687269942,131.550621421989));
#66553=CARTESIAN_POINT('Ctrl Pts',(81.6010178352607,9.4608126267098,131.551094025884));
#66554=CARTESIAN_POINT('Ctrl Pts',(81.5974863252881,9.47288847268219,131.551936147182));
#66555=CARTESIAN_POINT('Ctrl Pts',(81.5959213167361,9.47814351044607,131.552304652405));
#66556=CARTESIAN_POINT('Ctrl Pts',(81.5924649087459,9.48954351131489,131.553108601247));
#66557=CARTESIAN_POINT('Ctrl Pts',(81.5905639020135,9.49568518757177,131.553544564653));
#66558=CARTESIAN_POINT('Ctrl Pts',(81.5850372752455,9.51318115885471,131.554794324178));
#66559=CARTESIAN_POINT('Ctrl Pts',(81.5813253758679,9.52450748422618,131.555612809863));
#66560=CARTESIAN_POINT('Ctrl Pts',(81.5468873364763,9.62590072140347,131.563018922027));
#66561=CARTESIAN_POINT('Ctrl Pts',(81.5086211631642,9.7132114143114,131.569948916389));
#66562=CARTESIAN_POINT('Ctrl Pts',(81.4053325592501,9.9028818180346,131.585670156419));
#66563=CARTESIAN_POINT('Ctrl Pts',(81.3361640812508,10.00241250003,131.594394165559));
#66564=CARTESIAN_POINT('Ctrl Pts',(81.2430374545382,10.1094390286121,131.604153492306));
#66565=CARTESIAN_POINT('Ctrl Pts',(81.2289526489535,10.1250211233254,131.605586164094));
#66566=CARTESIAN_POINT('Ctrl Pts',(81.2059740737672,10.1494957515072,131.607856493799));
#66567=CARTESIAN_POINT('Ctrl Pts',(81.1972681514024,10.1585607183027,131.608701962165));
#66568=CARTESIAN_POINT('Ctrl Pts',(81.1815984830226,10.1745113438437,131.610198217245));
#66569=CARTESIAN_POINT('Ctrl Pts',(81.1746751269483,10.1814356626849,131.610850715529));
#66570=CARTESIAN_POINT('Ctrl Pts',(81.1600370231907,10.1958199100198,131.612212683915));
#66571=CARTESIAN_POINT('Ctrl Pts',(81.1523104119806,10.2032671673007,131.6129215828));
#66572=CARTESIAN_POINT('Ctrl Pts',(81.131714897616,10.2227377198584,131.614785471104));
#66573=CARTESIAN_POINT('Ctrl Pts',(81.1187261602245,10.2346327219037,131.615934968153));
#66574=CARTESIAN_POINT('Ctrl Pts',(81.0511480862688,10.2945780019843,131.621789276029));
#66575=CARTESIAN_POINT('Ctrl Pts',(80.9936403080464,10.3392256561434,131.626352594241));
#66576=CARTESIAN_POINT('Ctrl Pts',(80.8485778984843,10.4373433972192,131.637165141609));
#66577=CARTESIAN_POINT('Ctrl Pts',(80.7586595416916,10.4867665338019,131.643313510126));
#66578=CARTESIAN_POINT('Ctrl Pts',(80.6169705487816,10.5484255305124,131.652921882488));
#66579=CARTESIAN_POINT('Ctrl Pts',(80.5682186142069,10.566971835703,131.656217855357));
#66580=CARTESIAN_POINT('Ctrl Pts',(80.5082087672168,10.5866320739973,131.660353885233));
#66581=CARTESIAN_POINT('Ctrl Pts',(80.4977008951034,10.5899595253757,131.661080997133));
#66582=CARTESIAN_POINT('Ctrl Pts',(80.4811345117288,10.5950251714944,131.662232998727));
#66583=CARTESIAN_POINT('Ctrl Pts',(80.4750976102733,10.5968337338346,131.662653969603));
#66584=CARTESIAN_POINT('Ctrl Pts',(80.4637671335971,10.6001582313595,131.663446527335));
#66585=CARTESIAN_POINT('Ctrl Pts',(80.4584761280154,10.6016822269449,131.663817648866));
#66586=CARTESIAN_POINT('Ctrl Pts',(80.4460317459932,10.6051999337018,131.664692836212));
#66587=CARTESIAN_POINT('Ctrl Pts',(80.4388724950879,10.6071720733584,131.665198102675));
#66588=CARTESIAN_POINT('Ctrl Pts',(80.4151459553601,10.6135376083416,131.666877918186));
#66589=CARTESIAN_POINT('Ctrl Pts',(80.3985246743736,10.6177230308913,131.668063214499));
#66590=CARTESIAN_POINT('Ctrl Pts',(80.3578759335465,10.6272944002076,131.670977878784));
#66591=CARTESIAN_POINT('Ctrl Pts',(80.3337883352276,10.632405423534,131.672718462475));
#66592=CARTESIAN_POINT('Ctrl Pts',(80.2325830586402,10.6515461023721,131.680064701137));
#66593=CARTESIAN_POINT('Ctrl Pts',(80.1546396322059,10.6606580387945,131.685797011849));
#66594=CARTESIAN_POINT('Ctrl Pts',(79.9725432637179,10.6690117288328,131.69904745732));
#66595=CARTESIAN_POINT('Ctrl Pts',(79.8685057633726,10.6640522683722,131.706499814795));
#66596=CARTESIAN_POINT('Ctrl Pts',(79.7422480369526,10.6461093451544,131.715278623998));
#66597=CARTESIAN_POINT('Ctrl Pts',(79.7189739821184,10.642296114171,131.716886726127));
#66598=CARTESIAN_POINT('Ctrl Pts',(79.6838685515317,10.6357762293792,131.719298042399));
#66599=CARTESIAN_POINT('Ctrl Pts',(79.6719736992034,10.6334324977711,131.720112586589));
#66600=CARTESIAN_POINT('Ctrl Pts',(79.6505892027233,10.628975930472,131.721572800149));
#66601=CARTESIAN_POINT('Ctrl Pts',(79.6410905644552,10.6269094969481,131.722219912869));
#66602=CARTESIAN_POINT('Ctrl Pts',(79.6207717061567,10.6223025048802,131.723601221309));
#66603=CARTESIAN_POINT('Ctrl Pts',(79.609957679577,10.6197365571404,131.724334571447));
#66604=CARTESIAN_POINT('Ctrl Pts',(79.5803374208064,10.612394422509,131.726338856894));
#66605=CARTESIAN_POINT('Ctrl Pts',(79.5615873069736,10.6073975288431,131.727602684996));
#66606=CARTESIAN_POINT('Ctrl Pts',(79.5200082929675,10.5955350318481,131.730397250035));
#66607=CARTESIAN_POINT('Ctrl Pts',(79.4972306424051,10.5885046851489,131.731922683992));
#66608=CARTESIAN_POINT('Ctrl Pts',(79.4247113591903,10.5644052901091,131.736771743078));
#66609=CARTESIAN_POINT('Ctrl Pts',(79.3756226218998,10.545469005002,131.740041452459));
#66610=CARTESIAN_POINT('Ctrl Pts',(79.2414178545118,10.4862582188833,131.749071251283));
#66611=CARTESIAN_POINT('Ctrl Pts',(79.1587034679735,10.4410514571943,131.754736443701));
#66612=CARTESIAN_POINT('Ctrl Pts',(79.0358843578375,10.3597309657736,131.763888191661));
#66613=CARTESIAN_POINT('Ctrl Pts',(78.9929556689949,10.3282498900722,131.767248903843));
#66614=CARTESIAN_POINT('Ctrl Pts',(78.9429732560593,10.2877787074443,131.771460298706));
#66615=CARTESIAN_POINT('Ctrl Pts',(78.9344056817388,10.2806983521752,131.77219338812));
#66616=CARTESIAN_POINT('Ctrl Pts',(78.9210764556528,10.2694565629013,131.773352805125));
#66617=CARTESIAN_POINT('Ctrl Pts',(78.9162663805771,10.2653526854059,131.77377513105));
#66618=CARTESIAN_POINT('Ctrl Pts',(78.9077330343718,10.2579878266643,131.77453164724));
#66619=CARTESIAN_POINT('Ctrl Pts',(78.904000769313,10.2547374945224,131.774865061432));
#66620=CARTESIAN_POINT('Ctrl Pts',(78.9002486109599,10.2514403239504,131.775202801851));
#66621=CARTESIAN_POINT('Ctrl Pts',(78.9002141507659,10.2514100398866,131.77520590391));
#66622=CARTESIAN_POINT('Ctrl Pts',(78.9001468073939,10.2513508527311,131.77521196649));
#66623=CARTESIAN_POINT('Ctrl Pts',(78.9001139241717,10.2513219498258,131.775214926997));
#66624=CARTESIAN_POINT('Ctrl Pts',(78.9000496414552,10.2512654436549,131.775220714815));
#66625=CARTESIAN_POINT('Ctrl Pts',(78.9000182418703,10.2512378405123,131.775223542118));
#66626=CARTESIAN_POINT('Ctrl Pts',(78.8999568403929,10.2511838588304,131.775229071223));
#66627=CARTESIAN_POINT('Ctrl Pts',(78.899926838313,10.2511574803085,131.775231773027));
#66628=CARTESIAN_POINT('Ctrl Pts',(78.8998681519487,10.2511058781583,131.775237058285));
#66629=CARTESIAN_POINT('Ctrl Pts',(78.8998394675703,10.2510806546114,131.775239641733));
#66630=CARTESIAN_POINT('Ctrl Pts',(78.8997608113842,10.2510114836653,131.775246726285));
#66631=CARTESIAN_POINT('Ctrl Pts',(78.8997108412508,10.2509675341781,131.775251227545));
#66632=CARTESIAN_POINT('Ctrl Pts',(78.8996112950469,10.2508799712089,131.775260195478));
#66633=CARTESIAN_POINT('Ctrl Pts',(78.8995617190306,10.250836357857,131.775264662139));
#66634=CARTESIAN_POINT('Ctrl Pts',(78.8994629441931,10.2507494525646,131.775273562371));
#66635=CARTESIAN_POINT('Ctrl Pts',(78.899413745256,10.2507061606002,131.775277995947));
#66636=CARTESIAN_POINT('Ctrl Pts',(78.8993157076356,10.2506198834079,131.775286831516));
#66637=CARTESIAN_POINT('Ctrl Pts',(78.8992668690136,10.250576898308,131.775291233497));
#66638=CARTESIAN_POINT('Ctrl Pts',(78.8991695359932,10.2504912209563,131.775300007303));
#66639=CARTESIAN_POINT('Ctrl Pts',(78.8991210415293,10.2504485287171,131.775304379128));
#66640=CARTESIAN_POINT('Ctrl Pts',(78.8990243810791,10.2503634234336,131.775313094022));
#66641=CARTESIAN_POINT('Ctrl Pts',(78.8989762150178,10.2503210103899,131.775317437092));
#66642=CARTESIAN_POINT('Ctrl Pts',(78.8988801961044,10.2502364502506,131.775326095836));
#66643=CARTESIAN_POINT('Ctrl Pts',(78.8988323431614,10.2501943031381,131.775330411514));
#66644=CARTESIAN_POINT('Ctrl Pts',(78.8987369353573,10.2501102617251,131.77533901682));
#66645=CARTESIAN_POINT('Ctrl Pts',(78.898689380537,10.2500683675202,131.775343306441));
#66646=CARTESIAN_POINT('Ctrl Pts',(78.8985945544824,10.2499848193294,131.775351860926));
#66647=CARTESIAN_POINT('Ctrl Pts',(78.8985472832385,10.2499431653913,131.775356125787));
#66648=CARTESIAN_POINT('Ctrl Pts',(78.8984530101794,10.2498600854266,131.775364632016));
#66649=CARTESIAN_POINT('Ctrl Pts',(78.8984060083371,10.2498186594292,131.775368873381));
#66650=CARTESIAN_POINT('Ctrl Pts',(78.898312260135,10.2497360232124,131.775377333865));
#66651=CARTESIAN_POINT('Ctrl Pts',(78.8982655138022,10.2496948130667,131.775381552976));
#66652=CARTESIAN_POINT('Ctrl Pts',(78.8981722631248,10.2496125968062,131.775389970154));
#66653=CARTESIAN_POINT('Ctrl Pts',(78.8981257587633,10.2495715907235,131.775394168219));
#66654=CARTESIAN_POINT('Ctrl Pts',(78.8980329788979,10.2494897711508,131.775402544478));
#66655=CARTESIAN_POINT('Ctrl Pts',(78.8979867033324,10.2494489576509,131.775406722675));
#66656=CARTESIAN_POINT('Ctrl Pts',(78.8926578890969,10.2447485955114,131.775887903631));
#66657=CARTESIAN_POINT('Ctrl Pts',(78.8874050709824,10.2400556987704,131.776367328106));
#66658=CARTESIAN_POINT('Ctrl Pts',(78.8700641490564,10.22436435013,131.777966616281));
#66659=CARTESIAN_POINT('Ctrl Pts',(78.8581085679564,10.2132217426786,131.779096272608));
#66660=CARTESIAN_POINT('Ctrl Pts',(78.8292729705187,10.1855431385927,131.781883749071));
#66661=CARTESIAN_POINT('Ctrl Pts',(78.8125774324182,10.168820705091,131.783552145622));
#66662=CARTESIAN_POINT('Ctrl Pts',(78.7460516622809,10.0992910289822,131.790406928328));
#66663=CARTESIAN_POINT('Ctrl Pts',(78.6993444134696,10.0436097549103,131.795706010284));
#66664=CARTESIAN_POINT('Ctrl Pts',(78.5903691088932,9.89497245956752,131.809116088394));
#66665=CARTESIAN_POINT('Ctrl Pts',(78.5335362523315,9.79845297575904,131.817152867725));
#66666=CARTESIAN_POINT('Ctrl Pts',(78.4769926821523,9.67568706995518,131.826455327091));
#66667=CARTESIAN_POINT('Ctrl Pts',(78.4676459179303,9.65421355116837,131.828051949695));
#66668=CARTESIAN_POINT('Ctrl Pts',(78.4541646053471,9.62136549156057,131.830449632312));
#66669=CARTESIAN_POINT('Ctrl Pts',(78.4496964371472,9.61013196755477,131.83126183149));
#66670=CARTESIAN_POINT('Ctrl Pts',(78.4423621792914,9.59109182805984,131.832625701042));
#66671=CARTESIAN_POINT('Ctrl Pts',(78.4394316094756,9.583310750653,131.833179510178));
#66672=CARTESIAN_POINT('Ctrl Pts',(78.4365593737656,9.57550795671282,131.83373138687));
#66673=CARTESIAN_POINT('Origin',(80.,9.,134.));
#66674=CARTESIAN_POINT('',(78.4365593745624,9.57550795887745,132.531716954706));
#66675=CARTESIAN_POINT('',(78.4365593734337,9.57550795581125,132.340765796073));
#66676=CARTESIAN_POINT('',(78.4365593737638,9.57550795670799,134.));
#66677=CARTESIAN_POINT('',(78.3340003204331,9.00103328753322,131.67971837006));
#66678=CARTESIAN_POINT('Ctrl Pts',(78.4365593734337,9.57550795581125,132.340765796073));
#66679=CARTESIAN_POINT('Ctrl Pts',(78.4390138527709,9.58217586139625,132.340304604494));
#66680=CARTESIAN_POINT('Ctrl Pts',(78.4415110860817,9.58882832869225,132.339841377572));
#66681=CARTESIAN_POINT('Ctrl Pts',(78.4479889033644,9.60575485622253,132.338654312622));
#66682=CARTESIAN_POINT('Ctrl Pts',(78.4520287230219,9.61600511328503,132.337927491696));
#66683=CARTESIAN_POINT('Ctrl Pts',(78.4585385959357,9.63205415596764,132.336775781979));
#66684=CARTESIAN_POINT('Ctrl Pts',(78.4609404859263,9.63788049441641,132.336354807383));
#66685=CARTESIAN_POINT('Ctrl Pts',(78.4655035584109,9.64877346727423,132.33556211255));
#66686=CARTESIAN_POINT('Ctrl Pts',(78.4676568817167,9.65384318105349,132.335190856561));
#66687=CARTESIAN_POINT('Ctrl Pts',(78.4727743996705,9.66572756575533,132.33431516263));
#66688=CARTESIAN_POINT('Ctrl Pts',(78.4757590914988,9.6725331766438,132.333809521163));
#66689=CARTESIAN_POINT('Ctrl Pts',(78.485788061143,9.69499124181602,132.332127626535));
#66690=CARTESIAN_POINT('Ctrl Pts',(78.4930284404067,9.71055420855854,132.330940593191));
#66691=CARTESIAN_POINT('Ctrl Pts',(78.5112573689462,9.74820444751152,132.328020888363));
#66692=CARTESIAN_POINT('Ctrl Pts',(78.5224983779539,9.7701644913867,132.326276955941));
#66693=CARTESIAN_POINT('Ctrl Pts',(78.5716048551329,9.86106272255202,132.318907798201));
#66694=CARTESIAN_POINT('Ctrl Pts',(78.6138391705723,9.92752304124814,132.313155275592));
#66695=CARTESIAN_POINT('Ctrl Pts',(78.7221886185351,10.074000497477,132.299912297943));
#66696=CARTESIAN_POINT('Ctrl Pts',(78.791406265167,10.1513412954622,132.292486963747));
#66697=CARTESIAN_POINT('Ctrl Pts',(78.8846665958901,10.2377979294419,132.283732607803));
#66698=CARTESIAN_POINT('Ctrl Pts',(78.9023029743275,10.2534646604678,132.282124112159));
#66699=CARTESIAN_POINT('Ctrl Pts',(78.929501555907,10.2766111866273,132.279712197102));
#66700=CARTESIAN_POINT('Ctrl Pts',(78.9388219389407,10.2843691746692,132.278897442431));
#66701=CARTESIAN_POINT('Ctrl Pts',(78.9557669456565,10.2981632668954,132.277436841167));
#66702=CARTESIAN_POINT('Ctrl Pts',(78.9633612055754,10.3042356213783,132.276789550596));
#66703=CARTESIAN_POINT('Ctrl Pts',(78.9797514805819,10.3171076450253,132.275407846758));
#66704=CARTESIAN_POINT('Ctrl Pts',(78.988563311556,10.323886485052,132.274674279711));
#66705=CARTESIAN_POINT('Ctrl Pts',(79.0129439059284,10.3422566746645,132.272669345638));
#66706=CARTESIAN_POINT('Ctrl Pts',(79.0286487147295,10.3536651894777,132.271405091017));
#66707=CARTESIAN_POINT('Ctrl Pts',(79.0640824399794,10.378471191151,132.268609540911));
#66708=CARTESIAN_POINT('Ctrl Pts',(79.0839070112697,10.3917249099864,132.267083552912));
#66709=CARTESIAN_POINT('Ctrl Pts',(79.1483620682851,10.4328420827666,132.262232387711));
#66710=CARTESIAN_POINT('Ctrl Pts',(79.1940314019558,10.4590198230951,132.258961176229));
#66711=CARTESIAN_POINT('Ctrl Pts',(79.326296364182,10.5267253240894,132.249814538132));
#66712=CARTESIAN_POINT('Ctrl Pts',(79.4153417702033,10.5629907794155,132.24403963887));
#66713=CARTESIAN_POINT('Ctrl Pts',(79.5562149503113,10.6066313642942,132.234865176505));
#66714=CARTESIAN_POINT('Ctrl Pts',(79.606095684983,10.6195825953491,132.231607110909));
#66715=CARTESIAN_POINT('Ctrl Pts',(79.6672460723956,10.6324679611317,132.22751368908));
#66716=CARTESIAN_POINT('Ctrl Pts',(79.678023533096,10.6346277739441,132.22678854052));
#66717=CARTESIAN_POINT('Ctrl Pts',(79.6950066511224,10.6378567396888,132.225638905835));
#66718=CARTESIAN_POINT('Ctrl Pts',(79.7011985728069,10.6389976651727,132.225218310871));
#66719=CARTESIAN_POINT('Ctrl Pts',(79.7128206281102,10.6410711026307,132.224425902874));
#66720=CARTESIAN_POINT('Ctrl Pts',(79.7182491008089,10.6420118095776,132.224054549673));
#66721=CARTESIAN_POINT('Ctrl Pts',(79.7310207883624,10.6441598353183,132.22317804452));
#66722=CARTESIAN_POINT('Ctrl Pts',(79.7383675299625,10.6453448956663,132.222671682156));
#66723=CARTESIAN_POINT('Ctrl Pts',(79.7627451334605,10.6491097096597,132.220984874354));
#66724=CARTESIAN_POINT('Ctrl Pts',(79.7798074146923,10.6514744544618,132.219793565263));
#66725=CARTESIAN_POINT('Ctrl Pts',(79.8215033733309,10.6565956930603,132.216861147464));
#66726=CARTESIAN_POINT('Ctrl Pts',(79.8461673992109,10.6590677308374,132.215108658155));
#66727=CARTESIAN_POINT('Ctrl Pts',(79.9500013399327,10.6671397031637,132.207679049791));
#66728=CARTESIAN_POINT('Ctrl Pts',(80.0294620111311,10.6676287937855,132.201872894601));
#66729=CARTESIAN_POINT('Ctrl Pts',(80.2110512464068,10.6557607959364,132.188647894191));
#66730=CARTESIAN_POINT('Ctrl Pts',(80.31262824295,10.6396208285482,132.181292363647));
#66731=CARTESIAN_POINT('Ctrl Pts',(80.4349492535965,10.6083941848069,132.172601673988));
#66732=CARTESIAN_POINT('Ctrl Pts',(80.4576850996068,10.6020727684417,132.170992601716));
#66733=CARTESIAN_POINT('Ctrl Pts',(80.4918928920256,10.5917739992773,132.168580002099));
#66734=CARTESIAN_POINT('Ctrl Pts',(80.5034674828791,10.5881509969698,132.167765129868));
#66735=CARTESIAN_POINT('Ctrl Pts',(80.5242487849829,10.5813961405454,132.166304401418));
#66736=CARTESIAN_POINT('Ctrl Pts',(80.5334694928912,10.5783094908542,132.165657100138));
#66737=CARTESIAN_POINT('Ctrl Pts',(80.5531725091705,10.5715214725207,132.164275462519));
#66738=CARTESIAN_POINT('Ctrl Pts',(80.563645905216,10.5677955437813,132.163541971584));
#66739=CARTESIAN_POINT('Ctrl Pts',(80.5922965609809,10.5572788059536,132.161537476843));
#66740=CARTESIAN_POINT('Ctrl Pts',(80.6103940656554,10.5502746954223,132.16027358011));
#66741=CARTESIAN_POINT('Ctrl Pts',(80.6504398833067,10.5339661147666,132.157478940686));
#66742=CARTESIAN_POINT('Ctrl Pts',(80.6723193690304,10.5245034713234,132.155953500046));
#66743=CARTESIAN_POINT('Ctrl Pts',(80.7417880472896,10.4926724087618,132.151104742971));
#66744=CARTESIAN_POINT('Ctrl Pts',(80.7885256086428,10.4685191231564,132.147835328958));
#66745=CARTESIAN_POINT('Ctrl Pts',(80.9171323419402,10.3941436674144,132.138689894579));
#66746=CARTESIAN_POINT('Ctrl Pts',(80.9959075317428,10.3390052677834,132.132914549906));
#66747=CARTESIAN_POINT('Ctrl Pts',(81.1090204913883,10.2443018063335,132.123737490756));
#66748=CARTESIAN_POINT('Ctrl Pts',(81.1469850496162,10.2093955559901,132.120477113869));
#66749=CARTESIAN_POINT('Ctrl Pts',(81.191005572531,10.1649817966471,132.116381097494));
#66750=CARTESIAN_POINT('Ctrl Pts',(81.1986668823445,10.1570974676378,132.11565583174));
#66751=CARTESIAN_POINT('Ctrl Pts',(81.21059251829,10.1445791376865,132.114506051638));
#66752=CARTESIAN_POINT('Ctrl Pts',(81.2149097154227,10.1399956262496,132.114085430065));
#66753=CARTESIAN_POINT('Ctrl Pts',(81.2229554854038,10.1313559277382,132.113293002017));
#66754=CARTESIAN_POINT('Ctrl Pts',(81.2266900463082,10.1273055846822,132.112921655684));
#66755=CARTESIAN_POINT('Ctrl Pts',(81.2354212509468,10.1177413395842,132.112045207636));
#66756=CARTESIAN_POINT('Ctrl Pts',(81.2404011139916,10.1122124080508,132.111538895995));
#66757=CARTESIAN_POINT('Ctrl Pts',(81.2567827326659,10.09377772971,132.109852434224));
#66758=CARTESIAN_POINT('Ctrl Pts',(81.2680209863795,10.0807290499715,132.108661426332));
#66759=CARTESIAN_POINT('Ctrl Pts',(81.2949308813777,10.0484864983784,132.105729904596));
#66760=CARTESIAN_POINT('Ctrl Pts',(81.3103801893936,10.0291129931921,132.103978018607));
#66761=CARTESIAN_POINT('Ctrl Pts',(81.3734456722168,9.94630524212548,132.096552687401));
#66762=CARTESIAN_POINT('Ctrl Pts',(81.41693141149,9.87985859548995,132.090750329207));
#66763=CARTESIAN_POINT('Ctrl Pts',(81.5054772720264,9.72085934380122,132.077524055374));
#66764=CARTESIAN_POINT('Ctrl Pts',(81.5470432090717,9.62670867912194,132.070163587505));
#66765=CARTESIAN_POINT('Ctrl Pts',(81.5871737825231,9.50694384516692,132.061468394675));
#66766=CARTESIAN_POINT('Ctrl Pts',(81.5941942172462,9.48441467218927,132.059859364991));
#66767=CARTESIAN_POINT('Ctrl Pts',(81.6040952861907,9.45009042620961,132.057446815933));
#66768=CARTESIAN_POINT('Ctrl Pts',(81.6073292721404,9.43840130400958,132.056631952383));
#66769=CARTESIAN_POINT('Ctrl Pts',(81.6129256186727,9.41727867226319,132.055171233327));
#66770=CARTESIAN_POINT('Ctrl Pts',(81.6153335460166,9.4078579209575,132.054523932838));
#66771=CARTESIAN_POINT('Ctrl Pts',(81.6203172453292,9.38762299975282,132.053142290333));
#66772=CARTESIAN_POINT('Ctrl Pts',(81.6228675478002,9.37680299603075,132.05240879378));
#66773=CARTESIAN_POINT('Ctrl Pts',(81.6295717328665,9.34702806679832,132.050404266611));
#66774=CARTESIAN_POINT('Ctrl Pts',(81.6335031438414,9.32802445305044,132.049140343462));
#66775=CARTESIAN_POINT('Ctrl Pts',(81.6415219697934,9.28553412545088,132.046345636821));
#66776=CARTESIAN_POINT('Ctrl Pts',(81.6454391542386,9.26201944358941,132.044820155781));
#66777=CARTESIAN_POINT('Ctrl Pts',(81.6563754912358,9.18638909082043,132.039971220987));
#66778=CARTESIAN_POINT('Ctrl Pts',(81.6614330282506,9.13402080964627,132.036701674323));
#66779=CARTESIAN_POINT('Ctrl Pts',(81.6687006183625,8.98563262243248,132.027556155132));
#66780=CARTESIAN_POINT('Ctrl Pts',(81.6651025899473,8.88954566138587,132.021780847144));
#66781=CARTESIAN_POINT('Ctrl Pts',(81.6468889545434,8.74315389156069,132.012603980365));
#66782=CARTESIAN_POINT('Ctrl Pts',(81.6381546073884,8.69232888696934,132.009343770407));
#66783=CARTESIAN_POINT('Ctrl Pts',(81.6247175973539,8.63125945939537,132.00524794143));
#66784=CARTESIAN_POINT('Ctrl Pts',(81.6222490815676,8.62054676320443,132.004522684149));
#66785=CARTESIAN_POINT('Ctrl Pts',(81.6182002831897,8.60373810317127,132.003372914561));
#66786=CARTESIAN_POINT('Ctrl Pts',(81.6166910924922,8.59762510567916,132.002952294911));
#66787=CARTESIAN_POINT('Ctrl Pts',(81.6137964673571,8.58617960837191,132.002159868313));
#66788=CARTESIAN_POINT('Ctrl Pts',(81.6124191900852,8.58084524756849,132.001788521483));
#66789=CARTESIAN_POINT('Ctrl Pts',(81.6091195679808,8.56832235842835,132.000912069307));
#66790=CARTESIAN_POINT('Ctrl Pts',(81.6071754942407,8.56113977656776,132.000405753999));
#66791=CARTESIAN_POINT('Ctrl Pts',(81.6005728762602,8.53737808358832,131.998719267217));
#66792=CARTESIAN_POINT('Ctrl Pts',(81.5957055606148,8.52085881433693,131.997528237554));
#66793=CARTESIAN_POINT('Ctrl Pts',(81.5832126218306,8.48076233898569,131.994596651056));
#66794=CARTESIAN_POINT('Ctrl Pts',(81.5753154773496,8.45727449844457,131.992844721464));
#66795=CARTESIAN_POINT('Ctrl Pts',(81.5399497935568,8.35937386944984,131.985419081214));
#66796=CARTESIAN_POINT('Ctrl Pts',(81.5077097119981,8.28679752008612,131.979616448682));
#66797=CARTESIAN_POINT('Ctrl Pts',(81.4221538810516,8.12617085872966,131.966390266842));
#66798=CARTESIAN_POINT('Ctrl Pts',(81.3656016229424,8.04018872417165,131.959030155715));
#66799=CARTESIAN_POINT('Ctrl Pts',(81.2867522254879,7.94151930090832,131.950335288274));
#66800=CARTESIAN_POINT('Ctrl Pts',(81.2716324412234,7.92340178644546,131.948726255539));
#66801=CARTESIAN_POINT('Ctrl Pts',(81.2481656183724,7.89646673440405,131.946313702858));
#66802=CARTESIAN_POINT('Ctrl Pts',(81.240099244862,7.88740979891581,131.945498838686));
#66803=CARTESIAN_POINT('Ctrl Pts',(81.2253887654404,7.87125161561904,131.944038118956));
#66804=CARTESIAN_POINT('Ctrl Pts',(81.2187800927997,7.86411900536034,131.94339081841));
#66805=CARTESIAN_POINT('Ctrl Pts',(81.2044831308971,7.84895701527119,131.942009176253));
#66806=CARTESIAN_POINT('Ctrl Pts',(81.1967761263927,7.84094586896147,131.941275680102));
#66807=CARTESIAN_POINT('Ctrl Pts',(81.1753974676037,7.81916415039868,131.939271155252));
#66808=CARTESIAN_POINT('Ctrl Pts',(81.1615642451314,7.80555407572372,131.938007233993));
#66809=CARTESIAN_POINT('Ctrl Pts',(81.1302160269946,7.77577132682943,131.935212532161));
#66810=CARTESIAN_POINT('Ctrl Pts',(81.1125852054254,7.75972649888601,131.933687054013));
#66811=CARTESIAN_POINT('Ctrl Pts',(81.0549774627006,7.70951823043555,131.928838131937));
#66812=CARTESIAN_POINT('Ctrl Pts',(81.0137243817552,7.67686578690892,131.925568594767));
#66813=CARTESIAN_POINT('Ctrl Pts',(80.8930004882725,7.5902772216071,131.916423081668));
#66814=CARTESIAN_POINT('Ctrl Pts',(80.8103231358185,7.54118430901875,131.910647771076));
#66815=CARTESIAN_POINT('Ctrl Pts',(80.6774556564384,7.47708601493515,131.901470890533));
#66816=CARTESIAN_POINT('Ctrl Pts',(80.6300183734611,7.45685745929915,131.898210668606));
#66817=CARTESIAN_POINT('Ctrl Pts',(80.5714237646628,7.43502340630212,131.894114826193));
#66818=CARTESIAN_POINT('Ctrl Pts',(80.5610847910996,7.43128692905135,131.893389568305));
#66819=CARTESIAN_POINT('Ctrl Pts',(80.5447672804534,7.42557176804789,131.892239797962));
#66820=CARTESIAN_POINT('Ctrl Pts',(80.5388129917335,7.42352411877329,131.891819178175));
#66821=CARTESIAN_POINT('Ctrl Pts',(80.5276272616244,7.41974817596469,131.891026751472));
#66822=CARTESIAN_POINT('Ctrl Pts',(80.522398681053,7.41801201993512,131.890655404678));
#66823=CARTESIAN_POINT('Ctrl Pts',(80.5100881416732,7.41399197418184,131.889778952799));
#66824=CARTESIAN_POINT('Ctrl Pts',(80.5029993933729,7.41172956483827,131.889272637754));
#66825=CARTESIAN_POINT('Ctrl Pts',(80.4794553039468,7.4043887752591,131.887586152767));
#66826=CARTESIAN_POINT('Ctrl Pts',(80.462937004629,7.39951824722721,131.886395124666));
#66827=CARTESIAN_POINT('Ctrl Pts',(80.4224747686478,7.38826645432181,131.883463542814));
#66828=CARTESIAN_POINT('Ctrl Pts',(80.3984586434108,7.38216177243315,131.881711616348));
#66829=CARTESIAN_POINT('Ctrl Pts',(80.2970277363352,7.35877433359403,131.874285998263));
#66830=CARTESIAN_POINT('Ctrl Pts',(80.2185678234387,7.34649632054733,131.868483385404));
#66831=CARTESIAN_POINT('Ctrl Pts',(80.0372161823935,7.3312537473824,131.855257196962));
#66832=CARTESIAN_POINT('Ctrl Pts',(79.9343065701634,7.33213012454231,131.847897060247));
#66833=CARTESIAN_POINT('Ctrl Pts',(79.8086444248078,7.34485779346857,131.839202169469));
#66834=CARTESIAN_POINT('Ctrl Pts',(79.7852226313434,7.34773384082206,131.837593136954));
#66835=CARTESIAN_POINT('Ctrl Pts',(79.7498656640781,7.35284005235047,131.835180584534));
#66836=CARTESIAN_POINT('Ctrl Pts',(79.7378815914028,7.35470457591523,131.834365720408));
#66837=CARTESIAN_POINT('Ctrl Pts',(79.7163278933248,7.3582994555634,131.832905000728));
#66838=CARTESIAN_POINT('Ctrl Pts',(79.7067511376011,7.35998303262163,131.832257700187));
#66839=CARTESIAN_POINT('Ctrl Pts',(79.6862586570776,7.36377081829597,131.830876058008));
#66840=CARTESIAN_POINT('Ctrl Pts',(79.6753481000852,7.36590063971851,131.830142561829));
#66841=CARTESIAN_POINT('Ctrl Pts',(79.6454531915931,7.37204758322549,131.828138036817));
#66842=CARTESIAN_POINT('Ctrl Pts',(79.626516048026,7.37628749487896,131.826874115426));
#66843=CARTESIAN_POINT('Ctrl Pts',(79.5844919138071,7.38647059451865,131.824079413257));
#66844=CARTESIAN_POINT('Ctrl Pts',(79.5614495093685,7.39258043304805,131.822553934905));
#66845=CARTESIAN_POINT('Ctrl Pts',(79.4880225626582,7.41374663145598,131.817705011935));
#66846=CARTESIAN_POINT('Ctrl Pts',(79.4382152952725,7.43069467128549,131.814435474097));
#66847=CARTESIAN_POINT('Ctrl Pts',(79.3010761743782,7.48472736583335,131.805361753301));
#66848=CARTESIAN_POINT('Ctrl Pts',(79.2159943864409,7.52694888187069,131.799654645729));
#66849=CARTESIAN_POINT('Ctrl Pts',(79.0900528403074,7.60346348141398,131.790494747482));
#66850=CARTESIAN_POINT('Ctrl Pts',(79.0464580256391,7.63285896594573,131.78717364008));
#66851=CARTESIAN_POINT('Ctrl Pts',(78.9954457554362,7.67088392042171,131.783006955854));
#66852=CARTESIAN_POINT('Ctrl Pts',(78.9866281861097,7.67759448963587,131.782276059823));
#66853=CARTESIAN_POINT('Ctrl Pts',(78.9728906244354,7.68826747139531,131.781119294417));
#66854=CARTESIAN_POINT('Ctrl Pts',(78.9679249266102,7.69217090735795,131.78069739561));
#66855=CARTESIAN_POINT('Ctrl Pts',(78.9588177569431,7.6994140391134,131.779916408637));
#66856=CARTESIAN_POINT('Ctrl Pts',(78.9546699320347,7.70274545643338,131.779557897802));
#66857=CARTESIAN_POINT('Ctrl Pts',(78.9504874664583,7.70613777928122,131.77919356162));
#66858=CARTESIAN_POINT('Ctrl Pts',(78.9504367514988,7.70617891821937,131.779189143399));
#66859=CARTESIAN_POINT('Ctrl Pts',(78.9503356591736,7.70626093210177,131.779180335527));
#66860=CARTESIAN_POINT('Ctrl Pts',(78.9502852816959,7.7063018070723,131.779175945872));
#66861=CARTESIAN_POINT('Ctrl Pts',(78.9501848475955,7.70638330640876,131.779167193691));
#66862=CARTESIAN_POINT('Ctrl Pts',(78.9501347909267,7.70642393075108,131.779162831165));
#66863=CARTESIAN_POINT('Ctrl Pts',(78.9500349822592,7.70650494178493,131.779154131848));
#66864=CARTESIAN_POINT('Ctrl Pts',(78.9499852302099,7.70654532845987,131.779149795057));
#66865=CARTESIAN_POINT('Ctrl Pts',(78.9498860149407,7.70662587684671,131.779141145843));
#66866=CARTESIAN_POINT('Ctrl Pts',(78.949836551719,7.70666603850583,131.779136833424));
#66867=CARTESIAN_POINT('Ctrl Pts',(78.9497378986349,7.70674614926079,131.779128231619));
#66868=CARTESIAN_POINT('Ctrl Pts',(78.9496887088085,7.70678609827639,131.77912394224));
#66869=CARTESIAN_POINT('Ctrl Pts',(78.9495905875734,7.70686579572739,131.779115385226));
#66870=CARTESIAN_POINT('Ctrl Pts',(78.9495416561191,7.70690554415188,131.77911111759));
#66871=CARTESIAN_POINT('Ctrl Pts',(78.9494440371514,7.70698485203819,131.779102602812));
#66872=CARTESIAN_POINT('Ctrl Pts',(78.9493953494971,7.70702441156951,131.779098355661));
#66873=CARTESIAN_POINT('Ctrl Pts',(78.9492982035649,7.70710335336997,131.779089880592));
#66874=CARTESIAN_POINT('Ctrl Pts',(78.9492497453263,7.70714273556504,131.779085652682));
#66875=CARTESIAN_POINT('Ctrl Pts',(78.9491530441415,7.70722133401415,131.779077214877));
#66876=CARTESIAN_POINT('Ctrl Pts',(78.9491048012547,7.70726055018061,131.779073004991));
#66877=CARTESIAN_POINT('Ctrl Pts',(78.9435936542307,7.71174101956509,131.778592034527));
#66878=CARTESIAN_POINT('Ctrl Pts',(78.9381590781216,7.71621675497583,131.778112854273));
#66879=CARTESIAN_POINT('Ctrl Pts',(78.9263376052806,7.72607893967102,131.777060077229));
#66880=CARTESIAN_POINT('Ctrl Pts',(78.919962564018,7.73147923322922,131.776485574723));
#66881=CARTESIAN_POINT('Ctrl Pts',(78.9025202450491,7.74648140544285,131.774895603843));
#66882=CARTESIAN_POINT('Ctrl Pts',(78.8915388603403,7.7561814648169,131.773874226398));
#66883=CARTESIAN_POINT('Ctrl Pts',(78.8558974833036,7.78851099972673,131.770495534403));
#66884=CARTESIAN_POINT('Ctrl Pts',(78.8317923897985,7.81173787721554,131.768108160864));
#66885=CARTESIAN_POINT('Ctrl Pts',(78.7191948906083,7.92697242573903,131.756513342766));
#66886=CARTESIAN_POINT('Ctrl Pts',(78.6407610399778,8.02823593192158,131.747098873635));
#66887=CARTESIAN_POINT('Ctrl Pts',(78.5472856779196,8.18270375317607,131.734313248665));
#66888=CARTESIAN_POINT('Ctrl Pts',(78.522076365869,8.22922451973882,131.730633166426));
#66889=CARTESIAN_POINT('Ctrl Pts',(78.4919275287124,8.29179943941586,131.725900959521));
#66890=CARTESIAN_POINT('Ctrl Pts',(78.4849576008098,8.30683539055494,131.724779638178));
#66891=CARTESIAN_POINT('Ctrl Pts',(78.4739354608275,8.33157387107286,131.722959726897));
#66892=CARTESIAN_POINT('Ctrl Pts',(78.4697488337423,8.34121487230785,131.722256581635));
#66893=CARTESIAN_POINT('Ctrl Pts',(78.461807386397,8.35998676841101,131.720899031883));
#66894=CARTESIAN_POINT('Ctrl Pts',(78.4580419495825,8.36911266374234,131.720244290199));
#66895=CARTESIAN_POINT('Ctrl Pts',(78.4493891406325,8.3906239025751,131.718712880616));
#66896=CARTESIAN_POINT('Ctrl Pts',(78.4445686360912,8.40303555003665,131.717838485136));
#66897=CARTESIAN_POINT('Ctrl Pts',(78.42900136871,8.44458679033562,131.71494047257));
#66898=CARTESIAN_POINT('Ctrl Pts',(78.4189202622286,8.47396996969817,131.712938811937));
#66899=CARTESIAN_POINT('Ctrl Pts',(78.3964472039559,8.54597050419559,131.708133198753));
#66900=CARTESIAN_POINT('Ctrl Pts',(78.3849248036476,8.58883471803644,131.70535523583));
#66901=CARTESIAN_POINT('Ctrl Pts',(78.3477145017679,8.75318296227013,131.694918523051));
#66902=CARTESIAN_POINT('Ctrl Pts',(78.333923345181,8.87692383949796,131.687524599961));
#66903=CARTESIAN_POINT('Ctrl Pts',(78.3340003204331,9.00103328753322,131.67971837006));
#66904=CARTESIAN_POINT('Ctrl Pts',(78.3340003219602,9.00103574665424,131.679718215386));
#66905=CARTESIAN_POINT('Ctrl Pts',(78.3340235477417,9.03839444284753,131.677368428309));
#66906=CARTESIAN_POINT('Ctrl Pts',(78.3353033761624,9.07573933155099,131.674981797394));
#66907=CARTESIAN_POINT('Ctrl Pts',(78.3383818254571,9.12101870446789,131.67200839924));
#66908=CARTESIAN_POINT('Ctrl Pts',(78.338984433172,9.12902622004195,131.671479522037));
#66909=CARTESIAN_POINT('Ctrl Pts',(78.3401157666353,9.1427343912963,131.670568437123));
#66910=CARTESIAN_POINT('Ctrl Pts',(78.3406160393469,9.14843733822041,131.670187712284));
#66911=CARTESIAN_POINT('Ctrl Pts',(78.3416182455442,9.15922325460433,131.669464259105));
#66912=CARTESIAN_POINT('Ctrl Pts',(78.3421141834323,9.16430674360668,131.669121861723));
#66913=CARTESIAN_POINT('Ctrl Pts',(78.3431534772886,9.17447566293804,131.668433932483));
#66914=CARTESIAN_POINT('Ctrl Pts',(78.3436968892138,9.1795610207734,131.668088404159));
#66915=CARTESIAN_POINT('Ctrl Pts',(78.3450460613825,9.19165931192057,131.667262926474));
#66916=CARTESIAN_POINT('Ctrl Pts',(78.3458729885,9.19866971623309,131.666781836851));
#66917=CARTESIAN_POINT('Ctrl Pts',(78.3489767353649,9.22361829732525,131.665060389841));
#66918=CARTESIAN_POINT('Ctrl Pts',(78.3515009223379,9.24152368075207,131.663807692287));
#66919=CARTESIAN_POINT('Ctrl Pts',(78.3619153610792,9.30759910931665,131.65912951612));
#66920=CARTESIAN_POINT('Ctrl Pts',(78.3716295252477,9.35545367340081,131.65563257661));
#66921=CARTESIAN_POINT('Ctrl Pts',(78.3980044333927,9.4613027324769,131.647742105841));
#66922=CARTESIAN_POINT('Ctrl Pts',(78.4157414300658,9.51895336013236,131.643338258236));
#66923=CARTESIAN_POINT('Ctrl Pts',(78.4365593658221,9.57550793513344,131.638964603241));
#66924=CARTESIAN_POINT('',(78.3340002424278,8.99871136581395,131.870599642122));
#66925=CARTESIAN_POINT('Ctrl Pts',(78.4365593737656,9.57550795671282,131.83373138687));
#66926=CARTESIAN_POINT('Ctrl Pts',(78.4360745518862,9.57419087635994,131.833824541444));
#66927=CARTESIAN_POINT('Ctrl Pts',(78.4355913920686,9.57287317725898,131.833917640984));
#66928=CARTESIAN_POINT('Ctrl Pts',(78.4312888554247,9.56109303599931,131.834749065508));
#66929=CARTESIAN_POINT('Ctrl Pts',(78.4275727469838,9.55059294788695,131.835483950254));
#66930=CARTESIAN_POINT('Ctrl Pts',(78.417635866271,9.52159429691574,131.837497098183));
#66931=CARTESIAN_POINT('Ctrl Pts',(78.4116342732758,9.50302209926302,131.83876814628));
#66932=CARTESIAN_POINT('Ctrl Pts',(78.3737904607603,9.37847418408069,131.847179937131));
#66933=CARTESIAN_POINT('Ctrl Pts',(78.3522467171661,9.26965446890637,131.853967829947));
#66934=CARTESIAN_POINT('Ctrl Pts',(78.3365122009242,9.106050039411,131.864005637014));
#66935=CARTESIAN_POINT('Ctrl Pts',(78.3339590443037,9.05239520490956,131.867276149316));
#66936=CARTESIAN_POINT('Ctrl Pts',(78.3340004966975,8.99871353358091,131.870599064419));
#66937=CARTESIAN_POINT('Ctrl Pts',(78.3340004983938,8.99871133866798,131.870599200285));
#66938=CARTESIAN_POINT('Ctrl Pts',(78.3340316402379,8.95845072455788,131.87309134809));
#66939=CARTESIAN_POINT('Ctrl Pts',(78.3355221838307,8.91820640698278,131.875611367354));
#66940=CARTESIAN_POINT('Ctrl Pts',(78.3399331311568,8.85810475873496,131.879468884735));
#66941=CARTESIAN_POINT('Ctrl Pts',(78.3417567416082,8.83818070644958,131.880763270043));
#66942=CARTESIAN_POINT('Ctrl Pts',(78.3447889344087,8.81054521362256,131.882586340663));
#66943=CARTESIAN_POINT('Ctrl Pts',(78.3456936612383,8.8028013193423,131.883100227923));
#66944=CARTESIAN_POINT('Ctrl Pts',(78.3473458863135,8.78947176722082,131.883990456338));
#66945=CARTESIAN_POINT('Ctrl Pts',(78.3480674427875,8.78388294740192,131.884365434232));
#66946=CARTESIAN_POINT('Ctrl Pts',(78.3495612860912,8.77275716531181,131.885115537949));
#66947=CARTESIAN_POINT('Ctrl Pts',(78.3503331210716,8.76722018570077,131.88549064018));
#66948=CARTESIAN_POINT('Ctrl Pts',(78.3519976259096,8.75570360970529,131.886274744676));
#66949=CARTESIAN_POINT('Ctrl Pts',(78.3528949894902,8.74972488590105,131.886683983951));
#66950=CARTESIAN_POINT('Ctrl Pts',(78.3553845610003,8.73373155311702,131.887784315166));
#66951=CARTESIAN_POINT('Ctrl Pts',(78.3570356655544,8.72372656494716,131.888478540562));
#66952=CARTESIAN_POINT('Ctrl Pts',(78.365108168319,8.67744466039859,131.891715353203));
#66953=CARTESIAN_POINT('Ctrl Pts',(78.3726399727852,8.64137466936291,131.894310308466));
#66954=CARTESIAN_POINT('Ctrl Pts',(78.3955410670832,8.54739034158854,131.901214182282));
#66955=CARTESIAN_POINT('Ctrl Pts',(78.4128495312938,8.49000322142901,131.905572920464));
#66956=CARTESIAN_POINT('Ctrl Pts',(78.4688726432898,8.33500992385575,131.917569925703));
#66957=CARTESIAN_POINT('Ctrl Pts',(78.5137809246817,8.23992008586034,131.925169288583));
#66958=CARTESIAN_POINT('Ctrl Pts',(78.5853165251336,8.11939407162546,131.934939051558));
#66959=CARTESIAN_POINT('Ctrl Pts',(78.6042471911213,8.08968656230755,131.937361611782));
#66960=CARTESIAN_POINT('Ctrl Pts',(78.6319775211428,8.04907132466332,131.940696381739));
#66961=CARTESIAN_POINT('Ctrl Pts',(78.6399931891947,8.03764229966226,131.941637427042));
#66962=CARTESIAN_POINT('Ctrl Pts',(78.6539847138118,8.01821669597899,131.943241905762));
#66963=CARTESIAN_POINT('Ctrl Pts',(78.6598904165466,8.01017076295418,131.943907976668));
#66964=CARTESIAN_POINT('Ctrl Pts',(78.6713122039051,7.99489932823909,131.945175327185));
#66965=CARTESIAN_POINT('Ctrl Pts',(78.6768157979363,7.98766497994507,131.945777060179));
#66966=CARTESIAN_POINT('Ctrl Pts',(78.691304412121,7.96894005623519,131.947338404459));
#66967=CARTESIAN_POINT('Ctrl Pts',(78.7003817418318,7.95752162868693,131.948294341491));
#66968=CARTESIAN_POINT('Ctrl Pts',(78.732919426878,7.91767791575345,131.951645497409));
#66969=CARTESIAN_POINT('Ctrl Pts',(78.7571727634297,7.88991214301204,131.954008857723));
#66970=CARTESIAN_POINT('Ctrl Pts',(78.8792664844338,7.75915896415067,131.965332882698));
#66971=CARTESIAN_POINT('Ctrl Pts',(78.9890744921864,7.66817486594924,131.973770183453));
#66972=CARTESIAN_POINT('Ctrl Pts',(79.1405664360587,7.57230344207744,131.984898644657));
#66973=CARTESIAN_POINT('Ctrl Pts',(79.1726994951628,7.55344650036948,131.987237301765));
#66974=CARTESIAN_POINT('Ctrl Pts',(79.2192568135953,7.5281836525115,131.990633834411));
#66975=CARTESIAN_POINT('Ctrl Pts',(79.2331833508589,7.52088016999526,131.991650840466));
#66976=CARTESIAN_POINT('Ctrl Pts',(79.2580880975047,7.50826563903372,131.993475055217));
#66977=CARTESIAN_POINT('Ctrl Pts',(79.2690253408589,7.50287585648964,131.994278035975));
#66978=CARTESIAN_POINT('Ctrl Pts',(79.2858700142636,7.4948035210287,131.995519054706));
#66979=CARTESIAN_POINT('Ctrl Pts',(79.2917358664506,7.4920344863332,131.995952013122));
#66980=CARTESIAN_POINT('Ctrl Pts',(79.3025832041484,7.48699114344993,131.996754392575));
#66981=CARTESIAN_POINT('Ctrl Pts',(79.3075599132548,7.48470705460791,131.997123213011));
#66982=CARTESIAN_POINT('Ctrl Pts',(79.3189412437748,7.4795513046145,131.99796821665));
#66983=CARTESIAN_POINT('Ctrl Pts',(79.3253528106485,7.47669555565565,131.998445325647));
#66984=CARTESIAN_POINT('Ctrl Pts',(79.3457764474946,7.46775297954117,131.999968120125));
#66985=CARTESIAN_POINT('Ctrl Pts',(79.3598538234333,7.46181853483207,132.001022184795));
#66986=CARTESIAN_POINT('Ctrl Pts',(79.494265610946,7.40732066936147,132.011115255864));
#66987=CARTESIAN_POINT('Ctrl Pts',(79.6197987020533,7.37278169333299,132.020719015859));
#66988=CARTESIAN_POINT('Ctrl Pts',(79.8363958854486,7.33964605483098,132.036546682854));
#66989=CARTESIAN_POINT('Ctrl Pts',(79.9256855260011,7.3332596019077,132.042876337841));
#66990=CARTESIAN_POINT('Ctrl Pts',(80.0334757976223,7.33423465614544,132.050241616456));
#66991=CARTESIAN_POINT('Ctrl Pts',(80.0518784187392,7.3347061860848,132.051489870549));
#66992=CARTESIAN_POINT('Ctrl Pts',(80.0811619853997,7.33594243591086,132.053462284287));
#66993=CARTESIAN_POINT('Ctrl Pts',(80.0920493070806,7.33650915863104,132.05419254896));
#66994=CARTESIAN_POINT('Ctrl Pts',(80.1126639561657,7.33778523169112,132.055569742338));
#66995=CARTESIAN_POINT('Ctrl Pts',(80.1223920969227,7.33847320680039,132.056217309416));
#66996=CARTESIAN_POINT('Ctrl Pts',(80.1445324500483,7.34023448362968,132.057686067956));
#66997=CARTESIAN_POINT('Ctrl Pts',(80.1569398846019,7.34136167742539,132.058505540383));
#66998=CARTESIAN_POINT('Ctrl Pts',(80.1893777119806,7.34467585208633,132.060639275625));
#66999=CARTESIAN_POINT('Ctrl Pts',(80.2093834837405,7.34708724814287,132.061946535181));
#67000=CARTESIAN_POINT('Ctrl Pts',(80.3593515745496,7.36793026703697,132.071692469615));
#67001=CARTESIAN_POINT('Ctrl Pts',(80.4867709206836,7.40129956560474,132.079622332589));
#67002=CARTESIAN_POINT('Ctrl Pts',(80.6884719389161,7.48050692875075,132.092884394717));
#67003=CARTESIAN_POINT('Ctrl Pts',(80.7654527719295,7.51779526018346,132.098150772127));
#67004=CARTESIAN_POINT('Ctrl Pts',(80.8499776377055,7.56708375628951,132.104540859735));
#67005=CARTESIAN_POINT('Ctrl Pts',(80.8606597016236,7.57347421984896,132.105360257314));
#67006=CARTESIAN_POINT('Ctrl Pts',(80.8768427248161,7.58340351503491,132.106621384711));
#67007=CARTESIAN_POINT('Ctrl Pts',(80.8823963837906,7.58685620564829,132.107057777122));
#67008=CARTESIAN_POINT('Ctrl Pts',(80.8925583992115,7.59325715477464,132.107863198879));
#67009=CARTESIAN_POINT('Ctrl Pts',(80.8971727370576,7.59619552444934,132.108231590072));
#67010=CARTESIAN_POINT('Ctrl Pts',(80.9077140146641,7.60298131803264,132.109079273762));
#67011=CARTESIAN_POINT('Ctrl Pts',(80.9136309872968,7.60684374721721,132.109559526849));
#67012=CARTESIAN_POINT('Ctrl Pts',(80.9321372734362,7.61909271525781,132.111075141032));
#67013=CARTESIAN_POINT('Ctrl Pts',(80.9446366313429,7.62761287522598,132.112118650243));
#67014=CARTESIAN_POINT('Ctrl Pts',(81.0414571257971,7.69555966590559,132.120347731364));
#67015=CARTESIAN_POINT('Ctrl Pts',(81.1202029629156,7.76252701759398,132.127902356081));
#67016=CARTESIAN_POINT('Ctrl Pts',(81.2720493961906,7.91810320028777,132.143711605378));
#67017=CARTESIAN_POINT('Ctrl Pts',(81.3432449235341,8.00787473158587,132.151902768764));
#67018=CARTESIAN_POINT('Ctrl Pts',(81.4151571255812,8.12064528610795,132.161055483773));
#67019=CARTESIAN_POINT('Ctrl Pts',(81.4253284738023,8.1372293466144,132.1623761801));
#67020=CARTESIAN_POINT('Ctrl Pts',(81.4408565097413,8.16357171793795,132.164435478899));
#67021=CARTESIAN_POINT('Ctrl Pts',(81.4464095889559,8.173211596557,132.165181147888));
#67022=CARTESIAN_POINT('Ctrl Pts',(81.4566326609653,8.19137662933929,132.166571776055));
#67023=CARTESIAN_POINT('Ctrl Pts',(81.4613253804112,8.19988838029911,132.167217529178));
#67024=CARTESIAN_POINT('Ctrl Pts',(81.471696135259,8.21909470273719,132.168661797515));
#67025=CARTESIAN_POINT('Ctrl Pts',(81.4773326514158,8.22981116094054,132.16945881738));
#67026=CARTESIAN_POINT('Ctrl Pts',(81.4935672642219,8.26151139583161,132.171791457617));
#67027=CARTESIAN_POINT('Ctrl Pts',(81.5038389294672,8.28265966646983,132.173315723502));
#67028=CARTESIAN_POINT('Ctrl Pts',(81.5589401013627,8.40249692472199,132.181790095452));
#67029=CARTESIAN_POINT('Ctrl Pts',(81.5945039144788,8.5051616567703,132.188417050114));
#67030=CARTESIAN_POINT('Ctrl Pts',(81.6373836568384,8.68351817009856,132.199618286142));
#67031=CARTESIAN_POINT('Ctrl Pts',(81.6499732336384,8.75756913489963,132.204190154683));
#67032=CARTESIAN_POINT('Ctrl Pts',(81.6611300541824,8.86778302629311,132.211182924309));
#67033=CARTESIAN_POINT('Ctrl Pts',(81.6635846515538,8.90345951991959,132.213475852723));
#67034=CARTESIAN_POINT('Ctrl Pts',(81.6652439400975,8.94888411694041,132.216463659033));
#67035=CARTESIAN_POINT('Ctrl Pts',(81.665513475106,8.9585866373357,132.217105805608));
#67036=CARTESIAN_POINT('Ctrl Pts',(81.6658114644099,8.97424008198021,132.218148996003));
#67037=CARTESIAN_POINT('Ctrl Pts',(81.6658928438257,8.98018994112299,132.218547187023));
#67038=CARTESIAN_POINT('Ctrl Pts',(81.6659887292251,8.99171515339399,132.219321971851));
#67039=CARTESIAN_POINT('Ctrl Pts',(81.666007124468,8.99729033951679,132.219698350734));
#67040=CARTESIAN_POINT('Ctrl Pts',(81.665985689979,9.00975289296879,132.220543094886));
#67041=CARTESIAN_POINT('Ctrl Pts',(81.6659311330671,9.01664012762671,132.221012249005));
#67042=CARTESIAN_POINT('Ctrl Pts',(81.6656404977047,9.03721890758763,132.222420604055));
#67043=CARTESIAN_POINT('Ctrl Pts',(81.665278322262,9.05090770671635,132.223366080099));
#67044=CARTESIAN_POINT('Ctrl Pts',(81.6607645858142,9.16724520156487,132.231466498603));
#67045=CARTESIAN_POINT('Ctrl Pts',(81.647295466524,9.26930309814728,132.238988805981));
#67046=CARTESIAN_POINT('Ctrl Pts',(81.599077192505,9.48131831528588,132.254801181296));
#67047=CARTESIAN_POINT('Ctrl Pts',(81.5621485844486,9.59026791946311,132.263026282082));
#67048=CARTESIAN_POINT('Ctrl Pts',(81.5062203774433,9.71220246970613,132.272205682261));
#67049=CARTESIAN_POINT('Ctrl Pts',(81.4978266860374,9.72968997323268,132.273522418533));
#67050=CARTESIAN_POINT('Ctrl Pts',(81.484146496828,9.75696014383506,132.275576974645));
#67051=CARTESIAN_POINT('Ctrl Pts',(81.4790644303846,9.76684281605324,132.276321806964));
#67052=CARTESIAN_POINT('Ctrl Pts',(81.469352088897,9.78527379261788,132.277711676659));
#67053=CARTESIAN_POINT('Ctrl Pts',(81.4647451642479,9.79383379946791,132.278357499702));
#67054=CARTESIAN_POINT('Ctrl Pts',(81.4542240237014,9.81297940041972,132.279802957133));
#67055=CARTESIAN_POINT('Ctrl Pts',(81.4482685927552,9.82354181000819,132.280601085136));
#67056=CARTESIAN_POINT('Ctrl Pts',(81.4303880215247,9.8544604408534,132.2829402422));
#67057=CARTESIAN_POINT('Ctrl Pts',(81.4181449152866,9.87462999372215,132.284469818896));
#67058=CARTESIAN_POINT('Ctrl Pts',(81.3503007304635,9.9812257093451,132.29258715386));
#67059=CARTESIAN_POINT('Ctrl Pts',(81.2872199585986,10.0626307269221,132.298888921183));
#67060=CARTESIAN_POINT('Ctrl Pts',(81.1628992427004,10.1956191483002,132.310007381257));
#67061=CARTESIAN_POINT('Ctrl Pts',(81.1047053011346,10.249585629033,132.31482549069));
#67062=CARTESIAN_POINT('Ctrl Pts',(81.0235809200499,10.3147058921622,132.321384825536));
#67063=CARTESIAN_POINT('Ctrl Pts',(81.0039232110396,10.3297772517555,132.32296360362));
#67064=CARTESIAN_POINT('Ctrl Pts',(80.9700457038409,10.3545714092684,132.325680424689));
#67065=CARTESIAN_POINT('Ctrl Pts',(80.955997367388,10.3645223879495,132.326805922499));
#67066=CARTESIAN_POINT('Ctrl Pts',(80.9356618043696,10.3784586774781,132.328437511756));
#67067=CARTESIAN_POINT('Ctrl Pts',(80.929497613732,10.3826226956406,132.328932392836));
#67068=CARTESIAN_POINT('Ctrl Pts',(80.9187212437622,10.3897976877807,132.329798477217));
#67069=CARTESIAN_POINT('Ctrl Pts',(80.9141216894636,10.3928272945879,132.330168437248));
#67070=CARTESIAN_POINT('Ctrl Pts',(80.9042330880757,10.3992705766097,132.330964577414));
#67071=CARTESIAN_POINT('Ctrl Pts',(80.8989397800303,10.4026770450561,132.331391178623));
#67072=CARTESIAN_POINT('Ctrl Pts',(80.8843522353673,10.4119482647905,132.332567733544));
#67073=CARTESIAN_POINT('Ctrl Pts',(80.8750192688317,10.4177510506833,132.333321484732));
#67074=CARTESIAN_POINT('Ctrl Pts',(80.8216179422312,10.4502252726654,132.337636985714));
#67075=CARTESIAN_POINT('Ctrl Pts',(80.7763926772353,10.4749314245003,132.341301353216));
#67076=CARTESIAN_POINT('Ctrl Pts',(80.6437992502714,10.5395768613531,132.351931419868));
#67077=CARTESIAN_POINT('Ctrl Pts',(80.5540210821498,10.5741143838078,132.358983560135));
#67078=CARTESIAN_POINT('Ctrl Pts',(80.4112411560208,10.6153023841077,132.369670191623));
#67079=CARTESIAN_POINT('Ctrl Pts',(80.3600519300265,10.6274779806804,132.373404753369));
#67080=CARTESIAN_POINT('Ctrl Pts',(80.284945051806,10.6416243251809,132.378731226177));
#67081=CARTESIAN_POINT('Ctrl Pts',(80.2614289582662,10.6455330766647,132.38037777149));
#67082=CARTESIAN_POINT('Ctrl Pts',(80.2186318806754,10.6517059582119,132.383336576203));
#67083=CARTESIAN_POINT('Ctrl Pts',(80.1993801440945,10.6541402857695,132.38465382758));
#67084=CARTESIAN_POINT('Ctrl Pts',(80.1690407853044,10.6574392089392,132.386709000647));
#67085=CARTESIAN_POINT('Ctrl Pts',(80.1579800544197,10.6585300211921,132.387453941836));
#67086=CARTESIAN_POINT('Ctrl Pts',(80.1372264187758,10.6603672476535,132.388843910055));
#67087=CARTESIAN_POINT('Ctrl Pts',(80.1275363505881,10.6611396609605,132.389489723832));
#67088=CARTESIAN_POINT('Ctrl Pts',(80.1057474801884,10.6626847062135,132.390935025706));
#67089=CARTESIAN_POINT('Ctrl Pts',(80.0936458045795,10.663410183357,132.39173300886));
#67090=CARTESIAN_POINT('Ctrl Pts',(80.057985194326,10.6651575713348,132.394071313556));
#67091=CARTESIAN_POINT('Ctrl Pts',(80.0344106400923,10.665811519179,132.395600195557));
#67092=CARTESIAN_POINT('Ctrl Pts',(79.9068353858666,10.6666407882894,132.403796237536));
#67093=CARTESIAN_POINT('Ctrl Pts',(79.8030026316509,10.6575785293874,132.410169498754));
#67094=CARTESIAN_POINT('Ctrl Pts',(79.6236308687163,10.624819163601,132.421304916774));
#67095=CARTESIAN_POINT('Ctrl Pts',(79.5476725897228,10.6053315036096,132.426068225049));
#67096=CARTESIAN_POINT('Ctrl Pts',(79.4500218943596,10.5727955602315,132.432559806305));
#67097=CARTESIAN_POINT('Ctrl Pts',(79.4268475886982,10.564499273461,132.434128998003));
#67098=CARTESIAN_POINT('Ctrl Pts',(79.3878662049638,10.5495618187369,132.436830921199));
#67099=CARTESIAN_POINT('Ctrl Pts',(79.3719618943802,10.5431842712598,132.437951287413));
#67100=CARTESIAN_POINT('Ctrl Pts',(79.3493112470958,10.5336933462092,132.439576735811));
#67101=CARTESIAN_POINT('Ctrl Pts',(79.3424823723078,10.5307781346188,132.440070722904));
#67102=CARTESIAN_POINT('Ctrl Pts',(79.3306239248811,10.5256218363943,132.440935799553));
#67103=CARTESIAN_POINT('Ctrl Pts',(79.3255856122922,10.5234013096555,132.441305654924));
#67104=CARTESIAN_POINT('Ctrl Pts',(79.3148036778202,10.5185854345541,132.442102225564));
#67105=CARTESIAN_POINT('Ctrl Pts',(79.3090638427345,10.5159825016311,132.442529367695));
#67106=CARTESIAN_POINT('Ctrl Pts',(79.2933248836194,10.508737158965,132.443708834835));
#67107=CARTESIAN_POINT('Ctrl Pts',(79.2833570677149,10.5040280669959,132.444464986975));
#67108=CARTESIAN_POINT('Ctrl Pts',(79.2264912904439,10.47646936916,132.44882856354));
#67109=CARTESIAN_POINT('Ctrl Pts',(79.1806446818053,10.4515279060208,132.452541212418));
#67110=CARTESIAN_POINT('Ctrl Pts',(79.0487711760485,10.3715462288854,132.463659331384));
#67111=CARTESIAN_POINT('Ctrl Pts',(78.9665372428196,10.310698981517,132.471162290542));
#67112=CARTESIAN_POINT('Ctrl Pts',(78.8359641791022,10.1941107694014,132.483711465315));
#67113=CARTESIAN_POINT('Ctrl Pts',(78.7847831231749,10.1419853373315,132.488839161652));
#67114=CARTESIAN_POINT('Ctrl Pts',(78.7256827106888,10.0733042909583,132.495022751646));
#67115=CARTESIAN_POINT('Ctrl Pts',(78.7143987446615,10.0597622886962,132.496216934413));
#67116=CARTESIAN_POINT('Ctrl Pts',(78.6965917611611,10.0376888659565,132.498124359699));
#67117=CARTESIAN_POINT('Ctrl Pts',(78.6899328695039,10.0292693245814,132.498843026617));
#67118=CARTESIAN_POINT('Ctrl Pts',(78.6773568393692,10.0130483328765,132.500210995867));
#67119=CARTESIAN_POINT('Ctrl Pts',(78.671426216,10.005257958216,132.500860813736));
#67120=CARTESIAN_POINT('Ctrl Pts',(78.6580440461882,9.98735404511676,132.502338258425));
#67121=CARTESIAN_POINT('Ctrl Pts',(78.6506374605169,9.9772075234007,132.50316411518));
#67122=CARTESIAN_POINT('Ctrl Pts',(78.6311691993435,9.94989388027907,132.505357799955));
#67123=CARTESIAN_POINT('Ctrl Pts',(78.6193156080722,9.93258072973556,132.506717755246));
#67124=CARTESIAN_POINT('Ctrl Pts',(78.5412033247309,9.81373602995264,132.515861037351));
#67125=CARTESIAN_POINT('Ctrl Pts',(78.4858706795807,9.70545752468266,132.523222986965));
#67126=CARTESIAN_POINT('Ctrl Pts',(78.4406741477407,9.58659514057224,132.530993796469));
#67127=CARTESIAN_POINT('Ctrl Pts',(78.4386019183015,9.58105678893567,132.531355281971));
#67128=CARTESIAN_POINT('Ctrl Pts',(78.4365593745624,9.57550795887745,132.531716954706));
#67129=CARTESIAN_POINT('Origin',(80.,9.,134.));
#67130=CARTESIAN_POINT('',(78.4365593737643,9.57550795670927,133.231048988662));
#67131=CARTESIAN_POINT('',(78.4365593647824,9.57550793230875,133.038342764662));
#67132=CARTESIAN_POINT('',(78.4365593737638,9.57550795670799,134.));
#67133=CARTESIAN_POINT('Ctrl Pts',(78.4365593647824,9.57550793230875,133.038342764662));
#67134=CARTESIAN_POINT('Ctrl Pts',(78.458363872793,9.63474265687277,133.034409061954));
#67135=CARTESIAN_POINT('Ctrl Pts',(78.4835221810049,9.69270400732193,133.03055199272));
#67136=CARTESIAN_POINT('Ctrl Pts',(78.5536676740876,9.83204591991857,133.021025947317));
#67137=CARTESIAN_POINT('Ctrl Pts',(78.6022744362798,9.91133808078974,133.015379540216));
#67138=CARTESIAN_POINT('Ctrl Pts',(78.6705019239503,10.0042380022328,133.007981824922));
#67139=CARTESIAN_POINT('Ctrl Pts',(78.6841418566152,10.0220451687343,133.006524471428));
#67140=CARTESIAN_POINT('Ctrl Pts',(78.703280559747,10.0460127435335,133.004499984223));
#67141=CARTESIAN_POINT('Ctrl Pts',(78.708472471434,10.0524165536073,133.003952747093));
#67142=CARTESIAN_POINT('Ctrl Pts',(78.7172966634518,10.0631368554165,133.003025421484));
#67143=CARTESIAN_POINT('Ctrl Pts',(78.720903820544,10.0674740209847,133.00264710751));
#67144=CARTESIAN_POINT('Ctrl Pts',(78.7283635648206,10.0763513512869,133.001866101055));
#67145=CARTESIAN_POINT('Ctrl Pts',(78.7322185525966,10.0808892882716,133.001463249547));
#67146=CARTESIAN_POINT('Ctrl Pts',(78.7424299066295,10.0927799074118,133.000398336395));
#67147=CARTESIAN_POINT('Ctrl Pts',(78.7488263220688,10.1000976693339,132.999733473148));
#67148=CARTESIAN_POINT('Ctrl Pts',(78.7768041857642,10.1315458613859,132.996836376631));
#67149=CARTESIAN_POINT('Ctrl Pts',(78.7990209686983,10.1550987294904,132.994563863957));
#67150=CARTESIAN_POINT('Ctrl Pts',(78.9053963006527,10.2614835050117,132.98386801059));
#67151=CARTESIAN_POINT('Ctrl Pts',(78.9975233571079,10.3358665182641,132.975148044204));
#67152=CARTESIAN_POINT('Ctrl Pts',(79.1407783152589,10.428299923245,132.962889069126));
#67153=CARTESIAN_POINT('Ctrl Pts',(79.1861342775254,10.454622302091,132.959167508737));
#67154=CARTESIAN_POINT('Ctrl Pts',(79.2537714238063,10.4897196495944,132.953857224597));
#67155=CARTESIAN_POINT('Ctrl Pts',(79.2751162906602,10.5002217931661,132.952214243424));
#67156=CARTESIAN_POINT('Ctrl Pts',(79.3142408113898,10.5184418360883,132.949261112801));
#67157=CARTESIAN_POINT('Ctrl Pts',(79.3319438478213,10.5263133055979,132.947946001921));
#67158=CARTESIAN_POINT('Ctrl Pts',(79.3600090145075,10.5382103086532,132.945893264854));
#67159=CARTESIAN_POINT('Ctrl Pts',(79.3702805318703,10.5424437808128,132.945148649509));
#67160=CARTESIAN_POINT('Ctrl Pts',(79.3896208082384,10.5501896009276,132.943758777155));
#67161=CARTESIAN_POINT('Ctrl Pts',(79.3986794091948,10.5537258800983,132.943112738267));
#67162=CARTESIAN_POINT('Ctrl Pts',(79.4191131867078,10.5614973022901,132.94166626658));
#67163=CARTESIAN_POINT('Ctrl Pts',(79.4305048074356,10.5656878851088,132.94086734672));
#67164=CARTESIAN_POINT('Ctrl Pts',(79.4642169670935,10.5776727961898,132.938524156423));
#67165=CARTESIAN_POINT('Ctrl Pts',(79.4866593494814,10.5851171492447,132.936991395942));
#67166=CARTESIAN_POINT('Ctrl Pts',(79.6072911402031,10.6223009381666,132.928882423234));
#67167=CARTESIAN_POINT('Ctrl Pts',(79.7079143655427,10.6434019228162,132.922590953249));
#67168=CARTESIAN_POINT('Ctrl Pts',(79.8886678491112,10.6641681096812,132.911478889195));
#67169=CARTESIAN_POINT('Ctrl Pts',(79.9680269647158,10.6675809779561,132.90665692751));
#67170=CARTESIAN_POINT('Ctrl Pts',(80.0720917264687,10.664623944309,132.900092760462));
#67171=CARTESIAN_POINT('Ctrl Pts',(80.0968425491642,10.6633675131114,132.898513227839));
#67172=CARTESIAN_POINT('Ctrl Pts',(80.1387315127585,10.6603030405283,132.895795178828));
#67173=CARTESIAN_POINT('Ctrl Pts',(80.1558869045101,10.6587802251282,132.894669220452));
#67174=CARTESIAN_POINT('Ctrl Pts',(80.1804159037325,10.6562190300862,132.893037000909));
#67175=CARTESIAN_POINT('Ctrl Pts',(80.187811598653,10.6553966811942,132.892541959607));
#67176=CARTESIAN_POINT('Ctrl Pts',(80.2006728660645,10.6538793048184,132.891675608485));
#67177=CARTESIAN_POINT('Ctrl Pts',(80.2061408962968,10.6532066670416,132.891305542858));
#67178=CARTESIAN_POINT('Ctrl Pts',(80.2178511219851,10.6517071575515,132.890509180806));
#67179=CARTESIAN_POINT('Ctrl Pts',(80.2240918929547,10.650872031951,132.890082463133));
#67180=CARTESIAN_POINT('Ctrl Pts',(80.2412149955069,10.6484817772762,132.888905586246));
#67181=CARTESIAN_POINT('Ctrl Pts',(80.2520866734937,10.6468543156574,132.888151627584));
#67182=CARTESIAN_POINT('Ctrl Pts',(80.313829722362,10.6369858625775,132.883834271339));
#67183=CARTESIAN_POINT('Ctrl Pts',(80.3643085811822,10.6264962272298,132.880168168151));
#67184=CARTESIAN_POINT('Ctrl Pts',(80.5071904680114,10.589820087356,132.869537877139));
#67185=CARTESIAN_POINT('Ctrl Pts',(80.5979306311228,10.5579634488277,132.862487426011));
#67186=CARTESIAN_POINT('Ctrl Pts',(80.7333469544304,10.4968375459011,132.851802904118));
#67187=CARTESIAN_POINT('Ctrl Pts',(80.780221154801,10.4729481433787,132.848068813194));
#67188=CARTESIAN_POINT('Ctrl Pts',(80.8465905447746,10.4350639495914,132.842742818878));
#67189=CARTESIAN_POINT('Ctrl Pts',(80.8670352406487,10.4228050043596,132.841096298208));
#67190=CARTESIAN_POINT('Ctrl Pts',(80.9036340885582,10.399777816193,132.83813746538));
#67191=CARTESIAN_POINT('Ctrl Pts',(80.9198762138907,10.3891581288892,132.836820162547));
#67192=CARTESIAN_POINT('Ctrl Pts',(80.9451257723535,10.3720119673865,132.834764799998));
#67193=CARTESIAN_POINT('Ctrl Pts',(80.9542592831434,10.3656752158268,132.834019721275));
#67194=CARTESIAN_POINT('Ctrl Pts',(80.9712618462955,10.3536251208314,132.832629430069));
#67195=CARTESIAN_POINT('Ctrl Pts',(80.979145578467,10.3479334126121,132.831983431115));
#67196=CARTESIAN_POINT('Ctrl Pts',(80.9967495577334,10.3349881647595,132.83053762395));
#67197=CARTESIAN_POINT('Ctrl Pts',(81.0064414060493,10.3276967989957,132.829739322518));
#67198=CARTESIAN_POINT('Ctrl Pts',(81.0347515316582,10.3059103975364,132.827399773135));
#67199=CARTESIAN_POINT('Ctrl Pts',(81.0531429809031,10.2911245679799,132.825869980262));
#67200=CARTESIAN_POINT('Ctrl Pts',(81.1498161991498,10.2099633976874,132.817760985217));
#67201=CARTESIAN_POINT('Ctrl Pts',(81.2221553308757,10.1368502033465,132.811466923631));
#67202=CARTESIAN_POINT('Ctrl Pts',(81.3376911383935,9.99621144904232,132.800350683934));
#67203=CARTESIAN_POINT('Ctrl Pts',(81.3836202198775,9.93136897466239,132.795527081024));
#67204=CARTESIAN_POINT('Ctrl Pts',(81.4375969469632,9.84230952789956,132.788960886304));
#67205=CARTESIAN_POINT('Ctrl Pts',(81.4499682725651,9.82083019024092,132.787381068504));
#67206=CARTESIAN_POINT('Ctrl Pts',(81.4701170511469,9.7839697424649,132.784662576486));
#67207=CARTESIAN_POINT('Ctrl Pts',(81.4781436031578,9.76872890725481,132.783536465656));
#67208=CARTESIAN_POINT('Ctrl Pts',(81.4892972088397,9.74672967247109,132.78190406371));
#67209=CARTESIAN_POINT('Ctrl Pts',(81.4926177976683,9.74006991889102,132.781408995896));
#67210=CARTESIAN_POINT('Ctrl Pts',(81.4983189134259,9.72844134171625,132.780542614862));
#67211=CARTESIAN_POINT('Ctrl Pts',(81.5007195881627,9.72348259920487,132.780172546106));
#67212=CARTESIAN_POINT('Ctrl Pts',(81.5058111313507,9.71283131207421,132.779376196705));
#67213=CARTESIAN_POINT('Ctrl Pts',(81.5084942956302,9.70713548880917,132.778949494983));
#67214=CARTESIAN_POINT('Ctrl Pts',(81.5157728976149,9.69145451380474,132.777772703947));
#67215=CARTESIAN_POINT('Ctrl Pts',(81.5203018039857,9.68143908787989,132.777018816058));
#67216=CARTESIAN_POINT('Ctrl Pts',(81.5454904102591,9.62423473801289,132.772703008399));
#67217=CARTESIAN_POINT('Ctrl Pts',(81.5640498655995,9.57615670261246,132.769038467298));
#67218=CARTESIAN_POINT('Ctrl Pts',(81.6107309039638,9.43625119684255,132.758410176252));
#67219=CARTESIAN_POINT('Ctrl Pts',(81.633185923138,9.34274473930579,132.751360068374));
#67220=CARTESIAN_POINT('Ctrl Pts',(81.6552883978274,9.19581245952426,132.740674530224));
#67221=CARTESIAN_POINT('Ctrl Pts',(81.6606453380057,9.14345783522433,132.736939172299));
#67222=CARTESIAN_POINT('Ctrl Pts',(81.664817715732,9.06712900057565,132.731611589903));
#67223=CARTESIAN_POINT('Ctrl Pts',(81.6656078919411,9.04329871517843,132.72996471171));
#67224=CARTESIAN_POINT('Ctrl Pts',(81.6661130279278,9.00005310832927,132.727005302984));
#67225=CARTESIAN_POINT('Ctrl Pts',(81.6660006131039,8.98064445695825,132.725687778819));
#67226=CARTESIAN_POINT('Ctrl Pts',(81.6652904696519,8.95012785388706,132.723632151177));
#67227=CARTESIAN_POINT('Ctrl Pts',(81.6649206134033,8.93901688177521,132.722887025676));
#67228=CARTESIAN_POINT('Ctrl Pts',(81.6640188300732,8.91819612781828,132.721496692136));
#67229=CARTESIAN_POINT('Ctrl Pts',(81.6635130563646,8.90848574701562,132.720850697161));
#67230=CARTESIAN_POINT('Ctrl Pts',(81.6621855176908,8.88667585372414,132.719404956828));
#67231=CARTESIAN_POINT('Ctrl Pts',(81.6613165906193,8.87457968240863,132.718606717627));
#67232=CARTESIAN_POINT('Ctrl Pts',(81.6583686253788,8.83898453849543,132.71626753446));
#67233=CARTESIAN_POINT('Ctrl Pts',(81.6559224325431,8.81551839268672,132.714738040061));
#67234=CARTESIAN_POINT('Ctrl Pts',(81.6401040686105,8.68974245662752,132.70659421783));
#67235=CARTESIAN_POINT('Ctrl Pts',(81.6177478784738,8.588786859531,132.700268507794));
#67236=CARTESIAN_POINT('Ctrl Pts',(81.5620501834658,8.41537375840546,132.689144835628));
#67237=CARTESIAN_POINT('Ctrl Pts',(81.5325977294016,8.34202501550044,132.684345510267));
#67238=CARTESIAN_POINT('Ctrl Pts',(81.4872447500361,8.24882094365922,132.677809317136));
#67239=CARTESIAN_POINT('Ctrl Pts',(81.47593727185,8.22684027417586,132.676233727817));
#67240=CARTESIAN_POINT('Ctrl Pts',(81.4559441687673,8.1900135426461,132.673521805443));
#67241=CARTESIAN_POINT('Ctrl Pts',(81.4475097464026,8.17503517572367,132.672397956209));
#67242=CARTESIAN_POINT('Ctrl Pts',(81.4350972443057,8.1537688321937,132.670768260328));
#67243=CARTESIAN_POINT('Ctrl Pts',(81.4313061285966,8.14737226705228,132.67027358608));
#67244=CARTESIAN_POINT('Ctrl Pts',(81.4246320752865,8.13628141372444,132.66940764892));
#67245=CARTESIAN_POINT('Ctrl Pts',(81.4217684719951,8.13157570436811,132.669037626473));
#67246=CARTESIAN_POINT('Ctrl Pts',(81.4155799852824,8.12151892965444,132.66824108861));
#67247=CARTESIAN_POINT('Ctrl Pts',(81.4122481294619,8.11617258289667,132.667814149577));
#67248=CARTESIAN_POINT('Ctrl Pts',(81.4030116158703,8.10153711316241,132.666636081175));
#67249=CARTESIAN_POINT('Ctrl Pts',(81.3970452206595,8.09228760692123,132.665881140234));
#67250=CARTESIAN_POINT('Ctrl Pts',(81.3624652782639,8.03982803140378,132.6615426165));
#67251=CARTESIAN_POINT('Ctrl Pts',(81.3319420159483,7.99791656764431,132.6578551749));
#67252=CARTESIAN_POINT('Ctrl Pts',(81.2370259884891,7.87959983081459,132.64692275476));
#67253=CARTESIAN_POINT('Ctrl Pts',(81.1676541732336,7.80747534998635,132.639583951734));
#67254=CARTESIAN_POINT('Ctrl Pts',(81.0544636093322,7.70919989812938,132.628824437386));
#67255=CARTESIAN_POINT('Ctrl Pts',(81.0152296014073,7.67811950467839,132.625278632196));
#67256=CARTESIAN_POINT('Ctrl Pts',(80.947216176168,7.62905798695339,132.619440996194));
#67257=CARTESIAN_POINT('Ctrl Pts',(80.9191812762621,7.61010555936394,132.617115978724));
#67258=CARTESIAN_POINT('Ctrl Pts',(80.8789638676492,7.58466694315366,132.613890476227));
#67259=CARTESIAN_POINT('Ctrl Pts',(80.867250037415,7.57745912721672,132.612963624196));
#67260=CARTESIAN_POINT('Ctrl Pts',(80.8469136238374,7.56529019362384,132.611375674988));
#67261=CARTESIAN_POINT('Ctrl Pts',(80.8383335497348,7.56025982151991,132.610712080168));
#67262=CARTESIAN_POINT('Ctrl Pts',(80.8207217280619,7.55014509270155,132.609362661168));
#67263=CARTESIAN_POINT('Ctrl Pts',(80.8116865425432,7.54506757132803,132.608677104587));
#67264=CARTESIAN_POINT('Ctrl Pts',(80.7886903129719,7.53242523036049,132.606948759544));
#67265=CARTESIAN_POINT('Ctrl Pts',(80.7746672163916,7.52497496746674,132.605910059923));
#67266=CARTESIAN_POINT('Ctrl Pts',(80.7192406366863,7.49653616491054,132.601861223339));
#67267=CARTESIAN_POINT('Ctrl Pts',(80.6770719202831,7.47708016938978,132.598904060902));
#67268=CARTESIAN_POINT('Ctrl Pts',(80.5298633247235,7.41648573299649,132.588912002858));
#67269=CARTESIAN_POINT('Ctrl Pts',(80.4214979948379,7.3842610085533,132.582135825225));
#67270=CARTESIAN_POINT('Ctrl Pts',(80.2467533101099,7.35108938536976,132.571192963126));
#67271=CARTESIAN_POINT('Ctrl Pts',(80.1821502317034,7.34270919025295,132.567137837064));
#67272=CARTESIAN_POINT('Ctrl Pts',(80.1021383017193,7.33706504119916,132.561927496987));
#67273=CARTESIAN_POINT('Ctrl Pts',(80.0870328818012,7.3362060981031,132.560935575747));
#67274=CARTESIAN_POINT('Ctrl Pts',(80.0648573137609,7.3352479215985,132.559464514824));
#67275=CARTESIAN_POINT('Ctrl Pts',(80.0577943998456,7.33498776085358,132.558993771697));
#67276=CARTESIAN_POINT('Ctrl Pts',(80.0457810338617,7.33462178050525,132.558188996733));
#67277=CARTESIAN_POINT('Ctrl Pts',(80.040831418933,7.33449307675643,132.557856234753));
#67278=CARTESIAN_POINT('Ctrl Pts',(80.0295620456989,7.33425030825084,132.557095814404));
#67279=CARTESIAN_POINT('Ctrl Pts',(80.0232423093397,7.33415014426926,132.556667416102));
#67280=CARTESIAN_POINT('Ctrl Pts',(80.0058231099533,7.33397320073411,132.555481483936));
#67281=CARTESIAN_POINT('Ctrl Pts',(79.9947234507573,7.33397138501693,132.554720058067));
#67282=CARTESIAN_POINT('Ctrl Pts',(79.9308568333433,7.33459915665192,132.550308949639));
#67283=CARTESIAN_POINT('Ctrl Pts',(79.8781483343874,7.3376246616884,132.54655177365));
#67284=CARTESIAN_POINT('Ctrl Pts',(79.7250433324634,7.35373322060475,132.535450183526));
#67285=CARTESIAN_POINT('Ctrl Pts',(79.6255752407566,7.37346893563222,132.528013862693));
#67286=CARTESIAN_POINT('Ctrl Pts',(79.4584095292679,7.42279417085371,132.515518140212));
#67287=CARTESIAN_POINT('Ctrl Pts',(79.3897350897818,7.44807285472084,132.510381181652));
#67288=CARTESIAN_POINT('Ctrl Pts',(79.3068207310512,7.48495230233739,132.504188110223));
#67289=CARTESIAN_POINT('Ctrl Pts',(79.2908212127828,7.49237520769528,132.50299320216));
#67290=CARTESIAN_POINT('Ctrl Pts',(79.265274118672,7.50472437723302,132.501084777423));
#67291=CARTESIAN_POINT('Ctrl Pts',(79.2556514276604,7.50949118723549,132.500365828569));
#67292=CARTESIAN_POINT('Ctrl Pts',(79.2373424597085,7.51878246756278,132.498997417226));
#67293=CARTESIAN_POINT('Ctrl Pts',(79.2286487099196,7.52329112671427,132.498347438041));
#67294=CARTESIAN_POINT('Ctrl Pts',(79.2088942347118,7.53375803780484,132.496869749779));
#67295=CARTESIAN_POINT('Ctrl Pts',(79.1978600494055,7.539765314201,132.496043810347));
#67296=CARTESIAN_POINT('Ctrl Pts',(79.1685849889021,7.55613534359005,132.493850164165));
#67297=CARTESIAN_POINT('Ctrl Pts',(79.1504697574567,7.56671897498553,132.492490327151));
#67298=CARTESIAN_POINT('Ctrl Pts',(79.0289990837983,7.64079928182422,132.483343087422));
#67299=CARTESIAN_POINT('Ctrl Pts',(78.9326446897258,7.71507748669581,132.475977566467));
#67300=CARTESIAN_POINT('Ctrl Pts',(78.7769423582714,7.86481079633191,132.462777109716));
#67301=CARTESIAN_POINT('Ctrl Pts',(78.7144130612452,7.93614588721792,132.456972520335));
#67302=CARTESIAN_POINT('Ctrl Pts',(78.6512058941246,8.02201572094275,132.450001560231));
#67303=CARTESIAN_POINT('Ctrl Pts',(78.6442262120951,8.03171481164655,132.449214309078));
#67304=CARTESIAN_POINT('Ctrl Pts',(78.6336484468648,8.04675246438208,132.447992506668));
#67305=CARTESIAN_POINT('Ctrl Pts',(78.6299758001279,8.05203844001826,132.447562792655));
#67306=CARTESIAN_POINT('Ctrl Pts',(78.6232309133811,8.06186730250599,132.4467630783));
#67307=CARTESIAN_POINT('Ctrl Pts',(78.6201503620369,8.06640423662196,132.446393641615));
#67308=CARTESIAN_POINT('Ctrl Pts',(78.61313702902,8.07684377994631,132.445542937354));
#67309=CARTESIAN_POINT('Ctrl Pts',(78.6092194980376,8.08275635861927,132.445060696256));
#67310=CARTESIAN_POINT('Ctrl Pts',(78.5967639032098,8.10181835731779,132.443505037225));
#67311=CARTESIAN_POINT('Ctrl Pts',(78.588373953011,8.11506290296182,132.442422743279));
#67312=CARTESIAN_POINT('Ctrl Pts',(78.5325283523124,8.20603724123565,132.434989446076));
#67313=CARTESIAN_POINT('Ctrl Pts',(78.4913328088637,8.28742005575831,132.428352542801));
#67314=CARTESIAN_POINT('Ctrl Pts',(78.4247983181732,8.45083157997319,132.415509623882));
#67315=CARTESIAN_POINT('Ctrl Pts',(78.3987241872377,8.53227695919785,132.409321369037));
#67316=CARTESIAN_POINT('Ctrl Pts',(78.3680020355095,8.6617527578773,132.399941832053));
#67317=CARTESIAN_POINT('Ctrl Pts',(78.3589911652403,8.70859076932037,132.396636476905));
#67318=CARTESIAN_POINT('Ctrl Pts',(78.3497214906526,8.77113624633401,132.392336251937));
#67319=CARTESIAN_POINT('Ctrl Pts',(78.3476572785426,8.78654898576195,132.39128552387));
#67320=CARTESIAN_POINT('Ctrl Pts',(78.3445854612189,8.81221103466813,132.389550395346));
#67321=CARTESIAN_POINT('Ctrl Pts',(78.3434565920573,8.82244455366229,132.388862228165));
#67322=CARTESIAN_POINT('Ctrl Pts',(78.3414309106954,8.84251319908358,132.38751981382));
#67323=CARTESIAN_POINT('Ctrl Pts',(78.3405265445635,8.85234711549764,132.386865356495));
#67324=CARTESIAN_POINT('Ctrl Pts',(78.3385587767958,8.87605391770599,132.385295374785));
#67325=CARTESIAN_POINT('Ctrl Pts',(78.3375816034244,8.8899333674968,132.384382577325));
#67326=CARTESIAN_POINT('Ctrl Pts',(78.3349117757002,8.9361039845083,132.381365790222));
#67327=CARTESIAN_POINT('Ctrl Pts',(78.3339852171911,8.9684332389627,132.379285502678));
#67328=CARTESIAN_POINT('Ctrl Pts',(78.334022550631,9.04912758001036,132.374154844899));
#67329=CARTESIAN_POINT('Ctrl Pts',(78.3361502741554,9.09746277210266,132.371137465754));
#67330=CARTESIAN_POINT('Ctrl Pts',(78.3493322671356,9.24767666778614,132.361827880112));
#67331=CARTESIAN_POINT('Ctrl Pts',(78.3676768809818,9.34866524845633,132.355677482683));
#67332=CARTESIAN_POINT('Ctrl Pts',(78.4072396823514,9.49060039028313,132.346514737682));
#67333=CARTESIAN_POINT('Ctrl Pts',(78.4210455027179,9.53336255103003,132.343680820218));
#67334=CARTESIAN_POINT('Ctrl Pts',(78.4365593734337,9.57550795581125,132.340765796073));
#67335=CARTESIAN_POINT('Ctrl Pts',(78.4365593745624,9.57550795887745,132.531716954706));
#67336=CARTESIAN_POINT('Ctrl Pts',(78.4158153041906,9.51915405124514,132.535390102318));
#67337=CARTESIAN_POINT('Ctrl Pts',(78.3981331275018,9.46171927848792,132.5390813048));
#67338=CARTESIAN_POINT('Ctrl Pts',(78.3781664940499,9.38172466887552,132.544300095684));
#67339=CARTESIAN_POINT('Ctrl Pts',(78.3731815460984,9.35988784635904,132.54573262462));
#67340=CARTESIAN_POINT('Ctrl Pts',(78.365398621124,9.3223188212678,132.548220991885));
#67341=CARTESIAN_POINT('Ctrl Pts',(78.3623839053814,9.30663426281379,132.549266886095));
#67342=CARTESIAN_POINT('Ctrl Pts',(78.3583344197384,9.28379968614592,132.550802957639));
#67343=CARTESIAN_POINT('Ctrl Pts',(78.3571198293399,9.27668190998204,132.551283647918));
#67344=CARTESIAN_POINT('Ctrl Pts',(78.3550723079505,9.26419390574105,132.552130660832));
#67345=CARTESIAN_POINT('Ctrl Pts',(78.3542193240584,9.25882715735029,132.552495857473));
#67346=CARTESIAN_POINT('Ctrl Pts',(78.3524177218625,9.24712284102455,132.553295001798));
#67347=CARTESIAN_POINT('Ctrl Pts',(78.3514794201271,9.24078404445869,132.5537294835));
#67348=CARTESIAN_POINT('Ctrl Pts',(78.3489603434048,9.22306087866001,132.554948689038));
#67349=CARTESIAN_POINT('Ctrl Pts',(78.3474608131118,9.21166558704167,132.555737654615));
#67350=CARTESIAN_POINT('Ctrl Pts',(78.3380833661921,9.13421699267986,132.561130159692));
#67351=CARTESIAN_POINT('Ctrl Pts',(78.3340507254895,9.06776530077335,132.565903956972));
#67352=CARTESIAN_POINT('Ctrl Pts',(78.3338866237805,8.85057454433804,132.581651623519));
#67353=CARTESIAN_POINT('Ctrl Pts',(78.3542177053222,8.70053264545152,132.592678381093));
#67354=CARTESIAN_POINT('Ctrl Pts',(78.399968049702,8.53537156616134,132.604461594223));
#67355=CARTESIAN_POINT('Ctrl Pts',(78.4058459399267,8.51558827180375,132.605868735997));
#67356=CARTESIAN_POINT('Ctrl Pts',(78.4158613425301,8.48403869741446,132.608106732611));
#67357=CARTESIAN_POINT('Ctrl Pts',(78.4197658644806,8.47220132299353,132.608945050402));
#67358=CARTESIAN_POINT('Ctrl Pts',(78.4269697471796,8.45115810670466,132.610433193698));
#67359=CARTESIAN_POINT('Ctrl Pts',(78.4302179670185,8.44193550905234,132.611084665797));
#67360=CARTESIAN_POINT('Ctrl Pts',(78.4372192219823,8.42260192085466,132.612449055518));
#67361=CARTESIAN_POINT('Ctrl Pts',(78.4409896335776,8.41249766932211,132.613161361915));
#67362=CARTESIAN_POINT('Ctrl Pts',(78.4512640226325,8.38575913052174,132.615044776518));
#67363=CARTESIAN_POINT('Ctrl Pts',(78.4579379342537,8.36919131360153,132.616210178117));
#67364=CARTESIAN_POINT('Ctrl Pts',(78.4948474479269,8.28165297370368,132.622364571122));
#67365=CARTESIAN_POINT('Ctrl Pts',(78.5297202375517,8.21273493904726,132.627192781898));
#67366=CARTESIAN_POINT('Ctrl Pts',(78.6234638765606,8.05559383548338,132.638466358107));
#67367=CARTESIAN_POINT('Ctrl Pts',(78.6862116460568,7.97009100919123,132.64481399731));
#67368=CARTESIAN_POINT('Ctrl Pts',(78.7863054113061,7.85785818900112,132.654221210498));
#67369=CARTESIAN_POINT('Ctrl Pts',(78.8172908938107,7.82580202834366,132.657055872879));
#67370=CARTESIAN_POINT('Ctrl Pts',(78.8572844312582,7.78761707820762,132.660681139094));
#67371=CARTESIAN_POINT('Ctrl Pts',(78.8651192803846,7.78027996758507,132.661389843263));
#67372=CARTESIAN_POINT('Ctrl Pts',(78.8775723371469,7.76884189568672,132.662515013205));
#67373=CARTESIAN_POINT('Ctrl Pts',(78.8821435488544,7.76468988197728,132.662927769796));
#67374=CARTESIAN_POINT('Ctrl Pts',(78.8908594572922,7.75686124980466,132.663714512337));
#67375=CARTESIAN_POINT('Ctrl Pts',(78.8949995433564,7.75317977126558,132.664088130795));
#67376=CARTESIAN_POINT('Ctrl Pts',(78.9049152154767,7.74445065761625,132.664982647011));
#67377=CARTESIAN_POINT('Ctrl Pts',(78.9107073957882,7.73942217491663,132.66550490769));
#67378=CARTESIAN_POINT('Ctrl Pts',(78.930670049947,7.72233191020739,132.667303349307));
#67379=CARTESIAN_POINT('Ctrl Pts',(78.9450072054279,7.71046813870667,132.66859238136));
#67380=CARTESIAN_POINT('Ctrl Pts',(78.981044202202,7.68165131457063,132.671819860232));
#67381=CARTESIAN_POINT('Ctrl Pts',(79.00297095642,7.66499172682218,132.673772646311));
#67382=CARTESIAN_POINT('Ctrl Pts',(79.104958054512,7.59141779231284,132.682772151182));
#67383=CARTESIAN_POINT('Ctrl Pts',(79.18954183518,7.54110946450824,132.68999384812));
#67384=CARTESIAN_POINT('Ctrl Pts',(79.3572778212561,7.46045801028231,132.703433474745));
#67385=CARTESIAN_POINT('Ctrl Pts',(79.4393906520102,7.42869387562057,132.709657774871));
#67386=CARTESIAN_POINT('Ctrl Pts',(79.5415669179649,7.39820565346661,132.716946633924));
#67387=CARTESIAN_POINT('Ctrl Pts',(79.5595840734671,7.39315841462845,132.718215799916));
#67388=CARTESIAN_POINT('Ctrl Pts',(79.5882910603853,7.38563572707629,132.72021332017));
#67389=CARTESIAN_POINT('Ctrl Pts',(79.5989264398569,7.38296064798719,132.720948051151));
#67390=CARTESIAN_POINT('Ctrl Pts',(79.6181099836043,7.37833638960376,132.72226404378));
#67391=CARTESIAN_POINT('Ctrl Pts',(79.6266485037331,7.37634932477325,132.722846501165));
#67392=CARTESIAN_POINT('Ctrl Pts',(79.6467822340523,7.37183107322512,132.724212416469));
#67393=CARTESIAN_POINT('Ctrl Pts',(79.6583896953554,7.36935618351344,132.724994051237));
#67394=CARTESIAN_POINT('Ctrl Pts',(79.6926342373903,7.36243643230209,132.727283650897));
#67395=CARTESIAN_POINT('Ctrl Pts',(79.7153389039482,7.35833733830105,132.728780659801));
#67396=CARTESIAN_POINT('Ctrl Pts',(79.8216456865524,7.34141667968682,132.735703231742));
#67397=CARTESIAN_POINT('Ctrl Pts',(79.9060648788887,7.33450082558079,132.740943671897));
#67398=CARTESIAN_POINT('Ctrl Pts',(80.079759781727,7.33352626246292,132.75158616841));
#67399=CARTESIAN_POINT('Ctrl Pts',(80.1687582859573,7.3401761214123,132.756965490504));
#67400=CARTESIAN_POINT('Ctrl Pts',(80.300961109487,7.36079997074128,132.765334522732));
#67401=CARTESIAN_POINT('Ctrl Pts',(80.3448301471471,7.36946458966138,132.768177321253));
#67402=CARTESIAN_POINT('Ctrl Pts',(80.3987399752409,7.38238514037267,132.771811771643));
#67403=CARTESIAN_POINT('Ctrl Pts',(80.4091618593135,7.38498979572191,132.772521023632));
#67404=CARTESIAN_POINT('Ctrl Pts',(80.4255356819421,7.38925062710553,132.773646868134));
#67405=CARTESIAN_POINT('Ctrl Pts',(80.4315050567109,7.39083949159219,132.774059744041));
#67406=CARTESIAN_POINT('Ctrl Pts',(80.4428107206027,7.39391614325671,132.774846564453));
#67407=CARTESIAN_POINT('Ctrl Pts',(80.4481485987269,7.39539739533989,132.775220140005));
#67408=CARTESIAN_POINT('Ctrl Pts',(80.4608560055704,7.3989920303435,132.776114345397));
#67409=CARTESIAN_POINT('Ctrl Pts',(80.4682184572554,7.40112969653713,132.776636335574));
#67410=CARTESIAN_POINT('Ctrl Pts',(80.4933772252836,7.40862314091016,132.778432840137));
#67411=CARTESIAN_POINT('Ctrl Pts',(80.5110978173229,7.41422563282207,132.779720169746));
#67412=CARTESIAN_POINT('Ctrl Pts',(80.5547852935542,7.42884604008863,132.782942437674));
#67413=CARTESIAN_POINT('Ctrl Pts',(80.5806292618344,7.43821224947295,132.784891660076));
#67414=CARTESIAN_POINT('Ctrl Pts',(80.6973664294046,7.48381731998525,132.79386016481));
#67415=CARTESIAN_POINT('Ctrl Pts',(80.7851896293361,7.52738084349259,132.801053515718));
#67416=CARTESIAN_POINT('Ctrl Pts',(80.9440628477874,7.62446181479534,132.814500316631));
#67417=CARTESIAN_POINT('Ctrl Pts',(81.0156701985821,7.67645230122932,132.820757441908));
#67418=CARTESIAN_POINT('Ctrl Pts',(81.0970494899205,7.74605075065364,132.828077414278));
#67419=CARTESIAN_POINT('Ctrl Pts',(81.1110679049416,7.75845480812324,132.82934710576));
#67420=CARTESIAN_POINT('Ctrl Pts',(81.1329650929628,7.77849830523119,132.831345256668));
#67421=CARTESIAN_POINT('Ctrl Pts',(81.1409821960153,7.78598355425947,132.8320800997));
#67422=CARTESIAN_POINT('Ctrl Pts',(81.1552730838317,7.799593007555,132.833396189896));
#67423=CARTESIAN_POINT('Ctrl Pts',(81.1615734909718,7.80568853483234,132.833978633909));
#67424=CARTESIAN_POINT('Ctrl Pts',(81.1762878604293,7.8201510018893,132.835344384885));
#67425=CARTESIAN_POINT('Ctrl Pts',(81.1846612032995,7.82855873620775,132.836125870133));
#67426=CARTESIAN_POINT('Ctrl Pts',(81.2090387759521,7.85356515834883,132.838414560437));
#67427=CARTESIAN_POINT('Ctrl Pts',(81.2247894917678,7.87040786441079,132.839910823041));
#67428=CARTESIAN_POINT('Ctrl Pts',(81.296596289534,7.9504614586341,132.846826731609));
#67429=CARTESIAN_POINT('Ctrl Pts',(81.348144591726,8.01755322883263,132.852061692706));
#67430=CARTESIAN_POINT('Ctrl Pts',(81.4430437050401,8.16269090499177,132.862686835265));
#67431=CARTESIAN_POINT('Ctrl Pts',(81.4856639088488,8.24088027471099,132.868054516755));
#67432=CARTESIAN_POINT('Ctrl Pts',(81.5401297620792,8.36315096492667,132.876424772968));
#67433=CARTESIAN_POINT('Ctrl Pts',(81.5567488133593,8.40492964441232,132.879282540408));
#67434=CARTESIAN_POINT('Ctrl Pts',(81.5752319570369,8.45749063800833,132.882935024104));
#67435=CARTESIAN_POINT('Ctrl Pts',(81.5787079938222,8.46769070877485,132.883646453979));
#67436=CARTESIAN_POINT('Ctrl Pts',(81.5840228006412,8.48379653591062,132.884774980131));
#67437=CARTESIAN_POINT('Ctrl Pts',(81.5859281190037,8.48968024971342,132.885188330221));
#67438=CARTESIAN_POINT('Ctrl Pts',(81.5894772090753,8.50085186032292,132.885975462202));
#67439=CARTESIAN_POINT('Ctrl Pts',(81.5911274321993,8.50613751481145,132.886348869353));
#67440=CARTESIAN_POINT('Ctrl Pts',(81.5949950355936,8.51874603587493,132.887241849074));
#67441=CARTESIAN_POINT('Ctrl Pts',(81.5971883567455,8.52607607266579,132.887762771786));
#67442=CARTESIAN_POINT('Ctrl Pts',(81.6045093512998,8.5511708333037,132.889551648223));
#67443=CARTESIAN_POINT('Ctrl Pts',(81.6093915283186,8.56900496838309,132.890832276323));
#67444=CARTESIAN_POINT('Ctrl Pts',(81.6207432476791,8.61335765598293,132.894034057287));
#67445=CARTESIAN_POINT('Ctrl Pts',(81.6268596610508,8.63996048416184,132.895969278331));
#67446=CARTESIAN_POINT('Ctrl Pts',(81.6516012192961,8.76113097272919,132.904817256898));
#67447=CARTESIAN_POINT('Ctrl Pts',(81.6626520440427,8.85705548287418,132.9119005437));
#67448=CARTESIAN_POINT('Ctrl Pts',(81.6678678671305,9.04344174628777,132.925375603963));
#67449=CARTESIAN_POINT('Ctrl Pts',(81.6630809982746,9.13355432024879,132.931760868367));
#67450=CARTESIAN_POINT('Ctrl Pts',(81.6485207269419,9.24142648951733,132.939202037549));
#67451=CARTESIAN_POINT('Ctrl Pts',(81.6457000626636,9.2599590170741,132.940473640124));
#67452=CARTESIAN_POINT('Ctrl Pts',(81.6407330911091,9.28925999589201,132.942474084478));
#67453=CARTESIAN_POINT('Ctrl Pts',(81.6387921577502,9.30006115235657,132.943209334939));
#67454=CARTESIAN_POINT('Ctrl Pts',(81.6351091696299,9.3194539624201,132.944525780391));
#67455=CARTESIAN_POINT('Ctrl Pts',(81.6334057748133,9.32805245089953,132.945108176281));
#67456=CARTESIAN_POINT('Ctrl Pts',(81.6292387070813,9.34824965727235,132.946473332182));
#67457=CARTESIAN_POINT('Ctrl Pts',(81.626718893194,9.35983641161602,132.947254275684));
#67458=CARTESIAN_POINT('Ctrl Pts',(81.618945099474,9.39383043447905,132.949539672752));
#67459=CARTESIAN_POINT('Ctrl Pts',(81.6133501500741,9.41615744984906,132.951033232815));
#67460=CARTESIAN_POINT('Ctrl Pts',(81.5851541067631,9.51954074054812,132.957925055547));
#67461=CARTESIAN_POINT('Ctrl Pts',(81.5568947983073,9.59892996510389,132.96314021144));
#67462=CARTESIAN_POINT('Ctrl Pts',(81.486972424395,9.75647134086693,132.973702274399));
#67463=CARTESIAN_POINT('Ctrl Pts',(81.4448467058316,9.83411769014553,132.979027543099));
#67464=CARTESIAN_POINT('Ctrl Pts',(81.3717116908379,9.94661376218597,132.987411067292));
#67465=CARTESIAN_POINT('Ctrl Pts',(81.3450645485001,9.98410929651989,132.990332342853));
#67466=CARTESIAN_POINT('Ctrl Pts',(81.3102761597338,10.0290041139942,132.994055219915));
#67467=CARTESIAN_POINT('Ctrl Pts',(81.3035655322302,10.0374921538753,132.994769510685));
#67468=CARTESIAN_POINT('Ctrl Pts',(81.2928842066497,10.0507353597904,132.995901559221));
#67469=CARTESIAN_POINT('Ctrl Pts',(81.2889687111907,10.0555349480552,132.996315531793));
#67470=CARTESIAN_POINT('Ctrl Pts',(81.2815042354324,10.0645813849687,132.997103077801));
#67471=CARTESIAN_POINT('Ctrl Pts',(81.2779607444216,10.0688325231977,132.997476268929));
#67472=CARTESIAN_POINT('Ctrl Pts',(81.2694808793058,10.0789033944355,132.998367662583));
#67473=CARTESIAN_POINT('Ctrl Pts',(81.2645256185513,10.084706961251,132.998887202043));
#67474=CARTESIAN_POINT('Ctrl Pts',(81.2475082721929,10.1043624776593,133.000666231312));
#67475=CARTESIAN_POINT('Ctrl Pts',(81.2352575425769,10.1180483466645,133.001938214848));
#67476=CARTESIAN_POINT('Ctrl Pts',(81.2044133177024,10.1513800982963,133.005113628517));
#67477=CARTESIAN_POINT('Ctrl Pts',(81.1855631956721,10.1707806438628,133.007030851371));
#67478=CARTESIAN_POINT('Ctrl Pts',(81.0987425745169,10.2558890770279,133.015726770152));
#67479=CARTESIAN_POINT('Ctrl Pts',(81.0257261485521,10.3161984274356,133.022671525339));
#67480=CARTESIAN_POINT('Ctrl Pts',(80.8721094917607,10.4224963304983,133.036182186964));
#67481=CARTESIAN_POINT('Ctrl Pts',(80.7919880086041,10.4686152851551,133.042729455884));
#67482=CARTESIAN_POINT('Ctrl Pts',(80.6914477481183,10.5158524799551,133.050323749649));
#67483=CARTESIAN_POINT('Ctrl Pts',(80.6743149201014,10.5235511701283,133.051597922004));
#67484=CARTESIAN_POINT('Ctrl Pts',(80.6469634889915,10.5352898225739,133.053601450012));
#67485=CARTESIAN_POINT('Ctrl Pts',(80.6368292535379,10.5395210642342,133.054337248131));
#67486=CARTESIAN_POINT('Ctrl Pts',(80.6185331535562,10.5469484635262,133.055654172333));
#67487=CARTESIAN_POINT('Ctrl Pts',(80.6103865831932,10.5501809684458,133.056236504754));
#67488=CARTESIAN_POINT('Ctrl Pts',(80.591170014908,10.5576310007113,133.057600866738));
#67489=CARTESIAN_POINT('Ctrl Pts',(80.5800796958838,10.561795082413,133.058381086744));
#67490=CARTESIAN_POINT('Ctrl Pts',(80.5473686047823,10.5736806046241,133.060662089585));
#67491=CARTESIAN_POINT('Ctrl Pts',(80.5256310053261,10.5810740539564,133.062152044061));
#67492=CARTESIAN_POINT('Ctrl Pts',(80.4239698308709,10.6133227661132,133.069011839254));
#67493=CARTESIAN_POINT('Ctrl Pts',(80.342394898151,10.6325834949729,133.074200659079));
#67494=CARTESIAN_POINT('Ctrl Pts',(80.1735305712101,10.6592332406143,133.084678021482));
#67495=CARTESIAN_POINT('Ctrl Pts',(80.0864208569186,10.6660425575278,133.089946105605));
#67496=CARTESIAN_POINT('Ctrl Pts',(79.9518613333301,10.6659766059245,133.098344000836));
#67497=CARTESIAN_POINT('Ctrl Pts',(79.904566299961,10.6639371671559,133.101346949218));
#67498=CARTESIAN_POINT('Ctrl Pts',(79.8465579274791,10.6589546537889,133.105162493006));
#67499=CARTESIAN_POINT('Ctrl Pts',(79.8356984302451,10.6579143498844,133.105882533594));
#67500=CARTESIAN_POINT('Ctrl Pts',(79.8186712560455,10.6561142755856,133.107021660441));
#67501=CARTESIAN_POINT('Ctrl Pts',(79.8124960503494,10.6554264927497,133.107436882593));
#67502=CARTESIAN_POINT('Ctrl Pts',(79.8008336670123,10.6540614677923,133.10822527644));
#67503=CARTESIAN_POINT('Ctrl Pts',(79.7953458341789,10.653391434642,133.108598050728));
#67504=CARTESIAN_POINT('Ctrl Pts',(79.7823299136031,10.6517364729172,133.109486336782));
#67505=CARTESIAN_POINT('Ctrl Pts',(79.7748051027522,10.6507273836479,133.110003159542));
#67506=CARTESIAN_POINT('Ctrl Pts',(79.7493361657147,10.6471345756428,133.111762971197));
#67507=CARTESIAN_POINT('Ctrl Pts',(79.7314281207907,10.6443095046291,133.113018105082));
#67508=CARTESIAN_POINT('Ctrl Pts',(79.6873970552532,10.6366249795273,133.116142316988));
#67509=CARTESIAN_POINT('Ctrl Pts',(79.6613378592204,10.6314318013803,133.118024660605));
#67510=CARTESIAN_POINT('Ctrl Pts',(79.5465476998577,10.6056873085211,133.126434521699));
#67511=CARTESIAN_POINT('Ctrl Pts',(79.4594659785083,10.5785034939415,133.133119685991));
#67512=CARTESIAN_POINT('Ctrl Pts',(79.2854473896917,10.5080824350587,133.146715054857));
#67513=CARTESIAN_POINT('Ctrl Pts',(79.1991638130289,10.4640919567255,133.153585283214));
#67514=CARTESIAN_POINT('Ctrl Pts',(79.1012915543917,10.4029361026397,133.161474505971));
#67515=CARTESIAN_POINT('Ctrl Pts',(79.0855806718509,10.3927468974138,133.162744706175));
#67516=CARTESIAN_POINT('Ctrl Pts',(79.0609429621842,10.3761715759078,133.164743467601));
#67517=CARTESIAN_POINT('Ctrl Pts',(79.0519021111862,10.3699586598858,133.165478419101));
#67518=CARTESIAN_POINT('Ctrl Pts',(79.0351461343413,10.3581985463208,133.166843640303));
#67519=CARTESIAN_POINT('Ctrl Pts',(79.0274158771078,10.352673797925,133.167474726944));
#67520=CARTESIAN_POINT('Ctrl Pts',(79.0192318271128,10.3467182984905,133.168144321731));
#67521=CARTESIAN_POINT('Ctrl Pts',(79.0187306902262,10.3463531951666,133.168185329153));
#67522=CARTESIAN_POINT('Ctrl Pts',(79.0177834489313,10.3456622726275,133.168262851953));
#67523=CARTESIAN_POINT('Ctrl Pts',(79.0173373026378,10.3453365112047,133.168299369537));
#67524=CARTESIAN_POINT('Ctrl Pts',(79.0164831042801,10.3447121519121,133.168369295703));
#67525=CARTESIAN_POINT('Ctrl Pts',(79.0160750260463,10.3444135901194,133.16840270566));
#67526=CARTESIAN_POINT('Ctrl Pts',(79.01528530826,10.3438352576828,133.168467368711));
#67527=CARTESIAN_POINT('Ctrl Pts',(79.0149036519001,10.3435555101599,133.168498622686));
#67528=CARTESIAN_POINT('Ctrl Pts',(79.0141582335067,10.3430086429776,133.168559672112));
#67529=CARTESIAN_POINT('Ctrl Pts',(79.0137944607681,10.3427415380721,133.168589468123));
#67530=CARTESIAN_POINT('Ctrl Pts',(79.0130781715019,10.342215145173,133.168648144478));
#67531=CARTESIAN_POINT('Ctrl Pts',(79.0127256485115,10.3419558660371,133.168677025161));
#67532=CARTESIAN_POINT('Ctrl Pts',(79.0120264045867,10.3414411504904,133.168734317195));
#67533=CARTESIAN_POINT('Ctrl Pts',(79.0116796804819,10.3411857184935,133.16876272871));
#67534=CARTESIAN_POINT('Ctrl Pts',(79.0109872994469,10.3406752263985,133.168819470176));
#67535=CARTESIAN_POINT('Ctrl Pts',(79.0106416420438,10.3404201669912,133.168847800151));
#67536=CARTESIAN_POINT('Ctrl Pts',(79.0099470572966,10.3399072202583,133.168904734023));
#67537=CARTESIAN_POINT('Ctrl Pts',(79.0095981319571,10.3396493302479,133.168933337814));
#67538=CARTESIAN_POINT('Ctrl Pts',(78.998242932863,10.3312498645064,133.169864299206));
#67539=CARTESIAN_POINT('Ctrl Pts',(78.9873370692588,10.3229728759129,133.170761420092));
#67540=CARTESIAN_POINT('Ctrl Pts',(78.9459345373154,10.2907385122996,133.17418046036));
#67541=CARTESIAN_POINT('Ctrl Pts',(78.9161743683087,10.2658523905039,133.176665711008));
#67542=CARTESIAN_POINT('Ctrl Pts',(78.8418332495801,10.1991409403637,133.182981079369));
#67543=CARTESIAN_POINT('Ctrl Pts',(78.798635466005,10.1558604189858,133.186755962853));
#67544=CARTESIAN_POINT('Ctrl Pts',(78.6995289695442,10.0449905032841,133.195869447882));
#67545=CARTESIAN_POINT('Ctrl Pts',(78.6463923762766,9.9751794567776,133.201158779527));
#67546=CARTESIAN_POINT('Ctrl Pts',(78.5736601763062,9.86214986167906,133.209550700495));
#67547=CARTESIAN_POINT('Ctrl Pts',(78.5500002320452,9.82173443354892,133.212522689878));
#67548=CARTESIAN_POINT('Ctrl Pts',(78.5229781739841,9.77076646661656,133.216303496342));
#67549=CARTESIAN_POINT('Ctrl Pts',(78.517975303888,9.76110262464493,133.217021778711));
#67550=CARTESIAN_POINT('Ctrl Pts',(78.5102679143547,9.7458504186802,133.218158741245));
#67551=CARTESIAN_POINT('Ctrl Pts',(78.5074992479223,9.740294560261,133.218573581508));
#67552=CARTESIAN_POINT('Ctrl Pts',(78.5023227456048,9.7297598427144,133.219361713918));
#67553=CARTESIAN_POINT('Ctrl Pts',(78.4999085718602,9.72478430576832,133.219734613259));
#67554=CARTESIAN_POINT('Ctrl Pts',(78.4942339071059,9.71293919491742,133.220623838431));
#67555=CARTESIAN_POINT('Ctrl Pts',(78.4909956222077,9.70605920738418,133.221141483102));
#67556=CARTESIAN_POINT('Ctrl Pts',(78.4801663088353,9.68263667605853,133.222907091899));
#67557=CARTESIAN_POINT('Ctrl Pts',(78.4727996201629,9.66599265205912,133.224167305683));
#67558=CARTESIAN_POINT('Ctrl Pts',(78.4554074491306,9.62489074762251,133.22728720334));
#67559=CARTESIAN_POINT('Ctrl Pts',(78.4456887246787,9.60030900062951,133.229159777037));
#67560=CARTESIAN_POINT('Ctrl Pts',(78.4365593737642,9.57550795670914,133.231048988662));
#67561=CARTESIAN_POINT('Origin',(80.,9.,134.));
#67562=CARTESIAN_POINT('',(78.4365594251401,9.5755080962782,133.933539779158));
#67563=CARTESIAN_POINT('',(78.4365593568557,9.5755079107748,133.73811642446));
#67564=CARTESIAN_POINT('',(78.4365593737638,9.57550795670799,134.));
#67565=CARTESIAN_POINT('',(78.3340006446003,8.99853445987493,133.077925722171));
#67566=CARTESIAN_POINT('Ctrl Pts',(78.4365593568556,9.5755079107748,133.73811642446));
#67567=CARTESIAN_POINT('Ctrl Pts',(78.4533138724376,9.62102368931857,133.734685168399));
#67568=CARTESIAN_POINT('Ctrl Pts',(78.4720530953956,9.66579994160906,133.731307672136));
#67569=CARTESIAN_POINT('Ctrl Pts',(78.5003899641021,9.72598161132062,133.726765519516));
#67570=CARTESIAN_POINT('Ctrl Pts',(78.5083159725748,9.74213096291014,133.725546268158));
#67571=CARTESIAN_POINT('Ctrl Pts',(78.5214232527383,9.76777844344069,133.723608574949));
#67572=CARTESIAN_POINT('Ctrl Pts',(78.5264379851748,9.77735959102491,133.722884398203));
#67573=CARTESIAN_POINT('Ctrl Pts',(78.5361622240781,9.79550643991229,133.721511936369));
#67574=CARTESIAN_POINT('Ctrl Pts',(78.5408544996839,9.80408080813696,133.720863078475));
#67575=CARTESIAN_POINT('Ctrl Pts',(78.5517810140162,9.82363657562874,133.719382073356));
#67576=CARTESIAN_POINT('Ctrl Pts',(78.5580652359074,9.83458947440356,133.718551752309));
#67577=CARTESIAN_POINT('Ctrl Pts',(78.5782078655825,9.86878971091871,133.715955453846));
#67578=CARTESIAN_POINT('Ctrl Pts',(78.5925089713435,9.89177215287589,133.7142054799));
#67579=CARTESIAN_POINT('Ctrl Pts',(78.6585091620241,9.9922910884067,133.706509917165));
#67580=CARTESIAN_POINT('Ctrl Pts',(78.7161010395514,10.0657604531942,133.700783869137));
#67581=CARTESIAN_POINT('Ctrl Pts',(78.8564192981992,10.2167724206075,133.688188810723));
#67582=CARTESIAN_POINT('Ctrl Pts',(78.9415014299337,10.291466357208,133.681367664958));
#67583=CARTESIAN_POINT('Ctrl Pts',(79.0451948644778,10.3653243084814,133.67308643364));
#67584=CARTESIAN_POINT('Ctrl Pts',(79.0570298032732,10.3735248406953,133.672141472186));
#67585=CARTESIAN_POINT('Ctrl Pts',(79.0747155131244,10.3854431192072,133.670727260796));
#67586=CARTESIAN_POINT('Ctrl Pts',(79.0804859589658,10.3892796486917,133.67026551086));
#67587=CARTESIAN_POINT('Ctrl Pts',(79.0908495931465,10.3960771474094,133.669435312735));
#67588=CARTESIAN_POINT('Ctrl Pts',(79.0954336441448,10.3990516680198,133.669067769173));
#67589=CARTESIAN_POINT('Ctrl Pts',(79.1056325019292,10.4055984715684,133.668249257963));
#67590=CARTESIAN_POINT('Ctrl Pts',(79.1112540481959,10.4091596482241,133.667797611525));
#67591=CARTESIAN_POINT('Ctrl Pts',(79.1279243777179,10.4195806572977,133.666457195611));
#67592=CARTESIAN_POINT('Ctrl Pts',(79.1390320226525,10.4263447162064,133.665562660636));
#67593=CARTESIAN_POINT('Ctrl Pts',(79.1649197523285,10.4416966258473,133.663476619749));
#67594=CARTESIAN_POINT('Ctrl Pts',(79.1797549276294,10.4501883162241,133.66228029872));
#67595=CARTESIAN_POINT('Ctrl Pts',(79.2317890482612,10.4789189353703,133.658087669552));
#67596=CARTESIAN_POINT('Ctrl Pts',(79.2696253079559,10.4979658318823,133.655045411505));
#67597=CARTESIAN_POINT('Ctrl Pts',(79.4026924223626,10.5587116994226,133.64445562282));
#67598=CARTESIAN_POINT('Ctrl Pts',(79.5010822267611,10.5929352068715,133.636830784168));
#67599=CARTESIAN_POINT('Ctrl Pts',(79.6614132789467,10.6323773405461,133.625069981759));
#67600=CARTESIAN_POINT('Ctrl Pts',(79.7215692931465,10.6437076041462,133.620793936258));
#67601=CARTESIAN_POINT('Ctrl Pts',(79.7994482501544,10.6539761184316,133.615435179758));
#67602=CARTESIAN_POINT('Ctrl Pts',(79.8167124446517,10.6559781751258,133.614258088955));
#67603=CARTESIAN_POINT('Ctrl Pts',(79.8446351488687,10.6587742124256,133.612371093816));
#67604=CARTESIAN_POINT('Ctrl Pts',(79.8552751094234,10.6597363766622,133.611655974854));
#67605=CARTESIAN_POINT('Ctrl Pts',(79.8757008890263,10.6613855499246,133.610290401294));
#67606=CARTESIAN_POINT('Ctrl Pts',(79.8854849257758,10.6620886015135,133.609639472008));
#67607=CARTESIAN_POINT('Ctrl Pts',(79.9081435129188,10.6635157489398,133.608139079746));
#67608=CARTESIAN_POINT('Ctrl Pts',(79.9210215096234,10.6641768760487,133.607291615217));
#67609=CARTESIAN_POINT('Ctrl Pts',(79.9624541130472,10.665821891718,133.604580927236));
#67610=CARTESIAN_POINT('Ctrl Pts',(79.9910277185034,10.6662208503361,133.602735846403));
#67611=CARTESIAN_POINT('Ctrl Pts',(80.1115597627914,10.664802809602,133.595034966983));
#67612=CARTESIAN_POINT('Ctrl Pts',(80.2032771081441,10.6561083420529,133.58938773939));
#67613=CARTESIAN_POINT('Ctrl Pts',(80.4037797510479,10.6201845954713,133.576943439944));
#67614=CARTESIAN_POINT('Ctrl Pts',(80.5114673801259,10.5894748100621,133.570191623868));
#67615=CARTESIAN_POINT('Ctrl Pts',(80.6287550814395,10.5428655388323,133.56198388557));
#67616=CARTESIAN_POINT('Ctrl Pts',(80.642183530831,10.5373247220364,133.561030685729));
#67617=CARTESIAN_POINT('Ctrl Pts',(80.6619303445797,10.5288729763663,133.55960648604));
#67618=CARTESIAN_POINT('Ctrl Pts',(80.6683061046653,10.5260967548224,133.559143140018));
#67619=CARTESIAN_POINT('Ctrl Pts',(80.6796617030663,10.5210673371442,133.558311287544));
#67620=CARTESIAN_POINT('Ctrl Pts',(80.6846480901018,10.5188294392895,133.557943702163));
#67621=CARTESIAN_POINT('Ctrl Pts',(80.6956620371813,10.5138211038266,133.557126602584));
#67622=CARTESIAN_POINT('Ctrl Pts',(80.7016840283085,10.5110392201949,133.556676424345));
#67623=CARTESIAN_POINT('Ctrl Pts',(80.7193684552058,10.5027413167849,133.555344657496));
#67624=CARTESIAN_POINT('Ctrl Pts',(80.7309833048455,10.4971258537808,133.554457410651));
#67625=CARTESIAN_POINT('Ctrl Pts',(80.7576742745415,10.4838368663137,133.552391268937));
#67626=CARTESIAN_POINT('Ctrl Pts',(80.7727008972842,10.4760675550503,133.551207679084));
#67627=CARTESIAN_POINT('Ctrl Pts',(80.8243225568881,10.448373033997,133.547076835809));
#67628=CARTESIAN_POINT('Ctrl Pts',(80.8602849963634,10.4273056449414,133.544084930005));
#67629=CARTESIAN_POINT('Ctrl Pts',(81.0035553774474,10.3359927194376,133.531789739167));
#67630=CARTESIAN_POINT('Ctrl Pts',(81.1033920987968,10.2548044069588,133.522371856285));
#67631=CARTESIAN_POINT('Ctrl Pts',(81.222315669571,10.1328162409611,133.510411830442));
#67632=CARTESIAN_POINT('Ctrl Pts',(81.2505512563477,10.1015672157563,133.507500443784));
#67633=CARTESIAN_POINT('Ctrl Pts',(81.287427847411,10.0575070721881,133.503594197743));
#67634=CARTESIAN_POINT('Ctrl Pts',(81.2971179331146,10.0455987590924,133.502557106785));
#67635=CARTESIAN_POINT('Ctrl Pts',(81.3123683107769,10.0263189588971,133.500907091755));
#67636=CARTESIAN_POINT('Ctrl Pts',(81.3180341397578,10.0190324827392,133.500289980404));
#67637=CARTESIAN_POINT('Ctrl Pts',(81.3296378919313,10.0038509129828,133.499017364066));
#67638=CARTESIAN_POINT('Ctrl Pts',(81.335566747811,9.99594932022478,133.498362232117));
#67639=CARTESIAN_POINT('Ctrl Pts',(81.3493443699952,9.97724311005353,133.496827857507));
#67640=CARTESIAN_POINT('Ctrl Pts',(81.3571342766735,9.9663958284583,133.49595091345));
#67641=CARTESIAN_POINT('Ctrl Pts',(81.3827439718924,9.92981440211319,133.493034652759));
#67642=CARTESIAN_POINT('Ctrl Pts',(81.3999694987182,9.90367102323536,133.491017685084));
#67643=CARTESIAN_POINT('Ctrl Pts',(81.4400596235266,9.83892533369479,133.486167047121));
#67644=CARTESIAN_POINT('Ctrl Pts',(81.4621218896997,9.79985464409008,133.483360052284));
#67645=CARTESIAN_POINT('Ctrl Pts',(81.5152312361153,9.69624243644612,133.476151763462));
#67646=CARTESIAN_POINT('Ctrl Pts',(81.5437424461656,9.63050677051844,133.471806924921));
#67647=CARTESIAN_POINT('Ctrl Pts',(81.5756433514638,9.54168600879277,133.466032482952));
#67648=CARTESIAN_POINT('Ctrl Pts',(81.5829078849972,9.52007528178697,133.464634395126));
#67649=CARTESIAN_POINT('Ctrl Pts',(81.6092253763279,9.43611840251818,133.459207297491));
#67650=CARTESIAN_POINT('Ctrl Pts',(81.6250541268509,9.37283053315452,133.455126576894));
#67651=CARTESIAN_POINT('Ctrl Pts',(81.639258153691,9.29752325179486,133.450112335241));
#67652=CARTESIAN_POINT('Ctrl Pts',(81.6412662424835,9.28623850756035,133.449356803423));
#67653=CARTESIAN_POINT('Ctrl Pts',(81.6442141586173,9.26862015119077,133.448169494538));
#67654=CARTESIAN_POINT('Ctrl Pts',(81.6452342252854,9.26230006776009,133.447742036189));
#67655=CARTESIAN_POINT('Ctrl Pts',(81.6470532161736,9.25060180701274,133.446947707024));
#67656=CARTESIAN_POINT('Ctrl Pts',(81.6478622696715,9.24522540570564,133.446581403729));
#67657=CARTESIAN_POINT('Ctrl Pts',(81.6496865516487,9.23268567794725,133.445724220559));
#67658=CARTESIAN_POINT('Ctrl Pts',(81.6506814460104,9.22551962736021,133.445232240536));
#67659=CARTESIAN_POINT('Ctrl Pts',(81.6537323062779,9.20244223321678,133.443641527536));
#67660=CARTESIAN_POINT('Ctrl Pts',(81.6556050439919,9.18650814890319,133.442533504518));
#67661=CARTESIAN_POINT('Ctrl Pts',(81.6595538068366,9.14813777846912,133.439845912231));
#67662=CARTESIAN_POINT('Ctrl Pts',(81.6614053059014,9.1256819228667,133.438257154254));
#67663=CARTESIAN_POINT('Ctrl Pts',(81.6669297984497,9.03666611442462,133.431913202917));
#67664=CARTESIAN_POINT('Ctrl Pts',(81.6670619414313,8.96995118471119,133.427059445446));
#67665=CARTESIAN_POINT('Ctrl Pts',(81.6562298535306,8.78342873645697,133.413459104192));
#67666=CARTESIAN_POINT('Ctrl Pts',(81.6362979099804,8.66453087580806,133.40478355916));
#67667=CARTESIAN_POINT('Ctrl Pts',(81.5980391094291,8.5285451938593,133.395065365251));
#67668=CARTESIAN_POINT('Ctrl Pts',(81.591957854287,8.50840169879939,133.393630108704));
#67669=CARTESIAN_POINT('Ctrl Pts',(81.5816331484603,8.47640584367857,133.391356389004));
#67670=CARTESIAN_POINT('Ctrl Pts',(81.5776343069374,8.46447757704711,133.390510081107));
#67671=CARTESIAN_POINT('Ctrl Pts',(81.5702821479644,8.443343980226,133.389012723388));
#67672=CARTESIAN_POINT('Ctrl Pts',(81.5669820676809,8.43412090056489,133.388359955569));
#67673=CARTESIAN_POINT('Ctrl Pts',(81.559897123907,8.41485720853457,133.386997800567));
#67674=CARTESIAN_POINT('Ctrl Pts',(81.5560962079875,8.4048229472242,133.386288981656));
#67675=CARTESIAN_POINT('Ctrl Pts',(81.5458068996314,8.37843211267489,133.384426150809));
#67676=CARTESIAN_POINT('Ctrl Pts',(81.5391557514839,8.36214012463879,133.383277617252));
#67677=CARTESIAN_POINT('Ctrl Pts',(81.5038164425773,8.27934971206428,133.377443688775));
#67678=CARTESIAN_POINT('Ctrl Pts',(81.4710707443097,8.21466345169506,133.372898514549));
#67679=CARTESIAN_POINT('Ctrl Pts',(81.382636583747,8.06504129781753,133.362166260359));
#67680=CARTESIAN_POINT('Ctrl Pts',(81.3232036310128,7.98266892405917,133.356077249446));
#67681=CARTESIAN_POINT('Ctrl Pts',(81.2216520015338,7.8659960643519,133.346467892483));
#67682=CARTESIAN_POINT('Ctrl Pts',(81.1847418375529,7.82748812570972,133.343100781389));
#67683=CARTESIAN_POINT('Ctrl Pts',(81.137982467524,7.78316986629655,133.338882124724));
#67684=CARTESIAN_POINT('Ctrl Pts',(81.1298349306032,7.77560109283501,133.338148645584));
#67685=CARTESIAN_POINT('Ctrl Pts',(81.1169353792254,7.76385625084447,133.33698867596));
#67686=CARTESIAN_POINT('Ctrl Pts',(81.1122341339775,7.7596245577064,133.336566191956));
#67687=CARTESIAN_POINT('Ctrl Pts',(81.1038106281421,7.75212877017414,133.335809430434));
#67688=CARTESIAN_POINT('Ctrl Pts',(81.1000977552134,7.74885435076932,133.335475929858));
#67689=CARTESIAN_POINT('Ctrl Pts',(81.0910541402644,7.74095007441324,133.334663797175));
#67690=CARTESIAN_POINT('Ctrl Pts',(81.0857085436646,7.73633754278862,133.334183930127));
#67691=CARTESIAN_POINT('Ctrl Pts',(81.0688457511456,7.72197319877986,133.332671173776));
#67692=CARTESIAN_POINT('Ctrl Pts',(81.0572256459197,7.71234413052489,133.331630180348));
#67693=CARTESIAN_POINT('Ctrl Pts',(80.9950755335242,7.66225143474915,133.326077067913));
#67694=CARTESIAN_POINT('Ctrl Pts',(80.9423541323211,7.62460421608266,133.321418823345));
#67695=CARTESIAN_POINT('Ctrl Pts',(80.7930096781042,7.53058499202765,133.308610104847));
#67696=CARTESIAN_POINT('Ctrl Pts',(80.692673764837,7.48070636574628,133.300432383108));
#67697=CARTESIAN_POINT('Ctrl Pts',(80.5435792296822,7.42445530223334,133.289194010673));
#67698=CARTESIAN_POINT('Ctrl Pts',(80.4983636167282,7.40957428498924,133.285892949317));
#67699=CARTESIAN_POINT('Ctrl Pts',(80.4371689976208,7.39230123550686,133.281565046485));
#67700=CARTESIAN_POINT('Ctrl Pts',(80.4217068877066,7.38817638008139,133.280483087125));
#67701=CARTESIAN_POINT('Ctrl Pts',(80.396111129377,7.38174170220755,133.278710484611));
#67702=CARTESIAN_POINT('Ctrl Pts',(80.3860113234091,7.37930286239629,133.278015732056));
#67703=CARTESIAN_POINT('Ctrl Pts',(80.3662143577409,7.37471797324053,133.276662841383));
#67704=CARTESIAN_POINT('Ctrl Pts',(80.3565195384294,7.37256384201751,133.276004469798));
#67705=CARTESIAN_POINT('Ctrl Pts',(80.3334367970526,7.36765116167709,133.274446466998));
#67706=CARTESIAN_POINT('Ctrl Pts',(80.320032911397,7.36497040343789,133.273549343527));
#67707=CARTESIAN_POINT('Ctrl Pts',(80.273883789589,7.35632991367169,133.270485152579));
#67708=CARTESIAN_POINT('Ctrl Pts',(80.2409925708943,7.35118633459383,133.268343755974));
#67709=CARTESIAN_POINT('Ctrl Pts',(80.1594722961909,7.34092990068269,133.263121066018));
#67710=CARTESIAN_POINT('Ctrl Pts',(80.1107298446527,7.33696529155995,133.260072534283));
#67711=CARTESIAN_POINT('Ctrl Pts',(79.994797432476,7.3326562114703,133.252912883531));
#67712=CARTESIAN_POINT('Ctrl Pts',(79.9276247423833,7.33421959505197,133.2488379159));
#67713=CARTESIAN_POINT('Ctrl Pts',(79.8475185863583,7.34093967521996,133.243916685164));
#67714=CARTESIAN_POINT('Ctrl Pts',(79.834321991487,7.34220552101315,133.243103843953));
#67715=CARTESIAN_POINT('Ctrl Pts',(79.7494057928624,7.3513749262557,133.23785260614));
#67716=CARTESIAN_POINT('Ctrl Pts',(79.6782573197369,7.36377229963186,133.233358685601));
#67717=CARTESIAN_POINT('Ctrl Pts',(79.596880594906,7.3834650976776,133.227882121798));
#67718=CARTESIAN_POINT('Ctrl Pts',(79.5856441738791,7.38630871102959,133.227118283983));
#67719=CARTESIAN_POINT('Ctrl Pts',(79.5682214248156,7.39091186844713,133.225920686043));
#67720=CARTESIAN_POINT('Ctrl Pts',(79.5620138161878,7.3925904528052,133.225491364874));
#67721=CARTESIAN_POINT('Ctrl Pts',(79.5505800575376,7.39575337596857,133.224695484106));
#67722=CARTESIAN_POINT('Ctrl Pts',(79.5453512593809,7.39722739137678,133.224329512885));
#67723=CARTESIAN_POINT('Ctrl Pts',(79.5332174538534,7.40071210346732,133.223475629999));
#67724=CARTESIAN_POINT('Ctrl Pts',(79.5263181941017,7.40274195467925,133.222986646803));
#67725=CARTESIAN_POINT('Ctrl Pts',(79.5042997382551,7.40937526951419,133.221415464369));
#67726=CARTESIAN_POINT('Ctrl Pts',(79.4892333363723,7.41414907614173,133.220324279785));
#67727=CARTESIAN_POINT('Ctrl Pts',(79.4062442277734,7.44174951580364,133.214232923631));
#67728=CARTESIAN_POINT('Ctrl Pts',(79.3397868037485,7.46872373334628,133.209056317954));
#67729=CARTESIAN_POINT('Ctrl Pts',(79.1566026461127,7.55722206374598,133.194265949274));
#67730=CARTESIAN_POINT('Ctrl Pts',(79.0451257459542,7.62844818435537,133.18466760681));
#67731=CARTESIAN_POINT('Ctrl Pts',(78.9220022433216,7.72947695119266,133.173657076169));
#67732=CARTESIAN_POINT('Ctrl Pts',(78.9012348759895,7.74739338269677,133.171781552192));
#67733=CARTESIAN_POINT('Ctrl Pts',(78.8716170469183,7.77424898564333,133.169077864142));
#67734=CARTESIAN_POINT('Ctrl Pts',(78.8624113398681,7.78278773694922,133.168233252829));
#67735=CARTESIAN_POINT('Ctrl Pts',(78.8461994172958,7.79816968845228,133.166737825009));
#67736=CARTESIAN_POINT('Ctrl Pts',(78.8391554475851,7.80497204444058,133.166085305943));
#67737=CARTESIAN_POINT('Ctrl Pts',(78.8291895817662,7.81476734387068,133.165157971275));
#67738=CARTESIAN_POINT('Ctrl Pts',(78.8262184568082,7.81770969131757,133.164880970341));
#67739=CARTESIAN_POINT('Ctrl Pts',(78.8231266848953,7.82079465960108,133.164592150359));
#67740=CARTESIAN_POINT('Ctrl Pts',(78.8229949739282,7.82092612477736,133.164579845402));
#67741=CARTESIAN_POINT('Ctrl Pts',(78.8225491598063,7.82137125608858,133.16453819201));
#67742=CARTESIAN_POINT('Ctrl Pts',(78.8222351597612,7.82168502591829,133.164508848104));
#67743=CARTESIAN_POINT('Ctrl Pts',(78.8216202401235,7.82229998608254,133.164451370525));
#67744=CARTESIAN_POINT('Ctrl Pts',(78.8213193105538,7.8226011663013,133.164423236417));
#67745=CARTESIAN_POINT('Ctrl Pts',(78.8207286263011,7.82319279595478,133.164368001706));
#67746=CARTESIAN_POINT('Ctrl Pts',(78.8204388634105,7.82348323710768,133.164340900744));
#67747=CARTESIAN_POINT('Ctrl Pts',(78.8198688482503,7.82405500878748,133.16428757784));
#67748=CARTESIAN_POINT('Ctrl Pts',(78.8195885891986,7.82433633256011,133.1642613556));
#67749=CARTESIAN_POINT('Ctrl Pts',(78.8190361133961,7.82489130395431,133.164209653719));
#67750=CARTESIAN_POINT('Ctrl Pts',(78.8187638911407,7.82516494599789,133.164184173839));
#67751=CARTESIAN_POINT('Ctrl Pts',(78.8103067761803,7.83367208039258,133.163392444313));
#67752=CARTESIAN_POINT('Ctrl Pts',(78.8022079079764,7.84199097652383,133.162629964288));
#67753=CARTESIAN_POINT('Ctrl Pts',(78.7745942068553,7.87095455071802,133.16001441712));
#67754=CARTESIAN_POINT('Ctrl Pts',(78.7555201524743,7.89201396843054,133.158180071095));
#67755=CARTESIAN_POINT('Ctrl Pts',(78.7111292342008,7.94361886288451,133.153831508313));
#67756=CARTESIAN_POINT('Ctrl Pts',(78.6863461381593,7.97460114388211,133.151337370668));
#67757=CARTESIAN_POINT('Ctrl Pts',(78.6103912907225,8.0768346359254,133.143414767314));
#67758=CARTESIAN_POINT('Ctrl Pts',(78.5637312761252,8.15124842426908,133.138110163814));
#67759=CARTESIAN_POINT('Ctrl Pts',(78.4858206463559,8.30048486186269,133.1277908407));
#67760=CARTESIAN_POINT('Ctrl Pts',(78.4537418747022,8.3745858561639,133.122797735055));
#67761=CARTESIAN_POINT('Ctrl Pts',(78.4233197365001,8.46169631532066,133.116762967672));
#67762=CARTESIAN_POINT('Ctrl Pts',(78.4195970652688,8.47272582514927,133.115995892229));
#67763=CARTESIAN_POINT('Ctrl Pts',(78.4139944305792,8.48991781992767,133.11479428497));
#67764=CARTESIAN_POINT('Ctrl Pts',(78.4120340360187,8.4960539806568,133.114364239368));
#67765=CARTESIAN_POINT('Ctrl Pts',(78.4084708698339,8.50743417084807,133.113564244413));
#67766=CARTESIAN_POINT('Ctrl Pts',(78.4068583423584,8.51267493013052,133.113194862411));
#67767=CARTESIAN_POINT('Ctrl Pts',(78.4031865025385,8.52482152306541,133.112336540812));
#67768=CARTESIAN_POINT('Ctrl Pts',(78.4011461048203,8.53173282449425,133.111846547559));
#67769=CARTESIAN_POINT('Ctrl Pts',(78.3947518778829,8.55392064054761,133.110268800813));
#67770=CARTESIAN_POINT('Ctrl Pts',(78.3905718240015,8.56924574432102,133.109171960131));
#67771=CARTESIAN_POINT('Ctrl Pts',(78.3517969808658,8.71985486158714,133.0983387757));
#67772=CARTESIAN_POINT('Ctrl Pts',(78.3341234680228,8.85891102740731,133.087968181546));
#67773=CARTESIAN_POINT('Ctrl Pts',(78.3340006446003,8.99853445987493,133.077925722171));
#67774=CARTESIAN_POINT('Ctrl Pts',(78.334000643305,8.99853593313598,133.077925616206));
#67775=CARTESIAN_POINT('Ctrl Pts',(78.3339316737719,9.07701813953855,133.072280759997));
#67776=CARTESIAN_POINT('Ctrl Pts',(78.3394083941732,9.15541856497152,133.066746213697));
#67777=CARTESIAN_POINT('Ctrl Pts',(78.3522801515502,9.24648871189249,133.060461213954));
#67778=CARTESIAN_POINT('Ctrl Pts',(78.354326636417,9.25980104488598,133.059545931238));
#67779=CARTESIAN_POINT('Ctrl Pts',(78.3581585251793,9.28286170761914,133.057966092966));
#67780=CARTESIAN_POINT('Ctrl Pts',(78.3598698652317,9.29262146617993,133.057299246906));
#67781=CARTESIAN_POINT('Ctrl Pts',(78.3634800552974,9.31218285113474,133.055966075389));
#67782=CARTESIAN_POINT('Ctrl Pts',(78.3653801422347,9.32198383503753,133.055299819179));
#67783=CARTESIAN_POINT('Ctrl Pts',(78.3694200787876,9.34186442003407,133.053951612522));
#67784=CARTESIAN_POINT('Ctrl Pts',(78.3715655716086,9.3519424408267,133.053269873584));
#67785=CARTESIAN_POINT('Ctrl Pts',(78.3771917656863,9.37721672002002,133.051564068158));
#67786=CARTESIAN_POINT('Ctrl Pts',(78.3807925684521,9.39238544805761,133.050543871151));
#67787=CARTESIAN_POINT('Ctrl Pts',(78.3953380363042,9.45004571296821,133.046677012386));
#67788=CARTESIAN_POINT('Ctrl Pts',(78.4077473246361,9.49215149384497,133.043877153545));
#67789=CARTESIAN_POINT('Ctrl Pts',(78.4265388761537,9.54771743668607,133.04018773218));
#67790=CARTESIAN_POINT('Ctrl Pts',(78.4314573090839,9.56164754784783,133.039263215163));
#67791=CARTESIAN_POINT('Ctrl Pts',(78.4365593647824,9.57550793230875,133.038342764662));
#67792=CARTESIAN_POINT('',(78.3340000765189,9.00050493656018,133.272970309233));
#67793=CARTESIAN_POINT('Ctrl Pts',(78.4365593737642,9.57550795670914,133.231048988662));
#67794=CARTESIAN_POINT('Ctrl Pts',(78.436461916935,9.57524320282636,133.231069156205));
#67795=CARTESIAN_POINT('Ctrl Pts',(78.4363645272696,9.57497842395342,133.23108932565));
#67796=CARTESIAN_POINT('Ctrl Pts',(78.407498131545,9.49643612376326,133.237072257336));
#67797=CARTESIAN_POINT('Ctrl Pts',(78.3846480814157,9.41611127630672,133.243182772986));
#67798=CARTESIAN_POINT('Ctrl Pts',(78.3513888497726,9.25379191329365,133.255206136156));
#67799=CARTESIAN_POINT('Ctrl Pts',(78.3408639956099,9.17204636037335,133.261103741288));
#67800=CARTESIAN_POINT('Ctrl Pts',(78.334817626086,9.06009551836616,133.26889834066));
#67801=CARTESIAN_POINT('Ctrl Pts',(78.3340091080431,9.03030376633059,133.270946591912));
#67802=CARTESIAN_POINT('Ctrl Pts',(78.3340000765189,9.00050493656018,133.272970309233));
#67803=CARTESIAN_POINT('Ctrl Pts',(78.3340000762184,9.0005039440939,133.272970376634));
#67804=CARTESIAN_POINT('Ctrl Pts',(78.3339976906018,8.99261728163465,133.273505980588));
#67805=CARTESIAN_POINT('Ctrl Pts',(78.3340513068531,8.98473055887474,133.274039846394));
#67806=CARTESIAN_POINT('Ctrl Pts',(78.3342826460377,8.96808778940267,133.275162829666));
#67807=CARTESIAN_POINT('Ctrl Pts',(78.3344734091631,8.95933216535589,133.275751521671));
#67808=CARTESIAN_POINT('Ctrl Pts',(78.3350069258589,8.9413552901423,133.276956035385));
#67809=CARTESIAN_POINT('Ctrl Pts',(78.3353572678109,8.93213455223497,133.277571598656));
#67810=CARTESIAN_POINT('Ctrl Pts',(78.3362616313914,8.91260940516593,133.278870483235));
#67811=CARTESIAN_POINT('Ctrl Pts',(78.3368348210835,8.90230623868865,133.279553178857));
#67812=CARTESIAN_POINT('Ctrl Pts',(78.3385195583362,8.87637013403552,133.281265291819));
#67813=CARTESIAN_POINT('Ctrl Pts',(78.3397560479465,8.8607460991998,133.282290776303));
#67814=CARTESIAN_POINT('Ctrl Pts',(78.3453906963644,8.80038986588423,133.286231969989));
#67815=CARTESIAN_POINT('Ctrl Pts',(78.3513780475261,8.7558230969127,133.289098279209));
#67816=CARTESIAN_POINT('Ctrl Pts',(78.3747357773466,8.6229534732413,133.29757661396));
#67817=CARTESIAN_POINT('Ctrl Pts',(78.397460520862,8.53576261080013,133.303042613918));
#67818=CARTESIAN_POINT('Ctrl Pts',(78.4582638678523,8.36161531908081,133.314314205));
#67819=CARTESIAN_POINT('Ctrl Pts',(78.4969421837066,8.27522597289918,133.320105329415));
#67820=CARTESIAN_POINT('Ctrl Pts',(78.5486304022539,8.181934737297,133.327074563826));
#67821=CARTESIAN_POINT('Ctrl Pts',(78.5546524440025,8.17134150318087,133.327877037898));
#67822=CARTESIAN_POINT('Ctrl Pts',(78.5640565095659,8.15521343058383,133.329117435649));
#67823=CARTESIAN_POINT('Ctrl Pts',(78.5673557102706,8.14963043849194,133.329550287636));
#67824=CARTESIAN_POINT('Ctrl Pts',(78.5735008530715,8.13936873575705,133.330352574247));
#67825=CARTESIAN_POINT('Ctrl Pts',(78.5763373699455,8.13468462286057,133.33072140944));
#67826=CARTESIAN_POINT('Ctrl Pts',(78.5828633261871,8.12402685924504,133.331566579186));
#67827=CARTESIAN_POINT('Ctrl Pts',(78.586567468122,8.11806249147503,133.332043840979));
#67828=CARTESIAN_POINT('Ctrl Pts',(78.5984572801371,8.0991849465474,133.333567619908));
#67829=CARTESIAN_POINT('Ctrl Pts',(78.6067827912849,8.08636138206777,133.334622530965));
#67830=CARTESIAN_POINT('Ctrl Pts',(78.6718552790283,7.98908990652449,133.342766654373));
#67831=CARTESIAN_POINT('Ctrl Pts',(78.7360499709074,7.90989242480569,133.350213830109));
#67832=CARTESIAN_POINT('Ctrl Pts',(78.8877362334637,7.75429427524032,133.366018514977));
#67833=CARTESIAN_POINT('Ctrl Pts',(78.9768190667109,7.68014256855238,133.374308265934));
#67834=CARTESIAN_POINT('Ctrl Pts',(79.0889714252201,7.60502396866075,133.383544518744));
#67835=CARTESIAN_POINT('Ctrl Pts',(79.1052522183433,7.59452582583626,133.384859482924));
#67836=CARTESIAN_POINT('Ctrl Pts',(79.1311511046681,7.57845824542435,133.386911916442));
#67837=CARTESIAN_POINT('Ctrl Pts',(79.1406477113292,7.57269729306556,133.387656374132));
#67838=CARTESIAN_POINT('Ctrl Pts',(79.1585629022349,7.56207298066403,133.389045905185));
#67839=CARTESIAN_POINT('Ctrl Pts',(79.1669677696563,7.55718753384629,133.389691760503));
#67840=CARTESIAN_POINT('Ctrl Pts',(79.185957562513,7.54637070897763,133.391137755132));
#67841=CARTESIAN_POINT('Ctrl Pts',(79.1965655630021,7.54048079005655,133.391936383075));
#67842=CARTESIAN_POINT('Ctrl Pts',(79.2280194530625,7.52346339045191,133.394278483317));
#67843=CARTESIAN_POINT('Ctrl Pts',(79.2490393430912,7.51266261193098,133.39581045891));
#67844=CARTESIAN_POINT('Ctrl Pts',(79.3674336652126,7.45497744089553,133.404270765032));
#67845=CARTESIAN_POINT('Ctrl Pts',(79.4689628593109,7.41720564843457,133.410878524406));
#67846=CARTESIAN_POINT('Ctrl Pts',(79.6460681417884,7.37029686375471,133.422065944804));
#67847=CARTESIAN_POINT('Ctrl Pts',(79.7199038650213,7.35599737471142,133.426643271146));
#67848=CARTESIAN_POINT('Ctrl Pts',(79.829951825236,7.34231494403922,133.433643316259));
#67849=CARTESIAN_POINT('Ctrl Pts',(79.8655873782694,7.33904577276688,133.435937755948));
#67850=CARTESIAN_POINT('Ctrl Pts',(79.91098881767,7.33635121984644,133.438927283502));
#67851=CARTESIAN_POINT('Ctrl Pts',(79.9206847846028,7.33586078114829,133.439569566155));
#67852=CARTESIAN_POINT('Ctrl Pts',(79.9363299482605,7.33520645774564,133.440612924074));
#67853=CARTESIAN_POINT('Ctrl Pts',(79.9422768741108,7.33498965415705,133.441011144881));
#67854=CARTESIAN_POINT('Ctrl Pts',(79.9537971150287,7.33463145968591,133.441785941147));
#67855=CARTESIAN_POINT('Ctrl Pts',(79.9593701742531,7.33448617677437,133.442162301269));
#67856=CARTESIAN_POINT('Ctrl Pts',(79.971828684925,7.33422396438118,133.443006954968));
#67857=CARTESIAN_POINT('Ctrl Pts',(79.9787143388054,7.33412175105805,133.443476036851));
#67858=CARTESIAN_POINT('Ctrl Pts',(79.9992891360013,7.33394391043794,133.444884026227));
#67859=CARTESIAN_POINT('Ctrl Pts',(80.0129784042471,7.33399431859728,133.445829204494));
#67860=CARTESIAN_POINT('Ctrl Pts',(80.1294256411956,7.33585833849934,133.4539321431));
#67861=CARTESIAN_POINT('Ctrl Pts',(80.2318047428464,7.3470082965904,133.461457592154));
#67862=CARTESIAN_POINT('Ctrl Pts',(80.4448668856639,7.39040352061597,133.477270424917));
#67863=CARTESIAN_POINT('Ctrl Pts',(80.5545948611097,7.42483615666219,133.485492956991));
#67864=CARTESIAN_POINT('Ctrl Pts',(80.6777392382939,7.47796133305972,133.49467001486));
#67865=CARTESIAN_POINT('Ctrl Pts',(80.6954131319735,7.48595481909441,133.495986743098));
#67866=CARTESIAN_POINT('Ctrl Pts',(80.7229874500541,7.49901078287701,133.498041289588));
#67867=CARTESIAN_POINT('Ctrl Pts',(80.7329831997019,7.50386660949968,133.498786120209));
#67868=CARTESIAN_POINT('Ctrl Pts',(80.751630419617,7.51315696763973,133.500175988367));
#67869=CARTESIAN_POINT('Ctrl Pts',(80.7602930577058,7.51756788896651,133.500821811555));
#67870=CARTESIAN_POINT('Ctrl Pts',(80.7796731770337,7.52765060040558,133.502267271415));
#67871=CARTESIAN_POINT('Ctrl Pts',(80.7903684174145,7.53336412317115,133.503065401678));
#67872=CARTESIAN_POINT('Ctrl Pts',(80.8216861517258,7.55053650848381,133.505404572047));
#67873=CARTESIAN_POINT('Ctrl Pts',(80.8421292587959,7.56231750854899,133.506934159587));
#67874=CARTESIAN_POINT('Ctrl Pts',(80.9502247758351,7.62770818984177,133.515050247536));
#67875=CARTESIAN_POINT('Ctrl Pts',(81.0330295487542,7.6889068623411,133.521350881295));
#67876=CARTESIAN_POINT('Ctrl Pts',(81.1688136589222,7.81016101826928,133.532469075745));
#67877=CARTESIAN_POINT('Ctrl Pts',(81.2241022440341,7.8671213138598,133.537288054666));
#67878=CARTESIAN_POINT('Ctrl Pts',(81.2910637399378,7.94675547761684,133.543848463834));
#67879=CARTESIAN_POINT('Ctrl Pts',(81.3065802203259,7.96606692551881,133.545427393132));
#67880=CARTESIAN_POINT('Ctrl Pts',(81.3321413301288,7.99937425055244,133.548144449112));
#67881=CARTESIAN_POINT('Ctrl Pts',(81.3424102336148,8.01319347291886,133.549270027772));
#67882=CARTESIAN_POINT('Ctrl Pts',(81.3568066038894,8.03320778833813,133.550901713761));
#67883=CARTESIAN_POINT('Ctrl Pts',(81.3611099608627,8.03927578874542,133.551396608904));
#67884=CARTESIAN_POINT('Ctrl Pts',(81.3685284940726,8.04988627106338,133.552262709149));
#67885=CARTESIAN_POINT('Ctrl Pts',(81.3716620131375,8.0544157056535,133.55263267084));
#67886=CARTESIAN_POINT('Ctrl Pts',(81.3783286277925,8.0641550254371,133.553428804293));
#67887=CARTESIAN_POINT('Ctrl Pts',(81.3818546168129,8.06936933356374,133.553855397039));
#67888=CARTESIAN_POINT('Ctrl Pts',(81.391455070299,8.08374154619191,133.555031906416));
#67889=CARTESIAN_POINT('Ctrl Pts',(81.3974684746196,8.09293957578421,133.555785620058));
#67890=CARTESIAN_POINT('Ctrl Pts',(81.4311433328127,8.14557798363366,133.5601002991));
#67891=CARTESIAN_POINT('Ctrl Pts',(81.4568672269784,8.1902191553164,133.563763837486));
#67892=CARTESIAN_POINT('Ctrl Pts',(81.5245100564812,8.32129316163141,133.574392839356));
#67893=CARTESIAN_POINT('Ctrl Pts',(81.5610830164513,8.41025873016334,133.581444794114));
#67894=CARTESIAN_POINT('Ctrl Pts',(81.605515542038,8.55206932932379,133.592131964013));
#67895=CARTESIAN_POINT('Ctrl Pts',(81.6188562365306,8.60297680582893,133.595867200292));
#67896=CARTESIAN_POINT('Ctrl Pts',(81.63471145473,8.67775367372426,133.601194518558));
#67897=CARTESIAN_POINT('Ctrl Pts',(81.6391550674477,8.70117731183862,133.602841254199));
#67898=CARTESIAN_POINT('Ctrl Pts',(81.6463013028563,8.74382709388512,133.605800365489));
#67899=CARTESIAN_POINT('Ctrl Pts',(81.6491734675297,8.76302011298758,133.607117734688));
#67900=CARTESIAN_POINT('Ctrl Pts',(81.6531623562786,8.7932785685513,133.609173048873));
#67901=CARTESIAN_POINT('Ctrl Pts',(81.6545046780016,8.80431196440993,133.609918014963));
#67902=CARTESIAN_POINT('Ctrl Pts',(81.6568138218278,8.82501872640462,133.611308005724));
#67903=CARTESIAN_POINT('Ctrl Pts',(81.6578065795981,8.83468866404034,133.611953817388));
#67904=CARTESIAN_POINT('Ctrl Pts',(81.6598470942018,8.85643617030607,133.613399083718));
#67905=CARTESIAN_POINT('Ctrl Pts',(81.6608477843686,8.86851768388437,133.61419703377));
#67906=CARTESIAN_POINT('Ctrl Pts',(81.663406183093,8.9041262700719,133.616535143697));
#67907=CARTESIAN_POINT('Ctrl Pts',(81.6645964743734,8.92767732745032,133.618063866961));
#67908=CARTESIAN_POINT('Ctrl Pts',(81.6683370307246,9.05544504806204,133.626275643631));
#67909=CARTESIAN_POINT('Ctrl Pts',(81.6616018430605,9.15970381562065,133.632663200137));
#67910=CARTESIAN_POINT('Ctrl Pts',(81.632845300703,9.33982027825646,133.643802078366));
#67911=CARTESIAN_POINT('Ctrl Pts',(81.6151137661839,9.41601371610997,133.6485544592));
#67912=CARTESIAN_POINT('Ctrl Pts',(81.584863594433,9.51416693766071,133.655032520303));
#67913=CARTESIAN_POINT('Ctrl Pts',(81.5771051039896,9.53749382917846,133.65659978726));
#67914=CARTESIAN_POINT('Ctrl Pts',(81.5630729797701,9.57675984626653,133.659298718012));
#67915=CARTESIAN_POINT('Ctrl Pts',(81.5570642676673,9.59278990453277,133.66041805248));
#67916=CARTESIAN_POINT('Ctrl Pts',(81.5480979086607,9.61563297300678,133.662042265941));
#67917=CARTESIAN_POINT('Ctrl Pts',(81.5453398245459,9.62252382582609,133.66253607295));
#67918=CARTESIAN_POINT('Ctrl Pts',(81.5404558248239,9.63449362926699,133.663400946802));
#67919=CARTESIAN_POINT('Ctrl Pts',(81.5383506316102,9.63958083696979,133.663770781289));
#67920=CARTESIAN_POINT('Ctrl Pts',(81.5337808304227,9.65047068038874,133.664567439537));
#67921=CARTESIAN_POINT('Ctrl Pts',(81.5313085340496,9.65626969460908,133.664994691331));
#67922=CARTESIAN_POINT('Ctrl Pts',(81.5244197079475,9.6721772405201,133.666174749137));
#67923=CARTESIAN_POINT('Ctrl Pts',(81.5199356908112,9.68225594037223,133.666931388306));
#67924=CARTESIAN_POINT('Ctrl Pts',(81.4936353726453,9.73982473044721,133.671301950198));
#67925=CARTESIAN_POINT('Ctrl Pts',(81.4696960734452,9.78630756238536,133.675021462593));
#67926=CARTESIAN_POINT('Ctrl Pts',(81.3925518833272,9.92022858523847,133.686163104619));
#67927=CARTESIAN_POINT('Ctrl Pts',(81.3334282287822,10.0039882219303,133.693682715429));
#67928=CARTESIAN_POINT('Ctrl Pts',(81.2198088715287,10.137058927403,133.706224759534));
#67929=CARTESIAN_POINT('Ctrl Pts',(81.1690523623575,10.1891828613474,133.711330843185));
#67930=CARTESIAN_POINT('Ctrl Pts',(81.1019642253685,10.249616292301,133.717492787095));
#67931=CARTESIAN_POINT('Ctrl Pts',(81.0886953332371,10.2611933018708,133.718685747098));
#67932=CARTESIAN_POINT('Ctrl Pts',(81.0670487487982,10.2794835309093,133.720591701858));
#67933=CARTESIAN_POINT('Ctrl Pts',(81.0587856766769,10.2863296771672,133.721310105985));
#67934=CARTESIAN_POINT('Ctrl Pts',(81.0428569413904,10.2992695160165,133.722677877021));
#67935=CARTESIAN_POINT('Ctrl Pts',(81.0352025995274,10.3053763673253,133.723327756611));
#67936=CARTESIAN_POINT('Ctrl Pts',(81.0176007656893,10.3191674132863,133.724805753231));
#67937=CARTESIAN_POINT('Ctrl Pts',(81.0076191828995,10.3268072879126,133.725632095427));
#67938=CARTESIAN_POINT('Ctrl Pts',(80.9807273846552,10.3469116774754,133.727827989257));
#67939=CARTESIAN_POINT('Ctrl Pts',(80.9636659512391,10.3591708014653,133.729189642396));
#67940=CARTESIAN_POINT('Ctrl Pts',(80.8469854273796,10.4397071305131,133.738304247379));
#67941=CARTESIAN_POINT('Ctrl Pts',(80.7404283258063,10.4973011311402,133.745639610053));
#67942=CARTESIAN_POINT('Ctrl Pts',(80.5671851459957,10.5678809492911,133.757070391546));
#67943=CARTESIAN_POINT('Ctrl Pts',(80.5043657798887,10.5892021750872,133.761131682327));
#67944=CARTESIAN_POINT('Ctrl Pts',(80.4187903515136,10.6126608373729,133.766747645376));
#67945=CARTESIAN_POINT('Ctrl Pts',(80.3970152165322,10.6181591862726,133.768183883208));
#67946=CARTESIAN_POINT('Ctrl Pts',(80.3595441017168,10.62681902944,133.77067807578));
#67947=CARTESIAN_POINT('Ctrl Pts',(80.343901062721,10.6301975734692,133.771726024234));
#67948=CARTESIAN_POINT('Ctrl Pts',(80.3211276038736,10.6347737716873,133.773264567756));
#67949=CARTESIAN_POINT('Ctrl Pts',(80.3140336848583,10.6361512957294,133.773745633039));
#67950=CARTESIAN_POINT('Ctrl Pts',(80.3015893065327,10.6384838810663,133.774593059245));
#67951=CARTESIAN_POINT('Ctrl Pts',(80.2962427951625,10.6394589788814,133.774958290382));
#67952=CARTESIAN_POINT('Ctrl Pts',(80.2845856993941,10.6415261170223,133.775757207788));
#67953=CARTESIAN_POINT('Ctrl Pts',(80.2782736606913,10.6426079201925,133.776191425318));
#67954=CARTESIAN_POINT('Ctrl Pts',(80.2606330000671,10.6455267095962,133.777409192905));
#67955=CARTESIAN_POINT('Ctrl Pts',(80.2492916556214,10.6472830251457,133.778196969373));
#67956=CARTESIAN_POINT('Ctrl Pts',(80.1727704439156,10.6583247589852,133.783540864829));
#67957=CARTESIAN_POINT('Ctrl Pts',(80.1071142619588,10.6638555325745,133.788263817613));
#67958=CARTESIAN_POINT('Ctrl Pts',(80.0205159427081,10.666003543698,133.794543326326));
#67959=CARTESIAN_POINT('Ctrl Pts',(79.9997129860433,10.6661298304552,133.796055813938));
#67960=CARTESIAN_POINT('Ctrl Pts',(79.9107607700668,10.6650038671956,133.802529662383));
#67961=CARTESIAN_POINT('Ctrl Pts',(79.8427218693291,10.6599596401399,133.807494384476));
#67962=CARTESIAN_POINT('Ctrl Pts',(79.7041211212561,10.6410834274608,133.817515485007));
#67963=CARTESIAN_POINT('Ctrl Pts',(79.6337528996968,10.6268265761426,133.82255224343));
#67964=CARTESIAN_POINT('Ctrl Pts',(79.5475739026474,10.6034882697754,133.828644654542));
#67965=CARTESIAN_POINT('Ctrl Pts',(79.5307070329419,10.598633215237,133.829833626625));
#67966=CARTESIAN_POINT('Ctrl Pts',(79.5036679138261,10.5903852781821,133.831734785228));
#67967=CARTESIAN_POINT('Ctrl Pts',(79.4934465879558,10.5871592619694,133.832452332212));
#67968=CARTESIAN_POINT('Ctrl Pts',(79.473944928724,10.5807966361743,133.833819460409));
#67969=CARTESIAN_POINT('Ctrl Pts',(79.4646597712293,10.5776763893161,133.834469544958));
#67970=CARTESIAN_POINT('Ctrl Pts',(79.4435003638077,10.5703575275151,133.835949359433));
#67971=CARTESIAN_POINT('Ctrl Pts',(79.4316450288256,10.5661057596879,133.836777298828));
#67972=CARTESIAN_POINT('Ctrl Pts',(79.4000644477015,10.5543739317494,133.838980466862));
#67973=CARTESIAN_POINT('Ctrl Pts',(79.3804307589017,10.5466528395429,133.840347711874));
#67974=CARTESIAN_POINT('Ctrl Pts',(79.2509904481143,10.4928889183974,133.849357420134));
#67975=CARTESIAN_POINT('Ctrl Pts',(79.1462430747107,10.4355610645967,133.856595880305));
#67976=CARTESIAN_POINT('Ctrl Pts',(78.9699041148057,10.3128689198404,133.869720206282));
#67977=CARTESIAN_POINT('Ctrl Pts',(78.8961850138629,10.2515229050092,133.875580330368));
#67978=CARTESIAN_POINT('Ctrl Pts',(78.8192428280163,10.175383162731,133.882648386722));
#67979=CARTESIAN_POINT('Ctrl Pts',(78.8104343491552,10.166467581056,133.883473288501));
#67980=CARTESIAN_POINT('Ctrl Pts',(78.7971720486753,10.1527375744529,133.88474115286));
#67981=CARTESIAN_POINT('Ctrl Pts',(78.7926444570711,10.1479945929044,133.885178690297));
#67982=CARTESIAN_POINT('Ctrl Pts',(78.7843920613262,10.1392467913437,133.885985145762));
#67983=CARTESIAN_POINT('Ctrl Pts',(78.7806588340017,10.1352502059921,133.886353413212));
#67984=CARTESIAN_POINT('Ctrl Pts',(78.7721628194211,10.1260645927159,133.887199406111));
#67985=CARTESIAN_POINT('Ctrl Pts',(78.7674132319093,10.1208637132067,133.887678076848));
#67986=CARTESIAN_POINT('Ctrl Pts',(78.7526487673841,10.1044890467979,133.889183682213));
#67987=CARTESIAN_POINT('Ctrl Pts',(78.7427521035009,10.093210336394,133.890218618129));
#67988=CARTESIAN_POINT('Ctrl Pts',(78.6650788248194,10.0022403777949,133.898538900544));
#67989=CARTESIAN_POINT('Ctrl Pts',(78.6047986749672,9.91646607616967,133.906204482806));
#67990=CARTESIAN_POINT('Ctrl Pts',(78.5073026724441,9.74558706254934,133.920508699118));
#67991=CARTESIAN_POINT('Ctrl Pts',(78.4683717547555,9.66193031557139,133.927135282778));
#67992=CARTESIAN_POINT('Ctrl Pts',(78.4365594251401,9.5755080962782,133.933539779158));
#67993=CARTESIAN_POINT('Origin',(80.,9.,134.));
#67994=CARTESIAN_POINT('',(78.4365593788086,9.57550797041272,134.632696244622));
#67995=CARTESIAN_POINT('',(78.4365593695155,9.57550794516687,134.440654960983));
#67996=CARTESIAN_POINT('',(78.4365593737638,9.57550795670799,134.));
#67997=CARTESIAN_POINT('Ctrl Pts',(78.4365593695155,9.57550794516687,134.440654960983));
#67998=CARTESIAN_POINT('Ctrl Pts',(78.4717534098169,9.67111703800434,134.433522190505));
#67999=CARTESIAN_POINT('Ctrl Pts',(78.5156454552651,9.76330196577179,134.426050259462));
#68000=CARTESIAN_POINT('Ctrl Pts',(78.6055725715436,9.91467496779458,134.413255774226));
#68001=CARTESIAN_POINT('Ctrl Pts',(78.6476779773201,9.97585109071723,134.407912451059));
#68002=CARTESIAN_POINT('Ctrl Pts',(78.7208950245598,10.0683458166058,134.399623746152));
#68003=CARTESIAN_POINT('Ctrl Pts',(78.7494092000487,10.101587755822,134.396595232034));
#68004=CARTESIAN_POINT('Ctrl Pts',(78.7882311734735,10.1433933553685,134.392717792511));
#68005=CARTESIAN_POINT('Ctrl Pts',(78.7973761238583,10.1530081891617,134.391820944744));
#68006=CARTESIAN_POINT('Ctrl Pts',(78.8138136955503,10.1698819958327,134.390237530461));
#68007=CARTESIAN_POINT('Ctrl Pts',(78.8210604278832,10.1771844912938,134.389549030466));
#68008=CARTESIAN_POINT('Ctrl Pts',(78.8353519540154,10.1913216413596,134.388209505794));
#68009=CARTESIAN_POINT('Ctrl Pts',(78.8423904069475,10.1981620763861,134.387558241358));
#68010=CARTESIAN_POINT('Ctrl Pts',(78.8586848634129,10.2137204861971,134.386069439706));
#68011=CARTESIAN_POINT('Ctrl Pts',(78.8679811180378,10.2223955682949,134.385233767959));
#68012=CARTESIAN_POINT('Ctrl Pts',(78.8983105698349,10.2500556642151,134.382550090482));
#68013=CARTESIAN_POINT('Ctrl Pts',(78.9197296884904,10.2686114338002,134.380719977311));
#68014=CARTESIAN_POINT('Ctrl Pts',(79.0426548317125,10.3697315291208,134.370548321813));
#68015=CARTESIAN_POINT('Ctrl Pts',(79.1531340971381,10.4406577670204,134.3626819129));
#68016=CARTESIAN_POINT('Ctrl Pts',(79.3349163426839,10.5291527269294,134.350277274017));
#68017=CARTESIAN_POINT('Ctrl Pts',(79.4009847355871,10.5562206511986,134.345855173336));
#68018=CARTESIAN_POINT('Ctrl Pts',(79.4835238801607,10.584000374267,134.340204787391));
#68019=CARTESIAN_POINT('Ctrl Pts',(79.4985423529536,10.5888187284823,134.339171656379));
#68020=CARTESIAN_POINT('Ctrl Pts',(79.5204991763432,10.5955207920101,134.33765087529));
#68021=CARTESIAN_POINT('Ctrl Pts',(79.52738540625,10.5975741230538,134.337172448045));
#68022=CARTESIAN_POINT('Ctrl Pts',(79.5395001725956,10.6011013139814,134.336327831701));
#68023=CARTESIAN_POINT('Ctrl Pts',(79.5447229565041,10.6025942471699,134.335962744969));
#68024=CARTESIAN_POINT('Ctrl Pts',(79.5561484430879,10.6057998628139,134.335161876589));
#68025=CARTESIAN_POINT('Ctrl Pts',(79.5623536995695,10.6075021356771,134.334725542647));
#68026=CARTESIAN_POINT('Ctrl Pts',(79.5797810505691,10.6121745538988,134.333496551393));
#68027=CARTESIAN_POINT('Ctrl Pts',(79.5910242985964,10.6150633469108,134.33269954875));
#68028=CARTESIAN_POINT('Ctrl Pts',(79.6770221111404,10.6362037307128,134.326576764937));
#68029=CARTESIAN_POINT('Ctrl Pts',(79.7529225796494,10.6493718284977,134.321023978802));
#68030=CARTESIAN_POINT('Ctrl Pts',(79.8863716847609,10.6631051806393,134.311272788271));
#68031=CARTESIAN_POINT('Ctrl Pts',(79.9435573553131,10.666026628933,134.307097168952));
#68032=CARTESIAN_POINT('Ctrl Pts',(80.0835683615011,10.665961027129,134.296979523559));
#68033=CARTESIAN_POINT('Ctrl Pts',(80.1662478239518,10.6597515104948,134.291100279272));
#68034=CARTESIAN_POINT('Ctrl Pts',(80.2707236121087,10.6440153912872,134.283836629884));
#68035=CARTESIAN_POINT('Ctrl Pts',(80.2932420642366,10.6401484879565,134.282280374805));
#68036=CARTESIAN_POINT('Ctrl Pts',(80.3272859169139,10.633578821394,134.279940686102));
#68037=CARTESIAN_POINT('Ctrl Pts',(80.3388730360393,10.6312145521252,134.279146661994));
#68038=CARTESIAN_POINT('Ctrl Pts',(80.3590024547347,10.6268835391473,134.277770999319));
#68039=CARTESIAN_POINT('Ctrl Pts',(80.3675561022312,10.6249724087513,134.277187615218));
#68040=CARTESIAN_POINT('Ctrl Pts',(80.3868119500423,10.6205102742645,134.275876783885));
#68041=CARTESIAN_POINT('Ctrl Pts',(80.3975048341847,10.6179205636449,134.275150604561));
#68042=CARTESIAN_POINT('Ctrl Pts',(80.426462197628,10.6106029639376,134.273188219848));
#68043=CARTESIAN_POINT('Ctrl Pts',(80.4446736378678,10.6056703635157,134.271958618735));
#68044=CARTESIAN_POINT('Ctrl Pts',(80.5580078175167,10.5728973886081,134.264327463464));
#68045=CARTESIAN_POINT('Ctrl Pts',(80.6505763286658,10.53692323142,134.258203402104));
#68046=CARTESIAN_POINT('Ctrl Pts',(80.8035679698344,10.4611505315518,134.247760058908));
#68047=CARTESIAN_POINT('Ctrl Pts',(80.8656108827619,10.425271703696,134.243418208718));
#68048=CARTESIAN_POINT('Ctrl Pts',(80.955803724873,10.3650471629056,134.236683650588));
#68049=CARTESIAN_POINT('Ctrl Pts',(80.985766829958,10.3435690989589,134.234368599642));
#68050=CARTESIAN_POINT('Ctrl Pts',(81.0273755962566,10.3116018045944,134.231003249736));
#68051=CARTESIAN_POINT('Ctrl Pts',(81.039625270246,10.3019136564475,134.229993002769));
#68052=CARTESIAN_POINT('Ctrl Pts',(81.0611431150497,10.2843980711431,134.228179755869));
#68053=CARTESIAN_POINT('Ctrl Pts',(81.0704655439687,10.2766387953932,134.227380910594));
#68054=CARTESIAN_POINT('Ctrl Pts',(81.0846327705929,10.2645828047962,134.226144889673));
#68055=CARTESIAN_POINT('Ctrl Pts',(81.0895388497703,10.2603582857805,134.225712728893));
#68056=CARTESIAN_POINT('Ctrl Pts',(81.0985512418213,10.2525059645829,134.224910922071));
#68057=CARTESIAN_POINT('Ctrl Pts',(81.1026644322755,10.2488863715036,134.224541866833));
#68058=CARTESIAN_POINT('Ctrl Pts',(81.1120218309677,10.2405696318755,134.223695163274));
#68059=CARTESIAN_POINT('Ctrl Pts',(81.1172541714244,10.235859488779,134.22321657594));
#68060=CARTESIAN_POINT('Ctrl Pts',(81.133827277232,10.2207491483756,134.221684661446));
#68061=CARTESIAN_POINT('Ctrl Pts',(81.1450534976661,10.2102252779089,134.220622820074));
#68062=CARTESIAN_POINT('Ctrl Pts',(81.2492013953704,10.1098468775308,134.210555269639));
#68063=CARTESIAN_POINT('Ctrl Pts',(81.3315103269491,10.0096247672927,134.200990320769));
#68064=CARTESIAN_POINT('Ctrl Pts',(81.4498942791623,9.82547168943415,134.1851748068));
#68065=CARTESIAN_POINT('Ctrl Pts',(81.4922220469123,9.74624058084547,134.178822287609));
#68066=CARTESIAN_POINT('Ctrl Pts',(81.5353121423154,9.64707956838064,134.171434710219));
#68067=CARTESIAN_POINT('Ctrl Pts',(81.5423733435618,9.63006337658953,134.170185456192));
#68068=CARTESIAN_POINT('Ctrl Pts',(81.5531637218669,9.60279134563995,134.168211714246));
#68069=CARTESIAN_POINT('Ctrl Pts',(81.5570767196664,9.59261037129318,134.167481109577));
#68070=CARTESIAN_POINT('Ctrl Pts',(81.5642994349045,9.57325249807744,134.166103419677));
#68071=CARTESIAN_POINT('Ctrl Pts',(81.567629063061,9.56408357195772,134.16545569432));
#68072=CARTESIAN_POINT('Ctrl Pts',(81.5750273495003,9.54313907051892,134.163986767324));
#68073=CARTESIAN_POINT('Ctrl Pts',(81.5790448685575,9.53134595013395,134.163167283554));
#68074=CARTESIAN_POINT('Ctrl Pts',(81.5910806614151,9.49467318798527,134.160641522239));
#68075=CARTESIAN_POINT('Ctrl Pts',(81.5986462271919,9.46964837359512,134.158949999286));
#68076=CARTESIAN_POINT('Ctrl Pts',(81.6411775401056,9.31600138516183,134.148736305119));
#68077=CARTESIAN_POINT('Ctrl Pts',(81.6611923991752,9.18374758227627,134.14072090391));
#68078=CARTESIAN_POINT('Ctrl Pts',(81.6674194862762,8.97846918028418,134.128123847904));
#68079=CARTESIAN_POINT('Ctrl Pts',(81.6649268959898,8.90636581012944,134.123658054442));
#68080=CARTESIAN_POINT('Ctrl Pts',(81.6562025417169,8.81889162830616,134.117955261184));
#68081=CARTESIAN_POINT('Ctrl Pts',(81.6544050883785,8.80314761834793,134.116917400582));
#68082=CARTESIAN_POINT('Ctrl Pts',(81.6514648583346,8.78029189447922,134.115390923116));
#68083=CARTESIAN_POINT('Ctrl Pts',(81.6505000343227,8.77315762769281,134.114911626281));
#68084=CARTESIAN_POINT('Ctrl Pts',(81.6487259548289,8.76065036311876,134.114066056469));
#68085=CARTESIAN_POINT('Ctrl Pts',(81.6479366085231,8.75527473396422,134.113700894662));
#68086=CARTESIAN_POINT('Ctrl Pts',(81.6461563682749,8.74355020220027,134.112900574557));
#68087=CARTESIAN_POINT('Ctrl Pts',(81.6451550526002,8.73720324008348,134.112464870509));
#68088=CARTESIAN_POINT('Ctrl Pts',(81.6422483126799,8.71944644920624,134.111239316501));
#68089=CARTESIAN_POINT('Ctrl Pts',(81.640260772931,8.70805070045029,134.110445158203));
#68090=CARTESIAN_POINT('Ctrl Pts',(81.6253827006515,8.62769878644319,134.104795786829));
#68091=CARTESIAN_POINT('Ctrl Pts',(81.6082679814573,8.55960358964008,134.099751553034));
#68092=CARTESIAN_POINT('Ctrl Pts',(81.5821724444974,8.47795678547016,134.09353028303));
#68093=CARTESIAN_POINT('Ctrl Pts',(81.5772210400791,8.46318294905379,134.092397282145));
#68094=CARTESIAN_POINT('Ctrl Pts',(81.5500165615117,8.38563866339634,134.08641730424));
#68095=CARTESIAN_POINT('Ctrl Pts',(81.524220608712,8.32417197039541,134.0815651552));
#68096=CARTESIAN_POINT('Ctrl Pts',(81.4622342756303,8.19820736482847,134.071496195681));
#68097=CARTESIAN_POINT('Ctrl Pts',(81.4252893935586,8.13423248932816,134.066308633628));
#68098=CARTESIAN_POINT('Ctrl Pts',(81.3743818047362,8.0582234247988,134.060064952454));
#68099=CARTESIAN_POINT('Ctrl Pts',(81.3643117476438,8.04369358475773,134.058867228155));
#68100=CARTESIAN_POINT('Ctrl Pts',(81.3477504420116,8.02059189175592,134.056955416699));
#68101=CARTESIAN_POINT('Ctrl Pts',(81.3414043902598,8.01191813720221,134.056235862665));
#68102=CARTESIAN_POINT('Ctrl Pts',(81.3291174349257,7.99546095138826,134.054866992511));
#68103=CARTESIAN_POINT('Ctrl Pts',(81.3231910023655,7.98766733024652,134.05421715313));
#68104=CARTESIAN_POINT('Ctrl Pts',(81.3095146325956,7.97000737072319,134.052740724637));
#68105=CARTESIAN_POINT('Ctrl Pts',(81.3017212023016,7.96017534403954,134.051915894276));
#68106=CARTESIAN_POINT('Ctrl Pts',(81.2806399739871,7.93418821513339,134.049727291466));
#68107=CARTESIAN_POINT('Ctrl Pts',(81.2671574883132,7.91819342487992,134.048371330096));
#68108=CARTESIAN_POINT('Ctrl Pts',(81.1728115718415,7.8104519499025,134.039163307409));
#68109=CARTESIAN_POINT('Ctrl Pts',(81.0823604792179,7.72759629044802,134.031741275172));
#68110=CARTESIAN_POINT('Ctrl Pts',(80.9309654286274,7.6168442623512,134.020277141289));
#68111=CARTESIAN_POINT('Ctrl Pts',(80.8760692804462,7.58143811939194,134.016275171723));
#68112=CARTESIAN_POINT('Ctrl Pts',(80.790461102991,7.53309175100642,134.010050577342));
#68113=CARTESIAN_POINT('Ctrl Pts',(80.7612045315729,7.51769912582214,134.007925635897));
#68114=CARTESIAN_POINT('Ctrl Pts',(80.7230090107625,7.49903246561289,134.005129409953));
#68115=CARTESIAN_POINT('Ctrl Pts',(80.7144710260588,7.49494959836549,134.004502972021));
#68116=CARTESIAN_POINT('Ctrl Pts',(80.7005562138335,7.48844061238148,134.003479042104));
#68117=CARTESIAN_POINT('Ctrl Pts',(80.6952003287852,7.48596985130118,134.003084213235));
#68118=CARTESIAN_POINT('Ctrl Pts',(80.6847248401779,7.48120463262235,134.002310368956));
#68119=CARTESIAN_POINT('Ctrl Pts',(80.6796065806318,7.47890750875482,134.001931519594));
#68120=CARTESIAN_POINT('Ctrl Pts',(80.6668202692552,7.47324630488577,134.000983382627));
#68121=CARTESIAN_POINT('Ctrl Pts',(80.6591383430751,7.46991413498947,134.000412230716));
#68122=CARTESIAN_POINT('Ctrl Pts',(80.6315242939161,7.45818259653272,133.998354540622));
#68123=CARTESIAN_POINT('Ctrl Pts',(80.6114550711116,7.45011406010067,133.996850570291));
#68124=CARTESIAN_POINT('Ctrl Pts',(80.4916245280058,7.40462750030144,133.987843672003));
#68125=CARTESIAN_POINT('Ctrl Pts',(80.388621751089,7.37646093642236,133.980010302708));
#68126=CARTESIAN_POINT('Ctrl Pts',(80.1990335284948,7.34370480911231,133.966054588333));
#68127=CARTESIAN_POINT('Ctrl Pts',(80.1134128065259,7.33564746488484,133.959912346471));
#68128=CARTESIAN_POINT('Ctrl Pts',(79.9985594831699,7.33374847760258,133.951957176601));
#68129=CARTESIAN_POINT('Ctrl Pts',(79.9695680245425,7.33402572411456,133.949972205689));
#68130=CARTESIAN_POINT('Ctrl Pts',(79.9276388698942,7.3355217058213,133.94713316799));
#68131=CARTESIAN_POINT('Ctrl Pts',(79.9146863464289,7.33613530539314,133.946260517242));
#68132=CARTESIAN_POINT('Ctrl Pts',(79.891940011496,7.33747918723407,133.944735342234));
#68133=CARTESIAN_POINT('Ctrl Pts',(79.8821431766625,7.33814495509189,133.944080837117));
#68134=CARTESIAN_POINT('Ctrl Pts',(79.8617332644356,7.33971335414146,133.942722033578));
#68135=CARTESIAN_POINT('Ctrl Pts',(79.8511217790143,7.34063122821057,133.942018242842));
#68136=CARTESIAN_POINT('Ctrl Pts',(79.8233708843971,7.34329998063211,133.940184256715));
#68137=CARTESIAN_POINT('Ctrl Pts',(79.8062482696252,7.34521508897377,133.939059229406));
#68138=CARTESIAN_POINT('Ctrl Pts',(79.729846399537,7.35496256964079,133.934064647661));
#68139=CARTESIAN_POINT('Ctrl Pts',(79.6709813137082,7.36571759223016,133.930286982939));
#68140=CARTESIAN_POINT('Ctrl Pts',(79.5110234161314,7.40393879256718,133.92006358903));
#68141=CARTESIAN_POINT('Ctrl Pts',(79.4117517666636,7.43779866347004,133.913776385343));
#68142=CARTESIAN_POINT('Ctrl Pts',(79.2771189196786,7.49838544137152,133.904658568878));
#68143=CARTESIAN_POINT('Ctrl Pts',(79.2386239628447,7.51753267652199,133.901975605468));
#68144=CARTESIAN_POINT('Ctrl Pts',(79.185772786292,7.54642239771882,133.89812611215));
#68145=CARTESIAN_POINT('Ctrl Pts',(79.1707606110715,7.55493398517142,133.897013152933));
#68146=CARTESIAN_POINT('Ctrl Pts',(79.144589270734,7.57031467942988,133.895033377468));
#68147=CARTESIAN_POINT('Ctrl Pts',(79.1333736616278,7.57708524674022,133.894171889332));
#68148=CARTESIAN_POINT('Ctrl Pts',(79.1165669096028,7.58750344509526,133.89285923895));
#68149=CARTESIAN_POINT('Ctrl Pts',(79.1109156271945,7.59105375652308,133.892414100823));
#68150=CARTESIAN_POINT('Ctrl Pts',(79.1006767501204,7.5975722664739,133.891600454173));
#68151=CARTESIAN_POINT('Ctrl Pts',(79.0960822335142,7.60052919843287,133.891232676755));
#68152=CARTESIAN_POINT('Ctrl Pts',(79.0857122386401,7.60727547479778,133.890396526846));
#68153=CARTESIAN_POINT('Ctrl Pts',(79.0799457689899,7.61107814424571,133.889927301711));
#68154=CARTESIAN_POINT('Ctrl Pts',(79.0623277990385,7.62285408349946,133.888480972167));
#68155=CARTESIAN_POINT('Ctrl Pts',(79.0505554172563,7.63094376228111,133.887496710809));
#68156=CARTESIAN_POINT('Ctrl Pts',(78.9457899123003,7.7049370416856,133.878586364187));
#68157=CARTESIAN_POINT('Ctrl Pts',(78.8596916831411,7.78006546219407,133.870204991479));
#68158=CARTESIAN_POINT('Ctrl Pts',(78.7209618818999,7.92873594493842,133.85544274897));
#68159=CARTESIAN_POINT('Ctrl Pts',(78.6653321864532,7.99889503028003,133.84903941248));
#68160=CARTESIAN_POINT('Ctrl Pts',(78.5994406429063,8.09731914270485,133.840836179085));
#68161=CARTESIAN_POINT('Ctrl Pts',(78.5839190152081,8.12186899017604,133.838847548913));
#68162=CARTESIAN_POINT('Ctrl Pts',(78.5624013561224,8.15795813791738,133.836004308962));
#68163=CARTESIAN_POINT('Ctrl Pts',(78.5558867540909,8.16918033972146,133.835131038241));
#68164=CARTESIAN_POINT('Ctrl Pts',(78.5446730298935,8.18902783685474,133.833605155122));
#68165=CARTESIAN_POINT('Ctrl Pts',(78.5399179056304,8.19762058593297,133.832950556056));
#68166=CARTESIAN_POINT('Ctrl Pts',(78.5301664535987,8.21561572017753,133.831591912922));
#68167=CARTESIAN_POINT('Ctrl Pts',(78.5251837085998,8.22502498874853,133.830888373463));
#68168=CARTESIAN_POINT('Ctrl Pts',(78.5123837571888,8.24976665037211,133.829055830354));
#68169=CARTESIAN_POINT('Ctrl Pts',(78.5047131914249,8.26517378864806,133.827931979447));
#68170=CARTESIAN_POINT('Ctrl Pts',(78.4715818485716,8.33438952014141,133.822955704477));
#68171=CARTESIAN_POINT('Ctrl Pts',(78.4487755266755,8.3894239231307,133.819194279212));
#68172=CARTESIAN_POINT('Ctrl Pts',(78.3874605661852,8.56316532165436,133.807739248082));
#68173=CARTESIAN_POINT('Ctrl Pts',(78.3592967448776,8.68504337033533,133.800310442124));
#68174=CARTESIAN_POINT('Ctrl Pts',(78.3415069564533,8.83912280758562,133.79060816018));
#68175=CARTESIAN_POINT('Ctrl Pts',(78.3388471401507,8.86941820951917,133.788684127488));
#68176=CARTESIAN_POINT('Ctrl Pts',(78.3358148753454,8.91972728041939,133.785437379776));
#68177=CARTESIAN_POINT('Ctrl Pts',(78.3349713560226,8.93970599466852,133.784134560203));
#68178=CARTESIAN_POINT('Ctrl Pts',(78.3342967629445,8.96758129161905,133.782291999451));
#68179=CARTESIAN_POINT('Ctrl Pts',(78.3341619212957,8.97546969345619,133.78176780665));
#68180=CARTESIAN_POINT('Ctrl Pts',(78.3340274107861,8.98893507310451,133.780867837847));
#68181=CARTESIAN_POINT('Ctrl Pts',(78.3339997062066,8.99451175506259,133.780493595106));
#68182=CARTESIAN_POINT('Ctrl Pts',(78.3340003253419,9.00617081158276,133.779707828496));
#68183=CARTESIAN_POINT('Ctrl Pts',(78.3340339570425,9.01225298347197,133.779296039333));
#68184=CARTESIAN_POINT('Ctrl Pts',(78.3342142740156,9.0286366550134,133.778181977064));
#68185=CARTESIAN_POINT('Ctrl Pts',(78.3344232112333,9.03893700301425,133.777476439763));
#68186=CARTESIAN_POINT('Ctrl Pts',(78.3360154195585,9.09279080067836,133.773763074316));
#68187=CARTESIAN_POINT('Ctrl Pts',(78.3390114485997,9.13627592012142,133.770680929117));
#68188=CARTESIAN_POINT('Ctrl Pts',(78.3559301549065,9.29231160739358,133.7594283155));
#68189=CARTESIAN_POINT('Ctrl Pts',(78.3796274787048,9.4034931184064,133.751070147562));
#68190=CARTESIAN_POINT('Ctrl Pts',(78.4213757555641,9.5329283937359,133.741325712562));
#68191=CARTESIAN_POINT('Ctrl Pts',(78.428752080249,9.5542984480888,133.739715322682));
#68192=CARTESIAN_POINT('Ctrl Pts',(78.4365593568556,9.5755079107748,133.73811642446));
#68193=CARTESIAN_POINT('Ctrl Pts',(78.4365594251401,9.5755080962782,133.933539779158));
#68194=CARTESIAN_POINT('Ctrl Pts',(78.4292827696383,9.55574014073706,133.935004724177));
#68195=CARTESIAN_POINT('Ctrl Pts',(78.4223785847212,9.5358275358506,133.936458722568));
#68196=CARTESIAN_POINT('Ctrl Pts',(78.4098685575793,9.49740473250551,133.939223437784));
#68197=CARTESIAN_POINT('Ctrl Pts',(78.4042055386525,9.47892542613148,133.940535321508));
#68198=CARTESIAN_POINT('Ctrl Pts',(78.3957986621001,9.44968569135736,133.942584064875));
#68199=CARTESIAN_POINT('Ctrl Pts',(78.3928387794976,9.43898972102187,133.943327871012));
#68200=CARTESIAN_POINT('Ctrl Pts',(78.3874866924185,9.41886914002329,133.944716814553));
#68201=CARTESIAN_POINT('Ctrl Pts',(78.3850697044886,9.40945167123947,133.945362727448));
#68202=CARTESIAN_POINT('Ctrl Pts',(78.379818829415,9.38822224508079,133.94680966347));
#68203=CARTESIAN_POINT('Ctrl Pts',(78.3770313841504,9.37639928547213,133.947609166515));
#68204=CARTESIAN_POINT('Ctrl Pts',(78.3691885495291,9.34142565176383,133.949956423171));
#68205=CARTESIAN_POINT('Ctrl Pts',(78.3644973321265,9.31819581511957,133.951492602172));
#68206=CARTESIAN_POINT('Ctrl Pts',(78.3427139805689,9.19706531134075,133.959398109159));
#68207=CARTESIAN_POINT('Ctrl Pts',(78.333910218766,9.09787589607775,133.965502739526));
#68208=CARTESIAN_POINT('Ctrl Pts',(78.3341019470699,8.88724216840797,133.978370404461));
#68209=CARTESIAN_POINT('Ctrl Pts',(78.3453445218236,8.77630641058436,133.985095466586));
#68210=CARTESIAN_POINT('Ctrl Pts',(78.3704604189554,8.65305748572697,133.993274686661));
#68211=CARTESIAN_POINT('Ctrl Pts',(78.373557302935,8.63881795150663,133.994230825064));
#68212=CARTESIAN_POINT('Ctrl Pts',(78.3784090194991,8.61783883427495,133.995658511274));
#68213=CARTESIAN_POINT('Ctrl Pts',(78.3800200632685,8.61106624615768,133.996122349285));
#68214=CARTESIAN_POINT('Ctrl Pts',(78.3829713986039,8.59899580431812,133.996954615568));
#68215=CARTESIAN_POINT('Ctrl Pts',(78.3842953744662,8.59369417438305,133.997322116891));
#68216=CARTESIAN_POINT('Ctrl Pts',(78.3872818226931,8.58198092045737,133.998138437268));
#68217=CARTESIAN_POINT('Ctrl Pts',(78.3889564365218,8.57557273526007,133.998587914231));
#68218=CARTESIAN_POINT('Ctrl Pts',(78.3939939260773,8.55675538646089,133.999915916189));
#68219=CARTESIAN_POINT('Ctrl Pts',(78.3974621993928,8.5443752977656,134.000800054597));
#68220=CARTESIAN_POINT('Ctrl Pts',(78.4058039318622,8.51587342677483,134.002857798219));
#68221=CARTESIAN_POINT('Ctrl Pts',(78.4107792279849,8.49978311450435,134.0040360492));
#68222=CARTESIAN_POINT('Ctrl Pts',(78.428821732205,8.44442122607083,134.008141407812));
#68223=CARTESIAN_POINT('Ctrl Pts',(78.4431072005666,8.40556472504274,134.011112642033));
#68224=CARTESIAN_POINT('Ctrl Pts',(78.5067069662335,8.25064794641112,134.023229987836));
#68225=CARTESIAN_POINT('Ctrl Pts',(78.5676843445167,8.13980698015248,134.032491073314));
#68226=CARTESIAN_POINT('Ctrl Pts',(78.6660831901528,8.00091694717258,134.044461408363));
#68227=CARTESIAN_POINT('Ctrl Pts',(78.6929988890228,7.96595468162453,134.047515227136));
#68228=CARTESIAN_POINT('Ctrl Pts',(78.7312816391157,7.9201141106541,134.051577554172));
#68229=CARTESIAN_POINT('Ctrl Pts',(78.7414587805668,7.90827025272771,134.052632795706));
#68230=CARTESIAN_POINT('Ctrl Pts',(78.7586276623913,7.88884881788925,134.054373205629));
#68231=CARTESIAN_POINT('Ctrl Pts',(78.7655257267966,7.88119013808065,134.055062190782));
#68232=CARTESIAN_POINT('Ctrl Pts',(78.7792396077382,7.86624535739449,134.05641218649));
#68233=CARTESIAN_POINT('Ctrl Pts',(78.7860506671652,7.85895550059733,134.05707335696));
#68234=CARTESIAN_POINT('Ctrl Pts',(78.8025323136292,7.84162986995193,134.058651505359));
#68235=CARTESIAN_POINT('Ctrl Pts',(78.8122642524354,7.83165329138682,134.059565793758));
#68236=CARTESIAN_POINT('Ctrl Pts',(78.8469171865273,7.79700979063132,134.062761953827));
#68237=CARTESIAN_POINT('Ctrl Pts',(78.8724915709273,7.77300756384942,134.065014972303));
#68238=CARTESIAN_POINT('Ctrl Pts',(78.9383230163171,7.71502094328138,134.070581454987));
#68239=CARTESIAN_POINT('Ctrl Pts',(78.9794700518876,7.6821045395804,134.073855840616));
#68240=CARTESIAN_POINT('Ctrl Pts',(79.0998222603495,7.59484888620787,134.083006360312));
#68241=CARTESIAN_POINT('Ctrl Pts',(79.1822547195393,7.54533134956343,134.088782132031));
#68242=CARTESIAN_POINT('Ctrl Pts',(79.314691453025,7.48060774315112,134.097952739101));
#68243=CARTESIAN_POINT('Ctrl Pts',(79.3619109959993,7.4601811976655,134.101205579418));
#68244=CARTESIAN_POINT('Ctrl Pts',(79.4202678761006,7.43808215511817,134.105293019905));
#68245=CARTESIAN_POINT('Ctrl Pts',(79.4305796641964,7.43429340073857,134.106017783195));
#68246=CARTESIAN_POINT('Ctrl Pts',(79.4468567163556,7.42849495057426,134.107166870708));
#68247=CARTESIAN_POINT('Ctrl Pts',(79.4527974057639,7.4264165321767,134.10758730846));
#68248=CARTESIAN_POINT('Ctrl Pts',(79.4639589770602,7.42258237566908,134.10837946313));
#68249=CARTESIAN_POINT('Ctrl Pts',(79.469176962349,7.42081880742468,134.108750720923));
#68250=CARTESIAN_POINT('Ctrl Pts',(79.4814640972008,7.41673379388088,134.109627046339));
#68251=CARTESIAN_POINT('Ctrl Pts',(79.4885401527792,7.41443379787537,134.110133324271));
#68252=CARTESIAN_POINT('Ctrl Pts',(79.5120478338653,7.40696660971541,134.111820031297));
#68253=CARTESIAN_POINT('Ctrl Pts',(79.5285435615917,7.40200705012318,134.113011324654));
#68254=CARTESIAN_POINT('Ctrl Pts',(79.5689576453855,7.39053645909651,134.115943816239));
#68255=CARTESIAN_POINT('Ctrl Pts',(79.5929497358112,7.38430189950451,134.117696397838));
#68256=CARTESIAN_POINT('Ctrl Pts',(79.6943259687317,7.36035958894112,134.125127285409));
#68257=CARTESIAN_POINT('Ctrl Pts',(79.7727835603266,7.34765949977901,134.130934681421));
#68258=CARTESIAN_POINT('Ctrl Pts',(79.9540430108181,7.3314761693961,134.144159920278));
#68259=CARTESIAN_POINT('Ctrl Pts',(80.0568808706016,7.33181091585703,134.151514475538));
#68260=CARTESIAN_POINT('Ctrl Pts',(80.1825333510307,7.34386166571305,134.160204110095));
#68261=CARTESIAN_POINT('Ctrl Pts',(80.2059685914751,7.34661267553775,134.161813033239));
#68262=CARTESIAN_POINT('Ctrl Pts',(80.2413484885229,7.35152982092665,134.1642253242));
#68263=CARTESIAN_POINT('Ctrl Pts',(80.253340092762,7.3533300770676,134.16504003577));
#68264=CARTESIAN_POINT('Ctrl Pts',(80.2749078495667,7.35680915130232,134.166500430426));
#68265=CARTESIAN_POINT('Ctrl Pts',(80.2844908825668,7.35844115682495,134.167147558405));
#68266=CARTESIAN_POINT('Ctrl Pts',(80.3049968846645,7.36211832573745,134.168528772613));
#68267=CARTESIAN_POINT('Ctrl Pts',(80.3159148288969,7.36418909727171,134.169262014424));
#68268=CARTESIAN_POINT('Ctrl Pts',(80.3458290817464,7.37017350912847,134.171265674622));
#68269=CARTESIAN_POINT('Ctrl Pts',(80.3647794256104,7.37430994167322,134.172528993386));
#68270=CARTESIAN_POINT('Ctrl Pts',(80.4949918326228,7.40512401197013,134.181177420844));
#68271=CARTESIAN_POINT('Ctrl Pts',(80.6033237838827,7.44287085822383,134.188181742833));
#68272=CARTESIAN_POINT('Ctrl Pts',(80.8003166559047,7.53518514326631,134.201466172693));
#68273=CARTESIAN_POINT('Ctrl Pts',(80.8894137990673,7.58751050261682,134.207730718492));
#68274=CARTESIAN_POINT('Ctrl Pts',(80.985371672674,7.65656128276603,134.215410054106));
#68275=CARTESIAN_POINT('Ctrl Pts',(80.9975311542382,7.6655651094126,134.216401997883));
#68276=CARTESIAN_POINT('Ctrl Pts',(81.0151872144262,7.67901519384399,134.217873010427));
#68277=CARTESIAN_POINT('Ctrl Pts',(81.0207812013519,7.68333312000774,134.218343681427));
#68278=CARTESIAN_POINT('Ctrl Pts',(81.0306567116587,7.69105665848395,134.219183150422));
#68279=CARTESIAN_POINT('Ctrl Pts',(81.0349491721654,7.69444795658702,134.219550951431));
#68280=CARTESIAN_POINT('Ctrl Pts',(81.0443358553451,7.70193937711952,134.220361760343));
#68281=CARTESIAN_POINT('Ctrl Pts',(81.0494226004676,7.7060483156635,134.220805366688));
#68282=CARTESIAN_POINT('Ctrl Pts',(81.0641202472575,7.718064357426,134.222099107279));
#68283=CARTESIAN_POINT('Ctrl Pts',(81.0736666537819,7.72604914307242,134.222954440932));
#68284=CARTESIAN_POINT('Ctrl Pts',(81.1511393244527,7.79233796605027,134.23001380237));
#68285=CARTESIAN_POINT('Ctrl Pts',(81.2143478908648,7.85591734582821,134.236517821913));
#68286=CARTESIAN_POINT('Ctrl Pts',(81.3536801647676,8.02068697694039,134.252224711899));
#68287=CARTESIAN_POINT('Ctrl Pts',(81.4240099031207,8.12609427616564,134.261361197319));
#68288=CARTESIAN_POINT('Ctrl Pts',(81.4911808132693,8.25679019836835,134.271464199248));
#68289=CARTESIAN_POINT('Ctrl Pts',(81.5002638658933,8.2753004582786,134.272869995471));
#68290=CARTESIAN_POINT('Ctrl Pts',(81.5143382192573,8.30538186762996,134.275115400431));
#68291=CARTESIAN_POINT('Ctrl Pts',(81.5195456956089,8.31684885552939,134.275962358245));
#68292=CARTESIAN_POINT('Ctrl Pts',(81.5285604575656,8.33731279343818,134.277458306956));
#68293=CARTESIAN_POINT('Ctrl Pts',(81.5324195237557,8.34628613570786,134.278109040574));
#68294=CARTESIAN_POINT('Ctrl Pts',(81.540389176041,8.36527612225781,134.27947541763));
#68295=CARTESIAN_POINT('Ctrl Pts',(81.5444814996683,8.37529997506769,134.280190418696));
#68296=CARTESIAN_POINT('Ctrl Pts',(81.5551375599044,8.40214615932136,134.282089272543));
#68297=CARTESIAN_POINT('Ctrl Pts',(81.5615261301565,8.41903680727938,134.283267247005));
#68298=CARTESIAN_POINT('Ctrl Pts',(81.5950770012891,8.51229623372557,134.289685905848));
#68299=CARTESIAN_POINT('Ctrl Pts',(81.6169146373465,8.59046963469517,134.294747577581));
#68300=CARTESIAN_POINT('Ctrl Pts',(81.6405770225901,8.70753636567241,134.302093818309));
#68301=CARTESIAN_POINT('Ctrl Pts',(81.6468769238953,8.74539360741391,134.304435841777));
#68302=CARTESIAN_POINT('Ctrl Pts',(81.6648733724003,8.88266271293565,134.312889590771));
#68303=CARTESIAN_POINT('Ctrl Pts',(81.6689133593665,8.98284781760037,134.318980025011));
#68304=CARTESIAN_POINT('Ctrl Pts',(81.6631858489151,9.09798325804285,134.326464228381));
#68305=CARTESIAN_POINT('Ctrl Pts',(81.6622208071392,9.11318054263232,134.327462062326));
#68306=CARTESIAN_POINT('Ctrl Pts',(81.6604995116557,9.13545472222088,134.32894198442));
#68307=CARTESIAN_POINT('Ctrl Pts',(81.6599059739023,9.14254389913312,134.329415593353));
#68308=CARTESIAN_POINT('Ctrl Pts',(81.6587744483283,9.15509163005926,134.330258819551));
#68309=CARTESIAN_POINT('Ctrl Pts',(81.6582548812689,9.16055164785982,134.330627414616));
#68310=CARTESIAN_POINT('Ctrl Pts',(81.6570687683985,9.17239575021775,134.331430717949));
#68311=CARTESIAN_POINT('Ctrl Pts',(81.6563922993576,9.17877848038597,134.331865938271));
#68312=CARTESIAN_POINT('Ctrl Pts',(81.6543599356357,9.19695193197278,134.333111456928));
#68313=CARTESIAN_POINT('Ctrl Pts',(81.6529149367816,9.20873200953898,134.333926396938));
#68314=CARTESIAN_POINT('Ctrl Pts',(81.6493342434214,9.23554872486521,134.335797389002));
#68315=CARTESIAN_POINT('Ctrl Pts',(81.6471185599384,9.25057346553193,134.336857041338));
#68316=CARTESIAN_POINT('Ctrl Pts',(81.6215515157509,9.40891522731972,134.348130798183));
#68317=CARTESIAN_POINT('Ctrl Pts',(81.5797647521216,9.54862355016414,134.35893263322));
#68318=CARTESIAN_POINT('Ctrl Pts',(81.4935541903558,9.74105368209058,134.373993201831));
#68319=CARTESIAN_POINT('Ctrl Pts',(81.4631973685814,9.79932477347735,134.378592525845));
#68320=CARTESIAN_POINT('Ctrl Pts',(81.4204118118372,9.87080296011738,134.384277892558));
#68321=CARTESIAN_POINT('Ctrl Pts',(81.4111065614483,9.88580236193422,134.385473753312));
#68322=CARTESIAN_POINT('Ctrl Pts',(81.3957586771143,9.90968623527289,134.38738319654));
#68323=CARTESIAN_POINT('Ctrl Pts',(81.3898656277605,9.91866472529193,134.388102224063));
#68324=CARTESIAN_POINT('Ctrl Pts',(81.3784357055735,9.93571728264751,134.389470466152));
#68325=CARTESIAN_POINT('Ctrl Pts',(81.3729137001607,9.94380072384735,134.39012020017));
#68326=CARTESIAN_POINT('Ctrl Pts',(81.3600278108871,9.96231143156325,134.391611003564));
#68327=CARTESIAN_POINT('Ctrl Pts',(81.3526146325724,9.97270376196015,134.39245015694));
#68328=CARTESIAN_POINT('Ctrl Pts',(81.3286529132681,10.0054913097682,134.395105720157));
#68329=CARTESIAN_POINT('Ctrl Pts',(81.3116615214287,10.0275580448526,134.396905031995));
#68330=CARTESIAN_POINT('Ctrl Pts',(81.2483226798764,10.1056834158241,134.403335698931));
#68331=CARTESIAN_POINT('Ctrl Pts',(81.1988686984716,10.1591206750026,134.407846467255));
#68332=CARTESIAN_POINT('Ctrl Pts',(81.0506790659567,10.299579119196,134.420372121352));
#68333=CARTESIAN_POINT('Ctrl Pts',(80.9449318739748,10.3783779499106,134.428212585468));
#68334=CARTESIAN_POINT('Ctrl Pts',(80.8182619913302,10.4512825090272,134.437709817667));
#68335=CARTESIAN_POINT('Ctrl Pts',(80.8053801951284,10.4584705386873,134.438677099889));
#68336=CARTESIAN_POINT('Ctrl Pts',(80.7862288879123,10.4688258697336,134.440119853789));
#68337=CARTESIAN_POINT('Ctrl Pts',(80.7800316637102,10.4721263189549,134.440587434949));
#68338=CARTESIAN_POINT('Ctrl Pts',(80.7689642403079,10.4779309814886,134.441424078927));
#68339=CARTESIAN_POINT('Ctrl Pts',(80.7641022939745,10.4804504962472,134.44179217973));
#68340=CARTESIAN_POINT('Ctrl Pts',(80.753455623245,10.4859013010626,134.442599551497));
#68341=CARTESIAN_POINT('Ctrl Pts',(80.7476662611274,10.4888227601342,134.443039382238));
#68342=CARTESIAN_POINT('Ctrl Pts',(80.7309504769168,10.4971358848322,134.444311311855));
#68343=CARTESIAN_POINT('Ctrl Pts',(80.7199820400186,10.5024414456951,134.445148354278));
#68344=CARTESIAN_POINT('Ctrl Pts',(80.6251959938193,10.5470143114208,134.452396553142));
#68345=CARTESIAN_POINT('Ctrl Pts',(80.5383071566729,10.5793495783025,134.459129988765));
#68346=CARTESIAN_POINT('Ctrl Pts',(80.3305015798915,10.637533839283,134.474838723062));
#68347=CARTESIAN_POINT('Ctrl Pts',(80.2084656950573,10.6574984451795,134.483746324709));
#68348=CARTESIAN_POINT('Ctrl Pts',(80.0645052553556,10.6648813030621,134.493660293738));
#68349=CARTESIAN_POINT('Ctrl Pts',(80.0436646238897,10.665558209756,134.495082319254));
#68350=CARTESIAN_POINT('Ctrl Pts',(80.0102924973982,10.6660152851486,134.49733917295));
#68351=CARTESIAN_POINT('Ctrl Pts',(79.997767239054,10.6660455862611,134.498181665826));
#68352=CARTESIAN_POINT('Ctrl Pts',(79.9754573623775,10.6658479570174,134.499674539596));
#68353=CARTESIAN_POINT('Ctrl Pts',(79.965672976613,10.6656750641851,134.500326605001));
#68354=CARTESIAN_POINT('Ctrl Pts',(79.9451414961652,10.665131276112,134.501689551222));
#68355=CARTESIAN_POINT('Ctrl Pts',(79.9343952942363,10.6647425187863,134.502399844363));
#68356=CARTESIAN_POINT('Ctrl Pts',(79.905959282621,10.6634380312737,134.504271723231));
#68357=CARTESIAN_POINT('Ctrl Pts',(79.8882787166219,10.6623441684622,134.505427729311));
#68358=CARTESIAN_POINT('Ctrl Pts',(79.796375038728,10.6551853055709,134.511400849813));
#68359=CARTESIAN_POINT('Ctrl Pts',(79.7225978722295,10.6444304813611,134.51606901182));
#68360=CARTESIAN_POINT('Ctrl Pts',(79.5852682836288,10.6149017989144,134.524734195293));
#68361=CARTESIAN_POINT('Ctrl Pts',(79.5216372751277,10.5972099006477,134.528740413662));
#68362=CARTESIAN_POINT('Ctrl Pts',(79.3843706418594,10.5501029584372,134.537624458055));
#68363=CARTESIAN_POINT('Ctrl Pts',(79.3114526527675,10.5191175787064,134.542505410142));
#68364=CARTESIAN_POINT('Ctrl Pts',(79.2269807790108,10.4758882291769,134.548662012659));
#68365=CARTESIAN_POINT('Ctrl Pts',(79.2130432063088,10.4685039127005,134.549695170748));
#68366=CARTESIAN_POINT('Ctrl Pts',(79.1929796770627,10.4575063395732,134.551210853761));
#68367=CARTESIAN_POINT('Ctrl Pts',(79.1867682276615,10.454049727965,134.551684103978));
#68368=CARTESIAN_POINT('Ctrl Pts',(79.1758041225414,10.4478560817909,134.55252693549));
#68369=CARTESIAN_POINT('Ctrl Pts',(79.1710425819683,10.4451351756224,134.55289549816));
#68370=CARTESIAN_POINT('Ctrl Pts',(79.1607340955242,10.4391768439629,134.553699030435));
#68371=CARTESIAN_POINT('Ctrl Pts',(79.1551924934083,10.4359308896811,134.554134514844));
#68372=CARTESIAN_POINT('Ctrl Pts',(79.1394483284626,10.4265861727884,134.55538153999));
#68373=CARTESIAN_POINT('Ctrl Pts',(79.1292923235012,10.4204102962432,134.556197739389));
#68374=CARTESIAN_POINT('Ctrl Pts',(79.0384128396547,10.3638055169821,134.563602268254));
#68375=CARTESIAN_POINT('Ctrl Pts',(78.9620914784457,10.3066588842547,134.570533367854));
#68376=CARTESIAN_POINT('Ctrl Pts',(78.8008697701194,10.162863868255,134.586259005378));
#68377=CARTESIAN_POINT('Ctrl Pts',(78.7196727220553,10.0728177145332,134.594986297006));
#68378=CARTESIAN_POINT('Ctrl Pts',(78.6366415339469,9.95773204050071,134.604748412558));
#68379=CARTESIAN_POINT('Ctrl Pts',(78.6246776784905,9.94047091927356,134.60618091296));
#68380=CARTESIAN_POINT('Ctrl Pts',(78.6060805321219,9.91252531414578,134.608451025808));
#68381=CARTESIAN_POINT('Ctrl Pts',(78.5992366254061,9.90198443185305,134.609296446346));
#68382=CARTESIAN_POINT('Ctrl Pts',(78.5872737879914,9.88309485330583,134.610792647012));
#68383=CARTESIAN_POINT('Ctrl Pts',(78.5821080271373,9.87477667456243,134.611445138275));
#68384=CARTESIAN_POINT('Ctrl Pts',(78.5714349500713,9.85724737267127,134.612807122053));
#68385=CARTESIAN_POINT('Ctrl Pts',(78.5659426808873,9.84802757880847,134.613516043089));
#68386=CARTESIAN_POINT('Ctrl Pts',(78.551672706782,9.82353764321999,134.615380058359));
#68387=CARTESIAN_POINT('Ctrl Pts',(78.5430472517491,9.80818000839586,134.61652965884));
#68388=CARTESIAN_POINT('Ctrl Pts',(78.5000523691766,9.72870127932335,134.622385815212));
#68389=CARTESIAN_POINT('Ctrl Pts',(78.4696638823641,9.66251168730783,134.626950764182));
#68390=CARTESIAN_POINT('Ctrl Pts',(78.4412789673489,9.5882097138014,134.631861484381));
#68391=CARTESIAN_POINT('Ctrl Pts',(78.4388996016047,9.58186548337547,134.632279173869));
#68392=CARTESIAN_POINT('Ctrl Pts',(78.4365593788086,9.57550797041271,134.632696244622));
#68393=CARTESIAN_POINT('Origin',(80.,9.,134.));
#68394=CARTESIAN_POINT('',(78.4365593737638,9.57550795670805,135.330578607084));
#68395=CARTESIAN_POINT('',(78.436559333852,9.57550784828241,135.139259993339));
#68396=CARTESIAN_POINT('',(78.4365593737638,9.57550795670799,134.));
#68397=CARTESIAN_POINT('',(78.3340007521426,9.00139877871345,134.47795709598));
#68398=CARTESIAN_POINT('Ctrl Pts',(78.436559333852,9.57550784828241,135.139259993339));
#68399=CARTESIAN_POINT('Ctrl Pts',(78.4595768295332,9.63803781879155,135.135190034949));
#68400=CARTESIAN_POINT('Ctrl Pts',(78.48633467882,9.69915708210112,135.131135418933));
#68401=CARTESIAN_POINT('Ctrl Pts',(78.5389125131787,9.80197250901578,135.123936741731));
#68402=CARTESIAN_POINT('Ctrl Pts',(78.5630224575881,9.84441170149945,135.120844198812));
#68403=CARTESIAN_POINT('Ctrl Pts',(78.5947306342489,9.89492566985977,135.116936366758));
#68404=CARTESIAN_POINT('Ctrl Pts',(78.600594089363,9.90406693714173,135.11621972521));
#68405=CARTESIAN_POINT('Ctrl Pts',(78.6099809912233,9.91839121479723,135.115080647939));
#68406=CARTESIAN_POINT('Ctrl Pts',(78.6134451542317,9.92361297339697,135.114661987101));
#68407=CARTESIAN_POINT('Ctrl Pts',(78.6200142168467,9.9333947030339,135.113871014238));
#68408=CARTESIAN_POINT('Ctrl Pts',(78.6231124072684,9.93795894725437,135.113499139384));
#68409=CARTESIAN_POINT('Ctrl Pts',(78.6304738652055,9.94868875603311,135.112618382558));
#68410=CARTESIAN_POINT('Ctrl Pts',(78.6347561394962,9.954841026381,135.112108254196));
#68411=CARTESIAN_POINT('Ctrl Pts',(78.6491993564279,9.97529555597973,135.110395607681));
#68412=CARTESIAN_POINT('Ctrl Pts',(78.6595442915055,9.98946562995298,135.109181781516));
#68413=CARTESIAN_POINT('Ctrl Pts',(78.6854148977695,10.0237517388748,135.106182152998));
#68414=CARTESIAN_POINT('Ctrl Pts',(78.7011804707563,10.0436806524863,135.104384326804));
#68415=CARTESIAN_POINT('Ctrl Pts',(78.770530949551,10.1273393577573,135.09662654426));
#68416=CARTESIAN_POINT('Ctrl Pts',(78.8283957107909,10.1873629637841,135.090528050799));
#68417=CARTESIAN_POINT('Ctrl Pts',(78.969608427744,10.3134284072819,135.07678436002));
#68418=CARTESIAN_POINT('Ctrl Pts',(79.0552882169735,10.3763459205111,135.069214044058));
#68419=CARTESIAN_POINT('Ctrl Pts',(79.1624700284796,10.4402952614068,135.060679223039));
#68420=CARTESIAN_POINT('Ctrl Pts',(79.1787177532822,10.4496214727164,135.059408011729));
#68421=CARTESIAN_POINT('Ctrl Pts',(79.2048192615853,10.4640240143684,135.057400675318));
#68422=CARTESIAN_POINT('Ctrl Pts',(79.2145719524751,10.4692792497745,135.056658220562));
#68423=CARTESIAN_POINT('Ctrl Pts',(79.2329037893004,10.4789226616873,135.055276467085));
#68424=CARTESIAN_POINT('Ctrl Pts',(79.2414699375459,10.4833344150064,135.054636357071));
#68425=CARTESIAN_POINT('Ctrl Pts',(79.260911613389,10.4931348418625,135.053195808424));
#68426=CARTESIAN_POINT('Ctrl Pts',(79.271808799099,10.498479525102,135.052396930061));
#68427=CARTESIAN_POINT('Ctrl Pts',(79.3048180336016,10.5142242530074,135.050001816641));
#68428=CARTESIAN_POINT('Ctrl Pts',(79.3271020192118,10.524257675576,135.04841816174));
#68429=CARTESIAN_POINT('Ctrl Pts',(79.3791778856433,10.5463402248736,135.044786816533));
#68430=CARTESIAN_POINT('Ctrl Pts',(79.4091140021764,10.5580250691894,135.04275081985));
#68431=CARTESIAN_POINT('Ctrl Pts',(79.5208019710125,10.5979371338126,135.035310974151));
#68432=CARTESIAN_POINT('Ctrl Pts',(79.6043765441966,10.6206532697851,135.030054517818));
#68433=CARTESIAN_POINT('Ctrl Pts',(79.6942272612181,10.6377068638952,135.024466413443));
#68434=CARTESIAN_POINT('Ctrl Pts',(79.699118059475,10.6386124610672,135.024162405358));
#68435=CARTESIAN_POINT('Ctrl Pts',(79.7870407308366,10.6544856197643,135.018699181239));
#68436=CARTESIAN_POINT('Ctrl Pts',(79.8710774225485,10.6631445377566,135.013513524576));
#68437=CARTESIAN_POINT('Ctrl Pts',(79.9712133501961,10.6658264270786,135.007014882455));
#68438=CARTESIAN_POINT('Ctrl Pts',(79.9870348609031,10.6660246747404,135.005978529663));
#68439=CARTESIAN_POINT('Ctrl Pts',(80.0099746926268,10.6659853481699,135.004458930245));
#68440=CARTESIAN_POINT('Ctrl Pts',(80.0170929929726,10.6659275193683,135.003985023274));
#68441=CARTESIAN_POINT('Ctrl Pts',(80.0296966550466,10.665744341872,135.003141378851));
#68442=CARTESIAN_POINT('Ctrl Pts',(80.035182089349,10.6656375125257,135.002772665828));
#68443=CARTESIAN_POINT('Ctrl Pts',(80.0470838781903,10.6653469034605,135.001969232211));
#68444=CARTESIAN_POINT('Ctrl Pts',(80.0534996296835,10.6651531420862,135.001534000457));
#68445=CARTESIAN_POINT('Ctrl Pts',(80.0717706408757,10.6644956407054,135.000288753083));
#68446=CARTESIAN_POINT('Ctrl Pts',(80.08362200275,10.6639423377607,134.999474100277));
#68447=CARTESIAN_POINT('Ctrl Pts',(80.1904844336595,10.6578087718802,134.992071838171));
#68448=CARTESIAN_POINT('Ctrl Pts',(80.2848507584234,10.6442233634993,134.985141304991));
#68449=CARTESIAN_POINT('Ctrl Pts',(80.4952998086151,10.595260035669,134.969412834063));
#68450=CARTESIAN_POINT('Ctrl Pts',(80.6097575305606,10.555114898904,134.960682148722));
#68451=CARTESIAN_POINT('Ctrl Pts',(80.7378176643581,10.4938614507758,134.950917010713));
#68452=CARTESIAN_POINT('Ctrl Pts',(80.7565884822857,10.4844429521204,134.949484556792));
#68453=CARTESIAN_POINT('Ctrl Pts',(80.786302232231,10.4688236010766,134.947214383048));
#68454=CARTESIAN_POINT('Ctrl Pts',(80.797361201076,10.4628496510365,134.946368857043));
#68455=CARTESIAN_POINT('Ctrl Pts',(80.8169154517957,10.4519989884945,134.944872389066));
#68456=CARTESIAN_POINT('Ctrl Pts',(80.8254372134439,10.447171493526,134.944219736213));
#68457=CARTESIAN_POINT('Ctrl Pts',(80.8432096442333,10.4368955219991,134.942857330438));
#68458=CARTESIAN_POINT('Ctrl Pts',(80.852451242863,10.4314321964071,134.942148150075));
#68459=CARTESIAN_POINT('Ctrl Pts',(80.876721843206,10.4167658062093,134.940283247379));
#68460=CARTESIAN_POINT('Ctrl Pts',(80.891659004499,10.4074128030831,134.939133025982));
#68461=CARTESIAN_POINT('Ctrl Pts',(80.9675789591181,10.3581810806092,134.9332690082));
#68462=CARTESIAN_POINT('Ctrl Pts',(81.0260502414299,10.3145675022484,134.928697289946));
#68463=CARTESIAN_POINT('Ctrl Pts',(81.1593619892043,10.2007988837498,134.917877567722));
#68464=CARTESIAN_POINT('Ctrl Pts',(81.2309443048808,10.127303340571,134.911729872304));
#68465=CARTESIAN_POINT('Ctrl Pts',(81.3280267478551,10.0072759803649,134.902129804689));
#68466=CARTESIAN_POINT('Ctrl Pts',(81.3588137561803,9.96534137660396,134.898842181923));
#68467=CARTESIAN_POINT('Ctrl Pts',(81.3936832742374,9.91286597158227,134.894715513996));
#68468=CARTESIAN_POINT('Ctrl Pts',(81.3996886516148,9.90363101625349,134.893988807344));
#68469=CARTESIAN_POINT('Ctrl Pts',(81.4089846636838,9.88902076959058,134.892837239411));
#68470=CARTESIAN_POINT('Ctrl Pts',(81.4123372547927,9.88368500423325,134.89241629075));
#68471=CARTESIAN_POINT('Ctrl Pts',(81.4185634844085,9.8736498055683,134.891623615563));
#68472=CARTESIAN_POINT('Ctrl Pts',(81.4214441854525,9.86895498512908,134.891252352986));
#68473=CARTESIAN_POINT('Ctrl Pts',(81.4281569679721,9.85789213274889,134.890376603875));
#68474=CARTESIAN_POINT('Ctrl Pts',(81.431969772634,9.85151265497805,134.889870913347));
#68475=CARTESIAN_POINT('Ctrl Pts',(81.444448788892,9.83031226637494,134.888188684681));
#68476=CARTESIAN_POINT('Ctrl Pts',(81.4529282546458,9.81538346376594,134.887001360695));
#68477=CARTESIAN_POINT('Ctrl Pts',(81.4730292090426,9.77868469899812,134.884080792212));
#68478=CARTESIAN_POINT('Ctrl Pts',(81.4844004177947,9.75678278312836,134.882336278665));
#68479=CARTESIAN_POINT('Ctrl Pts',(81.5299828212697,9.6640044249349,134.87496302992));
#68480=CARTESIAN_POINT('Ctrl Pts',(81.559635482426,9.59100389808208,134.869206879877));
#68481=CARTESIAN_POINT('Ctrl Pts',(81.6160813514976,9.41778818137742,134.85596512143));
#68482=CARTESIAN_POINT('Ctrl Pts',(81.6389125309935,9.31660417435719,134.848544516602));
#68483=CARTESIAN_POINT('Ctrl Pts',(81.6552351362672,9.190549172048,134.839794471824));
#68484=CARTESIAN_POINT('Ctrl Pts',(81.657767096704,9.16709486871849,134.838185936527));
#68485=CARTESIAN_POINT('Ctrl Pts',(81.6608454107353,9.13151260438395,134.835773974394));
#68486=CARTESIAN_POINT('Ctrl Pts',(81.6617586641462,9.1194202624968,134.834959211637));
#68487=CARTESIAN_POINT('Ctrl Pts',(81.6631661659548,9.09761579739518,134.833498601627));
#68488=CARTESIAN_POINT('Ctrl Pts',(81.6637075580421,9.08790738119863,134.83285131032));
#68489=CARTESIAN_POINT('Ctrl Pts',(81.6646857187853,9.06708983388079,134.831469611039));
#68490=CARTESIAN_POINT('Ctrl Pts',(81.6650963482185,9.05597990141252,134.830736049229));
#68491=CARTESIAN_POINT('Ctrl Pts',(81.6659184384813,9.02546477680437,134.828731145386));
#68492=CARTESIAN_POINT('Ctrl Pts',(81.6661020643355,9.00605481777819,134.827466915392));
#68493=CARTESIAN_POINT('Ctrl Pts',(81.6657553517935,8.96280345461606,134.824671427951));
#68494=CARTESIAN_POINT('Ctrl Pts',(81.6650524306856,8.93896752365867,134.823145477617));
#68495=CARTESIAN_POINT('Ctrl Pts',(81.6611589647097,8.86261631701194,134.818294478144));
#68496=CARTESIAN_POINT('Ctrl Pts',(81.6559928557438,8.81023259395848,134.815023390367));
#68497=CARTESIAN_POINT('Ctrl Pts',(81.6344255122983,8.66322093320718,134.805876838922));
#68498=CARTESIAN_POINT('Ctrl Pts',(81.612316427257,8.56964984982452,134.800101912622));
#68499=CARTESIAN_POINT('Ctrl Pts',(81.5661516753972,8.42958022776165,134.790927272234));
#68500=CARTESIAN_POINT('Ctrl Pts',(81.5477674300288,8.38143339017847,134.787669044119));
#68501=CARTESIAN_POINT('Ctrl Pts',(81.522792307153,8.32414468076876,134.783575439866));
#68502=CARTESIAN_POINT('Ctrl Pts',(81.5183001488764,8.3141126438614,134.782850283073));
#68503=CARTESIAN_POINT('Ctrl Pts',(81.5110793056081,8.2984054054304,134.781700638172));
#68504=CARTESIAN_POINT('Ctrl Pts',(81.5084170545687,8.29269976022694,134.781280041339));
#68505=CARTESIAN_POINT('Ctrl Pts',(81.50336467134,8.28202993069098,134.780487631935));
#68506=CARTESIAN_POINT('Ctrl Pts',(81.5009821783954,8.27706234566539,134.780116279215));
#68507=CARTESIAN_POINT('Ctrl Pts',(81.4953237456508,8.26541285384464,134.779239778075));
#68508=CARTESIAN_POINT('Ctrl Pts',(81.4920276294024,8.25874098493878,134.778733419276));
#68509=CARTESIAN_POINT('Ctrl Pts',(81.48095434106,8.23669997016199,134.77704663579));
#68510=CARTESIAN_POINT('Ctrl Pts',(81.4729838095861,8.22142994231128,134.775855347865));
#68511=CARTESIAN_POINT('Ctrl Pts',(81.4529702350702,8.18449536905194,134.772922993039));
#68512=CARTESIAN_POINT('Ctrl Pts',(81.4406778902115,8.16297109229459,134.77117054613));
#68513=CARTESIAN_POINT('Ctrl Pts',(81.3870267135645,8.07371117513843,134.763741238432));
#68514=CARTESIAN_POINT('Ctrl Pts',(81.341336430295,8.00870296076878,134.757935350165));
#68515=CARTESIAN_POINT('Ctrl Pts',(81.2263388287413,7.86766591825471,134.744710260202));
#68516=CARTESIAN_POINT('Ctrl Pts',(81.1542689103373,7.79428149358286,134.737354382563));
#68517=CARTESIAN_POINT('Ctrl Pts',(81.0578765739544,7.71275105004603,134.728663376349));
#68518=CARTESIAN_POINT('Ctrl Pts',(81.0395393957121,7.69789760444843,134.727054307098));
#68519=CARTESIAN_POINT('Ctrl Pts',(81.0113080575839,7.67600638428667,134.724641711067));
#68520=CARTESIAN_POINT('Ctrl Pts',(81.0016430053057,7.66867945813251,134.723826839451));
#68521=CARTESIAN_POINT('Ctrl Pts',(80.9840864605018,7.65566954206517,134.722366111667));
#68522=CARTESIAN_POINT('Ctrl Pts',(80.97622367182,7.64994893010276,134.721718810443));
#68523=CARTESIAN_POINT('Ctrl Pts',(80.9592655601433,7.63783659249082,134.720337172478));
#68524=CARTESIAN_POINT('Ctrl Pts',(80.9501554004482,7.6314663728264,134.719603681144));
#68525=CARTESIAN_POINT('Ctrl Pts',(80.9249698491532,7.61422827459938,134.717599184103));
#68526=CARTESIAN_POINT('Ctrl Pts',(80.9087669674189,7.60354908903928,134.716335285497));
#68527=CARTESIAN_POINT('Ctrl Pts',(80.8722537008129,7.58038823382266,134.713540641305));
#68528=CARTESIAN_POINT('Ctrl Pts',(80.8518543935338,7.56805437866129,134.712015197801));
#68529=CARTESIAN_POINT('Ctrl Pts',(80.7856299839704,7.52992994320918,134.707166428122));
#68530=CARTESIAN_POINT('Ctrl Pts',(80.7388449438088,7.50586840734171,134.703897004702));
#68531=CARTESIAN_POINT('Ctrl Pts',(80.603661743914,7.4442491239965,134.69475156433));
#68532=CARTESIAN_POINT('Ctrl Pts',(80.513053586177,7.41206331113077,134.688976222279));
#68533=CARTESIAN_POINT('Ctrl Pts',(80.3702990586206,7.37485630706935,134.679799176776));
#68534=CARTESIAN_POINT('Ctrl Pts',(80.3198439569555,7.36417845165627,134.676538811708));
#68535=CARTESIAN_POINT('Ctrl Pts',(80.2581314695191,7.35408232145139,134.672442808601));
#68536=CARTESIAN_POINT('Ctrl Pts',(80.2472651147339,7.3524148558345,134.671717543446));
#68537=CARTESIAN_POINT('Ctrl Pts',(80.230150472288,7.34996169503671,134.67056776409));
#68538=CARTESIAN_POINT('Ctrl Pts',(80.2239126446682,7.34910364588566,134.670147142652));
#68539=CARTESIAN_POINT('Ctrl Pts',(80.2122079664861,7.34756115590539,134.669354714707));
#68540=CARTESIAN_POINT('Ctrl Pts',(80.2067424029856,7.34686844752748,134.668983368338));
#68541=CARTESIAN_POINT('Ctrl Pts',(80.19388701471,7.34530389645441,134.668106919998));
#68542=CARTESIAN_POINT('Ctrl Pts',(80.1864946807959,7.34445444088535,134.667600608097));
#68543=CARTESIAN_POINT('Ctrl Pts',(80.1619759648962,7.34180328468377,134.665914144554));
#68544=CARTESIAN_POINT('Ctrl Pts',(80.1448279913955,7.34021767842525,134.66472313512));
#68545=CARTESIAN_POINT('Ctrl Pts',(80.1029546813816,7.33699962101212,134.661791608797));
#68546=CARTESIAN_POINT('Ctrl Pts',(80.0782119829312,7.33565247579054,134.660039719719));
#68547=CARTESIAN_POINT('Ctrl Pts',(79.9741769426422,7.3323130279938,134.652614366621));
#68548=CARTESIAN_POINT('Ctrl Pts',(79.8948266089783,7.33543267728944,134.646811988994));
#68549=CARTESIAN_POINT('Ctrl Pts',(79.7140227875555,7.3555239420664,134.633591198007));
#68550=CARTESIAN_POINT('Ctrl Pts',(79.6132923451326,7.37625491741082,134.626236039483));
#68551=CARTESIAN_POINT('Ctrl Pts',(79.4924794818541,7.41300983157092,134.617542352806));
#68552=CARTESIAN_POINT('Ctrl Pts',(79.470010608614,7.42037149447115,134.615930088245));
#68553=CARTESIAN_POINT('Ctrl Pts',(79.4362541554326,7.43223281902356,134.613513699278));
#68554=CARTESIAN_POINT('Ctrl Pts',(79.4248473719495,7.43638151105058,134.612698176615));
#68555=CARTESIAN_POINT('Ctrl Pts',(79.4043851854499,7.44407791036834,134.611236744118));
#68556=CARTESIAN_POINT('Ctrl Pts',(79.395313677967,7.44758091510655,134.610589383219));
#68557=CARTESIAN_POINT('Ctrl Pts',(79.3759451212478,7.45525570856294,134.609208110183));
#68558=CARTESIAN_POINT('Ctrl Pts',(79.3656580385916,7.45945149259336,134.608475038938));
#68559=CARTESIAN_POINT('Ctrl Pts',(79.337549692951,7.47124531524862,134.606472966311));
#68560=CARTESIAN_POINT('Ctrl Pts',(79.3198174265426,7.47905193612013,134.605211042645));
#68561=CARTESIAN_POINT('Ctrl Pts',(79.2002987474682,7.534178404984,134.596703849676));
#68562=CARTESIAN_POINT('Ctrl Pts',(79.1033803906839,7.59137206742112,134.589823415652));
#68563=CARTESIAN_POINT('Ctrl Pts',(78.9278811533166,7.72044313864304,134.576519626134));
#68564=CARTESIAN_POINT('Ctrl Pts',(78.8489726735374,7.79093652603735,134.57011457457));
#68565=CARTESIAN_POINT('Ctrl Pts',(78.7672402454537,7.87925129477731,134.562295530178));
#68566=CARTESIAN_POINT('Ctrl Pts',(78.7573504110862,7.8902269442982,134.56132680261));
#68567=CARTESIAN_POINT('Ctrl Pts',(78.7429742663424,7.90661457736231,134.559882215023));
#68568=CARTESIAN_POINT('Ctrl Pts',(78.7383738375851,7.91192610573639,134.559414272181));
#68569=CARTESIAN_POINT('Ctrl Pts',(78.7302470677872,7.9214298816747,134.558577143894));
#68570=CARTESIAN_POINT('Ctrl Pts',(78.7267076060679,7.92561064453025,134.558208923318));
#68571=CARTESIAN_POINT('Ctrl Pts',(78.7190235218901,7.93477828291706,134.557401479233));
#68572=CARTESIAN_POINT('Ctrl Pts',(78.7148874323616,7.93977185052571,134.556961697435));
#68573=CARTESIAN_POINT('Ctrl Pts',(78.7030686725898,7.95421159584004,134.555690391752));
#68574=CARTESIAN_POINT('Ctrl Pts',(78.6954604622114,7.96371778601726,134.554853933028));
#68575=CARTESIAN_POINT('Ctrl Pts',(78.62665966037,8.05164037652404,134.547128469293));
#68576=CARTESIAN_POINT('Ctrl Pts',(78.5725065577799,8.13529879337757,134.539869065089));
#68577=CARTESIAN_POINT('Ctrl Pts',(78.4880026369898,8.29564766771051,134.526677331998));
#68578=CARTESIAN_POINT('Ctrl Pts',(78.4552417606265,8.37073639724606,134.520753607426));
#68579=CARTESIAN_POINT('Ctrl Pts',(78.4124015647396,8.49271341237347,134.511636873155));
#68580=CARTESIAN_POINT('Ctrl Pts',(78.3985939950807,8.53814715393391,134.508344061591));
#68581=CARTESIAN_POINT('Ctrl Pts',(78.3827529244764,8.59959576188696,134.504024965509));
#68582=CARTESIAN_POINT('Ctrl Pts',(78.3789844705253,8.61513594432263,134.502943853637));
#68583=CARTESIAN_POINT('Ctrl Pts',(78.3731378917345,8.64085717013506,134.501172268919));
#68584=CARTESIAN_POINT('Ctrl Pts',(78.3709303090874,8.65100738955739,134.5004776961));
#68585=CARTESIAN_POINT('Ctrl Pts',(78.3667977765972,8.67090252478805,134.499124894524));
#68586=CARTESIAN_POINT('Ctrl Pts',(78.3648647659361,8.68064530015661,134.498466434605));
#68587=CARTESIAN_POINT('Ctrl Pts',(78.3611942719982,8.70005300453407,134.497162480892));
#68588=CARTESIAN_POINT('Ctrl Pts',(78.3594548795604,8.70971715708942,134.496516951246));
#68589=CARTESIAN_POINT('Ctrl Pts',(78.3555736685381,8.73243147202584,134.495008221625));
#68590=CARTESIAN_POINT('Ctrl Pts',(78.3535015709651,8.74549299401506,134.494147213189));
#68591=CARTESIAN_POINT('Ctrl Pts',(78.3474319850282,8.78693577934105,134.491434719267));
#68592=CARTESIAN_POINT('Ctrl Pts',(78.3440110778587,8.81539706561595,134.489600685518));
#68593=CARTESIAN_POINT('Ctrl Pts',(78.3364011152609,8.89627585539281,134.484454790613));
#68594=CARTESIAN_POINT('Ctrl Pts',(78.3339564019042,8.94882309198879,134.481190393475));
#68595=CARTESIAN_POINT('Ctrl Pts',(78.334000588343,9.00140012801338,134.477956726976));
#68596=CARTESIAN_POINT('Ctrl Pts',(78.334000587195,9.00139876132414,134.477956811032));
#68597=CARTESIAN_POINT('Ctrl Pts',(78.3341144029438,9.13695939446217,134.469619369734));
#68598=CARTESIAN_POINT('Ctrl Pts',(78.3507729491612,9.27198368688069,134.461562220848));
#68599=CARTESIAN_POINT('Ctrl Pts',(78.3865043312805,9.41512871033398,134.452015614116));
#68600=CARTESIAN_POINT('Ctrl Pts',(78.3895374774457,9.42674414342167,134.451233266144));
#68601=CARTESIAN_POINT('Ctrl Pts',(78.3952949355229,9.44785628193003,134.449795506627));
#68602=CARTESIAN_POINT('Ctrl Pts',(78.3979787300738,9.45736356674616,134.449142174374));
#68603=CARTESIAN_POINT('Ctrl Pts',(78.4024251895845,9.47259559702508,134.448085140636));
#68604=CARTESIAN_POINT('Ctrl Pts',(78.4041345039162,9.47833585352387,134.44768442901));
#68605=CARTESIAN_POINT('Ctrl Pts',(78.4074892318674,9.48938362278601,134.446908425406));
#68606=CARTESIAN_POINT('Ctrl Pts',(78.4091303015437,9.49469230413346,134.446533381212));
#68607=CARTESIAN_POINT('Ctrl Pts',(78.4128412140502,9.50648726034336,134.445695424521));
#68608=CARTESIAN_POINT('Ctrl Pts',(78.4149243241241,9.51296925290203,134.445231765119));
#68609=CARTESIAN_POINT('Ctrl Pts',(78.4212156623015,9.5321416841275,134.443851358949));
#68610=CARTESIAN_POINT('Ctrl Pts',(78.4255368765548,9.5447940916601,134.442928665735));
#68611=CARTESIAN_POINT('Ctrl Pts',(78.4321583095151,9.56344447363863,134.441552517316));
#68612=CARTESIAN_POINT('Ctrl Pts',(78.4343415699454,9.56948301017296,134.441104442064));
#68613=CARTESIAN_POINT('Ctrl Pts',(78.4365593695155,9.57550794516687,134.440654960983));
#68614=CARTESIAN_POINT('',(78.33399962793,9.00042833786235,134.670001209792));
#68615=CARTESIAN_POINT('Ctrl Pts',(78.4365593788086,9.57550797041271,134.632696244622));
#68616=CARTESIAN_POINT('Ctrl Pts',(78.3964895291875,9.46665312599119,134.639837428959));
#68617=CARTESIAN_POINT('Ctrl Pts',(78.3678945384663,9.35390299944845,134.646774484532));
#68618=CARTESIAN_POINT('Ctrl Pts',(78.3463552045929,9.20536770540159,134.656260408587));
#68619=CARTESIAN_POINT('Ctrl Pts',(78.342501337998,9.171507483015,134.658447247285));
#68620=CARTESIAN_POINT('Ctrl Pts',(78.338872193526,9.12770335501346,134.661335059154));
#68621=CARTESIAN_POINT('Ctrl Pts',(78.3381436654843,9.11784416823972,134.661988859751));
#68622=CARTESIAN_POINT('Ctrl Pts',(78.3371147150437,9.10200200404197,134.663046400438));
#68623=CARTESIAN_POINT('Ctrl Pts',(78.3367587310335,9.09602269583068,134.663447144266));
#68624=CARTESIAN_POINT('Ctrl Pts',(78.3361542697455,9.0848549763065,134.664198821945));
#68625=CARTESIAN_POINT('Ctrl Pts',(78.3358978010449,9.07966711689634,134.664549308398));
#68626=CARTESIAN_POINT('Ctrl Pts',(78.3354160271824,9.06890111970038,134.665279246728));
#68627=CARTESIAN_POINT('Ctrl Pts',(78.335194491578,9.06332285323331,134.665658898888));
#68628=CARTESIAN_POINT('Ctrl Pts',(78.3346997106691,9.04905618855536,134.666633389127));
#68629=CARTESIAN_POINT('Ctrl Pts',(78.3344664262952,9.04036669725143,134.667230258446));
#68630=CARTESIAN_POINT('Ctrl Pts',(78.3341030873326,9.02126033511182,134.668549398473));
#68631=CARTESIAN_POINT('Ctrl Pts',(78.3340027210372,9.01084335607688,134.669273015857));
#68632=CARTESIAN_POINT('Ctrl Pts',(78.3340000545804,9.00042645273249,134.670000601306));
#68633=CARTESIAN_POINT('Ctrl Pts',(78.3340000550508,9.00042828629872,134.670000473238));
#68634=CARTESIAN_POINT('Ctrl Pts',(78.3339655643716,8.86626226295517,134.679371509964));
#68635=CARTESIAN_POINT('Ctrl Pts',(78.3501373438938,8.73258081952499,134.689320485778));
#68636=CARTESIAN_POINT('Ctrl Pts',(78.3979867997652,8.53793954488717,134.70375480757));
#68637=CARTESIAN_POINT('Ctrl Pts',(78.4176301614395,8.47459188357303,134.708453036327));
#68638=CARTESIAN_POINT('Ctrl Pts',(78.4507577524891,8.38667242062074,134.714950171927));
#68639=CARTESIAN_POINT('Ctrl Pts',(78.4611626488001,8.36101484640449,134.716843815114));
#68640=CARTESIAN_POINT('Ctrl Pts',(78.4772814611657,8.32394789450348,134.719577511883));
#68641=CARTESIAN_POINT('Ctrl Pts',(78.4824941151857,8.31232703772465,134.720434277576));
#68642=CARTESIAN_POINT('Ctrl Pts',(78.4919466359459,8.29188503438602,134.721941261321));
#68643=CARTESIAN_POINT('Ctrl Pts',(78.4961318749502,8.28303945517025,134.722593313147));
#68644=CARTESIAN_POINT('Ctrl Pts',(78.5050794805669,8.26455164845712,134.723956291029));
#68645=CARTESIAN_POINT('Ctrl Pts',(78.5098577732733,8.25491759483874,134.724666628887));
#68646=CARTESIAN_POINT('Ctrl Pts',(78.5227541482814,8.22953614636296,134.726538763998));
#68647=CARTESIAN_POINT('Ctrl Pts',(78.531030845559,8.21387054585789,134.727694978796));
#68648=CARTESIAN_POINT('Ctrl Pts',(78.5717445858448,8.13969933644567,134.733177471293));
#68649=CARTESIAN_POINT('Ctrl Pts',(78.6074377376139,8.08304708015765,134.737386447034));
#68650=CARTESIAN_POINT('Ctrl Pts',(78.7306339541458,7.91136886111357,134.750467103729));
#68651=CARTESIAN_POINT('Ctrl Pts',(78.8297057385005,7.80550903048326,134.758995701262));
#68652=CARTESIAN_POINT('Ctrl Pts',(78.9526798341496,7.70427666301174,134.769227894363));
#68653=CARTESIAN_POINT('Ctrl Pts',(78.9643223946167,7.69495197031709,134.770194072015));
#68654=CARTESIAN_POINT('Ctrl Pts',(78.9827584636376,7.68058832899099,134.771722870912));
#68655=CARTESIAN_POINT('Ctrl Pts',(78.9894680948451,7.67544242763187,134.772279029694));
#68656=CARTESIAN_POINT('Ctrl Pts',(79.0019141360088,7.66604663756914,134.773310855872));
#68657=CARTESIAN_POINT('Ctrl Pts',(79.0076392904091,7.66178208707062,134.773785562536));
#68658=CARTESIAN_POINT('Ctrl Pts',(79.0134457612967,7.65751471567714,134.774267280301));
#68659=CARTESIAN_POINT('Ctrl Pts',(79.0134999791126,7.6574748742329,134.774271778355));
#68660=CARTESIAN_POINT('Ctrl Pts',(79.0136085086173,7.65739513248702,134.774280782299));
#68661=CARTESIAN_POINT('Ctrl Pts',(79.0136628203814,7.65735523214674,134.774285288196));
#68662=CARTESIAN_POINT('Ctrl Pts',(79.0137715540034,7.65727536074349,134.774294309169));
#68663=CARTESIAN_POINT('Ctrl Pts',(79.0138259757974,7.65723538974719,134.774298824242));
#68664=CARTESIAN_POINT('Ctrl Pts',(79.0139349458008,7.65715536510478,134.774307864923));
#68665=CARTESIAN_POINT('Ctrl Pts',(79.0139894941712,7.65711531136321,134.774312390546));
#68666=CARTESIAN_POINT('Ctrl Pts',(79.0140987341401,7.65703510895518,134.774321453723));
#68667=CARTESIAN_POINT('Ctrl Pts',(79.0141534256526,7.65699496037784,134.77432599127));
#68668=CARTESIAN_POINT('Ctrl Pts',(79.0142372940766,7.65693340115975,134.774332949553));
#68669=CARTESIAN_POINT('Ctrl Pts',(79.0142664693503,7.65691198804299,134.774335370135));
#68670=CARTESIAN_POINT('Ctrl Pts',(79.0143255417741,7.65686863495178,134.774340271206));
#68671=CARTESIAN_POINT('Ctrl Pts',(79.014355439047,7.65684669496034,134.774342751704));
#68672=CARTESIAN_POINT('Ctrl Pts',(79.0144159916862,7.65680226176421,134.774347775614));
#68673=CARTESIAN_POINT('Ctrl Pts',(79.0144466469614,7.65677976870502,134.774350319018));
#68674=CARTESIAN_POINT('Ctrl Pts',(79.01450875407,7.65673420138942,134.77435547193));
#68675=CARTESIAN_POINT('Ctrl Pts',(79.0145402059464,7.65671112718616,134.774358081442));
#68676=CARTESIAN_POINT('Ctrl Pts',(79.014603947371,7.65666436767768,134.774363369984));
#68677=CARTESIAN_POINT('Ctrl Pts',(79.0146362368861,7.65664068248822,134.774366049012));
#68678=CARTESIAN_POINT('Ctrl Pts',(79.014701697453,7.65659266910958,134.774371480224));
#68679=CARTESIAN_POINT('Ctrl Pts',(79.0147348686655,7.65656834090136,134.774374232423));
#68680=CARTESIAN_POINT('Ctrl Pts',(79.0148021397554,7.65651900722135,134.774379813891));
#68681=CARTESIAN_POINT('Ctrl Pts',(79.014836239638,7.65649400185285,134.774382643161));
#68682=CARTESIAN_POINT('Ctrl Pts',(79.0149054185573,7.65644327715413,134.774388382961));
#68683=CARTESIAN_POINT('Ctrl Pts',(79.0149404976944,7.65641755786645,134.7743912935));
#68684=CARTESIAN_POINT('Ctrl Pts',(79.0192893423312,7.65322933803952,134.774752121319));
#68685=CARTESIAN_POINT('Ctrl Pts',(79.0236181254127,7.6500877643364,134.775111452968));
#68686=CARTESIAN_POINT('Ctrl Pts',(79.0330801844961,7.64329008805398,134.775897371685));
#68687=CARTESIAN_POINT('Ctrl Pts',(79.0382190092707,7.63964231271351,134.77632447413));
#68688=CARTESIAN_POINT('Ctrl Pts',(79.0524019646582,7.62969512779834,134.77750372754));
#68689=CARTESIAN_POINT('Ctrl Pts',(79.0614879140347,7.62345631103728,134.778259703456));
#68690=CARTESIAN_POINT('Ctrl Pts',(79.1133508313759,7.58859706382759,134.782574758738));
#68691=CARTESIAN_POINT('Ctrl Pts',(79.1573702490982,7.56188351848903,134.786236178465));
#68692=CARTESIAN_POINT('Ctrl Pts',(79.2868521186522,7.49129355265541,134.79686349874));
#68693=CARTESIAN_POINT('Ctrl Pts',(79.374969956264,7.45270766917598,134.803915883256));
#68694=CARTESIAN_POINT('Ctrl Pts',(79.5157219516368,7.4050722027638,134.81460187366));
#68695=CARTESIAN_POINT('Ctrl Pts',(79.5662936761663,7.39058407485569,134.81833561118));
#68696=CARTESIAN_POINT('Ctrl Pts',(79.6406651938631,7.37303889138632,134.823661050877));
#68697=CARTESIAN_POINT('Ctrl Pts',(79.6639759107463,7.36806499446573,134.825307363598));
#68698=CARTESIAN_POINT('Ctrl Pts',(79.7064425619118,7.35995231119174,134.828265793654));
#68699=CARTESIAN_POINT('Ctrl Pts',(79.7255615497273,7.35664490044277,134.829582901039));
#68700=CARTESIAN_POINT('Ctrl Pts',(79.7557168877124,7.35196927526038,134.831637901646));
#68701=CARTESIAN_POINT('Ctrl Pts',(79.7667160914956,7.35037636503631,134.832382812402));
#68702=CARTESIAN_POINT('Ctrl Pts',(79.787364243718,7.34759674316542,134.833772753076));
#68703=CARTESIAN_POINT('Ctrl Pts',(79.7970091768313,7.34638419800633,134.834418569438));
#68704=CARTESIAN_POINT('Ctrl Pts',(79.8187058503884,7.34384921928543,134.83586391477));
#68705=CARTESIAN_POINT('Ctrl Pts',(79.8307626083924,7.34257377376927,134.836661938393));
#68706=CARTESIAN_POINT('Ctrl Pts',(79.8663104509477,7.33920522971412,134.839000481215));
#68707=CARTESIAN_POINT('Ctrl Pts',(79.8898338919031,7.33747911813372,134.840529557292));
#68708=CARTESIAN_POINT('Ctrl Pts',(80.0169191278567,7.33086319106281,134.848704969525));
#68709=CARTESIAN_POINT('Ctrl Pts',(80.120732423455,7.33514835686051,134.855059492965));
#68710=CARTESIAN_POINT('Ctrl Pts',(80.3013471321691,7.35959770217609,134.866190415333));
#68711=CARTESIAN_POINT('Ctrl Pts',(80.3783618299464,7.37563230934988,134.870968067021));
#68712=CARTESIAN_POINT('Ctrl Pts',(80.4776725496375,7.40375667796768,134.877477389854));
#68713=CARTESIAN_POINT('Ctrl Pts',(80.5012401771179,7.41099969654625,134.879049101299));
#68714=CARTESIAN_POINT('Ctrl Pts',(80.5409205188762,7.42416519602091,134.88175494137));
#68715=CARTESIAN_POINT('Ctrl Pts',(80.5571187043268,7.42981879060742,134.882876657556));
#68716=CARTESIAN_POINT('Ctrl Pts',(80.5802011360544,7.43827728810236,134.884503721651));
#68717=CARTESIAN_POINT('Ctrl Pts',(80.587159019503,7.4408799059292,134.884997944199));
#68718=CARTESIAN_POINT('Ctrl Pts',(80.5992436735831,7.44549257245466,134.885863286103));
#68719=CARTESIAN_POINT('Ctrl Pts',(80.604378255201,7.44748164382845,134.88623316888));
#68720=CARTESIAN_POINT('Ctrl Pts',(80.6153667197088,7.4518012090293,134.887029625428));
#68721=CARTESIAN_POINT('Ctrl Pts',(80.6212171751045,7.45413942603265,134.887456624532));
#68722=CARTESIAN_POINT('Ctrl Pts',(80.6372592945784,7.46065665748178,134.888635321439));
#68723=CARTESIAN_POINT('Ctrl Pts',(80.6474227784382,7.46490356510367,134.889390838519));
#68724=CARTESIAN_POINT('Ctrl Pts',(80.7053387281912,7.48978172973047,134.893743378003));
#68725=CARTESIAN_POINT('Ctrl Pts',(80.7521418935547,7.51253793236193,134.897445033514));
#68726=CARTESIAN_POINT('Ctrl Pts',(80.8876317634994,7.58644525919441,134.908569778452));
#68727=CARTESIAN_POINT('Ctrl Pts',(80.9727652378245,7.64362368216281,134.916091786867));
#68728=CARTESIAN_POINT('Ctrl Pts',(81.1086268706204,7.75428135027503,134.928652989111));
#68729=CARTESIAN_POINT('Ctrl Pts',(81.1620649880607,7.80397487713806,134.933774979999));
#68730=CARTESIAN_POINT('Ctrl Pts',(81.2241714733357,7.86983598770199,134.939952857166));
#68731=CARTESIAN_POINT('Ctrl Pts',(81.2360566858485,7.8828471896814,134.941146718081));
#68732=CARTESIAN_POINT('Ctrl Pts',(81.2548457660713,7.90408335100636,134.943053756302));
#68733=CARTESIAN_POINT('Ctrl Pts',(81.2618801817239,7.91219045119758,134.94377235405));
#68734=CARTESIAN_POINT('Ctrl Pts',(81.2751807585309,7.92782189281806,134.945140271076));
#68735=CARTESIAN_POINT('Ctrl Pts',(81.2814598683829,7.93533457219946,134.945790105141));
#68736=CARTESIAN_POINT('Ctrl Pts',(81.2956442187441,7.9526128219236,134.947267694861));
#68737=CARTESIAN_POINT('Ctrl Pts',(81.3035060145859,7.96241341244177,134.948093679199));
#68738=CARTESIAN_POINT('Ctrl Pts',(81.3242023253096,7.98882017335116,134.950287944473));
#68739=CARTESIAN_POINT('Ctrl Pts',(81.3368354399322,8.00558182350233,134.951648345913));
#68740=CARTESIAN_POINT('Ctrl Pts',(81.4202054119589,8.12065857266002,134.960784214748));
#68741=CARTESIAN_POINT('Ctrl Pts',(81.4803566264465,8.22619584699319,134.968139287296));
#68742=CARTESIAN_POINT('Ctrl Pts',(81.5548111698802,8.39793574788531,134.979577599606));
#68743=CARTESIAN_POINT('Ctrl Pts',(81.5774554675545,8.46004432938995,134.983625386728));
#68744=CARTESIAN_POINT('Ctrl Pts',(81.602764709373,8.5448037509964,134.989224360882));
#68745=CARTESIAN_POINT('Ctrl Pts',(81.6087430956234,8.56640584542373,134.990657848497));
#68746=CARTESIAN_POINT('Ctrl Pts',(81.6182342449221,8.60360463697743,134.993147721655));
#68747=CARTESIAN_POINT('Ctrl Pts',(81.6219617264688,8.61914377097646,134.994194147028));
#68748=CARTESIAN_POINT('Ctrl Pts',(81.6270484136842,8.64177992750096,134.995730857786));
#68749=CARTESIAN_POINT('Ctrl Pts',(81.6285859996696,8.64883650862056,134.996211645075));
#68750=CARTESIAN_POINT('Ctrl Pts',(81.6312000630023,8.66122000055998,134.997058764868));
#68751=CARTESIAN_POINT('Ctrl Pts',(81.6322964316461,8.66654251908276,134.997423970398));
#68752=CARTESIAN_POINT('Ctrl Pts',(81.6346286589376,8.67815190451848,134.998223055866));
#68753=CARTESIAN_POINT('Ctrl Pts',(81.6358542801932,8.6844404656776,134.998657469107));
#68754=CARTESIAN_POINT('Ctrl Pts',(81.6391763465296,8.70202532500559,134.99987630194));
#68755=CARTESIAN_POINT('Ctrl Pts',(81.6411922067568,8.71333621756289,135.000664959297));
#68756=CARTESIAN_POINT('Ctrl Pts',(81.6540547720352,8.7900954033791,135.006044639556));
#68757=CARTESIAN_POINT('Ctrl Pts',(81.6610996002016,8.85611365607817,135.010805013117));
#68758=CARTESIAN_POINT('Ctrl Pts',(81.665209496978,8.94421690254066,135.017199631535));
#68759=CARTESIAN_POINT('Ctrl Pts',(81.6657983350307,8.96608376369899,135.018790384712));
#68760=CARTESIAN_POINT('Ctrl Pts',(81.6664768275813,9.05993177730709,135.025620917735));
#68761=CARTESIAN_POINT('Ctrl Pts',(81.662332170408,9.13187027488392,135.0308608838));
#68762=CARTESIAN_POINT('Ctrl Pts',(81.6453814388771,9.2697271088658,135.040783878553));
#68763=CARTESIAN_POINT('Ctrl Pts',(81.6332219646552,9.33559034233666,135.045471709918));
#68764=CARTESIAN_POINT('Ctrl Pts',(81.6129873141637,9.41728292185814,135.051211768597));
#68765=CARTESIAN_POINT('Ctrl Pts',(81.608583542799,9.43394946380289,135.05237908819));
#68766=CARTESIAN_POINT('Ctrl Pts',(81.6010414288129,9.46079906787661,135.054254202118));
#68767=CARTESIAN_POINT('Ctrl Pts',(81.5980627804573,9.47102526106106,135.054967094336));
#68768=CARTESIAN_POINT('Ctrl Pts',(81.5921510532064,9.4906193687477,135.056330834542));
#68769=CARTESIAN_POINT('Ctrl Pts',(81.5892328582637,9.49999127038626,135.056982134395));
#68770=CARTESIAN_POINT('Ctrl Pts',(81.5823384505464,9.52146257453709,135.058472316146));
#68771=CARTESIAN_POINT('Ctrl Pts',(81.5783059521219,9.53354336766289,135.059309318231));
#68772=CARTESIAN_POINT('Ctrl Pts',(81.5648133893197,9.57247301044821,135.062002881108));
#68773=CARTESIAN_POINT('Ctrl Pts',(81.5548033520058,9.59912684920207,135.063841354955));
#68774=CARTESIAN_POINT('Ctrl Pts',(81.4950347547579,9.74666919824612,135.074012539877));
#68775=CARTESIAN_POINT('Ctrl Pts',(81.4318677430366,9.86162693812818,135.081871730983));
#68776=CARTESIAN_POINT('Ctrl Pts',(81.3144981211259,10.0260261801304,135.094265552378));
#68777=CARTESIAN_POINT('Ctrl Pts',(81.2694138767051,10.0813052834377,135.098683841434));
#68778=CARTESIAN_POINT('Ctrl Pts',(81.2102100137371,10.1450747715085,135.104329553291));
#68779=CARTESIAN_POINT('Ctrl Pts',(81.1993213311166,10.156474301575,135.105362159929));
#68780=CARTESIAN_POINT('Ctrl Pts',(81.1832381854639,10.1728405671852,135.106882232634));
#68781=CARTESIAN_POINT('Ctrl Pts',(81.1781703771917,10.177931304084,135.107360485816));
#68782=CARTESIAN_POINT('Ctrl Pts',(81.1692137682067,10.1868128141315,135.108204821734));
#68783=CARTESIAN_POINT('Ctrl Pts',(81.1653391169179,10.1906175846407,135.108569803132));
#68784=CARTESIAN_POINT('Ctrl Pts',(81.1568337888374,10.1988882221994,135.109370462327));
#68785=CARTESIAN_POINT('Ctrl Pts',(81.1521958984812,10.2033461648048,135.109806692327));
#68786=CARTESIAN_POINT('Ctrl Pts',(81.1391183099488,10.2157714354649,135.11103542964));
#68787=CARTESIAN_POINT('Ctrl Pts',(81.1306211943769,10.2236774098439,135.111832280922));
#68788=CARTESIAN_POINT('Ctrl Pts',(81.0651948577583,10.283288863595,135.117951756461));
#68789=CARTESIAN_POINT('Ctrl Pts',(81.0048352230073,10.331079969485,135.123501132967));
#68790=CARTESIAN_POINT('Ctrl Pts',(80.8942455523406,10.406821720891,135.133244006134));
#68791=CARTESIAN_POINT('Ctrl Pts',(80.8454599825917,10.4366698097108,135.137414680222));
#68792=CARTESIAN_POINT('Ctrl Pts',(80.7224007237856,10.5035170862845,135.147535074295));
#68793=CARTESIAN_POINT('Ctrl Pts',(80.6467054064323,10.5375962292472,135.153421747104));
#68794=CARTESIAN_POINT('Ctrl Pts',(80.5472951364979,10.5737046696924,135.160693101657));
#68795=CARTESIAN_POINT('Ctrl Pts',(80.5256541130962,10.5810648934162,135.162250076072));
#68796=CARTESIAN_POINT('Ctrl Pts',(80.492595949516,10.5915542938227,135.164590482353));
#68797=CARTESIAN_POINT('Ctrl Pts',(80.4812863703349,10.5950107466402,135.165384517732));
#68798=CARTESIAN_POINT('Ctrl Pts',(80.4615343328447,10.6008181768382,135.166760054414));
#68799=CARTESIAN_POINT('Ctrl Pts',(80.4531084734992,10.603223469129,135.167343302369));
#68800=CARTESIAN_POINT('Ctrl Pts',(80.4340667845741,10.60849710561,135.168653637365));
#68801=CARTESIAN_POINT('Ctrl Pts',(80.4234406749298,10.6113270669855,135.1693794589));
#68802=CARTESIAN_POINT('Ctrl Pts',(80.3945261603837,10.6187218356989,135.1713403868));
#68803=CARTESIAN_POINT('Ctrl Pts',(80.376186701251,10.6230819096126,135.172568903385));
#68804=CARTESIAN_POINT('Ctrl Pts',(80.257825845632,10.6491073300895,135.180407936744));
#68805=CARTESIAN_POINT('Ctrl Pts',(80.1560575540375,10.6618300337175,135.186720343809));
#68806=CARTESIAN_POINT('Ctrl Pts',(79.9711508904763,10.6677991590036,135.198030615194));
#68807=CARTESIAN_POINT('Ctrl Pts',(79.8884694665592,10.6643153573151,135.203037381399));
#68808=CARTESIAN_POINT('Ctrl Pts',(79.7785227195045,10.6514512508697,135.209983518382));
#68809=CARTESIAN_POINT('Ctrl Pts',(79.7507402310437,10.647486815931,135.211764281708));
#68810=CARTESIAN_POINT('Ctrl Pts',(79.704468073352,10.6396868145213,135.214792621852));
#68811=CARTESIAN_POINT('Ctrl Pts',(79.6859189679776,10.6362350079938,135.216023557846));
#68812=CARTESIAN_POINT('Ctrl Pts',(79.6598766766881,10.6309296734533,135.217780840331));
#68813=CARTESIAN_POINT('Ctrl Pts',(79.652330865977,10.6293377925579,135.218293479883));
#68814=CARTESIAN_POINT('Ctrl Pts',(79.6393774296913,10.6265110289581,135.219179887729));
#68815=CARTESIAN_POINT('Ctrl Pts',(79.6339644523312,10.625301431283,135.21955223185));
#68816=CARTESIAN_POINT('Ctrl Pts',(79.6225562905157,10.6226922518594,135.220341200459));
#68817=CARTESIAN_POINT('Ctrl Pts',(79.616562882159,10.6212864866049,135.220758140634));
#68818=CARTESIAN_POINT('Ctrl Pts',(79.600227109927,10.6173592548224,135.221900991594));
#68819=CARTESIAN_POINT('Ctrl Pts',(79.5899011146247,10.6147718762332,135.222630451623));
#68820=CARTESIAN_POINT('Ctrl Pts',(79.5378582464754,10.6012001597168,135.226340226601));
#68821=CARTESIAN_POINT('Ctrl Pts',(79.4965578283731,10.5886982831219,135.22939244255));
#68822=CARTESIAN_POINT('Ctrl Pts',(79.3705372398145,10.5451438203399,135.238953074695));
#68823=CARTESIAN_POINT('Ctrl Pts',(79.2878164753645,10.5088032830177,135.245574547554));
#68824=CARTESIAN_POINT('Ctrl Pts',(79.126556758386,10.4217290802034,135.258830502727));
#68825=CARTESIAN_POINT('Ctrl Pts',(79.0485067711148,10.3707233603725,135.26543372522));
#68826=CARTESIAN_POINT('Ctrl Pts',(78.9605025005847,10.3020539474665,135.273062215689));
#68827=CARTESIAN_POINT('Ctrl Pts',(78.9460807894463,10.2904084156567,135.27431932258));
#68828=CARTESIAN_POINT('Ctrl Pts',(78.9234687965993,10.2715172078411,135.276302367087));
#68829=CARTESIAN_POINT('Ctrl Pts',(78.9151506769188,10.264427695755,135.277034524169));
#68830=CARTESIAN_POINT('Ctrl Pts',(78.8995470943713,10.2508614659861,135.278413302258));
#68831=CARTESIAN_POINT('Ctrl Pts',(78.8922475758704,10.244401694923,135.279060581157));
#68832=CARTESIAN_POINT('Ctrl Pts',(78.8757834475827,10.2295719472118,135.280526008271));
#68833=CARTESIAN_POINT('Ctrl Pts',(78.8666547623747,10.2211628131991,135.281342467502));
#68834=CARTESIAN_POINT('Ctrl Pts',(78.8430725753683,10.1989472090883,135.283462807994));
#68835=CARTESIAN_POINT('Ctrl Pts',(78.8287717965673,10.1849810236034,135.284759832465));
#68836=CARTESIAN_POINT('Ctrl Pts',(78.7067132658651,10.061409291051,135.295942556402));
#68837=CARTESIAN_POINT('Ctrl Pts',(78.6143579187439,9.93764471136762,135.305096360121));
#68838=CARTESIAN_POINT('Ctrl Pts',(78.5113757384388,9.75043263522426,135.318278407621));
#68839=CARTESIAN_POINT('Ctrl Pts',(78.4853363743524,9.69637913181366,135.322029156211));
#68840=CARTESIAN_POINT('Ctrl Pts',(78.4566660025697,9.62760516086039,135.326874455342));
#68841=CARTESIAN_POINT('Ctrl Pts',(78.4512393376177,9.61409155740559,135.327829956955));
#68842=CARTESIAN_POINT('Ctrl Pts',(78.4434820923841,9.59401720648724,135.329256871534));
#68843=CARTESIAN_POINT('Ctrl Pts',(78.4410142084785,9.58750977509323,135.329720586687));
#68844=CARTESIAN_POINT('Ctrl Pts',(78.4379080630576,9.57916195781168,135.330317158519));
#68845=CARTESIAN_POINT('Ctrl Pts',(78.4372321137202,9.57733554043893,135.330447786867));
#68846=CARTESIAN_POINT('Ctrl Pts',(78.4365593737638,9.57550795670805,135.330578607084));
#68847=CARTESIAN_POINT('Origin',(80.,9.,134.));
#68848=CARTESIAN_POINT('',(78.4365593745323,9.57550795879571,136.032852165095));
#68849=CARTESIAN_POINT('',(78.4365593737294,9.5755079566144,135.837694135948));
#68850=CARTESIAN_POINT('',(78.4365593737638,9.57550795670799,134.));
#68851=CARTESIAN_POINT('Ctrl Pts',(78.4365593737294,9.5755079566144,135.837694135948));
#68852=CARTESIAN_POINT('Ctrl Pts',(78.4371889020499,9.57721815043606,135.837570608446));
#68853=CARTESIAN_POINT('Ctrl Pts',(78.4378212447466,9.57892733385798,135.837447172522));
#68854=CARTESIAN_POINT('Ctrl Pts',(78.4430078465044,9.59287602418787,135.836439956826));
#68855=CARTESIAN_POINT('Ctrl Pts',(78.4477031699583,9.60506290119926,135.835560896534));
#68856=CARTESIAN_POINT('Ctrl Pts',(78.456184053024,9.62632659361785,135.834028387693));
#68857=CARTESIAN_POINT('Ctrl Pts',(78.4599075277412,9.63542730821962,135.833372898105));
#68858=CARTESIAN_POINT('Ctrl Pts',(78.4678162009344,9.65427929313463,135.832015684355));
#68859=CARTESIAN_POINT('Ctrl Pts',(78.4720144386067,9.66402463848485,135.831314436495));
#68860=CARTESIAN_POINT('Ctrl Pts',(78.4831971227381,9.6893151977885,135.82949506286));
#68861=CARTESIAN_POINT('Ctrl Pts',(78.4903275987439,9.70479478308494,135.828381950611));
#68862=CARTESIAN_POINT('Ctrl Pts',(78.5220251521166,9.77091790502434,135.823625425996));
#68863=CARTESIAN_POINT('Ctrl Pts',(78.5489137951427,9.82041080652283,135.820062437349));
#68864=CARTESIAN_POINT('Ctrl Pts',(78.6423744983455,9.97341519189136,135.808892894365));
#68865=CARTESIAN_POINT('Ctrl Pts',(78.717911922364,10.0709491270467,135.801557481335));
#68866=CARTESIAN_POINT('Ctrl Pts',(78.8269160378371,10.18345392699,135.791796678314));
#68867=CARTESIAN_POINT('Ctrl Pts',(78.8510660309233,10.2069132665183,135.789674860879));
#68868=CARTESIAN_POINT('Ctrl Pts',(78.8867641540232,10.2395476136788,135.786566292188));
#68869=CARTESIAN_POINT('Ctrl Pts',(78.8977504725858,10.2493271317726,135.785613198198));
#68870=CARTESIAN_POINT('Ctrl Pts',(78.9151944838268,10.2644457919935,135.78410274589));
#68871=CARTESIAN_POINT('Ctrl Pts',(78.9215656914436,10.2698840908047,135.783551656952));
#68872=CARTESIAN_POINT('Ctrl Pts',(78.9333776871248,10.2798135064164,135.78253043967));
#68873=CARTESIAN_POINT('Ctrl Pts',(78.9388065511281,10.2843185855315,135.782061266588));
#68874=CARTESIAN_POINT('Ctrl Pts',(78.944311691745,10.2888282273662,135.781585494046));
#68875=CARTESIAN_POINT('Ctrl Pts',(78.944359643814,10.2888675037541,135.781581349868));
#68876=CARTESIAN_POINT('Ctrl Pts',(78.9444557602574,10.2889462214621,135.781573043163));
#68877=CARTESIAN_POINT('Ctrl Pts',(78.9445039246395,10.2889856627496,135.781568880635));
#68878=CARTESIAN_POINT('Ctrl Pts',(78.9446004792839,10.2890647212547,135.781560536056));
#68879=CARTESIAN_POINT('Ctrl Pts',(78.9446488698297,10.2891043386629,135.781556353981));
#68880=CARTESIAN_POINT('Ctrl Pts',(78.9447458910764,10.2891837609702,135.781547969073));
#68881=CARTESIAN_POINT('Ctrl Pts',(78.9447945217013,10.2892235657627,135.781543766247));
#68882=CARTESIAN_POINT('Ctrl Pts',(78.9448920376513,10.2893033746091,135.781535338581));
#68883=CARTESIAN_POINT('Ctrl Pts',(78.9449409229435,10.2893433785888,135.781531113744));
#68884=CARTESIAN_POINT('Ctrl Pts',(78.9450389629839,10.289423597741,135.78152264078));
#68885=CARTESIAN_POINT('Ctrl Pts',(78.9450881177422,10.2894638128714,135.781518392651));
#68886=CARTESIAN_POINT('Ctrl Pts',(78.9492752585669,10.2928890513312,135.781156525011));
#68887=CARTESIAN_POINT('Ctrl Pts',(78.9534293415932,10.2962540019012,135.780797496679));
#68888=CARTESIAN_POINT('Ctrl Pts',(78.9624494181203,10.3034889497047,135.780017748647));
#68889=CARTESIAN_POINT('Ctrl Pts',(78.9673208142496,10.3073516543394,135.779596563731));
#68890=CARTESIAN_POINT('Ctrl Pts',(78.9808088158269,10.3179243531187,135.7784304457));
#68891=CARTESIAN_POINT('Ctrl Pts',(78.9894697747196,10.3245768827743,135.777681728199));
#68892=CARTESIAN_POINT('Ctrl Pts',(79.0359779336887,10.3595784389727,135.773664349366));
#68893=CARTESIAN_POINT('Ctrl Pts',(79.0749506047345,10.3863891275557,135.770309329564));
#68894=CARTESIAN_POINT('Ctrl Pts',(79.1888177813669,10.4577823086992,135.7606469809));
#68895=CARTESIAN_POINT('Ctrl Pts',(79.2661448503083,10.4981997819734,135.754255358622));
#68896=CARTESIAN_POINT('Ctrl Pts',(79.4233562643577,10.5652668334709,135.74189897358));
#68897=CARTESIAN_POINT('Ctrl Pts',(79.5028145895219,10.5922903771581,135.735944638444));
#68898=CARTESIAN_POINT('Ctrl Pts',(79.6062258886722,10.6189582228513,135.728601378606));
#68899=CARTESIAN_POINT('Ctrl Pts',(79.6285887039478,10.6242344407781,135.727036168204));
#68900=CARTESIAN_POINT('Ctrl Pts',(79.6626425303537,10.6315288478536,135.724685904037));
#68901=CARTESIAN_POINT('Ctrl Pts',(79.6742569685117,10.6338873687392,135.723890113654));
#68902=CARTESIAN_POINT('Ctrl Pts',(79.6945054233707,10.6377746854809,135.72251250527));
#68903=CARTESIAN_POINT('Ctrl Pts',(79.7031280474857,10.6393596022848,135.721928925997));
#68904=CARTESIAN_POINT('Ctrl Pts',(79.7225806466558,10.642776654463,135.720619073461));
#68905=CARTESIAN_POINT('Ctrl Pts',(79.7334171079582,10.6445699150402,135.719894055633));
#68906=CARTESIAN_POINT('Ctrl Pts',(79.7628286326272,10.6491386990061,135.717938345507));
#68907=CARTESIAN_POINT('Ctrl Pts',(79.781434530142,10.6517075672982,135.716714179264));
#68908=CARTESIAN_POINT('Ctrl Pts',(79.8914918128947,10.6650105351748,135.709542605456));
#68909=CARTESIAN_POINT('Ctrl Pts',(79.9836672967324,10.6684635269506,135.70383092974));
#68910=CARTESIAN_POINT('Ctrl Pts',(80.1702715709164,10.6599795974664,135.692386144377));
#68911=CARTESIAN_POINT('Ctrl Pts',(80.2643313114565,10.6476198988377,135.686675985887));
#68912=CARTESIAN_POINT('Ctrl Pts',(80.3832678283266,10.621540816857,135.679024852909));
#68913=CARTESIAN_POINT('Ctrl Pts',(80.4095641042411,10.6150993561976,135.677304690945));
#68914=CARTESIAN_POINT('Ctrl Pts',(80.4534309272396,10.6032137196487,135.674369289443));
#68915=CARTESIAN_POINT('Ctrl Pts',(80.4710899431191,10.5981138989459,135.673169399217));
#68916=CARTESIAN_POINT('Ctrl Pts',(80.495958918979,10.5904839007493,135.671448951928));
#68917=CARTESIAN_POINT('Ctrl Pts',(80.5032421119597,10.5881944650987,135.670941340366));
#68918=CARTESIAN_POINT('Ctrl Pts',(80.5157789344344,10.5841586850526,135.670060658604));
#68919=CARTESIAN_POINT('Ctrl Pts',(80.5210400278227,10.5824360768028,135.669688960555));
#68920=CARTESIAN_POINT('Ctrl Pts',(80.5321708221944,10.5787300593399,135.668897925723));
#68921=CARTESIAN_POINT('Ctrl Pts',(80.5380379820997,10.5767401532695,135.668478244052));
#68922=CARTESIAN_POINT('Ctrl Pts',(80.5541224476665,10.5711847185626,135.667320493298));
#68923=CARTESIAN_POINT('Ctrl Pts',(80.5643161112282,10.5675523653185,135.666578725591));
#68924=CARTESIAN_POINT('Ctrl Pts',(80.6173642992726,10.548064989706,135.662679060297));
#68925=CARTESIAN_POINT('Ctrl Pts',(80.6595849349259,10.5305524484115,135.659440510941));
#68926=CARTESIAN_POINT('Ctrl Pts',(80.7954511837306,10.4675310484174,135.648683421257));
#68927=CARTESIAN_POINT('Ctrl Pts',(80.8855625271718,10.4149806455776,135.641024428585));
#68928=CARTESIAN_POINT('Ctrl Pts',(81.0332169965827,10.3092099344154,135.627972585677));
#68929=CARTESIAN_POINT('Ctrl Pts',(81.0930285014872,10.2597062551331,135.622511354908));
#68930=CARTESIAN_POINT('Ctrl Pts',(81.1621294348974,10.1938722759951,135.615995350205));
#68931=CARTESIAN_POINT('Ctrl Pts',(81.1748786032305,10.1813281279153,135.614783283866));
#68932=CARTESIAN_POINT('Ctrl Pts',(81.1949931638495,10.1608892250598,135.612854227821));
#68933=CARTESIAN_POINT('Ctrl Pts',(81.2024878104736,10.153124247273,135.612131593229));
#68934=CARTESIAN_POINT('Ctrl Pts',(81.2166293532872,10.13818480507,135.610760346202));
#68935=CARTESIAN_POINT('Ctrl Pts',(81.2232895281687,10.1310235943625,135.610111177375));
#68936=CARTESIAN_POINT('Ctrl Pts',(81.2382912286932,10.114605796552,135.608640963039));
#68937=CARTESIAN_POINT('Ctrl Pts',(81.246592802831,10.1053133703756,135.607821622425));
#68938=CARTESIAN_POINT('Ctrl Pts',(81.2724752762651,10.0756790851664,135.605247713919));
#68939=CARTESIAN_POINT('Ctrl Pts',(81.2896689976927,10.0550037108813,135.603508996473));
#68940=CARTESIAN_POINT('Ctrl Pts',(81.388552741998,9.93006435616154,135.593309988638));
#68941=CARTESIAN_POINT('Ctrl Pts',(81.4580714713327,9.8167794409514,135.585345574692));
#68942=CARTESIAN_POINT('Ctrl Pts',(81.5434655964223,9.63121112141915,135.57281469744));
#68943=CARTESIAN_POINT('Ctrl Pts',(81.5692342064941,9.56410563174356,135.568364281595));
#68944=CARTESIAN_POINT('Ctrl Pts',(81.595296918562,9.48045189419966,135.562679933504));
#68945=CARTESIAN_POINT('Ctrl Pts',(81.5997871089906,9.46528211039712,135.561643733308));
#68946=CARTESIAN_POINT('Ctrl Pts',(81.6060039428389,9.44312424672617,135.560119255425));
#68947=CARTESIAN_POINT('Ctrl Pts',(81.607902550172,9.43618476227067,135.559640263588));
#68948=CARTESIAN_POINT('Ctrl Pts',(81.6111558893842,9.42398374722654,135.558795028424));
#68949=CARTESIAN_POINT('Ctrl Pts',(81.6125299211568,9.41872756049863,135.558429893178));
#68950=CARTESIAN_POINT('Ctrl Pts',(81.6154737145086,9.4072370390653,135.557629381805));
#68951=CARTESIAN_POINT('Ctrl Pts',(81.6170330850204,9.40100040737403,135.557193457639));
#68952=CARTESIAN_POINT('Ctrl Pts',(81.6213006324686,9.38350280744024,135.555966702875));
#68953=CARTESIAN_POINT('Ctrl Pts',(81.6239274687256,9.37222265080472,135.555171551032));
#68954=CARTESIAN_POINT('Ctrl Pts',(81.6418716392339,9.29135891068976,135.54944506218));
#68955=CARTESIAN_POINT('Ctrl Pts',(81.6528271685414,9.22089036318195,135.544318813724));
#68956=CARTESIAN_POINT('Ctrl Pts',(81.6605271818987,9.13568532352874,135.538107697812));
#68957=CARTESIAN_POINT('Ctrl Pts',(81.6616320165991,9.1214086708507,135.537066427058));
#68958=CARTESIAN_POINT('Ctrl Pts',(81.6667939648985,9.04129254314559,135.531224458975));
#68959=CARTESIAN_POINT('Ctrl Pts',(81.6671221653112,8.97526858400889,135.52641825763));
#68960=CARTESIAN_POINT('Ctrl Pts',(81.6594838417457,8.83502385270356,135.516341107659));
#68961=CARTESIAN_POINT('Ctrl Pts',(81.6504498133135,8.76099797400832,135.511102797069));
#68962=CARTESIAN_POINT('Ctrl Pts',(81.6331693527157,8.67041276363314,135.504808441865));
#68963=CARTESIAN_POINT('Ctrl Pts',(81.6295720065072,8.65306340820967,135.503607945659));
#68964=CARTESIAN_POINT('Ctrl Pts',(81.6233470671427,8.62527879573648,135.50169280095));
#68965=CARTESIAN_POINT('Ctrl Pts',(81.62089403588,8.61480626282599,135.500972651338));
#68966=CARTESIAN_POINT('Ctrl Pts',(81.6160151736116,8.59484969448182,135.499603326994));
#68967=CARTESIAN_POINT('Ctrl Pts',(81.6136068461751,8.58536188747445,135.498953622558));
#68968=CARTESIAN_POINT('Ctrl Pts',(81.607925652204,8.56377979931247,135.49747842109));
#68969=CARTESIAN_POINT('Ctrl Pts',(81.6045996705743,8.55170001343006,135.496654672192));
#68970=CARTESIAN_POINT('Ctrl Pts',(81.5953745508907,8.51961363783677,135.494470982989));
#68971=CARTESIAN_POINT('Ctrl Pts',(81.589235335494,8.49967797878135,135.493118796825));
#68972=CARTESIAN_POINT('Ctrl Pts',(81.5442627613074,8.36283131153741,135.483856233414));
#68973=CARTESIAN_POINT('Ctrl Pts',(81.4929411815564,8.25042551509475,135.476383324012));
#68974=CARTESIAN_POINT('Ctrl Pts',(81.3823894100486,8.06563168265518,135.463221266979));
#68975=CARTESIAN_POINT('Ctrl Pts',(81.3286182436084,7.99063711854755,135.457567557998));
#68976=CARTESIAN_POINT('Ctrl Pts',(81.2608470093163,7.91097446152881,135.450737524056));
#68977=CARTESIAN_POINT('Ctrl Pts',(81.2526526459669,7.90155877259471,135.449915906257));
#68978=CARTESIAN_POINT('Ctrl Pts',(81.2399998363058,7.88734584060681,135.448651989517));
#68979=CARTESIAN_POINT('Ctrl Pts',(81.2356174078701,7.882481100754,135.448215062634));
#68980=CARTESIAN_POINT('Ctrl Pts',(81.2275203207019,7.87359873861287,135.44740904312));
#68981=CARTESIAN_POINT('Ctrl Pts',(81.2238144068862,7.86957342830091,135.447040593474));
#68982=CARTESIAN_POINT('Ctrl Pts',(81.2152813085664,7.86039604004827,135.446193269992));
#68983=CARTESIAN_POINT('Ctrl Pts',(81.2104411737599,7.85525635848035,135.445713440452));
#68984=CARTESIAN_POINT('Ctrl Pts',(81.195154867592,7.83922935100644,135.444200921511));
#68985=CARTESIAN_POINT('Ctrl Pts',(81.1845937089885,7.82845343159333,135.443160131475));
#68986=CARTESIAN_POINT('Ctrl Pts',(81.1004040028163,7.74485403017175,135.434906390445));
#68987=CARTESIAN_POINT('Ctrl Pts',(81.0202827741972,7.67890198977009,135.427321282152));
#68988=CARTESIAN_POINT('Ctrl Pts',(80.8402202887424,7.55688726559962,135.411504619801));
#68989=CARTESIAN_POINT('Ctrl Pts',(80.7395468894221,7.50279461738319,135.403335481153));
#68990=CARTESIAN_POINT('Ctrl Pts',(80.6161604699399,7.45200790544327,135.394204948353));
#68991=CARTESIAN_POINT('Ctrl Pts',(80.5980709950718,7.44492945826397,135.392886308833));
#68992=CARTESIAN_POINT('Ctrl Pts',(80.5694364482698,7.43429830858088,135.390829345355));
#68993=CARTESIAN_POINT('Ctrl Pts',(80.5589730075605,7.43053230605684,135.390083984161));
#68994=CARTESIAN_POINT('Ctrl Pts',(80.5392916128432,7.4236703741662,135.388693437174));
#68995=CARTESIAN_POINT('Ctrl Pts',(80.5300827980014,7.42054985293012,135.388047462111));
#68996=CARTESIAN_POINT('Ctrl Pts',(80.5093328045889,7.41372037989788,135.386602057814));
#68997=CARTESIAN_POINT('Ctrl Pts',(80.4977773224061,7.41005638802945,135.385804131618));
#68998=CARTESIAN_POINT('Ctrl Pts',(80.463642341964,7.39964155929411,135.383466789958));
#68999=CARTESIAN_POINT('Ctrl Pts',(80.4409578348283,7.39324313065237,135.381938796362));
#69000=CARTESIAN_POINT('Ctrl Pts',(80.3161449279824,7.36088081709177,135.3736550935));
#69001=CARTESIAN_POINT('Ctrl Pts',(80.2118627864795,7.34416881613139,135.367202248805));
#69002=CARTESIAN_POINT('Ctrl Pts',(80.0295733591696,7.33247099956887,135.356047607247));
#69003=CARTESIAN_POINT('Ctrl Pts',(79.9522106782296,7.33289410774803,135.351345341874));
#69004=CARTESIAN_POINT('Ctrl Pts',(79.8507929580685,7.34051498721274,135.344929256771));
#69005=CARTESIAN_POINT('Ctrl Pts',(79.8264674895346,7.34288214316547,135.34337078917));
#69006=CARTESIAN_POINT('Ctrl Pts',(79.7852787299223,7.34780711061536,135.340685489222));
#69007=CARTESIAN_POINT('Ctrl Pts',(79.7683861076351,7.3500904517831,135.339570821136));
#69008=CARTESIAN_POINT('Ctrl Pts',(79.7442041198344,7.35373775124611,135.337952115254));
#69009=CARTESIAN_POINT('Ctrl Pts',(79.7368835629395,7.35489190040628,135.337459044359));
#69010=CARTESIAN_POINT('Ctrl Pts',(79.7241384735539,7.35698851781325,135.336594912208));
#69011=CARTESIAN_POINT('Ctrl Pts',(79.7187105267668,7.35790909399508,135.336225075123));
#69012=CARTESIAN_POINT('Ctrl Pts',(79.7070675909919,7.35994315140387,135.335427754671));
#69013=CARTESIAN_POINT('Ctrl Pts',(79.7008544413295,7.36106504269217,135.334999837235));
#69014=CARTESIAN_POINT('Ctrl Pts',(79.6837663099493,7.3642510035482,135.333816498112));
#69015=CARTESIAN_POINT('Ctrl Pts',(79.6729055217632,7.36638813912674,135.333057211024));
#69016=CARTESIAN_POINT('Ctrl Pts',(79.6106135659066,7.37929173353919,135.328664026149));
#69017=CARTESIAN_POINT('Ctrl Pts',(79.5596980648687,7.39237748693745,135.324923475073));
#69018=CARTESIAN_POINT('Ctrl Pts',(79.4119690862255,7.43788958409844,135.31377785942));
#69019=CARTESIAN_POINT('Ctrl Pts',(79.3174062356663,7.47683327946542,135.306277611792));
#69020=CARTESIAN_POINT('Ctrl Pts',(79.1627104763143,7.55785936185751,135.293761005204));
#69021=CARTESIAN_POINT('Ctrl Pts',(79.1006811008133,7.59570249196534,135.288661579771));
#69022=CARTESIAN_POINT('Ctrl Pts',(79.0269119947805,7.64760742475122,135.282506098413));
#69023=CARTESIAN_POINT('Ctrl Pts',(79.0126747578349,7.65796615133012,135.281313313264));
#69024=CARTESIAN_POINT('Ctrl Pts',(78.9900273114165,7.6749994959794,135.279407441579));
#69025=CARTESIAN_POINT('Ctrl Pts',(78.9815130756263,7.68153287430435,135.278688948962));
#69026=CARTESIAN_POINT('Ctrl Pts',(78.9653497315866,7.69418578672538,135.277320881687));
#69027=CARTESIAN_POINT('Ctrl Pts',(78.9576903320825,7.70029137854909,135.276670795295));
#69028=CARTESIAN_POINT('Ctrl Pts',(78.9403207273325,7.71438964180317,135.27519214855));
#69029=CARTESIAN_POINT('Ctrl Pts',(78.9306462081757,7.72242548696557,135.274365366127));
#69030=CARTESIAN_POINT('Ctrl Pts',(78.9050436415752,7.74418608268522,135.272167883603));
#69031=CARTESIAN_POINT('Ctrl Pts',(78.8892825334564,7.75810435436498,135.270805098002));
#69032=CARTESIAN_POINT('Ctrl Pts',(78.785007142001,7.85376114434714,135.261708171914));
#69033=CARTESIAN_POINT('Ctrl Pts',(78.7053200499514,7.94459541896909,135.254389280659));
#69034=CARTESIAN_POINT('Ctrl Pts',(78.5979475730788,8.0976566520055,135.242965088757));
#69035=CARTESIAN_POINT('Ctrl Pts',(78.5630673382307,8.15430633410518,135.238892842738));
#69036=CARTESIAN_POINT('Ctrl Pts',(78.521038709007,8.23270897647865,135.233263027437));
#69037=CARTESIAN_POINT('Ctrl Pts',(78.5108140012874,8.25274704738411,135.231824481991));
#69038=CARTESIAN_POINT('Ctrl Pts',(78.4940058489315,8.28740306060595,135.22932661385));
#69039=CARTESIAN_POINT('Ctrl Pts',(78.4872217666789,8.301920669576,135.228277335055));
#69040=CARTESIAN_POINT('Ctrl Pts',(78.4776817992591,8.32312808515022,135.226737113721));
#69041=CARTESIAN_POINT('Ctrl Pts',(78.474758190257,8.32974205681834,135.226255727875));
#69042=CARTESIAN_POINT('Ctrl Pts',(78.4697121624634,8.34136148585165,135.22540785943));
#69043=CARTESIAN_POINT('Ctrl Pts',(78.4675710458501,8.34635861719915,135.225042509136));
#69044=CARTESIAN_POINT('Ctrl Pts',(78.4629609830329,8.35726516019802,135.224243469643));
#69045=CARTESIAN_POINT('Ctrl Pts',(78.4605016781524,8.36317826077445,135.223809250165));
#69046=CARTESIAN_POINT('Ctrl Pts',(78.453732180635,8.37972309185749,135.222591783484));
#69047=CARTESIAN_POINT('Ctrl Pts',(78.4494977200106,8.39038514328856,135.221804314434));
#69048=CARTESIAN_POINT('Ctrl Pts',(78.4217951048182,8.4622944255158,135.216477948403));
#69049=CARTESIAN_POINT('Ctrl Pts',(78.4018538499882,8.52483167063241,135.211773462402));
#69050=CARTESIAN_POINT('Ctrl Pts',(78.3800892829802,8.61018958902758,135.205388320628));
#69051=CARTESIAN_POINT('Ctrl Pts',(78.3749694611813,8.63211603112233,135.203751007043));
#69052=CARTESIAN_POINT('Ctrl Pts',(78.3556833935058,8.72299245558801,135.196989681015));
#69053=CARTESIAN_POINT('Ctrl Pts',(78.3454484854014,8.79270639435171,135.191865066245));
#69054=CARTESIAN_POINT('Ctrl Pts',(78.3359116036228,8.90817036100321,135.183580455327));
#69055=CARTESIAN_POINT('Ctrl Pts',(78.3340252029878,8.95361618722017,135.180369783187));
#69056=CARTESIAN_POINT('Ctrl Pts',(78.3339832799616,9.03001090103268,135.175064120421));
#69057=CARTESIAN_POINT('Ctrl Pts',(78.3348273798225,9.06093218182135,135.172941591376));
#69058=CARTESIAN_POINT('Ctrl Pts',(78.3372103810584,9.10410698033752,135.170011188523));
#69059=CARTESIAN_POINT('Ctrl Pts',(78.3380251523274,9.11639243985792,135.169181086744));
#69060=CARTESIAN_POINT('Ctrl Pts',(78.3396793292485,9.13774683111602,135.167744448532));
#69061=CARTESIAN_POINT('Ctrl Pts',(78.3404570351457,9.14681986477141,135.167136010918));
#69062=CARTESIAN_POINT('Ctrl Pts',(78.3422420221702,9.16581283062367,135.165866268476));
#69063=CARTESIAN_POINT('Ctrl Pts',(78.3432640475013,9.17573104138504,135.165205451804));
#69064=CARTESIAN_POINT('Ctrl Pts',(78.3459230598327,9.19944540806841,135.163630504336));
#69065=CARTESIAN_POINT('Ctrl Pts',(78.347643710537,9.21323158013467,135.162719032102));
#69066=CARTESIAN_POINT('Ctrl Pts',(78.3542717295818,9.26142340818167,135.159545705797));
#69067=CARTESIAN_POINT('Ctrl Pts',(78.3600831440737,9.29569699801195,135.157312135275));
#69068=CARTESIAN_POINT('Ctrl Pts',(78.377253028677,9.38072420582431,135.151806446648));
#69069=CARTESIAN_POINT('Ctrl Pts',(78.389923300544,9.43117546839901,135.148572236091));
#69070=CARTESIAN_POINT('Ctrl Pts',(78.4145339668366,9.51279575799008,135.143322369138));
#69071=CARTESIAN_POINT('Ctrl Pts',(78.4250816317236,9.54432720267512,135.141289483025));
#69072=CARTESIAN_POINT('Ctrl Pts',(78.436559333852,9.57550784828241,135.139259993339));
#69073=CARTESIAN_POINT('Ctrl Pts',(78.4365593737638,9.57550795670805,135.330578607084));
#69074=CARTESIAN_POINT('Ctrl Pts',(78.4355262723798,9.57270140528524,135.33077950276));
#69075=CARTESIAN_POINT('Ctrl Pts',(78.4345007395636,9.56989210354653,135.330980854609));
#69076=CARTESIAN_POINT('Ctrl Pts',(78.4313071287389,9.56106998627476,135.331613968312));
#69077=CARTESIAN_POINT('Ctrl Pts',(78.4291661450982,9.55504761120526,135.332047319095));
#69078=CARTESIAN_POINT('Ctrl Pts',(78.4232962754902,9.53823024994616,135.333260372946));
#69079=CARTESIAN_POINT('Ctrl Pts',(78.4196437447625,9.52740925797726,135.33404425235));
#69080=CARTESIAN_POINT('Ctrl Pts',(78.3963374997551,9.45594559517682,135.339239229933));
#69081=CARTESIAN_POINT('Ctrl Pts',(78.3800690873393,9.39426112985148,135.343806896006));
#69082=CARTESIAN_POINT('Ctrl Pts',(78.3452668265791,9.22301847979288,135.356465476987));
#69083=CARTESIAN_POINT('Ctrl Pts',(78.334083988153,9.11228258671161,135.364607419398));
#69084=CARTESIAN_POINT('Ctrl Pts',(78.3339601059339,8.9475905634631,135.37627703322));
#69085=CARTESIAN_POINT('Ctrl Pts',(78.3365124686746,8.89395279681553,135.380013427585));
#69086=CARTESIAN_POINT('Ctrl Pts',(78.3432447661313,8.82394431812517,135.384805757513));
#69087=CARTESIAN_POINT('Ctrl Pts',(78.3450880334805,8.80738658885369,135.385933100535));
#69088=CARTESIAN_POINT('Ctrl Pts',(78.3485009066364,8.78041502197843,135.387760125986));
#69089=CARTESIAN_POINT('Ctrl Pts',(78.3499213969916,8.76998384700473,135.388464434486));
#69090=CARTESIAN_POINT('Ctrl Pts',(78.3528637810574,8.74980904945305,135.38982244397));
#69091=CARTESIAN_POINT('Ctrl Pts',(78.3543734980957,8.74006412552131,135.390476498127));
#69092=CARTESIAN_POINT('Ctrl Pts',(78.3581156922323,8.71724976331965,135.392003588042));
#69093=CARTESIAN_POINT('Ctrl Pts',(78.3604178571507,8.7041923088771,135.392874387061));
#69094=CARTESIAN_POINT('Ctrl Pts',(78.3685721522937,8.66096687825507,135.39574766828));
#69095=CARTESIAN_POINT('Ctrl Pts',(78.3751032246534,8.63093233611292,135.397728715485));
#69096=CARTESIAN_POINT('Ctrl Pts',(78.3929307120513,8.55864300837883,135.402474127848));
#69097=CARTESIAN_POINT('Ctrl Pts',(78.4050672459156,8.51661856466896,135.405213399711));
#69098=CARTESIAN_POINT('Ctrl Pts',(78.4417660192211,8.40606709352683,135.412431961071));
#69099=CARTESIAN_POINT('Ctrl Pts',(78.4691873764116,8.33859052489656,135.416848633756));
#69100=CARTESIAN_POINT('Ctrl Pts',(78.5082913556486,8.25794485264148,135.422331579828));
#69101=CARTESIAN_POINT('Ctrl Pts',(78.5158807852211,8.24288001844525,135.423365202029));
#69102=CARTESIAN_POINT('Ctrl Pts',(78.5569119677471,8.16442251607549,135.428809918712));
#69103=CARTESIAN_POINT('Ctrl Pts',(78.594186073562,8.10312910721448,135.433275373539));
#69104=CARTESIAN_POINT('Ctrl Pts',(78.6419287132801,8.03494426001742,135.438720104484));
#69105=CARTESIAN_POINT('Ctrl Pts',(78.6486718058958,8.02552460550151,135.439483540475));
#69106=CARTESIAN_POINT('Ctrl Pts',(78.6593083991554,8.0109886991139,135.440680571152));
#69107=CARTESIAN_POINT('Ctrl Pts',(78.6631343644788,8.00582315911466,135.441109732105));
#69108=CARTESIAN_POINT('Ctrl Pts',(78.6702479503188,7.99633422592931,135.441905355014));
#69109=CARTESIAN_POINT('Ctrl Pts',(78.6735269361245,7.99200460944198,135.442271229362));
#69110=CARTESIAN_POINT('Ctrl Pts',(78.6811961254307,7.98198033279288,135.443124925565));
#69111=CARTESIAN_POINT('Ctrl Pts',(78.6856020646813,7.97629800956047,135.443613818828));
#69112=CARTESIAN_POINT('Ctrl Pts',(78.6998089939681,7.95821830353017,135.445184849795));
#69113=CARTESIAN_POINT('Ctrl Pts',(78.7097493242125,7.94593221112157,135.446275972561));
#69114=CARTESIAN_POINT('Ctrl Pts',(78.7657260411902,7.878724162347,135.4523678497));
#69115=CARTESIAN_POINT('Ctrl Pts',(78.815090538436,7.82668024068256,135.457545086332));
#69116=CARTESIAN_POINT('Ctrl Pts',(78.9644277739157,7.68830054279848,135.472346573717));
#69117=CARTESIAN_POINT('Ctrl Pts',(79.0715402208265,7.61041741960888,135.481955240158));
#69118=CARTESIAN_POINT('Ctrl Pts',(79.210581360526,7.53264839284583,135.492967592059));
#69119=CARTESIAN_POINT('Ctrl Pts',(79.2347530466752,7.51989872622275,135.494836149405));
#69120=CARTESIAN_POINT('Ctrl Pts',(79.2704570670618,7.50217482543893,135.497531655256));
#69121=CARTESIAN_POINT('Ctrl Pts',(79.2817482452908,7.49672771052085,135.498374914482));
#69122=CARTESIAN_POINT('Ctrl Pts',(79.3019624432637,7.48725568726848,135.499868658341));
#69123=CARTESIAN_POINT('Ctrl Pts',(79.3108613630338,7.48318104825195,135.500520834452));
#69124=CARTESIAN_POINT('Ctrl Pts',(79.329606366152,7.47479710343564,135.501883524849));
#69125=CARTESIAN_POINT('Ctrl Pts',(79.3394593108189,7.47050416572711,135.502593455724));
#69126=CARTESIAN_POINT('Ctrl Pts',(79.365634982382,7.45939952365756,135.504463258595));
#69127=CARTESIAN_POINT('Ctrl Pts',(79.3820261018241,7.45275176411336,135.505617573671));
#69128=CARTESIAN_POINT('Ctrl Pts',(79.4675358538586,7.41964720720809,135.511559328879));
#69129=CARTESIAN_POINT('Ctrl Pts',(79.5382595516358,7.39755475181327,135.516199808249));
#69130=CARTESIAN_POINT('Ctrl Pts',(79.6749399046776,7.36466444374126,135.524873926533));
#69131=CARTESIAN_POINT('Ctrl Pts',(79.7405293754179,7.3529840330421,135.528914746655));
#69132=CARTESIAN_POINT('Ctrl Pts',(79.8206920456076,7.34361696822805,135.53385549727));
#69133=CARTESIAN_POINT('Ctrl Pts',(79.8347620036837,7.34215426290705,135.534722882639));
#69134=CARTESIAN_POINT('Ctrl Pts',(79.919920544765,7.33439608424094,135.539982085897));
#69135=CARTESIAN_POINT('Ctrl Pts',(79.9913263135815,7.33249548365123,135.54442948329));
#69136=CARTESIAN_POINT('Ctrl Pts',(80.0741971893372,7.33561275340795,135.54985408425));
#69137=CARTESIAN_POINT('Ctrl Pts',(80.0857651839337,7.33616874523279,135.550617320797));
#69138=CARTESIAN_POINT('Ctrl Pts',(80.103742584287,7.3372207635344,135.551814104463));
#69139=CARTESIAN_POINT('Ctrl Pts',(80.110156765949,7.33763337483366,135.552243220755));
#69140=CARTESIAN_POINT('Ctrl Pts',(80.1219864120354,7.33846311626056,135.553038806115));
#69141=CARTESIAN_POINT('Ctrl Pts',(80.1274024210042,7.33886962559536,135.553404688075));
#69142=CARTESIAN_POINT('Ctrl Pts',(80.1399848731861,7.33987592262087,135.554258461848));
#69143=CARTESIAN_POINT('Ctrl Pts',(80.1471494855941,7.34049563390066,135.554747425744));
#69144=CARTESIAN_POINT('Ctrl Pts',(80.1700509906115,7.34262599477267,135.556318915199));
#69145=CARTESIAN_POINT('Ctrl Pts',(80.1857699441369,7.34431421607951,135.557410432914));
#69146=CARTESIAN_POINT('Ctrl Pts',(80.2726560108602,7.3548986234757,135.56350670515));
#69147=CARTESIAN_POINT('Ctrl Pts',(80.3432091811378,7.36815893093811,135.568688199619));
#69148=CARTESIAN_POINT('Ctrl Pts',(80.5406863706064,7.41864906966731,135.583506964158));
#69149=CARTESIAN_POINT('Ctrl Pts',(80.6643696174399,7.46649499200883,135.593128129855));
#69150=CARTESIAN_POINT('Ctrl Pts',(80.8027309224151,7.53993897976176,135.603954121002));
#69151=CARTESIAN_POINT('Ctrl Pts',(80.8240961288433,7.55189061297607,135.605629646067));
#69152=CARTESIAN_POINT('Ctrl Pts',(80.8557933317578,7.57055075849263,135.608122311018));
#69153=CARTESIAN_POINT('Ctrl Pts',(80.8663262234286,7.57690961304857,135.608951799932));
#69154=CARTESIAN_POINT('Ctrl Pts',(80.8845276031981,7.58817502206136,135.610387567001));
#69155=CARTESIAN_POINT('Ctrl Pts',(80.8922279884972,7.59302875958053,135.610995742188));
#69156=CARTESIAN_POINT('Ctrl Pts',(80.9082777442465,7.60333006208968,135.612265113588));
#69157=CARTESIAN_POINT('Ctrl Pts',(80.9166187988983,7.60878996517094,135.612925820588));
#69158=CARTESIAN_POINT('Ctrl Pts',(80.9364673964996,7.62203850458377,135.614500826786));
#69159=CARTESIAN_POINT('Ctrl Pts',(80.9479276130456,7.62989696471609,135.615412464521));
#69160=CARTESIAN_POINT('Ctrl Pts',(80.9877284052998,7.65792749639774,135.618588065335));
#69161=CARTESIAN_POINT('Ctrl Pts',(81.015535505028,7.67884371973154,135.620823683606));
#69162=CARTESIAN_POINT('Ctrl Pts',(81.0832734073492,7.73319888802652,135.626335958627));
#69163=CARTESIAN_POINT('Ctrl Pts',(81.1223302056246,7.76766812399154,135.629574577227));
#69164=CARTESIAN_POINT('Ctrl Pts',(81.2309739037552,7.87300760811763,135.638893173755));
#69165=CARTESIAN_POINT('Ctrl Pts',(81.2959154866832,7.94832989600981,135.644859765391));
#69166=CARTESIAN_POINT('Ctrl Pts',(81.3825097768175,8.06905684535266,135.654117567324));
#69167=CARTESIAN_POINT('Ctrl Pts',(81.4094588894118,8.11038599325179,135.657242339616));
#69168=CARTESIAN_POINT('Ctrl Pts',(81.4400674820342,8.1622171387033,135.661186180796));
#69169=CARTESIAN_POINT('Ctrl Pts',(81.4455101231757,8.17164322670767,135.661904399419));
#69170=CARTESIAN_POINT('Ctrl Pts',(81.4539421455483,8.18658278726268,135.663045365083));
#69171=CARTESIAN_POINT('Ctrl Pts',(81.4569935343459,8.19206116430724,135.66346431519));
#69172=CARTESIAN_POINT('Ctrl Pts',(81.4626695039906,8.2023883644143,135.664255362671));
#69173=CARTESIAN_POINT('Ctrl Pts',(81.4653010320628,8.2072331484142,135.664627018325));
#69174=CARTESIAN_POINT('Ctrl Pts',(81.4714469492169,8.21868325443794,135.665506598766));
#69175=CARTESIAN_POINT('Ctrl Pts',(81.4749409411293,8.22529928613699,135.666015761414));
#69176=CARTESIAN_POINT('Ctrl Pts',(81.4864437598857,8.24744029100124,135.667722237322));
#69177=CARTESIAN_POINT('Ctrl Pts',(81.4942526464905,8.26306707550487,135.668930754027));
#69178=CARTESIAN_POINT('Ctrl Pts',(81.5127500832846,8.30158649940001,135.671914618186));
#69179=CARTESIAN_POINT('Ctrl Pts',(81.5231661820241,8.32460465184501,135.673701839157));
#69180=CARTESIAN_POINT('Ctrl Pts',(81.5652864053762,8.42361949908233,135.681382280979));
#69181=CARTESIAN_POINT('Ctrl Pts',(81.5918557215902,8.5016722043508,135.68741180965));
#69182=CARTESIAN_POINT('Ctrl Pts',(81.6373024528799,8.67672963025059,135.700546199591));
#69183=CARTESIAN_POINT('Ctrl Pts',(81.6535550730723,8.77411413891817,135.707597502603));
#69184=CARTESIAN_POINT('Ctrl Pts',(81.6629257119012,8.89608075737983,135.71602037739));
#69185=CARTESIAN_POINT('Ctrl Pts',(81.6642393184605,8.91982067431672,135.7176418433));
#69186=CARTESIAN_POINT('Ctrl Pts',(81.6654563090048,8.95573707809814,135.720069018246));
#69187=CARTESIAN_POINT('Ctrl Pts',(81.665735071334,8.96789689741178,135.720886281368));
#69188=CARTESIAN_POINT('Ctrl Pts',(81.665997040466,8.98978188462742,135.722349441641));
#69189=CARTESIAN_POINT('Ctrl Pts',(81.6660283044952,8.99950580976594,135.722996807222));
#69190=CARTESIAN_POINT('Ctrl Pts',(81.6659130142133,9.02031603070605,135.724376609691));
#69191=CARTESIAN_POINT('Ctrl Pts',(81.66574093169,9.03140175975677,135.725108219727));
#69192=CARTESIAN_POINT('Ctrl Pts',(81.6649666818517,9.06175307058747,135.727102466855));
#69193=CARTESIAN_POINT('Ctrl Pts',(81.6641408185409,9.08101160115348,135.72835811806));
#69194=CARTESIAN_POINT('Ctrl Pts',(81.6615587931183,9.12384220092693,135.731131890408));
#69195=CARTESIAN_POINT('Ctrl Pts',(81.6596348364403,9.14740015750329,135.732644831843));
#69196=CARTESIAN_POINT('Ctrl Pts',(81.651886303822,9.22253291145368,135.737439086954));
#69197=CARTESIAN_POINT('Ctrl Pts',(81.6441529643126,9.27388116766472,135.740667914712));
#69198=CARTESIAN_POINT('Ctrl Pts',(81.6143575210505,9.42378454711294,135.750080428851));
#69199=CARTESIAN_POINT('Ctrl Pts',(81.5857260250495,9.52078278621531,135.756144397367));
#69200=CARTESIAN_POINT('Ctrl Pts',(81.530774782337,9.65923586281198,135.765435689647));
#69201=CARTESIAN_POINT('Ctrl Pts',(81.5111337397708,9.70309120762843,135.768482149024));
#69202=CARTESIAN_POINT('Ctrl Pts',(81.4847261831156,9.75582007881523,135.77234650148));
#69203=CARTESIAN_POINT('Ctrl Pts',(81.4797280760176,9.76555903475263,135.77306896099));
#69204=CARTESIAN_POINT('Ctrl Pts',(81.4717394179309,9.78075463082542,135.774211065236));
#69205=CARTESIAN_POINT('Ctrl Pts',(81.4688135424138,9.78624517951265,135.774626812462));
#69206=CARTESIAN_POINT('Ctrl Pts',(81.463230742399,9.79658165709692,135.77541556904));
#69207=CARTESIAN_POINT('Ctrl Pts',(81.4605803742529,9.80143091317351,135.775788174682));
#69208=CARTESIAN_POINT('Ctrl Pts',(81.454239459696,9.81289666766545,135.776675184424));
#69209=CARTESIAN_POINT('Ctrl Pts',(81.4505278485402,9.81950128338884,135.777190888842));
#69210=CARTESIAN_POINT('Ctrl Pts',(81.4378304522403,9.8417391122704,135.778942836025));
#69211=CARTESIAN_POINT('Ctrl Pts',(81.4286363033025,9.85725106568938,135.780191082515));
#69212=CARTESIAN_POINT('Ctrl Pts',(81.4053782746448,9.89507738748669,135.783294438228));
#69213=CARTESIAN_POINT('Ctrl Pts',(81.3910330153885,9.9172124186111,135.785162601277));
#69214=CARTESIAN_POINT('Ctrl Pts',(81.3256058612948,10.0131007982961,135.793459217994));
#69215=CARTESIAN_POINT('Ctrl Pts',(81.2691408661249,10.0829981997379,135.800041990791));
#69216=CARTESIAN_POINT('Ctrl Pts',(81.1397406665309,10.2190842941631,135.813648349463));
#69217=CARTESIAN_POINT('Ctrl Pts',(81.0660031271714,10.2840633393234,135.820625335516));
#69218=CARTESIAN_POINT('Ctrl Pts',(80.9717595732041,10.3533645055372,135.82862382769));
#69219=CARTESIAN_POINT('Ctrl Pts',(80.9563662710091,10.3642858056406,135.829904297675));
#69220=CARTESIAN_POINT('Ctrl Pts',(80.9317110782607,10.381155852343,135.831915381344));
#69221=CARTESIAN_POINT('Ctrl Pts',(80.9225705091458,10.3872781579476,135.832652520586));
#69222=CARTESIAN_POINT('Ctrl Pts',(80.9060423576129,10.3981130176164,135.833970623002));
#69223=CARTESIAN_POINT('Ctrl Pts',(80.8986770458846,10.4028586300952,135.834552805803));
#69224=CARTESIAN_POINT('Ctrl Pts',(80.8812895413516,10.4138686004615,135.835915252056));
#69225=CARTESIAN_POINT('Ctrl Pts',(80.8712373615092,10.4200849083835,135.836693722761));
#69226=CARTESIAN_POINT('Ctrl Pts',(80.8415842486195,10.4379891213393,135.838964119111));
#69227=CARTESIAN_POINT('Ctrl Pts',(80.8218078298927,10.4493821900743,135.840445372837));
#69228=CARTESIAN_POINT('Ctrl Pts',(80.7293814862687,10.5001281731556,135.847228376951));
#69229=CARTESIAN_POINT('Ctrl Pts',(80.654098593684,10.5344507911214,135.852354049634));
#69230=CARTESIAN_POINT('Ctrl Pts',(80.5227686740386,10.582895324556,135.86093616232));
#69231=CARTESIAN_POINT('Ctrl Pts',(80.4679769501478,10.5999506848582,135.864419714101));
#69232=CARTESIAN_POINT('Ctrl Pts',(80.3377702569209,10.633218563853,135.872667132635));
#69233=CARTESIAN_POINT('Ctrl Pts',(80.2619015467661,10.6470871492649,135.877449139394));
#69234=CARTESIAN_POINT('Ctrl Pts',(80.173821971105,10.6569479918808,135.883246274229));
#69235=CARTESIAN_POINT('Ctrl Pts',(80.1622741205884,10.658118758322,135.884011169932));
#69236=CARTESIAN_POINT('Ctrl Pts',(80.1443085207512,10.6597507154383,135.885210008354));
#69237=CARTESIAN_POINT('Ctrl Pts',(80.1378984781843,10.6602955739268,135.885639496073));
#69238=CARTESIAN_POINT('Ctrl Pts',(80.1260198425192,10.6612360039375,135.886438895678));
#69239=CARTESIAN_POINT('Ctrl Pts',(80.1205522586141,10.6616417216824,135.886808245399));
#69240=CARTESIAN_POINT('Ctrl Pts',(80.1078860378463,10.6625187652172,135.887667066783));
#69241=CARTESIAN_POINT('Ctrl Pts',(80.1006862709663,10.6629703280143,135.888157598022));
#69242=CARTESIAN_POINT('Ctrl Pts',(80.077574998257,10.6642692133135,135.889739284605));
#69243=CARTESIAN_POINT('Ctrl Pts',(80.0616547356785,10.6649349962972,135.890839590619));
#69244=CARTESIAN_POINT('Ctrl Pts',(80.0234091746146,10.6659851504276,135.893504900459));
#69245=CARTESIAN_POINT('Ctrl Pts',(80.0010812613823,10.6661492253617,135.895078907019));
#69246=CARTESIAN_POINT('Ctrl Pts',(79.9131523002241,10.6650280120699,135.901332136934));
#69247=CARTESIAN_POINT('Ctrl Pts',(79.8476567622816,10.6603166690618,135.906107479269));
#69248=CARTESIAN_POINT('Ctrl Pts',(79.6619254928567,10.6358727075662,135.919744178876));
#69249=CARTESIAN_POINT('Ctrl Pts',(79.5433200779141,10.6068066586641,135.92853648176));
#69250=CARTESIAN_POINT('Ctrl Pts',(79.4092286288398,10.5578783178132,135.938355106246));
#69251=CARTESIAN_POINT('Ctrl Pts',(79.3896674785021,10.5503193053925,135.939785442954));
#69252=CARTESIAN_POINT('Ctrl Pts',(79.3586268708904,10.5376456746956,135.942052817809));
#69253=CARTESIAN_POINT('Ctrl Pts',(79.3470540734671,10.5327672177043,135.942897634334));
#69254=CARTESIAN_POINT('Ctrl Pts',(79.3265595088388,10.523853585934,135.944393147976));
#69255=CARTESIAN_POINT('Ctrl Pts',(79.3176161856124,10.519869791592,135.945045550733));
#69256=CARTESIAN_POINT('Ctrl Pts',(79.2989405155616,10.5113526569068,135.946407729794));
#69257=CARTESIAN_POINT('Ctrl Pts',(79.2892157983496,10.5068035977015,135.947116931299));
#69258=CARTESIAN_POINT('Ctrl Pts',(79.2636366710297,10.4945353687164,135.948982554098));
#69259=CARTESIAN_POINT('Ctrl Pts',(79.2478593963666,10.4866578192775,135.950133464123));
#69260=CARTESIAN_POINT('Ctrl Pts',(79.1673402747877,10.4448448283746,135.956013131467));
#69261=CARTESIAN_POINT('Ctrl Pts',(79.1047536180214,10.4069238260739,135.960598823203));
#69262=CARTESIAN_POINT('Ctrl Pts',(78.9618238360485,10.3069107756024,135.971367229113));
#69263=CARTESIAN_POINT('Ctrl Pts',(78.8842717425862,10.2413599753503,135.977454361145));
#69264=CARTESIAN_POINT('Ctrl Pts',(78.7959791055502,10.1517330206466,135.985274076365));
#69265=CARTESIAN_POINT('Ctrl Pts',(78.7791866299631,10.1339179362806,135.986807656105));
#69266=CARTESIAN_POINT('Ctrl Pts',(78.741903796181,10.0925762592732,135.990337665404));
#69267=CARTESIAN_POINT('Ctrl Pts',(78.7216703511934,10.0688320524545,135.992344934213));
#69268=CARTESIAN_POINT('Ctrl Pts',(78.6961022820835,10.037062565829,135.995026271725));
#69269=CARTESIAN_POINT('Ctrl Pts',(78.6901526190616,10.0295376885197,135.995661063656));
#69270=CARTESIAN_POINT('Ctrl Pts',(78.680633553061,10.0172823066178,135.996695201466));
#69271=CARTESIAN_POINT('Ctrl Pts',(78.6770237243328,10.0125832725887,135.997091783689));
#69272=CARTESIAN_POINT('Ctrl Pts',(78.6700171507486,10.0033611596313,135.997870449096));
#69273=CARTESIAN_POINT('Ctrl Pts',(78.6666182534952,9.99883988229195,135.998252377929));
#69274=CARTESIAN_POINT('Ctrl Pts',(78.6582720049682,9.98761903026825,135.999200510252));
#69275=CARTESIAN_POINT('Ctrl Pts',(78.653351783978,9.98089955478689,135.999768517035));
#69276=CARTESIAN_POINT('Ctrl Pts',(78.6350024287481,9.95544183230182,136.001920485684));
#69277=CARTESIAN_POINT('Ctrl Pts',(78.6219130226321,9.93646335570433,136.003524716942));
#69278=CARTESIAN_POINT('Ctrl Pts',(78.5887353552704,9.88615620575833,136.007764765068));
#69279=CARTESIAN_POINT('Ctrl Pts',(78.5692960739808,9.85441596795094,136.010427614625));
#69280=CARTESIAN_POINT('Ctrl Pts',(78.5061596399335,9.74312315643574,136.019662196131));
#69281=CARTESIAN_POINT('Ctrl Pts',(78.4679062115829,9.66066563172754,136.026320752444));
#69282=CARTESIAN_POINT('Ctrl Pts',(78.4365593745323,9.57550795879571,136.032852165095));
#69283=CARTESIAN_POINT('Origin',(80.,9.,134.));
#69284=CARTESIAN_POINT('',(78.436559386885,9.57550799235334,136.733447166179));
#69285=CARTESIAN_POINT('',(78.4365593610507,9.57550792217121,136.539851329404));
#69286=CARTESIAN_POINT('',(78.4365593737638,9.57550795670799,134.));
#69287=CARTESIAN_POINT('',(78.3340002443602,8.99909766519367,135.879690700183));
#69288=CARTESIAN_POINT('Ctrl Pts',(78.4365593610507,9.57550792217122,136.539851329404));
#69289=CARTESIAN_POINT('Ctrl Pts',(78.4458980275004,9.60087760011751,136.537889809312));
#69290=CARTESIAN_POINT('Ctrl Pts',(78.4558546510834,9.62602120168908,136.535921262459));
#69291=CARTESIAN_POINT('Ctrl Pts',(78.513413053214,9.76163062536091,136.525197504869));
#69292=CARTESIAN_POINT('Ctrl Pts',(78.5722644735132,9.86695051212577,136.516515201914));
#69293=CARTESIAN_POINT('Ctrl Pts',(78.6541410523814,9.98217214453261,136.506791241766));
#69294=CARTESIAN_POINT('Ctrl Pts',(78.6666490069173,9.99908639648936,136.505356318561));
#69295=CARTESIAN_POINT('Ctrl Pts',(78.6871436490772,10.0257301910071,136.503083020575));
#69296=CARTESIAN_POINT('Ctrl Pts',(78.694925708194,10.0356135045628,136.502236805642));
#69297=CARTESIAN_POINT('Ctrl Pts',(78.7089655592686,10.0530346707326,136.500739553739));
#69298=CARTESIAN_POINT('Ctrl Pts',(78.7151792245619,10.060607150158,136.500086799618));
#69299=CARTESIAN_POINT('Ctrl Pts',(78.7283389195473,10.0763592497235,136.498724614947));
#69300=CARTESIAN_POINT('Ctrl Pts',(78.7352979370172,10.0845274726714,136.498015753178));
#69301=CARTESIAN_POINT('Ctrl Pts',(78.7538775446772,10.1059134442187,136.496152676661));
#69302=CARTESIAN_POINT('Ctrl Pts',(78.7656296915254,10.1190155047002,136.495003942963));
#69303=CARTESIAN_POINT('Ctrl Pts',(78.8268276349446,10.185105430601,136.489166463528));
#69304=CARTESIAN_POINT('Ctrl Pts',(78.879488287366,10.2350156611454,136.484618156925));
#69305=CARTESIAN_POINT('Ctrl Pts',(79.0133919326892,10.3462861007539,136.473867741119));
#69306=CARTESIAN_POINT('Ctrl Pts',(79.0973198710174,10.4039405144166,136.467764442186));
#69307=CARTESIAN_POINT('Ctrl Pts',(79.2322433804078,10.4794992547448,136.458155545519));
#69308=CARTESIAN_POINT('Ctrl Pts',(79.2797188993223,10.5031840215815,136.454805680345));
#69309=CARTESIAN_POINT('Ctrl Pts',(79.3384037901551,10.529042145102,136.450606265239));
#69310=CARTESIAN_POINT('Ctrl Pts',(79.3486145731024,10.5334198497632,136.44987349627));
#69311=CARTESIAN_POINT('Ctrl Pts',(79.3647039479201,10.5401282105118,136.448714407541));
#69312=CARTESIAN_POINT('Ctrl Pts',(79.370553547515,10.5425281646531,136.448292084374));
#69313=CARTESIAN_POINT('Ctrl Pts',(79.3810077458325,10.5467479118295,136.44753545195));
#69314=CARTESIAN_POINT('Ctrl Pts',(79.3856069953906,10.5485805587497,136.447201917851));
#69315=CARTESIAN_POINT('Ctrl Pts',(79.3967884586408,10.552978345497,136.446389492731));
#69316=CARTESIAN_POINT('Ctrl Pts',(79.4033788396736,10.5555221283219,136.445909364363));
#69317=CARTESIAN_POINT('Ctrl Pts',(79.4241170173408,10.56337556062,136.444394953272));
#69318=CARTESIAN_POINT('Ctrl Pts',(79.438320538265,10.5685345057026,136.443352542089));
#69319=CARTESIAN_POINT('Ctrl Pts',(79.5139094505476,10.5948313099461,136.437784753802));
#69320=CARTESIAN_POINT('Ctrl Pts',(79.5764159518748,10.6125587759403,136.433112458027));
#69321=CARTESIAN_POINT('Ctrl Pts',(79.749410282889,10.6508684561015,136.420251466739));
#69322=CARTESIAN_POINT('Ctrl Pts',(79.861217992052,10.6640032544479,136.412036239531));
#69323=CARTESIAN_POINT('Ctrl Pts',(80.0204682490802,10.666536310738,136.400809113303));
#69324=CARTESIAN_POINT('Ctrl Pts',(80.0674469135898,10.6652969361736,136.397551199577));
#69325=CARTESIAN_POINT('Ctrl Pts',(80.1302143102675,10.6609799004612,136.393269371992));
#69326=CARTESIAN_POINT('Ctrl Pts',(80.1460979604029,10.6596582217318,136.392191852024));
#69327=CARTESIAN_POINT('Ctrl Pts',(80.172287697451,10.6571000615169,136.390424580544));
#69328=CARTESIAN_POINT('Ctrl Pts',(80.1826052506413,10.6559948657601,136.389730768935));
#69329=CARTESIAN_POINT('Ctrl Pts',(80.2027836034663,10.6536425196755,136.388378339198));
#69330=CARTESIAN_POINT('Ctrl Pts',(80.2126448787324,10.6524033816069,136.387719499716));
#69331=CARTESIAN_POINT('Ctrl Pts',(80.2360839112888,10.6492447993141,136.386158204223));
#69332=CARTESIAN_POINT('Ctrl Pts',(80.2496503598245,10.6472458036534,136.385258285195));
#69333=CARTESIAN_POINT('Ctrl Pts',(80.2963336744391,10.6397770917644,136.382173098446));
#69334=CARTESIAN_POINT('Ctrl Pts',(80.3293102520229,10.6334740770935,136.380013993463));
#69335=CARTESIAN_POINT('Ctrl Pts',(80.4103597203438,10.6154280592734,136.3747374412));
#69336=CARTESIAN_POINT('Ctrl Pts',(80.4581431700007,10.6025318396699,136.371653699907));
#69337=CARTESIAN_POINT('Ctrl Pts',(80.5681771776301,10.5675097634719,136.364530377955));
#69338=CARTESIAN_POINT('Ctrl Pts',(80.6298245739275,10.5437724303144,136.36052327146));
#69339=CARTESIAN_POINT('Ctrl Pts',(80.7032614684615,10.5103624497923,136.355584336946));
#69340=CARTESIAN_POINT('Ctrl Pts',(80.7165401282959,10.5041082605296,136.35468429641));
#69341=CARTESIAN_POINT('Ctrl Pts',(80.7934727348447,10.4666233640757,136.349419896146));
#69342=CARTESIAN_POINT('Ctrl Pts',(80.8551559140994,10.4315337576631,136.344999977038));
#69343=CARTESIAN_POINT('Ctrl Pts',(80.9240868982668,10.3862732260957,136.339605906287));
#69344=CARTESIAN_POINT('Ctrl Pts',(80.9336983409376,10.3798179019983,136.338842882871));
#69345=CARTESIAN_POINT('Ctrl Pts',(80.9485397695367,10.369623898227,136.337646293559));
#69346=CARTESIAN_POINT('Ctrl Pts',(80.953816932243,10.3659540890121,136.337217154765));
#69347=CARTESIAN_POINT('Ctrl Pts',(80.9635152417125,10.3591261526397,136.336421427271));
#69348=CARTESIAN_POINT('Ctrl Pts',(80.9679423382045,10.3559768237714,136.336055424912));
#69349=CARTESIAN_POINT('Ctrl Pts',(80.9781970595739,10.3486060558101,136.335201225032));
#69350=CARTESIAN_POINT('Ctrl Pts',(80.9840127922328,10.3443684766607,136.334711953221));
#69351=CARTESIAN_POINT('Ctrl Pts',(81.0025319991253,10.330690083646,136.333138896977));
#69352=CARTESIAN_POINT('Ctrl Pts',(81.015128026274,10.3211061852551,136.332046098187));
#69353=CARTESIAN_POINT('Ctrl Pts',(81.0841690520176,10.2670048330408,136.325936764934));
#69354=CARTESIAN_POINT('Ctrl Pts',(81.1378185215559,10.2190532234388,136.3207427415));
#69355=CARTESIAN_POINT('Ctrl Pts',(81.2811849946705,10.0731816316372,136.305872598001));
#69356=CARTESIAN_POINT('Ctrl Pts',(81.3625569574922,9.96778336794194,136.296214151952));
#69357=CARTESIAN_POINT('Ctrl Pts',(81.4442407137162,9.83092508232392,136.285205243351));
#69358=CARTESIAN_POINT('Ctrl Pts',(81.4573618852194,9.80769066449269,136.283381715138));
#69359=CARTESIAN_POINT('Ctrl Pts',(81.4758303629881,9.77307077235363,136.280729067577));
#69360=CARTESIAN_POINT('Ctrl Pts',(81.4816153784461,9.76192490753418,136.279884613378));
#69361=CARTESIAN_POINT('Ctrl Pts',(81.4916744330505,9.74199646418387,136.278391315488));
#69362=CARTESIAN_POINT('Ctrl Pts',(81.4959982425564,9.73323981910587,136.277740753512));
#69363=CARTESIAN_POINT('Ctrl Pts',(81.5049633818357,9.71467402722417,136.276372962746));
#69364=CARTESIAN_POINT('Ctrl Pts',(81.5095863899686,9.70485650061991,136.275656392404));
#69365=CARTESIAN_POINT('Ctrl Pts',(81.5216898386558,9.67848795092658,136.273749143768));
#69366=CARTESIAN_POINT('Ctrl Pts',(81.528996238272,9.66185830061692,136.272564435488));
#69367=CARTESIAN_POINT('Ctrl Pts',(81.5682750111704,9.56833445083818,136.265996175822));
#69368=CARTESIAN_POINT('Ctrl Pts',(81.5947210065873,9.48924235382752,136.260802471226));
#69369=CARTESIAN_POINT('Ctrl Pts',(81.6324281079547,9.34015279512863,136.251351667603));
#69370=CARTESIAN_POINT('Ctrl Pts',(81.6453576294033,9.27078321913306,136.247080789718));
#69371=CARTESIAN_POINT('Ctrl Pts',(81.6624622758917,9.1299065981701,136.238353015175));
#69372=CARTESIAN_POINT('Ctrl Pts',(81.6665015166774,9.05853763611416,136.233902556347));
#69373=CARTESIAN_POINT('Ctrl Pts',(81.6658609443739,8.97555613782454,136.228474420203));
#69374=CARTESIAN_POINT('Ctrl Pts',(81.6656507162538,8.96397415633981,136.227711019224));
#69375=CARTESIAN_POINT('Ctrl Pts',(81.6651360325248,8.9459692040301,136.226513962298));
#69376=CARTESIAN_POINT('Ctrl Pts',(81.6649151318616,8.93954395020537,136.226084738945));
#69377=CARTESIAN_POINT('Ctrl Pts',(81.6644389495642,8.92769162615402,136.225288940422));
#69378=CARTESIAN_POINT('Ctrl Pts',(81.664194303583,8.92226432882691,136.224922952537));
#69379=CARTESIAN_POINT('Ctrl Pts',(81.6635640161367,8.90965334753726,136.224068899793));
#69380=CARTESIAN_POINT('Ctrl Pts',(81.663158387874,8.90247089955206,136.223579761925));
#69381=CARTESIAN_POINT('Ctrl Pts',(81.6617121751876,8.87950594198288,136.222007575483));
#69382=CARTESIAN_POINT('Ctrl Pts',(81.6604933809911,8.86373607440735,136.220915526025));
#69383=CARTESIAN_POINT('Ctrl Pts',(81.6525008293375,8.77650657570113,136.214814543334));
#69384=CARTESIAN_POINT('Ctrl Pts',(81.6413392147133,8.70553122657962,136.209628611462));
#69385=CARTESIAN_POINT('Ctrl Pts',(81.5966894584062,8.50639479706589,136.194791421912));
#69386=CARTESIAN_POINT('Ctrl Pts',(81.5524567974861,8.38116773129696,136.185156833187));
#69387=CARTESIAN_POINT('Ctrl Pts',(81.4819160569234,8.23828547885221,136.174146397751));
#69388=CARTESIAN_POINT('Ctrl Pts',(81.4693832552013,8.21438100318894,136.172301411733));
#69389=CARTESIAN_POINT('Ctrl Pts',(81.4502138693321,8.17988328371215,136.169633008825));
#69390=CARTESIAN_POINT('Ctrl Pts',(81.4440306759922,8.169044455681,136.168793745769));
#69391=CARTESIAN_POINT('Ctrl Pts',(81.4327841307596,8.14983453727094,136.167304384201));
#69392=CARTESIAN_POINT('Ctrl Pts',(81.4277677824247,8.1414367548883,136.166652631738));
#69393=CARTESIAN_POINT('Ctrl Pts',(81.4170672044347,8.1238762711815,136.165288113281));
#69394=CARTESIAN_POINT('Ctrl Pts',(81.4113673827893,8.11472356289231,136.164575954843));
#69395=CARTESIAN_POINT('Ctrl Pts',(81.3960019106015,8.09057549888803,136.1626939861));
#69396=CARTESIAN_POINT('Ctrl Pts',(81.3861834043846,8.07567869924814,136.161529863921));
#69397=CARTESIAN_POINT('Ctrl Pts',(81.3328896409876,7.99758022478432,136.155404556238));
#69398=CARTESIAN_POINT('Ctrl Pts',(81.2853248028695,7.93727589449194,136.150602200035));
#69399=CARTESIAN_POINT('Ctrl Pts',(81.1619942589528,7.80136202703497,136.139292518966));
#69400=CARTESIAN_POINT('Ctrl Pts',(81.0827859129208,7.72935611213826,136.132888141231));
#69401=CARTESIAN_POINT('Ctrl Pts',(80.9619007348197,7.63902654463295,136.123444441762));
#69402=CARTESIAN_POINT('Ctrl Pts',(80.9255337584337,7.61403885768261,136.12063792134));
#69403=CARTESIAN_POINT('Ctrl Pts',(80.8791641576979,7.58481767525403,136.117044303455));
#69404=CARTESIAN_POINT('Ctrl Pts',(80.8700517176677,7.57919719092472,136.116337384099));
#69405=CARTESIAN_POINT('Ctrl Pts',(80.8556032078558,7.57047657391985,136.115214342057));
#69406=CARTESIAN_POINT('Ctrl Pts',(80.8503028131598,7.56731748183787,136.114801903797));
#69407=CARTESIAN_POINT('Ctrl Pts',(80.8402069969403,7.56137602564292,136.114015220141));
#69408=CARTESIAN_POINT('Ctrl Pts',(80.835415081637,7.55858806203347,136.113641337107));
#69409=CARTESIAN_POINT('Ctrl Pts',(80.823945821088,7.55199158285998,136.11274541065));
#69410=CARTESIAN_POINT('Ctrl Pts',(80.8172559187656,7.54820530045358,136.112221993922));
#69411=CARTESIAN_POINT('Ctrl Pts',(80.7941987094058,7.53536548380102,136.110415779378));
#69412=CARTESIAN_POINT('Ctrl Pts',(80.7777059411348,7.52654173717698,136.109119988525));
#69413=CARTESIAN_POINT('Ctrl Pts',(80.7364041228524,7.5053315541547,136.105871934395));
#69414=CARTESIAN_POINT('Ctrl Pts',(80.7114282203446,7.49328353415353,136.103905115514));
#69415=CARTESIAN_POINT('Ctrl Pts',(80.6071193867698,7.44613815221024,136.095711658995));
#69416=CARTESIAN_POINT('Ctrl Pts',(80.5254062658984,7.41664014416357,136.089349800247));
#69417=CARTESIAN_POINT('Ctrl Pts',(80.3465548666147,7.36745376822056,136.075907222767));
#69418=CARTESIAN_POINT('Ctrl Pts',(80.2491871353681,7.34978201894724,136.068880472038));
#69419=CARTESIAN_POINT('Ctrl Pts',(80.1320200842002,7.33913192770637,136.060836249827));
#69420=CARTESIAN_POINT('Ctrl Pts',(80.1131998031606,7.33774312707843,136.059555958063));
#69421=CARTESIAN_POINT('Ctrl Pts',(80.0833746162996,7.33605116518116,136.057544960696));
#69422=CARTESIAN_POINT('Ctrl Pts',(80.0723838103143,7.33553682960693,136.056807733068));
#69423=CARTESIAN_POINT('Ctrl Pts',(80.0526302741536,7.33480846003855,136.055489367396));
#69424=CARTESIAN_POINT('Ctrl Pts',(80.0438695133671,7.33455462973606,136.054907010221));
#69425=CARTESIAN_POINT('Ctrl Pts',(80.0232854957997,7.33412077387957,136.053544016591));
#69426=CARTESIAN_POINT('Ctrl Pts',(80.011461414904,7.3339974614781,136.052765175393));
#69427=CARTESIAN_POINT('Ctrl Pts',(79.9767976902504,7.33400501918422,136.050493189432));
#69428=CARTESIAN_POINT('Ctrl Pts',(79.9539602954211,7.33447964568401,136.049010736823));
#69429=CARTESIAN_POINT('Ctrl Pts',(79.8484624695344,7.33884393409024,136.04221843503));
#69430=CARTESIAN_POINT('Ctrl Pts',(79.7661508423424,7.34841894270687,136.037085242915));
#69431=CARTESIAN_POINT('Ctrl Pts',(79.6286599096413,7.37490279584805,136.028501166937));
#69432=CARTESIAN_POINT('Ctrl Pts',(79.5730324592314,7.38862387123253,136.025023027446));
#69433=CARTESIAN_POINT('Ctrl Pts',(79.444500014626,7.42745215560983,136.016782791305));
#69434=CARTESIAN_POINT('Ctrl Pts',(79.3724200242907,7.45480512372725,136.012002410027));
#69435=CARTESIAN_POINT('Ctrl Pts',(79.2919795314778,7.49188951860505,136.00620841966));
#69436=CARTESIAN_POINT('Ctrl Pts',(79.281510138081,7.49684914002765,136.005444964198));
#69437=CARTESIAN_POINT('Ctrl Pts',(79.2653123770348,7.50473031435706,136.004247839794));
#69438=CARTESIAN_POINT('Ctrl Pts',(79.2595475269933,7.5075766458903,136.003818604241));
#69439=CARTESIAN_POINT('Ctrl Pts',(79.2489418620964,7.51288965071559,136.003022795464));
#69440=CARTESIAN_POINT('Ctrl Pts',(79.2440964610611,7.51534672257244,136.002656809662));
#69441=CARTESIAN_POINT('Ctrl Pts',(79.2328632502145,7.52111225695536,136.001802778125));
#69442=CARTESIAN_POINT('Ctrl Pts',(79.2264847928044,7.52443842255551,136.001313659565));
#69443=CARTESIAN_POINT('Ctrl Pts',(79.2061527485013,7.53520900332105,135.999741598483));
#69444=CARTESIAN_POINT('Ctrl Pts',(79.1922840230788,7.5428105895762,135.998649657017));
#69445=CARTESIAN_POINT('Ctrl Pts',(79.1160927714381,7.58599360479228,135.992549877015));
#69446=CARTESIAN_POINT('Ctrl Pts',(79.056016814999,7.62537285193159,135.987365110413));
#69447=CARTESIAN_POINT('Ctrl Pts',(78.8929628019962,7.74799401685066,135.972532659081));
#69448=CARTESIAN_POINT('Ctrl Pts',(78.7970750631929,7.83981291272444,135.962901499605));
#69449=CARTESIAN_POINT('Ctrl Pts',(78.6958864665773,7.96290092295109,135.951890834227));
#69450=CARTESIAN_POINT('Ctrl Pts',(78.6792313709984,7.98419638691527,135.950042753144));
#69451=CARTESIAN_POINT('Ctrl Pts',(78.6556507015866,8.01590810574452,135.947370770852));
#69452=CARTESIAN_POINT('Ctrl Pts',(78.6483131203581,8.02601104389264,135.946530963027));
#69453=CARTESIAN_POINT('Ctrl Pts',(78.6354302502559,8.04417517413303,135.945040984802));
#69454=CARTESIAN_POINT('Ctrl Pts',(78.6298411583723,8.05220442320869,135.944389155505));
#69455=CARTESIAN_POINT('Ctrl Pts',(78.6182437384799,8.06918219062246,135.943024828332));
#69456=CARTESIAN_POINT('Ctrl Pts',(78.612250854005,8.07814074962577,135.942312934921));
#69457=CARTESIAN_POINT('Ctrl Pts',(78.5965809579962,8.10206427868909,135.940432484722));
#69458=CARTESIAN_POINT('Ctrl Pts',(78.5870562300029,8.11712769340393,135.939269599304));
#69459=CARTESIAN_POINT('Ctrl Pts',(78.5380114395936,8.19751962447847,135.933168598142));
#69460=CARTESIAN_POINT('Ctrl Pts',(78.5027728281628,8.2653584214726,135.92838770591));
#69461=CARTESIAN_POINT('Ctrl Pts',(78.4371865697683,8.41611517413024,135.91825484369));
#69462=CARTESIAN_POINT('Ctrl Pts',(78.408519948634,8.49950227648941,135.912944595744));
#69463=CARTESIAN_POINT('Ctrl Pts',(78.3742897727855,8.63250494513716,135.904457920536));
#69464=CARTESIAN_POINT('Ctrl Pts',(78.3641286570108,8.68076577835562,135.90137319221));
#69465=CARTESIAN_POINT('Ctrl Pts',(78.3529714810313,8.74854529491676,135.896946601538));
#69466=CARTESIAN_POINT('Ctrl Pts',(78.3501550515473,8.7677415701127,135.895682464896));
#69467=CARTESIAN_POINT('Ctrl Pts',(78.3466497920386,8.7949309109591,135.893871644247));
#69468=CARTESIAN_POINT('Ctrl Pts',(78.3456823718366,8.80288729081993,135.893339297453));
#69469=CARTESIAN_POINT('Ctrl Pts',(78.3441430496019,8.81635771375061,135.892433404305));
#69470=CARTESIAN_POINT('Ctrl Pts',(78.3435411760049,8.82186832690684,135.892061506298));
#69471=CARTESIAN_POINT('Ctrl Pts',(78.342438082413,8.83245737806811,135.891344210993));
#69472=CARTESIAN_POINT('Ctrl Pts',(78.3419326783328,8.83753524738031,135.890999078881));
#69473=CARTESIAN_POINT('Ctrl Pts',(78.340884149257,8.84858484071975,135.890245654511));
#69474=CARTESIAN_POINT('Ctrl Pts',(78.3403499229025,8.85455731196778,135.88983689008));
#69475=CARTESIAN_POINT('Ctrl Pts',(78.3391176720687,8.86922540738591,135.888829448641));
#69476=CARTESIAN_POINT('Ctrl Pts',(78.3384556917618,8.87792377279871,135.888228975868));
#69477=CARTESIAN_POINT('Ctrl Pts',(78.3353083420516,8.92406629268983,135.88502886214));
#69478=CARTESIAN_POINT('Ctrl Pts',(78.3340205656214,8.96157809269317,135.88237599935));
#69479=CARTESIAN_POINT('Ctrl Pts',(78.3340002443602,8.99909766519367,135.879690700183));
#69480=CARTESIAN_POINT('Ctrl Pts',(78.3340002456947,8.99909520463398,135.879690876287));
#69481=CARTESIAN_POINT('Ctrl Pts',(78.3339311639518,9.12629542146476,135.870587082321));
#69482=CARTESIAN_POINT('Ctrl Pts',(78.3484291209228,9.25309503966349,135.86118595031));
#69483=CARTESIAN_POINT('Ctrl Pts',(78.3865895332018,9.41734411656879,135.849173887942));
#69484=CARTESIAN_POINT('Ctrl Pts',(78.3974571739415,9.45730340847634,135.846260812617));
#69485=CARTESIAN_POINT('Ctrl Pts',(78.4180656644503,9.52326615740673,135.841471980529));
#69486=CARTESIAN_POINT('Ctrl Pts',(78.4269871736021,9.54950385642816,135.83957241518));
#69487=CARTESIAN_POINT('Ctrl Pts',(78.4365593737294,9.5755079566144,135.837694135948));
#69488=CARTESIAN_POINT('',(78.3340003883633,8.99886244719965,136.072462051176));
#69489=CARTESIAN_POINT('Ctrl Pts',(78.4365593745323,9.57550795879571,136.032852165095));
#69490=CARTESIAN_POINT('Ctrl Pts',(78.4356277148595,9.57297698670518,136.033046285279));
#69491=CARTESIAN_POINT('Ctrl Pts',(78.4347021561404,9.57044363022435,136.03324030345));
#69492=CARTESIAN_POINT('Ctrl Pts',(78.4095803158231,9.50116081178708,136.038538509474));
#69493=CARTESIAN_POINT('Ctrl Pts',(78.3896669089255,9.43292796125389,136.043552730623));
#69494=CARTESIAN_POINT('Ctrl Pts',(78.3698143382183,9.34416329481746,136.049800240416));
#69495=CARTESIAN_POINT('Ctrl Pts',(78.365811465529,9.32462525924818,136.051159038004));
#69496=CARTESIAN_POINT('Ctrl Pts',(78.3598903716904,9.29283119587528,136.053344580382));
#69497=CARTESIAN_POINT('Ctrl Pts',(78.3577566142742,9.28061785155142,136.054178056609));
#69498=CARTESIAN_POINT('Ctrl Pts',(78.3541893803237,9.25876317691845,136.055658992162));
#69499=CARTESIAN_POINT('Ctrl Pts',(78.3527038212801,9.24913105802732,136.056308069511));
#69500=CARTESIAN_POINT('Ctrl Pts',(78.3499924352749,9.23046504336666,136.057559132773));
#69501=CARTESIAN_POINT('Ctrl Pts',(78.3487560728268,9.22143305627928,136.058161428655));
#69502=CARTESIAN_POINT('Ctrl Pts',(78.3462230634299,9.20172621449645,136.059469152917));
#69503=CARTESIAN_POINT('Ctrl Pts',(78.344955499794,9.19104798557724,136.060173652948));
#69504=CARTESIAN_POINT('Ctrl Pts',(78.3412526870132,9.15704544821936,136.0624046368));
#69505=CARTESIAN_POINT('Ctrl Pts',(78.33920639662,9.13368101662976,136.063919147197));
#69506=CARTESIAN_POINT('Ctrl Pts',(78.3351936433969,9.07319343063213,136.067799234268));
#69507=CARTESIAN_POINT('Ctrl Pts',(78.3339750077718,9.03603351786301,136.070143150966));
#69508=CARTESIAN_POINT('Ctrl Pts',(78.3340003883633,8.99886244719965,136.072462051176));
#69509=CARTESIAN_POINT('Ctrl Pts',(78.3340003869984,8.99886444785471,136.072461926366));
#69510=CARTESIAN_POINT('Ctrl Pts',(78.3340531441327,8.92146301309155,136.077290581301));
#69511=CARTESIAN_POINT('Ctrl Pts',(78.3394999121662,8.84415419702371,136.081997861543));
#69512=CARTESIAN_POINT('Ctrl Pts',(78.3596031876968,8.70151152241477,136.090799621358));
#69513=CARTESIAN_POINT('Ctrl Pts',(78.3728537644019,8.63614436901105,136.0948817902));
#69514=CARTESIAN_POINT('Ctrl Pts',(78.395771922399,8.54998256302621,136.100524008562));
#69515=CARTESIAN_POINT('Ctrl Pts',(78.4020028876724,8.52833428565311,136.101964483626));
#69516=CARTESIAN_POINT('Ctrl Pts',(78.4134188217244,8.49149881699858,136.104465329264));
#69517=CARTESIAN_POINT('Ctrl Pts',(78.4183879553125,8.47624759472493,136.105515622285));
#69518=CARTESIAN_POINT('Ctrl Pts',(78.4259160897696,8.45422700585422,136.107056986682));
#69519=CARTESIAN_POINT('Ctrl Pts',(78.4283003909941,8.44739828827664,136.10753847939));
#69520=CARTESIAN_POINT('Ctrl Pts',(78.4325542090003,8.43546546783966,136.108386377101));
#69521=CARTESIAN_POINT('Ctrl Pts',(78.4344043529058,8.43035465917388,136.108751647994));
#69522=CARTESIAN_POINT('Ctrl Pts',(78.438487381553,8.41924592080844,136.109550308729));
#69523=CARTESIAN_POINT('Ctrl Pts',(78.4407297901262,8.41325187071367,136.109984226704));
#69524=CARTESIAN_POINT('Ctrl Pts',(78.4470829225921,8.39656332434912,136.111200364459));
#69525=CARTESIAN_POINT('Ctrl Pts',(78.4512694246017,8.385898332915,136.111986793306));
#69526=CARTESIAN_POINT('Ctrl Pts',(78.4799752666411,8.31493192506949,136.117277844626));
#69527=CARTESIAN_POINT('Ctrl Pts',(78.507898388204,8.25607503662913,136.121945620769));
#69528=CARTESIAN_POINT('Ctrl Pts',(78.5496654896484,8.17990204110557,136.128241573454));
#69529=CARTESIAN_POINT('Ctrl Pts',(78.5605161495456,8.16100233712507,136.129825995778));
#69530=CARTESIAN_POINT('Ctrl Pts',(78.607265245597,8.08315253400646,136.136434473902));
#69531=CARTESIAN_POINT('Ctrl Pts',(78.64644051915,8.02624589460323,136.141461378754));
#69532=CARTESIAN_POINT('Ctrl Pts',(78.7180407219012,7.93494324859615,136.14976933578));
#69533=CARTESIAN_POINT('Ctrl Pts',(78.748601331274,7.89919687992975,136.153093131371));
#69534=CARTESIAN_POINT('Ctrl Pts',(78.7957310356929,7.84857346821893,136.157900575771));
#69535=CARTESIAN_POINT('Ctrl Pts',(78.8111492200505,7.83266084637885,136.159427611635));
#69536=CARTESIAN_POINT('Ctrl Pts',(78.8396995303685,7.80434756730253,136.162174621035));
#69537=CARTESIAN_POINT('Ctrl Pts',(78.8527244032876,7.79184410387257,136.163398921305));
#69538=CARTESIAN_POINT('Ctrl Pts',(78.8736862199784,7.7723661856787,136.165324871146));
#69539=CARTESIAN_POINT('Ctrl Pts',(78.8814903602932,7.76525156088244,136.166032473925));
#69540=CARTESIAN_POINT('Ctrl Pts',(78.8966095250413,7.75172919220106,136.167385612255));
#69541=CARTESIAN_POINT('Ctrl Pts',(78.9039140122308,7.74531037140608,136.168031596976));
#69542=CARTESIAN_POINT('Ctrl Pts',(78.9204810008802,7.73100722187497,136.169479679248));
#69543=CARTESIAN_POINT('Ctrl Pts',(78.9297745554825,7.72315958264297,136.170280246122));
#69544=CARTESIAN_POINT('Ctrl Pts',(78.957486111298,7.70027461065848,136.172633779232));
#69545=CARTESIAN_POINT('Ctrl Pts',(78.976141478408,7.68552857954004,136.174175075683));
#69546=CARTESIAN_POINT('Ctrl Pts',(79.0768085212832,7.60940081325571,136.182281295892));
#69547=CARTESIAN_POINT('Ctrl Pts',(79.1640373786691,7.55527912932194,136.188562885749));
#69548=CARTESIAN_POINT('Ctrl Pts',(79.3266333773447,7.47408365318616,136.199662664586));
#69549=CARTESIAN_POINT('Ctrl Pts',(79.4000062528873,7.44377088487217,136.204482058647));
#69550=CARTESIAN_POINT('Ctrl Pts',(79.4987636390716,7.41099661009946,136.211042980748));
#69551=CARTESIAN_POINT('Ctrl Pts',(79.5224448305711,7.40371976366654,136.212621982234));
#69552=CARTESIAN_POINT('Ctrl Pts',(79.5628446199963,7.3922849728829,136.215339150357));
#69553=CARTESIAN_POINT('Ctrl Pts',(79.5794819977325,7.38785329831413,136.216464767613));
#69554=CARTESIAN_POINT('Ctrl Pts',(79.6034016650233,7.3818772904637,136.21809649978));
#69555=CARTESIAN_POINT('Ctrl Pts',(79.6106308998602,7.38012252283014,136.218591401636));
#69556=CARTESIAN_POINT('Ctrl Pts',(79.6232325458451,7.37715292691006,136.219457509455));
#69557=CARTESIAN_POINT('Ctrl Pts',(79.6285996162931,7.37591623026215,136.219827471938));
#69558=CARTESIAN_POINT('Ctrl Pts',(79.6401136592124,7.37332319018451,136.220623602186));
#69559=CARTESIAN_POINT('Ctrl Pts',(79.64626211335,7.3719750843008,136.221050190894));
#69560=CARTESIAN_POINT('Ctrl Pts',(79.663165244482,7.36836918738495,136.222226678532));
#69561=CARTESIAN_POINT('Ctrl Pts',(79.6739346251001,7.36618296116407,136.222980374254));
#69562=CARTESIAN_POINT('Ctrl Pts',(79.7352883383868,7.35435866547006,136.227294660842));
#69563=CARTESIAN_POINT('Ctrl Pts',(79.786271870605,7.34696434852525,136.230957803344));
#69564=CARTESIAN_POINT('Ctrl Pts',(79.9330610803652,7.33257898529598,136.241586302096));
#69565=CARTESIAN_POINT('Ctrl Pts',(80.0292434301914,7.33149182043701,136.248638173744));
#69566=CARTESIAN_POINT('Ctrl Pts',(80.1774362924461,7.3426409991384,136.259325602428));
#69567=CARTESIAN_POINT('Ctrl Pts',(80.2296730923483,7.34906885175078,136.263061157461));
#69568=CARTESIAN_POINT('Ctrl Pts',(80.3050186510509,7.36198659414462,136.268388875245));
#69569=CARTESIAN_POINT('Ctrl Pts',(80.328426569488,7.36651893711743,136.27003570082));
#69570=CARTESIAN_POINT('Ctrl Pts',(80.3706981806889,7.37564922888482,136.272994956971));
#69571=CARTESIAN_POINT('Ctrl Pts',(80.3895937887019,7.38007737720623,136.274312381842));
#69572=CARTESIAN_POINT('Ctrl Pts',(80.41918371063,7.38755944389731,136.276367762707));
#69573=CARTESIAN_POINT('Ctrl Pts',(80.4299316748906,7.39039188138417,136.277112740561));
#69574=CARTESIAN_POINT('Ctrl Pts',(80.4500249318149,7.39590273153883,136.278502741974));
#69575=CARTESIAN_POINT('Ctrl Pts',(80.4593766296121,7.39855577526023,136.279148552641));
#69576=CARTESIAN_POINT('Ctrl Pts',(80.4803371515214,7.40470091698071,136.280593802181));
#69577=CARTESIAN_POINT('Ctrl Pts',(80.4919322395702,7.40823819996467,136.281391736597));
#69578=CARTESIAN_POINT('Ctrl Pts',(80.5259619131412,7.41902690972052,136.283729754519));
#69579=CARTESIAN_POINT('Ctrl Pts',(80.5482829454949,7.42662854120583,136.2852584028));
#69580=CARTESIAN_POINT('Ctrl Pts',(80.6684827181651,7.4704325131571,136.29347727327));
#69581=CARTESIAN_POINT('Ctrl Pts',(80.7629594290216,7.5152972863955,136.299871275994));
#69582=CARTESIAN_POINT('Ctrl Pts',(80.919683081142,7.60865842096054,136.311011723616));
#69583=CARTESIAN_POINT('Ctrl Pts',(80.983845328925,7.65326505081037,136.315759181713));
#69584=CARTESIAN_POINT('Ctrl Pts',(81.0637776959932,7.71760514161585,136.322231150989));
#69585=CARTESIAN_POINT('Ctrl Pts',(81.082571443264,7.73343041943481,136.323797549425));
#69586=CARTESIAN_POINT('Ctrl Pts',(81.1138497761565,7.76097316930884,136.326495129723));
#69587=CARTESIAN_POINT('Ctrl Pts',(81.1265165492664,7.77247842400972,136.327613998469));
#69588=CARTESIAN_POINT('Ctrl Pts',(81.1444191234065,7.7892498425877,136.329237654458));
#69589=CARTESIAN_POINT('Ctrl Pts',(81.1498008982252,7.79435952169334,136.32973138014));
#69590=CARTESIAN_POINT('Ctrl Pts',(81.1591155133244,7.80332229114611,136.330596162431));
#69591=CARTESIAN_POINT('Ctrl Pts',(81.1630636771064,7.80715919164722,136.330965987508));
#69592=CARTESIAN_POINT('Ctrl Pts',(81.1714924574114,7.81543207327504,136.331762685419));
#69593=CARTESIAN_POINT('Ctrl Pts',(81.1759668595373,7.81987386573971,136.332189986815));
#69594=CARTESIAN_POINT('Ctrl Pts',(81.188202586242,7.83215909805313,136.333370311814));
#69595=CARTESIAN_POINT('Ctrl Pts',(81.1959112004824,7.84005425019851,136.334127171301));
#69596=CARTESIAN_POINT('Ctrl Pts',(81.2397026746054,7.88580595563019,136.338500511347));
#69597=CARTESIAN_POINT('Ctrl Pts',(81.2740621717922,7.92526489625351,136.342222723922));
#69598=CARTESIAN_POINT('Ctrl Pts',(81.36972325798,8.0461685123325,136.353337187766));
#69599=CARTESIAN_POINT('Ctrl Pts',(81.4254825206518,8.13170417319068,136.360825746992));
#69600=CARTESIAN_POINT('Ctrl Pts',(81.5071779949745,8.28634739173715,136.373364231176));
#69601=CARTESIAN_POINT('Ctrl Pts',(81.5370027634574,8.35307596322642,136.378494736779));
#69602=CARTESIAN_POINT('Ctrl Pts',(81.5684768422049,8.4380861890499,136.384681139292));
#69603=CARTESIAN_POINT('Ctrl Pts',(81.5743347196586,8.45471386648205,136.385875480287));
#69604=CARTESIAN_POINT('Ctrl Pts',(81.5833335102568,8.48161189689634,136.387783095859));
#69605=CARTESIAN_POINT('Ctrl Pts',(81.5866408293228,8.49182471705531,136.388501796782));
#69606=CARTESIAN_POINT('Ctrl Pts',(81.5927754208663,8.51141192076544,136.389869791718));
#69607=CARTESIAN_POINT('Ctrl Pts',(81.5956192040493,8.52078061898938,136.390519601639));
#69608=CARTESIAN_POINT('Ctrl Pts',(81.6019224727224,8.5422247721688,136.391996975092));
#69609=CARTESIAN_POINT('Ctrl Pts',(81.6053283402842,8.5543154679845,136.392822769176));
#69610=CARTESIAN_POINT('Ctrl Pts',(81.614056014618,8.5866972282222,136.395016168822));
#69611=CARTESIAN_POINT('Ctrl Pts',(81.6191319958297,8.60705262120181,136.396375904976));
#69612=CARTESIAN_POINT('Ctrl Pts',(81.6509426179813,8.74572292910676,136.405522797681));
#69613=CARTESIAN_POINT('Ctrl Pts',(81.6650720831742,8.86655650291308,136.41288809779));
#69614=CARTESIAN_POINT('Ctrl Pts',(81.6664361104077,9.05379667937085,136.424330348604));
#69615=CARTESIAN_POINT('Ctrl Pts',(81.6630018453198,9.11969544808851,136.428371150736));
#69616=CARTESIAN_POINT('Ctrl Pts',(81.6531837064261,9.20746310136646,136.433961334851));
#69617=CARTESIAN_POINT('Ctrl Pts',(81.6502464055033,9.22966063418458,136.435393396896));
#69618=CARTESIAN_POINT('Ctrl Pts',(81.6444495977984,9.26757518884687,136.437881030727));
#69619=CARTESIAN_POINT('Ctrl Pts',(81.6418096589256,9.28332306541428,136.438926666206));
#69620=CARTESIAN_POINT('Ctrl Pts',(81.6376479925338,9.30613262049103,136.44046242638));
#69621=CARTESIAN_POINT('Ctrl Pts',(81.6363059433073,9.31322672916653,136.440943069394));
#69622=CARTESIAN_POINT('Ctrl Pts',(81.633873045942,9.32564459283121,136.441790030242));
#69623=CARTESIAN_POINT('Ctrl Pts',(81.6328021976409,9.33097207322808,136.44215522256));
#69624=CARTESIAN_POINT('Ctrl Pts',(81.6304116884145,9.34257086014009,136.442954395602));
#69625=CARTESIAN_POINT('Ctrl Pts',(81.6290819233892,9.34883972159588,136.44338891069));
#69626=CARTESIAN_POINT('Ctrl Pts',(81.6252657802977,9.36633222086151,136.444608298));
#69627=CARTESIAN_POINT('Ctrl Pts',(81.6226994066407,9.37753777297932,136.445397413902));
#69628=CARTESIAN_POINT('Ctrl Pts',(81.6044757219645,9.45348711802887,136.450796223447));
#69629=CARTESIAN_POINT('Ctrl Pts',(81.5850651386949,9.51726147192289,136.455576621685));
#69630=CARTESIAN_POINT('Ctrl Pts',(81.5543651901998,9.59997740745913,136.461973961768));
#69631=CARTESIAN_POINT('Ctrl Pts',(81.5464431899345,9.62011085810467,136.463547373611));
#69632=CARTESIAN_POINT('Ctrl Pts',(81.5104525822664,9.70659681239344,136.470365206775));
#69633=CARTESIAN_POINT('Ctrl Pts',(81.4784869358484,9.77124809500272,136.475609756227));
#69634=CARTESIAN_POINT('Ctrl Pts',(81.4090013952113,9.89147934437659,136.485530128629));
#69635=CARTESIAN_POINT('Ctrl Pts',(81.3721150591305,9.94727117582283,136.490211221038));
#69636=CARTESIAN_POINT('Ctrl Pts',(81.3216223477074,10.0144788123303,136.495944434571));
#69637=CARTESIAN_POINT('Ctrl Pts',(81.3110592185517,10.0280936994288,136.497111309044));
#69638=CARTESIAN_POINT('Ctrl Pts',(81.2936287115666,10.0498543541593,136.498985887513));
#69639=CARTESIAN_POINT('Ctrl Pts',(81.2868913353451,10.0581021257214,136.499698684046));
#69640=CARTESIAN_POINT('Ctrl Pts',(81.273792821711,10.0738268935684,136.501062356521));
#69641=CARTESIAN_POINT('Ctrl Pts',(81.2674437998601,10.0813133547781,136.501713683256));
#69642=CARTESIAN_POINT('Ctrl Pts',(81.2527042578371,10.0983853185433,136.503204087334));
#69643=CARTESIAN_POINT('Ctrl Pts',(81.2442691547377,10.1079316545407,136.504041282955));
#69644=CARTESIAN_POINT('Ctrl Pts',(81.2166216463029,10.138507382077,136.506736170426));
#69645=CARTESIAN_POINT('Ctrl Pts',(81.1969786102493,10.159141773007,136.508575749744));
#69646=CARTESIAN_POINT('Ctrl Pts',(81.0842992880271,10.271587167455,136.518746647065));
#69647=CARTESIAN_POINT('Ctrl Pts',(80.9812427320881,10.3527024702783,136.52660468837));
#69648=CARTESIAN_POINT('Ctrl Pts',(80.8089796364339,10.4581447509026,136.538997006382));
#69649=CARTESIAN_POINT('Ctrl Pts',(80.745882777515,10.491405619886,136.54341493937));
#69650=CARTESIAN_POINT('Ctrl Pts',(80.6664719944726,10.5269641682872,136.549060224161));
#69651=CARTESIAN_POINT('Ctrl Pts',(80.6519948407415,10.5332016090782,136.550092792081));
#69652=CARTESIAN_POINT('Ctrl Pts',(80.6307954172729,10.5419807844289,136.551612818145));
#69653=CARTESIAN_POINT('Ctrl Pts',(80.6241412643118,10.5446861414027,136.552091064196));
#69654=CARTESIAN_POINT('Ctrl Pts',(80.6124261410438,10.5493610661181,136.552935392305));
#69655=CARTESIAN_POINT('Ctrl Pts',(80.607372724284,10.5513490464612,136.553300373097));
#69656=CARTESIAN_POINT('Ctrl Pts',(80.5963115518121,10.555638106521,136.554101036828));
#69657=CARTESIAN_POINT('Ctrl Pts',(80.5903002527089,10.5579290720182,136.554537272025));
#69658=CARTESIAN_POINT('Ctrl Pts',(80.5734064698385,10.5642556490202,136.555766037709));
#69659=CARTESIAN_POINT('Ctrl Pts',(80.5624951096833,10.5682123414605,136.556562912473));
#69660=CARTESIAN_POINT('Ctrl Pts',(80.4788922277897,10.5975437926729,136.562688499604));
#69661=CARTESIAN_POINT('Ctrl Pts',(80.4045691098785,10.6179632513618,136.568244476519));
#69662=CARTESIAN_POINT('Ctrl Pts',(80.2729626348254,10.644484111067,136.578002871392));
#69663=CARTESIAN_POINT('Ctrl Pts',(80.216267404747,10.6528960245061,136.582182529251));
#69664=CARTESIAN_POINT('Ctrl Pts',(80.0769170039275,10.6662776354405,136.592298421443));
#69665=CARTESIAN_POINT('Ctrl Pts',(79.994098936278,10.6680426113408,136.598172072534));
#69666=CARTESIAN_POINT('Ctrl Pts',(79.8886810548849,10.662433584049,136.605429609091));
#69667=CARTESIAN_POINT('Ctrl Pts',(79.8659071031743,10.6607517917005,136.606985022737));
#69668=CARTESIAN_POINT('Ctrl Pts',(79.8314054840249,10.6574895544519,136.609323585377));
#69669=CARTESIAN_POINT('Ctrl Pts',(79.8196489842142,10.6562515683095,136.610117312495));
#69670=CARTESIAN_POINT('Ctrl Pts',(79.7992030873229,10.6538782808652,136.611492509951));
#69671=CARTESIAN_POINT('Ctrl Pts',(79.7905077515289,10.6527993740684,136.612075724195));
#69672=CARTESIAN_POINT('Ctrl Pts',(79.770916709222,10.6502114496122,136.613386231962));
#69673=CARTESIAN_POINT('Ctrl Pts',(79.7600265500876,10.6486630145815,136.614112257789));
#69674=CARTESIAN_POINT('Ctrl Pts',(79.7305036901016,10.6441665295293,136.616074359909));
#69675=CARTESIAN_POINT('Ctrl Pts',(79.7119040793561,10.6410096359875,136.617303832634));
#69676=CARTESIAN_POINT('Ctrl Pts',(79.5960403487304,10.6193134693007,136.624928541129));
#69677=CARTESIAN_POINT('Ctrl Pts',(79.5005320938761,10.5924493635285,136.631046890396));
#69678=CARTESIAN_POINT('Ctrl Pts',(79.3412551908745,10.5318957765152,136.641470337049));
#69679=CARTESIAN_POINT('Ctrl Pts',(79.2762465790241,10.5022748303543,136.645798286387));
#69680=CARTESIAN_POINT('Ctrl Pts',(79.1806609743707,10.4510733646507,136.652530398233));
#69681=CARTESIAN_POINT('Ctrl Pts',(79.1485772869746,10.4324836322335,136.654858373179));
#69682=CARTESIAN_POINT('Ctrl Pts',(79.1038484739672,10.4045334396655,136.658240769282));
#69683=CARTESIAN_POINT('Ctrl Pts',(79.0906728703663,10.3960393524008,136.659254690725));
#69684=CARTESIAN_POINT('Ctrl Pts',(79.0674902914687,10.3806265241495,136.661073882843));
#69685=CARTESIAN_POINT('Ctrl Pts',(79.0574353909328,10.3737816028056,136.661874958807));
#69686=CARTESIAN_POINT('Ctrl Pts',(79.0421399378135,10.3631221875605,136.663113642967));
#69687=CARTESIAN_POINT('Ctrl Pts',(79.0368449483351,10.3593860157656,136.663546201151));
#69688=CARTESIAN_POINT('Ctrl Pts',(79.027115580287,10.3524355440393,136.664348231931));
#69689=CARTESIAN_POINT('Ctrl Pts',(79.0226750903932,10.3492301556437,136.664717108332));
#69690=CARTESIAN_POINT('Ctrl Pts',(79.0125730778852,10.3418619357556,136.665562738655));
#69691=CARTESIAN_POINT('Ctrl Pts',(79.0069220354718,10.3376851397204,136.666040423824));
#69692=CARTESIAN_POINT('Ctrl Pts',(78.9890335633866,10.324287597794,136.667566932692));
#69693=CARTESIAN_POINT('Ctrl Pts',(78.9768972461405,10.3149340253902,136.668624191239));
#69694=CARTESIAN_POINT('Ctrl Pts',(78.8854012954304,10.2423837757863,136.676750572399));
#69695=CARTESIAN_POINT('Ctrl Pts',(78.8118406528033,10.1722293634422,136.684175373678));
#69696=CARTESIAN_POINT('Ctrl Pts',(78.6690376031109,10.0086999071987,136.699966323611));
#69697=CARTESIAN_POINT('Ctrl Pts',(78.6022200081783,9.91386921074871,136.708264360951));
#69698=CARTESIAN_POINT('Ctrl Pts',(78.5362713505037,9.79588488873858,136.717513992661));
#69699=CARTESIAN_POINT('Ctrl Pts',(78.527079001614,9.77874135861699,136.718834533187));
#69700=CARTESIAN_POINT('Ctrl Pts',(78.5131044699187,9.75154602302515,136.720893645411));
#69701=CARTESIAN_POINT('Ctrl Pts',(78.5081194252236,9.74160104038382,136.721639281496));
#69702=CARTESIAN_POINT('Ctrl Pts',(78.4989661081055,9.72287462326264,136.723029879778));
#69703=CARTESIAN_POINT('Ctrl Pts',(78.4947743800461,9.71410524816181,136.723675635595));
#69704=CARTESIAN_POINT('Ctrl Pts',(78.4855334627877,9.69432969248777,136.72511995042));
#69705=CARTESIAN_POINT('Ctrl Pts',(78.4805270036655,9.68330406155704,136.725917013648));
#69706=CARTESIAN_POINT('Ctrl Pts',(78.4661546710695,9.65071287997985,136.72824990872));
#69707=CARTESIAN_POINT('Ctrl Pts',(78.45712432468,9.62900197491221,136.729774382256));
#69708=CARTESIAN_POINT('Ctrl Pts',(78.4444496037559,9.59661206619143,136.732009064827));
#69709=CARTESIAN_POINT('Ctrl Pts',(78.4404505189736,9.58607874726763,136.732729698797));
#69710=CARTESIAN_POINT('Ctrl Pts',(78.436559386885,9.57550799235334,136.733447166179));
#69711=CARTESIAN_POINT('Origin',(80.,9.,134.));
#69712=CARTESIAN_POINT('',(78.4365593900224,9.5755080008764,137.430947520545));
#69713=CARTESIAN_POINT('',(78.4365593610394,9.57550792214055,137.240217191853));
#69714=CARTESIAN_POINT('',(78.4365593737638,9.57550795670799,134.));
#69715=CARTESIAN_POINT('Ctrl Pts',(78.4365593610394,9.57550792214055,137.240217191853));
#69716=CARTESIAN_POINT('Ctrl Pts',(78.4441567507286,9.59614719978225,137.238854438564));
#69717=CARTESIAN_POINT('Ctrl Pts',(78.452164058202,9.61663935851914,137.23748249975));
#69718=CARTESIAN_POINT('Ctrl Pts',(78.4751003999289,9.67207150003121,137.233704427405));
#69719=CARTESIAN_POINT('Ctrl Pts',(78.4908185278503,9.70666093137332,137.231273238148));
#69720=CARTESIAN_POINT('Ctrl Pts',(78.5121018738559,9.7495418921171,137.228128061239));
#69721=CARTESIAN_POINT('Ctrl Pts',(78.5165791146514,9.75836425742755,137.227473783099));
#69722=CARTESIAN_POINT('Ctrl Pts',(78.5238939653149,9.77246545940252,137.22641558442));
#69723=CARTESIAN_POINT('Ctrl Pts',(78.5266820284786,9.77776992970115,137.226014665493));
#69724=CARTESIAN_POINT('Ctrl Pts',(78.5321095974894,9.78796232448249,137.225238569216));
#69725=CARTESIAN_POINT('Ctrl Pts',(78.5347450217788,9.79285225846006,137.224863642427));
#69726=CARTESIAN_POINT('Ctrl Pts',(78.5412736012842,9.80482207728492,137.223939667203));
#69727=CARTESIAN_POINT('Ctrl Pts',(78.5451938711188,9.8118869398309,137.223388953042));
#69728=CARTESIAN_POINT('Ctrl Pts',(78.558908288206,9.83618392116839,137.221477110259));
#69729=CARTESIAN_POINT('Ctrl Pts',(78.5689580529981,9.85326885122324,137.220101504471));
#69730=CARTESIAN_POINT('Ctrl Pts',(78.6358228215016,9.96243624264813,137.211127292575));
#69731=CARTESIAN_POINT('Ctrl Pts',(78.7011862165201,10.0489724589298,137.203171911928));
#69732=CARTESIAN_POINT('Ctrl Pts',(78.8422075956884,10.2021111029538,137.188068368296));
#69733=CARTESIAN_POINT('Ctrl Pts',(78.9164366201114,10.2694293964965,137.180934778744));
#69734=CARTESIAN_POINT('Ctrl Pts',(79.0126836258733,10.3420824796925,137.172669483643));
#69735=CARTESIAN_POINT('Ctrl Pts',(79.029327568455,10.3541691553361,137.17127149212));
#69736=CARTESIAN_POINT('Ctrl Pts',(79.053897604199,10.3713258513728,137.169251906349));
#69737=CARTESIAN_POINT('Ctrl Pts',(79.0616490111354,10.3766414790926,137.168621001937));
#69738=CARTESIAN_POINT('Ctrl Pts',(79.0773649264363,10.3872244542846,137.167354179846));
#69739=CARTESIAN_POINT('Ctrl Pts',(79.0853305657053,10.3924894965559,137.166718365568));
#69740=CARTESIAN_POINT('Ctrl Pts',(79.1025455082022,10.4036565835148,137.165357454539));
#69741=CARTESIAN_POINT('Ctrl Pts',(79.1118087782443,10.4095363537644,137.16463320721));
#69742=CARTESIAN_POINT('Ctrl Pts',(79.1370363126506,10.4252018319677,137.162681922915));
#69743=CARTESIAN_POINT('Ctrl Pts',(79.1531088633351,10.4348108015295,137.161461360357));
#69744=CARTESIAN_POINT('Ctrl Pts',(79.255317963956,10.4936004893069,137.153832918091));
#69745=CARTESIAN_POINT('Ctrl Pts',(79.3455445039721,10.5352802477523,137.147703388719));
#69746=CARTESIAN_POINT('Ctrl Pts',(79.5059607040737,10.5926535732133,137.137281713342));
#69747=CARTESIAN_POINT('Ctrl Pts',(79.5744316013533,10.6122999311012,137.132966095825));
#69748=CARTESIAN_POINT('Ctrl Pts',(79.6803413395232,10.6354700730709,137.126236506467));
#69749=CARTESIAN_POINT('Ctrl Pts',(79.7169912342135,10.6422087862814,137.123897445164));
#69750=CARTESIAN_POINT('Ctrl Pts',(79.7693891997842,10.6500369799307,137.120500313191));
#69751=CARTESIAN_POINT('Ctrl Pts',(79.7849762807276,10.6521404714815,137.119483123625));
#69752=CARTESIAN_POINT('Ctrl Pts',(79.8126981119374,10.6554826291982,137.117658570102));
#69753=CARTESIAN_POINT('Ctrl Pts',(79.8248212730772,10.6568093206845,137.116855435411));
#69754=CARTESIAN_POINT('Ctrl Pts',(79.8434145542836,10.6586377227587,137.115614156822));
#69755=CARTESIAN_POINT('Ctrl Pts',(79.8498751598587,10.6592349520136,137.115181094226));
#69756=CARTESIAN_POINT('Ctrl Pts',(79.8617961764518,10.660266757952,137.114378503731));
#69757=CARTESIAN_POINT('Ctrl Pts',(79.867255441798,10.6607121615801,137.114009576577));
#69758=CARTESIAN_POINT('Ctrl Pts',(79.879717665427,10.6616670725899,137.113164293621));
#69759=CARTESIAN_POINT('Ctrl Pts',(79.8867217125316,10.6621592358291,137.112687011154));
#69760=CARTESIAN_POINT('Ctrl Pts',(79.9089820012279,10.6635820820643,137.111163518315));
#69761=CARTESIAN_POINT('Ctrl Pts',(79.9242475335512,10.6643470618944,137.11010892025));
#69762=CARTESIAN_POINT('Ctrl Pts',(80.0412447323588,10.668597104661,137.10196180995));
#69763=CARTESIAN_POINT('Ctrl Pts',(80.1430844532501,10.6629614691322,137.09451097101));
#69764=CARTESIAN_POINT('Ctrl Pts',(80.3581200602769,10.631155894574,137.07870094813));
#69765=CARTESIAN_POINT('Ctrl Pts',(80.470425302254,10.6023822883109,137.070409584079));
#69766=CARTESIAN_POINT('Ctrl Pts',(80.5969898265088,10.5554847758582,137.061174597286));
#69767=CARTESIAN_POINT('Ctrl Pts',(80.6150000626136,10.5484523623587,137.059862232195));
#69768=CARTESIAN_POINT('Ctrl Pts',(80.6431531455503,10.5368907768096,137.057812784356));
#69769=CARTESIAN_POINT('Ctrl Pts',(80.6533796047633,10.5325711503486,137.057068749769));
#69770=CARTESIAN_POINT('Ctrl Pts',(80.6724826551113,10.5242761081943,137.055679401051));
#69771=CARTESIAN_POINT('Ctrl Pts',(80.6813690377307,10.5203245761071,137.055033310805));
#69772=CARTESIAN_POINT('Ctrl Pts',(80.7012782375894,10.5112618713821,137.053585999822));
#69773=CARTESIAN_POINT('Ctrl Pts',(80.7122808458653,10.5061074397518,137.052786299797));
#69774=CARTESIAN_POINT('Ctrl Pts',(80.7445770879048,10.4905444205572,137.050438512168));
#69775=CARTESIAN_POINT('Ctrl Pts',(80.7657066730077,10.4798010309386,137.048902004));
#69776=CARTESIAN_POINT('Ctrl Pts',(80.8741629807096,10.4217108576275,137.040999131004));
#69777=CARTESIAN_POINT('Ctrl Pts',(80.95735954906,10.3670729803495,137.034897172586));
#69778=CARTESIAN_POINT('Ctrl Pts',(81.0992953801532,10.254510936634,137.023830527725));
#69779=CARTESIAN_POINT('Ctrl Pts',(81.1595555584995,10.1990317287867,137.01886543544));
#69780=CARTESIAN_POINT('Ctrl Pts',(81.2327128834758,10.1209857011942,137.012124713097));
#69781=CARTESIAN_POINT('Ctrl Pts',(81.249513077078,10.1022281660943,137.010520676842));
#69782=CARTESIAN_POINT('Ctrl Pts',(81.2772104621868,10.0698565956479,137.00776459678));
#69783=CARTESIAN_POINT('Ctrl Pts',(81.2883310684674,10.0564386869723,137.00662557701));
#69784=CARTESIAN_POINT('Ctrl Pts',(81.3039183880279,10.0370191561546,137.004977737447));
#69785=CARTESIAN_POINT('Ctrl Pts',(81.3085587520806,10.0311575436909,137.004480433655));
#69786=CARTESIAN_POINT('Ctrl Pts',(81.3165527052162,10.020918889011,137.003611524914));
#69787=CARTESIAN_POINT('Ctrl Pts',(81.3199242697735,10.0165561099329,137.003241187156));
#69788=CARTESIAN_POINT('Ctrl Pts',(81.3270879085903,10.0071906900113,137.002445881928));
#69789=CARTESIAN_POINT('Ctrl Pts',(81.3308733237961,10.0021834143096,137.002020507632));
#69790=CARTESIAN_POINT('Ctrl Pts',(81.3411588937267,9.98841681493098,137.000850854266));
#69791=CARTESIAN_POINT('Ctrl Pts',(81.3476013271066,9.97961503953268,137.000102848898));
#69792=CARTESIAN_POINT('Ctrl Pts',(81.3829464792416,9.93031732360164,136.995915217375));
#69793=CARTESIAN_POINT('Ctrl Pts',(81.4101077302643,9.8886092939543,136.99237983895));
#69794=CARTESIAN_POINT('Ctrl Pts',(81.4861778279224,9.75950789100241,136.98159180925));
#69795=CARTESIAN_POINT('Ctrl Pts',(81.5291201290991,9.66885700191761,136.974233533431));
#69796=CARTESIAN_POINT('Ctrl Pts',(81.5902754412872,9.50252003513767,136.961501041081));
#69797=CARTESIAN_POINT('Ctrl Pts',(81.6118311849855,9.42837563872173,136.956070830108));
#69798=CARTESIAN_POINT('Ctrl Pts',(81.6319586796834,9.33553822559325,136.949585577354));
#69799=CARTESIAN_POINT('Ctrl Pts',(81.6354623509377,9.31802197222772,136.948375063007));
#69800=CARTESIAN_POINT('Ctrl Pts',(81.6406290638025,9.2898424152369,136.946447872807));
#69801=CARTESIAN_POINT('Ctrl Pts',(81.6424713083734,9.27921382720119,136.945725571437));
#69802=CARTESIAN_POINT('Ctrl Pts',(81.64578689093,9.25891536543541,136.944354584762));
#69803=CARTESIAN_POINT('Ctrl Pts',(81.6472785455074,9.2492489865344,136.943705346627));
#69804=CARTESIAN_POINT('Ctrl Pts',(81.6504780457373,9.22723048957915,136.942234475678));
#69805=CARTESIAN_POINT('Ctrl Pts',(81.652132528817,9.21487111519411,136.94141455346));
#69806=CARTESIAN_POINT('Ctrl Pts',(81.656922081295,9.17575769578835,136.938836791272));
#69807=CARTESIAN_POINT('Ctrl Pts',(81.6595472699879,9.14894475857101,136.937094871233));
#69808=CARTESIAN_POINT('Ctrl Pts',(81.6712224189802,8.99004308033938,136.926896824456));
#69809=CARTESIAN_POINT('Ctrl Pts',(81.6651515597865,8.85732401881156,136.918935842363));
#69810=CARTESIAN_POINT('Ctrl Pts',(81.6316554657435,8.65589040181983,136.906409426386));
#69811=CARTESIAN_POINT('Ctrl Pts',(81.6153131106448,8.58590802729544,136.901960051444));
#69812=CARTESIAN_POINT('Ctrl Pts',(81.5899272799326,8.50206680169757,136.896276951877));
#69813=CARTESIAN_POINT('Ctrl Pts',(81.5851280112728,8.4869937927546,136.895240864237));
#69814=CARTESIAN_POINT('Ctrl Pts',(81.5778349735574,8.46516866762161,136.89371652191));
#69815=CARTESIAN_POINT('Ctrl Pts',(81.5755107528314,8.45836024811325,136.89323755076));
#69816=CARTESIAN_POINT('Ctrl Pts',(81.5713540664811,8.44643707202731,136.892392338283));
#69817=CARTESIAN_POINT('Ctrl Pts',(81.5695405691288,8.44131590494413,136.892027204831));
#69818=CARTESIAN_POINT('Ctrl Pts',(81.5655263782726,8.4301539769805,136.891226680444));
#69819=CARTESIAN_POINT('Ctrl Pts',(81.5633157933471,8.42411714923985,136.890790741317));
#69820=CARTESIAN_POINT('Ctrl Pts',(81.5570246087822,8.4072399016705,136.889563904925));
#69821=CARTESIAN_POINT('Ctrl Pts',(81.5528659058478,8.39642926986835,136.888768685536));
#69822=CARTESIAN_POINT('Ctrl Pts',(81.5222892163702,8.31935279925682,136.883036021022));
#69823=CARTESIAN_POINT('Ctrl Pts',(81.4917543439312,8.25480757612961,136.877903187313));
#69824=CARTESIAN_POINT('Ctrl Pts',(81.4502898035044,8.17998923869833,136.871692828559));
#69825=CARTESIAN_POINT('Ctrl Pts',(81.4432387155267,8.16764180305702,136.870658858038));
#69826=CARTESIAN_POINT('Ctrl Pts',(81.4020137165864,8.09755017501308,136.864741651403));
#69827=CARTESIAN_POINT('Ctrl Pts',(81.3645323426622,8.04181919621046,136.859852864129));
#69828=CARTESIAN_POINT('Ctrl Pts',(81.279182604106,7.93011871742011,136.849772279195));
#69829=CARTESIAN_POINT('Ctrl Pts',(81.2307568765635,7.87474700498699,136.844607678291));
#69830=CARTESIAN_POINT('Ctrl Pts',(81.1663483333201,7.81025238864768,136.8383869511));
#69831=CARTESIAN_POINT('Ctrl Pts',(81.1536721564451,7.79795656880646,136.837190498154));
#69832=CARTESIAN_POINT('Ctrl Pts',(81.1329732538303,7.7785078724003,136.835280215567));
#69833=CARTESIAN_POINT('Ctrl Pts',(81.1250729326946,7.77122731266041,136.834560934724));
#69834=CARTESIAN_POINT('Ctrl Pts',(81.1098383097247,7.75745792706753,136.833192272027));
#69835=CARTESIAN_POINT('Ctrl Pts',(81.1025161719375,7.75095637612602,136.832542369872));
#69836=CARTESIAN_POINT('Ctrl Pts',(81.0856769838456,7.7362678007032,136.831065374322));
#69837=CARTESIAN_POINT('Ctrl Pts',(81.0761237914023,7.72812296792738,136.830240044582));
#69838=CARTESIAN_POINT('Ctrl Pts',(81.0503887938214,7.70667945261632,136.828049171444));
#69839=CARTESIAN_POINT('Ctrl Pts',(81.0340464230124,7.69357636496063,136.826691465504));
#69840=CARTESIAN_POINT('Ctrl Pts',(80.9209696590145,7.60636456397531,136.817510131877));
#69841=CARTESIAN_POINT('Ctrl Pts',(80.8166041346293,7.54275383490075,136.810112937507));
#69842=CARTESIAN_POINT('Ctrl Pts',(80.6468474133552,7.46330148471858,136.798658618166));
#69843=CARTESIAN_POINT('Ctrl Pts',(80.5858862609422,7.43904197648147,136.794639866934));
#69844=CARTESIAN_POINT('Ctrl Pts',(80.5024725214716,7.41142344598125,136.789077368489));
#69845=CARTESIAN_POINT('Ctrl Pts',(80.4811476814525,7.40483514568857,136.78764973846));
#69846=CARTESIAN_POINT('Ctrl Pts',(80.4443864797406,7.39428196086315,136.785169016454));
#69847=CARTESIAN_POINT('Ctrl Pts',(80.4290133520928,7.3901064436533,136.784125785631));
#69848=CARTESIAN_POINT('Ctrl Pts',(80.406594820929,7.38436121002614,136.782592842662));
#69849=CARTESIAN_POINT('Ctrl Pts',(80.3995948267126,7.38261568644368,136.782112561499));
#69850=CARTESIAN_POINT('Ctrl Pts',(80.3872541589689,7.37962341033284,136.781262619434));
#69851=CARTESIAN_POINT('Ctrl Pts',(80.381918337216,7.37835748132305,136.780894052722));
#69852=CARTESIAN_POINT('Ctrl Pts',(80.3703065362092,7.37566305993886,136.780089559));
#69853=CARTESIAN_POINT('Ctrl Pts',(80.3640285949764,7.37424460507,136.779653108145));
#69854=CARTESIAN_POINT('Ctrl Pts',(80.3463976223474,7.37036825622229,136.778423478526));
#69855=CARTESIAN_POINT('Ctrl Pts',(80.3350271334523,7.36799272854395,136.777625947544));
#69856=CARTESIAN_POINT('Ctrl Pts',(80.2466940468641,7.3505001320761,136.771400025706));
#69857=CARTESIAN_POINT('Ctrl Pts',(80.1687834258318,7.34071788543422,136.765735938482));
#69858=CARTESIAN_POINT('Ctrl Pts',(80.0841050236893,7.33611203704654,136.759570310174));
#69859=CARTESIAN_POINT('Ctrl Pts',(80.0777243878536,7.33580177639229,136.759105630035));
#69860=CARTESIAN_POINT('Ctrl Pts',(80.0049687431653,7.33268334361355,136.753806824493));
#69861=CARTESIAN_POINT('Ctrl Pts',(79.9384815145451,7.333811005712,136.748965503485));
#69862=CARTESIAN_POINT('Ctrl Pts',(79.7977697960227,7.34463383993467,136.738838859056));
#69863=CARTESIAN_POINT('Ctrl Pts',(79.7237636951394,7.3553631071429,136.73358567604));
#69864=CARTESIAN_POINT('Ctrl Pts',(79.6333835584968,7.37474227366125,136.727276485483));
#69865=CARTESIAN_POINT('Ctrl Pts',(79.6161091430804,7.3787356340346,136.726075186789));
#69866=CARTESIAN_POINT('Ctrl Pts',(79.588459588512,7.38559415740954,136.724159077109));
#69867=CARTESIAN_POINT('Ctrl Pts',(79.5780431392189,7.38828533793717,136.723438755088));
#69868=CARTESIAN_POINT('Ctrl Pts',(79.5582009220473,7.39361730171117,136.722069298777));
#69869=CARTESIAN_POINT('Ctrl Pts',(79.5487709702345,7.39624061395898,136.721419632922));
#69870=CARTESIAN_POINT('Ctrl Pts',(79.5273289595814,7.40240964810455,136.719944784321));
#69871=CARTESIAN_POINT('Ctrl Pts',(79.5153325728377,7.40600804763197,136.719121346653));
#69872=CARTESIAN_POINT('Ctrl Pts',(79.4834852018927,7.41595367384657,136.716939070755));
#69873=CARTESIAN_POINT('Ctrl Pts',(79.4637104247722,7.42253879498198,136.715587970325));
#69874=CARTESIAN_POINT('Ctrl Pts',(79.3277038545238,7.47068312921476,136.706310434162));
#69875=CARTESIAN_POINT('Ctrl Pts',(79.2162803033471,7.52467647500018,136.698823529851));
#69876=CARTESIAN_POINT('Ctrl Pts',(79.0335694217868,7.63980673795968,136.685623092476));
#69877=CARTESIAN_POINT('Ctrl Pts',(78.9595576862316,7.69555042192493,136.679945541948));
#69878=CARTESIAN_POINT('Ctrl Pts',(78.8815147889027,7.76521500198143,136.673108825756));
#69879=CARTESIAN_POINT('Ctrl Pts',(78.8725537632234,7.77339161877224,136.672309866105));
#69880=CARTESIAN_POINT('Ctrl Pts',(78.8589482264551,7.78608123331161,136.671073704971));
#69881=CARTESIAN_POINT('Ctrl Pts',(78.8542391888395,7.79052487330223,136.670641520119));
#69882=CARTESIAN_POINT('Ctrl Pts',(78.8455932049895,7.79877938189214,136.669839692465));
#69883=CARTESIAN_POINT('Ctrl Pts',(78.8416490114791,7.80258235939275,136.669470640732));
#69884=CARTESIAN_POINT('Ctrl Pts',(78.832680139837,7.81131589518588,136.668623975459));
#69885=CARTESIAN_POINT('Ctrl Pts',(78.8276679044773,7.81625889221227,136.668145423239));
#69886=CARTESIAN_POINT('Ctrl Pts',(78.8118018459658,7.83210538182189,136.666613735772));
#69887=CARTESIAN_POINT('Ctrl Pts',(78.801068026262,7.84312715792007,136.665552089735));
#69888=CARTESIAN_POINT('Ctrl Pts',(78.7015875533203,7.94814790205874,136.655483836516));
#69889=CARTESIAN_POINT('Ctrl Pts',(78.6239167938436,8.05202297935756,136.645917844602));
#69890=CARTESIAN_POINT('Ctrl Pts',(78.5140361434025,8.24137836753594,136.630102035964));
#69891=CARTESIAN_POINT('Ctrl Pts',(78.4753621461088,8.322445951564,136.623750161606));
#69892=CARTESIAN_POINT('Ctrl Pts',(78.4368323551965,8.42345664111919,136.616363206657));
#69893=CARTESIAN_POINT('Ctrl Pts',(78.4305529141594,8.44077623220499,136.615113974666));
#69894=CARTESIAN_POINT('Ctrl Pts',(78.421014869428,8.46851066873512,136.613140259184));
#69895=CARTESIAN_POINT('Ctrl Pts',(78.4175692373393,8.4788590948793,136.612409659228));
#69896=CARTESIAN_POINT('Ctrl Pts',(78.4112349102624,8.49852553556778,136.611031973253));
#69897=CARTESIAN_POINT('Ctrl Pts',(78.4083259638667,8.50783649215256,136.610384247156));
#69898=CARTESIAN_POINT('Ctrl Pts',(78.4018883932622,8.52909608521878,136.608915311756));
#69899=CARTESIAN_POINT('Ctrl Pts',(78.3984116560258,8.54105992217274,136.608095820398));
#69900=CARTESIAN_POINT('Ctrl Pts',(78.3896655882493,8.57246658091112,136.605962403692));
#69901=CARTESIAN_POINT('Ctrl Pts',(78.3846140015559,8.59196829271555,136.60465547565));
#69902=CARTESIAN_POINT('Ctrl Pts',(78.3492974616268,8.73926351182668,136.594905585127));
#69903=CARTESIAN_POINT('Ctrl Pts',(78.3338838504094,8.87014160580966,136.586972037662));
#69904=CARTESIAN_POINT('Ctrl Pts',(78.3340197490512,9.02294677687804,136.577620043621));
#69905=CARTESIAN_POINT('Ctrl Pts',(78.3344536791785,9.04440920217299,136.576303249206));
#69906=CARTESIAN_POINT('Ctrl Pts',(78.3378839391261,9.13111758901513,136.570951054929));
#69907=CARTESIAN_POINT('Ctrl Pts',(78.3443007902142,9.19616240125983,136.566863007183));
#69908=CARTESIAN_POINT('Ctrl Pts',(78.3563104862453,9.27197837462577,136.56184054762));
#69909=CARTESIAN_POINT('Ctrl Pts',(78.3582210861192,9.2832833103782,136.561084807116));
#69910=CARTESIAN_POINT('Ctrl Pts',(78.361380210246,9.30086903943918,136.559897239663));
#69911=CARTESIAN_POINT('Ctrl Pts',(78.3625485693222,9.30716413041022,136.559469734436));
#69912=CARTESIAN_POINT('Ctrl Pts',(78.3647761199494,9.31879213203793,136.558675366611));
#69913=CARTESIAN_POINT('Ctrl Pts',(78.3658251665951,9.32412678388195,136.55830907206));
#69914=CARTESIAN_POINT('Ctrl Pts',(78.36833079584,9.33654707787777,136.557451973668));
#69915=CARTESIAN_POINT('Ctrl Pts',(78.3698074289554,9.34362843866692,136.556960070411));
#69916=CARTESIAN_POINT('Ctrl Pts',(78.374706053551,9.36637793164341,136.555369859755));
#69917=CARTESIAN_POINT('Ctrl Pts',(78.3783080674557,9.38200579814046,136.554262270216));
#69918=CARTESIAN_POINT('Ctrl Pts',(78.3875090109046,9.41944717148081,136.551575936862));
#69919=CARTESIAN_POINT('Ctrl Pts',(78.3933256591598,9.44120355757371,136.549988014995));
#69920=CARTESIAN_POINT('Ctrl Pts',(78.4105689193626,9.50082844584118,136.545573123226));
#69921=CARTESIAN_POINT('Ctrl Pts',(78.422903446365,9.53840988900929,136.542719656609));
#69922=CARTESIAN_POINT('Ctrl Pts',(78.4365593610507,9.57550792217122,136.539851329404));
#69923=CARTESIAN_POINT('Ctrl Pts',(78.436559386885,9.57550799235334,136.733447166179));
#69924=CARTESIAN_POINT('Ctrl Pts',(78.4030736853152,9.48453982772584,136.7396214358));
#69925=CARTESIAN_POINT('Ctrl Pts',(78.3775820235553,9.3907985152114,136.745546815303));
#69926=CARTESIAN_POINT('Ctrl Pts',(78.3470673792254,9.22139434210338,136.756057559526));
#69927=CARTESIAN_POINT('Ctrl Pts',(78.3387660613633,9.14663529075277,136.760635517436));
#69928=CARTESIAN_POINT('Ctrl Pts',(78.3345040615497,9.04752667892352,136.766897315785));
#69929=CARTESIAN_POINT('Ctrl Pts',(78.3339912587269,9.02345761297898,136.768433258204));
#69930=CARTESIAN_POINT('Ctrl Pts',(78.3340063127332,8.98253179884407,136.771083427609));
#69931=CARTESIAN_POINT('Ctrl Pts',(78.3342683081362,8.96567826665469,136.772185903033));
#69932=CARTESIAN_POINT('Ctrl Pts',(78.3350100826247,8.94153772320898,136.773784708654));
#69933=CARTESIAN_POINT('Ctrl Pts',(78.3352821544608,8.93424475258736,136.774270287832));
#69934=CARTESIAN_POINT('Ctrl Pts',(78.3358435545575,8.92145291171762,136.77512687663));
#69935=CARTESIAN_POINT('Ctrl Pts',(78.336112240968,8.91595332062918,136.775496744943));
#69936=CARTESIAN_POINT('Ctrl Pts',(78.3367468940995,8.90416255723736,136.776293261581));
#69937=CARTESIAN_POINT('Ctrl Pts',(78.3371212853714,8.89787220329512,136.776720336044));
#69938=CARTESIAN_POINT('Ctrl Pts',(78.3382678817186,8.88029006601136,136.777919737365));
#69939=CARTESIAN_POINT('Ctrl Pts',(78.3391194664742,8.86900405722907,136.778696199416));
#69940=CARTESIAN_POINT('Ctrl Pts',(78.345620941244,8.79315013695945,136.783955179707));
#69941=CARTESIAN_POINT('Ctrl Pts',(78.3549191936476,8.72895721360702,136.788600550031));
#69942=CARTESIAN_POINT('Ctrl Pts',(78.3892328775846,8.56154782536482,136.800982578253));
#69943=CARTESIAN_POINT('Ctrl Pts',(78.4204160779959,8.45988032602276,136.808760913248));
#69944=CARTESIAN_POINT('Ctrl Pts',(78.4829024545348,8.30918647951376,136.820349849389));
#69945=CARTESIAN_POINT('Ctrl Pts',(78.5074387888753,8.25765869026001,136.824328711338));
#69946=CARTESIAN_POINT('Ctrl Pts',(78.5427106751217,8.19243793920472,136.829384750903));
#69947=CARTESIAN_POINT('Ctrl Pts',(78.5510801249017,8.17751602332318,136.830543104393));
#69948=CARTESIAN_POINT('Ctrl Pts',(78.565016929048,8.15354123986161,136.832407432349));
#69949=CARTESIAN_POINT('Ctrl Pts',(78.5704434701634,8.14440840141322,136.833118397418));
#69950=CARTESIAN_POINT('Ctrl Pts',(78.5810561805067,8.12693015172603,136.834480789204));
#69951=CARTESIAN_POINT('Ctrl Pts',(78.5862295314058,8.11857751785878,136.835132646085));
#69952=CARTESIAN_POINT('Ctrl Pts',(78.5984298129583,8.09926334226122,136.836642101561));
#69953=CARTESIAN_POINT('Ctrl Pts',(78.6055120194309,8.0883373409974,136.837497619059));
#69954=CARTESIAN_POINT('Ctrl Pts',(78.6289517611519,8.05308826193487,136.840264121129));
#69955=CARTESIAN_POINT('Ctrl Pts',(78.6458237677389,8.02911277069109,136.842155863237));
#69956=CARTESIAN_POINT('Ctrl Pts',(78.687779516564,7.97271591149635,136.846642829469));
#69957=CARTESIAN_POINT('Ctrl Pts',(78.7134443739473,7.94075018576501,136.849216611562));
#69958=CARTESIAN_POINT('Ctrl Pts',(78.7883700637603,7.85417587290556,136.856329726646));
#69959=CARTESIAN_POINT('Ctrl Pts',(78.8401043991311,7.80183360512246,136.860796614085));
#69960=CARTESIAN_POINT('Ctrl Pts',(78.9595934886699,7.69595660826427,136.870555998891));
#69961=CARTESIAN_POINT('Ctrl Pts',(79.0283848665807,7.64392655417022,136.875844112729));
#69962=CARTESIAN_POINT('Ctrl Pts',(79.1141666863909,7.58893498888015,136.882455019426));
#69963=CARTESIAN_POINT('Ctrl Pts',(79.127574218344,7.5806063490936,136.883488876303));
#69964=CARTESIAN_POINT('Ctrl Pts',(79.1471901595856,7.56880401922944,136.88500539939));
#69965=CARTESIAN_POINT('Ctrl Pts',(79.1533061405205,7.56517734092202,136.885478776532));
#69966=CARTESIAN_POINT('Ctrl Pts',(79.1641803132638,7.55882286604679,136.886321747656));
#69967=CARTESIAN_POINT('Ctrl Pts',(79.1689290337283,7.55607925150957,136.886690321747));
#69968=CARTESIAN_POINT('Ctrl Pts',(79.1792668997422,7.55017435272811,136.887493772831));
#69969=CARTESIAN_POINT('Ctrl Pts',(79.1848607139052,7.54702196502059,136.887929163654));
#69970=CARTESIAN_POINT('Ctrl Pts',(79.2008557751368,7.53812940244398,136.88917565485));
#69971=CARTESIAN_POINT('Ctrl Pts',(79.2113001410009,7.53246817806658,136.889991407863));
#69972=CARTESIAN_POINT('Ctrl Pts',(79.2352491944495,7.51981641808843,136.891864572921));
#69973=CARTESIAN_POINT('Ctrl Pts',(79.2487907110497,7.51289818820773,136.892925596629));
#69974=CARTESIAN_POINT('Ctrl Pts',(79.3926812392006,7.44185269648364,136.904205504012));
#69975=CARTESIAN_POINT('Ctrl Pts',(79.5307891946342,7.39485083645149,136.91501211988));
#69976=CARTESIAN_POINT('Ctrl Pts',(79.7375241832035,7.35350096951997,136.930069769281));
#69977=CARTESIAN_POINT('Ctrl Pts',(79.8025087289686,7.34444820210943,136.934662444953));
#69978=CARTESIAN_POINT('Ctrl Pts',(79.88545485719,7.33784875794428,136.940341161207));
#69979=CARTESIAN_POINT('Ctrl Pts',(79.903065819285,7.33672878116685,136.94153669007));
#69980=CARTESIAN_POINT('Ctrl Pts',(79.9314178969884,7.3353775790235,136.943445734171));
#69981=CARTESIAN_POINT('Ctrl Pts',(79.9421488409848,7.3349701017669,136.944164690372));
#69982=CARTESIAN_POINT('Ctrl Pts',(79.9626687076319,7.33438953908708,136.945532878419));
#69983=CARTESIAN_POINT('Ctrl Pts',(79.9724566431502,7.33419893043463,136.946182628945));
#69984=CARTESIAN_POINT('Ctrl Pts',(79.9950119682409,7.33395855055136,136.947673585971));
#69985=CARTESIAN_POINT('Ctrl Pts',(80.0077794925974,7.33396924208447,136.948512875108));
#69986=CARTESIAN_POINT('Ctrl Pts',(80.0484006518734,7.33447024037042,136.951169344954));
#69987=CARTESIAN_POINT('Ctrl Pts',(80.076243568615,7.33551237129322,136.952969410681));
#69988=CARTESIAN_POINT('Ctrl Pts',(80.1770792879234,7.34182229840092,136.959429254076));
#69989=CARTESIAN_POINT('Ctrl Pts',(80.2497335226601,7.35119888417629,136.963966667801));
#69990=CARTESIAN_POINT('Ctrl Pts',(80.4498370468105,7.39055937721553,136.976475842704));
#69991=CARTESIAN_POINT('Ctrl Pts',(80.5746952596342,7.43080668921727,136.984278205149));
#69992=CARTESIAN_POINT('Ctrl Pts',(80.7072561045526,7.49150001316877,136.993749635824));
#69993=CARTESIAN_POINT('Ctrl Pts',(80.7208808831035,7.49796334230454,136.994738366762));
#69994=CARTESIAN_POINT('Ctrl Pts',(80.7407501115925,7.50772151433877,136.996205496484));
#69995=CARTESIAN_POINT('Ctrl Pts',(80.7470647878348,7.51087273718508,136.996675560369));
#69996=CARTESIAN_POINT('Ctrl Pts',(80.7582379682765,7.516537460813,136.997514382947));
#69997=CARTESIAN_POINT('Ctrl Pts',(80.7631043855971,7.51903490358137,136.997882150861));
#69998=CARTESIAN_POINT('Ctrl Pts',(80.7737677952332,7.5245738742949,136.998693420935));
#69999=CARTESIAN_POINT('Ctrl Pts',(80.7795591139725,7.52762557835944,136.999137526626));
#70000=CARTESIAN_POINT('Ctrl Pts',(80.7963388836133,7.53659433490796,137.000434164659));
#70001=CARTESIAN_POINT('Ctrl Pts',(80.8072787359053,7.5426006801379,137.001291930846));
#70002=CARTESIAN_POINT('Ctrl Pts',(80.8322664331978,7.55668742064324,137.003278070515));
#70003=CARTESIAN_POINT('Ctrl Pts',(80.846265765879,7.56485093877536,137.00441067271));
#70004=CARTESIAN_POINT('Ctrl Pts',(80.8935450089723,7.59335346502885,137.008298515055));
#70005=CARTESIAN_POINT('Ctrl Pts',(80.9262273734105,7.61465541325279,137.011093449451));
#70006=CARTESIAN_POINT('Ctrl Pts',(81.0157500518482,7.67758981040091,137.019000471824));
#70007=CARTESIAN_POINT('Ctrl Pts',(81.0707431456563,7.72170971288379,137.024153825553));
#70008=CARTESIAN_POINT('Ctrl Pts',(81.1942227452502,7.83435010290942,137.036260037415));
#70009=CARTESIAN_POINT('Ctrl Pts',(81.2598665593812,7.90562817839676,137.043136301701));
#70010=CARTESIAN_POINT('Ctrl Pts',(81.3304312911098,7.99707379042736,137.05103540341));
#70011=CARTESIAN_POINT('Ctrl Pts',(81.3416480347789,8.01212905548655,137.052309403241));
#70012=CARTESIAN_POINT('Ctrl Pts',(81.3590799344955,8.03637112370215,137.054319988779));
#70013=CARTESIAN_POINT('Ctrl Pts',(81.3654616852998,8.0454355569973,137.055062941595));
#70014=CARTESIAN_POINT('Ctrl Pts',(81.3772182215592,8.06249334398771,137.056444941151));
#70015=CARTESIAN_POINT('Ctrl Pts',(81.3826150441936,8.07047086861635,137.057084805771));
#70016=CARTESIAN_POINT('Ctrl Pts',(81.394645433703,8.08859066904249,137.058523918968));
#70017=CARTESIAN_POINT('Ctrl Pts',(81.4012381752752,8.09875949746397,137.059321617668));
#70018=CARTESIAN_POINT('Ctrl Pts',(81.4207421221415,8.12957439531984,137.061710067042));
#70019=CARTESIAN_POINT('Ctrl Pts',(81.4333125873483,8.15043303020283,137.063288340336));
#70020=CARTESIAN_POINT('Ctrl Pts',(81.4613258109241,8.19930917774067,137.066905332146));
#70021=CARTESIAN_POINT('Ctrl Pts',(81.4764281202986,8.22751109276889,137.068932489297));
#70022=CARTESIAN_POINT('Ctrl Pts',(81.5290033459996,8.33287168606672,137.076320011856));
#70023=CARTESIAN_POINT('Ctrl Pts',(81.5613147843599,8.41245538300326,137.081535407693));
#70024=CARTESIAN_POINT('Ctrl Pts',(81.6148198800948,8.58036312745446,137.092302034073));
#70025=CARTESIAN_POINT('Ctrl Pts',(81.6352154788742,8.66863238517132,137.097840102902));
#70026=CARTESIAN_POINT('Ctrl Pts',(81.6506322174938,8.77368769325163,137.104729507002));
#70027=CARTESIAN_POINT('Ctrl Pts',(81.652697507866,8.78929907209232,137.105761031409));
#70028=CARTESIAN_POINT('Ctrl Pts',(81.6553728835853,8.8119918009125,137.107274750262));
#70029=CARTESIAN_POINT('Ctrl Pts',(81.6561594996812,8.81905201392687,137.10774770353));
#70030=CARTESIAN_POINT('Ctrl Pts',(81.6574732822563,8.83157081142447,137.108590208591));
#70031=CARTESIAN_POINT('Ctrl Pts',(81.6580186866952,8.83702728371803,137.10895874472));
#70032=CARTESIAN_POINT('Ctrl Pts',(81.6591446599214,8.84888320875113,137.109762467733));
#70033=CARTESIAN_POINT('Ctrl Pts',(81.6597151408411,8.85528325970895,137.110198171706));
#70034=CARTESIAN_POINT('Ctrl Pts',(81.661236646562,8.87354665634267,137.111446449934));
#70035=CARTESIAN_POINT('Ctrl Pts',(81.6620975663473,8.88541682635254,137.112263697002));
#70036=CARTESIAN_POINT('Ctrl Pts',(81.6686518303634,8.99153249930862,137.11961669387));
#70037=CARTESIAN_POINT('Ctrl Pts',(81.6664502117914,9.08608453758049,137.126489790719));
#70038=CARTESIAN_POINT('Ctrl Pts',(81.6431119020496,9.30091395812051,137.142220075137));
#70039=CARTESIAN_POINT('Ctrl Pts',(81.616749530842,9.42011567995595,137.151009721228));
#70040=CARTESIAN_POINT('Ctrl Pts',(81.5708940626847,9.55523578336539,137.160824648851));
#70041=CARTESIAN_POINT('Ctrl Pts',(81.5637873314049,9.5749471129144,137.162253763344));
#70042=CARTESIAN_POINT('Ctrl Pts',(81.5518306590445,9.6062468085746,137.16451959139));
#70043=CARTESIAN_POINT('Ctrl Pts',(81.547218424341,9.61792293177251,137.165364066556));
#70044=CARTESIAN_POINT('Ctrl Pts',(81.5387753200797,9.63860969892447,137.166859192072));
#70045=CARTESIAN_POINT('Ctrl Pts',(81.5349962149629,9.64764068767145,137.167511544957));
#70046=CARTESIAN_POINT('Ctrl Pts',(81.5269053177683,9.66650690800216,137.16887383513));
#70047=CARTESIAN_POINT('Ctrl Pts',(81.5225775820687,9.67633484571877,137.169583195738));
#70048=CARTESIAN_POINT('Ctrl Pts',(81.5108883537846,9.702199197676,137.171449730414));
#70049=CARTESIAN_POINT('Ctrl Pts',(81.5033664766593,9.71816196390955,137.172601383266));
#70050=CARTESIAN_POINT('Ctrl Pts',(81.4633015131445,9.79979769045396,137.178494476378));
#70051=CARTESIAN_POINT('Ctrl Pts',(81.4267022120965,9.86339470417785,137.18309201408));
#70052=CARTESIAN_POINT('Ctrl Pts',(81.3312272227854,10.006551182847,137.193712905817));
#70053=CARTESIAN_POINT('Ctrl Pts',(81.2692294400598,10.0836819981732,137.199650714628));
#70054=CARTESIAN_POINT('Ctrl Pts',(81.1627542193764,10.1943893051936,137.209183141753));
#70055=CARTESIAN_POINT('Ctrl Pts',(81.1228165717532,10.2320084490749,137.2126423618));
#70056=CARTESIAN_POINT('Ctrl Pts',(81.0725947826126,10.2748417351893,137.216964011017));
#70057=CARTESIAN_POINT('Ctrl Pts',(81.064015015251,10.2820113291743,137.217701391912));
#70058=CARTESIAN_POINT('Ctrl Pts',(81.0504599681644,10.2931086668703,137.218866131505));
#70059=CARTESIAN_POINT('Ctrl Pts',(81.0455331445941,10.2970954511045,137.219289428603));
#70060=CARTESIAN_POINT('Ctrl Pts',(81.0367206717318,10.3041436726657,137.220046729303));
#70061=CARTESIAN_POINT('Ctrl Pts',(81.0328439664583,10.3072160528096,137.220379946082));
#70062=CARTESIAN_POINT('Ctrl Pts',(81.0234193004885,10.3146172269441,137.221190164059));
#70063=CARTESIAN_POINT('Ctrl Pts',(81.0178575820266,10.3189281467118,137.221668385616));
#70064=CARTESIAN_POINT('Ctrl Pts',(81.0003786265952,10.3322997865969,137.223171157498));
#70065=CARTESIAN_POINT('Ctrl Pts',(80.9883668463439,10.3412348996587,137.224203667787));
#70066=CARTESIAN_POINT('Ctrl Pts',(80.9246734000024,10.3872938528503,137.22967064186));
#70067=CARTESIAN_POINT('Ctrl Pts',(80.8710209325088,10.4215927877309,137.234246628945));
#70068=CARTESIAN_POINT('Ctrl Pts',(80.7207611093635,10.5059464438477,137.246749508099));
#70069=CARTESIAN_POINT('Ctrl Pts',(80.6209860253325,10.5497587407792,137.254707430096));
#70070=CARTESIAN_POINT('Ctrl Pts',(80.4690607933605,10.5994220790315,137.266011218455));
#70071=CARTESIAN_POINT('Ctrl Pts',(80.4197640777349,10.6130617125935,137.269565251839));
#70072=CARTESIAN_POINT('Ctrl Pts',(80.3539378517031,10.6280517334369,137.274163338005));
#70073=CARTESIAN_POINT('Ctrl Pts',(80.3379091313229,10.6314539227006,137.275271741466));
#70074=CARTESIAN_POINT('Ctrl Pts',(80.31156082702,10.6366415136901,137.277075992327));
#70075=CARTESIAN_POINT('Ctrl Pts',(80.3012703047201,10.6385669975331,137.27777624808));
#70076=CARTESIAN_POINT('Ctrl Pts',(80.2812275607659,10.6421220423068,137.279131825288));
#70077=CARTESIAN_POINT('Ctrl Pts',(80.2714776606844,10.6437620356028,137.27978745126));
#70078=CARTESIAN_POINT('Ctrl Pts',(80.2484623751338,10.6474229829796,137.281326461368));
#70079=CARTESIAN_POINT('Ctrl Pts',(80.2351859027425,10.6493706815928,137.282207503514));
#70080=CARTESIAN_POINT('Ctrl Pts',(80.1904607809732,10.6553809635095,137.285154198034));
#70081=CARTESIAN_POINT('Ctrl Pts',(80.1589188923718,10.6587062542882,137.287196833749));
#70082=CARTESIAN_POINT('Ctrl Pts',(80.0817652431223,10.6646188745619,137.292123523469));
#70083=CARTESIAN_POINT('Ctrl Pts',(80.0361045469151,10.6662348184673,137.294979714829));
#70084=CARTESIAN_POINT('Ctrl Pts',(79.9202871807467,10.6655696888832,137.302145286982));
#70085=CARTESIAN_POINT('Ctrl Pts',(79.850236043801,10.6607370501646,137.30640394688));
#70086=CARTESIAN_POINT('Ctrl Pts',(79.7581933805297,10.6485147712397,137.312085024652));
#70087=CARTESIAN_POINT('Ctrl Pts',(79.7357524450302,10.645066743442,137.31347727211));
#70088=CARTESIAN_POINT('Ctrl Pts',(79.6490469979864,10.6299245969132,137.318906036174));
#70089=CARTESIAN_POINT('Ctrl Pts',(79.5854286126961,10.6149150765957,137.322994359479));
#70090=CARTESIAN_POINT('Ctrl Pts',(79.5118803014772,10.5929301840218,137.328017006247));
#70091=CARTESIAN_POINT('Ctrl Pts',(79.5009315690447,10.5895339237011,137.32877262626));
#70092=CARTESIAN_POINT('Ctrl Pts',(79.4839251983947,10.584065584103,137.329959974923));
#70093=CARTESIAN_POINT('Ctrl Pts',(79.4778427368079,10.5820710365412,137.330387382962));
#70094=CARTESIAN_POINT('Ctrl Pts',(79.4666170529393,10.5783181478392,137.331181545506));
#70095=CARTESIAN_POINT('Ctrl Pts',(79.4614707563206,10.5765696288291,137.33154773202));
#70096=CARTESIAN_POINT('Ctrl Pts',(79.4494980113515,10.5724362778149,137.332404532393));
#70097=CARTESIAN_POINT('Ctrl Pts',(79.4426784654646,10.570032161951,137.332896244569));
#70098=CARTESIAN_POINT('Ctrl Pts',(79.4207932614516,10.562156352059,137.334485643967));
#70099=CARTESIAN_POINT('Ctrl Pts',(79.405791369107,10.5565117956628,137.335592602676));
#70100=CARTESIAN_POINT('Ctrl Pts',(79.3699279742725,10.5424239612572,137.338277211525));
#70101=CARTESIAN_POINT('Ctrl Pts',(79.349151891389,10.5337728223931,137.33986402686));
#70102=CARTESIAN_POINT('Ctrl Pts',(79.267674636542,10.4978922777206,137.346196413881));
#70103=CARTESIAN_POINT('Ctrl Pts',(79.2084545190922,10.4674592182152,137.351040247954));
#70104=CARTESIAN_POINT('Ctrl Pts',(79.0474882485134,10.3721546951768,137.364657209239));
#70105=CARTESIAN_POINT('Ctrl Pts',(78.9507143056559,10.2996525362347,137.373359192585));
#70106=CARTESIAN_POINT('Ctrl Pts',(78.847302217206,10.2030304697436,137.383094040994));
#70107=CARTESIAN_POINT('Ctrl Pts',(78.8322718237093,10.1884466605559,137.384522420273));
#70108=CARTESIAN_POINT('Ctrl Pts',(78.808678873446,10.1646748412572,137.386787317785));
#70109=CARTESIAN_POINT('Ctrl Pts',(78.7999387177852,10.1556671001299,137.387631587554));
#70110=CARTESIAN_POINT('Ctrl Pts',(78.7845640397795,10.1394591927282,137.389126479589));
#70111=CARTESIAN_POINT('Ctrl Pts',(78.7778897106595,10.1322977845993,137.389778802522));
#70112=CARTESIAN_POINT('Ctrl Pts',(78.7640260963101,10.1171570388989,137.391141159827));
#70113=CARTESIAN_POINT('Ctrl Pts',(78.7568500483043,10.1091661493547,137.391850616386));
#70114=CARTESIAN_POINT('Ctrl Pts',(78.7407313745033,10.0908642412796,137.393454409272));
#70115=CARTESIAN_POINT('Ctrl Pts',(78.7318371039949,10.0805115229938,137.394346731238));
#70116=CARTESIAN_POINT('Ctrl Pts',(78.6919672881274,10.0329334559382,137.398382610261));
#70117=CARTESIAN_POINT('Ctrl Pts',(78.6624949279325,9.99447571999671,137.401465951503));
#70118=CARTESIAN_POINT('Ctrl Pts',(78.5842718581045,9.88262336604409,137.410024479372));
#70119=CARTESIAN_POINT('Ctrl Pts',(78.539605694465,9.80657283152094,137.415372364282));
#70120=CARTESIAN_POINT('Ctrl Pts',(78.4771203097745,9.67780902984256,137.424120149123));
#70121=CARTESIAN_POINT('Ctrl Pts',(78.4555629954577,9.62713370969076,137.427494595459));
#70122=CARTESIAN_POINT('Ctrl Pts',(78.4365593900224,9.5755080008764,137.430947520545));
#70123=CARTESIAN_POINT('Origin',(80.,9.,134.));
#70124=CARTESIAN_POINT('',(78.4365594482967,9.57550815918599,138.131873589273));
#70125=CARTESIAN_POINT('',(78.4365593728781,9.57550795430191,137.937814872615));
#70126=CARTESIAN_POINT('',(78.4365593737638,9.57550795670799,134.));
#70127=CARTESIAN_POINT('',(78.3340004536037,8.99997160195063,137.276979806444));
#70128=CARTESIAN_POINT('Ctrl Pts',(78.4365593728781,9.5755079543019,137.937814872615));
#70129=CARTESIAN_POINT('Ctrl Pts',(78.4603180243237,9.64005135572325,137.933372005971));
#70130=CARTESIAN_POINT('Ctrl Pts',(78.4880535272684,9.70306961636733,137.929060117645));
#70131=CARTESIAN_POINT('Ctrl Pts',(78.5665915402355,9.85521111305201,137.918489348387));
#70132=CARTESIAN_POINT('Ctrl Pts',(78.6218618578815,9.94168978399369,137.912339466934));
#70133=CARTESIAN_POINT('Ctrl Pts',(78.7166757234652,10.0636472777365,137.902733472706));
#70134=CARTESIAN_POINT('Ctrl Pts',(78.7505375248075,10.1032266780965,137.899441897796));
#70135=CARTESIAN_POINT('Ctrl Pts',(78.7937404694485,10.1491803062351,137.895310756722));
#70136=CARTESIAN_POINT('Ctrl Pts',(78.8013677233108,10.1571335621185,137.894583814464));
#70137=CARTESIAN_POINT('Ctrl Pts',(78.8134803147446,10.1695156083388,137.893431954189));
#70138=CARTESIAN_POINT('Ctrl Pts',(78.8179130109011,10.1739957702526,137.89301095204));
#70139=CARTESIAN_POINT('Ctrl Pts',(78.8262671585949,10.1823440941879,137.892218236306));
#70140=CARTESIAN_POINT('Ctrl Pts',(78.830182502229,10.1862180905868,137.89184698729));
#70141=CARTESIAN_POINT('Ctrl Pts',(78.8394248791861,10.1952726065343,137.890971351862));
#70142=CARTESIAN_POINT('Ctrl Pts',(78.8447674349128,10.2004369747196,137.890465762424));
#70143=CARTESIAN_POINT('Ctrl Pts',(78.8625618331006,10.2174090883994,137.888784221988));
#70144=CARTESIAN_POINT('Ctrl Pts',(78.8751610930413,10.2290597415161,137.887597496814));
#70145=CARTESIAN_POINT('Ctrl Pts',(78.906299149686,10.256973567291,137.884678707655));
#70146=CARTESIAN_POINT('Ctrl Pts',(78.9250231240445,10.2730234425448,137.882935391324));
#70147=CARTESIAN_POINT('Ctrl Pts',(79.0048908929729,10.3384661040631,137.875570568485));
#70148=CARTESIAN_POINT('Ctrl Pts',(79.0691330440637,10.3839145534009,137.869821889228));
#70149=CARTESIAN_POINT('Ctrl Pts',(79.2249486631411,10.4783735349723,137.856577618796));
#70150=CARTESIAN_POINT('Ctrl Pts',(79.3183881013215,10.523714118291,137.849147271953));
#70151=CARTESIAN_POINT('Ctrl Pts',(79.4375354745546,10.5683577223649,137.840388347377));
#70152=CARTESIAN_POINT('Ctrl Pts',(79.4597959030243,10.5761636717191,137.838779894225));
#70153=CARTESIAN_POINT('Ctrl Pts',(79.4937410006874,10.5872633250951,137.836368029617));
#70154=CARTESIAN_POINT('Ctrl Pts',(79.505307451961,10.5909061361305,137.835553283614));
#70155=CARTESIAN_POINT('Ctrl Pts',(79.5262182959437,10.5972418213938,137.834092691733));
#70156=CARTESIAN_POINT('Ctrl Pts',(79.5355483451059,10.5999797518256,137.833445401957));
#70157=CARTESIAN_POINT('Ctrl Pts',(79.5555963636861,10.6056727561798,137.83206369325));
#70158=CARTESIAN_POINT('Ctrl Pts',(79.5663210667442,10.6086025565167,137.831330120601));
#70159=CARTESIAN_POINT('Ctrl Pts',(79.595848217657,10.6163520861527,137.829325154166));
#70160=CARTESIAN_POINT('Ctrl Pts',(79.6147071949879,10.6209510279663,137.82806087318));
#70161=CARTESIAN_POINT('Ctrl Pts',(79.6569032110071,10.6304628571024,137.825265255981));
#70162=CARTESIAN_POINT('Ctrl Pts',(79.6802742251072,10.6352064239638,137.823739227656));
#70163=CARTESIAN_POINT('Ctrl Pts',(79.7555116219636,10.6488023737964,137.818887885018));
#70164=CARTESIAN_POINT('Ctrl Pts',(79.8076998245706,10.6557007887152,137.815616541092));
#70165=CARTESIAN_POINT('Ctrl Pts',(79.9557638262409,10.6681756114588,137.806469809281));
#70166=CARTESIAN_POINT('Ctrl Pts',(80.0519101902268,10.6679540340626,137.800694938082));
#70167=CARTESIAN_POINT('Ctrl Pts',(80.1988056810736,10.6548974336841,137.791520665853));
#70168=CARTESIAN_POINT('Ctrl Pts',(80.2498684314536,10.6479605163513,137.788262774791));
#70169=CARTESIAN_POINT('Ctrl Pts',(80.3113335506969,10.6366881919472,137.784169548875));
#70170=CARTESIAN_POINT('Ctrl Pts',(80.3221247004967,10.6345985681234,137.783444409162));
#70171=CARTESIAN_POINT('Ctrl Pts',(80.3390632597283,10.6311443063431,137.782294785459));
#70172=CARTESIAN_POINT('Ctrl Pts',(80.34522518396,10.6298512850267,137.78187419251));
#70173=CARTESIAN_POINT('Ctrl Pts',(80.3567651574653,10.6273613544703,137.781081786038));
#70174=CARTESIAN_POINT('Ctrl Pts',(80.3621447783337,10.6261726573734,137.780710432324));
#70175=CARTESIAN_POINT('Ctrl Pts',(80.3747768455679,10.6233156492839,137.77983392288));
#70176=CARTESIAN_POINT('Ctrl Pts',(80.3820241120107,10.6216254048738,137.779327556701));
#70177=CARTESIAN_POINT('Ctrl Pts',(80.406008334227,10.6158619835251,137.77764072285));
#70178=CARTESIAN_POINT('Ctrl Pts',(80.4226928029456,10.6115779390934,137.77644939108));
#70179=CARTESIAN_POINT('Ctrl Pts',(80.4632161898438,10.6005002744246,137.773516905807));
#70180=CARTESIAN_POINT('Ctrl Pts',(80.486975284828,10.5934319274754,137.771764371064));
#70181=CARTESIAN_POINT('Ctrl Pts',(80.5861154510812,10.5615133489777,137.764334440491));
#70182=CARTESIAN_POINT('Ctrl Pts',(80.659826748801,10.5318234463411,137.758527999245));
#70183=CARTESIAN_POINT('Ctrl Pts',(80.8233419338781,10.4519619417108,137.745303094737));
#70184=CARTESIAN_POINT('Ctrl Pts',(80.9112011989396,10.398500708682,137.737947936093));
#70185=CARTESIAN_POINT('Ctrl Pts',(81.0125321908413,10.323212481663,137.729257585613));
#70186=CARTESIAN_POINT('Ctrl Pts',(81.031171164287,10.3087394079502,137.727648510103));
#70187=CARTESIAN_POINT('Ctrl Pts',(81.058916096021,10.2862347312287,137.725235906644));
#70188=CARTESIAN_POINT('Ctrl Pts',(81.0682514393932,10.2784920640967,137.724421033757));
#70189=CARTESIAN_POINT('Ctrl Pts',(81.0849174965081,10.2643593506877,137.722960304602));
#70190=CARTESIAN_POINT('Ctrl Pts',(81.0922783077409,10.2580058216151,137.722313003266));
#70191=CARTESIAN_POINT('Ctrl Pts',(81.1079340706472,10.2442514450235,137.720931366033));
#70192=CARTESIAN_POINT('Ctrl Pts',(81.1162114601229,10.236831253529,137.720197875534));
#70193=CARTESIAN_POINT('Ctrl Pts',(81.1387318021035,10.2162328630918,137.718193383288));
#70194=CARTESIAN_POINT('Ctrl Pts',(81.152820052104,10.2028875562101,137.716929488585));
#70195=CARTESIAN_POINT('Ctrl Pts',(81.1836870087352,10.1726078398235,137.714134854323));
#70196=CARTESIAN_POINT('Ctrl Pts',(81.2003420349938,10.1555531855752,137.712609416785));
#70197=CARTESIAN_POINT('Ctrl Pts',(81.2525450193666,10.0997506005858,137.70776067334));
#70198=CARTESIAN_POINT('Ctrl Pts',(81.2866279749678,10.0596742360916,137.704491269499));
#70199=CARTESIAN_POINT('Ctrl Pts',(81.3774118913886,9.94207472581671,137.695345841588));
#70200=CARTESIAN_POINT('Ctrl Pts',(81.4293852737237,9.86117632790724,137.689570494069));
#70201=CARTESIAN_POINT('Ctrl Pts',(81.4981227772977,9.73064464780243,137.680393420181));
#70202=CARTESIAN_POINT('Ctrl Pts',(81.5200097938617,9.68394631594964,137.677133030546));
#70203=CARTESIAN_POINT('Ctrl Pts',(81.5438938451707,9.62615385919302,137.673036999861));
#70204=CARTESIAN_POINT('Ctrl Pts',(81.5479919678399,9.61595268662903,137.672311733463));
#70205=CARTESIAN_POINT('Ctrl Pts',(81.5542779886716,9.59984629841822,137.671161952565));
#70206=CARTESIAN_POINT('Ctrl Pts',(81.5565339582423,9.59396774437959,137.670741330847));
#70207=CARTESIAN_POINT('Ctrl Pts',(81.5607012833398,9.58292182896472,137.66994890269));
#70208=CARTESIAN_POINT('Ctrl Pts',(81.5626203961725,9.57775760352184,137.669577556394));
#70209=CARTESIAN_POINT('Ctrl Pts',(81.5670712353594,9.56559624535191,137.668701108659));
#70210=CARTESIAN_POINT('Ctrl Pts',(81.5695817342217,9.55859157150085,137.668194797296));
#70211=CARTESIAN_POINT('Ctrl Pts',(81.5777465593237,9.53532079435447,137.666508337432));
#70212=CARTESIAN_POINT('Ctrl Pts',(81.5831953865827,9.51898445876916,137.6653173312));
#70213=CARTESIAN_POINT('Ctrl Pts',(81.5958641434518,9.47894421199637,137.662385814406));
#70214=CARTESIAN_POINT('Ctrl Pts',(81.6028102189478,9.45515842657444,137.660633931746));
#70215=CARTESIAN_POINT('Ctrl Pts',(81.6297523872076,9.35461773490232,137.653208624139));
#70216=CARTESIAN_POINT('Ctrl Pts',(81.6447841101506,9.27664229544041,137.647406286896));
#70217=CARTESIAN_POINT('Ctrl Pts',(81.6664020734281,9.09593859837252,137.634180006056));
#70218=CARTESIAN_POINT('Ctrl Pts',(81.6691489838036,8.99305708989231,137.62681951096));
#70219=CARTESIAN_POINT('Ctrl Pts',(81.6608518954632,8.86702007947374,137.618124293289));
#70220=CARTESIAN_POINT('Ctrl Pts',(81.6588020259686,8.84351161250257,137.616515263834));
#70221=CARTESIAN_POINT('Ctrl Pts',(81.6549434674822,8.80799687927613,137.614102715043));
#70222=CARTESIAN_POINT('Ctrl Pts',(81.6535019120037,8.79595461430971,137.613287851536));
#70223=CARTESIAN_POINT('Ctrl Pts',(81.6506679017083,8.77428774963148,137.611827132523));
#70224=CARTESIAN_POINT('Ctrl Pts',(81.6493224477173,8.76465767055056,137.611179832034));
#70225=CARTESIAN_POINT('Ctrl Pts',(81.646258296431,8.74404456072636,137.609798189491));
#70226=CARTESIAN_POINT('Ctrl Pts',(81.6445138201669,8.7330657930999,137.609064692901));
#70227=CARTESIAN_POINT('Ctrl Pts',(81.6394229111241,8.70297301421987,137.607060165533));
#70228=CARTESIAN_POINT('Ctrl Pts',(81.6358521643053,8.68389834012931,137.605796242225));
#70229=CARTESIAN_POINT('Ctrl Pts',(81.6271545090234,8.64154174850958,137.60300153518));
#70230=CARTESIAN_POINT('Ctrl Pts',(81.6218594829965,8.61829852407933,137.601476053899));
#70231=CARTESIAN_POINT('Ctrl Pts',(81.6032907977022,8.54417187390974,137.596627118047));
#70232=CARTESIAN_POINT('Ctrl Pts',(81.5881062991737,8.49379878635708,137.593357570595));
#70233=CARTESIAN_POINT('Ctrl Pts',(81.5385449084026,8.35374328700117,137.584212050977));
#70234=CARTESIAN_POINT('Ctrl Pts',(81.4987685533963,8.26620192264929,137.57843674328));
#70235=CARTESIAN_POINT('Ctrl Pts',(81.4263874947732,8.13765907838286,137.569259877718));
#70236=CARTESIAN_POINT('Ctrl Pts',(81.3990272130029,8.09394542818712,137.565999668745));
#70237=CARTESIAN_POINT('Ctrl Pts',(81.3634298489296,8.04253673466349,137.561903840873));
#70238=CARTESIAN_POINT('Ctrl Pts',(81.357082326405,8.03356096886301,137.561178583639));
#70239=CARTESIAN_POINT('Ctrl Pts',(81.3469603297793,8.01954422976199,137.560028814107));
#70240=CARTESIAN_POINT('Ctrl Pts',(81.3432451735803,8.01446052957018,137.559608194465));
#70241=CARTESIAN_POINT('Ctrl Pts',(81.3362254231235,8.00496835568891,137.558815767872));
#70242=CARTESIAN_POINT('Ctrl Pts',(81.3329276705251,8.00055506595402,137.558444421038));
#70243=CARTESIAN_POINT('Ctrl Pts',(81.325124518436,7.99021963727935,137.557567968835));
#70244=CARTESIAN_POINT('Ctrl Pts',(81.3206012694709,7.98431124251789,137.557061653504));
#70245=CARTESIAN_POINT('Ctrl Pts',(81.3054789153626,7.96482978627866,137.555375166562));
#70246=CARTESIAN_POINT('Ctrl Pts',(81.2947093396599,7.951391284682,137.554184136761));
#70247=CARTESIAN_POINT('Ctrl Pts',(81.2679408337498,7.919030066635,137.551252549849));
#70248=CARTESIAN_POINT('Ctrl Pts',(81.2517245712348,7.90029302940611,137.549500619978));
#70249=CARTESIAN_POINT('Ctrl Pts',(81.1818666631113,7.82312345585774,137.542074977754));
#70250=CARTESIAN_POINT('Ctrl Pts',(81.1245066502778,7.76820003645204,137.536272343468));
#70251=CARTESIAN_POINT('Ctrl Pts',(80.9844165234301,7.65202999601314,137.523046162218));
#70252=CARTESIAN_POINT('Ctrl Pts',(80.8994762689304,7.59392464172677,137.515686053372));
#70253=CARTESIAN_POINT('Ctrl Pts',(80.7890927180304,7.53253778157291,137.506991188015));
#70254=CARTESIAN_POINT('Ctrl Pts',(80.7682306276826,7.52150939072891,137.505382155263));
#70255=CARTESIAN_POINT('Ctrl Pts',(80.7363006692908,7.50548857362456,137.502969602562));
#70256=CARTESIAN_POINT('Ctrl Pts',(80.7254016843756,7.5001681797742,137.502154738387));
#70257=CARTESIAN_POINT('Ctrl Pts',(80.705661514236,7.49079743936208,137.500694018656));
#70258=CARTESIAN_POINT('Ctrl Pts',(80.6968412180264,7.48670463377182,137.500046718111));
#70259=CARTESIAN_POINT('Ctrl Pts',(80.677861533278,7.47809878539718,137.49866507596));
#70260=CARTESIAN_POINT('Ctrl Pts',(80.6676917443785,7.47360971246924,137.497931579813));
#70261=CARTESIAN_POINT('Ctrl Pts',(80.6396486332997,7.46156503664912,137.495927054985));
#70262=CARTESIAN_POINT('Ctrl Pts',(80.6216866964267,7.45421922218457,137.494663133743));
#70263=CARTESIAN_POINT('Ctrl Pts',(80.581384165052,7.43855305421675,137.491868431954));
#70264=CARTESIAN_POINT('Ctrl Pts',(80.5589848945867,7.4303949272185,137.490342953831));
#70265=CARTESIAN_POINT('Ctrl Pts',(80.4866375721685,7.4057903156756,137.485494031866));
#70266=CARTESIAN_POINT('Ctrl Pts',(80.436081874529,7.39122597404735,137.482224494779));
#70267=CARTESIAN_POINT('Ctrl Pts',(80.291535630357,7.35690074541331,137.473078981691));
#70268=CARTESIAN_POINT('Ctrl Pts',(80.1964152774299,7.34283741180767,137.467303671037));
#70269=CARTESIAN_POINT('Ctrl Pts',(80.049163857556,7.33392794644519,137.45812679033));
#70270=CARTESIAN_POINT('Ctrl Pts',(79.9975986803697,7.33320478592516,137.454866568298));
#70271=CARTESIAN_POINT('Ctrl Pts',(79.9351010014767,7.33522825058939,137.450770725768));
#70272=CARTESIAN_POINT('Ctrl Pts',(79.9241173822381,7.33569273567307,137.450045467875));
#70273=CARTESIAN_POINT('Ctrl Pts',(79.9068514718617,7.33659415681977,137.448895697529));
#70274=CARTESIAN_POINT('Ctrl Pts',(79.9005654573009,7.33695808355034,137.448475077741));
#70275=CARTESIAN_POINT('Ctrl Pts',(79.8887833918301,7.33770723979103,137.447682651039));
#70276=CARTESIAN_POINT('Ctrl Pts',(79.8832870055806,7.33808410923743,137.447311304246));
#70277=CARTESIAN_POINT('Ctrl Pts',(79.870371598657,7.33903406181835,137.446434852372));
#70278=CARTESIAN_POINT('Ctrl Pts',(79.8629544437138,7.33962959540837,137.445928537331));
#70279=CARTESIAN_POINT('Ctrl Pts',(79.8383853890871,7.34176802390877,137.444242052367));
#70280=CARTESIAN_POINT('Ctrl Pts',(79.8212540776608,7.34352711870955,137.443051024286));
#70281=CARTESIAN_POINT('Ctrl Pts',(79.7795477081114,7.34846412712838,137.440119442494));
#70282=CARTESIAN_POINT('Ctrl Pts',(79.7550107682784,7.35192533621856,137.438367516069));
#70283=CARTESIAN_POINT('Ctrl Pts',(79.6522888318208,7.36875994801261,137.430941898269));
#70284=CARTESIAN_POINT('Ctrl Pts',(79.5750351830167,7.38716051164576,137.425139285665));
#70285=CARTESIAN_POINT('Ctrl Pts',(79.4015807794382,7.44180668854913,137.411922708435));
#70286=CARTESIAN_POINT('Ctrl Pts',(79.3068122953559,7.48158991550364,137.404571845428));
#70287=CARTESIAN_POINT('Ctrl Pts',(79.1953997081614,7.54098152746416,137.395879555419));
#70288=CARTESIAN_POINT('Ctrl Pts',(79.1747461884986,7.55256337641308,137.394264843608));
#70289=CARTESIAN_POINT('Ctrl Pts',(79.1438820430329,7.57074651293147,137.391845550211));
#70290=CARTESIAN_POINT('Ctrl Pts',(79.1334859649914,7.57702532446266,137.391029529376));
#70291=CARTESIAN_POINT('Ctrl Pts',(79.1148905181638,7.58853559284854,137.38956755723));
#70292=CARTESIAN_POINT('Ctrl Pts',(79.1066666315337,7.59372617632354,137.388920150257));
#70293=CARTESIAN_POINT('Ctrl Pts',(79.0908010514225,7.60393523127913,137.387669294185));
#70294=CARTESIAN_POINT('Ctrl Pts',(79.0831543084549,7.60894516640444,137.387065559858));
#70295=CARTESIAN_POINT('Ctrl Pts',(79.0613035831744,7.62351961376397,137.385337573908));
#70296=CARTESIAN_POINT('Ctrl Pts',(79.0472050347962,7.63324069184258,137.384219211252));
#70297=CARTESIAN_POINT('Ctrl Pts',(78.9801076315827,7.68104787299922,137.378875786567));
#70298=CARTESIAN_POINT('Ctrl Pts',(78.9292242924007,7.72201094963783,137.374762688965));
#70299=CARTESIAN_POINT('Ctrl Pts',(78.8264135681483,7.81524048778105,137.366159302839));
#70300=CARTESIAN_POINT('Ctrl Pts',(78.7752832935954,7.86817423451628,137.361697125596));
#70301=CARTESIAN_POINT('Ctrl Pts',(78.7157297954127,7.93860636357451,137.356054407551));
#70302=CARTESIAN_POINT('Ctrl Pts',(78.7038852369026,7.95310319767985,137.354907078642));
#70303=CARTESIAN_POINT('Ctrl Pts',(78.6490951958397,8.02251742219506,137.349464305369));
#70304=CARTESIAN_POINT('Ctrl Pts',(78.6093852501464,8.07988904640922,137.345114750604));
#70305=CARTESIAN_POINT('Ctrl Pts',(78.567418680568,8.14947050178401,137.339799275742));
#70306=CARTESIAN_POINT('Ctrl Pts',(78.5615510904945,8.15943210830667,137.339037337228));
#70307=CARTESIAN_POINT('Ctrl Pts',(78.5525852701964,8.17502250403875,137.33784209163));
#70308=CARTESIAN_POINT('Ctrl Pts',(78.5494149920936,8.18060973872479,137.337413195881));
#70309=CARTESIAN_POINT('Ctrl Pts',(78.5436229645985,8.19095645574832,137.336617672193));
#70310=CARTESIAN_POINT('Ctrl Pts',(78.5409920890399,8.19571060035635,137.336251627882));
#70311=CARTESIAN_POINT('Ctrl Pts',(78.5349285124989,8.20679548813728,137.335397003523));
#70312=CARTESIAN_POINT('Ctrl Pts',(78.5315135705612,8.21313567696747,137.334907345496));
#70313=CARTESIAN_POINT('Ctrl Pts',(78.5207105506204,8.23350785641826,137.333331779417));
#70314=CARTESIAN_POINT('Ctrl Pts',(78.5134819306624,8.2476227907738,137.332236818073));
#70315=CARTESIAN_POINT('Ctrl Pts',(78.4744667230697,8.32656335934003,137.326103332673));
#70316=CARTESIAN_POINT('Ctrl Pts',(78.4467215596323,8.39329354004269,137.320885898191));
#70317=CARTESIAN_POINT('Ctrl Pts',(78.3781212144582,8.59417900957207,137.305451726776));
#70318=CARTESIAN_POINT('Ctrl Pts',(78.3497413654723,8.7319640815458,137.295262916405));
#70319=CARTESIAN_POINT('Ctrl Pts',(78.3373025928241,8.89299608217247,137.284174441421));
#70320=CARTESIAN_POINT('Ctrl Pts',(78.3360669841584,8.91432912615348,137.28272012647));
#70321=CARTESIAN_POINT('Ctrl Pts',(78.3347977471238,8.94718053836917,137.280502133071));
#70322=CARTESIAN_POINT('Ctrl Pts',(78.3344726075072,8.95868468939974,137.279729470816));
#70323=CARTESIAN_POINT('Ctrl Pts',(78.3341612575565,8.97608330710807,137.278566801402));
#70324=CARTESIAN_POINT('Ctrl Pts',(78.3340870825413,8.98197565526008,137.27817406287));
#70325=CARTESIAN_POINT('Ctrl Pts',(78.3340147926857,8.99190271330143,137.277514077583));
#70326=CARTESIAN_POINT('Ctrl Pts',(78.3340000686845,8.99593720572022,137.277246316743));
#70327=CARTESIAN_POINT('Ctrl Pts',(78.3340000002397,8.99997173673522,137.276979010776));
#70328=CARTESIAN_POINT('Ctrl Pts',(78.3340000002429,8.99997155004477,137.276979023145));
#70329=CARTESIAN_POINT('Ctrl Pts',(78.3339999112415,9.00518337813501,137.276633715891));
#70330=CARTESIAN_POINT('Ctrl Pts',(78.3340242788548,9.01039523950057,137.276289169831));
#70331=CARTESIAN_POINT('Ctrl Pts',(78.3341549983631,9.02434857171807,137.275368731287));
#70332=CARTESIAN_POINT('Ctrl Pts',(78.3343056973382,9.03308953525333,137.274794220308));
#70333=CARTESIAN_POINT('Ctrl Pts',(78.3350293907745,9.06190427622381,137.2729068771));
#70334=CARTESIAN_POINT('Ctrl Pts',(78.3358965351355,9.08196940223928,137.271603123381));
#70335=CARTESIAN_POINT('Ctrl Pts',(78.3432383809184,9.20164398891471,137.263880528597));
#70336=CARTESIAN_POINT('Ctrl Pts',(78.3582917109302,9.30052728128795,137.257736897948));
#70337=CARTESIAN_POINT('Ctrl Pts',(78.3969323077997,9.45780953315502,137.247839398521));
#70338=CARTESIAN_POINT('Ctrl Pts',(78.4151125289883,9.51724486873033,137.244064136938));
#70339=CARTESIAN_POINT('Ctrl Pts',(78.4365593610394,9.57550792214055,137.240217191853));
#70340=CARTESIAN_POINT('',(78.3340007164138,9.00153000900957,137.471592617802));
#70341=CARTESIAN_POINT('Ctrl Pts',(78.4365593900224,9.5755080008764,137.430947520545));
#70342=CARTESIAN_POINT('Ctrl Pts',(78.4254741421113,9.54539351640444,137.432961692578));
#70343=CARTESIAN_POINT('Ctrl Pts',(78.4152578407775,9.51495565961625,137.435002791709));
#70344=CARTESIAN_POINT('Ctrl Pts',(78.401326629796,9.46909459877583,137.43811228276));
#70345=CARTESIAN_POINT('Ctrl Pts',(78.396944381392,9.45389307791809,137.439148496163));
#70346=CARTESIAN_POINT('Ctrl Pts',(78.3909056497913,9.43176616931305,137.440667851912));
#70347=CARTESIAN_POINT('Ctrl Pts',(78.3890758906659,9.42488841146042,137.441141656688));
#70348=CARTESIAN_POINT('Ctrl Pts',(78.3859140581865,9.41268954428143,137.44198509852));
#70349=CARTESIAN_POINT('Ctrl Pts',(78.3845641129672,9.40737327005085,137.442353711423));
#70350=CARTESIAN_POINT('Ctrl Pts',(78.3816919415351,9.39582344462313,137.443156890438));
#70351=CARTESIAN_POINT('Ctrl Pts',(78.3801794888434,9.38958783293473,137.443591967108));
#70352=CARTESIAN_POINT('Ctrl Pts',(78.3771195253297,9.37664616117294,137.44449772603));
#70353=CARTESIAN_POINT('Ctrl Pts',(78.3755774747087,9.3699389423902,137.444968691075));
#70354=CARTESIAN_POINT('Ctrl Pts',(78.3716952592679,9.35256066034583,137.446192601775));
#70355=CARTESIAN_POINT('Ctrl Pts',(78.369418460985,9.34187596857764,137.446948646952));
#70356=CARTESIAN_POINT('Ctrl Pts',(78.345237229499,9.22265629376286,137.45541838206));
#70357=CARTESIAN_POINT('Ctrl Pts',(78.3341023880633,9.11223104855113,137.463553888552));
#70358=CARTESIAN_POINT('Ctrl Pts',(78.3340007028448,9.00153031966764,137.471592615215));
#70359=CARTESIAN_POINT('Ctrl Pts',(78.3340007025608,9.00153001046496,137.471592637669));
#70360=CARTESIAN_POINT('Ctrl Pts',(78.3339287513718,8.92318372917125,137.47728188952));
#70361=CARTESIAN_POINT('Ctrl Pts',(78.3393833622202,8.84492220646431,137.482910887098));
#70362=CARTESIAN_POINT('Ctrl Pts',(78.3549525496431,8.73453511273653,137.490701819754));
#70363=CARTESIAN_POINT('Ctrl Pts',(78.3605546094469,8.70188626702482,137.492988332332));
#70364=CARTESIAN_POINT('Ctrl Pts',(78.3695663929548,8.65737273930555,137.49608242935));
#70365=CARTESIAN_POINT('Ctrl Pts',(78.3721395827095,8.64534853356166,137.496915889869));
#70366=CARTESIAN_POINT('Ctrl Pts',(78.3769359582418,8.62408867414977,137.498385630189));
#70367=CARTESIAN_POINT('Ctrl Pts',(78.3791054258978,8.61484159793951,137.499023588584));
#70368=CARTESIAN_POINT('Ctrl Pts',(78.3836666407023,8.59612140612928,137.500312608937));
#70369=CARTESIAN_POINT('Ctrl Pts',(78.3860628785508,8.58664975872747,137.500963498353));
#70370=CARTESIAN_POINT('Ctrl Pts',(78.391287589648,8.56673634341967,137.502329436818));
#70371=CARTESIAN_POINT('Ctrl Pts',(78.3941347336951,8.55629990859409,137.503043850255));
#70372=CARTESIAN_POINT('Ctrl Pts',(78.4019934698906,8.52856005056862,137.504939337139));
#70373=CARTESIAN_POINT('Ctrl Pts',(78.40718448228,8.51130862107592,137.506114569891));
#70374=CARTESIAN_POINT('Ctrl Pts',(78.4343862111914,8.42595120347724,137.511916816552));
#70375=CARTESIAN_POINT('Ctrl Pts',(78.46049114693,8.35922478435311,137.516407989382));
#70376=CARTESIAN_POINT('Ctrl Pts',(78.5371894315996,8.1951819621097,137.52759031137));
#70377=CARTESIAN_POINT('Ctrl Pts',(78.5932321632432,8.10080659771329,137.534149370386));
#70378=CARTESIAN_POINT('Ctrl Pts',(78.6841730731729,7.97721594606461,137.543736304128));
#70379=CARTESIAN_POINT('Ctrl Pts',(78.711609931341,7.9428632827288,137.54652636555));
#70380=CARTESIAN_POINT('Ctrl Pts',(78.7479791615948,7.90084805569639,137.550159052374));
#70381=CARTESIAN_POINT('Ctrl Pts',(78.7556800360156,7.89213765062358,137.550924784073));
#70382=CARTESIAN_POINT('Ctrl Pts',(78.767867220488,7.87864018135803,137.552132599807));
#70383=CARTESIAN_POINT('Ctrl Pts',(78.7722918866621,7.87379761410806,137.55257030158));
#70384=CARTESIAN_POINT('Ctrl Pts',(78.7804577469815,7.86496581416413,137.553376906155));
#70385=CARTESIAN_POINT('Ctrl Pts',(78.7841901274287,7.86096871823972,137.5537451566));
#70386=CARTESIAN_POINT('Ctrl Pts',(78.7927722180932,7.85186819306799,137.554590910183));
#70387=CARTESIAN_POINT('Ctrl Pts',(78.7976346243268,7.84677709771279,137.555069356436));
#70388=CARTESIAN_POINT('Ctrl Pts',(78.812949288948,7.83094429383044,137.556573545334));
#70389=CARTESIAN_POINT('Ctrl Pts',(78.8235139908239,7.82031306444383,137.557607268595));
#70390=CARTESIAN_POINT('Ctrl Pts',(78.9091693881078,7.73641326926946,137.565946867398));
#70391=CARTESIAN_POINT('Ctrl Pts',(78.9908790518476,7.67025030826881,137.573635216038));
#70392=CARTESIAN_POINT('Ctrl Pts',(79.1721446481223,7.54985705249177,137.58945608513));
#70393=CARTESIAN_POINT('Ctrl Pts',(79.272131820779,7.49717740518232,137.597530761659));
#70394=CARTESIAN_POINT('Ctrl Pts',(79.3947319766863,7.44771616568219,137.606577657256));
#70395=CARTESIAN_POINT('Ctrl Pts',(79.4129004286917,7.44075382592577,137.607898495035));
#70396=CARTESIAN_POINT('Ctrl Pts',(79.4416437058296,7.43031276647969,137.609957963222));
#70397=CARTESIAN_POINT('Ctrl Pts',(79.4521380532596,7.4266192259896,137.61070366208));
#70398=CARTESIAN_POINT('Ctrl Pts',(79.4718686805701,7.41989627774148,137.612094317371));
#70399=CARTESIAN_POINT('Ctrl Pts',(79.481095943743,7.41684206381599,137.612740068047));
#70400=CARTESIAN_POINT('Ctrl Pts',(79.5018762998957,7.41016498895068,137.614184294179));
#70401=CARTESIAN_POINT('Ctrl Pts',(79.513443300426,7.40658694181847,137.61498127468));
#70402=CARTESIAN_POINT('Ctrl Pts',(79.5475774495274,7.39643450794926,137.617313683611));
#70403=CARTESIAN_POINT('Ctrl Pts',(79.5702464859399,7.39021105195353,137.618837761028));
#70404=CARTESIAN_POINT('Ctrl Pts',(79.6830467970281,7.3617961508521,137.626311547409));
#70405=CARTESIAN_POINT('Ctrl Pts',(79.7747948485177,7.34668313218989,137.632034142422));
#70406=CARTESIAN_POINT('Ctrl Pts',(79.9437118458753,7.33318910940777,137.642395696399));
#70407=CARTESIAN_POINT('Ctrl Pts',(80.0204164978586,7.33236425947121,137.647040535184));
#70408=CARTESIAN_POINT('Ctrl Pts',(80.1292101070493,7.3387028727825,137.653841168167));
#70409=CARTESIAN_POINT('Ctrl Pts',(80.1614551903792,7.3415261947357,137.655884159614));
#70410=CARTESIAN_POINT('Ctrl Pts',(80.2143589252237,7.34771574145885,137.659310584514));
#70411=CARTESIAN_POINT('Ctrl Pts',(80.2350736061321,7.3505354438978,137.660671196879));
#70412=CARTESIAN_POINT('Ctrl Pts',(80.2636582052659,7.35497576089786,137.662581896315));
#70413=CARTESIAN_POINT('Ctrl Pts',(80.2715786388843,7.35626479235752,137.663114869811));
#70414=CARTESIAN_POINT('Ctrl Pts',(80.285009157298,7.3585502956289,137.664025119953));
#70415=CARTESIAN_POINT('Ctrl Pts',(80.290524224223,7.35951744114007,137.664400771594));
#70416=CARTESIAN_POINT('Ctrl Pts',(80.3019657698684,7.36158338531573,137.665184157333));
#70417=CARTESIAN_POINT('Ctrl Pts',(80.3078912684435,7.36268656227587,137.66559211338));
#70418=CARTESIAN_POINT('Ctrl Pts',(80.3236871490699,7.36571613070729,137.666685384723));
#70419=CARTESIAN_POINT('Ctrl Pts',(80.333546110018,7.36769974702247,137.667373766445));
#70420=CARTESIAN_POINT('Ctrl Pts',(80.378503331374,7.37716940001516,137.670538517282));
#70421=CARTESIAN_POINT('Ctrl Pts',(80.4133694492256,7.3856985426999,137.673064548523));
#70422=CARTESIAN_POINT('Ctrl Pts',(80.5397860150075,7.42098699538215,137.682424452084));
#70423=CARTESIAN_POINT('Ctrl Pts',(80.6292683281143,7.45446713406057,137.689430037614));
#70424=CARTESIAN_POINT('Ctrl Pts',(80.8021709727264,7.53667825828746,137.703292062072));
#70425=CARTESIAN_POINT('Ctrl Pts',(80.8852284541493,7.58537458060474,137.710119491605));
#70426=CARTESIAN_POINT('Ctrl Pts',(80.9788302865691,7.6517440023957,137.717962194055));
#70427=CARTESIAN_POINT('Ctrl Pts',(80.9938439023537,7.66277252809275,137.719225694971));
#70428=CARTESIAN_POINT('Ctrl Pts',(81.017383868299,7.68067974389455,137.721216415677));
#70429=CARTESIAN_POINT('Ctrl Pts',(81.0260324088749,7.68739443110717,137.721949938113));
#70430=CARTESIAN_POINT('Ctrl Pts',(81.0422513000252,7.70024495962461,137.723329872008));
#70431=CARTESIAN_POINT('Ctrl Pts',(81.0498351960297,7.70636287721292,137.723976955361));
#70432=CARTESIAN_POINT('Ctrl Pts',(81.0669304055423,7.72040290784581,137.725440040069));
#70433=CARTESIAN_POINT('Ctrl Pts',(81.0764080507875,7.7283652527157,137.726254373629));
#70434=CARTESIAN_POINT('Ctrl Pts',(81.1053015397203,7.75319372240697,137.728747786565));
#70435=CARTESIAN_POINT('Ctrl Pts',(81.1244168571189,7.77040484955706,137.730412662811));
#70436=CARTESIAN_POINT('Ctrl Pts',(81.2404340440021,7.87983397813105,137.740635202132));
#70437=CARTESIAN_POINT('Ctrl Pts',(81.3263327863133,7.98299817522528,137.748679835144));
#70438=CARTESIAN_POINT('Ctrl Pts',(81.4381964934003,8.15598342027225,137.761314867289));
#70439=CARTESIAN_POINT('Ctrl Pts',(81.473428334307,8.21911608842373,137.765789522364));
#70440=CARTESIAN_POINT('Ctrl Pts',(81.5112621464553,8.29864827394566,137.771502842678));
#70441=CARTESIAN_POINT('Ctrl Pts',(81.5178697891846,8.31306566758462,137.772541547719));
#70442=CARTESIAN_POINT('Ctrl Pts',(81.5271765651335,8.33416249251169,137.774068965174));
#70443=CARTESIAN_POINT('Ctrl Pts',(81.5300400073809,8.34076907042324,137.774548339349));
#70444=CARTESIAN_POINT('Ctrl Pts',(81.5350076882618,8.35243730498534,137.775397199345));
#70445=CARTESIAN_POINT('Ctrl Pts',(81.5371299066947,8.35749109295909,137.775765599455));
#70446=CARTESIAN_POINT('Ctrl Pts',(81.5416921792717,8.36850753872899,137.776570348652));
#70447=CARTESIAN_POINT('Ctrl Pts',(81.544122563974,8.37447381494852,137.777007227026));
#70448=CARTESIAN_POINT('Ctrl Pts',(81.5508499438202,8.39126677958626,137.778239506254));
#70449=CARTESIAN_POINT('Ctrl Pts',(81.5550679850582,8.4021244069886,137.779039289344));
#70450=CARTESIAN_POINT('Ctrl Pts',(81.5878017294627,8.48907449138211,137.785463319868));
#70451=CARTESIAN_POINT('Ctrl Pts',(81.6108262378961,8.56710848663504,137.791340103224));
#70452=CARTESIAN_POINT('Ctrl Pts',(81.6310452013371,8.66022818212903,137.79827098935));
#70453=CARTESIAN_POINT('Ctrl Pts',(81.6338521471435,8.67399310328744,137.799293625379));
#70454=CARTESIAN_POINT('Ctrl Pts',(81.6455914630325,8.73552644289922,137.803853633398));
#70455=CARTESIAN_POINT('Ctrl Pts',(81.6526056327334,8.78363815439648,137.807387361721));
#70456=CARTESIAN_POINT('Ctrl Pts',(81.66570866662,8.91290568798445,137.816741005222));
#70457=CARTESIAN_POINT('Ctrl Pts',(81.6679754656164,8.99432400382189,137.822479946779));
#70458=CARTESIAN_POINT('Ctrl Pts',(81.6634641980402,9.09364501107874,137.829269764892));
#70459=CARTESIAN_POINT('Ctrl Pts',(81.662350622459,9.11168249155662,137.830494710364));
#70460=CARTESIAN_POINT('Ctrl Pts',(81.6601006884897,9.14049548262302,137.832439120203));
#70461=CARTESIAN_POINT('Ctrl Pts',(81.6591523447306,9.15128378339317,137.833164392343));
#70462=CARTESIAN_POINT('Ctrl Pts',(81.6571487606078,9.17178294113825,137.8345375067));
#70463=CARTESIAN_POINT('Ctrl Pts',(81.6561131865902,9.18149521698174,137.83518593514));
#70464=CARTESIAN_POINT('Ctrl Pts',(81.6535475865648,9.20370281359891,137.836663983932));
#70465=CARTESIAN_POINT('Ctrl Pts',(81.6519612191109,9.21619112454287,137.837491801894));
#70466=CARTESIAN_POINT('Ctrl Pts',(81.6474063716617,9.24906326446204,137.839662789551));
#70467=CARTESIAN_POINT('Ctrl Pts',(81.6442010948644,9.26941247645857,137.840998540815));
#70468=CARTESIAN_POINT('Ctrl Pts',(81.6186182888777,9.4142932730626,137.850462352303));
#70469=CARTESIAN_POINT('Ctrl Pts',(81.5824965813417,9.53597810194223,137.858124406919));
#70470=CARTESIAN_POINT('Ctrl Pts',(81.4979964629142,9.73452480618185,137.871319775353));
#70471=CARTESIAN_POINT('Ctrl Pts',(81.4565123747977,9.81368752299305,137.87680683921));
#70472=CARTESIAN_POINT('Ctrl Pts',(81.4022259737074,9.89970805908838,137.883449050135));
#70473=CARTESIAN_POINT('Ctrl Pts',(81.395435760577,9.91020398158919,137.884271877212));
#70474=CARTESIAN_POINT('Ctrl Pts',(81.3849085623913,9.92608162862454,137.885537202478));
#70475=CARTESIAN_POINT('Ctrl Pts',(81.3812567023457,9.93151963351911,137.885974308671));
#70476=CARTESIAN_POINT('Ctrl Pts',(81.3744968329581,9.94145864187024,137.886780373674));
#70477=CARTESIAN_POINT('Ctrl Pts',(81.3713986110425,9.94596604850566,137.887148686581));
#70478=CARTESIAN_POINT('Ctrl Pts',(81.3642551315529,9.9562497921903,137.887995311226));
#70479=CARTESIAN_POINT('Ctrl Pts',(81.3601953706312,9.9620157369843,137.888474573981));
#70480=CARTESIAN_POINT('Ctrl Pts',(81.3473565354114,9.98000657517159,137.889983919264));
#70481=CARTESIAN_POINT('Ctrl Pts',(81.3384486144671,9.992137988303,137.891022057793));
#70482=CARTESIAN_POINT('Ctrl Pts',(81.2667091256282,10.0871130683613,137.899301629979));
#70483=CARTESIAN_POINT('Ctrl Pts',(81.1964164928546,10.1640235873545,137.906918442772));
#70484=CARTESIAN_POINT('Ctrl Pts',(81.0352408581541,10.3102487629109,137.922742541798));
#70485=CARTESIAN_POINT('Ctrl Pts',(80.9434500740638,10.3778194409555,137.930888542775));
#70486=CARTESIAN_POINT('Ctrl Pts',(80.8287674670517,10.4453638055376,137.939995778718));
#70487=CARTESIAN_POINT('Ctrl Pts',(80.8118871670219,10.4549128248653,137.941312267555));
#70488=CARTESIAN_POINT('Ctrl Pts',(80.7850779599095,10.4694665914661,137.943366527283));
#70489=CARTESIAN_POINT('Ctrl Pts',(80.7752595745072,10.4746701560225,137.944111307281));
#70490=CARTESIAN_POINT('Ctrl Pts',(80.7567555227279,10.4842410757629,137.945501129611));
#70491=CARTESIAN_POINT('Ctrl Pts',(80.7480823187248,10.4886313658591,137.946146957093));
#70492=CARTESIAN_POINT('Ctrl Pts',(80.7285044915405,10.4983271501057,137.947592489253));
#70493=CARTESIAN_POINT('Ctrl Pts',(80.7175792934883,10.5035900416917,137.948390686852));
#70494=CARTESIAN_POINT('Ctrl Pts',(80.6852284939717,10.5187411552836,137.950730253628));
#70495=CARTESIAN_POINT('Ctrl Pts',(80.6636486154599,10.5282942748456,137.95226016427));
#70496=CARTESIAN_POINT('Ctrl Pts',(80.5475559826864,10.5767639656207,137.960342116054));
#70497=CARTESIAN_POINT('Ctrl Pts',(80.4498125073947,10.6073811523825,137.966611684753));
#70498=CARTESIAN_POINT('Ctrl Pts',(80.2719511564401,10.6455849840024,137.977722604372));
#70499=CARTESIAN_POINT('Ctrl Pts',(80.1929377981737,10.6567077628697,137.982565383274));
#70500=CARTESIAN_POINT('Ctrl Pts',(80.08865782956,10.6638247270237,137.989155191184));
#70501=CARTESIAN_POINT('Ctrl Pts',(80.06384390888,10.6649614883015,137.990738248872));
#70502=CARTESIAN_POINT('Ctrl Pts',(80.0217687601418,10.6659470953656,137.993461717335));
#70503=CARTESIAN_POINT('Ctrl Pts',(80.0045178912742,10.66608317173,137.994589502206));
#70504=CARTESIAN_POINT('Ctrl Pts',(79.979824035363,10.6658944621728,137.996223827633));
#70505=CARTESIAN_POINT('Ctrl Pts',(79.9723798522388,10.6657876667918,137.996719106262));
#70506=CARTESIAN_POINT('Ctrl Pts',(79.9594293769094,10.6655150464119,137.997585639382));
#70507=CARTESIAN_POINT('Ctrl Pts',(79.9539227914281,10.6653718008705,137.997955646565));
#70508=CARTESIAN_POINT('Ctrl Pts',(79.9421285358687,10.6650064488473,137.998751598054));
#70509=CARTESIAN_POINT('Ctrl Pts',(79.93584148749,10.6647760399084,137.999177960879));
#70510=CARTESIAN_POINT('Ctrl Pts',(79.9185910485487,10.6640459815483,138.000353232378));
#70511=CARTESIAN_POINT('Ctrl Pts',(79.9076312849937,10.663473609809,138.001105925484));
#70512=CARTESIAN_POINT('Ctrl Pts',(79.8455854960802,10.6596182451507,138.005398170394));
#70513=CARTESIAN_POINT('Ctrl Pts',(79.7946711079838,10.6540905455986,138.009039077295));
#70514=CARTESIAN_POINT('Ctrl Pts',(79.6484020627057,10.631353365934,138.019704308045));
#70515=CARTESIAN_POINT('Ctrl Pts',(79.554184957195,10.6081619860541,138.026818643538));
#70516=CARTESIAN_POINT('Ctrl Pts',(79.4130223831853,10.5600471704601,138.037541472249));
#70517=CARTESIAN_POINT('Ctrl Pts',(79.3643495247312,10.5408566599295,138.041254083757));
#70518=CARTESIAN_POINT('Ctrl Pts',(79.2949977090718,10.5096660990511,138.046553032325));
#70519=CARTESIAN_POINT('Ctrl Pts',(79.2735493110557,10.4994630556862,138.048193373808));
#70520=CARTESIAN_POINT('Ctrl Pts',(79.2350357843055,10.4801216409016,138.051142183353));
#70521=CARTESIAN_POINT('Ctrl Pts',(79.2178981042715,10.4711379957743,138.052455592176));
#70522=CARTESIAN_POINT('Ctrl Pts',(79.1911784230002,10.4565324966649,138.054506162777));
#70523=CARTESIAN_POINT('Ctrl Pts',(79.1814899617597,10.4511101215595,138.055250291754));
#70524=CARTESIAN_POINT('Ctrl Pts',(79.1634206093619,10.4407586322126,138.056639526508));
#70525=CARTESIAN_POINT('Ctrl Pts',(79.1550273102227,10.4358522464081,138.057285410977));
#70526=CARTESIAN_POINT('Ctrl Pts',(79.1362508773537,10.4246546339289,138.058731880603));
#70527=CARTESIAN_POINT('Ctrl Pts',(79.1258925211453,10.4183227775366,138.059530949999));
#70528=CARTESIAN_POINT('Ctrl Pts',(79.095551065719,10.3993169870543,138.061875649637));
#70529=CARTESIAN_POINT('Ctrl Pts',(79.0757671930687,10.3863295834404,138.063409743942));
#70530=CARTESIAN_POINT('Ctrl Pts',(78.9739598577287,10.3163482767935,138.071345537865));
#70531=CARTESIAN_POINT('Ctrl Pts',(78.8969042495098,10.2524831793467,138.077479404025));
#70532=CARTESIAN_POINT('Ctrl Pts',(78.7682487685487,10.1247114646343,138.088555960527));
#70533=CARTESIAN_POINT('Ctrl Pts',(78.7147591971933,10.0631750674789,138.093499383091));
#70534=CARTESIAN_POINT('Ctrl Pts',(78.6509400881766,9.97786721061838,138.100213338924));
#70535=CARTESIAN_POINT('Ctrl Pts',(78.6363511293087,9.95741764666495,138.101813627696));
#70536=CARTESIAN_POINT('Ctrl Pts',(78.6124511771225,9.9222618100677,138.10456383958));
#70537=CARTESIAN_POINT('Ctrl Pts',(78.6028979092562,9.90772477759486,138.105700809082));
#70538=CARTESIAN_POINT('Ctrl Pts',(78.589570516647,9.88673584902199,138.107346118212));
#70539=CARTESIAN_POINT('Ctrl Pts',(78.5856091176666,9.88040344168236,138.107842987693));
#70540=CARTESIAN_POINT('Ctrl Pts',(78.5787988305795,9.86935241191356,138.108711319212));
#70541=CARTESIAN_POINT('Ctrl Pts',(78.5759305606735,9.86464594549603,138.109081517776));
#70542=CARTESIAN_POINT('Ctrl Pts',(78.5698452684304,9.85454833355674,138.109876726172));
#70543=CARTESIAN_POINT('Ctrl Pts',(78.5666353998263,9.84915330201386,138.110302144389));
#70544=CARTESIAN_POINT('Ctrl Pts',(78.5579283427053,9.83432875449606,138.111472338454));
#70545=CARTESIAN_POINT('Ctrl Pts',(78.5524933254307,9.82486335028105,138.112220847355));
#70546=CARTESIAN_POINT('Ctrl Pts',(78.5227117142183,9.77179608591075,138.11642191868));
#70547=CARTESIAN_POINT('Ctrl Pts',(78.5002443780857,9.72717394337924,138.119970955635));
#70548=CARTESIAN_POINT('Ctrl Pts',(78.4641777346591,9.64673575538072,138.12631815485));
#70549=CARTESIAN_POINT('Ctrl Pts',(78.4497513016068,9.61134549370152,138.129094408613));
#70550=CARTESIAN_POINT('Ctrl Pts',(78.4365594482967,9.57550815918599,138.131873589273));
#70551=CARTESIAN_POINT('Origin',(80.,9.,134.));
#70552=CARTESIAN_POINT('',(78.4365593737687,9.57550795672114,138.833737829798));
#70553=CARTESIAN_POINT('',(78.4365593294404,9.57550783629781,138.638847722432));
#70554=CARTESIAN_POINT('',(78.4365593737638,9.57550795670799,134.));
#70555=CARTESIAN_POINT('Ctrl Pts',(78.4365593294404,9.57550783629781,138.638847722432));
#70556=CARTESIAN_POINT('Ctrl Pts',(78.4698751475928,9.66601451889556,138.631860971438));
#70557=CARTESIAN_POINT('Ctrl Pts',(78.5110043344498,9.75350400925092,138.624997573652));
#70558=CARTESIAN_POINT('Ctrl Pts',(78.56925966871,9.85376521116878,138.617062797006));
#70559=CARTESIAN_POINT('Ctrl Pts',(78.5793064228173,9.87038080542856,138.615744725277));
#70560=CARTESIAN_POINT('Ctrl Pts',(78.595560026213,9.89622986845154,138.61368844008));
#70561=CARTESIAN_POINT('Ctrl Pts',(78.6015725411225,9.90558283426176,138.612943197163));
#70562=CARTESIAN_POINT('Ctrl Pts',(78.6130177193405,9.92300091580669,138.61155275464));
#70563=CARTESIAN_POINT('Ctrl Pts',(78.6184282007808,9.93107996858373,138.610906766962));
#70564=CARTESIAN_POINT('Ctrl Pts',(78.6307436256256,9.94912590423244,138.609461184705));
#70565=CARTESIAN_POINT('Ctrl Pts',(78.6376873154159,9.95906577628718,138.608663094773));
#70566=CARTESIAN_POINT('Ctrl Pts',(78.6584519768842,9.98810973039291,138.606324798227));
#70567=CARTESIAN_POINT('Ctrl Pts',(78.6725710537013,10.0069977257062,138.604796027743));
#70568=CARTESIAN_POINT('Ctrl Pts',(78.7513426715646,10.1078384642751,138.596575410555));
#70569=CARTESIAN_POINT('Ctrl Pts',(78.8231888943482,10.1838793037918,138.590179940072));
#70570=CARTESIAN_POINT('Ctrl Pts',(78.9603567424553,10.304141881122,138.579039582531));
#70571=CARTESIAN_POINT('Ctrl Pts',(79.0225638155637,10.3513922269045,138.574293696002));
#70572=CARTESIAN_POINT('Ctrl Pts',(79.1084026561718,10.4075558902805,138.567823600148));
#70573=CARTESIAN_POINT('Ctrl Pts',(79.1292519552094,10.4205481770095,138.566257394367));
#70574=CARTESIAN_POINT('Ctrl Pts',(79.1650984130671,10.441800307635,138.563560057599));
#70575=CARTESIAN_POINT('Ctrl Pts',(79.1799499811963,10.4502988305529,138.562441234675));
#70576=CARTESIAN_POINT('Ctrl Pts',(79.2014272070227,10.4621534065749,138.560817553085));
#70577=CARTESIAN_POINT('Ctrl Pts',(79.2079490717549,10.4656965620156,138.560323754007));
#70578=CARTESIAN_POINT('Ctrl Pts',(79.2193507606788,10.4717924761891,138.559458801605));
#70579=CARTESIAN_POINT('Ctrl Pts',(79.224219912497,10.4743648064948,138.559088879836));
#70580=CARTESIAN_POINT('Ctrl Pts',(79.2346933188503,10.4798315668086,138.558291914412));
#70581=CARTESIAN_POINT('Ctrl Pts',(79.2403011901216,10.4827182798151,138.557864441443));
#70582=CARTESIAN_POINT('Ctrl Pts',(79.2557703539077,10.4905704058508,138.556683498593));
#70583=CARTESIAN_POINT('Ctrl Pts',(79.2656646161706,10.4954696348169,138.555926187831));
#70584=CARTESIAN_POINT('Ctrl Pts',(79.3227321057375,10.523024220578,138.551550041503));
#70585=CARTESIAN_POINT('Ctrl Pts',(79.3708990178427,10.5435431320813,138.547825355627));
#70586=CARTESIAN_POINT('Ctrl Pts',(79.5154078606454,10.5972152414325,138.536711882098));
#70587=CARTESIAN_POINT('Ctrl Pts',(79.6139265359875,10.6238457737905,138.529227113014));
#70588=CARTESIAN_POINT('Ctrl Pts',(79.7861823776582,10.6538342419194,138.516692139568));
#70589=CARTESIAN_POINT('Ctrl Pts',(79.8588582831123,10.6616158826775,138.511561555687));
#70590=CARTESIAN_POINT('Ctrl Pts',(79.9494358320328,10.6653258261224,138.505374865551));
#70591=CARTESIAN_POINT('Ctrl Pts',(79.967062684725,10.6657676959816,138.504180316125));
#70592=CARTESIAN_POINT('Ctrl Pts',(79.9954304593155,10.666028332329,138.502272322725));
#70593=CARTESIAN_POINT('Ctrl Pts',(80.0061679972251,10.6660231841036,138.501553450984));
#70594=CARTESIAN_POINT('Ctrl Pts',(80.0266977190896,10.665814857622,138.500185097982));
#70595=CARTESIAN_POINT('Ctrl Pts',(80.0364895890604,10.6656291378804,138.499535100863));
#70596=CARTESIAN_POINT('Ctrl Pts',(80.0588395816359,10.6650080428592,138.498057251417));
#70597=CARTESIAN_POINT('Ctrl Pts',(80.0713956557027,10.6645169130661,138.497231170131));
#70598=CARTESIAN_POINT('Ctrl Pts',(80.1049042047268,10.6628263598905,138.495036878493));
#70599=CARTESIAN_POINT('Ctrl Pts',(80.1258420023163,10.6613730011019,138.493676545403));
#70600=CARTESIAN_POINT('Ctrl Pts',(80.2674420411157,10.6488516692777,138.484537467913));
#70601=CARTESIAN_POINT('Ctrl Pts',(80.3866140790496,10.6250447616171,138.477179522494));
#70602=CARTESIAN_POINT('Ctrl Pts',(80.5651040283222,10.5686208468811,138.465740446354));
#70603=CARTESIAN_POINT('Ctrl Pts',(80.6268057216803,10.5450007293215,138.46169497969));
#70604=CARTESIAN_POINT('Ctrl Pts',(80.7073518884925,10.5085461089418,138.456098851407));
#70605=CARTESIAN_POINT('Ctrl Pts',(80.7275756528225,10.4988968030965,138.454665755171));
#70606=CARTESIAN_POINT('Ctrl Pts',(80.7618759593436,10.4816734783529,138.452176444966));
#70607=CARTESIAN_POINT('Ctrl Pts',(80.7760497639094,10.4742991527802,138.451130183467));
#70608=CARTESIAN_POINT('Ctrl Pts',(80.7964736589637,10.4632969218808,138.44959359307));
#70609=CARTESIAN_POINT('Ctrl Pts',(80.8028101492682,10.4598301375242,138.44911275806));
#70610=CARTESIAN_POINT('Ctrl Pts',(80.8138754647173,10.4536823162074,138.448265497098));
#70611=CARTESIAN_POINT('Ctrl Pts',(80.8186140150488,10.451019173433,138.447900197882));
#70612=CARTESIAN_POINT('Ctrl Pts',(80.8289118836179,10.4451651028096,138.447100826664));
#70613=CARTESIAN_POINT('Ctrl Pts',(80.8344657583841,10.4419653185167,138.446666220341));
#70614=CARTESIAN_POINT('Ctrl Pts',(80.8499296717283,10.4329367526867,138.445446647146));
#70615=CARTESIAN_POINT('Ctrl Pts',(80.8597978180775,10.4270374479311,138.444657435966));
#70616=CARTESIAN_POINT('Ctrl Pts',(80.9263981430245,10.3862813619017,138.439260270069));
#70617=CARTESIAN_POINT('Ctrl Pts',(80.9810517778842,10.348156133496,138.434481746895));
#70618=CARTESIAN_POINT('Ctrl Pts',(81.0502562035274,10.2934398789512,138.428084980723));
#70619=CARTESIAN_POINT('Ctrl Pts',(81.0669773043952,10.2796812991607,138.426510261427));
#70620=CARTESIAN_POINT('Ctrl Pts',(81.1371848469924,10.219579705752,138.419783885405));
#70621=CARTESIAN_POINT('Ctrl Pts',(81.1879605471258,10.1701772831467,138.414631882007));
#70622=CARTESIAN_POINT('Ctrl Pts',(81.2810227128656,10.0673109733487,138.404715591331));
#70623=CARTESIAN_POINT('Ctrl Pts',(81.3234830320867,10.01418278992,138.399952975223));
#70624=CARTESIAN_POINT('Ctrl Pts',(81.3725447586744,9.944445091565,138.394136853282));
#70625=CARTESIAN_POINT('Ctrl Pts',(81.3822840009549,9.93013258491287,138.392964465253));
#70626=CARTESIAN_POINT('Ctrl Pts',(81.397662282159,9.90675793808567,138.391083127421));
#70627=CARTESIAN_POINT('Ctrl Pts',(81.4034402037986,9.89778918280856,138.390369019844));
#70628=CARTESIAN_POINT('Ctrl Pts',(81.4143668755396,9.88046501591153,138.389004176543));
#70629=CARTESIAN_POINT('Ctrl Pts',(81.4195287092893,9.87211842853965,138.388352977357));
#70630=CARTESIAN_POINT('Ctrl Pts',(81.4312045339081,9.85286051276188,138.386864718679));
#70631=CARTESIAN_POINT('Ctrl Pts',(81.4376680921694,9.84191920261341,138.386029519993));
#70632=CARTESIAN_POINT('Ctrl Pts',(81.4581156391399,9.80638398624396,138.383349066478));
#70633=CARTESIAN_POINT('Ctrl Pts',(81.4715990360857,9.78150673601723,138.381521642392));
#70634=CARTESIAN_POINT('Ctrl Pts',(81.5438698071603,9.63965525522469,138.371347682696));
#70635=CARTESIAN_POINT('Ctrl Pts',(81.5893418100884,9.51641830732505,138.363477085657));
#70636=CARTESIAN_POINT('Ctrl Pts',(81.636579003702,9.31976948397194,138.351068475344));
#70637=CARTESIAN_POINT('Ctrl Pts',(81.6487655171531,9.24942593473739,138.346646775582));
#70638=CARTESIAN_POINT('Ctrl Pts',(81.6580970524159,9.16284628102584,138.340996870565));
#70639=CARTESIAN_POINT('Ctrl Pts',(81.6595643024016,9.14714288426201,138.339963783403));
#70640=CARTESIAN_POINT('Ctrl Pts',(81.6613751850065,9.12425832140393,138.338443055351));
#70641=CARTESIAN_POINT('Ctrl Pts',(81.6618956694207,9.11709148135974,138.337964636403));
#70642=CARTESIAN_POINT('Ctrl Pts',(81.6627281742232,9.10450132613928,138.337120029267));
#70643=CARTESIAN_POINT('Ctrl Pts',(81.6630600580564,9.09907951625501,138.336754943365));
#70644=CARTESIAN_POINT('Ctrl Pts',(81.6637271597607,9.08723154786881,138.335954070026));
#70645=CARTESIAN_POINT('Ctrl Pts',(81.6640516611493,9.08080513966375,138.335517730234));
#70646=CARTESIAN_POINT('Ctrl Pts',(81.6648571887898,9.06277983209842,138.334288707313));
#70647=CARTESIAN_POINT('Ctrl Pts',(81.665254208477,9.05117781458003,138.333491678512));
#70648=CARTESIAN_POINT('Ctrl Pts',(81.6673600431489,8.96254844721634,138.32736223425));
#70649=CARTESIAN_POINT('Ctrl Pts',(81.6638445707235,8.88549809884345,138.321802255384));
#70650=CARTESIAN_POINT('Ctrl Pts',(81.6484360905783,8.75199969873759,138.312034124754));
#70651=CARTESIAN_POINT('Ctrl Pts',(81.6389215378767,8.69539836439753,138.307848689915));
#70652=CARTESIAN_POINT('Ctrl Pts',(81.608628840787,8.55876150375631,138.297735945525));
#70653=CARTESIAN_POINT('Ctrl Pts',(81.5847771185521,8.47955478599375,138.291870908533));
#70654=CARTESIAN_POINT('Ctrl Pts',(81.5469582248326,8.38113247558281,138.284622337968));
#70655=CARTESIAN_POINT('Ctrl Pts',(81.5383358630638,8.36000029365466,138.283067787426));
#70656=CARTESIAN_POINT('Ctrl Pts',(81.524592182781,8.32820062675729,138.280730112098));
#70657=CARTESIAN_POINT('Ctrl Pts',(81.5197872560296,8.31740024129588,138.279936424551));
#70658=CARTESIAN_POINT('Ctrl Pts',(81.5112203994609,8.2986828759621,138.278561131887));
#70659=CARTESIAN_POINT('Ctrl Pts',(81.5075102403455,8.29074286432606,138.277977784237));
#70660=CARTESIAN_POINT('Ctrl Pts',(81.4990001690529,8.27289917888247,138.276666762775));
#70661=CARTESIAN_POINT('Ctrl Pts',(81.494164399837,8.26301298048575,138.275940359269));
#70662=CARTESIAN_POINT('Ctrl Pts',(81.480766566296,8.23629658245513,138.273976686895));
#70663=CARTESIAN_POINT('Ctrl Pts',(81.4720156051569,8.2195625334724,138.272746037432));
#70664=CARTESIAN_POINT('Ctrl Pts',(81.4174770794252,8.11945350495147,138.265372266942));
#70665=CARTESIAN_POINT('Ctrl Pts',(81.3649004322941,8.03997208345693,138.259482296623));
#70666=CARTESIAN_POINT('Ctrl Pts',(81.2486346798971,7.89322663979722,138.248020525256));
#70667=CARTESIAN_POINT('Ctrl Pts',(81.1855669134947,7.82591962859444,138.242461164671));
#70668=CARTESIAN_POINT('Ctrl Pts',(81.0974522237328,7.74625834087843,138.234993167515));
#70669=CARTESIAN_POINT('Ctrl Pts',(81.0772105399731,7.72882462809436,138.233295021015));
#70670=CARTESIAN_POINT('Ctrl Pts',(81.0424867113786,7.7003428333551,138.230393501992));
#70671=CARTESIAN_POINT('Ctrl Pts',(81.0282262033174,7.68903161642448,138.229205023145));
#70672=CARTESIAN_POINT('Ctrl Pts',(81.0077487757175,7.673328885167,138.227498164455));
#70673=CARTESIAN_POINT('Ctrl Pts',(81.0016820985551,7.66874239542077,138.226992455909));
#70674=CARTESIAN_POINT('Ctrl Pts',(80.9911489474787,7.660891951698,138.226113961521));
#70675=CARTESIAN_POINT('Ctrl Pts',(80.9866972650644,7.65760843739858,138.225742528422));
#70676=CARTESIAN_POINT('Ctrl Pts',(80.9772133866843,7.65068589299375,138.224950768147));
#70677=CARTESIAN_POINT('Ctrl Pts',(80.972177254307,7.64705286669271,138.224530085084));
#70678=CARTESIAN_POINT('Ctrl Pts',(80.9582555253865,7.6371277046653,138.223366762406));
#70679=CARTESIAN_POINT('Ctrl Pts',(80.949328562139,7.63089452169851,138.222620367147));
#70680=CARTESIAN_POINT('Ctrl Pts',(80.9016376259835,7.59828536161688,138.218633231472));
#70681=CARTESIAN_POINT('Ctrl Pts',(80.8618374981891,7.57346938281445,138.215307560432));
#70682=CARTESIAN_POINT('Ctrl Pts',(80.7448733383006,7.50722280179509,138.205645885225));
#70683=CARTESIAN_POINT('Ctrl Pts',(80.6654169334357,7.47015018279518,138.199222597692));
#70684=CARTESIAN_POINT('Ctrl Pts',(80.5121119517632,7.41283519098589,138.18739024551));
#70685=CARTESIAN_POINT('Ctrl Pts',(80.4390579909328,7.39109305294282,138.181970522357));
#70686=CARTESIAN_POINT('Ctrl Pts',(80.3375008399328,7.36830459358104,138.174770807004));
#70687=CARTESIAN_POINT('Ctrl Pts',(80.3100865663232,7.36287349267407,138.172858984433));
#70688=CARTESIAN_POINT('Ctrl Pts',(80.2699484838518,7.35596616727004,138.170104156736));
#70689=CARTESIAN_POINT('Ctrl Pts',(80.2573249825108,7.3539431066078,138.169244075488));
#70690=CARTESIAN_POINT('Ctrl Pts',(80.2349914171841,7.35062710259901,138.167733194048));
#70691=CARTESIAN_POINT('Ctrl Pts',(80.2252910321334,7.34927413580797,138.167080530441));
#70692=CARTESIAN_POINT('Ctrl Pts',(80.2049346504632,7.34661770215669,138.165718148428));
#70693=CARTESIAN_POINT('Ctrl Pts',(80.194276820789,7.34533152571712,138.165009002177));
#70694=CARTESIAN_POINT('Ctrl Pts',(80.1660947666925,7.34220659288969,138.163144294905));
#70695=CARTESIAN_POINT('Ctrl Pts',(80.1485522221125,7.340542640482,138.161994232691));
#70696=CARTESIAN_POINT('Ctrl Pts',(80.0661765790623,7.33404590401942,138.156639177914));
#70697=CARTESIAN_POINT('Ctrl Pts',(80.0011191323809,7.33273200050666,138.152544385492));
#70698=CARTESIAN_POINT('Ctrl Pts',(79.7905807369824,7.34080750592639,138.139488284622));
#70699=CARTESIAN_POINT('Ctrl Pts',(79.6463990940175,7.36545665094281,138.130891323677));
#70700=CARTESIAN_POINT('Ctrl Pts',(79.4858549650214,7.41516124815858,138.120104771471));
#70701=CARTESIAN_POINT('Ctrl Pts',(79.4645682704295,7.42222570358287,138.118647577626));
#70702=CARTESIAN_POINT('Ctrl Pts',(79.435661751426,7.43247127561186,138.116623277611));
#70703=CARTESIAN_POINT('Ctrl Pts',(79.4279123143807,7.43528289025306,138.11607606326));
#70704=CARTESIAN_POINT('Ctrl Pts',(79.4148958097335,7.44011509760981,138.11514876498));
#70705=CARTESIAN_POINT('Ctrl Pts',(79.4096174245005,7.44210519111252,138.114770455316));
#70706=CARTESIAN_POINT('Ctrl Pts',(79.3987883762957,7.44625097279439,138.113989445477));
#70707=CARTESIAN_POINT('Ctrl Pts',(79.393239034047,7.44840965992862,138.113586586177));
#70708=CARTESIAN_POINT('Ctrl Pts',(79.3786618957416,7.45417030825552,138.112521630125));
#70709=CARTESIAN_POINT('Ctrl Pts',(79.3696540024839,7.45782154478325,138.111856731377));
#70710=CARTESIAN_POINT('Ctrl Pts',(79.3307794633611,7.47397633421778,138.108959257332));
#70711=CARTESIAN_POINT('Ctrl Pts',(79.3012509123767,7.48726944246051,138.106686390145));
#70712=CARTESIAN_POINT('Ctrl Pts',(79.2485890456955,7.51284750779756,138.102524107678));
#70713=CARTESIAN_POINT('Ctrl Pts',(79.2253208989838,7.52483453793934,138.100645156923));
#70714=CARTESIAN_POINT('Ctrl Pts',(79.1163595061494,7.58425706699978,138.091683336236));
#70715=CARTESIAN_POINT('Ctrl Pts',(79.0346701850194,7.63864458735291,138.08449167424));
#70716=CARTESIAN_POINT('Ctrl Pts',(78.9010169556137,7.7457401561245,138.072211211653));
#70717=CARTESIAN_POINT('Ctrl Pts',(78.8468840825302,7.79531836101649,138.067057827598));
#70718=CARTESIAN_POINT('Ctrl Pts',(78.7839868269093,7.86106213638394,138.060848319867));
#70719=CARTESIAN_POINT('Ctrl Pts',(78.7719891260512,7.87400851273935,138.059652491979));
#70720=CARTESIAN_POINT('Ctrl Pts',(78.7530241926725,7.89513679310415,138.057742961111));
#70721=CARTESIAN_POINT('Ctrl Pts',(78.7459267067906,7.90319940070358,138.057023814628));
#70722=CARTESIAN_POINT('Ctrl Pts',(78.7325087096955,7.91874253020877,138.055655253828));
#70723=CARTESIAN_POINT('Ctrl Pts',(78.7261752349649,7.92621121166902,138.055005320669));
#70724=CARTESIAN_POINT('Ctrl Pts',(78.7118711209733,7.9433838576828,138.053528045512));
#70725=CARTESIAN_POINT('Ctrl Pts',(78.7039435452367,7.9531230437098,138.052702469588));
#70726=CARTESIAN_POINT('Ctrl Pts',(78.6830809368851,7.97935343687659,138.050510476768));
#70727=CARTESIAN_POINT('Ctrl Pts',(78.6703454409366,7.99600097512323,138.049151910357));
#70728=CARTESIAN_POINT('Ctrl Pts',(78.5858580460651,8.1108693065002,138.03998413505));
#70729=CARTESIAN_POINT('Ctrl Pts',(78.5247346361114,8.21645241547501,138.032599543878));
#70730=CARTESIAN_POINT('Ctrl Pts',(78.4491360791845,8.38787732964649,138.021150156936));
#70731=CARTESIAN_POINT('Ctrl Pts',(78.4262054996706,8.44950686764995,138.017122855687));
#70732=CARTESIAN_POINT('Ctrl Pts',(78.4004337782013,8.53369187129784,138.011549591999));
#70733=CARTESIAN_POINT('Ctrl Pts',(78.394323335799,8.55518799531768,138.010120209386));
#70734=CARTESIAN_POINT('Ctrl Pts',(78.3845969613144,8.59222154197438,138.007636733414));
#70735=CARTESIAN_POINT('Ctrl Pts',(78.3807683358447,8.60770034367379,138.006592530437));
#70736=CARTESIAN_POINT('Ctrl Pts',(78.3755304552818,8.6302611924448,138.005058417337));
#70737=CARTESIAN_POINT('Ctrl Pts',(78.3739440164941,8.63730174906978,138.004577958352));
#70738=CARTESIAN_POINT('Ctrl Pts',(78.3712431197804,8.6496622096962,138.00373111118));
#70739=CARTESIAN_POINT('Ctrl Pts',(78.370108874352,8.65497759567742,138.003365845923));
#70740=CARTESIAN_POINT('Ctrl Pts',(78.3676928823558,8.66657743321451,138.002566244546));
#70741=CARTESIAN_POINT('Ctrl Pts',(78.3664214283584,8.67286366579006,138.002131371326));
#70742=CARTESIAN_POINT('Ctrl Pts',(78.3629688718115,8.6904557147033,138.000910345724));
#70743=CARTESIAN_POINT('Ctrl Pts',(78.3608686842504,8.70177677730762,138.000119933529));
#70744=CARTESIAN_POINT('Ctrl Pts',(78.3472941136256,8.77943044674238,137.994670723471));
#70745=CARTESIAN_POINT('Ctrl Pts',(78.3397332555545,8.84637714545199,137.989837644452));
#70746=CARTESIAN_POINT('Ctrl Pts',(78.3347732333155,8.94187762843282,137.982902275693));
#70747=CARTESIAN_POINT('Ctrl Pts',(78.3340257364443,8.97019868153111,137.980840122181));
#70748=CARTESIAN_POINT('Ctrl Pts',(78.3338937192958,9.11928312173196,137.969987770784));
#70749=CARTESIAN_POINT('Ctrl Pts',(78.346916648822,9.23971673357786,137.961268923042));
#70750=CARTESIAN_POINT('Ctrl Pts',(78.3773635453077,9.37821719681774,137.951513842782));
#70751=CARTESIAN_POINT('Ctrl Pts',(78.3822617974017,9.39864832833047,137.950080771153));
#70752=CARTESIAN_POINT('Ctrl Pts',(78.3907068943763,9.43114931819787,137.94780981578));
#70753=CARTESIAN_POINT('Ctrl Pts',(78.3940061035281,9.44328055892653,137.946964117364));
#70754=CARTESIAN_POINT('Ctrl Pts',(78.4001194494637,9.46479473827414,137.945467453211));
#70755=CARTESIAN_POINT('Ctrl Pts',(78.402879583022,9.47419226630688,137.944814775025));
#70756=CARTESIAN_POINT('Ctrl Pts',(78.4088380738411,9.49383696006755,137.943452424694));
#70757=CARTESIAN_POINT('Ctrl Pts',(78.4120529265984,9.50407868389715,137.942743324161));
#70758=CARTESIAN_POINT('Ctrl Pts',(78.4208047007412,9.53104476374886,137.940878879167));
#70759=CARTESIAN_POINT('Ctrl Pts',(78.4265083827096,9.54771388805996,137.939729030653));
#70760=CARTESIAN_POINT('Ctrl Pts',(78.433823501066,9.56803434018546,137.938329395143));
#70761=CARTESIAN_POINT('Ctrl Pts',(78.4351847809449,9.57177370031289,137.938071921239));
#70762=CARTESIAN_POINT('Ctrl Pts',(78.4365593728781,9.5755079543019,137.937814872615));
#70763=CARTESIAN_POINT('Ctrl Pts',(78.4365594482967,9.57550815918599,138.131873589273));
#70764=CARTESIAN_POINT('Ctrl Pts',(78.414637849384,9.51595536892372,138.136491900461));
#70765=CARTESIAN_POINT('Ctrl Pts',(78.3961254178195,9.45516788459882,138.14111638968));
#70766=CARTESIAN_POINT('Ctrl Pts',(78.3633053651022,9.32012388879201,138.151092520531));
#70767=CARTESIAN_POINT('Ctrl Pts',(78.3504862686607,9.24567456191019,138.156401286859));
#70768=CARTESIAN_POINT('Ctrl Pts',(78.3409385833685,9.15292782700929,138.162765649055));
#70769=CARTESIAN_POINT('Ctrl Pts',(78.3394018998885,9.13522461606615,138.163969701031));
#70770=CARTESIAN_POINT('Ctrl Pts',(78.3373894606692,9.10676175426065,138.165888993768));
#70771=CARTESIAN_POINT('Ctrl Pts',(78.3367343264427,9.09601659357096,138.166609780825));
#70772=CARTESIAN_POINT('Ctrl Pts',(78.3356827063292,9.07549597672171,138.167979367341));
#70773=CARTESIAN_POINT('Ctrl Pts',(78.3352680907964,9.06572194426203,138.168628705263));
#70774=CARTESIAN_POINT('Ctrl Pts',(78.3345197768597,9.04345014518695,138.170101784909));
#70775=CARTESIAN_POINT('Ctrl Pts',(78.3342406128081,9.0309510410592,138.170923794325));
#70776=CARTESIAN_POINT('Ctrl Pts',(78.3338721747492,8.99768326344809,138.173100002262));
#70777=CARTESIAN_POINT('Ctrl Pts',(78.3340304986832,8.97691365807849,138.174446530418));
#70778=CARTESIAN_POINT('Ctrl Pts',(78.3378513864377,8.83179078941756,138.183782698973));
#70779=CARTESIAN_POINT('Ctrl Pts',(78.3550437260773,8.70818656399838,138.191324616436));
#70780=CARTESIAN_POINT('Ctrl Pts',(78.4084928740364,8.49896359949546,138.204525774198));
#70781=CARTESIAN_POINT('Ctrl Pts',(78.4384117498405,8.41231826870576,138.210146095496));
#70782=CARTESIAN_POINT('Ctrl Pts',(78.4802104555524,8.31739833167442,138.216922874802));
#70783=CARTESIAN_POINT('Ctrl Pts',(78.485257448758,8.30627074519,138.217727500129));
#70784=CARTESIAN_POINT('Ctrl Pts',(78.4931726195924,8.28931765787036,138.21897053404));
#70785=CARTESIAN_POINT('Ctrl Pts',(78.4959533468624,8.2834514619487,138.219403837487));
#70786=CARTESIAN_POINT('Ctrl Pts',(78.5011424516177,8.27266786802886,138.220206518164));
#70787=CARTESIAN_POINT('Ctrl Pts',(78.5035408713517,8.26774590899586,138.220575290997));
#70788=CARTESIAN_POINT('Ctrl Pts',(78.5090660378454,8.25654785934247,138.221419757373));
#70789=CARTESIAN_POINT('Ctrl Pts',(78.5122081713514,8.25027962872683,138.221896372034));
#70790=CARTESIAN_POINT('Ctrl Pts',(78.5223042246101,8.23045247212741,138.223415985597));
#70791=CARTESIAN_POINT('Ctrl Pts',(78.5294044201984,8.2169694756745,138.224467316182));
#70792=CARTESIAN_POINT('Ctrl Pts',(78.5855325897473,8.1138408899625,138.232637376182));
#70793=CARTESIAN_POINT('Ctrl Pts',(78.6425252244934,8.02878693163967,138.240117459765));
#70794=CARTESIAN_POINT('Ctrl Pts',(78.7795628508592,7.86010829693086,138.255923485067));
#70795=CARTESIAN_POINT('Ctrl Pts',(78.8612687627697,7.77847618599563,138.264182945378));
#70796=CARTESIAN_POINT('Ctrl Pts',(78.9658258335971,7.69370139811592,138.273393669623));
#70797=CARTESIAN_POINT('Ctrl Pts',(78.9811053750318,7.6817488698564,138.274710513945));
#70798=CARTESIAN_POINT('Ctrl Pts',(79.0054617482289,7.66337246904914,138.276765199439));
#70799=CARTESIAN_POINT('Ctrl Pts',(79.0143996700174,7.65676826622106,138.277510054563));
#70800=CARTESIAN_POINT('Ctrl Pts',(79.0312785371243,7.64455571226963,138.278899944832));
#70801=CARTESIAN_POINT('Ctrl Pts',(79.0392037391194,7.63892651127807,138.279545765869));
#70802=CARTESIAN_POINT('Ctrl Pts',(79.0571237790144,7.62643258739501,138.280991190476));
#70803=CARTESIAN_POINT('Ctrl Pts',(79.0671452704098,7.61960691412703,138.281789287962));
#70804=CARTESIAN_POINT('Ctrl Pts',(79.0968805489473,7.59982583747257,138.284128265636));
#70805=CARTESIAN_POINT('Ctrl Pts',(79.1167964965988,7.58717867746819,138.28565769616));
#70806=CARTESIAN_POINT('Ctrl Pts',(79.225102628248,7.52158699880848,138.293792071544));
#70807=CARTESIAN_POINT('Ctrl Pts',(79.317994307088,7.4765031953814,138.300109324374));
#70808=CARTESIAN_POINT('Ctrl Pts',(79.4884867459653,7.41249832585567,138.311231414377));
#70809=CARTESIAN_POINT('Ctrl Pts',(79.5643873148481,7.39001639114764,138.316037638715));
#70810=CARTESIAN_POINT('Ctrl Pts',(79.6657466595042,7.36768798256059,138.322582286372));
#70811=CARTESIAN_POINT('Ctrl Pts',(79.6900166995516,7.36290560993512,138.324158994922));
#70812=CARTESIAN_POINT('Ctrl Pts',(79.7313263464648,7.3557171038693,138.326872600835));
#70813=CARTESIAN_POINT('Ctrl Pts',(79.7483136567872,7.35303135951741,138.327996991992));
#70814=CARTESIAN_POINT('Ctrl Pts',(79.7727005126892,7.34956180462178,138.329627257385));
#70815=CARTESIAN_POINT('Ctrl Pts',(79.7800691084418,7.34856374891355,138.33012194618));
#70816=CARTESIAN_POINT('Ctrl Pts',(79.7929064676546,7.34691240354196,138.330987814442));
#70817=CARTESIAN_POINT('Ctrl Pts',(79.7983721830943,7.34623685034833,138.331357752602));
#70818=CARTESIAN_POINT('Ctrl Pts',(79.8100939733911,7.34484703225218,138.33215398822));
#70819=CARTESIAN_POINT('Ctrl Pts',(79.816350673941,7.34414113906587,138.33258070801));
#70820=CARTESIAN_POINT('Ctrl Pts',(79.8335459591911,7.34229978744588,138.333757895499));
#70821=CARTESIAN_POINT('Ctrl Pts',(79.8444917892242,7.34123717106693,138.334512167061));
#70822=CARTESIAN_POINT('Ctrl Pts',(79.9069181891597,7.3358001443225,138.338838958122));
#70823=CARTESIAN_POINT('Ctrl Pts',(79.9585650469178,7.33371448078588,138.342514709301));
#70824=CARTESIAN_POINT('Ctrl Pts',(80.1062897031846,7.33462066696945,138.353161094629));
#70825=CARTESIAN_POINT('Ctrl Pts',(80.2021297567767,7.34351864753318,138.360217535047));
#70826=CARTESIAN_POINT('Ctrl Pts',(80.3482770337563,7.36996643463314,138.370897266388));
#70827=CARTESIAN_POINT('Ctrl Pts',(80.3994163169786,7.38173741146202,138.374621449589));
#70828=CARTESIAN_POINT('Ctrl Pts',(80.4728290324852,7.40232830237056,138.379934912268));
#70829=CARTESIAN_POINT('Ctrl Pts',(80.4955994412264,7.40924438087714,138.381578527507));
#70830=CARTESIAN_POINT('Ctrl Pts',(80.5366303837534,7.42267337305199,138.384532612724));
#70831=CARTESIAN_POINT('Ctrl Pts',(80.554939950649,7.42902159052957,138.385848050426));
#70832=CARTESIAN_POINT('Ctrl Pts',(80.583565628269,7.43950951519255,138.387901052862));
#70833=CARTESIAN_POINT('Ctrl Pts',(80.5939576958954,7.44343530121392,138.388645612348));
#70834=CARTESIAN_POINT('Ctrl Pts',(80.6133689848682,7.45099096569337,138.390035238025));
#70835=CARTESIAN_POINT('Ctrl Pts',(80.6223971505771,7.45459639777722,138.390681087156));
#70836=CARTESIAN_POINT('Ctrl Pts',(80.6426192887695,7.46287814195678,138.392126944959));
#70837=CARTESIAN_POINT('Ctrl Pts',(80.6537948611912,7.46759814368206,138.392925443575));
#70838=CARTESIAN_POINT('Ctrl Pts',(80.6865744247106,7.48186647011733,138.395266773831));
#70839=CARTESIAN_POINT('Ctrl Pts',(80.7080286210067,7.49175286609609,138.396798120448));
#70840=CARTESIAN_POINT('Ctrl Pts',(80.8199922498526,7.54626310536275,138.404797826564));
#70841=CARTESIAN_POINT('Ctrl Pts',(80.9065217582138,7.59858650179525,138.410991884992));
#70842=CARTESIAN_POINT('Ctrl Pts',(81.05276059186,7.70626109595913,138.422084629955));
#70843=CARTESIAN_POINT('Ctrl Pts',(81.1141641228485,7.75874993612572,138.426984504078));
#70844=CARTESIAN_POINT('Ctrl Pts',(81.1892927783001,7.83305373898671,138.433644775243));
#70845=CARTESIAN_POINT('Ctrl Pts',(81.2066673559814,7.85102887431014,138.435237653497));
#70846=CARTESIAN_POINT('Ctrl Pts',(81.2353929821131,7.88211779770212,138.437976368323));
#70847=CARTESIAN_POINT('Ctrl Pts',(81.2469559886809,7.89503070495842,138.43910939277));
#70848=CARTESIAN_POINT('Ctrl Pts',(81.2632034314202,7.91375475706185,138.440749985354));
#70849=CARTESIAN_POINT('Ctrl Pts',(81.268053988071,7.91942112040923,138.441246173031));
#70850=CARTESIAN_POINT('Ctrl Pts',(81.2764214767593,7.92932984601704,138.442113732601));
#70851=CARTESIAN_POINT('Ctrl Pts',(81.2799556739122,7.93355739170006,138.442483847944));
#70852=CARTESIAN_POINT('Ctrl Pts',(81.2874751356204,7.94264326842464,138.443279368357));
#70853=CARTESIAN_POINT('Ctrl Pts',(81.2914538419781,7.94750655421665,138.443705186116));
#70854=CARTESIAN_POINT('Ctrl Pts',(81.302284331078,7.96089884401729,138.444877535578));
#70855=CARTESIAN_POINT('Ctrl Pts',(81.3090796168231,7.96947283769105,138.445627822173));
#70856=CARTESIAN_POINT('Ctrl Pts',(81.3467455593922,8.01797179417796,138.449867410779));
#70857=CARTESIAN_POINT('Ctrl Pts',(81.3758712214113,8.05921291139832,138.453455236175));
#70858=CARTESIAN_POINT('Ctrl Pts',(81.454966856042,8.18275540357339,138.464020380551));
#70859=CARTESIAN_POINT('Ctrl Pts',(81.499736688283,8.26814746189261,138.471089924749));
#70860=CARTESIAN_POINT('Ctrl Pts',(81.5573988258966,8.40595520346095,138.481837139326));
#70861=CARTESIAN_POINT('Ctrl Pts',(81.5755563232026,8.45593795418796,138.485613081212));
#70862=CARTESIAN_POINT('Ctrl Pts',(81.6017424851114,8.54041095075611,138.491778221743));
#70863=CARTESIAN_POINT('Ctrl Pts',(81.6111176165792,8.57443985920846,138.494205727242));
#70864=CARTESIAN_POINT('Ctrl Pts',(81.6226860975378,8.62232161223749,138.497546023901));
#70865=CARTESIAN_POINT('Ctrl Pts',(81.6257958881495,8.63594109481123,138.498487778727));
#70866=CARTESIAN_POINT('Ctrl Pts',(81.630833587254,8.65935729333653,138.500093088662));
#70867=CARTESIAN_POINT('Ctrl Pts',(81.6328453675909,8.66913498835969,138.500759288286));
#70868=CARTESIAN_POINT('Ctrl Pts',(81.6365205099671,8.68784746929808,138.502026634361));
#70869=CARTESIAN_POINT('Ctrl Pts',(81.6381988751599,8.69677890419265,138.502628236285));
#70870=CARTESIAN_POINT('Ctrl Pts',(81.6423784664736,8.72006896456704,138.50418869879));
#70871=CARTESIAN_POINT('Ctrl Pts',(81.6447645414857,8.73444767558111,138.505143893466));
#70872=CARTESIAN_POINT('Ctrl Pts',(81.652506158067,8.78521599040884,138.508489501857));
#70873=CARTESIAN_POINT('Ctrl Pts',(81.6568453408311,8.82175128228929,138.510848200184));
#70874=CARTESIAN_POINT('Ctrl Pts',(81.6703115006988,8.97961742097151,138.520878132781));
#70875=CARTESIAN_POINT('Ctrl Pts',(81.667343736401,9.10159783692041,138.528188075259));
#70876=CARTESIAN_POINT('Ctrl Pts',(81.6411898648129,9.29596637601409,138.540236404648));
#70877=CARTESIAN_POINT('Ctrl Pts',(81.6263253019061,9.36900325051639,138.544867531466));
#70878=CARTESIAN_POINT('Ctrl Pts',(81.6035664506266,9.45195651606326,138.550495984455));
#70879=CARTESIAN_POINT('Ctrl Pts',(81.6003868868736,9.46308945989816,138.551259258554));
#70880=CARTESIAN_POINT('Ctrl Pts',(81.5952822719424,9.48028208892552,138.55245155244));
#70881=CARTESIAN_POINT('Ctrl Pts',(81.5934380574184,9.48636567100102,138.552876092584));
#70882=CARTESIAN_POINT('Ctrl Pts',(81.5899348447478,9.4976880410318,138.553671426601));
#70883=CARTESIAN_POINT('Ctrl Pts',(81.5882846901683,9.50292935519285,138.554041714052));
#70884=CARTESIAN_POINT('Ctrl Pts',(81.5844103219732,9.5150260917976,138.554901151823));
#70885=CARTESIAN_POINT('Ctrl Pts',(81.5821675232111,9.52187533691655,138.555391351295));
#70886=CARTESIAN_POINT('Ctrl Pts',(81.5748930757631,9.54361270621935,138.556958027052));
#70887=CARTESIAN_POINT('Ctrl Pts',(81.5696953432664,9.55844378346109,138.558043326547));
#70888=CARTESIAN_POINT('Ctrl Pts',(81.5345844752285,9.65426319935507,138.565152192615));
#70889=CARTESIAN_POINT('Ctrl Pts',(81.4986263975882,9.73288878810961,138.571431825343));
#70890=CARTESIAN_POINT('Ctrl Pts',(81.4212058917595,9.87240697068342,138.58304676143));
#70891=CARTESIAN_POINT('Ctrl Pts',(81.3814820678671,9.93403898360383,138.588369654603));
#70892=CARTESIAN_POINT('Ctrl Pts',(81.3134507173293,10.025707793532,138.596497657231));
#70893=CARTESIAN_POINT('Ctrl Pts',(81.2878698570919,10.0576487845835,138.599375111348));
#70894=CARTESIAN_POINT('Ctrl Pts',(81.2420094106939,10.1107769901602,138.604237184161));
#70895=CARTESIAN_POINT('Ctrl Pts',(81.2222999374128,10.1324292245238,138.606242214442));
#70896=CARTESIAN_POINT('Ctrl Pts',(81.1930184007679,10.1629412899006,138.609104133544));
#70897=CARTESIAN_POINT('Ctrl Pts',(81.18389790651,10.172224855551,138.609980031773));
#70898=CARTESIAN_POINT('Ctrl Pts',(81.1677031341513,10.1883273518583,138.611508775063));
#70899=CARTESIAN_POINT('Ctrl Pts',(81.1606756730323,10.195192241366,138.612163632632));
#70900=CARTESIAN_POINT('Ctrl Pts',(81.1459214810457,10.2093522501043,138.613521175951));
#70901=CARTESIAN_POINT('Ctrl Pts',(81.1381848320589,10.2166364298585,138.614223371539));
#70902=CARTESIAN_POINT('Ctrl Pts',(81.1178023519147,10.23546226283,138.616048792409));
#70903=CARTESIAN_POINT('Ctrl Pts',(81.1050471662243,10.2468840750931,138.61716693801));
#70904=CARTESIAN_POINT('Ctrl Pts',(81.048942768151,10.2955862776625,138.62198550762));
#70905=CARTESIAN_POINT('Ctrl Pts',(81.0038643175851,10.3308201250184,138.625602725255));
#70906=CARTESIAN_POINT('Ctrl Pts',(80.8703213163117,10.4245441518146,138.635760662698));
#70907=CARTESIAN_POINT('Ctrl Pts',(80.7779759666654,10.4770031489307,138.642126353889));
#70908=CARTESIAN_POINT('Ctrl Pts',(80.6269437164868,10.5446818877417,138.652339500227));
#70909=CARTESIAN_POINT('Ctrl Pts',(80.5713525655898,10.5660955565402,138.65606496528));
#70910=CARTESIAN_POINT('Ctrl Pts',(80.5009374305427,10.5889708463977,138.660879948062));
#70911=CARTESIAN_POINT('Ctrl Pts',(80.4870760012602,10.5932744879666,138.661832344571));
#70912=CARTESIAN_POINT('Ctrl Pts',(80.4664963302561,10.599370340004,138.663255498536));
#70913=CARTESIAN_POINT('Ctrl Pts',(80.4598198222796,10.6013026064257,138.663718616607));
#70914=CARTESIAN_POINT('Ctrl Pts',(80.4483802827232,10.60453591428,138.664514851499));
#70915=CARTESIAN_POINT('Ctrl Pts',(80.4436232513506,10.6058576487229,138.664846772434));
#70916=CARTESIAN_POINT('Ctrl Pts',(80.4326875975321,10.608843804261,138.665611735535));
#70917=CARTESIAN_POINT('Ctrl Pts',(80.4265053484731,10.6104937528121,138.66604557398));
#70918=CARTESIAN_POINT('Ctrl Pts',(80.4092327514541,10.6149971187187,138.667261232166));
#70919=CARTESIAN_POINT('Ctrl Pts',(80.3981225082043,10.6177717974687,138.668047255481));
#70920=CARTESIAN_POINT('Ctrl Pts',(80.3238895414408,10.6354998147202,138.67332221061));
#70921=CARTESIAN_POINT('Ctrl Pts',(80.2599746108758,10.6468683642374,138.677973173226));
#70922=CARTESIAN_POINT('Ctrl Pts',(80.1726390973349,10.6571918445905,138.684346254378));
#70923=CARTESIAN_POINT('Ctrl Pts',(80.149656848923,10.6594251631363,138.686025218517));
#70924=CARTESIAN_POINT('Ctrl Pts',(80.0553326270621,10.666615732976,138.692909975694));
#70925=CARTESIAN_POINT('Ctrl Pts',(79.9837491995658,10.6674551721576,138.698116437658));
#70926=CARTESIAN_POINT('Ctrl Pts',(79.8674834373629,10.661328437191,138.706437658304));
#70927=CARTESIAN_POINT('Ctrl Pts',(79.822747614529,10.6571526768007,138.709607725067));
#70928=CARTESIAN_POINT('Ctrl Pts',(79.7471814059211,10.6470034241371,138.71490139837));
#70929=CARTESIAN_POINT('Ctrl Pts',(79.7162531253605,10.6419578133436,138.717050629039));
#70930=CARTESIAN_POINT('Ctrl Pts',(79.6723672323591,10.6335210951386,138.720077218468));
#70931=CARTESIAN_POINT('Ctrl Pts',(79.6592812856565,10.6308418606453,138.720976763044));
#70932=CARTESIAN_POINT('Ctrl Pts',(79.6365771357627,10.6259081683505,138.722532760185));
#70933=CARTESIAN_POINT('Ctrl Pts',(79.6269443021032,10.623725039425,138.723191448666));
#70934=CARTESIAN_POINT('Ctrl Pts',(79.6083520929794,10.6193372203495,138.724460123332));
#70935=CARTESIAN_POINT('Ctrl Pts',(79.5993905232437,10.617143521526,138.725070434654));
#70936=CARTESIAN_POINT('Ctrl Pts',(79.5755792743885,10.6111046924307,138.726689157048));
#70937=CARTESIAN_POINT('Ctrl Pts',(79.5607634601316,10.6071286725431,138.727693334503));
#70938=CARTESIAN_POINT('Ctrl Pts',(79.505572949772,10.5914973175549,138.731424960401));
#70939=CARTESIAN_POINT('Ctrl Pts',(79.465587071244,10.578519907278,138.734109837021));
#70940=CARTESIAN_POINT('Ctrl Pts',(79.3592437811039,10.5395011582675,138.74124610156));
#70941=CARTESIAN_POINT('Ctrl Pts',(79.2939954713438,10.5106922254269,138.745617493715));
#70942=CARTESIAN_POINT('Ctrl Pts',(79.1302274333835,10.4254487935235,138.756898446319));
#70943=CARTESIAN_POINT('Ctrl Pts',(79.0352854784983,10.3629846025207,138.763743707595));
#70944=CARTESIAN_POINT('Ctrl Pts',(78.9363102086356,10.2823127455362,138.772050382616));
#70945=CARTESIAN_POINT('Ctrl Pts',(78.925304322394,10.2731029480145,138.772992294661));
#70946=CARTESIAN_POINT('Ctrl Pts',(78.9091705562749,10.2592438213694,138.774402735372));
#70947=CARTESIAN_POINT('Ctrl Pts',(78.9039501303199,10.2547025766547,138.774863819975));
#70948=CARTESIAN_POINT('Ctrl Pts',(78.8946591181166,10.2465181012451,138.775693220494));
#70949=CARTESIAN_POINT('Ctrl Pts',(78.890577956397,10.242887190852,138.776060637702));
#70950=CARTESIAN_POINT('Ctrl Pts',(78.8815611664521,10.2347853751436,138.776879346046));
#70951=CARTESIAN_POINT('Ctrl Pts',(78.8766345121527,10.2303049719124,138.777331320272));
#70952=CARTESIAN_POINT('Ctrl Pts',(78.8621441286129,10.2169675135089,138.778674130992));
#70953=CARTESIAN_POINT('Ctrl Pts',(78.8526575987415,10.2080278560539,138.779570765341));
#70954=CARTESIAN_POINT('Ctrl Pts',(78.830937882052,10.1870736052995,138.781662644502));
#70955=CARTESIAN_POINT('Ctrl Pts',(78.8187834772551,10.1749797684339,138.782862741672));
#70956=CARTESIAN_POINT('Ctrl Pts',(78.7771190701015,10.1322231168403,138.787074156149));
#70957=CARTESIAN_POINT('Ctrl Pts',(78.7486002214435,10.100620318275,138.79013183154));
#70958=CARTESIAN_POINT('Ctrl Pts',(78.6545313762142,9.98799134945566,138.800756752041));
#70959=CARTESIAN_POINT('Ctrl Pts',(78.5953819310225,9.90192232857178,138.808400266586));
#70960=CARTESIAN_POINT('Ctrl Pts',(78.5150811796408,9.75780283068197,138.820148096467));
#70961=CARTESIAN_POINT('Ctrl Pts',(78.4884265097267,9.70313312068178,138.824395576988));
#70962=CARTESIAN_POINT('Ctrl Pts',(78.4581005186763,9.63119009899751,138.829720882919));
#70963=CARTESIAN_POINT('Ctrl Pts',(78.4516327232602,9.6151534499893,138.830891885378));
#70964=CARTESIAN_POINT('Ctrl Pts',(78.442404467417,9.59120410005916,138.832617607355));
#70965=CARTESIAN_POINT('Ctrl Pts',(78.4394523293198,9.58336703874729,138.8331787035));
#70966=CARTESIAN_POINT('Ctrl Pts',(78.4365593737687,9.57550795672114,138.833737829798));
#70967=CARTESIAN_POINT('Origin',(80.,9.,134.));
#70968=CARTESIAN_POINT('',(78.4365593737676,9.57550795671827,139.531855288841));
#70969=CARTESIAN_POINT('',(78.4365593737638,9.57550795670799,139.340802412607));
#70970=CARTESIAN_POINT('',(78.4365593737638,9.57550795670799,134.));
#70971=CARTESIAN_POINT('',(81.2690708798525,10.0793586530483,140.));
#70972=CARTESIAN_POINT('Ctrl Pts',(78.4365593737676,9.57550795671827,139.531855288841));
#70973=CARTESIAN_POINT('Ctrl Pts',(78.4053667308162,9.49076917133665,139.537370123103));
#70974=CARTESIAN_POINT('Ctrl Pts',(78.3811187428276,9.40364475628102,139.542897610453));
#70975=CARTESIAN_POINT('Ctrl Pts',(78.3610876164748,9.29961255398156,139.549772227858));
#70976=CARTESIAN_POINT('Ctrl Pts',(78.3583425323577,9.28418690792652,139.550798653398));
#70977=CARTESIAN_POINT('Ctrl Pts',(78.3546746539356,9.26174516760808,139.552305209109));
#70978=CARTESIAN_POINT('Ctrl Pts',(78.3535782721426,9.25475776074172,139.552776147149));
#70979=CARTESIAN_POINT('Ctrl Pts',(78.3517117452004,9.24234652681836,139.55361628133));
#70980=CARTESIAN_POINT('Ctrl Pts',(78.3509238114044,9.23692558411675,139.55398447884));
#70981=CARTESIAN_POINT('Ctrl Pts',(78.3492663990445,9.22511369656628,139.554789527723));
#70982=CARTESIAN_POINT('Ctrl Pts',(78.3484073002293,9.21872162274131,139.555226917024));
#70983=CARTESIAN_POINT('Ctrl Pts',(78.3460625052061,9.2004732948317,139.556480224361));
#70984=CARTESIAN_POINT('Ctrl Pts',(78.3446672560414,9.18860611061177,139.557300839175));
#70985=CARTESIAN_POINT('Ctrl Pts',(78.333364075957,9.0826516048928,139.564671223018));
#70986=CARTESIAN_POINT('Ctrl Pts',(78.3313608875267,8.98790384756586,139.571558498935));
#70987=CARTESIAN_POINT('Ctrl Pts',(78.3451972873752,8.77188127659991,139.58731651004));
#70988=CARTESIAN_POINT('Ctrl Pts',(78.3663122964101,8.65145308166225,139.596119420761));
#70989=CARTESIAN_POINT('Ctrl Pts',(78.4062640967921,8.51419734399615,139.605954073373));
#70990=CARTESIAN_POINT('Ctrl Pts',(78.4125241826993,8.49411567631456,139.607388987131));
#70991=CARTESIAN_POINT('Ctrl Pts',(78.4231442968658,8.46218851940609,139.609664788115));
#70992=CARTESIAN_POINT('Ctrl Pts',(78.4272613658869,8.4502652448208,139.610513451837));
#70993=CARTESIAN_POINT('Ctrl Pts',(78.4348319556892,8.42912181998497,139.612016513195));
#70994=CARTESIAN_POINT('Ctrl Pts',(78.4382324971456,8.41988347938466,139.612672616458));
#70995=CARTESIAN_POINT('Ctrl Pts',(78.4455376008314,8.40056740148135,139.614043338092));
#70996=CARTESIAN_POINT('Ctrl Pts',(78.4494587539753,8.39049639524773,139.614757370607));
#70997=CARTESIAN_POINT('Ctrl Pts',(78.4600904688232,8.36395687939928,139.616637826442));
#70998=CARTESIAN_POINT('Ctrl Pts',(78.4669672952011,8.34755614732925,139.617798664051));
#70999=CARTESIAN_POINT('Ctrl Pts',(78.5040857977424,8.26286014614947,139.623792192387));
#71000=CARTESIAN_POINT('Ctrl Pts',(78.5386341911395,8.19654093875735,139.628475965896));
#71001=CARTESIAN_POINT('Ctrl Pts',(78.6273025671526,8.05110419380196,139.638990034171));
#71002=CARTESIAN_POINT('Ctrl Pts',(78.6840202632315,7.97389190749445,139.644750830598));
#71003=CARTESIAN_POINT('Ctrl Pts',(78.7788109362275,7.86572660845065,139.65367678295));
#71004=CARTESIAN_POINT('Ctrl Pts',(78.812131143485,7.83087827413104,139.656709975096));
#71005=CARTESIAN_POINT('Ctrl Pts',(78.857393958366,7.7874743897082,139.660776866668));
#71006=CARTESIAN_POINT('Ctrl Pts',(78.8680069505943,7.77756038009546,139.661726901642));
#71007=CARTESIAN_POINT('Ctrl Pts',(78.8840134712842,7.76299524890752,139.663156978034));
#71008=CARTESIAN_POINT('Ctrl Pts',(78.8893097257908,7.75823762466625,139.66362972244));
#71009=CARTESIAN_POINT('Ctrl Pts',(78.8988844390412,7.7497469210675,139.664483924752));
#71010=CARTESIAN_POINT('Ctrl Pts',(78.9031518593805,7.74600143721624,139.664864490509));
#71011=CARTESIAN_POINT('Ctrl Pts',(78.9119754231542,7.73833655872414,139.66565123698));
#71012=CARTESIAN_POINT('Ctrl Pts',(78.9165337119192,7.73441992800407,139.6660575779));
#71013=CARTESIAN_POINT('Ctrl Pts',(78.9284546333327,7.72428868574962,139.667119774126));
#71014=CARTESIAN_POINT('Ctrl Pts',(78.9358500406632,7.71811323302088,139.667778264676));
#71015=CARTESIAN_POINT('Ctrl Pts',(78.9693822239564,7.69060268948958,139.670760313008));
#71016=CARTESIAN_POINT('Ctrl Pts',(78.9961081467314,7.67000183951041,139.673127018181));
#71017=CARTESIAN_POINT('Ctrl Pts',(79.078295038691,7.61053954222738,139.680332728223));
#71018=CARTESIAN_POINT('Ctrl Pts',(79.1355172652143,7.57423383202161,139.685252406462));
#71019=CARTESIAN_POINT('Ctrl Pts',(79.2942426688896,7.48660346930289,139.698407037452));
#71020=CARTESIAN_POINT('Ctrl Pts',(79.3990703762787,7.44200311167996,139.706573674443));
#71021=CARTESIAN_POINT('Ctrl Pts',(79.5277093152694,7.40220809819103,139.71583196675));
#71022=CARTESIAN_POINT('Ctrl Pts',(79.5478979744556,7.3963786982033,139.717264747969));
#71023=CARTESIAN_POINT('Ctrl Pts',(79.5803929030306,7.38765839275512,139.719539488006));
#71024=CARTESIAN_POINT('Ctrl Pts',(79.5926306120503,7.38452305150594,139.720389118694));
#71025=CARTESIAN_POINT('Ctrl Pts',(79.6145046399116,7.37918322722211,139.721895582784));
#71026=CARTESIAN_POINT('Ctrl Pts',(79.6241270252903,7.37692477142474,139.722554103203));
#71027=CARTESIAN_POINT('Ctrl Pts',(79.6443814771264,7.37236066433221,139.723931733666));
#71028=CARTESIAN_POINT('Ctrl Pts',(79.6550172081869,7.37007324595036,139.724650237993));
#71029=CARTESIAN_POINT('Ctrl Pts',(79.6832792183942,7.36428398969517,139.726547021515));
#71030=CARTESIAN_POINT('Ctrl Pts',(79.7009413603169,7.36096281600217,139.727719579448));
#71031=CARTESIAN_POINT('Ctrl Pts',(79.7944212245474,7.34494637327114,139.733863415645));
#71032=CARTESIAN_POINT('Ctrl Pts',(79.8710008794541,7.33722323910122,139.738675901439));
#71033=CARTESIAN_POINT('Ctrl Pts',(80.0546353883884,7.33147201806204,139.749995122743));
#71034=CARTESIAN_POINT('Ctrl Pts',(80.1614895001244,7.33840756221315,139.756398196994));
#71035=CARTESIAN_POINT('Ctrl Pts',(80.3114471576711,7.36274926557926,139.765895226437));
#71036=CARTESIAN_POINT('Ctrl Pts',(80.355640800178,7.37177761697455,139.768761519963));
#71037=CARTESIAN_POINT('Ctrl Pts',(80.409741442029,7.38513740138604,139.772414688513));
#71038=CARTESIAN_POINT('Ctrl Pts',(80.4200485064856,7.38778770027444,139.773117257217));
#71039=CARTESIAN_POINT('Ctrl Pts',(80.436323379197,7.39213918253426,139.774238093289));
#71040=CARTESIAN_POINT('Ctrl Pts',(80.4423084959807,7.39377532990872,139.774652754427));
#71041=CARTESIAN_POINT('Ctrl Pts',(80.4534063064654,7.39687586103046,139.775426471519));
#71042=CARTESIAN_POINT('Ctrl Pts',(80.4585214575859,7.3983313839014,139.775785009602));
#71043=CARTESIAN_POINT('Ctrl Pts',(80.4704166120831,7.4017778182161,139.776623426204));
#71044=CARTESIAN_POINT('Ctrl Pts',(80.4771909418797,7.40378737900399,139.777104405194));
#71045=CARTESIAN_POINT('Ctrl Pts',(80.4996779315145,7.41061393702509,139.778712154311));
#71046=CARTESIAN_POINT('Ctrl Pts',(80.5153314671278,7.41562014743402,139.779849528432));
#71047=CARTESIAN_POINT('Ctrl Pts',(80.55322384788,7.4283595574259,139.782642847223));
#71048=CARTESIAN_POINT('Ctrl Pts',(80.5753773386563,7.43633408313875,139.784309913187));
#71049=CARTESIAN_POINT('Ctrl Pts',(80.6654046790929,7.4709130715592,139.791204241041));
#71050=CARTESIAN_POINT('Ctrl Pts',(80.7316635856436,7.50148824087596,139.796557027201));
#71051=CARTESIAN_POINT('Ctrl Pts',(80.9013281874108,7.59372222585803,139.810707967327));
#71052=CARTESIAN_POINT('Ctrl Pts',(81.0004470399118,7.66241778458007,139.819419383229));
#71053=CARTESIAN_POINT('Ctrl Pts',(81.1092751016174,7.75676652829245,139.829342478444));
#71054=CARTESIAN_POINT('Ctrl Pts',(81.1268962507127,7.77271614438428,139.830963459691));
#71055=CARTESIAN_POINT('Ctrl Pts',(81.1526837625225,7.7970813390071,139.833358730681));
#71056=CARTESIAN_POINT('Ctrl Pts',(81.1611116817903,7.80521431360711,139.83414539553));
#71057=CARTESIAN_POINT('Ctrl Pts',(81.1760953042924,7.81998186305234,139.835551254031));
#71058=CARTESIAN_POINT('Ctrl Pts',(81.1826823077608,7.82658381913668,139.836171886201));
#71059=CARTESIAN_POINT('Ctrl Pts',(81.1966248066269,7.84079464412579,139.837491383799));
#71060=CARTESIAN_POINT('Ctrl Pts',(81.2039639681868,7.8484190183791,139.83818949429));
#71061=CARTESIAN_POINT('Ctrl Pts',(81.2237527349007,7.86937279243841,139.840082081726));
#71062=CARTESIAN_POINT('Ctrl Pts',(81.2360571416266,7.88283778028323,139.841270150687));
#71063=CARTESIAN_POINT('Ctrl Pts',(81.3155034313595,7.97269749339213,139.849024342637));
#71064=CARTESIAN_POINT('Ctrl Pts',(81.3757536331803,8.05490450313513,139.855287060513));
#71065=CARTESIAN_POINT('Ctrl Pts',(81.4828978778062,8.23326696583813,139.867989113746));
#71066=CARTESIAN_POINT('Ctrl Pts',(81.5287990176698,8.32945273557691,139.874398074938));
#71067=CARTESIAN_POINT('Ctrl Pts',(81.5722470710693,8.44862322547404,139.882558428744));
#71068=CARTESIAN_POINT('Ctrl Pts',(81.5789196238383,8.468032025565,139.883894545287));
#71069=CARTESIAN_POINT('Ctrl Pts',(81.5877128975135,8.49523388460554,139.885783694033));
#71070=CARTESIAN_POINT('Ctrl Pts',(81.5901383567808,8.50292749457657,139.886319835288));
#71071=CARTESIAN_POINT('Ctrl Pts',(81.5941215369148,8.5158897763245,139.887226693119));
#71072=CARTESIAN_POINT('Ctrl Pts',(81.5957092256296,8.52114903315197,139.887595635095));
#71073=CARTESIAN_POINT('Ctrl Pts',(81.5989613818557,8.53211768075396,139.888367229068));
#71074=CARTESIAN_POINT('Ctrl Pts',(81.600621290968,8.53782812135838,139.888770105643));
#71075=CARTESIAN_POINT('Ctrl Pts',(81.6045716412018,8.55169472712968,139.889751057349));
#71076=CARTESIAN_POINT('Ctrl Pts',(81.606830482858,8.55985961202684,139.890330872933));
#71077=CARTESIAN_POINT('Ctrl Pts',(81.6162178053412,8.59482695740804,139.892822511523));
#71078=CARTESIAN_POINT('Ctrl Pts',(81.622738220569,8.62178625974415,139.89476473738));
#71079=CARTESIAN_POINT('Ctrl Pts',(81.6388046100089,8.69630909345912,139.900170835777));
#71080=CARTESIAN_POINT('Ctrl Pts',(81.6469506220005,8.74414514010715,139.903681742951));
#71081=CARTESIAN_POINT('Ctrl Pts',(81.6663865506929,8.89880131909011,139.915050442486));
#71082=CARTESIAN_POINT('Ctrl Pts',(81.6694453861322,9.00639326269799,139.92296815897));
#71083=CARTESIAN_POINT('Ctrl Pts',(81.6574866644886,9.18146727647585,139.935529580012));
#71084=CARTESIAN_POINT('Ctrl Pts',(81.6486856361659,9.24905865828822,139.940304728758));
#71085=CARTESIAN_POINT('Ctrl Pts',(81.6321457760444,9.33469610208402,139.946265985266));
#71086=CARTESIAN_POINT('Ctrl Pts',(81.6281984719859,9.35339934954393,139.947562687596));
#71087=CARTESIAN_POINT('Ctrl Pts',(81.6212939304409,9.38353793248474,139.949644961515));
#71088=CARTESIAN_POINT('Ctrl Pts',(81.6185355334317,9.395016573005,139.950436311492));
#71089=CARTESIAN_POINT('Ctrl Pts',(81.6129949985425,9.41703960326716,139.951951763404));
#71090=CARTESIAN_POINT('Ctrl Pts',(81.610230892546,9.42758785929924,139.952676349238));
#71091=CARTESIAN_POINT('Ctrl Pts',(81.6035551209315,9.4520804060029,139.954356363082));
#71092=CARTESIAN_POINT('Ctrl Pts',(81.5995647671019,9.46600246207649,139.955309460251));
#71093=CARTESIAN_POINT('Ctrl Pts',(81.5858025496379,9.51175673215393,139.958437569274));
#71094=CARTESIAN_POINT('Ctrl Pts',(81.5752576500616,9.54334907755491,139.960590535652));
#71095=CARTESIAN_POINT('Ctrl Pts',(81.5337731745299,9.65624785971019,139.968291296163));
#71096=CARTESIAN_POINT('Ctrl Pts',(81.4974257178194,9.73541750188746,139.973698039324));
#71097=CARTESIAN_POINT('Ctrl Pts',(81.4141641539465,9.88472987117062,139.98435684324));
#71098=CARTESIAN_POINT('Ctrl Pts',(81.3677849887947,9.95486588117745,139.989595164794));
#71099=CARTESIAN_POINT('Ctrl Pts',(81.3077170231935,10.0322932224563,139.995972388889));
#71100=CARTESIAN_POINT('Ctrl Pts',(81.298971634533,10.0432764629132,139.99689214452));
#71101=CARTESIAN_POINT('Ctrl Pts',(81.2863139832169,10.0587671730338,139.998213014843));
#71102=CARTESIAN_POINT('Ctrl Pts',(81.2825144776254,10.0633664479793,139.99860821659));
#71103=CARTESIAN_POINT('Ctrl Pts',(81.2755009163509,10.0717640454966,139.999335560135));
#71104=CARTESIAN_POINT('Ctrl Pts',(81.2722943743604,10.075568584752,139.999667279677));
#71105=CARTESIAN_POINT('Ctrl Pts',(81.2690708798525,10.0793586530483,140.));
#71106=CARTESIAN_POINT('',(78.7475355302757,10.0985848861505,140.));
#71107=CARTESIAN_POINT('Origin',(80.,9.,140.));
#71108=CARTESIAN_POINT('Ctrl Pts',(78.7475355302756,10.0985848861504,140.));
#71109=CARTESIAN_POINT('Ctrl Pts',(78.7492750986987,10.1005681171869,139.999818410898));
#71110=CARTESIAN_POINT('Ctrl Pts',(78.7510193658275,10.1025472028964,139.999636522787));
#71111=CARTESIAN_POINT('Ctrl Pts',(78.770908215588,10.1250057874456,139.997564813153));
#71112=CARTESIAN_POINT('Ctrl Pts',(78.7895488081928,10.1450381433428,139.995644440404));
#71113=CARTESIAN_POINT('Ctrl Pts',(78.8882628677563,10.2460175613479,139.98562143943));
#71114=CARTESIAN_POINT('Ctrl Pts',(78.9759871769111,10.3190590992091,139.977218838742));
#71115=CARTESIAN_POINT('Ctrl Pts',(79.1419499639817,10.4306376570869,139.962791329009));
#71116=CARTESIAN_POINT('Ctrl Pts',(79.2170533914007,10.4730827499196,139.956701369571));
#71117=CARTESIAN_POINT('Ctrl Pts',(79.3118014922645,10.5173259355423,139.949558030066));
#71118=CARTESIAN_POINT('Ctrl Pts',(79.3286173003773,10.5248411387034,139.948309317913));
#71119=CARTESIAN_POINT('Ctrl Pts',(79.3556487262977,10.5363879435193,139.946331440542));
#71120=CARTESIAN_POINT('Ctrl Pts',(79.3657851517762,10.5405998874096,139.945596259446));
#71121=CARTESIAN_POINT('Ctrl Pts',(79.3851089845753,10.5484063894291,139.944206726716));
#71122=CARTESIAN_POINT('Ctrl Pts',(79.394288092677,10.5520201029836,139.94355176061));
#71123=CARTESIAN_POINT('Ctrl Pts',(79.4153287694979,10.5600884833331,139.942061691837));
#71124=CARTESIAN_POINT('Ctrl Pts',(79.4272102356773,10.5644898286818,139.941228374794));
#71125=CARTESIAN_POINT('Ctrl Pts',(79.4585943042953,10.5757102123304,139.939047594908));
#71126=CARTESIAN_POINT('Ctrl Pts',(79.4781758977839,10.5823028996122,139.937707454102));
#71127=CARTESIAN_POINT('Ctrl Pts',(79.6370549675723,10.6325235681068,139.926984125458));
#71128=CARTESIAN_POINT('Ctrl Pts',(79.7814057183628,10.6580351361542,139.918235640159));
#71129=CARTESIAN_POINT('Ctrl Pts',(79.9881845593757,10.6670746420004,139.90544526783));
#71130=CARTESIAN_POINT('Ctrl Pts',(80.0492243989363,10.6663891718741,139.9016274265));
#71131=CARTESIAN_POINT('Ctrl Pts',(80.1248166860646,10.6613834150736,139.896700584619));
#71132=CARTESIAN_POINT('Ctrl Pts',(80.1395369390971,10.6602118731241,139.89573171006));
#71133=CARTESIAN_POINT('Ctrl Pts',(80.1599038879926,10.6583181583504,139.894375639909));
#71134=CARTESIAN_POINT('Ctrl Pts',(80.1655658804903,10.6577624391401,139.893996986679));
#71135=CARTESIAN_POINT('Ctrl Pts',(80.1714021636216,10.6571594160172,139.893604854225));
#71136=CARTESIAN_POINT('Ctrl Pts',(80.171579509769,10.6571410632821,139.893592936825));
#71137=CARTESIAN_POINT('Ctrl Pts',(80.1719340651294,10.6571043144563,139.893569107748));
#71138=CARTESIAN_POINT('Ctrl Pts',(80.1721112743328,10.6570859184089,139.893557196074));
#71139=CARTESIAN_POINT('Ctrl Pts',(80.1724681775636,10.6570488104965,139.893533202193));
#71140=CARTESIAN_POINT('Ctrl Pts',(80.1726478715362,10.6570300978238,139.893521119941));
#71141=CARTESIAN_POINT('Ctrl Pts',(80.1730128166048,10.6569920337717,139.893496578145));
#71142=CARTESIAN_POINT('Ctrl Pts',(80.1731980674868,10.6569726805567,139.893484118503));
#71143=CARTESIAN_POINT('Ctrl Pts',(80.1735779686894,10.6569329277586,139.893458563112));
#71144=CARTESIAN_POINT('Ctrl Pts',(80.1737726186638,10.6569125249414,139.893445467188));
#71145=CARTESIAN_POINT('Ctrl Pts',(80.1741764645885,10.6568701226802,139.893418292312));
#71146=CARTESIAN_POINT('Ctrl Pts',(80.1743856599498,10.6568481179187,139.893404213072));
#71147=CARTESIAN_POINT('Ctrl Pts',(80.1748260242303,10.6568017127244,139.893374570582));
#71148=CARTESIAN_POINT('Ctrl Pts',(80.175057192188,10.6567773035316,139.893359006855));
#71149=CARTESIAN_POINT('Ctrl Pts',(80.1755531972879,10.6567248250234,139.893325606149));
#71150=CARTESIAN_POINT('Ctrl Pts',(80.1758180327483,10.6566967405916,139.893307768348));
#71151=CARTESIAN_POINT('Ctrl Pts',(80.1764020011204,10.6566346721597,139.893268426891));
#71152=CARTESIAN_POINT('Ctrl Pts',(80.176721130876,10.6566006594537,139.893246921666));
#71153=CARTESIAN_POINT('Ctrl Pts',(80.1774569200864,10.6565220243359,139.893197325737));
#71154=CARTESIAN_POINT('Ctrl Pts',(80.1778735723233,10.6564773369607,139.893169231475));
#71155=CARTESIAN_POINT('Ctrl Pts',(80.1786073295496,10.6563983589592,139.89311973797));
#71156=CARTESIAN_POINT('Ctrl Pts',(80.1789244418834,10.6563641344306,139.893098342367));
#71157=CARTESIAN_POINT('Ctrl Pts',(80.1845614758536,10.6557541166304,139.892717909549));
#71158=CARTESIAN_POINT('Ctrl Pts',(80.1898783580145,10.6551528146369,139.892357455688));
#71159=CARTESIAN_POINT('Ctrl Pts',(80.2022343165761,10.653695123613,139.891516011902));
#71160=CARTESIAN_POINT('Ctrl Pts',(80.2092708314008,10.6528194079281,139.891033993502));
#71161=CARTESIAN_POINT('Ctrl Pts',(80.2319915260492,10.6498443361182,139.889468874148));
#71162=CARTESIAN_POINT('Ctrl Pts',(80.2476509081041,10.6475665037098,139.888376764884));
#71163=CARTESIAN_POINT('Ctrl Pts',(80.3411772974491,10.6325986329934,139.881782820596));
#71164=CARTESIAN_POINT('Ctrl Pts',(80.418088524781,10.614614450719,139.876068361954));
#71165=CARTESIAN_POINT('Ctrl Pts',(80.5564340513755,10.5717151770512,139.865536547396));
#71166=CARTESIAN_POINT('Ctrl Pts',(80.6182268478162,10.5484520551824,139.860733731884));
#71167=CARTESIAN_POINT('Ctrl Pts',(80.7461488655859,10.4914112409354,139.850690609429));
#71168=CARTESIAN_POINT('Ctrl Pts',(80.8117374630785,10.4567534612047,139.845481557463));
#71169=CARTESIAN_POINT('Ctrl Pts',(80.8899158582108,10.4085172618325,139.839211264558));
#71170=CARTESIAN_POINT('Ctrl Pts',(80.9048735959079,10.3989549417533,139.838008313772));
#71171=CARTESIAN_POINT('Ctrl Pts',(80.9286833317609,10.3831919451638,139.836087464075));
#71172=CARTESIAN_POINT('Ctrl Pts',(80.937632473553,10.3771412570411,139.83536409414));
#71173=CARTESIAN_POINT('Ctrl Pts',(80.9546271750259,10.3654083472983,139.833987438966));
#71174=CARTESIAN_POINT('Ctrl Pts',(80.9626824004861,10.3597410051297,139.833333632863));
#71175=CARTESIAN_POINT('Ctrl Pts',(80.9809536269438,10.346642326696,139.831847381941));
#71176=CARTESIAN_POINT('Ctrl Pts',(80.9911363918032,10.3391655019623,139.831016715976));
#71177=CARTESIAN_POINT('Ctrl Pts',(81.0180920377573,10.3188970796573,139.828810584563));
#71178=CARTESIAN_POINT('Ctrl Pts',(81.0347090196051,10.30590130274,139.827443034891));
#71179=CARTESIAN_POINT('Ctrl Pts',(81.1448734339632,10.2163208233676,139.818312653203));
#71180=CARTESIAN_POINT('Ctrl Pts',(81.2300929659983,10.1300649017884,139.810966409533));
#71181=CARTESIAN_POINT('Ctrl Pts',(81.3644670124966,9.96066167524757,139.797749486242));
#71182=CARTESIAN_POINT('Ctrl Pts',(81.4171750095174,9.88105099238715,139.791907767027));
#71183=CARTESIAN_POINT('Ctrl Pts',(81.4685531305597,9.78679926524852,139.784889721542));
#71184=CARTESIAN_POINT('Ctrl Pts',(81.4742087798991,9.77615065143372,139.784095347322));
#71185=CARTESIAN_POINT('Ctrl Pts',(81.4827223790021,9.75969220912737,139.782863862527));
#71186=CARTESIAN_POINT('Ctrl Pts',(81.4856630076555,9.75392528141965,139.782431667568));
#71187=CARTESIAN_POINT('Ctrl Pts',(81.4910294417248,9.74324773934362,139.781629910425));
#71188=CARTESIAN_POINT('Ctrl Pts',(81.4934647279951,9.73834213053225,139.781260939473));
#71189=CARTESIAN_POINT('Ctrl Pts',(81.4989767863981,9.72709986391266,139.78041395824));
#71190=CARTESIAN_POINT('Ctrl Pts',(81.5020375687078,9.72075568393222,139.779935008673));
#71191=CARTESIAN_POINT('Ctrl Pts',(81.5114663439987,9.70089145713497,139.778432744825));
#71192=CARTESIAN_POINT('Ctrl Pts',(81.5176925032422,9.68730544199477,139.777401506352));
#71193=CARTESIAN_POINT('Ctrl Pts',(81.5653593419637,9.57948550333323,139.769198242541));
#71194=CARTESIAN_POINT('Ctrl Pts',(81.5981641547459,9.48168577394389,139.761657185607));
#71195=CARTESIAN_POINT('Ctrl Pts',(81.6480358012736,9.26968123022381,139.74581391735));
#71196=CARTESIAN_POINT('Ctrl Pts',(81.6627089976902,9.15542873537538,139.737577113301));
#71197=CARTESIAN_POINT('Ctrl Pts',(81.6659732073318,9.02138184528976,139.728404304849));
#71198=CARTESIAN_POINT('Ctrl Pts',(81.6661089783952,9.00219922893443,139.727102401817));
#71199=CARTESIAN_POINT('Ctrl Pts',(81.6658009943218,8.97198667939606,139.725068057421));
#71200=CARTESIAN_POINT('Ctrl Pts',(81.6655789773034,8.96095669877791,139.724328745244));
#71201=CARTESIAN_POINT('Ctrl Pts',(81.6649566872603,8.94026054187571,139.722947618986));
#71202=CARTESIAN_POINT('Ctrl Pts',(81.6645817507167,8.93059412650554,139.722305038663));
#71203=CARTESIAN_POINT('Ctrl Pts',(81.6635486081921,8.90885003708972,139.720864934414));
#71204=CARTESIAN_POINT('Ctrl Pts',(81.6628430220334,8.89677507769214,139.720068930335));
#71205=CARTESIAN_POINT('Ctrl Pts',(81.6603716121573,8.86114797964545,139.717730493693));
#71206=CARTESIAN_POINT('Ctrl Pts',(81.6582363706974,8.83762388309946,139.716199637637));
#71207=CARTESIAN_POINT('Ctrl Pts',(81.6442645692347,8.71315789442467,139.708156235552));
#71208=CARTESIAN_POINT('Ctrl Pts',(81.6237101542136,8.61340845804988,139.701924276533));
#71209=CARTESIAN_POINT('Ctrl Pts',(81.5707057125444,8.43877123795905,139.690787681328));
#71210=CARTESIAN_POINT('Ctrl Pts',(81.5416217936874,8.36321544518455,139.685881605787));
#71211=CARTESIAN_POINT('Ctrl Pts',(81.4965111736758,8.2674455312216,139.679212331265));
#71212=CARTESIAN_POINT('Ctrl Pts',(81.4853439508587,8.24505963413609,139.677618983377));
#71213=CARTESIAN_POINT('Ctrl Pts',(81.4655964689787,8.20760920551813,139.674880336749));
#71214=CARTESIAN_POINT('Ctrl Pts',(81.4572771121725,8.19241127962502,139.673747993319));
#71215=CARTESIAN_POINT('Ctrl Pts',(81.4450533848761,8.1708848495053,139.672109901386));
#71216=CARTESIAN_POINT('Ctrl Pts',(81.4413409920195,8.16444787272541,139.671615621108));
#71217=CARTESIAN_POINT('Ctrl Pts',(81.4348113091426,8.15329896353987,139.6707513724));
#71218=CARTESIAN_POINT('Ctrl Pts',(81.4320135987525,8.14857578744658,139.670382656971));
#71219=CARTESIAN_POINT('Ctrl Pts',(81.4259695167432,8.13848605742688,139.669589357307));
#71220=CARTESIAN_POINT('Ctrl Pts',(81.4227162194236,8.13312406212703,139.669164355312));
#71221=CARTESIAN_POINT('Ctrl Pts',(81.4137344797883,8.118507353448,139.667996697368));
#71222=CARTESIAN_POINT('Ctrl Pts',(81.407945615409,8.10929039880981,139.667250335225));
#71223=CARTESIAN_POINT('Ctrl Pts',(81.3754565030873,8.05866978534001,139.663098084314));
#71224=CARTESIAN_POINT('Ctrl Pts',(81.3470224720968,8.01841319804142,139.659598300316));
#71225=CARTESIAN_POINT('Ctrl Pts',(81.2642198516651,7.91156707465608,139.649869030341));
#71226=CARTESIAN_POINT('Ctrl Pts',(81.2064152620534,7.84782792978545,139.643566876989));
#71227=CARTESIAN_POINT('Ctrl Pts',(81.0835143179181,7.73174766910833,139.631348866015));
#71228=CARTESIAN_POINT('Ctrl Pts',(81.0188815933741,7.67926111943427,139.625444129004));
#71229=CARTESIAN_POINT('Ctrl Pts',(80.9317796281978,7.61874426909228,139.618152116356));
#71230=CARTESIAN_POINT('Ctrl Pts',(80.9127002713673,7.60606349685692,139.616591653707));
#71231=CARTESIAN_POINT('Ctrl Pts',(80.8833640619185,7.58742635245284,139.614246262621));
#71232=CARTESIAN_POINT('Ctrl Pts',(80.873295797785,7.58117977257087,139.613450695429));
#71233=CARTESIAN_POINT('Ctrl Pts',(80.8556535575413,7.57049307713706,139.612072572033));
#71234=CARTESIAN_POINT('Ctrl Pts',(80.8481096451488,7.56600450213261,139.611488264746));
#71235=CARTESIAN_POINT('Ctrl Pts',(80.8310200940209,7.55601837457729,139.610175603773));
#71236=CARTESIAN_POINT('Ctrl Pts',(80.821454637414,7.55055540992867,139.609448517601));
#71237=CARTESIAN_POINT('Ctrl Pts',(80.7953476009133,7.53598678289165,139.607484166069));
#71238=CARTESIAN_POINT('Ctrl Pts',(80.7787039561566,7.52706663359772,139.606253500638));
#71239=CARTESIAN_POINT('Ctrl Pts',(80.6672312942661,7.46974069865266,139.598145144544));
#71240=CARTESIAN_POINT('Ctrl Pts',(80.5680972936347,7.43023547044236,139.591592283712));
#71241=CARTESIAN_POINT('Ctrl Pts',(80.3866011081683,7.37737548465106,139.580037400198));
#71242=CARTESIAN_POINT('Ctrl Pts',(80.3057421837066,7.36021629637196,139.575027261048));
#71243=CARTESIAN_POINT('Ctrl Pts',(80.1866818205355,7.34406507866575,139.567456166848));
#71244=CARTESIAN_POINT('Ctrl Pts',(80.149255105943,7.34027321812248,139.565047941981));
#71245=CARTESIAN_POINT('Ctrl Pts',(80.1018795857936,7.33708865866905,139.561928092699));
#71246=CARTESIAN_POINT('Ctrl Pts',(80.0920182106946,7.33651383645002,139.561274784604));
#71247=CARTESIAN_POINT('Ctrl Pts',(80.0761608197798,7.3357309356564,139.560217137779));
#71248=CARTESIAN_POINT('Ctrl Pts',(80.0701675992035,7.33546748479596,139.559815775111));
#71249=CARTESIAN_POINT('Ctrl Pts',(80.0586099431458,7.33502196097285,139.559038396566));
#71250=CARTESIAN_POINT('Ctrl Pts',(80.0530458311416,7.3348354039381,139.5586626271));
#71251=CARTESIAN_POINT('Ctrl Pts',(80.0406526779747,7.33448205531283,139.557822405884));
#71252=CARTESIAN_POINT('Ctrl Pts',(80.0338233404751,7.33432937173224,139.557357199541));
#71253=CARTESIAN_POINT('Ctrl Pts',(80.0135473697047,7.33400080666893,139.555969883116));
#71254=CARTESIAN_POINT('Ctrl Pts',(80.0000996997849,7.33394573753342,139.555041755501));
#71255=CARTESIAN_POINT('Ctrl Pts',(79.8797815025852,7.33490965958925,139.546674444081));
#71256=CARTESIAN_POINT('Ctrl Pts',(79.7732490591185,7.3460475246641,139.538836936621));
#71257=CARTESIAN_POINT('Ctrl Pts',(79.5949919508074,7.3822377378563,139.525617369195));
#71258=CARTESIAN_POINT('Ctrl Pts',(79.5225431689758,7.40211911086728,139.52020977534));
#71259=CARTESIAN_POINT('Ctrl Pts',(79.4099453776348,7.44136454264681,139.511829421572));
#71260=CARTESIAN_POINT('Ctrl Pts',(79.3688075776359,7.4575650095866,139.508771661348));
#71261=CARTESIAN_POINT('Ctrl Pts',(79.3144889245214,7.48149406073892,139.504737646618));
#71262=CARTESIAN_POINT('Ctrl Pts',(79.3007022349305,7.48779353780562,139.503714000649));
#71263=CARTESIAN_POINT('Ctrl Pts',(79.27776794372,7.49865351527179,139.502011045577));
#71264=CARTESIAN_POINT('Ctrl Pts',(79.2685731154254,7.50311151688941,139.501328263302));
#71265=CARTESIAN_POINT('Ctrl Pts',(79.2505173739298,7.51207172159102,139.499987186907));
#71266=CARTESIAN_POINT('Ctrl Pts',(79.2416545925398,7.51656917292258,139.499328762384));
#71267=CARTESIAN_POINT('Ctrl Pts',(79.2201912948159,7.52770343183762,139.49773354055));
#71268=CARTESIAN_POINT('Ctrl Pts',(79.2076344596344,7.534423092265,139.496799692401));
#71269=CARTESIAN_POINT('Ctrl Pts',(79.1648697993957,7.55801846394256,139.493615639117));
#71270=CARTESIAN_POINT('Ctrl Pts',(79.1351011633426,7.57567438042733,139.491393086056));
#71271=CARTESIAN_POINT('Ctrl Pts',(79.0013945651311,7.66071538902914,139.481340113618));
#71272=CARTESIAN_POINT('Ctrl Pts',(78.9046264916226,7.7386299123878,139.473897338724));
#71273=CARTESIAN_POINT('Ctrl Pts',(78.7643433145804,7.88000915540193,139.461665691532));
#71274=CARTESIAN_POINT('Ctrl Pts',(78.7149939414714,7.93699322549024,139.456984746963));
#71275=CARTESIAN_POINT('Ctrl Pts',(78.6626904070687,8.00637349674128,139.451299675603));
#71276=CARTESIAN_POINT('Ctrl Pts',(78.6558042869799,8.01570916803908,139.450534934193));
#71277=CARTESIAN_POINT('Ctrl Pts',(78.6452926771124,8.0302760365412,139.449340714995));
#71278=CARTESIAN_POINT('Ctrl Pts',(78.6415985710281,8.03545759533834,139.448915736125));
#71279=CARTESIAN_POINT('Ctrl Pts',(78.6347704093569,8.04515218274614,139.448120005445));
#71280=CARTESIAN_POINT('Ctrl Pts',(78.6316288854985,8.04965970361618,139.447749764622));
#71281=CARTESIAN_POINT('Ctrl Pts',(78.6244223298619,8.06010962891752,139.446890876136));
#71282=CARTESIAN_POINT('Ctrl Pts',(78.6203734702877,8.06606291971006,139.446401184483));
#71283=CARTESIAN_POINT('Ctrl Pts',(78.6076290978192,8.08506548486369,139.4448373713));
#71284=CARTESIAN_POINT('Ctrl Pts',(78.5990794698452,8.09821093365397,139.443754464852));
#71285=CARTESIAN_POINT('Ctrl Pts',(78.5460191682421,8.18236943841616,139.436824183178));
#71286=CARTESIAN_POINT('Ctrl Pts',(78.5067388158411,8.25652951784427,139.430735061346));
#71287=CARTESIAN_POINT('Ctrl Pts',(78.4427463578755,8.40308167274243,139.419094545706));
#71288=CARTESIAN_POINT('Ctrl Pts',(78.4171000601497,8.47485264748105,139.413558033869));
#71289=CARTESIAN_POINT('Ctrl Pts',(78.385402981615,8.58733593744271,139.405238400553));
#71290=CARTESIAN_POINT('Ctrl Pts',(78.3757958706539,8.62693625566892,139.402373492433));
#71291=CARTESIAN_POINT('Ctrl Pts',(78.3618143819876,8.69544236650391,139.397530264804));
#71292=CARTESIAN_POINT('Ctrl Pts',(78.3567311470748,8.72418278881758,139.395531728685));
#71293=CARTESIAN_POINT('Ctrl Pts',(78.3504789670484,8.76589483573377,139.39267745763));
#71294=CARTESIAN_POINT('Ctrl Pts',(78.3487030801407,8.77876852581196,139.391802837263));
#71295=CARTESIAN_POINT('Ctrl Pts',(78.345850162255,8.80140314295193,139.390275746978));
#71296=CARTESIAN_POINT('Ctrl Pts',(78.3447084797235,8.81115512359756,139.389621273678));
#71297=CARTESIAN_POINT('Ctrl Pts',(78.3425106275818,8.83148313808281,139.388263988864));
#71298=CARTESIAN_POINT('Ctrl Pts',(78.3414693157658,8.84206035732694,139.387561672131));
#71299=CARTESIAN_POINT('Ctrl Pts',(78.3390131433626,8.86972146348093,139.385734767674));
#71300=CARTESIAN_POINT('Ctrl Pts',(78.3377605825241,8.88681877531719,139.384615282217));
#71301=CARTESIAN_POINT('Ctrl Pts',(78.333402225627,8.96227584006357,139.379713452031));
#71302=CARTESIAN_POINT('Ctrl Pts',(78.3331042628764,9.02075953004453,139.376018566448));
#71303=CARTESIAN_POINT('Ctrl Pts',(78.3408872562269,9.18441018408281,139.36582617507));
#71304=CARTESIAN_POINT('Ctrl Pts',(78.3558701181429,9.28896149901275,139.359496157283));
#71305=CARTESIAN_POINT('Ctrl Pts',(78.3957051395104,9.45377587821222,139.3490300654));
#71306=CARTESIAN_POINT('Ctrl Pts',(78.4143721582719,9.51522510607317,139.345008208124));
#71307=CARTESIAN_POINT('Ctrl Pts',(78.4365419166502,9.5754605308294,139.340805721476));
#71308=CARTESIAN_POINT('Ctrl Pts',(78.4365506449801,9.5754842438558,139.340804067081));
#71309=CARTESIAN_POINT('Ctrl Pts',(78.4365593737638,9.57550795670799,139.340802412607));
#71310=CARTESIAN_POINT('Origin',(80.,-9.,141.545925280538));
#71311=CARTESIAN_POINT('',(81.2520391107128,-7.37076839346109,129.106054343781));
#71312=CARTESIAN_POINT('',(81.2492121870567,-7.37445590553645,129.047846843673));
#71313=CARTESIAN_POINT('',(81.2520391107129,-7.37076839346111,141.545925280538));
#71314=CARTESIAN_POINT('',(81.8174278887594,-8.04137941204074,129.));
#71315=CARTESIAN_POINT('Ctrl Pts',(81.2492121870567,-7.37445590553645,129.047846843673));
#71316=CARTESIAN_POINT('Ctrl Pts',(81.4831295299336,-7.55380834072825,129.031897895782));
#71317=CARTESIAN_POINT('Ctrl Pts',(81.6801942371869,-7.78120112171703,129.015948947891));
#71318=CARTESIAN_POINT('Ctrl Pts',(81.8174278887595,-8.04137941204082,129.));
#71319=CARTESIAN_POINT('',(82.0533682620167,-9.07534150942548,129.000000008563));
#71320=CARTESIAN_POINT('Origin',(80.,-9.,129.));
#71321=CARTESIAN_POINT('Ctrl Pts',(81.2520391107129,-7.37076839346109,129.106054343781));
#71322=CARTESIAN_POINT('Ctrl Pts',(81.3081324823019,-7.41387527574805,129.102199425929));
#71323=CARTESIAN_POINT('Ctrl Pts',(81.3621028898732,-7.45996383129776,129.098344508077));
#71324=CARTESIAN_POINT('Ctrl Pts',(81.4136153569759,-7.50879606189431,129.094489590225));
#71325=CARTESIAN_POINT('Ctrl Pts',(81.4662255514254,-7.55866890417088,129.090552524322));
#71326=CARTESIAN_POINT('Ctrl Pts',(81.5162713772154,-7.61140346509638,129.08661545842));
#71327=CARTESIAN_POINT('Ctrl Pts',(81.5634292255428,-7.66670085156455,129.082678392517));
#71328=CARTESIAN_POINT('Ctrl Pts',(81.6094922174622,-7.72071440723755,129.078832732859));
#71329=CARTESIAN_POINT('Ctrl Pts',(81.6527995488012,-7.77717267636535,129.074987073202));
#71330=CARTESIAN_POINT('Ctrl Pts',(81.6930864251896,-7.83575950966368,129.071141413544));
#71331=CARTESIAN_POINT('Ctrl Pts',(81.7333528037562,-7.89431653418604,129.067297710544));
#71332=CARTESIAN_POINT('Ctrl Pts',(81.7706014995003,-7.95499957180025,129.063454007545));
#71333=CARTESIAN_POINT('Ctrl Pts',(81.804609430456,-8.01746126488105,129.059610304545));
#71334=CARTESIAN_POINT('Ctrl Pts',(81.8386116248341,-8.07991242170324,129.055767249915));
#71335=CARTESIAN_POINT('Ctrl Pts',(81.8693739064979,-8.14414120838439,129.051924195285));
#71336=CARTESIAN_POINT('Ctrl Pts',(81.8967186837959,-8.20977484408587,129.048081140655));
#71337=CARTESIAN_POINT('Ctrl Pts',(81.9252282934647,-8.27820434031468,129.044074379647));
#71338=CARTESIAN_POINT('Ctrl Pts',(81.9500224558933,-8.348160541956,129.04006761864));
#71339=CARTESIAN_POINT('Ctrl Pts',(81.9709560850656,-8.41919911050101,129.036060857632));
#71340=CARTESIAN_POINT('Ctrl Pts',(81.9910610267401,-8.48742551622748,129.03221270996));
#71341=CARTESIAN_POINT('Ctrl Pts',(82.0076052835568,-8.55664969729867,129.028364562288));
#71342=CARTESIAN_POINT('Ctrl Pts',(82.0205122847536,-8.62646597255455,129.024516414616));
#71343=CARTESIAN_POINT('Ctrl Pts',(82.0334284198522,-8.6963316547163,129.020665543725));
#71344=CARTESIAN_POINT('Ctrl Pts',(82.0427021171196,-8.7667897800782,129.016814672833));
#71345=CARTESIAN_POINT('Ctrl Pts',(82.0483086557833,-8.83742935952861,129.012963801941));
#71346=CARTESIAN_POINT('Ctrl Pts',(82.0539242775961,-8.90818338210834,129.009106692256));
#71347=CARTESIAN_POINT('Ctrl Pts',(82.0558608834404,-8.9791189577832,129.005249582572));
#71348=CARTESIAN_POINT('Ctrl Pts',(82.0541457913538,-9.04982600087946,129.001392472887));
#71349=CARTESIAN_POINT('Ctrl Pts',(82.0539394015318,-9.05833470670729,129.000928318112));
#71350=CARTESIAN_POINT('Ctrl Pts',(82.05368019249,-9.06684011174075,129.000464163338));
#71351=CARTESIAN_POINT('Ctrl Pts',(82.0533682620167,-9.07534150942548,129.000000008563));
#71352=CARTESIAN_POINT('Origin',(80.,-9.,141.545925280538));
#71353=CARTESIAN_POINT('',(81.2520391107129,-7.37076839346111,129.806138766351));
#71354=CARTESIAN_POINT('',(81.2520391107129,-7.37076839346113,129.747865110012));
#71355=CARTESIAN_POINT('',(81.2520391107129,-7.37076839346111,141.545925280538));
#71356=CARTESIAN_POINT('',(77.9454433123729,-9.00149860204779,129.295925300346));
#71357=CARTESIAN_POINT('Ctrl Pts',(81.2520391107129,-7.37076839346113,129.747865110012));
#71358=CARTESIAN_POINT('Ctrl Pts',(81.3085193358146,-7.41417256664642,129.744007244271));
#71359=CARTESIAN_POINT('Ctrl Pts',(81.3627900147932,-7.46055568534263,129.740149378531));
#71360=CARTESIAN_POINT('Ctrl Pts',(81.4145261450971,-7.50965998935252,129.73629151279));
#71361=CARTESIAN_POINT('Ctrl Pts',(81.4662398813796,-7.55874303852898,129.732435316929));
#71362=CARTESIAN_POINT('Ctrl Pts',(81.5154208944419,-7.61054460151153,129.728579121068));
#71363=CARTESIAN_POINT('Ctrl Pts',(81.5617787946249,-7.66476797553387,129.724722925207));
#71364=CARTESIAN_POINT('Ctrl Pts',(81.6081321217098,-7.71898600054751,129.720867109751));
#71365=CARTESIAN_POINT('Ctrl Pts',(81.6516625743354,-7.77562499232182,129.717011294294));
#71366=CARTESIAN_POINT('Ctrl Pts',(81.6921192009196,-7.83435418227522,129.713155478838));
#71367=CARTESIAN_POINT('Ctrl Pts',(81.7326518844035,-7.89319378084367,129.709292414597));
#71368=CARTESIAN_POINT('Ctrl Pts',(81.7700988981036,-7.95413104048772,129.705429350357));
#71369=CARTESIAN_POINT('Ctrl Pts',(81.8042518642402,-8.01680481445141,129.701566286116));
#71370=CARTESIAN_POINT('Ctrl Pts',(81.8383883949273,-8.07944842788261,129.6977050809));
#71371=CARTESIAN_POINT('Ctrl Pts',(81.8692338552675,-8.14382643622838,129.693843875683));
#71372=CARTESIAN_POINT('Ctrl Pts',(81.8966275669693,-8.2095561786488,129.689982670467));
#71373=CARTESIAN_POINT('Ctrl Pts',(81.9240726505379,-8.2754091851093,129.68611422427));
#71374=CARTESIAN_POINT('Ctrl Pts',(81.94805288481,-8.34261853290929,129.682245778074));
#71375=CARTESIAN_POINT('Ctrl Pts',(81.9684568199746,-8.41078415636068,129.678377331878));
#71376=CARTESIAN_POINT('Ctrl Pts',(81.9888137867372,-8.47879286741362,129.674517790568));
#71377=CARTESIAN_POINT('Ctrl Pts',(82.0056108665842,-8.5477529730635,129.670658249259));
#71378=CARTESIAN_POINT('Ctrl Pts',(82.0187884996638,-8.61725915278709,129.666798707949));
#71379=CARTESIAN_POINT('Ctrl Pts',(82.0319999878966,-8.68694390345363,129.662929250947));
#71380=CARTESIAN_POINT('Ctrl Pts',(82.0416249747741,-8.75744965513442,129.659059793944));
#71381=CARTESIAN_POINT('Ctrl Pts',(82.0475698224613,-8.82837428908914,129.655190336942));
#71382=CARTESIAN_POINT('Ctrl Pts',(82.0535058275942,-8.89919342750028,129.651326635492));
#71383=CARTESIAN_POINT('Ctrl Pts',(82.0557725190415,-8.97042973138174,129.647462934043));
#71384=CARTESIAN_POINT('Ctrl Pts',(82.0543273941934,-9.04167157264538,129.643599232593));
#71385=CARTESIAN_POINT('Ctrl Pts',(82.0528839599576,-9.11283007000717,129.639740051183));
#71386=CARTESIAN_POINT('Ctrl Pts',(82.0477373446454,-9.18399360866671,129.635880869773));
#71387=CARTESIAN_POINT('Ctrl Pts',(82.0388970253626,-9.25474788020187,129.632021688364));
#71388=CARTESIAN_POINT('Ctrl Pts',(82.030062258362,-9.32545771356014,129.628164930765));
#71389=CARTESIAN_POINT('Ctrl Pts',(82.0175384501078,-9.39575830898987,129.624308173166));
#71390=CARTESIAN_POINT('Ctrl Pts',(82.0013870127015,-9.4652392802525,129.620451415567));
#71391=CARTESIAN_POINT('Ctrl Pts',(81.9852403197715,-9.53469984151569,129.616595790889));
#71392=CARTESIAN_POINT('Ctrl Pts',(81.9654682231559,-9.60334078380567,129.612740166211));
#71393=CARTESIAN_POINT('Ctrl Pts',(81.9421831305996,-9.67076243910528,129.608884541532));
#71394=CARTESIAN_POINT('Ctrl Pts',(81.9188970937224,-9.73818682867246,129.60502876049));
#71395=CARTESIAN_POINT('Ctrl Pts',(81.8920979386739,-9.80439137473934,129.601172979448));
#71396=CARTESIAN_POINT('Ctrl Pts',(81.8619472202092,-9.86899373510695,129.597317198406));
#71397=CARTESIAN_POINT('Ctrl Pts',(81.831764901583,-9.9336638034805,129.593457376223));
#71398=CARTESIAN_POINT('Ctrl Pts',(81.7982242132673,-9.9967278930938,129.58959755404));
#71399=CARTESIAN_POINT('Ctrl Pts',(81.7615335686011,-10.0578265685789,129.585737731857));
#71400=CARTESIAN_POINT('Ctrl Pts',(81.7248221155494,-10.1189598949895,129.581875720651));
#71401=CARTESIAN_POINT('Ctrl Pts',(81.6849574213982,-10.1781251853909,129.578013709445));
#71402=CARTESIAN_POINT('Ctrl Pts',(81.6421907782822,-10.2349927166687,129.574151698238));
#71403=CARTESIAN_POINT('Ctrl Pts',(81.5993493071618,-10.2919597480142,129.570282929743));
#71404=CARTESIAN_POINT('Ctrl Pts',(81.5535960615509,-10.3466206209628,129.566414161247));
#71405=CARTESIAN_POINT('Ctrl Pts',(81.5052216076061,-10.3986799042296,129.562545392751));
#71406=CARTESIAN_POINT('Ctrl Pts',(81.4765469614202,-10.4295387854496,129.560252125153));
#71407=CARTESIAN_POINT('Ctrl Pts',(81.4469520009933,-10.4594842601665,129.557958857556));
#71408=CARTESIAN_POINT('Ctrl Pts',(81.4165027389574,-10.4884614717977,129.555665589958));
#71409=CARTESIAN_POINT('Ctrl Pts',(81.3651794348254,-10.5373035831004,129.551800206612));
#71410=CARTESIAN_POINT('Ctrl Pts',(81.31122528226,-10.5835848618398,129.547934823266));
#71411=CARTESIAN_POINT('Ctrl Pts',(81.254926402395,-10.6270086929921,129.544069439919));
#71412=CARTESIAN_POINT('Ctrl Pts',(81.1987116344752,-10.6703676478465,129.540209831553));
#71413=CARTESIAN_POINT('Ctrl Pts',(81.1401594746294,-10.7108773337765,129.536350223187));
#71414=CARTESIAN_POINT('Ctrl Pts',(81.0795918236439,-10.7482788841661,129.532490614821));
#71415=CARTESIAN_POINT('Ctrl Pts',(81.019095246917,-10.7856365449972,129.528635535586));
#71416=CARTESIAN_POINT('Ctrl Pts',(80.9565882888255,-10.819893060054,129.524780456351));
#71417=CARTESIAN_POINT('Ctrl Pts',(80.892423346155,-10.850831741066,129.520925377115));
#71418=CARTESIAN_POINT('Ctrl Pts',(80.8282988035791,-10.8817509421941,129.517072725149));
#71419=CARTESIAN_POINT('Ctrl Pts',(80.762518784844,-10.9093562425956,129.513220073182));
#71420=CARTESIAN_POINT('Ctrl Pts',(80.6954606021694,-10.9334766906612,129.509367421215));
#71421=CARTESIAN_POINT('Ctrl Pts',(80.6284220946006,-10.9575900617029,129.50551589963));
#71422=CARTESIAN_POINT('Ctrl Pts',(80.5601066253927,-10.9782204454682,129.501664378046));
#71423=CARTESIAN_POINT('Ctrl Pts',(80.4909101913095,-10.9952455354087,129.497812856461));
#71424=CARTESIAN_POINT('Ctrl Pts',(80.421710794651,-11.0122713542612,129.493961169977));
#71425=CARTESIAN_POINT('Ctrl Pts',(80.3516308314874,-11.0256914586866,129.490109483493));
#71426=CARTESIAN_POINT('Ctrl Pts',(80.2810784152267,-11.0354342256614,129.486257797009));
#71427=CARTESIAN_POINT('Ctrl Pts',(80.2104512222903,-11.045187318742,129.482402028222));
#71428=CARTESIAN_POINT('Ctrl Pts',(80.1393510599224,-11.0512552274711,129.478546259435));
#71429=CARTESIAN_POINT('Ctrl Pts',(80.0681922209285,-11.0536181201735,129.474690490649));
#71430=CARTESIAN_POINT('Ctrl Pts',(79.9969926693478,-11.0559823647736,129.470832515835));
#71431=CARTESIAN_POINT('Ctrl Pts',(79.9257348612537,-11.0546373832113,129.466974541022));
#71432=CARTESIAN_POINT('Ctrl Pts',(79.8548313680584,-11.0496154836457,129.463116566208));
#71433=CARTESIAN_POINT('Ctrl Pts',(79.7838023847573,-11.0445846959607,129.459251763273));
#71434=CARTESIAN_POINT('Ctrl Pts',(79.7131294516034,-11.0358640575065,129.455386960338));
#71435=CARTESIAN_POINT('Ctrl Pts',(79.6432176148211,-11.0235374699091,129.451522157403));
#71436=CARTESIAN_POINT('Ctrl Pts',(79.6010712876026,-11.0161063907345,129.449192262257));
#71437=CARTESIAN_POINT('Ctrl Pts',(79.5592013425454,-11.0073657984892,129.446862367112));
#71438=CARTESIAN_POINT('Ctrl Pts',(79.5176937268385,-10.9973427901512,129.444532471966));
#71439=CARTESIAN_POINT('Ctrl Pts',(79.4486461692916,-10.980669602997,129.440656711665));
#71440=CARTESIAN_POINT('Ctrl Pts',(79.3803310897322,-10.9603796507532,129.436780951364));
#71441=CARTESIAN_POINT('Ctrl Pts',(79.3131544468131,-10.9365538331189,129.432905191063));
#71442=CARTESIAN_POINT('Ctrl Pts',(79.2460779854487,-10.9127635472906,129.429035210743));
#71443=CARTESIAN_POINT('Ctrl Pts',(79.1801370428466,-10.8854480245579,129.425165230423));
#71444=CARTESIAN_POINT('Ctrl Pts',(79.1157251296031,-10.8547386651721,129.421295250102));
#71445=CARTESIAN_POINT('Ctrl Pts',(79.0513895511559,-10.8240656995616,129.41742985611));
#71446=CARTESIAN_POINT('Ctrl Pts',(78.9885798369927,-10.7900070947805,129.413564462118));
#71447=CARTESIAN_POINT('Ctrl Pts',(78.9276704924502,-10.752742704945,129.409699068125));
#71448=CARTESIAN_POINT('Ctrl Pts',(78.8668000421066,-10.7155021106142,129.405836142414));
#71449=CARTESIAN_POINT('Ctrl Pts',(78.8078279653701,-10.6750600450864,129.401973216703));
#71450=CARTESIAN_POINT('Ctrl Pts',(78.7511037956164,-10.6316420665012,129.398110290992));
#71451=CARTESIAN_POINT('Ctrl Pts',(78.6943970463681,-10.5882374219697,129.394248551621));
#71452=CARTESIAN_POINT('Ctrl Pts',(78.6399372174938,-10.5418589729753,129.390386812249));
#71453=CARTESIAN_POINT('Ctrl Pts',(78.5880430834521,-10.4927743393804,129.386525072878));
#71454=CARTESIAN_POINT('Ctrl Pts',(78.5361476869729,-10.4436885116952,129.382663239561));
#71455=CARTESIAN_POINT('Ctrl Pts',(78.4868184593472,-10.3918967028469,129.378801406244));
#71456=CARTESIAN_POINT('Ctrl Pts',(78.4403381714333,-10.3377042060979,129.374939572927));
#71457=CARTESIAN_POINT('Ctrl Pts',(78.393810886182,-10.2834569140116,129.371073834818));
#71458=CARTESIAN_POINT('Ctrl Pts',(78.3501386070332,-10.2268044562488,129.367208096709));
#71459=CARTESIAN_POINT('Ctrl Pts',(78.3095639575526,-10.1680854202047,129.3633423586));
#71460=CARTESIAN_POINT('Ctrl Pts',(78.2689670491438,-10.109334171367,129.359474499777));
#71461=CARTESIAN_POINT('Ctrl Pts',(78.2314714082485,-10.0485144990275,129.355606640955));
#71462=CARTESIAN_POINT('Ctrl Pts',(78.1972749688131,-9.98599189876595,129.351738782133));
#71463=CARTESIAN_POINT('Ctrl Pts',(78.1630202938598,-9.92336282437823,129.347864336462));
#71464=CARTESIAN_POINT('Ctrl Pts',(78.1320762482958,-9.859025468056,129.343989890791));
#71465=CARTESIAN_POINT('Ctrl Pts',(78.1045933769319,-9.79336706241788,129.340115445121));
#71466=CARTESIAN_POINT('Ctrl Pts',(78.0887134735239,-9.75542891812244,129.337876748072));
#71467=CARTESIAN_POINT('Ctrl Pts',(78.0739882226127,-9.71705005416845,129.335638051023));
#71468=CARTESIAN_POINT('Ctrl Pts',(78.0604390161882,-9.67830727002969,129.333399353975));
#71469=CARTESIAN_POINT('Ctrl Pts',(78.0332608353717,-9.60059361214667,129.328908780042));
#71470=CARTESIAN_POINT('Ctrl Pts',(78.0107314285335,-9.52117080928538,129.324418206109));
#71471=CARTESIAN_POINT('Ctrl Pts',(77.9930364419773,-9.44056195849032,129.319927632176));
#71472=CARTESIAN_POINT('Ctrl Pts',(77.9754996317223,-9.36067367393154,129.315477199691));
#71473=CARTESIAN_POINT('Ctrl Pts',(77.9627112852818,-9.27962060760744,129.311026767205));
#71474=CARTESIAN_POINT('Ctrl Pts',(77.9548055732078,-9.19793261256783,129.30657633472));
#71475=CARTESIAN_POINT('Ctrl Pts',(77.9484987710017,-9.13276580374609,129.303025990722));
#71476=CARTESIAN_POINT('Ctrl Pts',(77.9452984673716,-9.06719534548324,129.299475646723));
#71477=CARTESIAN_POINT('Ctrl Pts',(77.9452505466265,-9.00149878663961,129.295925302725));
#71478=CARTESIAN_POINT('Ctrl Pts',(77.94704827473,-9.00149706514133,129.295925280538));
#71479=CARTESIAN_POINT('Ctrl Pts',(77.9500644504662,-8.54755626783022,129.271372265686));
#71480=CARTESIAN_POINT('Ctrl Pts',(78.3217621619307,-7.40396017493601,129.209774878171));
#71481=CARTESIAN_POINT('Ctrl Pts',(79.9094070337756,-6.71505827450504,129.127082065883));
#71482=CARTESIAN_POINT('Ctrl Pts',(80.9398133637899,-7.13722923514124,129.068942268446));
#71483=CARTESIAN_POINT('Ctrl Pts',(81.2492121870567,-7.37445590553645,129.047846843673));
#71484=CARTESIAN_POINT('',(77.9452508134305,-8.99817166960857,129.354074719499));
#71485=CARTESIAN_POINT('Ctrl Pts',(77.9452508134311,-8.99817166892661,129.354074719462));
#71486=CARTESIAN_POINT('Ctrl Pts',(77.9453406300956,-8.89723222694866,129.34859460346));
#71487=CARTESIAN_POINT('Ctrl Pts',(77.952871897115,-8.79661291965776,129.343114487457));
#71488=CARTESIAN_POINT('Ctrl Pts',(77.9676835787623,-8.69720051772217,129.337634371454));
#71489=CARTESIAN_POINT('Ctrl Pts',(77.9734619030679,-8.65841781147318,129.335496471906));
#71490=CARTESIAN_POINT('Ctrl Pts',(77.9803477788761,-8.61981845206601,129.333358572358));
#71491=CARTESIAN_POINT('Ctrl Pts',(77.988329837195,-8.58145404245158,129.331220672811));
#71492=CARTESIAN_POINT('Ctrl Pts',(78.0027616152757,-8.51209014862456,129.327355292404));
#71493=CARTESIAN_POINT('Ctrl Pts',(78.0208137903994,-8.44333610135341,129.323489911997));
#71494=CARTESIAN_POINT('Ctrl Pts',(78.042419743995,-8.3755986036216,129.31962453159));
#71495=CARTESIAN_POINT('Ctrl Pts',(78.0639934177053,-8.3079623075629,129.315764926167));
#71496=CARTESIAN_POINT('Ctrl Pts',(78.0891101847324,-8.24134000650113,129.311905320744));
#71497=CARTESIAN_POINT('Ctrl Pts',(78.1176525274556,-8.17612770704076,129.308045715321));
#71498=CARTESIAN_POINT('Ctrl Pts',(78.1461613766581,-8.11099193211538,129.30419063902));
#71499=CARTESIAN_POINT('Ctrl Pts',(78.17808762317,-8.04726331621047,129.30033556272));
#71500=CARTESIAN_POINT('Ctrl Pts',(78.2132646763425,-7.98532052070883,129.29648048642));
#71501=CARTESIAN_POINT('Ctrl Pts',(78.24841958107,-7.92341672610333,129.292627837382));
#71502=CARTESIAN_POINT('Ctrl Pts',(78.2868209921103,-7.8632969435781,129.288775188345));
#71503=CARTESIAN_POINT('Ctrl Pts',(78.3282558117856,-7.80531638846454,129.284922539307));
#71504=CARTESIAN_POINT('Ctrl Pts',(78.369678474441,-7.74735284490711,129.281071020641));
#71505=CARTESIAN_POINT('Ctrl Pts',(78.4141324960515,-7.69152767864704,129.277219501974));
#71506=CARTESIAN_POINT('Ctrl Pts',(78.4613617424586,-7.63816672278501,129.273367983308));
#71507=CARTESIAN_POINT('Ctrl Pts',(78.5085930111155,-7.58480348212737,129.269516299728));
#71508=CARTESIAN_POINT('Ctrl Pts',(78.5585994161696,-7.53390502441321,129.265664616149));
#71509=CARTESIAN_POINT('Ctrl Pts',(78.6110860295267,-7.4857623881556,129.261812932569));
#71510=CARTESIAN_POINT('Ctrl Pts',(78.6636282726897,-7.43756872621102,129.257957166645));
#71511=CARTESIAN_POINT('Ctrl Pts',(78.7186556121075,-7.39213704604406,129.254101400722));
#71512=CARTESIAN_POINT('Ctrl Pts',(78.7758385789269,-7.34971930337404,129.250245634798));
#71513=CARTESIAN_POINT('Ctrl Pts',(78.8330542625269,-7.30727729172922,129.246387662829));
#71514=CARTESIAN_POINT('Ctrl Pts',(78.8924276226871,-7.26785291933302,129.242529690859));
#71515=CARTESIAN_POINT('Ctrl Pts',(78.9536009498714,-7.23165427860104,129.23867171889));
#71516=CARTESIAN_POINT('Ctrl Pts',(79.0148825470524,-7.19539157029434,129.234806918738));
#71517=CARTESIAN_POINT('Ctrl Pts',(79.0779700401004,-7.16236621772688,129.230942118587));
#71518=CARTESIAN_POINT('Ctrl Pts',(79.1424825630927,-7.13273959826168,129.227077318435));
#71519=CARTESIAN_POINT('Ctrl Pts',(79.1813743788247,-7.11487898807997,129.22474739723));
#71520=CARTESIAN_POINT('Ctrl Pts',(79.2207837219093,-7.09825266193998,129.222417476024));
#71521=CARTESIAN_POINT('Ctrl Pts',(79.2606244867228,-7.08288721957572,129.220087554819));
#71522=CARTESIAN_POINT('Ctrl Pts',(79.3268985355705,-7.05732721633333,129.216211793083));
#71523=CARTESIAN_POINT('Ctrl Pts',(79.3946273063918,-7.03515857174183,129.212336031348));
#71524=CARTESIAN_POINT('Ctrl Pts',(79.4634308896462,-7.01654565156791,129.208460269612));
#71525=CARTESIAN_POINT('Ctrl Pts',(79.5321318648481,-6.99796048918509,129.204590287872));
#71526=CARTESIAN_POINT('Ctrl Pts',(79.6019040070276,-6.98292064977586,129.200720306131));
#71527=CARTESIAN_POINT('Ctrl Pts',(79.6723489208654,-6.97154188289679,129.196850324391));
#71528=CARTESIAN_POINT('Ctrl Pts',(79.742710349704,-6.96017660111254,129.192984929006));
#71529=CARTESIAN_POINT('Ctrl Pts',(79.8137424907851,-6.95246384924864,129.189119533621));
#71530=CARTESIAN_POINT('Ctrl Pts',(79.8850350203369,-6.94846871436211,129.185254138236));
#71531=CARTESIAN_POINT('Ctrl Pts',(79.9562820251037,-6.94447613062165,129.18139121115));
#71532=CARTESIAN_POINT('Ctrl Pts',(80.0277886063581,-6.94419648043532,129.177528284064));
#71533=CARTESIAN_POINT('Ctrl Pts',(80.0991389834618,-6.94764305627453,129.173665356978));
#71534=CARTESIAN_POINT('Ctrl Pts',(80.1704674478651,-6.95108857362201,129.169803616252));
#71535=CARTESIAN_POINT('Ctrl Pts',(80.2416393202463,-6.95825802149985,129.165941875525));
#71536=CARTESIAN_POINT('Ctrl Pts',(80.3122401944723,-6.96911260197522,129.162080134798));
#71537=CARTESIAN_POINT('Ctrl Pts',(80.3828427858252,-6.97996744645144,129.158218300147));
#71538=CARTESIAN_POINT('Ctrl Pts',(80.4528738734421,-6.99450752577777,129.154356465497));
#71539=CARTESIAN_POINT('Ctrl Pts',(80.5219272353851,-7.01264257782771,129.150494630846));
#71540=CARTESIAN_POINT('Ctrl Pts',(80.5910504180819,-7.03079596646503,129.146628891445));
#71541=CARTESIAN_POINT('Ctrl Pts',(80.6591934325206,-7.05255146114117,129.142763152043));
#71542=CARTESIAN_POINT('Ctrl Pts',(80.7259641399556,-7.07776858052977,129.138897412641));
#71543=CARTESIAN_POINT('Ctrl Pts',(80.792771476884,-7.10299953368385,129.135029552548));
#71544=CARTESIAN_POINT('Ctrl Pts',(80.858204564293,-7.13169569834081,129.131161692454));
#71545=CARTESIAN_POINT('Ctrl Pts',(80.9218927148622,-7.16366904268754,129.127293832361));
#71546=CARTESIAN_POINT('Ctrl Pts',(80.9856893236471,-7.1956968362819,129.123419385466));
#71547=CARTESIAN_POINT('Ctrl Pts',(81.0477346416405,-7.23101271315047,129.119544938571));
#71548=CARTESIAN_POINT('Ctrl Pts',(81.1076845945461,-7.2693838087244,129.115670491676));
#71549=CARTESIAN_POINT('Ctrl Pts',(81.1423241343156,-7.29155492023849,129.113431806726));
#71550=CARTESIAN_POINT('Ctrl Pts',(81.1762646743719,-7.31474525825012,129.111193121777));
#71551=CARTESIAN_POINT('Ctrl Pts',(81.2094449384984,-7.33890382480706,129.108954436827));
#71552=CARTESIAN_POINT('Ctrl Pts',(81.2237726733701,-7.34933585558259,129.107987739145));
#71553=CARTESIAN_POINT('Ctrl Pts',(81.2379725769056,-7.35995848134784,129.107021041463));
#71554=CARTESIAN_POINT('Ctrl Pts',(81.2520391107129,-7.37076839346109,129.106054343781));
#71555=CARTESIAN_POINT('Ctrl Pts',(81.2520391107129,-7.37076839346111,129.806138766351));
#71556=CARTESIAN_POINT('Ctrl Pts',(81.3085777008962,-7.41421741930245,129.80227718848));
#71557=CARTESIAN_POINT('Ctrl Pts',(81.3628020023102,-7.46057451897514,129.798415610609));
#71558=CARTESIAN_POINT('Ctrl Pts',(81.4144129914842,-7.50955260004903,129.794554032738));
#71559=CARTESIAN_POINT('Ctrl Pts',(81.4661146722451,-7.55861674612496,129.790685669245));
#71560=CARTESIAN_POINT('Ctrl Pts',(81.5151935371269,-7.61031071703995,129.786817305753));
#71561=CARTESIAN_POINT('Ctrl Pts',(81.5613890771163,-7.66431226989174,129.78294894226));
#71562=CARTESIAN_POINT('Ctrl Pts',(81.590032865033,-7.69779621720377,129.780550343099));
#71563=CARTESIAN_POINT('Ctrl Pts',(81.6175689183534,-7.73216671299117,129.778151743938));
#71564=CARTESIAN_POINT('Ctrl Pts',(81.6439435864093,-7.76734147177588,129.775753144777));
#71565=CARTESIAN_POINT('Ctrl Pts',(81.6864883346646,-7.82408157004983,129.771883985277));
#71566=CARTESIAN_POINT('Ctrl Pts',(81.7261753868327,-7.88313796797225,129.768014825776));
#71567=CARTESIAN_POINT('Ctrl Pts',(81.7627435659047,-7.94419098158735,129.764145666276));
#71568=CARTESIAN_POINT('Ctrl Pts',(81.7992572713571,-8.00515304786175,129.760282270452));
#71569=CARTESIAN_POINT('Ctrl Pts',(81.8326610783687,-8.06810541268281,129.756418874627));
#71570=CARTESIAN_POINT('Ctrl Pts',(81.8627355243751,-8.1326973257674,129.752555478803));
#71571=CARTESIAN_POINT('Ctrl Pts',(81.8927747030353,-8.1972134939701,129.748696613459));
#71572=CARTESIAN_POINT('Ctrl Pts',(81.9194920717898,-8.26336495317575,129.744837748116));
#71573=CARTESIAN_POINT('Ctrl Pts',(81.9427136505352,-8.33077564709266,129.740978882773));
#71574=CARTESIAN_POINT('Ctrl Pts',(81.9659206058334,-8.39814389011814,129.737122447493));
#71575=CARTESIAN_POINT('Ctrl Pts',(81.9856359808804,-8.46676933639469,129.733266012214));
#71576=CARTESIAN_POINT('Ctrl Pts',(82.0017341467539,-8.53625657069942,129.729409576934));
#71577=CARTESIAN_POINT('Ctrl Pts',(82.0178275595263,-8.60572328839044,129.725554280295));
#71578=CARTESIAN_POINT('Ctrl Pts',(82.030305773847,-8.67605081598735,129.721698983657));
#71579=CARTESIAN_POINT('Ctrl Pts',(82.0390936631195,-8.74683089539595,129.717843687018));
#71580=CARTESIAN_POINT('Ctrl Pts',(82.0478818969737,-8.81761375016064,129.713988239209));
#71581=CARTESIAN_POINT('Ctrl Pts',(82.0529794608286,-8.88884870963739,129.7101327914));
#71582=CARTESIAN_POINT('Ctrl Pts',(82.0543629818976,-8.9601214204246,129.706277343591));
#71583=CARTESIAN_POINT('Ctrl Pts',(82.0557479511442,-9.0314687347381,129.702417860156));
#71584=CARTESIAN_POINT('Ctrl Pts',(82.0534111076121,-9.10285339258064,129.698558376722));
#71585=CARTESIAN_POINT('Ctrl Pts',(82.04738123642,-9.17386096530035,129.694698893287));
#71586=CARTESIAN_POINT('Ctrl Pts',(82.0413479508545,-9.24490874557463,129.690837224446));
#71587=CARTESIAN_POINT('Ctrl Pts',(82.0316175410741,-9.31557853422141,129.686975555605));
#71588=CARTESIAN_POINT('Ctrl Pts',(82.0182703747424,-9.38546369081551,129.683113886764));
#71589=CARTESIAN_POINT('Ctrl Pts',(82.0048998596312,-9.45547110055874,129.679245462537));
#71590=CARTESIAN_POINT('Ctrl Pts',(81.987900071923,-9.52469066594064,129.675377038311));
#71591=CARTESIAN_POINT('Ctrl Pts',(81.9674017425439,-9.59272923492526,129.671508614084));
#71592=CARTESIAN_POINT('Ctrl Pts',(81.9552344686409,-9.63311515562621,129.669212418318));
#71593=CARTESIAN_POINT('Ctrl Pts',(81.9418354955515,-9.67308530827785,129.666916222551));
#71594=CARTESIAN_POINT('Ctrl Pts',(81.9272400721396,-9.7125610618322,129.664620026785));
#71595=CARTESIAN_POINT('Ctrl Pts',(81.9026497177558,-9.77906977090307,129.660751398515));
#71596=CARTESIAN_POINT('Ctrl Pts',(81.8745642853651,-9.84443451853481,129.656882770244));
#71597=CARTESIAN_POINT('Ctrl Pts',(81.8431105990524,-9.9082625623468,129.653014141974));
#71598=CARTESIAN_POINT('Ctrl Pts',(81.8117037902735,-9.97199547895319,129.649151279379));
#71599=CARTESIAN_POINT('Ctrl Pts',(81.7769389049626,-10.0341958054905,129.645288416785));
#71600=CARTESIAN_POINT('Ctrl Pts',(81.7389914953888,-10.0944889864523,129.64142555419));
#71601=CARTESIAN_POINT('Ctrl Pts',(81.7010885954797,-10.1547114477181,129.637567222464));
#71602=CARTESIAN_POINT('Ctrl Pts',(81.6600108435754,-10.213030797469,129.633708890737));
#71603=CARTESIAN_POINT('Ctrl Pts',(81.6159797248073,-10.2690969590664,129.629850559011));
#71604=CARTESIAN_POINT('Ctrl Pts',(81.5719763372501,-10.3251278096703,129.625994657298));
#71605=CARTESIAN_POINT('Ctrl Pts',(81.5250235725302,-10.3789079062814,129.622138755585));
#71606=CARTESIAN_POINT('Ctrl Pts',(81.4753854079039,-10.4301172891215,129.618282853872));
#71607=CARTESIAN_POINT('Ctrl Pts',(81.4257618905939,-10.4813115610074,129.614428089966));
#71608=CARTESIAN_POINT('Ctrl Pts',(81.3734548845351,-10.5299362763718,129.610573326059));
#71609=CARTESIAN_POINT('Ctrl Pts',(81.3187665507146,-10.575706935701,129.606718562153));
#71610=CARTESIAN_POINT('Ctrl Pts',(81.2640760492417,-10.6214794092176,129.602863645457));
#71611=CARTESIAN_POINT('Ctrl Pts',(81.2070044066542,-10.6643972919325,129.599008728761));
#71612=CARTESIAN_POINT('Ctrl Pts',(81.1478869763645,-10.7042162574019,129.595153812065));
#71613=CARTESIAN_POINT('Ctrl Pts',(81.0887075634526,-10.744076971707,129.59129485362));
#71614=CARTESIAN_POINT('Ctrl Pts',(81.0274784849117,-10.7808320108207,129.587435895174));
#71615=CARTESIAN_POINT('Ctrl Pts',(80.964563447489,-10.8142808267377,129.583576936729));
#71616=CARTESIAN_POINT('Ctrl Pts',(80.9016127366326,-10.8477486084563,129.579715790217));
#71617=CARTESIAN_POINT('Ctrl Pts',(80.8369746044577,-10.8779062296208,129.575854643705));
#71618=CARTESIAN_POINT('Ctrl Pts',(80.7710341896528,-10.9046007037924,129.571993497193));
#71619=CARTESIAN_POINT('Ctrl Pts',(80.7049782381157,-10.9313419503769,129.568125585417));
#71620=CARTESIAN_POINT('Ctrl Pts',(80.6376159077565,-10.9546077765723,129.564257673642));
#71621=CARTESIAN_POINT('Ctrl Pts',(80.5693483188029,-10.9742948245833,129.560389761867));
#71622=CARTESIAN_POINT('Ctrl Pts',(80.528737160153,-10.9860062947315,129.558088810843));
#71623=CARTESIAN_POINT('Ctrl Pts',(80.4878058768319,-10.9964522641733,129.555787859818));
#71624=CARTESIAN_POINT('Ctrl Pts',(80.446640193328,-11.0056196299907,129.553486908794));
#71625=CARTESIAN_POINT('Ctrl Pts',(80.3774071770919,-11.0210374326956,129.549617137516));
#71626=CARTESIAN_POINT('Ctrl Pts',(80.3072395029954,-11.0328963456036,129.545747366239));
#71627=CARTESIAN_POINT('Ctrl Pts',(80.2365361341041,-11.041089958763,129.541877594962));
#71628=CARTESIAN_POINT('Ctrl Pts',(80.1659381343249,-11.0492713609945,129.538013590798));
#71629=CARTESIAN_POINT('Ctrl Pts',(80.0948065029077,-11.0537982508364,129.534149586634));
#71630=CARTESIAN_POINT('Ctrl Pts',(80.0235513380866,-11.0546150240311,129.53028558247));
#71631=CARTESIAN_POINT('Ctrl Pts',(79.95237986535,-11.0554308378926,129.526426116736));
#71632=CARTESIAN_POINT('Ctrl Pts',(79.8810856306334,-11.0525451855223,129.522566651002));
#71633=CARTESIAN_POINT('Ctrl Pts',(79.8100830674483,-11.0459543301917,129.518707185268));
#71634=CARTESIAN_POINT('Ctrl Pts',(79.7391253061563,-11.0393676336235,129.514850154818));
#71635=CARTESIAN_POINT('Ctrl Pts',(79.6684593336303,-11.0290804173782,129.510993124368));
#71636=CARTESIAN_POINT('Ctrl Pts',(79.5984973212508,-11.0151409780601,129.507136093917));
#71637=CARTESIAN_POINT('Ctrl Pts',(79.5285560722597,-11.0012056757013,129.50328020816));
#71638=CARTESIAN_POINT('Ctrl Pts',(79.4593188446184,-10.9836203969911,129.499424322402));
#71639=CARTESIAN_POINT('Ctrl Pts',(79.3911887258673,-10.9624847502564,129.495568436644));
#71640=CARTESIAN_POINT('Ctrl Pts',(79.3230560578231,-10.941348312668,129.491712406607));
#71641=CARTESIAN_POINT('Ctrl Pts',(79.2560310440557,-10.9166613892836,129.48785637657));
#71642=CARTESIAN_POINT('Ctrl Pts',(79.1905010257898,-10.8885732639357,129.484000346533));
#71643=CARTESIAN_POINT('Ctrl Pts',(79.1249026706106,-10.8604558473432,129.480140295298));
#71644=CARTESIAN_POINT('Ctrl Pts',(79.0608028703654,-10.8289303400641,129.476280244063));
#71645=CARTESIAN_POINT('Ctrl Pts',(78.998567567296,-10.7941935919037,129.472420192828));
#71646=CARTESIAN_POINT('Ctrl Pts',(78.9362971464976,-10.7594372427188,129.468557963468));
#71647=CARTESIAN_POINT('Ctrl Pts',(78.8758937286265,-10.7214663039507,129.464695734108));
#71648=CARTESIAN_POINT('Ctrl Pts',(78.8176949311995,-10.6805214330049,129.460833504749));
#71649=CARTESIAN_POINT('Ctrl Pts',(78.7593946027653,-10.6395051314768,129.456964537517));
#71650=CARTESIAN_POINT('Ctrl Pts',(78.7033069558238,-10.595504839164,129.453095570286));
#71651=CARTESIAN_POINT('Ctrl Pts',(78.6497365892073,-10.5488015637823,129.449226603054));
#71652=CARTESIAN_POINT('Ctrl Pts',(78.6180158870127,-10.521147082705,129.446935665637));
#71653=CARTESIAN_POINT('Ctrl Pts',(78.5871771037121,-10.4925456023546,129.444644728219));
#71654=CARTESIAN_POINT('Ctrl Pts',(78.5572770056771,-10.4630611484664,129.442353790802));
#71655=CARTESIAN_POINT('Ctrl Pts',(78.5075191974749,-10.4139950283555,129.438541361007));
#71656=CARTESIAN_POINT('Ctrl Pts',(78.4601566106289,-10.3622781813274,129.434728931212));
#71657=CARTESIAN_POINT('Ctrl Pts',(78.4154907210218,-10.3081773225874,129.430916501417));
#71658=CARTESIAN_POINT('Ctrl Pts',(78.370884322811,-10.2541485218687,129.427109149474));
#71659=CARTESIAN_POINT('Ctrl Pts',(78.328967820547,-10.1977423834135,129.423301797531));
#71660=CARTESIAN_POINT('Ctrl Pts',(78.2900066717981,-10.1392630863875,129.419494445588));
#71661=CARTESIAN_POINT('Ctrl Pts',(78.2510834935506,-10.080840781732,129.415690804189));
#71662=CARTESIAN_POINT('Ctrl Pts',(78.2151102356859,-10.0203497381726,129.41188716279));
#71663=CARTESIAN_POINT('Ctrl Pts',(78.182311540293,-9.958126414388,129.408083521391));
#71664=CARTESIAN_POINT('Ctrl Pts',(78.1495330966884,-9.89594151083817,129.404282228577));
#71665=CARTESIAN_POINT('Ctrl Pts',(78.1199255604223,-9.83202689089695,129.400480935764));
#71666=CARTESIAN_POINT('Ctrl Pts',(78.093668727308,-9.76674548662288,129.39667964295));
#71667=CARTESIAN_POINT('Ctrl Pts',(78.0674079984643,-9.70145439653907,129.392877786139));
#71668=CARTESIAN_POINT('Ctrl Pts',(78.044499168057,-9.63479657590548,129.389075929327));
#71669=CARTESIAN_POINT('Ctrl Pts',(78.0250741537879,-9.56715559105353,129.385274072515));
#71670=CARTESIAN_POINT('Ctrl Pts',(78.0056484039667,-9.49951204489265,129.381472071741));
#71671=CARTESIAN_POINT('Ctrl Pts',(77.9897068601131,-9.4308857455588,129.377670070968));
#71672=CARTESIAN_POINT('Ctrl Pts',(77.9773310417072,-9.36167367565081,129.373868070194));
#71673=CARTESIAN_POINT('Ctrl Pts',(77.9649417578525,-9.29238629988788,129.370061932672));
#71674=CARTESIAN_POINT('Ctrl Pts',(77.9561260209403,-9.22251237727799,129.36625579515));
#71675=CARTESIAN_POINT('Ctrl Pts',(77.9509136980301,-9.15245618904848,129.362449657627));
#71676=CARTESIAN_POINT('Ctrl Pts',(77.9470906725768,-9.10107284320192,129.359658011585));
#71677=CARTESIAN_POINT('Ctrl Pts',(77.9452050596103,-9.04959160188904,129.356866365542));
#71678=CARTESIAN_POINT('Ctrl Pts',(77.9452508134305,-8.99817166960858,129.354074719499));
#71679=CARTESIAN_POINT('Origin',(80.,-9.,141.545925280538));
#71680=CARTESIAN_POINT('',(81.2520391107129,-7.37076839346111,130.506052881321));
#71681=CARTESIAN_POINT('',(81.2520391107129,-7.37076839346112,130.44794571257));
#71682=CARTESIAN_POINT('',(81.2520391107129,-7.37076839346111,141.545925280538));
#71683=CARTESIAN_POINT('',(77.9452500565798,-9.00048219782007,129.995925280508));
#71684=CARTESIAN_POINT('Ctrl Pts',(81.2520391107129,-7.37076839346111,130.44794571257));
#71685=CARTESIAN_POINT('Ctrl Pts',(81.2676313194312,-7.38275076297777,130.446873986343));
#71686=CARTESIAN_POINT('Ctrl Pts',(81.2830435643931,-7.39495088616389,130.445802260117));
#71687=CARTESIAN_POINT('Ctrl Pts',(81.2982695699414,-7.40736266329582,130.44473053389));
#71688=CARTESIAN_POINT('Ctrl Pts',(81.3532376875177,-7.45217100272229,130.440861444716));
#71689=CARTESIAN_POINT('Ctrl Pts',(81.4059909768369,-7.49991619016276,130.436992355542));
#71690=CARTESIAN_POINT('Ctrl Pts',(81.4561988949054,-7.55035095937804,130.433123266368));
#71691=CARTESIAN_POINT('Ctrl Pts',(81.5063320052026,-7.60071058282287,130.429259941981));
#71692=CARTESIAN_POINT('Ctrl Pts',(81.553926932326,-7.65375149205841,130.425396617594));
#71693=CARTESIAN_POINT('Ctrl Pts',(81.5986861257916,-7.70918621261568,130.421533293207));
#71694=CARTESIAN_POINT('Ctrl Pts',(81.6433928156937,-7.76455590697052,130.417674500588));
#71695=CARTESIAN_POINT('Ctrl Pts',(81.6852700755659,-7.8223134588909,130.413815707969));
#71696=CARTESIAN_POINT('Ctrl Pts',(81.7240583935174,-7.88213586771812,130.40995691535));
#71697=CARTESIAN_POINT('Ctrl Pts',(81.7628222770737,-7.94192059189048,130.406100553547));
#71698=CARTESIAN_POINT('Ctrl Pts',(81.7985008155955,-8.0037671856847,130.402244191744));
#71699=CARTESIAN_POINT('Ctrl Pts',(81.8308767539392,-8.06732220226645,130.398387829941));
#71700=CARTESIAN_POINT('Ctrl Pts',(81.8632431275178,-8.13085844290422,130.394532607416));
#71701=CARTESIAN_POINT('Ctrl Pts',(81.892308617534,-8.19610167170972,130.390677384892));
#71702=CARTESIAN_POINT('Ctrl Pts',(81.9179018845683,-8.2626738010423,130.386822162367));
#71703=CARTESIAN_POINT('Ctrl Pts',(81.9434961516872,-8.32924853175284,130.382966789195));
#71704=CARTESIAN_POINT('Ctrl Pts',(81.9656177541859,-8.39715181186872,130.379111416023));
#71705=CARTESIAN_POINT('Ctrl Pts',(81.9841441099778,-8.4659871599481,130.375256042851));
#71706=CARTESIAN_POINT('Ctrl Pts',(82.0026898570007,-8.53489455685084,130.371396634324));
#71707=CARTESIAN_POINT('Ctrl Pts',(82.0176327188452,-8.60473549914392,130.367537225796));
#71708=CARTESIAN_POINT('Ctrl Pts',(82.0289007144961,-8.67510085685347,130.363677817269));
#71709=CARTESIAN_POINT('Ctrl Pts',(82.0401750899228,-8.74550605440905,130.3598162236));
#71710=CARTESIAN_POINT('Ctrl Pts',(82.0477704054632,-8.81643577520147,130.355954629932));
#71711=CARTESIAN_POINT('Ctrl Pts',(82.0516666187413,-8.8874760112566,130.352093036263));
#71712=CARTESIAN_POINT('Ctrl Pts',(82.0555696483801,-8.95864053102955,130.348224686801));
#71713=CARTESIAN_POINT('Ctrl Pts',(82.0557606538846,-9.02991546614981,130.344356337338));
#71714=CARTESIAN_POINT('Ctrl Pts',(82.0522717225159,-9.10088775674808,130.340487987875));
#71715=CARTESIAN_POINT('Ctrl Pts',(82.0502001471195,-9.14302800987866,130.33819113055));
#71716=CARTESIAN_POINT('Ctrl Pts',(82.0468322168565,-9.1850616621623,130.335894273224));
#71717=CARTESIAN_POINT('Ctrl Pts',(82.0421831982172,-9.22690382856912,130.333597415899));
#71718=CARTESIAN_POINT('Ctrl Pts',(82.0343518468729,-9.29738767291675,130.329728320484));
#71719=CARTESIAN_POINT('Ctrl Pts',(82.0228518583727,-9.36760364829802,130.325859225068));
#71720=CARTESIAN_POINT('Ctrl Pts',(82.0077116910824,-9.43713994096954,130.321990129653));
#71721=CARTESIAN_POINT('Ctrl Pts',(81.9925940813417,-9.50657263053435,130.318126798858));
#71722=CARTESIAN_POINT('Ctrl Pts',(81.9738471609236,-9.57532717671738,130.314263468062));
#71723=CARTESIAN_POINT('Ctrl Pts',(81.951551062922,-9.64299767597408,130.310400137267));
#71724=CARTESIAN_POINT('Ctrl Pts',(81.9292811174798,-9.71058880005251,130.306541338027));
#71725=CARTESIAN_POINT('Ctrl Pts',(81.9034704149883,-9.77709794379142,130.302682538786));
#71726=CARTESIAN_POINT('Ctrl Pts',(81.8742495666074,-9.84213189262258,130.298823739545));
#71727=CARTESIAN_POINT('Ctrl Pts',(81.8450471246696,-9.90712487605568,130.294967370993));
#71728=CARTESIAN_POINT('Ctrl Pts',(81.8124389972207,-9.97064406611448,130.29111100244));
#71729=CARTESIAN_POINT('Ctrl Pts',(81.7766042934178,-10.032315236306,130.287254633888));
#71730=CARTESIAN_POINT('Ctrl Pts',(81.7407801750932,-10.0939681889942,130.283399404497));
#71731=CARTESIAN_POINT('Ctrl Pts',(81.7017316165523,-10.1537737857869,130.279544175106));
#71732=CARTESIAN_POINT('Ctrl Pts',(81.6596833322111,-10.2113830109757,130.275688945714));
#71733=CARTESIAN_POINT('Ctrl Pts',(81.6176334036367,-10.2689944888843,130.27183356557));
#71734=CARTESIAN_POINT('Ctrl Pts',(81.5725838045506,-10.3244090335942,130.267978185426));
#71735=CARTESIAN_POINT('Ctrl Pts',(81.5248011475405,-10.3773086157283,130.264122805282));
#71736=CARTESIAN_POINT('Ctrl Pts',(81.4769684759247,-10.4302635684068,130.260263389672));
#71737=CARTESIAN_POINT('Ctrl Pts',(81.4263973620334,-10.4806979423454,130.256403974061));
#71738=CARTESIAN_POINT('Ctrl Pts',(81.3733924898514,-10.5283293595688,130.252544558451));
#71739=CARTESIAN_POINT('Ctrl Pts',(81.3203576061274,-10.5759877458653,130.248682957626));
#71740=CARTESIAN_POINT('Ctrl Pts',(81.2648865988595,-10.6208397105533,130.244821356801));
#71741=CARTESIAN_POINT('Ctrl Pts',(81.2073164206213,-10.6626438653536,130.240959755975));
#71742=CARTESIAN_POINT('Ctrl Pts',(81.1496455239559,-10.7045211560874,130.23709139932));
#71743=CARTESIAN_POINT('Ctrl Pts',(81.0898685316552,-10.7433397265681,130.233223042664));
#71744=CARTESIAN_POINT('Ctrl Pts',(81.0283498737814,-10.7789024986192,130.229354686009));
#71745=CARTESIAN_POINT('Ctrl Pts',(80.991823818404,-10.8000175200812,130.227057889975));
#71746=CARTESIAN_POINT('Ctrl Pts',(80.9546842389192,-10.8199856735525,130.224761093941));
#71747=CARTESIAN_POINT('Ctrl Pts',(80.9170107237101,-10.8387737476647,130.222464297907));
#71748=CARTESIAN_POINT('Ctrl Pts',(80.8535484476817,-10.870422876734,130.218595269411));
#71749=CARTESIAN_POINT('Ctrl Pts',(80.7883214528133,-10.8988447018783,130.214726240915));
#71750=CARTESIAN_POINT('Ctrl Pts',(80.7216911380469,-10.9238397708137,130.210857212419));
#71751=CARTESIAN_POINT('Ctrl Pts',(80.6551601017931,-10.9487975973426,130.206993948738));
#71752=CARTESIAN_POINT('Ctrl Pts',(80.5872303472227,-10.9703386333542,130.203130685056));
#71753=CARTESIAN_POINT('Ctrl Pts',(80.5182863363069,-10.988310045264,130.199267421374));
#71754=CARTESIAN_POINT('Ctrl Pts',(80.4494231951227,-11.0062603771229,130.195408689212));
#71755=CARTESIAN_POINT('Ctrl Pts',(80.3795486285444,-11.0206492799013,130.191549957049));
#71756=CARTESIAN_POINT('Ctrl Pts',(80.3090638173179,-11.0313732102509,130.187691224887));
#71757=CARTESIAN_POINT('Ctrl Pts',(80.2386234047366,-11.0420903855567,130.183834923354));
#71758=CARTESIAN_POINT('Ctrl Pts',(80.1675739892765,-11.0491470957167,130.179978621821));
#71759=CARTESIAN_POINT('Ctrl Pts',(80.0963271041859,-11.0524908407833,130.176122320288));
#71760=CARTESIAN_POINT('Ctrl Pts',(80.0251012627136,-11.0558335982348,130.17226715776));
#71761=CARTESIAN_POINT('Ctrl Pts',(79.9536785524018,-11.0554655450204,130.168411995232));
#71762=CARTESIAN_POINT('Ctrl Pts',(79.882474061892,-11.0513861694893,130.164556832704));
#71763=CARTESIAN_POINT('Ctrl Pts',(79.8112667822854,-11.047306634168,130.160701519168));
#71764=CARTESIAN_POINT('Ctrl Pts',(79.740278224328,-11.0395155178963,130.156846205632));
#71765=CARTESIAN_POINT('Ctrl Pts',(79.6699201689214,-11.0280643154533,130.152990892097));
#71766=CARTESIAN_POINT('Ctrl Pts',(79.5994884522895,-11.0166011241969,130.149131542248));
#71767=CARTESIAN_POINT('Ctrl Pts',(79.5296890363937,-11.0014702756004,130.145272192399));
#71768=CARTESIAN_POINT('Ctrl Pts',(79.4609243994404,-10.9827745861245,130.141412842551));
#71769=CARTESIAN_POINT('Ctrl Pts',(79.392120820313,-10.964068309073,130.13755130711));
#71770=CARTESIAN_POINT('Ctrl Pts',(79.3243536484091,-10.9417933240919,130.133689771669));
#71771=CARTESIAN_POINT('Ctrl Pts',(79.2580084266242,-10.9161017894515,130.129828236228));
#71772=CARTESIAN_POINT('Ctrl Pts',(79.1915471101499,-10.8903652982844,130.12595994365));
#71773=CARTESIAN_POINT('Ctrl Pts',(79.12651315498,-10.8612005201156,130.122091651072));
#71774=CARTESIAN_POINT('Ctrl Pts',(79.0632697805276,-10.8288067307475,130.118223358494));
#71775=CARTESIAN_POINT('Ctrl Pts',(79.0257093132346,-10.809567942865,130.115925965634));
#71776=CARTESIAN_POINT('Ctrl Pts',(78.9887799256528,-10.7891910807889,130.113628572775));
#71777=CARTESIAN_POINT('Ctrl Pts',(78.9525527426241,-10.7677250367395,130.111331179916));
#71778=CARTESIAN_POINT('Ctrl Pts',(78.8915407846791,-10.7315730296748,130.107462029052));
#71779=CARTESIAN_POINT('Ctrl Pts',(78.8322831872935,-10.6921878298015,130.103592878188));
#71780=CARTESIAN_POINT('Ctrl Pts',(78.7751435457919,-10.6497649011555,130.099723727324));
#71781=CARTESIAN_POINT('Ctrl Pts',(78.7180890430305,-10.6074051831739,130.095860341541));
#71782=CARTESIAN_POINT('Ctrl Pts',(78.6631466188576,-10.5620170081236,130.091996955758));
#71783=CARTESIAN_POINT('Ctrl Pts',(78.6106532103293,-10.5138405003605,130.088133569974));
#71784=CARTESIAN_POINT('Ctrl Pts',(78.5582213866318,-10.4657205128761,130.084274716683));
#71785=CARTESIAN_POINT('Ctrl Pts',(78.5082332276439,-10.4148190173584,130.080415863392));
#71786=CARTESIAN_POINT('Ctrl Pts',(78.4609933270415,-10.3614169174391,130.0765570101));
#71787=CARTESIAN_POINT('Ctrl Pts',(78.4137831902294,-10.3080484638416,130.072700588103));
#71788=CARTESIAN_POINT('Ctrl Pts',(78.369318197509,-10.2521828946335,130.068844166106));
#71789=CARTESIAN_POINT('Ctrl Pts',(78.327865673879,-10.1941374953949,130.064987744109));
#71790=CARTESIAN_POINT('Ctrl Pts',(78.2864254023504,-10.1361092526054,130.061132461953));
#71791=CARTESIAN_POINT('Ctrl Pts',(78.2479961143842,-10.0759028539788,130.057277179797));
#71792=CARTESIAN_POINT('Ctrl Pts',(78.2128033861742,-10.0138667693684,130.05342189764));
#71793=CARTESIAN_POINT('Ctrl Pts',(78.177609288703,-9.95182827108889,130.049566465484));
#71794=CARTESIAN_POINT('Ctrl Pts',(78.1456522387718,-9.88796036908939,130.045711033329));
#71795=CARTESIAN_POINT('Ctrl Pts',(78.117112326338,-9.82263696177101,130.041855601173));
#71796=CARTESIAN_POINT('Ctrl Pts',(78.0885425523607,-9.7572452060379,130.037996135047));
#71797=CARTESIAN_POINT('Ctrl Pts',(78.0633972480212,-9.69039535096697,130.034136668921));
#71798=CARTESIAN_POINT('Ctrl Pts',(78.0418083407976,-9.62248131564733,130.030277202795));
#71799=CARTESIAN_POINT('Ctrl Pts',(78.0202072143132,-9.55452884117498,130.026415552222));
#71800=CARTESIAN_POINT('Ctrl Pts',(78.0021666149461,-9.48551145760912,130.02255390165));
#71801=CARTESIAN_POINT('Ctrl Pts',(77.9877678314391,-9.41583561933637,130.018692251077));
#71802=CARTESIAN_POINT('Ctrl Pts',(77.9733438642384,-9.34603791695104,130.014823846418));
#71803=CARTESIAN_POINT('Ctrl Pts',(77.9625745033955,-9.27557994090165,130.010955441758));
#71804=CARTESIAN_POINT('Ctrl Pts',(77.9554893450192,-9.20487494763926,130.007087037099));
#71805=CARTESIAN_POINT('Ctrl Pts',(77.9512835216487,-9.16290373157261,130.004790712041));
#71806=CARTESIAN_POINT('Ctrl Pts',(77.948374915081,-9.12084552646747,130.002494386983));
#71807=CARTESIAN_POINT('Ctrl Pts',(77.9467610336941,-9.07878648198151,130.000198061924));
#71808=CARTESIAN_POINT('Ctrl Pts',(77.9457600484714,-9.05270000353759,129.998773801462));
#71809=CARTESIAN_POINT('Ctrl Pts',(77.9452561844424,-9.02659432475927,129.997349541));
#71810=CARTESIAN_POINT('Ctrl Pts',(77.9452500565799,-9.00048219837867,129.995925280538));
#71811=CARTESIAN_POINT('Ctrl Pts',(77.9452500565798,-9.00048219782009,129.995925280508));
#71812=CARTESIAN_POINT('Ctrl Pts',(77.9452335129531,-8.92998620069327,129.99208014511));
#71813=CARTESIAN_POINT('Ctrl Pts',(77.94884919308,-8.85934488793869,129.988235009713));
#71814=CARTESIAN_POINT('Ctrl Pts',(77.9561158551286,-8.78896643668981,129.984389874316));
#71815=CARTESIAN_POINT('Ctrl Pts',(77.9636220283225,-8.71626829266497,129.980418002216));
#71816=CARTESIAN_POINT('Ctrl Pts',(77.9750241783424,-8.64385116603616,129.976446130117));
#71817=CARTESIAN_POINT('Ctrl Pts',(77.9902844923641,-8.57216692406059,129.972474258018));
#71818=CARTESIAN_POINT('Ctrl Pts',(78.005019200792,-8.50295167705567,129.968639187703));
#71819=CARTESIAN_POINT('Ctrl Pts',(78.0233505262677,-8.43442018110653,129.964804117388));
#71820=CARTESIAN_POINT('Ctrl Pts',(78.0451918525315,-8.36697340570031,129.960969047074));
#71821=CARTESIAN_POINT('Ctrl Pts',(78.0670205792052,-8.29956553826654,129.957136189093));
#71822=CARTESIAN_POINT('Ctrl Pts',(78.0923551392775,-8.23324161778643,129.953303331113));
#71823=CARTESIAN_POINT('Ctrl Pts',(78.121058669008,-8.1683888906526,129.949470473133));
#71824=CARTESIAN_POINT('Ctrl Pts',(78.1497555440784,-8.10355119905121,129.945638503767));
#71825=CARTESIAN_POINT('Ctrl Pts',(78.1818196388573,-8.040184473733,129.941806534401));
#71826=CARTESIAN_POINT('Ctrl Pts',(78.2170660967416,-7.97865566085095,129.937974565034));
#71827=CARTESIAN_POINT('Ctrl Pts',(78.2523165439689,-7.91711988387786,129.93414216195));
#71828=CARTESIAN_POINT('Ctrl Pts',(78.2907498217624,-7.85742285789769,129.930309758865));
#71829=CARTESIAN_POINT('Ctrl Pts',(78.332136214679,-7.7999050220442,129.926477355781));
#71830=CARTESIAN_POINT('Ctrl Pts',(78.3735674182597,-7.74232490938332,129.922640803204));
#71831=CARTESIAN_POINT('Ctrl Pts',(78.4179578264847,-7.68692909327009,129.918804250627));
#71832=CARTESIAN_POINT('Ctrl Pts',(78.4650362993757,-7.63402635447611,129.91496769805));
#71833=CARTESIAN_POINT('Ctrl Pts',(78.5121454593173,-7.58108913221403,129.911128644702));
#71834=CARTESIAN_POINT('Ctrl Pts',(78.5619458225972,-7.53064856875079,129.907289591353));
#71835=CARTESIAN_POINT('Ctrl Pts',(78.6141300949471,-7.48297588391985,129.903450538005));
#71836=CARTESIAN_POINT('Ctrl Pts',(78.6664000147489,-7.4352249562814,129.89960518381));
#71837=CARTESIAN_POINT('Ctrl Pts',(78.7210612665847,-7.39025127784402,129.895759829614));
#71838=CARTESIAN_POINT('Ctrl Pts',(78.7777751369244,-7.34828454430555,129.891914475419));
#71839=CARTESIAN_POINT('Ctrl Pts',(78.7917840726457,-7.33791830992497,129.89096463159));
#71840=CARTESIAN_POINT('Ctrl Pts',(78.8059181218404,-7.32773532710005,129.890014787761));
#71841=CARTESIAN_POINT('Ctrl Pts',(78.8201719453355,-7.3177386279396,129.889064943932));
#71842=CARTESIAN_POINT('Ctrl Pts',(78.8782264908607,-7.27702296826328,129.885196315152));
#71843=CARTESIAN_POINT('Ctrl Pts',(78.9385050111917,-7.2392361583561,129.881327686372));
#71844=CARTESIAN_POINT('Ctrl Pts',(79.0006798082348,-7.20462908655889,129.877459057592));
#71845=CARTESIAN_POINT('Ctrl Pts',(79.0627619420393,-7.17007359198433,129.873596194486));
#71846=CARTESIAN_POINT('Ctrl Pts',(79.1267343216675,-7.13868866324636,129.869733331381));
#71847=CARTESIAN_POINT('Ctrl Pts',(79.192239515353,-7.11068251425472,129.865870468276));
#71848=CARTESIAN_POINT('Ctrl Pts',(79.257667876001,-7.08270921452855,129.86201213604));
#71849=CARTESIAN_POINT('Ctrl Pts',(79.3246250349128,-7.05810701269977,129.858153803805));
#71850=CARTESIAN_POINT('Ctrl Pts',(79.3927297045678,-7.03703786312989,129.854295471569));
#71851=CARTESIAN_POINT('Ctrl Pts',(79.4607914812494,-7.01598198311225,129.850439569349));
#71852=CARTESIAN_POINT('Ctrl Pts',(79.5299988717297,-6.99845488399779,129.846583667128));
#71853=CARTESIAN_POINT('Ctrl Pts',(79.5999527695071,-6.98456958049281,129.842727764907));
#71854=CARTESIAN_POINT('Ctrl Pts',(79.6698860251347,-6.97068837429367,129.838873000494));
#71855=CARTESIAN_POINT('Ctrl Pts',(79.7405648743919,-6.96044692483719,129.835018236082));
#71856=CARTESIAN_POINT('Ctrl Pts',(79.8115789746446,-6.95390736287332,129.831163471669));
#71857=CARTESIAN_POINT('Ctrl Pts',(79.8825958895971,-6.94736754170876,129.827308554469));
#71858=CARTESIAN_POINT('Ctrl Pts',(79.9539475978615,-6.94452994170624,129.82345363727));
#71859=CARTESIAN_POINT('Ctrl Pts',(80.0252193065267,-6.94540477244828,129.819598720071));
#71860=CARTESIAN_POINT('Ctrl Pts',(80.0965657410168,-6.94628052041891,129.815739761129));
#71861=CARTESIAN_POINT('Ctrl Pts',(80.1678315216015,-6.95087646314228,129.811880802188));
#71862=CARTESIAN_POINT('Ctrl Pts',(80.2386034358576,-6.9591506760917,129.808021843246));
#71863=CARTESIAN_POINT('Ctrl Pts',(80.3094154784047,-6.96742958059185,129.804160696241));
#71864=CARTESIAN_POINT('Ctrl Pts',(80.3797326179328,-6.97939082554255,129.800299549237));
#71865=CARTESIAN_POINT('Ctrl Pts',(80.4491510670373,-6.99494117755133,129.796438402232));
#71866=CARTESIAN_POINT('Ctrl Pts',(80.5186911466634,-7.01051877588222,129.792570489975));
#71867=CARTESIAN_POINT('Ctrl Pts',(80.5873289239613,-7.02969790579128,129.788702577718));
#71868=CARTESIAN_POINT('Ctrl Pts',(80.6546756951435,-7.05233542500554,129.784834665461));
#71869=CARTESIAN_POINT('Ctrl Pts',(80.6947389922348,-7.06580204919211,129.782533718954));
#71870=CARTESIAN_POINT('Ctrl Pts',(80.7343457867761,-7.08049160587811,129.780232772447));
#71871=CARTESIAN_POINT('Ctrl Pts',(80.7734181194189,-7.09636611317867,129.777931825941));
#71872=CARTESIAN_POINT('Ctrl Pts',(80.8391271617478,-7.12306271923229,129.774062259392));
#71873=CARTESIAN_POINT('Ctrl Pts',(80.9035808241524,-7.15321771156363,129.770192692842));
#71874=CARTESIAN_POINT('Ctrl Pts',(80.9663905023612,-7.18669170865896,129.766323126293));
#71875=CARTESIAN_POINT('Ctrl Pts',(81.0291002102201,-7.22011242722627,129.762459718698));
#71876=CARTESIAN_POINT('Ctrl Pts',(81.0901707053912,-7.25684143326172,129.758596311103));
#71877=CARTESIAN_POINT('Ctrl Pts',(81.1492332295155,-7.29669129436928,129.754732903508));
#71878=CARTESIAN_POINT('Ctrl Pts',(81.1842307637733,-7.32030435358001,129.752443639009));
#71879=CARTESIAN_POINT('Ctrl Pts',(81.2185236431271,-7.34501227869952,129.750154374511));
#71880=CARTESIAN_POINT('Ctrl Pts',(81.2520391107129,-7.37076839346113,129.747865110012));
#71881=CARTESIAN_POINT('',(77.9452500005989,-9.00004961080126,130.054074719503));
#71882=CARTESIAN_POINT('Ctrl Pts',(77.9452500005989,-9.0000496100482,130.054074719462));
#71883=CARTESIAN_POINT('Ctrl Pts',(77.9452481959175,-8.92530327730347,130.05004413849));
#71884=CARTESIAN_POINT('Ctrl Pts',(77.9493293030799,-8.85063229326303,130.046013557518));
#71885=CARTESIAN_POINT('Ctrl Pts',(77.9574429753664,-8.77648632341645,130.041982976546));
#71886=CARTESIAN_POINT('Ctrl Pts',(77.9655784946025,-8.70214070744002,130.037941542793));
#71887=CARTESIAN_POINT('Ctrl Pts',(77.977768229183,-8.62832334710428,130.033900109041));
#71888=CARTESIAN_POINT('Ctrl Pts',(77.9939102844703,-8.55547596718978,130.029858675289));
#71889=CARTESIAN_POINT('Ctrl Pts',(78.0100750999784,-8.48252587281739,130.025811543135));
#71890=CARTESIAN_POINT('Ctrl Pts',(78.0302032326271,-8.41054888741118,130.021764410981));
#71891=CARTESIAN_POINT('Ctrl Pts',(78.0541430544742,-8.33997097787378,130.017717278826));
#71892=CARTESIAN_POINT('Ctrl Pts',(78.0781473948008,-8.26920285892522,130.013659239539));
#71893=CARTESIAN_POINT('Ctrl Pts',(78.1059838015981,-8.19984174114008,130.009601200252));
#71894=CARTESIAN_POINT('Ctrl Pts',(78.1374525227725,-8.13229356486568,130.005543160965));
#71895=CARTESIAN_POINT('Ctrl Pts',(78.1569006457639,-8.0905478188995,130.00303523423));
#71896=CARTESIAN_POINT('Ctrl Pts',(78.1777351877113,-8.04949402479317,130.000527307495));
#71897=CARTESIAN_POINT('Ctrl Pts',(78.1999006272447,-8.00922262303484,129.99801938076));
#71898=CARTESIAN_POINT('Ctrl Pts',(78.234095691327,-7.94709513119158,129.994150352343));
#71899=CARTESIAN_POINT('Ctrl Pts',(78.2715778605616,-7.88661829432888,129.990281323926));
#71900=CARTESIAN_POINT('Ctrl Pts',(78.312163336166,-7.82816171818907,129.986412295509));
#71901=CARTESIAN_POINT('Ctrl Pts',(78.3526883398097,-7.76979224177453,129.982549031907));
#71902=CARTESIAN_POINT('Ctrl Pts',(78.3963071967288,-7.71343744678505,129.978685768304));
#71903=CARTESIAN_POINT('Ctrl Pts',(78.4427906230037,-7.65944171380172,129.974822504702));
#71904=CARTESIAN_POINT('Ctrl Pts',(78.4892195252959,-7.60550931656296,129.970963772618));
#71905=CARTESIAN_POINT('Ctrl Pts',(78.5385060073011,-7.55393085126767,129.967105040534));
#71906=CARTESIAN_POINT('Ctrl Pts',(78.5903789984731,-7.50501966750249,129.963246308451));
#71907=CARTESIAN_POINT('Ctrl Pts',(78.6422193146569,-7.45613929307212,129.959390006997));
#71908=CARTESIAN_POINT('Ctrl Pts',(78.6966425549832,-7.40992319930734,129.955533705543));
#71909=CARTESIAN_POINT('Ctrl Pts',(78.7533401012571,-7.36664864179006,129.951677404088));
#71910=CARTESIAN_POINT('Ctrl Pts',(78.8100209012381,-7.32338686592666,129.947822241639));
#71911=CARTESIAN_POINT('Ctrl Pts',(78.8689742876135,-7.28306519605176,129.943967079189));
#71912=CARTESIAN_POINT('Ctrl Pts',(78.929859147609,-7.24592015046527,129.940111916739));
#71913=CARTESIAN_POINT('Ctrl Pts',(78.990746392486,-7.20877364989418,129.936256603281));
#71914=CARTESIAN_POINT('Ctrl Pts',(79.0535648453302,-7.17480427177923,129.932401289823));
#71915=CARTESIAN_POINT('Ctrl Pts',(79.117946533292,-7.1442038785555,129.928545976366));
#71916=CARTESIAN_POINT('Ctrl Pts',(79.1823956255543,-7.11357144830132,129.924686626594));
#71917=CARTESIAN_POINT('Ctrl Pts',(79.2484107803471,-7.08631525289264,129.920827276822));
#71918=CARTESIAN_POINT('Ctrl Pts',(79.3156024849781,-7.06257965223553,129.91696792705));
#71919=CARTESIAN_POINT('Ctrl Pts',(79.3828322410247,-7.03883060984165,129.913106391685));
#71920=CARTESIAN_POINT('Ctrl Pts',(79.4512394072066,-7.01860626893441,129.90924485632));
#71921=CARTESIAN_POINT('Ctrl Pts',(79.5204203348216,-7.00200077396226,129.905383320956));
#71922=CARTESIAN_POINT('Ctrl Pts',(79.5897223192403,-6.98536622173092,129.901515028452));
#71923=CARTESIAN_POINT('Ctrl Pts',(79.6598002905396,-6.9723632470331,129.897646735948));
#71924=CARTESIAN_POINT('Ctrl Pts',(79.7302421608351,-6.96303454356508,129.893778443445));
#71925=CARTESIAN_POINT('Ctrl Pts',(79.7720778542155,-6.9574941912677,129.891481049886));
#71926=CARTESIAN_POINT('Ctrl Pts',(79.8140418177163,-6.95324883831699,129.889183656327));
#71927=CARTESIAN_POINT('Ctrl Pts',(79.856047742892,-6.95029872660099,129.886886262768));
#71928=CARTESIAN_POINT('Ctrl Pts',(79.9267744990955,-6.94533152658724,129.883018065759));
#71929=CARTESIAN_POINT('Ctrl Pts',(79.9978971276319,-6.94401963059411,129.87914986875));
#71930=CARTESIAN_POINT('Ctrl Pts',(80.0690057038552,-6.94640905355145,129.87528167174));
#71931=CARTESIAN_POINT('Ctrl Pts',(80.1400164928976,-6.94879519061914,129.871418794203));
#71932=CARTESIAN_POINT('Ctrl Pts',(80.2110127869314,-6.95487253311624,129.867555916666));
#71933=CARTESIAN_POINT('Ctrl Pts',(80.2815810444504,-6.96463524696279,129.863693039128));
#71934=CARTESIAN_POINT('Ctrl Pts',(80.3520758709569,-6.97438780204975,129.859834181175));
#71935=CARTESIAN_POINT('Ctrl Pts',(80.4221430662193,-6.98781805163217,129.855975323221));
#71936=CARTESIAN_POINT('Ctrl Pts',(80.4913723285457,-7.00486822559522,129.852116465267));
#71937=CARTESIAN_POINT('Ctrl Pts',(80.5605648400204,-7.02190934835083,129.848259655816));
#71938=CARTESIAN_POINT('Ctrl Pts',(80.6289198289698,-7.04256647320145,129.844402846365));
#71939=CARTESIAN_POINT('Ctrl Pts',(80.6960368317509,-7.06673067283781,129.840546036914));
#71940=CARTESIAN_POINT('Ctrl Pts',(80.7631293991516,-7.09088607498043,129.836690631616));
#71941=CARTESIAN_POINT('Ctrl Pts',(80.828984419639,-7.11854584861426,129.832835226319));
#71942=CARTESIAN_POINT('Ctrl Pts',(80.8932181129685,-7.14955168535705,129.828979821022));
#71943=CARTESIAN_POINT('Ctrl Pts',(80.9574849838627,-7.18057353703062,129.825122424356));
#71944=CARTESIAN_POINT('Ctrl Pts',(81.0201284140811,-7.21494469754726,129.82126502769));
#71945=CARTESIAN_POINT('Ctrl Pts',(81.0807870621434,-7.25245976046229,129.817407631025));
#71946=CARTESIAN_POINT('Ctrl Pts',(81.1398557515114,-7.2889914944976,129.8136513428));
#71947=CARTESIAN_POINT('Ctrl Pts',(81.1970420997478,-7.32850404723543,129.809895054576));
#71948=CARTESIAN_POINT('Ctrl Pts',(81.2520391107129,-7.37076839346111,129.806138766351));
#71949=CARTESIAN_POINT('Ctrl Pts',(81.2520391107129,-7.37076839346111,130.506052881321));
#71950=CARTESIAN_POINT('Ctrl Pts',(81.3085807246794,-7.41421974303275,130.50219771141));
#71951=CARTESIAN_POINT('Ctrl Pts',(81.362873206473,-7.46062977900589,130.498342541498));
#71952=CARTESIAN_POINT('Ctrl Pts',(81.4145999487785,-7.5097300421011,130.494487371586));
#71953=CARTESIAN_POINT('Ctrl Pts',(81.4663306422551,-7.55883405574272,130.490631907195));
#71954=CARTESIAN_POINT('Ctrl Pts',(81.5154948564782,-7.6106283683093,130.486776442805));
#71955=CARTESIAN_POINT('Ctrl Pts',(81.561812211972,-7.66480706374127,130.482920978414));
#71956=CARTESIAN_POINT('Ctrl Pts',(81.6081791212523,-7.71904372361176,130.479061389158));
#71957=CARTESIAN_POINT('Ctrl Pts',(81.651692776919,-7.77566948756278,130.475201799901));
#71958=CARTESIAN_POINT('Ctrl Pts',(81.6921131557005,-7.83434540673269,130.471342210645));
#71959=CARTESIAN_POINT('Ctrl Pts',(81.7325577723832,-7.89305651065771,130.467480307003));
#71960=CARTESIAN_POINT('Ctrl Pts',(81.7699051661614,-7.95381980266632,130.463618403362));
#71961=CARTESIAN_POINT('Ctrl Pts',(81.8039601860705,-8.01626974755644,130.45975649972));
#71962=CARTESIAN_POINT('Ctrl Pts',(81.8380736285783,-8.0788268275497,130.455887970845));
#71963=CARTESIAN_POINT('Ctrl Pts',(81.8688832138848,-8.14307589792443,130.45201944197));
#71964=CARTESIAN_POINT('Ctrl Pts',(81.8962413478652,-8.20863010346207,130.448150913095));
#71965=CARTESIAN_POINT('Ctrl Pts',(81.9094401501915,-8.24025641983182,130.446284559639));
#71966=CARTESIAN_POINT('Ctrl Pts',(81.9218363544097,-8.27218626462339,130.444418206182));
#71967=CARTESIAN_POINT('Ctrl Pts',(81.9334175758367,-8.30437507236593,130.442551852726));
#71968=CARTESIAN_POINT('Ctrl Pts',(81.9574262793432,-8.37110478185256,130.438682768014));
#71969=CARTESIAN_POINT('Ctrl Pts',(81.9780233007512,-8.43920959718742,130.434813683301));
#71970=CARTESIAN_POINT('Ctrl Pts',(81.9950528338328,-8.50830725781688,130.430944598589));
#71971=CARTESIAN_POINT('Ctrl Pts',(82.0120569938305,-8.57730196666607,130.427081278604));
#71972=CARTESIAN_POINT('Ctrl Pts',(82.0255041010556,-8.64728611664166,130.423217958619));
#71973=CARTESIAN_POINT('Ctrl Pts',(82.0352873460395,-8.71785999654176,130.419354638634));
#71974=CARTESIAN_POINT('Ctrl Pts',(82.0450591153133,-8.78835109354143,130.415495850309));
#71975=CARTESIAN_POINT('Ctrl Pts',(82.0511754926477,-8.85943006756781,130.411637061983));
#71976=CARTESIAN_POINT('Ctrl Pts',(82.053580576256,-8.93068636985202,130.407778273658));
#71977=CARTESIAN_POINT('Ctrl Pts',(82.0559841448421,-9.00189778601412,130.40392191608));
#71978=CARTESIAN_POINT('Ctrl Pts',(82.0546810415849,-9.07328582445763,130.400065558502));
#71979=CARTESIAN_POINT('Ctrl Pts',(82.0496672686969,-9.14443562625877,130.396209200924));
#71980=CARTESIAN_POINT('Ctrl Pts',(82.0446549769234,-9.21556440975503,130.39235398255));
#71981=CARTESIAN_POINT('Ctrl Pts',(82.0359342258414,-9.28645461201044,130.388498764175));
#71982=CARTESIAN_POINT('Ctrl Pts',(82.0235530649265,-9.3566939247121,130.3846435458));
#71983=CARTESIAN_POINT('Ctrl Pts',(82.0111714199462,-9.42693598355592,130.380788176699));
#71984=CARTESIAN_POINT('Ctrl Pts',(81.9951291675039,-9.49652662429819,130.376932807597));
#71985=CARTESIAN_POINT('Ctrl Pts',(81.9755256195375,-9.56506290716236,130.373077438495));
#71986=CARTESIAN_POINT('Ctrl Pts',(81.9559015520805,-9.63367092855154,130.369218033888));
#71987=CARTESIAN_POINT('Ctrl Pts',(81.9327088816582,-9.70122192097859,130.365358629282));
#71988=CARTESIAN_POINT('Ctrl Pts',(81.9060968013722,-9.7673281868266,130.361499224675));
#71989=CARTESIAN_POINT('Ctrl Pts',(81.8794696531574,-9.83347188246193,130.357637634849));
#71990=CARTESIAN_POINT('Ctrl Pts',(81.8494194456522,-9.89816878232024,130.353776045023));
#71991=CARTESIAN_POINT('Ctrl Pts',(81.8161423941771,-9.96105377923019,130.349914455197));
#71992=CARTESIAN_POINT('Ctrl Pts',(81.7828071235772,-10.0240487951869,130.346046109413));
#71993=CARTESIAN_POINT('Ctrl Pts',(81.7462339870473,-10.0852251621662,130.342177763628));
#71994=CARTESIAN_POINT('Ctrl Pts',(81.7066633828725,-10.1442454544643,130.338309417844));
#71995=CARTESIAN_POINT('Ctrl Pts',(81.683167681349,-10.1792897304005,130.336012523474));
#71996=CARTESIAN_POINT('Ctrl Pts',(81.6586159996239,-10.2135744578996,130.333715629104));
#71997=CARTESIAN_POINT('Ctrl Pts',(81.6330651749265,-10.2470347617216,130.331418734734));
#71998=CARTESIAN_POINT('Ctrl Pts',(81.5900252789422,-10.3033980303506,130.327549658259));
#71999=CARTESIAN_POINT('Ctrl Pts',(81.5439796921779,-10.3576408743815,130.323680581783));
#72000=CARTESIAN_POINT('Ctrl Pts',(81.4951650564802,-10.4094250658977,130.319811505308));
#72001=CARTESIAN_POINT('Ctrl Pts',(81.4464231523288,-10.4611321013668,130.315948193577));
#72002=CARTESIAN_POINT('Ctrl Pts',(81.3949207192542,-10.5103874052188,130.312084881846));
#72003=CARTESIAN_POINT('Ctrl Pts',(81.3409356349291,-10.5568844483382,130.308221570115));
#72004=CARTESIAN_POINT('Ctrl Pts',(81.2870138748539,-10.6033269506447,130.304362790031));
#72005=CARTESIAN_POINT('Ctrl Pts',(81.2306156143129,-10.647017303385,130.300504009947));
#72006=CARTESIAN_POINT('Ctrl Pts',(81.1720554473805,-10.6876858685092,130.296645229862));
#72007=CARTESIAN_POINT('Ctrl Pts',(81.113532168842,-10.7283288155703,130.292788880512));
#72008=CARTESIAN_POINT('Ctrl Pts',(81.0528500838303,-10.7659534750732,130.288932531162));
#72009=CARTESIAN_POINT('Ctrl Pts',(80.9903555592917,-10.8003314774452,130.285076181812));
#72010=CARTESIAN_POINT('Ctrl Pts',(80.9278794958464,-10.8346993244394,130.281220971641));
#72011=CARTESIAN_POINT('Ctrl Pts',(80.8635924811966,-10.8658221843169,130.277365761469));
#72012=CARTESIAN_POINT('Ctrl Pts',(80.7978669688866,-10.8935167975119,130.273510551298));
#72013=CARTESIAN_POINT('Ctrl Pts',(80.7321388862765,-10.9212124937485,130.269655190362));
#72014=CARTESIAN_POINT('Ctrl Pts',(80.6649726428412,-10.9454794905282,130.265799829427));
#72015=CARTESIAN_POINT('Ctrl Pts',(80.5967606250719,-10.9661826768802,130.261944468491));
#72016=CARTESIAN_POINT('Ctrl Pts',(80.528477206057,-10.9869075343884,130.258085071938));
#72017=CARTESIAN_POINT('Ctrl Pts',(80.4591462933012,-11.0040609933093,130.254225675386));
#72018=CARTESIAN_POINT('Ctrl Pts',(80.3891745224171,-11.0175581165363,130.250366278833));
#72019=CARTESIAN_POINT('Ctrl Pts',(80.3191631320623,-11.0310628821149,130.24650469701));
#72020=CARTESIAN_POINT('Ctrl Pts',(80.2485106425874,-11.0409071236151,130.242643115187));
#72021=CARTESIAN_POINT('Ctrl Pts',(80.1776302144995,-11.0470576614734,130.238781533364));
#72022=CARTESIAN_POINT('Ctrl Pts',(80.106625775804,-11.0532189601575,130.234913195415));
#72023=CARTESIAN_POINT('Ctrl Pts',(80.035393087939,-11.0556736360794,130.231044857466));
#72024=CARTESIAN_POINT('Ctrl Pts',(79.9643460192144,-11.0544406431324,130.227176519517));
#72025=CARTESIAN_POINT('Ctrl Pts',(79.9221592153547,-11.05370850833,130.224879551926));
#72026=CARTESIAN_POINT('Ctrl Pts',(79.8800377937428,-11.051677162781,130.222582584334));
#72027=CARTESIAN_POINT('Ctrl Pts',(79.8380670939317,-11.0483591717353,130.220285616743));
#72028=CARTESIAN_POINT('Ctrl Pts',(79.7673702407754,-11.0427702364356,130.216416527563));
#72029=CARTESIAN_POINT('Ctrl Pts',(79.6968246044294,-11.03350602237,130.212547438383));
#72030=CARTESIAN_POINT('Ctrl Pts',(79.6268426933459,-11.0205818931661,130.208678349203));
#72031=CARTESIAN_POINT('Ctrl Pts',(79.5569650524864,-11.0076770203932,130.20481502481));
#72032=CARTESIAN_POINT('Ctrl Pts',(79.4876499434675,-10.9911231442897,130.200951700417));
#72033=CARTESIAN_POINT('Ctrl Pts',(79.41930560889,-10.9709874648595,130.197088376024));
#72034=CARTESIAN_POINT('Ctrl Pts',(79.3510414437919,-10.9508754050453,130.193229583399));
#72035=CARTESIAN_POINT('Ctrl Pts',(79.283746254927,-10.9271900242032,130.189370790774));
#72036=CARTESIAN_POINT('Ctrl Pts',(79.2178172056323,-10.9000493779623,130.18551199815));
#72037=CARTESIAN_POINT('Ctrl Pts',(79.151929687824,-10.8729258287583,130.181655636341));
#72038=CARTESIAN_POINT('Ctrl Pts',(79.0874070503361,-10.8423515170163,130.177799274533));
#72039=CARTESIAN_POINT('Ctrl Pts',(79.0246290184254,-10.8084935749961,130.173942912724));
#72040=CARTESIAN_POINT('Ctrl Pts',(78.9618695329172,-10.7746456355676,130.170087690194));
#72041=CARTESIAN_POINT('Ctrl Pts',(78.9008540570915,-10.7375162222038,130.166232467664));
#72042=CARTESIAN_POINT('Ctrl Pts',(78.8419385666496,-10.6973188501535,130.162377245133));
#72043=CARTESIAN_POINT('Ctrl Pts',(78.7830207740229,-10.6571199073485,130.158521871956));
#72044=CARTESIAN_POINT('Ctrl Pts',(78.7262035297341,-10.6138530434507,130.154666498779));
#72045=CARTESIAN_POINT('Ctrl Pts',(78.6718131695291,-10.5677746349089,130.150811125601));
#72046=CARTESIAN_POINT('Ctrl Pts',(78.6173658798344,-10.5216479968595,130.146951717069));
#72047=CARTESIAN_POINT('Ctrl Pts',(78.5653509164017,-10.4727042543346,130.143092308536));
#72048=CARTESIAN_POINT('Ctrl Pts',(78.5160601907348,-10.4212389682871,130.139232900004));
#72049=CARTESIAN_POINT('Ctrl Pts',(78.4667415573744,-10.3697445433417,130.13537130633));
#72050=CARTESIAN_POINT('Ctrl Pts',(78.4201505496984,-10.3157261008707,130.131509712656));
#72051=CARTESIAN_POINT('Ctrl Pts',(78.3765391350539,-10.2595127559848,130.127648118983));
#72052=CARTESIAN_POINT('Ctrl Pts',(78.3328514229635,-10.2032010667853,130.123779769515));
#72053=CARTESIAN_POINT('Ctrl Pts',(78.2921539887692,-10.1446872075429,130.119911420047));
#72054=CARTESIAN_POINT('Ctrl Pts',(78.2546553847502,-10.0843291642848,130.11604307058));
#72055=CARTESIAN_POINT('Ctrl Pts',(78.2323903484066,-10.0484911894607,130.113746213303));
#72056=CARTESIAN_POINT('Ctrl Pts',(78.2112521765726,-10.0120035409388,130.111449356027));
#72057=CARTESIAN_POINT('Ctrl Pts',(78.1912765943959,-9.97494471869947,130.109152498751));
#72058=CARTESIAN_POINT('Ctrl Pts',(78.155830663704,-9.9091852112667,130.105076810588));
#72059=CARTESIAN_POINT('Ctrl Pts',(78.1239212019008,-9.84139127309731,130.101001122426));
#72060=CARTESIAN_POINT('Ctrl Pts',(78.0957732939458,-9.77195739160262,130.096925434263));
#72061=CARTESIAN_POINT('Ctrl Pts',(78.0677085507469,-9.70272865685746,130.092861787976));
#72062=CARTESIAN_POINT('Ctrl Pts',(78.0433833815986,-9.63187000592221,130.088798141689));
#72063=CARTESIAN_POINT('Ctrl Pts',(78.0229762170244,-9.55979864598709,130.084734495402));
#72064=CARTESIAN_POINT('Ctrl Pts',(78.0026057685884,-9.4878569553155,130.080678160342));
#72065=CARTESIAN_POINT('Ctrl Pts',(77.9861394179744,-9.41470728619444,130.076621825281));
#72066=CARTESIAN_POINT('Ctrl Pts',(77.9737071028153,-9.34078535373292,130.07256549022));
#72067=CARTESIAN_POINT('Ctrl Pts',(77.96130303065,-9.26703135271886,130.0685183701));
#72068=CARTESIAN_POINT('Ctrl Pts',(77.9529148139121,-9.19250898403491,130.06447124998));
#72069=CARTESIAN_POINT('Ctrl Pts',(77.9486218581334,-9.11766597457222,130.06042412986));
#72070=CARTESIAN_POINT('Ctrl Pts',(77.946376826516,-9.07852629290516,130.058307659741));
#72071=CARTESIAN_POINT('Ctrl Pts',(77.9452509482569,-9.03929913360494,130.056191189622));
#72072=CARTESIAN_POINT('Ctrl Pts',(77.9452500005989,-9.00004961080127,130.054074719503));
#72073=CARTESIAN_POINT('Origin',(80.,-9.,141.545925280538));
#72074=CARTESIAN_POINT('',(81.2520391107129,-7.37076839346111,131.206019331682));
#72075=CARTESIAN_POINT('',(81.2520391107129,-7.3707683934611,131.147979657963));
#72076=CARTESIAN_POINT('',(81.2520391107129,-7.37076839346111,141.545925280538));
#72077=CARTESIAN_POINT('',(77.9452508472645,-8.99813403300313,130.695925280507));
#72078=CARTESIAN_POINT('Ctrl Pts',(81.2520391107129,-7.3707683934611,131.147979657963));
#72079=CARTESIAN_POINT('Ctrl Pts',(81.3086037747096,-7.4142374566219,131.144119415677));
#72080=CARTESIAN_POINT('Ctrl Pts',(81.362864049299,-7.46062653621925,131.14025917339));
#72081=CARTESIAN_POINT('Ctrl Pts',(81.4145173037714,-7.50965159783651,131.136398931104));
#72082=CARTESIAN_POINT('Ctrl Pts',(81.4662067801097,-7.55871103829843,131.132535981821));
#72083=CARTESIAN_POINT('Ctrl Pts',(81.5152852658367,-7.61040978588829,131.128673032539));
#72084=CARTESIAN_POINT('Ctrl Pts',(81.5614888520647,-7.66442891339409,131.124810083256));
#72085=CARTESIAN_POINT('Ctrl Pts',(81.607767173866,-7.71853541832652,131.120940885546));
#72086=CARTESIAN_POINT('Ctrl Pts',(81.6511610284125,-7.77496940355062,131.117071687836));
#72087=CARTESIAN_POINT('Ctrl Pts',(81.6914490147046,-7.83338189918263,131.113202490127));
#72088=CARTESIAN_POINT('Ctrl Pts',(81.6972565756089,-7.8418021295584,131.112644740698));
#72089=CARTESIAN_POINT('Ctrl Pts',(81.7029996757573,-7.85026343058691,131.112086991269));
#72090=CARTESIAN_POINT('Ctrl Pts',(81.7086777314096,-7.85876471633363,131.11152924184));
#72091=CARTESIAN_POINT('Ctrl Pts',(81.748066149928,-7.91773775595226,131.107660158956));
#72092=CARTESIAN_POINT('Ctrl Pts',(81.7844750515849,-7.97886786377236,131.103791076072));
#72093=CARTESIAN_POINT('Ctrl Pts',(81.8176610664465,-8.04182161889099,131.099921993188));
#72094=CARTESIAN_POINT('Ctrl Pts',(81.8507976357948,-8.10468157604252,131.096058675046));
#72095=CARTESIAN_POINT('Ctrl Pts',(81.8807206253814,-8.16935936080732,131.092195356903));
#72096=CARTESIAN_POINT('Ctrl Pts',(81.9072300095338,-8.2354928036743,131.088332038761));
#72097=CARTESIAN_POINT('Ctrl Pts',(81.9337082981801,-8.30154867201683,131.08447325229));
#72098=CARTESIAN_POINT('Ctrl Pts',(81.9567807551404,-8.36905635809634,131.080614465819));
#72099=CARTESIAN_POINT('Ctrl Pts',(81.9762941479208,-8.43763090110313,131.076755679349));
#72100=CARTESIAN_POINT('Ctrl Pts',(81.9957952486906,-8.50616224716216,131.072899323631));
#72101=CARTESIAN_POINT('Ctrl Pts',(82.0117416006339,-8.57575865069783,131.069042967914));
#72102=CARTESIAN_POINT('Ctrl Pts',(82.0240293050706,-8.64601845427297,131.065186612197));
#72103=CARTESIAN_POINT('Ctrl Pts',(82.0363133795937,-8.71625750238318,131.061331395686));
#72104=CARTESIAN_POINT('Ctrl Pts',(82.0449408686595,-8.78715908320829,131.057476179176));
#72105=CARTESIAN_POINT('Ctrl Pts',(82.0498590005135,-8.8583114665404,131.053620962666));
#72106=CARTESIAN_POINT('Ctrl Pts',(82.0547773246505,-8.92946663170095,131.049765595429));
#72107=CARTESIAN_POINT('Ctrl Pts',(82.0559859723494,-9.00087213405753,131.045910228192));
#72108=CARTESIAN_POINT('Ctrl Pts',(82.0534841808734,-9.07211297666065,131.042054860955));
#72109=CARTESIAN_POINT('Ctrl Pts',(82.0509797707049,-9.14342838896989,131.038195458202));
#72110=CARTESIAN_POINT('Ctrl Pts',(82.0447571854772,-9.21457831099044,131.034336055448));
#72111=CARTESIAN_POINT('Ctrl Pts',(82.0348677469965,-9.28515051242027,131.030476652695));
#72112=CARTESIAN_POINT('Ctrl Pts',(82.0249727090402,-9.35576267236917,131.026615064718));
#72113=CARTESIAN_POINT('Ctrl Pts',(82.0114067771824,-9.42579598340886,131.022753476741));
#72114=CARTESIAN_POINT('Ctrl Pts',(81.9942723547638,-9.49484880269107,131.018891888764));
#72115=CARTESIAN_POINT('Ctrl Pts',(81.9771079550666,-9.56402243232522,131.015023544803));
#72116=CARTESIAN_POINT('Ctrl Pts',(81.9563627415182,-9.63221168044898,131.011155200841));
#72117=CARTESIAN_POINT('Ctrl Pts',(81.9321886708894,-9.69903111703738,131.007286856879));
#72118=CARTESIAN_POINT('Ctrl Pts',(81.9178348053739,-9.73870657018487,131.004989945869));
#72119=CARTESIAN_POINT('Ctrl Pts',(81.9022729705369,-9.77789946020317,131.002693034859));
#72120=CARTESIAN_POINT('Ctrl Pts',(81.8855426871365,-9.81653312087521,131.000396123848));
#72121=CARTESIAN_POINT('Ctrl Pts',(81.8573609872102,-9.88161045435812,130.996527040743));
#72122=CARTESIAN_POINT('Ctrl Pts',(81.8257510312545,-9.94535454821874,130.992657957637));
#72123=CARTESIAN_POINT('Ctrl Pts',(81.7908609381868,-10.0073800983624,130.988788874532));
#72124=CARTESIAN_POINT('Ctrl Pts',(81.7560228296013,-10.0693132335588,130.984925556166));
#72125=CARTESIAN_POINT('Ctrl Pts',(81.7179145211625,-10.1295324877013,130.9810622378));
#72126=CARTESIAN_POINT('Ctrl Pts',(81.6767317935167,-10.1876733789685,130.977198919433));
#72127=CARTESIAN_POINT('Ctrl Pts',(81.635597373182,-10.2457460710103,130.973340132737));
#72128=CARTESIAN_POINT('Ctrl Pts',(81.5913959763829,-10.3017448482196,130.96948134604));
#72129=CARTESIAN_POINT('Ctrl Pts',(81.5443679111866,-10.3553321797246,130.965622559344));
#72130=CARTESIAN_POINT('Ctrl Pts',(81.4973694702163,-10.4088857551478,130.961766203399));
#72131=CARTESIAN_POINT('Ctrl Pts',(81.4475482131879,-10.4600305343499,130.957909847455));
#72132=CARTESIAN_POINT('Ctrl Pts',(81.395185233245,-10.5084613775086,130.954053491511));
#72133=CARTESIAN_POINT('Ctrl Pts',(81.3428377218496,-10.5568779137122,130.950198274772));
#72134=CARTESIAN_POINT('Ctrl Pts',(81.2879503346217,-10.6025817758474,130.946343058034));
#72135=CARTESIAN_POINT('Ctrl Pts',(81.2308403574089,-10.6453053142422,130.942487841296));
#72136=CARTESIAN_POINT('Ctrl Pts',(81.1737281473731,-10.6880305229949,130.93863247383));
#72137=CARTESIAN_POINT('Ctrl Pts',(81.1143935651329,-10.7277748874385,130.934777106365));
#72138=CARTESIAN_POINT('Ctrl Pts',(81.0531848497,-10.764312680582,130.9309217389));
#72139=CARTESIAN_POINT('Ctrl Pts',(80.991912065475,-10.8008887188063,130.927062335918));
#72140=CARTESIAN_POINT('Ctrl Pts',(80.9287616500267,-10.8342512360934,130.923202932937));
#72141=CARTESIAN_POINT('Ctrl Pts',(80.8641077676447,-10.8642197639753,130.919343529956));
#72142=CARTESIAN_POINT('Ctrl Pts',(80.7994172777452,-10.8942052602645,130.915481941752));
#72143=CARTESIAN_POINT('Ctrl Pts',(80.7332220772815,-10.9207927604884,130.911620353548));
#72144=CARTESIAN_POINT('Ctrl Pts',(80.6659151412917,-10.9438504538926,130.907758765343));
#72145=CARTESIAN_POINT('Ctrl Pts',(80.598490449488,-10.9669484875295,130.903890421157));
#72146=CARTESIAN_POINT('Ctrl Pts',(80.5299506061597,-10.9865042514215,130.90002207697));
#72147=CARTESIAN_POINT('Ctrl Pts',(80.4607018422215,-11.0024363598062,130.896153732784));
#72148=CARTESIAN_POINT('Ctrl Pts',(80.4195839634142,-11.0118963770606,130.893856823808));
#72149=CARTESIAN_POINT('Ctrl Pts',(80.3782163235417,-11.0200798088441,130.891559914832));
#72150=CARTESIAN_POINT('Ctrl Pts',(80.3366847674755,-11.0269782756236,130.889263005857));
#72151=CARTESIAN_POINT('Ctrl Pts',(80.2667259651641,-11.0385985595567,130.885393923738));
#72152=CARTESIAN_POINT('Ctrl Pts',(80.196027842885,-11.0466155311481,130.881524841618));
#72153=CARTESIAN_POINT('Ctrl Pts',(80.124994443943,-11.0509446485665,130.877655759499));
#72154=CARTESIAN_POINT('Ctrl Pts',(80.0540668812426,-11.0552673158145,130.873792442121));
#72155=CARTESIAN_POINT('Ctrl Pts',(79.9828055143971,-11.0559130064459,130.869929124742));
#72156=CARTESIAN_POINT('Ctrl Pts',(79.9116227440299,-11.0528485144129,130.866065807363));
#72157=CARTESIAN_POINT('Ctrl Pts',(79.840523470976,-11.0497876170257,130.862207021652));
#72158=CARTESIAN_POINT('Ctrl Pts',(79.7695030942512,-11.0430252023924,130.85834823594));
#72159=CARTESIAN_POINT('Ctrl Pts',(79.6989755229046,-11.0325800910885,130.854489450228));
#72160=CARTESIAN_POINT('Ctrl Pts',(79.628492378718,-11.0221415594332,130.850633095267));
#72161=CARTESIAN_POINT('Ctrl Pts',(79.5585019034254,-11.0080250046074,130.846776740305));
#72162=CARTESIAN_POINT('Ctrl Pts',(79.489412914315,-10.9903010803473,130.842920385343));
#72163=CARTESIAN_POINT('Ctrl Pts',(79.4203443347233,-10.9725823918964,130.839065169584));
#72164=CARTESIAN_POINT('Ctrl Pts',(79.35217718291,-10.9512585702692,130.835209953825));
#72165=CARTESIAN_POINT('Ctrl Pts',(79.2853084096626,-10.9264510098108,130.831354738066));
#72166=CARTESIAN_POINT('Ctrl Pts',(79.2184370219655,-10.901642479421,130.827499371575));
#72167=CARTESIAN_POINT('Ctrl Pts',(79.1528645683048,-10.8733501108095,130.823644005084));
#72168=CARTESIAN_POINT('Ctrl Pts',(79.0889695672252,-10.8417440411355,130.819788638592));
#72169=CARTESIAN_POINT('Ctrl Pts',(79.0250076852926,-10.8101048884212,130.815929236571));
#72170=CARTESIAN_POINT('Ctrl Pts',(78.9627271973097,-10.7751453264637,130.81206983455));
#72171=CARTESIAN_POINT('Ctrl Pts',(78.9024826599988,-10.7370818204382,130.808210432529));
#72172=CARTESIAN_POINT('Ctrl Pts',(78.842204011663,-10.6989967624967,130.804348845277));
#72173=CARTESIAN_POINT('Ctrl Pts',(78.7839640056126,-10.6578045425288,130.800487258026));
#72174=CARTESIAN_POINT('Ctrl Pts',(78.7280865221899,-10.6137638202243,130.796625670775));
#72175=CARTESIAN_POINT('Ctrl Pts',(78.672111278851,-10.5696460468958,130.792757327521));
#72176=CARTESIAN_POINT('Ctrl Pts',(78.6185071759079,-10.5226701416633,130.788888984267));
#72177=CARTESIAN_POINT('Ctrl Pts',(78.5675629197205,-10.473133250436,130.785020641013));
#72178=CARTESIAN_POINT('Ctrl Pts',(78.5373135967212,-10.4437195827283,130.782723723297));
#72179=CARTESIAN_POINT('Ctrl Pts',(78.5080013169699,-10.4134036807332,130.780426805581));
#72180=CARTESIAN_POINT('Ctrl Pts',(78.4796796815619,-10.3822531214811,130.778129887865));
#72181=CARTESIAN_POINT('Ctrl Pts',(78.432491033328,-10.3303510063079,130.774302833369));
#72182=CARTESIAN_POINT('Ctrl Pts',(78.3878608320509,-10.2759167409365,130.770475778873));
#72183=CARTESIAN_POINT('Ctrl Pts',(78.3460767383655,-10.2192355831111,130.766648724377));
#72184=CARTESIAN_POINT('Ctrl Pts',(78.3043498473697,-10.1626320221507,130.762826909143));
#72185=CARTESIAN_POINT('Ctrl Pts',(78.2654616325306,-10.1037880620617,130.759005093909));
#72186=CARTESIAN_POINT('Ctrl Pts',(78.2296616569659,-10.043024311166,130.755183278674));
#72187=CARTESIAN_POINT('Ctrl Pts',(78.1938980883374,-9.98232235422308,130.751365350051));
#72188=CARTESIAN_POINT('Ctrl Pts',(78.1612167818143,-9.91970490401357,130.747547421428));
#72189=CARTESIAN_POINT('Ctrl Pts',(78.1318247421453,-9.85552251194209,130.743729492805));
#72190=CARTESIAN_POINT('Ctrl Pts',(78.1011566442909,-9.78855363524112,130.73974580845));
#72191=CARTESIAN_POINT('Ctrl Pts',(78.0740702736535,-9.71988128861933,130.735762124094));
#72192=CARTESIAN_POINT('Ctrl Pts',(78.0507474289142,-9.6499322861771,130.731778439738));
#72193=CARTESIAN_POINT('Ctrl Pts',(78.0284112294296,-9.58294239323039,130.72796328042));
#72194=CARTESIAN_POINT('Ctrl Pts',(78.0095266831817,-9.5147822055705,130.724148121101));
#72195=CARTESIAN_POINT('Ctrl Pts',(77.9942033860666,-9.44584471067081,130.720332961782));
#72196=CARTESIAN_POINT('Ctrl Pts',(77.978879928244,-9.37690649276972,130.71651776245));
#72197=CARTESIAN_POINT('Ctrl Pts',(77.9671178912741,-9.30719143896892,130.712702563119));
#72198=CARTESIAN_POINT('Ctrl Pts',(77.958975811088,-9.23710297926417,130.708887363787));
#72199=CARTESIAN_POINT('Ctrl Pts',(77.9508281237988,-9.16696625262999,130.705069537091));
#72200=CARTESIAN_POINT('Ctrl Pts',(77.9463054071666,-9.09645610237582,130.701251710395));
#72201=CARTESIAN_POINT('Ctrl Pts',(77.9454142484556,-9.0259798393166,130.697433883698));
#72202=CARTESIAN_POINT('Ctrl Pts',(77.9452968688612,-9.01669700891443,130.696931015978));
#72203=CARTESIAN_POINT('Ctrl Pts',(77.9452424192122,-9.00741476447613,130.696428148258));
#72204=CARTESIAN_POINT('Ctrl Pts',(77.945250847264,-8.99813403357328,130.695925280538));
#72205=CARTESIAN_POINT('Ctrl Pts',(77.9452508472645,-8.99813403300313,130.695925280507));
#72206=CARTESIAN_POINT('Ctrl Pts',(77.9453334654873,-8.90715722391885,130.690995787233));
#72207=CARTESIAN_POINT('Ctrl Pts',(77.9514620741457,-8.81644963145446,130.686066293958));
#72208=CARTESIAN_POINT('Ctrl Pts',(77.9635073127305,-8.72669596197999,130.681136800683));
#72209=CARTESIAN_POINT('Ctrl Pts',(77.9750243886388,-8.64087783416966,130.67642345708));
#72210=CARTESIAN_POINT('Ctrl Pts',(77.9919501516155,-8.55593137583548,130.671710113477));
#72211=CARTESIAN_POINT('Ctrl Pts',(78.014131603958,-8.47243552422342,130.666996769874));
#72212=CARTESIAN_POINT('Ctrl Pts',(78.0323398920176,-8.40389553439494,130.663127685166));
#72213=CARTESIAN_POINT('Ctrl Pts',(78.0541363781932,-8.33616506606054,130.659258600459));
#72214=CARTESIAN_POINT('Ctrl Pts',(78.079431785375,-8.26964714317534,130.655389515751));
#72215=CARTESIAN_POINT('Ctrl Pts',(78.1046895037667,-8.20322832840126,130.651526195771));
#72216=CARTESIAN_POINT('Ctrl Pts',(78.133435623837,-8.13801892333169,130.64766287579));
#72217=CARTESIAN_POINT('Ctrl Pts',(78.1655306436996,-8.0744084360288,130.64379955581));
#72218=CARTESIAN_POINT('Ctrl Pts',(78.1975880162222,-8.01087256359274,130.639940767489));
#72219=CARTESIAN_POINT('Ctrl Pts',(78.2329862679424,-7.94893231509545,130.636081979169));
#72220=CARTESIAN_POINT('Ctrl Pts',(78.2715378619355,-7.88895715664184,130.632223190848));
#72221=CARTESIAN_POINT('Ctrl Pts',(78.3100651713178,-7.82901977803666,130.628366833275));
#72222=CARTESIAN_POINT('Ctrl Pts',(78.3517416199971,-7.77104544125757,130.624510475702));
#72223=CARTESIAN_POINT('Ctrl Pts',(78.39633452927,-7.71537763506611,130.620654118128));
#72224=CARTESIAN_POINT('Ctrl Pts',(78.4409142653881,-7.65972627365573,130.616798899759));
#72225=CARTESIAN_POINT('Ctrl Pts',(78.4884084481412,-7.60638046905467,130.612943681389));
#72226=CARTESIAN_POINT('Ctrl Pts',(78.538543041537,-7.55565200832347,130.609088463019));
#72227=CARTESIAN_POINT('Ctrl Pts',(78.588679595042,-7.50492156426463,130.605233093922));
#72228=CARTESIAN_POINT('Ctrl Pts',(78.6414564211046,-7.45680901120684,130.601377724824));
#72229=CARTESIAN_POINT('Ctrl Pts',(78.6965626498843,-7.41158927325979,130.597522355727));
#72230=CARTESIAN_POINT('Ctrl Pts',(78.7517265596389,-7.36632220275835,130.593662951125));
#72231=CARTESIAN_POINT('Ctrl Pts',(78.8092243630841,-7.32395430067749,130.589803546523));
#72232=CARTESIAN_POINT('Ctrl Pts',(78.8687128334742,-7.28471958288035,130.585944141922));
#72233=CARTESIAN_POINT('Ctrl Pts',(78.9282349866143,-7.24546265013672,130.5820825521));
#72234=CARTESIAN_POINT('Ctrl Pts',(78.9897496313597,-7.20934267930978,130.578220962279));
#72235=CARTESIAN_POINT('Ctrl Pts',(79.0528877151142,-7.1765483603017,130.574359372458));
#72236=CARTESIAN_POINT('Ctrl Pts',(79.1161362606994,-7.14369666672193,130.570491026678));
#72237=CARTESIAN_POINT('Ctrl Pts',(79.1810134736196,-7.11418244262259,130.566622680898));
#72238=CARTESIAN_POINT('Ctrl Pts',(79.2471297063824,-7.08814647959419,130.562754335118));
#72239=CARTESIAN_POINT('Ctrl Pts',(79.2863873152439,-7.07268719508579,130.560457440706));
#72240=CARTESIAN_POINT('Ctrl Pts',(79.3260814289308,-7.0584532561107,130.558160546294));
#72241=CARTESIAN_POINT('Ctrl Pts',(79.3661283994563,-7.04546569318312,130.555863651882));
#72242=CARTESIAN_POINT('Ctrl Pts',(79.4335880972261,-7.02358795665611,130.551994500213));
#72243=CARTESIAN_POINT('Ctrl Pts',(79.5023139048528,-7.00516397119918,130.548125348544));
#72244=CARTESIAN_POINT('Ctrl Pts',(79.5719187854035,-6.9903373327323,130.544256196876));
#72245=CARTESIAN_POINT('Ctrl Pts',(79.6441103182617,-6.97495970763487,130.54024326003));
#72246=CARTESIAN_POINT('Ctrl Pts',(79.7172470800461,-6.96345231053239,130.536230323184));
#72247=CARTESIAN_POINT('Ctrl Pts',(79.7908772299262,-6.95591946598558,130.532217386337));
#72248=CARTESIAN_POINT('Ctrl Pts',(79.8616761607451,-6.94867627361388,130.528358754532));
#72249=CARTESIAN_POINT('Ctrl Pts',(79.9329306947213,-6.94510762601367,130.524500122727));
#72250=CARTESIAN_POINT('Ctrl Pts',(80.004228495175,-6.9452543509406,130.520641490922));
#72251=CARTESIAN_POINT('Ctrl Pts',(80.0754817362487,-6.94540098416803,130.516785270667));
#72252=CARTESIAN_POINT('Ctrl Pts',(80.1467777054929,-6.94925838149796,130.512929050412));
#72253=CARTESIAN_POINT('Ctrl Pts',(80.2177016824627,-6.95681534364784,130.509072830158));
#72254=CARTESIAN_POINT('Ctrl Pts',(80.2886050591163,-6.96437011083043,130.505217729966));
#72255=CARTESIAN_POINT('Ctrl Pts',(80.3591361753002,-6.9756222575018,130.501362629775));
#72256=CARTESIAN_POINT('Ctrl Pts',(80.4288847876532,-6.99050867097674,130.497507529584));
#72257=CARTESIAN_POINT('Ctrl Pts',(80.4986364724683,-7.00539574020581,130.493652259574));
#72258=CARTESIAN_POINT('Ctrl Pts',(80.5676051105877,-7.02391728997555,130.489796989563));
#72259=CARTESIAN_POINT('Ctrl Pts',(80.6353917187032,-7.04595933350828,130.485941719553));
#72260=CARTESIAN_POINT('Ctrl Pts',(80.7032436165698,-7.06802260718628,130.482082736278));
#72261=CARTESIAN_POINT('Ctrl Pts',(80.7699107501882,-7.09361298979535,130.478223753003));
#72262=CARTESIAN_POINT('Ctrl Pts',(80.8350113131769,-7.12256726635372,130.474364769728));
#72263=CARTESIAN_POINT('Ctrl Pts',(80.9001492847591,-7.1515381808444,130.470503568973));
#72264=CARTESIAN_POINT('Ctrl Pts',(80.9637184610631,-7.18387661662423,130.466642368219));
#72265=CARTESIAN_POINT('Ctrl Pts',(81.025361334346,-7.21937322930149,130.462781167465));
#72266=CARTESIAN_POINT('Ctrl Pts',(81.0870986711808,-7.25492423814713,130.458914049681));
#72267=CARTESIAN_POINT('Ctrl Pts',(81.1469034085351,-7.29364281593865,130.455046931896));
#72268=CARTESIAN_POINT('Ctrl Pts',(81.2044475328565,-7.33527668872698,130.451179814112));
#72269=CARTESIAN_POINT('Ctrl Pts',(81.2204890700428,-7.34688293569694,130.450101780265));
#72270=CARTESIAN_POINT('Ctrl Pts',(81.2363551343962,-7.35871550197462,130.449023746417));
#72271=CARTESIAN_POINT('Ctrl Pts',(81.2520391107129,-7.37076839346111,130.44794571257));
#72272=CARTESIAN_POINT('',(77.9452507933687,-9.00180564337554,130.754074719418));
#72273=CARTESIAN_POINT('Ctrl Pts',(77.9452507933687,-9.00180564337555,130.754074719418));
#72274=CARTESIAN_POINT('Ctrl Pts',(77.9451892124666,-8.93172906490193,130.75026907596));
#72275=CARTESIAN_POINT('Ctrl Pts',(77.9487167666403,-8.86153512362492,130.746463432502));
#72276=CARTESIAN_POINT('Ctrl Pts',(77.9558428519795,-8.79162745695133,130.742657789045));
#72277=CARTESIAN_POINT('Ctrl Pts',(77.9629627689979,-8.72178030217006,130.738855439742));
#72278=CARTESIAN_POINT('Ctrl Pts',(77.9736749941492,-8.65221942719567,130.735053090439));
#72279=CARTESIAN_POINT('Ctrl Pts',(77.9879368905025,-8.5833471398165,130.731250741136));
#72280=CARTESIAN_POINT('Ctrl Pts',(78.0021915378923,-8.51450985848987,130.727450324471));
#72281=CARTESIAN_POINT('Ctrl Pts',(78.0199921779358,-8.44636096084695,130.723649907807));
#72282=CARTESIAN_POINT('Ctrl Pts',(78.0412447589193,-8.37929437892127,130.719849491143));
#72283=CARTESIAN_POINT('Ctrl Pts',(78.0624941303822,-8.31223792525093,130.716049648409));
#72284=CARTESIAN_POINT('Ctrl Pts',(78.0871942556725,-8.24626394027792,130.712249805676));
#72285=CARTESIAN_POINT('Ctrl Pts',(78.1152012631972,-8.18175108662069,130.708449962943));
#72286=CARTESIAN_POINT('Ctrl Pts',(78.1432332471445,-8.11718070092245,130.70464673154));
#72287=CARTESIAN_POINT('Ctrl Pts',(78.1745778040796,-8.05407451019606,130.700843500138));
#72288=CARTESIAN_POINT('Ctrl Pts',(78.2090433737826,-7.99279002908629,130.697040268735));
#72289=CARTESIAN_POINT('Ctrl Pts',(78.2435240047018,-7.93147876708109,130.693235375347));
#72290=CARTESIAN_POINT('Ctrl Pts',(78.281128094716,-7.87199122326443,130.689430481959));
#72291=CARTESIAN_POINT('Ctrl Pts',(78.3216202127564,-7.81465665215848,130.685625588571));
#72292=CARTESIAN_POINT('Ctrl Pts',(78.3621848365631,-7.75721941694875,130.681813882086));
#72293=CARTESIAN_POINT('Ctrl Pts',(78.4056475048417,-7.70194324737498,130.678002175601));
#72294=CARTESIAN_POINT('Ctrl Pts',(78.4517323843917,-7.64912437546652,130.674190469116));
#72295=CARTESIAN_POINT('Ctrl Pts',(78.4895041823922,-7.60583330516712,130.671066342314));
#72296=CARTESIAN_POINT('Ctrl Pts',(78.5290366712978,-7.56419239373585,130.667942215512));
#72297=CARTESIAN_POINT('Ctrl Pts',(78.5701610019991,-7.52434489046531,130.664818088709));
#72298=CARTESIAN_POINT('Ctrl Pts',(78.6210915251772,-7.47499565719387,130.660949006592));
#72299=CARTESIAN_POINT('Ctrl Pts',(78.6746796484665,-7.42818957462096,130.657079924474));
#72300=CARTESIAN_POINT('Ctrl Pts',(78.7306411390617,-7.38422599208386,130.653210842356));
#72301=CARTESIAN_POINT('Ctrl Pts',(78.7865192498114,-7.34032791310425,130.649347524979));
#72302=CARTESIAN_POINT('Ctrl Pts',(78.8447633297201,-7.29926422509389,130.645484207602));
#72303=CARTESIAN_POINT('Ctrl Pts',(78.9050530730376,-7.2612968080677,130.641620890225));
#72304=CARTESIAN_POINT('Ctrl Pts',(78.9652720965509,-7.22337392678093,130.637762104515));
#72305=CARTESIAN_POINT('Ctrl Pts',(79.0275316080639,-7.18854035986118,130.633903318805));
#72306=CARTESIAN_POINT('Ctrl Pts',(79.0914804690462,-7.15701605422743,130.630044533095));
#72307=CARTESIAN_POINT('Ctrl Pts',(79.1553890469699,-7.12551160657752,130.626188178135));
#72308=CARTESIAN_POINT('Ctrl Pts',(79.2209844283878,-7.09731249870358,130.622331823175));
#72309=CARTESIAN_POINT('Ctrl Pts',(79.2878901805766,-7.07259314944127,130.618475468214));
#72310=CARTESIAN_POINT('Ctrl Pts',(79.354776168195,-7.04788110250054,130.614620252457));
#72311=CARTESIAN_POINT('Ctrl Pts',(79.4229713026635,-7.02664694166551,130.610765036699));
#72312=CARTESIAN_POINT('Ctrl Pts',(79.4920800506123,-7.00901660290348,130.606909820942));
#72313=CARTESIAN_POINT('Ctrl Pts',(79.5611915005902,-6.99138557482657,130.603054454452));
#72314=CARTESIAN_POINT('Ctrl Pts',(79.6312161637148,-6.97735876651486,130.599199087962));
#72315=CARTESIAN_POINT('Ctrl Pts',(79.70174594251,-6.96701153970546,130.595343721472));
#72316=CARTESIAN_POINT('Ctrl Pts',(79.7723495469836,-6.95665348213704,130.591484319453));
#72317=CARTESIAN_POINT('Ctrl Pts',(79.8434588409484,-6.94998276524663,130.587624917433));
#72318=CARTESIAN_POINT('Ctrl Pts',(79.9146590843218,-6.94702301751549,130.583765515413));
#72319=CARTESIAN_POINT('Ctrl Pts',(79.9858996419443,-6.94406159394727,130.579903928163));
#72320=CARTESIAN_POINT('Ctrl Pts',(80.0572307655028,-6.94481531721578,130.576042340914));
#72321=CARTESIAN_POINT('Ctrl Pts',(80.1282389460113,-6.94925566312475,130.572180753664));
#72322=CARTESIAN_POINT('Ctrl Pts',(80.199371358203,-6.95370377759844,130.568312410411));
#72323=CARTESIAN_POINT('Ctrl Pts',(80.2701792165508,-6.96185133656276,130.564444067159));
#72324=CARTESIAN_POINT('Ctrl Pts',(80.3402560516066,-6.97361815497545,130.560575723906));
#72325=CARTESIAN_POINT('Ctrl Pts',(80.381865783308,-6.98060497389702,130.558278806176));
#72326=CARTESIAN_POINT('Ctrl Pts',(80.4232179919651,-6.9888668452408,130.555981888447));
#72327=CARTESIAN_POINT('Ctrl Pts',(80.4642301545167,-6.99837867563882,130.553684970717));
#72328=CARTESIAN_POINT('Ctrl Pts',(80.5351039378127,-7.01481622402536,130.549715629934));
#72329=CARTESIAN_POINT('Ctrl Pts',(80.605246038444,-7.03505572659329,130.545746289151));
#72330=CARTESIAN_POINT('Ctrl Pts',(80.6742185442106,-7.05901393174951,130.541776948368));
#72331=CARTESIAN_POINT('Ctrl Pts',(80.7413369803834,-7.08232810956167,130.537914308567));
#72332=CARTESIAN_POINT('Ctrl Pts',(80.8073474059089,-7.10916343562223,130.534051668765));
#72333=CARTESIAN_POINT('Ctrl Pts',(80.8718566425127,-7.13939161632369,130.530189028963));
#72334=CARTESIAN_POINT('Ctrl Pts',(80.939038869302,-7.17087232510634,130.52616633769));
#72335=CARTESIAN_POINT('Ctrl Pts',(81.0045922551066,-7.20603309031259,130.522143646416));
#72336=CARTESIAN_POINT('Ctrl Pts',(81.068092810446,-7.24467230672629,130.518120955142));
#72337=CARTESIAN_POINT('Ctrl Pts',(81.1315933657854,-7.28331152314,130.514098263869));
#72338=CARTESIAN_POINT('Ctrl Pts',(81.1930405549278,-7.32542892237426,130.510075572595));
#72339=CARTESIAN_POINT('Ctrl Pts',(81.2520391107129,-7.37076839346111,130.506052881321));
#72340=CARTESIAN_POINT('Ctrl Pts',(81.2520391107129,-7.37076839346111,131.206019331682));
#72341=CARTESIAN_POINT('Ctrl Pts',(81.3108254762814,-7.41594479967191,131.201991466223));
#72342=CARTESIAN_POINT('Ctrl Pts',(81.3672518683302,-7.46437480581457,131.197963600765));
#72343=CARTESIAN_POINT('Ctrl Pts',(81.420942732416,-7.51577652838455,131.193935735306));
#72344=CARTESIAN_POINT('Ctrl Pts',(81.4723686497498,-7.56500987153721,131.190077785176));
#72345=CARTESIAN_POINT('Ctrl Pts',(81.5212847957304,-7.61696888104173,131.186219835045));
#72346=CARTESIAN_POINT('Ctrl Pts',(81.5673942501132,-7.67136429853329,131.182361884915));
#72347=CARTESIAN_POINT('Ctrl Pts',(81.6134791222044,-7.72573071624524,131.17850599157));
#72348=CARTESIAN_POINT('Ctrl Pts',(81.6567599581888,-7.78253059464984,131.174650098225));
#72349=CARTESIAN_POINT('Ctrl Pts',(81.6969781583872,-7.84143938766383,131.17079420488));
#72350=CARTESIAN_POINT('Ctrl Pts',(81.7371883706359,-7.90033648049054,131.166939077374));
#72351=CARTESIAN_POINT('Ctrl Pts',(81.7743368814707,-7.96134125486396,131.163083949868));
#72352=CARTESIAN_POINT('Ctrl Pts',(81.8082077333116,-8.02409920806872,131.159228822363));
#72353=CARTESIAN_POINT('Ctrl Pts',(81.8420831878268,-8.0868656893855,131.155373170988));
#72354=CARTESIAN_POINT('Ctrl Pts',(81.8726798707601,-8.15138539377557,131.151517519613));
#72355=CARTESIAN_POINT('Ctrl Pts',(81.899828028585,-8.21727972793427,131.147661868238));
#72356=CARTESIAN_POINT('Ctrl Pts',(81.9270062103126,-8.28324693646923,131.143801952791));
#72357=CARTESIAN_POINT('Ctrl Pts',(81.9507280728954,-8.35059135785771,131.139942037344));
#72358=CARTESIAN_POINT('Ctrl Pts',(81.9708725888309,-8.41891583992077,131.136082121897));
#72359=CARTESIAN_POINT('Ctrl Pts',(81.9910302592243,-8.4872849381727,131.132219685908));
#72360=CARTESIAN_POINT('Ctrl Pts',(82.0076058223155,-8.55663489829064,131.12835724992));
#72361=CARTESIAN_POINT('Ctrl Pts',(82.0205292093832,-8.62655753250442,131.124494813931));
#72362=CARTESIAN_POINT('Ctrl Pts',(82.0334740890637,-8.69659645357762,131.120625954406));
#72363=CARTESIAN_POINT('Ctrl Pts',(82.0427546124962,-8.76720946810902,131.116757094882));
#72364=CARTESIAN_POINT('Ctrl Pts',(82.0483525478946,-8.83798332791455,131.112888235357));
#72365=CARTESIAN_POINT('Ctrl Pts',(82.0500587935554,-8.85955513655416,131.111709010463));
#72366=CARTESIAN_POINT('Ctrl Pts',(82.051423284175,-8.88114189500333,131.110529785569));
#72367=CARTESIAN_POINT('Ctrl Pts',(82.0524464644487,-8.90273195246212,131.109350560675));
#72368=CARTESIAN_POINT('Ctrl Pts',(82.0558035588436,-8.97356977326592,131.105481477794));
#72369=CARTESIAN_POINT('Ctrl Pts',(82.055495594845,-9.04472034164982,131.101612394913));
#72370=CARTESIAN_POINT('Ctrl Pts',(82.0514858739564,-9.1157724987093,131.097743312031));
#72371=CARTESIAN_POINT('Ctrl Pts',(82.0474821273517,-9.18671879160199,131.09387999389));
#72372=CARTESIAN_POINT('Ctrl Pts',(82.0397875989869,-9.25756648316244,131.090016675749));
#72373=CARTESIAN_POINT('Ctrl Pts',(82.0284175513188,-9.32790211954455,131.086153357608));
#72374=CARTESIAN_POINT('Ctrl Pts',(82.017060840712,-9.398155252254,131.082294571138));
#72375=CARTESIAN_POINT('Ctrl Pts',(82.002037251814,-9.46789704563033,131.078435784667));
#72376=CARTESIAN_POINT('Ctrl Pts',(81.9834138929834,-9.53671863356917,131.074576998197));
#72377=CARTESIAN_POINT('Ctrl Pts',(81.9648022655031,-9.60549686895472,131.070720642479));
#72378=CARTESIAN_POINT('Ctrl Pts',(81.9425954935463,-9.67335558113362,131.066864286761));
#72379=CARTESIAN_POINT('Ctrl Pts',(81.9169115671826,-9.73989702398478,131.063007931043));
#72380=CARTESIAN_POINT('Ctrl Pts',(81.8912352281081,-9.80641880982698,131.059152714531));
#72381=CARTESIAN_POINT('Ctrl Pts',(81.8620839487075,-9.87162364593301,131.05529749802));
#72382=CARTESIAN_POINT('Ctrl Pts',(81.8296247232369,-9.93513150659159,131.051442281508));
#72383=CARTESIAN_POINT('Ctrl Pts',(81.7971642287085,-9.99864185021608,131.047586914269));
#72384=CARTESIAN_POINT('Ctrl Pts',(81.7613957543859,-10.0604546551141,131.043731547029));
#72385=CARTESIAN_POINT('Ctrl Pts',(81.7225325466069,-10.1202139029578,131.03987617979));
#72386=CARTESIAN_POINT('Ctrl Pts',(81.683628659651,-10.1800357024321,131.036016777033));
#72387=CARTESIAN_POINT('Ctrl Pts',(81.6416238381699,-10.2377992458656,131.032157374276));
#72388=CARTESIAN_POINT('Ctrl Pts',(81.5967745355417,-10.2931777314606,131.02829797152));
#72389=CARTESIAN_POINT('Ctrl Pts',(81.5518998388882,-10.3485875727865,131.024436383539));
#72390=CARTESIAN_POINT('Ctrl Pts',(81.5041777800796,-10.4016093067255,131.020574795558));
#72391=CARTESIAN_POINT('Ctrl Pts',(81.4539031289799,-10.4519515329522,131.016713207577));
#72392=CARTESIAN_POINT('Ctrl Pts',(81.403540520585,-10.5023818346994,131.01284486361));
#72393=CARTESIAN_POINT('Ctrl Pts',(81.3506167645223,-10.5501229437333,131.008976519643));
#72394=CARTESIAN_POINT('Ctrl Pts',(81.2954607381983,-10.5949228941509,131.005108175676));
#72395=CARTESIAN_POINT('Ctrl Pts',(81.2627106817069,-10.6215238116711,131.002811264679));
#72396=CARTESIAN_POINT('Ctrl Pts',(81.2291741999367,-10.6470885862042,131.000514353681));
#72397=CARTESIAN_POINT('Ctrl Pts',(81.1949246752987,-10.6715718898277,130.998217442684));
#72398=CARTESIAN_POINT('Ctrl Pts',(81.1372323025235,-10.712813334617,130.994348359918));
#72399=CARTESIAN_POINT('Ctrl Pts',(81.0772893247062,-10.7511452709508,130.990479277153));
#72400=CARTESIAN_POINT('Ctrl Pts',(81.0154212654763,-10.7863138627124,130.986610194388));
#72401=CARTESIAN_POINT('Ctrl Pts',(80.9536453865701,-10.8214300550256,130.982746876363));
#72402=CARTESIAN_POINT('Ctrl Pts',(80.8899505385777,-10.8533920202796,130.978883558338));
#72403=CARTESIAN_POINT('Ctrl Pts',(80.8246923557848,-10.8819883317412,130.975020240313));
#72404=CARTESIAN_POINT('Ctrl Pts',(80.7595107208086,-10.9105510997434,130.971161453958));
#72405=CARTESIAN_POINT('Ctrl Pts',(80.6927698363414,-10.9357558618127,130.967302667603));
#72406=CARTESIAN_POINT('Ctrl Pts',(80.6248496025533,-10.9574372369731,130.963443881248));
#72407=CARTESIAN_POINT('Ctrl Pts',(80.5569721535271,-10.9791049544587,130.959587525646));
#72408=CARTESIAN_POINT('Ctrl Pts',(80.4879172907714,-10.9972535410618,130.955731170043));
#72409=CARTESIAN_POINT('Ctrl Pts',(80.4180831694305,-11.011766394475,130.951874814441));
#72410=CARTESIAN_POINT('Ctrl Pts',(80.3482696777804,-11.0262749606476,130.948019598044));
#72411=CARTESIAN_POINT('Ctrl Pts',(80.2776778599192,-11.0371498270919,130.944164381647));
#72412=CARTESIAN_POINT('Ctrl Pts',(80.2067175623955,-11.0443251727397,130.94030916525));
#72413=CARTESIAN_POINT('Ctrl Pts',(80.1357544905257,-11.0515007989232,130.936453798125));
#72414=CARTESIAN_POINT('Ctrl Pts',(80.0644233939313,-11.0549765704646,130.932598431));
#72415=CARTESIAN_POINT('Ctrl Pts',(79.9931390359827,-11.0547385453319,130.928743063875));
#72416=CARTESIAN_POINT('Ctrl Pts',(79.9217800627219,-11.0545002710517,130.92488366123));
#72417=CARTESIAN_POINT('Ctrl Pts',(79.850468412543,-11.0505404417333,130.921024258585));
#72418=CARTESIAN_POINT('Ctrl Pts',(79.7796177376916,-11.0428972614793,130.917164855941));
#72419=CARTESIAN_POINT('Ctrl Pts',(79.7087269466182,-11.0352497535952,130.913303268072));
#72420=CARTESIAN_POINT('Ctrl Pts',(79.6382981302969,-11.0239148203288,130.909441680202));
#72421=CARTESIAN_POINT('Ctrl Pts',(79.568735981132,-11.0089820577919,130.905580092333));
#72422=CARTESIAN_POINT('Ctrl Pts',(79.4990521304568,-10.9940231698437,130.901711748475));
#72423=CARTESIAN_POINT('Ctrl Pts',(79.4302384433608,-10.9754540120118,130.897843404617));
#72424=CARTESIAN_POINT('Ctrl Pts',(79.3626849813448,-10.9534142237366,130.893975060759));
#72425=CARTESIAN_POINT('Ctrl Pts',(79.322573666333,-10.940327627374,130.891678148737));
#72426=CARTESIAN_POINT('Ctrl Pts',(79.282906308109,-10.9260183444643,130.889381236715));
#72427=CARTESIAN_POINT('Ctrl Pts',(79.2437607894409,-10.9105234410791,130.887084324692));
#72428=CARTESIAN_POINT('Ctrl Pts',(79.1778212781382,-10.8844227176334,130.883215241808));
#72429=CARTESIAN_POINT('Ctrl Pts',(79.1131054573431,-10.8548531261454,130.879346158925));
#72430=CARTESIAN_POINT('Ctrl Pts',(79.0500031407997,-10.8219504740826,130.875477076041));
#72431=CARTESIAN_POINT('Ctrl Pts',(78.9869948435725,-10.7890968453364,130.871613757898));
#72432=CARTESIAN_POINT('Ctrl Pts',(78.9255957058774,-10.7529202363441,130.867750439756));
#72433=CARTESIAN_POINT('Ctrl Pts',(78.8661762433591,-10.7136047535464,130.863887121613));
#72434=CARTESIAN_POINT('Ctrl Pts',(78.8068264798667,-10.6743353878076,130.860028335142));
#72435=CARTESIAN_POINT('Ctrl Pts',(78.7494521821209,-10.6319347285184,130.856169548672));
#72436=CARTESIAN_POINT('Ctrl Pts',(78.6943983425402,-10.5866322430035,130.852310762201));
#72437=CARTESIAN_POINT('Ctrl Pts',(78.6393791828529,-10.5413582947419,130.848454406484));
#72438=CARTESIAN_POINT('Ctrl Pts',(78.5866779555273,-10.493186454796,130.844598050766));
#72439=CARTESIAN_POINT('Ctrl Pts',(78.5366085735479,-10.4423879836876,130.840741695049));
#72440=CARTESIAN_POINT('Ctrl Pts',(78.4865539825763,-10.3916045189674,130.836886478539));
#72441=CARTESIAN_POINT('Ctrl Pts',(78.4391300342721,-10.3381963093146,130.833031262028));
#72442=CARTESIAN_POINT('Ctrl Pts',(78.3946143198086,-10.2824719803318,130.829176045518));
#72443=CARTESIAN_POINT('Ctrl Pts',(78.3500968649242,-10.2267454727075,130.825320678281));
#72444=CARTESIAN_POINT('Ctrl Pts',(78.3084881711024,-10.1687030468921,130.821465311044));
#72445=CARTESIAN_POINT('Ctrl Pts',(78.2700249110102,-10.1086855974418,130.817609943807));
#72446=CARTESIAN_POINT('Ctrl Pts',(78.2315213903893,-10.048605326113,130.813750541054));
#72447=CARTESIAN_POINT('Ctrl Pts',(78.1961701385383,-9.98654631417253,130.8098911383));
#72448=CARTESIAN_POINT('Ctrl Pts',(78.1641634157798,-9.92287680572152,130.806031735547));
#72449=CARTESIAN_POINT('Ctrl Pts',(78.1321385705706,-9.85917124710896,130.80217014757));
#72450=CARTESIAN_POINT('Ctrl Pts',(78.103462219597,-9.7938538217371,130.798308559593));
#72451=CARTESIAN_POINT('Ctrl Pts',(78.0782785874139,-9.72731312026404,130.794446971617));
#72452=CARTESIAN_POINT('Ctrl Pts',(78.0530508955748,-9.66065600347805,130.790578627655));
#72453=CARTESIAN_POINT('Ctrl Pts',(78.0313282706817,-9.59277180050978,130.786710283693));
#72454=CARTESIAN_POINT('Ctrl Pts',(78.0132049587201,-9.52406395262953,130.782841939732));
#72455=CARTESIAN_POINT('Ctrl Pts',(78.0024438590867,-9.48326721535527,130.780545028721));
#72456=CARTESIAN_POINT('Ctrl Pts',(77.9929507711792,-9.44218030000125,130.778248117711));
#72457=CARTESIAN_POINT('Ctrl Pts',(77.9847367966347,-9.40088874224893,130.775951206701));
#72458=CARTESIAN_POINT('Ctrl Pts',(77.9647646110824,-9.3004887898615,130.77036629374));
#72459=CARTESIAN_POINT('Ctrl Pts',(77.9522903129557,-9.19855146660896,130.764781380779));
#72460=CARTESIAN_POINT('Ctrl Pts',(77.9474937711085,-9.09599866072768,130.759196467817));
#72461=CARTESIAN_POINT('Ctrl Pts',(77.9460275184567,-9.06464934108068,130.757489218366));
#72462=CARTESIAN_POINT('Ctrl Pts',(77.945278419186,-9.03324269326322,130.755781968914));
#72463=CARTESIAN_POINT('Ctrl Pts',(77.9452507933694,-9.00180564418067,130.754074719462));
#72464=CARTESIAN_POINT('Origin',(80.,-9.,141.545925280538));
#72465=CARTESIAN_POINT('',(81.2520391107129,-7.3707683934611,131.906140964161));
#72466=CARTESIAN_POINT('',(81.2520391107129,-7.37076839346113,131.847886939579));
#72467=CARTESIAN_POINT('',(81.2520391107129,-7.37076839346111,141.545925280538));
#72468=CARTESIAN_POINT('',(77.9452501035681,-9.00065239039587,131.39592528057));
#72469=CARTESIAN_POINT('Ctrl Pts',(81.2520391107129,-7.37076839346113,131.847886939579));
#72470=CARTESIAN_POINT('Ctrl Pts',(81.3085634825606,-7.41420649273306,131.844031409821));
#72471=CARTESIAN_POINT('Ctrl Pts',(81.3628520478468,-7.46061066578053,131.840175880064));
#72472=CARTESIAN_POINT('Ctrl Pts',(81.4145852360442,-7.50971607655934,131.836320350307));
#72473=CARTESIAN_POINT('Ctrl Pts',(81.4663133131985,-7.55881663590943,131.832465201462));
#72474=CARTESIAN_POINT('Ctrl Pts',(81.5154861631145,-7.6106175677554,131.828610052616));
#72475=CARTESIAN_POINT('Ctrl Pts',(81.5618198988355,-7.66481605533116,131.824754903771));
#72476=CARTESIAN_POINT('Ctrl Pts',(81.6083190592735,-7.71920804704219,131.820885990939));
#72477=CARTESIAN_POINT('Ctrl Pts',(81.6519584670128,-7.77601437920203,131.817017078107));
#72478=CARTESIAN_POINT('Ctrl Pts',(81.6924922190995,-7.83489586268532,131.813148165275));
#72479=CARTESIAN_POINT('Ctrl Pts',(81.7329383906802,-7.89365012206901,131.80928761193));
#72480=CARTESIAN_POINT('Ctrl Pts',(81.7702920867994,-7.95447014009036,131.805427058584));
#72481=CARTESIAN_POINT('Ctrl Pts',(81.8043538921319,-8.01699206796262,131.801566505239));
#72482=CARTESIAN_POINT('Ctrl Pts',(81.8385263315502,-8.07971706951997,131.797693412664));
#72483=CARTESIAN_POINT('Ctrl Pts',(81.8693852591814,-8.14415460682124,131.793820320089));
#72484=CARTESIAN_POINT('Ctrl Pts',(81.8967778292422,-8.2099168214706,131.789947227514));
#72485=CARTESIAN_POINT('Ctrl Pts',(81.9241703993031,-8.27567903611997,131.786074134939));
#72486=CARTESIAN_POINT('Ctrl Pts',(81.9480965076543,-8.3427654484236,131.782201042364));
#72487=CARTESIAN_POINT('Ctrl Pts',(81.9684540117226,-8.41077477461233,131.778327949789));
#72488=CARTESIAN_POINT('Ctrl Pts',(81.9887904401113,-8.47871369222997,131.774458866942));
#72489=CARTESIAN_POINT('Ctrl Pts',(82.0056453207931,-8.54783974469615,131.770589784096));
#72490=CARTESIAN_POINT('Ctrl Pts',(82.0188839110767,-8.61776274894318,131.766720701249));
#72491=CARTESIAN_POINT('Ctrl Pts',(82.0321027765211,-8.68758157140082,131.762857383143));
#72492=CARTESIAN_POINT('Ctrl Pts',(82.0417159571494,-8.75819451523129,131.758994065037));
#72493=CARTESIAN_POINT('Ctrl Pts',(82.0476385852171,-8.82919664280217,131.75513074693));
#72494=CARTESIAN_POINT('Ctrl Pts',(82.0535542660443,-8.90011548490451,131.751271960495));
#72495=CARTESIAN_POINT('Ctrl Pts',(82.0557879530187,-8.97142212220669,131.747413174059));
#72496=CARTESIAN_POINT('Ctrl Pts',(82.0543062010365,-9.04270356991117,131.743554387624));
#72497=CARTESIAN_POINT('Ctrl Pts',(82.0528253824494,-9.11394011553025,131.739698031941));
#72498=CARTESIAN_POINT('Ctrl Pts',(82.0476337784022,-9.18515101850258,131.735841676258));
#72499=CARTESIAN_POINT('Ctrl Pts',(82.0387500055478,-9.25592181888014,131.731985320575));
#72500=CARTESIAN_POINT('Ctrl Pts',(82.0298688570489,-9.32667171285441,131.728130104098));
#72501=CARTESIAN_POINT('Ctrl Pts',(82.0172977655642,-9.39698128060341,131.724274887621));
#72502=CARTESIAN_POINT('Ctrl Pts',(82.001107178664,-9.46644144541354,131.720419671144));
#72503=CARTESIAN_POINT('Ctrl Pts',(81.9849159587603,-9.53590432590819,131.71656430394));
#72504=CARTESIAN_POINT('Ctrl Pts',(81.9651050749101,-9.60451726493085,131.712708936735));
#72505=CARTESIAN_POINT('Ctrl Pts',(81.941795650409,-9.67188333403389,131.708853569531));
#72506=CARTESIAN_POINT('Ctrl Pts',(81.9184618272967,-9.73931991704135,131.704994166809));
#72507=CARTESIAN_POINT('Ctrl Pts',(81.8916223124967,-9.80550656477264,131.701134764086));
#72508=CARTESIAN_POINT('Ctrl Pts',(81.8614472056882,-9.8700642866682,131.697275361364));
#72509=CARTESIAN_POINT('Ctrl Pts',(81.8312550134973,-9.93465856165302,131.693413773417));
#72510=CARTESIAN_POINT('Ctrl Pts',(81.7977236980533,-9.99762164579254,131.68955218547));
#72511=CARTESIAN_POINT('Ctrl Pts',(81.7610690802575,-10.0585996679864,131.685690597524));
#72512=CARTESIAN_POINT('Ctrl Pts',(81.7243503338942,-10.1196843734156,131.68182225359));
#72513=CARTESIAN_POINT('Ctrl Pts',(81.684497647197,-10.1787766802047,131.677953909657));
#72514=CARTESIAN_POINT('Ctrl Pts',(81.6417694498063,-10.2355527654384,131.674085565724));
#72515=CARTESIAN_POINT('Ctrl Pts',(81.6163986757783,-10.2692647710139,131.671788654415));
#72516=CARTESIAN_POINT('Ctrl Pts',(81.5900148690266,-10.3021607970392,131.669491743107));
#72517=CARTESIAN_POINT('Ctrl Pts',(81.5626783192385,-10.3341791607884,131.667194831798));
#72518=CARTESIAN_POINT('Ctrl Pts',(81.516630665768,-10.3881131989183,131.663325748947));
#72519=CARTESIAN_POINT('Ctrl Pts',(81.4676973380779,-10.4397661522298,131.659456666095));
#72520=CARTESIAN_POINT('Ctrl Pts',(81.4161330600869,-10.4888131913134,131.655587583244));
#72521=CARTESIAN_POINT('Ctrl Pts',(81.3646456102982,-10.5377871527552,131.651724265133));
#72522=CARTESIAN_POINT('Ctrl Pts',(81.310535340387,-10.5841625749118,131.647860947022));
#72523=CARTESIAN_POINT('Ctrl Pts',(81.254096421259,-10.6276485273809,131.643997628911));
#72524=CARTESIAN_POINT('Ctrl Pts',(81.1977237049614,-10.6710834708446,131.640138842471));
#72525=CARTESIAN_POINT('Ctrl Pts',(81.1390281480807,-10.711635381957,131.636280056031));
#72526=CARTESIAN_POINT('Ctrl Pts',(81.0783385728406,-10.7490521675536,131.632421269591));
#72527=CARTESIAN_POINT('Ctrl Pts',(81.0176872275828,-10.786445383319,131.628564913903));
#72528=CARTESIAN_POINT('Ctrl Pts',(80.9550447685521,-10.8207071373998,131.624708558215));
#72529=CARTESIAN_POINT('Ctrl Pts',(80.8907694945673,-10.8516282753426,131.620852202528));
#72530=CARTESIAN_POINT('Ctrl Pts',(80.8265132081422,-10.8825402788716,131.616996986046));
#72531=CARTESIAN_POINT('Ctrl Pts',(80.760625501884,-10.9101134149559,131.613141769564));
#72532=CARTESIAN_POINT('Ctrl Pts',(80.6934882640478,-10.9341849937707,131.609286553083));
#72533=CARTESIAN_POINT('Ctrl Pts',(80.6263484013468,-10.9582575137122,131.605431185874));
#72534=CARTESIAN_POINT('Ctrl Pts',(80.5579593680992,-10.9788280427057,131.601575818665));
#72535=CARTESIAN_POINT('Ctrl Pts',(80.4887203319164,-10.99578305426,131.597720451456));
#72536=CARTESIAN_POINT('Ctrl Pts',(80.4194088213442,-11.0127558130878,131.593861048728));
#72537=CARTESIAN_POINT('Ctrl Pts',(80.3492460045624,-11.0261053840647,131.590001646001));
#72538=CARTESIAN_POINT('Ctrl Pts',(80.2786425427956,-11.0357691165366,131.586142243274));
#72539=CARTESIAN_POINT('Ctrl Pts',(80.2079991047945,-11.0454383206898,131.582280655323));
#72540=CARTESIAN_POINT('Ctrl Pts',(80.1369150094404,-11.0514174911261,131.578419067372));
#72541=CARTESIAN_POINT('Ctrl Pts',(80.0658046125601,-11.0536960134026,131.57455747942));
#72542=CARTESIAN_POINT('Ctrl Pts',(79.9945698054933,-11.0559785220355,131.570689135483));
#72543=CARTESIAN_POINT('Ctrl Pts',(79.9233090908679,-11.0545474659095,131.566820791545));
#72544=CARTESIAN_POINT('Ctrl Pts',(79.8524346901784,-11.0494443251372,131.562952447607));
#72545=CARTESIAN_POINT('Ctrl Pts',(79.810351511404,-11.0464142270575,131.56065553634));
#72546=CARTESIAN_POINT('Ctrl Pts',(79.7684044150229,-11.0420904754752,131.558358625073));
#72547=CARTESIAN_POINT('Ctrl Pts',(79.7266779226688,-11.036490266253,131.556061713806));
#72548=CARTESIAN_POINT('Ctrl Pts',(79.6563908124203,-11.0270568703262,131.552192630968));
#72549=CARTESIAN_POINT('Ctrl Pts',(79.5864549840659,-11.0139619085453,131.54832354813));
#72550=CARTESIAN_POINT('Ctrl Pts',(79.5172814947751,-10.9972432018193,131.544454465292));
#72551=CARTESIAN_POINT('Ctrl Pts',(79.4482110705339,-10.9805494051327,131.540591147194));
#72552=CARTESIAN_POINT('Ctrl Pts',(79.3799011990718,-10.9602426939566,131.536727829097));
#72553=CARTESIAN_POINT('Ctrl Pts',(79.3127558531514,-10.9364124160732,131.532864510999));
#72554=CARTESIAN_POINT('Ctrl Pts',(79.2456892686947,-10.9126100910961,131.529005724572));
#72555=CARTESIAN_POINT('Ctrl Pts',(79.179784952049,-10.8852925709212,131.525146938145));
#72556=CARTESIAN_POINT('Ctrl Pts',(79.1154330417219,-10.8545993796027,131.521288151718));
#72557=CARTESIAN_POINT('Ctrl Pts',(79.0511216683789,-10.8239255227437,131.517431796044));
#72558=CARTESIAN_POINT('Ctrl Pts',(78.9883611986391,-10.78988042217,131.513575440369));
#72559=CARTESIAN_POINT('Ctrl Pts',(78.9275216843035,-10.75265165531,131.509719084695));
#72560=CARTESIAN_POINT('Ctrl Pts',(78.8667001425688,-10.7154338861999,131.505863868226));
#72561=CARTESIAN_POINT('Ctrl Pts',(78.8077988437895,-10.6750345713477,131.502008651758));
#72562=CARTESIAN_POINT('Ctrl Pts',(78.7511615977412,-10.6316863079476,131.498153435289));
#72563=CARTESIAN_POINT('Ctrl Pts',(78.6945221373449,-10.5883363497592,131.494298068093));
#72564=CARTESIAN_POINT('Ctrl Pts',(78.6401472898436,-10.5420375111187,131.490442700897));
#72565=CARTESIAN_POINT('Ctrl Pts',(78.588348933253,-10.4930635714034,131.486587333701));
#72566=CARTESIAN_POINT('Ctrl Pts',(78.5364963579054,-10.4440383693257,131.482727930987));
#72567=CARTESIAN_POINT('Ctrl Pts',(78.487226010765,-10.3923328109689,131.478868528272));
#72568=CARTESIAN_POINT('Ctrl Pts',(78.4408132612832,-10.3382579259282,131.475009125558));
#72569=CARTESIAN_POINT('Ctrl Pts',(78.3943742325369,-10.2841524232615,131.471147537619));
#72570=CARTESIAN_POINT('Ctrl Pts',(78.3507963192775,-10.2276753081196,131.467285949681));
#72571=CARTESIAN_POINT('Ctrl Pts',(78.310313177494,-10.169168937472,131.463424361742));
#72572=CARTESIAN_POINT('Ctrl Pts',(78.2697592090004,-10.1105602078285,131.459556017817));
#72573=CARTESIAN_POINT('Ctrl Pts',(78.2323110773254,-10.0499155479552,131.455687673892));
#72574=CARTESIAN_POINT('Ctrl Pts',(78.1981575144787,-9.98760377675981,131.451819329966));
#72575=CARTESIAN_POINT('Ctrl Pts',(78.1778781109871,-9.95060483887392,131.449522418582));
#72576=CARTESIAN_POINT('Ctrl Pts',(78.1587593571235,-9.91301857604652,131.447225507198));
#72577=CARTESIAN_POINT('Ctrl Pts',(78.1408326489501,-9.87492532440782,131.444928595814));
#72578=CARTESIAN_POINT('Ctrl Pts',(78.1081554784628,-9.80548816582994,131.440741738743));
#72579=CARTESIAN_POINT('Ctrl Pts',(78.0793295383054,-9.73412774208689,131.436554881671));
#72580=CARTESIAN_POINT('Ctrl Pts',(78.0545656017943,-9.66127344176059,131.432368024599));
#72581=CARTESIAN_POINT('Ctrl Pts',(78.0298638437661,-9.58860206751596,131.42819168009));
#72582=CARTESIAN_POINT('Ctrl Pts',(78.0092039024853,-9.51444461665576,131.42401533558));
#72583=CARTESIAN_POINT('Ctrl Pts',(77.9927491649568,-9.43925123530684,131.41983899107));
#72584=CARTESIAN_POINT('Ctrl Pts',(77.9763607882809,-9.36436110382013,131.415679489478));
#72585=CARTESIAN_POINT('Ctrl Pts',(77.964143907639,-9.28844370983482,131.411519987886));
#72586=CARTESIAN_POINT('Ctrl Pts',(77.9562120164592,-9.21196282889739,131.407360486294));
#72587=CARTESIAN_POINT('Ctrl Pts',(77.948943292438,-9.14187633832032,131.403548751052));
#72588=CARTESIAN_POINT('Ctrl Pts',(77.9452725398498,-9.07131705349499,131.399737015811));
#72589=CARTESIAN_POINT('Ctrl Pts',(77.9452501035681,-9.00065239039586,131.39592528057));
#72590=CARTESIAN_POINT('Ctrl Pts',(77.9452501035679,-9.00065238980674,131.395925280538));
#72591=CARTESIAN_POINT('Ctrl Pts',(77.9452268384226,-8.92737709575494,131.391972724785));
#72592=CARTESIAN_POINT('Ctrl Pts',(77.9491275646018,-8.85413490590009,131.388020169032));
#72593=CARTESIAN_POINT('Ctrl Pts',(77.9569155176319,-8.78136020397297,131.384067613279));
#72594=CARTESIAN_POINT('Ctrl Pts',(77.9647095603039,-8.70852859725101,131.3801119669));
#72595=CARTESIAN_POINT('Ctrl Pts',(77.9763968270617,-8.63616565292411,131.376156320522));
#72596=CARTESIAN_POINT('Ctrl Pts',(77.9918890690412,-8.56469774700355,131.372200674143));
#72597=CARTESIAN_POINT('Ctrl Pts',(78.0074099266821,-8.49309783298509,131.368237721305));
#72598=CARTESIAN_POINT('Ctrl Pts',(78.0267496922354,-8.42239669799367,131.364274768467));
#72599=CARTESIAN_POINT('Ctrl Pts',(78.0497697059512,-8.35300744774416,131.360311815629));
#72600=CARTESIAN_POINT('Ctrl Pts',(78.0728143784025,-8.28354386864407,131.356344617728));
#72601=CARTESIAN_POINT('Ctrl Pts',(78.0995469862571,-8.21539539157083,131.352377419827));
#72602=CARTESIAN_POINT('Ctrl Pts',(78.1297809942058,-8.14895450599507,131.348410221926));
#72603=CARTESIAN_POINT('Ctrl Pts',(78.160077328868,-8.08237665405856,131.344434845737));
#72604=CARTESIAN_POINT('Ctrl Pts',(78.1938892656029,-8.01751381958153,131.340459469549));
#72605=CARTESIAN_POINT('Ctrl Pts',(78.2309848912298,-7.95473299705641,131.336484093361));
#72606=CARTESIAN_POINT('Ctrl Pts',(78.2393476952122,-7.94057974572926,131.335587888181));
#72607=CARTESIAN_POINT('Ctrl Pts',(78.2478772169343,-7.92653218314774,131.334691683002));
#72608=CARTESIAN_POINT('Ctrl Pts',(78.2565705111978,-7.9125942891106,131.333795477822));
#72609=CARTESIAN_POINT('Ctrl Pts',(78.2941010642335,-7.85242183255806,131.329926394941));
#72610=CARTESIAN_POINT('Ctrl Pts',(78.3348239566215,-7.79407678770886,131.32605731206));
#72611=CARTESIAN_POINT('Ctrl Pts',(78.3785355099981,-7.73791819989232,131.322188229179));
#72612=CARTESIAN_POINT('Ctrl Pts',(78.4221819353426,-7.68184328556781,131.318324911038));
#72613=CARTESIAN_POINT('Ctrl Pts',(78.4688078867317,-7.62794874203111,131.314461592897));
#72614=CARTESIAN_POINT('Ctrl Pts',(78.518165643408,-7.57656594739218,131.310598274756));
#72615=CARTESIAN_POINT('Ctrl Pts',(78.5674655034558,-7.52524342475045,131.306739488286));
#72616=CARTESIAN_POINT('Ctrl Pts',(78.61949046886,-7.47642714733036,131.302880701815));
#72617=CARTESIAN_POINT('Ctrl Pts',(78.6739527858865,-7.43041523056516,131.299021915345));
#72618=CARTESIAN_POINT('Ctrl Pts',(78.7283807956474,-7.38443229793316,131.295165559627));
#72619=CARTESIAN_POINT('Ctrl Pts',(78.7852427407113,-7.34125053392767,131.291309203909));
#72620=CARTESIAN_POINT('Ctrl Pts',(78.8442153428599,-7.30112996706057,131.287452848192));
#72621=CARTESIAN_POINT('Ctrl Pts',(78.903170523911,-7.26102125221097,131.28359763168));
#72622=CARTESIAN_POINT('Ctrl Pts',(78.9642347227805,-7.22397221229798,131.279742415168));
#72623=CARTESIAN_POINT('Ctrl Pts',(79.0270544352444,-7.19020042807984,131.275887198657));
#72624=CARTESIAN_POINT('Ctrl Pts',(79.0898766037698,-7.1564273234867,131.272031831417));
#72625=CARTESIAN_POINT('Ctrl Pts',(79.1544539932407,-7.12593195705841,131.268176464178));
#72626=CARTESIAN_POINT('Ctrl Pts',(79.2204087129456,-7.09888585622828,131.264321096939));
#72627=CARTESIAN_POINT('Ctrl Pts',(79.2864324692501,-7.07181144550855,131.260461694183));
#72628=CARTESIAN_POINT('Ctrl Pts',(79.3538359833414,-7.04819369232281,131.256602291426));
#72629=CARTESIAN_POINT('Ctrl Pts',(79.4222224454191,-7.02815551832237,131.252742888669));
#72630=CARTESIAN_POINT('Ctrl Pts',(79.4906476284457,-7.00810599855131,131.248881300688));
#72631=CARTESIAN_POINT('Ctrl Pts',(79.5600563944949,-6.99164020485382,131.245019712707));
#72632=CARTESIAN_POINT('Ctrl Pts',(79.6300405550026,-6.97883014777154,131.241158124726));
#72633=CARTESIAN_POINT('Ctrl Pts',(79.7001471552952,-6.96599767903749,131.23728978076));
#72634=CARTESIAN_POINT('Ctrl Pts',(79.770830677994,-6.95683377887449,131.233421436793));
#72635=CARTESIAN_POINT('Ctrl Pts',(79.8416773114535,-6.95135862367485,131.229553092826));
#72636=CARTESIAN_POINT('Ctrl Pts',(79.8837439976099,-6.9481076345425,131.227256181828));
#72637=CARTESIAN_POINT('Ctrl Pts',(79.9258681602479,-6.94615616588539,131.224959270829));
#72638=CARTESIAN_POINT('Ctrl Pts',(79.9679636615179,-6.94549976015658,131.222662359831));
#72639=CARTESIAN_POINT('Ctrl Pts',(80.0388583887718,-6.94439428086052,131.21879403961));
#72640=CARTESIAN_POINT('Ctrl Pts',(80.1099492315829,-6.9469604939641,131.21492571939));
#72641=CARTESIAN_POINT('Ctrl Pts',(80.1808243171314,-6.95322201281283,131.211057399169));
#72642=CARTESIAN_POINT('Ctrl Pts',(80.2516008675007,-6.95947482648855,131.20719445694));
#72643=CARTESIAN_POINT('Ctrl Pts',(80.3221617761498,-6.96941271114748,131.203331514712));
#72644=CARTESIAN_POINT('Ctrl Pts',(80.3920944026438,-6.98300730246355,131.199468572483));
#72645=CARTESIAN_POINT('Ctrl Pts',(80.4619532083238,-6.99658754334194,131.195609707972));
#72646=CARTESIAN_POINT('Ctrl Pts',(80.5311845737719,-7.01381673726949,131.191750843462));
#72647=CARTESIAN_POINT('Ctrl Pts',(80.5993819433181,-7.03461483456188,131.187891978951));
#72648=CARTESIAN_POINT('Ctrl Pts',(80.6675362532688,-7.05539980000383,131.184035550915));
#72649=CARTESIAN_POINT('Ctrl Pts',(80.734657399007,-7.07974905664672,131.180179122878));
#72650=CARTESIAN_POINT('Ctrl Pts',(80.800351555953,-7.10753204799037,131.176322694842));
#72651=CARTESIAN_POINT('Ctrl Pts',(80.8660214074106,-7.13530476019795,131.172467693605));
#72652=CARTESIAN_POINT('Ctrl Pts',(80.9302648728479,-7.16650849170464,131.168612692368));
#72653=CARTESIAN_POINT('Ctrl Pts',(80.9927074781101,-7.2009643068009,131.164757691131));
#72654=CARTESIAN_POINT('Ctrl Pts',(81.0551657820356,-7.23542878441596,131.16090172071));
#72655=CARTESIAN_POINT('Ctrl Pts',(81.1158218958355,-7.27314674404535,131.157045750289));
#72656=CARTESIAN_POINT('Ctrl Pts',(81.1743265826277,-7.31389364515938,131.153189779868));
#72657=CARTESIAN_POINT('Ctrl Pts',(81.2006767631621,-7.33224581930889,131.151453072566));
#72658=CARTESIAN_POINT('Ctrl Pts',(81.2265908984792,-7.3512118387721,131.149716365264));
#72659=CARTESIAN_POINT('Ctrl Pts',(81.2520391107129,-7.3707683934611,131.147979657963));
#72660=CARTESIAN_POINT('',(77.9452503396332,-8.99881859296011,131.454074719514));
#72661=CARTESIAN_POINT('Ctrl Pts',(77.9452503396338,-8.99881859201236,131.454074719462));
#72662=CARTESIAN_POINT('Ctrl Pts',(77.9452901831621,-8.92952121357853,131.450299784525));
#72663=CARTESIAN_POINT('Ctrl Pts',(77.9488353855607,-8.86032618901156,131.446524849588));
#72664=CARTESIAN_POINT('Ctrl Pts',(77.955856695627,-8.7914916939617,131.44274991465));
#72665=CARTESIAN_POINT('Ctrl Pts',(77.9630531190942,-8.72094044770435,131.438880831799));
#72666=CARTESIAN_POINT('Ctrl Pts',(77.9739204176304,-8.65062402026964,131.435011748947));
#72667=CARTESIAN_POINT('Ctrl Pts',(77.9884338439667,-8.58095446261622,131.431142666096));
#72668=CARTESIAN_POINT('Ctrl Pts',(78.0029256460216,-8.5113887091287,131.427279347985));
#72669=CARTESIAN_POINT('Ctrl Pts',(78.0210526941546,-8.44246838399812,131.423416029874));
#72670=CARTESIAN_POINT('Ctrl Pts',(78.0427385152252,-8.37460009376617,131.419552711764));
#72671=CARTESIAN_POINT('Ctrl Pts',(78.0643988988361,-8.30681141301247,131.415693925323));
#72672=CARTESIAN_POINT('Ctrl Pts',(78.0896096163957,-8.24007277643222,131.411835138883));
#72673=CARTESIAN_POINT('Ctrl Pts',(78.1182436044466,-8.1747785568141,131.407976352443));
#72674=CARTESIAN_POINT('Ctrl Pts',(78.1468595551847,-8.1095254677665,131.404119996755));
#72675=CARTESIAN_POINT('Ctrl Pts',(78.1788943034942,-8.04571543433216,131.400263641067));
#72676=CARTESIAN_POINT('Ctrl Pts',(78.2141721188595,-7.98372427882916,131.39640728538));
#72677=CARTESIAN_POINT('Ctrl Pts',(78.2494395128048,-7.92175143613432,131.392552068898));
#72678=CARTESIAN_POINT('Ctrl Pts',(78.2879478317048,-7.86159682662655,131.388696852416));
#72679=CARTESIAN_POINT('Ctrl Pts',(78.3294755145793,-7.80361147359645,131.384841635935));
#72680=CARTESIAN_POINT('Ctrl Pts',(78.3710048210619,-7.74562385351272,131.380986268726));
#72681=CARTESIAN_POINT('Ctrl Pts',(78.4155534412473,-7.68980605195061,131.377130901517));
#72682=CARTESIAN_POINT('Ctrl Pts',(78.4628576386407,-7.63647848443282,131.373275534308));
#72683=CARTESIAN_POINT('Ctrl Pts',(78.5102113506287,-7.58309509749437,131.36941613158));
#72684=CARTESIAN_POINT('Ctrl Pts',(78.5603260745858,-7.53220751210493,131.365556728853));
#72685=CARTESIAN_POINT('Ctrl Pts',(78.6128996831315,-7.48410083665061,131.361697326126));
#72686=CARTESIAN_POINT('Ctrl Pts',(78.6655030592671,-7.43596692281909,131.357835738175));
#72687=CARTESIAN_POINT('Ctrl Pts',(78.7205677163503,-7.39061736238294,131.353974150224));
#72688=CARTESIAN_POINT('Ctrl Pts',(78.7777588906715,-7.34829656621796,131.350112562272));
#72689=CARTESIAN_POINT('Ctrl Pts',(78.8350501230007,-7.30590172830415,131.346244218335));
#72690=CARTESIAN_POINT('Ctrl Pts',(78.8944748953435,-7.26654650244283,131.342375874397));
#72691=CARTESIAN_POINT('Ctrl Pts',(78.9556705686811,-7.23043123858347,131.338507530459));
#72692=CARTESIAN_POINT('Ctrl Pts',(78.9920067977859,-7.20898703460304,131.336210619192));
#72693=CARTESIAN_POINT('Ctrl Pts',(79.0289669160089,-7.18868424210409,131.333913707925));
#72694=CARTESIAN_POINT('Ctrl Pts',(79.0664716248486,-7.16955679266272,131.331616796658));
#72695=CARTESIAN_POINT('Ctrl Pts',(79.129647258756,-7.13733713862794,131.32774771382));
#72696=CARTESIAN_POINT('Ctrl Pts',(79.1946166239916,-7.10832886924695,131.323878630982));
#72697=CARTESIAN_POINT('Ctrl Pts',(79.2610201204866,-7.08273468185169,131.320009548144));
#72698=CARTESIAN_POINT('Ctrl Pts',(79.3273246790835,-7.05717862851921,131.316146230047));
#72699=CARTESIAN_POINT('Ctrl Pts',(79.395058677896,-7.03502673327756,131.312282911949));
#72700=CARTESIAN_POINT('Ctrl Pts',(79.4638390357952,-7.01643528389846,131.308419593851));
#72701=CARTESIAN_POINT('Ctrl Pts',(79.532538714362,-6.99786564228206,131.304560807425));
#72702=CARTESIAN_POINT('Ctrl Pts',(79.602281847348,-6.98284827692435,131.300702020998));
#72703=CARTESIAN_POINT('Ctrl Pts',(79.6726681924121,-6.9714903376515,131.296843234571));
#72704=CARTESIAN_POINT('Ctrl Pts',(79.7430101992408,-6.96013955304743,131.292986878896));
#72705=CARTESIAN_POINT('Ctrl Pts',(79.8139941358381,-6.95244369831161,131.289130523222));
#72706=CARTESIAN_POINT('Ctrl Pts',(79.8852089486723,-6.94845897505434,131.285274167547));
#72707=CARTESIAN_POINT('Ctrl Pts',(79.9564027239387,-6.94447542892417,131.281418951079));
#72708=CARTESIAN_POINT('Ctrl Pts',(80.0278267552795,-6.94420086492617,131.27756373461));
#72709=CARTESIAN_POINT('Ctrl Pts',(80.0990659661041,-6.9476395304772,131.273708518142));
#72710=CARTESIAN_POINT('Ctrl Pts',(80.17030796217,-6.95107833046982,131.269853150946));
#72711=CARTESIAN_POINT('Ctrl Pts',(80.2413646382617,-6.95823062261835,131.26599778375));
#72712=CARTESIAN_POINT('Ctrl Pts',(80.3118237572176,-6.96904862024353,131.262142416554));
#72713=CARTESIAN_POINT('Ctrl Pts',(80.3823566276609,-6.97987794136278,131.258283013839));
#72714=CARTESIAN_POINT('Ctrl Pts',(80.452290211231,-6.9943805535867,131.254423611125));
#72715=CARTESIAN_POINT('Ctrl Pts',(80.521221110999,-7.01245726688732,131.250564208411));
#72716=CARTESIAN_POINT('Ctrl Pts',(80.5901910399853,-7.0305442153654,131.246702620472));
#72717=CARTESIAN_POINT('Ctrl Pts',(80.6581566919426,-7.05220914584597,131.242841032534));
#72718=CARTESIAN_POINT('Ctrl Pts',(80.7247311599638,-7.0773033759125,131.238979444595));
#72719=CARTESIAN_POINT('Ctrl Pts',(80.7914221024071,-7.1024415092355,131.23511110067));
#72720=CARTESIAN_POINT('Ctrl Pts',(80.8567165563495,-7.13102072583423,131.231242756745));
#72721=CARTESIAN_POINT('Ctrl Pts',(80.9202495129067,-7.16284502654378,131.227374412819));
#72722=CARTESIAN_POINT('Ctrl Pts',(80.9579735555477,-7.18174138116103,131.225077501435));
#72723=CARTESIAN_POINT('Ctrl Pts',(80.9950770457654,-7.20178096490513,131.222780590051));
#72724=CARTESIAN_POINT('Ctrl Pts',(81.0314884665626,-7.22291556029309,131.220483678667));
#72725=CARTESIAN_POINT('Ctrl Pts',(81.0928208329711,-7.25851523533601,131.216614699991));
#72726=CARTESIAN_POINT('Ctrl Pts',(81.1524281864619,-7.29736350009924,131.212745721315));
#72727=CARTESIAN_POINT('Ctrl Pts',(81.2099452235106,-7.3392681978706,131.208876742639));
#72728=CARTESIAN_POINT('Ctrl Pts',(81.2241048442314,-7.34958435213222,131.20792427232));
#72729=CARTESIAN_POINT('Ctrl Pts',(81.238137884631,-7.36008551775973,131.206971802001));
#72730=CARTESIAN_POINT('Ctrl Pts',(81.2520391107129,-7.37076839346111,131.206019331682));
#72731=CARTESIAN_POINT('Ctrl Pts',(81.2520391107129,-7.3707683934611,131.906140964161));
#72732=CARTESIAN_POINT('Ctrl Pts',(81.3085547243609,-7.41419976219301,131.902272668884));
#72733=CARTESIAN_POINT('Ctrl Pts',(81.3627348190519,-7.46051906654932,131.898404373607));
#72734=CARTESIAN_POINT('Ctrl Pts',(81.4142868175889,-7.50943287299956,131.89453607833));
#72735=CARTESIAN_POINT('Ctrl Pts',(81.4465096511469,-7.54000669144819,131.892118181092));
#72736=CARTESIAN_POINT('Ctrl Pts',(81.4777064491362,-7.57159343467494,131.889700283854));
#72737=CARTESIAN_POINT('Ctrl Pts',(81.5078138187364,-7.60411495798271,131.887282386616));
#72738=CARTESIAN_POINT('Ctrl Pts',(81.5559911794038,-7.65615541115613,131.883413303769));
#72739=CARTESIAN_POINT('Ctrl Pts',(81.6015655640654,-7.71079489866968,131.879544220922));
#72740=CARTESIAN_POINT('Ctrl Pts',(81.6442441695771,-7.76774244846634,131.875675138076));
#72741=CARTESIAN_POINT('Ctrl Pts',(81.686859186095,-7.82460514925387,131.871811819969));
#72742=CARTESIAN_POINT('Ctrl Pts',(81.7265866988018,-7.88376870064298,131.867948501863));
#72743=CARTESIAN_POINT('Ctrl Pts',(81.763172185142,-7.94490691972623,131.864085183757));
#72744=CARTESIAN_POINT('Ctrl Pts',(81.7997147567208,-8.00597342370201,131.860226397321));
#72745=CARTESIAN_POINT('Ctrl Pts',(81.8331223745401,-8.06900957962136,131.856367610885));
#72746=CARTESIAN_POINT('Ctrl Pts',(81.8631831399905,-8.13365933412124,131.852508824449));
#72747=CARTESIAN_POINT('Ctrl Pts',(81.8932249693628,-8.19826836401633,131.848652468766));
#72748=CARTESIAN_POINT('Ctrl Pts',(81.9199239248084,-8.26448853642176,131.844796113083));
#72749=CARTESIAN_POINT('Ctrl Pts',(81.9431141996678,-8.33193954648609,131.8409397574));
#72750=CARTESIAN_POINT('Ctrl Pts',(81.9662976238879,-8.39937063084663,131.837084540923));
#72751=CARTESIAN_POINT('Ctrl Pts',(81.9859742674042,-8.46803137187562,131.833229324446));
#72752=CARTESIAN_POINT('Ctrl Pts',(82.0020272285703,-8.53752347241913,131.829374107968));
#72753=CARTESIAN_POINT('Ctrl Pts',(82.0180808173591,-8.6070182898959,131.825518740764));
#72754=CARTESIAN_POINT('Ctrl Pts',(82.0305103353282,-8.67734405760476,131.821663373559));
#72755=CARTESIAN_POINT('Ctrl Pts',(82.0392497279014,-8.74809106853049,131.817808006355));
#72756=CARTESIAN_POINT('Ctrl Pts',(82.0479982682355,-8.81891213228487,131.813948603632));
#72757=CARTESIAN_POINT('Ctrl Pts',(82.0530489129702,-8.89015483633853,131.810089200909));
#72758=CARTESIAN_POINT('Ctrl Pts',(82.054387478561,-8.96140401015755,131.806229798187));
#72759=CARTESIAN_POINT('Ctrl Pts',(82.0557268020581,-9.03269352581846,131.80236821024));
#72760=CARTESIAN_POINT('Ctrl Pts',(82.0533498785534,-9.10398903279388,131.798506622293));
#72761=CARTESIAN_POINT('Ctrl Pts',(82.0472946356544,-9.17487777823574,131.794645034346));
#72762=CARTESIAN_POINT('Ctrl Pts',(82.0412287988909,-9.24589054607866,131.790776690413));
#72763=CARTESIAN_POINT('Ctrl Pts',(82.0314718608921,-9.31649465020871,131.786908346479));
#72764=CARTESIAN_POINT('Ctrl Pts',(82.0181132365229,-9.38628555120693,131.783040002546));
#72765=CARTESIAN_POINT('Ctrl Pts',(82.0101812697978,-9.42772537982472,131.780743091239));
#72766=CARTESIAN_POINT('Ctrl Pts',(82.0009804488129,-9.46887873542872,131.778446179932));
#72767=CARTESIAN_POINT('Ctrl Pts',(81.9905377382803,-9.50966368811404,131.776149268625));
#72768=CARTESIAN_POINT('Ctrl Pts',(81.972947284492,-9.57836480007402,131.772280185777));
#72769=CARTESIAN_POINT('Ctrl Pts',(81.9517614930239,-9.64628873086806,131.76841110293));
#72770=CARTESIAN_POINT('Ctrl Pts',(81.9270660084628,-9.71303166937197,131.764542020082));
#72771=CARTESIAN_POINT('Ctrl Pts',(81.902407318942,-9.77967516422618,131.760678701975));
#72772=CARTESIAN_POINT('Ctrl Pts',(81.8742494834813,-9.84514070770194,131.756815383868));
#72773=CARTESIAN_POINT('Ctrl Pts',(81.8427284911057,-9.90903755179161,131.752952065761));
#72774=CARTESIAN_POINT('Ctrl Pts',(81.811244472842,-9.97285944490778,131.749093279325));
#72775=CARTESIAN_POINT('Ctrl Pts',(81.7764053476041,-10.0351158601245,131.745234492889));
#72776=CARTESIAN_POINT('Ctrl Pts',(81.7383953179643,-10.0954356580739,131.741375706452));
#72777=CARTESIAN_POINT('Ctrl Pts',(81.700409231856,-10.1557174589736,131.737519350769));
#72778=CARTESIAN_POINT('Ctrl Pts',(81.6592564626003,-10.2140646529026,131.733662995085));
#72779=CARTESIAN_POINT('Ctrl Pts',(81.6151665866136,-10.2701316703346,131.729806639401));
#72780=CARTESIAN_POINT('Ctrl Pts',(81.5710897352177,-10.3261821250083,131.725951422923));
#72781=CARTESIAN_POINT('Ctrl Pts',(81.5240777997389,-10.3799533587932,131.722096206445));
#72782=CARTESIAN_POINT('Ctrl Pts',(81.4744019976384,-10.4311311302113,131.718240989968));
#72783=CARTESIAN_POINT('Ctrl Pts',(81.4247242533627,-10.4823109025271,131.714385622762));
#72784=CARTESIAN_POINT('Ctrl Pts',(81.3723827756188,-10.5308966641232,131.710530255557));
#72785=CARTESIAN_POINT('Ctrl Pts',(81.3176859461205,-10.5766107033433,131.706674888352));
#72786=CARTESIAN_POINT('Ctrl Pts',(81.2629318639568,-10.6223725926967,131.702815485629));
#72787=CARTESIAN_POINT('Ctrl Pts',(81.2058178820311,-10.6652564470385,131.698956082905));
#72788=CARTESIAN_POINT('Ctrl Pts',(81.1466851059664,-10.7050251699769,131.695096680182));
#72789=CARTESIAN_POINT('Ctrl Pts',(81.0875188484595,-10.7448164102786,131.691235092235));
#72790=CARTESIAN_POINT('Ctrl Pts',(81.026331938212,-10.7814887581191,131.687373504287));
#72791=CARTESIAN_POINT('Ctrl Pts',(80.9634917137323,-10.814850208714,131.68351191634));
#72792=CARTESIAN_POINT('Ctrl Pts',(80.9005415480276,-10.8482700263625,131.679643572406));
#72793=CARTESIAN_POINT('Ctrl Pts',(80.8359327335556,-10.8783671766135,131.675775228472));
#72794=CARTESIAN_POINT('Ctrl Pts',(80.7700536341266,-10.904997365633,131.671906884538));
#72795=CARTESIAN_POINT('Ctrl Pts',(80.73093652081,-10.9208096054866,131.669609973236));
#72796=CARTESIAN_POINT('Ctrl Pts',(80.6913718813707,-10.9354004615867,131.667313061935));
#72797=CARTESIAN_POINT('Ctrl Pts',(80.6514431729604,-10.948748150712,131.665016150633));
#72798=CARTESIAN_POINT('Ctrl Pts',(80.5841843803941,-10.9712319597269,131.661147067787));
#72799=CARTESIAN_POINT('Ctrl Pts',(80.515628483031,-10.9902736788646,131.657277984941));
#72800=CARTESIAN_POINT('Ctrl Pts',(80.446161187892,-11.0057262417685,131.653408902095));
#72801=CARTESIAN_POINT('Ctrl Pts',(80.3767973955581,-11.0211557811243,131.64954558399));
#72802=CARTESIAN_POINT('Ctrl Pts',(80.3065253712461,-11.0330066745891,131.645682265884));
#72803=CARTESIAN_POINT('Ctrl Pts',(80.2357471530527,-11.0411812370114,131.641818947779));
#72804=CARTESIAN_POINT('Ctrl Pts',(80.1650519576818,-11.0493462106752,131.637960161344));
#72805=CARTESIAN_POINT('Ctrl Pts',(80.0938522280816,-11.053843363589,131.634101374909));
#72806=CARTESIAN_POINT('Ctrl Pts',(80.0225596785612,-11.0546261517374,131.630242588474));
#72807=CARTESIAN_POINT('Ctrl Pts',(79.9513120381194,-11.0554084467867,131.626386232792));
#72808=CARTESIAN_POINT('Ctrl Pts',(79.879972178366,-11.0524810138315,131.622529877109));
#72809=CARTESIAN_POINT('Ctrl Pts',(79.8089549414209,-11.0458492975028,131.618673521427));
#72810=CARTESIAN_POINT('Ctrl Pts',(79.7379586836785,-11.0392195402494,131.614818304951));
#72811=CARTESIAN_POINT('Ctrl Pts',(79.6672853429508,-11.0288877172192,131.610963088474));
#72812=CARTESIAN_POINT('Ctrl Pts',(79.5973460269111,-11.0149112487789,131.607107871998));
#72813=CARTESIAN_POINT('Ctrl Pts',(79.5274039764532,-11.0009342339005,131.603252504794));
#72814=CARTESIAN_POINT('Ctrl Pts',(79.4581964835926,-10.983312388063,131.599397137591));
#72815=CARTESIAN_POINT('Ctrl Pts',(79.3901241232501,-10.9621541676073,131.595541770387));
#72816=CARTESIAN_POINT('Ctrl Pts',(79.3219805097085,-10.9409738002642,131.591682367665));
#72817=CARTESIAN_POINT('Ctrl Pts',(79.2549748653891,-10.9162498135222,131.587822964943));
#72818=CARTESIAN_POINT('Ctrl Pts',(79.1894913917903,-10.8881401850811,131.583963562221));
#72819=CARTESIAN_POINT('Ctrl Pts',(79.1239708409342,-10.8600146407475,131.580101974275));
#72820=CARTESIAN_POINT('Ctrl Pts',(79.0599746125186,-10.8284998533183,131.576240386329));
#72821=CARTESIAN_POINT('Ctrl Pts',(78.9978632532916,-10.7938002964089,131.572378798383));
#72822=CARTESIAN_POINT('Ctrl Pts',(78.935643228015,-10.7590400313807,131.568510454451));
#72823=CARTESIAN_POINT('Ctrl Pts',(78.875315067074,-10.721084131254,131.564642110518));
#72824=CARTESIAN_POINT('Ctrl Pts',(78.8172106373791,-10.6801806111757,131.560773766585));
#72825=CARTESIAN_POINT('Ctrl Pts',(78.7827098989956,-10.6558932779622,131.558476855271));
#72826=CARTESIAN_POINT('Ctrl Pts',(78.748992556151,-10.6305675087266,131.556179943956));
#72827=CARTESIAN_POINT('Ctrl Pts',(78.7161221751681,-10.6042616037931,131.553883032642));
#72828=CARTESIAN_POINT('Ctrl Pts',(78.6614508986843,-10.5605086152737,131.550062721779));
#72829=CARTESIAN_POINT('Ctrl Pts',(78.608898578427,-10.5138612905726,131.546242410916));
#72830=CARTESIAN_POINT('Ctrl Pts',(78.5587935921191,-10.464555103908,131.542422100053));
#72831=CARTESIAN_POINT('Ctrl Pts',(78.5087739526719,-10.4153329034604,131.538608296557));
#72832=CARTESIAN_POINT('Ctrl Pts',(78.4611937228879,-10.3634611802395,131.534794493061));
#72833=CARTESIAN_POINT('Ctrl Pts',(78.4163489115401,-10.3092160984802,131.530980689565));
#72834=CARTESIAN_POINT('Ctrl Pts',(78.3715467866426,-10.2550226510107,131.527170516316));
#72835=CARTESIAN_POINT('Ctrl Pts',(78.329475236033,-10.1984607050715,131.523360343067));
#72836=CARTESIAN_POINT('Ctrl Pts',(78.2903930042303,-10.1398427446431,131.519550169818));
#72837=CARTESIAN_POINT('Ctrl Pts',(78.2513341075912,-10.0812597837433,131.515742271541));
#72838=CARTESIAN_POINT('Ctrl Pts',(78.2152612668582,-10.0206236570601,131.511934373265));
#72839=CARTESIAN_POINT('Ctrl Pts',(78.1823913627716,-9.95827783255842,131.508126474989));
#72840=CARTESIAN_POINT('Ctrl Pts',(78.1495294250015,-9.8959471181271,131.504319499591));
#72841=CARTESIAN_POINT('Ctrl Pts',(78.1198691151505,-9.83190797011655,131.500512524193));
#72842=CARTESIAN_POINT('Ctrl Pts',(78.0935816345597,-9.76652891557465,131.496705548795));
#72843=CARTESIAN_POINT('Ctrl Pts',(78.0672753510514,-9.7011030966816,131.492895850343));
#72844=CARTESIAN_POINT('Ctrl Pts',(78.0443469047302,-9.63433592002832,131.48908615189));
#72845=CARTESIAN_POINT('Ctrl Pts',(78.0249190681298,-9.56661527958821,131.485276453437));
#72846=CARTESIAN_POINT('Ctrl Pts',(78.0054843153251,-9.4988705309676,131.481465398753));
#72847=CARTESIAN_POINT('Ctrl Pts',(77.9895527685954,-9.43017212917455,131.477654344068));
#72848=CARTESIAN_POINT('Ctrl Pts',(77.9771963820948,-9.36091977763721,131.473843289384));
#72849=CARTESIAN_POINT('Ctrl Pts',(77.9648204879244,-9.29155809381223,131.470026217989));
#72850=CARTESIAN_POINT('Ctrl Pts',(77.9560310883201,-9.22164120977054,131.466209146595));
#72851=CARTESIAN_POINT('Ctrl Pts',(77.9508483050221,-9.15157471249978,131.4623920752));
#72852=CARTESIAN_POINT('Ctrl Pts',(77.947083896162,-9.10068334236886,131.459619623304));
#72853=CARTESIAN_POINT('Ctrl Pts',(77.9452210770952,-9.04971315177238,131.456847171409));
#72854=CARTESIAN_POINT('Ctrl Pts',(77.9452503396332,-8.99881859296011,131.454074719514));
#72855=CARTESIAN_POINT('Origin',(80.,-9.,141.545925280538));
#72856=CARTESIAN_POINT('',(81.2520391107129,-7.37076839346111,132.606087908702));
#72857=CARTESIAN_POINT('',(81.2520391107129,-7.3707683934611,132.547886797565));
#72858=CARTESIAN_POINT('',(81.2520391107129,-7.37076839346111,141.545925280538));
#72859=CARTESIAN_POINT('',(77.9452505617457,-9.00151937274232,132.095925280492));
#72860=CARTESIAN_POINT('Ctrl Pts',(81.2520391107129,-7.3707683934611,132.547886797565));
#72861=CARTESIAN_POINT('Ctrl Pts',(81.3083538607612,-7.41404540164551,132.544022016873));
#72862=CARTESIAN_POINT('Ctrl Pts',(81.3625154605356,-7.4603173375776,132.540157236181));
#72863=CARTESIAN_POINT('Ctrl Pts',(81.4141896923186,-7.50934072416269,132.536292455488));
#72864=CARTESIAN_POINT('Ctrl Pts',(81.4657959242599,-7.55829959924148,132.53243276059));
#72865=CARTESIAN_POINT('Ctrl Pts',(81.5149209399992,-7.61000240004589,132.528573065691));
#72866=CARTESIAN_POINT('Ctrl Pts',(81.5612632581667,-7.66416520437648,132.524713370792));
#72867=CARTESIAN_POINT('Ctrl Pts',(81.6075720611851,-7.71828883771727,132.520856467256));
#72868=CARTESIAN_POINT('Ctrl Pts',(81.6511018440891,-7.77486857728232,132.516999563721));
#72869=CARTESIAN_POINT('Ctrl Pts',(81.69158870253,-7.83358445484778,132.513142660186));
#72870=CARTESIAN_POINT('Ctrl Pts',(81.7320598241879,-7.89227751021701,132.509287255785));
#72871=CARTESIAN_POINT('Ctrl Pts',(81.7694900933409,-7.95310465610614,132.505431851384));
#72872=CARTESIAN_POINT('Ctrl Pts',(81.8036576222462,-8.01571511023833,132.501576446984));
#72873=CARTESIAN_POINT('Ctrl Pts',(81.8378232999895,-8.07832217219966,132.497721251465));
#72874=CARTESIAN_POINT('Ctrl Pts',(81.8687263571848,-8.14271192338244,132.493866055946));
#72875=CARTESIAN_POINT('Ctrl Pts',(81.8961906155537,-8.20850855217127,132.490010860427));
#72876=CARTESIAN_POINT('Ctrl Pts',(81.9236819791242,-8.27437011738988,132.486151860114));
#72877=CARTESIAN_POINT('Ctrl Pts',(81.9477275771208,-8.34164088432177,132.482292859801));
#72878=CARTESIAN_POINT('Ctrl Pts',(81.9681995653047,-8.4099253999414,132.478433859488));
#72879=CARTESIAN_POINT('Ctrl Pts',(81.9886814325063,-8.47824286712054,132.474572996965));
#72880=CARTESIAN_POINT('Ctrl Pts',(82.0055861392755,-8.54757458485537,132.470712134443));
#72881=CARTESIAN_POINT('Ctrl Pts',(82.0188366084774,-8.61751299267635,132.46685127192));
#72882=CARTESIAN_POINT('Ctrl Pts',(82.0321114365273,-8.68757997096613,132.462983311825));
#72883=CARTESIAN_POINT('Ctrl Pts',(82.0417185398173,-8.75825538508629,132.459115351731));
#72884=CARTESIAN_POINT('Ctrl Pts',(82.0476326158688,-8.82912509566834,132.455247391636));
#72885=CARTESIAN_POINT('Ctrl Pts',(82.05279078611,-8.89093661600497,132.45187381367));
#72886=CARTESIAN_POINT('Ctrl Pts',(82.055140463518,-8.95289567740437,132.448500235704));
#72887=CARTESIAN_POINT('Ctrl Pts',(82.0546972072604,-9.01472918789744,132.445126657738));
#72888=CARTESIAN_POINT('Ctrl Pts',(82.0541888463451,-9.08564468984679,132.441257574891));
#72889=CARTESIAN_POINT('Ctrl Pts',(82.0500038297876,-9.15667273902183,132.437388492044));
#72890=CARTESIAN_POINT('Ctrl Pts',(82.0421279206532,-9.22740078757216,132.433519409197));
#72891=CARTESIAN_POINT('Ctrl Pts',(82.0342637462307,-9.29802345485751,132.429656091091));
#72892=CARTESIAN_POINT('Ctrl Pts',(82.0227196484063,-9.36834652990705,132.425792772985));
#72893=CARTESIAN_POINT('Ctrl Pts',(82.007533399049,-9.43795800506769,132.421929454878));
#72894=CARTESIAN_POINT('Ctrl Pts',(81.9923649631563,-9.50748782599476,132.418070668442));
#72895=CARTESIAN_POINT('Ctrl Pts',(81.9735629648898,-9.57630723272567,132.414211882007));
#72896=CARTESIAN_POINT('Ctrl Pts',(81.9512166949537,-9.64401162398986,132.410353095571));
#72897=CARTESIAN_POINT('Ctrl Pts',(81.928884501529,-9.7116733664521,132.406496739888));
#72898=CARTESIAN_POINT('Ctrl Pts',(81.9030126178373,-9.7782210267392,132.402640384204));
#72899=CARTESIAN_POINT('Ctrl Pts',(81.8737405346709,-9.8432638799516,132.398784028521));
#72900=CARTESIAN_POINT('Ctrl Pts',(81.8444770987711,-9.90828751885387,132.394928812044));
#72901=CARTESIAN_POINT('Ctrl Pts',(81.8118156567702,-9.97180679045934,132.391073595567));
#72902=CARTESIAN_POINT('Ctrl Pts',(81.7759436651096,-10.0334513345375,132.38721837909));
#72903=CARTESIAN_POINT('Ctrl Pts',(81.7400702709614,-10.0950982887329,132.383363011885));
#72904=CARTESIAN_POINT('Ctrl Pts',(81.7009863241764,-10.1548699511211,132.37950764468));
#72905=CARTESIAN_POINT('Ctrl Pts',(81.6589241562073,-10.2124224537891,132.375652277476));
#72906=CARTESIAN_POINT('Ctrl Pts',(81.616817960618,-10.2700351982336,132.371792874753));
#72907=CARTESIAN_POINT('Ctrl Pts',(81.5717276080723,-10.3254237530131,132.36793347203));
#72908=CARTESIAN_POINT('Ctrl Pts',(81.5239269806332,-10.3782757779915,132.364074069307));
#72909=CARTESIAN_POINT('Ctrl Pts',(81.4760992881035,-10.4311577282016,132.360212481361));
#72910=CARTESIAN_POINT('Ctrl Pts',(81.4255586101456,-10.4814999465868,132.356350893414));
#72911=CARTESIAN_POINT('Ctrl Pts',(81.3726151590844,-10.5290275300176,132.352489305467));
#72912=CARTESIAN_POINT('Ctrl Pts',(81.3195790815579,-10.5766382646591,132.348620961533));
#72913=CARTESIAN_POINT('Ctrl Pts',(81.2641322160707,-10.6214242274925,132.3447526176));
#72914=CARTESIAN_POINT('Ctrl Pts',(81.2066166827356,-10.6631517499748,132.340884273666));
#72915=CARTESIAN_POINT('Ctrl Pts',(81.1724656141925,-10.6879283520124,132.33858736236));
#72916=CARTESIAN_POINT('Ctrl Pts',(81.1375857558048,-10.7116274925515,132.336290451053));
#72917=CARTESIAN_POINT('Ctrl Pts',(81.1020528512105,-10.7342079101535,132.333993539747));
#72918=CARTESIAN_POINT('Ctrl Pts',(81.0421986673429,-10.7722439919877,132.3301244569));
#72919=CARTESIAN_POINT('Ctrl Pts',(80.9802557831637,-10.8072522372018,132.326255374053));
#72920=CARTESIAN_POINT('Ctrl Pts',(80.9165630719349,-10.8389969270407,132.322386291206));
#72921=CARTESIAN_POINT('Ctrl Pts',(80.8529652596694,-10.870694318875,132.318522973099));
#72922=CARTESIAN_POINT('Ctrl Pts',(80.7876232267181,-10.8991375924029,132.314659654993));
#72923=CARTESIAN_POINT('Ctrl Pts',(80.7209036010568,-10.9241350161783,132.310796336886));
#72924=CARTESIAN_POINT('Ctrl Pts',(80.6542622374908,-10.9491031179851,132.30693755045));
#72925=CARTESIAN_POINT('Ctrl Pts',(80.586246943666,-10.9706332291725,132.303078764015));
#72926=CARTESIAN_POINT('Ctrl Pts',(80.517246068014,-10.9885809180478,132.299219977579));
#72927=CARTESIAN_POINT('Ctrl Pts',(80.4482886578541,-11.0065173011952,132.295363621895));
#72928=CARTESIAN_POINT('Ctrl Pts',(80.3783473666403,-11.0208756172173,132.291507266212));
#72929=CARTESIAN_POINT('Ctrl Pts',(80.3078261123459,-11.0315611354468,132.287650910529));
#72930=CARTESIAN_POINT('Ctrl Pts',(80.2373256907361,-11.0422434970673,132.283795694051));
#72931=CARTESIAN_POINT('Ctrl Pts',(80.1662461262163,-11.0492551421476,132.279940477574));
#72932=CARTESIAN_POINT('Ctrl Pts',(80.0950002433515,-11.0525526829446,132.276085261097));
#72933=CARTESIAN_POINT('Ctrl Pts',(80.0237515749859,-11.0558503526656,132.272229893892));
#72934=CARTESIAN_POINT('Ctrl Pts',(79.9523370607307,-11.0554336095476,132.268374526687));
#72935=CARTESIAN_POINT('Ctrl Pts',(79.8811716074018,-11.0513111357404,132.264519159483));
#72936=CARTESIAN_POINT('Ctrl Pts',(79.809931663249,-11.0471843468272,132.26065975676));
#72937=CARTESIAN_POINT('Ctrl Pts',(79.7389417863995,-11.0393441122429,132.256800354037));
#72938=CARTESIAN_POINT('Ctrl Pts',(79.668612932374,-11.0278511222253,132.252940951314));
#72939=CARTESIAN_POINT('Ctrl Pts',(79.598244257599,-11.0163516247864,132.249079363367));
#72940=CARTESIAN_POINT('Ctrl Pts',(79.5285378256335,-11.0011953579895,132.24521777542));
#72941=CARTESIAN_POINT('Ctrl Pts',(79.4598928447498,-10.9824938394224,132.241356187473));
#72942=CARTESIAN_POINT('Ctrl Pts',(79.3911277670117,-10.9637596018781,132.23748784354));
#72943=CARTESIAN_POINT('Ctrl Pts',(79.3234283095606,-10.9414678809868,132.233619499606));
#72944=CARTESIAN_POINT('Ctrl Pts',(79.257176344285,-10.9157793659527,132.229751155673));
#72945=CARTESIAN_POINT('Ctrl Pts',(79.2178378338809,-10.9005262649808,132.227454244367));
#72946=CARTESIAN_POINT('Ctrl Pts',(79.1790092532521,-10.8840764896419,132.225157333061));
#72947=CARTESIAN_POINT('Ctrl Pts',(79.1407663493566,-10.8664712952794,132.222860421755));
#72948=CARTESIAN_POINT('Ctrl Pts',(79.0763472474527,-10.836815837818,132.218991338908));
#72949=CARTESIAN_POINT('Ctrl Pts',(79.0133390613033,-10.8037633551402,132.215122256061));
#72950=CARTESIAN_POINT('Ctrl Pts',(78.95212362422,-10.7674706966686,132.211253173215));
#72951=CARTESIAN_POINT('Ctrl Pts',(78.8909993950849,-10.7312321124482,132.207389855108));
#72952=CARTESIAN_POINT('Ctrl Pts',(78.8316630274035,-10.691763181006,132.203526537002));
#72953=CARTESIAN_POINT('Ctrl Pts',(78.7744744529048,-10.6492679272686,132.199663218896));
#72954=CARTESIAN_POINT('Ctrl Pts',(78.717352960582,-10.6068225204476,132.19580443246));
#72955=CARTESIAN_POINT('Ctrl Pts',(78.6623746451655,-10.5613581309169,132.191945646024));
#72956=CARTESIAN_POINT('Ctrl Pts',(78.6098714810446,-10.5131226861318,132.188086859589));
#72957=CARTESIAN_POINT('Ctrl Pts',(78.5574013900671,-10.46491762614,132.184230503905));
#72958=CARTESIAN_POINT('Ctrl Pts',(78.5074037139146,-10.4139453019374,132.180374148222));
#72959=CARTESIAN_POINT('Ctrl Pts',(78.4601771161138,-10.3604936783243,132.176517792539));
#72960=CARTESIAN_POINT('Ctrl Pts',(78.4129644695228,-10.307057844856,132.172662576062));
#72961=CARTESIAN_POINT('Ctrl Pts',(78.3685215975989,-10.2511445298601,132.168807359585));
#72962=CARTESIAN_POINT('Ctrl Pts',(78.3271088597401,-10.1930770282508,132.164952143108));
#72963=CARTESIAN_POINT('Ctrl Pts',(78.285694502767,-10.1350072563759,132.161096775903));
#72964=CARTESIAN_POINT('Ctrl Pts',(78.2473107953373,-10.0747835274586,132.157241408699));
#72965=CARTESIAN_POINT('Ctrl Pts',(78.2121754805814,-10.012759127466,132.153386041494));
#72966=CARTESIAN_POINT('Ctrl Pts',(78.1770033887319,-9.95066980483986,132.149526638771));
#72967=CARTESIAN_POINT('Ctrl Pts',(78.1450867170067,-9.88677647217476,132.145667236049));
#72968=CARTESIAN_POINT('Ctrl Pts',(78.1165973717166,-9.8214573039879,132.141807833326));
#72969=CARTESIAN_POINT('Ctrl Pts',(78.0880918955353,-9.7561011515749,132.137946245379));
#72970=CARTESIAN_POINT('Ctrl Pts',(78.0630177797161,-9.68931801151647,132.134084657432));
#72971=CARTESIAN_POINT('Ctrl Pts',(78.0414978573553,-9.62150375683197,132.130223069485));
#72972=CARTESIAN_POINT('Ctrl Pts',(78.019940285119,-9.55357085867815,132.126354725552));
#72973=CARTESIAN_POINT('Ctrl Pts',(78.0019494437881,-9.48460371441895,132.122486381619));
#72974=CARTESIAN_POINT('Ctrl Pts',(77.9875974528442,-9.41501030192132,132.118618037685));
#72975=CARTESIAN_POINT('Ctrl Pts',(77.9790756536328,-9.37368773628851,132.116321126378));
#72976=CARTESIAN_POINT('Ctrl Pts',(77.9718357960167,-9.33214452690067,132.114024215071));
#72977=CARTESIAN_POINT('Ctrl Pts',(77.9658843036767,-9.29046668736917,132.111727303764));
#72978=CARTESIAN_POINT('Ctrl Pts',(77.9522361754433,-9.19488990327605,132.106459962688));
#72979=CARTESIAN_POINT('Ctrl Pts',(77.9453221472454,-9.09832918085083,132.101192621613));
#72980=CARTESIAN_POINT('Ctrl Pts',(77.9452505617463,-9.00151937358667,132.095925280538));
#72981=CARTESIAN_POINT('Ctrl Pts',(77.9452505617457,-9.00151937274232,132.095925280492));
#72982=CARTESIAN_POINT('Ctrl Pts',(77.9451965787833,-8.92851460007613,132.091953151545));
#72983=CARTESIAN_POINT('Ctrl Pts',(77.9490383631329,-8.85536232529461,132.087981022599));
#72984=CARTESIAN_POINT('Ctrl Pts',(77.9567917436018,-8.78251992393294,132.084008893652));
#72985=CARTESIAN_POINT('Ctrl Pts',(77.9642163077101,-8.71276672648809,132.080205220386));
#72986=CARTESIAN_POINT('Ctrl Pts',(77.9752273595376,-8.64329821470206,132.07640154712));
#72987=CARTESIAN_POINT('Ctrl Pts',(77.989785708765,-8.57451666799445,132.072597873854));
#72988=CARTESIAN_POINT('Ctrl Pts',(78.0043341072356,-8.50578213406467,132.068796800431));
#72989=CARTESIAN_POINT('Ctrl Pts',(78.0224248939572,-8.4377341234779,132.064995727008));
#72990=CARTESIAN_POINT('Ctrl Pts',(78.0439673846338,-8.37076715746578,132.061194653586));
#72991=CARTESIAN_POINT('Ctrl Pts',(78.0655028484981,-8.30382203499575,132.057394820012));
#72992=CARTESIAN_POINT('Ctrl Pts',(78.090487629481,-8.23795773444723,132.053594986438));
#72993=CARTESIAN_POINT('Ctrl Pts',(78.1187810484404,-8.17355410413447,132.049795152864));
#72994=CARTESIAN_POINT('Ctrl Pts',(78.1470753477331,-8.10914846994011,132.04599520106));
#72995=CARTESIAN_POINT('Ctrl Pts',(78.1786782846806,-8.04620405373723,132.042195249257));
#72996=CARTESIAN_POINT('Ctrl Pts',(78.2134016340244,-7.9850793916797,132.038395297453));
#72997=CARTESIAN_POINT('Ctrl Pts',(78.2481601793031,-7.92389277305208,132.03459149398));
#72998=CARTESIAN_POINT('Ctrl Pts',(78.2860451976124,-7.8645300241073,132.030787690508));
#72999=CARTESIAN_POINT('Ctrl Pts',(78.3268238180267,-7.80732274836095,132.026983887035));
#73000=CARTESIAN_POINT('Ctrl Pts',(78.3676269245136,-7.7500811217344,132.023177799517));
#73001=CARTESIAN_POINT('Ctrl Pts',(78.4113267751391,-7.69499793290784,132.019371711999));
#73002=CARTESIAN_POINT('Ctrl Pts',(78.4576505098363,-7.64237132739038,132.015565624481));
#73003=CARTESIAN_POINT('Ctrl Pts',(78.5040502056943,-7.58965842533244,132.011753295782));
#73004=CARTESIAN_POINT('Ctrl Pts',(78.5530820149241,-7.53941049549435,132.007940967083));
#73005=CARTESIAN_POINT('Ctrl Pts',(78.6044374301091,-7.4918877110707,132.004128638384));
#73006=CARTESIAN_POINT('Ctrl Pts',(78.6203081568685,-7.47720140927148,132.002950487513));
#73007=CARTESIAN_POINT('Ctrl Pts',(78.6364005734966,-7.4627750674,132.001772336643));
#73008=CARTESIAN_POINT('Ctrl Pts',(78.6527050052883,-7.44861553452252,132.000594185772));
#73009=CARTESIAN_POINT('Ctrl Pts',(78.7062492490401,-7.40211520323282,131.996725102925));
#73010=CARTESIAN_POINT('Ctrl Pts',(78.7623085494611,-7.35829907639647,131.992856020077));
#73011=CARTESIAN_POINT('Ctrl Pts',(78.8205827822767,-7.3174505686198,131.98898693723));
#73012=CARTESIAN_POINT('Ctrl Pts',(78.8787701893918,-7.27666292308245,131.985123619123));
#73013=CARTESIAN_POINT('Ctrl Pts',(78.9391655836702,-7.23883439640809,131.981260301016));
#73014=CARTESIAN_POINT('Ctrl Pts',(79.0014348634829,-7.20420902367991,131.977396982909));
#73015=CARTESIAN_POINT('Ctrl Pts',(79.0636311014544,-7.1696242665006,131.973538196473));
#73016=CARTESIAN_POINT('Ctrl Pts',(79.1276964363551,-7.13823543493536,131.969679410036));
#73017=CARTESIAN_POINT('Ctrl Pts',(79.1932682648411,-7.11024301298091,131.9658206236));
#73018=CARTESIAN_POINT('Ctrl Pts',(79.2587987878832,-7.08226822419972,131.961964267916));
#73019=CARTESIAN_POINT('Ctrl Pts',(79.3258334760286,-7.05768579059293,131.958107912232));
#73020=CARTESIAN_POINT('Ctrl Pts',(79.3939869504898,-7.03664935726617,131.954251556549));
#73021=CARTESIAN_POINT('Ctrl Pts',(79.4621202917322,-7.01561913831244,131.950396340071));
#73022=CARTESIAN_POINT('Ctrl Pts',(79.5313712992331,-6.99813298320813,131.946541123593));
#73023=CARTESIAN_POINT('Ctrl Pts',(79.6013381641286,-6.98429508530646,131.942685907115));
#73024=CARTESIAN_POINT('Ctrl Pts',(79.6713077645193,-6.97045664638438,131.93883053991));
#73025=CARTESIAN_POINT('Ctrl Pts',(79.7419928008914,-6.9602668399403,131.934975172705));
#73026=CARTESIAN_POINT('Ctrl Pts',(79.8129816751026,-6.95377867554544,131.9311198055));
#73027=CARTESIAN_POINT('Ctrl Pts',(79.8840448553072,-6.94728371981171,131.927260402776));
#73028=CARTESIAN_POINT('Ctrl Pts',(79.9554120234629,-6.94449818502207,131.923401000053));
#73029=CARTESIAN_POINT('Ctrl Pts',(80.0266677680113,-6.945423062368,131.91954159733));
#73030=CARTESIAN_POINT('Ctrl Pts',(80.0979638581219,-6.94634846338675,131.915680009382));
#73031=CARTESIAN_POINT('Ctrl Pts',(80.1691479140509,-6.95098842710182,131.911818421435));
#73032=CARTESIAN_POINT('Ctrl Pts',(80.2398085956787,-6.95929193662136,131.907956833487));
#73033=CARTESIAN_POINT('Ctrl Pts',(80.3105929007015,-6.9676099734284,131.904088489553));
#73034=CARTESIAN_POINT('Ctrl Pts',(80.3808515242713,-6.97960427102286,131.90022014562));
#73035=CARTESIAN_POINT('Ctrl Pts',(80.4501829707131,-6.99517261207356,131.896351801686));
#73036=CARTESIAN_POINT('Ctrl Pts',(80.4913499883317,-7.00441664495069,131.894054890384));
#73037=CARTESIAN_POINT('Ctrl Pts',(80.5321903805204,-7.01491979407838,131.891757979082));
#73038=CARTESIAN_POINT('Ctrl Pts',(80.5726231150619,-7.02665250637483,131.889461067781));
#73039=CARTESIAN_POINT('Ctrl Pts',(80.6407129225889,-7.04641070801747,131.885593007651));
#73040=CARTESIAN_POINT('Ctrl Pts',(80.7079122298124,-7.06973586291902,131.881724947521));
#73041=CARTESIAN_POINT('Ctrl Pts',(80.7738204657345,-7.09652963004138,131.877856887391));
#73042=CARTESIAN_POINT('Ctrl Pts',(80.8396428369124,-7.12328849044943,131.87399386654));
#73043=CARTESIAN_POINT('Ctrl Pts',(80.9041770260992,-7.15350682139415,131.870130845689));
#73044=CARTESIAN_POINT('Ctrl Pts',(80.967036885349,-7.18703634209772,131.866267824838));
#73045=CARTESIAN_POINT('Ctrl Pts',(81.0298266373812,-7.22052846753132,131.86240911239));
#73046=CARTESIAN_POINT('Ctrl Pts',(81.0909453409531,-7.25732422244068,131.858550399943));
#73047=CARTESIAN_POINT('Ctrl Pts',(81.1500279067684,-7.29722773802429,131.854691687496));
#73048=CARTESIAN_POINT('Ctrl Pts',(81.184758141456,-7.32068403925214,131.85242343819));
#73049=CARTESIAN_POINT('Ctrl Pts',(81.2187852194779,-7.34521329605046,131.850155188884));
#73050=CARTESIAN_POINT('Ctrl Pts',(81.2520391107129,-7.37076839346113,131.847886939579));
#73051=CARTESIAN_POINT('',(77.945250271645,-8.99894343713344,132.154074719416));
#73052=CARTESIAN_POINT('Ctrl Pts',(77.945250271645,-8.99894343713344,132.154074719416));
#73053=CARTESIAN_POINT('Ctrl Pts',(77.945290872253,-8.91998543955825,132.14981310901));
#73054=CARTESIAN_POINT('Ctrl Pts',(77.9498868100455,-8.84118478791793,132.145551498605));
#73055=CARTESIAN_POINT('Ctrl Pts',(77.9589591217714,-8.76304072944942,132.141289888199));
#73056=CARTESIAN_POINT('Ctrl Pts',(77.9680642943239,-8.68461362533253,132.137012841811));
#73057=CARTESIAN_POINT('Ctrl Pts',(77.981678191433,-8.60684816261152,132.132735795423));
#73058=CARTESIAN_POINT('Ctrl Pts',(77.999671050668,-8.53023233725138,132.128458749035));
#73059=CARTESIAN_POINT('Ctrl Pts',(78.017750965159,-8.45324581981796,132.124161008917));
#73060=CARTESIAN_POINT('Ctrl Pts',(78.0402521766357,-8.37742036596183,132.119863268799));
#73061=CARTESIAN_POINT('Ctrl Pts',(78.0669947748154,-8.30323005094278,132.115565528682));
#73062=CARTESIAN_POINT('Ctrl Pts',(78.0794747989853,-8.2686075016157,132.113559893321));
#73063=CARTESIAN_POINT('Ctrl Pts',(78.0928778545041,-8.23434073399828,132.11155425796));
#73064=CARTESIAN_POINT('Ctrl Pts',(78.1071822245976,-8.20047612191953,132.109548622599));
#73065=CARTESIAN_POINT('Ctrl Pts',(78.1347768681954,-8.13514770166873,132.105679539752));
#73066=CARTESIAN_POINT('Ctrl Pts',(78.1658116320372,-8.07112160100121,132.101810456905));
#73067=CARTESIAN_POINT('Ctrl Pts',(78.2001418722771,-8.00878444192498,132.097941374058));
#73068=CARTESIAN_POINT('Ctrl Pts',(78.2344209621713,-7.94654016210686,132.094078055952));
#73069=CARTESIAN_POINT('Ctrl Pts',(78.2719855496262,-7.8859802508739,132.090214737845));
#73070=CARTESIAN_POINT('Ctrl Pts',(78.3126431435273,-7.8274709379233,132.086351419739));
#73071=CARTESIAN_POINT('Ctrl Pts',(78.3532530460864,-7.76903025637427,132.082492633303));
#73072=CARTESIAN_POINT('Ctrl Pts',(78.3969484726024,-7.71263579225423,132.078633846867));
#73073=CARTESIAN_POINT('Ctrl Pts',(78.4434921636943,-7.65862722630175,132.074775060431));
#73074=CARTESIAN_POINT('Ctrl Pts',(78.4900065356737,-7.60465268178554,132.070918704748));
#73075=CARTESIAN_POINT('Ctrl Pts',(78.5393652961915,-7.55306142074469,132.067062349065));
#73076=CARTESIAN_POINT('Ctrl Pts',(78.5912901108142,-7.50416110138486,132.063205993381));
#73077=CARTESIAN_POINT('Ctrl Pts',(78.6431995863267,-7.45527522766904,132.059350776904));
#73078=CARTESIAN_POINT('Ctrl Pts',(78.6976732575751,-7.40907905034047,132.055495560427));
#73079=CARTESIAN_POINT('Ctrl Pts',(78.7543962613515,-7.36584306482982,132.05164034395));
#73080=CARTESIAN_POINT('Ctrl Pts',(78.8111214828275,-7.3226053889215,132.047784976745));
#73081=CARTESIAN_POINT('Ctrl Pts',(78.870095823747,-7.28232842734014,132.04392960954));
#73082=CARTESIAN_POINT('Ctrl Pts',(78.9309730915482,-7.2452410332168,132.040074242335));
#73083=CARTESIAN_POINT('Ctrl Pts',(78.9919140812485,-7.20811481870503,132.036214839613));
#73084=CARTESIAN_POINT('Ctrl Pts',(79.0547615582912,-7.17418508951644,132.03235543689));
#73085=CARTESIAN_POINT('Ctrl Pts',(79.11914299841,-7.14363567550713,132.028496034167));
#73086=CARTESIAN_POINT('Ctrl Pts',(79.1835608918059,-7.11306896417964,132.02463444622));
#73087=CARTESIAN_POINT('Ctrl Pts',(79.2495140279317,-7.08588656333384,132.020772858273));
#73088=CARTESIAN_POINT('Ctrl Pts',(79.3166106344542,-7.06222381644346,132.016911270326));
#73089=CARTESIAN_POINT('Ctrl Pts',(79.3838246288948,-7.03851967072926,132.013042926392));
#73090=CARTESIAN_POINT('Ctrl Pts',(79.4521856218024,-7.01834761064219,132.009174582459));
#73091=CARTESIAN_POINT('Ctrl Pts',(79.5212881315132,-7.00179267605439,132.005306238525));
#73092=CARTESIAN_POINT('Ctrl Pts',(79.5623192131711,-6.99196283230839,132.00300932722));
#73093=CARTESIAN_POINT('Ctrl Pts',(79.6036115398418,-6.98340727619076,132.000712415914));
#73094=CARTESIAN_POINT('Ctrl Pts',(79.6450793453083,-6.97613515980606,131.998415504608));
#73095=CARTESIAN_POINT('Ctrl Pts',(79.7149081391761,-6.96388944025815,131.994547671615));
#73096=CARTESIAN_POINT('Ctrl Pts',(79.7855081655632,-6.95523790608877,131.990679838623));
#73097=CARTESIAN_POINT('Ctrl Pts',(79.8564765514174,-6.95026865609003,131.98681200563));
#73098=CARTESIAN_POINT('Ctrl Pts',(79.9273493904374,-6.94530609633936,131.982949380016));
#73099=CARTESIAN_POINT('Ctrl Pts',(79.9985891252929,-6.9440160213747,131.979086754401));
#73100=CARTESIAN_POINT('Ctrl Pts',(80.0697838953175,-6.94643535031051,131.975224128786));
#73101=CARTESIAN_POINT('Ctrl Pts',(80.1409066359354,-6.9488522315549,131.97136541108));
#73102=CARTESIAN_POINT('Ctrl Pts',(80.2119840191086,-6.9549710540467,131.967506693374));
#73103=CARTESIAN_POINT('Ctrl Pts',(80.2826020050066,-6.96477675198364,131.963647975667));
#73104=CARTESIAN_POINT('Ctrl Pts',(80.353172170657,-6.97457580981471,131.959791870962));
#73105=CARTESIAN_POINT('Ctrl Pts',(80.4232830766715,-6.98805672020389,131.955935766256));
#73106=CARTESIAN_POINT('Ctrl Pts',(80.4925253618697,-7.00515255460095,131.95207966155));
#73107=CARTESIAN_POINT('Ctrl Pts',(80.561770301311,-7.02224904432734,131.948223409029));
#73108=CARTESIAN_POINT('Ctrl Pts',(80.6301460772589,-7.0429606369905,131.944367156508));
#73109=CARTESIAN_POINT('Ctrl Pts',(80.6972543344538,-7.06716944467827,131.940510903988));
#73110=CARTESIAN_POINT('Ctrl Pts',(80.7643590610103,-7.09137697871429,131.936654854349));
#73111=CARTESIAN_POINT('Ctrl Pts',(80.8301959465034,-7.11908118996674,131.93279880471));
#73112=CARTESIAN_POINT('Ctrl Pts',(80.894384749111,-7.15011527844093,131.928942755071));
#73113=CARTESIAN_POINT('Ctrl Pts',(80.9586397009929,-7.18118134885509,131.925082731609));
#73114=CARTESIAN_POINT('Ctrl Pts',(81.0212427411819,-7.21558393418775,131.921222708148));
#73115=CARTESIAN_POINT('Ctrl Pts',(81.0818372046269,-7.25310966996064,131.917362684687));
#73116=CARTESIAN_POINT('Ctrl Pts',(81.140556548437,-7.28947415699949,131.913622111178));
#73117=CARTESIAN_POINT('Ctrl Pts',(81.1973895061473,-7.32877102364184,131.90988153767));
#73118=CARTESIAN_POINT('Ctrl Pts',(81.2520391107129,-7.3707683934611,131.906140964161));
#73119=CARTESIAN_POINT('Ctrl Pts',(81.2520391107129,-7.37076839346111,132.606087908702));
#73120=CARTESIAN_POINT('Ctrl Pts',(81.3085934782384,-7.4142295439442,132.602232450567));
#73121=CARTESIAN_POINT('Ctrl Pts',(81.3628750382077,-7.46063328907426,132.598376992433));
#73122=CARTESIAN_POINT('Ctrl Pts',(81.4145730951239,-7.50970455242875,132.594521534299));
#73123=CARTESIAN_POINT('Ctrl Pts',(81.4663263971359,-7.55882825385944,132.590661956181));
#73124=CARTESIAN_POINT('Ctrl Pts',(81.5154903332362,-7.61062482749505,132.586802378063));
#73125=CARTESIAN_POINT('Ctrl Pts',(81.5617909053502,-7.66478214119745,132.582942799945));
#73126=CARTESIAN_POINT('Ctrl Pts',(81.6081191558986,-7.71897183008615,132.579080914575));
#73127=CARTESIAN_POINT('Ctrl Pts',(81.6515803396647,-7.77552468259948,132.575219029205));
#73128=CARTESIAN_POINT('Ctrl Pts',(81.6919423194437,-7.83409745253926,132.571357143836));
#73129=CARTESIAN_POINT('Ctrl Pts',(81.7323736167915,-7.89277081521586,132.567488626073));
#73130=CARTESIAN_POINT('Ctrl Pts',(81.7696948321811,-7.95347060574031,132.56362010831));
#73131=CARTESIAN_POINT('Ctrl Pts',(81.8037189057658,-8.01582741783614,132.559751590548));
#73132=CARTESIAN_POINT('Ctrl Pts',(81.8203431345088,-8.04629507790004,132.55786142522));
#73133=CARTESIAN_POINT('Ctrl Pts',(81.8361809521596,-8.07715799347721,132.555971259893));
#73134=CARTESIAN_POINT('Ctrl Pts',(81.8512147628779,-8.10837145390982,132.554081094566));
#73135=CARTESIAN_POINT('Ctrl Pts',(81.8819882927562,-8.1722639942131,132.550212011719));
#73136=CARTESIAN_POINT('Ctrl Pts',(81.9095104472025,-8.23787671514327,132.546342928872));
#73137=CARTESIAN_POINT('Ctrl Pts',(81.9335867653229,-8.3048454966928,132.542473846025));
#73138=CARTESIAN_POINT('Ctrl Pts',(81.9576272109299,-8.37171449809755,132.538610527919));
#73139=CARTESIAN_POINT('Ctrl Pts',(81.9782318482963,-8.43993509614539,132.534747209812));
#73140=CARTESIAN_POINT('Ctrl Pts',(81.9952531484605,-8.5091207520598,132.530883891706));
#73141=CARTESIAN_POINT('Ctrl Pts',(82.0122544826462,-8.57822525322665,132.52702510527));
#73142=CARTESIAN_POINT('Ctrl Pts',(82.0256807132234,-8.64829209427239,132.523166318834));
#73143=CARTESIAN_POINT('Ctrl Pts',(82.0354338270112,-8.71891869795672,132.519307532398));
#73144=CARTESIAN_POINT('Ctrl Pts',(82.0451807970526,-8.78950081205954,132.515451176715));
#73145=CARTESIAN_POINT('Ctrl Pts',(82.0512591745401,-8.86064150915053,132.511594821032));
#73146=CARTESIAN_POINT('Ctrl Pts',(82.053622127359,-8.9319285631008,132.507738465349));
#73147=CARTESIAN_POINT('Ctrl Pts',(82.0559843821379,-9.00319455814147,132.503883248871));
#73148=CARTESIAN_POINT('Ctrl Pts',(82.0546333751519,-9.07460633895539,132.500028032394));
#73149=CARTESIAN_POINT('Ctrl Pts',(82.0495743065814,-9.14574883979362,132.496172815917));
#73150=CARTESIAN_POINT('Ctrl Pts',(82.0445150402166,-9.2168941220909,132.492317448712));
#73151=CARTESIAN_POINT('Ctrl Pts',(82.0357474610954,-9.28776961910727,132.488462081508));
#73152=CARTESIAN_POINT('Ctrl Pts',(82.0233287253966,-9.35796428800237,132.484606714303));
#73153=CARTESIAN_POINT('Ctrl Pts',(82.0108969906679,-9.42823243157463,132.48074731158));
#73154=CARTESIAN_POINT('Ctrl Pts',(81.9948065550646,-9.4978178450992,132.476887908857));
#73155=CARTESIAN_POINT('Ctrl Pts',(81.9751657636102,-9.56631949353887,132.473028506135));
#73156=CARTESIAN_POINT('Ctrl Pts',(81.9555138513854,-9.63485992814995,132.469166918188));
#73157=CARTESIAN_POINT('Ctrl Pts',(81.9323077396484,-9.70231491653813,132.465305330241));
#73158=CARTESIAN_POINT('Ctrl Pts',(81.9057048777051,-9.76830103578668,132.461443742294));
#73159=CARTESIAN_POINT('Ctrl Pts',(81.8790554731013,-9.83440260011612,132.45757539836));
#73160=CARTESIAN_POINT('Ctrl Pts',(81.8489976583775,-9.89902972393679,132.453707054427));
#73161=CARTESIAN_POINT('Ctrl Pts',(81.8157356889678,-9.96182195353851,132.449838710493));
#73162=CARTESIAN_POINT('Ctrl Pts',(81.7959856887283,-9.99910617247326,132.447541799187));
#73163=CARTESIAN_POINT('Ctrl Pts',(81.7751068783501,-10.0357439816394,132.44524488788));
#73164=CARTESIAN_POINT('Ctrl Pts',(81.7531490904376,-10.0716649799251,132.442947976574));
#73165=CARTESIAN_POINT('Ctrl Pts',(81.7161618108983,-10.1321728967617,132.439078893727));
#73166=CARTESIAN_POINT('Ctrl Pts',(81.6759658686669,-10.1908822176689,132.43520981088));
#73167=CARTESIAN_POINT('Ctrl Pts',(81.632761701244,-10.2474320780912,132.431340728033));
#73168=CARTESIAN_POINT('Ctrl Pts',(81.5896219058757,-10.3038976820418,132.427477409927));
#73169=CARTESIAN_POINT('Ctrl Pts',(81.5434830746863,-10.3582098292608,132.42361409182));
#73170=CARTESIAN_POINT('Ctrl Pts',(81.494589934882,-10.4100349247623,132.419750773714));
#73171=CARTESIAN_POINT('Ctrl Pts',(81.445754146712,-10.4617992294466,132.415891987278));
#73172=CARTESIAN_POINT('Ctrl Pts',(81.3941707991378,-10.5110819255448,132.412033200842));
#73173=CARTESIAN_POINT('Ctrl Pts',(81.3401249501949,-10.5575823189691,132.408174414406));
#73174=CARTESIAN_POINT('Ctrl Pts',(81.2861131461739,-10.6040534205552,132.404318058723));
#73175=CARTESIAN_POINT('Ctrl Pts',(81.2296422857039,-10.6477453806082,132.40046170304));
#73176=CARTESIAN_POINT('Ctrl Pts',(81.1710332927739,-10.6883952705795,132.396605347356));
#73177=CARTESIAN_POINT('Ctrl Pts',(81.1124416135272,-10.7290331521662,132.392750130879));
#73178=CARTESIAN_POINT('Ctrl Pts',(81.0517134547251,-10.7666304710523,132.388894914402));
#73179=CARTESIAN_POINT('Ctrl Pts',(80.9892003473083,-10.8009664725877,132.385039697925));
#73180=CARTESIAN_POINT('Ctrl Pts',(80.9266847958159,-10.8353038165582,132.38118433072));
#73181=CARTESIAN_POINT('Ctrl Pts',(80.8623845840018,-10.8663793580925,132.377328963515));
#73182=CARTESIAN_POINT('Ctrl Pts',(80.796676042939,-10.8940181744395,132.373473596311));
#73183=CARTESIAN_POINT('Ctrl Pts',(80.7308987229515,-10.9216859210905,132.369614193588));
#73184=CARTESIAN_POINT('Ctrl Pts',(80.6637105797083,-10.9459095727734,132.365754790865));
#73185=CARTESIAN_POINT('Ctrl Pts',(80.5955073002182,-10.9665626402144,132.361895388142));
#73186=CARTESIAN_POINT('Ctrl Pts',(80.5272654034954,-10.9872274015843,132.358033800195));
#73187=CARTESIAN_POINT('Ctrl Pts',(80.4580076981792,-11.0043174377093,132.354172212249));
#73188=CARTESIAN_POINT('Ctrl Pts',(80.3881417079494,-11.017757065915,132.350310624302));
#73189=CARTESIAN_POINT('Ctrl Pts',(80.3181534846656,-11.031220207232,132.346442280368));
#73190=CARTESIAN_POINT('Ctrl Pts',(80.247555333052,-11.0410201229495,132.342573936435));
#73191=CARTESIAN_POINT('Ctrl Pts',(80.1767608663214,-11.0471329118153,132.338705592501));
#73192=CARTESIAN_POINT('Ctrl Pts',(80.1347251492659,-11.0507625099329,132.336408681195));
#73193=CARTESIAN_POINT('Ctrl Pts',(80.0926202580343,-11.0530931573773,132.334111769889));
#73194=CARTESIAN_POINT('Ctrl Pts',(80.0505323671532,-11.0541285359904,132.331814858582));
#73195=CARTESIAN_POINT('Ctrl Pts',(79.9796364922361,-11.0558726023028,132.327945775735));
#73196=CARTESIAN_POINT('Ctrl Pts',(79.9085113617542,-11.0539454419162,132.324076692888));
#73197=CARTESIAN_POINT('Ctrl Pts',(79.8375688633132,-11.0483197231718,132.320207610042));
#73198=CARTESIAN_POINT('Ctrl Pts',(79.7667320656567,-11.0427023864678,132.316344291935));
#73199=CARTESIAN_POINT('Ctrl Pts',(79.6960778402228,-11.0333974680175,132.312480973829));
#73200=CARTESIAN_POINT('Ctrl Pts',(79.6260191864144,-11.0204296358868,132.308617655722));
#73201=CARTESIAN_POINT('Ctrl Pts',(79.5560427113801,-11.0074770150183,132.304758869287));
#73202=CARTESIAN_POINT('Ctrl Pts',(79.4866608956555,-10.9908701029518,132.300900082851));
#73203=CARTESIAN_POINT('Ctrl Pts',(79.4182809721587,-10.9706852958165,132.297041296415));
#73204=CARTESIAN_POINT('Ctrl Pts',(79.3499441229995,-10.9505132036296,132.293184940732));
#73205=CARTESIAN_POINT('Ctrl Pts',(79.2826083787457,-10.9267678251053,132.289328585049));
#73206=CARTESIAN_POINT('Ctrl Pts',(79.2166686972241,-10.8995761718318,132.285472229365));
#73207=CARTESIAN_POINT('Ctrl Pts',(79.1507484949446,-10.872392551245,132.281617012888));
#73208=CARTESIAN_POINT('Ctrl Pts',(79.0862239854993,-10.8417648621427,132.277761796411));
#73209=CARTESIAN_POINT('Ctrl Pts',(79.0234712956362,-10.8078687043183,132.273906579934));
#73210=CARTESIAN_POINT('Ctrl Pts',(78.9607161523306,-10.7739712212555,132.270051212729));
#73211=CARTESIAN_POINT('Ctrl Pts',(78.8997333925077,-10.7368052485742,132.266195845525));
#73212=CARTESIAN_POINT('Ctrl Pts',(78.8408740891248,-10.6965920797993,132.26234047832));
#73213=CARTESIAN_POINT('Ctrl Pts',(78.7819531761015,-10.6563368188023,132.258481075597));
#73214=CARTESIAN_POINT('Ctrl Pts',(78.7251605584144,-10.6130282691899,132.254621672874));
#73215=CARTESIAN_POINT('Ctrl Pts',(78.6708171167331,-10.5669302554135,132.250762270152));
#73216=CARTESIAN_POINT('Ctrl Pts',(78.6164429053683,-10.5208061405797,132.246900682205));
#73217=CARTESIAN_POINT('Ctrl Pts',(78.5645209843352,-10.4718897507229,132.243039094258));
#73218=CARTESIAN_POINT('Ctrl Pts',(78.5153359699761,-10.4204824111735,132.239177506311));
#73219=CARTESIAN_POINT('Ctrl Pts',(78.4660649046714,-10.3689851326409,132.235309162378));
#73220=CARTESIAN_POINT('Ctrl Pts',(78.4195406232412,-10.31498857167,132.231440818444));
#73221=CARTESIAN_POINT('Ctrl Pts',(78.3760075415848,-10.2588272548331,132.227572474511));
#73222=CARTESIAN_POINT('Ctrl Pts',(78.3501588504697,-10.2254802810766,132.225275563204));
#73223=CARTESIAN_POINT('Ctrl Pts',(78.3253639320698,-10.1913706665246,132.222978651898));
#73224=CARTESIAN_POINT('Ctrl Pts',(78.3016664325153,-10.1565728062058,132.220681740591));
#73225=CARTESIAN_POINT('Ctrl Pts',(78.2611561583561,-10.0970867469942,132.216755228997));
#73226=CARTESIAN_POINT('Ctrl Pts',(78.22369963522,-10.0353595220403,132.212828717404));
#73227=CARTESIAN_POINT('Ctrl Pts',(78.1895485268499,-9.97173197223746,132.20890220581));
#73228=CARTESIAN_POINT('Ctrl Pts',(78.1554524650247,-9.90820698065173,132.204982023173));
#73229=CARTESIAN_POINT('Ctrl Pts',(78.1246514562146,-9.8427881549543,132.201061840536));
#73230=CARTESIAN_POINT('Ctrl Pts',(78.0973541022689,-9.77584544230588,132.1971416579));
#73231=CARTESIAN_POINT('Ctrl Pts',(78.0700989505557,-9.70900622437492,132.19322753594));
#73232=CARTESIAN_POINT('Ctrl Pts',(78.0463368576597,-9.64064823422256,132.189313413981));
#73233=CARTESIAN_POINT('Ctrl Pts',(78.0262298521903,-9.57116457008041,132.185399292022));
#73234=CARTESIAN_POINT('Ctrl Pts',(78.0061411816448,-9.5017442658303,132.181488739223));
#73235=CARTESIAN_POINT('Ctrl Pts',(77.9897011084485,-9.43120077295633,132.177578186424));
#73236=CARTESIAN_POINT('Ctrl Pts',(77.977022638429,-9.35994465834536,132.173667633625));
#73237=CARTESIAN_POINT('Ctrl Pts',(77.9643515390457,-9.28872996851899,132.169759354228));
#73238=CARTESIAN_POINT('Ctrl Pts',(77.9554377814959,-9.21680393863984,132.165851074832));
#73239=CARTESIAN_POINT('Ctrl Pts',(77.9503434953968,-9.14458829702956,132.161942795435));
#73240=CARTESIAN_POINT('Ctrl Pts',(77.9469249211355,-9.09612723126452,132.159320103444));
#73241=CARTESIAN_POINT('Ctrl Pts',(77.9452252851269,-9.04753598590096,132.156697411453));
#73242=CARTESIAN_POINT('Ctrl Pts',(77.9452502716446,-8.99894343798261,132.154074719462));
#73243=CARTESIAN_POINT('Origin',(80.,-9.,141.545925280538));
#73244=CARTESIAN_POINT('',(81.2520391107129,-7.37076839346112,133.306011340568));
#73245=CARTESIAN_POINT('',(81.2520391107129,-7.3707683934611,133.247993489751));
#73246=CARTESIAN_POINT('',(81.2520391107129,-7.37076839346111,141.545925280538));
#73247=CARTESIAN_POINT('',(77.9452506345969,-8.99838510821483,132.795925280579));
#73248=CARTESIAN_POINT('Ctrl Pts',(81.2520391107129,-7.3707683934611,133.247993489751));
#73249=CARTESIAN_POINT('Ctrl Pts',(81.3085458581026,-7.4141929486116,133.244130558908));
#73250=CARTESIAN_POINT('Ctrl Pts',(81.362730023197,-7.46051391564537,133.240267628065));
#73251=CARTESIAN_POINT('Ctrl Pts',(81.4142959525366,-7.50944154051626,133.236404697222));
#73252=CARTESIAN_POINT('Ctrl Pts',(81.4659453720001,-7.55844838384621,133.232535511929));
#73253=CARTESIAN_POINT('Ctrl Pts',(81.5149677691851,-7.61006994974573,133.228666326635));
#73254=CARTESIAN_POINT('Ctrl Pts',(81.5611066401294,-7.66398217802155,133.224797141341));
#73255=CARTESIAN_POINT('Ctrl Pts',(81.5680176300305,-7.67205751357997,133.224217588787));
#73256=CARTESIAN_POINT('Ctrl Pts',(81.5748640036943,-7.6801841888825,133.223638036233));
#73257=CARTESIAN_POINT('Ctrl Pts',(81.5816449834366,-7.68836106002075,133.223058483679));
#73258=CARTESIAN_POINT('Ctrl Pts',(81.6269146871557,-7.74294971060641,133.219189400832));
#73259=CARTESIAN_POINT('Ctrl Pts',(81.6694436428744,-7.79999167812778,133.215320317985));
#73260=CARTESIAN_POINT('Ctrl Pts',(81.7089553397541,-7.85918046596933,133.211451235138));
#73261=CARTESIAN_POINT('Ctrl Pts',(81.7484081661759,-7.9182810654689,133.207587917032));
#73262=CARTESIAN_POINT('Ctrl Pts',(81.7848523898165,-7.97952173530745,133.203724598926));
#73263=CARTESIAN_POINT('Ctrl Pts',(81.8180516424325,-8.04256290653195,133.199861280819));
#73264=CARTESIAN_POINT('Ctrl Pts',(81.8512119523379,-8.10553013048689,133.196002494383));
#73265=CARTESIAN_POINT('Ctrl Pts',(81.8811346266599,-8.17029323296865,133.192143707948));
#73266=CARTESIAN_POINT('Ctrl Pts',(81.9076274856162,-8.23648514184629,133.188284921512));
#73267=CARTESIAN_POINT('Ctrl Pts',(81.934103656014,-8.30263535467497,133.184428565829));
#73268=CARTESIAN_POINT('Ctrl Pts',(81.9571541174251,-8.37021213829343,133.180572210145));
#73269=CARTESIAN_POINT('Ctrl Pts',(81.9766340351603,-8.43882671700644,133.176715854462));
#73270=CARTESIAN_POINT('Ctrl Pts',(81.9961081983328,-8.50742102628585,133.172860637985));
#73271=CARTESIAN_POINT('Ctrl Pts',(82.0120137792493,-8.57705205496281,133.169005421508));
#73272=CARTESIAN_POINT('Ctrl Pts',(82.0242557560878,-8.6473157269663,133.16515020503));
#73273=CARTESIAN_POINT('Ctrl Pts',(82.036498211551,-8.71758214606921,133.161294837826));
#73274=CARTESIAN_POINT('Ctrl Pts',(82.0450766973487,-8.78848077865394,133.157439470621));
#73275=CARTESIAN_POINT('Ctrl Pts',(82.0499475849728,-8.85959892676965,133.153584103417));
#73276=CARTESIAN_POINT('Ctrl Pts',(82.054823571088,-8.93079151619345,133.149724700694));
#73277=CARTESIAN_POINT('Ctrl Pts',(82.055984178733,-9.00220359418581,133.145865297971));
#73278=CARTESIAN_POINT('Ctrl Pts',(82.0534378710938,-9.073419834225,133.142005895248));
#73279=CARTESIAN_POINT('Ctrl Pts',(82.0508901217152,-9.14467639745873,133.138144307301));
#73280=CARTESIAN_POINT('Ctrl Pts',(82.0446313214623,-9.21573641786266,133.134282719354));
#73281=CARTESIAN_POINT('Ctrl Pts',(82.0347218354742,-9.28618982292246,133.130421131407));
#73282=CARTESIAN_POINT('Ctrl Pts',(82.0247950124852,-9.35676648873972,133.126552787474));
#73283=CARTESIAN_POINT('Ctrl Pts',(82.0112048445784,-9.42673394328516,133.122684443541));
#73284=CARTESIAN_POINT('Ctrl Pts',(81.9940626600268,-9.49569312118169,133.118816099607));
#73285=CARTESIAN_POINT('Ctrl Pts',(81.9838841241492,-9.53663909654412,133.116519188301));
#73286=CARTESIAN_POINT('Ctrl Pts',(81.972454231622,-9.57722987554718,133.114222276994));
#73287=CARTESIAN_POINT('Ctrl Pts',(81.9598043720399,-9.61738511954302,133.111925365688));
#73288=CARTESIAN_POINT('Ctrl Pts',(81.9384960374134,-9.68502550483927,133.108056282841));
#73289=CARTESIAN_POINT('Ctrl Pts',(81.9136400623009,-9.75169392790778,133.104187199994));
#73290=CARTESIAN_POINT('Ctrl Pts',(81.8853439706104,-9.81699184511425,133.100318117147));
#73291=CARTESIAN_POINT('Ctrl Pts',(81.8570900386852,-9.88219247168061,133.096454799041));
#73292=CARTESIAN_POINT('Ctrl Pts',(81.8254063559398,-9.94602620356839,133.092591480934));
#73293=CARTESIAN_POINT('Ctrl Pts',(81.7904500040003,-10.0081102844804,133.088728162828));
#73294=CARTESIAN_POINT('Ctrl Pts',(81.7555346558482,-10.0701215407895,133.084869376392));
#73295=CARTESIAN_POINT('Ctrl Pts',(81.7173545009176,-10.1303868015217,133.081010589956));
#73296=CARTESIAN_POINT('Ctrl Pts',(81.6761136941161,-10.1885455173853,133.07715180352));
#73297=CARTESIAN_POINT('Ctrl Pts',(81.6348988659987,-10.2466675975224,133.073295447837));
#73298=CARTESIAN_POINT('Ctrl Pts',(81.5906274914361,-10.3026853701469,133.069439092154));
#73299=CARTESIAN_POINT('Ctrl Pts',(81.5435476382644,-10.3562662905596,133.065582736471));
#73300=CARTESIAN_POINT('Ctrl Pts',(81.4964816929528,-10.4098313826319,133.061727519993));
#73301=CARTESIAN_POINT('Ctrl Pts',(81.4466092365965,-10.4609606869092,133.057872303516));
#73302=CARTESIAN_POINT('Ctrl Pts',(81.3942182089022,-10.5093552095069,133.054017087039));
#73303=CARTESIAN_POINT('Ctrl Pts',(81.3418251328754,-10.5577516241857,133.050161719834));
#73304=CARTESIAN_POINT('Ctrl Pts',(81.28691364835,-10.6034127169036,133.04630635263));
#73305=CARTESIAN_POINT('Ctrl Pts',(81.2298068132815,-10.6460779946608,133.042450985425));
#73306=CARTESIAN_POINT('Ctrl Pts',(81.1726402029288,-10.6887879313296,133.038591582702));
#73307=CARTESIAN_POINT('Ctrl Pts',(81.1132740448054,-10.7284955019295,133.034732179979));
#73308=CARTESIAN_POINT('Ctrl Pts',(81.0520618587254,-10.7649825517311,133.030872777257));
#73309=CARTESIAN_POINT('Ctrl Pts',(80.9908150138248,-10.8014902607869,133.02701118931));
#73310=CARTESIAN_POINT('Ctrl Pts',(80.9277204900953,-10.8347735922872,133.023149601363));
#73311=CARTESIAN_POINT('Ctrl Pts',(80.8631555438839,-10.8646608457204,133.019288013416));
#73312=CARTESIAN_POINT('Ctrl Pts',(80.7984776389848,-10.8946003879747,133.015419669482));
#73313=CARTESIAN_POINT('Ctrl Pts',(80.732324626437,-10.9211318087839,133.011551325549));
#73314=CARTESIAN_POINT('Ctrl Pts',(80.6650921565283,-10.9441321935055,133.007682981616));
#73315=CARTESIAN_POINT('Ctrl Pts',(80.6251714506786,-10.9577891600597,133.005386070309));
#73316=CARTESIAN_POINT('Ctrl Pts',(80.5848704458191,-10.9702021689855,133.003089159003));
#73317=CARTESIAN_POINT('Ctrl Pts',(80.5442736622039,-10.981354017618,133.000792247696));
#73318=CARTESIAN_POINT('Ctrl Pts',(80.4758895157697,-11.0001389947021,132.996923164849));
#73319=CARTESIAN_POINT('Ctrl Pts',(80.4063977765706,-11.0154163084819,132.993054082002));
#73320=CARTESIAN_POINT('Ctrl Pts',(80.3361915931483,-11.027060131125,132.989184999155));
#73321=CARTESIAN_POINT('Ctrl Pts',(80.266090013438,-11.038686605053,132.985321681049));
#73322=CARTESIAN_POINT('Ctrl Pts',(80.1952765778128,-11.0466902550951,132.981458362943));
#73323=CARTESIAN_POINT('Ctrl Pts',(80.1241580504815,-11.0509954512384,132.977595044836));
#73324=CARTESIAN_POINT('Ctrl Pts',(80.0531229451553,-11.0552955973883,132.9737362584));
#73325=CARTESIAN_POINT('Ctrl Pts',(79.9817839415209,-11.0559058777313,132.969877471965));
#73326=CARTESIAN_POINT('Ctrl Pts',(79.9105546785685,-11.0528022547177,132.966018685529));
#73327=CARTESIAN_POINT('Ctrl Pts',(79.8393702848288,-11.049700586759,132.962162329846));
#73328=CARTESIAN_POINT('Ctrl Pts',(79.7682959787965,-11.0428896780456,132.958305974162));
#73329=CARTESIAN_POINT('Ctrl Pts',(79.6977456893856,-11.0323975728718,132.954449618479));
#73330=CARTESIAN_POINT('Ctrl Pts',(79.6272162412367,-11.0219085671709,132.950594402002));
#73331=CARTESIAN_POINT('Ctrl Pts',(79.5572109826255,-11.0077405953441,132.946739185525));
#73332=CARTESIAN_POINT('Ctrl Pts',(79.4881372810349,-10.9899733966648,132.942883969048));
#73333=CARTESIAN_POINT('Ctrl Pts',(79.4190608788692,-10.9722055033412,132.939028601843));
#73334=CARTESIAN_POINT('Ctrl Pts',(79.3509165759533,-10.9508382269336,132.935173234638));
#73335=CARTESIAN_POINT('Ctrl Pts',(79.28409844135,-10.92600169284,132.931317867434));
#73336=CARTESIAN_POINT('Ctrl Pts',(79.2172103663801,-10.9011391616677,132.927458464711));
#73337=CARTESIAN_POINT('Ctrl Pts',(79.1516516870319,-10.8728002933874,132.923599061988));
#73338=CARTESIAN_POINT('Ctrl Pts',(79.0877974244997,-10.8411637688567,132.919739659265));
#73339=CARTESIAN_POINT('Ctrl Pts',(79.0239070071824,-10.8095093314772,132.915878071318));
#73340=CARTESIAN_POINT('Ctrl Pts',(78.9617233514698,-10.7745537590656,132.912016483371));
#73341=CARTESIAN_POINT('Ctrl Pts',(78.9015953250592,-10.7365208701793,132.908154895425));
#73342=CARTESIAN_POINT('Ctrl Pts',(78.8413621025112,-10.6984214413906,132.904286551491));
#73343=CARTESIAN_POINT('Ctrl Pts',(78.7831920861634,-10.6572342278724,132.900418207558));
#73344=CARTESIAN_POINT('Ctrl Pts',(78.7274031336022,-10.6132249620355,132.896549863624));
#73345=CARTESIAN_POINT('Ctrl Pts',(78.6942772590379,-10.5870935264582,132.894252952318));
#73346=CARTESIAN_POINT('Ctrl Pts',(78.661990207726,-10.5599678909665,132.891956041011));
#73347=CARTESIAN_POINT('Ctrl Pts',(78.6306022743163,-10.5319097334348,132.889659129705));
#73348=CARTESIAN_POINT('Ctrl Pts',(78.5772314750468,-10.4842007532368,132.885753552658));
#73349=CARTESIAN_POINT('Ctrl Pts',(78.5262345230158,-10.4335895840301,132.881847975611));
#73350=CARTESIAN_POINT('Ctrl Pts',(78.4779491498061,-10.3803473374206,132.877942398564));
#73351=CARTESIAN_POINT('Ctrl Pts',(78.4309056772216,-10.3284744823049,132.874137273026));
#73352=CARTESIAN_POINT('Ctrl Pts',(78.386436362009,-10.2741046430855,132.870332147487));
#73353=CARTESIAN_POINT('Ctrl Pts',(78.3448201620121,-10.2175291645042,132.866527021949));
#73354=CARTESIAN_POINT('Ctrl Pts',(78.3032434930469,-10.1610074267026,132.862725510881));
#73355=CARTESIAN_POINT('Ctrl Pts',(78.264514863504,-10.102284603711,132.858923999814));
#73356=CARTESIAN_POINT('Ctrl Pts',(78.2288739527537,-10.0416861750382,132.855122488746));
#73357=CARTESIAN_POINT('Ctrl Pts',(78.1932541443473,-9.981123625608,132.851323228485));
#73358=CARTESIAN_POINT('Ctrl Pts',(78.1607186828808,-9.91868810415967,132.847523968224));
#73359=CARTESIAN_POINT('Ctrl Pts',(78.1314636677263,-9.85473360614478,132.843724707962));
#73360=CARTESIAN_POINT('Ctrl Pts',(78.1007916228991,-9.78768133426415,132.839741422347));
#73361=CARTESIAN_POINT('Ctrl Pts',(78.073726197892,-9.71895970058232,132.835758136732));
#73362=CARTESIAN_POINT('Ctrl Pts',(78.0504379098929,-9.64900325062141,132.831774851116));
#73363=CARTESIAN_POINT('Ctrl Pts',(78.02821733148,-9.58225412840588,132.827974189155));
#73364=CARTESIAN_POINT('Ctrl Pts',(78.0094352320241,-9.51438146381125,132.824173527193));
#73365=CARTESIAN_POINT('Ctrl Pts',(77.9941886715373,-9.44577850678409,132.820372865231));
#73366=CARTESIAN_POINT('Ctrl Pts',(77.9789361563188,-9.37714875602829,132.816570718874));
#73367=CARTESIAN_POINT('Ctrl Pts',(77.967222012663,-9.30778863950404,132.812768572516));
#73368=CARTESIAN_POINT('Ctrl Pts',(77.9590918603005,-9.23809982740112,132.808966426159));
#73369=CARTESIAN_POINT('Ctrl Pts',(77.9509517006751,-9.16832523655263,132.805159599806));
#73370=CARTESIAN_POINT('Ctrl Pts',(77.9464043599199,-9.09822164285832,132.801352773453));
#73371=CARTESIAN_POINT('Ctrl Pts',(77.9454434209989,-9.02819266187148,132.797545947101));
#73372=CARTESIAN_POINT('Ctrl Pts',(77.9453070553061,-9.01825493294981,132.797005724927));
#73373=CARTESIAN_POINT('Ctrl Pts',(77.9452428274764,-9.00831870003405,132.796465502753));
#73374=CARTESIAN_POINT('Ctrl Pts',(77.9452506345969,-8.99838510821483,132.795925280579));
#73375=CARTESIAN_POINT('Ctrl Pts',(77.9452506345975,-8.99838510746551,132.795925280538));
#73376=CARTESIAN_POINT('Ctrl Pts',(77.9453344508848,-8.8917393341807,132.790125524263));
#73377=CARTESIAN_POINT('Ctrl Pts',(77.9537227446016,-8.7854126555166,132.784325767988));
#73378=CARTESIAN_POINT('Ctrl Pts',(77.9702575839437,-8.68040136583243,132.778526011713));
#73379=CARTESIAN_POINT('Ctrl Pts',(77.9812881618236,-8.61034714969089,132.774656928866));
#73380=CARTESIAN_POINT('Ctrl Pts',(77.9959713625728,-8.54072745600456,132.770787846019));
#73381=CARTESIAN_POINT('Ctrl Pts',(78.0142600200556,-8.47195237473287,132.766918763172));
#73382=CARTESIAN_POINT('Ctrl Pts',(78.0325214283508,-8.40327976490233,132.763055445066));
#73383=CARTESIAN_POINT('Ctrl Pts',(78.0543775063822,-8.33544973518021,132.75919212696));
#73384=CARTESIAN_POINT('Ctrl Pts',(78.0797297357171,-8.26886412028216,132.755328808853));
#73385=CARTESIAN_POINT('Ctrl Pts',(78.1050522268967,-8.20235661028468,132.751470022417));
#73386=CARTESIAN_POINT('Ctrl Pts',(78.1338625514209,-8.13709106744276,132.747611235982));
#73387=CARTESIAN_POINT('Ctrl Pts',(78.1660123424268,-8.07345435386632,132.743752449546));
#73388=CARTESIAN_POINT('Ctrl Pts',(78.1981418814219,-8.00985772675313,132.739896093862));
#73389=CARTESIAN_POINT('Ctrl Pts',(78.2336064948159,-7.94788832581778,132.736039738179));
#73390=CARTESIAN_POINT('Ctrl Pts',(78.2722102319604,-7.88791183804621,132.732183382496));
#73391=CARTESIAN_POINT('Ctrl Pts',(78.3108025651744,-7.82795306792971,132.728328166019));
#73392=CARTESIAN_POINT('Ctrl Pts',(78.352531918358,-7.76998645045226,132.724472949542));
#73393=CARTESIAN_POINT('Ctrl Pts',(78.3971579299849,-7.71435041279142,132.720617733064));
#73394=CARTESIAN_POINT('Ctrl Pts',(78.4417856863553,-7.65871219992794,132.71676236586));
#73395=CARTESIAN_POINT('Ctrl Pts',(78.4893100203424,-7.60540512535013,132.712906998655));
#73396=CARTESIAN_POINT('Ctrl Pts',(78.5394501256201,-7.55473475550368,132.709051631451));
#73397=CARTESIAN_POINT('Ctrl Pts',(78.5896427139156,-7.50401134759714,132.705192228728));
#73398=CARTESIAN_POINT('Ctrl Pts',(78.6424561967729,-7.45593049983249,132.701332826005));
#73399=CARTESIAN_POINT('Ctrl Pts',(78.6975733581745,-7.41076043179036,132.697473423282));
#73400=CARTESIAN_POINT('Ctrl Pts',(78.7527217273459,-7.36556478810086,132.693611835335));
#73401=CARTESIAN_POINT('Ctrl Pts',(78.8101759802005,-7.32328349307188,132.689750247388));
#73402=CARTESIAN_POINT('Ctrl Pts',(78.8695885307939,-7.28414235066328,132.685888659441));
#73403=CARTESIAN_POINT('Ctrl Pts',(78.9291050257741,-7.24493272942309,132.682020315508));
#73404=CARTESIAN_POINT('Ctrl Pts',(78.9905862396583,-7.20887447518602,132.678151971575));
#73405=CARTESIAN_POINT('Ctrl Pts',(79.0536591538174,-7.1761478773359,132.674283627641));
#73406=CARTESIAN_POINT('Ctrl Pts',(79.091110035165,-7.1567157653218,132.671986716335));
#73407=CARTESIAN_POINT('Ctrl Pts',(79.1291216747153,-7.13845736884238,132.669689805028));
#73408=CARTESIAN_POINT('Ctrl Pts',(79.1676130426289,-7.1214022474999,132.667392893722));
#73409=CARTESIAN_POINT('Ctrl Pts',(79.2324506752053,-7.0926733726614,132.663523810875));
#73410=CARTESIAN_POINT('Ctrl Pts',(79.2989043618555,-7.06724886354418,132.659654728028));
#73411=CARTESIAN_POINT('Ctrl Pts',(79.3666039904559,-7.04531151904103,132.655785645181));
#73412=CARTESIAN_POINT('Ctrl Pts',(79.4342027499861,-7.02340686008714,132.651922327075));
#73413=CARTESIAN_POINT('Ctrl Pts',(79.503043308219,-7.0049792009511,132.648059008968));
#73414=CARTESIAN_POINT('Ctrl Pts',(79.5727346360592,-6.99016372028054,132.644195690862));
#73415=CARTESIAN_POINT('Ctrl Pts',(79.6423442159988,-6.97536561816309,132.640336904426));
#73416=CARTESIAN_POINT('Ctrl Pts',(79.7128021104156,-6.96417137875143,132.63647811799));
#73417=CARTESIAN_POINT('Ctrl Pts',(79.7837028323883,-6.95666618053164,132.632619331554));
#73418=CARTESIAN_POINT('Ctrl Pts',(79.8545588921051,-6.94916571003639,132.628762975871));
#73419=CARTESIAN_POINT('Ctrl Pts',(79.9258567440053,-6.9453497213157,132.624906620188));
#73420=CARTESIAN_POINT('Ctrl Pts',(79.9971828825805,-6.94525193117272,132.621050264504));
#73421=CARTESIAN_POINT('Ctrl Pts',(80.0684879507002,-6.94515416991792,132.617195048027));
#73422=CARTESIAN_POINT('Ctrl Pts',(80.1398208033875,-6.9487724272913,132.61333983155));
#73423=CARTESIAN_POINT('Ctrl Pts',(80.2107667494145,-6.95608832386494,132.609484615073));
#73424=CARTESIAN_POINT('Ctrl Pts',(80.2817154692159,-6.96340450646825,132.605629247868));
#73425=CARTESIAN_POINT('Ctrl Pts',(80.3522767693298,-6.97441856326924,132.601773880663));
#73426=CARTESIAN_POINT('Ctrl Pts',(80.422041629453,-6.98906031281177,132.597918513459));
#73427=CARTESIAN_POINT('Ctrl Pts',(80.4918795143608,-7.00371738827347,132.594059110736));
#73428=CARTESIAN_POINT('Ctrl Pts',(80.5609188187151,-7.02200963656564,132.590199708013));
#73429=CARTESIAN_POINT('Ctrl Pts',(80.6287621506491,-7.04381603104128,132.58634030529));
#73430=CARTESIAN_POINT('Ctrl Pts',(80.6966438960106,-7.06563477246877,132.582478717343));
#73431=CARTESIAN_POINT('Ctrl Pts',(80.7633278665928,-7.09097144841154,132.578617129396));
#73432=CARTESIAN_POINT('Ctrl Pts',(80.8284358332442,-7.11965651204441,132.57475554145));
#73433=CARTESIAN_POINT('Ctrl Pts',(80.8936577086169,-7.14839176122426,132.570887197516));
#73434=CARTESIAN_POINT('Ctrl Pts',(80.9572976411984,-7.18048687518794,132.567018853583));
#73435=CARTESIAN_POINT('Ctrl Pts',(81.0190018459504,-7.21572625406032,132.563150509649));
#73436=CARTESIAN_POINT('Ctrl Pts',(81.0556400270383,-7.23665038313284,132.560853598343));
#73437=CARTESIAN_POINT('Ctrl Pts',(81.0915962750952,-7.25868222392753,132.558556687036));
#73438=CARTESIAN_POINT('Ctrl Pts',(81.1268018071313,-7.28176973314236,132.55625977573));
#73439=CARTESIAN_POINT('Ctrl Pts',(81.1695802911759,-7.3098235243353,132.553468783008));
#73440=CARTESIAN_POINT('Ctrl Pts',(81.211370811523,-7.33951543903302,132.550677790287));
#73441=CARTESIAN_POINT('Ctrl Pts',(81.2520391107129,-7.3707683934611,132.547886797565));
#73442=CARTESIAN_POINT('',(77.9452507493435,-9.00175482953772,132.854074719498));
#73443=CARTESIAN_POINT('Ctrl Pts',(77.945250749343,-9.00175482886545,132.854074719462));
#73444=CARTESIAN_POINT('Ctrl Pts',(77.9451902335234,-8.93089616152734,132.850240467841));
#73445=CARTESIAN_POINT('Ctrl Pts',(77.9487993838056,-8.85997312348533,132.846406216221));
#73446=CARTESIAN_POINT('Ctrl Pts',(77.9560714877068,-8.78939658327859,132.8425719646));
#73447=CARTESIAN_POINT('Ctrl Pts',(77.9633409049725,-8.7188461171535,132.838739129521));
#73448=CARTESIAN_POINT('Ctrl Pts',(77.9742705404255,-8.64864238372495,132.834906294442));
#73449=CARTESIAN_POINT('Ctrl Pts',(77.9888017188309,-8.57919239987539,132.831073459363));
#73450=CARTESIAN_POINT('Ctrl Pts',(78.0033325301935,-8.50974417026249,132.827240721097));
#73451=CARTESIAN_POINT('Ctrl Pts',(78.0214646012841,-8.4410501334779,132.823407982832));
#73452=CARTESIAN_POINT('Ctrl Pts',(78.0430882613476,-8.37350657655141,132.819575244566));
#73453=CARTESIAN_POINT('Ctrl Pts',(78.0647340638347,-8.30589385566048,132.815738581613));
#73454=CARTESIAN_POINT('Ctrl Pts',(78.0898784440367,-8.23943443646795,132.811901918659));
#73455=CARTESIAN_POINT('Ctrl Pts',(78.1183622815556,-8.17450798972523,132.808065255706));
#73456=CARTESIAN_POINT('Ctrl Pts',(78.1468610721472,-8.10954745874536,132.804226578632));
#73457=CARTESIAN_POINT('Ctrl Pts',(78.178702588492,-8.04612194192218,132.800387901557));
#73458=CARTESIAN_POINT('Ctrl Pts',(78.2136813665786,-7.98458712712931,132.796549224483));
#73459=CARTESIAN_POINT('Ctrl Pts',(78.2487243400167,-7.92293937960173,132.792703502416));
#73460=CARTESIAN_POINT('Ctrl Pts',(78.2869158076438,-7.86318967817087,132.788857780349));
#73461=CARTESIAN_POINT('Ctrl Pts',(78.3280069113267,-7.80566475647388,132.785012058282));
#73462=CARTESIAN_POINT('Ctrl Pts',(78.3588674553701,-7.76246196510268,132.782123815704));
#73463=CARTESIAN_POINT('Ctrl Pts',(78.3913626087628,-7.72051343395676,132.779235573126));
#73464=CARTESIAN_POINT('Ctrl Pts',(78.4253729722412,-7.67994421104584,132.776347330549));
#73465=CARTESIAN_POINT('Ctrl Pts',(78.4709331737854,-7.62559777709811,132.772478247702));
#73466=CARTESIAN_POINT('Ctrl Pts',(78.5193994699273,-7.57350635485296,132.768609164855));
#73467=CARTESIAN_POINT('Ctrl Pts',(78.5705200716172,-7.52399705391533,132.764740082008));
#73468=CARTESIAN_POINT('Ctrl Pts',(78.62156450616,-7.47456151936696,132.760876763902));
#73469=CARTESIAN_POINT('Ctrl Pts',(78.675255050003,-7.42770080468091,132.757013445795));
#73470=CARTESIAN_POINT('Ctrl Pts',(78.7313001635042,-7.38370847698331,132.753150127689));
#73471=CARTESIAN_POINT('Ctrl Pts',(78.7872795361089,-7.33976775226914,132.749291341253));
#73472=CARTESIAN_POINT('Ctrl Pts',(78.8456076120165,-7.29868902976494,132.745432554817));
#73473=CARTESIAN_POINT('Ctrl Pts',(78.905957852007,-7.26072735291014,132.741573768381));
#73474=CARTESIAN_POINT('Ctrl Pts',(78.9662700757718,-7.22278958912815,132.737717412698));
#73475=CARTESIAN_POINT('Ctrl Pts',(79.0286015261643,-7.18796523346361,132.733861057015));
#73476=CARTESIAN_POINT('Ctrl Pts',(79.0925958019738,-7.15646665777254,132.730004701331));
#73477=CARTESIAN_POINT('Ctrl Pts',(79.1565711732334,-7.1249773870761,132.726149484854));
#73478=CARTESIAN_POINT('Ctrl Pts',(79.2222079591014,-7.09681216029129,132.722294268377));
#73479=CARTESIAN_POINT('Ctrl Pts',(79.2891257515506,-7.07213709891199,132.7184390519));
#73480=CARTESIAN_POINT('Ctrl Pts',(79.3560461602854,-7.04746107281158,132.714583684695));
#73481=CARTESIAN_POINT('Ctrl Pts',(79.424247218489,-7.02627564902794,132.710728317491));
#73482=CARTESIAN_POINT('Ctrl Pts',(79.4933307968454,-7.00869794328568,132.706872950286));
#73483=CARTESIAN_POINT('Ctrl Pts',(79.56248668687,-6.99110183847875,132.703013547563));
#73484=CARTESIAN_POINT('Ctrl Pts',(79.6325264693278,-6.97712111008018,132.69915414484));
#73485=CARTESIAN_POINT('Ctrl Pts',(79.7030400637036,-6.96682210352,132.695294742118));
#73486=CARTESIAN_POINT('Ctrl Pts',(79.7735935834305,-6.9565172655814,132.691433154171));
#73487=CARTESIAN_POINT('Ctrl Pts',(79.8446209652136,-6.94989834441169,132.687571566224));
#73488=CARTESIAN_POINT('Ctrl Pts',(79.9157079655863,-6.94697968460261,132.683709978277));
#73489=CARTESIAN_POINT('Ctrl Pts',(79.9869193352142,-6.94405591849357,132.679841634343));
#73490=CARTESIAN_POINT('Ctrl Pts',(80.0581900457724,-6.94484533336773,132.67597329041));
#73491=CARTESIAN_POINT('Ctrl Pts',(80.129107519016,-6.94931016215676,132.672104946476));
#73492=CARTESIAN_POINT('Ctrl Pts',(80.1712162738,-6.95196124900504,132.66980803517));
#73493=CARTESIAN_POINT('Ctrl Pts',(80.2132005988818,-6.95590716216112,132.667511123864));
#73494=CARTESIAN_POINT('Ctrl Pts',(80.2549758212292,-6.96113146743384,132.665214212557));
#73495=CARTESIAN_POINT('Ctrl Pts',(80.3253420978987,-6.96993129875895,132.661345290086));
#73496=CARTESIAN_POINT('Ctrl Pts',(80.3953900995648,-6.98239540609979,132.657476367615));
#73497=CARTESIAN_POINT('Ctrl Pts',(80.4647084963175,-6.99848967628185,132.653607445144));
#73498=CARTESIAN_POINT('Ctrl Pts',(80.5356580114459,-7.01496265775943,132.649647483774));
#73499=CARTESIAN_POINT('Ctrl Pts',(80.6058426319329,-7.03523884401316,132.645687522404));
#73500=CARTESIAN_POINT('Ctrl Pts',(80.6748265781646,-7.05922524441845,132.641727561034));
#73501=CARTESIAN_POINT('Ctrl Pts',(80.7420453191852,-7.08259786551268,132.63786892968));
#73502=CARTESIAN_POINT('Ctrl Pts',(80.8081236067996,-7.10949292659595,132.634010298327));
#73503=CARTESIAN_POINT('Ctrl Pts',(80.872670498717,-7.1397731957718,132.630151666974));
#73504=CARTESIAN_POINT('Ctrl Pts',(80.9397599518661,-7.17124623250323,132.626141040595));
#73505=CARTESIAN_POINT('Ctrl Pts',(81.0051943257724,-7.20637657914342,132.622130414216));
#73506=CARTESIAN_POINT('Ctrl Pts',(81.0685566253344,-7.24495461569964,132.618119787838));
#73507=CARTESIAN_POINT('Ctrl Pts',(81.1319189248964,-7.28353265225587,132.614109161459));
#73508=CARTESIAN_POINT('Ctrl Pts',(81.1932086344546,-7.3255580888724,132.61009853508));
#73509=CARTESIAN_POINT('Ctrl Pts',(81.2520391107129,-7.37076839346111,132.606087908702));
#73510=CARTESIAN_POINT('Ctrl Pts',(81.2520391107129,-7.37076839346111,133.306011340568));
#73511=CARTESIAN_POINT('Ctrl Pts',(81.3084857799458,-7.41414677948397,133.302153261449));
#73512=CARTESIAN_POINT('Ctrl Pts',(81.3627336375113,-7.46050680788434,133.298295182331));
#73513=CARTESIAN_POINT('Ctrl Pts',(81.414455974713,-7.50959339168848,133.294437103213));
#73514=CARTESIAN_POINT('Ctrl Pts',(81.4661499207835,-7.55865303116414,133.29058114185));
#73515=CARTESIAN_POINT('Ctrl Pts',(81.5153207454392,-7.61043592261164,133.286725180486));
#73516=CARTESIAN_POINT('Ctrl Pts',(81.5616759656113,-7.66464770905503,133.282869219123));
#73517=CARTESIAN_POINT('Ctrl Pts',(81.6080212472215,-7.71884787248822,133.279014084478));
#73518=CARTESIAN_POINT('Ctrl Pts',(81.6515518076407,-7.77547552757596,133.275158949833));
#73519=CARTESIAN_POINT('Ctrl Pts',(81.6920142694605,-7.83420187234587,133.271303815188));
#73520=CARTESIAN_POINT('Ctrl Pts',(81.7324815910096,-7.89293527042191,133.267448217523));
#73521=CARTESIAN_POINT('Ctrl Pts',(81.7698798089391,-7.95376745712211,133.263592619859));
#73522=CARTESIAN_POINT('Ctrl Pts',(81.8039988352567,-8.0163406255758,133.259737022194));
#73523=CARTESIAN_POINT('Ctrl Pts',(81.8381552721333,-8.07898240376049,133.255877196974));
#73524=CARTESIAN_POINT('Ctrl Pts',(81.8690251105619,-8.14336854525437,133.252017371755));
#73525=CARTESIAN_POINT('Ctrl Pts',(81.8964446627459,-8.20911745268799,133.248157546535));
#73526=CARTESIAN_POINT('Ctrl Pts',(81.9238817319164,-8.27490836382467,133.244295255465));
#73527=CARTESIAN_POINT('Ctrl Pts',(81.9478639656512,-8.342063315957,133.240432964395));
#73528=CARTESIAN_POINT('Ctrl Pts',(81.968277124051,-8.41018415972663,133.236570673326));
#73529=CARTESIAN_POINT('Ctrl Pts',(81.9887245108757,-8.47841922732844,133.232701906034));
#73530=CARTESIAN_POINT('Ctrl Pts',(82.005590767028,-8.54762294683034,133.228833138743));
#73531=CARTESIAN_POINT('Ctrl Pts',(82.0188126251097,-8.61738642575352,133.224964371451));
#73532=CARTESIAN_POINT('Ctrl Pts',(82.023465751608,-8.64193806519704,133.223602848472));
#73533=CARTESIAN_POINT('Ctrl Pts',(82.0276679805648,-8.66655898766611,133.222241325494));
#73534=CARTESIAN_POINT('Ctrl Pts',(82.0314180869268,-8.69123128622436,133.220879802515));
#73535=CARTESIAN_POINT('Ctrl Pts',(82.0420748826076,-8.7613433362115,133.217010719668));
#73536=CARTESIAN_POINT('Ctrl Pts',(82.0491185350753,-8.83214506707416,133.213141636821));
#73537=CARTESIAN_POINT('Ctrl Pts',(82.0524700687833,-8.90323131059755,133.209272553974));
#73538=CARTESIAN_POINT('Ctrl Pts',(82.0558166088733,-8.97421163916328,133.205409235868));
#73539=CARTESIAN_POINT('Ctrl Pts',(82.0554819269895,-9.0454751576497,133.201545917761));
#73540=CARTESIAN_POINT('Ctrl Pts',(82.0514384934808,-9.11660904752696,133.197682599655));
#73541=CARTESIAN_POINT('Ctrl Pts',(82.0473998029181,-9.18765949737885,133.193823813219));
#73542=CARTESIAN_POINT('Ctrl Pts',(82.0396610294618,-9.2585801380065,133.189965026783));
#73543=CARTESIAN_POINT('Ctrl Pts',(82.0282466859119,-9.32895735831159,133.186106240347));
#73544=CARTESIAN_POINT('Ctrl Pts',(82.0168395325615,-9.39929024612842,133.182249884664));
#73545=CARTESIAN_POINT('Ctrl Pts',(82.0017614803033,-9.46907991438652,133.178393528981));
#73546=CARTESIAN_POINT('Ctrl Pts',(81.9830888001475,-9.53791855631631,133.174537173298));
#73547=CARTESIAN_POINT('Ctrl Pts',(81.9644216360885,-9.60673686262192,133.17068195682));
#73548=CARTESIAN_POINT('Ctrl Pts',(81.9421620793816,-9.67460423176284,133.166826740343));
#73549=CARTESIAN_POINT('Ctrl Pts',(81.9164369736022,-9.74112542036437,133.162971523866));
#73550=CARTESIAN_POINT('Ctrl Pts',(81.8907108620482,-9.8076492097454,133.159116156661));
#73551=CARTESIAN_POINT('Ctrl Pts',(81.8615191096899,-9.87282626180524,133.155260789457));
#73552=CARTESIAN_POINT('Ctrl Pts',(81.8290370447409,-9.9362804341999,133.151405422252));
#73553=CARTESIAN_POINT('Ctrl Pts',(81.7965209799272,-9.99980102581,133.147546019529));
#73554=CARTESIAN_POINT('Ctrl Pts',(81.7607079492157,-10.0615947044879,133.143686616806));
#73555=CARTESIAN_POINT('Ctrl Pts',(81.7218192748204,-10.1213099247562,133.139827214084));
#73556=CARTESIAN_POINT('Ctrl Pts',(81.6829085813523,-10.1810589562513,133.135965626137));
#73557=CARTESIAN_POINT('Ctrl Pts',(81.6409190635822,-10.2387267937158,133.13210403819));
#73558=CARTESIAN_POINT('Ctrl Pts',(81.5961138122492,-10.2939931455951,133.128242450243));
#73559=CARTESIAN_POINT('Ctrl Pts',(81.551230172523,-10.349356187938,133.124374106309));
#73560=CARTESIAN_POINT('Ctrl Pts',(81.5035212891509,-10.4023089952922,133.120505762376));
#73561=CARTESIAN_POINT('Ctrl Pts',(81.4532882515811,-10.4525669761895,133.116637418443));
#73562=CARTESIAN_POINT('Ctrl Pts',(81.4234613194531,-10.4824087189476,133.114340507136));
#73563=CARTESIAN_POINT('Ctrl Pts',(81.392745133871,-10.5113011007561,133.11204359583));
#73564=CARTESIAN_POINT('Ctrl Pts',(81.3612080022368,-10.5391914556502,133.109746684523));
#73565=CARTESIAN_POINT('Ctrl Pts',(81.3080845861498,-10.5861719783254,133.105877601676));
#73566=CARTESIAN_POINT('Ctrl Pts',(81.2524220485734,-10.6304910492068,133.102008518829));
#73567=CARTESIAN_POINT('Ctrl Pts',(81.1945179499447,-10.6718625630595,133.098139435982));
#73568=CARTESIAN_POINT('Ctrl Pts',(81.136700125535,-10.7131724354199,133.094276117876));
#73569=CARTESIAN_POINT('Ctrl Pts',(81.0766477615528,-10.7515431880736,133.09041279977));
#73570=CARTESIAN_POINT('Ctrl Pts',(81.0146927489592,-10.7867277878036,133.086549481663));
#73571=CARTESIAN_POINT('Ctrl Pts',(80.9528104095716,-10.8218711160117,133.082690695227));
#73572=CARTESIAN_POINT('Ctrl Pts',(80.8890302750626,-10.8538354762219,133.078831908792));
#73573=CARTESIAN_POINT('Ctrl Pts',(80.8237131290574,-10.8824171279285,133.074973122356));
#73574=CARTESIAN_POINT('Ctrl Pts',(80.7584371280646,-10.9109807752904,133.071116766673));
#73575=CARTESIAN_POINT('Ctrl Pts',(80.6916264804665,-10.9361657474567,133.067260410989));
#73576=CARTESIAN_POINT('Ctrl Pts',(80.6236651661146,-10.9578149358597,133.063404055306));
#73577=CARTESIAN_POINT('Ctrl Pts',(80.5557239282157,-10.9794577288756,133.059548838829));
#73578=CARTESIAN_POINT('Ctrl Pts',(80.486633161009,-10.9975666643961,133.055693622352));
#73579=CARTESIAN_POINT('Ctrl Pts',(80.4167937189864,-11.0120339356764,133.051838405874));
#73580=CARTESIAN_POINT('Ctrl Pts',(80.3469515464505,-11.0265017725837,133.04798303867));
#73581=CARTESIAN_POINT('Ctrl Pts',(80.2763611171161,-11.0373275661965,133.044127671465));
#73582=CARTESIAN_POINT('Ctrl Pts',(80.2054335351808,-11.0444546033412,133.040272304261));
#73583=CARTESIAN_POINT('Ctrl Pts',(80.1344317114082,-11.0515891005504,133.036412901538));
#73584=CARTESIAN_POINT('Ctrl Pts',(80.0630925148929,-11.0550170640636,133.032553498815));
#73585=CARTESIAN_POINT('Ctrl Pts',(79.9918313314322,-11.0547337626451,133.028694096092));
#73586=CARTESIAN_POINT('Ctrl Pts',(79.9205297993297,-11.0544503008192,133.024832508145));
#73587=CARTESIAN_POINT('Ctrl Pts',(79.8493068534627,-11.050451418172,133.020970920198));
#73588=CARTESIAN_POINT('Ctrl Pts',(79.7785742766001,-11.0427844261,133.017109332251));
#73589=CARTESIAN_POINT('Ctrl Pts',(79.7077179505589,-11.0351040203506,133.013240988318));
#73590=CARTESIAN_POINT('Ctrl Pts',(79.6373541861036,-11.0237427699366,133.009372644385));
#73591=CARTESIAN_POINT('Ctrl Pts',(79.5678853829314,-11.0087992732515,133.005504300451));
#73592=CARTESIAN_POINT('Ctrl Pts',(79.526636806746,-10.9999262549563,133.003207389145));
#73593=CARTESIAN_POINT('Ctrl Pts',(79.4857035065239,-10.989791230724,133.000910477838));
#73594=CARTESIAN_POINT('Ctrl Pts',(79.4451667772748,-10.9784230228797,132.998613566532));
#73595=CARTESIAN_POINT('Ctrl Pts',(79.3768837907402,-10.9592735947553,132.994744483685));
#73596=CARTESIAN_POINT('Ctrl Pts',(79.309459608366,-10.9365474476032,132.990875400838));
#73597=CARTESIAN_POINT('Ctrl Pts',(79.2432959875487,-10.9103393939403,132.987006317991));
#73598=CARTESIAN_POINT('Ctrl Pts',(79.1772309472266,-10.8841703889702,132.983142999885));
#73599=CARTESIAN_POINT('Ctrl Pts',(79.1124231883006,-10.8545299527042,132.979279681778));
#73600=CARTESIAN_POINT('Ctrl Pts',(79.0492602626734,-10.8215629317617,132.975416363672));
#73601=CARTESIAN_POINT('Ctrl Pts',(78.9861714271336,-10.7886345811219,132.971557577236));
#73602=CARTESIAN_POINT('Ctrl Pts',(78.9247240210361,-10.7523876203454,132.9676987908));
#73603=CARTESIAN_POINT('Ctrl Pts',(78.8652848954573,-10.7130146508488,132.963840004364));
#73604=CARTESIAN_POINT('Ctrl Pts',(78.8058832121691,-10.6736664834359,132.959983648681));
#73605=CARTESIAN_POINT('Ctrl Pts',(78.7484877035544,-10.6311964817129,132.956127292998));
#73606=CARTESIAN_POINT('Ctrl Pts',(78.6934386248326,-10.5858420272589,132.952270937314));
#73607=CARTESIAN_POINT('Ctrl Pts',(78.6384058081598,-10.5405009709649,132.948415720837));
#73608=CARTESIAN_POINT('Ctrl Pts',(78.5857184199869,-10.4922774623159,132.94456050436));
#73609=CARTESIAN_POINT('Ctrl Pts',(78.5356844479139,-10.441449800173,132.940705287883));
#73610=CARTESIAN_POINT('Ctrl Pts',(78.4856485196625,-10.3906201508208,132.936849920678));
#73611=CARTESIAN_POINT('Ctrl Pts',(78.4382665526913,-10.3371864935733,132.932994553474));
#73612=CARTESIAN_POINT('Ctrl Pts',(78.3938091684396,-10.2814634505562,132.929139186269));
#73613=CARTESIAN_POINT('Ctrl Pts',(78.3493052494292,-10.2256820807076,132.925279783546));
#73614=CARTESIAN_POINT('Ctrl Pts',(78.3077323276445,-10.1676069219255,132.921420380823));
#73615=CARTESIAN_POINT('Ctrl Pts',(78.2693196750343,-10.1075843874291,132.917560978101));
#73616=CARTESIAN_POINT('Ctrl Pts',(78.2308852728786,-10.0475278677022,132.913699390154));
#73617=CARTESIAN_POINT('Ctrl Pts',(78.1956149422799,-9.98552219973657,132.909837802207));
#73618=CARTESIAN_POINT('Ctrl Pts',(78.1636922782394,-9.92193899662742,132.90597621426));
#73619=CARTESIAN_POINT('Ctrl Pts',(78.1317137643539,-9.85824455242537,132.902107870326));
#73620=CARTESIAN_POINT('Ctrl Pts',(78.1030948055356,-9.79296750779668,132.898239526393));
#73621=CARTESIAN_POINT('Ctrl Pts',(78.0779708196895,-9.72649940986562,132.894371182459));
#73622=CARTESIAN_POINT('Ctrl Pts',(78.0630529198994,-9.68703256609916,132.892074271153));
#73623=CARTESIAN_POINT('Ctrl Pts',(78.0493662725192,-9.64714610891388,132.889777359846));
#73624=CARTESIAN_POINT('Ctrl Pts',(78.0369307557737,-9.60692396959823,132.88748044854));
#73625=CARTESIAN_POINT('Ctrl Pts',(78.0114354604795,-9.52446054325239,132.88277132119));
#73626=CARTESIAN_POINT('Ctrl Pts',(77.9911203973392,-9.44032478764207,132.878062193839));
#73627=CARTESIAN_POINT('Ctrl Pts',(77.9761678835394,-9.35510720477408,132.873353066489));
#73628=CARTESIAN_POINT('Ctrl Pts',(77.9614177985698,-9.27104330722287,132.868707691839));
#73629=CARTESIAN_POINT('Ctrl Pts',(77.951886094498,-9.18592667450051,132.86406231719));
#73630=CARTESIAN_POINT('Ctrl Pts',(77.9477016670826,-9.10034498096334,132.85941694254));
#73631=CARTESIAN_POINT('Ctrl Pts',(77.9460976239039,-9.06753840598652,132.857636201526));
#73632=CARTESIAN_POINT('Ctrl Pts',(77.945278854709,-9.03466371179541,132.855855460512));
#73633=CARTESIAN_POINT('Ctrl Pts',(77.9452507493435,-9.00175482953773,132.854074719498));
#73634=CARTESIAN_POINT('Origin',(80.,-9.,141.545925280538));
#73635=CARTESIAN_POINT('',(81.2520391107129,-7.3707683934611,134.006113615385));
#73636=CARTESIAN_POINT('',(81.2520391107129,-7.37076839346111,133.947919788834));
#73637=CARTESIAN_POINT('',(81.2520391107129,-7.37076839346111,141.545925280538));
#73638=CARTESIAN_POINT('',(77.94525006034,-8.99950203698838,133.495925280488));
#73639=CARTESIAN_POINT('Ctrl Pts',(81.2520391107129,-7.37076839346111,133.947919788834));
#73640=CARTESIAN_POINT('Ctrl Pts',(81.3085900102766,-7.41422687886956,133.944064641566));
#73641=CARTESIAN_POINT('Ctrl Pts',(81.3628803154506,-7.46063677639288,133.940209494297));
#73642=CARTESIAN_POINT('Ctrl Pts',(81.4145961687758,-7.50972645404108,133.936354347029));
#73643=CARTESIAN_POINT('Ctrl Pts',(81.4665751616528,-7.5590659087875,133.932479584079));
#73644=CARTESIAN_POINT('Ctrl Pts',(81.5159530604065,-7.61111216160157,133.928604821129));
#73645=CARTESIAN_POINT('Ctrl Pts',(81.5624487563918,-7.66555200695202,133.924730058179));
#73646=CARTESIAN_POINT('Ctrl Pts',(81.6087738176557,-7.71979206331893,133.920869515235));
#73647=CARTESIAN_POINT('Ctrl Pts',(81.652237532106,-7.77640775807705,133.917008972292));
#73648=CARTESIAN_POINT('Ctrl Pts',(81.6926037674573,-7.83505792037144,133.913148429348));
#73649=CARTESIAN_POINT('Ctrl Pts',(81.7331930315904,-7.89403213255886,133.909266556395));
#73650=CARTESIAN_POINT('Ctrl Pts',(81.7706502273261,-7.95506293762194,133.905384683441));
#73651=CARTESIAN_POINT('Ctrl Pts',(81.8047817874466,-8.01777789568704,133.901502810488));
#73652=CARTESIAN_POINT('Ctrl Pts',(81.8389133475671,-8.08049285375215,133.897620937535));
#73653=CARTESIAN_POINT('Ctrl Pts',(81.8697191170293,-8.14489149318802,133.893739064581));
#73654=CARTESIAN_POINT('Ctrl Pts',(81.8970550143789,-8.21058259778507,133.889857191628));
#73655=CARTESIAN_POINT('Ctrl Pts',(81.9243008446297,-8.2760572614461,133.885988108781));
#73656=CARTESIAN_POINT('Ctrl Pts',(81.9482063861372,-8.34307235839047,133.882119025934));
#73657=CARTESIAN_POINT('Ctrl Pts',(81.9685973105307,-8.41125371213795,133.878249943087));
#73658=CARTESIAN_POINT('Ctrl Pts',(81.9889578534638,-8.47933347906872,133.874386624981));
#73659=CARTESIAN_POINT('Ctrl Pts',(82.0058140357402,-8.54857559196324,133.870523306875));
#73660=CARTESIAN_POINT('Ctrl Pts',(82.0190396129381,-8.61858604654963,133.866659988768));
#73661=CARTESIAN_POINT('Ctrl Pts',(82.0322496765391,-8.68851437889975,133.862801202332));
#73662=CARTESIAN_POINT('Ctrl Pts',(82.0418375045425,-8.7592087877014,133.858942415897));
#73663=CARTESIAN_POINT('Ctrl Pts',(82.0477271687752,-8.83026195252723,133.855083629461));
#73664=CARTESIAN_POINT('Ctrl Pts',(82.0536131229513,-8.9012703590693,133.851227273778));
#73665=CARTESIAN_POINT('Ctrl Pts',(82.0558054951567,-8.97263659029657,133.847370918094));
#73666=CARTESIAN_POINT('Ctrl Pts',(82.0542799880628,-9.04394648045941,133.843514562411));
#73667=CARTESIAN_POINT('Ctrl Pts',(82.052754931619,-9.11523530496674,133.839659345934));
#73668=CARTESIAN_POINT('Ctrl Pts',(82.047514186688,-9.1864673360446,133.835804129457));
#73669=CARTESIAN_POINT('Ctrl Pts',(82.0385855656644,-9.25722840816021,133.831948912979));
#73670=CARTESIAN_POINT('Ctrl Pts',(82.0296565955584,-9.32799224682206,133.828093545775));
#73671=CARTESIAN_POINT('Ctrl Pts',(82.017039526099,-9.3982846082792,133.82423817857));
#73672=CARTESIAN_POINT('Ctrl Pts',(82.0008138292302,-9.46769817538806,133.820382811366));
#73673=CARTESIAN_POINT('Ctrl Pts',(81.9845711484813,-9.53718439957352,133.816523408643));
#73674=CARTESIAN_POINT('Ctrl Pts',(81.9647124108874,-9.60578951916727,133.81266400592));
#73675=CARTESIAN_POINT('Ctrl Pts',(81.9413676557693,-9.67311899960777,133.808804603197));
#73676=CARTESIAN_POINT('Ctrl Pts',(81.9180096826674,-9.74048660252897,133.80494301525));
#73677=CARTESIAN_POINT('Ctrl Pts',(81.8911619457095,-9.80657667818826,133.801081427303));
#73678=CARTESIAN_POINT('Ctrl Pts',(81.8610025557139,-9.87101495401993,133.797219839356));
#73679=CARTESIAN_POINT('Ctrl Pts',(81.8307904007844,-9.93556596692488,133.793351495423));
#73680=CARTESIAN_POINT('Ctrl Pts',(81.7972552538553,-9.99845898147934,133.78948315149));
#73681=CARTESIAN_POINT('Ctrl Pts',(81.7606207105567,-10.0593452109953,133.785614807556));
#73682=CARTESIAN_POINT('Ctrl Pts',(81.7388681729964,-10.0954977019287,133.78331789625));
#73683=CARTESIAN_POINT('Ctrl Pts',(81.7160237303534,-10.1309432266616,133.781020984943));
#73684=CARTESIAN_POINT('Ctrl Pts',(81.6921409778438,-10.165614204444,133.778724073637));
#73685=CARTESIAN_POINT('Ctrl Pts',(81.6519111492854,-10.2240164967084,133.77485499079));
#73686=CARTESIAN_POINT('Ctrl Pts',(81.6085754448934,-10.2804480026079,133.770985907943));
#73687=CARTESIAN_POINT('Ctrl Pts',(81.5623536704284,-10.3345593171527,133.767116825096));
#73688=CARTESIAN_POINT('Ctrl Pts',(81.5162007641022,-10.3885900085374,133.76325350699));
#73689=CARTESIAN_POINT('Ctrl Pts',(81.4671706362291,-10.4403070041942,133.759390188883));
#73690=CARTESIAN_POINT('Ctrl Pts',(81.4155258303407,-10.4893905418453,133.755526870777));
#73691=CARTESIAN_POINT('Ctrl Pts',(81.3639416037897,-10.5384165045258,133.751668084341));
#73692=CARTESIAN_POINT('Ctrl Pts',(81.3097491417684,-10.5848148120564,133.747809297905));
#73693=CARTESIAN_POINT('Ctrl Pts',(81.2532494656944,-10.6283007520838,133.743950511469));
#73694=CARTESIAN_POINT('Ctrl Pts',(81.1967853802733,-10.6717592991577,133.740094155786));
#73695=CARTESIAN_POINT('Ctrl Pts',(81.1380173483262,-10.71230882291,133.736237800103));
#73696=CARTESIAN_POINT('Ctrl Pts',(81.0772801458063,-10.7497042749995,133.73238144442));
#73697=CARTESIAN_POINT('Ctrl Pts',(81.0165608856641,-10.787088680098,133.728526227942));
#73698=CARTESIAN_POINT('Ctrl Pts',(80.9538740232493,-10.8213206087536,133.724671011465));
#73699=CARTESIAN_POINT('Ctrl Pts',(80.8895825976209,-10.8521987918444,133.720815794988));
#73700=CARTESIAN_POINT('Ctrl Pts',(80.8252886583901,-10.8830781821799,133.716960427783));
#73701=CARTESIAN_POINT('Ctrl Pts',(80.7593904702462,-10.9106033582973,133.713105060579));
#73702=CARTESIAN_POINT('Ctrl Pts',(80.692273337813,-10.934620166403,133.709249693374));
#73703=CARTESIAN_POINT('Ctrl Pts',(80.625085952044,-10.9586621135578,133.705390290651));
#73704=CARTESIAN_POINT('Ctrl Pts',(80.5566775333181,-10.9791881979556,133.701530887928));
#73705=CARTESIAN_POINT('Ctrl Pts',(80.487450073939,-10.9960936821494,133.697671485206));
#73706=CARTESIAN_POINT('Ctrl Pts',(80.4181834174287,-11.0130087383612,133.693809897259));
#73707=CARTESIAN_POINT('Ctrl Pts',(80.3480972745911,-11.0262990228787,133.689948309312));
#73708=CARTESIAN_POINT('Ctrl Pts',(80.2776026879915,-11.035911174418,133.686086721365));
#73709=CARTESIAN_POINT('Ctrl Pts',(80.2069847685858,-11.0455401427608,133.682218377431));
#73710=CARTESIAN_POINT('Ctrl Pts',(80.1359574629724,-11.0514780899316,133.678350033498));
#73711=CARTESIAN_POINT('Ctrl Pts',(80.0649350722543,-11.0537236909797,133.674481689565));
#73712=CARTESIAN_POINT('Ctrl Pts',(80.0227640204922,-11.0550570642593,133.672184778258));
#73713=CARTESIAN_POINT('Ctrl Pts',(79.9805946865914,-11.055089647407,133.669887866952));
#73714=CARTESIAN_POINT('Ctrl Pts',(79.9385129163662,-11.0538298130678,133.667590955645));
#73715=CARTESIAN_POINT('Ctrl Pts',(79.8676273515257,-11.0517076573634,133.663721872798));
#73716=CARTESIAN_POINT('Ctrl Pts',(79.7967129435705,-11.0459072368963,133.659852789951));
#73717=CARTESIAN_POINT('Ctrl Pts',(79.7261824575087,-11.0364237073664,133.655983707104));
#73718=CARTESIAN_POINT('Ctrl Pts',(79.6557570583534,-11.0269543078226,133.652120388998));
#73719=CARTESIAN_POINT('Ctrl Pts',(79.585714923167,-11.0138127562554,133.648257070892));
#73720=CARTESIAN_POINT('Ctrl Pts',(79.5164670932608,-10.9970461914038,133.644393752785));
#73721=CARTESIAN_POINT('Ctrl Pts',(79.4473004910326,-10.9802992937263,133.640534966349));
#73722=CARTESIAN_POINT('Ctrl Pts',(79.3789268132231,-10.9599359427143,133.636676179914));
#73723=CARTESIAN_POINT('Ctrl Pts',(79.3117485241908,-10.9360546140402,133.632817393478));
#73724=CARTESIAN_POINT('Ctrl Pts',(79.2446125525545,-10.9121883288521,133.628961037795));
#73725=CARTESIAN_POINT('Ctrl Pts',(79.1786709323801,-10.8848086249775,133.625104682111));
#73726=CARTESIAN_POINT('Ctrl Pts',(79.1143111127732,-10.8540638493706,133.621248326428));
#73727=CARTESIAN_POINT('Ctrl Pts',(79.0499703057015,-10.8233281560783,133.617393109951));
#73728=CARTESIAN_POINT('Ctrl Pts',(78.9872108096157,-10.7892295738504,133.613537893474));
#73729=CARTESIAN_POINT('Ctrl Pts',(78.9263986226034,-10.7519639393983,133.609682676996));
#73730=CARTESIAN_POINT('Ctrl Pts',(78.8655840580166,-10.7146968479715,133.605827309792));
#73731=CARTESIAN_POINT('Ctrl Pts',(78.8067173667049,-10.6742627141862,133.601971942587));
#73732=CARTESIAN_POINT('Ctrl Pts',(78.7501370400148,-10.6309016352181,133.598116575382));
#73733=CARTESIAN_POINT('Ctrl Pts',(78.6934974891512,-10.5874951690243,133.59425717266));
#73734=CARTESIAN_POINT('Ctrl Pts',(78.6391494666403,-10.5411559378864,133.590397769937));
#73735=CARTESIAN_POINT('Ctrl Pts',(78.5873989985902,-10.4921648613059,133.586538367214));
#73736=CARTESIAN_POINT('Ctrl Pts',(78.5356192290186,-10.443146045593,133.582676779267));
#73737=CARTESIAN_POINT('Ctrl Pts',(78.4864402767899,-10.3914727474777,133.57881519132));
#73738=CARTESIAN_POINT('Ctrl Pts',(78.4401299138821,-10.3374613553051,133.574953603373));
#73739=CARTESIAN_POINT('Ctrl Pts',(78.3937385293345,-10.2833554682659,133.57108525944));
#73740=CARTESIAN_POINT('Ctrl Pts',(78.3502260507417,-10.226903705087,133.567216915506));
#73741=CARTESIAN_POINT('Ctrl Pts',(78.3098183000035,-10.1684534152019,133.563348571573));
#73742=CARTESIAN_POINT('Ctrl Pts',(78.2858253404492,-10.1337473151214,133.561051660267));
#73743=CARTESIAN_POINT('Ctrl Pts',(78.2629261494461,-10.0983371353048,133.55875474896));
#73744=CARTESIAN_POINT('Ctrl Pts',(78.2411602539382,-10.0622995388182,133.556457837654));
#73745=CARTESIAN_POINT('Ctrl Pts',(78.2033015192917,-9.99961717400613,133.552462681303));
#73746=CARTESIAN_POINT('Ctrl Pts',(78.1687336620036,-9.9348033260882,133.548467524953));
#73747=CARTESIAN_POINT('Ctrl Pts',(78.1376942678546,-9.86822515657996,133.544472368603));
#73748=CARTESIAN_POINT('Ctrl Pts',(78.1062630365257,-9.80080651312272,133.540426777931));
#73749=CARTESIAN_POINT('Ctrl Pts',(78.0784502909621,-9.73157903424725,133.536381187259));
#73750=CARTESIAN_POINT('Ctrl Pts',(78.0544569760339,-9.66095378385848,133.532335596587));
#73751=CARTESIAN_POINT('Ctrl Pts',(78.0308540830868,-9.59147775566983,133.528355836231));
#73752=CARTESIAN_POINT('Ctrl Pts',(78.0109474205578,-9.52064953469732,133.524376075876));
#73753=CARTESIAN_POINT('Ctrl Pts',(77.9948811787216,-9.44888314187016,133.520396315521));
#73754=CARTESIAN_POINT('Ctrl Pts',(77.97841630266,-9.37533608741029,133.51631780969));
#73755=CARTESIAN_POINT('Ctrl Pts',(77.9659851790174,-9.3008041087637,133.51223930386));
#73756=CARTESIAN_POINT('Ctrl Pts',(77.9576890084772,-9.22575069524891,133.508160798029));
#73757=CARTESIAN_POINT('Ctrl Pts',(77.9493928379371,-9.15069728173412,133.504082292199));
#73758=CARTESIAN_POINT('Ctrl Pts',(77.9452317338588,-9.07512292632964,133.500003786368));
#73759=CARTESIAN_POINT('Ctrl Pts',(77.9452500603398,-8.99950203790955,133.495925280538));
#73760=CARTESIAN_POINT('Ctrl Pts',(77.94525006034,-8.99950203698839,133.495925280488));
#73761=CARTESIAN_POINT('Ctrl Pts',(77.9452690078821,-8.92131859753172,133.491708567086));
#73762=CARTESIAN_POINT('Ctrl Pts',(77.9497549266111,-8.84325445761002,133.487491853684));
#73763=CARTESIAN_POINT('Ctrl Pts',(77.9586394355346,-8.76581074246384,133.483275140282));
#73764=CARTESIAN_POINT('Ctrl Pts',(77.9673566235425,-8.68982551573053,133.479137839749));
#73765=CARTESIAN_POINT('Ctrl Pts',(77.9803079746392,-8.61443788697709,133.475000539216));
#73766=CARTESIAN_POINT('Ctrl Pts',(77.9973777224886,-8.54010699492684,133.470863238684));
#73767=CARTESIAN_POINT('Ctrl Pts',(78.0149389348737,-8.46363600112062,133.466606818847));
#73768=CARTESIAN_POINT('Ctrl Pts',(78.0368591598541,-8.38828393878643,133.46235039901));
#73769=CARTESIAN_POINT('Ctrl Pts',(78.0629590532119,-8.31452940765756,133.458093979173));
#73770=CARTESIAN_POINT('Ctrl Pts',(78.0890589465697,-8.24077487652868,133.453837559336));
#73771=CARTESIAN_POINT('Ctrl Pts',(78.1193382663649,-8.16861823146456,133.449581139499));
#73772=CARTESIAN_POINT('Ctrl Pts',(78.1535669543638,-8.09851091493974,133.445324719662));
#73773=CARTESIAN_POINT('Ctrl Pts',(78.1846808093607,-8.03478341008652,133.441455636815));
#73774=CARTESIAN_POINT('Ctrl Pts',(78.2191586994743,-7.97254376655812,133.437586553968));
#73775=CARTESIAN_POINT('Ctrl Pts',(78.2568351259752,-7.91217014911979,133.433717471121));
#73776=CARTESIAN_POINT('Ctrl Pts',(78.2944554164795,-7.85188648536049,133.429854153015));
#73777=CARTESIAN_POINT('Ctrl Pts',(78.3352645285792,-7.79346373766178,133.425990834909));
#73778=CARTESIAN_POINT('Ctrl Pts',(78.3790502987056,-7.73725710123816,133.422127516802));
#73779=CARTESIAN_POINT('Ctrl Pts',(78.4227847081404,-7.68111639517741,133.418268730366));
#73780=CARTESIAN_POINT('Ctrl Pts',(78.4694885429766,-7.62718701827358,133.41440994393));
#73781=CARTESIAN_POINT('Ctrl Pts',(78.5189063847534,-7.57579521648899,133.410551157495));
#73782=CARTESIAN_POINT('Ctrl Pts',(78.5682930969135,-7.52443578777113,133.406694801811));
#73783=CARTESIAN_POINT('Ctrl Pts',(78.6203900882303,-7.47561111213256,133.402838446128));
#73784=CARTESIAN_POINT('Ctrl Pts',(78.6749026713714,-7.42961322211333,133.398982090445));
#73785=CARTESIAN_POINT('Ctrl Pts',(78.7293991509495,-7.3836289203314,133.395126873968));
#73786=CARTESIAN_POINT('Ctrl Pts',(78.7863094346098,-7.34047005944964,133.39127165749));
#73787=CARTESIAN_POINT('Ctrl Pts',(78.8453043857987,-7.30038957374219,133.387416441013));
#73788=CARTESIAN_POINT('Ctrl Pts',(78.9043016435137,-7.26030752100764,133.383561073809));
#73789=CARTESIAN_POINT('Ctrl Pts',(78.9653833275144,-7.22330435356743,133.379705706604));
#73790=CARTESIAN_POINT('Ctrl Pts',(79.0281912878424,-7.18958971791626,133.375850339399));
#73791=CARTESIAN_POINT('Ctrl Pts',(79.0910649909779,-7.15583979223511,133.371990936677));
#73792=CARTESIAN_POINT('Ctrl Pts',(79.1556681486058,-7.12538549996297,133.368131533954));
#73793=CARTESIAN_POINT('Ctrl Pts',(79.2216187718385,-7.09839009622221,133.364272131231));
#73794=CARTESIAN_POINT('Ctrl Pts',(79.2876067368321,-7.0713794074718,133.360410543284));
#73795=CARTESIAN_POINT('Ctrl Pts',(79.35494322745,-7.04783166635548,133.356548955337));
#73796=CARTESIAN_POINT('Ctrl Pts',(79.4232296777164,-7.02786066470118,133.35268736739));
#73797=CARTESIAN_POINT('Ctrl Pts',(79.4916355975752,-7.00785472306364,133.348819023457));
#73798=CARTESIAN_POINT('Ctrl Pts',(79.5609943224181,-6.99143812635553,133.344950679524));
#73799=CARTESIAN_POINT('Ctrl Pts',(79.6308963387199,-6.97867369043749,133.34108233559));
#73800=CARTESIAN_POINT('Ctrl Pts',(79.672402144395,-6.97109453571783,133.338785424284));
#73801=CARTESIAN_POINT('Ctrl Pts',(79.7140993616812,-6.96480201206941,133.336488512977));
#73802=CARTESIAN_POINT('Ctrl Pts',(79.7559018530522,-6.95980058397306,133.334191601671));
#73803=CARTESIAN_POINT('Ctrl Pts',(79.8262968740992,-6.95137822385623,133.330323623604));
#73804=CARTESIAN_POINT('Ctrl Pts',(79.8972661514778,-6.94658701062118,133.326455645537));
#73805=CARTESIAN_POINT('Ctrl Pts',(79.9684025636867,-6.94549296313728,133.32258766747));
#73806=CARTESIAN_POINT('Ctrl Pts',(80.0394421231407,-6.94440040520718,133.318724955685));
#73807=CARTESIAN_POINT('Ctrl Pts',(80.1106478848647,-6.94699503549171,133.314862243899));
#73808=CARTESIAN_POINT('Ctrl Pts',(80.1816065604025,-6.95329127140211,133.310999532113));
#73809=CARTESIAN_POINT('Ctrl Pts',(80.2524923697579,-6.95958104182157,133.307140786876));
#73810=CARTESIAN_POINT('Ctrl Pts',(80.3231311151167,-6.96956483233156,133.303282041639));
#73811=CARTESIAN_POINT('Ctrl Pts',(80.3931101843536,-6.98320503137837,133.299423296402));
#73812=CARTESIAN_POINT('Ctrl Pts',(80.4630408059895,-6.99683578710266,133.295567222635));
#73813=CARTESIAN_POINT('Ctrl Pts',(80.5323121827187,-7.01411783254821,133.291711148868));
#73814=CARTESIAN_POINT('Ctrl Pts',(80.6005192195216,-7.03496202848769,133.2878550751));
#73815=CARTESIAN_POINT('Ctrl Pts',(80.6687201287411,-7.05580435182643,133.283999347755));
#73816=CARTESIAN_POINT('Ctrl Pts',(80.735856419764,-7.08020806062568,133.280143620409));
#73817=CARTESIAN_POINT('Ctrl Pts',(80.8015369135476,-7.10803379028046,133.276287893064));
#73818=CARTESIAN_POINT('Ctrl Pts',(80.867213554729,-7.1358578877692,133.272432391883));
#73819=CARTESIAN_POINT('Ctrl Pts',(80.9314341240364,-7.16710341035558,133.268576890702));
#73820=CARTESIAN_POINT('Ctrl Pts',(80.9938281893639,-7.20158317052866,133.26472138952));
#73821=CARTESIAN_POINT('Ctrl Pts',(81.0562666112049,-7.23608744267965,133.260863147428));
#73822=CARTESIAN_POINT('Ctrl Pts',(81.1168755162799,-7.27383029855921,133.257004905336));
#73823=CARTESIAN_POINT('Ctrl Pts',(81.1753108603495,-7.31457959427192,133.253146663244));
#73824=CARTESIAN_POINT('Ctrl Pts',(81.2013268074122,-7.3327215516264,133.251428938746));
#73825=CARTESIAN_POINT('Ctrl Pts',(81.2269123279116,-7.35145885228397,133.249711214249));
#73826=CARTESIAN_POINT('Ctrl Pts',(81.2520391107129,-7.3707683934611,133.247993489751));
#73827=CARTESIAN_POINT('',(77.9452500001325,-9.00002333775544,133.554074719471));
#73828=CARTESIAN_POINT('Ctrl Pts',(77.9452500001325,-9.00002333758729,133.554074719462));
#73829=CARTESIAN_POINT('Ctrl Pts',(77.9452491949294,-8.92912950095486,133.550206920375));
#73830=CARTESIAN_POINT('Ctrl Pts',(77.948921710863,-8.85809631169957,133.546339121287));
#73831=CARTESIAN_POINT('Ctrl Pts',(77.9562848605137,-8.78733596652337,133.5424713222));
#73832=CARTESIAN_POINT('Ctrl Pts',(77.9636370380662,-8.71668106392196,133.538609286661));
#73833=CARTESIAN_POINT('Ctrl Pts',(77.97466888319,-8.64629867796401,133.534747251122));
#73834=CARTESIAN_POINT('Ctrl Pts',(77.9893456969755,-8.57660085471362,133.530885215583));
#73835=CARTESIAN_POINT('Ctrl Pts',(78.0040053078095,-8.50698472550769,133.527027706804));
#73836=CARTESIAN_POINT('Ctrl Pts',(78.0223013014783,-8.43805203863106,133.523170198025));
#73837=CARTESIAN_POINT('Ctrl Pts',(78.0441474066621,-8.37020781551908,133.519312689246));
#73838=CARTESIAN_POINT('Ctrl Pts',(78.0659797748482,-8.30240625337239,133.515457606098));
#73839=CARTESIAN_POINT('Ctrl Pts',(78.0913576770541,-8.23569225876866,133.51160252295));
#73840=CARTESIAN_POINT('Ctrl Pts',(78.1201445418238,-8.17045734355309,133.507747439802));
#73841=CARTESIAN_POINT('Ctrl Pts',(78.1489229525421,-8.10524158635715,133.503893488805));
#73842=CARTESIAN_POINT('Ctrl Pts',(78.1811081421473,-8.04150449073841,133.500039537807));
#73843=CARTESIAN_POINT('Ctrl Pts',(78.2165154281123,-7.9796175499654,133.49618558681));
#73844=CARTESIAN_POINT('Ctrl Pts',(78.2519241814885,-7.91772804436478,133.49233147609));
#73845=CARTESIAN_POINT('Ctrl Pts',(78.2905550529745,-7.857689266697,133.488477365371));
#73846=CARTESIAN_POINT('Ctrl Pts',(78.3321782980712,-7.79984653769805,133.484623254651));
#73847=CARTESIAN_POINT('Ctrl Pts',(78.3738451508805,-7.7419432082079,133.480765106069));
#73848=CARTESIAN_POINT('Ctrl Pts',(78.4185103508029,-7.68624091544602,133.476906957487));
#73849=CARTESIAN_POINT('Ctrl Pts',(78.4659023851083,-7.63305374264985,133.473048808904));
#73850=CARTESIAN_POINT('Ctrl Pts',(78.513321406382,-7.57983628289573,133.469188463334));
#73851=CARTESIAN_POINT('Ctrl Pts',(78.5634700109468,-7.52913713982456,133.465328117764));
#73852=CARTESIAN_POINT('Ctrl Pts',(78.6160400988869,-7.48123321256654,133.461467772193));
#73853=CARTESIAN_POINT('Ctrl Pts',(78.6687019134685,-7.43324570039295,133.457600690919));
#73854=CARTESIAN_POINT('Ctrl Pts',(78.7237932705989,-7.3880634493979,133.453733609645));
#73855=CARTESIAN_POINT('Ctrl Pts',(78.7809738927824,-7.34592233785049,133.449866528371));
#73856=CARTESIAN_POINT('Ctrl Pts',(78.8140980817257,-7.32151039394591,133.44762636508));
#73857=CARTESIAN_POINT('Ctrl Pts',(78.8479228431124,-7.29811817395487,133.445386201789));
#73858=CARTESIAN_POINT('Ctrl Pts',(78.8823781830246,-7.27578451557798,133.443146038498));
#73859=CARTESIAN_POINT('Ctrl Pts',(78.9418874898534,-7.23721108886549,133.439276955651));
#73860=CARTESIAN_POINT('Ctrl Pts',(79.0035126729261,-7.20164657081051,133.435407872804));
#73861=CARTESIAN_POINT('Ctrl Pts',(79.0669169949675,-7.16932972159936,133.431538789957));
#73862=CARTESIAN_POINT('Ctrl Pts',(79.1302268477313,-7.13706102288172,133.427675471851));
#73863=CARTESIAN_POINT('Ctrl Pts',(79.1953101483624,-7.10803060679747,133.423812153744));
#73864=CARTESIAN_POINT('Ctrl Pts',(79.2618020099645,-7.08243349789177,133.419948835638));
#73865=CARTESIAN_POINT('Ctrl Pts',(79.3282158766384,-7.05686641438503,133.416090049202));
#73866=CARTESIAN_POINT('Ctrl Pts',(79.3960345712222,-7.03472481221642,133.412231262766));
#73867=CARTESIAN_POINT('Ctrl Pts',(79.4648710613896,-7.01615661365074,133.40837247633));
#73868=CARTESIAN_POINT('Ctrl Pts',(79.5336641896158,-6.99760011168859,133.404516120647));
#73869=CARTESIAN_POINT('Ctrl Pts',(79.60347337351,-6.9826126736317,133.400659764964));
#73870=CARTESIAN_POINT('Ctrl Pts',(79.6738955643609,-6.97129266291155,133.39680340928));
#73871=CARTESIAN_POINT('Ctrl Pts',(79.7442969517914,-6.95997599623592,133.392948192803));
#73872=CARTESIAN_POINT('Ctrl Pts',(79.8153105073031,-6.95232468311315,133.389092976326));
#73873=CARTESIAN_POINT('Ctrl Pts',(79.8865238136966,-6.94838582632064,133.385237759849));
#73874=CARTESIAN_POINT('Ctrl Pts',(79.9577399043173,-6.94444681553062,133.381382392644));
#73875=CARTESIAN_POINT('Ctrl Pts',(80.0291552761617,-6.94422057386752,133.37752702544));
#73876=CARTESIAN_POINT('Ctrl Pts',(80.1003549610624,-6.94770215507345,133.373671658235));
#73877=CARTESIAN_POINT('Ctrl Pts',(80.1716291726179,-6.95118738054552,133.369812255512));
#73878=CARTESIAN_POINT('Ctrl Pts',(80.242686760354,-6.95838815261647,133.365952852789));
#73879=CARTESIAN_POINT('Ctrl Pts',(80.3131162389923,-6.96924748347334,133.362093450067));
#73880=CARTESIAN_POINT('Ctrl Pts',(80.3835855953545,-6.98011296296865,133.35823186212));
#73881=CARTESIAN_POINT('Ctrl Pts',(80.4534256588216,-6.99464102599578,133.354370274173));
#73882=CARTESIAN_POINT('Ctrl Pts',(80.5222362332727,-7.01272375368768,133.350508686226));
#73883=CARTESIAN_POINT('Ctrl Pts',(80.5911671942902,-7.03083811775983,133.346640342292));
#73884=CARTESIAN_POINT('Ctrl Pts',(80.6590646073802,-7.05251941511445,133.342771998359));
#73885=CARTESIAN_POINT('Ctrl Pts',(80.7255451693952,-7.07761040117585,133.338903654425));
#73886=CARTESIAN_POINT('Ctrl Pts',(80.7650194139755,-7.0925087066433,133.336606743119));
#73887=CARTESIAN_POINT('Ctrl Pts',(80.8039945234929,-7.10860822903842,133.334309831813));
#73888=CARTESIAN_POINT('Ctrl Pts',(80.8423943826247,-7.1258683966641,133.332012920506));
#73889=CARTESIAN_POINT('Ctrl Pts',(80.9070806959083,-7.15494393588762,133.328143668699));
#73890=CARTESIAN_POINT('Ctrl Pts',(80.9703866144571,-7.18742936372782,133.324274416891));
#73891=CARTESIAN_POINT('Ctrl Pts',(81.0319288584345,-7.22317125371349,133.320405165084));
#73892=CARTESIAN_POINT('Ctrl Pts',(81.093372977261,-7.25885615555375,133.316542082549));
#73893=CARTESIAN_POINT('Ctrl Pts',(81.1530585893493,-7.2977869662659,133.312679000015));
#73894=CARTESIAN_POINT('Ctrl Pts',(81.210624007114,-7.33976294587214,133.308815917481));
#73895=CARTESIAN_POINT('Ctrl Pts',(81.2245547338712,-7.34992105685204,133.30788105851));
#73896=CARTESIAN_POINT('Ctrl Pts',(81.2383614038783,-7.36025728881951,133.306946199539));
#73897=CARTESIAN_POINT('Ctrl Pts',(81.2520391107129,-7.37076839346111,133.306011340568));
#73898=CARTESIAN_POINT('Ctrl Pts',(81.2520391107129,-7.3707683934611,134.006113615385));
#73899=CARTESIAN_POINT('Ctrl Pts',(81.2874945677546,-7.39801535989994,134.003679619742));
#73900=CARTESIAN_POINT('Ctrl Pts',(81.3220223716194,-7.42639116812375,134.001245624099));
#73901=CARTESIAN_POINT('Ctrl Pts',(81.3555499459166,-7.45582322688577,133.998811628456));
#73902=CARTESIAN_POINT('Ctrl Pts',(81.4088454244803,-7.5026084682794,133.994942545609));
#73903=CARTESIAN_POINT('Ctrl Pts',(81.4598203372147,-7.55224773101518,133.991073462762));
#73904=CARTESIAN_POINT('Ctrl Pts',(81.5081533895656,-7.60448184675306,133.987204379915));
#73905=CARTESIAN_POINT('Ctrl Pts',(81.5564144280789,-7.65663813626349,133.983341061809));
#73906=CARTESIAN_POINT('Ctrl Pts',(81.6020410922966,-7.71138125082055,133.979477743702));
#73907=CARTESIAN_POINT('Ctrl Pts',(81.6447465261169,-7.76841304516227,133.975614425596));
#73908=CARTESIAN_POINT('Ctrl Pts',(81.6874018664798,-7.8253779412312,133.97175563916));
#73909=CARTESIAN_POINT('Ctrl Pts',(81.7271424930792,-7.88462579755637,133.967896852724));
#73910=CARTESIAN_POINT('Ctrl Pts',(81.7637208600582,-7.94582435510224,133.964038066288));
#73911=CARTESIAN_POINT('Ctrl Pts',(81.8002761853482,-8.00698436204436,133.960181710605));
#73912=CARTESIAN_POINT('Ctrl Pts',(81.8336729544594,-8.07009221629728,133.956325354922));
#73913=CARTESIAN_POINT('Ctrl Pts',(81.8637069616787,-8.1347867757076,133.952468999239));
#73914=CARTESIAN_POINT('Ctrl Pts',(81.8937320965514,-8.19946222369726,133.948613782761));
#73915=CARTESIAN_POINT('Ctrl Pts',(81.9203962372521,-8.26572300591116,133.944758566284));
#73916=CARTESIAN_POINT('Ctrl Pts',(81.9435419628082,-8.33318503218383,133.940903349807));
#73917=CARTESIAN_POINT('Ctrl Pts',(81.9666885932929,-8.40064969601996,133.937047982602));
#73918=CARTESIAN_POINT('Ctrl Pts',(81.9863163799621,-8.4693152369516,133.933192615398));
#73919=CARTESIAN_POINT('Ctrl Pts',(82.0023172982288,-8.53878096340919,133.929337248193));
#73920=CARTESIAN_POINT('Ctrl Pts',(82.0183349650936,-8.60831940153999,133.92547784547));
#73921=CARTESIAN_POINT('Ctrl Pts',(82.0307180759414,-8.6786592228294,133.921618442747));
#73922=CARTESIAN_POINT('Ctrl Pts',(82.0394096353205,-8.74938894305702,133.917759040025));
#73923=CARTESIAN_POINT('Ctrl Pts',(82.0481061159287,-8.82015871100782,133.913897452078));
#73924=CARTESIAN_POINT('Ctrl Pts',(82.053106850083,-8.89131833255214,133.910035864131));
#73925=CARTESIAN_POINT('Ctrl Pts',(82.0544069244437,-8.96245334505461,133.906174276184));
#73926=CARTESIAN_POINT('Ctrl Pts',(82.0557092733312,-9.0337128108112,133.90230593225));
#73927=CARTESIAN_POINT('Ctrl Pts',(82.0532980524677,-9.10494709590801,133.898437588317));
#73928=CARTESIAN_POINT('Ctrl Pts',(82.0472204087786,-9.17574458848055,133.894569244383));
#73929=CARTESIAN_POINT('Ctrl Pts',(82.0436116788554,-9.21778210219532,133.892272333077));
#73930=CARTESIAN_POINT('Ctrl Pts',(82.0387112898198,-9.25966575020436,133.889975421771));
#73931=CARTESIAN_POINT('Ctrl Pts',(82.0325375986326,-9.30131125542311,133.887678510464));
#73932=CARTESIAN_POINT('Ctrl Pts',(82.0221381885172,-9.37146194406432,133.883809427617));
#73933=CARTESIAN_POINT('Ctrl Pts',(82.0080823914302,-9.44121101360281,133.87994034477));
#73934=CARTESIAN_POINT('Ctrl Pts',(81.9904136794236,-9.51014796604846,133.876071261923));
#73935=CARTESIAN_POINT('Ctrl Pts',(81.9727712929167,-9.57898220587301,133.872207943817));
#73936=CARTESIAN_POINT('Ctrl Pts',(81.9515267963479,-9.64700626370974,133.868344625711));
#73937=CARTESIAN_POINT('Ctrl Pts',(81.9267750863095,-9.71381743413647,133.864481307604));
#73938=CARTESIAN_POINT('Ctrl Pts',(81.9020524100173,-9.78055023508601,133.860622521168));
#73939=CARTESIAN_POINT('Ctrl Pts',(81.8738308599146,-9.84607252130558,133.856763734733));
#73940=CARTESIAN_POINT('Ctrl Pts',(81.8422553138061,-9.90999611057039,133.852904948297));
#73941=CARTESIAN_POINT('Ctrl Pts',(81.8106996579763,-9.97387943266128,133.849048592614));
#73942=CARTESIAN_POINT('Ctrl Pts',(81.7757944124788,-10.0361656212767,133.84519223693));
#73943=CARTESIAN_POINT('Ctrl Pts',(81.7377322276223,-10.0964872400455,133.841335881247));
#73944=CARTESIAN_POINT('Ctrl Pts',(81.6996812867164,-10.1567910392041,133.83748066477));
#73945=CARTESIAN_POINT('Ctrl Pts',(81.6584755169942,-10.2151310100689,133.833625448293));
#73946=CARTESIAN_POINT('Ctrl Pts',(81.6143522232711,-10.2711665751268,133.829770231815));
#73947=CARTESIAN_POINT('Ctrl Pts',(81.5702272044592,-10.3272043310076,133.825914864611));
#73948=CARTESIAN_POINT('Ctrl Pts',(81.5231847374418,-10.3809371219074,133.822059497406));
#73949=CARTESIAN_POINT('Ctrl Pts',(81.4735028660502,-10.4320568655754,133.818204130202));
#73950=CARTESIAN_POINT('Ctrl Pts',(81.4237689912869,-10.4832301176754,133.814344727479));
#73951=CARTESIAN_POINT('Ctrl Pts',(81.3713905363678,-10.5317845134968,133.810485324756));
#73952=CARTESIAN_POINT('Ctrl Pts',(81.3166822895861,-10.5774489883322,133.806625922033));
#73953=CARTESIAN_POINT('Ctrl Pts',(81.2619430665654,-10.6231393187519,133.802764334086));
#73954=CARTESIAN_POINT('Ctrl Pts',(81.2048718145003,-10.6659361792457,133.798902746139));
#73955=CARTESIAN_POINT('Ctrl Pts',(81.1458140722615,-10.7056106455776,133.795041158192));
#73956=CARTESIAN_POINT('Ctrl Pts',(81.0866530063858,-10.7453545238104,133.791172814259));
#73957=CARTESIAN_POINT('Ctrl Pts',(81.0254989284647,-10.7819648517648,133.787304470326));
#73958=CARTESIAN_POINT('Ctrl Pts',(80.9627232188053,-10.8152579889573,133.783436126392));
#73959=CARTESIAN_POINT('Ctrl Pts',(80.9254488089373,-10.835026495729,133.781139215086));
#73960=CARTESIAN_POINT('Ctrl Pts',(80.8876030962552,-10.8536263832245,133.778842303779));
#73961=CARTESIAN_POINT('Ctrl Pts',(80.8492668411798,-10.8710273635018,133.776545392473));
#73962=CARTESIAN_POINT('Ctrl Pts',(80.7846904918397,-10.900338828042,133.772676309626));
#73963=CARTESIAN_POINT('Ctrl Pts',(80.7184684036561,-10.9263606106449,133.768807226779));
#73964=CARTESIAN_POINT('Ctrl Pts',(80.6509690279542,-10.9489065875881,133.764938143932));
#73965=CARTESIAN_POINT('Ctrl Pts',(80.5835702229558,-10.9714189721501,133.761074825826));
#73966=CARTESIAN_POINT('Ctrl Pts',(80.5148983650355,-10.9904656781335,133.757211507719));
#73967=CARTESIAN_POINT('Ctrl Pts',(80.4453432503833,-11.0059080118086,133.753348189613));
#73968=CARTESIAN_POINT('Ctrl Pts',(80.3758697238538,-11.0213322316323,133.749489403177));
#73969=CARTESIAN_POINT('Ctrl Pts',(80.3055154704923,-11.0331603724661,133.745630616741));
#73970=CARTESIAN_POINT('Ctrl Pts',(80.2346851938962,-11.0413036085467,133.741771830305));
#73971=CARTESIAN_POINT('Ctrl Pts',(80.1638995351806,-11.0494417149858,133.737915474622));
#73972=CARTESIAN_POINT('Ctrl Pts',(80.0926389296107,-11.0538994665824,133.734059118939));
#73973=CARTESIAN_POINT('Ctrl Pts',(80.0213165623721,-11.0546394249767,133.730202763256));
#73974=CARTESIAN_POINT('Ctrl Pts',(79.9500152644751,-11.0553791647799,133.726347546778));
#73975=CARTESIAN_POINT('Ctrl Pts',(79.878652726623,-11.0524032867213,133.722492330301));
#73976=CARTESIAN_POINT('Ctrl Pts',(79.8076437887121,-11.0457264358851,133.718637113824));
#73977=CARTESIAN_POINT('Ctrl Pts',(79.7366320745641,-11.0390493240039,133.714781746619));
#73978=CARTESIAN_POINT('Ctrl Pts',(79.6659744712478,-11.0286709997384,133.710926379415));
#73979=CARTESIAN_POINT('Ctrl Pts',(79.596080614355,-11.0146579591584,133.70707101221));
#73980=CARTESIAN_POINT('Ctrl Pts',(79.5261135976531,-11.000630250746,133.703211609487));
#73981=CARTESIAN_POINT('Ctrl Pts',(79.4569124005049,-10.9829603269613,133.699352206764));
#73982=CARTESIAN_POINT('Ctrl Pts',(79.3888754883127,-10.9617656316989,133.695492804042));
#73983=CARTESIAN_POINT('Ctrl Pts',(79.3208000530864,-10.9405589358335,133.691631216095));
#73984=CARTESIAN_POINT('Ctrl Pts',(79.2538906709944,-10.915823664085,133.687769628148));
#73985=CARTESIAN_POINT('Ctrl Pts',(79.1885270823431,-10.8877259510875,133.683908040201));
#73986=CARTESIAN_POINT('Ctrl Pts',(79.1230491377505,-10.8595790801341,133.680039696267));
#73987=CARTESIAN_POINT('Ctrl Pts',(79.0591228218862,-10.8280582378338,133.676171352334));
#73988=CARTESIAN_POINT('Ctrl Pts',(78.9971038465646,-10.7933758300826,133.6723030084));
#73989=CARTESIAN_POINT('Ctrl Pts',(78.9602787637695,-10.7727824144328,133.670006097094));
#73990=CARTESIAN_POINT('Ctrl Pts',(78.9241256132804,-10.7510751922943,133.667709185788));
#73991=CARTESIAN_POINT('Ctrl Pts',(78.8887136438621,-10.7283055855843,133.665412274481));
#73992=CARTESIAN_POINT('Ctrl Pts',(78.8290631719137,-10.6899508199882,133.661543191634));
#73993=CARTESIAN_POINT('Ctrl Pts',(78.7712838542151,-10.6484291560101,133.657674108787));
#73994=CARTESIAN_POINT('Ctrl Pts',(78.7157319002099,-10.6039491919514,133.65380502594));
#73995=CARTESIAN_POINT('Ctrl Pts',(78.6602627158456,-10.5595355008208,133.649941707834));
#73996=CARTESIAN_POINT('Ctrl Pts',(78.6070146838405,-10.5121725599639,133.646078389728));
#73997=CARTESIAN_POINT('Ctrl Pts',(78.5563157431669,-10.4621126253036,133.642215071621));
#73998=CARTESIAN_POINT('Ctrl Pts',(78.5056762723312,-10.4121114109275,133.638356285185));
#73999=CARTESIAN_POINT('Ctrl Pts',(78.4575802975038,-10.3594198263333,133.63449749875));
#74000=CARTESIAN_POINT('Ctrl Pts',(78.4123219474133,-10.3043296990541,133.630638712314));
#74001=CARTESIAN_POINT('Ctrl Pts',(78.3670921067648,-10.2492742745156,133.626782356631));
#74002=CARTESIAN_POINT('Ctrl Pts',(78.3246966521302,-10.1918236793768,133.622926000947));
#74003=CARTESIAN_POINT('Ctrl Pts',(78.2853911402273,-10.1323047383497,133.619069645264));
#74004=CARTESIAN_POINT('Ctrl Pts',(78.2460972395663,-10.0728033798137,133.615214428787));
#74005=CARTESIAN_POINT('Ctrl Pts',(78.2098917370287,-10.0112352935604,133.61135921231));
#74006=CARTESIAN_POINT('Ctrl Pts',(78.1769873297906,-9.94795694351372,133.607503995832));
#74007=CARTESIAN_POINT('Ctrl Pts',(78.1440816360885,-9.88467611947279,133.603648628628));
#74008=CARTESIAN_POINT('Ctrl Pts',(78.1144775160846,-9.81968533089659,133.599793261423));
#74009=CARTESIAN_POINT('Ctrl Pts',(78.0883412825142,-9.7533647923553,133.595937894219));
#74010=CARTESIAN_POINT('Ctrl Pts',(78.0621776914343,-9.68697483429487,133.592078491496));
#74011=CARTESIAN_POINT('Ctrl Pts',(78.0394894114196,-9.61925280063322,133.588219088773));
#74012=CARTESIAN_POINT('Ctrl Pts',(78.020393893762,-9.55059715459226,133.58435968605));
#74013=CARTESIAN_POINT('Ctrl Pts',(78.0012875640722,-9.48190263518528,133.580498098103));
#74014=CARTESIAN_POINT('Ctrl Pts',(77.9857781519716,-9.41227392546944,133.576636510156));
#74015=CARTESIAN_POINT('Ctrl Pts',(77.9739320459272,-9.34212016599325,133.572774922209));
#74016=CARTESIAN_POINT('Ctrl Pts',(77.9620652146957,-9.27184367000021,133.568906578276));
#74017=CARTESIAN_POINT('Ctrl Pts',(77.9538745412824,-9.20104077296669,133.565038234342));
#74018=CARTESIAN_POINT('Ctrl Pts',(77.949374507556,-9.13012552493194,133.561169890409));
#74019=CARTESIAN_POINT('Ctrl Pts',(77.946702517029,-9.08801809141209,133.558872979102));
#74020=CARTESIAN_POINT('Ctrl Pts',(77.9453307150346,-9.04587106372851,133.556576067796));
#74021=CARTESIAN_POINT('Ctrl Pts',(77.9452534594865,-9.00377051029501,133.55427915649));
#74022=CARTESIAN_POINT('Ctrl Pts',(77.9452511674388,-9.00252145466656,133.55421101083));
#74023=CARTESIAN_POINT('Ctrl Pts',(77.9452500143197,-9.0012723969475,133.55414286517));
#74024=CARTESIAN_POINT('Ctrl Pts',(77.9452500001325,-9.00002333845969,133.55407471951));
#74025=CARTESIAN_POINT('Origin',(80.,-9.,141.545925280538));
#74026=CARTESIAN_POINT('',(81.2520391107129,-7.37076839346111,134.706120114083));
#74027=CARTESIAN_POINT('',(81.2520391107129,-7.37076839346112,134.647862573676));
#74028=CARTESIAN_POINT('',(81.2520391107129,-7.37076839346111,141.545925280538));
#74029=CARTESIAN_POINT('',(77.9452508583196,-9.00187810112593,134.19592528059));
#74030=CARTESIAN_POINT('Ctrl Pts',(81.2520391107129,-7.37076839346111,134.647862573676));
#74031=CARTESIAN_POINT('Ctrl Pts',(81.3084423634553,-7.41411341458736,134.644002866637));
#74032=CARTESIAN_POINT('Ctrl Pts',(81.3626623275803,-7.46044482548973,134.640143159597));
#74033=CARTESIAN_POINT('Ctrl Pts',(81.4143696957603,-7.50951151422936,134.636283452558));
#74034=CARTESIAN_POINT('Ctrl Pts',(81.4660396077081,-7.55854265961508,134.632426541446));
#74035=CARTESIAN_POINT('Ctrl Pts',(81.5152001830901,-7.61030481882812,134.628569630335));
#74036=CARTESIAN_POINT('Ctrl Pts',(81.5615557483562,-7.66450712945533,134.624712719223));
#74037=CARTESIAN_POINT('Ctrl Pts',(81.6078932410243,-7.7186883082816,134.620857311802));
#74038=CARTESIAN_POINT('Ctrl Pts',(81.6514275786264,-7.77530738151462,134.617001904381));
#74039=CARTESIAN_POINT('Ctrl Pts',(81.6919016799579,-7.83403847925596,134.613146496959));
#74040=CARTESIAN_POINT('Ctrl Pts',(81.7323735406718,-7.89276632568549,134.609291302971));
#74041=CARTESIAN_POINT('Ctrl Pts',(81.7697852271571,-7.95360556357426,134.605436108982));
#74042=CARTESIAN_POINT('Ctrl Pts',(81.8039225237931,-8.01620068578403,134.601580914993));
#74043=CARTESIAN_POINT('Ctrl Pts',(81.8380934850055,-8.07885753632238,134.597721919196));
#74044=CARTESIAN_POINT('Ctrl Pts',(81.868983373165,-8.14327330249264,134.593862923398));
#74045=CARTESIAN_POINT('Ctrl Pts',(81.896424007617,-8.20906792590404,134.590003927601));
#74046=CARTESIAN_POINT('Ctrl Pts',(81.923877854851,-8.27489422970581,134.586143073681));
#74047=CARTESIAN_POINT('Ctrl Pts',(81.9478789761604,-8.34210025519686,134.58228221976));
#74048=CARTESIAN_POINT('Ctrl Pts',(81.9683084278477,-8.41028863385224,134.57842136584));
#74049=CARTESIAN_POINT('Ctrl Pts',(81.9887754594446,-8.47860244480755,134.574553409892));
#74050=CARTESIAN_POINT('Ctrl Pts',(82.0056575794369,-8.54790174613055,134.570685453943));
#74051=CARTESIAN_POINT('Ctrl Pts',(82.0188866566306,-8.61777725057383,134.566817497995));
#74052=CARTESIAN_POINT('Ctrl Pts',(82.0304714636668,-8.67896777986658,134.563430298522));
#74053=CARTESIAN_POINT('Ctrl Pts',(82.0392556566401,-8.74059983008632,134.56004309905));
#74054=CARTESIAN_POINT('Ctrl Pts',(82.0452262841889,-8.80239683969454,134.556655899578));
#74055=CARTESIAN_POINT('Ctrl Pts',(82.052046329133,-8.87298546366857,134.552786816731));
#74056=CARTESIAN_POINT('Ctrl Pts',(82.0552210145704,-8.94406583722984,134.548917733884));
#74057=CARTESIAN_POINT('Ctrl Pts',(82.0546935628721,-9.0152290903256,134.545048651037));
#74058=CARTESIAN_POINT('Ctrl Pts',(82.0541668970505,-9.08628631372333,134.541185332931));
#74059=CARTESIAN_POINT('Ctrl Pts',(82.0499490467711,-9.15742568972607,134.537322014825));
#74060=CARTESIAN_POINT('Ctrl Pts',(82.0420350207688,-9.22823351299477,134.533458696718));
#74061=CARTESIAN_POINT('Ctrl Pts',(82.0341302779158,-9.29895827871404,134.529599910282));
#74062=CARTESIAN_POINT('Ctrl Pts',(82.0225380250317,-9.36935178377462,134.525741123847));
#74063=CARTESIAN_POINT('Ctrl Pts',(82.0073052791557,-9.43900236761729,134.521882337411));
#74064=CARTESIAN_POINT('Ctrl Pts',(81.9920821287927,-9.5086090766994,134.518025981728));
#74065=CARTESIAN_POINT('Ctrl Pts',(81.9732231387407,-9.57747331959585,134.514169626044));
#74066=CARTESIAN_POINT('Ctrl Pts',(81.9508266910127,-9.64519205213054,134.510313270361));
#74067=CARTESIAN_POINT('Ctrl Pts',(81.9284368594196,-9.71289077987354,134.506458053884));
#74068=CARTESIAN_POINT('Ctrl Pts',(81.9025117972192,-9.77944420810088,134.502602837407));
#74069=CARTESIAN_POINT('Ctrl Pts',(81.8731996991641,-9.84446459342684,134.498747620929));
#74070=CARTESIAN_POINT('Ctrl Pts',(81.8438864550936,-9.90948752085537,134.494892253725));
#74071=CARTESIAN_POINT('Ctrl Pts',(81.8111861139161,-9.97297684442902,134.49103688652));
#74072=CARTESIAN_POINT('Ctrl Pts',(81.7752942420166,-10.0345665356866,134.487181519316));
#74073=CARTESIAN_POINT('Ctrl Pts',(81.7393648011145,-10.0962206945562,134.483322116593));
#74074=CARTESIAN_POINT('Ctrl Pts',(81.7002374058725,-10.1559708312496,134.47946271387));
#74075=CARTESIAN_POINT('Ctrl Pts',(81.6581522078642,-10.2134779841657,134.475603311147));
#74076=CARTESIAN_POINT('Ctrl Pts',(81.6160431808863,-10.2710176980836,134.4717417232));
#74077=CARTESIAN_POINT('Ctrl Pts',(81.5709733243342,-10.3263115233336,134.467880135253));
#74078=CARTESIAN_POINT('Ctrl Pts',(81.5232227929821,-10.3790539820615,134.464018547306));
#74079=CARTESIAN_POINT('Ctrl Pts',(81.4753887203639,-10.4318887156115,134.460150203373));
#74080=CARTESIAN_POINT('Ctrl Pts',(81.4248649538139,-10.4821628279647,134.45628185944));
#74081=CARTESIAN_POINT('Ctrl Pts',(81.3719676447898,-10.5296085591255,134.452413515506));
#74082=CARTESIAN_POINT('Ctrl Pts',(81.3405587449436,-10.5577804689193,134.4501166042));
#74083=CARTESIAN_POINT('Ctrl Pts',(81.3083136507051,-10.5849559667216,134.447819692893));
#74084=CARTESIAN_POINT('Ctrl Pts',(81.2753034381164,-10.6110861873992,134.445522781587));
#74085=CARTESIAN_POINT('Ctrl Pts',(81.219698658366,-10.6551018132211,134.44165369874));
#74086=CARTESIAN_POINT('Ctrl Pts',(81.1617035722651,-10.6963215672399,134.437784615893));
#74087=CARTESIAN_POINT('Ctrl Pts',(81.1016308900006,-10.7344759856212,134.433915533046));
#74088=CARTESIAN_POINT('Ctrl Pts',(81.0416477130367,-10.7725735558219,134.43005221494));
#74089=CARTESIAN_POINT('Ctrl Pts',(80.9795934911439,-10.8076145978201,134.426188896833));
#74090=CARTESIAN_POINT('Ctrl Pts',(80.9158130846978,-10.8393705326541,134.422325578727));
#74091=CARTESIAN_POINT('Ctrl Pts',(80.8521074926439,-10.8710892177889,134.418466792291));
#74092=CARTESIAN_POINT('Ctrl Pts',(80.7866801707553,-10.8995302345098,134.414608005855));
#74093=CARTESIAN_POINT('Ctrl Pts',(80.7199024698014,-10.9245098068012,134.410749219419));
#74094=CARTESIAN_POINT('Ctrl Pts',(80.6531668339025,-10.9494736437936,134.406892863736));
#74095=CARTESIAN_POINT('Ctrl Pts',(80.5850829605107,-10.9709801925506,134.403036508053));
#74096=CARTESIAN_POINT('Ctrl Pts',(80.5160428208376,-10.9888935038262,134.39918015237));
#74097=CARTESIAN_POINT('Ctrl Pts',(80.4470230763131,-11.0068015233302,134.395324935892));
#74098=CARTESIAN_POINT('Ctrl Pts',(80.3770480962869,-11.0211182907457,134.391469719415));
#74099=CARTESIAN_POINT('Ctrl Pts',(80.3065240147203,-11.0317580050045,134.387614502938));
#74100=CARTESIAN_POINT('Ctrl Pts',(80.235997175873,-11.0423981352443,134.383759135733));
#74101=CARTESIAN_POINT('Ctrl Pts',(80.1649216735389,-11.0493608566172,134.379903768529));
#74102=CARTESIAN_POINT('Ctrl Pts',(80.0937110916941,-11.0526119442782,134.376048401324));
#74103=CARTESIAN_POINT('Ctrl Pts',(80.0224259717883,-11.0558664349414,134.372188998601));
#74104=CARTESIAN_POINT('Ctrl Pts',(79.9510059763948,-11.0554015142251,134.368329595878));
#74105=CARTESIAN_POINT('Ctrl Pts',(79.8798661318538,-11.0512350953082,134.364470193156));
#74106=CARTESIAN_POINT('Ctrl Pts',(79.808686007374,-11.0470663173323,134.360608605209));
#74107=CARTESIAN_POINT('Ctrl Pts',(79.7377868325604,-11.0391919226788,134.356747017262));
#74108=CARTESIAN_POINT('Ctrl Pts',(79.6675771998992,-11.0276815934641,134.352885429315));
#74109=CARTESIAN_POINT('Ctrl Pts',(79.5972447329689,-11.0161511265159,134.349017085381));
#74110=CARTESIAN_POINT('Ctrl Pts',(79.5276046915497,-11.0009721281821,134.345148741448));
#74111=CARTESIAN_POINT('Ctrl Pts',(79.4590535039995,-10.9822649800076,134.341280397514));
#74112=CARTESIAN_POINT('Ctrl Pts',(79.4183497815635,-10.9711572137665,134.338983486208));
#74113=CARTESIAN_POINT('Ctrl Pts',(79.3780296424184,-10.9588064987021,134.336686574902));
#74114=CARTESIAN_POINT('Ctrl Pts',(79.3381726900255,-10.9452460446617,134.334389663595));
#74115=CARTESIAN_POINT('Ctrl Pts',(79.271034768591,-10.9224038391411,134.330520580748));
#74116=CARTESIAN_POINT('Ctrl Pts',(79.2049492964155,-10.8960370323457,134.326651497901));
#74117=CARTESIAN_POINT('Ctrl Pts',(79.1403122668311,-10.8662621905667,134.322782415054));
#74118=CARTESIAN_POINT('Ctrl Pts',(79.075771543197,-10.836531711817,134.318919096948));
#74119=CARTESIAN_POINT('Ctrl Pts',(79.0126754159974,-10.8034034789718,134.315055778841));
#74120=CARTESIAN_POINT('Ctrl Pts',(78.9514029674593,-10.7670432439097,134.311192460735));
#74121=CARTESIAN_POINT('Ctrl Pts',(78.8902023914798,-10.7307256593893,134.307333674299));
#74122=CARTESIAN_POINT('Ctrl Pts',(78.8308216607734,-10.6911838498401,134.303474887863));
#74123=CARTESIAN_POINT('Ctrl Pts',(78.7736165849993,-10.6486301228327,134.299616101428));
#74124=CARTESIAN_POINT('Ctrl Pts',(78.7164475442282,-10.6061032015529,134.295759745744));
#74125=CARTESIAN_POINT('Ctrl Pts',(78.6614518281798,-10.5605684162585,134.291903390061));
#74126=CARTESIAN_POINT('Ctrl Pts',(78.6089562497838,-10.5122813387345,134.288047034378));
#74127=CARTESIAN_POINT('Ctrl Pts',(78.5564761791074,-10.4640085256966,134.284191817901));
#74128=CARTESIAN_POINT('Ctrl Pts',(78.5064951371636,-10.4129853632591,134.280336601423));
#74129=CARTESIAN_POINT('Ctrl Pts',(78.459305487336,-10.3595065211859,134.276481384946));
#74130=CARTESIAN_POINT('Ctrl Pts',(78.4121139925342,-10.30602558825,134.272626017742));
#74131=CARTESIAN_POINT('Ctrl Pts',(78.3677144262841,-10.2500891507715,134.268770650537));
#74132=CARTESIAN_POINT('Ctrl Pts',(78.3263598618196,-10.1920261114469,134.264915283332));
#74133=CARTESIAN_POINT('Ctrl Pts',(78.2849620104029,-10.1339022959532,134.261055880609));
#74134=CARTESIAN_POINT('Ctrl Pts',(78.2466158057055,-10.0736478315659,134.257196477887));
#74135=CARTESIAN_POINT('Ctrl Pts',(78.2115313003927,-10.0116211113973,134.253337075164));
#74136=CARTESIAN_POINT('Ctrl Pts',(78.1764269299573,-9.94955927121262,134.249475487217));
#74137=CARTESIAN_POINT('Ctrl Pts',(78.144588152236,-9.8857236125756,134.24561389927));
#74138=CARTESIAN_POINT('Ctrl Pts',(78.1161780375013,-9.82049520175772,134.241752311323));
#74139=CARTESIAN_POINT('Ctrl Pts',(78.0877182182525,-9.75515267149706,134.23788396739));
#74140=CARTESIAN_POINT('Ctrl Pts',(78.0626992088762,-9.68841297919082,134.234015623456));
#74141=CARTESIAN_POINT('Ctrl Pts',(78.0412348877942,-9.62067446999657,134.230147279523));
#74142=CARTESIAN_POINT('Ctrl Pts',(78.0284899916253,-9.58045329258207,134.227850368216));
#74143=CARTESIAN_POINT('Ctrl Pts',(78.0169973859048,-9.53988022519759,134.22555345691));
#74144=CARTESIAN_POINT('Ctrl Pts',(78.0067723452924,-9.49904015771159,134.223256545603));
#74145=CARTESIAN_POINT('Ctrl Pts',(77.9843222460634,-9.40937170529799,134.218213447125));
#74146=CARTESIAN_POINT('Ctrl Pts',(77.967913679714,-9.31813449884541,134.213170348647));
#74147=CARTESIAN_POINT('Ctrl Pts',(77.9577201042085,-9.22603183347914,134.208127250169));
#74148=CARTESIAN_POINT('Ctrl Pts',(77.9494988556529,-9.15174986007309,134.204059926976));
#74149=CARTESIAN_POINT('Ctrl Pts',(77.9453194352602,-9.07690516324679,134.199992603783));
#74150=CARTESIAN_POINT('Ctrl Pts',(77.9452508583196,-9.00187810112594,134.19592528059));
#74151=CARTESIAN_POINT('Ctrl Pts',(77.9452508583188,-9.00187810017601,134.195925280538));
#74152=CARTESIAN_POINT('Ctrl Pts',(77.9451865584667,-8.93153037992358,134.192111631088));
#74153=CARTESIAN_POINT('Ctrl Pts',(77.9487392155753,-8.86108771113924,134.188297981638));
#74154=CARTESIAN_POINT('Ctrl Pts',(77.9559113871452,-8.79095621201019,134.184484332188));
#74155=CARTESIAN_POINT('Ctrl Pts',(77.9630788626377,-8.72087063243831,134.180673179777));
#74156=CARTESIAN_POINT('Ctrl Pts',(77.9738611037571,-8.65109631311334,134.176862027366));
#74157=CARTESIAN_POINT('Ctrl Pts',(77.9882086454291,-8.58203695357894,134.173050874956));
#74158=CARTESIAN_POINT('Ctrl Pts',(78.0025518660922,-8.51299839245752,134.169240870339));
#74159=CARTESIAN_POINT('Ctrl Pts',(78.0204581554943,-8.44467485161844,134.165430865722));
#74160=CARTESIAN_POINT('Ctrl Pts',(78.0418267999905,-8.37746061870398,134.161620861105));
#74161=CARTESIAN_POINT('Ctrl Pts',(78.0631965645668,-8.31024286262121,134.15781065678));
#74162=CARTESIAN_POINT('Ctrl Pts',(78.0880288903436,-8.24413500386008,134.154000452454));
#74163=CARTESIAN_POINT('Ctrl Pts',(78.1161735511138,-8.17951509887334,134.150190248128));
#74164=CARTESIAN_POINT('Ctrl Pts',(78.1443474516825,-8.11482805955463,134.146376085339));
#74165=CARTESIAN_POINT('Ctrl Pts',(78.1758403520862,-8.05163251518824,134.14256192255));
#74166=CARTESIAN_POINT('Ctrl Pts',(78.210454788899,-7.99028444603172,134.138747759761));
#74167=CARTESIAN_POINT('Ctrl Pts',(78.2450904309211,-7.92889879432974,134.134931260371));
#74168=CARTESIAN_POINT('Ctrl Pts',(78.2828511440636,-7.86936328817681,134.131114760981));
#74169=CARTESIAN_POINT('Ctrl Pts',(78.3234961567948,-7.81200487113028,134.127298261591));
#74170=CARTESIAN_POINT('Ctrl Pts',(78.3642086074958,-7.75455128533028,134.123475429888));
#74171=CARTESIAN_POINT('Ctrl Pts',(78.407814592662,-7.69928238170397,134.119652598184));
#74172=CARTESIAN_POINT('Ctrl Pts',(78.4540338348352,-7.64649116047744,134.115829766481));
#74173=CARTESIAN_POINT('Ctrl Pts',(78.4689707705123,-7.62943032090719,134.114594320191));
#74174=CARTESIAN_POINT('Ctrl Pts',(78.4841803654163,-7.61262795755886,134.113358873901));
#74175=CARTESIAN_POINT('Ctrl Pts',(78.4996524028237,-7.5960930763946,134.112123427611));
#74176=CARTESIAN_POINT('Ctrl Pts',(78.5481066294738,-7.54431031123745,134.108254344765));
#74177=CARTESIAN_POINT('Ctrl Pts',(78.5993397400987,-7.49493758081945,134.104385261918));
#74178=CARTESIAN_POINT('Ctrl Pts',(78.6530824932534,-7.44828778682404,134.100516179071));
#74179=CARTESIAN_POINT('Ctrl Pts',(78.7067451723861,-7.40170749869516,134.096652860964));
#74180=CARTESIAN_POINT('Ctrl Pts',(78.7629097078898,-7.35784240972122,134.092789542858));
#74181=CARTESIAN_POINT('Ctrl Pts',(78.8212689947725,-7.31696976265564,134.088926224751));
#74182=CARTESIAN_POINT('Ctrl Pts',(78.8795598262342,-7.27614505918933,134.085067438316));
#74183=CARTESIAN_POINT('Ctrl Pts',(78.9400398993904,-7.23830610264095,134.08120865188));
#74184=CARTESIAN_POINT('Ctrl Pts',(79.0023692611183,-7.20368976194578,134.077349865444));
#74185=CARTESIAN_POINT('Ctrl Pts',(79.0646593599188,-7.16909522700693,134.073493509761));
#74186=CARTESIAN_POINT('Ctrl Pts',(79.1287960124367,-7.13771951571177,134.069637154078));
#74187=CARTESIAN_POINT('Ctrl Pts',(79.1944117734195,-7.10975526142912,134.065780798394));
#74188=CARTESIAN_POINT('Ctrl Pts',(79.2600081508495,-7.0817992680672,134.061925581917));
#74189=CARTESIAN_POINT('Ctrl Pts',(79.3270823226429,-7.05725292135065,134.05807036544));
#74190=CARTESIAN_POINT('Ctrl Pts',(79.3952453929246,-7.03626136471245,134.054215148963));
#74191=CARTESIAN_POINT('Ctrl Pts',(79.4634111281785,-7.01526898736714,134.050359781758));
#74192=CARTESIAN_POINT('Ctrl Pts',(79.5326653815287,-6.99783181690051,134.046504414553));
#74193=CARTESIAN_POINT('Ctrl Pts',(79.6026042328258,-6.98404509804113,134.042649047349));
#74194=CARTESIAN_POINT('Ctrl Pts',(79.6726162910286,-6.97024394824659,134.038789644626));
#74195=CARTESIAN_POINT('Ctrl Pts',(79.7433139000598,-6.96010097183086,134.034930241903));
#74196=CARTESIAN_POINT('Ctrl Pts',(79.8142839731725,-6.95366006736921,134.03107083918));
#74197=CARTESIAN_POINT('Ctrl Pts',(79.8852942300982,-6.94721551601684,134.027209251233));
#74198=CARTESIAN_POINT('Ctrl Pts',(79.9565767725572,-6.94447722804744,134.023347663287));
#74199=CARTESIAN_POINT('Ctrl Pts',(80.0277171909406,-6.94543695160592,134.01948607534));
#74200=CARTESIAN_POINT('Ctrl Pts',(80.0989820720358,-6.94639835423517,134.015617731406));
#74201=CARTESIAN_POINT('Ctrl Pts',(80.1701038477248,-6.95107065368359,134.011749387473));
#74202=CARTESIAN_POINT('Ctrl Pts',(80.2406726110882,-6.95939365462812,134.007881043539));
#74203=CARTESIAN_POINT('Ctrl Pts',(80.2825743119812,-6.96433561307386,134.005584132233));
#74204=CARTESIAN_POINT('Ctrl Pts',(80.3242812036117,-6.97056369253628,134.003287220926));
#74205=CARTESIAN_POINT('Ctrl Pts',(80.3657096343967,-6.97805686879937,134.00099030962));
#74206=CARTESIAN_POINT('Ctrl Pts',(80.435496785936,-6.99067929782875,133.997121109306));
#74207=CARTESIAN_POINT('Ctrl Pts',(80.5047663681027,-7.00694373601728,133.993251908991));
#74208=CARTESIAN_POINT('Ctrl Pts',(80.5731094334077,-7.02679369050293,133.989382708677));
#74209=CARTESIAN_POINT('Ctrl Pts',(80.6413358826972,-7.04660977435969,133.985520110506));
#74210=CARTESIAN_POINT('Ctrl Pts',(80.7086384934941,-7.0699990848956,133.981657512335));
#74211=CARTESIAN_POINT('Ctrl Pts',(80.7746179998118,-7.09685404740793,133.977794914165));
#74212=CARTESIAN_POINT('Ctrl Pts',(80.8405321010276,-7.12368238875172,133.973936144965));
#74213=CARTESIAN_POINT('Ctrl Pts',(80.9051252521817,-7.15396938460669,133.970077375765));
#74214=CARTESIAN_POINT('Ctrl Pts',(80.9680140702184,-7.18755791199851,133.966218606566));
#74215=CARTESIAN_POINT('Ctrl Pts',(81.030862599658,-7.22112492150066,133.962362309417));
#74216=CARTESIAN_POINT('Ctrl Pts',(81.0920085350432,-7.25798903737295,133.958506012269));
#74217=CARTESIAN_POINT('Ctrl Pts',(81.1510907558965,-7.29794605426575,133.954649715121));
#74218=CARTESIAN_POINT('Ctrl Pts',(81.1854604267632,-7.32119009451308,133.952406406359));
#74219=CARTESIAN_POINT('Ctrl Pts',(81.2191321632765,-7.34547991695526,133.950163097596));
#74220=CARTESIAN_POINT('Ctrl Pts',(81.2520391107129,-7.37076839346111,133.947919788834));
#74221=CARTESIAN_POINT('',(77.9452507619582,-8.99823046142755,134.254074719427));
#74222=CARTESIAN_POINT('Ctrl Pts',(77.9452507619582,-8.99823046142755,134.254074719427));
#74223=CARTESIAN_POINT('Ctrl Pts',(77.9453248874363,-8.91215758797735,134.249416661534));
#74224=CARTESIAN_POINT('Ctrl Pts',(77.9508111829309,-8.82632098520286,134.24475860364));
#74225=CARTESIAN_POINT('Ctrl Pts',(77.9615982093287,-8.74131930437674,134.240100545746));
#74226=CARTESIAN_POINT('Ctrl Pts',(77.9725417920147,-8.65508396126522,134.235374883656));
#74227=CARTESIAN_POINT('Ctrl Pts',(77.9889410126122,-8.56970793661434,134.230649221565));
#74228=CARTESIAN_POINT('Ctrl Pts',(78.0106307458957,-8.48579426945562,134.225923559475));
#74229=CARTESIAN_POINT('Ctrl Pts',(78.0180442984579,-8.45711257134388,134.224308327796));
#74230=CARTESIAN_POINT('Ctrl Pts',(78.0260755171318,-8.42860153023918,134.222693096118));
#74231=CARTESIAN_POINT('Ctrl Pts',(78.0347165430364,-8.40028465395229,134.221077864439));
#74232=CARTESIAN_POINT('Ctrl Pts',(78.0554150258306,-8.33245516436548,134.217208781592));
#74233=CARTESIAN_POINT('Ctrl Pts',(78.0796697562115,-8.26556565706135,134.213339698745));
#74234=CARTESIAN_POINT('Ctrl Pts',(78.1073768028461,-8.20001562759332,134.209470615898));
#74235=CARTESIAN_POINT('Ctrl Pts',(78.135042567363,-8.13456326440015,134.205607297792));
#74236=CARTESIAN_POINT('Ctrl Pts',(78.1661502502832,-8.07044686133226,134.201743979686));
#74237=CARTESIAN_POINT('Ctrl Pts',(78.2005462224255,-8.0080505734299,134.197880661579));
#74238=CARTESIAN_POINT('Ctrl Pts',(78.2349018481057,-7.94572747634918,134.194021875143));
#74239=CARTESIAN_POINT('Ctrl Pts',(78.2725378680003,-7.88512090997112,134.190163088708));
#74240=CARTESIAN_POINT('Ctrl Pts',(78.3132533816179,-7.82659324704664,134.186304302272));
#74241=CARTESIAN_POINT('Ctrl Pts',(78.3539432474475,-7.76810245225814,134.182447946588));
#74242=CARTESIAN_POINT('Ctrl Pts',(78.3977084815971,-7.71168836062039,134.178591590905));
#74243=CARTESIAN_POINT('Ctrl Pts',(78.4443040202919,-7.65768573678892,134.174735235222));
#74244=CARTESIAN_POINT('Ctrl Pts',(78.4908857941979,-7.60369906587329,134.170880018745));
#74245=CARTESIAN_POINT('Ctrl Pts',(78.5402958955815,-7.55212281610491,134.167024802267));
#74246=CARTESIAN_POINT('Ctrl Pts',(78.5922490883443,-7.50325856166388,134.16316958579));
#74247=CARTESIAN_POINT('Ctrl Pts',(78.6442043123216,-7.45439239677664,134.159314218586));
#74248=CARTESIAN_POINT('Ctrl Pts',(78.6987024697097,-7.40823876894237,134.155458851381));
#74249=CARTESIAN_POINT('Ctrl Pts',(78.7554228609497,-7.36506106919762,134.151603484176));
#74250=CARTESIAN_POINT('Ctrl Pts',(78.8122026229723,-7.32183817417522,134.147744081453));
#74251=CARTESIAN_POINT('Ctrl Pts',(78.8712088748859,-7.28159772029608,134.143884678731));
#74252=CARTESIAN_POINT('Ctrl Pts',(78.932090075322,-7.24456103630057,134.140025276008));
#74253=CARTESIAN_POINT('Ctrl Pts',(78.9930057471719,-7.20750338184365,134.136163688061));
#74254=CARTESIAN_POINT('Ctrl Pts',(79.0557980530734,-7.17365333900788,134.132302100114));
#74255=CARTESIAN_POINT('Ctrl Pts',(79.120091297845,-7.14318599790613,134.128440512167));
#74256=CARTESIAN_POINT('Ctrl Pts',(79.1844970259528,-7.11266535309906,134.124572168233));
#74257=CARTESIAN_POINT('Ctrl Pts',(79.2504084863379,-7.08553941073387,134.1207038243));
#74258=CARTESIAN_POINT('Ctrl Pts',(79.3174311513888,-7.06193464263828,134.116835480367));
#74259=CARTESIAN_POINT('Ctrl Pts',(79.3572272811514,-7.04791881062928,134.11453856906));
#74260=CARTESIAN_POINT('Ctrl Pts',(79.3974148942614,-7.03514346187569,134.112241657754));
#74261=CARTESIAN_POINT('Ctrl Pts',(79.4379096287717,-7.02362655930808,134.109944746447));
#74262=CARTESIAN_POINT('Ctrl Pts',(79.5061249302259,-7.00422579054222,134.10607549038));
#74263=CARTESIAN_POINT('Ctrl Pts',(79.5754794623163,-6.98832288444096,134.102206234313));
#74264=CARTESIAN_POINT('Ctrl Pts',(79.645581172235,-6.97604721966502,134.098336978247));
#74265=CARTESIAN_POINT('Ctrl Pts',(79.7155609766724,-6.96379290202634,134.094474450739));
#74266=CARTESIAN_POINT('Ctrl Pts',(79.7862849026504,-6.95515337539077,134.090611923232));
#74267=CARTESIAN_POINT('Ctrl Pts',(79.8573471332508,-6.95020788319687,134.086749395724));
#74268=CARTESIAN_POINT('Ctrl Pts',(79.9283395278624,-6.94526725115633,134.082890664093));
#74269=CARTESIAN_POINT('Ctrl Pts',(79.9996690856365,-6.94401348583595,134.079031932462));
#74270=CARTESIAN_POINT('Ctrl Pts',(80.0709224192402,-6.94647435541965,134.07517320083));
#74271=CARTESIAN_POINT('Ctrl Pts',(80.1421295659897,-6.94893362985238,134.071316970453));
#74272=CARTESIAN_POINT('Ctrl Pts',(80.2132601023311,-6.95510274416918,134.067460740076));
#74273=CARTESIAN_POINT('Ctrl Pts',(80.2838999035947,-6.9649573942448,134.063604509698));
#74274=CARTESIAN_POINT('Ctrl Pts',(80.3545175459512,-6.97480895302809,134.059749488977));
#74275=CARTESIAN_POINT('Ctrl Pts',(80.4246442782307,-6.9883436841954,134.055894468255));
#74276=CARTESIAN_POINT('Ctrl Pts',(80.4938720915139,-7.0054855428642,134.052039447534));
#74277=CARTESIAN_POINT('Ctrl Pts',(80.5631419758923,-7.02263781897557,134.048182084041));
#74278=CARTESIAN_POINT('Ctrl Pts',(80.6315113758258,-7.04340149176895,134.044324720548));
#74279=CARTESIAN_POINT('Ctrl Pts',(80.6985844526089,-7.06764979233238,134.040467357055));
#74280=CARTESIAN_POINT('Ctrl Pts',(80.7656748958074,-7.09190437121314,134.036608994821));
#74281=CARTESIAN_POINT('Ctrl Pts',(80.831467895916,-7.11964519319846,134.032750632588));
#74282=CARTESIAN_POINT('Ctrl Pts',(80.8955871455516,-7.15069709695175,134.028892270355));
#74283=CARTESIAN_POINT('Ctrl Pts',(80.9598054148642,-7.18179695431484,134.025027949634));
#74284=CARTESIAN_POINT('Ctrl Pts',(81.0223443385685,-7.21621788193465,134.021163628913));
#74285=CARTESIAN_POINT('Ctrl Pts',(81.0828523129242,-7.25373872776877,134.017299308192));
#74286=CARTESIAN_POINT('Ctrl Pts',(81.141234597276,-7.28994143846816,134.013570743923));
#74287=CARTESIAN_POINT('Ctrl Pts',(81.1977259690068,-7.32902959010821,134.009842179654));
#74288=CARTESIAN_POINT('Ctrl Pts',(81.2520391107129,-7.3707683934611,134.006113615385));
#74289=CARTESIAN_POINT('Ctrl Pts',(81.2520391107129,-7.37076839346111,134.706120114083));
#74290=CARTESIAN_POINT('Ctrl Pts',(81.308617435007,-7.41424795434766,134.702260546292));
#74291=CARTESIAN_POINT('Ctrl Pts',(81.3628983050282,-7.46065513417077,134.6984009785));
#74292=CARTESIAN_POINT('Ctrl Pts',(81.4145767289439,-7.50970800162167,134.694541410709));
#74293=CARTESIAN_POINT('Ctrl Pts',(81.4662859532541,-7.55879010463279,134.690679542611));
#74294=CARTESIAN_POINT('Ctrl Pts',(81.5153893099384,-7.61052068126371,134.686817674514));
#74295=CARTESIAN_POINT('Ctrl Pts',(81.5616202022989,-7.66458249739198,134.682955806416));
#74296=CARTESIAN_POINT('Ctrl Pts',(81.6079305750915,-7.71873725692424,134.679087298971));
#74297=CARTESIAN_POINT('Ctrl Pts',(81.6513583306771,-7.77523087073858,134.675218791526));
#74298=CARTESIAN_POINT('Ctrl Pts',(81.691678980054,-7.83371539024845,134.671350284081));
#74299=CARTESIAN_POINT('Ctrl Pts',(81.711621074086,-7.86264110958842,134.669436968189));
#74300=CARTESIAN_POINT('Ctrl Pts',(81.7308038121415,-7.8920534289855,134.667523652297));
#74301=CARTESIAN_POINT('Ctrl Pts',(81.7492042338686,-7.9219081158287,134.665610336405));
#74302=CARTESIAN_POINT('Ctrl Pts',(81.7864133305879,-7.98227988049495,134.661741253558));
#74303=CARTESIAN_POINT('Ctrl Pts',(81.8205661439275,-8.04469849530034,134.657872170711));
#74304=CARTESIAN_POINT('Ctrl Pts',(81.8514316391579,-8.10882187637653,134.654003087864));
#74305=CARTESIAN_POINT('Ctrl Pts',(81.8822511463398,-8.17284971681296,134.650139769758));
#74306=CARTESIAN_POINT('Ctrl Pts',(81.9097928487125,-8.2385768475084,134.646276451652));
#74307=CARTESIAN_POINT('Ctrl Pts',(81.9338700765014,-8.30563403761968,134.642413133545));
#74308=CARTESIAN_POINT('Ctrl Pts',(81.9579190617114,-8.37261256967272,134.638554347109));
#74309=CARTESIAN_POINT('Ctrl Pts',(81.9785114811098,-8.44091760715137,134.634695560674));
#74310=CARTESIAN_POINT('Ctrl Pts',(81.995508258998,-8.51015885149286,134.630836774238));
#74311=CARTESIAN_POINT('Ctrl Pts',(82.0124943301625,-8.57935647892769,134.626980418555));
#74312=CARTESIAN_POINT('Ctrl Pts',(82.0258891379882,-8.64948867252513,134.623124062871));
#74313=CARTESIAN_POINT('Ctrl Pts',(82.035603517282,-8.72015024936765,134.619267707188));
#74314=CARTESIAN_POINT('Ctrl Pts',(82.0453150268509,-8.79079095207278,134.615412490711));
#74315=CARTESIAN_POINT('Ctrl Pts',(82.0513482002261,-8.86196024656078,134.611557274234));
#74316=CARTESIAN_POINT('Ctrl Pts',(82.0536653328037,-8.93324475046548,134.607702057756));
#74317=CARTESIAN_POINT('Ctrl Pts',(82.0559825559742,-9.0045320413811,134.603846690552));
#74318=CARTESIAN_POINT('Ctrl Pts',(82.0545834363202,-9.07593406505799,134.599991323347));
#74319=CARTESIAN_POINT('Ctrl Pts',(82.0494823628482,-9.14703607337761,134.596135956143));
#74320=CARTESIAN_POINT('Ctrl Pts',(82.0443759499432,-9.21821250611137,134.59227655342));
#74321=CARTESIAN_POINT('Ctrl Pts',(82.0355598828126,-9.28908781107467,134.588417150697));
#74322=CARTESIAN_POINT('Ctrl Pts',(82.0231004992737,-9.35925190652057,134.584557747974));
#74323=CARTESIAN_POINT('Ctrl Pts',(82.0106340611339,-9.42945572942843,134.580696160027));
#74324=CARTESIAN_POINT('Ctrl Pts',(81.9945203098238,-9.49894706773126,134.57683457208));
#74325=CARTESIAN_POINT('Ctrl Pts',(81.9748762440994,-9.56732828502722,134.572972984133));
#74326=CARTESIAN_POINT('Ctrl Pts',(81.9551978103779,-9.63582913771395,134.5691046402));
#74327=CARTESIAN_POINT('Ctrl Pts',(81.9319768891766,-9.70321553231904,134.565236296267));
#74328=CARTESIAN_POINT('Ctrl Pts',(81.905379407727,-9.76910784361488,134.561367952333));
#74329=CARTESIAN_POINT('Ctrl Pts',(81.8895865886511,-9.80823280184666,134.559071041027));
#74330=CARTESIAN_POINT('Ctrl Pts',(81.8726042233082,-9.84683141646728,134.55677412972));
#74331=CARTESIAN_POINT('Ctrl Pts',(81.8544746051535,-9.88482851521686,134.554477218414));
#74332=CARTESIAN_POINT('Ctrl Pts',(81.82393577049,-9.94883356521285,134.550608135567));
#74333=CARTESIAN_POINT('Ctrl Pts',(81.7900196413615,-10.0113811016805,134.54673905272));
#74334=CARTESIAN_POINT('Ctrl Pts',(81.7528883050505,-10.0720914851435,134.542869969873));
#74335=CARTESIAN_POINT('Ctrl Pts',(81.7158122925787,-10.132711413163,134.539006651767));
#74336=CARTESIAN_POINT('Ctrl Pts',(81.6755308333298,-10.1914992105347,134.53514333366));
#74337=CARTESIAN_POINT('Ctrl Pts',(81.6322528843363,-10.2480977862635,134.531280015554));
#74338=CARTESIAN_POINT('Ctrl Pts',(81.5890257003603,-10.3046299718848,134.527421229118));
#74339=CARTESIAN_POINT('Ctrl Pts',(81.5428093020267,-10.35897765267,134.523562442682));
#74340=CARTESIAN_POINT('Ctrl Pts',(81.4938561601465,-10.4108122962649,134.519703656246));
#74341=CARTESIAN_POINT('Ctrl Pts',(81.4449338551562,-10.4626142878352,134.515847300563));
#74342=CARTESIAN_POINT('Ctrl Pts',(81.3932785596599,-10.5119060305783,134.51199094488));
#74343=CARTESIAN_POINT('Ctrl Pts',(81.3391823197829,-10.5583928506255,134.508134589197));
#74344=CARTESIAN_POINT('Ctrl Pts',(81.2851020604768,-10.6048659380007,134.504279372719));
#74345=CARTESIAN_POINT('Ctrl Pts',(81.2285826565668,-10.6485354312491,134.500424156242));
#74346=CARTESIAN_POINT('Ctrl Pts',(81.1699509540173,-10.6891454430255,134.496568939765));
#74347=CARTESIAN_POINT('Ctrl Pts',(81.1113169591439,-10.7297570425318,134.49271357256));
#74348=CARTESIAN_POINT('Ctrl Pts',(81.0505709022714,-10.767308648295,134.488858205356));
#74349=CARTESIAN_POINT('Ctrl Pts',(80.9880690313273,-10.8015873977778,134.485002838151));
#74350=CARTESIAN_POINT('Ctrl Pts',(80.9255017379676,-10.8359020277641,134.481143435428));
#74351=CARTESIAN_POINT('Ctrl Pts',(80.8611753885617,-10.8669367287521,134.477284032705));
#74352=CARTESIAN_POINT('Ctrl Pts',(80.7954704866765,-10.894524813067,134.473424629983));
#74353=CARTESIAN_POINT('Ctrl Pts',(80.7297283821598,-10.922128517972,134.469563042036));
#74354=CARTESIAN_POINT('Ctrl Pts',(80.6626066286419,-10.9462815568095,134.465701454089));
#74355=CARTESIAN_POINT('Ctrl Pts',(80.5945027514398,-10.9668665539458,134.461839866142));
#74356=CARTESIAN_POINT('Ctrl Pts',(80.5262797240634,-10.9874875652724,134.457971522208));
#74357=CARTESIAN_POINT('Ctrl Pts',(80.4570716142915,-11.0045279555587,134.454103178275));
#74358=CARTESIAN_POINT('Ctrl Pts',(80.3872873535,-11.0179212245078,134.450234834341));
#74359=CARTESIAN_POINT('Ctrl Pts',(80.3458514676581,-11.025873762185,134.447937923035));
#74360=CARTESIAN_POINT('Ctrl Pts',(80.3042125940091,-11.0325414442796,134.445641011729));
#74361=CARTESIAN_POINT('Ctrl Pts',(80.2624568263926,-11.0379190309676,134.443344100422));
#74362=CARTESIAN_POINT('Ctrl Pts',(80.1921204038274,-11.0469774253227,134.439475017575));
#74363=CARTESIAN_POINT('Ctrl Pts',(80.1211767085351,-11.0524079162304,134.435605934728));
#74364=CARTESIAN_POINT('Ctrl Pts',(80.0500326011497,-11.0541407695974,134.431736851881));
#74365=CARTESIAN_POINT('Ctrl Pts',(79.9789944949364,-11.0558710410993,134.427873533775));
#74366=CARTESIAN_POINT('Ctrl Pts',(79.9077570510336,-11.0539145991276,134.424010215668));
#74367=CARTESIAN_POINT('Ctrl Pts',(79.8367336075802,-11.0482533162688,134.420146897562));
#74368=CARTESIAN_POINT('Ctrl Pts',(79.7657934745984,-11.0425986740926,134.416288111126));
#74369=CARTESIAN_POINT('Ctrl Pts',(79.6950673253476,-11.0332478616258,134.41242932469));
#74370=CARTESIAN_POINT('Ctrl Pts',(79.6249681059247,-11.0202347984644,134.408570538255));
#74371=CARTESIAN_POINT('Ctrl Pts',(79.5549130438699,-11.0072299325785,134.404714182571));
#74372=CARTESIAN_POINT('Ctrl Pts',(79.4854846046223,-10.9905674814048,134.400857826888));
#74373=CARTESIAN_POINT('Ctrl Pts',(79.4170887535173,-10.9703329772462,134.397001471205));
#74374=CARTESIAN_POINT('Ctrl Pts',(79.3487131072313,-10.9501044505627,134.393146254728));
#74375=CARTESIAN_POINT('Ctrl Pts',(79.2813699090765,-10.9263061035359,134.38929103825));
#74376=CARTESIAN_POINT('Ctrl Pts',(79.2154514132945,-10.8990737420117,134.385435821773));
#74377=CARTESIAN_POINT('Ctrl Pts',(79.1495303402965,-10.8718403157837,134.381580454569));
#74378=CARTESIAN_POINT('Ctrl Pts',(79.0850345283964,-10.8411727960219,134.377725087364));
#74379=CARTESIAN_POINT('Ctrl Pts',(79.0223360323177,-10.8072550259428,134.373869720159));
#74380=CARTESIAN_POINT('Ctrl Pts',(78.9595719080107,-10.7733017532076,134.370010317437));
#74381=CARTESIAN_POINT('Ctrl Pts',(78.8986092831664,-10.7360916703621,134.366150914714));
#74382=CARTESIAN_POINT('Ctrl Pts',(78.83979457526,-10.6958540429247,134.362291511991));
#74383=CARTESIAN_POINT('Ctrl Pts',(78.7809465660041,-10.6555936326265,134.358429924044));
#74384=CARTESIAN_POINT('Ctrl Pts',(78.7242492809845,-10.6123025602003,134.354568336097));
#74385=CARTESIAN_POINT('Ctrl Pts',(78.6700169412625,-10.5662511375802,134.35070674815));
#74386=CARTESIAN_POINT('Ctrl Pts',(78.6156897201183,-10.5201191463456,134.346838404217));
#74387=CARTESIAN_POINT('Ctrl Pts',(78.5638364078437,-10.4712174964199,134.342970060283));
#74388=CARTESIAN_POINT('Ctrl Pts',(78.5147346698684,-10.4198536761262,134.33910171635));
#74389=CARTESIAN_POINT('Ctrl Pts',(78.4855794708835,-10.3893553177577,134.336804805043));
#74390=CARTESIAN_POINT('Ctrl Pts',(78.4573936249819,-10.3579895422356,134.334507893737));
#74391=CARTESIAN_POINT('Ctrl Pts',(78.4302282299173,-10.3258258378653,134.332210982431));
#74392=CARTESIAN_POINT('Ctrl Pts',(78.3847678948151,-10.2720010075869,134.328367181984));
#74393=CARTESIAN_POINT('Ctrl Pts',(78.3419831696141,-10.2157215771965,134.324523381537));
#74394=CARTESIAN_POINT('Ctrl Pts',(78.3021523840387,-10.1572860646679,134.32067958109));
#74395=CARTESIAN_POINT('Ctrl Pts',(78.2623775799222,-10.0989326822102,134.316841183036));
#74396=CARTESIAN_POINT('Ctrl Pts',(78.2255487573435,-10.0384296294759,134.313002784982));
#74397=CARTESIAN_POINT('Ctrl Pts',(78.1919047913618,-9.97610925566744,134.309164386928));
#74398=CARTESIAN_POINT('Ctrl Pts',(78.1582964950696,-9.91385495458019,134.305330058384));
#74399=CARTESIAN_POINT('Ctrl Pts',(78.1278665893411,-9.8497875856462,134.301495729841));
#74400=CARTESIAN_POINT('Ctrl Pts',(78.1008102845208,-9.78426780318845,134.297661401297));
#74401=CARTESIAN_POINT('Ctrl Pts',(78.0737690938031,-9.71878462117251,134.293829214673));
#74402=CARTESIAN_POINT('Ctrl Pts',(78.0500979587486,-9.65185108679847,134.289997028049));
#74403=CARTESIAN_POINT('Ctrl Pts',(78.029945075938,-9.58385028789842,134.286164841426));
#74404=CARTESIAN_POINT('Ctrl Pts',(78.0097994694122,-9.51587404097869,134.282334038429));
#74405=CARTESIAN_POINT('Ctrl Pts',(77.9931697296341,-9.4468317675747,134.278503235433));
#74406=CARTESIAN_POINT('Ctrl Pts',(77.9801543906818,-9.37712236345498,134.274672432436));
#74407=CARTESIAN_POINT('Ctrl Pts',(77.9671331495257,-9.30738134747254,134.270839892245));
#74408=CARTESIAN_POINT('Ctrl Pts',(77.9577296763164,-9.23697308077803,134.267007352054));
#74409=CARTESIAN_POINT('Ctrl Pts',(77.9519912481155,-9.1663060873945,134.263174811862));
#74410=CARTESIAN_POINT('Ctrl Pts',(77.9474494190888,-9.11037484794392,134.260141447729));
#74411=CARTESIAN_POINT('Ctrl Pts',(77.9452024908778,-9.05428179787052,134.257108083595));
#74412=CARTESIAN_POINT('Ctrl Pts',(77.9452507619577,-8.99823046207066,134.254074719462));
#74413=CARTESIAN_POINT('Origin',(80.,-9.,141.545925280538));
#74414=CARTESIAN_POINT('',(81.2520391107129,-7.37076839346111,135.406026966566));
#74415=CARTESIAN_POINT('',(81.2520391107129,-7.37076839346111,135.347982838348));
#74416=CARTESIAN_POINT('',(81.2520391107129,-7.37076839346111,141.545925280538));
#74417=CARTESIAN_POINT('',(77.9452501039006,-8.99934656332038,134.895925280576));
#74418=CARTESIAN_POINT('Ctrl Pts',(81.2520391107129,-7.37076839346111,135.347982838348));
#74419=CARTESIAN_POINT('Ctrl Pts',(81.3084942669191,-7.41415330159074,135.344113662368));
#74420=CARTESIAN_POINT('Ctrl Pts',(81.3626078704091,-7.46041147904279,135.340244486388));
#74421=CARTESIAN_POINT('Ctrl Pts',(81.4140911496352,-7.50924724282546,135.336375310408));
#74422=CARTESIAN_POINT('Ctrl Pts',(81.4220196881186,-7.51676805809484,135.335779448778));
#74423=CARTESIAN_POINT('Ctrl Pts',(81.4298859208187,-7.52434994013014,135.335183587148));
#74424=CARTESIAN_POINT('Ctrl Pts',(81.4376888783051,-7.53199173990814,135.334587725519));
#74425=CARTESIAN_POINT('Ctrl Pts',(81.4883554885787,-7.5816119117233,135.330718642672));
#74426=CARTESIAN_POINT('Ctrl Pts',(81.5365494452544,-7.63395539912312,135.326849559825));
#74427=CARTESIAN_POINT('Ctrl Pts',(81.5819640552087,-7.68874590924272,135.322980476978));
#74428=CARTESIAN_POINT('Ctrl Pts',(81.6273109996591,-7.74345478423476,135.319117158872));
#74429=CARTESIAN_POINT('Ctrl Pts',(81.6698865098525,-7.80060307389247,135.315253840765));
#74430=CARTESIAN_POINT('Ctrl Pts',(81.7094204040751,-7.85987744315283,135.311390522659));
#74431=CARTESIAN_POINT('Ctrl Pts',(81.748907925055,-7.91908228360087,135.307531736223));
#74432=CARTESIAN_POINT('Ctrl Pts',(81.7853606487122,-7.98040784776143,135.303672949787));
#74433=CARTESIAN_POINT('Ctrl Pts',(81.8185495042662,-8.04350887979387,135.299814163351));
#74434=CARTESIAN_POINT('Ctrl Pts',(81.8517174532748,-8.10657016280314,135.295957807668));
#74435=CARTESIAN_POINT('Ctrl Pts',(81.8816253876486,-8.17140426584292,135.292101451985));
#74436=CARTESIAN_POINT('Ctrl Pts',(81.9080890863941,-8.23763945479594,135.288245096302));
#74437=CARTESIAN_POINT('Ctrl Pts',(81.934544967498,-8.30385507721092,135.284389879824));
#74438=CARTESIAN_POINT('Ctrl Pts',(81.9575584527788,-8.37147051297918,135.280534663347));
#74439=CARTESIAN_POINT('Ctrl Pts',(81.9769932870615,-8.44009366371367,135.27667944687));
#74440=CARTESIAN_POINT('Ctrl Pts',(81.9964288811882,-8.50871949740812,135.272824079665));
#74441=CARTESIAN_POINT('Ctrl Pts',(82.0122854162816,-8.5783526562895,135.268968712461));
#74442=CARTESIAN_POINT('Ctrl Pts',(82.0244768648761,-8.64858715720481,135.265113345256));
#74443=CARTESIAN_POINT('Ctrl Pts',(82.0366810745929,-8.71889517449053,135.261253942533));
#74444=CARTESIAN_POINT('Ctrl Pts',(82.0452124563531,-8.78980531070922,135.25739453981));
#74445=CARTESIAN_POINT('Ctrl Pts',(82.0500365241631,-8.86090358704329,135.253535137088));
#74446=CARTESIAN_POINT('Ctrl Pts',(82.0548633233981,-8.93204211977993,135.249673549141));
#74447=CARTESIAN_POINT('Ctrl Pts',(82.0559786224031,-9.0033685187395,135.245811961194));
#74448=CARTESIAN_POINT('Ctrl Pts',(82.0534001022136,-9.07446866944749,135.241950373247));
#74449=CARTESIAN_POINT('Ctrl Pts',(82.0508170708106,-9.14569321241763,135.238082029313));
#74450=CARTESIAN_POINT('Ctrl Pts',(82.0445273605926,-9.21669023281058,135.23421368538));
#74451=CARTESIAN_POINT('Ctrl Pts',(82.0346004801354,-9.28705129982747,135.230345341446));
#74452=CARTESIAN_POINT('Ctrl Pts',(82.0287061841907,-9.32882967660675,135.22804843014));
#74453=CARTESIAN_POINT('Ctrl Pts',(82.0215305338992,-9.37038402446779,135.225751518834));
#74454=CARTESIAN_POINT('Ctrl Pts',(82.0130964518113,-9.41163119197237,135.223454607527));
#74455=CARTESIAN_POINT('Ctrl Pts',(81.9988894764508,-9.48111089187594,135.21958552468));
#74456=CARTESIAN_POINT('Ctrl Pts',(81.9810534349364,-9.54999030648095,135.215716441833));
#74457=CARTESIAN_POINT('Ctrl Pts',(81.9596541057285,-9.61786191693714,135.211847358986));
#74458=CARTESIAN_POINT('Ctrl Pts',(81.9382866604539,-9.68563240207868,135.20798404088));
#74459=CARTESIAN_POINT('Ctrl Pts',(81.9133666108288,-9.75239760413573,135.204120722774));
#74460=CARTESIAN_POINT('Ctrl Pts',(81.8850106587594,-9.81776058774157,135.200257404667));
#74461=CARTESIAN_POINT('Ctrl Pts',(81.8566879682109,-9.8830469005928,135.196398618231));
#74462=CARTESIAN_POINT('Ctrl Pts',(81.8249375731792,-9.94693381863534,135.192539831796));
#74463=CARTESIAN_POINT('Ctrl Pts',(81.7899252910331,-10.0090416319559,135.18868104536));
#74464=CARTESIAN_POINT('Ctrl Pts',(81.7549350640573,-10.0711103219083,135.184824689677));
#74465=CARTESIAN_POINT('Ctrl Pts',(81.7166872645516,-10.1314017084278,135.180968333993));
#74466=CARTESIAN_POINT('Ctrl Pts',(81.6753942808026,-10.1895594000949,135.17711197831));
#74467=CARTESIAN_POINT('Ctrl Pts',(81.6341134954144,-10.2476999113974,135.173256761833));
#74468=CARTESIAN_POINT('Ctrl Pts',(81.5897895927768,-10.3037075833172,135.169401545356));
#74469=CARTESIAN_POINT('Ctrl Pts',(81.542678085589,-10.357255276926,135.165546328878));
#74470=CARTESIAN_POINT('Ctrl Pts',(81.4955647364821,-10.4108050640894,135.161690961674));
#74471=CARTESIAN_POINT('Ctrl Pts',(81.4456638889813,-10.4618943187293,135.157835594469));
#74472=CARTESIAN_POINT('Ctrl Pts',(81.393269963358,-10.5102305690538,135.153980227265));
#74473=CARTESIAN_POINT('Ctrl Pts',(81.3408211955816,-10.5586174142517,135.150120824542));
#74474=CARTESIAN_POINT('Ctrl Pts',(81.2858744981699,-10.6042451726542,135.146261421819));
#74475=CARTESIAN_POINT('Ctrl Pts',(81.2287589638966,-10.6468603374736,135.142402019096));
#74476=CARTESIAN_POINT('Ctrl Pts',(81.1716110903591,-10.6894996313342,135.138540431149));
#74477=CARTESIAN_POINT('Ctrl Pts',(81.1122923395104,-10.7291226660256,135.134678843202));
#74478=CARTESIAN_POINT('Ctrl Pts',(81.0511602124642,-10.7655196884295,135.130817255255));
#74479=CARTESIAN_POINT('Ctrl Pts',(80.9899211325705,-10.8019803887287,135.126948911322));
#74480=CARTESIAN_POINT('Ctrl Pts',(80.9268627722774,-10.8352035817788,135.123080567389));
#74481=CARTESIAN_POINT('Ctrl Pts',(80.8623659678924,-10.8650261392058,135.119212223455));
#74482=CARTESIAN_POINT('Ctrl Pts',(80.8240696215051,-10.8827339155875,135.116915312149));
#74483=CARTESIAN_POINT('Ctrl Pts',(80.7852665078416,-10.8992436749217,135.114618400842));
#74484=CARTESIAN_POINT('Ctrl Pts',(80.7460389179157,-10.9145295754976,135.112321489536));
#74485=CARTESIAN_POINT('Ctrl Pts',(80.6799611399521,-10.9402782474436,135.108452406689));
#74486=CARTESIAN_POINT('Ctrl Pts',(80.6124193474613,-10.9626524379399,135.104583323842));
#74487=CARTESIAN_POINT('Ctrl Pts',(80.5437915874517,-10.9814863794426,135.100714240995));
#74488=CARTESIAN_POINT('Ctrl Pts',(80.4752660793819,-11.0002922593118,135.096850922889));
#74489=CARTESIAN_POINT('Ctrl Pts',(80.4056582801986,-11.0155682329928,135.092987604782));
#74490=CARTESIAN_POINT('Ctrl Pts',(80.3353649652505,-11.0271970556861,135.089124286676));
#74491=CARTESIAN_POINT('Ctrl Pts',(80.2651541043339,-11.0388122377749,135.08526550024));
#74492=CARTESIAN_POINT('Ctrl Pts',(80.1942598018297,-11.0467886877423,135.081406713804));
#74493=CARTESIAN_POINT('Ctrl Pts',(80.1230910006735,-11.0510597670602,135.077547927368));
#74494=CARTESIAN_POINT('Ctrl Pts',(80.0519670306435,-11.0553281559114,135.073691571685));
#74495=CARTESIAN_POINT('Ctrl Pts',(79.9805693887847,-11.0558957759222,135.069835216002));
#74496=CARTESIAN_POINT('Ctrl Pts',(79.9093126865443,-11.0527477618252,135.065978860319));
#74497=CARTESIAN_POINT('Ctrl Pts',(79.8380770342472,-11.049600677683,135.062123643841));
#74498=CARTESIAN_POINT('Ctrl Pts',(79.7669827239569,-11.0427401599728,135.058268427364));
#74499=CARTESIAN_POINT('Ctrl Pts',(79.6964431809677,-11.0322034396484,135.054413210887));
#74500=CARTESIAN_POINT('Ctrl Pts',(79.6259008800933,-11.0216663073698,135.050557843682));
#74501=CARTESIAN_POINT('Ctrl Pts',(79.5559138697092,-11.0074527610684,135.046702476478));
#74502=CARTESIAN_POINT('Ctrl Pts',(79.4868875528033,-10.9896515220088,135.042847109273));
#74503=CARTESIAN_POINT('Ctrl Pts',(79.4177889841661,-10.971831649906,135.03898770655));
#74504=CARTESIAN_POINT('Ctrl Pts',(79.3496535877346,-10.9504167101113,135.035128303828));
#74505=CARTESIAN_POINT('Ctrl Pts',(79.2828728363905,-10.9255456872568,135.031268901105));
#74506=CARTESIAN_POINT('Ctrl Pts',(79.2160542732604,-10.9006605822338,135.027407313158));
#74507=CARTESIAN_POINT('Ctrl Pts',(79.150592328098,-10.8723156917601,135.023545725211));
#74508=CARTESIAN_POINT('Ctrl Pts',(79.0868571230049,-10.840697598383,135.019684137264));
#74509=CARTESIAN_POINT('Ctrl Pts',(79.0230104108859,-10.8090241880183,135.015815793331));
#74510=CARTESIAN_POINT('Ctrl Pts',(78.9608968938107,-10.7740663797939,135.011947449397));
#74511=CARTESIAN_POINT('Ctrl Pts',(78.9008601794405,-10.7360556492694,135.008079105464));
#74512=CARTESIAN_POINT('Ctrl Pts',(78.8652121061538,-10.7134859713377,135.005782194157));
#74513=CARTESIAN_POINT('Ctrl Pts',(78.8302956660188,-10.6898407605847,135.003485282851));
#74514=CARTESIAN_POINT('Ctrl Pts',(78.7961772025379,-10.6651751363777,135.001188371544));
#74515=CARTESIAN_POINT('Ctrl Pts',(78.7391631807264,-10.6239573823215,134.99735009344));
#74516=CARTESIAN_POINT('Ctrl Pts',(78.6841480871177,-10.5797208791893,134.993511815336));
#74517=CARTESIAN_POINT('Ctrl Pts',(78.6314732100564,-10.5326878311342,134.989673537232));
#74518=CARTESIAN_POINT('Ctrl Pts',(78.5778665128153,-10.4848227670261,134.985767359871));
#74519=CARTESIAN_POINT('Ctrl Pts',(78.5266841028897,-10.4340614803725,134.981861182511));
#74520=CARTESIAN_POINT('Ctrl Pts',(78.4782549032979,-10.3806844038965,134.97795500515));
#74521=CARTESIAN_POINT('Ctrl Pts',(78.4307943615624,-10.3283749503611,134.974126957294));
#74522=CARTESIAN_POINT('Ctrl Pts',(78.3859782647131,-10.2735537602863,134.970298909439));
#74523=CARTESIAN_POINT('Ctrl Pts',(78.3440811368767,-10.2165238514935,134.966470861583));
#74524=CARTESIAN_POINT('Ctrl Pts',(78.3022091390412,-10.159528149381,134.9626451098));
#74525=CARTESIAN_POINT('Ctrl Pts',(78.263252930074,-10.1003267534489,134.958819358016));
#74526=CARTESIAN_POINT('Ctrl Pts',(78.2274466135477,-10.0392555290575,134.954993606233));
#74527=CARTESIAN_POINT('Ctrl Pts',(78.1916493141246,-9.97819968422998,134.951168817889));
#74528=CARTESIAN_POINT('Ctrl Pts',(78.1590005823022,-9.9152753720847,134.947344029545));
#74529=CARTESIAN_POINT('Ctrl Pts',(78.1296900536078,-9.85084561873846,134.9435192412));
#74530=CARTESIAN_POINT('Ctrl Pts',(78.0992961245193,-9.7840343587023,134.939553077815));
#74531=CARTESIAN_POINT('Ctrl Pts',(78.0724922819995,-9.71560468558299,134.93558691443));
#74532=CARTESIAN_POINT('Ctrl Pts',(78.0494357340079,-9.64598498955847,134.931620751044));
#74533=CARTESIAN_POINT('Ctrl Pts',(78.0271754962614,-9.57876976783858,134.927791568118));
#74534=CARTESIAN_POINT('Ctrl Pts',(78.0084080033322,-9.5104458945301,134.923962385192));
#74535=CARTESIAN_POINT('Ctrl Pts',(77.9932234204898,-9.441412870711,134.920133202266));
#74536=CARTESIAN_POINT('Ctrl Pts',(77.9780288922086,-9.37233463236631,134.916301511343));
#74537=CARTESIAN_POINT('Ctrl Pts',(77.9664220204801,-9.30254680699824,134.912469820419));
#74538=CARTESIAN_POINT('Ctrl Pts',(77.9584413426124,-9.23245604088901,134.908638129495));
#74539=CARTESIAN_POINT('Ctrl Pts',(77.9504482845427,-9.16225654493767,134.904800494576));
#74540=CARTESIAN_POINT('Ctrl Pts',(77.9460926623442,-9.09175366297,134.900962859657));
#74541=CARTESIAN_POINT('Ctrl Pts',(77.9453609729324,-9.02135488119547,134.897125224738));
#74542=CARTESIAN_POINT('Ctrl Pts',(77.9452847118622,-9.01401749684174,134.896725243351));
#74543=CARTESIAN_POINT('Ctrl Pts',(77.9452477713803,-9.00668123844234,134.896325261963));
#74544=CARTESIAN_POINT('Ctrl Pts',(77.9452501039006,-8.99934656332038,134.895925280576));
#74545=CARTESIAN_POINT('Ctrl Pts',(77.9452501039008,-8.99934656262625,134.895925280538));
#74546=CARTESIAN_POINT('Ctrl Pts',(77.9452615144079,-8.96346594230785,134.893968604876));
#74547=CARTESIAN_POINT('Ctrl Pts',(77.9462127014812,-8.92760146641289,134.892011929214));
#74548=CARTESIAN_POINT('Ctrl Pts',(77.948101493401,-8.89178687179018,134.890055253553));
#74549=CARTESIAN_POINT('Ctrl Pts',(77.9518363445886,-8.82096796376281,134.886186170706));
#74550=CARTESIAN_POINT('Ctrl Pts',(77.9592491642671,-8.75020393167272,134.882317087859));
#74551=CARTESIAN_POINT('Ctrl Pts',(77.9703354015928,-8.67990754386781,134.878448005012));
#74552=CARTESIAN_POINT('Ctrl Pts',(77.9814051209779,-8.6097158941748,134.874584686905));
#74553=CARTESIAN_POINT('Ctrl Pts',(77.996137318782,-8.53999098164773,134.870721368799));
#74554=CARTESIAN_POINT('Ctrl Pts',(78.0144755138151,-8.47114266833102,134.866858050692));
#74555=CARTESIAN_POINT('Ctrl Pts',(78.0327921981524,-8.4023751140594,134.862999264257));
#74556=CARTESIAN_POINT('Ctrl Pts',(78.0547063534121,-8.33448258368312,134.859140477821));
#74557=CARTESIAN_POINT('Ctrl Pts',(78.080110369965,-8.26786519616665,134.855281691385));
#74558=CARTESIAN_POINT('Ctrl Pts',(78.1054983838503,-8.20128977271945,134.851425335702));
#74559=CARTESIAN_POINT('Ctrl Pts',(78.1343717248418,-8.13598835133011,134.847568980018));
#74560=CARTESIAN_POINT('Ctrl Pts',(78.1665732666696,-8.07234490460657,134.843712624335));
#74561=CARTESIAN_POINT('Ctrl Pts',(78.1987652958395,-8.00872025879446,134.839857407858));
#74562=CARTESIAN_POINT('Ctrl Pts',(78.2342833547564,-7.94675304851614,134.836002191381));
#74563=CARTESIAN_POINT('Ctrl Pts',(78.2729233278852,-7.88680472012461,134.832146974903));
#74564=CARTESIAN_POINT('Ctrl Pts',(78.3115648117214,-7.82685404793276,134.828291607699));
#74565=CARTESIAN_POINT('Ctrl Pts',(78.3533281870658,-7.76892282145853,134.824436240494));
#74566=CARTESIAN_POINT('Ctrl Pts',(78.3979657153935,-7.71334398013873,134.82058087329));
#74567=CARTESIAN_POINT('Ctrl Pts',(78.4426499670412,-7.65770696292771,134.816721470567));
#74568=CARTESIAN_POINT('Ctrl Pts',(78.4902140724076,-7.60442762571345,134.812862067844));
#74569=CARTESIAN_POINT('Ctrl Pts',(78.5403702200733,-7.55380552205067,134.809002665121));
#74570=CARTESIAN_POINT('Ctrl Pts',(78.5905547665438,-7.50315475575514,134.805141077174));
#74571=CARTESIAN_POINT('Ctrl Pts',(78.6433339173323,-7.45516454506113,134.801279489227));
#74572=CARTESIAN_POINT('Ctrl Pts',(78.6983852719671,-7.41009539208548,134.797417901281));
#74573=CARTESIAN_POINT('Ctrl Pts',(78.7535329409201,-7.36494738901126,134.793549557347));
#74574=CARTESIAN_POINT('Ctrl Pts',(78.8109603589956,-7.3227309347253,134.789681213414));
#74575=CARTESIAN_POINT('Ctrl Pts',(78.8703151273709,-7.28366388750543,134.78581286948));
#74576=CARTESIAN_POINT('Ctrl Pts',(78.9055582807505,-7.26046699911813,134.783515958174));
#74577=CARTESIAN_POINT('Ctrl Pts',(78.9414804390346,-7.23837961974738,134.781219046867));
#74578=CARTESIAN_POINT('Ctrl Pts',(78.9780040594418,-7.2174395213675,134.778922135561));
#74579=CARTESIAN_POINT('Ctrl Pts',(79.0395270763861,-7.18216651137894,134.775053052714));
#74580=CARTESIAN_POINT('Ctrl Pts',(79.1029988479682,-7.15001324800689,134.771183969867));
#74581=CARTESIAN_POINT('Ctrl Pts',(79.1680701255574,-7.1211997853657,134.76731488702));
#74582=CARTESIAN_POINT('Ctrl Pts',(79.2330444501883,-7.09242925334685,134.763451568914));
#74583=CARTESIAN_POINT('Ctrl Pts',(79.299613109705,-7.06698883964769,134.759588250807));
#74584=CARTESIAN_POINT('Ctrl Pts',(79.3674011311609,-7.04505339365916,134.755724932701));
#74585=CARTESIAN_POINT('Ctrl Pts',(79.4351096372938,-7.02314367794034,134.751866146265));
#74586=CARTESIAN_POINT('Ctrl Pts',(79.5040342043391,-7.00473091228001,134.74800735983));
#74587=CARTESIAN_POINT('Ctrl Pts',(79.5737803137747,-6.98994170692142,134.744148573394));
#74588=CARTESIAN_POINT('Ctrl Pts',(79.6434824882756,-6.97516181767775,134.74029221771));
#74589=CARTESIAN_POINT('Ctrl Pts',(79.7140047043385,-6.96400106066667,134.736435862027));
#74590=CARTESIAN_POINT('Ctrl Pts',(79.7849391516779,-6.95653568809755,134.732579506344));
#74591=CARTESIAN_POINT('Ctrl Pts',(79.8558526442712,-6.94907252087423,134.728724289867));
#74592=CARTESIAN_POINT('Ctrl Pts',(79.9271776435276,-6.94530262167439,134.72486907339));
#74593=CARTESIAN_POINT('Ctrl Pts',(79.9984997781608,-6.94525054767389,134.721013856912));
#74594=CARTESIAN_POINT('Ctrl Pts',(80.0698247012761,-6.94519847163746,134.717158489708));
#74595=CARTESIAN_POINT('Ctrl Pts',(80.1411462737612,-6.94886450753711,134.713303122503));
#74596=CARTESIAN_POINT('Ctrl Pts',(80.2120504136819,-6.95622110184166,134.709447755299));
#74597=CARTESIAN_POINT('Ctrl Pts',(80.2830287709025,-6.96358539649439,134.705588352576));
#74598=CARTESIAN_POINT('Ctrl Pts',(80.3535883391531,-6.97464791074666,134.701728949853));
#74599=CARTESIAN_POINT('Ctrl Pts',(80.4233213503342,-6.98932931665794,134.69786954713));
#74600=CARTESIAN_POINT('Ctrl Pts',(80.493093844894,-7.00401903529657,134.694007959183));
#74601=CARTESIAN_POINT('Ctrl Pts',(80.5620383810086,-7.02233159984533,134.690146371236));
#74602=CARTESIAN_POINT('Ctrl Pts',(80.6297612385618,-7.04413744222527,134.686284783289));
#74603=CARTESIAN_POINT('Ctrl Pts',(80.6976025796817,-7.06598143470804,134.682416439356));
#74604=CARTESIAN_POINT('Ctrl Pts',(80.7642175207548,-7.09133073420804,134.678548095423));
#74605=CARTESIAN_POINT('Ctrl Pts',(80.8292318976491,-7.12000744086013,134.674679751489));
#74606=CARTESIAN_POINT('Ctrl Pts',(80.8678355636978,-7.13703484402624,134.672382840183));
#74607=CARTESIAN_POINT('Ctrl Pts',(80.9058753734192,-7.15523447752825,134.670085928876));
#74608=CARTESIAN_POINT('Ctrl Pts',(80.9432775356496,-7.17456168188603,134.66778901757));
#74609=CARTESIAN_POINT('Ctrl Pts',(81.00626540739,-7.20711005333276,134.663920857385));
#74610=CARTESIAN_POINT('Ctrl Pts',(81.0676899896171,-7.24298613757157,134.6600526972));
#74611=CARTESIAN_POINT('Ctrl Pts',(81.1271772473667,-7.28201600254284,134.656184537015));
#74612=CARTESIAN_POINT('Ctrl Pts',(81.1698375608372,-7.31000563153863,134.653410549236));
#74613=CARTESIAN_POINT('Ctrl Pts',(81.2115018543262,-7.339616143386,134.650636561456));
#74614=CARTESIAN_POINT('Ctrl Pts',(81.2520391107129,-7.37076839346111,134.647862573676));
#74615=CARTESIAN_POINT('',(77.9452502540764,-9.00102182517148,134.954074719507));
#74616=CARTESIAN_POINT('Ctrl Pts',(77.9452502540759,-9.00102182433968,134.954074719462));
#74617=CARTESIAN_POINT('Ctrl Pts',(77.9452142125462,-8.92854721091016,134.950163294815));
#74618=CARTESIAN_POINT('Ctrl Pts',(77.9490169737962,-8.8560783559993,134.946251870168));
#74619=CARTESIAN_POINT('Ctrl Pts',(77.9566303437358,-8.78404164670334,134.942340445521));
#74620=CARTESIAN_POINT('Ctrl Pts',(77.9642467236715,-8.71197645721814,134.938427474467));
#74621=CARTESIAN_POINT('Ctrl Pts',(77.9756766562268,-8.6403442159496,134.934514503412));
#74622=CARTESIAN_POINT('Ctrl Pts',(77.9908402897156,-8.56956438220089,134.930601532358));
#74623=CARTESIAN_POINT('Ctrl Pts',(78.00602657836,-8.49867880017356,134.926682715147));
#74624=CARTESIAN_POINT('Ctrl Pts',(78.0249576060862,-8.42864862450627,134.922763897937));
#74625=CARTESIAN_POINT('Ctrl Pts',(78.047502858124,-8.35988089118828,134.918845080726));
#74626=CARTESIAN_POINT('Ctrl Pts',(78.0700662114443,-8.291057945173,134.914923117149));
#74627=CARTESIAN_POINT('Ctrl Pts',(78.0962493989041,-8.22349989413301,134.911001153572));
#74628=CARTESIAN_POINT('Ctrl Pts',(78.1258736804293,-8.15759386232501,134.907079189996));
#74629=CARTESIAN_POINT('Ctrl Pts',(78.1555587274254,-8.09155264374307,134.903149181668));
#74630=CARTESIAN_POINT('Ctrl Pts',(78.1886987529193,-8.02717062698403,134.89921917334));
#74631=CARTESIAN_POINT('Ctrl Pts',(78.2250691444905,-7.9648101523583,134.895289165013));
#74632=CARTESIAN_POINT('Ctrl Pts',(78.2479358387258,-7.92560304338773,134.892818300805));
#74633=CARTESIAN_POINT('Ctrl Pts',(78.2720785667058,-7.88719445512439,134.890347436597));
#74634=CARTESIAN_POINT('Ctrl Pts',(78.2974332054889,-7.84966792936633,134.887876572388));
#74635=CARTESIAN_POINT('Ctrl Pts',(78.3371355888423,-7.79090580207634,134.884007489541));
#74636=CARTESIAN_POINT('Ctrl Pts',(78.3799614657705,-7.73408641807268,134.880138406695));
#74637=CARTESIAN_POINT('Ctrl Pts',(78.4256941852279,-7.67956114716557,134.876269323848));
#74638=CARTESIAN_POINT('Ctrl Pts',(78.4713587652141,-7.62511711619277,134.872406005741));
#74639=CARTESIAN_POINT('Ctrl Pts',(78.5199212810797,-7.57296078261917,134.868542687635));
#74640=CARTESIAN_POINT('Ctrl Pts',(78.571122078857,-7.52341425952635,134.864679369528));
#74641=CARTESIAN_POINT('Ctrl Pts',(78.6222628181182,-7.47392585448606,134.860820583093));
#74642=CARTESIAN_POINT('Ctrl Pts',(78.6760353447623,-7.42704151531016,134.856961796657));
#74643=CARTESIAN_POINT('Ctrl Pts',(78.7321412129293,-7.3830486530054,134.853103010221));
#74644=CARTESIAN_POINT('Ctrl Pts',(78.7882117385135,-7.33908350297803,134.849246654538));
#74645=CARTESIAN_POINT('Ctrl Pts',(78.8466123081177,-7.29800651519423,134.845390298854));
#74646=CARTESIAN_POINT('Ctrl Pts',(78.9070103656066,-7.26006574215906,134.841533943171));
#74647=CARTESIAN_POINT('Ctrl Pts',(78.9673905809044,-7.22213617720819,134.837678726694));
#74648=CARTESIAN_POINT('Ctrl Pts',(79.0297667014881,-7.18734124597068,134.833823510217));
#74649=CARTESIAN_POINT('Ctrl Pts',(79.0937775151035,-7.15588547796834,134.82996829374));
#74650=CARTESIAN_POINT('Ctrl Pts',(79.1577908313503,-7.12442848013955,134.826112926535));
#74651=CARTESIAN_POINT('Ctrl Pts',(79.2234385305605,-7.09631111701001,134.82225755933));
#74652=CARTESIAN_POINT('Ctrl Pts',(79.2903367116233,-7.07169100514715,134.818402192126));
#74653=CARTESIAN_POINT('Ctrl Pts',(79.3573049168394,-7.04704512274075,134.814542789403));
#74654=CARTESIAN_POINT('Ctrl Pts',(79.4255257599688,-7.02590396723754,134.81068338668));
#74655=CARTESIAN_POINT('Ctrl Pts',(79.4945982079856,-7.0083758911058,134.806823983957));
#74656=CARTESIAN_POINT('Ctrl Pts',(79.563709765365,-6.99083789043967,134.80296239601));
#74657=CARTESIAN_POINT('Ctrl Pts',(79.6336734108451,-6.97691713645357,134.799100808063));
#74658=CARTESIAN_POINT('Ctrl Pts',(79.7040785989494,-6.96667068901757,134.795239220117));
#74659=CARTESIAN_POINT('Ctrl Pts',(79.774606963454,-6.95640631505451,134.791370876183));
#74660=CARTESIAN_POINT('Ctrl Pts',(79.8455779290268,-6.94982912682779,134.78750253225));
#74661=CARTESIAN_POINT('Ctrl Pts',(79.9165772232856,-6.94694417932068,134.783634188316));
#74662=CARTESIAN_POINT('Ctrl Pts',(79.9587345610346,-6.94523118051251,134.78133727701));
#74663=CARTESIAN_POINT('Ctrl Pts',(80.0009018924247,-6.94481893458073,134.779040365703));
#74664=CARTESIAN_POINT('Ctrl Pts',(80.0429932997395,-6.94569984211715,134.776743454397));
#74665=CARTESIAN_POINT('Ctrl Pts',(80.1138837197782,-6.94718346809346,134.772874992454));
#74666=CARTESIAN_POINT('Ctrl Pts',(80.1848360783876,-6.95234376833629,134.769006530512));
#74667=CARTESIAN_POINT('Ctrl Pts',(80.2554378698441,-6.96118930325802,134.765138068569));
#74668=CARTESIAN_POINT('Ctrl Pts',(80.325940790493,-6.97002245088528,134.761275024024));
#74669=CARTESIAN_POINT('Ctrl Pts',(80.3960936402553,-6.98253053403551,134.757411979479));
#74670=CARTESIAN_POINT('Ctrl Pts',(80.4654850568473,-6.99867013604657,134.753548934934));
#74671=CARTESIAN_POINT('Ctrl Pts',(80.536481586217,-7.01518306782501,134.749596533196));
#74672=CARTESIAN_POINT('Ctrl Pts',(80.6066804960061,-7.03549762531567,134.745644131458));
#74673=CARTESIAN_POINT('Ctrl Pts',(80.675648520014,-7.05951123685221,134.741691729721));
#74674=CARTESIAN_POINT('Ctrl Pts',(80.7429382618448,-7.08294049619321,134.737835506546));
#74675=CARTESIAN_POINT('Ctrl Pts',(80.8090558650348,-7.10989063762988,134.73397928337));
#74676=CARTESIAN_POINT('Ctrl Pts',(80.8736130183895,-7.14021564244656,134.730123060195));
#74677=CARTESIAN_POINT('Ctrl Pts',(80.9405853642445,-7.17167515707978,134.726122569176));
#74678=CARTESIAN_POINT('Ctrl Pts',(81.0058776664664,-7.20676688624266,134.722122078158));
#74679=CARTESIAN_POINT('Ctrl Pts',(81.0690801890059,-7.24527349368194,134.718121587139));
#74680=CARTESIAN_POINT('Ctrl Pts',(81.1322827115453,-7.28378010112123,134.71412109612));
#74681=CARTESIAN_POINT('Ctrl Pts',(81.1933949592345,-7.32570127656327,134.710120605101));
#74682=CARTESIAN_POINT('Ctrl Pts',(81.2520391107129,-7.37076839346111,134.706120114083));
#74683=CARTESIAN_POINT('Ctrl Pts',(81.2520391107129,-7.37076839346111,135.406026966566));
#74684=CARTESIAN_POINT('Ctrl Pts',(81.3085478694585,-7.41419449430732,135.402170997473));
#74685=CARTESIAN_POINT('Ctrl Pts',(81.3628300813749,-7.46059120030964,135.39831502838));
#74686=CARTESIAN_POINT('Ctrl Pts',(81.4145642490411,-7.50969615586794,135.394459059287));
#74687=CARTESIAN_POINT('Ctrl Pts',(81.4662872342288,-7.55879049725901,135.390603923672));
#74688=CARTESIAN_POINT('Ctrl Pts',(81.515462916766,-7.61059159127112,135.386748788057));
#74689=CARTESIAN_POINT('Ctrl Pts',(81.56180511097,-7.66479875754703,135.382893652442));
#74690=CARTESIAN_POINT('Ctrl Pts',(81.6081527898687,-7.71901233935326,135.379038060564));
#74691=CARTESIAN_POINT('Ctrl Pts',(81.6516660009943,-7.77563218785869,135.375182468686));
#74692=CARTESIAN_POINT('Ctrl Pts',(81.6920985972817,-7.83432427340303,135.371326876807));
#74693=CARTESIAN_POINT('Ctrl Pts',(81.7325754841388,-7.89308065127935,135.367467061447));
#74694=CARTESIAN_POINT('Ctrl Pts',(81.7699647470556,-7.95391339462022,135.363607246086));
#74695=CARTESIAN_POINT('Ctrl Pts',(81.8040639134633,-8.016459986254,135.359747430725));
#74696=CARTESIAN_POINT('Ctrl Pts',(81.8381848105413,-8.07904643749463,135.355885155587));
#74697=CARTESIAN_POINT('Ctrl Pts',(81.8690112291951,-8.14334847244807,135.352022880448));
#74698=CARTESIAN_POINT('Ctrl Pts',(81.8963881558205,-8.20898196925509,135.34816060531));
#74699=CARTESIAN_POINT('Ctrl Pts',(81.9238110295093,-8.27472561964063,135.344291848063));
#74700=CARTESIAN_POINT('Ctrl Pts',(81.9477726968834,-8.34180473375835,135.340423090816));
#74701=CARTESIAN_POINT('Ctrl Pts',(81.9681677230269,-8.4098192001299,135.336554333569));
#74702=CARTESIAN_POINT('Ctrl Pts',(81.9754519986149,-8.43411120708983,135.335172570498));
#74703=CARTESIAN_POINT('Ctrl Pts',(81.9822817781762,-8.45852243441226,135.333790807426));
#74704=CARTESIAN_POINT('Ctrl Pts',(81.9886538483545,-8.48303439773548,135.332409044355));
#74705=CARTESIAN_POINT('Ctrl Pts',(82.0064963192771,-8.55167048939985,135.328539961508));
#74706=CARTESIAN_POINT('Ctrl Pts',(82.0208162221759,-8.6213658157439,135.324670878661));
#74707=CARTESIAN_POINT('Ctrl Pts',(82.031493149485,-8.69172553447344,135.320801795814));
#74708=CARTESIAN_POINT('Ctrl Pts',(82.0421541687048,-8.76198042073116,135.316938477708));
#74709=CARTESIAN_POINT('Ctrl Pts',(82.0491829141827,-8.83289725805528,135.313075159601));
#74710=CARTESIAN_POINT('Ctrl Pts',(82.0525093587264,-8.90406828032084,135.309211841495));
#74711=CARTESIAN_POINT('Ctrl Pts',(82.0558319013519,-8.97515581900462,135.305353055059));
#74712=CARTESIAN_POINT('Ctrl Pts',(82.0554607467397,-9.04649646748708,135.301494268623));
#74713=CARTESIAN_POINT('Ctrl Pts',(82.0513775498521,-9.11767629524553,135.297635482187));
#74714=CARTESIAN_POINT('Ctrl Pts',(82.0472969250792,-9.18881128493185,135.293779126504));
#74715=CARTESIAN_POINT('Ctrl Pts',(82.0395089249653,-9.25978517104288,135.289922770821));
#74716=CARTESIAN_POINT('Ctrl Pts',(82.0280472853772,-9.33018444962502,135.286066415137));
#74717=CARTESIAN_POINT('Ctrl Pts',(82.0165890316722,-9.40056293155539,135.28221119866));
#74718=CARTESIAN_POINT('Ctrl Pts',(82.001459370995,-9.47036666373856,135.278355982183));
#74719=CARTESIAN_POINT('Ctrl Pts',(81.982743639037,-9.53918941417479,135.274500765706));
#74720=CARTESIAN_POINT('Ctrl Pts',(81.9640271753499,-9.60801485537473,135.270645398501));
#74721=CARTESIAN_POINT('Ctrl Pts',(81.9417244916246,-9.6758587705007,135.266790031297));
#74722=CARTESIAN_POINT('Ctrl Pts',(81.915971121969,-9.74232891785301,135.262934664092));
#74723=CARTESIAN_POINT('Ctrl Pts',(81.890190795558,-9.80886864132405,135.259075261369));
#74724=CARTESIAN_POINT('Ctrl Pts',(81.8609527488611,-9.87403127262947,135.255215858646));
#74725=CARTESIAN_POINT('Ctrl Pts',(81.8284408048189,-9.93744428409014,135.251356455924));
#74726=CARTESIAN_POINT('Ctrl Pts',(81.7959104522586,-10.000893200496,135.247494867977));
#74727=CARTESIAN_POINT('Ctrl Pts',(81.7601027561565,-10.0625901046345,135.24363328003));
#74728=CARTESIAN_POINT('Ctrl Pts',(81.7212463131005,-10.1221892407869,135.239771692083));
#74729=CARTESIAN_POINT('Ctrl Pts',(81.6823218893047,-10.1818926477641,135.235903348149));
#74730=CARTESIAN_POINT('Ctrl Pts',(81.6403383555224,-10.2394905665673,135.232035004216));
#74731=CARTESIAN_POINT('Ctrl Pts',(81.5955657916373,-10.2946688252433,135.228166660282));
#74732=CARTESIAN_POINT('Ctrl Pts',(81.5689811316447,-10.3274320873529,135.225869748976));
#74733=CARTESIAN_POINT('Ctrl Pts',(81.5414139051124,-10.3593429288424,135.223572837669));
#74734=CARTESIAN_POINT('Ctrl Pts',(81.5129266135238,-10.3903419092409,135.221275926363));
#74735=CARTESIAN_POINT('Ctrl Pts',(81.4649405676835,-10.4425588246247,135.217406843516));
#74736=CARTESIAN_POINT('Ctrl Pts',(81.4141540521792,-10.4923908221379,135.213537760669));
#74737=CARTESIAN_POINT('Ctrl Pts',(81.3608334803885,-10.5395225887118,135.209668677822));
#74738=CARTESIAN_POINT('Ctrl Pts',(81.3075923535905,-10.5865841313039,135.205805359716));
#74739=CARTESIAN_POINT('Ctrl Pts',(81.2518250260106,-10.6309531098095,135.201942041609));
#74740=CARTESIAN_POINT('Ctrl Pts',(81.1938360940875,-10.6723495277465,135.198078723503));
#74741=CARTESIAN_POINT('Ctrl Pts',(81.1359151831591,-10.7136973877013,135.194219937067));
#74742=CARTESIAN_POINT('Ctrl Pts',(81.075778237626,-10.7520793322013,135.190361150631));
#74743=CARTESIAN_POINT('Ctrl Pts',(81.0137630642248,-10.7872554412041,135.186502364195));
#74744=CARTESIAN_POINT('Ctrl Pts',(80.9517869558356,-10.8224093918375,135.182646008512));
#74745=CARTESIAN_POINT('Ctrl Pts',(80.8879353884644,-10.8543612744068,135.178789652829));
#74746=CARTESIAN_POINT('Ctrl Pts',(80.8225740581306,-10.8829151551227,135.174933297146));
#74747=CARTESIAN_POINT('Ctrl Pts',(80.7572320361883,-10.9114606007363,135.171078080668));
#74748=CARTESIAN_POINT('Ctrl Pts',(80.6903815816309,-10.9366098429589,135.167222864191));
#74749=CARTESIAN_POINT('Ctrl Pts',(80.6224102677982,-10.9582142428854,135.163367647714));
#74750=CARTESIAN_POINT('Ctrl Pts',(80.5544362964903,-10.9798194874795,135.159512280509));
#74751=CARTESIAN_POINT('Ctrl Pts',(80.4853418425312,-10.9978794695692,135.155656913305));
#74752=CARTESIAN_POINT('Ctrl Pts',(80.4155299521801,-11.0122953116631,135.1518015461));
#74753=CARTESIAN_POINT('Ctrl Pts',(80.3456449878167,-11.0267262432126,135.147942143377));
#74754=CARTESIAN_POINT('Ctrl Pts',(80.2750415646969,-11.0375053218868,135.144082740654));
#74755=CARTESIAN_POINT('Ctrl Pts',(80.2041323575917,-11.0445849317365,135.140223337932));
#74756=CARTESIAN_POINT('Ctrl Pts',(80.1331830011365,-11.051668550117,135.136361749985));
#74757=CARTESIAN_POINT('Ctrl Pts',(80.0619280015,-11.0550485068064,135.132500162038));
#74758=CARTESIAN_POINT('Ctrl Pts',(79.990781825789,-11.0547293222622,135.128638574091));
#74759=CARTESIAN_POINT('Ctrl Pts',(79.9195111772936,-11.0544095792932,135.124770230157));
#74760=CARTESIAN_POINT('Ctrl Pts',(79.848350218004,-11.0503778014863,135.120901886224));
#74761=CARTESIAN_POINT('Ctrl Pts',(79.7777093801838,-11.0426904912007,135.11703354229));
#74762=CARTESIAN_POINT('Ctrl Pts',(79.7357648835527,-11.0381259875746,135.114736630984));
#74763=CARTESIAN_POINT('Ctrl Pts',(79.6940036089263,-11.0322736611288,135.112439719677));
#74764=CARTESIAN_POINT('Ctrl Pts',(79.6525093937848,-11.0251537820848,135.110142808371));
#74765=CARTESIAN_POINT('Ctrl Pts',(79.5826135490471,-11.013160544991,135.106273725524));
#74766=CARTESIAN_POINT('Ctrl Pts',(79.513202433067,-10.997521008181,135.102404642677));
#74767=CARTESIAN_POINT('Ctrl Pts',(79.4446854481566,-10.9782879747425,135.09853555983));
#74768=CARTESIAN_POINT('Ctrl Pts',(79.3762705501363,-10.9590835975646,135.094672241724));
#74769=CARTESIAN_POINT('Ctrl Pts',(79.3087476026802,-10.9362964817773,135.090808923617));
#74770=CARTESIAN_POINT('Ctrl Pts',(79.2425170472081,-10.9100306643428,135.086945605511));
#74771=CARTESIAN_POINT('Ctrl Pts',(79.1763641801522,-10.883795656702,135.083086819075));
#74772=CARTESIAN_POINT('Ctrl Pts',(79.1115011432172,-10.8540902309144,135.079228032639));
#74773=CARTESIAN_POINT('Ctrl Pts',(79.0483127208927,-10.8210680616839,135.075369246204));
#74774=CARTESIAN_POINT('Ctrl Pts',(78.9851641026408,-10.7880666939987,135.07151289052));
#74775=CARTESIAN_POINT('Ctrl Pts',(78.9236884356437,-10.7517529524849,135.067656534837));
#74776=CARTESIAN_POINT('Ctrl Pts',(78.8642486766826,-10.7123277998335,135.063800179154));
#74777=CARTESIAN_POINT('Ctrl Pts',(78.8048264768216,-10.6729142937671,135.059944962676));
#74778=CARTESIAN_POINT('Ctrl Pts',(78.7474393956033,-10.6303914696825,135.056089746199));
#74779=CARTESIAN_POINT('Ctrl Pts',(78.6924225216405,-10.5850043219458,135.052234529722));
#74780=CARTESIAN_POINT('Ctrl Pts',(78.6374034966826,-10.5396153997074,135.048379162517));
#74781=CARTESIAN_POINT('Ctrl Pts',(78.5847552362845,-10.4913622423186,135.044523795313));
#74782=CARTESIAN_POINT('Ctrl Pts',(78.5347794150567,-10.4405298330678,135.040668428108));
#74783=CARTESIAN_POINT('Ctrl Pts',(78.4847512827717,-10.3896442161458,135.036809025385));
#74784=CARTESIAN_POINT('Ctrl Pts',(78.4374015149919,-10.3361743051257,135.032949622663));
#74785=CARTESIAN_POINT('Ctrl Pts',(78.3929939421255,-10.2804409757793,135.02909021994));
#74786=CARTESIAN_POINT('Ctrl Pts',(78.3485612253426,-10.224676089784,135.025228631993));
#74787=CARTESIAN_POINT('Ctrl Pts',(78.3070743024084,-10.1666456296284,135.021367044046));
#74788=CARTESIAN_POINT('Ctrl Pts',(78.2687541743393,-10.1067002546455,135.017505456099));
#74789=CARTESIAN_POINT('Ctrl Pts',(78.2303670038326,-10.0466500030804,135.013637112166));
#74790=CARTESIAN_POINT('Ctrl Pts',(78.1951579298455,-9.98467857040146,135.009768768232));
#74791=CARTESIAN_POINT('Ctrl Pts',(78.1633020932596,-9.92116142009714,135.005900424299));
#74792=CARTESIAN_POINT('Ctrl Pts',(78.1443870142261,-9.88344676411107,135.003603512992));
#74793=CARTESIAN_POINT('Ctrl Pts',(78.1266532537514,-9.8451875492383,135.001306601686));
#74794=CARTESIAN_POINT('Ctrl Pts',(78.110129253951,-9.80646520428854,134.999009690379));
#74795=CARTESIAN_POINT('Ctrl Pts',(78.0793053040283,-9.73423235291849,134.994725020811));
#74796=CARTESIAN_POINT('Ctrl Pts',(78.052590491782,-9.66014619425519,134.990440351243));
#74797=CARTESIAN_POINT('Ctrl Pts',(78.0301869119698,-9.58466568286928,134.986155681675));
#74798=CARTESIAN_POINT('Ctrl Pts',(78.0078542859392,-9.50942422380289,134.98188458197));
#74799=CARTESIAN_POINT('Ctrl Pts',(77.9898057879736,-9.43279749448197,134.977613482265));
#74800=CARTESIAN_POINT('Ctrl Pts',(77.9761951891263,-9.3552627900365,134.97334238256));
#74801=CARTESIAN_POINT('Ctrl Pts',(77.9626561574425,-9.27813577807579,134.969093741125));
#74802=CARTESIAN_POINT('Ctrl Pts',(77.953508604126,-9.20011059760666,134.964845099689));
#74803=CARTESIAN_POINT('Ctrl Pts',(77.9488557708441,-9.12167544411387,134.960596458253));
#74804=CARTESIAN_POINT('Ctrl Pts',(77.9464750440831,-9.08154233432821,134.958422545337));
#74805=CARTESIAN_POINT('Ctrl Pts',(77.9452702854505,-9.04130216095229,134.956248632422));
#74806=CARTESIAN_POINT('Ctrl Pts',(77.9452502540763,-9.00102182517148,134.954074719507));
#74807=CARTESIAN_POINT('Origin',(80.,-9.,141.545925280538));
#74808=CARTESIAN_POINT('',(81.2520391107129,-7.37076839346112,136.106053391332));
#74809=CARTESIAN_POINT('',(81.2520391107129,-7.37076839346112,136.047954616434));
#74810=CARTESIAN_POINT('',(81.2520391107129,-7.37076839346111,141.545925280538));
#74811=CARTESIAN_POINT('',(77.9452505223076,-8.99853493254343,135.595925280489));
#74812=CARTESIAN_POINT('Ctrl Pts',(81.2520391107129,-7.37076839346111,136.047954616434));
#74813=CARTESIAN_POINT('Ctrl Pts',(81.3089518218122,-7.41450492539866,136.044073934521));
#74814=CARTESIAN_POINT('Ctrl Pts',(81.3635519299052,-7.46121314581298,136.040193252607));
#74815=CARTESIAN_POINT('Ctrl Pts',(81.4155258488792,-7.51060947577379,136.036312570693));
#74816=CARTESIAN_POINT('Ctrl Pts',(81.4672299062672,-7.55974932763548,136.03245203825));
#74817=CARTESIAN_POINT('Ctrl Pts',(81.516334682387,-7.61154904832071,136.028591505807));
#74818=CARTESIAN_POINT('Ctrl Pts',(81.5625698796666,-7.66569383810955,136.024730973364));
#74819=CARTESIAN_POINT('Ctrl Pts',(81.6091670534803,-7.72026252883326,136.020840216715));
#74820=CARTESIAN_POINT('Ctrl Pts',(81.6528492126412,-7.77721277184851,136.016949460066));
#74821=CARTESIAN_POINT('Ctrl Pts',(81.6933836048278,-7.83619179870548,136.013058703416));
#74822=CARTESIAN_POINT('Ctrl Pts',(81.7339179970144,-7.89517082556246,136.009167946767));
#74823=CARTESIAN_POINT('Ctrl Pts',(81.7713044167982,-7.95617817802814,136.005277190118));
#74824=CARTESIAN_POINT('Ctrl Pts',(81.8053578201977,-8.01883706574744,136.001386433468));
#74825=CARTESIAN_POINT('Ctrl Pts',(81.8392215261155,-8.08114690661623,135.997517350621));
#74826=CARTESIAN_POINT('Ctrl Pts',(81.8699219428301,-8.14533399680408,135.993648267774));
#74827=CARTESIAN_POINT('Ctrl Pts',(81.897247021578,-8.21104417004908,135.989779184927));
#74828=CARTESIAN_POINT('Ctrl Pts',(81.9245313873213,-8.27665643841313,135.985915866821));
#74829=CARTESIAN_POINT('Ctrl Pts',(81.9484502126878,-8.34378684040901,135.982052548715));
#74830=CARTESIAN_POINT('Ctrl Pts',(81.9688372273746,-8.41205652091058,135.978189230608));
#74831=CARTESIAN_POINT('Ctrl Pts',(81.989200328101,-8.48024612110317,135.974330444172));
#74832=CARTESIAN_POINT('Ctrl Pts',(82.0060397088494,-8.54957188209905,135.970471657737));
#74833=CARTESIAN_POINT('Ctrl Pts',(82.0192377707971,-8.61963650610701,135.966612871301));
#74834=CARTESIAN_POINT('Ctrl Pts',(82.0324275189334,-8.6896569945394,135.962756515618));
#74835=CARTESIAN_POINT('Ctrl Pts',(82.0419804093478,-8.76041494632014,135.958900159934));
#74836=CARTESIAN_POINT('Ctrl Pts',(82.0478294907081,-8.83150092140787,135.955043804251));
#74837=CARTESIAN_POINT('Ctrl Pts',(82.0536768441911,-8.90256589698681,135.951188587774));
#74838=CARTESIAN_POINT('Ctrl Pts',(82.0558225209815,-8.97395821961339,135.947333371297));
#74839=CARTESIAN_POINT('Ctrl Pts',(82.0542514007093,-9.0452630664432,135.943478154819));
#74840=CARTESIAN_POINT('Ctrl Pts',(82.052680219011,-9.11657070107929,135.939622787615));
#74841=CARTESIAN_POINT('Ctrl Pts',(82.0473919646485,-9.18779036751191,135.93576742041));
#74842=CARTESIAN_POINT('Ctrl Pts',(82.0384236078768,-9.25850871813237,135.931912053206));
#74843=CARTESIAN_POINT('Ctrl Pts',(82.0294458636811,-9.32930109158191,135.928052650483));
#74844=CARTESIAN_POINT('Ctrl Pts',(82.0167803887356,-9.39959061880823,135.92419324776));
#74845=CARTESIAN_POINT('Ctrl Pts',(82.0005157706015,-9.46897144270698,135.920333845037));
#74846=CARTESIAN_POINT('Ctrl Pts',(81.9842419433129,-9.53839155057324,135.91647225709));
#74847=CARTESIAN_POINT('Ctrl Pts',(81.964365051502,-9.60690146410664,135.912610669143));
#74848=CARTESIAN_POINT('Ctrl Pts',(81.9410235901457,-9.67411051393499,135.908749081196));
#74849=CARTESIAN_POINT('Ctrl Pts',(81.9176412920663,-9.74143714840501,135.904880737263));
#74850=CARTESIAN_POINT('Ctrl Pts',(81.8907825058248,-9.80745792514187,135.90101239333));
#74851=CARTESIAN_POINT('Ctrl Pts',(81.8606336006024,-9.87180282564891,135.897144049396));
#74852=CARTESIAN_POINT('Ctrl Pts',(81.8427320482915,-9.91000897588458,135.89484713809));
#74853=CARTESIAN_POINT('Ctrl Pts',(81.8236714017529,-9.94762473769756,135.892550226783));
#74854=CARTESIAN_POINT('Ctrl Pts',(81.8034979882718,-9.98457735541688,135.890253315477));
#74855=CARTESIAN_POINT('Ctrl Pts',(81.7695164375494,-10.0468230063339,135.88638423263));
#74856=CARTESIAN_POINT('Ctrl Pts',(81.7322420417681,-10.1074292564437,135.882515149783));
#74857=CARTESIAN_POINT('Ctrl Pts',(81.6918573366432,-10.1660258637554,135.878646066936));
#74858=CARTESIAN_POINT('Ctrl Pts',(81.6515328027148,-10.2245351650446,135.87478274883));
#74859=CARTESIAN_POINT('Ctrl Pts',(81.6081074316388,-10.2810403703443,135.870919430723));
#74860=CARTESIAN_POINT('Ctrl Pts',(81.561809330398,-10.3351963069084,135.867056112617));
#74861=CARTESIAN_POINT('Ctrl Pts',(81.5155655368123,-10.3892887185796,135.863197326181));
#74862=CARTESIAN_POINT('Ctrl Pts',(81.4664560205841,-10.441036967801,135.859338539745));
#74863=CARTESIAN_POINT('Ctrl Pts',(81.4147507814426,-10.4901267694084,135.855479753309));
#74864=CARTESIAN_POINT('Ctrl Pts',(81.3630781128103,-10.5391856480405,135.851623397626));
#74865=CARTESIAN_POINT('Ctrl Pts',(81.3088133167697,-10.5855890678083,135.847767041943));
#74866=CARTESIAN_POINT('Ctrl Pts',(81.2522640643579,-10.6290587084626,135.84391068626));
#74867=CARTESIAN_POINT('Ctrl Pts',(81.1957315171616,-10.6725155077497,135.840055469782));
#74868=CARTESIAN_POINT('Ctrl Pts',(81.1369162382928,-10.7130399526008,135.836200253305));
#74869=CARTESIAN_POINT('Ctrl Pts',(81.0761585331535,-10.7503943481459,135.832345036828));
#74870=CARTESIAN_POINT('Ctrl Pts',(81.0153984525695,-10.7877502041362,135.828489669623));
#74871=CARTESIAN_POINT('Ctrl Pts',(80.9526962099212,-10.8219355122066,135.824634302419));
#74872=CARTESIAN_POINT('Ctrl Pts',(80.888419124146,-10.852757140683,135.820778935214));
#74873=CARTESIAN_POINT('Ctrl Pts',(80.8240747577897,-10.8836110309996,135.816919532491));
#74874=CARTESIAN_POINT('Ctrl Pts',(80.7581526965937,-10.911094002836,135.813060129768));
#74875=CARTESIAN_POINT('Ctrl Pts',(80.691041962686,-10.9350603526265,135.809200727045));
#74876=CARTESIAN_POINT('Ctrl Pts',(80.6238932301537,-10.9590402723526,135.805339139099));
#74877=CARTESIAN_POINT('Ctrl Pts',(80.5555549506982,-10.9794994668986,135.801477551152));
#74878=CARTESIAN_POINT('Ctrl Pts',(80.4864304555317,-10.9963423990967,135.797615963205));
#74879=CARTESIAN_POINT('Ctrl Pts',(80.4171850245831,-11.0132147986085,135.793747619271));
#74880=CARTESIAN_POINT('Ctrl Pts',(80.3471511091485,-11.0264582138856,135.789879275338));
#74881=CARTESIAN_POINT('Ctrl Pts',(80.2767406569824,-11.0360285290911,135.786010931404));
#74882=CARTESIAN_POINT('Ctrl Pts',(80.234932956723,-11.0417111068504,135.783714020098));
#74883=CARTESIAN_POINT('Ctrl Pts',(80.1929925914078,-11.0460996761472,135.781417108791));
#74884=CARTESIAN_POINT('Ctrl Pts',(80.1510058124904,-11.0491936968218,135.779120197485));
#74885=CARTESIAN_POINT('Ctrl Pts',(80.0802802578498,-11.0544054881029,135.775251114638));
#74886=CARTESIAN_POINT('Ctrl Pts',(80.0091460436975,-11.0559616725954,135.771382031791));
#74887=CARTESIAN_POINT('Ctrl Pts',(79.9380132263567,-11.0538147926221,135.767512948944));
#74888=CARTESIAN_POINT('Ctrl Pts',(79.8669863933663,-11.0516711113929,135.763649630838));
#74889=CARTESIAN_POINT('Ctrl Pts',(79.7959614346627,-11.0458353320829,135.759786312731));
#74890=CARTESIAN_POINT('Ctrl Pts',(79.7253520620256,-11.0363118800092,135.755922994625));
#74891=CARTESIAN_POINT('Ctrl Pts',(79.6548255141554,-11.026799598941,135.752064208189));
#74892=CARTESIAN_POINT('Ctrl Pts',(79.5847140631344,-11.0136083019093,135.748205421753));
#74893=CARTESIAN_POINT('Ctrl Pts',(79.5154281928644,-10.9967943625294,135.744346635318));
#74894=CARTESIAN_POINT('Ctrl Pts',(79.4461859676121,-10.9799910146984,135.740490279634));
#74895=CARTESIAN_POINT('Ctrl Pts',(79.3777687622945,-10.959569666261,135.736633923951));
#74896=CARTESIAN_POINT('Ctrl Pts',(79.3105772776748,-10.9356378464066,135.732777568268));
#74897=CARTESIAN_POINT('Ctrl Pts',(79.2434056420925,-10.9117130962514,135.72892235179));
#74898=CARTESIAN_POINT('Ctrl Pts',(79.177459465732,-10.8842800963727,135.725067135313));
#74899=CARTESIAN_POINT('Ctrl Pts',(79.113123018869,-10.8534958275756,135.721211918836));
#74900=CARTESIAN_POINT('Ctrl Pts',(79.0487840566434,-10.8227103552056,135.717356551631));
#74901=CARTESIAN_POINT('Ctrl Pts',(78.9860553861175,-10.7885735654471,135.713501184427));
#74902=CARTESIAN_POINT('Ctrl Pts',(78.9252984901619,-10.7512893042704,135.709645817222));
#74903=CARTESIAN_POINT('Ctrl Pts',(78.864477998304,-10.7139660166391,135.705786414499));
#74904=CARTESIAN_POINT('Ctrl Pts',(78.8056338159311,-10.6734889355417,135.701927011777));
#74905=CARTESIAN_POINT('Ctrl Pts',(78.7490993513748,-10.6301058645895,135.698067609054));
#74906=CARTESIAN_POINT('Ctrl Pts',(78.6925328765606,-10.5866982298017,135.694206021107));
#74907=CARTESIAN_POINT('Ctrl Pts',(78.6382790925866,-10.5403816452458,135.69034443316));
#74908=CARTESIAN_POINT('Ctrl Pts',(78.5866370222996,-10.4914431453347,135.686482845213));
#74909=CARTESIAN_POINT('Ctrl Pts',(78.5349046023597,-10.4424190257639,135.68261450128));
#74910=CARTESIAN_POINT('Ctrl Pts',(78.4857933536458,-10.390764184664,135.678746157346));
#74911=CARTESIAN_POINT('Ctrl Pts',(78.4395637716867,-10.336800785408,135.674877813413));
#74912=CARTESIAN_POINT('Ctrl Pts',(78.412113976291,-10.3047588718613,135.672580902106));
#74913=CARTESIAN_POINT('Ctrl Pts',(78.3856793652921,-10.2719036572887,135.6702839908));
#74914=CARTESIAN_POINT('Ctrl Pts',(78.360307173587,-10.2383073114174,135.667987079493));
#74915=CARTESIAN_POINT('Ctrl Pts',(78.3174433117301,-10.1815495371952,135.664106670182));
#74916=CARTESIAN_POINT('Ctrl Pts',(78.2774445565979,-10.1224505980396,135.660226260871));
#74917=CARTESIAN_POINT('Ctrl Pts',(78.2405752223932,-10.0613303041199,135.65634585156));
#74918=CARTESIAN_POINT('Ctrl Pts',(78.2037608188311,-10.0003010717042,135.652471223568));
#74919=CARTESIAN_POINT('Ctrl Pts',(78.1700668305629,-9.93725686913624,135.648596595576));
#74920=CARTESIAN_POINT('Ctrl Pts',(78.1397161676285,-9.87254892442625,135.644721967583));
#74921=CARTESIAN_POINT('Ctrl Pts',(78.1078633935518,-9.8046384623624,135.640655576996));
#74922=CARTESIAN_POINT('Ctrl Pts',(78.0796937990201,-9.7348957272421,135.636589186409));
#74923=CARTESIAN_POINT('Ctrl Pts',(78.0554121444881,-9.66375871722748,135.632522795822));
#74924=CARTESIAN_POINT('Ctrl Pts',(78.0323224526799,-9.59611375361004,135.62865602038));
#74925=CARTESIAN_POINT('Ctrl Pts',(78.0127481522004,-9.52720869452225,135.624789244939));
#74926=CARTESIAN_POINT('Ctrl Pts',(77.9968162204212,-9.45744104290337,135.620922469497));
#74927=CARTESIAN_POINT('Ctrl Pts',(77.9808915414106,-9.38770515194222,135.617057454346));
#74928=CARTESIAN_POINT('Ctrl Pts',(77.968606042256,-9.31710791801235,135.613192439195));
#74929=CARTESIAN_POINT('Ctrl Pts',(77.9600362376923,-9.2460597711358,135.609327424043));
#74930=CARTESIAN_POINT('Ctrl Pts',(77.9514663540314,-9.17501096850289,135.605462373219));
#74931=CARTESIAN_POINT('Ctrl Pts',(77.946612293274,-9.10351172242717,135.601597322395));
#74932=CARTESIAN_POINT('Ctrl Pts',(77.945498864882,-9.03197887269597,135.59773227157));
#74933=CARTESIAN_POINT('Ctrl Pts',(77.9453253479641,-9.02083117815062,135.597129941226));
#74934=CARTESIAN_POINT('Ctrl Pts',(77.9452425738058,-9.00968267177878,135.596527610882));
#74935=CARTESIAN_POINT('Ctrl Pts',(77.9452505223069,-8.99853493345712,135.595925280538));
#74936=CARTESIAN_POINT('Ctrl Pts',(77.9452505223076,-8.99853493254344,135.595925280489));
#74937=CARTESIAN_POINT('Ctrl Pts',(77.9453088390013,-8.91674607330211,135.591506096049));
#74938=CARTESIAN_POINT('Ctrl Pts',(77.9502545524831,-8.83515245773087,135.587086911609));
#74939=CARTESIAN_POINT('Ctrl Pts',(77.9599940449637,-8.75429028119236,135.582667727169));
#74940=CARTESIAN_POINT('Ctrl Pts',(77.9698223745246,-8.67269053442832,135.57820823391));
#74941=CARTESIAN_POINT('Ctrl Pts',(77.9845322237854,-8.59183581843483,135.573748740651));
#74942=CARTESIAN_POINT('Ctrl Pts',(78.0039776882017,-8.51225775936117,135.569289247392));
#74943=CARTESIAN_POINT('Ctrl Pts',(78.0220522312958,-8.43829001926129,135.565144152095));
#74944=CARTESIAN_POINT('Ctrl Pts',(78.0442176079845,-8.36542517061296,135.560999056799));
#74945=CARTESIAN_POINT('Ctrl Pts',(78.0703199470975,-8.29407333530297,135.556853961502));
#74946=CARTESIAN_POINT('Ctrl Pts',(78.0946841909334,-8.22747265610305,135.552984878655));
#74947=CARTESIAN_POINT('Ctrl Pts',(78.1225481710407,-8.16200436801017,135.549115795808));
#74948=CARTESIAN_POINT('Ctrl Pts',(78.1537863391279,-8.0980617089239,135.545246712961));
#74949=CARTESIAN_POINT('Ctrl Pts',(78.1849779639025,-8.03421432121068,135.541383394855));
#74950=CARTESIAN_POINT('Ctrl Pts',(78.2195335859642,-7.97188848336657,135.537520076748));
#74951=CARTESIAN_POINT('Ctrl Pts',(78.2572788690438,-7.91145940717916,135.533656758642));
#74952=CARTESIAN_POINT('Ctrl Pts',(78.2949798769208,-7.85110121427484,135.529797972206));
#74953=CARTESIAN_POINT('Ctrl Pts',(78.3358628578839,-7.79263577363492,135.52593918577));
#74954=CARTESIAN_POINT('Ctrl Pts',(78.3797074616774,-7.73641397097142,135.522080399334));
#74955=CARTESIAN_POINT('Ctrl Pts',(78.4235244465856,-7.68022758392105,135.518224043651));
#74956=CARTESIAN_POINT('Ctrl Pts',(78.4702990549624,-7.62628241299098,135.514367687968));
#74957=CARTESIAN_POINT('Ctrl Pts',(78.5197683434641,-7.57489937004817,135.510511332285));
#74958=CARTESIAN_POINT('Ctrl Pts',(78.5692230182428,-7.52353150617074,135.506656115807));
#74959=CARTESIAN_POINT('Ctrl Pts',(78.6213704560568,-7.47472461743221,135.50280089933));
#74960=CARTESIAN_POINT('Ctrl Pts',(78.6759094097281,-7.42876428526668,135.498945682853));
#74961=CARTESIAN_POINT('Ctrl Pts',(78.7304504957095,-7.38280215618959,135.495090315648));
#74962=CARTESIAN_POINT('Ctrl Pts',(78.7873829102919,-7.33968711599724,135.491234948444));
#74963=CARTESIAN_POINT('Ctrl Pts',(78.8463720764142,-7.29966468706224,135.487379581239));
#74964=CARTESIAN_POINT('Ctrl Pts',(78.9054229881079,-7.25960036555775,135.483520178516));
#74965=CARTESIAN_POINT('Ctrl Pts',(78.9665345461123,-7.22263539062787,135.479660775793));
#74966=CARTESIAN_POINT('Ctrl Pts',(79.0293436696696,-7.18897160406316,135.475801373071));
#74967=CARTESIAN_POINT('Ctrl Pts',(79.0921883562461,-7.15528875679807,135.471939785124));
#74968=CARTESIAN_POINT('Ctrl Pts',(79.1567320820357,-7.12491102578324,135.468078197177));
#74969=CARTESIAN_POINT('Ctrl Pts',(79.2225901682402,-7.09799276657967,135.46421660923));
#74970=CARTESIAN_POINT('Ctrl Pts',(79.2885634755271,-7.07102741291679,135.460348265296));
#74971=CARTESIAN_POINT('Ctrl Pts',(79.3558552755072,-7.04753377516652,135.456479921363));
#74972=CARTESIAN_POINT('Ctrl Pts',(79.4240647345015,-7.02761663653966,135.452611577429));
#74973=CARTESIAN_POINT('Ctrl Pts',(79.4645655483546,-7.01579041278846,135.450314666123));
#74974=CARTESIAN_POINT('Ctrl Pts',(79.5053896608541,-7.00522416360188,135.448017754817));
#74975=CARTESIAN_POINT('Ctrl Pts',(79.5464518564912,-6.99593122772204,135.44572084351));
#74976=CARTESIAN_POINT('Ctrl Pts',(79.6192550066374,-6.9794548801799,135.441648426628));
#74977=CARTESIAN_POINT('Ctrl Pts',(79.6931072768256,-6.9669168711275,135.437576009747));
#74978=CARTESIAN_POINT('Ctrl Pts',(79.7675435326616,-6.95844139116886,135.433503592865));
#74979=CARTESIAN_POINT('Ctrl Pts',(79.8381398313005,-6.95040313739657,135.429641260523));
#74980=CARTESIAN_POINT('Ctrl Pts',(79.9092607958587,-6.94601875938677,135.42577892818));
#74981=CARTESIAN_POINT('Ctrl Pts',(79.980496462632,-6.9453425651632,135.421916595838));
#74982=CARTESIAN_POINT('Ctrl Pts',(80.0516622919897,-6.94466703386116,135.418058050016));
#74983=CARTESIAN_POINT('Ctrl Pts',(80.1229421172637,-6.94769247846982,135.414199504194));
#74984=CARTESIAN_POINT('Ctrl Pts',(80.1939215987489,-6.95442135911652,135.410340958372));
#74985=CARTESIAN_POINT('Ctrl Pts',(80.264855239782,-6.96114589407173,135.406484904502));
#74986=CARTESIAN_POINT('Ctrl Pts',(80.3354884395999,-6.97156907186203,135.402628850632));
#74987=CARTESIAN_POINT('Ctrl Pts',(80.4054093394314,-6.98564133531246,135.398772796763));
#74988=CARTESIAN_POINT('Ctrl Pts',(80.4753084723093,-6.99970921795104,135.394917943314));
#74989=CARTESIAN_POINT('Ctrl Pts',(80.5444952700206,-7.01742383308555,135.391063089866));
#74990=CARTESIAN_POINT('Ctrl Pts',(80.6125671730664,-7.03868436477413,135.387208236418));
#74991=CARTESIAN_POINT('Ctrl Pts',(80.6806707825929,-7.05995479917745,135.383351587459));
#74992=CARTESIAN_POINT('Ctrl Pts',(80.7476579949989,-7.08477430739439,135.3794949385));
#74993=CARTESIAN_POINT('Ctrl Pts',(80.8131416938626,-7.11299227659179,135.375638289541));
#74994=CARTESIAN_POINT('Ctrl Pts',(80.8786429816968,-7.14121782515682,135.371780604683));
#74995=CARTESIAN_POINT('Ctrl Pts',(80.9426395127162,-7.17284344390741,135.367922919825));
#74996=CARTESIAN_POINT('Ctrl Pts',(81.004766625319,-7.20767146115866,135.364065234967));
#74997=CARTESIAN_POINT('Ctrl Pts',(81.06696585699,-7.24253990784641,135.36020307199));
#74998=CARTESIAN_POINT('Ctrl Pts',(81.1272909249947,-7.2806179182745,135.356340909013));
#74999=CARTESIAN_POINT('Ctrl Pts',(81.1854050203164,-7.32166377018525,135.352478746035));
#75000=CARTESIAN_POINT('Ctrl Pts',(81.2079550446943,-7.33759080055679,135.35098011014));
#75001=CARTESIAN_POINT('Ctrl Pts',(81.2301725106883,-7.35396425196326,135.349481474244));
#75002=CARTESIAN_POINT('Ctrl Pts',(81.2520391107129,-7.37076839346111,135.347982838348));
#75003=CARTESIAN_POINT('',(77.945250359968,-9.00121625991051,135.654074719411));
#75004=CARTESIAN_POINT('Ctrl Pts',(77.945250359968,-9.00121625991051,135.654074719411));
#75005=CARTESIAN_POINT('Ctrl Pts',(77.9452088811236,-8.93114189521501,135.650257838806));
#75006=CARTESIAN_POINT('Ctrl Pts',(77.9487563144495,-8.86092442684195,135.646440958201));
#75007=CARTESIAN_POINT('Ctrl Pts',(77.9559102037764,-8.79096778364445,135.642624077596));
#75008=CARTESIAN_POINT('Ctrl Pts',(77.9630536357837,-8.72111340076158,135.638812776381));
#75009=CARTESIAN_POINT('Ctrl Pts',(77.9737930081513,-8.65151957937679,135.635001475166));
#75010=CARTESIAN_POINT('Ctrl Pts',(77.9880938466836,-8.5825898986039,135.631190173951));
#75011=CARTESIAN_POINT('Ctrl Pts',(78.0023832068387,-8.51371554331888,135.627381931827));
#75012=CARTESIAN_POINT('Ctrl Pts',(78.0202282665398,-8.44550475924146,135.623573689702));
#75013=CARTESIAN_POINT('Ctrl Pts',(78.0415429670004,-8.37835411012833,135.619765447577));
#75014=CARTESIAN_POINT('Ctrl Pts',(78.0628481279409,-8.31123351468479,135.615958909853));
#75015=CARTESIAN_POINT('Ctrl Pts',(78.0876196992428,-8.24517258878994,135.61215237213));
#75016=CARTESIAN_POINT('Ctrl Pts',(78.1157214210871,-8.18055396788435,135.608345834406));
#75017=CARTESIAN_POINT('Ctrl Pts',(78.1438205431129,-8.11594132514243,135.604539648843));
#75018=CARTESIAN_POINT('Ctrl Pts',(78.1752490033444,-8.05277117987547,135.60073346328));
#75019=CARTESIAN_POINT('Ctrl Pts',(78.209822671994,-7.99140558359992,135.596927277716));
#75020=CARTESIAN_POINT('Ctrl Pts',(78.2444287085066,-7.92998253686311,135.593117528803));
#75021=CARTESIAN_POINT('Ctrl Pts',(78.2821855870687,-7.87036784851871,135.589307779889));
#75022=CARTESIAN_POINT('Ctrl Pts',(78.3228640638333,-7.81289738686239,135.585498030976));
#75023=CARTESIAN_POINT('Ctrl Pts',(78.3635622899698,-7.75539902333731,135.581686432432));
#75024=CARTESIAN_POINT('Ctrl Pts',(78.407184627001,-7.70004735028743,135.577874833887));
#75025=CARTESIAN_POINT('Ctrl Pts',(78.4534612670308,-7.64714542173745,135.574063235343));
#75026=CARTESIAN_POINT('Ctrl Pts',(78.4998192121047,-7.59415054794265,135.570244940069));
#75027=CARTESIAN_POINT('Ctrl Pts',(78.5488404216445,-7.54361436930265,135.566426644794));
#75028=CARTESIAN_POINT('Ctrl Pts',(78.6002185439983,-7.4958027263907,135.56260834952));
#75029=CARTESIAN_POINT('Ctrl Pts',(78.6358004088325,-7.46269082315915,135.559963993126));
#75030=CARTESIAN_POINT('Ctrl Pts',(78.6725119658444,-7.43088485820555,135.557319636732));
#75031=CARTESIAN_POINT('Ctrl Pts',(78.7102431226447,-7.4004610789935,135.554675280338));
#75032=CARTESIAN_POINT('Ctrl Pts',(78.765449361827,-7.35594660940278,135.550806197491));
#75033=CARTESIAN_POINT('Ctrl Pts',(78.823070982614,-7.31420637759796,135.546937114644));
#75034=CARTESIAN_POINT('Ctrl Pts',(78.8827977135628,-7.27551265192246,135.543068031797));
#75035=CARTESIAN_POINT('Ctrl Pts',(78.942435454661,-7.23687657796856,135.539204713691));
#75036=CARTESIAN_POINT('Ctrl Pts',(79.0041716756558,-7.201278262049,135.535341395584));
#75037=CARTESIAN_POINT('Ctrl Pts',(79.067663588119,-7.16894937874977,135.531478077478));
#75038=CARTESIAN_POINT('Ctrl Pts',(79.1310810245934,-7.13665841721817,135.527619291042));
#75039=CARTESIAN_POINT('Ctrl Pts',(79.1962496310247,-7.10762948996541,135.523760504606));
#75040=CARTESIAN_POINT('Ctrl Pts',(79.2627997262892,-7.08204970894948,135.51990171817));
#75041=CARTESIAN_POINT('Ctrl Pts',(79.3293078998736,-7.05648604131993,135.516045362487));
#75042=CARTESIAN_POINT('Ctrl Pts',(79.3971953833863,-7.03436738318268,135.512189006804));
#75043=CARTESIAN_POINT('Ctrl Pts',(79.4660714454971,-7.01583320731686,135.50833265112));
#75044=CARTESIAN_POINT('Ctrl Pts',(79.5349271609297,-6.99730450663215,135.504477434643));
#75045=CARTESIAN_POINT('Ctrl Pts',(79.6047704063476,-6.9823583121868,135.500622218166));
#75046=CARTESIAN_POINT('Ctrl Pts',(79.6751958367452,-6.97108407812636,135.496767001689));
#75047=CARTESIAN_POINT('Ctrl Pts',(79.7456240205664,-6.95980940327711,135.492911634484));
#75048=CARTESIAN_POINT('Ctrl Pts',(79.816633954534,-6.95220704845246,135.48905626728));
#75049=CARTESIAN_POINT('Ctrl Pts',(79.8878123795719,-6.94831496074015,135.485200900075));
#75050=CARTESIAN_POINT('Ctrl Pts',(79.9590653090116,-6.94441879907333,135.481341497352));
#75051=CARTESIAN_POINT('Ctrl Pts',(80.0304865955319,-6.94424068370814,135.477482094629));
#75052=CARTESIAN_POINT('Ctrl Pts',(80.1016610683356,-6.9477664388075,135.473622691907));
#75053=CARTESIAN_POINT('Ctrl Pts',(80.172875840685,-6.95129419021709,135.46976110396));
#75054=CARTESIAN_POINT('Ctrl Pts',(80.2438430376165,-6.95852993759325,135.465899516013));
#75055=CARTESIAN_POINT('Ctrl Pts',(80.3141534558341,-6.96940768033377,135.462037928066));
#75056=CARTESIAN_POINT('Ctrl Pts',(80.3845868846486,-6.98030445407512,135.458169584132));
#75057=CARTESIAN_POINT('Ctrl Pts',(80.4543607649208,-6.9948558454545,135.454301240199));
#75058=CARTESIAN_POINT('Ctrl Pts',(80.5230776005261,-7.01294504697834,135.450432896265));
#75059=CARTESIAN_POINT('Ctrl Pts',(80.5638796800099,-7.02368589428125,135.448135984959));
#75060=CARTESIAN_POINT('Ctrl Pts',(80.6043093824187,-7.03567309355378,135.445839073653));
#75061=CARTESIAN_POINT('Ctrl Pts',(80.6442868085185,-7.04887415299036,135.443542162346));
#75062=CARTESIAN_POINT('Ctrl Pts',(80.7116141902558,-7.07110651897124,135.439673853667));
#75063=CARTESIAN_POINT('Ctrl Pts',(80.7779213073233,-7.09687140314609,135.435805544988));
#75064=CARTESIAN_POINT('Ctrl Pts',(80.8428113700394,-7.1260558820946,135.431937236309));
#75065=CARTESIAN_POINT('Ctrl Pts',(80.907616628674,-7.15520222018102,135.428073983079));
#75066=CARTESIAN_POINT('Ctrl Pts',(80.9710080660985,-7.18775909376035,135.424210729848));
#75067=CARTESIAN_POINT('Ctrl Pts',(81.0326051384994,-7.22356418904463,135.420347476618));
#75068=CARTESIAN_POINT('Ctrl Pts',(81.0941310956293,-7.25932794650305,135.416488683604));
#75069=CARTESIAN_POINT('Ctrl Pts',(81.1538663843257,-7.29833223449443,135.41262989059));
#75070=CARTESIAN_POINT('Ctrl Pts',(81.2114532906711,-7.34036796637863,135.408771097577));
#75071=CARTESIAN_POINT('Ctrl Pts',(81.2251040198816,-7.35033235636819,135.40785638724));
#75072=CARTESIAN_POINT('Ctrl Pts',(81.2386341418168,-7.36046688367673,135.406941676903));
#75073=CARTESIAN_POINT('Ctrl Pts',(81.2520391107129,-7.37076839346111,135.406026966566));
#75074=CARTESIAN_POINT('Ctrl Pts',(81.2520391107129,-7.37076839346111,136.106053391332));
#75075=CARTESIAN_POINT('Ctrl Pts',(81.3083146859017,-7.41401529637627,136.102186604392));
#75076=CARTESIAN_POINT('Ctrl Pts',(81.3624484341154,-7.46025936207125,136.098319817451));
#75077=CARTESIAN_POINT('Ctrl Pts',(81.4141045137042,-7.50925991976423,136.094453030511));
#75078=CARTESIAN_POINT('Ctrl Pts',(81.467120080933,-7.55955007692093,136.090484477253));
#75079=CARTESIAN_POINT('Ctrl Pts',(81.5175252609129,-7.61274362222067,136.086515923994));
#75080=CARTESIAN_POINT('Ctrl Pts',(81.5649910403901,-7.66853441426421,136.082547370735));
#75081=CARTESIAN_POINT('Ctrl Pts',(81.6111305654479,-7.72276634041901,136.078689703917));
#75082=CARTESIAN_POINT('Ctrl Pts',(81.6544924636885,-7.77945187547075,136.074832037098));
#75083=CARTESIAN_POINT('Ctrl Pts',(81.6948115872083,-7.83827230111163,136.070974370279));
#75084=CARTESIAN_POINT('Ctrl Pts',(81.7351106664465,-7.89706348471872,136.067118621264));
#75085=CARTESIAN_POINT('Ctrl Pts',(81.7723696984119,-7.95798705275809,136.063262872248));
#75086=CARTESIAN_POINT('Ctrl Pts',(81.8063653527452,-8.02069321716743,136.059407123233));
#75087=CARTESIAN_POINT('Ctrl Pts',(81.8403554784318,-8.08338918379615,136.055552001271));
#75088=CARTESIAN_POINT('Ctrl Pts',(81.8710830494685,-8.14786674381296,136.051696879308));
#75089=CARTESIAN_POINT('Ctrl Pts',(81.8983702885415,-8.21375079645013,136.047841757346));
#75090=CARTESIAN_POINT('Ctrl Pts',(81.927056966845,-8.28301374453645,136.043788923592));
#75091=CARTESIAN_POINT('Ctrl Pts',(81.9519407108041,-8.3538307905123,136.039736089839));
#75092=CARTESIAN_POINT('Ctrl Pts',(81.9728728500854,-8.4257437158411,136.035683256085));
#75093=CARTESIAN_POINT('Ctrl Pts',(81.9928102665477,-8.49423924427389,136.031823018328));
#75094=CARTESIAN_POINT('Ctrl Pts',(82.0091630513749,-8.56372835764467,136.027962780571));
#75095=CARTESIAN_POINT('Ctrl Pts',(82.0218549347861,-8.63380307868442,136.024102542813));
#75096=CARTESIAN_POINT('Ctrl Pts',(82.0345557101281,-8.703926894058,136.020239600574));
#75097=CARTESIAN_POINT('Ctrl Pts',(82.0435904207257,-8.77463665202572,136.016376658335));
#75098=CARTESIAN_POINT('Ctrl Pts',(82.0489346542456,-8.84551911078864,136.012513716096));
#75099=CARTESIAN_POINT('Ctrl Pts',(82.0542875354261,-8.91651626653303,136.008644523117));
#75100=CARTESIAN_POINT('Ctrl Pts',(82.0559380205708,-8.98768619634296,136.004775330138));
#75101=CARTESIAN_POINT('Ctrl Pts',(82.0539137429452,-9.05861654238137,136.000906137159));
#75102=CARTESIAN_POINT('Ctrl Pts',(82.0536175569377,-9.06899485004974,136.000340008874));
#75103=CARTESIAN_POINT('Ctrl Pts',(82.0532427894454,-9.07936804108318,135.999773880589));
#75104=CARTESIAN_POINT('Ctrl Pts',(82.0527896193309,-9.0897348386495,135.999207752304));
#75105=CARTESIAN_POINT('Ctrl Pts',(82.0496925249742,-9.16058450240403,135.995338669457));
#75106=CARTESIAN_POINT('Ctrl Pts',(82.0429171171316,-9.23141240638119,135.99146958661));
#75107=CARTESIAN_POINT('Ctrl Pts',(82.0324642301758,-9.30180575799021,135.987600503763));
#75108=CARTESIAN_POINT('Ctrl Pts',(82.0220269175002,-9.37209422701601,135.983737185657));
#75109=CARTESIAN_POINT('Ctrl Pts',(82.0079230726634,-9.44194895226674,135.97987386755));
#75110=CARTESIAN_POINT('Ctrl Pts',(81.9902054844461,-9.51095957979161,135.976010549444));
#75111=CARTESIAN_POINT('Ctrl Pts',(81.9725086789529,-9.57988925787698,135.972151763008));
#75112=CARTESIAN_POINT('Ctrl Pts',(81.9512066702234,-9.64797633672259,135.968292976572));
#75113=CARTESIAN_POINT('Ctrl Pts',(81.926403461125,-9.71481974473689,135.964434190136));
#75114=CARTESIAN_POINT('Ctrl Pts',(81.9016158762296,-9.78162104630555,135.960577834453));
#75115=CARTESIAN_POINT('Ctrl Pts',(81.8733316352398,-9.84717977697588,135.95672147877));
#75116=CARTESIAN_POINT('Ctrl Pts',(81.8417044010277,-9.91111056504417,135.952865123087));
#75117=CARTESIAN_POINT('Ctrl Pts',(81.8100865098174,-9.97502246731751,135.949009906609));
#75118=CARTESIAN_POINT('Ctrl Pts',(81.7751278012401,-10.037306946552,135.945154690132));
#75119=CARTESIAN_POINT('Ctrl Pts',(81.73702912834,-10.0976007333262,135.941299473655));
#75120=CARTESIAN_POINT('Ctrl Pts',(81.6989289658958,-10.1578968774073,135.93744410645));
#75121=CARTESIAN_POINT('Ctrl Pts',(81.6576888567552,-10.2162017650157,135.933588739246));
#75122=CARTESIAN_POINT('Ctrl Pts',(81.6135535318411,-10.2721802397393,135.929733372041));
#75123=CARTESIAN_POINT('Ctrl Pts',(81.5693720092769,-10.3282173086614,135.925873969318));
#75124=CARTESIAN_POINT('Ctrl Pts',(81.5222895227638,-10.3819227213963,135.922014566595));
#75125=CARTESIAN_POINT('Ctrl Pts',(81.4725911750785,-10.4329943452717,135.918155163873));
#75126=CARTESIAN_POINT('Ctrl Pts',(81.4228646877985,-10.4840948863017,135.914293575926));
#75127=CARTESIAN_POINT('Ctrl Pts',(81.370519747522,-10.5325583396234,135.910431987979));
#75128=CARTESIAN_POINT('Ctrl Pts',(81.3158763962692,-10.5781213110029,135.906570400032));
#75129=CARTESIAN_POINT('Ctrl Pts',(81.2611374445147,-10.623763996434,135.902702056098));
#75130=CARTESIAN_POINT('Ctrl Pts',(81.204092442359,-10.6664957772108,135.898833712165));
#75131=CARTESIAN_POINT('Ctrl Pts',(81.1450918128935,-10.7060956311251,135.894965368231));
#75132=CARTESIAN_POINT('Ctrl Pts',(81.1100589370072,-10.7296088847949,135.892668456925));
#75133=CARTESIAN_POINT('Ctrl Pts',(81.0743370944697,-10.7520187877172,135.890371545619));
#75134=CARTESIAN_POINT('Ctrl Pts',(81.0380034848463,-10.7732868713062,135.888074634312));
#75135=CARTESIAN_POINT('Ctrl Pts',(80.9768005357524,-10.8091123632051,135.884205551465));
#75136=CARTESIAN_POINT('Ctrl Pts',(80.9136208229209,-10.8418357801991,135.880336468618));
#75137=CARTESIAN_POINT('Ctrl Pts',(80.848811599609,-10.871233932695,135.876467385771));
#75138=CARTESIAN_POINT('Ctrl Pts',(80.7840989388076,-10.9005882834098,135.872604067665));
#75139=CARTESIAN_POINT('Ctrl Pts',(80.7177620256113,-10.9266270050879,135.868740749559));
#75140=CARTESIAN_POINT('Ctrl Pts',(80.6501742435435,-10.9491718794228,135.864877431452));
#75141=CARTESIAN_POINT('Ctrl Pts',(80.5826657419181,-10.9716903086288,135.861018645016));
#75142=CARTESIAN_POINT('Ctrl Pts',(80.5139097444996,-10.9907228780985,135.857159858581));
#75143=CARTESIAN_POINT('Ctrl Pts',(80.4442996139071,-11.006139430743,135.853301072145));
#75144=CARTESIAN_POINT('Ctrl Pts',(80.3747333325926,-11.0215462720898,135.849444716462));
#75145=CARTESIAN_POINT('Ctrl Pts',(80.3043144587391,-11.0333415109886,135.845588360778));
#75146=CARTESIAN_POINT('Ctrl Pts',(80.2334500995799,-11.041445226673,135.841732005095));
#75147=CARTESIAN_POINT('Ctrl Pts',(80.162606674462,-11.0495465484388,135.837876788618));
#75148=CARTESIAN_POINT('Ctrl Pts',(80.0913185076772,-11.053958456799,135.834021572141));
#75149=CARTESIAN_POINT('Ctrl Pts',(80.0199997326211,-11.0546526648548,135.830166355663));
#75150=CARTESIAN_POINT('Ctrl Pts',(79.9486781692142,-11.0553469000522,135.826310988459));
#75151=CARTESIAN_POINT('Ctrl Pts',(79.8773264809416,-11.0523231438444,135.822455621254));
#75152=CARTESIAN_POINT('Ctrl Pts',(79.8063589810277,-11.0456052205329,135.81860025405));
#75153=CARTESIAN_POINT('Ctrl Pts',(79.7353171974932,-11.0388802653875,135.814740851327));
#75154=CARTESIAN_POINT('Ctrl Pts',(79.6646608896919,-11.0284534700421,135.810881448604));
#75155=CARTESIAN_POINT('Ctrl Pts',(79.5947985234111,-11.0144004879542,135.807022045881));
#75156=CARTESIAN_POINT('Ctrl Pts',(79.5248966005098,-11.0003395489575,135.803160457934));
#75157=CARTESIAN_POINT('Ctrl Pts',(79.4557899848465,-10.9826484565105,135.799298869987));
#75158=CARTESIAN_POINT('Ctrl Pts',(79.3878735471228,-10.9614532286516,135.79543728204));
#75159=CARTESIAN_POINT('Ctrl Pts',(79.3198382871569,-10.9402209189819,135.791568938107));
#75160=CARTESIAN_POINT('Ctrl Pts',(79.2529978181222,-10.9154724026927,135.787700594174));
#75161=CARTESIAN_POINT('Ctrl Pts',(79.1877278906751,-10.8873822037184,135.78383225024));
#75162=CARTESIAN_POINT('Ctrl Pts',(79.1489724860621,-10.870703051933,135.781535338934));
#75163=CARTESIAN_POINT('Ctrl Pts',(79.1107703609553,-10.8528466407429,135.779238427627));
#75164=CARTESIAN_POINT('Ctrl Pts',(79.0731957056113,-10.8338569634523,135.776941516321));
#75165=CARTESIAN_POINT('Ctrl Pts',(79.0099022497155,-10.8018693832321,135.773072433474));
#75166=CARTESIAN_POINT('Ctrl Pts',(78.9481427918078,-10.7665385540289,135.769203350627));
#75167=CARTESIAN_POINT('Ctrl Pts',(78.888293184181,-10.7280351611473,135.76533426778));
#75168=CARTESIAN_POINT('Ctrl Pts',(78.8285327494848,-10.689589136401,135.761470949674));
#75169=CARTESIAN_POINT('Ctrl Pts',(78.7706769218817,-10.6479801915525,135.757607631567));
#75170=CARTESIAN_POINT('Ctrl Pts',(78.7150779443411,-10.6034253563485,135.753744313461));
#75171=CARTESIAN_POINT('Ctrl Pts',(78.6595441843798,-10.5589227839491,135.749885527025));
#75172=CARTESIAN_POINT('Ctrl Pts',(78.6062623933193,-10.5114814873496,135.746026740589));
#75173=CARTESIAN_POINT('Ctrl Pts',(78.555555272579,-10.4613613488545,135.742167954153));
#75174=CARTESIAN_POINT('Ctrl Pts',(78.5048800936066,-10.4112727823714,135.73831159847));
#75175=CARTESIAN_POINT('Ctrl Pts',(78.4567767119,-10.3585090626023,135.734455242787));
#75176=CARTESIAN_POINT('Ctrl Pts',(78.4115330784901,-10.3033688663494,135.730598887103));
#75177=CARTESIAN_POINT('Ctrl Pts',(78.3663028105026,-10.2482449590626,135.726743670626));
#75178=CARTESIAN_POINT('Ctrl Pts',(78.3239309216268,-10.1907463443663,135.722888454149));
#75179=CARTESIAN_POINT('Ctrl Pts',(78.2846657944256,-10.1312056071672,135.719033237672));
#75180=CARTESIAN_POINT('Ctrl Pts',(78.2453991320754,-10.0716625421035,135.715177870467));
#75181=CARTESIAN_POINT('Ctrl Pts',(78.2092397381529,-10.0100776027747,135.711322503263));
#75182=CARTESIAN_POINT('Ctrl Pts',(78.176392312414,-9.94681178925757,135.707467136058));
#75183=CARTESIAN_POINT('Ctrl Pts',(78.1435105043773,-9.88347975368548,135.703607733335));
#75184=CARTESIAN_POINT('Ctrl Pts',(78.1139478091927,-9.81846376375441,135.699748330612));
#75185=CARTESIAN_POINT('Ctrl Pts',(78.0878622116925,-9.75214801803009,135.69588892789));
#75186=CARTESIAN_POINT('Ctrl Pts',(78.0617618443221,-9.68579472380968,135.692027339943));
#75187=CARTESIAN_POINT('Ctrl Pts',(78.0391426479369,-9.61814066971615,135.688165751996));
#75188=CARTESIAN_POINT('Ctrl Pts',(78.020112920712,-9.54958594939138,135.684304164049));
#75189=CARTESIAN_POINT('Ctrl Pts',(78.0010499002972,-9.4809112901261,135.680435820115));
#75190=CARTESIAN_POINT('Ctrl Pts',(77.9855889924593,-9.41133329297089,135.676567476182));
#75191=CARTESIAN_POINT('Ctrl Pts',(77.9737873736295,-9.34126229682866,135.672699132248));
#75192=CARTESIAN_POINT('Ctrl Pts',(77.9667799119894,-9.29965615578732,135.670402220942));
#75193=CARTESIAN_POINT('Ctrl Pts',(77.9610615928321,-9.25787632082747,135.668105309635));
#75194=CARTESIAN_POINT('Ctrl Pts',(77.9566356952625,-9.21600898274021,135.665808398329));
#75195=CARTESIAN_POINT('Ctrl Pts',(77.9490991887904,-9.14471644614228,135.66189717204));
#75196=CARTESIAN_POINT('Ctrl Pts',(77.94529286412,-9.07302272422374,135.657985945751));
#75197=CARTESIAN_POINT('Ctrl Pts',(77.9452503599685,-9.00121626084845,135.654074719462));
#75198=CARTESIAN_POINT('Origin',(80.,-9.,141.545925280538));
#75199=CARTESIAN_POINT('',(81.2520391107129,-7.37076839346112,136.806140361831));
#75200=CARTESIAN_POINT('',(81.2520391107129,-7.37076839346111,136.747866921905));
#75201=CARTESIAN_POINT('',(81.2520391107129,-7.37076839346111,141.545925280538));
#75202=CARTESIAN_POINT('',(77.9452505319477,-9.0014785258654,136.295925280587));
#75203=CARTESIAN_POINT('Ctrl Pts',(81.2520391107129,-7.37076839346111,136.747866921905));
#75204=CARTESIAN_POINT('Ctrl Pts',(81.3085184556658,-7.41417189026582,136.74401000071));
#75205=CARTESIAN_POINT('Ctrl Pts',(81.3627855884167,-7.46055213904031,136.740153079514));
#75206=CARTESIAN_POINT('Ctrl Pts',(81.4145162201043,-7.50965056930868,136.736296158318));
#75207=CARTESIAN_POINT('Ctrl Pts',(81.4662266025468,-7.5587297806711,136.732440746861));
#75208=CARTESIAN_POINT('Ctrl Pts',(81.5154021025145,-7.61052472766807,136.728585335404));
#75209=CARTESIAN_POINT('Ctrl Pts',(81.5617531766557,-7.66473801158507,136.724729923947));
#75210=CARTESIAN_POINT('Ctrl Pts',(81.6081016121926,-7.71894820932962,136.720874731965));
#75211=CARTESIAN_POINT('Ctrl Pts',(81.6516256266796,-7.77557610039535,136.717019539983));
#75212=CARTESIAN_POINT('Ctrl Pts',(81.6920752305164,-7.83429035485974,136.713164348002));
#75213=CARTESIAN_POINT('Ctrl Pts',(81.7325646822271,-7.89306245014317,136.709305358178));
#75214=CARTESIAN_POINT('Ctrl Pts',(81.7699733971474,-7.95392461339505,136.705446368354));
#75215=CARTESIAN_POINT('Ctrl Pts',(81.8040946199613,-8.01651631191624,136.70158737853));
#75216=CARTESIAN_POINT('Ctrl Pts',(81.8382322243345,-8.07913806063906,136.69772653601));
#75217=CARTESIAN_POINT('Ctrl Pts',(81.8690789820362,-8.14349056008712,136.693865693489));
#75218=CARTESIAN_POINT('Ctrl Pts',(81.8964753095992,-8.2091909442978,136.690004850969));
#75219=CARTESIAN_POINT('Ctrl Pts',(81.9239220747863,-8.27501228527817,136.686136900498));
#75220=CARTESIAN_POINT('Ctrl Pts',(81.9479055541882,-8.34218601034174,136.682268950028));
#75221=CARTESIAN_POINT('Ctrl Pts',(81.9683154627715,-8.41031211517045,136.678400999558));
#75222=CARTESIAN_POINT('Ctrl Pts',(81.9862840426306,-8.47028932428496,136.674995713511));
#75223=CARTESIAN_POINT('Ctrl Pts',(82.0014835403753,-8.53100427227776,136.671590427464));
#75224=CARTESIAN_POINT('Ctrl Pts',(82.0138717544801,-8.59217881491123,136.668185141417));
#75225=CARTESIAN_POINT('Ctrl Pts',(82.0279472318517,-8.66168527349155,136.66431605857));
#75226=CARTESIAN_POINT('Ctrl Pts',(82.0384476506382,-8.73205742237571,136.660446975723));
#75227=CARTESIAN_POINT('Ctrl Pts',(82.045274300028,-8.80289444415531,136.656577892876));
#75228=CARTESIAN_POINT('Ctrl Pts',(82.0520907780507,-8.87362592230528,136.65271457477));
#75229=CARTESIAN_POINT('Ctrl Pts',(82.0552443056657,-8.94482041888086,136.648851256664));
#75230=CARTESIAN_POINT('Ctrl Pts',(82.0546871818792,-9.01606695744053,136.644987938557));
#75231=CARTESIAN_POINT('Ctrl Pts',(82.0541307115987,-9.08722992383783,136.641129152121));
#75232=CARTESIAN_POINT('Ctrl Pts',(82.0498722394196,-9.15844432755198,136.637270365686));
#75233=CARTESIAN_POINT('Ctrl Pts',(82.0419160056416,-9.22929585343982,136.63341157925));
#75234=CARTESIAN_POINT('Ctrl Pts',(82.0339647837074,-9.30010274806166,136.629555223566));
#75235=CARTESIAN_POINT('Ctrl Pts',(82.022320475588,-9.37054673676131,136.625698867883));
#75236=CARTESIAN_POINT('Ctrl Pts',(82.0070393018439,-9.44021676859681,136.6218425122));
#75237=CARTESIAN_POINT('Ctrl Pts',(81.9917626423116,-9.50986621920728,136.617987295723));
#75238=CARTESIAN_POINT('Ctrl Pts',(81.9728513540896,-9.57874169261185,136.614132079245));
#75239=CARTESIAN_POINT('Ctrl Pts',(81.9504127845803,-9.64644221106426,136.610276862768));
#75240=CARTESIAN_POINT('Ctrl Pts',(81.9279733377901,-9.7141453764044,136.606421495564));
#75241=CARTESIAN_POINT('Ctrl Pts',(81.9020064908407,-9.78067303516738,136.602566128359));
#75242=CARTESIAN_POINT('Ctrl Pts',(81.8726689525193,-9.84564091479191,136.598710761154));
#75243=CARTESIAN_POINT('Ctrl Pts',(81.8433007057953,-9.91067679807057,136.594851358432));
#75244=CARTESIAN_POINT('Ctrl Pts',(81.8105549249676,-9.97414919940608,136.590991955709));
#75245=CARTESIAN_POINT('Ctrl Pts',(81.7746354615352,-10.0356961625697,136.587132552986));
#75246=CARTESIAN_POINT('Ctrl Pts',(81.7386956602205,-10.0972779741073,136.583270965039));
#75247=CARTESIAN_POINT('Ctrl Pts',(81.6995788656065,-10.1569317707976,136.579409377092));
#75248=CARTESIAN_POINT('Ctrl Pts',(81.657532177304,-10.2143247686273,136.575547789145));
#75249=CARTESIAN_POINT('Ctrl Pts',(81.6154119268133,-10.2718181775639,136.571679445212));
#75250=CARTESIAN_POINT('Ctrl Pts',(81.5703518557309,-10.3270425141682,136.567811101278));
#75251=CARTESIAN_POINT('Ctrl Pts',(81.5226387640878,-10.3796987919823,136.563942757345));
#75252=CARTESIAN_POINT('Ctrl Pts',(81.4943081033344,-10.4109645744313,136.561645846039));
#75253=CARTESIAN_POINT('Ctrl Pts',(81.4650427907927,-10.441325655851,136.559348934732));
#75254=CARTESIAN_POINT('Ctrl Pts',(81.4349084744057,-10.4707260902625,136.557052023426));
#75255=CARTESIAN_POINT('Ctrl Pts',(81.3841480613615,-10.520250299647,136.553182940579));
#75256=CARTESIAN_POINT('Ctrl Pts',(81.3307213118379,-10.5672405174436,136.549313857732));
#75257=CARTESIAN_POINT('Ctrl Pts',(81.2749114269963,-10.61139641796,136.545444774885));
#75258=CARTESIAN_POINT('Ctrl Pts',(81.2191846960997,-10.6554865283868,136.541581456779));
#75259=CARTESIAN_POINT('Ctrl Pts',(81.1610822558933,-10.696750405096,136.537718138672));
#75260=CARTESIAN_POINT('Ctrl Pts',(81.1009235091993,-10.734925067371,136.533854820566));
#75261=CARTESIAN_POINT('Ctrl Pts',(81.040835328692,-10.7730549507819,136.52999603413));
#75262=CARTESIAN_POINT('Ctrl Pts',(80.9786960410183,-10.8081025585325,136.526137247694));
#75263=CARTESIAN_POINT('Ctrl Pts',(80.9148560258896,-10.8398467366587,136.522278461258));
#75264=CARTESIAN_POINT('Ctrl Pts',(80.8510562252893,-10.8715709182803,136.518422105575));
#75265=CARTESIAN_POINT('Ctrl Pts',(80.7855582566906,-10.8999955830086,136.514565749892));
#75266=CARTESIAN_POINT('Ctrl Pts',(80.7187379505123,-10.9249450176546,136.510709394209));
#75267=CARTESIAN_POINT('Ctrl Pts',(80.6519373837214,-10.9498870819879,136.506854177731));
#75268=CARTESIAN_POINT('Ctrl Pts',(80.5838157097101,-10.971355784529,136.502998961254));
#75269=CARTESIAN_POINT('Ctrl Pts',(80.5147680262649,-10.9892238289432,136.499143744777));
#75270=CARTESIAN_POINT('Ctrl Pts',(80.445717643262,-11.0070925719444,136.495288377572));
#75271=CARTESIAN_POINT('Ctrl Pts',(80.3757416497898,-11.0213602577598,136.491433010368));
#75272=CARTESIAN_POINT('Ctrl Pts',(80.3052478817002,-11.0319501207504,136.487577643163));
#75273=CARTESIAN_POINT('Ctrl Pts',(80.234680325858,-11.0425510684398,136.48371824044));
#75274=CARTESIAN_POINT('Ctrl Pts',(80.1635943948841,-11.0494664361707,136.479858837718));
#75275=CARTESIAN_POINT('Ctrl Pts',(80.0924047452201,-11.0526711683952,136.475999434995));
#75276=CARTESIAN_POINT('Ctrl Pts',(80.0211747874173,-11.0558777151642,136.472137847048));
#75277=CARTESIAN_POINT('Ctrl Pts',(79.9498414800191,-11.0553694474645,136.468276259101));
#75278=CARTESIAN_POINT('Ctrl Pts',(79.8788184278489,-11.0511734663531,136.464414671154));
#75279=CARTESIAN_POINT('Ctrl Pts',(79.8076711183032,-11.0469701442224,136.46054632722));
#75280=CARTESIAN_POINT('Ctrl Pts',(79.7368356306459,-11.039066281392,136.456677983287));
#75281=CARTESIAN_POINT('Ctrl Pts',(79.6667187079824,-11.0275406636837,136.452809639354));
#75282=CARTESIAN_POINT('Ctrl Pts',(79.6250852970937,-11.0206970835669,136.450512728047));
#75283=CARTESIAN_POINT('Ctrl Pts',(79.5837050187289,-11.0125775795324,136.448215816741));
#75284=CARTESIAN_POINT('Ctrl Pts',(79.542660481108,-11.0032069605908,136.445918905434));
#75285=CARTESIAN_POINT('Ctrl Pts',(79.4735221055763,-10.9874224150972,136.442049822587));
#75286=CARTESIAN_POINT('Ctrl Pts',(79.4050664517629,-10.9680234049621,136.43818073974));
#75287=CARTESIAN_POINT('Ctrl Pts',(79.3376994359524,-10.9450849661036,136.434311656893));
#75288=CARTESIAN_POINT('Ctrl Pts',(79.2704327936357,-10.922180704375,136.430448338787));
#75289=CARTESIAN_POINT('Ctrl Pts',(79.2042520257743,-10.8957476371235,136.426585020681));
#75290=CARTESIAN_POINT('Ctrl Pts',(79.1395513089721,-10.8659114696599,136.422721702574));
#75291=CARTESIAN_POINT('Ctrl Pts',(79.0749264860859,-10.8361103000093,136.418862916138));
#75292=CARTESIAN_POINT('Ctrl Pts',(79.011778704775,-10.8029141617227,136.415004129703));
#75293=CARTESIAN_POINT('Ctrl Pts',(78.9504838028598,-10.7664974708276,136.411145343267));
#75294=CARTESIAN_POINT('Ctrl Pts',(78.8892275122382,-10.7301037197774,136.407288987584));
#75295=CARTESIAN_POINT('Ctrl Pts',(78.8298222019966,-10.6904936885913,136.4034326319));
#75296=CARTESIAN_POINT('Ctrl Pts',(78.7726193376199,-10.6478878214597,136.399576276217));
#75297=CARTESIAN_POINT('Ctrl Pts',(78.715433371542,-10.605294540528,136.39572105974));
#75298=CARTESIAN_POINT('Ctrl Pts',(78.6604489490394,-10.5597074706402,136.391865843263));
#75299=CARTESIAN_POINT('Ctrl Pts',(78.6079873092376,-10.5113895034889,136.388010626785));
#75300=CARTESIAN_POINT('Ctrl Pts',(78.5555236183424,-10.4630696472495,136.384155259581));
#75301=CARTESIAN_POINT('Ctrl Pts',(78.505583261801,-10.4120190124883,136.380299892376));
#75302=CARTESIAN_POINT('Ctrl Pts',(78.458451935106,-10.3585385994228,136.376444525171));
#75303=CARTESIAN_POINT('Ctrl Pts',(78.4112712747642,-10.3050022069484,136.372585122449));
#75304=CARTESIAN_POINT('Ctrl Pts',(78.3669058355862,-10.2490313243411,136.368725719726));
#75305=CARTESIAN_POINT('Ctrl Pts',(78.3256015690602,-10.1909607285575,136.364866317003));
#75306=CARTESIAN_POINT('Ctrl Pts',(78.284273915734,-10.1328572527464,136.361004729056));
#75307=CARTESIAN_POINT('Ctrl Pts',(78.246011146134,-10.0726521072607,136.357143141109));
#75308=CARTESIAN_POINT('Ctrl Pts',(78.211014822882,-10.0107074742734,136.353281553162));
#75309=CARTESIAN_POINT('Ctrl Pts',(78.1759572723082,-9.94865446693053,136.349413209229));
#75310=CARTESIAN_POINT('Ctrl Pts',(78.1441777944373,-9.88485633102083,136.345544865295));
#75311=CARTESIAN_POINT('Ctrl Pts',(78.11583080815,-9.81969751676059,136.341676521362));
#75312=CARTESIAN_POINT('Ctrl Pts',(78.0989991834482,-9.78100808796084,136.339379610055));
#75313=CARTESIAN_POINT('Ctrl Pts',(78.0833767987335,-9.74183928814454,136.337082698749));
#75314=CARTESIAN_POINT('Ctrl Pts',(78.0689876162083,-9.7022739751288,136.334785787443));
#75315=CARTESIAN_POINT('Ctrl Pts',(78.0409616303172,-9.62521213353946,136.330312065342));
#75316=CARTESIAN_POINT('Ctrl Pts',(78.0175257042645,-9.54639696143254,136.325838343242));
#75317=CARTESIAN_POINT('Ctrl Pts',(77.9988702448821,-9.46634457826986,136.321364621142));
#75318=CARTESIAN_POINT('Ctrl Pts',(77.980378474062,-9.38699459858276,136.316930152813));
#75319=CARTESIAN_POINT('Ctrl Pts',(77.9665837380255,-9.30642919168824,136.312495684485));
#75320=CARTESIAN_POINT('Ctrl Pts',(77.9576251286369,-9.22517203939353,136.308061216156));
#75321=CARTESIAN_POINT('Ctrl Pts',(77.9494527016197,-9.15104578631668,136.3040159043));
#75322=CARTESIAN_POINT('Ctrl Pts',(77.9453044026692,-9.07634420048478,136.299970592443));
#75323=CARTESIAN_POINT('Ctrl Pts',(77.9452505319477,-9.0014785258654,136.295925280587));
#75324=CARTESIAN_POINT('Ctrl Pts',(77.945250531947,-9.0014785249549,136.295925280538));
#75325=CARTESIAN_POINT('Ctrl Pts',(77.9451990745752,-8.92996670708856,136.292061191873));
#75326=CARTESIAN_POINT('Ctrl Pts',(77.9488851993071,-8.85842205612611,136.288197103208));
#75327=CARTESIAN_POINT('Ctrl Pts',(77.9562925982608,-8.78726161940889,136.284333014543));
#75328=CARTESIAN_POINT('Ctrl Pts',(77.963699599031,-8.71610500790984,136.280469133592));
#75329=CARTESIAN_POINT('Ctrl Pts',(77.9748274258945,-8.64533304915,136.276605252641));
#75330=CARTESIAN_POINT('Ctrl Pts',(77.9896079183788,-8.57535751430792,136.272741371689));
#75331=CARTESIAN_POINT('Ctrl Pts',(78.004392467588,-8.505362773645,136.268876430239));
#75332=CARTESIAN_POINT('Ctrl Pts',(78.0228315710416,-8.43616536208909,136.265011488788));
#75333=CARTESIAN_POINT('Ctrl Pts',(78.0448063606777,-8.36816505695425,136.261146547337));
#75334=CARTESIAN_POINT('Ctrl Pts',(78.0668090603739,-8.3000783850039,136.257276697046));
#75335=CARTESIAN_POINT('Ctrl Pts',(78.0923562553075,-8.23319231170985,136.253406846754));
#75336=CARTESIAN_POINT('Ctrl Pts',(78.1212800534333,-8.16788887468532,136.249536996462));
#75337=CARTESIAN_POINT('Ctrl Pts',(78.150225897606,-8.10253566264064,136.245664196527));
#75338=CARTESIAN_POINT('Ctrl Pts',(78.1825532470501,-8.03876791594965,136.241791396591));
#75339=CARTESIAN_POINT('Ctrl Pts',(78.218048415587,-7.97694276147033,136.237918596656));
#75340=CARTESIAN_POINT('Ctrl Pts',(78.2536056682715,-7.91500946939994,136.234039022855));
#75341=CARTESIAN_POINT('Ctrl Pts',(78.2923415309161,-7.85502595047044,136.230159449055));
#75342=CARTESIAN_POINT('Ctrl Pts',(78.3339997518957,-7.79731935418567,136.226279875254));
#75343=CARTESIAN_POINT('Ctrl Pts',(78.3434032521695,-7.78429325798648,136.225404139987));
#75344=CARTESIAN_POINT('Ctrl Pts',(78.3529555021339,-7.7713830389363,136.224528404719));
#75345=CARTESIAN_POINT('Ctrl Pts',(78.3626532888616,-7.75859220639458,136.223652669452));
#75346=CARTESIAN_POINT('Ctrl Pts',(78.4054990456459,-7.70208107498526,136.219783586605));
#75347=CARTESIAN_POINT('Ctrl Pts',(78.4513577800799,-7.64768002160084,136.215914503758));
#75348=CARTESIAN_POINT('Ctrl Pts',(78.4999940143903,-7.59572808700198,136.212045420911));
#75349=CARTESIAN_POINT('Ctrl Pts',(78.5485577831372,-7.54385355819469,136.208182102805));
#75350=CARTESIAN_POINT('Ctrl Pts',(78.5998905079846,-7.49442125662193,136.204318784698));
#75351=CARTESIAN_POINT('Ctrl Pts',(78.653715366554,-7.4477386662526,136.200455466592));
#75352=CARTESIAN_POINT('Ctrl Pts',(78.7074770885851,-7.40111083454381,136.196596680156));
#75353=CARTESIAN_POINT('Ctrl Pts',(78.7637247725266,-7.35722662402505,136.19273789372));
#75354=CARTESIAN_POINT('Ctrl Pts',(78.8221447529236,-7.31635675410897,136.188879107284));
#75355=CARTESIAN_POINT('Ctrl Pts',(78.8805279330166,-7.27551262921406,136.185022751601));
#75356=CARTESIAN_POINT('Ctrl Pts',(78.9410802976006,-7.23767935551522,136.181166395918));
#75357=CARTESIAN_POINT('Ctrl Pts',(79.0034562665656,-7.20308649349707,136.177310040234));
#75358=CARTESIAN_POINT('Ctrl Pts',(79.0658138090448,-7.16850385055676,136.173454823757));
#75359=CARTESIAN_POINT('Ctrl Pts',(79.1299934618201,-7.13715995436414,136.16959960728));
#75360=CARTESIAN_POINT('Ctrl Pts',(79.1956234031311,-7.10923934541951,136.165744390803));
#75361=CARTESIAN_POINT('Ctrl Pts',(79.2612559103764,-7.08131764486262,136.161889023598));
#75362=CARTESIAN_POINT('Ctrl Pts',(79.3283383708565,-7.05681968541932,136.158033656394));
#75363=CARTESIAN_POINT('Ctrl Pts',(79.3964788642983,-7.0358819278716,136.154178289189));
#75364=CARTESIAN_POINT('Ctrl Pts',(79.464690682256,-7.01492225420114,136.150318886466));
#75365=CARTESIAN_POINT('Ctrl Pts',(79.5339622786305,-6.99753036445279,136.146459483743));
#75366=CARTESIAN_POINT('Ctrl Pts',(79.6038873114514,-6.98379259487751,136.142600081021));
#75367=CARTESIAN_POINT('Ctrl Pts',(79.6738519363752,-6.97004704686918,136.138738493074));
#75368=CARTESIAN_POINT('Ctrl Pts',(79.7444702531337,-6.95995980648334,136.134876905127));
#75369=CARTESIAN_POINT('Ctrl Pts',(79.8153292167477,-6.95356547519522,136.13101531718));
#75370=CARTESIAN_POINT('Ctrl Pts',(79.8863121506583,-6.94715995679532,136.127146973246));
#75371=CARTESIAN_POINT('Ctrl Pts',(79.9575360864152,-6.94446026522219,136.123278629313));
#75372=CARTESIAN_POINT('Ctrl Pts',(80.0285870917951,-6.94544887124153,136.119410285379));
#75373=CARTESIAN_POINT('Ctrl Pts',(80.0707751341201,-6.94603587704622,136.117113374073));
#75374=CARTESIAN_POINT('Ctrl Pts',(80.1129022677805,-6.94792224733129,136.114816462766));
#75375=CARTESIAN_POINT('Ctrl Pts',(80.1548831168874,-6.95109571170265,136.11251955146));
#75376=CARTESIAN_POINT('Ctrl Pts',(80.2255915701652,-6.9564407859926,136.108650857776));
#75377=CARTESIAN_POINT('Ctrl Pts',(80.2961614847423,-6.96546088698956,136.104782164092));
#75378=CARTESIAN_POINT('Ctrl Pts',(80.3661804272604,-6.97814207789188,136.100913470407));
#75379=CARTESIAN_POINT('Ctrl Pts',(80.436100256216,-6.99080531825163,136.097050252956));
#75380=CARTESIAN_POINT('Ctrl Pts',(80.5054701866994,-7.00711927976587,136.093187035504));
#75381=CARTESIAN_POINT('Ctrl Pts',(80.5738817794945,-7.02701817908419,136.089323818053));
#75382=CARTESIAN_POINT('Ctrl Pts',(80.6422141511602,-7.04689403533025,136.085465074235));
#75383=CARTESIAN_POINT('Ctrl Pts',(80.7095899251629,-7.07034644905535,136.081606330418));
#75384=CARTESIAN_POINT('Ctrl Pts',(80.77561154664,-7.09725874296618,136.077747586601));
#75385=CARTESIAN_POINT('Ctrl Pts',(80.8415882785365,-7.12415273860499,136.07389146643));
#75386=CARTESIAN_POINT('Ctrl Pts',(80.9062122370551,-7.15450176135287,136.070035346259));
#75387=CARTESIAN_POINT('Ctrl Pts',(80.9691031912749,-7.18814002550948,136.066179226088));
#75388=CARTESIAN_POINT('Ctrl Pts',(81.0319836313122,-7.22177266598216,136.062323750588));
#75389=CARTESIAN_POINT('Ctrl Pts',(81.0931312103806,-7.25869323415421,136.058468275088));
#75390=CARTESIAN_POINT('Ctrl Pts',(81.1521891448271,-7.29868940606292,136.054612799588));
#75391=CARTESIAN_POINT('Ctrl Pts',(81.1861856902748,-7.32171309777801,136.052393405203));
#75392=CARTESIAN_POINT('Ctrl Pts',(81.2194902560995,-7.34575510571162,136.050174010819));
#75393=CARTESIAN_POINT('Ctrl Pts',(81.2520391107129,-7.37076839346111,136.047954616434));
#75394=CARTESIAN_POINT('',(77.9452507823625,-8.99820692503895,136.35407471951));
#75395=CARTESIAN_POINT('Ctrl Pts',(77.9452507823632,-8.99820692415778,136.354074719462));
#75396=CARTESIAN_POINT('Ctrl Pts',(77.9453413919223,-8.89437421594169,136.348435142862));
#75397=CARTESIAN_POINT('Ctrl Pts',(77.9533058453998,-8.79087359259561,136.342795566261));
#75398=CARTESIAN_POINT('Ctrl Pts',(77.9689745018475,-8.68865936925234,136.337155989661));
#75399=CARTESIAN_POINT('Ctrl Pts',(77.9731872821077,-8.66117736632162,136.3356396952));
#75400=CARTESIAN_POINT('Ctrl Pts',(77.9779567533565,-8.6337881827006,136.334123400739));
#75401=CARTESIAN_POINT('Ctrl Pts',(77.9832790921583,-8.60651004793739,136.332607106279));
#75402=CARTESIAN_POINT('Ctrl Pts',(77.9968599435675,-8.53690525411839,136.328738023432));
#75403=CARTESIAN_POINT('Ctrl Pts',(78.0140751186039,-8.46786804761569,136.324868940585));
#75404=CARTESIAN_POINT('Ctrl Pts',(78.0348625104967,-8.39980652298718,136.320999857738));
#75405=CARTESIAN_POINT('Ctrl Pts',(78.0556189302123,-8.33184640663594,136.317136539631));
#75406=CARTESIAN_POINT('Ctrl Pts',(78.0799368611765,-8.26485954738233,136.313273221525));
#75407=CARTESIAN_POINT('Ctrl Pts',(78.10770317995,-8.19924391520985,136.309409903418));
#75408=CARTESIAN_POINT('Ctrl Pts',(78.1354369288421,-8.13370525014871,136.305551116983));
#75409=CARTESIAN_POINT('Ctrl Pts',(78.1666108424926,-8.06953506244951,136.301692330547));
#75410=CARTESIAN_POINT('Ctrl Pts',(78.2010625289041,-8.00711453954285,136.297833544111));
#75411=CARTESIAN_POINT('Ctrl Pts',(78.2354925132795,-7.94473333698852,136.293977188428));
#75412=CARTESIAN_POINT('Ctrl Pts',(78.2731959397886,-7.88410003685616,136.290120832745));
#75413=CARTESIAN_POINT('Ctrl Pts',(78.31396363746,-7.82557292832084,136.286264477061));
#75414=CARTESIAN_POINT('Ctrl Pts',(78.3547192919453,-7.76706310927942,136.282409260584));
#75415=CARTESIAN_POINT('Ctrl Pts',(78.3985371429807,-7.71065864500986,136.278554044107));
#75416=CARTESIAN_POINT('Ctrl Pts',(78.4451646335603,-7.65668896164434,136.27469882763));
#75417=CARTESIAN_POINT('Ctrl Pts',(78.4917939471352,-7.60271716822562,136.270843460425));
#75418=CARTESIAN_POINT('Ctrl Pts',(78.5412327990923,-7.55118071085677,136.26698809322));
#75419=CARTESIAN_POINT('Ctrl Pts',(78.5931894143107,-7.50237470023623,136.263132726016));
#75420=CARTESIAN_POINT('Ctrl Pts',(78.6452004139374,-7.45351760303132,136.259273323293));
#75421=CARTESIAN_POINT('Ctrl Pts',(78.6997340829042,-7.40739699112836,136.25541392057));
#75422=CARTESIAN_POINT('Ctrl Pts',(78.7564636241791,-7.36426932396856,136.251554517847));
#75423=CARTESIAN_POINT('Ctrl Pts',(78.8132252861659,-7.32111723758483,136.2476929299));
#75424=CARTESIAN_POINT('Ctrl Pts',(78.8721848938302,-7.28096174301087,136.243831341954));
#75425=CARTESIAN_POINT('Ctrl Pts',(78.9329868490229,-7.24401580356145,136.239969754007));
#75426=CARTESIAN_POINT('Ctrl Pts',(78.9938951794156,-7.20700522586667,136.236101410073));
#75427=CARTESIAN_POINT('Ctrl Pts',(79.0566518647923,-7.17321564463468,136.23223306614));
#75428=CARTESIAN_POINT('Ctrl Pts',(79.1208775529782,-7.14281361041968,136.228364722206));
#75429=CARTESIAN_POINT('Ctrl Pts',(79.1590129183687,-7.12476175739713,136.2260678109));
#75430=CARTESIAN_POINT('Ctrl Pts',(79.1976658166295,-7.10790331027639,136.223770899593));
#75431=CARTESIAN_POINT('Ctrl Pts',(79.2367541927432,-7.09226485061344,136.221473988287));
#75432=CARTESIAN_POINT('Ctrl Pts',(79.3025974689338,-7.06592230274737,136.21760490544));
#75433=CARTESIAN_POINT('Ctrl Pts',(79.3699350818581,-7.042940918566,136.213735822593));
#75434=CARTESIAN_POINT('Ctrl Pts',(79.4383904922889,-7.02348986257381,136.209866739746));
#75435=CARTESIAN_POINT('Ctrl Pts',(79.5067439075722,-7.00406778768498,136.20600342164));
#75436=CARTESIAN_POINT('Ctrl Pts',(79.576211350986,-6.98816573169893,136.202140103533));
#75437=CARTESIAN_POINT('Ctrl Pts',(79.646397118856,-6.97590450695954,136.198276785427));
#75438=CARTESIAN_POINT('Ctrl Pts',(79.7165005588474,-6.96365766463206,136.194417998991));
#75439=CARTESIAN_POINT('Ctrl Pts',(79.787320173404,-6.95504325370055,136.190559212555));
#75440=CARTESIAN_POINT('Ctrl Pts',(79.8584476361331,-6.95013159183725,136.186700426119));
#75441=CARTESIAN_POINT('Ctrl Pts',(79.9295302937763,-6.94522302396076,136.182844070436));
#75442=CARTESIAN_POINT('Ctrl Pts',(80.0009199313708,-6.94401261097418,136.178987714753));
#75443=CARTESIAN_POINT('Ctrl Pts',(80.0722020881108,-6.94651895042286,136.17513135907));
#75444=CARTESIAN_POINT('Ctrl Pts',(80.1434631873879,-6.94902454947377,136.171276142592));
#75445=CARTESIAN_POINT('Ctrl Pts',(80.2146163836262,-6.95524470413217,136.167420926115));
#75446=CARTESIAN_POINT('Ctrl Pts',(80.2852479330856,-6.96514590715442,136.163565709638));
#75447=CARTESIAN_POINT('Ctrl Pts',(80.3558822440273,-6.9750474972841,136.159710342433));
#75448=CARTESIAN_POINT('Ctrl Pts',(80.4259943869255,-6.98863035188814,136.155854975229));
#75449=CARTESIAN_POINT('Ctrl Pts',(80.4951781764373,-7.00580940327154,136.151999608024));
#75450=CARTESIAN_POINT('Ctrl Pts',(80.5644343825113,-7.02300643643724,136.148140205301));
#75451=CARTESIAN_POINT('Ctrl Pts',(80.6327598229708,-7.04380706333403,136.144280802578));
#75452=CARTESIAN_POINT('Ctrl Pts',(80.6997617894774,-7.06807582951935,136.140421399856));
#75453=CARTESIAN_POINT('Ctrl Pts',(80.7668016930238,-7.09235833687073,136.136559811909));
#75454=CARTESIAN_POINT('Ctrl Pts',(80.8325161831507,-7.12011270351405,136.132698223962));
#75455=CARTESIAN_POINT('Ctrl Pts',(80.8965334728951,-7.1511556867928,136.128836636015));
#75456=CARTESIAN_POINT('Ctrl Pts',(80.9606627631826,-7.18225298088349,136.124968292081));
#75457=CARTESIAN_POINT('Ctrl Pts',(81.0230884991664,-7.21665014422836,136.121099948148));
#75458=CARTESIAN_POINT('Ctrl Pts',(81.0834650030631,-7.25411880426027,136.117231604214));
#75459=CARTESIAN_POINT('Ctrl Pts',(81.1193148335923,-7.27636661633304,136.114934692908));
#75460=CARTESIAN_POINT('Ctrl Pts',(81.1544427439922,-7.29969650476408,136.112637781602));
#75461=CARTESIAN_POINT('Ctrl Pts',(81.1887818971918,-7.32405394973193,136.110340870295));
#75462=CARTESIAN_POINT('Ctrl Pts',(81.2101480388384,-7.3392093793463,136.108911710641));
#75463=CARTESIAN_POINT('Ctrl Pts',(81.231239727959,-7.3547843918115,136.107482550986));
#75464=CARTESIAN_POINT('Ctrl Pts',(81.2520391107129,-7.37076839346111,136.106053391332));
#75465=CARTESIAN_POINT('Ctrl Pts',(81.2520391107129,-7.37076839346113,136.806140361831));
#75466=CARTESIAN_POINT('Ctrl Pts',(81.3085695514287,-7.41421115656367,136.802278511048));
#75467=CARTESIAN_POINT('Ctrl Pts',(81.3627835844241,-7.46055901156867,136.798416660265));
#75468=CARTESIAN_POINT('Ctrl Pts',(81.414383045544,-7.50952418235728,136.794554809483));
#75469=CARTESIAN_POINT('Ctrl Pts',(81.4660713106751,-7.55857362347511,136.790686312355));
#75470=CARTESIAN_POINT('Ctrl Pts',(81.5151356879525,-7.61024901931506,136.786817815227));
#75471=CARTESIAN_POINT('Ctrl Pts',(81.5613166927242,-7.66422765879788,136.782949318099));
#75472=CARTESIAN_POINT('Ctrl Pts',(81.584435026541,-7.69124950929039,136.781012738148));
#75473=CARTESIAN_POINT('Ctrl Pts',(81.6068314370808,-7.71884807176579,136.779076158196));
#75474=CARTESIAN_POINT('Ctrl Pts',(81.6284774886262,-7.74698019507359,136.777139578245));
#75475=CARTESIAN_POINT('Ctrl Pts',(81.6717240205759,-7.80318521550851,136.773270495398));
#75476=CARTESIAN_POINT('Ctrl Pts',(81.7121420629601,-7.86174185461321,136.769401412551));
#75477=CARTESIAN_POINT('Ctrl Pts',(81.74946647925,-7.92233372490335,136.765532329704));
#75478=CARTESIAN_POINT('Ctrl Pts',(81.7867352840211,-7.98283531632865,136.761669011597));
#75479=CARTESIAN_POINT('Ctrl Pts',(81.8209193594215,-8.04536570948455,136.757805693491));
#75480=CARTESIAN_POINT('Ctrl Pts',(81.8517948922016,-8.1095769321744,136.753942375384));
#75481=CARTESIAN_POINT('Ctrl Pts',(81.8826342079938,-8.17371283512477,136.750083588949));
#75482=CARTESIAN_POINT('Ctrl Pts',(81.9101724804935,-8.23952521564348,136.746224802513));
#75483=CARTESIAN_POINT('Ctrl Pts',(81.9342310595732,-8.30664022997986,136.742366016077));
#75484=CARTESIAN_POINT('Ctrl Pts',(81.9582744835122,-8.37371296677855,136.738509660393));
#75485=CARTESIAN_POINT('Ctrl Pts',(81.9788423992928,-8.4420862532001,136.73465330471));
#75486=CARTESIAN_POINT('Ctrl Pts',(81.9958042626971,-8.51136628493326,136.730796949027));
#75487=CARTESIAN_POINT('Ctrl Pts',(82.0127611153972,-8.58062585065134,136.726941732549));
#75488=CARTESIAN_POINT('Ctrl Pts',(82.0261139151062,-8.65079115831113,136.723086516072));
#75489=CARTESIAN_POINT('Ctrl Pts',(82.0357824558691,-8.72145493205695,136.719231299595));
#75490=CARTESIAN_POINT('Ctrl Pts',(82.0454513746432,-8.79212146854498,136.71537593239));
#75491=CARTESIAN_POINT('Ctrl Pts',(82.0514356848208,-8.86328602821354,136.711520565186));
#75492=CARTESIAN_POINT('Ctrl Pts',(82.0537068542763,-8.93453459540696,136.707665197981));
#75493=CARTESIAN_POINT('Ctrl Pts',(82.0559804010269,-9.00585774042168,136.703805795258));
#75494=CARTESIAN_POINT('Ctrl Pts',(82.0545330329304,-9.07726458196395,136.699946392535));
#75495=CARTESIAN_POINT('Ctrl Pts',(82.0493883707933,-9.14834037938871,136.696086989812));
#75496=CARTESIAN_POINT('Ctrl Pts',(82.0442407957081,-9.2194564204883,136.692225401865));
#75497=CARTESIAN_POINT('Ctrl Pts',(82.0353918194841,-9.29024056207635,136.688363813918));
#75498=CARTESIAN_POINT('Ctrl Pts',(82.022916738459,-9.36028520891424,136.684502225971));
#75499=CARTESIAN_POINT('Ctrl Pts',(82.0104198318325,-9.43045240137242,136.680633882038));
#75500=CARTESIAN_POINT('Ctrl Pts',(81.9942842644375,-9.49987704270607,136.676765538104));
#75501=CARTESIAN_POINT('Ctrl Pts',(81.9746358599068,-9.56816439810169,136.672897194171));
#75502=CARTESIAN_POINT('Ctrl Pts',(81.9629692027315,-9.60871146458532,136.670600282865));
#75503=CARTESIAN_POINT('Ctrl Pts',(81.9500649911238,-9.64885788541115,136.668303371559));
#75504=CARTESIAN_POINT('Ctrl Pts',(81.9359575268557,-9.68852452150279,136.666006460253));
#75505=CARTESIAN_POINT('Ctrl Pts',(81.9121938979014,-9.75534186046859,136.662137377406));
#75506=CARTESIAN_POINT('Ctrl Pts',(81.8849204792404,-9.82105836347765,136.658268294559));
#75507=CARTESIAN_POINT('Ctrl Pts',(81.8542592736282,-9.8852796782169,136.654399211712));
#75508=CARTESIAN_POINT('Ctrl Pts',(81.8236437516832,-9.94940530640005,136.650535893606));
#75509=CARTESIAN_POINT('Ctrl Pts',(81.7896506697926,-10.0120397335354,136.6466725755));
#75510=CARTESIAN_POINT('Ctrl Pts',(81.7524509790069,-10.0728061934375,136.642809257393));
#75511=CARTESIAN_POINT('Ctrl Pts',(81.7152949234441,-10.1335013743055,136.638950470957));
#75512=CARTESIAN_POINT('Ctrl Pts',(81.6749399827043,-10.1923325279531,136.635091684522));
#75513=CARTESIAN_POINT('Ctrl Pts',(81.631603338975,-10.2489467990054,136.631232898086));
#75514=CARTESIAN_POINT('Ctrl Pts',(81.5882939941534,-10.3055254072183,136.627376542403));
#75515=CARTESIAN_POINT('Ctrl Pts',(81.5420069673467,-10.3598895185864,136.623520186719));
#75516=CARTESIAN_POINT('Ctrl Pts',(81.4930023019683,-10.4117158668859,136.619663831036));
#75517=CARTESIAN_POINT('Ctrl Pts',(81.4440121130588,-10.4635269051631,136.615808614559));
#75518=CARTESIAN_POINT('Ctrl Pts',(81.3923062129689,-10.5128013159132,136.611953398082));
#75519=CARTESIAN_POINT('Ctrl Pts',(81.3381832654853,-10.5592508170513,136.608098181605));
#75520=CARTESIAN_POINT('Ctrl Pts',(81.2840582019563,-10.605702134226,136.6042428144));
#75521=CARTESIAN_POINT('Ctrl Pts',(81.2275162734896,-10.6493280078128,136.600387447195));
#75522=CARTESIAN_POINT('Ctrl Pts',(81.1688898330688,-10.689879913085,136.596532079991));
#75523=CARTESIAN_POINT('Ctrl Pts',(81.1102020267516,-10.7304742651441,136.592672677268));
#75524=CARTESIAN_POINT('Ctrl Pts',(81.0494257532268,-10.7679879489103,136.588813274545));
#75525=CARTESIAN_POINT('Ctrl Pts',(80.9869222612899,-10.8022158618408,136.584953871822));
#75526=CARTESIAN_POINT('Ctrl Pts',(80.9243833793849,-10.8364631548843,136.581092283876));
#75527=CARTESIAN_POINT('Ctrl Pts',(80.8601157701031,-10.8674207626341,136.577230695929));
#75528=CARTESIAN_POINT('Ctrl Pts',(80.7945027069387,-10.894930872398,136.573369107982));
#75529=CARTESIAN_POINT('Ctrl Pts',(80.7287748513685,-10.922489112085,136.569500764048));
#75530=CARTESIAN_POINT('Ctrl Pts',(80.6616972995672,-10.9465876473852,136.565632420115));
#75531=CARTESIAN_POINT('Ctrl Pts',(80.5936699255709,-10.9671180905001,136.561764076181));
#75532=CARTESIAN_POINT('Ctrl Pts',(80.5532772285473,-10.9793084768076,136.559467164875));
#75533=CARTESIAN_POINT('Ctrl Pts',(80.5125499020237,-10.9902418503799,136.557170253568));
#75534=CARTESIAN_POINT('Ctrl Pts',(80.4715730379621,-10.9999041057929,136.554873342262));
#75535=CARTESIAN_POINT('Ctrl Pts',(80.4025486566509,-11.0161799047645,136.551004259415));
#75536=CARTESIAN_POINT('Ctrl Pts',(80.3325454831752,-11.028909941549,136.547135176568));
#75537=CARTESIAN_POINT('Ctrl Pts',(80.261960997851,-11.037982825763,136.543266093721));
#75538=CARTESIAN_POINT('Ctrl Pts',(80.1914816798898,-11.047042191832,136.539402775615));
#75539=CARTESIAN_POINT('Ctrl Pts',(80.1204232472095,-11.052455159967,136.535539457508));
#75540=CARTESIAN_POINT('Ctrl Pts',(80.0491949540307,-11.0541610012358,136.531676139402));
#75541=CARTESIAN_POINT('Ctrl Pts',(79.9780502116125,-11.0558648415534,136.527817352966));
#75542=CARTESIAN_POINT('Ctrl Pts',(79.9067364877533,-11.0538701809413,136.52395856653));
#75543=CARTESIAN_POINT('Ctrl Pts',(79.8356680232695,-11.0481680995279,136.520099780094));
#75544=CARTESIAN_POINT('Ctrl Pts',(79.7646443267072,-11.0424696100077,136.516243424411));
#75545=CARTESIAN_POINT('Ctrl Pts',(79.6938660660862,-11.0330683718492,136.512387068728));
#75546=CARTESIAN_POINT('Ctrl Pts',(79.6237458704838,-11.0200075228875,136.508530713045));
#75547=CARTESIAN_POINT('Ctrl Pts',(79.5536463890894,-11.0069505322314,136.504675496567));
#75548=CARTESIAN_POINT('Ctrl Pts',(79.4842050640868,-10.9902361659327,136.50082028009));
#75549=CARTESIAN_POINT('Ctrl Pts',(79.4158260801514,-10.9699589827884,136.496965063613));
#75550=CARTESIAN_POINT('Ctrl Pts',(79.3474444228022,-10.9496810068669,136.493109696408));
#75551=CARTESIAN_POINT('Ctrl Pts',(79.2801256540917,-10.9258400777689,136.489254329204));
#75552=CARTESIAN_POINT('Ctrl Pts',(79.214258829581,-10.8985806213086,136.485398961999));
#75553=CARTESIAN_POINT('Ctrl Pts',(79.1483230604661,-10.8712926316308,136.481539559276));
#75554=CARTESIAN_POINT('Ctrl Pts',(79.0838427191728,-10.8405791577151,136.477680156553));
#75555=CARTESIAN_POINT('Ctrl Pts',(79.021186053369,-10.8066324530409,136.473820753831));
#75556=CARTESIAN_POINT('Ctrl Pts',(78.9584939108687,-10.7726665274758,136.469959165884));
#75557=CARTESIAN_POINT('Ctrl Pts',(78.8976279140911,-10.7354639802963,136.466097577937));
#75558=CARTESIAN_POINT('Ctrl Pts',(78.838928526699,-10.6952612177439,136.46223598999));
#75559=CARTESIAN_POINT('Ctrl Pts',(78.7801264426247,-10.6549881190175,136.458367646056));
#75560=CARTESIAN_POINT('Ctrl Pts',(78.7234989219708,-10.6117046202694,136.454499302123));
#75561=CARTESIAN_POINT('Ctrl Pts',(78.6693539087199,-10.5656878814952,136.450630958189));
#75562=CARTESIAN_POINT('Ctrl Pts',(78.6372041580082,-10.5383644662566,136.448334046883));
#75563=CARTESIAN_POINT('Ctrl Pts',(78.605928968819,-10.5100781387365,136.446037135576));
#75564=CARTESIAN_POINT('Ctrl Pts',(78.5755863437915,-10.4808927370025,136.44374022427));
#75565=CARTESIAN_POINT('Ctrl Pts',(78.5252398783671,-10.4324664120564,136.439929038996));
#75566=CARTESIAN_POINT('Ctrl Pts',(78.4772533655966,-10.3813612335529,136.436117853722));
#75567=CARTESIAN_POINT('Ctrl Pts',(78.4319314969758,-10.3278398745042,136.432306668448));
#75568=CARTESIAN_POINT('Ctrl Pts',(78.3866698572087,-10.2743896407247,136.428500547911));
#75569=CARTESIAN_POINT('Ctrl Pts',(78.3440661660638,-10.2185299668056,136.424694427373));
#75570=CARTESIAN_POINT('Ctrl Pts',(78.3043895848264,-10.160561451391,136.420888306836));
#75571=CARTESIAN_POINT('Ctrl Pts',(78.2647515349153,-10.1026492312446,136.417085882556));
#75572=CARTESIAN_POINT('Ctrl Pts',(78.2280352419789,-10.0426326403597,136.413283458277));
#75573=CARTESIAN_POINT('Ctrl Pts',(78.1944694698461,-9.98084507807418,136.409481033997));
#75574=CARTESIAN_POINT('Ctrl Pts',(78.1609242933767,-9.91909542809487,136.405680942852));
#75575=CARTESIAN_POINT('Ctrl Pts',(78.1305260421695,-9.85557740152834,136.401880851706));
#75576=CARTESIAN_POINT('Ctrl Pts',(78.1034589744874,-9.79065144093181,136.398080760561));
#75577=CARTESIAN_POINT('Ctrl Pts',(78.0763869021235,-9.72571347557106,136.394279966781));
#75578=CARTESIAN_POINT('Ctrl Pts',(78.0526474523868,-9.65936751256437,136.390479173001));
#75579=CARTESIAN_POINT('Ctrl Pts',(78.0323772815509,-9.59199527054117,136.386678379222));
#75580=CARTESIAN_POINT('Ctrl Pts',(78.0121062978096,-9.52462032665303,136.382877433017));
#75581=CARTESIAN_POINT('Ctrl Pts',(77.9953050033776,-9.45621950575168,136.379076486812));
#75582=CARTESIAN_POINT('Ctrl Pts',(77.982059819869,-9.38718857409885,136.375275540607));
#75583=CARTESIAN_POINT('Ctrl Pts',(77.9687990309019,-9.31807631029025,136.371470116132));
#75584=CARTESIAN_POINT('Ctrl Pts',(77.9591028023245,-9.24833294891454,136.367664691657));
#75585=CARTESIAN_POINT('Ctrl Pts',(77.9530059961545,-9.17836230184846,136.363859267182));
#75586=CARTESIAN_POINT('Ctrl Pts',(77.9477806053111,-9.11839254583255,136.360597751292));
#75587=CARTESIAN_POINT('Ctrl Pts',(77.9451983804903,-9.05825611876819,136.357336235401));
#75588=CARTESIAN_POINT('Ctrl Pts',(77.9452507823624,-8.99820692503894,136.35407471951));
#75589=CARTESIAN_POINT('Origin',(80.,-9.,141.545925280538));
#75590=CARTESIAN_POINT('',(81.2520391107129,-7.37076839346112,137.506056941207));
#75591=CARTESIAN_POINT('',(81.2520391107129,-7.37076839346111,137.447938222965));
#75592=CARTESIAN_POINT('',(81.2520391107129,-7.37076839346111,141.545925280538));
#75593=CARTESIAN_POINT('',(77.9452500969073,-9.00063106298383,136.9959252805));
#75594=CARTESIAN_POINT('Ctrl Pts',(81.2520391107129,-7.37076839346111,137.447938222965));
#75595=CARTESIAN_POINT('Ctrl Pts',(81.2608674563024,-7.37755283952553,137.447331137763));
#75596=CARTESIAN_POINT('Ctrl Pts',(81.2696380423385,-7.38440703668142,137.446724052561));
#75597=CARTESIAN_POINT('Ctrl Pts',(81.278349723312,-7.39132988235372,137.446116967359));
#75598=CARTESIAN_POINT('Ctrl Pts',(81.3338711151901,-7.43545064718095,137.442247884513));
#75599=CARTESIAN_POINT('Ctrl Pts',(81.3872144048877,-7.48253558718294,137.438378801667));
#75600=CARTESIAN_POINT('Ctrl Pts',(81.4380459985655,-7.53234156953681,137.434509718821));
#75601=CARTESIAN_POINT('Ctrl Pts',(81.4888018557037,-7.58207334346069,137.430646400715));
#75602=CARTESIAN_POINT('Ctrl Pts',(81.5370531010313,-7.63451777501446,137.426783082609));
#75603=CARTESIAN_POINT('Ctrl Pts',(81.5824986302664,-7.68939111566231,137.422919764504));
#75604=CARTESIAN_POINT('Ctrl Pts',(81.627890851913,-7.74420008990238,137.419060978069));
#75605=CARTESIAN_POINT('Ctrl Pts',(81.6704835863641,-7.80143194162259,137.415202191634));
#75606=CARTESIAN_POINT('Ctrl Pts',(81.7100133228627,-7.86076692545724,137.411343405199));
#75607=CARTESIAN_POINT('Ctrl Pts',(81.7495181585258,-7.92006453260271,137.407487049517));
#75608=CARTESIAN_POINT('Ctrl Pts',(81.7859635555627,-7.98146224011746,137.403630693834));
#75609=CARTESIAN_POINT('Ctrl Pts',(81.8191278778122,-8.04460933296025,137.399774338152));
#75610=CARTESIAN_POINT('Ctrl Pts',(81.8522824029886,-8.10773777151931,137.395919121676));
#75611=CARTESIAN_POINT('Ctrl Pts',(81.8821575518824,-8.17261413959968,137.392063905199));
#75612=CARTESIAN_POINT('Ctrl Pts',(81.9085772938749,-8.2388625118909,137.388208688723));
#75613=CARTESIAN_POINT('Ctrl Pts',(81.9349980688003,-8.30511347429516,137.384353321519));
#75614=CARTESIAN_POINT('Ctrl Pts',(81.9579629907074,-8.37273609536695,137.380497954316));
#75615=CARTESIAN_POINT('Ctrl Pts',(81.977344553654,-8.44133545070856,137.376642587112));
#75616=CARTESIAN_POINT('Ctrl Pts',(81.9967464038118,-8.51000661086893,137.37278318439));
#75617=CARTESIAN_POINT('Ctrl Pts',(82.0125572752224,-8.57965607774693,137.368923781668));
#75618=CARTESIAN_POINT('Ctrl Pts',(82.0247001017075,-8.64987564973897,137.365064378946));
#75619=CARTESIAN_POINT('Ctrl Pts',(82.0368498035563,-8.72013498060414,137.361202791));
#75620=CARTESIAN_POINT('Ctrl Pts',(82.0453272683024,-8.79096457660569,137.357341203054));
#75621=CARTESIAN_POINT('Ctrl Pts',(82.0501073036935,-8.86195071227024,137.353479615108));
#75622=CARTESIAN_POINT('Ctrl Pts',(82.0548957019278,-8.93306104072356,137.349611271176));
#75623=CARTESIAN_POINT('Ctrl Pts',(82.0559737483448,-9.00432796975142,137.345742927243));
#75624=CARTESIAN_POINT('Ctrl Pts',(82.0533683880917,-9.07533807328007,137.341874583311));
#75625=CARTESIAN_POINT('Ctrl Pts',(82.0518214001433,-9.11750182942235,137.339577671996));
#75626=CARTESIAN_POINT('Ctrl Pts',(82.0489767704361,-9.15957512116204,137.337280760682));
#75627=CARTESIAN_POINT('Ctrl Pts',(82.0448487092084,-9.2014728739772,137.334983849367));
#75628=CARTESIAN_POINT('Ctrl Pts',(82.0378951055636,-9.27204846639731,137.33111476652));
#75629=CARTESIAN_POINT('Ctrl Pts',(82.0272698405453,-9.34240187340793,137.327245683672));
#75630=CARTESIAN_POINT('Ctrl Pts',(82.0129962433475,-9.41212096133174,137.323376600825));
#75631=CARTESIAN_POINT('Ctrl Pts',(81.9987439130975,-9.48173617129175,137.319513282718));
#75632=CARTESIAN_POINT('Ctrl Pts',(81.9808541372859,-9.55071846613516,137.315649964611));
#75633=CARTESIAN_POINT('Ctrl Pts',(81.9594019894067,-9.618660978573,137.311786646504));
#75634=CARTESIAN_POINT('Ctrl Pts',(81.9379750048887,-9.68652379447008,137.307927860067));
#75635=CARTESIAN_POINT('Ctrl Pts',(81.9129940940926,-9.75334878963518,137.304069073631));
#75636=CARTESIAN_POINT('Ctrl Pts',(81.8845849626281,-9.81874115637112,137.300210287195));
#75637=CARTESIAN_POINT('Ctrl Pts',(81.8561937268333,-9.88409233071111,137.296353931511));
#75638=CARTESIAN_POINT('Ctrl Pts',(81.8243787479481,-9.94801222257079,137.292497575827));
#75639=CARTESIAN_POINT('Ctrl Pts',(81.7893144621876,-10.0101244071432,137.288641220143));
#75640=CARTESIAN_POINT('Ctrl Pts',(81.7542605347681,-10.0722182431544,137.284786003665));
#75641=CARTESIAN_POINT('Ctrl Pts',(81.7159594447803,-10.1325050092476,137.280930787188));
#75642=CARTESIAN_POINT('Ctrl Pts',(81.6746315439693,-10.1906329217869,137.27707557071));
#75643=CARTESIAN_POINT('Ctrl Pts',(81.633302027361,-10.2487631069539,137.273220203505));
#75644=CARTESIAN_POINT('Ctrl Pts',(81.5889457482666,-10.3047338763535,137.2693648363));
#75645=CARTESIAN_POINT('Ctrl Pts',(81.5418253390224,-10.3582239088046,137.265509469094));
#75646=CARTESIAN_POINT('Ctrl Pts',(81.4946556075589,-10.4117699307336,137.261650066371));
#75647=CARTESIAN_POINT('Ctrl Pts',(81.4447162920578,-10.4628296669441,137.257790663648));
#75648=CARTESIAN_POINT('Ctrl Pts',(81.3923085370105,-10.5111169710739,137.253931260924));
#75649=CARTESIAN_POINT('Ctrl Pts',(81.3398711082806,-10.5594316158546,137.250069672977));
#75650=CARTESIAN_POINT('Ctrl Pts',(81.2849628318101,-10.6049703933609,137.246208085029));
#75651=CARTESIAN_POINT('Ctrl Pts',(81.2279176282725,-10.6474877421935,137.242346497082));
#75652=CARTESIAN_POINT('Ctrl Pts',(81.1707726221066,-10.6900794766517,137.238478153148));
#75653=CARTESIAN_POINT('Ctrl Pts',(81.1114836288107,-10.7296389588855,137.234609809214));
#75654=CARTESIAN_POINT('Ctrl Pts',(81.0504125958223,-10.7659645922378,137.23074146528));
#75655=CARTESIAN_POINT('Ctrl Pts',(81.0141503739875,-10.7875337079128,137.228444553978));
#75656=CARTESIAN_POINT('Ctrl Pts',(80.9772603389445,-10.8079635657243,137.226147642677));
#75657=CARTESIAN_POINT('Ctrl Pts',(80.9398216719654,-10.8272199614179,137.223850731375));
#75658=CARTESIAN_POINT('Ctrl Pts',(80.8767572845336,-10.859656821396,137.219981648528));
#75659=CARTESIAN_POINT('Ctrl Pts',(80.8118881255425,-10.8888884882119,137.216112565681));
#75660=CARTESIAN_POINT('Ctrl Pts',(80.7455730954224,-10.914711028297,137.212243482835));
#75661=CARTESIAN_POINT('Ctrl Pts',(80.6793568713899,-10.9404950940853,137.208380164728));
#75662=CARTESIAN_POINT('Ctrl Pts',(80.6116995013939,-10.9628799408364,137.204516846622));
#75663=CARTESIAN_POINT('Ctrl Pts',(80.5429835264878,-10.9817079634656,137.200653528516));
#75664=CARTESIAN_POINT('Ctrl Pts',(80.4743481553937,-11.0005139008315,137.19679474208));
#75665=CARTESIAN_POINT('Ctrl Pts',(80.4046571121525,-11.0157711736357,137.192935955644));
#75666=CARTESIAN_POINT('Ctrl Pts',(80.3343102680188,-11.0273712553938,137.189077169208));
#75667=CARTESIAN_POINT('Ctrl Pts',(80.2640077372386,-11.038964029951,137.185220813525));
#75668=CARTESIAN_POINT('Ctrl Pts',(80.1930507033399,-11.0469041052396,137.181364457842));
#75669=CARTESIAN_POINT('Ctrl Pts',(80.1218500240242,-11.0511338654864,137.177508102159));
#75670=CARTESIAN_POINT('Ctrl Pts',(80.0506703781022,-11.0553623762197,137.173652885682));
#75671=CARTESIAN_POINT('Ctrl Pts',(79.9792477143182,-11.055882719111,137.169797669205));
#75672=CARTESIAN_POINT('Ctrl Pts',(79.9079970921908,-11.052689218429,137.165942452728));
#75673=CARTESIAN_POINT('Ctrl Pts',(79.8367436843772,-11.0494955928907,137.162087085523));
#75674=CARTESIAN_POINT('Ctrl Pts',(79.7656628167716,-11.0425878594553,137.158231718318));
#75675=CARTESIAN_POINT('Ctrl Pts',(79.6951668885374,-11.0320123859504,137.154376351114));
#75676=CARTESIAN_POINT('Ctrl Pts',(79.6245971702895,-11.0214258428086,137.150516948391));
#75677=CARTESIAN_POINT('Ctrl Pts',(79.5546140950367,-11.0071639680623,137.146657545668));
#75678=CARTESIAN_POINT('Ctrl Pts',(79.4856213986487,-10.9893245630042,137.142798142946));
#75679=CARTESIAN_POINT('Ctrl Pts',(79.4165896380539,-10.9714750571348,137.138936554999));
#75680=CARTESIAN_POINT('Ctrl Pts',(79.3485498361865,-10.9500441345683,137.135074967052));
#75681=CARTESIAN_POINT('Ctrl Pts',(79.2818894093021,-10.9251791454375,137.131213379105));
#75682=CARTESIAN_POINT('Ctrl Pts',(79.2151123576116,-10.900270654117,137.127345035172));
#75683=CARTESIAN_POINT('Ctrl Pts',(79.149719944888,-10.8719162943588,137.123476691239));
#75684=CARTESIAN_POINT('Ctrl Pts',(79.0860778523182,-10.8403108081182,137.119608347305));
#75685=CARTESIAN_POINT('Ctrl Pts',(79.048289009199,-10.8215443799097,137.117311435998));
#75686=CARTESIAN_POINT('Ctrl Pts',(79.0111167807689,-10.801632594008,137.115014524691));
#75687=CARTESIAN_POINT('Ctrl Pts',(78.9746328495178,-10.780623421505,137.112717613384));
#75688=CARTESIAN_POINT('Ctrl Pts',(78.9131766878655,-10.7452340580989,137.108848530537));
#75689=CARTESIAN_POINT('Ctrl Pts',(78.853434442433,-10.7065900127146,137.10497944769));
#75690=CARTESIAN_POINT('Ctrl Pts',(78.7957721050871,-10.664882199921,137.101110364844));
#75691=CARTESIAN_POINT('Ctrl Pts',(78.7381956817481,-10.6232365296883,137.097247046737));
#75692=CARTESIAN_POINT('Ctrl Pts',(78.6826934055514,-10.5785364355522,137.093383728631));
#75693=CARTESIAN_POINT('Ctrl Pts',(78.629605168481,-10.5310178210086,137.089520410524));
#75694=CARTESIAN_POINT('Ctrl Pts',(78.5765792038922,-10.4835549457817,137.085661624089));
#75695=CARTESIAN_POINT('Ctrl Pts',(78.5259620139863,-10.4332804396436,137.081802837653));
#75696=CARTESIAN_POINT('Ctrl Pts',(78.4780616577515,-10.3804713850326,137.077944051217));
#75697=CARTESIAN_POINT('Ctrl Pts',(78.4301914752288,-10.3276955962538,137.074087695534));
#75698=CARTESIAN_POINT('Ctrl Pts',(78.3850350565736,-10.2723887855567,137.070231339851));
#75699=CARTESIAN_POINT('Ctrl Pts',(78.3428636478343,-10.2148648784252,137.066374984168));
#75700=CARTESIAN_POINT('Ctrl Pts',(78.3007046969516,-10.157357964432,137.062519767691));
#75701=CARTESIAN_POINT('Ctrl Pts',(78.2615292924248,-10.0976356458329,137.058664551214));
#75702=CARTESIAN_POINT('Ctrl Pts',(78.2255673227381,-10.0360435494539,137.054809334737));
#75703=CARTESIAN_POINT('Ctrl Pts',(78.1896039470459,-9.97444904500807,137.050953967532));
#75704=CARTESIAN_POINT('Ctrl Pts',(78.1568544986654,-9.91098503826771,137.047098600327));
#75705=CARTESIAN_POINT('Ctrl Pts',(78.1275036996413,-9.84602314840838,137.043243233123));
#75706=CARTESIAN_POINT('Ctrl Pts',(78.0981221783341,-9.78099326116471,137.0393838304));
#75707=CARTESIAN_POINT('Ctrl Pts',(78.072146608295,-9.7144628045736,137.035524427677));
#75708=CARTESIAN_POINT('Ctrl Pts',(78.0497138018131,-9.64682401599008,137.031665024955));
#75709=CARTESIAN_POINT('Ctrl Pts',(78.0272682936999,-9.57914692979317,137.027803437008));
#75710=CARTESIAN_POINT('Ctrl Pts',(78.0083696711111,-9.5103607309998,137.023941849061));
#75711=CARTESIAN_POINT('Ctrl Pts',(77.993104267279,-9.44087082063364,137.020080261114));
#75712=CARTESIAN_POINT('Ctrl Pts',(77.9778121560757,-9.37125933517854,137.016211917181));
#75713=CARTESIAN_POINT('Ctrl Pts',(77.9661660338547,-9.30094215949368,137.012343573247));
#75714=CARTESIAN_POINT('Ctrl Pts',(77.9582006297367,-9.23033213864404,137.008475229314));
#75715=CARTESIAN_POINT('Ctrl Pts',(77.953471001994,-9.18840594022715,137.006178318007));
#75716=CARTESIAN_POINT('Ctrl Pts',(77.9500380668079,-9.14637656073434,137.003881406699));
#75717=CARTESIAN_POINT('Ctrl Pts',(77.9479004012492,-9.10433024157265,137.001584495392));
#75718=CARTESIAN_POINT('Ctrl Pts',(77.9461447814819,-9.06979848389885,136.999698090441));
#75719=CARTESIAN_POINT('Ctrl Pts',(77.9452607206379,-9.03522204066764,136.997811685489));
#75720=CARTESIAN_POINT('Ctrl Pts',(77.9452500969075,-9.00063106367537,136.995925280538));
#75721=CARTESIAN_POINT('Ctrl Pts',(77.9452500969073,-9.00063106298383,136.9959252805));
#75722=CARTESIAN_POINT('Ctrl Pts',(77.9452284795406,-8.93024461476221,136.992086783991));
#75723=CARTESIAN_POINT('Ctrl Pts',(77.9488278088239,-8.85971198196666,136.988248287481));
#75724=CARTESIAN_POINT('Ctrl Pts',(77.956066989778,-8.78944024072726,136.984409790972));
#75725=CARTESIAN_POINT('Ctrl Pts',(77.9634503271985,-8.71776915252224,136.980494857073));
#75726=CARTESIAN_POINT('Ctrl Pts',(77.9746201460017,-8.6463699740825,136.976579923174));
#75727=CARTESIAN_POINT('Ctrl Pts',(77.9895405666956,-8.57567650367051,136.972664989275));
#75728=CARTESIAN_POINT('Ctrl Pts',(78.0041321582484,-8.50654103712668,136.968836336077));
#75729=CARTESIAN_POINT('Ctrl Pts',(78.0223106191684,-8.43808100216141,136.965007682879));
#75730=CARTESIAN_POINT('Ctrl Pts',(78.0439901438109,-8.37069641269804,136.961179029681));
#75731=CARTESIAN_POINT('Ctrl Pts',(78.0656575011448,-8.30334964182633,136.957352525257));
#75732=CARTESIAN_POINT('Ctrl Pts',(78.0908218742364,-8.23707758891418,136.953526020833));
#75733=CARTESIAN_POINT('Ctrl Pts',(78.1193471946889,-8.17226659583193,136.949699516409));
#75734=CARTESIAN_POINT('Ctrl Pts',(78.1478664215464,-8.1074694477107,136.945873829405));
#75735=CARTESIAN_POINT('Ctrl Pts',(78.1797449711963,-8.04413319186299,136.942048142401));
#75736=CARTESIAN_POINT('Ctrl Pts',(78.2147987712684,-7.98262389676421,136.938222455397));
#75737=CARTESIAN_POINT('Ctrl Pts',(78.2512749609404,-7.91861871872357,136.934241532231));
#75738=CARTESIAN_POINT('Ctrl Pts',(78.2911893552543,-7.85659246133984,136.930260609065));
#75739=CARTESIAN_POINT('Ctrl Pts',(78.3342831480842,-7.79692688013413,136.926279685898));
#75740=CARTESIAN_POINT('Ctrl Pts',(78.3757481853334,-7.73951639512645,136.922449224095));
#75741=CARTESIAN_POINT('Ctrl Pts',(78.4201562185497,-7.68429169388733,136.918618762292));
#75742=CARTESIAN_POINT('Ctrl Pts',(78.4672353624941,-7.63155923456245,136.914788300489));
#75743=CARTESIAN_POINT('Ctrl Pts',(78.51434688584,-7.57879050768187,136.910955204227));
#75744=CARTESIAN_POINT('Ctrl Pts',(78.5641328247559,-7.528517780551,136.907122107966));
#75745=CARTESIAN_POINT('Ctrl Pts',(78.6162853882318,-7.48100973153902,136.903289011704));
#75746=CARTESIAN_POINT('Ctrl Pts',(78.6685215402373,-7.43342553808277,136.899449771873));
#75747=CARTESIAN_POINT('Ctrl Pts',(78.7231314966095,-7.38861516648557,136.895610532042));
#75748=CARTESIAN_POINT('Ctrl Pts',(78.7797764230507,-7.34680552119327,136.891771292211));
#75749=CARTESIAN_POINT('Ctrl Pts',(78.7862678537047,-7.34201419335271,136.891331320608));
#75750=CARTESIAN_POINT('Ctrl Pts',(78.7927859814812,-7.33726222463984,136.890891349004));
#75751=CARTESIAN_POINT('Ctrl Pts',(78.7993302756117,-7.33254991815727,136.8904513774));
#75752=CARTESIAN_POINT('Ctrl Pts',(78.8568803901062,-7.29111018879981,136.886582294554));
#75753=CARTESIAN_POINT('Ctrl Pts',(78.9166911084275,-7.25257220614516,136.882713211707));
#75754=CARTESIAN_POINT('Ctrl Pts',(78.9784377823447,-7.21719092498409,136.87884412886));
#75755=CARTESIAN_POINT('Ctrl Pts',(79.0400924567971,-7.18186236016741,136.874980810753));
#75756=CARTESIAN_POINT('Ctrl Pts',(79.1036769431805,-7.14968140041849,136.871117492647));
#75757=CARTESIAN_POINT('Ctrl Pts',(79.1688363368496,-7.12086069500995,136.867254174541));
#75758=CARTESIAN_POINT('Ctrl Pts',(79.2339192985751,-7.09207379627775,136.863395388105));
#75759=CARTESIAN_POINT('Ctrl Pts',(79.3005730559836,-7.06663951812903,136.859536601669));
#75760=CARTESIAN_POINT('Ctrl Pts',(79.3684182802396,-7.04472454785405,136.855677815233));
#75761=CARTESIAN_POINT('Ctrl Pts',(79.4362207669793,-7.02282338240339,136.85182145955));
#75762=CARTESIAN_POINT('Ctrl Pts',(79.5052127703408,-7.00443727548517,136.847965103867));
#75763=CARTESIAN_POINT('Ctrl Pts',(79.574996538769,-6.98968419882803,136.844108748183));
#75764=CARTESIAN_POINT('Ctrl Pts',(79.6447596923733,-6.97493548037747,136.840253531706));
#75765=CARTESIAN_POINT('Ctrl Pts',(79.715313671678,-6.96381776194594,136.836398315229));
#75766=CARTESIAN_POINT('Ctrl Pts',(79.7862488590475,-6.95639827455506,136.832543098752));
#75767=CARTESIAN_POINT('Ctrl Pts',(79.8571868197706,-6.94897849708443,136.828687731547));
#75768=CARTESIAN_POINT('Ctrl Pts',(79.928505534772,-6.94525728606247,136.824832364343));
#75769=CARTESIAN_POINT('Ctrl Pts',(79.9997902910996,-6.9452500107015,136.820976997138));
#75770=CARTESIAN_POINT('Ctrl Pts',(80.0711496631286,-6.94524272772522,136.817117594415));
#75771=CARTESIAN_POINT('Ctrl Pts',(80.1424745187488,-6.94895714073665,136.813258191692));
#75772=CARTESIAN_POINT('Ctrl Pts',(80.2133510766837,-6.95635646929855,136.80939878897));
#75773=CARTESIAN_POINT('Ctrl Pts',(80.2842677654826,-6.96375998741841,136.805537201023));
#75774=CARTESIAN_POINT('Ctrl Pts',(80.3547351711984,-6.97485249894931,136.801675613076));
#75775=CARTESIAN_POINT('Ctrl Pts',(80.424348295495,-6.98954580091699,136.797814025129));
#75776=CARTESIAN_POINT('Ctrl Pts',(80.4940832104476,-7.00426480934311,136.793945681196));
#75777=CARTESIAN_POINT('Ctrl Pts',(80.5629603903894,-7.02259706077393,136.790077337262));
#75778=CARTESIAN_POINT('Ctrl Pts',(80.6305892955939,-7.04440425885554,136.786208993329));
#75779=CARTESIAN_POINT('Ctrl Pts',(80.6707453933162,-7.05735274552062,136.783912082022));
#75780=CARTESIAN_POINT('Ctrl Pts',(80.7104617445907,-7.07152543845114,136.781615170715));
#75781=CARTESIAN_POINT('Ctrl Pts',(80.7496603396343,-7.08688553983841,136.779318259409));
#75782=CARTESIAN_POINT('Ctrl Pts',(80.8156837929553,-7.11275705221844,136.775449497882));
#75783=CARTESIAN_POINT('Ctrl Pts',(80.8804957013765,-7.14210104542521,136.771580736354));
#75784=CARTESIAN_POINT('Ctrl Pts',(80.9437058827517,-7.17478308977812,136.767711974827));
#75785=CARTESIAN_POINT('Ctrl Pts',(81.0068160594631,-7.20741342795354,136.763849334057));
#75786=CARTESIAN_POINT('Ctrl Pts',(81.0683291135876,-7.24337110879749,136.759986693287));
#75787=CARTESIAN_POINT('Ctrl Pts',(81.1278740897058,-7.28247340624075,136.756124052517));
#75788=CARTESIAN_POINT('Ctrl Pts',(81.1703036669818,-7.31033627661527,136.753371675647));
#75789=CARTESIAN_POINT('Ctrl Pts',(81.2117343093368,-7.33979478144065,136.750619298776));
#75790=CARTESIAN_POINT('Ctrl Pts',(81.2520391107129,-7.37076839346111,136.747866921905));
#75791=CARTESIAN_POINT('',(77.9452500020166,-8.99990896698627,137.054074719424));
#75792=CARTESIAN_POINT('Ctrl Pts',(77.9452500020166,-8.99990896698627,137.054074719424));
#75793=CARTESIAN_POINT('Ctrl Pts',(77.9452533307477,-8.92477457357937,137.050023196181));
#75794=CARTESIAN_POINT('Ctrl Pts',(77.9493820167298,-8.84972529838846,137.045971672937));
#75795=CARTESIAN_POINT('Ctrl Pts',(77.9575824977975,-8.77521497114594,137.041920149694));
#75796=CARTESIAN_POINT('Ctrl Pts',(77.9658071971075,-8.70048459472072,137.037856661204));
#75797=CARTESIAN_POINT('Ctrl Pts',(77.978127678062,-8.62629675433766,137.033793172715));
#75798=CARTESIAN_POINT('Ctrl Pts',(77.9944388833354,-8.55309713603182,137.029729684225));
#75799=CARTESIAN_POINT('Ctrl Pts',(78.0107756928437,-8.47978261387955,137.025659817145));
#75800=CARTESIAN_POINT('Ctrl Pts',(78.0311156065384,-8.40745979942027,137.021589950064));
#75801=CARTESIAN_POINT('Ctrl Pts',(78.0553039258151,-8.33655841135058,137.017520082983));
#75802=CARTESIAN_POINT('Ctrl Pts',(78.0795588774132,-8.26546170900407,137.013439004511));
#75803=CARTESIAN_POINT('Ctrl Pts',(78.1076832711748,-8.19579463867159,137.00935792604));
#75804=CARTESIAN_POINT('Ctrl Pts',(78.1394743984723,-8.12796671591055,137.005276847569));
#75805=CARTESIAN_POINT('Ctrl Pts',(78.1547192877522,-8.09544100007468,137.003319836455));
#75806=CARTESIAN_POINT('Ctrl Pts',(78.1708066784999,-8.06333781496755,137.001362825341));
#75807=CARTESIAN_POINT('Ctrl Pts',(78.1877106415427,-8.03170002389624,136.999405814228));
#75808=CARTESIAN_POINT('Ctrl Pts',(78.2211303973098,-7.96915094898812,136.995536731381));
#75809=CARTESIAN_POINT('Ctrl Pts',(78.2578576247281,-7.90821156189568,136.991667648534));
#75810=CARTESIAN_POINT('Ctrl Pts',(78.2977131288887,-7.84925373303147,136.987798565687));
#75811=CARTESIAN_POINT('Ctrl Pts',(78.3375092503357,-7.79038374839189,136.983935247581));
#75812=CARTESIAN_POINT('Ctrl Pts',(78.3804241267733,-7.733489860678,136.980071929474));
#75813=CARTESIAN_POINT('Ctrl Pts',(78.4262327681652,-7.67891928236645,136.976208611368));
#75814=CARTESIAN_POINT('Ctrl Pts',(78.4719876760385,-7.62441271532224,136.972349824932));
#75815=CARTESIAN_POINT('Ctrl Pts',(78.5206292956542,-7.57222441469258,136.968491038496));
#75816=CARTESIAN_POINT('Ctrl Pts',(78.5718904678376,-7.52267108379792,136.964632252061));
#75817=CARTESIAN_POINT('Ctrl Pts',(78.6231193492412,-7.47314896786815,136.960775896378));
#75818=CARTESIAN_POINT('Ctrl Pts',(78.6769641609443,-7.42625886541624,136.956919540694));
#75819=CARTESIAN_POINT('Ctrl Pts',(78.7331197501868,-7.38228185547259,136.953063185011));
#75820=CARTESIAN_POINT('Ctrl Pts',(78.7892587505059,-7.33831783677804,136.949207968534));
#75821=CARTESIAN_POINT('Ctrl Pts',(78.8477067909087,-7.29726550149995,136.945352752057));
#75822=CARTESIAN_POINT('Ctrl Pts',(78.9081257198297,-7.25936559875358,136.94149753558));
#75823=CARTESIAN_POINT('Ctrl Pts',(78.96854701095,-7.22146421423439,136.937642168375));
#75824=CARTESIAN_POINT('Ctrl Pts',(79.0309389308821,-7.18671576321925,136.933786801171));
#75825=CARTESIAN_POINT('Ctrl Pts',(79.0949359144031,-7.15531667664539,136.929931433966));
#75826=CARTESIAN_POINT('Ctrl Pts',(79.1589998853148,-7.12388472378996,136.926072031243));
#75827=CARTESIAN_POINT('Ctrl Pts',(79.2246718365866,-7.09580934829369,136.922212628521));
#75828=CARTESIAN_POINT('Ctrl Pts',(79.291564073674,-7.07123975030834,136.918353225798));
#75829=CARTESIAN_POINT('Ctrl Pts',(79.3584941856716,-7.04665624082359,136.914491637851));
#75830=CARTESIAN_POINT('Ctrl Pts',(79.4266454946026,-7.02558260394684,136.910630049904));
#75831=CARTESIAN_POINT('Ctrl Pts',(79.4956155457542,-7.00811800429464,136.906768461957));
#75832=CARTESIAN_POINT('Ctrl Pts',(79.5647062624825,-6.99062284969934,136.902900118024));
#75833=CARTESIAN_POINT('Ctrl Pts',(79.6346181046537,-6.97674943327319,136.899031774091));
#75834=CARTESIAN_POINT('Ctrl Pts',(79.704939538399,-6.9665455779635,136.895163430157));
#75835=CARTESIAN_POINT('Ctrl Pts',(79.7466943820948,-6.96048682232018,136.89286651885));
#75836=CARTESIAN_POINT('Ctrl Pts',(79.7885935358446,-6.95572082826681,136.890569607543));
#75837=CARTESIAN_POINT('Ctrl Pts',(79.830550756554,-6.95224891249068,136.888272696236));
#75838=CARTESIAN_POINT('Ctrl Pts',(79.901208363859,-6.94640206998401,136.884404607397));
#75839=CARTESIAN_POINT('Ctrl Pts',(79.9723072994879,-6.94420512848996,136.880536518558));
#75840=CARTESIAN_POINT('Ctrl Pts',(80.0434382677722,-6.94570920281647,136.876668429718));
#75841=CARTESIAN_POINT('Ctrl Pts',(80.1144716684083,-6.94721121406134,136.87280564659));
#75842=CARTESIAN_POINT('Ctrl Pts',(80.1855365333489,-6.95240416047176,136.868942863461));
#75843=CARTESIAN_POINT('Ctrl Pts',(80.256219300306,-6.96128735898099,136.865080080333));
#75844=CARTESIAN_POINT('Ctrl Pts',(80.3268287676249,-6.97016134541117,136.861221302998));
#75845=CARTESIAN_POINT('Ctrl Pts',(80.3970564438626,-6.98271792913604,136.857362525663));
#75846=CARTESIAN_POINT('Ctrl Pts',(80.4664913551475,-6.99890445553626,136.853503748329));
#75847=CARTESIAN_POINT('Ctrl Pts',(80.5375128267714,-7.01546083768106,136.849556799454));
#75848=CARTESIAN_POINT('Ctrl Pts',(80.607704334842,-7.03581507458642,136.845609850579));
#75849=CARTESIAN_POINT('Ctrl Pts',(80.6766354069122,-7.0598551372094,136.841662901704));
#75850=CARTESIAN_POINT('Ctrl Pts',(80.7439678387922,-7.08333766592015,136.837807489939));
#75851=CARTESIAN_POINT('Ctrl Pts',(80.8100972024929,-7.11033669413166,136.833952078174));
#75852=CARTESIAN_POINT('Ctrl Pts',(80.8746382145517,-7.14069756194807,136.830096666409));
#75853=CARTESIAN_POINT('Ctrl Pts',(80.9414777739727,-7.17213969407085,136.826103948979));
#75854=CARTESIAN_POINT('Ctrl Pts',(81.0066131920739,-7.20718744927472,136.822111231549));
#75855=CARTESIAN_POINT('Ctrl Pts',(81.0696421225511,-7.2456159792781,136.81811851412));
#75856=CARTESIAN_POINT('Ctrl Pts',(81.1326710530283,-7.28404450928148,136.81412579669));
#75857=CARTESIAN_POINT('Ctrl Pts',(81.1935930213483,-7.32585348421251,136.81013307926));
#75858=CARTESIAN_POINT('Ctrl Pts',(81.2520391107129,-7.37076839346113,136.806140361831));
#75859=CARTESIAN_POINT('Ctrl Pts',(81.2520391107129,-7.37076839346111,137.506056941207));
#75860=CARTESIAN_POINT('Ctrl Pts',(81.3085836343695,-7.41422197908427,137.50220180446));
#75861=CARTESIAN_POINT('Ctrl Pts',(81.3628760679797,-7.46063245916092,137.498346667712));
#75862=CARTESIAN_POINT('Ctrl Pts',(81.4146004952369,-7.50973056081275,137.494491530965));
#75863=CARTESIAN_POINT('Ctrl Pts',(81.4663309415066,-7.55883437585964,137.490635945607));
#75864=CARTESIAN_POINT('Ctrl Pts',(81.5154924376303,-7.61062609708868,137.486780360249));
#75865=CARTESIAN_POINT('Ctrl Pts',(81.561805417557,-7.66479911616659,137.482924774891));
#75866=CARTESIAN_POINT('Ctrl Pts',(81.6081690741475,-7.71903141253303,137.479064970668));
#75867=CARTESIAN_POINT('Ctrl Pts',(81.6516776792929,-7.77564983589475,137.475205166445));
#75868=CARTESIAN_POINT('Ctrl Pts',(81.6920921389353,-7.8343148985025,137.471345362222));
#75869=CARTESIAN_POINT('Ctrl Pts',(81.7325322819063,-7.89301724266961,137.467483105099));
#75870=CARTESIAN_POINT('Ctrl Pts',(81.769874112489,-7.95376840044712,137.463620847977));
#75871=CARTESIAN_POINT('Ctrl Pts',(81.8039234895922,-8.01620245670292,137.459758590854));
#75872=CARTESIAN_POINT('Ctrl Pts',(81.8380300713486,-8.07874140528959,137.455889844947));
#75873=CARTESIAN_POINT('Ctrl Pts',(81.8688329530289,-8.14296845639921,137.452021099039));
#75874=CARTESIAN_POINT('Ctrl Pts',(81.8961856379346,-8.20849662730306,137.448152353132));
#75875=CARTESIAN_POINT('Ctrl Pts',(81.9061170255109,-8.23228901421703,137.446747664153));
#75876=CARTESIAN_POINT('Ctrl Pts',(81.9155940431147,-8.2562527808878,137.445342975173));
#75877=CARTESIAN_POINT('Ctrl Pts',(81.9246113195382,-8.28036896175498,137.443938286194));
#75878=CARTESIAN_POINT('Ctrl Pts',(81.9494485540355,-8.34679469955542,137.440069203343));
#75879=CARTESIAN_POINT('Ctrl Pts',(81.9708914866249,-8.41463789219201,137.436200120492));
#75880=CARTESIAN_POINT('Ctrl Pts',(81.9887795660641,-8.48351824804187,137.432331037641));
#75881=CARTESIAN_POINT('Ctrl Pts',(82.0066409931575,-8.55229597559809,137.42846771953));
#75882=CARTESIAN_POINT('Ctrl Pts',(82.0209579595018,-8.62210733259121,137.424604401419));
#75883=CARTESIAN_POINT('Ctrl Pts',(82.0316186896447,-8.69255396833502,137.420741083309));
#75884=CARTESIAN_POINT('Ctrl Pts',(82.0422669147554,-8.76291797020327,137.416882296868));
#75885=CARTESIAN_POINT('Ctrl Pts',(82.0492673502678,-8.83391529265563,137.413023510428));
#75886=CARTESIAN_POINT('Ctrl Pts',(82.0525589895964,-8.90513611473707,137.409164723988));
#75887=CARTESIAN_POINT('Ctrl Pts',(82.0558485554335,-8.97631207292382,137.405308368301));
#75888=CARTESIAN_POINT('Ctrl Pts',(82.0554339378344,-9.0477107672997,137.401452012613));
#75889=CARTESIAN_POINT('Ctrl Pts',(82.0513059765539,-9.11891742115505,137.397595656925));
#75890=CARTESIAN_POINT('Ctrl Pts',(82.0471792347145,-9.19010303985237,137.393740440444));
#75891=CARTESIAN_POINT('Ctrl Pts',(82.0393413550608,-9.26109624595062,137.389885223962));
#75892=CARTESIAN_POINT('Ctrl Pts',(82.027835252322,-9.3314841654442,137.38603000748));
#75893=CARTESIAN_POINT('Ctrl Pts',(82.0163286997288,-9.40187483689556,137.382174640271));
#75894=CARTESIAN_POINT('Ctrl Pts',(82.0011537198591,-9.4716596956942,137.378319273062));
#75895=CARTESIAN_POINT('Ctrl Pts',(81.9824046025214,-9.5404345977099,137.374463905853));
#75896=CARTESIAN_POINT('Ctrl Pts',(81.9636358599706,-9.60928148829397,137.370604503126));
#75897=CARTESIAN_POINT('Ctrl Pts',(81.9412856398145,-9.67711584214869,137.366745100399));
#75898=CARTESIAN_POINT('Ctrl Pts',(81.9154982988431,-9.74354813538135,137.362885697672));
#75899=CARTESIAN_POINT('Ctrl Pts',(81.8896963568767,-9.8100180431004,137.35902410972));
#75900=CARTESIAN_POINT('Ctrl Pts',(81.8604536191945,-9.8750838665717,137.355162521769));
#75901=CARTESIAN_POINT('Ctrl Pts',(81.8279617422849,-9.93837808544472,137.351300933817));
#75902=CARTESIAN_POINT('Ctrl Pts',(81.7954130196723,-10.0017830398218,137.347432589879));
#75903=CARTESIAN_POINT('Ctrl Pts',(81.7596040527335,-10.0634097812331,137.343564245942));
#75904=CARTESIAN_POINT('Ctrl Pts',(81.7207710219745,-10.1229179188315,137.339695902004));
#75905=CARTESIAN_POINT('Ctrl Pts',(81.6977130862498,-10.1582521377946,137.337398990737));
#75906=CARTESIAN_POINT('Ctrl Pts',(81.673589784248,-10.1928399972618,137.33510207947));
#75907=CARTESIAN_POINT('Ctrl Pts',(81.6484571427742,-10.2266159182632,137.332805168203));
#75908=CARTESIAN_POINT('Ctrl Pts',(81.6061219104928,-10.2835105133897,137.328936085356));
#75909=CARTESIAN_POINT('Ctrl Pts',(81.5607548249677,-10.3383222428234,137.32506700251));
#75910=CARTESIAN_POINT('Ctrl Pts',(81.5125883019348,-10.3907099594631,137.321197919663));
#75911=CARTESIAN_POINT('Ctrl Pts',(81.4644935446192,-10.4430196210176,137.317334601557));
#75912=CARTESIAN_POINT('Ctrl Pts',(81.4136079552723,-10.4929120841274,137.313471283451));
#75913=CARTESIAN_POINT('Ctrl Pts',(81.3602055766754,-10.5400773849651,137.309607965345));
#75914=CARTESIAN_POINT('Ctrl Pts',(81.3068658390478,-10.5871873609233,137.305749178909));
#75915=CARTESIAN_POINT('Ctrl Pts',(81.2510155385621,-10.6315762088092,137.301890392473));
#75916=CARTESIAN_POINT('Ctrl Pts',(81.192965890586,-10.6729703961512,137.298031606038));
#75917=CARTESIAN_POINT('Ctrl Pts',(81.1349528096313,-10.7143385081907,137.294175250355));
#75918=CARTESIAN_POINT('Ctrl Pts',(81.074743524441,-10.7527154209336,137.290318894672));
#75919=CARTESIAN_POINT('Ctrl Pts',(81.0126815343111,-10.7878684718305,137.286462538989));
#75920=CARTESIAN_POINT('Ctrl Pts',(80.9506378779143,-10.8230111381642,137.282607322512));
#75921=CARTESIAN_POINT('Ctrl Pts',(80.8867430255922,-10.8549315940657,137.278752106035));
#75922=CARTESIAN_POINT('Ctrl Pts',(80.8213671225575,-10.8834419588831,137.274896889558));
#75923=CARTESIAN_POINT('Ctrl Pts',(80.7559886635204,-10.9119534383706,137.271041522354));
#75924=CARTESIAN_POINT('Ctrl Pts',(80.6891294849716,-10.937054369908,137.267186155149));
#75925=CARTESIAN_POINT('Ctrl Pts',(80.6211802626988,-10.9586047696596,137.263330787945));
#75926=CARTESIAN_POINT('Ctrl Pts',(80.5531599161191,-10.9801777268033,137.259471385222));
#75927=CARTESIAN_POINT('Ctrl Pts',(80.4840477121677,-10.9981925861569,137.2556119825));
#75928=CARTESIAN_POINT('Ctrl Pts',(80.4142491990326,-11.012559356541,137.251752579777));
#75929=CARTESIAN_POINT('Ctrl Pts',(80.3444111654309,-11.0269342615035,137.247890991831));
#75930=CARTESIAN_POINT('Ctrl Pts',(80.2738865295666,-11.0376568925161,137.244029403884));
#75931=CARTESIAN_POINT('Ctrl Pts',(80.2030880081496,-11.044688930729,137.240167815937));
#75932=CARTESIAN_POINT('Ctrl Pts',(80.1321656221815,-11.0517332717449,137.236299472004));
#75933=CARTESIAN_POINT('Ctrl Pts',(80.0609688793818,-11.0550741059518,137.232431128071));
#75934=CARTESIAN_POINT('Ctrl Pts',(79.9899118530182,-11.0547252351082,137.228562784137));
#75935=CARTESIAN_POINT('Ctrl Pts',(79.9477202355612,-11.0545180856407,137.226265872829));
#75936=CARTESIAN_POINT('Ctrl Pts',(79.9055778257029,-11.0530110759741,137.22396896152));
#75937=CARTESIAN_POINT('Ctrl Pts',(79.8635701063467,-11.0502157073386,137.221672050211));
#75938=CARTESIAN_POINT('Ctrl Pts',(79.7928092782111,-11.0455069870694,137.217802967365));
#75939=CARTESIAN_POINT('Ctrl Pts',(79.7221539169065,-11.0371214012433,137.213933884519));
#75940=CARTESIAN_POINT('Ctrl Pts',(79.6520166891183,-11.0250691785339,137.210064801673));
#75941=CARTESIAN_POINT('Ctrl Pts',(79.5819839623019,-11.0130349130352,137.206201483567));
#75942=CARTESIAN_POINT('Ctrl Pts',(79.5124683114827,-10.9973449363675,137.202338165462));
#75943=CARTESIAN_POINT('Ctrl Pts',(79.4438787829363,-10.9780613626558,137.198474847356));
#75944=CARTESIAN_POINT('Ctrl Pts',(79.3753697098809,-10.9588004085687,137.194616060921));
#75945=CARTESIAN_POINT('Ctrl Pts',(79.30778506664,-10.9359543612667,137.190757274486));
#75946=CARTESIAN_POINT('Ctrl Pts',(79.2415234539812,-10.9096363244449,137.186898488051));
#75947=CARTESIAN_POINT('Ctrl Pts',(79.1753035812799,-10.8833348660565,137.183042132369));
#75948=CARTESIAN_POINT('Ctrl Pts',(79.1104055360921,-10.853565936213,137.179185776687));
#75949=CARTESIAN_POINT('Ctrl Pts',(79.0472110931796,-10.8204919284468,137.175329421004));
#75950=CARTESIAN_POINT('Ctrl Pts',(78.9840353185384,-10.7874276910737,137.171474204528));
#75951=CARTESIAN_POINT('Ctrl Pts',(78.9225625772248,-10.7510605392452,137.167618988052));
#75952=CARTESIAN_POINT('Ctrl Pts',(78.8631514734681,-10.7115995414297,137.163763771576));
#75953=CARTESIAN_POINT('Ctrl Pts',(78.8037380469151,-10.6721370008073,137.159908404372));
#75954=CARTESIAN_POINT('Ctrl Pts',(78.7463868213841,-10.6295806446556,137.156053037168));
#75955=CARTESIAN_POINT('Ctrl Pts',(78.6914272967846,-10.5841827681488,137.152197669964));
#75956=CARTESIAN_POINT('Ctrl Pts',(78.6364102445497,-10.5387373724448,137.148338267243));
#75957=CARTESIAN_POINT('Ctrl Pts',(78.58379026601,-10.4904448290285,137.144478864521));
#75958=CARTESIAN_POINT('Ctrl Pts',(78.5338629270879,-10.4395970429022,137.140619461799));
#75959=CARTESIAN_POINT('Ctrl Pts',(78.4839073189144,-10.3887204663601,137.136757873853));
#75960=CARTESIAN_POINT('Ctrl Pts',(78.4366477073388,-10.3352861310318,137.132896285907));
#75961=CARTESIAN_POINT('Ctrl Pts',(78.3923401347156,-10.2796199904869,137.129034697961));
#75962=CARTESIAN_POINT('Ctrl Pts',(78.3479550444059,-10.2238564600339,137.125166354028));
#75963=CARTESIAN_POINT('Ctrl Pts',(78.3065325869227,-10.1658537241226,137.121298010096));
#75964=CARTESIAN_POINT('Ctrl Pts',(78.2682857521435,-10.105967145204,137.117429666163));
#75965=CARTESIAN_POINT('Ctrl Pts',(78.2455758822133,-10.0704082178926,137.115132754849));
#75966=CARTESIAN_POINT('Ctrl Pts',(78.2239847570716,-10.034185612918,137.112835843534));
#75967=CARTESIAN_POINT('Ctrl Pts',(78.2035490783993,-9.99737738533625,137.11053893222));
#75968=CARTESIAN_POINT('Ctrl Pts',(78.1674867936405,-9.93242291008696,137.106485635472));
#75969=CARTESIAN_POINT('Ctrl Pts',(78.1348950465757,-9.8654094674081,137.102432338725));
#75970=CARTESIAN_POINT('Ctrl Pts',(78.1060020779535,-9.79672418927981,137.098379041977));
#75971=CARTESIAN_POINT('Ctrl Pts',(78.0771900219366,-9.72823125915408,137.094337096186));
#75972=CARTESIAN_POINT('Ctrl Pts',(78.0520562805304,-9.65807620028567,137.090295150394));
#75973=CARTESIAN_POINT('Ctrl Pts',(78.0307828211536,-9.5866696387545,137.086253204602));
#75974=CARTESIAN_POINT('Ctrl Pts',(78.0095451555341,-9.51538322266288,137.082218059604));
#75975=CARTESIAN_POINT('Ctrl Pts',(77.9921549775743,-9.44284988951571,137.078182914607));
#75976=CARTESIAN_POINT('Ctrl Pts',(77.978745992917,-9.36949939289633,137.074147769609));
#75977=CARTESIAN_POINT('Ctrl Pts',(77.9653646220904,-9.29629995083135,137.070120934399));
#75978=CARTESIAN_POINT('Ctrl Pts',(77.9559481961507,-9.22228710632508,137.066094099189));
#75979=CARTESIAN_POINT('Ctrl Pts',(77.9505800370191,-9.1479032718887,137.062067263979));
#75980=CARTESIAN_POINT('Ctrl Pts',(77.9470284265033,-9.09869042217371,137.059403082473));
#75981=CARTESIAN_POINT('Ctrl Pts',(77.945247813142,-9.04931548698807,137.056738900968));
#75982=CARTESIAN_POINT('Ctrl Pts',(77.9452500020165,-8.99990896768397,137.054074719462));
#75983=CARTESIAN_POINT('Origin',(80.,-9.,141.545925280538));
#75984=CARTESIAN_POINT('',(81.2520391107129,-7.37076839346111,138.206016809128));
#75985=CARTESIAN_POINT('',(81.2520391107129,-7.37076839346111,138.147982307182));
#75986=CARTESIAN_POINT('',(81.2520391107129,-7.37076839346111,141.545925280538));
#75987=CARTESIAN_POINT('',(77.9452508576385,-8.99812264423968,137.695925280507));
#75988=CARTESIAN_POINT('Ctrl Pts',(81.2520391107129,-7.37076839346111,138.147982307182));
#75989=CARTESIAN_POINT('Ctrl Pts',(81.30859831624,-7.41423326187304,138.144121802281));
#75990=CARTESIAN_POINT('Ctrl Pts',(81.3628508305885,-7.46061547005432,138.14026129738));
#75991=CARTESIAN_POINT('Ctrl Pts',(81.4144948396281,-7.50963027702341,138.136400792478));
#75992=CARTESIAN_POINT('Ctrl Pts',(81.4668569716313,-7.55932664723847,138.132486606283));
#75993=CARTESIAN_POINT('Ctrl Pts',(81.5165371353892,-7.61172902392757,138.128572420088));
#75994=CARTESIAN_POINT('Ctrl Pts',(81.5632621184245,-7.66650492629369,138.124658233893));
#75995=CARTESIAN_POINT('Ctrl Pts',(81.6099871014597,-7.72128082865981,138.120744047698));
#75996=CARTESIAN_POINT('Ctrl Pts',(81.6537566440181,-7.77842980912718,138.116829861503));
#75997=CARTESIAN_POINT('Ctrl Pts',(81.6943435741599,-7.83758982488841,138.112915675308));
#75998=CARTESIAN_POINT('Ctrl Pts',(81.7344628184555,-7.89606813592506,138.109046592536));
#75999=CARTESIAN_POINT('Ctrl Pts',(81.7716296199628,-7.9567404259928,138.105177509764));
#76000=CARTESIAN_POINT('Ctrl Pts',(81.8055964784098,-8.01927632859497,138.101308426992));
#76001=CARTESIAN_POINT('Ctrl Pts',(81.8395127279186,-8.08171905579692,138.097445108962));
#76002=CARTESIAN_POINT('Ctrl Pts',(81.8702382682593,-8.14601946047875,138.093581790932));
#76003=CARTESIAN_POINT('Ctrl Pts',(81.897568582308,-8.21181789037196,138.089718472901));
#76004=CARTESIAN_POINT('Ctrl Pts',(81.9248668378963,-8.27753913870203,138.085859686544));
#76005=CARTESIAN_POINT('Ctrl Pts',(81.9487775925488,-8.34475447543659,138.082000900186));
#76006=CARTESIAN_POINT('Ctrl Pts',(81.9691428350753,-8.41308087646445,138.078142113828));
#76007=CARTESIAN_POINT('Ctrl Pts',(81.9894952489868,-8.48136423685131,138.074285758224));
#76008=CARTESIAN_POINT('Ctrl Pts',(82.0063064433988,-8.55075680851853,138.070429402619));
#76009=CARTESIAN_POINT('Ctrl Pts',(82.0194675293368,-8.62085825809528,138.066573047015));
#76010=CARTESIAN_POINT('Ctrl Pts',(82.0326247273551,-8.69093899898543,138.062717830618));
#76011=CARTESIAN_POINT('Ctrl Pts',(82.0421338679957,-8.76172772486692,138.05886261422));
#76012=CARTESIAN_POINT('Ctrl Pts',(82.0479370599022,-8.83281339413957,138.055007397823));
#76013=CARTESIAN_POINT('Ctrl Pts',(82.053740478695,-8.90390184263526,138.051152030699));
#76014=CARTESIAN_POINT('Ctrl Pts',(82.0558376237614,-8.9752867732197,138.047296663575));
#76015=CARTESIAN_POINT('Ctrl Pts',(82.054222568083,-9.04655323058885,138.043441296451));
#76016=CARTESIAN_POINT('Ctrl Pts',(82.052605821882,-9.11789428449572,138.039581893809));
#76017=CARTESIAN_POINT('Ctrl Pts',(82.047269129314,-9.18911613098387,138.035722491168));
#76018=CARTESIAN_POINT('Ctrl Pts',(82.0382586782996,-9.25980593302764,138.031863088526));
#76019=CARTESIAN_POINT('Ctrl Pts',(82.029243125498,-9.33053576018485,138.028001500661));
#76020=CARTESIAN_POINT('Ctrl Pts',(82.0165497598728,-9.40073246494944,138.024139912796));
#76021=CARTESIAN_POINT('Ctrl Pts',(82.0002759786768,-9.46999316125715,138.020278324931));
#76022=CARTESIAN_POINT('Ctrl Pts',(81.9839737259161,-9.5393750316407,138.016409981079));
#76023=CARTESIAN_POINT('Ctrl Pts',(81.9640786868404,-9.60781715746944,138.012541637227));
#76024=CARTESIAN_POINT('Ctrl Pts',(81.9407380100524,-9.67493224759071,138.008673293375));
#76025=CARTESIAN_POINT('Ctrl Pts',(81.9268789832666,-9.71478326991421,138.006376381355));
#76026=CARTESIAN_POINT('Ctrl Pts',(81.9118060744727,-9.75416679838156,138.004079469336));
#76027=CARTESIAN_POINT('Ctrl Pts',(81.8955578473674,-9.79300568080172,138.001782557316));
#76028=CARTESIAN_POINT('Ctrl Pts',(81.868188171565,-9.85842867209067,137.997913474436));
#76029=CARTESIAN_POINT('Ctrl Pts',(81.8373739143581,-9.92256118941954,137.994044391556));
#76030=CARTESIAN_POINT('Ctrl Pts',(81.8032583883211,-9.98501611532485,137.990175308676));
#76031=CARTESIAN_POINT('Ctrl Pts',(81.7691936927123,-10.0473779865129,137.986311990536));
#76032=CARTESIAN_POINT('Ctrl Pts',(81.7318377227877,-10.1080668049176,137.982448672396));
#76033=CARTESIAN_POINT('Ctrl Pts',(81.6913817082797,-10.1667156806167,137.978585354256));
#76034=CARTESIAN_POINT('Ctrl Pts',(81.6509731486556,-10.2252957612152,137.974726567787));
#76035=CARTESIAN_POINT('Ctrl Pts',(81.6074720419677,-10.2818402541869,137.970867781317));
#76036=CARTESIAN_POINT('Ctrl Pts',(81.5611144773083,-10.3360086643576,137.967008994847));
#76037=CARTESIAN_POINT('Ctrl Pts',(81.5147861145119,-10.3901429524059,137.96315263913));
#76038=CARTESIAN_POINT('Ctrl Pts',(81.4656051787558,-10.4419037589918,137.959296283412));
#76039=CARTESIAN_POINT('Ctrl Pts',(81.4138489441355,-10.4909824699395,137.955439927694));
#76040=CARTESIAN_POINT('Ctrl Pts',(81.3621079988221,-10.5400466825475,137.951584711183));
#76041=CARTESIAN_POINT('Ctrl Pts',(81.3077936172875,-10.5864300384086,137.947729494671));
#76042=CARTESIAN_POINT('Ctrl Pts',(81.2512197300677,-10.6298609602016,137.94387427816));
#76043=CARTESIAN_POINT('Ctrl Pts',(81.1946436309757,-10.6732935800156,137.94001891092));
#76044=CARTESIAN_POINT('Ctrl Pts',(81.1358082374835,-10.7137732425222,137.936163543681));
#76045=CARTESIAN_POINT('Ctrl Pts',(81.0750589525922,-10.7510699046444,137.932308176442));
#76046=CARTESIAN_POINT('Ctrl Pts',(81.0142460797654,-10.7884056062014,137.928448773684));
#76047=CARTESIAN_POINT('Ctrl Pts',(80.9515157312946,-10.8225514018019,137.924589370927));
#76048=CARTESIAN_POINT('Ctrl Pts',(80.8872397966611,-10.8533221807664,137.920729968169));
#76049=CARTESIAN_POINT('Ctrl Pts',(80.8229274684877,-10.8841103823881,137.916868380188));
#76050=CARTESIAN_POINT('Ctrl Pts',(80.7570682607569,-10.9115195764983,137.913006792206));
#76051=CARTESIAN_POINT('Ctrl Pts',(80.6900534777516,-10.9354130722776,137.909145204224));
#76052=CARTESIAN_POINT('Ctrl Pts',(80.6229214499872,-10.959348370582,137.905276860257));
#76053=CARTESIAN_POINT('Ctrl Pts',(80.5546302761199,-10.9797555510984,137.901408516289));
#76054=CARTESIAN_POINT('Ctrl Pts',(80.485585142784,-10.996548179135,137.897540172321));
#76055=CARTESIAN_POINT('Ctrl Pts',(80.4445881354143,-11.0065191569884,137.895243261322));
#76056=CARTESIAN_POINT('Ctrl Pts',(80.4033254996451,-11.0152167540812,137.892946350323));
#76057=CARTESIAN_POINT('Ctrl Pts',(80.3618829696563,-11.0226315232322,137.890649439325));
#76058=CARTESIAN_POINT('Ctrl Pts',(80.2920741777511,-11.0351214961376,137.886780356478));
#76059=CARTESIAN_POINT('Ctrl Pts',(80.2214812825332,-11.0440176346564,137.88291127363));
#76060=CARTESIAN_POINT('Ctrl Pts',(80.1505072441012,-11.0492303755247,137.879042190783));
#76061=CARTESIAN_POINT('Ctrl Pts',(80.0796389534447,-11.0544353496693,137.875178872676));
#76062=CARTESIAN_POINT('Ctrl Pts',(80.0083911273402,-11.0559677845549,137.871315554569));
#76063=CARTESIAN_POINT('Ctrl Pts',(79.9371757213841,-11.0537893447275,137.867452236462));
#76064=CARTESIAN_POINT('Ctrl Pts',(79.8660438510692,-11.0516134602092,137.863593450026));
#76065=CARTESIAN_POINT('Ctrl Pts',(79.7949448085641,-11.0457353620015,137.85973466359));
#76066=CARTESIAN_POINT('Ctrl Pts',(79.724292705199,-11.0361687184744,137.855875877153));
#76067=CARTESIAN_POINT('Ctrl Pts',(79.6536851074765,-11.0266081012309,137.852019521469));
#76068=CARTESIAN_POINT('Ctrl Pts',(79.5835243705776,-11.0133636135099,137.848163165785));
#76069=CARTESIAN_POINT('Ctrl Pts',(79.5142201594866,-10.9965008161909,137.844306810101));
#76070=CARTESIAN_POINT('Ctrl Pts',(79.4449364215517,-10.9796430003106,137.840451593623));
#76071=CARTESIAN_POINT('Ctrl Pts',(79.3765091788521,-10.9591691116506,137.836596377145));
#76072=CARTESIAN_POINT('Ctrl Pts',(79.3093368622182,-10.9351955954397,137.832741160667));
#76073=CARTESIAN_POINT('Ctrl Pts',(79.2421619193459,-10.9112211419355,137.828885793462));
#76074=CARTESIAN_POINT('Ctrl Pts',(79.1762424567267,-10.8837469545931,137.825030426256));
#76075=CARTESIAN_POINT('Ctrl Pts',(79.1119590809446,-10.8529384470573,137.821175059051));
#76076=CARTESIAN_POINT('Ctrl Pts',(79.0476084179951,-10.8220976914142,137.817315656327));
#76077=CARTESIAN_POINT('Ctrl Pts',(78.9848976994584,-10.7879158588881,137.813456253603));
#76078=CARTESIAN_POINT('Ctrl Pts',(78.9241841484707,-10.7506049857401,137.809596850879));
#76079=CARTESIAN_POINT('Ctrl Pts',(78.8634362209924,-10.713272986882,137.805735262931));
#76080=CARTESIAN_POINT('Ctrl Pts',(78.8046881124177,-10.6728086962058,137.801873674983));
#76081=CARTESIAN_POINT('Ctrl Pts',(78.7482668969634,-10.6294667229687,137.798012087035));
#76082=CARTESIAN_POINT('Ctrl Pts',(78.6917469705685,-10.5860489213944,137.7941437431));
#76083=CARTESIAN_POINT('Ctrl Pts',(78.6375624345439,-10.5397437012184,137.790275399166));
#76084=CARTESIAN_POINT('Ctrl Pts',(78.5860056707852,-10.4908445926549,137.786407055231));
#76085=CARTESIAN_POINT('Ctrl Pts',(78.5553927482461,-10.4618097092846,137.784110143932));
#76086=CARTESIAN_POINT('Ctrl Pts',(78.5257055636268,-10.4318610058014,137.781813232633));
#76087=CARTESIAN_POINT('Ctrl Pts',(78.4969985543702,-10.401065386388,137.779516321333));
#76088=CARTESIAN_POINT('Ctrl Pts',(78.4492223163319,-10.3498131353968,137.775693638866));
#76089=CARTESIAN_POINT('Ctrl Pts',(78.4039661357283,-10.2960019555863,137.771870956398));
#76090=CARTESIAN_POINT('Ctrl Pts',(78.3615208436963,-10.2399127456633,137.768048273931));
#76091=CARTESIAN_POINT('Ctrl Pts',(78.3191332469998,-10.1838997770766,137.764230787586));
#76092=CARTESIAN_POINT('Ctrl Pts',(78.279549263615,-10.1256153088631,137.760413301241));
#76093=CARTESIAN_POINT('Ctrl Pts',(78.2430220975309,-10.0653760898084,137.756595814896));
#76094=CARTESIAN_POINT('Ctrl Pts',(78.2065316626794,-10.0051974465115,137.752782167365));
#76095=CARTESIAN_POINT('Ctrl Pts',(78.1730922068983,-9.94306837371643,137.748968519833));
#76096=CARTESIAN_POINT('Ctrl Pts',(78.1429147652313,-9.87933610940529,137.745154872302));
#76097=CARTESIAN_POINT('Ctrl Pts',(78.1127570014886,-9.81564540324506,137.741343711551));
#76098=CARTESIAN_POINT('Ctrl Pts',(78.0858572438916,-9.75035402913312,137.7375325508));
#76099=CARTESIAN_POINT('Ctrl Pts',(78.0623806013098,-9.68383377243263,137.733721390049));
#76100=CARTESIAN_POINT('Ctrl Pts',(78.038904093185,-9.61731389671139,137.729910251125));
#76101=CARTESIAN_POINT('Ctrl Pts',(78.0188508409781,-9.54956561720769,137.726099112202));
#76102=CARTESIAN_POINT('Ctrl Pts',(78.0023372240674,-9.48097920553086,137.722287973278));
#76103=CARTESIAN_POINT('Ctrl Pts',(77.985823466128,-9.41239220811633,137.718476801807));
#76104=CARTESIAN_POINT('Ctrl Pts',(77.972849509985,-9.34296755130379,137.714665630336));
#76105=CARTESIAN_POINT('Ctrl Pts',(77.9634808603819,-9.27310685906643,137.710854458865));
#76106=CARTESIAN_POINT('Ctrl Pts',(77.954104932819,-9.20319189611444,137.707040326716));
#76107=CARTESIAN_POINT('Ctrl Pts',(77.9483399514159,-9.13284071762486,137.703226194567));
#76108=CARTESIAN_POINT('Ctrl Pts',(77.9461995397871,-9.06245984413321,137.699412062418));
#76109=CARTESIAN_POINT('Ctrl Pts',(77.9455473032982,-9.0410130470818,137.698249801791));
#76110=CARTESIAN_POINT('Ctrl Pts',(77.9452312678571,-9.01956349172712,137.697087541165));
#76111=CARTESIAN_POINT('Ctrl Pts',(77.945250857638,-8.99812264480472,137.695925280538));
#76112=CARTESIAN_POINT('Ctrl Pts',(77.9452508576385,-8.99812264423968,137.695925280507));
#76113=CARTESIAN_POINT('Ctrl Pts',(77.9453355911812,-8.90538253720821,137.690898045562));
#76114=CARTESIAN_POINT('Ctrl Pts',(77.9517027473503,-8.81292196311298,137.685870810616));
#76115=CARTESIAN_POINT('Ctrl Pts',(77.9642171232013,-8.72145800849217,137.68084357567));
#76116=CARTESIAN_POINT('Ctrl Pts',(77.9745563908271,-8.64589129096623,137.676690118227));
#76117=CARTESIAN_POINT('Ctrl Pts',(77.9890907794789,-8.57100419652186,137.672536660784));
#76118=CARTESIAN_POINT('Ctrl Pts',(78.0077202195897,-8.49718906230229,137.668383203341));
#76119=CARTESIAN_POINT('Ctrl Pts',(78.0250741586275,-8.4284278256959,137.66451412049));
#76120=CARTESIAN_POINT('Ctrl Pts',(78.0460260884595,-8.36043139357307,137.660645037639));
#76121=CARTESIAN_POINT('Ctrl Pts',(78.0704917545785,-8.29360386938326,137.656775954788));
#76122=CARTESIAN_POINT('Ctrl Pts',(78.0949209680755,-8.22687591487056,137.652912636677));
#76123=CARTESIAN_POINT('Ctrl Pts',(78.1228533603049,-8.16131386369155,137.649049318567));
#76124=CARTESIAN_POINT('Ctrl Pts',(78.1541542876671,-8.09730892949901,137.645186000456));
#76125=CARTESIAN_POINT('Ctrl Pts',(78.1854184990542,-8.03337907306842,137.641327214016));
#76126=CARTESIAN_POINT('Ctrl Pts',(78.2200431845955,-7.97100313985777,137.637468427576));
#76127=CARTESIAN_POINT('Ctrl Pts',(78.2578454199538,-7.91055290090612,137.633609641135));
#76128=CARTESIAN_POINT('Ctrl Pts',(78.2956238426761,-7.85014074117173,137.629753285448));
#76129=CARTESIAN_POINT('Ctrl Pts',(78.3365755870682,-7.79165227993754,137.62589692976));
#76130=CARTESIAN_POINT('Ctrl Pts',(78.3804722672276,-7.73543387469017,137.622040574073));
#76131=CARTESIAN_POINT('Ctrl Pts',(78.4243559798685,-7.67923207692214,137.618185357591));
#76132=CARTESIAN_POINT('Ctrl Pts',(78.4711826023524,-7.62529938649872,137.614330141109));
#76133=CARTESIAN_POINT('Ctrl Pts',(78.520682000174,-7.57395097633683,137.610474924628));
#76134=CARTESIAN_POINT('Ctrl Pts',(78.5701833332742,-7.52260055860539,137.606619557419));
#76135=CARTESIAN_POINT('Ctrl Pts',(78.6223573104465,-7.47383496994327,137.60276419021));
#76136=CARTESIAN_POINT('Ctrl Pts',(78.676896507449,-7.42793298154968,137.598908823001));
#76137=CARTESIAN_POINT('Ctrl Pts',(78.7314927921186,-7.38198294629104,137.595049420273));
#76138=CARTESIAN_POINT('Ctrl Pts',(78.7884588663218,-7.33890280824862,137.591190017546));
#76139=CARTESIAN_POINT('Ctrl Pts',(78.8474544423378,-7.29893083620532,137.587330614819));
#76140=CARTESIAN_POINT('Ctrl Pts',(78.9064834221125,-7.25893623171735,137.583469026868));
#76141=CARTESIAN_POINT('Ctrl Pts',(78.9675437752331,-7.22205354786824,137.579607438916));
#76142=CARTESIAN_POINT('Ctrl Pts',(79.030268826082,-7.18847605237149,137.575745850965));
#76143=CARTESIAN_POINT('Ctrl Pts',(79.093103616655,-7.15483981184317,137.571877507027));
#76144=CARTESIAN_POINT('Ctrl Pts',(79.1576084799626,-7.12452051139249,137.568009163089));
#76145=CARTESIAN_POINT('Ctrl Pts',(79.2233955510299,-7.09766378041636,137.564140819151));
#76146=CARTESIAN_POINT('Ctrl Pts',(79.262458019929,-7.08171702672345,137.561843907884));
#76147=CARTESIAN_POINT('Ctrl Pts',(79.3019722152477,-7.06699010951289,137.559546996617));
#76148=CARTESIAN_POINT('Ctrl Pts',(79.3418547552918,-7.05350509906448,137.55725008535));
#76149=CARTESIAN_POINT('Ctrl Pts',(79.4090365153636,-7.03078972698665,137.553380960127));
#76150=CARTESIAN_POINT('Ctrl Pts',(79.4775272460006,-7.01151203626851,137.549511834903));
#76151=CARTESIAN_POINT('Ctrl Pts',(79.5469417357709,-6.99582042428487,137.54564270968));
#76152=CARTESIAN_POINT('Ctrl Pts',(79.6162525807633,-6.98015224189991,137.54177936156));
#76153=CARTESIAN_POINT('Ctrl Pts',(79.6864839770011,-6.96805961584166,137.537916013439));
#76154=CARTESIAN_POINT('Ctrl Pts',(79.7572342153366,-6.95964161572121,137.534052665318));
#76155=CARTESIAN_POINT('Ctrl Pts',(79.8279006001617,-6.95123359265351,137.530193896055));
#76156=CARTESIAN_POINT('Ctrl Pts',(79.8990841254847,-6.94649160115844,137.526335126793));
#76157=CARTESIAN_POINT('Ctrl Pts',(79.9703732449642,-6.94546360025283,137.52247635753));
#76158=CARTESIAN_POINT('Ctrl Pts',(80.0416171339064,-6.94443625157907,137.518620036526));
#76159=CARTESIAN_POINT('Ctrl Pts',(80.1129659995101,-6.94711822512923,137.514763715522));
#76160=CARTESIAN_POINT('Ctrl Pts',(80.1840049945603,-6.95350550343352,137.510907394518));
#76161=CARTESIAN_POINT('Ctrl Pts',(80.2550226814983,-6.95989086587679,137.507052230216));
#76162=CARTESIAN_POINT('Ctrl Pts',(80.3257301988895,-6.96997928287426,137.503197065914));
#76163=CARTESIAN_POINT('Ctrl Pts',(80.3957162605865,-6.9837147514284,137.499341901611));
#76164=CARTESIAN_POINT('Ctrl Pts',(80.4657047407188,-6.99745069462477,137.49548660409));
#76165=CARTESIAN_POINT('Ctrl Pts',(80.5349712394912,-7.01483384359809,137.491631306569));
#76166=CARTESIAN_POINT('Ctrl Pts',(80.6031148326335,-7.03575712775699,137.487776009048));
#76167=CARTESIAN_POINT('Ctrl Pts',(80.67132616268,-7.05670121032744,137.483916879238));
#76168=CARTESIAN_POINT('Ctrl Pts',(80.7384118941889,-7.08119230845913,137.480057749428));
#76169=CARTESIAN_POINT('Ctrl Pts',(80.8039873646176,-7.10907380365194,137.476198619618));
#76170=CARTESIAN_POINT('Ctrl Pts',(80.8695998450386,-7.1369710348192,137.472337311763));
#76171=CARTESIAN_POINT('Ctrl Pts',(80.9336999310067,-7.1682622590305,137.468476003907));
#76172=CARTESIAN_POINT('Ctrl Pts',(80.9959264492284,-7.20274429470169,137.464614696052));
#76173=CARTESIAN_POINT('Ctrl Pts',(81.0582543739519,-7.23728252349944,137.460747095675));
#76174=CARTESIAN_POINT('Ctrl Pts',(81.1187022253211,-7.27502168482671,137.456879495297));
#76175=CARTESIAN_POINT('Ctrl Pts',(81.1769374678791,-7.31571505997286,137.45301189492));
#76176=CARTESIAN_POINT('Ctrl Pts',(81.2024025701055,-7.33350945581485,137.451320670935));
#76177=CARTESIAN_POINT('Ctrl Pts',(81.2274450179012,-7.35186821624316,137.44962944695));
#76178=CARTESIAN_POINT('Ctrl Pts',(81.2520391107129,-7.37076839346111,137.447938222965));
#76179=CARTESIAN_POINT('',(77.9452508246239,-9.00184086701729,137.754074719432));
#76180=CARTESIAN_POINT('Ctrl Pts',(77.9452508246239,-9.00184086701728,137.754074719432));
#76181=CARTESIAN_POINT('Ctrl Pts',(77.9451879957237,-8.93171215608289,137.750267950527));
#76182=CARTESIAN_POINT('Ctrl Pts',(77.9487196432091,-8.86147127332159,137.746461181623));
#76183=CARTESIAN_POINT('Ctrl Pts',(77.9558535710242,-8.79152232876057,137.742654412718));
#76184=CARTESIAN_POINT('Ctrl Pts',(77.9629816800021,-8.72163043853593,137.73885074883));
#76185=CARTESIAN_POINT('Ctrl Pts',(77.9737061958363,-8.65203051067417,137.735047084943));
#76186=CARTESIAN_POINT('Ctrl Pts',(77.9879828890365,-8.58312506948712,137.731243421055));
#76187=CARTESIAN_POINT('Ctrl Pts',(78.0022530301476,-8.5142512514906,137.727441502806));
#76188=CARTESIAN_POINT('Ctrl Pts',(78.0200720145936,-8.44607177785787,137.723639584557));
#76189=CARTESIAN_POINT('Ctrl Pts',(78.0413442350505,-8.37898055028048,137.719837666308));
#76190=CARTESIAN_POINT('Ctrl Pts',(78.0626142800848,-8.3118961838471,137.716036136865));
#76191=CARTESIAN_POINT('Ctrl Pts',(78.0873367072432,-8.24590031936901,137.712234607422));
#76192=CARTESIAN_POINT('Ctrl Pts',(78.1153661610127,-8.18137135681427,137.70843307798));
#76193=CARTESIAN_POINT('Ctrl Pts',(78.1434216019787,-8.1167825669493,137.704628023991));
#76194=CARTESIAN_POINT('Ctrl Pts',(78.1747899917197,-8.05366385490174,137.700822970003));
#76195=CARTESIAN_POINT('Ctrl Pts',(78.2092783941065,-7.99237224498024,137.697017916015));
#76196=CARTESIAN_POINT('Ctrl Pts',(78.2437833388229,-7.93105123659601,137.693211036936));
#76197=CARTESIAN_POINT('Ctrl Pts',(78.2814110055525,-7.87155949732334,137.689404157857));
#76198=CARTESIAN_POINT('Ctrl Pts',(78.3219247244651,-7.81422559812649,137.685597278778));
#76199=CARTESIAN_POINT('Ctrl Pts',(78.3625095297396,-7.75679109946812,137.681783720056));
#76200=CARTESIAN_POINT('Ctrl Pts',(78.4059901860581,-7.70152239258478,137.677970161334));
#76201=CARTESIAN_POINT('Ctrl Pts',(78.4520898455688,-7.64871479090879,137.674156602612));
#76202=CARTESIAN_POINT('Ctrl Pts',(78.4841323747948,-7.61200976666302,137.671505909134));
#76203=CARTESIAN_POINT('Ctrl Pts',(78.5174393844108,-7.576493026584,137.668855215655));
#76204=CARTESIAN_POINT('Ctrl Pts',(78.5519082624525,-7.54225246282259,137.666204522177));
#76205=CARTESIAN_POINT('Ctrl Pts',(78.6022207357351,-7.49227324831671,137.66233543933));
#76206=CARTESIAN_POINT('Ctrl Pts',(78.6552222517713,-7.44480391681055,137.658466356483));
#76207=CARTESIAN_POINT('Ctrl Pts',(78.7106323248068,-7.40014733157491,137.654597273636));
#76208=CARTESIAN_POINT('Ctrl Pts',(78.7659598395983,-7.35555728242294,137.650733955529));
#76209=CARTESIAN_POINT('Ctrl Pts',(78.8236884129031,-7.31377196316542,137.646870637422));
#76210=CARTESIAN_POINT('Ctrl Pts',(78.8835010225438,-7.27505721954632,137.643007319315));
#76211=CARTESIAN_POINT('Ctrl Pts',(78.9432434720188,-7.23638788830505,137.639148532878));
#76212=CARTESIAN_POINT('Ctrl Pts',(79.0050646962477,-7.20078224102097,137.635289746442));
#76213=CARTESIAN_POINT('Ctrl Pts',(79.06861632084,-7.16846457727558,137.631430960006));
#76214=CARTESIAN_POINT('Ctrl Pts',(79.1321279125703,-7.13616727128783,137.627574604322));
#76215=CARTESIAN_POINT('Ctrl Pts',(79.1973673100838,-7.1071540593101,137.623718248638));
#76216=CARTESIAN_POINT('Ctrl Pts',(79.2639602801964,-7.08160403113136,137.619861892954));
#76217=CARTESIAN_POINT('Ctrl Pts',(79.3305335780805,-7.05606155068615,137.616006676476));
#76218=CARTESIAN_POINT('Ctrl Pts',(79.3984592014336,-7.03398039690303,137.612151459998));
#76219=CARTESIAN_POINT('Ctrl Pts',(79.4673432145724,-7.01549141814958,137.60829624352));
#76220=CARTESIAN_POINT('Ctrl Pts',(79.5362299208718,-6.99700171653192,137.604440876314));
#76221=CARTESIAN_POINT('Ctrl Pts',(79.6060746216013,-6.98210459257871,137.600585509109));
#76222=CARTESIAN_POINT('Ctrl Pts',(79.6764701885847,-6.97088048069475,137.596730141903));
#76223=CARTESIAN_POINT('Ctrl Pts',(79.7469394405332,-6.95964462022593,137.592870739179));
#76224=CARTESIAN_POINT('Ctrl Pts',(79.8179602290655,-6.95208952323919,137.589011336456));
#76225=CARTESIAN_POINT('Ctrl Pts',(79.8891181401292,-6.94824397755201,137.585151933732));
#76226=CARTESIAN_POINT('Ctrl Pts',(79.9603163413626,-6.94439625448658,137.581290345784));
#76227=CARTESIAN_POINT('Ctrl Pts',(80.0316513336722,-6.94426226483673,137.577428757836));
#76228=CARTESIAN_POINT('Ctrl Pts',(80.1027092849991,-6.94781863246082,137.573567169888));
#76229=CARTESIAN_POINT('Ctrl Pts',(80.1738915547607,-6.95138122207764,137.569698825953));
#76230=CARTESIAN_POINT('Ctrl Pts',(80.2447953324307,-6.95864700984184,137.565830482018));
#76231=CARTESIAN_POINT('Ctrl Pts',(80.3150131820552,-6.96954087516358,137.561962138084));
#76232=CARTESIAN_POINT('Ctrl Pts',(80.3567065203249,-6.97600933887123,137.559665226784));
#76233=CARTESIAN_POINT('Ctrl Pts',(80.3981582238856,-6.9837559538072,137.557368315485));
#76234=CARTESIAN_POINT('Ctrl Pts',(80.4392854645027,-6.99275665571495,137.555071404186));
#76235=CARTESIAN_POINT('Ctrl Pts',(80.5085688299926,-7.00791932917862,137.551202004181));
#76236=CARTESIAN_POINT('Ctrl Pts',(80.5772019369491,-7.02670306183723,137.547332604176));
#76237=CARTESIAN_POINT('Ctrl Pts',(80.644778110245,-7.04903645573556,137.543463204171));
#76238=CARTESIAN_POINT('Ctrl Pts',(80.7122373862133,-7.0713312159863,137.539600497687));
#76239=CARTESIAN_POINT('Ctrl Pts',(80.7786429038342,-7.09716328564512,137.535737791203));
#76240=CARTESIAN_POINT('Ctrl Pts',(80.8435995584078,-7.1264105712419,137.531875084719));
#76241=CARTESIAN_POINT('Ctrl Pts',(80.9084915578482,-7.15562874531559,137.528016223011));
#76242=CARTESIAN_POINT('Ctrl Pts',(80.9719371146362,-7.18825519303851,137.524157361303));
#76243=CARTESIAN_POINT('Ctrl Pts',(81.0335588124515,-7.22411888244065,137.520298499595));
#76244=CARTESIAN_POINT('Ctrl Pts',(81.0951364101866,-7.25995690569538,137.516442399514));
#76245=CARTESIAN_POINT('Ctrl Pts',(81.1548923224176,-7.29902732574741,137.512586299433));
#76246=CARTESIAN_POINT('Ctrl Pts',(81.2124731810425,-7.34111291892647,137.508730199351));
#76247=CARTESIAN_POINT('Ctrl Pts',(81.2257792412245,-7.35083825906566,137.507839113303));
#76248=CARTESIAN_POINT('Ctrl Pts',(81.2389692666534,-7.36072442189331,137.506948027255));
#76249=CARTESIAN_POINT('Ctrl Pts',(81.2520391107129,-7.37076839346111,137.506056941207));
#76250=CARTESIAN_POINT('Ctrl Pts',(81.2520391107129,-7.37076839346111,138.206016809128));
#76251=CARTESIAN_POINT('Ctrl Pts',(81.3100004179798,-7.41531075521925,138.202046816837));
#76252=CARTESIAN_POINT('Ctrl Pts',(81.3656646502486,-7.46301363829869,138.198076824546));
#76253=CARTESIAN_POINT('Ctrl Pts',(81.4186724490077,-7.51360636272669,138.194106832255));
#76254=CARTESIAN_POINT('Ctrl Pts',(81.470180544976,-7.56276771192698,138.190249159447));
#76255=CARTESIAN_POINT('Ctrl Pts',(81.5191801491463,-7.61465719146405,138.186391486638));
#76256=CARTESIAN_POINT('Ctrl Pts',(81.5653745141076,-7.66898527690999,138.182533813829));
#76257=CARTESIAN_POINT('Ctrl Pts',(81.6115458735347,-7.72328630609853,138.178678062203));
#76258=CARTESIAN_POINT('Ctrl Pts',(81.6549144517787,-7.78002316174998,138.174822310578));
#76259=CARTESIAN_POINT('Ctrl Pts',(81.6952218735085,-7.8388710829204,138.170966558952));
#76260=CARTESIAN_POINT('Ctrl Pts',(81.7355227048577,-7.89770938228475,138.167111437753));
#76261=CARTESIAN_POINT('Ctrl Pts',(81.7727630996661,-7.95865766065981,138.163256316554));
#76262=CARTESIAN_POINT('Ctrl Pts',(81.8067273668012,-8.02136125942632,138.159401195355));
#76263=CARTESIAN_POINT('Ctrl Pts',(81.8424556842878,-8.08732158400432,138.155345845254));
#76264=CARTESIAN_POINT('Ctrl Pts',(81.8745580065639,-8.15522401595865,138.151290495153));
#76265=CARTESIAN_POINT('Ctrl Pts',(81.9028386326526,-8.22462737952329,138.147235145052));
#76266=CARTESIAN_POINT('Ctrl Pts',(81.9297585778696,-8.29069150197893,138.143374912177));
#76267=CARTESIAN_POINT('Ctrl Pts',(81.9532159966933,-8.35811495349229,138.139514679302));
#76268=CARTESIAN_POINT('Ctrl Pts',(81.9730927843165,-8.42649984570362,138.135654446427));
#76269=CARTESIAN_POINT('Ctrl Pts',(81.9929834859348,-8.49493260817794,138.131791511342));
#76270=CARTESIAN_POINT('Ctrl Pts',(82.0092884595855,-8.56432767786134,138.127928576256));
#76271=CARTESIAN_POINT('Ctrl Pts',(82.0219406340872,-8.63427655977905,138.124065641171));
#76272=CARTESIAN_POINT('Ctrl Pts',(82.0346132883302,-8.70433866610792,138.120196453255));
#76273=CARTESIAN_POINT('Ctrl Pts',(82.0436212919721,-8.77495589200382,138.116327265338));
#76274=CARTESIAN_POINT('Ctrl Pts',(82.0489494313871,-8.84571523043957,138.112458077422));
#76275=CARTESIAN_POINT('Ctrl Pts',(82.0497394482973,-8.85620689921254,138.111884382996));
#76276=CARTESIAN_POINT('Ctrl Pts',(82.0504486576644,-8.86670169549341,138.11131068857));
#76277=CARTESIAN_POINT('Ctrl Pts',(82.0510771072001,-8.87719827843336,138.110736994144));
#76278=CARTESIAN_POINT('Ctrl Pts',(82.0553154671481,-8.94798884187682,138.106867911045));
#76279=CARTESIAN_POINT('Ctrl Pts',(82.0558929439494,-9.01913773756604,138.102998827945));
#76280=CARTESIAN_POINT('Ctrl Pts',(82.0527677254119,-9.09023429507291,138.099129744846));
#76281=CARTESIAN_POINT('Ctrl Pts',(82.0496471632914,-9.16122492231617,138.095266426484));
#76282=CARTESIAN_POINT('Ctrl Pts',(82.0428348777429,-9.23216288480688,138.091403108122));
#76283=CARTESIAN_POINT('Ctrl Pts',(82.032340984946,-9.30263457074262,138.087539789761));
#76284=CARTESIAN_POINT('Ctrl Pts',(82.021859401472,-9.37302359348072,138.083681003066));
#76285=CARTESIAN_POINT('Ctrl Pts',(82.0077048599954,-9.44294694792222,138.079822216372));
#76286=CARTESIAN_POINT('Ctrl Pts',(81.9899393756735,-9.51199496447144,138.075963429678));
#76287=CARTESIAN_POINT('Ctrl Pts',(81.9721850822951,-9.58099948586839,138.072107073734));
#76288=CARTESIAN_POINT('Ctrl Pts',(81.9508244796561,-9.64912929399013,138.068250717791));
#76289=CARTESIAN_POINT('Ctrl Pts',(81.9259705990646,-9.71598520518144,138.064394361847));
#76290=CARTESIAN_POINT('Ctrl Pts',(81.9011240605487,-9.78282136649287,138.060539145108));
#76291=CARTESIAN_POINT('Ctrl Pts',(81.8727864619641,-9.84838392288732,138.056683928369));
#76292=CARTESIAN_POINT('Ctrl Pts',(81.8411200555273,-9.91229079992897,138.052828711631));
#76293=CARTESIAN_POINT('Ctrl Pts',(81.8094524110205,-9.97620017555506,138.048973344163));
#76294=CARTESIAN_POINT('Ctrl Pts',(81.7744559179282,-10.0384533090118,138.045117976696));
#76295=CARTESIAN_POINT('Ctrl Pts',(81.7363393757206,-10.0986915558164,138.041262609229));
#76296=CARTESIAN_POINT('Ctrl Pts',(81.6981829358925,-10.1589928556307,138.037403206243));
#76297=CARTESIAN_POINT('Ctrl Pts',(81.6569001878845,-10.2172746473378,138.033543803258));
#76298=CARTESIAN_POINT('Ctrl Pts',(81.6127434984387,-10.2732069630439,138.029684400273));
#76299=CARTESIAN_POINT('Ctrl Pts',(81.5685618071274,-10.329170948068,138.025822812063));
#76300=CARTESIAN_POINT('Ctrl Pts',(81.5215032556432,-10.3827824436303,138.021961223854));
#76301=CARTESIAN_POINT('Ctrl Pts',(81.4718589647921,-10.4337464037482,138.018099635644));
#76302=CARTESIAN_POINT('Ctrl Pts',(81.4221278195125,-10.4847995271025,138.01423129145));
#76303=CARTESIAN_POINT('Ctrl Pts',(81.3698022596313,-10.5331955372286,138.010362947257));
#76304=CARTESIAN_POINT('Ctrl Pts',(81.3152080015881,-10.5786783950694,138.006494603063));
#76305=CARTESIAN_POINT('Ctrl Pts',(81.2827915373983,-10.6056847778885,138.004197694093));
#76306=CARTESIAN_POINT('Ctrl Pts',(81.2495758162233,-10.6316648862377,138.001900785122));
#76307=CARTESIAN_POINT('Ctrl Pts',(81.2156336505187,-10.6565724826359,137.999603876152));
#76308=CARTESIAN_POINT('Ctrl Pts',(81.1584589632516,-10.6985286750322,137.995734793277));
#76309=CARTESIAN_POINT('Ctrl Pts',(81.0989976384083,-10.7376035912017,137.991865710402));
#76310=CARTESIAN_POINT('Ctrl Pts',(81.0375720156334,-10.7735393637792,137.987996627528));
#76311=CARTESIAN_POINT('Ctrl Pts',(80.9762379139521,-10.8094215938601,137.984133309392));
#76312=CARTESIAN_POINT('Ctrl Pts',(80.9129457396517,-10.8421737210908,137.980269991257));
#76313=CARTESIAN_POINT('Ctrl Pts',(80.8480484684536,-10.8715799095025,137.976406673121));
#76314=CARTESIAN_POINT('Ctrl Pts',(80.7832273216993,-10.9009516044803,137.972547886654));
#76315=CARTESIAN_POINT('Ctrl Pts',(80.7168052582111,-10.9269849570654,137.968689100188));
#76316=CARTESIAN_POINT('Ctrl Pts',(80.6491600907199,-10.9495098715104,137.964830313721));
#76317=CARTESIAN_POINT('Ctrl Pts',(80.5815575347049,-10.9720205969173,137.960973958006));
#76318=CARTESIAN_POINT('Ctrl Pts',(80.512733863091,-10.9910271157927,137.957117602291));
#76319=CARTESIAN_POINT('Ctrl Pts',(80.4430857491828,-11.0064078801109,137.953261246575));
#76320=CARTESIAN_POINT('Ctrl Pts',(80.3734582100062,-11.0217841008014,137.949406030065));
#76321=CARTESIAN_POINT('Ctrl Pts',(80.3030071861419,-11.0335365886353,137.945550813555));
#76322=CARTESIAN_POINT('Ctrl Pts',(80.2321416733279,-11.0415944274034,137.941695597045));
#76323=CARTESIAN_POINT('Ctrl Pts',(80.1612733898664,-11.0496525812109,137.937840229806));
#76324=CARTESIAN_POINT('Ctrl Pts',(80.0899910682031,-11.0540157464709,137.933984862568));
#76325=CARTESIAN_POINT('Ctrl Pts',(80.0187092661134,-11.0546648208069,137.930129495329));
#76326=CARTESIAN_POINT('Ctrl Pts',(79.9473528513915,-11.055314574547,137.926270092571));
#76327=CARTESIAN_POINT('Ctrl Pts',(79.875997444087,-11.052242472327,137.922410689813));
#76328=CARTESIAN_POINT('Ctrl Pts',(79.8050571398559,-11.0454815676947,137.918551287055));
#76329=CARTESIAN_POINT('Ctrl Pts',(79.7340766686535,-11.0387168349838,137.914689699072));
#76330=CARTESIAN_POINT('Ctrl Pts',(79.6635122491684,-11.0282592132919,137.910828111089));
#76331=CARTESIAN_POINT('Ctrl Pts',(79.5937696574455,-11.0141932556952,137.906966523106));
#76332=CARTESIAN_POINT('Ctrl Pts',(79.5239050485444,-11.0001026891986,137.903098179136));
#76333=CARTESIAN_POINT('Ctrl Pts',(79.454865608743,-10.9823913036386,137.899229835166));
#76334=CARTESIAN_POINT('Ctrl Pts',(79.3870431070684,-10.9611938736157,137.895361491195));
#76335=CARTESIAN_POINT('Ctrl Pts',(79.3467720628869,-10.948607451412,137.893064580184));
#76336=CARTESIAN_POINT('Ctrl Pts',(79.3069297253047,-10.9347929137085,137.890767669172));
#76337=CARTESIAN_POINT('Ctrl Pts',(79.2675944322142,-10.9197863544614,137.88847075816));
#76338=CARTESIAN_POINT('Ctrl Pts',(79.2013352240665,-10.8945082224174,137.884601675388));
#76339=CARTESIAN_POINT('Ctrl Pts',(79.1362564439906,-10.8657462631716,137.880732592617));
#76340=CARTESIAN_POINT('Ctrl Pts',(79.072749565558,-10.8336314227039,137.876863509845));
#76341=CARTESIAN_POINT('Ctrl Pts',(79.0093373092316,-10.8015644317593,137.873000191815));
#76342=CARTESIAN_POINT('Ctrl Pts',(78.9474927356075,-10.7661546932086,137.869136873785));
#76343=CARTESIAN_POINT('Ctrl Pts',(78.8875886226998,-10.7275816884168,137.865273555755));
#76344=CARTESIAN_POINT('Ctrl Pts',(78.8277547773211,-10.6890539297625,137.861414769397));
#76345=CARTESIAN_POINT('Ctrl Pts',(78.7698572778851,-10.6473705369187,137.85755598304));
#76346=CARTESIAN_POINT('Ctrl Pts',(78.7142439456413,-10.602756666241,137.853697196682));
#76347=CARTESIAN_POINT('Ctrl Pts',(78.658665645734,-10.5581708990425,137.849840841078));
#76348=CARTESIAN_POINT('Ctrl Pts',(78.6053690363735,-10.5106586196787,137.845984485474));
#76349=CARTESIAN_POINT('Ctrl Pts',(78.5546713818689,-10.4604871612278,137.84212812987));
#76350=CARTESIAN_POINT('Ctrl Pts',(78.5039887039709,-10.4103305239398,137.838272913473));
#76351=CARTESIAN_POINT('Ctrl Pts',(78.455903801816,-10.357516608615,137.834417697076));
#76352=CARTESIAN_POINT('Ctrl Pts',(78.4106980856967,-10.3023505625184,137.830562480679));
#76353=CARTESIAN_POINT('Ctrl Pts',(78.3654906021781,-10.2471823596053,137.826707113555));
#76354=CARTESIAN_POINT('Ctrl Pts',(78.3231628343794,-10.1896622204827,137.822851746431));
#76355=CARTESIAN_POINT('Ctrl Pts',(78.2839556788196,-10.1301280680721,137.818996379307));
#76356=CARTESIAN_POINT('Ctrl Pts',(78.2447074840645,-10.0705315996463,137.815136976666));
#76357=CARTESIAN_POINT('Ctrl Pts',(78.2085866898057,-10.0089173161854,137.811277574025));
#76358=CARTESIAN_POINT('Ctrl Pts',(78.175790124002,-9.94565104071822,137.807418171383));
#76359=CARTESIAN_POINT('Ctrl Pts',(78.1429749885287,-9.88234894339576,137.803556583518));
#76360=CARTESIAN_POINT('Ctrl Pts',(78.1134880292955,-9.81739343458066,137.799694995653));
#76361=CARTESIAN_POINT('Ctrl Pts',(78.0874782954112,-9.75117128005319,137.795833407788));
#76362=CARTESIAN_POINT('Ctrl Pts',(78.0614230565633,-9.68483326748785,137.791965063936));
#76363=CARTESIAN_POINT('Ctrl Pts',(78.0388573428529,-9.61722464575904,137.788096720084));
#76364=CARTESIAN_POINT('Ctrl Pts',(78.0198804134945,-9.54874765205621,137.784228376233));
#76365=CARTESIAN_POINT('Ctrl Pts',(78.0086124552047,-9.50808797027721,137.781931464211));
#76366=CARTESIAN_POINT('Ctrl Pts',(77.9986088005102,-9.46712235311462,137.77963455219));
#76367=CARTESIAN_POINT('Ctrl Pts',(77.9898816146324,-9.42593619159094,137.777337640169));
#76368=CARTESIAN_POINT('Ctrl Pts',(77.9692978091794,-9.32879514887455,137.771920179047));
#76369=CARTESIAN_POINT('Ctrl Pts',(77.9557497500277,-9.23011503383561,137.766502717926));
#76370=CARTESIAN_POINT('Ctrl Pts',(77.949413941794,-9.13074547943003,137.761085256805));
#76371=CARTESIAN_POINT('Ctrl Pts',(77.94668096293,-9.08788198326621,137.758748411024));
#76372=CARTESIAN_POINT('Ctrl Pts',(77.9452893931581,-9.04489049479503,137.756411565243));
#76373=CARTESIAN_POINT('Ctrl Pts',(77.9452508246244,-9.00184086757116,137.754074719462));
#76374=CARTESIAN_POINT('Origin',(80.,-9.,141.545925280538));
#76375=CARTESIAN_POINT('',(81.2520391107129,-7.37076839346111,138.906139397208));
#76376=CARTESIAN_POINT('',(81.2520391107129,-7.37076839346111,138.847890491337));
#76377=CARTESIAN_POINT('',(81.2520391107129,-7.37076839346111,141.545925280538));
#76378=CARTESIAN_POINT('',(77.9452500654425,-9.00051859011398,138.39592528059));
#76379=CARTESIAN_POINT('Ctrl Pts',(81.2520391107129,-7.37076839346111,138.847890491337));
#76380=CARTESIAN_POINT('Ctrl Pts',(81.3085681377711,-7.4142100701898,138.844035068992));
#76381=CARTESIAN_POINT('Ctrl Pts',(81.3628582559677,-7.46061620714495,138.840179646647));
#76382=CARTESIAN_POINT('Ctrl Pts',(81.4145905616516,-7.50972113167154,138.836324224303));
#76383=CARTESIAN_POINT('Ctrl Pts',(81.4663198262433,-7.55882316955704,138.832469028599));
#76384=CARTESIAN_POINT('Ctrl Pts',(81.5154912256335,-7.61062334443875,138.828613832896));
#76385=CARTESIAN_POINT('Ctrl Pts',(81.5618216651866,-7.66481812150793,138.824758637193));
#76386=CARTESIAN_POINT('Ctrl Pts',(81.6081976898814,-7.71906622154602,138.820899648311));
#76387=CARTESIAN_POINT('Ctrl Pts',(81.6517268546166,-7.77571326004013,138.817040659429));
#76388=CARTESIAN_POINT('Ctrl Pts',(81.6921660259195,-7.83442215908853,138.813181670547));
#76389=CARTESIAN_POINT('Ctrl Pts',(81.7326245444005,-7.8931591460401,138.809320835421));
#76390=CARTESIAN_POINT('Ctrl Pts',(81.7699898695783,-7.95395954422761,138.805460000296));
#76391=CARTESIAN_POINT('Ctrl Pts',(81.8040634605908,-8.01645915557045,138.801599165171));
#76392=CARTESIAN_POINT('Ctrl Pts',(81.8381998457058,-8.0790739472301,138.797731214926));
#76393=CARTESIAN_POINT('Ctrl Pts',(81.8690321655762,-8.14339376955236,138.793863264681));
#76394=CARTESIAN_POINT('Ctrl Pts',(81.8964091261853,-8.20903224552375,138.789995314436));
#76395=CARTESIAN_POINT('Ctrl Pts',(81.9206649231915,-8.26718747946997,138.786568337376));
#76396=CARTESIAN_POINT('Ctrl Pts',(81.9422089601469,-8.32637733301329,138.783141360317));
#76397=CARTESIAN_POINT('Ctrl Pts',(81.9609690692731,-8.38632429422847,138.779714383257));
#76398=CARTESIAN_POINT('Ctrl Pts',(81.9821493409331,-8.45400476000776,138.775845306345));
#76399=CARTESIAN_POINT('Ctrl Pts',(81.9998631210085,-8.52291559440797,138.771976229432));
#76400=CARTESIAN_POINT('Ctrl Pts',(82.0139708208754,-8.59266832290836,138.76810715252));
#76401=CARTESIAN_POINT('Ctrl Pts',(82.0280575005765,-8.6623171213604,138.764243840448));
#76402=CARTESIAN_POINT('Ctrl Pts',(82.0385486697698,-8.73280485169113,138.760380528376));
#76403=CARTESIAN_POINT('Ctrl Pts',(82.0453544272477,-8.80372766512275,138.756517216304));
#76404=CARTESIAN_POINT('Ctrl Pts',(82.0521522013523,-8.87456728380361,138.752658436021));
#76405=CARTESIAN_POINT('Ctrl Pts',(82.0552731047176,-8.94584049060809,138.748799655739));
#76406=CARTESIAN_POINT('Ctrl Pts',(82.0546785546254,-9.01713475014791,138.744940875457));
#76407=CARTESIAN_POINT('Ctrl Pts',(82.0540843790675,-9.08838409816279,138.741084525997));
#76408=CARTESIAN_POINT('Ctrl Pts',(82.049779397677,-9.15965398798164,138.737228176538));
#76409=CARTESIAN_POINT('Ctrl Pts',(82.0417770670953,-9.23052976116694,138.733371827078));
#76410=CARTESIAN_POINT('Ctrl Pts',(82.0337771006125,-9.30138459578544,138.729516616886));
#76411=CARTESIAN_POINT('Ctrl Pts',(82.0220820079176,-9.37184506246619,138.725661406693));
#76412=CARTESIAN_POINT('Ctrl Pts',(82.0067571395565,-9.44150124047278,138.721806196501));
#76413=CARTESIAN_POINT('Ctrl Pts',(81.9914316722434,-9.51116014089782,138.717950835633));
#76414=CARTESIAN_POINT('Ctrl Pts',(81.9724762541412,-9.58001421627456,138.714095474765));
#76415=CARTESIAN_POINT('Ctrl Pts',(81.9500070587942,-9.64766506247656,138.710240113896));
#76416=CARTESIAN_POINT('Ctrl Pts',(81.9275143444946,-9.71538672016182,138.706380717546));
#76417=CARTESIAN_POINT('Ctrl Pts',(81.9015006643918,-9.78190217257416,138.702521321195));
#76418=CARTESIAN_POINT('Ctrl Pts',(81.8721313878705,-9.84683034254225,138.698661924844));
#76419=CARTESIAN_POINT('Ctrl Pts',(81.8427454824318,-9.91179527491291,138.694800343298));
#76420=CARTESIAN_POINT('Ctrl Pts',(81.8100004214718,-9.97517070397781,138.690938761753));
#76421=CARTESIAN_POINT('Ctrl Pts',(81.7741076046741,-10.0366001010696,138.687077180207));
#76422=CARTESIAN_POINT('Ctrl Pts',(81.7381519917931,-10.0981369716305,138.683208842653));
#76423=CARTESIAN_POINT('Ctrl Pts',(81.6990378945876,-10.1577206064699,138.679340505098));
#76424=CARTESIAN_POINT('Ctrl Pts',(81.6570196921329,-10.2150239925137,138.675472167544));
#76425=CARTESIAN_POINT('Ctrl Pts',(81.6320698419778,-10.249049981529,138.673175200118));
#76426=CARTESIAN_POINT('Ctrl Pts',(81.6060968321676,-10.2822726221546,138.670878232692));
#76427=CARTESIAN_POINT('Ctrl Pts',(81.579160184669,-10.3146294815103,138.668581265266));
#76428=CARTESIAN_POINT('Ctrl Pts',(81.5337872424589,-10.3691324002469,138.664712180582));
#76429=CARTESIAN_POINT('Ctrl Pts',(81.4855004608265,-10.421390317654,138.660843095898));
#76430=CARTESIAN_POINT('Ctrl Pts',(81.4345505021733,-10.4710752595344,138.656974011214));
#76431=CARTESIAN_POINT('Ctrl Pts',(81.3836764561363,-10.5206861736036,138.653110691252));
#76432=CARTESIAN_POINT('Ctrl Pts',(81.330147454379,-10.5677313853259,138.649247371289));
#76433=CARTESIAN_POINT('Ctrl Pts',(81.2742540250556,-10.6119163260324,138.645384051327));
#76434=CARTESIAN_POINT('Ctrl Pts',(81.218426158404,-10.656049438057,138.641525263017));
#76435=CARTESIAN_POINT('Ctrl Pts',(81.1602397524556,-10.6973286435976,138.637666474707));
#76436=CARTESIAN_POINT('Ctrl Pts',(81.100020467273,-10.7354977770313,138.633807686397));
#76437=CARTESIAN_POINT('Ctrl Pts',(81.0398391156441,-10.773642866824,138.629951328829));
#76438=CARTESIAN_POINT('Ctrl Pts',(80.977627834725,-10.8086815118984,138.626094971261));
#76439=CARTESIAN_POINT('Ctrl Pts',(80.9137422932057,-10.8404001152215,138.622238613693));
#76440=CARTESIAN_POINT('Ctrl Pts',(80.8498756239809,-10.8721093486182,138.618383395324));
#76441=CARTESIAN_POINT('Ctrl Pts',(80.7843361109232,-10.900500271449,138.614528176955));
#76442=CARTESIAN_POINT('Ctrl Pts',(80.717503588529,-10.9254054541701,138.610672958585));
#76443=CARTESIAN_POINT('Ctrl Pts',(80.6506684531029,-10.9503116106392,138.606817589484));
#76444=CARTESIAN_POINT('Ctrl Pts',(80.5825406639435,-10.9717315888527,138.602962220382));
#76445=CARTESIAN_POINT('Ctrl Pts',(80.5135179453508,-10.9895469037705,138.599106851281));
#76446=CARTESIAN_POINT('Ctrl Pts',(80.4444229789358,-11.0073808664281,138.595247446667));
#76447=CARTESIAN_POINT('Ctrl Pts',(80.374431684465,-11.0216025121984,138.591388042053));
#76448=CARTESIAN_POINT('Ctrl Pts',(80.3039539120623,-11.0321440849118,138.58752863744));
#76449=CARTESIAN_POINT('Ctrl Pts',(80.2334362346204,-11.0426916263421,138.583667047602));
#76450=CARTESIAN_POINT('Ctrl Pts',(80.1624320146735,-11.0495548999817,138.579805457765));
#76451=CARTESIAN_POINT('Ctrl Pts',(80.0913554442118,-11.0527181358659,138.575943867928));
#76452=CARTESIAN_POINT('Ctrl Pts',(80.020154523198,-11.0558869059244,138.572075522125));
#76453=CARTESIAN_POINT('Ctrl Pts',(79.9488814848721,-11.0553427177614,138.568207176323));
#76454=CARTESIAN_POINT('Ctrl Pts',(79.8779490353346,-11.0511219184934,138.564338830521));
#76455=CARTESIAN_POINT('Ctrl Pts',(79.8358317181288,-11.0486157489929,138.562041936105));
#76456=CARTESIAN_POINT('Ctrl Pts',(79.7938343727432,-11.0448143517772,138.559745041689));
#76457=CARTESIAN_POINT('Ctrl Pts',(79.752041726348,-11.0397338691671,138.557448147274));
#76458=CARTESIAN_POINT('Ctrl Pts',(79.6816426567301,-11.0311758744047,138.553579063983));
#76459=CARTESIAN_POINT('Ctrl Pts',(79.6115492768518,-11.0189522248678,138.549709980692));
#76460=CARTESIAN_POINT('Ctrl Pts',(79.5421730827928,-11.0030956233741,138.5458408974));
#76461=CARTESIAN_POINT('Ctrl Pts',(79.4729002555399,-10.9872626473657,138.541977578836));
#76462=CARTESIAN_POINT('Ctrl Pts',(79.4043429627404,-10.9678075712217,138.538114260271));
#76463=CARTESIAN_POINT('Ctrl Pts',(79.33690625781,-10.9448147088009,138.534250941706));
#76464=CARTESIAN_POINT('Ctrl Pts',(79.2695486557729,-10.9218488168845,138.530392154793));
#76465=CARTESIAN_POINT('Ctrl Pts',(79.2033094882355,-10.8953535376155,138.526533367881));
#76466=CARTESIAN_POINT('Ctrl Pts',(79.1385805998206,-10.8654635293928,138.522674580968));
#76467=CARTESIAN_POINT('Ctrl Pts',(79.0738924856648,-10.8355923495939,138.518818224796));
#76468=CARTESIAN_POINT('Ctrl Pts',(79.0107132031364,-10.8023308866084,138.514961868625));
#76469=CARTESIAN_POINT('Ctrl Pts',(78.9494151096807,-10.7658620984473,138.511105512453));
#76470=CARTESIAN_POINT('Ctrl Pts',(78.8881351241254,-10.7294040834302,138.507250295477));
#76471=CARTESIAN_POINT('Ctrl Pts',(78.8287356416474,-10.6897408724661,138.503395078501));
#76472=CARTESIAN_POINT('Ctrl Pts',(78.7715633399238,-10.6471007664016,138.499539861525));
#76473=CARTESIAN_POINT('Ctrl Pts',(78.714388802788,-10.6044589931275,138.495684493812));
#76474=CARTESIAN_POINT('Ctrl Pts',(78.6594420073859,-10.5588403858577,138.491829126099));
#76475=CARTESIAN_POINT('Ctrl Pts',(78.6070382145787,-10.5105148217928,138.487973758385));
#76476=CARTESIAN_POINT('Ctrl Pts',(78.5545795691395,-10.4621386739011,138.484114355142));
#76477=CARTESIAN_POINT('Ctrl Pts',(78.5046695977665,-10.4110502430044,138.480254951899));
#76478=CARTESIAN_POINT('Ctrl Pts',(78.4575875191282,-10.357557107952,138.476395548656));
#76479=CARTESIAN_POINT('Ctrl Pts',(78.410478782161,-10.3040336845683,138.472533960182));
#76480=CARTESIAN_POINT('Ctrl Pts',(78.3662014270504,-10.248103227629,138.468672371707));
#76481=CARTESIAN_POINT('Ctrl Pts',(78.3249933520731,-10.1901051600177,138.464810783232));
#76482=CARTESIAN_POINT('Ctrl Pts',(78.2837131820377,-10.1320056226324,138.460942438765));
#76483=CARTESIAN_POINT('Ctrl Pts',(78.24551327357,-10.0718316626621,138.457074094298));
#76484=CARTESIAN_POINT('Ctrl Pts',(78.2105869337417,-10.009949721919,138.453205749831));
#76485=CARTESIAN_POINT('Ctrl Pts',(78.1898487213452,-9.97320608267847,138.450908842982));
#76486=CARTESIAN_POINT('Ctrl Pts',(78.1702637553136,-9.93586072306953,138.448611936132));
#76487=CARTESIAN_POINT('Ctrl Pts',(78.1518644288019,-9.89799358181013,138.446315029283));
#76488=CARTESIAN_POINT('Ctrl Pts',(78.1182272557188,-9.82876585307291,138.442115883558));
#76489=CARTESIAN_POINT('Ctrl Pts',(78.0884378127264,-9.75755151755703,138.437916737834));
#76490=CARTESIAN_POINT('Ctrl Pts',(78.0627161720044,-9.68478385807979,138.433717592109));
#76491=CARTESIAN_POINT('Ctrl Pts',(78.0373092445397,-9.61290653632974,138.429569824399));
#76492=CARTESIAN_POINT('Ctrl Pts',(78.015871306733,-9.53951403357927,138.425422056689));
#76493=CARTESIAN_POINT('Ctrl Pts',(77.9985686429311,-9.46504847644219,138.421274288979));
#76494=CARTESIAN_POINT('Ctrl Pts',(77.9809444893882,-9.38919932236631,138.417049454248));
#76495=CARTESIAN_POINT('Ctrl Pts',(77.9676110562636,-9.31223716100421,138.412824619516));
#76496=CARTESIAN_POINT('Ctrl Pts',(77.9586923529769,-9.23465006436166,138.408599784785));
#76497=CARTESIAN_POINT('Ctrl Pts',(77.9497736496901,-9.15706296771911,138.404374950053));
#76498=CARTESIAN_POINT('Ctrl Pts',(77.9452698355286,-9.07885132744909,138.400150115321));
#76499=CARTESIAN_POINT('Ctrl Pts',(77.9452500654424,-9.00051859011397,138.39592528059));
#76500=CARTESIAN_POINT('Ctrl Pts',(77.9452500654422,-9.00051858915731,138.395925280538));
#76501=CARTESIAN_POINT('Ctrl Pts',(77.945231494911,-8.92693857444419,138.391956781386));
#76502=CARTESIAN_POINT('Ctrl Pts',(77.9491695788627,-8.85340118457614,138.387988282233));
#76503=CARTESIAN_POINT('Ctrl Pts',(77.9570245321441,-8.7803439046172,138.384019783081));
#76504=CARTESIAN_POINT('Ctrl Pts',(77.9650800376502,-8.70542133030115,138.379949960432));
#76505=CARTESIAN_POINT('Ctrl Pts',(77.9772551019408,-8.63100421160297,138.375880137783));
#76506=CARTESIAN_POINT('Ctrl Pts',(77.9934509662018,-8.55755391575534,138.371810315134));
#76507=CARTESIAN_POINT('Ctrl Pts',(78.009290174775,-8.48572109862694,138.367830115698));
#76508=CARTESIAN_POINT('Ctrl Pts',(78.0289746941044,-8.41481336367742,138.363849916262));
#76509=CARTESIAN_POINT('Ctrl Pts',(78.0523617931341,-8.34524586472757,138.359869716826));
#76510=CARTESIAN_POINT('Ctrl Pts',(78.076538812492,-8.2733286608601,138.35575508257));
#76511=CARTESIAN_POINT('Ctrl Pts',(78.1046727995094,-8.20284433337413,138.351640448314));
#76512=CARTESIAN_POINT('Ctrl Pts',(78.1365533044576,-8.13422637175051,138.347525814058));
#76513=CARTESIAN_POINT('Ctrl Pts',(78.1684338094059,-8.06560841012688,138.343411179803));
#76514=CARTESIAN_POINT('Ctrl Pts',(78.2040605214212,-7.9988572326398,138.339296545547));
#76515=CARTESIAN_POINT('Ctrl Pts',(78.2431735357102,-7.93437420410772,138.335181911291));
#76516=CARTESIAN_POINT('Ctrl Pts',(78.2799523824106,-7.87373936262925,138.331312828192));
#76517=CARTESIAN_POINT('Ctrl Pts',(78.3199460624041,-7.81489206535987,138.327443745094));
#76518=CARTESIAN_POINT('Ctrl Pts',(78.3629553810999,-7.75819386447393,138.323574661995));
#76519=CARTESIAN_POINT('Ctrl Pts',(78.4059006180928,-7.70158014103087,138.319711343634));
#76520=CARTESIAN_POINT('Ctrl Pts',(78.4518522838164,-7.64710954187769,138.315848025273));
#76521=CARTESIAN_POINT('Ctrl Pts',(78.5005668004012,-7.5951165021822,138.311984706912));
#76522=CARTESIAN_POINT('Ctrl Pts',(78.54922417492,-7.54318445025606,138.308125920218));
#76523=CARTESIAN_POINT('Ctrl Pts',(78.600637632403,-7.49372453791673,138.304267133525));
#76524=CARTESIAN_POINT('Ctrl Pts',(78.6545231511768,-7.44703843840848,138.300408346831));
#76525=CARTESIAN_POINT('Ctrl Pts',(78.7083747260523,-7.4003817476959,138.296551990888));
#76526=CARTESIAN_POINT('Ctrl Pts',(78.7646949064437,-7.35649572054899,138.292695634945));
#76527=CARTESIAN_POINT('Ctrl Pts',(78.8231636749831,-7.31564438831321,138.288839279003));
#76528=CARTESIAN_POINT('Ctrl Pts',(78.8816151712853,-7.27480512395438,138.284984062264));
#76529=CARTESIAN_POINT('Ctrl Pts',(78.9422135976551,-7.23699905282433,138.281128845526));
#76530=CARTESIAN_POINT('Ctrl Pts',(79.0046081848307,-7.20244813794041,138.277273628788));
#76531=CARTESIAN_POINT('Ctrl Pts',(79.0670052114642,-7.16789587221007,138.273418261321));
#76532=CARTESIAN_POINT('Ctrl Pts',(79.1311981122825,-7.13659924880211,138.269562893855));
#76533=CARTESIAN_POINT('Ctrl Pts',(79.1968111603265,-7.10873448444593,138.265707526388));
#76534=CARTESIAN_POINT('Ctrl Pts',(79.2624928873308,-7.08084055328374,138.261848123404));
#76535=CARTESIAN_POINT('Ctrl Pts',(79.329597280913,-7.05638584232824,138.257988720419));
#76536=CARTESIAN_POINT('Ctrl Pts',(79.3977290916283,-7.03549820172414,138.254129317435));
#76537=CARTESIAN_POINT('Ctrl Pts',(79.4658994791117,-7.01459873437332,138.250267729226));
#76538=CARTESIAN_POINT('Ctrl Pts',(79.5350979703206,-6.99727047603946,138.246406141017));
#76539=CARTESIAN_POINT('Ctrl Pts',(79.6049173043764,-6.98359051130015,138.242544552808));
#76540=CARTESIAN_POINT('Ctrl Pts',(79.6748587898068,-6.96988661298257,138.238676208615));
#76541=CARTESIAN_POINT('Ctrl Pts',(79.7454228055971,-6.95984382020474,138.234807864422));
#76542=CARTESIAN_POINT('Ctrl Pts',(79.8161958231854,-6.95348745738378,138.230939520229));
#76543=CARTESIAN_POINT('Ctrl Pts',(79.8582187589169,-6.94971323614222,138.228642611253));
#76544=CARTESIAN_POINT('Ctrl Pts',(79.9003153380999,-6.94723771720572,138.226345702276));
#76545=CARTESIAN_POINT('Ctrl Pts',(79.9423993743177,-6.94605751530842,138.224048793299));
#76546=CARTESIAN_POINT('Ctrl Pts',(80.0132740183771,-6.9440699115302,138.220180518752));
#76547=CARTESIAN_POINT('Ctrl Pts',(80.08439044857,-6.94575118859824,138.216312244204));
#76548=CARTESIAN_POINT('Ctrl Pts',(80.155337132446,-6.95113008275697,138.212443969656));
#76549=CARTESIAN_POINT('Ctrl Pts',(80.2261854267694,-6.95650151741286,138.20858105967));
#76550=CARTESIAN_POINT('Ctrl Pts',(80.2968639617738,-6.96556035954378,138.204718149683));
#76551=CARTESIAN_POINT('Ctrl Pts',(80.3669597863483,-6.97828338343298,138.200855239696));
#76552=CARTESIAN_POINT('Ctrl Pts',(80.4369818596955,-6.99099302080975,138.196996394065));
#76553=CARTESIAN_POINT('Ctrl Pts',(80.5064219639399,-7.00735910187849,138.193137548434));
#76554=CARTESIAN_POINT('Ctrl Pts',(80.5748725845537,-7.0273066447041,138.189278702803));
#76555=CARTESIAN_POINT('Ctrl Pts',(80.6432814451583,-7.04724201803346,138.185422211356));
#76556=CARTESIAN_POINT('Ctrl Pts',(80.7107015541041,-7.07075438381265,138.18156571991));
#76557=CARTESIAN_POINT('Ctrl Pts',(80.7767374728927,-7.09771809115886,138.177709228464));
#76558=CARTESIAN_POINT('Ctrl Pts',(80.8427490507323,-7.12467185963791,138.173854158527));
#76559=CARTESIAN_POINT('Ctrl Pts',(80.9073770035231,-7.15507425641064,138.16999908859));
#76560=CARTESIAN_POINT('Ctrl Pts',(80.9702446392712,-7.18875101036175,138.166144018653));
#76561=CARTESIAN_POINT('Ctrl Pts',(81.0331314679084,-7.22243804550443,138.1622877718));
#76562=CARTESIAN_POINT('Ctrl Pts',(81.0942564769351,-7.25940120604435,138.158431524947));
#76563=CARTESIAN_POINT('Ctrl Pts',(81.1532675878582,-7.29942026552831,138.154575278094));
#76564=CARTESIAN_POINT('Ctrl Pts',(81.1868977428242,-7.32222693957645,138.152377621123));
#76565=CARTESIAN_POINT('Ctrl Pts',(81.2198418371831,-7.34602529029772,138.150179964153));
#76566=CARTESIAN_POINT('Ctrl Pts',(81.2520391107129,-7.37076839346111,138.147982307182));
#76567=CARTESIAN_POINT('',(77.9452502723122,-8.998942140427,138.454074719513));
#76568=CARTESIAN_POINT('Ctrl Pts',(77.9452502723127,-8.99894213949946,138.454074719462));
#76569=CARTESIAN_POINT('Ctrl Pts',(77.9452815714104,-8.93814791146918,138.450761929014));
#76570=CARTESIAN_POINT('Ctrl Pts',(77.9480107215814,-8.87742515330738,138.447449138566));
#76571=CARTESIAN_POINT('Ctrl Pts',(77.9534202484156,-8.8169456831852,138.444136348118));
#76572=CARTESIAN_POINT('Ctrl Pts',(77.95973816009,-8.74631030932362,138.440267263429));
#76573=CARTESIAN_POINT('Ctrl Pts',(77.9697295884145,-8.67586405616008,138.436398178741));
#76574=CARTESIAN_POINT('Ctrl Pts',(77.9833749153706,-8.60601925104963,138.432529094052));
#76575=CARTESIAN_POINT('Ctrl Pts',(77.9969999115456,-8.53627851082886,138.428665774085));
#76576=CARTESIAN_POINT('Ctrl Pts',(78.0142679075652,-8.46713791276437,138.424802454119));
#76577=CARTESIAN_POINT('Ctrl Pts',(78.0351074957963,-8.39900498386093,138.420939134152));
#76578=CARTESIAN_POINT('Ctrl Pts',(78.0559226393103,-8.33095197449105,138.417080345837));
#76579=CARTESIAN_POINT('Ctrl Pts',(78.0803009119579,-8.26390474873362,138.413221557523));
#76580=CARTESIAN_POINT('Ctrl Pts',(78.1081201674743,-8.19825923031046,138.409362769208));
#76581=CARTESIAN_POINT('Ctrl Pts',(78.1359218989831,-8.13265506355303,138.405506411635));
#76582=CARTESIAN_POINT('Ctrl Pts',(78.1671601238633,-8.06845129855351,138.401650054063));
#76583=CARTESIAN_POINT('Ctrl Pts',(78.2016638017234,-8.00602591559542,138.39779369649));
#76584=CARTESIAN_POINT('Ctrl Pts',(78.2361572869241,-7.94361897358904,138.393938478116));
#76585=CARTESIAN_POINT('Ctrl Pts',(78.2739140751586,-7.88298979559202,138.390083259742));
#76586=CARTESIAN_POINT('Ctrl Pts',(78.3147169905254,-7.82449213508538,138.386228041368));
#76587=CARTESIAN_POINT('Ctrl Pts',(78.3555215012133,-7.76599218742458,138.382372672262));
#76588=CARTESIAN_POINT('Ctrl Pts',(78.3993720957678,-7.70962431988504,138.378517303156));
#76589=CARTESIAN_POINT('Ctrl Pts',(78.4460090451571,-7.6557122053792,138.374661934049));
#76590=CARTESIAN_POINT('Ctrl Pts',(78.4926948106186,-7.60174365970214,138.370802529431));
#76591=CARTESIAN_POINT('Ctrl Pts',(78.5421724345315,-7.55023636649636,138.366943124813));
#76592=CARTESIAN_POINT('Ctrl Pts',(78.5941433605884,-7.50147917200917,138.363083720194));
#76593=CARTESIAN_POINT('Ctrl Pts',(78.6461437129704,-7.45269437083563,138.359222130352));
#76594=CARTESIAN_POINT('Ctrl Pts',(78.7006398065214,-7.40666308175431,138.35536054051));
#76595=CARTESIAN_POINT('Ctrl Pts',(78.7572999446834,-7.36363386278741,138.351498950668));
#76596=CARTESIAN_POINT('Ctrl Pts',(78.814059211424,-7.320529362936,138.347630604861));
#76597=CARTESIAN_POINT('Ctrl Pts',(78.8729896799775,-7.28043769271993,138.343762259054));
#76598=CARTESIAN_POINT('Ctrl Pts',(78.9337312323303,-7.24356369953473,138.339893913247));
#76599=CARTESIAN_POINT('Ctrl Pts',(78.9697975347749,-7.22166915553571,138.337597018874));
#76600=CARTESIAN_POINT('Ctrl Pts',(79.0065018723974,-7.20090815423955,138.3353001245));
#76601=CARTESIAN_POINT('Ctrl Pts',(79.0437653768922,-7.18131561064877,138.333003230127));
#76602=CARTESIAN_POINT('Ctrl Pts',(79.1065351778409,-7.14831227191436,138.329134146835));
#76603=CARTESIAN_POINT('Ctrl Pts',(79.171138534669,-7.11849774863183,138.325265063544));
#76604=CARTESIAN_POINT('Ctrl Pts',(79.2372183974205,-7.09207919732861,138.321395980252));
#76605=CARTESIAN_POINT('Ctrl Pts',(79.3031998047232,-7.06570000824887,138.317532661687));
#76606=CARTESIAN_POINT('Ctrl Pts',(79.3706529037847,-7.0427069264209,138.313669343122));
#76607=CARTESIAN_POINT('Ctrl Pts',(79.4391965878916,-7.02326099460056,138.309806024557));
#76608=CARTESIAN_POINT('Ctrl Pts',(79.5076598706248,-7.00383787275389,138.305947237644));
#76609=CARTESIAN_POINT('Ctrl Pts',(79.5772107323073,-6.98795376812263,138.30208845073));
#76610=CARTESIAN_POINT('Ctrl Pts',(79.647450294872,-6.97572080287472,138.298229663817));
#76611=CARTESIAN_POINT('Ctrl Pts',(79.7176456118739,-6.96349554346113,138.294373307645));
#76612=CARTESIAN_POINT('Ctrl Pts',(79.7885282916002,-6.95491694354026,138.290516951473));
#76613=CARTESIAN_POINT('Ctrl Pts',(79.859688011633,-6.9500463155426,138.286660595301));
#76614=CARTESIAN_POINT('Ctrl Pts',(79.9308267105698,-6.94517712636366,138.282805378325));
#76615=CARTESIAN_POINT('Ctrl Pts',(80.0022418029535,-6.94401376766526,138.278950161348));
#76616=CARTESIAN_POINT('Ctrl Pts',(80.0735182971014,-6.94656565176987,138.275094944372));
#76617=CARTESIAN_POINT('Ctrl Pts',(80.1447975781293,-6.94911763565204,138.271239576658));
#76618=CARTESIAN_POINT('Ctrl Pts',(80.2159377647695,-6.95538513115795,138.267384208944));
#76619=CARTESIAN_POINT('Ctrl Pts',(80.286526057035,-6.96532548520901,138.263528841231));
#76620=CARTESIAN_POINT('Ctrl Pts',(80.3571882361979,-6.97527624412885,138.259669437987));
#76621=CARTESIAN_POINT('Ctrl Pts',(80.4272968857762,-6.98890746818216,138.255810034744));
#76622=CARTESIAN_POINT('Ctrl Pts',(80.4964474056642,-7.00612499491335,138.2519506315));
#76623=CARTESIAN_POINT('Ctrl Pts',(80.5656370792465,-7.02335227037497,138.248089043025));
#76624=CARTESIAN_POINT('Ctrl Pts',(80.6338670783263,-7.04416974898001,138.24422745455));
#76625=CARTESIAN_POINT('Ctrl Pts',(80.7007486756555,-7.06843357451339,138.240365866075));
#76626=CARTESIAN_POINT('Ctrl Pts',(80.7677472848243,-7.09273985051112,138.236497521607));
#76627=CARTESIAN_POINT('Ctrl Pts',(80.8333923347223,-7.12050432223672,138.232629177139));
#76628=CARTESIAN_POINT('Ctrl Pts',(80.8973164056134,-7.15153554788925,138.228760832672));
#76629=CARTESIAN_POINT('Ctrl Pts',(80.9352726003762,-7.1699609583517,138.226463925826));
#76630=CARTESIAN_POINT('Ctrl Pts',(80.9726225197316,-7.18953722705832,138.224167018981));
#76631=CARTESIAN_POINT('Ctrl Pts',(81.0092940526334,-7.21021703052608,138.221870112135));
#76632=CARTESIAN_POINT('Ctrl Pts',(81.0710608673403,-7.24504856026857,138.218001372317));
#76633=CARTESIAN_POINT('Ctrl Pts',(81.1311434378208,-7.28314949063208,138.214132632499));
#76634=CARTESIAN_POINT('Ctrl Pts',(81.1891741648745,-7.3243322620236,138.210263892681));
#76635=CARTESIAN_POINT('Ctrl Pts',(81.2104094471644,-7.3394023433474,138.208848198163));
#76636=CARTESIAN_POINT('Ctrl Pts',(81.2313701776481,-7.35488464036548,138.207432503646));
#76637=CARTESIAN_POINT('Ctrl Pts',(81.2520391107129,-7.37076839346111,138.206016809128));
#76638=CARTESIAN_POINT('Ctrl Pts',(81.2520391107129,-7.37076839346111,138.906139397208));
#76639=CARTESIAN_POINT('Ctrl Pts',(81.3085407539465,-7.41418902614719,138.902270840233));
#76640=CARTESIAN_POINT('Ctrl Pts',(81.3627052412802,-7.46049401748224,138.898402283257));
#76641=CARTESIAN_POINT('Ctrl Pts',(81.4142409454556,-7.50938934973049,138.894533726281));
#76642=CARTESIAN_POINT('Ctrl Pts',(81.4402844264973,-7.53409852327941,138.892578757549));
#76643=CARTESIAN_POINT('Ctrl Pts',(81.465657188517,-7.55946864892284,138.890623788816));
#76644=CARTESIAN_POINT('Ctrl Pts',(81.4903255362227,-7.58545860485367,138.888668820084));
#76645=CARTESIAN_POINT('Ctrl Pts',(81.5391460717293,-7.63689470351241,138.884799788338));
#76646=CARTESIAN_POINT('Ctrl Pts',(81.5853962807173,-7.69096197875137,138.880930756591));
#76647=CARTESIAN_POINT('Ctrl Pts',(81.6287797614883,-7.74737313973151,138.877061724845));
#76648=CARTESIAN_POINT('Ctrl Pts',(81.6720985929598,-7.80370023779242,138.873198458661));
#76649=CARTESIAN_POINT('Ctrl Pts',(81.7125588821633,-7.86236390650683,138.869335192478));
#76650=CARTESIAN_POINT('Ctrl Pts',(81.7499020657528,-7.92304116941539,138.865471926294));
#76651=CARTESIAN_POINT('Ctrl Pts',(81.7872014358446,-7.98364724173804,138.86161319275));
#76652=CARTESIAN_POINT('Ctrl Pts',(81.8213907113594,-8.04626180385324,138.857754459207));
#76653=CARTESIAN_POINT('Ctrl Pts',(81.8522535771044,-8.11053147970038,138.853895725663));
#76654=CARTESIAN_POINT('Ctrl Pts',(81.8830969966853,-8.17476066032353,138.850039423442));
#76655=CARTESIAN_POINT('Ctrl Pts',(81.9106179549556,-8.24064244877835,138.84618312122));
#76656=CARTESIAN_POINT('Ctrl Pts',(81.9346459227277,-8.3077986447766,138.842326818998));
#76657=CARTESIAN_POINT('Ctrl Pts',(81.9586667892483,-8.37493499336037,138.838471656473));
#76658=CARTESIAN_POINT('Ctrl Pts',(81.9791965511485,-8.44334454460101,138.834616493947));
#76659=CARTESIAN_POINT('Ctrl Pts',(81.9961133562055,-8.51263049779648,138.830761331421));
#76660=CARTESIAN_POINT('Ctrl Pts',(82.0130308208679,-8.58191915252996,138.826906018578));
#76661=CARTESIAN_POINT('Ctrl Pts',(82.0263349359147,-8.6520838046047,138.823050705735));
#76662=CARTESIAN_POINT('Ctrl Pts',(82.0359545500872,-8.72271561082636,138.819195392892));
#76663=CARTESIAN_POINT('Ctrl Pts',(82.0455842328843,-8.79342134570424,138.815336044783));
#76664=CARTESIAN_POINT('Ctrl Pts',(82.0515216507147,-8.86459472846081,138.811476696675));
#76665=CARTESIAN_POINT('Ctrl Pts',(82.0537474512825,-8.93582080671598,138.807617348566));
#76666=CARTESIAN_POINT('Ctrl Pts',(82.0559745120042,-9.00708721015571,138.803755815458));
#76667=CARTESIAN_POINT('Ctrl Pts',(82.0544857824498,-9.07840588256192,138.79989428235));
#76668=CARTESIAN_POINT('Ctrl Pts',(82.0493140475513,-9.14936364018326,138.796032749242));
#76669=CARTESIAN_POINT('Ctrl Pts',(82.0441332640688,-9.22044554709946,138.792164459909));
#76670=CARTESIAN_POINT('Ctrl Pts',(82.0352566703983,-9.29116479632561,138.788296170576));
#76671=CARTESIAN_POINT('Ctrl Pts',(82.0227686370176,-9.36111577589204,138.784427881242));
#76672=CARTESIAN_POINT('Ctrl Pts',(82.0153519422922,-9.40265995225419,138.782130488192));
#76673=CARTESIAN_POINT('Ctrl Pts',(82.006662387559,-9.44393336415556,138.779833095143));
#76674=CARTESIAN_POINT('Ctrl Pts',(81.9967259333069,-9.48485369933577,138.777535702093));
#76675=CARTESIAN_POINT('Ctrl Pts',(81.979991708908,-9.55376863156547,138.773666606553));
#76676=CARTESIAN_POINT('Ctrl Pts',(81.9596527303735,-9.62195117122628,138.769797511013));
#76677=CARTESIAN_POINT('Ctrl Pts',(81.9357896130199,-9.68899647069068,138.765928415473));
#76678=CARTESIAN_POINT('Ctrl Pts',(81.9119620497925,-9.75594187804965,138.762065084575));
#76679=CARTESIAN_POINT('Ctrl Pts',(81.884620931774,-9.821752954616,138.758201753676));
#76680=CARTESIAN_POINT('Ctrl Pts',(81.8538973773168,-9.88603728864983,138.754338422778));
#76681=CARTESIAN_POINT('Ctrl Pts',(81.82320986079,-9.9502462188316,138.750479623466));
#76682=CARTESIAN_POINT('Ctrl Pts',(81.7891479971028,-10.0129315275076,138.746620824154));
#76683=CARTESIAN_POINT('Ctrl Pts',(81.7518913583523,-10.0737198102999,138.742762024842));
#76684=CARTESIAN_POINT('Ctrl Pts',(81.7146581880431,-10.1344698017623,138.738905656238));
#76685=CARTESIAN_POINT('Ctrl Pts',(81.6742344885484,-10.1933247249269,138.735049287634));
#76686=CARTESIAN_POINT('Ctrl Pts',(81.6308455204021,-10.2499361788045,138.73119291903));
#76687=CARTESIAN_POINT('Ctrl Pts',(81.5874693694662,-10.306530909516,138.727337689607));
#76688=CARTESIAN_POINT('Ctrl Pts',(81.5411299842249,-10.3608831012861,138.723482460184));
#76689=CARTESIAN_POINT('Ctrl Pts',(81.4920946528018,-10.4126751606722,138.719627230761));
#76690=CARTESIAN_POINT('Ctrl Pts',(81.4430574041797,-10.4644692450408,138.715771850605));
#76691=CARTESIAN_POINT('Ctrl Pts',(81.3913243356852,-10.5137026470529,138.711916470449));
#76692=CARTESIAN_POINT('Ctrl Pts',(81.3372003513379,-10.560093837845,138.708061090293));
#76693=CARTESIAN_POINT('Ctrl Pts',(81.2830197152762,-10.6065335864164,138.7042016747));
#76694=CARTESIAN_POINT('Ctrl Pts',(81.226443537245,-10.6501248683155,138.700342259108));
#76695=CARTESIAN_POINT('Ctrl Pts',(81.1678099480159,-10.6906263596121,138.696482843515));
#76696=CARTESIAN_POINT('Ctrl Pts',(81.1091431605051,-10.731150782814,138.692621242726));
#76697=CARTESIAN_POINT('Ctrl Pts',(81.0484170565591,-10.7685816778062,138.688759641936));
#76698=CARTESIAN_POINT('Ctrl Pts',(80.9859965589404,-10.8027224823188,138.684898041146));
#76699=CARTESIAN_POINT('Ctrl Pts',(80.9234668577401,-10.8369230155788,138.681029684552));
#76700=CARTESIAN_POINT('Ctrl Pts',(80.8592372824306,-10.8678217557705,138.677161327959));
#76701=CARTESIAN_POINT('Ctrl Pts',(80.7936943731894,-10.8952695862245,138.673292971365));
#76702=CARTESIAN_POINT('Ctrl Pts',(80.7547789650431,-10.9115664448353,138.670996175611));
#76703=CARTESIAN_POINT('Ctrl Pts',(80.7154009145431,-10.9266477050085,138.668699379856));
#76704=CARTESIAN_POINT('Ctrl Pts',(80.6756433883521,-10.9404905499064,138.666402584101));
#76705=CARTESIAN_POINT('Ctrl Pts',(80.6086694833266,-10.963809641115,138.662533495768));
#76706=CARTESIAN_POINT('Ctrl Pts',(80.5403557402951,-10.9837030370275,138.658664407435));
#76707=CARTESIAN_POINT('Ctrl Pts',(80.4710860079057,-11.0000188838247,138.654795319102));
#76708=CARTESIAN_POINT('Ctrl Pts',(80.401919481237,-11.016310421466,138.650931995365));
#76709=CARTESIAN_POINT('Ctrl Pts',(80.3318002614742,-11.0290348798839,138.647068671628));
#76710=CARTESIAN_POINT('Ctrl Pts',(80.2611291413822,-11.0380895794888,138.643205347892));
#76711=CARTESIAN_POINT('Ctrl Pts',(80.1905409149407,-11.0471336583889,138.639346555638));
#76712=CARTESIAN_POINT('Ctrl Pts',(80.1194025535331,-11.0525164671184,138.635487763385));
#76713=CARTESIAN_POINT('Ctrl Pts',(80.0481251616243,-11.0541863428907,138.631628971132));
#76714=CARTESIAN_POINT('Ctrl Pts',(79.9768926670995,-11.055855166814,138.627772609519));
#76715=CARTESIAN_POINT('Ctrl Pts',(79.905521800321,-11.0538156865004,138.623916247905));
#76716=CARTESIAN_POINT('Ctrl Pts',(79.8344274401024,-11.0480681848779,138.620059886292));
#76717=CARTESIAN_POINT('Ctrl Pts',(79.763354079924,-11.0423223809676,138.616204663781));
#76718=CARTESIAN_POINT('Ctrl Pts',(79.6925575480956,-11.0328707693168,138.61234944127));
#76719=CARTESIAN_POINT('Ctrl Pts',(79.6224496359158,-11.0197656510298,138.608494218759));
#76720=CARTESIAN_POINT('Ctrl Pts',(79.552338981,-11.0066600200492,138.604638845425));
#76721=CARTESIAN_POINT('Ctrl Pts',(79.4829174763242,-10.9899006900868,138.600783472092));
#76722=CARTESIAN_POINT('Ctrl Pts',(79.4145870162218,-10.9695911253161,138.596928098758));
#76723=CARTESIAN_POINT('Ctrl Pts',(79.3461850310351,-10.9492603014564,138.593068689802));
#76724=CARTESIAN_POINT('Ctrl Pts',(79.2788768368191,-10.9253719630721,138.589209280847));
#76725=CARTESIAN_POINT('Ctrl Pts',(79.2130485719069,-10.8980792955834,138.585349871891));
#76726=CARTESIAN_POINT('Ctrl Pts',(79.1471830334149,-10.8707711743162,138.581488277644));
#76727=CARTESIAN_POINT('Ctrl Pts',(79.0827995310201,-10.8400550959288,138.577626683396));
#76728=CARTESIAN_POINT('Ctrl Pts',(79.0202611286595,-10.8061310324792,138.573765089148));
#76729=CARTESIAN_POINT('Ctrl Pts',(78.9576133126571,-10.7721476174122,138.569896738874));
#76730=CARTESIAN_POINT('Ctrl Pts',(78.8968174561364,-10.7349452653864,138.5660283886));
#76731=CARTESIAN_POINT('Ctrl Pts',(78.8382084871952,-10.6947678434744,138.562160038327));
#76732=CARTESIAN_POINT('Ctrl Pts',(78.8034090417435,-10.670912245475,138.559863180921));
#76733=CARTESIAN_POINT('Ctrl Pts',(78.7693799732322,-10.6460085938022,138.557566323515));
#76734=CARTESIAN_POINT('Ctrl Pts',(78.7361855638824,-10.6201143890358,138.55526946611));
#76735=CARTESIAN_POINT('Ctrl Pts',(78.6809217159353,-10.5770043164979,138.551445533679));
#76736=CARTESIAN_POINT('Ctrl Pts',(78.6277456593305,-10.5309690669994,138.547621601249));
#76737=CARTESIAN_POINT('Ctrl Pts',(78.5769890148234,-10.4822406345013,138.543797668819));
#76738=CARTESIAN_POINT('Ctrl Pts',(78.5263187089004,-10.4335950905374,138.539980241013));
#76739=CARTESIAN_POINT('Ctrl Pts',(78.4780599997091,-10.3822658016579,138.536162813207));
#76740=CARTESIAN_POINT('Ctrl Pts',(78.4325126206117,-10.3285258288638,138.532345385401));
#76741=CARTESIAN_POINT('Ctrl Pts',(78.3870085971723,-10.2748370100972,138.52853159133));
#76742=CARTESIAN_POINT('Ctrl Pts',(78.3442111089203,-10.2187424334804,138.524717797259));
#76743=CARTESIAN_POINT('Ctrl Pts',(78.3043830641576,-10.1605519244671,138.520904003188));
#76744=CARTESIAN_POINT('Ctrl Pts',(78.2645788526164,-10.102396236829,138.517092491303));
#76745=CARTESIAN_POINT('Ctrl Pts',(78.2277408418242,-10.0421475141073,138.513280979417));
#76746=CARTESIAN_POINT('Ctrl Pts',(78.1940904592992,-9.98014707738473,138.509469467532));
#76747=CARTESIAN_POINT('Ctrl Pts',(78.1604483206664,-9.91816182993723,138.505658889416));
#76748=CARTESIAN_POINT('Ctrl Pts',(78.1299924973061,-9.85442615832262,138.5018483113));
#76749=CARTESIAN_POINT('Ctrl Pts',(78.1028990537304,-9.78930701388173,138.498037733184));
#76750=CARTESIAN_POINT('Ctrl Pts',(78.0757855811533,-9.72413972969709,138.494224338074));
#76751=CARTESIAN_POINT('Ctrl Pts',(78.0520396486506,-9.6575873893915,138.490410942963));
#76752=CARTESIAN_POINT('Ctrl Pts',(78.0317891516039,-9.59003696388962,138.486597547853));
#76753=CARTESIAN_POINT('Ctrl Pts',(78.0115315638732,-9.52246288569773,138.482782817488));
#76754=CARTESIAN_POINT('Ctrl Pts',(77.994771969706,-9.45389051055339,138.478968087122));
#76755=CARTESIAN_POINT('Ctrl Pts',(77.9815875950891,-9.38471928233684,138.475153356757));
#76756=CARTESIAN_POINT('Ctrl Pts',(77.9683814173209,-9.31543366486841,138.471332317928));
#76757=CARTESIAN_POINT('Ctrl Pts',(77.9587623379457,-9.24554771071851,138.4675112791));
#76758=CARTESIAN_POINT('Ctrl Pts',(77.9527558266144,-9.17546753841907,138.463690240271));
#76759=CARTESIAN_POINT('Ctrl Pts',(77.9477174293809,-9.11668270862904,138.460485066685));
#76760=CARTESIAN_POINT('Ctrl Pts',(77.9452199900004,-9.05776145210071,138.457279893099));
#76761=CARTESIAN_POINT('Ctrl Pts',(77.9452502723122,-8.998942140427,138.454074719513));
#76762=CARTESIAN_POINT('Origin',(80.,-9.,141.545925280538));
#76763=CARTESIAN_POINT('',(81.2520391107129,-7.37076839346112,139.606097362913));
#76764=CARTESIAN_POINT('',(81.2520391107129,-7.37076839346111,139.547882946156));
#76765=CARTESIAN_POINT('',(81.2520391107129,-7.37076839346111,141.545925280538));
#76766=CARTESIAN_POINT('',(77.9455903633547,-9.00215277156236,139.85407487124));
#76767=CARTESIAN_POINT('Ctrl Pts',(77.9452511251707,-9.00215032272264,139.854074719462));
#76768=CARTESIAN_POINT('Ctrl Pts',(77.9451772141952,-8.93152441513387,139.850255486395));
#76769=CARTESIAN_POINT('Ctrl Pts',(77.9487489191035,-8.8608346373683,139.846436253328));
#76770=CARTESIAN_POINT('Ctrl Pts',(77.9559591751019,-8.79048945456173,139.842617020261));
#76771=CARTESIAN_POINT('Ctrl Pts',(77.9631670371951,-8.72016762733346,139.838799055232));
#76772=CARTESIAN_POINT('Ctrl Pts',(77.9740110032964,-8.65019066081581,139.834981090203));
#76773=CARTESIAN_POINT('Ctrl Pts',(77.9884320510566,-8.58096306930816,139.831163125175));
#76774=CARTESIAN_POINT('Ctrl Pts',(78.0028533540946,-8.51173425235067,139.827345092561));
#76775=CARTESIAN_POINT('Ctrl Pts',(78.0208517611104,-8.44325532150668,139.823527059948));
#76776=CARTESIAN_POINT('Ctrl Pts',(78.042317286345,-8.3759199128665,139.819709027335));
#76777=CARTESIAN_POINT('Ctrl Pts',(78.0638059335618,-8.3085119726624,139.815886882058));
#76778=CARTESIAN_POINT('Ctrl Pts',(78.0887690027399,-8.24225048659746,139.812064736781));
#76779=CARTESIAN_POINT('Ctrl Pts',(78.117047128281,-8.17751228253237,139.808242591504));
#76780=CARTESIAN_POINT('Ctrl Pts',(78.1453414305068,-8.11273704455875,139.804418259744));
#76781=CARTESIAN_POINT('Ctrl Pts',(78.1769543394074,-8.04948726524998,139.800593927984));
#76782=CARTESIAN_POINT('Ctrl Pts',(78.211680274969,-7.988115558196,139.796769596225));
#76783=CARTESIAN_POINT('Ctrl Pts',(78.246470364294,-7.92663047115926,139.792938199277));
#76784=CARTESIAN_POINT('Ctrl Pts',(78.2843846938144,-7.86703080006613,139.789106802328));
#76785=CARTESIAN_POINT('Ctrl Pts',(78.3251745145668,-7.80963990496851,139.78527540538));
#76786=CARTESIAN_POINT('Ctrl Pts',(78.3519377903433,-7.77198422705121,139.782761524926));
#76787=CARTESIAN_POINT('Ctrl Pts',(78.3799381149203,-7.73527877551538,139.780247644471));
#76788=CARTESIAN_POINT('Ctrl Pts',(78.4090964455802,-7.69960642764035,139.777733764017));
#76789=CARTESIAN_POINT('Ctrl Pts',(78.4539904848238,-7.64468298898069,139.773863232157));
#76790=CARTESIAN_POINT('Ctrl Pts',(78.5018203572766,-7.59197912134451,139.769992700298));
#76791=CARTESIAN_POINT('Ctrl Pts',(78.5523383786184,-7.54182532168506,139.766122168439));
#76792=CARTESIAN_POINT('Ctrl Pts',(78.6027804379957,-7.49174693632431,139.762257456547));
#76793=CARTESIAN_POINT('Ctrl Pts',(78.6559022811376,-7.44421134674237,139.758392744654));
#76794=CARTESIAN_POINT('Ctrl Pts',(78.7114160407119,-7.39951602870717,139.754528032762));
#76795=CARTESIAN_POINT('Ctrl Pts',(78.766863418076,-7.35487415641255,139.750667942212));
#76796=CARTESIAN_POINT('Ctrl Pts',(78.8246966540222,-7.3130661119175,139.746807851663));
#76797=CARTESIAN_POINT('Ctrl Pts',(78.8845923882131,-7.27435130398223,139.742947761113));
#76798=CARTESIAN_POINT('Ctrl Pts',(78.9444495327706,-7.23566143922973,139.739090157544));
#76799=CARTESIAN_POINT('Ctrl Pts',(79.0063661324868,-7.20006111986884,139.735232553974));
#76800=CARTESIAN_POINT('Ctrl Pts',(79.0699884040452,-7.16776748367202,139.731374950404));
#76801=CARTESIAN_POINT('Ctrl Pts',(79.1335909260111,-7.13548387204895,139.72751854431));
#76802=CARTESIAN_POINT('Ctrl Pts',(79.198897636093,-7.10650512532283,139.723662138215));
#76803=CARTESIAN_POINT('Ctrl Pts',(79.2655301301099,-7.0810024563008,139.719805732121));
#76804=CARTESIAN_POINT('Ctrl Pts',(79.3321641853529,-7.05549918974097,139.715949235669));
#76805=CARTESIAN_POINT('Ctrl Pts',(79.4001236321068,-7.0334723340365,139.712092739217));
#76806=CARTESIAN_POINT('Ctrl Pts',(79.4690116881436,-7.01504433924285,139.708236242766));
#76807=CARTESIAN_POINT('Ctrl Pts',(79.5379700295608,-6.9965975426612,139.704375811593));
#76808=CARTESIAN_POINT('Ctrl Pts',(79.6078584017997,-6.98175706283591,139.700515380419));
#76809=CARTESIAN_POINT('Ctrl Pts',(79.6782673968351,-6.97059474363528,139.696654949246));
#76810=CARTESIAN_POINT('Ctrl Pts',(79.7487152375011,-6.95942626602652,139.692792388219));
#76811=CARTESIAN_POINT('Ctrl Pts',(79.8196837898523,-6.9519400401992,139.688929827192));
#76812=CARTESIAN_POINT('Ctrl Pts',(79.8907587707328,-6.94815597173465,139.685067266165));
#76813=CARTESIAN_POINT('Ctrl Pts',(79.9619562493202,-6.94436538142931,139.681198048015));
#76814=CARTESIAN_POINT('Ctrl Pts',(80.0332600370826,-6.94428968860846,139.677328829865));
#76815=CARTESIAN_POINT('Ctrl Pts',(80.1042568089757,-6.94789666919957,139.673459611715));
#76816=CARTESIAN_POINT('Ctrl Pts',(80.1462088178506,-6.95002803486219,139.671173289818));
#76817=CARTESIAN_POINT('Ctrl Pts',(80.1880537235075,-6.95344426405484,139.668886967922));
#76818=CARTESIAN_POINT('Ctrl Pts',(80.2297077973158,-6.95813029545166,139.666600646025));
#76819=CARTESIAN_POINT('Ctrl Pts',(80.3003043866995,-6.96607232378442,139.662725718236));
#76820=CARTESIAN_POINT('Ctrl Pts',(80.3706220099204,-6.97769490534872,139.658850790447));
#76821=CARTESIAN_POINT('Ctrl Pts',(80.4402478318877,-6.99296751171832,139.654975862658));
#76822=CARTESIAN_POINT('Ctrl Pts',(80.5097766496484,-7.00821883996117,139.651106333502));
#76823=CARTESIAN_POINT('Ctrl Pts',(80.5786151099305,-7.02710999796615,139.647236804346));
#76824=CARTESIAN_POINT('Ctrl Pts',(80.6463564866655,-7.04955880513012,139.643367275191));
#76825=CARTESIAN_POINT('Ctrl Pts',(80.7140192485418,-7.07198156012497,139.63950223668));
#76826=CARTESIAN_POINT('Ctrl Pts',(80.7805869991265,-7.09795360980493,139.63563719817));
#76827=CARTESIAN_POINT('Ctrl Pts',(80.8456659697587,-7.12734236175106,139.631772159659));
#76828=CARTESIAN_POINT('Ctrl Pts',(80.9107019062309,-7.15671168007311,139.627909676947));
#76829=CARTESIAN_POINT('Ctrl Pts',(80.9742505775629,-7.18949301568476,139.624047194234));
#76830=CARTESIAN_POINT('Ctrl Pts',(81.0359374810629,-7.22550539650608,139.620184711521));
#76831=CARTESIAN_POINT('Ctrl Pts',(81.0976087027791,-7.2615086224122,139.616323210713));
#76832=CARTESIAN_POINT('Ctrl Pts',(81.1574186781938,-7.30074101982408,139.612461709904));
#76833=CARTESIAN_POINT('Ctrl Pts',(81.2150182692663,-7.34297611126178,139.608600209095));
#76834=CARTESIAN_POINT('Ctrl Pts',(81.2274627326795,-7.35210105538665,139.607765927035));
#76835=CARTESIAN_POINT('Ctrl Pts',(81.2398041258756,-7.3613659982008,139.606931644974));
#76836=CARTESIAN_POINT('Ctrl Pts',(81.2520391107129,-7.37076839346111,139.606097362913));
#76837=CARTESIAN_POINT('',(79.4698297828115,-10.9851743256717,140.));
#76838=CARTESIAN_POINT('Ctrl Pts',(79.4698297828115,-10.9851743256717,140.));
#76839=CARTESIAN_POINT('Ctrl Pts',(78.809740437582,-10.8088876857538,139.962955627336));
#76840=CARTESIAN_POINT('Ctrl Pts',(78.075115219758,-10.1125316678232,139.914314179016));
#76841=CARTESIAN_POINT('Ctrl Pts',(77.945732886822,-9.21640413993257,139.865672730697));
#76842=CARTESIAN_POINT('Ctrl Pts',(77.947342226875,-9.00216541764168,139.85407565504));
#76843=CARTESIAN_POINT('',(80.5303700197491,-10.9851209546653,139.99999999143));
#76844=CARTESIAN_POINT('Origin',(80.,-9.,140.));
#76845=CARTESIAN_POINT('',(77.9452505498836,-8.99849675473629,139.795925280583));
#76846=CARTESIAN_POINT('Ctrl Pts',(80.5303700197491,-10.9851209546653,139.99999999143));
#76847=CARTESIAN_POINT('Ctrl Pts',(80.4620741507688,-11.0033677427488,139.996143015247));
#76848=CARTESIAN_POINT('Ctrl Pts',(80.3926968367418,-11.0181229590247,139.992286039064));
#76849=CARTESIAN_POINT('Ctrl Pts',(80.322629557872,-11.0292628540648,139.988429062881));
#76850=CARTESIAN_POINT('Ctrl Pts',(80.2526675158343,-11.0403860176536,139.984577879644));
#76851=CARTESIAN_POINT('Ctrl Pts',(80.182018044633,-11.0479045602196,139.980726696407));
#76852=CARTESIAN_POINT('Ctrl Pts',(80.1110860698619,-11.0517449762538,139.976875513169));
#76853=CARTESIAN_POINT('Ctrl Pts',(80.0402379061024,-11.055580854572,139.97302888037));
#76854=CARTESIAN_POINT('Ctrl Pts',(79.9691083877808,-11.055747211313,139.969182247571));
#76855=CARTESIAN_POINT('Ctrl Pts',(79.8981090915934,-11.0522221627504,139.965335614772));
#76856=CARTESIAN_POINT('Ctrl Pts',(79.8271544971697,-11.0486993335886,139.961491403846));
#76857=CARTESIAN_POINT('Ctrl Pts',(79.7563304496936,-11.0414897336107,139.95764719292));
#76858=CARTESIAN_POINT('Ctrl Pts',(79.6860485460449,-11.0306235611406,139.953802981993));
#76859=CARTESIAN_POINT('Ctrl Pts',(79.6157869882531,-11.0197605343108,139.949959883925));
#76860=CARTESIAN_POINT('Ctrl Pts',(79.5460677459476,-11.0052431110503,139.946116785857));
#76861=CARTESIAN_POINT('Ctrl Pts',(79.4772955407152,-10.9871531422474,139.942273687788));
#76862=CARTESIAN_POINT('Ctrl Pts',(79.4085198539763,-10.9690622576626,139.938430395168));
#76863=CARTESIAN_POINT('Ctrl Pts',(79.3406917719253,-10.9473985954838,139.934587102547));
#76864=CARTESIAN_POINT('Ctrl Pts',(79.2742023673069,-10.922294295595,139.930743809927));
#76865=CARTESIAN_POINT('Ctrl Pts',(79.2076443016715,-10.897164071474,139.926896548488));
#76866=CARTESIAN_POINT('Ctrl Pts',(79.1424281306179,-10.8685862925332,139.923049287049));
#76867=CARTESIAN_POINT('Ctrl Pts',(79.0789254608646,-10.8367414776872,139.91920202561));
#76868=CARTESIAN_POINT('Ctrl Pts',(79.0153854805086,-10.8048779526163,139.915352503736));
#76869=CARTESIAN_POINT('Ctrl Pts',(78.953561429991,-10.7697438138146,139.911502981863));
#76870=CARTESIAN_POINT('Ctrl Pts',(78.893798374401,-10.7315644735389,139.907653459989));
#76871=CARTESIAN_POINT('Ctrl Pts',(78.8339351963667,-10.6933211705219,139.903797488921));
#76872=CARTESIAN_POINT('Ctrl Pts',(78.7761403009812,-10.6520227697349,139.899941517853));
#76873=CARTESIAN_POINT('Ctrl Pts',(78.7207272530863,-10.6079361932315,139.896085546786));
#76874=CARTESIAN_POINT('Ctrl Pts',(78.6965845362067,-10.5887282670274,139.894405552248));
#76875=CARTESIAN_POINT('Ctrl Pts',(78.6728934890379,-10.5689915700536,139.89272555771));
#76876=CARTESIAN_POINT('Ctrl Pts',(78.6496778127435,-10.5487503198072,139.891045563173));
#76877=CARTESIAN_POINT('Ctrl Pts',(78.594908743558,-10.5009983430355,139.887082218065));
#76878=CARTESIAN_POINT('Ctrl Pts',(78.5425524721368,-10.4502296884911,139.883118872957));
#76879=CARTESIAN_POINT('Ctrl Pts',(78.4929635830642,-10.3967243108536,139.879155527849));
#76880=CARTESIAN_POINT('Ctrl Pts',(78.4452783531287,-10.3452729417435,139.875344330899));
#76881=CARTESIAN_POINT('Ctrl Pts',(78.400152313208,-10.2912915243667,139.871533133949));
#76882=CARTESIAN_POINT('Ctrl Pts',(78.3578674259957,-10.2350701080886,139.867721936999));
#76883=CARTESIAN_POINT('Ctrl Pts',(78.3156213067393,-10.1789002371624,139.86391423426));
#76884=CARTESIAN_POINT('Ctrl Pts',(78.2762114760096,-10.1204948355065,139.860106531521));
#76885=CARTESIAN_POINT('Ctrl Pts',(78.2398808613688,-10.0601783719376,139.856298828782));
#76886=CARTESIAN_POINT('Ctrl Pts',(78.2035706331938,-9.99989575419088,139.852493262687));
#76887=CARTESIAN_POINT('Ctrl Pts',(78.1703364516158,-9.93770462878445,139.848687696592));
#76888=CARTESIAN_POINT('Ctrl Pts',(78.1403778803837,-9.87395831407092,139.844882130498));
#76889=CARTESIAN_POINT('Ctrl Pts',(78.1104254664197,-9.81022510088838,139.841077346546));
#76890=CARTESIAN_POINT('Ctrl Pts',(78.0837475373579,-9.74493778587895,139.837272562595));
#76891=CARTESIAN_POINT('Ctrl Pts',(78.0604967798146,-9.67847241756049,139.833467778643));
#76892=CARTESIAN_POINT('Ctrl Pts',(78.0372308347851,-9.6119636338024,139.829660509392));
#76893=CARTESIAN_POINT('Ctrl Pts',(78.0173966958587,-9.54427573298083,139.82585324014));
#76894=CARTESIAN_POINT('Ctrl Pts',(78.0010976872857,-9.47580154132315,139.822045970889));
#76895=CARTESIAN_POINT('Ctrl Pts',(77.9847922388687,-9.4073002950685,139.818237197361));
#76896=CARTESIAN_POINT('Ctrl Pts',(77.9720247926029,-9.33801263115874,139.814428423833));
#76897=CARTESIAN_POINT('Ctrl Pts',(77.962847357618,-9.26834059352989,139.810619650305));
#76898=CARTESIAN_POINT('Ctrl Pts',(77.9536577730378,-9.19857632020982,139.806805834512));
#76899=CARTESIAN_POINT('Ctrl Pts',(77.9480677192538,-9.12842715583003,139.802992018719));
#76900=CARTESIAN_POINT('Ctrl Pts',(77.9460771917355,-9.05829802904844,139.799178202926));
#76901=CARTESIAN_POINT('Ctrl Pts',(77.9455112640845,-9.03835958980393,139.798093895478));
#76902=CARTESIAN_POINT('Ctrl Pts',(77.9452359721152,-9.01842275238194,139.79700958803));
#76903=CARTESIAN_POINT('Ctrl Pts',(77.9452505498836,-8.99849675473629,139.795925280583));
#76904=CARTESIAN_POINT('Ctrl Pts',(77.9452505498842,-8.9984967539153,139.795925280538));
#76905=CARTESIAN_POINT('Ctrl Pts',(77.9453223104453,-8.90040903895431,139.790587668752));
#76906=CARTESIAN_POINT('Ctrl Pts',(77.9524183451655,-8.80257549275452,139.785250056967));
#76907=CARTESIAN_POINT('Ctrl Pts',(77.9664267198136,-8.70575983175005,139.779912445181));
#76908=CARTESIAN_POINT('Ctrl Pts',(77.976571754963,-8.63564475354966,139.776046881864));
#76909=CARTESIAN_POINT('Ctrl Pts',(77.9903674947664,-8.56591523418777,139.772181318546));
#76910=CARTESIAN_POINT('Ctrl Pts',(78.0077726664933,-8.49698129843022,139.768315755229));
#76911=CARTESIAN_POINT('Ctrl Pts',(78.0251516536356,-8.4281510678534,139.764456007319));
#76912=CARTESIAN_POINT('Ctrl Pts',(78.0461291766953,-8.36011451330124,139.760596259409));
#76913=CARTESIAN_POINT('Ctrl Pts',(78.0706124987683,-8.29327414608565,139.756736511499));
#76914=CARTESIAN_POINT('Ctrl Pts',(78.0950667072662,-8.22651325999793,139.752881353288));
#76915=CARTESIAN_POINT('Ctrl Pts',(78.1230182678931,-8.16094619082245,139.749026195076));
#76916=CARTESIAN_POINT('Ctrl Pts',(78.1543243910515,-8.09696118077206,139.745171036865));
#76917=CARTESIAN_POINT('Ctrl Pts',(78.1856104997258,-8.0330170773187,139.741318343315));
#76918=CARTESIAN_POINT('Ctrl Pts',(78.2202467029164,-7.9706534626749,139.737465649765));
#76919=CARTESIAN_POINT('Ctrl Pts',(78.2580423382098,-7.91023806864503,139.733612956215));
#76920=CARTESIAN_POINT('Ctrl Pts',(78.295826518032,-7.84984098590428,139.729761430377));
#76921=CARTESIAN_POINT('Ctrl Pts',(78.3367679709835,-7.79139136406186,139.72590990454));
#76922=CARTESIAN_POINT('Ctrl Pts',(78.3806312563075,-7.73523028402328,139.722058378702));
#76923=CARTESIAN_POINT('Ctrl Pts',(78.4244959947189,-7.67906734350036,139.718206725272));
#76924=CARTESIAN_POINT('Ctrl Pts',(78.471282456273,-7.62519347759648,139.714355071842));
#76925=CARTESIAN_POINT('Ctrl Pts',(78.5207143194315,-7.57391745057829,139.710503418413));
#76926=CARTESIAN_POINT('Ctrl Pts',(78.5701978474364,-7.52258783124362,139.706647739339));
#76927=CARTESIAN_POINT('Ctrl Pts',(78.6223319578652,-7.473861822142,139.702792060265));
#76928=CARTESIAN_POINT('Ctrl Pts',(78.6768034311584,-7.42801132233532,139.698936381191));
#76929=CARTESIAN_POINT('Ctrl Pts',(78.7313056172835,-7.38213497048893,139.695078528157));
#76930=CARTESIAN_POINT('Ctrl Pts',(78.7881474011765,-7.33913764908114,139.691220675123));
#76931=CARTESIAN_POINT('Ctrl Pts',(78.8469846502084,-7.29924923470695,139.687362822089));
#76932=CARTESIAN_POINT('Ctrl Pts',(78.9059252833125,-7.25929073162568,139.683498190347));
#76933=CARTESIAN_POINT('Ctrl Pts',(78.9668679650895,-7.222452293824,139.679633558604));
#76934=CARTESIAN_POINT('Ctrl Pts',(79.0294425512897,-7.1889186099866,139.675768926861));
#76935=CARTESIAN_POINT('Ctrl Pts',(79.0671668276065,-7.16870219255865,139.673439060304));
#76936=CARTESIAN_POINT('Ctrl Pts',(79.1054837830116,-7.14968597763149,139.671109193747));
#76937=CARTESIAN_POINT('Ctrl Pts',(79.1443091147733,-7.13190185711778,139.66877932719));
#76938=CARTESIAN_POINT('Ctrl Pts',(79.2087912972159,-7.10236549898486,139.664909820515));
#76939=CARTESIAN_POINT('Ctrl Pts',(79.2749307389754,-7.0761139131,139.66104031384));
#76940=CARTESIAN_POINT('Ctrl Pts',(79.3423595470498,-7.05333449274319,139.657170807165));
#76941=CARTESIAN_POINT('Ctrl Pts',(79.4096878660436,-7.03058902053217,139.653307067212));
#76942=CARTESIAN_POINT('Ctrl Pts',(79.4783012807501,-7.01130559658793,139.649443327259));
#76943=CARTESIAN_POINT('Ctrl Pts',(79.5478103944463,-6.99562425600158,139.645579587305));
#76944=CARTESIAN_POINT('Ctrl Pts',(79.6172378912085,-6.9799613282948,139.641720384118));
#76945=CARTESIAN_POINT('Ctrl Pts',(79.6875585264096,-6.96789218894587,139.637861180932));
#76946=CARTESIAN_POINT('Ctrl Pts',(79.7583678281001,-6.9595070556351,139.634001977745));
#76947=CARTESIAN_POINT('Ctrl Pts',(79.8291324677329,-6.95112721113948,139.630145208701));
#76948=CARTESIAN_POINT('Ctrl Pts',(79.9003846811958,-6.94642681955575,139.626288439657));
#76949=CARTESIAN_POINT('Ctrl Pts',(79.9717113396144,-6.94544474053541,139.622431670613));
#76950=CARTESIAN_POINT('Ctrl Pts',(80.0430168551677,-6.94446295262593,139.618576044804));
#76951=CARTESIAN_POINT('Ctrl Pts',(80.1143962865175,-6.94719729578647,139.614720418995));
#76952=CARTESIAN_POINT('Ctrl Pts',(80.1854346706739,-6.95363455233137,139.610864793186));
#76953=CARTESIAN_POINT('Ctrl Pts',(80.2564757458479,-6.96007205272711,139.607009021322));
#76954=CARTESIAN_POINT('Ctrl Pts',(80.3271752646984,-6.97021269897574,139.603153249457));
#76955=CARTESIAN_POINT('Ctrl Pts',(80.397123288252,-6.9839914046741,139.599297477593));
#76956=CARTESIAN_POINT('Ctrl Pts',(80.4671443389033,-6.99778449560931,139.595437680227));
#76957=CARTESIAN_POINT('Ctrl Pts',(80.536411850583,-7.01522313403648,139.591577882862));
#76958=CARTESIAN_POINT('Ctrl Pts',(80.604526877104,-7.03619124725474,139.587718085497));
#76959=CARTESIAN_POINT('Ctrl Pts',(80.6726803776316,-7.05717120407593,139.583856107968));
#76960=CARTESIAN_POINT('Ctrl Pts',(80.7396796407864,-7.08168443741847,139.57999413044));
#76961=CARTESIAN_POINT('Ctrl Pts',(80.8051442726936,-7.10956611788491,139.576132152911));
#76962=CARTESIAN_POINT('Ctrl Pts',(80.8707232169427,-7.13749648449068,139.572263431716));
#76963=CARTESIAN_POINT('Ctrl Pts',(80.9347617433241,-7.16880682822043,139.56839471052));
#76964=CARTESIAN_POINT('Ctrl Pts',(80.9969033225346,-7.20328596376068,139.564525989324));
#76965=CARTESIAN_POINT('Ctrl Pts',(81.0337389571915,-7.22372414470459,139.562232729282));
#76966=CARTESIAN_POINT('Ctrl Pts',(81.0699085748146,-7.24527491322266,139.55993946924));
#76967=CARTESIAN_POINT('Ctrl Pts',(81.105343077467,-7.2678873467364,139.557646209198));
#76968=CARTESIAN_POINT('Ctrl Pts',(81.1556290406518,-7.29997720024298,139.554391788184));
#76969=CARTESIAN_POINT('Ctrl Pts',(81.2045988689083,-7.33431130662179,139.55113736717));
#76970=CARTESIAN_POINT('Ctrl Pts',(81.2520391107129,-7.37076839346111,139.547882946156));
#76971=CARTESIAN_POINT('Origin',(80.,-9.,134.));
#76972=CARTESIAN_POINT('',(78.4365593938057,-8.4244919888458,129.733376828424));
#76973=CARTESIAN_POINT('',(78.4365593669558,-8.42449206178673,129.539973210016));
#76974=CARTESIAN_POINT('',(78.4365593749993,-8.42449203993574,134.));
#76975=CARTESIAN_POINT('',(79.2300979593296,-10.4774325188554,129.));
#76976=CARTESIAN_POINT('Ctrl Pts',(78.4365593669558,-8.42449206178673,129.539973210016));
#76977=CARTESIAN_POINT('Ctrl Pts',(78.4421051495214,-8.40942623692262,129.538809960763));
#76978=CARTESIAN_POINT('Ctrl Pts',(78.4478692931931,-8.39443896491615,129.537643380814));
#76979=CARTESIAN_POINT('Ctrl Pts',(78.5031573253039,-8.25666554449912,129.526842962418));
#76980=CARTESIAN_POINT('Ctrl Pts',(78.566945264484,-8.14008694623375,129.517194430966));
#76981=CARTESIAN_POINT('Ctrl Pts',(78.6598156206824,-8.00994194088386,129.506139863644));
#76982=CARTESIAN_POINT('Ctrl Pts',(78.676306699791,-7.9879993410312,129.504262795112));
#76983=CARTESIAN_POINT('Ctrl Pts',(78.7011001312814,-7.95665351983249,129.501560125491));
#76984=CARTESIAN_POINT('Ctrl Pts',(78.7089776205111,-7.94692166614924,129.500717927568));
#76985=CARTESIAN_POINT('Ctrl Pts',(78.7231795512279,-7.9297755008893,129.499228174938));
#76986=CARTESIAN_POINT('Ctrl Pts',(78.7294606651604,-7.92232623559256,129.498578906769));
#76987=CARTESIAN_POINT('Ctrl Pts',(78.7427539217707,-7.90683849740872,129.497224481522));
#76988=CARTESIAN_POINT('Ctrl Pts',(78.7497786592342,-7.89881137853938,129.496519885272));
#76989=CARTESIAN_POINT('Ctrl Pts',(78.7685132743193,-7.8778138430891,129.494669362884));
#76990=CARTESIAN_POINT('Ctrl Pts',(78.7803511513633,-7.86495900949914,129.49352885744));
#76991=CARTESIAN_POINT('Ctrl Pts',(78.841554047578,-7.80056171704367,129.487771341444));
#76992=CARTESIAN_POINT('Ctrl Pts',(78.8939951307454,-7.75203994922801,129.483290817009));
#76993=CARTESIAN_POINT('Ctrl Pts',(79.0025415416958,-7.66384038981644,129.474652767779));
#76994=CARTESIAN_POINT('Ctrl Pts',(79.0583029557258,-7.6239721065796,129.470497234));
#76995=CARTESIAN_POINT('Ctrl Pts',(79.1346995757809,-7.57617446652224,129.464983869449));
#76996=CARTESIAN_POINT('Ctrl Pts',(79.1532601749058,-7.56505902057212,129.463657217349));
#76997=CARTESIAN_POINT('Ctrl Pts',(79.2285893136379,-7.52191694293435,129.458304193105));
#76998=CARTESIAN_POINT('Ctrl Pts',(79.2869924491519,-7.49287620261494,129.454224907383));
#76999=CARTESIAN_POINT('Ctrl Pts',(79.3574421351471,-7.46285792580099,129.449214025385));
#77000=CARTESIAN_POINT('Ctrl Pts',(79.3679915115582,-7.45849047400551,129.448461352988));
#77001=CARTESIAN_POINT('Ctrl Pts',(79.3845012182123,-7.45185339398491,129.447278551668));
#77002=CARTESIAN_POINT('Ctrl Pts',(79.3904313386674,-7.44950888173565,129.446852729747));
#77003=CARTESIAN_POINT('Ctrl Pts',(79.4009824191374,-7.44540732738616,129.446093120303));
#77004=CARTESIAN_POINT('Ctrl Pts',(79.4055979580861,-7.44363672301757,129.445760148423));
#77005=CARTESIAN_POINT('Ctrl Pts',(79.4167433589534,-7.43941795366539,129.444954516762));
#77006=CARTESIAN_POINT('Ctrl Pts',(79.4232807587345,-7.4369902287469,129.444480676272));
#77007=CARTESIAN_POINT('Ctrl Pts',(79.4435055772063,-7.42962370903896,129.443011187527));
#77008=CARTESIAN_POINT('Ctrl Pts',(79.4572421835039,-7.42482329415341,129.442008104407));
#77009=CARTESIAN_POINT('Ctrl Pts',(79.5275840643049,-7.40127083481238,129.436852221769));
#77010=CARTESIAN_POINT('Ctrl Pts',(79.5850991855127,-7.38538931416034,129.432574509866));
#77011=CARTESIAN_POINT('Ctrl Pts',(79.746891747963,-7.3499299248934,129.420573036073));
#77012=CARTESIAN_POINT('Ctrl Pts',(79.8523888785454,-7.33716821499544,129.412800023091));
#77013=CARTESIAN_POINT('Ctrl Pts',(80.0157945475274,-7.33308541577284,129.401185023904));
#77014=CARTESIAN_POINT('Ctrl Pts',(80.0732430980142,-7.33462002079192,129.3971774228));
#77015=CARTESIAN_POINT('Ctrl Pts',(80.1476576745716,-7.34046714864326,129.392086436276));
#77016=CARTESIAN_POINT('Ctrl Pts',(80.1647902112465,-7.34208073228306,129.390921102206));
#77017=CARTESIAN_POINT('Ctrl Pts',(80.192516992695,-7.34512617092939,129.38904548791));
#77018=CARTESIAN_POINT('Ctrl Pts',(80.2031274764858,-7.34639502296655,129.388330184557));
#77019=CARTESIAN_POINT('Ctrl Pts',(80.2235279836516,-7.34903393664873,129.386959360675));
#77020=CARTESIAN_POINT('Ctrl Pts',(80.2333194283543,-7.35038921156909,129.386303408469));
#77021=CARTESIAN_POINT('Ctrl Pts',(80.2560618285666,-7.35374362688137,129.384784169683));
#77022=CARTESIAN_POINT('Ctrl Pts',(80.2690025291913,-7.35580859947425,129.383922981935));
#77023=CARTESIAN_POINT('Ctrl Pts',(80.3110274492081,-7.36302404559621,129.381135778116));
#77024=CARTESIAN_POINT('Ctrl Pts',(80.3400003117498,-7.36879544286572,129.379229198639));
#77025=CARTESIAN_POINT('Ctrl Pts',(80.4091469975403,-7.38449202983201,129.374702170212));
#77026=CARTESIAN_POINT('Ctrl Pts',(80.4491348849155,-7.39514939011828,129.372103483886));
#77027=CARTESIAN_POINT('Ctrl Pts',(80.5603451229927,-7.42927161059155,129.3648744392));
#77028=CARTESIAN_POINT('Ctrl Pts',(80.6304397707747,-7.45606979612854,129.36031892819));
#77029=CARTESIAN_POINT('Ctrl Pts',(80.7739311678776,-7.52233584460262,129.350643978906));
#77030=CARTESIAN_POINT('Ctrl Pts',(80.8466493666071,-7.5627657409146,129.345529800997));
#77031=CARTESIAN_POINT('Ctrl Pts',(80.9294110477657,-7.61724644598969,129.339103104612));
#77032=CARTESIAN_POINT('Ctrl Pts',(80.9426546507233,-7.62624075958579,129.338054795383));
#77033=CARTESIAN_POINT('Ctrl Pts',(80.9616544589108,-7.63954846245772,129.336518536545));
#77034=CARTESIAN_POINT('Ctrl Pts',(80.9675160335009,-7.6437107961181,129.336040046828));
#77035=CARTESIAN_POINT('Ctrl Pts',(80.9778647884257,-7.65116072216811,129.335186811843));
#77036=CARTESIAN_POINT('Ctrl Pts',(80.9823627046248,-7.65443303533248,129.334813083378));
#77037=CARTESIAN_POINT('Ctrl Pts',(80.9921302395696,-7.6616141688067,129.333995152748));
#77038=CARTESIAN_POINT('Ctrl Pts',(80.9973931481054,-7.66553158527528,129.333550397849));
#77039=CARTESIAN_POINT('Ctrl Pts',(81.0123582500058,-7.67680875431978,129.332274468473));
#77040=CARTESIAN_POINT('Ctrl Pts',(81.0220028404786,-7.68424376423163,129.331438516697));
#77041=CARTESIAN_POINT('Ctrl Pts',(81.0438463582184,-7.70146797988907,129.329515389397));
#77042=CARTESIAN_POINT('Ctrl Pts',(81.0559905513174,-7.71132449998642,129.32842447879));
#77043=CARTESIAN_POINT('Ctrl Pts',(81.096211033922,-7.74491870195875,129.324742713934));
#77044=CARTESIAN_POINT('Ctrl Pts',(81.1236388480168,-7.7694135093637,129.322117430346));
#77045=CARTESIAN_POINT('Ctrl Pts',(81.2005140827859,-7.84278218217326,129.314467617277));
#77046=CARTESIAN_POINT('Ctrl Pts',(81.2477431818303,-7.89386976861539,129.309398873089));
#77047=CARTESIAN_POINT('Ctrl Pts',(81.3523823720482,-8.02231596145479,129.297428709378));
#77048=CARTESIAN_POINT('Ctrl Pts',(81.4065602181387,-8.10200331115536,129.290600396389));
#77049=CARTESIAN_POINT('Ctrl Pts',(81.4627734102828,-8.20237534866955,129.282738285493));
#77050=CARTESIAN_POINT('Ctrl Pts',(81.471702417144,-8.21897299693459,129.281460096307));
#77051=CARTESIAN_POINT('Ctrl Pts',(81.4854250621002,-8.2455526155487,129.279446908675));
#77052=CARTESIAN_POINT('Ctrl Pts',(81.4904039112463,-8.2554365960657,129.278705532416));
#77053=CARTESIAN_POINT('Ctrl Pts',(81.4996262667756,-8.27420799716288,129.27731090634));
#77054=CARTESIAN_POINT('Ctrl Pts',(81.503890154147,-8.2830848148542,129.276656976824));
#77055=CARTESIAN_POINT('Ctrl Pts',(81.51339256266,-8.30332539064225,129.275178243855));
#77056=CARTESIAN_POINT('Ctrl Pts',(81.5185823110353,-8.31471149230558,129.274355132529));
#77057=CARTESIAN_POINT('Ctrl Pts',(81.5341697356079,-8.34995651944988,129.27183307611));
#77058=CARTESIAN_POINT('Ctrl Pts',(81.5441373349323,-8.37400214563419,129.270148596857));
#77059=CARTESIAN_POINT('Ctrl Pts',(81.5661022838081,-8.43071117584757,129.2662515433));
#77060=CARTESIAN_POINT('Ctrl Pts',(81.5776481178226,-8.46353678720286,129.2640531434));
#77061=CARTESIAN_POINT('Ctrl Pts',(81.6148612060515,-8.5809626793549,129.25635058614));
#77062=CARTESIAN_POINT('Ctrl Pts',(81.6348164241211,-8.66721605467108,129.25099239051));
#77063=CARTESIAN_POINT('Ctrl Pts',(81.66016419167,-8.83745719085409,129.240470953946));
#77064=CARTESIAN_POINT('Ctrl Pts',(81.6662327280654,-8.92106763900409,129.235324432262));
#77065=CARTESIAN_POINT('Ctrl Pts',(81.6659483645958,-9.02042572749627,129.228879170295));
#77066=CARTESIAN_POINT('Ctrl Pts',(81.6656828216231,-9.03608127190637,129.227853784274));
#77067=CARTESIAN_POINT('Ctrl Pts',(81.6649735763235,-9.05891196765729,129.226341071643));
#77068=CARTESIAN_POINT('Ctrl Pts',(81.6647040113192,-9.06609220629656,129.22586281435));
#77069=CARTESIAN_POINT('Ctrl Pts',(81.6641482873134,-9.07871587838213,129.225017213397));
#77070=CARTESIAN_POINT('Ctrl Pts',(81.6638818410816,-9.0841601353511,129.224650966338));
#77071=CARTESIAN_POINT('Ctrl Pts',(81.6632663094816,-9.09558824289128,129.223878707916));
#77072=CARTESIAN_POINT('Ctrl Pts',(81.6629116461076,-9.1015715547018,129.223472360227));
#77073=CARTESIAN_POINT('Ctrl Pts',(81.6618279054598,-9.11832377081192,129.222329174227));
#77074=CARTESIAN_POINT('Ctrl Pts',(81.6610264630458,-9.12908746975198,129.221588322054));
#77075=CARTESIAN_POINT('Ctrl Pts',(81.6550402791469,-9.20015174065917,129.216658629842));
#77076=CARTESIAN_POINT('Ctrl Pts',(81.6466779519982,-9.26013263890496,129.212316204664));
#77077=CARTESIAN_POINT('Ctrl Pts',(81.6120320563035,-9.4374265982666,129.199179546184));
#77078=CARTESIAN_POINT('Ctrl Pts',(81.5763006516239,-9.55251362934102,129.190280518424));
#77079=CARTESIAN_POINT('Ctrl Pts',(81.505826795098,-9.71504511962773,129.177663005555));
#77080=CARTESIAN_POINT('Ctrl Pts',(81.48048531832,-9.76613867419146,129.173682126311));
#77081=CARTESIAN_POINT('Ctrl Pts',(81.4443832378883,-9.83041715376138,129.168654599245));
#77082=CARTESIAN_POINT('Ctrl Pts',(81.435975776323,-9.84487229446125,129.16752250497));
#77083=CARTESIAN_POINT('Ctrl Pts',(81.422061095598,-9.86798818177181,129.165709029961));
#77084=CARTESIAN_POINT('Ctrl Pts',(81.4166891873383,-9.87672857729801,129.165022602217));
#77085=CARTESIAN_POINT('Ctrl Pts',(81.4062436001058,-9.89337741507283,129.163713427037));
#77086=CARTESIAN_POINT('Ctrl Pts',(81.4011831040058,-9.90129361699914,129.163090209504));
#77087=CARTESIAN_POINT('Ctrl Pts',(81.3893422940441,-9.91947557533854,129.161656832144));
#77088=CARTESIAN_POINT('Ctrl Pts',(81.3825146399891,-9.9297099697401,129.160848533992));
#77089=CARTESIAN_POINT('Ctrl Pts',(81.3603535257935,-9.96214458099085,129.158281169335));
#77090=CARTESIAN_POINT('Ctrl Pts',(81.3445934268057,-9.9840490647939,129.156538710523));
#77091=CARTESIAN_POINT('Ctrl Pts',(81.2908335459066,-10.0550637218277,129.150846887588));
#77092=CARTESIAN_POINT('Ctrl Pts',(81.2506197507949,-10.1024345952231,129.146982423801));
#77093=CARTESIAN_POINT('Ctrl Pts',(81.1436257940824,-10.2150603749868,129.137431388163));
#77094=CARTESIAN_POINT('Ctrl Pts',(81.0738399867031,-10.277152343676,129.131825983486));
#77095=CARTESIAN_POINT('Ctrl Pts',(80.9566353766147,-10.3650048822894,129.122733375139));
#77096=CARTESIAN_POINT('Ctrl Pts',(80.9125403291373,-10.3948686158705,129.119372292501));
#77097=CARTESIAN_POINT('Ctrl Pts',(80.8578135471789,-10.428226216401,129.115170830819));
#77098=CARTESIAN_POINT('Ctrl Pts',(80.8484750257994,-10.4337936816692,129.11445287116));
#77099=CARTESIAN_POINT('Ctrl Pts',(80.833755681823,-10.4423749475326,129.113318488733));
#77100=CARTESIAN_POINT('Ctrl Pts',(80.8284112515301,-10.4454510790768,129.112906048126));
#77101=CARTESIAN_POINT('Ctrl Pts',(80.8182622725121,-10.4512178251095,129.112121526084));
#77102=CARTESIAN_POINT('Ctrl Pts',(80.8134612205255,-10.4539144276564,129.11174985938));
#77103=CARTESIAN_POINT('Ctrl Pts',(80.8038690255773,-10.4592396837431,129.111006339217));
#77104=CARTESIAN_POINT('Ctrl Pts',(80.799078134191,-10.4618686665421,129.110634512434));
#77105=CARTESIAN_POINT('Ctrl Pts',(80.7836859065697,-10.4702168200401,129.109438594242));
#77106=CARTESIAN_POINT('Ctrl Pts',(80.7730357413556,-10.4758444428702,129.10860913776));
#77107=CARTESIAN_POINT('Ctrl Pts',(80.7480249590674,-10.4887153316269,129.106658139892));
#77108=CARTESIAN_POINT('Ctrl Pts',(80.7336188013687,-10.4958670024119,129.10553201283));
#77109=CARTESIAN_POINT('Ctrl Pts',(80.6847384433017,-10.5192568402237,129.101708096936));
#77110=CARTESIAN_POINT('Ctrl Pts',(80.6498129233082,-10.5345197474586,129.098971190258));
#77111=CARTESIAN_POINT('Ctrl Pts',(80.507882362411,-10.5908308757962,129.087901487725));
#77112=CARTESIAN_POINT('Ctrl Pts',(80.3972812718764,-10.6219919419258,129.079417142815));
#77113=CARTESIAN_POINT('Ctrl Pts',(80.2098310726684,-10.6544630165915,129.065738018543));
#77114=CARTESIAN_POINT('Ctrl Pts',(80.1345031853498,-10.6622841871778,129.060414502622));
#77115=CARTESIAN_POINT('Ctrl Pts',(80.0392875853344,-10.6656522439802,129.053897824544));
#77116=CARTESIAN_POINT('Ctrl Pts',(80.0196692971777,-10.6659994251104,129.052566049396));
#77117=CARTESIAN_POINT('Ctrl Pts',(79.9881339529254,-10.6660003479618,129.050441511476));
#77118=CARTESIAN_POINT('Ctrl Pts',(79.9762192521891,-10.6658728793751,129.049642532108));
#77119=CARTESIAN_POINT('Ctrl Pts',(79.9534345908827,-10.6653846161134,129.04812127416));
#77120=CARTESIAN_POINT('Ctrl Pts',(79.9425648355876,-10.6650451848089,129.047398428518));
#77121=CARTESIAN_POINT('Ctrl Pts',(79.9174608320011,-10.6640151297221,129.045735185369));
#77122=CARTESIAN_POINT('Ctrl Pts',(79.9032304499663,-10.6632482493494,129.044796968387));
#77123=CARTESIAN_POINT('Ctrl Pts',(79.8572148200931,-10.6601758694142,129.04177623738));
#77124=CARTESIAN_POINT('Ctrl Pts',(79.8254844654185,-10.6571409217714,129.039713673389));
#77125=CARTESIAN_POINT('Ctrl Pts',(79.7061279291857,-10.6422580968799,129.032003191899));
#77126=CARTESIAN_POINT('Ctrl Pts',(79.6194042500843,-10.6243523978704,129.026506258357));
#77127=CARTESIAN_POINT('Ctrl Pts',(79.4530587979164,-10.5759463542871,129.015705200889));
#77128=CARTESIAN_POINT('Ctrl Pts',(79.3735468198919,-10.5460612398616,129.010415206558));
#77129=CARTESIAN_POINT('Ctrl Pts',(79.2839673137288,-10.5043434987173,129.003983026668));
#77130=CARTESIAN_POINT('Ctrl Pts',(79.2713460464801,-10.4982708572166,129.003065253333));
#77131=CARTESIAN_POINT('Ctrl Pts',(79.253473921207,-10.489392568874,129.001747290998));
#77132=CARTESIAN_POINT('Ctrl Pts',(79.2481589036594,-10.4867166422333,129.001352998794));
#77133=CARTESIAN_POINT('Ctrl Pts',(79.2385954444432,-10.481837375072,129.000639121319));
#77134=CARTESIAN_POINT('Ctrl Pts',(79.234341920028,-10.4796440811167,129.0003200235));
#77135=CARTESIAN_POINT('Ctrl Pts',(79.2300979593296,-10.4774325188555,129.));
#77136=CARTESIAN_POINT('',(78.6641544596132,-8.00193394365392,128.999128947666));
#77137=CARTESIAN_POINT('Origin',(80.,-9.,129.));
#77138=CARTESIAN_POINT('',(78.4365593804234,-8.42449202520043,129.032769696));
#77139=CARTESIAN_POINT('Ctrl Pts',(78.6653336475789,-8.00289332179799,128.998257895331));
#77140=CARTESIAN_POINT('Ctrl Pts',(78.6630695895503,-8.00592385216835,128.998515381112));
#77141=CARTESIAN_POINT('Ctrl Pts',(78.6608158838452,-8.00896205294451,128.998773542407));
#77142=CARTESIAN_POINT('Ctrl Pts',(78.6540156321242,-8.01819496474882,128.99955808582));
#77143=CARTESIAN_POINT('Ctrl Pts',(78.6495016584439,-8.02441337142469,129.000086487955));
#77144=CARTESIAN_POINT('Ctrl Pts',(78.6275129566489,-8.05514984269038,129.002697449622));
#77145=CARTESIAN_POINT('Ctrl Pts',(78.6106631800488,-8.08010574189685,129.004814697559));
#77146=CARTESIAN_POINT('Ctrl Pts',(78.5348728686095,-8.19919303571354,129.014858057607));
#77147=CARTESIAN_POINT('Ctrl Pts',(78.484764080392,-8.29860885504514,129.023048835688));
#77148=CARTESIAN_POINT('Ctrl Pts',(78.4420795996736,-8.40965885144952,129.031630802593));
#77149=CARTESIAN_POINT('Ctrl Pts',(78.4392928985672,-8.41706607545248,129.032200782898));
#77150=CARTESIAN_POINT('Ctrl Pts',(78.4365593804234,-8.42449202520042,129.032769696));
#77151=CARTESIAN_POINT('',(78.4365593749993,-8.42449203993574,128.));
#77152=CARTESIAN_POINT('',(78.4365593749993,-8.42449203993574,134.));
#77153=CARTESIAN_POINT('Origin',(80.,-9.,128.));
#77154=CARTESIAN_POINT('Ctrl Pts',(78.4365593804234,-8.42449202520042,129.032769696));
#77155=CARTESIAN_POINT('Ctrl Pts',(78.4096421356088,-8.49761614467909,129.038371844014));
#77156=CARTESIAN_POINT('Ctrl Pts',(78.3878815483186,-8.57255645732196,129.043863517686));
#77157=CARTESIAN_POINT('Ctrl Pts',(78.3675657998122,-8.66675351310855,129.050446145633));
#77158=CARTESIAN_POINT('Ctrl Pts',(78.3639843431817,-8.68480568466688,129.051693840243));
#77159=CARTESIAN_POINT('Ctrl Pts',(78.3587462013066,-8.71370935642439,129.053670362302));
#77160=CARTESIAN_POINT('Ctrl Pts',(78.3568964522487,-8.72452385664356,129.054405193902));
#77161=CARTESIAN_POINT('Ctrl Pts',(78.3535870427762,-8.74509289096038,129.055794215036));
#77162=CARTESIAN_POINT('Ctrl Pts',(78.3521069179843,-8.75484360653624,129.056449017273));
#77163=CARTESIAN_POINT('Ctrl Pts',(78.3489233111293,-8.77714962911568,129.057938911605));
#77164=CARTESIAN_POINT('Ctrl Pts',(78.3472762808697,-8.78971247513152,129.058772216853));
#77165=CARTESIAN_POINT('Ctrl Pts',(78.3433203235853,-8.82281225660801,129.060953369334));
#77166=CARTESIAN_POINT('Ctrl Pts',(78.3412498728459,-8.84337585894582,129.062293887701));
#77167=CARTESIAN_POINT('Ctrl Pts',(78.3276469462407,-9.00942286243062,129.073015574458));
#77168=CARTESIAN_POINT('Ctrl Pts',(78.3348930193932,-9.15580098927435,129.081762368785));
#77169=CARTESIAN_POINT('Ctrl Pts',(78.3720834551145,-9.35939909493017,129.094552020351));
#77170=CARTESIAN_POINT('Ctrl Pts',(78.3863380897752,-9.41877639812151,129.09837109746));
#77171=CARTESIAN_POINT('Ctrl Pts',(78.4080452696062,-9.49137990511416,129.103299314955));
#77172=CARTESIAN_POINT('Ctrl Pts',(78.4124631859569,-9.50547097133187,129.104268228217));
#77173=CARTESIAN_POINT('Ctrl Pts',(78.4188413398983,-9.52490536890206,129.1056242622));
#77174=CARTESIAN_POINT('Ctrl Pts',(78.4206426747747,-9.53030066157981,129.106002839049));
#77175=CARTESIAN_POINT('Ctrl Pts',(78.4225463402344,-9.53590671330397,129.106398519546));
#77176=CARTESIAN_POINT('Ctrl Pts',(78.4226211554302,-9.53612688309365,129.106414063065));
#77177=CARTESIAN_POINT('Ctrl Pts',(78.422770798915,-9.53656695873192,129.106445138926));
#77178=CARTESIAN_POINT('Ctrl Pts',(78.4228456270988,-9.53678686459003,129.106460671261));
#77179=CARTESIAN_POINT('Ctrl Pts',(78.4229967420417,-9.5372306584089,129.106492024724));
#77180=CARTESIAN_POINT('Ctrl Pts',(78.4230730304888,-9.53745454577447,129.106507845947));
#77181=CARTESIAN_POINT('Ctrl Pts',(78.4232288600846,-9.53791154756071,129.106540148343));
#77182=CARTESIAN_POINT('Ctrl Pts',(78.4233084052583,-9.53814466060712,129.106556629747));
#77183=CARTESIAN_POINT('Ctrl Pts',(78.4234731817409,-9.53862720019305,129.106590754658));
#77184=CARTESIAN_POINT('Ctrl Pts',(78.4235584205148,-9.5388766240504,129.106608398588));
#77185=CARTESIAN_POINT('Ctrl Pts',(78.4237382273484,-9.5394023631487,129.1066455989));
#77186=CARTESIAN_POINT('Ctrl Pts',(78.423832808883,-9.53967867378591,129.106665156056));
#77187=CARTESIAN_POINT('Ctrl Pts',(78.4240374452184,-9.54027598602979,129.10670744644));
#77188=CARTESIAN_POINT('Ctrl Pts',(78.424147525423,-9.54059697883303,129.106730181126));
#77189=CARTESIAN_POINT('Ctrl Pts',(78.4243953955544,-9.54131904667906,129.106781340535));
#77190=CARTESIAN_POINT('Ctrl Pts',(78.4245332404916,-9.54172010257193,129.106809768427));
#77191=CARTESIAN_POINT('Ctrl Pts',(78.4248089410281,-9.54252125010253,129.106866581082));
#77192=CARTESIAN_POINT('Ctrl Pts',(78.4249467959659,-9.54292134194454,129.106894965805));
#77193=CARTESIAN_POINT('Ctrl Pts',(78.4268295298595,-9.54837878633416,129.107282319114));
#77194=CARTESIAN_POINT('Ctrl Pts',(78.428598525952,-9.55342752580425,129.107642699987));
#77195=CARTESIAN_POINT('Ctrl Pts',(78.4327683479179,-9.56514707022418,129.108483982786));
#77196=CARTESIAN_POINT('Ctrl Pts',(78.4351874402871,-9.57181107953126,129.1089659129));
#77197=CARTESIAN_POINT('Ctrl Pts',(78.4431430177107,-9.59329816599076,129.110530889108));
#77198=CARTESIAN_POINT('Ctrl Pts',(78.4488479811817,-9.6080573545679,129.111622943353));
#77199=CARTESIAN_POINT('Ctrl Pts',(78.4845977626891,-9.69676628128776,129.118281279102));
#77200=CARTESIAN_POINT('Ctrl Pts',(78.5197126889738,-9.76855332466226,129.124065225017));
#77201=CARTESIAN_POINT('Ctrl Pts',(78.5940700406345,-9.89641236903334,129.134820673432));
#77202=CARTESIAN_POINT('Ctrl Pts',(78.6318872286945,-9.95313300038912,129.139777824227));
#77203=CARTESIAN_POINT('Ctrl Pts',(78.7017399623389,-10.0451433854631,129.148049068867));
#77204=CARTESIAN_POINT('Ctrl Pts',(78.7320089393397,-10.081666844528,129.151401916215));
#77205=CARTESIAN_POINT('Ctrl Pts',(78.7856439840373,-10.1410335191105,129.156963574378));
#77206=CARTESIAN_POINT('Ctrl Pts',(78.8081968196041,-10.164570075073,129.159201282403));
#77207=CARTESIAN_POINT('Ctrl Pts',(78.8411224095579,-10.1969727520342,129.162331499006));
#77208=CARTESIAN_POINT('Ctrl Pts',(78.8509345237074,-10.2063952871565,129.163248053969));
#77209=CARTESIAN_POINT('Ctrl Pts',(78.8681298696912,-10.2225077629295,129.164826817197));
#77210=CARTESIAN_POINT('Ctrl Pts',(78.8754596089702,-10.2292534883524,129.165491384624));
#77211=CARTESIAN_POINT('Ctrl Pts',(78.8906336128491,-10.242969153047,129.16685030353));
#77212=CARTESIAN_POINT('Ctrl Pts',(78.8984841204855,-10.2499315469333,129.167544321678));
#77213=CARTESIAN_POINT('Ctrl Pts',(78.9187041954616,-10.2675256996774,129.169309383794));
#77214=CARTESIAN_POINT('Ctrl Pts',(78.9311652512517,-10.278050987555,129.170376048325));
#77215=CARTESIAN_POINT('Ctrl Pts',(78.9823649599522,-10.3200243931331,129.174677221132));
#77216=CARTESIAN_POINT('Ctrl Pts',(79.0223546163069,-10.3499095162561,129.177850029573));
#77217=CARTESIAN_POINT('Ctrl Pts',(79.1633883788147,-10.4457470422045,129.188528116886));
#77218=CARTESIAN_POINT('Ctrl Pts',(79.2702099834336,-10.5025010153419,129.195744032815));
#77219=CARTESIAN_POINT('Ctrl Pts',(79.4330600782967,-10.5675240858282,129.206598739541));
#77220=CARTESIAN_POINT('Ctrl Pts',(79.4848635012946,-10.58530306482,129.210037212744));
#77221=CARTESIAN_POINT('Ctrl Pts',(79.5512169646293,-10.604479785553,129.214531661322));
#77222=CARTESIAN_POINT('Ctrl Pts',(79.5650420669351,-10.6082826734889,129.215472970861));
#77223=CARTESIAN_POINT('Ctrl Pts',(79.5856206905315,-10.6136585257693,129.216883661276));
#77224=CARTESIAN_POINT('Ctrl Pts',(79.5923381451511,-10.6153686445306,129.217345651641));
#77225=CARTESIAN_POINT('Ctrl Pts',(79.6038586880922,-10.6182250905566,129.218140845998));
#77226=CARTESIAN_POINT('Ctrl Pts',(79.6086565176863,-10.6193920651842,129.218472869485));
#77227=CARTESIAN_POINT('Ctrl Pts',(79.6196893173018,-10.6220236750174,129.219238427623));
#77228=CARTESIAN_POINT('Ctrl Pts',(79.625927440841,-10.6234736630792,129.219672763043));
#77229=CARTESIAN_POINT('Ctrl Pts',(79.6434351589962,-10.6274368912019,129.220895590287));
#77230=CARTESIAN_POINT('Ctrl Pts',(79.6547224906052,-10.6298689344806,129.221688395545));
#77231=CARTESIAN_POINT('Ctrl Pts',(79.7354173412039,-10.6463801635573,129.22738353793));
#77232=CARTESIAN_POINT('Ctrl Pts',(79.8056280414769,-10.6561367382867,129.232479283037));
#77233=CARTESIAN_POINT('Ctrl Pts',(79.8909017485095,-10.6624890395765,129.23868862336));
#77234=CARTESIAN_POINT('Ctrl Pts',(79.9055797847451,-10.6633872227276,129.239758284618));
#77235=CARTESIAN_POINT('Ctrl Pts',(79.9872832888677,-10.6673019181041,129.245712372193));
#77236=CARTESIAN_POINT('Ctrl Pts',(80.0544349201842,-10.6664618395219,129.250602377746));
#77237=CARTESIAN_POINT('Ctrl Pts',(80.1947253237735,-10.6562155437339,129.260692005127));
#77238=CARTESIAN_POINT('Ctrl Pts',(80.2676679650444,-10.6460025706391,129.265864060174));
#77239=CARTESIAN_POINT('Ctrl Pts',(80.3569385338475,-10.6274092066713,129.272087197347));
#77240=CARTESIAN_POINT('Ctrl Pts',(80.3741136599144,-10.6235469977397,129.273279810671));
#77241=CARTESIAN_POINT('Ctrl Pts',(80.401618131403,-10.6169023468378,129.275182799228));
#77242=CARTESIAN_POINT('Ctrl Pts',(80.411987114148,-10.6142914698798,129.275898631705));
#77243=CARTESIAN_POINT('Ctrl Pts',(80.4317456122551,-10.6091135631706,129.277259908056));
#77244=CARTESIAN_POINT('Ctrl Pts',(80.441139131806,-10.6065637261465,129.277905877371));
#77245=CARTESIAN_POINT('Ctrl Pts',(80.462505068764,-10.6005624935669,129.279372687967));
#77246=CARTESIAN_POINT('Ctrl Pts',(80.4744622886533,-10.5970587920311,129.280191790036));
#77247=CARTESIAN_POINT('Ctrl Pts',(80.5062136229817,-10.5873669456274,129.282362892754));
#77248=CARTESIAN_POINT('Ctrl Pts',(80.5259337868642,-10.5809426824809,129.283707181825));
#77249=CARTESIAN_POINT('Ctrl Pts',(80.6640028537375,-10.5330942043162,129.293102046469));
#77250=CARTESIAN_POINT('Ctrl Pts',(80.7774638600435,-10.478793938927,129.300693851854));
#77251=CARTESIAN_POINT('Ctrl Pts',(80.9619418148984,-10.3633518960431,129.313985497023));
#77252=CARTESIAN_POINT('Ctrl Pts',(81.0359088301449,-10.308032274021,129.319644951935));
#77253=CARTESIAN_POINT('Ctrl Pts',(81.1137263748375,-10.2390756053764,129.326443735746));
#77254=CARTESIAN_POINT('Ctrl Pts',(81.1224602857129,-10.2311692334273,129.327219994112));
#77255=CARTESIAN_POINT('Ctrl Pts',(81.1357899796162,-10.2188427978369,129.328426612819));
#77256=CARTESIAN_POINT('Ctrl Pts',(81.1404456733377,-10.2144876723935,129.328852252722));
#77257=CARTESIAN_POINT('Ctrl Pts',(81.1490514031147,-10.2063444057755,129.329647130337));
#77258=CARTESIAN_POINT('Ctrl Pts',(81.1530079164191,-10.2025633844024,129.330015834876));
#77259=CARTESIAN_POINT('Ctrl Pts',(81.1620623576548,-10.1938247958838,129.330867054166));
#77260=CARTESIAN_POINT('Ctrl Pts',(81.1671472619829,-10.1888539988368,129.331350567942));
#77261=CARTESIAN_POINT('Ctrl Pts',(81.1830096500442,-10.1731477201653,129.332875735517));
#77262=CARTESIAN_POINT('Ctrl Pts',(81.1936716612685,-10.1622974360859,129.333925595327));
#77263=CARTESIAN_POINT('Ctrl Pts',(81.2719261072152,-10.0804487223339,129.341807328732));
#77264=CARTESIAN_POINT('Ctrl Pts',(81.3332772576937,-10.0037598843842,129.348971688738));
#77265=CARTESIAN_POINT('Ctrl Pts',(81.4322556200153,-9.85482767619449,129.361983145366));
#77266=CARTESIAN_POINT('Ctrl Pts',(81.4720327621261,-9.78435230836564,129.367825855314));
#77267=CARTESIAN_POINT('Ctrl Pts',(81.5197616983309,-9.68325652546844,129.375696198326));
#77268=CARTESIAN_POINT('Ctrl Pts',(81.5322005865692,-9.65488676243698,129.377853500018));
#77269=CARTESIAN_POINT('Ctrl Pts',(81.5527754565263,-9.60415998945305,129.381621185544));
#77270=CARTESIAN_POINT('Ctrl Pts',(81.5612369029593,-9.58194531104749,129.383241664363));
#77271=CARTESIAN_POINT('Ctrl Pts',(81.5732563253708,-9.54823801654378,129.385657666451));
#77272=CARTESIAN_POINT('Ctrl Pts',(81.5771696907278,-9.53687630591745,129.386464827723));
#77273=CARTESIAN_POINT('Ctrl Pts',(81.5840276294898,-9.516243226196,129.387917987705));
#77274=CARTESIAN_POINT('Ctrl Pts',(81.5870145492163,-9.50698661424842,129.388565352295));
#77275=CARTESIAN_POINT('Ctrl Pts',(81.5932726818051,-9.48699495679227,129.389953920819));
#77276=CARTESIAN_POINT('Ctrl Pts',(81.5965168544273,-9.47625189804618,129.390694215873));
#77277=CARTESIAN_POINT('Ctrl Pts',(81.6052025035908,-9.44640288524095,129.392735409332));
#77278=CARTESIAN_POINT('Ctrl Pts',(81.6104113000333,-9.42723074879825,129.394028776547));
#77279=CARTESIAN_POINT('Ctrl Pts',(81.6415714534823,-9.30385811828331,129.40224810757));
#77280=CARTESIAN_POINT('Ctrl Pts',(81.6577413694293,-9.19744403187217,129.408846045515));
#77281=CARTESIAN_POINT('Ctrl Pts',(81.6694756847925,-8.98103396986609,129.422090064455));
#77282=CARTESIAN_POINT('Ctrl Pts',(81.6646339036772,-8.87156324183172,129.428709153294));
#77283=CARTESIAN_POINT('Ctrl Pts',(81.6470201250653,-8.7488084117633,129.436771650201));
#77284=CARTESIAN_POINT('Ctrl Pts',(81.6447374542312,-8.73427236363221,129.437736932729));
#77285=CARTESIAN_POINT('Ctrl Pts',(81.6410853627971,-8.71286968180983,129.439176362717));
#77286=CARTESIAN_POINT('Ctrl Pts',(81.6398646308326,-8.70597793321021,129.439642656321));
#77287=CARTESIAN_POINT('Ctrl Pts',(81.6376114368216,-8.69370802893159,129.44047814703));
#77288=CARTESIAN_POINT('Ctrl Pts',(81.6365958330058,-8.68832698657475,129.440846399267));
#77289=CARTESIAN_POINT('Ctrl Pts',(81.6342945821157,-8.67645557646187,129.441662960924));
#77290=CARTESIAN_POINT('Ctrl Pts',(81.6329968127525,-8.66996790930031,129.442111915263));
#77291=CARTESIAN_POINT('Ctrl Pts',(81.6290744137912,-8.65094918562685,129.443435648521));
#77292=CARTESIAN_POINT('Ctrl Pts',(81.6263440055483,-8.63844078303207,129.444315979006));
#77293=CARTESIAN_POINT('Ctrl Pts',(81.6197100478641,-8.60964656151575,129.446363090263));
#77294=CARTESIAN_POINT('Ctrl Pts',(81.6157045896166,-8.59338583630867,129.447534446949));
#77295=CARTESIAN_POINT('Ctrl Pts',(81.6010465372756,-8.53751976987163,129.451605685435));
#77296=CARTESIAN_POINT('Ctrl Pts',(81.5891775745634,-8.49825087460818,129.454548939693));
#77297=CARTESIAN_POINT('Ctrl Pts',(81.5358427326902,-8.34275946089723,129.466440042762));
#77298=CARTESIAN_POINT('Ctrl Pts',(81.4829659982357,-8.23084681331225,129.475503008274));
#77299=CARTESIAN_POINT('Ctrl Pts',(81.3937203127852,-8.0860644898412,129.487488889464));
#77300=CARTESIAN_POINT('Ctrl Pts',(81.3675685043992,-8.04737649300279,129.490725641308));
#77301=CARTESIAN_POINT('Ctrl Pts',(81.3303695542058,-7.9970414275945,129.494985033702));
#77302=CARTESIAN_POINT('Ctrl Pts',(81.3207321185703,-7.98438405380397,129.496060508078));
#77303=CARTESIAN_POINT('Ctrl Pts',(81.3045140640033,-7.96370533916564,129.497825438851));
#77304=CARTESIAN_POINT('Ctrl Pts',(81.298037363818,-7.95560420443892,129.498518929313));
#77305=CARTESIAN_POINT('Ctrl Pts',(81.2852030999192,-7.9398547793325,129.499871453844));
#77306=CARTESIAN_POINT('Ctrl Pts',(81.278851880996,-7.93220190545565,129.500530702896));
#77307=CARTESIAN_POINT('Ctrl Pts',(81.2635644684063,-7.91411346252924,129.502094122966));
#77308=CARTESIAN_POINT('Ctrl Pts',(81.2545668775261,-7.90373055019752,129.502995741496));
#77309=CARTESIAN_POINT('Ctrl Pts',(81.2230440369481,-7.86825071776,129.506092836269));
#77310=CARTESIAN_POINT('Ctrl Pts',(81.1998850866693,-7.8437261650007,129.50826188435));
#77311=CARTESIAN_POINT('Ctrl Pts',(81.1407295831974,-7.78477536566424,129.513568249281));
#77312=CARTESIAN_POINT('Ctrl Pts',(81.1039034746794,-7.7512275759412,129.516671347967));
#77313=CARTESIAN_POINT('Ctrl Pts',(81.0147299416358,-7.67702475430291,129.523826243238));
#77314=CARTESIAN_POINT('Ctrl Pts',(80.9613524648524,-7.63774380970178,129.527845788089));
#77315=CARTESIAN_POINT('Ctrl Pts',(80.8995878948306,-7.59773325471521,129.532351577536));
#77316=CARTESIAN_POINT('Ctrl Pts',(80.8933707509953,-7.59376420688563,129.532803598771));
#77317=CARTESIAN_POINT('Ctrl Pts',(80.8215182851377,-7.54856214254918,129.538012374849));
#77318=CARTESIAN_POINT('Ctrl Pts',(80.7531168654114,-7.51192205848376,129.542822035831));
#77319=CARTESIAN_POINT('Ctrl Pts',(80.6718314202186,-7.47542354097248,129.548650215978));
#77320=CARTESIAN_POINT('Ctrl Pts',(80.6611892936752,-7.47077812728171,129.549415434918));
#77321=CARTESIAN_POINT('Ctrl Pts',(80.6445756303972,-7.46373190289868,129.550614723483));
#77322=CARTESIAN_POINT('Ctrl Pts',(80.6386370294827,-7.46125370818591,129.551044334992));
#77323=CARTESIAN_POINT('Ctrl Pts',(80.6276137023138,-7.45672844739292,129.551843758788));
#77324=CARTESIAN_POINT('Ctrl Pts',(80.6225330520719,-7.45467199587074,129.552213006875));
#77325=CARTESIAN_POINT('Ctrl Pts',(80.6107467266368,-7.44996890161242,129.553071395728));
#77326=CARTESIAN_POINT('Ctrl Pts',(80.6040339591825,-7.44734068727761,129.553561593192));
#77327=CARTESIAN_POINT('Ctrl Pts',(80.5824443388883,-7.43904901152836,129.555141884271));
#77328=CARTESIAN_POINT('Ctrl Pts',(80.5675038080964,-7.43355537033496,129.556241114139));
#77329=CARTESIAN_POINT('Ctrl Pts',(80.4837467766038,-7.40411334087662,129.562425890288));
#77330=CARTESIAN_POINT('Ctrl Pts',(80.4135013021998,-7.38448776983677,129.567693500649));
#77331=CARTESIAN_POINT('Ctrl Pts',(80.2093058802686,-7.34163116108932,129.582866015755));
#77332=CARTESIAN_POINT('Ctrl Pts',(80.0734667500323,-7.3300860907803,129.592743571448));
#77333=CARTESIAN_POINT('Ctrl Pts',(79.9140801323266,-7.33604890318619,129.603724393727));
#77334=CARTESIAN_POINT('Ctrl Pts',(79.8904639400111,-7.3374364891958,129.605337553233));
#77335=CARTESIAN_POINT('Ctrl Pts',(79.8547895173569,-7.34029606937242,129.607754563777));
#77336=CARTESIAN_POINT('Ctrl Pts',(79.8427055028622,-7.34139767385291,129.608569839626));
#77337=CARTESIAN_POINT('Ctrl Pts',(79.8209688406627,-7.34361893242463,129.610030476796));
#77338=CARTESIAN_POINT('Ctrl Pts',(79.8113120165988,-7.34469119230794,129.61067729217));
#77339=CARTESIAN_POINT('Ctrl Pts',(79.7906497720514,-7.34716862309817,129.61205700983));
#77340=CARTESIAN_POINT('Ctrl Pts',(79.7796478468959,-7.34859937717827,129.612789075835));
#77341=CARTESIAN_POINT('Ctrl Pts',(79.7495184947372,-7.35282403856453,129.614787336265));
#77342=CARTESIAN_POINT('Ctrl Pts',(79.7304237325863,-7.35584115154222,129.616046485166));
#77343=CARTESIAN_POINT('Ctrl Pts',(79.594608376844,-7.37973077332341,129.624959911134));
#77344=CARTESIAN_POINT('Ctrl Pts',(79.4803543478131,-7.41267907807416,129.632201026817));
#77345=CARTESIAN_POINT('Ctrl Pts',(79.2790812601726,-7.49481130831862,129.645474050551));
#77346=CARTESIAN_POINT('Ctrl Pts',(79.1911208241831,-7.54019656438399,129.651491358508));
#77347=CARTESIAN_POINT('Ctrl Pts',(79.0947278034089,-7.60133112420974,129.658902404308));
#77348=CARTESIAN_POINT('Ctrl Pts',(79.0818595543526,-7.60974446418748,129.659910003334));
#77349=CARTESIAN_POINT('Ctrl Pts',(79.0632768808135,-7.62226444085727,129.661394741468));
#77350=CARTESIAN_POINT('Ctrl Pts',(79.057468692785,-7.62623138651246,129.661863114736));
#77351=CARTESIAN_POINT('Ctrl Pts',(79.04734102478,-7.63324296103815,129.662687713331));
#77352=CARTESIAN_POINT('Ctrl Pts',(79.0430106498823,-7.63627154124793,129.663042863947));
#77353=CARTESIAN_POINT('Ctrl Pts',(79.038631193083,-7.6393655806482,129.663404695187));
#77354=CARTESIAN_POINT('Ctrl Pts',(79.0385677336052,-7.63941042074669,129.663409938779));
#77355=CARTESIAN_POINT('Ctrl Pts',(79.0384037054441,-7.6395263392985,129.663423493717));
#77356=CARTESIAN_POINT('Ctrl Pts',(79.0383031414642,-7.63959742449208,129.663431805524));
#77357=CARTESIAN_POINT('Ctrl Pts',(79.0381073036602,-7.63973588801838,129.66344799465));
#77358=CARTESIAN_POINT('Ctrl Pts',(79.0380120290431,-7.6398032652035,129.66345587189));
#77359=CARTESIAN_POINT('Ctrl Pts',(79.0378262514459,-7.63993467440556,129.663471234329));
#77360=CARTESIAN_POINT('Ctrl Pts',(79.0377357477108,-7.6399987054943,129.663478719467));
#77361=CARTESIAN_POINT('Ctrl Pts',(79.0375590601058,-7.64012373784807,129.663493334703));
#77362=CARTESIAN_POINT('Ctrl Pts',(79.0374728757355,-7.64018473820744,129.663500464735));
#77363=CARTESIAN_POINT('Ctrl Pts',(79.0373044317979,-7.6403039850307,129.66351440213));
#77364=CARTESIAN_POINT('Ctrl Pts',(79.0372221716709,-7.64036223079924,129.663521209448));
#77365=CARTESIAN_POINT('Ctrl Pts',(79.0370612283736,-7.64047621153728,129.663534529926));
#77366=CARTESIAN_POINT('Ctrl Pts',(79.0369825447501,-7.64053194587682,129.663541043045));
#77367=CARTESIAN_POINT('Ctrl Pts',(79.0368284467748,-7.6406411189091,129.663553800361));
#77368=CARTESIAN_POINT('Ctrl Pts',(79.036753032093,-7.6406945570031,129.663560044514));
#77369=CARTESIAN_POINT('Ctrl Pts',(79.0366051991417,-7.6407993284438,129.663572286284));
#77370=CARTESIAN_POINT('Ctrl Pts',(79.036532780421,-7.64085066137814,129.663578283876));
#77371=CARTESIAN_POINT('Ctrl Pts',(79.0363906955298,-7.64095139320473,129.663590052536));
#77372=CARTESIAN_POINT('Ctrl Pts',(79.036321029128,-7.64100079161436,129.663595823569));
#77373=CARTESIAN_POINT('Ctrl Pts',(79.0361842307604,-7.64109780714756,129.66360715702));
#77374=CARTESIAN_POINT('Ctrl Pts',(79.0361170985661,-7.64114542385967,129.663612719407));
#77375=CARTESIAN_POINT('Ctrl Pts',(79.0359851727473,-7.64123901323716,129.663623651653));
#77376=CARTESIAN_POINT('Ctrl Pts',(79.0359203788248,-7.64128498560353,129.663629021493));
#77377=CARTESIAN_POINT('Ctrl Pts',(79.0357929526966,-7.64137541026624,129.663639583173));
#77378=CARTESIAN_POINT('Ctrl Pts',(79.0357303202857,-7.64141986225229,129.663644774991));
#77379=CARTESIAN_POINT('Ctrl Pts',(79.035607057197,-7.64150735835607,129.663654993776));
#77380=CARTESIAN_POINT('Ctrl Pts',(79.0355464263586,-7.64155040217933,129.663660020722));
#77381=CARTESIAN_POINT('Ctrl Pts',(79.0354270213497,-7.6416351837396,129.663669921687));
#77382=CARTESIAN_POINT('Ctrl Pts',(79.0353682469778,-7.64167692125265,129.663674795693));
#77383=CARTESIAN_POINT('Ctrl Pts',(79.0352524227304,-7.6417591829689,129.663684401647));
#77384=CARTESIAN_POINT('Ctrl Pts',(79.0351953726902,-7.6417997069583,129.663689133582));
#77385=CARTESIAN_POINT('Ctrl Pts',(79.0350828765919,-7.64187962625542,129.663698465307));
#77386=CARTESIAN_POINT('Ctrl Pts',(79.0350274303308,-7.64191902140844,129.66370306509));
#77387=CARTESIAN_POINT('Ctrl Pts',(79.0349180313275,-7.64199676063556,129.663712141603));
#77388=CARTESIAN_POINT('Ctrl Pts',(79.0348640784739,-7.6420351045181,129.663716618319));
#77389=CARTESIAN_POINT('Ctrl Pts',(79.0347575647386,-7.64211081257364,129.663725457055));
#77390=CARTESIAN_POINT('Ctrl Pts',(79.0347050038745,-7.64214817648842,129.663729819053));
#77391=CARTESIAN_POINT('Ctrl Pts',(79.0346011812592,-7.64222198989296,129.663738435999));
#77392=CARTESIAN_POINT('Ctrl Pts',(79.0345499192983,-7.64225843930835,129.663742690946));
#77393=CARTESIAN_POINT('Ctrl Pts',(79.0344486084306,-7.64233048424501,129.663751100877));
#77394=CARTESIAN_POINT('Ctrl Pts',(79.034398559412,-7.64236607964214,129.663755255853));
#77395=CARTESIAN_POINT('Ctrl Pts',(79.034299594889,-7.64243647250967,129.663763472395));
#77396=CARTESIAN_POINT('Ctrl Pts',(79.0342506793253,-7.64247126983627,129.66376753395));
#77397=CARTESIAN_POINT('Ctrl Pts',(79.0341539082047,-7.64254011830429,129.663775569707));
#77398=CARTESIAN_POINT('Ctrl Pts',(79.0341060525173,-7.64257416936841,129.663779543906));
#77399=CARTESIAN_POINT('Ctrl Pts',(79.034011332843,-7.64264157341076,129.66378741058));
#77400=CARTESIAN_POINT('Ctrl Pts',(79.0339644687292,-7.64267492632344,129.663791303053));
#77401=CARTESIAN_POINT('Ctrl Pts',(79.0338716684268,-7.64274097899074,129.663799011534));
#77402=CARTESIAN_POINT('Ctrl Pts',(79.0338257322336,-7.64277367860572,129.663802827531));
#77403=CARTESIAN_POINT('Ctrl Pts',(79.0337347285458,-7.64283846641518,129.663810387944));
#77404=CARTESIAN_POINT('Ctrl Pts',(79.0336896609904,-7.64287055452182,129.663814132354));
#77405=CARTESIAN_POINT('Ctrl Pts',(79.0336003391557,-7.64293415838738,129.663821554167));
#77406=CARTESIAN_POINT('Ctrl Pts',(79.0335560848077,-7.64296567407474,129.663825231565));
#77407=CARTESIAN_POINT('Ctrl Pts',(79.0334683376524,-7.64302816958831,129.663832523621));
#77408=CARTESIAN_POINT('Ctrl Pts',(79.0334248447051,-7.64305914940331,129.663836138282));
#77409=CARTESIAN_POINT('Ctrl Pts',(79.0333385715155,-7.64312060762961,129.663843308896));
#77410=CARTESIAN_POINT('Ctrl Pts',(79.0332957912819,-7.64315108593262,129.66384686484));
#77411=CARTESIAN_POINT('Ctrl Pts',(79.0332108974944,-7.64321157362305,129.663853921819));
#77412=CARTESIAN_POINT('Ctrl Pts',(79.0331687840547,-7.6432415828351,129.663857422837));
#77413=CARTESIAN_POINT('Ctrl Pts',(79.0330851814234,-7.64330116230142,129.66386437347));
#77414=CARTESIAN_POINT('Ctrl Pts',(79.0330436919574,-7.64333073266457,129.6638678231));
#77415=CARTESIAN_POINT('Ctrl Pts',(79.0329612958847,-7.64338946367549,129.663874674375));
#77416=CARTESIAN_POINT('Ctrl Pts',(79.0329203894405,-7.64341862412765,129.663878076001));
#77417=CARTESIAN_POINT('Ctrl Pts',(79.0328391216176,-7.64347656202198,129.663884834391));
#77418=CARTESIAN_POINT('Ctrl Pts',(79.0327987599985,-7.64350533956201,129.663888191169));
#77419=CARTESIAN_POINT('Ctrl Pts',(79.0327185448268,-7.64356253779469,129.663894862922));
#77420=CARTESIAN_POINT('Ctrl Pts',(79.0326786914107,-7.64359095832226,129.663898177881));
#77421=CARTESIAN_POINT('Ctrl Pts',(79.0325994583428,-7.64364746679155,129.663904768832));
#77422=CARTESIAN_POINT('Ctrl Pts',(79.0325600786426,-7.64367555470543,129.663908044823));
#77423=CARTESIAN_POINT('Ctrl Pts',(79.0324817599268,-7.64373142135731,129.663914560576));
#77424=CARTESIAN_POINT('Ctrl Pts',(79.0324428209724,-7.64375919999428,129.663917800328));
#77425=CARTESIAN_POINT('Ctrl Pts',(79.0265053569533,-7.6479953096944,129.664411834297));
#77426=CARTESIAN_POINT('Ctrl Pts',(79.0206344838947,-7.65224197882215,129.664905186614));
#77427=CARTESIAN_POINT('Ctrl Pts',(79.0078784053937,-7.66159638528165,129.665987455159));
#77428=CARTESIAN_POINT('Ctrl Pts',(79.0010045819552,-7.66671921875005,129.666577306224));
#77429=CARTESIAN_POINT('Ctrl Pts',(78.9186701944317,-7.7290744669457,129.673720143616));
#77430=CARTESIAN_POINT('Ctrl Pts',(78.8481909104483,-7.79258213981179,129.680615370289));
#77431=CARTESIAN_POINT('Ctrl Pts',(78.7005474443368,-7.95037244048865,129.696345603662));
#77432=CARTESIAN_POINT('Ctrl Pts',(78.6275229733317,-8.04783825080116,129.705113144021));
#77433=CARTESIAN_POINT('Ctrl Pts',(78.555065254074,-8.17044627079254,129.714909670994));
#77434=CARTESIAN_POINT('Ctrl Pts',(78.5447370037935,-8.18870135529724,129.716340242617));
#77435=CARTESIAN_POINT('Ctrl Pts',(78.5287781334731,-8.2181944043214,129.71860800874));
#77436=CARTESIAN_POINT('Ctrl Pts',(78.5229254807155,-8.22930897925426,129.719452982495));
#77437=CARTESIAN_POINT('Ctrl Pts',(78.5127348142947,-8.24920431973421,129.720948788938));
#77438=CARTESIAN_POINT('Ctrl Pts',(78.5083475285705,-8.25795903237727,129.721601327405));
#77439=CARTESIAN_POINT('Ctrl Pts',(78.4993114788223,-8.27639425773511,129.722963808336));
#77440=CARTESIAN_POINT('Ctrl Pts',(78.4946785956039,-8.28608208706773,129.723673175715));
#77441=CARTESIAN_POINT('Ctrl Pts',(78.4826844209806,-8.31179906385109,129.72553929064));
#77442=CARTESIAN_POINT('Ctrl Pts',(78.4754833271746,-8.32790175732582,129.726690524951));
#77443=CARTESIAN_POINT('Ctrl Pts',(78.4571826872773,-8.37063298275656,129.72970300732));
#77444=CARTESIAN_POINT('Ctrl Pts',(78.4465195527456,-8.39743395206965,129.731549510502));
#77445=CARTESIAN_POINT('Ctrl Pts',(78.4365593938057,-8.42449198884581,129.733376828424));
#77446=CARTESIAN_POINT('Origin',(80.,-9.,134.));
#77447=CARTESIAN_POINT('',(78.4345148344113,-8.42372400280583,130.432124665727));
#77448=CARTESIAN_POINT('',(78.4365593712355,-8.42449205016053,130.240113128671));
#77449=CARTESIAN_POINT('',(78.4365593749993,-8.42449203993574,134.));
#77450=CARTESIAN_POINT('Ctrl Pts',(78.4365593712355,-8.42449205016054,130.240113128671));
#77451=CARTESIAN_POINT('Ctrl Pts',(78.4562489674097,-8.37100275495381,130.236594916316));
#77452=CARTESIAN_POINT('Ctrl Pts',(78.4786723687427,-8.3185543893542,130.233028078192));
#77453=CARTESIAN_POINT('Ctrl Pts',(78.5107180139043,-8.25310858487162,130.2283009661));
#77454=CARTESIAN_POINT('Ctrl Pts',(78.5178965700835,-8.23896320842644,130.227262057371));
#77455=CARTESIAN_POINT('Ctrl Pts',(78.5286264146443,-8.21854773312112,130.225734315427));
#77456=CARTESIAN_POINT('Ctrl Pts',(78.5320183854576,-8.21219428303662,130.22525482372));
#77457=CARTESIAN_POINT('Ctrl Pts',(78.5380414429338,-8.20108654908569,130.22440904851));
#77458=CARTESIAN_POINT('Ctrl Pts',(78.5406547529564,-8.19632284260615,130.224043878242));
#77459=CARTESIAN_POINT('Ctrl Pts',(78.54640817077,-8.18595574479711,130.223243721417));
#77460=CARTESIAN_POINT('Ctrl Pts',(78.5495573437357,-8.18035778973985,130.222808190793));
#77461=CARTESIAN_POINT('Ctrl Pts',(78.5584637423665,-8.16473788328814,130.221583495256));
#77462=CARTESIAN_POINT('Ctrl Pts',(78.5642928754636,-8.15475765626252,130.220790030511));
#77463=CARTESIAN_POINT('Ctrl Pts',(78.6059234670989,-8.08515393390818,130.215183224136));
#77464=CARTESIAN_POINT('Ctrl Pts',(78.6453202268297,-8.02776893801363,130.210184040967));
#77465=CARTESIAN_POINT('Ctrl Pts',(78.6998429395048,-7.95812404811907,130.203765394012));
#77466=CARTESIAN_POINT('Ctrl Pts',(78.7117572784247,-7.94342791983462,130.202389324106));
#77467=CARTESIAN_POINT('Ctrl Pts',(78.7712000470168,-7.87260683263331,130.195659711576));
#77468=CARTESIAN_POINT('Ctrl Pts',(78.8221620006092,-7.81946468673388,130.190306651402));
#77469=CARTESIAN_POINT('Ctrl Pts',(78.9246253009635,-7.7258813575024,130.180402885944));
#77470=CARTESIAN_POINT('Ctrl Pts',(78.9753245989724,-7.68476188212218,130.175837625116));
#77471=CARTESIAN_POINT('Ctrl Pts',(79.0422169721025,-7.63673159185644,130.170222167182));
#77472=CARTESIAN_POINT('Ctrl Pts',(79.0562766590351,-7.62696126242622,130.169062960979));
#77473=CARTESIAN_POINT('Ctrl Pts',(79.0780706460221,-7.61230917767639,130.167297435918));
#77474=CARTESIAN_POINT('Ctrl Pts',(79.0856983464037,-7.60727172640133,130.166685282373));
#77475=CARTESIAN_POINT('Ctrl Pts',(79.101525269002,-7.5970054476837,130.165426768109));
#77476=CARTESIAN_POINT('Ctrl Pts',(79.109729602413,-7.59178510798048,130.164780740794));
#77477=CARTESIAN_POINT('Ctrl Pts',(79.1282824555546,-7.58020705066821,130.163333799139));
#77478=CARTESIAN_POINT('Ctrl Pts',(79.1386558078989,-7.57389001404572,130.162534402935));
#77479=CARTESIAN_POINT('Ctrl Pts',(79.1694559694582,-7.55559238631713,130.160188241922));
#77480=CARTESIAN_POINT('Ctrl Pts',(79.1900707086901,-7.54393290856342,130.158653033531));
#77481=CARTESIAN_POINT('Ctrl Pts',(79.302175072845,-7.48364570286396,130.150476769271));
#77482=CARTESIAN_POINT('Ctrl Pts',(79.3978041221713,-7.44319125698328,130.144126799862));
#77483=CARTESIAN_POINT('Ctrl Pts',(79.5714126844545,-7.38815902626617,130.133004543948));
#77484=CARTESIAN_POINT('Ctrl Pts',(79.6478218321723,-7.36975853676477,130.128231134946));
#77485=CARTESIAN_POINT('Ctrl Pts',(79.7495424799942,-7.35274947236639,130.121726987987));
#77486=CARTESIAN_POINT('Ctrl Pts',(79.773933799732,-7.34922526822217,130.120155954105));
#77487=CARTESIAN_POINT('Ctrl Pts',(79.8154182317847,-7.34416796195394,130.117451122044));
#77488=CARTESIAN_POINT('Ctrl Pts',(79.8324737224539,-7.34235556960559,130.116329723554));
#77489=CARTESIAN_POINT('Ctrl Pts',(79.8569518546057,-7.34013602473691,130.114702977381));
#77490=CARTESIAN_POINT('Ctrl Pts',(79.8643546127382,-7.33951467577272,130.114208748101));
#77491=CARTESIAN_POINT('Ctrl Pts',(79.8772524414581,-7.33851892234612,130.113343325437));
#77492=CARTESIAN_POINT('Ctrl Pts',(79.8827456069124,-7.33812222446614,130.112973368173));
#77493=CARTESIAN_POINT('Ctrl Pts',(79.8945297572386,-7.33732993115931,130.112176652894));
#77494=CARTESIAN_POINT('Ctrl Pts',(79.9008209460103,-7.33694280258446,130.111749468479));
#77495=CARTESIAN_POINT('Ctrl Pts',(79.9181195111698,-7.33597683807036,130.110570073436));
#77496=CARTESIAN_POINT('Ctrl Pts',(79.9291304381353,-7.33547154219307,130.109814037617));
#77497=CARTESIAN_POINT('Ctrl Pts',(79.9922258798403,-7.33320323179177,130.105454305496));
#77498=CARTESIAN_POINT('Ctrl Pts',(80.0443606165131,-7.33377584956241,130.10174559877));
#77499=CARTESIAN_POINT('Ctrl Pts',(80.1986023738523,-7.3427135963045,130.090608413702));
#77500=CARTESIAN_POINT('Ctrl Pts',(80.3000714787427,-7.35804993281389,130.083081385085));
#77501=CARTESIAN_POINT('Ctrl Pts',(80.4701068503262,-7.40004793807312,130.070526767085));
#77502=CARTESIAN_POINT('Ctrl Pts',(80.5395138421777,-7.42209807379113,130.065415467588));
#77503=CARTESIAN_POINT('Ctrl Pts',(80.6236694280322,-7.45503956353026,130.059248047805));
#77504=CARTESIAN_POINT('Ctrl Pts',(80.6399706537873,-7.46172047098607,130.058054549339));
#77505=CARTESIAN_POINT('Ctrl Pts',(80.6660298674103,-7.4728865674394,130.056147801498));
#77506=CARTESIAN_POINT('Ctrl Pts',(80.675855429789,-7.47720957858888,130.055429137591));
#77507=CARTESIAN_POINT('Ctrl Pts',(80.6945653749809,-7.48565827062489,130.054060908962));
#77508=CARTESIAN_POINT('Ctrl Pts',(80.7034564604505,-7.48976791562052,130.053410830928));
#77509=CARTESIAN_POINT('Ctrl Pts',(80.7236761314824,-7.49933117622764,130.051932427284));
#77510=CARTESIAN_POINT('Ctrl Pts',(80.7349803515376,-7.50483513979877,130.051105877068));
#77511=CARTESIAN_POINT('Ctrl Pts',(80.7650064928709,-7.51987753605714,130.048909509002));
#77512=CARTESIAN_POINT('Ctrl Pts',(80.7836124663331,-7.5296432377673,130.047547591853));
#77513=CARTESIAN_POINT('Ctrl Pts',(80.9078369461697,-7.59787284045522,130.038436056632));
#77514=CARTESIAN_POINT('Ctrl Pts',(81.0070169636583,-7.66731505112715,130.031103578709));
#77515=CARTESIAN_POINT('Ctrl Pts',(81.1477032665413,-7.79056635603684,130.019674552662));
#77516=CARTESIAN_POINT('Ctrl Pts',(81.1949209082573,-7.83719507999336,130.015611970953));
#77517=CARTESIAN_POINT('Ctrl Pts',(81.2542447687083,-7.90321804288564,130.009994306451));
#77518=CARTESIAN_POINT('Ctrl Pts',(81.2689181879826,-7.92022820337079,130.00855770085));
#77519=CARTESIAN_POINT('Ctrl Pts',(81.2934513075985,-7.94985907261235,130.006062863773));
#77520=CARTESIAN_POINT('Ctrl Pts',(81.3034814413055,-7.96233515116671,130.005014641894));
#77521=CARTESIAN_POINT('Ctrl Pts',(81.3177775368196,-7.98065186508941,130.003475666234));
#77522=CARTESIAN_POINT('Ctrl Pts',(81.3221880394496,-7.98637924241827,130.002994445667));
#77523=CARTESIAN_POINT('Ctrl Pts',(81.3298504479927,-7.99646457391867,130.002146696995));
#77524=CARTESIAN_POINT('Ctrl Pts',(81.3331185044392,-8.00081001940362,130.001781298783));
#77525=CARTESIAN_POINT('Ctrl Pts',(81.3401922272381,-8.01031223782528,130.000981901113));
#77526=CARTESIAN_POINT('Ctrl Pts',(81.3439893690652,-8.01547491401748,130.00054736898));
#77527=CARTESIAN_POINT('Ctrl Pts',(81.3545090794997,-8.02995200871444,129.999328574087));
#77528=CARTESIAN_POINT('Ctrl Pts',(81.3611650884005,-8.03931402857036,129.998540078512));
#77529=CARTESIAN_POINT('Ctrl Pts',(81.4054685847778,-8.1030139381261,129.993176928803));
#77530=CARTESIAN_POINT('Ctrl Pts',(81.439946061721,-8.15947675384267,129.988434194037));
#77531=CARTESIAN_POINT('Ctrl Pts',(81.4813324729098,-8.23730949777258,129.982043702622));
#77532=CARTESIAN_POINT('Ctrl Pts',(81.4913019513496,-8.25699181158267,129.980439347805));
#77533=CARTESIAN_POINT('Ctrl Pts',(81.5315342487989,-8.34049467232167,129.973693641993));
#77534=CARTESIAN_POINT('Ctrl Pts',(81.5581154647473,-8.40601201963876,129.968551867066));
#77535=CARTESIAN_POINT('Ctrl Pts',(81.6019915139492,-8.53760052806315,129.958635381771));
#77536=CARTESIAN_POINT('Ctrl Pts',(81.6195482075004,-8.60344501003612,129.953863125404));
#77537=CARTESIAN_POINT('Ctrl Pts',(81.6364567550507,-8.68716568887623,129.948037086216));
#77538=CARTESIAN_POINT('Ctrl Pts',(81.6396208598089,-8.70419686821001,129.946863960421));
#77539=CARTESIAN_POINT('Ctrl Pts',(81.6443043490202,-8.73179653056876,129.944981636755));
#77540=CARTESIAN_POINT('Ctrl Pts',(81.6459887029334,-8.74233531052925,129.944267274214));
#77541=CARTESIAN_POINT('Ctrl Pts',(81.6490275276901,-8.76259623442835,129.942902065167));
#77542=CARTESIAN_POINT('Ctrl Pts',(81.6503975686912,-8.77231555328744,129.942250753972));
#77543=CARTESIAN_POINT('Ctrl Pts',(81.6533440220763,-8.79464419258868,129.940762403013));
#77544=CARTESIAN_POINT('Ctrl Pts',(81.6548622395854,-8.80726067908265,129.939927222597));
#77545=CARTESIAN_POINT('Ctrl Pts',(81.6592931853532,-8.84800710326969,129.937247506579));
#77546=CARTESIAN_POINT('Ctrl Pts',(81.6616342006517,-8.8761951142858,129.935420781766));
#77547=CARTESIAN_POINT('Ctrl Pts',(81.6707675273531,-9.03514811038791,129.92524571895));
#77548=CARTESIAN_POINT('Ctrl Pts',(81.6628435021933,-9.16629323540851,129.917373557133));
#77549=CARTESIAN_POINT('Ctrl Pts',(81.6270065293568,-9.36536842599655,129.904962964013));
#77550=CARTESIAN_POINT('Ctrl Pts',(81.6098741333425,-9.43468066079452,129.900540853335));
#77551=CARTESIAN_POINT('Ctrl Pts',(81.5835972696578,-9.51771079301962,129.8948904473));
#77552=CARTESIAN_POINT('Ctrl Pts',(81.5786251621711,-9.5326793883301,129.893857296503));
#77553=CARTESIAN_POINT('Ctrl Pts',(81.5710795984695,-9.55436137685456,129.892336480976));
#77554=CARTESIAN_POINT('Ctrl Pts',(81.5686738463451,-9.56113278278878,129.891858038952));
#77555=CARTESIAN_POINT('Ctrl Pts',(81.5643731923813,-9.57299390013294,129.891013494545));
#77556=CARTESIAN_POINT('Ctrl Pts',(81.5624970978877,-9.57809022867613,129.890648495646));
#77557=CARTESIAN_POINT('Ctrl Pts',(81.558345404965,-9.58920025362453,129.889848050222));
#77558=CARTESIAN_POINT('Ctrl Pts',(81.556059938379,-9.59520988291922,129.889412053678));
#77559=CARTESIAN_POINT('Ctrl Pts',(81.5495543095432,-9.61202284606181,129.888184092584));
#77560=CARTESIAN_POINT('Ctrl Pts',(81.5452561288073,-9.62279531141073,129.887387787092));
#77561=CARTESIAN_POINT('Ctrl Pts',(81.5123599439697,-9.70280513425765,129.881406707882));
#77562=CARTESIAN_POINT('Ctrl Pts',(81.4792364637049,-9.77008090094177,129.87600647646));
#77563=CARTESIAN_POINT('Ctrl Pts',(81.4365724877883,-9.84375373036876,129.869820280643));
#77564=CARTESIAN_POINT('Ctrl Pts',(81.4313589715068,-9.85256809889896,129.869075423762));
#77565=CARTESIAN_POINT('Ctrl Pts',(81.3984151400417,-9.90711144748691,129.864438456259));
#77566=CARTESIAN_POINT('Ctrl Pts',(81.3685767550498,-9.95153247332523,129.860540925779));
#77567=CARTESIAN_POINT('Ctrl Pts',(81.285101803817,-10.0637330909048,129.850450789761));
#77568=CARTESIAN_POINT('Ctrl Pts',(81.2282345042584,-10.1289193882629,129.844341959158));
#77569=CARTESIAN_POINT('Ctrl Pts',(81.1535026628115,-10.2022154777481,129.837190979985));
#77570=CARTESIAN_POINT('Ctrl Pts',(81.140235942271,-10.2148055360057,129.835950952778));
#77571=CARTESIAN_POINT('Ctrl Pts',(81.1187545223984,-10.2345292857427,129.833988588503));
#77572=CARTESIAN_POINT('Ctrl Pts',(81.1106729435498,-10.2418050816921,129.833260246867));
#77573=CARTESIAN_POINT('Ctrl Pts',(81.0952084443737,-10.2554559296427,129.831884923769));
#77574=CARTESIAN_POINT('Ctrl Pts',(81.0878396792485,-10.2618462533395,129.831237321222));
#77575=CARTESIAN_POINT('Ctrl Pts',(81.0709033206699,-10.2762751343051,129.82976609731));
#77576=CARTESIAN_POINT('Ctrl Pts',(81.0613004804071,-10.2842715620653,129.828944221658));
#77577=CARTESIAN_POINT('Ctrl Pts',(81.0358744784454,-10.3049642077827,129.826799254864));
#77578=CARTESIAN_POINT('Ctrl Pts',(81.0199075182236,-10.3174810169984,129.825483298234));
#77579=CARTESIAN_POINT('Ctrl Pts',(80.8821314384003,-10.4214801146542,129.814374562119));
#77580=CARTESIAN_POINT('Ctrl Pts',(80.7485423448441,-10.4961441767399,129.805297172332));
#77581=CARTESIAN_POINT('Ctrl Pts',(80.550173775588,-10.5737038009776,129.792162596528));
#77582=CARTESIAN_POINT('Ctrl Pts',(80.4925264962668,-10.5926866937094,129.788370789343));
#77583=CARTESIAN_POINT('Ctrl Pts',(80.4198457033443,-10.6122964668454,129.783476238388));
#77584=CARTESIAN_POINT('Ctrl Pts',(80.4056626676359,-10.615923288962,129.782515797768));
#77585=CARTESIAN_POINT('Ctrl Pts',(80.3846560582215,-10.6210010319848,129.78108295452));
#77586=CARTESIAN_POINT('Ctrl Pts',(80.3778677649744,-10.6225968620248,129.780618348246));
#77587=CARTESIAN_POINT('Ctrl Pts',(80.3662539665188,-10.6252502683978,129.779820459057));
#77588=CARTESIAN_POINT('Ctrl Pts',(80.3614334607402,-10.6263290735062,129.779488387));
#77589=CARTESIAN_POINT('Ctrl Pts',(80.3503725239455,-10.6287528493538,129.778724314905));
#77590=CARTESIAN_POINT('Ctrl Pts',(80.3441292484284,-10.6300833741772,129.778291529286));
#77591=CARTESIAN_POINT('Ctrl Pts',(80.3267383617414,-10.6336852425491,129.777082082871));
#77592=CARTESIAN_POINT('Ctrl Pts',(80.3155751473921,-10.635878277052,129.776301286539));
#77593=CARTESIAN_POINT('Ctrl Pts',(80.2469302582341,-10.6486349439905,129.771476303066));
#77594=CARTESIAN_POINT('Ctrl Pts',(80.1889535691919,-10.6562810178661,129.767300688954));
#77595=CARTESIAN_POINT('Ctrl Pts',(79.9813673613194,-10.6726170396098,129.752245137594));
#77596=CARTESIAN_POINT('Ctrl Pts',(79.8310928637872,-10.6641759328561,129.741233574809));
#77597=CARTESIAN_POINT('Ctrl Pts',(79.6555558801329,-10.6302611308564,129.728852681626));
#77598=CARTESIAN_POINT('Ctrl Pts',(79.6272948034205,-10.6240332890535,129.726871439424));
#77599=CARTESIAN_POINT('Ctrl Pts',(79.58662838514,-10.6139541177168,129.724036402142));
#77600=CARTESIAN_POINT('Ctrl Pts',(79.5740846003788,-10.6106893166929,129.723164111496));
#77601=CARTESIAN_POINT('Ctrl Pts',(79.5521038005499,-10.60469357567,129.721639071754));
#77602=CARTESIAN_POINT('Ctrl Pts',(79.5426505969199,-10.6020249710547,129.720984348335));
#77603=CARTESIAN_POINT('Ctrl Pts',(79.5229870827171,-10.5962857952125,129.719624616609));
#77604=CARTESIAN_POINT('Ctrl Pts',(79.5127815089568,-10.5932004940225,129.718920120408));
#77605=CARTESIAN_POINT('Ctrl Pts',(79.4861318556273,-10.5848638704819,129.717083220198));
#77606=CARTESIAN_POINT('Ctrl Pts',(79.4697382693343,-10.5794544916105,129.715956007674));
#77607=CARTESIAN_POINT('Ctrl Pts',(79.3965460899949,-10.5540352598911,129.710931718787));
#77608=CARTESIAN_POINT('Ctrl Pts',(79.3407701251768,-10.5312084679691,129.707127905271));
#77609=CARTESIAN_POINT('Ctrl Pts',(79.1920039237619,-10.4606845608547,129.696895632408));
#77610=CARTESIAN_POINT('Ctrl Pts',(79.1020761755456,-10.4071920085322,129.690622684558));
#77611=CARTESIAN_POINT('Ctrl Pts',(78.9832026449799,-10.3204197492197,129.681531252842));
#77612=CARTESIAN_POINT('Ctrl Pts',(78.949644131555,-10.2938845495352,129.678860827546));
#77613=CARTESIAN_POINT('Ctrl Pts',(78.904070107656,-10.2549062598838,129.67502759815));
#77614=CARTESIAN_POINT('Ctrl Pts',(78.89116877281,-10.2435213347824,129.673917796747));
#77615=CARTESIAN_POINT('Ctrl Pts',(78.868779355724,-10.2231380823707,129.671942991095));
#77616=CARTESIAN_POINT('Ctrl Pts',(78.8592163837481,-10.2142238794662,129.67108326768));
#77617=CARTESIAN_POINT('Ctrl Pts',(78.8449328651977,-10.200591701573,129.669772532845));
#77618=CARTESIAN_POINT('Ctrl Pts',(78.840133879012,-10.1959561435628,129.669327506683));
#77619=CARTESIAN_POINT('Ctrl Pts',(78.8314480425868,-10.1874646512513,129.668513242234));
#77620=CARTESIAN_POINT('Ctrl Pts',(78.8275521905069,-10.1836182266586,129.66814472639));
#77621=CARTESIAN_POINT('Ctrl Pts',(78.8187624937985,-10.174854070225,129.667305794942));
#77622=CARTESIAN_POINT('Ctrl Pts',(78.8138803874055,-10.1699249517288,129.666834512977));
#77623=CARTESIAN_POINT('Ctrl Pts',(78.7989692463701,-10.1546809549692,129.665379091345));
#77624=CARTESIAN_POINT('Ctrl Pts',(78.7890432290859,-10.1442668584192,129.66438770624));
#77625=CARTESIAN_POINT('Ctrl Pts',(78.7025441790252,-10.051128486279,129.655556852204));
#77626=CARTESIAN_POINT('Ctrl Pts',(78.634421708776,-9.96096568098782,129.647274342617));
#77627=CARTESIAN_POINT('Ctrl Pts',(78.5208163862279,-9.77385308810089,129.631386140596));
#77628=CARTESIAN_POINT('Ctrl Pts',(78.4745008520548,-9.67800633567131,129.62380605576));
#77629=CARTESIAN_POINT('Ctrl Pts',(78.4310551098949,-9.56064758164267,129.615249424404));
#77630=CARTESIAN_POINT('Ctrl Pts',(78.4247907092429,-9.54279786328208,129.613966020551));
#77631=CARTESIAN_POINT('Ctrl Pts',(78.4153590588307,-9.51438368671037,129.611950596357));
#77632=CARTESIAN_POINT('Ctrl Pts',(78.4119905242534,-9.50388828584718,129.61121202972));
#77633=CARTESIAN_POINT('Ctrl Pts',(78.4061271503014,-9.48497667464124,129.609891471137));
#77634=CARTESIAN_POINT('Ctrl Pts',(78.4035942225085,-9.47657280092303,129.609308256));
#77635=CARTESIAN_POINT('Ctrl Pts',(78.3978012868829,-9.45678815845285,129.607943486356));
#77636=CARTESIAN_POINT('Ctrl Pts',(78.394595904774,-9.44539178386632,129.607163727866));
#77637=CARTESIAN_POINT('Ctrl Pts',(78.3855587994676,-9.41189559073053,129.604889752691));
#77638=CARTESIAN_POINT('Ctrl Pts',(78.3800598963578,-9.38970823716448,129.603406229091));
#77639=CARTESIAN_POINT('Ctrl Pts',(78.3567710078587,-9.28670722237465,129.596613029166));
#77640=CARTESIAN_POINT('Ctrl Pts',(78.3445596094683,-9.20474858965247,129.591479866595));
#77641=CARTESIAN_POINT('Ctrl Pts',(78.3342832475888,-9.06504004771183,129.582891624144));
#77642=CARTESIAN_POINT('Ctrl Pts',(78.3330316961664,-9.00768799540359,129.579409293732));
#77643=CARTESIAN_POINT('Ctrl Pts',(78.3370332642402,-8.87337796289595,129.571163206144));
#77644=CARTESIAN_POINT('Ctrl Pts',(78.3446663050754,-8.79663152608362,129.566381266975));
#77645=CARTESIAN_POINT('Ctrl Pts',(78.3595251353606,-8.70925440496168,129.560584047531));
#77646=CARTESIAN_POINT('Ctrl Pts',(78.3615909663109,-8.69783017632925,129.559818991777));
#77647=CARTESIAN_POINT('Ctrl Pts',(78.3649870959763,-8.68010906475886,129.558619886321));
#77648=CARTESIAN_POINT('Ctrl Pts',(78.3662348218431,-8.67379646547043,129.558190293493));
#77649=CARTESIAN_POINT('Ctrl Pts',(78.3686091834629,-8.66213932360055,129.557392187906));
#77650=CARTESIAN_POINT('Ctrl Pts',(78.3697255679078,-8.65679291054558,129.557024251764));
#77651=CARTESIAN_POINT('Ctrl Pts',(78.3723670093262,-8.64444667106826,129.556170222869));
#77652=CARTESIAN_POINT('Ctrl Pts',(78.3739109302899,-8.63745116931079,129.555683093661));
#77653=CARTESIAN_POINT('Ctrl Pts',(78.379004616887,-8.61505892765786,129.554113930225));
#77654=CARTESIAN_POINT('Ctrl Pts',(78.3827282008986,-8.5997031808566,129.553022833416));
#77655=CARTESIAN_POINT('Ctrl Pts',(78.4006109934767,-8.53028283862264,129.548028822059));
#77656=CARTESIAN_POINT('Ctrl Pts',(78.4172634050794,-8.47691200050206,129.544020612337));
#77657=CARTESIAN_POINT('Ctrl Pts',(78.4365593669558,-8.42449206178673,129.539973210016));
#77658=CARTESIAN_POINT('',(78.3314565003769,-9.00039636157243,129.771406545978));
#77659=CARTESIAN_POINT('Ctrl Pts',(78.4365593938057,-8.42449198884581,129.733376828424));
#77660=CARTESIAN_POINT('Ctrl Pts',(78.4212621561002,-8.4660488779381,129.736183301371));
#77661=CARTESIAN_POINT('Ctrl Pts',(78.4076230942358,-8.5082121619528,129.738944145127));
#77662=CARTESIAN_POINT('Ctrl Pts',(78.3774921208378,-8.61584510834271,129.745843697833));
#77663=CARTESIAN_POINT('Ctrl Pts',(78.3632688753793,-8.68185193517039,129.749938839626));
#77664=CARTESIAN_POINT('Ctrl Pts',(78.3435271826576,-8.81114823422785,129.757946195357));
#77665=CARTESIAN_POINT('Ctrl Pts',(78.3375464657446,-8.87424579974563,129.761848452997));
#77666=CARTESIAN_POINT('Ctrl Pts',(78.3343844978591,-8.95850538309094,129.767222862207));
#77667=CARTESIAN_POINT('Ctrl Pts',(78.3339938900017,-8.97949774424152,129.768575424904));
#77668=CARTESIAN_POINT('Ctrl Pts',(78.3340000722425,-9.00049062409868,129.769946575773));
#77669=CARTESIAN_POINT('Ctrl Pts',(78.331327895087,-9.000391595574,129.77148036339));
#77670=CARTESIAN_POINT('Ctrl Pts',(78.3312607934084,-9.02159739328517,129.772904623852));
#77671=CARTESIAN_POINT('Ctrl Pts',(78.3316301189342,-9.0428007934763,129.774328884314));
#77672=CARTESIAN_POINT('Ctrl Pts',(78.3535891091806,-9.6150351256133,129.81279751744));
#77673=CARTESIAN_POINT('Ctrl Pts',(78.9961810223348,-10.6940907034897,129.886886262768));
#77674=CARTESIAN_POINT('Ctrl Pts',(80.8788147299153,-10.762182300724,129.99801938076));
#77675=CARTESIAN_POINT('Ctrl Pts',(81.9571171311415,-9.21745201145648,130.10915249875));
#77676=CARTESIAN_POINT('Ctrl Pts',(81.2441915797765,-7.47370268910709,130.220285616743));
#77677=CARTESIAN_POINT('Ctrl Pts',(79.4504429588567,-7.13772696278846,130.327943005734));
#77678=CARTESIAN_POINT('Ctrl Pts',(78.6106062169705,-7.95554246370299,130.398556022063));
#77679=CARTESIAN_POINT('Ctrl Pts',(78.4345148344113,-8.42372400280583,130.432124665727));
#77680=CARTESIAN_POINT('Origin',(80.,-9.,134.));
#77681=CARTESIAN_POINT('',(78.4365594227781,-8.42449191013859,131.131996270822));
#77682=CARTESIAN_POINT('',(78.4365593749572,-8.42449204005001,130.937771468334));
#77683=CARTESIAN_POINT('',(78.4365593749993,-8.42449203993574,134.));
#77684=CARTESIAN_POINT('',(78.3340004597058,-9.00014280943258,130.276978848223));
#77685=CARTESIAN_POINT('Ctrl Pts',(78.4365593749572,-8.42449204005001,130.937771468334));
#77686=CARTESIAN_POINT('Ctrl Pts',(78.4379751786435,-8.42064582912985,130.937505217487));
#77687=CARTESIAN_POINT('Ctrl Pts',(78.4394051976635,-8.41680478221285,130.937239411317));
#77688=CARTESIAN_POINT('Ctrl Pts',(78.4707357895122,-8.3335909330545,130.931482490514));
#77689=CARTESIAN_POINT('Ctrl Pts',(78.5066420832507,-8.25660581212541,130.926197191765));
#77690=CARTESIAN_POINT('Ctrl Pts',(78.5811686898538,-8.12422985648461,130.916866704775));
#77691=CARTESIAN_POINT('Ctrl Pts',(78.6175766910789,-8.0678190663728,130.912799700205));
#77692=CARTESIAN_POINT('Ctrl Pts',(78.700583954414,-7.95480933705074,130.904182065975));
#77693=CARTESIAN_POINT('Ctrl Pts',(78.7477116502163,-7.89878397792025,130.899629813918));
#77694=CARTESIAN_POINT('Ctrl Pts',(78.8063923604581,-7.83767849066319,130.894088350327));
#77695=CARTESIAN_POINT('Ctrl Pts',(78.8145118151106,-7.82939834561506,130.893324114215));
#77696=CARTESIAN_POINT('Ctrl Pts',(78.8272678033789,-7.81665872811047,130.892126023023));
#77697=CARTESIAN_POINT('Ctrl Pts',(78.8318450286061,-7.81214002084199,130.891696612699));
#77698=CARTESIAN_POINT('Ctrl Pts',(78.8403363115843,-7.80385383711295,130.890900657176));
#77699=CARTESIAN_POINT('Ctrl Pts',(78.8442427715019,-7.80007886138395,130.890534701351));
#77700=CARTESIAN_POINT('Ctrl Pts',(78.8533621386253,-7.79135228168231,130.88968097387));
#77701=CARTESIAN_POINT('Ctrl Pts',(78.8585886828827,-7.78641527181206,130.889192132031));
#77702=CARTESIAN_POINT('Ctrl Pts',(78.8753978949519,-7.77074187647731,130.887621865087));
#77703=CARTESIAN_POINT('Ctrl Pts',(78.8871009469279,-7.76013666828329,130.886531468779));
#77704=CARTESIAN_POINT('Ctrl Pts',(78.952643580292,-7.70241807934173,130.880448871238));
#77705=CARTESIAN_POINT('Ctrl Pts',(79.0093195000568,-7.65864827724601,130.875280748648));
#77706=CARTESIAN_POINT('Ctrl Pts',(79.1777138439869,-7.54510769288029,130.86051577728));
#77707=CARTESIAN_POINT('Ctrl Pts',(79.295152273063,-7.48472191251716,130.850933429242));
#77708=CARTESIAN_POINT('Ctrl Pts',(79.4444116480076,-7.42912671411549,130.839919206391));
#77709=CARTESIAN_POINT('Ctrl Pts',(79.4705734664749,-7.42011740900082,130.838026779079));
#77710=CARTESIAN_POINT('Ctrl Pts',(79.5089588858195,-7.40795938078234,130.835303590602));
#77711=CARTESIAN_POINT('Ctrl Pts',(79.5210118700461,-7.40429166338219,130.834456045037));
#77712=CARTESIAN_POINT('Ctrl Pts',(79.5425107821774,-7.39801510220942,130.832957278427));
#77713=CARTESIAN_POINT('Ctrl Pts',(79.5519401807672,-7.39535224967844,130.832304328109));
#77714=CARTESIAN_POINT('Ctrl Pts',(79.5717351409171,-7.38995026702352,130.830942566229));
#77715=CARTESIAN_POINT('Ctrl Pts',(79.5821047842792,-7.38722768813281,130.830234316185));
#77716=CARTESIAN_POINT('Ctrl Pts',(79.6095211552821,-7.38031162845498,130.828374743925));
#77717=CARTESIAN_POINT('Ctrl Pts',(79.6266094179509,-7.37628707571677,130.827228864698));
#77718=CARTESIAN_POINT('Ctrl Pts',(79.7138357034984,-7.35719383769863,130.821441595589));
#77719=CARTESIAN_POINT('Ctrl Pts',(79.7848351438677,-7.34639544267265,130.816937575108));
#77720=CARTESIAN_POINT('Ctrl Pts',(79.9242063943786,-7.33433051378958,130.808296276992));
#77721=CARTESIAN_POINT('Ctrl Pts',(79.9923925808898,-7.33262426702841,130.804159512606));
#77722=CARTESIAN_POINT('Ctrl Pts',(80.0813617029876,-7.33585686431539,130.798710670584));
#77723=CARTESIAN_POINT('Ctrl Pts',(80.1022146132505,-7.33700744116704,130.797429602586));
#77724=CARTESIAN_POINT('Ctrl Pts',(80.18861058098,-7.34340556530168,130.792087469822));
#77725=CARTESIAN_POINT('Ctrl Pts',(80.2538284915496,-7.35213833318391,130.787973315768));
#77726=CARTESIAN_POINT('Ctrl Pts',(80.3296165436456,-7.36689233412866,130.782921575209));
#77727=CARTESIAN_POINT('Ctrl Pts',(80.3408583982308,-7.36920165299669,130.782165102061));
#77728=CARTESIAN_POINT('Ctrl Pts',(80.3583356545238,-7.37298045944227,130.78097662716));
#77729=CARTESIAN_POINT('Ctrl Pts',(80.364588208444,-7.37437013391965,130.780548957687));
#77730=CARTESIAN_POINT('Ctrl Pts',(80.3761326966877,-7.37700592996078,130.779754454781));
#77731=CARTESIAN_POINT('Ctrl Pts',(80.3814267353306,-7.37824194180872,130.779388191247));
#77732=CARTESIAN_POINT('Ctrl Pts',(80.3937470006999,-7.38118204522755,130.778531391237));
#77733=CARTESIAN_POINT('Ctrl Pts',(80.4007682535684,-7.38290597882792,130.778039757918));
#77734=CARTESIAN_POINT('Ctrl Pts',(80.4233066214429,-7.38859563955571,130.776451311067));
#77735=CARTESIAN_POINT('Ctrl Pts',(80.4387773078315,-7.3927393068761,130.775345243089));
#77736=CARTESIAN_POINT('Ctrl Pts',(80.475812514774,-7.40323334535298,130.772663327211));
#77737=CARTESIAN_POINT('Ctrl Pts',(80.4973125926134,-7.40979832050611,130.771078338583));
#77738=CARTESIAN_POINT('Ctrl Pts',(80.5817605968819,-7.4374642587155,130.764757789034));
#77739=CARTESIAN_POINT('Ctrl Pts',(80.6435539932315,-7.46188404670908,130.759924299184));
#77740=CARTESIAN_POINT('Ctrl Pts',(80.8130252587442,-7.54086063983661,130.746314159855));
#77741=CARTESIAN_POINT('Ctrl Pts',(80.9164942383467,-7.60352368730289,130.73760809624));
#77742=CARTESIAN_POINT('Ctrl Pts',(81.0289942761497,-7.68959224325825,130.727863888625));
#77743=CARTESIAN_POINT('Ctrl Pts',(81.0454438793713,-7.70267780631879,130.726430157856));
#77744=CARTESIAN_POINT('Ctrl Pts',(81.071332361068,-7.72408422160583,130.724158368675));
#77745=CARTESIAN_POINT('Ctrl Pts',(81.0809317845535,-7.7322064073299,130.72331248652));
#77746=CARTESIAN_POINT('Ctrl Pts',(81.0978435890471,-7.74684742117823,130.721815613545));
#77747=CARTESIAN_POINT('Ctrl Pts',(81.1051920659364,-7.75332344360976,130.721162908601));
#77748=CARTESIAN_POINT('Ctrl Pts',(81.1204722978016,-7.76703081163949,130.719800618051));
#77749=CARTESIAN_POINT('Ctrl Pts',(81.1283921664166,-7.77427477897728,130.719091603048));
#77750=CARTESIAN_POINT('Ctrl Pts',(81.1491205100005,-7.7936053016993,130.71722764733));
#77751=CARTESIAN_POINT('Ctrl Pts',(81.1618085235067,-7.80581948273725,130.716078197239));
#77752=CARTESIAN_POINT('Ctrl Pts',(81.2258416721733,-7.86944808258024,130.710227964373));
#77753=CARTESIAN_POINT('Ctrl Pts',(81.2739803943592,-7.92398359149619,130.705668406939));
#77754=CARTESIAN_POINT('Ctrl Pts',(81.3809287815911,-8.06242335177976,130.694867304089));
#77755=CARTESIAN_POINT('Ctrl Pts',(81.4358613894735,-8.14893308402113,130.68872635182));
#77756=CARTESIAN_POINT('Ctrl Pts',(81.5063768868028,-8.28647324729803,130.679116775095));
#77757=CARTESIAN_POINT('Ctrl Pts',(81.528031873874,-8.33411023384711,130.675810695852));
#77758=CARTESIAN_POINT('Ctrl Pts',(81.5514980860824,-8.39293205122977,130.671662912455));
#77759=CARTESIAN_POINT('Ctrl Pts',(81.5554854683014,-8.40322303379583,130.670934873472));
#77760=CARTESIAN_POINT('Ctrl Pts',(81.5615900748789,-8.41945524887713,130.669781652355));
#77761=CARTESIAN_POINT('Ctrl Pts',(81.5637763884082,-8.42537040296432,130.669360401225));
#77762=CARTESIAN_POINT('Ctrl Pts',(81.5678090009686,-8.43647425306369,130.668567494961));
#77763=CARTESIAN_POINT('Ctrl Pts',(81.5696632186497,-8.4416598639921,130.668196307275));
#77764=CARTESIAN_POINT('Ctrl Pts',(81.5739565745366,-8.45385732919949,130.667321194772));
#77765=CARTESIAN_POINT('Ctrl Pts',(81.5763745887056,-8.46087639059137,130.666816071392));
#77766=CARTESIAN_POINT('Ctrl Pts',(81.5842136674819,-8.48413549877322,130.665137709382));
#77767=CARTESIAN_POINT('Ctrl Pts',(81.5894310989104,-8.50044234283363,130.663953750486));
#77768=CARTESIAN_POINT('Ctrl Pts',(81.6015258094516,-8.54035292144257,130.661043178718));
#77769=CARTESIAN_POINT('Ctrl Pts',(81.6081335736433,-8.5640336758851,130.659305390575));
#77770=CARTESIAN_POINT('Ctrl Pts',(81.6335455273103,-8.66356154161786,130.651979361482));
#77771=CARTESIAN_POINT('Ctrl Pts',(81.6475251687453,-8.74053560742116,130.646265062631));
#77772=CARTESIAN_POINT('Ctrl Pts',(81.6674238403131,-8.92179965718661,130.633009243394));
#77773=CARTESIAN_POINT('Ctrl Pts',(81.6690521899081,-9.026249960386,130.625534035596));
#77774=CARTESIAN_POINT('Ctrl Pts',(81.6590634112011,-9.15368997235432,130.61673426691));
#77775=CARTESIAN_POINT('Ctrl Pts',(81.656721920953,-9.17715695103335,130.615126224066));
#77776=CARTESIAN_POINT('Ctrl Pts',(81.6524232451519,-9.21260392185124,130.612714844952));
#77777=CARTESIAN_POINT('Ctrl Pts',(81.6508321809667,-9.22462442536748,130.611900181043));
#77778=CARTESIAN_POINT('Ctrl Pts',(81.6477289998494,-9.24625125571113,130.610439675983));
#77779=CARTESIAN_POINT('Ctrl Pts',(81.646263752607,-9.25586363870974,130.609792391712));
#77780=CARTESIAN_POINT('Ctrl Pts',(81.6429428379427,-9.27643885969083,130.608410630332));
#77781=CARTESIAN_POINT('Ctrl Pts',(81.6410614019871,-9.28739710659669,130.607677000098));
#77782=CARTESIAN_POINT('Ctrl Pts',(81.6355939044603,-9.31743577248257,130.605671708726));
#77783=CARTESIAN_POINT('Ctrl Pts',(81.6317837427775,-9.3364740077268,130.604407164274));
#77784=CARTESIAN_POINT('Ctrl Pts',(81.6037188544358,-9.46498887986672,130.595905374797));
#77785=CARTESIAN_POINT('Ctrl Pts',(81.5687976423735,-9.57184534855465,130.589031974806));
#77786=CARTESIAN_POINT('Ctrl Pts',(81.4806404119436,-9.77098524382982,130.575732493722));
#77787=CARTESIAN_POINT('Ctrl Pts',(81.4287966779467,-9.86327755070613,130.569324840339));
#77788=CARTESIAN_POINT('Ctrl Pts',(81.3601531717696,-9.96216296114336,130.561502913589));
#77789=CARTESIAN_POINT('Ctrl Pts',(81.3515687945304,-9.97418477274017,130.560534312451));
#77790=CARTESIAN_POINT('Ctrl Pts',(81.3386226105081,-9.99181446921927,130.559084894736));
#77791=CARTESIAN_POINT('Ctrl Pts',(81.3343826924601,-9.99751153386184,130.558611943584));
#77792=CARTESIAN_POINT('Ctrl Pts',(81.3268100611465,-10.0075519999819,130.557769943426));
#77793=CARTESIAN_POINT('Ctrl Pts',(81.323492177072,-10.0119063329974,130.557401913929));
#77794=CARTESIAN_POINT('Ctrl Pts',(81.3161780712314,-10.0214077266664,130.556592461005));
#77795=CARTESIAN_POINT('Ctrl Pts',(81.3121731502927,-10.0265476507736,130.556150456456));
#77796=CARTESIAN_POINT('Ctrl Pts',(81.3005032256842,-10.041344985319,130.554866324836));
#77797=CARTESIAN_POINT('Ctrl Pts',(81.2927612267938,-10.0509407245668,130.554019113226));
#77798=CARTESIAN_POINT('Ctrl Pts',(81.2236904824365,-10.1346316171562,130.546507932999));
#77799=CARTESIAN_POINT('Ctrl Pts',(81.1561643678984,-10.2033650622613,130.539498089612));
#77800=CARTESIAN_POINT('Ctrl Pts',(80.9927268640371,-10.3432029953362,130.523841081859));
#77801=CARTESIAN_POINT('Ctrl Pts',(80.8943225059096,-10.4106373831664,130.515260103051));
#77802=CARTESIAN_POINT('Ctrl Pts',(80.7709777360487,-10.4770222091074,130.505622964162));
#77803=CARTESIAN_POINT('Ctrl Pts',(80.7522074186084,-10.4866692119515,130.504183328547));
#77804=CARTESIAN_POINT('Ctrl Pts',(80.7219462400565,-10.5015020239545,130.501904073351));
#77805=CARTESIAN_POINT('Ctrl Pts',(80.7105715758021,-10.50691829648,130.501056548512));
#77806=CARTESIAN_POINT('Ctrl Pts',(80.6902430406924,-10.516316767711,130.499557809267));
#77807=CARTESIAN_POINT('Ctrl Pts',(80.681313531692,-10.5203499182258,130.498904865735));
#77808=CARTESIAN_POINT('Ctrl Pts',(80.6625399329366,-10.5286306846625,130.497543108927));
#77809=CARTESIAN_POINT('Ctrl Pts',(80.6526893485531,-10.5328625366215,130.496834857243));
#77810=CARTESIAN_POINT('Ctrl Pts',(80.6266031420297,-10.5437722189913,130.494975260309));
#77811=CARTESIAN_POINT('Ctrl Pts',(80.6103013627048,-10.550289149343,130.493829358415));
#77812=CARTESIAN_POINT('Ctrl Pts',(80.5268691621918,-10.5821226218604,130.488041613524));
#77813=CARTESIAN_POINT('Ctrl Pts',(80.458252622996,-10.6033432241656,130.483537170095));
#77814=CARTESIAN_POINT('Ctrl Pts',(80.3222154669893,-10.6359632846762,130.474895848719));
#77815=CARTESIAN_POINT('Ctrl Pts',(80.255044083031,-10.6477716441688,130.470759456356));
#77816=CARTESIAN_POINT('Ctrl Pts',(80.1665936209609,-10.6577811642385,130.465311399429));
#77817=CARTESIAN_POINT('Ctrl Pts',(80.1458076476477,-10.6597385119645,130.464030743268));
#77818=CARTESIAN_POINT('Ctrl Pts',(80.0594209790125,-10.6662379399585,130.458688733597));
#77819=CARTESIAN_POINT('Ctrl Pts',(79.9936243433958,-10.6672843127791,130.454574285287));
#77820=CARTESIAN_POINT('Ctrl Pts',(79.9164807371749,-10.663944785375,130.449522215874));
#77821=CARTESIAN_POINT('Ctrl Pts',(79.9050205399134,-10.6633299733551,130.448765737469));
#77822=CARTESIAN_POINT('Ctrl Pts',(79.887175888407,-10.6621876387491,130.447577257663));
#77823=CARTESIAN_POINT('Ctrl Pts',(79.8807863206327,-10.6617415929644,130.447149588667));
#77824=CARTESIAN_POINT('Ctrl Pts',(79.8689784955862,-10.660848855838,130.446355088328));
#77825=CARTESIAN_POINT('Ctrl Pts',(79.8635596581383,-10.6604124748095,130.445988826901));
#77826=CARTESIAN_POINT('Ctrl Pts',(79.8509395571915,-10.6593339791497,130.445132034986));
#77827=CARTESIAN_POINT('Ctrl Pts',(79.8437402666757,-10.6586715048006,130.444640407693));
#77828=CARTESIAN_POINT('Ctrl Pts',(79.8206074879546,-10.6563909024663,130.443051995644));
#77829=CARTESIAN_POINT('Ctrl Pts',(79.8046934963907,-10.6545899243362,130.44194595692));
#77830=CARTESIAN_POINT('Ctrl Pts',(79.7665119627536,-10.6497104593924,130.439264125732));
#77831=CARTESIAN_POINT('Ctrl Pts',(79.7442762870278,-10.6464101990776,130.437679193191));
#77832=CARTESIAN_POINT('Ctrl Pts',(79.6566617277263,-10.6315886771896,130.431358999439));
#77833=CARTESIAN_POINT('Ctrl Pts',(79.5919317840731,-10.6166144268172,130.426525817943));
#77834=CARTESIAN_POINT('Ctrl Pts',(79.4126685246305,-10.5636900643682,130.412919849561));
#77835=CARTESIAN_POINT('Ctrl Pts',(79.3010903760441,-10.5171091710704,130.40421751504));
#77836=CARTESIAN_POINT('Ctrl Pts',(79.177069215543,-10.4487180775746,130.394474164678));
#77837=CARTESIAN_POINT('Ctrl Pts',(79.1588289082504,-10.4382038829372,130.393038054886));
#77838=CARTESIAN_POINT('Ctrl Pts',(79.1300111278939,-10.4208566804488,130.390763254938));
#77839=CARTESIAN_POINT('Ctrl Pts',(79.1193038486856,-10.4142449038642,130.389916708291));
#77840=CARTESIAN_POINT('Ctrl Pts',(79.1003962927541,-10.4022714174054,130.388419077895));
#77841=CARTESIAN_POINT('Ctrl Pts',(79.0921665732345,-10.3969575635843,130.387766273986));
#77842=CARTESIAN_POINT('Ctrl Pts',(79.0763844252012,-10.3865688044735,130.386512336961));
#77843=CARTESIAN_POINT('Ctrl Pts',(79.0688257856487,-10.3815040237468,130.385910857295));
#77844=CARTESIAN_POINT('Ctrl Pts',(79.0481156161052,-10.3673796630799,130.384259983483));
#77845=CARTESIAN_POINT('Ctrl Pts',(79.0350520407655,-10.3581923605481,130.383215437355));
#77846=CARTESIAN_POINT('Ctrl Pts',(78.9802666599839,-10.3184735901038,130.378818164374));
#77847=CARTESIAN_POINT('Ctrl Pts',(78.9398435683865,-10.2861951013431,130.37553308263));
#77848=CARTESIAN_POINT('Ctrl Pts',(78.8350349486768,-10.1941995420655,130.36681005697));
#77849=CARTESIAN_POINT('Ctrl Pts',(78.7737617404019,-10.1311926192413,130.361487607277));
#77850=CARTESIAN_POINT('Ctrl Pts',(78.664474129254,-9.99944280630085,130.351018855969));
#77851=CARTESIAN_POINT('Ctrl Pts',(78.6161177349635,-9.9313333045399,130.345888803918));
#77852=CARTESIAN_POINT('Ctrl Pts',(78.5649535755764,-9.84643077202604,130.339459110195));
#77853=CARTESIAN_POINT('Ctrl Pts',(78.5570283715056,-9.83284820206149,130.338429382553));
#77854=CARTESIAN_POINT('Ctrl Pts',(78.5457517353161,-9.81287758797118,130.336910672011));
#77855=CARTESIAN_POINT('Ctrl Pts',(78.5422473808255,-9.80657627343514,130.336430803434));
#77856=CARTESIAN_POINT('Ctrl Pts',(78.5361437305159,-9.79543135338164,130.335580539162));
#77857=CARTESIAN_POINT('Ctrl Pts',(78.5335273354806,-9.79059733034208,130.335211227187));
#77858=CARTESIAN_POINT('Ctrl Pts',(78.5279358262035,-9.78014325702492,130.334411331313));
#77859=CARTESIAN_POINT('Ctrl Pts',(78.5249689973576,-9.77451918705533,130.333980280205));
#77860=CARTESIAN_POINT('Ctrl Pts',(78.516690140713,-9.75860527313978,130.332758829244));
#77861=CARTESIAN_POINT('Ctrl Pts',(78.5114532225692,-9.74827706884176,130.331964057096));
#77862=CARTESIAN_POINT('Ctrl Pts',(78.4733556629172,-9.67115857451692,130.326019101976));
#77863=CARTESIAN_POINT('Ctrl Pts',(78.4449001050395,-9.60229440920325,130.320655598117));
#77864=CARTESIAN_POINT('Ctrl Pts',(78.3797244376846,-9.40878356916902,130.305821591508));
#77865=CARTESIAN_POINT('Ctrl Pts',(78.3528067216336,-9.28135729323273,130.29634947586));
#77866=CARTESIAN_POINT('Ctrl Pts',(78.3381320600553,-9.12127693737839,130.285186056999));
#77867=CARTESIAN_POINT('Ctrl Pts',(78.336166388487,-9.09039402050533,130.283062852791));
#77868=CARTESIAN_POINT('Ctrl Pts',(78.3346320841121,-9.04744096532827,130.280150357049));
#77869=CARTESIAN_POINT('Ctrl Pts',(78.334332733261,-9.03540494588075,130.279338626029));
#77870=CARTESIAN_POINT('Ctrl Pts',(78.3340552946905,-9.0156258602895,130.278011637488));
#77871=CARTESIAN_POINT('Ctrl Pts',(78.3340006704557,-9.00788450869137,130.277494013668));
#77872=CARTESIAN_POINT('Ctrl Pts',(78.334000006134,-9.00014296370202,130.276978071365));
#77873=CARTESIAN_POINT('Ctrl Pts',(78.3340000061253,-9.00014286169838,130.276978064567));
#77874=CARTESIAN_POINT('Ctrl Pts',(78.3339997367268,-8.99700123680821,130.276768688126));
#77875=CARTESIAN_POINT('Ctrl Pts',(78.3340083537072,-8.99385959459696,130.276559589479));
#77876=CARTESIAN_POINT('Ctrl Pts',(78.3340569686603,-8.98513399509389,130.275979602651));
#77877=CARTESIAN_POINT('Ctrl Pts',(78.3341161544701,-8.97955015239747,130.275609316099));
#77878=CARTESIAN_POINT('Ctrl Pts',(78.334372662962,-8.9631369346624,130.274523376322));
#77879=CARTESIAN_POINT('Ctrl Pts',(78.3346475204383,-8.95230891536532,130.273810149919));
#77880=CARTESIAN_POINT('Ctrl Pts',(78.3357842883398,-8.91996407050541,130.271688564743));
#77881=CARTESIAN_POINT('Ctrl Pts',(78.3369577962785,-8.89845994695566,130.270289889103));
#77882=CARTESIAN_POINT('Ctrl Pts',(78.3488699338953,-8.73757508373254,130.259900036097));
#77883=CARTESIAN_POINT('Ctrl Pts',(78.3766951673673,-8.60002230815777,130.251496490578));
#77884=CARTESIAN_POINT('Ctrl Pts',(78.4262408798902,-8.45312708993837,130.241988178509));
#77885=CARTESIAN_POINT('Ctrl Pts',(78.4313026982203,-8.43877247177136,130.241052411112));
#77886=CARTESIAN_POINT('Ctrl Pts',(78.4365593712355,-8.42449205016054,130.240113128671));
#77887=CARTESIAN_POINT('',(78.3344014643664,-8.99848374960743,130.471480117348));
#77888=CARTESIAN_POINT('Ctrl Pts',(78.4345148344113,-8.42372400280583,130.432124665727));
#77889=CARTESIAN_POINT('Ctrl Pts',(78.4162821667148,-8.47219996057315,130.435600394726));
#77890=CARTESIAN_POINT('Ctrl Pts',(78.3564961095336,-8.65837616141247,130.4487188786));
#77891=CARTESIAN_POINT('Ctrl Pts',(78.3331165493187,-8.85422408541304,130.461837362474));
#77892=CARTESIAN_POINT('Ctrl Pts',(78.3344014643664,-8.99848374960743,130.471480117348));
#77893=CARTESIAN_POINT('Ctrl Pts',(78.3340007022079,-8.99847037383078,130.471710616873));
#77894=CARTESIAN_POINT('Ctrl Pts',(78.3339349962914,-9.07003427155384,130.476898790049));
#77895=CARTESIAN_POINT('Ctrl Pts',(78.3384804025895,-9.14153633045385,130.482027598063));
#77896=CARTESIAN_POINT('Ctrl Pts',(78.3517548529112,-9.24474170582688,130.489298976558));
#77897=CARTESIAN_POINT('Ctrl Pts',(78.3568386683126,-9.27682423362049,130.491541426185));
#77898=CARTESIAN_POINT('Ctrl Pts',(78.3651641916091,-9.32097168702806,130.494603337894));
#77899=CARTESIAN_POINT('Ctrl Pts',(78.3676080353816,-9.33317777945166,130.495447392491));
#77900=CARTESIAN_POINT('Ctrl Pts',(78.3721676567293,-9.35469566604922,130.496931158938));
#77901=CARTESIAN_POINT('Ctrl Pts',(78.3742270887476,-9.36401868212237,130.49757262701));
#77902=CARTESIAN_POINT('Ctrl Pts',(78.3785607079475,-9.38286615914597,130.498866758121));
#77903=CARTESIAN_POINT('Ctrl Pts',(78.3808389486926,-9.39238930999188,130.499519262949));
#77904=CARTESIAN_POINT('Ctrl Pts',(78.3857896109931,-9.41230566956377,130.500881216119));
#77905=CARTESIAN_POINT('Ctrl Pts',(78.3884787640826,-9.42269428717302,130.501590093497));
#77906=CARTESIAN_POINT('Ctrl Pts',(78.395845467767,-9.45006035456796,130.50345385919));
#77907=CARTESIAN_POINT('Ctrl Pts',(78.4006922195962,-9.46699116488763,130.504603256466));
#77908=CARTESIAN_POINT('Ctrl Pts',(78.4246464313182,-9.54591694311443,130.509948632133));
#77909=CARTESIAN_POINT('Ctrl Pts',(78.4470968889685,-9.60684226960879,130.514034925297));
#77910=CARTESIAN_POINT('Ctrl Pts',(78.5114041204336,-9.75421267713005,130.523999465394));
#77911=CARTESIAN_POINT('Ctrl Pts',(78.5572802094065,-9.83863802790201,130.529775232375));
#77912=CARTESIAN_POINT('Ctrl Pts',(78.6438709655651,-9.96964258787924,130.539459137901));
#77913=CARTESIAN_POINT('Ctrl Pts',(78.6803554417283,-10.0187390846018,130.543280858618));
#77914=CARTESIAN_POINT('Ctrl Pts',(78.7284371630885,-10.0765135101543,130.548170346282));
#77915=CARTESIAN_POINT('Ctrl Pts',(78.7375602322723,-10.0871978600399,130.549092228681));
#77916=CARTESIAN_POINT('Ctrl Pts',(78.751459540794,-10.1030649862324,130.55049035203));
#77917=CARTESIAN_POINT('Ctrl Pts',(78.7561355921269,-10.1083352256711,130.550959657423));
#77918=CARTESIAN_POINT('Ctrl Pts',(78.7641519328284,-10.1172555816057,130.551762745771));
#77919=CARTESIAN_POINT('Ctrl Pts',(78.7674752795892,-10.1209207342306,130.552095272333));
#77920=CARTESIAN_POINT('Ctrl Pts',(78.7750891478601,-10.1292428872085,130.552856242805));
#77921=CARTESIAN_POINT('Ctrl Pts',(78.7793898269372,-10.1338901604976,130.553285435664));
#77922=CARTESIAN_POINT('Ctrl Pts',(78.7913398032136,-10.1466564258724,130.554475964399));
#77923=CARTESIAN_POINT('Ctrl Pts',(78.7990441471252,-10.1547231066074,130.555241240959));
#77924=CARTESIAN_POINT('Ctrl Pts',(78.8446863825659,-10.2015610418966,130.559758495396));
#77925=CARTESIAN_POINT('Ctrl Pts',(78.8844151630289,-10.2385345094071,130.563624042726));
#77926=CARTESIAN_POINT('Ctrl Pts',(79.0023348661794,-10.3379933616657,130.574756164542));
#77927=CARTESIAN_POINT('Ctrl Pts',(79.0844569030679,-10.3954728708792,130.582104453583));
#77928=CARTESIAN_POINT('Ctrl Pts',(79.234327251112,-10.4814149119788,130.594488158848));
#77929=CARTESIAN_POINT('Ctrl Pts',(79.2997232162067,-10.5134265584611,130.59959835429));
#77930=CARTESIAN_POINT('Ctrl Pts',(79.3833014121684,-10.5477561184446,130.605764416584));
#77931=CARTESIAN_POINT('Ctrl Pts',(79.3996974180764,-10.5541888565728,130.606957609198));
#77932=CARTESIAN_POINT('Ctrl Pts',(79.4262434251179,-10.5641210139541,130.608863843208));
#77933=CARTESIAN_POINT('Ctrl Pts',(79.4363302411152,-10.5677842854651,130.609582296842));
#77934=CARTESIAN_POINT('Ctrl Pts',(79.4556870709455,-10.5746032219618,130.610950104293));
#77935=CARTESIAN_POINT('Ctrl Pts',(79.4649508511102,-10.5777751064724,130.611599971338));
#77936=CARTESIAN_POINT('Ctrl Pts',(79.4861676535505,-10.584831305075,130.613077860562));
#77937=CARTESIAN_POINT('Ctrl Pts',(79.4981378380038,-10.5886624344247,130.613904108824));
#77938=CARTESIAN_POINT('Ctrl Pts',(79.5302234525753,-10.5985327799545,130.61609957673));
#77939=CARTESIAN_POINT('Ctrl Pts',(79.5504120410543,-10.604327829163,130.617460902834));
#77940=CARTESIAN_POINT('Ctrl Pts',(79.6878855308817,-10.6409900307895,130.626607855615));
#77941=CARTESIAN_POINT('Ctrl Pts',(79.8081290242379,-10.6593532170167,130.633971881391));
#77942=CARTESIAN_POINT('Ctrl Pts',(79.9951672340737,-10.6672964652315,130.645411826756));
#77943=CARTESIAN_POINT('Ctrl Pts',(80.0611267486218,-10.6661822004068,130.649451503037));
#77944=CARTESIAN_POINT('Ctrl Pts',(80.1491626392878,-10.6594600465141,130.655040270119));
#77945=CARTESIAN_POINT('Ctrl Pts',(80.1714460790178,-10.6573060312199,130.656472101945));
#77946=CARTESIAN_POINT('Ctrl Pts',(80.2095354739301,-10.6528477797081,130.658959373959));
#77947=CARTESIAN_POINT('Ctrl Pts',(80.2253645281284,-10.6507639690004,130.660004881676));
#77948=CARTESIAN_POINT('Ctrl Pts',(80.2483040931285,-10.6474080250113,130.661540487815));
#77949=CARTESIAN_POINT('Ctrl Pts',(80.2554406826258,-10.6463165480506,130.6620211072));
#77950=CARTESIAN_POINT('Ctrl Pts',(80.2679360840632,-10.6443222876067,130.662868041826));
#77951=CARTESIAN_POINT('Ctrl Pts',(80.2732979144741,-10.6434396184187,130.663233231789));
#77952=CARTESIAN_POINT('Ctrl Pts',(80.2849738446537,-10.6414587959512,130.664032418627));
#77953=CARTESIAN_POINT('Ctrl Pts',(80.2912858560192,-10.6403504557155,130.66446695004));
#77954=CARTESIAN_POINT('Ctrl Pts',(80.3089030958394,-10.637152116998,130.665686426224));
#77955=CARTESIAN_POINT('Ctrl Pts',(80.3201930617965,-10.6349815172269,130.666475615621));
#77956=CARTESIAN_POINT('Ctrl Pts',(80.3967805439833,-10.6194332116624,130.67187752762));
#77957=CARTESIAN_POINT('Ctrl Pts',(80.4612401564026,-10.6022653519447,130.676661174944));
#77958=CARTESIAN_POINT('Ctrl Pts',(80.5449875676661,-10.5744875039766,130.683058938858));
#77959=CARTESIAN_POINT('Ctrl Pts',(80.5653502840295,-10.567291098561,130.684629520004));
#77960=CARTESIAN_POINT('Ctrl Pts',(80.6530219722544,-10.5343760330184,130.691445250736));
#77961=CARTESIAN_POINT('Ctrl Pts',(80.7187668878932,-10.5047002537558,130.696690519489));
#77962=CARTESIAN_POINT('Ctrl Pts',(80.8413634571602,-10.4394880833444,130.706610484027));
#77963=CARTESIAN_POINT('Ctrl Pts',(80.8984060004816,-10.4045950053442,130.711290522432));
#77964=CARTESIAN_POINT('Ctrl Pts',(80.9673362819525,-10.3565077860403,130.717022665434));
#77965=CARTESIAN_POINT('Ctrl Pts',(80.9813136869283,-10.3464309646386,130.718189470369));
#77966=CARTESIAN_POINT('Ctrl Pts',(81.0036733627508,-10.3297778704295,130.720063965301));
#77967=CARTESIAN_POINT('Ctrl Pts',(81.0121529828278,-10.3233350869063,130.720776746996));
#77968=CARTESIAN_POINT('Ctrl Pts',(81.0283289145614,-10.3107982281401,130.722140409185));
#77969=CARTESIAN_POINT('Ctrl Pts',(81.0360342555722,-10.3047165898122,130.722791740303));
#77970=CARTESIAN_POINT('Ctrl Pts',(81.0536148448369,-10.2905867024288,130.724282179668));
#77971=CARTESIAN_POINT('Ctrl Pts',(81.0634525138686,-10.2824925120503,130.725119405891));
#77972=CARTESIAN_POINT('Ctrl Pts',(81.0949848363604,-10.255936166672,130.727814502186));
#77973=CARTESIAN_POINT('Ctrl Pts',(81.1162998049607,-10.2370296464228,130.729654255701));
#77974=CARTESIAN_POINT('Ctrl Pts',(81.2326405640691,-10.1283772925202,130.739825103638));
#77975=CARTESIAN_POINT('Ctrl Pts',(81.3173305023669,-10.0282416172791,130.747682960545));
#77976=CARTESIAN_POINT('Ctrl Pts',(81.4287681531836,-9.85979973806537,130.760075036412));
#77977=CARTESIAN_POINT('Ctrl Pts',(81.464228715595,-9.79791350891299,130.764492911404));
#77978=CARTESIAN_POINT('Ctrl Pts',(81.5025598138242,-9.719804482804,130.770138126559));
#77979=CARTESIAN_POINT('Ctrl Pts',(81.5093029094214,-9.70555593044175,130.771170688264));
#77980=CARTESIAN_POINT('Ctrl Pts',(81.5188227689612,-9.68467875259524,130.772690706941));
#77981=CARTESIAN_POINT('Ctrl Pts',(81.5217606540628,-9.67812395974106,130.773168951957));
#77982=CARTESIAN_POINT('Ctrl Pts',(81.5268450210865,-9.66658065754449,130.77401327899));
#77983=CARTESIAN_POINT('Ctrl Pts',(81.5290096381502,-9.66160034506998,130.774378259752));
#77984=CARTESIAN_POINT('Ctrl Pts',(81.5336853733046,-9.65069698105437,130.775178924295));
#77985=CARTESIAN_POINT('Ctrl Pts',(81.5361865080277,-9.64477003225855,130.775615160342));
#77986=CARTESIAN_POINT('Ctrl Pts',(81.5431038140211,-9.62810933413548,130.77684393083));
#77987=CARTESIAN_POINT('Ctrl Pts',(81.5474421305327,-9.61734394814327,130.7776408096));
#77988=CARTESIAN_POINT('Ctrl Pts',(81.5797035290483,-9.53481119429368,130.783767442007));
#77989=CARTESIAN_POINT('Ctrl Pts',(81.6027298466803,-9.4612381194497,130.789324547852));
#77990=CARTESIAN_POINT('Ctrl Pts',(81.6338713713232,-9.33061058580814,130.799085601361));
#77991=CARTESIAN_POINT('Ctrl Pts',(81.6442748597005,-9.27422521883321,130.803266799623));
#77992=CARTESIAN_POINT('Ctrl Pts',(81.6625427760792,-9.13543976952625,130.813381921777));
#77993=CARTESIAN_POINT('Ctrl Pts',(81.6672167964606,-9.05276509734269,130.819253342362));
#77994=CARTESIAN_POINT('Ctrl Pts',(81.6653211370544,-8.94724904151348,130.826508511372));
#77995=CARTESIAN_POINT('Ctrl Pts',(81.664441948953,-8.92443386100817,130.828063657201));
#77996=CARTESIAN_POINT('Ctrl Pts',(81.662396235259,-8.88984341716917,130.830401903338));
#77997=CARTESIAN_POINT('Ctrl Pts',(81.6615728292183,-8.8780513983945,130.831195577415));
#77998=CARTESIAN_POINT('Ctrl Pts',(81.6599206693514,-8.85753548451438,130.83257071638));
#77999=CARTESIAN_POINT('Ctrl Pts',(81.6591484689769,-8.8488076402864,130.833153924702));
#78000=CARTESIAN_POINT('Ctrl Pts',(81.657251608415,-8.82913718673916,130.834464461788));
#78001=CARTESIAN_POINT('Ctrl Pts',(81.6560873480727,-8.81819873523137,130.835190522481));
#78002=CARTESIAN_POINT('Ctrl Pts',(81.6526323147927,-8.78853282324315,130.837152825602));
#78003=CARTESIAN_POINT('Ctrl Pts',(81.6501315873015,-8.76983109164512,130.838382462097));
#78004=CARTESIAN_POINT('Ctrl Pts',(81.6325665270246,-8.65354377805336,130.845989601109));
#78005=CARTESIAN_POINT('Ctrl Pts',(81.6091687584517,-8.5574111158663,130.852091928085));
#78006=CARTESIAN_POINT('Ctrl Pts',(81.5546416263406,-8.39697167087249,130.862457980312));
#78007=CARTESIAN_POINT('Ctrl Pts',(81.5276565773295,-8.33155519145757,130.866745363976));
#78008=CARTESIAN_POINT('Ctrl Pts',(81.4800461213261,-8.23420691757921,130.873469238923));
#78009=CARTESIAN_POINT('Ctrl Pts',(81.4623505494835,-8.20093425361032,130.875833686416));
#78010=CARTESIAN_POINT('Ctrl Pts',(81.4319356984658,-8.14814507655618,130.879739252365));
#78011=CARTESIAN_POINT('Ctrl Pts',(81.4199079247614,-8.12824429516696,130.881248666677));
#78012=CARTESIAN_POINT('Ctrl Pts',(81.4029979605197,-8.10154436312205,130.883334011098));
#78013=CARTESIAN_POINT('Ctrl Pts',(81.3984745951529,-8.09451968100571,130.883888458908));
#78014=CARTESIAN_POINT('Ctrl Pts',(81.3907978027002,-8.08279253905306,130.884824371434));
#78015=CARTESIAN_POINT('Ctrl Pts',(81.3876728141512,-8.07807147025708,130.885203984046));
#78016=CARTESIAN_POINT('Ctrl Pts',(81.3812325122673,-8.06844873248295,130.88598374448));
#78017=CARTESIAN_POINT('Ctrl Pts',(81.377915063145,-8.06354867027114,130.886384020439));
#78018=CARTESIAN_POINT('Ctrl Pts',(81.3691722055018,-8.05078201105671,130.887435104111));
#78019=CARTESIAN_POINT('Ctrl Pts',(81.3637051862832,-8.04294437312531,130.888088589271));
#78020=CARTESIAN_POINT('Ctrl Pts',(81.3403033530246,-8.01000262850932,130.890868655212));
#78021=CARTESIAN_POINT('Ctrl Pts',(81.3217415758271,-7.98535385856593,130.893031748975));
#78022=CARTESIAN_POINT('Ctrl Pts',(81.285084696454,-7.93938971865251,130.897205550448));
#78023=CARTESIAN_POINT('Ctrl Pts',(81.2671154623649,-7.91798562025579,130.899210828371));
#78024=CARTESIAN_POINT('Ctrl Pts',(81.1837249630317,-7.8235821568325,130.908305867638));
#78025=CARTESIAN_POINT('Ctrl Pts',(81.112471366274,-7.75598519805464,130.915503351778));
#78026=CARTESIAN_POINT('Ctrl Pts',(80.9782578558318,-7.64946555261912,130.927789459145));
#78027=CARTESIAN_POINT('Ctrl Pts',(80.9178753618898,-7.60772156917584,130.932942943766));
#78028=CARTESIAN_POINT('Ctrl Pts',(80.8397846694581,-7.5610319318352,130.939152342283));
#78029=CARTESIAN_POINT('Ctrl Pts',(80.8244956027776,-7.55221740760362,130.940347971198));
#78030=CARTESIAN_POINT('Ctrl Pts',(80.7996816476042,-7.53843215060789,130.942257135475));
#78031=CARTESIAN_POINT('Ctrl Pts',(80.7902440582646,-7.53330792133854,130.942976113034));
#78032=CARTESIAN_POINT('Ctrl Pts',(80.7721096005433,-7.52368750058408,130.944344317003));
#78033=CARTESIAN_POINT('Ctrl Pts',(80.7634213915043,-7.51917603437965,130.944994062325));
#78034=CARTESIAN_POINT('Ctrl Pts',(80.7435029479819,-7.50905501954871,130.946470856878));
#78035=CARTESIAN_POINT('Ctrl Pts',(80.732247980091,-7.50349524611999,130.947296141659));
#78036=CARTESIAN_POINT('Ctrl Pts',(80.7020458272479,-7.48899818728424,130.949487225157));
#78037=CARTESIAN_POINT('Ctrl Pts',(80.682990739516,-7.48028998357588,130.950845181426));
#78038=CARTESIAN_POINT('Ctrl Pts',(80.5520955391911,-7.42343014636041,130.960020689904));
#78039=CARTESIAN_POINT('Ctrl Pts',(80.4354321426459,-7.3873051455299,130.967412568938));
#78040=CARTESIAN_POINT('Ctrl Pts',(80.2514272741726,-7.3517745597988,130.978865153797));
#78041=CARTESIAN_POINT('Ctrl Pts',(80.1863171475013,-7.34315134885402,130.982887875269));
#78042=CARTESIAN_POINT('Ctrl Pts',(80.0986023530793,-7.3367705492934,130.988455299123));
#78043=CARTESIAN_POINT('Ctrl Pts',(80.0763019554807,-7.33559844323361,130.989883661545));
#78044=CARTESIAN_POINT('Ctrl Pts',(80.038058757277,-7.33435854068887,130.992365482683));
#78045=CARTESIAN_POINT('Ctrl Pts',(80.0221257547304,-7.33407072618035,130.993409066881));
#78046=CARTESIAN_POINT('Ctrl Pts',(79.9989775909897,-7.33398469388084,130.994942358131));
#78047=CARTESIAN_POINT('Ctrl Pts',(79.9917634494024,-7.33400474191033,130.995422626066));
#78048=CARTESIAN_POINT('Ctrl Pts',(79.979067267385,-7.33412248895304,130.996272462684));
#78049=CARTESIAN_POINT('Ctrl Pts',(79.973585239474,-7.33420039613402,130.996640936562));
#78050=CARTESIAN_POINT('Ctrl Pts',(79.9616716768041,-7.33442852931824,130.997445117796));
#78051=CARTESIAN_POINT('Ctrl Pts',(79.9552406947495,-7.33458894401272,130.99788134771));
#78052=CARTESIAN_POINT('Ctrl Pts',(79.9372100727314,-7.33514320966316,130.99911008477));
#78053=CARTESIAN_POINT('Ctrl Pts',(79.92561364928,-7.33562102893979,130.999906935883));
#78054=CARTESIAN_POINT('Ctrl Pts',(79.8372212372407,-7.34018873811724,131.006026392456));
#78055=CARTESIAN_POINT('Ctrl Pts',(79.760794240132,-7.34947030524099,131.011575748592));
#78056=CARTESIAN_POINT('Ctrl Pts',(79.6291675076378,-7.37479057317232,131.021318573695));
#78057=CARTESIAN_POINT('Ctrl Pts',(79.5736352839467,-7.38846786895871,131.025489219892));
#78058=CARTESIAN_POINT('Ctrl Pts',(79.4395576803271,-7.42890772652891,131.035609628235));
#78059=CARTESIAN_POINT('Ctrl Pts',(79.3620876943569,-7.45873492602896,131.041496341761));
#78060=CARTESIAN_POINT('Ctrl Pts',(79.2664930760454,-7.50398999017591,131.048767739415));
#78061=CARTESIAN_POINT('Ctrl Pts',(79.246038392162,-7.51419370682019,131.050324718605));
#78062=CARTESIAN_POINT('Ctrl Pts',(79.2153282633118,-7.53031088130757,131.052665130445));
#78063=CARTESIAN_POINT('Ctrl Pts',(79.2049158712771,-7.53591766600507,131.053459166687));
#78064=CARTESIAN_POINT('Ctrl Pts',(79.1868936858972,-7.54587108630127,131.054834704235));
#78065=CARTESIAN_POINT('Ctrl Pts',(79.1792569649429,-7.55016771620758,131.055417952201));
#78066=CARTESIAN_POINT('Ctrl Pts',(79.162113886921,-7.55999174534771,131.056728286416));
#78067=CARTESIAN_POINT('Ctrl Pts',(79.1526275785951,-7.56555345127182,131.057454107168));
#78068=CARTESIAN_POINT('Ctrl Pts',(79.1270319199945,-7.58090239872992,131.059415030927));
#78069=CARTESIAN_POINT('Ctrl Pts',(79.1110321679757,-7.59086994525747,131.060643544204));
#78070=CARTESIAN_POINT('Ctrl Pts',(79.0091997788899,-7.65673452824745,131.068488277696));
#78071=CARTESIAN_POINT('Ctrl Pts',(78.9285035260769,-7.72017720525288,131.074805814438));
#78072=CARTESIAN_POINT('Ctrl Pts',(78.7941286541876,-7.84749654549597,131.08612265459));
#78073=CARTESIAN_POINT('Ctrl Pts',(78.7384386361225,-7.90873871294369,131.091130846483));
#78074=CARTESIAN_POINT('Ctrl Pts',(78.6702836766794,-7.99591122926426,131.098074883096));
#78075=CARTESIAN_POINT('Ctrl Pts',(78.653599824774,-8.01839613359637,131.099851652771));
#78076=CARTESIAN_POINT('Ctrl Pts',(78.6266524900329,-8.05669337869112,131.10287387624));
#78077=CARTESIAN_POINT('Ctrl Pts',(78.6160762103203,-8.07227933281521,131.104102775823));
#78078=CARTESIAN_POINT('Ctrl Pts',(78.6015482732039,-8.09449010836787,131.105857639076));
#78079=CARTESIAN_POINT('Ctrl Pts',(78.5973744748722,-8.10096884008838,131.106369946345));
#78080=CARTESIAN_POINT('Ctrl Pts',(78.590274796018,-8.11215901988406,131.107255969064));
#78081=CARTESIAN_POINT('Ctrl Pts',(78.5873272327987,-8.11685651863825,131.10762826374));
#78082=CARTESIAN_POINT('Ctrl Pts',(78.5811559200268,-8.12680162410432,131.108417344547));
#78083=CARTESIAN_POINT('Ctrl Pts',(78.5779378438558,-8.13205233572931,131.108834448185));
#78084=CARTESIAN_POINT('Ctrl Pts',(78.5692311393943,-8.14643686832164,131.109978205508));
#78085=CARTESIAN_POINT('Ctrl Pts',(78.5638010279701,-8.15560551268972,131.110708417531));
#78086=CARTESIAN_POINT('Ctrl Pts',(78.5367500253487,-8.2022964846864,131.114430542781));
#78087=CARTESIAN_POINT('Ctrl Pts',(78.5165118726414,-8.24059651117372,131.117494917529));
#78088=CARTESIAN_POINT('Ctrl Pts',(78.4751020078549,-8.32695065359558,131.12436273958));
#78089=CARTESIAN_POINT('Ctrl Pts',(78.4546708836615,-8.37528983399627,131.128179703618));
#78090=CARTESIAN_POINT('Ctrl Pts',(78.4365594227781,-8.42449191013859,131.131996270822));
#78091=CARTESIAN_POINT('Origin',(80.,-9.,134.));
#78092=CARTESIAN_POINT('',(78.4365593750065,-8.42449203991615,131.833731407018));
#78093=CARTESIAN_POINT('',(78.4365593409241,-8.42449213250519,131.638964580993));
#78094=CARTESIAN_POINT('',(78.4365593749993,-8.42449203993574,134.));
#78095=CARTESIAN_POINT('Ctrl Pts',(78.4365593409241,-8.42449213250519,131.638964580993));
#78096=CARTESIAN_POINT('Ctrl Pts',(78.4458655786914,-8.39921054848143,131.637009426607));
#78097=CARTESIAN_POINT('Ctrl Pts',(78.45578681441,-8.37414987847205,131.635060102878));
#78098=CARTESIAN_POINT('Ctrl Pts',(78.4868519260182,-8.30092644683857,131.629339976712));
#78099=CARTESIAN_POINT('Ctrl Pts',(78.5096700688799,-8.25351589953718,131.625605512207));
#78100=CARTESIAN_POINT('Ctrl Pts',(78.5460367147342,-8.18629555394418,131.620279049753));
#78101=CARTESIAN_POINT('Ctrl Pts',(78.5578278365022,-8.16557582110753,131.618632423778));
#78102=CARTESIAN_POINT('Ctrl Pts',(78.5800172557813,-8.12846024571771,131.615673421396));
#78103=CARTESIAN_POINT('Ctrl Pts',(78.5902650070094,-8.1119798189514,131.614356053443));
#78104=CARTESIAN_POINT('Ctrl Pts',(78.6068326692018,-8.08634560308722,131.612300613037));
#78105=CARTESIAN_POINT('Ctrl Pts',(78.6129600127437,-8.07707007160663,131.611555520689));
#78106=CARTESIAN_POINT('Ctrl Pts',(78.6246201136149,-8.05979751678223,131.610165217369));
#78107=CARTESIAN_POINT('Ctrl Pts',(78.6301309035784,-8.0517863073952,131.609519219788));
#78108=CARTESIAN_POINT('Ctrl Pts',(78.6426719589249,-8.03389252008994,131.608073432858));
#78109=CARTESIAN_POINT('Ctrl Pts',(78.6497406821475,-8.02403746928345,131.607275150101));
#78110=CARTESIAN_POINT('Ctrl Pts',(78.6708760989417,-7.99524018386758,131.604935709937));
#78111=CARTESIAN_POINT('Ctrl Pts',(78.6852386309918,-7.97651806824382,131.603406005969));
#78112=CARTESIAN_POINT('Ctrl Pts',(78.7642767000292,-7.8778996173458,131.595286882628));
#78113=CARTESIAN_POINT('Ctrl Pts',(78.8358459349932,-7.80381022204583,131.58898361292));
#78114=CARTESIAN_POINT('Ctrl Pts',(78.9738804213262,-7.68511820104678,131.577865215615));
#78115=CARTESIAN_POINT('Ctrl Pts',(79.0375709331692,-7.63780908912981,131.573048674426));
#78116=CARTESIAN_POINT('Ctrl Pts',(79.1252629771434,-7.58190110541228,131.566491204802));
#78117=CARTESIAN_POINT('Ctrl Pts',(79.1464387070191,-7.56905544365617,131.564912614831));
#78118=CARTESIAN_POINT('Ctrl Pts',(79.1828054296177,-7.54808905865068,131.562196030298));
#78119=CARTESIAN_POINT('Ctrl Pts',(79.1978508139614,-7.53972298034343,131.561070575995));
#78120=CARTESIAN_POINT('Ctrl Pts',(79.2195800071615,-7.52807745154977,131.559438959644));
#78121=CARTESIAN_POINT('Ctrl Pts',(79.2261609327953,-7.52460701957523,131.558944006111));
#78122=CARTESIAN_POINT('Ctrl Pts',(79.2376550203745,-7.51864370112384,131.558077754094));
#78123=CARTESIAN_POINT('Ctrl Pts',(79.2425576551244,-7.51613092040974,131.557707698912));
#78124=CARTESIAN_POINT('Ctrl Pts',(79.2530910098671,-7.51079799368046,131.556911295267));
#78125=CARTESIAN_POINT('Ctrl Pts',(79.2587251890072,-7.5079854871808,131.556484524989));
#78126=CARTESIAN_POINT('Ctrl Pts',(79.2742412935967,-7.50034963484902,131.555307364634));
#78127=CARTESIAN_POINT('Ctrl Pts',(79.2841550317748,-7.49559218196858,131.554553172224));
#78128=CARTESIAN_POINT('Ctrl Pts',(79.3407539751862,-7.46911730288394,131.550238673728));
#78129=CARTESIAN_POINT('Ctrl Pts',(79.3883748931019,-7.44947725096099,131.546575858626));
#78130=CARTESIAN_POINT('Ctrl Pts',(79.527155106851,-7.39962932382511,131.535949581446));
#78131=CARTESIAN_POINT('Ctrl Pts',(79.6201227032875,-7.37504987889197,131.528899677945));
#78132=CARTESIAN_POINT('Ctrl Pts',(79.7665216443112,-7.34960268970617,131.518213422867));
#78133=CARTESIAN_POINT('Ctrl Pts',(79.818752213746,-7.34305294148303,131.514477205166));
#78134=CARTESIAN_POINT('Ctrl Pts',(79.8949812530474,-7.33714235290396,131.509148545286));
#78135=CARTESIAN_POINT('Ctrl Pts',(79.9187907712315,-7.3358096106454,131.507501424643));
#78136=CARTESIAN_POINT('Ctrl Pts',(79.9620192377495,-7.33431990755659,131.504541625467));
#78137=CARTESIAN_POINT('Ctrl Pts',(79.9814275835736,-7.33399044742003,131.503223951292));
#78138=CARTESIAN_POINT('Ctrl Pts',(80.0119550658292,-7.33400580258322,131.50116814413));
#78139=CARTESIAN_POINT('Ctrl Pts',(80.0230720345102,-7.33412266927534,131.500422987071));
#78140=CARTESIAN_POINT('Ctrl Pts',(80.0439083220803,-7.33455033143151,131.499032625192));
#78141=CARTESIAN_POINT('Ctrl Pts',(80.0536276446551,-7.33483495656921,131.498386633122));
#78142=CARTESIAN_POINT('Ctrl Pts',(80.0754613864867,-7.33566571254057,131.496940938652));
#78143=CARTESIAN_POINT('Ctrl Pts',(80.0875735394324,-7.33625905579204,131.496142741986));
#78144=CARTESIAN_POINT('Ctrl Pts',(80.1232226992481,-7.33839580778805,131.493803808395));
#78145=CARTESIAN_POINT('Ctrl Pts',(80.1467352532577,-7.34030690181749,131.492274517283));
#78146=CARTESIAN_POINT('Ctrl Pts',(80.2732026987212,-7.35329490145321,131.484107156664));
#78147=CARTESIAN_POINT('Ctrl Pts',(80.3749988433689,-7.37345254427141,131.477760068691));
#78148=CARTESIAN_POINT('Ctrl Pts',(80.5496839388112,-7.42532807027902,131.466631331814));
#78149=CARTESIAN_POINT('Ctrl Pts',(80.6234075954246,-7.45303349692442,131.461848397888));
#78150=CARTESIAN_POINT('Ctrl Pts',(80.717314455519,-7.49613012789184,131.455332470186));
#78151=CARTESIAN_POINT('Ctrl Pts',(80.7395037349128,-7.50691637277533,131.453759748105));
#78152=CARTESIAN_POINT('Ctrl Pts',(80.7767119634748,-7.52603623361309,131.451052281686));
#78153=CARTESIAN_POINT('Ctrl Pts',(80.7918568923749,-7.53411689940639,131.449929967366));
#78154=CARTESIAN_POINT('Ctrl Pts',(80.8133753906402,-7.54602898834544,131.448302108394));
#78155=CARTESIAN_POINT('Ctrl Pts',(80.8198529382876,-7.54967162918538,131.447807701658));
#78156=CARTESIAN_POINT('Ctrl Pts',(80.8310887136411,-7.55608937584467,131.446942066126));
#78157=CARTESIAN_POINT('Ctrl Pts',(80.8358578947802,-7.55884493575117,131.446572075076));
#78158=CARTESIAN_POINT('Ctrl Pts',(80.846054397116,-7.56480396040778,131.445775408652));
#78159=CARTESIAN_POINT('Ctrl Pts',(80.8514771436474,-7.56801453028059,131.445348307929));
#78160=CARTESIAN_POINT('Ctrl Pts',(80.8663297020705,-7.57692226954918,131.444169368613));
#78161=CARTESIAN_POINT('Ctrl Pts',(80.8757212192001,-7.58268221290394,131.443413709574));
#78162=CARTESIAN_POINT('Ctrl Pts',(80.9291293800028,-7.61617162121528,131.439060719835));
#78163=CARTESIAN_POINT('Ctrl Pts',(80.9718811358459,-7.64585512972602,131.435358744385));
#78164=CARTESIAN_POINT('Ctrl Pts',(81.0944626015655,-7.739764039765,131.424228053455));
#78165=CARTESIAN_POINT('Ctrl Pts',(81.1698458319262,-7.80940957006429,131.416700270466));
#78166=CARTESIAN_POINT('Ctrl Pts',(81.2870595185933,-7.93965356445614,131.404139782459));
#78167=CARTESIAN_POINT('Ctrl Pts',(81.3321685239625,-7.99691155836971,131.399023632875));
#78168=CARTESIAN_POINT('Ctrl Pts',(81.3833648212215,-8.07146987214609,131.39285139671));
#78169=CARTESIAN_POINT('Ctrl Pts',(81.3931074652497,-8.08615205937241,131.39165766225));
#78170=CARTESIAN_POINT('Ctrl Pts',(81.4084083175703,-8.11002402194833,131.389750649041));
#78171=CARTESIAN_POINT('Ctrl Pts',(81.4141135680451,-8.11911745589448,131.389031952547));
#78172=CARTESIAN_POINT('Ctrl Pts',(81.4248553339725,-8.13661179135328,131.387663731977));
#78173=CARTESIAN_POINT('Ctrl Pts',(81.4299064148513,-8.14500317349381,131.387013693947));
#78174=CARTESIAN_POINT('Ctrl Pts',(81.4412706341251,-8.16426501511268,131.385535477412));
#78175=CARTESIAN_POINT('Ctrl Pts',(81.4475353806834,-8.17516344538691,131.384709073121));
#78176=CARTESIAN_POINT('Ctrl Pts',(81.4639368455201,-8.20445863922648,131.382513311268));
#78177=CARTESIAN_POINT('Ctrl Pts',(81.4738502258437,-8.22297830189355,131.381151848116));
#78178=CARTESIAN_POINT('Ctrl Pts',(81.5384207042964,-8.34929003323565,131.372031869747));
#78179=CARTESIAN_POINT('Ctrl Pts',(81.5815596006821,-8.46256646799858,131.36469163028));
#78180=CARTESIAN_POINT('Ctrl Pts',(81.6360938151624,-8.67164530780132,131.351488360123));
#78181=CARTESIAN_POINT('Ctrl Pts',(81.6521779437584,-8.76564435143321,131.345654650789));
#78182=CARTESIAN_POINT('Ctrl Pts',(81.6611437627277,-8.87233346178025,131.338653936978));
#78183=CARTESIAN_POINT('Ctrl Pts',(81.662012479237,-8.88419048222527,131.337870598005));
#78184=CARTESIAN_POINT('Ctrl Pts',(81.6631549948394,-8.90246677499294,131.33665359572));
#78185=CARTESIAN_POINT('Ctrl Pts',(81.6635187004372,-8.90888031674602,131.336224710363));
#78186=CARTESIAN_POINT('Ctrl Pts',(81.6641242216537,-8.92077455626452,131.335425693152));
#78187=CARTESIAN_POINT('Ctrl Pts',(81.6643760691832,-8.92625453822107,131.3350561157));
#78188=CARTESIAN_POINT('Ctrl Pts',(81.6648922226903,-8.93884074479375,131.334204006438));
#78189=CARTESIAN_POINT('Ctrl Pts',(81.665138099408,-8.94594749838666,131.333720489071));
#78190=CARTESIAN_POINT('Ctrl Pts',(81.6657831315884,-8.96882974464267,131.332156478196));
#78191=CARTESIAN_POINT('Ctrl Pts',(81.6660036296677,-8.98460886358292,131.331066979627));
#78192=CARTESIAN_POINT('Ctrl Pts',(81.6659801411667,-9.08546423598645,131.324042817735));
#78193=CARTESIAN_POINT('Ctrl Pts',(81.6594435855025,-9.17040600857637,131.317858820687));
#78194=CARTESIAN_POINT('Ctrl Pts',(81.6351141222184,-9.32782176743634,131.306264204932));
#78195=CARTESIAN_POINT('Ctrl Pts',(81.618886649581,-9.40034081569565,131.300867342512));
#78196=CARTESIAN_POINT('Ctrl Pts',(81.5862231349415,-9.51102550919333,131.292648286159));
#78197=CARTESIAN_POINT('Ctrl Pts',(81.5731103827957,-9.5500682614269,131.28975159488));
#78198=CARTESIAN_POINT('Ctrl Pts',(81.5481723112403,-9.61610355189692,131.284860823126));
#78199=CARTESIAN_POINT('Ctrl Pts',(81.5370537016945,-9.6433406563753,131.282846009276));
#78200=CARTESIAN_POINT('Ctrl Pts',(81.5199730613387,-9.68220811855459,131.279972728956));
#78201=CARTESIAN_POINT('Ctrl Pts',(81.5145869422515,-9.69408388207942,131.279095046393));
#78202=CARTESIAN_POINT('Ctrl Pts',(81.5048969265439,-9.71479917633505,131.277564116494));
#78203=CARTESIAN_POINT('Ctrl Pts',(81.5006532446356,-9.72366599235934,131.276908841072));
#78204=CARTESIAN_POINT('Ctrl Pts',(81.4916623041498,-9.7420325712057,131.275551298613));
#78205=CARTESIAN_POINT('Ctrl Pts',(81.4869021803769,-9.75152556919881,131.274849514543));
#78206=CARTESIAN_POINT('Ctrl Pts',(81.4742495990483,-9.77616742562916,131.273027057211));
#78207=CARTESIAN_POINT('Ctrl Pts',(81.4662142349603,-9.79124181218071,131.271911429947));
#78208=CARTESIAN_POINT('Ctrl Pts',(81.4305063555684,-9.85581742277738,131.267125201772));
#78209=CARTESIAN_POINT('Ctrl Pts',(81.4005467730613,-9.90401418610575,131.263536343956));
#78210=CARTESIAN_POINT('Ctrl Pts',(81.3075764453768,-10.0378259725601,131.253388422396));
#78211=CARTESIAN_POINT('Ctrl Pts',(81.2387666897964,-10.1190601862772,131.247007538993));
#78212=CARTESIAN_POINT('Ctrl Pts',(81.1198762639925,-10.234911750383,131.236765125093));
#78213=CARTESIAN_POINT('Ctrl Pts',(81.0748501724917,-10.2742941017695,131.233025046109));
#78214=CARTESIAN_POINT('Ctrl Pts',(81.0163647980167,-10.3201401884637,131.228192440881));
#78215=CARTESIAN_POINT('Ctrl Pts',(81.0048021391684,-10.3289620557987,131.227238143958));
#78216=CARTESIAN_POINT('Ctrl Pts',(80.9875399316191,-10.3417784048487,131.225812614709));
#78217=CARTESIAN_POINT('Ctrl Pts',(80.9819281036176,-10.3458906342102,131.225349056806));
#78218=CARTESIAN_POINT('Ctrl Pts',(80.9722885688292,-10.3528619051586,131.224552264536));
#78219=CARTESIAN_POINT('Ctrl Pts',(80.9682736457543,-10.3557383749834,131.224220229837));
#78220=CARTESIAN_POINT('Ctrl Pts',(80.9590293973587,-10.3622993556297,131.223455284448));
#78221=CARTESIAN_POINT('Ctrl Pts',(80.9537917167311,-10.3659715505825,131.223021579553));
#78222=CARTESIAN_POINT('Ctrl Pts',(80.9391290419711,-10.3761262647808,131.221806911243));
#78223=CARTESIAN_POINT('Ctrl Pts',(80.9296584465635,-10.3825418651067,131.221021755724));
#78224=CARTESIAN_POINT('Ctrl Pts',(80.8664827686277,-10.4243959175322,131.215784141136));
#78225=CARTESIAN_POINT('Ctrl Pts',(80.8108346402948,-10.4567914972086,131.211172226164));
#78226=CARTESIAN_POINT('Ctrl Pts',(80.7325963960003,-10.4964644114896,131.204816264652));
#78227=CARTESIAN_POINT('Ctrl Pts',(80.711512535999,-10.5066031662938,131.203115255327));
#78228=CARTESIAN_POINT('Ctrl Pts',(80.6268215987685,-10.5451547711884,131.196343033857));
#78229=CARTESIAN_POINT('Ctrl Pts',(80.5616695724448,-10.570011748226,131.191270542404));
#78230=CARTESIAN_POINT('Ctrl Pts',(80.4510957057507,-10.6044305789594,131.18298462564));
#78231=CARTESIAN_POINT('Ctrl Pts',(80.406487887433,-10.6163084627075,131.17972436833));
#78232=CARTESIAN_POINT('Ctrl Pts',(80.3302571408869,-10.6332503440041,131.174299005777));
#78233=CARTESIAN_POINT('Ctrl Pts',(80.2988786767481,-10.6392828445552,131.172106551839));
#78234=CARTESIAN_POINT('Ctrl Pts',(80.2540607244863,-10.6465692401506,131.169030759013));
#78235=CARTESIAN_POINT('Ctrl Pts',(80.2407512512279,-10.6485678535705,131.168124238321));
#78236=CARTESIAN_POINT('Ctrl Pts',(80.217616082208,-10.6517557798064,131.166560018261));
#78237=CARTESIAN_POINT('Ctrl Pts',(80.2078014727354,-10.6530191984851,131.165900017342));
#78238=CARTESIAN_POINT('Ctrl Pts',(80.1875911714186,-10.655437990949,131.164548068667));
#78239=CARTESIAN_POINT('Ctrl Pts',(80.1771946705243,-10.6565830636122,131.163856472428));
#78240=CARTESIAN_POINT('Ctrl Pts',(80.1505403861338,-10.6592649714502,131.162092850528));
#78241=CARTESIAN_POINT('Ctrl Pts',(80.1342692930381,-10.660660844725,131.161025264474));
#78242=CARTESIAN_POINT('Ctrl Pts',(80.0675438935439,-10.6653979784359,131.156681027819));
#78243=CARTESIAN_POINT('Ctrl Pts',(80.0169679475903,-10.6666809673076,131.15346824237));
#78244=CARTESIAN_POINT('Ctrl Pts',(79.8572490463909,-10.6634598483811,131.143473349963));
#78245=CARTESIAN_POINT('Ctrl Pts',(79.7485734331196,-10.6505336684615,131.136911382521));
#78246=CARTESIAN_POINT('Ctrl Pts',(79.5796315275146,-10.6133558432963,131.126261859302));
#78247=CARTESIAN_POINT('Ctrl Pts',(79.5181659521544,-10.5960767188038,131.122283197339));
#78248=CARTESIAN_POINT('Ctrl Pts',(79.4436751154021,-10.5704404921533,131.117164532706));
#78249=CARTESIAN_POINT('Ctrl Pts',(79.4295675978083,-10.565371378551,131.116181545578));
#78250=CARTESIAN_POINT('Ctrl Pts',(79.4089367853213,-10.5576424053649,131.114721284565));
#78251=CARTESIAN_POINT('Ctrl Pts',(79.4023584382069,-10.5551302665283,131.114252232981));
#78252=CARTESIAN_POINT('Ctrl Pts',(79.3911848610749,-10.5507819360683,131.113449349733));
#78253=CARTESIAN_POINT('Ctrl Pts',(79.3865815679417,-10.548966853394,131.113116771407));
#78254=CARTESIAN_POINT('Ctrl Pts',(79.3761006664735,-10.5447801753478,131.112355345465));
#78255=CARTESIAN_POINT('Ctrl Pts',(79.3702285937258,-10.5423955851238,131.111925745568));
#78256=CARTESIAN_POINT('Ctrl Pts',(79.354039481854,-10.5357134886961,131.1107333257));
#78257=CARTESIAN_POINT('Ctrl Pts',(79.3437520859572,-10.531345672533,131.10996654682));
#78258=CARTESIAN_POINT('Ctrl Pts',(79.2833788371888,-10.5049923790786,131.105416241671));
#78259=CARTESIAN_POINT('Ctrl Pts',(79.2343610308612,-10.4806564974867,131.101517260273));
#78260=CARTESIAN_POINT('Ctrl Pts',(79.1002965325023,-10.4056587834121,131.090429413026));
#78261=CARTESIAN_POINT('Ctrl Pts',(79.0184266620057,-10.349762345456,131.08316342681));
#78262=CARTESIAN_POINT('Ctrl Pts',(78.8854050424377,-10.2404039613561,131.070816219604));
#78263=CARTESIAN_POINT('Ctrl Pts',(78.8319340291888,-10.1901884186516,131.065666602184));
#78264=CARTESIAN_POINT('Ctrl Pts',(78.7698978622216,-10.123706419606,131.059460863011));
#78265=CARTESIAN_POINT('Ctrl Pts',(78.7580643443188,-10.1106139093169,131.058265245751));
#78266=CARTESIAN_POINT('Ctrl Pts',(78.7393663531112,-10.0892539484748,131.056355968303));
#78267=CARTESIAN_POINT('Ctrl Pts',(78.7323702141229,-10.0811041074925,131.055636867204));
#78268=CARTESIAN_POINT('Ctrl Pts',(78.7191470513043,-10.0653955200778,131.054268340989));
#78269=CARTESIAN_POINT('Ctrl Pts',(78.7129069295663,-10.0578484416075,131.053618397522));
#78270=CARTESIAN_POINT('Ctrl Pts',(78.6988167754124,-10.0404979239043,131.052141028486));
#78271=CARTESIAN_POINT('Ctrl Pts',(78.6910102619647,-10.0306597856117,131.051315369808));
#78272=CARTESIAN_POINT('Ctrl Pts',(78.6665038325572,-9.99904799294626,131.048699381254));
#78273=CARTESIAN_POINT('Ctrl Pts',(78.6502297194569,-9.97694894903163,131.04692566924));
#78274=CARTESIAN_POINT('Ctrl Pts',(78.558979137228,-9.84640148887605,131.036736927588));
#78275=CARTESIAN_POINT('Ctrl Pts',(78.4965433845736,-9.72976528600962,131.028809827571));
#78276=CARTESIAN_POINT('Ctrl Pts',(78.4224131503897,-9.54028274575061,131.016327503265));
#78277=CARTESIAN_POINT('Ctrl Pts',(78.4006499410546,-9.47197748760387,131.011888444127));
#78278=CARTESIAN_POINT('Ctrl Pts',(78.379533148169,-9.3871599883793,131.006217717961));
#78279=CARTESIAN_POINT('Ctrl Pts',(78.3759342246032,-9.37177410770109,131.005182747008));
#78280=CARTESIAN_POINT('Ctrl Pts',(78.3710167274966,-9.3493153451493,131.003659749694));
#78281=CARTESIAN_POINT('Ctrl Pts',(78.3695241519386,-9.34228090303748,131.003180983918));
#78282=CARTESIAN_POINT('Ctrl Pts',(78.3669840164233,-9.32991561272275,131.002335996631));
#78283=CARTESIAN_POINT('Ctrl Pts',(78.3659169202432,-9.3245889728867,131.001970880914));
#78284=CARTESIAN_POINT('Ctrl Pts',(78.3636434814905,-9.31294520742212,131.001170226983));
#78285=CARTESIAN_POINT('Ctrl Pts',(78.3624476755718,-9.30662638468164,131.000734139032));
#78286=CARTESIAN_POINT('Ctrl Pts',(78.3591989068843,-9.28889818600297,130.999506490884));
#78287=CARTESIAN_POINT('Ctrl Pts',(78.3572284503758,-9.27747433401644,130.998710599833));
#78288=CARTESIAN_POINT('Ctrl Pts',(78.3438152459265,-9.19455302981011,130.992903208467));
#78289=CARTESIAN_POINT('Ctrl Pts',(78.3369264852316,-9.12240479457994,130.987690481246));
#78290=CARTESIAN_POINT('Ctrl Pts',(78.3342650542894,-9.03384832452713,130.981256601982));
#78291=CARTESIAN_POINT('Ctrl Pts',(78.3340146152127,-9.01764398355277,130.980077686109));
#78292=CARTESIAN_POINT('Ctrl Pts',(78.333889406962,-8.87265096241319,130.969524597057));
#78293=CARTESIAN_POINT('Ctrl Pts',(78.3487122814742,-8.74425940938005,130.960198804359));
#78294=CARTESIAN_POINT('Ctrl Pts',(78.3828536587066,-8.59898927122409,130.949942217047));
#78295=CARTESIAN_POINT('Ctrl Pts',(78.3878837061593,-8.57922332198349,130.948551940134));
#78296=CARTESIAN_POINT('Ctrl Pts',(78.3965884154774,-8.54746899448516,130.946326160262));
#78297=CARTESIAN_POINT('Ctrl Pts',(78.4000375342468,-8.53542154225168,130.945483516037));
#78298=CARTESIAN_POINT('Ctrl Pts',(78.4064150735652,-8.51405927323683,130.943992239616));
#78299=CARTESIAN_POINT('Ctrl Pts',(78.4092900336537,-8.50472924816484,130.943341905896));
#78300=CARTESIAN_POINT('Ctrl Pts',(78.4155376869815,-8.48506967678336,130.941973412031));
#78301=CARTESIAN_POINT('Ctrl Pts',(78.4189297690752,-8.47474673399138,130.941255920823));
#78302=CARTESIAN_POINT('Ctrl Pts',(78.4269651601825,-8.45107643519932,130.939612795179));
#78303=CARTESIAN_POINT('Ctrl Pts',(78.4316777696174,-8.43775354229633,130.938689485125));
#78304=CARTESIAN_POINT('Ctrl Pts',(78.4365593749572,-8.42449204005001,130.937771468334));
#78305=CARTESIAN_POINT('Ctrl Pts',(78.4365594227781,-8.42449191013859,131.131996270822));
#78306=CARTESIAN_POINT('Ctrl Pts',(78.4235761673907,-8.45976256689324,131.134732188538));
#78307=CARTESIAN_POINT('Ctrl Pts',(78.4117849555462,-8.49547663369563,131.13746816417));
#78308=CARTESIAN_POINT('Ctrl Pts',(78.3772965578482,-8.61318938570139,131.146340231324));
#78309=CARTESIAN_POINT('Ctrl Pts',(78.3596657873488,-8.69652602544283,131.152387296996));
#78310=CARTESIAN_POINT('Ctrl Pts',(78.3454336264977,-8.80378322644139,131.159828485104));
#78311=CARTESIAN_POINT('Ctrl Pts',(78.342869015249,-8.82677211793479,131.161404455124));
#78312=CARTESIAN_POINT('Ctrl Pts',(78.3397128484832,-8.86163924033204,131.163767284688));
#78313=CARTESIAN_POINT('Ctrl Pts',(78.3387684394046,-8.87348185874766,131.164565058941));
#78314=CARTESIAN_POINT('Ctrl Pts',(78.33734731046,-8.89408066677514,131.16594472061));
#78315=CARTESIAN_POINT('Ctrl Pts',(78.3368129066966,-8.9028322641114,131.166528387983));
#78316=CARTESIAN_POINT('Ctrl Pts',(78.3357660830759,-8.92253034850817,131.167836685924));
#78317=CARTESIAN_POINT('Ctrl Pts',(78.3352925225985,-8.93347856370225,131.168560077128));
#78318=CARTESIAN_POINT('Ctrl Pts',(78.3343042584106,-8.96309090897862,131.170507039486));
#78319=CARTESIAN_POINT('Ctrl Pts',(78.333995210254,-8.98176069142106,131.171724185505));
#78320=CARTESIAN_POINT('Ctrl Pts',(78.334025399594,-9.09808660637892,131.17925069829));
#78321=CARTESIAN_POINT('Ctrl Pts',(78.3426363912761,-9.19555512328972,131.185291057286));
#78322=CARTESIAN_POINT('Ctrl Pts',(78.3768931288007,-9.38817213921979,131.197262568064));
#78323=CARTESIAN_POINT('Ctrl Pts',(78.4025200085894,-9.48291617632865,131.203173327976));
#78324=CARTESIAN_POINT('Ctrl Pts',(78.4474708800055,-9.60518932489194,131.211423092386));
#78325=CARTESIAN_POINT('Ctrl Pts',(78.4595036544767,-9.63519404434482,131.213500940887));
#78326=CARTESIAN_POINT('Ctrl Pts',(78.4762762779447,-9.67373314656306,131.216263628589));
#78327=CARTESIAN_POINT('Ctrl Pts',(78.4802298261564,-9.68260452784972,131.21690617709));
#78328=CARTESIAN_POINT('Ctrl Pts',(78.4867307953796,-9.69685560833873,131.217949862233));
#78329=CARTESIAN_POINT('Ctrl Pts',(78.4892299457115,-9.70225726396787,131.218348141172));
#78330=CARTESIAN_POINT('Ctrl Pts',(78.4941536457533,-9.71275140764668,131.219127370169));
#78331=CARTESIAN_POINT('Ctrl Pts',(78.4965751935204,-9.71784514993842,131.219508141732));
#78332=CARTESIAN_POINT('Ctrl Pts',(78.5025999086656,-9.73035397842765,131.220449321646));
#78333=CARTESIAN_POINT('Ctrl Pts',(78.5062323140834,-9.73775474295358,131.221011476393));
#78334=CARTESIAN_POINT('Ctrl Pts',(78.51995583963,-9.76519856179563,131.223115091475));
#78335=CARTESIAN_POINT('Ctrl Pts',(78.5303961715476,-9.7850630686603,131.224675703936));
#78336=CARTESIAN_POINT('Ctrl Pts',(78.6115818772415,-9.93223539752564,131.236492773686));
#78337=CARTESIAN_POINT('Ctrl Pts',(78.6983472001639,-10.0499863844994,131.247328008473));
#78338=CARTESIAN_POINT('Ctrl Pts',(78.8443874629582,-10.2018074825112,131.262368685855));
#78339=CARTESIAN_POINT('Ctrl Pts',(78.8921595598234,-10.2459827527107,131.266922037966));
#78340=CARTESIAN_POINT('Ctrl Pts',(78.9560088661246,-10.298440930226,131.27256140148));
#78341=CARTESIAN_POINT('Ctrl Pts',(78.9697973586504,-10.3094078417488,131.273754960245));
#78342=CARTESIAN_POINT('Ctrl Pts',(78.992261899242,-10.3267008322504,131.275661634988));
#78343=CARTESIAN_POINT('Ctrl Pts',(79.0008293452605,-10.3331651023197,131.276380167694));
#78344=CARTESIAN_POINT('Ctrl Pts',(79.0173313533483,-10.3453676807137,131.277748035452));
#78345=CARTESIAN_POINT('Ctrl Pts',(79.0252551776222,-10.3511196851692,131.278397884586));
#78346=CARTESIAN_POINT('Ctrl Pts',(79.0436370499541,-10.3642174392655,131.279889757032));
#78347=CARTESIAN_POINT('Ctrl Pts',(79.0541299186394,-10.3715134407402,131.280729854853));
#78348=CARTESIAN_POINT('Ctrl Pts',(79.0878176531082,-10.3943670044879,131.283391730513));
#78349=CARTESIAN_POINT('Ctrl Pts',(79.1113209476974,-10.4094628994058,131.285196291933));
#78350=CARTESIAN_POINT('Ctrl Pts',(79.1999437245756,-10.46328565117,131.291825258049));
#78351=CARTESIAN_POINT('Ctrl Pts',(79.2673038185802,-10.4981498450688,131.296516757853));
#78352=CARTESIAN_POINT('Ctrl Pts',(79.416482708141,-10.5628841241907,131.306483853868));
#78353=CARTESIAN_POINT('Ctrl Pts',(79.4987338297728,-10.5911725396823,131.311728429494));
#78354=CARTESIAN_POINT('Ctrl Pts',(79.6291678118446,-10.6249099219855,131.320132968678));
#78355=CARTESIAN_POINT('Ctrl Pts',(79.6760158950084,-10.6348951472366,131.323170146666));
#78356=CARTESIAN_POINT('Ctrl Pts',(79.7340106057263,-10.6446657105387,131.327024088314));
#78357=CARTESIAN_POINT('Ctrl Pts',(79.7448146754482,-10.6463766554863,131.327746036344));
#78358=CARTESIAN_POINT('Ctrl Pts',(79.7617870313953,-10.6488933465009,131.328887510982));
#78359=CARTESIAN_POINT('Ctrl Pts',(79.7679445454255,-10.6497711809184,131.329303147153));
#78360=CARTESIAN_POINT('Ctrl Pts',(79.7795826196477,-10.6513638986268,131.330091826584));
#78361=CARTESIAN_POINT('Ctrl Pts',(79.7850620002083,-10.6520860146524,131.330464467462));
#78362=CARTESIAN_POINT('Ctrl Pts',(79.7980641877281,-10.6537337686017,131.331351745269));
#78363=CARTESIAN_POINT('Ctrl Pts',(79.8055898381186,-10.6546353474618,131.331867684759));
#78364=CARTESIAN_POINT('Ctrl Pts',(79.8310594385515,-10.6575104728943,131.333621283196));
#78365=CARTESIAN_POINT('Ctrl Pts',(79.8490285195014,-10.6592436310399,131.334870975461));
#78366=CARTESIAN_POINT('Ctrl Pts',(79.8933524806792,-10.6627928567919,131.337978705836));
#78367=CARTESIAN_POINT('Ctrl Pts',(79.9197286972502,-10.6642746593209,131.339849842052));
#78368=CARTESIAN_POINT('Ctrl Pts',(80.0360758048018,-10.6680388818661,131.348170062387));
#78369=CARTESIAN_POINT('Ctrl Pts',(80.1261097839662,-10.6636559212747,131.354774159003));
#78370=CARTESIAN_POINT('Ctrl Pts',(80.3122473496333,-10.639392174998,131.368373760117));
#78371=CARTESIAN_POINT('Ctrl Pts',(80.4078616449494,-10.6182583080106,131.375324199531));
#78372=CARTESIAN_POINT('Ctrl Pts',(80.5188754329337,-10.583247373121,131.383283266209));
#78373=CARTESIAN_POINT('Ctrl Pts',(80.5365704813197,-10.5773383045695,131.384549040968));
#78374=CARTESIAN_POINT('Ctrl Pts',(80.5645920115753,-10.567454672806,131.386549670926));
#78375=CARTESIAN_POINT('Ctrl Pts',(80.574984154071,-10.5636724476731,131.387290786442));
#78376=CARTESIAN_POINT('Ctrl Pts',(80.5935342361823,-10.556711195946,131.388612428773));
#78377=CARTESIAN_POINT('Ctrl Pts',(80.6017061452099,-10.5535708406523,131.389194214383));
#78378=CARTESIAN_POINT('Ctrl Pts',(80.6207784810072,-10.5460685340735,131.390551208275));
#78379=CARTESIAN_POINT('Ctrl Pts',(80.6316583985691,-10.5416554458963,131.39132467192));
#78380=CARTESIAN_POINT('Ctrl Pts',(80.6631859808786,-10.5284774979807,131.393564847808));
#78381=CARTESIAN_POINT('Ctrl Pts',(80.6837049159427,-10.5194100080589,131.395021327691));
#78382=CARTESIAN_POINT('Ctrl Pts',(80.7761932494394,-10.4762854738253,131.401589414786));
#78383=CARTESIAN_POINT('Ctrl Pts',(80.8458510199626,-10.4375092917663,131.406538348014));
#78384=CARTESIAN_POINT('Ctrl Pts',(80.9505202713853,-10.3689904747214,131.414216655985));
#78385=CARTESIAN_POINT('Ctrl Pts',(80.9875301199682,-10.3425379004362,131.416985736688));
#78386=CARTESIAN_POINT('Ctrl Pts',(81.0913849026212,-10.2616875882799,131.425031432797));
#78387=CARTESIAN_POINT('Ctrl Pts',(81.1551434834546,-10.2035848077741,131.430320106844));
#78388=CARTESIAN_POINT('Ctrl Pts',(81.2249261328506,-10.1293188931778,131.436931767804));
#78389=CARTESIAN_POINT('Ctrl Pts',(81.2355712479461,-10.1176622210156,131.437965763383));
#78390=CARTESIAN_POINT('Ctrl Pts',(81.2507687089481,-10.100538141771,131.439482453151));
#78391=CARTESIAN_POINT('Ctrl Pts',(81.2554545663262,-10.0951896603187,131.439955855419));
#78392=CARTESIAN_POINT('Ctrl Pts',(81.2636936620114,-10.0856631195614,131.440798854115));
#78393=CARTESIAN_POINT('Ctrl Pts',(81.2672607192338,-10.081497271752,131.441167430399));
#78394=CARTESIAN_POINT('Ctrl Pts',(81.2749591810721,-10.0724161097713,131.441970865179));
#78395=CARTESIAN_POINT('Ctrl Pts',(81.2790826974783,-10.0674945786423,131.44240623731));
#78396=CARTESIAN_POINT('Ctrl Pts',(81.2907536941616,-10.0534002121502,131.443652622143));
#78397=CARTESIAN_POINT('Ctrl Pts',(81.2982314766246,-10.0441705410988,131.444468286287));
#78398=CARTESIAN_POINT('Ctrl Pts',(81.364718549674,-9.96028866936057,131.451870606439));
#78399=CARTESIAN_POINT('Ctrl Pts',(81.417323390191,-9.88079602607164,131.458799941915));
#78400=CARTESIAN_POINT('Ctrl Pts',(81.5207126166027,-9.69109221364698,131.474526837408));
#78401=CARTESIAN_POINT('Ctrl Pts',(81.5668546688677,-9.57892302507623,131.483257135814));
#78402=CARTESIAN_POINT('Ctrl Pts',(81.6062809044694,-9.44255906873708,131.493021805051));
#78403=CARTESIAN_POINT('Ctrl Pts',(81.6117311683976,-9.42227903554291,131.494454147757));
#78404=CARTESIAN_POINT('Ctrl Pts',(81.6198283065318,-9.38970523881117,131.496724060969));
#78405=CARTESIAN_POINT('Ctrl Pts',(81.622721789246,-9.37747572839121,131.497569437401));
#78406=CARTESIAN_POINT('Ctrl Pts',(81.6276230902474,-9.35566127757586,131.499065587766));
#78407=CARTESIAN_POINT('Ctrl Pts',(81.6296852686911,-9.34608929529792,131.499718072435));
#78408=CARTESIAN_POINT('Ctrl Pts',(81.6338305478312,-9.32598912190236,131.501080070041));
#78409=CARTESIAN_POINT('Ctrl Pts',(81.6358965527004,-9.31545783328286,131.50178901126));
#78410=CARTESIAN_POINT('Ctrl Pts',(81.6410843510511,-9.2875906866489,131.503653142698));
#78411=CARTESIAN_POINT('Ctrl Pts',(81.6440332810671,-9.27022372137051,131.504802837899));
#78412=CARTESIAN_POINT('Ctrl Pts',(81.6577496825342,-9.18088135407764,131.510660690822));
#78413=CARTESIAN_POINT('Ctrl Pts',(81.6640689195304,-9.10829878055827,131.51522713665));
#78414=CARTESIAN_POINT('Ctrl Pts',(81.6678057759094,-8.9331077850239,131.526045686722));
#78415=CARTESIAN_POINT('Ctrl Pts',(81.6605390429065,-8.83070946241532,131.532196929265));
#78416=CARTESIAN_POINT('Ctrl Pts',(81.6354696537977,-8.67828090631664,131.541803043561));
#78417=CARTESIAN_POINT('Ctrl Pts',(81.6246237696407,-8.62735992939889,131.545093133628));
#78418=CARTESIAN_POINT('Ctrl Pts',(81.6086178020925,-8.56638020405897,131.549222479066));
#78419=CARTESIAN_POINT('Ctrl Pts',(81.6057154340369,-8.55575312092573,131.549949213593));
#78420=CARTESIAN_POINT('Ctrl Pts',(81.6009877848167,-8.53909457336029,131.551100746918));
#78421=CARTESIAN_POINT('Ctrl Pts',(81.5992332453044,-8.53304312482268,131.551521632101));
#78422=CARTESIAN_POINT('Ctrl Pts',(81.5958810622113,-8.52172188209529,131.552314124717));
#78423=CARTESIAN_POINT('Ctrl Pts',(81.5942915669891,-8.516449879853,131.552685267818));
#78424=CARTESIAN_POINT('Ctrl Pts',(81.5904964731112,-8.50408453429794,131.553560636681));
#78425=CARTESIAN_POINT('Ctrl Pts',(81.5882695383499,-8.49699796383648,131.554066064633));
#78426=CARTESIAN_POINT('Ctrl Pts',(81.5807435135289,-8.47359693470009,131.555746979429));
#78427=CARTESIAN_POINT('Ctrl Pts',(81.5752400472542,-8.45735003999213,131.556933232162));
#78428=CARTESIAN_POINT('Ctrl Pts',(81.5612194476903,-8.41797132363961,131.559850737597));
#78429=CARTESIAN_POINT('Ctrl Pts',(81.5524380276693,-8.39493836296873,131.561593232655));
#78430=CARTESIAN_POINT('Ctrl Pts',(81.5135494387733,-8.29936286523725,131.568952897489));
#78431=CARTESIAN_POINT('Ctrl Pts',(81.478843571217,-8.22880279889845,131.574697108613));
#78432=CARTESIAN_POINT('Ctrl Pts',(81.3870631378972,-8.07136297374987,131.587943537972));
#78433=CARTESIAN_POINT('Ctrl Pts',(81.3265750604024,-7.9868286864708,131.595380353435));
#78434=CARTESIAN_POINT('Ctrl Pts',(81.2431564103606,-7.89064240074824,131.604145006203));
#78435=CARTESIAN_POINT('Ctrl Pts',(81.2273281456317,-7.8731557936916,131.605753245688));
#78436=CARTESIAN_POINT('Ctrl Pts',(81.2028085054054,-7.84719703572044,131.60816472492));
#78437=CARTESIAN_POINT('Ctrl Pts',(81.1943876600075,-7.83847466397561,131.608979297008));
#78438=CARTESIAN_POINT('Ctrl Pts',(81.1790447382035,-7.8229256636898,131.61043954062));
#78439=CARTESIAN_POINT('Ctrl Pts',(81.1721567735728,-7.81606630552004,131.61108665575));
#78440=CARTESIAN_POINT('Ctrl Pts',(81.1572659430072,-7.80149466126838,131.612467948047));
#78441=CARTESIAN_POINT('Ctrl Pts',(81.1492451103219,-7.79380134460412,131.613201279828));
#78442=CARTESIAN_POINT('Ctrl Pts',(81.1270125253147,-7.7728996904679,131.615205459814));
#78443=CARTESIAN_POINT('Ctrl Pts',(81.1126458151924,-7.75985817632879,131.616469202088));
#78444=CARTESIAN_POINT('Ctrl Pts',(81.0801308284989,-7.73136239645004,131.619263548815));
#78445=CARTESIAN_POINT('Ctrl Pts',(81.0618719698616,-7.7160405067067,131.620788851588));
#78446=CARTESIAN_POINT('Ctrl Pts',(81.0022999140359,-7.66819105936158,131.625637333851));
#78447=CARTESIAN_POINT('Ctrl Pts',(80.9597724559267,-7.63722429268645,131.628906612746));
#78448=CARTESIAN_POINT('Ctrl Pts',(80.8356512413603,-7.55554158194246,131.638053474279));
#78449=CARTESIAN_POINT('Ctrl Pts',(80.7510454521757,-7.5097978437155,131.643830285086));
#78450=CARTESIAN_POINT('Ctrl Pts',(80.6156941667761,-7.45108656384421,131.653008226286));
#78451=CARTESIAN_POINT('Ctrl Pts',(80.5674915627972,-7.4327845247519,131.656267849422));
#78452=CARTESIAN_POINT('Ctrl Pts',(80.5080786521613,-7.41332647039939,131.660362902791));
#78453=CARTESIAN_POINT('Ctrl Pts',(80.4976001181492,-7.41000914692264,131.661088009249));
#78454=CARTESIAN_POINT('Ctrl Pts',(80.4810698832316,-7.40495536264248,131.662237522514));
#78455=CARTESIAN_POINT('Ctrl Pts',(80.475039631697,-7.40314904491215,131.662658038131));
#78456=CARTESIAN_POINT('Ctrl Pts',(80.4637142778653,-7.39982644524963,131.663450251357));
#78457=CARTESIAN_POINT('Ctrl Pts',(80.4584217175928,-7.39830219388272,131.663821488933));
#78458=CARTESIAN_POINT('Ctrl Pts',(80.4459637650599,-7.39478112073818,131.664697646789));
#78459=CARTESIAN_POINT('Ctrl Pts',(80.4387924570966,-7.39280601531959,131.665203775957));
#78460=CARTESIAN_POINT('Ctrl Pts',(80.4149835504506,-7.3864198436843,131.666889468489));
#78461=CARTESIAN_POINT('Ctrl Pts',(80.398291452127,-7.38221876341182,131.668079878854));
#78462=CARTESIAN_POINT('Ctrl Pts',(80.3574334262281,-7.37260621180815,131.671009743737));
#78463=CARTESIAN_POINT('Ctrl Pts',(80.3332065603375,-7.36747359805217,131.672760556846));
#78464=CARTESIAN_POINT('Ctrl Pts',(80.2310169164863,-7.34819342649752,131.680178911411));
#78465=CARTESIAN_POINT('Ctrl Pts',(80.1522124578486,-7.33907727904711,131.685975182024));
#78466=CARTESIAN_POINT('Ctrl Pts',(79.9703617869121,-7.33109461967067,131.69920415078));
#78467=CARTESIAN_POINT('Ctrl Pts',(79.8674501388419,-7.33610078564603,131.706573173012));
#78468=CARTESIAN_POINT('Ctrl Pts',(79.7422862257752,-7.35388453218234,131.715276002977));
#78469=CARTESIAN_POINT('Ctrl Pts',(79.7190022121216,-7.3576989116387,131.716884802495));
#78470=CARTESIAN_POINT('Ctrl Pts',(79.6838848389204,-7.36422060771146,131.719296946586));
#78471=CARTESIAN_POINT('Ctrl Pts',(79.671987941799,-7.36656462678864,131.720111632849));
#78472=CARTESIAN_POINT('Ctrl Pts',(79.6506012380265,-7.37102148708713,131.721571999992));
#78473=CARTESIAN_POINT('Ctrl Pts',(79.6411024292714,-7.37308788467288,131.722219125531));
#78474=CARTESIAN_POINT('Ctrl Pts',(79.6207847896032,-7.37769444667959,131.723600353556));
#78475=CARTESIAN_POINT('Ctrl Pts',(79.6099721449218,-7.38025996948403,131.724333611448));
#78476=CARTESIAN_POINT('Ctrl Pts',(79.5803598111892,-7.38759983181462,131.726337364952));
#78477=CARTESIAN_POINT('Ctrl Pts',(79.5616161868808,-7.3925946765683,131.727600759806));
#78478=CARTESIAN_POINT('Ctrl Pts',(79.4326016501931,-7.42939946325379,131.736271980696));
#78479=CARTESIAN_POINT('Ctrl Pts',(79.3257842115861,-7.47220274965911,131.743296386014));
#78480=CARTESIAN_POINT('Ctrl Pts',(79.1332954069401,-7.57348958976585,131.756578319682));
#78481=CARTESIAN_POINT('Ctrl Pts',(79.0470175050946,-7.62962508976139,131.762820577318));
#78482=CARTESIAN_POINT('Ctrl Pts',(78.9545835844362,-7.70273742655758,131.770475763271));
#78483=CARTESIAN_POINT('Ctrl Pts',(78.9428268756396,-7.71230026327776,131.771469287838));
#78484=CARTESIAN_POINT('Ctrl Pts',(78.9257784149653,-7.72655821118568,131.772942210409));
#78485=CARTESIAN_POINT('Ctrl Pts',(78.9203831267429,-7.7311290823351,131.773413179627));
#78486=CARTESIAN_POINT('Ctrl Pts',(78.9108654703834,-7.73929705782073,131.774252966508));
#78487=CARTESIAN_POINT('Ctrl Pts',(78.906731489144,-7.7428803184892,131.774620784136));
#78488=CARTESIAN_POINT('Ctrl Pts',(78.8977049489005,-7.75078256160792,131.775430719388));
#78489=CARTESIAN_POINT('Ctrl Pts',(78.8928201569517,-7.75510989257313,131.775873426714));
#78490=CARTESIAN_POINT('Ctrl Pts',(78.8793626175268,-7.76717349180127,131.777105029212));
#78491=CARTESIAN_POINT('Ctrl Pts',(78.8708448783743,-7.77497019009992,131.777898133249));
#78492=CARTESIAN_POINT('Ctrl Pts',(78.8512754153641,-7.79326056051038,131.779750676825));
#78493=CARTESIAN_POINT('Ctrl Pts',(78.8402853948725,-7.80381847351903,131.780814087352));
#78494=CARTESIAN_POINT('Ctrl Pts',(78.8041695486948,-7.83947986989369,131.784381958025));
#78495=CARTESIAN_POINT('Ctrl Pts',(78.7797028735409,-7.86523480392826,131.78691993339));
#78496=CARTESIAN_POINT('Ctrl Pts',(78.6924711721465,-7.96314530765645,131.796372403422));
#78497=CARTESIAN_POINT('Ctrl Pts',(78.6351267542301,-8.03988469725625,131.803394937501));
#78498=CARTESIAN_POINT('Ctrl Pts',(78.543502771379,-8.18743333640404,131.815883981024));
#78499=CARTESIAN_POINT('Ctrl Pts',(78.5070315460716,-8.25656396350369,131.821386784816));
#78500=CARTESIAN_POINT('Ctrl Pts',(78.4681182441537,-8.34484144003548,131.827978433095));
#78501=CARTESIAN_POINT('Ctrl Pts',(78.4609767564664,-8.36179787248843,131.82922601524));
#78502=CARTESIAN_POINT('Ctrl Pts',(78.4500537133038,-8.38898338197496,131.831197621849));
#78503=CARTESIAN_POINT('Ctrl Pts',(78.4460893481639,-8.39913687496472,131.831927742689));
#78504=CARTESIAN_POINT('Ctrl Pts',(78.440311810998,-8.41437395314495,131.833014313653));
#78505=CARTESIAN_POINT('Ctrl Pts',(78.4384233036404,-8.41942844053872,131.833373268318));
#78506=CARTESIAN_POINT('Ctrl Pts',(78.4365593750065,-8.42449203991602,131.833731407018));
#78507=CARTESIAN_POINT('Origin',(80.,-9.,134.));
#78508=CARTESIAN_POINT('',(78.4365593757978,-8.42449203776636,132.531716974833));
#78509=CARTESIAN_POINT('',(78.4365593746692,-8.42449204083249,132.34076576841));
#78510=CARTESIAN_POINT('',(78.4365593749993,-8.42449203993574,134.));
#78511=CARTESIAN_POINT('',(78.3340003204321,-8.99896671418601,131.679718342728));
#78512=CARTESIAN_POINT('Ctrl Pts',(78.4365593746692,-8.42449204083248,132.34076576841));
#78513=CARTESIAN_POINT('Ctrl Pts',(78.4390138554722,-8.4178241313095,132.340304576558));
#78514=CARTESIAN_POINT('Ctrl Pts',(78.4415110902992,-8.4111716600942,132.339841349361));
#78515=CARTESIAN_POINT('Ctrl Pts',(78.4479889080622,-8.39424513180157,132.338654284345));
#78516=CARTESIAN_POINT('Ctrl Pts',(78.4520287265719,-8.38399487785357,132.337927463635));
#78517=CARTESIAN_POINT('Ctrl Pts',(78.4585385975825,-8.36794584003524,132.336775754262));
#78518=CARTESIAN_POINT('Ctrl Pts',(78.4609404868607,-8.36211950334775,132.336354779793));
#78519=CARTESIAN_POINT('Ctrl Pts',(78.4655035579377,-8.3512265338598,132.335562085204));
#78520=CARTESIAN_POINT('Ctrl Pts',(78.4676568805521,-8.34615682169059,132.335190829334));
#78521=CARTESIAN_POINT('Ctrl Pts',(78.4727743967095,-8.3342724410677,132.334315135706));
#78522=CARTESIAN_POINT('Ctrl Pts',(78.4757590874159,-8.32746683263963,132.333809494426));
#78523=CARTESIAN_POINT('Ctrl Pts',(78.4857880525261,-8.30500877715541,132.332127600537));
#78524=CARTESIAN_POINT('Ctrl Pts',(78.4930284281871,-8.28944581755006,132.330940567757));
#78525=CARTESIAN_POINT('Ctrl Pts',(78.5112573464877,-8.25179559762374,132.328020864471));
#78526=CARTESIAN_POINT('Ctrl Pts',(78.5224983485425,-8.22983556547231,132.326276933038));
#78527=CARTESIAN_POINT('Ctrl Pts',(78.5716047804195,-8.13893740803797,132.318907781584));
#78528=CARTESIAN_POINT('Ctrl Pts',(78.6138390492161,-8.07247714628997,132.313155264429));
#78529=CARTESIAN_POINT('Ctrl Pts',(78.7221884903929,-7.92599964484594,132.299912284184));
#78530=CARTESIAN_POINT('Ctrl Pts',(78.7914062011884,-7.84865876223397,132.292486942134));
#78531=CARTESIAN_POINT('Ctrl Pts',(78.8846666075101,-7.76220206015346,132.283732579222));
#78532=CARTESIAN_POINT('Ctrl Pts',(78.9023029834943,-7.74653533156957,132.282124083819));
#78533=CARTESIAN_POINT('Ctrl Pts',(78.929501560374,-7.72338880965422,132.279712169194));
#78534=CARTESIAN_POINT('Ctrl Pts',(78.9388219412196,-7.71563082347502,132.278897414716));
#78535=CARTESIAN_POINT('Ctrl Pts',(78.9557669434384,-7.70183673491072,132.27743681384));
#78536=CARTESIAN_POINT('Ctrl Pts',(78.9633612010551,-7.6957643822364,132.276789523463));
#78537=CARTESIAN_POINT('Ctrl Pts',(78.9797514704731,-7.68289236283971,132.275407820087));
#78538=CARTESIAN_POINT('Ctrl Pts',(78.9885632981431,-7.67611352522975,132.274674253307));
#78539=CARTESIAN_POINT('Ctrl Pts',(79.0129438815596,-7.65774334339052,132.272669320105));
#78540=CARTESIAN_POINT('Ctrl Pts',(79.0286486825662,-7.64633483373563,132.271405066081));
#78541=CARTESIAN_POINT('Ctrl Pts',(79.0640823888214,-7.62152884380707,132.268609517381));
#78542=CARTESIAN_POINT('Ctrl Pts',(79.0839069487887,-7.60827513136339,132.267083530185));
#78543=CARTESIAN_POINT('Ctrl Pts',(79.1483619602897,-7.56715798283446,132.26223236815));
#78544=CARTESIAN_POINT('Ctrl Pts',(79.1940312582562,-7.54098025767199,132.258961158955));
#78545=CARTESIAN_POINT('Ctrl Pts',(79.3262962095248,-7.47327474193002,132.249814520825));
#78546=CARTESIAN_POINT('Ctrl Pts',(79.4153416452689,-7.43700926514236,132.244039619524));
#78547=CARTESIAN_POINT('Ctrl Pts',(79.5562148879313,-7.39336865188749,132.234865153142));
#78548=CARTESIAN_POINT('Ctrl Pts',(79.6060956539418,-7.38041741116058,132.231607085556));
#78549=CARTESIAN_POINT('Ctrl Pts',(79.6672460728669,-7.36753203877562,132.227513661619));
#78550=CARTESIAN_POINT('Ctrl Pts',(79.6780235330704,-7.36537222606435,132.226788513093));
#78551=CARTESIAN_POINT('Ctrl Pts',(79.6950066493537,-7.3621432606454,132.225638878526));
#78552=CARTESIAN_POINT('Ctrl Pts',(79.7011985697911,-7.36100233538198,132.225218283648));
#78553=CARTESIAN_POINT('Ctrl Pts',(79.7128206219749,-7.3589288984493,132.224425875865));
#78554=CARTESIAN_POINT('Ctrl Pts',(79.7182490928005,-7.35798819180292,132.224054522793));
#78555=CARTESIAN_POINT('Ctrl Pts',(79.7310207746876,-7.35584016693622,132.223178018032));
#78556=CARTESIAN_POINT('Ctrl Pts',(79.7383675124889,-7.35465510712965,132.222671655933));
#78557=CARTESIAN_POINT('Ctrl Pts',(79.762745097692,-7.35089029563906,132.220984849409));
#78558=CARTESIAN_POINT('Ctrl Pts',(79.7798073643738,-7.34852555239971,132.219793541349));
#78559=CARTESIAN_POINT('Ctrl Pts',(79.8215032819806,-7.34340431717928,132.216861126487));
#78560=CARTESIAN_POINT('Ctrl Pts',(79.846167281314,-7.34093228049031,132.215108639107));
#78561=CARTESIAN_POINT('Ctrl Pts',(79.9500010431229,-7.33286031298507,132.207679043735));
#78562=CARTESIAN_POINT('Ctrl Pts',(80.0294615613863,-7.33237120551508,132.201872899958));
#78563=CARTESIAN_POINT('Ctrl Pts',(80.2110508572643,-7.34423914152668,132.188647894957));
#78564=CARTESIAN_POINT('Ctrl Pts',(80.3126280641072,-7.36037912427822,132.181292348828));
#78565=CARTESIAN_POINT('Ctrl Pts',(80.4349492723316,-7.39160582032479,132.172601645145));
#78566=CARTESIAN_POINT('Ctrl Pts',(80.4576851139909,-7.39792723573308,132.170992573184));
#78567=CARTESIAN_POINT('Ctrl Pts',(80.4918928991399,-7.40822600294466,132.168579974081));
#78568=CARTESIAN_POINT('Ctrl Pts',(80.5034674870425,-7.41184900437356,132.167765102057));
#78569=CARTESIAN_POINT('Ctrl Pts',(80.5242487834139,-7.41860385895263,132.166304374011));
#78570=CARTESIAN_POINT('Ctrl Pts',(80.5334694885374,-7.42169050769239,132.165657072925));
#78571=CARTESIAN_POINT('Ctrl Pts',(80.5531724983306,-7.42847852369167,132.164275435761));
#78572=CARTESIAN_POINT('Ctrl Pts',(80.5636458906848,-7.43220445102253,132.163541945084));
#78573=CARTESIAN_POINT('Ctrl Pts',(80.5922965347342,-7.44272118417166,132.16153745116));
#78574=CARTESIAN_POINT('Ctrl Pts',(80.610394031465,-7.44972529122425,132.160273554981));
#78575=CARTESIAN_POINT('Ctrl Pts',(80.6504398305175,-7.46603386303442,132.157478916854));
#78576=CARTESIAN_POINT('Ctrl Pts',(80.6723193056744,-7.47549650092215,132.155953476952));
#78577=CARTESIAN_POINT('Ctrl Pts',(80.7417879430125,-7.5073275406437,132.151104722753));
#78578=CARTESIAN_POINT('Ctrl Pts',(80.7885254753155,-7.53148080649983,132.14783531081));
#78579=CARTESIAN_POINT('Ctrl Pts',(80.9171322188888,-7.60585624908078,132.13868987609));
#78580=CARTESIAN_POINT('Ctrl Pts',(80.9959074435753,-7.66099466397898,132.132914529277));
#78581=CARTESIAN_POINT('Ctrl Pts',(81.1090204556218,-7.75569816072375,132.123737466394));
#78582=CARTESIAN_POINT('Ctrl Pts',(81.1469850335465,-7.79060442767444,132.120477087942));
#78583=CARTESIAN_POINT('Ctrl Pts',(81.1910055738852,-7.83501820474529,132.116381069937));
#78584=CARTESIAN_POINT('Ctrl Pts',(81.1986668831073,-7.84290253316042,132.115655804238));
#78585=CARTESIAN_POINT('Ctrl Pts',(81.2105925175451,-7.85542086153305,132.114506024282));
#78586=CARTESIAN_POINT('Ctrl Pts',(81.2149097137643,-7.86000437199037,132.114085402798));
#78587=CARTESIAN_POINT('Ctrl Pts',(81.2229554815718,-7.86864406812863,132.113292974968));
#78588=CARTESIAN_POINT('Ctrl Pts',(81.2266900412187,-7.87269440978877,132.112921628763));
#78589=CARTESIAN_POINT('Ctrl Pts',(81.2354212421437,-7.88225865071046,132.112045181097));
#78590=CARTESIAN_POINT('Ctrl Pts',(81.2404011027583,-7.88778757944596,132.111538869711));
#78591=CARTESIAN_POINT('Ctrl Pts',(81.2567827100098,-7.9062222444754,132.109852409155));
#78592=CARTESIAN_POINT('Ctrl Pts',(81.2680209550141,-7.91927091344793,132.108661402239));
#78593=CARTESIAN_POINT('Ctrl Pts',(81.2949308263346,-7.95151343423113,132.105729883274));
#78594=CARTESIAN_POINT('Ctrl Pts',(81.3103801199245,-7.97088691895358,132.103977999103));
#78595=CARTESIAN_POINT('Ctrl Pts',(81.3734455078844,-8.05369453133679,132.096552680094));
#78596=CARTESIAN_POINT('Ctrl Pts',(81.4169311826397,-8.1201410488441,132.090750332607));
#78597=CARTESIAN_POINT('Ctrl Pts',(81.5054771231403,-8.27914031728263,132.077524054422));
#78598=CARTESIAN_POINT('Ctrl Pts',(81.5470431553519,-8.37329115606433,132.070163571888));
#78599=CARTESIAN_POINT('Ctrl Pts',(81.587173788204,-8.4930561728192,132.061468365871));
#78600=CARTESIAN_POINT('Ctrl Pts',(81.5941942214222,-8.51558534176302,132.059859336487));
#78601=CARTESIAN_POINT('Ctrl Pts',(81.6040952881193,-8.54990958074568,132.05744678793));
#78602=CARTESIAN_POINT('Ctrl Pts',(81.6073292732164,-8.56159870001947,132.056631924586));
#78603=CARTESIAN_POINT('Ctrl Pts',(81.6129256181999,-8.58272132597783,132.055171205931));
#78604=CARTESIAN_POINT('Ctrl Pts',(81.6153335448347,-8.59214207443145,132.054523905637));
#78605=CARTESIAN_POINT('Ctrl Pts',(81.620317242589,-8.6123769889062,132.053142263587));
#78606=CARTESIAN_POINT('Ctrl Pts',(81.6228675442374,-8.62319698874166,132.052408767294));
#78607=CARTESIAN_POINT('Ctrl Pts',(81.6295717268579,-8.65297190547595,132.05040424095));
#78608=CARTESIAN_POINT('Ctrl Pts',(81.633503136431,-8.67197551056528,132.049140318361));
#78609=CARTESIAN_POINT('Ctrl Pts',(81.6415219596932,-8.71446581748976,132.046345613033));
#78610=CARTESIAN_POINT('Ctrl Pts',(81.6454391430599,-8.73798048730697,132.04482013274));
#78611=CARTESIAN_POINT('Ctrl Pts',(81.6563754769981,-8.81361079262504,132.039971200864));
#78612=CARTESIAN_POINT('Ctrl Pts',(81.6614330148538,-8.86597903814657,132.036701656302));
#78613=CARTESIAN_POINT('Ctrl Pts',(81.6687006217978,-9.01436722626628,132.027556136803));
#78614=CARTESIAN_POINT('Ctrl Pts',(81.6651025996308,-9.11045422485917,132.021780826678));
#78615=CARTESIAN_POINT('Ctrl Pts',(81.6468889631369,-9.25684605866391,132.012603956121));
#78616=CARTESIAN_POINT('Ctrl Pts',(81.6381546126156,-9.30767108964271,132.009343744548));
#78617=CARTESIAN_POINT('Ctrl Pts',(81.6247175969581,-9.36874054232483,132.005247913885));
#78618=CARTESIAN_POINT('Ctrl Pts',(81.6222490813424,-9.37945323773523,132.004522656656));
#78619=CARTESIAN_POINT('Ctrl Pts',(81.618200283463,-9.39626189569163,132.00337288721));
#78620=CARTESIAN_POINT('Ctrl Pts',(81.616691093091,-9.40237489189451,132.00295226765));
#78621=CARTESIAN_POINT('Ctrl Pts',(81.6137964687685,-9.41382038609896,132.002159841269));
#78622=CARTESIAN_POINT('Ctrl Pts',(81.6124191919873,-9.41915474508975,132.001788494566));
#78623=CARTESIAN_POINT('Ctrl Pts',(81.609119571383,-9.43167762882553,132.000912042774));
#78624=CARTESIAN_POINT('Ctrl Pts',(81.6071754986794,-9.43886020711391,132.000405727722));
#78625=CARTESIAN_POINT('Ctrl Pts',(81.60057288572,-9.46262188316392,131.998719242162));
#78626=CARTESIAN_POINT('Ctrl Pts',(81.5957055744258,-9.47914113916711,131.997528213483));
#78627=CARTESIAN_POINT('Ctrl Pts',(81.583212648774,-9.51923757766001,131.994596629776));
#78628=CARTESIAN_POINT('Ctrl Pts',(81.5753155137285,-9.54272539481332,131.992844702014));
#78629=CARTESIAN_POINT('Ctrl Pts',(81.5399498954958,-9.64062586768529,131.985419074057));
#78630=CARTESIAN_POINT('Ctrl Pts',(81.5077098880013,-9.71320209183247,131.979616452315));
#78631=CARTESIAN_POINT('Ctrl Pts',(81.4221540866066,-9.87382882997936,131.966390266095));
#78632=CARTESIAN_POINT('Ctrl Pts',(81.3656017331419,-9.95981114022294,131.959030140193));
#78633=CARTESIAN_POINT('Ctrl Pts',(81.2867522134217,-10.0584807136639,131.950335259466));
#78634=CARTESIAN_POINT('Ctrl Pts',(81.2716324317419,-10.0765982246591,131.948726227032));
#78635=CARTESIAN_POINT('Ctrl Pts',(81.2481656135652,-10.1035332709996,131.946313674854));
#78636=CARTESIAN_POINT('Ctrl Pts',(81.2400992420526,-10.1125902041824,131.945498810888));
#78637=CARTESIAN_POINT('Ctrl Pts',(81.2253887666518,-10.1287483830406,131.944038091559));
#78638=CARTESIAN_POINT('Ctrl Pts',(81.2187800960244,-10.1358809911544,131.943390791208));
#78639=CARTESIAN_POINT('Ctrl Pts',(81.2044831389323,-10.1510429762822,131.942009149506));
#78640=CARTESIAN_POINT('Ctrl Pts',(81.1967761372451,-10.1590541197949,131.941275653614));
#78641=CARTESIAN_POINT('Ctrl Pts',(81.1753974876219,-10.1808358295315,131.939271129589));
#78642=CARTESIAN_POINT('Ctrl Pts',(81.161564271656,-10.1944458983397,131.938007208889));
#78643=CARTESIAN_POINT('Ctrl Pts',(81.1302160694115,-10.2242286337766,131.935212508369));
#78644=CARTESIAN_POINT('Ctrl Pts',(81.112585257366,-10.2402734542893,131.933687030967));
#78645=CARTESIAN_POINT('Ctrl Pts',(81.0549775527976,-10.2904816944714,131.928838111805));
#78646=CARTESIAN_POINT('Ctrl Pts',(81.0137245022189,-10.3231341193944,131.925568576734));
#78647=CARTESIAN_POINT('Ctrl Pts',(80.8930006170416,-10.4097226993484,131.916423063324));
#78648=CARTESIAN_POINT('Ctrl Pts',(80.8103232364147,-10.4588156375441,131.910647750595));
#78649=CARTESIAN_POINT('Ctrl Pts',(80.6774557027464,-10.5229139653606,131.901470866278));
#78650=CARTESIAN_POINT('Ctrl Pts',(80.6300183958495,-10.5431425324435,131.898210642741));
#78651=CARTESIAN_POINT('Ctrl Pts',(80.5714237629889,-10.5649765943034,131.894114798647));
#78652=CARTESIAN_POINT('Ctrl Pts',(80.561084790177,-10.568713071273,131.893389540811));
#78653=CARTESIAN_POINT('Ctrl Pts',(80.5447672815434,-10.5744282315696,131.892239770611));
#78654=CARTESIAN_POINT('Ctrl Pts',(80.5388129940871,-10.576475880417,131.891819150913));
#78655=CARTESIAN_POINT('Ctrl Pts',(80.5276272670334,-10.5802518222227,131.891026724428));
#78656=CARTESIAN_POINT('Ctrl Pts',(80.5223986882551,-10.5819879776801,131.890655377762));
#78657=CARTESIAN_POINT('Ctrl Pts',(80.510088154221,-10.5860080217651,131.889778926266));
#78658=CARTESIAN_POINT('Ctrl Pts',(80.5029994094838,-10.5882704300421,131.889272611477));
#78659=CARTESIAN_POINT('Ctrl Pts',(80.4794553369939,-10.5956112146605,131.887586127711));
#78660=CARTESIAN_POINT('Ctrl Pts',(80.4629370511585,-10.6004817391643,131.886395100593));
#78661=CARTESIAN_POINT('Ctrl Pts',(80.422474853255,-10.6117335231138,131.883463521531));
#78662=CARTESIAN_POINT('Ctrl Pts',(80.3984587527755,-10.6178382002461,131.881711596896));
#78663=CARTESIAN_POINT('Ctrl Pts',(80.2970280123449,-10.6412256095007,131.874285991096));
#78664=CARTESIAN_POINT('Ctrl Pts',(80.2185682447507,-10.6535036168591,131.868483389024));
#78665=CARTESIAN_POINT('Ctrl Pts',(80.0372165552375,-10.6687462564714,131.855257196203));
#78666=CARTESIAN_POINT('Ctrl Pts',(79.9343067437774,-10.6678698944816,131.84789704472));
#78667=CARTESIAN_POINT('Ctrl Pts',(79.8086444060226,-10.6551422042981,131.839202140661));
#78668=CARTESIAN_POINT('Ctrl Pts',(79.7852226168708,-10.652266157235,131.837593108446));
#78669=CARTESIAN_POINT('Ctrl Pts',(79.7498656569269,-10.6471599465411,131.83518055653));
#78670=CARTESIAN_POINT('Ctrl Pts',(79.7378815872724,-10.6452954234043,131.83436569261));
#78671=CARTESIAN_POINT('Ctrl Pts',(79.7163278951061,-10.641700544727,131.832904973331));
#78672=CARTESIAN_POINT('Ctrl Pts',(79.7067511422757,-10.6400169681968,131.832257672985));
#78673=CARTESIAN_POINT('Ctrl Pts',(79.6862586685287,-10.6362291838728,131.830876031261));
#78674=CARTESIAN_POINT('Ctrl Pts',(79.6753481154141,-10.6340993632999,131.830142535341));
#78675=CARTESIAN_POINT('Ctrl Pts',(79.6454532193076,-10.6279524227061,131.828138011154));
#78676=CARTESIAN_POINT('Ctrl Pts',(79.626516084198,-10.6237125133367,131.826874090322));
#78677=CARTESIAN_POINT('Ctrl Pts',(79.5844919699034,-10.6135294197492,131.824079389465));
#78678=CARTESIAN_POINT('Ctrl Pts',(79.5614495768711,-10.6074195851901,131.822553911859));
#78679=CARTESIAN_POINT('Ctrl Pts',(79.4880226746003,-10.5862534035045,131.817704991802));
#78680=CARTESIAN_POINT('Ctrl Pts',(79.4382154393115,-10.5693053790952,131.814435456063));
#78681=CARTESIAN_POINT('Ctrl Pts',(79.3010763505116,-10.5152727150492,131.805361737594));
#78682=CARTESIAN_POINT('Ctrl Pts',(79.2159945627614,-10.4730512116047,131.799654630386));
#78683=CARTESIAN_POINT('Ctrl Pts',(79.0900529554257,-10.3965365960898,131.790494728809));
#78684=CARTESIAN_POINT('Ctrl Pts',(79.046458083827,-10.3671410771866,131.787173617382));
#78685=CARTESIAN_POINT('Ctrl Pts',(78.9954457596652,-10.3291160827815,131.783006928775));
#78686=CARTESIAN_POINT('Ctrl Pts',(78.9866281896581,-10.3224055130902,131.782276032691));
#78687=CARTESIAN_POINT('Ctrl Pts',(78.9728906280675,-10.311732531444,131.781119267297));
#78688=CARTESIAN_POINT('Ctrl Pts',(78.9679249309892,-10.3078290960931,131.780697368555));
#78689=CARTESIAN_POINT('Ctrl Pts',(78.9588177635487,-10.3005859661669,131.779916381778));
#78690=CARTESIAN_POINT('Ctrl Pts',(78.9546699401155,-10.2972545500703,131.779557871074));
#78691=CARTESIAN_POINT('Ctrl Pts',(78.9504874760473,-10.2938622284968,131.779193535027));
#78692=CARTESIAN_POINT('Ctrl Pts',(78.9504367611324,-10.2938210895955,131.77918911681));
#78693=CARTESIAN_POINT('Ctrl Pts',(78.9503356688527,-10.2937390757512,131.779180308942));
#78694=CARTESIAN_POINT('Ctrl Pts',(78.9502852914157,-10.2936982008144,131.779175919291));
#78695=CARTESIAN_POINT('Ctrl Pts',(78.9501848574102,-10.2936167015562,131.779167167118));
#78696=CARTESIAN_POINT('Ctrl Pts',(78.9501348008209,-10.293576077279,131.779162804599));
#78697=CARTESIAN_POINT('Ctrl Pts',(78.9500349921428,-10.2934950662379,131.779154105282));
#78698=CARTESIAN_POINT('Ctrl Pts',(78.9499852401427,-10.2934546796035,131.779149768495));
#78699=CARTESIAN_POINT('Ctrl Pts',(78.9498860248407,-10.2933741311912,131.779141119278));
#78700=CARTESIAN_POINT('Ctrl Pts',(78.9498365615822,-10.2933339695029,131.779136806856));
#78701=CARTESIAN_POINT('Ctrl Pts',(78.9497379087235,-10.2932538589322,131.77912820507));
#78702=CARTESIAN_POINT('Ctrl Pts',(78.9496887189448,-10.293213909956,131.779123915696));
#78703=CARTESIAN_POINT('Ctrl Pts',(78.9495905977843,-10.2931342125669,131.779115358688));
#78704=CARTESIAN_POINT('Ctrl Pts',(78.9495416663926,-10.2930944641939,131.779111091058));
#78705=CARTESIAN_POINT('Ctrl Pts',(78.9494440474455,-10.2930151563256,131.779102576282));
#78706=CARTESIAN_POINT('Ctrl Pts',(78.9493953598266,-10.2929755968237,131.779098329134));
#78707=CARTESIAN_POINT('Ctrl Pts',(78.9492982139278,-10.2928966550517,131.779089854068));
#78708=CARTESIAN_POINT('Ctrl Pts',(78.9492497556804,-10.2928572728501,131.779085626157));
#78709=CARTESIAN_POINT('Ctrl Pts',(78.9491530546733,-10.2927786745468,131.779077188368));
#78710=CARTESIAN_POINT('Ctrl Pts',(78.9491048118317,-10.2927394584177,131.779072978486));
#78711=CARTESIAN_POINT('Ctrl Pts',(78.9435936679568,-10.2882589916685,131.778592008303));
#78712=CARTESIAN_POINT('Ctrl Pts',(78.9381590949362,-10.2837832589096,131.778112828331));
#78713=CARTESIAN_POINT('Ctrl Pts',(78.9263376294428,-10.2739210806555,131.777060051966));
#78714=CARTESIAN_POINT('Ctrl Pts',(78.9199625924164,-10.2685207909121,131.77648554986));
#78715=CARTESIAN_POINT('Ctrl Pts',(78.902520287083,-10.253518631209,131.774895580284));
#78716=CARTESIAN_POINT('Ctrl Pts',(78.8915389116066,-10.2438185807195,131.773874203754));
#78717=CARTESIAN_POINT('Ctrl Pts',(78.8558975721785,-10.2114890830967,131.770495515559));
#78718=CARTESIAN_POINT('Ctrl Pts',(78.8317925055993,-10.1882622355015,131.768108144967));
#78719=CARTESIAN_POINT('Ctrl Pts',(78.7191904794858,-10.0730230819379,131.756512862521));
#78720=CARTESIAN_POINT('Ctrl Pts',(78.6407531864533,-9.97175393740744,131.747097908635));
#78721=CARTESIAN_POINT('Ctrl Pts',(78.54727896112,-9.81728396794897,131.734312245805));
#78722=CARTESIAN_POINT('Ctrl Pts',(78.5220724739797,-9.77076765711,131.730632540249));
#78723=CARTESIAN_POINT('Ctrl Pts',(78.4919262977753,-9.70819792594375,131.725900734967));
#78724=CARTESIAN_POINT('Ctrl Pts',(78.4849566348642,-9.69316248446617,131.72477945326));
#78725=CARTESIAN_POINT('Ctrl Pts',(78.4739348051216,-9.66842462994766,131.722959589786));
#78726=CARTESIAN_POINT('Ctrl Pts',(78.4697482366556,-9.6587837387716,131.722256453152));
#78727=CARTESIAN_POINT('Ctrl Pts',(78.4618068342,-9.64001190520926,131.720898908933));
#78728=CARTESIAN_POINT('Ctrl Pts',(78.4580413866192,-9.63088596108174,131.720244164257));
#78729=CARTESIAN_POINT('Ctrl Pts',(78.449388458603,-9.60937436899457,131.718712730757));
#78730=CARTESIAN_POINT('Ctrl Pts',(78.4445678521679,-9.5969624145978,131.717838314566));
#78731=CARTESIAN_POINT('Ctrl Pts',(78.4289998366686,-9.55540898736597,131.714940153122));
#78732=CARTESIAN_POINT('Ctrl Pts',(78.4189181815305,-9.52602389371686,131.712938367513));
#78733=CARTESIAN_POINT('Ctrl Pts',(78.3964437244496,-9.45401759116544,131.708132387151));
#78734=CARTESIAN_POINT('Ctrl Pts',(78.3849206709727,-9.41114947304623,131.705354187579));
#78735=CARTESIAN_POINT('Ctrl Pts',(78.3477129961438,-9.24680354893202,131.69491768606));
#78736=CARTESIAN_POINT('Ctrl Pts',(78.3339233495109,-9.12306938570736,131.687524146382));
#78737=CARTESIAN_POINT('Ctrl Pts',(78.3340003204321,-8.99896671418601,131.679718342728));
#78738=CARTESIAN_POINT('Ctrl Pts',(78.3340003219591,-8.998964255121,131.679718188058));
#78739=CARTESIAN_POINT('Ctrl Pts',(78.3340235477069,-8.96160554903245,131.677368400364));
#78740=CARTESIAN_POINT('Ctrl Pts',(78.3353033767596,-8.92426065044466,131.674981768813));
#78741=CARTESIAN_POINT('Ctrl Pts',(78.3383818272231,-8.87898127153856,131.672008370228));
#78742=CARTESIAN_POINT('Ctrl Pts',(78.3389844347566,-8.87097375979838,131.671479493273));
#78743=CARTESIAN_POINT('Ctrl Pts',(78.3401157678519,-8.85726559464761,131.670568408757));
#78744=CARTESIAN_POINT('Ctrl Pts',(78.3406160404092,-8.85156264999074,131.670187684067));
#78745=CARTESIAN_POINT('Ctrl Pts',(78.3416182463319,-8.84077673723529,131.669464231128));
#78746=CARTESIAN_POINT('Ctrl Pts',(78.3421141841099,-8.83569324959901,131.669121833836));
#78747=CARTESIAN_POINT('Ctrl Pts',(78.3431534777294,-8.82552433291402,131.668433904773));
#78748=CARTESIAN_POINT('Ctrl Pts',(78.3436968895286,-8.82043897635919,131.668088376536));
#78749=CARTESIAN_POINT('Ctrl Pts',(78.3450460614502,-8.80834068753394,131.667262899008));
#78750=CARTESIAN_POINT('Ctrl Pts',(78.345872988445,-8.8013302842618,131.666781809456));
#78751=CARTESIAN_POINT('Ctrl Pts',(78.3489767353076,-8.77638170300056,131.665060362435));
#78752=CARTESIAN_POINT('Ctrl Pts',(78.351500922452,-8.75847631837876,131.663807664797));
#78753=CARTESIAN_POINT('Ctrl Pts',(78.3619153581104,-8.69240090991068,131.659129490043));
#78754=CARTESIAN_POINT('Ctrl Pts',(78.3716295171211,-8.64454636678423,131.655632552103));
#78755=CARTESIAN_POINT('Ctrl Pts',(78.3980065525462,-8.53868875348034,131.647741443782));
#78756=CARTESIAN_POINT('Ctrl Pts',(78.4157446379831,-8.48103793269769,131.643337557353));
#78757=CARTESIAN_POINT('Ctrl Pts',(78.4365593409241,-8.42449213250519,131.638964580993));
#78758=CARTESIAN_POINT('',(78.3340002424327,-9.00128863288225,131.870599662366));
#78759=CARTESIAN_POINT('Ctrl Pts',(78.4365593750065,-8.42449203991602,131.833731407018));
#78760=CARTESIAN_POINT('Ctrl Pts',(78.435054346559,-8.42858064125575,131.834020585971));
#78761=CARTESIAN_POINT('Ctrl Pts',(78.4335653428238,-8.43267518337795,131.834309232973));
#78762=CARTESIAN_POINT('Ctrl Pts',(78.4278795475944,-8.4485033348739,131.835421421153));
#78763=CARTESIAN_POINT('Ctrl Pts',(78.4237983197513,-8.46027825154674,131.836241125397));
#78764=CARTESIAN_POINT('Ctrl Pts',(78.4115574972136,-8.49691828400013,131.838769040101));
#78765=CARTESIAN_POINT('Ctrl Pts',(78.4038510981433,-8.52193138397899,131.840462454949));
#78766=CARTESIAN_POINT('Ctrl Pts',(78.3871741035046,-8.58097003216267,131.844392686761));
#78767=CARTESIAN_POINT('Ctrl Pts',(78.3786855856983,-8.61511911372465,131.846614795668));
#78768=CARTESIAN_POINT('Ctrl Pts',(78.346405873371,-8.76512322839677,131.856205052507));
#78769=CARTESIAN_POINT('Ctrl Pts',(78.333909190809,-8.88304341633613,131.863279796691));
#78770=CARTESIAN_POINT('Ctrl Pts',(78.3340004966965,-9.00128646516507,131.870599084676));
#78771=CARTESIAN_POINT('Ctrl Pts',(78.3340004983928,-9.0012886600276,131.870599220539));
#78772=CARTESIAN_POINT('Ctrl Pts',(78.3340321196368,-9.04216909052046,131.873129735217));
#78773=CARTESIAN_POINT('Ctrl Pts',(78.3355684237451,-9.08303249464215,131.87568896695));
#78774=CARTESIAN_POINT('Ctrl Pts',(78.3400975380125,-9.14381523758201,131.879593155217));
#78775=CARTESIAN_POINT('Ctrl Pts',(78.3419509048717,-9.16380513354296,131.880892980567));
#78776=CARTESIAN_POINT('Ctrl Pts',(78.3449992886001,-9.19127433863501,131.882706986491));
#78777=CARTESIAN_POINT('Ctrl Pts',(78.3458848578507,-9.19878711905922,131.883205992588));
#78778=CARTESIAN_POINT('Ctrl Pts',(78.3475086460371,-9.21179970775164,131.884075702536));
#78779=CARTESIAN_POINT('Ctrl Pts',(78.3482232444392,-9.21730241307577,131.884445159621));
#78780=CARTESIAN_POINT('Ctrl Pts',(78.3497070429375,-9.22829787079051,131.885186948462));
#78781=CARTESIAN_POINT('Ctrl Pts',(78.3504761918229,-9.2337904346705,131.885559272398));
#78782=CARTESIAN_POINT('Ctrl Pts',(78.3521570865827,-9.24537245666064,131.886348286418));
#78783=CARTESIAN_POINT('Ctrl Pts',(78.353075152663,-9.25146064089973,131.886765292928));
#78784=CARTESIAN_POINT('Ctrl Pts',(78.3556732395593,-9.26806514286679,131.887908511837));
#78785=CARTESIAN_POINT('Ctrl Pts',(78.3574203499857,-9.27857044804912,131.888638277172));
#78786=CARTESIAN_POINT('Ctrl Pts',(78.3667644898343,-9.33160905197933,131.892353057818));
#78787=CARTESIAN_POINT('Ctrl Pts',(78.3759127776337,-9.37384861842069,131.895410201041));
#78788=CARTESIAN_POINT('Ctrl Pts',(78.4088204323466,-9.50156735091101,131.904867664855));
#78789=CARTESIAN_POINT('Ctrl Pts',(78.4377723653983,-9.5855483814739,131.911376125597));
#78790=CARTESIAN_POINT('Ctrl Pts',(78.5110634565282,-9.75335190586252,131.924626964921));
#78791=CARTESIAN_POINT('Ctrl Pts',(78.5561479364638,-9.83652123578932,131.931330721001));
#78792=CARTESIAN_POINT('Ctrl Pts',(78.6182535411965,-9.93095533943586,131.93905542961));
#78793=CARTESIAN_POINT('Ctrl Pts',(78.6287207077375,-9.94630559099729,131.940315497481));
#78794=CARTESIAN_POINT('Ctrl Pts',(78.6457553790043,-9.97041081411814,131.942302096822));
#78795=CARTESIAN_POINT('Ctrl Pts',(78.6521558848247,-9.97928131439143,131.943034886225));
#78796=CARTESIAN_POINT('Ctrl Pts',(78.6644233302848,-9.99593470284866,131.944414198127));
#78797=CARTESIAN_POINT('Ctrl Pts',(78.6702720760128,-10.003730356265,131.945061385013));
#78798=CARTESIAN_POINT('Ctrl Pts',(78.6837146170901,-10.0213238653724,131.946525720378));
#78799=CARTESIAN_POINT('Ctrl Pts',(78.6913500901491,-10.0310892660324,131.94734118974));
#78800=CARTESIAN_POINT('Ctrl Pts',(78.7152193585032,-10.0609245907382,131.949841873932));
#78801=CARTESIAN_POINT('Ctrl Pts',(78.7318116063492,-10.0807037514705,131.951512761807));
#78802=CARTESIAN_POINT('Ctrl Pts',(78.8371123049505,-10.2004631756827,131.96173330062));
#78803=CARTESIAN_POINT('Ctrl Pts',(78.937122555842,-10.2898503742027,131.969771336136));
#78804=CARTESIAN_POINT('Ctrl Pts',(79.1059551663074,-10.4076406214928,131.98239783046));
#78805=CARTESIAN_POINT('Ctrl Pts',(79.1677812414,-10.4450528791687,131.986870517345));
#78806=CARTESIAN_POINT('Ctrl Pts',(79.2459000760047,-10.485644883087,131.992581476702));
#78807=CARTESIAN_POINT('Ctrl Pts',(79.26007304626,-10.4927543241237,131.993619969719));
#78808=CARTESIAN_POINT('Ctrl Pts',(79.280825733421,-10.5027961315938,131.995147131803));
#78809=CARTESIAN_POINT('Ctrl Pts',(79.2873268972639,-10.5058900632867,131.995626467001));
#78810=CARTESIAN_POINT('Ctrl Pts',(79.2988124666569,-10.5112650626089,131.996475284383));
#78811=CARTESIAN_POINT('Ctrl Pts',(79.3037883786177,-10.5135638154085,131.99684368125));
#78812=CARTESIAN_POINT('Ctrl Pts',(79.3146377432341,-10.5185111413832,131.997648455186));
#78813=CARTESIAN_POINT('Ctrl Pts',(79.3205151546212,-10.5211501736821,131.998085361834));
#78814=CARTESIAN_POINT('Ctrl Pts',(79.3370629895589,-10.5284653233663,131.999317795776));
#78815=CARTESIAN_POINT('Ctrl Pts',(79.3477671251166,-10.5330635937391,132.000117706979));
#78816=CARTESIAN_POINT('Ctrl Pts',(79.4295022931189,-10.5671643727818,132.00624139629));
#78817=CARTESIAN_POINT('Ctrl Pts',(79.5024443227339,-10.5918252023334,132.011791715511));
#78818=CARTESIAN_POINT('Ctrl Pts',(79.6322218136303,-10.6259078611341,132.021544744789));
#78819=CARTESIAN_POINT('Ctrl Pts',(79.6883394136397,-10.6375912532945,132.025724771962));
#78820=CARTESIAN_POINT('Ctrl Pts',(79.8266839939385,-10.6590234117932,132.035840904689));
#78821=CARTESIAN_POINT('Ctrl Pts',(79.9092591257557,-10.6655830223465,132.04171443686));
#78822=CARTESIAN_POINT('Ctrl Pts',(80.0148230932484,-10.6660905123571,132.048971847056));
#78823=CARTESIAN_POINT('Ctrl Pts',(80.0376560194855,-10.665730900642,132.050527246296));
#78824=CARTESIAN_POINT('Ctrl Pts',(80.0722884332743,-10.6644729241821,132.052865791811));
#78825=CARTESIAN_POINT('Ctrl Pts',(80.0840968650154,-10.6639181057682,132.053659515976));
#78826=CARTESIAN_POINT('Ctrl Pts',(80.104645865219,-10.6627332951643,132.05503471007));
#78827=CARTESIAN_POINT('Ctrl Pts',(80.1133890952879,-10.6621599459911,132.05561792388));
#78828=CARTESIAN_POINT('Ctrl Pts',(80.1330971801894,-10.6607113306497,132.056928432906));
#78829=CARTESIAN_POINT('Ctrl Pts',(80.1440587804744,-10.6597963913257,132.057654460407));
#78830=CARTESIAN_POINT('Ctrl Pts',(80.173792706204,-10.6570177844738,132.059616572637));
#78831=CARTESIAN_POINT('Ctrl Pts',(80.1925440956127,-10.6549437032903,132.060846053678));
#78832=CARTESIAN_POINT('Ctrl Pts',(80.3094567004957,-10.6399979732241,132.068469883845));
#78833=CARTESIAN_POINT('Ctrl Pts',(80.4063476699741,-10.6187161656053,132.074587432156));
#78834=CARTESIAN_POINT('Ctrl Pts',(80.568823531528,-10.5675090846156,132.085008159284));
#78835=CARTESIAN_POINT('Ctrl Pts',(80.6354111525916,-10.5417188122892,132.089334227471));
#78836=CARTESIAN_POINT('Ctrl Pts',(80.7338037839405,-10.4961498845915,132.096065986805));
#78837=CARTESIAN_POINT('Ctrl Pts',(80.7669370175872,-10.4794389900358,132.098395687312));
#78838=CARTESIAN_POINT('Ctrl Pts',(80.8132427379196,-10.4541108070232,132.101780367295));
#78839=CARTESIAN_POINT('Ctrl Pts',(80.8268953831342,-10.4463906721799,132.102794787423));
#78840=CARTESIAN_POINT('Ctrl Pts',(80.8509431208304,-10.4323406986326,132.104614791611));
#78841=CARTESIAN_POINT('Ctrl Pts',(80.8613818395354,-10.4260874367043,132.105416175597));
#78842=CARTESIAN_POINT('Ctrl Pts',(80.8772741086849,-10.4163291100904,132.106655237239));
#78843=CARTESIAN_POINT('Ctrl Pts',(80.8827775151652,-10.4129054692478,132.10708786011));
#78844=CARTESIAN_POINT('Ctrl Pts',(80.8928939731447,-10.4065298952878,132.10788994706));
#78845=CARTESIAN_POINT('Ctrl Pts',(80.8975126161732,-10.4035872236395,132.108258814229));
#78846=CARTESIAN_POINT('Ctrl Pts',(80.9080233227687,-10.3968174567629,132.109104342529));
#78847=CARTESIAN_POINT('Ctrl Pts',(80.913905741243,-10.3929758267279,132.10958193402));
#78848=CARTESIAN_POINT('Ctrl Pts',(80.932533132624,-10.3806420636811,132.111107838917));
#78849=CARTESIAN_POINT('Ctrl Pts',(80.9451849632606,-10.37201162356,132.11216457811));
#78850=CARTESIAN_POINT('Ctrl Pts',(81.0407800692325,-10.3048517451646,132.120294978693));
#78851=CARTESIAN_POINT('Ctrl Pts',(81.1183298665335,-10.2390303195043,132.127724832671));
#78852=CARTESIAN_POINT('Ctrl Pts',(81.2703564375848,-10.0840282279089,132.143516198847));
#78853=CARTESIAN_POINT('Ctrl Pts',(81.342514178779,-9.9932712513982,132.15180978059));
#78854=CARTESIAN_POINT('Ctrl Pts',(81.4151572946302,-9.8793544402138,132.161055526028));
#78855=CARTESIAN_POINT('Ctrl Pts',(81.4253286015919,-9.86277044061573,132.162376217263));
#78856=CARTESIAN_POINT('Ctrl Pts',(81.4408565887629,-9.83642814570942,132.164435509861));
#78857=CARTESIAN_POINT('Ctrl Pts',(81.4464096585687,-9.82678828142979,132.165181177672));
#78858=CARTESIAN_POINT('Ctrl Pts',(81.456632720532,-9.80862326335147,132.166571804607));
#78859=CARTESIAN_POINT('Ctrl Pts',(81.4613254390525,-9.80011151259059,132.167217557667));
#78860=CARTESIAN_POINT('Ctrl Pts',(81.4716962007195,-9.78090517417354,132.168661827098));
#78861=CARTESIAN_POINT('Ctrl Pts',(81.4773327242669,-9.77018869960252,132.169458848109));
#78862=CARTESIAN_POINT('Ctrl Pts',(81.4935673849794,-9.73848836294817,132.171791495594));
#78863=CARTESIAN_POINT('Ctrl Pts',(81.5038390874986,-9.71734000532881,132.173315767468));
#78864=CARTESIAN_POINT('Ctrl Pts',(81.5589385377694,-9.59750640443749,132.181789878686));
#78865=CARTESIAN_POINT('Ctrl Pts',(81.5945013405354,-9.49484573089368,132.188416594995));
#78866=CARTESIAN_POINT('Ctrl Pts',(81.637382106173,-9.31649057665,132.199617765142));
#78867=CARTESIAN_POINT('Ctrl Pts',(81.6499725231119,-9.24243664599759,132.204189811422));
#78868=CARTESIAN_POINT('Ctrl Pts',(81.6611299141817,-9.13221894674011,132.21118281793));
#78869=CARTESIAN_POINT('Ctrl Pts',(81.6635845998015,-9.09654166499363,132.213475795502));
#78870=CARTESIAN_POINT('Ctrl Pts',(81.6652439304393,-9.05111621041222,132.216463657714));
#78871=CARTESIAN_POINT('Ctrl Pts',(81.665513469019,-9.0414136231496,132.217105808627));
#78872=CARTESIAN_POINT('Ctrl Pts',(81.6658114616797,-9.02576009777273,132.218149004307));
#78873=CARTESIAN_POINT('Ctrl Pts',(81.6658928419021,-9.01981022479718,132.218547196219));
#78874=CARTESIAN_POINT('Ctrl Pts',(81.6659887283855,-9.00828500870662,132.219321981245));
#78875=CARTESIAN_POINT('Ctrl Pts',(81.6660071241545,-9.00270983260339,132.21969835942));
#78876=CARTESIAN_POINT('Ctrl Pts',(81.6659856911072,-8.99024732520934,132.220543100376));
#78877=CARTESIAN_POINT('Ctrl Pts',(81.6659311354573,-8.98336012657935,132.221012251989));
#78878=CARTESIAN_POINT('Ctrl Pts',(81.6656405062171,-8.96278152621034,132.222420594565));
#78879=CARTESIAN_POINT('Ctrl Pts',(81.6652783387284,-8.94909287055782,132.223366060494));
#78880=CARTESIAN_POINT('Ctrl Pts',(81.6607646042034,-8.83275412547422,132.231466563769));
#78881=CARTESIAN_POINT('Ctrl Pts',(81.6472952179804,-8.73069485031223,132.238988976958));
#78882=CARTESIAN_POINT('Ctrl Pts',(81.599076449266,-8.518679487388,132.254801368189));
#78883=CARTESIAN_POINT('Ctrl Pts',(81.5621480966043,-8.40973101139748,132.263026382946));
#78884=CARTESIAN_POINT('Ctrl Pts',(81.5062203657711,-8.28779750578302,132.272205704492));
#78885=CARTESIAN_POINT('Ctrl Pts',(81.4978266768859,-8.27031000815241,132.273522440321));
#78886=CARTESIAN_POINT('Ctrl Pts',(81.4841464916188,-8.2430398459942,132.275576995798));
#78887=CARTESIAN_POINT('Ctrl Pts',(81.4790644264461,-8.2331571763924,132.27632182792));
#78888=CARTESIAN_POINT('Ctrl Pts',(81.4693520872585,-8.21472620434297,132.277711697275));
#78889=CARTESIAN_POINT('Ctrl Pts',(81.4647451636199,-8.20616619939979,132.278357520174));
#78890=CARTESIAN_POINT('Ctrl Pts',(81.4542240252029,-8.18702060229962,132.279802977315));
#78891=CARTESIAN_POINT('Ctrl Pts',(81.4482685953857,-8.1764581946507,132.28060110517));
#78892=CARTESIAN_POINT('Ctrl Pts',(81.4303880270165,-8.14553956842806,132.282940261883));
#78893=CARTESIAN_POINT('Ctrl Pts',(81.4181449225842,-8.12537001819633,132.284469838377));
#78894=CARTESIAN_POINT('Ctrl Pts',(81.3503006574022,-8.01877417389043,132.292587183117));
#78895=CARTESIAN_POINT('Ctrl Pts',(81.2872197795695,-7.93736904122788,132.298888959422));
#78896=CARTESIAN_POINT('Ctrl Pts',(81.1628989994817,-7.8043806226364,132.310007421919));
#78897=CARTESIAN_POINT('Ctrl Pts',(81.104705132187,-7.75041422878135,132.314825524784));
#78898=CARTESIAN_POINT('Ctrl Pts',(81.0235808504587,-7.68529405402791,132.321384851457));
#78899=CARTESIAN_POINT('Ctrl Pts',(81.0039231563842,-7.670222707349,132.32296362833));
#78900=CARTESIAN_POINT('Ctrl Pts',(80.9700456731267,-7.64542856887439,132.325680447472));
#78901=CARTESIAN_POINT('Ctrl Pts',(80.9559973453454,-7.63547759674423,132.326805944588));
#78902=CARTESIAN_POINT('Ctrl Pts',(80.9356617934914,-7.62154131515328,132.328437532949));
#78903=CARTESIAN_POINT('Ctrl Pts',(80.9294976051768,-7.61737729862326,132.328932413844));
#78904=CARTESIAN_POINT('Ctrl Pts',(80.9187212386999,-7.61020230887844,132.329798497944));
#78905=CARTESIAN_POINT('Ctrl Pts',(80.9141216855576,-7.60717270285408,132.330168457883));
#78906=CARTESIAN_POINT('Ctrl Pts',(80.9042330860898,-7.60072942211105,132.330964597894));
#78907=CARTESIAN_POINT('Ctrl Pts',(80.89893977881,-7.59732295416597,132.331391199042));
#78908=CARTESIAN_POINT('Ctrl Pts',(80.884352235185,-7.58805173509775,132.33256775388));
#78909=CARTESIAN_POINT('Ctrl Pts',(80.8750192689168,-7.58224894937167,132.333321505046));
#78910=CARTESIAN_POINT('Ctrl Pts',(80.8216179210651,-7.54977471444806,132.337637007748));
#78911=CARTESIAN_POINT('Ctrl Pts',(80.7763926333708,-7.52506855153028,132.341301377097));
#78912=CARTESIAN_POINT('Ctrl Pts',(80.6437991547922,-7.46042309691272,132.351931447797));
#78913=CARTESIAN_POINT('Ctrl Pts',(80.5540209569969,-7.42588557037395,132.358983590216));
#78914=CARTESIAN_POINT('Ctrl Pts',(80.4112410286266,-7.38469758446319,132.369670221335));
#78915=CARTESIAN_POINT('Ctrl Pts',(80.3600518318519,-7.37252199859724,132.373404780799));
#78916=CARTESIAN_POINT('Ctrl Pts',(80.28494499347,-7.35837566484272,132.378731250655));
#78917=CARTESIAN_POINT('Ctrl Pts',(80.2614289099509,-7.35446691580834,132.380377795236));
#78918=CARTESIAN_POINT('Ctrl Pts',(80.2186318496623,-7.34829403776919,132.383336598715));
#78919=CARTESIAN_POINT('Ctrl Pts',(80.1993801203271,-7.34585971145186,132.384653849583));
#78920=CARTESIAN_POINT('Ctrl Pts',(80.169040771893,-7.34256078971381,132.386709021938));
#78921=CARTESIAN_POINT('Ctrl Pts',(80.1579800440934,-7.34146997784515,132.387453962916));
#78922=CARTESIAN_POINT('Ctrl Pts',(80.137226413665,-7.33963275193658,132.388843930783));
#78923=CARTESIAN_POINT('Ctrl Pts',(80.127536347605,-7.338860338823,132.389489744417));
#78924=CARTESIAN_POINT('Ctrl Pts',(80.1057474812901,-7.33731529387086,132.390935046019));
#78925=CARTESIAN_POINT('Ctrl Pts',(80.0936458076379,-7.33658981682944,132.391733029045));
#78926=CARTESIAN_POINT('Ctrl Pts',(80.0579852011558,-7.33484242892865,132.394071333496));
#78927=CARTESIAN_POINT('Ctrl Pts',(80.0344106487367,-7.33418848102524,132.395600215382));
#78928=CARTESIAN_POINT('Ctrl Pts',(79.9068353987634,-7.33335921114161,132.403796257104));
#78929=CARTESIAN_POINT('Ctrl Pts',(79.8030026469127,-7.3424214689515,132.410169518184));
#78930=CARTESIAN_POINT('Ctrl Pts',(79.6236308787605,-7.37518083371644,132.421304936487));
#78931=CARTESIAN_POINT('Ctrl Pts',(79.5476725925114,-7.39466849524455,132.426068245187));
#78932=CARTESIAN_POINT('Ctrl Pts',(79.4500218901552,-7.42720444123743,132.432559826914));
#78933=CARTESIAN_POINT('Ctrl Pts',(79.4268475844415,-7.43550072809721,132.434129018617));
#78934=CARTESIAN_POINT('Ctrl Pts',(79.3878662013054,-7.45043818271576,132.436830941777));
#78935=CARTESIAN_POINT('Ctrl Pts',(79.3719618913626,-7.45681572997584,132.437951307948));
#78936=CARTESIAN_POINT('Ctrl Pts',(79.3493112457265,-7.46630665437703,132.43957675623));
#78937=CARTESIAN_POINT('Ctrl Pts',(79.342482371947,-7.46922186554151,132.44007074325));
#78938=CARTESIAN_POINT('Ctrl Pts',(79.3306239265987,-7.47437816285633,132.440935819748));
#78939=CARTESIAN_POINT('Ctrl Pts',(79.3255856150809,-7.47659868911413,132.441305675039));
#78940=CARTESIAN_POINT('Ctrl Pts',(79.314803683406,-7.48141456293347,132.44210224547));
#78941=CARTESIAN_POINT('Ctrl Pts',(79.3090638500406,-7.48401749504684,132.442529387471));
#78942=CARTESIAN_POINT('Ctrl Pts',(79.2933248968458,-7.49126283487397,132.443708854159));
#78943=CARTESIAN_POINT('Ctrl Pts',(79.283357085113,-7.49597192474842,132.444465005974));
#78944=CARTESIAN_POINT('Ctrl Pts',(79.226491354791,-7.52353059882319,132.448828578866));
#78945=CARTESIAN_POINT('Ctrl Pts',(79.1806447868976,-7.54847203637923,132.452541224214));
#78946=CARTESIAN_POINT('Ctrl Pts',(79.0487712547293,-7.62845371138045,132.463659344451));
#78947=CARTESIAN_POINT('Ctrl Pts',(78.9665372630134,-7.68930099715414,132.47116230885));
#78948=CARTESIAN_POINT('Ctrl Pts',(78.8359641567243,-7.80588925293691,132.483711487921));
#78949=CARTESIAN_POINT('Ctrl Pts',(78.7847831076796,-7.8580146797057,132.488839183625));
#78950=CARTESIAN_POINT('Ctrl Pts',(78.725682703302,-7.92669571786026,132.495022772812));
#78951=CARTESIAN_POINT('Ctrl Pts',(78.7143987392386,-7.94023771793119,132.496216955377));
#78952=CARTESIAN_POINT('Ctrl Pts',(78.6965917590267,-7.96231113674697,132.498124380316));
#78953=CARTESIAN_POINT('Ctrl Pts',(78.6899328687333,-7.97073067642218,132.498843047088));
#78954=CARTESIAN_POINT('Ctrl Pts',(78.6773568413267,-7.98695166459002,132.50021101604));
#78955=CARTESIAN_POINT('Ctrl Pts',(78.6714262193241,-7.99474203741312,132.500860833758));
#78956=CARTESIAN_POINT('Ctrl Pts',(78.6580440528446,-8.01264594587972,132.502338278073));
#78957=CARTESIAN_POINT('Ctrl Pts',(78.6506374691082,-8.0227924647801,132.503164134606));
#78958=CARTESIAN_POINT('Ctrl Pts',(78.6311692136781,-8.05010609921862,132.505357818712));
#78959=CARTESIAN_POINT('Ctrl Pts',(78.6193156260609,-8.06741924378956,132.506717773559));
#78960=CARTESIAN_POINT('Ctrl Pts',(78.5412032923739,-8.1862640141107,132.515861061319));
#78961=CARTESIAN_POINT('Ctrl Pts',(78.4858706108274,-8.29454260679863,132.523223016254));
#78962=CARTESIAN_POINT('Ctrl Pts',(78.4406740918851,-8.41340500872868,132.530993826561));
#78963=CARTESIAN_POINT('Ctrl Pts',(78.4386018914004,-8.41894328418144,132.531355307084));
#78964=CARTESIAN_POINT('Ctrl Pts',(78.4365593757978,-8.42449203776637,132.531716974833));
#78965=CARTESIAN_POINT('Origin',(80.,-9.,134.));
#78966=CARTESIAN_POINT('',(78.4365594153165,-8.4244919304089,133.231049000392));
#78967=CARTESIAN_POINT('',(78.4365593697901,-8.4244920540871,133.038342736257));
#78968=CARTESIAN_POINT('',(78.4365593749993,-8.42449203993574,134.));
#78969=CARTESIAN_POINT('Ctrl Pts',(78.4365593697901,-8.4244920540871,133.038342736257));
#78970=CARTESIAN_POINT('Ctrl Pts',(78.4628061193141,-8.35318941629014,133.03360761879));
#78971=CARTESIAN_POINT('Ctrl Pts',(78.4939041984131,-8.28375384386915,133.02898652258));
#78972=CARTESIAN_POINT('Ctrl Pts',(78.561214954218,-8.1574070897627,133.020239035207));
#78973=CARTESIAN_POINT('Ctrl Pts',(78.5963402310007,-8.10010937121719,133.016124919609));
#78974=CARTESIAN_POINT('Ctrl Pts',(78.6535462851658,-8.01832521231255,133.009803734371));
#78975=CARTESIAN_POINT('Ctrl Pts',(78.6730506737764,-7.99211699782551,133.007703247721));
#78976=CARTESIAN_POINT('Ctrl Pts',(78.6991841628878,-7.95907551198317,133.004932413371));
#78977=CARTESIAN_POINT('Ctrl Pts',(78.7051202654679,-7.95170037940832,133.004305759935));
#78978=CARTESIAN_POINT('Ctrl Pts',(78.7148565738052,-7.93981267045829,133.003281565034));
#78979=CARTESIAN_POINT('Ctrl Pts',(78.7186185588224,-7.93526886065503,133.002886689248));
#78980=CARTESIAN_POINT('Ctrl Pts',(78.7260049108909,-7.92644330276556,133.002112831928));
#78981=CARTESIAN_POINT('Ctrl Pts',(78.7296269035633,-7.92215972345916,133.001734017121));
#78982=CARTESIAN_POINT('Ctrl Pts',(78.7387075861672,-7.91152973305655,133.000786086764));
#78983=CARTESIAN_POINT('Ctrl Pts',(78.7441925567266,-7.90520607728211,133.000215108605));
#78984=CARTESIAN_POINT('Ctrl Pts',(78.7640094902605,-7.88270388410603,132.99815869683));
#78985=CARTESIAN_POINT('Ctrl Pts',(78.7786076633492,-7.86676401301595,132.996655858209));
#78986=CARTESIAN_POINT('Ctrl Pts',(78.8874916271528,-7.7524208418627,132.985560771926));
#78987=CARTESIAN_POINT('Ctrl Pts',(78.9932244310413,-7.66563394739609,132.975447055159));
#78988=CARTESIAN_POINT('Ctrl Pts',(79.1502573126506,-7.56613988581271,132.962107931343));
#78989=CARTESIAN_POINT('Ctrl Pts',(79.1933347581965,-7.54147011898524,132.958592383899));
#78990=CARTESIAN_POINT('Ctrl Pts',(79.2673572284867,-7.50336315150526,132.95279812802));
#78991=CARTESIAN_POINT('Ctrl Pts',(79.2977228468922,-7.48887645458893,132.950486878261));
#78992=CARTESIAN_POINT('Ctrl Pts',(79.3410671274373,-7.46978701217852,132.947276870002));
#78993=CARTESIAN_POINT('Ctrl Pts',(79.3536941822265,-7.46441114613154,132.946352084262));
#78994=CARTESIAN_POINT('Ctrl Pts',(79.3755799234528,-7.4554112591725,132.944766555005));
#78995=CARTESIAN_POINT('Ctrl Pts',(79.3848071100372,-7.45171303506075,132.944103333911));
#78996=CARTESIAN_POINT('Ctrl Pts',(79.4037294557153,-7.44432489458287,132.942753704367));
#78997=CARTESIAN_POINT('Ctrl Pts',(79.413427095572,-7.44064249396593,132.942067571759));
#78998=CARTESIAN_POINT('Ctrl Pts',(79.438095306397,-7.43153813951464,132.940335843413));
#78999=CARTESIAN_POINT('Ctrl Pts',(79.4531105909201,-7.42623969568196,132.939294369759));
#79000=CARTESIAN_POINT('Ctrl Pts',(79.5125729198906,-7.40621105941954,132.935216709227));
#79001=CARTESIAN_POINT('Ctrl Pts',(79.5575589068905,-7.39314131368899,132.932234517607));
#79002=CARTESIAN_POINT('Ctrl Pts',(79.7122185630681,-7.35519744060681,132.922242261325));
#79003=CARTESIAN_POINT('Ctrl Pts',(79.8238262386276,-7.33953113110188,132.91548705435));
#79004=CARTESIAN_POINT('Ctrl Pts',(80.0010847397146,-7.33273401068903,132.90457282982));
#79005=CARTESIAN_POINT('Ctrl Pts',(80.0660898201429,-7.33404462124014,132.900525133508));
#79006=CARTESIAN_POINT('Ctrl Pts',(80.1459140896061,-7.34033329199974,132.895323701359));
#79007=CARTESIAN_POINT('Ctrl Pts',(80.1609662175044,-7.34172549294908,132.894332642906));
#79008=CARTESIAN_POINT('Ctrl Pts',(80.183022414331,-7.34406862638646,132.892862624704));
#79009=CARTESIAN_POINT('Ctrl Pts',(80.1900431875613,-7.34485967344103,132.892392044608));
#79010=CARTESIAN_POINT('Ctrl Pts',(80.2019749655849,-7.34628097086639,132.891587452357));
#79011=CARTESIAN_POINT('Ctrl Pts',(80.2068885363969,-7.34688849539379,132.891254708467));
#79012=CARTESIAN_POINT('Ctrl Pts',(80.2180703928207,-7.34832167942787,132.890494193003));
#79013=CARTESIAN_POINT('Ctrl Pts',(80.2243365903599,-7.3491611036296,132.890065680317));
#79014=CARTESIAN_POINT('Ctrl Pts',(80.241597854255,-7.35157352510601,132.888879130739));
#79015=CARTESIAN_POINT('Ctrl Pts',(80.2525819664453,-7.35322081020548,132.888117195497));
#79016=CARTESIAN_POINT('Ctrl Pts',(80.3158419436076,-7.36335566787966,132.883692413098));
#79017=CARTESIAN_POINT('Ctrl Pts',(80.3677010739732,-7.37422155243195,132.879921299376));
#79018=CARTESIAN_POINT('Ctrl Pts',(80.5173538371733,-7.41310421819481,132.868770245084));
#79019=CARTESIAN_POINT('Ctrl Pts',(80.6132187608485,-7.44762834092024,132.861298328387));
#79020=CARTESIAN_POINT('Ctrl Pts',(80.7709996605853,-7.52136256312843,132.848816183098));
#79021=CARTESIAN_POINT('Ctrl Pts',(80.8345968220762,-7.55630339480565,132.843723893006));
#79022=CARTESIAN_POINT('Ctrl Pts',(80.910562799522,-7.60474334819562,132.837575563113));
#79023=CARTESIAN_POINT('Ctrl Pts',(80.9252516028103,-7.61444045633709,132.836383185083));
#79024=CARTESIAN_POINT('Ctrl Pts',(80.9486446301411,-7.63042177810377,132.834477803156));
#79025=CARTESIAN_POINT('Ctrl Pts',(80.9574462568691,-7.6365603003019,132.833759398177));
#79026=CARTESIAN_POINT('Ctrl Pts',(80.974167790149,-7.64846418437229,132.832391397068));
#79027=CARTESIAN_POINT('Ctrl Pts',(80.9820973253557,-7.65421517514561,132.831741290156));
#79028=CARTESIAN_POINT('Ctrl Pts',(81.0000926800359,-7.66751028188434,132.830262459357));
#79029=CARTESIAN_POINT('Ctrl Pts',(81.010124784145,-7.67509919147521,132.829435514994));
#79030=CARTESIAN_POINT('Ctrl Pts',(81.0366998609108,-7.6956795651641,132.827237294747));
#79031=CARTESIAN_POINT('Ctrl Pts',(81.0530846964875,-7.70887216597268,132.825873941988));
#79032=CARTESIAN_POINT('Ctrl Pts',(81.1614825713486,-7.79958772097864,132.816787169467));
#79033=CARTESIAN_POINT('Ctrl Pts',(81.2451155205109,-7.8865716972318,132.809477672488));
#79034=CARTESIAN_POINT('Ctrl Pts',(81.3593481732068,-8.03451473641377,132.79805701234));
#79035=CARTESIAN_POINT('Ctrl Pts',(81.396841794092,-8.08960394667465,132.79397828883));
#79036=CARTESIAN_POINT('Ctrl Pts',(81.4424673892459,-8.16612302913608,132.788340328566));
#79037=CARTESIAN_POINT('Ctrl Pts',(81.4536048178128,-8.18569299163068,132.78690046957));
#79038=CARTESIAN_POINT('Ctrl Pts',(81.4719891491043,-8.21957633963112,132.784400539124));
#79039=CARTESIAN_POINT('Ctrl Pts',(81.4794323780598,-8.23378009873849,132.783350533682));
#79040=CARTESIAN_POINT('Ctrl Pts',(81.4899337485244,-8.25454326224539,132.781809438179));
#79041=CARTESIAN_POINT('Ctrl Pts',(81.4931562564454,-8.26101913972246,132.781327919972));
#79042=CARTESIAN_POINT('Ctrl Pts',(81.4987268566032,-8.27239889389514,132.780479905602));
#79043=CARTESIAN_POINT('Ctrl Pts',(81.5010932703707,-8.27729359159184,132.780114543085));
#79044=CARTESIAN_POINT('Ctrl Pts',(81.5061944370699,-8.28797800974474,132.77931558338));
#79045=CARTESIAN_POINT('Ctrl Pts',(81.5089197422572,-8.29377184646675,132.778881456882));
#79046=CARTESIAN_POINT('Ctrl Pts',(81.5164321597137,-8.30998479734562,132.777664495741));
#79047=CARTESIAN_POINT('Ctrl Pts',(81.5211450968081,-8.32043760316743,132.776877444629));
#79048=CARTESIAN_POINT('Ctrl Pts',(81.5519978182549,-8.39079508451345,132.771567455939));
#79049=CARTESIAN_POINT('Ctrl Pts',(81.5746980614344,-8.45213873188183,132.766880069889));
#79050=CARTESIAN_POINT('Ctrl Pts',(81.5999803136546,-8.53515745502293,132.760590050769));
#79051=CARTESIAN_POINT('Ctrl Pts',(81.6058293379807,-8.55578415835092,132.759031289682));
#79052=CARTESIAN_POINT('Ctrl Pts',(81.62874740918,-8.64298355937333,132.752469936565));
#79053=CARTESIAN_POINT('Ctrl Pts',(81.6420877587951,-8.71047005477192,132.747464313843));
#79054=CARTESIAN_POINT('Ctrl Pts',(81.6606685882657,-8.84904153065469,132.737451629434));
#79055=CARTESIAN_POINT('Ctrl Pts',(81.665597880524,-8.92003264419149,132.732460942705));
#79056=CARTESIAN_POINT('Ctrl Pts',(81.6660696298094,-9.00864433451294,132.726414619291));
#79057=CARTESIAN_POINT('Ctrl Pts',(81.6658866973958,-9.02615889899833,132.725228151296));
#79058=CARTESIAN_POINT('Ctrl Pts',(81.6651468317012,-9.05437624418066,132.723329877337));
#79059=CARTESIAN_POINT('Ctrl Pts',(81.6647627797226,-9.06508182215686,132.72261274267));
#79060=CARTESIAN_POINT('Ctrl Pts',(81.6638296949817,-9.08557331172566,132.721245690273));
#79061=CARTESIAN_POINT('Ctrl Pts',(81.6632975133836,-9.09535950165407,132.720595275641));
#79062=CARTESIAN_POINT('Ctrl Pts',(81.661882833037,-9.11773106072618,132.719113731521));
#79063=CARTESIAN_POINT('Ctrl Pts',(81.660943665876,-9.13031234301575,132.718284404982));
#79064=CARTESIAN_POINT('Ctrl Pts',(81.6575690410271,-9.16951538422329,132.715711295771));
#79065=CARTESIAN_POINT('Ctrl Pts',(81.654635644927,-9.19609080034345,132.71398301054));
#79066=CARTESIAN_POINT('Ctrl Pts',(81.6333961878039,-9.35363799821407,132.70380948757));
#79067=CARTESIAN_POINT('Ctrl Pts',(81.6001896077223,-9.48211904785678,132.695857850917));
#79068=CARTESIAN_POINT('Ctrl Pts',(81.526068531088,-9.67217472149256,132.683343587908));
#79069=CARTESIAN_POINT('Ctrl Pts',(81.4957106024904,-9.73725941700626,132.67889705109));
#79070=CARTESIAN_POINT('Ctrl Pts',(81.4536619545557,-9.81404729330117,132.673217355844));
#79071=CARTESIAN_POINT('Ctrl Pts',(81.4458698862522,-9.8278081307099,132.672181575324));
#79072=CARTESIAN_POINT('Ctrl Pts',(81.4342502574912,-9.84766381558653,132.67065760297));
#79073=CARTESIAN_POINT('Ctrl Pts',(81.4305769479412,-9.85384854431348,132.670178688358));
#79074=CARTESIAN_POINT('Ctrl Pts',(81.4240592521183,-9.8646622247977,132.669333537986));
#79075=CARTESIAN_POINT('Ctrl Pts',(81.421232103019,-9.86930134281507,132.668968409527));
#79076=CARTESIAN_POINT('Ctrl Pts',(81.4150095455925,-9.87940054833436,132.668167849903));
#79077=CARTESIAN_POINT('Ctrl Pts',(81.4116052587202,-9.88485474999599,132.66773187012));
#79078=CARTESIAN_POINT('Ctrl Pts',(81.4019783332577,-9.90008165213583,132.666504811552));
#79079=CARTESIAN_POINT('Ctrl Pts',(81.3956853393783,-9.90980912402503,132.66570940825));
#79080=CARTESIAN_POINT('Ctrl Pts',(81.3497800994107,-9.97917057965944,132.659958986398));
#79081=CARTESIAN_POINT('Ctrl Pts',(81.306465701874,-10.0362559502864,132.654807202752));
#79082=CARTESIAN_POINT('Ctrl Pts',(81.2505036866459,-10.1009044360093,132.64859897745));
#79083=CARTESIAN_POINT('Ctrl Pts',(81.2412549610045,-10.1113218097621,132.647585963284));
#79084=CARTESIAN_POINT('Ctrl Pts',(81.1872493633575,-10.1706361286461,132.641748751946));
#79085=CARTESIAN_POINT('Ctrl Pts',(81.1397343722851,-10.2169454933137,132.636918942927));
#79086=CARTESIAN_POINT('Ctrl Pts',(81.0522763581015,-10.2925566698174,132.628625216851));
#79087=CARTESIAN_POINT('Ctrl Pts',(81.0135515415972,-10.3231410746955,132.625131381835));
#79088=CARTESIAN_POINT('Ctrl Pts',(80.9463433485087,-10.3715363970818,132.619368298839));
#79089=CARTESIAN_POINT('Ctrl Pts',(80.9185775920956,-10.390285333292,132.617066968719));
#79090=CARTESIAN_POINT('Ctrl Pts',(80.8786826620773,-10.4155071540131,132.613868131652));
#79091=CARTESIAN_POINT('Ctrl Pts',(80.8670115371286,-10.4226857480351,132.612944840979));
#79092=CARTESIAN_POINT('Ctrl Pts',(80.8467255689278,-10.4348207365521,132.611361061483));
#79093=CARTESIAN_POINT('Ctrl Pts',(80.8381526449522,-10.439845438317,132.61069810958));
#79094=CARTESIAN_POINT('Ctrl Pts',(80.820533788081,-10.4499613913401,132.609348321176));
#79095=CARTESIAN_POINT('Ctrl Pts',(80.8114841907148,-10.4550454117424,132.608661766522));
#79096=CARTESIAN_POINT('Ctrl Pts',(80.788406512914,-10.4677280652419,132.60692756251));
#79097=CARTESIAN_POINT('Ctrl Pts',(80.774315510965,-10.4752105007322,132.605884059613));
#79098=CARTESIAN_POINT('Ctrl Pts',(80.7181887881325,-10.5039884274052,132.601785206916));
#79099=CARTESIAN_POINT('Ctrl Pts',(80.6753630391188,-10.5237000079728,132.598784609546));
#79100=CARTESIAN_POINT('Ctrl Pts',(80.5279728255844,-10.5841024462646,132.58879214491));
#79101=CARTESIAN_POINT('Ctrl Pts',(80.4201624656764,-10.6160444892451,132.58205231361));
#79102=CARTESIAN_POINT('Ctrl Pts',(80.2462147002532,-10.6489825153716,132.57115911966));
#79103=CARTESIAN_POINT('Ctrl Pts',(80.1818266400267,-10.6573177808013,132.567116903301));
#79104=CARTESIAN_POINT('Ctrl Pts',(80.1020555385948,-10.6629398275944,132.561922041275));
#79105=CARTESIAN_POINT('Ctrl Pts',(80.0869734191753,-10.6637967989842,132.560931619842));
#79106=CARTESIAN_POINT('Ctrl Pts',(80.0648255313732,-10.6647532978196,132.559462371492));
#79107=CARTESIAN_POINT('Ctrl Pts',(80.0577669669406,-10.665013172659,132.558991911758));
#79108=CARTESIAN_POINT('Ctrl Pts',(80.0457584732086,-10.6653788379769,132.558187454295));
#79109=CARTESIAN_POINT('Ctrl Pts',(80.0408093794307,-10.6655074618602,132.557854723654));
#79110=CARTESIAN_POINT('Ctrl Pts',(80.02953766703,-10.6657501350732,132.557094137516));
#79111=CARTESIAN_POINT('Ctrl Pts',(80.0232150695413,-10.6658502464163,132.556665540036));
#79112=CARTESIAN_POINT('Ctrl Pts',(80.0057803210671,-10.6660270328463,132.555478532953));
#79113=CARTESIAN_POINT('Ctrl Pts',(79.9946679747136,-10.6660285229165,132.554716220296));
#79114=CARTESIAN_POINT('Ctrl Pts',(79.9304589107186,-10.6653947580465,132.550281336751));
#79115=CARTESIAN_POINT('Ctrl Pts',(79.8774216670898,-10.6623324111577,132.546499926768));
#79116=CARTESIAN_POINT('Ctrl Pts',(79.7243947393697,-10.6461339093797,132.535401447877));
#79117=CARTESIAN_POINT('Ctrl Pts',(79.6253248774927,-10.6264486999272,132.527995105171));
#79118=CARTESIAN_POINT('Ctrl Pts',(79.4584982207439,-10.5772381492018,132.515524753495));
#79119=CARTESIAN_POINT('Ctrl Pts',(79.3897847196958,-10.551948559544,132.510384861366));
#79120=CARTESIAN_POINT('Ctrl Pts',(79.3068310585781,-10.5150524504498,132.504188854034));
#79121=CARTESIAN_POINT('Ctrl Pts',(79.2908293375031,-10.5076286419254,132.5029937815));
#79122=CARTESIAN_POINT('Ctrl Pts',(79.2652795958838,-10.4952783177129,132.501085159112));
#79123=CARTESIAN_POINT('Ctrl Pts',(79.2556564327779,-10.4905113159321,132.500366175053));
#79124=CARTESIAN_POINT('Ctrl Pts',(79.2373471100845,-10.4812199258996,132.49899773735));
#79125=CARTESIAN_POINT('Ctrl Pts',(79.2286534721638,-10.4767113598669,132.498347766625));
#79126=CARTESIAN_POINT('Ctrl Pts',(79.2088999899896,-10.4662450586745,132.496870152935));
#79127=CARTESIAN_POINT('Ctrl Pts',(79.1978666759877,-10.4602383171276,132.496044278973));
#79128=CARTESIAN_POINT('Ctrl Pts',(79.1685955698161,-10.4438706967361,132.49385093017));
#79129=CARTESIAN_POINT('Ctrl Pts',(79.1504833642781,-10.4332890371368,132.492491321604));
#79130=CARTESIAN_POINT('Ctrl Pts',(79.028962818056,-10.3591802558185,132.483340344464));
#79131=CARTESIAN_POINT('Ctrl Pts',(78.9325628869623,-10.2848603187997,132.475971354361));
#79132=CARTESIAN_POINT('Ctrl Pts',(78.7768704876421,-10.1351072236162,132.462770402837));
#79133=CARTESIAN_POINT('Ctrl Pts',(78.714380758827,-10.0638102341602,132.456968930806));
#79134=CARTESIAN_POINT('Ctrl Pts',(78.6512058662437,-9.97798424046067,132.450001529669));
#79135=CARTESIAN_POINT('Ctrl Pts',(78.6442261913598,-9.96828515917442,132.44921427928));
#79136=CARTESIAN_POINT('Ctrl Pts',(78.6336484352558,-9.95324751895324,132.447992477885));
#79137=CARTESIAN_POINT('Ctrl Pts',(78.6299757906708,-9.94796154628915,132.447562764113));
#79138=CARTESIAN_POINT('Ctrl Pts',(78.6232309069204,-9.93813268800382,132.4467630501));
#79139=CARTESIAN_POINT('Ctrl Pts',(78.6201503564435,-9.93359575510221,132.446393613512));
#79140=CARTESIAN_POINT('Ctrl Pts',(78.6131370243566,-9.92315621304728,132.445542909355));
#79141=CARTESIAN_POINT('Ctrl Pts',(78.6092194934486,-9.917243634422,132.44506066826));
#79142=CARTESIAN_POINT('Ctrl Pts',(78.5967638951246,-9.89818163016667,132.443505008774));
#79143=CARTESIAN_POINT('Ctrl Pts',(78.5883739415129,-9.88493707881446,132.44242271436));
#79144=CARTESIAN_POINT('Ctrl Pts',(78.5325282458581,-9.79396258240091,132.434989404229));
#79145=CARTESIAN_POINT('Ctrl Pts',(78.4913326360921,-9.71257960117055,132.428352487438));
#79146=CARTESIAN_POINT('Ctrl Pts',(78.4247981823295,-9.54916801018671,132.415509565079));
#79147=CARTESIAN_POINT('Ctrl Pts',(78.3987241090773,-9.46772274949642,132.409321320066));
#79148=CARTESIAN_POINT('Ctrl Pts',(78.3680020106449,-9.33824711606812,132.399941795619));
#79149=CARTESIAN_POINT('Ctrl Pts',(78.3589911515499,-9.29140914651757,132.396636443554));
#79150=CARTESIAN_POINT('Ctrl Pts',(78.3497214859849,-9.22886371949396,132.392336222087));
#79151=CARTESIAN_POINT('Ctrl Pts',(78.3476572751646,-9.21345098753675,132.39128549454));
#79152=CARTESIAN_POINT('Ctrl Pts',(78.344585459482,-9.18778894981642,132.389550366783));
#79153=CARTESIAN_POINT('Ctrl Pts',(78.3434565908137,-9.17755543451907,132.388862199855));
#79154=CARTESIAN_POINT('Ctrl Pts',(78.3414309101958,-9.15748679548525,132.387519785941));
#79155=CARTESIAN_POINT('Ctrl Pts',(78.3405265443351,-9.14765288175546,132.386865328795));
#79156=CARTESIAN_POINT('Ctrl Pts',(78.3385587769912,-9.12394608464232,132.385295347423));
#79157=CARTESIAN_POINT('Ctrl Pts',(78.3375816037598,-9.11006663726376,132.384382550121));
#79158=CARTESIAN_POINT('Ctrl Pts',(78.3349117758727,-9.06389602089076,132.381365763054));
#79159=CARTESIAN_POINT('Ctrl Pts',(78.3339852172248,-9.0315667646501,132.379285475395));
#79160=CARTESIAN_POINT('Ctrl Pts',(78.3340225505802,-8.95087241551319,132.374154817107));
#79161=CARTESIAN_POINT('Ctrl Pts',(78.3361502746032,-8.90253721712625,132.371137437581));
#79162=CARTESIAN_POINT('Ctrl Pts',(78.3493322717099,-8.75232329209449,132.361827850156));
#79163=CARTESIAN_POINT('Ctrl Pts',(78.3676768928935,-8.65133468893829,132.355677451397));
#79164=CARTESIAN_POINT('Ctrl Pts',(78.4072397004561,-8.50939955348026,132.346514706518));
#79165=CARTESIAN_POINT('Ctrl Pts',(78.4210455134462,-8.46663741954607,132.343680790756));
#79166=CARTESIAN_POINT('Ctrl Pts',(78.4365593746692,-8.42449204083248,132.34076576841));
#79167=CARTESIAN_POINT('Ctrl Pts',(78.4365593757978,-8.42449203776637,132.531716974833));
#79168=CARTESIAN_POINT('Ctrl Pts',(78.4158152968604,-8.48084596829506,132.535390123933));
#79169=CARTESIAN_POINT('Ctrl Pts',(78.3981331141248,-8.53828076475871,132.539081327909));
#79170=CARTESIAN_POINT('Ctrl Pts',(78.3781664810635,-8.61827538701239,132.544300119671));
#79171=CARTESIAN_POINT('Ctrl Pts',(78.3731815364889,-8.64011219783514,132.545732647857));
#79172=CARTESIAN_POINT('Ctrl Pts',(78.3653986161774,-8.67768120417352,132.548221013902));
#79173=CARTESIAN_POINT('Ctrl Pts',(78.3623839019968,-8.69336575563498,132.549266907653));
#79174=CARTESIAN_POINT('Ctrl Pts',(78.3583344181542,-8.71620032307511,132.550802978582));
#79175=CARTESIAN_POINT('Ctrl Pts',(78.3571198281678,-8.72331809703613,132.551283668714));
#79176=CARTESIAN_POINT('Ctrl Pts',(78.3550723073871,-8.7358060977931,132.552130681393));
#79177=CARTESIAN_POINT('Ctrl Pts',(78.3542193237079,-8.74117284490548,132.552495877947));
#79178=CARTESIAN_POINT('Ctrl Pts',(78.3524177218992,-8.75287715876222,132.553295022104));
#79179=CARTESIAN_POINT('Ctrl Pts',(78.3514794203367,-8.75921595413856,132.553729503724));
#79180=CARTESIAN_POINT('Ctrl Pts',(78.3489603439765,-8.77693911718939,132.554948709072));
#79181=CARTESIAN_POINT('Ctrl Pts',(78.3474608138544,-8.78833440724614,132.55573767454));
#79182=CARTESIAN_POINT('Ctrl Pts',(78.3380833665429,-8.8657830019875,132.561130179634));
#79183=CARTESIAN_POINT('Ctrl Pts',(78.3340507255463,-8.9322346958779,132.56590397706));
#79184=CARTESIAN_POINT('Ctrl Pts',(78.3338866236568,-9.14942545685867,132.58165164396));
#79185=CARTESIAN_POINT('Ctrl Pts',(78.3542177057676,-9.2994673582841,132.592678401743));
#79186=CARTESIAN_POINT('Ctrl Pts',(78.3999680512033,-9.46462843896716,132.604461614973));
#79187=CARTESIAN_POINT('Ctrl Pts',(78.40584594122,-9.48441173241258,132.605868756683));
#79188=CARTESIAN_POINT('Ctrl Pts',(78.4158613430934,-9.51596130427402,132.608106753117));
#79189=CARTESIAN_POINT('Ctrl Pts',(78.4197658645175,-9.52779867707683,132.608945070794));
#79190=CARTESIAN_POINT('Ctrl Pts',(78.426969745976,-9.54884188980903,132.610433213838));
#79191=CARTESIAN_POINT('Ctrl Pts',(78.4302179651041,-9.55806448552675,132.611084685801));
#79192=CARTESIAN_POINT('Ctrl Pts',(78.4372192182297,-9.57739806893125,132.612449075184));
#79193=CARTESIAN_POINT('Ctrl Pts',(78.4409896286756,-9.58750231761332,132.613161381381));
#79194=CARTESIAN_POINT('Ctrl Pts',(78.451264013806,-9.61424084701655,132.615044795323));
#79195=CARTESIAN_POINT('Ctrl Pts',(78.4579379224952,-9.63080865745263,132.616210196466));
#79196=CARTESIAN_POINT('Ctrl Pts',(78.4948473974399,-9.71834691112663,132.62236458341));
#79197=CARTESIAN_POINT('Ctrl Pts',(78.5297201404637,-9.78726487106699,132.627192788968));
#79198=CARTESIAN_POINT('Ctrl Pts',(78.6205084632086,-9.93945208313728,132.638110963633));
#79199=CARTESIAN_POINT('Ctrl Pts',(78.679402675396,-10.0205822827333,132.644123620688));
#79200=CARTESIAN_POINT('Ctrl Pts',(78.7779661704362,-10.1334319031237,132.653456651628));
#79201=CARTESIAN_POINT('Ctrl Pts',(78.8123770773947,-10.1694380403403,132.656609753309));
#79202=CARTESIAN_POINT('Ctrl Pts',(78.8562259004477,-10.2113858928923,132.660585351344));
#79203=CARTESIAN_POINT('Ctrl Pts',(78.8641811817914,-10.2188480499981,132.661305043859));
#79204=CARTESIAN_POINT('Ctrl Pts',(78.8768283138518,-10.2304798872114,132.662447838725));
#79205=CARTESIAN_POINT('Ctrl Pts',(78.8814716054946,-10.2347022381293,132.662867124056));
#79206=CARTESIAN_POINT('Ctrl Pts',(78.8902376889261,-10.24258359811,132.663658418623));
#79207=CARTESIAN_POINT('Ctrl Pts',(78.8943549179573,-10.2462485042515,132.664029982204));
#79208=CARTESIAN_POINT('Ctrl Pts',(78.9040963971883,-10.2548335080476,132.664908818345));
#79209=CARTESIAN_POINT('Ctrl Pts',(78.9097356442377,-10.2597362695311,132.665417322477));
#79210=CARTESIAN_POINT('Ctrl Pts',(78.9286252058328,-10.2759370151046,132.667119270985));
#79211=CARTESIAN_POINT('Ctrl Pts',(78.9420191451869,-10.2870647486891,132.668323840663));
#79212=CARTESIAN_POINT('Ctrl Pts',(78.9751817009875,-10.3137488990789,132.671295909271));
#79213=CARTESIAN_POINT('Ctrl Pts',(78.9951326397183,-10.3290711672589,132.673075168257));
#79214=CARTESIAN_POINT('Ctrl Pts',(79.081288061803,-10.3921893680708,132.680697551053));
#79215=CARTESIAN_POINT('Ctrl Pts',(79.150610370743,-10.4355345063037,132.686675298426));
#79216=CARTESIAN_POINT('Ctrl Pts',(79.3108758938014,-10.5200567631612,132.699835811052));
#79217=CARTESIAN_POINT('Ctrl Pts',(79.4029201945575,-10.558514106641,132.706962339044));
#79218=CARTESIAN_POINT('Ctrl Pts',(79.5204474213307,-10.595664884564,132.715448553096));
#79219=CARTESIAN_POINT('Ctrl Pts',(79.5431840538902,-10.6023221869954,132.717064097743));
#79220=CARTESIAN_POINT('Ctrl Pts',(79.5777816762202,-10.6116560383882,132.719484247576));
#79221=CARTESIAN_POINT('Ctrl Pts',(79.5895418734781,-10.6146911899588,132.720300307338));
#79222=CARTESIAN_POINT('Ctrl Pts',(79.6107742212711,-10.6199240149705,132.721762162006));
#79223=CARTESIAN_POINT('Ctrl Pts',(79.6202343090276,-10.6221678544288,132.722409414242));
#79224=CARTESIAN_POINT('Ctrl Pts',(79.6405345976397,-10.6267955624123,132.723789876356));
#79225=CARTESIAN_POINT('Ctrl Pts',(79.6513801166758,-10.6291541867961,132.724522251137));
#79226=CARTESIAN_POINT('Ctrl Pts',(79.6811777265671,-10.6353232178694,132.726520909046));
#79227=CARTESIAN_POINT('Ctrl Pts',(79.7001742110378,-10.6389125100781,132.727780153089));
#79228=CARTESIAN_POINT('Ctrl Pts',(79.7426115828233,-10.6461682494264,132.730563058112));
#79229=CARTESIAN_POINT('Ctrl Pts',(79.7660771718582,-10.6496662987064,132.732081485437));
#79230=CARTESIAN_POINT('Ctrl Pts',(79.8413897075775,-10.659253845929,132.736899769277));
#79231=CARTESIAN_POINT('Ctrl Pts',(79.893452634329,-10.6634087961407,132.740146515545));
#79232=CARTESIAN_POINT('Ctrl Pts',(80.0433753531649,-10.6683043262529,132.749382744675));
#79233=CARTESIAN_POINT('Ctrl Pts',(80.1412090102354,-10.6628828131774,132.75526419388));
#79234=CARTESIAN_POINT('Ctrl Pts',(80.2879360713108,-10.6417047856632,132.764493801283));
#79235=CARTESIAN_POINT('Ctrl Pts',(80.3375160720623,-10.6322327119384,132.767687695366));
#79236=CARTESIAN_POINT('Ctrl Pts',(80.3972256713105,-10.6179887037877,132.771709025876));
#79237=CARTESIAN_POINT('Ctrl Pts',(80.4078412782409,-10.6153455220601,132.772430811117));
#79238=CARTESIAN_POINT('Ctrl Pts',(80.4245117554956,-10.6110199411952,132.773576203108));
#79239=CARTESIAN_POINT('Ctrl Pts',(80.4305846738193,-10.6094074427887,132.773995964239));
#79240=CARTESIAN_POINT('Ctrl Pts',(80.4419661222363,-10.6063163801216,132.774787611976));
#79241=CARTESIAN_POINT('Ctrl Pts',(80.4472766148384,-10.6048457846498,132.775159047355));
#79242=CARTESIAN_POINT('Ctrl Pts',(80.4597583884856,-10.601322536176,132.77603683814));
#79243=CARTESIAN_POINT('Ctrl Pts',(80.4669232826222,-10.5992480368798,132.776544416275));
#79244=CARTESIAN_POINT('Ctrl Pts',(80.4906918612159,-10.5921928237475,132.778240012906));
#79245=CARTESIAN_POINT('Ctrl Pts',(80.5072310923569,-10.5870012762234,132.779439047536));
#79246=CARTESIAN_POINT('Ctrl Pts',(80.5474189323835,-10.5736942357623,132.782394597509));
#79247=CARTESIAN_POINT('Ctrl Pts',(80.5709712463872,-10.5653027619819,132.784162714937));
#79248=CARTESIAN_POINT('Ctrl Pts',(80.6697101985818,-10.5275980949115,132.791704560633));
#79249=CARTESIAN_POINT('Ctrl Pts',(80.7429019767104,-10.4933732013583,132.797610581001));
#79250=CARTESIAN_POINT('Ctrl Pts',(80.9013573331191,-10.4047369775956,132.810801329379));
#79251=CARTESIAN_POINT('Ctrl Pts',(80.9847498232759,-10.3475922769379,132.818026556118));
#79252=CARTESIAN_POINT('Ctrl Pts',(81.0806643418262,-10.2681792279019,132.826599076604));
#79253=CARTESIAN_POINT('Ctrl Pts',(81.0985371963692,-10.2527290613549,132.828210017449));
#79254=CARTESIAN_POINT('Ctrl Pts',(81.1250830171934,-10.2287763723764,132.830624703444));
#79255=CARTESIAN_POINT('Ctrl Pts',(81.1340009452007,-10.2205511208777,132.831439826067));
#79256=CARTESIAN_POINT('Ctrl Pts',(81.1499018020704,-10.2055605939398,132.832900665503));
#79257=CARTESIAN_POINT('Ctrl Pts',(81.1569167861001,-10.1988302869793,132.833547830998));
#79258=CARTESIAN_POINT('Ctrl Pts',(81.1718204224324,-10.1842788032407,132.834928814232));
#79259=CARTESIAN_POINT('Ctrl Pts',(81.1796906051357,-10.1764393194891,132.835661790403));
#79260=CARTESIAN_POINT('Ctrl Pts',(81.2010713519051,-10.1547116490995,132.837663918047));
#79261=CARTESIAN_POINT('Ctrl Pts',(81.2144192453219,-10.1406653025051,132.838925988465));
#79262=CARTESIAN_POINT('Ctrl Pts',(81.3034428476702,-10.0436488817863,132.84743652416));
#79263=CARTESIAN_POINT('Ctrl Pts',(81.3708096935066,-9.95344185250607,132.854319798004));
#79264=CARTESIAN_POINT('Ctrl Pts',(81.4828880313821,-9.76663934118246,132.867623192274));
#79265=CARTESIAN_POINT('Ctrl Pts',(81.5284536881442,-9.67120483582628,132.874025086864));
#79266=CARTESIAN_POINT('Ctrl Pts',(81.5697578165006,-9.55824251204767,132.881840561365));
#79267=CARTESIAN_POINT('Ctrl Pts',(81.5746466927612,-9.54429960590879,132.882809358926));
#79268=CARTESIAN_POINT('Ctrl Pts',(81.5815856872882,-9.5236335346917,132.884253958279));
#79269=CARTESIAN_POINT('Ctrl Pts',(81.5837798873492,-9.51695902049629,132.884721840826));
#79270=CARTESIAN_POINT('Ctrl Pts',(81.5876091580003,-9.50505757560984,132.88555881122));
#79271=CARTESIAN_POINT('Ctrl Pts',(81.5892607675465,-9.49983617773504,132.885926934036));
#79272=CARTESIAN_POINT('Ctrl Pts',(81.5928108435998,-9.48841746952314,132.886734090532));
#79273=CARTESIAN_POINT('Ctrl Pts',(81.5946988731554,-9.48221728340004,132.887173681521));
#79274=CARTESIAN_POINT('Ctrl Pts',(81.6000271977416,-9.46434579991353,132.888444232073));
#79275=CARTESIAN_POINT('Ctrl Pts',(81.6033757833033,-9.45264791101363,132.889280119208));
#79276=CARTESIAN_POINT('Ctrl Pts',(81.6310851294426,-9.35168120120261,132.89652509023));
#79277=CARTESIAN_POINT('Ctrl Pts',(81.6480949869689,-9.26057178358526,132.903256408156));
#79278=CARTESIAN_POINT('Ctrl Pts',(81.6699287213006,-9.04584574233947,132.918967736365));
#79279=CARTESIAN_POINT('Ctrl Pts',(81.668745261142,-8.92213018775728,132.927880056535));
#79280=CARTESIAN_POINT('Ctrl Pts',(81.6514041694624,-8.77896884929953,132.937797963883));
#79281=CARTESIAN_POINT('Ctrl Pts',(81.6485093423848,-8.75832352879022,132.939219687155));
#79282=CARTESIAN_POINT('Ctrl Pts',(81.6432562627092,-8.72536990308967,132.941476158024));
#79283=CARTESIAN_POINT('Ctrl Pts',(81.6411453937733,-8.71302500731883,132.942318566198));
#79284=CARTESIAN_POINT('Ctrl Pts',(81.6371375406534,-8.69107860761379,132.943811343712));
#79285=CARTESIAN_POINT('Ctrl Pts',(81.6352947993765,-8.68146792964494,132.944463396795));
#79286=CARTESIAN_POINT('Ctrl Pts',(81.6312495242113,-8.66133109774449,132.945826371088));
#79287=CARTESIAN_POINT('Ctrl Pts',(81.6290295289294,-8.65080887952893,132.946536704153));
#79288=CARTESIAN_POINT('Ctrl Pts',(81.6228829379358,-8.62301085719126,132.948408812287));
#79289=CARTESIAN_POINT('Ctrl Pts',(81.6187823319621,-8.60577462670225,132.949565005195));
#79290=CARTESIAN_POINT('Ctrl Pts',(81.596005957803,-8.51639462779842,132.955541616139));
#79291=CARTESIAN_POINT('Ctrl Pts',(81.5727790716396,-8.44549373641885,132.960212859109));
#79292=CARTESIAN_POINT('Ctrl Pts',(81.5202038506543,-8.31525051526367,132.968876971414));
#79293=CARTESIAN_POINT('Ctrl Pts',(81.4919216806215,-8.25564024213442,132.972879261933));
#79294=CARTESIAN_POINT('Ctrl Pts',(81.453052511677,-8.18488427490483,132.977821225375));
#79295=CARTESIAN_POINT('Ctrl Pts',(81.4457506773648,-8.17200228397415,132.978729230212));
#79296=CARTESIAN_POINT('Ctrl Pts',(81.4025542259513,-8.09810843123554,132.983994794105));
#79297=CARTESIAN_POINT('Ctrl Pts',(81.3629760745773,-8.03934373853891,132.988407911037));
#79298=CARTESIAN_POINT('Ctrl Pts',(81.3127238305807,-7.9741120342173,132.993794268414));
#79299=CARTESIAN_POINT('Ctrl Pts',(81.3055649526431,-7.9650168553237,132.994557070523));
#79300=CARTESIAN_POINT('Ctrl Pts',(81.2942852564308,-7.95098952877681,132.99575331608));
#79301=CARTESIAN_POINT('Ctrl Pts',(81.2902295199812,-7.94600518214882,132.996182335017));
#79302=CARTESIAN_POINT('Ctrl Pts',(81.2826926133445,-7.93685129790907,132.996977838491));
#79303=CARTESIAN_POINT('Ctrl Pts',(81.2792197636935,-7.93267516839633,132.997343737002));
#79304=CARTESIAN_POINT('Ctrl Pts',(81.2710999887562,-7.92300762888036,132.998197679754));
#79305=CARTESIAN_POINT('Ctrl Pts',(81.2664378755928,-7.91752928384904,132.998686797546));
#79306=CARTESIAN_POINT('Ctrl Pts',(81.2514089112804,-7.9000990697772,133.000259286629));
#79307=CARTESIAN_POINT('Ctrl Pts',(81.2409075799827,-7.88826502619166,133.001351665555));
#79308=CARTESIAN_POINT('Ctrl Pts',(81.1817937264921,-7.82353019701535,133.007457531567));
#79309=CARTESIAN_POINT('Ctrl Pts',(81.1299711988407,-7.77367187492198,133.012648321675));
#79310=CARTESIAN_POINT('Ctrl Pts',(80.9738691934974,-7.64180453156737,133.027504891379));
#79311=CARTESIAN_POINT('Ctrl Pts',(80.8627775051936,-7.56865679934544,133.037153419174));
#79312=CARTESIAN_POINT('Ctrl Pts',(80.7225627058335,-7.49865302733902,133.047980017715));
#79313=CARTESIAN_POINT('Ctrl Pts',(80.700715915299,-7.48833306982371,133.049633197859));
#79314=CARTESIAN_POINT('Ctrl Pts',(80.6674859339321,-7.47351121929718,133.052098572088));
#79315=CARTESIAN_POINT('Ctrl Pts',(80.6562657614842,-7.46865394709259,133.052922742239));
#79316=CARTESIAN_POINT('Ctrl Pts',(80.6366176807033,-7.46040380629872,133.054351926406));
#79317=CARTESIAN_POINT('Ctrl Pts',(80.6282137286017,-7.45695559756736,133.054958794181));
#79318=CARTESIAN_POINT('Ctrl Pts',(80.610512616879,-7.44986127581422,133.056227947113));
#79319=CARTESIAN_POINT('Ctrl Pts',(80.6012100040343,-7.44622966368224,133.056889723907));
#79320=CARTESIAN_POINT('Ctrl Pts',(80.5787978814287,-7.43771170102919,133.058471955769));
#79321=CARTESIAN_POINT('Ctrl Pts',(80.5656582357957,-7.43290635358832,133.059389684776));
#79322=CARTESIAN_POINT('Ctrl Pts',(80.5190371530316,-7.41651918778691,133.062612715534));
#79323=CARTESIAN_POINT('Ctrl Pts',(80.4852471041173,-7.40583985045085,133.06488849212));
#79324=CARTESIAN_POINT('Ctrl Pts',(80.399684714473,-7.38177093524388,133.07052624976));
#79325=CARTESIAN_POINT('Ctrl Pts',(80.3475600776867,-7.36978043965928,133.073847758025));
#79326=CARTESIAN_POINT('Ctrl Pts',(80.1997407208815,-7.3431907309335,133.08308835023));
#79327=CARTESIAN_POINT('Ctrl Pts',(80.1032298667384,-7.33439039792309,133.088908042074));
#79328=CARTESIAN_POINT('Ctrl Pts',(79.996351570097,-7.33397305178477,133.09556666818));
#79329=CARTESIAN_POINT('Ctrl Pts',(79.9861976747816,-7.33402623287396,133.096201508343));
#79330=CARTESIAN_POINT('Ctrl Pts',(79.9356214334154,-7.33475352949348,133.099377492607));
#79331=CARTESIAN_POINT('Ctrl Pts',(79.8952359291423,-7.33680599233644,133.101957553004));
#79332=CARTESIAN_POINT('Ctrl Pts',(79.8445503188952,-7.34123516684255,133.10529549855));
#79333=CARTESIAN_POINT('Ctrl Pts',(79.8341409004791,-7.34224364867037,133.105986353036));
#79334=CARTESIAN_POINT('Ctrl Pts',(79.8176609755389,-7.34399701764252,133.107089538914));
#79335=CARTESIAN_POINT('Ctrl Pts',(79.8115836845716,-7.34467746753537,133.107498399673));
#79336=CARTESIAN_POINT('Ctrl Pts',(79.7999869807061,-7.34604059245775,133.108282722863));
#79337=CARTESIAN_POINT('Ctrl Pts',(79.7944670607851,-7.34671746613816,133.108657866207));
#79338=CARTESIAN_POINT('Ctrl Pts',(79.7812096785281,-7.34841055437289,133.10956309663));
#79339=CARTESIAN_POINT('Ctrl Pts',(79.7734758308322,-7.34945351583315,133.110094635323));
#79340=CARTESIAN_POINT('Ctrl Pts',(79.7464936842369,-7.35328544547661,133.111960526385));
#79341=CARTESIAN_POINT('Ctrl Pts',(79.7272879575286,-7.35635699230105,133.113309011756));
#79342=CARTESIAN_POINT('Ctrl Pts',(79.6793318054228,-7.36489016132777,133.116720128808));
#79343=CARTESIAN_POINT('Ctrl Pts',(79.6506638199184,-7.37077432188388,133.118799111772));
#79344=CARTESIAN_POINT('Ctrl Pts',(79.512140613932,-7.40303051728754,133.128995819326));
#79345=CARTESIAN_POINT('Ctrl Pts',(79.4050039016121,-7.43977567209337,133.137323087963));
#79346=CARTESIAN_POINT('Ctrl Pts',(79.2374776266775,-7.51702070433264,133.150543957348));
#79347=CARTESIAN_POINT('Ctrl Pts',(79.1745369284178,-7.55111036764585,133.155568501978));
#79348=CARTESIAN_POINT('Ctrl Pts',(79.0986876842548,-7.59874415685813,133.161684964036));
#79349=CARTESIAN_POINT('Ctrl Pts',(79.0835579239352,-7.60859215390399,133.162908572599));
#79350=CARTESIAN_POINT('Ctrl Pts',(79.0596151996061,-7.62473652923424,133.164851375605));
#79351=CARTESIAN_POINT('Ctrl Pts',(79.0506987498941,-7.63087607100305,133.16557636095));
#79352=CARTESIAN_POINT('Ctrl Pts',(79.0340463431707,-7.64258320490658,133.166933392714));
#79353=CARTESIAN_POINT('Ctrl Pts',(79.026297134487,-7.648131086651,133.167566152538));
#79354=CARTESIAN_POINT('Ctrl Pts',(79.0181373382699,-7.65407948399196,133.168233908238));
#79355=CARTESIAN_POINT('Ctrl Pts',(79.0176790286989,-7.65441394505793,133.168271418884));
#79356=CARTESIAN_POINT('Ctrl Pts',(79.0168042104152,-7.65505304728113,133.168343028467));
#79357=CARTESIAN_POINT('Ctrl Pts',(79.0163876722894,-7.65535764789969,133.16837712895));
#79358=CARTESIAN_POINT('Ctrl Pts',(79.0155836537838,-7.65594617367591,133.168442959062));
#79359=CARTESIAN_POINT('Ctrl Pts',(79.0151961546095,-7.65623007294442,133.168474689675));
#79360=CARTESIAN_POINT('Ctrl Pts',(79.0144410161087,-7.65678382333709,133.1685365317));
#79361=CARTESIAN_POINT('Ctrl Pts',(79.0140733647186,-7.65705365787708,133.168566643743));
#79362=CARTESIAN_POINT('Ctrl Pts',(79.0133508791919,-7.65758437644078,133.16862582447));
#79363=CARTESIAN_POINT('Ctrl Pts',(79.0129960376394,-7.65784525025894,133.168654893542));
#79364=CARTESIAN_POINT('Ctrl Pts',(79.0122934669367,-7.65836219826909,133.168712455094));
#79365=CARTESIAN_POINT('Ctrl Pts',(79.0119457338286,-7.65861826701337,133.16874094778));
#79366=CARTESIAN_POINT('Ctrl Pts',(79.0112524962273,-7.65912917918932,133.168797756442));
#79367=CARTESIAN_POINT('Ctrl Pts',(79.0109069905987,-7.65938402102904,133.168826072476));
#79368=CARTESIAN_POINT('Ctrl Pts',(79.010213794509,-7.65989573006845,133.168882889498));
#79369=CARTESIAN_POINT('Ctrl Pts',(79.0098661054437,-7.66015259909183,133.168911390412));
#79370=CARTESIAN_POINT('Ctrl Pts',(79.0091643422305,-7.66067147670592,133.16896892168));
#79371=CARTESIAN_POINT('Ctrl Pts',(79.0088102719173,-7.66093349046409,133.168997951835));
#79372=CARTESIAN_POINT('Ctrl Pts',(79.0001405132159,-7.66735447687778,133.169708860074));
#79373=CARTESIAN_POINT('Ctrl Pts',(78.9918821330406,-7.67359076529657,133.170387756767));
#79374=CARTESIAN_POINT('Ctrl Pts',(78.9720939428277,-7.68882532764748,133.17201910786));
#79375=CARTESIAN_POINT('Ctrl Pts',(78.960623345634,-7.69789936038672,133.172968600568));
#79376=CARTESIAN_POINT('Ctrl Pts',(78.8635035999248,-7.77682901625709,133.181046251922));
#79377=CARTESIAN_POINT('Ctrl Pts',(78.7848792030455,-7.85489874582346,133.187820102659));
#79378=CARTESIAN_POINT('Ctrl Pts',(78.6473993478902,-8.02164764340797,133.201017862272));
#79379=CARTESIAN_POINT('Ctrl Pts',(78.5881436278529,-8.10929395911782,133.207422190819));
#79380=CARTESIAN_POINT('Ctrl Pts',(78.5305081129846,-8.21490902219319,133.215240360801));
#79381=CARTESIAN_POINT('Ctrl Pts',(78.5236044191713,-8.2279700124642,133.216209038305));
#79382=CARTESIAN_POINT('Ctrl Pts',(78.5136753631901,-8.24737497135535,133.217653491449));
#79383=CARTESIAN_POINT('Ctrl Pts',(78.510514778311,-8.25364945926426,133.218121350122));
#79384=CARTESIAN_POINT('Ctrl Pts',(78.5049612861768,-8.26485019412939,133.218958294643));
#79385=CARTESIAN_POINT('Ctrl Pts',(78.5025528484962,-8.26976851619361,133.219326415699));
#79386=CARTESIAN_POINT('Ctrl Pts',(78.4973468395443,-8.28053388479694,133.220133589179));
#79387=CARTESIAN_POINT('Ctrl Pts',(78.4945591657769,-8.28638532621985,133.220573199109));
#79388=CARTESIAN_POINT('Ctrl Pts',(78.486636108547,-8.30326919173247,133.221843858602));
#79389=CARTESIAN_POINT('Ctrl Pts',(78.4815874937763,-8.31434153801031,133.222679837));
#79390=CARTESIAN_POINT('Ctrl Pts',(78.4622319575474,-8.3580533818118,133.22598786149));
#79391=CARTESIAN_POINT('Ctrl Pts',(78.4488589367769,-8.3910787220815,133.228503759881));
#79392=CARTESIAN_POINT('Ctrl Pts',(78.4365594153165,-8.4244919304089,133.231049000392));
#79393=CARTESIAN_POINT('Origin',(80.,-9.,134.));
#79394=CARTESIAN_POINT('',(78.4365594263723,-8.42449190037431,133.93353979929));
#79395=CARTESIAN_POINT('',(78.4365593580908,-8.42449208586977,133.738116396704));
#79396=CARTESIAN_POINT('',(78.4365593749993,-8.42449203993574,134.));
#79397=CARTESIAN_POINT('',(78.3340006446021,-9.00146554209231,133.077925694822));
#79398=CARTESIAN_POINT('Ctrl Pts',(78.4365593580908,-8.42449208586977,133.738116396704));
#79399=CARTESIAN_POINT('Ctrl Pts',(78.4533138667674,-8.37897632638644,133.734685142075));
#79400=CARTESIAN_POINT('Ctrl Pts',(78.4720530811991,-8.3342000924349,133.731307647191));
#79401=CARTESIAN_POINT('Ctrl Pts',(78.5003899433233,-8.27401843136631,133.726765495222));
#79402=CARTESIAN_POINT('Ctrl Pts',(78.508315955554,-8.25786907107223,133.725546243208));
#79403=CARTESIAN_POINT('Ctrl Pts',(78.5214232395522,-8.23222158195401,133.723608549351));
#79404=CARTESIAN_POINT('Ctrl Pts',(78.526437971788,-8.22264043435211,133.722884372604));
#79405=CARTESIAN_POINT('Ctrl Pts',(78.5361622085575,-8.20449358869406,133.721511911016));
#79406=CARTESIAN_POINT('Ctrl Pts',(78.5408544821735,-8.19591922368459,133.720863053366));
#79407=CARTESIAN_POINT('Ctrl Pts',(78.5517809892182,-8.17636346813049,133.719382049155));
#79408=CARTESIAN_POINT('Ctrl Pts',(78.5580652056686,-8.16541057799479,133.718551728765));
#79409=CARTESIAN_POINT('Ctrl Pts',(78.5782078064762,-8.13121038717511,133.715955433786));
#79410=CARTESIAN_POINT('Ctrl Pts',(78.5925088871898,-8.1082279812748,133.714205462608));
#79411=CARTESIAN_POINT('Ctrl Pts',(78.6587528887146,-8.00733769276167,133.706481469928));
#79412=CARTESIAN_POINT('Ctrl Pts',(78.716649758199,-7.9335399405343,133.700729428705));
#79413=CARTESIAN_POINT('Ctrl Pts',(78.8570283046628,-7.78270480563669,133.688140393348));
#79414=CARTESIAN_POINT('Ctrl Pts',(78.94173087951,-7.70839205729023,133.681349333308));
#79415=CARTESIAN_POINT('Ctrl Pts',(79.0450251742556,-7.63479377606791,133.673099955543));
#79416=CARTESIAN_POINT('Ctrl Pts',(79.0569058825938,-7.62655964717383,133.672151347801));
#79417=CARTESIAN_POINT('Ctrl Pts',(79.0746469987598,-7.6146025869256,133.670732714913));
#79418=CARTESIAN_POINT('Ctrl Pts',(79.0804263238281,-7.61075976920946,133.670270257671));
#79419=CARTESIAN_POINT('Ctrl Pts',(79.090799158767,-7.60395569599645,133.669439327743));
#79420=CARTESIAN_POINT('Ctrl Pts',(79.0953834588731,-7.60098077921779,133.669071766976));
#79421=CARTESIAN_POINT('Ctrl Pts',(79.1055745161043,-7.59443847044575,133.668253887085));
#79422=CARTESIAN_POINT('Ctrl Pts',(79.111187948624,-7.59088208687161,133.667802895745));
#79423=CARTESIAN_POINT('Ctrl Pts',(79.1278103623157,-7.58048981561205,133.666466342105));
#79424=CARTESIAN_POINT('Ctrl Pts',(79.138877701091,-7.57374886917976,133.665575062322));
#79425=CARTESIAN_POINT('Ctrl Pts',(79.1646552465304,-7.55845755486214,133.663497914242));
#79426=CARTESIAN_POINT('Ctrl Pts',(79.1794198870932,-7.55000216985275,133.662307284708));
#79427=CARTESIAN_POINT('Ctrl Pts',(79.2311098041938,-7.52144278988786,133.658142329133));
#79428=CARTESIAN_POINT('Ctrl Pts',(79.2686630154529,-7.50251233089856,133.655122636084));
#79429=CARTESIAN_POINT('Ctrl Pts',(79.4010492882962,-7.44194482434151,133.644584745545));
#79430=CARTESIAN_POINT('Ctrl Pts',(79.4990293222452,-7.40773457687879,133.636987697878));
#79431=CARTESIAN_POINT('Ctrl Pts',(79.659642412605,-7.3679630070081,133.62519617809));
#79432=CARTESIAN_POINT('Ctrl Pts',(79.7205192921871,-7.35644281495842,133.620866630459));
#79433=CARTESIAN_POINT('Ctrl Pts',(79.7991860460248,-7.34605512179524,133.615453062732));
#79434=CARTESIAN_POINT('Ctrl Pts',(79.8165041720785,-7.34404431656801,133.614272198444));
#79435=CARTESIAN_POINT('Ctrl Pts',(79.8444925623591,-7.34123907335018,133.612380664533));
#79436=CARTESIAN_POINT('Ctrl Pts',(79.8551440994919,-7.34027497691531,133.611664734488));
#79437=CARTESIAN_POINT('Ctrl Pts',(79.8755779075552,-7.33862367653564,133.610298569988));
#79438=CARTESIAN_POINT('Ctrl Pts',(79.8853583706529,-7.33792014358867,133.609647851876));
#79439=CARTESIAN_POINT('Ctrl Pts',(79.9079878620645,-7.33649305068916,133.608149323691));
#79440=CARTESIAN_POINT('Ctrl Pts',(79.9208403101122,-7.33583193070292,133.60730349556));
#79441=CARTESIAN_POINT('Ctrl Pts',(79.9621010771884,-7.33418860475422,133.60460388092));
#79442=CARTESIAN_POINT('Ctrl Pts',(79.9905282571934,-7.33378441608296,133.602768023737));
#79443=CARTESIAN_POINT('Ctrl Pts',(80.108613025317,-7.33512789595377,133.595222295321));
#79444=CARTESIAN_POINT('Ctrl Pts',(80.1980481373214,-7.34338441258375,133.589709336541));
#79445=CARTESIAN_POINT('Ctrl Pts',(80.3994318352907,-7.37852618049508,133.577216721648));
#79446=CARTESIAN_POINT('Ctrl Pts',(80.5101149494159,-7.40987479005604,133.570293704643));
#79447=CARTESIAN_POINT('Ctrl Pts',(80.6298696552314,-7.457592218266,133.561904880392));
#79448=CARTESIAN_POINT('Ctrl Pts',(80.6429897545246,-7.46301539031032,133.560972878244));
#79449=CARTESIAN_POINT('Ctrl Pts',(80.6623723378939,-7.4713187489628,133.559574391791));
#79450=CARTESIAN_POINT('Ctrl Pts',(80.6686892332579,-7.47407136916926,133.559115168488));
#79451=CARTESIAN_POINT('Ctrl Pts',(80.6799837145581,-7.47907659704441,133.558287568766));
#79452=CARTESIAN_POINT('Ctrl Pts',(80.6849675398563,-7.48131460891143,133.557920070878));
#79453=CARTESIAN_POINT('Ctrl Pts',(80.6960289018128,-7.4863472947156,133.55709923453));
#79454=CARTESIAN_POINT('Ctrl Pts',(80.7021005901423,-7.48915404432202,133.55664519331));
#79455=CARTESIAN_POINT('Ctrl Pts',(80.7200811974411,-7.49759770140704,133.555290607492));
#79456=CARTESIAN_POINT('Ctrl Pts',(80.7319400008513,-7.50333924825636,133.554384119599));
#79457=CARTESIAN_POINT('Ctrl Pts',(80.8135332625971,-7.54404498544958,133.548062214842));
#79458=CARTESIAN_POINT('Ctrl Pts',(80.880798166495,-7.58372553925565,133.542422279533));
#79459=CARTESIAN_POINT('Ctrl Pts',(81.0596299720167,-7.70690117389728,133.526630021248));
#79460=CARTESIAN_POINT('Ctrl Pts',(81.1639156222914,-7.79990173560627,133.516518126028));
#79461=CARTESIAN_POINT('Ctrl Pts',(81.268077763225,-7.91930347475049,133.505646075288));
#79462=CARTESIAN_POINT('Ctrl Pts',(81.2804743458944,-7.93402078045473,133.504336079165));
#79463=CARTESIAN_POINT('Ctrl Pts',(81.3003063633836,-7.95841080825115,133.502212788022));
#79464=CARTESIAN_POINT('Ctrl Pts',(81.3078951421285,-7.96795591473291,133.5013933793));
#79465=CARTESIAN_POINT('Ctrl Pts',(81.3213490360387,-7.98526487630589,133.499927728057));
#79466=CARTESIAN_POINT('Ctrl Pts',(81.3272521618083,-7.99299833556981,133.499279998614));
#79467=CARTESIAN_POINT('Ctrl Pts',(81.3397273052546,-8.00964182630015,133.497900842285));
#79468=CARTESIAN_POINT('Ctrl Pts',(81.3462789592926,-8.01856658994189,133.497170229755));
#79469=CARTESIAN_POINT('Ctrl Pts',(81.3639433363302,-8.04313904535226,133.495182333228));
#79470=CARTESIAN_POINT('Ctrl Pts',(81.3748756347908,-8.05891480218871,133.493931956197));
#79471=CARTESIAN_POINT('Ctrl Pts',(81.4490298851866,-8.16997368240963,133.485298333208));
#79472=CARTESIAN_POINT('Ctrl Pts',(81.5025702479063,-8.27135852524312,133.478296078032));
#79473=CARTESIAN_POINT('Ctrl Pts',(81.584030613147,-8.4735580082545,133.464984553828));
#79474=CARTESIAN_POINT('Ctrl Pts',(81.6136963320868,-8.57306628377615,133.458691042137));
#79475=CARTESIAN_POINT('Ctrl Pts',(81.6368714642679,-8.68945972023276,133.450981231153));
#79476=CARTESIAN_POINT('Ctrl Pts',(81.6396154513551,-8.70428968812911,133.449992398164));
#79477=CARTESIAN_POINT('Ctrl Pts',(81.6433475588429,-8.72611201604772,133.448525069648));
#79478=CARTESIAN_POINT('Ctrl Pts',(81.6444932392356,-8.73307714878011,133.448054910248));
#79479=CARTESIAN_POINT('Ctrl Pts',(81.646448341435,-8.74545374286702,133.447215891084));
#79480=CARTESIAN_POINT('Ctrl Pts',(81.6472754164775,-8.75086220936775,133.44684802229));
#79481=CARTESIAN_POINT('Ctrl Pts',(81.6490338786682,-8.76275297262645,133.446036486262));
#79482=CARTESIAN_POINT('Ctrl Pts',(81.6499536813191,-8.769236634588,133.445592214764));
#79483=CARTESIAN_POINT('Ctrl Pts',(81.6525161717919,-8.78809855523841,133.444294962084));
#79484=CARTESIAN_POINT('Ctrl Pts',(81.6540579064927,-8.80048975198712,133.443436741255));
#79485=CARTESIAN_POINT('Ctrl Pts',(81.6652741972421,-8.89972967002329,133.436521535527));
#79486=CARTESIAN_POINT('Ctrl Pts',(81.6682400733814,-8.98719112720432,133.430178651183));
#79487=CARTESIAN_POINT('Ctrl Pts',(81.6585796053075,-9.2030909417412,133.414448977104));
#79488=CARTESIAN_POINT('Ctrl Pts',(81.6379329755294,-9.33063558207947,133.405126136297));
#79489=CARTESIAN_POINT('Ctrl Pts',(81.5972277975585,-9.47416812168722,133.394871923007));
#79490=CARTESIAN_POINT('Ctrl Pts',(81.5913026016324,-9.49368830132768,133.393481387875));
#79491=CARTESIAN_POINT('Ctrl Pts',(81.5811606216304,-9.52501822420807,133.391255279489));
#79492=CARTESIAN_POINT('Ctrl Pts',(81.5771665661634,-9.53689727566338,133.390412561551));
#79493=CARTESIAN_POINT('Ctrl Pts',(81.5698232211865,-9.55794835265927,133.388921203123));
#79494=CARTESIAN_POINT('Ctrl Pts',(81.5665266656359,-9.56713801039342,133.388270860424));
#79495=CARTESIAN_POINT('Ctrl Pts',(81.5593911015059,-9.58649248814824,133.386902396314));
#79496=CARTESIAN_POINT('Ctrl Pts',(81.5555330375977,-9.59664983405357,133.38618494341));
#79497=CARTESIAN_POINT('Ctrl Pts',(81.5449375126894,-9.62374377315015,133.384272635885));
#79498=CARTESIAN_POINT('Ctrl Pts',(81.5380208976747,-9.64060906451234,133.383083808359));
#79499=CARTESIAN_POINT('Ctrl Pts',(81.4973875955961,-9.73523425063597,133.376416282509));
#79500=CARTESIAN_POINT('Ctrl Pts',(81.4580507379254,-9.81045035137135,133.371134848421));
#79501=CARTESIAN_POINT('Ctrl Pts',(81.3774428705731,-9.93954983153217,133.361786631262));
#79502=CARTESIAN_POINT('Ctrl Pts',(81.3382915470587,-9.99452417956614,133.357698706954));
#79503=CARTESIAN_POINT('Ctrl Pts',(81.2501271176305,-10.1036517789193,133.349075651628));
#79504=CARTESIAN_POINT('Ctrl Pts',(81.2006738992874,-10.1572573309112,133.344539786208));
#79505=CARTESIAN_POINT('Ctrl Pts',(81.1394751862315,-10.2154368580119,133.339016543279));
#79506=CARTESIAN_POINT('Ctrl Pts',(81.1309883502346,-10.223337970069,133.338252397329));
#79507=CARTESIAN_POINT('Ctrl Pts',(81.1176670964474,-10.235482751097,133.337054417855));
#79508=CARTESIAN_POINT('Ctrl Pts',(81.1128892127569,-10.2397882736169,133.336625027775));
#79509=CARTESIAN_POINT('Ctrl Pts',(81.1040298489659,-10.2476792882462,133.335829089156));
#79510=CARTESIAN_POINT('Ctrl Pts',(81.0999556148451,-10.2512726145808,133.335463129761));
#79511=CARTESIAN_POINT('Ctrl Pts',(81.0904481941125,-10.2595754978366,133.334609366828));
#79512=CARTESIAN_POINT('Ctrl Pts',(81.0850020450138,-10.2642698510644,133.334120492799));
#79513=CARTESIAN_POINT('Ctrl Pts',(81.0674947060846,-10.2791640088564,133.332550018255));
#79514=CARTESIAN_POINT('Ctrl Pts',(81.0553191839195,-10.2892272429027,133.331459443341));
#79515=CARTESIAN_POINT('Ctrl Pts',(80.9871956723876,-10.3439206347133,133.325374864325));
#79516=CARTESIAN_POINT('Ctrl Pts',(80.9285645041819,-10.3850790283139,133.320204823061));
#79517=CARTESIAN_POINT('Ctrl Pts',(80.7550820010143,-10.490885120868,133.305432089289));
#79518=CARTESIAN_POINT('Ctrl Pts',(80.6349367190937,-10.5458830875849,133.295844128403));
#79519=CARTESIAN_POINT('Ctrl Pts',(80.4832858219372,-10.5946009090372,133.284830343213));
#79520=CARTESIAN_POINT('Ctrl Pts',(80.4568105127833,-10.6023862073558,133.28294304469));
#79521=CARTESIAN_POINT('Ctrl Pts',(80.4179942487842,-10.6127601162185,133.280225770502));
#79522=CARTESIAN_POINT('Ctrl Pts',(80.4057991744592,-10.6158717243573,133.279379113084));
#79523=CARTESIAN_POINT('Ctrl Pts',(80.3840509535066,-10.6211590999533,133.27788135762));
#79524=CARTESIAN_POINT('Ctrl Pts',(80.3745117956259,-10.6233893199827,133.277228538393));
#79525=CARTESIAN_POINT('Ctrl Pts',(80.3544868502458,-10.627885174799,133.275866495089));
#79526=CARTESIAN_POINT('Ctrl Pts',(80.3439977050833,-10.6301339384558,133.275157837372));
#79527=CARTESIAN_POINT('Ctrl Pts',(80.3162592978414,-10.6358011040009,133.273295929878));
#79528=CARTESIAN_POINT('Ctrl Pts',(80.2989760801053,-10.6390480582314,133.272148148442));
#79529=CARTESIAN_POINT('Ctrl Pts',(80.2104583092256,-10.6542308808987,133.266327520544));
#79530=CARTESIAN_POINT('Ctrl Pts',(80.1385489362517,-10.6617998031448,133.261794078396));
#79531=CARTESIAN_POINT('Ctrl Pts',(79.9661868862269,-10.6686715815886,133.251141285174));
#79532=CARTESIAN_POINT('Ctrl Pts',(79.8658543605867,-10.6636141132819,133.245116553544));
#79533=CARTESIAN_POINT('Ctrl Pts',(79.7125740712422,-10.6419251886125,133.235507371677));
#79534=CARTESIAN_POINT('Ctrl Pts',(79.6589731910374,-10.6316345816674,133.232065388663));
#79535=CARTESIAN_POINT('Ctrl Pts',(79.5951269918162,-10.6160936262512,133.227763037117));
#79536=CARTESIAN_POINT('Ctrl Pts',(79.5843014074159,-10.6133429347415,133.22702639555));
#79537=CARTESIAN_POINT('Ctrl Pts',(79.5673794441732,-10.608861586405,133.225862503675));
#79538=CARTESIAN_POINT('Ctrl Pts',(79.5612636566299,-10.6072045816297,133.225439304001));
#79539=CARTESIAN_POINT('Ctrl Pts',(79.5503885638563,-10.6041913994828,133.224681965123));
#79540=CARTESIAN_POINT('Ctrl Pts',(79.5456256389454,-10.6028488473074,133.224348610791));
#79541=CARTESIAN_POINT('Ctrl Pts',(79.5340975556181,-10.5995438507754,133.223537766283));
#79542=CARTESIAN_POINT('Ctrl Pts',(79.5273388434327,-10.5975597155602,133.22305905178));
#79543=CARTESIAN_POINT('Ctrl Pts',(79.5062251447896,-10.591215719854,133.221553579368));
#79544=CARTESIAN_POINT('Ctrl Pts',(79.491916801865,-10.5867049188131,133.220518824025));
#79545=CARTESIAN_POINT('Ctrl Pts',(79.4169826766383,-10.5619639881928,133.215029935782));
#79546=CARTESIAN_POINT('Ctrl Pts',(79.357502492438,-10.5384524778238,133.210433125733));
#79547=CARTESIAN_POINT('Ctrl Pts',(79.2002897335136,-10.4655995671432,133.197859911223));
#79548=CARTESIAN_POINT('Ctrl Pts',(79.1058112361221,-10.4099467186223,133.189853435972));
#79549=CARTESIAN_POINT('Ctrl Pts',(78.9768541114127,-10.3157725403069,133.178567637458));
#79550=CARTESIAN_POINT('Ctrl Pts',(78.9376028078378,-10.2842889098674,133.175072915361));
#79551=CARTESIAN_POINT('Ctrl Pts',(78.8875912623926,-10.2403098502144,133.170537671087));
#79552=CARTESIAN_POINT('Ctrl Pts',(78.8755083612627,-10.2293658166959,133.169435029025));
#79553=CARTESIAN_POINT('Ctrl Pts',(78.8559440647082,-10.211115717106,133.16763757602));
#79554=CARTESIAN_POINT('Ctrl Pts',(78.8483676071161,-10.2039136611744,133.16693842334));
#79555=CARTESIAN_POINT('Ctrl Pts',(78.8337497379333,-10.1897538817642,133.16558320609));
#79556=CARTESIAN_POINT('Ctrl Pts',(78.8267015804713,-10.1828037871409,133.164926852764));
#79557=CARTESIAN_POINT('Ctrl Pts',(78.8194395798959,-10.1755140354318,133.164247384722));
#79558=CARTESIAN_POINT('Ctrl Pts',(78.819163606737,-10.1752368124594,133.164221558479));
#79559=CARTESIAN_POINT('Ctrl Pts',(78.8186190150012,-10.1746893689219,133.164170584649));
#79560=CARTESIAN_POINT('Ctrl Pts',(78.8183503914444,-10.1744191533587,133.164145436845));
#79561=CARTESIAN_POINT('Ctrl Pts',(78.809839362714,-10.165851807505,133.163348510929));
#79562=CARTESIAN_POINT('Ctrl Pts',(78.8016842923687,-10.1574680367095,133.162580557559));
#79563=CARTESIAN_POINT('Ctrl Pts',(78.7735959120466,-10.1279768717481,133.159919264611));
#79564=CARTESIAN_POINT('Ctrl Pts',(78.7541258342425,-10.1064341533194,133.158045584328));
#79565=CARTESIAN_POINT('Ctrl Pts',(78.7086527321511,-10.0533969751689,133.153585636621));
#79566=CARTESIAN_POINT('Ctrl Pts',(78.683224887093,-10.0214336026417,133.151020900114));
#79567=CARTESIAN_POINT('Ctrl Pts',(78.607652409245,-9.91891847405607,133.143107382217));
#79568=CARTESIAN_POINT('Ctrl Pts',(78.5618131373326,-9.84537676647108,133.137873794813));
#79569=CARTESIAN_POINT('Ctrl Pts',(78.4850924529382,-9.69783518671517,133.127677489305));
#79570=CARTESIAN_POINT('Ctrl Pts',(78.4534269397785,-9.62452156485839,133.122735946446));
#79571=CARTESIAN_POINT('Ctrl Pts',(78.4233032485605,-9.5382551271212,133.11675956546));
#79572=CARTESIAN_POINT('Ctrl Pts',(78.4195847571195,-9.52723701436853,133.115993273416));
#79573=CARTESIAN_POINT('Ctrl Pts',(78.4139869965921,-9.51005903082281,133.11479263629));
#79574=CARTESIAN_POINT('Ctrl Pts',(78.4120275077825,-9.50392541350993,133.114362765966));
#79575=CARTESIAN_POINT('Ctrl Pts',(78.4084651663653,-9.4925474044237,133.113562919594));
#79576=CARTESIAN_POINT('Ctrl Pts',(78.4068525911845,-9.48730627214856,133.113193508944));
#79577=CARTESIAN_POINT('Ctrl Pts',(78.4031796413574,-9.4751554799136,133.112334885332));
#79578=CARTESIAN_POINT('Ctrl Pts',(78.4011382270982,-9.46824033805653,133.111844616063));
#79579=CARTESIAN_POINT('Ctrl Pts',(78.3947372325598,-9.44602743814125,133.11026507179));
#79580=CARTESIAN_POINT('Ctrl Pts',(78.3905519857202,-9.43068093903555,133.109166681608));
#79581=CARTESIAN_POINT('Ctrl Pts',(78.3517886860116,-9.28007998761419,133.098333863763));
#79582=CARTESIAN_POINT('Ctrl Pts',(78.3341234393601,-9.14105620196211,133.087965797041));
#79583=CARTESIAN_POINT('Ctrl Pts',(78.3340006446021,-9.00146554209231,133.077925694822));
#79584=CARTESIAN_POINT('Ctrl Pts',(78.3340006433067,-9.00146406876337,133.077925588852));
#79585=CARTESIAN_POINT('Ctrl Pts',(78.3339557795667,-8.95041253084761,133.074253691684));
#79586=CARTESIAN_POINT('Ctrl Pts',(78.3362574875391,-8.89938133463348,133.070625660202));
#79587=CARTESIAN_POINT('Ctrl Pts',(78.3434724212921,-8.82035306990941,133.06508751588));
#79588=CARTESIAN_POINT('Ctrl Pts',(78.3467625632695,-8.79224345465086,133.063133300972));
#79589=CARTESIAN_POINT('Ctrl Pts',(78.3526326291935,-8.75118184671486,133.060300908169));
#79590=CARTESIAN_POINT('Ctrl Pts',(78.3546527512714,-8.73815619881368,133.059405695518));
#79591=CARTESIAN_POINT('Ctrl Pts',(78.358444577942,-8.71548655266099,133.057853137201));
#79592=CARTESIAN_POINT('Ctrl Pts',(78.3601472018672,-8.70583182872112,133.057193654487));
#79593=CARTESIAN_POINT('Ctrl Pts',(78.363744613137,-8.68643535616325,133.055872052782));
#79594=CARTESIAN_POINT('Ctrl Pts',(78.3656414214097,-8.67669438478769,133.055210027292));
#79595=CARTESIAN_POINT('Ctrl Pts',(78.369704743846,-8.65677761962082,133.053859646418));
#79596=CARTESIAN_POINT('Ctrl Pts',(78.3718797665199,-8.64660399228132,133.053171593961));
#79597=CARTESIAN_POINT('Ctrl Pts',(78.3776557214902,-8.62077297136029,133.051428621622));
#79598=CARTESIAN_POINT('Ctrl Pts',(78.3813881513399,-8.60514583689018,133.050377934898));
#79599=CARTESIAN_POINT('Ctrl Pts',(78.39721509255,-8.54288108328702,133.046203830266));
#79600=CARTESIAN_POINT('Ctrl Pts',(78.4111046198013,-8.49672145218842,133.043137896813));
#79601=CARTESIAN_POINT('Ctrl Pts',(78.4300953670899,-8.44228584116502,133.039524165461));
#79602=CARTESIAN_POINT('Ctrl Pts',(78.4332897259278,-8.4333744580521,133.038932605405));
#79603=CARTESIAN_POINT('Ctrl Pts',(78.4365593697901,-8.4244920540871,133.038342736257));
#79604=CARTESIAN_POINT('',(78.3340000765193,-8.99949506206163,133.272970329525));
#79605=CARTESIAN_POINT('Ctrl Pts',(78.4365594153165,-8.4244919304089,133.231049000392));
#79606=CARTESIAN_POINT('Ctrl Pts',(78.4169016046737,-8.47789486355425,133.235116951829));
#79607=CARTESIAN_POINT('Ctrl Pts',(78.3999859734769,-8.53228865755636,133.239258820952));
#79608=CARTESIAN_POINT('Ctrl Pts',(78.3591291913327,-8.69214623975658,133.251269527389));
#79609=CARTESIAN_POINT('Ctrl Pts',(78.3426173016183,-8.79920153575082,133.259095417802));
#79610=CARTESIAN_POINT('Ctrl Pts',(78.3348735958138,-8.93787647209043,133.268758890274));
#79611=CARTESIAN_POINT('Ctrl Pts',(78.3340094155008,-8.96868188443447,133.270877725158));
#79612=CARTESIAN_POINT('Ctrl Pts',(78.3340000765193,-8.99949506206163,133.272970329525));
#79613=CARTESIAN_POINT('Ctrl Pts',(78.3340000762188,-8.99949605454145,133.272970396927));
#79614=CARTESIAN_POINT('Ctrl Pts',(78.3339976905965,-9.00738271465986,133.273506000723));
#79615=CARTESIAN_POINT('Ctrl Pts',(78.3340513068087,-9.01526943507976,133.274039866371));
#79616=CARTESIAN_POINT('Ctrl Pts',(78.3342826459358,-9.03191220643399,133.275162849773));
#79617=CARTESIAN_POINT('Ctrl Pts',(78.3344734091424,-9.04066783470319,133.275751542062));
#79618=CARTESIAN_POINT('Ctrl Pts',(78.3350069259462,-9.05864471200285,133.276956055915));
#79619=CARTESIAN_POINT('Ctrl Pts',(78.3353572678232,-9.06786544777664,133.277571619044));
#79620=CARTESIAN_POINT('Ctrl Pts',(78.3362616311666,-9.08739059026412,133.278870503318));
#79621=CARTESIAN_POINT('Ctrl Pts',(78.3368348206864,-9.0976937542916,133.279553198778));
#79622=CARTESIAN_POINT('Ctrl Pts',(78.3385195573599,-9.12362985231068,133.281265311306));
#79623=CARTESIAN_POINT('Ctrl Pts',(78.3397560464906,-9.13925388296953,133.28229079552));
#79624=CARTESIAN_POINT('Ctrl Pts',(78.3453906920561,-9.19961009437805,133.286231987792));
#79625=CARTESIAN_POINT('Ctrl Pts',(78.3513780395266,-9.24417684578525,133.289098295909));
#79626=CARTESIAN_POINT('Ctrl Pts',(78.3744558474355,-9.37545417849947,133.297475027547));
#79627=CARTESIAN_POINT('Ctrl Pts',(78.3966464648053,-9.46110554478804,133.302846601555));
#79628=CARTESIAN_POINT('Ctrl Pts',(78.4567536615628,-9.63488025455061,133.314080558537));
#79629=CARTESIAN_POINT('Ctrl Pts',(78.4956850759552,-9.72229745089437,133.319928689779));
#79630=CARTESIAN_POINT('Ctrl Pts',(78.5479448248526,-9.81685300266526,133.326983012949));
#79631=CARTESIAN_POINT('Ctrl Pts',(78.5541303718902,-9.82775241168547,133.3278078664));
#79632=CARTESIAN_POINT('Ctrl Pts',(78.563738514104,-9.84424637288987,133.329075671561));
#79633=CARTESIAN_POINT('Ctrl Pts',(78.567072318361,-9.84989249292746,133.3295131989));
#79634=CARTESIAN_POINT('Ctrl Pts',(78.5732478247967,-9.86021168489491,133.330319645113));
#79635=CARTESIAN_POINT('Ctrl Pts',(78.5760793146266,-9.86489062383157,133.330687913518));
#79636=CARTESIAN_POINT('Ctrl Pts',(78.5826101205488,-9.87556355643477,133.331533920798));
#79637=CARTESIAN_POINT('Ctrl Pts',(78.5863244316876,-9.8815480671857,133.332012605091));
#79638=CARTESIAN_POINT('Ctrl Pts',(78.5980705246104,-9.90020827004241,133.333518296356));
#79639=CARTESIAN_POINT('Ctrl Pts',(78.6062354311041,-9.91279870220469,133.334553305873));
#79640=CARTESIAN_POINT('Ctrl Pts',(78.6726614972274,-10.012259489797,133.342872497762));
#79641=CARTESIAN_POINT('Ctrl Pts',(78.7388115647394,-10.0935707540443,133.350536788483));
#79642=CARTESIAN_POINT('Ctrl Pts',(78.8914760175719,-10.2488127460606,133.366367480931));
#79643=CARTESIAN_POINT('Ctrl Pts',(78.9788374196915,-10.321209509879,133.374474519769));
#79644=CARTESIAN_POINT('Ctrl Pts',(79.0889731347742,-10.394977141385,133.383544677698));
#79645=CARTESIAN_POINT('Ctrl Pts',(79.10525355026,-10.4054750157039,133.384859609808));
#79646=CARTESIAN_POINT('Ctrl Pts',(79.1311519693164,-10.421542282271,133.386912004808));
#79647=CARTESIAN_POINT('Ctrl Pts',(79.1406484940575,-10.4273031774243,133.387656455614));
#79648=CARTESIAN_POINT('Ctrl Pts',(79.1585636120169,-10.4379274347415,133.389045980287));
#79649=CARTESIAN_POINT('Ctrl Pts',(79.166968489529,-10.4428128818439,133.389691836043));
#79650=CARTESIAN_POINT('Ctrl Pts',(79.1859584148176,-10.4536297694642,133.391137839997));
#79651=CARTESIAN_POINT('Ctrl Pts',(79.1965665390288,-10.4595197483663,133.391936476739));
#79652=CARTESIAN_POINT('Ctrl Pts',(79.2280211556656,-10.4765375105128,133.394278629311));
#79653=CARTESIAN_POINT('Ctrl Pts',(79.2490416603501,-10.4873385687717,133.395810647642));
#79654=CARTESIAN_POINT('Ctrl Pts',(79.3673976897871,-10.5450047946258,133.40426820204));
#79655=CARTESIAN_POINT('Ctrl Pts',(79.4688845300493,-10.5827651065281,133.410873462124));
#79656=CARTESIAN_POINT('Ctrl Pts',(79.6459756401576,-10.6296845394323,133.422060215578));
#79657=CARTESIAN_POINT('Ctrl Pts',(79.719842632773,-10.6439936733598,133.426639428557));
#79658=CARTESIAN_POINT('Ctrl Pts',(79.8299308669531,-10.6576830873738,133.433641988216));
#79659=CARTESIAN_POINT('Ctrl Pts',(79.8655747645331,-10.6609533874633,133.435936949813));
#79660=CARTESIAN_POINT('Ctrl Pts',(79.9109853092113,-10.663648596655,133.438927071686));
#79661=CARTESIAN_POINT('Ctrl Pts',(79.9206819974643,-10.6641390902288,133.439569401219));
#79662=CARTESIAN_POINT('Ctrl Pts',(79.9363280405427,-10.6647934698571,133.440612816794));
#79663=CARTESIAN_POINT('Ctrl Pts',(79.9422751239601,-10.6650102857316,133.441011047805));
#79664=CARTESIAN_POINT('Ctrl Pts',(79.9537954300195,-10.6653684932562,133.44178584785));
#79665=CARTESIAN_POINT('Ctrl Pts',(79.9593683966915,-10.6655137795521,133.442162201405));
#79666=CARTESIAN_POINT('Ctrl Pts',(79.9718264543493,-10.6657759964044,133.443006823653));
#79667=CARTESIAN_POINT('Ctrl Pts',(79.9787117477343,-10.6658782143431,133.443475880464));
#79668=CARTESIAN_POINT('Ctrl Pts',(79.9992847199339,-10.6660560756403,133.444883743139));
#79669=CARTESIAN_POINT('Ctrl Pts',(80.0129725238945,-10.6660057151717,133.445828818276));
#79670=CARTESIAN_POINT('Ctrl Pts',(80.1294326774497,-10.6641420020371,133.4539326332));
#79671=CARTESIAN_POINT('Ctrl Pts',(80.2318260645922,-10.6529896068574,133.461459174235));
#79672=CARTESIAN_POINT('Ctrl Pts',(80.4448897550273,-10.6095893145318,133.477272165677));
#79673=CARTESIAN_POINT('Ctrl Pts',(80.554605962369,-10.5751590714603,133.485493804684));
#79674=CARTESIAN_POINT('Ctrl Pts',(80.6777394093593,-10.5220385902219,133.49467004799));
#79675=CARTESIAN_POINT('Ctrl Pts',(80.695413263213,-10.5140451200776,133.495986773261));
#79676=CARTESIAN_POINT('Ctrl Pts',(80.7229875321801,-10.5009891774864,133.498041316093));
#79677=CARTESIAN_POINT('Ctrl Pts',(80.7329832720138,-10.4961333549944,133.498786145984));
#79678=CARTESIAN_POINT('Ctrl Pts',(80.7516304808649,-10.4868430013897,133.500176013319));
#79679=CARTESIAN_POINT('Ctrl Pts',(80.7602931176226,-10.4824320802956,133.500821836409));
#79680=CARTESIAN_POINT('Ctrl Pts',(80.7796732432428,-10.4723493646066,133.502267296741));
#79681=CARTESIAN_POINT('Ctrl Pts',(80.7903684911444,-10.4666358371689,133.503065427567));
#79682=CARTESIAN_POINT('Ctrl Pts',(80.8216862765814,-10.4494634215597,133.505404601765));
#79683=CARTESIAN_POINT('Ctrl Pts',(80.8421294262872,-10.4376823941721,133.50693419251));
#79684=CARTESIAN_POINT('Ctrl Pts',(80.950219864591,-10.3722947635359,133.515049899328));
#79685=CARTESIAN_POINT('Ctrl Pts',(81.033020121515,-10.311100097151,133.521350186711));
#79686=CARTESIAN_POINT('Ctrl Pts',(81.1688044771587,-10.1898483065746,133.532468300325));
#79687=CARTESIAN_POINT('Ctrl Pts',(81.2240966347742,-10.1328850677276,133.537287545242));
#79688=CARTESIAN_POINT('Ctrl Pts',(81.2910617499602,-10.0532469793383,133.54384828301));
#79689=CARTESIAN_POINT('Ctrl Pts',(81.3065787328773,-10.0339349721425,133.545427258493));
#79690=CARTESIAN_POINT('Ctrl Pts',(81.332140567466,-10.0006267714197,133.548144386176));
#79691=CARTESIAN_POINT('Ctrl Pts',(81.3424097099089,-9.98680724623321,133.549269989483));
#79692=CARTESIAN_POINT('Ctrl Pts',(81.3568063492455,-9.96679256953123,133.550901704897));
#79693=CARTESIAN_POINT('Ctrl Pts',(81.3611097452609,-9.96072451721202,133.551396604261));
#79694=CARTESIAN_POINT('Ctrl Pts',(81.368528321773,-9.95011397715609,133.552262709199));
#79695=CARTESIAN_POINT('Ctrl Pts',(81.3716618457523,-9.94558453719693,133.552632671317));
#79696=CARTESIAN_POINT('Ctrl Pts',(81.378328444134,-9.93584524479607,133.553428802512));
#79697=CARTESIAN_POINT('Ctrl Pts',(81.3818544123961,-9.9306309697025,133.553855392544));
#79698=CARTESIAN_POINT('Ctrl Pts',(81.3914547540172,-9.91625893209888,133.555031887564));
#79699=CARTESIAN_POINT('Ctrl Pts',(81.3974680696614,-9.90706104607363,133.555785589418));
#79700=CARTESIAN_POINT('Ctrl Pts',(81.4311409713177,-9.85442575994328,133.560100012507));
#79701=CARTESIAN_POINT('Ctrl Pts',(81.456863273399,-9.80978773403668,133.563763292817));
#79702=CARTESIAN_POINT('Ctrl Pts',(81.5245050487877,-9.67871798065568,133.57439196795));
#79703=CARTESIAN_POINT('Ctrl Pts',(81.5610783934606,-9.5897533848694,133.581443869823));
#79704=CARTESIAN_POINT('Ctrl Pts',(81.605512699765,-9.44794118776061,133.592131209116));
#79705=CARTESIAN_POINT('Ctrl Pts',(81.6188543971261,-9.39703106633235,133.595866652682));
#79706=CARTESIAN_POINT('Ctrl Pts',(81.6347106047286,-9.32225069886422,133.601194230665));
#79707=CARTESIAN_POINT('Ctrl Pts',(81.6391544272509,-9.29882626531135,133.602841024702));
#79708=CARTESIAN_POINT('Ctrl Pts',(81.6463009563173,-9.2561751725945,133.605800229999));
#79709=CARTESIAN_POINT('Ctrl Pts',(81.6491732215023,-9.23698164179548,133.607117635293));
#79710=CARTESIAN_POINT('Ctrl Pts',(81.6531622152748,-9.20672256491316,133.609172992605));
#79711=CARTESIAN_POINT('Ctrl Pts',(81.6545045573501,-9.19568906185629,133.609917966219));
#79712=CARTESIAN_POINT('Ctrl Pts',(81.6568137231118,-9.17498220747502,133.611307963631));
#79713=CARTESIAN_POINT('Ctrl Pts',(81.6578064848816,-9.16531228495021,133.611953774496));
#79714=CARTESIAN_POINT('Ctrl Pts',(81.6598469955976,-9.14356495602038,133.613399029516));
#79715=CARTESIAN_POINT('Ctrl Pts',(81.6608476811531,-9.13148360493405,133.614196969158));
#79716=CARTESIAN_POINT('Ctrl Pts',(81.663406043482,-9.0958759604373,133.616535018348));
#79717=CARTESIAN_POINT('Ctrl Pts',(81.6645963324937,-9.07232568382532,133.618063692197));
#79718=CARTESIAN_POINT('Ctrl Pts',(81.6683393113823,-8.94448516801164,133.626280156226));
#79719=CARTESIAN_POINT('Ctrl Pts',(81.6615926852596,-8.84015289178326,133.63267197218));
#79720=CARTESIAN_POINT('Ctrl Pts',(81.6328099509266,-8.66002277642012,133.643811887084));
#79721=CARTESIAN_POINT('Ctrl Pts',(81.6150850942583,-8.58388549538828,133.648561015107));
#79722=CARTESIAN_POINT('Ctrl Pts',(81.5848512902794,-8.48579558324173,133.655035050917));
#79723=CARTESIAN_POINT('Ctrl Pts',(81.5770952560203,-8.46247770207241,133.65660174401));
#79724=CARTESIAN_POINT('Ctrl Pts',(81.5630673980937,-8.42322516993826,133.659299782432));
#79725=CARTESIAN_POINT('Ctrl Pts',(81.55706024496,-8.40719966818956,133.660418809146));
#79726=CARTESIAN_POINT('Ctrl Pts',(81.5480958593724,-8.38436188376008,133.66204265416));
#79727=CARTESIAN_POINT('Ctrl Pts',(81.5453380614535,-8.37747180739011,133.662536407364));
#79728=CARTESIAN_POINT('Ctrl Pts',(81.5404543857011,-8.36550287767333,133.663401220569));
#79729=CARTESIAN_POINT('Ctrl Pts',(81.5383492209843,-8.36041577103342,133.663771048759));
#79730=CARTESIAN_POINT('Ctrl Pts',(81.5337792555254,-8.34952560154517,133.664567732996));
#79731=CARTESIAN_POINT('Ctrl Pts',(81.5313067605332,-8.34372616266693,133.664995017425));
#79732=CARTESIAN_POINT('Ctrl Pts',(81.5244168750763,-8.32781630079384,133.666175251278));
#79733=CARTESIAN_POINT('Ctrl Pts',(81.5199319644061,-8.31773572438035,133.666932035656));
#79734=CARTESIAN_POINT('Ctrl Pts',(81.4936202128274,-8.26014293276102,133.671304452874));
#79735=CARTESIAN_POINT('Ctrl Pts',(81.4696683382951,-8.21363897157253,133.67502577066));
#79736=CARTESIAN_POINT('Ctrl Pts',(81.3925143860814,-8.07971673871163,133.686167987996));
#79737=CARTESIAN_POINT('Ctrl Pts',(81.3333986547187,-7.99597439332068,133.693686184765));
#79738=CARTESIAN_POINT('Ctrl Pts',(81.2197946781932,-7.86292640181156,133.706226215633));
#79739=CARTESIAN_POINT('Ctrl Pts',(81.1690437497628,-7.81080920323398,133.711331666761));
#79740=CARTESIAN_POINT('Ctrl Pts',(81.1019623501586,-7.75038206141623,133.717492976774));
#79741=CARTESIAN_POINT('Ctrl Pts',(81.0886938358631,-7.7388054128458,133.718685900679));
#79742=CARTESIAN_POINT('Ctrl Pts',(81.0670477209241,-7.72051561282908,133.720591811923));
#79743=CARTESIAN_POINT('Ctrl Pts',(81.0587847309792,-7.71366954537114,133.721310208189));
#79744=CARTESIAN_POINT('Ctrl Pts',(81.042856053203,-7.70072977086798,133.722677973116));
#79745=CARTESIAN_POINT('Ctrl Pts',(81.0352016849585,-7.69462290718215,133.723327854375));
#79746=CARTESIAN_POINT('Ctrl Pts',(81.0175996463144,-7.68083172114363,133.724805866862));
#79747=CARTESIAN_POINT('Ctrl Pts',(81.0076178823878,-7.67319172236144,133.725632223117));
#79748=CARTESIAN_POINT('Ctrl Pts',(80.9807252600766,-7.65308676336552,133.727828181275));
#79749=CARTESIAN_POINT('Ctrl Pts',(80.9636631693813,-7.6408272140896,133.729189883931));
#79750=CARTESIAN_POINT('Ctrl Pts',(80.8469932920619,-7.56029866769342,133.738303631306));
#79751=CARTESIAN_POINT('Ctrl Pts',(80.7404491586042,-7.50271029738933,133.745638199615));
#79752=CARTESIAN_POINT('Ctrl Pts',(80.567211869434,-7.43212832413474,133.757068679495));
#79753=CARTESIAN_POINT('Ctrl Pts',(80.5043839556051,-7.41080320475072,133.761130515969));
#79754=CARTESIAN_POINT('Ctrl Pts',(80.4187979439278,-7.38734110932624,133.766747165373));
#79755=CARTESIAN_POINT('Ctrl Pts',(80.3970210918388,-7.3818422303494,133.768183514117));
#79756=CARTESIAN_POINT('Ctrl Pts',(80.3595473180854,-7.37318167199245,133.770677880824));
#79757=CARTESIAN_POINT('Ctrl Pts',(80.3439033485443,-7.36980289934193,133.771725890636));
#79758=CARTESIAN_POINT('Ctrl Pts',(80.3211287868474,-7.36522645993465,133.773264507926));
#79759=CARTESIAN_POINT('Ctrl Pts',(80.3140347007547,-7.36384889850058,133.773745584339));
#79760=CARTESIAN_POINT('Ctrl Pts',(80.3015901391559,-7.36151627213661,133.774593022745));
#79761=CARTESIAN_POINT('Ctrl Pts',(80.2962436119711,-7.36054116865741,133.774958254838));
#79762=CARTESIAN_POINT('Ctrl Pts',(80.2845866141595,-7.35847404201647,133.775757165277));
#79763=CARTESIAN_POINT('Ctrl Pts',(80.2782746894911,-7.35739225454501,133.7761913748));
#79764=CARTESIAN_POINT('Ctrl Pts',(80.2606346489957,-7.35447355514359,133.777409099069));
#79765=CARTESIAN_POINT('Ctrl Pts',(80.2492938120254,-7.35271730475782,133.778196839765));
#79766=CARTESIAN_POINT('Ctrl Pts',(80.1727929469362,-7.34167838063601,133.783539309828));
#79767=CARTESIAN_POINT('Ctrl Pts',(80.1071568807101,-7.33614800363321,133.788260773178));
#79768=CARTESIAN_POINT('Ctrl Pts',(80.0205526783311,-7.33399658439232,133.794540674751));
#79769=CARTESIAN_POINT('Ctrl Pts',(79.9997237292618,-7.33386984308063,133.796055051637));
#79770=CARTESIAN_POINT('Ctrl Pts',(79.9107261756953,-7.33499719451583,133.802532202975));
#79771=CARTESIAN_POINT('Ctrl Pts',(79.8426680396476,-7.34004466542439,133.807498326553));
#79772=CARTESIAN_POINT('Ctrl Pts',(79.704070582836,-7.35892664007696,133.81751912812));
#79773=CARTESIAN_POINT('Ctrl Pts',(79.6337241988074,-7.37318084949938,133.822554296935));
#79774=CARTESIAN_POINT('Ctrl Pts',(79.547567710075,-7.39651349216286,133.828645111702));
#79775=CARTESIAN_POINT('Ctrl Pts',(79.5307021467986,-7.40136823387309,133.829833990993));
#79776=CARTESIAN_POINT('Ctrl Pts',(79.503664606551,-7.40961575591624,133.83173503789));
#79777=CARTESIAN_POINT('Ctrl Pts',(79.4934435631474,-7.41284170537806,133.832452564826));
#79778=CARTESIAN_POINT('Ctrl Pts',(79.4739421152303,-7.41920429961048,133.833819677867));
#79779=CARTESIAN_POINT('Ctrl Pts',(79.4646568886899,-7.42232458830664,133.834469767091));
#79780=CARTESIAN_POINT('Ctrl Pts',(79.4434968735197,-7.42964370472721,133.835949623724));
#79781=CARTESIAN_POINT('Ctrl Pts',(79.4316410038073,-7.43389569638078,133.836777600236));
#79782=CARTESIAN_POINT('Ctrl Pts',(79.4000579845595,-7.44562853488086,133.838980937765));
#79783=CARTESIAN_POINT('Ctrl Pts',(79.3804224162109,-7.45335047437402,133.840348313163));
#79784=CARTESIAN_POINT('Ctrl Pts',(79.2510204840719,-7.50709945962742,133.84935534867));
#79785=CARTESIAN_POINT('Ctrl Pts',(79.1463095077185,-7.56440301348871,133.856591346483));
#79786=CARTESIAN_POINT('Ctrl Pts',(78.9699650840164,-7.68708038064582,133.869715375268));
#79787=CARTESIAN_POINT('Ctrl Pts',(78.8962134430123,-7.74844901882281,133.875577743605));
#79788=CARTESIAN_POINT('Ctrl Pts',(78.8192432211413,-7.82461644085024,133.882648370344));
#79789=CARTESIAN_POINT('Ctrl Pts',(78.8104346410356,-7.83353211977652,133.883473281171));
#79790=CARTESIAN_POINT('Ctrl Pts',(78.7971722212994,-7.84726224526244,133.884741156544));
#79791=CARTESIAN_POINT('Ctrl Pts',(78.7926446096592,-7.8520052464573,133.885178695802));
#79792=CARTESIAN_POINT('Ctrl Pts',(78.7843921961703,-7.86075306479148,133.885985152824));
#79793=CARTESIAN_POINT('Ctrl Pts',(78.7806589708722,-7.86474964701672,133.886353419989));
#79794=CARTESIAN_POINT('Ctrl Pts',(78.7721629845168,-7.87393522751475,133.887199409881));
#79795=CARTESIAN_POINT('Ctrl Pts',(78.7674134228655,-7.87913607705212,133.887678077869));
#79796=CARTESIAN_POINT('Ctrl Pts',(78.7526491198931,-7.89551055790167,133.889183666216));
#79797=CARTESIAN_POINT('Ctrl Pts',(78.7427525878823,-7.90678910937542,133.890218587618));
#79798=CARTESIAN_POINT('Ctrl Pts',(78.6650772264852,-7.9977614030156,133.898539084728));
#79799=CARTESIAN_POINT('Ctrl Pts',(78.6047953550745,-8.08353859734886,133.906204921304));
#79800=CARTESIAN_POINT('Ctrl Pts',(78.5073001242087,-8.25441841247182,133.920509154064));
#79801=CARTESIAN_POINT('Ctrl Pts',(78.4683707136649,-8.33807251325376,133.927135512778));
#79802=CARTESIAN_POINT('Ctrl Pts',(78.4365594263723,-8.4244919003743,133.93353979929));
#79803=CARTESIAN_POINT('Origin',(80.,-9.,134.));
#79804=CARTESIAN_POINT('',(78.4365594680555,-8.42449178713676,134.632696249083));
#79805=CARTESIAN_POINT('',(78.4365593695135,-8.4244920548384,134.440654933552));
#79806=CARTESIAN_POINT('',(78.4365593749993,-8.42449203993574,134.));
#79807=CARTESIAN_POINT('Ctrl Pts',(78.4365593695135,-8.4244920548384,134.440654933552));
#79808=CARTESIAN_POINT('Ctrl Pts',(78.4604281544172,-8.35964946068749,134.435817450756));
#79809=CARTESIAN_POINT('Ctrl Pts',(78.4883094068626,-8.2963502231991,134.430817626444));
#79810=CARTESIAN_POINT('Ctrl Pts',(78.5600797186349,-8.15751128644456,134.419450966649));
#79811=CARTESIAN_POINT('Ctrl Pts',(78.6061381558519,-8.0833162960484,134.413091474615));
#79812=CARTESIAN_POINT('Ctrl Pts',(78.6815254624746,-7.98079172361757,134.404038301892));
#79813=CARTESIAN_POINT('Ctrl Pts',(78.7064132363256,-7.94938383223044,134.40122264318));
#79814=CARTESIAN_POINT('Ctrl Pts',(78.7509808543772,-7.89712825121749,134.396467114652));
#79815=CARTESIAN_POINT('Ctrl Pts',(78.7701096548337,-7.87583593969998,134.39450753354));
#79816=CARTESIAN_POINT('Ctrl Pts',(78.7977805476383,-7.84658768869443,134.391782711849));
#79817=CARTESIAN_POINT('Ctrl Pts',(78.8058711457575,-7.83821350372441,134.390998558487));
#79818=CARTESIAN_POINT('Ctrl Pts',(78.8143192790629,-7.82965074612878,134.390192421115));
#79819=CARTESIAN_POINT('Ctrl Pts',(78.8145895998778,-7.82937694738164,134.390166639819));
#79820=CARTESIAN_POINT('Ctrl Pts',(78.815138042624,-7.82882183317268,134.390114360048));
#79821=CARTESIAN_POINT('Ctrl Pts',(78.8154161699469,-7.82854052307942,134.390087861815));
#79822=CARTESIAN_POINT('Ctrl Pts',(78.8159816583395,-7.82796897079121,134.390034014012));
#79823=CARTESIAN_POINT('Ctrl Pts',(78.8162690260306,-7.82767873512303,134.390006664733));
#79824=CARTESIAN_POINT('Ctrl Pts',(78.8168546160354,-7.82708773567737,134.389950963421));
#79825=CARTESIAN_POINT('Ctrl Pts',(78.8171528463984,-7.82678697986582,134.389922611745));
#79826=CARTESIAN_POINT('Ctrl Pts',(78.8177620141437,-7.82617312200096,134.389864733003));
#79827=CARTESIAN_POINT('Ctrl Pts',(78.8180729612844,-7.82586002969489,134.389835206373));
#79828=CARTESIAN_POINT('Ctrl Pts',(78.8185020571743,-7.82542831673484,134.389794484572));
#79829=CARTESIAN_POINT('Ctrl Pts',(78.8186200992656,-7.82530959050026,134.389783284704));
#79830=CARTESIAN_POINT('Ctrl Pts',(78.818890796289,-7.82503740665418,134.389757606603));
#79831=CARTESIAN_POINT('Ctrl Pts',(78.8190434632945,-7.82488396093598,134.389743128897));
#79832=CARTESIAN_POINT('Ctrl Pts',(78.8193957159969,-7.8245300494634,134.389709733695));
#79833=CARTESIAN_POINT('Ctrl Pts',(78.8195953228865,-7.82432960474896,134.389690817135));
#79834=CARTESIAN_POINT('Ctrl Pts',(78.8200596899689,-7.82386352602137,134.389646826012));
#79835=CARTESIAN_POINT('Ctrl Pts',(78.8203244889154,-7.82359793046469,134.389621753158));
#79836=CARTESIAN_POINT('Ctrl Pts',(78.8209475382402,-7.82297342868785,134.3895627882));
#79837=CARTESIAN_POINT('Ctrl Pts',(78.8213058630013,-7.82261459642031,134.389528899379));
#79838=CARTESIAN_POINT('Ctrl Pts',(78.8278609207265,-7.81605624611889,134.388909366331));
#79839=CARTESIAN_POINT('Ctrl Pts',(78.8341064206742,-7.80990546583899,134.388325889288));
#79840=CARTESIAN_POINT('Ctrl Pts',(78.8482931346758,-7.79615277661807,134.387015531196));
#79841=CARTESIAN_POINT('Ctrl Pts',(78.8562616819097,-7.78857954847971,134.386289912049));
#79842=CARTESIAN_POINT('Ctrl Pts',(78.8780776085952,-7.76825306473355,134.384330746181));
#79843=CARTESIAN_POINT('Ctrl Pts',(78.8920673884735,-7.75565449334599,134.383103765968));
#79844=CARTESIAN_POINT('Ctrl Pts',(78.9752609182827,-7.68324972529538,134.375969508528));
#79845=CARTESIAN_POINT('Ctrl Pts',(79.0490852196478,-7.62898370000524,134.370294372178));
#79846=CARTESIAN_POINT('Ctrl Pts',(79.2080289381381,-7.53119477209854,134.358859043487));
#79847=CARTESIAN_POINT('Ctrl Pts',(79.2931735232444,-7.48837803039206,134.353123925114));
#79848=CARTESIAN_POINT('Ctrl Pts',(79.4066903535852,-7.44299143420336,134.345442532917));
#79849=CARTESIAN_POINT('Ctrl Pts',(79.4321218958737,-7.43353700798298,134.343718797002));
#79850=CARTESIAN_POINT('Ctrl Pts',(79.4751783966695,-7.41871660149663,134.340777900067));
#79851=CARTESIAN_POINT('Ctrl Pts',(79.4926825959062,-7.41301421406123,134.339576162977));
#79852=CARTESIAN_POINT('Ctrl Pts',(79.5175786461641,-7.40535772122652,134.337853517496));
#79853=CARTESIAN_POINT('Ctrl Pts',(79.5248956886389,-7.4031624229224,134.337345599253));
#79854=CARTESIAN_POINT('Ctrl Pts',(79.5375414843708,-7.39946297209523,134.336464564497));
#79855=CARTESIAN_POINT('Ctrl Pts',(79.5428630738136,-7.3979349307168,134.336092823265));
#79856=CARTESIAN_POINT('Ctrl Pts',(79.5541534482153,-7.39475384810932,134.335301903068));
#79857=CARTESIAN_POINT('Ctrl Pts',(79.5601237688585,-7.39310757857471,134.334882380969));
#79858=CARTESIAN_POINT('Ctrl Pts',(79.5765409583558,-7.38867901434732,134.333725517092));
#79859=CARTESIAN_POINT('Ctrl Pts',(79.5870057298549,-7.38596511928022,134.33298448573));
#79860=CARTESIAN_POINT('Ctrl Pts',(79.6419335895716,-7.37228946970346,134.329078673721));
#79861=CARTESIAN_POINT('Ctrl Pts',(79.686804531605,-7.363063559037,134.325832839242));
#79862=CARTESIAN_POINT('Ctrl Pts',(79.8191738558044,-7.34148856145347,134.316199696814));
#79863=CARTESIAN_POINT('Ctrl Pts',(79.9073450160713,-7.33423489150616,134.309717824102));
#79864=CARTESIAN_POINT('Ctrl Pts',(80.0798740565613,-7.33378705899995,134.297242989146));
#79865=CARTESIAN_POINT('Ctrl Pts',(80.1639779990175,-7.33995168353664,134.291258941342));
#79866=CARTESIAN_POINT('Ctrl Pts',(80.2700353051403,-7.3558689111397,134.283884221775));
#79867=CARTESIAN_POINT('Ctrl Pts',(80.2927319233199,-7.35975787872547,134.282315493636));
#79868=CARTESIAN_POINT('Ctrl Pts',(80.3269881800399,-7.36636129700816,134.27996107715));
#79869=CARTESIAN_POINT('Ctrl Pts',(80.338610651751,-7.36873070250928,134.279164594538));
#79870=CARTESIAN_POINT('Ctrl Pts',(80.3587789966513,-7.37306714767717,134.277786222555));
#79871=CARTESIAN_POINT('Ctrl Pts',(80.3673363535131,-7.37497788235475,134.277202565745));
#79872=CARTESIAN_POINT('Ctrl Pts',(80.38657166401,-7.379432559903,134.275893090737));
#79873=CARTESIAN_POINT('Ctrl Pts',(80.3972404324327,-7.38201467007062,134.275168523132));
#79874=CARTESIAN_POINT('Ctrl Pts',(80.4260600425129,-7.38929198554653,134.273215398645));
#79875=CARTESIAN_POINT('Ctrl Pts',(80.4441587602555,-7.39418851992955,134.271993337626));
#79876=CARTESIAN_POINT('Ctrl Pts',(80.548757120659,-7.42439099280467,134.264949947773));
#79877=CARTESIAN_POINT('Ctrl Pts',(80.6331766852885,-7.45637813520837,134.259353444285));
#79878=CARTESIAN_POINT('Ctrl Pts',(80.8016359315266,-7.53636808914985,134.247921545156));
#79879=CARTESIAN_POINT('Ctrl Pts',(80.8849137526741,-7.58516296545013,134.242116811753));
#79880=CARTESIAN_POINT('Ctrl Pts',(80.9857665153195,-7.65665895948425,134.23435110281));
#79881=CARTESIAN_POINT('Ctrl Pts',(81.007637769759,-7.6729857829191,134.232617502212));
#79882=CARTESIAN_POINT('Ctrl Pts',(81.0436369081636,-7.70126220900221,134.229661443933));
#79883=CARTESIAN_POINT('Ctrl Pts',(81.0579850350533,-7.71292368440036,134.228454617076));
#79884=CARTESIAN_POINT('Ctrl Pts',(81.0779925931422,-7.72974548715713,134.226725914759));
#79885=CARTESIAN_POINT('Ctrl Pts',(81.0838156553143,-7.73471023955476,134.226217152874));
#79886=CARTESIAN_POINT('Ctrl Pts',(81.0937940908496,-7.74333729081661,134.225335146039));
#79887=CARTESIAN_POINT('Ctrl Pts',(81.097965752787,-7.74698049389898,134.224963284983));
#79888=CARTESIAN_POINT('Ctrl Pts',(81.1067589691621,-7.75473743221446,134.2241726757));
#79889=CARTESIAN_POINT('Ctrl Pts',(81.1113757270145,-7.75885606442307,134.223753589144));
#79890=CARTESIAN_POINT('Ctrl Pts',(81.1239751415644,-7.7702227281193,134.222599145985));
#79891=CARTESIAN_POINT('Ctrl Pts',(81.1319103766087,-7.77752253954141,134.221860124429));
#79892=CARTESIAN_POINT('Ctrl Pts',(81.1727162984845,-7.81579879091319,134.217999861508));
#79893=CARTESIAN_POINT('Ctrl Pts',(81.2043854110169,-7.84802299561058,134.214799800512));
#79894=CARTESIAN_POINT('Ctrl Pts',(81.3060463051857,-7.96024468216313,134.203927798364));
#79895=CARTESIAN_POINT('Ctrl Pts',(81.3696915784666,-8.0456444655024,134.196105403601));
#79896=CARTESIAN_POINT('Ctrl Pts',(81.4642161464865,-8.20161456954474,134.183009233408));
#79897=CARTESIAN_POINT('Ctrl Pts',(81.4991597275764,-8.26933502185664,134.177652493886));
#79898=CARTESIAN_POINT('Ctrl Pts',(81.5364164067653,-8.35556402601269,134.171240195187));
#79899=CARTESIAN_POINT('Ctrl Pts',(81.5432169680661,-8.37202346241667,134.170033431159));
#79900=CARTESIAN_POINT('Ctrl Pts',(81.5537069007831,-8.39861246578579,134.168110750083));
#79901=CARTESIAN_POINT('Ctrl Pts',(81.5575639864799,-8.40867391626479,134.167389254215));
#79902=CARTESIAN_POINT('Ctrl Pts',(81.564736436126,-8.42794091311735,134.166018893941));
#79903=CARTESIAN_POINT('Ctrl Pts',(81.5680688371174,-8.43713958883738,134.165369485333));
#79904=CARTESIAN_POINT('Ctrl Pts',(81.575471012176,-8.45814843702911,134.163897012699));
#79905=CARTESIAN_POINT('Ctrl Pts',(81.5794894106835,-8.46997618715963,134.163075673167));
#79906=CARTESIAN_POINT('Ctrl Pts',(81.59179053065,-8.50756610365097,134.160488502339));
#79907=CARTESIAN_POINT('Ctrl Pts',(81.5995790915591,-8.53348622888576,134.158738761298));
#79908=CARTESIAN_POINT('Ctrl Pts',(81.6416951053189,-8.68713521954408,134.148543042906));
#79909=CARTESIAN_POINT('Ctrl Pts',(81.6613452972767,-8.81839159700811,134.140590427004));
#79910=CARTESIAN_POINT('Ctrl Pts',(81.6673951326799,-9.02232081244227,134.128074890246));
#79911=CARTESIAN_POINT('Ctrl Pts',(81.6648867296921,-9.09409867496912,134.12362805577));
#79912=CARTESIAN_POINT('Ctrl Pts',(81.656190220502,-9.18121822000287,134.117948003497));
#79913=CARTESIAN_POINT('Ctrl Pts',(81.6543955005055,-9.19693037611636,134.116912190772));
#79914=CARTESIAN_POINT('Ctrl Pts',(81.6514594466223,-9.21974859007526,134.115388179631));
#79915=CARTESIAN_POINT('Ctrl Pts',(81.6504952355611,-9.22687710176757,134.114909259099));
#79916=CARTESIAN_POINT('Ctrl Pts',(81.6487218285582,-9.23937804550147,134.114064102235));
#79917=CARTESIAN_POINT('Ctrl Pts',(81.6479324730694,-9.24475309920712,134.113698973264));
#79918=CARTESIAN_POINT('Ctrl Pts',(81.6461515386529,-9.25648089505401,134.112898417369));
#79919=CARTESIAN_POINT('Ctrl Pts',(81.6451494878438,-9.26283168928598,134.112462441872));
#79920=CARTESIAN_POINT('Ctrl Pts',(81.6422388684703,-9.28060955064329,134.111235406685));
#79921=CARTESIAN_POINT('Ctrl Pts',(81.6402478692286,-9.29202248166598,134.110440022732));
#79922=CARTESIAN_POINT('Ctrl Pts',(81.6251048208468,-9.3737802784709,134.104691538413));
#79923=CARTESIAN_POINT('Ctrl Pts',(81.6075525216211,-9.44322674926886,134.09954182347));
#79924=CARTESIAN_POINT('Ctrl Pts',(81.5813084429264,-9.52460893271757,134.093333368532));
#79925=CARTESIAN_POINT('Ctrl Pts',(81.5768565989234,-9.53784215703743,134.092318070302));
#79926=CARTESIAN_POINT('Ctrl Pts',(81.5503241928956,-9.61354803164934,134.086480605595));
#79927=CARTESIAN_POINT('Ctrl Pts',(81.5246975025853,-9.67471815677951,134.08165283596));
#79928=CARTESIAN_POINT('Ctrl Pts',(81.4627725835815,-9.80085300514316,134.071572383585));
#79929=CARTESIAN_POINT('Ctrl Pts',(81.4256277807417,-9.86524989328049,134.06635102227));
#79930=CARTESIAN_POINT('Ctrl Pts',(81.37445416223,-9.94167147444477,134.060073582733));
#79931=CARTESIAN_POINT('Ctrl Pts',(81.3643698508529,-9.95622401242201,134.058874006735));
#79932=CARTESIAN_POINT('Ctrl Pts',(81.3477906294414,-9.97935286749778,134.05695996871));
#79933=CARTESIAN_POINT('Ctrl Pts',(81.3414415277462,-9.98803150602629,134.056240016948));
#79934=CARTESIAN_POINT('Ctrl Pts',(81.3291526136429,-10.0044924866336,134.054870844027));
#79935=CARTESIAN_POINT('Ctrl Pts',(81.3232273836548,-10.0122851002471,134.054221095302));
#79936=CARTESIAN_POINT('Ctrl Pts',(81.3095595133667,-10.0299354286428,134.052745488531));
#79937=CARTESIAN_POINT('Ctrl Pts',(81.3017735584805,-10.039758973486,134.05192138213));
#79938=CARTESIAN_POINT('Ctrl Pts',(81.2807260566603,-10.0657075604624,134.049736068617));
#79939=CARTESIAN_POINT('Ctrl Pts',(81.2672707744724,-10.0816730942799,134.048382634449));
#79940=CARTESIAN_POINT('Ctrl Pts',(81.1725655472882,-10.1898530541529,134.039137657389));
#79941=CARTESIAN_POINT('Ctrl Pts',(81.0816286729673,-10.2730842594732,134.031681170422));
#79942=CARTESIAN_POINT('Ctrl Pts',(80.9299564152572,-10.383815781604,134.020203215644));
#79943=CARTESIAN_POINT('Ctrl Pts',(80.8753715402846,-10.4189744542783,134.0162243749));
#79944=CARTESIAN_POINT('Ctrl Pts',(80.7901965573352,-10.467048148943,134.010031333431));
#79945=CARTESIAN_POINT('Ctrl Pts',(80.7610410287725,-10.4823822315928,134.00791366116));
#79946=CARTESIAN_POINT('Ctrl Pts',(80.7229594434782,-10.5009913400821,134.005125747321));
#79947=CARTESIAN_POINT('Ctrl Pts',(80.7144313054781,-10.5050691875502,134.004500025969));
#79948=CARTESIAN_POINT('Ctrl Pts',(80.7005285650467,-10.5115721921344,134.003476977466));
#79949=CARTESIAN_POINT('Ctrl Pts',(80.6951748352517,-10.5140418449269,134.003082304922));
#79950=CARTESIAN_POINT('Ctrl Pts',(80.6847000029934,-10.518806570568,134.002308504491));
#79951=CARTESIAN_POINT('Ctrl Pts',(80.6795802263952,-10.5211042717181,134.001929540396));
#79952=CARTESIAN_POINT('Ctrl Pts',(80.6667847319004,-10.5267692614012,134.00098071632));
#79953=CARTESIAN_POINT('Ctrl Pts',(80.6590950970591,-10.5301045395165,134.000408986378));
#79954=CARTESIAN_POINT('Ctrl Pts',(80.6314237885211,-10.5418593175358,133.998347009341));
#79955=CARTESIAN_POINT('Ctrl Pts',(80.6113042784857,-10.5499461685438,133.996839238729));
#79956=CARTESIAN_POINT('Ctrl Pts',(80.4914623485628,-10.5954192898092,133.987831306368));
#79957=CARTESIAN_POINT('Ctrl Pts',(80.3885033330421,-10.6235642845263,133.980001452305));
#79958=CARTESIAN_POINT('Ctrl Pts',(80.1989852292527,-10.6562996949848,133.966051091097));
#79959=CARTESIAN_POINT('Ctrl Pts',(80.113389406705,-10.6643528356489,133.959910700826));
#79960=CARTESIAN_POINT('Ctrl Pts',(79.9985607754945,-10.6662515301852,133.951957237713));
#79961=CARTESIAN_POINT('Ctrl Pts',(79.9695689329967,-10.665974299154,133.949972239948));
#79962=CARTESIAN_POINT('Ctrl Pts',(79.9276393308621,-10.6644783147152,133.947133171567));
#79963=CARTESIAN_POINT('Ctrl Pts',(79.9146867435558,-10.6638647154661,133.946260516424));
#79964=CARTESIAN_POINT('Ctrl Pts',(79.8919403380547,-10.6625208340308,133.944735336558));
#79965=CARTESIAN_POINT('Ctrl Pts',(79.8821434964361,-10.6618550676255,133.944080830936));
#79966=CARTESIAN_POINT('Ctrl Pts',(79.861733610264,-10.6602866744464,133.942722029031));
#79967=CARTESIAN_POINT('Ctrl Pts',(79.8511221576218,-10.6593688055455,133.94201824041));
#79968=CARTESIAN_POINT('Ctrl Pts',(79.8233714391934,-10.6567000770141,133.940184265758));
#79969=CARTESIAN_POINT('Ctrl Pts',(79.8062489674001,-10.6547849912203,133.93905924769));
#79970=CARTESIAN_POINT('Ctrl Pts',(79.7298492782139,-10.6450378282656,133.93406480769));
#79971=CARTESIAN_POINT('Ctrl Pts',(79.670986197031,-10.6342833155264,133.930287268569));
#79972=CARTESIAN_POINT('Ctrl Pts',(79.5110290925058,-10.5960630171867,133.920063922536));
#79973=CARTESIAN_POINT('Ctrl Pts',(79.4117563054396,-10.5622031178988,133.913776654347));
#79974=CARTESIAN_POINT('Ctrl Pts',(79.2771215662817,-10.5016158568823,133.904658725152));
#79975=CARTESIAN_POINT('Ctrl Pts',(79.238625823429,-10.4824683035283,133.901975711185));
#79976=CARTESIAN_POINT('Ctrl Pts',(79.1857736944808,-10.4535781135716,133.898126151816));
#79977=CARTESIAN_POINT('Ctrl Pts',(79.1707613264984,-10.4450664279501,133.897013179087));
#79978=CARTESIAN_POINT('Ctrl Pts',(79.1445896861132,-10.4296855702496,133.895033381867));
#79979=CARTESIAN_POINT('Ctrl Pts',(79.1333739678954,-10.4229149409468,133.894171885651));
#79980=CARTESIAN_POINT('Ctrl Pts',(79.1165670873087,-10.4124966661632,133.892859225489));
#79981=CARTESIAN_POINT('Ctrl Pts',(79.1109157840619,-10.4089463425788,133.892414085797));
#79982=CARTESIAN_POINT('Ctrl Pts',(79.1006768882704,-10.402427822106,133.891600437776));
#79983=CARTESIAN_POINT('Ctrl Pts',(79.0960823736167,-10.3994708920489,133.891232660568));
#79984=CARTESIAN_POINT('Ctrl Pts',(79.085712406993,-10.3927246355635,133.890396513062));
#79985=CARTESIAN_POINT('Ctrl Pts',(79.0799459634399,-10.3889219844041,133.889927290139));
#79986=CARTESIAN_POINT('Ctrl Pts',(79.0623281501129,-10.3771461538933,133.88848097378));
#79987=CARTESIAN_POINT('Ctrl Pts',(79.0505558967655,-10.3690565686035,133.887496723574));
#79988=CARTESIAN_POINT('Ctrl Pts',(78.9457893431323,-10.295062618417,133.878586293032));
#79989=CARTESIAN_POINT('Ctrl Pts',(78.8596901102479,-10.2199331985886,133.870204812937));
#79990=CARTESIAN_POINT('Ctrl Pts',(78.7209604058106,-10.0712622015278,133.855442551632));
#79991=CARTESIAN_POINT('Ctrl Pts',(78.6653314691638,-10.0011039158258,133.8490392964));
#79992=CARTESIAN_POINT('Ctrl Pts',(78.5994405667938,-9.90268073790606,133.84083614186));
#79993=CARTESIAN_POINT('Ctrl Pts',(78.5839189624327,-9.87813092338495,133.838847514511));
#79994=CARTESIAN_POINT('Ctrl Pts',(78.5624013300585,-9.84204181744154,133.836004277962));
#79995=CARTESIAN_POINT('Ctrl Pts',(78.555886733001,-9.83081962347559,133.835131007876));
#79996=CARTESIAN_POINT('Ctrl Pts',(78.5446730156189,-9.81097213748313,133.833605125644));
#79997=CARTESIAN_POINT('Ctrl Pts',(78.5399178933261,-9.80237939163076,133.832950526835));
#79998=CARTESIAN_POINT('Ctrl Pts',(78.5301664438174,-9.78438426147971,133.831591884029));
#79999=CARTESIAN_POINT('Ctrl Pts',(78.5251836994121,-9.77497499375271,133.830888344641));
#80000=CARTESIAN_POINT('Ctrl Pts',(78.5123837464134,-9.75023332837819,133.829055801276));
#80001=CARTESIAN_POINT('Ctrl Pts',(78.5047131786277,-9.73482618543004,133.827931950045));
#80002=CARTESIAN_POINT('Ctrl Pts',(78.4715817838219,-9.66561034177503,133.82295566711));
#80003=CARTESIAN_POINT('Ctrl Pts',(78.4487754234425,-9.61057582615569,133.819194234605));
#80004=CARTESIAN_POINT('Ctrl Pts',(78.3874605002678,-9.43683440399255,133.807739203704));
#80005=CARTESIAN_POINT('Ctrl Pts',(78.35929672025,-9.31495645834477,133.800310403973));
#80006=CARTESIAN_POINT('Ctrl Pts',(78.3415069515466,-9.16087713967949,133.790608129399));
#80007=CARTESIAN_POINT('Ctrl Pts',(78.3388471370996,-9.13058174901709,133.788684097398));
#80008=CARTESIAN_POINT('Ctrl Pts',(78.3358148742834,-9.08027269593718,133.785437350806));
#80009=CARTESIAN_POINT('Ctrl Pts',(78.3349713554805,-9.06029398819754,133.784134531648));
#80010=CARTESIAN_POINT('Ctrl Pts',(78.3342967627965,-9.03241870018604,133.782291971479));
#80011=CARTESIAN_POINT('Ctrl Pts',(78.3341619212222,-9.02453030077042,133.781767778837));
#80012=CARTESIAN_POINT('Ctrl Pts',(78.3340274107809,-9.0110649252554,133.780867810309));
#80013=CARTESIAN_POINT('Ctrl Pts',(78.3339997062126,-9.00548824500956,133.780493567682));
#80014=CARTESIAN_POINT('Ctrl Pts',(78.3340003253352,-8.99382919224086,133.779707801327));
#80015=CARTESIAN_POINT('Ctrl Pts',(78.3340339570069,-8.98774702239071,133.779296012302));
#80016=CARTESIAN_POINT('Ctrl Pts',(78.3342142738354,-8.97136335691666,133.77818195045));
#80017=CARTESIAN_POINT('Ctrl Pts',(78.3344232108852,-8.96106301293832,133.777476413428));
#80018=CARTESIAN_POINT('Ctrl Pts',(78.3360154175545,-8.90720924942272,133.773763050365));
#80019=CARTESIAN_POINT('Ctrl Pts',(78.3390114428183,-8.86372415998546,133.770680907367));
#80020=CARTESIAN_POINT('Ctrl Pts',(78.3559301161319,-8.7076886804988,133.759428309044));
#80021=CARTESIAN_POINT('Ctrl Pts',(78.379627376782,-8.59650734151485,133.751070154554));
#80022=CARTESIAN_POINT('Ctrl Pts',(78.4213756147411,-8.46707201417176,133.741325715804));
#80023=CARTESIAN_POINT('Ctrl Pts',(78.4287520063035,-8.44570175265309,133.739715310315));
#80024=CARTESIAN_POINT('Ctrl Pts',(78.4365593580908,-8.42449208586977,133.738116396704));
#80025=CARTESIAN_POINT('Ctrl Pts',(78.4365594263723,-8.4244919003743,133.93353979929));
#80026=CARTESIAN_POINT('Ctrl Pts',(78.4292827658715,-8.44425986936527,133.93500474531));
#80027=CARTESIAN_POINT('Ctrl Pts',(78.4223785765527,-8.4641724876544,133.936458744668));
#80028=CARTESIAN_POINT('Ctrl Pts',(78.4098685482923,-8.50259529746954,133.939223460302));
#80029=CARTESIAN_POINT('Ctrl Pts',(78.4042055318288,-8.52107459690236,133.940535343517));
#80030=CARTESIAN_POINT('Ctrl Pts',(78.3957986584612,-8.55031432170058,133.94258408617));
#80031=CARTESIAN_POINT('Ctrl Pts',(78.3928387767658,-8.5610102890579,133.943327892097));
#80032=CARTESIAN_POINT('Ctrl Pts',(78.3874866911236,-8.58113086501106,133.944716835285));
#80033=CARTESIAN_POINT('Ctrl Pts',(78.3850697037473,-8.59054833173501,133.945362748037));
#80034=CARTESIAN_POINT('Ctrl Pts',(78.3798188296641,-8.61177775394053,133.946809683789));
#80035=CARTESIAN_POINT('Ctrl Pts',(78.377031384831,-8.62360071165609,133.947609186707));
#80036=CARTESIAN_POINT('Ctrl Pts',(78.3691885509082,-8.6585743417681,133.949956443125));
#80037=CARTESIAN_POINT('Ctrl Pts',(78.3644973337424,-8.68180417670322,133.951492622017));
#80038=CARTESIAN_POINT('Ctrl Pts',(78.3427139812442,-8.80293468151543,133.959398129095));
#80039=CARTESIAN_POINT('Ctrl Pts',(78.333910218843,-8.90212409965979,133.965502759633));
#80040=CARTESIAN_POINT('Ctrl Pts',(78.3341019469804,-9.11275783268123,133.97837042487));
#80041=CARTESIAN_POINT('Ctrl Pts',(78.3453445221357,-9.22369359293837,133.985095487123));
#80042=CARTESIAN_POINT('Ctrl Pts',(78.3704604199684,-9.34694251898306,133.993274707298));
#80043=CARTESIAN_POINT('Ctrl Pts',(78.3735573037419,-9.36118205208093,133.994230845626));
#80044=CARTESIAN_POINT('Ctrl Pts',(78.3784090198239,-9.38216116708226,133.995658531687));
#80045=CARTESIAN_POINT('Ctrl Pts',(78.3800200633337,-9.3889337540938,133.996122369623));
#80046=CARTESIAN_POINT('Ctrl Pts',(78.3829713981018,-9.40100419364035,133.996954635746));
#80047=CARTESIAN_POINT('Ctrl Pts',(78.3842953736583,-9.40630582238773,133.997322136986));
#80048=CARTESIAN_POINT('Ctrl Pts',(78.3872818210453,-9.41801907315317,133.998138457141));
#80049=CARTESIAN_POINT('Ctrl Pts',(78.3889564343288,-9.42442725638386,133.998587933964));
#80050=CARTESIAN_POINT('Ctrl Pts',(78.3939939217679,-9.44324459776028,133.99991593539));
#80051=CARTESIAN_POINT('Ctrl Pts',(78.3974621934096,-9.45562468102995,134.000800073401));
#80052=CARTESIAN_POINT('Ctrl Pts',(78.4058039213543,-9.48412653831921,134.002857816002));
#80053=CARTESIAN_POINT('Ctrl Pts',(78.4107792144989,-9.50021684235532,134.004036066356));
#80054=CARTESIAN_POINT('Ctrl Pts',(78.4288217049656,-9.55557869467189,134.008141422183));
#80055=CARTESIAN_POINT('Ctrl Pts',(78.4431071607122,-9.59443516849589,134.011112654195));
#80056=CARTESIAN_POINT('Ctrl Pts',(78.5067068162444,-9.74935171683419,134.023229981363));
#80057=CARTESIAN_POINT('Ctrl Pts',(78.5676840530407,-9.86019250148546,134.032491050464));
#80058=CARTESIAN_POINT('Ctrl Pts',(78.6660828270149,-9.99908257765676,134.044461387281));
#80059=CARTESIAN_POINT('Ctrl Pts',(78.6929986494428,-10.034045024901,134.047515221621));
#80060=CARTESIAN_POINT('Ctrl Pts',(78.7312815510882,-10.079885786275,134.051577565385));
#80061=CARTESIAN_POINT('Ctrl Pts',(78.7414587074118,-10.0917296632852,134.052632808588));
#80062=CARTESIAN_POINT('Ctrl Pts',(78.7586276065021,-10.1111511197035,134.054373220408));
#80063=CARTESIAN_POINT('Ctrl Pts',(78.7655256728305,-10.1188098024058,134.055062205806));
#80064=CARTESIAN_POINT('Ctrl Pts',(78.7792395513224,-10.1337545818071,134.056412201371));
#80065=CARTESIAN_POINT('Ctrl Pts',(78.786050606249,-10.1410444345415,134.057073371456));
#80066=CARTESIAN_POINT('Ctrl Pts',(78.8025322309468,-10.1583700442849,134.058651517908));
#80067=CARTESIAN_POINT('Ctrl Pts',(78.8122641521326,-10.1683466063583,134.059565804759));
#80068=CARTESIAN_POINT('Ctrl Pts',(78.8469169595075,-10.2029899873905,134.062761953608));
#80069=CARTESIAN_POINT('Ctrl Pts',(78.8724912286758,-10.2269921173564,134.065014962686));
#80070=CARTESIAN_POINT('Ctrl Pts',(78.9383222979008,-10.2849784499329,134.070581416209));
#80071=CARTESIAN_POINT('Ctrl Pts',(78.9794690594892,-10.3178946790545,134.073855782634));
#80072=CARTESIAN_POINT('Ctrl Pts',(79.099820970463,-10.4051502913865,134.083006287883));
#80073=CARTESIAN_POINT('Ctrl Pts',(79.1822534347788,-10.4546679320136,134.088782062847));
#80074=CARTESIAN_POINT('Ctrl Pts',(79.314690556998,-10.5193918674606,134.097952697684));
#80075=CARTESIAN_POINT('Ctrl Pts',(79.3619104914205,-10.5398186077943,134.101205564474));
#80076=CARTESIAN_POINT('Ctrl Pts',(79.4202677956596,-10.5619178151596,134.105293034575));
#80077=CARTESIAN_POINT('Ctrl Pts',(79.4305796015699,-10.5657065766197,134.106017799103));
#80078=CARTESIAN_POINT('Ctrl Pts',(79.4468566749004,-10.5715050348482,134.107166888096));
#80079=CARTESIAN_POINT('Ctrl Pts',(79.4527973675493,-10.5735834545484,134.107587326072));
#80080=CARTESIAN_POINT('Ctrl Pts',(79.4639589397967,-10.5774176116596,134.108379480801));
#80081=CARTESIAN_POINT('Ctrl Pts',(79.4691769227751,-10.5791811792647,134.108750738425));
#80082=CARTESIAN_POINT('Ctrl Pts',(79.4814640451072,-10.5832661890077,134.109627062937));
#80083=CARTESIAN_POINT('Ctrl Pts',(79.488540090438,-10.5855661819649,134.110133340128));
#80084=CARTESIAN_POINT('Ctrl Pts',(79.5120477068619,-10.5930333507688,134.111820042482));
#80085=CARTESIAN_POINT('Ctrl Pts',(79.5285433797077,-10.5979928956034,134.113011331831));
#80086=CARTESIAN_POINT('Ctrl Pts',(79.5689573023215,-10.6094634473464,134.115943811591));
#80087=CARTESIAN_POINT('Ctrl Pts',(79.5929492856933,-10.6156979854235,134.117696385264));
#80088=CARTESIAN_POINT('Ctrl Pts',(79.6943247637283,-10.6396401545466,134.125127217116));
#80089=CARTESIAN_POINT('Ctrl Pts',(79.7727816911643,-10.6523402115628,134.130934563748));
#80090=CARTESIAN_POINT('Ctrl Pts',(79.9540413246789,-10.6685238374717,134.144159819736));
#80091=CARTESIAN_POINT('Ctrl Pts',(80.0568800574186,-10.6681891652364,134.151514439752));
#80092=CARTESIAN_POINT('Ctrl Pts',(80.1825333909696,-10.6561383297429,134.160204133224));
#80093=CARTESIAN_POINT('Ctrl Pts',(80.2059686214435,-10.6533873205866,134.161813055674));
#80094=CARTESIAN_POINT('Ctrl Pts',(80.2413485049412,-10.6484701766428,134.164225345702));
#80095=CARTESIAN_POINT('Ctrl Pts',(80.2533401055619,-10.6466699209363,134.165040057024));
#80096=CARTESIAN_POINT('Ctrl Pts',(80.2749078565126,-10.6431908475222,134.166500451282));
#80097=CARTESIAN_POINT('Ctrl Pts',(80.2844908872714,-10.6415588423463,134.167147579108));
#80098=CARTESIAN_POINT('Ctrl Pts',(80.3049968852284,-10.6378816741444,134.168528793037));
#80099=CARTESIAN_POINT('Ctrl Pts',(80.3159148275612,-10.6358109029731,134.16926203472));
#80100=CARTESIAN_POINT('Ctrl Pts',(80.3458290767552,-10.6298264919091,134.171265694674));
#80101=CARTESIAN_POINT('Ctrl Pts',(80.3647794188693,-10.6256900598178,134.172529013322));
#80102=CARTESIAN_POINT('Ctrl Pts',(80.4949920291305,-10.594875942142,134.181177454284));
#80103=CARTESIAN_POINT('Ctrl Pts',(80.6033241737846,-10.557129006175,134.188181788303));
#80104=CARTESIAN_POINT('Ctrl Pts',(80.8003169804827,-10.4648146621754,134.201466215994));
#80105=CARTESIAN_POINT('Ctrl Pts',(80.8894139033819,-10.4124894138518,134.207730747794));
#80106=CARTESIAN_POINT('Ctrl Pts',(80.9853716031139,-10.3434387685317,134.215410068768));
#80107=CARTESIAN_POINT('Ctrl Pts',(80.9975311048848,-10.3344349277599,134.216402014125));
#80108=CARTESIAN_POINT('Ctrl Pts',(81.0151871878791,-10.3209848265773,134.217873028519));
#80109=CARTESIAN_POINT('Ctrl Pts',(81.0207811777829,-10.3166668982845,134.218343699755));
#80110=CARTESIAN_POINT('Ctrl Pts',(81.0306566903959,-10.3089433582546,134.219183168925));
#80111=CARTESIAN_POINT('Ctrl Pts',(81.0349491502649,-10.3055520607704,134.219550969869));
#80112=CARTESIAN_POINT('Ctrl Pts',(81.0443358284447,-10.2980606444942,134.220361778326));
#80113=CARTESIAN_POINT('Ctrl Pts',(81.0494225692489,-10.2939517096269,134.220805384279));
#80114=CARTESIAN_POINT('Ctrl Pts',(81.0641201940356,-10.2819356865279,134.222099122877));
#80115=CARTESIAN_POINT('Ctrl Pts',(81.073666583166,-10.2739509162153,134.222954454908));
#80116=CARTESIAN_POINT('Ctrl Pts',(81.1510007894549,-10.2077805783689,134.230001198648));
#80117=CARTESIAN_POINT('Ctrl Pts',(81.2140906708677,-10.1443413753495,134.236491412577));
#80118=CARTESIAN_POINT('Ctrl Pts',(81.3534985039486,-9.97959189862281,134.252200637322));
#80119=CARTESIAN_POINT('Ctrl Pts',(81.4239632906421,-9.87401288515521,134.261353426494));
#80120=CARTESIAN_POINT('Ctrl Pts',(81.4912166869833,-9.74313731362072,134.271469742676));
#80121=CARTESIAN_POINT('Ctrl Pts',(81.5002908954914,-9.7246430632648,134.272874266104));
#80122=CARTESIAN_POINT('Ctrl Pts',(81.5143544762918,-9.69458259381862,134.275118052451));
#80123=CARTESIAN_POINT('Ctrl Pts',(81.5195595239156,-9.68312028799751,134.275964647412));
#80124=CARTESIAN_POINT('Ctrl Pts',(81.5285715573802,-9.66266159373057,134.277460189477));
#80125=CARTESIAN_POINT('Ctrl Pts',(81.5324302254004,-9.65368876776061,134.278110875941));
#80126=CARTESIAN_POINT('Ctrl Pts',(81.5404004165549,-9.63469664577142,134.279477387173));
#80127=CARTESIAN_POINT('Ctrl Pts',(81.5444936163413,-9.62467011605464,134.28019256751));
#80128=CARTESIAN_POINT('Ctrl Pts',(81.5551549834062,-9.59780891275826,134.28209244906));
#80129=CARTESIAN_POINT('Ctrl Pts',(81.5615476367147,-9.58090579129727,134.283271260448));
#80130=CARTESIAN_POINT('Ctrl Pts',(81.5951923770168,-9.48737232862071,134.289708546599));
#80131=CARTESIAN_POINT('Ctrl Pts',(81.617081706908,-9.40892510205804,134.294786678539));
#80132=CARTESIAN_POINT('Ctrl Pts',(81.6427292892478,-9.28168176460839,134.30276976461));
#80133=CARTESIAN_POINT('Ctrl Pts',(81.6502270476375,-9.23378391083949,134.305721165263));
#80134=CARTESIAN_POINT('Ctrl Pts',(81.6561283783128,-9.18114937776188,134.308957527548));
#80135=CARTESIAN_POINT('Ctrl Pts',(81.6566122533579,-9.17666959113448,134.309232930461));
#80136=CARTESIAN_POINT('Ctrl Pts',(81.665819090058,-9.08806611875033,134.314679870135));
#80137=CARTESIAN_POINT('Ctrl Pts',(81.6681407894447,-9.0034108967471,134.319877501067));
#80138=CARTESIAN_POINT('Ctrl Pts',(81.6632588291239,-8.90317093516773,134.326388483428));
#80139=CARTESIAN_POINT('Ctrl Pts',(81.662265418857,-8.88739701077373,134.327423710482));
#80140=CARTESIAN_POINT('Ctrl Pts',(81.6604996645589,-8.86454713856628,134.328941880589));
#80141=CARTESIAN_POINT('Ctrl Pts',(81.6599061125614,-8.85745770260244,134.329415506386));
#80142=CARTESIAN_POINT('Ctrl Pts',(81.658774571574,-8.84490968721675,134.330258751075));
#80143=CARTESIAN_POINT('Ctrl Pts',(81.6582550064039,-8.83944964373234,134.330627347597));
#80144=CARTESIAN_POINT('Ctrl Pts',(81.657068918047,-8.8276056949357,134.331430639946));
#80145=CARTESIAN_POINT('Ctrl Pts',(81.6563924739572,-8.82122314378105,134.331865847696));
#80146=CARTESIAN_POINT('Ctrl Pts',(81.6543602448719,-8.80305071695764,134.333111294929));
#80147=CARTESIAN_POINT('Ctrl Pts',(81.6529153717143,-8.79127148312748,134.333926175283));
#80148=CARTESIAN_POINT('Ctrl Pts',(81.6387310570383,-8.68503944927931,134.341337928602));
#80149=CARTESIAN_POINT('Ctrl Pts',(81.6180353018436,-8.59183635437831,134.348278623742));
#80150=CARTESIAN_POINT('Ctrl Pts',(81.5533134672623,-8.38570580150564,134.364005803122));
#80151=CARTESIAN_POINT('Ctrl Pts',(81.5047095036511,-8.2747417854604,134.372725095181));
#80152=CARTESIAN_POINT('Ctrl Pts',(81.4340586983671,-8.15178253447627,134.382480412671));
#80153=CARTESIAN_POINT('Ctrl Pts',(81.4232499552787,-8.13376859112513,134.383913329452));
#80154=CARTESIAN_POINT('Ctrl Pts',(81.4054335571921,-8.10530983544477,134.38618396905));
#80155=CARTESIAN_POINT('Ctrl Pts',(81.39864363339,-8.09473209708972,134.387029505684));
#80156=CARTESIAN_POINT('Ctrl Pts',(81.3863522606568,-8.07605233703291,134.38852583832));
#80157=CARTESIAN_POINT('Ctrl Pts',(81.380897929932,-8.06792018116672,134.389178346512));
#80158=CARTESIAN_POINT('Ctrl Pts',(81.3693166942414,-8.05097790725196,134.390540292577));
#80159=CARTESIAN_POINT('Ctrl Pts',(81.3631757100119,-8.04217792133702,134.391249159608));
#80160=CARTESIAN_POINT('Ctrl Pts',(81.3467340951886,-8.01909565391363,134.39311286582));
#80161=CARTESIAN_POINT('Ctrl Pts',(81.3362911425038,-8.00491604360166,134.394262214612));
#80162=CARTESIAN_POINT('Ctrl Pts',(81.2816007757981,-7.93307061648487,134.400113877658));
#80163=CARTESIAN_POINT('Ctrl Pts',(81.2338361142941,-7.87817594252731,134.404674862731));
#80164=CARTESIAN_POINT('Ctrl Pts',(81.1105600652069,-7.7539328981265,134.41548111725));
#80165=CARTESIAN_POINT('Ctrl Pts',(81.0319516515263,-7.68809252785914,134.42162563817));
#80166=CARTESIAN_POINT('Ctrl Pts',(80.9048458900799,-7.60016488358483,134.431235225722));
#80167=CARTESIAN_POINT('Ctrl Pts',(80.8605188925679,-7.57248799874148,134.434537085882));
#80168=CARTESIAN_POINT('Ctrl Pts',(80.8053511394162,-7.5415463042026,134.438679869126));
#80169=CARTESIAN_POINT('Ctrl Pts',(80.7956787335038,-7.53624695471797,134.439407424297));
#80170=CARTESIAN_POINT('Ctrl Pts',(80.7803966829641,-7.52807039814425,134.440559975802));
#80171=CARTESIAN_POINT('Ctrl Pts',(80.7748218995872,-7.52512822379691,134.440981047197));
#80172=CARTESIAN_POINT('Ctrl Pts',(80.7643467318049,-7.51967557967916,134.441773681179));
#80173=CARTESIAN_POINT('Ctrl Pts',(80.7594504365315,-7.51715767974026,134.442144777272));
#80174=CARTESIAN_POINT('Ctrl Pts',(80.7479235359005,-7.51130208252279,134.44301975126));
#80175=CARTESIAN_POINT('Ctrl Pts',(80.7412830120814,-7.50798438486794,134.443524827989));
#80176=CARTESIAN_POINT('Ctrl Pts',(80.7192513201532,-7.49716043065008,134.445203353457));
#80177=CARTESIAN_POINT('Ctrl Pts',(80.7037671705056,-7.48984737672318,134.446387527633));
#80178=CARTESIAN_POINT('Ctrl Pts',(80.6657785498853,-7.47261672975433,134.449298859705));
#80179=CARTESIAN_POINT('Ctrl Pts',(80.6431622682002,-7.46295644185148,134.451037202124));
#80180=CARTESIAN_POINT('Ctrl Pts',(80.547770340733,-7.42468479288244,134.458367726801));
#80181=CARTESIAN_POINT('Ctrl Pts',(80.4732420488356,-7.40071533541414,134.46408611378));
#80182=CARTESIAN_POINT('Ctrl Pts',(80.2961574665958,-7.35722933801795,134.477341278724));
#80183=CARTESIAN_POINT('Ctrl Pts',(80.1928842189041,-7.3419266974643,134.484811850572));
#80184=CARTESIAN_POINT('Ctrl Pts',(80.065298487664,-7.33511320407712,134.493607237537));
#80185=CARTESIAN_POINT('Ctrl Pts',(80.0417287266177,-7.33435575594236,134.495215169867));
#80186=CARTESIAN_POINT('Ctrl Pts',(80.0060280428315,-7.33396680231363,134.497626284443));
#80187=CARTESIAN_POINT('Ctrl Pts',(79.993904991723,-7.33396704191,134.498440793903));
#80188=CARTESIAN_POINT('Ctrl Pts',(79.972062903696,-7.33420589352749,134.499900969763));
#80189=CARTESIAN_POINT('Ctrl Pts',(79.9623440119483,-7.3343972502591,134.500548079191));
#80190=CARTESIAN_POINT('Ctrl Pts',(79.9415175349273,-7.33498969216655,134.501929406787));
#80191=CARTESIAN_POINT('Ctrl Pts',(79.9304111187463,-7.33541689255676,134.502662779132));
#80192=CARTESIAN_POINT('Ctrl Pts',(79.8999282801208,-7.33689502169682,134.504667193256));
#80193=CARTESIAN_POINT('Ctrl Pts',(79.8805642575413,-7.33817339278846,134.505931126263));
#80194=CARTESIAN_POINT('Ctrl Pts',(79.8374722021615,-7.34177537256366,134.508725958328));
#80195=CARTESIAN_POINT('Ctrl Pts',(79.8137626135259,-7.34427057735474,134.51025155281));
#80196=CARTESIAN_POINT('Ctrl Pts',(79.7379413646647,-7.35389941536268,134.515101318387));
#80197=CARTESIAN_POINT('Ctrl Pts',(79.6861094692054,-7.3629919909374,134.51837155516));
#80198=CARTESIAN_POINT('Ctrl Pts',(79.5411252078008,-7.39556671760973,134.527519029308));
#80199=CARTESIAN_POINT('Ctrl Pts',(79.4494578137711,-7.42466697126672,134.533295575406));
#80200=CARTESIAN_POINT('Ctrl Pts',(79.3132519982137,-7.48125533530951,134.542470969164));
#80201=CARTESIAN_POINT('Ctrl Pts',(79.2666405046927,-7.5032064579193,134.545728190481));
#80202=CARTESIAN_POINT('Ctrl Pts',(79.2114010581597,-7.53242079546742,134.54982124773));
#80203=CARTESIAN_POINT('Ctrl Pts',(79.2017281898612,-7.5376597133766,134.550546960634));
#80204=CARTESIAN_POINT('Ctrl Pts',(79.1866010131659,-7.54604754457162,134.551697226376));
#80205=CARTESIAN_POINT('Ctrl Pts',(79.1811112670207,-7.54913236504575,134.552117879677));
#80206=CARTESIAN_POINT('Ctrl Pts',(79.1708533227672,-7.55497331540321,134.552910196809));
#80207=CARTESIAN_POINT('Ctrl Pts',(79.1660811426601,-7.5577220561197,134.553281399005));
#80208=CARTESIAN_POINT('Ctrl Pts',(79.1548988444578,-7.56423702828533,134.554157262092));
#80209=CARTESIAN_POINT('Ctrl Pts',(79.148500218352,-7.56802255931892,134.554663129371));
#80210=CARTESIAN_POINT('Ctrl Pts',(79.127391119667,-7.58070254978715,134.556347036359));
#80211=CARTESIAN_POINT('Ctrl Pts',(79.1127935337693,-7.58978152791956,134.55753589272));
#80212=CARTESIAN_POINT('Ctrl Pts',(79.0775530574905,-7.61246307526759,134.560461136249));
#80213=CARTESIAN_POINT('Ctrl Pts',(79.0570677708726,-7.6263021584186,134.562208838476));
#80214=CARTESIAN_POINT('Ctrl Pts',(78.9724600075178,-7.68624424950195,134.569605193289));
#80215=CARTESIAN_POINT('Ctrl Pts',(78.9113510744778,-7.73641966397281,134.575381941928));
#80216=CARTESIAN_POINT('Ctrl Pts',(78.7791702891653,-7.86168177330922,134.588617446902));
#80217=CARTESIAN_POINT('Ctrl Pts',(78.7110461167117,-7.93943506442631,134.596011862628));
#80218=CARTESIAN_POINT('Ctrl Pts',(78.6367110615838,-8.0421087470549,134.604737857928));
#80219=CARTESIAN_POINT('Ctrl Pts',(78.6232851714385,-8.06150718613825,134.606346449602));
#80220=CARTESIAN_POINT('Ctrl Pts',(78.6035884391703,-8.09129886476789,134.608758346948));
#80221=CARTESIAN_POINT('Ctrl Pts',(78.5970121880381,-8.10148555194778,134.60957299084));
#80222=CARTESIAN_POINT('Ctrl Pts',(78.585364884483,-8.11996705776851,134.611033312138));
#80223=CARTESIAN_POINT('Ctrl Pts',(78.5802541766147,-8.1282361023082,134.611680433811));
#80224=CARTESIAN_POINT('Ctrl Pts',(78.5694565408014,-8.14605333597346,134.613061685677));
#80225=CARTESIAN_POINT('Ctrl Pts',(78.5637921615218,-8.15561469197104,134.613794970981));
#80226=CARTESIAN_POINT('Ctrl Pts',(78.548504349547,-8.18201916551864,134.615798882702));
#80227=CARTESIAN_POINT('Ctrl Pts',(78.5390785519315,-8.1989751299592,134.617062406442));
#80228=CARTESIAN_POINT('Ctrl Pts',(78.4940698695076,-8.28337919127685,134.623244806254));
#80229=CARTESIAN_POINT('Ctrl Pts',(78.4628720992874,-8.35301021093932,134.62800685597));
#80230=CARTESIAN_POINT('Ctrl Pts',(78.4365594680555,-8.42449178713676,134.632696249083));
#80231=CARTESIAN_POINT('Origin',(80.,-9.,134.));
#80232=CARTESIAN_POINT('',(78.4365593749993,-8.42449203993567,135.330578627164));
#80233=CARTESIAN_POINT('',(78.4365593350865,-8.42449214836376,135.139259965645));
#80234=CARTESIAN_POINT('',(78.4365593749993,-8.42449203993574,134.));
#80235=CARTESIAN_POINT('',(78.3340005883416,-8.9985998736709,134.47795669959));
#80236=CARTESIAN_POINT('Ctrl Pts',(78.4365593350865,-8.42449214836376,135.139259965645));
#80237=CARTESIAN_POINT('Ctrl Pts',(78.4595770340976,-8.36196162589672,135.135189971337));
#80238=CARTESIAN_POINT('Ctrl Pts',(78.4863351525883,-8.30084183598527,135.13113531974));
#80239=CARTESIAN_POINT('Ctrl Pts',(78.5389131195365,-8.19802641900077,135.123936636303));
#80240=CARTESIAN_POINT('Ctrl Pts',(78.5630228224522,-8.15558770865141,135.120844126155));
#80241=CARTESIAN_POINT('Ctrl Pts',(78.5947307026104,-8.10507422314614,135.116936330962));
#80242=CARTESIAN_POINT('Ctrl Pts',(78.6005941427007,-8.09593298064479,135.116219691288));
#80243=CARTESIAN_POINT('Ctrl Pts',(78.6099810250474,-8.08160873406148,135.115080616419));
#80244=CARTESIAN_POINT('Ctrl Pts',(78.6134451839667,-8.07638698201634,135.114661956085));
#80245=CARTESIAN_POINT('Ctrl Pts',(78.6200142423709,-8.06660525923144,135.113870983743));
#80246=CARTESIAN_POINT('Ctrl Pts',(78.6231124327411,-8.06204101535449,135.113499108902));
#80247=CARTESIAN_POINT('Ctrl Pts',(78.6304738953643,-8.05131120036578,135.11261835153));
#80248=CARTESIAN_POINT('Ctrl Pts',(78.6347561744854,-8.04515892352745,135.112108222604));
#80249=CARTESIAN_POINT('Ctrl Pts',(78.6491994291896,-8.02470434223818,135.110395571658));
#80250=CARTESIAN_POINT('Ctrl Pts',(78.6595443985481,-8.01053422404222,135.109181741546));
#80251=CARTESIAN_POINT('Ctrl Pts',(78.6854151106593,-7.97624798498357,135.106182101068));
#80252=CARTESIAN_POINT('Ctrl Pts',(78.7011807578211,-7.95631898755379,135.104384266743));
#80253=CARTESIAN_POINT('Ctrl Pts',(78.7705317998867,-7.87265966126243,135.096626423372));
#80254=CARTESIAN_POINT('Ctrl Pts',(78.8283971268501,-7.81263558804286,135.090527875419));
#80255=CARTESIAN_POINT('Ctrl Pts',(78.9696097783315,-7.68657062137669,135.076784213937));
#80256=CARTESIAN_POINT('Ctrl Pts',(79.0552887227416,-7.62365381658308,135.069213978658));
#80257=CARTESIAN_POINT('Ctrl Pts',(79.1624696559496,-7.55970495399906,135.060679224766));
#80258=CARTESIAN_POINT('Ctrl Pts',(79.1787174599824,-7.55037869224015,135.059408006955));
#80259=CARTESIAN_POINT('Ctrl Pts',(79.2048190648998,-7.53597609231756,135.057400662815));
#80260=CARTESIAN_POINT('Ctrl Pts',(79.2145717717768,-7.5307208466782,135.056658206746));
#80261=CARTESIAN_POINT('Ctrl Pts',(79.2329036191681,-7.52107742659557,135.055276452319));
#80262=CARTESIAN_POINT('Ctrl Pts',(79.2414697617659,-7.51666567491935,135.054636342653));
#80263=CARTESIAN_POINT('Ctrl Pts',(79.2609113985985,-7.50686526475417,135.053195796726));
#80264=CARTESIAN_POINT('Ctrl Pts',(79.2718085506382,-7.50152059593467,135.052396920712));
#80265=CARTESIAN_POINT('Ctrl Pts',(79.3048175879237,-7.4857759544867,135.050001821179));
#80266=CARTESIAN_POINT('Ctrl Pts',(79.3271014070675,-7.47574259752548,135.048418177598));
#80267=CARTESIAN_POINT('Ctrl Pts',(79.3791768156469,-7.45366021107353,135.04478686273));
#80268=CARTESIAN_POINT('Ctrl Pts',(79.4091126373617,-7.44197545474172,135.042750884785));
#80269=CARTESIAN_POINT('Ctrl Pts',(79.5207988426877,-7.40206388665551,135.035311150927));
#80270=CARTESIAN_POINT('Ctrl Pts',(79.6043718861882,-7.37934794847096,135.030054782485));
#80271=CARTESIAN_POINT('Ctrl Pts',(79.7073523961798,-7.35980192515111,135.023650091205));
#80272=CARTESIAN_POINT('Ctrl Pts',(79.7254255209208,-7.35667982746918,135.022528339556));
#80273=CARTESIAN_POINT('Ctrl Pts',(79.8200902975363,-7.34193194448609,135.016649596042));
#80274=CARTESIAN_POINT('Ctrl Pts',(79.8973630934295,-7.3353619991716,135.011842704575));
#80275=CARTESIAN_POINT('Ctrl Pts',(79.9864107022758,-7.33401496225293,135.006017625944));
#80276=CARTESIAN_POINT('Ctrl Pts',(79.9980214807866,-7.33396072017218,135.005252480809));
#80277=CARTESIAN_POINT('Ctrl Pts',(80.0160665085711,-7.33406504378312,135.004053263937));
#80278=CARTESIAN_POINT('Ctrl Pts',(80.0225011376284,-7.33413952974075,135.003623650212));
#80279=CARTESIAN_POINT('Ctrl Pts',(80.034366383432,-7.33434563606311,135.002827523103));
#80280=CARTESIAN_POINT('Ctrl Pts',(80.0397969859595,-7.33446654034419,135.002461601358));
#80281=CARTESIAN_POINT('Ctrl Pts',(80.0524093383324,-7.33480905382207,135.001608224779));
#80282=CARTESIAN_POINT('Ctrl Pts',(80.0595903096703,-7.33505056647917,135.001119702819));
#80283=CARTESIAN_POINT('Ctrl Pts',(80.0825245838325,-7.3359704568226,134.999551511326));
#80284=CARTESIAN_POINT('Ctrl Pts',(80.0982693737121,-7.33682601251735,134.998462902655));
#80285=CARTESIAN_POINT('Ctrl Pts',(80.1851183459718,-7.34278276466411,134.992400142951));
#80286=CARTESIAN_POINT('Ctrl Pts',(80.2558446351054,-7.35221989060694,134.987251230197));
#80287=CARTESIAN_POINT('Ctrl Pts',(80.4539862530033,-7.39172361223971,134.97256368386));
#80288=CARTESIAN_POINT('Ctrl Pts',(80.5787995948267,-7.43230774268162,134.963037279015));
#80289=CARTESIAN_POINT('Ctrl Pts',(80.7233827361843,-7.49897369665789,134.952018346345));
#80290=CARTESIAN_POINT('Ctrl Pts',(80.7488659444659,-7.51152342479597,134.950074444951));
#80291=CARTESIAN_POINT('Ctrl Pts',(80.7852864668139,-7.53063172832563,134.947292001966));
#80292=CARTESIAN_POINT('Ctrl Pts',(80.7964878339778,-7.53667327684771,134.946435629892));
#80293=CARTESIAN_POINT('Ctrl Pts',(80.8162048154638,-7.54760127492435,134.944926772722));
#80294=CARTESIAN_POINT('Ctrl Pts',(80.8247484102004,-7.55243569249882,134.944272477817));
#80295=CARTESIAN_POINT('Ctrl Pts',(80.842479489308,-7.56267681544452,134.94291330907));
#80296=CARTESIAN_POINT('Ctrl Pts',(80.8516588370472,-7.56809676969414,134.94220894986));
#80297=CARTESIAN_POINT('Ctrl Pts',(80.8755715024308,-7.58252732676567,134.940371699113));
#80298=CARTESIAN_POINT('Ctrl Pts',(80.8902180870378,-7.59167971358375,134.939244010435));
#80299=CARTESIAN_POINT('Ctrl Pts',(80.9612666525135,-7.63762807468132,134.93375756812));
#80300=CARTESIAN_POINT('Ctrl Pts',(81.015547792024,-7.67759495096403,134.929518629652));
#80301=CARTESIAN_POINT('Ctrl Pts',(81.122311087216,-7.76666597919458,134.920909803424));
#80302=CARTESIAN_POINT('Ctrl Pts',(81.1743361769062,-7.81609551483648,134.916558264143));
#80303=CARTESIAN_POINT('Ctrl Pts',(81.2383180250598,-7.88526581017985,134.910793193035));
#80304=CARTESIAN_POINT('Ctrl Pts',(81.2532829691558,-7.90211766856884,134.909411218824));
#80305=CARTESIAN_POINT('Ctrl Pts',(81.3103994202164,-7.96912594926011,134.903981163259));
#80306=CARTESIAN_POINT('Ctrl Pts',(81.3499147443503,-8.02144184902819,134.899881128447));
#80307=CARTESIAN_POINT('Ctrl Pts',(81.392605451346,-8.08548502962895,134.894845224273));
#80308=CARTESIAN_POINT('Ctrl Pts',(81.3988687358981,-8.09509458175673,134.894089145168));
#80309=CARTESIAN_POINT('Ctrl Pts',(81.4084732152304,-8.11016843659735,134.892901158263));
#80310=CARTESIAN_POINT('Ctrl Pts',(81.4118831098485,-8.11558884564656,134.892473577062));
#80311=CARTESIAN_POINT('Ctrl Pts',(81.4181300451258,-8.12564724829787,134.891679146676));
#80312=CARTESIAN_POINT('Ctrl Pts',(81.4209757364171,-8.13027963537631,134.891312866394));
#80313=CARTESIAN_POINT('Ctrl Pts',(81.4275538993163,-8.1411064291571,134.890455905735));
#80314=CARTESIAN_POINT('Ctrl Pts',(81.4312687480956,-8.14731127172097,134.88996412713));
#80315=CARTESIAN_POINT('Ctrl Pts',(81.4430862385932,-8.16734461569995,134.888374731461));
#80316=CARTESIAN_POINT('Ctrl Pts',(81.4510294824002,-8.18126544286772,134.887267845065));
#80317=CARTESIAN_POINT('Ctrl Pts',(81.4696384076648,-8.21499985460932,134.884583553367));
#80318=CARTESIAN_POINT('Ctrl Pts',(81.4801057423278,-8.23491884976268,134.882996987279));
#80319=CARTESIAN_POINT('Ctrl Pts',(81.519902073269,-8.31452493314344,134.876666651372));
#80320=CARTESIAN_POINT('Ctrl Pts',(81.5460485064376,-8.37573123773124,134.87182468724));
#80321=CARTESIAN_POINT('Ctrl Pts',(81.6090637709776,-8.5517024548868,134.858218677217));
#80322=CARTESIAN_POINT('Ctrl Pts',(81.6372573948194,-8.66915996472706,134.849525409811));
#80323=CARTESIAN_POINT('Ctrl Pts',(81.6552067644714,-8.80950415929666,134.839792101912));
#80324=CARTESIAN_POINT('Ctrl Pts',(81.6574792126088,-8.83040982282763,134.838357725663));
#80325=CARTESIAN_POINT('Ctrl Pts',(81.660477499567,-8.86388005071383,134.836085119794));
#80326=CARTESIAN_POINT('Ctrl Pts',(81.6614577644362,-8.87641893667384,134.835239057551));
#80327=CARTESIAN_POINT('Ctrl Pts',(81.6629487579776,-8.89874108815865,134.833741979593));
#80328=CARTESIAN_POINT('Ctrl Pts',(81.6635153548643,-8.90851989254091,134.833089248116));
#80329=CARTESIAN_POINT('Ctrl Pts',(81.6645219276044,-8.9290217347799,134.831727015136));
#80330=CARTESIAN_POINT('Ctrl Pts',(81.6649446026819,-8.93974520184122,134.831018083247));
#80331=CARTESIAN_POINT('Ctrl Pts',(81.6657869838347,-8.9680684317809,134.829154604133));
#80332=CARTESIAN_POINT('Ctrl Pts',(81.6660314095419,-8.98567235349846,134.828005542342));
#80333=CARTESIAN_POINT('Ctrl Pts',(81.6658540375682,-9.07583549934513,134.822162228331));
#80334=CARTESIAN_POINT('Ctrl Pts',(81.6609714707634,-9.14831175867685,134.817608774634));
#80335=CARTESIAN_POINT('Ctrl Pts',(81.6378978560055,-9.32131475564214,134.806832053501));
#80336=CARTESIAN_POINT('Ctrl Pts',(81.6151690677491,-9.42092759131997,134.800708601513));
#80337=CARTESIAN_POINT('Ctrl Pts',(81.5763225683016,-9.53971583289705,134.792940495281));
#80338=CARTESIAN_POINT('Ctrl Pts',(81.5687141664789,-9.56144617366989,134.791498863826));
#80339=CARTESIAN_POINT('Ctrl Pts',(81.5493296563802,-9.61333643402813,134.787991250943));
#80340=CARTESIAN_POINT('Ctrl Pts',(81.5371204641159,-9.64332287388392,134.78591034512));
#80341=CARTESIAN_POINT('Ctrl Pts',(81.5201208374032,-9.68182336657085,134.783144035793));
#80342=CARTESIAN_POINT('Ctrl Pts',(81.5161174225967,-9.69067967481296,134.782501054123));
#80343=CARTESIAN_POINT('Ctrl Pts',(81.5095368241562,-9.70490427073001,134.781456765782));
#80344=CARTESIAN_POINT('Ctrl Pts',(81.5070078751695,-9.71029480904442,134.781058321519));
#80345=CARTESIAN_POINT('Ctrl Pts',(81.5020267713931,-9.72076584433124,134.780278852064));
#80346=CARTESIAN_POINT('Ctrl Pts',(81.4995776259497,-9.72584761789911,134.779898006205));
#80347=CARTESIAN_POINT('Ctrl Pts',(81.493485822658,-9.73832517572923,134.77895675164));
#80348=CARTESIAN_POINT('Ctrl Pts',(81.48981401351,-9.74570648760143,134.778394597122));
#80349=CARTESIAN_POINT('Ctrl Pts',(81.4759487384856,-9.77306820235624,134.776291644873));
#80350=CARTESIAN_POINT('Ctrl Pts',(81.4654073624579,-9.79286837816158,134.774731713571));
#80351=CARTESIAN_POINT('Ctrl Pts',(81.3834394928083,-9.9396097685221,134.76291457146));
#80352=CARTESIAN_POINT('Ctrl Pts',(81.2960409403727,-10.0569072463972,134.752078366232));
#80353=CARTESIAN_POINT('Ctrl Pts',(81.1491877331454,-10.2079521638097,134.737037184466));
#80354=CARTESIAN_POINT('Ctrl Pts',(81.10118473183,-10.2518685882026,134.732484196918));
#80355=CARTESIAN_POINT('Ctrl Pts',(81.0370589315132,-10.3039843576651,134.726844988755));
#80356=CARTESIAN_POINT('Ctrl Pts',(81.0232100676481,-10.3148793219644,134.725651243418));
#80357=CARTESIAN_POINT('Ctrl Pts',(81.0006495310242,-10.3320554595426,134.723744217125));
#80358=CARTESIAN_POINT('Ctrl Pts',(80.9920457458399,-10.3384754307517,134.723025518288));
#80359=CARTESIAN_POINT('Ctrl Pts',(80.9754745608034,-10.3505929448306,134.721657295945));
#80360=CARTESIAN_POINT('Ctrl Pts',(80.9675178243394,-10.3563042387219,134.721007258458));
#80361=CARTESIAN_POINT('Ctrl Pts',(80.9490601134014,-10.3693079764402,134.719514893307));
#80362=CARTESIAN_POINT('Ctrl Pts',(80.938524552036,-10.3765504398901,134.718674492941));
#80363=CARTESIAN_POINT('Ctrl Pts',(80.9046989976945,-10.3992342621798,134.716011371556));
#80364=CARTESIAN_POINT('Ctrl Pts',(80.8811027039194,-10.4142117832447,134.714205886392));
#80365=CARTESIAN_POINT('Ctrl Pts',(80.7918224145945,-10.4677790839561,134.707549490834));
#80366=CARTESIAN_POINT('Ctrl Pts',(80.7238909448072,-10.5024452759759,134.702833216025));
#80367=CARTESIAN_POINT('Ctrl Pts',(80.5732190554284,-10.566733879394,134.692794054025));
#80368=CARTESIAN_POINT('Ctrl Pts',(80.490035263764,-10.5947097196123,134.687502989554));
#80369=CARTESIAN_POINT('Ctrl Pts',(80.359676118395,-10.6273833155937,134.679111837194));
#80370=CARTESIAN_POINT('Ctrl Pts',(80.3138558079837,-10.6368375086744,134.67614267141));
#80371=CARTESIAN_POINT('Ctrl Pts',(80.2569633293007,-10.6460997097192,134.672364915299));
#80372=CARTESIAN_POINT('Ctrl Pts',(80.2462067104766,-10.6477428947505,134.671646672907));
#80373=CARTESIAN_POINT('Ctrl Pts',(80.2292889368182,-10.6501579102668,134.670509689661));
#80374=CARTESIAN_POINT('Ctrl Pts',(80.2231380210954,-10.6510008981709,134.670094787554));
#80375=CARTESIAN_POINT('Ctrl Pts',(80.2114974742476,-10.652530007249,134.669306469576));
#80376=CARTESIAN_POINT('Ctrl Pts',(80.2060089587909,-10.6532231887014,134.668933446066));
#80377=CARTESIAN_POINT('Ctrl Pts',(80.1929643506541,-10.6548047145764,134.668043817711));
#80378=CARTESIAN_POINT('Ctrl Pts',(80.1854055028075,-10.6556686497899,134.667525892015));
#80379=CARTESIAN_POINT('Ctrl Pts',(80.1597269056849,-10.658425525904,134.665758804767));
#80380=CARTESIAN_POINT('Ctrl Pts',(80.1415828476452,-10.6600729318058,134.664497369311));
#80381=CARTESIAN_POINT('Ctrl Pts',(80.096744043622,-10.6634037180127,134.661354170434));
#80382=CARTESIAN_POINT('Ctrl Pts',(80.0700293014619,-10.6647423454954,134.659458949532));
#80383=CARTESIAN_POINT('Ctrl Pts',(79.9510027949963,-10.6678366140256,134.650945512812));
#80384=CARTESIAN_POINT('Ctrl Pts',(79.8586724262388,-10.662560037362,134.644166627032));
#80385=CARTESIAN_POINT('Ctrl Pts',(79.6731949992742,-10.6363917693144,134.630607560278));
#80386=CARTESIAN_POINT('Ctrl Pts',(79.5804286110354,-10.6150990359347,134.623859740041));
#80387=CARTESIAN_POINT('Ctrl Pts',(79.4720877813883,-10.5802586871293,134.61607940845));
#80388=CARTESIAN_POINT('Ctrl Pts',(79.4543038474139,-10.5742060182796,134.614805053408));
#80389=CARTESIAN_POINT('Ctrl Pts',(79.4262884620084,-10.5641392906645,134.612801178886));
#80390=CARTESIAN_POINT('Ctrl Pts',(79.4159882727425,-10.5603227108047,134.612065215707));
#80391=CARTESIAN_POINT('Ctrl Pts',(79.3975363748909,-10.5532773208182,134.610747960638));
#80392=CARTESIAN_POINT('Ctrl Pts',(79.3893710645594,-10.5500855341478,134.610165462149));
#80393=CARTESIAN_POINT('Ctrl Pts',(79.370228935208,-10.5424282239076,134.608800660836));
#80394=CARTESIAN_POINT('Ctrl Pts',(79.3592737166715,-10.5379097053935,134.608020169134));
#80395=CARTESIAN_POINT('Ctrl Pts',(79.3272287948392,-10.5242908037662,134.605738173161));
#80396=CARTESIAN_POINT('Ctrl Pts',(79.3062774531805,-10.5148705093417,134.604247508801));
#80397=CARTESIAN_POINT('Ctrl Pts',(79.2098572990438,-10.4690972710692,134.597382672941));
#80398=CARTESIAN_POINT('Ctrl Pts',(79.137000274639,-10.4275174697447,134.592189834619));
#80399=CARTESIAN_POINT('Ctrl Pts',(78.9951464206837,-10.3317145130248,134.581699221926));
#80400=CARTESIAN_POINT('Ctrl Pts',(78.9266847645311,-10.2771793958034,134.576422095966));
#80401=CARTESIAN_POINT('Ctrl Pts',(78.828397737918,-10.1853787209171,134.568027029418));
#80402=CARTESIAN_POINT('Ctrl Pts',(78.7953576185797,-10.1517857530904,134.565037550925));
#80403=CARTESIAN_POINT('Ctrl Pts',(78.7564814841443,-10.1087544805613,134.561237001151));
#80404=CARTESIAN_POINT('Ctrl Pts',(78.7492545818048,-10.1005956027413,134.560517599131));
#80405=CARTESIAN_POINT('Ctrl Pts',(78.738035145519,-10.0876761005289,134.559379188394));
#80406=CARTESIAN_POINT('Ctrl Pts',(78.7339881522555,-10.0829628764776,134.558964034378));
#80407=CARTESIAN_POINT('Ctrl Pts',(78.7263879463462,-10.0740106753153,134.558175544376));
#80408=CARTESIAN_POINT('Ctrl Pts',(78.7228293658957,-10.0697765007617,134.557802603789));
#80409=CARTESIAN_POINT('Ctrl Pts',(78.7144310524679,-10.0596821439433,134.556913596875));
#80410=CARTESIAN_POINT('Ctrl Pts',(78.7096102584103,-10.0538064690579,134.55639621489));
#80411=CARTESIAN_POINT('Ctrl Pts',(78.6934007142733,-10.033771968731,134.554632965941));
#80412=CARTESIAN_POINT('Ctrl Pts',(78.6822039181712,-10.0194604437154,134.553374894496));
#80413=CARTESIAN_POINT('Ctrl Pts',(78.6141843361677,-9.92952593831224,134.545492669597));
#80414=CARTESIAN_POINT('Ctrl Pts',(78.5636581467632,-9.84936612425774,134.538579423431));
#80415=CARTESIAN_POINT('Ctrl Pts',(78.483742814344,-9.69485337883322,134.525923075884));
#80416=CARTESIAN_POINT('Ctrl Pts',(78.4523584077222,-9.62182386272021,134.520184681434));
#80417=CARTESIAN_POINT('Ctrl Pts',(78.4112168365699,-9.50342376969325,134.511356299255));
#80418=CARTESIAN_POINT('Ctrl Pts',(78.3979356800917,-9.45941054467738,134.508171022092));
#80419=CARTESIAN_POINT('Ctrl Pts',(78.3825486164873,-9.39957168790171,134.503966904184));
#80420=CARTESIAN_POINT('Ctrl Pts',(78.378825451367,-9.38418696580942,134.502896957911));
#80421=CARTESIAN_POINT('Ctrl Pts',(78.3730304226634,-9.3586546838525,134.501138778493));
#80422=CARTESIAN_POINT('Ctrl Pts',(78.3708329841123,-9.34853698588228,134.500446568906));
#80423=CARTESIAN_POINT('Ctrl Pts',(78.3667085381386,-9.32865489412879,134.499094892106));
#80424=CARTESIAN_POINT('Ctrl Pts',(78.364774431335,-9.31889243597133,134.498435224417));
#80425=CARTESIAN_POINT('Ctrl Pts',(78.3610995940139,-9.29943038570299,134.497127873068));
#80426=CARTESIAN_POINT('Ctrl Pts',(78.359357214964,-9.28973152308358,134.496480161984));
#80427=CARTESIAN_POINT('Ctrl Pts',(78.3554622532095,-9.2668876302688,134.494963169856));
#80428=CARTESIAN_POINT('Ctrl Pts',(78.3533810378689,-9.25373099502853,134.494096130788));
#80429=CARTESIAN_POINT('Ctrl Pts',(78.3397677171448,-9.16043609987433,134.487991767609));
#80430=CARTESIAN_POINT('Ctrl Pts',(78.3339325374407,-9.07957311045808,134.482936828984));
#80431=CARTESIAN_POINT('Ctrl Pts',(78.3340005883416,-8.9985998736709,134.47795669959));
#80432=CARTESIAN_POINT('Ctrl Pts',(78.3340005871935,-8.99860124042719,134.47795678365));
#80433=CARTESIAN_POINT('Ctrl Pts',(78.3341161231815,-8.86099153826944,134.469493317637));
#80434=CARTESIAN_POINT('Ctrl Pts',(78.3512803163155,-8.72394302691231,134.46132014703));
#80435=CARTESIAN_POINT('Ctrl Pts',(78.3889956810779,-8.57517810429444,134.451364961208));
#80436=CARTESIAN_POINT('Ctrl Pts',(78.3931211871174,-8.55983072105692,134.45032415857));
#80437=CARTESIAN_POINT('Ctrl Pts',(78.3994358404868,-8.53761236960593,134.448794138787));
#80438=CARTESIAN_POINT('Ctrl Pts',(78.4014511939541,-8.5306923617065,134.448314302381));
#80439=CARTESIAN_POINT('Ctrl Pts',(78.4050787622014,-8.51853108705294,134.447464846563));
#80440=CARTESIAN_POINT('Ctrl Pts',(78.4066720452708,-8.51328437842448,134.447096316818));
#80441=CARTESIAN_POINT('Ctrl Pts',(78.4101931791924,-8.50189182130291,134.446291541461));
#80442=CARTESIAN_POINT('Ctrl Pts',(78.4121307473039,-8.49574935002067,134.445854768662));
#80443=CARTESIAN_POINT('Ctrl Pts',(78.4176688187356,-8.47854103727911,134.444623380188));
#80444=CARTESIAN_POINT('Ctrl Pts',(78.4213496353584,-8.46750171431008,134.443824393295));
#80445=CARTESIAN_POINT('Ctrl Pts',(78.4288419455592,-8.44579178596344,134.442236434915));
#80446=CARTESIAN_POINT('Ctrl Pts',(78.4326467504955,-8.43512118271736,134.441447903419));
#80447=CARTESIAN_POINT('Ctrl Pts',(78.4365593695135,-8.4244920548384,134.440654933552));
#80448=CARTESIAN_POINT('',(78.3339996279362,-8.9995716607509,134.670001230007));
#80449=CARTESIAN_POINT('Ctrl Pts',(78.4365594680555,-8.42449178713676,134.632696249083));
#80450=CARTESIAN_POINT('Ctrl Pts',(78.4230664091285,-8.46114738084474,134.635100959469));
#80451=CARTESIAN_POINT('Ctrl Pts',(78.4108580173571,-8.49828954855501,134.637487701189));
#80452=CARTESIAN_POINT('Ctrl Pts',(78.3785500153332,-8.60966343661029,134.644568869371));
#80453=CARTESIAN_POINT('Ctrl Pts',(78.3622729774936,-8.68486328966597,134.649250240163));
#80454=CARTESIAN_POINT('Ctrl Pts',(78.3463552023685,-8.79463231339255,134.656260430122));
#80455=CARTESIAN_POINT('Ctrl Pts',(78.3425013367062,-8.8284925305262,134.658447268492));
#80456=CARTESIAN_POINT('Ctrl Pts',(78.338872193042,-8.87229665142323,134.661335079901));
#80457=CARTESIAN_POINT('Ctrl Pts',(78.3381436651677,-8.88215583637794,134.661988880378));
#80458=CARTESIAN_POINT('Ctrl Pts',(78.3371147149533,-8.89799799750504,134.663046420861));
#80459=CARTESIAN_POINT('Ctrl Pts',(78.3367587310208,-8.90397730446751,134.663447164606));
#80460=CARTESIAN_POINT('Ctrl Pts',(78.3361542698538,-8.91514502163804,134.664198842126));
#80461=CARTESIAN_POINT('Ctrl Pts',(78.3358978011997,-8.92033287994357,134.664549328504));
#80462=CARTESIAN_POINT('Ctrl Pts',(78.3354160274224,-8.9310988746163,134.665279266662));
#80463=CARTESIAN_POINT('Ctrl Pts',(78.3351944918527,-8.93667713966902,134.665658918725));
#80464=CARTESIAN_POINT('Ctrl Pts',(78.3346997108799,-8.95094380408305,134.666633408942));
#80465=CARTESIAN_POINT('Ctrl Pts',(78.3344664264399,-8.95963329653432,134.667230278338));
#80466=CARTESIAN_POINT('Ctrl Pts',(78.3341030873741,-8.97873966103855,134.668549418527));
#80467=CARTESIAN_POINT('Ctrl Pts',(78.3340027210467,-8.98915664129192,134.669273035995));
#80468=CARTESIAN_POINT('Ctrl Pts',(78.3340000545808,-8.99957354585502,134.670000621529));
#80469=CARTESIAN_POINT('Ctrl Pts',(78.3340000550511,-8.99957171231383,134.670000493463));
#80470=CARTESIAN_POINT('Ctrl Pts',(78.3339655640915,-9.13373839219119,134.679371576049));
#80471=CARTESIAN_POINT('Ctrl Pts',(78.3501375019262,-9.26742048515377,134.689320602716));
#80472=CARTESIAN_POINT('Ctrl Pts',(78.3979871940484,-9.46206173214905,134.703754922728));
#80473=CARTESIAN_POINT('Ctrl Pts',(78.4176304081814,-9.52540878035722,134.70845310578));
#80474=CARTESIAN_POINT('Ctrl Pts',(78.4507577760545,-9.61332763812592,134.714950196648));
#80475=CARTESIAN_POINT('Ctrl Pts',(78.4611626667193,-9.63898519600179,134.716843838627));
#80476=CARTESIAN_POINT('Ctrl Pts',(78.4772814709453,-9.67605212743428,134.719577533887));
#80477=CARTESIAN_POINT('Ctrl Pts',(78.4824941231686,-9.68767297980347,134.720434299254));
#80478=CARTESIAN_POINT('Ctrl Pts',(78.4919466410799,-9.70811497651373,134.721941282511));
#80479=CARTESIAN_POINT('Ctrl Pts',(78.4961318790929,-9.71696055348584,134.722593334171));
#80480=CARTESIAN_POINT('Ctrl Pts',(78.505079483049,-9.73544835656566,134.723956311786));
#80481=CARTESIAN_POINT('Ctrl Pts',(78.5098577750967,-9.74508240878569,134.72466664954));
#80482=CARTESIAN_POINT('Ctrl Pts',(78.52275414945,-9.77046385587785,134.726538784549));
#80483=CARTESIAN_POINT('Ctrl Pts',(78.5310308467589,-9.78612945638457,134.727694999347));
#80484=CARTESIAN_POINT('Ctrl Pts',(78.5717446085006,-9.86030070461446,134.733177494711));
#80485=CARTESIAN_POINT('Ctrl Pts',(78.6074377863159,-9.91695299704115,134.737386473143));
#80486=CARTESIAN_POINT('Ctrl Pts',(78.7306340209266,-10.0886312118089,134.750467129965));
#80487=CARTESIAN_POINT('Ctrl Pts',(78.8297057845599,-10.1944910101378,134.758995725453));
#80488=CARTESIAN_POINT('Ctrl Pts',(78.952679850075,-10.2957233498186,134.769227916008));
#80489=CARTESIAN_POINT('Ctrl Pts',(78.9643224077977,-10.3050480401016,134.77019409343));
#80490=CARTESIAN_POINT('Ctrl Pts',(78.982758472502,-10.3194116778307,134.771722891968));
#80491=CARTESIAN_POINT('Ctrl Pts',(78.98946810218,-10.3245575779515,134.772279050622));
#80492=CARTESIAN_POINT('Ctrl Pts',(79.0019141405984,-10.3339533658567,134.773310876572));
#80493=CARTESIAN_POINT('Ctrl Pts',(79.0076392937887,-10.3382179154274,134.773785583136));
#80494=CARTESIAN_POINT('Ctrl Pts',(79.0134457632717,-10.3424852857742,134.774267300784));
#80495=CARTESIAN_POINT('Ctrl Pts',(79.0134999811191,-10.3425251272416,134.774271798841));
#80496=CARTESIAN_POINT('Ctrl Pts',(79.0136085108232,-10.3426048691337,134.774280802802));
#80497=CARTESIAN_POINT('Ctrl Pts',(79.0136628224429,-10.3426447693677,134.774285308686));
#80498=CARTESIAN_POINT('Ctrl Pts',(79.0137715557547,-10.3427246405428,134.774294329634));
#80499=CARTESIAN_POINT('Ctrl Pts',(79.013825977572,-10.3427646115562,134.774298844709));
#80500=CARTESIAN_POINT('Ctrl Pts',(79.0139349477684,-10.3428446363401,134.774307885406));
#80501=CARTESIAN_POINT('Ctrl Pts',(79.0139894959941,-10.3428846899752,134.774312411017));
#80502=CARTESIAN_POINT('Ctrl Pts',(79.0140987356719,-10.3429648921693,134.774321474169));
#80503=CARTESIAN_POINT('Ctrl Pts',(79.0141534271985,-10.3430050407569,134.774326011718));
#80504=CARTESIAN_POINT('Ctrl Pts',(79.0142372954618,-10.3430665998569,134.774332969988));
#80505=CARTESIAN_POINT('Ctrl Pts',(79.0142664706427,-10.3430880129055,134.774335390562));
#80506=CARTESIAN_POINT('Ctrl Pts',(79.0143255429488,-10.3431313659103,134.774340291623));
#80507=CARTESIAN_POINT('Ctrl Pts',(79.0143554400502,-10.3431533057758,134.774342772107));
#80508=CARTESIAN_POINT('Ctrl Pts',(79.0144159922831,-10.3431977386738,134.774347795983));
#80509=CARTESIAN_POINT('Ctrl Pts',(79.0144466474883,-10.3432202316816,134.774350339381));
#80510=CARTESIAN_POINT('Ctrl Pts',(79.0145087542789,-10.3432657987639,134.774355492267));
#80511=CARTESIAN_POINT('Ctrl Pts',(79.0145402060875,-10.3432888729174,134.774358101774));
#80512=CARTESIAN_POINT('Ctrl Pts',(79.0146039474237,-10.3433356323609,134.774363390308));
#80513=CARTESIAN_POINT('Ctrl Pts',(79.0146362367528,-10.343359317414,134.77436606932));
#80514=CARTESIAN_POINT('Ctrl Pts',(79.0147016970534,-10.3434073305974,134.774371500511));
#80515=CARTESIAN_POINT('Ctrl Pts',(79.0147348681049,-10.3434316586875,134.774374252696));
#80516=CARTESIAN_POINT('Ctrl Pts',(79.0148021388393,-10.3434809921068,134.774379834135));
#80517=CARTESIAN_POINT('Ctrl Pts',(79.0148362386128,-10.3435059973954,134.774382663395));
#80518=CARTESIAN_POINT('Ctrl Pts',(79.0149054174014,-10.3435567219983,134.774388403185));
#80519=CARTESIAN_POINT('Ctrl Pts',(79.0149404963375,-10.3435824411387,134.774391313707));
#80520=CARTESIAN_POINT('Ctrl Pts',(79.0192893398945,-10.3467706601818,134.774752141436));
#80521=CARTESIAN_POINT('Ctrl Pts',(79.0236181220911,-10.3499122332568,134.775111473011));
#80522=CARTESIAN_POINT('Ctrl Pts',(79.0330801786284,-10.3567099077547,134.775897391517));
#80523=CARTESIAN_POINT('Ctrl Pts',(79.0382190017326,-10.3603576819476,134.776324493823));
#80524=CARTESIAN_POINT('Ctrl Pts',(79.0524019511165,-10.3703048627952,134.777503746734));
#80525=CARTESIAN_POINT('Ctrl Pts',(79.061487896114,-10.3765436767027,134.778259722285));
#80526=CARTESIAN_POINT('Ctrl Pts',(79.1133507500622,-10.4114028825208,134.782574772295));
#80527=CARTESIAN_POINT('Ctrl Pts',(79.1573701053193,-10.4381163947461,134.786236186844));
#80528=CARTESIAN_POINT('Ctrl Pts',(79.2868519069303,-10.5087063475569,134.79686350198));
#80529=CARTESIAN_POINT('Ctrl Pts',(79.374969743379,-10.5472922451104,134.803915886907));
#80530=CARTESIAN_POINT('Ctrl Pts',(79.5157217824108,-10.5949277474463,134.814601881482));
#80531=CARTESIAN_POINT('Ctrl Pts',(79.5662935521673,-10.6094158933086,134.818335622565));
#80532=CARTESIAN_POINT('Ctrl Pts',(79.6406651286282,-10.6269610943946,134.823661066639));
#80533=CARTESIAN_POINT('Ctrl Pts',(79.6639758579436,-10.6319349948502,134.825307380278));
#80534=CARTESIAN_POINT('Ctrl Pts',(79.7064425288364,-10.6400476829755,134.828265811755));
#80535=CARTESIAN_POINT('Ctrl Pts',(79.725561523881,-10.6433550953282,134.829582919654));
#80536=CARTESIAN_POINT('Ctrl Pts',(79.7557168691385,-10.6480307219866,134.831637920771));
#80537=CARTESIAN_POINT('Ctrl Pts',(79.7667160729204,-10.649623632337,134.832382831533));
#80538=CARTESIAN_POINT('Ctrl Pts',(79.7873642226649,-10.6524032541108,134.83377277205));
#80539=CARTESIAN_POINT('Ctrl Pts',(79.7970091532958,-10.6536157990899,134.83441858825));
#80540=CARTESIAN_POINT('Ctrl Pts',(79.8187058179514,-10.6561507771167,134.835863933002));
#80541=CARTESIAN_POINT('Ctrl Pts',(79.8307625695265,-10.6574262222151,134.83666195621));
#80542=CARTESIAN_POINT('Ctrl Pts',(79.866310382155,-10.6607947644141,134.839000497099));
#80543=CARTESIAN_POINT('Ctrl Pts',(79.8898337995487,-10.6625208754126,134.840529571684));
#80544=CARTESIAN_POINT('Ctrl Pts',(80.0169213852895,-10.6691369336915,134.848705135352));
#80545=CARTESIAN_POINT('Ctrl Pts',(80.1207370622526,-10.6648514547836,134.855059796419));
#80546=CARTESIAN_POINT('Ctrl Pts',(80.3013522301192,-10.6404012746056,134.866190751969));
#80547=CARTESIAN_POINT('Ctrl Pts',(80.3783651080232,-10.6243668395529,134.870968298552));
#80548=CARTESIAN_POINT('Ctrl Pts',(80.4776737703714,-10.5962429520857,134.877477491342));
#80549=CARTESIAN_POINT('Ctrl Pts',(80.501241105463,-10.589000005949,134.879049184282));
#80550=CARTESIAN_POINT('Ctrl Pts',(80.5409210087273,-10.5758346341372,134.881754995544));
#80551=CARTESIAN_POINT('Ctrl Pts',(80.5571190456132,-10.5701810865987,134.882876701772));
#80552=CARTESIAN_POINT('Ctrl Pts',(80.5802013040859,-10.56172264934,134.884503753885));
#80553=CARTESIAN_POINT('Ctrl Pts',(80.5871591613581,-10.5591200405168,134.884997974632));
#80554=CARTESIAN_POINT('Ctrl Pts',(80.5992437850293,-10.5545073845682,134.885863314436));
#80555=CARTESIAN_POINT('Ctrl Pts',(80.6043783622986,-10.5525183144636,134.886233196932));
#80556=CARTESIAN_POINT('Ctrl Pts',(80.6153668345606,-10.5481987453737,134.887029654107));
#80557=CARTESIAN_POINT('Ctrl Pts',(80.6212173019891,-10.5458605230313,134.88745665413));
#80558=CARTESIAN_POINT('Ctrl Pts',(80.6372594904589,-10.5393432618707,134.888635356231));
#80559=CARTESIAN_POINT('Ctrl Pts',(80.6474230308605,-10.5350963288823,134.889390877641));
#80560=CARTESIAN_POINT('Ctrl Pts',(80.7053400824852,-10.5102176771152,134.893743500901));
#80561=CARTESIAN_POINT('Ctrl Pts',(80.7521442491115,-10.4874609164817,134.897445240398));
#80562=CARTESIAN_POINT('Ctrl Pts',(80.8876327028721,-10.4135539652158,134.908569889407));
#80563=CARTESIAN_POINT('Ctrl Pts',(80.9727640360823,-10.3563769860894,134.916091705519));
#80564=CARTESIAN_POINT('Ctrl Pts',(81.108624851904,-10.2457205151263,134.928652816149));
#80565=CARTESIAN_POINT('Ctrl Pts',(81.1620638983282,-10.1960262534107,134.933774892698));
#80566=CARTESIAN_POINT('Ctrl Pts',(81.2241712531038,-10.1301642519014,134.939952855472));
#80567=CARTESIAN_POINT('Ctrl Pts',(81.2360565134369,-10.1171530021458,134.941146721057));
#80568=CARTESIAN_POINT('Ctrl Pts',(81.2548456494016,-10.0959167827094,134.943053764791));
#80569=CARTESIAN_POINT('Ctrl Pts',(81.2618800743664,-10.0878096734668,134.943772363441));
#80570=CARTESIAN_POINT('Ctrl Pts',(81.2751806568171,-10.0721782280951,134.94514028096));
#80571=CARTESIAN_POINT('Ctrl Pts',(81.2814597632777,-10.0646655542489,134.945790114628));
#80572=CARTESIAN_POINT('Ctrl Pts',(81.2956440900474,-10.047387336875,134.947267701777));
#80573=CARTESIAN_POINT('Ctrl Pts',(81.3035058661933,-10.0375867735755,134.94809368396));
#80574=CARTESIAN_POINT('Ctrl Pts',(81.3242020903954,-10.0111801319241,134.950287939771));
#80575=CARTESIAN_POINT('Ctrl Pts',(81.3368351410188,-9.99441857593888,134.951648334009));
#80576=CARTESIAN_POINT('Ctrl Pts',(81.4202062247464,-9.87934038134007,134.960784321498));
#80577=CARTESIAN_POINT('Ctrl Pts',(81.4803582617905,-9.77380132754669,134.968139504169));
#80578=CARTESIAN_POINT('Ctrl Pts',(81.5548125319775,-9.60206059398917,134.979577859045));
#80579=CARTESIAN_POINT('Ctrl Pts',(81.5774562682301,-9.53995317480335,134.98362557116));
#80580=CARTESIAN_POINT('Ctrl Pts',(81.60276500431,-9.45519519827983,134.989224450874));
#80581=CARTESIAN_POINT('Ctrl Pts',(81.6087433117181,-9.43359333996628,134.990657923125));
#80582=CARTESIAN_POINT('Ctrl Pts',(81.6182343533038,-9.39639491518517,134.993147772109));
#80583=CARTESIAN_POINT('Ctrl Pts',(81.6219618000273,-9.38085591015712,134.994194188927));
#80584=CARTESIAN_POINT('Ctrl Pts',(81.6270484498644,-9.35821990766349,134.995730889327));
#80585=CARTESIAN_POINT('Ctrl Pts',(81.6285860298727,-9.35116335079337,134.99621167499));
#80586=CARTESIAN_POINT('Ctrl Pts',(81.6312000864178,-9.33877988663787,134.99705879292));
#80587=CARTESIAN_POINT('Ctrl Pts',(81.6322964539683,-9.33345737158956,134.997423998227));
#80588=CARTESIAN_POINT('Ctrl Pts',(81.6346286825067,-9.32184797605086,134.998223084424));
#80589=CARTESIAN_POINT('Ctrl Pts',(81.6358543059121,-9.31555940127625,134.998657498626));
#80590=CARTESIAN_POINT('Ctrl Pts',(81.6391763853969,-9.29797446371018,134.999876336945));
#80591=CARTESIAN_POINT('Ctrl Pts',(81.6411922554431,-9.28666350632705,135.000664998887));
#80592=CARTESIAN_POINT('Ctrl Pts',(81.6540552666921,-9.20990156134054,135.006044873079));
#80593=CARTESIAN_POINT('Ctrl Pts',(81.661100209379,-9.14388056898265,135.010805449705));
#80594=CARTESIAN_POINT('Ctrl Pts',(81.6652096704722,-9.05577697596238,135.017200097133));
#80595=CARTESIAN_POINT('Ctrl Pts',(81.665798379235,-9.03391251562046,135.018790675824));
#80596=CARTESIAN_POINT('Ctrl Pts',(81.6664767850191,-8.94006623175308,135.025621083104));
#80597=CARTESIAN_POINT('Ctrl Pts',(81.6623319886287,-8.86812706646643,135.030861097291));
#80598=CARTESIAN_POINT('Ctrl Pts',(81.645381018262,-8.73027056741288,135.040784064559));
#80599=CARTESIAN_POINT('Ctrl Pts',(81.6332216477549,-8.66440831011032,135.045471825213));
#80600=CARTESIAN_POINT('Ctrl Pts',(81.612987228798,-8.58271675104982,135.051211811907));
#80601=CARTESIAN_POINT('Ctrl Pts',(81.6085834722453,-8.56605027743998,135.052379126672));
#80602=CARTESIAN_POINT('Ctrl Pts',(81.6010413784179,-8.5392007574084,135.05425423469));
#80603=CARTESIAN_POINT('Ctrl Pts',(81.5980627336176,-8.52897458039818,135.054967125767));
#80604=CARTESIAN_POINT('Ctrl Pts',(81.5921510087143,-8.50938048682056,135.056330864971));
#80605=CARTESIAN_POINT('Ctrl Pts',(81.5892328122197,-8.50000858321588,135.05698216495));
#80606=CARTESIAN_POINT('Ctrl Pts',(81.5823383932591,-8.47853725094815,135.058472348632));
#80607=CARTESIAN_POINT('Ctrl Pts',(81.5783058845753,-8.46645643185838,135.059309352503));
#80608=CARTESIAN_POINT('Ctrl Pts',(81.5648132508347,-8.4275266024776,135.062002928243));
#80609=CARTESIAN_POINT('Ctrl Pts',(81.5548031451842,-8.40087260591408,135.063841412918));
#80610=CARTESIAN_POINT('Ctrl Pts',(81.4950344855907,-8.25333029494713,135.074012595117));
#80611=CARTESIAN_POINT('Ctrl Pts',(81.4318675300645,-8.13837273581656,135.081871775029));
#80612=CARTESIAN_POINT('Ctrl Pts',(81.3144980280403,-7.97397370461078,135.094265581886));
#80613=CARTESIAN_POINT('Ctrl Pts',(81.2694138161518,-7.91869464926673,135.09868386757));
#80614=CARTESIAN_POINT('Ctrl Pts',(81.210209995916,-7.85492520975466,135.104329575303));
#80615=CARTESIAN_POINT('Ctrl Pts',(81.1993213180594,-7.84352568498104,135.105362181486));
#80616=CARTESIAN_POINT('Ctrl Pts',(81.1832381788494,-7.82715942615533,135.106882253578));
#80617=CARTESIAN_POINT('Ctrl Pts',(81.1781703721315,-7.8220686908685,135.107360506613));
#80618=CARTESIAN_POINT('Ctrl Pts',(81.1692137656287,-7.81318718333462,135.108204842296));
#80619=CARTESIAN_POINT('Ctrl Pts',(81.165339115256,-7.80938241373852,135.108569823608));
#80620=CARTESIAN_POINT('Ctrl Pts',(81.156833788951,-7.80111177791663,135.109370482636));
#80621=CARTESIAN_POINT('Ctrl Pts',(81.1521958994567,-7.79665383613564,135.109806712555));
#80622=CARTESIAN_POINT('Ctrl Pts',(81.1391183129126,-7.7842285673267,135.111035449682));
#80623=CARTESIAN_POINT('Ctrl Pts',(81.1306211984808,-7.7763225939623,135.111832300858));
#80624=CARTESIAN_POINT('Ctrl Pts',(81.0651948429934,-7.71671112250744,135.117951778171));
#80625=CARTESIAN_POINT('Ctrl Pts',(81.0048351857145,-7.66892000078039,135.123501156732));
#80626=CARTESIAN_POINT('Ctrl Pts',(80.8942454603738,-7.59317821923879,135.133244034475));
#80627=CARTESIAN_POINT('Ctrl Pts',(80.8454598586471,-7.56333011596693,135.137414711098));
#80628=CARTESIAN_POINT('Ctrl Pts',(80.7224006028771,-7.49648285817966,135.147535104135));
#80629=CARTESIAN_POINT('Ctrl Pts',(80.6467053257672,-7.46240373932795,135.153421773494));
#80630=CARTESIAN_POINT('Ctrl Pts',(80.5472951060551,-7.42629531983579,135.160693124238));
#80631=CARTESIAN_POINT('Ctrl Pts',(80.5256540900555,-7.41893509903838,135.162250098101));
#80632=CARTESIAN_POINT('Ctrl Pts',(80.4925959369778,-7.40844570232025,135.16459050362));
#80633=CARTESIAN_POINT('Ctrl Pts',(80.4812863608128,-7.40498925051011,135.165384538784));
#80634=CARTESIAN_POINT('Ctrl Pts',(80.4615343282968,-7.39918182186175,135.166760075115));
#80635=CARTESIAN_POINT('Ctrl Pts',(80.4531084708974,-7.3967765301468,135.167343322934));
#80636=CARTESIAN_POINT('Ctrl Pts',(80.434066786017,-7.39150289479416,135.168653657651));
#80637=CARTESIAN_POINT('Ctrl Pts',(80.4234406784741,-7.38867293396076,135.169379479044));
#80638=CARTESIAN_POINT('Ctrl Pts',(80.3945261688822,-7.38127816640636,135.171340406612));
#80639=CARTESIAN_POINT('Ctrl Pts',(80.3761867126155,-7.37691809305534,135.172568923011));
#80640=CARTESIAN_POINT('Ctrl Pts',(80.2578261671444,-7.35089273968766,135.180407935869));
#80641=CARTESIAN_POINT('Ctrl Pts',(80.1560581931952,-7.33817004567148,135.186720324653));
#80642=CARTESIAN_POINT('Ctrl Pts',(79.9711519344295,-7.33220082725675,135.198030572033));
#80643=CARTESIAN_POINT('Ctrl Pts',(79.8884705956017,-7.33568457134481,135.203037332583));
#80644=CARTESIAN_POINT('Ctrl Pts',(79.7785236846193,-7.34854861557631,135.209983476996));
#80645=CARTESIAN_POINT('Ctrl Pts',(79.7507409538766,-7.35251307057591,135.211764255161));
#80646=CARTESIAN_POINT('Ctrl Pts',(79.7044684385107,-7.36031311830765,135.214792617982));
#80647=CARTESIAN_POINT('Ctrl Pts',(79.6859192166138,-7.36376494292112,135.216023561489));
#80648=CARTESIAN_POINT('Ctrl Pts',(79.6598767919797,-7.36907030241892,135.21778085283));
#80649=CARTESIAN_POINT('Ctrl Pts',(79.6523309637325,-7.37066218649873,135.21829349354));
#80650=CARTESIAN_POINT('Ctrl Pts',(79.6393775081506,-7.37348895364017,135.219179902661));
#80651=CARTESIAN_POINT('Ctrl Pts',(79.6339645289813,-7.37469855144849,135.219552246888));
#80652=CARTESIAN_POINT('Ctrl Pts',(79.6225563755177,-7.37730772840862,135.22034121488));
#80653=CARTESIAN_POINT('Ctrl Pts',(79.6165629772903,-7.37871349093621,135.220758154326));
#80654=CARTESIAN_POINT('Ctrl Pts',(79.6002272580043,-7.38264070886757,135.221901001507));
#80655=CARTESIAN_POINT('Ctrl Pts',(79.5899013053382,-7.38522807562341,135.222630458448));
#80656=CARTESIAN_POINT('Ctrl Pts',(79.5378591172056,-7.3987996067678,135.226340184451));
#80657=CARTESIAN_POINT('Ctrl Pts',(79.4965593227174,-7.41130126126427,135.229392352303));
#80658=CARTESIAN_POINT('Ctrl Pts',(79.3705388583657,-7.4548554930012,135.238952966392));
#80659=CARTESIAN_POINT('Ctrl Pts',(79.2878176306945,-7.49119614370717,135.245574474084));
#80660=CARTESIAN_POINT('Ctrl Pts',(79.1265572284294,-7.5782706138291,135.258830483274));
#80661=CARTESIAN_POINT('Ctrl Pts',(79.0485070069298,-7.62927645808574,135.265433725204));
#80662=CARTESIAN_POINT('Ctrl Pts',(78.9605025230795,-7.69794603449026,135.273062234116));
#80663=CARTESIAN_POINT('Ctrl Pts',(78.9460808071472,-7.70959156980129,135.274319341418));
#80664=CARTESIAN_POINT('Ctrl Pts',(78.9234688097721,-7.72848278100851,135.276302386316));
#80665=CARTESIAN_POINT('Ctrl Pts',(78.9151506902299,-7.73557229282677,135.277034543382));
#80666=CARTESIAN_POINT('Ctrl Pts',(78.8995471097111,-7.74913852053893,135.278413321286));
#80667=CARTESIAN_POINT('Ctrl Pts',(78.8922475930745,-7.75559828978252,135.279060600017));
#80668=CARTESIAN_POINT('Ctrl Pts',(78.8757834713942,-7.77042803108348,135.280526026533));
#80669=CARTESIAN_POINT('Ctrl Pts',(78.8666547908596,-7.77883716043145,135.281342485338));
#80670=CARTESIAN_POINT('Ctrl Pts',(78.8430726209364,-7.80105274723584,135.283462824265));
#80671=CARTESIAN_POINT('Ctrl Pts',(78.8287718542016,-7.81501891972989,135.284759847613));
#80672=CARTESIAN_POINT('Ctrl Pts',(78.7067132739332,-7.93859068784639,135.295942575706));
#80673=CARTESIAN_POINT('Ctrl Pts',(78.6143578809276,-8.06235533176093,135.305096383721));
#80674=CARTESIAN_POINT('Ctrl Pts',(78.5113756955332,-8.24956745276767,135.318278434067));
#80675=CARTESIAN_POINT('Ctrl Pts',(78.4853363497141,-8.30362092487862,135.322029180513));
#80676=CARTESIAN_POINT('Ctrl Pts',(78.4566659949515,-8.37239485799929,135.326874476996));
#80677=CARTESIAN_POINT('Ctrl Pts',(78.4512393321645,-8.38590845647614,135.327829978261));
#80678=CARTESIAN_POINT('Ctrl Pts',(78.4434820897048,-8.4059828005563,135.329256892356));
#80679=CARTESIAN_POINT('Ctrl Pts',(78.4410142065181,-8.4124902301322,135.329720607381));
#80680=CARTESIAN_POINT('Ctrl Pts',(78.4379080626342,-8.42083804333813,135.330317178921));
#80681=CARTESIAN_POINT('Ctrl Pts',(78.4372321141303,-8.42266445845914,135.330447807108));
#80682=CARTESIAN_POINT('Ctrl Pts',(78.4365593749993,-8.42449203993567,135.330578627164));
#80683=CARTESIAN_POINT('Origin',(80.,-9.,134.));
#80684=CARTESIAN_POINT('',(78.4365593762033,-8.4244920366647,136.032852185112));
#80685=CARTESIAN_POINT('',(78.4365593748807,-8.42449204025778,135.837694108205));
#80686=CARTESIAN_POINT('',(78.4365593749993,-8.42449203993574,134.));
#80687=CARTESIAN_POINT('Ctrl Pts',(78.4365593748807,-8.42449204025778,135.837694108205));
#80688=CARTESIAN_POINT('Ctrl Pts',(78.4383939076403,-8.41950829851134,135.837334131949));
#80689=CARTESIAN_POINT('Ctrl Pts',(78.4402523135159,-8.41453321100119,135.836974938851));
#80690=CARTESIAN_POINT('Ctrl Pts',(78.4463332781694,-8.39848850480445,135.835817009369));
#80691=CARTESIAN_POINT('Ctrl Pts',(78.4506501675972,-8.3874549234687,135.835021458479));
#80692=CARTESIAN_POINT('Ctrl Pts',(78.4583654957885,-8.36833877271354,135.83364411433));
#80693=CARTESIAN_POINT('Ctrl Pts',(78.4617106704672,-8.3602353602156,135.833060561932));
#80694=CARTESIAN_POINT('Ctrl Pts',(78.4693916474057,-8.34203741850409,135.831750578648));
#80695=CARTESIAN_POINT('Ctrl Pts',(78.4737636770115,-8.33195854634371,135.831025404877));
#80696=CARTESIAN_POINT('Ctrl Pts',(78.4858836455377,-8.30475845833332,135.829068798149));
#80697=CARTESIAN_POINT('Ctrl Pts',(78.4938222333095,-8.28772356648408,135.827843901735));
#80698=CARTESIAN_POINT('Ctrl Pts',(78.5459111333964,-8.1807165988968,135.820145019594));
#80699=CARTESIAN_POINT('Ctrl Pts',(78.5978179491005,-8.09474370543545,135.813955697692));
#80700=CARTESIAN_POINT('Ctrl Pts',(78.7020167114911,-7.9528404496892,135.80318867182));
#80701=CARTESIAN_POINT('Ctrl Pts',(78.7510052880733,-7.89486881111581,135.798593382761));
#80702=CARTESIAN_POINT('Ctrl Pts',(78.8271405395223,-7.81632593121283,135.791776868014));
#80703=CARTESIAN_POINT('Ctrl Pts',(78.8512349740222,-7.79292823306179,135.789660066913));
#80704=CARTESIAN_POINT('Ctrl Pts',(78.8868571773618,-7.76036913385192,135.786558188611));
#80705=CARTESIAN_POINT('Ctrl Pts',(78.8978261777244,-7.75060636264791,135.78560660933));
#80706=CARTESIAN_POINT('Ctrl Pts',(78.9152457023473,-7.73551032921353,135.784098287101));
#80707=CARTESIAN_POINT('Ctrl Pts',(78.9216100735742,-7.73007828054375,135.783547791416));
#80708=CARTESIAN_POINT('Ctrl Pts',(78.9334104480814,-7.72015922539667,135.782527580717));
#80709=CARTESIAN_POINT('Ctrl Pts',(78.9388345663148,-7.71565830150089,135.782058818015));
#80710=CARTESIAN_POINT('Ctrl Pts',(78.9443349429914,-7.71115272772209,135.781583457167));
#80711=CARTESIAN_POINT('Ctrl Pts',(78.9443829285015,-7.71111342539069,135.781579310099));
#80712=CARTESIAN_POINT('Ctrl Pts',(78.9444791139154,-7.71103465410426,135.781570997433));
#80713=CARTESIAN_POINT('Ctrl Pts',(78.9445273138624,-7.71099518515308,135.781566831832));
#80714=CARTESIAN_POINT('Ctrl Pts',(78.9446239420666,-7.71091606935077,135.781558480895));
#80715=CARTESIAN_POINT('Ctrl Pts',(78.9446723703386,-7.71087642252949,135.781554295559));
#80716=CARTESIAN_POINT('Ctrl Pts',(78.9447694693343,-7.71079693953716,135.781545903931));
#80717=CARTESIAN_POINT('Ctrl Pts',(78.9448181401431,-7.71075710334139,135.781541697632));
#80718=CARTESIAN_POINT('Ctrl Pts',(78.9449157387769,-7.7106772298155,135.781533262819));
#80719=CARTESIAN_POINT('Ctrl Pts',(78.9449646665673,-7.71063719256158,135.781529034309));
#80720=CARTESIAN_POINT('Ctrl Pts',(78.945062793984,-7.71055690493771,135.781520553792));
#80721=CARTESIAN_POINT('Ctrl Pts',(78.9451119936912,-7.71051665455248,135.781516301779));
#80722=CARTESIAN_POINT('Ctrl Pts',(78.9452106802047,-7.71043592833354,135.781507772938));
#80723=CARTESIAN_POINT('Ctrl Pts',(78.945260166977,-7.71039545258179,135.781503496112));
#80724=CARTESIAN_POINT('Ctrl Pts',(78.9453594432432,-7.71031426301585,135.781494916296));
#80725=CARTESIAN_POINT('Ctrl Pts',(78.945409232749,-7.71027354924947,135.781490613305));
#80726=CARTESIAN_POINT('Ctrl Pts',(78.9455091304601,-7.710191870763,135.781481979774));
#80727=CARTESIAN_POINT('Ctrl Pts',(78.9455592387293,-7.71015090605151,135.78147764923));
#80728=CARTESIAN_POINT('Ctrl Pts',(78.9456597904758,-7.71006871236304,135.781468959168));
#80729=CARTESIAN_POINT('Ctrl Pts',(78.9457102339212,-7.71002748347658,135.781464599653));
#80730=CARTESIAN_POINT('Ctrl Pts',(78.9498796479072,-7.70662010879387,135.781104262798));
#80731=CARTESIAN_POINT('Ctrl Pts',(78.9540145362725,-7.7032738509777,135.780746886022));
#80732=CARTESIAN_POINT('Ctrl Pts',(78.9630893941307,-7.69600145301667,135.779962392012));
#80733=CARTESIAN_POINT('Ctrl Pts',(78.968035577044,-7.6920836259374,135.779534738161));
#80734=CARTESIAN_POINT('Ctrl Pts',(78.9817064309062,-7.6813808879947,135.77835281934));
#80735=CARTESIAN_POINT('Ctrl Pts',(78.9904763642322,-7.67465469863019,135.777594703506));
#80736=CARTESIAN_POINT('Ctrl Pts',(79.0408342507606,-7.63682200865986,135.773245076621));
#80737=CARTESIAN_POINT('Ctrl Pts',(79.0837880996224,-7.60758920742123,135.769549402611));
#80738=CARTESIAN_POINT('Ctrl Pts',(79.2150509514012,-7.52696222425652,135.758445590601));
#80739=CARTESIAN_POINT('Ctrl Pts',(79.3068069189079,-7.48162244657397,135.750938797174));
#80740=CARTESIAN_POINT('Ctrl Pts',(79.470350793193,-7.41874456707789,135.738376910084));
#80741=CARTESIAN_POINT('Ctrl Pts',(79.5402243519671,-7.39703211563662,135.733240668417));
#80742=CARTESIAN_POINT('Ctrl Pts',(79.6284561167797,-7.37586264519249,135.727048314786));
#80743=CARTESIAN_POINT('Ctrl Pts',(79.6456695425891,-7.37202058584756,135.725853447226));
#80744=CARTESIAN_POINT('Ctrl Pts',(79.6734573218843,-7.366279955023,135.723945071337));
#80745=CARTESIAN_POINT('Ctrl Pts',(79.683994289227,-7.36420914965044,135.723226131327));
#80746=CARTESIAN_POINT('Ctrl Pts',(79.7041777537373,-7.36044484649549,135.721857726924));
#80747=CARTESIAN_POINT('Ctrl Pts',(79.7138205634914,-7.35873425677817,135.721207745928));
#80748=CARTESIAN_POINT('Ctrl Pts',(79.7358668438709,-7.35502355471972,135.719730040084));
#80749=CARTESIAN_POINT('Ctrl Pts',(79.7482790759779,-7.35307850202868,135.718904085037));
#80750=CARTESIAN_POINT('Ctrl Pts',(79.7814735289224,-7.3482608303342,135.716710367351));
#80751=CARTESIAN_POINT('Ctrl Pts',(79.8022904084353,-7.34563997765474,135.715350475287));
#80752=CARTESIAN_POINT('Ctrl Pts',(79.9437506440844,-7.33053847234002,135.706204142184));
#80753=CARTESIAN_POINT('Ctrl Pts',(80.0653963566273,-7.33087060094516,135.698839462544));
#80754=CARTESIAN_POINT('Ctrl Pts',(80.2514621884996,-7.35176752148609,135.68739780262));
#80755=CARTESIAN_POINT('Ctrl Pts',(80.3164868468536,-7.36300935972011,135.683356945727));
#80756=CARTESIAN_POINT('Ctrl Pts',(80.4024681817477,-7.38318933156897,135.677766619055));
#80757=CARTESIAN_POINT('Ctrl Pts',(80.4241607993943,-7.38874431226376,135.676334464093));
#80758=CARTESIAN_POINT('Ctrl Pts',(80.4611207594921,-7.39900697722901,135.673846632523));
#80759=CARTESIAN_POINT('Ctrl Pts',(80.4764448366359,-7.40350030204292,135.672800892618));
#80760=CARTESIAN_POINT('Ctrl Pts',(80.4986010621413,-7.4103443358034,135.671264929807));
#80761=CARTESIAN_POINT('Ctrl Pts',(80.5054867739309,-7.4125204673926,135.670784189941));
#80762=CARTESIAN_POINT('Ctrl Pts',(80.5175302329767,-7.41641293106894,135.669937033602));
#80763=CARTESIAN_POINT('Ctrl Pts',(80.5226940575881,-7.41810984329749,135.669571742901));
#80764=CARTESIAN_POINT('Ctrl Pts',(80.5339300780641,-7.4218631968693,135.668772313184));
#80765=CARTESIAN_POINT('Ctrl Pts',(80.539998641126,-7.42392939188108,135.668337639144));
#80766=CARTESIAN_POINT('Ctrl Pts',(80.5569211369628,-7.42980028934295,135.667117697882));
#80767=CARTESIAN_POINT('Ctrl Pts',(80.5677475731315,-7.433682356924,135.666328182428));
#80768=CARTESIAN_POINT('Ctrl Pts',(80.6411436826058,-7.46086112485284,135.660918140859));
#80769=CARTESIAN_POINT('Ctrl Pts',(80.7022977614075,-7.48778653667888,135.656126132143));
#80770=CARTESIAN_POINT('Ctrl Pts',(80.7807771079322,-7.52812876505948,135.649727624631));
#80771=CARTESIAN_POINT('Ctrl Pts',(80.7996977670178,-7.53832244032269,135.648164671113));
#80772=CARTESIAN_POINT('Ctrl Pts',(80.8801006239151,-7.58366874245671,135.641446320003));
#80773=CARTESIAN_POINT('Ctrl Pts',(80.9395080190151,-7.62235812846393,135.636290611703));
#80774=CARTESIAN_POINT('Ctrl Pts',(81.0324153518665,-7.69167750951371,135.628004396148));
#80775=CARTESIAN_POINT('Ctrl Pts',(81.067448260924,-7.7201000033821,135.624820979092));
#80776=CARTESIAN_POINT('Ctrl Pts',(81.1248650608886,-7.77068232619236,135.619507681416));
#80777=CARTESIAN_POINT('Ctrl Pts',(81.1478516576813,-7.79211749273543,135.617351926669));
#80778=CARTESIAN_POINT('Ctrl Pts',(81.1797385270572,-7.82358516594212,135.614317790017));
#80779=CARTESIAN_POINT('Ctrl Pts',(81.1891442511561,-7.83309348186384,135.61341707404));
#80780=CARTESIAN_POINT('Ctrl Pts',(81.2052988242849,-7.84982245432557,135.611859592708));
#80781=CARTESIAN_POINT('Ctrl Pts',(81.212099691251,-7.85699169377217,135.611200581259));
#80782=CARTESIAN_POINT('Ctrl Pts',(81.225987020049,-7.87189458022222,135.609847710728));
#80783=CARTESIAN_POINT('Ctrl Pts',(81.2330650526035,-7.87963550751747,135.609154228349));
#80784=CARTESIAN_POINT('Ctrl Pts',(81.2510679210011,-7.89970172342409,135.607379663128));
#80785=CARTESIAN_POINT('Ctrl Pts',(81.2618841183515,-7.91212328642472,135.606303130617));
#80786=CARTESIAN_POINT('Ctrl Pts',(81.3060213017579,-7.96435559340015,135.601863161036));
#80787=CARTESIAN_POINT('Ctrl Pts',(81.3376584174224,-8.00555455425008,135.598567361822));
#80788=CARTESIAN_POINT('Ctrl Pts',(81.4290417440531,-8.13682809789294,135.588570167249));
#80789=CARTESIAN_POINT('Ctrl Pts',(81.4819902394504,-8.23127956995287,135.582076927784));
#80790=CARTESIAN_POINT('Ctrl Pts',(81.5509065263991,-8.38822986804488,135.571521770207));
#80791=CARTESIAN_POINT('Ctrl Pts',(81.573054799165,-8.44766804635366,135.567567768311));
#80792=CARTESIAN_POINT('Ctrl Pts',(81.5961730984153,-8.52249523526723,135.5624786694));
#80793=CARTESIAN_POINT('Ctrl Pts',(81.6003922334336,-8.53683262034233,135.561498590011));
#80794=CARTESIAN_POINT('Ctrl Pts',(81.6063123207462,-8.55799751651901,135.560041845528));
#80795=CARTESIAN_POINT('Ctrl Pts',(81.6081639473392,-8.56478260467207,135.559573346392));
#80796=CARTESIAN_POINT('Ctrl Pts',(81.6112447696592,-8.57636009491999,135.558771079305));
#80797=CARTESIAN_POINT('Ctrl Pts',(81.6124956694893,-8.58114657470802,135.558438559297));
#80798=CARTESIAN_POINT('Ctrl Pts',(81.6153018703657,-8.59208320856258,135.557676796998));
#80799=CARTESIAN_POINT('Ctrl Pts',(81.6168433421262,-8.59823658105232,135.557246798334));
#80800=CARTESIAN_POINT('Ctrl Pts',(81.6210095297212,-8.61527986235172,135.556052223295));
#80801=CARTESIAN_POINT('Ctrl Pts',(81.6235595546928,-8.62618743317122,135.555283665678));
#80802=CARTESIAN_POINT('Ctrl Pts',(81.6380311793001,-8.69103206495627,135.550694045268));
#80803=CARTESIAN_POINT('Ctrl Pts',(81.6473730459765,-8.74550424502651,135.546755266948));
#80804=CARTESIAN_POINT('Ctrl Pts',(81.6657735937353,-8.89793009896356,135.535670640689));
#80805=CARTESIAN_POINT('Ctrl Pts',(81.6688943965567,-8.99638484146893,135.528451610779));
#80806=CARTESIAN_POINT('Ctrl Pts',(81.6591558999855,-9.16772160325569,135.516146491686));
#80807=CARTESIAN_POINT('Ctrl Pts',(81.6501708767704,-9.24055684332047,135.510994424597));
#80808=CARTESIAN_POINT('Ctrl Pts',(81.6331039422934,-9.32990751788484,135.504786234551));
#80809=CARTESIAN_POINT('Ctrl Pts',(81.6295174824161,-9.34718910235691,135.503590480379));
#80810=CARTESIAN_POINT('Ctrl Pts',(81.6233075931183,-9.37489174863058,135.501681038262));
#80811=CARTESIAN_POINT('Ctrl Pts',(81.6208568648414,-9.38534970884734,135.50096190772));
#80812=CARTESIAN_POINT('Ctrl Pts',(81.6159788225714,-9.40529536531078,135.499593359175));
#80813=CARTESIAN_POINT('Ctrl Pts',(81.6135686677059,-9.41478675210875,135.498943422501));
#80814=CARTESIAN_POINT('Ctrl Pts',(81.6078770675369,-9.43640007808269,135.497466114757));
#80815=CARTESIAN_POINT('Ctrl Pts',(81.6045419437463,-9.44850736624858,135.496640510046));
#80816=CARTESIAN_POINT('Ctrl Pts',(81.5952758385749,-9.48071851561596,135.494448385969));
#80817=CARTESIAN_POINT('Ctrl Pts',(81.5891017239668,-9.50075050282238,135.493089718617));
#80818=CARTESIAN_POINT('Ctrl Pts',(81.5445459236425,-9.63617791969349,135.483923553231));
#80819=CARTESIAN_POINT('Ctrl Pts',(81.4940074647466,-9.74718806594842,135.476540457815));
#80820=CARTESIAN_POINT('Ctrl Pts',(81.3837790771595,-9.93249414058302,135.463364246062));
#80821=CARTESIAN_POINT('Ctrl Pts',(81.3289859381131,-10.0090496467401,135.457602280899));
#80822=CARTESIAN_POINT('Ctrl Pts',(81.2601244677779,-10.0898584100671,135.450664997258));
#80823=CARTESIAN_POINT('Ctrl Pts',(81.2521049461546,-10.0990624234618,135.449861081478));
#80824=CARTESIAN_POINT('Ctrl Pts',(81.2396678243958,-10.1130237261968,135.448618845724));
#80825=CARTESIAN_POINT('Ctrl Pts',(81.2353221572715,-10.1178449329456,135.44818561919));
#80826=CARTESIAN_POINT('Ctrl Pts',(81.227257594154,-10.1266875338113,135.447382885672));
#80827=CARTESIAN_POINT('Ctrl Pts',(81.2235469049681,-10.1307161312871,135.447013981236));
#80828=CARTESIAN_POINT('Ctrl Pts',(81.2150363999968,-10.1398648162468,135.446168953998));
#80829=CARTESIAN_POINT('Ctrl Pts',(81.2102240540331,-10.1449729198564,135.445691906759));
#80830=CARTESIAN_POINT('Ctrl Pts',(81.1952123087992,-10.1607068855986,135.444206627641));
#80831=CARTESIAN_POINT('Ctrl Pts',(81.1849044847329,-10.1712276731728,135.443190763733));
#80832=CARTESIAN_POINT('Ctrl Pts',(81.0988458232378,-10.256765517001,135.434752255089));
#80833=CARTESIAN_POINT('Ctrl Pts',(81.0161997778977,-10.3244833604926,135.426934312391));
#80834=CARTESIAN_POINT('Ctrl Pts',(80.8353061284195,-10.4457460442801,135.411104789846));
#80835=CARTESIAN_POINT('Ctrl Pts',(80.7369720946791,-10.4982651805633,135.403144920433));
#80836=CARTESIAN_POINT('Ctrl Pts',(80.6161605284524,-10.547992071442,135.394204925114));
#80837=CARTESIAN_POINT('Ctrl Pts',(80.598071040794,-10.5550705243262,135.392886284624));
#80838=CARTESIAN_POINT('Ctrl Pts',(80.5694364803041,-10.5657016797744,135.390829320125));
#80839=CARTESIAN_POINT('Ctrl Pts',(80.5589730388702,-10.5694676827981,135.390083958867));
#80840=CARTESIAN_POINT('Ctrl Pts',(80.5392916467636,-10.5763296142076,135.388693412042));
#80841=CARTESIAN_POINT('Ctrl Pts',(80.5300828352837,-10.5794501345361,135.388047437203));
#80842=CARTESIAN_POINT('Ctrl Pts',(80.5093328547878,-10.586279603908,135.386602033777));
#80843=CARTESIAN_POINT('Ctrl Pts',(80.4977773822075,-10.5899435931722,135.385804108222));
#80844=CARTESIAN_POINT('Ctrl Pts',(80.463642447802,-10.600358409488,135.383466769636));
#80845=CARTESIAN_POINT('Ctrl Pts',(80.4409579774769,-10.6067568296459,135.381938778431));
#80846=CARTESIAN_POINT('Ctrl Pts',(80.3161426684702,-10.6391197809079,135.373654915505));
#80847=CARTESIAN_POINT('Ctrl Pts',(80.2118579831632,-10.6558319590356,135.367201924982));
#80848=CARTESIAN_POINT('Ctrl Pts',(80.0295678783465,-10.667529009758,135.35604724617));
#80849=CARTESIAN_POINT('Ctrl Pts',(79.9522071013403,-10.667105701846,135.351345090981));
#80850=CARTESIAN_POINT('Ctrl Pts',(79.8507915989673,-10.6594848858688,135.344929142454));
#80851=CARTESIAN_POINT('Ctrl Pts',(79.8264664511588,-10.6571177433717,135.343370694582));
#80852=CARTESIAN_POINT('Ctrl Pts',(79.7852781773838,-10.6521928158553,135.340685425391));
#80853=CARTESIAN_POINT('Ctrl Pts',(79.768385721024,-10.649909492222,135.339570767969));
#80854=CARTESIAN_POINT('Ctrl Pts',(79.7442039282953,-10.6462622188573,135.337952074943));
#80855=CARTESIAN_POINT('Ctrl Pts',(79.7368834012025,-10.6451080735904,135.337459006005));
#80856=CARTESIAN_POINT('Ctrl Pts',(79.7241383466785,-10.6430114608672,135.336594876149));
#80857=CARTESIAN_POINT('Ctrl Pts',(79.7187104050076,-10.6420908851305,135.336225039383));
#80858=CARTESIAN_POINT('Ctrl Pts',(79.7070674607948,-10.6400568253947,135.335427718297));
#80859=CARTESIAN_POINT('Ctrl Pts',(79.7008542976147,-10.6389349311296,135.334999799894));
#80860=CARTESIAN_POINT('Ctrl Pts',(79.6837660876834,-10.6357489539311,135.333816455222));
#80861=CARTESIAN_POINT('Ctrl Pts',(79.6729052346935,-10.6336118038436,135.333057163494));
#80862=CARTESIAN_POINT('Ctrl Pts',(79.6106132183702,-10.6207081829048,135.328663973521));
#80863=CARTESIAN_POINT('Ctrl Pts',(79.5596977218537,-10.6076224190586,135.324923422212));
#80864=CARTESIAN_POINT('Ctrl Pts',(79.4119688331959,-10.5621103152775,135.313777811983));
#80865=CARTESIAN_POINT('Ctrl Pts',(79.3174060645967,-10.5231666383592,135.30627757059));
#80866=CARTESIAN_POINT('Ctrl Pts',(79.1627104076536,-10.4421405968979,135.29376097206));
#80867=CARTESIAN_POINT('Ctrl Pts',(79.1006810571642,-10.4042974786623,135.288661548636));
#80868=CARTESIAN_POINT('Ctrl Pts',(79.0269119784182,-10.3523925634111,135.282506069526));
#80869=CARTESIAN_POINT('Ctrl Pts',(79.0126747455877,-10.3420338395948,135.281313284718));
#80870=CARTESIAN_POINT('Ctrl Pts',(78.9900273057665,-10.3250004996883,135.279407413584));
#80871=CARTESIAN_POINT('Ctrl Pts',(78.9815130725154,-10.3184671232668,135.278688921181));
#80872=CARTESIAN_POINT('Ctrl Pts',(78.9653497333927,-10.3058142146827,135.277320854322));
#80873=CARTESIAN_POINT('Ctrl Pts',(78.9576903362711,-10.2997086247869,135.276670768132));
#80874=CARTESIAN_POINT('Ctrl Pts',(78.9403207371306,-10.2856103662315,135.275192121867));
#80875=CARTESIAN_POINT('Ctrl Pts',(78.9306462211732,-10.2775745238718,135.274365339721));
#80876=CARTESIAN_POINT('Ctrl Pts',(78.9050436637096,-10.2558139364783,135.272167857993));
#80877=CARTESIAN_POINT('Ctrl Pts',(78.889282561388,-10.2418956704791,135.270805072906));
#80878=CARTESIAN_POINT('Ctrl Pts',(78.7850070921004,-10.14623881434,135.261708140156));
#80879=CARTESIAN_POINT('Ctrl Pts',(78.7053199332686,-10.0554044504728,135.254389242633));
#80880=CARTESIAN_POINT('Ctrl Pts',(78.5979474577496,-9.90234316385511,135.242965047997));
#80881=CARTESIAN_POINT('Ctrl Pts',(78.5630672644076,-9.84569353518899,135.238892805906));
#80882=CARTESIAN_POINT('Ctrl Pts',(78.5210386775775,-9.76729096251886,135.233262995623));
#80883=CARTESIAN_POINT('Ctrl Pts',(78.5108139771359,-9.74725290405196,135.231824451065));
#80884=CARTESIAN_POINT('Ctrl Pts',(78.4940058356331,-9.71259691109633,135.229326584376));
#80885=CARTESIAN_POINT('Ctrl Pts',(78.4872217572517,-9.69807930979763,135.228277306131));
#80886=CARTESIAN_POINT('Ctrl Pts',(78.4776817946995,-9.67687190456469,135.226737085544));
#80887=CARTESIAN_POINT('Ctrl Pts',(78.4747581868851,-9.67025793547792,135.226255699886));
#80888=CARTESIAN_POINT('Ctrl Pts',(78.4697121609575,-9.65863851063518,135.225407831745));
#80889=CARTESIAN_POINT('Ctrl Pts',(78.4675710450408,-9.65364138088882,135.225042481567));
#80890=CARTESIAN_POINT('Ctrl Pts',(78.4629609835975,-9.64273484113436,135.224243442312));
#80891=CARTESIAN_POINT('Ctrl Pts',(78.4605016793919,-9.63682174220386,135.223809222955));
#80892=CARTESIAN_POINT('Ctrl Pts',(78.4537321835503,-9.62027691535868,135.222591756587));
#80893=CARTESIAN_POINT('Ctrl Pts',(78.4494977238917,-9.60961486653051,135.22180428773));
#80894=CARTESIAN_POINT('Ctrl Pts',(78.4217951171761,-9.5377056080225,135.216477923464));
#80895=CARTESIAN_POINT('Ctrl Pts',(78.4018538674087,-9.47516838486711,135.211773439132));
#80896=CARTESIAN_POINT('Ctrl Pts',(78.3800892955835,-9.38981046480314,135.205388297193));
#80897=CARTESIAN_POINT('Ctrl Pts',(78.3749694674895,-9.36788399828525,135.203750981773));
#80898=CARTESIAN_POINT('Ctrl Pts',(78.3556833956392,-9.27700755545551,135.19698965436));
#80899=CARTESIAN_POINT('Ctrl Pts',(78.3454484878604,-9.20729362310927,135.191865040038));
#80900=CARTESIAN_POINT('Ctrl Pts',(78.3359116043374,-9.09182965559912,135.183580428998));
#80901=CARTESIAN_POINT('Ctrl Pts',(78.3340252030434,-9.04638382201416,135.180369756322));
#80902=CARTESIAN_POINT('Ctrl Pts',(78.3339832799272,-8.96998909899421,135.175064092908));
#80903=CARTESIAN_POINT('Ctrl Pts',(78.3348273798544,-8.93906781637886,135.172941563736));
#80904=CARTESIAN_POINT('Ctrl Pts',(78.3372103811871,-8.89589301781814,135.170011160881));
#80905=CARTESIAN_POINT('Ctrl Pts',(78.3380251523454,-8.88360756007382,135.169181059222));
#80906=CARTESIAN_POINT('Ctrl Pts',(78.3396793289291,-8.86225317288682,135.167744421283));
#80907=CARTESIAN_POINT('Ctrl Pts',(78.3404570346014,-8.85318014152402,135.167135983822));
#80908=CARTESIAN_POINT('Ctrl Pts',(78.3422420209813,-8.8341871814754,135.165866241765));
#80909=CARTESIAN_POINT('Ctrl Pts',(78.3432640458672,-8.82426897422111,135.165205425325));
#80910=CARTESIAN_POINT('Ctrl Pts',(78.3459230567602,-8.80055461789486,135.163630478538));
#80911=CARTESIAN_POINT('Ctrl Pts',(78.3476437063625,-8.78676845266505,135.162719006752));
#80912=CARTESIAN_POINT('Ctrl Pts',(78.3542717192831,-8.73857666057836,135.159545682791));
#80913=CARTESIAN_POINT('Ctrl Pts',(78.3600831270989,-8.70430309960197,135.157312114117));
#80914=CARTESIAN_POINT('Ctrl Pts',(78.3772529875,-8.61927597781728,135.151806430982));
#80915=CARTESIAN_POINT('Ctrl Pts',(78.3899232382344,-8.56882477145895,135.148572223972));
#80916=CARTESIAN_POINT('Ctrl Pts',(78.4145339022593,-8.48720443493499,135.143322354091));
#80917=CARTESIAN_POINT('Ctrl Pts',(78.4250815971791,-8.45567289096299,135.141289461639));
#80918=CARTESIAN_POINT('Ctrl Pts',(78.4365593350865,-8.42449214836376,135.139259965645));
#80919=CARTESIAN_POINT('Ctrl Pts',(78.4365593749993,-8.42449203993567,135.330578627164));
#80920=CARTESIAN_POINT('Ctrl Pts',(78.4355262731809,-8.42729859251999,135.330779522923));
#80921=CARTESIAN_POINT('Ctrl Pts',(78.4345007399363,-8.43010789542315,135.330980874855));
#80922=CARTESIAN_POINT('Ctrl Pts',(78.4313071291383,-8.4389300126237,135.331613988554));
#80923=CARTESIAN_POINT('Ctrl Pts',(78.4291661459327,-8.44495238644834,135.332047339247));
#80924=CARTESIAN_POINT('Ctrl Pts',(78.4232962774157,-8.46176974445812,135.333260392863));
#80925=CARTESIAN_POINT('Ctrl Pts',(78.4196437473155,-8.47259073441824,135.33404427212));
#80926=CARTESIAN_POINT('Ctrl Pts',(78.3963375081978,-8.54405437768576,135.339239248275));
#80927=CARTESIAN_POINT('Ctrl Pts',(78.380069099068,-8.60573882491424,135.343806912988));
#80928=CARTESIAN_POINT('Ctrl Pts',(78.3452668310428,-8.77698147651284,135.356465494113));
#80929=CARTESIAN_POINT('Ctrl Pts',(78.3340839882609,-8.88771739067351,135.364607438158));
#80930=CARTESIAN_POINT('Ctrl Pts',(78.333960105889,-9.05240943781643,135.376277053692));
#80931=CARTESIAN_POINT('Ctrl Pts',(78.3365124688393,-9.10604720710605,135.380013448242));
#80932=CARTESIAN_POINT('Ctrl Pts',(78.3432447666648,-9.17605568673706,135.38480577823));
#80933=CARTESIAN_POINT('Ctrl Pts',(78.3450880338692,-9.19261341434206,135.385933121138));
#80934=CARTESIAN_POINT('Ctrl Pts',(78.3485009066,-9.21958497765593,135.387760146348));
#80935=CARTESIAN_POINT('Ctrl Pts',(78.3499213966887,-9.23001615073439,135.38846445472));
#80936=CARTESIAN_POINT('Ctrl Pts',(78.3528637800764,-9.25019094399288,135.389822463916));
#80937=CARTESIAN_POINT('Ctrl Pts',(78.3543734966964,-9.25993586552764,135.390476517913));
#80938=CARTESIAN_POINT('Ctrl Pts',(78.3581156895823,-9.2827502210897,135.392003607387));
#80939=CARTESIAN_POINT('Ctrl Pts',(78.3604178536093,-9.29580767130029,135.392874406126));
#80940=CARTESIAN_POINT('Ctrl Pts',(78.3685721444306,-9.33903308249695,135.395747686064));
#80941=CARTESIAN_POINT('Ctrl Pts',(78.3751032126185,-9.36906760960462,135.397728732291));
#80942=CARTESIAN_POINT('Ctrl Pts',(78.3929306864518,-9.44135689561609,135.402474141945));
#80943=CARTESIAN_POINT('Ctrl Pts',(78.4050672096251,-9.48338131303913,135.405213412114));
#80944=CARTESIAN_POINT('Ctrl Pts',(78.4417659737733,-9.59393279114656,135.412431973884));
#80945=CARTESIAN_POINT('Ctrl Pts',(78.469187338651,-9.66140939121931,135.416848648503));
#80946=CARTESIAN_POINT('Ctrl Pts',(78.5082912027581,-9.74205483343944,135.422331578807));
#80947=CARTESIAN_POINT('Ctrl Pts',(78.515880497758,-9.75711941162343,135.423365183253));
#80948=CARTESIAN_POINT('Ctrl Pts',(78.5569116448512,-9.83557695259039,135.428809900326));
#80949=CARTESIAN_POINT('Ctrl Pts',(78.5941858934046,-9.8968706349051,135.433275373302));
#80950=CARTESIAN_POINT('Ctrl Pts',(78.6419287095258,-9.96505573471517,135.438720124378));
#80951=CARTESIAN_POINT('Ctrl Pts',(78.6486718028772,-9.97447539032831,135.439483560455));
#80952=CARTESIAN_POINT('Ctrl Pts',(78.6593083965521,-9.98901129735335,135.440680591179));
#80953=CARTESIAN_POINT('Ctrl Pts',(78.663134361529,-9.99417683691514,135.441109752094));
#80954=CARTESIAN_POINT('Ctrl Pts',(78.6702479461729,-10.0036657685702,135.441905374871));
#80955=CARTESIAN_POINT('Ctrl Pts',(78.6735269311231,-10.007995383969,135.442271249124));
#80956=CARTESIAN_POINT('Ctrl Pts',(78.681196117597,-10.0180196570363,135.443124945014));
#80957=CARTESIAN_POINT('Ctrl Pts',(78.6856020548501,-10.0237019777944,135.443613838057));
#80958=CARTESIAN_POINT('Ctrl Pts',(78.6998089743626,-10.0417816718146,135.445184867954));
#80959=CARTESIAN_POINT('Ctrl Pts',(78.7097492965875,-10.0540677548791,135.446275989853));
#80960=CARTESIAN_POINT('Ctrl Pts',(78.765725932875,-10.1212757113765,135.452367858337));
#80961=CARTESIAN_POINT('Ctrl Pts',(78.8150903471115,-10.1733195593721,135.457545086692));
#80962=CARTESIAN_POINT('Ctrl Pts',(78.9644272114544,-10.3116989777376,135.472346540187));
#80963=CARTESIAN_POINT('Ctrl Pts',(79.071539327848,-10.3895819502659,135.48195518204));
#80964=CARTESIAN_POINT('Ctrl Pts',(79.2105803728829,-10.4673510817889,135.492967535828));
#80965=CARTESIAN_POINT('Ctrl Pts',(79.2347523357253,-10.4801009121257,135.49483611561));
#80966=CARTESIAN_POINT('Ctrl Pts',(79.2704566879891,-10.4978249903886,135.497531647256));
#80967=CARTESIAN_POINT('Ctrl Pts',(79.2817479146326,-10.5032721319534,135.498374910287));
#80968=CARTESIAN_POINT('Ctrl Pts',(79.3019621659085,-10.5127441847858,135.499868658346));
#80969=CARTESIAN_POINT('Ctrl Pts',(79.3108610900638,-10.5168188277655,135.500520834889));
#80970=CARTESIAN_POINT('Ctrl Pts',(79.3296060676239,-10.5252027651225,135.501883523649));
#80971=CARTESIAN_POINT('Ctrl Pts',(79.3394589820578,-10.5294956920664,135.502593452478));
#80972=CARTESIAN_POINT('Ctrl Pts',(79.3656344908504,-10.5406002723171,135.504463244113));
#80973=CARTESIAN_POINT('Ctrl Pts',(79.3820254762902,-10.5472479844239,135.505617550118));
#80974=CARTESIAN_POINT('Ctrl Pts',(79.4675328256897,-10.5803516593296,135.511559140819));
#80975=CARTESIAN_POINT('Ctrl Pts',(79.5382541497404,-10.6024435799612,135.516199475138));
#80976=CARTESIAN_POINT('Ctrl Pts',(79.6749347772821,-10.6353346536221,135.524873631087));
#80977=CARTESIAN_POINT('Ctrl Pts',(79.740527048473,-10.6470157161123,135.528914623565));
#80978=CARTESIAN_POINT('Ctrl Pts',(79.8206909608897,-10.6563829005471,135.533855450762));
#80979=CARTESIAN_POINT('Ctrl Pts',(79.8347593096595,-10.6578454547886,135.534722736919));
#80980=CARTESIAN_POINT('Ctrl Pts',(79.9199176347961,-10.6656038366701,135.539981924922));
#80981=CARTESIAN_POINT('Ctrl Pts',(79.9913248241879,-10.6675045693128,135.544429406272));
#80982=CARTESIAN_POINT('Ctrl Pts',(80.0741971314396,-10.6643872492668,135.549854100756));
#80983=CARTESIAN_POINT('Ctrl Pts',(80.0857651395046,-10.6638312571511,135.550617338171));
#80984=CARTESIAN_POINT('Ctrl Pts',(80.1037425554612,-10.6627792382724,135.551814122857));
#80985=CARTESIAN_POINT('Ctrl Pts',(80.1101567392705,-10.6623666269425,135.552243239286));
#80986=CARTESIAN_POINT('Ctrl Pts',(80.121986385737,-10.6615368856644,135.553038824661));
#80987=CARTESIAN_POINT('Ctrl Pts',(80.1274023929413,-10.6611303765512,135.553404706496));
#80988=CARTESIAN_POINT('Ctrl Pts',(80.1399848362193,-10.6601240804651,135.554258479652));
#80989=CARTESIAN_POINT('Ctrl Pts',(80.1471494414926,-10.6595043699788,135.55474744305));
#80990=CARTESIAN_POINT('Ctrl Pts',(80.1700509051904,-10.6573740136638,135.556318929629));
#80991=CARTESIAN_POINT('Ctrl Pts',(80.1857698246274,-10.6556857970013,135.557410444924));
#80992=CARTESIAN_POINT('Ctrl Pts',(80.2726555271094,-10.645101442159,135.563506691196));
#80993=CARTESIAN_POINT('Ctrl Pts',(80.343208373796,-10.6318412242077,135.568688160618));
#80994=CARTESIAN_POINT('Ctrl Pts',(80.5406842505535,-10.5813515668489,135.583506823124));
#80995=CARTESIAN_POINT('Ctrl Pts',(80.6643665785313,-10.533506233294,135.593127914921));
#80996=CARTESIAN_POINT('Ctrl Pts',(80.8027279036113,-10.4600626944706,135.603953904724));
#80997=CARTESIAN_POINT('Ctrl Pts',(80.8240938879187,-10.4481106769402,135.605629490446));
#80998=CARTESIAN_POINT('Ctrl Pts',(80.8557920351668,-10.4294500195427,135.608122229329));
#80999=CARTESIAN_POINT('Ctrl Pts',(80.8663251096201,-10.4230910667889,135.608951732539));
#81000=CARTESIAN_POINT('Ctrl Pts',(80.8845267145437,-10.4118255350073,135.610387517227));
#81001=CARTESIAN_POINT('Ctrl Pts',(80.8922271441489,-10.4069717761769,135.610995695854));
#81002=CARTESIAN_POINT('Ctrl Pts',(80.9082769064928,-10.3966704823726,135.612265067652));
#81003=CARTESIAN_POINT('Ctrl Pts',(80.9166179243367,-10.3912106107022,135.612925771662));
#81004=CARTESIAN_POINT('Ctrl Pts',(80.9364662765708,-10.3779622539267,135.614500758185));
#81005=CARTESIAN_POINT('Ctrl Pts',(80.9479262877194,-10.3701039496195,135.615412379409));
#81006=CARTESIAN_POINT('Ctrl Pts',(80.9877255006586,-10.3420745969456,135.618587853349));
#81007=CARTESIAN_POINT('Ctrl Pts',(81.0155312863061,-10.3211594779654,135.620823364375));
#81008=CARTESIAN_POINT('Ctrl Pts',(81.0832652078284,-10.2668079721503,135.626335306234));
#81009=CARTESIAN_POINT('Ctrl Pts',(81.122319498465,-10.2323414716649,135.629573705253));
#81010=CARTESIAN_POINT('Ctrl Pts',(81.2309895076531,-10.1269787610188,135.638894482858));
#81011=CARTESIAN_POINT('Ctrl Pts',(81.2959547269485,-10.0516254042706,135.644863331075));
#81012=CARTESIAN_POINT('Ctrl Pts',(81.382547020713,-9.93088625497374,135.654121892469));
#81013=CARTESIAN_POINT('Ctrl Pts',(81.409478425099,-9.88958139409313,135.657244839241));
#81014=CARTESIAN_POINT('Ctrl Pts',(81.4400707768826,-9.83777717851968,135.661186634006));
#81015=CARTESIAN_POINT('Ctrl Pts',(81.4455126450187,-9.8283523531352,135.661904756946));
#81016=CARTESIAN_POINT('Ctrl Pts',(81.4539437423657,-9.81341435590741,135.663045603797));
#81017=CARTESIAN_POINT('Ctrl Pts',(81.4569949572909,-9.80793626701459,135.663464532077));
#81018=CARTESIAN_POINT('Ctrl Pts',(81.4626707874389,-9.79760928253296,135.664255563397));
#81019=CARTESIAN_POINT('Ctrl Pts',(81.4653023458829,-9.79276442375454,135.664627224973));
#81020=CARTESIAN_POINT('Ctrl Pts',(81.4714485719595,-9.78131369534124,135.665506853635));
#81021=CARTESIAN_POINT('Ctrl Pts',(81.4749428358345,-9.77469711248493,135.666016058988));
#81022=CARTESIAN_POINT('Ctrl Pts',(81.4864475524603,-9.75255230236352,135.667722829231));
#81023=CARTESIAN_POINT('Ctrl Pts',(81.4942579700291,-9.73692221625749,135.668931602659));
#81024=CARTESIAN_POINT('Ctrl Pts',(81.5127597045187,-9.69839291856715,135.671916234599));
#81025=CARTESIAN_POINT('Ctrl Pts',(81.5231783781498,-9.67536810898402,135.673703974035));
#81026=CARTESIAN_POINT('Ctrl Pts',(81.5653168624551,-9.57630423285464,135.681388211939));
#81027=CARTESIAN_POINT('Ctrl Pts',(81.5918958839658,-9.49820694710658,135.687421128465));
#81028=CARTESIAN_POINT('Ctrl Pts',(81.6373188618132,-9.3231666259707,135.700553726765));
#81029=CARTESIAN_POINT('Ctrl Pts',(81.6535561297683,-9.22584859002855,135.707600033417));
#81030=CARTESIAN_POINT('Ctrl Pts',(81.6629242930125,-9.10394338421816,135.716018745893));
#81031=CARTESIAN_POINT('Ctrl Pts',(81.6642385471,-9.08019720024782,135.717640650187));
#81032=CARTESIAN_POINT('Ctrl Pts',(81.6654560444901,-9.0442732278568,135.720068345016));
#81033=CARTESIAN_POINT('Ctrl Pts',(81.6657349069284,-9.03211212056762,135.720885697022));
#81034=CARTESIAN_POINT('Ctrl Pts',(81.665996994287,-9.01022574073723,135.722348953673));
#81035=CARTESIAN_POINT('Ctrl Pts',(81.6660283028545,-9.00050171167892,135.722996327569));
#81036=CARTESIAN_POINT('Ctrl Pts',(81.6659131095358,-8.97969226939058,135.72437608127));
#81037=CARTESIAN_POINT('Ctrl Pts',(81.6657410988884,-8.9686074226696,135.725107634832));
#81038=CARTESIAN_POINT('Ctrl Pts',(81.6649671608321,-8.93826114098241,135.727101556844));
#81039=CARTESIAN_POINT('Ctrl Pts',(81.664141663783,-8.9190067518587,135.728356943319));
#81040=CARTESIAN_POINT('Ctrl Pts',(81.6615608590606,-8.87618676336635,135.731130043053));
#81041=CARTESIAN_POINT('Ctrl Pts',(81.6596378892046,-8.85263526330765,135.732642580561));
#81042=CARTESIAN_POINT('Ctrl Pts',(81.6518941871683,-8.7775307674222,135.73743506905));
#81043=CARTESIAN_POINT('Ctrl Pts',(81.644166459128,-8.72620404349717,135.740662579849));
#81044=CARTESIAN_POINT('Ctrl Pts',(81.6143429736189,-8.5761085532356,135.750087170798));
#81045=CARTESIAN_POINT('Ctrl Pts',(81.5856374198292,-8.4789056373043,135.756163698559));
#81046=CARTESIAN_POINT('Ctrl Pts',(81.5306223575826,-8.34042224827635,135.765459430542));
#81047=CARTESIAN_POINT('Ctrl Pts',(81.5110408417259,-8.29672035167029,135.768495872958));
#81048=CARTESIAN_POINT('Ctrl Pts',(81.484709148366,-8.24414658279281,135.772348989523));
#81049=CARTESIAN_POINT('Ctrl Pts',(81.4797147453269,-8.23441532126142,135.773070896926));
#81050=CARTESIAN_POINT('Ctrl Pts',(81.4717307334529,-8.21922901368865,135.77421232156));
#81051=CARTESIAN_POINT('Ctrl Pts',(81.4688056690406,-8.21374012674534,135.774627948916));
#81052=CARTESIAN_POINT('Ctrl Pts',(81.4632234080043,-8.20340486698522,135.775416622239));
#81053=CARTESIAN_POINT('Ctrl Pts',(81.4605727448325,-8.19855517904087,135.775789265932));
#81054=CARTESIAN_POINT('Ctrl Pts',(81.4542296989428,-8.18708583695093,135.776676565089));
#81055=CARTESIAN_POINT('Ctrl Pts',(81.4505162124318,-8.18047808713489,135.777192523295));
#81056=CARTESIAN_POINT('Ctrl Pts',(81.4378056838691,-8.15821810702523,135.778946253225));
#81057=CARTESIAN_POINT('Ctrl Pts',(81.4285997029371,-8.14268747666244,135.780196060627));
#81058=CARTESIAN_POINT('Ctrl Pts',(81.4053049045252,-8.10480612435782,135.783304139457));
#81059=CARTESIAN_POINT('Ctrl Pts',(81.3909335584144,-8.08263549696637,135.785175512523));
#81060=CARTESIAN_POINT('Ctrl Pts',(81.3252956707159,-7.98646626025524,135.793497616316));
#81061=CARTESIAN_POINT('Ctrl Pts',(81.26860812812,-7.91635236270762,135.800103414872));
#81062=CARTESIAN_POINT('Ctrl Pts',(81.1391697945811,-7.78041330523172,135.813702478902));
#81063=CARTESIAN_POINT('Ctrl Pts',(81.0657024735681,-7.71571665043239,135.820650802584));
#81064=CARTESIAN_POINT('Ctrl Pts',(80.9717693841213,-7.64664250173487,135.828623028917));
#81065=CARTESIAN_POINT('Ctrl Pts',(80.9563739679159,-7.63571955288704,135.829903684356));
#81066=CARTESIAN_POINT('Ctrl Pts',(80.9317161631004,-7.61884757330649,135.831914990394));
#81067=CARTESIAN_POINT('Ctrl Pts',(80.9225751423151,-7.61272491870699,135.832652169005));
#81068=CARTESIAN_POINT('Ctrl Pts',(80.9060466132159,-7.60188974071801,135.83397030598));
#81069=CARTESIAN_POINT('Ctrl Pts',(80.8986813826161,-7.59714414853699,135.834552484362));
#81070=CARTESIAN_POINT('Ctrl Pts',(80.8812946553441,-7.5861345938802,135.835914874432));
#81071=CARTESIAN_POINT('Ctrl Pts',(80.8712431798858,-7.57991866792703,135.836693293865));
#81072=CARTESIAN_POINT('Ctrl Pts',(80.8415942605421,-7.56201680171253,135.838963380257));
#81073=CARTESIAN_POINT('Ctrl Pts',(80.8218214048979,-7.55062557014839,135.84044437985));
#81074=CARTESIAN_POINT('Ctrl Pts',(80.7294265454685,-7.49989545581792,135.84722515247));
#81075=CARTESIAN_POINT('Ctrl Pts',(80.654173556158,-7.46558284756121,135.852348990203));
#81076=CARTESIAN_POINT('Ctrl Pts',(80.5228555594444,-7.41713257439729,135.860930630532));
#81077=CARTESIAN_POINT('Ctrl Pts',(80.4680435725637,-7.40006801321869,135.864415508163));
#81078=CARTESIAN_POINT('Ctrl Pts',(80.3378013276486,-7.36678712508914,135.87266519345));
#81079=CARTESIAN_POINT('Ctrl Pts',(80.261917391431,-7.3529146397612,135.877448117471));
#81080=CARTESIAN_POINT('Ctrl Pts',(80.1738222333491,-7.34305203519499,135.883246277199));
#81081=CARTESIAN_POINT('Ctrl Pts',(80.1622743212221,-7.34188126087881,135.88401117691));
#81082=CARTESIAN_POINT('Ctrl Pts',(80.1443086467896,-7.34024929546995,135.885210020238));
#81083=CARTESIAN_POINT('Ctrl Pts',(80.1378985913507,-7.33970443542221,135.885639508796));
#81084=CARTESIAN_POINT('Ctrl Pts',(80.1260719757006,-7.33876812311061,135.886435407561));
#81085=CARTESIAN_POINT('Ctrl Pts',(80.1206564601087,-7.33836601280564,135.886801226508));
#81086=CARTESIAN_POINT('Ctrl Pts',(80.1080733090859,-7.33749353220929,135.88765435572));
#81087=CARTESIAN_POINT('Ctrl Pts',(80.10090453398,-7.33704303548779,135.888142732459));
#81088=CARTESIAN_POINT('Ctrl Pts',(80.0779955381416,-7.33575207444401,135.889710413694));
#81089=CARTESIAN_POINT('Ctrl Pts',(80.0622467464349,-7.33508866325179,135.890798651506));
#81090=CARTESIAN_POINT('Ctrl Pts',(79.9752685816344,-7.33266049192449,135.896858503602));
#81091=CARTESIAN_POINT('Ctrl Pts',(79.903998064701,-7.33524346902666,135.902004727388));
#81092=CARTESIAN_POINT('Ctrl Pts',(79.7031389500549,-7.35546489389957,135.916680042758));
#81093=CARTESIAN_POINT('Ctrl Pts',(79.5751233401283,-7.38379657932082,135.926197246953));
#81094=CARTESIAN_POINT('Ctrl Pts',(79.4247905605017,-7.43618944298602,135.937216846116));
#81095=CARTESIAN_POINT('Ctrl Pts',(79.3981039063056,-7.4462655878706,135.939169120612));
#81096=CARTESIAN_POINT('Ctrl Pts',(79.3598841193415,-7.46182898078638,135.941961042852));
#81097=CARTESIAN_POINT('Ctrl Pts',(79.3481358788281,-7.46677085593219,135.942818695584));
#81098=CARTESIAN_POINT('Ctrl Pts',(79.3274407337455,-7.47575710545454,135.944328877299));
#81099=CARTESIAN_POINT('Ctrl Pts',(79.318470826052,-7.47974661311075,135.944983228999));
#81100=CARTESIAN_POINT('Ctrl Pts',(79.2998474467593,-7.48822761314794,135.946341605517));
#81101=CARTESIAN_POINT('Ctrl Pts',(79.29020068965,-7.49273283875478,135.947045123891));
#81102=CARTESIAN_POINT('Ctrl Pts',(79.2650683210252,-7.50476494852482,135.948878148297));
#81103=CARTESIAN_POINT('Ctrl Pts',(79.2496547838107,-7.51244007699564,135.950002494021));
#81104=CARTESIAN_POINT('Ctrl Pts',(79.1751894718625,-7.55097185824301,135.955439589461));
#81105=CARTESIAN_POINT('Ctrl Pts',(79.1179023373438,-7.58511476559386,135.959635254769));
#81106=CARTESIAN_POINT('Ctrl Pts',(79.003133893035,-7.66320395638896,135.968233678969));
#81107=CARTESIAN_POINT('Ctrl Pts',(78.9461595717073,-7.70764309423015,135.972615160241));
#81108=CARTESIAN_POINT('Ctrl Pts',(78.8767632322408,-7.7694209105575,135.978299452942));
#81109=CARTESIAN_POINT('Ctrl Pts',(78.861538488781,-7.78349225383452,135.979570351591));
#81110=CARTESIAN_POINT('Ctrl Pts',(78.7978289407144,-7.84461894982535,135.985009900097));
#81111=CARTESIAN_POINT('Ctrl Pts',(78.7519736357233,-7.89431081429408,135.989231822588));
#81112=CARTESIAN_POINT('Ctrl Pts',(78.7019843304581,-7.95556523047784,135.994404286884));
#81113=CARTESIAN_POINT('Ctrl Pts',(78.6947948037225,-7.96456383893094,135.995163433037));
#81114=CARTESIAN_POINT('Ctrl Pts',(78.6837483313387,-7.97868776737917,135.996355150152));
#81115=CARTESIAN_POINT('Ctrl Pts',(78.679826545077,-7.98376224374992,135.996783349626));
#81116=CARTESIAN_POINT('Ctrl Pts',(78.6726364699279,-7.99317748214126,135.997578167998));
#81117=CARTESIAN_POINT('Ctrl Pts',(78.6693599973233,-7.99751174392324,135.997944210028));
#81118=CARTESIAN_POINT('Ctrl Pts',(78.6617836346137,-8.00763666952269,135.998799593189));
#81119=CARTESIAN_POINT('Ctrl Pts',(78.6575001050023,-8.01343928349378,135.999290020375));
#81120=CARTESIAN_POINT('Ctrl Pts',(78.6438794019379,-8.03214331960909,136.00087102896));
#81121=CARTESIAN_POINT('Ctrl Pts',(78.6346898176738,-8.04515043595365,136.001970750449));
#81122=CARTESIAN_POINT('Ctrl Pts',(78.6130766642929,-8.07669209918186,136.004634366466));
#81123=CARTESIAN_POINT('Ctrl Pts',(78.6008364311504,-8.09534811887406,136.006207249543));
#81124=CARTESIAN_POINT('Ctrl Pts',(78.5275463265607,-8.21210045116397,136.016009681774));
#81125=CARTESIAN_POINT('Ctrl Pts',(78.4764681494425,-8.31607477521382,136.024536811395));
#81126=CARTESIAN_POINT('Ctrl Pts',(78.4365593762033,-8.4244920366647,136.032852185112));
#81127=CARTESIAN_POINT('Origin',(80.,-9.,134.));
#81128=CARTESIAN_POINT('',(78.4365593881204,-8.4244920042904,136.733447186333));
#81129=CARTESIAN_POINT('',(78.4365593622862,-8.42449207447235,136.539851301691));
#81130=CARTESIAN_POINT('',(78.4365593749993,-8.42449203993574,134.));
#81131=CARTESIAN_POINT('',(78.3340002443612,-9.00090233676016,135.879690672883));
#81132=CARTESIAN_POINT('Ctrl Pts',(78.4365593622862,-8.42449207447235,136.539851301691));
#81133=CARTESIAN_POINT('Ctrl Pts',(78.4458979984507,-8.39912247896779,136.537889787967));
#81134=CARTESIAN_POINT('Ctrl Pts',(78.455854587738,-8.37397895835581,136.535921247526));
#81135=CARTESIAN_POINT('Ctrl Pts',(78.5134129738292,-8.23836951363643,136.52519748894));
#81136=CARTESIAN_POINT('Ctrl Pts',(78.5722644369613,-8.13304953404382,136.516515178362));
#81137=CARTESIAN_POINT('Ctrl Pts',(78.6541410729474,-8.01782782744679,136.506791211876));
#81138=CARTESIAN_POINT('Ctrl Pts',(78.6666490233352,-8.00091358175776,136.505356289194));
#81139=CARTESIAN_POINT('Ctrl Pts',(78.6871436587462,-7.97426979666754,136.503082992003));
#81140=CARTESIAN_POINT('Ctrl Pts',(78.6949257154184,-7.96438648638276,136.502236777347));
#81141=CARTESIAN_POINT('Ctrl Pts',(78.7089655621025,-7.94696532582124,136.500739525924));
#81142=CARTESIAN_POINT('Ctrl Pts',(78.7151792254797,-7.93939284875827,136.500086772006));
#81143=CARTESIAN_POINT('Ctrl Pts',(78.7283389164118,-7.92364075401344,136.498724587753));
#81144=CARTESIAN_POINT('Ctrl Pts',(78.7352979317373,-7.91547253351798,136.498015726198));
#81145=CARTESIAN_POINT('Ctrl Pts',(78.7538775336075,-7.89408656833953,136.496152650241));
#81146=CARTESIAN_POINT('Ctrl Pts',(78.7656296767321,-7.88098451170213,136.495003916887));
#81147=CARTESIAN_POINT('Ctrl Pts',(78.826827592354,-7.81489461363774,136.48916643996));
#81148=CARTESIAN_POINT('Ctrl Pts',(78.8794882176982,-7.76498440405701,136.484618135389));
#81149=CARTESIAN_POINT('Ctrl Pts',(79.0133917116924,-7.65371407264057,136.473867730857));
#81150=CARTESIAN_POINT('Ctrl Pts',(79.0973195120229,-7.59605972736649,136.467764440725));
#81151=CARTESIAN_POINT('Ctrl Pts',(79.2322430241922,-7.52050092347646,136.458155543224));
#81152=CARTESIAN_POINT('Ctrl Pts',(79.2797187045284,-7.49681606523634,136.454805666835));
#81153=CARTESIAN_POINT('Ctrl Pts',(79.3384037686755,-7.47095786415576,136.450606239352));
#81154=CARTESIAN_POINT('Ctrl Pts',(79.3486145561412,-7.46658015740575,136.449873470062));
#81155=CARTESIAN_POINT('Ctrl Pts',(79.3647039354683,-7.45987179462465,136.448714381012));
#81156=CARTESIAN_POINT('Ctrl Pts',(79.3705535350147,-7.45747184044791,136.448292057849));
#81157=CARTESIAN_POINT('Ctrl Pts',(79.3810077314937,-7.45325209391485,136.447535425562));
#81158=CARTESIAN_POINT('Ctrl Pts',(79.3856069792557,-7.45141944765787,136.447201891594));
#81159=CARTESIAN_POINT('Ctrl Pts',(79.3967884356634,-7.44702166345237,136.446389466975));
#81160=CARTESIAN_POINT('Ctrl Pts',(79.40337881163,-7.4444778824587,136.44590933898));
#81161=CARTESIAN_POINT('Ctrl Pts',(79.4241169634453,-7.43662445944628,136.444394929788));
#81162=CARTESIAN_POINT('Ctrl Pts',(79.438320463404,-7.43146552131711,136.443352520157));
#81163=CARTESIAN_POINT('Ctrl Pts',(79.5139091748129,-7.40516878178558,136.437784746751));
#81164=CARTESIAN_POINT('Ctrl Pts',(79.5764154898566,-7.38744135302447,136.43311246509));
#81165=CARTESIAN_POINT('Ctrl Pts',(79.7494091035494,-7.34913175896596,136.420251526671));
#81166=CARTESIAN_POINT('Ctrl Pts',(79.8612162704327,-7.33599692494895,136.412036337478));
#81167=CARTESIAN_POINT('Ctrl Pts',(80.0204666113632,-7.33346365173211,136.400809199551));
#81168=CARTESIAN_POINT('Ctrl Pts',(80.0674458954969,-7.3347030051546,136.397551241812));
#81169=CARTESIAN_POINT('Ctrl Pts',(80.1302139726367,-7.33902007246642,136.393269367407));
#81170=CARTESIAN_POINT('Ctrl Pts',(80.1460976857024,-7.34034175348256,136.392191843095));
#81171=CARTESIAN_POINT('Ctrl Pts',(80.1722874966879,-7.34289991754057,136.390424566541));
#81172=CARTESIAN_POINT('Ctrl Pts',(80.18260506101,-7.34400511326013,136.389730754153));
#81173=CARTESIAN_POINT('Ctrl Pts',(80.2027834139771,-7.34635745715489,136.388378324355));
#81174=CARTESIAN_POINT('Ctrl Pts',(80.2126446782996,-7.34759659266697,136.387719485578));
#81175=CARTESIAN_POINT('Ctrl Pts',(80.2360836498065,-7.35075516367826,136.386158194084));
#81176=CARTESIAN_POINT('Ctrl Pts',(80.2496500483913,-7.35275414957019,136.385258278319));
#81177=CARTESIAN_POINT('Ctrl Pts',(80.2963330040623,-7.360222793522,136.382173115089));
#81178=CARTESIAN_POINT('Ctrl Pts',(80.329309275834,-7.36652573256676,136.380014029814));
#81179=CARTESIAN_POINT('Ctrl Pts',(80.4103578132057,-7.38457147628857,136.374737537394));
#81180=CARTESIAN_POINT('Ctrl Pts',(80.4581406483268,-7.39746745960658,136.371653835184));
#81181=CARTESIAN_POINT('Ctrl Pts',(80.568175295527,-7.43248950156114,136.364530472941));
#81182=CARTESIAN_POINT('Ctrl Pts',(80.6298238840813,-7.45622723466822,136.360523291078));
#81183=CARTESIAN_POINT('Ctrl Pts',(80.7032606024939,-7.48963716094518,136.355584367573));
#81184=CARTESIAN_POINT('Ctrl Pts',(80.7165379694341,-7.49589072502501,136.354684415188));
#81185=CARTESIAN_POINT('Ctrl Pts',(80.7934704966602,-7.53337536449922,136.349420029075));
#81186=CARTESIAN_POINT('Ctrl Pts',(80.8551548081927,-7.56846551973307,136.345000035879));
#81187=CARTESIAN_POINT('Ctrl Pts',(80.9240868512756,-7.61372674247104,136.339605882579));
#81188=CARTESIAN_POINT('Ctrl Pts',(80.9336983049727,-7.62018207355534,136.338842858322));
#81189=CARTESIAN_POINT('Ctrl Pts',(80.9485397459497,-7.63037608542951,136.337646268045));
#81190=CARTESIAN_POINT('Ctrl Pts',(80.9538169101488,-7.63404589555177,136.33721712914));
#81191=CARTESIAN_POINT('Ctrl Pts',(80.963515219306,-7.64087383148488,136.33642140169));
#81192=CARTESIAN_POINT('Ctrl Pts',(80.9679423140171,-7.64402315897177,136.336055399488));
#81193=CARTESIAN_POINT('Ctrl Pts',(80.9781970271658,-7.65139392072596,136.335201200318));
#81194=CARTESIAN_POINT('Ctrl Pts',(80.9840127534341,-7.65563149498363,136.334711929063));
#81195=CARTESIAN_POINT('Ctrl Pts',(81.0025319242982,-7.66930986042372,136.333138875958));
#81196=CARTESIAN_POINT('Ctrl Pts',(81.0151279223944,-7.67889373537157,136.332046079795));
#81197=CARTESIAN_POINT('Ctrl Pts',(81.0841686419274,-7.73299483639653,136.325936774487));
#81198=CARTESIAN_POINT('Ctrl Pts',(81.1378178635452,-7.78094618354147,136.320742777989));
#81199=CARTESIAN_POINT('Ctrl Pts',(81.2811833912345,-7.92681659573577,136.305872744793));
#81200=CARTESIAN_POINT('Ctrl Pts',(81.3625548330531,-8.03221379828502,136.29621437872));
#81201=CARTESIAN_POINT('Ctrl Pts',(81.4442389121655,-8.1690717533662,136.285205465082));
#81202=CARTESIAN_POINT('Ctrl Pts',(81.4573606332714,-8.19230704256972,136.283381865019));
#81203=CARTESIAN_POINT('Ctrl Pts',(81.4758297153299,-8.22692798822632,136.280729134223));
#81204=CARTESIAN_POINT('Ctrl Pts',(81.4816148248892,-8.23807401298346,136.279884667254));
#81205=CARTESIAN_POINT('Ctrl Pts',(81.4916739838878,-8.25800263259035,136.278391355258));
#81206=CARTESIAN_POINT('Ctrl Pts',(81.495997807099,-8.26675929219515,136.277740791827));
#81207=CARTESIAN_POINT('Ctrl Pts',(81.5049629191842,-8.28532500014035,136.276373006485));
#81208=CARTESIAN_POINT('Ctrl Pts',(81.509585888601,-8.29514242724521,136.275656442947));
#81209=CARTESIAN_POINT('Ctrl Pts',(81.5216891100965,-8.32151042812492,136.273749232637));
#81210=CARTESIAN_POINT('Ctrl Pts',(81.5289953339168,-8.33813962355231,136.272564555453));
#81211=CARTESIAN_POINT('Ctrl Pts',(81.5682698759759,-8.43165296703818,136.265997024199));
#81212=CARTESIAN_POINT('Ctrl Pts',(81.5947133211053,-8.51073444073599,136.260803963161));
#81213=CARTESIAN_POINT('Ctrl Pts',(81.6324170442734,-8.65979738498129,136.251354757236));
#81214=CARTESIAN_POINT('Ctrl Pts',(81.6453461156356,-8.72915093698868,136.24708481809));
#81215=CARTESIAN_POINT('Ctrl Pts',(81.662459100545,-8.87003789992456,136.238356449962));
#81216=CARTESIAN_POINT('Ctrl Pts',(81.6665016739439,-8.94143385250075,136.233904390947));
#81217=CARTESIAN_POINT('Ctrl Pts',(81.6658609637158,-9.02444267643055,136.228474470825));
#81218=CARTESIAN_POINT('Ctrl Pts',(81.6656507377964,-9.03602493747524,136.227711051804));
#81219=CARTESIAN_POINT('Ctrl Pts',(81.6651360511147,-9.05403023032443,136.226513972609));
#81220=CARTESIAN_POINT('Ctrl Pts',(81.6649151504188,-9.06045554523203,136.226084745294));
#81221=CARTESIAN_POINT('Ctrl Pts',(81.6644389692623,-9.07230791960864,136.225288943578));
#81222=CARTESIAN_POINT('Ctrl Pts',(81.6641943252666,-9.07773520620492,136.224922956507));
#81223=CARTESIAN_POINT('Ctrl Pts',(81.6635640467441,-9.09034608125817,136.224068911169));
#81224=CARTESIAN_POINT('Ctrl Pts',(81.6631584265527,-9.09752843379783,136.223579779953));
#81225=CARTESIAN_POINT('Ctrl Pts',(81.6617122631881,-9.12049277594965,136.222007636225));
#81226=CARTESIAN_POINT('Ctrl Pts',(81.6604935238163,-9.13626212460825,136.220915623487));
#81227=CARTESIAN_POINT('Ctrl Pts',(81.6525016212957,-9.22348588014215,136.214815048416));
#81228=CARTESIAN_POINT('Ctrl Pts',(81.6413412605934,-9.29445608866452,136.20962951134));
#81229=CARTESIAN_POINT('Ctrl Pts',(81.5966984547348,-9.49357164199205,136.194793927766));
#81230=CARTESIAN_POINT('Ctrl Pts',(81.5524746229044,-9.61878398600857,136.185160501482));
#81231=CARTESIAN_POINT('Ctrl Pts',(81.4819404287675,-9.76166763579994,136.174149988258));
#81232=CARTESIAN_POINT('Ctrl Pts',(81.4694013042364,-9.78558575376171,136.172303953241));
#81233=CARTESIAN_POINT('Ctrl Pts',(81.4502237978625,-9.82009920015295,136.169634337258));
#81234=CARTESIAN_POINT('Ctrl Pts',(81.4440393996247,-9.83094042447244,136.168794889648));
#81235=CARTESIAN_POINT('Ctrl Pts',(81.4327914956574,-9.85015305454894,136.167305319371));
#81236=CARTESIAN_POINT('Ctrl Pts',(81.4277750405684,-9.85855117886512,136.166653541075));
#81237=CARTESIAN_POINT('Ctrl Pts',(81.4170751623764,-9.8761108398764,136.165289088098));
#81238=CARTESIAN_POINT('Ctrl Pts',(81.4113761758909,-9.88526240116317,136.164577019924));
#81239=CARTESIAN_POINT('Ctrl Pts',(81.3960152590079,-9.90940388130542,136.162695567703));
#81240=CARTESIAN_POINT('Ctrl Pts',(81.3862006265654,-9.92429534542364,136.161531866083));
#81241=CARTESIAN_POINT('Ctrl Pts',(81.3329812732045,-10.0022885708619,136.155414844941));
#81242=CARTESIAN_POINT('Ctrl Pts',(81.2855004283773,-10.0625028316024,136.150619806194));
#81243=CARTESIAN_POINT('Ctrl Pts',(81.1622164359776,-10.1984316536936,136.139310742078));
#81244=CARTESIAN_POINT('Ctrl Pts',(81.0829428853939,-10.2705186946937,136.132900500656));
#81245=CARTESIAN_POINT('Ctrl Pts',(80.9619576739437,-10.3609341645832,136.12344881136));
#81246=CARTESIAN_POINT('Ctrl Pts',(80.9255672361524,-10.3859397219893,136.12064048653));
#81247=CARTESIAN_POINT('Ctrl Pts',(80.8791713301346,-10.4151778832335,136.117044832342));
#81248=CARTESIAN_POINT('Ctrl Pts',(80.8700573069079,-10.4207994006373,136.116337790711));
#81249=CARTESIAN_POINT('Ctrl Pts',(80.8556068528442,-10.4295212462321,136.115214598171));
#81250=CARTESIAN_POINT('Ctrl Pts',(80.8503061137683,-10.4326805609976,136.114802133344));
#81251=CARTESIAN_POINT('Ctrl Pts',(80.8402100744248,-10.4386221764665,136.114015432708));
#81252=CARTESIAN_POINT('Ctrl Pts',(80.8354182834395,-10.441410081732,136.113641559589));
#81253=CARTESIAN_POINT('Ctrl Pts',(80.8239499223941,-10.4480060787172,136.112745703874));
#81254=CARTESIAN_POINT('Ctrl Pts',(80.8172608006503,-10.451791946709,136.112222348559));
#81255=CARTESIAN_POINT('Ctrl Pts',(80.7942092016864,-10.4646287567196,136.110416574757));
#81256=CARTESIAN_POINT('Ctrl Pts',(80.7777213447462,-10.473450062993,136.109121171448));
#81257=CARTESIAN_POINT('Ctrl Pts',(80.7364346084739,-10.4946532188458,136.105874305914));
#81258=CARTESIAN_POINT('Ctrl Pts',(80.7114690359023,-10.5066969882113,136.103908300771));
#81259=CARTESIAN_POINT('Ctrl Pts',(80.6072361076533,-10.5538123090927,136.095720779249));
#81260=CARTESIAN_POINT('Ctrl Pts',(80.5255923794135,-10.5832942288402,136.089364194733));
#81261=CARTESIAN_POINT('Ctrl Pts',(80.3467292457091,-10.6325146990658,136.075919808714));
#81262=CARTESIAN_POINT('Ctrl Pts',(80.2492730306803,-10.6502104482126,136.068886331677));
#81263=CARTESIAN_POINT('Ctrl Pts',(80.1320163222917,-10.6608683617966,136.060835965956));
#81264=CARTESIAN_POINT('Ctrl Pts',(80.1131968745165,-10.6622570628442,136.059555732243));
#81265=CARTESIAN_POINT('Ctrl Pts',(80.0833727029531,-10.663948929493,136.057544804656));
#81266=CARTESIAN_POINT('Ctrl Pts',(80.0723820770744,-10.6644632445714,136.056807589525));
#81267=CARTESIAN_POINT('Ctrl Pts',(80.0526286996157,-10.6651915898383,136.055489235069));
#81268=CARTESIAN_POINT('Ctrl Pts',(80.0438679172225,-10.6654454124197,136.054906876735));
#81269=CARTESIAN_POINT('Ctrl Pts',(80.0232836338115,-10.6658792538787,136.053543866153));
#81270=CARTESIAN_POINT('Ctrl Pts',(80.0114593086445,-10.6660025547435,136.052765009314));
#81271=CARTESIAN_POINT('Ctrl Pts',(79.9767941044868,-10.6659949478093,136.050492927875));
#81272=CARTESIAN_POINT('Ctrl Pts',(79.9539554752603,-10.6655202380111,136.049010396839));
#81273=CARTESIAN_POINT('Ctrl Pts',(79.848446760731,-10.6611551149451,136.042217403857));
#81274=CARTESIAN_POINT('Ctrl Pts',(79.7661255982622,-10.6515779678433,136.037083643217));
#81275=CARTESIAN_POINT('Ctrl Pts',(79.6286323979852,-10.625090677726,136.028499419117));
#81276=CARTESIAN_POINT('Ctrl Pts',(79.5730117706789,-10.6113704050205,136.025021688911));
#81277=CARTESIAN_POINT('Ctrl Pts',(79.4444914013148,-10.5725445346539,136.016782191104));
#81278=CARTESIAN_POINT('Ctrl Pts',(79.3724166335505,-10.5451932275107,136.012002132342));
#81279=CARTESIAN_POINT('Ctrl Pts',(79.2919807624931,-10.5081110617897,136.006208481804));
#81280=CARTESIAN_POINT('Ctrl Pts',(79.2815110756145,-10.5031513105747,136.005445005633));
#81281=CARTESIAN_POINT('Ctrl Pts',(79.2653129595804,-10.4952699721735,136.004247855657));
#81282=CARTESIAN_POINT('Ctrl Pts',(79.2595480455056,-10.4924236116674,136.003818615544));
#81283=CARTESIAN_POINT('Ctrl Pts',(79.2489423270313,-10.4871105840532,136.003022803071));
#81284=CARTESIAN_POINT('Ctrl Pts',(79.2440969360405,-10.4846535192165,136.002656818186));
#81285=CARTESIAN_POINT('Ctrl Pts',(79.2328638313419,-10.4788880439583,136.00180279509));
#81286=CARTESIAN_POINT('Ctrl Pts',(79.2264854694499,-10.4755619316208,136.001313684126));
#81287=CARTESIAN_POINT('Ctrl Pts',(79.2061540431883,-10.4647916918972,135.999741671881));
#81288=CARTESIAN_POINT('Ctrl Pts',(79.192285832796,-10.4571904070715,135.998649772408));
#81289=CARTESIAN_POINT('Ctrl Pts',(79.1161002628295,-10.4140107729154,135.99255045869));
#81290=CARTESIAN_POINT('Ctrl Pts',(79.0560290753016,-10.3746352535461,135.987366143711));
#81291=CARTESIAN_POINT('Ctrl Pts',(78.8929935452841,-10.2520311570916,135.972535528709));
#81292=CARTESIAN_POINT('Ctrl Pts',(78.7971169914575,-10.1602283871828,135.962905698296));
#81293=CARTESIAN_POINT('Ctrl Pts',(78.6959238483847,-10.03714652932,135.951894942957));
#81294=CARTESIAN_POINT('Ctrl Pts',(78.6792575030176,-10.0158380468731,135.950045661469));
#81295=CARTESIAN_POINT('Ctrl Pts',(78.6556642597566,-9.98411045439296,135.947372291279));
#81296=CARTESIAN_POINT('Ctrl Pts',(78.6483247491142,-9.97400513336739,135.946532272485));
#81297=CARTESIAN_POINT('Ctrl Pts',(78.6354396923509,-9.95583830969484,135.94504205554));
#81298=CARTESIAN_POINT('Ctrl Pts',(78.6298502933984,-9.94780878662706,135.944390196573));
#81299=CARTESIAN_POINT('Ctrl Pts',(78.6182533960129,-9.93083212674594,135.943025943599));
#81300=CARTESIAN_POINT('Ctrl Pts',(78.6122613093948,-9.92187497070461,135.942314152859));
#81301=CARTESIAN_POINT('Ctrl Pts',(78.5965961061624,-9.89795924788947,135.940434290283));
#81302=CARTESIAN_POINT('Ctrl Pts',(78.5870750962848,-9.88290234815893,135.93927188334));
#81303=CARTESIAN_POINT('Ctrl Pts',(78.5381038896986,-9.80263568816844,135.933180222101));
#81304=CARTESIAN_POINT('Ctrl Pts',(78.5029188790437,-9.73492485512945,135.928407576921));
#81305=CARTESIAN_POINT('Ctrl Pts',(78.4372856302942,-9.58417285838609,135.918273188005));
#81306=CARTESIAN_POINT('Ctrl Pts',(78.4085578727547,-9.5006450862159,135.91295397125));
#81307=CARTESIAN_POINT('Ctrl Pts',(78.3742897703535,-9.36749504146005,135.904457892236));
#81308=CARTESIAN_POINT('Ctrl Pts',(78.364128658753,-9.31923422752997,135.901373165135));
#81309=CARTESIAN_POINT('Ctrl Pts',(78.3529714837076,-9.25145472319147,135.896946575299));
#81310=CARTESIAN_POINT('Ctrl Pts',(78.3501550529687,-9.2322584406095,135.895682438179));
#81311=CARTESIAN_POINT('Ctrl Pts',(78.346649792503,-9.20506909276868,135.893871617067));
#81312=CARTESIAN_POINT('Ctrl Pts',(78.3456823723338,-9.19711271333548,135.893339270303));
#81313=CARTESIAN_POINT('Ctrl Pts',(78.3441430502629,-9.18364229216901,135.892433377276));
#81314=CARTESIAN_POINT('Ctrl Pts',(78.3435411767897,-9.17813168034955,135.89206147936));
#81315=CARTESIAN_POINT('Ctrl Pts',(78.3424380834556,-9.16754263219605,135.891344184262));
#81316=CARTESIAN_POINT('Ctrl Pts',(78.3419326795074,-9.16246476455477,135.890999052264));
#81317=CARTESIAN_POINT('Ctrl Pts',(78.3408841507623,-9.1514151756644,135.890245628202));
#81318=CARTESIAN_POINT('Ctrl Pts',(78.3403499245922,-9.14544270719875,135.889836863965));
#81319=CARTESIAN_POINT('Ctrl Pts',(78.3391176742243,-9.13077461965185,135.888829423074));
#81320=CARTESIAN_POINT('Ctrl Pts',(78.3384556941492,-9.12207625933092,135.888228950659));
#81321=CARTESIAN_POINT('Ctrl Pts',(78.3353083429498,-9.07593373282946,135.885028836512));
#81322=CARTESIAN_POINT('Ctrl Pts',(78.3340205656728,-9.03842192104802,135.882375972897));
#81323=CARTESIAN_POINT('Ctrl Pts',(78.3340002443612,-9.00090233676016,135.879690672883));
#81324=CARTESIAN_POINT('Ctrl Pts',(78.3340002456957,-9.00090479726252,135.879690848982));
#81325=CARTESIAN_POINT('Ctrl Pts',(78.3339486782985,-8.90595394516173,135.872895160915));
#81326=CARTESIAN_POINT('Ctrl Pts',(78.3420143785496,-8.81117037196368,135.86591863175));
#81327=CARTESIAN_POINT('Ctrl Pts',(78.3722930491939,-8.63513663529914,135.853006356088));
#81328=CARTESIAN_POINT('Ctrl Pts',(78.392666927927,-8.55386180232306,135.847062253801));
#81329=CARTESIAN_POINT('Ctrl Pts',(78.424631626278,-8.45770686105293,135.840094980782));
#81330=CARTESIAN_POINT('Ctrl Pts',(78.430463714507,-8.44105167753812,135.838890212765));
#81331=CARTESIAN_POINT('Ctrl Pts',(78.4365593748807,-8.42449204025778,135.837694108205));
#81332=CARTESIAN_POINT('',(78.3340003883624,-9.00113755153436,136.072462071471));
#81333=CARTESIAN_POINT('Ctrl Pts',(78.4365593762033,-8.4244920366647,136.032852185112));
#81334=CARTESIAN_POINT('Ctrl Pts',(78.4356277258545,-8.42702298340278,136.033046303352));
#81335=CARTESIAN_POINT('Ctrl Pts',(78.4347021631167,-8.42955635039758,136.033240322336));
#81336=CARTESIAN_POINT('Ctrl Pts',(78.4095803139013,-8.49883919715719,136.038538530477));
#81337=CARTESIAN_POINT('Ctrl Pts',(78.3896669126106,-8.56707202833529,136.04355275021));
#81338=CARTESIAN_POINT('Ctrl Pts',(78.3698143433768,-8.65583668041469,136.049800259074));
#81339=CARTESIAN_POINT('Ctrl Pts',(78.3658114692678,-8.67537472157639,136.051159057064));
#81340=CARTESIAN_POINT('Ctrl Pts',(78.3598903740665,-8.70716879080624,136.053344599856));
#81341=CARTESIAN_POINT('Ctrl Pts',(78.3577566165095,-8.71938213535617,136.054178076104));
#81342=CARTESIAN_POINT('Ctrl Pts',(78.3541893826516,-8.74123680834678,136.055659011553));
#81343=CARTESIAN_POINT('Ctrl Pts',(78.3527038238034,-8.75086892536187,136.056308088779));
#81344=CARTESIAN_POINT('Ctrl Pts',(78.3499924381886,-8.76953493586363,136.057559151771));
#81345=CARTESIAN_POINT('Ctrl Pts',(78.3487560759312,-8.77856692066546,136.058161447505));
#81346=CARTESIAN_POINT('Ctrl Pts',(78.3462230670659,-8.79827375592153,136.059469171345));
#81347=CARTESIAN_POINT('Ctrl Pts',(78.3449555037265,-8.80895198059508,136.060173671105));
#81348=CARTESIAN_POINT('Ctrl Pts',(78.3412526903109,-8.84295451651808,136.062404654891));
#81349=CARTESIAN_POINT('Ctrl Pts',(78.3392063991886,-8.86631895095113,136.063919165488));
#81350=CARTESIAN_POINT('Ctrl Pts',(78.3351936440725,-8.9268065492008,136.067799253375));
#81351=CARTESIAN_POINT('Ctrl Pts',(78.3339750077928,-8.96396647141597,136.070143170673));
#81352=CARTESIAN_POINT('Ctrl Pts',(78.3340003883624,-9.00113755153436,136.072462071471));
#81353=CARTESIAN_POINT('Ctrl Pts',(78.3340003869976,-9.0011355508379,136.072461946658));
#81354=CARTESIAN_POINT('Ctrl Pts',(78.3340531440873,-9.07853700943008,136.077290603074));
#81355=CARTESIAN_POINT('Ctrl Pts',(78.3394999153977,-9.15584584925452,136.081997884715));
#81356=CARTESIAN_POINT('Ctrl Pts',(78.3596031981819,-9.29848853188085,136.090799645083));
#81357=CARTESIAN_POINT('Ctrl Pts',(78.3728537737941,-9.36385567026177,136.094881813052));
#81358=CARTESIAN_POINT('Ctrl Pts',(78.3957719282622,-9.45001745767704,136.100524030258));
#81359=CARTESIAN_POINT('Ctrl Pts',(78.4020028926957,-9.47166573117722,136.101964505079));
#81360=CARTESIAN_POINT('Ctrl Pts',(78.4134188250564,-9.50850119330994,136.104465350293));
#81361=CARTESIAN_POINT('Ctrl Pts',(78.4183879578705,-9.5237524129145,136.105515643136));
#81362=CARTESIAN_POINT('Ctrl Pts',(78.4259160910296,-9.54577299776072,136.107057007256));
#81363=CARTESIAN_POINT('Ctrl Pts',(78.428300391788,-9.55260171396246,136.107538499868));
#81364=CARTESIAN_POINT('Ctrl Pts',(78.432554208905,-9.56453453188385,136.1083863974));
#81365=CARTESIAN_POINT('Ctrl Pts',(78.4344043523939,-9.56964533940766,136.108751668212));
#81366=CARTESIAN_POINT('Ctrl Pts',(78.438487380011,-9.58075407502649,136.109550328748));
#81367=CARTESIAN_POINT('Ctrl Pts',(78.4407297879627,-9.58674812351805,136.109984246605));
#81368=CARTESIAN_POINT('Ctrl Pts',(78.4470829183529,-9.6034366646677,136.111200383974));
#81369=CARTESIAN_POINT('Ctrl Pts',(78.4512694188528,-9.6141016525141,136.111986812549));
#81370=CARTESIAN_POINT('Ctrl Pts',(78.4799752262506,-9.68506797711475,136.1172778576));
#81371=CARTESIAN_POINT('Ctrl Pts',(78.5078983054853,-9.74392478991529,136.121945627329));
#81372=CARTESIAN_POINT('Ctrl Pts',(78.5496654074353,-9.82009781652399,136.128241581835));
#81373=CARTESIAN_POINT('Ctrl Pts',(78.5605161227628,-9.8389976198774,136.129826012431));
#81374=CARTESIAN_POINT('Ctrl Pts',(78.6072653212665,-9.91684758692653,136.136434504642));
#81375=CARTESIAN_POINT('Ctrl Pts',(78.6464406462863,-9.97375428776186,136.141461415257));
#81376=CARTESIAN_POINT('Ctrl Pts',(78.7180408791542,-10.0650569381424,136.149769373454));
#81377=CARTESIAN_POINT('Ctrl Pts',(78.7486014556983,-10.1008032590583,136.153093164816));
#81378=CARTESIAN_POINT('Ctrl Pts',(78.7957311118314,-10.1514266110471,136.157900603742));
#81379=CARTESIAN_POINT('Ctrl Pts',(78.8111492838832,-10.1673392182684,136.159427638254));
#81380=CARTESIAN_POINT('Ctrl Pts',(78.8396995725587,-10.1956524734418,136.162174645403));
#81381=CARTESIAN_POINT('Ctrl Pts',(78.8527244363873,-10.2081559273629,136.163398944764));
#81382=CARTESIAN_POINT('Ctrl Pts',(78.8736862406611,-10.2276338332598,136.165324893413));
#81383=CARTESIAN_POINT('Ctrl Pts',(78.8814903778884,-10.2347484550194,136.166032495897));
#81384=CARTESIAN_POINT('Ctrl Pts',(78.8966095381082,-10.248270819334,136.1673856338));
#81385=CARTESIAN_POINT('Ctrl Pts',(78.9039140238905,-10.2546896387645,136.168031618388));
#81386=CARTESIAN_POINT('Ctrl Pts',(78.9204810112987,-10.2689927869896,136.169479700536));
#81387=CARTESIAN_POINT('Ctrl Pts',(78.9297745660913,-10.2768404262507,136.170280267417));
#81388=CARTESIAN_POINT('Ctrl Pts',(78.9574861288122,-10.299725403546,136.172633801087));
#81389=CARTESIAN_POINT('Ctrl Pts',(78.9761415028634,-10.3144714396632,136.17417509808));
#81390=CARTESIAN_POINT('Ctrl Pts',(79.0768073905316,-10.3905983285773,136.182281225029));
#81391=CARTESIAN_POINT('Ctrl Pts',(79.1640349305834,-10.4447193506548,136.188562730292));
#81392=CARTESIAN_POINT('Ctrl Pts',(79.3266304206723,-10.5259151006111,136.199662489825));
#81393=CARTESIAN_POINT('Ctrl Pts',(79.4000042932717,-10.5562284169969,136.204481949268));
#81394=CARTESIAN_POINT('Ctrl Pts',(79.4987629040837,-10.5890031609177,136.211042952097));
#81395=CARTESIAN_POINT('Ctrl Pts',(79.5224442681842,-10.5962800709341,136.212621964881));
#81396=CARTESIAN_POINT('Ctrl Pts',(79.5628443217163,-10.6077149470157,136.215339150513));
#81397=CARTESIAN_POINT('Ctrl Pts',(79.5794817893799,-10.6121466483397,136.216464773764));
#81398=CARTESIAN_POINT('Ctrl Pts',(79.6034015617999,-10.6181226843057,136.218096513039));
#81399=CARTESIAN_POINT('Ctrl Pts',(79.6106308111568,-10.6198774559174,136.218591415872));
#81400=CARTESIAN_POINT('Ctrl Pts',(79.6232324725035,-10.6228470560656,136.219457524723));
#81401=CARTESIAN_POINT('Ctrl Pts',(79.6285995437493,-10.6240837531513,136.219827487251));
#81402=CARTESIAN_POINT('Ctrl Pts',(79.6401135767127,-10.6266767915208,136.22062361679));
#81403=CARTESIAN_POINT('Ctrl Pts',(79.646262020066,-10.628024895388,136.221050204735));
#81404=CARTESIAN_POINT('Ctrl Pts',(79.663165096473,-10.6316307817585,136.222226688523));
#81405=CARTESIAN_POINT('Ctrl Pts',(79.6739344330024,-10.6338170001975,136.222980381118));
#81406=CARTESIAN_POINT('Ctrl Pts',(79.7352872076183,-10.6456411241806,136.227294601405));
#81407=CARTESIAN_POINT('Ctrl Pts',(79.7862698313537,-10.6530353594936,136.230957677139));
#81408=CARTESIAN_POINT('Ctrl Pts',(79.9330579404276,-10.6674208787999,136.241586092992));
#81409=CARTESIAN_POINT('Ctrl Pts',(80.0292401159734,-10.6685082277759,136.248637952651));
#81410=CARTESIAN_POINT('Ctrl Pts',(80.177433543744,-10.657359317835,136.259325425901));
#81411=CARTESIAN_POINT('Ctrl Pts',(80.2296710641545,-10.6509314532033,136.26306103374));
#81412=CARTESIAN_POINT('Ctrl Pts',(80.3050175434361,-10.6380136151343,136.268388817616));
#81413=CARTESIAN_POINT('Ctrl Pts',(80.328425668977,-10.6334812469752,136.270035658001));
#81414=CARTESIAN_POINT('Ctrl Pts',(80.3706976159592,-10.6243509015645,136.272994937952));
#81415=CARTESIAN_POINT('Ctrl Pts',(80.3895933533836,-10.6199227290637,136.274312371937));
#81416=CARTESIAN_POINT('Ctrl Pts',(80.4191834297355,-10.6124406293078,136.276367763611));
#81417=CARTESIAN_POINT('Ctrl Pts',(80.4299314199239,-10.6096081869,136.277112743289));
#81418=CARTESIAN_POINT('Ctrl Pts',(80.4500246977973,-10.6040973340813,136.27850274619));
#81419=CARTESIAN_POINT('Ctrl Pts',(80.4593763907743,-10.6014442932179,136.279148556542));
#81420=CARTESIAN_POINT('Ctrl Pts',(80.4803368661032,-10.5952991686223,136.280593802909));
#81421=CARTESIAN_POINT('Ctrl Pts',(80.4919319126449,-10.5917619007353,136.281391734493));
#81422=CARTESIAN_POINT('Ctrl Pts',(80.5259613500972,-10.580973274519,136.283729736273));
#81423=CARTESIAN_POINT('Ctrl Pts',(80.5482821903339,-10.573371718859,136.285258371482));
#81424=CARTESIAN_POINT('Ctrl Pts',(80.6684995754837,-10.5295614105909,136.293478446592));
#81425=CARTESIAN_POINT('Ctrl Pts',(80.7629927560757,-10.4846869174966,136.299873544174));
#81426=CARTESIAN_POINT('Ctrl Pts',(80.919717190734,-10.3913182249627,136.311014259237));
#81427=CARTESIAN_POINT('Ctrl Pts',(80.9838666726462,-10.3467185230584,136.315760881859));
#81428=CARTESIAN_POINT('Ctrl Pts',(81.0637854840536,-10.2823883520391,136.322231817124));
#81429=CARTESIAN_POINT('Ctrl Pts',(81.0825773122126,-10.266564517711,136.323798067999));
#81430=CARTESIAN_POINT('Ctrl Pts',(81.113852828467,-10.2390240696416,136.326495418802));
#81431=CARTESIAN_POINT('Ctrl Pts',(81.126518660641,-10.2275196210859,136.327614208366));
#81432=CARTESIAN_POINT('Ctrl Pts',(81.1444201587758,-10.2107491774557,136.329237769508));
#81433=CARTESIAN_POINT('Ctrl Pts',(81.1498017746462,-10.2056396411621,136.329731481296));
#81434=CARTESIAN_POINT('Ctrl Pts',(81.1591162105398,-10.1966770333956,136.330596247874));
#81435=CARTESIAN_POINT('Ctrl Pts',(81.1630643522751,-10.1928401499102,136.330966071275));
#81436=CARTESIAN_POINT('Ctrl Pts',(81.1714931933473,-10.1845671995464,136.331762775723));
#81437=CARTESIAN_POINT('Ctrl Pts',(81.1759676771506,-10.1801253201649,136.332190085424));
#81438=CARTESIAN_POINT('Ctrl Pts',(81.1882038535997,-10.1678396175123,136.333370455408));
#81439=CARTESIAN_POINT('Ctrl Pts',(81.1959128292911,-10.1599440755418,136.334127352037));
#81440=CARTESIAN_POINT('Ctrl Pts',(81.2397086768444,-10.1141876432716,136.338501141757));
#81441=CARTESIAN_POINT('Ctrl Pts',(81.2740717816077,-10.0747239988735,136.342223789743));
#81442=CARTESIAN_POINT('Ctrl Pts',(81.3697297132629,-9.95382130089555,136.353338096539));
#81443=CARTESIAN_POINT('Ctrl Pts',(81.425483861494,-9.86829261827158,136.36082600959));
#81444=CARTESIAN_POINT('Ctrl Pts',(81.5071765192192,-9.71365588212225,136.373363998937));
#81445=CARTESIAN_POINT('Ctrl Pts',(81.5370020297739,-9.64692595342673,136.378494616416));
#81446=CARTESIAN_POINT('Ctrl Pts',(81.568476699323,-9.56191421255803,136.384681130756));
#81447=CARTESIAN_POINT('Ctrl Pts',(81.5743346100442,-9.5452864528588,136.385875477882));
#81448=CARTESIAN_POINT('Ctrl Pts',(81.5833334383259,-9.5183883231667,136.387783100725));
#81449=CARTESIAN_POINT('Ctrl Pts',(81.5866407641407,-9.50817548682752,136.388501802862));
#81450=CARTESIAN_POINT('Ctrl Pts',(81.5927753609326,-9.48858827446242,136.389869798529));
#81451=CARTESIAN_POINT('Ctrl Pts',(81.5956191430648,-9.47921958390969,136.390519607981));
#81452=CARTESIAN_POINT('Ctrl Pts',(81.601922400416,-9.45777547969089,136.39199697821));
#81453=CARTESIAN_POINT('Ctrl Pts',(81.6053282585027,-9.445684825389,136.392822769564));
#81454=CARTESIAN_POINT('Ctrl Pts',(81.614055890675,-9.4133032484279,136.39501615713));
#81455=CARTESIAN_POINT('Ctrl Pts',(81.6191318435975,-9.39294799830358,136.396375884072));
#81456=CARTESIAN_POINT('Ctrl Pts',(81.6509430449827,-9.25427546454901,136.405522926466));
#81457=CARTESIAN_POINT('Ctrl Pts',(81.6650725882106,-9.13343941731572,136.412888365569));
#81458=CARTESIAN_POINT('Ctrl Pts',(81.6664358878596,-8.94619840577459,136.424330670322));
#81459=CARTESIAN_POINT('Ctrl Pts',(81.6630015445271,-8.88030126193085,136.428371377915));
#81460=CARTESIAN_POINT('Ctrl Pts',(81.6531835309658,-8.79253553429311,136.433961442991));
#81461=CARTESIAN_POINT('Ctrl Pts',(81.6502462549271,-8.77033831438495,136.435393485661));
#81462=CARTESIAN_POINT('Ctrl Pts',(81.6444495029706,-8.73242423840711,136.437881089014));
#81463=CARTESIAN_POINT('Ctrl Pts',(81.6418095872274,-8.71667652858781,136.438926713713));
#81464=CARTESIAN_POINT('Ctrl Pts',(81.6376479532972,-8.69386717035036,136.44046246085));
#81465=CARTESIAN_POINT('Ctrl Pts',(81.6363059090365,-8.68677309252152,136.440943101831));
#81466=CARTESIAN_POINT('Ctrl Pts',(81.6338730173725,-8.67435526389663,136.441790060367));
#81467=CARTESIAN_POINT('Ctrl Pts',(81.6328021694493,-8.66902778776265,136.442155252426));
#81468=CARTESIAN_POINT('Ctrl Pts',(81.6304116565038,-8.65742898765019,136.442954426446));
#81469=CARTESIAN_POINT('Ctrl Pts',(81.6290818871377,-8.65116010877972,136.443388942784));
#81470=CARTESIAN_POINT('Ctrl Pts',(81.6252657202622,-8.63366751014333,136.44460833716));
#81471=CARTESIAN_POINT('Ctrl Pts',(81.6226993256684,-8.62246187642905,136.445397458953));
#81472=CARTESIAN_POINT('Ctrl Pts',(81.6044747703193,-8.54650899196724,136.450796521397));
#81473=CARTESIAN_POINT('Ctrl Pts',(81.5850629263057,-8.48273129030787,136.455577184603));
#81474=CARTESIAN_POINT('Ctrl Pts',(81.5543622918707,-8.40001519832784,136.461974559569));
#81475=CARTESIAN_POINT('Ctrl Pts',(81.5464413774292,-8.3798847325863,136.463547740871));
#81476=CARTESIAN_POINT('Ctrl Pts',(81.5104515909371,-8.29340098473167,136.470365403037));
#81477=CARTESIAN_POINT('Ctrl Pts',(81.4784854695449,-8.22874901729802,136.4756100113));
#81478=CARTESIAN_POINT('Ctrl Pts',(81.4089998191959,-8.10851825372225,136.485530350487));
#81479=CARTESIAN_POINT('Ctrl Pts',(81.3721140638212,-8.05272746631147,136.490211356849));
#81480=CARTESIAN_POINT('Ctrl Pts',(81.3216220970021,-7.98552086249892,136.4959444828));
#81481=CARTESIAN_POINT('Ctrl Pts',(81.3110590167478,-7.97190604464337,136.49711135142));
#81482=CARTESIAN_POINT('Ctrl Pts',(81.2936285718628,-7.95014547389772,136.498985922746));
#81483=CARTESIAN_POINT('Ctrl Pts',(81.2868912070567,-7.94189771844929,136.499698717918));
#81484=CARTESIAN_POINT('Ctrl Pts',(81.2737927021483,-7.92617296457323,136.501062389236));
#81485=CARTESIAN_POINT('Ctrl Pts',(81.2674436772684,-7.91868650149739,136.50171371616));
#81486=CARTESIAN_POINT('Ctrl Pts',(81.2527041082732,-7.90161451047526,136.503204122685));
#81487=CARTESIAN_POINT('Ctrl Pts',(81.2442689806765,-7.89206814957792,136.50404132054));
#81488=CARTESIAN_POINT('Ctrl Pts',(81.2166213009232,-7.86149224353199,136.506736223956));
#81489=CARTESIAN_POINT('Ctrl Pts',(81.1969781106936,-7.84085770590956,136.508575816671));
#81490=CARTESIAN_POINT('Ctrl Pts',(81.0842987360328,-7.7284123852319,136.518746710605));
#81491=CARTESIAN_POINT('Ctrl Pts',(80.981242331743,-7.64729726130296,136.526604738046));
#81492=CARTESIAN_POINT('Ctrl Pts',(80.808979475236,-7.54185516316771,136.538997038029));
#81493=CARTESIAN_POINT('Ctrl Pts',(80.7458826769845,-7.50859433325969,136.543414966816));
#81494=CARTESIAN_POINT('Ctrl Pts',(80.6664719662814,-7.47303581949627,136.549060246491));
#81495=CARTESIAN_POINT('Ctrl Pts',(80.6519948202777,-7.46679838230708,136.550092813866));
#81496=CARTESIAN_POINT('Ctrl Pts',(80.6307954069113,-7.45801921134401,136.551612839209));
#81497=CARTESIAN_POINT('Ctrl Pts',(80.6241412562447,-7.45531385534933,136.552091085096));
#81498=CARTESIAN_POINT('Ctrl Pts',(80.6124261365001,-7.4506389320905,136.552935412953));
#81499=CARTESIAN_POINT('Ctrl Pts',(80.6073727209619,-7.44865095224276,136.553300393657));
#81500=CARTESIAN_POINT('Ctrl Pts',(80.596311550661,-7.44436189304197,136.554101057231));
#81501=CARTESIAN_POINT('Ctrl Pts',(80.5903002525085,-7.44207092791004,136.554537292359));
#81502=CARTESIAN_POINT('Ctrl Pts',(80.5734064712943,-7.43574435151897,136.555766057923));
#81503=CARTESIAN_POINT('Ctrl Pts',(80.5624951118452,-7.43178765932048,136.556562932635));
#81504=CARTESIAN_POINT('Ctrl Pts',(80.4788920153318,-7.40245613263875,136.562688535492));
#81505=CARTESIAN_POINT('Ctrl Pts',(80.4045686724083,-7.382036628393,136.568244529526));
#81506=CARTESIAN_POINT('Ctrl Pts',(80.2729616517355,-7.35551571470066,136.578002964458));
#81507=CARTESIAN_POINT('Ctrl Pts',(80.2162661012459,-7.34710379394236,136.582182645411));
#81508=CARTESIAN_POINT('Ctrl Pts',(80.0769158166393,-7.33372233195937,136.5922985263));
#81509=CARTESIAN_POINT('Ctrl Pts',(79.9940981971669,-7.33195741347212,136.598172144181));
#81510=CARTESIAN_POINT('Ctrl Pts',(79.8886808228571,-7.33756643230204,136.605429645344));
#81511=CARTESIAN_POINT('Ctrl Pts',(79.8659069304871,-7.33924822305783,136.606985054866));
#81512=CARTESIAN_POINT('Ctrl Pts',(79.8314053839323,-7.34251045582481,136.609323612528));
#81513=CARTESIAN_POINT('Ctrl Pts',(79.8196488975306,-7.34374844122533,136.610117338724));
#81514=CARTESIAN_POINT('Ctrl Pts',(79.7992030170704,-7.34612172768013,136.611492535054));
#81515=CARTESIAN_POINT('Ctrl Pts',(79.7905076843217,-7.34720063446611,136.612075749085));
#81516=CARTESIAN_POINT('Ctrl Pts',(79.7709166399991,-7.34978855996296,136.61338625697));
#81517=CARTESIAN_POINT('Ctrl Pts',(79.7600264758242,-7.35133699619361,136.614112283122));
#81518=CARTESIAN_POINT('Ctrl Pts',(79.7305035798678,-7.35583348817845,136.616074387602));
#81519=CARTESIAN_POINT('Ctrl Pts',(79.7119039383535,-7.35899038840539,136.617303862332));
#81520=CARTESIAN_POINT('Ctrl Pts',(79.5960436052583,-7.38068593144789,136.624928347029));
#81521=CARTESIAN_POINT('Ctrl Pts',(79.5005386444308,-7.4075487987189,136.631046492309));
#81522=CARTESIAN_POINT('Ctrl Pts',(79.3412720498868,-7.46809734382974,136.641469246738));
#81523=CARTESIAN_POINT('Ctrl Pts',(79.2762702912745,-7.49771412304658,136.645796717367));
#81524=CARTESIAN_POINT('Ctrl Pts',(79.1806842162881,-7.54891332608269,136.652528739725));
#81525=CARTESIAN_POINT('Ctrl Pts',(79.1485939632716,-7.56750626756389,136.654857154041));
#81526=CARTESIAN_POINT('Ctrl Pts',(79.1038570540067,-7.59546106337106,136.658240131652));
#81527=CARTESIAN_POINT('Ctrl Pts',(79.0906797036811,-7.60395617395465,136.659254180049));
#81528=CARTESIAN_POINT('Ctrl Pts',(79.0674943722164,-7.61937070891527,136.661073578881));
#81529=CARTESIAN_POINT('Ctrl Pts',(79.0574384495355,-7.62621628790698,136.66187473324));
#81530=CARTESIAN_POINT('Ctrl Pts',(79.0421417763418,-7.63687651931365,136.663113513431));
#81531=CARTESIAN_POINT('Ctrl Pts',(79.0368465755623,-7.6406128301045,136.663546088036));
#81532=CARTESIAN_POINT('Ctrl Pts',(79.0271170197089,-7.64756342062821,136.664348132998));
#81533=CARTESIAN_POINT('Ctrl Pts',(79.0226765514367,-7.65076878616497,136.664717006978));
#81534=CARTESIAN_POINT('Ctrl Pts',(79.0125748345348,-7.6581367733994,136.665562611119));
#81535=CARTESIAN_POINT('Ctrl Pts',(79.0069240637365,-7.6623133563403,136.6660402723));
#81536=CARTESIAN_POINT('Ctrl Pts',(78.989037355094,-7.67570952944139,136.66756662675));
#81537=CARTESIAN_POINT('Ctrl Pts',(78.9769025005247,-7.68506190836095,136.66862375255));
#81538=CARTESIAN_POINT('Ctrl Pts',(78.8853942567783,-7.7576211424056,136.676751167105));
#81539=CARTESIAN_POINT('Ctrl Pts',(78.8118218810881,-7.82778818382988,136.684177266436));
#81540=CARTESIAN_POINT('Ctrl Pts',(78.6690211389724,-7.99132345046157,136.699968396462));
#81541=CARTESIAN_POINT('Ctrl Pts',(78.6022130327686,-8.08614326269147,136.708265359407));
#81542=CARTESIAN_POINT('Ctrl Pts',(78.5362713348221,-8.2041151402908,136.717514015289));
#81543=CARTESIAN_POINT('Ctrl Pts',(78.5270789898906,-8.22125866375,136.718834555279));
#81544=CARTESIAN_POINT('Ctrl Pts',(78.5131044634775,-8.24845398976563,136.720893666757));
#81545=CARTESIAN_POINT('Ctrl Pts',(78.5081194202886,-8.2583989695918,136.721639302626));
#81546=CARTESIAN_POINT('Ctrl Pts',(78.4989661055957,-8.27712538197755,136.72302990055));
#81547=CARTESIAN_POINT('Ctrl Pts',(78.4947743784798,-8.28589475516883,136.723675656225));
#81548=CARTESIAN_POINT('Ctrl Pts',(78.4855334629231,-8.30567030724916,136.725119970786));
#81549=CARTESIAN_POINT('Ctrl Pts',(78.4805270045569,-8.31669593649359,136.725917033893));
#81550=CARTESIAN_POINT('Ctrl Pts',(78.4661546731418,-8.34928711518128,136.728249928762));
#81551=CARTESIAN_POINT('Ctrl Pts',(78.4571243271641,-8.37099801904214,136.729774402218));
#81552=CARTESIAN_POINT('Ctrl Pts',(78.4444496060379,-8.40338792783224,136.7320090848));
#81553=CARTESIAN_POINT('Ctrl Pts',(78.440450520719,-8.41392124806094,136.732729718861));
#81554=CARTESIAN_POINT('Ctrl Pts',(78.4365593881204,-8.4244920042904,136.733447186333));
#81555=CARTESIAN_POINT('Origin',(80.,-9.,134.));
#81556=CARTESIAN_POINT('',(78.4365593939729,-8.42449198839149,137.430947540156));
#81557=CARTESIAN_POINT('',(78.4365593749625,-8.42449204003552,137.240217161908));
#81558=CARTESIAN_POINT('',(78.4365593749993,-8.42449203993574,134.));
#81559=CARTESIAN_POINT('Ctrl Pts',(78.4365593749625,-8.42449204003557,137.240217161908));
#81560=CARTESIAN_POINT('Ctrl Pts',(78.4426950514193,-8.40782369397956,137.239116598015));
#81561=CARTESIAN_POINT('Ctrl Pts',(78.4490997416212,-8.39124680179114,137.238009742291));
#81562=CARTESIAN_POINT('Ctrl Pts',(78.4662907046562,-8.34878773177696,137.235135251636));
#81563=CARTESIAN_POINT('Ctrl Pts',(78.4774630443045,-8.32307854127335,137.233356454132));
#81564=CARTESIAN_POINT('Ctrl Pts',(78.4972254658144,-8.28056959083472,137.230331063815));
#81565=CARTESIAN_POINT('Ctrl Pts',(78.5054622762946,-8.26361128913567,137.229101067464));
#81566=CARTESIAN_POINT('Ctrl Pts',(78.5174707414679,-8.23991944152322,137.227344819163));
#81567=CARTESIAN_POINT('Ctrl Pts',(78.5210044754583,-8.2330660456309,137.22683224986));
#81568=CARTESIAN_POINT('Ctrl Pts',(78.5271621613846,-8.22132453607942,137.225945842083));
#81569=CARTESIAN_POINT('Ctrl Pts',(78.5297631723509,-8.21642457495041,137.225573426403));
#81570=CARTESIAN_POINT('Ctrl Pts',(78.5353037595954,-8.20611155528073,137.224784156948));
#81571=CARTESIAN_POINT('Ctrl Pts',(78.5382488512281,-8.20070186082715,137.224366986071));
#81572=CARTESIAN_POINT('Ctrl Pts',(78.5463706967688,-8.18597825767548,137.223223174653));
#81573=CARTESIAN_POINT('Ctrl Pts',(78.5516068147169,-8.1766976774988,137.222492976522));
#81574=CARTESIAN_POINT('Ctrl Pts',(78.5785566029695,-8.12998427163418,137.218773010506));
#81575=CARTESIAN_POINT('Ctrl Pts',(78.6016321182466,-8.09336045565965,137.215710889432));
#81576=CARTESIAN_POINT('Ctrl Pts',(78.6990757537441,-7.95128837297588,137.203356731949));
#81577=CARTESIAN_POINT('Ctrl Pts',(78.7841597555164,-7.85372877195035,137.193826034099));
#81578=CARTESIAN_POINT('Ctrl Pts',(78.9225828363449,-7.72795764263543,137.180540971547));
#81579=CARTESIAN_POINT('Ctrl Pts',(78.9675177481265,-7.69122145478909,137.176496460323));
#81580=CARTESIAN_POINT('Ctrl Pts',(79.0276261909263,-7.64710712299797,137.17141694395));
#81581=CARTESIAN_POINT('Ctrl Pts',(79.0411155400122,-7.63751308705435,137.170296981442));
#81582=CARTESIAN_POINT('Ctrl Pts',(79.0622524086141,-7.62294932916238,137.168572142088));
#81583=CARTESIAN_POINT('Ctrl Pts',(79.0698012045732,-7.61783890160981,137.167961950662));
#81584=CARTESIAN_POINT('Ctrl Pts',(79.0850382616431,-7.60770500590972,137.166741735859));
#81585=CARTESIAN_POINT('Ctrl Pts',(79.0927268726588,-7.60268263755114,137.166131768532));
#81586=CARTESIAN_POINT('Ctrl Pts',(79.1106804612623,-7.5911656255291,137.1647204928));
#81587=CARTESIAN_POINT('Ctrl Pts',(79.1209758071485,-7.5847191027587,137.163920987391));
#81588=CARTESIAN_POINT('Ctrl Pts',(79.1515521806562,-7.5660358063852,137.161574346328));
#81589=CARTESIAN_POINT('Ctrl Pts',(79.172025225386,-7.55411795988559,137.160038772768));
#81590=CARTESIAN_POINT('Ctrl Pts',(79.2823685526551,-7.49299711604768,137.151936177905));
#81591=CARTESIAN_POINT('Ctrl Pts',(79.3763824843039,-7.45172448025189,137.145652897398));
#81592=CARTESIAN_POINT('Ctrl Pts',(79.5489222105686,-7.3942642999744,137.134546062335));
#81593=CARTESIAN_POINT('Ctrl Pts',(79.6259336842268,-7.374598219539,137.129721188107));
#81594=CARTESIAN_POINT('Ctrl Pts',(79.7284421092199,-7.35609403781579,137.123153422847));
#81595=CARTESIAN_POINT('Ctrl Pts',(79.7529309360415,-7.35223568187565,137.121573384306));
#81596=CARTESIAN_POINT('Ctrl Pts',(79.794567906668,-7.34662453757074,137.118854549447));
#81597=CARTESIAN_POINT('Ctrl Pts',(79.8116742817811,-7.34458883300667,137.117728320681));
#81598=CARTESIAN_POINT('Ctrl Pts',(79.8362110084004,-7.34205411701391,137.116095777721));
#81599=CARTESIAN_POINT('Ctrl Pts',(79.8436185684363,-7.34133902581075,137.115600689487));
#81600=CARTESIAN_POINT('Ctrl Pts',(79.8565179687512,-7.34018095510876,137.11473428551));
#81601=CARTESIAN_POINT('Ctrl Pts',(79.8620076124977,-7.33971554995454,137.114364214438));
#81602=CARTESIAN_POINT('Ctrl Pts',(79.8737757401039,-7.33877663250152,137.113567875109));
#81603=CARTESIAN_POINT('Ctrl Pts',(79.8800545256124,-7.33831148514745,137.113141185907));
#81604=CARTESIAN_POINT('Ctrl Pts',(79.8973011623914,-7.33713206982759,137.111964461905));
#81605=CARTESIAN_POINT('Ctrl Pts',(79.9082734499359,-7.3364907489447,137.111210629211));
#81606=CARTESIAN_POINT('Ctrl Pts',(79.9706870801465,-7.33346207287906,137.106896027397));
#81607=CARTESIAN_POINT('Ctrl Pts',(80.0222062908539,-7.33335255587465,137.103232702536));
#81608=CARTESIAN_POINT('Ctrl Pts',(80.1695302163405,-7.33987107846556,137.092605930355));
#81609=CARTESIAN_POINT('Ctrl Pts',(80.2648731906396,-7.35239210199664,137.085556050158));
#81610=CARTESIAN_POINT('Ctrl Pts',(80.409985060169,-7.38437757452937,137.074869708017));
#81611=CARTESIAN_POINT('Ctrl Pts',(80.4607981217731,-7.39812935833552,137.071133387273));
#81612=CARTESIAN_POINT('Ctrl Pts',(80.5335741141651,-7.42157573007627,137.06580459824));
#81613=CARTESIAN_POINT('Ctrl Pts',(80.5561102154883,-7.42937399787028,137.064157448522));
#81614=CARTESIAN_POINT('Ctrl Pts',(80.5966738226919,-7.4443930226246,137.061197602513));
#81615=CARTESIAN_POINT('Ctrl Pts',(80.6147569525622,-7.4514501418102,137.059879910339));
#81616=CARTESIAN_POINT('Ctrl Pts',(80.642997515347,-7.46304398699626,137.057824081614));
#81617=CARTESIAN_POINT('Ctrl Pts',(80.6532394096869,-7.46736896982468,137.057078920747));
#81618=CARTESIAN_POINT('Ctrl Pts',(80.672356381081,-7.47566820016619,137.055688555415));
#81619=CARTESIAN_POINT('Ctrl Pts',(80.6812413888095,-7.47961823340645,137.055042563662));
#81620=CARTESIAN_POINT('Ctrl Pts',(80.7011282510186,-7.48866872758541,137.053596874606));
#81621=CARTESIAN_POINT('Ctrl Pts',(80.7121101008661,-7.49381201154106,137.052798682987));
#81622=CARTESIAN_POINT('Ctrl Pts',(80.7442842046183,-7.50931112236119,137.050459779111));
#81623=CARTESIAN_POINT('Ctrl Pts',(80.7653143711202,-7.51999786823467,137.04893051222));
#81624=CARTESIAN_POINT('Ctrl Pts',(80.8774414618012,-7.58000608229351,137.040760427582));
#81625=CARTESIAN_POINT('Ctrl Pts',(80.9640177691385,-7.63729704266457,137.034410865706));
#81626=CARTESIAN_POINT('Ctrl Pts',(81.1059702794231,-7.75157350076364,137.023281539753));
#81627=CARTESIAN_POINT('Ctrl Pts',(81.1636488216443,-7.80515328309771,137.018500501604));
#81628=CARTESIAN_POINT('Ctrl Pts',(81.2341633547055,-7.88062286609127,137.011986918203));
#81629=CARTESIAN_POINT('Ctrl Pts',(81.2505991737976,-7.89901592559647,137.010414528358));
#81630=CARTESIAN_POINT('Ctrl Pts',(81.2777687528396,-7.93081452611746,137.007707578318));
#81631=CARTESIAN_POINT('Ctrl Pts',(81.2887149114812,-7.94403390962229,137.006585441913));
#81632=CARTESIAN_POINT('Ctrl Pts',(81.3041047672187,-7.9632155586324,137.004957795859));
#81633=CARTESIAN_POINT('Ctrl Pts',(81.3087162183797,-7.96904264090452,137.004463420134));
#81634=CARTESIAN_POINT('Ctrl Pts',(81.3166776270797,-7.97924225881998,137.003597819541));
#81635=CARTESIAN_POINT('Ctrl Pts',(81.3200451289696,-7.98360086762118,137.003227832105));
#81636=CARTESIAN_POINT('Ctrl Pts',(81.3272193920897,-7.99298242140102,137.002431150676));
#81637=CARTESIAN_POINT('Ctrl Pts',(81.3310192225362,-7.99801020749411,137.002004031134));
#81638=CARTESIAN_POINT('Ctrl Pts',(81.3413838291799,-8.01188723885079,137.000824990503));
#81639=CARTESIAN_POINT('Ctrl Pts',(81.347889344664,-8.02078005318047,137.000069247937));
#81640=CARTESIAN_POINT('Ctrl Pts',(81.3846160984488,-8.07204371315929,136.99571468891));
#81641=CARTESIAN_POINT('Ctrl Pts',(81.4129241435148,-8.11574389506282,136.992011142933));
#81642=CARTESIAN_POINT('Ctrl Pts',(81.4906692313515,-8.24905122007465,136.980887321945));
#81643=CARTESIAN_POINT('Ctrl Pts',(81.533956939151,-8.34197514854748,136.973368375761));
#81644=CARTESIAN_POINT('Ctrl Pts',(81.5930243260781,-8.50690503324851,136.96080970814));
#81645=CARTESIAN_POINT('Ctrl Pts',(81.6130734390434,-8.57707462971653,136.95568737143));
#81646=CARTESIAN_POINT('Ctrl Pts',(81.6321832050295,-8.66556825751299,136.949508938956));
#81647=CARTESIAN_POINT('Ctrl Pts',(81.6356298002149,-8.68285365641989,136.948314854678));
#81648=CARTESIAN_POINT('Ctrl Pts',(81.6407335345188,-8.71075145200543,136.946407420768));
#81649=CARTESIAN_POINT('Ctrl Pts',(81.642563407467,-8.72133045449254,136.94568864909));
#81650=CARTESIAN_POINT('Ctrl Pts',(81.6458668126839,-8.7415926652274,136.944320371805));
#81651=CARTESIAN_POINT('Ctrl Pts',(81.6473574585509,-8.75127258594335,136.943670351426));
#81652=CARTESIAN_POINT('Ctrl Pts',(81.6505659021743,-8.77340310262026,136.942192292773));
#81653=CARTESIAN_POINT('Ctrl Pts',(81.6522283581794,-8.78586121756385,136.94136602735));
#81654=CARTESIAN_POINT('Ctrl Pts',(81.6562911740907,-8.81917862691827,136.939170897462));
#81655=CARTESIAN_POINT('Ctrl Pts',(81.6584385088627,-8.84006689597057,136.937809920035));
#81656=CARTESIAN_POINT('Ctrl Pts',(81.6702856578205,-8.98155785591697,136.928681678237));
#81657=CARTESIAN_POINT('Ctrl Pts',(81.6672181616441,-9.10286759374759,136.92133377957));
#81658=CARTESIAN_POINT('Ctrl Pts',(81.6421933819359,-9.28832325615413,136.909898570094));
#81659=CARTESIAN_POINT('Ctrl Pts',(81.6294561155291,-9.35327172153023,136.905846244306));
#81660=CARTESIAN_POINT('Ctrl Pts',(81.6072764738956,-9.43900046420705,136.900241485791));
#81661=CARTESIAN_POINT('Ctrl Pts',(81.6012209198121,-9.46059802079472,136.898806991174));
#81662=CARTESIAN_POINT('Ctrl Pts',(81.5901049388938,-9.49737103224749,136.896315484499));
#81663=CARTESIAN_POINT('Ctrl Pts',(81.5852584361791,-9.51260833480376,136.895268448324));
#81664=CARTESIAN_POINT('Ctrl Pts',(81.577904757381,-9.53462583093099,136.893730925547));
#81665=CARTESIAN_POINT('Ctrl Pts',(81.57557140313,-9.54146371187931,136.893249948932));
#81666=CARTESIAN_POINT('Ctrl Pts',(81.5714046680247,-9.55341929879982,136.892402531769));
#81667=CARTESIAN_POINT('Ctrl Pts',(81.5695906049574,-9.55854353687809,136.892037219388));
#81668=CARTESIAN_POINT('Ctrl Pts',(81.565583310173,-9.56968935902594,136.891237933373));
#81669=CARTESIAN_POINT('Ctrl Pts',(81.5633804395223,-9.57570709978228,136.890803426458));
#81670=CARTESIAN_POINT('Ctrl Pts',(81.5571307728611,-9.59247936082111,136.889584395084));
#81671=CARTESIAN_POINT('Ctrl Pts',(81.5530074393112,-9.60320470152957,136.888795632103));
#81672=CARTESIAN_POINT('Ctrl Pts',(81.5243353306837,-9.67554157651748,136.88341713847));
#81673=CARTESIAN_POINT('Ctrl Pts',(81.4962397283866,-9.73567610515647,136.878658160536));
#81674=CARTESIAN_POINT('Ctrl Pts',(81.4542098855688,-9.81320879768197,136.872264086088));
#81675=CARTESIAN_POINT('Ctrl Pts',(81.4434022627158,-9.83224084803977,136.870672475403));
#81676=CARTESIAN_POINT('Ctrl Pts',(81.3961142480812,-9.91182094501964,136.863935160198));
#81677=CARTESIAN_POINT('Ctrl Pts',(81.356172711813,-9.97023146690618,136.858789052242));
#81678=CARTESIAN_POINT('Ctrl Pts',(81.2707344875501,-10.0795464616061,136.848870215821));
#81679=CARTESIAN_POINT('Ctrl Pts',(81.2255795816743,-10.1305501149061,136.844099710361));
#81680=CARTESIAN_POINT('Ctrl Pts',(81.1651733223514,-10.1908933739795,136.838275596081));
#81681=CARTESIAN_POINT('Ctrl Pts',(81.1527310720011,-10.2029409853636,136.837102701328));
#81682=CARTESIAN_POINT('Ctrl Pts',(81.1323226691134,-10.2220946034857,136.835220753704));
#81683=CARTESIAN_POINT('Ctrl Pts',(81.1244724042254,-10.2293216292539,136.83450653695));
#81684=CARTESIAN_POINT('Ctrl Pts',(81.1092701341845,-10.2430495013136,136.833141614853));
#81685=CARTESIAN_POINT('Ctrl Pts',(81.1019290860147,-10.2495617590704,136.832490444838));
#81686=CARTESIAN_POINT('Ctrl Pts',(81.0849533051084,-10.2643550578846,136.831002433068));
#81687=CARTESIAN_POINT('Ctrl Pts',(81.075280455923,-10.2725915851624,136.830167449989));
#81688=CARTESIAN_POINT('Ctrl Pts',(81.0437811266256,-10.2987979864457,136.827488467548));
#81689=CARTESIAN_POINT('Ctrl Pts',(81.0215904795059,-10.3163237796437,136.825662270724));
#81690=CARTESIAN_POINT('Ctrl Pts',(80.8941829600746,-10.4117843904456,136.815487987002));
#81691=CARTESIAN_POINT('Ctrl Pts',(80.7805155922315,-10.477665785899,136.807616109418));
#81692=CARTESIAN_POINT('Ctrl Pts',(80.5948102165628,-10.5578334716761,136.795205826581));
#81693=CARTESIAN_POINT('Ctrl Pts',(80.5275786266557,-10.5818668656425,136.790783731773));
#81694=CARTESIAN_POINT('Ctrl Pts',(80.4438609717809,-10.6058618263717,136.785133352981));
#81695=CARTESIAN_POINT('Ctrl Pts',(80.428638808202,-10.6099917687636,136.784100222729));
#81696=CARTESIAN_POINT('Ctrl Pts',(80.406399766443,-10.6156877382123,136.782579442641));
#81697=CARTESIAN_POINT('Ctrl Pts',(80.3994272362334,-10.6174255827648,136.782101015622));
#81698=CARTESIAN_POINT('Ctrl Pts',(80.387164519408,-10.6203978349666,136.781256399625));
#81699=CARTESIAN_POINT('Ctrl Pts',(80.3818792114243,-10.6216515579059,136.780891313014));
#81700=CARTESIAN_POINT('Ctrl Pts',(80.3703196916429,-10.6243339342483,136.780090444845));
#81701=CARTESIAN_POINT('Ctrl Pts',(80.3640434023766,-10.6257520726284,136.779654110995));
#81702=CARTESIAN_POINT('Ctrl Pts',(80.3464214875973,-10.629626616931,136.778425119894));
#81703=CARTESIAN_POINT('Ctrl Pts',(80.3350584324346,-10.6320007921896,136.777628117311));
#81704=CARTESIAN_POINT('Ctrl Pts',(80.2481873668732,-10.6492060058914,136.771505309369));
#81705=CARTESIAN_POINT('Ctrl Pts',(80.1717659562092,-10.6589066249809,136.765952496989));
#81706=CARTESIAN_POINT('Ctrl Pts',(80.0378293131449,-10.6665530998448,136.756201245071));
#81707=CARTESIAN_POINT('Ctrl Pts',(79.9805694525012,-10.6668692240055,136.752025590368));
#81708=CARTESIAN_POINT('Ctrl Pts',(79.8407066776633,-10.6604322746638,136.741907962373));
#81709=CARTESIAN_POINT('Ctrl Pts',(79.7583961203379,-10.6504668633876,136.736028769055));
#81710=CARTESIAN_POINT('Ctrl Pts',(79.6547453997424,-10.6299929870419,136.728765173955));
#81711=CARTESIAN_POINT('Ctrl Pts',(79.6324263275546,-10.6251054002649,136.727208925176));
#81712=CARTESIAN_POINT('Ctrl Pts',(79.5987168025749,-10.6169933927209,136.724869244062));
#81713=CARTESIAN_POINT('Ctrl Pts',(79.5872492926389,-10.6141043035424,136.724075221344));
#81714=CARTESIAN_POINT('Ctrl Pts',(79.5673378331323,-10.6088617907514,136.722699560353));
#81715=CARTESIAN_POINT('Ctrl Pts',(79.5588800167884,-10.606563406102,136.722116176556));
#81716=CARTESIAN_POINT('Ctrl Pts',(79.5398471622232,-10.601229652412,136.720805344988));
#81717=CARTESIAN_POINT('Ctrl Pts',(79.5292831919322,-10.5981560406459,136.720079165132));
#81718=CARTESIAN_POINT('Ctrl Pts',(79.5006887586706,-10.589528294682,136.718116776693));
#81719=CARTESIAN_POINT('Ctrl Pts',(79.482720595688,-10.5837720733188,136.716887172434));
#81720=CARTESIAN_POINT('Ctrl Pts',(79.3710001194815,-10.5458774279842,136.709256356354));
#81721=CARTESIAN_POINT('Ctrl Pts',(79.2801691849516,-10.5057307623201,136.703132604211));
#81722=CARTESIAN_POINT('Ctrl Pts',(79.1307980769976,-10.423084225761,136.692690283821));
#81723=CARTESIAN_POINT('Ctrl Pts',(79.0704611377027,-10.384426766757,136.688349133291));
#81724=CARTESIAN_POINT('Ctrl Pts',(78.9831009961099,-10.3201635222736,136.681614700908));
#81725=CARTESIAN_POINT('Ctrl Pts',(78.9541373767744,-10.2973381718092,136.679299001643));
#81726=CARTESIAN_POINT('Ctrl Pts',(78.9140155203406,-10.2635021618502,136.675932793283));
#81727=CARTESIAN_POINT('Ctrl Pts',(78.902217052264,-10.2532647623231,136.674922358475));
#81728=CARTESIAN_POINT('Ctrl Pts',(78.881514870769,-10.2347850724395,136.673108805605));
#81729=CARTESIAN_POINT('Ctrl Pts',(78.8725538246555,-10.2266084379607,136.672309844211));
#81730=CARTESIAN_POINT('Ctrl Pts',(78.8589482644406,-10.2139188024175,136.67107368102));
#81731=CARTESIAN_POINT('Ctrl Pts',(78.8542392234489,-10.2094751595079,136.670641495881));
#81732=CARTESIAN_POINT('Ctrl Pts',(78.8455932379682,-10.2012206497899,136.669839668113));
#81733=CARTESIAN_POINT('Ctrl Pts',(78.8416490461505,-10.197417674136,136.669470616557));
#81734=CARTESIAN_POINT('Ctrl Pts',(78.8326801841062,-10.1886841482209,136.668623952236));
#81735=CARTESIAN_POINT('Ctrl Pts',(78.8276679565666,-10.1837411593081,136.668145400797));
#81736=CARTESIAN_POINT('Ctrl Pts',(78.8118019440852,-10.1678947172797,136.666613717909));
#81737=CARTESIAN_POINT('Ctrl Pts',(78.8010681616062,-10.1568729816143,136.665552075737));
#81738=CARTESIAN_POINT('Ctrl Pts',(78.7015875274873,-10.0518520987993,136.655483808707));
#81739=CARTESIAN_POINT('Ctrl Pts',(78.6239166161286,-9.94797679901163,136.645917796238));
#81740=CARTESIAN_POINT('Ctrl Pts',(78.5140359773491,-9.75862128761004,136.630101981317));
#81741=CARTESIAN_POINT('Ctrl Pts',(78.4753620663599,-9.67755384702874,136.623750119211));
#81742=CARTESIAN_POINT('Ctrl Pts',(78.4368323410281,-9.57654332016253,136.616363176341));
#81743=CARTESIAN_POINT('Ctrl Pts',(78.4305529036133,-9.55922373788411,136.615113945007));
#81744=CARTESIAN_POINT('Ctrl Pts',(78.4210148636928,-9.53148931414127,136.613140230456));
#81745=CARTESIAN_POINT('Ctrl Pts',(78.4175692330125,-9.52114089189607,136.612409630781));
#81746=CARTESIAN_POINT('Ctrl Pts',(78.4112349081996,-9.50147445784116,136.611031945276));
#81747=CARTESIAN_POINT('Ctrl Pts',(78.4083259626888,-9.49216350398151,136.610384219371));
#81748=CARTESIAN_POINT('Ctrl Pts',(78.4018883936778,-9.47090391612322,136.608915284332));
#81749=CARTESIAN_POINT('Ctrl Pts',(78.3984116571421,-9.45894008165288,136.608095793143));
#81750=CARTESIAN_POINT('Ctrl Pts',(78.3896655905076,-9.42753342749442,136.605962376743));
#81751=CARTESIAN_POINT('Ctrl Pts',(78.3846140042365,-9.40803171779105,136.604655448837));
#81752=CARTESIAN_POINT('Ctrl Pts',(78.3492974627889,-9.26073649740845,136.594905558187));
#81753=CARTESIAN_POINT('Ctrl Pts',(78.3338838505488,-9.12985839975195,136.586972010518));
#81754=CARTESIAN_POINT('Ctrl Pts',(78.334019749062,-8.97705318451493,136.5776200138));
#81755=CARTESIAN_POINT('Ctrl Pts',(78.3344536807646,-8.95559071879492,136.576303216903));
#81756=CARTESIAN_POINT('Ctrl Pts',(78.3378839471517,-8.86888232659901,136.570951022189));
#81757=CARTESIAN_POINT('Ctrl Pts',(78.3443007974377,-8.80383754936091,136.566862976514));
#81758=CARTESIAN_POINT('Ctrl Pts',(78.3563104882211,-8.72802161356447,136.561840519403));
#81759=CARTESIAN_POINT('Ctrl Pts',(78.3582210876476,-8.7167166808898,136.561084779101));
#81760=CARTESIAN_POINT('Ctrl Pts',(78.361380210958,-8.69913095672272,136.559897211975));
#81761=CARTESIAN_POINT('Ctrl Pts',(78.3625485697071,-8.69283586757687,136.559469706871));
#81762=CARTESIAN_POINT('Ctrl Pts',(78.3647761196605,-8.68120786947389,136.558675339287));
#81763=CARTESIAN_POINT('Ctrl Pts',(78.3658251659638,-8.67587321933013,136.558309044853));
#81764=CARTESIAN_POINT('Ctrl Pts',(78.3683307942889,-8.66345292970111,136.557451946765));
#81765=CARTESIAN_POINT('Ctrl Pts',(78.3698074268084,-8.65637157157594,136.556960043696));
#81766=CARTESIAN_POINT('Ctrl Pts',(78.3747060489727,-8.63362208901498,136.555369833779));
#81767=CARTESIAN_POINT('Ctrl Pts',(78.3783080608523,-8.61799423022668,136.5542622448));
#81768=CARTESIAN_POINT('Ctrl Pts',(78.3875089984116,-8.58055287725605,136.551575912956));
#81769=CARTESIAN_POINT('Ctrl Pts',(78.3933256425078,-8.55879650374042,136.549987992049));
#81770=CARTESIAN_POINT('Ctrl Pts',(78.4105689037284,-8.49917160166134,136.545573099394));
#81771=CARTESIAN_POINT('Ctrl Pts',(78.4229034382648,-8.46159013275024,136.542719630848));
#81772=CARTESIAN_POINT('Ctrl Pts',(78.4365593622862,-8.42449207447235,136.539851301691));
#81773=CARTESIAN_POINT('Ctrl Pts',(78.4365593881204,-8.4244920042904,136.733447186333));
#81774=CARTESIAN_POINT('Ctrl Pts',(78.4030736945878,-8.51546014648167,136.739621454435));
#81775=CARTESIAN_POINT('Ctrl Pts',(78.3775820369106,-8.6092014352621,136.745546832545));
#81776=CARTESIAN_POINT('Ctrl Pts',(78.3470673853013,-8.7786056050962,136.756057576631));
#81777=CARTESIAN_POINT('Ctrl Pts',(78.3387660631224,-8.85336467809191,136.760635535814));
#81778=CARTESIAN_POINT('Ctrl Pts',(78.3345040617009,-8.95247331443709,136.766897335687));
#81779=CARTESIAN_POINT('Ctrl Pts',(78.3339912587448,-8.976542383031,136.768433278269));
#81780=CARTESIAN_POINT('Ctrl Pts',(78.3340063127194,-9.01746820049141,136.771083447886));
#81781=CARTESIAN_POINT('Ctrl Pts',(78.3342683081296,-9.03432173335585,136.772185923354));
#81782=CARTESIAN_POINT('Ctrl Pts',(78.3350100826228,-9.05846227663029,136.773784728963));
#81783=CARTESIAN_POINT('Ctrl Pts',(78.3352821544246,-9.06575524640231,136.774270308084));
#81784=CARTESIAN_POINT('Ctrl Pts',(78.3358435544196,-9.07854708528083,136.775126896748));
#81785=CARTESIAN_POINT('Ctrl Pts',(78.3361122407625,-9.0840466752278,136.775496764983));
#81786=CARTESIAN_POINT('Ctrl Pts',(78.3367468936854,-9.09583743544319,136.776293281405));
#81787=CARTESIAN_POINT('Ctrl Pts',(78.3371212848046,-9.10212778735096,136.776720355728));
#81788=CARTESIAN_POINT('Ctrl Pts',(78.3382678805403,-9.11970991711179,136.77791975653));
#81789=CARTESIAN_POINT('Ctrl Pts',(78.3391194647483,-9.1309959204132,136.778696218196));
#81790=CARTESIAN_POINT('Ctrl Pts',(78.3456209276976,-9.20684971771665,136.783955189898));
#81791=CARTESIAN_POINT('Ctrl Pts',(78.3549191552492,-9.27104252512709,136.788600551448));
#81792=CARTESIAN_POINT('Ctrl Pts',(78.3892327549589,-9.43845169740273,136.800982562631));
#81793=CARTESIAN_POINT('Ctrl Pts',(78.4204158893562,-9.54011910056802,136.808760889797));
#81794=CARTESIAN_POINT('Ctrl Pts',(78.4829022374298,-9.690813060589,136.820349834248));
#81795=CARTESIAN_POINT('Ctrl Pts',(78.5074386473511,-9.74234104091414,136.824328710901));
#81796=CARTESIAN_POINT('Ctrl Pts',(78.5427106347886,-9.80756198835594,136.829384765667));
#81797=CARTESIAN_POINT('Ctrl Pts',(78.5510800918421,-9.82248391877545,136.83054312028));
#81798=CARTESIAN_POINT('Ctrl Pts',(78.5650169043896,-9.8464587183596,136.832407449484));
#81799=CARTESIAN_POINT('Ctrl Pts',(78.5704434462281,-9.85559155861872,136.833118414691));
#81800=CARTESIAN_POINT('Ctrl Pts',(78.5810561551776,-9.87306980706646,136.834480806376));
#81801=CARTESIAN_POINT('Ctrl Pts',(78.5862295038704,-9.881422437934,136.83513266302));
#81802=CARTESIAN_POINT('Ctrl Pts',(78.5984297757597,-9.90073659966631,136.836642117404));
#81803=CARTESIAN_POINT('Ctrl Pts',(78.6055119745721,-9.91166259019809,136.837497634055));
#81804=CARTESIAN_POINT('Ctrl Pts',(78.6289516698963,-9.94691160386154,136.840264130959));
#81805=CARTESIAN_POINT('Ctrl Pts',(78.6458236350977,-9.9708870422807,136.842155868848));
#81806=CARTESIAN_POINT('Ctrl Pts',(78.687779259035,-10.0272837545402,136.846642823129));
#81807=CARTESIAN_POINT('Ctrl Pts',(78.7134440285047,-10.0592493898091,136.849216597647));
#81808=CARTESIAN_POINT('Ctrl Pts',(78.7883692976428,-10.1458232872106,136.856329676963));
#81809=CARTESIAN_POINT('Ctrl Pts',(78.8401032628258,-10.1981652664024,136.860796537195));
#81810=CARTESIAN_POINT('Ctrl Pts',(78.9595922688885,-10.3040424533988,136.870555924798));
#81811=CARTESIAN_POINT('Ctrl Pts',(79.028384029632,-10.3560728796528,136.87584406862));
#81812=CARTESIAN_POINT('Ctrl Pts',(79.114166368779,-10.4110648129433,136.882455015258));
#81813=CARTESIAN_POINT('Ctrl Pts',(79.1275739912358,-10.4193935125204,136.883488879084));
#81814=CARTESIAN_POINT('Ctrl Pts',(79.1471900400681,-10.4311959096451,136.885005410462));
#81815=CARTESIAN_POINT('Ctrl Pts',(79.1533060366019,-10.4348225978468,136.885478788803));
#81816=CARTESIAN_POINT('Ctrl Pts',(79.1641802255776,-10.4411770831021,136.886321761173));
#81817=CARTESIAN_POINT('Ctrl Pts',(79.1689289465603,-10.4439206983225,136.886690335297));
#81818=CARTESIAN_POINT('Ctrl Pts',(79.1792667995152,-10.449825590466,136.887493785354));
#81819=CARTESIAN_POINT('Ctrl Pts',(79.18486060001,-10.4529779710146,136.887929175106));
#81820=CARTESIAN_POINT('Ctrl Pts',(79.2008555866187,-10.4618704939397,136.889175660464));
#81821=CARTESIAN_POINT('Ctrl Pts',(79.211299890914,-10.4675316869695,136.889991408645));
#81822=CARTESIAN_POINT('Ctrl Pts',(79.2352487806186,-10.48018336694,136.891864560845));
#81823=CARTESIAN_POINT('Ctrl Pts',(79.2487901943231,-10.4871015496115,136.89292557646));
#81824=CARTESIAN_POINT('Ctrl Pts',(79.3926802361372,-10.5581468755979,136.904205445557));
#81825=CARTESIAN_POINT('Ctrl Pts',(79.5307877751497,-10.6051487126799,136.915012031052));
#81826=CARTESIAN_POINT('Ctrl Pts',(79.7375228892412,-10.646498846995,136.930069698027));
#81827=CARTESIAN_POINT('Ctrl Pts',(79.8025079980723,-10.6555517333834,136.934662415066));
#81828=CARTESIAN_POINT('Ctrl Pts',(79.8854547239337,-10.6621512331637,136.940341172531));
#81829=CARTESIAN_POINT('Ctrl Pts',(79.9030657133278,-10.6632712129491,136.941536703293));
#81830=CARTESIAN_POINT('Ctrl Pts',(79.9314178227011,-10.6646224179439,136.943445749573));
#81831=CARTESIAN_POINT('Ctrl Pts',(79.942148771015,-10.66502989583,136.944164706079));
#81832=CARTESIAN_POINT('Ctrl Pts',(79.9626686379264,-10.6656104593268,136.945532894171));
#81833=CARTESIAN_POINT('Ctrl Pts',(79.9724565693854,-10.6658010683219,136.946182644441));
#81834=CARTESIAN_POINT('Ctrl Pts',(79.9950118735277,-10.6660414490357,136.947673600115));
#81835=CARTESIAN_POINT('Ctrl Pts',(80.0077793809961,-10.6660307583072,136.948512888166));
#81836=CARTESIAN_POINT('Ctrl Pts',(80.0484004376635,-10.6655297644201,136.951169351394));
#81837=CARTESIAN_POINT('Ctrl Pts',(80.0762432688115,-10.6644876410038,136.952969411709));
#81838=CARTESIAN_POINT('Ctrl Pts',(80.17707580758,-10.6581779363621,136.959429051887));
#81839=CARTESIAN_POINT('Ctrl Pts',(80.2497269836236,-10.6488019685092,136.963966280212));
#81840=CARTESIAN_POINT('Ctrl Pts',(80.4498323691207,-10.6094423174595,136.976475569173));
#81841=CARTESIAN_POINT('Ctrl Pts',(80.5746952258867,-10.5691937199781,136.984278196408));
#81842=CARTESIAN_POINT('Ctrl Pts',(80.7072593246362,-10.5084984670799,136.993749889294));
#81843=CARTESIAN_POINT('Ctrl Pts',(80.7208831856639,-10.5020355425522,136.994738555911));
#81844=CARTESIAN_POINT('Ctrl Pts',(80.7407513367565,-10.4922778766141,136.996205607827));
#81845=CARTESIAN_POINT('Ctrl Pts',(80.7470658423804,-10.4891267328796,136.996675659482));
#81846=CARTESIAN_POINT('Ctrl Pts',(80.7582388396376,-10.4834620937601,136.997514468975));
#81847=CARTESIAN_POINT('Ctrl Pts',(80.7631052433752,-10.4809646543762,136.997882236156));
#81848=CARTESIAN_POINT('Ctrl Pts',(80.7737687639961,-10.4754256182811,136.998693515298));
#81849=CARTESIAN_POINT('Ctrl Pts',(80.7795602064822,-10.4723738438356,136.999137630889));
#81850=CARTESIAN_POINT('Ctrl Pts',(80.7963407056481,-10.4634046795101,137.000434326687));
#81851=CARTESIAN_POINT('Ctrl Pts',(80.8072811569883,-10.4573979847158,137.001292141429));
#81852=CARTESIAN_POINT('Ctrl Pts',(80.8970833642042,-10.4067720101496,137.008430061082));
#81853=CARTESIAN_POINT('Ctrl Pts',(80.9722441434968,-10.3559144171397,137.01501705316));
#81854=CARTESIAN_POINT('Ctrl Pts',(81.1403180900579,-10.2209993084927,137.030705606517));
#81855=CARTESIAN_POINT('Ctrl Pts',(81.2286584273756,-10.1320663474827,137.039739972988));
#81856=CARTESIAN_POINT('Ctrl Pts',(81.3190964111585,-10.0178262180048,137.049759134163));
#81857=CARTESIAN_POINT('Ctrl Pts',(81.3316568116364,-10.0013369837524,137.051172559126));
#81858=CARTESIAN_POINT('Ctrl Pts',(81.3512882083391,-9.97454203031362,137.053418518639));
#81859=CARTESIAN_POINT('Ctrl Pts',(81.3585563025847,-9.96438414456928,137.054258601021));
#81860=CARTESIAN_POINT('Ctrl Pts',(81.3713113262891,-9.94612732341943,137.055748741476));
#81861=CARTESIAN_POINT('Ctrl Pts',(81.3768423814852,-9.93806008831394,137.056400462165));
#81862=CARTESIAN_POINT('Ctrl Pts',(81.388314362337,-9.92100773224648,137.057764231038));
#81863=CARTESIAN_POINT('Ctrl Pts',(81.39423985985,-9.91201273780734,137.058475678021));
#81864=CARTESIAN_POINT('Ctrl Pts',(81.4097237013106,-9.88800440344568,137.06035416898));
#81865=CARTESIAN_POINT('Ctrl Pts',(81.4191295884013,-9.87289402885515,137.061515560676));
#81866=CARTESIAN_POINT('Ctrl Pts',(81.4674035912919,-9.79249929604251,137.067591076656));
#81867=CARTESIAN_POINT('Ctrl Pts',(81.5020166326017,-9.7247596804068,137.072349634004));
#81868=CARTESIAN_POINT('Ctrl Pts',(81.5734663343402,-9.55762699477199,137.083554347229));
#81869=CARTESIAN_POINT('Ctrl Pts',(81.6056856278077,-9.45663511974328,137.089898723803));
#81870=CARTESIAN_POINT('Ctrl Pts',(81.6378182559004,-9.30854847151764,137.09936819472));
#81871=CARTESIAN_POINT('Ctrl Pts',(81.6456753667433,-9.26344366715188,137.102276282563));
#81872=CARTESIAN_POINT('Ctrl Pts',(81.6530800128923,-9.20736267157802,137.105984314004));
#81873=CARTESIAN_POINT('Ctrl Pts',(81.6543903865843,-9.19663478889484,137.106697782848));
#81874=CARTESIAN_POINT('Ctrl Pts',(81.6562871041937,-9.17974248924931,137.107828819388));
#81875=CARTESIAN_POINT('Ctrl Pts',(81.6569436381821,-9.17358603264176,137.108242613114));
#81876=CARTESIAN_POINT('Ctrl Pts',(81.6581221064551,-9.16191886877446,137.109030039472));
#81877=CARTESIAN_POINT('Ctrl Pts',(81.6586509120692,-9.15640904111595,137.109403291966));
#81878=CARTESIAN_POINT('Ctrl Pts',(81.6598439596103,-9.14329115099583,137.110295138221));
#81879=CARTESIAN_POINT('Ctrl Pts',(81.6604833562444,-9.1356810308897,137.110815072687));
#81880=CARTESIAN_POINT('Ctrl Pts',(81.6624850134589,-9.10971888398158,137.112596910054));
#81881=CARTESIAN_POINT('Ctrl Pts',(81.663595457097,-9.09134954271517,137.113871358065));
#81882=CARTESIAN_POINT('Ctrl Pts',(81.6655890493043,-9.0458747670624,137.117054282046));
#81883=CARTESIAN_POINT('Ctrl Pts',(81.6661150297035,-9.0187594914234,137.118976628921));
#81884=CARTESIAN_POINT('Ctrl Pts',(81.665502353316,-8.89659148234794,137.127715518917));
#81885=CARTESIAN_POINT('Ctrl Pts',(81.6568917014446,-8.80175481881864,137.134699384888));
#81886=CARTESIAN_POINT('Ctrl Pts',(81.6241860233122,-8.61793103655888,137.148200103104));
#81887=CARTESIAN_POINT('Ctrl Pts',(81.6007092506829,-8.52915839469721,137.154701657713));
#81888=CARTESIAN_POINT('Ctrl Pts',(81.5637647548798,-8.42506688566657,137.162252692951));
#81889=CARTESIAN_POINT('Ctrl Pts',(81.5571880318334,-8.40748520854705,137.163526063361));
#81890=CARTESIAN_POINT('Ctrl Pts',(81.5462955055341,-8.37980103947063,137.165528628987));
#81891=CARTESIAN_POINT('Ctrl Pts',(81.5421746800608,-8.36962407466295,137.166264256121));
#81892=CARTESIAN_POINT('Ctrl Pts',(81.5345838467956,-8.35139747600969,137.167581030549));
#81893=CARTESIAN_POINT('Ctrl Pts',(81.5311503807921,-8.34333316408331,137.168163382486));
#81894=CARTESIAN_POINT('Ctrl Pts',(81.522925753619,-8.32443094134723,137.169527991053));
#81895=CARTESIAN_POINT('Ctrl Pts',(81.5180822481688,-8.31361621233241,137.170308435965));
#81896=CARTESIAN_POINT('Ctrl Pts',(81.5035097039028,-8.28198717541995,137.172590804864));
#81897=CARTESIAN_POINT('Ctrl Pts',(81.4934647746397,-8.26132084362126,137.174081880258));
#81898=CARTESIAN_POINT('Ctrl Pts',(81.4447953142107,-8.16624307054402,137.180951620334));
#81899=CARTESIAN_POINT('Ctrl Pts',(81.4010152041951,-8.09460346171918,137.186148617948));
#81900=CARTESIAN_POINT('Ctrl Pts',(81.3008705401275,-7.95551164674379,137.196652378125));
#81901=CARTESIAN_POINT('Ctrl Pts',(81.2442006213366,-7.88861193906081,137.20193831183));
#81902=CARTESIAN_POINT('Ctrl Pts',(81.1495068912117,-7.79319049627619,137.21033118623));
#81903=CARTESIAN_POINT('Ctrl Pts',(81.1150857141232,-7.76131592118927,137.213308127978));
#81904=CARTESIAN_POINT('Ctrl Pts',(81.0710771882292,-7.72388551734343,137.217094491853));
#81905=CARTESIAN_POINT('Ctrl Pts',(81.0627158218324,-7.71691403930226,137.217813057695));
#81906=CARTESIAN_POINT('Ctrl Pts',(81.0494797805833,-7.70609631889675,137.218950369127));
#81907=CARTESIAN_POINT('Ctrl Pts',(81.0446507239971,-7.70219438761639,137.219365270916));
#81908=CARTESIAN_POINT('Ctrl Pts',(81.0354791978529,-7.69486804724877,137.220153445191));
#81909=CARTESIAN_POINT('Ctrl Pts',(81.0311413471601,-7.69143815516734,137.220526324128));
#81910=CARTESIAN_POINT('Ctrl Pts',(81.0207998958806,-7.68334462915329,137.221415396917));
#81911=CARTESIAN_POINT('Ctrl Pts',(81.0147813537242,-7.67870041568294,137.221932908338));
#81912=CARTESIAN_POINT('Ctrl Pts',(80.9942551414701,-7.66308430727233,137.22369757671));
#81913=CARTESIAN_POINT('Ctrl Pts',(80.9796002248323,-7.65230931297159,137.224956966311));
#81914=CARTESIAN_POINT('Ctrl Pts',(80.9430135399167,-7.6263210689669,137.228094086435));
#81915=CARTESIAN_POINT('Ctrl Pts',(80.9208873689399,-7.61139111429586,137.229985214478));
#81916=CARTESIAN_POINT('Ctrl Pts',(80.8209939379261,-7.54742418886821,137.238466092561));
#81917=CARTESIAN_POINT('Ctrl Pts',(80.7396056100558,-7.50434271516757,137.245215577464));
#81918=CARTESIAN_POINT('Ctrl Pts',(80.5674640664469,-7.43072593788484,137.258770013421));
#81919=CARTESIAN_POINT('Ctrl Pts',(80.4767826088042,-7.40083757849732,137.265540872448));
#81920=CARTESIAN_POINT('Ctrl Pts',(80.3656505449698,-7.37451164804401,137.273349923768));
#81921=CARTESIAN_POINT('Ctrl Pts',(80.3471992399141,-7.37047079126015,137.274631403468));
#81922=CARTESIAN_POINT('Ctrl Pts',(80.3178947134579,-7.36457343749752,137.276643698277));
#81923=CARTESIAN_POINT('Ctrl Pts',(80.3070854331381,-7.36250934750913,137.277381052308));
#81924=CARTESIAN_POINT('Ctrl Pts',(80.2876348235573,-7.35899452629569,137.278699344028));
#81925=CARTESIAN_POINT('Ctrl Pts',(80.2790010878172,-7.35750459529958,137.279281503469));
#81926=CARTESIAN_POINT('Ctrl Pts',(80.2586983642431,-7.35416564350015,137.280643646055));
#81927=CARTESIAN_POINT('Ctrl Pts',(80.2470205646876,-7.35237248586113,137.281421839117));
#81928=CARTESIAN_POINT('Ctrl Pts',(80.2127545332068,-7.34748334988967,137.283690554916));
#81929=CARTESIAN_POINT('Ctrl Pts',(80.1901200915037,-7.34472654753425,137.285170430414));
#81930=CARTESIAN_POINT('Ctrl Pts',(80.0854031239648,-7.33414879322847,137.291941335192));
#81931=CARTESIAN_POINT('Ctrl Pts',(80.002864225,-7.33196281932455,137.297057058166));
#81932=CARTESIAN_POINT('Ctrl Pts',(79.7919194644137,-7.34204107561868,137.310005486723));
#81933=CARTESIAN_POINT('Ctrl Pts',(79.664509127047,-7.3630633913947,137.317694886708));
#81934=CARTESIAN_POINT('Ctrl Pts',(79.5273692636888,-7.40238562815179,137.326955958689));
#81935=CARTESIAN_POINT('Ctrl Pts',(79.5139785017933,-7.40640828107118,137.327871331792));
#81936=CARTESIAN_POINT('Ctrl Pts',(79.4940024158347,-7.41268438603332,137.329255760459));
#81937=CARTESIAN_POINT('Ctrl Pts',(79.4873776210148,-7.4148114604742,137.329718024127));
#81938=CARTESIAN_POINT('Ctrl Pts',(79.4754516813434,-7.41872319071898,137.330556189795));
#81939=CARTESIAN_POINT('Ctrl Pts',(79.4701457492388,-7.42049319157249,137.330931250759));
#81940=CARTESIAN_POINT('Ctrl Pts',(79.4592424670526,-7.42419152855173,137.331706602901));
#81941=CARTESIAN_POINT('Ctrl Pts',(79.4536463463172,-7.42612302562506,137.332107063082));
#81942=CARTESIAN_POINT('Ctrl Pts',(79.4390329966833,-7.43125414116497,137.333159158438));
#81943=CARTESIAN_POINT('Ctrl Pts',(79.4300329836935,-7.43450163274381,137.333813480159));
#81944=CARTESIAN_POINT('Ctrl Pts',(79.3889993801016,-7.44970860057302,137.33682431057));
#81945=CARTESIAN_POINT('Ctrl Pts',(79.3573129913227,-7.46257416219897,137.339226467524));
#81946=CARTESIAN_POINT('Ctrl Pts',(79.2627235372162,-7.50441517704138,137.346588336996));
#81947=CARTESIAN_POINT('Ctrl Pts',(79.2012105148663,-7.53634533445654,137.351635606992));
#81948=CARTESIAN_POINT('Ctrl Pts',(79.0420267517058,-7.63200485642804,137.365152648743));
#81949=CARTESIAN_POINT('Ctrl Pts',(78.9487381917789,-7.70231699241491,137.373548315926));
#81950=CARTESIAN_POINT('Ctrl Pts',(78.8480522834023,-7.79624712134135,137.383022913099));
#81951=CARTESIAN_POINT('Ctrl Pts',(78.8328425060737,-7.81098864997468,137.384467923748));
#81952=CARTESIAN_POINT('Ctrl Pts',(78.8090260155006,-7.83496945372168,137.386753858893));
#81953=CARTESIAN_POINT('Ctrl Pts',(78.8002364893233,-7.84402303692085,137.387602764272));
#81954=CARTESIAN_POINT('Ctrl Pts',(78.784805559936,-7.86028315769854,137.389102934962));
#81955=CARTESIAN_POINT('Ctrl Pts',(78.7781233786036,-7.86744998480212,137.389755943137));
#81956=CARTESIAN_POINT('Ctrl Pts',(78.76427297701,-7.88257020400818,137.391116832424));
#81957=CARTESIAN_POINT('Ctrl Pts',(78.7571173950721,-7.89053460454368,137.391824161008));
#81958=CARTESIAN_POINT('Ctrl Pts',(78.7410372318918,-7.90878318484026,137.393423843834));
#81959=CARTESIAN_POINT('Ctrl Pts',(78.7321608837218,-7.91910898683019,137.394314188008));
#81960=CARTESIAN_POINT('Ctrl Pts',(78.6928012258623,-7.96604787071688,137.398297492482));
#81961=CARTESIAN_POINT('Ctrl Pts',(78.6637685887258,-8.00385146548987,137.401332334813));
#81962=CARTESIAN_POINT('Ctrl Pts',(78.5872532638754,-8.11285925199138,137.409688507001));
#81963=CARTESIAN_POINT('Ctrl Pts',(78.5435757492815,-8.18654959279615,137.414890615171));
#81964=CARTESIAN_POINT('Ctrl Pts',(78.4798579573421,-8.31578365342842,137.423693429284));
#81965=CARTESIAN_POINT('Ctrl Pts',(78.4567655212686,-8.36959947731005,137.427276118832));
#81966=CARTESIAN_POINT('Ctrl Pts',(78.4365593939729,-8.42449198839149,137.430947540156));
#81967=CARTESIAN_POINT('Origin',(80.,-9.,134.));
#81968=CARTESIAN_POINT('',(78.4365594354234,-8.4244918757859,138.13187361233));
#81969=CARTESIAN_POINT('',(78.4365593741136,-8.42449204234183,137.937814844869));
#81970=CARTESIAN_POINT('',(78.4365593749993,-8.42449203993574,134.));
#81971=CARTESIAN_POINT('',(78.3340004536119,-9.00002839986701,137.276979779061));
#81972=CARTESIAN_POINT('Ctrl Pts',(78.4365593741136,-8.42449204234183,137.937814844869));
#81973=CARTESIAN_POINT('Ctrl Pts',(78.4603179885632,-8.35994874185208,137.933371985177));
#81974=CARTESIAN_POINT('Ctrl Pts',(78.4880534421214,-8.29693057726159,137.929060103377));
#81975=CARTESIAN_POINT('Ctrl Pts',(78.5665913610029,-8.14478919144876,137.918489342388));
#81976=CARTESIAN_POINT('Ctrl Pts',(78.6218616409535,-8.05831053718337,137.912339462922));
#81977=CARTESIAN_POINT('Ctrl Pts',(78.7166755345118,-7.93635294388492,137.902733463664));
#81978=CARTESIAN_POINT('Ctrl Pts',(78.7505374150341,-7.89677344010222,137.899441880882));
#81979=CARTESIAN_POINT('Ctrl Pts',(78.7937404515054,-7.8508197125464,137.895310731004));
#81980=CARTESIAN_POINT('Ctrl Pts',(78.8013677090719,-7.84286645257854,137.894583788391));
#81981=CARTESIAN_POINT('Ctrl Pts',(78.8134803043143,-7.83048440224266,137.893431927752));
#81982=CARTESIAN_POINT('Ctrl Pts',(78.8179130004964,-7.82600424022333,137.8930109256));
#81983=CARTESIAN_POINT('Ctrl Pts',(78.8262671466301,-7.81765591769989,137.892218210012));
#81984=CARTESIAN_POINT('Ctrl Pts',(78.8301824886623,-7.81378192280248,137.891846961148));
#81985=CARTESIAN_POINT('Ctrl Pts',(78.8394248594893,-7.80472741262935,137.890971326298));
#81986=CARTESIAN_POINT('Ctrl Pts',(78.8447674106453,-7.79956304867256,137.890465737291));
#81987=CARTESIAN_POINT('Ctrl Pts',(78.8625617832787,-7.78259095855185,137.888784199261));
#81988=CARTESIAN_POINT('Ctrl Pts',(78.8751610216921,-7.77094032418107,137.8875974761));
#81989=CARTESIAN_POINT('Ctrl Pts',(78.9062990152035,-7.74302655077145,137.884678692788));
#81990=CARTESIAN_POINT('Ctrl Pts',(78.9250229469967,-7.72697670799429,137.882935380343));
#81991=CARTESIAN_POINT('Ctrl Pts',(79.0048904208475,-7.66153426535988,137.875570584162));
#81992=CARTESIAN_POINT('Ctrl Pts',(79.0691322943938,-7.61608596866158,137.869821928419));
#81993=CARTESIAN_POINT('Ctrl Pts',(79.2249479352132,-7.52162681719461,137.856577649312));
#81994=CARTESIAN_POINT('Ctrl Pts',(79.3183877378418,-7.47628601570247,137.849147271052));
#81995=CARTESIAN_POINT('Ctrl Pts',(79.4375354997769,-7.43164226868499,137.840388318034));
#81996=CARTESIAN_POINT('Ctrl Pts',(79.4597959223641,-7.42383632174753,137.838779865323));
#81997=CARTESIAN_POINT('Ctrl Pts',(79.4937410107878,-7.41273667170991,137.836368001387));
#81998=CARTESIAN_POINT('Ctrl Pts',(79.5053074587709,-7.40909386177838,137.835553255619));
#81999=CARTESIAN_POINT('Ctrl Pts',(79.5262182966011,-7.40275817842931,137.83409266417));
#82000=CARTESIAN_POINT('Ctrl Pts',(79.5355483429084,-7.40002024883038,137.833445374592));
#82001=CARTESIAN_POINT('Ctrl Pts',(79.5555963550732,-7.39432724622947,137.832063666324));
#82002=CARTESIAN_POINT('Ctrl Pts',(79.5663210545656,-7.39139744679201,137.831330093915));
#82003=CARTESIAN_POINT('Ctrl Pts',(79.5958481947151,-7.38364791967222,137.829325128198));
#82004=CARTESIAN_POINT('Ctrl Pts',(79.6147071648056,-7.37904897929614,137.828060847683));
#82005=CARTESIAN_POINT('Ctrl Pts',(79.6569031637806,-7.3695371529798,137.825265231572));
#82006=CARTESIAN_POINT('Ctrl Pts',(79.6802741680488,-7.36479358733659,137.823739203859));
#82007=CARTESIAN_POINT('Ctrl Pts',(79.755511527174,-7.35119764114957,137.818887863544));
#82008=CARTESIAN_POINT('Ctrl Pts',(79.8076997016165,-7.34429922645207,137.815616521277));
#82009=CARTESIAN_POINT('Ctrl Pts',(79.9557637071104,-7.3318243898085,137.806469789002));
#82010=CARTESIAN_POINT('Ctrl Pts',(80.0519101041761,-7.33204596136709,137.800694915909));
#82011=CARTESIAN_POINT('Ctrl Pts',(80.1988056473655,-7.34510256166756,137.791520640568));
#82012=CARTESIAN_POINT('Ctrl Pts',(80.249868416941,-7.35203948084721,137.788262748334));
#82013=CARTESIAN_POINT('Ctrl Pts',(80.3113335539439,-7.36331180867816,137.784169521228));
#82014=CARTESIAN_POINT('Ctrl Pts',(80.3221247026131,-7.36540143230137,137.78344438159));
#82015=CARTESIAN_POINT('Ctrl Pts',(80.3390632593351,-7.36885569358066,137.782294758058));
#82016=CARTESIAN_POINT('Ctrl Pts',(80.3452251821864,-7.37014871460305,137.781874165202));
#82017=CARTESIAN_POINT('Ctrl Pts',(80.356765152495,-7.37263864444638,137.781081758952));
#82018=CARTESIAN_POINT('Ctrl Pts',(80.3621447715477,-7.3738273411217,137.780710405365));
#82019=CARTESIAN_POINT('Ctrl Pts',(80.374776833488,-7.37668434794355,137.779833896293));
#82020=CARTESIAN_POINT('Ctrl Pts',(80.3820240964597,-7.3783745914791,137.779327530361));
#82021=CARTESIAN_POINT('Ctrl Pts',(80.4060083025106,-7.3841380086455,137.777640697665));
#82022=CARTESIAN_POINT('Ctrl Pts',(80.4226927586246,-7.38842204942205,137.776449366821));
#82023=CARTESIAN_POINT('Ctrl Pts',(80.463216110517,-7.39949970298187,137.773516884167));
#82024=CARTESIAN_POINT('Ctrl Pts',(80.486975183291,-7.4065680418602,137.77176435114));
#82025=CARTESIAN_POINT('Ctrl Pts',(80.586115201697,-7.43848656424449,137.764334432047));
#82026=CARTESIAN_POINT('Ctrl Pts',(80.6598263802082,-7.46817640185108,137.758528000872));
#82027=CARTESIAN_POINT('Ctrl Pts',(80.8233416366015,-7.54803787661784,137.745303092223));
#82028=CARTESIAN_POINT('Ctrl Pts',(80.9112010692431,-7.60149919320195,137.737947919739));
#82029=CARTESIAN_POINT('Ctrl Pts',(81.0125322055783,-7.67678752968935,137.729257556827));
#82030=CARTESIAN_POINT('Ctrl Pts',(81.0311711755371,-7.69126060099015,137.727648481611));
#82031=CARTESIAN_POINT('Ctrl Pts',(81.0589161014918,-7.71376527330377,137.725235878649));
#82032=CARTESIAN_POINT('Ctrl Pts',(81.0682514425024,-7.72150793853002,137.724421005967));
#82033=CARTESIAN_POINT('Ctrl Pts',(81.0849174950513,-7.7356406480849,137.722960277211));
#82034=CARTESIAN_POINT('Ctrl Pts',(81.0922783040723,-7.74199417522227,137.722312976071));
#82035=CARTESIAN_POINT('Ctrl Pts',(81.1079340618461,-7.75574854717508,137.720931339293));
#82036=CARTESIAN_POINT('Ctrl Pts',(81.1162114484187,-7.76316873594401,137.720197849054));
#82037=CARTESIAN_POINT('Ctrl Pts',(81.1387317812083,-7.78376711748497,137.718193357637));
#82038=CARTESIAN_POINT('Ctrl Pts',(81.1528200250781,-7.79711241803091,137.716929463497));
#82039=CARTESIAN_POINT('Ctrl Pts',(81.1836869676044,-7.82739211890354,137.714134830555));
#82040=CARTESIAN_POINT('Ctrl Pts',(81.2003419860459,-7.84444676382978,137.712609393769));
#82041=CARTESIAN_POINT('Ctrl Pts',(81.252544940583,-7.90024931138634,137.707760653262));
#82042=CARTESIAN_POINT('Ctrl Pts',(81.2866278763551,-7.94032564594187,137.704491251537));
#82043=CARTESIAN_POINT('Ctrl Pts',(81.3774118072201,-8.05792514731249,137.695345823314));
#82044=CARTESIAN_POINT('Ctrl Pts',(81.4293852163419,-8.13882357268403,137.689570473641));
#82045=CARTESIAN_POINT('Ctrl Pts',(81.4981227558006,-8.26935530624059,137.680393395951));
#82046=CARTESIAN_POINT('Ctrl Pts',(81.5200097847314,-8.31605366175291,137.677133004696));
#82047=CARTESIAN_POINT('Ctrl Pts',(81.5438938458182,-8.37384614241747,137.673036972318));
#82048=CARTESIAN_POINT('Ctrl Pts',(81.5479919681851,-8.38404731425259,137.672311705972));
#82049=CARTESIAN_POINT('Ctrl Pts',(81.5542779882448,-8.40015370048978,137.671161925215));
#82050=CARTESIAN_POINT('Ctrl Pts',(81.556533957345,-8.40603225328301,137.670741303586));
#82051=CARTESIAN_POINT('Ctrl Pts',(81.5607012813342,-8.41707816568329,137.669948875646));
#82052=CARTESIAN_POINT('Ctrl Pts',(81.5626203935325,-8.42224238935577,137.669577529478));
#82053=CARTESIAN_POINT('Ctrl Pts',(81.5670712308611,-8.43440374223383,137.668701082127));
#82054=CARTESIAN_POINT('Ctrl Pts',(81.5695817285307,-8.44140841255747,137.66819477102));
#82055=CARTESIAN_POINT('Ctrl Pts',(81.577746548073,-8.46467917293505,137.666508312379));
#82056=CARTESIAN_POINT('Ctrl Pts',(81.5831953713264,-8.4810154951532,137.665317307131));
#82057=CARTESIAN_POINT('Ctrl Pts',(81.595864117891,-8.52105570413708,137.662385793131));
#82058=CARTESIAN_POINT('Ctrl Pts',(81.6028101877545,-8.5448414649516,137.660633912303));
#82059=CARTESIAN_POINT('Ctrl Pts',(81.6297523205309,-8.64538199089007,137.653208617));
#82060=CARTESIAN_POINT('Ctrl Pts',(81.6447840326573,-8.72335728513493,137.647406290558));
#82061=CARTESIAN_POINT('Ctrl Pts',(81.6664020641407,-8.90406102835186,137.634180005334));
#82062=CARTESIAN_POINT('Ctrl Pts',(81.6691489967224,-9.00694273567105,137.62681949545));
#82063=CARTESIAN_POINT('Ctrl Pts',(81.6608518938923,-9.13297993938015,137.618124264481));
#82064=CARTESIAN_POINT('Ctrl Pts',(81.6588020245364,-9.15648840202831,137.616515235326));
#82065=CARTESIAN_POINT('Ctrl Pts',(81.6549434666265,-9.19200312790644,137.614102687039));
#82066=CARTESIAN_POINT('Ctrl Pts',(81.6535019114694,-9.20404538983951,137.613287823738));
#82067=CARTESIAN_POINT('Ctrl Pts',(81.6506679019358,-9.22571224857844,137.611827105126));
#82068=CARTESIAN_POINT('Ctrl Pts',(81.6493224483708,-9.23534232474823,137.611179804832));
#82069=CARTESIAN_POINT('Ctrl Pts',(81.6462582981961,-9.25595542774813,137.609798162744));
#82070=CARTESIAN_POINT('Ctrl Pts',(81.6445138226447,-9.26693419147022,137.609064666414));
#82071=CARTESIAN_POINT('Ctrl Pts',(81.6394229160776,-9.29702695786795,137.607060139871));
#82072=CARTESIAN_POINT('Ctrl Pts',(81.6358521712444,-9.31610162342348,137.605796217122));
#82073=CARTESIAN_POINT('Ctrl Pts',(81.6271545213111,-9.35845819491181,137.603001511389));
#82074=CARTESIAN_POINT('Ctrl Pts',(81.6218594988519,-9.3817014077988,137.601476030854));
#82075=CARTESIAN_POINT('Ctrl Pts',(81.6032908287108,-9.45582801295078,137.596627097917));
#82076=CARTESIAN_POINT('Ctrl Pts',(81.5881063444686,-9.50620106787074,137.593357552564));
#82077=CARTESIAN_POINT('Ctrl Pts',(81.5385449689,-9.64625657447896,137.584212032637));
#82078=CARTESIAN_POINT('Ctrl Pts',(81.4987686054243,-9.7337979759346,137.578436722803));
#82079=CARTESIAN_POINT('Ctrl Pts',(81.4263875215395,-9.86234087892624,137.569259853466));
#82080=CARTESIAN_POINT('Ctrl Pts',(81.3990272266733,-9.90605455221021,137.565999642882));
#82081=CARTESIAN_POINT('Ctrl Pts',(81.3634298479079,-9.95746326678215,137.561903813327));
#82082=CARTESIAN_POINT('Ctrl Pts',(81.3570823258384,-9.96643903192347,137.561178556145));
#82083=CARTESIAN_POINT('Ctrl Pts',(81.3469603304609,-9.98045576929294,137.560028786756));
#82084=CARTESIAN_POINT('Ctrl Pts',(81.3432451750532,-9.98553946841378,137.559608167204));
#82085=CARTESIAN_POINT('Ctrl Pts',(81.3362254265296,-9.99503163972663,137.558815740828));
#82086=CARTESIAN_POINT('Ctrl Pts',(81.332927675076,-9.99944492796627,137.558444394122));
#82087=CARTESIAN_POINT('Ctrl Pts',(81.3251245264176,-10.0097803522191,137.557567942302));
#82088=CARTESIAN_POINT('Ctrl Pts',(81.3206012797656,-10.0156887440696,137.557061627227));
#82089=CARTESIAN_POINT('Ctrl Pts',(81.3054789367246,-10.0351701865493,137.555375141507));
#82090=CARTESIAN_POINT('Ctrl Pts',(81.2947093700716,-10.0486086775402,137.554184112689));
#82091=CARTESIAN_POINT('Ctrl Pts',(81.2679408902936,-10.0809698664641,137.551252528568));
#82092=CARTESIAN_POINT('Ctrl Pts',(81.2517246453798,-10.0997068856325,137.549500600528));
#82093=CARTESIAN_POINT('Ctrl Pts',(81.1818668571275,-10.1768763396028,137.542074970595));
#82094=CARTESIAN_POINT('Ctrl Pts',(81.1245069603111,-10.2317996712501,137.536272347099));
#82095=CARTESIAN_POINT('Ctrl Pts',(80.9844168316786,-10.3479697939445,137.523046161468));
#82096=CARTESIAN_POINT('Ctrl Pts',(80.8994764223209,-10.4060752746079,137.515686037849));
#82097=CARTESIAN_POINT('Ctrl Pts',(80.7890927013382,-10.4674622273336,137.506991159206));
#82098=CARTESIAN_POINT('Ctrl Pts',(80.7682306146954,-10.4784906159504,137.505382126755));
#82099=CARTESIAN_POINT('Ctrl Pts',(80.7363006627894,-10.4945114295537,137.502969574557));
#82100=CARTESIAN_POINT('Ctrl Pts',(80.7254016805974,-10.4998318220285,137.502154710589));
#82101=CARTESIAN_POINT('Ctrl Pts',(80.7056615158633,-10.5092025598581,137.500693991258));
#82102=CARTESIAN_POINT('Ctrl Pts',(80.6968412223297,-10.5132953642277,137.500046690908));
#82103=CARTESIAN_POINT('Ctrl Pts',(80.6778615439137,-10.5219012098366,137.498665049212));
#82104=CARTESIAN_POINT('Ctrl Pts',(80.6676917586815,-10.5263902812453,137.497931553325));
#82105=CARTESIAN_POINT('Ctrl Pts',(80.6396486594298,-10.5384349523762,137.495927029322));
#82106=CARTESIAN_POINT('Ctrl Pts',(80.6216867308017,-10.5457807638806,137.494663108639));
#82107=CARTESIAN_POINT('Ctrl Pts',(80.5813842192337,-10.5614469254257,137.491868408161));
#82108=CARTESIAN_POINT('Ctrl Pts',(80.5589849603961,-10.5696050491619,137.490342930784));
#82109=CARTESIAN_POINT('Ctrl Pts',(80.4866376839961,-10.5942096490248,137.485494011733));
#82110=CARTESIAN_POINT('Ctrl Pts',(80.4360820215044,-10.6087739849591,137.482224476744));
#82111=CARTESIAN_POINT('Ctrl Pts',(80.2915357794526,-10.6430992302992,137.473078963344));
#82112=CARTESIAN_POINT('Ctrl Pts',(80.196415390744,-10.6571625769103,137.467303650553));
#82113=CARTESIAN_POINT('Ctrl Pts',(80.0491639078534,-10.6660720528888,137.458126766072));
#82114=CARTESIAN_POINT('Ctrl Pts',(79.9975987042039,-10.6667952149265,137.454866542431));
#82115=CARTESIAN_POINT('Ctrl Pts',(79.9351009996958,-10.6647717493359,137.450770698221));
#82116=CARTESIAN_POINT('Ctrl Pts',(79.9241173812591,-10.664307264277,137.45004544038));
#82117=CARTESIAN_POINT('Ctrl Pts',(79.906851473015,-10.6634058432398,137.448895670176));
#82118=CARTESIAN_POINT('Ctrl Pts',(79.9005654597846,-10.6630419165931,137.448475050478));
#82119=CARTESIAN_POINT('Ctrl Pts',(79.8887833975199,-10.6622927605834,137.447682623994));
#82120=CARTESIAN_POINT('Ctrl Pts',(79.8832870131459,-10.6619158912876,137.447311277329));
#82121=CARTESIAN_POINT('Ctrl Pts',(79.8703716118011,-10.6609659391908,137.446434825838));
#82122=CARTESIAN_POINT('Ctrl Pts',(79.8629544605581,-10.6603704059653,137.445928511053));
#82123=CARTESIAN_POINT('Ctrl Pts',(79.8383854234812,-10.6582319792987,137.44424202731));
#82124=CARTESIAN_POINT('Ctrl Pts',(79.821254125865,-10.6564728863473,137.443051000212));
#82125=CARTESIAN_POINT('Ctrl Pts',(79.7795477949342,-10.6515358840836,137.440119421209));
#82126=CARTESIAN_POINT('Ctrl Pts',(79.7550108798058,-10.6480746799821,137.438367496614));
#82127=CARTESIAN_POINT('Ctrl Pts',(79.6522891087164,-10.6312401040158,137.430941891097));
#82128=CARTESIAN_POINT('Ctrl Pts',(79.5750355964759,-10.6128395902213,137.425139289275));
#82129=CARTESIAN_POINT('Ctrl Pts',(79.4015811272432,-10.5581934577351,137.411922708001));
#82130=CARTESIAN_POINT('Ctrl Pts',(79.3068124572052,-10.518410171439,137.404571830552));
#82131=CARTESIAN_POINT('Ctrl Pts',(79.1953997011355,-10.4590184686371,137.395879527354));
#82132=CARTESIAN_POINT('Ctrl Pts',(79.1747461828208,-10.4474366203254,137.394264815647));
#82133=CARTESIAN_POINT('Ctrl Pts',(79.1438820408187,-10.4292534857213,137.391845522519));
#82134=CARTESIAN_POINT('Ctrl Pts',(79.1334859648963,-10.4229746754583,137.39102950185));
#82135=CARTESIAN_POINT('Ctrl Pts',(79.1148905226113,-10.4114644099205,137.389567530062));
#82136=CARTESIAN_POINT('Ctrl Pts',(79.1066666384071,-10.4062738280228,137.38892012328));
#82137=CARTESIAN_POINT('Ctrl Pts',(79.0908010631536,-10.3960647763414,137.387669267592));
#82138=CARTESIAN_POINT('Ctrl Pts',(79.0831543226182,-10.3910548429111,137.387065533458));
#82139=CARTESIAN_POINT('Ctrl Pts',(79.0613036065022,-10.3764804020417,137.385337548237));
#82140=CARTESIAN_POINT('Ctrl Pts',(79.0472050647388,-10.3667593289274,137.384219186112));
#82141=CARTESIAN_POINT('Ctrl Pts',(78.980107724224,-10.3189521951582,137.378875766461));
#82142=CARTESIAN_POINT('Ctrl Pts',(78.9292244362571,-10.2779891673023,137.37476267311));
#82143=CARTESIAN_POINT('Ctrl Pts',(78.826413713766,-10.1847596594816,137.366159287972));
#82144=CARTESIAN_POINT('Ctrl Pts',(78.7752833995031,-10.1318258832438,137.361697107771));
#82145=CARTESIAN_POINT('Ctrl Pts',(78.715730127043,-10.0613940305427,137.356054411611));
#82146=CARTESIAN_POINT('Ctrl Pts',(78.7038858188533,-10.0468975155575,137.354907107612));
#82147=CARTESIAN_POINT('Ctrl Pts',(78.6490957049875,-9.97748331239432,137.349464333658));
#82148=CARTESIAN_POINT('Ctrl Pts',(78.6093854884828,-9.92011134664481,137.345114753188));
#82149=CARTESIAN_POINT('Ctrl Pts',(78.5674186914343,-9.85052951658297,137.339799249718));
#82150=CARTESIAN_POINT('Ctrl Pts',(78.5615510988413,-9.84056790604222,137.339037310898));
#82151=CARTESIAN_POINT('Ctrl Pts',(78.5525852761224,-9.8249775063575,137.337842065));
#82152=CARTESIAN_POINT('Ctrl Pts',(78.5494149980306,-9.81939027178488,137.33741316926));
#82153=CARTESIAN_POINT('Ctrl Pts',(78.5436229714813,-9.80904355662836,137.336617645717));
#82154=CARTESIAN_POINT('Ctrl Pts',(78.5409920968417,-9.80428941378284,137.336251601543));
#82155=CARTESIAN_POINT('Ctrl Pts',(78.5349285236896,-9.79320453248398,137.335396977686));
#82156=CARTESIAN_POINT('Ctrl Pts',(78.5315135841764,-9.78686434839327,137.334907320027));
#82157=CARTESIAN_POINT('Ctrl Pts',(78.5207105767518,-9.76649219355298,137.333331755857));
#82158=CARTESIAN_POINT('Ctrl Pts',(78.5134819663801,-9.75237727932634,137.332236796082));
#82159=CARTESIAN_POINT('Ctrl Pts',(78.4744668556548,-9.67343691879679,137.326103326881));
#82160=CARTESIAN_POINT('Ctrl Pts',(78.4467217555122,-9.60670693680316,137.32088590796));
#82161=CARTESIAN_POINT('Ctrl Pts',(78.3781212857171,-9.40582138687903,137.305451728632));
#82162=CARTESIAN_POINT('Ctrl Pts',(78.349741350932,-9.26803599819419,137.295262893656));
#82163=CARTESIAN_POINT('Ctrl Pts',(78.3373025807438,-9.10700372058145,137.284174400434));
#82164=CARTESIAN_POINT('Ctrl Pts',(78.3360669770646,-9.0856707241575,137.282720088802));
#82165=CARTESIAN_POINT('Ctrl Pts',(78.3347977443621,-9.05281937188488,137.280502099517));
#82166=CARTESIAN_POINT('Ctrl Pts',(78.3344726056708,-9.04131523314185,137.279729438107));
#82167=CARTESIAN_POINT('Ctrl Pts',(78.3341612568167,-9.02391663867215,137.278566770269));
#82168=CARTESIAN_POINT('Ctrl Pts',(78.3340870821118,-9.01802430146893,137.278174032471));
#82169=CARTESIAN_POINT('Ctrl Pts',(78.3340147926115,-9.00809726575708,137.277514048675));
#82170=CARTESIAN_POINT('Ctrl Pts',(78.3340000686888,-9.00406278471672,137.277246288591));
#82171=CARTESIAN_POINT('Ctrl Pts',(78.3340000002398,-9.00002826508004,137.276978983378));
#82172=CARTESIAN_POINT('Ctrl Pts',(78.334000000243,-9.0000284517738,137.276978995747));
#82173=CARTESIAN_POINT('Ctrl Pts',(78.3339998559323,-8.99157830878331,137.276419135442));
#82174=CARTESIAN_POINT('Ctrl Pts',(78.3340640017322,-8.98312812680701,137.275861279928));
#82175=CARTESIAN_POINT('Ctrl Pts',(78.3344125114647,-8.9602008431423,137.274352894817));
#82176=CARTESIAN_POINT('Ctrl Pts',(78.3348213222679,-8.94572617903658,137.273406244807));
#82177=CARTESIAN_POINT('Ctrl Pts',(78.337191248607,-8.88833837798755,137.269673328737));
#82178=CARTESIAN_POINT('Ctrl Pts',(78.340623104397,-8.84550060921749,137.266932401451));
#82179=CARTESIAN_POINT('Ctrl Pts',(78.3611175763466,-8.67353914507015,137.256037782249));
#82180=CARTESIAN_POINT('Ctrl Pts',(78.3916241621003,-8.54656426521876,137.248277246748));
#82181=CARTESIAN_POINT('Ctrl Pts',(78.4365593749625,-8.42449204003557,137.240217161908));
#82182=CARTESIAN_POINT('',(78.3340007164175,-8.99846998957594,137.471592638051));
#82183=CARTESIAN_POINT('Ctrl Pts',(78.4365593939729,-8.42449198839149,137.430947540156));
#82184=CARTESIAN_POINT('Ctrl Pts',(78.4253966868889,-8.45481689990651,137.432975786351));
#82185=CARTESIAN_POINT('Ctrl Pts',(78.4151148644401,-8.48547039210586,137.435031381114));
#82186=CARTESIAN_POINT('Ctrl Pts',(78.4011804947077,-8.53140879447188,137.438146593564));
#82187=CARTESIAN_POINT('Ctrl Pts',(78.396844163587,-8.54646626464699,137.439173120898));
#82188=CARTESIAN_POINT('Ctrl Pts',(78.3908552708693,-8.56842207113429,137.440680830275));
#82189=CARTESIAN_POINT('Ctrl Pts',(78.3890332220193,-8.57527384863215,137.441152873332));
#82190=CARTESIAN_POINT('Ctrl Pts',(78.3858798945934,-8.58744413339833,137.441994379246));
#82191=CARTESIAN_POINT('Ctrl Pts',(78.3845310535768,-8.5927578857862,137.442362835515));
#82192=CARTESIAN_POINT('Ctrl Pts',(78.3816559318007,-8.60432350412263,137.443167149854));
#82193=CARTESIAN_POINT('Ctrl Pts',(78.3801396609965,-8.61057749026454,137.443603532063));
#82194=CARTESIAN_POINT('Ctrl Pts',(78.3770706379162,-8.6235640505564,137.444512487288));
#82195=CARTESIAN_POINT('Ctrl Pts',(78.375523461572,-8.63029780852984,137.444985348976));
#82196=CARTESIAN_POINT('Ctrl Pts',(78.3716235762703,-8.64776848626763,137.446215862591));
#82197=CARTESIAN_POINT('Ctrl Pts',(78.369335201114,-8.65851923128557,137.446976657879));
#82198=CARTESIAN_POINT('Ctrl Pts',(78.3452056092581,-8.77765714383894,137.455441551978));
#82199=CARTESIAN_POINT('Ctrl Pts',(78.3341022436752,-8.88792624741543,137.463565331214));
#82200=CARTESIAN_POINT('Ctrl Pts',(78.3340007028461,-8.99846967886182,137.471592635464));
#82201=CARTESIAN_POINT('Ctrl Pts',(78.3340007025621,-8.99846998812028,137.471592657922));
#82202=CARTESIAN_POINT('Ctrl Pts',(78.333928799091,-9.07676423789923,137.477278131424));
#82203=CARTESIAN_POINT('Ctrl Pts',(78.3393761194856,-9.15497390237208,137.48290344457));
#82204=CARTESIAN_POINT('Ctrl Pts',(78.3549267449954,-9.26530406909678,137.49069054483));
#82205=CARTESIAN_POINT('Ctrl Pts',(78.3605243789937,-9.29794666877342,137.492976680033));
#82206=CARTESIAN_POINT('Ctrl Pts',(78.3695335593229,-9.34247161202522,137.496071652893));
#82207=CARTESIAN_POINT('Ctrl Pts',(78.3721093407894,-9.35451323671659,137.496906339278));
#82208=CARTESIAN_POINT('Ctrl Pts',(78.3769092493717,-9.37579613030707,137.49837769819));
#82209=CARTESIAN_POINT('Ctrl Pts',(78.3790793717241,-9.38504887956074,137.499016058276));
#82210=CARTESIAN_POINT('Ctrl Pts',(78.3836412988074,-9.4037772197593,137.500305658421));
#82211=CARTESIAN_POINT('Ctrl Pts',(78.3860375411522,-9.41325135515755,137.500956727615));
#82212=CARTESIAN_POINT('Ctrl Pts',(78.3912590264513,-9.43315732682523,137.50232217255));
#82213=CARTESIAN_POINT('Ctrl Pts',(78.3941027030309,-9.44358389355644,137.503035920355));
#82214=CARTESIAN_POINT('Ctrl Pts',(78.4019431644165,-9.47126754270717,137.504927593944));
#82215=CARTESIAN_POINT('Ctrl Pts',(78.4071180554961,-9.48847302714551,137.506099721521));
#82216=CARTESIAN_POINT('Ctrl Pts',(78.4340621327363,-9.57307053966714,137.511850440935));
#82217=CARTESIAN_POINT('Ctrl Pts',(78.4598359086686,-9.63911470235923,137.516296272916));
#82218=CARTESIAN_POINT('Ctrl Pts',(78.5347471334781,-9.79997299598436,137.527257932845));
#82219=CARTESIAN_POINT('Ctrl Pts',(78.5889268678075,-9.89207260534004,137.533650556547));
#82220=CARTESIAN_POINT('Ctrl Pts',(78.672937597443,-10.0078641137908,137.542564276164));
#82221=CARTESIAN_POINT('Ctrl Pts',(78.6953047169174,-10.0366554612219,137.544863923682));
#82222=CARTESIAN_POINT('Ctrl Pts',(78.7308642089458,-10.0794530321035,137.548451471454));
#82223=CARTESIAN_POINT('Ctrl Pts',(78.7433857141227,-10.0940040971263,137.549702827015));
#82224=CARTESIAN_POINT('Ctrl Pts',(78.7614188355533,-10.1142420296484,137.551493914495));
#82225=CARTESIAN_POINT('Ctrl Pts',(78.7667243878721,-10.1201115390208,137.552019566283));
#82226=CARTESIAN_POINT('Ctrl Pts',(78.775842217388,-10.1300552436493,137.552921171226));
#82227=CARTESIAN_POINT('Ctrl Pts',(78.7796336043926,-10.1341485749341,137.553295575405));
#82228=CARTESIAN_POINT('Ctrl Pts',(78.787592956522,-10.142655684411,137.554080695178));
#82229=CARTESIAN_POINT('Ctrl Pts',(78.7917645480015,-10.1470657966119,137.554491667892));
#82230=CARTESIAN_POINT('Ctrl Pts',(78.8030469045565,-10.1588634199501,137.555601545504));
#82231=CARTESIAN_POINT('Ctrl Pts',(78.8102017874062,-10.1662081027249,137.556303675397));
#82232=CARTESIAN_POINT('Ctrl Pts',(78.8442657579952,-10.2005359431904,137.559636446087));
#82233=CARTESIAN_POINT('Ctrl Pts',(78.8720256879978,-10.2266546519448,137.562323142642));
#82234=CARTESIAN_POINT('Ctrl Pts',(78.971029704128,-10.3136014398985,137.571736541764));
#82235=CARTESIAN_POINT('Ctrl Pts',(79.0464903694629,-10.3693602933498,137.578615294642));
#82236=CARTESIAN_POINT('Ctrl Pts',(79.2073280405334,-10.4684339838284,137.592289005479));
#82237=CARTESIAN_POINT('Ctrl Pts',(79.2925659184523,-10.5113470108072,137.599053773995));
#82238=CARTESIAN_POINT('Ctrl Pts',(79.3982889066405,-10.5536556263566,137.606836743984));
#82239=CARTESIAN_POINT('Ctrl Pts',(79.415674729862,-10.5602775626645,137.608098534098));
#82240=CARTESIAN_POINT('Ctrl Pts',(79.4434589669027,-10.5703304863871,137.610087200981));
#82241=CARTESIAN_POINT('Ctrl Pts',(79.4537861306055,-10.5739524061321,137.6108203581));
#82242=CARTESIAN_POINT('Ctrl Pts',(79.4733751346673,-10.5806065943856,137.612199981537));
#82243=CARTESIAN_POINT('Ctrl Pts',(79.4826293032467,-10.5836598511153,137.61284711601));
#82244=CARTESIAN_POINT('Ctrl Pts',(79.5037063460114,-10.5904093923997,137.614310821788));
#82245=CARTESIAN_POINT('Ctrl Pts',(79.5155448122557,-10.5940553978139,137.615125719673));
#82246=CARTESIAN_POINT('Ctrl Pts',(79.546509046066,-10.6032149271836,137.617239131014));
#82247=CARTESIAN_POINT('Ctrl Pts',(79.5656952382616,-10.6085184413274,137.618530862869));
#82248=CARTESIAN_POINT('Ctrl Pts',(79.7142085101317,-10.6467198437046,137.628405089555));
#82249=CARTESIAN_POINT('Ctrl Pts',(79.8469694289449,-10.6643162175775,137.636458087175));
#82250=CARTESIAN_POINT('Ctrl Pts',(80.0639419874605,-10.6668667430825,137.649743502432));
#82251=CARTESIAN_POINT('Ctrl Pts',(80.1474113668569,-10.6615653646854,137.654899393087));
#82252=CARTESIAN_POINT('Ctrl Pts',(80.2425442890156,-10.6482978077173,137.66117112114));
#82253=CARTESIAN_POINT('Ctrl Pts',(80.2549493250267,-10.646424675946,137.661996836986));
#82254=CARTESIAN_POINT('Ctrl Pts',(80.2738062985884,-10.6433591028779,137.66326569746));
#82255=CARTESIAN_POINT('Ctrl Pts',(80.2802746228279,-10.6422682979004,137.663703403915));
#82256=CARTESIAN_POINT('Ctrl Pts',(80.2921235769085,-10.6401980751279,137.664510012672));
#82257=CARTESIAN_POINT('Ctrl Pts',(80.2975060326865,-10.6392303277792,137.664878262565));
#82258=CARTESIAN_POINT('Ctrl Pts',(80.3098063428566,-10.6369561973641,137.665724009077));
#82259=CARTESIAN_POINT('Ctrl Pts',(80.3167207214058,-10.6356324594103,137.666202448748));
#82260=CARTESIAN_POINT('Ctrl Pts',(80.3383281723918,-10.6313536304051,137.66770659632));
#82261=CARTESIAN_POINT('Ctrl Pts',(80.352989417361,-10.6282441622426,137.668740284237));
#82262=CARTESIAN_POINT('Ctrl Pts',(80.4699427903108,-10.601786055276,137.677080485071));
#82263=CARTESIAN_POINT('Ctrl Pts',(80.5698548258405,-10.5690209530326,137.68476954026));
#82264=CARTESIAN_POINT('Ctrl Pts',(80.7694879020487,-10.4819540977734,137.700604123405));
#82265=CARTESIAN_POINT('Ctrl Pts',(80.8681249163085,-10.426417731538,137.708691301777));
#82266=CARTESIAN_POINT('Ctrl Pts',(80.9762107936308,-10.3501640350449,137.717741998127));
#82267=CARTESIAN_POINT('Ctrl Pts',(80.9918273040628,-10.3387341367218,137.719055607483));
#82268=CARTESIAN_POINT('Ctrl Pts',(81.0160854915727,-10.3203217579863,137.721106418013));
#82269=CARTESIAN_POINT('Ctrl Pts',(81.0248621149918,-10.313520813076,137.721850589115));
#82270=CARTESIAN_POINT('Ctrl Pts',(81.0411949528946,-10.3006012385433,137.7232398614));
#82271=CARTESIAN_POINT('Ctrl Pts',(81.0487668203291,-10.294503254171,137.723885741696));
#82272=CARTESIAN_POINT('Ctrl Pts',(81.0656721227355,-10.2806429158128,137.725332148854));
#82273=CARTESIAN_POINT('Ctrl Pts',(81.0749750347802,-10.2728440747457,137.726131160526));
#82274=CARTESIAN_POINT('Ctrl Pts',(81.1021548697266,-10.2495480551742,137.728475521489));
#82275=CARTESIAN_POINT('Ctrl Pts',(81.1197883473678,-10.2337705809647,137.73000933995));
#82276=CARTESIAN_POINT('Ctrl Pts',(81.2076057492842,-10.1517620098186,137.737727760093));
#82277=CARTESIAN_POINT('Ctrl Pts',(81.2722792657677,-10.079896229531,137.743664699698));
#82278=CARTESIAN_POINT('Ctrl Pts',(81.3809915161687,-9.9356762384391,137.754701511532));
#82279=CARTESIAN_POINT('Ctrl Pts',(81.426449643025,-9.86479308503417,137.759799131248));
#82280=CARTESIAN_POINT('Ctrl Pts',(81.4784810001691,-9.76831115862205,137.766702765309));
#82281=CARTESIAN_POINT('Ctrl Pts',(81.490083118573,-9.7455603688608,137.768328752891));
#82282=CARTESIAN_POINT('Ctrl Pts',(81.5087939315282,-9.7066872858138,137.77111878787));
#82283=CARTESIAN_POINT('Ctrl Pts',(81.5161783075457,-9.69070205376934,137.772269385));
#82284=CARTESIAN_POINT('Ctrl Pts',(81.5263467600307,-9.66774089378601,137.773930977843));
#82285=CARTESIAN_POINT('Ctrl Pts',(81.5293394500616,-9.66085790772632,137.774430191044));
#82286=CARTESIAN_POINT('Ctrl Pts',(81.5344508870818,-9.64888127413629,137.775301181211));
#82287=CARTESIAN_POINT('Ctrl Pts',(81.5365910089567,-9.64379694239568,137.775671670876));
#82288=CARTESIAN_POINT('Ctrl Pts',(81.5411051628852,-9.6329218301072,137.776465826167));
#82289=CARTESIAN_POINT('Ctrl Pts',(81.5434717912701,-9.62712836996598,137.776889885529));
#82290=CARTESIAN_POINT('Ctrl Pts',(81.5498442235546,-9.61127419997591,137.778052783553));
#82291=CARTESIAN_POINT('Ctrl Pts',(81.5537845831316,-9.60118775654959,137.778795281941));
#82292=CARTESIAN_POINT('Ctrl Pts',(81.5747287407027,-9.54599378242774,137.782870021529));
#82293=CARTESIAN_POINT('Ctrl Pts',(81.5898654126192,-9.50020682099157,137.786292169078));
#82294=CARTESIAN_POINT('Ctrl Pts',(81.630423819106,-9.35694952861181,137.797001885396));
#82295=CARTESIAN_POINT('Ctrl Pts',(81.6490137744856,-9.25777810040102,137.804405290629));
#82296=CARTESIAN_POINT('Ctrl Pts',(81.6634452195096,-9.1058401491153,137.815375771247));
#82297=CARTESIAN_POINT('Ctrl Pts',(81.6659361032245,-9.05394345424891,137.819061643048));
#82298=CARTESIAN_POINT('Ctrl Pts',(81.666027321704,-8.97836960669219,137.824327029546));
#82299=CARTESIAN_POINT('Ctrl Pts',(81.6655526361715,-8.95472944170512,137.825959785858));
#82300=CARTESIAN_POINT('Ctrl Pts',(81.6637776570495,-8.91184327006092,137.828896368364));
#82301=CARTESIAN_POINT('Ctrl Pts',(81.6626460493423,-8.89259483289745,137.830205073067));
#82302=CARTESIAN_POINT('Ctrl Pts',(81.6603377686136,-8.8623140109963,137.832250007524));
#82303=CARTESIAN_POINT('Ctrl Pts',(81.659384642876,-8.85126683379036,137.832993140685));
#82304=CARTESIAN_POINT('Ctrl Pts',(81.6573887946023,-8.83055110062724,137.834381479127));
#82305=CARTESIAN_POINT('Ctrl Pts',(81.6563715768038,-8.82088061975106,137.835027453212));
#82306=CARTESIAN_POINT('Ctrl Pts',(81.6538917617682,-8.79913705486678,137.836475370358));
#82307=CARTESIAN_POINT('Ctrl Pts',(81.6523815114681,-8.78706987996542,137.837275784262));
#82308=CARTESIAN_POINT('Ctrl Pts',(81.6475300510807,-8.75147339223351,137.839628415047));
#82309=CARTESIAN_POINT('Ctrl Pts',(81.6438172994119,-8.72799720293559,137.841168975842));
#82310=CARTESIAN_POINT('Ctrl Pts',(81.6221296287628,-8.60761778319821,137.849025220927));
#82311=CARTESIAN_POINT('Ctrl Pts',(81.596083933701,-8.51236537276604,137.855081390981));
#82312=CARTESIAN_POINT('Ctrl Pts',(81.5330995677683,-8.34277745190497,137.86613379942));
#82313=CARTESIAN_POINT('Ctrl Pts',(81.4987514403605,-8.26782650995303,137.871129874108));
#82314=CARTESIAN_POINT('Ctrl Pts',(81.4468114002514,-8.17360362600286,137.877908668892));
#82315=CARTESIAN_POINT('Ctrl Pts',(81.4341147571109,-8.15176128260955,137.879517827212));
#82316=CARTESIAN_POINT('Ctrl Pts',(81.4118071508072,-8.11531829323692,137.88228179177));
#82317=CARTESIAN_POINT('Ctrl Pts',(81.4024538216986,-8.10056441459199,137.883423474044));
#82318=CARTESIAN_POINT('Ctrl Pts',(81.3887657623159,-8.07970567877433,137.885074416134));
#82319=CARTESIAN_POINT('Ctrl Pts',(81.3846188239005,-8.07347817757043,137.885572098233));
#82320=CARTESIAN_POINT('Ctrl Pts',(81.3773434370146,-8.06271058116893,137.88644135031));
#82321=CARTESIAN_POINT('Ctrl Pts',(81.3742341711195,-8.05815774139058,137.886811648553));
#82322=CARTESIAN_POINT('Ctrl Pts',(81.3675400249508,-8.04845935182042,137.887606486348));
#82323=CARTESIAN_POINT('Ctrl Pts',(81.3639487349722,-8.04331866847154,137.888031429168));
#82324=CARTESIAN_POINT('Ctrl Pts',(81.3540446631058,-8.02931079687984,137.889199068998));
#82325=CARTESIAN_POINT('Ctrl Pts',(81.3476739977762,-8.02048519215416,137.889945473316));
#82326=CARTESIAN_POINT('Ctrl Pts',(81.3119591728061,-7.97201563722908,137.894101656577));
#82327=CARTESIAN_POINT('Ctrl Pts',(81.2809547211809,-7.93363104604614,137.897605550045));
#82328=CARTESIAN_POINT('Ctrl Pts',(81.1805132342218,-7.81999125222122,137.908521974782));
#82329=CARTESIAN_POINT('Ctrl Pts',(81.1058056445215,-7.74970903512104,137.916048330052));
#82330=CARTESIAN_POINT('Ctrl Pts',(80.9655955866681,-7.64026376568088,137.928816752154));
#82331=CARTESIAN_POINT('Ctrl Pts',(80.9029777016017,-7.59789741857565,137.934129787077));
#82332=CARTESIAN_POINT('Ctrl Pts',(80.8223309766096,-7.55098530545667,137.940498399085));
#82333=CARTESIAN_POINT('Ctrl Pts',(80.8068270766963,-7.54229566410665,137.941702676221));
#82334=CARTESIAN_POINT('Ctrl Pts',(80.7817126420186,-7.52874297347771,137.943622239956));
#82335=CARTESIAN_POINT('Ctrl Pts',(80.7721891980258,-7.52372233484165,137.944343075639));
#82336=CARTESIAN_POINT('Ctrl Pts',(80.7539203346258,-7.51431637884403,137.945712700113));
#82337=CARTESIAN_POINT('Ctrl Pts',(80.7451836834685,-7.50991511047496,137.946362027887));
#82338=CARTESIAN_POINT('Ctrl Pts',(80.7251958640092,-7.50006559668248,137.947835011013));
#82339=CARTESIAN_POINT('Ctrl Pts',(80.7139210395036,-7.49466647584213,137.948656934899));
#82340=CARTESIAN_POINT('Ctrl Pts',(80.6837599198264,-7.48063846516974,137.950832754035));
#82341=CARTESIAN_POINT('Ctrl Pts',(80.664770911554,-7.47223470462493,137.952178983401));
#82342=CARTESIAN_POINT('Ctrl Pts',(80.5308887424507,-7.41595293988394,137.961518941402));
#82343=CARTESIAN_POINT('Ctrl Pts',(80.4111035743345,-7.38072680830335,137.969064414489));
#82344=CARTESIAN_POINT('Ctrl Pts',(80.1983317311004,-7.34331578888048,137.982271404312));
#82345=CARTESIAN_POINT('Ctrl Pts',(80.1070201845569,-7.33492342684084,137.987893836029));
#82346=CARTESIAN_POINT('Ctrl Pts',(80.0033286260467,-7.33395888718647,137.994670080333));
#82347=CARTESIAN_POINT('Ctrl Pts',(79.9911603387355,-7.33397901919427,137.99547145766));
#82348=CARTESIAN_POINT('Ctrl Pts',(79.9725128395491,-7.33421415974513,137.996710511161));
#82349=CARTESIAN_POINT('Ctrl Pts',(79.9660325437043,-7.33433370150281,137.997143132654));
#82350=CARTESIAN_POINT('Ctrl Pts',(79.9540782141347,-7.33462401144572,137.997945218567));
#82351=CARTESIAN_POINT('Ctrl Pts',(79.948604125208,-7.33478396156473,137.998314086096));
#82352=CARTESIAN_POINT('Ctrl Pts',(79.9361091842425,-7.33521072614168,137.999159617112));
#82353=CARTESIAN_POINT('Ctrl Pts',(79.9290891657766,-7.33549496492269,137.999637210981));
#82354=CARTESIAN_POINT('Ctrl Pts',(79.9073131556326,-7.33651467401116,138.001126184783));
#82355=CARTESIAN_POINT('Ctrl Pts',(79.8925654632131,-7.3374020137617,138.002145250694));
#82356=CARTESIAN_POINT('Ctrl Pts',(79.7725952931103,-7.34622317902403,138.010511833729));
#82357=CARTESIAN_POINT('Ctrl Pts',(79.6683405938783,-7.36394096014155,138.018246555101));
#82358=CARTESIAN_POINT('Ctrl Pts',(79.4580716482882,-7.42060974519864,138.034078191174));
#82359=CARTESIAN_POINT('Ctrl Pts',(79.3528848377405,-7.460711014358,138.042119080553));
#82360=CARTESIAN_POINT('Ctrl Pts',(79.2351910414667,-7.51979760909405,138.051130306956));
#82361=CARTESIAN_POINT('Ctrl Pts',(79.2180173470157,-7.52879809454356,138.052446467466));
#82362=CARTESIAN_POINT('Ctrl Pts',(79.1912545939545,-7.54342514353333,138.054500334068));
#82363=CARTESIAN_POINT('Ctrl Pts',(79.1815585142408,-7.54885114856061,138.055245044792));
#82364=CARTESIAN_POINT('Ctrl Pts',(79.16348225366,-7.5592055821618,138.056634804679));
#82365=CARTESIAN_POINT('Ctrl Pts',(79.155089574531,-7.56411112052619,138.057280638303));
#82366=CARTESIAN_POINT('Ctrl Pts',(79.1363239101879,-7.57530119325411,138.058726270384));
#82367=CARTESIAN_POINT('Ctrl Pts',(79.1259755728194,-7.58162614528763,138.059524560838));
#82368=CARTESIAN_POINT('Ctrl Pts',(79.0956931542708,-7.6005921803549,138.061864673503));
#82369=CARTESIAN_POINT('Ctrl Pts',(79.0759570725515,-7.61354485292491,138.063395028967));
#82370=CARTESIAN_POINT('Ctrl Pts',(78.972722802962,-7.68448087179511,138.071441705272));
#82371=CARTESIAN_POINT('Ctrl Pts',(78.8943842881878,-7.74959758800389,138.077679052033));
#82372=CARTESIAN_POINT('Ctrl Pts',(78.7657869538816,-7.87808503629385,138.088782369142));
#82373=CARTESIAN_POINT('Ctrl Pts',(78.7132728669344,-7.93872410145422,138.093649710774));
#82374=CARTESIAN_POINT('Ctrl Pts',(78.6504216108429,-8.02285388397609,138.100269843259));
#82375=CARTESIAN_POINT('Ctrl Pts',(78.635964887324,-8.04313823348432,138.101857140033));
#82376=CARTESIAN_POINT('Ctrl Pts',(78.6122543102871,-8.07803648285834,138.104587190866));
#82377=CARTESIAN_POINT('Ctrl Pts',(78.6027631538214,-8.09248473037824,138.105717238794));
#82378=CARTESIAN_POINT('Ctrl Pts',(78.5895054421188,-8.11336782102481,138.107354271195));
#82379=CARTESIAN_POINT('Ctrl Pts',(78.5855542415546,-8.11968488041981,138.107849942608));
#82380=CARTESIAN_POINT('Ctrl Pts',(78.5787554361119,-8.13071854765846,138.108716919122));
#82381=CARTESIAN_POINT('Ctrl Pts',(78.5758886399612,-8.13542311678905,138.109086972922));
#82382=CARTESIAN_POINT('Ctrl Pts',(78.5697998012233,-8.14552768918537,138.109882738041));
#82383=CARTESIAN_POINT('Ctrl Pts',(78.5665850315755,-8.15093164966051,138.11030886536));
#82384=CARTESIAN_POINT('Ctrl Pts',(78.5578510209819,-8.16580431479997,138.111482871798));
#82385=CARTESIAN_POINT('Ctrl Pts',(78.5523946208913,-8.17530928871096,138.11223452253));
#82386=CARTESIAN_POINT('Ctrl Pts',(78.5221398794056,-8.22923810541439,138.116503867796));
#82387=CARTESIAN_POINT('Ctrl Pts',(78.4992951965933,-8.27472179707336,138.120121681014));
#82388=CARTESIAN_POINT('Ctrl Pts',(78.4634101512892,-8.35514979643572,138.126466083823));
#82389=CARTESIAN_POINT('Ctrl Pts',(78.4494000929481,-8.38960860654049,138.129168419324));
#82390=CARTESIAN_POINT('Ctrl Pts',(78.4365594354234,-8.42449187578589,138.13187361233));
#82391=CARTESIAN_POINT('Origin',(80.,-9.,134.));
#82392=CARTESIAN_POINT('',(78.4365593750041,-8.42449203992252,138.833737849951));
#82393=CARTESIAN_POINT('',(78.436559345854,-8.42449211911253,138.638847691527));
#82394=CARTESIAN_POINT('',(78.4365593749993,-8.42449203993574,134.));
#82395=CARTESIAN_POINT('Ctrl Pts',(78.436559345854,-8.42449211911253,138.638847691527));
#82396=CARTESIAN_POINT('Ctrl Pts',(78.4434608386264,-8.40574333263555,138.63740036079));
#82397=CARTESIAN_POINT('Ctrl Pts',(78.4507011944744,-8.38711431632311,138.635956897866));
#82398=CARTESIAN_POINT('Ctrl Pts',(78.478217800435,-8.31992405170581,138.630735319541));
#82399=CARTESIAN_POINT('Ctrl Pts',(78.5004548885466,-8.27220215182169,138.626998446861));
#82400=CARTESIAN_POINT('Ctrl Pts',(78.5359994117821,-8.20449582377853,138.621668964208));
#82401=CARTESIAN_POINT('Ctrl Pts',(78.5475358445659,-8.18362227306315,138.620021657096));
#82402=CARTESIAN_POINT('Ctrl Pts',(78.5692688525915,-8.14621949086728,138.617061556459));
#82403=CARTESIAN_POINT('Ctrl Pts',(78.5793136655477,-8.12960746307735,138.615743765781));
#82404=CARTESIAN_POINT('Ctrl Pts',(78.5955648023106,-8.10376265788315,138.613687817337));
#82405=CARTESIAN_POINT('Ctrl Pts',(78.6015768985399,-8.09441044750361,138.612942633952));
#82406=CARTESIAN_POINT('Ctrl Pts',(78.6130217290521,-8.07699305790112,138.611552245553));
#82407=CARTESIAN_POINT('Ctrl Pts',(78.6184322973563,-8.06891395182371,138.610906253053));
#82408=CARTESIAN_POINT('Ctrl Pts',(78.6307485453104,-8.05086698277575,138.609460586652));
#82409=CARTESIAN_POINT('Ctrl Pts',(78.6376929919388,-8.04092614501287,138.608662418179));
#82410=CARTESIAN_POINT('Ctrl Pts',(78.6584620210802,-8.01187649078897,138.606323658837));
#82411=CARTESIAN_POINT('Ctrl Pts',(78.6725848901082,-7.99298389592706,138.604794511063));
#82412=CARTESIAN_POINT('Ctrl Pts',(78.750998140174,-7.89260552361618,138.596611537474));
#82413=CARTESIAN_POINT('Ctrl Pts',(78.8223970604525,-7.81696032970234,138.590250266556));
#82414=CARTESIAN_POINT('Ctrl Pts',(78.9593334832886,-7.69664747395032,138.579118180237));
#82415=CARTESIAN_POINT('Ctrl Pts',(79.0218699622572,-7.64908382375167,138.574346148211));
#82416=CARTESIAN_POINT('Ctrl Pts',(79.1081348243836,-7.59261249238801,138.567843704408));
#82417=CARTESIAN_POINT('Ctrl Pts',(79.1290454399641,-7.57957713537964,138.566272894509));
#82418=CARTESIAN_POINT('Ctrl Pts',(79.1649872963638,-7.55826358366812,138.563568399681));
#82419=CARTESIAN_POINT('Ctrl Pts',(79.1798718133722,-7.54974491525152,138.562447108845));
#82420=CARTESIAN_POINT('Ctrl Pts',(79.2013882609893,-7.53786783131661,138.560820473376));
#82421=CARTESIAN_POINT('Ctrl Pts',(79.2079158569174,-7.53432135396445,138.560326243612));
#82422=CARTESIAN_POINT('Ctrl Pts',(79.219323999269,-7.52822171547543,138.559460806323));
#82423=CARTESIAN_POINT('Ctrl Pts',(79.2241938354606,-7.52564891190675,138.559090834731));
#82424=CARTESIAN_POINT('Ctrl Pts',(79.2346645379832,-7.52018333386636,138.558294079285));
#82425=CARTESIAN_POINT('Ctrl Pts',(79.2402689975685,-7.51729823112319,138.557866868923));
#82426=CARTESIAN_POINT('Ctrl Pts',(79.2557197346365,-7.5094549924992,138.556687340246));
#82427=CARTESIAN_POINT('Ctrl Pts',(79.2655988547602,-7.50456278151904,138.555931195485));
#82428=CARTESIAN_POINT('Ctrl Pts',(79.3223560191607,-7.47715425293571,138.551578890084));
#82429=CARTESIAN_POINT('Ctrl Pts',(79.370215206549,-7.45674676918163,138.547878181303));
#82430=CARTESIAN_POINT('Ctrl Pts',(79.5149160171262,-7.40289776301465,138.53674916697));
#82431=CARTESIAN_POINT('Ctrl Pts',(79.6139828650921,-7.37610512135498,138.529221755229));
#82432=CARTESIAN_POINT('Ctrl Pts',(79.786623253287,-7.34611715486538,138.516660911712));
#82433=CARTESIAN_POINT('Ctrl Pts',(79.8591121163593,-7.3383708786738,138.511544095369));
#82434=CARTESIAN_POINT('Ctrl Pts',(79.9494895583125,-7.33467266240074,138.505371191486));
#82435=CARTESIAN_POINT('Ctrl Pts',(79.967105186019,-7.33423158311541,138.504177419419));
#82436=CARTESIAN_POINT('Ctrl Pts',(79.9954593124748,-7.3339716043367,138.50227036102));
#82437=CARTESIAN_POINT('Ctrl Pts',(80.0061944363775,-7.33397692954553,138.50155165648));
#82438=CARTESIAN_POINT('Ctrl Pts',(80.0267223977116,-7.33418553422263,138.500183429913));
#82439=CARTESIAN_POINT('Ctrl Pts',(80.0365149210737,-7.33437141341169,138.499533393843));
#82440=CARTESIAN_POINT('Ctrl Pts',(80.0588703600664,-7.33499300885727,138.498055194475));
#82441=CARTESIAN_POINT('Ctrl Pts',(80.0714312232682,-7.33548457664384,138.497228805245));
#82442=CARTESIAN_POINT('Ctrl Pts',(80.1049615143958,-7.33717704190505,138.495033111872));
#82443=CARTESIAN_POINT('Ctrl Pts',(80.1259162276642,-7.33863240784865,138.493671701344));
#82444=CARTESIAN_POINT('Ctrl Pts',(80.2672375367983,-7.35113690819438,138.484550788982));
#82445=CARTESIAN_POINT('Ctrl Pts',(80.3861216598723,-7.37486021889751,138.477209685945));
#82446=CARTESIAN_POINT('Ctrl Pts',(80.5645438658497,-7.43116916736222,138.465777060569));
#82447=CARTESIAN_POINT('Ctrl Pts',(80.62643700612,-7.45484131225998,138.461720066128));
#82448=CARTESIAN_POINT('Ctrl Pts',(80.7072016229514,-7.49138287629356,138.456109433669));
#82449=CARTESIAN_POINT('Ctrl Pts',(80.7274605479272,-7.501046761181,138.454673988079));
#82450=CARTESIAN_POINT('Ctrl Pts',(80.7618138964147,-7.51829439139616,138.452180987866));
#82451=CARTESIAN_POINT('Ctrl Pts',(80.7760059856607,-7.52567758361189,138.451133425087));
#82452=CARTESIAN_POINT('Ctrl Pts',(80.7964511678912,-7.53669081840668,138.449595268841));
#82453=CARTESIAN_POINT('Ctrl Pts',(80.8027909110374,-7.54015926481604,138.449114196331));
#82454=CARTESIAN_POINT('Ctrl Pts',(80.8138598112878,-7.54630891859968,138.448266673758));
#82455=CARTESIAN_POINT('Ctrl Pts',(80.8185987148561,-7.54897219344509,138.447901352834));
#82456=CARTESIAN_POINT('Ctrl Pts',(80.828894873633,-7.55482515148955,138.447102125861));
#82457=CARTESIAN_POINT('Ctrl Pts',(80.8344467008278,-7.55802366374395,138.446667687241));
#82458=CARTESIAN_POINT('Ctrl Pts',(80.849899348852,-7.56704534861054,138.445449026636));
#82459=CARTESIAN_POINT('Ctrl Pts',(80.8597583783436,-7.57293887702075,138.444660570075));
#82460=CARTESIAN_POINT('Ctrl Pts',(80.9259763525672,-7.61345788121388,138.439294622351));
#82461=CARTESIAN_POINT('Ctrl Pts',(80.9802851901333,-7.65130795039124,138.434548768141));
#82462=CARTESIAN_POINT('Ctrl Pts',(81.0494939380594,-7.70593500960563,138.428156629021));
#82463=CARTESIAN_POINT('Ctrl Pts',(81.0665206734937,-7.71993150217568,138.426553800348));
#82464=CARTESIAN_POINT('Ctrl Pts',(81.1369212003291,-7.78018280586612,138.41980969693));
#82465=CARTESIAN_POINT('Ctrl Pts',(81.187606613277,-7.82947215992488,138.414667977005));
#82466=CARTESIAN_POINT('Ctrl Pts',(81.2807389945504,-7.93233655596453,138.404747316231));
#82467=CARTESIAN_POINT('Ctrl Pts',(81.323329006124,-7.9856035669354,138.399971005538));
#82468=CARTESIAN_POINT('Ctrl Pts',(81.3725098713493,-8.05550397657339,138.394141012636));
#82469=CARTESIAN_POINT('Ctrl Pts',(81.3822567335077,-8.06982665742033,138.392967746781));
#82470=CARTESIAN_POINT('Ctrl Pts',(81.3976439983137,-8.09321384810194,138.391085353149));
#82471=CARTESIAN_POINT('Ctrl Pts',(81.4034235669459,-8.10218477836519,138.390371057));
#82472=CARTESIAN_POINT('Ctrl Pts',(81.4143515263168,-8.11951033732702,138.389006078594));
#82473=CARTESIAN_POINT('Ctrl Pts',(81.4195130574064,-8.1278561053661,138.388354930774));
#82474=CARTESIAN_POINT('Ctrl Pts',(81.4311857622385,-8.1471080739557,138.386867102131));
#82475=CARTESIAN_POINT('Ctrl Pts',(81.4376466055814,-8.15804419602341,138.386032278416));
#82476=CARTESIAN_POINT('Ctrl Pts',(81.458075420221,-8.19354447769681,138.383354379379));
#82477=CARTESIAN_POINT('Ctrl Pts',(81.4715441897384,-8.21839121760763,138.381529085882));
#82478=CARTESIAN_POINT('Ctrl Pts',(81.5438289532878,-8.36023867017505,138.371354561212));
#82479=CARTESIAN_POINT('Ctrl Pts',(81.5893207665385,-8.48350766445429,138.363481739732));
#82480=CARTESIAN_POINT('Ctrl Pts',(81.6365740009059,-8.68020229686246,138.351070222903));
#82481=CARTESIAN_POINT('Ctrl Pts',(81.6487634832857,-8.75055726931617,138.346647835921));
#82482=CARTESIAN_POINT('Ctrl Pts',(81.6580966694744,-8.83714970725488,138.340997106757));
#82483=CARTESIAN_POINT('Ctrl Pts',(81.6595640601898,-8.85285425929765,138.33996394504));
#82484=CARTESIAN_POINT('Ctrl Pts',(81.6613750744937,-8.87574018888127,138.338443127261));
#82485=CARTESIAN_POINT('Ctrl Pts',(81.6618955800766,-8.88290723770163,138.337964694672));
#82486=CARTESIAN_POINT('Ctrl Pts',(81.6627281080705,-8.89549762033381,138.337120072694));
#82487=CARTESIAN_POINT('Ctrl Pts',(81.6630599964519,-8.90091944868504,138.336754985731));
#82488=CARTESIAN_POINT('Ctrl Pts',(81.6637270982145,-8.91276728910201,138.33595412142));
#82489=CARTESIAN_POINT('Ctrl Pts',(81.6640515969898,-8.9191935507508,138.335517791822));
#82490=CARTESIAN_POINT('Ctrl Pts',(81.6648571046909,-8.93721805853627,138.334288824208));
#82491=CARTESIAN_POINT('Ctrl Pts',(81.6652541190076,-8.94881942246295,138.333491841116));
#82492=CARTESIAN_POINT('Ctrl Pts',(81.6673560871115,-9.03727841390818,138.327374187734));
#82493=CARTESIAN_POINT('Ctrl Pts',(81.6638602753966,-9.11415912409219,138.321826942408));
#82494=CARTESIAN_POINT('Ctrl Pts',(81.6485394998224,-9.24725678906403,138.312088770737));
#82495=CARTESIAN_POINT('Ctrl Pts',(81.6390939687503,-9.3036274436794,138.30792068187));
#82496=CARTESIAN_POINT('Ctrl Pts',(81.6088803119067,-9.44038431505247,138.297799254905));
#82497=CARTESIAN_POINT('Ctrl Pts',(81.5849649046377,-9.51992698704693,138.29190908635));
#82498=CARTESIAN_POINT('Ctrl Pts',(81.5470215729409,-9.61871075116403,138.284633845712));
#82499=CARTESIAN_POINT('Ctrl Pts',(81.5383847161538,-9.63988381438838,138.283076281886));
#82500=CARTESIAN_POINT('Ctrl Pts',(81.5246220019957,-9.67173184891744,138.280735047203));
#82501=CARTESIAN_POINT('Ctrl Pts',(81.5198140171293,-9.68254032237748,138.279940764566));
#82502=CARTESIAN_POINT('Ctrl Pts',(81.5112438553686,-9.70126658874638,138.278564817294));
#82503=CARTESIAN_POINT('Ctrl Pts',(81.5075336055757,-9.70920748161489,138.277981404823));
#82504=CARTESIAN_POINT('Ctrl Pts',(81.499026415129,-9.72704661579931,138.276670717998));
#82505=CARTESIAN_POINT('Ctrl Pts',(81.4941937393209,-9.73692744143512,138.275944709717));
#82506=CARTESIAN_POINT('Ctrl Pts',(81.4808128369563,-9.76361297905029,138.273983308478));
#82507=CARTESIAN_POINT('Ctrl Pts',(81.4720764779417,-9.78032193991025,138.272754508241));
#82508=CARTESIAN_POINT('Ctrl Pts',(81.4178318295768,-9.87991424152801,138.265418864789));
#82509=CARTESIAN_POINT('Ctrl Pts',(81.3656165050383,-9.95895311903628,138.259561907776));
#82510=CARTESIAN_POINT('Ctrl Pts',(81.2495545732988,-10.1057764438651,138.248102500175));
#82511=CARTESIAN_POINT('Ctrl Pts',(81.186188023533,-10.1734921905774,138.242514313668));
#82512=CARTESIAN_POINT('Ctrl Pts',(81.0976679062517,-10.2535543146676,138.235011266274));
#82513=CARTESIAN_POINT('Ctrl Pts',(81.0773761295718,-10.2710364939648,138.233308855011));
#82514=CARTESIAN_POINT('Ctrl Pts',(81.0425742000378,-10.2995874716513,138.230400768338));
#82515=CARTESIAN_POINT('Ctrl Pts',(81.0282871355572,-10.3109210728568,138.229210074329));
#82516=CARTESIAN_POINT('Ctrl Pts',(81.0077780479651,-10.3266489115807,138.227500577077));
#82517=CARTESIAN_POINT('Ctrl Pts',(81.0017069209194,-10.3312389595983,138.226994498134));
#82518=CARTESIAN_POINT('Ctrl Pts',(80.9911686592186,-10.339093461734,138.22611557854));
#82519=CARTESIAN_POINT('Ctrl Pts',(80.986716357711,-10.3423775321488,138.225744094408));
#82520=CARTESIAN_POINT('Ctrl Pts',(80.9772341857389,-10.3492990304779,138.224952477717));
#82521=CARTESIAN_POINT('Ctrl Pts',(80.9722004020218,-10.3529304869702,138.224531991428));
#82522=CARTESIAN_POINT('Ctrl Pts',(80.9582917627374,-10.3628467116179,138.223369763879));
#82523=CARTESIAN_POINT('Ctrl Pts',(80.9493756678044,-10.3690727108579,138.222624278211));
#82524=CARTESIAN_POINT('Ctrl Pts',(80.9018947684799,-10.4015412007286,138.218654700848));
#82525=CARTESIAN_POINT('Ctrl Pts',(80.8623047052113,-10.4262403921482,138.215346547015));
#82526=CARTESIAN_POINT('Ctrl Pts',(80.7454339453908,-10.4925072199919,138.205691384427));
#82527=CARTESIAN_POINT('Ctrl Pts',(80.6658362202949,-10.5296770218662,138.199255542834));
#82528=CARTESIAN_POINT('Ctrl Pts',(80.5122979459122,-10.587109161112,138.187404044057));
#82529=CARTESIAN_POINT('Ctrl Pts',(80.4391581917112,-10.6088839199372,138.181977622184));
#82530=CARTESIAN_POINT('Ctrl Pts',(80.3375096411757,-10.631693630497,138.174771394722));
#82531=CARTESIAN_POINT('Ctrl Pts',(80.3100928388688,-10.6371253636595,138.172859390139));
#82532=CARTESIAN_POINT('Ctrl Pts',(80.2699517562068,-10.6440332989691,138.170104352569));
#82533=CARTESIAN_POINT('Ctrl Pts',(80.2573278065656,-10.6460564554662,138.16924423978));
#82534=CARTESIAN_POINT('Ctrl Pts',(80.2349937357081,-10.6493725674169,138.167733322795));
#82535=CARTESIAN_POINT('Ctrl Pts',(80.2252932949809,-10.6507255557019,138.167080654889));
#82536=CARTESIAN_POINT('Ctrl Pts',(80.2049370835632,-10.653381994793,138.165718283175));
#82537=CARTESIAN_POINT('Ctrl Pts',(80.1942794804908,-10.6546681605338,138.165009151354));
#82538=CARTESIAN_POINT('Ctrl Pts',(80.1660986948024,-10.6577930024467,138.163144526125));
#82539=CARTESIAN_POINT('Ctrl Pts',(80.1485571947301,-10.6594569032775,138.161994530635));
#82540=CARTESIAN_POINT('Ctrl Pts',(80.0662023256179,-10.6659523016728,138.156640816002));
#82541=CARTESIAN_POINT('Ctrl Pts',(80.0011647255404,-10.6672671971632,138.152547223699));
#82542=CARTESIAN_POINT('Ctrl Pts',(79.7906320968475,-10.6592001775789,138.139491356231));
#82543=CARTESIAN_POINT('Ctrl Pts',(79.6464361269822,-10.6345525797856,138.130893657106));
#82544=CARTESIAN_POINT('Ctrl Pts',(79.4858722721177,-10.584844454118,138.120105926452));
#82545=CARTESIAN_POINT('Ctrl Pts',(79.4645796308183,-10.5777782396883,138.118648339947));
#82546=CARTESIAN_POINT('Ctrl Pts',(79.4356664268688,-10.5675304121401,138.116623579734));
#82547=CARTESIAN_POINT('Ctrl Pts',(79.4279161747799,-10.564718525695,138.116076309569));
#82548=CARTESIAN_POINT('Ctrl Pts',(79.4148987023142,-10.5598859879694,138.115148944494));
#82549=CARTESIAN_POINT('Ctrl Pts',(79.4096201605108,-10.5578958463197,138.114770624443));
#82550=CARTESIAN_POINT('Ctrl Pts',(79.3987912128859,-10.553750123733,138.113989623443));
#82551=CARTESIAN_POINT('Ctrl Pts',(79.3932421260253,-10.5515915481405,138.113586783608));
#82552=CARTESIAN_POINT('Ctrl Pts',(79.3786664088957,-10.545831497834,138.112521934093));
#82553=CARTESIAN_POINT('Ctrl Pts',(79.3696596741634,-10.5421807654733,138.111857123389));
#82554=CARTESIAN_POINT('Ctrl Pts',(79.3307974762706,-10.5260313066563,138.108960583435));
#82555=CARTESIAN_POINT('Ctrl Pts',(79.3012798319572,-10.5127436550002,138.106688593166));
#82556=CARTESIAN_POINT('Ctrl Pts',(79.2486156407491,-10.4871661761695,138.102526226925));
#82557=CARTESIAN_POINT('Ctrl Pts',(79.2253348701368,-10.4751730474593,138.100646276896));
#82558=CARTESIAN_POINT('Ctrl Pts',(79.1163605275306,-10.4157436165353,138.091683399061));
#82559=CARTESIAN_POINT('Ctrl Pts',(79.0346706200088,-10.3613557689784,138.08449168696));
#82560=CARTESIAN_POINT('Ctrl Pts',(78.9010168983634,-10.2542597921801,138.072211178715));
#82561=CARTESIAN_POINT('Ctrl Pts',(78.8468840465849,-10.2046816029801,138.067057796581));
#82562=CARTESIAN_POINT('Ctrl Pts',(78.783986813428,-10.1389378491472,138.060848291008));
#82563=CARTESIAN_POINT('Ctrl Pts',(78.7719891160083,-10.1259914762317,138.059652463455));
#82564=CARTESIAN_POINT('Ctrl Pts',(78.753024188109,-10.1048632017148,138.057742933131));
#82565=CARTESIAN_POINT('Ctrl Pts',(78.7459267043359,-10.0968005964589,138.05702378686));
#82566=CARTESIAN_POINT('Ctrl Pts',(78.7325087113124,-10.0812574716588,138.055655226475));
#82567=CARTESIAN_POINT('Ctrl Pts',(78.7261752385491,-10.0737887925549,138.055005293519));
#82568=CARTESIAN_POINT('Ctrl Pts',(78.7118711291791,-10.05661615227,138.053528018844));
#82569=CARTESIAN_POINT('Ctrl Pts',(78.7039435560626,-10.0468769696414,138.052702443199));
#82570=CARTESIAN_POINT('Ctrl Pts',(78.683080955167,-10.0206465865431,138.050510451186));
#82571=CARTESIAN_POINT('Ctrl Pts',(78.670345463884,-10.0039990550955,138.049151885297));
#82572=CARTESIAN_POINT('Ctrl Pts',(78.5858580102951,-9.88913065055669,138.039984103861));
#82573=CARTESIAN_POINT('Ctrl Pts',(78.5247345555471,-9.78354744866699,138.032599506894));
#82574=CARTESIAN_POINT('Ctrl Pts',(78.4491360085769,-9.61212248495406,138.021150117326));
#82575=CARTESIAN_POINT('Ctrl Pts',(78.4262054564742,-9.5504930016204,138.017122819631));
#82576=CARTESIAN_POINT('Ctrl Pts',(78.4004337605245,-9.46630806743096,138.011549560494));
#82577=CARTESIAN_POINT('Ctrl Pts',(78.3943233224832,-9.44481195594943,138.010120178699));
#82578=CARTESIAN_POINT('Ctrl Pts',(78.3845969542231,-9.40777842962082,138.007636704069));
#82579=CARTESIAN_POINT('Ctrl Pts',(78.3807683309085,-9.39229963562683,138.006592501605));
#82580=CARTESIAN_POINT('Ctrl Pts',(78.375530452953,-9.36973879727022,138.005058389208));
#82581=CARTESIAN_POINT('Ctrl Pts',(78.3739440148056,-9.36269824330599,138.004577930402));
#82582=CARTESIAN_POINT('Ctrl Pts',(78.3712431190839,-9.35033778703886,138.003731083528));
#82583=CARTESIAN_POINT('Ctrl Pts',(78.3701088740253,-9.34502240275204,138.003365818387));
#82584=CARTESIAN_POINT('Ctrl Pts',(78.3676928827579,-9.33342256871863,138.002566217251));
#82585=CARTESIAN_POINT('Ctrl Pts',(78.3664214291154,-9.32713633795341,138.002131344157));
#82586=CARTESIAN_POINT('Ctrl Pts',(78.3629688734555,-9.30954429387675,138.000910318892));
#82587=CARTESIAN_POINT('Ctrl Pts',(78.3608686863847,-9.29822323430471,138.000119906912));
#82588=CARTESIAN_POINT('Ctrl Pts',(78.3472941221451,-9.22056960548436,137.994670699723));
#82589=CARTESIAN_POINT('Ctrl Pts',(78.3397332654653,-9.15362294499791,137.989837623539));
#82590=CARTESIAN_POINT('Ctrl Pts',(78.3347732356146,-9.05812245807967,137.982902254536));
#82591=CARTESIAN_POINT('Ctrl Pts',(78.3340257365145,-9.02980136265055,137.980840097936));
#82592=CARTESIAN_POINT('Ctrl Pts',(78.3338937191599,-8.88071687455458,137.969987743028));
#82593=CARTESIAN_POINT('Ctrl Pts',(78.3469166497543,-8.76028325719652,137.96126889487));
#82594=CARTESIAN_POINT('Ctrl Pts',(78.3773635481472,-8.62178279113277,137.951513814421));
#82595=CARTESIAN_POINT('Ctrl Pts',(78.3822617998227,-8.60135166197025,137.950080742957));
#82596=CARTESIAN_POINT('Ctrl Pts',(78.3907068956839,-8.56885067699838,137.947809787927));
#82597=CARTESIAN_POINT('Ctrl Pts',(78.3940061041705,-8.55671943882072,137.946964089689));
#82598=CARTESIAN_POINT('Ctrl Pts',(78.4001194486049,-8.53520526474169,137.945467425903));
#82599=CARTESIAN_POINT('Ctrl Pts',(78.4028795813367,-8.52580773942798,137.944814747905));
#82600=CARTESIAN_POINT('Ctrl Pts',(78.4088380700724,-8.50616305216194,137.943452398024));
#82601=CARTESIAN_POINT('Ctrl Pts',(78.4120529215466,-8.49592133210179,137.942743297751));
#82602=CARTESIAN_POINT('Ctrl Pts',(78.4208046914339,-8.46895526421802,137.940878853581));
#82603=CARTESIAN_POINT('Ctrl Pts',(78.4265083702413,-8.45228614804004,137.939729005626));
#82604=CARTESIAN_POINT('Ctrl Pts',(78.433823490773,-8.43196568807629,137.938329369574));
#82605=CARTESIAN_POINT('Ctrl Pts',(78.4351847763598,-8.42822631211844,137.938071894579));
#82606=CARTESIAN_POINT('Ctrl Pts',(78.4365593741136,-8.42449204234183,137.937814844869));
#82607=CARTESIAN_POINT('Ctrl Pts',(78.4365594354234,-8.42449187578589,138.13187361233));
#82608=CARTESIAN_POINT('Ctrl Pts',(78.4162408380163,-8.4796899139457,138.136154213031));
#82609=CARTESIAN_POINT('Ctrl Pts',(78.3988502582591,-8.53595084181721,138.140440641763));
#82610=CARTESIAN_POINT('Ctrl Pts',(78.3715300080598,-8.64440579812346,138.148485977305));
#82611=CARTESIAN_POINT('Ctrl Pts',(78.3610470722338,-8.69636212694456,138.152248990963));
#82612=CARTESIAN_POINT('Ctrl Pts',(78.3494451869366,-8.77240761653733,138.157611105667));
#82613=CARTESIAN_POINT('Ctrl Pts',(78.3463441283616,-8.7961573093358,138.159265662141));
#82614=CARTESIAN_POINT('Ctrl Pts',(78.3416515914771,-8.83932701747486,138.162237367125));
#82615=CARTESIAN_POINT('Ctrl Pts',(78.339886678227,-8.85872344118776,138.163559574137));
#82616=CARTESIAN_POINT('Ctrl Pts',(78.337648209532,-8.88924630923566,138.16562068145));
#82617=CARTESIAN_POINT('Ctrl Pts',(78.3369454406017,-8.90035363447742,138.16636666894));
#82618=CARTESIAN_POINT('Ctrl Pts',(78.3358375461699,-8.92117245425774,138.167757585857));
#82619=CARTESIAN_POINT('Ctrl Pts',(78.3354060060516,-8.93088200769565,138.168403312385));
#82620=CARTESIAN_POINT('Ctrl Pts',(78.3346279522514,-8.95268846264312,138.169847129197));
#82621=CARTESIAN_POINT('Ctrl Pts',(78.3343282238388,-8.96478656519042,138.170643728318));
#82622=CARTESIAN_POINT('Ctrl Pts',(78.3338346509293,-9.00036039841419,138.172973899075));
#82623=CARTESIAN_POINT('Ctrl Pts',(78.334005132081,-9.02383880690506,138.174496153192));
#82624=CARTESIAN_POINT('Ctrl Pts',(78.3372811617206,-9.13916410223909,138.181909022735));
#82625=CARTESIAN_POINT('Ctrl Pts',(78.3474859608974,-9.23065282536611,138.187577559313));
#82626=CARTESIAN_POINT('Ctrl Pts',(78.3797605383403,-9.39510428146941,138.197826704273));
#82627=CARTESIAN_POINT('Ctrl Pts',(78.3993774358818,-9.46828379149291,138.202414086921));
#82628=CARTESIAN_POINT('Ctrl Pts',(78.4347717964449,-9.57161383638414,138.209220657374));
#82629=CARTESIAN_POINT('Ctrl Pts',(78.4466000024374,-9.60301730952699,138.211335740606));
#82630=CARTESIAN_POINT('Ctrl Pts',(78.467528952769,-9.65387184785785,138.214870435589));
#82631=CARTESIAN_POINT('Ctrl Pts',(78.4760722519293,-9.67354288487014,138.216265358164));
#82632=CARTESIAN_POINT('Ctrl Pts',(78.4883633259994,-9.70041147377598,138.218216451382));
#82633=CARTESIAN_POINT('Ctrl Pts',(78.4917879523247,-9.70775566359377,138.218754544787));
#82634=CARTESIAN_POINT('Ctrl Pts',(78.4976753745127,-9.72014459103995,138.219670874305));
#82635=CARTESIAN_POINT('Ctrl Pts',(78.5001103985647,-9.72520251988738,138.22004743184));
#82636=CARTESIAN_POINT('Ctrl Pts',(78.5052004481131,-9.73564005329026,138.220829765833));
#82637=CARTESIAN_POINT('Ctrl Pts',(78.5078590190368,-9.74101773149138,138.221235740676));
#82638=CARTESIAN_POINT('Ctrl Pts',(78.5149940884378,-9.7552562456191,138.222318122792));
#82639=CARTESIAN_POINT('Ctrl Pts',(78.5195207618503,-9.76409146524403,138.222997494212));
#82640=CARTESIAN_POINT('Ctrl Pts',(78.5401181263322,-9.80342344633525,138.226054891001));
#82641=CARTESIAN_POINT('Ctrl Pts',(78.5570529769975,-9.83345534985851,138.228478683909));
#82642=CARTESIAN_POINT('Ctrl Pts',(78.5872318929872,-9.88329417236705,138.23262873011));
#82643=CARTESIAN_POINT('Ctrl Pts',(78.5999925923471,-9.9033833621558,138.234338253884));
#82644=CARTESIAN_POINT('Ctrl Pts',(78.6663398912396,-10.0030504792924,138.242984226519));
#82645=CARTESIAN_POINT('Ctrl Pts',(78.7263031982461,-10.0781731988061,138.250026907009));
#82646=CARTESIAN_POINT('Ctrl Pts',(78.8267376140599,-10.1838479474004,138.260489784493));
#82647=CARTESIAN_POINT('Ctrl Pts',(78.8626831996413,-10.2184218720492,138.264022441926));
#82648=CARTESIAN_POINT('Ctrl Pts',(78.9254731741463,-10.2736116935564,138.269841119918));
#82649=CARTESIAN_POINT('Ctrl Pts',(78.951490614769,-10.2951150526434,138.272160049775));
#82650=CARTESIAN_POINT('Ctrl Pts',(78.9889948813682,-10.3242406758455,138.27537855041));
#82651=CARTESIAN_POINT('Ctrl Pts',(78.999948857413,-10.3325323445636,138.276304339618));
#82652=CARTESIAN_POINT('Ctrl Pts',(79.0190041344841,-10.346588998651,138.277890905895));
#82653=CARTESIAN_POINT('Ctrl Pts',(79.0270566402004,-10.3524185910603,138.278554171431));
#82654=CARTESIAN_POINT('Ctrl Pts',(79.0436103339799,-10.3641782238089,138.279903295275));
#82655=CARTESIAN_POINT('Ctrl Pts',(79.0521156581689,-10.3701017123973,138.280588882975));
#82656=CARTESIAN_POINT('Ctrl Pts',(79.0737995389116,-10.3849047634619,138.282318041019));
#82657=CARTESIAN_POINT('Ctrl Pts',(79.0870510677369,-10.3936759930543,138.28335751218));
#82658=CARTESIAN_POINT('Ctrl Pts',(79.1396108269839,-10.4273940525248,138.287415930332));
#82659=CARTESIAN_POINT('Ctrl Pts',(79.179833989079,-10.4508796050651,138.290381556378));
#82660=CARTESIAN_POINT('Ctrl Pts',(79.32056975265,-10.5253265657428,138.300373902286));
#82661=CARTESIAN_POINT('Ctrl Pts',(79.4252318929986,-10.5677655049789,138.307143184363));
#82662=CARTESIAN_POINT('Ctrl Pts',(79.5958292560824,-10.6175395647836,138.318076734668));
#82663=CARTESIAN_POINT('Ctrl Pts',(79.6592880574734,-10.6320850874439,138.322129520577));
#82664=CARTESIAN_POINT('Ctrl Pts',(79.738340761138,-10.6453933188223,138.327336953533));
#82665=CARTESIAN_POINT('Ctrl Pts',(79.7532876126986,-10.647700728144,138.328328495682));
#82666=CARTESIAN_POINT('Ctrl Pts',(79.7752600163266,-10.6507870431205,138.329799023082));
#82667=CARTESIAN_POINT('Ctrl Pts',(79.7822629023838,-10.6517253021591,138.330269618447));
#82668=CARTESIAN_POINT('Ctrl Pts',(79.7941816947229,-10.6532450902334,138.331074150936));
#82669=CARTESIAN_POINT('Ctrl Pts',(79.7990945678788,-10.6538493007611,138.331406819084));
#82670=CARTESIAN_POINT('Ctrl Pts',(79.810285203852,-10.6551749831075,138.33216702983));
#82671=CARTESIAN_POINT('Ctrl Pts',(79.8165642818435,-10.6558826234256,138.332595312));
#82672=CARTESIAN_POINT('Ctrl Pts',(79.8338809064756,-10.6577344732874,138.333780918482));
#82673=CARTESIAN_POINT('Ctrl Pts',(79.8449258580662,-10.6588041268058,138.334542132722));
#82674=CARTESIAN_POINT('Ctrl Pts',(79.9085243171649,-10.6643226433761,138.338950985471));
#82675=CARTESIAN_POINT('Ctrl Pts',(79.9612500247842,-10.6663837943462,138.342706003469));
#82676=CARTESIAN_POINT('Ctrl Pts',(80.1158374726023,-10.6650866694285,138.353853764988));
#82677=CARTESIAN_POINT('Ctrl Pts',(80.2174106677104,-10.6548916397337,138.361340095339));
#82678=CARTESIAN_POINT('Ctrl Pts',(80.3886112914624,-10.6216648825184,138.373839403056));
#82679=CARTESIAN_POINT('Ctrl Pts',(80.4588362841796,-10.6032116494468,138.378934977978));
#82680=CARTESIAN_POINT('Ctrl Pts',(80.544336970477,-10.5746628182562,138.38508639419));
#82681=CARTESIAN_POINT('Ctrl Pts',(80.5609412639335,-10.5688246136208,138.386278758174));
#82682=CARTESIAN_POINT('Ctrl Pts',(80.5875138613088,-10.5590056323754,138.388183997746));
#82683=CARTESIAN_POINT('Ctrl Pts',(80.5975412679014,-10.5551898731265,138.388902275348));
#82684=CARTESIAN_POINT('Ctrl Pts',(80.6166491724863,-10.5477065885507,138.390269954034));
#82685=CARTESIAN_POINT('Ctrl Pts',(80.6257355252957,-10.5440553570189,138.390919866397));
#82686=CARTESIAN_POINT('Ctrl Pts',(80.6464137681153,-10.5355335612935,138.392398140205));
#82687=CARTESIAN_POINT('Ctrl Pts',(80.6579838635581,-10.5306114226591,138.393224724461));
#82688=CARTESIAN_POINT('Ctrl Pts',(80.6887451802089,-10.5171116982725,138.395421714864));
#82689=CARTESIAN_POINT('Ctrl Pts',(80.7078320268624,-10.5083009359409,138.396784209767));
#82690=CARTESIAN_POINT('Ctrl Pts',(80.8352048575512,-10.4465532195802,138.405884162082));
#82691=CARTESIAN_POINT('Ctrl Pts',(80.9376382540033,-10.3823609225986,138.413205954785));
#82692=CARTESIAN_POINT('Ctrl Pts',(81.0844094952207,-10.2665018248198,138.424631601502));
#82693=CARTESIAN_POINT('Ctrl Pts',(81.1340493662402,-10.222252669018,138.42870222721));
#82694=CARTESIAN_POINT('Ctrl Pts',(81.1967735684444,-10.1592216096295,138.434329931317));
#82695=CARTESIAN_POINT('Ctrl Pts',(81.2123110473044,-10.1429626144115,138.435768066381));
#82696=CARTESIAN_POINT('Ctrl Pts',(81.2383451425973,-10.1145913818378,138.43826523838));
#82697=CARTESIAN_POINT('Ctrl Pts',(81.2490050868428,-10.1026327073994,138.439314237175));
#82698=CARTESIAN_POINT('Ctrl Pts',(81.2642226788876,-10.0850572719499,138.440854044841));
#82699=CARTESIAN_POINT('Ctrl Pts',(81.2689191772768,-10.0795611987909,138.441335302064));
#82700=CARTESIAN_POINT('Ctrl Pts',(81.2770836122515,-10.0698798945819,138.442182939146));
#82701=CARTESIAN_POINT('Ctrl Pts',(81.280567065107,-10.0657079956872,138.442548187269));
#82702=CARTESIAN_POINT('Ctrl Pts',(81.2881093726586,-10.0565847016777,138.443346985021));
#82703=CARTESIAN_POINT('Ctrl Pts',(81.2921600560248,-10.0516270127352,138.443781064482));
#82704=CARTESIAN_POINT('Ctrl Pts',(81.3033865396136,-10.0377239711607,138.444998089986));
#82705=CARTESIAN_POINT('Ctrl Pts',(81.3104985386231,-10.0287278911602,138.445785254614));
#82706=CARTESIAN_POINT('Ctrl Pts',(81.3576051003872,-9.96786081399175,138.451105045985));
#82707=CARTESIAN_POINT('Ctrl Pts',(81.3945994656451,-9.91374864267551,138.455802824427));
#82708=CARTESIAN_POINT('Ctrl Pts',(81.4392456805557,-9.83939219079096,138.462089307413));
#82709=CARTESIAN_POINT('Ctrl Pts',(81.4498327865488,-9.82097031100142,138.463634071691));
#82710=CARTESIAN_POINT('Ctrl Pts',(81.4930625739267,-9.74230366163525,138.470166397353));
#82711=CARTESIAN_POINT('Ctrl Pts',(81.522326526334,-9.68027453639487,138.475157104236));
#82712=CARTESIAN_POINT('Ctrl Pts',(81.5740833076893,-9.55036673136398,138.485172991431));
#82713=CARTESIAN_POINT('Ctrl Pts',(81.5962000233244,-9.48248291686422,138.49018060228));
#82714=CARTESIAN_POINT('Ctrl Pts',(81.6182480663619,-9.39640425338043,138.496243725862));
#82715=CARTESIAN_POINT('Ctrl Pts',(81.6223285704271,-9.37935891541123,138.497430985418));
#82716=CARTESIAN_POINT('Ctrl Pts',(81.6284687982065,-9.35179558137282,138.499330080579));
#82717=CARTESIAN_POINT('Ctrl Pts',(81.6306972451329,-9.34131695210185,138.50004725577));
#82718=CARTESIAN_POINT('Ctrl Pts',(81.6347697947028,-9.32121595399975,138.501414100116));
#82719=CARTESIAN_POINT('Ctrl Pts',(81.6366303867693,-9.31159742436894,138.502064268603));
#82720=CARTESIAN_POINT('Ctrl Pts',(81.6406906590706,-9.28956698441122,138.50354485532));
#82721=CARTESIAN_POINT('Ctrl Pts',(81.6428345543528,-9.27714530261816,138.50437347627));
#82722=CARTESIAN_POINT('Ctrl Pts',(81.6481949467874,-9.24383602047196,138.506579763343));
#82723=CARTESIAN_POINT('Ctrl Pts',(81.6511554036219,-9.22290914042401,138.507949409065));
#82724=CARTESIAN_POINT('Ctrl Pts',(81.6680483973525,-9.08456358618208,138.51690793204));
#82725=CARTESIAN_POINT('Ctrl Pts',(81.6698456203906,-8.9660018533556,138.5240992852));
#82726=CARTESIAN_POINT('Ctrl Pts',(81.6501770088163,-8.75098256066482,138.537289425265));
#82727=CARTESIAN_POINT('Ctrl Pts',(81.6327473246685,-8.65471109099327,138.543263811233));
#82728=CARTESIAN_POINT('Ctrl Pts',(81.6038688700322,-8.54911094842004,138.550422975132));
#82729=CARTESIAN_POINT('Ctrl Pts',(81.6006228756811,-8.53772012885398,138.551203440306));
#82730=CARTESIAN_POINT('Ctrl Pts',(81.5954325132745,-8.52021647805795,138.552416843218));
#82731=CARTESIAN_POINT('Ctrl Pts',(81.5935737520238,-8.51407837488094,138.552845045651));
#82732=CARTESIAN_POINT('Ctrl Pts',(81.5900594521317,-8.50271031434071,138.553643365241));
#82733=CARTESIAN_POINT('Ctrl Pts',(81.5884134676726,-8.49747761716935,138.554012934576));
#82734=CARTESIAN_POINT('Ctrl Pts',(81.5845712890876,-8.48547056017931,138.554865747976));
#82735=CARTESIAN_POINT('Ctrl Pts',(81.5823574762219,-8.47870207421528,138.555349985149));
#82736=CARTESIAN_POINT('Ctrl Pts',(81.5750782316615,-8.45692024145689,138.556919160484));
#82737=CARTESIAN_POINT('Ctrl Pts',(81.5698421648651,-8.441965420673,138.558013186098));
#82738=CARTESIAN_POINT('Ctrl Pts',(81.534719793454,-8.34606021026865,138.565127151807));
#82739=CARTESIAN_POINT('Ctrl Pts',(81.4987980591139,-8.26746762889686,138.571403106748));
#82740=CARTESIAN_POINT('Ctrl Pts',(81.421387860257,-8.12788116124493,138.58302200605));
#82741=CARTESIAN_POINT('Ctrl Pts',(81.3816206262326,-8.0661581589655,138.588352384458));
#82742=CARTESIAN_POINT('Ctrl Pts',(81.3135217447979,-7.97438210084636,138.59648960147));
#82743=CARTESIAN_POINT('Ctrl Pts',(81.287926120545,-7.94241869640054,138.599369002259));
#82744=CARTESIAN_POINT('Ctrl Pts',(81.2420410227901,-7.88925798838842,138.604233970561));
#82745=CARTESIAN_POINT('Ctrl Pts',(81.2223226334362,-7.86759491075819,138.606239982383));
#82746=CARTESIAN_POINT('Ctrl Pts',(81.1930300845942,-7.83707066942061,138.60910302719));
#82747=CARTESIAN_POINT('Ctrl Pts',(81.1839079980817,-7.8277853100051,138.609979090436));
#82748=CARTESIAN_POINT('Ctrl Pts',(81.1677113960768,-7.81168076386031,138.611508022467));
#82749=CARTESIAN_POINT('Ctrl Pts',(81.1606837334129,-7.80481558343157,138.612162905309));
#82750=CARTESIAN_POINT('Ctrl Pts',(81.1459301255889,-7.79065595012923,138.613520407573));
#82751=CARTESIAN_POINT('Ctrl Pts',(81.1381942801273,-7.78337241803148,138.614222537639));
#82752=CARTESIAN_POINT('Ctrl Pts',(81.1178162367899,-7.76455036630309,138.616047582469));
#82753=CARTESIAN_POINT('Ctrl Pts',(81.1050647698006,-7.75313159209656,138.617165421521));
#82754=CARTESIAN_POINT('Ctrl Pts',(81.0490050659694,-7.70446651354744,138.621980260943));
#82755=CARTESIAN_POINT('Ctrl Pts',(81.0039709766193,-7.66926262617503,138.62559422336));
#82756=CARTESIAN_POINT('Ctrl Pts',(80.8704583063733,-7.57553737992661,138.635751020503));
#82757=CARTESIAN_POINT('Ctrl Pts',(80.7780919607908,-7.52305585898818,138.642118464408));
#82758=CARTESIAN_POINT('Ctrl Pts',(80.6270110757672,-7.4553443511373,138.652335002728));
#82759=CARTESIAN_POINT('Ctrl Pts',(80.5713939399396,-7.43391845206384,138.656062169448));
#82760=CARTESIAN_POINT('Ctrl Pts',(80.5009487293594,-7.4110326858951,138.660879192669));
#82761=CARTESIAN_POINT('Ctrl Pts',(80.487084210346,-7.40672799191786,138.661831798766));
#82762=CARTESIAN_POINT('Ctrl Pts',(80.4665008344863,-7.40063097107062,138.663255206706));
#82763=CARTESIAN_POINT('Ctrl Pts',(80.4598237340371,-7.3986985141548,138.663718365233));
#82764=CARTESIAN_POINT('Ctrl Pts',(80.4483835429749,-7.39546499659551,138.664514644571));
#82765=CARTESIAN_POINT('Ctrl Pts',(80.4436264545524,-7.39414323598432,138.6648465691));
#82766=CARTESIAN_POINT('Ctrl Pts',(80.4326911864844,-7.39115716278059,138.665611504384));
#82767=CARTESIAN_POINT('Ctrl Pts',(80.426509381775,-7.38950731713928,138.666045311097));
#82768=CARTESIAN_POINT('Ctrl Pts',(80.4092392091179,-7.38500453207709,138.667260796942));
#82769=CARTESIAN_POINT('Ctrl Pts',(80.3981309546554,-7.38223029558075,138.668046677816));
#82770=CARTESIAN_POINT('Ctrl Pts',(80.3239741758767,-7.36451996800702,138.673316204635));
#82771=CARTESIAN_POINT('Ctrl Pts',(80.2601352780521,-7.35316000409785,138.677961507062));
#82772=CARTESIAN_POINT('Ctrl Pts',(80.1728225135298,-7.34282650960915,138.684332877029));
#82773=CARTESIAN_POINT('Ctrl Pts',(80.1497859762565,-7.34058572493441,138.686015810713));
#82774=CARTESIAN_POINT('Ctrl Pts',(80.0554444741208,-7.33338957486402,138.692901841891));
#82775=CARTESIAN_POINT('Ctrl Pts',(79.98389831609,-7.33254497208265,138.698105649573));
#82776=CARTESIAN_POINT('Ctrl Pts',(79.867632732577,-7.33865868101431,138.706427078755));
#82777=CARTESIAN_POINT('Ctrl Pts',(79.8228604510651,-7.34283427505929,138.709599800144));
#82778=CARTESIAN_POINT('Ctrl Pts',(79.7472398062837,-7.35298726597787,138.714897355868));
#82779=CARTESIAN_POINT('Ctrl Pts',(79.7162933957214,-7.35803488049326,138.71704786435));
#82780=CARTESIAN_POINT('Ctrl Pts',(79.6723866033942,-7.36647499557967,138.720075906184));
#82781=CARTESIAN_POINT('Ctrl Pts',(79.6592977296486,-7.36915467970334,138.72097565453));
#82782=CARTESIAN_POINT('Ctrl Pts',(79.6365901829645,-7.37408891250029,138.722531887723));
#82783=CARTESIAN_POINT('Ctrl Pts',(79.6269568673208,-7.37627207083083,138.723190610427));
#82784=CARTESIAN_POINT('Ctrl Pts',(79.6083649157451,-7.38065968284363,138.724459269741));
#82785=CARTESIAN_POINT('Ctrl Pts',(79.5994040807519,-7.38285312439915,138.725069532154));
#82786=CARTESIAN_POINT('Ctrl Pts',(79.575597584752,-7.3888905239227,138.726687934529));
#82787=CARTESIAN_POINT('Ctrl Pts',(79.5607857617665,-7.39286527240194,138.727691844057));
#82788=CARTESIAN_POINT('Ctrl Pts',(79.5056283885136,-7.40848626607871,138.731421240146));
#82789=CARTESIAN_POINT('Ctrl Pts',(79.4656710068684,-7.42145249105214,138.7341042228));
#82790=CARTESIAN_POINT('Ctrl Pts',(79.3594316509531,-7.46042450719096,138.741233517957));
#82791=CARTESIAN_POINT('Ctrl Pts',(79.2942554315006,-7.48919023149188,138.74560004529));
#82792=CARTESIAN_POINT('Ctrl Pts',(79.1304105993628,-7.57442764320174,138.756885153246));
#82793=CARTESIAN_POINT('Ctrl Pts',(79.0353381914595,-7.6369657403136,138.763738793941));
#82794=CARTESIAN_POINT('Ctrl Pts',(78.9362642613365,-7.71772555263,138.772054323678));
#82795=CARTESIAN_POINT('Ctrl Pts',(78.9252712137089,-7.72692518593542,138.772995183921));
#82796=CARTESIAN_POINT('Ctrl Pts',(78.9091524749974,-7.74077185919534,138.774404348627));
#82797=CARTESIAN_POINT('Ctrl Pts',(78.9039344851552,-7.74531110776139,138.774865228488));
#82798=CARTESIAN_POINT('Ctrl Pts',(78.8946460068597,-7.75349352568745,138.775694417824));
#82799=CARTESIAN_POINT('Ctrl Pts',(78.8905649680532,-7.75712440338631,138.7760618307));
#82800=CARTESIAN_POINT('Ctrl Pts',(78.8815462931104,-7.7652280820378,138.776880724837));
#82801=CARTESIAN_POINT('Ctrl Pts',(78.8766176535488,-7.76971040658603,138.777332891113));
#82802=CARTESIAN_POINT('Ctrl Pts',(78.8621153960861,-7.78305920548846,138.778676836857));
#82803=CARTESIAN_POINT('Ctrl Pts',(78.8526191752965,-7.79200849095004,138.779574428366));
#82804=CARTESIAN_POINT('Ctrl Pts',(78.8308736699423,-7.81298929850626,138.781668925739));
#82805=CARTESIAN_POINT('Ctrl Pts',(78.8187034532117,-7.82510034502003,138.782870699949));
#82806=CARTESIAN_POINT('Ctrl Pts',(78.7769632552624,-7.86794179975979,138.787090302782));
#82807=CARTESIAN_POINT('Ctrl Pts',(78.748389024546,-7.89961636345954,138.790154663125));
#82808=CARTESIAN_POINT('Ctrl Pts',(78.6542158893786,-8.01242624549054,138.800794974995));
#82809=CARTESIAN_POINT('Ctrl Pts',(78.5950305976655,-8.09861169058053,138.808446732508));
#82810=CARTESIAN_POINT('Ctrl Pts',(78.5148468736009,-8.24267426842422,138.82018529873));
#82811=CARTESIAN_POINT('Ctrl Pts',(78.4883035625149,-8.29715043875238,138.824416774424));
#82812=CARTESIAN_POINT('Ctrl Pts',(78.4580734001981,-8.36887655595176,138.829725783489));
#82813=CARTESIAN_POINT('Ctrl Pts',(78.4516117542697,-8.38489974774697,138.83089576422));
#82814=CARTESIAN_POINT('Ctrl Pts',(78.442394503203,-8.40882235253628,138.83261952162));
#82815=CARTESIAN_POINT('Ctrl Pts',(78.4394474475768,-8.41664622318104,138.833179667397));
#82816=CARTESIAN_POINT('Ctrl Pts',(78.4365593750041,-8.42449203992252,138.833737849951));
#82817=CARTESIAN_POINT('Origin',(80.,-9.,134.));
#82818=CARTESIAN_POINT('',(78.4365593777415,-8.42449203248626,139.531855306428));
#82819=CARTESIAN_POINT('',(78.4365593749993,-8.42449203993574,139.340802385574));
#82820=CARTESIAN_POINT('',(78.4365593749993,-8.42449203993574,134.));
#82821=CARTESIAN_POINT('',(81.2690708798523,-7.92064134695145,140.));
#82822=CARTESIAN_POINT('Ctrl Pts',(78.4365593777415,-8.42449203248626,139.531855306428));
#82823=CARTESIAN_POINT('Ctrl Pts',(78.4333404532528,-8.43323665044058,139.532424409646));
#82824=CARTESIAN_POINT('Ctrl Pts',(78.4301945868942,-8.44200910936127,139.532993870147));
#82825=CARTESIAN_POINT('Ctrl Pts',(78.419533560236,-8.47254216118274,139.534972166137));
#82826=CARTESIAN_POINT('Ctrl Pts',(78.4123963589365,-8.49443043612462,139.53638376207));
#82827=CARTESIAN_POINT('Ctrl Pts',(78.3869901806648,-8.57819727689475,139.541783446891));
#82828=CARTESIAN_POINT('Ctrl Pts',(78.3718694226088,-8.64096375128971,139.545823316546));
#82829=CARTESIAN_POINT('Ctrl Pts',(78.3584038607409,-8.71566193855221,139.550790121101));
#82830=CARTESIAN_POINT('Ctrl Pts',(78.3564963028477,-8.72690368481098,139.551541807271));
#82831=CARTESIAN_POINT('Ctrl Pts',(78.3537028346285,-8.74445694919823,139.552723318112));
#82832=CARTESIAN_POINT('Ctrl Pts',(78.3527374544938,-8.75075572163072,139.55314884938));
#82833=CARTESIAN_POINT('Ctrl Pts',(78.3510874949719,-8.76194962470796,139.553908104212));
#82834=CARTESIAN_POINT('Ctrl Pts',(78.3503885288946,-8.76684249475162,139.554241014478));
#82835=CARTESIAN_POINT('Ctrl Pts',(78.3487556593623,-8.77864783270122,139.555046693432));
#82836=CARTESIAN_POINT('Ctrl Pts',(78.3478433887019,-8.78556310529877,139.555520644395));
#82837=CARTESIAN_POINT('Ctrl Pts',(78.3451603527288,-8.80693553532605,139.556991210515));
#82838=CARTESIAN_POINT('Ctrl Pts',(78.3435357886257,-8.82140989323287,139.55799527747));
#82839=CARTESIAN_POINT('Ctrl Pts',(78.3362143639208,-8.89537946819798,139.563161766661));
#82840=CARTESIAN_POINT('Ctrl Pts',(78.3335328311396,-8.95512395476671,139.567449646769));
#82841=CARTESIAN_POINT('Ctrl Pts',(78.3350143225227,-9.12102457025296,139.579471606928));
#82842=CARTESIAN_POINT('Ctrl Pts',(78.3461055098331,-9.2268498508276,139.587254390769));
#82843=CARTESIAN_POINT('Ctrl Pts',(78.3785495197234,-9.38694126747906,139.598859494532));
#82844=CARTESIAN_POINT('Ctrl Pts',(78.3927843424843,-9.44236223395556,139.602849199311));
#82845=CARTESIAN_POINT('Ctrl Pts',(78.414967988087,-9.51334659543113,139.607921300435));
#82846=CARTESIAN_POINT('Ctrl Pts',(78.4203465767135,-9.52966622165135,139.609084890794));
#82847=CARTESIAN_POINT('Ctrl Pts',(78.4294758192753,-9.55598905041998,139.610958279747));
#82848=CARTESIAN_POINT('Ctrl Pts',(78.4330717802038,-9.56604415867437,139.611673081819));
#82849=CARTESIAN_POINT('Ctrl Pts',(78.4401816178468,-9.58533775889907,139.613043317199));
#82850=CARTESIAN_POINT('Ctrl Pts',(78.4436815065165,-9.59458088707646,139.61369917853));
#82851=CARTESIAN_POINT('Ctrl Pts',(78.4520149054745,-9.61601138314027,139.615218747307));
#82852=CARTESIAN_POINT('Ctrl Pts',(78.4569104788238,-9.62817403868894,139.616080350495));
#82853=CARTESIAN_POINT('Ctrl Pts',(78.4733198428754,-9.66759197542188,139.618871246148));
#82854=CARTESIAN_POINT('Ctrl Pts',(78.4854165423551,-9.69459950202579,139.620781023888));
#82855=CARTESIAN_POINT('Ctrl Pts',(78.5161794770682,-9.75865156375282,139.625317420193));
#82856=CARTESIAN_POINT('Ctrl Pts',(78.5355223305134,-9.79534964308775,139.627922145527));
#82857=CARTESIAN_POINT('Ctrl Pts',(78.5938125526467,-9.8965881322203,139.635181163493));
#82858=CARTESIAN_POINT('Ctrl Pts',(78.6357970808385,-9.95926234849222,139.639759744868));
#82859=CARTESIAN_POINT('Ctrl Pts',(78.7324626387119,-10.0843181441866,139.64943615499));
#82860=CARTESIAN_POINT('Ctrl Pts',(78.7878422340391,-10.145891371441,139.654528457406));
#82861=CARTESIAN_POINT('Ctrl Pts',(78.8590300667545,-10.2140824047719,139.660923745035));
#82862=CARTESIAN_POINT('Ctrl Pts',(78.8706606701187,-10.2249086118572,139.661964395625));
#82863=CARTESIAN_POINT('Ctrl Pts',(78.8877588598309,-10.2403737368211,139.66349137245));
#82864=CARTESIAN_POINT('Ctrl Pts',(78.8931047534505,-10.2451466858936,139.663968395241));
#82865=CARTESIAN_POINT('Ctrl Pts',(78.902651876943,-10.2535605298944,139.664819947933));
#82866=CARTESIAN_POINT('Ctrl Pts',(78.9068407711754,-10.2572150984051,139.665193475063));
#82867=CARTESIAN_POINT('Ctrl Pts',(78.9160225930382,-10.2651451251798,139.666012050725));
#82868=CARTESIAN_POINT('Ctrl Pts',(78.9210225264198,-10.2694119955457,139.666457661981));
#82869=CARTESIAN_POINT('Ctrl Pts',(78.9354062854157,-10.2815405124402,139.667738863739));
#82870=CARTESIAN_POINT('Ctrl Pts',(78.9448514640773,-10.289328277783,139.668579292777));
#82871=CARTESIAN_POINT('Ctrl Pts',(79.0247596891575,-10.3537483479579,139.675676174776));
#82872=CARTESIAN_POINT('Ctrl Pts',(79.0996323539212,-10.4046576322554,139.682231424069));
#82873=CARTESIAN_POINT('Ctrl Pts',(79.2831586925251,-10.5087204662582,139.697540687089));
#82874=CARTESIAN_POINT('Ctrl Pts',(79.3942290091503,-10.5566470847077,139.70623242643));
#82875=CARTESIAN_POINT('Ctrl Pts',(79.5292493320315,-10.598241575332,139.715941521078));
#82876=CARTESIAN_POINT('Ctrl Pts',(79.5490938718281,-10.6039532578404,139.717348999701));
#82877=CARTESIAN_POINT('Ctrl Pts',(79.5812738151483,-10.6125708589054,139.719600829134));
#82878=CARTESIAN_POINT('Ctrl Pts',(79.5935446215182,-10.6157074095775,139.720452417016));
#82879=CARTESIAN_POINT('Ctrl Pts',(79.6154318062779,-10.6210368758597,139.721959161735));
#82880=CARTESIAN_POINT('Ctrl Pts',(79.6250340115783,-10.6232848681485,139.722616040514));
#82881=CARTESIAN_POINT('Ctrl Pts',(79.6453625097835,-10.6278540093104,139.723998184974));
#82882=CARTESIAN_POINT('Ctrl Pts',(79.6560929535699,-10.6301547098796,139.724722774618));
#82883=CARTESIAN_POINT('Ctrl Pts',(79.6848887083222,-10.6360317814155,139.726654451821));
#82884=CARTESIAN_POINT('Ctrl Pts',(79.7029922193621,-10.6394149986532,139.727855427068));
#82885=CARTESIAN_POINT('Ctrl Pts',(79.80609941461,-10.6569197897013,139.734625618059));
#82886=CARTESIAN_POINT('Ctrl Pts',(79.8920465002447,-10.6647310559526,139.73999125171));
#82887=CARTESIAN_POINT('Ctrl Pts',(80.0471568259668,-10.6667588570442,139.749512297185));
#82888=CARTESIAN_POINT('Ctrl Pts',(80.1160802829024,-10.6633803019553,139.753688354109));
#82889=CARTESIAN_POINT('Ctrl Pts',(80.255326852766,-10.6478559797584,139.762303379854));
#82890=CARTESIAN_POINT('Ctrl Pts',(80.3254717545605,-10.6354469398585,139.766738371423));
#82891=CARTESIAN_POINT('Ctrl Pts',(80.4048523298509,-10.6160946675892,139.772083026492));
#82892=CARTESIAN_POINT('Ctrl Pts',(80.4150815615746,-10.6134976501151,139.772778121658));
#82893=CARTESIAN_POINT('Ctrl Pts',(80.4317945780882,-10.6090850720961,139.773925300364));
#82894=CARTESIAN_POINT('Ctrl Pts',(80.4382934288413,-10.6073270336747,139.774374244738));
#82895=CARTESIAN_POINT('Ctrl Pts',(80.4499604164394,-10.6040949178373,139.775185664697));
#82896=CARTESIAN_POINT('Ctrl Pts',(80.4551324609957,-10.6026351183594,139.775547309249));
#82897=CARTESIAN_POINT('Ctrl Pts',(80.4664515220898,-10.5993811248984,139.776343207569));
#82898=CARTESIAN_POINT('Ctrl Pts',(80.4725953572075,-10.5975764860549,139.776778100029));
#82899=CARTESIAN_POINT('Ctrl Pts',(80.4910290637525,-10.592046287383,139.778091308662));
#82900=CARTESIAN_POINT('Ctrl Pts',(80.5032860892827,-10.5882140939152,139.778975718084));
#82901=CARTESIAN_POINT('Ctrl Pts',(80.5316807680756,-10.5789747317609,139.781048723281));
#82902=CARTESIAN_POINT('Ctrl Pts',(80.5477820863235,-10.5734612723499,139.782242558027));
#82903=CARTESIAN_POINT('Ctrl Pts',(80.6040227226354,-10.5532353608266,139.786470410536));
#82904=CARTESIAN_POINT('Ctrl Pts',(80.6436755877561,-10.5372263174946,139.789555500521));
#82905=CARTESIAN_POINT('Ctrl Pts',(80.8031867408985,-10.4655727008004,139.802285631473));
#82906=CARTESIAN_POINT('Ctrl Pts',(80.916861725362,-10.3972782344416,139.812067228599));
#82907=CARTESIAN_POINT('Ctrl Pts',(81.0569037537876,-10.2886209102246,139.824567590418));
#82908=CARTESIAN_POINT('Ctrl Pts',(81.09139649508,-10.2595411021694,139.827694743806));
#82909=CARTESIAN_POINT('Ctrl Pts',(81.1360059875825,-10.218721668253,139.831808648112));
#82910=CARTESIAN_POINT('Ctrl Pts',(81.1471984318728,-10.2081919942998,139.832847146247));
#82911=CARTESIAN_POINT('Ctrl Pts',(81.1654081336394,-10.1905793642854,139.8345478695));
#82912=CARTESIAN_POINT('Ctrl Pts',(81.1725101327028,-10.1835857962451,139.835214050844));
#82913=CARTESIAN_POINT('Ctrl Pts',(81.1862643397577,-10.1697962802914,139.836510136405));
#82914=CARTESIAN_POINT('Ctrl Pts',(81.1929219523482,-10.1630062955044,139.837140275669));
#82915=CARTESIAN_POINT('Ctrl Pts',(81.2085741248112,-10.1467670900775,139.838628692959));
#82916=CARTESIAN_POINT('Ctrl Pts',(81.2175166437438,-10.1372683996353,139.839484625874));
#82917=CARTESIAN_POINT('Ctrl Pts',(81.2476218982996,-10.1045286482221,139.842386641424));
#82918=CARTESIAN_POINT('Ctrl Pts',(81.2682389071128,-10.0807933287107,139.844409213305));
#82919=CARTESIAN_POINT('Ctrl Pts',(81.317167239161,-10.0211351116341,139.849315314171));
#82920=CARTESIAN_POINT('Ctrl Pts',(81.3446951156404,-9.9846024383433,139.852169779538));
#82921=CARTESIAN_POINT('Ctrl Pts',(81.409852720479,-9.89029153035011,139.859248722404));
#82922=CARTESIAN_POINT('Ctrl Pts',(81.4454646417108,-9.8312255412782,139.863425417562));
#82923=CARTESIAN_POINT('Ctrl Pts',(81.4839812445956,-9.75733976711819,139.868518094815));
#82924=CARTESIAN_POINT('Ctrl Pts',(81.4904794658724,-9.74446948335571,139.869400718296));
#82925=CARTESIAN_POINT('Ctrl Pts',(81.5285336112064,-9.66660410584125,139.874722682628));
#82926=CARTESIAN_POINT('Ctrl Pts',(81.5559972010636,-9.59970490934644,139.87921868466));
#82927=CARTESIAN_POINT('Ctrl Pts',(81.582651234163,-9.52048060172039,139.884691847716));
#82928=CARTESIAN_POINT('Ctrl Pts',(81.5861624602782,-9.50967991654074,139.885441157944));
#82929=CARTESIAN_POINT('Ctrl Pts',(81.5914414359383,-9.49285851692904,139.886614321777));
#82930=CARTESIAN_POINT('Ctrl Pts',(81.593286137095,-9.48686203767098,139.887033737411));
#82931=CARTESIAN_POINT('Ctrl Pts',(81.5966781112051,-9.47561015774045,139.887823253749));
#82932=CARTESIAN_POINT('Ctrl Pts',(81.5982334227164,-9.47035724404381,139.888192863062));
#82933=CARTESIAN_POINT('Ctrl Pts',(81.6017740074708,-9.45817892996487,139.889051990876));
#82934=CARTESIAN_POINT('Ctrl Pts',(81.6037403070411,-9.4512481862311,139.889542587414));
#82935=CARTESIAN_POINT('Ctrl Pts',(81.6096079798025,-9.43004316939073,139.891048240973));
#82936=CARTESIAN_POINT('Ctrl Pts',(81.613364050977,-9.41572993291234,139.892070949335));
#82937=CARTESIAN_POINT('Ctrl Pts',(81.6219042834181,-9.38132533032869,139.894541696425));
#82938=CARTESIAN_POINT('Ctrl Pts',(81.6265063838393,-9.36119165346352,139.89599768361));
#82939=CARTESIAN_POINT('Ctrl Pts',(81.6422617977123,-9.28584128035031,139.901472849812));
#82940=CARTESIAN_POINT('Ctrl Pts',(81.6509861812045,-9.23015824787884,139.90556977086));
#82941=CARTESIAN_POINT('Ctrl Pts',(81.6677889480927,-9.07029076048419,139.917325727882));
#82942=CARTESIAN_POINT('Ctrl Pts',(81.6689168362063,-8.96562969149369,139.924999074863));
#82943=CARTESIAN_POINT('Ctrl Pts',(81.6551768070528,-8.800869347878,139.936777989476));
#82944=CARTESIAN_POINT('Ctrl Pts',(81.6467937830021,-8.74051000832748,139.941032702189));
#82945=CARTESIAN_POINT('Ctrl Pts',(81.6315698865677,-8.662539577122,139.946457704903));
#82946=CARTESIAN_POINT('Ctrl Pts',(81.6277127861067,-8.64440055848037,139.947714881212));
#82947=CARTESIAN_POINT('Ctrl Pts',(81.6209329203193,-8.61494288553508,139.949749699927));
#82948=CARTESIAN_POINT('Ctrl Pts',(81.6181925528292,-8.60358432602193,139.950532639646));
#82949=CARTESIAN_POINT('Ctrl Pts',(81.6126529634537,-8.58163853294764,139.95204256836));
#82950=CARTESIAN_POINT('Ctrl Pts',(81.6098684122609,-8.57104825252114,139.952769942825));
#82951=CARTESIAN_POINT('Ctrl Pts',(81.6030790560553,-8.54622456803031,139.954472453299));
#82952=CARTESIAN_POINT('Ctrl Pts',(81.5989887458851,-8.53201537012094,139.95544506176));
#82953=CARTESIAN_POINT('Ctrl Pts',(81.5845145593896,-8.48414083252938,139.958717660399));
#82954=CARTESIAN_POINT('Ctrl Pts',(81.5732519240165,-8.45074988184117,139.960992615474));
#82955=CARTESIAN_POINT('Ctrl Pts',(81.5311907017559,-8.33799111482543,139.968685337612));
#82956=CARTESIAN_POINT('Ctrl Pts',(81.4953746470215,-8.2606377492648,139.973974787409));
#82957=CARTESIAN_POINT('Ctrl Pts',(81.4131957273197,-8.11380195118367,139.984466512586));
#82958=CARTESIAN_POINT('Ctrl Pts',(81.3672181484585,-8.0443948701926,139.989655600748));
#82959=CARTESIAN_POINT('Ctrl Pts',(81.3076666935999,-7.96764335815803,139.995977687977));
#82960=CARTESIAN_POINT('Ctrl Pts',(81.2989362273536,-7.95667978529728,139.996895849814));
#82961=CARTESIAN_POINT('Ctrl Pts',(81.286298471537,-7.94121402256193,139.998214628889));
#82962=CARTESIAN_POINT('Ctrl Pts',(81.2825035135694,-7.93662036906806,139.998609354866));
#82963=CARTESIAN_POINT('Ctrl Pts',(81.2754966558533,-7.92823089946848,139.999336000877));
#82964=CARTESIAN_POINT('Ctrl Pts',(81.2722922328498,-7.92442889733726,139.999667500718));
#82965=CARTESIAN_POINT('Ctrl Pts',(81.2690708798523,-7.92064134695143,140.));
#82966=CARTESIAN_POINT('',(78.7475353758638,-7.90141528989,140.));
#82967=CARTESIAN_POINT('Origin',(80.,-9.,140.));
#82968=CARTESIAN_POINT('Ctrl Pts',(78.7475353758638,-7.90141528989007,140.));
#82969=CARTESIAN_POINT('Ctrl Pts',(78.7493539374217,-7.89934200050503,139.999810165109));
#82970=CARTESIAN_POINT('Ctrl Pts',(78.7511776339592,-7.89727324164226,139.999620003453));
#82971=CARTESIAN_POINT('Ctrl Pts',(78.7714683906298,-7.87437077097766,139.99750663889));
#82972=CARTESIAN_POINT('Ctrl Pts',(78.7904485659617,-7.85399991429323,139.995551875342));
#82973=CARTESIAN_POINT('Ctrl Pts',(78.8893648755144,-7.75303154664668,139.985514608203));
#82974=CARTESIAN_POINT('Ctrl Pts',(78.9768777152484,-7.68027976303666,139.977138092156));
#82975=CARTESIAN_POINT('Ctrl Pts',(79.142409596094,-7.56910092884384,139.962753900001));
#82976=CARTESIAN_POINT('Ctrl Pts',(79.2173174159119,-7.52679071308032,139.956681272142));
#82977=CARTESIAN_POINT('Ctrl Pts',(79.3118446016702,-7.48265463169636,139.949554808457));
#82978=CARTESIAN_POINT('Ctrl Pts',(79.3286516293955,-7.47514386544472,139.948306776368));
#82979=CARTESIAN_POINT('Ctrl Pts',(79.3556723006463,-7.46360218460404,139.94632971417));
#82980=CARTESIAN_POINT('Ctrl Pts',(79.3658068692669,-7.45939118718801,139.945594676906));
#82981=CARTESIAN_POINT('Ctrl Pts',(79.3851293206591,-7.45158553196245,139.944205258331));
#82982=CARTESIAN_POINT('Ctrl Pts',(79.3943089232454,-7.44797176451418,139.943550264081));
#82983=CARTESIAN_POINT('Ctrl Pts',(79.4153537960536,-7.43990210610232,139.942059914676));
#82984=CARTESIAN_POINT('Ctrl Pts',(79.4272389915304,-7.43549961199141,139.941226347614));
#82985=CARTESIAN_POINT('Ctrl Pts',(79.4586396099145,-7.42427404545535,139.939044453311));
#82986=CARTESIAN_POINT('Ctrl Pts',(79.4782341544611,-7.417677713767,139.937703460455));
#82987=CARTESIAN_POINT('Ctrl Pts',(79.6370652727423,-7.36748004867061,139.926983720903));
#82988=CARTESIAN_POINT('Ctrl Pts',(79.7813497621902,-7.34197805747743,139.918238931225));
#82989=CARTESIAN_POINT('Ctrl Pts',(79.988096548862,-7.33292471575854,139.905450729332));
#82990=CARTESIAN_POINT('Ctrl Pts',(80.0491711394147,-7.33360798749068,139.901630822285));
#82991=CARTESIAN_POINT('Ctrl Pts',(80.1248019355846,-7.33861544217696,139.896701509358));
#82992=CARTESIAN_POINT('Ctrl Pts',(80.1395260822402,-7.33978717976292,139.895732384367));
#82993=CARTESIAN_POINT('Ctrl Pts',(80.1598973328611,-7.34168120815393,139.89437603223));
#82994=CARTESIAN_POINT('Ctrl Pts',(80.1655597417161,-7.34223694634459,139.893997352313));
#82995=CARTESIAN_POINT('Ctrl Pts',(80.1713966207971,-7.34284001067116,139.893605180919));
#82996=CARTESIAN_POINT('Ctrl Pts',(80.1715741468675,-7.34285838143518,139.89359325146));
#82997=CARTESIAN_POINT('Ctrl Pts',(80.1719290400283,-7.34289516415132,139.89356939974));
#82998=CARTESIAN_POINT('Ctrl Pts',(80.1721064070974,-7.34291357605161,139.893557477482));
#82999=CARTESIAN_POINT('Ctrl Pts',(80.1724636059533,-7.34295071367453,139.893533463782));
#83000=CARTESIAN_POINT('Ctrl Pts',(80.1726434376896,-7.34296944019948,139.893521372293));
#83001=CARTESIAN_POINT('Ctrl Pts',(80.1730086392265,-7.34300753004428,139.8934968133));
#83002=CARTESIAN_POINT('Ctrl Pts',(80.1731940087945,-7.34302689519276,139.8934843457));
#83003=CARTESIAN_POINT('Ctrl Pts',(80.1735741281947,-7.34306666990928,139.893458775678));
#83004=CARTESIAN_POINT('Ctrl Pts',(80.1737688776887,-7.34308708270748,139.893445673082));
#83005=CARTESIAN_POINT('Ctrl Pts',(80.1741729016833,-7.34312950276752,139.893418486269));
#83006=CARTESIAN_POINT('Ctrl Pts',(80.1743821755901,-7.34315151534109,139.893404401766));
#83007=CARTESIAN_POINT('Ctrl Pts',(80.1748226712495,-7.34319793346448,139.893374750478));
#83008=CARTESIAN_POINT('Ctrl Pts',(80.1750538920419,-7.3432223477666,139.893359183218));
#83009=CARTESIAN_POINT('Ctrl Pts',(80.1755499662663,-7.34327483260521,139.893325777907));
#83010=CARTESIAN_POINT('Ctrl Pts',(80.1758148180392,-7.34330291824578,139.893307939033));
#83011=CARTESIAN_POINT('Ctrl Pts',(80.1763987565177,-7.34336498236033,139.893268599647));
#83012=CARTESIAN_POINT('Ctrl Pts',(80.1767178400715,-7.34339898950561,139.893247097567));
#83013=CARTESIAN_POINT('Ctrl Pts',(80.1774533982222,-7.34347759843096,139.89319751729));
#83014=CARTESIAN_POINT('Ctrl Pts',(80.1778698656223,-7.34352226506263,139.893169435538));
#83015=CARTESIAN_POINT('Ctrl Pts',(80.1786060166775,-7.34360149897452,139.893119780657));
#83016=CARTESIAN_POINT('Ctrl Pts',(80.1789257074836,-7.34363600178163,139.893098211078));
#83017=CARTESIAN_POINT('Ctrl Pts',(80.1845660015237,-7.34424638561685,139.892717557303));
#83018=CARTESIAN_POINT('Ctrl Pts',(80.1898835646255,-7.34484778045083,139.892357056154));
#83019=CARTESIAN_POINT('Ctrl Pts',(80.202241442798,-7.34630574251937,139.891515478632));
#83020=CARTESIAN_POINT('Ctrl Pts',(80.2092791952211,-7.34718164570595,139.891033373285));
#83021=CARTESIAN_POINT('Ctrl Pts',(80.2320080471498,-7.35015791997912,139.889467683694));
#83022=CARTESIAN_POINT('Ctrl Pts',(80.2476743224481,-7.35243694878018,139.888375082349));
#83023=CARTESIAN_POINT('Ctrl Pts',(80.3436670236751,-7.36780133731417,139.88160715832));
#83024=CARTESIAN_POINT('Ctrl Pts',(80.4229709614544,-7.386534002239,139.875705596791));
#83025=CARTESIAN_POINT('Ctrl Pts',(80.5733653283458,-7.43391200677015,139.86423832153));
#83026=CARTESIAN_POINT('Ctrl Pts',(80.6444937978286,-7.46181645134146,139.858687852615));
#83027=CARTESIAN_POINT('Ctrl Pts',(80.7511590581591,-7.51236554098703,139.850279500871));
#83028=CARTESIAN_POINT('Ctrl Pts',(80.7881741408623,-7.53164097920583,139.847343477006));
#83029=CARTESIAN_POINT('Ctrl Pts',(80.8502528406159,-7.56699294134065,139.842392437584));
#83030=CARTESIAN_POINT('Ctrl Pts',(80.8756797404288,-7.58238781401237,139.840356228927));
#83031=CARTESIAN_POINT('Ctrl Pts',(80.9117323051127,-7.60555648306264,139.837455245878));
#83032=CARTESIAN_POINT('Ctrl Pts',(80.92269787575,-7.61278798835659,139.83657096411));
#83033=CARTESIAN_POINT('Ctrl Pts',(80.9417675197182,-7.62569008931478,139.835029367443));
#83034=CARTESIAN_POINT('Ctrl Pts',(80.9499086298742,-7.63130449189569,139.834370000928));
#83035=CARTESIAN_POINT('Ctrl Pts',(80.9667309752048,-7.64312818410487,139.833004693084));
#83036=CARTESIAN_POINT('Ctrl Pts',(80.9754035235131,-7.64934909084074,139.832299231685));
#83037=CARTESIAN_POINT('Ctrl Pts',(80.9978512458042,-7.66578005352087,139.830468599966));
#83038=CARTESIAN_POINT('Ctrl Pts',(81.011529865795,-7.67612034519384,139.829348479924));
#83039=CARTESIAN_POINT('Ctrl Pts',(81.0706009549604,-7.72222501529789,139.824486973085));
#83040=CARTESIAN_POINT('Ctrl Pts',(81.1142773684257,-7.7601280995592,139.82083041753));
#83041=CARTESIAN_POINT('Ctrl Pts',(81.2321348644005,-7.87367583325694,139.810639881814));
#83042=CARTESIAN_POINT('Ctrl Pts',(81.301194414478,-7.95422028329682,139.804277854754));
#83043=CARTESIAN_POINT('Ctrl Pts',(81.3964412667812,-8.08947486500636,139.794065804642));
#83044=CARTESIAN_POINT('Ctrl Pts',(81.428097786748,-8.13997707231692,139.790337199806));
#83045=CARTESIAN_POINT('Ctrl Pts',(81.4640323750513,-8.20477881642482,139.785517398176));
#83046=CARTESIAN_POINT('Ctrl Pts',(81.4709184258613,-8.21758931795455,139.784562892861));
#83047=CARTESIAN_POINT('Ctrl Pts',(81.4808560567645,-8.23667179246633,139.783136125072));
#83048=CARTESIAN_POINT('Ctrl Pts',(81.4840375926609,-8.24287581434837,139.782671497275));
#83049=CARTESIAN_POINT('Ctrl Pts',(81.4894081394236,-8.25351233634473,139.781873301335));
#83050=CARTESIAN_POINT('Ctrl Pts',(81.491616518262,-8.25793490886457,139.781540938579));
#83051=CARTESIAN_POINT('Ctrl Pts',(81.4966290701098,-8.2680859999423,139.780776879659));
#83052=CARTESIAN_POINT('Ctrl Pts',(81.4994199852038,-8.27382069602188,139.78034440212));
#83053=CARTESIAN_POINT('Ctrl Pts',(81.5071171990913,-8.28987028125186,139.779132004655));
#83054=CARTESIAN_POINT('Ctrl Pts',(81.5119503355289,-8.30021958151238,139.778347884258));
#83055=CARTESIAN_POINT('Ctrl Pts',(81.5437425051465,-8.37016395834686,139.773036908064));
#83056=CARTESIAN_POINT('Ctrl Pts',(81.5672753021543,-8.43124647300328,139.768344596779));
#83057=CARTESIAN_POINT('Ctrl Pts',(81.5936445312741,-8.51388391484801,139.76205551411));
#83058=CARTESIAN_POINT('Ctrl Pts',(81.5997426392731,-8.53434432298382,139.760502821396));
#83059=CARTESIAN_POINT('Ctrl Pts',(81.6236911077188,-8.62072795225309,139.753977179407));
#83060=CARTESIAN_POINT('Ctrl Pts',(81.6378733378574,-8.68760290840882,139.749001061225));
#83061=CARTESIAN_POINT('Ctrl Pts',(81.658428839337,-8.82595425033272,139.738979311701));
#83062=CARTESIAN_POINT('Ctrl Pts',(81.6643753463769,-8.89735807836616,139.733952586272));
#83063=CARTESIAN_POINT('Ctrl Pts',(81.6660363813183,-8.98641542707321,139.727874803751));
#83064=CARTESIAN_POINT('Ctrl Pts',(81.6660872038639,-9.00390311487463,139.726690230643));
#83065=CARTESIAN_POINT('Ctrl Pts',(81.6657257179225,-9.03205716930825,139.724796787155));
#83066=CARTESIAN_POINT('Ctrl Pts',(81.6654862641975,-9.042724026385,139.724082559602));
#83067=CARTESIAN_POINT('Ctrl Pts',(81.6648321378074,-9.06312586766012,139.722722273661));
#83068=CARTESIAN_POINT('Ctrl Pts',(81.6644345034237,-9.07286091527993,139.722075709121));
#83069=CARTESIAN_POINT('Ctrl Pts',(81.6633310817852,-9.09509113086167,139.720604732979));
#83070=CARTESIAN_POINT('Ctrl Pts',(81.6625698515538,-9.10758305536424,139.719782094138));
#83071=CARTESIAN_POINT('Ctrl Pts',(81.6596923497431,-9.1474067527764,139.717171187968));
#83072=CARTESIAN_POINT('Ctrl Pts',(81.6570421866931,-9.17469624225397,139.715399629821));
#83073=CARTESIAN_POINT('Ctrl Pts',(81.6376675935821,-9.33338213563908,139.705176503311));
#83074=CARTESIAN_POINT('Ctrl Pts',(81.6059960250623,-9.46246963972847,139.697221498124));
#83075=CARTESIAN_POINT('Ctrl Pts',(81.5340375636779,-9.65380674706418,139.684692600514));
#83076=CARTESIAN_POINT('Ctrl Pts',(81.5043714871238,-9.71944321177551,139.680236223466));
#83077=CARTESIAN_POINT('Ctrl Pts',(81.4631342160772,-9.79689645532444,139.674544848725));
#83078=CARTESIAN_POINT('Ctrl Pts',(81.4555103463818,-9.8107374923517,139.67351001607));
#83079=CARTESIAN_POINT('Ctrl Pts',(81.4441457382448,-9.83069272989906,139.671988907977));
#83080=CARTESIAN_POINT('Ctrl Pts',(81.4405603271241,-9.83689501371369,139.67151197667));
#83081=CARTESIAN_POINT('Ctrl Pts',(81.4341711126735,-9.84778479128826,139.67066689137));
#83082=CARTESIAN_POINT('Ctrl Pts',(81.4313840996893,-9.8524819002305,139.670299812345));
#83083=CARTESIAN_POINT('Ctrl Pts',(81.4252633112822,-9.86268296529061,139.66949693088));
#83084=CARTESIAN_POINT('Ctrl Pts',(81.4219207676737,-9.8681812783333,139.669060589968));
#83085=CARTESIAN_POINT('Ctrl Pts',(81.4124587001724,-9.88354467303419,139.667831556611));
#83086=CARTESIAN_POINT('Ctrl Pts',(81.4062679313666,-9.89336512989974,139.667034518386));
#83087=CARTESIAN_POINT('Ctrl Pts',(81.3582665633542,-9.96777467357826,139.660912350089));
#83088=CARTESIAN_POINT('Ctrl Pts',(81.3121335585872,-10.0294555433507,139.655360272685));
#83089=CARTESIAN_POINT('Ctrl Pts',(81.224574894705,-10.1310360235524,139.64561226723));
#83090=CARTESIAN_POINT('Ctrl Pts',(81.1850326540324,-10.1724009684961,139.641439164999));
#83091=CARTESIAN_POINT('Ctrl Pts',(81.0831203649265,-10.2685761049912,139.631312567974));
#83092=CARTESIAN_POINT('Ctrl Pts',(81.0186258244716,-10.3209239592282,139.625422222657));
#83093=CARTESIAN_POINT('Ctrl Pts',(80.9316990406666,-10.3813096806829,139.61814547709));
#83094=CARTESIAN_POINT('Ctrl Pts',(80.9126396640306,-10.3939757781732,139.616586736671));
#83095=CARTESIAN_POINT('Ctrl Pts',(80.88332798228,-10.4125961682517,139.614243379646));
#83096=CARTESIAN_POINT('Ctrl Pts',(80.8732637576959,-10.4188399067106,139.613448152337));
#83097=CARTESIAN_POINT('Ctrl Pts',(80.8556259343521,-10.4295234538503,139.612070402855));
#83098=CARTESIAN_POINT('Ctrl Pts',(80.8480823472263,-10.4340116394292,139.611486132631));
#83099=CARTESIAN_POINT('Ctrl Pts',(80.8309899761645,-10.4439989849271,139.610173280854));
#83100=CARTESIAN_POINT('Ctrl Pts',(80.8214213359579,-10.4494634895677,139.60944596923));
#83101=CARTESIAN_POINT('Ctrl Pts',(80.7952964116793,-10.4640412386552,139.607480322099));
#83102=CARTESIAN_POINT('Ctrl Pts',(80.7786378300618,-10.4729685358751,139.606248601722));
#83103=CARTESIAN_POINT('Ctrl Pts',(80.6672862837081,-10.5302244591373,139.598149482522));
#83104=CARTESIAN_POINT('Ctrl Pts',(80.5683018071055,-10.5696799064406,139.591605797225));
#83105=CARTESIAN_POINT('Ctrl Pts',(80.3868728384437,-10.6225647751614,139.580054269002));
#83106=CARTESIAN_POINT('Ctrl Pts',(80.3059193113103,-10.6397556394334,139.575038406747));
#83107=CARTESIAN_POINT('Ctrl Pts',(80.1867389325085,-10.6559290088295,139.567459809341));
#83108=CARTESIAN_POINT('Ctrl Pts',(80.1492892276118,-10.6597242386087,139.565050148035));
#83109=CARTESIAN_POINT('Ctrl Pts',(80.1018887090753,-10.6629107935685,139.56192866627));
#83110=CARTESIAN_POINT('Ctrl Pts',(80.0920254534338,-10.6634857740933,139.561275235901));
#83111=CARTESIAN_POINT('Ctrl Pts',(80.0761657650853,-10.6642688395286,139.560217438356));
#83112=CARTESIAN_POINT('Ctrl Pts',(80.0701721292605,-10.664532325736,139.55981604875));
#83113=CARTESIAN_POINT('Ctrl Pts',(80.0586142721602,-10.6649778859173,139.559038658183));
#83114=CARTESIAN_POINT('Ctrl Pts',(80.0530503747249,-10.6651644505984,139.558662903994));
#83115=CARTESIAN_POINT('Ctrl Pts',(80.0406583130797,-10.6655178035376,139.557822758591));
#83116=CARTESIAN_POINT('Ctrl Pts',(80.0338298527203,-10.6656704924212,139.55735761325));
#83117=CARTESIAN_POINT('Ctrl Pts',(80.0135582978902,-10.6659990758735,139.555970603341));
#83118=CARTESIAN_POINT('Ctrl Pts',(80.0001141668264,-10.666054232988,139.555042724803));
#83119=CARTESIAN_POINT('Ctrl Pts',(79.8797192190196,-10.6650909972192,139.546670132137));
#83120=CARTESIAN_POINT('Ctrl Pts',(79.7731070624113,-10.6539381911227,139.538826489691));
#83121=CARTESIAN_POINT('Ctrl Pts',(79.5948262185852,-10.6177183907781,139.525604967858));
#83122=CARTESIAN_POINT('Ctrl Pts',(79.5224286645308,-10.5978442683703,139.520201217202));
#83123=CARTESIAN_POINT('Ctrl Pts',(79.4098980719767,-10.5586170294244,139.511825874485));
#83124=CARTESIAN_POINT('Ctrl Pts',(79.3687777189582,-10.5424222471287,139.508769413966));
#83125=CARTESIAN_POINT('Ctrl Pts',(79.3144780077489,-10.5185009892293,139.504736806741));
#83126=CARTESIAN_POINT('Ctrl Pts',(79.3006933409563,-10.51220232744,139.50371331105));
#83127=CARTESIAN_POINT('Ctrl Pts',(79.2777614702244,-10.5013433675697,139.502010535763));
#83128=CARTESIAN_POINT('Ctrl Pts',(79.268567060679,-10.4968855215201,139.501327784579));
#83129=CARTESIAN_POINT('Ctrl Pts',(79.250511446633,-10.4879252950346,139.4999867176));
#83130=CARTESIAN_POINT('Ctrl Pts',(79.2416483802354,-10.4834276535451,139.499328271847));
#83131=CARTESIAN_POINT('Ctrl Pts',(79.2201831894907,-10.4722922929816,139.497732909068));
#83132=CARTESIAN_POINT('Ctrl Pts',(79.2076247658292,-10.4655716846842,139.496798942487));
#83133=CARTESIAN_POINT('Ctrl Pts',(79.1648496281197,-10.4419701014166,139.493614107054));
#83134=CARTESIAN_POINT('Ctrl Pts',(79.1350724031962,-10.4243084060242,139.49139090862));
#83135=CARTESIAN_POINT('Ctrl Pts',(79.0013682029356,-10.339263981473,139.481338055479));
#83136=CARTESIAN_POINT('Ctrl Pts',(78.9046097132845,-10.2613544837943,139.473895916739));
#83137=CARTESIAN_POINT('Ctrl Pts',(78.7643378022569,-10.1199844952839,139.461665141977));
#83138=CARTESIAN_POINT('Ctrl Pts',(78.7149912630022,-10.0630032548102,139.456984431318));
#83139=CARTESIAN_POINT('Ctrl Pts',(78.6626901949287,-9.99362621672947,139.451299624925));
#83140=CARTESIAN_POINT('Ctrl Pts',(78.655804128079,-9.984290613936,139.450534889118));
#83141=CARTESIAN_POINT('Ctrl Pts',(78.6452925823987,-9.96972383101064,139.44934067692));
#83142=CARTESIAN_POINT('Ctrl Pts',(78.6415984885356,-9.96454228835086,139.448915699367));
#83143=CARTESIAN_POINT('Ctrl Pts',(78.6347703390119,-9.95484771667766,139.448119969966));
#83144=CARTESIAN_POINT('Ctrl Pts',(78.6316288152713,-9.95034019526756,139.447749729091));
#83145=CARTESIAN_POINT('Ctrl Pts',(78.6244222472155,-9.93989025030038,139.446890838975));
#83146=CARTESIAN_POINT('Ctrl Pts',(78.6203733753413,-9.93393694020989,139.446401145726));
#83147=CARTESIAN_POINT('Ctrl Pts',(78.607628919214,-9.91493424557989,139.44483732186));
#83148=CARTESIAN_POINT('Ctrl Pts',(78.5990792227414,-9.90178868475456,139.443754406159));
#83149=CARTESIAN_POINT('Ctrl Pts',(78.5460195224288,-9.81763106810065,139.436824197599));
#83150=CARTESIAN_POINT('Ctrl Pts',(78.5067396813834,-9.74347208501618,139.430735165811));
#83151=CARTESIAN_POINT('Ctrl Pts',(78.4427471723247,-9.59692053708474,139.41909468941));
#83152=CARTESIAN_POINT('Ctrl Pts',(78.4171005623256,-9.52514896290282,139.413558127237));
#83153=CARTESIAN_POINT('Ctrl Pts',(78.3854031808042,-9.4126648612746,139.405238430763));
#83154=CARTESIAN_POINT('Ctrl Pts',(78.375796006304,-9.37306435634014,139.402373508329));
#83155=CARTESIAN_POINT('Ctrl Pts',(78.3618144405452,-9.30455795812348,139.39753025958));
#83156=CARTESIAN_POINT('Ctrl Pts',(78.3567311832555,-9.27581743740151,139.395531716406));
#83157=CARTESIAN_POINT('Ctrl Pts',(78.3504789830638,-9.23410527786678,139.392677437512));
#83158=CARTESIAN_POINT('Ctrl Pts',(78.348703093463,-9.22123157442661,139.391802816204));
#83159=CARTESIAN_POINT('Ctrl Pts',(78.3458501729191,-9.19859694577888,139.390275725099));
#83160=CARTESIAN_POINT('Ctrl Pts',(78.3447084900745,-9.18884496703559,139.389621251908));
#83161=CARTESIAN_POINT('Ctrl Pts',(78.3425106384797,-9.16851696823571,139.388263968104));
#83162=CARTESIAN_POINT('Ctrl Pts',(78.3414693272939,-9.15793976280069,139.387561652264));
#83163=CARTESIAN_POINT('Ctrl Pts',(78.3390131582086,-9.13027871935646,139.385734751878));
#83164=CARTESIAN_POINT('Ctrl Pts',(78.337760598814,-9.11318145650967,139.384615269562));
#83165=CARTESIAN_POINT('Ctrl Pts',(78.333402259759,-9.03772492201462,139.379713473445));
#83166=CARTESIAN_POINT('Ctrl Pts',(78.3331042642608,-8.97924171468461,139.376018617256));
#83167=CARTESIAN_POINT('Ctrl Pts',(78.3408870781395,-8.81559126377517,139.365826235957));
#83168=CARTESIAN_POINT('Ctrl Pts',(78.3558698957589,-8.71103966773445,139.359496202171));
#83169=CARTESIAN_POINT('Ctrl Pts',(78.3957049617281,-8.54622470714689,139.349030076711));
#83170=CARTESIAN_POINT('Ctrl Pts',(78.4143720525308,-8.48477518134467,139.345008201278));
#83171=CARTESIAN_POINT('Ctrl Pts',(78.4365419168178,-8.42453946871522,139.340805694646));
#83172=CARTESIAN_POINT('Ctrl Pts',(78.4365506456816,-8.42451575423836,139.340804040149));
#83173=CARTESIAN_POINT('Ctrl Pts',(78.4365593749993,-8.42449203993574,139.340802385574));
#83174=CARTESIAN_POINT('Origin',(-1.54592528053767,-30.,55.));
#83175=CARTESIAN_POINT('',(9.49394873724561,-31.2520475724682,56.6292251037768));
#83176=CARTESIAN_POINT('',(9.55204617751071,-31.254042933277,56.631836765028));
#83177=CARTESIAN_POINT('',(-1.54592528053767,-31.2520475724682,56.6292251037768));
#83178=CARTESIAN_POINT('',(10.,-27.9466241674713,54.9248651020699));
#83179=CARTESIAN_POINT('Ctrl Pts',(9.55204617751071,-31.254042933277,56.631836765028));
#83180=CARTESIAN_POINT('Ctrl Pts',(9.5531837572224,-31.2706395868589,56.6191575655763));
#83181=CARTESIAN_POINT('Ctrl Pts',(9.5913664272136,-31.8206121569964,56.184448873392));
#83182=CARTESIAN_POINT('Ctrl Pts',(9.66659418748433,-32.4128254657117,54.7282396369248));
#83183=CARTESIAN_POINT('Ctrl Pts',(9.77772945832288,-31.081050325948,52.8236098971708));
#83184=CARTESIAN_POINT('Ctrl Pts',(9.88886472916145,-28.7562331488978,52.91517862984));
#83185=CARTESIAN_POINT('Ctrl Pts',(9.96295490972048,-27.9716077196437,54.242084880697));
#83186=CARTESIAN_POINT('Ctrl Pts',(10.,-27.9466241674713,54.9248651020699));
#83187=CARTESIAN_POINT('',(9.99999281491357,-28.1818141229585,55.9591738002264));
#83188=CARTESIAN_POINT('Origin',(10.,-30.,55.));
#83189=CARTESIAN_POINT('',(9.9459252805888,-27.9452500000283,55.0000107795145));
#83190=CARTESIAN_POINT('Ctrl Pts',(9.9459252805888,-27.9452500000283,55.0000107795145));
#83191=CARTESIAN_POINT('Ctrl Pts',(9.94992922500024,-27.9452503895637,55.0742625308859));
#83192=CARTESIAN_POINT('Ctrl Pts',(9.95393316941168,-27.9492798952893,55.1484430447576));
#83193=CARTESIAN_POINT('Ctrl Pts',(9.95793711382313,-27.9572896739692,55.222108276359));
#83194=CARTESIAN_POINT('Ctrl Pts',(9.96195101270092,-27.9653193662803,55.295956651879));
#83195=CARTESIAN_POINT('Ctrl Pts',(9.96596491157871,-27.9773490514669,55.3692867586229));
#83196=CARTESIAN_POINT('Ctrl Pts',(9.9699788104565,-27.9932783699437,55.4416626110102));
#83197=CARTESIAN_POINT('Ctrl Pts',(9.97399811839586,-28.009229154498,55.5141359958598));
#83198=CARTESIAN_POINT('Ctrl Pts',(9.97801742633522,-28.0290899299268,55.5856521509838));
#83199=CARTESIAN_POINT('Ctrl Pts',(9.98203673427458,-28.0527106422095,55.6557909114464));
#83200=CARTESIAN_POINT('Ctrl Pts',(9.98606633320141,-28.0763918326784,55.7261092543437));
#83201=CARTESIAN_POINT('Ctrl Pts',(9.99009593212824,-28.1038520364647,55.7950427573651));
#83202=CARTESIAN_POINT('Ctrl Pts',(9.99412553105508,-28.1348932435125,55.8621915966911));
#83203=CARTESIAN_POINT('Ctrl Pts',(9.9960804898642,-28.1499528765593,55.8947688375892));
#83204=CARTESIAN_POINT('Ctrl Pts',(9.99803544867332,-28.1658546891076,55.9269264110958));
#83205=CARTESIAN_POINT('Ctrl Pts',(9.99999040748243,-28.1825723553983,55.9586210508524));
#83206=CARTESIAN_POINT('Ctrl Pts',(9.49394873724561,-31.2520475724682,56.6292251037768));
#83207=CARTESIAN_POINT('Ctrl Pts',(9.49780465159691,-31.3085979756072,56.5857665327002));
#83208=CARTESIAN_POINT('Ctrl Pts',(9.50166056594821,-31.3628989655048,56.5393479980115));
#83209=CARTESIAN_POINT('Ctrl Pts',(9.50551648029951,-31.4146337209008,56.4902378998638));
#83210=CARTESIAN_POINT('Ctrl Pts',(9.50937266007019,-31.4663720374253,56.4411244212542));
#83211=CARTESIAN_POINT('Ctrl Pts',(9.51322883984087,-31.515543418208,56.3893193473735));
#83212=CARTESIAN_POINT('Ctrl Pts',(9.51708501961154,-31.56186724767,56.3351285567898));
#83213=CARTESIAN_POINT('Ctrl Pts',(9.52094529470732,-31.6082402737858,56.2808802147127));
#83214=CARTESIAN_POINT('Ctrl Pts',(9.52480556980309,-31.651759396774,56.2242414689498));
#83215=CARTESIAN_POINT('Ctrl Pts',(9.52866584489886,-31.692184336313,56.1655512577476));
#83216=CARTESIAN_POINT('Ctrl Pts',(9.53252840685189,-31.7326332239033,56.1068262780038));
#83217=CARTESIAN_POINT('Ctrl Pts',(9.53639096880491,-31.7699840254071,56.0460478276773));
#83218=CARTESIAN_POINT('Ctrl Pts',(9.54025353075794,-31.8040413147177,55.9835814644916));
#83219=CARTESIAN_POINT('Ctrl Pts',(9.54412271723623,-31.8381570143209,55.9210079677488));
#83220=CARTESIAN_POINT('Ctrl Pts',(9.54799190371453,-31.8689677171337,55.8567412175391));
#83221=CARTESIAN_POINT('Ctrl Pts',(9.55186109019283,-31.8963255363346,55.7911681381005));
#83222=CARTESIAN_POINT('Ctrl Pts',(9.55378515750059,-31.9099300203342,55.7585599867167));
#83223=CARTESIAN_POINT('Ctrl Pts',(9.55570922480834,-31.922681421013,55.7256290564944));
#83224=CARTESIAN_POINT('Ctrl Pts',(9.5576332921161,-31.9345661853751,55.6924241741181));
#83225=CARTESIAN_POINT('Ctrl Pts',(9.56150301975733,-31.9584690919815,55.6256417644604));
#83226=CARTESIAN_POINT('Ctrl Pts',(9.56537274739856,-31.9789565387339,55.557489844211));
#83227=CARTESIAN_POINT('Ctrl Pts',(9.5692424750398,-31.9958734322516,55.4883511082534));
#83228=CARTESIAN_POINT('Ctrl Pts',(9.57310644880504,-32.0127651721366,55.4193151742885));
#83229=CARTESIAN_POINT('Ctrl Pts',(9.57697042257028,-32.0260967827392,55.3492958050351));
#83230=CARTESIAN_POINT('Ctrl Pts',(9.58083439633552,-32.0357622033577,55.2786930459845));
#83231=CARTESIAN_POINT('Ctrl Pts',(9.58469385125523,-32.0454163204464,55.2081728555487));
#83232=CARTESIAN_POINT('Ctrl Pts',(9.58855330617495,-32.0514126985859,55.1370711093101));
#83233=CARTESIAN_POINT('Ctrl Pts',(9.59241276109466,-32.0536962063712,55.0657985899276));
#83234=CARTESIAN_POINT('Ctrl Pts',(9.59626979277466,-32.0559782804083,54.9945708204913));
#83235=CARTESIAN_POINT('Ctrl Pts',(9.60012682445465,-32.0545520937131,54.9231729748411));
#83236=CARTESIAN_POINT('Ctrl Pts',(9.60398385613465,-32.0494144274265,54.8520200447484));
#83237=CARTESIAN_POINT('Ctrl Pts',(9.60783975505705,-32.0442782700023,54.7808880113007));
#83238=CARTESIAN_POINT('Ctrl Pts',(9.61169565397945,-32.0354328319464,54.7100012346741));
#83239=CARTESIAN_POINT('Ctrl Pts',(9.61555155290186,-32.0229269368548,54.6397720573759));
#83240=CARTESIAN_POINT('Ctrl Pts',(9.61940760794305,-32.0104205354208,54.5695400366178));
#83241=CARTESIAN_POINT('Ctrl Pts',(9.62326366298424,-31.9942534700028,54.4999661457278));
#83242=CARTESIAN_POINT('Ctrl Pts',(9.62711971802543,-31.9745258093191,54.4314532641615));
#83243=CARTESIAN_POINT('Ctrl Pts',(9.63097981215373,-31.9547774845788,54.3628686176712));
#83244=CARTESIAN_POINT('Ctrl Pts',(9.63483990628203,-31.9314612540917,54.2953476666301));
#83245=CARTESIAN_POINT('Ctrl Pts',(9.63870000041033,-31.9047270402197,54.2292779588231));
#83246=CARTESIAN_POINT('Ctrl Pts',(9.64256228268184,-31.8779776717203,54.1631707985661));
#83247=CARTESIAN_POINT('Ctrl Pts',(9.64642456495335,-31.8478066682151,54.0985169594539));
#83248=CARTESIAN_POINT('Ctrl Pts',(9.65028684722486,-31.8144109346917,54.0356813169023));
#83249=CARTESIAN_POINT('Ctrl Pts',(9.65415588300166,-31.7809568060931,53.9727358012717));
#83250=CARTESIAN_POINT('Ctrl Pts',(9.65802491877847,-31.7442669396311,53.9116152461669));
#83251=CARTESIAN_POINT('Ctrl Pts',(9.66189395455528,-31.7045823754473,53.8526567698311));
#83252=CARTESIAN_POINT('Ctrl Pts',(9.6641854906884,-31.6810781697485,53.817737093025));
#83253=CARTESIAN_POINT('Ctrl Pts',(9.66647702682152,-31.6565242523107,53.7835752583064));
#83254=CARTESIAN_POINT('Ctrl Pts',(9.66876856295464,-31.6309771514931,53.750235584677));
#83255=CARTESIAN_POINT('Ctrl Pts',(9.67263320043979,-31.5878923918726,53.6940087809235));
#83256=CARTESIAN_POINT('Ctrl Pts',(9.67649783792494,-31.5418110729999,53.6399009041512));
#83257=CARTESIAN_POINT('Ctrl Pts',(9.68036247541009,-31.4929694991081,53.5882494422764));
#83258=CARTESIAN_POINT('Ctrl Pts',(9.68422133661275,-31.444200926301,53.536675181287));
#83259=CARTESIAN_POINT('Ctrl Pts',(9.68808019781541,-31.3926806189403,53.4875503988675));
#83260=CARTESIAN_POINT('Ctrl Pts',(9.69193905901806,-31.3386861089886,53.441180875117));
#83261=CARTESIAN_POINT('Ctrl Pts',(9.69579339263811,-31.2847549505261,53.3948657564974));
#83262=CARTESIAN_POINT('Ctrl Pts',(9.69964772625817,-31.2283557229377,53.3512997914991));
#83263=CARTESIAN_POINT('Ctrl Pts',(9.70350205987822,-31.1698026561876,53.3107518512438));
#83264=CARTESIAN_POINT('Ctrl Pts',(9.70735396752099,-31.1112864436448,53.2702294324902));
#83265=CARTESIAN_POINT('Ctrl Pts',(9.71120587516376,-31.050619480747,53.2327215466549));
#83266=CARTESIAN_POINT('Ctrl Pts',(9.71505778280652,-30.988147735328,53.1984557691619));
#83267=CARTESIAN_POINT('Ctrl Pts',(9.7189085623831,-30.925694285328,53.1642000267135));
#83268=CARTESIAN_POINT('Ctrl Pts',(9.72275934195968,-30.8614375288067,53.1331847418678));
#83269=CARTESIAN_POINT('Ctrl Pts',(9.72661012153625,-30.7957494675024,53.1055923491841));
#83270=CARTESIAN_POINT('Ctrl Pts',(9.73046106935284,-30.730058536296,53.0779987509928));
#83271=CARTESIAN_POINT('Ctrl Pts',(9.73431201716944,-30.6629366260364,53.0538285284208));
#83272=CARTESIAN_POINT('Ctrl Pts',(9.73816296498603,-30.5947755996095,53.0332159374733));
#83273=CARTESIAN_POINT('Ctrl Pts',(9.74201800536427,-30.5265421356383,53.0125814406721));
#83274=CARTESIAN_POINT('Ctrl Pts',(9.74587304574251,-30.4572678182304,52.9955122640044));
#83275=CARTESIAN_POINT('Ctrl Pts',(9.74972808612076,-30.3873586781989,52.982092465715));
#83276=CARTESIAN_POINT('Ctrl Pts',(9.75358533703476,-30.3174094512581,52.9686649723198));
#83277=CARTESIAN_POINT('Ctrl Pts',(9.75744258794876,-30.2468251597645,52.9588910892792));
#83278=CARTESIAN_POINT('Ctrl Pts',(9.76129983886276,-30.1760182474746,52.9528031020305));
#83279=CARTESIAN_POINT('Ctrl Pts',(9.76516393339993,-30.1050857079345,52.946704313335));
#83280=CARTESIAN_POINT('Ctrl Pts',(9.76902802793711,-30.0339302458983,52.9443044929261));
#83281=CARTESIAN_POINT('Ctrl Pts',(9.77289212247429,-29.9629649002034,52.9455837900067));
#83282=CARTESIAN_POINT('Ctrl Pts',(9.77522935958062,-29.9200407849609,52.9463575859318));
#83283=CARTESIAN_POINT('Ctrl Pts',(9.77756659668694,-29.8771861604196,52.9484763944796));
#83284=CARTESIAN_POINT('Ctrl Pts',(9.77990383379327,-29.8344910055602,52.9519266772746));
#83285=CARTESIAN_POINT('Ctrl Pts',(9.78377991894163,-29.7636851574035,52.9576486426939));
#83286=CARTESIAN_POINT('Ctrl Pts',(9.78765600408998,-29.6930399153945,52.9670577757194));
#83287=CARTESIAN_POINT('Ctrl Pts',(9.79153208923833,-29.6229689292378,52.9801373476942));
#83288=CARTESIAN_POINT('Ctrl Pts',(9.79540239074575,-29.5530024984272,52.9931974031865));
#83289=CARTESIAN_POINT('Ctrl Pts',(9.79927269225317,-29.483609094309,53.0099169371265));
#83290=CARTESIAN_POINT('Ctrl Pts',(9.80314299376058,-29.4151979308667,53.0302273982925));
#83291=CARTESIAN_POINT('Ctrl Pts',(9.8070087021416,-29.3468679551871,53.0505137557769));
#83292=CARTESIAN_POINT('Ctrl Pts',(9.81087441052261,-29.2795183660661,53.0743824373223));
#83293=CARTESIAN_POINT('Ctrl Pts',(9.81474011890363,-29.2135471460565,53.1017140702665));
#83294=CARTESIAN_POINT('Ctrl Pts',(9.81860335462269,-29.1476181238822,53.1290282208033));
#83295=CARTESIAN_POINT('Ctrl Pts',(9.82246659034176,-29.0830661673647,53.1598007427907));
#83296=CARTESIAN_POINT('Ctrl Pts',(9.82632982606082,-29.0202717074698,53.1938632290671));
#83297=CARTESIAN_POINT('Ctrl Pts',(9.83019187065583,-28.9574966085452,53.2279152130988));
#83298=CARTESIAN_POINT('Ctrl Pts',(9.83405391525085,-28.8964783554352,53.2652549167899));
#83299=CARTESIAN_POINT('Ctrl Pts',(9.83791595984586,-28.8375735449655,53.3056675948516));
#83300=CARTESIAN_POINT('Ctrl Pts',(9.84177809319259,-28.7786673808338,53.3460812016169));
#83301=CARTESIAN_POINT('Ctrl Pts',(9.84564022653931,-28.7218751535432,53.3895676474181));
#83302=CARTESIAN_POINT('Ctrl Pts',(9.84950235988604,-28.6675237625811,53.4358693663207));
#83303=CARTESIAN_POINT('Ctrl Pts',(9.85336838840979,-28.6131175552078,53.482217783091));
#83304=CARTESIAN_POINT('Ctrl Pts',(9.85723441693354,-28.5611574676679,53.5313868268505));
#83305=CARTESIAN_POINT('Ctrl Pts',(9.8611004454573,-28.5119359268435,53.5830797917028));
#83306=CARTESIAN_POINT('Ctrl Pts',(9.86496858955252,-28.462687450965,53.6348010440241));
#83307=CARTESIAN_POINT('Ctrl Pts',(9.86883673364774,-28.4161808209744,53.6890486000156));
#83308=CARTESIAN_POINT('Ctrl Pts',(9.87270487774297,-28.372668511454,53.7454922125046));
#83309=CARTESIAN_POINT('Ctrl Pts',(9.87657959820511,-28.329082225136,53.8020317867512));
#83310=CARTESIAN_POINT('Ctrl Pts',(9.88045431866725,-28.2885006989418,53.8607744738912));
#83311=CARTESIAN_POINT('Ctrl Pts',(9.88432903912939,-28.2511329827409,53.9213611733099));
#83312=CARTESIAN_POINT('Ctrl Pts',(9.8865657276302,-28.2295624096003,53.956334941151));
#83313=CARTESIAN_POINT('Ctrl Pts',(9.88880241613101,-28.2090618900528,53.9919226987536));
#83314=CARTESIAN_POINT('Ctrl Pts',(9.89103910463182,-28.1896644294155,54.0280521184876));
#83315=CARTESIAN_POINT('Ctrl Pts',(9.89510093082391,-28.1544386419854,54.0936631426994));
#83316=CARTESIAN_POINT('Ctrl Pts',(9.899162757016,-28.1227297888941,54.1612912760284));
#83317=CARTESIAN_POINT('Ctrl Pts',(9.9032245832081,-28.094761105567,54.2305441418511));
#83318=CARTESIAN_POINT('Ctrl Pts',(9.90727491540929,-28.0668715668848,54.2996010387249));
#83319=CARTESIAN_POINT('Ctrl Pts',(9.91132524761048,-28.0427012767271,54.3702731296961));
#83320=CARTESIAN_POINT('Ctrl Pts',(9.91537557981167,-28.0224268197389,54.442145288438));
#83321=CARTESIAN_POINT('Ctrl Pts',(9.91941896482588,-28.0021871377856,54.5138941710383));
#83322=CARTESIAN_POINT('Ctrl Pts',(9.92346234984009,-27.985830114662,54.5868386314102));
#83323=CARTESIAN_POINT('Ctrl Pts',(9.9275057348543,-27.9734837874876,54.6605451386057));
#83324=CARTESIAN_POINT('Ctrl Pts',(9.9315405950777,-27.9611634904479,54.7340962481446));
#83325=CARTESIAN_POINT('Ctrl Pts',(9.93557545530109,-27.9528371217764,54.8084057976557));
#83326=CARTESIAN_POINT('Ctrl Pts',(9.93961031552448,-27.9485821515478,54.8830283215822));
#83327=CARTESIAN_POINT('Ctrl Pts',(9.94171530386221,-27.9463623317244,54.9219589248499));
#83328=CARTESIAN_POINT('Ctrl Pts',(9.94382029219994,-27.9452497952564,54.9609745046743));
#83329=CARTESIAN_POINT('Ctrl Pts',(9.94592528053768,-27.9452500000283,55.0000107785665));
#83330=CARTESIAN_POINT('Origin',(-1.54592528053767,-30.,55.));
#83331=CARTESIAN_POINT('',(8.79398090556005,-31.2520475724682,56.6292251037768));
#83332=CARTESIAN_POINT('',(8.85202116861107,-31.2520475724682,56.6292251037768));
#83333=CARTESIAN_POINT('',(-1.54592528053767,-31.2520475724682,56.6292251037768));
#83334=CARTESIAN_POINT('',(9.30407471946232,-27.9452508243762,55.0018405904705));
#83335=CARTESIAN_POINT('Ctrl Pts',(8.85202116861107,-31.2520475724682,56.6292251037768));
#83336=CARTESIAN_POINT('Ctrl Pts',(8.85588129510045,-31.308611520277,56.5857561237206));
#83337=CARTESIAN_POINT('Ctrl Pts',(8.85974142158982,-31.3628714284232,56.5393669395893));
#83338=CARTESIAN_POINT('Ctrl Pts',(8.8636015480792,-31.4145245822312,56.4903414940086));
#83339=CARTESIAN_POINT('Ctrl Pts',(8.86746436482228,-31.4662137348823,56.4412818809242));
#83340=CARTESIAN_POINT('Ctrl Pts',(8.87132718156535,-31.5152921853506,56.3895827035034));
#83341=CARTESIAN_POINT('Ctrl Pts',(8.87518999830842,-31.5614959281433,56.3355628135329));
#83342=CARTESIAN_POINT('Ctrl Pts',(8.87905908132929,-31.6077746228446,56.2814552922664));
#83343=CARTESIAN_POINT('Ctrl Pts',(8.88292816435016,-31.6511690154702,56.2250199351042));
#83344=CARTESIAN_POINT('Ctrl Pts',(8.88679724737102,-31.6914575926751,56.166605663745));
#83345=CARTESIAN_POINT('Ctrl Pts',(8.88741392878548,-31.6978790668702,56.1572951901025));
#83346=CARTESIAN_POINT('Ctrl Pts',(8.88803061019994,-31.7042217349627,56.1479344948192));
#83347=CARTESIAN_POINT('Ctrl Pts',(8.8886472916144,-31.7104848088554,56.1385250463537));
#83348=CARTESIAN_POINT('Ctrl Pts',(8.89251644611531,-31.7497803024012,56.0794887124745));
#83349=CARTESIAN_POINT('Ctrl Pts',(8.89638560061622,-31.7860927622602,56.0182999805595));
#83350=CARTESIAN_POINT('Ctrl Pts',(8.90025475511712,-31.8191793429239,55.9552926676046));
#83351=CARTESIAN_POINT('Ctrl Pts',(8.90411814418484,-31.8522166212218,55.8923792419455));
#83352=CARTESIAN_POINT('Ctrl Pts',(8.90798153325255,-31.8820373378707,55.8276530408393));
#83353=CARTESIAN_POINT('Ctrl Pts',(8.91184492232026,-31.9084420372948,55.7614765608907));
#83354=CARTESIAN_POINT('Ctrl Pts',(8.91570377839669,-31.9348157555596,55.6953777271231));
#83355=CARTESIAN_POINT('Ctrl Pts',(8.91956263447312,-31.9577812388704,55.6278324435397));
#83356=CARTESIAN_POINT('Ctrl Pts',(8.92342149054955,-31.9771858609769,55.5592259236239));
#83357=CARTESIAN_POINT('Ctrl Pts',(8.92727791500854,-31.9965782554656,55.4906626353825));
#83358=CARTESIAN_POINT('Ctrl Pts',(8.93113433946754,-32.0124141086027,55.4210399038763));
#83359=CARTESIAN_POINT('Ctrl Pts',(8.93499076392654,-32.0245901542657,55.3507595611677));
#83360=CARTESIAN_POINT('Ctrl Pts',(8.93884604822064,-32.0367626000397,55.2804999970795));
#83361=CARTESIAN_POINT('Ctrl Pts',(8.94270133251474,-32.0452773036021,55.2095836861502));
#83362=CARTESIAN_POINT('Ctrl Pts',(8.94655661680884,-32.0500821415544,55.1384224525854));
#83363=CARTESIAN_POINT('Ctrl Pts',(8.95041205077674,-32.054887166045,55.0672584563261));
#83364=CARTESIAN_POINT('Ctrl Pts',(8.95426748474464,-32.055982008449,54.9958500033625));
#83365=CARTESIAN_POINT('Ctrl Pts',(8.95812291871254,-32.0533665594502,54.9246121028825));
#83366=CARTESIAN_POINT('Ctrl Pts',(8.96198238635905,-32.0507483740847,54.8532996710272));
#83367=CARTESIAN_POINT('Ctrl Pts',(8.96584185400557,-32.044412166173,54.782158634289));
#83368=CARTESIAN_POINT('Ctrl Pts',(8.96970132165209,-32.0344099065248,54.7116011533762));
#83369=CARTESIAN_POINT('Ctrl Pts',(8.97356297345388,-32.0244019863839,54.6410037424761));
#83370=CARTESIAN_POINT('Ctrl Pts',(8.97742462525567,-32.0107239775958,54.5709910218015));
#83371=CARTESIAN_POINT('Ctrl Pts',(8.98128627705745,-31.9934789159077,54.5019644848691));
#83372=CARTESIAN_POINT('Ctrl Pts',(8.98515468302837,-31.9762036919809,54.4328172180189));
#83373=CARTESIAN_POINT('Ctrl Pts',(8.98902308899929,-31.9553491011636,54.3646600433246));
#83374=CARTESIAN_POINT('Ctrl Pts',(8.99289149497021,-31.9310677072978,54.2978781641827));
#83375=CARTESIAN_POINT('Ctrl Pts',(8.99518851746446,-31.9166496476834,54.2582237225985));
#83376=CARTESIAN_POINT('Ctrl Pts',(8.99748553995872,-31.9010242638133,54.2190538077006));
#83377=CARTESIAN_POINT('Ctrl Pts',(8.99978256245297,-31.8842312012679,54.1804450337722));
#83378=CARTESIAN_POINT('Ctrl Pts',(9.00365176190955,-31.8559442738922,54.1154108221018));
#83379=CARTESIAN_POINT('Ctrl Pts',(9.00752096136614,-31.8242310367163,54.0517155014003));
#83380=CARTESIAN_POINT('Ctrl Pts',(9.01139016082272,-31.7892402531975,53.9897441517923));
#83381=CARTESIAN_POINT('Ctrl Pts',(9.01525359672947,-31.7543015918623,53.9278651145518));
#83382=CARTESIAN_POINT('Ctrl Pts',(9.01911703263621,-31.7160953121696,53.8677053704774));
#83383=CARTESIAN_POINT('Ctrl Pts',(9.02298046854296,-31.6748178047568,53.8096290984027));
#83384=CARTESIAN_POINT('Ctrl Pts',(9.02683937399512,-31.6335887013754,53.7516209294154));
#83385=CARTESIAN_POINT('Ctrl Pts',(9.03069827944728,-31.589295804072,53.6956917734453));
#83386=CARTESIAN_POINT('Ctrl Pts',(9.03455718489944,-31.5421799864629,53.6421787850187));
#83387=CARTESIAN_POINT('Ctrl Pts',(9.03841366026827,-31.4950938392783,53.5886994955316));
#83388=CARTESIAN_POINT('Ctrl Pts',(9.0422701356371,-31.4451886189367,53.5376337185791));
#83389=CARTESIAN_POINT('Ctrl Pts',(9.04612661100593,-31.3927459309374,53.4892861507362));
#83390=CARTESIAN_POINT('Ctrl Pts',(9.04998194765525,-31.3403187279357,53.4409528587057));
#83391=CARTESIAN_POINT('Ctrl Pts',(9.05383728430456,-31.2853559016916,53.3953365114308));
#83392=CARTESIAN_POINT('Ctrl Pts',(9.05769262095387,-31.2281751891768,53.3527042563065));
#83393=CARTESIAN_POINT('Ctrl Pts',(9.06154810863517,-31.1709922366198,53.3100703310729));
#83394=CARTESIAN_POINT('Ctrl Pts',(9.06540359631647,-31.1115916160343,53.2704210186607));
#83395=CARTESIAN_POINT('Ctrl Pts',(9.06925908399777,-31.0503219494664,53.2339814935938));
#83396=CARTESIAN_POINT('Ctrl Pts',(9.07311860703276,-30.9889881548826,53.197503829027));
#83397=CARTESIAN_POINT('Ctrl Pts',(9.07697813006775,-30.9257818275672,53.1642429069912));
#83398=CARTESIAN_POINT('Ctrl Pts',(9.08083765310275,-30.8610774416811,53.1343786016643));
#83399=CARTESIAN_POINT('Ctrl Pts',(9.08469936132035,-30.7963364215018,53.1044973877816));
#83400=CARTESIAN_POINT('Ctrl Pts',(9.08856106953795,-30.7300961055593,53.0780167993037));
#83401=CARTESIAN_POINT('Ctrl Pts',(9.09242277775555,-30.6627497006221,53.0550680225712));
#83402=CARTESIAN_POINT('Ctrl Pts',(9.09629124113087,-30.5952854888593,53.0320791023069));
#83403=CARTESIAN_POINT('Ctrl Pts',(9.10015970450618,-30.5267117925989,53.0126344610694));
#83404=CARTESIAN_POINT('Ctrl Pts',(9.10402816788149,-30.4574349938009,52.9968148390759));
#83405=CARTESIAN_POINT('Ctrl Pts',(9.10632472301817,-30.4163080726706,52.9874233493229));
#83406=CARTESIAN_POINT('Ctrl Pts',(9.10862127815485,-30.3749335317263,52.9793084532619));
#83407=CARTESIAN_POINT('Ctrl Pts',(9.11091783329152,-30.3333971860964,52.9724783900528));
#83408=CARTESIAN_POINT('Ctrl Pts',(9.11478631670382,-30.2634303642635,52.9609733380697));
#83409=CARTESIAN_POINT('Ctrl Pts',(9.11865480011613,-30.1927300179298,52.9530716431946));
#83410=CARTESIAN_POINT('Ctrl Pts',(9.12252328352843,-30.1217002072108,52.9488572399599));
#83411=CARTESIAN_POINT('Ctrl Pts',(9.12638600086703,-30.0507762682456,52.9446491184013));
#83412=CARTESIAN_POINT('Ctrl Pts',(9.13024871820564,-29.9795243207904,52.9441174077245));
#83413=CARTESIAN_POINT('Ctrl Pts',(9.13411143554424,-29.9083567087272,52.9472946948808));
#83414=CARTESIAN_POINT('Ctrl Pts',(9.13796962214508,-29.8372725720414,52.9504682552681));
#83415=CARTESIAN_POINT('Ctrl Pts',(9.14182780874593,-29.7662730573655,52.9573421505805));
#83416=CARTESIAN_POINT('Ctrl Pts',(9.14568599534678,-29.6957719407134,52.9678969390204));
#83417=CARTESIAN_POINT('Ctrl Pts',(9.14954175207606,-29.6253152254023,52.9784450800937));
#83418=CARTESIAN_POINT('Ctrl Pts',(9.15339750880534,-29.5553567648275,52.9926694432706));
#83419=CARTESIAN_POINT('Ctrl Pts',(9.15725326553462,-29.4863051646889,53.0104987613287));
#83420=CARTESIAN_POINT('Ctrl Pts',(9.16110788480679,-29.4172739349313,53.0283228196969));
#83421=CARTESIAN_POINT('Ctrl Pts',(9.16496250407896,-29.3491495047654,53.0497496002636));
#83422=CARTESIAN_POINT('Ctrl Pts',(9.16881712335113,-29.2823285343048,53.0746571136998));
#83423=CARTESIAN_POINT('Ctrl Pts',(9.17267189596913,-29.2155049055486,53.0995656180154));
#83424=CARTESIAN_POINT('Ctrl Pts',(9.17652666858713,-29.1499852940231,53.1279549583208));
#83425=CARTESIAN_POINT('Ctrl Pts',(9.18038144120513,-29.0861478495278,53.1596544320217));
#83426=CARTESIAN_POINT('Ctrl Pts',(9.18424025761134,-29.0222434373716,53.1913871595538));
#83427=CARTESIAN_POINT('Ctrl Pts',(9.18809907401755,-28.9600251510098,53.2264367356658));
#83428=CARTESIAN_POINT('Ctrl Pts',(9.19195789042377,-28.8998471034632,53.2645861684481));
#83429=CARTESIAN_POINT('Ctrl Pts',(9.19581889570076,-28.839634920587,53.3027572410728));
#83430=CARTESIAN_POINT('Ctrl Pts',(9.19967990097776,-28.7814656768177,53.3440313893116));
#83431=CARTESIAN_POINT('Ctrl Pts',(9.20354090625475,-28.7256627373057,53.3881494785779));
#83432=CARTESIAN_POINT('Ctrl Pts',(9.20740868014233,-28.6697619713626,53.4323449099207));
#83433=CARTESIAN_POINT('Ctrl Pts',(9.2112764540299,-28.6162361569351,53.4793939152693));
#83434=CARTESIAN_POINT('Ctrl Pts',(9.21514422791748,-28.5653734201062,53.52899893312));
#83435=CARTESIAN_POINT('Ctrl Pts',(9.21744718665501,-28.5350886134965,53.558534865831));
#83436=CARTESIAN_POINT('Ctrl Pts',(9.21975014539255,-28.5057472096071,53.5889762917178));
#83437=CARTESIAN_POINT('Ctrl Pts',(9.22205310413009,-28.4774031176423,53.6202549886538));
#83438=CARTESIAN_POINT('Ctrl Pts',(9.22588186911175,-28.4302798822223,53.6722571272716));
#83439=CARTESIAN_POINT('Ctrl Pts',(9.22971063409341,-28.3857218334432,53.7267889522));
#83440=CARTESIAN_POINT('Ctrl Pts',(9.23353939907507,-28.3440162798996,53.7835644360417));
#83441=CARTESIAN_POINT('Ctrl Pts',(9.23736291406493,-28.302367912894,53.8402620694994));
#83442=CARTESIAN_POINT('Ctrl Pts',(9.2411864290548,-28.2635645787771,53.8991968672192));
#83443=CARTESIAN_POINT('Ctrl Pts',(9.24500994404467,-28.2278554195201,53.9600475259052));
#83444=CARTESIAN_POINT('Ctrl Pts',(9.24882955990619,-28.1921826756022,54.0208361305575));
#83445=CARTESIAN_POINT('Ctrl Pts',(9.25264917576771,-28.1595980989182,54.0835362956583));
#83446=CARTESIAN_POINT('Ctrl Pts',(9.25646879162923,-28.1303082181272,54.1477968532696));
#83447=CARTESIAN_POINT('Ctrl Pts',(9.26043595228199,-28.0998869226853,54.2145396789678));
#83448=CARTESIAN_POINT('Ctrl Pts',(9.26440311293475,-28.0730203785571,54.2829654537267));
#83449=CARTESIAN_POINT('Ctrl Pts',(9.26837027358751,-28.0498874430765,54.3526526605991));
#83450=CARTESIAN_POINT('Ctrl Pts',(9.27218706938689,-28.0276313010401,54.4196985560749));
#83451=CARTESIAN_POINT('Ctrl Pts',(9.27600386518627,-28.0088309596904,54.4879114610378));
#83452=CARTESIAN_POINT('Ctrl Pts',(9.27982066098565,-27.9935957073492,54.5568980061743));
#83453=CARTESIAN_POINT('Ctrl Pts',(9.28363747690964,-27.9783603746778,54.6258849150525));
#83454=CARTESIAN_POINT('Ctrl Pts',(9.28745429283363,-27.9666902652569,54.6956449850153));
#83455=CARTESIAN_POINT('Ctrl Pts',(9.29127110875762,-27.9586435999298,54.765774445475));
#83456=CARTESIAN_POINT('Ctrl Pts',(9.29509049516895,-27.9505915154649,54.8359511355874));
#83457=CARTESIAN_POINT('Ctrl Pts',(9.29890988158028,-27.9461677832664,54.9064972176053));
#83458=CARTESIAN_POINT('Ctrl Pts',(9.30272926799162,-27.9453786732185,54.977005086767));
#83459=CARTESIAN_POINT('Ctrl Pts',(9.30317775181519,-27.9452860135467,54.9852843325273));
#83460=CARTESIAN_POINT('Ctrl Pts',(9.30362623563875,-27.945243409575,54.9935630529975));
#83461=CARTESIAN_POINT('Ctrl Pts',(9.30407471946232,-27.9452508243762,55.0018405904705));
#83462=CARTESIAN_POINT('Ctrl Pts',(9.30407500815832,-27.9458343182313,55.0018453946623));
#83463=CARTESIAN_POINT('Ctrl Pts',(9.31377946376176,-27.9442447038212,55.180908445478));
#83464=CARTESIAN_POINT('Ctrl Pts',(9.36052900964471,-28.0476742131919,56.041715898022));
#83465=CARTESIAN_POINT('Ctrl Pts',(9.44318606609553,-29.2381700604055,57.2943385069855));
#83466=CARTESIAN_POINT('Ctrl Pts',(9.51613866694288,-30.7301723791876,57.0320535442367));
#83467=CARTESIAN_POINT('Ctrl Pts',(9.55204617751071,-31.254042933277,56.631836765028));
#83468=CARTESIAN_POINT('',(9.24592528058113,-27.9452507889202,54.9981994259027));
#83469=CARTESIAN_POINT('Ctrl Pts',(9.24592528058113,-27.9452507889202,54.9981994259027));
#83470=CARTESIAN_POINT('Ctrl Pts',(9.24973102059823,-27.9451893827432,55.0682739060629));
#83471=CARTESIAN_POINT('Ctrl Pts',(9.25353676061533,-27.9487168964303,55.1384663033952));
#83472=CARTESIAN_POINT('Ctrl Pts',(9.25734250063243,-27.9558428982201,55.2083729966738));
#83473=CARTESIAN_POINT('Ctrl Pts',(9.26114492409795,-27.9629626899818,55.27821876904));
#83474=CARTESIAN_POINT('Ctrl Pts',(9.26494734756347,-27.9736747051185,55.3477788345256));
#83475=CARTESIAN_POINT('Ctrl Pts',(9.26874977102899,-27.9879364790639,55.416650873296));
#83476=CARTESIAN_POINT('Ctrl Pts',(9.27255023950047,-28.0021909204007,55.4854875019058));
#83477=CARTESIAN_POINT('Ctrl Pts',(9.27635070797195,-28.0199914006488,55.5536363151698));
#83478=CARTESIAN_POINT('Ctrl Pts',(9.28015117644343,-28.0412440363914,55.6207033409992));
#83479=CARTESIAN_POINT('Ctrl Pts',(9.28395104864064,-28.062493337703,55.6877598443519));
#83480=CARTESIAN_POINT('Ctrl Pts',(9.28775092083786,-28.0871935671388,55.7537344197391));
#83481=CARTESIAN_POINT('Ctrl Pts',(9.29155079303508,-28.1152010131206,55.8182483373392));
#83482=CARTESIAN_POINT('Ctrl Pts',(9.29535403744921,-28.1432333144602,55.8828195081608));
#83483=CARTESIAN_POINT('Ctrl Pts',(9.29915728186334,-28.1745784953574,55.9459269708964));
#83484=CARTESIAN_POINT('Ctrl Pts',(9.30296052627747,-28.209045142649,56.0072131161929));
#83485=CARTESIAN_POINT('Ctrl Pts',(9.30676541262342,-28.2435266698375,56.0685257198656));
#83486=CARTESIAN_POINT('Ctrl Pts',(9.31057029896936,-28.2811320775326,56.128015016866));
#83487=CARTESIAN_POINT('Ctrl Pts',(9.3143751853153,-28.3216260647905,56.1853516339506));
#83488=CARTESIAN_POINT('Ctrl Pts',(9.31818690208205,-28.3621927456712,56.2427911800549));
#83489=CARTESIAN_POINT('Ctrl Pts',(9.32199861884879,-28.405658051256,56.2980699343737));
#83490=CARTESIAN_POINT('Ctrl Pts',(9.32581033561554,-28.4517462499833,56.3508915160216));
#83491=CARTESIAN_POINT('Ctrl Pts',(9.32899447389002,-28.490246276756,56.3950163107365));
#83492=CARTESIAN_POINT('Ctrl Pts',(9.3321786121645,-28.5305757983056,56.4374269739367));
#83493=CARTESIAN_POINT('Ctrl Pts',(9.33536275043899,-28.5725559515922,56.4779719385581));
#83494=CARTESIAN_POINT('Ctrl Pts',(9.33923123501024,-28.6235586283883,56.5272309708483));
#83495=CARTESIAN_POINT('Ctrl Pts',(9.34309971958148,-28.6772141652392,56.573943517376));
#83496=CARTESIAN_POINT('Ctrl Pts',(9.34696820415272,-28.7332379698518,56.6178107186797));
#83497=CARTESIAN_POINT('Ctrl Pts',(9.35083092265192,-28.7891782695964,56.6616125348336));
#83498=CARTESIAN_POINT('Ctrl Pts',(9.35469364115112,-28.8474794508072,56.7025771269198));
#83499=CARTESIAN_POINT('Ctrl Pts',(9.35855635965032,-28.9078209020442,56.7404431563508));
#83500=CARTESIAN_POINT('Ctrl Pts',(9.36241454740881,-28.968091576322,56.7782647711653));
#83501=CARTESIAN_POINT('Ctrl Pts',(9.36627273516731,-29.0303973575254,56.8129947854112));
#83502=CARTESIAN_POINT('Ctrl Pts',(9.3701309229258,-29.0943868629872,56.8444138387493));
#83503=CARTESIAN_POINT('Ctrl Pts',(9.3739866808103,-29.1583360680684,56.8758131044706));
#83504=CARTESIAN_POINT('Ctrl Pts',(9.3778424386948,-29.223966458435,56.9039053326329));
#83505=CARTESIAN_POINT('Ctrl Pts',(9.3816981965793,-29.290901426245,56.9285167293022));
#83506=CARTESIAN_POINT('Ctrl Pts',(9.38555281700262,-29.3578166480206,56.9531208655291));
#83507=CARTESIAN_POINT('Ctrl Pts',(9.38940743742595,-29.4260352273575,56.9742460412247));
#83508=CARTESIAN_POINT('Ctrl Pts',(9.39326205784927,-29.4951615313425,56.9917669750911));
#83509=CARTESIAN_POINT('Ctrl Pts',(9.39711683161271,-29.5642905852315,57.0092886059553));
#83510=CARTESIAN_POINT('Ctrl Pts',(9.40097160537615,-29.634326963864,57.0232055930722));
#83511=CARTESIAN_POINT('Ctrl Pts',(9.40482637913959,-29.704862551242,57.0334432494763));
#83512=CARTESIAN_POINT('Ctrl Pts',(9.40868519667478,-29.7754721325385,57.0436916454849));
#83513=CARTESIAN_POINT('Ctrl Pts',(9.41254401420997,-29.8465814860722,57.05025293598));
#83514=CARTESIAN_POINT('Ctrl Pts',(9.41640283174516,-29.9177759369013,57.0531041780552));
#83515=CARTESIAN_POINT('Ctrl Pts',(9.42026383814357,-29.9890107718411,57.0559570374597));
#83516=CARTESIAN_POINT('Ctrl Pts',(9.42412484454199,-30.0603303140259,57.055095665034));
#83517=CARTESIAN_POINT('Ctrl Pts',(9.4279858509404,-30.1313212078869,57.0505492685764));
#83518=CARTESIAN_POINT('Ctrl Pts',(9.43185362592536,-30.2024365532404,57.0459949020004));
#83519=CARTESIAN_POINT('Ctrl Pts',(9.43572140091031,-30.2732216171642,57.0377426700059));
#83520=CARTESIAN_POINT('Ctrl Pts',(9.43958917589527,-30.3432701708816,57.0258734294824));
#83521=CARTESIAN_POINT('Ctrl Pts',(9.44189212435604,-30.3849784423271,57.0188062527981));
#83522=CARTESIAN_POINT('Ctrl Pts',(9.4441950728168,-30.4264258160014,57.010457737578));
#83523=CARTESIAN_POINT('Ctrl Pts',(9.44649802127757,-30.4675291496378,57.0008533321408));
#83524=CARTESIAN_POINT('Ctrl Pts',(9.45045224760824,-30.5381047126224,56.9843623018302));
#83525=CARTESIAN_POINT('Ctrl Pts',(9.45440647393891,-30.6079477242885,56.9640996491157));
#83526=CARTESIAN_POINT('Ctrl Pts',(9.45836070026958,-30.6766255095933,56.9401483145027));
#83527=CARTESIAN_POINT('Ctrl Pts',(9.46222412309782,-30.7437262017013,56.9167469901543));
#83528=CARTESIAN_POINT('Ctrl Pts',(9.46608754592607,-30.8097141140611,56.8898247287655));
#83529=CARTESIAN_POINT('Ctrl Pts',(9.46995096875432,-30.8741961087912,56.8595103457293));
#83530=CARTESIAN_POINT('Ctrl Pts',(9.4739505968362,-30.9409514209492,56.8281272269079));
#83531=CARTESIAN_POINT('Ctrl Pts',(9.47795022491808,-31.0060921252477,56.7931084436052));
#83532=CARTESIAN_POINT('Ctrl Pts',(9.48194985299997,-31.0692017699715,56.7546524264337));
#83533=CARTESIAN_POINT('Ctrl Pts',(9.48594948108185,-31.1323114146954,56.7161964092622));
#83534=CARTESIAN_POINT('Ctrl Pts',(9.48994910916373,-31.1933894800341,56.6743034186563));
#83535=CARTESIAN_POINT('Ctrl Pts',(9.49394873724561,-31.2520475724682,56.6292251037768));
#83536=CARTESIAN_POINT('Ctrl Pts',(8.79398090556005,-31.2520475724682,56.6292251037768));
#83537=CARTESIAN_POINT('Ctrl Pts',(8.79801593729024,-31.3109357776389,56.5839699489427));
#83538=CARTESIAN_POINT('Ctrl Pts',(8.80205096902044,-31.3674561592778,56.5354495907487));
#83539=CARTESIAN_POINT('Ctrl Pts',(8.80608600075064,-31.421231125295,56.4839473208281));
#83540=CARTESIAN_POINT('Ctrl Pts',(8.80994398323754,-31.4726465517402,56.4347048690519));
#83541=CARTESIAN_POINT('Ctrl Pts',(8.81380196572444,-31.5215520411688,56.3827370741503));
#83542=CARTESIAN_POINT('Ctrl Pts',(8.81765994821134,-31.56765065383,56.3283331622927));
#83543=CARTESIAN_POINT('Ctrl Pts',(8.82151585711969,-31.6137244895268,56.2739584913103));
#83544=CARTESIAN_POINT('Ctrl Pts',(8.82537176602805,-31.6569941284217,56.2171506714122));
#83545=CARTESIAN_POINT('Ctrl Pts',(8.8292276749364,-31.6972009450905,56.1582342226354));
#83546=CARTESIAN_POINT('Ctrl Pts',(8.83308280124164,-31.7373996013021,56.0993297316608));
#83547=CARTESIAN_POINT('Ctrl Pts',(8.83693792754688,-31.7745363962181,56.0383178629856));
#83548=CARTESIAN_POINT('Ctrl Pts',(8.84079305385212,-31.8083953414219,55.9755531003609));
#83549=CARTESIAN_POINT('Ctrl Pts',(8.84464868727536,-31.8422587405603,55.91278008142));
#83550=CARTESIAN_POINT('Ctrl Pts',(8.84850432069861,-31.8728432056857,55.8482541395236));
#83551=CARTESIAN_POINT('Ctrl Pts',(8.85235995412186,-31.8999789486164,55.7823538568414));
#83552=CARTESIAN_POINT('Ctrl Pts',(8.85621984162051,-31.9271446315033,55.7163808637275));
#83553=CARTESIAN_POINT('Ctrl Pts',(8.86007972911915,-31.9508538154152,55.649030954446));
#83554=CARTESIAN_POINT('Ctrl Pts',(8.86393961661779,-31.9709854350814,55.5807012805194));
#83555=CARTESIAN_POINT('Ctrl Pts',(8.86780200960935,-31.9911301223903,55.5123272530943));
#83556=CARTESIAN_POINT('Ctrl Pts',(8.8716644026009,-32.0076925122235,55.4429726678314));
#83557=CARTESIAN_POINT('Ctrl Pts',(8.87552679559246,-32.0206024973771,55.3730457211834));
#83558=CARTESIAN_POINT('Ctrl Pts',(8.87939562662056,-32.0335340015621,55.3030022166817));
#83559=CARTESIAN_POINT('Ctrl Pts',(8.88326445764865,-32.0428008922359,55.2323849281591));
#83560=CARTESIAN_POINT('Ctrl Pts',(8.88713328867675,-32.0483848997645,55.1616071313926));
#83561=CARTESIAN_POINT('Ctrl Pts',(8.88836274814608,-32.0501594179285,55.1391149543445));
#83562=CARTESIAN_POINT('Ctrl Pts',(8.88959220761542,-32.0515624047983,55.1166065609287));
#83563=CARTESIAN_POINT('Ctrl Pts',(8.89082166708475,-32.052594374007,55.0940951555338));
#83564=CARTESIAN_POINT('Ctrl Pts',(8.89469076155227,-32.0558419689506,55.0232520279301));
#83565=CARTESIAN_POINT('Ctrl Pts',(8.89855985601979,-32.0554240053786,54.9521018207862));
#83566=CARTESIAN_POINT('Ctrl Pts',(8.90242895048731,-32.0513044211451,54.8810557513345));
#83567=CARTESIAN_POINT('Ctrl Pts',(8.90629228017547,-32.0471909749095,54.810115537379));
#83568=CARTESIAN_POINT('Ctrl Pts',(8.91015560986364,-32.039386883526,54.7392796341407));
#83569=CARTESIAN_POINT('Ctrl Pts',(8.9140189395518,-32.0279080492904,54.6689614733551));
#83570=CARTESIAN_POINT('Ctrl Pts',(8.91787773748938,-32.0164426799201,54.5987257969528));
#83571=CARTESIAN_POINT('Ctrl Pts',(8.92173653542695,-32.001311207765,54.5290071337659));
#83572=CARTESIAN_POINT('Ctrl Pts',(8.92559533336452,-31.9825813738596,54.4602142475714));
#83573=CARTESIAN_POINT('Ctrl Pts',(8.92945170047951,-31.9638633386813,54.3914646969712));
#83574=CARTESIAN_POINT('Ctrl Pts',(8.93330806759449,-31.9415515662884,54.3236402339398));
#83575=CARTESIAN_POINT('Ctrl Pts',(8.93716443470947,-31.9157646621692,54.2571384236051));
#83576=CARTESIAN_POINT('Ctrl Pts',(8.94101966253136,-31.8899853763189,54.1906562600135));
#83577=CARTESIAN_POINT('Ctrl Pts',(8.94487489035324,-31.8607331724859,54.1254964260389));
#83578=CARTESIAN_POINT('Ctrl Pts',(8.94873011817513,-31.8281756328998,54.0620386906853));
#83579=CARTESIAN_POINT('Ctrl Pts',(8.95258549662043,-31.7956168212935,53.9985784760435));
#83580=CARTESIAN_POINT('Ctrl Pts',(8.95644087506573,-31.7597526412559,53.9368209232596));
#83581=CARTESIAN_POINT('Ctrl Pts',(8.96029625351103,-31.7207968899626,53.8771217225384));
#83582=CARTESIAN_POINT('Ctrl Pts',(8.96415566745054,-31.6818003629812,53.8173600335862));
#83583=CARTESIAN_POINT('Ctrl Pts',(8.96801508139005,-31.6397060709665,53.7596614052524));
#83584=CARTESIAN_POINT('Ctrl Pts',(8.97187449532956,-31.5947709730042,53.7043522445652));
#83585=CARTESIAN_POINT('Ctrl Pts',(8.97573609436686,-31.5498104339814,53.6490117692984));
#83586=CARTESIAN_POINT('Ctrl Pts',(8.97959769340417,-31.5020062128951,53.5960638155294));
#83587=CARTESIAN_POINT('Ctrl Pts',(8.98345929244148,-31.4516535306604,53.5457993297274));
#83588=CARTESIAN_POINT('Ctrl Pts',(8.98732764769787,-31.4012127518238,53.4954469016312));
#83589=CARTESIAN_POINT('Ctrl Pts',(8.99119600295426,-31.3482149711079,53.4477876400769));
#83590=CARTESIAN_POINT('Ctrl Pts',(8.99506435821066,-31.2929894562316,53.4030730046198));
#83591=CARTESIAN_POINT('Ctrl Pts',(8.99736188478154,-31.260189447078,53.3765157066829));
#83592=CARTESIAN_POINT('Ctrl Pts',(8.99965941135243,-31.2266041943995,53.3509963236269));
#83593=CARTESIAN_POINT('Ctrl Pts',(9.00195693792331,-31.1923072097097,53.3265601055986));
#83594=CARTESIAN_POINT('Ctrl Pts',(9.00582593499164,-31.1345516499269,53.2854099151674));
#83595=CARTESIAN_POINT('Ctrl Pts',(9.00969493205998,-31.0745501065352,53.2471725977323));
#83596=CARTESIAN_POINT('Ctrl Pts',(9.01356392912831,-31.0126284809632,53.2121014788187));
#83597=CARTESIAN_POINT('Ctrl Pts',(9.01742716115078,-30.9507991224581,53.1770826180499));
#83598=CARTESIAN_POINT('Ctrl Pts',(9.02129039317326,-30.887055780123,53.1452208285152));
#83599=CARTESIAN_POINT('Ctrl Pts',(9.02515362519573,-30.8217544008784,53.1167269801919));
#83600=CARTESIAN_POINT('Ctrl Pts',(9.02901232554179,-30.756529621931,53.0882665559292));
#83601=CARTESIAN_POINT('Ctrl Pts',(9.03287102588784,-30.6897508794427,53.0631664188339));
#83602=CARTESIAN_POINT('Ctrl Pts',(9.03672972623389,-30.6217983152514,53.0415913558068));
#83603=CARTESIAN_POINT('Ctrl Pts',(9.04058599585565,-30.5538885566509,53.0200298836329));
#83604=CARTESIAN_POINT('Ctrl Pts',(9.04444226547741,-30.4848069052957,53.0019892266398));
#83605=CARTESIAN_POINT('Ctrl Pts',(9.04829853509917,-30.4149516824997,52.9875853648687));
#83606=CARTESIAN_POINT('Ctrl Pts',(9.05215366566829,-30.345117093317,52.9731857576644));
#83607=CARTESIAN_POINT('Ctrl Pts',(9.05600879623741,-30.2745098618575,52.9624209111053));
#83608=CARTESIAN_POINT('Ctrl Pts',(9.05986392680652,-30.2035399219365,52.9553560058832));
#83609=CARTESIAN_POINT('Ctrl Pts',(9.06371920838183,-30.1325672021095,52.9482908239274));
#83610=CARTESIAN_POINT('Ctrl Pts',(9.06757448995713,-30.0612322292501,52.944925916974));
#83611=CARTESIAN_POINT('Ctrl Pts',(9.07142977153244,-29.9899497730715,52.9452745790645));
#83612=CARTESIAN_POINT('Ctrl Pts',(9.07528908984937,-29.9185926793205,52.9456236062278));
#83613=CARTESIAN_POINT('Ctrl Pts',(9.0791484081663,-29.8472886988166,52.9496939620888));
#83614=CARTESIAN_POINT('Ctrl Pts',(9.08300772648323,-29.7764514087396,52.9574467963244));
#83615=CARTESIAN_POINT('Ctrl Pts',(9.08686923045711,-29.7055740012111,52.9652040212411));
#83616=CARTESIAN_POINT('Ctrl Pts',(9.09073073443099,-29.6351642899932,52.9766477981494));
#83617=CARTESIAN_POINT('Ctrl Pts',(9.09459223840487,-29.5656268115988,52.9916878988319));
#83618=CARTESIAN_POINT('Ctrl Pts',(9.09846050051131,-29.4959676336023,53.0067543216405));
#83619=CARTESIAN_POINT('Ctrl Pts',(9.10232876261775,-29.4271842051521,53.025429507103));
#83620=CARTESIAN_POINT('Ctrl Pts',(9.1061970247242,-29.3596663533093,53.0475732066436));
#83621=CARTESIAN_POINT('Ctrl Pts',(9.10849541940342,-29.3195494565847,53.0607302678257));
#83622=CARTESIAN_POINT('Ctrl Pts',(9.11079381408265,-29.2798789969184,53.0751109003345));
#83623=CARTESIAN_POINT('Ctrl Pts',(9.11309220876187,-29.2407329502307,53.0906778402704));
#83624=CARTESIAN_POINT('Ctrl Pts',(9.11696136315485,-29.1748338686332,53.1168834761355));
#83625=CARTESIAN_POINT('Ctrl Pts',(9.12083051754782,-29.1101640263347,53.1465561390878));
#83626=CARTESIAN_POINT('Ctrl Pts',(9.12469967194079,-29.0471130310267,53.1795593976016));
#83627=CARTESIAN_POINT('Ctrl Pts',(9.12856306090183,-28.9841559880878,53.2125134779173));
#83628=CARTESIAN_POINT('Ctrl Pts',(9.13242644986287,-28.9228134307589,53.2487880790794));
#83629=CARTESIAN_POINT('Ctrl Pts',(9.13628983882391,-28.8634555918223,53.2881985013618));
#83630=CARTESIAN_POINT('Ctrl Pts',(9.14014869479598,-28.8041673985856,53.3275626826338));
#83631=CARTESIAN_POINT('Ctrl Pts',(9.14400755076807,-28.7468597008544,53.3700551092534));
#83632=CARTESIAN_POINT('Ctrl Pts',(9.14786640674014,-28.691877136126,53.4154457612596));
#83633=CARTESIAN_POINT('Ctrl Pts',(9.15172283109628,-28.6369292180602,53.4608078108423));
#83634=CARTESIAN_POINT('Ctrl Pts',(9.15557925545242,-28.5843038998644,53.5090641539634));
#83635=CARTESIAN_POINT('Ctrl Pts',(9.15943567980856,-28.5343146735652,53.5599430266917));
#83636=CARTESIAN_POINT('Ctrl Pts',(9.16329096400142,-28.4843402267287,53.6108068569308));
#83637=CARTESIAN_POINT('Ctrl Pts',(9.16714624819429,-28.4370006647841,53.664291331159));
#83638=CARTESIAN_POINT('Ctrl Pts',(9.17100153238715,-28.3925730990924,53.7200873776939));
#83639=CARTESIAN_POINT('Ctrl Pts',(9.17485696625558,-28.3481438085678,53.7758855904256));
#83640=CARTESIAN_POINT('Ctrl Pts',(9.178712400124,-28.3066270396117,53.8339951722531));
#83641=CARTESIAN_POINT('Ctrl Pts',(9.18256783399242,-28.2682589344091,53.894074846906));
#83642=CARTESIAN_POINT('Ctrl Pts',(9.18642730154279,-28.2298506872306,53.954217378894));
#83643=CARTESIAN_POINT('Ctrl Pts',(9.19028676909316,-28.1945979418333,54.0163337080404));
#83644=CARTESIAN_POINT('Ctrl Pts',(9.19414623664353,-28.1626923851445,54.0800552783488));
#83645=CARTESIAN_POINT('Ctrl Pts',(9.1980078883509,-28.1307687724041,54.1438129100859));
#83646=CARTESIAN_POINT('Ctrl Pts',(9.20186954005828,-28.1021963139035,54.2091771461072));
#83647=CARTESIAN_POINT('Ctrl Pts',(9.20573119176565,-28.0771186290985,54.2757591588843));
#83648=CARTESIAN_POINT('Ctrl Pts',(9.20959959764587,-28.0519970824875,54.3424576260849));
#83649=CARTESIAN_POINT('Ctrl Pts',(9.2134680035261,-28.0303826606991,54.4103776594867));
#83650=CARTESIAN_POINT('Ctrl Pts',(9.21733640940633,-28.0123689814919,54.4791156589371));
#83651=CARTESIAN_POINT('Ctrl Pts',(9.21963343280437,-28.0016726264804,54.5199316430815));
#83652=CARTESIAN_POINT('Ctrl Pts',(9.2219304562024,-27.9922448704791,54.5610358236325));
#83653=CARTESIAN_POINT('Ctrl Pts',(9.22422747960044,-27.9840966829305,54.6023426365223));
#83654=CARTESIAN_POINT('Ctrl Pts',(9.22983463137485,-27.9642065397518,54.7031746826342));
#83655=CARTESIAN_POINT('Ctrl Pts',(9.23544178314927,-27.9518767132062,54.8055436423064));
#83656=CARTESIAN_POINT('Ctrl Pts',(9.24104893492368,-27.947287515211,54.9085176667792));
#83657=CARTESIAN_POINT('Ctrl Pts',(9.24267438346168,-27.9459571597165,54.938368647146));
#83658=CARTESIAN_POINT('Ctrl Pts',(9.24429983199968,-27.9452770157847,54.9682703020373));
#83659=CARTESIAN_POINT('Ctrl Pts',(9.24592528053768,-27.9452507889209,54.9981994251026));
#83660=CARTESIAN_POINT('Origin',(-1.54592528053767,-30.,55.));
#83661=CARTESIAN_POINT('',(8.09385946080458,-31.2520475724682,56.6292251037768));
#83662=CARTESIAN_POINT('',(8.15211404571458,-31.2520475724682,56.6292251037768));
#83663=CARTESIAN_POINT('',(-1.54592528053767,-31.2520475724682,56.6292251037768));
#83664=CARTESIAN_POINT('',(8.60407471942946,-27.9452501088858,54.9993310708367));
#83665=CARTESIAN_POINT('Ctrl Pts',(8.15211404571458,-31.2520475724682,56.6292251037768));
#83666=CARTESIAN_POINT('Ctrl Pts',(8.15596957845487,-31.308571006352,56.5857872583755));
#83667=CARTESIAN_POINT('Ctrl Pts',(8.15982511119515,-31.362858995009,56.5393831792067));
#83668=CARTESIAN_POINT('Ctrl Pts',(8.16368064393543,-31.4145918930459,56.4902776045518));
#83669=CARTESIAN_POINT('Ctrl Pts',(8.1675357777639,-31.4663194385503,56.4411771105941));
#83670=CARTESIAN_POINT('Ctrl Pts',(8.17139091159237,-31.515492066891,56.3893760114549));
#83671=CARTESIAN_POINT('Ctrl Pts',(8.17524604542084,-31.5618258017338,56.3351770397736));
#83672=CARTESIAN_POINT('Ctrl Pts',(8.17912851385102,-31.608488063223,56.2805937734425));
#83673=CARTESIAN_POINT('Ctrl Pts',(8.18301098228121,-31.6522706727025,56.2235788607262));
#83674=CARTESIAN_POINT('Ctrl Pts',(8.18689345071139,-31.6929251008616,56.1644750600046));
#83675=CARTESIAN_POINT('Ctrl Pts',(8.1907539689977,-31.7333496828382,56.1057054118854));
#83676=CARTESIAN_POINT('Ctrl Pts',(8.19461448728401,-31.7706811538646,56.0448708815817));
#83677=CARTESIAN_POINT('Ctrl Pts',(8.19847500557032,-31.8047201484561,55.9823353542739));
#83678=CARTESIAN_POINT('Ctrl Pts',(8.20236844907244,-31.8390494515399,55.9192664799956));
#83679=CARTESIAN_POINT('Ctrl Pts',(8.20626189257456,-31.8700296290214,55.8544679084298));
#83680=CARTESIAN_POINT('Ctrl Pts',(8.21015533607669,-31.8975055949884,55.788333736109));
#83681=CARTESIAN_POINT('Ctrl Pts',(8.21404877957881,-31.9249815609555,55.7221995637882));
#83682=CARTESIAN_POINT('Ctrl Pts',(8.21794222308093,-31.9489532088339,55.6547302832358));
#83683=CARTESIAN_POINT('Ctrl Pts',(8.22183566658305,-31.9693172416555,55.5863336628732));
#83684=CARTESIAN_POINT('Ctrl Pts',(8.22570474058959,-31.9895538137326,55.5183651445588));
#83685=CARTESIAN_POINT('Ctrl Pts',(8.22957381459614,-32.0063071206436,55.449214604025));
#83686=CARTESIAN_POINT('Ctrl Pts',(8.23344288860268,-32.01944299116,55.3792724191852));
#83687=CARTESIAN_POINT('Ctrl Pts',(8.23730619764667,-32.0325592890859,55.3094344489653));
#83688=CARTESIAN_POINT('Ctrl Pts',(8.24116950669066,-32.0420687607178,55.2388076493788));
#83689=CARTESIAN_POINT('Ctrl Pts',(8.24503281573465,-32.0478871312764,55.1677970799878));
#83690=CARTESIAN_POINT('Ctrl Pts',(8.24889159285783,-32.0536986764959,55.0968698107608));
#83691=CARTESIAN_POINT('Ctrl Pts',(8.252750369981,-32.0558276818286,55.0255601477677));
#83692=CARTESIAN_POINT('Ctrl Pts',(8.25660914710418,-32.0542413068434,54.9542811225153));
#83693=CARTESIAN_POINT('Ctrl Pts',(8.26046549331127,-32.0526559312277,54.8830470009523));
#83694=CARTESIAN_POINT('Ctrl Pts',(8.26432183951836,-32.0473598297511,54.8118439633547));
#83695=CARTESIAN_POINT('Ctrl Pts',(8.26817818572546,-32.0383722258364,54.7410864402188));
#83696=CARTESIAN_POINT('Ctrl Pts',(8.2720333925775,-32.0293872773037,54.6703498223484));
#83697=CARTESIAN_POINT('Ctrl Pts',(8.27588859942954,-32.0167130527585,54.6000589392748));
#83698=CARTESIAN_POINT('Ctrl Pts',(8.27974380628158,-32.0004205986065,54.5306227624065));
#83699=CARTESIAN_POINT('Ctrl Pts',(8.28359916372655,-31.9841275080351,54.4611838732073));
#83700=CARTESIAN_POINT('Ctrl Pts',(8.28745452117151,-31.9642160203678,54.3926002289364));
#83701=CARTESIAN_POINT('Ctrl Pts',(8.29130987861647,-31.9408078398956,54.3252685785442));
#83702=CARTESIAN_POINT('Ctrl Pts',(8.29516927165503,-31.9173751569214,54.2578664487783));
#83703=CARTESIAN_POINT('Ctrl Pts',(8.2990286646936,-31.8904386344849,54.1917193887793));
#83704=CARTESIAN_POINT('Ctrl Pts',(8.30288805773216,-31.8601689269621,54.1272061379314));
#83705=CARTESIAN_POINT('Ctrl Pts',(8.3067496358931,-31.8298820812483,54.0626563607835));
#83706=CARTESIAN_POINT('Ctrl Pts',(8.31061121405404,-31.7962585227126,53.9997426628865));
#83707=CARTESIAN_POINT('Ctrl Pts',(8.31447279221498,-31.7595145901036,53.9388185971698));
#83708=CARTESIAN_POINT('Ctrl Pts',(8.31834112686172,-31.7227063677537,53.8777879344692));
#83709=CARTESIAN_POINT('Ctrl Pts',(8.32220946150847,-31.6827671433323,53.8187542567448));
#83710=CARTESIAN_POINT('Ctrl Pts',(8.32607779615521,-31.6399558203565,53.7620410064227));
#83711=CARTESIAN_POINT('Ctrl Pts',(8.32837550991068,-31.6145267469504,53.7283544649824));
#83712=CARTESIAN_POINT('Ctrl Pts',(8.33067322366614,-31.5880851306643,53.6954859602816));
#83713=CARTESIAN_POINT('Ctrl Pts',(8.33297093742161,-31.5606914159249,53.6634971504862));
#83714=CARTESIAN_POINT('Ctrl Pts',(8.33684001407394,-31.514563658772,53.6096317998433));
#83715=CARTESIAN_POINT('Ctrl Pts',(8.34070909072628,-31.4655536320953,53.5580518103859));
#83716=CARTESIAN_POINT('Ctrl Pts',(8.34457816737861,-31.4139165404304,53.5090816322825));
#83717=CARTESIAN_POINT('Ctrl Pts',(8.34844147909947,-31.3623563881289,53.4601844198363));
#83718=CARTESIAN_POINT('Ctrl Pts',(8.35230479082034,-31.30817729029,53.41388963149));
#83719=CARTESIAN_POINT('Ctrl Pts',(8.3561681025412,-31.2516738481402,53.3704877599779));
#83720=CARTESIAN_POINT('Ctrl Pts',(8.36002688237409,-31.1952366877943,53.3271368013699));
#83721=CARTESIAN_POINT('Ctrl Pts',(8.36388566220698,-31.1364809824483,53.2866723133255));
#83722=CARTESIAN_POINT('Ctrl Pts',(8.36774444203987,-31.0757359270089,53.2493459000013));
#83723=CARTESIAN_POINT('Ctrl Pts',(8.37160079097541,-31.0150291388458,53.2120430010218));
#83724=CARTESIAN_POINT('Ctrl Pts',(8.37545713991095,-30.9523358998726,53.1778745083927));
#83725=CARTESIAN_POINT('Ctrl Pts',(8.3793134888465,-30.8880148178725,53.1470490438927));
#83726=CARTESIAN_POINT('Ctrl Pts',(8.38316869844154,-30.8237127392392,53.116232686634));
#83727=CARTESIAN_POINT('Ctrl Pts',(8.38702390803659,-30.7577842102125,53.088757606512));
#83728=CARTESIAN_POINT('Ctrl Pts',(8.39087911763163,-30.690611359049,53.06478592573));
#83729=CARTESIAN_POINT('Ctrl Pts',(8.39473447783001,-30.6234358837856,53.040813308497));
#83730=CARTESIAN_POINT('Ctrl Pts',(8.39858983802839,-30.5550164481427,53.0203445235216));
#83731=CARTESIAN_POINT('Ctrl Pts',(8.40244519822677,-30.4857523867497,53.0034925040794));
#83732=CARTESIAN_POINT('Ctrl Pts',(8.40630459401537,-30.4164158233452,52.9866228448212));
#83733=CARTESIAN_POINT('Ctrl Pts',(8.41016398980398,-30.3462333422905,52.9733776235643));
#83734=CARTESIAN_POINT('Ctrl Pts',(8.41402338559259,-30.2756156963431,52.9638188807404));
#83735=CARTESIAN_POINT('Ctrl Pts',(8.4178849665058,-30.204958067879,52.954254725918));
#83736=CARTESIAN_POINT('Ctrl Pts',(8.42174654741902,-30.1338652684148,52.9483812445603));
#83737=CARTESIAN_POINT('Ctrl Pts',(8.42560812833224,-30.0627516680271,52.9462084354395));
#83738=CARTESIAN_POINT('Ctrl Pts',(8.42947646570466,-29.9915136429154,52.9440318246384));
#83739=CARTESIAN_POINT('Ctrl Pts',(8.43334480307707,-29.9202552300438,52.9455688029681));
#83740=CARTESIAN_POINT('Ctrl Pts',(8.43721314044949,-29.8493885879424,52.95077727783));
#83741=CARTESIAN_POINT('Ctrl Pts',(8.43951082971972,-29.8072956918226,52.9538709730411));
#83742=CARTESIAN_POINT('Ctrl Pts',(8.44180851898994,-29.7653408945803,52.9582589957021));
#83743=CARTESIAN_POINT('Ctrl Pts',(8.44410620826017,-29.7236087780448,52.9639240056112));
#83744=CARTESIAN_POINT('Ctrl Pts',(8.44797527191515,-29.6533363450292,52.9734632780571));
#83745=CARTESIAN_POINT('Ctrl Pts',(8.45184433557013,-29.5834206956311,52.9866635450178));
#83746=CARTESIAN_POINT('Ctrl Pts',(8.45571339922511,-29.514272826168,53.0034863699185));
#83747=CARTESIAN_POINT('Ctrl Pts',(8.45957669792241,-29.4452279879746,53.0202841285804));
#83748=CARTESIAN_POINT('Ctrl Pts',(8.46343999661971,-29.3769491270779,53.040693617078));
#83749=CARTESIAN_POINT('Ctrl Pts',(8.46730329531701,-29.3098400782369,53.0646248826411));
#83750=CARTESIAN_POINT('Ctrl Pts',(8.47116206214992,-29.2428097520452,53.0885280754978));
#83751=CARTESIAN_POINT('Ctrl Pts',(8.47502082898283,-29.1769469674925,53.1159446770033));
#83752=CARTESIAN_POINT('Ctrl Pts',(8.47887959581574,-29.1126416498874,53.1467345789161));
#83753=CARTESIAN_POINT('Ctrl Pts',(8.48273593177282,-29.048376842178,53.1775050843658));
#83754=CARTESIAN_POINT('Ctrl Pts',(8.48659226772991,-28.9856679919586,53.2116444648626));
#83755=CARTESIAN_POINT('Ctrl Pts',(8.49044860368699,-28.9248848657667,53.248964588981));
#83756=CARTESIAN_POINT('Ctrl Pts',(8.49430380034396,-28.8641196970928,53.2862736873947));
#83757=CARTESIAN_POINT('Ctrl Pts',(8.49815899700094,-28.8052795367251,53.3267614098114));
#83758=CARTESIAN_POINT('Ctrl Pts',(8.50201419365791,-28.748707841602,53.3701946444953));
#83759=CARTESIAN_POINT('Ctrl Pts',(8.50586954097745,-28.6921339356353,53.4136295765668));
#83760=CARTESIAN_POINT('Ctrl Pts',(8.509724888297,-28.6378290549019,53.4600099518644));
#83761=CARTESIAN_POINT('Ctrl Pts',(8.51358023561654,-28.5861046627145,53.509061524508));
#83762=CARTESIAN_POINT('Ctrl Pts',(8.51743961870478,-28.5343261255524,53.558164444225));
#83763=CARTESIAN_POINT('Ctrl Pts',(8.52129900179303,-28.4851338224501,53.6099438081762));
#83764=CARTESIAN_POINT('Ctrl Pts',(8.52515838488127,-28.4388026522076,53.6640881751606));
#83765=CARTESIAN_POINT('Ctrl Pts',(8.5290199531756,-28.3924452489757,53.7182631990135));
#83766=CARTESIAN_POINT('Ctrl Pts',(8.53288152146993,-28.3489524998295,53.7748055063574));
#83767=CARTESIAN_POINT('Ctrl Pts',(8.53674308976426,-28.3085575429557,53.8333723914599));
#83768=CARTESIAN_POINT('Ctrl Pts',(8.54061141478311,-28.2680919055774,53.8920417531414));
#83769=CARTESIAN_POINT('Ctrl Pts',(8.54447973980196,-28.2307351369873,53.9527423513882));
#83770=CARTESIAN_POINT('Ctrl Pts',(8.54834806482081,-28.1966754116349,54.0151050860635));
#83771=CARTESIAN_POINT('Ctrl Pts',(8.55064586958012,-28.1764437613382,54.0521488680213));
#83772=CARTESIAN_POINT('Ctrl Pts',(8.55294367433942,-28.1573745478791,54.0897786837591));
#83773=CARTESIAN_POINT('Ctrl Pts',(8.55524147909873,-28.1394990816289,54.1279140551298));
#83774=CARTESIAN_POINT('Ctrl Pts',(8.55943211157693,-28.1068986141053,54.1974636220317));
#83775=CARTESIAN_POINT('Ctrl Pts',(8.56362274405514,-28.0781594760249,54.2689335413495));
#83776=CARTESIAN_POINT('Ctrl Pts',(8.56781337653335,-28.0534920738987,54.3418932790764));
#83777=CARTESIAN_POINT('Ctrl Pts',(8.5719933930468,-28.0288871607341,54.4146681907637));
#83778=CARTESIAN_POINT('Ctrl Pts',(8.57617340956025,-28.0083335647055,54.4889250761304));
#83779=CARTESIAN_POINT('Ctrl Pts',(8.5803534260737,-27.9919942666101,54.5642127386292));
#83780=CARTESIAN_POINT('Ctrl Pts',(8.58451639467447,-27.9757216072291,54.6391933455236));
#83781=CARTESIAN_POINT('Ctrl Pts',(8.58867936327524,-27.9636290821987,54.7151960112602));
#83782=CARTESIAN_POINT('Ctrl Pts',(8.59284233187601,-27.9558297509936,54.7917560191092));
#83783=CARTESIAN_POINT('Ctrl Pts',(8.59658646106049,-27.948815116394,54.8606132667231));
#83784=CARTESIAN_POINT('Ctrl Pts',(8.60033059024498,-27.9452727055362,54.9299209337767));
#83785=CARTESIAN_POINT('Ctrl Pts',(8.60407471942946,-27.9452501088858,54.9993310708368));
#83786=CARTESIAN_POINT('Ctrl Pts',(8.60407471946233,-27.9452501088856,54.9993310714461));
#83787=CARTESIAN_POINT('Ctrl Pts',(8.60802536616343,-27.9452262658779,55.0725697113247));
#83788=CARTESIAN_POINT('Ctrl Pts',(8.61197601286453,-27.9491224942341,55.1457764209575));
#83789=CARTESIAN_POINT('Ctrl Pts',(8.61592665956562,-27.9569024004591,55.2185171875399));
#83790=CARTESIAN_POINT('Ctrl Pts',(8.61988032372518,-27.964688248887,55.2913135126822));
#83791=CARTESIAN_POINT('Ctrl Pts',(8.62383398788475,-27.9763636264396,55.3636427387966));
#83792=CARTESIAN_POINT('Ctrl Pts',(8.62778765204431,-27.9918406472823,55.4350788165292));
#83793=CARTESIAN_POINT('Ctrl Pts',(8.63174855419895,-28.0073460019935,55.5066456726886));
#83794=CARTESIAN_POINT('Ctrl Pts',(8.63570945635358,-28.0266667958937,55.5773156752853));
#83795=CARTESIAN_POINT('Ctrl Pts',(8.63967035850822,-28.0496647215581,55.6466760117438));
#83796=CARTESIAN_POINT('Ctrl Pts',(8.64363545525019,-28.072687001979,55.7161098006577));
#83797=CARTESIAN_POINT('Ctrl Pts',(8.64760055199216,-28.0993940051616,55.7842307419675));
#83798=CARTESIAN_POINT('Ctrl Pts',(8.65156564873413,-28.1295995338212,55.8506466120653));
#83799=CARTESIAN_POINT('Ctrl Pts',(8.65553891552182,-28.1598673006975,55.9171993314586));
#83800=CARTESIAN_POINT('Ctrl Pts',(8.6595121823095,-28.1936477762703,55.9820395665411));
#83801=CARTESIAN_POINT('Ctrl Pts',(8.66348544909719,-28.2307093656716,56.0448005617236));
#83802=CARTESIAN_POINT('Ctrl Pts',(8.66444921604389,-28.2396991307103,56.0600240480715));
#83803=CARTESIAN_POINT('Ctrl Pts',(8.66541298299059,-28.2488817522033,56.0751253418758));
#83804=CARTESIAN_POINT('Ctrl Pts',(8.66637674993729,-28.2582535611019,56.090099493205));
#83805=CARTESIAN_POINT('Ctrl Pts',(8.67024584448533,-28.2958771949471,56.1502140338289));
#83806=CARTESIAN_POINT('Ctrl Pts',(8.67411493903338,-28.3366903556877,56.208496216297));
#83807=CARTESIAN_POINT('Ctrl Pts',(8.67798403358143,-28.3804888083777,56.2645873092476));
#83808=CARTESIAN_POINT('Ctrl Pts',(8.6818473633506,-28.4242220033203,56.3205948289634));
#83809=CARTESIAN_POINT('Ctrl Pts',(8.68571069311978,-28.4709313646131,56.3744173595926));
#83810=CARTESIAN_POINT('Ctrl Pts',(8.68957402288896,-28.5203686578006,56.4257239051378));
#83811=CARTESIAN_POINT('Ctrl Pts',(8.69343282090788,-28.5697479602187,56.4769702672493));
#83812=CARTESIAN_POINT('Ctrl Pts',(8.6972916189268,-28.6218485029957,56.5257061584302));
#83813=CARTESIAN_POINT('Ctrl Pts',(8.70115041694573,-28.6763820702183,56.5716339072635));
#83814=CARTESIAN_POINT('Ctrl Pts',(8.70500678414222,-28.7308812844071,56.6175327242373));
#83815=CARTESIAN_POINT('Ctrl Pts',(8.70886315133872,-28.7878101115706,56.6606265962843));
#83816=CARTESIAN_POINT('Ctrl Pts',(8.71271951853521,-28.84684487025,56.7006559937951));
#83817=CARTESIAN_POINT('Ctrl Pts',(8.71657474643865,-28.9058621881913,56.7406735653536));
#83818=CARTESIAN_POINT('Ctrl Pts',(8.72042997434208,-28.9669838006437,56.7776281872548));
#83819=CARTESIAN_POINT('Ctrl Pts',(8.72428520224552,-29.0298558657819,56.8113028243069));
#83820=CARTESIAN_POINT('Ctrl Pts',(8.7281405807723,-29.0927303873249,56.8449787770235));
#83821=CARTESIAN_POINT('Ctrl Pts',(8.73199595929907,-29.1573550680685,56.8753742630506));
#83822=CARTESIAN_POINT('Ctrl Pts',(8.73585133782585,-29.2233517508641,56.9023183381375));
#83823=CARTESIAN_POINT('Ctrl Pts',(8.73971075184615,-29.2894175135656,56.9292906160687));
#83824=CARTESIAN_POINT('Ctrl Pts',(8.74357016586645,-29.3568576944318,56.9528040874015));
#83825=CARTESIAN_POINT('Ctrl Pts',(8.74742957988676,-29.4252752922519,56.9727364428134));
#83826=CARTESIAN_POINT('Ctrl Pts',(8.7512911790046,-29.4937316262956,56.9926800833945));
#83827=CARTESIAN_POINT('Ctrl Pts',(8.75515277812243,-29.5631660058587,57.0090384604104));
#83828=CARTESIAN_POINT('Ctrl Pts',(8.75901437724027,-29.6331701295281,57.0217401931578));
#83829=CARTESIAN_POINT('Ctrl Pts',(8.76288273257591,-29.7032967317593,57.0344641487383));
#83830=CARTESIAN_POINT('Ctrl Pts',(8.76675108791155,-29.7739945862777,57.0435186252626));
#83831=CARTESIAN_POINT('Ctrl Pts',(8.77061944324719,-29.8448498484024,57.048884084803));
#83832=CARTESIAN_POINT('Ctrl Pts',(8.77291696909007,-29.8869327962474,57.0520707832533));
#83833=CARTESIAN_POINT('Ctrl Pts',(8.77521449493296,-29.9290712407228,57.0539571768661));
#83834=CARTESIAN_POINT('Ctrl Pts',(8.77751202077585,-29.9711789821164,57.0545478605835));
#83835=CARTESIAN_POINT('Ctrl Pts',(8.78138026094705,-30.0420738785901,57.0555423679972));
#83836=CARTESIAN_POINT('Ctrl Pts',(8.78524850111824,-30.1131591787548,57.0528650336868));
#83837=CARTESIAN_POINT('Ctrl Pts',(8.78911674128944,-30.1840229876492,57.046492878687));
#83838=CARTESIAN_POINT('Ctrl Pts',(8.79297960149185,-30.2547882387852,57.0401295861139));
#83839=CARTESIAN_POINT('Ctrl Pts',(8.79684246169427,-30.3253321302883,57.0300817109936));
#83840=CARTESIAN_POINT('Ctrl Pts',(8.80070532189668,-30.3952420799265,57.0163782533928));
#83841=CARTESIAN_POINT('Ctrl Pts',(8.80456410253959,-30.4650781977964,57.0026892679882));
#83842=CARTESIAN_POINT('Ctrl Pts',(8.8084228831825,-30.5342812283326,56.9853524557353));
#83843=CARTESIAN_POINT('Ctrl Pts',(8.81228166382541,-30.602444754302,56.9644484927109));
#83844=CARTESIAN_POINT('Ctrl Pts',(8.81613799809855,-30.6705650663122,56.9435577822727));
#83845=CARTESIAN_POINT('Ctrl Pts',(8.81999433237169,-30.7376467179062,56.919104550155));
#83846=CARTESIAN_POINT('Ctrl Pts',(8.82385066664483,-30.8032961041465,56.8912199585355));
#83847=CARTESIAN_POINT('Ctrl Pts',(8.82770557351924,-30.868921190665,56.8633456882283));
#83848=CARTESIAN_POINT('Ctrl Pts',(8.83156048039366,-30.9331146192322,56.8320427739045));
#83849=CARTESIAN_POINT('Ctrl Pts',(8.83541538726808,-30.9955022105465,56.7974907263452));
#83850=CARTESIAN_POINT('Ctrl Pts',(8.83927123894508,-31.0579050924915,56.7629302103936));
#83851=CARTESIAN_POINT('Ctrl Pts',(8.84312709062208,-31.1185008279476,56.7251192060502));
#83852=CARTESIAN_POINT('Ctrl Pts',(8.84698294229908,-31.176940552369,56.6842827846562));
#83853=CARTESIAN_POINT('Ctrl Pts',(8.84866235106974,-31.2023938617725,56.6664965599784));
#83854=CARTESIAN_POINT('Ctrl Pts',(8.85034175984041,-31.2274385369056,56.6481369675613));
#83855=CARTESIAN_POINT('Ctrl Pts',(8.85202116861107,-31.2520475724682,56.6292251037768));
#83856=CARTESIAN_POINT('',(8.54592528048674,-27.9452503479084,55.0011957129338));
#83857=CARTESIAN_POINT('Ctrl Pts',(8.54592528053768,-27.9452503479089,55.0011957138689));
#83858=CARTESIAN_POINT('Ctrl Pts',(8.54975547188148,-27.9452912658151,55.0715102394494));
#83859=CARTESIAN_POINT('Ctrl Pts',(8.55358566322528,-27.9489412102894,55.1417182661176));
#83860=CARTESIAN_POINT('Ctrl Pts',(8.55741585456908,-27.956169205503,55.21154963003));
#83861=CARTESIAN_POINT('Ctrl Pts',(8.56128493120739,-27.9634705815735,55.2820899436809));
#83862=CARTESIAN_POINT('Ctrl Pts',(8.5651540078457,-27.974442464725,55.3523899847241));
#83863=CARTESIAN_POINT('Ctrl Pts',(8.56902308448401,-27.9890594966833,55.4220377407537));
#83864=CARTESIAN_POINT('Ctrl Pts',(8.57288639619077,-28.0036547492363,55.4915817214946));
#83865=CARTESIAN_POINT('Ctrl Pts',(8.57674970789754,-28.0218842706945,55.5604748748738));
#83866=CARTESIAN_POINT('Ctrl Pts',(8.58061301960431,-28.0436709850475,55.6283107095657));
#83867=CARTESIAN_POINT('Ctrl Pts',(8.58447179942306,-28.0654321423248,55.6960669689011));
#83868=CARTESIAN_POINT('Ctrl Pts',(8.58833057924181,-28.0907420560937,55.7627679129253));
#83869=CARTESIAN_POINT('Ctrl Pts',(8.59218935906055,-28.1194730782315,55.8280193590755));
#83870=CARTESIAN_POINT('Ctrl Pts',(8.59604570798193,-28.1481860008224,55.8932296990791));
#83871=CARTESIAN_POINT('Ctrl Pts',(8.59990205690332,-28.1803155606427,55.9569919093067));
#83872=CARTESIAN_POINT('Ctrl Pts',(8.6037584058247,-28.2156854700809,56.0189304298232));
#83873=CARTESIAN_POINT('Ctrl Pts',(8.60761361540559,-28.2510449296426,56.0808506508897));
#83874=CARTESIAN_POINT('Ctrl Pts',(8.61146882498649,-28.2896425974598,56.1409478302951));
#83875=CARTESIAN_POINT('Ctrl Pts',(8.61532403456738,-28.3312563923001,56.1988712751003));
#83876=CARTESIAN_POINT('Ctrl Pts',(8.61917939475162,-28.3728718127788,56.2567969826786));
#83877=CARTESIAN_POINT('Ctrl Pts',(8.62303475493585,-28.4175033089793,56.3125483938257));
#83878=CARTESIAN_POINT('Ctrl Pts',(8.62689011512009,-28.4648866696248,56.3658054859329));
#83879=CARTESIAN_POINT('Ctrl Pts',(8.6307495108947,-28.512319628706,56.4191183247921));
#83880=CARTESIAN_POINT('Ctrl Pts',(8.6346089066693,-28.5625098788081,56.4699312689458));
#83881=CARTESIAN_POINT('Ctrl Pts',(8.63846830244391,-28.6151548701809,56.5179596598449));
#83882=CARTESIAN_POINT('Ctrl Pts',(8.64232988334319,-28.6678296682582,56.5660152436072));
#83883=CARTESIAN_POINT('Ctrl Pts',(8.64619146424246,-28.7229615987137,56.6112828272418));
#83884=CARTESIAN_POINT('Ctrl Pts',(8.65005304514174,-28.7802155359329,56.6535184981489));
#83885=CARTESIAN_POINT('Ctrl Pts',(8.65392138250044,-28.8375696481618,56.6958280671833));
#83886=CARTESIAN_POINT('Ctrl Pts',(8.65778971985915,-28.8970527743099,56.7350948645475));
#83887=CARTESIAN_POINT('Ctrl Pts',(8.66165805721786,-28.9583019787723,56.7711190798674));
#83888=CARTESIAN_POINT('Ctrl Pts',(8.66395574661445,-28.9946823754629,56.7925165046227));
#83889=CARTESIAN_POINT('Ctrl Pts',(8.66625343601104,-29.031685386149,56.8127708165083));
#83890=CARTESIAN_POINT('Ctrl Pts',(8.66855112540763,-29.0692315807068,56.8318481684207));
#83891=CARTESIAN_POINT('Ctrl Pts',(8.67242018909353,-29.1324553646189,56.8639723927031));
#83892=CARTESIAN_POINT('Ctrl Pts',(8.67628925277942,-29.1974680298235,56.8928825728788));
#83893=CARTESIAN_POINT('Ctrl Pts',(8.68015831646531,-29.2639096761121,56.9183765526034));
#83894=CARTESIAN_POINT('Ctrl Pts',(8.68402161519355,-29.3302523234416,56.9438325459506));
#83895=CARTESIAN_POINT('Ctrl Pts',(8.68788491392178,-29.3980192755995,56.9658822701096));
#83896=CARTESIAN_POINT('Ctrl Pts',(8.69174821265001,-29.4668272208466,56.9843700133972));
#83897=CARTESIAN_POINT('Ctrl Pts',(8.69560697951371,-29.5355544505424,57.0028360695324));
#83898=CARTESIAN_POINT('Ctrl Pts',(8.69946574637741,-29.605319780853,57.0177483190721));
#83899=CARTESIAN_POINT('Ctrl Pts',(8.70332451324111,-29.6757228125058,57.0290002139406));
#83900=CARTESIAN_POINT('Ctrl Pts',(8.70718084922889,-29.7460814929344,57.0402450205445));
#83901=CARTESIAN_POINT('Ctrl Pts',(8.71103718521667,-29.8170765991176,57.0478339708275));
#83902=CARTESIAN_POINT('Ctrl Pts',(8.71489352120445,-29.8882969970362,57.0517114810881));
#83903=CARTESIAN_POINT('Ctrl Pts',(8.71874871789197,-29.9594963538895,57.0555878457929));
#83904=CARTESIAN_POINT('Ctrl Pts',(8.7226039145795,-30.0309203855335,57.0557549209219));
#83905=CARTESIAN_POINT('Ctrl Pts',(8.72645911126702,-30.1021540129104,57.0522090829509));
#83906=CARTESIAN_POINT('Ctrl Pts',(8.73031445861694,-30.1733904241217,57.0486631064074));
#83907=CARTESIAN_POINT('Ctrl Pts',(8.73416980596685,-30.2444359312142,57.0414039550345));
#83908=CARTESIAN_POINT('Ctrl Pts',(8.73802515331677,-30.3148783727667,57.0304800350813));
#83909=CARTESIAN_POINT('Ctrl Pts',(8.74188453643489,-30.3853945532952,57.0195446799954));
#83910=CARTESIAN_POINT('Ctrl Pts',(8.74574391955302,-30.4553059270577,57.0049369728678));
#83911=CARTESIAN_POINT('Ctrl Pts',(8.74960330267114,-30.5242092501069,56.9867567099679));
#83912=CARTESIAN_POINT('Ctrl Pts',(8.75346487099512,-30.5931515866305,56.9685661532941));
#83913=CARTESIAN_POINT('Ctrl Pts',(8.75732643931909,-30.6610842733858,56.9467991623766));
#83914=CARTESIAN_POINT('Ctrl Pts',(8.76118800764307,-30.727620630972,56.9216050010041));
#83915=CARTESIAN_POINT('Ctrl Pts',(8.76505633269088,-30.7942734095965,56.8963667565087));
#83916=CARTESIAN_POINT('Ctrl Pts',(8.7689246577387,-30.8595245362443,56.8676895646065));
#83917=CARTESIAN_POINT('Ctrl Pts',(8.77279298278651,-30.9230093006504,56.8357699729032));
#83918=CARTESIAN_POINT('Ctrl Pts',(8.77509078727307,-30.9607195692233,56.8168095752844));
#83919=CARTESIAN_POINT('Ctrl Pts',(8.77738859175963,-30.9978070811695,56.7967059942276));
#83920=CARTESIAN_POINT('Ctrl Pts',(8.77968639624619,-31.0342003092193,56.7755076127437));
#83921=CARTESIAN_POINT('Ctrl Pts',(8.78355540384214,-31.0954786627907,56.7398141064151));
#83922=CARTESIAN_POINT('Ctrl Pts',(8.78742441143808,-31.155027029067,56.7008746007601));
#83923=CARTESIAN_POINT('Ctrl Pts',(8.79129341903402,-31.2124803894351,56.6588818124675));
#83924=CARTESIAN_POINT('Ctrl Pts',(8.79218924787603,-31.2257831230203,56.6491588150383));
#83925=CARTESIAN_POINT('Ctrl Pts',(8.79308507671804,-31.2389736349695,56.6392723290926));
#83926=CARTESIAN_POINT('Ctrl Pts',(8.79398090556005,-31.2520475724682,56.6292251037768));
#83927=CARTESIAN_POINT('Ctrl Pts',(8.09385946080458,-31.2520475724682,56.6292251037768));
#83928=CARTESIAN_POINT('Ctrl Pts',(8.09772772586411,-31.3085644633221,56.5857922866461));
#83929=CARTESIAN_POINT('Ctrl Pts',(8.10159599092365,-31.3627460064793,56.5394711533693));
#83930=CARTESIAN_POINT('Ctrl Pts',(8.10546425598318,-31.4142995210562,56.4905550735347));
#83931=CARTESIAN_POINT('Ctrl Pts',(8.10793442772706,-31.4472202317744,56.4593185588778));
#83932=CARTESIAN_POINT('Ctrl Pts',(8.11040459947095,-31.4790700476866,56.4270246328561));
#83933=CARTESIAN_POINT('Ctrl Pts',(8.11287477121484,-31.509781418586,56.3937566611832));
#83934=CARTESIAN_POINT('Ctrl Pts',(8.11674384460076,-31.5578851782077,56.3416484528685));
#83935=CARTESIAN_POINT('Ctrl Pts',(8.12061291798669,-31.6033823195331,56.286944893517));
#83936=CARTESIAN_POINT('Ctrl Pts',(8.12448199137262,-31.6459804498429,56.2299373647609));
#83937=CARTESIAN_POINT('Ctrl Pts',(8.12834529980472,-31.6885151085589,56.1730147777307));
#83938=CARTESIAN_POINT('Ctrl Pts',(8.13220860823683,-31.7281590420354,56.1137954215491));
#83939=CARTESIAN_POINT('Ctrl Pts',(8.13607191666893,-31.7646581875197,56.0526058349257));
#83940=CARTESIAN_POINT('Ctrl Pts',(8.13993069319594,-31.8011145171983,55.9914880275569));
#83941=CARTESIAN_POINT('Ctrl Pts',(8.14378946972296,-31.8344331389063,55.9284049957583));
#83942=CARTESIAN_POINT('Ctrl Pts',(8.14764824624997,-31.8644026557454,55.8637130887913));
#83943=CARTESIAN_POINT('Ctrl Pts',(8.1515045918709,-31.8943532927452,55.7990619356616));
#83944=CARTESIAN_POINT('Ctrl Pts',(8.15536093749182,-31.9209588070259,55.7328043579523));
#83945=CARTESIAN_POINT('Ctrl Pts',(8.15921728311275,-31.9440539276629,55.6653208916294));
#83946=CARTESIAN_POINT('Ctrl Pts',(8.16307248938938,-31.9671422249244,55.5978573630688));
#83947=CARTESIAN_POINT('Ctrl Pts',(8.16692769566601,-31.9867220303301,55.5291691242961));
#83948=CARTESIAN_POINT('Ctrl Pts',(8.17078290194264,-32.0026770032117,55.4596546348149));
#83949=CARTESIAN_POINT('Ctrl Pts',(8.17463825882374,-32.0186325993778,55.3901374297353));
#83950=CARTESIAN_POINT('Ctrl Pts',(8.17849361570483,-32.0309629753566,55.3197943838317));
#83951=CARTESIAN_POINT('Ctrl Pts',(8.18234897258592,-32.0396026535511,55.2490352949432));
#83952=CARTESIAN_POINT('Ctrl Pts',(8.18620836508193,-32.0482513753737,55.1782021386094));
#83953=CARTESIAN_POINT('Ctrl Pts',(8.19006775757793,-32.0532016284849,55.1069525531374));
#83954=CARTESIAN_POINT('Ctrl Pts',(8.19392715007394,-32.0544398139621,55.0357017269505));
#83955=CARTESIAN_POINT('Ctrl Pts',(8.19778872770351,-32.0556787004825,54.9644105595513));
#83956=CARTESIAN_POINT('Ctrl Pts',(8.20165030533308,-32.0532013523708,54.8931186357618));
#83957=CARTESIAN_POINT('Ctrl Pts',(8.20551188296266,-32.0470462784205,54.8222386529506));
#83958=CARTESIAN_POINT('Ctrl Pts',(8.20938021710133,-32.040880435086,54.7512346531456));
#83959=CARTESIAN_POINT('Ctrl Pts',(8.21324855124,-32.0310240857909,54.680644514615));
#83960=CARTESIAN_POINT('Ctrl Pts',(8.21711688537867,-32.0175672150315,54.6108726489568));
#83961=CARTESIAN_POINT('Ctrl Pts',(8.21941460427025,-32.0095740828313,54.5694294519433));
#83962=CARTESIAN_POINT('Ctrl Pts',(8.22171232316183,-32.0003116078501,54.5282747183277));
#83963=CARTESIAN_POINT('Ctrl Pts',(8.2240100420534,-31.9898069000022,54.4874904262323));
#83964=CARTESIAN_POINT('Ctrl Pts',(8.2278791158888,-31.9721182739341,54.4188147331265));
#83965=CARTESIAN_POINT('Ctrl Pts',(8.23174818972419,-31.9508354434352,54.3509213488541));
#83966=CARTESIAN_POINT('Ctrl Pts',(8.23561726355958,-31.9260446276857,54.2842139602764));
#83967=CARTESIAN_POINT('Ctrl Pts',(8.239480572445,-31.9012907504436,54.2176059662243));
#83968=CARTESIAN_POINT('Ctrl Pts',(8.24334388133041,-31.8730394310988,54.1521809117855));
#83969=CARTESIAN_POINT('Ctrl Pts',(8.24720719021583,-31.8414272146186,54.0883293490729));
#83970=CARTESIAN_POINT('Ctrl Pts',(8.25106596719964,-31.8098520812346,54.0245526882147));
#83971=CARTESIAN_POINT('Ctrl Pts',(8.25492474418344,-31.774924096428,53.9623462859312));
#83972=CARTESIAN_POINT('Ctrl Pts',(8.25878352116725,-31.7368279907332,53.9020810170574));
#83973=CARTESIAN_POINT('Ctrl Pts',(8.26263986724686,-31.6987558843479,53.841853713346));
#83974=CARTESIAN_POINT('Ctrl Pts',(8.26649621332647,-31.657519875693,53.7835655265795));
#83975=CARTESIAN_POINT('Ctrl Pts',(8.27035255940609,-31.6133500326752,53.7275616971473));
#83976=CARTESIAN_POINT('Ctrl Pts',(8.27420776614261,-31.5691932394731,53.6715744138379));
#83977=CARTESIAN_POINT('Ctrl Pts',(8.27806297287914,-31.5221046333941,53.6178705292117));
#83978=CARTESIAN_POINT('Ctrl Pts',(8.28191817961566,-31.4723558787003,53.5667638962973));
#83979=CARTESIAN_POINT('Ctrl Pts',(8.28577353695716,-31.4226051805542,53.5156552668848));
#83980=CARTESIAN_POINT('Ctrl Pts',(8.28962889429866,-31.3701944678999,53.4671444371841));
#83981=CARTESIAN_POINT('Ctrl Pts',(8.29348425164016,-31.3154325171293,53.4215086774458));
#83982=CARTESIAN_POINT('Ctrl Pts',(8.29734364459416,-31.2606132440424,53.3758251482724));
#83983=CARTESIAN_POINT('Ctrl Pts',(8.30120303754816,-31.2034381937461,53.3330230083174));
#83984=CARTESIAN_POINT('Ctrl Pts',(8.30506243050216,-31.1442488086253,53.2933388659551));
#83985=CARTESIAN_POINT('Ctrl Pts',(8.30892400858906,-31.0850259113242,53.2536322550009));
#83986=CARTESIAN_POINT('Ctrl Pts',(8.31278558667596,-31.0237868260713,53.2170474051958));
#83987=CARTESIAN_POINT('Ctrl Pts',(8.31664716476286,-30.960899163762,53.1837757958937));
#83988=CARTESIAN_POINT('Ctrl Pts',(8.32051549935281,-30.8979014685404,53.1504459721195));
#83989=CARTESIAN_POINT('Ctrl Pts',(8.32438383394277,-30.8332498781125,53.1204411674763));
#83990=CARTESIAN_POINT('Ctrl Pts',(8.32825216853272,-30.76733296071,53.0939051204339));
#83991=CARTESIAN_POINT('Ctrl Pts',(8.33054988331913,-30.7281796061413,53.0781432295622));
#83992=CARTESIAN_POINT('Ctrl Pts',(8.33284759810555,-30.6885801579557,53.0636042166874));
#83993=CARTESIAN_POINT('Ctrl Pts',(8.33514531289196,-30.648618192526,53.0503097674696));
#83994=CARTESIAN_POINT('Ctrl Pts',(8.33901438504392,-30.5813271046607,53.027923532438));
#83995=CARTESIAN_POINT('Ctrl Pts',(8.34288345719589,-30.5127439015,53.0089812381448));
#83996=CARTESIAN_POINT('Ctrl Pts',(8.34675252934785,-30.4432544997986,52.99362939343));
#83997=CARTESIAN_POINT('Ctrl Pts',(8.3506158365476,-30.3738686379293,52.9783004231015));
#83998=CARTESIAN_POINT('Ctrl Pts',(8.35447914374734,-30.3035797281994,52.9665513870857));
#83999=CARTESIAN_POINT('Ctrl Pts',(8.35834245094709,-30.2327899472138,52.9584793895294));
#84000=CARTESIAN_POINT('Ctrl Pts',(8.36220122624996,-30.1620832069936,52.9504168609225));
#84001=CARTESIAN_POINT('Ctrl Pts',(8.36606000155283,-30.0908772429123,52.9460228576887));
#84002=CARTESIAN_POINT('Ctrl Pts',(8.36991877685571,-30.0195838339789,52.9453433289363));
#84003=CARTESIAN_POINT('Ctrl Pts',(8.37377512125821,-29.9483353375269,52.9446642282644));
#84004=CARTESIAN_POINT('Ctrl Pts',(8.37763146566071,-29.8769999901311,52.9476949641797));
#84005=CARTESIAN_POINT('Ctrl Pts',(8.38148781006321,-29.8059926235627,52.9544294926872));
#84006=CARTESIAN_POINT('Ctrl Pts',(8.38534301512887,-29.7350062357504,52.9611620315134));
#84007=CARTESIAN_POINT('Ctrl Pts',(8.38919822019453,-29.6643481197445,52.9715961446681));
#84008=CARTESIAN_POINT('Ctrl Pts',(8.3930534252602,-29.5944292978043,52.9856738178685));
#84009=CARTESIAN_POINT('Ctrl Pts',(8.39690878093952,-29.5245077443027,52.9997520410499));
#84010=CARTESIAN_POINT('Ctrl Pts',(8.40076413661884,-29.4553260180037,53.0174740088399));
#84011=CARTESIAN_POINT('Ctrl Pts',(8.40461949229815,-29.3872845346697,53.0387306862531));
#84012=CARTESIAN_POINT('Ctrl Pts',(8.40847888361457,-29.3191718281447,53.0600096143335));
#84013=CARTESIAN_POINT('Ctrl Pts',(8.41233827493098,-29.2522022118387,53.0848304929071));
#84014=CARTESIAN_POINT('Ctrl Pts',(8.41619766624739,-29.1867596565612,53.1130347893235));
#84015=CARTESIAN_POINT('Ctrl Pts',(8.42005924270809,-29.1212800484394,53.1412550546977));
#84016=CARTESIAN_POINT('Ctrl Pts',(8.42392081916879,-29.0573296582121,53.172862336044));
#84017=CARTESIAN_POINT('Ctrl Pts',(8.42778239562949,-28.9952687346829,53.2076516390516));
#84018=CARTESIAN_POINT('Ctrl Pts',(8.43165072862884,-28.9330992241472,53.242501812347));
#84019=CARTESIAN_POINT('Ctrl Pts',(8.43551906162818,-28.8728261917055,53.2805448636724));
#84020=CARTESIAN_POINT('Ctrl Pts',(8.43938739462753,-28.8147811434618,53.3215322986109));
#84021=CARTESIAN_POINT('Ctrl Pts',(8.44168512432852,-28.7803032866259,53.3458781981604));
#84022=CARTESIAN_POINT('Ctrl Pts',(8.44398285402952,-28.7466108877596,53.3712621390403));
#84023=CARTESIAN_POINT('Ctrl Pts',(8.44628058373051,-28.713767495987,53.39762566542));
#84024=CARTESIAN_POINT('Ctrl Pts',(8.45010049356798,-28.6591662975635,53.4414542731647));
#84025=CARTESIAN_POINT('Ctrl Pts',(8.45392040340544,-28.6066877347304,53.4881735901039));
#84026=CARTESIAN_POINT('Ctrl Pts',(8.4577403132429,-28.5566598033146,53.5375477309901));
#84027=CARTESIAN_POINT('Ctrl Pts',(8.46155371487502,-28.5067171074317,53.5868377502448));
#84028=CARTESIAN_POINT('Ctrl Pts',(8.46536711650714,-28.4592171051878,53.6387732652591));
#84029=CARTESIAN_POINT('Ctrl Pts',(8.46918051813926,-28.4144553668289,53.6930777457238));
#84030=CARTESIAN_POINT('Ctrl Pts',(8.47299028959279,-28.3697362395348,53.7473305308832));
#84031=CARTESIAN_POINT('Ctrl Pts',(8.47680006104632,-28.3277505256955,53.803947428803));
#84032=CARTESIAN_POINT('Ctrl Pts',(8.48060983249986,-28.2887564798592,53.8626156422404));
#84033=CARTESIAN_POINT('Ctrl Pts',(8.48441732945581,-28.2497857141235,53.9212488297686));
#84034=CARTESIAN_POINT('Ctrl Pts',(8.48822482641176,-28.2138033505418,53.98193048944));
#84035=CARTESIAN_POINT('Ctrl Pts',(8.49203232336772,-28.1810257351875,54.0443169006151));
#84036=CARTESIAN_POINT('Ctrl Pts',(8.49583889832167,-28.1482560570759,54.1066882046485));
#84037=CARTESIAN_POINT('Ctrl Pts',(8.49964547327562,-28.1186898182962,54.1707629985846));
#84038=CARTESIAN_POINT('Ctrl Pts',(8.50345204822957,-28.0924976487741,54.2361725701655));
#84039=CARTESIAN_POINT('Ctrl Pts',(8.50726133448231,-28.0662868234265,54.3016287308442));
#84040=CARTESIAN_POINT('Ctrl Pts',(8.51107062073505,-28.0434550559848,54.3684211046283));
#84041=CARTESIAN_POINT('Ctrl Pts',(8.51487990698779,-28.0241245176057,54.4361616893354));
#84042=CARTESIAN_POINT('Ctrl Pts',(8.51869055154789,-28.0047870863836,54.503926428839));
#84043=CARTESIAN_POINT('Ctrl Pts',(8.52250119610798,-27.988953484362,54.5726395657635));
#84044=CARTESIAN_POINT('Ctrl Pts',(8.52631184066808,-27.9766950474164,54.6419013664494));
#84045=CARTESIAN_POINT('Ctrl Pts',(8.53012846727584,-27.9644173668618,54.7112718960882));
#84046=CARTESIAN_POINT('Ctrl Pts',(8.5339450938836,-27.9557261209346,54.7811923133063));
#84047=CARTESIAN_POINT('Ctrl Pts',(8.53776172049136,-27.9506408049551,54.8512570936646));
#84048=CARTESIAN_POINT('Ctrl Pts',(8.54048290715649,-27.9470150654072,54.9012120317815));
#84049=CARTESIAN_POINT('Ctrl Pts',(8.54320409382162,-27.9452212775139,54.95124025844));
#84050=CARTESIAN_POINT('Ctrl Pts',(8.54592528048675,-27.9452503479084,55.0011957129338));
#84051=CARTESIAN_POINT('Origin',(-1.54592528053767,-30.,55.));
#84052=CARTESIAN_POINT('',(7.39391310379067,-31.2520475724682,56.6292251037768));
#84053=CARTESIAN_POINT('',(7.45211324645396,-31.2520475724682,56.6292251037768));
#84054=CARTESIAN_POINT('',(-1.54592528053767,-31.2520475724682,56.6292251037768));
#84055=CARTESIAN_POINT('',(7.9040747195078,-27.9452505543666,54.9984906394943));
#84056=CARTESIAN_POINT('Ctrl Pts',(7.45211324645396,-31.2520475724682,56.6292251037768));
#84057=CARTESIAN_POINT('Ctrl Pts',(7.45597808729066,-31.3083605687531,56.5859489781306));
#84058=CARTESIAN_POINT('Ctrl Pts',(7.45984292812737,-31.362520824477,56.5396778615538));
#84059=CARTESIAN_POINT('Ctrl Pts',(7.46370776896407,-31.4141940637171,56.4906551286757));
#84060=CARTESIAN_POINT('Ctrl Pts',(7.4675674980657,-31.4657989586397,56.4416972344893));
#84061=CARTESIAN_POINT('Ctrl Pts',(7.47142722716733,-31.5149230210412,56.3899952859469));
#84062=CARTESIAN_POINT('Ctrl Pts',(7.47528695626896,-31.561264698516,56.3358331122066));
#84063=CARTESIAN_POINT('Ctrl Pts',(7.47914387729268,-31.6075726609198,56.2817103432016));
#84064=CARTESIAN_POINT('Ctrl Pts',(7.4830007983164,-31.6511019392643,56.2251312676947));
#84065=CARTESIAN_POINT('Ctrl Pts',(7.48685771934013,-31.6915885447453,56.1664157739788));
#84066=CARTESIAN_POINT('Ctrl Pts',(7.49071312456391,-31.7320592386756,56.1077233559083));
#84067=CARTESIAN_POINT('Ctrl Pts',(7.49456852978768,-31.7694893575694,56.0468965856172));
#84068=CARTESIAN_POINT('Ctrl Pts',(7.49842393501146,-31.8036569179452,55.9842861803603));
#84069=CARTESIAN_POINT('Ctrl Pts',(7.5022791147205,-31.8378224797533,55.9216794373824));
#84070=CARTESIAN_POINT('Ctrl Pts',(7.50613429442953,-31.8687256306425,55.8572896937603));
#84071=CARTESIAN_POINT('Ctrl Pts',(7.50998947413857,-31.8961900876794,55.7914927124658));
#84072=CARTESIAN_POINT('Ctrl Pts',(7.51384844789869,-31.9236815736905,55.7256309774823));
#84073=CARTESIAN_POINT('Ctrl Pts',(7.51770742165881,-31.947727418207,55.658359687754));
#84074=CARTESIAN_POINT('Ctrl Pts',(7.52156639541893,-31.9681996651815,55.5900742669186));
#84075=CARTESIAN_POINT('Ctrl Pts',(7.52542721647184,-31.9886817122315,55.5217561578159));
#84076=CARTESIAN_POINT('Ctrl Pts',(7.52928803752475,-32.0055866384878,55.4524234231595));
#84077=CARTESIAN_POINT('Ctrl Pts',(7.53314885857766,-32.018837251576,55.3824836129156));
#84078=CARTESIAN_POINT('Ctrl Pts',(7.53701679393931,-32.032112281479,55.3124149250582));
#84079=CARTESIAN_POINT('Ctrl Pts',(7.54088472930095,-32.0417194785206,55.2417374091514));
#84080=CARTESIAN_POINT('Ctrl Pts',(7.5447526646626,-32.0476334237151,55.1708652234503));
#84081=CARTESIAN_POINT('Ctrl Pts',(7.54817645695896,-32.0528682888576,55.1081310718315));
#84082=CARTESIAN_POINT('Ctrl Pts',(7.55160024925533,-32.0552101424747,55.0452446703328));
#84083=CARTESIAN_POINT('Ctrl Pts',(7.55502404155169,-32.054675403713,54.9824914912987));
#84084=CARTESIAN_POINT('Ctrl Pts',(7.55889311489863,-32.0540711195416,54.9115769522672));
#84085=CARTESIAN_POINT('Ctrl Pts',(7.56276218824557,-32.049790052573,54.840554831208));
#84086=CARTESIAN_POINT('Ctrl Pts',(7.5666312615925,-32.0418185215203,54.7698376927544));
#84087=CARTESIAN_POINT('Ctrl Pts',(7.57049456998682,-32.0338588681175,54.6992259234463));
#84088=CARTESIAN_POINT('Ctrl Pts',(7.57435787838114,-32.0222197196123,54.6289187135154));
#84089=CARTESIAN_POINT('Ctrl Pts',(7.57822118677546,-32.0069394027378,54.5593280174115));
#84090=CARTESIAN_POINT('Ctrl Pts',(7.58207996326664,-31.9916770106337,54.4898189555605));
#84091=CARTESIAN_POINT('Ctrl Pts',(7.58593873975781,-31.9727820381229,54.4210252101677));
#84092=CARTESIAN_POINT('Ctrl Pts',(7.58979751624899,-31.9503443207461,54.3533512599304));
#84093=CARTESIAN_POINT('Ctrl Pts',(7.59365386183529,-31.9279207384083,54.2857199421016));
#84094=CARTESIAN_POINT('Ctrl Pts',(7.5975102074216,-31.9019589916094,54.2192074798691));
#84095=CARTESIAN_POINT('Ctrl Pts',(7.6013665530079,-31.8725990972371,54.1542044079526));
#84096=CARTESIAN_POINT('Ctrl Pts',(7.60522175925117,-31.843247877137,54.0892205409531));
#84097=CARTESIAN_POINT('Ctrl Pts',(7.60907696549444,-31.8105007024769,54.0257456214283));
#84098=CARTESIAN_POINT('Ctrl Pts',(7.61293217173771,-31.7745455283029,53.9641497548004));
#84099=CARTESIAN_POINT('Ctrl Pts',(7.61678752858674,-31.7385889495202,53.902551481896));
#84100=CARTESIAN_POINT('Ctrl Pts',(7.62064288543577,-31.6994243692117,53.8428328260564));
#84101=CARTESIAN_POINT('Ctrl Pts',(7.6244982422848,-31.6572845816706,53.7853373398935));
#84102=CARTESIAN_POINT('Ctrl Pts',(7.62835763475092,-31.615100684063,53.7277816699978));
#84103=CARTESIAN_POINT('Ctrl Pts',(7.63221702721703,-31.5699356501099,53.6724542078444));
#84104=CARTESIAN_POINT('Ctrl Pts',(7.63607641968315,-31.522063782187,53.6196669222776));
#84105=CARTESIAN_POINT('Ctrl Pts',(7.63993799728402,-31.4741648098732,53.5668497492782));
#84106=CARTESIAN_POINT('Ctrl Pts',(7.64379957488489,-31.4235562975153,53.5165759584269));
#84107=CARTESIAN_POINT('Ctrl Pts',(7.64766115248575,-31.3705488271908,53.4691200325349));
#84108=CARTESIAN_POINT('Ctrl Pts',(7.65152948659789,-31.3174486109455,53.4215810741284));
#84109=CARTESIAN_POINT('Ctrl Pts',(7.65539782071002,-31.2619414349407,53.3768701291034));
#84110=CARTESIAN_POINT('Ctrl Pts',(7.65926615482215,-31.2043697334878,53.3352204027084));
#84111=CARTESIAN_POINT('Ctrl Pts',(7.66156387401152,-31.1701732035712,53.3104812326171));
#84112=CARTESIAN_POINT('Ctrl Pts',(7.66386159320088,-31.135248827559,53.286821267397));
#84113=CARTESIAN_POINT('Ctrl Pts',(7.66615931239025,-31.0996724855831,53.2642817086429));
#84114=CARTESIAN_POINT('Ctrl Pts',(7.6700283858083,-31.0397663492338,53.2263278942544));
#84115=CARTESIAN_POINT('Ctrl Pts',(7.67389745922635,-30.9777756735512,53.1914047567586));
#84116=CARTESIAN_POINT('Ctrl Pts',(7.67776653264439,-30.9140396518326,53.1597475506394));
#84117=CARTESIAN_POINT('Ctrl Pts',(7.68162984111029,-30.8503985973261,53.1281375140253));
#84118=CARTESIAN_POINT('Ctrl Pts',(7.68549314957619,-30.7850177903921,53.0997839637252));
#84119=CARTESIAN_POINT('Ctrl Pts',(7.68935645804209,-30.7182641189677,53.0748781290777));
#84120=CARTESIAN_POINT('Ctrl Pts',(7.69321523460519,-30.6515887537808,53.0500015105341));
#84121=CARTESIAN_POINT('Ctrl Pts',(7.69707401116829,-30.5835441759438,53.0285647431122));
#84122=CARTESIAN_POINT('Ctrl Pts',(7.70093278773139,-30.5145189292144,53.0107117267776));
#84123=CARTESIAN_POINT('Ctrl Pts',(7.7047891333898,-30.4455371661628,52.9928699572672));
#84124=CARTESIAN_POINT('Ctrl Pts',(7.7086454790482,-30.3755764291012,52.9786075810634));
#84125=CARTESIAN_POINT('Ctrl Pts',(7.7125018247066,-30.3050407634035,52.9680187758835));
#84126=CARTESIAN_POINT('Ctrl Pts',(7.71635703102204,-30.2345259372057,52.9574330991265));
#84127=CARTESIAN_POINT('Ctrl Pts',(7.72021223733748,-30.1634369997333,52.950518910766));
#84128=CARTESIAN_POINT('Ctrl Pts',(7.72406744365292,-30.0921868327526,52.947319033467));
#84129=CARTESIAN_POINT('Ctrl Pts',(7.72792280057407,-30.0209338823456,52.9441190311629));
#84130=CARTESIAN_POINT('Ctrl Pts',(7.73177815749522,-29.949520175321,52.944633647595));
#84131=CARTESIAN_POINT('Ctrl Pts',(7.73563351441637,-29.8783606044694,52.9488536327324));
#84132=CARTESIAN_POINT('Ctrl Pts',(7.73949290695406,-29.8071265469369,52.953078035163));
#84133=CARTESIAN_POINT('Ctrl Pts',(7.74335229949174,-29.7361476425378,52.9610155200702));
#84134=CARTESIAN_POINT('Ctrl Pts',(7.74721169202943,-29.6658347616567,52.9726048347737));
#84135=CARTESIAN_POINT('Ctrl Pts',(7.75107326970165,-29.5954820705973,52.9842007111865));
#84136=CARTESIAN_POINT('Ctrl Pts',(7.75493484737387,-29.5257966285102,52.9994524294679));
#84137=CARTESIAN_POINT('Ctrl Pts',(7.7587964250461,-29.4571774889379,53.018247925702));
#84138=CARTESIAN_POINT('Ctrl Pts',(7.76266475922848,-29.3884382880972,53.0370763079667));
#84139=CARTESIAN_POINT('Ctrl Pts',(7.76653309341087,-29.3207695760174,53.0594606949769));
#84140=CARTESIAN_POINT('Ctrl Pts',(7.77040142759325,-29.2545530026706,53.0852398749001));
#84141=CARTESIAN_POINT('Ctrl Pts',(7.77269914613844,-29.2152215898702,53.1005522282275));
#84142=CARTESIAN_POINT('Ctrl Pts',(7.77499686468362,-29.1764021062297,53.1170613980521));
#84143=CARTESIAN_POINT('Ctrl Pts',(7.77729458322881,-29.1381703215976,53.1347259804724));
#84144=CARTESIAN_POINT('Ctrl Pts',(7.78116365643188,-29.0737927355196,53.1644709475523));
#84145=CARTESIAN_POINT('Ctrl Pts',(7.78503272963494,-29.010830773603,53.1976109569));
#84146=CARTESIAN_POINT('Ctrl Pts',(7.78890180283801,-28.9496660496235,53.233988631071));
#84147=CARTESIAN_POINT('Ctrl Pts',(7.79276511108878,-28.8885924616079,53.2703121021951));
#84148=CARTESIAN_POINT('Ctrl Pts',(7.79662841933955,-28.8293112100936,53.3098634160455));
#84149=CARTESIAN_POINT('Ctrl Pts',(7.80049172759033,-28.772181941995,53.3524380500458));
#84150=CARTESIAN_POINT('Ctrl Pts',(7.80435050393912,-28.7151196900976,53.3949627413402));
#84151=CARTESIAN_POINT('Ctrl Pts',(7.80820928028792,-28.6602047949092,53.4405034192765));
#84152=CARTESIAN_POINT('Ctrl Pts',(7.81206805663672,-28.6077688852181,53.4888116975264));
#84153=CARTESIAN_POINT('Ctrl Pts',(7.81592440208143,-28.5553660084511,53.5370895431262));
#84154=CARTESIAN_POINT('Ctrl Pts',(7.81978074752615,-28.5054393752643,53.5881312015924));
#84155=CARTESIAN_POINT('Ctrl Pts',(7.82363709297087,-28.4582872481402,53.6416482954504));
#84156=CARTESIAN_POINT('Ctrl Pts',(7.82749229907355,-28.4111490519259,53.6951495778943));
#84157=CARTESIAN_POINT('Ctrl Pts',(7.83134750517623,-28.3667840553773,53.751124479488));
#84158=CARTESIAN_POINT('Ctrl Pts',(7.83520271127891,-28.3254521679029,53.8092493457827));
#84159=CARTESIAN_POINT('Ctrl Pts',(7.83905806798854,-28.2841186657627,53.8673764827754));
#84160=CARTESIAN_POINT('Ctrl Pts',(7.84291342469817,-28.2458187876686,53.9276533540459));
#84161=CARTESIAN_POINT('Ctrl Pts',(7.8467687814078,-28.2107697851967,53.9897263732359));
#84162=CARTESIAN_POINT('Ctrl Pts',(7.85062817373729,-28.1756840949522,54.0518643677649));
#84163=CARTESIAN_POINT('Ctrl Pts',(7.85448756606678,-28.1438563125732,54.1158018394962));
#84164=CARTESIAN_POINT('Ctrl Pts',(7.85834695839627,-28.1154578183361,54.1811603771009));
#84165=CARTESIAN_POINT('Ctrl Pts',(7.86220853586187,-28.087043245253,54.2465559198318));
#84166=CARTESIAN_POINT('Ctrl Pts',(7.86607011332747,-28.0620619956734,54.3133736748834));
#84167=CARTESIAN_POINT('Ctrl Pts',(7.86993169079306,-28.0406363521104,54.3812176005826));
#84168=CARTESIAN_POINT('Ctrl Pts',(7.87380002477352,-28.0191732205828,54.4491802312659));
#84169=CARTESIAN_POINT('Ctrl Pts',(7.87766835875397,-28.0012782378103,54.5181721469249));
#84170=CARTESIAN_POINT('Ctrl Pts',(7.88153669273442,-27.9870229559283,54.5877852713206));
#84171=CARTESIAN_POINT('Ctrl Pts',(7.88383441317874,-27.978555576228,54.6291342085956));
#84172=CARTESIAN_POINT('Ctrl Pts',(7.88613213362306,-27.9713713483028,54.6707021625493));
#84173=CARTESIAN_POINT('Ctrl Pts',(7.88842985406737,-27.9654765817855,54.7124030194235));
#84174=CARTESIAN_POINT('Ctrl Pts',(7.89364480919903,-27.9520976944732,54.8070481700501));
#84175=CARTESIAN_POINT('Ctrl Pts',(7.89885976433068,-27.9453209576453,54.9026480509693));
#84176=CARTESIAN_POINT('Ctrl Pts',(7.90407471946233,-27.9452505543672,54.9984906386586));
#84177=CARTESIAN_POINT('Ctrl Pts',(7.9040747195078,-27.9452505543666,54.9984906394943));
#84178=CARTESIAN_POINT('Ctrl Pts',(7.90805348639939,-27.9451968399875,55.0716140518884));
#84179=CARTESIAN_POINT('Ctrl Pts',(7.91203225329098,-27.9490515818689,55.1448858516351));
#84180=CARTESIAN_POINT('Ctrl Pts',(7.91601102018257,-27.9568307713825,55.2178464269405));
#84181=CARTESIAN_POINT('Ctrl Pts',(7.91981486835398,-27.9642679640135,55.2875994329654));
#84182=CARTESIAN_POINT('Ctrl Pts',(7.92361871652539,-27.9752917462574,55.3570674381771));
#84183=CARTESIAN_POINT('Ctrl Pts',(7.9274225646968,-27.989862959598,55.4258481434781));
#84184=CARTESIAN_POINT('Ctrl Pts',(7.93122379837303,-28.004424157721,55.4945815738054));
#84185=CARTESIAN_POINT('Ctrl Pts',(7.93502503204926,-28.022527850686,55.5626281516843));
#84186=CARTESIAN_POINT('Ctrl Pts',(7.93882626572548,-28.0440833851904,55.6295933278012));
#84187=CARTESIAN_POINT('Ctrl Pts',(7.94262624479675,-28.0656318052465,55.6965364019246));
#84188=CARTESIAN_POINT('Ctrl Pts',(7.94642622386803,-28.0906296533896,55.7623983055293));
#84189=CARTESIAN_POINT('Ctrl Pts',(7.9502262029393,-28.1189362790883,55.8267991535855));
#84190=CARTESIAN_POINT('Ctrl Pts',(7.95402628536166,-28.147243674665,55.8912017532035));
#84191=CARTESIAN_POINT('Ctrl Pts',(7.95782636778403,-28.1788598217366,55.954142760903));
#84192=CARTESIAN_POINT('Ctrl Pts',(7.96162645020639,-28.2135965196232,56.0152635952291));
#84193=CARTESIAN_POINT('Ctrl Pts',(7.96543037542274,-28.2483683446356,56.0764462373657));
#84194=CARTESIAN_POINT('Ctrl Pts',(7.96923430063909,-28.2862667667487,56.1358045983047));
#84195=CARTESIAN_POINT('Ctrl Pts',(7.97303822585543,-28.3270589327906,56.1930070193189));
#84196=CARTESIAN_POINT('Ctrl Pts',(7.97684442148116,-28.3678754460295,56.2502435821487));
#84197=CARTESIAN_POINT('Ctrl Pts',(7.98065061710689,-28.4115888246903,56.3053212553387));
#84198=CARTESIAN_POINT('Ctrl Pts',(7.98445681273261,-28.4579262184841,56.3579418304409));
#84199=CARTESIAN_POINT('Ctrl Pts',(7.98826926304463,-28.5043397580912,56.4106488764506));
#84200=CARTESIAN_POINT('Ctrl Pts',(7.99208171335666,-28.5533855611436,56.460890416352));
#84201=CARTESIAN_POINT('Ctrl Pts',(7.99589416366868,-28.6047551136808,56.5084062018237));
#84202=CARTESIAN_POINT('Ctrl Pts',(7.99711781741443,-28.6212428158763,56.5236569891432));
#84203=CARTESIAN_POINT('Ctrl Pts',(7.99834147116018,-28.6379696641195,56.5386273004937));
#84204=CARTESIAN_POINT('Ctrl Pts',(7.99956512490593,-28.6549248140595,56.5533094690586));
#84205=CARTESIAN_POINT('Ctrl Pts',(8.00343419874366,-28.7085353450415,56.5997330545484));
#84206=CARTESIAN_POINT('Ctrl Pts',(8.00730327258139,-28.7646570840593,56.6434688627344));
#84207=CARTESIAN_POINT('Ctrl Pts',(8.01117234641911,-28.8229895049232,56.6842339080362));
#84208=CARTESIAN_POINT('Ctrl Pts',(8.01503565530687,-28.8812350100284,56.724938213105));
#84209=CARTESIAN_POINT('Ctrl Pts',(8.01889896419463,-28.941684263671,56.7626802656851));
#84210=CARTESIAN_POINT('Ctrl Pts',(8.02276227308239,-29.0040028183901,56.7972165080271));
#84211=CARTESIAN_POINT('Ctrl Pts',(8.02662105006854,-29.0662482695686,56.8317122372088));
#84212=CARTESIAN_POINT('Ctrl Pts',(8.0304798270547,-29.1303582433312,56.8630093916739));
#84213=CARTESIAN_POINT('Ctrl Pts',(8.03433860404085,-29.1959698525558,56.8909080052982));
#84214=CARTESIAN_POINT('Ctrl Pts',(8.03819495012281,-29.2615401285971,56.9187890437019));
#84215=CARTESIAN_POINT('Ctrl Pts',(8.04205129620478,-29.3286097172951,56.9432755992752));
#84216=CARTESIAN_POINT('Ctrl Pts',(8.04590764228674,-29.3967930228278,56.964214577176));
#84217=CARTESIAN_POINT('Ctrl Pts',(8.0497628490256,-29.4649561838567,56.9851473687338));
#84218=CARTESIAN_POINT('Ctrl Pts',(8.05361805576447,-29.5342319443494,57.0025345208916));
#84219=CARTESIAN_POINT('Ctrl Pts',(8.05747326250334,-29.6042183489008,57.0162724139246));
#84220=CARTESIAN_POINT('Ctrl Pts',(8.06132861984717,-29.6742074874951,57.030010843633));
#84221=CARTESIAN_POINT('Ctrl Pts',(8.06518397719101,-29.7449068481516,57.0400996397737));
#84222=CARTESIAN_POINT('Ctrl Pts',(8.06903933453485,-29.8159047591773,57.046486380313));
#84223=CARTESIAN_POINT('Ctrl Pts',(8.07289872749117,-29.8869769875828,57.0528798062013));
#84224=CARTESIAN_POINT('Ctrl Pts',(8.07675812044748,-29.9583479053718,57.0555633972186));
#84225=CARTESIAN_POINT('Ctrl Pts',(8.0806175134038,-30.029602101583,57.0545367551061));
#84226=CARTESIAN_POINT('Ctrl Pts',(8.084479091493,-30.1008966408971,57.0535095317236));
#84227=CARTESIAN_POINT('Ctrl Pts',(8.0883406695822,-30.1720738421352,57.0487679257093));
#84228=CARTESIAN_POINT('Ctrl Pts',(8.0922022476714,-30.2427224400021,57.0403635410435));
#84229=CARTESIAN_POINT('Ctrl Pts',(8.09607058226361,-30.3134946498881,57.0319444514438));
#84230=CARTESIAN_POINT('Ctrl Pts',(8.09993891685583,-30.3837359309531,57.0198498705582));
#84231=CARTESIAN_POINT('Ctrl Pts',(8.10380725144805,-30.4530449352733,57.0041825887686));
#84232=CARTESIAN_POINT('Ctrl Pts',(8.10610496621353,-30.4942131224637,56.9948765311242));
#84233=CARTESIAN_POINT('Ctrl Pts',(8.10840268097901,-30.5350526561088,56.984310943053));
#84234=CARTESIAN_POINT('Ctrl Pts',(8.11070039574449,-30.5754824614278,56.9725155256902));
#84235=CARTESIAN_POINT('Ctrl Pts',(8.11456845415834,-30.6435434979776,56.952658681812));
#84236=CARTESIAN_POINT('Ctrl Pts',(8.11843651257219,-30.7107088762612,56.9292361830766));
#84237=CARTESIAN_POINT('Ctrl Pts',(8.12230457098605,-30.7765781669856,56.9023469486561));
#84238=CARTESIAN_POINT('Ctrl Pts',(8.12616758929688,-30.8423616296342,56.8754927510674));
#84239=CARTESIAN_POINT('Ctrl Pts',(8.13003060760772,-30.9068519077994,56.8451809567541));
#84240=CARTESIAN_POINT('Ctrl Pts',(8.13389362591856,-30.9696630675606,56.8115604041569));
#84241=CARTESIAN_POINT('Ctrl Pts',(8.13775232708986,-31.0324040323294,56.777977424412));
#84242=CARTESIAN_POINT('Ctrl Pts',(8.14161102826117,-31.0934691786952,56.7410932568684));
#84243=CARTESIAN_POINT('Ctrl Pts',(8.14546972943248,-31.1524937026271,56.7011042965982));
#84244=CARTESIAN_POINT('Ctrl Pts',(8.14768450152651,-31.1863719074076,56.6781519016487));
#84245=CARTESIAN_POINT('Ctrl Pts',(8.14989927362054,-31.2195782530622,56.6541775381873));
#84246=CARTESIAN_POINT('Ctrl Pts',(8.15211404571458,-31.2520475724682,56.6292251037768));
#84247=CARTESIAN_POINT('',(7.84592528058377,-27.9452502651294,55.0010438147507));
#84248=CARTESIAN_POINT('Ctrl Pts',(7.84592528058377,-27.9452502651294,55.0010438147507));
#84249=CARTESIAN_POINT('Ctrl Pts',(7.85018308153832,-27.945290341015,55.0799332108689));
#84250=CARTESIAN_POINT('Ctrl Pts',(7.85444088249287,-27.9498778523315,55.1586663192291));
#84251=CARTESIAN_POINT('Ctrl Pts',(7.85869868344743,-27.9589342275273,55.2367447463844));
#84252=CARTESIAN_POINT('Ctrl Pts',(7.86297170270191,-27.9680229721636,55.3151022426966));
#84253=CARTESIAN_POINT('Ctrl Pts',(7.86724472195638,-27.981612447429,55.3928000839964));
#84254=CARTESIAN_POINT('Ctrl Pts',(7.87151774121087,-27.9995732784147,55.4693511415428));
#84255=CARTESIAN_POINT('Ctrl Pts',(7.87581130775173,-28.0176204760456,55.5462703033284));
#84256=CARTESIAN_POINT('Ctrl Pts',(7.88010487429258,-28.0400810290445,55.6220313489469));
#84257=CARTESIAN_POINT('Ctrl Pts',(7.88439844083344,-28.0667754154102,55.6961610934531));
#84258=CARTESIAN_POINT('Ctrl Pts',(7.8864670370682,-28.0796364964253,55.7318760425309));
#84259=CARTESIAN_POINT('Ctrl Pts',(7.88853563330296,-28.0934796387085,55.7672126691396));
#84260=CARTESIAN_POINT('Ctrl Pts',(7.89060422953772,-28.1082809506136,55.8021200662548));
#84261=CARTESIAN_POINT('Ctrl Pts',(7.89447330295539,-28.1359651170432,55.8674103727869));
#84262=CARTESIAN_POINT('Ctrl Pts',(7.89834237637307,-28.167087596891,55.9313936569422));
#84263=CARTESIAN_POINT('Ctrl Pts',(7.90221144979074,-28.2015032190154,55.9936834965361));
#84264=CARTESIAN_POINT('Ctrl Pts',(7.90607475825627,-28.2358675615715,56.0558805237416));
#84265=CARTESIAN_POINT('Ctrl Pts',(7.90993806672179,-28.2735150735108,56.1163886932215));
#84266=CARTESIAN_POINT('Ctrl Pts',(7.91380137518732,-28.3142527643123,56.1748420403915));
#84267=CARTESIAN_POINT('Ctrl Pts',(7.91766015175004,-28.354942667251,56.2332268181242));
#84268=CARTESIAN_POINT('Ctrl Pts',(7.92151892831277,-28.3987152722196,56.2895611648753));
#84269=CARTESIAN_POINT('Ctrl Pts',(7.9253777048755,-28.4453328567444,56.3435057261439));
#84270=CARTESIAN_POINT('Ctrl Pts',(7.92923405053353,-28.4919210736956,56.39741630408));
#84271=CARTESIAN_POINT('Ctrl Pts',(7.93309039619156,-28.5413503975354,56.4489397167099));
#84272=CARTESIAN_POINT('Ctrl Pts',(7.93694674184959,-28.5933420745337,56.4977686881568));
#84273=CARTESIAN_POINT('Ctrl Pts',(7.94080194816466,-28.6453183907847,56.5465832332658));
#84274=CARTESIAN_POINT('Ctrl Pts',(7.94465715447972,-28.6998552033538,56.5927045852142));
#84275=CARTESIAN_POINT('Ctrl Pts',(7.94851236079479,-28.7566372805762,56.6358626808039));
#84276=CARTESIAN_POINT('Ctrl Pts',(7.95236771771557,-28.8134215760212,56.679022462388));
#84277=CARTESIAN_POINT('Ctrl Pts',(7.95622307463635,-28.872450922176,56.7192184655813));
#84278=CARTESIAN_POINT('Ctrl Pts',(7.96007843155713,-28.9333788150103,56.7562223123031));
#84279=CARTESIAN_POINT('Ctrl Pts',(7.96393782409444,-28.9943704844591,56.7932648930095));
#84280=CARTESIAN_POINT('Ctrl Pts',(7.96779721663176,-29.0572642516549,56.8271083943555));
#84281=CARTESIAN_POINT('Ctrl Pts',(7.97165660916908,-29.1216873424442,56.8575694975094));
#84282=CARTESIAN_POINT('Ctrl Pts',(7.97551818684094,-29.1861469086943,56.8880478473175));
#84283=CARTESIAN_POINT('Ctrl Pts',(7.9793797645128,-29.25213707264,56.9151398020442));
#84284=CARTESIAN_POINT('Ctrl Pts',(7.98324134218466,-29.3192658784659,56.9387105555702));
#84285=CARTESIAN_POINT('Ctrl Pts',(7.98710967636669,-29.386512137959,56.9623225502803));
#84286=CARTESIAN_POINT('Ctrl Pts',(7.99097801054871,-29.4549005506657,56.9824009063602));
#84287=CARTESIAN_POINT('Ctrl Pts',(7.99484634473073,-29.5240255201802,56.9988611400146));
#84288=CARTESIAN_POINT('Ctrl Pts',(7.99714406327925,-29.5650844662653,57.0086382126253));
#84289=CARTESIAN_POINT('Ctrl Pts',(7.99944178182776,-29.6064030937439,57.0171397434781));
#84290=CARTESIAN_POINT('Ctrl Pts',(8.00173950037628,-29.6478955330734,57.0243566896351));
#84291=CARTESIAN_POINT('Ctrl Pts',(8.00560732707807,-29.717741147918,57.0365052171688));
#84292=CARTESIAN_POINT('Ctrl Pts',(8.00947515377985,-29.7883529993774,57.0450585066243));
#84293=CARTESIAN_POINT('Ctrl Pts',(8.01334298048164,-29.8593280936835,57.0499290176182));
#84294=CARTESIAN_POINT('Ctrl Pts',(8.01720559810006,-29.9302076006711,57.054792969141));
#84295=CARTESIAN_POINT('Ctrl Pts',(8.02106821571849,-30.0014489001652,57.0559839468319));
#84296=CARTESIAN_POINT('Ctrl Pts',(8.02493083333691,-30.0726400820925,57.0534656025786));
#84297=CARTESIAN_POINT('Ctrl Pts',(8.02878954136419,-30.1437592070777,57.0509498072954));
#84298=CARTESIAN_POINT('Ctrl Pts',(8.03264824939147,-30.2148278322896,57.0447321564718));
#84299=CARTESIAN_POINT('Ctrl Pts',(8.03650695741876,-30.2854319409786,57.0348282899471));
#84300=CARTESIAN_POINT('Ctrl Pts',(8.04036305078271,-30.355988208273,57.0249311342896));
#84301=CARTESIAN_POINT('Ctrl Pts',(8.04421914414666,-30.4260801040577,57.011352788786));
#84302=CARTESIAN_POINT('Ctrl Pts',(8.04807523751061,-30.4952983625841,56.9941607494185));
#84303=CARTESIAN_POINT('Ctrl Pts',(8.05193146499299,-30.5645190285843,56.9769681120964));
#84304=CARTESIAN_POINT('Ctrl Pts',(8.05578769247537,-30.6328655206172,56.9561616284351));
#84305=CARTESIAN_POINT('Ctrl Pts',(8.05964391995774,-30.6999396536652,56.9318597370739));
#84306=CARTESIAN_POINT('Ctrl Pts',(8.06349994384164,-30.7670102453788,56.9075591287873));
#84307=CARTESIAN_POINT('Ctrl Pts',(8.06735596772554,-30.8328081570226,56.8797636523508));
#84308=CARTESIAN_POINT('Ctrl Pts',(8.07121199160944,-30.8969533847305,56.8486406324975));
#84309=CARTESIAN_POINT('Ctrl Pts',(8.07507195420201,-30.9611641331332,56.8174858222528));
#84310=CARTESIAN_POINT('Ctrl Pts',(8.07893191679458,-31.0237183897864,56.7829968969806));
#84311=CARTESIAN_POINT('Ctrl Pts',(8.08279187938714,-31.0842598013465,56.7453877064091));
#84312=CARTESIAN_POINT('Ctrl Pts',(8.08648107319296,-31.1421227974679,56.7094423858081));
#84313=CARTESIAN_POINT('Ctrl Pts',(8.09017026699877,-31.1981469838444,56.6706473117852));
#84314=CARTESIAN_POINT('Ctrl Pts',(8.09385946080458,-31.2520475724682,56.6292251037768));
#84315=CARTESIAN_POINT('Ctrl Pts',(7.39391310379067,-31.2520475724682,56.6292251037768));
#84316=CARTESIAN_POINT('Ctrl Pts',(7.39776854030701,-31.3086015795504,56.5857637630962));
#84317=CARTESIAN_POINT('Ctrl Pts',(7.40162397682335,-31.3628830545341,56.5393596382812));
#84318=CARTESIAN_POINT('Ctrl Pts',(7.40547941333968,-31.414581229404,56.4902877265541));
#84319=CARTESIAN_POINT('Ctrl Pts',(7.40933896024307,-31.4663345211219,56.4411634979105));
#84320=CARTESIAN_POINT('Ctrl Pts',(7.41319850714646,-31.5154986629533,56.3893661408871));
#84321=CARTESIAN_POINT('Ctrl Pts',(7.41705805404985,-31.5617995710039,56.335207722608));
#84322=CARTESIAN_POINT('Ctrl Pts',(7.42091989399772,-31.6081279874757,56.2810171275823));
#84323=CARTESIAN_POINT('Ctrl Pts',(7.42478173394559,-31.6515894883817,56.2244630645941));
#84324=CARTESIAN_POINT('Ctrl Pts',(7.42864357389346,-31.691951840923,56.1658887298954));
#84325=CARTESIAN_POINT('Ctrl Pts',(7.43251206089659,-31.7323836657343,56.1072135761974));
#84326=CARTESIAN_POINT('Ctrl Pts',(7.43638054789972,-31.7697054404123,56.0465116235778));
#84327=CARTESIAN_POINT('Ctrl Pts',(7.44024903490285,-31.8037299979096,55.9841522530284));
#84328=CARTESIAN_POINT('Ctrl Pts',(7.44218707199639,-31.8207756424906,55.9529114156785));
#84329=CARTESIAN_POINT('Ctrl Pts',(7.44412510908994,-31.8369944921675,55.9212549384705));
#84330=CARTESIAN_POINT('Ctrl Pts',(7.44606314618348,-31.8523676042235,55.8892310280929));
#84331=CARTESIAN_POINT('Ctrl Pts',(7.44993221953076,-31.8830582955001,55.8252988884398));
#84332=CARTESIAN_POINT('Ctrl Pts',(7.45380129287804,-31.9104954100641,55.7596507813513));
#84333=CARTESIAN_POINT('Ctrl Pts',(7.45767036622532,-31.9344849573745,55.6926510753559));
#84334=CARTESIAN_POINT('Ctrl Pts',(7.46153367462015,-31.9584387600538,55.6257511994968));
#84335=CARTESIAN_POINT('Ctrl Pts',(7.46539698301498,-31.9789550296681,55.5575041758803));
#84336=CARTESIAN_POINT('Ctrl Pts',(7.4692602914098,-31.9958867364297,55.488296731347));
#84337=CARTESIAN_POINT('Ctrl Pts',(7.47311906790172,-32.0127985812379,55.419170471484));
#84338=CARTESIAN_POINT('Ctrl Pts',(7.47697784439365,-32.0261341006974,55.3490864981594));
#84339=CARTESIAN_POINT('Ctrl Pts',(7.48083662088557,-32.0357958014218,55.2784475128517));
#84340=CARTESIAN_POINT('Ctrl Pts',(7.48469296647276,-32.0454514155864,55.2078530278264));
#84341=CARTESIAN_POINT('Ctrl Pts',(7.48854931205996,-32.0514377370475,55.1367047046642));
#84342=CARTESIAN_POINT('Ctrl Pts',(7.49240565764715,-32.053708465876,55.0654148277488));
#84343=CARTESIAN_POINT('Ctrl Pts',(7.49626086389146,-32.055978523826,54.994146013161));
#84344=CARTESIAN_POINT('Ctrl Pts',(7.50011607013577,-32.0545351530398,54.9227362131225));
#84345=CARTESIAN_POINT('Ctrl Pts',(7.50397127638008,-32.0493840895025,54.8516004845229));
#84346=CARTESIAN_POINT('Ctrl Pts',(7.50782663323027,-32.044232824736,54.7804619769644));
#84347=CARTESIAN_POINT('Ctrl Pts',(7.51168199008047,-32.0353736169328,54.7095980464599));
#84348=CARTESIAN_POINT('Ctrl Pts',(7.51553734693067,-32.0228641528445,54.6394196599415));
#84349=CARTESIAN_POINT('Ctrl Pts',(7.51939673939817,-32.0103415944016,54.5691678137871));
#84350=CARTESIAN_POINT('Ctrl Pts',(7.52325613186567,-31.9941612376679,54.4996034233314));
#84351=CARTESIAN_POINT('Ctrl Pts',(7.52711552433317,-31.9744319452988,54.4311273816719));
#84352=CARTESIAN_POINT('Ctrl Pts',(7.53097710193553,-31.9546914824762,54.3626125698208));
#84353=CARTESIAN_POINT('Ctrl Pts',(7.53483867953788,-31.9313982427059,54.2951877928218));
#84354=CARTESIAN_POINT('Ctrl Pts',(7.53870025714024,-31.9047101701479,54.2292362682149));
#84355=CARTESIAN_POINT('Ctrl Pts',(7.54256859125404,-31.8779754020975,54.1631693497778));
#84356=CARTESIAN_POINT('Ctrl Pts',(7.54643692536784,-31.8478341476564,54.0985812705662));
#84357=CARTESIAN_POINT('Ctrl Pts',(7.55030525948163,-31.8144911274965,54.0358322185758));
#84358=CARTESIAN_POINT('Ctrl Pts',(7.55260297866177,-31.7946859879477,53.9985604379972));
#84359=CARTESIAN_POINT('Ctrl Pts',(7.5549006978419,-31.7737520802405,53.9619369825755));
#84360=CARTESIAN_POINT('Ctrl Pts',(7.55719841702204,-31.7517393817971,53.9260322627001));
#84361=CARTESIAN_POINT('Ctrl Pts',(7.56106749037986,-31.7146727350905,53.8655731794967));
#84362=CARTESIAN_POINT('Ctrl Pts',(7.56493656373769,-31.6743998062233,53.8069168887164));
#84363=CARTESIAN_POINT('Ctrl Pts',(7.56880563709551,-31.6311215035676,53.7504239906675));
#84364=CARTESIAN_POINT('Ctrl Pts',(7.57266894550093,-31.5879076859531,53.6940152675199));
#84365=CARTESIAN_POINT('Ctrl Pts',(7.57653225390636,-31.5416976763381,53.6397639210884));
#84366=CARTESIAN_POINT('Ctrl Pts',(7.58039556231178,-31.4927366371123,53.588003224252));
#84367=CARTESIAN_POINT('Ctrl Pts',(7.58425433881433,-31.4438330322539,53.5363032459569));
#84368=CARTESIAN_POINT('Ctrl Pts',(7.58811311531688,-31.3921851401621,53.4870884649974));
#84369=CARTESIAN_POINT('Ctrl Pts',(7.59197189181942,-31.3380784109807,53.440659200634));
#84370=CARTESIAN_POINT('Ctrl Pts',(7.59582823741726,-31.2840057672932,53.3942591852094));
#84371=CARTESIAN_POINT('Ctrl Pts',(7.59968458301509,-31.2274777274727,53.3506415205165));
#84372=CARTESIAN_POINT('Ctrl Pts',(7.60354092861292,-31.1688155581712,53.310068713386));
#84373=CARTESIAN_POINT('Ctrl Pts',(7.60739613486786,-31.1101707203885,53.2695078933397));
#84374=CARTESIAN_POINT('Ctrl Pts',(7.6112513411228,-31.0493934042002,53.231990421099));
#84375=CARTESIAN_POINT('Ctrl Pts',(7.61510654737773,-30.9868354279729,53.1977365895637));
#84376=CARTESIAN_POINT('Ctrl Pts',(7.61896190423855,-30.9242750078818,53.1634814198825));
#84377=CARTESIAN_POINT('Ctrl Pts',(7.62281726109936,-30.8599342167953,53.1324903754099));
#84378=CARTESIAN_POINT('Ctrl Pts',(7.62667261796017,-30.7941896131577,53.1049378846981));
#84379=CARTESIAN_POINT('Ctrl Pts',(7.63053201043819,-30.7283761909742,53.0773565532565));
#84380=CARTESIAN_POINT('Ctrl Pts',(7.6343914029162,-30.6611564718399,53.0532211487873));
#84381=CARTESIAN_POINT('Ctrl Pts',(7.63825079539421,-30.5929263067048,53.0326576410504));
#84382=CARTESIAN_POINT('Ctrl Pts',(7.64211237300705,-30.5246575105906,53.0120824905388));
#84383=CARTESIAN_POINT('Ctrl Pts',(7.6459739506199,-30.4553776016146,52.9950833784695));
#84384=CARTESIAN_POINT('Ctrl Pts',(7.64983552823274,-30.3854942007663,52.9817354525049));
#84385=CARTESIAN_POINT('Ctrl Pts',(7.65370386235683,-30.3154885265802,52.9683641719892));
#84386=CARTESIAN_POINT('Ctrl Pts',(7.65757219648092,-30.2448777337682,52.9586568983752));
#84387=CARTESIAN_POINT('Ctrl Pts',(7.661440530605,-30.1740754650965,52.9526369899426));
#84388=CARTESIAN_POINT('Ctrl Pts',(7.6637382496902,-30.132020224059,52.9490612754223));
#84389=CARTESIAN_POINT('Ctrl Pts',(7.6660359687754,-30.0898974659227,52.9467855163727));
#84390=CARTESIAN_POINT('Ctrl Pts',(7.6683336878606,-30.0477934514707,52.9458059126517));
#84391=CARTESIAN_POINT('Ctrl Pts',(7.67220276119183,-29.9768955246948,52.9441563817512));
#84392=CARTESIAN_POINT('Ctrl Pts',(7.67607183452307,-29.9057732300604,52.9461783579695));
#84393=CARTESIAN_POINT('Ctrl Pts',(7.6799409078543,-29.8348384890744,52.9518986260908));
#84394=CARTESIAN_POINT('Ctrl Pts',(7.68380421623315,-29.7640094414595,52.9576103709636));
#84395=CARTESIAN_POINT('Ctrl Pts',(7.687667524612,-29.6933678730486,52.9670094308489));
#84396=CARTESIAN_POINT('Ctrl Pts',(7.69153083299085,-29.6233267481749,52.980070589387));
#84397=CARTESIAN_POINT('Ctrl Pts',(7.69538960946695,-29.5533677859286,52.9931164263678));
#84398=CARTESIAN_POINT('Ctrl Pts',(7.69924838594304,-29.4840083433624,53.009815740327));
#84399=CARTESIAN_POINT('Ctrl Pts',(7.70310716241913,-29.4156555496703,53.0300915945484));
#84400=CARTESIAN_POINT('Ctrl Pts',(7.70696350799061,-29.3473458160319,53.0503546756361));
#84401=CARTESIAN_POINT('Ctrl Pts',(7.71081985356208,-29.2800419377385,53.0741896890378));
#84402=CARTESIAN_POINT('Ctrl Pts',(7.71467619913355,-29.2141387017029,53.1014690989245));
#84403=CARTESIAN_POINT('Ctrl Pts',(7.71853140536226,-29.1482549365299,53.1287404492123));
#84404=CARTESIAN_POINT('Ctrl Pts',(7.72238661159097,-29.0837714406864,53.1594539900072));
#84405=CARTESIAN_POINT('Ctrl Pts',(7.72624181781968,-29.0210641054759,53.1934336223343));
#84406=CARTESIAN_POINT('Ctrl Pts',(7.73009717465446,-28.9583543205637,53.2274145820972));
#84407=CARTESIAN_POINT('Ctrl Pts',(7.73395253148923,-28.8974212601037,53.2646616533317));
#84408=CARTESIAN_POINT('Ctrl Pts',(7.737807888324,-28.8386157008929,53.3049530766709));
#84409=CARTESIAN_POINT('Ctrl Pts',(7.74166728077639,-28.7797485866145,53.3452866752962));
#84410=CARTESIAN_POINT('Ctrl Pts',(7.74552667322878,-28.7230138206927,53.3886707122444));
#84411=CARTESIAN_POINT('Ctrl Pts',(7.74938606568117,-28.6687319311445,53.4348409373658));
#84412=CARTESIAN_POINT('Ctrl Pts',(7.75324764326858,-28.6144193079356,53.4810373034349));
#84413=CARTESIAN_POINT('Ctrl Pts',(7.757109220856,-28.56256267905,53.5300226642511));
#84414=CARTESIAN_POINT('Ctrl Pts',(7.76097079844341,-28.5134462582933,53.5814953170617));
#84415=CARTESIAN_POINT('Ctrl Pts',(7.76483913254268,-28.4642438996857,53.6330580303673));
#84416=CARTESIAN_POINT('Ctrl Pts',(7.76870746664195,-28.4177916382251,53.6871163559143));
#84417=CARTESIAN_POINT('Ctrl Pts',(7.77257580074122,-28.374333443196,53.7433354430919));
#84418=CARTESIAN_POINT('Ctrl Pts',(7.77487352006053,-28.3485200745111,53.7767285470501));
#84419=CARTESIAN_POINT('Ctrl Pts',(7.77717123937985,-28.323762236405,53.8108834243806));
#84420=CARTESIAN_POINT('Ctrl Pts',(7.77946895869916,-28.3001035209765,53.8457255425578));
#84421=CARTESIAN_POINT('Ctrl Pts',(7.78339694508641,-28.2596585843988,53.905288677512));
#84422=CARTESIAN_POINT('Ctrl Pts',(7.78732493147366,-28.2222729068542,53.9670902448233));
#84423=CARTESIAN_POINT('Ctrl Pts',(7.79125291786091,-28.1881978041484,54.0307887920545));
#84424=CARTESIAN_POINT('Ctrl Pts',(7.79517455595449,-28.1541777726005,54.094384391606));
#84425=CARTESIAN_POINT('Ctrl Pts',(7.79909619404806,-28.1234579082038,54.1598704747613));
#84426=CARTESIAN_POINT('Ctrl Pts',(7.80301783214163,-28.0962464206018,54.2268765483904));
#84427=CARTESIAN_POINT('Ctrl Pts',(7.80693336842876,-28.0690772722537,54.2937783650529));
#84428=CARTESIAN_POINT('Ctrl Pts',(7.81084890471589,-28.0454058198635,54.3621950395434));
#84429=CARTESIAN_POINT('Ctrl Pts',(7.81476444100302,-28.0253936651134,54.4317329987358));
#84430=CARTESIAN_POINT('Ctrl Pts',(7.81867638568786,-28.0053998669039,54.5012071728743));
#84431=CARTESIAN_POINT('Ctrl Pts',(7.82258833037271,-27.9890588284757,54.5718001425285));
#84432=CARTESIAN_POINT('Ctrl Pts',(7.82650027505756,-27.9764831073348,54.6431009279941));
#84433=CARTESIAN_POINT('Ctrl Pts',(7.83040988908206,-27.9639148785634,54.7143592338423));
#84434=CARTESIAN_POINT('Ctrl Pts',(7.83431950310656,-27.9551075922549,54.7863240593652));
#84435=CARTESIAN_POINT('Ctrl Pts',(7.83822911713106,-27.9501229158777,54.8585733317576));
#84436=CARTESIAN_POINT('Ctrl Pts',(7.84079450493327,-27.9468520999107,54.9059814392977));
#84437=CARTESIAN_POINT('Ctrl Pts',(7.84335989273547,-27.9452261188372,54.9535117905147));
#84438=CARTESIAN_POINT('Ctrl Pts',(7.84592528053768,-27.945250265129,55.0010438138967));
#84439=CARTESIAN_POINT('Origin',(-1.54592528053767,-30.,55.));
#84440=CARTESIAN_POINT('',(6.69398930341886,-31.2520475724682,56.6292251037768));
#84441=CARTESIAN_POINT('',(6.75200712063213,-31.2520475724682,56.6292251037768));
#84442=CARTESIAN_POINT('',(-1.54592528053767,-31.2520475724682,56.6292251037768));
#84443=CARTESIAN_POINT('',(7.20407471942299,-27.945250640964,55.0016229729599));
#84444=CARTESIAN_POINT('Ctrl Pts',(6.75200712063213,-31.2520475724682,56.6292251037768));
#84445=CARTESIAN_POINT('Ctrl Pts',(6.75587000360825,-31.3085547924693,56.5857997186257));
#84446=CARTESIAN_POINT('Ctrl Pts',(6.75973288658436,-31.3627396230512,56.5394776578832));
#84447=CARTESIAN_POINT('Ctrl Pts',(6.76359576956048,-31.4143063307506,56.490548612189));
#84448=CARTESIAN_POINT('Ctrl Pts',(6.76746491972785,-31.4659567009429,56.4415401833789));
#84449=CARTESIAN_POINT('Ctrl Pts',(6.77133406989522,-31.5149801444479,56.3899166863317));
#84450=CARTESIAN_POINT('Ctrl Pts',(6.77520322006258,-31.5611200623353,56.3360021382745));
#84451=CARTESIAN_POINT('Ctrl Pts',(6.77582786193565,-31.5685689654498,56.3272980862665));
#84452=CARTESIAN_POINT('Ctrl Pts',(6.77645250380871,-31.575942805177,56.318534383896));
#84453=CARTESIAN_POINT('Ctrl Pts',(6.77707714568177,-31.5832406084852,56.3097124639185));
#84454=CARTESIAN_POINT('Ctrl Pts',(6.78094621902978,-31.6284436880358,56.2550689042481));
#84455=CARTESIAN_POINT('Ctrl Pts',(6.78481529237778,-31.6709030568371,56.1979753737613));
#84456=CARTESIAN_POINT('Ctrl Pts',(6.78868436572578,-31.7103425768957,56.1387387023185));
#84457=CARTESIAN_POINT('Ctrl Pts',(6.79254767412136,-31.7497233317315,56.0795902940235));
#84458=CARTESIAN_POINT('Ctrl Pts',(6.79641098251693,-31.7860929023769,56.0183054844465));
#84459=CARTESIAN_POINT('Ctrl Pts',(6.80027429091251,-31.8192153334279,55.9552241271664));
#84460=CARTESIAN_POINT('Ctrl Pts',(6.80413306740521,-31.8522989097914,55.8922167682719));
#84461=CARTESIAN_POINT('Ctrl Pts',(6.80799184389792,-31.8821426879791,55.8274174758218));
#84462=CARTESIAN_POINT('Ctrl Pts',(6.81185062039062,-31.9085549343264,55.7611935530194));
#84463=CARTESIAN_POINT('Ctrl Pts',(6.81570696597862,-31.9349505418106,55.6950113491521));
#84464=CARTESIAN_POINT('Ctrl Pts',(6.81956331156662,-31.9579187268033,55.6274067456564));
#84465=CARTESIAN_POINT('Ctrl Pts',(6.82341965715462,-31.9773151269939,55.5587686919119));
#84466=CARTESIAN_POINT('Ctrl Pts',(6.82727486339975,-31.9967057965908,55.4901509170234));
#84467=CARTESIAN_POINT('Ctrl Pts',(6.83113006964488,-32.0125266443568,55.4205007652728));
#84468=CARTESIAN_POINT('Ctrl Pts',(6.83498527589,-32.0246831393636,55.3502224260052));
#84469=CARTESIAN_POINT('Ctrl Pts',(6.83884063274105,-32.036840109271,55.2799413412726));
#84470=CARTESIAN_POINT('Ctrl Pts',(6.84269598959209,-32.0453323615838,55.2090324993541));
#84471=CARTESIAN_POINT('Ctrl Pts',(6.84655134644314,-32.0501167691132,55.1379086491154));
#84472=CARTESIAN_POINT('Ctrl Pts',(6.8504107389115,-32.0549061847492,55.0667103495708));
#84473=CARTESIAN_POINT('Ctrl Pts',(6.85427013137986,-32.0559799751667,54.995297078117));
#84474=CARTESIAN_POINT('Ctrl Pts',(6.85812952384822,-32.0533471080334,54.9240841490139));
#84475=CARTESIAN_POINT('Ctrl Pts',(6.86199110145146,-32.0507127502069,54.8528309001309));
#84476=CARTESIAN_POINT('Ctrl Pts',(6.8658526790547,-32.0443676002785,54.7817787034946));
#84477=CARTESIAN_POINT('Ctrl Pts',(6.86971425665794,-32.0343725214679,54.7113375563115));
#84478=CARTESIAN_POINT('Ctrl Pts',(6.87358259077263,-32.0243599545033,54.6407731599113));
#84479=CARTESIAN_POINT('Ctrl Pts',(6.87745092488731,-32.0106848016684,54.5708224244431));
#84480=CARTESIAN_POINT('Ctrl Pts',(6.88131925900199,-31.993458875977,54.501884278216));
#84481=CARTESIAN_POINT('Ctrl Pts',(6.88361697817477,-31.983226993581,54.4609362898505));
#84482=CARTESIAN_POINT('Ctrl Pts',(6.88591469734756,-31.9717433059069,54.4203452700944));
#84483=CARTESIAN_POINT('Ctrl Pts',(6.88821241652034,-31.9590393346448,54.3801916039498));
#84484=CARTESIAN_POINT('Ctrl Pts',(6.89208148986834,-31.9376474268756,54.3125778235781));
#84485=CARTESIAN_POINT('Ctrl Pts',(6.89595056321633,-31.9127091017352,54.2459403779375));
#84486=CARTESIAN_POINT('Ctrl Pts',(6.89981963656433,-31.8843323730244,54.1806776760809));
#84487=CARTESIAN_POINT('Ctrl Pts',(6.90368294495989,-31.8559979258825,54.1155122162092));
#84488=CARTESIAN_POINT('Ctrl Pts',(6.90754625335546,-31.8242354368057,54.051717876011));
#84489=CARTESIAN_POINT('Ctrl Pts',(6.91140956175102,-31.7892024578523,53.9896772162743));
#84490=CARTESIAN_POINT('Ctrl Pts',(6.9152683382437,-31.7542105747789,53.9277093341199));
#84491=CARTESIAN_POINT('Ctrl Pts',(6.91912711473639,-31.715956060097,53.8674914671294));
#84492=CARTESIAN_POINT('Ctrl Pts',(6.92298589122908,-31.6746435117732,53.8093839111721));
#84493=CARTESIAN_POINT('Ctrl Pts',(6.92684223681705,-31.6333569890222,53.7513129611006));
#84494=CARTESIAN_POINT('Ctrl Pts',(6.93069858240503,-31.5890165355209,53.6953500794837));
#84495=CARTESIAN_POINT('Ctrl Pts',(6.93455492799301,-31.5418706276525,53.6418275035614));
#84496=CARTESIAN_POINT('Ctrl Pts',(6.93841013423812,-31.4947386488662,53.5883207406838));
#84497=CARTESIAN_POINT('Ctrl Pts',(6.94226534048322,-31.4448031821568,53.5372532164894));
#84498=CARTESIAN_POINT('Ctrl Pts',(6.94612054672832,-31.3923525344185,53.4889235683135));
#84499=CARTESIAN_POINT('Ctrl Pts',(6.94997590357934,-31.3398998376646,53.4405920321113));
#84500=CARTESIAN_POINT('Ctrl Pts',(6.95383126043035,-31.2849321235481,53.3949989118376));
#84501=CARTESIAN_POINT('Ctrl Pts',(6.95768661728136,-31.2277727697314,53.3524043006835));
#84502=CARTESIAN_POINT('Ctrl Pts',(6.96154600974969,-31.1705535840271,53.3097651033713));
#84503=CARTESIAN_POINT('Ctrl Pts',(6.96540540221802,-31.1111385693846,53.270130971609));
#84504=CARTESIAN_POINT('Ctrl Pts',(6.96926479468635,-31.049881513145,53.2337196228072));
#84505=CARTESIAN_POINT('Ctrl Pts',(6.97312637228955,-30.9885897740035,53.1972876584011));
#84506=CARTESIAN_POINT('Ctrl Pts',(6.97698794989275,-30.9254543472475,53.1640823355941));
#84507=CARTESIAN_POINT('Ctrl Pts',(6.98084952749596,-30.8608526994133,53.1342748883041));
#84508=CARTESIAN_POINT('Ctrl Pts',(6.9847178616106,-30.7961380195966,53.1044152876251));
#84509=CARTESIAN_POINT('Ctrl Pts',(6.98858619572524,-30.7299524480231,53.0779656125225));
#84510=CARTESIAN_POINT('Ctrl Pts',(6.99245452983988,-30.662691785105,53.0550482884004));
#84511=CARTESIAN_POINT('Ctrl Pts',(6.99475224901289,-30.6227401909056,53.0414358202245));
#84512=CARTESIAN_POINT('Ctrl Pts',(6.99704996818589,-30.5824095673591,53.029068655143));
#84513=CARTESIAN_POINT('Ctrl Pts',(6.9993476873589,-30.5417845456398,53.0179639083493));
#84514=CARTESIAN_POINT('Ctrl Pts',(7.00321676070842,-30.4733770610767,52.9992648957034));
#84515=CARTESIAN_POINT('Ctrl Pts',(7.00708583405794,-30.4038663884346,52.984074911664));
#84516=CARTESIAN_POINT('Ctrl Pts',(7.01095490740745,-30.3336458313196,52.9725192918937));
#84517=CARTESIAN_POINT('Ctrl Pts',(7.01481821580455,-30.2635299034361,52.9609808900959));
#84518=CARTESIAN_POINT('Ctrl Pts',(7.01868152420164,-30.1927066660855,52.9530661817184));
#84519=CARTESIAN_POINT('Ctrl Pts',(7.02254483259873,-30.121582975828,52.9488502876463));
#84520=CARTESIAN_POINT('Ctrl Pts',(7.02640360909295,-30.0505427181167,52.9446393390821));
#84521=CARTESIAN_POINT('Ctrl Pts',(7.03026238558716,-29.9792031901646,52.9441186148241));
#84522=CARTESIAN_POINT('Ctrl Pts',(7.03412116208138,-29.9079780588148,52.9473116347481));
#84523=CARTESIAN_POINT('Ctrl Pts',(7.03797750767089,-29.8367977970001,52.9505026431725));
#84524=CARTESIAN_POINT('Ctrl Pts',(7.0418338532604,-29.7657322729608,52.9574027324669));
#84525=CARTESIAN_POINT('Ctrl Pts',(7.04569019884991,-29.6951953783404,52.9679833403451));
#84526=CARTESIAN_POINT('Ctrl Pts',(7.04954540509654,-29.6246793235816,52.9785608222223));
#84527=CARTESIAN_POINT('Ctrl Pts',(7.05340061134318,-29.5546920683275,52.9928165918795));
#84528=CARTESIAN_POINT('Ctrl Pts',(7.05725581758981,-29.4856408781172,53.0106704003017));
#84529=CARTESIAN_POINT('Ctrl Pts',(7.06111117444235,-29.4165869903813,53.0285249061934));
#84530=CARTESIAN_POINT('Ctrl Pts',(7.06496653129489,-29.3484697100577,53.0499776061749));
#84531=CARTESIAN_POINT('Ctrl Pts',(7.06882188814743,-29.2816829411958,53.0748978817915));
#84532=CARTESIAN_POINT('Ctrl Pts',(7.07268128061727,-29.2148262628937,53.0998442428521));
#84533=CARTESIAN_POINT('Ctrl Pts',(7.07654067308711,-29.1493033323038,53.1282652550815));
#84534=CARTESIAN_POINT('Ctrl Pts',(7.08040006555694,-29.0854889448541,53.1599817684284));
#84535=CARTESIAN_POINT('Ctrl Pts',(7.08426164316165,-29.0216384265771,53.1917162392283));
#84536=CARTESIAN_POINT('Ctrl Pts',(7.08812322076635,-28.9594988005098,53.2267496868236));
#84537=CARTESIAN_POINT('Ctrl Pts',(7.09198479837105,-28.8994186520185,53.2648578562621));
#84538=CARTESIAN_POINT('Ctrl Pts',(7.09585313248717,-28.839233382706,53.3030327026674));
#84539=CARTESIAN_POINT('Ctrl Pts',(7.09972146660328,-28.7811151815409,53.3442927304759));
#84540=CARTESIAN_POINT('Ctrl Pts',(7.1035898007194,-28.7253815713666,53.3883718096632));
#84541=CARTESIAN_POINT('Ctrl Pts',(7.10588751987875,-28.6922768342696,53.4145539701838));
#84542=CARTESIAN_POINT('Ctrl Pts',(7.10818523903811,-28.6600127586308,53.4417299774308));
#84543=CARTESIAN_POINT('Ctrl Pts',(7.11048295819746,-28.6286496245778,53.4698380117356));
#84544=CARTESIAN_POINT('Ctrl Pts',(7.11438261491519,-28.5754205535222,53.5175425731711));
#84545=CARTESIAN_POINT('Ctrl Pts',(7.11828227163292,-28.524561791378,53.5681375184189));
#84546=CARTESIAN_POINT('Ctrl Pts',(7.12218192835065,-28.476409230357,53.6213525725703));
#84547=CARTESIAN_POINT('Ctrl Pts',(7.12598698948115,-28.4294247259409,53.6732767671252));
#84548=CARTESIAN_POINT('Ctrl Pts',(7.12979205061164,-28.3850169998589,53.7276950180236));
#84549=CARTESIAN_POINT('Ctrl Pts',(7.13359711174214,-28.3434646904989,53.7843156944025));
#84550=CARTESIAN_POINT('Ctrl Pts',(7.13739855500299,-28.3019518892661,53.8408825355815));
#84551=CARTESIAN_POINT('Ctrl Pts',(7.14119999826383,-28.2632894190354,53.8996472498018));
#84552=CARTESIAN_POINT('Ctrl Pts',(7.14500144152468,-28.2277166035742,53.9602841132053));
#84553=CARTESIAN_POINT('Ctrl Pts',(7.14880063065914,-28.1921648815811,54.0208850210138));
#84554=CARTESIAN_POINT('Ctrl Pts',(7.15259981979359,-28.1596994343324,54.0833554448165));
#84555=CARTESIAN_POINT('Ctrl Pts',(7.15639900892805,-28.1305159753065,54.1473411913809));
#84556=CARTESIAN_POINT('Ctrl Pts',(7.16037198480262,-28.0999975739994,54.2142538452186));
#84557=CARTESIAN_POINT('Ctrl Pts',(7.1643449606772,-28.0730689420862,54.2828232869358));
#84558=CARTESIAN_POINT('Ctrl Pts',(7.16831793655178,-28.0498988920081,54.3526181720895));
#84559=CARTESIAN_POINT('Ctrl Pts',(7.1721185069018,-28.0277342959684,54.4193843391825));
#84560=CARTESIAN_POINT('Ctrl Pts',(7.17591907725183,-28.009008924759,54.4872712685952));
#84561=CARTESIAN_POINT('Ctrl Pts',(7.17971964760185,-27.9938195467796,54.5558856547957));
#84562=CARTESIAN_POINT('Ctrl Pts',(7.18352169694533,-27.9786242578476,54.6245267423119));
#84563=CARTESIAN_POINT('Ctrl Pts',(7.18732374628881,-27.9669677847835,54.6938953556263));
#84564=CARTESIAN_POINT('Ctrl Pts',(7.1911257956323,-27.9588954503991,54.7635898054259));
#84565=CARTESIAN_POINT('Ctrl Pts',(7.19493249872832,-27.9508132353837,54.8333695620411));
#84566=CARTESIAN_POINT('Ctrl Pts',(7.19873920182434,-27.9463239372981,54.9034754508827));
#84567=CARTESIAN_POINT('Ctrl Pts',(7.20254590492036,-27.9454208415896,54.9735038809335));
#84568=CARTESIAN_POINT('Ctrl Pts',(7.20305550975457,-27.9452999438134,54.9828786142883));
#84569=CARTESIAN_POINT('Ctrl Pts',(7.20356511458877,-27.9452432391406,54.9922519653909));
#84570=CARTESIAN_POINT('Ctrl Pts',(7.20407471942298,-27.945250640964,55.0016229729598));
#84571=CARTESIAN_POINT('Ctrl Pts',(7.20407471946233,-27.9452506409646,55.0016229736833));
#84572=CARTESIAN_POINT('Ctrl Pts',(7.20992255598689,-27.9453355786842,55.109157511533));
#84573=CARTESIAN_POINT('Ctrl Pts',(7.21577039251146,-27.953864093232,55.2163661668599));
#84574=CARTESIAN_POINT('Ctrl Pts',(7.22161822903602,-27.9706730699848,55.3222262770401));
#84575=CARTESIAN_POINT('Ctrl Pts',(7.22548730238329,-27.9817943049366,55.3922659454058));
#84576=CARTESIAN_POINT('Ctrl Pts',(7.22935637573056,-27.9965675768626,55.4618663739711));
#84577=CARTESIAN_POINT('Ctrl Pts',(7.23322544907783,-28.0149451914136,55.5306175359032));
#84578=CARTESIAN_POINT('Ctrl Pts',(7.23708875747265,-28.0332954231614,55.5992662580147));
#84579=CARTESIAN_POINT('Ctrl Pts',(7.24095206586747,-28.0552392128128,55.6670677598203));
#84580=CARTESIAN_POINT('Ctrl Pts',(7.24481537426229,-28.0806775244038,55.7336203358492));
#84581=CARTESIAN_POINT('Ctrl Pts',(7.2486741507542,-28.1060859952609,55.8000948415347));
#84582=CARTESIAN_POINT('Ctrl Pts',(7.25253292724611,-28.1349806728731,55.8653228799988));
#84583=CARTESIAN_POINT('Ctrl Pts',(7.25639170373802,-28.1672126921902,55.9289177826004));
#84584=CARTESIAN_POINT('Ctrl Pts',(7.26024804932521,-28.1994244063747,55.9924726224646));
#84585=CARTESIAN_POINT('Ctrl Pts',(7.2641043949124,-28.2349690720051,56.0543959353494));
#84586=CARTESIAN_POINT('Ctrl Pts',(7.26796074049958,-28.273650267584,56.1143222890561));
#84587=CARTESIAN_POINT('Ctrl Pts',(7.27181594674388,-28.3123200349483,56.1742309377457));
#84588=CARTESIAN_POINT('Ctrl Pts',(7.27567115298818,-28.3541242292472,56.2321433906359));
#84589=CARTESIAN_POINT('Ctrl Pts',(7.27952635923247,-28.3988220533025,56.2877215325953));
#84590=CARTESIAN_POINT('Ctrl Pts',(7.28338171608267,-28.4435216235047,56.3433018457475));
#84591=CARTESIAN_POINT('Ctrl Pts',(7.28723707293288,-28.4911147417313,56.396547289749));
#84592=CARTESIAN_POINT('Ctrl Pts',(7.29109242978307,-28.5413202084445,56.4471526623711));
#84593=CARTESIAN_POINT('Ctrl Pts',(7.29495182225056,-28.5915782280232,56.4978110064623));
#84594=CARTESIAN_POINT('Ctrl Pts',(7.29881121471805,-28.6444537119087,56.5458234170178));
#84595=CARTESIAN_POINT('Ctrl Pts',(7.30267060718554,-28.6996290990732,56.5909220856229));
#84596=CARTESIAN_POINT('Ctrl Pts',(7.3065321847879,-28.754835725782,56.6360462884731));
#84597=CARTESIAN_POINT('Ctrl Pts',(7.31039376239025,-28.8123444561797,56.6782531777261));
#84598=CARTESIAN_POINT('Ctrl Pts',(7.31425533999261,-28.871807414128,56.717317399808));
#84599=CARTESIAN_POINT('Ctrl Pts',(7.31812367410639,-28.931374413014,56.7564499716398));
#84600=CARTESIAN_POINT('Ctrl Pts',(7.32199200822018,-28.9929020466295,56.7924286527882));
#84601=CARTESIAN_POINT('Ctrl Pts',(7.32586034233397,-29.0560170648301,56.8250736370371));
#84602=CARTESIAN_POINT('Ctrl Pts',(7.32815806151417,-29.0935062225947,56.8444641561184));
#84603=CARTESIAN_POINT('Ctrl Pts',(7.33045578069437,-29.1315550145839,56.8626794081666));
#84604=CARTESIAN_POINT('Ctrl Pts',(7.33275349987457,-29.1700822865709,56.8796899083191));
#84605=CARTESIAN_POINT('Ctrl Pts',(7.33662257323245,-29.2349574213919,56.9083334751706));
#84606=CARTESIAN_POINT('Ctrl Pts',(7.34049164659033,-29.3014442654214,56.9336705787694));
#84607=CARTESIAN_POINT('Ctrl Pts',(7.34436071994821,-29.3691724695526,56.9555189053879));
#84608=CARTESIAN_POINT('Ctrl Pts',(7.34822402835369,-29.4367997580803,56.9773346778129));
#84609=CARTESIAN_POINT('Ctrl Pts',(7.35208733675917,-29.5056642766728,56.9956718438265));
#84610=CARTESIAN_POINT('Ctrl Pts',(7.35595064516465,-29.5753748215141,57.0103957372358));
#84611=CARTESIAN_POINT('Ctrl Pts',(7.35980942166726,-29.6450035915175,57.0251023585954));
#84612=CARTESIAN_POINT('Ctrl Pts',(7.36366819816986,-29.7154759434518,57.0362040267315));
#84613=CARTESIAN_POINT('Ctrl Pts',(7.36752697467247,-29.7863862810899,57.0436160944741));
#84614=CARTESIAN_POINT('Ctrl Pts',(7.37138332027036,-29.8572519475029,57.0510234928531));
#84615=CARTESIAN_POINT('Ctrl Pts',(7.37523966586826,-29.9285545701936,57.0547458518867));
#84616=CARTESIAN_POINT('Ctrl Pts',(7.37909601146615,-29.9998806016868,57.054749996531));
#84617=CARTESIAN_POINT('Ctrl Pts',(7.38295121772115,-30.0711855601706,57.0547541399507));
#84618=CARTESIAN_POINT('Ctrl Pts',(7.38680642397615,-30.1425134282052,57.0510422498442));
#84619=CARTESIAN_POINT('Ctrl Pts',(7.39066163023115,-30.2134495407978,57.0436332489058));
#84620=CARTESIAN_POINT('Ctrl Pts',(7.39451698709202,-30.2843884245509,57.0362239585305));
#84621=CARTESIAN_POINT('Ctrl Pts',(7.39837234395289,-30.3549350395487,57.0251173232316));
#84622=CARTESIAN_POINT('Ctrl Pts',(7.40222770081377,-30.4246804595726,57.0103840602624));
#84623=CARTESIAN_POINT('Ctrl Pts',(7.40608709329184,-30.4944988860202,56.9956353751646));
#84624=CARTESIAN_POINT('Ctrl Pts',(7.40994648576991,-30.5635139670784,56.9772525849503));
#84625=CARTESIAN_POINT('Ctrl Pts',(7.41380587824798,-30.6313284715343,56.9553572368062));
#84626=CARTESIAN_POINT('Ctrl Pts',(7.41766745586088,-30.6991813716279,56.9334494918177));
#84627=CARTESIAN_POINT('Ctrl Pts',(7.42152903347377,-30.7658318878465,56.9080254031064));
#84628=CARTESIAN_POINT('Ctrl Pts',(7.42539061108667,-30.8309020153114,56.8792550128845));
#84629=CARTESIAN_POINT('Ctrl Pts',(7.42925894521082,-30.8960859944432,56.8504342837896));
#84630=CARTESIAN_POINT('Ctrl Pts',(7.43312727933496,-30.9596836304835,56.8182557830043));
#84631=CARTESIAN_POINT('Ctrl Pts',(7.43699561345911,-31.0213414229231,56.7829355738));
#84632=CARTESIAN_POINT('Ctrl Pts',(7.43929333254379,-31.0579650138179,56.7619560213211));
#84633=CARTESIAN_POINT('Ctrl Pts',(7.44159105162846,-31.0939047372455,56.7398688732165));
#84634=CARTESIAN_POINT('Ctrl Pts',(7.44388877071314,-31.1290918065592,56.7167263191496));
#84635=CARTESIAN_POINT('Ctrl Pts',(7.44663026262674,-31.1710747742032,56.6891140991626));
#84636=CARTESIAN_POINT('Ctrl Pts',(7.44937175454035,-31.2121024284199,56.6599226547301));
#84637=CARTESIAN_POINT('Ctrl Pts',(7.45211324645396,-31.2520475724682,56.6292251037768));
#84638=CARTESIAN_POINT('',(7.14592528050079,-27.9452507538412,54.9982399120147));
#84639=CARTESIAN_POINT('Ctrl Pts',(7.14592528053768,-27.9452507538406,54.9982399126965));
#84640=CARTESIAN_POINT('Ctrl Pts',(7.14975890798127,-27.9451900689549,55.0690842525566));
#84641=CARTESIAN_POINT('Ctrl Pts',(7.15359253542486,-27.948797567142,55.1399937211669));
#84642=CARTESIAN_POINT('Ctrl Pts',(7.15742616286845,-27.9560667657204,55.2105575843025));
#84643=CARTESIAN_POINT('Ctrl Pts',(7.16125834634855,-27.9633332263026,55.281094869049));
#84644=CARTESIAN_POINT('Ctrl Pts',(7.16509052982866,-27.9742586004218,55.3512863175633));
#84645=CARTESIAN_POINT('Ctrl Pts',(7.16892271330876,-27.9887844405815,55.420725012393));
#84646=CARTESIAN_POINT('Ctrl Pts',(7.1727547734992,-28.0033098134134,55.4901614732291));
#84647=CARTESIAN_POINT('Ctrl Pts',(7.17658683368964,-28.0214353197262,55.5588447472065));
#84648=CARTESIAN_POINT('Ctrl Pts',(7.18041889388008,-28.0430515099035,55.6263786152231));
#84649=CARTESIAN_POINT('Ctrl Pts',(7.184254856409,-28.0646897127022,55.693981255649));
#84650=CARTESIAN_POINT('Ctrl Pts',(7.18809081893791,-28.0898255470869,55.7604316831495));
#84651=CARTESIAN_POINT('Ctrl Pts',(7.19192678146683,-28.1183001035102,55.8253502662811));
#84652=CARTESIAN_POINT('Ctrl Pts',(7.19576473620228,-28.1467894481899,55.8903025648687));
#84653=CARTESIAN_POINT('Ctrl Pts',(7.19960269093773,-28.1786207452875,55.9537209954183));
#84654=CARTESIAN_POINT('Ctrl Pts',(7.20344064567318,-28.2135887279427,56.0152498852827));
#84655=CARTESIAN_POINT('Ctrl Pts',(7.20728565488564,-28.2486209846309,56.0768918703159));
#84656=CARTESIAN_POINT('Ctrl Pts',(7.2111306640981,-28.2868011751235,56.13663696377));
#84657=CARTESIAN_POINT('Ctrl Pts',(7.21497567331056,-28.3278806170888,56.1941584198894));
#84658=CARTESIAN_POINT('Ctrl Pts',(7.21791465037583,-28.3592801615682,56.2381256072106));
#84659=CARTESIAN_POINT('Ctrl Pts',(7.2208536274411,-28.3923726831846,56.280794230244));
#84660=CARTESIAN_POINT('Ctrl Pts',(7.22379260450636,-28.4270322754391,56.3220325638916));
#84661=CARTESIAN_POINT('Ctrl Pts',(7.22766167785587,-28.472660567773,56.3763215679058));
#84662=CARTESIAN_POINT('Ctrl Pts',(7.23153075120538,-28.521192108488,56.4283519319452));
#84663=CARTESIAN_POINT('Ctrl Pts',(7.23539982455489,-28.5723747010563,56.4777968630078));
#84664=CARTESIAN_POINT('Ctrl Pts',(7.23926313295198,-28.6234810311232,56.5271681206997));
#84665=CARTESIAN_POINT('Ctrl Pts',(7.24312644134906,-28.6772302256901,56.5739612573856));
#84666=CARTESIAN_POINT('Ctrl Pts',(7.24698974974614,-28.7333303795716,56.6178830721606));
#84667=CARTESIAN_POINT('Ctrl Pts',(7.25084852624035,-28.7893647244566,56.6617533638942));
#84668=CARTESIAN_POINT('Ctrl Pts',(7.25470730273456,-28.8477441700428,56.7027587261681));
#84669=CARTESIAN_POINT('Ctrl Pts',(7.25856607922877,-28.9081418597549,56.7406445254792));
#84670=CARTESIAN_POINT('Ctrl Pts',(7.26242242481827,-28.968501500871,56.7785064579589));
#84671=CARTESIAN_POINT('Ctrl Pts',(7.26627877040777,-29.0308764530672,56.8132524689205));
#84672=CARTESIAN_POINT('Ctrl Pts',(7.27013511599727,-29.0949100511598,56.844670633747));
#84673=CARTESIAN_POINT('Ctrl Pts',(7.27399032224389,-29.1589247307653,56.8760795161942));
#84674=CARTESIAN_POINT('Ctrl Pts',(7.27784552849051,-29.2245966475194,56.9041622905641));
#84675=CARTESIAN_POINT('Ctrl Pts',(7.28170073473713,-29.2915451873075,56.9287533126019));
#84676=CARTESIAN_POINT('Ctrl Pts',(7.28555609158967,-29.3584963424798,56.9533452953025));
#84677=CARTESIAN_POINT('Ctrl Pts',(7.2894114484422,-29.4267237629434,56.9744450894259));
#84678=CARTESIAN_POINT('Ctrl Pts',(7.29326680529473,-29.4958291746578,56.9919360786365));
#84679=CARTESIAN_POINT('Ctrl Pts',(7.29712619776456,-29.5650069228655,57.0094453766422));
#84680=CARTESIAN_POINT('Ctrl Pts',(7.30098559023439,-29.6350640250389,57.0233382094805));
#84681=CARTESIAN_POINT('Ctrl Pts',(7.30484498270421,-29.7055903194803,57.0335487460389));
#84682=CARTESIAN_POINT('Ctrl Pts',(7.30870656030891,-29.7761565449383,57.0437650636625));
#84683=CARTESIAN_POINT('Ctrl Pts',(7.3125681379136,-29.8471920075161,57.0502948901935));
#84684=CARTESIAN_POINT('Ctrl Pts',(7.3164297155183,-29.9182824477439,57.0531244005547));
#84685=CARTESIAN_POINT('Ctrl Pts',(7.3202980496344,-29.9894972732411,57.0559588616436));
#84686=CARTESIAN_POINT('Ctrl Pts',(7.32416638375051,-30.0607667825374,57.0550800863142));
#84687=CARTESIAN_POINT('Ctrl Pts',(7.32803471786662,-30.1316784465509,57.0505263590634));
#84688=CARTESIAN_POINT('Ctrl Pts',(7.33033243702605,-30.1737986678505,57.047821529016));
#84689=CARTESIAN_POINT('Ctrl Pts',(7.33263015618548,-30.2157927466636,57.0438211176024));
#84690=CARTESIAN_POINT('Ctrl Pts',(7.33492787534492,-30.2575759412518,57.0385416838976));
#84691=CARTESIAN_POINT('Ctrl Pts',(7.33879679455246,-30.3279308422981,57.0296521281913));
#84692=CARTESIAN_POINT('Ctrl Pts',(7.34266571376,-30.397962804919,57.0170987141503));
#84693=CARTESIAN_POINT('Ctrl Pts',(7.34653463296754,-30.4672605428605,57.0009160770971));
#84694=CARTESIAN_POINT('Ctrl Pts',(7.35048283886946,-30.5379784160581,56.98440180536));
#84695=CARTESIAN_POINT('Ctrl Pts',(7.35443104477139,-30.6079311216361,56.9641078764496));
#84696=CARTESIAN_POINT('Ctrl Pts',(7.35837925067332,-30.6766868505021,56.9401269208115));
#84697=CARTESIAN_POINT('Ctrl Pts',(7.36223788201552,-30.7438826900678,56.9166900309076));
#84698=CARTESIAN_POINT('Ctrl Pts',(7.36609651335773,-30.8099348054257,56.8897318132154));
#84699=CARTESIAN_POINT('Ctrl Pts',(7.36995514469993,-30.8744523799092,56.8593898455599));
#84700=CARTESIAN_POINT('Ctrl Pts',(7.37394813788172,-30.9412165281709,56.8279913368074));
#84701=CARTESIAN_POINT('Ctrl Pts',(7.37794113106351,-31.0063367702874,56.7929692085721));
#84702=CARTESIAN_POINT('Ctrl Pts',(7.3819341242453,-31.0694017134189,56.7545305747797));
#84703=CARTESIAN_POINT('Ctrl Pts',(7.38592711742709,-31.1324666565503,56.7160919409874));
#84704=CARTESIAN_POINT('Ctrl Pts',(7.38992011060888,-31.1934757962958,56.6742370852408));
#84705=CARTESIAN_POINT('Ctrl Pts',(7.39391310379067,-31.2520475724682,56.6292251037768));
#84706=CARTESIAN_POINT('Ctrl Pts',(6.69398930341885,-31.2520475724682,56.6292251037768));
#84707=CARTESIAN_POINT('Ctrl Pts',(6.69784740330321,-31.308493025076,56.5858471864156));
#84708=CARTESIAN_POINT('Ctrl Pts',(6.70170550318757,-31.3627399888065,56.5394875421447));
#84709=CARTESIAN_POINT('Ctrl Pts',(6.70556360307192,-31.414461700709,56.4904011740895));
#84710=CARTESIAN_POINT('Ctrl Pts',(6.70941957071704,-31.4661548277986,56.4413419343833));
#84711=CARTESIAN_POINT('Ctrl Pts',(6.71327553836214,-31.5153251205055,56.389559294783));
#84712=CARTESIAN_POINT('Ctrl Pts',(6.71713150600726,-31.5616800291382,56.3353475386921));
#84713=CARTESIAN_POINT('Ctrl Pts',(6.72098663248669,-31.6080248256118,56.2811476087037));
#84714=CARTESIAN_POINT('Ctrl Pts',(6.72484175896612,-31.6515551421313,56.2245199837088));
#84715=CARTESIAN_POINT('Ctrl Pts',(6.72869688544555,-31.6920175240008,56.1657934040705));
#84716=CARTESIAN_POINT('Ctrl Pts',(6.73255246051975,-31.7324846142015,56.1070599908209));
#84717=CARTESIAN_POINT('Ctrl Pts',(6.73640803559394,-31.7698827875426,56.0462275395085));
#84718=CARTESIAN_POINT('Ctrl Pts',(6.74026361066813,-31.8040018700035,55.9836538087783));
#84719=CARTESIAN_POINT('Ctrl Pts',(6.74412340477226,-31.8381582878624,55.9210116056574));
#84720=CARTESIAN_POINT('Ctrl Pts',(6.74798319887639,-31.8690282224839,55.8566247484985));
#84721=CARTESIAN_POINT('Ctrl Pts',(6.75184299298052,-31.8964478925107,55.7908748026658));
#84722=CARTESIAN_POINT('Ctrl Pts',(6.75570523999021,-31.9238849877834,55.7250830726333));
#84723=CARTESIAN_POINT('Ctrl Pts',(6.7595674869999,-31.947867292199,55.6579269875362));
#84724=CARTESIAN_POINT('Ctrl Pts',(6.7634297340096,-31.9682804681214,55.5898046806459));
#84725=CARTESIAN_POINT('Ctrl Pts',(6.76729847021428,-31.9887279414562,55.5215679173444));
#84726=CARTESIAN_POINT('Ctrl Pts',(6.77116720641896,-32.0055942063419,55.4523621643166));
#84727=CARTESIAN_POINT('Ctrl Pts',(6.77503594262364,-32.018815894643,55.3825963225603));
#84728=CARTESIAN_POINT('Ctrl Pts',(6.77644113546647,-32.0236182437276,55.3572561452198));
#84729=CARTESIAN_POINT('Ctrl Pts',(6.7778463283093,-32.0279402711051,55.3318421247497));
#84730=CARTESIAN_POINT('Ctrl Pts',(6.77925152115213,-32.0317806392833,55.3063739485232));
#84731=CARTESIAN_POINT('Ctrl Pts',(6.78312059450031,-32.042354751044,55.2362495934447));
#84732=CARTESIAN_POINT('Ctrl Pts',(6.78698966784849,-32.0493149318717,55.1654398123004));
#84733=CARTESIAN_POINT('Ctrl Pts',(6.79085874119666,-32.0525826818245,55.094349863667));
#84734=CARTESIAN_POINT('Ctrl Pts',(6.79472204959242,-32.0558455628019,55.0233658396658));
#84735=CARTESIAN_POINT('Ctrl Pts',(6.79858535798817,-32.0554269116062,54.9521029581258));
#84736=CARTESIAN_POINT('Ctrl Pts',(6.80244866638393,-32.0512996831102,54.8809740676497));
#84737=CARTESIAN_POINT('Ctrl Pts',(6.8063074428768,-32.0471772961119,54.8099286158201));
#84738=CARTESIAN_POINT('Ctrl Pts',(6.81016621936967,-32.0393550011702,54.7390173254582));
#84739=CARTESIAN_POINT('Ctrl Pts',(6.81402499586255,-32.0278577964953,54.6686537767027));
#84740=CARTESIAN_POINT('Ctrl Pts',(6.81788134145071,-32.0163678346884,54.5983345547129));
#84741=CARTESIAN_POINT('Ctrl Pts',(6.82173768703888,-32.0012076343708,54.5285628680314));
#84742=CARTESIAN_POINT('Ctrl Pts',(6.82559403262705,-31.982453945114,54.4597464317546));
#84743=CARTESIAN_POINT('Ctrl Pts',(6.82944923887234,-31.9637057965646,54.3909503270365));
#84744=CARTESIAN_POINT('Ctrl Pts',(6.83330444511763,-31.9413663944681,54.3231093808663));
#84745=CARTESIAN_POINT('Ctrl Pts',(6.83715965136292,-31.9155630461784,54.2566186855888));
#84746=CARTESIAN_POINT('Ctrl Pts',(6.84101500821413,-31.8897586898656,54.1901253928129));
#84747=CARTESIAN_POINT('Ctrl Pts',(6.84487036506534,-31.8604902965015,54.1249829077371));
#84748=CARTESIAN_POINT('Ctrl Pts',(6.84872572191655,-31.8279336356115,54.0615671647368));
#84749=CARTESIAN_POINT('Ctrl Pts',(6.85258511438507,-31.7953428958465,53.998085040937));
#84750=CARTESIAN_POINT('Ctrl Pts',(6.85644450685359,-31.7594572398435,53.9363337003911));
#84751=CARTESIAN_POINT('Ctrl Pts',(6.8603038993221,-31.7204984022283,53.876664426616));
#84752=CARTESIAN_POINT('Ctrl Pts',(6.8641654769255,-31.6815175066557,53.8169613689197));
#84753=CARTESIAN_POINT('Ctrl Pts',(6.8680270545289,-31.6394602522241,53.7593431172581));
#84754=CARTESIAN_POINT('Ctrl Pts',(6.87188863213229,-31.5945901053133,53.7041296521114));
#84755=CARTESIAN_POINT('Ctrl Pts',(6.87575696624712,-31.5496414501626,53.6488195812642));
#84756=CARTESIAN_POINT('Ctrl Pts',(6.87962530036195,-31.501870402007,53.5959230581635));
#84757=CARTESIAN_POINT('Ctrl Pts',(6.88349363447679,-31.4515783840528,53.5457243186209));
#84758=CARTESIAN_POINT('Ctrl Pts',(6.88579135364809,-31.4217058522635,53.515907192489));
#84759=CARTESIAN_POINT('Ctrl Pts',(6.88808907281939,-31.3909445592811,53.4870411428943));
#84760=CARTESIAN_POINT('Ctrl Pts',(6.89038679199069,-31.3593629475622,53.4591788100837));
#84761=CARTESIAN_POINT('Ctrl Pts',(6.89425586533907,-31.306183440803,53.4122621064901));
#84762=CARTESIAN_POINT('Ctrl Pts',(6.89812493868745,-31.2504680114044,53.3680098732096));
#84763=CARTESIAN_POINT('Ctrl Pts',(6.90199401203584,-31.1925145591998,53.3267078591601));
#84764=CARTESIAN_POINT('Ctrl Pts',(6.9058573204318,-31.1346474581352,53.2854673854652));
#84765=CARTESIAN_POINT('Ctrl Pts',(6.90972062882776,-31.0745493458754,53.2471686849971));
#84766=CARTESIAN_POINT('Ctrl Pts',(6.91358393722373,-31.0125524062089,53.2120583938002));
#84767=CARTESIAN_POINT('Ctrl Pts',(6.91744271371681,-30.9506281928385,53.1769892891753));
#84768=CARTESIAN_POINT('Ctrl Pts',(6.92130149020989,-30.8868099971729,53.1451014027383));
#84769=CARTESIAN_POINT('Ctrl Pts',(6.92516026670297,-30.8214588440329,53.1165980434171));
#84770=CARTESIAN_POINT('Ctrl Pts',(6.92901661229135,-30.7561488600111,53.0881126402929));
#84771=CARTESIAN_POINT('Ctrl Pts',(6.93287295787973,-30.6893082786984,53.0630077278985));
#84772=CARTESIAN_POINT('Ctrl Pts',(6.93672930346811,-30.6213212655178,53.0414399556012));
#84773=CARTESIAN_POINT('Ctrl Pts',(6.94058450971361,-30.553354338846,53.0198785554216));
#84774=CARTESIAN_POINT('Ctrl Pts',(6.94443971595911,-30.4842421155299,53.001852367469));
#84775=CARTESIAN_POINT('Ctrl Pts',(6.94829492220461,-30.4143855767945,52.9874687191885));
#84776=CARTESIAN_POINT('Ctrl Pts',(6.95215027905603,-30.3445263090721,52.9730845090023));
#84777=CARTESIAN_POINT('Ctrl Pts',(6.95600563590744,-30.2739231444505,52.9623432168141));
#84778=CARTESIAN_POINT('Ctrl Pts',(6.95986099275886,-30.2029872528514,52.9553010642934));
#84779=CARTESIAN_POINT('Ctrl Pts',(6.96372038522758,-30.1319771086933,52.9482515403583));
#84780=CARTESIAN_POINT('Ctrl Pts',(6.96757977769631,-30.0606340267051,52.9449089337532));
#84781=CARTESIAN_POINT('Ctrl Pts',(6.97143917016503,-29.9893733963683,52.9452774791239));
#84782=CARTESIAN_POINT('Ctrl Pts',(6.97530074776863,-29.9180724192437,52.94564623316));
#84783=CARTESIAN_POINT('Ctrl Pts',(6.97916232537224,-29.846854471921,52.9497302941936));
#84784=CARTESIAN_POINT('Ctrl Pts',(6.98302390297584,-29.7761312786414,52.9574818585635));
#84785=CARTESIAN_POINT('Ctrl Pts',(6.98689223709087,-29.7052843426554,52.965246985663));
#84786=CARTESIAN_POINT('Ctrl Pts',(6.9907605712059,-29.6349343686608,52.9766923496816));
#84787=CARTESIAN_POINT('Ctrl Pts',(6.99462890532094,-29.5654836366656,52.9917188711501));
#84788=CARTESIAN_POINT('Ctrl Pts',(6.99692662449037,-29.5242311818642,53.0006443479578));
#84789=CARTESIAN_POINT('Ctrl Pts',(6.99922434365981,-29.4832957357369,53.0108323415112));
#84790=CARTESIAN_POINT('Ctrl Pts',(7.00152206282925,-29.4427586443784,53.0222539005006));
#84791=CARTESIAN_POINT('Ctrl Pts',(7.00539113617725,-29.3744992235288,53.0414863855086));
#84792=CARTESIAN_POINT('Ctrl Pts',(7.00926020952525,-29.3071029468862,53.0642945225907));
#84793=CARTESIAN_POINT('Ctrl Pts',(7.01312928287325,-29.2409714547338,53.0905830130715));
#84794=CARTESIAN_POINT('Ctrl Pts',(7.01699259126881,-29.1749384990712,53.1168323334763));
#84795=CARTESIAN_POINT('Ctrl Pts',(7.02085589966438,-29.1101670348887,53.1465515357107));
#84796=CARTESIAN_POINT('Ctrl Pts',(7.02471920805995,-29.0470444364269,53.1795953042372));
#84797=CARTESIAN_POINT('Ctrl Pts',(7.02857798455265,-28.983995884729,53.2126003103524));
#84798=CARTESIAN_POINT('Ctrl Pts',(7.03243676104536,-28.9225927850239,53.2489219119851));
#84799=CARTESIAN_POINT('Ctrl Pts',(7.03629553753807,-28.8632017528946,53.2883670639187));
#84800=CARTESIAN_POINT('Ctrl Pts',(7.04015188312606,-28.8038481351997,53.3277873666791));
#84801=CARTESIAN_POINT('Ctrl Pts',(7.04400822871406,-28.7465044740157,53.3703270476567));
#84802=CARTESIAN_POINT('Ctrl Pts',(7.04786457430206,-28.6915107348276,53.4157483137366));
#84803=CARTESIAN_POINT('Ctrl Pts',(7.05171978054718,-28.636533243334,53.4611561602734));
#84804=CARTESIAN_POINT('Ctrl Pts',(7.0555749867923,-28.5839046698531,53.5094435925543));
#84805=CARTESIAN_POINT('Ctrl Pts',(7.05943019303743,-28.5339326626621,53.5603319393378));
#84806=CARTESIAN_POINT('Ctrl Pts',(7.06328554988848,-28.4839587032848,53.6112222741048));
#84807=CARTESIAN_POINT('Ctrl Pts',(7.06714090673953,-28.4366418550357,53.6647133769478));
#84808=CARTESIAN_POINT('Ctrl Pts',(7.07099626359058,-28.3922523559867,53.72049029872));
#84809=CARTESIAN_POINT('Ctrl Pts',(7.07485565605895,-28.3478163919701,53.776325605311));
#84810=CARTESIAN_POINT('Ctrl Pts',(7.07871504852731,-28.3063141971478,53.8344511263024));
#84811=CARTESIAN_POINT('Ctrl Pts',(7.08257444099567,-28.2679746215663,53.894520171617));
#84812=CARTESIAN_POINT('Ctrl Pts',(7.08643601859892,-28.2296133386449,53.9546232271981));
#84813=CARTESIAN_POINT('Ctrl Pts',(7.09029759620216,-28.1944184793473,54.0166715749077));
#84814=CARTESIAN_POINT('Ctrl Pts',(7.0941591738054,-28.1625731861767,54.0802933802874));
#84815=CARTESIAN_POINT('Ctrl Pts',(7.09802750792009,-28.1306721740462,54.1440265032425));
#84816=CARTESIAN_POINT('Ctrl Pts',(7.10189584203478,-28.1021326235921,54.2093381351123));
#84817=CARTESIAN_POINT('Ctrl Pts',(7.10576417614946,-28.0770894760653,54.2758365657938));
#84818=CARTESIAN_POINT('Ctrl Pts',(7.10806189532224,-28.0622143079664,54.3153354080879));
#84819=CARTESIAN_POINT('Ctrl Pts',(7.11035961449502,-28.0485717693018,54.3552526613278));
#84820=CARTESIAN_POINT('Ctrl Pts',(7.1126573336678,-28.0361816560159,54.3955042809652));
#84821=CARTESIAN_POINT('Ctrl Pts',(7.11737359946004,-28.0107498851777,54.4781241846623));
#84822=CARTESIAN_POINT('Ctrl Pts',(7.12208986525227,-27.9905162579312,54.5624145979724));
#84823=CARTESIAN_POINT('Ctrl Pts',(7.12680613104451,-27.9756629418006,54.6477826845532));
#84824=CARTESIAN_POINT('Ctrl Pts',(7.13145774528264,-27.9610132380222,54.7319805276169));
#84825=CARTESIAN_POINT('Ctrl Pts',(7.13610935952078,-27.9515973927135,54.8172267077131));
#84826=CARTESIAN_POINT('Ctrl Pts',(7.14076097375891,-27.9475440844109,54.9029315856555));
#84827=CARTESIAN_POINT('Ctrl Pts',(7.14248240933954,-27.9460440655413,54.9346486238212));
#84828=CARTESIAN_POINT('Ctrl Pts',(7.14420384492016,-27.9452780035318,54.9664282743128));
#84829=CARTESIAN_POINT('Ctrl Pts',(7.14592528050078,-27.9452507538412,54.9982399120147));
#84830=CARTESIAN_POINT('Origin',(-1.54592528053767,-30.,55.));
#84831=CARTESIAN_POINT('',(5.99388650793247,-31.2520475724682,56.6292251037768));
#84832=CARTESIAN_POINT('',(6.05208116158501,-31.2520475724682,56.6292251037768));
#84833=CARTESIAN_POINT('',(-1.54592528053767,-31.2520475724682,56.6292251037768));
#84834=CARTESIAN_POINT('',(6.50407471951138,-27.9452500572952,55.0004852364684));
#84835=CARTESIAN_POINT('Ctrl Pts',(6.05208116158501,-31.2520475724682,56.6292251037768));
#84836=CARTESIAN_POINT('Ctrl Pts',(6.0559362959734,-31.3085979670454,56.5857665392798));
#84837=CARTESIAN_POINT('Ctrl Pts',(6.05979143036179,-31.3628880122941,56.5393564204563));
#84838=CARTESIAN_POINT('Ctrl Pts',(6.06364656475018,-31.4146037916008,56.4902663101904));
#84839=CARTESIAN_POINT('Ctrl Pts',(6.06753147774187,-31.4667190443164,56.4407970082357));
#84840=CARTESIAN_POINT('Ctrl Pts',(6.07141639073356,-31.5162197110505,56.3886064605778));
#84841=CARTESIAN_POINT('Ctrl Pts',(6.07530130372524,-31.5628224452354,56.3340103324819));
#84842=CARTESIAN_POINT('Ctrl Pts',(6.07916181883121,-31.6091325066665,56.2797570769541));
#84843=CARTESIAN_POINT('Ctrl Pts',(6.08302233393717,-31.6525806774308,56.22312879422));
#84844=CARTESIAN_POINT('Ctrl Pts',(6.08688284904313,-31.6929308605673,56.1644666864445));
#84845=CARTESIAN_POINT('Ctrl Pts',(6.09077996097768,-31.7336635545073,56.1052484748735));
#84846=CARTESIAN_POINT('Ctrl Pts',(6.09467707291223,-31.7712389448945,56.0439581022323));
#84847=CARTESIAN_POINT('Ctrl Pts',(6.09857418484678,-31.8054613055032,55.9809724954507));
#84848=CARTESIAN_POINT('Ctrl Pts',(6.10247129678132,-31.8396836661119,55.917986888669));
#84849=CARTESIAN_POINT('Ctrl Pts',(6.10636840871587,-31.8705528390726,55.8533065288065));
#84850=CARTESIAN_POINT('Ctrl Pts',(6.11026552065042,-31.8979233773647,55.7873273881637));
#84851=CARTESIAN_POINT('Ctrl Pts',(6.11413459399863,-31.9250969925984,55.7218229482382));
#84852=CARTESIAN_POINT('Ctrl Pts',(6.11800366734685,-31.9489286475827,55.6547817560974));
#84853=CARTESIAN_POINT('Ctrl Pts',(6.12187274069506,-31.9692444247994,55.5865781771397));
#84854=CARTESIAN_POINT('Ctrl Pts',(6.12573604909085,-31.989529931334,55.5184762220989));
#84855=CARTESIAN_POINT('Ctrl Pts',(6.12959935748663,-32.0063098212,55.4492157799231));
#84856=CARTESIAN_POINT('Ctrl Pts',(6.13346266588242,-32.0194582824912,55.379190991161));
#84857=CARTESIAN_POINT('Ctrl Pts',(6.13732144237533,-32.0325913198133,55.3092483458648));
#84858=CARTESIAN_POINT('Ctrl Pts',(6.14118021886824,-32.0421013009359,55.2385436101106));
#84859=CARTESIAN_POINT('Ctrl Pts',(6.14503899536115,-32.0479127447516,55.167484185474));
#84860=CARTESIAN_POINT('Ctrl Pts',(6.14889534094935,-32.0537205275452,55.0964695259825));
#84861=CARTESIAN_POINT('Ctrl Pts',(6.15275168653756,-32.0558343561298,55.0251011039399));
#84862=CARTESIAN_POINT('Ctrl Pts',(6.15660803212577,-32.0542303877086,54.9537931096617));
#84863=CARTESIAN_POINT('Ctrl Pts',(6.1604632383711,-32.0526268931738,54.8825061830636));
#84864=CARTESIAN_POINT('Ctrl Pts',(6.16431844461643,-32.0473077931978,54.8112801341851));
#84865=CARTESIAN_POINT('Ctrl Pts',(6.16817365086176,-32.0383013546747,54.740529095983));
#84866=CARTESIAN_POINT('Ctrl Pts',(6.17202900771301,-32.0292945643097,54.6697752938498));
#84867=CARTESIAN_POINT('Ctrl Pts',(6.17588436456425,-32.0166002129385,54.5994970208538));
#84868=CARTESIAN_POINT('Ctrl Pts',(6.17973972141549,-32.0002982194621,54.5301015048793));
#84869=CARTESIAN_POINT('Ctrl Pts',(6.18359911388405,-31.9839791617788,54.460633348743));
#84870=CARTESIAN_POINT('Ctrl Pts',(6.18745850635261,-31.9640450349276,54.3920502680834));
#84871=CARTESIAN_POINT('Ctrl Pts',(6.19131789882116,-31.9406263111478,54.3247466527437));
#84872=CARTESIAN_POINT('Ctrl Pts',(6.19517947642459,-31.9171943280091,54.2574049310237));
#84873=CARTESIAN_POINT('Ctrl Pts',(6.19904105402802,-31.8902740038575,54.1913445667913));
#84874=CARTESIAN_POINT('Ctrl Pts',(6.20290263163145,-31.8600438601551,54.126939635077));
#84875=CARTESIAN_POINT('Ctrl Pts',(6.20677096574632,-31.8297608234817,54.0624220155696));
#84876=CARTESIAN_POINT('Ctrl Pts',(6.21063929986119,-31.7961566342393,53.9995660400106));
#84877=CARTESIAN_POINT('Ctrl Pts',(6.21450763397606,-31.7594552707764,53.9387202477022));
#84878=CARTESIAN_POINT('Ctrl Pts',(6.21680535314703,-31.7376553372842,53.9025789684568));
#84879=CARTESIAN_POINT('Ctrl Pts',(6.21910307231801,-31.7147635080574,53.8671463546765));
#84880=CARTESIAN_POINT('Ctrl Pts',(6.22140079148898,-31.6908335103588,53.8324899988661));
#84881=CARTESIAN_POINT('Ctrl Pts',(6.22526986483718,-31.6505383700789,53.7741330054153));
#84882=CARTESIAN_POINT('Ctrl Pts',(6.22913893818539,-31.60713957811,53.7177502591309));
#84883=CARTESIAN_POINT('Ctrl Pts',(6.2330080115336,-31.5608573285146,53.6636909180425));
#84884=CARTESIAN_POINT('Ctrl Pts',(6.23687131992938,-31.5146440398674,53.6097121258351));
#84885=CARTESIAN_POINT('Ctrl Pts',(6.24073462832517,-31.4655561351378,53.5580502330749));
#84886=CARTESIAN_POINT('Ctrl Pts',(6.24459793672096,-31.4138565131095,53.5090247075026));
#84887=CARTESIAN_POINT('Ctrl Pts',(6.24845671321387,-31.3622175379781,53.4600566919444));
#84888=CARTESIAN_POINT('Ctrl Pts',(6.25231548970677,-31.3079732818955,53.4137192332199));
#84889=CARTESIAN_POINT('Ctrl Pts',(6.25617426619967,-31.251425082429,53.3702967062783));
#84890=CARTESIAN_POINT('Ctrl Pts',(6.26003061178787,-31.194912506504,53.3269015341278));
#84891=CARTESIAN_POINT('Ctrl Pts',(6.26388695737607,-31.1360992511543,53.2864179457087));
#84892=CARTESIAN_POINT('Ctrl Pts',(6.26774330296427,-31.0753203642288,53.249090614345));
#84893=CARTESIAN_POINT('Ctrl Pts',(6.27159850920959,-31.014559434198,53.2117743112016));
#84894=CARTESIAN_POINT('Ctrl Pts',(6.27545371545491,-30.9518344392441,53.1776126679242));
#84895=CARTESIAN_POINT('Ctrl Pts',(6.27930892170023,-30.8875086414516,53.1468065471061));
#84896=CARTESIAN_POINT('Ctrl Pts',(6.28316427855146,-30.8231803307336,53.1159992228286));
#84897=CARTESIAN_POINT('Ctrl Pts',(6.2870196354027,-30.7572515321044,53.0885478891026));
#84898=CARTESIAN_POINT('Ctrl Pts',(6.29087499225394,-30.6901077205897,53.0646062683571));
#84899=CARTESIAN_POINT('Ctrl Pts',(6.29473438472249,-30.6228936258978,53.0406395865802));
#84900=CARTESIAN_POINT('Ctrl Pts',(6.29859377719104,-30.5544624379835,53.0201901150296));
#84901=CARTESIAN_POINT('Ctrl Pts',(6.30245316965959,-30.4852162643896,53.0033621411804));
#84902=CARTESIAN_POINT('Ctrl Pts',(6.30631474726301,-30.4159308845658,52.9865246395641));
#84903=CARTESIAN_POINT('Ctrl Pts',(6.31017632486644,-30.3458300780981,52.9733128074614));
#84904=CARTESIAN_POINT('Ctrl Pts',(6.31403790246986,-30.2753249453433,52.9637795460777));
#84905=CARTESIAN_POINT('Ctrl Pts',(6.31790623658473,-30.2046964514173,52.9542296045709));
#84906=CARTESIAN_POINT('Ctrl Pts',(6.32177457069959,-30.1336627030752,52.9483711240021));
#84907=CARTESIAN_POINT('Ctrl Pts',(6.32564290481446,-30.0626380011789,52.9462049656043));
#84908=CARTESIAN_POINT('Ctrl Pts',(6.32794062398548,-30.0204506372341,52.9449183074382));
#84909=CARTESIAN_POINT('Ctrl Pts',(6.33023834315651,-29.9782664489834,52.9449333531371));
#84910=CARTESIAN_POINT('Ctrl Pts',(6.33253606232754,-29.9361713635722,52.9462416238341));
#84911=CARTESIAN_POINT('Ctrl Pts',(6.33640513567578,-29.8652884745271,52.948444588996));
#84912=CARTESIAN_POINT('Ctrl Pts',(6.34027420902402,-29.7943809273119,52.9543258278911));
#84913=CARTESIAN_POINT('Ctrl Pts',(6.34414328237226,-29.7238614901472,52.9638897166714));
#84914=CARTESIAN_POINT('Ctrl Pts',(6.34800659076806,-29.6534471275482,52.9734393551756));
#84915=CARTESIAN_POINT('Ctrl Pts',(6.35186989916386,-29.5834202045728,52.986660686914));
#84916=CARTESIAN_POINT('Ctrl Pts',(6.35573320755966,-29.514191706844,53.0035061069964));
#84917=CARTESIAN_POINT('Ctrl Pts',(6.3595919840526,-29.4450444184816,53.0203317663452));
#84918=CARTESIAN_POINT('Ctrl Pts',(6.36345076054553,-29.3766941646777,53.0407729552545));
#84919=CARTESIAN_POINT('Ctrl Pts',(6.36730953703847,-29.3095432958884,53.0647307416674));
#84920=CARTESIAN_POINT('Ctrl Pts',(6.37116588262669,-29.2424347299802,53.0886734354476));
#84921=CARTESIAN_POINT('Ctrl Pts',(6.37502222821492,-29.1765245064967,53.1161281686743));
#84922=CARTESIAN_POINT('Ctrl Pts',(6.37887857380315,-29.1121999040753,53.1469461550791));
#84923=CARTESIAN_POINT('Ctrl Pts',(6.3827337800485,-29.047894306117,53.1777550364251));
#84924=CARTESIAN_POINT('Ctrl Pts',(6.38658898629385,-28.9851738370485,53.2119249884776));
#84925=CARTESIAN_POINT('Ctrl Pts',(6.3904441925392,-28.9244042705919,53.2492597595934));
#84926=CARTESIAN_POINT('Ctrl Pts',(6.39429954939044,-28.8636323301366,53.2865959892138));
#84927=CARTESIAN_POINT('Ctrl Pts',(6.39815490624169,-28.8048118563631,53.3270970271894));
#84928=CARTESIAN_POINT('Ctrl Pts',(6.40201026309293,-28.7482810659899,53.3705223926851));
#84929=CARTESIAN_POINT('Ctrl Pts',(6.40586965556151,-28.6916911016811,53.4139932139362));
#84930=CARTESIAN_POINT('Ctrl Pts',(6.4097290480301,-28.6373959912352,53.460394176726));
#84931=CARTESIAN_POINT('Ctrl Pts',(6.41358844049868,-28.5857014397924,53.5094440147734));
#84932=CARTESIAN_POINT('Ctrl Pts',(6.41745001810214,-28.5339776196065,53.5585216241637));
#84933=CARTESIAN_POINT('Ctrl Pts',(6.4213115957056,-28.4848576241816,53.6102507419261));
#84934=CARTESIAN_POINT('Ctrl Pts',(6.42517317330906,-28.4386088641938,53.6643146764579));
#84935=CARTESIAN_POINT('Ctrl Pts',(6.42904150742395,-28.3922791838392,53.7184732053833));
#84936=CARTESIAN_POINT('Ctrl Pts',(6.43290984153884,-28.3488310651725,53.7749743220315));
#84937=CARTESIAN_POINT('Ctrl Pts',(6.43677817565373,-28.3084899336607,53.8334704213039));
#84938=CARTESIAN_POINT('Ctrl Pts',(6.43907589482452,-28.2845280450304,53.8682160261878));
#84939=CARTESIAN_POINT('Ctrl Pts',(6.44137361399531,-28.2616614968995,53.9036649604587));
#84940=CARTESIAN_POINT('Ctrl Pts',(6.4436713331661,-28.2399297696001,53.9397404343464));
#84941=CARTESIAN_POINT('Ctrl Pts',(6.44766818401096,-28.2021277293329,54.0024932242084));
#84942=CARTESIAN_POINT('Ctrl Pts',(6.45166503485582,-28.1676219954086,54.0673751957459));
#84943=CARTESIAN_POINT('Ctrl Pts',(6.45566188570067,-28.1366498578021,54.1340185856088));
#84944=CARTESIAN_POINT('Ctrl Pts',(6.45969628851415,-28.1053867249134,54.2012881160463));
#84945=CARTESIAN_POINT('Ctrl Pts',(6.46373069132762,-28.0777242453427,54.2703519944481));
#84946=CARTESIAN_POINT('Ctrl Pts',(6.46776509414109,-28.0538611856042,54.3408025503673));
#84947=CARTESIAN_POINT('Ctrl Pts',(6.4717464869999,-28.0303116740595,54.4103274226233));
#84948=CARTESIAN_POINT('Ctrl Pts',(6.4757278798587,-28.0104625063917,54.4812023266614));
#84949=CARTESIAN_POINT('Ctrl Pts',(6.47970927271751,-27.9944576731887,54.5530128213601));
#84950=CARTESIAN_POINT('Ctrl Pts',(6.48377018050831,-27.9781331972706,54.6262574891748));
#84951=CARTESIAN_POINT('Ctrl Pts',(6.48783108829911,-27.9658084880446,54.7004751038003));
#84952=CARTESIAN_POINT('Ctrl Pts',(6.49189199608992,-27.9575832299835,54.7752083185357));
#84953=CARTESIAN_POINT('Ctrl Pts',(6.49595290388072,-27.9493579719225,54.8499415332711));
#84954=CARTESIAN_POINT('Ctrl Pts',(6.50001381167153,-27.9452322760607,54.9251898673996));
#84955=CARTESIAN_POINT('Ctrl Pts',(6.50407471946233,-27.9452500572949,55.000485235559));
#84956=CARTESIAN_POINT('Ctrl Pts',(6.50407471951138,-27.9452500572952,55.0004852364684));
#84957=CARTESIAN_POINT('Ctrl Pts',(6.50830237655248,-27.9452685686983,55.078872387755));
#84958=CARTESIAN_POINT('Ctrl Pts',(6.51253003359359,-27.9497773969995,55.1571404354878));
#84959=CARTESIAN_POINT('Ctrl Pts',(6.5167576906347,-27.9587077545003,55.2347840091714));
#84960=CARTESIAN_POINT('Ctrl Pts',(6.52089243721875,-27.9674418511433,55.3107212240261));
#84961=CARTESIAN_POINT('Ctrl Pts',(6.52502718380281,-27.9804049307443,55.3860607936642));
#84962=CARTESIAN_POINT('Ctrl Pts',(6.52916193038687,-27.9974813727946,55.4603441214953));
#84963=CARTESIAN_POINT('Ctrl Pts',(6.5334360426565,-28.0151333930587,55.537131241687));
#84964=CARTESIAN_POINT('Ctrl Pts',(6.53771015492613,-28.0371808331558,55.6127892221116));
#84965=CARTESIAN_POINT('Ctrl Pts',(6.54198426719577,-28.0634417891518,55.6868332101001));
#84966=CARTESIAN_POINT('Ctrl Pts',(6.5462583794654,-28.0897027451478,55.7608771980886));
#84967=CARTESIAN_POINT('Ctrl Pts',(6.55053249173503,-28.1201769686499,55.8333068289191));
#84968=CARTESIAN_POINT('Ctrl Pts',(6.55480660400466,-28.1546308748034,55.903664956868));
#84969=CARTESIAN_POINT('Ctrl Pts',(6.55867567735284,-28.1858197349993,55.967355552833));
#84970=CARTESIAN_POINT('Ctrl Pts',(6.56254475070101,-28.2203708581139,56.0295543399142));
#84971=CARTESIAN_POINT('Ctrl Pts',(6.56641382404919,-28.2581183028436,56.0898833495433));
#84972=CARTESIAN_POINT('Ctrl Pts',(6.57027713244494,-28.2958095035574,56.1501224684313));
#84973=CARTESIAN_POINT('Ctrl Pts',(6.57414044084069,-28.3366873167933,56.2084969315059));
#84974=CARTESIAN_POINT('Ctrl Pts',(6.57800374923644,-28.3805391633643,56.2646517944095));
#84975=CARTESIAN_POINT('Ctrl Pts',(6.58186252572931,-28.4243395689709,56.3207407841395));
#84976=CARTESIAN_POINT('Ctrl Pts',(6.58572130222218,-28.4711067805808,56.3746149645711));
#84977=CARTESIAN_POINT('Ctrl Pts',(6.58958007871506,-28.5205849981006,56.4259483913014));
#84978=CARTESIAN_POINT('Ctrl Pts',(6.59343642430322,-28.5700320459395,56.4772494796288));
#84979=CARTESIAN_POINT('Ctrl Pts',(6.59729276989139,-28.622186375022,56.5260126408675));
#84980=CARTESIAN_POINT('Ctrl Pts',(6.60114911547956,-28.6767529565492,56.5719461900774));
#84981=CARTESIAN_POINT('Ctrl Pts',(6.60500432172485,-28.7313034165841,56.6178661683919));
#84982=CARTESIAN_POINT('Ctrl Pts',(6.60885952797014,-28.7882643427362,56.6609578816927));
#84983=CARTESIAN_POINT('Ctrl Pts',(6.61271473421543,-28.8473063029057,56.7009687837168));
#84984=CARTESIAN_POINT('Ctrl Pts',(6.61657009106664,-28.9063505695843,56.7409812487906));
#84985=CARTESIAN_POINT('Ctrl Pts',(6.62042544791785,-28.9674756283041,56.7779123929436));
#84986=CARTESIAN_POINT('Ctrl Pts',(6.62428080476905,-29.0303230844249,56.8115529917451));
#84987=CARTESIAN_POINT('Ctrl Pts',(6.62814019723757,-29.0932363264876,56.84522880404));
#84988=CARTESIAN_POINT('Ctrl Pts',(6.63199958970609,-29.157875135837,56.87560696547));
#84989=CARTESIAN_POINT('Ctrl Pts',(6.63585898217461,-29.2238573333837,56.9025246709459));
#84990=CARTESIAN_POINT('Ctrl Pts',(6.639720559778,-29.2898768891422,56.929457616856));
#84991=CARTESIAN_POINT('Ctrl Pts',(6.64358213738139,-29.3572408882721,56.9529260466306));
#84992=CARTESIAN_POINT('Ctrl Pts',(6.64744371498479,-29.425550632775,56.9728166379557));
#84993=CARTESIAN_POINT('Ctrl Pts',(6.65131204909962,-29.4939798972298,56.9927420313802));
#84994=CARTESIAN_POINT('Ctrl Pts',(6.65518038321445,-29.5633577378047,57.0090769765956));
#84995=CARTESIAN_POINT('Ctrl Pts',(6.65904871732928,-29.633274568757,57.0217591401004));
#84996=CARTESIAN_POINT('Ctrl Pts',(6.6613464365006,-29.6748038777845,57.0292921114917));
#84997=CARTESIAN_POINT('Ctrl Pts',(6.6636441556719,-29.7165232177405,57.0355373207604));
#84998=CARTESIAN_POINT('Ctrl Pts',(6.66594187484321,-29.7583463546465,57.0404904013955));
#84999=CARTESIAN_POINT('Ctrl Pts',(6.66980984683663,-29.8287512693327,57.048828399101));
#85000=CARTESIAN_POINT('Ctrl Pts',(6.67367781883005,-29.8997260959449,57.0535345806531));
#85001=CARTESIAN_POINT('Ctrl Pts',(6.67754579082347,-29.9708636354741,57.0545434127227));
#85002=CARTESIAN_POINT('Ctrl Pts',(6.68140849503898,-30.04190429303,57.0555508708674));
#85003=CARTESIAN_POINT('Ctrl Pts',(6.68527119925449,-30.1131067427456,57.0528709610101));
#85004=CARTESIAN_POINT('Ctrl Pts',(6.68913390347,-30.184057680519,57.0464897587679));
#85005=CARTESIAN_POINT('Ctrl Pts',(6.69299263966152,-30.2549357328196,57.0401151117167));
#85006=CARTESIAN_POINT('Ctrl Pts',(6.69685137585305,-30.3255623046268,57.0300467605916));
#85007=CARTESIAN_POINT('Ctrl Pts',(6.70071011204457,-30.3955248305998,57.0163228091947));
#85008=CARTESIAN_POINT('Ctrl Pts',(6.70456617531123,-30.4654388939246,57.0026083643018));
#85009=CARTESIAN_POINT('Ctrl Pts',(6.7084222385779,-30.5346893492482,56.9852434401783));
#85010=CARTESIAN_POINT('Ctrl Pts',(6.71227830184456,-30.6028712102003,56.9643176592424));
#85011=CARTESIAN_POINT('Ctrl Pts',(6.71613400849585,-30.6710467655764,56.9433938135588));
#85012=CARTESIAN_POINT('Ctrl Pts',(6.71998971514715,-30.7381534548819,56.9189098952706));
#85013=CARTESIAN_POINT('Ctrl Pts',(6.72384542179844,-30.803800270683,56.8910057343514));
#85014=CARTESIAN_POINT('Ctrl Pts',(6.72770090164934,-30.8694432250069,56.8631032148109));
#85015=CARTESIAN_POINT('Ctrl Pts',(6.73155638150024,-30.9336260323887,56.8317810498497));
#85016=CARTESIAN_POINT('Ctrl Pts',(6.73541186135113,-30.9959784893288,56.797226866952));
#85017=CARTESIAN_POINT('Ctrl Pts',(6.7392700583216,-31.0583748886803,56.7626483322615));
#85018=CARTESIAN_POINT('Ctrl Pts',(6.74312825529208,-31.1189379422677,56.7248334770738));
#85019=CARTESIAN_POINT('Ctrl Pts',(6.74698645226255,-31.1773238940585,56.6840148488));
#85020=CARTESIAN_POINT('Ctrl Pts',(6.74866000838574,-31.2026497568582,56.666309100283));
#85021=CARTESIAN_POINT('Ctrl Pts',(6.75033356450893,-31.2275663741968,56.6480387255383));
#85022=CARTESIAN_POINT('Ctrl Pts',(6.75200712063213,-31.2520475724682,56.6292251037768));
#85023=CARTESIAN_POINT('',(6.44592528053626,-27.9452500000201,54.999990915418));
#85024=CARTESIAN_POINT('Ctrl Pts',(6.44592528053768,-27.9452500000201,54.999990915444));
#85025=CARTESIAN_POINT('Ctrl Pts',(6.44979385259826,-27.9452496865186,55.0708988474439));
#85026=CARTESIAN_POINT('Ctrl Pts',(6.45366242465885,-27.9489241543316,55.1419458653842));
#85027=CARTESIAN_POINT('Ctrl Pts',(6.45753099671943,-27.9562906464585,55.2127196294351));
#85028=CARTESIAN_POINT('Ctrl Pts',(6.4613938042328,-27.9636461617984,55.28338793372));
#85029=CARTESIAN_POINT('Ctrl Pts',(6.46525661174617,-27.9746827313674,55.3537833129638));
#85030=CARTESIAN_POINT('Ctrl Pts',(6.46911941925954,-27.9893655867764,55.4234935877451));
#85031=CARTESIAN_POINT('Ctrl Pts',(6.47297769671014,-28.0040312230369,55.493122110609));
#85032=CARTESIAN_POINT('Ctrl Pts',(6.47683597416074,-28.0223345516742,55.5620666517312));
#85033=CARTESIAN_POINT('Ctrl Pts',(6.48069425161134,-28.0441892329501,55.6299220634266));
#85034=CARTESIAN_POINT('Ctrl Pts',(6.48455010010934,-28.0660301557584,55.6977347572041));
#85035=CARTESIAN_POINT('Ctrl Pts',(6.48840594860733,-28.0914178469666,55.7644592204328));
#85036=CARTESIAN_POINT('Ctrl Pts',(6.49226179710533,-28.1202156677511,55.8297038186796));
#85037=CARTESIAN_POINT('Ctrl Pts',(6.4961165089705,-28.1490049994706,55.8949291840255));
#85038=CARTESIAN_POINT('Ctrl Pts',(6.49997122083567,-28.1812022689765,55.958675106127));
#85039=CARTESIAN_POINT('Ctrl Pts',(6.50382593270084,-28.2166227266648,56.020569969895));
#85040=CARTESIAN_POINT('Ctrl Pts',(6.5076807986421,-28.2520446001387,56.0824673076531));
#85041=CARTESIAN_POINT('Ctrl Pts',(6.51153566458336,-28.2906896742964,56.1425130195333));
#85042=CARTESIAN_POINT('Ctrl Pts',(6.51539053052463,-28.3323281363288,56.2003616611753));
#85043=CARTESIAN_POINT('Ctrl Pts',(6.519249432972,-28.3740101988156,56.2582708772701));
#85044=CARTESIAN_POINT('Ctrl Pts',(6.52310833541937,-28.4186916216786,56.3139780354875));
#85045=CARTESIAN_POINT('Ctrl Pts',(6.52696723786674,-28.4661008192273,56.3671689236246));
#85046=CARTESIAN_POINT('Ctrl Pts',(6.53082833001039,-28.5135369186594,56.4203899944086));
#85047=CARTESIAN_POINT('Ctrl Pts',(6.53468942215403,-28.5637035320734,56.471091607219));
#85048=CARTESIAN_POINT('Ctrl Pts',(6.53855051429768,-28.6162924800363,56.5189967286653));
#85049=CARTESIAN_POINT('Ctrl Pts',(6.54241835505556,-28.6689733456508,56.5669855811318));
#85050=CARTESIAN_POINT('Ctrl Pts',(6.54628619581344,-28.724084622834,56.6121678755227));
#85051=CARTESIAN_POINT('Ctrl Pts',(6.55015403657131,-28.7812859390421,56.6543075893326));
#85052=CARTESIAN_POINT('Ctrl Pts',(6.55242968420588,-28.8149403855593,56.6791005283536));
#85053=CARTESIAN_POINT('Ctrl Pts',(6.55470533184044,-28.8493177649882,56.7028410824421));
#85054=CARTESIAN_POINT('Ctrl Pts',(6.55698097947501,-28.884344705424,56.7254885760806));
#85055=CARTESIAN_POINT('Ctrl Pts',(6.56085005282324,-28.9438977749117,56.7639940163386));
#85056=CARTESIAN_POINT('Ctrl Pts',(6.56471912617148,-29.0055632836953,56.7994881602144));
#85057=CARTESIAN_POINT('Ctrl Pts',(6.56858819951972,-29.0690042255801,56.8317326307385));
#85058=CARTESIAN_POINT('Ctrl Pts',(6.57245150791552,-29.132350639918,56.8639290567254));
#85059=CARTESIAN_POINT('Ctrl Pts',(6.57631481631132,-29.1974668067599,56.8928852023626));
#85060=CARTESIAN_POINT('Ctrl Pts',(6.58017812470713,-29.2639876198707,56.9184064581825));
#85061=CARTESIAN_POINT('Ctrl Pts',(6.58403690120006,-29.3304303998987,56.9438977759699));
#85062=CARTESIAN_POINT('Ctrl Pts',(6.587895677693,-29.3982741018804,56.9659620344099));
#85063=CARTESIAN_POINT('Ctrl Pts',(6.59175445418593,-29.4671315275863,56.9844517513932));
#85064=CARTESIAN_POINT('Ctrl Pts',(6.59561079977416,-29.5359455753353,57.0029298204513));
#85065=CARTESIAN_POINT('Ctrl Pts',(6.59946714536239,-29.6057716117535,57.0178376899947));
#85066=CARTESIAN_POINT('Ctrl Pts',(6.60332349095062,-29.6762064784604,57.0290774548816));
#85067=CARTESIAN_POINT('Ctrl Pts',(6.60717869719598,-29.7466205354494,57.0403138990221));
#85068=CARTESIAN_POINT('Ctrl Pts',(6.61103390344134,-29.8176425861672,57.0478843134957));
#85069=CARTESIAN_POINT('Ctrl Pts',(6.61488910968669,-29.8888601619433,57.0517420644167));
#85070=CARTESIAN_POINT('Ctrl Pts',(6.61874446653797,-29.9600805198763,57.0555999660429));
#85071=CARTESIAN_POINT('Ctrl Pts',(6.62259982338924,-30.0314959328385,57.0557448920874));
#85072=CARTESIAN_POINT('Ctrl Pts',(6.62645518024051,-30.1026914403188,57.0521822605668));
#85073=CARTESIAN_POINT('Ctrl Pts',(6.63031457270909,-30.1739614721126,57.0486158998409));
#85074=CARTESIAN_POINT('Ctrl Pts',(6.63417396517767,-30.2450106527457,57.0413342587147));
#85075=CARTESIAN_POINT('Ctrl Pts',(6.63803335764625,-30.3154275636869,57.0303947927845));
#85076=CARTESIAN_POINT('Ctrl Pts',(6.64189493524971,-30.3858843437134,57.0194491330794));
#85077=CARTESIAN_POINT('Ctrl Pts',(6.64575651285316,-30.4557076656982,57.0048416253513));
#85078=CARTESIAN_POINT('Ctrl Pts',(6.64961809045662,-30.524497458196,56.9866806433964));
#85079=CARTESIAN_POINT('Ctrl Pts',(6.65348642457151,-30.5934076105746,56.9684878855988));
#85080=CARTESIAN_POINT('Ctrl Pts',(6.65735475868641,-30.6612801603151,56.9467293886402));
#85081=CARTESIAN_POINT('Ctrl Pts',(6.6612230928013,-30.7277319849103,56.9215628328625));
#85082=CARTESIAN_POINT('Ctrl Pts',(6.66352081197206,-30.7672031440111,56.9066143625508));
#85083=CARTESIAN_POINT('Ctrl Pts',(6.66581853114281,-30.8061734483572,56.890464398356));
#85084=CARTESIAN_POINT('Ctrl Pts',(6.66811625031357,-30.8445667488952,56.8731536427001));
#85085=CARTESIAN_POINT('Ctrl Pts',(6.67198550519571,-30.9092193258676,56.8440031152172));
#85086=CARTESIAN_POINT('Ctrl Pts',(6.67585476007784,-30.9724875627591,56.8114442962675));
#85087=CARTESIAN_POINT('Ctrl Pts',(6.67972401495998,-31.0339883551208,56.7756310551392));
#85088=CARTESIAN_POINT('Ctrl Pts',(6.68358710202869,-31.0953911117043,56.7398749023641));
#85089=CARTESIAN_POINT('Ctrl Pts',(6.68745018909739,-31.1550316024593,56.7008748722445));
#85090=CARTESIAN_POINT('Ctrl Pts',(6.6913132761661,-31.2125483695227,56.6588321235338));
#85091=CARTESIAN_POINT('Ctrl Pts',(6.69220528525035,-31.2258293227616,56.6491242103779));
#85092=CARTESIAN_POINT('Ctrl Pts',(6.6930972943346,-31.238997144019,56.6392542625601));
#85093=CARTESIAN_POINT('Ctrl Pts',(6.69398930341885,-31.2520475724682,56.6292251037768));
#85094=CARTESIAN_POINT('Ctrl Pts',(5.99388650793247,-31.2520475724682,56.6292251037768));
#85095=CARTESIAN_POINT('Ctrl Pts',(5.99635921371572,-31.2880679719405,56.6015436903158));
#85096=CARTESIAN_POINT('Ctrl Pts',(5.99883191949896,-31.3231309837129,56.5726970835974));
#85097=CARTESIAN_POINT('Ctrl Pts',(6.00130462528221,-31.3571605423515,56.5427614283434));
#85098=CARTESIAN_POINT('Ctrl Pts',(6.00517369863043,-31.4104070139992,56.4959207379994));
#85099=CARTESIAN_POINT('Ctrl Pts',(6.00904277197864,-31.4613299633521,56.4462284604087));
#85100=CARTESIAN_POINT('Ctrl Pts',(6.01291184532686,-31.509608366483,56.3939440958463));
#85101=CARTESIAN_POINT('Ctrl Pts',(6.01677515372265,-31.5578148343796,56.3417376354349));
#85102=CARTESIAN_POINT('Ctrl Pts',(6.02063846211843,-31.6033842507581,56.2869471084688));
#85103=CARTESIAN_POINT('Ctrl Pts',(6.02450177051422,-31.6460300705182,56.2298709564218));
#85104=CARTESIAN_POINT('Ctrl Pts',(6.02836054700713,-31.688625864059,56.1728617582782));
#85105=CARTESIAN_POINT('Ctrl Pts',(6.03221932350004,-31.7283045838956,56.1135726480542));
#85106=CARTESIAN_POINT('Ctrl Pts',(6.03607809999295,-31.7648190305379,56.0523361401906));
#85107=CARTESIAN_POINT('Ctrl Pts',(6.03993444558116,-31.8013104742567,55.9911382093516));
#85108=CARTESIAN_POINT('Ctrl Pts',(6.04379079116937,-31.8346413514287,55.9279957310735));
#85109=CARTESIAN_POINT('Ctrl Pts',(6.04764713675758,-31.8646078326563,55.8632700579175));
#85110=CARTESIAN_POINT('Ctrl Pts',(6.05150234300291,-31.8945654603992,55.7985635077193));
#85111=CARTESIAN_POINT('Ctrl Pts',(6.05535754924824,-31.9211604615754,55.7322751318466));
#85112=CARTESIAN_POINT('Ctrl Pts',(6.05921275549357,-31.9442358153366,55.6647891822694));
#85113=CARTESIAN_POINT('Ctrl Pts',(6.06306811234482,-31.9673120705502,55.5973005963137));
#85114=CARTESIAN_POINT('Ctrl Pts',(6.06692346919606,-31.9868682502803,55.5286148041408));
#85115=CARTESIAN_POINT('Ctrl Pts',(6.07077882604731,-32.0027967472951,55.4591326077771));
#85116=CARTESIAN_POINT('Ctrl Pts',(6.07463821851587,-32.0187419175572,55.3895776805184));
#85117=CARTESIAN_POINT('Ctrl Pts',(6.07849761098443,-32.0310517160728,55.3192251594079));
#85118=CARTESIAN_POINT('Ctrl Pts',(6.08235700345299,-32.0396695759423,55.2484865861077));
#85119=CARTESIAN_POINT('Ctrl Pts',(6.08621858105642,-32.0482923151253,55.1777079616013));
#85120=CARTESIAN_POINT('Ctrl Pts',(6.09008015865986,-32.0532189209047,55.1065433346406));
#85121=CARTESIAN_POINT('Ctrl Pts',(6.09394173626329,-32.0544449115844,55.0354071710931));
#85122=CARTESIAN_POINT('Ctrl Pts',(6.09781007037817,-32.0556730473512,54.9641465422746));
#85123=CARTESIAN_POINT('Ctrl Pts',(6.10167840449304,-32.0531876576792,54.8929149619447));
#85124=CARTESIAN_POINT('Ctrl Pts',(6.10554673860791,-32.0470363181879,54.8221239911635));
#85125=CARTESIAN_POINT('Ctrl Pts',(6.10784445777886,-32.0433825358991,54.7800754591949));
#85126=CARTESIAN_POINT('Ctrl Pts',(6.11014217694982,-32.0384363455578,54.7381822477433));
#85127=CARTESIAN_POINT('Ctrl Pts',(6.11243989612077,-32.0322162126119,54.6965287036682));
#85128=CARTESIAN_POINT('Ctrl Pts',(6.11630896946898,-32.0217422822432,54.626389315323));
#85129=CARTESIAN_POINT('Ctrl Pts',(6.12017804281719,-32.0076124141733,54.5566554207575));
#85130=CARTESIAN_POINT('Ctrl Pts',(6.12404711616541,-31.9898705140381,54.4877374697857));
#85131=CARTESIAN_POINT('Ctrl Pts',(6.12791042456119,-31.9721550494861,54.4189222071512));
#85132=CARTESIAN_POINT('Ctrl Pts',(6.13177373295698,-31.9508383560286,54.3509209414693));
#85133=CARTESIAN_POINT('Ctrl Pts',(6.13563704135276,-31.9260157555761,54.2841362756973));
#85134=CARTESIAN_POINT('Ctrl Pts',(6.13949581784567,-31.9012222735897,54.2174299525239));
#85135=CARTESIAN_POINT('Ctrl Pts',(6.14335459433858,-31.8729312221433,54.1519378476021));
#85136=CARTESIAN_POINT('Ctrl Pts',(6.1472133708315,-31.8412878889772,54.088047987882));
#85137=CARTESIAN_POINT('Ctrl Pts',(6.1510697164197,-31.8096644900901,54.0241983767125));
#85138=CARTESIAN_POINT('Ctrl Pts',(6.15492606200791,-31.7746932144135,53.9619494424752));
#85139=CARTESIAN_POINT('Ctrl Pts',(6.15878240759611,-31.7365671002288,53.9016684157766));
#85140=CARTESIAN_POINT('Ctrl Pts',(6.16263761384144,-31.698452250262,53.8414051988816));
#85141=CARTESIAN_POINT('Ctrl Pts',(6.16649282008677,-31.6571846717615,53.7831091456009));
#85142=CARTESIAN_POINT('Ctrl Pts',(6.1703480263321,-31.6130020290762,53.727120580457));
#85143=CARTESIAN_POINT('Ctrl Pts',(6.17420338318335,-31.5688176603697,53.6711298280867));
#85144=CARTESIAN_POINT('Ctrl Pts',(6.17805874003459,-31.5217183040516,53.617447122804));
#85145=CARTESIAN_POINT('Ctrl Pts',(6.18191409688583,-31.4719823290645,53.5663802507562));
#85146=CARTESIAN_POINT('Ctrl Pts',(6.18577348935439,-31.4221942926549,53.5152599241617));
#85147=CARTESIAN_POINT('Ctrl Pts',(6.18963288182295,-31.3697644678361,53.4667612454627));
#85148=CARTESIAN_POINT('Ctrl Pts',(6.19349227429151,-31.3150079288294,53.4211549443927));
#85149=CARTESIAN_POINT('Ctrl Pts',(6.19735385189494,-31.2602203874244,53.3755228216629));
#85150=CARTESIAN_POINT('Ctrl Pts',(6.20121542949838,-31.2031038985306,53.3327866277354));
#85151=CARTESIAN_POINT('Ctrl Pts',(6.20507700710181,-31.144004242266,53.2931749192793));
#85152=CARTESIAN_POINT('Ctrl Pts',(6.20894534121668,-31.084801180724,53.2534939031493));
#85153=CARTESIAN_POINT('Ctrl Pts',(6.21281367533155,-31.0236084412542,53.2169485363527));
#85154=CARTESIAN_POINT('Ctrl Pts',(6.21668200944642,-30.9607975975375,53.1837220644774));
#85155=CARTESIAN_POINT('Ctrl Pts',(6.21897972861739,-30.9234891139714,53.1639861525462));
#85156=CARTESIAN_POINT('Ctrl Pts',(6.22127744778836,-30.8856101662258,53.1454202891853));
#85157=CARTESIAN_POINT('Ctrl Pts',(6.22357516695934,-30.8472416327671,53.1280547074751));
#85158=CARTESIAN_POINT('Ctrl Pts',(6.22744424030755,-30.7826337937888,53.0988132273933));
#85159=CARTESIAN_POINT('Ctrl Pts',(6.23131331365577,-30.7163837784897,53.0728631850843));
#85160=CARTESIAN_POINT('Ctrl Pts',(6.23518238700399,-30.6488602364774,53.050390306749));
#85161=CARTESIAN_POINT('Ctrl Pts',(6.23904569539978,-30.5814373051211,53.0279509131948));
#85162=CARTESIAN_POINT('Ctrl Pts',(6.24290900379557,-30.5127450708393,53.0089785516209));
#85163=CARTESIAN_POINT('Ctrl Pts',(6.24677231219135,-30.4431734770941,52.9936114953229));
#85164=CARTESIAN_POINT('Ctrl Pts',(6.25063108868427,-30.3736834951887,52.9782624655451));
#85165=CARTESIAN_POINT('Ctrl Pts',(6.25448986517719,-30.3033166748645,52.9665104445909));
#85166=CARTESIAN_POINT('Ctrl Pts',(6.2583486416701,-30.2324778133167,52.9584438217831));
#85167=CARTESIAN_POINT('Ctrl Pts',(6.26220498725831,-30.1616835779663,52.9503822806875));
#85168=CARTESIAN_POINT('Ctrl Pts',(6.26606133284652,-30.0904183728966,52.9460015863917));
#85169=CARTESIAN_POINT('Ctrl Pts',(6.26991767843473,-30.019095421567,52.9453387317187));
#85170=CARTESIAN_POINT('Ctrl Pts',(6.27377288468006,-29.9477935423365,52.9446760728837));
#85171=CARTESIAN_POINT('Ctrl Pts',(6.2776280909254,-29.8764344362172,52.9477290775123));
#85172=CARTESIAN_POINT('Ctrl Pts',(6.28148329717073,-29.8054329252716,52.9544826532313));
#85173=CARTESIAN_POINT('Ctrl Pts',(6.28533865402198,-29.73442864061,52.9612364927828));
#85174=CARTESIAN_POINT('Ctrl Pts',(6.28919401087323,-29.6637824622517,52.971691142247));
#85175=CARTESIAN_POINT('Ctrl Pts',(6.29304936772448,-29.5939039520625,52.9857796639023));
#85176=CARTESIAN_POINT('Ctrl Pts',(6.29690876019304,-29.5239522961346,52.9998829327999));
#85177=CARTESIAN_POINT('Ctrl Pts',(6.30076815266161,-29.4547703896441,53.0176275708756));
#85178=CARTESIAN_POINT('Ctrl Pts',(6.30462754513017,-29.3867565693747,53.038895704636));
#85179=CARTESIAN_POINT('Ctrl Pts',(6.30848912273361,-29.3187042406167,53.060175880121));
#85180=CARTESIAN_POINT('Ctrl Pts',(6.31235070033705,-29.251821770313,53.0849833536128));
#85181=CARTESIAN_POINT('Ctrl Pts',(6.31621227794049,-29.1864887175942,53.1131515811018));
#85182=CARTESIAN_POINT('Ctrl Pts',(6.32008061205536,-29.121041353171,53.1413690938754));
#85183=CARTESIAN_POINT('Ctrl Pts',(6.32394894617024,-29.0571492544873,53.1729588853264));
#85184=CARTESIAN_POINT('Ctrl Pts',(6.32781728028511,-28.995167902363,53.2077081660459));
#85185=CARTESIAN_POINT('Ctrl Pts',(6.33011499945604,-28.9583521215161,53.2283485983649));
#85186=CARTESIAN_POINT('Ctrl Pts',(6.33241271862696,-28.9222099501555,53.2501028948124));
#85187=CARTESIAN_POINT('Ctrl Pts',(6.33471043779788,-28.8868106539845,53.2729195032027));
#85188=CARTESIAN_POINT('Ctrl Pts',(6.3385795111461,-28.8272026413545,53.3113398343453));
#85189=CARTESIAN_POINT('Ctrl Pts',(6.34244858449431,-28.7694692515091,53.352924986983));
#85190=CARTESIAN_POINT('Ctrl Pts',(6.34631765784252,-28.7139664634267,53.3974659737439));
#85191=CARTESIAN_POINT('Ctrl Pts',(6.35018096623831,-28.6585463749739,53.441940594053));
#85192=CARTESIAN_POINT('Ctrl Pts',(6.35404427463409,-28.6053506667861,53.4893620046678));
#85193=CARTESIAN_POINT('Ctrl Pts',(6.35790758302988,-28.5547069996109,53.53947759157));
#85194=CARTESIAN_POINT('Ctrl Pts',(6.36176635952279,-28.5041227406313,53.5895343897478));
#85195=CARTESIAN_POINT('Ctrl Pts',(6.3656251360157,-28.4560849197777,53.6422787464759));
#85196=CARTESIAN_POINT('Ctrl Pts',(6.36948391250861,-28.4108873442306,53.6974185131926));
#85197=CARTESIAN_POINT('Ctrl Pts',(6.37334025809681,-28.365718241698,53.752523543635));
#85198=CARTESIAN_POINT('Ctrl Pts',(6.37719660368501,-28.3233861418328,53.8100206153616));
#85199=CARTESIAN_POINT('Ctrl Pts',(6.38105294927322,-28.2841462414807,53.8695826249233));
#85200=CARTESIAN_POINT('Ctrl Pts',(6.38490815551855,-28.2449179344104,53.9291270371122));
#85201=CARTESIAN_POINT('Ctrl Pts',(6.38876336176388,-28.2087802802552,53.9907347705192));
#85202=CARTESIAN_POINT('Ctrl Pts',(6.39261856800921,-28.1759455838436,54.0540491294996));
#85203=CARTESIAN_POINT('Ctrl Pts',(6.39647392486045,-28.1431096047252,54.1173659618929));
#85204=CARTESIAN_POINT('Ctrl Pts',(6.4003292817117,-28.1135770612139,54.1823891199659));
#85205=CARTESIAN_POINT('Ctrl Pts',(6.40418463856294,-28.0875138476605,54.248738208339));
#85206=CARTESIAN_POINT('Ctrl Pts',(6.40804403103149,-28.0614233522861,54.315156748008));
#85207=CARTESIAN_POINT('Ctrl Pts',(6.41190342350005,-28.0388096142203,54.3829035355095));
#85208=CARTESIAN_POINT('Ctrl Pts',(6.4157628159686,-28.0197896463723,54.4515799804112));
#85209=CARTESIAN_POINT('Ctrl Pts',(6.41962439357204,-28.0007589096804,54.5202953089704));
#85210=CARTESIAN_POINT('Ctrl Pts',(6.42348597117547,-27.9853260988985,54.5899408682425));
#85211=CARTESIAN_POINT('Ctrl Pts',(6.42734754877891,-27.9735571523901,54.6601074465793));
#85212=CARTESIAN_POINT('Ctrl Pts',(6.43121588289378,-27.9617676140331,54.7303967937266));
#85213=CARTESIAN_POINT('Ctrl Pts',(6.43508421700865,-27.9536547941648,54.8012084972218));
#85214=CARTESIAN_POINT('Ctrl Pts',(6.43895255112351,-27.9492327191636,54.8721284928109));
#85215=CARTESIAN_POINT('Ctrl Pts',(6.44125027029449,-27.9466060881116,54.9142536631379));
#85216=CARTESIAN_POINT('Ctrl Pts',(6.44354798946547,-27.9452806044252,54.9564170246933));
#85217=CARTESIAN_POINT('Ctrl Pts',(6.44584570863644,-27.9452505240975,54.9985324242889));
#85218=CARTESIAN_POINT('Ctrl Pts',(6.44587223260258,-27.9452501768621,54.9990185878926));
#85219=CARTESIAN_POINT('Ctrl Pts',(6.44589875656871,-27.9452500021695,54.9995047516196));
#85220=CARTESIAN_POINT('Ctrl Pts',(6.44592528053485,-27.9452500000201,54.999990915392));
#85221=CARTESIAN_POINT('Origin',(-1.54592528053767,-30.,55.));
#85222=CARTESIAN_POINT('',(5.29388070614408,-31.2520475724682,56.6292251037768));
#85223=CARTESIAN_POINT('',(5.35213793236373,-31.2520475724682,56.6292251037768));
#85224=CARTESIAN_POINT('',(-1.54592528053767,-31.2520475724682,56.6292251037768));
#85225=CARTESIAN_POINT('',(5.80407471943462,-27.9452508587686,54.9981214077886));
#85226=CARTESIAN_POINT('Ctrl Pts',(5.35213793236373,-31.2520475724682,56.6292251037768));
#85227=CARTESIAN_POINT('Ctrl Pts',(5.35599766139006,-31.3084496151558,56.5858805466216));
#85228=CARTESIAN_POINT('Ctrl Pts',(5.35985739041638,-31.362668650072,56.5395495461331));
#85229=CARTESIAN_POINT('Ctrl Pts',(5.3637171194427,-31.4143753267133,56.4904831423685));
#85230=CARTESIAN_POINT('Ctrl Pts',(5.36757404042557,-31.466044385534,56.441452435564));
#85231=CARTESIAN_POINT('Ctrl Pts',(5.37143096140844,-31.5152043607371,56.3896906066652));
#85232=CARTESIAN_POINT('Ctrl Pts',(5.37528788239131,-31.5615595250372,56.335488454561));
#85233=CARTESIAN_POINT('Ctrl Pts',(5.3791432876086,-31.6078964718101,56.2813076038413));
#85234=CARTESIAN_POINT('Ctrl Pts',(5.38299869282588,-31.6514304799869,56.2246887021999));
#85235=CARTESIAN_POINT('Ctrl Pts',(5.38685409804317,-31.6919044054673,56.165957565806));
#85236=CARTESIAN_POINT('Ctrl Pts',(5.39070927778001,-31.7323759638609,56.1072298642581));
#85237=CARTESIAN_POINT('Ctrl Pts',(5.39456445751685,-31.7697875205517,56.0463905741253));
#85238=CARTESIAN_POINT('Ctrl Pts',(5.39841963725369,-31.8039247894515,55.9837951598288));
#85239=CARTESIAN_POINT('Ctrl Pts',(5.40227861106393,-31.8380956545289,55.9211381422837));
#85240=CARTESIAN_POINT('Ctrl Pts',(5.40613758487416,-31.8689855617635,55.8567219757467));
#85241=CARTESIAN_POINT('Ctrl Pts',(5.40999655868439,-31.8964262535003,55.7909266891026));
#85242=CARTESIAN_POINT('Ctrl Pts',(5.41385737981818,-31.9238800813295,55.7250999056955));
#85243=CARTESIAN_POINT('Ctrl Pts',(5.41771820095197,-31.9478812405932,55.6578931451431));
#85244=CARTESIAN_POINT('Ctrl Pts',(5.42157902208576,-31.9683107067605,55.5897037596555));
#85245=CARTESIAN_POINT('Ctrl Pts',(5.42544695749405,-31.9887778179845,55.5213887226577));
#85246=CARTESIAN_POINT('Ctrl Pts',(5.42931489290235,-32.0056599709901,55.452087916219));
#85247=CARTESIAN_POINT('Ctrl Pts',(5.43318282831064,-32.0188889506662,55.3822106322144));
#85248=CARTESIAN_POINT('Ctrl Pts',(5.43660651741345,-32.0305985344048,55.3203590058229));
#85249=CARTESIAN_POINT('Ctrl Pts',(5.44003020651626,-32.0394466489614,55.2580560764145));
#85250=CARTESIAN_POINT('Ctrl Pts',(5.44345389561907,-32.0454200326909,55.1955874545234));
#85251=CARTESIAN_POINT('Ctrl Pts',(5.44732296896728,-32.0521704878556,55.1249923529236));
#85252=CARTESIAN_POINT('Ctrl Pts',(5.4511920423155,-32.0552751231039,55.0539090886279));
#85253=CARTESIAN_POINT('Ctrl Pts',(5.45506111566371,-32.0546775616078,54.9827465851108));
#85254=CARTESIAN_POINT('Ctrl Pts',(5.4589244240595,-32.0540808904835,54.9116901143335));
#85255=CARTESIAN_POINT('Ctrl Pts',(5.46278773245529,-32.0497929763707,54.8405551205058));
#85256=CARTESIAN_POINT('Ctrl Pts',(5.46665104085107,-32.0418092335022,54.7697553117114));
#85257=CARTESIAN_POINT('Ctrl Pts',(5.47050981734399,-32.0338348560645,54.69903855553));
#85258=CARTESIAN_POINT('Ctrl Pts',(5.4743685938369,-32.0221733156894,54.6286566837511));
#85259=CARTESIAN_POINT('Ctrl Pts',(5.47822737032981,-32.0068720328791,54.5590213087375));
#85260=CARTESIAN_POINT('Ctrl Pts',(5.48208371591802,-31.9915803893835,54.4894298017639));
#85261=CARTESIAN_POINT('Ctrl Pts',(5.48594006150623,-31.9726536565796,54.4205843318947));
#85262=CARTESIAN_POINT('Ctrl Pts',(5.48979640709443,-31.9501906114715,54.3528878447839));
#85263=CARTESIAN_POINT('Ctrl Pts',(5.49365161333977,-31.927734202986,54.2852113583468));
#85264=CARTESIAN_POINT('Ctrl Pts',(5.4975068195851,-31.9017437093017,54.2186836415556));
#85265=CARTESIAN_POINT('Ctrl Pts',(5.50136202583043,-31.8723677051339,54.1536922904336));
#85266=CARTESIAN_POINT('Ctrl Pts',(5.50521738268168,-31.8429905533751,54.0886984003859));
#85267=CARTESIAN_POINT('Ctrl Pts',(5.50907273953293,-31.8102278306458,54.025241436927));
#85268=CARTESIAN_POINT('Ctrl Pts',(5.51292809638417,-31.7742754619635,53.9636872346756));
#85269=CARTESIAN_POINT('Ctrl Pts',(5.51678748885273,-31.7382854599292,53.9020686002033));
#85270=CARTESIAN_POINT('Ctrl Pts',(5.52064688132129,-31.6990993924937,53.8423571232074));
#85271=CARTESIAN_POINT('Ctrl Pts',(5.52450627378985,-31.6569577433031,53.7848915277195));
#85272=CARTESIAN_POINT('Ctrl Pts',(5.52836785139329,-31.614792234091,53.7273933960027));
#85273=CARTESIAN_POINT('Ctrl Pts',(5.53222942899673,-31.5696681193188,53.6721440535542));
#85274=CARTESIAN_POINT('Ctrl Pts',(5.53609100660016,-31.5218658529192,53.6194487013448));
#85275=CARTESIAN_POINT('Ctrl Pts',(5.53995934071503,-31.4739799480193,53.5666611493181));
#85276=CARTESIAN_POINT('Ctrl Pts',(5.54382767482991,-31.4234068807573,53.5164368517537));
#85277=CARTESIAN_POINT('Ctrl Pts',(5.54769600894478,-31.3704630647951,53.469043256479));
#85278=CARTESIAN_POINT('Ctrl Pts',(5.54999372811573,-31.3390154138666,53.4408923343485));
#85279=CARTESIAN_POINT('Ctrl Pts',(5.55229144728667,-31.3067319607144,53.4137393489292));
#85280=CARTESIAN_POINT('Ctrl Pts',(5.55458916645762,-31.2736839053951,53.3876331460745));
#85281=CARTESIAN_POINT('Ctrl Pts',(5.55845823980584,-31.2180350899685,53.3436735469358));
#85282=CARTESIAN_POINT('Ctrl Pts',(5.56232731315406,-31.1599987860129,53.3025121980011));
#85283=CARTESIAN_POINT('Ctrl Pts',(5.56619638650227,-31.0998879711845,53.2644182493055));
#85284=CARTESIAN_POINT('Ctrl Pts',(5.57005969489806,-31.039866721985,53.2263810609198));
#85285=CARTESIAN_POINT('Ctrl Pts',(5.57392300329384,-30.977777504523,53.1914024584711));
#85286=CARTESIAN_POINT('Ctrl Pts',(5.57778631168963,-30.9139654058247,53.1597106750688));
#85287=CARTESIAN_POINT('Ctrl Pts',(5.58164508818254,-30.8502281627174,53.1280560681146));
#85288=CARTESIAN_POINT('Ctrl Pts',(5.58550386467545,-30.7847724858293,53.099680836624));
#85289=CARTESIAN_POINT('Ctrl Pts',(5.58936264116837,-30.7179699078131,53.0747683843301));
#85290=CARTESIAN_POINT('Ctrl Pts',(5.59321898675657,-30.6512094132659,53.0498716260775));
#85291=CARTESIAN_POINT('Ctrl Pts',(5.59707533234478,-30.5831041550984,53.0284334884236));
#85292=CARTESIAN_POINT('Ctrl Pts',(5.60093167793299,-30.5140462386054,53.0105895277556));
#85293=CARTESIAN_POINT('Ctrl Pts',(5.60478688417832,-30.4450087250154,52.9927508390191));
#85294=CARTESIAN_POINT('Ctrl Pts',(5.60864209042365,-30.3750195819568,52.9785043405957));
#85295=CARTESIAN_POINT('Ctrl Pts',(5.61249729666899,-30.3044850273214,52.9679354265582));
#85296=CARTESIAN_POINT('Ctrl Pts',(5.61635265352023,-30.2339477172119,52.9573660996399));
#85297=CARTESIAN_POINT('Ctrl Pts',(5.62020801037148,-30.1628654339729,52.9504747121478));
#85298=CARTESIAN_POINT('Ctrl Pts',(5.62406336722272,-30.0916517938954,52.9472950744991));
#85299=CARTESIAN_POINT('Ctrl Pts',(5.62792275969128,-30.0203636105239,52.944112108546));
#85300=CARTESIAN_POINT('Ctrl Pts',(5.63178215215984,-29.948944282133,52.9446486700726));
#85301=CARTESIAN_POINT('Ctrl Pts',(5.6356415446284,-29.8778088152285,52.9488864300424));
#85302=CARTESIAN_POINT('Ctrl Pts',(5.63950312223184,-29.8066330724021,52.9531265893736));
#85303=CARTESIAN_POINT('Ctrl Pts',(5.64336469983527,-29.7357419939951,52.9610720646429));
#85304=CARTESIAN_POINT('Ctrl Pts',(5.64722627743871,-29.6655441007778,52.9726527643308));
#85305=CARTESIAN_POINT('Ctrl Pts',(5.65109461155358,-29.5952233839591,52.9842537264964));
#85306=CARTESIAN_POINT('Ctrl Pts',(5.65496294566845,-29.5255987485088,52.9995025079733));
#85307=CARTESIAN_POINT('Ctrl Pts',(5.65883127978332,-29.4570665004026,53.0182783299578));
#85308=CARTESIAN_POINT('Ctrl Pts',(5.66112899895428,-29.4163596080747,53.0294308221788));
#85309=CARTESIAN_POINT('Ctrl Pts',(5.66342671812523,-29.3760378167379,53.0418267532859));
#85310=CARTESIAN_POINT('Ctrl Pts',(5.66572443729619,-29.3361807802747,53.0554327972468));
#85311=CARTESIAN_POINT('Ctrl Pts',(5.66959351064441,-29.2690664873413,53.0783436832807));
#85312=CARTESIAN_POINT('Ctrl Pts',(5.67346258399262,-29.2030082382591,53.1047780728359));
#85313=CARTESIAN_POINT('Ctrl Pts',(5.67733165734084,-29.1384019055368,53.1346189970632));
#85314=CARTESIAN_POINT('Ctrl Pts',(5.68119496573662,-29.0738918368037,53.1644154580578));
#85315=CARTESIAN_POINT('Ctrl Pts',(5.68505827413241,-29.0108298276283,53.1976081764318));
#85316=CARTESIAN_POINT('Ctrl Pts',(5.68892158252819,-28.9495947893964,53.2340310149845));
#85317=CARTESIAN_POINT('Ctrl Pts',(5.69278035902111,-28.888431583702,53.2704111272649));
#85318=CARTESIAN_POINT('Ctrl Pts',(5.69663913551402,-28.8290915074133,53.310013586091));
#85319=CARTESIAN_POINT('Ctrl Pts',(5.70049791200693,-28.7719301519625,53.3526257222959));
#85320=CARTESIAN_POINT('Ctrl Pts',(5.70435425759514,-28.7148048063217,53.3952110142296));
#85321=CARTESIAN_POINT('Ctrl Pts',(5.70821060318334,-28.6598558470069,53.4408019322546));
#85322=CARTESIAN_POINT('Ctrl Pts',(5.71206694877155,-28.6074098246734,53.489142572549));
#85323=CARTESIAN_POINT('Ctrl Pts',(5.71592215501688,-28.554979297321,53.5374689307821));
#85324=CARTESIAN_POINT('Ctrl Pts',(5.71977736126222,-28.5050505958746,53.5885430693972));
#85325=CARTESIAN_POINT('Ctrl Pts',(5.72363256750755,-28.4579157816097,53.6420700217273));
#85326=CARTESIAN_POINT('Ctrl Pts',(5.7274879243588,-28.4107791259953,53.6955990651196));
#85327=CARTESIAN_POINT('Ctrl Pts',(5.73134328121005,-28.3664368936453,53.7515807464295));
#85328=CARTESIAN_POINT('Ctrl Pts',(5.7351986380613,-28.3251418207853,53.8096859061502));
#85329=CARTESIAN_POINT('Ctrl Pts',(5.73905803052986,-28.2838035220665,53.8678518877862));
#85330=CARTESIAN_POINT('Ctrl Pts',(5.74291742299841,-28.2455190320516,53.9281453881854));
#85331=CARTESIAN_POINT('Ctrl Pts',(5.74677681546697,-28.210498036343,53.9902078012939));
#85332=CARTESIAN_POINT('Ctrl Pts',(5.75063839307041,-28.1754572122287,54.0523053532862));
#85333=CARTESIAN_POINT('Ctrl Pts',(5.75449997067384,-28.1436837771895,54.1161733765903));
#85334=CARTESIAN_POINT('Ctrl Pts',(5.75836154827728,-28.1153404112806,54.1814306399896));
#85335=CARTESIAN_POINT('Ctrl Pts',(5.76222988239215,-28.0869474536515,54.2468020824865));
#85336=CARTESIAN_POINT('Ctrl Pts',(5.76609821650702,-28.061996717454,54.3135671628903));
#85337=CARTESIAN_POINT('Ctrl Pts',(5.76996655062189,-28.0406016732822,54.3813274212027));
#85338=CARTESIAN_POINT('Ctrl Pts',(5.77226426979284,-28.0278934113543,54.4215757658208));
#85339=CARTESIAN_POINT('Ctrl Pts',(5.77456198896379,-28.0164386815437,54.4621749669161));
#85340=CARTESIAN_POINT('Ctrl Pts',(5.77685970813473,-28.0062526866041,54.5030400289492));
#85341=CARTESIAN_POINT('Ctrl Pts',(5.78191177765104,-27.9838564098189,54.5928913636073));
#85342=CARTESIAN_POINT('Ctrl Pts',(5.78696384716734,-27.9675248955209,54.6843103064913));
#85343=CARTESIAN_POINT('Ctrl Pts',(5.79201591668364,-27.9574316008769,54.7765902925033));
#85344=CARTESIAN_POINT('Ctrl Pts',(5.79603551760063,-27.9494010272129,54.8500114351059));
#85345=CARTESIAN_POINT('Ctrl Pts',(5.80005511851763,-27.9453186462865,54.9239774059998));
#85346=CARTESIAN_POINT('Ctrl Pts',(5.80407471943462,-27.9452508587686,54.9981214077886));
#85347=CARTESIAN_POINT('Ctrl Pts',(5.80407471946232,-27.9452508587681,54.9981214082995));
#85348=CARTESIAN_POINT('Ctrl Pts',(5.80788808427066,-27.9451865492831,55.0684612587007));
#85349=CARTESIAN_POINT('Ctrl Pts',(5.81170144907901,-27.9487383877838,55.1388965966684));
#85350=CARTESIAN_POINT('Ctrl Pts',(5.81551481388735,-27.9559090953207,55.209021376676));
#85351=CARTESIAN_POINT('Ctrl Pts',(5.81932566294071,-27.9630750721948,55.2790998939277));
#85352=CARTESIAN_POINT('Ctrl Pts',(5.82313651199406,-27.9738551346034,55.3488677648099));
#85353=CARTESIAN_POINT('Ctrl Pts',(5.82694736104741,-27.9881999804144,55.4179213367314));
#85354=CARTESIAN_POINT('Ctrl Pts',(5.8307570439826,-28.0025404367088,55.4869537782898));
#85355=CARTESIAN_POINT('Ctrl Pts',(5.83456672691779,-28.0204434107704,55.5552718667557));
#85356=CARTESIAN_POINT('Ctrl Pts',(5.83837640985297,-28.0418083477083,55.622481337387));
#85357=CARTESIAN_POINT('Ctrl Pts',(5.8421862745413,-28.0631743039291,55.6896940144616));
#85358=CARTESIAN_POINT('Ctrl Pts',(5.84599613922963,-28.0880023967574,55.7557974946326));
#85359=CARTESIAN_POINT('Ctrl Pts',(5.84980600391796,-28.1161425514219,55.8204137224211));
#85360=CARTESIAN_POINT('Ctrl Pts',(5.85361981396671,-28.1443118470301,55.8850968644778));
#85361=CARTESIAN_POINT('Ctrl Pts',(5.85743362401546,-28.1757998467947,55.9482892241738));
#85362=CARTESIAN_POINT('Ctrl Pts',(5.8612474340642,-28.2104092282856,56.0096348014479));
#85363=CARTESIAN_POINT('Ctrl Pts',(5.86506356527384,-28.2450396737366,56.0710177148643));
#85364=CARTESIAN_POINT('Ctrl Pts',(5.86887969648348,-28.2827950106825,56.1305511908721));
#85365=CARTESIAN_POINT('Ctrl Pts',(5.87269582769311,-28.3234345959172,56.1879082491222));
#85366=CARTESIAN_POINT('Ctrl Pts',(5.87651830066247,-28.3641417172167,56.2453606250284));
#85367=CARTESIAN_POINT('Ctrl Pts',(5.88034077363183,-28.4077423369056,56.3006289805386));
#85368=CARTESIAN_POINT('Ctrl Pts',(5.88416324660119,-28.453956286233,56.3534202590554));
#85369=CARTESIAN_POINT('Ctrl Pts',(5.88544049072523,-28.4693982516047,56.371059978375));
#85370=CARTESIAN_POINT('Ctrl Pts',(5.88671773484926,-28.4851317023626,56.3884234488368));
#85371=CARTESIAN_POINT('Ctrl Pts',(5.8879949789733,-28.5011453432884,56.4055007223598));
#85372=CARTESIAN_POINT('Ctrl Pts',(5.89186405232151,-28.5496544341879,56.4572318069697));
#85373=CARTESIAN_POINT('Ctrl Pts',(5.89573312566972,-28.6009398356743,56.5065499255198));
#85374=CARTESIAN_POINT('Ctrl Pts',(5.89960219901794,-28.6547319770887,56.5531424625682));
#85375=CARTESIAN_POINT('Ctrl Pts',(5.90346550741372,-28.7084439677517,56.5996655763374));
#85376=CARTESIAN_POINT('Ctrl Pts',(5.90732881580951,-28.7646549201418,56.6434708543949));
#85377=CARTESIAN_POINT('Ctrl Pts',(5.9111921242053,-28.8230574377306,56.6842813801793));
#85378=CARTESIAN_POINT('Ctrl Pts',(5.91505090069821,-28.881391445506,56.7250440326592));
#85379=CARTESIAN_POINT('Ctrl Pts',(5.91890967719112,-28.9419115156489,56.7628186340326));
#85380=CARTESIAN_POINT('Ctrl Pts',(5.92276845368403,-29.0042774461901,56.7973686762415));
#85381=CARTESIAN_POINT('Ctrl Pts',(5.92662479927223,-29.0666040882069,56.8318969530385));
#85382=CARTESIAN_POINT('Ctrl Pts',(5.93048114486044,-29.1307738596501,56.8632044660195));
#85383=CARTESIAN_POINT('Ctrl Pts',(5.93433749044864,-29.1964191132021,56.8910989717286));
#85384=CARTESIAN_POINT('Ctrl Pts',(5.93819269669397,-29.2620449721096,56.9189852361104));
#85385=CARTESIAN_POINT('Ctrl Pts',(5.9420479029393,-29.3291450008409,56.9434603052146));
#85386=CARTESIAN_POINT('Ctrl Pts',(5.94590310918463,-29.3973301517084,56.9643794481872));
#85387=CARTESIAN_POINT('Ctrl Pts',(5.94975846603587,-29.4655179662692,56.9852994083785));
#85388=CARTESIAN_POINT('Ctrl Pts',(5.95361382288712,-29.5347905220613,57.002663026264));
#85389=CARTESIAN_POINT('Ctrl Pts',(5.95746917973836,-29.6047437999568,57.0163754855749));
#85390=CARTESIAN_POINT('Ctrl Pts',(5.96132857220692,-29.6747703018546,57.0301022984827));
#85391=CARTESIAN_POINT('Ctrl Pts',(5.96518796467547,-29.7454784705751,57.0401702298633));
#85392=CARTESIAN_POINT('Ctrl Pts',(5.96904735714403,-29.8164551747293,57.046535819285));
#85393=CARTESIAN_POINT('Ctrl Pts',(5.97290893474746,-29.8874720649161,57.0529050128157));
#85394=CARTESIAN_POINT('Ctrl Pts',(5.9767705123509,-29.9587573075259,57.0555676733289));
#85395=CARTESIAN_POINT('Ctrl Pts',(5.98063208995433,-30.0298965035958,57.0545324922164));
#85396=CARTESIAN_POINT('Ctrl Pts',(5.9845004240692,-30.1011601702425,57.0534954998718));
#85397=CARTESIAN_POINT('Ctrl Pts',(5.98836875818407,-30.1722767953068,57.0487477806749));
#85398=CARTESIAN_POINT('Ctrl Pts',(5.99223709229894,-30.2428365374342,57.0403499647332));
#85399=CARTESIAN_POINT('Ctrl Pts',(5.99453481146991,-30.2847477238444,57.0353618168353));
#85400=CARTESIAN_POINT('Ctrl Pts',(5.99683253064089,-30.3264625982631,57.0290868493545));
#85401=CARTESIAN_POINT('Ctrl Pts',(5.99913024981186,-30.3678974432214,57.0215461987724));
#85402=CARTESIAN_POINT('Ctrl Pts',(6.00299944641651,-30.437670792137,57.0088482764164));
#85403=CARTESIAN_POINT('Ctrl Pts',(6.00686864302115,-30.5069226410627,56.9925089162004));
#85404=CARTESIAN_POINT('Ctrl Pts',(6.0107378396258,-30.5752441037058,56.9725850510565));
#85405=CARTESIAN_POINT('Ctrl Pts',(6.01460043061989,-30.6434489258622,56.9526952005435));
#85406=CARTESIAN_POINT('Ctrl Pts',(6.01846302161398,-30.7107260550316,56.9292331382206));
#85407=CARTESIAN_POINT('Ctrl Pts',(6.02232561260807,-30.7766763424025,56.9023068684238));
#85408=CARTESIAN_POINT('Ctrl Pts',(6.02618437399535,-30.8425612426614,56.8754072949627));
#85409=CARTESIAN_POINT('Ctrl Pts',(6.03004313538263,-30.9071214635225,56.8450505102865));
#85410=CARTESIAN_POINT('Ctrl Pts',(6.03390189676991,-30.9699737925889,56.811394049949));
#85411=CARTESIAN_POINT('Ctrl Pts',(6.03775817547521,-31.0327856832016,56.7777592437847));
#85412=CARTESIAN_POINT('Ctrl Pts',(6.04161445418052,-31.0938914352708,56.7408292034246));
#85413=CARTESIAN_POINT('Ctrl Pts',(6.04547073288583,-31.1529301526205,56.7008085211682));
#85414=CARTESIAN_POINT('Ctrl Pts',(6.04767420911889,-31.1866648539873,56.677940718055));
#85415=CARTESIAN_POINT('Ctrl Pts',(6.04987768535195,-31.2197251064094,56.6540646824644));
#85416=CARTESIAN_POINT('Ctrl Pts',(6.05208116158501,-31.2520475724682,56.6292251037768));
#85417=CARTESIAN_POINT('',(5.74592528057396,-27.9452507587439,55.0017658022555));
#85418=CARTESIAN_POINT('Ctrl Pts',(5.74592528057397,-27.9452507587439,55.0017658022555));
#85419=CARTESIAN_POINT('Ctrl Pts',(5.75057817989358,-27.9453246481722,55.0877461243749));
#85420=CARTESIAN_POINT('Ctrl Pts',(5.75523107921319,-27.9507990871283,55.1734909003221));
#85421=CARTESIAN_POINT('Ctrl Pts',(5.75988397853281,-27.9615629769875,55.2584029135126));
#85422=CARTESIAN_POINT('Ctrl Pts',(5.76460377517754,-27.9724816252865,55.3445357540116));
#85423=CARTESIAN_POINT('Ctrl Pts',(5.76932357182228,-27.9888428428115,55.4298117229022));
#85424=CARTESIAN_POINT('Ctrl Pts',(5.77404336846702,-28.0104818888369,55.5136294849929));
#85425=CARTESIAN_POINT('Ctrl Pts',(5.77570694017971,-28.0181089345694,55.5431724650257));
#85426=CARTESIAN_POINT('Ctrl Pts',(5.7773705118924,-28.0263912273234,55.5725344843005));
#85427=CARTESIAN_POINT('Ctrl Pts',(5.77903408360509,-28.0353201550615,55.6016898448475));
#85428=CARTESIAN_POINT('Ctrl Pts',(5.7829031569533,-28.0560867238101,55.6694983003469));
#85429=CARTESIAN_POINT('Ctrl Pts',(5.78677223030152,-28.080408575338,55.7363632146234));
#85430=CARTESIAN_POINT('Ctrl Pts',(5.79064130364973,-28.1081813798379,55.8018851980852));
#85431=CARTESIAN_POINT('Ctrl Pts',(5.79450461204551,-28.1359128026213,55.8673095532304));
#85432=CARTESIAN_POINT('Ctrl Pts',(5.7983679204413,-28.1670847837136,55.9313945058252));
#85433=CARTESIAN_POINT('Ctrl Pts',(5.80223122883708,-28.2015433108007,55.9937560563711));
#85434=CARTESIAN_POINT('Ctrl Pts',(5.80609000532999,-28.2359614158759,56.0560444529099));
#85435=CARTESIAN_POINT('Ctrl Pts',(5.80994878182291,-28.2736581751631,56.1166130399684));
#85436=CARTESIAN_POINT('Ctrl Pts',(5.81380755831582,-28.314432326825,56.1750996475394));
#85437=CARTESIAN_POINT('Ctrl Pts',(5.81766390390403,-28.3551807920867,56.2335494104344));
#85438=CARTESIAN_POINT('Ctrl Pts',(5.82152024949223,-28.3990025262958,56.2899193984337));
#85439=CARTESIAN_POINT('Ctrl Pts',(5.82537659508044,-28.4456521319429,56.3438750937368));
#85440=CARTESIAN_POINT('Ctrl Pts',(5.82923180132577,-28.4922879551384,56.3978148480317));
#85441=CARTESIAN_POINT('Ctrl Pts',(5.8330870075711,-28.5417496735576,56.4493413584357));
#85442=CARTESIAN_POINT('Ctrl Pts',(5.83694221381643,-28.5937517505766,56.4981533377774));
#85443=CARTESIAN_POINT('Ctrl Pts',(5.84079757066768,-28.6457558590875,56.546967223988));
#85444=CARTESIAN_POINT('Ctrl Pts',(5.84465292751893,-28.7003001675251,56.5930660377377));
#85445=CARTESIAN_POINT('Ctrl Pts',(5.84850828437018,-28.7570637140299,56.63618671047));
#85446=CARTESIAN_POINT('Ctrl Pts',(5.85236767683874,-28.8138866781086,56.6793525200184));
#85447=CARTESIAN_POINT('Ctrl Pts',(5.8562270693073,-28.8729331298637,56.7195336710872));
#85448=CARTESIAN_POINT('Ctrl Pts',(5.86008646177586,-28.9338513077055,56.7565091882535));
#85449=CARTESIAN_POINT('Ctrl Pts',(5.86394803937929,-28.9948039765808,56.7935056404484));
#85450=CARTESIAN_POINT('Ctrl Pts',(5.86780961698273,-29.0576300531253,56.8272926154683));
#85451=CARTESIAN_POINT('Ctrl Pts',(5.87167119458616,-29.1219536682789,56.8576954007186));
#85452=CARTESIAN_POINT('Ctrl Pts',(5.87553952870103,-29.1863898289479,56.8881513810067));
#85453=CARTESIAN_POINT('Ctrl Pts',(5.87940786281591,-29.2523283099901,56.9152111651145));
#85454=CARTESIAN_POINT('Ctrl Pts',(5.88327619693078,-29.3193744584956,56.9387486775629));
#85455=CARTESIAN_POINT('Ctrl Pts',(5.88557391610173,-29.3591986350495,56.9527295261616));
#85456=CARTESIAN_POINT('Ctrl Pts',(5.88787163527269,-29.3994133254085,56.9654686251861));
#85457=CARTESIAN_POINT('Ctrl Pts',(5.89016935444365,-29.4399340600699,56.9769480785873));
#85458=CARTESIAN_POINT('Ctrl Pts',(5.89403860384479,-29.5081690429625,56.9962789301377));
#85459=CARTESIAN_POINT('Ctrl Pts',(5.89790785324593,-29.5775396769516,57.0121107721141));
#85460=CARTESIAN_POINT('Ctrl Pts',(5.90177710264707,-29.6476537787499,57.0243146254648));
#85461=CARTESIAN_POINT('Ctrl Pts',(5.90563962090613,-29.7176459065084,57.0364972483747));
#85462=CARTESIAN_POINT('Ctrl Pts',(5.9095021391652,-29.788378457524,57.0450643409053));
#85463=CARTESIAN_POINT('Ctrl Pts',(5.91336465742426,-29.8594455361168,57.049937073469));
#85464=CARTESIAN_POINT('Ctrl Pts',(5.91722337851854,-29.9304427500797,57.0548050157463));
#85465=CARTESIAN_POINT('Ctrl Pts',(5.92108209961282,-30.001773357262,57.0559857693842));
#85466=CARTESIAN_POINT('Ctrl Pts',(5.92494082070709,-30.0730239443259,57.0534519877648));
#85467=CARTESIAN_POINT('Ctrl Pts',(5.9287970392771,-30.1442283227317,57.0509198493971));
#85468=CARTESIAN_POINT('Ctrl Pts',(5.9326532578471,-30.2153522997328,57.044677973616));
#85469=CARTESIAN_POINT('Ctrl Pts',(5.93650947641711,-30.2859817780574,57.0347510867718));
#85470=CARTESIAN_POINT('Ctrl Pts',(5.94036448407723,-30.3565890776771,57.0248273171175));
#85471=CARTESIAN_POINT('Ctrl Pts',(5.94421949173735,-30.426701706356,57.0112209023426));
#85472=CARTESIAN_POINT('Ctrl Pts',(5.94807449939747,-30.4959117356517,56.9940083031279));
#85473=CARTESIAN_POINT('Ctrl Pts',(5.95193183773627,-30.5651636082728,56.9767852974389));
#85474=CARTESIAN_POINT('Ctrl Pts',(5.95578917607507,-30.6335113173793,56.9559518624058));
#85475=CARTESIAN_POINT('Ctrl Pts',(5.95964651441388,-30.7005591600954,56.9316351688935));
#85476=CARTESIAN_POINT('Ctrl Pts',(5.96350485094006,-30.7676243531979,56.9073121827996));
#85477=CARTESIAN_POINT('Ctrl Pts',(5.96736318746624,-30.8333885587031,56.8795043250434));
#85478=CARTESIAN_POINT('Ctrl Pts',(5.97122152399242,-30.8974756542452,56.8483871381659));
#85479=CARTESIAN_POINT('Ctrl Pts',(5.97508578920568,-30.9616612254731,56.8172221368838));
#85480=CARTESIAN_POINT('Ctrl Pts',(5.97895005441895,-31.0241641074325,56.7827378750177));
#85481=CARTESIAN_POINT('Ctrl Pts',(5.98281431963221,-31.0846329359057,56.7451558546012));
#85482=CARTESIAN_POINT('Ctrl Pts',(5.98650504906563,-31.1423862402814,56.7092615613103));
#85483=CARTESIAN_POINT('Ctrl Pts',(5.99019577849905,-31.1982839789842,56.6705420320225));
#85484=CARTESIAN_POINT('Ctrl Pts',(5.99388650793247,-31.2520475724682,56.6292251037768));
#85485=CARTESIAN_POINT('Ctrl Pts',(5.29388070614408,-31.2520475724682,56.6292251037768));
#85486=CARTESIAN_POINT('Ctrl Pts',(5.29774024882555,-31.3086258322378,56.5857451250834));
#85487=CARTESIAN_POINT('Ctrl Pts',(5.30159979150703,-31.3629068090275,56.5393373691093));
#85488=CARTESIAN_POINT('Ctrl Pts',(5.3054593341885,-31.4145854558055,56.4902837148421));
#85489=CARTESIAN_POINT('Ctrl Pts',(5.30932116705353,-31.4662947677677,56.4412009530143));
#85490=CARTESIAN_POINT('Ctrl Pts',(5.31318299991856,-31.5153983418367,56.3894695204074));
#85491=CARTESIAN_POINT('Ctrl Pts',(5.31704483278359,-31.5616295181324,56.3354066087143));
#85492=CARTESIAN_POINT('Ctrl Pts',(5.3209133155756,-31.6079403027274,56.281250602776));
#85493=CARTESIAN_POINT('Ctrl Pts',(5.32478179836762,-31.6513685208432,56.2247554891651));
#85494=CARTESIAN_POINT('Ctrl Pts',(5.32865028115963,-31.6916896102803,56.1662691906115));
#85495=CARTESIAN_POINT('Ctrl Pts',(5.33059785419004,-31.7119891102565,56.1368244848094));
#85496=CARTESIAN_POINT('Ctrl Pts',(5.33254542722045,-31.7315017941742,56.1068755173923));
#85497=CARTESIAN_POINT('Ctrl Pts',(5.33449300025085,-31.7502034628656,56.0764689503526));
#85498=CARTESIAN_POINT('Ctrl Pts',(5.33836207359907,-31.7873564357047,56.0160628776113));
#85499=CARTESIAN_POINT('Ctrl Pts',(5.34223114694728,-31.8214512506892,55.9536127950323));
#85500=CARTESIAN_POINT('Ctrl Pts',(5.34610022029549,-31.852257189563,55.8894609975778));
#85501=CARTESIAN_POINT('Ctrl Pts',(5.34996352869128,-31.8830172273241,55.8254047868509));
#85502=CARTESIAN_POINT('Ctrl Pts',(5.35382683708707,-31.9104979076634,55.7596523286277));
#85503=CARTESIAN_POINT('Ctrl Pts',(5.35769014548285,-31.9345129022427,55.6925730239886));
#85504=CARTESIAN_POINT('Ctrl Pts',(5.36154892197577,-31.9584997257282,55.6255724075779));
#85505=CARTESIAN_POINT('Ctrl Pts',(5.36540769846868,-31.9790287759016,55.5572484915747));
#85506=CARTESIAN_POINT('Ctrl Pts',(5.36926647496159,-31.9959613378884,55.4879917009078));
#85507=CARTESIAN_POINT('Ctrl Pts',(5.3731228205498,-32.0128832329073,55.4187785397848));
#85508=CARTESIAN_POINT('Ctrl Pts',(5.37697916613801,-32.0262130196965,55.348634140719));
#85509=CARTESIAN_POINT('Ctrl Pts',(5.38083551172622,-32.0358619075835,55.2779637669743));
#85510=CARTESIAN_POINT('Ctrl Pts',(5.38469071797155,-32.0455079447426,55.2073142725271));
#85511=CARTESIAN_POINT('Ctrl Pts',(5.38854592421687,-32.0514751763228,55.1361395929657));
#85512=CARTESIAN_POINT('Ctrl Pts',(5.3924011304622,-32.0537262797841,55.0648531435188));
#85513=CARTESIAN_POINT('Ctrl Pts',(5.39625648731346,-32.055977471186,54.9935639092244));
#85514=CARTESIAN_POINT('Ctrl Pts',(5.40011184416471,-32.0545122331165,54.9221633819892));
#85515=CARTESIAN_POINT('Ctrl Pts',(5.40396720101597,-32.0493453378879,54.8510662946903));
#85516=CARTESIAN_POINT('Ctrl Pts',(5.40782659348453,-32.0441730341815,54.7798947860999));
#85517=CARTESIAN_POINT('Ctrl Pts',(5.41168598595309,-32.0352913737649,54.7090278370028));
#85518=CARTESIAN_POINT('Ctrl Pts',(5.41554537842165,-32.0227670734455,54.6388754659609));
#85519=CARTESIAN_POINT('Ctrl Pts',(5.41940695602509,-32.0102356820395,54.5686833756125));
#85520=CARTESIAN_POINT('Ctrl Pts',(5.42326853362853,-31.9940576553269,54.4992071420743));
#85521=CARTESIAN_POINT('Ctrl Pts',(5.42713011123197,-31.9743503595407,54.4308442917079));
#85522=CARTESIAN_POINT('Ctrl Pts',(5.43099844534684,-31.9546085823629,54.3623618284715));
#85523=CARTESIAN_POINT('Ctrl Pts',(5.43486677946171,-31.9313253661281,54.2949970970472));
#85524=CARTESIAN_POINT('Ctrl Pts',(5.43873511357658,-31.9046669889523,54.2291295675047));
#85525=CARTESIAN_POINT('Ctrl Pts',(5.44103283274752,-31.888832404223,54.1900054688932));
#85526=CARTESIAN_POINT('Ctrl Pts',(5.44333055191846,-31.8718079232593,54.1514091865266));
#85527=CARTESIAN_POINT('Ctrl Pts',(5.44562827108941,-31.8536359549886,54.1134159324275));
#85528=CARTESIAN_POINT('Ctrl Pts',(5.44949734443762,-31.8230366202179,54.0494400172218));
#85529=CARTESIAN_POINT('Ctrl Pts',(5.45336641778584,-31.7890613887607,53.9869247961122));
#85530=CARTESIAN_POINT('Ctrl Pts',(5.45723549113406,-31.7518727042285,53.9262497540493));
#85531=CARTESIAN_POINT('Ctrl Pts',(5.46109879952985,-31.7147394311547,53.8656651183187));
#85532=CARTESIAN_POINT('Ctrl Pts',(5.46496210792565,-31.6744024609844,53.8069156298799));
#85533=CARTESIAN_POINT('Ctrl Pts',(5.46882541632145,-31.6310710858572,53.7503581811652));
#85534=CARTESIAN_POINT('Ctrl Pts',(5.47268419281436,-31.5877905411488,53.6938670778826));
#85535=CARTESIAN_POINT('Ctrl Pts',(5.47654296930727,-31.5415228627517,53.6395632904017));
#85536=CARTESIAN_POINT('Ctrl Pts',(5.48040174580018,-31.492520829689,53.58777511159));
#85537=CARTESIAN_POINT('Ctrl Pts',(5.48425809138839,-31.4435496663262,53.5360195576603));
#85538=CARTESIAN_POINT('Ctrl Pts',(5.4881144369766,-31.3918478989097,53.486776820306));
#85539=CARTESIAN_POINT('Ctrl Pts',(5.49197078256481,-31.337707849888,53.440341296678));
#85540=CARTESIAN_POINT('Ctrl Pts',(5.49582598881014,-31.2835837963413,53.3939194922518));
#85541=CARTESIAN_POINT('Ctrl Pts',(5.49968119505547,-31.2270232598805,53.3503035710914));
#85542=CARTESIAN_POINT('Ctrl Pts',(5.50353640130079,-31.1683533262419,53.3097491110609));
#85543=CARTESIAN_POINT('Ctrl Pts',(5.50739175815205,-31.1096811006274,53.2691930667462));
#85544=CARTESIAN_POINT('Ctrl Pts',(5.5112471150033,-31.0488997150942,53.2316989954185));
#85545=CARTESIAN_POINT('Ctrl Pts',(5.51510247185456,-30.9863656167692,53.1974794224321));
#85546=CARTESIAN_POINT('Ctrl Pts',(5.51896186432312,-30.9237660605114,53.1632240299079));
#85547=CARTESIAN_POINT('Ctrl Pts',(5.52282125679167,-30.8594105560905,53.1322502116607));
#85548=CARTESIAN_POINT('Ctrl Pts',(5.52668064926023,-30.7936797627601,53.1047242953372));
#85549=CARTESIAN_POINT('Ctrl Pts',(5.53054222686366,-30.7279117535598,53.077182794219));
#85550=CARTESIAN_POINT('Ctrl Pts',(5.53440380446709,-30.6607673628243,53.0530932452879));
#85551=CARTESIAN_POINT('Ctrl Pts',(5.53826538207053,-30.5926442249953,53.0325726480808));
#85552=CARTESIAN_POINT('Ctrl Pts',(5.5421337161854,-30.5244018937155,53.0120161464678));
#85553=CARTESIAN_POINT('Ctrl Pts',(5.54600205030027,-30.4551778682624,52.9950411796584));
#85554=CARTESIAN_POINT('Ctrl Pts',(5.54987038441514,-30.3853811412491,52.9817138611016));
#85555=CARTESIAN_POINT('Ctrl Pts',(5.55216810358608,-30.343923171755,52.973797679501));
#85556=CARTESIAN_POINT('Ctrl Pts',(5.55446582275703,-30.3022632866961,52.9671674501318));
#85557=CARTESIAN_POINT('Ctrl Pts',(5.55676354192797,-30.2604876760479,52.9618283357069));
#85558=CARTESIAN_POINT('Ctrl Pts',(5.56063261527618,-30.1901427427731,52.9528379309675));
#85559=CARTESIAN_POINT('Ctrl Pts',(5.5645016886244,-30.1191940371152,52.9474759921008));
#85560=CARTESIAN_POINT('Ctrl Pts',(5.56837076197261,-30.0480484844917,52.9458118621611));
#85561=CARTESIAN_POINT('Ctrl Pts',(5.5722340703684,-29.977008939351,52.9441502117893));
#85562=CARTESIAN_POINT('Ctrl Pts',(5.57609737876418,-29.9057736111407,52.946175444879));
#85563=CARTESIAN_POINT('Ctrl Pts',(5.57996068715997,-29.8347558532785,52.9519052916249));
#85564=CARTESIAN_POINT('Ctrl Pts',(5.58381946365288,-29.7638214036972,52.9576284169014));
#85565=CARTESIAN_POINT('Ctrl Pts',(5.58767824014579,-29.6931044993658,52.967047484839));
#85566=CARTESIAN_POINT('Ctrl Pts',(5.5915370166387,-29.623018051686,52.9801281790308));
#85567=CARTESIAN_POINT('Ctrl Pts',(5.59539336222691,-29.5529757562073,52.9932006328072));
#85568=CARTESIAN_POINT('Ctrl Pts',(5.59924970781511,-29.4835636058177,53.0099300474539));
#85569=CARTESIAN_POINT('Ctrl Pts',(5.60310605340332,-29.4151874815847,53.0302305005903));
#85570=CARTESIAN_POINT('Ctrl Pts',(5.60696125964865,-29.3468315588217,53.0505249560337));
#85571=CARTESIAN_POINT('Ctrl Pts',(5.61081646589399,-29.2795115199829,53.074388217214));
#85572=CARTESIAN_POINT('Ctrl Pts',(5.61467167213932,-29.2136194867206,53.1016841014113));
#85573=CARTESIAN_POINT('Ctrl Pts',(5.61852702899056,-29.1477248793473,53.1289810519384));
#85574=CARTESIAN_POINT('Ctrl Pts',(5.62238238584179,-29.0832588362648,53.1597107037637));
#85575=CARTESIAN_POINT('Ctrl Pts',(5.62623774269303,-29.0205932334006,53.1936888562489));
#85576=CARTESIAN_POINT('Ctrl Pts',(5.63009713516159,-28.9578620349503,53.227702575564));
#85577=CARTESIAN_POINT('Ctrl Pts',(5.63395652763014,-28.8969354667709,53.2649713514488));
#85578=CARTESIAN_POINT('Ctrl Pts',(5.6378159200987,-28.8381597238713,53.3052655856255));
#85579=CARTESIAN_POINT('Ctrl Pts',(5.64167749770213,-28.7793507029555,53.3455826338427));
#85580=CARTESIAN_POINT('Ctrl Pts',(5.64553907530556,-28.7226953175213,53.3889282550317));
#85581=CARTESIAN_POINT('Ctrl Pts',(5.64940065290899,-28.6685075266163,53.4350318355243));
#85582=CARTESIAN_POINT('Ctrl Pts',(5.65326898702387,-28.614224924609,53.4812160823665));
#85583=CARTESIAN_POINT('Ctrl Pts',(5.65713732113874,-28.5624188903338,53.530167589093));
#85584=CARTESIAN_POINT('Ctrl Pts',(5.66100565525361,-28.5133667914838,53.5815786007548));
#85585=CARTESIAN_POINT('Ctrl Pts',(5.66330337442458,-28.4842307487953,53.6121157941787));
#85586=CARTESIAN_POINT('Ctrl Pts',(5.66560109359555,-28.45606557884,53.6435200799697));
#85587=CARTESIAN_POINT('Ctrl Pts',(5.66789881276653,-28.428922365385,53.6757218462451));
#85588=CARTESIAN_POINT('Ctrl Pts',(5.67174314546748,-28.3835088333867,53.7295988842594));
#85589=CARTESIAN_POINT('Ctrl Pts',(5.67558747816844,-28.3407741615804,53.7859284481419));
#85590=CARTESIAN_POINT('Ctrl Pts',(5.67943181086939,-28.3009964282985,53.844411653812));
#85591=CARTESIAN_POINT('Ctrl Pts',(5.68327073565046,-28.2612746513585,53.9028125896799));
#85592=CARTESIAN_POINT('Ctrl Pts',(5.68710966043153,-28.2245018386303,53.9633607567452));
#85593=CARTESIAN_POINT('Ctrl Pts',(5.6909485852126,-28.1909165779055,54.0257234815502));
#85594=CARTESIAN_POINT('Ctrl Pts',(5.69478343427785,-28.1573669740341,54.0880199969975));
#85595=CARTESIAN_POINT('Ctrl Pts',(5.6986182833431,-28.1269984405792,54.1521268173286));
#85596=CARTESIAN_POINT('Ctrl Pts',(5.70245313240835,-28.1000058717308,54.217683008594));
#85597=CARTESIAN_POINT('Ctrl Pts',(5.70628582152484,-28.0730285062359,54.2832022758471));
#85598=CARTESIAN_POINT('Ctrl Pts',(5.71011851064132,-28.0494235257525,54.350168842789));
#85599=CARTESIAN_POINT('Ctrl Pts',(5.71395119975781,-28.0293387874977,54.4181993915102));
#85600=CARTESIAN_POINT('Ctrl Pts',(5.71778249936709,-28.0092613307855,54.4862052763635));
#85601=CARTESIAN_POINT('Ctrl Pts',(5.72161379897638,-27.9927017184508,54.5552739041778));
#85602=CARTESIAN_POINT('Ctrl Pts',(5.72544509858566,-27.9797581310333,54.6250061955525));
#85603=CARTESIAN_POINT('Ctrl Pts',(5.7292781028654,-27.9668087845906,54.6947695131036));
#85604=CARTESIAN_POINT('Ctrl Pts',(5.73311110714515,-27.9574787693276,54.7651965997995));
#85605=CARTESIAN_POINT('Ctrl Pts',(5.73694411142489,-27.9518149998429,54.8358788020042));
#85606=CARTESIAN_POINT('Ctrl Pts',(5.73993783446249,-27.947391379114,54.8910843070453));
#85607=CARTESIAN_POINT('Ctrl Pts',(5.74293155750008,-27.9452032175471,54.9464451824547));
#85608=CARTESIAN_POINT('Ctrl Pts',(5.74592528053768,-27.9452507587434,55.001765801585));
#85609=CARTESIAN_POINT('Origin',(-1.54592528053767,-30.,55.));
#85610=CARTESIAN_POINT('',(4.59397380331217,-31.2520475724682,56.6292251037768));
#85611=CARTESIAN_POINT('',(4.65201752376309,-31.2520475724682,56.6292251037768));
#85612=CARTESIAN_POINT('',(-1.54592528053767,-31.2520475724682,56.6292251037768));
#85613=CARTESIAN_POINT('',(5.10407471942444,-27.9452501074214,55.0006644157262));
#85614=CARTESIAN_POINT('Ctrl Pts',(4.65201752376309,-31.2520475724682,56.6292251037768));
#85615=CARTESIAN_POINT('Ctrl Pts',(4.65588667239735,-31.3085034428774,56.5858391804114));
#85616=CARTESIAN_POINT('Ctrl Pts',(4.65975582103161,-31.3626178531137,56.5395797614622));
#85617=CARTESIAN_POINT('Ctrl Pts',(4.66362496966587,-31.4141019698079,56.490742493352));
#85618=CARTESIAN_POINT('Ctrl Pts',(4.66425231302696,-31.4224495991866,56.4828240237302));
#85619=CARTESIAN_POINT('Ctrl Pts',(4.66487965638806,-31.430728164715,56.4748378560675));
#85620=CARTESIAN_POINT('Ctrl Pts',(4.66550699974915,-31.4389365354664,56.4667853317374));
#85621=CARTESIAN_POINT('Ctrl Pts',(4.66937607309736,-31.4895607876317,56.417122245773));
#85622=CARTESIAN_POINT('Ctrl Pts',(4.67324514644558,-31.5377100925752,56.3647379575139));
#85623=CARTESIAN_POINT('Ctrl Pts',(4.67711421979379,-31.5830779920416,56.3099090173037));
#85624=CARTESIAN_POINT('Ctrl Pts',(4.68097752818958,-31.6283782929492,56.2551617726842));
#85625=CARTESIAN_POINT('Ctrl Pts',(4.68484083658537,-31.6709051075678,56.1979774777012));
#85626=CARTESIAN_POINT('Ctrl Pts',(4.68870414498115,-31.710388520268,56.1386696940885));
#85627=CARTESIAN_POINT('Ctrl Pts',(4.69256292147407,-31.7498256164505,56.0794314822229));
#85628=CARTESIAN_POINT('Ctrl Pts',(4.69642169796698,-31.7862261342444,56.0180751320759));
#85629=CARTESIAN_POINT('Ctrl Pts',(4.70028047445989,-31.8193612958817,55.9549460914354));
#85630=CARTESIAN_POINT('Ctrl Pts',(4.7041368200481,-31.852475583436,55.8918568200541));
#85631=CARTESIAN_POINT('Ctrl Pts',(4.7079931656363,-31.88232837079,55.8269975028873));
#85632=CARTESIAN_POINT('Ctrl Pts',(4.71184951122451,-31.9087357523067,55.7607400281082));
#85633=CARTESIAN_POINT('Ctrl Pts',(4.71570471746984,-31.9351353318614,55.6945021288521));
#85634=CARTESIAN_POINT('Ctrl Pts',(4.71955992371517,-31.9580913466993,55.626867343082));
#85635=CARTESIAN_POINT('Ctrl Pts',(4.72341512996051,-31.9774678741999,55.5582278826853));
#85636=CARTESIAN_POINT('Ctrl Pts',(4.72727048681175,-31.996845158656,55.4895857408473));
#85637=CARTESIAN_POINT('Ctrl Pts',(4.731125843663,-32.0126425482941,55.4199393145738));
#85638=CARTESIAN_POINT('Ctrl Pts',(4.73498120051425,-32.0247743599362,55.3496946580158));
#85639=CARTESIAN_POINT('Ctrl Pts',(4.7388405929828,-32.0369188706231,55.2793764724531));
#85640=CARTESIAN_POINT('Ctrl Pts',(4.74269998545136,-32.0453900610246,55.2084592862478));
#85641=CARTESIAN_POINT('Ctrl Pts',(4.74655937791992,-32.0501537961901,55.1373571056304));
#85642=CARTESIAN_POINT('Ctrl Pts',(4.75042095552336,-32.0549202285169,55.0662146679373));
#85643=CARTESIAN_POINT('Ctrl Pts',(4.7542825331268,-32.0559750197405,54.9948875132876));
#85644=CARTESIAN_POINT('Ctrl Pts',(4.75814411073023,-32.0533362020556,54.9237897393517));
#85645=CARTESIAN_POINT('Ctrl Pts',(4.7620124448451,-32.0506927672934,54.8525675673143));
#85646=CARTESIAN_POINT('Ctrl Pts',(4.76588077895997,-32.0443428641057,54.7815760612898));
#85647=CARTESIAN_POINT('Ctrl Pts',(4.76974911307484,-32.0343563474449,54.7112235914919));
#85648=CARTESIAN_POINT('Ctrl Pts',(4.7720468322458,-32.0284245405995,54.6694355210258));
#85649=CARTESIAN_POINT('Ctrl Pts',(4.77434455141676,-32.0212106673078,54.6278727252012));
#85650=CARTESIAN_POINT('Ctrl Pts',(4.77664227058771,-32.0127377461673,54.586618423665));
#85651=CARTESIAN_POINT('Ctrl Pts',(4.78051134393593,-31.9984704006273,54.5171513101072));
#85652=CARTESIAN_POINT('Ctrl Pts',(4.78438041728414,-31.9805745320216,54.4482876251215));
#85653=CARTESIAN_POINT('Ctrl Pts',(4.78824949063236,-31.9591162703888,54.3804348286113));
#85654=CARTESIAN_POINT('Ctrl Pts',(4.79211279902815,-31.9376899817496,54.3126831333491));
#85655=CARTESIAN_POINT('Ctrl Pts',(4.79597610742393,-31.9127119815914,54.2459397961355));
#85656=CARTESIAN_POINT('Ctrl Pts',(4.79983941581972,-31.8842993142413,54.180601649471));
#85657=CARTESIAN_POINT('Ctrl Pts',(4.80369819231263,-31.8559199767307,54.1153401485474));
#85658=CARTESIAN_POINT('Ctrl Pts',(4.80755696880554,-31.8241141679264,54.0514810072649));
#85659=CARTESIAN_POINT('Ctrl Pts',(4.81141574529846,-31.7890480327174,53.9894037902653));
#85660=CARTESIAN_POINT('Ctrl Pts',(4.81527209088666,-31.7540039880423,53.9273656799098));
#85661=CARTESIAN_POINT('Ctrl Pts',(4.81912843647487,-31.7157039302291,53.8671076886751));
#85662=CARTESIAN_POINT('Ctrl Pts',(4.82298478206308,-31.6743605549183,53.8089860224861));
#85663=CARTESIAN_POINT('Ctrl Pts',(4.82683998830841,-31.6330293943531,53.7508815281258));
#85664=CARTESIAN_POINT('Ctrl Pts',(4.83069519455374,-31.588656982753,53.694912501404));
#85665=CARTESIAN_POINT('Ctrl Pts',(4.83455040079908,-31.5414991148609,53.6414058584761));
#85666=CARTESIAN_POINT('Ctrl Pts',(4.83840575765032,-31.4943394047187,53.5878971252795));
#85667=CARTESIAN_POINT('Ctrl Pts',(4.84226111450157,-31.4443943450982,53.5368513298448));
#85668=CARTESIAN_POINT('Ctrl Pts',(4.84611647135282,-31.3919586083003,53.4885606875304));
#85669=CARTESIAN_POINT('Ctrl Pts',(4.84997586382138,-31.3394679840886,53.440219496704));
#85670=CARTESIAN_POINT('Ctrl Pts',(4.85383525628994,-31.2844818363485,53.3946395458178));
#85671=CARTESIAN_POINT('Ctrl Pts',(4.8576946487585,-31.2273294761762,53.3520740552413));
#85672=CARTESIAN_POINT('Ctrl Pts',(4.86155622636193,-31.1701447571246,53.30948446467));
#85673=CARTESIAN_POINT('Ctrl Pts',(4.86541780396537,-31.1107917884792,53.2699130016197));
#85674=CARTESIAN_POINT('Ctrl Pts',(4.8692793815688,-31.0496282517455,53.2335691081625));
#85675=CARTESIAN_POINT('Ctrl Pts',(4.87314771568367,-30.9883576986112,53.1971616246504));
#85676=CARTESIAN_POINT('Ctrl Pts',(4.87701604979855,-30.925270682684,53.1639932116718));
#85677=CARTESIAN_POINT('Ctrl Pts',(4.88088438391342,-30.8607481803857,53.1342266663759));
#85678=CARTESIAN_POINT('Ctrl Pts',(4.88318210308436,-30.8224230031684,53.1165458870667));
#85679=CARTESIAN_POINT('Ctrl Pts',(4.88547982225531,-30.7835917421944,53.1000644084989));
#85680=CARTESIAN_POINT('Ctrl Pts',(4.88777754142626,-30.7443367983747,53.0848080270935));
#85681=CARTESIAN_POINT('Ctrl Pts',(4.89164661477447,-30.6782363545785,53.0591181780328));
#85682=CARTESIAN_POINT('Ctrl Pts',(4.89551568812269,-30.6106748968163,53.0368040872381));
#85683=CARTESIAN_POINT('Ctrl Pts',(4.8993847614709,-30.5420306164589,53.0180311876013));
#85684=CARTESIAN_POINT('Ctrl Pts',(4.90324806986669,-30.4734886166672,52.9992862597457));
#85685=CARTESIAN_POINT('Ctrl Pts',(4.90711137826248,-30.403867461625,52.9840721766353));
#85686=CARTESIAN_POINT('Ctrl Pts',(4.91097468665826,-30.3335640282406,52.9725058319285));
#85687=CARTESIAN_POINT('Ctrl Pts',(4.91483346315117,-30.2633430651898,52.960953055269));
#85688=CARTESIAN_POINT('Ctrl Pts',(4.91869223964408,-30.1924418905885,52.9530395958994));
#85689=CARTESIAN_POINT('Ctrl Pts',(4.922551016137,-30.1212695042465,52.9488317304912));
#85690=CARTESIAN_POINT('Ctrl Pts',(4.9264073617252,-30.0501419542119,52.9446265159024));
#85691=CARTESIAN_POINT('Ctrl Pts',(4.93026370731341,-29.9787440152021,52.9441222924568));
#85692=CARTESIAN_POINT('Ctrl Pts',(4.93412005290161,-29.9074903098069,52.9473335585828));
#85693=CARTESIAN_POINT('Ctrl Pts',(4.93797525914695,-29.8362576560524,52.9505438759522));
#85694=CARTESIAN_POINT('Ctrl Pts',(4.94183046539228,-29.7651696363424,52.9574674817409));
#85695=CARTESIAN_POINT('Ctrl Pts',(4.94568567163761,-29.6946396410612,52.9680667792251));
#85696=CARTESIAN_POINT('Ctrl Pts',(4.94954102848885,-29.6241068904839,52.9786664907771));
#85697=CARTESIAN_POINT('Ctrl Pts',(4.9533963853401,-29.5541326876797,52.9929421047381));
#85698=CARTESIAN_POINT('Ctrl Pts',(4.95725174219134,-29.4851223551726,53.0108045411883));
#85699=CARTESIAN_POINT('Ctrl Pts',(4.9611111346599,-29.4160397856968,53.0286856752482));
#85700=CARTESIAN_POINT('Ctrl Pts',(4.96497052712846,-29.3479235718339,53.0501610047003));
#85701=CARTESIAN_POINT('Ctrl Pts',(4.96882991959702,-29.2811650615579,53.0750911985824));
#85702=CARTESIAN_POINT('Ctrl Pts',(4.97269149720045,-29.2143687535325,53.1000355075971));
#85703=CARTESIAN_POINT('Ctrl Pts',(4.97655307480389,-29.1489321251945,53.1284383815136));
#85704=CARTESIAN_POINT('Ctrl Pts',(4.98041465240732,-29.0852251315543,53.1601129103773));
#85705=CARTESIAN_POINT('Ctrl Pts',(4.98428298652219,-29.021406671287,53.1918428594186));
#85706=CARTESIAN_POINT('Ctrl Pts',(4.98815132063707,-28.9593243110823,53.2268556535021));
#85707=CARTESIAN_POINT('Ctrl Pts',(4.99201965475194,-28.8993214518452,53.2649195130681));
#85708=CARTESIAN_POINT('Ctrl Pts',(4.9943173739229,-28.8636808593091,53.2875287441346));
#85709=CARTESIAN_POINT('Ctrl Pts',(4.99661509309386,-28.8287733699117,53.3112136158591));
#85710=CARTESIAN_POINT('Ctrl Pts',(4.99891281226483,-28.7946653476447,53.3359188906993));
#85711=CARTESIAN_POINT('Ctrl Pts',(5.00275064676246,-28.7376953984199,53.3771836184579));
#85712=CARTESIAN_POINT('Ctrl Pts',(5.00658848126009,-28.6827265110719,53.4214646825556));
#85713=CARTESIAN_POINT('Ctrl Pts',(5.01042631575773,-28.6300997290131,53.4685396479014));
#85714=CARTESIAN_POINT('Ctrl Pts',(5.01432833257717,-28.5765928388975,53.5164018750681));
#85715=CARTESIAN_POINT('Ctrl Pts',(5.01823034939662,-28.5255075807004,53.5671520862871));
#85716=CARTESIAN_POINT('Ctrl Pts',(5.02213236621606,-28.477171663074,53.620510449929));
#85717=CARTESIAN_POINT('Ctrl Pts',(5.02595997436977,-28.4297574767738,53.6728513077967));
#85718=CARTESIAN_POINT('Ctrl Pts',(5.02978758252349,-28.3849890497206,53.7277013416823));
#85719=CARTESIAN_POINT('Ctrl Pts',(5.0336151906772,-28.3431406316787,53.7847573920793));
#85720=CARTESIAN_POINT('Ctrl Pts',(5.03744050268939,-28.3013173180588,53.841779215157));
#85721=CARTESIAN_POINT('Ctrl Pts',(5.04126581470158,-28.2624108313474,53.9010040323731));
#85722=CARTESIAN_POINT('Ctrl Pts',(5.04509112671377,-28.2266549764503,53.9620958666854));
#85723=CARTESIAN_POINT('Ctrl Pts',(5.04891547573736,-28.1909081227747,54.0231723216666));
#85724=CARTESIAN_POINT('Ctrl Pts',(5.05273982476095,-28.1583105759941,54.0861144340417));
#85725=CARTESIAN_POINT('Ctrl Pts',(5.05656417378455,-28.1290516520463,54.1505591004728));
#85726=CARTESIAN_POINT('Ctrl Pts',(5.06052338592121,-28.098760931695,54.2172763650067));
#85727=CARTESIAN_POINT('Ctrl Pts',(5.06448259805786,-28.0720489807079,54.2856036450338));
#85728=CARTESIAN_POINT('Ctrl Pts',(5.06844181019452,-28.0490719088945,54.3551146258167));
#85729=CARTESIAN_POINT('Ctrl Pts',(5.07227054686684,-28.0268520443261,54.4223348787524));
#85730=CARTESIAN_POINT('Ctrl Pts',(5.07609928353915,-28.0081247870476,54.4906615152341));
#85731=CARTESIAN_POINT('Ctrl Pts',(5.07992802021147,-27.9929800396064,54.5596950589858));
#85732=CARTESIAN_POINT('Ctrl Pts',(5.0839524700803,-27.9770611394391,54.632257384336));
#85733=CARTESIAN_POINT('Ctrl Pts',(5.08797691994913,-27.9651009153748,54.7056002068222));
#85734=CARTESIAN_POINT('Ctrl Pts',(5.09200136981795,-27.9571422025373,54.779252221198));
#85735=CARTESIAN_POINT('Ctrl Pts',(5.09602581968678,-27.9491834896999,54.8529042355738));
#85736=CARTESIAN_POINT('Ctrl Pts',(5.10005026955561,-27.9452262438762,54.9268648126139));
#85737=CARTESIAN_POINT('Ctrl Pts',(5.10407471942444,-27.9452501074214,55.0006644157262));
#85738=CARTESIAN_POINT('Ctrl Pts',(5.10407471946233,-27.9452501074216,55.000664416421));
#85739=CARTESIAN_POINT('Ctrl Pts',(5.10606584067601,-27.9452619140691,55.0371772219238));
#85740=CARTESIAN_POINT('Ctrl Pts',(5.1080569618897,-27.9462469037348,55.0736730530943));
#85741=CARTESIAN_POINT('Ctrl Pts',(5.11004808310338,-27.9482027488899,55.1101163150356));
#85742=CARTESIAN_POINT('Ctrl Pts',(5.1139171564516,-27.9520032751014,55.1809315183137));
#85743=CARTESIAN_POINT('Ctrl Pts',(5.11778622979981,-27.959481696,55.2516884433728));
#85744=CARTESIAN_POINT('Ctrl Pts',(5.12165530314803,-27.97063308038,55.32197432825));
#85745=CARTESIAN_POINT('Ctrl Pts',(5.12551861154382,-27.9817678491018,55.3921554865566));
#85746=CARTESIAN_POINT('Ctrl Pts',(5.1293819199396,-27.9965646425545,55.4618665219658));
#85747=CARTESIAN_POINT('Ctrl Pts',(5.13324522833539,-28.0149666018932,55.5306976266206));
#85748=CARTESIAN_POINT('Ctrl Pts',(5.1371040048283,-28.0333469745804,55.5994479880758));
#85749=CARTESIAN_POINT('Ctrl Pts',(5.14096278132121,-28.0553239879001,55.667320002077));
#85750=CARTESIAN_POINT('Ctrl Pts',(5.14482155781412,-28.0807896635758,55.733913650958));
#85751=CARTESIAN_POINT('Ctrl Pts',(5.14867790340233,-28.1062392966974,55.8004653479885));
#85752=CARTESIAN_POINT('Ctrl Pts',(5.15253424899053,-28.1351730587826,55.8657398249893));
#85753=CARTESIAN_POINT('Ctrl Pts',(5.15639059457874,-28.1674334698244,55.9293532562919));
#85754=CARTESIAN_POINT('Ctrl Pts',(5.16024580082407,-28.1996843496485,55.9929478932442));
#85755=CARTESIAN_POINT('Ctrl Pts',(5.16410100706941,-28.2352597076089,56.0548820257512));
#85756=CARTESIAN_POINT('Ctrl Pts',(5.16795621331474,-28.2739550952372,56.1147943977444));
#85757=CARTESIAN_POINT('Ctrl Pts',(5.17181157016599,-28.3126519945236,56.1747091102498));
#85758=CARTESIAN_POINT('Ctrl Pts',(5.17566692701723,-28.3544689000551,56.2326014985562));
#85759=CARTESIAN_POINT('Ctrl Pts',(5.17952228386848,-28.3991577667128,56.2881388537824));
#85760=CARTESIAN_POINT('Ctrl Pts',(5.18338167633704,-28.4438934117027,56.3437343430598));
#85761=CARTESIAN_POINT('Ctrl Pts',(5.1872410688056,-28.4915067137864,56.3969694990263));
#85762=CARTESIAN_POINT('Ctrl Pts',(5.19110046127416,-28.5417095857703,56.4475450356606));
#85763=CARTESIAN_POINT('Ctrl Pts',(5.19496203887759,-28.591940881929,56.4981492074674));
#85764=CARTESIAN_POINT('Ctrl Pts',(5.19882361648103,-28.6447643068034,56.5460904356484));
#85765=CARTESIAN_POINT('Ctrl Pts',(5.20268519408446,-28.6998572202674,56.5911085176094));
#85766=CARTESIAN_POINT('Ctrl Pts',(5.20655352819934,-28.7550465285054,56.6362053666489));
#85767=CARTESIAN_POINT('Ctrl Pts',(5.21042186231421,-28.812512861496,56.6783685706392));
#85768=CARTESIAN_POINT('Ctrl Pts',(5.21429019642908,-28.8719036200713,56.7173805984964));
#85769=CARTESIAN_POINT('Ctrl Pts',(5.21658791560004,-28.9071806360952,56.7405530240531));
#85770=CARTESIAN_POINT('Ctrl Pts',(5.21888563477099,-28.9431361072497,56.7626145303181));
#85771=CARTESIAN_POINT('Ctrl Pts',(5.22118335394195,-28.9796923731628,56.7835273782922));
#85772=CARTESIAN_POINT('Ctrl Pts',(5.22505242729016,-29.0412485789612,56.8187420136377));
#85773=CARTESIAN_POINT('Ctrl Pts',(5.22892150063838,-29.1047505806775,56.8508350814401));
#85774=CARTESIAN_POINT('Ctrl Pts',(5.2327905739866,-29.1698489244987,56.8795868573557));
#85775=CARTESIAN_POINT('Ctrl Pts',(5.23665388238238,-29.23485027123,56.9082957928788));
#85776=CARTESIAN_POINT('Ctrl Pts',(5.24051719077816,-29.3014427979312,56.9336731241379));
#85777=CARTESIAN_POINT('Ctrl Pts',(5.24438049917394,-29.3692513689758,56.9555443556619));
#85778=CARTESIAN_POINT('Ctrl Pts',(5.24823927566685,-29.436980396317,56.9773899308606));
#85779=CARTESIAN_POINT('Ctrl Pts',(5.25209805215977,-29.5059221744099,56.9957374274861));
#85780=CARTESIAN_POINT('Ctrl Pts',(5.25595682865268,-29.5756820674498,57.0104606075764));
#85781=CARTESIAN_POINT('Ctrl Pts',(5.25981317424088,-29.6453980140075,57.0251745125381));
#85782=CARTESIAN_POINT('Ctrl Pts',(5.26366951982909,-29.7159305788035,57.0362685307208));
#85783=CARTESIAN_POINT('Ctrl Pts',(5.2675258654173,-29.7868718816747,57.0436667946804));
#85784=CARTESIAN_POINT('Ctrl Pts',(5.27138107166263,-29.8577922252033,57.0510628728505));
#85785=CARTESIAN_POINT('Ctrl Pts',(5.27523627790796,-29.9291205841624,57.0547653141544));
#85786=CARTESIAN_POINT('Ctrl Pts',(5.27909148415329,-30.0004425660863,57.0547499523385));
#85787=CARTESIAN_POINT('Ctrl Pts',(5.28294684100454,-30.0717673342457,57.0547345899226));
#85788=CARTESIAN_POINT('Ctrl Pts',(5.28680219785578,-30.1430852390898,57.0510011383428));
#85789=CARTESIAN_POINT('Ctrl Pts',(5.29065755470703,-30.2139822266312,57.04357754176));
#85790=CARTESIAN_POINT('Ctrl Pts',(5.29451694717559,-30.2849534260086,57.0361461744842));
#85791=CARTESIAN_POINT('Ctrl Pts',(5.29837633964415,-30.3555023444169,57.0250170021201));
#85792=CARTESIAN_POINT('Ctrl Pts',(5.30223573211271,-30.4252212904858,57.0102697372784));
#85793=CARTESIAN_POINT('Ctrl Pts',(5.30609730971614,-30.4949797104621,56.9955141227385));
#85794=CARTESIAN_POINT('Ctrl Pts',(5.30995888731957,-30.5639067530248,56.9771364629712));
#85795=CARTESIAN_POINT('Ctrl Pts',(5.31382046492301,-30.6316088222237,56.9552666974582));
#85796=CARTESIAN_POINT('Ctrl Pts',(5.31768879903788,-30.6994293481395,56.9333586669313));
#85797=CARTESIAN_POINT('Ctrl Pts',(5.32155713315275,-30.766020167512,56.9079465050118));
#85798=CARTESIAN_POINT('Ctrl Pts',(5.32542546726762,-30.8310072858769,56.8792084645721));
#85799=CARTESIAN_POINT('Ctrl Pts',(5.32772318643858,-30.8696084364751,56.8621385981922));
#85800=CARTESIAN_POINT('Ctrl Pts',(5.33002090560954,-30.9076442250829,56.8438962093788));
#85801=CARTESIAN_POINT('Ctrl Pts',(5.3323186247805,-30.9450408253263,56.8245260757157));
#85802=CARTESIAN_POINT('Ctrl Pts',(5.33618678846697,-31.007997244408,56.7919168480152));
#85803=CARTESIAN_POINT('Ctrl Pts',(5.34005495215343,-31.069387166087,56.7559814127803));
#85804=CARTESIAN_POINT('Ctrl Pts',(5.34392311583989,-31.1288367206716,56.7168940621259));
#85805=CARTESIAN_POINT('Ctrl Pts',(5.34666138801451,-31.1709210465449,56.6892241356823));
#85806=CARTESIAN_POINT('Ctrl Pts',(5.34939966018912,-31.2120333271599,56.6599757585428));
#85807=CARTESIAN_POINT('Ctrl Pts',(5.35213793236373,-31.2520475724682,56.6292251037768));
#85808=CARTESIAN_POINT('',(5.04592528049197,-27.9452502582983,54.9989697199742));
#85809=CARTESIAN_POINT('Ctrl Pts',(5.04592528053768,-27.9452502582979,54.9989697208212));
#85810=CARTESIAN_POINT('Ctrl Pts',(5.04983580638859,-27.9452139274514,55.0714265840048));
#85811=CARTESIAN_POINT('Ctrl Pts',(5.0537463322395,-27.9490145212746,55.1438783326772));
#85812=CARTESIAN_POINT('Ctrl Pts',(5.05765685809041,-27.9566240457995,55.2158987547329));
#85813=CARTESIAN_POINT('Ctrl Pts',(5.06156889758459,-27.9642365157354,55.2879470536603));
#85814=CARTESIAN_POINT('Ctrl Pts',(5.06548093707878,-27.9756607961671,55.3595632307951));
#85815=CARTESIAN_POINT('Ctrl Pts',(5.06939297657296,-27.9908172317786,55.4303279753656));
#85816=CARTESIAN_POINT('Ctrl Pts',(5.07331083119316,-28.0059961969641,55.5011979095459));
#85817=CARTESIAN_POINT('Ctrl Pts',(5.07722868581337,-28.0249182944707,55.5712134277549));
#85818=CARTESIAN_POINT('Ctrl Pts',(5.08114654043358,-28.0474531999293,55.6399676210822));
#85819=CARTESIAN_POINT('Ctrl Pts',(5.08506751736907,-28.0700060644718,55.7087766077313));
#85820=CARTESIAN_POINT('Ctrl Pts',(5.08898849430456,-28.0961773017066,55.7763218332449));
#85821=CARTESIAN_POINT('Ctrl Pts',(5.09290947124006,-28.1257883534145,55.8422162823784));
#85822=CARTESIAN_POINT('Ctrl Pts',(5.09683849198264,-28.1554601516128,55.9082459126787));
#85823=CARTESIAN_POINT('Ctrl Pts',(5.10076751272523,-28.1885856454507,55.9726175877542));
#85824=CARTESIAN_POINT('Ctrl Pts',(5.10469653346781,-28.2249403918811,56.0349690575687));
#85825=CARTESIAN_POINT('Ctrl Pts',(5.10720517516979,-28.2481525454773,56.0747798673363));
#85826=CARTESIAN_POINT('Ctrl Pts',(5.10971381687176,-28.272680273511,56.1137676684776));
#85827=CARTESIAN_POINT('Ctrl Pts',(5.11222245857373,-28.2984564079793,56.1518450273163));
#85828=CARTESIAN_POINT('Ctrl Pts',(5.11609153192195,-28.3382108913768,56.2105716657746));
#85829=CARTESIAN_POINT('Ctrl Pts',(5.11996060527016,-28.3810871266736,56.2673528041018));
#85830=CARTESIAN_POINT('Ctrl Pts',(5.12382967861838,-28.4268681537415,56.3218372656221));
#85831=CARTESIAN_POINT('Ctrl Pts',(5.12769298701417,-28.472580966687,56.3762405448282));
#85832=CARTESIAN_POINT('Ctrl Pts',(5.13155629540996,-28.5211896701546,56.4283535710454));
#85833=CARTESIAN_POINT('Ctrl Pts',(5.13541960380575,-28.5724343269205,56.477854462234));
#85834=CARTESIAN_POINT('Ctrl Pts',(5.13927838029866,-28.6236188704922,56.5272972857749));
#85835=CARTESIAN_POINT('Ctrl Pts',(5.14313715679158,-28.6774328776295,56.5741337249527));
#85836=CARTESIAN_POINT('Ctrl Pts',(5.14699593328449,-28.7335776498748,56.6180766340329));
#85837=CARTESIAN_POINT('Ctrl Pts',(5.1508522788727,-28.7896870527249,56.6619918604981));
#85838=CARTESIAN_POINT('Ctrl Pts',(5.15470862446091,-28.8481239259431,56.703016874631));
#85839=CARTESIAN_POINT('Ctrl Pts',(5.15856497004911,-28.9085554955761,56.7409039193083));
#85840=CARTESIAN_POINT('Ctrl Pts',(5.16242017629444,-28.9689692109279,56.7787797703999));
#85841=CARTESIAN_POINT('Ctrl Pts',(5.16627538253978,-29.0313760413579,56.8135192346887));
#85842=CARTESIAN_POINT('Ctrl Pts',(5.17013058878511,-29.0954145952794,56.8449181033494));
#85843=CARTESIAN_POINT('Ctrl Pts',(5.17398594563635,-29.159455650905,56.8763181986256));
#85844=CARTESIAN_POINT('Ctrl Pts',(5.1778413024876,-29.225128119431,56.904377227293));
#85845=CARTESIAN_POINT('Ctrl Pts',(5.18169665933885,-29.2920479619277,56.9289379135393));
#85846=CARTESIAN_POINT('Ctrl Pts',(5.1855560518074,-29.3590378531605,56.9535243088274));
#85847=CARTESIAN_POINT('Ctrl Pts',(5.18941544427596,-29.4272772678509,56.9746048839808));
#85848=CARTESIAN_POINT('Ctrl Pts',(5.19327483674452,-29.4963650787195,56.9920716424283));
#85849=CARTESIAN_POINT('Ctrl Pts',(5.19713641434796,-29.5654920061554,57.0095482903138));
#85850=CARTESIAN_POINT('Ctrl Pts',(5.20099799195139,-29.6354678092425,57.0234069539317));
#85851=CARTESIAN_POINT('Ctrl Pts',(5.20485956955483,-29.7058818937089,57.0335909377384));
#85852=CARTESIAN_POINT('Ctrl Pts',(5.2087279036697,-29.7764191800413,57.0437927402219));
#85853=CARTESIAN_POINT('Ctrl Pts',(5.21259623778457,-29.8473957948861,57.0503069817964));
#85854=CARTESIAN_POINT('Ctrl Pts',(5.21646457189944,-29.918397463003,57.0531289751147));
#85855=CARTESIAN_POINT('Ctrl Pts',(5.21876229107039,-29.9605711453059,57.0548051871365));
#85856=CARTESIAN_POINT('Ctrl Pts',(5.22106001024135,-30.0027536735451,57.0551797214769));
#85857=CARTESIAN_POINT('Ctrl Pts',(5.2233577294123,-30.0448590459357,57.0542602630869));
#85858=CARTESIAN_POINT('Ctrl Pts',(5.22722618551046,-30.1157479459585,57.052712256498));
#85859=CARTESIAN_POINT('Ctrl Pts',(5.23109464160863,-30.1866954538954,57.0474875355491));
#85860=CARTESIAN_POINT('Ctrl Pts',(5.23496309770679,-30.2572890573119,57.0385779120474));
#85861=CARTESIAN_POINT('Ctrl Pts',(5.23882613522196,-30.3277837796012,57.0296807683395));
#85862=CARTESIAN_POINT('Ctrl Pts',(5.24268917273712,-30.3979251031771,57.0171090230145));
#85863=CARTESIAN_POINT('Ctrl Pts',(5.24655221025229,-30.467301706206,57.00090646405));
#85864=CARTESIAN_POINT('Ctrl Pts',(5.2504962515766,-30.538133063192,56.9843641545682));
#85865=CARTESIAN_POINT('Ctrl Pts',(5.25444029290092,-30.6081667459654,56.9640370267955));
#85866=CARTESIAN_POINT('Ctrl Pts',(5.25838433422523,-30.6769723099905,56.9400273333142));
#85867=CARTESIAN_POINT('Ctrl Pts',(5.26224054826836,-30.7442456878335,56.9165522960211));
#85868=CARTESIAN_POINT('Ctrl Pts',(5.26609676231149,-30.8103446016693,56.88955719285));
#85869=CARTESIAN_POINT('Ctrl Pts',(5.26995297635461,-30.8748808360116,56.859188286667));
#85870=CARTESIAN_POINT('Ctrl Pts',(5.27394093131952,-30.941621839826,56.8277818790254));
#85871=CARTESIAN_POINT('Ctrl Pts',(5.27792888628444,-31.0066909351777,56.792767130044));
#85872=CARTESIAN_POINT('Ctrl Pts',(5.28191684124935,-31.0696823161643,56.7543595141776));
#85873=CARTESIAN_POINT('Ctrl Pts',(5.28590479621426,-31.1326736971508,56.7159518983112));
#85874=CARTESIAN_POINT('Ctrl Pts',(5.28989275117917,-31.1935868763248,56.6741517210512));
#85875=CARTESIAN_POINT('Ctrl Pts',(5.29388070614408,-31.2520475724682,56.6292251037768));
#85876=CARTESIAN_POINT('Ctrl Pts',(4.59397380331217,-31.2520475724682,56.6292251037768));
#85877=CARTESIAN_POINT('Ctrl Pts',(4.59782977348395,-31.3085555898331,56.5857991058575));
#85878=CARTESIAN_POINT('Ctrl Pts',(4.60168574365573,-31.3628372624389,56.5394024325893));
#85879=CARTESIAN_POINT('Ctrl Pts',(4.60554171382751,-31.4145710538178,56.4902973851553));
#85880=CARTESIAN_POINT('Ctrl Pts',(4.60939684064206,-31.4662935302577,56.4412030777154));
#85881=CARTESIAN_POINT('Ctrl Pts',(4.61325196745661,-31.5154688799484,56.3894019068612));
#85882=CARTESIAN_POINT('Ctrl Pts',(4.61710709427116,-31.5618108701437,56.3351945058309));
#85883=CARTESIAN_POINT('Ctrl Pts',(4.62096266749001,-31.6081582265084,56.2809808278561));
#85884=CARTESIAN_POINT('Ctrl Pts',(4.62481824070887,-31.6516712583411,56.2243607374448));
#85885=CARTESIAN_POINT('Ctrl Pts',(4.62867381392772,-31.6921037647007,56.1656682255195));
#85886=CARTESIAN_POINT('Ctrl Pts',(4.63253360485403,-31.7325805011846,56.1069115083955));
#85887=CARTESIAN_POINT('Ctrl Pts',(4.63639339578033,-31.7699697123549,56.04607824704));
#85888=CARTESIAN_POINT('Ctrl Pts',(4.64025318670663,-31.8040688655624,55.9835309302754));
#85889=CARTESIAN_POINT('Ctrl Pts',(4.64411542856985,-31.8381896714642,55.9209438964562));
#85890=CARTESIAN_POINT('Ctrl Pts',(4.64797767043306,-31.8690160524473,55.8566410793345));
#85891=CARTESIAN_POINT('Ctrl Pts',(4.65183991229628,-31.8963929309228,55.7910065828084));
#85892=CARTESIAN_POINT('Ctrl Pts',(4.65570864526733,-31.9238158205691,55.7252617771379));
#85893=CARTESIAN_POINT('Ctrl Pts',(4.65957737823839,-31.947777476992,55.6581812831638));
#85894=CARTESIAN_POINT('Ctrl Pts',(4.66344611120945,-31.9681723975461,55.5901652107992));
#85895=CARTESIAN_POINT('Ctrl Pts',(4.66485786587946,-31.9756147887766,55.565345196465));
#85896=CARTESIAN_POINT('Ctrl Pts',(4.66626962054948,-31.982582718124,55.5404006983024));
#85897=CARTESIAN_POINT('Ctrl Pts',(4.6676813752195,-31.9890727647973,55.515351432366));
#85898=CARTESIAN_POINT('Ctrl Pts',(4.67155044856771,-32.0068594717553,55.4467010858964));
#85899=CARTESIAN_POINT('Ctrl Pts',(4.67541952191592,-32.0211227752712,55.3769943617174));
#85900=CARTESIAN_POINT('Ctrl Pts',(4.67928859526414,-32.0317425864936,55.3066261970678));
#85901=CARTESIAN_POINT('Ctrl Pts',(4.68315190365992,-32.0423465741064,55.2363628815863));
#85902=CARTESIAN_POINT('Ctrl Pts',(4.6870152120557,-32.0493177736078,55.1654405583601));
#85903=CARTESIAN_POINT('Ctrl Pts',(4.69087852045148,-32.0525864868934,55.0942670479159));
#85904=CARTESIAN_POINT('Ctrl Pts',(4.69473729694439,-32.0558513657733,55.02317702846));
#85905=CARTESIAN_POINT('Ctrl Pts',(4.69859607343731,-32.0554223634192,54.9518368899964));
#85906=CARTESIAN_POINT('Ctrl Pts',(4.70245484993022,-32.0512814688225,54.8806605758122));
#85907=CARTESIAN_POINT('Ctrl Pts',(4.70631119551842,-32.0471431828558,54.8095291004098));
#85908=CARTESIAN_POINT('Ctrl Pts',(4.71016754110663,-32.0392976720871,54.7385617283511));
#85909=CARTESIAN_POINT('Ctrl Pts',(4.71402388669483,-32.0277790060474,54.6681719343797));
#85910=CARTESIAN_POINT('Ctrl Pts',(4.71787909294016,-32.0162637431545,54.5978029368095));
#85911=CARTESIAN_POINT('Ctrl Pts',(4.7217342991855,-32.0010775578611,54.5280116577008));
#85912=CARTESIAN_POINT('Ctrl Pts',(4.72558950543083,-31.9823061136394,54.4592042582196));
#85913=CARTESIAN_POINT('Ctrl Pts',(4.72944486228207,-31.9635339361002,54.3903941707365));
#85914=CARTESIAN_POINT('Ctrl Pts',(4.73330021913332,-31.9411763515419,54.3225685072694));
#85915=CARTESIAN_POINT('Ctrl Pts',(4.73715557598456,-31.9153692105435,54.2561193981545));
#85916=CARTESIAN_POINT('Ctrl Pts',(4.74101496845312,-31.8895350557694,54.1896007330463));
#85917=CARTESIAN_POINT('Ctrl Pts',(4.74487436092168,-31.86024431273,54.1244619524446));
#85918=CARTESIAN_POINT('Ctrl Pts',(4.74873375339024,-31.8276811049241,54.0610754336991));
#85919=CARTESIAN_POINT('Ctrl Pts',(4.75259533099367,-31.7950994602784,53.9976530263795));
#85920=CARTESIAN_POINT('Ctrl Pts',(4.7564569085971,-31.7592419067675,53.9359852760462));
#85921=CARTESIAN_POINT('Ctrl Pts',(4.76031848620054,-31.720337319883,53.8764177518678));
#85922=CARTESIAN_POINT('Ctrl Pts',(4.76418682031541,-31.6813646625586,53.8167460037945));
#85923=CARTESIAN_POINT('Ctrl Pts',(4.76805515443027,-31.639334614274,53.7591822110137));
#85924=CARTESIAN_POINT('Ctrl Pts',(4.77192348854514,-31.5945175083743,53.7040403254778));
#85925=CARTESIAN_POINT('Ctrl Pts',(4.77422120771611,-31.5678969734476,53.6712870617325));
#85926=CARTESIAN_POINT('Ctrl Pts',(4.77651892688708,-31.5402938708371,53.6393876151711));
#85927=CARTESIAN_POINT('Ctrl Pts',(4.77881664605805,-31.5117708171909,53.6084014376301));
#85928=CARTESIAN_POINT('Ctrl Pts',(4.78268571940627,-31.4637415418701,53.5562245679752));
#85929=CARTESIAN_POINT('Ctrl Pts',(4.78655479275449,-31.4129137901361,53.5064349216958));
#85930=CARTESIAN_POINT('Ctrl Pts',(4.79042386610271,-31.3595542340858,53.4593475904412));
#85931=CARTESIAN_POINT('Ctrl Pts',(4.79428717449848,-31.3062741842312,53.4123304197136));
#85932=CARTESIAN_POINT('Ctrl Pts',(4.79815048289426,-31.2504701794635,53.3680078903843));
#85933=CARTESIAN_POINT('Ctrl Pts',(4.80201379129003,-31.1924470458222,53.3266597460738));
#85934=CARTESIAN_POINT('Ctrl Pts',(4.80587256778294,-31.134491976953,53.2853601057278));
#85935=CARTESIAN_POINT('Ctrl Pts',(4.80973134427586,-31.0743233436933,53.2470282003396));
#85936=CARTESIAN_POINT('Ctrl Pts',(4.81359012076877,-31.0122791493054,53.2119036697142));
#85937=CARTESIAN_POINT('Ctrl Pts',(4.81744646635698,-30.9502740407582,53.1768012664099));
#85938=CARTESIAN_POINT('Ctrl Pts',(4.82130281194519,-30.886396136989,53.1449024679027));
#85939=CARTESIAN_POINT('Ctrl Pts',(4.8251591575334,-30.8210112942301,53.1164029047467));
#85940=CARTESIAN_POINT('Ctrl Pts',(4.82901436377874,-30.7556457691784,53.0879117616801));
#85941=CARTESIAN_POINT('Ctrl Pts',(4.83286957002408,-30.6887746341001,53.0628180541669));
#85942=CARTESIAN_POINT('Ctrl Pts',(4.83672477626942,-30.6207855834735,53.041270099822));
#85943=CARTESIAN_POINT('Ctrl Pts',(4.84058013312066,-30.5527938768146,53.0197213036935));
#85944=CARTESIAN_POINT('Ctrl Pts',(4.8444354899719,-30.4836846316526,53.0017186804076));
#85945=CARTESIAN_POINT('Ctrl Pts',(4.84829084682314,-30.4138609742388,52.9873607733868));
#85946=CARTESIAN_POINT('Ctrl Pts',(4.8521502392917,-30.3439642285034,52.9729878371429));
#85947=CARTESIAN_POINT('Ctrl Pts',(4.85600963176026,-30.2733520545143,52.9622673310628));
#85948=CARTESIAN_POINT('Ctrl Pts',(4.85986902422882,-30.2024371646762,52.9552465290755));
#85949=CARTESIAN_POINT('Ctrl Pts',(4.86373060183226,-30.131482123804,52.9482217520068));
#85950=CARTESIAN_POINT('Ctrl Pts',(4.8675921794357,-30.0602245113805,52.944900871601));
#85951=CARTESIAN_POINT('Ctrl Pts',(4.87145375703914,-29.9890787889633,52.9452790238941));
#85952=CARTESIAN_POINT('Ctrl Pts',(4.87532209115401,-29.9178085845504,52.9456578378314));
#85953=CARTESIAN_POINT('Ctrl Pts',(4.87919042526888,-29.8466511461461,52.949748578334));
#85954=CARTESIAN_POINT('Ctrl Pts',(4.88305875938375,-29.7760168575584,52.9574944028468));
#85955=CARTESIAN_POINT('Ctrl Pts',(4.8853564785547,-29.734061391925,52.9620952798522));
#85956=CARTESIAN_POINT('Ctrl Pts',(4.88765419772566,-29.6922903458756,52.9679847345439));
#85957=CARTESIAN_POINT('Ctrl Pts',(4.88995191689662,-29.6507876285087,52.9751424044893));
#85958=CARTESIAN_POINT('Ctrl Pts',(4.89382099024483,-29.5809022135838,52.9871950305765));
#85959=CARTESIAN_POINT('Ctrl Pts',(4.89769006359305,-29.5115046159001,53.0028935228187));
#85960=CARTESIAN_POINT('Ctrl Pts',(4.90155913694126,-29.4430041910448,53.0221847327654));
#85961=CARTESIAN_POINT('Ctrl Pts',(4.90542244533705,-29.3746058324094,53.041447198644));
#85962=CARTESIAN_POINT('Ctrl Pts',(4.90928575373283,-29.3071024568889,53.0642916257024));
#85963=CARTESIAN_POINT('Ctrl Pts',(4.91314906212861,-29.2408944159804,53.0906136391997));
#85964=CARTESIAN_POINT('Ctrl Pts',(4.91700783862152,-29.1747640412532,53.1169047753256));
#85965=CARTESIAN_POINT('Ctrl Pts',(4.92086661511443,-29.1099264321078,53.1466652161715));
#85966=CARTESIAN_POINT('Ctrl Pts',(4.92472539160735,-29.046766241213,53.1797409624977));
#85967=CARTESIAN_POINT('Ctrl Pts',(4.92858173719555,-28.9836458392008,53.2127958721708));
#85968=CARTESIAN_POINT('Ctrl Pts',(4.93243808278376,-28.922201188255,53.2491617188718));
#85969=CARTESIAN_POINT('Ctrl Pts',(4.93629442837197,-28.8627950734064,53.2886372338305));
#85970=CARTESIAN_POINT('Ctrl Pts',(4.9401496346173,-28.803406509872,53.3281010858961));
#85971=CARTESIAN_POINT('Ctrl Pts',(4.94400484086263,-28.7460556911282,53.3706725135537));
#85972=CARTESIAN_POINT('Ctrl Pts',(4.94786004710796,-28.6910774968246,53.4161062399324));
#85973=CARTESIAN_POINT('Ctrl Pts',(4.95171540395921,-28.6360971547653,53.4615417412066));
#85974=CARTESIAN_POINT('Ctrl Pts',(4.95557076081046,-28.5834899942286,53.5098394520461));
#85975=CARTESIAN_POINT('Ctrl Pts',(4.95942611766171,-28.5335574470369,53.5607141349408));
#85976=CARTESIAN_POINT('Ctrl Pts',(4.96328551013027,-28.4835726326598,53.611642071207));
#85977=CARTESIAN_POINT('Ctrl Pts',(4.96714490259882,-28.4362683613669,53.6651520168576));
#85978=CARTESIAN_POINT('Ctrl Pts',(4.97100429506738,-28.3919081904314,53.7209228739054));
#85979=CARTESIAN_POINT('Ctrl Pts',(4.97486587267082,-28.3475229033779,53.7767253076446));
#85980=CARTESIAN_POINT('Ctrl Pts',(4.97872745027425,-28.3060853173042,53.8347908054496));
#85981=CARTESIAN_POINT('Ctrl Pts',(4.98258902787768,-28.267816134846,53.8947685220733));
#85982=CARTESIAN_POINT('Ctrl Pts',(4.98645736199256,-28.2294799937001,53.9548511802959));
#85983=CARTESIAN_POINT('Ctrl Pts',(4.99032569610743,-28.1943235639806,54.0168523145396));
#85984=CARTESIAN_POINT('Ctrl Pts',(4.9941940302223,-28.1625216672198,54.0803963141312));
#85985=CARTESIAN_POINT('Ctrl Pts',(4.99649174939326,-28.1436319266519,54.1181402787747));
#85986=CARTESIAN_POINT('Ctrl Pts',(4.99878946856422,-28.1259247988858,54.1564281827511));
#85987=CARTESIAN_POINT('Ctrl Pts',(5.00108718773517,-28.1094286858362,54.1951784865196));
#85988=CARTESIAN_POINT('Ctrl Pts',(5.00537446195647,-28.0786488755256,54.2674820040745));
#85989=CARTESIAN_POINT('Ctrl Pts',(5.00966173617776,-28.0519849253721,54.3416372137349));
#85990=CARTESIAN_POINT('Ctrl Pts',(5.01394901039905,-28.0296387343026,54.4171843815242));
#85991=CARTESIAN_POINT('Ctrl Pts',(5.01822262075576,-28.0073637622205,54.492490774822));
#85992=CARTESIAN_POINT('Ctrl Pts',(5.02249623111247,-27.9893792307943,54.5691800046957));
#85993=CARTESIAN_POINT('Ctrl Pts',(5.02676984146917,-27.9758386929292,54.6467740589123));
#85994=CARTESIAN_POINT('Ctrl Pts',(5.03102083155028,-27.9623698253084,54.7239574067835));
#85995=CARTESIAN_POINT('Ctrl Pts',(5.03527182163138,-27.9532981584277,54.8020357440809));
#85996=CARTESIAN_POINT('Ctrl Pts',(5.03952281171248,-27.9487267011557,54.88052022787));
#85997=CARTESIAN_POINT('Ctrl Pts',(5.04165696797231,-27.9464316583615,54.919922378706));
#85998=CARTESIAN_POINT('Ctrl Pts',(5.04379112423214,-27.9452700857513,54.9594266319027));
#85999=CARTESIAN_POINT('Ctrl Pts',(5.04592528049197,-27.9452502582983,54.9989697199742));
#86000=CARTESIAN_POINT('Origin',(-1.54592528053767,-30.,55.));
#86001=CARTESIAN_POINT('',(3.89394682683029,-31.2520475724682,56.6292251037768));
#86002=CARTESIAN_POINT('',(3.95204618803132,-31.2520475724682,56.6292251037768));
#86003=CARTESIAN_POINT('',(-1.54592528053767,-31.2520475724682,56.6292251037768));
#86004=CARTESIAN_POINT('',(4.4040747195126,-27.9452505182989,55.0014594345581));
#86005=CARTESIAN_POINT('Ctrl Pts',(3.95204618803132,-31.2520475724682,56.6292251037768));
#86006=CARTESIAN_POINT('Ctrl Pts',(3.9559336202552,-31.3090593123265,56.5854119988066));
#86007=CARTESIAN_POINT('Ctrl Pts',(3.95982105247907,-31.3637505089491,56.5386167090834));
#86008=CARTESIAN_POINT('Ctrl Pts',(3.96370848470294,-31.4158059227235,56.4891242902059));
#86009=CARTESIAN_POINT('Ctrl Pts',(3.96756899535413,-31.467500837967,56.4399746203913));
#86010=CARTESIAN_POINT('Ctrl Pts',(3.97142950600532,-31.5165960683909,56.3881654587326));
#86011=CARTESIAN_POINT('Ctrl Pts',(3.97529001665651,-31.5628213390034,56.3340116284559));
#86012=CARTESIAN_POINT('Ctrl Pts',(3.97919090966672,-31.609530142921,56.2792913292287));
#86013=CARTESIAN_POINT('Ctrl Pts',(3.98309180267694,-31.653308281332,56.2221774226634));
#86014=CARTESIAN_POINT('Ctrl Pts',(3.98699269568715,-31.6939212592051,56.1630255070775));
#86015=CARTESIAN_POINT('Ctrl Pts',(3.99089358869737,-31.7345342370783,56.1038735914916));
#86016=CARTESIAN_POINT('Ctrl Pts',(3.99479448170758,-31.7719818464491,56.0426841312037));
#86017=CARTESIAN_POINT('Ctrl Pts',(3.9986953747178,-31.8060778097422,55.9798369801435));
#86018=CARTESIAN_POINT('Ctrl Pts',(4.00256444806601,-31.8398956515835,55.9175024745466));
#86019=CARTESIAN_POINT('Ctrl Pts',(4.00643352141423,-31.8705488495701,55.8532930462969));
#86020=CARTESIAN_POINT('Ctrl Pts',(4.01030259476244,-31.8978256139735,55.7875630142701));
#86021=CARTESIAN_POINT('Ctrl Pts',(4.01416590315824,-31.9250617357643,55.7219309205539));
#86022=CARTESIAN_POINT('Ctrl Pts',(4.01802921155403,-31.9489312255174,55.6547831654668));
#86023=CARTESIAN_POINT('Ctrl Pts',(4.02189251994982,-31.9692680899005,55.5864987234424));
#86024=CARTESIAN_POINT('Ctrl Pts',(4.02575129644273,-31.9895810978671,55.5182943833482));
#86025=CARTESIAN_POINT('Ctrl Pts',(4.02961007293565,-32.0063695738439,55.4489564682266));
#86026=CARTESIAN_POINT('Ctrl Pts',(4.03346884942856,-32.0195162093906,55.378882359722));
#86027=CARTESIAN_POINT('Ctrl Pts',(4.03732519501676,-32.0326545629811,55.3088523956452));
#86028=CARTESIAN_POINT('Ctrl Pts',(4.04118154060496,-32.0421555385165,55.2380876346409));
#86029=CARTESIAN_POINT('Ctrl Pts',(4.04503788619317,-32.0479524838775,55.1669975636946));
#86030=CARTESIAN_POINT('Ctrl Pts',(4.0488930924385,-32.0537477165527,55.0959284960438));
#86031=CARTESIAN_POINT('Ctrl Pts',(4.05274829868383,-32.0558410521646,55.0245347931743));
#86032=CARTESIAN_POINT('Ctrl Pts',(4.05660350492916,-32.0542176734686,54.9532312870673));
#86033=CARTESIAN_POINT('Ctrl Pts',(4.06045886178041,-32.0525942313542,54.8819249954465));
#86034=CARTESIAN_POINT('Ctrl Pts',(4.06431421863166,-32.0472537999241,54.8107093931939));
#86035=CARTESIAN_POINT('Ctrl Pts',(4.06816957548291,-32.0382336514703,54.7399977990204));
#86036=CARTESIAN_POINT('Ctrl Pts',(4.07202896795147,-32.0292040611233,54.6692121870726));
#86037=CARTESIAN_POINT('Ctrl Pts',(4.07588836042003,-32.0164871263596,54.5989321192276));
#86038=CARTESIAN_POINT('Ctrl Pts',(4.07974775288859,-32.0001717313108,54.5295633860283));
#86039=CARTESIAN_POINT('Ctrl Pts',(4.08360933049202,-31.9838470987099,54.4601553772073));
#86040=CARTESIAN_POINT('Ctrl Pts',(4.08747090809546,-31.9639200857577,54.3916601968677));
#86041=CARTESIAN_POINT('Ctrl Pts',(4.09133248569889,-31.9405294728948,54.3244684113035));
#86042=CARTESIAN_POINT('Ctrl Pts',(4.09520081981376,-31.9170979340271,54.2571590618537));
#86043=CARTESIAN_POINT('Ctrl Pts',(4.09906915392864,-31.8901908793728,54.1911581102852));
#86044=CARTESIAN_POINT('Ctrl Pts',(4.10293748804351,-31.8599949485488,54.1268354371181));
#86045=CARTESIAN_POINT('Ctrl Pts',(4.10523520721445,-31.8420591221496,54.0886289547219));
#86046=CARTESIAN_POINT('Ctrl Pts',(4.1075329263854,-31.8229638179775,54.0510141262206));
#86047=CARTESIAN_POINT('Ctrl Pts',(4.10983064555634,-31.8027554667187,54.0140637496694));
#86048=CARTESIAN_POINT('Ctrl Pts',(4.11369971890456,-31.7687271162329,53.9518439105661));
#86049=CARTESIAN_POINT('Ctrl Pts',(4.11756879225277,-31.7314071723879,53.8912659359024));
#86050=CARTESIAN_POINT('Ctrl Pts',(4.12143786560099,-31.6909784467622,53.8326999292873));
#86051=CARTESIAN_POINT('Ctrl Pts',(4.12530117399678,-31.6506099602838,53.7742211865236));
#86052=CARTESIAN_POINT('Ctrl Pts',(4.12916448239257,-31.6071421603617,53.7177488576869));
#86053=CARTESIAN_POINT('Ctrl Pts',(4.13302779078836,-31.5608034111033,53.663627943128));
#86054=CARTESIAN_POINT('Ctrl Pts',(4.13688656728128,-31.514519020102,53.6095705157939));
#86055=CARTESIAN_POINT('Ctrl Pts',(4.14074534377419,-31.4653706837742,53.5578593909247));
#86056=CARTESIAN_POINT('Ctrl Pts',(4.14460412026711,-31.4136286358637,53.5088086499828));
#86057=CARTESIAN_POINT('Ctrl Pts',(4.14846046585532,-31.3619191837743,53.4597888094254));
#86058=CARTESIAN_POINT('Ctrl Pts',(4.15231681144352,-31.3076196135571,53.413426361147));
#86059=CARTESIAN_POINT('Ctrl Pts',(4.15617315703173,-31.2510378033498,53.3699993935308));
#86060=CARTESIAN_POINT('Ctrl Pts',(4.16002836327706,-31.1944727100266,53.3265852562499));
#86061=CARTESIAN_POINT('Ctrl Pts',(4.16388356952239,-31.1356271005005,53.2861051734572));
#86062=CARTESIAN_POINT('Ctrl Pts',(4.16773877576772,-31.074841456847,53.2487965837336));
#86063=CARTESIAN_POINT('Ctrl Pts',(4.17159413261897,-31.0140534385661,53.2114865365278));
#86064=CARTESIAN_POINT('Ctrl Pts',(4.17544948947023,-30.9513256508629,53.1773484806088));
#86065=CARTESIAN_POINT('Ctrl Pts',(4.17930484632148,-30.8870255559426,53.1465752711252));
#86066=CARTESIAN_POINT('Ctrl Pts',(4.18316423879004,-30.8226581545222,53.1157698496047));
#86067=CARTESIAN_POINT('Ctrl Pts',(4.1870236312586,-30.7567155995411,53.0883365157088));
#86068=CARTESIAN_POINT('Ctrl Pts',(4.19088302372716,-30.6895870208706,53.0644206802234));
#86069=CARTESIAN_POINT('Ctrl Pts',(4.1947446013306,-30.6224204349232,53.0404913039213));
#86070=CARTESIAN_POINT('Ctrl Pts',(4.19860617893403,-30.5540669542196,53.020083529651));
#86071=CARTESIAN_POINT('Ctrl Pts',(4.20246775653747,-30.4849299800429,53.0032925910501));
#86072=CARTESIAN_POINT('Ctrl Pts',(4.20633609065234,-30.4156720385299,52.9864722737391));
#86073=CARTESIAN_POINT('Ctrl Pts',(4.21020442476722,-30.3456283441276,52.9732815166488));
#86074=CARTESIAN_POINT('Ctrl Pts',(4.21407275888209,-30.2752108761978,52.9637641256175));
#86075=CARTESIAN_POINT('Ctrl Pts',(4.21637047805303,-30.2333841980396,52.9581109707501));
#86076=CARTESIAN_POINT('Ctrl Pts',(4.21866819722397,-30.1914257349881,52.9537528354883));
#86077=CARTESIAN_POINT('Ctrl Pts',(4.22096591639491,-30.1494218301972,52.9506901944409));
#86078=CARTESIAN_POINT('Ctrl Pts',(4.22483498974313,-30.0786924779758,52.9455330877756));
#86079=CARTESIAN_POINT('Ctrl Pts',(4.22870406309134,-30.0075572855653,52.9440318803733));
#86080=CARTESIAN_POINT('Ctrl Pts',(4.23257313643956,-29.9364263435633,52.9462337151693));
#86081=CARTESIAN_POINT('Ctrl Pts',(4.23643644483534,-29.8654013872743,52.9484322692126));
#86082=CARTESIAN_POINT('Ctrl Pts',(4.24029975323112,-29.7943811504202,52.9543228983359));
#86083=CARTESIAN_POINT('Ctrl Pts',(4.24416306162689,-29.7237793393138,52.963900859705));
#86084=CARTESIAN_POINT('Ctrl Pts',(4.24802183811981,-29.6532603485566,52.9734675855252));
#86085=CARTESIAN_POINT('Ctrl Pts',(4.25188061461272,-29.5831592876136,52.9867129867537));
#86086=CARTESIAN_POINT('Ctrl Pts',(4.25573939110563,-29.5138865950799,53.0035803747566));
#86087=CARTESIAN_POINT('Ctrl Pts',(4.25959573669383,-29.4446575421079,53.0204371368492));
#86088=CARTESIAN_POINT('Ctrl Pts',(4.26345208228203,-29.3762562930918,53.0409112441354));
#86089=CARTESIAN_POINT('Ctrl Pts',(4.26730842787023,-29.3090834642402,53.064894859933));
#86090=CARTESIAN_POINT('Ctrl Pts',(4.27116363411557,-29.2419304813494,53.0888713898611));
#86091=CARTESIAN_POINT('Ctrl Pts',(4.2750188403609,-29.1760056553523,53.1163552065662));
#86092=CARTESIAN_POINT('Ctrl Pts',(4.27887404660624,-29.1116931339928,53.1471890343846));
#86093=CARTESIAN_POINT('Ctrl Pts',(4.28272940345747,-29.0473781002269,53.1780240667447));
#86094=CARTESIAN_POINT('Ctrl Pts',(4.28658476030871,-28.9846759332392,53.2122091580431));
#86095=CARTESIAN_POINT('Ctrl Pts',(4.29044011715995,-28.9239479573436,53.2495401849814));
#86096=CARTESIAN_POINT('Ctrl Pts',(4.29429950962851,-28.8631564140842,53.2869102883904));
#86097=CARTESIAN_POINT('Ctrl Pts',(4.29815890209707,-28.8043436018006,53.3274326461376));
#86098=CARTESIAN_POINT('Ctrl Pts',(4.30201829456563,-28.7478427364951,53.3708591988561));
#86099=CARTESIAN_POINT('Ctrl Pts',(4.30587987216906,-28.6913098811777,53.4143103390906));
#86100=CARTESIAN_POINT('Ctrl Pts',(4.30974144977248,-28.6370919480339,53.4606686317744));
#86101=CARTESIAN_POINT('Ctrl Pts',(4.31360302737591,-28.5854877373587,53.5096468132227));
#86102=CARTESIAN_POINT('Ctrl Pts',(4.31747136149078,-28.5337932360106,53.5587106906423));
#86103=CARTESIAN_POINT('Ctrl Pts',(4.32133969560566,-28.484721922155,53.6104032563999));
#86104=CARTESIAN_POINT('Ctrl Pts',(4.32520802972053,-28.4385340417942,53.664402147402));
#86105=CARTESIAN_POINT('Ctrl Pts',(4.32750574889151,-28.4110992921008,53.6964764934597));
#86106=CARTESIAN_POINT('Ctrl Pts',(4.32980346806249,-28.3846810693941,53.7293639298705));
#86107=CARTESIAN_POINT('Ctrl Pts',(4.33210118723346,-28.3593266018392,53.7629921734008));
#86108=CARTESIAN_POINT('Ctrl Pts',(4.33598223894953,-28.3165006546754,53.8197932628943));
#86109=CARTESIAN_POINT('Ctrl Pts',(4.3398632906656,-28.276542709681,53.8789338902987));
#86110=CARTESIAN_POINT('Ctrl Pts',(4.34374434238166,-28.239716878203,53.9400939222665));
#86111=CARTESIAN_POINT('Ctrl Pts',(4.3476196054084,-28.202945973408,54.0011627324598));
#86112=CARTESIAN_POINT('Ctrl Pts',(4.35149486843514,-28.1692981577279,54.0642445616429));
#86113=CARTESIAN_POINT('Ctrl Pts',(4.35537013146187,-28.1389961109829,54.1289878947091));
#86114=CARTESIAN_POINT('Ctrl Pts',(4.35942884712858,-28.1072595834212,54.1967961385411));
#86115=CARTESIAN_POINT('Ctrl Pts',(4.36348756279528,-28.0791938035533,54.2664266821926));
#86116=CARTESIAN_POINT('Ctrl Pts',(4.36754627846199,-28.0550020434944,54.3374439558126));
#86117=CARTESIAN_POINT('Ctrl Pts',(4.37141366678501,-28.031950679948,54.4051134841278));
#86118=CARTESIAN_POINT('Ctrl Pts',(4.37528105510803,-28.0124165131011,54.4740414408055));
#86119=CARTESIAN_POINT('Ctrl Pts',(4.37914844343105,-27.9965263590061,54.5438301496782));
#86120=CARTESIAN_POINT('Ctrl Pts',(4.38301406018559,-27.9806434838534,54.6135868898248));
#86121=CARTESIAN_POINT('Ctrl Pts',(4.38687967694012,-27.9684014102057,54.6842031295399));
#86122=CARTESIAN_POINT('Ctrl Pts',(4.39074529369465,-27.9598764862882,54.7552682870977));
#86123=CARTESIAN_POINT('Ctrl Pts',(4.39461092103558,-27.9513515390242,54.8263336392748));
#86124=CARTESIAN_POINT('Ctrl Pts',(4.3984765483765,-27.9465438214084,54.8978474341102));
#86125=CARTESIAN_POINT('Ctrl Pts',(4.40234217571742,-27.9454779738573,54.9693927035768));
#86126=CARTESIAN_POINT('Ctrl Pts',(4.40291969029905,-27.9453187390298,54.980081379106));
#86127=CARTESIAN_POINT('Ctrl Pts',(4.40349720488069,-27.9452429264143,54.9907707532347));
#86128=CARTESIAN_POINT('Ctrl Pts',(4.40407471946232,-27.9452505182983,55.0014594336275));
#86129=CARTESIAN_POINT('Ctrl Pts',(4.4040747195126,-27.9452505182989,55.0014594345581));
#86130=CARTESIAN_POINT('Ctrl Pts',(4.4084909580683,-27.9453085732694,55.08319548757));
#86131=CARTESIAN_POINT('Ctrl Pts',(4.412907196624,-27.9502477237087,55.1647368982363));
#86132=CARTESIAN_POINT('Ctrl Pts',(4.4173234351797,-27.9599745962983,55.2455481923198));
#86133=CARTESIAN_POINT('Ctrl Pts',(4.42177971598848,-27.9697896629219,55.3270922063976));
#86134=CARTESIAN_POINT('Ctrl Pts',(4.42623599679726,-27.9844795567315,55.4078926142017));
#86135=CARTESIAN_POINT('Ctrl Pts',(4.43069227760603,-28.0038986271126,55.4874185795155));
#86136=CARTESIAN_POINT('Ctrl Pts',(4.4348736710947,-28.0221198249975,55.5620389564201));
#86137=CARTESIAN_POINT('Ctrl Pts',(4.43905506458337,-28.0445042064936,55.6355373428858));
#86138=CARTESIAN_POINT('Ctrl Pts',(4.44323645807203,-28.0708935156209,55.7074925684604));
#86139=CARTESIAN_POINT('Ctrl Pts',(4.44710553142025,-28.0953117323947,55.7740732541313));
#86140=CARTESIAN_POINT('Ctrl Pts',(4.45097460476847,-28.1232287475473,55.8395187237065));
#86141=CARTESIAN_POINT('Ctrl Pts',(4.45484367811668,-28.1545186966464,55.9034358424772));
#86142=CARTESIAN_POINT('Ctrl Pts',(4.45870698651247,-28.1857620234534,55.9672577241934));
#86143=CARTESIAN_POINT('Ctrl Pts',(4.46257029490826,-28.2203680964815,56.0295553426381));
#86144=CARTESIAN_POINT('Ctrl Pts',(4.46643360330405,-28.2581622778494,56.0899536284601));
#86145=CARTESIAN_POINT('Ctrl Pts',(4.47029237979696,-28.2959121242739,56.1502810633075));
#86146=CARTESIAN_POINT('Ctrl Pts',(4.47415115628987,-28.3368423939923,56.2087131813576));
#86147=CARTESIAN_POINT('Ctrl Pts',(4.47800993278279,-28.3807324547549,56.2648992763916));
#86148=CARTESIAN_POINT('Ctrl Pts',(4.48186627837099,-28.4245948661951,56.3210499759982));
#86149=CARTESIAN_POINT('Ctrl Pts',(4.4857226239592,-28.4714130710555,56.3749570778475));
#86150=CARTESIAN_POINT('Ctrl Pts',(4.48957896954741,-28.5209238681732,56.4262998838815));
#86151=CARTESIAN_POINT('Ctrl Pts',(4.49343417579274,-28.5704200375111,56.4776275208756));
#86152=CARTESIAN_POINT('Ctrl Pts',(4.49728938203808,-28.6226068827627,56.5263920166291));
#86153=CARTESIAN_POINT('Ctrl Pts',(4.50114458828341,-28.6771829274445,56.5723080344054));
#86154=CARTESIAN_POINT('Ctrl Pts',(4.50499994513465,-28.7317611041718,56.6182258459181));
#86155=CARTESIAN_POINT('Ctrl Pts',(4.5088553019859,-28.78872829249,56.6612946474706));
#86156=CARTESIAN_POINT('Ctrl Pts',(4.51271065883715,-28.8477497183875,56.7012691882897));
#86157=CARTESIAN_POINT('Ctrl Pts',(4.5165700513057,-28.9068329253074,56.741285572693));
#86158=CARTESIAN_POINT('Ctrl Pts',(4.52042944377426,-28.9679742592192,56.7782009577455));
#86159=CARTESIAN_POINT('Ctrl Pts',(4.52428883624282,-29.0308104776657,56.8118137962543));
#86160=CARTESIAN_POINT('Ctrl Pts',(4.52815041384626,-29.093682273114,56.8454456658895));
#86161=CARTESIAN_POINT('Ctrl Pts',(4.5320119914497,-29.1582504234921,56.875771060062));
#86162=CARTESIAN_POINT('Ctrl Pts',(4.53587356905313,-29.2241301267154,56.9026359352828));
#86163=CARTESIAN_POINT('Ctrl Pts',(4.53974190316801,-29.2901250981046,56.9295478153433));
#86164=CARTESIAN_POINT('Ctrl Pts',(4.54361023728288,-29.3574357450478,56.9529869280872));
#86165=CARTESIAN_POINT('Ctrl Pts',(4.54747857139775,-29.4256611505313,56.9728488154167));
#86166=CARTESIAN_POINT('Ctrl Pts',(4.5497762905687,-29.4661857839962,56.9846464104364));
#86167=CARTESIAN_POINT('Ctrl Pts',(4.55207400973964,-29.5070329226997,56.995182881589));
#86168=CARTESIAN_POINT('Ctrl Pts',(4.55437172891058,-29.5481172499469,57.0044449462892));
#86169=CARTESIAN_POINT('Ctrl Pts',(4.5584403036961,-29.6208653298829,57.0208452981589));
#86170=CARTESIAN_POINT('Ctrl Pts',(4.56250887848163,-29.694657290038,57.0333138861912));
#86171=CARTESIAN_POINT('Ctrl Pts',(4.56657745326715,-29.7690292171383,57.0417272246714));
#86172=CARTESIAN_POINT('Ctrl Pts',(4.57043978099225,-29.8396310300953,57.0497140682679));
#86173=CARTESIAN_POINT('Ctrl Pts',(4.57430210871735,-29.9107548818677,57.0540466921404));
#86174=CARTESIAN_POINT('Ctrl Pts',(4.57816443644246,-29.9819907734414,57.0546710759289));
#86175=CARTESIAN_POINT('Ctrl Pts',(4.58202297528157,-30.0531567836661,57.0552948472062));
#86176=CARTESIAN_POINT('Ctrl Pts',(4.58588151412069,-30.1244341324307,57.0522175912601));
#86177=CARTESIAN_POINT('Ctrl Pts',(4.5897400529598,-30.195408480989,57.0454371386228));
#86178=CARTESIAN_POINT('Ctrl Pts',(4.59359609750262,-30.2663369492122,57.0386610691105));
#86179=CARTESIAN_POINT('Ctrl Pts',(4.59745214204543,-30.3369623236069,57.0281866006375));
#86180=CARTESIAN_POINT('Ctrl Pts',(4.60130818658824,-30.4068727827817,57.0140635792178));
#86181=CARTESIAN_POINT('Ctrl Pts',(4.60516302838442,-30.4767614360441,56.9999449629381));
#86182=CARTESIAN_POINT('Ctrl Pts',(4.6090178701806,-30.5459351414517,56.9821801512765));
#86183=CARTESIAN_POINT('Ctrl Pts',(4.61287271197679,-30.6139914127986,56.9608702423948));
#86184=CARTESIAN_POINT('Ctrl Pts',(4.61672933960932,-30.6820792126415,56.9395504612507));
#86185=CARTESIAN_POINT('Ctrl Pts',(4.62058596724186,-30.7490480793185,56.9146824445157));
#86186=CARTESIAN_POINT('Ctrl Pts',(4.6244425948744,-30.8145110068051,56.8864170753821));
#86187=CARTESIAN_POINT('Ctrl Pts',(4.62830025678897,-30.8799914903373,56.8581441259565));
#86188=CARTESIAN_POINT('Ctrl Pts',(4.63215791870355,-30.9439647915131,56.8264722186575));
#86189=CARTESIAN_POINT('Ctrl Pts',(4.63601558061812,-31.0060663917418,56.7915992793891));
#86190=CARTESIAN_POINT('Ctrl Pts',(4.63987770191324,-31.0682397801868,56.7566860276956));
#86191=CARTESIAN_POINT('Ctrl Pts',(4.64373982320836,-31.1285367355297,56.7185646133584));
#86192=CARTESIAN_POINT('Ctrl Pts',(4.64760194450348,-31.1866206266542,56.6774769896779));
#86193=CARTESIAN_POINT('Ctrl Pts',(4.64907380425668,-31.208756477686,56.6618184396146));
#86194=CARTESIAN_POINT('Ctrl Pts',(4.65054566400989,-31.2305712397288,56.6457295083612));
#86195=CARTESIAN_POINT('Ctrl Pts',(4.65201752376309,-31.2520475724682,56.6292251037768));
#86196=CARTESIAN_POINT('',(4.34592528058805,-27.945250355841,54.9987907322123));
#86197=CARTESIAN_POINT('Ctrl Pts',(4.34592528058805,-27.945250355841,54.9987907322123));
#86198=CARTESIAN_POINT('Ctrl Pts',(4.34974237135585,-27.9452091140517,55.0688674784532));
#86199=CARTESIAN_POINT('Ctrl Pts',(4.35355946212366,-27.9487570283881,55.1390874484566));
#86200=CARTESIAN_POINT('Ctrl Pts',(4.35737655289147,-27.9559116838072,55.2090466888138));
#86201=CARTESIAN_POINT('Ctrl Pts',(4.36118805254387,-27.9630558593854,55.2789034557927));
#86202=CARTESIAN_POINT('Ctrl Pts',(4.36499955219628,-27.9737962381248,55.3484997581351));
#86203=CARTESIAN_POINT('Ctrl Pts',(4.36881105184868,-27.9880983872791,55.4174319863537));
#86204=CARTESIAN_POINT('Ctrl Pts',(4.37261948474161,-28.0023890288235,55.4863087512157));
#86205=CARTESIAN_POINT('Ctrl Pts',(4.37642791763454,-28.0202356597722,55.5545220139039));
#86206=CARTESIAN_POINT('Ctrl Pts',(4.38023635052746,-28.0415522620219,55.6216751725046));
#86207=CARTESIAN_POINT('Ctrl Pts',(4.38404307118795,-28.0628592805455,55.6887981397326));
#86208=CARTESIAN_POINT('Ctrl Pts',(4.38784979184843,-28.0876330256997,55.754861472588));
#86209=CARTESIAN_POINT('Ctrl Pts',(4.39165651250891,-28.1157372762022,55.8194824892615));
#86210=CARTESIAN_POINT('Ctrl Pts',(4.39546287300828,-28.1438388677079,55.8840973920172));
#86211=CARTESIAN_POINT('Ctrl Pts',(4.39926923350764,-28.1752701383301,55.94726979215));
#86212=CARTESIAN_POINT('Ctrl Pts',(4.40307559400701,-28.2098469931588,56.0086375833754));
#86213=CARTESIAN_POINT('Ctrl Pts',(4.40688551322989,-28.244456175316,56.0700627498815));
#86214=CARTESIAN_POINT('Ctrl Pts',(4.41069543245276,-28.2822165682394,56.1296795024771));
#86215=CARTESIAN_POINT('Ctrl Pts',(4.41450535167564,-28.3228989571176,56.187151908756));
#86216=CARTESIAN_POINT('Ctrl Pts',(4.41831711300167,-28.3636010160079,56.2446521030519));
#86217=CARTESIAN_POINT('Ctrl Pts',(4.42212887432769,-28.4072275723938,56.3000054956357));
#86218=CARTESIAN_POINT('Ctrl Pts',(4.42594063565372,-28.4535088401571,56.352908960362));
#86219=CARTESIAN_POINT('Ctrl Pts',(4.42975910316214,-28.4998715323844,56.4059055002451));
#86220=CARTESIAN_POINT('Ctrl Pts',(4.43357757067055,-28.5488979118374,56.4564431490458));
#86221=CARTESIAN_POINT('Ctrl Pts',(4.43739603817897,-28.6002816355939,56.5042559831506));
#86222=CARTESIAN_POINT('Ctrl Pts',(4.44006763663344,-28.6362323610277,56.5377083284741));
#86223=CARTESIAN_POINT('Ctrl Pts',(4.44273923508791,-28.673336292221,56.569827654895));
#86224=CARTESIAN_POINT('Ctrl Pts',(4.44541083354238,-28.7114798816251,56.6005353688822));
#86225=CARTESIAN_POINT('Ctrl Pts',(4.44927990689059,-28.766720348216,56.6450070212647));
#86226=CARTESIAN_POINT('Ctrl Pts',(4.45314898023881,-28.8243740439197,56.6867025917087));
#86227=CARTESIAN_POINT('Ctrl Pts',(4.45701805358702,-28.8841304900814,56.7253500512459));
#86228=CARTESIAN_POINT('Ctrl Pts',(4.46088136198281,-28.9437978986266,56.7639399257373));
#86229=CARTESIAN_POINT('Ctrl Pts',(4.4647446703786,-29.0055614338965,56.7994904428258));
#86230=CARTESIAN_POINT('Ctrl Pts',(4.46860797877438,-29.0690781313598,56.8317701921877));
#86231=CARTESIAN_POINT('Ctrl Pts',(4.4724667552673,-29.1325203197562,56.8640120753805));
#86232=CARTESIAN_POINT('Ctrl Pts',(4.47632553176021,-29.1977111543371,56.8929905930389));
#86233=CARTESIAN_POINT('Ctrl Pts',(4.48018430825312,-29.2642808120641,56.9185189180727));
#86234=CARTESIAN_POINT('Ctrl Pts',(4.48404065384133,-29.3308085330541,56.9440311610853));
#86235=CARTESIAN_POINT('Ctrl Pts',(4.48789699942954,-29.3987129013682,56.9660973501538));
#86236=CARTESIAN_POINT('Ctrl Pts',(4.49175334501774,-29.467603080323,56.984578313501));
#86237=CARTESIAN_POINT('Ctrl Pts',(4.49560855126307,-29.5364729059322,57.0030538167168));
#86238=CARTESIAN_POINT('Ctrl Pts',(4.4994637575084,-29.6063274950219,57.0179460712977));
#86239=CARTESIAN_POINT('Ctrl Pts',(4.50331896375372,-29.6767614356548,57.0291659353094));
#86240=CARTESIAN_POINT('Ctrl Pts',(4.50717432060498,-29.7471981278316,57.0403862376318));
#86241=CARTESIAN_POINT('Ctrl Pts',(4.51102967745623,-29.818213736402,57.0479337903106));
#86242=CARTESIAN_POINT('Ctrl Pts',(4.51488503430748,-29.8893949749598,57.0517709645416));
#86243=CARTESIAN_POINT('Ctrl Pts',(4.51874442677604,-29.9606507228948,57.0556121553571));
#86244=CARTESIAN_POINT('Ctrl Pts',(4.5226038192446,-30.0320719608352,57.0557351884641));
#86245=CARTESIAN_POINT('Ctrl Pts',(4.52646321171316,-30.1032435307008,57.0521545594493));
#86246=CARTESIAN_POINT('Ctrl Pts',(4.5303247893166,-30.1744553969293,57.0485719031316));
#86247=CARTESIAN_POINT('Ctrl Pts',(4.53418636692003,-30.2454168302103,57.0412814599577));
#86248=CARTESIAN_POINT('Ctrl Pts',(4.53804794452347,-30.3157186798858,57.0303495456869));
#86249=CARTESIAN_POINT('Ctrl Pts',(4.54191627863834,-30.3861435350528,57.0193985041031));
#86250=CARTESIAN_POINT('Ctrl Pts',(4.54578461275322,-30.4559060268755,57.0047933703203));
#86251=CARTESIAN_POINT('Ctrl Pts',(4.54965294686809,-30.5246087508623,56.9866512580266));
#86252=CARTESIAN_POINT('Ctrl Pts',(4.55195066603904,-30.5654169027212,56.9758751776828));
#86253=CARTESIAN_POINT('Ctrl Pts',(4.55424838520998,-30.6058514534182,56.9638521549951));
#86254=CARTESIAN_POINT('Ctrl Pts',(4.55654610438093,-30.6458324446948,56.9506147789555));
#86255=CARTESIAN_POINT('Ctrl Pts',(4.56041440940484,-30.7131420930502,56.9283291102433));
#86256=CARTESIAN_POINT('Ctrl Pts',(4.56428271442874,-30.7794286896822,56.90251174025));
#86257=CARTESIAN_POINT('Ctrl Pts',(4.56815101945265,-30.8442955339711,56.8732759043495));
#86258=CARTESIAN_POINT('Ctrl Pts',(4.57201426849278,-30.9090775954649,56.8440782805111));
#86259=CARTESIAN_POINT('Ctrl Pts',(4.57587751753291,-30.9724431452942,56.8114712484202));
#86260=CARTESIAN_POINT('Ctrl Pts',(4.57974076657305,-31.0340117676843,56.7756174212905));
#86261=CARTESIAN_POINT('Ctrl Pts',(4.58359955334054,-31.0955092748095,56.7398050073729));
#86262=CARTESIAN_POINT('Ctrl Pts',(4.58745834010803,-31.1552135590635,56.7007534901102));
#86263=CARTESIAN_POINT('Ctrl Pts',(4.59131712687552,-31.2127670719809,56.6586722375499));
#86264=CARTESIAN_POINT('Ctrl Pts',(4.59220268568774,-31.2259751147179,56.6490149472462));
#86265=CARTESIAN_POINT('Ctrl Pts',(4.59308824449995,-31.239069989523,56.6391982813232));
#86266=CARTESIAN_POINT('Ctrl Pts',(4.59397380331217,-31.2520475724682,56.6292251037768));
#86267=CARTESIAN_POINT('Ctrl Pts',(3.89394682683029,-31.2520475724682,56.6292251037768));
#86268=CARTESIAN_POINT('Ctrl Pts',(3.89781364274067,-31.3083220096347,56.585978610531));
#86269=CARTESIAN_POINT('Ctrl Pts',(3.90168045865106,-31.3624548341262,56.5397349396832));
#86270=CARTESIAN_POINT('Ctrl Pts',(3.90554727456145,-31.4141101763284,56.4907347086938));
#86271=CARTESIAN_POINT('Ctrl Pts',(3.90951904437923,-31.4671675583813,56.4404045034247));
#86272=CARTESIAN_POINT('Ctrl Pts',(3.91349081419701,-31.5176105505212,56.3871661673033));
#86273=CARTESIAN_POINT('Ctrl Pts',(3.91746258401478,-31.5651093206311,56.3313265478363));
#86274=CARTESIAN_POINT('Ctrl Pts',(3.92132025531689,-31.6112435758234,56.2770910539831));
#86275=CARTESIAN_POINT('Ctrl Pts',(3.925177926619,-31.6546001507359,56.2204021165531));
#86276=CARTESIAN_POINT('Ctrl Pts',(3.9290355979211,-31.6949138887671,56.1615784399533));
#86277=CARTESIAN_POINT('Ctrl Pts',(3.93289134398468,-31.7352075075202,56.102784120341));
#86278=CARTESIAN_POINT('Ctrl Pts',(3.93674709004826,-31.7724610285617,56.0418575757432));
#86279=CARTESIAN_POINT('Ctrl Pts',(3.94060283611184,-31.8064511104346,55.9791485832649));
#86280=CARTESIAN_POINT('Ctrl Pts',(3.94445794771281,-31.840435599243,55.9164499095448));
#86281=CARTESIAN_POINT('Ctrl Pts',(3.94831305931377,-31.8711574843615,55.8519697976937));
#86282=CARTESIAN_POINT('Ctrl Pts',(3.95216817091473,-31.8984389755367,55.7860833407873));
#86283=CARTESIAN_POINT('Ctrl Pts',(3.95622663585418,-31.9271595384907,55.7167214381973));
#86284=CARTESIAN_POINT('Ctrl Pts',(3.96028510079364,-31.9520664883309,55.6458012669927));
#86285=CARTESIAN_POINT('Ctrl Pts',(3.96434356573309,-31.9730105582645,55.573782972453));
#86286=CARTESIAN_POINT('Ctrl Pts',(3.96820378433556,-31.9929315603121,55.5052825999111));
#86287=CARTESIAN_POINT('Ctrl Pts',(3.97206400293803,-32.0092677198864,55.4357893832784));
#86288=CARTESIAN_POINT('Ctrl Pts',(3.9759242215405,-32.0219428275483,55.3657113132323));
#86289=CARTESIAN_POINT('Ctrl Pts',(3.97978713969793,-32.0346267992547,55.2955842357021));
#86290=CARTESIAN_POINT('Ctrl Pts',(3.98365005785536,-32.0436445648653,55.2248719723876));
#86291=CARTESIAN_POINT('Ctrl Pts',(3.98751297601278,-32.0489717734689,55.1539877723317));
#86292=CARTESIAN_POINT('Ctrl Pts',(3.99138214984943,-32.05430760905,55.0829887811258));
#86293=CARTESIAN_POINT('Ctrl Pts',(3.99525132368607,-32.0559409588887,55.0118177819486));
#86294=CARTESIAN_POINT('Ctrl Pts',(3.99912049752272,-32.0538995184525,54.9408871367581));
#86295=CARTESIAN_POINT('Ctrl Pts',(3.99970358174452,-32.053591873524,54.9301978935761));
#86296=CARTESIAN_POINT('Ctrl Pts',(4.00028666596633,-32.0532008679053,54.9195140956756));
#86297=CARTESIAN_POINT('Ctrl Pts',(4.00086975018814,-32.052726697614,54.90883713803));
#86298=CARTESIAN_POINT('Ctrl Pts',(4.00473882353635,-32.0495803260131,54.837989856074));
#86299=CARTESIAN_POINT('Ctrl Pts',(4.00860789688457,-32.0427556783592,54.7671668837602));
#86300=CARTESIAN_POINT('Ctrl Pts',(4.01247697023278,-32.0322538737086,54.6967810109899));
#86301=CARTESIAN_POINT('Ctrl Pts',(4.01634027862857,-32.021767716837,54.6265000137729));
#86302=CARTESIAN_POINT('Ctrl Pts',(4.02020358702435,-32.0076153497239,54.5566552998756));
#86303=CARTESIAN_POINT('Ctrl Pts',(4.02406689542014,-31.9898498441324,54.4876571847812));
#86304=CARTESIAN_POINT('Ctrl Pts',(4.02792567191305,-31.9721051785923,54.4187400088001));
#86305=CARTESIAN_POINT('Ctrl Pts',(4.03178444840596,-31.9507559140857,54.3506679271215));
#86306=CARTESIAN_POINT('Ctrl Pts',(4.03564322489888,-31.9259063300413,54.2838419375536));
#86307=CARTESIAN_POINT('Ctrl Pts',(4.03949957048708,-31.9010724004332,54.2170580462034));
#86308=CARTESIAN_POINT('Ctrl Pts',(4.04335591607529,-31.8727426950614,54.1515191437889));
#86309=CARTESIAN_POINT('Ctrl Pts',(4.04721226166349,-31.8410711425108,54.0876104939698));
#86310=CARTESIAN_POINT('Ctrl Pts',(4.05106746790882,-31.8094089472018,54.0237207257222));
#86311=CARTESIAN_POINT('Ctrl Pts',(4.05492267415416,-31.7744070804402,53.9614606888879));
#86312=CARTESIAN_POINT('Ctrl Pts',(4.05877788039949,-31.7362666457037,53.9011935122521));
#86313=CARTESIAN_POINT('Ctrl Pts',(4.06263323725073,-31.6981247209885,53.8409239812434));
#86314=CARTESIAN_POINT('Ctrl Pts',(4.06648859410198,-31.6568442465144,53.7826478743105));
#86315=CARTESIAN_POINT('Ctrl Pts',(4.07034395095323,-31.6126701841896,53.7267001768924));
#86316=CARTESIAN_POINT('Ctrl Pts',(4.07420334342179,-31.5684498824069,53.670693915895));
#86317=CARTESIAN_POINT('Ctrl Pts',(4.07806273589035,-31.5213302481,53.6170213118137));
#86318=CARTESIAN_POINT('Ctrl Pts',(4.0819221283589,-31.4715965922107,53.5659842984493));
#86319=CARTESIAN_POINT('Ctrl Pts',(4.08578370596234,-31.4218347778102,53.5149183886306));
#86320=CARTESIAN_POINT('Ctrl Pts',(4.08964528356578,-31.3694563524205,53.4664913700495));
#86321=CARTESIAN_POINT('Ctrl Pts',(4.09350686116921,-31.3147815393855,53.4209664138496));
#86322=CARTESIAN_POINT('Ctrl Pts',(4.09737519528408,-31.2600110631172,53.3753618037054));
#86323=CARTESIAN_POINT('Ctrl Pts',(4.10124352939895,-31.2029365664032,53.332669684726));
#86324=CARTESIAN_POINT('Ctrl Pts',(4.10511186351382,-31.1439086244318,53.2931108350421));
#86325=CARTESIAN_POINT('Ctrl Pts',(4.10740958268478,-31.1088471147839,53.2696136073983));
#86326=CARTESIAN_POINT('Ctrl Pts',(4.10970730185574,-31.0730969193769,53.2472209860021));
#86327=CARTESIAN_POINT('Ctrl Pts',(4.1120050210267,-31.036735346744,53.2259714254524));
#86328=CARTESIAN_POINT('Ctrl Pts',(4.11587409437492,-30.9755069802181,53.1901898080018));
#86329=CARTESIAN_POINT('Ctrl Pts',(4.11974316772313,-30.9123040724541,53.1575116551603));
#86330=CARTESIAN_POINT('Ctrl Pts',(4.12361224107135,-30.8474740331644,53.1281599091771));
#86331=CARTESIAN_POINT('Ctrl Pts',(4.12747554946714,-30.7827405911886,53.0988518975468));
#86332=CARTESIAN_POINT('Ctrl Pts',(4.13133885786292,-30.7163852690689,53.0728606532385));
#86333=CARTESIAN_POINT('Ctrl Pts',(4.13520216625871,-30.6487815749337,53.0503641287341));
#86334=CARTESIAN_POINT('Ctrl Pts',(4.13906094275162,-30.5812571841686,53.027893994063));
#86335=CARTESIAN_POINT('Ctrl Pts',(4.14291971924454,-30.5124877889161,53.008910588793));
#86336=CARTESIAN_POINT('Ctrl Pts',(4.14677849573745,-30.4428668423189,52.9935437900431));
#86337=CARTESIAN_POINT('Ctrl Pts',(4.15063484132565,-30.373289754672,52.9781866718808));
#86338=CARTESIAN_POINT('Ctrl Pts',(4.15449118691386,-30.3028626532351,52.9664417444936));
#86339=CARTESIAN_POINT('Ctrl Pts',(4.15834753250207,-30.2319927001259,52.9583886389451));
#86340=CARTESIAN_POINT('Ctrl Pts',(4.1622027387474,-30.1611436852792,52.9503379126565));
#86341=CARTESIAN_POINT('Ctrl Pts',(4.16605794499273,-30.0898525609284,52.9459768976138));
#86342=CARTESIAN_POINT('Ctrl Pts',(4.16991315123807,-30.018533478687,52.945333586037));
#86343=CARTESIAN_POINT('Ctrl Pts',(4.17376850808931,-29.9472116103234,52.9446902493287));
#86344=CARTESIAN_POINT('Ctrl Pts',(4.17762386494056,-29.8758622676869,52.9477649066092));
#86345=CARTESIAN_POINT('Ctrl Pts',(4.18147922179181,-29.8048997451773,52.9545334387803));
#86346=CARTESIAN_POINT('Ctrl Pts',(4.18533861426037,-29.7338629422326,52.9613090559519));
#86347=CARTESIAN_POINT('Ctrl Pts',(4.18919800672893,-29.6632142522808,52.9717862203667));
#86348=CARTESIAN_POINT('Ctrl Pts',(4.19305739919749,-29.5933620854676,52.9858889879243));
#86349=CARTESIAN_POINT('Ctrl Pts',(4.19691897680093,-29.5234703693193,52.9999997402747));
#86350=CARTESIAN_POINT('Ctrl Pts',(4.20078055440436,-29.4543765448197,53.0177400613253));
#86351=CARTESIAN_POINT('Ctrl Pts',(4.2046421320078,-29.3864753911509,53.0389836520731));
#86352=CARTESIAN_POINT('Ctrl Pts',(4.20851046612267,-29.3184554324318,53.0602644122316));
#86353=CARTESIAN_POINT('Ctrl Pts',(4.21237880023754,-29.251632766462,53.085060510933));
#86354=CARTESIAN_POINT('Ctrl Pts',(4.21624713435242,-29.1863830179574,53.11319715682));
#86355=CARTESIAN_POINT('Ctrl Pts',(4.21854485352336,-29.1476258698967,53.1299098059194));
#86356=CARTESIAN_POINT('Ctrl Pts',(4.22084257269431,-29.1094232312377,53.1478001486803));
#86357=CARTESIAN_POINT('Ctrl Pts',(4.22314029186526,-29.0718493387358,53.1668240912299));
#86358=CARTESIAN_POINT('Ctrl Pts',(4.22700936521348,-29.0085795763097,53.1988580447381));
#86359=CARTESIAN_POINT('Ctrl Pts',(4.23087843856169,-28.9468462494311,53.2342341040927));
#86360=CARTESIAN_POINT('Ctrl Pts',(4.23474751190991,-28.8870250841456,53.2727813111309));
#86361=CARTESIAN_POINT('Ctrl Pts',(4.2386108203057,-28.8272930529087,53.3112710825003));
#86362=CARTESIAN_POINT('Ctrl Pts',(4.24247412870148,-28.7694679328314,53.3529223615004));
#86363=CARTESIAN_POINT('Ctrl Pts',(4.24633743709726,-28.7139018069396,53.3975178627183));
#86364=CARTESIAN_POINT('Ctrl Pts',(4.25019621359018,-28.6584008635959,53.4420610506184));
#86365=CARTESIAN_POINT('Ctrl Pts',(4.25405499008309,-28.6051540277786,53.4895412978216));
#86366=CARTESIAN_POINT('Ctrl Pts',(4.25791376657601,-28.5544838097663,53.5396984878894));
#86367=CARTESIAN_POINT('Ctrl Pts',(4.26177011216421,-28.5038455123568,53.5898240805457));
#86368=CARTESIAN_POINT('Ctrl Pts',(4.26562645775242,-28.4557809568072,53.6426229293585));
#86369=CARTESIAN_POINT('Ctrl Pts',(4.26948280334063,-28.4105778747521,53.6977961487261));
#86370=CARTESIAN_POINT('Ctrl Pts',(4.27333800958596,-28.3653881477785,53.7529530673726));
#86371=CARTESIAN_POINT('Ctrl Pts',(4.27719321583129,-28.3230585236238,53.8104825883364));
#86372=CARTESIAN_POINT('Ctrl Pts',(4.28104842207662,-28.2838371407325,53.8700519467822));
#86373=CARTESIAN_POINT('Ctrl Pts',(4.28490377892787,-28.2446142256346,53.9296236323401));
#86374=CARTESIAN_POINT('Ctrl Pts',(4.28875913577911,-28.2085000581779,53.9912349066408));
#86375=CARTESIAN_POINT('Ctrl Pts',(4.29261449263036,-28.1756990732606,54.0545246215803));
#86376=CARTESIAN_POINT('Ctrl Pts',(4.29647388509892,-28.1428637537207,54.1178805853988));
#86377=CARTESIAN_POINT('Ctrl Pts',(4.30033327756748,-28.1133487638018,54.1829180648716));
#86378=CARTESIAN_POINT('Ctrl Pts',(4.30419267003604,-28.0873118065526,54.249252747493));
#86379=CARTESIAN_POINT('Ctrl Pts',(4.30805424763947,-28.0612601075366,54.3156249878983));
#86380=CARTESIAN_POINT('Ctrl Pts',(4.3119158252429,-28.0386905150585,54.3832954324832));
#86381=CARTESIAN_POINT('Ctrl Pts',(4.31577740284633,-28.0197110338744,54.4518639100176));
#86382=CARTESIAN_POINT('Ctrl Pts',(4.3196457369612,-28.0006983447388,54.5205523602032));
#86383=CARTESIAN_POINT('Ctrl Pts',(4.32351407107608,-27.9852884132227,54.5901415059717));
#86384=CARTESIAN_POINT('Ctrl Pts',(4.32738240519095,-27.973538114849,54.6602209680831));
#86385=CARTESIAN_POINT('Ctrl Pts',(4.32968012436191,-27.9665586541727,54.7018468770149));
#86386=CARTESIAN_POINT('Ctrl Pts',(4.33197784353286,-27.9608693712245,54.7436456571904));
#86387=CARTESIAN_POINT('Ctrl Pts',(4.33427556270382,-27.9564734841711,54.7855310241448));
#86388=CARTESIAN_POINT('Ctrl Pts',(4.33815880198177,-27.9490442554461,54.8563190056286));
#86389=CARTESIAN_POINT('Ctrl Pts',(4.34204204125972,-27.9452923123651,54.9274995857473));
#86390=CARTESIAN_POINT('Ctrl Pts',(4.34592528053768,-27.9452503558416,54.9987907312877));
#86391=CARTESIAN_POINT('Origin',(-1.54592528053767,-30.,55.));
#86392=CARTESIAN_POINT('',(3.19386027023256,-31.2520475724682,56.6292251037768));
#86393=CARTESIAN_POINT('',(3.25213375229793,-31.2520475724682,56.6292251037768));
#86394=CARTESIAN_POINT('',(-1.54592528053767,-31.2520475724682,56.6292251037768));
#86395=CARTESIAN_POINT('',(3.70407471941232,-27.9452505355246,54.9985165115458));
#86396=CARTESIAN_POINT('Ctrl Pts',(3.25213375229793,-31.2520475724682,56.6292251037768));
#86397=CARTESIAN_POINT('Ctrl Pts',(3.25599067575063,-31.3085261850896,56.5858217031878));
#86398=CARTESIAN_POINT('Ctrl Pts',(3.25984759920333,-31.3627927451719,56.5394415114278));
#86399=CARTESIAN_POINT('Ctrl Pts',(3.26370452265604,-31.414522935898,56.4903430565874));
#86400=CARTESIAN_POINT('Ctrl Pts',(3.26755992886839,-31.4662327769507,56.4412639161457));
#86401=CARTESIAN_POINT('Ctrl Pts',(3.27141533508075,-31.5154078769165,56.389468969029));
#86402=CARTESIAN_POINT('Ctrl Pts',(3.2752707412931,-31.5617586582873,56.3352555769458));
#86403=CARTESIAN_POINT('Ctrl Pts',(3.27912592055178,-31.6081067111569,56.2810453762069));
#86404=CARTESIAN_POINT('Ctrl Pts',(3.28298109981045,-31.6516304610639,56.2244173834216));
#86405=CARTESIAN_POINT('Ctrl Pts',(3.28683627906913,-31.6920798789517,56.1657028977174));
#86406=CARTESIAN_POINT('Ctrl Pts',(3.29069525143292,-31.7325690949614,56.1069306429184));
#86407=CARTESIAN_POINT('Ctrl Pts',(3.29455422379671,-31.769977660405,56.0460681954318));
#86408=CARTESIAN_POINT('Ctrl Pts',(3.29841319616051,-31.8040987756994,55.9834760647926));
#86409=CARTESIAN_POINT('Ctrl Pts',(3.30227401452487,-31.8382362133698,55.9208539922161));
#86410=CARTESIAN_POINT('Ctrl Pts',(3.30613483288923,-31.869082857657,55.8565010268448));
#86411=CARTESIAN_POINT('Ctrl Pts',(3.30999565125359,-31.8964790776824,55.7908000192291));
#86412=CARTESIAN_POINT('Ctrl Pts',(3.31386358533863,-31.9239257905907,55.724977920701));
#86413=CARTESIAN_POINT('Ctrl Pts',(3.31773151942368,-31.9479092094712,55.6578032745301));
#86414=CARTESIAN_POINT('Ctrl Pts',(3.32159945350872,-31.9683189986739,55.5896760822345));
#86415=CARTESIAN_POINT('Ctrl Pts',(3.32502755223462,-31.9864079243958,55.5292958544507));
#86416=CARTESIAN_POINT('Ctrl Pts',(3.32845565096053,-32.0016904370004,55.4681678305888));
#86417=CARTESIAN_POINT('Ctrl Pts',(3.33188374968643,-32.014123551826,55.4065757991813));
#86418=CARTESIAN_POINT('Ctrl Pts',(3.33575282303467,-32.0281560045216,55.3370608562826));
#86419=CARTESIAN_POINT('Ctrl Pts',(3.3396218963829,-32.0386128869442,55.2666824303766));
#86420=CARTESIAN_POINT('Ctrl Pts',(3.34349096973113,-32.0453957342307,55.1958413972863));
#86421=CARTESIAN_POINT('Ctrl Pts',(3.34735427812694,-32.0521684750165,55.125105917942));
#86422=CARTESIAN_POINT('Ctrl Pts',(3.35121758652275,-32.0552780011611,55.0539096792667));
#86423=CARTESIAN_POINT('Ctrl Pts',(3.35508089491855,-32.0546768638109,54.9826636849271));
#86424=CARTESIAN_POINT('Ctrl Pts',(3.35893967141149,-32.0540764316324,54.9115012666039));
#86425=CARTESIAN_POINT('Ctrl Pts',(3.36279844790443,-32.0497739862521,54.840289691963));
#86426=CARTESIAN_POINT('Ctrl Pts',(3.36665722439736,-32.041774022137,54.7694432715655));
#86427=CARTESIAN_POINT('Ctrl Pts',(3.37051356998559,-32.0337790977413,54.6986414821275));
#86428=CARTESIAN_POINT('Ctrl Pts',(3.37436991557382,-32.0220913303187,54.6282048721235));
#86429=CARTESIAN_POINT('Ctrl Pts',(3.37822626116204,-32.0067671925835,54.5585444560653));
#86430=CARTESIAN_POINT('Ctrl Pts',(3.38208146740739,-31.9914475823074,54.4889046209165));
#86431=CARTESIAN_POINT('Ctrl Pts',(3.38593667365274,-31.9724938389174,54.4200409986262));
#86432=CARTESIAN_POINT('Ctrl Pts',(3.38979187989809,-31.95001355578,54.3523544991478));
#86433=CARTESIAN_POINT('Ctrl Pts',(3.39364723674936,-31.927532394437,54.284665355456));
#86434=CARTESIAN_POINT('Ctrl Pts',(3.39750259360064,-31.901524575037,54.2181538862032));
#86435=CARTESIAN_POINT('Ctrl Pts',(3.40135795045191,-31.8721470420644,54.1532042658411));
#86436=CARTESIAN_POINT('Ctrl Pts',(3.40521734292049,-31.8427387579875,54.0881866590845));
#86437=CARTESIAN_POINT('Ctrl Pts',(3.40907673538907,-31.8099539197302,54.0247346083171));
#86438=CARTESIAN_POINT('Ctrl Pts',(3.41293612785765,-31.7739966007954,53.9632099427239));
#86439=CARTESIAN_POINT('Ctrl Pts',(3.41679770546111,-31.7380189233216,53.9016504427123));
#86440=CARTESIAN_POINT('Ctrl Pts',(3.42065928306457,-31.6988654562192,53.8420209065002));
#86441=CARTESIAN_POINT('Ctrl Pts',(3.42452086066803,-31.6567835031492,53.784653964423));
#86442=CARTESIAN_POINT('Ctrl Pts',(3.42838919478292,-31.6146279202765,53.7271866487577));
#86443=CARTESIAN_POINT('Ctrl Pts',(3.43225752889782,-31.5695339288584,53.6719902074217));
#86444=CARTESIAN_POINT('Ctrl Pts',(3.43612586301271,-31.5217885122851,53.6193634488479));
#86445=CARTESIAN_POINT('Ctrl Pts',(3.43842358218347,-31.4934286147897,53.5881041241675));
#86446=CARTESIAN_POINT('Ctrl Pts',(3.44072130135423,-31.4641339653967,53.5577507144535));
#86447=CARTESIAN_POINT('Ctrl Pts',(3.44301902052499,-31.4339703168495,53.5283591834641));
#86448=CARTESIAN_POINT('Ctrl Pts',(3.44688809387321,-31.383178483729,53.4788675002933));
#86449=CARTESIAN_POINT('Ctrl Pts',(3.45075716722142,-31.3297219400212,53.4319114872837));
#86450=CARTESIAN_POINT('Ctrl Pts',(3.45462624056964,-31.2738840751609,53.3877912897049));
#86451=CARTESIAN_POINT('Ctrl Pts',(3.45848954896542,-31.2181294091975,53.3437368315983));
#86452=CARTESIAN_POINT('Ctrl Pts',(3.4623528573612,-31.1600008431914,53.3025101003627));
#86453=CARTESIAN_POINT('Ctrl Pts',(3.46621616575699,-31.0998179446717,53.2643738734745));
#86454=CARTESIAN_POINT('Ctrl Pts',(3.47007494224989,-31.039705644464,53.2262823827706));
#86455=CARTESIAN_POINT('Ctrl Pts',(3.4739337187428,-30.9775442068879,53.1912744539901));
#86456=CARTESIAN_POINT('Ctrl Pts',(3.4777924952357,-30.9136841499305,53.1595710183042));
#86457=CARTESIAN_POINT('Ctrl Pts',(3.4816488408239,-30.8498643227489,53.1278875547601));
#86458=CARTESIAN_POINT('Ctrl Pts',(3.4855051864121,-30.7843484332854,53.099504669707));
#86459=CARTESIAN_POINT('Ctrl Pts',(3.4893615320003,-30.7175124215068,53.0745978374679));
#86460=CARTESIAN_POINT('Ctrl Pts',(3.49321673824563,-30.6506961561778,53.0496983638591));
#86461=CARTESIAN_POINT('Ctrl Pts',(3.49707194449096,-30.5825609977991,53.0282730737537));
#86462=CARTESIAN_POINT('Ctrl Pts',(3.50092715073629,-30.5135021230636,53.0104490124379));
#86463=CARTESIAN_POINT('Ctrl Pts',(3.50478250758753,-30.4444405505021,52.9926242548147));
#86464=CARTESIAN_POINT('Ctrl Pts',(3.50863786443877,-30.3744556608628,52.9784011245609));
#86465=CARTESIAN_POINT('Ctrl Pts',(3.51249322129001,-30.3039553368884,52.9678561282042));
#86466=CARTESIAN_POINT('Ctrl Pts',(3.51635261375857,-30.2333812162879,52.957300093811));
#86467=CARTESIAN_POINT('Ctrl Pts',(3.52021200622712,-30.1622910657473,52.9504299510044));
#86468=CARTESIAN_POINT('Ctrl Pts',(3.52407139869567,-30.0910995558641,52.9472704919008));
#86469=CARTESIAN_POINT('Ctrl Pts',(3.5279329762991,-30.0198677383285,52.9441092439549));
#86470=CARTESIAN_POINT('Ctrl Pts',(3.53179455390252,-29.9485349332096,52.9446628582596));
#86471=CARTESIAN_POINT('Ctrl Pts',(3.53565613150594,-29.8775147263652,52.9489039709846));
#86472=CARTESIAN_POINT('Ctrl Pts',(3.53952446562081,-29.8063702571363,52.9531525042848));
#86473=CARTESIAN_POINT('Ctrl Pts',(3.54339279973568,-29.735539961084,52.9611013632752));
#86474=CARTESIAN_POINT('Ctrl Pts',(3.54726113385054,-29.6654305296723,52.9726715036717));
#86475=CARTESIAN_POINT('Ctrl Pts',(3.54955885302155,-29.6237868195274,52.9795439538301));
#86476=CARTESIAN_POINT('Ctrl Pts',(3.55185657219255,-29.5823972321482,52.9876930655165));
#86477=CARTESIAN_POINT('Ctrl Pts',(3.55415429136356,-29.5413444470519,52.9970939497196));
#86478=CARTESIAN_POINT('Ctrl Pts',(3.55802336471177,-29.4722166621205,53.0129238696588));
#86479=CARTESIAN_POINT('Ctrl Pts',(3.56189243805998,-29.4037739608207,53.0323677854612));
#86480=CARTESIAN_POINT('Ctrl Pts',(3.5657615114082,-29.336422208519,53.0553503973329));
#86481=CARTESIAN_POINT('Ctrl Pts',(3.56962481980398,-29.2691708109051,53.0782987649162));
#86482=CARTESIAN_POINT('Ctrl Pts',(3.57348812819977,-29.2030075916814,53.1047752068269));
#86483=CARTESIAN_POINT('Ctrl Pts',(3.57735143659555,-29.1383266436026,53.1346537615298));
#86484=CARTESIAN_POINT('Ctrl Pts',(3.58121021308847,-29.0737215703296,53.1644972668155));
#86485=CARTESIAN_POINT('Ctrl Pts',(3.58506898958138,-29.0105957532292,53.197734754904));
#86486=CARTESIAN_POINT('Ctrl Pts',(3.58892776607429,-28.9493249145688,53.2341915654992));
#86487=CARTESIAN_POINT('Ctrl Pts',(3.59278411166249,-28.8880926745604,53.2706254094797));
#86488=CARTESIAN_POINT('Ctrl Pts',(3.59664045725069,-28.8287135110421,53.3102743044957));
#86489=CARTESIAN_POINT('Ctrl Pts',(3.60049680283889,-28.7715387439723,53.3529175779765));
#86490=CARTESIAN_POINT('Ctrl Pts',(3.60435200908422,-28.7143808689733,53.3955482526618));
#86491=CARTESIAN_POINT('Ctrl Pts',(3.60820721532955,-28.6594264866429,53.4411712592055));
#86492=CARTESIAN_POINT('Ctrl Pts',(3.61206242157488,-28.6069966629057,53.4895234972552));
#86493=CARTESIAN_POINT('Ctrl Pts',(3.61591777842612,-28.5545647909664,53.5378776242137));
#86494=CARTESIAN_POINT('Ctrl Pts',(3.61977313527735,-28.5046580290391,53.5889608634019));
#86495=CARTESIAN_POINT('Ctrl Pts',(3.62362849212859,-28.4575618745408,53.6424720291538));
#86496=CARTESIAN_POINT('Ctrl Pts',(3.62748788459715,-28.4104164218675,53.6960392080311));
#86497=CARTESIAN_POINT('Ctrl Pts',(3.6313472770657,-28.3660877711614,53.752039021358));
#86498=CARTESIAN_POINT('Ctrl Pts',(3.63520666953425,-28.3248216537988,53.8101365326565));
#86499=CARTESIAN_POINT('Ctrl Pts',(3.63906824713769,-28.2835321721287,53.868266937966));
#86500=CARTESIAN_POINT('Ctrl Pts',(3.64292982474112,-28.2453089360108,53.9284969952101));
#86501=CARTESIAN_POINT('Ctrl Pts',(3.64679140234455,-28.2103532700148,53.9904643917358));
#86502=CARTESIAN_POINT('Ctrl Pts',(3.65065973645941,-28.1753364429128,54.0525402111567));
#86503=CARTESIAN_POINT('Ctrl Pts',(3.65452807057428,-28.1435988168513,54.1163590037658));
#86504=CARTESIAN_POINT('Ctrl Pts',(3.65839640468915,-28.115294558128,54.1815362195686));
#86505=CARTESIAN_POINT('Ctrl Pts',(3.66069412386014,-28.0984823500927,54.2202502845419));
#86506=CARTESIAN_POINT('Ctrl Pts',(3.66299184303113,-28.0828805480779,54.2594432652727));
#86507=CARTESIAN_POINT('Ctrl Pts',(3.66528956220211,-28.0685130841418,54.2990322001912));
#86508=CARTESIAN_POINT('Ctrl Pts',(3.66976608681325,-28.0405217148215,54.3761612261093));
#86509=CARTESIAN_POINT('Ctrl Pts',(3.67424261142439,-28.0171274210087,54.4550424288448));
#86510=CARTESIAN_POINT('Ctrl Pts',(3.67871913603553,-27.9985204841622,54.535158833383));
#86511=CARTESIAN_POINT('Ctrl Pts',(3.68315616207699,-27.980077725435,54.6145683316352));
#86512=CARTESIAN_POINT('Ctrl Pts',(3.68759318811845,-27.9663383039406,54.6951911642614));
#86513=CARTESIAN_POINT('Ctrl Pts',(3.69203021415991,-27.9574411612528,54.7765029021317));
#86514=CARTESIAN_POINT('Ctrl Pts',(3.69604504924405,-27.9493905975919,54.8500776828302));
#86515=CARTESIAN_POINT('Ctrl Pts',(3.70005988432819,-27.9453041789034,54.9242161665679));
#86516=CARTESIAN_POINT('Ctrl Pts',(3.70407471941232,-27.9452505355246,54.9985165115458));
#86517=CARTESIAN_POINT('Ctrl Pts',(3.70407471946232,-27.9452505355239,54.9985165124711));
#86518=CARTESIAN_POINT('Ctrl Pts',(3.70793830290604,-27.9451989130944,55.0700177265206));
#86519=CARTESIAN_POINT('Ctrl Pts',(3.71180188634977,-27.94888376533,55.1415522381297));
#86520=CARTESIAN_POINT('Ctrl Pts',(3.71566546979349,-27.9562889262005,55.2127031013631));
#86521=CARTESIAN_POINT('Ctrl Pts',(3.71952882663493,-27.9636936527524,55.2838497915411));
#86522=CARTESIAN_POINT('Ctrl Pts',(3.72339218347637,-27.9748182037558,55.3546123983527));
#86523=CARTESIAN_POINT('Ctrl Pts',(3.72725554031781,-27.9895945586331,55.4245792315016));
#86524=CARTESIAN_POINT('Ctrl Pts',(3.73111993974998,-28.0043749011542,55.4945649463574));
#86525=CARTESIAN_POINT('Ctrl Pts',(3.73498433918215,-28.0228089023201,55.563753989815));
#86526=CARTESIAN_POINT('Ctrl Pts',(3.73884873861432,-28.0447778295687,55.6317466476002));
#86527=CARTESIAN_POINT('Ctrl Pts',(3.74271803189464,-28.0667745781118,55.6998254108072));
#86528=CARTESIAN_POINT('Ctrl Pts',(3.74658732517497,-28.0923150338194,55.7667043065627));
#86529=CARTESIAN_POINT('Ctrl Pts',(3.7504566184553,-28.12123143394,55.8320013447614));
#86530=CARTESIAN_POINT('Ctrl Pts',(3.75432884727621,-28.1501697722442,55.8973479222667));
#86531=CARTESIAN_POINT('Ctrl Pts',(3.75820107609713,-28.1824889322493,55.961109825256));
#86532=CARTESIAN_POINT('Ctrl Pts',(3.76207330491805,-28.2179753493682,56.022929961943));
#86533=CARTESIAN_POINT('Ctrl Pts',(3.76595231070722,-28.2535238729207,56.0848582929343));
#86534=CARTESIAN_POINT('Ctrl Pts',(3.76983131649638,-28.2922504492782,56.144837675185));
#86535=CARTESIAN_POINT('Ctrl Pts',(3.77371032228555,-28.3338989370465,56.202540980809));
#86536=CARTESIAN_POINT('Ctrl Pts',(3.77461515920393,-28.3436140783418,56.2160011518113));
#86537=CARTESIAN_POINT('Ctrl Pts',(3.7755199961223,-28.3534880425275,56.2293376254159));
#86538=CARTESIAN_POINT('Ctrl Pts',(3.77642483304068,-28.3635172836502,56.242546530955));
#86539=CARTESIAN_POINT('Ctrl Pts',(3.78029390638889,-28.4064022154458,56.2990276750626));
#86540=CARTESIAN_POINT('Ctrl Pts',(3.78416297973711,-28.4522986437702,56.3533966652134));
#86541=CARTESIAN_POINT('Ctrl Pts',(3.78803205308532,-28.5009708582321,56.4053146247836));
#86542=CARTESIAN_POINT('Ctrl Pts',(3.79189536148111,-28.5495705506776,56.4571552261493));
#86543=CARTESIAN_POINT('Ctrl Pts',(3.7957586698769,-28.6009374899869,56.5065516946496));
#86544=CARTESIAN_POINT('Ctrl Pts',(3.79962197827268,-28.6547946429132,56.5531967389114));
#86545=CARTESIAN_POINT('Ctrl Pts',(3.80348075476559,-28.7085886180236,56.5997870656129));
#86546=CARTESIAN_POINT('Ctrl Pts',(3.80733953125851,-28.7648666388802,56.6436320626764));
#86547=CARTESIAN_POINT('Ctrl Pts',(3.81119830775142,-28.8233148545278,56.6844612286797));
#86548=CARTESIAN_POINT('Ctrl Pts',(3.81505465333963,-28.8817262496851,56.7252646736255));
#86549=CARTESIAN_POINT('Ctrl Pts',(3.81891099892784,-28.9423047299241,56.7630557792996));
#86550=CARTESIAN_POINT('Ctrl Pts',(3.82276734451604,-29.0047045580452,56.797605225216));
#86551=CARTESIAN_POINT('Ctrl Pts',(3.82662255076137,-29.0670859503705,56.8321444636279));
#86552=CARTESIAN_POINT('Ctrl Pts',(3.8304777570067,-29.1312871975198,56.8634437084732));
#86553=CARTESIAN_POINT('Ctrl Pts',(3.83433296325203,-29.196936351747,56.8913186773663));
#86554=CARTESIAN_POINT('Ctrl Pts',(3.83818832010328,-29.2625880705973,56.9191947352115));
#86555=CARTESIAN_POINT('Ctrl Pts',(3.84204367695452,-29.3296873608164,56.9436460636853));
#86556=CARTESIAN_POINT('Ctrl Pts',(3.84589903380577,-29.3978422093976,56.9645364740103));
#86557=CARTESIAN_POINT('Ctrl Pts',(3.84975842627433,-29.4660683994648,56.9854487514944));
#86558=CARTESIAN_POINT('Ctrl Pts',(3.85361781874289,-29.5353518881371,57.0027925274235));
#86559=CARTESIAN_POINT('Ctrl Pts',(3.85747721121144,-29.6052862753475,57.0164817475174));
#86560=CARTESIAN_POINT('Ctrl Pts',(3.86133878881488,-29.6752602584451,57.0301787182593));
#86561=CARTESIAN_POINT('Ctrl Pts',(3.86520036641832,-29.7458853925299,57.0402169457162));
#86562=CARTESIAN_POINT('Ctrl Pts',(3.86906194402176,-29.8167486103775,57.0465621150362));
#86563=CARTESIAN_POINT('Ctrl Pts',(3.87293027813663,-29.8877358159293,57.0529183863495));
#86564=CARTESIAN_POINT('Ctrl Pts',(3.8767986122515,-29.958961451333,57.0555686805711));
#86565=CARTESIAN_POINT('Ctrl Pts',(3.88066694636637,-30.0300115980961,57.0545308141957));
#86566=CARTESIAN_POINT('Ctrl Pts',(3.88296466553733,-30.0722140758214,57.0539143406966));
#86567=CARTESIAN_POINT('Ctrl Pts',(3.88526238470828,-30.1143546997391,57.0519976298562));
#86568=CARTESIAN_POINT('Ctrl Pts',(3.88756010387923,-30.1563480122918,57.0487930255525));
#86569=CARTESIAN_POINT('Ctrl Pts',(3.89142879126951,-30.2270524747003,57.0433974087089));
#86570=CARTESIAN_POINT('Ctrl Pts',(3.89529747865978,-30.297615780284,57.0343268801616));
#86571=CARTESIAN_POINT('Ctrl Pts',(3.89916616605005,-30.3676255066587,57.0215956691074));
#86572=CARTESIAN_POINT('Ctrl Pts',(3.90302937622956,-30.4375361146533,57.008882482649));
#86573=CARTESIAN_POINT('Ctrl Pts',(3.90689258640907,-30.5068942246873,56.9925189834919));
#86574=CARTESIAN_POINT('Ctrl Pts',(3.91075579658857,-30.5752914454823,56.9725712446588));
#86575=CARTESIAN_POINT('Ctrl Pts',(3.91461452942219,-30.6436093959294,56.9526466246627));
#86576=CARTESIAN_POINT('Ctrl Pts',(3.91847326225581,-30.7109682049742,56.9291461509408));
#86577=CARTESIAN_POINT('Ctrl Pts',(3.92233199508943,-30.7769704028753,56.90218678251));
#86578=CARTESIAN_POINT('Ctrl Pts',(3.9261881038184,-30.8429277164369,56.8752457476118));
#86579=CARTESIAN_POINT('Ctrl Pts',(3.93004421254737,-30.9075298017762,56.8448506709041));
#86580=CARTESIAN_POINT('Ctrl Pts',(3.93390032127633,-30.9703965480012,56.8111676074089));
#86581=CARTESIAN_POINT('Ctrl Pts',(3.93775577559097,-31.0332526252066,56.7774902602151));
#86582=CARTESIAN_POINT('Ctrl Pts',(3.9416112299056,-31.0943735163416,56.7405262564677));
#86583=CARTESIAN_POINT('Ctrl Pts',(3.94546668422024,-31.1534025934277,56.7004881710774));
#86584=CARTESIAN_POINT('Ctrl Pts',(3.94765985215727,-31.1869811729291,56.6777125814913));
#86585=CARTESIAN_POINT('Ctrl Pts',(3.9498530200943,-31.2198833281314,56.6539430902286));
#86586=CARTESIAN_POINT('Ctrl Pts',(3.95204618803132,-31.2520475724682,56.6292251037768));
#86587=CARTESIAN_POINT('',(3.64592528049244,-27.9452507844795,55.001795499335));
#86588=CARTESIAN_POINT('Ctrl Pts',(3.64592528053768,-27.9452507844802,55.001795500168));
#86589=CARTESIAN_POINT('Ctrl Pts',(3.65155534725541,-27.9453413655908,55.1054554547427));
#86590=CARTESIAN_POINT('Ctrl Pts',(3.65718541397315,-27.9532796299172,55.2087840265977));
#86591=CARTESIAN_POINT('Ctrl Pts',(3.66281548069089,-27.968896452778,55.3108310521202));
#86592=CARTESIAN_POINT('Ctrl Pts',(3.66436496635141,-27.973194455679,55.3389160483864));
#86593=CARTESIAN_POINT('Ctrl Pts',(3.66591445201194,-27.9780738114728,55.3669041565418));
#86594=CARTESIAN_POINT('Ctrl Pts',(3.66746393767247,-27.9835304264076,55.3947759127352));
#86595=CARTESIAN_POINT('Ctrl Pts',(3.67133301102068,-27.9971556208533,55.4643718256261));
#86596=CARTESIAN_POINT('Ctrl Pts',(3.67520208436889,-28.0144147564084,55.5333978458128));
#86597=CARTESIAN_POINT('Ctrl Pts',(3.6790711577171,-28.0352454688278,55.6014459200446));
#86598=CARTESIAN_POINT('Ctrl Pts',(3.68293446611288,-28.0560451433073,55.6693926020628));
#86599=CARTESIAN_POINT('Ctrl Pts',(3.68679777450866,-28.0804056902296,55.7363637697989));
#86600=CARTESIAN_POINT('Ctrl Pts',(3.69066108290444,-28.1082137350863,55.8019615267479));
#86601=CARTESIAN_POINT('Ctrl Pts',(3.69451985939735,-28.1359891593636,55.8674823334168));
#86602=CARTESIAN_POINT('Ctrl Pts',(3.69837863589025,-28.1672038598827,55.9316324843949));
#86603=CARTESIAN_POINT('Ctrl Pts',(3.70223741238316,-28.201695204195,55.9940308968461));
#86604=CARTESIAN_POINT('Ctrl Pts',(3.70609375797136,-28.236164820073,56.0563900003104));
#86605=CARTESIAN_POINT('Ctrl Pts',(3.70995010355956,-28.2739067499908,56.1169991304989));
#86606=CARTESIAN_POINT('Ctrl Pts',(3.71380644914776,-28.3147115970108,56.1755001323905));
#86607=CARTESIAN_POINT('Ctrl Pts',(3.71766165539308,-28.3555043883915,56.23398385038));
#86608=CARTESIAN_POINT('Ctrl Pts',(3.72151686163841,-28.3993580225816,56.2903602783593));
#86609=CARTESIAN_POINT('Ctrl Pts',(3.72537206788373,-28.4460197348827,56.3443001517987));
#86610=CARTESIAN_POINT('Ctrl Pts',(3.72922742473497,-28.4926832700512,56.3982421324311));
#86611=CARTESIAN_POINT('Ctrl Pts',(3.73308278158621,-28.5421547816376,56.4497470035929));
#86612=CARTESIAN_POINT('Ctrl Pts',(3.73693813843745,-28.5941423085746,56.4985198410298));
#86613=CARTESIAN_POINT('Ctrl Pts',(3.74079753090601,-28.6461842537591,56.5473437317192));
#86614=CARTESIAN_POINT('Ctrl Pts',(3.74465692337456,-28.7007471166513,56.5934295468804));
#86615=CARTESIAN_POINT('Ctrl Pts',(3.74851631584311,-28.7575039387394,56.6365210356888));
#86616=CARTESIAN_POINT('Ctrl Pts',(3.75237789344654,-28.8142928957587,56.6796369223049));
#86617=CARTESIAN_POINT('Ctrl Pts',(3.75623947104997,-28.8732778829159,56.719754834327));
#86618=CARTESIAN_POINT('Ctrl Pts',(3.7601010486534,-28.9341031681986,56.7566620353544));
#86619=CARTESIAN_POINT('Ctrl Pts',(3.76396938276827,-28.9950348780511,56.7936338120428));
#86620=CARTESIAN_POINT('Ctrl Pts',(3.76783771688313,-29.0578128866956,56.8273834317255));
#86621=CARTESIAN_POINT('Ctrl Pts',(3.771706050998,-29.1220577374214,56.8577445858025));
#86622=CARTESIAN_POINT('Ctrl Pts',(3.774003770169,-29.1602179947229,56.8757785517695));
#86623=CARTESIAN_POINT('Ctrl Pts',(3.77630148934001,-29.1988953899806,56.8926179419242));
#86624=CARTESIAN_POINT('Ctrl Pts',(3.77859920851102,-29.2380077640327,56.9082361999568));
#86625=CARTESIAN_POINT('Ctrl Pts',(3.78246828185923,-29.303868138068,56.9345354042555));
#86626=CARTESIAN_POINT('Ctrl Pts',(3.78633735520744,-29.3712206395652,56.957472487004));
#86627=CARTESIAN_POINT('Ctrl Pts',(3.79020642855566,-29.4396886210873,56.9768785296929));
#86628=CARTESIAN_POINT('Ctrl Pts',(3.79406973695144,-29.5080545847304,56.996255657212));
#86629=CARTESIAN_POINT('Ctrl Pts',(3.79793304534722,-29.577532265659,57.0121120567743));
#86630=CARTESIAN_POINT('Ctrl Pts',(3.80179635374301,-29.647725883426,57.0243271744686));
#86631=CARTESIAN_POINT('Ctrl Pts',(3.80565513023592,-29.7178371596801,57.0365279630643));
#86632=CARTESIAN_POINT('Ctrl Pts',(3.80951390672883,-29.7886622282982,57.0450958714596));
#86633=CARTESIAN_POINT('Ctrl Pts',(3.81337268322174,-29.8597927189909,57.0499608486144));
#86634=CARTESIAN_POINT('Ctrl Pts',(3.81722902880994,-29.9308783997692,57.0548227609906));
#86635=CARTESIAN_POINT('Ctrl Pts',(3.82108537439815,-30.0022686373837,57.0559863371499));
#86636=CARTESIAN_POINT('Ctrl Pts',(3.82494171998635,-30.0735489608221,57.0534332501598));
#86637=CARTESIAN_POINT('Ctrl Pts',(3.82879692623168,-30.1448082247557,57.0508809174698));
#86638=CARTESIAN_POINT('Ctrl Pts',(3.83265213247701,-30.2159571537724,57.0446141189907));
#86639=CARTESIAN_POINT('Ctrl Pts',(3.83650733872234,-30.2865820279039,57.0346666321003));
#86640=CARTESIAN_POINT('Ctrl Pts',(3.84036269557359,-30.357209661038,57.0247187566055));
#86641=CARTESIAN_POINT('Ctrl Pts',(3.84421805242483,-30.4273127179108,57.0110899771617));
#86642=CARTESIAN_POINT('Ctrl Pts',(3.84807340927607,-30.4964850706127,56.9938656266556));
#86643=CARTESIAN_POINT('Ctrl Pts',(3.85193280174463,-30.565729829879,56.9766232464599));
#86644=CARTESIAN_POINT('Ctrl Pts',(3.85579219421319,-30.6340414678546,56.9557778996609));
#86645=CARTESIAN_POINT('Ctrl Pts',(3.85965158668174,-30.7010273665057,56.9314652971022));
#86646=CARTESIAN_POINT('Ctrl Pts',(3.86351316428518,-30.7680511916503,56.9071389290827));
#86647=CARTESIAN_POINT('Ctrl Pts',(3.86737474188861,-30.8337473356286,56.8793415867398));
#86648=CARTESIAN_POINT('Ctrl Pts',(3.87123631949205,-30.8977441330565,56.8482567554489));
#86649=CARTESIAN_POINT('Ctrl Pts',(3.87510465360692,-30.9618529041745,56.8171175357605));
#86650=CARTESIAN_POINT('Ctrl Pts',(3.87897298772178,-31.0242559669955,56.7826795777974));
#86651=CARTESIAN_POINT('Ctrl Pts',(3.88284132183665,-31.0846077947287,56.7451714798591));
#86652=CARTESIAN_POINT('Ctrl Pts',(3.88513904100763,-31.1204556681202,56.7228923609567));
#86653=CARTESIAN_POINT('Ctrl Pts',(3.8874367601786,-31.1555804033927,56.6995308769136));
#86654=CARTESIAN_POINT('Ctrl Pts',(3.88973447934958,-31.1899151292547,56.6751416500317));
#86655=CARTESIAN_POINT('Ctrl Pts',(3.89113859517648,-31.210896776013,56.66023760958));
#86656=CARTESIAN_POINT('Ctrl Pts',(3.89254271100338,-31.2316132332841,56.6449287439375));
#86657=CARTESIAN_POINT('Ctrl Pts',(3.89394682683029,-31.2520475724682,56.6292251037768));
#86658=CARTESIAN_POINT('Ctrl Pts',(3.19386027023256,-31.2520475724682,56.6292251037768));
#86659=CARTESIAN_POINT('Ctrl Pts',(3.1977220959346,-31.3085779768709,56.5857819015827));
#86660=CARTESIAN_POINT('Ctrl Pts',(3.20158392163664,-31.3627920617531,56.5394335086125));
#86661=CARTESIAN_POINT('Ctrl Pts',(3.20544574733867,-31.4143916292804,56.490467672082));
#86662=CARTESIAN_POINT('Ctrl Pts',(3.20931422587572,-31.4660800882896,56.4414174812444));
#86663=CARTESIAN_POINT('Ctrl Pts',(3.21318270441277,-31.5151447051828,56.3897411985227));
#86664=CARTESIAN_POINT('Ctrl Pts',(3.21705118294981,-31.5613259547182,56.3357615152501));
#86665=CARTESIAN_POINT('Ctrl Pts',(3.21900840673928,-31.5846909648513,56.3084509539436));
#86666=CARTESIAN_POINT('Ctrl Pts',(3.22096563052875,-31.6073185673067,56.280551271071));
#86667=CARTESIAN_POINT('Ctrl Pts',(3.22292285431822,-31.6291794168843,56.2521070202265));
#86668=CARTESIAN_POINT('Ctrl Pts',(3.2267919276666,-31.6723943169528,56.195877940318));
#86669=CARTESIAN_POINT('Ctrl Pts',(3.23066100101498,-31.7127794322327,56.1372988340834));
#86670=CARTESIAN_POINT('Ctrl Pts',(3.23453007436335,-31.750069802935,56.076686234404));
#86671=CARTESIAN_POINT('Ctrl Pts',(3.2383933827593,-31.7873046106655,56.0161639480173));
#86672=CARTESIAN_POINT('Ctrl Pts',(3.24225669115525,-31.8214535744354,55.9536145928793));
#86673=CARTESIAN_POINT('Ctrl Pts',(3.2461199995512,-31.8522930751998,55.8893862637049));
#86674=CARTESIAN_POINT('Ctrl Pts',(3.24997877604428,-31.883096399297,55.8252332783859));
#86675=CARTESIAN_POINT('Ctrl Pts',(3.25383755253736,-31.9105977625169,55.759405667002));
#86676=CARTESIAN_POINT('Ctrl Pts',(3.25769632903044,-31.9346187232656,55.6922773707773));
#86677=CARTESIAN_POINT('Ctrl Pts',(3.26155267461882,-31.9586245515839,55.6251913632135));
#86678=CARTESIAN_POINT('Ctrl Pts',(3.2654090202072,-31.9791541641155,55.5568067527675));
#86679=CARTESIAN_POINT('Ctrl Pts',(3.26926536579557,-31.996077236238,55.4875174145326));
#86680=CARTESIAN_POINT('Ctrl Pts',(3.27312057204107,-32.0129953085021,55.4182485475735));
#86681=CARTESIAN_POINT('Ctrl Pts',(3.27697577828658,-32.0263088405503,55.3480759551444));
#86682=CARTESIAN_POINT('Ctrl Pts',(3.28083098453208,-32.0359378534985,55.2774069559185));
#86683=CARTESIAN_POINT('Ctrl Pts',(3.2846863413835,-32.0455672426098,55.2067351959663));
#86684=CARTESIAN_POINT('Ctrl Pts',(3.28854169823492,-32.0515117634489,55.135567472352));
#86685=CARTESIAN_POINT('Ctrl Pts',(3.29239705508634,-32.0537431147051,55.0643178148044));
#86686=CARTESIAN_POINT('Ctrl Pts',(3.29625644755507,-32.0559768016414,54.9929935762614));
#86687=CARTESIAN_POINT('Ctrl Pts',(3.3001158400238,-32.0544895448673,54.9215877191223));
#86688=CARTESIAN_POINT('Ctrl Pts',(3.30397523249253,-32.0493051964124,54.8505149691207));
#86689=CARTESIAN_POINT('Ctrl Pts',(3.30783681009614,-32.0441179126508,54.7794019787067));
#86690=CARTESIAN_POINT('Ctrl Pts',(3.31169838769975,-32.035229430767,54.7086229531046));
#86691=CARTESIAN_POINT('Ctrl Pts',(3.31555996530336,-32.0227152743479,54.638585443819));
#86692=CARTESIAN_POINT('Ctrl Pts',(3.31942829941841,-32.0101792222039,54.5684253915519));
#86693=CARTESIAN_POINT('Ctrl Pts',(3.32329663353345,-31.9940049403023,54.499009919188));
#86694=CARTESIAN_POINT('Ctrl Pts',(3.3271649676485,-31.9743184724179,54.4307336897642));
#86695=CARTESIAN_POINT('Ctrl Pts',(3.32946268681792,-31.9626250733238,54.390178867844));
#86696=CARTESIAN_POINT('Ctrl Pts',(3.33176040598735,-31.9496934720379,54.3500256656002));
#86697=CARTESIAN_POINT('Ctrl Pts',(3.33405812515678,-31.9355580520016,54.310353286217));
#86698=CARTESIAN_POINT('Ctrl Pts',(3.33792719850496,-31.9117557624724,54.2435499327991));
#86699=CARTESIAN_POINT('Ctrl Pts',(3.34179627185313,-31.8844443398247,54.1778494349639));
#86700=CARTESIAN_POINT('Ctrl Pts',(3.3456653452013,-31.8537460124458,54.1136460730379));
#86701=CARTESIAN_POINT('Ctrl Pts',(3.34952865359705,-31.8230934258378,54.0495383746712));
#86702=CARTESIAN_POINT('Ctrl Pts',(3.3533919619928,-31.7890641595386,53.9869238189406));
#86703=CARTESIAN_POINT('Ctrl Pts',(3.35725527038854,-31.7518293801418,53.9261790720181));
#86704=CARTESIAN_POINT('Ctrl Pts',(3.36111404688141,-31.7146382794749,53.8655055824908));
#86705=CARTESIAN_POINT('Ctrl Pts',(3.36497282337429,-31.6742493875157,53.8066979570904));
#86706=CARTESIAN_POINT('Ctrl Pts',(3.36883159986716,-31.6308800882627,53.7501089246626));
#86707=CARTESIAN_POINT('Ctrl Pts',(3.37268794545532,-31.5875381102692,53.6935555414996));
#86708=CARTESIAN_POINT('Ctrl Pts',(3.37654429104349,-31.5412197448334,53.6392183630728));
#86709=CARTESIAN_POINT('Ctrl Pts',(3.38040063663165,-31.4921852201833,53.587420504479));
#86710=CARTESIAN_POINT('Ctrl Pts',(3.38425584287695,-31.4431651826,53.5356379493686));
#86711=CARTESIAN_POINT('Ctrl Pts',(3.38811104912224,-31.3914309127271,53.4863935772636));
#86712=CARTESIAN_POINT('Ctrl Pts',(3.39196625536753,-31.3372812390496,53.4399754969277));
#86713=CARTESIAN_POINT('Ctrl Pts',(3.39582161221873,-31.2831294499831,53.3935556032421));
#86714=CARTESIAN_POINT('Ctrl Pts',(3.39967696906994,-31.2265624400304,53.3499625350207));
#86715=CARTESIAN_POINT('Ctrl Pts',(3.40353232592114,-31.1679127039866,53.3094446242827));
#86716=CARTESIAN_POINT('Ctrl Pts',(3.40739171838966,-31.109201575989,53.2688843011849));
#86717=CARTESIAN_POINT('Ctrl Pts',(3.41125111085818,-31.0484037704212,53.231405837981));
#86718=CARTESIAN_POINT('Ctrl Pts',(3.4151105033267,-30.9858806529212,53.1972141278855));
#86719=CARTESIAN_POINT('Ctrl Pts',(3.41897208093009,-30.9233221356929,53.1630030589145));
#86720=CARTESIAN_POINT('Ctrl Pts',(3.42283365853349,-30.8590367999157,53.1320826582239));
#86721=CARTESIAN_POINT('Ctrl Pts',(3.42669523613688,-30.7934080086418,53.1046105164576));
#86722=CARTESIAN_POINT('Ctrl Pts',(3.43056357025171,-30.7276643882165,53.0770903073315));
#86723=CARTESIAN_POINT('Ctrl Pts',(3.43443190436654,-30.6605730766457,53.0530305668983));
#86724=CARTESIAN_POINT('Ctrl Pts',(3.43830023848138,-30.5925340091539,53.0325394513495));
#86725=CARTESIAN_POINT('Ctrl Pts',(3.4405979576527,-30.5521200570149,53.0203681063621));
#86726=CARTESIAN_POINT('Ctrl Pts',(3.44289567682402,-30.5113719666599,53.0094548530609));
#86727=CARTESIAN_POINT('Ctrl Pts',(3.44519339599535,-30.4703749284781,52.9998137613814));
#86728=CARTESIAN_POINT('Ctrl Pts',(3.44906246934355,-30.4013410144281,52.9835793619255));
#86729=CARTESIAN_POINT('Ctrl Pts',(3.45293154269174,-30.3313304296172,52.9708912873145));
#86730=CARTESIAN_POINT('Ctrl Pts',(3.45680061603994,-30.2607407184097,52.9618606916447));
#86731=CARTESIAN_POINT('Ctrl Pts',(3.46066392443571,-30.1902561864765,52.9528435516397));
#86732=CARTESIAN_POINT('Ctrl Pts',(3.46452723283147,-30.1191947189186,52.9474731342666));
#86733=CARTESIAN_POINT('Ctrl Pts',(3.46839054122724,-30.0479656040068,52.9458099252181));
#86734=CARTESIAN_POINT('Ctrl Pts',(3.47224931772014,-29.9768200453109,52.9441486672182));
#86735=CARTESIAN_POINT('Ctrl Pts',(3.47610809421303,-29.9055077131926,52.9461859906645));
#86736=CARTESIAN_POINT('Ctrl Pts',(3.47996687070592,-29.834442851793,52.9519305692488));
#86737=CARTESIAN_POINT('Ctrl Pts',(3.48382321629411,-29.7634227589635,52.9576715289339));
#86738=CARTESIAN_POINT('Ctrl Pts',(3.48767956188229,-29.6926503106142,52.9671150712111));
#86739=CARTESIAN_POINT('Ctrl Pts',(3.49153590747048,-29.6225381082574,52.9802178130348));
#86740=CARTESIAN_POINT('Ctrl Pts',(3.49539111371579,-29.5524466202884,52.9933166837024));
#86741=CARTESIAN_POINT('Ctrl Pts',(3.4992463199611,-29.4830154683081,53.0100725184488));
#86742=CARTESIAN_POINT('Ctrl Pts',(3.50310152620641,-29.4146487788767,53.0303905182932));
#86743=CARTESIAN_POINT('Ctrl Pts',(3.50695688305764,-29.34627941866,53.0507093118723));
#86744=CARTESIAN_POINT('Ctrl Pts',(3.51081223990887,-29.278975068581,53.0745904063289));
#86745=CARTESIAN_POINT('Ctrl Pts',(3.51466759676009,-29.2131246964214,53.1018891446709));
#86746=CARTESIAN_POINT('Ctrl Pts',(3.51852698922863,-29.1472053949999,53.1292164581269));
#86747=CARTESIAN_POINT('Ctrl Pts',(3.52238638169717,-29.0827435593446,53.1599683704247));
#86748=CARTESIAN_POINT('Ctrl Pts',(3.5262457741657,-29.0201073209133,53.1939524092726));
#86749=CARTESIAN_POINT('Ctrl Pts',(3.53010735176912,-28.9574356187063,53.2279556894153));
#86750=CARTESIAN_POINT('Ctrl Pts',(3.53396892937253,-28.896591985895,53.2651944853309));
#86751=CARTESIAN_POINT('Ctrl Pts',(3.53783050697594,-28.8379167435952,53.305432188526));
#86752=CARTESIAN_POINT('Ctrl Pts',(3.54169884109079,-28.7791388386051,53.3457402946833));
#86753=CARTESIAN_POINT('Ctrl Pts',(3.54556717520564,-28.7225372848209,53.3890574888132));
#86754=CARTESIAN_POINT('Ctrl Pts',(3.54943550932049,-28.6684198594727,53.4351064279468));
#86755=CARTESIAN_POINT('Ctrl Pts',(3.55173322849163,-28.6362751061957,53.4624586491139));
#86756=CARTESIAN_POINT('Ctrl Pts',(3.55403094766277,-28.6050061059768,53.4907739380974));
#86757=CARTESIAN_POINT('Ctrl Pts',(3.55632866683391,-28.5746708837891,53.5199883537683));
#86758=CARTESIAN_POINT('Ctrl Pts',(3.56013990426076,-28.5243537103042,53.5684464402949));
#86759=CARTESIAN_POINT('Ctrl Pts',(3.56395114168762,-28.4763982156425,53.6195819833469));
#86760=CARTESIAN_POINT('Ctrl Pts',(3.56776237911448,-28.4311089343791,53.673132114069));
#86761=CARTESIAN_POINT('Ctrl Pts',(3.57156855056509,-28.3858798525725,53.726611064841));
#86762=CARTESIAN_POINT('Ctrl Pts',(3.5753747220157,-28.3433102826234,53.7824978653988));
#86763=CARTESIAN_POINT('Ctrl Pts',(3.57918089346632,-28.3036692051413,53.8404917434904));
#86764=CARTESIAN_POINT('Ctrl Pts',(3.58298336737586,-28.264066637357,53.8984292828833));
#86765=CARTESIAN_POINT('Ctrl Pts',(3.5867858412854,-28.2273872042853,53.95846943092));
#86766=CARTESIAN_POINT('Ctrl Pts',(3.59058831519494,-28.1938594686743,54.0202786398151));
#86767=CARTESIAN_POINT('Ctrl Pts',(3.59438845464257,-28.1603523168263,54.0820499020345));
#86768=CARTESIAN_POINT('Ctrl Pts',(3.5981885940902,-28.1299932630392,54.1455876312835));
#86769=CARTESIAN_POINT('Ctrl Pts',(3.60198873353783,-28.1029663477994,54.2105312641285));
#86770=CARTESIAN_POINT('Ctrl Pts',(3.60578956781203,-28.0759344908939,54.2754867714223));
#86771=CARTESIAN_POINT('Ctrl Pts',(3.60959040208624,-28.0522361979825,54.3418482392768));
#86772=CARTESIAN_POINT('Ctrl Pts',(3.61339123636044,-28.0320078938971,54.4092338594531));
#86773=CARTESIAN_POINT('Ctrl Pts',(3.61719222217697,-28.0117787832929,54.4766221663485));
#86774=CARTESIAN_POINT('Ctrl Pts',(3.6209932079935,-27.995020070069,54.5450342228542));
#86775=CARTESIAN_POINT('Ctrl Pts',(3.62479419381004,-27.981817936286,54.6140742037604));
#86776=CARTESIAN_POINT('Ctrl Pts',(3.62859963984793,-27.968600310617,54.6831951988067));
#86777=CARTESIAN_POINT('Ctrl Pts',(3.63240508588582,-27.9589476807169,54.7529450939116));
#86778=CARTESIAN_POINT('Ctrl Pts',(3.63621053192372,-27.9528946642777,54.8229200548982));
#86779=CARTESIAN_POINT('Ctrl Pts',(3.63944878144662,-27.9477438416405,54.8824653438798));
#86780=CARTESIAN_POINT('Ctrl Pts',(3.64268703096953,-27.9451986849012,54.9421733287143));
#86781=CARTESIAN_POINT('Ctrl Pts',(3.64592528049244,-27.9452507844795,55.001795499335));
#86782=CARTESIAN_POINT('Origin',(-1.54592528053767,-30.,55.));
#86783=CARTESIAN_POINT('',(2.4939437805615,-31.2520475724682,56.6292251037768));
#86784=CARTESIAN_POINT('',(2.55206205584979,-31.2520475724682,56.6292251037768));
#86785=CARTESIAN_POINT('',(-1.54592528053767,-31.2520475724682,56.6292251037768));
#86786=CARTESIAN_POINT('',(3.00407471949931,-27.9452500948919,54.9993755336174));
#86787=CARTESIAN_POINT('Ctrl Pts',(2.55206205584979,-31.2520475724682,56.6292251037768));
#86788=CARTESIAN_POINT('Ctrl Pts',(2.55268698850536,-31.2611355765577,56.6222410391239));
#86789=CARTESIAN_POINT('Ctrl Pts',(2.55331192116094,-31.2701623751725,56.615183057574));
#86790=CARTESIAN_POINT('Ctrl Pts',(2.55393685381652,-31.279126718988,56.6080523621048));
#86791=CARTESIAN_POINT('Ctrl Pts',(2.55780592716298,-31.334626625123,56.563904911119));
#86792=CARTESIAN_POINT('Ctrl Pts',(2.56167500050945,-31.3879470171915,56.5167943495909));
#86793=CARTESIAN_POINT('Ctrl Pts',(2.56554407385591,-31.4387544190205,56.4669639682859));
#86794=CARTESIAN_POINT('Ctrl Pts',(2.56940738224991,-31.4894861173851,56.4172078346763));
#86795=CARTESIAN_POINT('Ctrl Pts',(2.5732706906439,-31.5377119139981,56.3647402628776));
#86796=CARTESIAN_POINT('Ctrl Pts',(2.5771339990379,-31.583130841571,56.3098451438879));
#86797=CARTESIAN_POINT('Ctrl Pts',(2.58099277552898,-31.6284964898948,56.2550144203138));
#86798=CARTESIAN_POINT('Ctrl Pts',(2.58485155202006,-31.6710615012904,56.1977621784434));
#86799=CARTESIAN_POINT('Ctrl Pts',(2.58871032851114,-31.7105625191579,56.1384082881603));
#86800=CARTESIAN_POINT('Ctrl Pts',(2.59256667409748,-31.7500386526582,56.0790917889138));
#86801=CARTESIAN_POINT('Ctrl Pts',(2.59642301968382,-31.7864543536427,56.0176766714479));
#86802=CARTESIAN_POINT('Ctrl Pts',(2.60027936527017,-31.8195881548854,55.9545137553229));
#86803=CARTESIAN_POINT('Ctrl Pts',(2.60413457151361,-31.8527121668703,55.8913695004457));
#86804=CARTESIAN_POINT('Ctrl Pts',(2.60798977775706,-31.8825559785433,55.8264789020223));
#86805=CARTESIAN_POINT('Ctrl Pts',(2.6118449840005,-31.9089437402716,55.7602179680708));
#86806=CARTESIAN_POINT('Ctrl Pts',(2.61570034084984,-31.9353325328533,55.6939544455971));
#86807=CARTESIAN_POINT('Ctrl Pts',(2.61955569769918,-31.9582648297553,55.626320933442));
#86808=CARTESIAN_POINT('Ctrl Pts',(2.62341105454852,-31.977613315118,55.5577124154687));
#86809=CARTESIAN_POINT('Ctrl Pts',(2.62727044701515,-31.9969820536207,55.4890320811287));
#86810=CARTESIAN_POINT('Ctrl Pts',(2.63112983948178,-32.0127593598703,55.4193751721447));
#86811=CARTESIAN_POINT('Ctrl Pts',(2.63498923194841,-32.0248683641302,55.3491499254542));
#86812=CARTESIAN_POINT('Ctrl Pts',(2.6388508095499,-32.0369842243416,55.2788849181961));
#86813=CARTESIAN_POINT('Ctrl Pts',(2.64271238715139,-32.0454275904864,55.2080514152564));
#86814=CARTESIAN_POINT('Ctrl Pts',(2.64657396475289,-32.0501734694218,55.1370631525213));
#86815=CARTESIAN_POINT('Ctrl Pts',(2.65044229886581,-32.0549276521099,55.0659506832939));
#86816=CARTESIAN_POINT('Ctrl Pts',(2.65431063297874,-32.0559714241148,54.9946833995398));
#86817=CARTESIAN_POINT('Ctrl Pts',(2.65817896709166,-32.053331929582,54.923674712847));
#86818=CARTESIAN_POINT('Ctrl Pts',(2.66047668627947,-32.051764118463,54.8814968613088));
#86819=CARTESIAN_POINT('Ctrl Pts',(2.66277440546727,-32.0488977950453,54.8394101629232));
#86820=CARTESIAN_POINT('Ctrl Pts',(2.66507212465508,-32.04474722679,54.7974997752229));
#86821=CARTESIAN_POINT('Ctrl Pts',(2.66894119800453,-32.0377581860459,54.726927894648));
#86822=CARTESIAN_POINT('Ctrl Pts',(2.67281027135398,-32.027097616907,54.6565800340403));
#86823=CARTESIAN_POINT('Ctrl Pts',(2.67667934470343,-32.012789053044,54.5868683134323));
#86824=CARTESIAN_POINT('Ctrl Pts',(2.68054265310047,-31.9985018090636,54.5172604638848));
#86825=CARTESIAN_POINT('Ctrl Pts',(2.68440596149751,-31.9805774566371,54.4482873448619));
#86826=CARTESIAN_POINT('Ctrl Pts',(2.68826926989455,-31.9590912711106,54.3803557843743));
#86827=CARTESIAN_POINT('Ctrl Pts',(2.69212804638873,-31.9376302902261,54.3125039118642));
#86828=CARTESIAN_POINT('Ctrl Pts',(2.69598682288292,-31.9126159214519,54.2456916318767));
#86829=CARTESIAN_POINT('Ctrl Pts',(2.69984559937711,-31.8841740662498,54.1803136877001));
#86830=CARTESIAN_POINT('Ctrl Pts',(2.7037019449666,-31.8557501284988,54.1149769295191));
#86831=CARTESIAN_POINT('Ctrl Pts',(2.70755829055609,-31.8239031814823,54.0510731588554));
#86832=CARTESIAN_POINT('Ctrl Pts',(2.71141463614558,-31.7888078481252,53.9889787119028));
#86833=CARTESIAN_POINT('Ctrl Pts',(2.71526984239221,-31.753722883553,53.9269026105221));
#86834=CARTESIAN_POINT('Ctrl Pts',(2.71912504863884,-31.7153916768536,53.8666351942883));
#86835=CARTESIAN_POINT('Ctrl Pts',(2.72298025488547,-31.6740347542169,53.8085281353829));
#86836=CARTESIAN_POINT('Ctrl Pts',(2.72683561173802,-31.6326762159473,53.7504188064907));
#86837=CARTESIAN_POINT('Ctrl Pts',(2.73069096859058,-31.5882920105504,53.6944703969831));
#86838=CARTESIAN_POINT('Ctrl Pts',(2.73454632544313,-31.5411449296255,53.6410040955214));
#86839=CARTESIAN_POINT('Ctrl Pts',(2.738405717913,-31.493948497218,53.5874818278961));
#86840=CARTESIAN_POINT('Ctrl Pts',(2.74226511038287,-31.4439837380421,53.5364472199356));
#86841=CARTESIAN_POINT('Ctrl Pts',(2.74612450285274,-31.3915519383472,53.4881862663072));
#86842=CARTESIAN_POINT('Ctrl Pts',(2.74998608045749,-31.3390904524892,53.4398979879914));
#86843=CARTESIAN_POINT('Ctrl Pts',(2.75384765806223,-31.2841595197586,53.3943868002742));
#86844=CARTESIAN_POINT('Ctrl Pts',(2.75770923566698,-31.2270931823125,53.3518980964691));
#86845=CARTESIAN_POINT('Ctrl Pts',(2.76157756978316,-31.1699269972392,53.3093350511792));
#86846=CARTESIAN_POINT('Ctrl Pts',(2.76544590389934,-31.1106183522403,53.2698053176905));
#86847=CARTESIAN_POINT('Ctrl Pts',(2.76931423801552,-31.0495292944085,53.2335103106221));
#86848=CARTESIAN_POINT('Ctrl Pts',(2.77161195717489,-31.013243520121,53.2119517454553));
#86849=CARTESIAN_POINT('Ctrl Pts',(2.77390967633427,-30.9763300611485,53.1915335551999));
#86850=CARTESIAN_POINT('Ctrl Pts',(2.77620739549364,-30.9388682001987,53.1722899395266));
#86851=CARTESIAN_POINT('Ctrl Pts',(2.78007646884163,-30.8757870846606,53.1398860836347));
#86852=CARTESIAN_POINT('Ctrl Pts',(2.78394554218962,-30.8109028729154,53.1106883390548));
#86853=CARTESIAN_POINT('Ctrl Pts',(2.7878146155376,-30.7445745687712,53.0849004532298));
#86854=CARTESIAN_POINT('Ctrl Pts',(2.79167792393316,-30.6783450943683,53.0591509915757));
#86855=CARTESIAN_POINT('Ctrl Pts',(2.79554123232871,-30.6106762477312,53.0368014781913));
#86856=CARTESIAN_POINT('Ctrl Pts',(2.79940454072427,-30.5419506494363,53.0180093198818));
#86857=CARTESIAN_POINT('Ctrl Pts',(2.80326331721695,-30.4733056705754,52.9992392059517));
#86858=CARTESIAN_POINT('Ctrl Pts',(2.80712209370964,-30.4036068687027,52.9840182856126));
#86859=CARTESIAN_POINT('Ctrl Pts',(2.81098087020232,-30.3332541692799,52.9724548781451));
#86860=CARTESIAN_POINT('Ctrl Pts',(2.81483721579029,-30.2629457897881,52.9608987552513));
#86861=CARTESIAN_POINT('Ctrl Pts',(2.81869356137827,-30.1919848082382,52.9529956525039));
#86862=CARTESIAN_POINT('Ctrl Pts',(2.82254990696625,-30.1207821102618,52.948802972813));
#86863=CARTESIAN_POINT('Ctrl Pts',(2.82640511321135,-30.0496004488561,52.9446115318336));
#86864=CARTESIAN_POINT('Ctrl Pts',(2.83026031945645,-29.9781776974827,52.9441283661294));
#86865=CARTESIAN_POINT('Ctrl Pts',(2.83411552570155,-29.9069289167445,52.9473589364037));
#86866=CARTESIAN_POINT('Ctrl Pts',(2.83797088255257,-29.8356773526305,52.9505896328822));
#86867=CARTESIAN_POINT('Ctrl Pts',(2.84182623940359,-29.7646002578324,52.9575343291709));
#86868=CARTESIAN_POINT('Ctrl Pts',(2.84568159625461,-29.6941100056602,52.968146443795));
#86869=CARTESIAN_POINT('Ctrl Pts',(2.84954098872294,-29.6235459674045,52.9787696667122));
#86870=CARTESIAN_POINT('Ctrl Pts',(2.85340038119128,-29.5535704793747,52.9930678987881));
#86871=CARTESIAN_POINT('Ctrl Pts',(2.85725977365961,-29.484587224989,53.0109431295573));
#86872=CARTESIAN_POINT('Ctrl Pts',(2.86112135126282,-29.4155649132344,53.028828481036));
#86873=CARTESIAN_POINT('Ctrl Pts',(2.86498292886603,-29.3475364169614,53.0502947165981));
#86874=CARTESIAN_POINT('Ctrl Pts',(2.86884450646924,-29.2808890742504,53.0751942853972));
#86875=CARTESIAN_POINT('Ctrl Pts',(2.87271284058389,-29.2141251202527,53.1001374203857));
#86876=CARTESIAN_POINT('Ctrl Pts',(2.87658117469855,-29.1487475903056,53.1285256886587));
#86877=CARTESIAN_POINT('Ctrl Pts',(2.8804495088132,-29.085122062944,53.1601641587391));
#86878=CARTESIAN_POINT('Ctrl Pts',(2.8827472279862,-29.047329672272,53.1789568268887));
#86879=CARTESIAN_POINT('Ctrl Pts',(2.8850449471592,-29.010154926613,53.1988953386928));
#86880=CARTESIAN_POINT('Ctrl Pts',(2.8873426663322,-28.9736695586947,53.2199316339674));
#86881=CARTESIAN_POINT('Ctrl Pts',(2.89121173968022,-28.9122327363604,53.2553541391823));
#86882=CARTESIAN_POINT('Ctrl Pts',(2.89508081302825,-28.8525115731673,53.2940303836906));
#86883=CARTESIAN_POINT('Ctrl Pts',(2.89894988637628,-28.7948719569891,53.3357692580508));
#86884=CARTESIAN_POINT('Ctrl Pts',(2.90281319477187,-28.7373182243329,53.3774459411307));
#86885=CARTESIAN_POINT('Ctrl Pts',(2.90667650316746,-28.6818402725092,53.4221759133552));
#86886=CARTESIAN_POINT('Ctrl Pts',(2.91053981156305,-28.6287778654904,53.4697230903098));
#86887=CARTESIAN_POINT('Ctrl Pts',(2.91439858805576,-28.5757777040006,53.5172144914459));
#86888=CARTESIAN_POINT('Ctrl Pts',(2.91825736454848,-28.52518781889,53.5675162103332));
#86889=CARTESIAN_POINT('Ctrl Pts',(2.92211614104119,-28.4773161191118,53.6203510006588));
#86890=CARTESIAN_POINT('Ctrl Pts',(2.9259724866292,-28.42947457696,53.6731525067709));
#86891=CARTESIAN_POINT('Ctrl Pts',(2.9298288322172,-28.3843481482349,53.7284835592293));
#86892=CARTESIAN_POINT('Ctrl Pts',(2.9336851778052,-28.3422079092312,53.7860300883941));
#86893=CARTESIAN_POINT('Ctrl Pts',(2.93754038405033,-28.3000801204035,53.8435596156521));
#86894=CARTESIAN_POINT('Ctrl Pts',(2.94139559029546,-28.2609370566215,53.9033029284216));
#86895=CARTESIAN_POINT('Ctrl Pts',(2.94525079654059,-28.2250084196241,53.9649142779003));
#86896=CARTESIAN_POINT('Ctrl Pts',(2.94910615339164,-28.1890783790533,54.0265280342628));
#86897=CARTESIAN_POINT('Ctrl Pts',(2.95296151024268,-28.1563632573901,54.0900095514638));
#86898=CARTESIAN_POINT('Ctrl Pts',(2.95681686709372,-28.1270475759819,54.1549871126044));
#86899=CARTESIAN_POINT('Ctrl Pts',(2.96067625956207,-28.0977012082128,54.2200326893867));
#86900=CARTESIAN_POINT('Ctrl Pts',(2.96453565203042,-28.0717615842208,54.2865769924694));
#86901=CARTESIAN_POINT('Ctrl Pts',(2.96839504449877,-28.0493653045325,54.3542277124725));
#86902=CARTESIAN_POINT('Ctrl Pts',(2.97225662210199,-28.0269563443791,54.4219167353818));
#86903=CARTESIAN_POINT('Ctrl Pts',(2.97611819970521,-28.0080948507467,54.4907129535368));
#86904=CARTESIAN_POINT('Ctrl Pts',(2.97997977730844,-27.992866938006,54.5602109210647));
#86905=CARTESIAN_POINT('Ctrl Pts',(2.9838481114231,-27.9776123813449,54.6298304875504));
#86906=CARTESIAN_POINT('Ctrl Pts',(2.98771644553776,-27.9660041778331,54.7001537753637));
#86907=CARTESIAN_POINT('Ctrl Pts',(2.99158477965242,-27.9580768337136,54.7707679222213));
#86908=CARTESIAN_POINT('Ctrl Pts',(2.99388249882519,-27.9533681374033,54.8127114240737));
#86909=CARTESIAN_POINT('Ctrl Pts',(2.99618021799797,-27.9499571027309,54.8547574798927));
#86910=CARTESIAN_POINT('Ctrl Pts',(2.99847793717075,-27.9478422574973,54.8968197577716));
#86911=CARTESIAN_POINT('Ctrl Pts',(3.00034353126794,-27.9461251447923,54.9309715106293));
#86912=CARTESIAN_POINT('Ctrl Pts',(3.00220912536513,-27.945260491498,54.9651664828388));
#86913=CARTESIAN_POINT('Ctrl Pts',(3.00407471946232,-27.9452500948921,54.999375532939));
#86914=CARTESIAN_POINT('Ctrl Pts',(3.00407471949931,-27.9452500948919,54.9993755336174));
#86915=CARTESIAN_POINT('Ctrl Pts',(3.00791348792943,-27.9452287021789,55.0697663124844));
#86916=CARTESIAN_POINT('Ctrl Pts',(3.01175225635953,-27.9488287016156,55.1403032604115));
#86917=CARTESIAN_POINT('Ctrl Pts',(3.01559102478965,-27.9560689985433,55.2105792577255));
#86918=CARTESIAN_POINT('Ctrl Pts',(3.01950861575713,-27.9634579625723,55.2822982523251));
#86919=CARTESIAN_POINT('Ctrl Pts',(3.02342620672462,-27.9746384824612,55.3537449447915));
#86920=CARTESIAN_POINT('Ctrl Pts',(3.02734379769211,-27.9895745963596,55.4244846980723));
#86921=CARTESIAN_POINT('Ctrl Pts',(3.03117271153813,-28.0041726219795,55.4936232127996));
#86922=CARTESIAN_POINT('Ctrl Pts',(3.03500162538416,-28.0223579037011,55.5620859435652));
#86923=CARTESIAN_POINT('Ctrl Pts',(3.03883053923018,-28.0440446045511,55.6294728377892));
#86924=CARTESIAN_POINT('Ctrl Pts',(3.04265730106962,-28.0657191165859,55.6968218578154));
#86925=CARTESIAN_POINT('Ctrl Pts',(3.04648406290905,-28.0908909937632,55.763095771083));
#86926=CARTESIAN_POINT('Ctrl Pts',(3.05031082474849,-28.1194241368905,55.8279081987697));
#86927=CARTESIAN_POINT('Ctrl Pts',(3.05413676563533,-28.1479511588223,55.8927067222909));
#86928=CARTESIAN_POINT('Ctrl Pts',(3.05796270652218,-28.1798378159302,55.9560439306859));
#86929=CARTESIAN_POINT('Ctrl Pts',(3.06178864740903,-28.2149000053524,56.0175537192744));
#86930=CARTESIAN_POINT('Ctrl Pts',(3.06577402745905,-28.2514233480716,56.0816268169964));
#86931=CARTESIAN_POINT('Ctrl Pts',(3.06975940750908,-28.2913924556521,56.1437163194019));
#86932=CARTESIAN_POINT('Ctrl Pts',(3.0737447875591,-28.3345476417928,56.2034392402785));
#86933=CARTESIAN_POINT('Ctrl Pts',(3.07757550004275,-28.3760280296626,56.2608443900235));
#86934=CARTESIAN_POINT('Ctrl Pts',(3.08140621252639,-28.4204513813226,56.3160629059914));
#86935=CARTESIAN_POINT('Ctrl Pts',(3.08523692501004,-28.467545737203,56.3687883309465));
#86936=CARTESIAN_POINT('Ctrl Pts',(3.0890702692227,-28.514672447269,56.421549978675));
#86937=CARTESIAN_POINT('Ctrl Pts',(3.09290361343535,-28.5644734622282,56.4718147802386));
#86938=CARTESIAN_POINT('Ctrl Pts',(3.09673695764801,-28.6166409204184,56.5193140621475));
#86939=CARTESIAN_POINT('Ctrl Pts',(3.10057644985478,-28.6688920458213,56.5668895243547));
#86940=CARTESIAN_POINT('Ctrl Pts',(3.10441594206155,-28.7235167987091,56.6116903146885));
#86941=CARTESIAN_POINT('Ctrl Pts',(3.10825543426832,-28.78017627537,56.6534895352949));
#86942=CARTESIAN_POINT('Ctrl Pts',(3.10870802551532,-28.7868551750304,56.6584167392997));
#86943=CARTESIAN_POINT('Ctrl Pts',(3.10916061676232,-28.793562318163,56.6633022876481));
#86944=CARTESIAN_POINT('Ctrl Pts',(3.10961320800932,-28.8002971269466,56.668145850604));
#86945=CARTESIAN_POINT('Ctrl Pts',(3.11348228135749,-28.8578710843358,56.7095520873956));
#86946=CARTESIAN_POINT('Ctrl Pts',(3.11735135470566,-28.9177039567794,56.7480552898337));
#86947=CARTESIAN_POINT('Ctrl Pts',(3.12122042805384,-28.9794709514127,56.783400690672));
#86948=CARTESIAN_POINT('Ctrl Pts',(3.12508373644957,-29.0411459126947,56.8186934265603));
#86949=CARTESIAN_POINT('Ctrl Pts',(3.12894704484531,-29.1047488575599,56.8508374611335));
#86950=CARTESIAN_POINT('Ctrl Pts',(3.13281035324104,-29.1699247609691,56.879620349977));
#86951=CARTESIAN_POINT('Ctrl Pts',(3.13666912973391,-29.2350242089589,56.9083694746881));
#86952=CARTESIAN_POINT('Ctrl Pts',(3.14052790622678,-29.3016925081184,56.9337650901779));
#86953=CARTESIAN_POINT('Ctrl Pts',(3.14438668271965,-29.3695502355939,56.9556407280123));
#86954=CARTESIAN_POINT('Ctrl Pts',(3.14824302830782,-29.4373652148903,56.9775025849005));
#86955=CARTESIAN_POINT('Ctrl Pts',(3.15209937389599,-29.5063676746395,56.9958487148634));
#86956=CARTESIAN_POINT('Ctrl Pts',(3.15595571948416,-29.5761597972383,57.0105613755921));
#86957=CARTESIAN_POINT('Ctrl Pts',(3.15981092572945,-29.6459313000157,57.0252696895203));
#86958=CARTESIAN_POINT('Ctrl Pts',(3.16366613197474,-29.7164915273919,57.0363465652489));
#86959=CARTESIAN_POINT('Ctrl Pts',(3.16752133822003,-29.7874308248523,57.0437250079884));
#86960=CARTESIAN_POINT('Ctrl Pts',(3.17137669507123,-29.8583728935984,57.0511037389711));
#86961=CARTESIAN_POINT('Ctrl Pts',(3.17523205192243,-29.9296935784217,57.0547837020508));
#86962=CARTESIAN_POINT('Ctrl Pts',(3.17908740877364,-30.0009781593421,57.0547497671747));
#86963=CARTESIAN_POINT('Ctrl Pts',(3.18294680124216,-30.0723373578141,57.054715796777));
#86964=CARTESIAN_POINT('Ctrl Pts',(3.18680619371068,-30.1436598901606,57.0509601682432));
#86965=CARTESIAN_POINT('Ctrl Pts',(3.1906655861792,-30.2145319980673,57.0435199006384));
#86966=CARTESIAN_POINT('Ctrl Pts',(3.19452716378259,-30.2854442327858,57.0360754204565));
#86967=CARTESIAN_POINT('Ctrl Pts',(3.19838874138599,-30.3559050553296,57.0249422240914));
#86968=CARTESIAN_POINT('Ctrl Pts',(3.20225031898938,-30.4255095200008,57.0102087480878));
#86969=CARTESIAN_POINT('Ctrl Pts',(3.20611865310422,-30.4952357699654,56.9954494932681));
#86970=CARTESIAN_POINT('Ctrl Pts',(3.20998698721905,-30.5641022010401,56.9770775072827));
#86971=CARTESIAN_POINT('Ctrl Pts',(3.21385532133388,-30.6317183549069,56.9552313117822));
#86972=CARTESIAN_POINT('Ctrl Pts',(3.21615304050521,-30.6718811041471,56.9422550742774));
#86973=CARTESIAN_POINT('Ctrl Pts',(3.21845075967654,-30.7116030891717,56.9280540225237));
#86974=CARTESIAN_POINT('Ctrl Pts',(3.22074847884787,-30.7508062394283,56.9126650395026));
#86975=CARTESIAN_POINT('Ctrl Pts',(3.22461723638002,-30.8168140809136,56.8867540209945));
#86976=CARTESIAN_POINT('Ctrl Pts',(3.22848599391216,-30.8816083095328,56.8573712555002));
#86977=CARTESIAN_POINT('Ctrl Pts',(3.23235475144431,-30.9447988231827,56.8246514040256));
#86978=CARTESIAN_POINT('Ctrl Pts',(3.23621738593945,-31.0078893259504,56.7919833378748));
#86979=CARTESIAN_POINT('Ctrl Pts',(3.24008002043459,-31.069380726473,56.755988895384));
#86980=CARTESIAN_POINT('Ctrl Pts',(3.24394265492973,-31.1289021786639,56.7168510225142));
#86981=CARTESIAN_POINT('Ctrl Pts',(3.24667302071913,-31.1709758817289,56.6891857828214));
#86982=CARTESIAN_POINT('Ctrl Pts',(3.24940338650853,-31.2120656351482,56.6599509300902));
#86983=CARTESIAN_POINT('Ctrl Pts',(3.25213375229793,-31.2520475724682,56.6292251037768));
#86984=CARTESIAN_POINT('',(2.94592528057331,-27.9452500017688,55.0000852584629));
#86985=CARTESIAN_POINT('Ctrl Pts',(2.94592528057331,-27.9452500017688,55.0000852584629));
#86986=CARTESIAN_POINT('Ctrl Pts',(2.94997591064045,-27.9452531186631,55.075203179736));
#86987=CARTESIAN_POINT('Ctrl Pts',(2.95402654070758,-27.9493797866683,55.1502363805526));
#86988=CARTESIAN_POINT('Ctrl Pts',(2.95807717077472,-27.9575765752355,55.2247312093882));
#86989=CARTESIAN_POINT('Ctrl Pts',(2.96213971867074,-27.9657974805257,55.2994452181063));
#86990=CARTESIAN_POINT('Ctrl Pts',(2.96620226656675,-27.9781123929304,55.3736172816542));
#86991=CARTESIAN_POINT('Ctrl Pts',(2.97026481446277,-27.9944163846147,55.4468018847295));
#86992=CARTESIAN_POINT('Ctrl Pts',(2.97433371205507,-28.0107458591727,55.5201008741491));
#86993=CARTESIAN_POINT('Ctrl Pts',(2.97840260964737,-28.0310767338397,55.5924089327701));
#86994=CARTESIAN_POINT('Ctrl Pts',(2.98247150723968,-28.0552544358868,55.6632965048618));
#86995=CARTESIAN_POINT('Ctrl Pts',(2.98655160384029,-28.0794986833015,55.7343791839796));
#86996=CARTESIAN_POINT('Ctrl Pts',(2.99063170044091,-28.1076107675264,55.804033182481));
#86997=CARTESIAN_POINT('Ctrl Pts',(2.99471179704152,-28.13938810136,55.8718491412735));
#86998=CARTESIAN_POINT('Ctrl Pts',(2.99669196890805,-28.1548104279885,55.9047619045846));
#86999=CARTESIAN_POINT('Ctrl Pts',(2.99867214077457,-28.1710953858869,55.9372421261635));
#87000=CARTESIAN_POINT('Ctrl Pts',(3.0006523126411,-28.1882160943968,55.9692453981822));
#87001=CARTESIAN_POINT('Ctrl Pts',(3.00452138598909,-28.2216683810969,56.0317768425021));
#87002=CARTESIAN_POINT('Ctrl Pts',(3.00839045933707,-28.2584272837304,56.0926968909224));
#87003=CARTESIAN_POINT('Ctrl Pts',(3.01225953268506,-28.2983134164957,56.1516337673156));
#87004=CARTESIAN_POINT('Ctrl Pts',(3.01612284108062,-28.3381401185816,56.2104828272582));
#87005=CARTESIAN_POINT('Ctrl Pts',(3.01998614947617,-28.3810845315726,56.2673541816168));
#87006=CARTESIAN_POINT('Ctrl Pts',(3.02384945787173,-28.4269214872472,56.3219007357647));
#87007=CARTESIAN_POINT('Ctrl Pts',(3.02770823436442,-28.4727046733,56.3763833033861));
#87008=CARTESIAN_POINT('Ctrl Pts',(3.0315670108571,-28.5213733511166,56.4285461177086));
#87009=CARTESIAN_POINT('Ctrl Pts',(3.03542578734979,-28.5726601990824,56.4780726150012));
#87010=CARTESIAN_POINT('Ctrl Pts',(3.03928213293776,-28.6239147379885,56.5275679121983));
#87011=CARTESIAN_POINT('Ctrl Pts',(3.04313847852574,-28.6777838261136,56.5744298507));
#87012=CARTESIAN_POINT('Ctrl Pts',(3.04699482411372,-28.7339621666515,56.6183775106663));
#87013=CARTESIAN_POINT('Ctrl Pts',(3.05085003035882,-28.790123909509,56.6623121864608));
#87014=CARTESIAN_POINT('Ctrl Pts',(3.05470523660392,-28.8485931678945,56.7033339939136));
#87015=CARTESIAN_POINT('Ctrl Pts',(3.05856044284903,-28.9090316670453,56.7412023601495));
#87016=CARTESIAN_POINT('Ctrl Pts',(3.06241579970005,-28.9694725272619,56.7790722057355));
#87017=CARTESIAN_POINT('Ctrl Pts',(3.06627115655107,-29.0318823681512,56.8137881094636));
#87018=CARTESIAN_POINT('Ctrl Pts',(3.07012651340209,-29.0958955242342,56.8451538308229));
#87019=CARTESIAN_POINT('Ctrl Pts',(3.07398590587042,-29.1599756864626,56.8765523844343));
#87020=CARTESIAN_POINT('Ctrl Pts',(3.07784529833876,-29.2256620769808,56.904593541083));
#87021=CARTESIAN_POINT('Ctrl Pts',(3.08170469080709,-29.2925669254098,56.9291283024921));
#87022=CARTESIAN_POINT('Ctrl Pts',(3.08556626841031,-29.3595096544428,56.9536769551452));
#87023=CARTESIAN_POINT('Ctrl Pts',(3.08942784601352,-29.4276717503139,56.9747151171569));
#87024=CARTESIAN_POINT('Ctrl Pts',(3.09328942361673,-29.496650708445,56.9921438334596));
#87025=CARTESIAN_POINT('Ctrl Pts',(3.09715775773139,-29.5657503574356,57.009603044377));
#87026=CARTESIAN_POINT('Ctrl Pts',(3.10102609184604,-29.6356692455197,57.0234401064427));
#87027=CARTESIAN_POINT('Ctrl Pts',(3.10489442596069,-29.7059958154604,57.0336074109752));
#87028=CARTESIAN_POINT('Ctrl Pts',(3.10719214513368,-29.747768501928,57.0396466024901));
#87029=CARTESIAN_POINT('Ctrl Pts',(3.10948986430668,-29.7896849274336,57.0443920466834));
#87030=CARTESIAN_POINT('Ctrl Pts',(3.11178758347967,-29.8316587568884,57.0478424715704));
#87031=CARTESIAN_POINT('Ctrl Pts',(3.11565566451452,-29.9023193387308,57.0536510678621));
#87032=CARTESIAN_POINT('Ctrl Pts',(3.11952374554936,-29.9734192805823,57.0558095440457));
#87033=CARTESIAN_POINT('Ctrl Pts',(3.12339182658421,-30.0445492609425,57.0542670045175));
#87034=CARTESIAN_POINT('Ctrl Pts',(3.1272546011206,-30.1155816603244,57.0527265811507));
#87035=CARTESIAN_POINT('Ctrl Pts',(3.13111737565698,-30.1866435352803,57.0474952245094));
#87036=CARTESIAN_POINT('Ctrl Pts',(3.13498015019336,-30.2573213255353,57.0385738392133));
#87037=CARTESIAN_POINT('Ctrl Pts',(3.13883891816664,-30.3279258070782,57.0296617073935));
#87038=CARTESIAN_POINT('Ctrl Pts',(3.14269768613993,-30.3981465150949,57.0170672030046));
#87039=CARTESIAN_POINT('Ctrl Pts',(3.14655645411321,-30.4675725057126,57.0008432008535));
#87040=CARTESIAN_POINT('Ctrl Pts',(3.15049843878983,-30.538495710494,56.9842693181231));
#87041=CARTESIAN_POINT('Ctrl Pts',(3.15444042346644,-30.6085889994615,56.9639075857685));
#87042=CARTESIAN_POINT('Ctrl Pts',(3.15838240814305,-30.6774235720076,56.9398698066078));
#87043=CARTESIAN_POINT('Ctrl Pts',(3.16223780659657,-30.7447461839188,56.9163600204961));
#87044=CARTESIAN_POINT('Ctrl Pts',(3.1660932050501,-30.8108643475105,56.8893342390793));
#87045=CARTESIAN_POINT('Ctrl Pts',(3.16994860350362,-30.8753928403272,56.8589472659556));
#87046=CARTESIAN_POINT('Ctrl Pts',(3.17393388129178,-30.9420951467751,56.8275366269519));
#87047=CARTESIAN_POINT('Ctrl Pts',(3.17791915907993,-31.0070982448223,56.792534472704));
#87048=CARTESIAN_POINT('Ctrl Pts',(3.18190443686809,-31.0700020867776,56.7541645010636));
#87049=CARTESIAN_POINT('Ctrl Pts',(3.18588971465625,-31.1329059287328,56.7157945294232));
#87050=CARTESIAN_POINT('Ctrl Pts',(3.1898749924444,-31.1937100444688,56.6740570672336));
#87051=CARTESIAN_POINT('Ctrl Pts',(3.19386027023256,-31.2520475724682,56.6292251037768));
#87052=CARTESIAN_POINT('Ctrl Pts',(2.4939437805615,-31.2520475724682,56.6292251037768));
#87053=CARTESIAN_POINT('Ctrl Pts',(2.4977989078397,-31.3085916391625,56.5857714022116));
#87054=CARTESIAN_POINT('Ctrl Pts',(2.5016540351179,-31.3628837135078,56.539360769282));
#87055=CARTESIAN_POINT('Ctrl Pts',(2.5055091623961,-31.4146078579625,56.490262450272));
#87056=CARTESIAN_POINT('Ctrl Pts',(2.50936473298036,-31.4663379502433,56.441158485383));
#87057=CARTESIAN_POINT('Ctrl Pts',(2.51322030356461,-31.5154991758658,56.3893665571315));
#87058=CARTESIAN_POINT('Ctrl Pts',(2.51707587414886,-31.5618119435276,56.3351932502655));
#87059=CARTESIAN_POINT('Ctrl Pts',(2.52093566056926,-31.6081753514347,56.2809607081241));
#87060=CARTESIAN_POINT('Ctrl Pts',(2.52479544698966,-31.6516837706464,56.2243419617214));
#87061=CARTESIAN_POINT('Ctrl Pts',(2.52865523341006,-31.6920980780379,56.1656764803325));
#87062=CARTESIAN_POINT('Ctrl Pts',(2.53251746798286,-31.7325380190715,56.1069737891027));
#87063=CARTESIAN_POINT('Ctrl Pts',(2.53637970255566,-31.7698796889665,56.0462221933922));
#87064=CARTESIAN_POINT('Ctrl Pts',(2.54024193712846,-31.8039289149859,55.9837875950518));
#87065=CARTESIAN_POINT('Ctrl Pts',(2.54411066551593,-31.838035390082,55.9212480215467));
#87066=CARTESIAN_POINT('Ctrl Pts',(2.5479793939034,-31.8688381659839,55.8570202365651));
#87067=CARTESIAN_POINT('Ctrl Pts',(2.55184812229087,-31.8961907114886,55.7914912179957));
#87068=CARTESIAN_POINT('Ctrl Pts',(2.5532691579562,-31.9062376671823,55.7674215332891));
#87069=CARTESIAN_POINT('Ctrl Pts',(2.55469019362154,-31.9158196056307,55.7431764396063));
#87070=CARTESIAN_POINT('Ctrl Pts',(2.55611122928687,-31.9249309694336,55.718775573747));
#87071=CARTESIAN_POINT('Ctrl Pts',(2.55998030264425,-31.9497386050189,55.6523390005514));
#87072=CARTESIAN_POINT('Ctrl Pts',(2.56384937600163,-31.9711513322486,55.5844864813544));
#87073=CARTESIAN_POINT('Ctrl Pts',(2.56771844935902,-31.9890087674208,55.5155983762805));
#87074=CARTESIAN_POINT('Ctrl Pts',(2.57158175776409,-32.0068395948623,55.4468129150708));
#87075=CARTESIAN_POINT('Ctrl Pts',(2.57544506616916,-32.021125524562,55.3769953972711));
#87076=CARTESIAN_POINT('Ctrl Pts',(2.57930837457424,-32.0317549564942,55.3065442207271));
#87077=CARTESIAN_POINT('Ctrl Pts',(2.58316715107659,-32.0423719194371,55.2361756878255));
#87078=CARTESIAN_POINT('Ctrl Pts',(2.58702592757895,-32.0493408324931,55.1651754506854));
#87079=CARTESIAN_POINT('Ctrl Pts',(2.5908847040813,-32.05260086952,55.0939533551597));
#87080=CARTESIAN_POINT('Ctrl Pts',(2.59474104967903,-32.0558588528288,55.0227761272549));
#87081=CARTESIAN_POINT('Ctrl Pts',(2.59859739527676,-32.0554125734715,54.951377802384));
#87082=CARTESIAN_POINT('Ctrl Pts',(2.6024537408745,-32.0512530538119,54.8801731594036));
#87083=CARTESIAN_POINT('Ctrl Pts',(2.60630894712943,-32.0470947630668,54.8089895535672));
#87084=CARTESIAN_POINT('Ctrl Pts',(2.61016415338436,-32.039225438307,54.7380000007136));
#87085=CARTESIAN_POINT('Ctrl Pts',(2.61401935963929,-32.0276881760292,54.6676173541059));
#87086=CARTESIAN_POINT('Ctrl Pts',(2.61787471650019,-32.0161504630412,54.5972319579573));
#87087=CARTESIAN_POINT('Ctrl Pts',(2.62173007336109,-32.000944608807,54.5274539941576));
#87088=CARTESIAN_POINT('Ctrl Pts',(2.625585430222,-31.9821650810571,54.458687563474));
#87089=CARTESIAN_POINT('Ctrl Pts',(2.62944482270023,-31.9633658957268,54.389849151127));
#87090=CARTESIAN_POINT('Ctrl Pts',(2.63330421517847,-31.9409856977157,54.3220248551406));
#87091=CARTESIAN_POINT('Ctrl Pts',(2.63716360765671,-31.9151690153129,54.2556041340218));
#87092=CARTESIAN_POINT('Ctrl Pts',(2.64102518526984,-31.8893377158598,54.189145806405));
#87093=CARTESIAN_POINT('Ctrl Pts',(2.64488676288298,-31.8600662581771,54.1240930788425));
#87094=CARTESIAN_POINT('Ctrl Pts',(2.64874834049612,-31.8275464605445,54.0608133853961));
#87095=CARTESIAN_POINT('Ctrl Pts',(2.65261667462063,-31.7949697637881,53.9974229729609));
#87096=CARTESIAN_POINT('Ctrl Pts',(2.65648500874514,-31.7591336240462,53.9358122083976));
#87097=CARTESIAN_POINT('Ctrl Pts',(2.66035334286965,-31.7202743717362,53.8763213767061));
#87098=CARTESIAN_POINT('Ctrl Pts',(2.66265106195491,-31.6971926929572,53.8409849205015));
#87099=CARTESIAN_POINT('Ctrl Pts',(2.66494878104017,-31.6730452280721,53.8063958214799));
#87100=CARTESIAN_POINT('Ctrl Pts',(2.66724650012543,-31.6478880931675,53.7726197024162));
#87101=CARTESIAN_POINT('Ctrl Pts',(2.67111557347257,-31.6055266048661,53.7157449160781));
#87102=CARTESIAN_POINT('Ctrl Pts',(2.67498464681972,-31.5601342423003,53.6609543818503));
#87103=CARTESIAN_POINT('Ctrl Pts',(2.67885372016687,-31.511943576216,53.6085891387375));
#87104=CARTESIAN_POINT('Ctrl Pts',(2.68271702856159,-31.4638247146368,53.5563019202854));
#87105=CARTESIAN_POINT('Ctrl Pts',(2.68658033695631,-31.4129161521506,53.5064331743893));
#87106=CARTESIAN_POINT('Ctrl Pts',(2.69044364535103,-31.3594920722925,53.4592927377747));
#87107=CARTESIAN_POINT('Ctrl Pts',(2.69430242184289,-31.3061306622283,53.4122075998466));
#87108=CARTESIAN_POINT('Ctrl Pts',(2.69816119833475,-31.2502599586848,53.367844733821));
#87109=CARTESIAN_POINT('Ctrl Pts',(2.70201997482661,-31.1921913010982,53.3264775280607));
#87110=CARTESIAN_POINT('Ctrl Pts',(2.70587632041377,-31.1341592248924,53.2851363823054));
#87111=CARTESIAN_POINT('Ctrl Pts',(2.70973266600094,-31.0739323364675,53.2467874338947));
#87112=CARTESIAN_POINT('Ctrl Pts',(2.7135890115881,-31.0118542404584,53.2116631864868));
#87113=CARTESIAN_POINT('Ctrl Pts',(2.7174442178324,-30.9497944851904,53.1765493164064));
#87114=CARTESIAN_POINT('Ctrl Pts',(2.72129942407669,-30.8858850307203,53.1446584949976));
#87115=CARTESIAN_POINT('Ctrl Pts',(2.72515463032099,-30.8204961070475,53.1161784317988));
#87116=CARTESIAN_POINT('Ctrl Pts',(2.72900998717122,-30.7551046289172,53.0876972560093));
#87117=CARTESIAN_POINT('Ctrl Pts',(2.73286534402146,-30.6882340130916,53.0626272949301));
#87118=CARTESIAN_POINT('Ctrl Pts',(2.73672070087169,-30.6202749981291,53.0411083518489));
#87119=CARTESIAN_POINT('Ctrl Pts',(2.74058009333926,-30.5522448466702,53.0195668836883));
#87120=CARTESIAN_POINT('Ctrl Pts',(2.74443948580683,-30.4831244858713,53.0015840005369));
#87121=CARTESIAN_POINT('Ctrl Pts',(2.7482988782744,-30.4133195037398,52.987249506191));
#87122=CARTESIAN_POINT('Ctrl Pts',(2.75216045587686,-30.3434749989882,52.9729068958518));
#87123=CARTESIAN_POINT('Ctrl Pts',(2.75602203347932,-30.2729455817938,52.9622168592576));
#87124=CARTESIAN_POINT('Ctrl Pts',(2.75988361108177,-30.2021439848606,52.9552175245556));
#87125=CARTESIAN_POINT('Ctrl Pts',(2.7637519451957,-30.1312185080393,52.9482059432823));
#87126=CARTESIAN_POINT('Ctrl Pts',(2.76762027930962,-30.0600203860959,52.9448979791087));
#87127=CARTESIAN_POINT('Ctrl Pts',(2.77148861342355,-29.9889636844098,52.9452796389196));
#87128=CARTESIAN_POINT('Ctrl Pts',(2.7737863326037,-29.9467573130019,52.9455063378143));
#87129=CARTESIAN_POINT('Ctrl Pts',(2.77608405178384,-29.9046007848128,52.9470337898437));
#87130=CARTESIAN_POINT('Ctrl Pts',(2.77838177096399,-29.8625796677549,52.9498504408737));
#87131=CARTESIAN_POINT('Ctrl Pts',(2.78225084431046,-29.7918213325315,52.9545933309191));
#87132=CARTESIAN_POINT('Ctrl Pts',(2.78611991765693,-29.7211702309432,52.9630130139421));
#87133=CARTESIAN_POINT('Ctrl Pts',(2.7899889910034,-29.6510390227326,52.9750990644368));
#87134=CARTESIAN_POINT('Ctrl Pts',(2.79385229939739,-29.5810123106239,52.9871671066127));
#87135=CARTESIAN_POINT('Ctrl Pts',(2.79771560779139,-29.5115044290717,53.0028905906901));
#87136=CARTESIAN_POINT('Ctrl Pts',(2.80157891618538,-29.4429243927077,53.0222072074507));
#87137=CARTESIAN_POINT('Ctrl Pts',(2.80543769267647,-29.3744248050251,53.0415011646091));
#87138=CARTESIAN_POINT('Ctrl Pts',(2.80929646916756,-29.3068513658813,53.0643797510297));
#87139=CARTESIAN_POINT('Ctrl Pts',(2.81315524565865,-29.2406026200768,53.0907296729206));
#87140=CARTESIAN_POINT('Ctrl Pts',(2.817011591245,-29.1743956088454,53.1170629952106));
#87141=CARTESIAN_POINT('Ctrl Pts',(2.82086793683135,-29.1095120856153,53.1468631352237));
#87142=CARTESIAN_POINT('Ctrl Pts',(2.8247242824177,-29.0463337456507,53.1799675173736));
#87143=CARTESIAN_POINT('Ctrl Pts',(2.82857948866115,-28.9831740714906,53.2130621189574));
#87144=CARTESIAN_POINT('Ctrl Pts',(2.83243469490461,-28.9217190104928,53.2494587992553));
#87145=CARTESIAN_POINT('Ctrl Pts',(2.83628990114806,-28.862327065072,53.2889483188307));
#87146=CARTESIAN_POINT('Ctrl Pts',(2.84014525799741,-28.8029327994699,53.3284393810874));
#87147=CARTESIAN_POINT('Ctrl Pts',(2.84400061484677,-28.745602212768,53.371023251697));
#87148=CARTESIAN_POINT('Ctrl Pts',(2.84785597169612,-28.6906646823592,53.4164474784591));
#87149=CARTESIAN_POINT('Ctrl Pts',(2.85171536416276,-28.6356696457698,53.4619192532957));
#87150=CARTESIAN_POINT('Ctrl Pts',(2.85557475662939,-28.5830730410599,53.5102370091905));
#87151=CARTESIAN_POINT('Ctrl Pts',(2.85943414909603,-28.5331702926792,53.5611087003456));
#87152=CARTESIAN_POINT('Ctrl Pts',(2.86329572669754,-28.4832392900495,53.6120091943517));
#87153=CARTESIAN_POINT('Ctrl Pts',(2.86715730429904,-28.4360055018113,53.6654661379536));
#87154=CARTESIAN_POINT('Ctrl Pts',(2.87101888190054,-28.3917248124773,53.7211534557661));
#87155=CARTESIAN_POINT('Ctrl Pts',(2.87488721601348,-28.3473666462636,53.7769382083678));
#87156=CARTESIAN_POINT('Ctrl Pts',(2.87875555012642,-28.3059721771753,53.8349607309138));
#87157=CARTESIAN_POINT('Ctrl Pts',(2.88262388423935,-28.2677542231778,53.8948655596799));
#87158=CARTESIAN_POINT('Ctrl Pts',(2.88492160342708,-28.2450534626819,53.9304479242005));
#87159=CARTESIAN_POINT('Ctrl Pts',(2.88721932261481,-28.2234725547324,53.9666938950509));
#87160=CARTESIAN_POINT('Ctrl Pts',(2.88951704180255,-28.2030482011612,54.0035253163528));
#87161=CARTESIAN_POINT('Ctrl Pts',(2.89357123056583,-28.167010644793,54.0685121673027));
#87162=CARTESIAN_POINT('Ctrl Pts',(2.89762541932912,-28.1344462576373,54.1355570099439));
#87163=CARTESIAN_POINT('Ctrl Pts',(2.90167960809241,-28.1055831555683,54.2042724197104));
#87164=CARTESIAN_POINT('Ctrl Pts',(2.9057224180279,-28.0768010631136,54.2727949670179));
#87165=CARTESIAN_POINT('Ctrl Pts',(2.9097652279634,-28.0516997313481,54.3429783611871));
#87166=CARTESIAN_POINT('Ctrl Pts',(2.9138080378989,-28.0304609873698,54.4144117144035));
#87167=CARTESIAN_POINT('Ctrl Pts',(2.91784402707854,-28.0092580759659,54.4857245500912));
#87168=CARTESIAN_POINT('Ctrl Pts',(2.92188001625818,-27.9919049146791,54.5582827532555));
#87169=CARTESIAN_POINT('Ctrl Pts',(2.92591600543781,-27.9785350595101,54.6316563332019));
#87170=CARTESIAN_POINT('Ctrl Pts',(2.92994364806252,-27.96519285363,54.7048781742343));
#87171=CARTESIAN_POINT('Ctrl Pts',(2.93397129068723,-27.9558176275774,54.7789116245549));
#87172=CARTESIAN_POINT('Ctrl Pts',(2.93799893331193,-27.9504925475353,54.8533140606889));
#87173=CARTESIAN_POINT('Ctrl Pts',(2.94064104905385,-27.9469993185879,54.9021217296069));
#87174=CARTESIAN_POINT('Ctrl Pts',(2.94328316479576,-27.9452479687193,54.9510878823304));
#87175=CARTESIAN_POINT('Ctrl Pts',(2.94592528053768,-27.9452500017688,55.0000852578022));
#87176=CARTESIAN_POINT('Origin',(-1.54592528053767,-30.,55.));
#87177=CARTESIAN_POINT('',(1.79398371971565,-31.2520475724682,56.6292251037768));
#87178=CARTESIAN_POINT('',(1.85198267751189,-31.2510897925305,56.6279533612582));
#87179=CARTESIAN_POINT('',(-1.54592528053767,-31.2520475724682,56.6292251037768));
#87180=CARTESIAN_POINT('',(2.30407472893164,-27.94525085778,55.0018775106036));
#87181=CARTESIAN_POINT('Ctrl Pts',(1.85198267751188,-31.2510897925303,56.6279533612584));
#87182=CARTESIAN_POINT('Ctrl Pts',(1.86369686126964,-31.4238148888446,56.4975418353466));
#87183=CARTESIAN_POINT('Ctrl Pts',(1.91245613530692,-32.0571540930741,55.8463606150952));
#87184=CARTESIAN_POINT('Ctrl Pts',(1.99826049962372,-32.2401039315954,54.0618361945102));
#87185=CARTESIAN_POINT('Ctrl Pts',(2.10939577046228,-30.4267596474104,52.6091647644781));
#87186=CARTESIAN_POINT('Ctrl Pts',(2.21133384374181,-28.4052057105241,53.2838821759632));
#87187=CARTESIAN_POINT('Ctrl Pts',(2.27622682674183,-27.9501900713887,54.4882110047797));
#87188=CARTESIAN_POINT('Ctrl Pts',(2.30407471946232,-27.9455375406346,55.0018770739853));
#87189=CARTESIAN_POINT('Ctrl Pts',(2.30407472893164,-27.94525085778,55.0018775106036));
#87190=CARTESIAN_POINT('Ctrl Pts',(2.30909837625683,-27.9453355391577,55.094552879717));
#87191=CARTESIAN_POINT('Ctrl Pts',(2.31412202358202,-27.951693882386,55.1869490611887));
#87192=CARTESIAN_POINT('Ctrl Pts',(2.3191456709072,-27.9641908887325,55.278350184085));
#87193=CARTESIAN_POINT('Ctrl Pts',(2.3233192179846,-27.9745731550298,55.354284433574));
#87194=CARTESIAN_POINT('Ctrl Pts',(2.327492765062,-27.9891913884281,55.4295325551457));
#87195=CARTESIAN_POINT('Ctrl Pts',(2.3316663121394,-28.0079438906639,55.5036963567039));
#87196=CARTESIAN_POINT('Ctrl Pts',(2.33553538549683,-28.0253283373804,55.5724496697427));
#87197=CARTESIAN_POINT('Ctrl Pts',(2.33940445885427,-28.0463104154775,55.6404365923651));
#87198=CARTESIAN_POINT('Ctrl Pts',(2.3432735322117,-28.070805693686,55.707253060075));
#87199=CARTESIAN_POINT('Ctrl Pts',(2.34713684061684,-28.095264473721,55.7739699706783));
#87200=CARTESIAN_POINT('Ctrl Pts',(2.35100014902197,-28.1232258972913,55.83951943575));
#87201=CARTESIAN_POINT('Ctrl Pts',(2.35486345742711,-28.1545551496884,55.9035103026299));
#87202=CARTESIAN_POINT('Ctrl Pts',(2.35872223392952,-28.1858476509101,55.9674261042151));
#87203=CARTESIAN_POINT('Ctrl Pts',(2.36258101043192,-28.2204999210114,56.0297865051127));
#87204=CARTESIAN_POINT('Ctrl Pts',(2.36643978693433,-28.2583288730812,56.0902198164395));
#87205=CARTESIAN_POINT('Ctrl Pts',(2.37029613253212,-28.2961339941324,56.1506150567312));
#87206=CARTESIAN_POINT('Ctrl Pts',(2.37415247812991,-28.3371115696483,56.2090852052227));
#87207=CARTESIAN_POINT('Ctrl Pts',(2.3780088237277,-28.3810330623122,56.2652840065273));
#87208=CARTESIAN_POINT('Ctrl Pts',(2.38186402998269,-28.4249415785363,56.3214662041075));
#87209=CARTESIAN_POINT('Ctrl Pts',(2.38571923623769,-28.4717919861991,56.3753780041934));
#87210=CARTESIAN_POINT('Ctrl Pts',(2.38957444249268,-28.5213140130926,56.4267043543158));
#87211=CARTESIAN_POINT('Ctrl Pts',(2.39342979935363,-28.5708379745941,56.4780327095331));
#87212=CARTESIAN_POINT('Ctrl Pts',(2.39728515621459,-28.6230334236482,56.5267750661973));
#87213=CARTESIAN_POINT('Ctrl Pts',(2.40114051307555,-28.6775928143398,56.5726527899744));
#87214=CARTESIAN_POINT('Ctrl Pts',(2.40499990555384,-28.7322093153926,56.6185785365271));
#87215=CARTESIAN_POINT('Ctrl Pts',(2.40885929803214,-28.7891943251104,56.6616333510855));
#87216=CARTESIAN_POINT('Ctrl Pts',(2.41271869051043,-28.848207451908,56.7015791161917));
#87217=CARTESIAN_POINT('Ctrl Pts',(2.41658026812362,-28.9072539911257,56.7415474980403));
#87218=CARTESIAN_POINT('Ctrl Pts',(2.42044184573681,-28.9683305171944,56.7784030751178));
#87219=CARTESIAN_POINT('Ctrl Pts',(2.42430342335001,-29.0310702705056,56.8119527427066));
#87220=CARTESIAN_POINT('Ctrl Pts',(2.42817175747458,-29.0939197980851,56.8455611113584));
#87221=CARTESIAN_POINT('Ctrl Pts',(2.43204009159915,-29.1584379231518,56.8758518155378));
#87222=CARTESIAN_POINT('Ctrl Pts',(2.43590842572371,-29.2242367176355,56.9026793981738));
#87223=CARTESIAN_POINT('Ctrl Pts',(2.43820614480846,-29.2633199873247,56.9186144871902));
#87224=CARTESIAN_POINT('Ctrl Pts',(2.44050386389321,-29.3028547612633,56.9333286803494));
#87225=CARTESIAN_POINT('Ctrl Pts',(2.44280158297796,-29.3427575594089,56.946799922125));
#87226=CARTESIAN_POINT('Ctrl Pts',(2.44667069995754,-29.4099496695596,56.9694840746987));
#87227=CARTESIAN_POINT('Ctrl Pts',(2.45053981693712,-29.4784491573178,56.9887299601906));
#87228=CARTESIAN_POINT('Ctrl Pts',(2.4544089339167,-29.5478707448616,57.0043893581707));
#87229=CARTESIAN_POINT('Ctrl Pts',(2.45827227321816,-29.6171886664814,57.0200253722724));
#87230=CARTESIAN_POINT('Ctrl Pts',(2.46213561251963,-29.6874254845863,57.032085423783));
#87231=CARTESIAN_POINT('Ctrl Pts',(2.4659989518211,-29.7581794462689,57.0404706276477));
#87232=CARTESIAN_POINT('Ctrl Pts',(2.46985771066891,-29.8288495206153,57.0488458898442));
#87233=CARTESIAN_POINT('Ctrl Pts',(2.47371646951672,-29.9000350404802,57.0535549025545));
#87234=CARTESIAN_POINT('Ctrl Pts',(2.47757522836452,-29.9713244395928,57.0545498958982));
#87235=CARTESIAN_POINT('Ctrl Pts',(2.48143153828646,-30.0425685955429,57.0555442577785));
#87236=CARTESIAN_POINT('Ctrl Pts',(2.4852878482084,-30.1139160153628,57.052829270212));
#87237=CARTESIAN_POINT('Ctrl Pts',(2.48914415813034,-30.1849518558916,57.046409141277));
#87238=CARTESIAN_POINT('Ctrl Pts',(2.49299931069925,-30.2559663771938,57.0399909391467));
#87239=CARTESIAN_POINT('Ctrl Pts',(2.49685446326816,-30.3266690213528,57.0298698472306));
#87240=CARTESIAN_POINT('Ctrl Pts',(2.50070961583707,-30.3966485302921,57.016102057416));
#87241=CARTESIAN_POINT('Ctrl Pts',(2.50456490098836,-30.4666304458936,57.0023337941139));
#87242=CARTESIAN_POINT('Ctrl Pts',(2.50842018613966,-30.5358887007757,56.9849186801404));
#87243=CARTESIAN_POINT('Ctrl Pts',(2.51227547129095,-30.6040224223521,56.963963970086));
#87244=CARTESIAN_POINT('Ctrl Pts',(2.51613458294686,-30.6722237690172,56.942988461753));
#87245=CARTESIAN_POINT('Ctrl Pts',(2.51999369460276,-30.7392978896813,56.9184664888671));
#87246=CARTESIAN_POINT('Ctrl Pts',(2.52385280625866,-30.8048601979397,56.8905548456135));
#87247=CARTESIAN_POINT('Ctrl Pts',(2.52771409565969,-30.8704595038312,56.8626274514693));
#87248=CARTESIAN_POINT('Ctrl Pts',(2.53157538506072,-30.934544862529,56.8313067925013));
#87249=CARTESIAN_POINT('Ctrl Pts',(2.53543667446175,-30.996755198201,56.7967962147554));
#87250=CARTESIAN_POINT('Ctrl Pts',(2.539304243646,-31.0590667092529,56.762229510953));
#87251=CARTESIAN_POINT('Ctrl Pts',(2.54317181283025,-31.1194966994414,56.7244627914467));
#87252=CARTESIAN_POINT('Ctrl Pts',(2.5470393820145,-31.1777127538234,56.683742923365));
#87253=CARTESIAN_POINT('Ctrl Pts',(2.54871360662626,-31.2029137900305,56.666115777713));
#87254=CARTESIAN_POINT('Ctrl Pts',(2.55038783123802,-31.2277003728419,56.6479357485599));
#87255=CARTESIAN_POINT('Ctrl Pts',(2.55206205584979,-31.2520475724682,56.6292251037768));
#87256=CARTESIAN_POINT('',(2.24592528056623,-27.9452508239567,54.9981598779332));
#87257=CARTESIAN_POINT('Ctrl Pts',(2.24592528056623,-27.9452508239567,54.9981598779332));
#87258=CARTESIAN_POINT('Ctrl Pts',(2.24973199312503,-27.9451880223023,55.0682865558788));
#87259=CARTESIAN_POINT('Ctrl Pts',(2.25353870568382,-27.9487194886746,55.1385255805472));
#87260=CARTESIAN_POINT('Ctrl Pts',(2.25734541824262,-27.9558530803982,55.2084728605418));
#87261=CARTESIAN_POINT('Ctrl Pts',(2.26114901960389,-27.962980841891,55.2783629731508));
#87262=CARTESIAN_POINT('Ctrl Pts',(2.26495262096516,-27.9737048438551,55.3479613175438));
#87263=CARTESIAN_POINT('Ctrl Pts',(2.26875622232642,-27.9879809101615,55.4168653794998));
#87264=CARTESIAN_POINT('Ctrl Pts',(2.27255807195645,-28.0022504016908,55.4857377080047));
#87265=CARTESIAN_POINT('Ctrl Pts',(2.27635992158647,-28.0200686123143,55.5539158983948));
#87266=CARTESIAN_POINT('Ctrl Pts',(2.2801617712165,-28.0413399868185,55.6210060509077));
#87267=CARTESIAN_POINT('Ctrl Pts',(2.28396322602616,-28.0626091523002,55.6880892361387));
#87268=CARTESIAN_POINT('Ctrl Pts',(2.28776468083582,-28.0873306169522,55.7540841309453));
#87269=CARTESIAN_POINT('Ctrl Pts',(2.29156613564548,-28.115359074996,55.8186123296774));
#87270=CARTESIAN_POINT('Ctrl Pts',(2.295371110743,-28.1434134884292,55.8832002839099));
#87271=CARTESIAN_POINT('Ctrl Pts',(2.29917608584051,-28.1747808101523,55.9463183697255));
#87272=CARTESIAN_POINT('Ctrl Pts',(2.30298106093803,-28.209268150215,56.0076095497095));
#87273=CARTESIAN_POINT('Ctrl Pts',(2.3067878558536,-28.2437719846523,56.0689300436293));
#87274=CARTESIAN_POINT('Ctrl Pts',(2.31059465076918,-28.281398538287,56.1284214698724));
#87275=CARTESIAN_POINT('Ctrl Pts',(2.31440144568475,-28.3219111830263,56.1857552381701));
#87276=CARTESIAN_POINT('Ctrl Pts',(2.31821492477245,-28.3624949620128,56.2431896761346));
#87277=CARTESIAN_POINT('Ctrl Pts',(2.32202840386014,-28.4059746382782,56.2984584996802));
#87278=CARTESIAN_POINT('Ctrl Pts',(2.32584188294784,-28.4520733984623,56.3512663685417));
#87279=CARTESIAN_POINT('Ctrl Pts',(2.32850815116848,-28.4843042450103,56.3881880191675));
#87280=CARTESIAN_POINT('Ctrl Pts',(2.33117441938912,-28.517814575004,56.4239073940283));
#87281=CARTESIAN_POINT('Ctrl Pts',(2.33384068760975,-28.5524999386103,56.458335055732));
#87282=CARTESIAN_POINT('Ctrl Pts',(2.33770976095524,-28.6028325400977,56.508293701008));
#87283=CARTESIAN_POINT('Ctrl Pts',(2.34157883430073,-28.6558531559513,56.5557413933927));
#87284=CARTESIAN_POINT('Ctrl Pts',(2.34544790764622,-28.7112811807228,56.6003753832588));
#87285=CARTESIAN_POINT('Ctrl Pts',(2.34931121603942,-28.7666266172646,56.6449428680993));
#87286=CARTESIAN_POINT('Ctrl Pts',(2.35317452443262,-28.8243719672316,56.6867046701006));
#87287=CARTESIAN_POINT('Ctrl Pts',(2.35703783282581,-28.8842001035252,56.7253950717232));
#87288=CARTESIAN_POINT('Ctrl Pts',(2.36089660931638,-28.943958057669,56.7640400870823));
#87289=CARTESIAN_POINT('Ctrl Pts',(2.36475538580694,-29.0057935391012,56.799620596212));
#87290=CARTESIAN_POINT('Ctrl Pts',(2.3686141622975,-29.0693580851263,56.8319124402602));
#87291=CARTESIAN_POINT('Ctrl Pts',(2.3724705078835,-29.1328825875402,56.8641839414896));
#87292=CARTESIAN_POINT('Ctrl Pts',(2.3763268534695,-29.1981335614045,56.8931706684583));
#87293=CARTESIAN_POINT('Ctrl Pts',(2.3801831990555,-29.264736703325,56.9186936824472));
#87294=CARTESIAN_POINT('Ctrl Pts',(2.38403840529877,-29.331320167599,56.944209155758));
#87295=CARTESIAN_POINT('Ctrl Pts',(2.38789361154204,-29.3992545534528,56.9662627739669));
#87296=CARTESIAN_POINT('Ctrl Pts',(2.39174881778531,-29.4681458743348,56.9847238476707));
#87297=CARTESIAN_POINT('Ctrl Pts',(2.39560417463466,-29.5370398864998,57.0031856425681));
#87298=CARTESIAN_POINT('Ctrl Pts',(2.399459531484,-29.6068904381121,57.0180544907098));
#87299=CARTESIAN_POINT('Ctrl Pts',(2.40331488833334,-29.6772903703766,57.0292501219535));
#87300=CARTESIAN_POINT('Ctrl Pts',(2.40717428080024,-29.747763994186,57.0404574722903));
#87301=CARTESIAN_POINT('Ctrl Pts',(2.41103367326713,-29.818787665871,57.0479838538703));
#87302=CARTESIAN_POINT('Ctrl Pts',(2.41489306573403,-29.8899469614783,57.0518006460697));
#87303=CARTESIAN_POINT('Ctrl Pts',(2.41875464333594,-29.9611465465016,57.0556195992845));
#87304=CARTESIAN_POINT('Ctrl Pts',(2.42261622093785,-30.0324814222935,57.0557247813156));
#87305=CARTESIAN_POINT('Ctrl Pts',(2.42647779853975,-30.103537767924,57.0521397352796));
#87306=CARTESIAN_POINT('Ctrl Pts',(2.43034613265333,-30.1747184391743,57.0485484165726));
#87307=CARTESIAN_POINT('Ctrl Pts',(2.43421446676691,-30.2456191238906,57.0412540285306));
#87308=CARTESIAN_POINT('Ctrl Pts',(2.43808280088049,-30.3158324179635,57.0303318561908));
#87309=CARTESIAN_POINT('Ctrl Pts',(2.44038052006976,-30.3575378209603,57.0238442870624));
#87310=CARTESIAN_POINT('Ctrl Pts',(2.44267823925904,-30.3990009022484,57.0160777639563));
#87311=CARTESIAN_POINT('Ctrl Pts',(2.44497595844831,-30.4401387559793,57.0070564112613));
#87312=CARTESIAN_POINT('Ctrl Pts',(2.44884535137329,-30.5094155069934,56.9918643205764));
#87313=CARTESIAN_POINT('Ctrl Pts',(2.45271474429828,-30.5780404718284,56.9730514624935));
#87314=CARTESIAN_POINT('Ctrl Pts',(2.45658413722326,-30.6456070065421,56.9506894052113));
#87315=CARTESIAN_POINT('Ctrl Pts',(2.46044683547002,-30.7130566401767,56.9283660379203));
#87316=CARTESIAN_POINT('Ctrl Pts',(2.46430953371679,-30.7794510248455,56.9025058240084));
#87317=CARTESIAN_POINT('Ctrl Pts',(2.46817223196355,-30.8443951085459,56.8732310223685));
#87318=CARTESIAN_POINT('Ctrl Pts',(2.4720310850811,-30.9092745435532,56.8439853623772));
#87319=CARTESIAN_POINT('Ctrl Pts',(2.47588993819866,-30.9727061011769,56.8113320565288));
#87320=CARTESIAN_POINT('Ctrl Pts',(2.47974879131621,-31.0343124383689,56.7754422948481));
#87321=CARTESIAN_POINT('Ctrl Pts',(2.48360488003591,-31.0958746421304,56.7395782438064));
#87322=CARTESIAN_POINT('Ctrl Pts',(2.48746096875562,-31.1556138035919,56.7004825855342));
#87323=CARTESIAN_POINT('Ctrl Pts',(2.49131705747533,-31.2131766480482,56.6583726912641));
#87324=CARTESIAN_POINT('Ctrl Pts',(2.49219263183739,-31.2262470295867,56.6488111001048));
#87325=CARTESIAN_POINT('Ctrl Pts',(2.49306820619944,-31.2392053155072,56.6390942842944));
#87326=CARTESIAN_POINT('Ctrl Pts',(2.4939437805615,-31.2520475724682,56.6292251037768));
#87327=CARTESIAN_POINT('Ctrl Pts',(1.79398371971565,-31.2520475724682,56.6292251037768));
#87328=CARTESIAN_POINT('Ctrl Pts',(1.79795521490481,-31.3100301074008,56.5846659498946));
#87329=CARTESIAN_POINT('Ctrl Pts',(1.80192671009397,-31.365713925972,56.5369438826613));
#87330=CARTESIAN_POINT('Ctrl Pts',(1.80589820528314,-31.4187392548253,56.4863298723089));
#87331=CARTESIAN_POINT('Ctrl Pts',(1.80975587414567,-31.4702448340343,56.4371665012244));
#87332=CARTESIAN_POINT('Ctrl Pts',(1.8136135430082,-31.5192418864264,56.3852750899823));
#87333=CARTESIAN_POINT('Ctrl Pts',(1.81747121187074,-31.565433662945,56.3309451564278));
#87334=CARTESIAN_POINT('Ctrl Pts',(1.82132695612579,-31.6116023941888,56.2766423283094));
#87335=CARTESIAN_POINT('Ctrl Pts',(1.82518270038085,-31.6549683125772,56.2199037615503));
#87336=CARTESIAN_POINT('Ctrl Pts',(1.8290384446359,-31.6952730400049,56.1610542116252));
#87337=CARTESIAN_POINT('Ctrl Pts',(1.83289355506024,-31.735571141896,56.1022143357474));
#87338=CARTESIAN_POINT('Ctrl Pts',(1.83674866548457,-31.7728087781897,56.0412645668965));
#87339=CARTESIAN_POINT('Ctrl Pts',(1.84060377590891,-31.8067702540875,55.9785595594773));
#87340=CARTESIAN_POINT('Ctrl Pts',(1.84466176160446,-31.8425189534045,55.912554699658));
#87341=CARTESIAN_POINT('Ctrl Pts',(1.84871974730001,-31.874636879848,55.8446052843981));
#87342=CARTESIAN_POINT('Ctrl Pts',(1.85277773299556,-31.902927962765,55.7751533596825));
#87343=CARTESIAN_POINT('Ctrl Pts',(1.85663795119261,-31.929840268841,55.7090862013134));
#87344=CARTESIAN_POINT('Ctrl Pts',(1.86049816938967,-31.953289919347,55.6416600649415));
#87345=CARTESIAN_POINT('Ctrl Pts',(1.86435838758672,-31.9731588391813,55.5732728476571));
#87346=CARTESIAN_POINT('Ctrl Pts',(1.8682213057675,-31.9930416560953,55.5048377977465));
#87347=CARTESIAN_POINT('Ctrl Pts',(1.87208422394829,-32.0093386495623,55.4354408020274));
#87348=CARTESIAN_POINT('Ctrl Pts',(1.87594714212907,-32.021982778969,55.3654903610944));
#87349=CARTESIAN_POINT('Ctrl Pts',(1.8798163155915,-32.034647383205,55.2954266483577));
#87350=CARTESIAN_POINT('Ctrl Pts',(1.88368548905393,-32.0436472670316,55.2248081835591));
#87351=CARTESIAN_POINT('Ctrl Pts',(1.88755466251637,-32.0489672479301,55.1540479776236));
#87352=CARTESIAN_POINT('Ctrl Pts',(1.88813630976275,-32.0497669929584,55.1434106982834));
#87353=CARTESIAN_POINT('Ctrl Pts',(1.88871795700913,-32.0504836729769,55.132770212495));
#87354=CARTESIAN_POINT('Ctrl Pts',(1.88929960425551,-32.0511173379966,55.1221279176511));
#87355=CARTESIAN_POINT('Ctrl Pts',(1.89316867807618,-32.0553324301403,55.05133617123));
#87356=CARTESIAN_POINT('Ctrl Pts',(1.89703775189685,-32.0558865433756,54.9801872886027));
#87357=CARTESIAN_POINT('Ctrl Pts',(1.90090682571751,-32.0527379982001,54.9090919517021));
#87358=CARTESIAN_POINT('Ctrl Pts',(1.90477013459152,-32.0495941443787,54.8381025473437));
#87359=CARTESIAN_POINT('Ctrl Pts',(1.90863344346552,-32.0427586045275,54.7671670117002));
#87360=CARTESIAN_POINT('Ctrl Pts',(1.91249675233952,-32.0322416284498,54.696698951377));
#87361=CARTESIAN_POINT('Ctrl Pts',(1.91635552931687,-32.0217369894257,54.6263135543812));
#87362=CARTESIAN_POINT('Ctrl Pts',(1.92021430629422,-32.0075595636329,54.5563950215758));
#87363=CARTESIAN_POINT('Ctrl Pts',(1.92407308327157,-31.9897714985709,54.4873530006183));
#87364=CARTESIAN_POINT('Ctrl Pts',(1.92792942934779,-31.9719946393981,54.4183544738372));
#87365=CARTESIAN_POINT('Ctrl Pts',(1.93178577542401,-31.9506117746052,54.3502318327127));
#87366=CARTESIAN_POINT('Ctrl Pts',(1.93564212150022,-31.9257360644493,54.2833842224878));
#87367=CARTESIAN_POINT('Ctrl Pts',(1.93949732823641,-31.9008677037095,54.2165563620875));
#87368=CARTESIAN_POINT('Ctrl Pts',(1.9433525349726,-31.8725087156346,54.1510032397652));
#87369=CARTESIAN_POINT('Ctrl Pts',(1.94720774170879,-31.8408214758495,54.087106875614));
#87370=CARTESIAN_POINT('Ctrl Pts',(1.95106309905301,-31.8091329981664,54.0232080152788));
#87371=CARTESIAN_POINT('Ctrl Pts',(1.95491845639722,-31.7741162284318,53.9609664758441));
#87372=CARTESIAN_POINT('Ctrl Pts',(1.95877381374144,-31.7359800819237,53.9007408323493));
#87373=CARTESIAN_POINT('Ctrl Pts',(1.9626332067028,-31.6978040161882,53.8404521473209));
#87374=CARTESIAN_POINT('Ctrl Pts',(1.96649259966416,-31.6565023159761,53.7821839818299));
#87375=CARTESIAN_POINT('Ctrl Pts',(1.97035199262551,-31.6123274545571,53.7262662202087));
#87376=CARTESIAN_POINT('Ctrl Pts',(1.97421357072239,-31.5681275819356,53.6703167987156));
#87377=CARTESIAN_POINT('Ctrl Pts',(1.97807514881927,-31.5210516304962,53.6167207953959));
#87378=CARTESIAN_POINT('Ctrl Pts',(1.98193672691615,-31.4713908162051,53.565773160031));
#87379=CARTESIAN_POINT('Ctrl Pts',(1.98580506152013,-31.421643111623,53.5147363828564));
#87380=CARTESIAN_POINT('Ctrl Pts',(1.9896733961241,-31.3693018714003,53.4663575549583));
#87381=CARTESIAN_POINT('Ctrl Pts',(1.99354173072807,-31.3146928945613,53.4208926079933));
#87382=CARTESIAN_POINT('Ctrl Pts',(1.99583944551674,-31.2822562347263,53.3938873223337));
#87383=CARTESIAN_POINT('Ctrl Pts',(1.99813716030541,-31.2490200918453,53.3679092936663));
#87384=CARTESIAN_POINT('Ctrl Pts',(2.00043487509407,-31.215057371021,53.3430047834627));
#87385=CARTESIAN_POINT('Ctrl Pts',(2.00430394846561,-31.1578682632107,53.3010686050758));
#87386=CARTESIAN_POINT('Ctrl Pts',(2.00817302183714,-31.0983935265725,53.262014475793));
#87387=CARTESIAN_POINT('Ctrl Pts',(2.01204209520867,-31.0369555873072,53.2261001515158));
#87388=CARTESIAN_POINT('Ctrl Pts',(2.01590540362962,-30.9756091910679,53.1902393398719));
#87389=CARTESIAN_POINT('Ctrl Pts',(2.01976871205056,-30.9123058145872,53.157509290031));
#87390=CARTESIAN_POINT('Ctrl Pts',(2.02363202047151,-30.8473985058096,53.1281257160665));
#87391=CARTESIAN_POINT('Ctrl Pts',(2.02749079699221,-30.7825673373284,53.0987766108555));
#87392=CARTESIAN_POINT('Ctrl Pts',(2.03134957351291,-30.7161364142718,53.0727663832749));
#87393=CARTESIAN_POINT('Ctrl Pts',(2.03520835003361,-30.6484836059538,53.0502649986962));
#87394=CARTESIAN_POINT('Ctrl Pts',(2.03906469565122,-30.5808734166941,53.0277777892544));
#87395=CARTESIAN_POINT('Ctrl Pts',(2.04292104126883,-30.5120433292085,53.0087951902573));
#87396=CARTESIAN_POINT('Ctrl Pts',(2.04677738688643,-30.44239005677,52.9934386129074));
#87397=CARTESIAN_POINT('Ctrl Pts',(2.05063259316274,-30.3727573631016,52.9780865725944));
#87398=CARTESIAN_POINT('Ctrl Pts',(2.05448779943904,-30.3023024414472,52.9663585316487));
#87399=CARTESIAN_POINT('Ctrl Pts',(2.05834300571534,-30.2314343101485,52.958325265233));
#87400=CARTESIAN_POINT('Ctrl Pts',(2.06219836259909,-30.160563410316,52.9502916849897));
#87401=CARTESIAN_POINT('Ctrl Pts',(2.06605371948284,-30.0892797517333,52.945953218372));
#87402=CARTESIAN_POINT('Ctrl Pts',(2.06990907636659,-30.0179978969706,52.9453288247983));
#87403=CARTESIAN_POINT('Ctrl Pts',(2.07376846886978,-29.9466414274711,52.9447037776366));
#87404=CARTESIAN_POINT('Ctrl Pts',(2.07762786137298,-29.8752872523237,52.9478005685648));
#87405=CARTESIAN_POINT('Ctrl Pts',(2.08148725387617,-29.8043494540794,52.9545860012259));
#87406=CARTESIAN_POINT('Ctrl Pts',(2.0853488315155,-29.7333714918078,52.9613752757078));
#87407=CARTESIAN_POINT('Ctrl Pts',(2.08921040915483,-29.6628108564796,52.9718572779855));
#87408=CARTESIAN_POINT('Ctrl Pts',(2.09307198679416,-29.5930732932551,52.9859473150293));
#87409=CARTESIAN_POINT('Ctrl Pts',(2.09694032094654,-29.5232137118297,53.0000620050849));
#87410=CARTESIAN_POINT('Ctrl Pts',(2.10080865509892,-29.454180548386,53.0177972128689));
#87411=CARTESIAN_POINT('Ctrl Pts',(2.1046769892513,-29.3863655238667,53.0390180285886));
#87412=CARTESIAN_POINT('Ctrl Pts',(2.10697470814507,-29.3460846543808,53.0516228003843));
#87413=CARTESIAN_POINT('Ctrl Pts',(2.10927242703885,-29.3062332188164,53.065456404428));
#87414=CARTESIAN_POINT('Ctrl Pts',(2.11157014593263,-29.2668896249878,53.0804826803205));
#87415=CARTESIAN_POINT('Ctrl Pts',(2.11543921914794,-29.2006398998848,53.1057850624959));
#87416=CARTESIAN_POINT('Ctrl Pts',(2.11930829236326,-29.1355718665169,53.1345708206531));
#87417=CARTESIAN_POINT('Ctrl Pts',(2.12317736557858,-29.0720769492189,53.1667088680929));
#87418=CARTESIAN_POINT('Ctrl Pts',(2.12704067383899,-29.0086766399354,53.1987990295446));
#87419=CARTESIAN_POINT('Ctrl Pts',(2.1309039820994,-28.9468452239291,53.2342313478661));
#87420=CARTESIAN_POINT('Ctrl Pts',(2.13476729035982,-28.8869554125041,53.2728262077179));
#87421=CARTESIAN_POINT('Ctrl Pts',(2.13862606671434,-28.8271358556305,53.3113757933485));
#87422=CARTESIAN_POINT('Ctrl Pts',(2.14248484306886,-28.7692537855618,53.3530802895987));
#87423=CARTESIAN_POINT('Ctrl Pts',(2.14634361942338,-28.7136569403488,53.3977144151597));
#87424=CARTESIAN_POINT('Ctrl Pts',(2.1501999648714,-28.6580951193817,53.4423204226397));
#87425=CARTESIAN_POINT('Ctrl Pts',(2.15405631031943,-28.6048160450079,53.4898520944433));
#87426=CARTESIAN_POINT('Ctrl Pts',(2.15791265576745,-28.5541368830964,53.5400419835906));
#87427=CARTESIAN_POINT('Ctrl Pts',(2.16176786187102,-28.5034726941752,53.5902170443018));
#87428=CARTESIAN_POINT('Ctrl Pts',(2.16562306797458,-28.4554072377314,53.6430484215505));
#87429=CARTESIAN_POINT('Ctrl Pts',(2.16947827407815,-28.4102218119229,53.6982308671603));
#87430=CARTESIAN_POINT('Ctrl Pts',(2.17333363078626,-28.365034620935,53.7534154684853));
#87431=CARTESIAN_POINT('Ctrl Pts',(2.17718898749436,-28.3227279900157,53.8109509432653));
#87432=CARTESIAN_POINT('Ctrl Pts',(2.18104434420247,-28.2835426916522,53.8704992823733));
#87433=CARTESIAN_POINT('Ctrl Pts',(2.18490373652677,-28.2443163758585,53.9301099540381));
#87434=CARTESIAN_POINT('Ctrl Pts',(2.18876312885106,-28.208218182415,53.9917372893924));
#87435=CARTESIAN_POINT('Ctrl Pts',(2.19262252117536,-28.1754448051268,54.0550153951724));
#87436=CARTESIAN_POINT('Ctrl Pts',(2.19648409863368,-28.1426528720102,54.1183293281319));
#87437=CARTESIAN_POINT('Ctrl Pts',(2.200345676092,-28.1131897031921,54.1832954494789));
#87438=CARTESIAN_POINT('Ctrl Pts',(2.20420725355032,-28.0872042059791,54.2495269406062));
#87439=CARTESIAN_POINT('Ctrl Pts',(2.2080755875203,-28.0611732425501,54.3158743154227));
#87440=CARTESIAN_POINT('Ctrl Pts',(2.21194392149028,-28.0386322528878,54.3834910193113));
#87441=CARTESIAN_POINT('Ctrl Pts',(2.21581225546026,-28.0196803487775,54.4519747802499));
#87442=CARTESIAN_POINT('Ctrl Pts',(2.21810997589723,-28.0084232603948,54.4926528960308));
#87443=CARTESIAN_POINT('Ctrl Pts',(2.22040769633421,-27.9984314787575,54.5336367006076));
#87444=CARTESIAN_POINT('Ctrl Pts',(2.22270541677119,-27.9897171495473,54.5748407078804));
#87445=CARTESIAN_POINT('Ctrl Pts',(2.22812785170408,-27.9691520353733,54.6720788421699));
#87446=CARTESIAN_POINT('Ctrl Pts',(2.23355028663696,-27.9556362036303,54.7708559975689));
#87447=CARTESIAN_POINT('Ctrl Pts',(2.23897272156985,-27.9493462554379,54.8703204626261));
#87448=CARTESIAN_POINT('Ctrl Pts',(2.24129024122579,-27.94665796526,54.9128310424102));
#87449=CARTESIAN_POINT('Ctrl Pts',(2.24360776088173,-27.9452890575006,54.9554668839035));
#87450=CARTESIAN_POINT('Ctrl Pts',(2.24592528053768,-27.9452508239571,54.9981598774073));
#87451=CARTESIAN_POINT('Origin',(-1.54592528053767,-30.,55.));
#87452=CARTESIAN_POINT('',(1.09386116309789,-31.2520475724682,56.6292251037768));
#87453=CARTESIAN_POINT('',(1.1521101573493,-31.2520475724682,56.6292251037768));
#87454=CARTESIAN_POINT('',(-1.54592528053767,-31.2520475724682,56.6292251037768));
#87455=CARTESIAN_POINT('',(1.60407469463954,-27.9455255624714,54.9994775006002));
#87456=CARTESIAN_POINT('Ctrl Pts',(1.15211015734929,-31.2520475724682,56.6292251037768));
#87457=CARTESIAN_POINT('Ctrl Pts',(1.15596557278302,-31.3085761712459,56.5857832891923));
#87458=CARTESIAN_POINT('Ctrl Pts',(1.15982098821674,-31.3628659140609,56.5393770070728));
#87459=CARTESIAN_POINT('Ctrl Pts',(1.16367640365046,-31.4145978871033,56.4902719148876));
#87460=CARTESIAN_POINT('Ctrl Pts',(1.1675315895544,-31.4663267803145,56.441169746144));
#87461=CARTESIAN_POINT('Ctrl Pts',(1.17138677545833,-31.5154978548606,56.3893694219266));
#87462=CARTESIAN_POINT('Ctrl Pts',(1.17524196136226,-31.5618280037784,56.3351744639236));
#87463=CARTESIAN_POINT('Ctrl Pts',(1.17910093874514,-31.6082037172392,56.2809262065344));
#87464=CARTESIAN_POINT('Ctrl Pts',(1.18295991612802,-31.6517326074729,56.2242789811046));
#87465=CARTESIAN_POINT('Ctrl Pts',(1.1868188935109,-31.6921715266186,56.1655698550501));
#87466=CARTESIAN_POINT('Ctrl Pts',(1.19067971455899,-31.7326297658641,56.1068326801208));
#87467=CARTESIAN_POINT('Ctrl Pts',(1.19454053560709,-31.7699948382545,56.0460320565788));
#87468=CARTESIAN_POINT('Ctrl Pts',(1.19840135665518,-31.8040681871318,55.9835321747045));
#87469=CARTESIAN_POINT('Ctrl Pts',(1.20226929615544,-31.8382043593054,55.9209170576472));
#87470=CARTESIAN_POINT('Ctrl Pts',(1.20613723565571,-31.869036471134,55.8565968616065));
#87471=CARTESIAN_POINT('Ctrl Pts',(1.21000517515597,-31.8964132111337,55.790957960411));
#87472=CARTESIAN_POINT('Ctrl Pts',(1.21344131802192,-31.9207337543677,55.7326466445138));
#87473=CARTESIAN_POINT('Ctrl Pts',(1.21687746088786,-31.9423279731226,55.6732951182633));
#87474=CARTESIAN_POINT('Ctrl Pts',(1.2203136037538,-31.961123148466,55.6131831366329));
#87475=CARTESIAN_POINT('Ctrl Pts',(1.22418266806599,-31.9822863378325,55.5454976148327));
#87476=CARTESIAN_POINT('Ctrl Pts',(1.22805173237817,-31.9999827568448,55.476582593894));
#87477=CARTESIAN_POINT('Ctrl Pts',(1.23192079669036,-32.0140729123918,55.4068265798466));
#87478=CARTESIAN_POINT('Ctrl Pts',(1.23578409589712,-32.0281420728801,55.3371745058588));
#87479=CARTESIAN_POINT('Ctrl Pts',(1.23964739510388,-32.0386155407856,55.266684398468));
#87480=CARTESIAN_POINT('Ctrl Pts',(1.24351069431064,-32.0454035141265,55.1957601259168));
#87481=CARTESIAN_POINT('Ctrl Pts',(1.2473694614317,-32.052183524409,55.1249190555366));
#87482=CARTESIAN_POINT('Ctrl Pts',(1.25122822855277,-32.0552865820036,55.0536453129186));
#87483=CARTESIAN_POINT('Ctrl Pts',(1.25508699567383,-32.0546742055237,54.9823514404111));
#87484=CARTESIAN_POINT('Ctrl Pts',(1.2589433317824,-32.0540622148393,54.9111024828439));
#87485=CARTESIAN_POINT('Ctrl Pts',(1.26279966789097,-32.0497394381791,54.8398339051697));
#87486=CARTESIAN_POINT('Ctrl Pts',(1.26665600399954,-32.0417194340277,54.7689603600819));
#87487=CARTESIAN_POINT('Ctrl Pts',(1.27051120067154,-32.0337017995573,54.6981077560912));
#87488=CARTESIAN_POINT('Ctrl Pts',(1.27436639734354,-32.0219891609535,54.6276504354089));
#87489=CARTESIAN_POINT('Ctrl Pts',(1.27822159401553,-32.0066469694416,54.5579983003076));
#87490=CARTESIAN_POINT('Ctrl Pts',(1.28207694121374,-31.9913041788936,54.4883434456378));
#87491=CARTESIAN_POINT('Ctrl Pts',(1.28593228841194,-31.9723316607293,54.4194943129083));
#87492=CARTESIAN_POINT('Ctrl Pts',(1.28978763561014,-31.9498456863397,54.3518492752742));
#87493=CARTESIAN_POINT('Ctrl Pts',(1.29364701837012,-31.92733617489,54.2841334305988));
#87494=CARTESIAN_POINT('Ctrl Pts',(1.29750640113009,-31.9013060192717,54.2176246589508));
#87495=CARTESIAN_POINT('Ctrl Pts',(1.30136578389007,-31.8719206824674,54.1527039944324));
#87496=CARTESIAN_POINT('Ctrl Pts',(1.30522735173892,-31.8425187083984,54.0877465734089));
#87497=CARTESIAN_POINT('Ctrl Pts',(1.30908891958777,-31.8097579947878,54.0243794811739));
#87498=CARTESIAN_POINT('Ctrl Pts',(1.31295048743662,-31.773850028845,53.962959191899));
#87499=CARTESIAN_POINT('Ctrl Pts',(1.31681881182973,-31.7378792351154,53.9014314361962));
#87500=CARTESIAN_POINT('Ctrl Pts',(1.32068713622285,-31.6987504615151,53.8418576903979));
#87501=CARTESIAN_POINT('Ctrl Pts',(1.32455546061596,-31.6567181674367,53.7845649025204));
#87502=CARTESIAN_POINT('Ctrl Pts',(1.32685326527476,-31.6317507677724,53.7505326907609));
#87503=CARTESIAN_POINT('Ctrl Pts',(1.32915106993356,-31.6057596613866,53.7173046689099));
#87504=CARTESIAN_POINT('Ctrl Pts',(1.33144887459237,-31.5788044520992,53.6849433226922));
#87505=CARTESIAN_POINT('Ctrl Pts',(1.33531795118106,-31.5334168823606,53.6304528217048));
#87506=CARTESIAN_POINT('Ctrl Pts',(1.33918702776976,-31.4851160905946,53.5782080927003));
#87507=CARTESIAN_POINT('Ctrl Pts',(1.34305610435845,-31.4341528251068,53.5285370420095));
#87508=CARTESIAN_POINT('Ctrl Pts',(1.34691941602998,-31.3832654947929,53.4789400010949));
#87509=CARTESIAN_POINT('Ctrl Pts',(1.35078272770152,-31.3297239103519,53.4319093628715));
#87510=CARTESIAN_POINT('Ctrl Pts',(1.35464603937305,-31.2738186770057,53.387739617614));
#87511=CARTESIAN_POINT('Ctrl Pts',(1.35850481917804,-31.2179790234208,53.3436216857768));
#87512=CARTESIAN_POINT('Ctrl Pts',(1.36236359898302,-31.1597816077401,53.3023582804948));
#87513=CARTESIAN_POINT('Ctrl Pts',(1.36622237878801,-31.0995521569077,53.2642054796896));
#87514=CARTESIAN_POINT('Ctrl Pts',(1.37007872770888,-31.0393606483322,53.2260767136938));
#87515=CARTESIAN_POINT('Ctrl Pts',(1.37393507662976,-30.9771400537194,53.191054923777));
#87516=CARTESIAN_POINT('Ctrl Pts',(1.37779142555063,-30.9132460973394,53.1593536113109));
#87517=CARTESIAN_POINT('Ctrl Pts',(1.38164663514423,-30.8493710179151,53.1276616647425));
#87518=CARTESIAN_POINT('Ctrl Pts',(1.38550184473782,-30.7838239931369,53.099288463844));
#87519=CARTESIAN_POINT('Ctrl Pts',(1.38935705433142,-30.7169849007977,53.0744013360702));
#87520=CARTESIAN_POINT('Ctrl Pts',(1.39321241454153,-30.6501431971683,53.0495132359985));
#87521=CARTESIAN_POINT('Ctrl Pts',(1.39706777475164,-30.5820097817782,53.0281116468946));
#87522=CARTESIAN_POINT('Ctrl Pts',(1.40092313496175,-30.512982409171,53.0103149469373));
#87523=CARTESIAN_POINT('Ctrl Pts',(1.40478253078214,-30.4438827819471,52.9924996182291));
#87524=CARTESIAN_POINT('Ctrl Pts',(1.40864192660254,-30.3738878009,52.9782968328076));
#87525=CARTESIAN_POINT('Ctrl Pts',(1.41250132242293,-30.3034073328994,52.9677742367437));
#87526=CARTESIAN_POINT('Ctrl Pts',(1.41636290337928,-30.2328869598431,52.9572456829329));
#87527=CARTESIAN_POINT('Ctrl Pts',(1.42022448433563,-30.1618810364133,52.9504015130578));
#87528=CARTESIAN_POINT('Ctrl Pts',(1.42408606529199,-30.0908037574162,52.9472573858033));
#87529=CARTESIAN_POINT('Ctrl Pts',(1.42795440272499,-30.0196021169253,52.9441077573764));
#87530=CARTESIAN_POINT('Ctrl Pts',(1.431822740158,-29.9483293575278,52.944671092936));
#87531=CARTESIAN_POINT('Ctrl Pts',(1.435691077591,-29.8773981743257,52.9489109344445));
#87532=CARTESIAN_POINT('Ctrl Pts',(1.43798876687098,-29.8352669429939,52.9514292872386));
#87533=CARTESIAN_POINT('Ctrl Pts',(1.44028645615095,-29.7932561152423,52.9552437332563));
#87534=CARTESIAN_POINT('Ctrl Pts',(1.44258414543093,-29.7514505018919,52.9603380894153));
#87535=CARTESIAN_POINT('Ctrl Pts',(1.44645321930508,-29.6810541224437,52.968916464434));
#87536=CARTESIAN_POINT('Ctrl Pts',(1.45032229317924,-29.6109644848074,52.9811603850238));
#87537=CARTESIAN_POINT('Ctrl Pts',(1.4541913670534,-29.5415930737697,52.9970370316743));
#87538=CARTESIAN_POINT('Ctrl Pts',(1.45805467599476,-29.4723250263626,53.012890022069));
#87539=CARTESIAN_POINT('Ctrl Pts',(1.46191798493612,-29.4037735510006,53.0323648868264));
#87540=CARTESIAN_POINT('Ctrl Pts',(1.46578129387748,-29.3363436752025,53.0553771972292));
#87541=CARTESIAN_POINT('Ctrl Pts',(1.4696400709426,-29.2689928983985,53.0783625129121));
#87542=CARTESIAN_POINT('Ctrl Pts',(1.47349884800773,-29.2027615652538,53.1048768755501));
#87543=CARTESIAN_POINT('Ctrl Pts',(1.47735762507285,-29.1380414802018,53.1347855156451));
#87544=CARTESIAN_POINT('Ctrl Pts',(1.48121397124943,-29.0733621664385,53.1646753143898));
#87545=CARTESIAN_POINT('Ctrl Pts',(1.48507031742601,-29.0101926518868,53.1979549449937));
#87546=CARTESIAN_POINT('Ctrl Pts',(1.48892666360258,-28.9489052400723,53.2344413438935));
#87547=CARTESIAN_POINT('Ctrl Pts',(1.49278187045159,-28.8876359351484,53.2709169631697));
#87548=CARTESIAN_POINT('Ctrl Pts',(1.4966370773006,-28.8282480462308,53.3105972214957));
#87549=CARTESIAN_POINT('Ctrl Pts',(1.50049228414961,-28.7710881841521,53.3532537197949));
#87550=CARTESIAN_POINT('Ctrl Pts',(1.50434764161902,-28.7139260888751,53.3959118846554));
#87551=CARTESIAN_POINT('Ctrl Pts',(1.50820299908843,-28.6589925812664,53.4415462280417));
#87552=CARTESIAN_POINT('Ctrl Pts',(1.51205835655784,-28.6066028434589,53.4898867835016));
#87553=CARTESIAN_POINT('Ctrl Pts',(1.51591774966253,-28.5541582661519,53.5382779399375));
#87554=CARTESIAN_POINT('Ctrl Pts',(1.51977714276722,-28.5042631317822,53.5893806331602));
#87555=CARTESIAN_POINT('Ctrl Pts',(1.52363653587191,-28.457196569526,53.6428872053445));
#87556=CARTESIAN_POINT('Ctrl Pts',(1.52749811412259,-28.4101033586993,53.6964240723622));
#87557=CARTESIAN_POINT('Ctrl Pts',(1.53135969237328,-28.3658422096494,53.7523671466232));
#87558=CARTESIAN_POINT('Ctrl Pts',(1.53522127062396,-28.3246509219981,53.8103769381279));
#87559=CARTESIAN_POINT('Ctrl Pts',(1.53908960539675,-28.2833875628186,53.8684882281426));
#87560=CARTESIAN_POINT('Ctrl Pts',(1.54295794016954,-28.2452050492593,53.9286730447033));
#87561=CARTESIAN_POINT('Ctrl Pts',(1.54682627494233,-28.2102965820227,53.9905648915457));
#87562=CARTESIAN_POINT('Ctrl Pts',(1.54912398871805,-28.1895616480602,54.0273274153309));
#87563=CARTESIAN_POINT('Ctrl Pts',(1.55142170249376,-28.1699809454479,54.0646917503864));
#87564=CARTESIAN_POINT('Ctrl Pts',(1.55371941626947,-28.1515868774171,54.1025778636766));
#87565=CARTESIAN_POINT('Ctrl Pts',(1.55791568927332,-28.1179941245144,54.1717685853846));
#87566=CARTESIAN_POINT('Ctrl Pts',(1.56211196227716,-28.0882444852697,54.242941908556));
#87567=CARTESIAN_POINT('Ctrl Pts',(1.56630823528101,-28.062557410543,54.3156654509246));
#87568=CARTESIAN_POINT('Ctrl Pts',(1.57045671771971,-28.0371628810861,54.3875607585274));
#87569=CARTESIAN_POINT('Ctrl Pts',(1.57460520015842,-28.0157390341105,54.4609708158));
#87570=CARTESIAN_POINT('Ctrl Pts',(1.57875368259713,-27.9984521149186,54.5354533110372));
#87571=CARTESIAN_POINT('Ctrl Pts',(1.58297385088354,-27.9808664774665,54.6112228650698));
#87572=CARTESIAN_POINT('Ctrl Pts',(1.58719401916996,-27.9675623121118,54.6881019450977));
#87573=CARTESIAN_POINT('Ctrl Pts',(1.59141418745637,-27.9586631451064,54.7656041652397));
#87574=CARTESIAN_POINT('Ctrl Pts',(1.59563435574278,-27.949763978101,54.8431063853816));
#87575=CARTESIAN_POINT('Ctrl Pts',(1.59985452402919,-27.9452699678385,54.9212313568782));
#87576=CARTESIAN_POINT('Ctrl Pts',(1.6040746923156,-27.9452500664616,54.9994773875089));
#87577=CARTESIAN_POINT('Ctrl Pts',(1.60407471946232,-27.94846822613,54.9994787085655));
#87578=CARTESIAN_POINT('Ctrl Pts',(1.62433470867756,-27.9493198488661,55.3745305565027));
#87579=CARTESIAN_POINT('Ctrl Pts',(1.68163978817232,-28.2273233735254,56.4365344918066));
#87580=CARTESIAN_POINT('Ctrl Pts',(1.76427577418884,-29.7210216460611,57.3046347470521));
#87581=CARTESIAN_POINT('Ctrl Pts',(1.82665177099012,-30.8775867504766,56.9099569767507));
#87582=CARTESIAN_POINT('Ctrl Pts',(1.85198267751188,-31.2510897925303,56.6279533612584));
#87583=CARTESIAN_POINT('',(1.54592528048776,-27.9452502738004,55.0010607462675));
#87584=CARTESIAN_POINT('Ctrl Pts',(1.54592528053768,-27.9452502738009,55.0010607471837));
#87585=CARTESIAN_POINT('Ctrl Pts',(1.54924811760506,-27.9452817536834,55.0620397260039));
#87586=CARTESIAN_POINT('Ctrl Pts',(1.55257095467244,-27.948027507084,55.1229466290489));
#87587=CARTESIAN_POINT('Ctrl Pts',(1.55589379173983,-27.9534698488702,55.1836080145764));
#87588=CARTESIAN_POINT('Ctrl Pts',(1.5597628683149,-27.9598068544746,55.2542414946407));
#87589=CARTESIAN_POINT('Ctrl Pts',(1.56363194488996,-27.9698173072335,55.3246848690047));
#87590=CARTESIAN_POINT('Ctrl Pts',(1.56750102146503,-27.9834814798758,55.3945258172747));
#87591=CARTESIAN_POINT('Ctrl Pts',(1.57136433312278,-27.9971252929249,55.4642627026542));
#87592=CARTESIAN_POINT('Ctrl Pts',(1.57522764478053,-28.0144119270837,55.5333984708159));
#87593=CARTESIAN_POINT('Ctrl Pts',(1.57909095643828,-28.0352698667458,55.6015256154004));
#87594=CARTESIAN_POINT('Ctrl Pts',(1.5829497362293,-28.0561033389532,55.6695728432794));
#87595=CARTESIAN_POINT('Ctrl Pts',(1.58680851602031,-28.0804996537178,55.7366133355057));
#87596=CARTESIAN_POINT('Ctrl Pts',(1.59066729581133,-28.1083365598858,55.8022512024517));
#87597=CARTESIAN_POINT('Ctrl Pts',(1.59452364471814,-28.1361559298637,55.867847720043));
#87598=CARTESIAN_POINT('Ctrl Pts',(1.59837999362495,-28.1674114018557,55.9320429192325));
#87599=CARTESIAN_POINT('Ctrl Pts',(1.60223634253175,-28.2019318353487,55.9944588668053));
#87600=CARTESIAN_POINT('Ctrl Pts',(1.6060915521112,-28.2364420700565,56.0568563740869));
#87601=CARTESIAN_POINT('Ctrl Pts',(1.60994676169065,-28.2742151162716,56.117475248475));
#87602=CARTESIAN_POINT('Ctrl Pts',(1.6138019712701,-28.315033704418,56.1759617958305));
#87603=CARTESIAN_POINT('Ctrl Pts',(1.61765733146601,-28.3558538872771,56.2344506281556));
#87604=CARTESIAN_POINT('Ctrl Pts',(1.62151269166191,-28.3997195684674,56.2908065709542));
#87605=CARTESIAN_POINT('Ctrl Pts',(1.62536805185782,-28.4463709333038,56.344706022005));
#87606=CARTESIAN_POINT('Ctrl Pts',(1.62922744766402,-28.4930711306015,56.3986618924741));
#87607=CARTESIAN_POINT('Ctrl Pts',(1.63308684347022,-28.5425625138155,56.4501557701598));
#87608=CARTESIAN_POINT('Ctrl Pts',(1.63694623927641,-28.5945464502454,56.4988988898462));
#87609=CARTESIAN_POINT('Ctrl Pts',(1.64080782021855,-28.6465598192532,56.5476696072054));
#87610=CARTESIAN_POINT('Ctrl Pts',(1.64466940116069,-28.7010681794651,56.593686152664));
#87611=CARTESIAN_POINT('Ctrl Pts',(1.64853098210283,-28.757739768715,56.6367000581254));
#87612=CARTESIAN_POINT('Ctrl Pts',(1.65239931952175,-28.8145105143163,56.6797892235536));
#87613=CARTESIAN_POINT('Ctrl Pts',(1.65626765694067,-28.8734516438254,56.7198649867566));
#87614=CARTESIAN_POINT('Ctrl Pts',(1.66013599435959,-28.9342029851873,56.7567225978271));
#87615=CARTESIAN_POINT('Ctrl Pts',(1.66243368376586,-28.9702876640422,56.7786150372205));
#87616=CARTESIAN_POINT('Ctrl Pts',(1.66473137317212,-29.0070105153468,56.799372976299));
#87617=CARTESIAN_POINT('Ctrl Pts',(1.66702906257839,-29.0442925787914,56.8189614859988));
#87618=CARTESIAN_POINT('Ctrl Pts',(1.67089813645202,-29.1070717591432,56.8519465321481));
#87619=CARTESIAN_POINT('Ctrl Pts',(1.67476721032565,-29.1716835679484,56.8817422542605));
#87620=CARTESIAN_POINT('Ctrl Pts',(1.67863628419928,-29.2377708981664,56.9081415982096));
#87621=CARTESIAN_POINT('Ctrl Pts',(1.68249959314005,-29.3037597580441,56.934501607049));
#87622=CARTESIAN_POINT('Ctrl Pts',(1.68636290208083,-29.3712193278617,56.9574751041645));
#87623=CARTESIAN_POINT('Ctrl Pts',(1.6902262110216,-29.4397684568758,56.9769011559986));
#87624=CARTESIAN_POINT('Ctrl Pts',(1.69408498808608,-29.5082371739482,56.9963044199933));
#87625=CARTESIAN_POINT('Ctrl Pts',(1.69794376515055,-29.5777924463391,57.012168372749));
#87626=CARTESIAN_POINT('Ctrl Pts',(1.70180254221503,-29.6480353658451,57.0243810063336));
#87627=CARTESIAN_POINT('Ctrl Pts',(1.70565888839091,-29.7182340348777,57.0365859464051));
#87628=CARTESIAN_POINT('Ctrl Pts',(1.70951523456679,-29.789119014104,57.0451440478454));
#87629=CARTESIAN_POINT('Ctrl Pts',(1.71337158074267,-29.8602799654172,57.0499941157077));
#87630=CARTESIAN_POINT('Ctrl Pts',(1.71722678759094,-29.9314198927785,57.054842750655));
#87631=CARTESIAN_POINT('Ctrl Pts',(1.7210819944392,-30.002835145962,57.0559854938997));
#87632=CARTESIAN_POINT('Ctrl Pts',(1.72493720128747,-30.0741107323921,57.0534130519319));
#87633=CARTESIAN_POINT('Ctrl Pts',(1.72879255875609,-30.1453891035115,57.0508405094605));
#87634=CARTESIAN_POINT('Ctrl Pts',(1.7326479162247,-30.2165273116536,57.0445525133233));
#87635=CARTESIAN_POINT('Ctrl Pts',(1.73650327369332,-30.2871125708193,57.0345918347859));
#87636=CARTESIAN_POINT('Ctrl Pts',(1.74036266679717,-30.3577717158337,57.0246207298055));
#87637=CARTESIAN_POINT('Ctrl Pts',(1.74422205990101,-30.4278762744413,57.0109693361209));
#87638=CARTESIAN_POINT('Ctrl Pts',(1.74808145300486,-30.4970216752217,56.993731932046));
#87639=CARTESIAN_POINT('Ctrl Pts',(1.75194303125466,-30.566206225368,56.9764847683423));
#87640=CARTESIAN_POINT('Ctrl Pts',(1.75580460950447,-30.6344300717935,56.9556476943948));
#87641=CARTESIAN_POINT('Ctrl Pts',(1.75966618775427,-30.7013045302177,56.9313646777334));
#87642=CARTESIAN_POINT('Ctrl Pts',(1.76353452252614,-30.7682959974722,56.9070391735895));
#87643=CARTESIAN_POINT('Ctrl Pts',(1.76740285729801,-30.8339329154279,56.8792558784943));
#87644=CARTESIAN_POINT('Ctrl Pts',(1.77127119206988,-30.8978479208636,56.8482063395359));
#87645=CARTESIAN_POINT('Ctrl Pts',(1.77356890585224,-30.9358121606592,56.8297635320212));
#87646=CARTESIAN_POINT('Ctrl Pts',(1.77586661963459,-30.9731693666111,56.8101692312376));
#87647=CARTESIAN_POINT('Ctrl Pts',(1.77816433341695,-31.0098473657377,56.7894708325124));
#87648=CARTESIAN_POINT('Ctrl Pts',(1.78203306890693,-31.0716033068006,56.7546202648094));
#87649=CARTESIAN_POINT('Ctrl Pts',(1.78590180439691,-31.1316740064266,56.7165008235736));
#87650=CARTESIAN_POINT('Ctrl Pts',(1.78977053988689,-31.1896919225454,56.6753001796485));
#87651=CARTESIAN_POINT('Ctrl Pts',(1.79117493316314,-31.210753060354,56.6603438954942));
#87652=CARTESIAN_POINT('Ctrl Pts',(1.7925793264394,-31.2315438885102,56.6449820348889));
#87653=CARTESIAN_POINT('Ctrl Pts',(1.79398371971565,-31.2520475724682,56.6292251037768));
#87654=CARTESIAN_POINT('Ctrl Pts',(1.09386116309789,-31.2520475724682,56.6292251037768));
#87655=CARTESIAN_POINT('Ctrl Pts',(1.09772972046203,-31.3085492190033,56.5858040017936));
#87656=CARTESIAN_POINT('Ctrl Pts',(1.10159827782616,-31.3627137126113,56.53949850154));
#87657=CARTESIAN_POINT('Ctrl Pts',(1.10546683519029,-31.4142494145056,56.4906026150757));
#87658=CARTESIAN_POINT('Ctrl Pts',(1.10742879292206,-31.4403859970288,56.4658048278205));
#87659=CARTESIAN_POINT('Ctrl Pts',(1.10939075065382,-31.4658470525731,56.4403413415681));
#87660=CARTESIAN_POINT('Ctrl Pts',(1.11135270838559,-31.4905985265509,56.4142537237512));
#87661=CARTESIAN_POINT('Ctrl Pts',(1.11522171018827,-31.5394087001283,56.3628086601157));
#87662=CARTESIAN_POINT('Ctrl Pts',(1.11909071199094,-31.5856481018848,56.3087329449302));
#87663=CARTESIAN_POINT('Ctrl Pts',(1.12295971379362,-31.6290203852074,56.2523139171465));
#87664=CARTESIAN_POINT('Ctrl Pts',(1.12682294948606,-31.672328029282,56.1959789726354));
#87665=CARTESIAN_POINT('Ctrl Pts',(1.1306861851785,-31.7127767429601,56.1373080296882));
#87666=CARTESIAN_POINT('Ctrl Pts',(1.13454942087094,-31.750108024177,56.0766241062745));
#87667=CARTESIAN_POINT('Ctrl Pts',(1.13840812329285,-31.7873954994213,56.016011391729));
#87668=CARTESIAN_POINT('Ctrl Pts',(1.14226682571477,-31.8215725551428,55.9533908004313));
#87669=CARTESIAN_POINT('Ctrl Pts',(1.14612552813668,-31.852422942802,55.8891157424547));
#87670=CARTESIAN_POINT('Ctrl Pts',(1.14998179884972,-31.8832538889098,55.8248811898634));
#87671=CARTESIAN_POINT('Ctrl Pts',(1.15383806956276,-31.9107621165093,55.7589946760764));
#87672=CARTESIAN_POINT('Ctrl Pts',(1.15769434027581,-31.934777167482,55.6918344272225));
#87673=CARTESIAN_POINT('Ctrl Pts',(1.16154947095325,-31.9587851188461,55.6246940330625));
#87674=CARTESIAN_POINT('Ctrl Pts',(1.16540460163069,-31.9793017802805,55.5562811085952));
#87675=CARTESIAN_POINT('Ctrl Pts',(1.16925973230813,-31.9962053739874,55.486992471568));
#87676=CARTESIAN_POINT('Ctrl Pts',(1.17311501300943,-32.013109625504,55.4177011381475));
#87677=CARTESIAN_POINT('Ctrl Pts',(1.17697029371072,-32.0264004171426,55.3475344969958));
#87678=CARTESIAN_POINT('Ctrl Pts',(1.18082557441202,-32.0360066742742,55.276901399077));
#87679=CARTESIAN_POINT('Ctrl Pts',(1.18468489036429,-32.0456229860975,55.2061943708015));
#87680=CARTESIAN_POINT('Ctrl Pts',(1.18854420631656,-32.0515469993018,55.1350203935007));
#87681=CARTESIAN_POINT('Ctrl Pts',(1.19240352226884,-32.0537594393593,55.0637944178004));
#87682=CARTESIAN_POINT('Ctrl Pts',(1.19626502303373,-32.05597313191,54.9925281200812));
#87683=CARTESIAN_POINT('Ctrl Pts',(1.20012652379863,-32.0544710787649,54.921210251292));
#87684=CARTESIAN_POINT('Ctrl Pts',(1.20398802456352,-32.0492861423162,54.8502539836562));
#87685=CARTESIAN_POINT('Ctrl Pts',(1.20785628216241,-32.0440921332926,54.7791735571116));
#87686=CARTESIAN_POINT('Ctrl Pts',(1.21172453976131,-32.0352024353683,54.7084564771461));
#87687=CARTESIAN_POINT('Ctrl Pts',(1.2155927973602,-32.0227014951234,54.638508334639));
#87688=CARTESIAN_POINT('Ctrl Pts',(1.21789119131485,-32.0152738394537,54.596947403453));
#87689=CARTESIAN_POINT('Ctrl Pts',(1.2201895852695,-32.0065722627379,54.5556577129014));
#87690=CARTESIAN_POINT('Ctrl Pts',(1.22248797922415,-31.9966227768528,54.514721678361));
#87691=CARTESIAN_POINT('Ctrl Pts',(1.22635707361176,-31.9798739075304,54.445810349574));
#87692=CARTESIAN_POINT('Ctrl Pts',(1.23022616799936,-31.9595204436173,54.3776321757481));
#87693=CARTESIAN_POINT('Ctrl Pts',(1.23409526238696,-31.9356430854709,54.3105919871595));
#87694=CARTESIAN_POINT('Ctrl Pts',(1.23795859201317,-31.9118013034203,54.2436516851728));
#87695=CARTESIAN_POINT('Ctrl Pts',(1.24182192163938,-31.8844462107573,54.1778464567112));
#87696=CARTESIAN_POINT('Ctrl Pts',(1.24568525126559,-31.8537090082601,54.1135686855739));
#87697=CARTESIAN_POINT('Ctrl Pts',(1.24954404916813,-31.8230078608041,54.0493663128948));
#87698=CARTESIAN_POINT('Ctrl Pts',(1.25340284707066,-31.7889326923645,53.9866882746953));
#87699=CARTESIAN_POINT('Ctrl Pts',(1.25726164497319,-31.7516631534684,53.9259079372413));
#87700=CARTESIAN_POINT('Ctrl Pts',(1.26111801206976,-31.7144170920955,53.8651658876715));
#87701=CARTESIAN_POINT('Ctrl Pts',(1.26497437916632,-31.6739809058884,53.8063195802681));
#87702=CARTESIAN_POINT('Ctrl Pts',(1.26883074626288,-31.6305799285602,53.7497173683216));
#87703=CARTESIAN_POINT('Ctrl Pts',(1.27268597408294,-31.5871917730699,53.6931318782195));
#87704=CARTESIAN_POINT('Ctrl Pts',(1.276541201903,-31.5408408607529,53.6387895526885));
#87705=CARTESIAN_POINT('Ctrl Pts',(1.28039642972305,-31.4917945464425,53.5870079286477));
#87706=CARTESIAN_POINT('Ctrl Pts',(1.28425180818311,-31.4427463156858,53.5352242812806));
#87707=CARTESIAN_POINT('Ctrl Pts',(1.28810718664316,-31.3910028094911,53.486001885227));
#87708=CARTESIAN_POINT('Ctrl Pts',(1.29196256510322,-31.3368689910113,53.4396222049221));
#87709=CARTESIAN_POINT('Ctrl Pts',(1.29582197908265,-31.2826785093335,53.393193977866));
#87710=CARTESIAN_POINT('Ctrl Pts',(1.29968139306208,-31.2260930904763,53.3496147231137));
#87711=CARTESIAN_POINT('Ctrl Pts',(1.30354080704151,-31.1674509159418,53.3091256932088));
#87712=CARTESIAN_POINT('Ctrl Pts',(1.30740240613298,-31.1087755395475,53.26861373934));
#87713=CARTESIAN_POINT('Ctrl Pts',(1.31126400522446,-31.0480415031214,53.2311957481936));
#87714=CARTESIAN_POINT('Ctrl Pts',(1.31512560431593,-30.9856137707499,53.1970682050038));
#87715=CARTESIAN_POINT('Ctrl Pts',(1.31899395964842,-30.9230768150242,53.1628809523773));
#87716=CARTESIAN_POINT('Ctrl Pts',(1.3228623149809,-30.8588406850115,53.1319958522056));
#87717=CARTESIAN_POINT('Ctrl Pts',(1.32673067031339,-30.7932919523926,53.1045619396116));
#87718=CARTESIAN_POINT('Ctrl Pts',(1.32902819689649,-30.7543606902058,53.0882681563249));
#87719=CARTESIAN_POINT('Ctrl Pts',(1.3313257234796,-30.7149667486081,53.0731908442583));
#87720=CARTESIAN_POINT('Ctrl Pts',(1.33362325006271,-30.6751933787958,53.0593528234812));
#87721=CARTESIAN_POINT('Ctrl Pts',(1.33749233009677,-30.608214240378,53.0360493238424));
#87722=CARTESIAN_POINT('Ctrl Pts',(1.34136141013084,-30.5398960582951,53.0161718100595));
#87723=CARTESIAN_POINT('Ctrl Pts',(1.3452304901649,-30.4706227140094,52.9998720482033));
#87724=CARTESIAN_POINT('Ctrl Pts',(1.34909380543655,-30.4014525840197,52.9835965722894));
#87725=CARTESIAN_POINT('Ctrl Pts',(1.35295712070819,-30.3313305857591,52.9708883773768));
#87726=CARTESIAN_POINT('Ctrl Pts',(1.35682043597984,-30.2606575336868,52.9618500514848));
#87727=CARTESIAN_POINT('Ctrl Pts',(1.36067921959847,-30.1900673808155,52.9528223275122));
#87728=CARTESIAN_POINT('Ctrl Pts',(1.3645380032171,-30.1189279375903,52.9474559832131));
#87729=CARTESIAN_POINT('Ctrl Pts',(1.36839678683573,-30.0476503185958,52.9458025874718));
#87730=CARTESIAN_POINT('Ctrl Pts',(1.37225313970019,-29.9764175993383,52.9441502332499));
#87731=CARTESIAN_POINT('Ctrl Pts',(1.37610949256465,-29.9050473615041,52.9462061985068));
#87732=CARTESIAN_POINT('Ctrl Pts',(1.37996584542911,-29.8339544822215,52.9519701055586));
#87733=CARTESIAN_POINT('Ctrl Pts',(1.38382105909059,-29.7628826044456,52.9577323098979));
#87734=CARTESIAN_POINT('Ctrl Pts',(1.38767627275206,-29.6920884064903,52.9672002422019));
#87735=CARTESIAN_POINT('Ctrl Pts',(1.39153148641353,-29.621983666113,52.9803215073149));
#87736=CARTESIAN_POINT('Ctrl Pts',(1.39538685081032,-29.5518761847048,52.9934432854573));
#87737=CARTESIAN_POINT('Ctrl Pts',(1.3992422152071,-29.4824586914817,53.010218588467));
#87738=CARTESIAN_POINT('Ctrl Pts',(1.40309757960388,-29.4141330555407,53.0305438603792));
#87739=CARTESIAN_POINT('Ctrl Pts',(1.40695697976471,-29.3457358968804,53.0508904086206));
#87740=CARTESIAN_POINT('Ctrl Pts',(1.41081637992554,-29.2784333436547,53.0747942050973));
#87741=CARTESIAN_POINT('Ctrl Pts',(1.41467578008637,-29.2126114976239,53.1021019761784));
#87742=CARTESIAN_POINT('Ctrl Pts',(1.41853736547651,-29.1467523826339,53.1294252091809));
#87743=CARTESIAN_POINT('Ctrl Pts',(1.42239895086665,-29.0823760824192,53.1601560442001));
#87744=CARTESIAN_POINT('Ctrl Pts',(1.42626053625679,-29.0198456135793,53.1940944262558));
#87745=CARTESIAN_POINT('Ctrl Pts',(1.43012887822424,-28.9572057358038,53.2280921899591));
#87746=CARTESIAN_POINT('Ctrl Pts',(1.43399722019169,-28.8964185518926,53.2653084519122));
#87747=CARTESIAN_POINT('Ctrl Pts',(1.43786556215914,-28.8378189326264,53.3054992684751));
#87748=CARTESIAN_POINT('Ctrl Pts',(1.44016321507319,-28.8030129131221,53.3293711359497));
#87749=CARTESIAN_POINT('Ctrl Pts',(1.44246086798723,-28.768978046545,53.3542916063209));
#87750=CARTESIAN_POINT('Ctrl Pts',(1.44475852090127,-28.7357786680281,53.3802031033839));
#87751=CARTESIAN_POINT('Ctrl Pts',(1.44858235440861,-28.6805271131827,53.423325913661));
#87752=CARTESIAN_POINT('Ctrl Pts',(1.45240618791595,-28.6273639390351,53.4693732488752));
#87753=CARTESIAN_POINT('Ctrl Pts',(1.45623002142328,-28.5766206997893,53.5181130507925));
#87754=CARTESIAN_POINT('Ctrl Pts',(1.4600473499653,-28.525963783081,53.5667699383463));
#87755=CARTESIAN_POINT('Ctrl Pts',(1.46386467850732,-28.4777189834451,53.6181098561307));
#87756=CARTESIAN_POINT('Ctrl Pts',(1.46768200704934,-28.4321859584129,53.6718596860639));
#87757=CARTESIAN_POINT('Ctrl Pts',(1.47149570176107,-28.3866962776419,53.7255583499112));
#87758=CARTESIAN_POINT('Ctrl Pts',(1.47530939647279,-28.3439135753923,53.7816620009685));
#87759=CARTESIAN_POINT('Ctrl Pts',(1.47912309118452,-28.3041006756,53.839860765253));
#87760=CARTESIAN_POINT('Ctrl Pts',(1.48293450371858,-28.2643116005019,53.8980247024393));
#87761=CARTESIAN_POINT('Ctrl Pts',(1.48674591625265,-28.2274890845337,53.958280856368));
#87762=CARTESIAN_POINT('Ctrl Pts',(1.49055732878671,-28.1938544633214,54.020287867363));
#87763=CARTESIAN_POINT('Ctrl Pts',(1.49436780766194,-28.1602280813803,54.0822796888729));
#87764=CARTESIAN_POINT('Ctrl Pts',(1.49817828653717,-28.1297882811194,54.1460210780293));
#87765=CARTESIAN_POINT('Ctrl Pts',(1.5019887654124,-28.1027110288688,54.2111450560945));
#87766=CARTESIAN_POINT('Ctrl Pts',(1.50580205935471,-28.0756137727595,54.2763171457942));
#87767=CARTESIAN_POINT('Ctrl Pts',(1.50961535329702,-28.0518842218103,54.3428734049702));
#87768=CARTESIAN_POINT('Ctrl Pts',(1.51342864723933,-28.031650167987,54.4104268482075));
#87769=CARTESIAN_POINT('Ctrl Pts',(1.51724327680651,-28.0114090270874,54.4780039523691));
#87770=CARTESIAN_POINT('Ctrl Pts',(1.5210579063737,-27.9946659420835,54.5465784518758));
#87771=CARTESIAN_POINT('Ctrl Pts',(1.52487253594088,-27.9814980324821,54.6157509015935));
#87772=CARTESIAN_POINT('Ctrl Pts',(1.52869346817071,-27.9683083664059,54.6850376404203));
#87773=CARTESIAN_POINT('Ctrl Pts',(1.53251440040054,-27.9587057437019,54.7549238082747));
#87774=CARTESIAN_POINT('Ctrl Pts',(1.53633533263036,-27.9527155258906,54.8250033012576));
#87775=CARTESIAN_POINT('Ctrl Pts',(1.53953198191616,-27.9477040197093,54.8836328575328));
#87776=CARTESIAN_POINT('Ctrl Pts',(1.54272863120196,-27.9452199894214,54.9423975000279));
#87777=CARTESIAN_POINT('Ctrl Pts',(1.54592528048776,-27.9452502738004,55.0010607462675));
#87778=CARTESIAN_POINT('Origin',(-1.54592528053767,-30.,55.));
#87779=CARTESIAN_POINT('',(0.393903215690563,-31.2520475724682,56.6292251037768));
#87780=CARTESIAN_POINT('',(0.452117492759457,-31.2520475724682,56.6292251037768));
#87781=CARTESIAN_POINT('',(-1.54592528053767,-31.2520475724682,56.6292251037768));
#87782=CARTESIAN_POINT('',(0.145925152667093,-27.9455328192711,54.9976432278968));
#87783=CARTESIAN_POINT('Ctrl Pts',(0.145925280537677,-27.9452513492555,
54.9976452678552));
#87784=CARTESIAN_POINT('Ctrl Pts',(0.149739558055857,-27.9451705070726,
55.0681884787126));
#87785=CARTESIAN_POINT('Ctrl Pts',(0.153553835574038,-27.9487267508694,
55.1387974637158));
#87786=CARTESIAN_POINT('Ctrl Pts',(0.157368113092218,-27.9559135127653,
55.209064571854));
#87787=CARTESIAN_POINT('Ctrl Pts',(0.161181088392145,-27.9630978210556,
55.279307690361));
#87788=CARTESIAN_POINT('Ctrl Pts',(0.164994063692073,-27.9739101382345,
55.3492086695877));
#87789=CARTESIAN_POINT('Ctrl Pts',(0.168807038992,-27.9882919346166,55.4183637438539));
#87790=CARTESIAN_POINT('Ctrl Pts',(0.172620052583361,-28.0026738754265,
55.4875195126033));
#87791=CARTESIAN_POINT('Ctrl Pts',(0.176433066174722,-28.0206252631438,
55.5559288755018));
#87792=CARTESIAN_POINT('Ctrl Pts',(0.180246079766083,-28.0420365947538,
55.6231988977981));
#87793=CARTESIAN_POINT('Ctrl Pts',(0.184063186873329,-28.0634709128085,
55.6905411387998));
#87794=CARTESIAN_POINT('Ctrl Pts',(0.187880293980576,-28.0883724380495,
55.7567411231829));
#87795=CARTESIAN_POINT('Ctrl Pts',(0.191697401087823,-28.1165822768063,
55.8214226941471));
#87796=CARTESIAN_POINT('Ctrl Pts',(0.195516676866285,-28.1448081428486,
55.8861410136376));
#87797=CARTESIAN_POINT('Ctrl Pts',(0.199335952644747,-28.1763458387153,
55.9493387592996));
#87798=CARTESIAN_POINT('Ctrl Pts',(0.203155228423209,-28.2109902488435,
56.0106639761894));
#87799=CARTESIAN_POINT('Ctrl Pts',(0.206981583712272,-28.2456988767667,
56.0721028671232));
#87800=CARTESIAN_POINT('Ctrl Pts',(0.210807939001335,-28.283525447051,56.1316618817862));
#87801=CARTESIAN_POINT('Ctrl Pts',(0.214634294290398,-28.324221670915,56.1890183153631));
#87802=CARTESIAN_POINT('Ctrl Pts',(0.217179710085972,-28.3512941206009,
56.2271736775747));
#87803=CARTESIAN_POINT('Ctrl Pts',(0.219725125881546,-28.3796356264345,
56.264354979052));
#87804=CARTESIAN_POINT('Ctrl Pts',(0.22227054167712,-28.4091638996304,56.3004760913838));
#87805=CARTESIAN_POINT('Ctrl Pts',(0.226143006984167,-28.4540867030981,
56.3554289028655));
#87806=CARTESIAN_POINT('Ctrl Pts',(0.230015472291213,-28.5019476711101,
56.4081582801573));
#87807=CARTESIAN_POINT('Ctrl Pts',(0.23388793759826,-28.5524985386363,56.4583336661581));
#87808=CARTESIAN_POINT('Ctrl Pts',(0.237754613392442,-28.602973830302,56.5084340376604));
#87809=CARTESIAN_POINT('Ctrl Pts',(0.241621289186625,-28.6561306971562,
56.5559876587984));
#87810=CARTESIAN_POINT('Ctrl Pts',(0.245487964980807,-28.7116807291363,
56.6006970415482));
#87811=CARTESIAN_POINT('Ctrl Pts',(0.249350054695347,-28.7671648758744,
56.6453533966327));
#87812=CARTESIAN_POINT('Ctrl Pts',(0.253212144409888,-28.8250361733924,
56.6871719121174));
#87813=CARTESIAN_POINT('Ctrl Pts',(0.257074234124429,-28.884970754992,56.7258932021643));
#87814=CARTESIAN_POINT('Ctrl Pts',(0.260933857400563,-28.9448670606931,
56.7645897637133));
#87815=CARTESIAN_POINT('Ctrl Pts',(0.264793480676698,-29.0068236298311,
56.8001927619133));
#87816=CARTESIAN_POINT('Ctrl Pts',(0.268653103952832,-29.070486209859,56.8324851094723));
#87817=CARTESIAN_POINT('Ctrl Pts',(0.272511547105436,-29.134129324332,56.8647675832803));
#87818=CARTESIAN_POINT('Ctrl Pts',(0.27636999025804,-29.1994769819466,56.8937411970124));
#87819=CARTESIAN_POINT('Ctrl Pts',(0.280228433410645,-29.2661503428946,
56.9192348067046));
#87820=CARTESIAN_POINT('Ctrl Pts',(0.284086981101935,-29.3328255102566,
56.9447291071076));
#87821=CARTESIAN_POINT('Ctrl Pts',(0.287945528793224,-29.4008259986621,
56.9667430451765));
#87822=CARTESIAN_POINT('Ctrl Pts',(0.291804076484514,-29.4697546186279,
56.9851542504384));
#87823=CARTESIAN_POINT('Ctrl Pts',(0.295666566280546,-29.5387536598665,
57.0035842656011));
#87824=CARTESIAN_POINT('Ctrl Pts',(0.299529056076578,-29.6086822562916,
57.0184040747128));
#87825=CARTESIAN_POINT('Ctrl Pts',(0.30339154587261,-29.679130615291,57.0295419188715));
#87826=CARTESIAN_POINT('Ctrl Pts',(0.307256172571424,-29.7496179494858,
57.0406859249856));
#87827=CARTESIAN_POINT('Ctrl Pts',(0.311120799270237,-29.8206251363632,
57.0481438597316));
#87828=CARTESIAN_POINT('Ctrl Pts',(0.31498542596905,-29.8917375229701,57.0518959034433));
#87829=CARTESIAN_POINT('Ctrl Pts',(0.318856698894589,-29.962972205747,57.0556543997661));
#87830=CARTESIAN_POINT('Ctrl Pts',(0.322727971820127,-30.0343119644734,
57.0556942799084));
#87831=CARTESIAN_POINT('Ctrl Pts',(0.326599244745665,-30.1053431155557,
57.0520478528789));
#87832=CARTESIAN_POINT('Ctrl Pts',(0.328868100669004,-30.1469726908851,
57.0499107734934));
#87833=CARTESIAN_POINT('Ctrl Pts',(0.331136956592343,-30.1884963605189,
57.0465084894332));
#87834=CARTESIAN_POINT('Ctrl Pts',(0.333405812515682,-30.2298323520304,
57.0418556884511));
#87835=CARTESIAN_POINT('Ctrl Pts',(0.337281012319212,-30.3004341141503,
57.0339087169108));
#87836=CARTESIAN_POINT('Ctrl Pts',(0.341156212122742,-30.3707563721026,
57.0222806500465));
#87837=CARTESIAN_POINT('Ctrl Pts',(0.345031411926271,-30.4403862442338,
57.0070021221687));
#87838=CARTESIAN_POINT('Ctrl Pts',(0.349104062239962,-30.5135639215033,
56.9909451174957));
#87839=CARTESIAN_POINT('Ctrl Pts',(0.353176712553653,-30.5859762357596,
56.9708557003268));
#87840=CARTESIAN_POINT('Ctrl Pts',(0.357249362867344,-30.6571493257187,
56.9468313553586));
#87841=CARTESIAN_POINT('Ctrl Pts',(0.361114528254948,-30.7246964369731,
56.9240309528004));
#87842=CARTESIAN_POINT('Ctrl Pts',(0.364979693642552,-30.7911269703477,
56.897686913658));
#87843=CARTESIAN_POINT('Ctrl Pts',(0.368844859030155,-30.8560479883579,
56.8679345288656));
#87844=CARTESIAN_POINT('Ctrl Pts',(0.372707534701384,-30.9209271879967,
56.8382013088417));
#87845=CARTESIAN_POINT('Ctrl Pts',(0.376570210372613,-30.9842983642662,
56.8050643040583));
#87846=CARTESIAN_POINT('Ctrl Pts',(0.380432886043842,-31.0457881929967,
56.7687070469381));
#87847=CARTESIAN_POINT('Ctrl Pts',(0.384294620004037,-31.107263030655,56.7323586536297));
#87848=CARTESIAN_POINT('Ctrl Pts',(0.388156353964232,-31.1668570150223,
56.692791812487));
#87849=CARTESIAN_POINT('Ctrl Pts',(0.392018087924427,-31.2242225181329,
56.6502353736956));
#87850=CARTESIAN_POINT('Ctrl Pts',(0.392646463846472,-31.2335569521676,
56.6433106497917));
#87851=CARTESIAN_POINT('Ctrl Pts',(0.393274839768517,-31.2428324444266,
56.6363068622567));
#87852=CARTESIAN_POINT('Ctrl Pts',(0.393903215690563,-31.2520475724682,
56.6292251037768));
#87853=CARTESIAN_POINT('',(0.,-29.4698297828114,53.0148256743283));
#87854=CARTESIAN_POINT('Ctrl Pts',(-2.77555756156289E-16,-29.4698297828114,
53.0148256743283));
#87855=CARTESIAN_POINT('Ctrl Pts',(0.0370450902795195,-28.8097276504722,
53.1911157292334));
#87856=CARTESIAN_POINT('Ctrl Pts',(0.085686536603176,-28.0750579168316,
53.887168576849));
#87857=CARTESIAN_POINT('Ctrl Pts',(0.134327982926832,-27.9457073141171,
54.7833755124352));
#87858=CARTESIAN_POINT('Ctrl Pts',(0.145924338970969,-27.9473239353676,
54.9976302467543));
#87859=CARTESIAN_POINT('',(5.31147209548166E-9,-30.5303401832825,53.0148710740871));
#87860=CARTESIAN_POINT('Origin',(0.,-30.,55.));
#87861=CARTESIAN_POINT('',(0.204074719418397,-27.9452505428834,55.0014936462286));
#87862=CARTESIAN_POINT('Ctrl Pts',(5.31147215099281E-9,-30.5303401832825,
53.0148710740871));
#87863=CARTESIAN_POINT('Ctrl Pts',(0.00385890060565744,-30.4620053990835,
52.9966149893042));
#87864=CARTESIAN_POINT('Ctrl Pts',(0.00771779589984257,-30.3925893645069,
52.9818548053524));
#87865=CARTESIAN_POINT('Ctrl Pts',(0.0115766911940278,-30.322484042902,
52.9707140160703));
#87866=CARTESIAN_POINT('Ctrl Pts',(0.0154298196873703,-30.2524834879199,
52.9595898757792));
#87867=CARTESIAN_POINT('Ctrl Pts',(0.0192829481807127,-30.1817961688685,
52.952074471318));
#87868=CARTESIAN_POINT('Ctrl Pts',(0.0231360766740552,-30.1108274410599,
52.9482410373516));
#87869=CARTESIAN_POINT('Ctrl Pts',(0.0269846844776238,-30.0399419774359,
52.9444121009683));
#87870=CARTESIAN_POINT('Ctrl Pts',(0.0308332922811925,-29.9687762463427,
52.9442565816047));
#87871=CARTESIAN_POINT('Ctrl Pts',(0.0346819000847611,-29.8977422088653,
52.947796085509));
#87872=CARTESIAN_POINT('Ctrl Pts',(0.0385281035507021,-29.8267525484244,
52.9513333781819));
#87873=CARTESIAN_POINT('Ctrl Pts',(0.042374307016643,-29.7558949052976,
52.9585610906355));
#87874=CARTESIAN_POINT('Ctrl Pts',(0.0462205104825839,-29.6855812197391,
52.9694487464929));
#87875=CARTESIAN_POINT('Ctrl Pts',(0.0500656158362666,-29.6152876091248,
52.9803332938646));
#87876=CARTESIAN_POINT('Ctrl Pts',(0.0539107211899489,-29.5455381304157,
52.9948756354664));
#87877=CARTESIAN_POINT('Ctrl Pts',(0.0577558265436315,-29.4767378155319,
53.012993646511));
#87878=CARTESIAN_POINT('Ctrl Pts',(0.0616011384233991,-29.4079338052853,
53.0311126306998));
#87879=CARTESIAN_POINT('Ctrl Pts',(0.0654464503031668,-29.3400795319328,
53.0528075386411));
#87880=CARTESIAN_POINT('Ctrl Pts',(0.0692917621829343,-29.2735663538694,
53.0779459632286));
#87881=CARTESIAN_POINT('Ctrl Pts',(0.0731410484831663,-29.2069844294093,
53.1031103702778));
#87882=CARTESIAN_POINT('Ctrl Pts',(0.0769903347833989,-29.1417468242309,
53.1317252233557));
#87883=CARTESIAN_POINT('Ctrl Pts',(0.0808396210836309,-29.0782254133911,
53.1636097435507));
#87884=CARTESIAN_POINT('Ctrl Pts',(0.0846911736894365,-29.0146666036892,
53.1955130360739));
#87885=CARTESIAN_POINT('Ctrl Pts',(0.0885427262952419,-28.9528264236558,
53.2306895847781));
#87886=CARTESIAN_POINT('Ctrl Pts',(0.0923942789010475,-28.8930501979511,
53.2689137230502));
#87887=CARTESIAN_POINT('Ctrl Pts',(0.0962522709070446,-28.8331740325393,
53.3072017681538));
#87888=CARTESIAN_POINT('Ctrl Pts',(0.100110262913041,-28.7753691044501,
53.3485472865186));
#87889=CARTESIAN_POINT('Ctrl Pts',(0.103968254919039,-28.719949233271,53.3926831061995));
#87890=CARTESIAN_POINT('Ctrl Pts',(0.105632468402095,-28.696042885953,53.4117218771676));
#87891=CARTESIAN_POINT('Ctrl Pts',(0.107296681885152,-28.6725798933521,
53.4312793816445));
#87892=CARTESIAN_POINT('Ctrl Pts',(0.108960895368209,-28.6495832862577,
53.4513321008862));
#87893=CARTESIAN_POINT('Ctrl Pts',(0.1129239713703,-28.594820299037,53.4990846586035));
#87894=CARTESIAN_POINT('Ctrl Pts',(0.116887047372392,-28.5424701409817,
53.549853287079));
#87895=CARTESIAN_POINT('Ctrl Pts',(0.120850123374483,-28.4928872821031,
53.6033580208037));
#87896=CARTESIAN_POINT('Ctrl Pts',(0.124661299720926,-28.4452048710549,
53.6548119862302));
#87897=CARTESIAN_POINT('Ctrl Pts',(0.128472476067368,-28.4000818931433,
53.708795745255));
#87898=CARTESIAN_POINT('Ctrl Pts',(0.132283652413811,-28.3578002588971,
53.7650192014361));
#87899=CARTESIAN_POINT('Ctrl Pts',(0.136091341654092,-28.3155573110128,
53.8211912149279));
#87900=CARTESIAN_POINT('Ctrl Pts',(0.139899030894372,-28.276150852727,53.879598466174));
#87901=CARTESIAN_POINT('Ctrl Pts',(0.143706720134652,-28.2398237521968,
53.939916447081));
#87902=CARTESIAN_POINT('Ctrl Pts',(0.147512279870369,-28.2035169681162,
54.0002006942961));
#87903=CARTESIAN_POINT('Ctrl Pts',(0.151317839606087,-28.1702863835626,
54.0623931243556));
#87904=CARTESIAN_POINT('Ctrl Pts',(0.155123399341804,-28.1403314967629,
54.1261403885246));
#87905=CARTESIAN_POINT('Ctrl Pts',(0.158928184118078,-28.1103827099391,
54.1898746712801));
#87906=CARTESIAN_POINT('Ctrl Pts',(0.162732968894353,-28.0837085076307,
54.2551627066053));
#87907=CARTESIAN_POINT('Ctrl Pts',(0.166537753670627,-28.0604615061024,
54.3216284254264));
#87908=CARTESIAN_POINT('Ctrl Pts',(0.170345033971954,-28.0371992570692,
54.3881377385311));
#87909=CARTESIAN_POINT('Ctrl Pts',(0.17415231427328,-28.0173688617457,54.4558258046817));
#87910=CARTESIAN_POINT('Ctrl Pts',(0.177959594574607,-28.001073570741,54.5242997867252));
#87911=CARTESIAN_POINT('Ctrl Pts',(0.181768385432865,-27.9847718145004,
54.5928009361533));
#87912=CARTESIAN_POINT('Ctrl Pts',(0.185577176291123,-27.9720080458716,
54.6620881305532));
#87913=CARTESIAN_POINT('Ctrl Pts',(0.189385967149382,-27.9628341983099,
54.7317593264916));
#87914=CARTESIAN_POINT('Ctrl Pts',(0.193199808147877,-27.9536481869885,
54.8015229006474));
#87915=CARTESIAN_POINT('Ctrl Pts',(0.197013649146372,-27.9480616306873,
54.8716709942671));
#87916=CARTESIAN_POINT('Ctrl Pts',(0.200827490144868,-27.9460744487514,
54.9417986904941));
#87917=CARTESIAN_POINT('Ctrl Pts',(0.201909899902711,-27.9455104647996,
54.9617016971274));
#87918=CARTESIAN_POINT('Ctrl Pts',(0.202992309660554,-27.945236083957,54.9816030786799));
#87919=CARTESIAN_POINT('Ctrl Pts',(0.204074719418397,-27.9452505428834,
55.0014936462286));
#87920=CARTESIAN_POINT('Ctrl Pts',(0.204074719462322,-27.945250542884,55.0014936470358));
#87921=CARTESIAN_POINT('Ctrl Pts',(0.209415201710472,-27.9453218815624,
55.0996313644095));
#87922=CARTESIAN_POINT('Ctrl Pts',(0.214755683958621,-27.9524246358466,
55.1975148488935));
#87923=CARTESIAN_POINT('Ctrl Pts',(0.22009616620677,-27.9664469146436,55.2943797063953));
#87924=CARTESIAN_POINT('Ctrl Pts',(0.223961020165476,-27.9765946985329,
55.3644798416603));
#87925=CARTESIAN_POINT('Ctrl Pts',(0.227825874124181,-27.9903917548322,
55.4341948503752));
#87926=CARTESIAN_POINT('Ctrl Pts',(0.231690728082887,-28.0077969414506,
55.5031148338168));
#87927=CARTESIAN_POINT('Ctrl Pts',(0.235549755777647,-28.0251758897655,
55.5719309204439));
#87928=CARTESIAN_POINT('Ctrl Pts',(0.239408783472407,-28.0461520542666,
55.6399538923791));
#87929=CARTESIAN_POINT('Ctrl Pts',(0.243267811167167,-28.0706328265759,
55.7067813471035));
#87930=CARTESIAN_POINT('Ctrl Pts',(0.247122236420484,-28.0950844020693,
55.7735291005479));
#87931=CARTESIAN_POINT('Ctrl Pts',(0.250976661673801,-28.1230321167656,
55.8390837137948));
#87932=CARTESIAN_POINT('Ctrl Pts',(0.254831086927118,-28.1543333061832,
55.9030570401892));
#87933=CARTESIAN_POINT('Ctrl Pts',(0.258683039994727,-28.1856144193642,
55.9669893348));
#87934=CARTESIAN_POINT('Ctrl Pts',(0.262534993062336,-28.220244526808,56.0293419181982));
#87935=CARTESIAN_POINT('Ctrl Pts',(0.266386946129945,-28.2580330866495,
56.0897471428235));
#87936=CARTESIAN_POINT('Ctrl Pts',(0.270237725008371,-28.2958101274207,
56.1501339541504));
#87937=CARTESIAN_POINT('Ctrl Pts',(0.274088503886798,-28.3367434512255,
56.2085741724364));
#87938=CARTESIAN_POINT('Ctrl Pts',(0.277939282765224,-28.3805977331326,
56.2647267928547));
#87939=CARTESIAN_POINT('Ctrl Pts',(0.281790183797984,-28.4244534061843,
56.3208811945454));
#87940=CARTESIAN_POINT('Ctrl Pts',(0.285641084830744,-28.4712299197825,
56.3747474718326));
#87941=CARTESIAN_POINT('Ctrl Pts',(0.289491985863504,-28.5206510640933,
56.4260169312921));
#87942=CARTESIAN_POINT('Ctrl Pts',(0.293346909493499,-28.5701238330386,
56.4773399461102));
#87943=CARTESIAN_POINT('Ctrl Pts',(0.297201833123494,-28.6222464086909,
56.5260603767546));
#87944=CARTESIAN_POINT('Ctrl Pts',(0.30105675675349,-28.6767056801163,56.5719063920805));
#87945=CARTESIAN_POINT('Ctrl Pts',(0.30491385131992,-28.7311956207916,56.6177782260203));
#87946=CARTESIAN_POINT('Ctrl Pts',(0.308770945886351,-28.7880244880892,
56.6607721284675));
#87947=CARTESIAN_POINT('Ctrl Pts',(0.312628040452781,-28.8468482568665,
56.7006582901359));
#87948=CARTESIAN_POINT('Ctrl Pts',(0.316491917659155,-28.9057754663131,
56.7406145909904));
#87949=CARTESIAN_POINT('Ctrl Pts',(0.320355794865529,-28.9667041640678,
56.7774519883196));
#87950=CARTESIAN_POINT('Ctrl Pts',(0.324219672071903,-29.0292643129354,
56.8109858608944));
#87951=CARTESIAN_POINT('Ctrl Pts',(0.326556927063046,-29.0671068768622,
56.8312704628269));
#87952=CARTESIAN_POINT('Ctrl Pts',(0.328894182054188,-29.1055459530557,
56.8503472123624));
#87953=CARTESIAN_POINT('Ctrl Pts',(0.33123143704533,-29.1444964052382,56.868183920777));
#87954=CARTESIAN_POINT('Ctrl Pts',(0.335101212232454,-29.208986370584,56.8977160222825));
#87955=CARTESIAN_POINT('Ctrl Pts',(0.338970987419577,-29.2751333583356,
56.9239626235659));
#87956=CARTESIAN_POINT('Ctrl Pts',(0.342840762606701,-29.3425693897772,
56.9467363856573));
#87957=CARTESIAN_POINT('Ctrl Pts',(0.346704773776642,-29.4099049754758,
56.9694762263063));
#87958=CARTESIAN_POINT('Ctrl Pts',(0.350568784946584,-29.4785253373009,
56.9887533416089));
#87959=CARTESIAN_POINT('Ctrl Pts',(0.354432796116526,-29.5480410034477,
57.0044277557287));
#87960=CARTESIAN_POINT('Ctrl Pts',(0.358292273241919,-29.6174750996629,
57.0200837774347));
#87961=CARTESIAN_POINT('Ctrl Pts',(0.362151750367312,-29.6878019420199,
57.0321453888722));
#87962=CARTESIAN_POINT('Ctrl Pts',(0.366011227492706,-29.7586169935523,
57.0405224347451));
#87963=CARTESIAN_POINT('Ctrl Pts',(0.369868271988589,-29.8293874103378,
57.0488942005637));
#87964=CARTESIAN_POINT('Ctrl Pts',(0.373725316484471,-29.9006449446999,
57.053585951543));
#87965=CARTESIAN_POINT('Ctrl Pts',(0.377582360980354,-29.9719764123368,
57.0545588920823));
#87966=CARTESIAN_POINT('Ctrl Pts',(0.381438263340815,-30.0432867575323,
57.0555315445176));
#87967=CARTESIAN_POINT('Ctrl Pts',(0.385294165701275,-30.1146705072659,
57.0527875661136));
#87968=CARTESIAN_POINT('Ctrl Pts',(0.389150068061736,-30.1857126517967,
57.0463402389296));
#87969=CARTESIAN_POINT('Ctrl Pts',(0.393006117165451,-30.2567574999633,
57.0398926663811));
#87970=CARTESIAN_POINT('Ctrl Pts',(0.396862166269167,-30.3274602337197,
57.0297415113169));
#87971=CARTESIAN_POINT('Ctrl Pts',(0.400718215372883,-30.3974108749329,
57.0159519237782));
#87972=CARTESIAN_POINT('Ctrl Pts',(0.404578289322704,-30.4674345288485,
57.0021479430184));
#87973=CARTESIAN_POINT('Ctrl Pts',(0.408438363272525,-30.5367040457586,
56.9846980427912));
#87974=CARTESIAN_POINT('Ctrl Pts',(0.412298437222346,-30.6048204469937,
56.9637183579623));
#87975=CARTESIAN_POINT('Ctrl Pts',(0.41616069125129,-30.6729753187727,56.9427268243002));
#87976=CARTESIAN_POINT('Ctrl Pts',(0.420022945280233,-30.7399753221862,
56.9182017044133));
#87977=CARTESIAN_POINT('Ctrl Pts',(0.423885199309177,-30.8054400360123,
56.8903078878555));
#87978=CARTESIAN_POINT('Ctrl Pts',(0.427754194419916,-30.8710190103161,
56.8623653861264));
#87979=CARTESIAN_POINT('Ctrl Pts',(0.431623189530655,-30.9350569086456,
56.8310426622144));
#87980=CARTESIAN_POINT('Ctrl Pts',(0.435492184641395,-30.9971971788319,
56.7965509592076));
#87981=CARTESIAN_POINT('Ctrl Pts',(0.437783692388893,-31.0340012859677,
56.7761223976813));
#87982=CARTESIAN_POINT('Ctrl Pts',(0.440075200136391,-31.070140249418,56.7545830404281));
#87983=CARTESIAN_POINT('Ctrl Pts',(0.44236670788389,-31.1055451381042,56.7319836922195));
#87984=CARTESIAN_POINT('Ctrl Pts',(0.445616969509079,-31.1557632319189,
56.6999289045728));
#87985=CARTESIAN_POINT('Ctrl Pts',(0.448867231134268,-31.204668249553,56.6656357667991));
#87986=CARTESIAN_POINT('Ctrl Pts',(0.452117492759457,-31.2520475724682,
56.6292251037768));
#87987=CARTESIAN_POINT('Origin',(-1.54592528053767,30.,55.));
#87988=CARTESIAN_POINT('',(9.49394873882619,28.7479524050421,56.6292250864936));
#87989=CARTESIAN_POINT('',(9.55204617709054,28.7459570691003,56.6318367151304));
#87990=CARTESIAN_POINT('',(-1.54592528053767,28.7479524050421,56.6292250864936));
#87991=CARTESIAN_POINT('',(10.,32.0533758325287,54.9248651020699));
#87992=CARTESIAN_POINT('Ctrl Pts',(9.55204617709054,28.7459570691003,56.6318367151304));
#87993=CARTESIAN_POINT('Ctrl Pts',(9.55318375694229,28.7293604144358,56.6191575145376));
#87994=CARTESIAN_POINT('Ctrl Pts',(9.59136642707355,28.1793878778151,56.1844488346597));
#87995=CARTESIAN_POINT('Ctrl Pts',(9.66659418748432,27.5871748102564,54.7282396850668));
#87996=CARTESIAN_POINT('Ctrl Pts',(9.77772945832289,28.9189493130402,52.8236099253744));
#87997=CARTESIAN_POINT('Ctrl Pts',(9.88886472916144,31.2437676373092,52.9151786827749));
#87998=CARTESIAN_POINT('Ctrl Pts',(9.96295490972048,32.0283922803563,54.2420848806971));
#87999=CARTESIAN_POINT('Ctrl Pts',(10.,32.0533758325287,54.92486510207));
#88000=CARTESIAN_POINT('',(9.99999281908575,31.8181858731057,55.9591737972435));
#88001=CARTESIAN_POINT('Origin',(10.,30.,55.));
#88002=CARTESIAN_POINT('',(9.94592528058885,32.054749999972,55.0000107214664));
#88003=CARTESIAN_POINT('Ctrl Pts',(9.94592528058884,32.054749999972,55.0000107214664));
#88004=CARTESIAN_POINT('Ctrl Pts',(9.94992923499555,32.0547496125334,55.0742626500147));
#88005=CARTESIAN_POINT('Ctrl Pts',(9.95393318940226,32.0507200896955,55.1484433401657));
#88006=CARTESIAN_POINT('Ctrl Pts',(9.95793714380898,32.0427102750594,55.2221087451377));
#88007=CARTESIAN_POINT('Ctrl Pts',(9.96195105284767,32.0346805464212,55.2959572970492));
#88008=CARTESIAN_POINT('Ctrl Pts',(9.96596496188636,32.0226508056886,55.3692875772289));
#88009=CARTESIAN_POINT('Ctrl Pts',(9.96997887092505,32.0067214128151,55.4416635980576));
#88010=CARTESIAN_POINT('Ctrl Pts',(9.97399818909952,31.9907705535238,55.514137152667));
#88011=CARTESIAN_POINT('Ctrl Pts',(9.978017507274,31.9709096843372,55.5856534725178));
#88012=CARTESIAN_POINT('Ctrl Pts',(9.98203682544847,31.9472888596583,55.6557923905861));
#88013=CARTESIAN_POINT('Ctrl Pts',(9.98606643459486,31.9236075567508,55.726110890764));
#88014=CARTESIAN_POINT('Ctrl Pts',(9.99009604374126,31.896147221868,55.7950445439403));
#88015=CARTESIAN_POINT('Ctrl Pts',(9.99412565288765,31.86510586548,55.8621935241303));
#88016=CARTESIAN_POINT('Ctrl Pts',(9.99608057294537,31.8500464966883,55.8947701049995));
#88017=CARTESIAN_POINT('Ctrl Pts',(9.99803549300309,31.8341449817694,55.9269270350611));
#88018=CARTESIAN_POINT('Ctrl Pts',(9.9999904130608,31.8174276447438,55.9586210505831));
#88019=CARTESIAN_POINT('Ctrl Pts',(9.49394873882619,28.7479524050421,56.6292250864936));
#88020=CARTESIAN_POINT('Ctrl Pts',(9.4978046533836,28.691402000007,56.5857665127182));
#88021=CARTESIAN_POINT('Ctrl Pts',(9.50166056794101,28.6371010084152,56.5393479750722));
#88022=CARTESIAN_POINT('Ctrl Pts',(9.50551648249842,28.5853662515599,56.4902378737216));
#88023=CARTESIAN_POINT('Ctrl Pts',(9.50937266247207,28.5336279336182,56.441124391949));
#88024=CARTESIAN_POINT('Ctrl Pts',(9.51322884244571,28.4844565516489,56.3893193146642));
#88025=CARTESIAN_POINT('Ctrl Pts',(9.51708502241936,28.4381327212654,56.3351285204497));
#88026=CARTESIAN_POINT('Ctrl Pts',(9.52094529771214,28.3917596943012,56.2808801748247));
#88027=CARTESIAN_POINT('Ctrl Pts',(9.52480557300492,28.3482405707212,56.2242414252943));
#88028=CARTESIAN_POINT('Ctrl Pts',(9.5286658482977,28.3078156308828,56.1655512101214));
#88029=CARTESIAN_POINT('Ctrl Pts',(9.53252841044457,28.2673667430272,56.1068262264544));
#88030=CARTESIAN_POINT('Ctrl Pts',(9.53639097259144,28.2300159415455,56.0460477720046));
#88031=CARTESIAN_POINT('Ctrl Pts',(9.54025353473831,28.1959586525825,55.9835814045152));
#88032=CARTESIAN_POINT('Ctrl Pts',(9.54412272140385,28.1618429533888,55.9210079035736));
#88033=CARTESIAN_POINT('Ctrl Pts',(9.54799190806938,28.1310322513002,55.8567411489902));
#88034=CARTESIAN_POINT('Ctrl Pts',(9.55186109473492,28.1036744331779,55.791168065026));
#88035=CARTESIAN_POINT('Ctrl Pts',(9.55378516052864,28.0900699610782,55.7585599386287));
#88036=CARTESIAN_POINT('Ctrl Pts',(9.55570922632237,28.0773185709614,55.7256290338948));
#88037=CARTESIAN_POINT('Ctrl Pts',(9.55763329211609,28.0654338157958,55.6924241773895));
#88038=CARTESIAN_POINT('Ctrl Pts',(9.56150302050322,28.0415309042693,55.6256417543415));
#88039=CARTESIAN_POINT('Ctrl Pts',(9.56537274889035,28.0210434541086,55.5574898205418));
#88040=CARTESIAN_POINT('Ctrl Pts',(9.56924247727748,28.0041265586444,55.4883510710455));
#88041=CARTESIAN_POINT('Ctrl Pts',(9.5731064517937,27.9872348167886,55.4193151234515));
#88042=CARTESIAN_POINT('Ctrl Pts',(9.57697042630992,27.9739032056838,55.3492957405771));
#88043=CARTESIAN_POINT('Ctrl Pts',(9.58083440082614,27.9642377859759,55.2786929680703));
#88044=CARTESIAN_POINT('Ctrl Pts',(9.58469385650073,27.9545836697849,55.2081727641071));
#88045=CARTESIAN_POINT('Ctrl Pts',(9.58855331217531,27.9485872939616,55.1370710045039));
#88046=CARTESIAN_POINT('Ctrl Pts',(9.5924127678499,27.9463037898525,55.0657984720641));
#88047=CARTESIAN_POINT('Ctrl Pts',(9.59626980028674,27.944021719488,54.9945706895333));
#88048=CARTESIAN_POINT('Ctrl Pts',(9.60012683272359,27.9454479112186,54.9231728310949));
#88049=CARTESIAN_POINT('Ctrl Pts',(9.60398386516044,27.9505855838444,54.8520198886547));
#88050=CARTESIAN_POINT('Ctrl Pts',(9.60783976484055,27.9557217476073,54.7808878428433));
#88051=CARTESIAN_POINT('Ctrl Pts',(9.61169566452066,27.9645671933069,54.7100010542932));
#88052=CARTESIAN_POINT('Ctrl Pts',(9.61555156420076,27.9770730972883,54.6397718656387));
#88053=CARTESIAN_POINT('Ctrl Pts',(9.6194076199994,27.9895795076116,54.5695398335291));
#88054=CARTESIAN_POINT('Ctrl Pts',(9.62326367579804,28.0057465831644,54.4999659318545));
#88055=CARTESIAN_POINT('Ctrl Pts',(9.62711973159668,28.0254742551705,54.4314530401933));
#88056=CARTESIAN_POINT('Ctrl Pts',(9.63097982647678,28.0452225912122,54.362868383712));
#88057=CARTESIAN_POINT('Ctrl Pts',(9.63483992135688,28.0685388341787,54.2953474233671));
#88058=CARTESIAN_POINT('Ctrl Pts',(9.63870001623698,28.0952730616512,54.229277707064));
#88059=CARTESIAN_POINT('Ctrl Pts',(9.64256229925823,28.1220224437418,54.1631705383484));
#88060=CARTESIAN_POINT('Ctrl Pts',(9.64642458227949,28.152193461956,54.098516691584));
#88061=CARTESIAN_POINT('Ctrl Pts',(9.65028686530075,28.185589211249,54.0356810423082));
#88062=CARTESIAN_POINT('Ctrl Pts',(9.65415590181592,28.2190433555348,53.9727355201483));
#88063=CARTESIAN_POINT('Ctrl Pts',(9.65802493833108,28.2557332387271,53.9116149594333));
#88064=CARTESIAN_POINT('Ctrl Pts',(9.66189397484625,28.2954178206257,53.8526564785299));
#88065=CARTESIAN_POINT('Ctrl Pts',(9.66418550421571,28.3189219629564,53.8177369087509));
#88066=CARTESIAN_POINT('Ctrl Pts',(9.66647703358517,28.3434758107717,53.7835751766599));
#88067=CARTESIAN_POINT('Ctrl Pts',(9.66876856295463,28.3690228362396,53.7502356006862));
#88068=CARTESIAN_POINT('Ctrl Pts',(9.67263319854557,28.4121075748347,53.6940088232283));
#88069=CARTESIAN_POINT('Ctrl Pts',(9.67649783413651,28.4581888703725,53.639900970039));
#88070=CARTESIAN_POINT('Ctrl Pts',(9.68036246972745,28.5070304189907,53.5882495288894));
#88071=CARTESIAN_POINT('Ctrl Pts',(9.68422132903282,28.5557989664874,53.5366752886731));
#88072=CARTESIAN_POINT('Ctrl Pts',(9.68808018833819,28.6073192465963,53.4875505241705));
#88073=CARTESIAN_POINT('Ctrl Pts',(9.69193904764356,28.6613137277076,53.4411810153594));
#88074=CARTESIAN_POINT('Ctrl Pts',(9.69579337937049,28.7152448573906,53.3948659116385));
#88075=CARTESIAN_POINT('Ctrl Pts',(9.69964771109743,28.7716440546169,53.3512999585715));
#88076=CARTESIAN_POINT('Ctrl Pts',(9.70350204282436,28.8301970897572,53.3107520271768));
#88077=CARTESIAN_POINT('Ctrl Pts',(9.70735394857745,28.8887132707444,53.2702296172545));
#88078=CARTESIAN_POINT('Ctrl Pts',(9.71120585433055,28.9493802008428,53.2327217371875));
#88079=CARTESIAN_POINT('Ctrl Pts',(9.71505776008364,29.0118519125401,53.1984559623064));
#88080=CARTESIAN_POINT('Ctrl Pts',(9.71890853777658,29.0743053289173,53.1642002224204));
#88081=CARTESIAN_POINT('Ctrl Pts',(9.72275931546952,29.1385620508987,53.133184936992));
#88082=CARTESIAN_POINT('Ctrl Pts',(9.72661009316246,29.2042500770591,53.105592540492));
#88083=CARTESIAN_POINT('Ctrl Pts',(9.73046103910404,29.2699409732687,53.0779989384217));
#88084=CARTESIAN_POINT('Ctrl Pts',(9.73431198504562,29.3370628479334,53.0538287087524));
#88085=CARTESIAN_POINT('Ctrl Pts',(9.7381629309872,29.4052238384774,53.0332161074016));
#88086=CARTESIAN_POINT('Ctrl Pts',(9.74201796951611,29.4734572670173,53.012581600038));
#88087=CARTESIAN_POINT('Ctrl Pts',(9.74587300804502,29.5427315487197,52.9955124095462));
#88088=CARTESIAN_POINT('Ctrl Pts',(9.74972804657392,29.6126406530814,52.982092594083));
#88089=CARTESIAN_POINT('Ctrl Pts',(9.75358529565015,29.6825898445608,52.9686650834601));
#88090=CARTESIAN_POINT('Ctrl Pts',(9.75744254472639,29.7531741006322,52.9588911798621));
#88091=CARTESIAN_POINT('Ctrl Pts',(9.76129979380262,29.8239809778604,52.9528031686364));
#88092=CARTESIAN_POINT('Ctrl Pts',(9.76516388654014,29.8949134830361,52.9467043558561));
#88093=CARTESIAN_POINT('Ctrl Pts',(9.76902797927766,29.966068911074,52.9443045080096));
#88094=CARTESIAN_POINT('Ctrl Pts',(9.77289207201518,30.0370342234693,52.9455837742093));
#88095=CARTESIAN_POINT('Ctrl Pts',(9.77522932594121,30.0799586474608,52.9463575573845));
#88096=CARTESIAN_POINT('Ctrl Pts',(9.77756657986724,30.1228135799402,52.9484763725428));
#88097=CARTESIAN_POINT('Ctrl Pts',(9.77990383379327,30.1655090399434,52.9519266809518));
#88098=CARTESIAN_POINT('Ctrl Pts',(9.78377991976378,30.2363148996234,52.9576486488858));
#88099=CARTESIAN_POINT('Ctrl Pts',(9.78765600573429,30.3069601528984,52.9670577856244));
#88100=CARTESIAN_POINT('Ctrl Pts',(9.79153209170481,30.3770311499455,52.9801373624747));
#88101=CARTESIAN_POINT('Ctrl Pts',(9.79540239402569,30.4469975914953,52.99319742281));
#88102=CARTESIAN_POINT('Ctrl Pts',(9.79927269634657,30.5163910059807,53.0099169627378));
#88103=CARTESIAN_POINT('Ctrl Pts',(9.80314299866746,30.5848021793035,53.0302274310007));
#88104=CARTESIAN_POINT('Ctrl Pts',(9.80700870784549,30.653132164578,53.0505137954924));
#88105=CARTESIAN_POINT('Ctrl Pts',(9.81087441702353,30.7204817628165,53.0743824851228));
#88106=CARTESIAN_POINT('Ctrl Pts',(9.81474012620157,30.7864529913537,53.1017141271951));
#88107=CARTESIAN_POINT('Ctrl Pts',(9.81860336270708,30.8523820218784,53.1290282867829));
#88108=CARTESIAN_POINT('Ctrl Pts',(9.82246659921258,30.9169339861647,53.1598008188452));
#88109=CARTESIAN_POINT('Ctrl Pts',(9.82632983571809,30.9797284531328,53.1938633161851));
#88110=CARTESIAN_POINT('Ctrl Pts',(9.83019188108792,31.0425035589435,53.2279153111765));
#88111=CARTESIAN_POINT('Ctrl Pts',(9.83405392645776,31.1035218182551,53.2652550267964));
#88112=CARTESIAN_POINT('Ctrl Pts',(9.83791597182759,31.1624266341236,53.3056677177189));
#88113=CARTESIAN_POINT('Ctrl Pts',(9.8417781059365,31.2213328034613,53.3460813372127));
#88114=CARTESIAN_POINT('Ctrl Pts',(9.84564024004541,31.2781250351691,53.3895677966547));
#88115=CARTESIAN_POINT('Ctrl Pts',(9.84950237415431,31.3324764296357,53.4358695300694));
#88116=CARTESIAN_POINT('Ctrl Pts',(9.85336840341607,31.386882640166,53.4822179610674));
#88117=CARTESIAN_POINT('Ctrl Pts',(9.85723443267783,31.43884272998,53.5313870198914));
#88118=CARTESIAN_POINT('Ctrl Pts',(9.86110046193959,31.4880642720665,53.5830800006002));
#88119=CARTESIAN_POINT('Ctrl Pts',(9.86496860676023,31.5373127490423,53.6348012686128));
#88120=CARTESIAN_POINT('Ctrl Pts',(9.86883675158086,31.5838193791356,53.6890488410715));
#88121=CARTESIAN_POINT('Ctrl Pts',(9.87270489640149,31.6273316876262,53.7454924707489));
#88122=CARTESIAN_POINT('Ctrl Pts',(9.87657961756178,31.6709179725922,53.8020320617973));
#88123=CARTESIAN_POINT('Ctrl Pts',(9.88045433872207,31.7114994963422,53.8607747664305));
#88124=CARTESIAN_POINT('Ctrl Pts',(9.88432905988236,31.7488672088626,53.9213614839692));
#88125=CARTESIAN_POINT('Ctrl Pts',(9.88656574146552,31.7704377092784,53.9563351478012));
#88126=CARTESIAN_POINT('Ctrl Pts',(9.88880242304867,31.7909381626963,53.991922797583));
#88127=CARTESIAN_POINT('Ctrl Pts',(9.89103910463183,31.8103355640854,54.0280521063824));
#88128=CARTESIAN_POINT('Ctrl Pts',(9.89510093122654,31.8455613563589,54.0936631385629));
#88129=CARTESIAN_POINT('Ctrl Pts',(9.89916275782125,31.8772702128551,54.1612912793214));
#88130=CARTESIAN_POINT('Ctrl Pts',(9.90322458441596,31.9052388984376,54.2305441517669));
#88131=CARTESIAN_POINT('Ctrl Pts',(9.90727491714547,31.9331284402423,54.2996010574072));
#88132=CARTESIAN_POINT('Ctrl Pts',(9.91132524987497,31.9572987321473,54.3702731564436));
#88133=CARTESIAN_POINT('Ctrl Pts',(9.91537558260448,31.9775731898177,54.4421453223156));
#88134=CARTESIAN_POINT('Ctrl Pts',(9.9194189682171,31.9978128728074,54.5138942132937));
#88135=CARTESIAN_POINT('Ctrl Pts',(9.92346235382972,32.0141698957701,54.5868386811531));
#88136=CARTESIAN_POINT('Ctrl Pts',(9.92750573944234,32.0265162219192,54.660545194763));
#88137=CARTESIAN_POINT('Ctrl Pts',(9.93154060036725,32.0388365182544,54.7340963126055));
#88138=CARTESIAN_POINT('Ctrl Pts',(9.93557546129217,32.0471628851546,54.8084058693907));
#88139=CARTESIAN_POINT('Ctrl Pts',(9.93961032221709,32.0514178528905,54.8830283994199));
#88140=CARTESIAN_POINT('Ctrl Pts',(9.94171530832395,32.0536376686749,54.9219589578441));
#88141=CARTESIAN_POINT('Ctrl Pts',(9.94382029443082,32.0547502036409,54.9609744922976));
#88142=CARTESIAN_POINT('Ctrl Pts',(9.94592528053769,32.054749999972,55.0000107205177));
#88143=CARTESIAN_POINT('Origin',(-1.54592528053767,30.,55.));
#88144=CARTESIAN_POINT('',(8.79398090709402,28.7479524050421,56.6292250864936));
#88145=CARTESIAN_POINT('',(8.85202117008686,28.7479524050421,56.6292250864936));
#88146=CARTESIAN_POINT('',(-1.54592528053767,28.7479524050421,56.6292250864936));
#88147=CARTESIAN_POINT('',(9.30407471946233,32.0547491756286,55.0018405851164));
#88148=CARTESIAN_POINT('Ctrl Pts',(8.85202117008686,28.7479524050421,56.6292250864936));
#88149=CARTESIAN_POINT('Ctrl Pts',(8.85588129653178,28.6913884584482,56.5857561061291));
#88150=CARTESIAN_POINT('Ctrl Pts',(8.8597414229767,28.6371285515222,56.5393669217963));
#88151=CARTESIAN_POINT('Ctrl Pts',(8.86360154942161,28.5854753989256,56.4903414761239));
#88152=CARTESIAN_POINT('Ctrl Pts',(8.86746436612079,28.5337862474788,56.4412818629403));
#88153=CARTESIAN_POINT('Ctrl Pts',(8.87132718281997,28.4847077982068,56.3895826855296));
#88154=CARTESIAN_POINT('Ctrl Pts',(8.87518999951914,28.4385040565871,56.3355627956802));
#88155=CARTESIAN_POINT('Ctrl Pts',(8.87905908249684,28.3922253630511,56.2814552745238));
#88156=CARTESIAN_POINT('Ctrl Pts',(8.88292816547454,28.3488309715686,56.2250199175821));
#88157=CARTESIAN_POINT('Ctrl Pts',(8.88679724845224,28.3085423954682,56.1666056465539));
#88158=CARTESIAN_POINT('Ctrl Pts',(8.8874139295063,28.3021209251303,56.1572951783015));
#88159=CARTESIAN_POINT('Ctrl Pts',(8.88803061056035,28.2957782608037,56.1479344884688));
#88160=CARTESIAN_POINT('Ctrl Pts',(8.88864729161441,28.2895151905841,56.1385250455118));
#88161=CARTESIAN_POINT('Ctrl Pts',(8.89251644614069,28.2502196968614,56.0794887113036));
#88162=CARTESIAN_POINT('Ctrl Pts',(8.89638560066697,28.2139072368597,56.0182999790416));
#88163=CARTESIAN_POINT('Ctrl Pts',(8.90025475519325,28.1808206560891,55.9552926657251));
#88164=CARTESIAN_POINT('Ctrl Pts',(8.90411814428605,28.1477833776866,55.8923792397089));
#88165=CARTESIAN_POINT('Ctrl Pts',(8.90798153337886,28.1179626609685,55.8276530382313));
#88166=CARTESIAN_POINT('Ctrl Pts',(8.91184492247166,28.091557961512,55.7614765579004));
#88167=CARTESIAN_POINT('Ctrl Pts',(8.91570377857263,28.0651842432186,55.69537772376));
#88168=CARTESIAN_POINT('Ctrl Pts',(8.91956263467359,28.0422187599149,55.6278324397933));
#88169=CARTESIAN_POINT('Ctrl Pts',(8.92342149077455,28.0228141378531,55.5592259194872));
#88170=CARTESIAN_POINT('Ctrl Pts',(8.92727791525774,28.0034217434107,55.4906626308618));
#88171=CARTESIAN_POINT('Ctrl Pts',(8.93113433974092,27.9875858903567,55.4210398989647));
#88172=CARTESIAN_POINT('Ctrl Pts',(8.9349907642241,27.9754098448151,55.3507595558618));
#88173=CARTESIAN_POINT('Ctrl Pts',(8.938846048542,27.9632373991636,55.2804999913863));
#88174=CARTESIAN_POINT('Ctrl Pts',(8.94270133285991,27.9547226957614,55.2095836800666));
#88175=CARTESIAN_POINT('Ctrl Pts',(8.94655661717781,27.9499178580085,55.1384224461116));
#88176=CARTESIAN_POINT('Ctrl Pts',(8.95041205116911,27.9451128337178,55.0672584494697));
#88177=CARTESIAN_POINT('Ctrl Pts',(8.95426748516041,27.9440179915521,54.9958499961239));
#88178=CARTESIAN_POINT('Ctrl Pts',(8.95812291915171,27.9466334408295,54.924612095266));
#88179=CARTESIAN_POINT('Ctrl Pts',(8.96198238682083,27.9492516264732,54.8532996630475));
#88180=CARTESIAN_POINT('Ctrl Pts',(8.96584185448996,27.9555878347017,54.7821586259505));
#88181=CARTESIAN_POINT('Ctrl Pts',(8.96970132215909,27.965590094707,54.7116011446873));
#88182=CARTESIAN_POINT('Ctrl Pts',(8.97356297398307,27.975598015204,54.6410037334444));
#88183=CARTESIAN_POINT('Ctrl Pts',(8.97742462580706,27.9892760243878,54.5709910124351));
#88184=CARTESIAN_POINT('Ctrl Pts',(8.98128627763105,28.0065210865127,54.5019644751812));
#88185=CARTESIAN_POINT('Ctrl Pts',(8.98515468362329,28.0237963108729,54.4328172080253));
#88186=CARTESIAN_POINT('Ctrl Pts',(8.98902308961553,28.044650902163,54.3646600330377));
#88187=CARTESIAN_POINT('Ctrl Pts',(8.99289149560777,28.0689322965427,54.29787815362));
#88188=CARTESIAN_POINT('Ctrl Pts',(8.9951885178895,28.0833503550488,54.2582237157596));
#88189=CARTESIAN_POINT('Ctrl Pts',(8.99748554017123,28.0989757375881,54.2190538044965));
#88190=CARTESIAN_POINT('Ctrl Pts',(8.99978256245296,28.1157687985927,54.1804450340928));
#88191=CARTESIAN_POINT('Ctrl Pts',(9.00365176201357,28.1440557267504,54.1154108205942));
#88192=CARTESIAN_POINT('Ctrl Pts',(9.00752096157417,28.1757689648771,54.0517154981927));
#88193=CARTESIAN_POINT('Ctrl Pts',(9.01139016113478,28.2107597494939,53.9897441470257));
#88194=CARTESIAN_POINT('Ctrl Pts',(9.01525359714625,28.2456984119333,53.9278651082145));
#88195=CARTESIAN_POINT('Ctrl Pts',(9.01911703315772,28.2839046928784,53.8677053627107));
#88196=CARTESIAN_POINT('Ctrl Pts',(9.02298046916919,28.3251822016714,53.8096290893584));
#88197=CARTESIAN_POINT('Ctrl Pts',(9.02683937472661,28.3664113064385,53.7516209190849));
#88198=CARTESIAN_POINT('Ctrl Pts',(9.03069828028404,28.4107042052559,53.6956917619807));
#88199=CARTESIAN_POINT('Ctrl Pts',(9.03455718584146,28.4578200244877,53.6421787725812));
#88200=CARTESIAN_POINT('Ctrl Pts',(9.03841366131584,28.5049061732982,53.5886994821171));
#88201=CARTESIAN_POINT('Ctrl Pts',(9.04227013679021,28.5548113953747,53.537633704349));
#88202=CARTESIAN_POINT('Ctrl Pts',(9.04612661226458,28.6072540851992,53.4892861358597));
#88203=CARTESIAN_POINT('Ctrl Pts',(9.04998194901956,28.6596812900275,53.4409528431812));
#88204=CARTESIAN_POINT('Ctrl Pts',(9.05383728577453,28.7146441181887,53.3953364954274));
#88205=CARTESIAN_POINT('Ctrl Pts',(9.05769262252951,28.771824832693,53.3527042400011));
#88206=CARTESIAN_POINT('Ctrl Pts',(9.06154811031643,28.8290077872388,53.3100703144658));
#88207=CARTESIAN_POINT('Ctrl Pts',(9.06540359810335,28.8884084098854,53.2704210019285));
#88208=CARTESIAN_POINT('Ctrl Pts',(9.06925908589027,28.9496780785689,53.2339814769201));
#88209=CARTESIAN_POINT('Ctrl Pts',(9.07311860903011,29.0110118752564,53.1975038124202));
#88210=CARTESIAN_POINT('Ctrl Pts',(9.07697813216994,29.0742182047295,53.1642428906337));
#88211=CARTESIAN_POINT('Ctrl Pts',(9.08083765530977,29.1389225928098,53.1343785857451));
#88212=CARTESIAN_POINT('Ctrl Pts',(9.08469936363192,29.2036636151786,53.1044973723037));
#88213=CARTESIAN_POINT('Ctrl Pts',(9.08856107195407,29.2699039333472,53.0780167844557));
#88214=CARTESIAN_POINT('Ctrl Pts',(9.09242278027622,29.3372503405294,53.0550680085485));
#88215=CARTESIAN_POINT('Ctrl Pts',(9.0962912437545,29.4047145545103,53.0320790891216));
#88216=CARTESIAN_POINT('Ctrl Pts',(9.10015970723278,29.4732882530069,53.0126344489143));
#88217=CARTESIAN_POINT('Ctrl Pts',(9.10402817071106,29.5425650540414,52.996814828151));
#88218=CARTESIAN_POINT('Ctrl Pts',(9.10632472490455,29.5836919585141,52.9874233432352));
#88219=CARTESIAN_POINT('Ctrl Pts',(9.10862127909803,29.6250664825843,52.9793084509649));
#88220=CARTESIAN_POINT('Ctrl Pts',(9.11091783329152,29.6666028112324,52.972478390492));
#88221=CARTESIAN_POINT('Ctrl Pts',(9.11478631643122,29.7365696282645,52.9609733392037));
#88222=CARTESIAN_POINT('Ctrl Pts',(9.11865479957092,29.8072699698205,52.9530716445104));
#88223=CARTESIAN_POINT('Ctrl Pts',(9.12252328271062,29.8782997758385,52.9488572409657));
#88224=CARTESIAN_POINT('Ctrl Pts',(9.1263859997762,29.9492237100945,52.9446491190983));
#88225=CARTESIAN_POINT('Ctrl Pts',(9.13024871684178,30.0204756529167,52.9441174076207));
#88226=CARTESIAN_POINT('Ctrl Pts',(9.13411143390736,30.0916432604721,52.9472946935057));
#88227=CARTESIAN_POINT('Ctrl Pts',(9.1379696202359,30.1627273926627,52.9504682526236));
#88228=CARTESIAN_POINT('Ctrl Pts',(9.14182780656444,30.2337269029682,52.957342146198));
#88229=CARTESIAN_POINT('Ctrl Pts',(9.14568599289298,30.3042280154203,52.9678969324531));
#88230=CARTESIAN_POINT('Ctrl Pts',(9.14954174935052,30.3746847265414,52.9784450713442));
#88231=CARTESIAN_POINT('Ctrl Pts',(9.15339750580807,30.4446431830962,52.9926694318933));
#88232=CARTESIAN_POINT('Ctrl Pts',(9.15725326226561,30.5136947794281,53.0104987468995));
#88233=CARTESIAN_POINT('Ctrl Pts',(9.16110788126701,30.5827260053959,53.0283228022209));
#88234=CARTESIAN_POINT('Ctrl Pts',(9.16496250026841,30.6508504319847,53.0497495793187));
#88235=CARTESIAN_POINT('Ctrl Pts',(9.1688171192698,30.7176713991228,53.0746570888849));
#88236=CARTESIAN_POINT('Ctrl Pts',(9.17267189161837,30.7844950245797,53.0995655893392));
#88237=CARTESIAN_POINT('Ctrl Pts',(9.17652666396692,30.8500146330596,53.1279549253845));
#88238=CARTESIAN_POINT('Ctrl Pts',(9.18038143631549,30.9138520748046,53.1596543944478));
#88239=CARTESIAN_POINT('Ctrl Pts',(9.18424025245614,30.9777564842764,53.1913871173716));
#88240=CARTESIAN_POINT('Ctrl Pts',(9.18809906859679,31.0399747682461,53.2264366885038));
#88241=CARTESIAN_POINT('Ctrl Pts',(9.19195788473744,31.1001528137344,53.2645861159561));
#88242=CARTESIAN_POINT('Ctrl Pts',(9.19581888975065,31.1603649945814,53.3027571832669));
#88243=CARTESIAN_POINT('Ctrl Pts',(9.19967989476387,31.2185342366537,53.3440313258441));
#88244=CARTESIAN_POINT('Ctrl Pts',(9.20354089977709,31.2743371748439,53.3881494091229));
#88245=CARTESIAN_POINT('Ctrl Pts',(9.20740867340654,31.3302379395512,53.4323448345376));
#88246=CARTESIAN_POINT('Ctrl Pts',(9.21127644703598,31.3837637531121,53.4793938336401));
#88247=CARTESIAN_POINT('Ctrl Pts',(9.21514422066542,31.4346264894879,53.5289988449496));
#88248=CARTESIAN_POINT('Ctrl Pts',(9.21744718182031,31.4649113296381,53.5585348067401));
#88249=CARTESIAN_POINT('Ctrl Pts',(9.2197501429752,31.4942527651073,53.5889762636244));
#88250=CARTESIAN_POINT('Ctrl Pts',(9.22205310413008,31.5225968865233,53.6202549932508));
#88251=CARTESIAN_POINT('Ctrl Pts',(9.2258818694665,31.5697201258097,53.6722571364507));
#88252=CARTESIAN_POINT('Ctrl Pts',(9.22971063480291,31.6142781779404,53.7267889663082));
#88253=CARTESIAN_POINT('Ctrl Pts',(9.23353940013933,31.6559837342967,53.7835644553677));
#88254=CARTESIAN_POINT('Ctrl Pts',(9.23736291548182,31.6976321040933,53.8402620940116));
#88255=CARTESIAN_POINT('Ctrl Pts',(9.24118643082432,31.7364354404661,53.8991968972038));
#88256=CARTESIAN_POINT('Ctrl Pts',(9.24500994616681,31.7721446014219,53.9600475615918));
#88257=CARTESIAN_POINT('Ctrl Pts',(9.24882956237847,31.8078173470169,54.0208361719064));
#88258=CARTESIAN_POINT('Ctrl Pts',(9.25264917859012,31.8404019248255,54.0835363428967));
#88259=CARTESIAN_POINT('Ctrl Pts',(9.25646879480177,31.8696918061671,54.1477969065701));
#88260=CARTESIAN_POINT('Ctrl Pts',(9.26043595519015,31.900113097365,54.2145397279986));
#88261=CARTESIAN_POINT('Ctrl Pts',(9.26440311557854,31.9269796377569,54.2829654981407));
#88262=CARTESIAN_POINT('Ctrl Pts',(9.26837027596692,31.9501125700655,54.3526527001891));
#88263=CARTESIAN_POINT('Ctrl Pts',(9.27218707210809,31.9723687125265,54.4196986014959));
#88264=CARTESIAN_POINT('Ctrl Pts',(9.27600386824927,31.991169053742,54.4879115124635));
#88265=CARTESIAN_POINT('Ctrl Pts',(9.27982066439045,32.0064043053609,54.5568980637264));
#88266=CARTESIAN_POINT('Ctrl Pts',(9.28363748065307,32.0216396372972,54.6258849786738));
#88267=CARTESIAN_POINT('Ctrl Pts',(9.2874542969157,32.0333097454008,54.6956450548262));
#88268=CARTESIAN_POINT('Ctrl Pts',(9.29127111317833,32.0413564087979,54.7657745215404));
#88269=CARTESIAN_POINT('Ctrl Pts',(9.29509049992236,32.0494084913186,54.8359512177981));
#88270=CARTESIAN_POINT('Ctrl Pts',(9.29890988666638,32.0538322209711,54.9064973060252));
#88271=CARTESIAN_POINT('Ctrl Pts',(9.30272927341042,32.0546213278406,54.9770051814002));
#88272=CARTESIAN_POINT('Ctrl Pts',(9.30317775542772,32.054713986758,54.9852843938245));
#88273=CARTESIAN_POINT('Ctrl Pts',(9.30362623744502,32.0547565903784,54.9935630809628));
#88274=CARTESIAN_POINT('Ctrl Pts',(9.30407471946233,32.0547491756286,55.0018405851164));
#88275=CARTESIAN_POINT('Ctrl Pts',(9.3040750081896,32.0541656181102,55.0018453898296));
#88276=CARTESIAN_POINT('Ctrl Pts',(9.31377946378262,32.0557552315022,55.1809084352921));
#88277=CARTESIAN_POINT('Ctrl Pts',(9.36052900965515,31.9523257255288,56.0417158650899));
#88278=CARTESIAN_POINT('Ctrl Pts',(9.44318606595545,30.7618299889055,57.2943384729));
#88279=CARTESIAN_POINT('Ctrl Pts',(9.51613866666276,29.2698275908187,57.0320534795199));
#88280=CARTESIAN_POINT('Ctrl Pts',(9.55204617709054,28.7459570691003,56.6318367151304));
#88281=CARTESIAN_POINT('',(9.24592528058114,32.0547492110797,54.998199425793));
#88282=CARTESIAN_POINT('Ctrl Pts',(9.24592528058114,32.0547492110797,54.998199425793));
#88283=CARTESIAN_POINT('Ctrl Pts',(9.2497310207861,32.0548106172635,55.0682739094095));
#88284=CARTESIAN_POINT('Ctrl Pts',(9.25353676099106,32.0512831032295,55.1384663101287));
#88285=CARTESIAN_POINT('Ctrl Pts',(9.25734250119601,32.0441571007588,55.2083730066908));
#88286=CARTESIAN_POINT('Ctrl Pts',(9.26114492485008,32.0370373083152,55.2782187823534));
#88287=CARTESIAN_POINT('Ctrl Pts',(9.26494734850415,32.0263252921618,55.3477788510323));
#88288=CARTESIAN_POINT('Ctrl Pts',(9.26874977215822,32.0120635168845,55.4166508928618));
#88289=CARTESIAN_POINT('Ctrl Pts',(9.27255024081877,31.9978090742142,55.4854875245403));
#88290=CARTESIAN_POINT('Ctrl Pts',(9.27635070947932,31.9800085923165,55.5536363407389));
#88291=CARTESIAN_POINT('Ctrl Pts',(9.28015117813986,31.9587559546279,55.6207033693399));
#88292=CARTESIAN_POINT('Ctrl Pts',(9.2839510505265,31.9375066513683,55.6877598754703));
#88293=CARTESIAN_POINT('Ctrl Pts',(9.28775092291313,31.9128064196875,55.753734453472));
#88294=CARTESIAN_POINT('Ctrl Pts',(9.29155079529976,31.8847989711826,55.8182483734961));
#88295=CARTESIAN_POINT('Ctrl Pts',(9.29535403990283,31.8567666673224,55.8828195467328));
#88296=CARTESIAN_POINT('Ctrl Pts',(9.29915728450591,31.825421483627,55.9459270116931));
#88297=CARTESIAN_POINT('Ctrl Pts',(9.30296052910898,31.7909548332783,56.0072131589972));
#88298=CARTESIAN_POINT('Ctrl Pts',(9.30676541564393,31.7564733030316,56.068525764678));
#88299=CARTESIAN_POINT('Ctrl Pts',(9.31057030217887,31.7188678920193,56.1280150634692));
#88300=CARTESIAN_POINT('Ctrl Pts',(9.31437518871381,31.6783739012035,56.1853516821007));
#88301=CARTESIAN_POINT('Ctrl Pts',(9.31818690566785,31.6378072167803,56.2427912297239));
#88302=CARTESIAN_POINT('Ctrl Pts',(9.32199862262189,31.5943419074146,56.2980699853191));
#88303=CARTESIAN_POINT('Ctrl Pts',(9.32581033957593,31.5482537046868,56.3508915679742));
#88304=CARTESIAN_POINT('Ctrl Pts',(9.32899447653029,31.5097536924258,56.3950163430684));
#88305=CARTESIAN_POINT('Ctrl Pts',(9.33217861348464,31.4694241869326,56.4374269880513));
#88306=CARTESIAN_POINT('Ctrl Pts',(9.335362750439,31.427444051006,56.4779719360487));
#88307=CARTESIAN_POINT('Ctrl Pts',(9.33923123464619,31.3764413789553,56.5272309639291));
#88308=CARTESIAN_POINT('Ctrl Pts',(9.34309971885338,31.3227858472138,56.5739435066278));
#88309=CARTESIAN_POINT('Ctrl Pts',(9.34696820306057,31.2667620480004,56.6178107047012));
#88310=CARTESIAN_POINT('Ctrl Pts',(9.35083092119519,31.2108217536625,56.6616125176175));
#88311=CARTESIAN_POINT('Ctrl Pts',(9.3546936393298,31.1525205781485,56.7025771070642));
#88312=CARTESIAN_POINT('Ctrl Pts',(9.35855635746442,31.0921791328281,56.7404431344675));
#88313=CARTESIAN_POINT('Ctrl Pts',(9.36241454485926,31.0319084644519,56.7782647472616));
#88314=CARTESIAN_POINT('Ctrl Pts',(9.3662727322541,30.9696026893691,56.8129947600966));
#88315=CARTESIAN_POINT('Ctrl Pts',(9.37013091964894,30.90561319018,56.844413812644));
#88316=CARTESIAN_POINT('Ctrl Pts',(9.37398667717055,30.8416639913588,56.8758130775795));
#88317=CARTESIAN_POINT('Ctrl Pts',(9.37784243469217,30.7760336074036,56.9039053055744));
#88318=CARTESIAN_POINT('Ctrl Pts',(9.38169819221378,30.709098646093,56.9285167027042));
#88319=CARTESIAN_POINT('Ctrl Pts',(9.38555281227549,30.6421834307945,56.9531208393988));
#88320=CARTESIAN_POINT('Ctrl Pts',(9.38940743233721,30.5739648580217,56.9742460161874));
#88321=CARTESIAN_POINT('Ctrl Pts',(9.39326205239892,30.5048385606257,56.9917669517806));
#88322=CARTESIAN_POINT('Ctrl Pts',(9.39711682580255,30.4357095132936,57.0092885843799));
#88323=CARTESIAN_POINT('Ctrl Pts',(9.40097159920618,30.3656731412421,57.0232055738624));
#88324=CARTESIAN_POINT('Ctrl Pts',(9.40482637260981,30.2951375604076,57.0334432332713));
#88325=CARTESIAN_POINT('Ctrl Pts',(9.40868518979036,30.2245279855601,57.0436916323025));
#88326=CARTESIAN_POINT('Ctrl Pts',(9.4125440069709,30.1534186384365,57.05025292645));
#88327=CARTESIAN_POINT('Ctrl Pts',(9.41640282415145,30.082224193917,57.0531041728161));
#88328=CARTESIAN_POINT('Ctrl Pts',(9.42026383019759,30.0109893652428,57.0559570365159));
#88329=CARTESIAN_POINT('Ctrl Pts',(9.42412483624374,29.939669829223,57.0550956690197));
#88330=CARTESIAN_POINT('Ctrl Pts',(9.42798584228988,29.8686789413621,57.0505492781346));
#88331=CARTESIAN_POINT('Ctrl Pts',(9.43185361693012,29.797563601869,57.0459949171313));
#88332=CARTESIAN_POINT('Ctrl Pts',(9.43572139157036,29.7267785436418,57.0377426913391));
#88333=CARTESIAN_POINT('Ctrl Pts',(9.4395891662106,29.6567299953908,57.0258734576561));
#88334=CARTESIAN_POINT('Ctrl Pts',(9.44189211789959,29.615021665017,57.0188062745083));
#88335=CARTESIAN_POINT('Ctrl Pts',(9.44419506958858,29.5735742331112,57.0104577492287));
#88336=CARTESIAN_POINT('Ctrl Pts',(9.44649802127757,29.5324708422954,57.0008533302559));
#88337=CARTESIAN_POINT('Ctrl Pts',(9.45045224773995,29.4618952777124,56.9843622992717));
#88338=CARTESIAN_POINT('Ctrl Pts',(9.45440647420234,29.3920522645419,56.9640996457197));
#88339=CARTESIAN_POINT('Ctrl Pts',(9.45836070066472,29.3233744778301,56.9401483101166));
#88340=CARTESIAN_POINT('Ctrl Pts',(9.46222412370766,29.2562737828537,56.91674698428));
#88341=CARTESIAN_POINT('Ctrl Pts',(9.4660875467506,29.1902858677679,56.8898247211004));
#88342=CARTESIAN_POINT('Ctrl Pts',(9.46995096979354,29.1258038704839,56.8595103359861));
#88343=CARTESIAN_POINT('Ctrl Pts',(9.47395059796565,29.0590485578855,56.8281272160492));
#88344=CARTESIAN_POINT('Ctrl Pts',(9.47795022613776,28.9939078532244,56.7931084315634));
#88345=CARTESIAN_POINT('Ctrl Pts',(9.48194985430987,28.9307982082082,56.7546524131375));
#88346=CARTESIAN_POINT('Ctrl Pts',(9.48594948248198,28.867688563192,56.7161963947116));
#88347=CARTESIAN_POINT('Ctrl Pts',(9.48994911065408,28.8066104976308,56.6743034027799));
#88348=CARTESIAN_POINT('Ctrl Pts',(9.49394873882619,28.7479524050421,56.6292250864936));
#88349=CARTESIAN_POINT('Ctrl Pts',(8.79398090709402,28.7479524050421,56.6292250864936));
#88350=CARTESIAN_POINT('Ctrl Pts',(8.7980159387603,28.6890642014229,56.5839699315589));
#88351=CARTESIAN_POINT('Ctrl Pts',(8.80205097042658,28.632543821309,56.5354495734022));
#88352=CARTESIAN_POINT('Ctrl Pts',(8.80608600209286,28.5787688567674,56.4839473036486));
#88353=CARTESIAN_POINT('Ctrl Pts',(8.80994398458318,28.5273534308732,56.4347048512085));
#88354=CARTESIAN_POINT('Ctrl Pts',(8.8138019670735,28.4784479420345,56.3827370556703));
#88355=CARTESIAN_POINT('Ctrl Pts',(8.81765994956382,28.4323493299988,56.328333143208));
#88356=CARTESIAN_POINT('Ctrl Pts',(8.82151585847565,28.3862754949263,56.2739584716203));
#88357=CARTESIAN_POINT('Ctrl Pts',(8.82537176738749,28.3430058566912,56.2171506511486));
#88358=CARTESIAN_POINT('Ctrl Pts',(8.82922767629933,28.3027990407137,56.1582342018338));
#88359=CARTESIAN_POINT('Ctrl Pts',(8.83308280260811,28.2626003851927,56.0993297103205));
#88360=CARTESIAN_POINT('Ctrl Pts',(8.8369379289169,28.2254635909987,56.0383178411421));
#88361=CARTESIAN_POINT('Ctrl Pts',(8.84079305522569,28.1916046465441,55.9755530780533));
#88362=CARTESIAN_POINT('Ctrl Pts',(8.84464868865254,28.1577412481544,55.9127800586474));
#88363=CARTESIAN_POINT('Ctrl Pts',(8.84850432207939,28.1271567838051,55.8482541163248));
#88364=CARTESIAN_POINT('Ctrl Pts',(8.85235995550625,28.1000210416728,55.7823538332582));
#88365=CARTESIAN_POINT('Ctrl Pts',(8.85621984300843,28.0728553595856,55.7163808397606));
#88366=CARTESIAN_POINT('Ctrl Pts',(8.8600797305106,28.0491461764957,55.6490309301374));
#88367=CARTESIAN_POINT('Ctrl Pts',(8.86393961801278,28.0290145576689,55.5807012559129));
#88368=CARTESIAN_POINT('Ctrl Pts',(8.86780201100793,28.0088698711997,55.512327228189));
#88369=CARTESIAN_POINT('Ctrl Pts',(8.87166440400307,27.9923074822234,55.4429726426712));
#88370=CARTESIAN_POINT('Ctrl Pts',(8.87552679699821,27.9793974979391,55.3730456958136));
#88371=CARTESIAN_POINT('Ctrl Pts',(8.87939562802961,27.9664659946257,55.3030021911072));
#88372=CARTESIAN_POINT('Ctrl Pts',(8.88326445906101,27.9571991048352,55.2323849024254));
#88373=CARTESIAN_POINT('Ctrl Pts',(8.8871332900924,27.9516150981964,55.161607105546));
#88374=CARTESIAN_POINT('Ctrl Pts',(8.88836274908986,27.9498405809977,55.1391149371139));
#88375=CARTESIAN_POINT('Ctrl Pts',(8.88959220808731,27.948437594808,55.1166065523314));
#88376=CARTESIAN_POINT('Ctrl Pts',(8.89082166708476,27.9474056259948,55.0940951555716));
#88377=CARTESIAN_POINT('Ctrl Pts',(8.89469076157756,27.9441580310279,55.0232520274891));
#88378=CARTESIAN_POINT('Ctrl Pts',(8.89855985607037,27.9445759946267,54.9521018198761));
#88379=CARTESIAN_POINT('Ctrl Pts',(8.90242895056317,27.948695578934,54.8810557499698));
#88380=CARTESIAN_POINT('Ctrl Pts',(8.90629228027677,27.9528090252435,54.8101155355569));
#88381=CARTESIAN_POINT('Ctrl Pts',(8.91015560999037,27.960613116748,54.7392796318758));
#88382=CARTESIAN_POINT('Ctrl Pts',(8.91401893970397,27.9720919511485,54.6689614706666));
#88383=CARTESIAN_POINT('Ctrl Pts',(8.91787773766708,27.9835573206839,54.5987257938387));
#88384=CARTESIAN_POINT('Ctrl Pts',(8.9217365356302,27.9986887930481,54.5290071302452));
#88385=CARTESIAN_POINT('Ctrl Pts',(8.92559533359331,28.0174186272033,54.4602142436673));
#88386=CARTESIAN_POINT('Ctrl Pts',(8.92945170073389,28.0361366626317,54.3914646926827));
#88387=CARTESIAN_POINT('Ctrl Pts',(8.93330806787446,28.0584484353156,54.3236402292901));
#88388=CARTESIAN_POINT('Ctrl Pts',(8.93716443501504,28.0842353397634,54.2571384186213));
#88389=CARTESIAN_POINT('Ctrl Pts',(8.94101966286253,28.1100146259423,54.1906562546951));
#88390=CARTESIAN_POINT('Ctrl Pts',(8.94487489071002,28.1392668301418,54.1254964204129));
#88391=CARTESIAN_POINT('Ctrl Pts',(8.94873011855751,28.1718243701289,54.0620386847821));
#88392=CARTESIAN_POINT('Ctrl Pts',(8.95258549702839,28.204383182136,53.9985784698635));
#88393=CARTESIAN_POINT('Ctrl Pts',(8.95644087549927,28.2402473626092,53.9368209168332));
#88394=CARTESIAN_POINT('Ctrl Pts',(8.96029625397015,28.2792031143695,53.8771217158995));
#88395=CARTESIAN_POINT('Ctrl Pts',(8.96415566793503,28.318199641816,53.8173600267382));
#88396=CARTESIAN_POINT('Ctrl Pts',(8.9680150818999,28.3602939343272,53.7596613982291));
#88397=CARTESIAN_POINT('Ctrl Pts',(8.97187449586478,28.4052290328142,53.7043522374035));
#88398=CARTESIAN_POINT('Ctrl Pts',(8.97573609492737,28.4501895723608,53.6490117619997));
#88399=CARTESIAN_POINT('Ctrl Pts',(8.97959769398996,28.4979937939993,53.5960638081306));
#88400=CARTESIAN_POINT('Ctrl Pts',(8.98345929305254,28.5483464768113,53.5457993222688));
#88401=CARTESIAN_POINT('Ctrl Pts',(8.98732764833382,28.5987872562203,53.4954468941186));
#88402=CARTESIAN_POINT('Ctrl Pts',(8.99119600361509,28.6517850375334,53.4477876325501));
#88403=CARTESIAN_POINT('Ctrl Pts',(8.99506435889637,28.7070105530286,53.4030729971221));
#88404=CARTESIAN_POINT('Ctrl Pts',(8.99736188523869,28.7398105590757,53.3765157020153));
#88405=CARTESIAN_POINT('Ctrl Pts',(8.999659411581,28.773395808489,53.3509963215848));
#88406=CARTESIAN_POINT('Ctrl Pts',(9.00195693792332,28.8076927897776,53.3265601059639));
#88407=CARTESIAN_POINT('Ctrl Pts',(9.00582593492974,28.8654483486545,53.2854099161514));
#88408=CARTESIAN_POINT('Ctrl Pts',(9.00969493193617,28.9254498910936,53.2471725992289));
#88409=CARTESIAN_POINT('Ctrl Pts',(9.0135639289426,28.9873715156788,53.2121014807206));
#88410=CARTESIAN_POINT('Ctrl Pts',(9.01742716090311,29.0492008731963,53.1770826203578));
#88411=CARTESIAN_POINT('Ctrl Pts',(9.02129039286362,29.1129442145097,53.1452208311218));
#88412=CARTESIAN_POINT('Ctrl Pts',(9.02515362482413,29.1782455927105,53.1167269829894));
#88413=CARTESIAN_POINT('Ctrl Pts',(9.02901232510842,29.2434703706178,53.0882665589162));
#88414=CARTESIAN_POINT('Ctrl Pts',(9.03287102539272,29.310249112044,53.063166421903));
#88415=CARTESIAN_POINT('Ctrl Pts',(9.03672972567701,29.3782016751627,53.0415913588504));
#88416=CARTESIAN_POINT('Ctrl Pts',(9.04058599523718,29.4461114326933,53.0200298866502));
#88417=CARTESIAN_POINT('Ctrl Pts',(9.04444226479734,29.5151930829683,53.0019892295235));
#88418=CARTESIAN_POINT('Ctrl Pts',(9.0482985343575,29.5850483046845,52.9875853675113));
#88419=CARTESIAN_POINT('Ctrl Pts',(9.05215366486527,29.6548828927918,52.9731857600651));
#88420=CARTESIAN_POINT('Ctrl Pts',(9.05600879537304,29.7254901231765,52.962420913157));
#88421=CARTESIAN_POINT('Ctrl Pts',(9.0598639258808,29.7964600620339,52.9553560074789));
#88422=CARTESIAN_POINT('Ctrl Pts',(9.06371920739509,29.8674327808034,52.9482908250664));
#88423=CARTESIAN_POINT('Ctrl Pts',(9.06757448890938,29.9387677526166,52.9449259175499));
#88424=CARTESIAN_POINT('Ctrl Pts',(9.07142977042368,30.0100502077706,52.9452745789708));
#88425=CARTESIAN_POINT('Ctrl Pts',(9.07528908868052,30.0814073005145,52.9456236054639));
#88426=CARTESIAN_POINT('Ctrl Pts',(9.07914840693737,30.1527112800329,52.9496939605497));
#88427=CARTESIAN_POINT('Ctrl Pts',(9.08300772519421,30.223548569157,52.9574467939053));
#88428=CARTESIAN_POINT('Ctrl Pts',(9.08686922910844,30.2944259757404,52.9652040179423));
#88429=CARTESIAN_POINT('Ctrl Pts',(9.09073073302266,30.3648356860456,52.9766477938668));
#88430=CARTESIAN_POINT('Ctrl Pts',(9.09459223693689,30.4343731635707,52.9916878934614));
#88431=CARTESIAN_POINT('Ctrl Pts',(9.098460498985,30.504032340722,53.0067543151856));
#88432=CARTESIAN_POINT('Ctrl Pts',(9.10232876103311,30.5728157683698,53.0254294994618));
#88433=CARTESIAN_POINT('Ctrl Pts',(9.10619702308123,30.6403336194645,53.0475731977143));
#88434=CARTESIAN_POINT('Ctrl Pts',(9.10849541830811,30.6804505259085,53.0607302614644));
#88435=CARTESIAN_POINT('Ctrl Pts',(9.11079381353499,30.7201209950869,53.0751108971256));
#88436=CARTESIAN_POINT('Ctrl Pts',(9.11309220876187,30.7592670510234,53.0906778407691));
#88437=CARTESIAN_POINT('Ctrl Pts',(9.11696136318876,30.8251661330657,53.1168834768612));
#88438=CARTESIAN_POINT('Ctrl Pts',(9.12083051761564,30.8898359757849,53.1465561400865));
#88439=CARTESIAN_POINT('Ctrl Pts',(9.12469967204252,30.9528869714854,53.1795593989165));
#88440=CARTESIAN_POINT('Ctrl Pts',(9.12856306103708,31.0158440148106,53.2125134795451));
#88441=CARTESIAN_POINT('Ctrl Pts',(9.13242645003163,31.0771865724978,53.2487880810627));
#88442=CARTESIAN_POINT('Ctrl Pts',(9.13628983902619,31.1365444117604,53.2881985037405));
#88443=CARTESIAN_POINT('Ctrl Pts',(9.14014869503105,31.195832605312,53.3275626854004));
#88444=CARTESIAN_POINT('Ctrl Pts',(9.14400755103591,31.2531403033267,53.3700551124467));
#88445=CARTESIAN_POINT('Ctrl Pts',(9.14786640704078,31.3081228683027,53.4154457649158));
#88446=CARTESIAN_POINT('Ctrl Pts',(9.15172283142924,31.3630707866097,53.4608078149557));
#88447=CARTESIAN_POINT('Ctrl Pts',(9.15557925581769,31.4156961050115,53.5090641585697));
#88448=CARTESIAN_POINT('Ctrl Pts',(9.15943568020615,31.4656853314769,53.5599430318236));
#88449=CARTESIAN_POINT('Ctrl Pts',(9.16329096443082,31.5156597784731,53.6108068625815));
#88450=CARTESIAN_POINT('Ctrl Pts',(9.1671462486555,31.5629993405386,53.6642913373607));
#88451=CARTESIAN_POINT('Ctrl Pts',(9.17100153288017,31.6074269063078,53.7200873844759));
#88452=CARTESIAN_POINT('Ctrl Pts',(9.17485696677985,31.6518561969035,53.77588559778));
#88453=CARTESIAN_POINT('Ctrl Pts',(9.17871240067954,31.693372965888,53.8339951802086));
#88454=CARTESIAN_POINT('Ctrl Pts',(9.18256783457922,31.7317410710717,53.8940748554882));
#88455=CARTESIAN_POINT('Ctrl Pts',(9.1864273021598,31.7701493182205,53.9542173880868));
#88456=CARTESIAN_POINT('Ctrl Pts',(9.19028676974038,31.8054020635424,54.0163337178684));
#88457=CARTESIAN_POINT('Ctrl Pts',(9.19414623732096,31.8373076201051,54.0800552888333));
#88458=CARTESIAN_POINT('Ctrl Pts',(9.198007889058,31.8692312327147,54.1438129212179));
#88459=CARTESIAN_POINT('Ctrl Pts',(9.20186954079504,31.8978036910347,54.2091771579076));
#88460=CARTESIAN_POINT('Ctrl Pts',(9.20573119253207,31.9228813756042,54.27575917137));
#88461=CARTESIAN_POINT('Ctrl Pts',(9.2095995984408,31.9480029219713,54.3424576392361));
#88462=CARTESIAN_POINT('Ctrl Pts',(9.21346800434952,31.9696173434629,54.4103776733197));
#88463=CARTESIAN_POINT('Ctrl Pts',(9.21733641025824,31.987631022315,54.4791156734637));
#88464=CARTESIAN_POINT('Ctrl Pts',(9.21963343337231,31.9983273757145,54.5199316526734));
#88465=CARTESIAN_POINT('Ctrl Pts',(9.22193045648637,32.0077551304157,54.5610358282184));
#88466=CARTESIAN_POINT('Ctrl Pts',(9.22422747960044,32.015903316979,54.6023426360634));
#88467=CARTESIAN_POINT('Ctrl Pts',(9.22983463068173,32.0357934577526,54.7031746698618));
#88468=CARTESIAN_POINT('Ctrl Pts',(9.23544178176301,32.0481232837319,54.8055436168192));
#88469=CARTESIAN_POINT('Ctrl Pts',(9.2410489328443,32.0527124830813,54.9085176284622));
#88470=CARTESIAN_POINT('Ctrl Pts',(9.24267438207543,32.0540428397002,54.9383686215289));
#88471=CARTESIAN_POINT('Ctrl Pts',(9.24429983130656,32.0547229842024,54.9682702891664));
#88472=CARTESIAN_POINT('Ctrl Pts',(9.24592528053769,32.054749211079,54.998199424993));
#88473=CARTESIAN_POINT('Origin',(-1.54592528053767,30.,55.));
#88474=CARTESIAN_POINT('',(8.09385946234359,28.7479524050421,56.6292250864936));
#88475=CARTESIAN_POINT('',(8.1521140472482,28.7479524050421,56.6292250864936));
#88476=CARTESIAN_POINT('',(-1.54592528053767,28.7479524050421,56.6292250864936));
#88477=CARTESIAN_POINT('',(8.60407471942946,32.0547498911142,54.9993310707398));
#88478=CARTESIAN_POINT('Ctrl Pts',(8.1521140472482,28.7479524050421,56.6292250864936));
#88479=CARTESIAN_POINT('Ctrl Pts',(8.15596957998729,28.6914289717662,56.5857872403185));
#88480=CARTESIAN_POINT('Ctrl Pts',(8.15982511272638,28.6371409837604,56.5393831604098));
#88481=CARTESIAN_POINT('Ctrl Pts',(8.16368064546547,28.5854080864135,56.4902775850545));
#88482=CARTESIAN_POINT('Ctrl Pts',(8.16753577929291,28.5336805415967,56.441177090394));
#88483=CARTESIAN_POINT('Ctrl Pts',(8.17139091312036,28.4845079139827,56.3893759905912));
#88484=CARTESIAN_POINT('Ctrl Pts',(8.17524604694781,28.4381741799003,56.33517701829));
#88485=CARTESIAN_POINT('Ctrl Pts',(8.17912851525075,28.3915119206939,56.2805937531091));
#88486=CARTESIAN_POINT('Ctrl Pts',(8.18301098355368,28.347729313344,56.2235788417456));
#88487=CARTESIAN_POINT('Ctrl Pts',(8.18689345185662,28.3070748871319,56.1644750425494));
#88488=CARTESIAN_POINT('Ctrl Pts',(8.19075397014214,28.2666503057745,56.1057053940328));
#88489=CARTESIAN_POINT('Ctrl Pts',(8.19461448842766,28.2293188353886,56.0448708633677));
#88490=CARTESIAN_POINT('Ctrl Pts',(8.19847500671318,28.1952798414538,55.9823353357366));
#88491=CARTESIAN_POINT('Ctrl Pts',(8.20236845002482,28.1609505407047,55.919266464205));
#88492=CARTESIAN_POINT('Ctrl Pts',(8.20626189333647,28.1299703652479,55.8544678955933));
#88493=CARTESIAN_POINT('Ctrl Pts',(8.21015533664811,28.1024944009687,55.7883337263779));
#88494=CARTESIAN_POINT('Ctrl Pts',(8.21404877995976,28.0750184366895,55.7221995571625));
#88495=CARTESIAN_POINT('Ctrl Pts',(8.2179422232714,28.0510467901622,55.6547302798665));
#88496=CARTESIAN_POINT('Ctrl Pts',(8.22183566658305,28.0306827583382,55.5863336628522));
#88497=CARTESIAN_POINT('Ctrl Pts',(8.22570474058982,28.0104461862614,55.5183651445359));
#88498=CARTESIAN_POINT('Ctrl Pts',(8.22957381459659,27.9936928793508,55.4492146040001));
#88499=CARTESIAN_POINT('Ctrl Pts',(8.23344288860335,27.9805570088349,55.3792724191582));
#88500=CARTESIAN_POINT('Ctrl Pts',(8.23730619764755,27.9674407109097,55.3094344489365));
#88501=CARTESIAN_POINT('Ctrl Pts',(8.24116950669174,27.9579312392786,55.2388076493481));
#88502=CARTESIAN_POINT('Ctrl Pts',(8.24503281573593,27.9521128687209,55.167797079955));
#88503=CARTESIAN_POINT('Ctrl Pts',(8.2488915928593,27.9463013235024,55.0968698107262));
#88504=CARTESIAN_POINT('Ctrl Pts',(8.25275036998267,27.9441723181709,55.0255601477312));
#88505=CARTESIAN_POINT('Ctrl Pts',(8.25660914710603,27.9457586931575,54.9542811224769));
#88506=CARTESIAN_POINT('Ctrl Pts',(8.26046549331331,27.9473440687745,54.8830470009119));
#88507=CARTESIAN_POINT('Ctrl Pts',(8.26432183952059,27.9526401702527,54.8118439633125));
#88508=CARTESIAN_POINT('Ctrl Pts',(8.26817818572786,27.9616277741692,54.7410864401745));
#88509=CARTESIAN_POINT('Ctrl Pts',(8.27203339258008,27.9706127227037,54.6703498223022));
#88510=CARTESIAN_POINT('Ctrl Pts',(8.27588859943229,27.983286947251,54.6000589392268));
#88511=CARTESIAN_POINT('Ctrl Pts',(8.27974380628451,27.9995794014052,54.5306227623565));
#88512=CARTESIAN_POINT('Ctrl Pts',(8.28359916372963,28.0158724919788,54.4611838731557));
#88513=CARTESIAN_POINT('Ctrl Pts',(8.28745452117475,28.0357839796486,54.392600228883));
#88514=CARTESIAN_POINT('Ctrl Pts',(8.29130987861986,28.0591921601236,54.325268578489));
#88515=CARTESIAN_POINT('Ctrl Pts',(8.29516927165858,28.0826248431004,54.2578664487216));
#88516=CARTESIAN_POINT('Ctrl Pts',(8.29902866469729,28.1095613655399,54.191719388721));
#88517=CARTESIAN_POINT('Ctrl Pts',(8.30288805773601,28.139831073066,54.1272061378716));
#88518=CARTESIAN_POINT('Ctrl Pts',(8.30674963589709,28.170117918783,54.0626563607222));
#88519=CARTESIAN_POINT('Ctrl Pts',(8.31061121405816,28.2037414773222,53.9997426628237));
#88520=CARTESIAN_POINT('Ctrl Pts',(8.31447279221924,28.2404854099351,53.9388185971057));
#88521=CARTESIAN_POINT('Ctrl Pts',(8.31834112686611,28.2772936322886,53.8777879344039));
#88522=CARTESIAN_POINT('Ctrl Pts',(8.32220946151299,28.3172328567141,53.8187542566786));
#88523=CARTESIAN_POINT('Ctrl Pts',(8.32607779615985,28.3600441796943,53.7620410063555));
#88524=CARTESIAN_POINT('Ctrl Pts',(8.32837550991377,28.3854732530849,53.7283544649385));
#88525=CARTESIAN_POINT('Ctrl Pts',(8.33067322366769,28.4119148693543,53.6954859602599));
#88526=CARTESIAN_POINT('Ctrl Pts',(8.3329709374216,28.4393085840758,53.6634971504855));
#88527=CARTESIAN_POINT('Ctrl Pts',(8.33684001407724,28.485436341269,53.6096317997955));
#88528=CARTESIAN_POINT('Ctrl Pts',(8.34070909073287,28.5344463679899,53.5580518102964));
#88529=CARTESIAN_POINT('Ctrl Pts',(8.3445781673885,28.5860834597022,53.5090816321568));
#88530=CARTESIAN_POINT('Ctrl Pts',(8.34844147911268,28.6376436120513,53.4601844196741));
#88531=CARTESIAN_POINT('Ctrl Pts',(8.35230479083687,28.691822709941,53.4138896312969));
#88532=CARTESIAN_POINT('Ctrl Pts',(8.35616810256105,28.7483261521441,53.3704877597595));
#88533=CARTESIAN_POINT('Ctrl Pts',(8.36002688239727,28.8047633125435,53.3271368011262));
#88534=CARTESIAN_POINT('Ctrl Pts',(8.36388566223349,28.8635190179454,53.286672313062));
#88535=CARTESIAN_POINT('Ctrl Pts',(8.36774444206971,28.9242640734426,53.2493458997239));
#88536=CARTESIAN_POINT('Ctrl Pts',(8.37160079100859,28.9849708616635,53.2120430007304));
#88537=CARTESIAN_POINT('Ctrl Pts',(8.37545713994746,29.0476641006963,53.1778745080932));
#88538=CARTESIAN_POINT('Ctrl Pts',(8.37931348888634,29.1119851827573,53.1470490435909));
#88539=CARTESIAN_POINT('Ctrl Pts',(8.38316869848472,29.1762872614515,53.1162326863298));
#88540=CARTESIAN_POINT('Ctrl Pts',(8.3870239080831,29.2422157905404,53.0887576062114));
#88541=CARTESIAN_POINT('Ctrl Pts',(8.39087911768149,29.3093886417666,53.064785925439));
#88542=CARTESIAN_POINT('Ctrl Pts',(8.39473447788319,29.3765641170926,53.0408133082155));
#88543=CARTESIAN_POINT('Ctrl Pts',(8.3985898380849,29.4449835527988,53.0203445232556));
#88544=CARTESIAN_POINT('Ctrl Pts',(8.40244519828661,29.514247614255,53.003492503835));
#88545=CARTESIAN_POINT('Ctrl Pts',(8.40630459407851,29.5835841777222,52.9866228445984));
#88546=CARTESIAN_POINT('Ctrl Pts',(8.41016398987041,29.6537666588396,52.9733776233692));
#88547=CARTESIAN_POINT('Ctrl Pts',(8.41402338566231,29.7243843048492,52.963818880579));
#88548=CARTESIAN_POINT('Ctrl Pts',(8.41788496657881,29.7950419333751,52.9542547257903));
#88549=CARTESIAN_POINT('Ctrl Pts',(8.42174654749532,29.8661347329007,52.9483812444725));
#88550=CARTESIAN_POINT('Ctrl Pts',(8.42560812841182,29.9372483333486,52.9462084353975));
#88551=CARTESIAN_POINT('Ctrl Pts',(8.42947646578746,30.0084863585194,52.9440318246423));
#88552=CARTESIAN_POINT('Ctrl Pts',(8.4333448031631,30.079744771449,52.945568803024));
#88553=CARTESIAN_POINT('Ctrl Pts',(8.43721314053875,30.1506114136066,52.9507772779438));
#88554=CARTESIAN_POINT('Ctrl Pts',(8.43951082977922,30.1927043091796,52.9538709731468));
#88555=CARTESIAN_POINT('Ctrl Pts',(8.44180851901969,30.2346591058783,52.958258995766));
#88556=CARTESIAN_POINT('Ctrl Pts',(8.44410620826017,30.2763912218767,52.9639240056006));
#88557=CARTESIAN_POINT('Ctrl Pts',(8.44797527190787,30.3466636547658,52.9734632780265));
#88558=CARTESIAN_POINT('Ctrl Pts',(8.45184433555557,30.4165793040417,52.9866635449544));
#88559=CARTESIAN_POINT('Ctrl Pts',(8.45571339920327,30.4857271733883,53.0034863698106));
#88560=CARTESIAN_POINT('Ctrl Pts',(8.45957669789329,30.5547720114652,53.0202841284279));
#88561=CARTESIAN_POINT('Ctrl Pts',(8.46343999658332,30.6230508722509,53.040693616869));
#88562=CARTESIAN_POINT('Ctrl Pts',(8.46730329527334,30.6901599209877,53.0646248823646));
#88563=CARTESIAN_POINT('Ctrl Pts',(8.471162062099,30.7571902470757,53.088528075154));
#88564=CARTESIAN_POINT('Ctrl Pts',(8.47502082892466,30.8230530315313,53.1159446765813));
#88565=CARTESIAN_POINT('Ctrl Pts',(8.47887959575032,30.887358349047,53.1467345784058));
#88566=CARTESIAN_POINT('Ctrl Pts',(8.48273593170018,30.9516231566673,53.1775050837675));
#88567=CARTESIAN_POINT('Ctrl Pts',(8.48659226765004,31.0143320068052,53.2116444641662));
#88568=CARTESIAN_POINT('Ctrl Pts',(8.4904486035999,31.0751151329243,53.2489645881773));
#88569=CARTESIAN_POINT('Ctrl Pts',(8.49430380024967,31.1358803015259,53.286273686484));
#88570=CARTESIAN_POINT('Ctrl Pts',(8.49815899689945,31.1947204618297,53.3267614087846));
#88571=CARTESIAN_POINT('Ctrl Pts',(8.50201419354923,31.2512921568985,53.3701946433441));
#88572=CARTESIAN_POINT('Ctrl Pts',(8.50586954086163,31.3078660628118,53.4136295752918));
#88573=CARTESIAN_POINT('Ctrl Pts',(8.50972488817404,31.362170943501,53.4600099504573));
#88574=CARTESIAN_POINT('Ctrl Pts',(8.51358023548644,31.4138953356547,53.5090615229615));
#88575=CARTESIAN_POINT('Ctrl Pts',(8.51743961856765,31.4656738727846,53.5581644425403));
#88576=CARTESIAN_POINT('Ctrl Pts',(8.52129900164886,31.5148661758648,53.6099438063461));
#88577=CARTESIAN_POINT('Ctrl Pts',(8.52515838473007,31.5611973460965,53.6640881731786));
#88578=CARTESIAN_POINT('Ctrl Pts',(8.52901995301741,31.6075547493181,53.7182631968803));
#88579=CARTESIAN_POINT('Ctrl Pts',(8.53288152130476,31.6510474984651,53.7748055040666));
#88580=CARTESIAN_POINT('Ctrl Pts',(8.5367430895921,31.6914424553517,53.8333723890059));
#88581=CARTESIAN_POINT('Ctrl Pts',(8.54061141460413,31.7319080927448,53.8920417505266));
#88582=CARTESIAN_POINT('Ctrl Pts',(8.54447973961616,31.7692648613614,53.9527423486073));
#88583=CARTESIAN_POINT('Ctrl Pts',(8.54834806462818,31.8033245867531,54.0151050831121));
#88584=CARTESIAN_POINT('Ctrl Pts',(8.5506458694517,31.8235562376743,54.0521488660691));
#88585=CARTESIAN_POINT('Ctrl Pts',(8.55294367427521,31.8426254516933,54.0897786828393));
#88586=CARTESIAN_POINT('Ctrl Pts',(8.55524147909873,31.8605009184363,54.1279140552688));
#88587=CARTESIAN_POINT('Ctrl Pts',(8.5594321115992,31.8931013861208,54.1974636225275));
#88588=CARTESIAN_POINT('Ctrl Pts',(8.56362274409967,31.9218405243209,54.2689335422176));
#88589=CARTESIAN_POINT('Ctrl Pts',(8.56781337660014,31.9465079265243,54.3418932803274));
#88590=CARTESIAN_POINT('Ctrl Pts',(8.57199339313536,31.9711128397633,54.414668192389));
#88591=CARTESIAN_POINT('Ctrl Pts',(8.57617340967057,31.9916664358248,54.4889250781403));
#88592=CARTESIAN_POINT('Ctrl Pts',(8.58035342620579,32.0080057339108,54.5642127410291));
#88593=CARTESIAN_POINT('Ctrl Pts',(8.5845163948271,32.0242783932778,54.6391933482917));
#88594=CARTESIAN_POINT('Ctrl Pts',(8.58867936344842,32.0363709182544,54.7151960144015));
#88595=CARTESIAN_POINT('Ctrl Pts',(8.59284233206974,32.0441702493645,54.7917560226244));
#88596=CARTESIAN_POINT('Ctrl Pts',(8.59658646118964,32.0511848837231,54.860613269047));
#88597=CARTESIAN_POINT('Ctrl Pts',(8.60033059030956,32.0547272944609,54.92992093489));
#88598=CARTESIAN_POINT('Ctrl Pts',(8.60407471942946,32.0547498911142,54.9993310707398));
#88599=CARTESIAN_POINT('Ctrl Pts',(8.60407471946233,32.0547498911144,54.9993310713492));
#88600=CARTESIAN_POINT('Ctrl Pts',(8.60802536615502,32.0547737341254,55.0725697110582));
#88601=CARTESIAN_POINT('Ctrl Pts',(8.61197601284772,32.0508775057908,55.1457764205272));
#88602=CARTESIAN_POINT('Ctrl Pts',(8.61592665954042,32.0430975996036,55.2185171869532));
#88603=CARTESIAN_POINT('Ctrl Pts',(8.61988032369122,32.0353117512143,55.2913135119326));
#88604=CARTESIAN_POINT('Ctrl Pts',(8.62383398784202,32.0236363737173,55.3636427378917));
#88605=CARTESIAN_POINT('Ctrl Pts',(8.62778765199282,32.0081593529454,55.435078815478));
#88606=CARTESIAN_POINT('Ctrl Pts',(8.63174855413826,31.9926539983069,55.5066456714832));
#88607=CARTESIAN_POINT('Ctrl Pts',(8.6357094562837,31.9733332044954,55.5773156739349));
#88608=CARTESIAN_POINT('Ctrl Pts',(8.63967035842913,31.9503352789342,55.6466760102591));
#88609=CARTESIAN_POINT('Ctrl Pts',(8.64363545516164,31.927312998618,55.7161097990342));
#88610=CARTESIAN_POINT('Ctrl Pts',(8.64760055189415,31.9006059955549,55.784230740216));
#88611=CARTESIAN_POINT('Ctrl Pts',(8.65156564862666,31.870400467028,55.850646610198));
#88612=CARTESIAN_POINT('Ctrl Pts',(8.65553891540463,31.8401327002866,55.917199329471));
#88613=CARTESIAN_POINT('Ctrl Pts',(8.6595121821826,31.8063522248623,55.9820395644455));
#88614=CARTESIAN_POINT('Ctrl Pts',(8.66348544896057,31.7692906356216,56.0448005595335));
#88615=CARTESIAN_POINT('Ctrl Pts',(8.66444921595281,31.7603008701752,56.0600240466151));
#88616=CARTESIAN_POINT('Ctrl Pts',(8.66541298294505,31.7511182482559,56.0751253411417));
#88617=CARTESIAN_POINT('Ctrl Pts',(8.66637674993729,31.7417464389131,56.0900994931811));
#88618=CARTESIAN_POINT('Ctrl Pts',(8.67024584450429,31.704122804878,56.1502140341101));
#88619=CARTESIAN_POINT('Ctrl Pts',(8.67411493907129,31.6633096439208,56.2084962168561));
#88620=CARTESIAN_POINT('Ctrl Pts',(8.6779840336383,31.6195111909914,56.2645873100556));
#88621=CARTESIAN_POINT('Ctrl Pts',(8.68184736342655,31.5757779958081,56.320594830022));
#88622=CARTESIAN_POINT('Ctrl Pts',(8.6857106932148,31.5290686342519,56.3744173608726));
#88623=CARTESIAN_POINT('Ctrl Pts',(8.68957402300305,31.479631340782,56.4257239066088));
#88624=CARTESIAN_POINT('Ctrl Pts',(8.69343282104112,31.4302520380805,56.4769702689124));
#88625=CARTESIAN_POINT('Ctrl Pts',(8.69729161907919,31.3781514950012,56.5257061602548));
#88626=CARTESIAN_POINT('Ctrl Pts',(8.70115041711727,31.3236179274611,56.5716339092179));
#88627=CARTESIAN_POINT('Ctrl Pts',(8.70500678433295,31.2691187129541,56.6175327263221));
#88628=CARTESIAN_POINT('Ctrl Pts',(8.70886315154863,31.2121898854573,56.6606265984677));
#88629=CARTESIAN_POINT('Ctrl Pts',(8.71271951876431,31.1531551264326,56.7006559960445));
#88630=CARTESIAN_POINT('Ctrl Pts',(8.71657474668694,31.0941378081461,56.7406735676691));
#88631=CARTESIAN_POINT('Ctrl Pts',(8.72042997460958,31.0330161953365,56.7776281896037));
#88632=CARTESIAN_POINT('Ctrl Pts',(8.72428520253221,30.9701441298328,56.8113028266557));
#88633=CARTESIAN_POINT('Ctrl Pts',(8.72814058107816,30.9072696079246,56.8449787793719));
#88634=CARTESIAN_POINT('Ctrl Pts',(8.73199595962412,30.8426449268075,56.8753742653652));
#88635=CARTESIAN_POINT('Ctrl Pts',(8.73585133817007,30.7766482436334,56.902318340384));
#88636=CARTESIAN_POINT('Ctrl Pts',(8.73971075220939,30.7105824805558,56.9292906182458));
#88637=CARTESIAN_POINT('Ctrl Pts',(8.74357016624872,30.6431422993087,56.9528040894751));
#88638=CARTESIAN_POINT('Ctrl Pts',(8.74742958028804,30.5747247011059,56.9727364447484));
#88639=CARTESIAN_POINT('Ctrl Pts',(8.75129117942483,30.5062683666808,56.9926800851906));
#88640=CARTESIAN_POINT('Ctrl Pts',(8.75515277856163,30.4368339867346,57.0090384620328));
#88641=CARTESIAN_POINT('Ctrl Pts',(8.75901437769842,30.3668298626838,57.0217401945709));
#88642=CARTESIAN_POINT('Ctrl Pts',(8.76288273305271,30.2967032600766,57.0344641499406));
#88643=CARTESIAN_POINT('Ctrl Pts',(8.766751088407,30.2260054051838,57.043518626219));
#88644=CARTESIAN_POINT('Ctrl Pts',(8.77061944376129,30.15515014269,57.0488840854776));
#88645=CARTESIAN_POINT('Ctrl Pts',(8.77291696943281,30.1130671979675,57.0520707835074));
#88646=CARTESIAN_POINT('Ctrl Pts',(8.77521449510433,30.0709287566252,57.0539571768937));
#88647=CARTESIAN_POINT('Ctrl Pts',(8.77751202077585,30.0288210183556,57.0545478605769));
#88648=CARTESIAN_POINT('Ctrl Pts',(8.78138026090062,29.9579261227046,57.0555423679953));
#88649=CARTESIAN_POINT('Ctrl Pts',(8.78524850102539,29.8868408233463,57.0528650337751));
#88650=CARTESIAN_POINT('Ctrl Pts',(8.78911674115016,29.8159770152335,57.0464928789462));
#88651=CARTESIAN_POINT('Ctrl Pts',(8.79297960130612,29.7452117648795,57.040129586544));
#88652=CARTESIAN_POINT('Ctrl Pts',(8.79684246146208,29.6746678741339,57.0300817116751));
#88653=CARTESIAN_POINT('Ctrl Pts',(8.80070532161804,29.6047579252208,57.0163782544017));
#88654=CARTESIAN_POINT('Ctrl Pts',(8.80456410221453,29.5349218080752,57.0026892693242));
#88655=CARTESIAN_POINT('Ctrl Pts',(8.80842288281104,29.465718778231,56.9853524574742));
#88656=CARTESIAN_POINT('Ctrl Pts',(8.81228166340753,29.3975552529139,56.9644484949238));
#88657=CARTESIAN_POINT('Ctrl Pts',(8.81613799763461,29.3294349415502,56.9435577849576));
#88658=CARTESIAN_POINT('Ctrl Pts',(8.81999433186168,29.2623532905634,56.9191045533825));
#88659=CARTESIAN_POINT('Ctrl Pts',(8.82385066608875,29.1967039048842,56.8912199623713));
#88660=CARTESIAN_POINT('Ctrl Pts',(8.82770557291724,29.1310788189245,56.8633456926713));
#88661=CARTESIAN_POINT('Ctrl Pts',(8.83156047974573,29.0668853908702,56.8320427790204));
#88662=CARTESIAN_POINT('Ctrl Pts',(8.83541538657421,29.0044978000164,56.7974907321952));
#88663=CARTESIAN_POINT('Ctrl Pts',(8.83927123820595,28.9420949185209,56.7629302169718));
#88664=CARTESIAN_POINT('Ctrl Pts',(8.84312708983769,28.8814991834627,56.7251192134167));
#88665=CARTESIAN_POINT('Ctrl Pts',(8.84698294146943,28.8230594593807,56.6842827928666));
#88666=CARTESIAN_POINT('Ctrl Pts',(8.84866235100857,28.7976061381791,56.6664965602088));
#88667=CARTESIAN_POINT('Ctrl Pts',(8.85034176054771,28.7725614516204,56.648136959284));
#88668=CARTESIAN_POINT('Ctrl Pts',(8.85202117008686,28.7479524050421,56.6292250864936));
#88669=CARTESIAN_POINT('',(8.54592528048675,32.0547496520916,55.001195712928));
#88670=CARTESIAN_POINT('Ctrl Pts',(8.54592528053768,32.0547496520911,55.001195713863));
#88671=CARTESIAN_POINT('Ctrl Pts',(8.54975547188148,32.0547087341851,55.0715102394462));
#88672=CARTESIAN_POINT('Ctrl Pts',(8.55358566322528,32.0510587897108,55.141718266117));
#88673=CARTESIAN_POINT('Ctrl Pts',(8.55741585456908,32.0438307944968,55.2115496300313));
#88674=CARTESIAN_POINT('Ctrl Pts',(8.56128493121179,32.0365294184178,55.2820899437643));
#88675=CARTESIAN_POINT('Ctrl Pts',(8.56515400785449,32.0255575352495,55.3523899848868));
#88676=CARTESIAN_POINT('Ctrl Pts',(8.5690230844972,32.0109405032667,55.422037740992));
#88677=CARTESIAN_POINT('Ctrl Pts',(8.57288639620839,31.9963452506891,55.4915817218089));
#88678=CARTESIAN_POINT('Ctrl Pts',(8.57674970791958,31.9781157291987,55.5604748752605));
#88679=CARTESIAN_POINT('Ctrl Pts',(8.58061301963077,31.9563290148064,55.6283107100206));
#88680=CARTESIAN_POINT('Ctrl Pts',(8.58447179945396,31.9345678574898,55.6960669694243));
#88681=CARTESIAN_POINT('Ctrl Pts',(8.58833057927715,31.9092579436745,55.7627679135125));
#88682=CARTESIAN_POINT('Ctrl Pts',(8.59218935910033,31.880526921484,55.8280193597217));
#88683=CARTESIAN_POINT('Ctrl Pts',(8.59604570802616,31.8518139988403,55.8932296997845));
#88684=CARTESIAN_POINT('Ctrl Pts',(8.59990205695198,31.8196844389608,55.9569919100661));
#88685=CARTESIAN_POINT('Ctrl Pts',(8.60375840587781,31.7843145294576,56.0189304306313));
#88686=CARTESIAN_POINT('Ctrl Pts',(8.60761361546314,31.7489550698309,56.0808506517465));
#88687=CARTESIAN_POINT('Ctrl Pts',(8.61146882504848,31.710357401943,56.140947831195));
#88688=CARTESIAN_POINT('Ctrl Pts',(8.61532403463381,31.6687436070267,56.1988712760374));
#88689=CARTESIAN_POINT('Ctrl Pts',(8.61917939482249,31.6271281864722,56.2567969836527));
#88690=CARTESIAN_POINT('Ctrl Pts',(8.62303475501116,31.5824966901905,56.3125483948307));
#88691=CARTESIAN_POINT('Ctrl Pts',(8.62689011519983,31.5351133294593,56.3658054869623));
#88692=CARTESIAN_POINT('Ctrl Pts',(8.63074951097883,31.487680370293,56.4191183258452));
#88693=CARTESIAN_POINT('Ctrl Pts',(8.63460890675783,31.4374901201012,56.4699312700161));
#88694=CARTESIAN_POINT('Ctrl Pts',(8.63846830253683,31.3848451286348,56.5179596609253));
#88695=CARTESIAN_POINT('Ctrl Pts',(8.64232988344048,31.3321703304641,56.5660152446976));
#88696=CARTESIAN_POINT('Ctrl Pts',(8.64619146434413,31.2770383999112,56.6112828283351));
#88697=CARTESIAN_POINT('Ctrl Pts',(8.65005304524778,31.2197844625913,56.6535184992375));
#88698=CARTESIAN_POINT('Ctrl Pts',(8.65392138261079,31.1624303502627,56.6958280682665));
#88699=CARTESIAN_POINT('Ctrl Pts',(8.6577897199738,31.1029472240117,56.7350948656177));
#88700=CARTESIAN_POINT('Ctrl Pts',(8.66165805733681,31.0416980194437,56.7711190809167));
#88701=CARTESIAN_POINT('Ctrl Pts',(8.66395574669375,31.0053176233586,56.7925165052665));
#88702=CARTESIAN_POINT('Ctrl Pts',(8.6662534360507,30.9683146132999,56.8127708167859));
#88703=CARTESIAN_POINT('Ctrl Pts',(8.66855112540764,30.9307684193872,56.831848168373));
#88704=CARTESIAN_POINT('Ctrl Pts',(8.67242018908383,30.8675446356291,56.8639723925812));
#88705=CARTESIAN_POINT('Ctrl Pts',(8.67628925276001,30.8025319705833,56.8928825727001));
#88706=CARTESIAN_POINT('Ctrl Pts',(8.6801583164362,30.7360903244563,56.9183765523853));
#88707=CARTESIAN_POINT('Ctrl Pts',(8.68402161515472,30.6697476772885,56.9438325456929));
#88708=CARTESIAN_POINT('Ctrl Pts',(8.68788491387324,30.6019807252953,56.9658822698298));
#88709=CARTESIAN_POINT('Ctrl Pts',(8.69174821259176,30.5331727802138,56.9843700131122));
#88710=CARTESIAN_POINT('Ctrl Pts',(8.69560697944579,30.4644455506829,57.0028360692425));
#88711=CARTESIAN_POINT('Ctrl Pts',(8.69946574629982,30.3946802205381,57.0177483187944));
#88712=CARTESIAN_POINT('Ctrl Pts',(8.70332451315385,30.3242771890504,57.0290002136919));
#88713=CARTESIAN_POINT('Ctrl Pts',(8.707180849132,30.2539185087863,57.0402450203249));
#88714=CARTESIAN_POINT('Ctrl Pts',(8.71103718511014,30.1829234027668,57.0478339706537));
#88715=CARTESIAN_POINT('Ctrl Pts',(8.71489352108828,30.1117030050094,57.0517114809768));
#88716=CARTESIAN_POINT('Ctrl Pts',(8.71874871776621,30.0405036483167,57.055587845744));
#88717=CARTESIAN_POINT('Ctrl Pts',(8.72260391444415,29.9690796168307,57.055754920952));
#88718=CARTESIAN_POINT('Ctrl Pts',(8.72645911112208,29.8978459896077,57.0522090830763));
#88719=CARTESIAN_POINT('Ctrl Pts',(8.73031445846246,29.8266095785493,57.048663106628));
#88720=CARTESIAN_POINT('Ctrl Pts',(8.73416980580284,29.7555640716055,57.0414039553665));
#88721=CARTESIAN_POINT('Ctrl Pts',(8.73802515314322,29.6851216301961,57.0304800355408));
#88722=CARTESIAN_POINT('Ctrl Pts',(8.74188453625196,29.6146054498077,57.0195446805819));
#88723=CARTESIAN_POINT('Ctrl Pts',(8.74574391936071,29.5446940761796,57.0049369735972));
#88724=CARTESIAN_POINT('Ctrl Pts',(8.74960330246945,29.4757907532576,56.9867567108556));
#88725=CARTESIAN_POINT('Ctrl Pts',(8.75346487078411,29.4068484168599,56.9685661543399));
#88726=CARTESIAN_POINT('Ctrl Pts',(8.75732643909878,29.3389157302231,56.9467991635959));
#88727=CARTESIAN_POINT('Ctrl Pts',(8.76118800741344,29.2723793727463,56.921605002412));
#88728=CARTESIAN_POINT('Ctrl Pts',(8.76505633245216,29.2057265942276,56.8963667581042));
#88729=CARTESIAN_POINT('Ctrl Pts',(8.76892465749088,29.1404754676766,56.8676895664043));
#88730=CARTESIAN_POINT('Ctrl Pts',(8.7727929825296,29.0769907033567,56.8357699749179));
#88731=CARTESIAN_POINT('Ctrl Pts',(8.7750907871018,29.0392804333409,56.8168095766768));
#88732=CARTESIAN_POINT('Ctrl Pts',(8.777388591674,29.0021929199974,56.7967059949121));
#88733=CARTESIAN_POINT('Ctrl Pts',(8.77968639624619,28.965799690604,56.7755076126407));
#88734=CARTESIAN_POINT('Ctrl Pts',(8.7835554038458,28.9045213369959,56.7398141062826));
#88735=CARTESIAN_POINT('Ctrl Pts',(8.78742441144541,28.8449729706854,56.7008746005939));
#88736=CARTESIAN_POINT('Ctrl Pts',(8.79129341904501,28.787519610286,56.6588818122636));
#88737=CARTESIAN_POINT('Ctrl Pts',(8.79218924839468,28.7742168691676,56.649158809325));
#88738=CARTESIAN_POINT('Ctrl Pts',(8.79308507774435,28.7610263498124,56.6392723176847));
#88739=CARTESIAN_POINT('Ctrl Pts',(8.79398090709402,28.7479524050421,56.6292250864936));
#88740=CARTESIAN_POINT('Ctrl Pts',(8.09385946234359,28.7479524050421,56.6292250864936));
#88741=CARTESIAN_POINT('Ctrl Pts',(8.09772772740314,28.6914355148067,56.5857922685974));
#88742=CARTESIAN_POINT('Ctrl Pts',(8.10159599246268,28.6372539723095,56.5394711345916));
#88743=CARTESIAN_POINT('Ctrl Pts',(8.10546425752223,28.5857004584289,56.4905550540694));
#88744=CARTESIAN_POINT('Ctrl Pts',(8.1079344287531,28.5527797549927,56.4593185454608));
#88745=CARTESIAN_POINT('Ctrl Pts',(8.11040459998397,28.5209299459321,56.4270246259437));
#88746=CARTESIAN_POINT('Ctrl Pts',(8.11287477121484,28.4902185814113,56.3937566611802));
#88747=CARTESIAN_POINT('Ctrl Pts',(8.11674384460076,28.4421148217901,56.3416484528659));
#88748=CARTESIAN_POINT('Ctrl Pts',(8.12061291798667,28.3966176804652,56.2869448935148));
#88749=CARTESIAN_POINT('Ctrl Pts',(8.12448199137259,28.3540195501558,56.2299373647591));
#88750=CARTESIAN_POINT('Ctrl Pts',(8.12834529980468,28.3114848914401,56.1730147777293));
#88751=CARTESIAN_POINT('Ctrl Pts',(8.13220860823678,28.271840957964,56.1137954215481));
#88752=CARTESIAN_POINT('Ctrl Pts',(8.13607191666887,28.23534181248,56.0526058349252));
#88753=CARTESIAN_POINT('Ctrl Pts',(8.13993069319587,28.1988854828017,55.9914880275569));
#88754=CARTESIAN_POINT('Ctrl Pts',(8.14378946972286,28.1655668610939,55.9284049957587));
#88755=CARTESIAN_POINT('Ctrl Pts',(8.14764824624986,28.135597344255,55.8637130887922));
#88756=CARTESIAN_POINT('Ctrl Pts',(8.15150459187077,28.1056467072554,55.7990619356629));
#88757=CARTESIAN_POINT('Ctrl Pts',(8.15536093749167,28.0790411929748,55.7328043579541));
#88758=CARTESIAN_POINT('Ctrl Pts',(8.15921728311258,28.0559460723379,55.6653208916317));
#88759=CARTESIAN_POINT('Ctrl Pts',(8.16307248938919,28.0328577750764,55.5978573630716));
#88760=CARTESIAN_POINT('Ctrl Pts',(8.16692769566581,28.0132779696707,55.5291691242994));
#88761=CARTESIAN_POINT('Ctrl Pts',(8.17078290194242,27.9973229967891,55.4596546348186));
#88762=CARTESIAN_POINT('Ctrl Pts',(8.17463825882349,27.9813674006231,55.3901374297395));
#88763=CARTESIAN_POINT('Ctrl Pts',(8.17849361570457,27.9690370246441,55.3197943838363));
#88764=CARTESIAN_POINT('Ctrl Pts',(8.18234897258564,27.9603973464495,55.2490352949481));
#88765=CARTESIAN_POINT('Ctrl Pts',(8.18620836508162,27.9517486246267,55.1782021386148));
#88766=CARTESIAN_POINT('Ctrl Pts',(8.1900677575776,27.9467983715154,55.1069525531432));
#88767=CARTESIAN_POINT('Ctrl Pts',(8.19392715007359,27.945560186038,55.0357017269566));
#88768=CARTESIAN_POINT('Ctrl Pts',(8.19778872770313,27.9443212995174,54.9644105595578));
#88769=CARTESIAN_POINT('Ctrl Pts',(8.20165030533268,27.9467986476289,54.8931186357687));
#88770=CARTESIAN_POINT('Ctrl Pts',(8.20551188296223,27.9529537215789,54.8222386529578));
#88771=CARTESIAN_POINT('Ctrl Pts',(8.20938021710087,27.9591195649131,54.7512346531531));
#88772=CARTESIAN_POINT('Ctrl Pts',(8.21324855123952,27.9689759142079,54.6806445146228));
#88773=CARTESIAN_POINT('Ctrl Pts',(8.21711688537817,27.9824327849669,54.6108726489648));
#88774=CARTESIAN_POINT('Ctrl Pts',(8.21941460426991,27.9904259171676,54.5694294519481));
#88775=CARTESIAN_POINT('Ctrl Pts',(8.22171232316166,27.9996883921494,54.5282747183294));
#88776=CARTESIAN_POINT('Ctrl Pts',(8.2240100420534,28.0101930999981,54.487490426231));
#88777=CARTESIAN_POINT('Ctrl Pts',(8.22787911588953,28.0278817260697,54.418814733112));
#88778=CARTESIAN_POINT('Ctrl Pts',(8.23174818972565,28.0491645565733,54.350921348827));
#88779=CARTESIAN_POINT('Ctrl Pts',(8.23561726356177,28.0739553723287,54.2842139602376));
#88780=CARTESIAN_POINT('Ctrl Pts',(8.23948057244793,28.0987092495767,54.2176059661738));
#88781=CARTESIAN_POINT('Ctrl Pts',(8.24334388133408,28.1269605689286,54.152180911724));
#88782=CARTESIAN_POINT('Ctrl Pts',(8.24720719022022,28.1585727854168,54.0883293490013));
#88783=CARTESIAN_POINT('Ctrl Pts',(8.25106596720477,28.1901479188089,54.024552688133));
#88784=CARTESIAN_POINT('Ctrl Pts',(8.25492474418931,28.2250759036248,53.9623462858401));
#88785=CARTESIAN_POINT('Ctrl Pts',(8.25878352117385,28.2631720093297,53.902081016958));
#88786=CARTESIAN_POINT('Ctrl Pts',(8.2626398672542,28.301244115725,53.8418537132383));
#88787=CARTESIAN_POINT('Ctrl Pts',(8.26649621333455,28.3424801243909,53.7835655264644));
#88788=CARTESIAN_POINT('Ctrl Pts',(8.2703525594149,28.3866499674206,53.7275616970258));
#88789=CARTESIAN_POINT('Ctrl Pts',(8.27420776615216,28.4308067606346,53.67157441371));
#88790=CARTESIAN_POINT('Ctrl Pts',(8.27806297288942,28.4778953667262,53.6178705290785));
#88791=CARTESIAN_POINT('Ctrl Pts',(8.28191817962669,28.5276441214334,53.56676389616));
#88792=CARTESIAN_POINT('Ctrl Pts',(8.28577353696892,28.5773948195928,53.5156552667433));
#88793=CARTESIAN_POINT('Ctrl Pts',(8.28962889431116,28.6298055322612,53.4671444370395));
#88794=CARTESIAN_POINT('Ctrl Pts',(8.29348425165339,28.6845674830464,53.4215086772994));
#88795=CARTESIAN_POINT('Ctrl Pts',(8.29734364460812,28.7393867561478,53.3758251481242));
#88796=CARTESIAN_POINT('Ctrl Pts',(8.30120303756285,28.7965618064593,53.3330230081686));
#88797=CARTESIAN_POINT('Ctrl Pts',(8.30506243051757,28.8557511915957,53.2933388658069));
#88798=CARTESIAN_POINT('Ctrl Pts',(8.3089240086052,28.9149740889123,53.2536322548534));
#88799=CARTESIAN_POINT('Ctrl Pts',(8.31278558669282,28.9762131741812,53.2170474050503));
#88800=CARTESIAN_POINT('Ctrl Pts',(8.31664716478044,29.039100836507,53.1837757957514));
#88801=CARTESIAN_POINT('Ctrl Pts',(8.3205154993711,29.1020985317447,53.1504459719806));
#88802=CARTESIAN_POINT('Ctrl Pts',(8.32438383396176,29.1667501221892,53.120441167342));
#88803=CARTESIAN_POINT('Ctrl Pts',(8.32825216855243,29.2326670396085,53.0939051203057));
#88804=CARTESIAN_POINT('Ctrl Pts',(8.33054988333227,29.271820394068,53.0781432294855));
#88805=CARTESIAN_POINT('Ctrl Pts',(8.33284759811211,29.3114198421419,53.0636042166553));
#88806=CARTESIAN_POINT('Ctrl Pts',(8.33514531289195,29.3513818074579,53.050309767475));
#88807=CARTESIAN_POINT('Ctrl Pts',(8.33901438504249,29.4186728952993,53.0279235324507));
#88808=CARTESIAN_POINT('Ctrl Pts',(8.34288345719303,29.4872560984358,53.0089812381622));
#88809=CARTESIAN_POINT('Ctrl Pts',(8.34675252934356,29.5567455001129,52.9936293934495));
#88810=CARTESIAN_POINT('Ctrl Pts',(8.35061583654187,29.6261313619579,52.9783004231232));
#88811=CARTESIAN_POINT('Ctrl Pts',(8.35447914374019,29.6964202716635,52.966551387107));
#88812=CARTESIAN_POINT('Ctrl Pts',(8.3583424509385,29.767210052625,52.9584793895478));
#88813=CARTESIAN_POINT('Ctrl Pts',(8.36220122623995,29.8379167928212,52.950416860938));
#88814=CARTESIAN_POINT('Ctrl Pts',(8.3660600015414,29.9091227568787,52.9460228576987));
#88815=CARTESIAN_POINT('Ctrl Pts',(8.36991877684285,29.9804161657888,52.9453433289385));
#88816=CARTESIAN_POINT('Ctrl Pts',(8.37377512124393,30.0516646622176,52.9446642282588));
#88817=CARTESIAN_POINT('Ctrl Pts',(8.37763146564502,30.1230000095906,52.9476949641638));
#88818=CARTESIAN_POINT('Ctrl Pts',(8.3814878100461,30.194007376137,52.9544294926587));
#88819=CARTESIAN_POINT('Ctrl Pts',(8.38534301511035,30.2649937639273,52.9611620314723));
#88820=CARTESIAN_POINT('Ctrl Pts',(8.3891982201746,30.3356518799121,52.9715961446121));
#88821=CARTESIAN_POINT('Ctrl Pts',(8.39305342523885,30.405570701832,52.9856738177953));
#88822=CARTESIAN_POINT('Ctrl Pts',(8.39690878091677,30.4754922553135,52.9997520409595));
#88823=CARTESIAN_POINT('Ctrl Pts',(8.40076413659469,30.5446739815933,53.0174740087301));
#88824=CARTESIAN_POINT('Ctrl Pts',(8.40461949227261,30.6127154649093,53.0387306861216));
#88825=CARTESIAN_POINT('Ctrl Pts',(8.40847888358764,30.6808281714167,53.0600096141804));
#88826=CARTESIAN_POINT('Ctrl Pts',(8.41233827490267,30.7477977877063,53.0848304927303));
#88827=CARTESIAN_POINT('Ctrl Pts',(8.41619766621771,30.8132403429686,53.1130347891208));
#88828=CARTESIAN_POINT('Ctrl Pts',(8.42005924267704,30.8787199510757,53.1412550544693));
#88829=CARTESIAN_POINT('Ctrl Pts',(8.42392081913638,30.9426703412895,53.1728623357878));
#88830=CARTESIAN_POINT('Ctrl Pts',(8.42778239559572,31.0047312648068,53.2076516387656));
#88831=CARTESIAN_POINT('Ctrl Pts',(8.43165072859373,31.0669007753313,53.2425018120314));
#88832=CARTESIAN_POINT('Ctrl Pts',(8.43551906159174,31.1271738077633,53.2805448633252));
#88833=CARTESIAN_POINT('Ctrl Pts',(8.43938739458976,31.1852188559992,53.3215322982303));
#88834=CARTESIAN_POINT('Ctrl Pts',(8.44168512430334,31.2196967130313,53.3458781979017));
#88835=CARTESIAN_POINT('Ctrl Pts',(8.44398285401693,31.2533891120851,53.3712621389149));
#88836=CARTESIAN_POINT('Ctrl Pts',(8.44628058373051,31.2862325040358,53.3976256654384));
#88837=CARTESIAN_POINT('Ctrl Pts',(8.45010049356877,31.3408337024676,53.441454273191));
#88838=CARTESIAN_POINT('Ctrl Pts',(8.45392040340703,31.3933122653082,53.488173590139));
#88839=CARTESIAN_POINT('Ctrl Pts',(8.45774031324528,31.4433401967307,53.5375477310348));
#88840=CARTESIAN_POINT('Ctrl Pts',(8.46155371487817,31.49328289262,53.5868377502989));
#88841=CARTESIAN_POINT('Ctrl Pts',(8.46536711651106,31.5407828948695,53.6387732653233));
#88842=CARTESIAN_POINT('Ctrl Pts',(8.46918051814395,31.585544633233,53.693077745799));
#88843=CARTESIAN_POINT('Ctrl Pts',(8.47299028959825,31.6302637605316,53.747330530969));
#88844=CARTESIAN_POINT('Ctrl Pts',(8.47680006105254,31.6722494743745,53.8039474289001));
#88845=CARTESIAN_POINT('Ctrl Pts',(8.48060983250683,31.7112435202134,53.8626156423496));
#88846=CARTESIAN_POINT('Ctrl Pts',(8.48441732946353,31.7502142859515,53.9212488298896));
#88847=CARTESIAN_POINT('Ctrl Pts',(8.48822482642023,31.7861966495347,53.9819304895735));
#88848=CARTESIAN_POINT('Ctrl Pts',(8.49203232337693,31.8189742648894,54.0443169007616));
#88849=CARTESIAN_POINT('Ctrl Pts',(8.49583889833161,31.8517439430014,54.1066882048078));
#88850=CARTESIAN_POINT('Ctrl Pts',(8.4996454732863,31.8813101817803,54.1707629987572));
#88851=CARTESIAN_POINT('Ctrl Pts',(8.50345204824098,31.9075023513006,54.236172570352));
#88852=CARTESIAN_POINT('Ctrl Pts',(8.50726133449443,31.9337131766461,54.301628731044));
#88853=CARTESIAN_POINT('Ctrl Pts',(8.51107062074788,31.9565449440846,54.3684211048419));
#88854=CARTESIAN_POINT('Ctrl Pts',(8.51487990700134,31.9758754824593,54.4361616895632));
#88855=CARTESIAN_POINT('Ctrl Pts',(8.51869055156213,31.995212913677,54.5039264290807));
#88856=CARTESIAN_POINT('Ctrl Pts',(8.52250119612292,32.0110465156929,54.5726395660196));
#88857=CARTESIAN_POINT('Ctrl Pts',(8.52631184068371,32.0233049526314,54.6419013667199));
#88858=CARTESIAN_POINT('Ctrl Pts',(8.53012846729214,32.035582633179,54.7112718963729));
#88859=CARTESIAN_POINT('Ctrl Pts',(8.53394509390057,32.0442738790978,54.7811923136052));
#88860=CARTESIAN_POINT('Ctrl Pts',(8.537761720509,32.0493591950676,54.8512570939779));
#88861=CARTESIAN_POINT('Ctrl Pts',(8.54048290716825,32.0529849346001,54.9012120319884));
#88862=CARTESIAN_POINT('Ctrl Pts',(8.5432040938275,32.0547787224859,54.9512402585401));
#88863=CARTESIAN_POINT('Ctrl Pts',(8.54592528048675,32.0547496520916,55.001195712928));
#88864=CARTESIAN_POINT('Origin',(-1.54592528053767,30.,55.));
#88865=CARTESIAN_POINT('',(7.39391310532386,28.7479524050421,56.6292250864936));
#88866=CARTESIAN_POINT('',(7.45211324799747,28.7479524050421,56.6292250864936));
#88867=CARTESIAN_POINT('',(-1.54592528053767,28.7479524050421,56.6292250864936));
#88868=CARTESIAN_POINT('',(7.9040747195078,32.0547494456334,54.9984906394957));
#88869=CARTESIAN_POINT('Ctrl Pts',(7.45211324799746,28.7479524050421,56.6292250864936));
#88870=CARTESIAN_POINT('Ctrl Pts',(7.45597808883343,28.6916394093406,56.5859489600594));
#88871=CARTESIAN_POINT('Ctrl Pts',(7.45984292966939,28.6374791542456,56.5396778427251));
#88872=CARTESIAN_POINT('Ctrl Pts',(7.46370777050535,28.585805915676,56.4906551091258));
#88873=CARTESIAN_POINT('Ctrl Pts',(7.4675674996065,28.5342010214195,56.4416972142158));
#88874=CARTESIAN_POINT('Ctrl Pts',(7.47142722870764,28.4850769597258,56.3899952649857));
#88875=CARTESIAN_POINT('Ctrl Pts',(7.47528695780879,28.4387352829959,56.3358330905986));
#88876=CARTESIAN_POINT('Ctrl Pts',(7.47914387883221,28.3924273213345,56.2817103209448));
#88877=CARTESIAN_POINT('Ctrl Pts',(7.48300079985563,28.3488980437697,56.2251312448299));
#88878=CARTESIAN_POINT('Ctrl Pts',(7.48685772087905,28.3084114391004,56.166415750551));
#88879=CARTESIAN_POINT('Ctrl Pts',(7.49071312610269,28.2679407459796,56.1077233319152));
#88880=CARTESIAN_POINT('Ctrl Pts',(7.49456853132634,28.2305106279276,56.0468965611038));
#88881=CARTESIAN_POINT('Ctrl Pts',(7.49842393654998,28.1963430684199,55.9842861553751));
#88882=CARTESIAN_POINT('Ctrl Pts',(7.50227911625905,28.1621775074785,55.9216794119227));
#88883=CARTESIAN_POINT('Ctrl Pts',(7.50613429596812,28.1312743574825,55.8572896678745));
#88884=CARTESIAN_POINT('Ctrl Pts',(7.5099894756772,28.1038099013592,55.7914926862055));
#88885=CARTESIAN_POINT('Ctrl Pts',(7.51384844943747,28.0763184162619,55.725630950845));
#88886=CARTESIAN_POINT('Ctrl Pts',(7.51770742319774,28.0522725726796,55.6583596607912));
#88887=CARTESIAN_POINT('Ctrl Pts',(7.52156639695801,28.0318003266534,55.5900742396838));
#88888=CARTESIAN_POINT('Ctrl Pts',(7.52542721801123,28.0113182805513,55.5217561303062));
#88889=CARTESIAN_POINT('Ctrl Pts',(7.52928803906444,27.9944133552572,55.4524233954285));
#88890=CARTESIAN_POINT('Ctrl Pts',(7.53314886011766,27.9811627431385,55.3824835850177));
#88891=CARTESIAN_POINT('Ctrl Pts',(7.53701679547944,27.9678877142075,55.3124148969963));
#88892=CARTESIAN_POINT('Ctrl Pts',(7.54088473084123,27.9582805181449,55.2417373809803));
#88893=CARTESIAN_POINT('Ctrl Pts',(7.54475266620301,27.9523665739296,55.1708651952251));
#88894=CARTESIAN_POINT('Ctrl Pts',(7.54817645798591,27.9471317104392,55.1081310529687));
#88895=CARTESIAN_POINT('Ctrl Pts',(7.5516002497688,27.9447898576055,55.0452446609213));
#88896=CARTESIAN_POINT('Ctrl Pts',(7.5550240415517,27.945324596287,54.9824914912983));
#88897=CARTESIAN_POINT('Ctrl Pts',(7.55889311489863,27.9459288804584,54.911576952267));
#88898=CARTESIAN_POINT('Ctrl Pts',(7.56276218824556,27.950209947427,54.840554831208));
#88899=CARTESIAN_POINT('Ctrl Pts',(7.56663126159248,27.9581814784797,54.7698376927546));
#88900=CARTESIAN_POINT('Ctrl Pts',(7.57049456998679,27.9661411318824,54.6992259234468));
#88901=CARTESIAN_POINT('Ctrl Pts',(7.5743578783811,27.9777802803876,54.628918713516));
#88902=CARTESIAN_POINT('Ctrl Pts',(7.57822118677541,27.993060597262,54.5593280174123));
#88903=CARTESIAN_POINT('Ctrl Pts',(7.58207996326658,28.0083229893661,54.4898189555615));
#88904=CARTESIAN_POINT('Ctrl Pts',(7.58593873975774,28.0272179618767,54.4210252101689));
#88905=CARTESIAN_POINT('Ctrl Pts',(7.58979751624891,28.0496556792535,54.3533512599318));
#88906=CARTESIAN_POINT('Ctrl Pts',(7.5936538618352,28.0720792615912,54.2857199421031));
#88907=CARTESIAN_POINT('Ctrl Pts',(7.5975102074215,28.0980410083899,54.2192074798708));
#88908=CARTESIAN_POINT('Ctrl Pts',(7.60136655300779,28.1274009027621,54.1542044079544));
#88909=CARTESIAN_POINT('Ctrl Pts',(7.60522175925105,28.1567521228621,54.0892205409551));
#88910=CARTESIAN_POINT('Ctrl Pts',(7.60907696549432,28.189499297522,54.0257456214304));
#88911=CARTESIAN_POINT('Ctrl Pts',(7.61293217173758,28.2254544716958,53.9641497548026));
#88912=CARTESIAN_POINT('Ctrl Pts',(7.6167875285866,28.2614110504783,53.9025514818982));
#88913=CARTESIAN_POINT('Ctrl Pts',(7.62064288543561,28.3005756307868,53.8428328260587));
#88914=CARTESIAN_POINT('Ctrl Pts',(7.62449824228463,28.3427154183277,53.7853373398959));
#88915=CARTESIAN_POINT('Ctrl Pts',(7.62835763475074,28.3848993159351,53.7277816700002));
#88916=CARTESIAN_POINT('Ctrl Pts',(7.63221702721685,28.430064349888,53.6724542078469));
#88917=CARTESIAN_POINT('Ctrl Pts',(7.63607641968296,28.4779362178107,53.6196669222801));
#88918=CARTESIAN_POINT('Ctrl Pts',(7.63993799728382,28.5258351901243,53.5668497492808));
#88919=CARTESIAN_POINT('Ctrl Pts',(7.64379957488468,28.576443702482,53.5165759584295));
#88920=CARTESIAN_POINT('Ctrl Pts',(7.64766115248553,28.6294511728063,53.4691200325375));
#88921=CARTESIAN_POINT('Ctrl Pts',(7.65152948659766,28.6825513890514,53.421581074131));
#88922=CARTESIAN_POINT('Ctrl Pts',(7.65539782070978,28.738058565056,53.376870129106));
#88923=CARTESIAN_POINT('Ctrl Pts',(7.6592661548219,28.7956302665086,53.3352204027109));
#88924=CARTESIAN_POINT('Ctrl Pts',(7.66156387401135,28.8298267964264,53.3104812326187));
#88925=CARTESIAN_POINT('Ctrl Pts',(7.6638615932008,28.86475117244,53.2868212673977));
#88926=CARTESIAN_POINT('Ctrl Pts',(7.66615931239025,28.9003275144172,53.2642817086427));
#88927=CARTESIAN_POINT('Ctrl Pts',(7.67002838580839,28.9602336507679,53.2263278942534));
#88928=CARTESIAN_POINT('Ctrl Pts',(7.67389745922652,29.0222243264519,53.1914047567569));
#88929=CARTESIAN_POINT('Ctrl Pts',(7.67776653264466,29.0859603481719,53.1597475506371));
#88930=CARTESIAN_POINT('Ctrl Pts',(7.68162984111065,29.14960140268,53.1281375140225));
#88931=CARTESIAN_POINT('Ctrl Pts',(7.68549314957663,29.2149822096154,53.099783963722));
#88932=CARTESIAN_POINT('Ctrl Pts',(7.68935645804262,29.2817358810413,53.0748781290743));
#88933=CARTESIAN_POINT('Ctrl Pts',(7.69321523460581,29.3484112462298,53.0500015105305));
#88934=CARTESIAN_POINT('Ctrl Pts',(7.69707401116899,29.4164558240683,53.0285647431085));
#88935=CARTESIAN_POINT('Ctrl Pts',(7.70093278773218,29.4854810707992,53.0107117267741));
#88936=CARTESIAN_POINT('Ctrl Pts',(7.70478913339068,29.5544628338524,52.9928699572638));
#88937=CARTESIAN_POINT('Ctrl Pts',(7.70864547904917,29.6244235709156,52.9786075810603));
#88938=CARTESIAN_POINT('Ctrl Pts',(7.71250182470766,29.6949592366148,52.9680187758807));
#88939=CARTESIAN_POINT('Ctrl Pts',(7.71635703102319,29.7654740628141,52.9574330991242));
#88940=CARTESIAN_POINT('Ctrl Pts',(7.72021223733871,29.836563000288,52.9505189107643));
#88941=CARTESIAN_POINT('Ctrl Pts',(7.72406744365423,29.9078131672703,52.9473190334659));
#88942=CARTESIAN_POINT('Ctrl Pts',(7.72792280057547,29.9790661176788,52.9441190311626));
#88943=CARTESIAN_POINT('Ctrl Pts',(7.73177815749672,30.0504798247049,52.9446336475956));
#88944=CARTESIAN_POINT('Ctrl Pts',(7.73563351441796,30.1216393955579,52.948853632734));
#88945=CARTESIAN_POINT('Ctrl Pts',(7.73949290695573,30.1928734530918,52.9530780351657));
#88946=CARTESIAN_POINT('Ctrl Pts',(7.7433522994935,30.2638523574922,52.961015520074));
#88947=CARTESIAN_POINT('Ctrl Pts',(7.74721169203127,30.3341652383747,52.9726048347789));
#88948=CARTESIAN_POINT('Ctrl Pts',(7.75107326970358,30.4045179294353,52.984200711193));
#88949=CARTESIAN_POINT('Ctrl Pts',(7.7549348473759,30.4742033715237,52.9994524294759));
#88950=CARTESIAN_POINT('Ctrl Pts',(7.75879642504821,30.5428225110972,53.0182479257117));
#88951=CARTESIAN_POINT('Ctrl Pts',(7.76266475923068,30.611561711939,53.037076307978));
#88952=CARTESIAN_POINT('Ctrl Pts',(7.76653309341314,30.6792304240199,53.0594606949899));
#88953=CARTESIAN_POINT('Ctrl Pts',(7.77040142759561,30.7454469973676,53.085239874915));
#88954=CARTESIAN_POINT('Ctrl Pts',(7.77269914614001,30.7847784101543,53.100552228238));
#88955=CARTESIAN_POINT('Ctrl Pts',(7.77499686468441,30.8235978937815,53.1170613980573));
#88956=CARTESIAN_POINT('Ctrl Pts',(7.77729458322882,30.8618296784007,53.1347259804716));
#88957=CARTESIAN_POINT('Ctrl Pts',(7.78116365643173,30.9262072644763,53.1644709475503));
#88958=CARTESIAN_POINT('Ctrl Pts',(7.78503272963465,30.9891692263907,53.1976109568967));
#88959=CARTESIAN_POINT('Ctrl Pts',(7.78890180283756,31.0503339503682,53.233988631066));
#88960=CARTESIAN_POINT('Ctrl Pts',(7.79276511108818,31.1114075383818,53.2703121021886));
#88961=CARTESIAN_POINT('Ctrl Pts',(7.79662841933881,31.1706887898942,53.3098634160372));
#88962=CARTESIAN_POINT('Ctrl Pts',(7.80049172758943,31.2278180579912,53.3524380500356));
#88963=CARTESIAN_POINT('Ctrl Pts',(7.80435050393808,31.284880309887,53.3949627413279));
#88964=CARTESIAN_POINT('Ctrl Pts',(7.80820928028672,31.3397952050739,53.4405034192621));
#88965=CARTESIAN_POINT('Ctrl Pts',(7.81206805663537,31.3922311147639,53.4888116975098));
#88966=CARTESIAN_POINT('Ctrl Pts',(7.81592440207993,31.4446339915296,53.5370895431073));
#88967=CARTESIAN_POINT('Ctrl Pts',(7.8197807475245,31.4945606247154,53.588131201571));
#88968=CARTESIAN_POINT('Ctrl Pts',(7.82363709296907,31.5417127518387,53.6416482954265));
#88969=CARTESIAN_POINT('Ctrl Pts',(7.8274922990716,31.5888509480522,53.6951495778678));
#88970=CARTESIAN_POINT('Ctrl Pts',(7.83134750517413,31.6332159446003,53.7511244794588));
#88971=CARTESIAN_POINT('Ctrl Pts',(7.83520271127665,31.6745478320743,53.8092493457506));
#88972=CARTESIAN_POINT('Ctrl Pts',(7.83905806798614,31.7158813342142,53.8673764827406));
#88973=CARTESIAN_POINT('Ctrl Pts',(7.84291342469562,31.7541812123083,53.9276533540082));
#88974=CARTESIAN_POINT('Ctrl Pts',(7.8467687814051,31.7892302147803,53.9897263731952));
#88975=CARTESIAN_POINT('Ctrl Pts',(7.85062817373444,31.824315905025,54.0518643677213));
#88976=CARTESIAN_POINT('Ctrl Pts',(7.85448756606379,31.8561436874045,54.1158018394496));
#88977=CARTESIAN_POINT('Ctrl Pts',(7.85834695839314,31.8845421816423,54.1811603770512));
#88978=CARTESIAN_POINT('Ctrl Pts',(7.86220853585858,31.9129567547261,54.246555919779));
#88979=CARTESIAN_POINT('Ctrl Pts',(7.86607011332404,31.9379380043066,54.3133736748274));
#88980=CARTESIAN_POINT('Ctrl Pts',(7.86993169078948,31.9593636478709,54.3812176005234));
#88981=CARTESIAN_POINT('Ctrl Pts',(7.8738000247698,31.9808267793997,54.4491802312037));
#88982=CARTESIAN_POINT('Ctrl Pts',(7.87766835875011,31.9987217621738,54.5181721468595));
#88983=CARTESIAN_POINT('Ctrl Pts',(7.88153669273042,32.0129770440577,54.587785271252));
#88984=CARTESIAN_POINT('Ctrl Pts',(7.88383441317607,32.0214444237642,54.6291342085506));
#88985=CARTESIAN_POINT('Ctrl Pts',(7.88613213362173,32.0286286516942,54.6707021625283));
#88986=CARTESIAN_POINT('Ctrl Pts',(7.88842985406738,32.0345234182149,54.7124030194264));
#88987=CARTESIAN_POINT('Ctrl Pts',(7.89364480919903,32.047902305527,54.8070481700526));
#88988=CARTESIAN_POINT('Ctrl Pts',(7.89885976433068,32.0546790423547,54.9026480509711));
#88989=CARTESIAN_POINT('Ctrl Pts',(7.90407471946233,32.0547494456328,54.99849063866));
#88990=CARTESIAN_POINT('Ctrl Pts',(7.9040747195078,32.0547494456334,54.9984906394957));
#88991=CARTESIAN_POINT('Ctrl Pts',(7.90805348639939,32.0548031600125,55.0716140518894));
#88992=CARTESIAN_POINT('Ctrl Pts',(7.91203225329098,32.050948418131,55.1448858516356));
#88993=CARTESIAN_POINT('Ctrl Pts',(7.91601102018257,32.0431692286174,55.2178464269408));
#88994=CARTESIAN_POINT('Ctrl Pts',(7.9198148683539,32.0357320359866,55.2875994329639));
#88995=CARTESIAN_POINT('Ctrl Pts',(7.92361871652522,32.0247082537432,55.3570674381738));
#88996=CARTESIAN_POINT('Ctrl Pts',(7.92742256469655,32.0101370404031,55.4258481434733));
#88997=CARTESIAN_POINT('Ctrl Pts',(7.93122379837268,31.9955758422806,55.4945815737987));
#88998=CARTESIAN_POINT('Ctrl Pts',(7.93502503204882,31.9774721493163,55.562628151676));
#88999=CARTESIAN_POINT('Ctrl Pts',(7.93882626572496,31.9559166148128,55.6295933277913));
#89000=CARTESIAN_POINT('Ctrl Pts',(7.94262624479613,31.9343681947576,55.6965364019132));
#89001=CARTESIAN_POINT('Ctrl Pts',(7.94642622386731,31.9093703466155,55.7623983055163));
#89002=CARTESIAN_POINT('Ctrl Pts',(7.95022620293848,31.881063720918,55.8267991535712));
#89003=CARTESIAN_POINT('Ctrl Pts',(7.95402628536076,31.8527563253424,55.891201753188));
#89004=CARTESIAN_POINT('Ctrl Pts',(7.95782636778304,31.821140178272,55.9541427608864));
#89005=CARTESIAN_POINT('Ctrl Pts',(7.96162645020532,31.7864034803868,56.0152635952116));
#89006=CARTESIAN_POINT('Ctrl Pts',(7.96543037542157,31.7516316553758,56.0764462373471));
#89007=CARTESIAN_POINT('Ctrl Pts',(7.96923430063783,31.7137332332642,56.1358045982852));
#89008=CARTESIAN_POINT('Ctrl Pts',(7.97303822585408,31.6729410672239,56.1930070192986));
#89009=CARTESIAN_POINT('Ctrl Pts',(7.97684442147971,31.6321245539866,56.2502435821276));
#89010=CARTESIAN_POINT('Ctrl Pts',(7.98065061710535,31.5884111753275,56.305321255317));
#89011=CARTESIAN_POINT('Ctrl Pts',(7.98445681273098,31.5420737815355,56.3579418304187));
#89012=CARTESIAN_POINT('Ctrl Pts',(7.98826926304291,31.4956602419301,56.4106488764279));
#89013=CARTESIAN_POINT('Ctrl Pts',(7.99208171335483,31.4466144388796,56.460890416329));
#89014=CARTESIAN_POINT('Ctrl Pts',(7.99589416366676,31.3952448863443,56.5084062018004));
#89015=CARTESIAN_POINT('Ctrl Pts',(7.99711781741315,31.3787571841404,56.5236569891282));
#89016=CARTESIAN_POINT('Ctrl Pts',(7.99834147115954,31.3620303358886,56.5386273004867));
#89017=CARTESIAN_POINT('Ctrl Pts',(7.99956512490593,31.3450751859396,56.5533094690593));
#89018=CARTESIAN_POINT('Ctrl Pts',(8.00343419874421,31.2914646549499,56.5997330545558));
#89019=CARTESIAN_POINT('Ctrl Pts',(8.00730327258249,31.2353429159238,56.6434688627475));
#89020=CARTESIAN_POINT('Ctrl Pts',(8.01117234642077,31.1770104950513,56.6842339080541));
#89021=CARTESIAN_POINT('Ctrl Pts',(8.01503565530908,31.1187649899374,56.7249382131276));
#89022=CARTESIAN_POINT('Ctrl Pts',(8.01889896419739,31.0583157362857,56.7626802657115));
#89023=CARTESIAN_POINT('Ctrl Pts',(8.0227622730857,30.9959971815572,56.7972165080563));
#89024=CARTESIAN_POINT('Ctrl Pts',(8.02662105007241,30.9337517303693,56.8317122372409));
#89025=CARTESIAN_POINT('Ctrl Pts',(8.03047982705912,30.8696417565971,56.8630093917077));
#89026=CARTESIAN_POINT('Ctrl Pts',(8.03433860404583,30.8040301473627,56.8909080053329));
#89027=CARTESIAN_POINT('Ctrl Pts',(8.03819495012834,30.7384598713115,56.9187890437374));
#89028=CARTESIAN_POINT('Ctrl Pts',(8.04205129621086,30.6713902826035,56.9432755993105));
#89029=CARTESIAN_POINT('Ctrl Pts',(8.04590764229338,30.6032069770608,56.9642145772102));
#89030=CARTESIAN_POINT('Ctrl Pts',(8.04976284903281,30.5350438160218,56.9851473687669));
#89031=CARTESIAN_POINT('Ctrl Pts',(8.05361805577223,30.4657680555189,57.0025345209226));
#89032=CARTESIAN_POINT('Ctrl Pts',(8.05747326251165,30.3957816509574,57.0162724139524));
#89033=CARTESIAN_POINT('Ctrl Pts',(8.06132861985604,30.3257925123531,57.0300108436577));
#89034=CARTESIAN_POINT('Ctrl Pts',(8.06518397720043,30.2550931516865,57.0400996397943));
#89035=CARTESIAN_POINT('Ctrl Pts',(8.06903933454482,30.184095240651,57.0464863803284));
#89036=CARTESIAN_POINT('Ctrl Pts',(8.07289872750168,30.1130230122358,57.0528798062116));
#89037=CARTESIAN_POINT('Ctrl Pts',(8.07675812045855,30.0416520944371,57.0555633972228));
#89038=CARTESIAN_POINT('Ctrl Pts',(8.08061751341541,29.9703978982166,57.0545367551032));
#89039=CARTESIAN_POINT('Ctrl Pts',(8.08447909150516,29.899103358893,57.0535095317136));
#89040=CARTESIAN_POINT('Ctrl Pts',(8.08834066959491,29.8279261576458,57.0487679256912));
#89041=CARTESIAN_POINT('Ctrl Pts',(8.09220224768466,29.75727755977,57.0403635410164));
#89042=CARTESIAN_POINT('Ctrl Pts',(8.09607058227741,29.6865053498754,57.0319444514077));
#89043=CARTESIAN_POINT('Ctrl Pts',(8.09993891687017,29.6162640688021,57.0198498705121));
#89044=CARTESIAN_POINT('Ctrl Pts',(8.10380725146292,29.546955064474,57.0041825887115));
#89045=CARTESIAN_POINT('Ctrl Pts',(8.10610496622344,29.5057868773735,56.9948765310819));
#89046=CARTESIAN_POINT('Ctrl Pts',(8.10840268098397,29.4649473438168,56.984310943031));
#89047=CARTESIAN_POINT('Ctrl Pts',(8.11070039574449,29.4245175385844,56.9725155256938));
#89048=CARTESIAN_POINT('Ctrl Pts',(8.11456845415719,29.356456502054,56.9526586818217));
#89049=CARTESIAN_POINT('Ctrl Pts',(8.11843651256988,29.2892911237888,56.9292361830943));
#89050=CARTESIAN_POINT('Ctrl Pts',(8.12230457098257,29.2234218330817,56.9023469486836));
#89051=CARTESIAN_POINT('Ctrl Pts',(8.12616758929226,29.1576383704503,56.8754927511046));
#89052=CARTESIAN_POINT('Ctrl Pts',(8.13003060760194,29.0931480923012,56.8451809568028));
#89053=CARTESIAN_POINT('Ctrl Pts',(8.13389362591162,29.0303369325548,56.8115604042186));
#89054=CARTESIAN_POINT('Ctrl Pts',(8.13775232708187,28.9675959677993,56.777977424486));
#89055=CARTESIAN_POINT('Ctrl Pts',(8.14161102825211,28.9065308214457,56.7410932569561));
#89056=CARTESIAN_POINT('Ctrl Pts',(8.14546972942235,28.8475062975245,56.7011042967009));
#89057=CARTESIAN_POINT('Ctrl Pts',(8.14768450203097,28.8136280848697,56.678151896421));
#89058=CARTESIAN_POINT('Ctrl Pts',(8.14989927463959,28.7804217316529,56.6541775271539));
#89059=CARTESIAN_POINT('Ctrl Pts',(8.1521140472482,28.7479524050421,56.6292250864936));
#89060=CARTESIAN_POINT('',(7.84592528058377,32.0547497348706,55.0010438147506));
#89061=CARTESIAN_POINT('Ctrl Pts',(7.84592528058377,32.0547497348706,55.0010438147506));
#89062=CARTESIAN_POINT('Ctrl Pts',(7.85018308153819,32.054709658985,55.0799332108663));
#89063=CARTESIAN_POINT('Ctrl Pts',(7.85444088249261,32.0501221476688,55.1586663192241));
#89064=CARTESIAN_POINT('Ctrl Pts',(7.85869868344703,32.0410657724735,55.2367447463771));
#89065=CARTESIAN_POINT('Ctrl Pts',(7.86297170270139,32.0319770278378,55.3151022426871));
#89066=CARTESIAN_POINT('Ctrl Pts',(7.86724472195574,32.0183875525732,55.3928000839848));
#89067=CARTESIAN_POINT('Ctrl Pts',(7.8715177412101,32.0004267215885,55.4693511415292));
#89068=CARTESIAN_POINT('Ctrl Pts',(7.87581130775081,31.9823795239587,55.5462703033123));
#89069=CARTESIAN_POINT('Ctrl Pts',(7.88010487429152,31.9599189709612,55.6220313489285));
#89070=CARTESIAN_POINT('Ctrl Pts',(7.88439844083223,31.9332245845972,55.6961610934325));
#89071=CARTESIAN_POINT('Ctrl Pts',(7.8864670370674,31.92036350358,55.7318760425174));
#89072=CARTESIAN_POINT('Ctrl Pts',(7.88853563330255,31.9065203612943,55.7672126691331));
#89073=CARTESIAN_POINT('Ctrl Pts',(7.89060422953771,31.8917190493863,55.802120066255));
#89074=CARTESIAN_POINT('Ctrl Pts',(7.89447330295551,31.8640348829558,55.8674103727891));
#89075=CARTESIAN_POINT('Ctrl Pts',(7.8983423763733,31.832912403107,55.9313936569463));
#89076=CARTESIAN_POINT('Ctrl Pts',(7.90221144979109,31.7984967809814,55.9936834965419));
#89077=CARTESIAN_POINT('Ctrl Pts',(7.90607475825673,31.7641324384241,56.055880523749));
#89078=CARTESIAN_POINT('Ctrl Pts',(7.90993806672237,31.7264849264835,56.1163886932305));
#89079=CARTESIAN_POINT('Ctrl Pts',(7.91380137518801,31.6857472356805,56.1748420404018));
#89080=CARTESIAN_POINT('Ctrl Pts',(7.91766015175086,31.6450573327403,56.233226818136));
#89081=CARTESIAN_POINT('Ctrl Pts',(7.9215189283137,31.6012847277701,56.2895611648883));
#89082=CARTESIAN_POINT('Ctrl Pts',(7.92537770487655,31.5546671432434,56.343505726158));
#89083=CARTESIAN_POINT('Ctrl Pts',(7.9292340505347,31.5080789262906,56.3974163040951));
#89084=CARTESIAN_POINT('Ctrl Pts',(7.93309039619284,31.4586496024489,56.4489397167259));
#89085=CARTESIAN_POINT('Ctrl Pts',(7.93694674185099,31.4066579254486,56.4977686881734));
#89086=CARTESIAN_POINT('Ctrl Pts',(7.94080194816617,31.3546816091956,56.5465832332832));
#89087=CARTESIAN_POINT('Ctrl Pts',(7.94465715448135,31.3001447966244,56.5927045852321));
#89088=CARTESIAN_POINT('Ctrl Pts',(7.94851236079653,31.2433627193998,56.6358626808222));
#89089=CARTESIAN_POINT('Ctrl Pts',(7.95236771771743,31.1865784239527,56.6790224624065));
#89090=CARTESIAN_POINT('Ctrl Pts',(7.95622307463832,31.1275490777957,56.7192184656));
#89091=CARTESIAN_POINT('Ctrl Pts',(7.96007843155922,31.066621184959,56.7562223123217));
#89092=CARTESIAN_POINT('Ctrl Pts',(7.96393782409665,31.0056295155079,56.7932648930281));
#89093=CARTESIAN_POINT('Ctrl Pts',(7.96779721663408,30.9427357483097,56.8271083943739));
#89094=CARTESIAN_POINT('Ctrl Pts',(7.97165660917151,30.8783126575179,56.8575694975273));
#89095=CARTESIAN_POINT('Ctrl Pts',(7.97551818684348,30.8138530912655,56.8880478473349));
#89096=CARTESIAN_POINT('Ctrl Pts',(7.97937976451545,30.7478629273174,56.9151398020609));
#89097=CARTESIAN_POINT('Ctrl Pts',(7.98324134218742,30.6807341214891,56.938710555586));
#89098=CARTESIAN_POINT('Ctrl Pts',(7.98710967636956,30.6134878619935,56.9623225502952));
#89099=CARTESIAN_POINT('Ctrl Pts',(7.9909780105517,30.5450994492843,56.982400906374));
#89100=CARTESIAN_POINT('Ctrl Pts',(7.99484634473384,30.4759744797673,56.998861140027));
#89101=CARTESIAN_POINT('Ctrl Pts',(7.99714406328132,30.4349155337004,57.0086382126324));
#89102=CARTESIAN_POINT('Ctrl Pts',(7.9994417818288,30.3935969062403,57.0171397434808));
#89103=CARTESIAN_POINT('Ctrl Pts',(8.00173950037628,30.3521044669293,57.0243566896346));
#89104=CARTESIAN_POINT('Ctrl Pts',(8.00560732707783,30.2822588520887,57.0365052171677));
#89105=CARTESIAN_POINT('Ctrl Pts',(8.00947515377938,30.2116470006334,57.0450585066231));
#89106=CARTESIAN_POINT('Ctrl Pts',(8.01334298048093,30.1406719063312,57.0499290176172));
#89107=CARTESIAN_POINT('Ctrl Pts',(8.01720559809914,30.0697923993474,57.0547929691402));
#89108=CARTESIAN_POINT('Ctrl Pts',(8.02106821571735,29.998551099857,57.0559839468317));
#89109=CARTESIAN_POINT('Ctrl Pts',(8.02493083333555,29.9273599179333,57.0534656025795));
#89110=CARTESIAN_POINT('Ctrl Pts',(8.02878954136263,29.8562407929515,57.0509498072973));
#89111=CARTESIAN_POINT('Ctrl Pts',(8.0326482493897,29.7851721677428,57.044732156475));
#89112=CARTESIAN_POINT('Ctrl Pts',(8.03650695741678,29.7145680590569,57.0348282899521));
#89113=CARTESIAN_POINT('Ctrl Pts',(8.04036305078054,29.6440117917654,57.0249311342962));
#89114=CARTESIAN_POINT('Ctrl Pts',(8.04421914414431,29.5739198959833,57.0113527887946));
#89115=CARTESIAN_POINT('Ctrl Pts',(8.04807523750807,29.5047016374595,56.9941607494294));
#89116=CARTESIAN_POINT('Ctrl Pts',(8.05193146499039,29.4354809714595,56.9769681121088));
#89117=CARTESIAN_POINT('Ctrl Pts',(8.05578769247272,29.3671344794266,56.9561616284492));
#89118=CARTESIAN_POINT('Ctrl Pts',(8.05964391995505,29.3000603463786,56.9318597370897));
#89119=CARTESIAN_POINT('Ctrl Pts',(8.0634999438389,29.2329897546648,56.9075591288049));
#89120=CARTESIAN_POINT('Ctrl Pts',(8.06735596772276,29.1671918430208,56.87976365237));
#89121=CARTESIAN_POINT('Ctrl Pts',(8.07121199160661,29.1030466153127,56.8486406325184));
#89122=CARTESIAN_POINT('Ctrl Pts',(8.07507195419949,29.0388358669038,56.8174858222726));
#89123=CARTESIAN_POINT('Ctrl Pts',(8.07893191679236,28.9762816102448,56.7829968969987));
#89124=CARTESIAN_POINT('Ctrl Pts',(8.08279187938524,28.9157401986791,56.745387706425));
#89125=CARTESIAN_POINT('Ctrl Pts',(8.08648107370469,28.8578771945009,56.7094423808202));
#89126=CARTESIAN_POINT('Ctrl Pts',(8.09017026802414,28.8018530005804,56.6706473009991));
#89127=CARTESIAN_POINT('Ctrl Pts',(8.09385946234359,28.7479524050421,56.6292250864936));
#89128=CARTESIAN_POINT('Ctrl Pts',(7.39391310532386,28.7479524050421,56.6292250864936));
#89129=CARTESIAN_POINT('Ctrl Pts',(7.39776854184031,28.6913983985599,56.5857637450324));
#89130=CARTESIAN_POINT('Ctrl Pts',(7.40162397835676,28.6371169242198,56.5393596194705));
#89131=CARTESIAN_POINT('Ctrl Pts',(7.40547941487322,28.5854187500326,56.4902877070354));
#89132=CARTESIAN_POINT('Ctrl Pts',(7.40933896177683,28.5336654589967,56.4411634776816));
#89133=CARTESIAN_POINT('Ctrl Pts',(7.41319850868044,28.4845013178865,56.3893661199868));
#89134=CARTESIAN_POINT('Ctrl Pts',(7.41705805558405,28.4382004105911,56.3352077010795));
#89135=CARTESIAN_POINT('Ctrl Pts',(7.42091989553231,28.3918719948729,56.2810171054231));
#89136=CARTESIAN_POINT('Ctrl Pts',(7.42478173548057,28.3484104947549,56.2244630418472));
#89137=CARTESIAN_POINT('Ctrl Pts',(7.42864357542883,28.30804814303,56.1658887066078));
#89138=CARTESIAN_POINT('Ctrl Pts',(7.43251206243218,28.2676163190382,56.1072135523706));
#89139=CARTESIAN_POINT('Ctrl Pts',(7.43638054943553,28.2302945452081,56.0465115992591));
#89140=CARTESIAN_POINT('Ctrl Pts',(7.44024903643888,28.1962699885805,55.9841522282678));
#89141=CARTESIAN_POINT('Ctrl Pts',(7.44218707302041,28.1792243489395,55.9529113989518));
#89142=CARTESIAN_POINT('Ctrl Pts',(7.44412510960195,28.163005503771,55.92125493001));
#89143=CARTESIAN_POINT('Ctrl Pts',(7.44606314618349,28.1476323957765,55.8892310280929));
#89144=CARTESIAN_POINT('Ctrl Pts',(7.44993221953076,28.1169417044999,55.8252988884398));
#89145=CARTESIAN_POINT('Ctrl Pts',(7.45380129287804,28.089504589936,55.7596507813514));
#89146=CARTESIAN_POINT('Ctrl Pts',(7.45767036622531,28.0655150426256,55.6926510753562));
#89147=CARTESIAN_POINT('Ctrl Pts',(7.46153367462014,28.0415612399463,55.6257511994971));
#89148=CARTESIAN_POINT('Ctrl Pts',(7.46539698301496,28.021044970332,55.5575041758807));
#89149=CARTESIAN_POINT('Ctrl Pts',(7.46926029140978,28.0041132635704,55.4882967313474));
#89150=CARTESIAN_POINT('Ctrl Pts',(7.4731190679017,27.9872014187622,55.4191704714845));
#89151=CARTESIAN_POINT('Ctrl Pts',(7.47697784439362,27.9738658993027,55.34908649816));
#89152=CARTESIAN_POINT('Ctrl Pts',(7.48083662088554,27.9642041985783,55.2784475128523));
#89153=CARTESIAN_POINT('Ctrl Pts',(7.48469296647273,27.9545485844137,55.2078530278271));
#89154=CARTESIAN_POINT('Ctrl Pts',(7.48854931205992,27.9485622629525,55.136704704665));
#89155=CARTESIAN_POINT('Ctrl Pts',(7.49240565764711,27.9462915341241,55.0654148277497));
#89156=CARTESIAN_POINT('Ctrl Pts',(7.49626086389141,27.944021476174,54.9941460131621));
#89157=CARTESIAN_POINT('Ctrl Pts',(7.50011607013571,27.9454648469601,54.9227362131237));
#89158=CARTESIAN_POINT('Ctrl Pts',(7.50397127638,27.9506159104974,54.8516004845243));
#89159=CARTESIAN_POINT('Ctrl Pts',(7.5078266332302,27.9557671752639,54.7804619769658));
#89160=CARTESIAN_POINT('Ctrl Pts',(7.51168199008039,27.964626383067,54.7095980464614));
#89161=CARTESIAN_POINT('Ctrl Pts',(7.51553734693059,27.9771358471552,54.639419659943));
#89162=CARTESIAN_POINT('Ctrl Pts',(7.51939673939808,27.9896584055981,54.5691678137887));
#89163=CARTESIAN_POINT('Ctrl Pts',(7.52325613186558,28.0058387623317,54.499603423333));
#89164=CARTESIAN_POINT('Ctrl Pts',(7.52711552433307,28.0255680547007,54.4311273816736));
#89165=CARTESIAN_POINT('Ctrl Pts',(7.53097710193543,28.0453085175232,54.3626125698226));
#89166=CARTESIAN_POINT('Ctrl Pts',(7.53483867953779,28.0686017572935,54.2951877928236));
#89167=CARTESIAN_POINT('Ctrl Pts',(7.53870025714014,28.0952898298514,54.2292362682168));
#89168=CARTESIAN_POINT('Ctrl Pts',(7.54256859125393,28.1220245979017,54.1631693497797));
#89169=CARTESIAN_POINT('Ctrl Pts',(7.54643692536773,28.1521658523427,54.0985812705681));
#89170=CARTESIAN_POINT('Ctrl Pts',(7.55030525948152,28.1855088725025,54.0358322185776));
#89171=CARTESIAN_POINT('Ctrl Pts',(7.5526029786617,28.2053140120516,53.9985604379984));
#89172=CARTESIAN_POINT('Ctrl Pts',(7.55490069784187,28.2262479197591,53.9619369825761));
#89173=CARTESIAN_POINT('Ctrl Pts',(7.55719841702204,28.2482606182029,53.9260322627001));
#89174=CARTESIAN_POINT('Ctrl Pts',(7.56106749037988,28.2853272649097,53.8655731794964));
#89175=CARTESIAN_POINT('Ctrl Pts',(7.56493656373772,28.3256001937771,53.8069168887159));
#89176=CARTESIAN_POINT('Ctrl Pts',(7.56880563709556,28.368878496433,53.7504239906667));
#89177=CARTESIAN_POINT('Ctrl Pts',(7.57266894550101,28.4120923140477,53.6940152675189));
#89178=CARTESIAN_POINT('Ctrl Pts',(7.57653225390645,28.458302323663,53.6397639210872));
#89179=CARTESIAN_POINT('Ctrl Pts',(7.58039556231189,28.507263362889,53.5880032242506));
#89180=CARTESIAN_POINT('Ctrl Pts',(7.58425433881445,28.5561669677477,53.5363032459553));
#89181=CARTESIAN_POINT('Ctrl Pts',(7.58811311531702,28.6078148598398,53.4870884649957));
#89182=CARTESIAN_POINT('Ctrl Pts',(7.59197189181958,28.6619215890214,53.4406592006322));
#89183=CARTESIAN_POINT('Ctrl Pts',(7.59582823741744,28.7159942327092,53.3942591852074));
#89184=CARTESIAN_POINT('Ctrl Pts',(7.5996845830153,28.7725222725302,53.3506415205144));
#89185=CARTESIAN_POINT('Ctrl Pts',(7.60354092861316,28.8311844418321,53.3100687133837));
#89186=CARTESIAN_POINT('Ctrl Pts',(7.60739613486812,28.8898292796153,53.2695078933373));
#89187=CARTESIAN_POINT('Ctrl Pts',(7.61125134112308,28.950606595804,53.2319904210965));
#89188=CARTESIAN_POINT('Ctrl Pts',(7.61510654737804,29.0131645720318,53.1977365895611));
#89189=CARTESIAN_POINT('Ctrl Pts',(7.61896190423888,29.0757249921232,53.1634814198799));
#89190=CARTESIAN_POINT('Ctrl Pts',(7.62281726109971,29.1400657832103,53.1324903754074));
#89191=CARTESIAN_POINT('Ctrl Pts',(7.62667261796054,29.2058103868482,53.1049378846956));
#89192=CARTESIAN_POINT('Ctrl Pts',(7.63053201043858,29.2716238090321,53.0773565532541));
#89193=CARTESIAN_POINT('Ctrl Pts',(7.63439140291661,29.3388435281668,53.053221148785));
#89194=CARTESIAN_POINT('Ctrl Pts',(7.63825079539464,29.4070736933023,53.0326576410483));
#89195=CARTESIAN_POINT('Ctrl Pts',(7.64211237300751,29.475342489417,53.0120824905368));
#89196=CARTESIAN_POINT('Ctrl Pts',(7.64597395062037,29.5446223983934,52.9950833784676));
#89197=CARTESIAN_POINT('Ctrl Pts',(7.64983552823323,29.6145057992422,52.9817354525033));
#89198=CARTESIAN_POINT('Ctrl Pts',(7.65370386235734,29.6845114734286,52.9683641719878));
#89199=CARTESIAN_POINT('Ctrl Pts',(7.65757219648145,29.7551222662411,52.9586568983741));
#89200=CARTESIAN_POINT('Ctrl Pts',(7.66144053060556,29.8259245349132,52.9526369899417));
#89201=CARTESIAN_POINT('Ctrl Pts',(7.66373824969057,29.8679797759474,52.9490612754219));
#89202=CARTESIAN_POINT('Ctrl Pts',(7.66603596877559,29.9101025340802,52.9467855163726));
#89203=CARTESIAN_POINT('Ctrl Pts',(7.6683336878606,29.9522065485288,52.9458059126518));
#89204=CARTESIAN_POINT('Ctrl Pts',(7.6722027611918,30.0231044753042,52.9441563817512));
#89205=CARTESIAN_POINT('Ctrl Pts',(7.676071834523,30.094226769938,52.9461783579694));
#89206=CARTESIAN_POINT('Ctrl Pts',(7.6799409078542,30.1651615109235,52.9518986260906));
#89207=CARTESIAN_POINT('Ctrl Pts',(7.68380421623302,30.2359905585378,52.9576103709633));
#89208=CARTESIAN_POINT('Ctrl Pts',(7.68766752461183,30.3066321269481,52.9670094308485));
#89209=CARTESIAN_POINT('Ctrl Pts',(7.69153083299065,30.3766732518212,52.9800705893863));
#89210=CARTESIAN_POINT('Ctrl Pts',(7.69538960946671,30.4466322140671,52.9931164263668));
#89211=CARTESIAN_POINT('Ctrl Pts',(7.69924838594278,30.5159916566329,53.0098157403258));
#89212=CARTESIAN_POINT('Ctrl Pts',(7.70310716241884,30.5843444503246,53.0300915945469));
#89213=CARTESIAN_POINT('Ctrl Pts',(7.70696350799029,30.6526541839626,53.0503546756343));
#89214=CARTESIAN_POINT('Ctrl Pts',(7.71081985356173,30.7199580622556,53.0741896890356));
#89215=CARTESIAN_POINT('Ctrl Pts',(7.71467619913318,30.7858612982909,53.1014690989219));
#89216=CARTESIAN_POINT('Ctrl Pts',(7.71853140536186,30.8517450634636,53.1287404492093));
#89217=CARTESIAN_POINT('Ctrl Pts',(7.72238661159054,30.9162285593068,53.1594539900038));
#89218=CARTESIAN_POINT('Ctrl Pts',(7.72624181781923,30.9789358945171,53.1934336223305));
#89219=CARTESIAN_POINT('Ctrl Pts',(7.73009717465397,31.0416456794291,53.2274145820929));
#89220=CARTESIAN_POINT('Ctrl Pts',(7.73395253148872,31.1025787398888,53.264661653327));
#89221=CARTESIAN_POINT('Ctrl Pts',(7.73780788832346,31.1613842990994,53.3049530766656));
#89222=CARTESIAN_POINT('Ctrl Pts',(7.74166728077582,31.2202514133776,53.3452866752904));
#89223=CARTESIAN_POINT('Ctrl Pts',(7.74552667322819,31.2769861792992,53.388670712238));
#89224=CARTESIAN_POINT('Ctrl Pts',(7.74938606568054,31.3312680688472,53.4348409373588));
#89225=CARTESIAN_POINT('Ctrl Pts',(7.75324764326794,31.3855806920561,53.4810373034274));
#89226=CARTESIAN_POINT('Ctrl Pts',(7.75710922085533,31.4374373209418,53.5300226642431));
#89227=CARTESIAN_POINT('Ctrl Pts',(7.76097079844273,31.4865537416984,53.5814953170531));
#89228=CARTESIAN_POINT('Ctrl Pts',(7.76483913254197,31.535756100306,53.633058030358));
#89229=CARTESIAN_POINT('Ctrl Pts',(7.76870746664122,31.5822083617667,53.6871163559044));
#89230=CARTESIAN_POINT('Ctrl Pts',(7.77257580074047,31.6256665567958,53.7433354430813));
#89231=CARTESIAN_POINT('Ctrl Pts',(7.77487352006003,31.6514799254838,53.7767285470431));
#89232=CARTESIAN_POINT('Ctrl Pts',(7.7771712393796,31.6762377635927,53.8108834243772));
#89233=CARTESIAN_POINT('Ctrl Pts',(7.77946895869917,31.6998964790238,53.8457255425582));
#89234=CARTESIAN_POINT('Ctrl Pts',(7.78339694508646,31.740341415602,53.9052886775131));
#89235=CARTESIAN_POINT('Ctrl Pts',(7.78732493147376,31.7777270931469,53.9670902448251));
#89236=CARTESIAN_POINT('Ctrl Pts',(7.79125291786106,31.811802195853,54.0307887920571));
#89237=CARTESIAN_POINT('Ctrl Pts',(7.79517455595466,31.845822227401,54.094384391609));
#89238=CARTESIAN_POINT('Ctrl Pts',(7.79909619404826,31.8765420917977,54.1598704747647));
#89239=CARTESIAN_POINT('Ctrl Pts',(7.80301783214186,31.9037535793997,54.2268765483943));
#89240=CARTESIAN_POINT('Ctrl Pts',(7.80693336842903,31.930922727748,54.2937783650575));
#89241=CARTESIAN_POINT('Ctrl Pts',(7.8108489047162,31.9545941801382,54.3621950395487));
#89242=CARTESIAN_POINT('Ctrl Pts',(7.81476444100337,31.9746063348883,54.4317329987417));
#89243=CARTESIAN_POINT('Ctrl Pts',(7.81867638568829,31.994600133098,54.5012071728815));
#89244=CARTESIAN_POINT('Ctrl Pts',(7.8225883303732,32.0109411715262,54.5718001425371));
#89245=CARTESIAN_POINT('Ctrl Pts',(7.82650027505812,32.0235168926669,54.643100928004));
#89246=CARTESIAN_POINT('Ctrl Pts',(7.83040988908265,32.0360851214381,54.7143592338528));
#89247=CARTESIAN_POINT('Ctrl Pts',(7.83431950310718,32.0448924077463,54.7863240593764));
#89248=CARTESIAN_POINT('Ctrl Pts',(7.83822911713171,32.0498770841231,54.8585733317694));
#89249=CARTESIAN_POINT('Ctrl Pts',(7.8407945049337,32.0531479000896,54.9059814393055));
#89250=CARTESIAN_POINT('Ctrl Pts',(7.84335989273569,32.0547738811628,54.9535117905185));
#89251=CARTESIAN_POINT('Ctrl Pts',(7.84592528053768,32.054749734871,55.0010438138966));
#89252=CARTESIAN_POINT('Origin',(-1.54592528053767,30.,55.));
#89253=CARTESIAN_POINT('',(6.69398930495604,28.7479524050421,56.6292250864936));
#89254=CARTESIAN_POINT('',(6.75200712216955,28.7479524050421,56.6292250864936));
#89255=CARTESIAN_POINT('',(-1.54592528053767,28.7479524050421,56.6292250864936));
#89256=CARTESIAN_POINT('',(7.20407471942299,32.054749359036,55.0016229729599));
#89257=CARTESIAN_POINT('Ctrl Pts',(6.75200712216955,28.7479524050421,56.6292250864936));
#89258=CARTESIAN_POINT('Ctrl Pts',(6.75587000514611,28.6914451856499,56.5857997005698));
#89259=CARTESIAN_POINT('Ctrl Pts',(6.75973288812266,28.6372603557193,56.5394776390901));
#89260=CARTESIAN_POINT('Ctrl Pts',(6.76359577109921,28.5856936487085,56.4905485926988));
#89261=CARTESIAN_POINT('Ctrl Pts',(6.76746492126687,28.5340432792079,56.4415401631923));
#89262=CARTESIAN_POINT('Ctrl Pts',(6.77133407143453,28.4850198364317,56.3899166654894));
#89263=CARTESIAN_POINT('Ctrl Pts',(6.77520322160219,28.4388799193048,56.336002116821));
#89264=CARTESIAN_POINT('Ctrl Pts',(6.77582786296206,28.4314310224336,56.3272980718661));
#89265=CARTESIAN_POINT('Ctrl Pts',(6.77645250432192,28.4240571888272,56.318534376648));
#89266=CARTESIAN_POINT('Ctrl Pts',(6.77707714568178,28.4167593915148,56.3097124639185));
#89267=CARTESIAN_POINT('Ctrl Pts',(6.78094621902979,28.3715563119641,56.2550689042481));
#89268=CARTESIAN_POINT('Ctrl Pts',(6.78481529237779,28.3290969431629,56.1979753737612));
#89269=CARTESIAN_POINT('Ctrl Pts',(6.78868436572579,28.2896574231043,56.1387387023184));
#89270=CARTESIAN_POINT('Ctrl Pts',(6.79254767412137,28.2502766682685,56.0795902940234));
#89271=CARTESIAN_POINT('Ctrl Pts',(6.79641098251694,28.2139070976231,56.0183054844465));
#89272=CARTESIAN_POINT('Ctrl Pts',(6.80027429091252,28.1807846665721,55.9552241271664));
#89273=CARTESIAN_POINT('Ctrl Pts',(6.80413306740522,28.1477010902086,55.8922167682719));
#89274=CARTESIAN_POINT('Ctrl Pts',(6.80799184389793,28.1178573120209,55.8274174758217));
#89275=CARTESIAN_POINT('Ctrl Pts',(6.81185062039063,28.0914450656736,55.7611935530194));
#89276=CARTESIAN_POINT('Ctrl Pts',(6.81570696597863,28.0650494581894,55.6950113491521));
#89277=CARTESIAN_POINT('Ctrl Pts',(6.81956331156663,28.0420812731967,55.6274067456564));
#89278=CARTESIAN_POINT('Ctrl Pts',(6.82341965715463,28.022684873006,55.5587686919118));
#89279=CARTESIAN_POINT('Ctrl Pts',(6.82727486339976,28.0032942034092,55.4901509170234));
#89280=CARTESIAN_POINT('Ctrl Pts',(6.83113006964489,27.9874733556432,55.4205007652727));
#89281=CARTESIAN_POINT('Ctrl Pts',(6.83498527589001,27.9753168606364,55.3502224260051));
#89282=CARTESIAN_POINT('Ctrl Pts',(6.83884063274106,27.963159890729,55.2799413412725));
#89283=CARTESIAN_POINT('Ctrl Pts',(6.8426959895921,27.9546676384162,55.209032499354));
#89284=CARTESIAN_POINT('Ctrl Pts',(6.84655134644315,27.9498832308868,55.1379086491153));
#89285=CARTESIAN_POINT('Ctrl Pts',(6.85041073891151,27.9450938152508,55.0667103495707));
#89286=CARTESIAN_POINT('Ctrl Pts',(6.85427013137987,27.9440200248333,54.9952970781169));
#89287=CARTESIAN_POINT('Ctrl Pts',(6.85812952384823,27.9466528919666,54.9240841490138));
#89288=CARTESIAN_POINT('Ctrl Pts',(6.86199110145147,27.9492872497931,54.8528309001307));
#89289=CARTESIAN_POINT('Ctrl Pts',(6.86585267905471,27.9556323997215,54.7817787034945));
#89290=CARTESIAN_POINT('Ctrl Pts',(6.86971425665795,27.9656274785321,54.7113375563115));
#89291=CARTESIAN_POINT('Ctrl Pts',(6.87358259077263,27.9756400454968,54.6407731599112));
#89292=CARTESIAN_POINT('Ctrl Pts',(6.87745092488731,27.9893151983316,54.570822424443));
#89293=CARTESIAN_POINT('Ctrl Pts',(6.881319259002,28.006541124023,54.5018842782159));
#89294=CARTESIAN_POINT('Ctrl Pts',(6.88361697817478,28.016773006419,54.4609362898504));
#89295=CARTESIAN_POINT('Ctrl Pts',(6.88591469734756,28.0282566940931,54.4203452700944));
#89296=CARTESIAN_POINT('Ctrl Pts',(6.88821241652034,28.0409606653552,54.3801916039498));
#89297=CARTESIAN_POINT('Ctrl Pts',(6.89208148986834,28.0623525731244,54.3125778235781));
#89298=CARTESIAN_POINT('Ctrl Pts',(6.89595056321633,28.0872908982648,54.2459403779374));
#89299=CARTESIAN_POINT('Ctrl Pts',(6.89981963656433,28.1156676269756,54.1806776760809));
#89300=CARTESIAN_POINT('Ctrl Pts',(6.90368294495989,28.1440020741175,54.1155122162092));
#89301=CARTESIAN_POINT('Ctrl Pts',(6.90754625335546,28.1757645631943,54.051717876011));
#89302=CARTESIAN_POINT('Ctrl Pts',(6.91140956175102,28.2107975421477,53.9896772162743));
#89303=CARTESIAN_POINT('Ctrl Pts',(6.9152683382437,28.2457894252211,53.9277093341199));
#89304=CARTESIAN_POINT('Ctrl Pts',(6.91912711473639,28.284043939903,53.8674914671293));
#89305=CARTESIAN_POINT('Ctrl Pts',(6.92298589122907,28.3253564882268,53.8093839111721));
#89306=CARTESIAN_POINT('Ctrl Pts',(6.92684223681705,28.3666430109778,53.7513129611006));
#89307=CARTESIAN_POINT('Ctrl Pts',(6.93069858240503,28.4109834644791,53.6953500794837));
#89308=CARTESIAN_POINT('Ctrl Pts',(6.93455492799301,28.4581293723475,53.6418275035614));
#89309=CARTESIAN_POINT('Ctrl Pts',(6.93841013423811,28.5052613511338,53.5883207406838));
#89310=CARTESIAN_POINT('Ctrl Pts',(6.94226534048321,28.5551968178432,53.5372532164894));
#89311=CARTESIAN_POINT('Ctrl Pts',(6.94612054672832,28.6076474655815,53.4889235683135));
#89312=CARTESIAN_POINT('Ctrl Pts',(6.94997590357933,28.6601001623354,53.4405920321113));
#89313=CARTESIAN_POINT('Ctrl Pts',(6.95383126043035,28.715067876452,53.3949989118376));
#89314=CARTESIAN_POINT('Ctrl Pts',(6.95768661728136,28.7722272302686,53.3524043006835));
#89315=CARTESIAN_POINT('Ctrl Pts',(6.96154600974969,28.8294464159729,53.3097651033713));
#89316=CARTESIAN_POINT('Ctrl Pts',(6.96540540221802,28.8888614306154,53.2701309716089));
#89317=CARTESIAN_POINT('Ctrl Pts',(6.96926479468635,28.950118486855,53.2337196228072));
#89318=CARTESIAN_POINT('Ctrl Pts',(6.97312637228955,29.0114102259965,53.1972876584011));
#89319=CARTESIAN_POINT('Ctrl Pts',(6.97698794989275,29.0745456527526,53.1640823355941));
#89320=CARTESIAN_POINT('Ctrl Pts',(6.98084952749596,29.1391473005867,53.1342748883041));
#89321=CARTESIAN_POINT('Ctrl Pts',(6.9847178616106,29.2038619804034,53.1044152876251));
#89322=CARTESIAN_POINT('Ctrl Pts',(6.98858619572524,29.2700475519769,53.0779656125225));
#89323=CARTESIAN_POINT('Ctrl Pts',(6.99245452983988,29.337308214895,53.0550482884004));
#89324=CARTESIAN_POINT('Ctrl Pts',(6.99475224901289,29.3772598090944,53.0414358202245));
#89325=CARTESIAN_POINT('Ctrl Pts',(6.99704996818589,29.4175904326409,53.029068655143));
#89326=CARTESIAN_POINT('Ctrl Pts',(6.9993476873589,29.4582154543603,53.0179639083493));
#89327=CARTESIAN_POINT('Ctrl Pts',(7.00321676070842,29.5266229389234,52.9992648957034));
#89328=CARTESIAN_POINT('Ctrl Pts',(7.00708583405794,29.5961336115655,52.984074911664));
#89329=CARTESIAN_POINT('Ctrl Pts',(7.01095490740746,29.6663541686804,52.9725192918937));
#89330=CARTESIAN_POINT('Ctrl Pts',(7.01481821580455,29.7364700965639,52.9609808900959));
#89331=CARTESIAN_POINT('Ctrl Pts',(7.01868152420164,29.8072933339145,52.9530661817184));
#89332=CARTESIAN_POINT('Ctrl Pts',(7.02254483259873,29.8784170241721,52.9488502876463));
#89333=CARTESIAN_POINT('Ctrl Pts',(7.02640360909295,29.9494572818834,52.9446393390821));
#89334=CARTESIAN_POINT('Ctrl Pts',(7.03026238558717,30.0207968098355,52.9441186148241));
#89335=CARTESIAN_POINT('Ctrl Pts',(7.03412116208139,30.0920219411853,52.9473116347481));
#89336=CARTESIAN_POINT('Ctrl Pts',(7.0379775076709,30.163202203,52.9505026431725));
#89337=CARTESIAN_POINT('Ctrl Pts',(7.04183385326041,30.2342677270393,52.9574027324669));
#89338=CARTESIAN_POINT('Ctrl Pts',(7.04569019884992,30.3048046216598,52.9679833403451));
#89339=CARTESIAN_POINT('Ctrl Pts',(7.04954540509655,30.3753206764185,52.9785608222224));
#89340=CARTESIAN_POINT('Ctrl Pts',(7.05340061134318,30.4453079316725,52.9928165918795));
#89341=CARTESIAN_POINT('Ctrl Pts',(7.05725581758981,30.5143591218829,53.0106704003017));
#89342=CARTESIAN_POINT('Ctrl Pts',(7.06111117444235,30.5834130096188,53.0285249061934));
#89343=CARTESIAN_POINT('Ctrl Pts',(7.0649665312949,30.6515302899424,53.0499776061749));
#89344=CARTESIAN_POINT('Ctrl Pts',(7.06882188814744,30.7183170588043,53.0748978817915));
#89345=CARTESIAN_POINT('Ctrl Pts',(7.07268128061728,30.7851737371063,53.0998442428521));
#89346=CARTESIAN_POINT('Ctrl Pts',(7.07654067308711,30.8506966676963,53.1282652550816));
#89347=CARTESIAN_POINT('Ctrl Pts',(7.08040006555695,30.914511055146,53.1599817684284));
#89348=CARTESIAN_POINT('Ctrl Pts',(7.08426164316165,30.978361573423,53.1917162392284));
#89349=CARTESIAN_POINT('Ctrl Pts',(7.08812322076636,31.0405011994903,53.2267496868237));
#89350=CARTESIAN_POINT('Ctrl Pts',(7.09198479837106,31.1005813479816,53.2648578562622));
#89351=CARTESIAN_POINT('Ctrl Pts',(7.09585313248718,31.1607666172941,53.3030327026675));
#89352=CARTESIAN_POINT('Ctrl Pts',(7.09972146660329,31.2188848184593,53.344292730476));
#89353=CARTESIAN_POINT('Ctrl Pts',(7.10358980071941,31.2746184286335,53.3883718096634));
#89354=CARTESIAN_POINT('Ctrl Pts',(7.10588751987876,31.3077231657305,53.4145539701839));
#89355=CARTESIAN_POINT('Ctrl Pts',(7.10818523903811,31.3399872413693,53.4417299774308));
#89356=CARTESIAN_POINT('Ctrl Pts',(7.11048295819746,31.3713503754222,53.4698380117356));
#89357=CARTESIAN_POINT('Ctrl Pts',(7.11438261491519,31.4245794464778,53.5175425731711));
#89358=CARTESIAN_POINT('Ctrl Pts',(7.11828227163292,31.475438208622,53.5681375184189));
#89359=CARTESIAN_POINT('Ctrl Pts',(7.12218192835065,31.523590769643,53.6213525725703));
#89360=CARTESIAN_POINT('Ctrl Pts',(7.12598698948115,31.5705752740591,53.6732767671252));
#89361=CARTESIAN_POINT('Ctrl Pts',(7.12979205061164,31.6149830001411,53.7276950180236));
#89362=CARTESIAN_POINT('Ctrl Pts',(7.13359711174214,31.6565353095011,53.7843156944025));
#89363=CARTESIAN_POINT('Ctrl Pts',(7.13739855500299,31.6980481107339,53.8408825355814));
#89364=CARTESIAN_POINT('Ctrl Pts',(7.14119999826383,31.7367105809646,53.8996472498017));
#89365=CARTESIAN_POINT('Ctrl Pts',(7.14500144152468,31.7722833964258,53.9602841132052));
#89366=CARTESIAN_POINT('Ctrl Pts',(7.14880063065913,31.8078351184189,54.0208850210137));
#89367=CARTESIAN_POINT('Ctrl Pts',(7.15259981979358,31.8403005656675,54.0833554448163));
#89368=CARTESIAN_POINT('Ctrl Pts',(7.15639900892804,31.8694840246935,54.1473411913808));
#89369=CARTESIAN_POINT('Ctrl Pts',(7.16037198480262,31.9000024260006,54.2142538452185));
#89370=CARTESIAN_POINT('Ctrl Pts',(7.16434496067719,31.9269310579137,54.2828232869357));
#89371=CARTESIAN_POINT('Ctrl Pts',(7.16831793655177,31.9501011079919,54.3526181720895));
#89372=CARTESIAN_POINT('Ctrl Pts',(7.1721185069018,31.9722657040316,54.4193843391825));
#89373=CARTESIAN_POINT('Ctrl Pts',(7.17591907725182,31.9909910752409,54.4872712685952));
#89374=CARTESIAN_POINT('Ctrl Pts',(7.17971964760184,32.0061804532204,54.5558856547957));
#89375=CARTESIAN_POINT('Ctrl Pts',(7.18352169694533,32.0213757421524,54.6245267423119));
#89376=CARTESIAN_POINT('Ctrl Pts',(7.18732374628882,32.0330322152166,54.6938953556266));
#89377=CARTESIAN_POINT('Ctrl Pts',(7.19112579563232,32.0411045496009,54.7635898054263));
#89378=CARTESIAN_POINT('Ctrl Pts',(7.19493249872834,32.0491867646163,54.8333695620416));
#89379=CARTESIAN_POINT('Ctrl Pts',(7.19873920182436,32.053676062702,54.9034754508831));
#89380=CARTESIAN_POINT('Ctrl Pts',(7.20254590492038,32.0545791584104,54.973503880934));
#89381=CARTESIAN_POINT('Ctrl Pts',(7.20305550975458,32.0547000561866,54.9828786142887));
#89382=CARTESIAN_POINT('Ctrl Pts',(7.20356511458878,32.0547567608594,54.9922519653911));
#89383=CARTESIAN_POINT('Ctrl Pts',(7.20407471942298,32.054749359036,55.0016229729599));
#89384=CARTESIAN_POINT('Ctrl Pts',(7.20407471946233,32.0547493590354,55.0016229736834));
#89385=CARTESIAN_POINT('Ctrl Pts',(7.20992255598689,32.0546644213158,55.1091575115331));
#89386=CARTESIAN_POINT('Ctrl Pts',(7.21577039251145,32.046135906768,55.2163661668599));
#89387=CARTESIAN_POINT('Ctrl Pts',(7.22161822903602,32.0293269300152,55.3222262770401));
#89388=CARTESIAN_POINT('Ctrl Pts',(7.22548730238329,32.0182056950634,55.3922659454058));
#89389=CARTESIAN_POINT('Ctrl Pts',(7.22935637573056,32.0034324231375,55.461866373971));
#89390=CARTESIAN_POINT('Ctrl Pts',(7.23322544907782,31.9850548085864,55.5306175359031));
#89391=CARTESIAN_POINT('Ctrl Pts',(7.23708875747264,31.9667045768386,55.5992662580145));
#89392=CARTESIAN_POINT('Ctrl Pts',(7.24095206586746,31.9447607871872,55.6670677598202));
#89393=CARTESIAN_POINT('Ctrl Pts',(7.24481537426228,31.9193224755962,55.733620335849));
#89394=CARTESIAN_POINT('Ctrl Pts',(7.24867415075418,31.8939140047392,55.8000948415345));
#89395=CARTESIAN_POINT('Ctrl Pts',(7.25253292724609,31.865019327127,55.8653228799985));
#89396=CARTESIAN_POINT('Ctrl Pts',(7.256391703738,31.83278730781,55.9289177826001));
#89397=CARTESIAN_POINT('Ctrl Pts',(7.26024804932519,31.8005755936255,55.9924726224643));
#89398=CARTESIAN_POINT('Ctrl Pts',(7.26410439491237,31.7650309279952,56.054395935349));
#89399=CARTESIAN_POINT('Ctrl Pts',(7.26796074049956,31.7263497324162,56.1143222890557));
#89400=CARTESIAN_POINT('Ctrl Pts',(7.27181594674385,31.687679965052,56.1742309377452));
#89401=CARTESIAN_POINT('Ctrl Pts',(7.27567115298815,31.6458757707532,56.2321433906354));
#89402=CARTESIAN_POINT('Ctrl Pts',(7.27952635923244,31.6011779466979,56.2877215325948));
#89403=CARTESIAN_POINT('Ctrl Pts',(7.28338171608263,31.5564783764959,56.3433018457469));
#89404=CARTESIAN_POINT('Ctrl Pts',(7.28723707293281,31.5088852582695,56.3965472897482));
#89405=CARTESIAN_POINT('Ctrl Pts',(7.291092429783,31.4586797915564,56.4471526623701));
#89406=CARTESIAN_POINT('Ctrl Pts',(7.29495182225048,31.4084217719779,56.4978110064613));
#89407=CARTESIAN_POINT('Ctrl Pts',(7.29881121471797,31.3555462880924,56.5458234170168));
#89408=CARTESIAN_POINT('Ctrl Pts',(7.30267060718546,31.300370900928,56.5909220856219));
#89409=CARTESIAN_POINT('Ctrl Pts',(7.30653218478781,31.2451642742193,56.6360462884721));
#89410=CARTESIAN_POINT('Ctrl Pts',(7.31039376239016,31.1876555438217,56.6782531777251));
#89411=CARTESIAN_POINT('Ctrl Pts',(7.31425533999251,31.1281925858735,56.717317399807));
#89412=CARTESIAN_POINT('Ctrl Pts',(7.31812367410629,31.0686255869876,56.7564499716388));
#89413=CARTESIAN_POINT('Ctrl Pts',(7.32199200822008,31.0070979533721,56.7924286527873));
#89414=CARTESIAN_POINT('Ctrl Pts',(7.32586034233386,30.9439829351717,56.8250736370362));
#89415=CARTESIAN_POINT('Ctrl Pts',(7.3281580615141,30.9064937774064,56.8444641561179));
#89416=CARTESIAN_POINT('Ctrl Pts',(7.33045578069434,30.8684449854165,56.8626794081664));
#89417=CARTESIAN_POINT('Ctrl Pts',(7.33275349987458,30.8299177134289,56.8796899083192));
#89418=CARTESIAN_POINT('Ctrl Pts',(7.33662257323247,30.7650425786077,56.9083334751708));
#89419=CARTESIAN_POINT('Ctrl Pts',(7.34049164659037,30.698555734578,56.9336705787696));
#89420=CARTESIAN_POINT('Ctrl Pts',(7.34436071994826,30.6308275304466,56.9555189053882));
#89421=CARTESIAN_POINT('Ctrl Pts',(7.34822402835375,30.5632002419187,56.9773346778132));
#89422=CARTESIAN_POINT('Ctrl Pts',(7.35208733675924,30.494335723326,56.9956718438268));
#89423=CARTESIAN_POINT('Ctrl Pts',(7.35595064516473,30.4246251784845,57.0103957372361));
#89424=CARTESIAN_POINT('Ctrl Pts',(7.35980942166735,30.3549964084809,57.0251023585957));
#89425=CARTESIAN_POINT('Ctrl Pts',(7.36366819816997,30.2845240565464,57.0362040267317));
#89426=CARTESIAN_POINT('Ctrl Pts',(7.36752697467258,30.2136137189081,57.0436160944743));
#89427=CARTESIAN_POINT('Ctrl Pts',(7.37138332027049,30.1427480524949,57.0510234928532));
#89428=CARTESIAN_POINT('Ctrl Pts',(7.37523966586839,30.0714454298039,57.0547458518868));
#89429=CARTESIAN_POINT('Ctrl Pts',(7.3790960114663,30.0001193983105,57.054749996531));
#89430=CARTESIAN_POINT('Ctrl Pts',(7.38295121772131,29.9288144398266,57.0547541399507));
#89431=CARTESIAN_POINT('Ctrl Pts',(7.38680642397632,29.8574865717917,57.051042249844));
#89432=CARTESIAN_POINT('Ctrl Pts',(7.39066163023133,29.786550459199,57.0436332489055));
#89433=CARTESIAN_POINT('Ctrl Pts',(7.39451698709222,29.7156115754456,57.03622395853));
#89434=CARTESIAN_POINT('Ctrl Pts',(7.39837234395311,29.6450649604476,57.0251173232309));
#89435=CARTESIAN_POINT('Ctrl Pts',(7.402227700814,29.5753195404234,57.0103840602616));
#89436=CARTESIAN_POINT('Ctrl Pts',(7.40608709329209,29.5055011139756,56.9956353751636));
#89437=CARTESIAN_POINT('Ctrl Pts',(7.40994648577017,29.4364860329173,56.977252584949));
#89438=CARTESIAN_POINT('Ctrl Pts',(7.41380587824825,29.3686715284612,56.9553572368047));
#89439=CARTESIAN_POINT('Ctrl Pts',(7.41766745586116,29.3008186283674,56.933449491816));
#89440=CARTESIAN_POINT('Ctrl Pts',(7.42152903347407,29.2341681121487,56.9080254031045));
#89441=CARTESIAN_POINT('Ctrl Pts',(7.42539061108697,29.1690979846837,56.8792550128823));
#89442=CARTESIAN_POINT('Ctrl Pts',(7.42925894521113,29.1039140055518,56.8504342837871));
#89443=CARTESIAN_POINT('Ctrl Pts',(7.43312727933529,29.0403163695113,56.8182557830016));
#89444=CARTESIAN_POINT('Ctrl Pts',(7.43699561345945,28.9786585770717,56.782935573797));
#89445=CARTESIAN_POINT('Ctrl Pts',(7.43929333254401,28.9420349861788,56.761956021319));
#89446=CARTESIAN_POINT('Ctrl Pts',(7.44159105162857,28.906095262753,56.7398688732154));
#89447=CARTESIAN_POINT('Ctrl Pts',(7.44388877071313,28.8709081934411,56.7167263191498));
#89448=CARTESIAN_POINT('Ctrl Pts',(7.44663026314124,28.8289252179179,56.6891140939806));
#89449=CARTESIAN_POINT('Ctrl Pts',(7.44937175556935,28.7878975561809,56.659922643773));
#89450=CARTESIAN_POINT('Ctrl Pts',(7.45211324799746,28.7479524050421,56.6292250864936));
#89451=CARTESIAN_POINT('',(7.1459252805008,32.0547492461588,54.9982399120147));
#89452=CARTESIAN_POINT('Ctrl Pts',(7.14592528053769,32.0547492461594,54.9982399126965));
#89453=CARTESIAN_POINT('Ctrl Pts',(7.14975890798128,32.0548099310451,55.0690842525566));
#89454=CARTESIAN_POINT('Ctrl Pts',(7.15359253542487,32.051202432858,55.1399937211669));
#89455=CARTESIAN_POINT('Ctrl Pts',(7.15742616286845,32.0439332342796,55.2105575843025));
#89456=CARTESIAN_POINT('Ctrl Pts',(7.16125834634856,32.0366667736974,55.2810948690491));
#89457=CARTESIAN_POINT('Ctrl Pts',(7.16509052982867,32.0257413995781,55.3512863175634));
#89458=CARTESIAN_POINT('Ctrl Pts',(7.16892271330877,32.0112155594184,55.4207250123931));
#89459=CARTESIAN_POINT('Ctrl Pts',(7.17275477349921,31.9966901865866,55.4901614732292));
#89460=CARTESIAN_POINT('Ctrl Pts',(7.17658683368964,31.9785646802737,55.5588447472066));
#89461=CARTESIAN_POINT('Ctrl Pts',(7.18041889388008,31.9569484900965,55.6263786152232));
#89462=CARTESIAN_POINT('Ctrl Pts',(7.184254856409,31.9353102872978,55.6939812556491));
#89463=CARTESIAN_POINT('Ctrl Pts',(7.18809081893792,31.910174452913,55.7604316831496));
#89464=CARTESIAN_POINT('Ctrl Pts',(7.19192678146684,31.8816998964897,55.8253502662812));
#89465=CARTESIAN_POINT('Ctrl Pts',(7.19576473620229,31.8532105518101,55.8903025648688));
#89466=CARTESIAN_POINT('Ctrl Pts',(7.19960269093774,31.8213792547125,55.9537209954185));
#89467=CARTESIAN_POINT('Ctrl Pts',(7.20344064567319,31.7864112720573,56.0152498852828));
#89468=CARTESIAN_POINT('Ctrl Pts',(7.20728565488565,31.751379015369,56.076891870316));
#89469=CARTESIAN_POINT('Ctrl Pts',(7.21113066409811,31.7131988248763,56.1366369637702));
#89470=CARTESIAN_POINT('Ctrl Pts',(7.21497567331057,31.672119382911,56.1941584198897));
#89471=CARTESIAN_POINT('Ctrl Pts',(7.21791465037584,31.6407198384317,56.2381256072108));
#89472=CARTESIAN_POINT('Ctrl Pts',(7.2208536274411,31.6076273168153,56.2807942302441));
#89473=CARTESIAN_POINT('Ctrl Pts',(7.22379260450636,31.5729677245609,56.3220325638916));
#89474=CARTESIAN_POINT('Ctrl Pts',(7.22766167785587,31.527339432227,56.3763215679058));
#89475=CARTESIAN_POINT('Ctrl Pts',(7.23153075120538,31.478807891512,56.4283519319452));
#89476=CARTESIAN_POINT('Ctrl Pts',(7.23539982455489,31.4276252989438,56.4777968630078));
#89477=CARTESIAN_POINT('Ctrl Pts',(7.23926313295197,31.3765189688769,56.5271681206996));
#89478=CARTESIAN_POINT('Ctrl Pts',(7.24312644134905,31.3227697743101,56.5739612573854));
#89479=CARTESIAN_POINT('Ctrl Pts',(7.24698974974612,31.2666696204287,56.6178830721603));
#89480=CARTESIAN_POINT('Ctrl Pts',(7.25084852624033,31.2106352755437,56.6617533638939));
#89481=CARTESIAN_POINT('Ctrl Pts',(7.25470730273454,31.1522558299576,56.7027587261679));
#89482=CARTESIAN_POINT('Ctrl Pts',(7.25856607922875,31.0918581402454,56.740644525479));
#89483=CARTESIAN_POINT('Ctrl Pts',(7.26242242481826,31.0314984991293,56.7785064579587));
#89484=CARTESIAN_POINT('Ctrl Pts',(7.26627877040776,30.969123546933,56.8132524689203));
#89485=CARTESIAN_POINT('Ctrl Pts',(7.27013511599726,30.9050899488404,56.8446706337469));
#89486=CARTESIAN_POINT('Ctrl Pts',(7.27399032224388,30.8410752692349,56.8760795161941));
#89487=CARTESIAN_POINT('Ctrl Pts',(7.27784552849051,30.7754033524808,56.9041622905641));
#89488=CARTESIAN_POINT('Ctrl Pts',(7.28170073473713,30.7084548126927,56.9287533126018));
#89489=CARTESIAN_POINT('Ctrl Pts',(7.28555609158966,30.6415036575203,56.9533452953024));
#89490=CARTESIAN_POINT('Ctrl Pts',(7.2894114484422,30.5732762370567,56.9744450894259));
#89491=CARTESIAN_POINT('Ctrl Pts',(7.29326680529474,30.5041708253421,56.9919360786365));
#89492=CARTESIAN_POINT('Ctrl Pts',(7.29712619776457,30.4349930771345,57.0094453766422));
#89493=CARTESIAN_POINT('Ctrl Pts',(7.30098559023439,30.364935974961,57.0233382094805));
#89494=CARTESIAN_POINT('Ctrl Pts',(7.30484498270422,30.2944096805196,57.0335487460389));
#89495=CARTESIAN_POINT('Ctrl Pts',(7.30870656030892,30.2238434550615,57.0437650636625));
#89496=CARTESIAN_POINT('Ctrl Pts',(7.31256813791362,30.1528079924837,57.0502948901935));
#89497=CARTESIAN_POINT('Ctrl Pts',(7.31642971551831,30.0817175522559,57.0531244005548));
#89498=CARTESIAN_POINT('Ctrl Pts',(7.32029804963442,30.0105027267586,57.0559588616436));
#89499=CARTESIAN_POINT('Ctrl Pts',(7.32416638375053,29.9392332174624,57.0550800863142));
#89500=CARTESIAN_POINT('Ctrl Pts',(7.32803471786664,29.8683215534489,57.0505263590634));
#89501=CARTESIAN_POINT('Ctrl Pts',(7.33033243702606,29.8262013321494,57.047821529016));
#89502=CARTESIAN_POINT('Ctrl Pts',(7.33263015618549,29.7842072533363,57.0438211176024));
#89503=CARTESIAN_POINT('Ctrl Pts',(7.33492787534492,29.7424240587483,57.0385416838977));
#89504=CARTESIAN_POINT('Ctrl Pts',(7.33879679455239,29.6720691577032,57.0296521281915));
#89505=CARTESIAN_POINT('Ctrl Pts',(7.34266571375985,29.6020371950836,57.0170987141508));
#89506=CARTESIAN_POINT('Ctrl Pts',(7.34653463296732,29.5327394571435,57.000916077098));
#89507=CARTESIAN_POINT('Ctrl Pts',(7.35048283899703,29.462021581657,56.9844018048266));
#89508=CARTESIAN_POINT('Ctrl Pts',(7.35443104502674,29.3920688738398,56.9641078751369));
#89509=CARTESIAN_POINT('Ctrl Pts',(7.35837925105645,29.3233131428259,56.9401269184844));
#89510=CARTESIAN_POINT('Ctrl Pts',(7.36223788239855,29.2561173033377,56.9166900283484));
#89511=CARTESIAN_POINT('Ctrl Pts',(7.36609651374064,29.1900651880705,56.889731810428));
#89512=CARTESIAN_POINT('Ctrl Pts',(7.36995514508274,29.1255476136902,56.8593898425497));
#89513=CARTESIAN_POINT('Ctrl Pts',(7.37394813845626,29.0587834623276,56.8279913320583));
#89514=CARTESIAN_POINT('Ctrl Pts',(7.37794113182978,28.9936632172819,56.7929692017413));
#89515=CARTESIAN_POINT('Ctrl Pts',(7.3819341252033,28.9305982714506,56.7545305655575));
#89516=CARTESIAN_POINT('Ctrl Pts',(7.38592711857682,28.8675333256194,56.7160919293738));
#89517=CARTESIAN_POINT('Ctrl Pts',(7.38992011195034,28.8065241834037,56.674237070926));
#89518=CARTESIAN_POINT('Ctrl Pts',(7.39391310532386,28.7479524050421,56.6292250864936));
#89519=CARTESIAN_POINT('Ctrl Pts',(6.69398930495604,28.7479524050421,56.6292250864936));
#89520=CARTESIAN_POINT('Ctrl Pts',(6.69784740484003,28.6915069530229,56.5858471683454));
#89521=CARTESIAN_POINT('Ctrl Pts',(6.70170550472402,28.6372599899261,56.5394875233192));
#89522=CARTESIAN_POINT('Ctrl Pts',(6.70556360460801,28.5855382786981,56.4904011545458));
#89523=CARTESIAN_POINT('Ctrl Pts',(6.70941957225292,28.5338451522805,56.4413419141198));
#89524=CARTESIAN_POINT('Ctrl Pts',(6.71327553989783,28.4846748602865,56.3895592738365));
#89525=CARTESIAN_POINT('Ctrl Pts',(6.71713150754274,28.4383199524028,56.3353475171044));
#89526=CARTESIAN_POINT('Ctrl Pts',(6.72098663402215,28.3919751566759,56.2811475864723));
#89527=CARTESIAN_POINT('Ctrl Pts',(6.72484176050156,28.3484448409394,56.2245199608754));
#89528=CARTESIAN_POINT('Ctrl Pts',(6.72869688698097,28.3079824598838,56.1657933806808));
#89529=CARTESIAN_POINT('Ctrl Pts',(6.73255246205531,28.2675153704954,56.1070599668723));
#89530=CARTESIAN_POINT('Ctrl Pts',(6.73640803712965,28.2301171979976,56.0462275150466));
#89531=CARTESIAN_POINT('Ctrl Pts',(6.74026361220398,28.1959981164053,55.9836537838522));
#89532=CARTESIAN_POINT('Ctrl Pts',(6.74412340630836,28.1618416994149,55.9210115802648));
#89533=CARTESIAN_POINT('Ctrl Pts',(6.74798320041274,28.1309717656873,55.8566247226886));
#89534=CARTESIAN_POINT('Ctrl Pts',(6.75184299451711,28.1035520965734,55.7908747764904));
#89535=CARTESIAN_POINT('Ctrl Pts',(6.75570524152721,28.076115002213,55.7250830460894));
#89536=CARTESIAN_POINT('Ctrl Pts',(6.75956748853731,28.052132698729,55.6579269606755));
#89537=CARTESIAN_POINT('Ctrl Pts',(6.76342973554741,28.0317195237508,55.5898046535219));
#89538=CARTESIAN_POINT('Ctrl Pts',(6.76729847175235,28.0112720513625,55.5215678899592));
#89539=CARTESIAN_POINT('Ctrl Pts',(6.77116720795728,27.9944057874356,55.4523621367241));
#89540=CARTESIAN_POINT('Ctrl Pts',(6.77503594416221,27.9811841000988,55.3825962948147));
#89541=CARTESIAN_POINT('Ctrl Pts',(6.77644113649218,27.9763817531175,55.3572561266689));
#89542=CARTESIAN_POINT('Ctrl Pts',(6.77784632882215,27.9720597274933,55.3318421154545));
#89543=CARTESIAN_POINT('Ctrl Pts',(6.77925152115212,27.9682193607167,55.3063739485233));
#89544=CARTESIAN_POINT('Ctrl Pts',(6.7831205945003,27.957645248956,55.2362495934447));
#89545=CARTESIAN_POINT('Ctrl Pts',(6.78698966784848,27.9506850681283,55.1654398123005));
#89546=CARTESIAN_POINT('Ctrl Pts',(6.79085874119666,27.9474173181755,55.094349863667));
#89547=CARTESIAN_POINT('Ctrl Pts',(6.79472204959241,27.9441544371981,55.023365839666));
#89548=CARTESIAN_POINT('Ctrl Pts',(6.79858535798816,27.9445730883938,54.952102958126));
#89549=CARTESIAN_POINT('Ctrl Pts',(6.80244866638391,27.9487003168898,54.8809740676499));
#89550=CARTESIAN_POINT('Ctrl Pts',(6.80630744287678,27.952822703888,54.8099286158204));
#89551=CARTESIAN_POINT('Ctrl Pts',(6.81016621936966,27.9606449988298,54.7390173254585));
#89552=CARTESIAN_POINT('Ctrl Pts',(6.81402499586253,27.9721422035047,54.668653776703));
#89553=CARTESIAN_POINT('Ctrl Pts',(6.8178813414507,27.9836321653116,54.5983345547132));
#89554=CARTESIAN_POINT('Ctrl Pts',(6.82173768703886,27.9987923656292,54.5285628680318));
#89555=CARTESIAN_POINT('Ctrl Pts',(6.82559403262703,28.0175460548859,54.4597464317549));
#89556=CARTESIAN_POINT('Ctrl Pts',(6.82944923887232,28.0362942034353,54.3909503270368));
#89557=CARTESIAN_POINT('Ctrl Pts',(6.83330444511761,28.0586336055317,54.3231093808666));
#89558=CARTESIAN_POINT('Ctrl Pts',(6.8371596513629,28.0844369538214,54.2566186855892));
#89559=CARTESIAN_POINT('Ctrl Pts',(6.84101500821412,28.1102413101343,54.1901253928131));
#89560=CARTESIAN_POINT('Ctrl Pts',(6.84487036506534,28.1395097034985,54.1249829077371));
#89561=CARTESIAN_POINT('Ctrl Pts',(6.84872572191656,28.1720663643886,54.0615671647367));
#89562=CARTESIAN_POINT('Ctrl Pts',(6.85258511438508,28.2046571041536,53.9980850409369));
#89563=CARTESIAN_POINT('Ctrl Pts',(6.8564445068536,28.2405427601566,53.936333700391));
#89564=CARTESIAN_POINT('Ctrl Pts',(6.86030389932212,28.2795015977718,53.8766644266159));
#89565=CARTESIAN_POINT('Ctrl Pts',(6.86416547692552,28.3184824933445,53.8169613689194));
#89566=CARTESIAN_POINT('Ctrl Pts',(6.86802705452891,28.3605397477762,53.7593431172579));
#89567=CARTESIAN_POINT('Ctrl Pts',(6.87188863213231,28.405409894687,53.704129652111));
#89568=CARTESIAN_POINT('Ctrl Pts',(6.87575696624714,28.4503585498376,53.648819581264));
#89569=CARTESIAN_POINT('Ctrl Pts',(6.87962530036197,28.4981295979932,53.5959230581633));
#89570=CARTESIAN_POINT('Ctrl Pts',(6.8834936344768,28.5484216159474,53.5457243186207));
#89571=CARTESIAN_POINT('Ctrl Pts',(6.8857913536481,28.5782941477366,53.5159071924889));
#89572=CARTESIAN_POINT('Ctrl Pts',(6.88808907281939,28.6090554407189,53.4870411428942));
#89573=CARTESIAN_POINT('Ctrl Pts',(6.89038679199069,28.6406370524378,53.4591788100837));
#89574=CARTESIAN_POINT('Ctrl Pts',(6.89425586533907,28.693816559197,53.4122621064901));
#89575=CARTESIAN_POINT('Ctrl Pts',(6.89812493868745,28.7495319885956,53.3680098732096));
#89576=CARTESIAN_POINT('Ctrl Pts',(6.90199401203584,28.8074854408002,53.3267078591601));
#89577=CARTESIAN_POINT('Ctrl Pts',(6.90585732043179,28.8653525418647,53.2854673854653));
#89578=CARTESIAN_POINT('Ctrl Pts',(6.90972062882775,28.9254506541244,53.2471686849973));
#89579=CARTESIAN_POINT('Ctrl Pts',(6.91358393722371,28.9874475937907,53.2120583938004));
#89580=CARTESIAN_POINT('Ctrl Pts',(6.91744271371679,29.0493718071612,53.1769892891755));
#89581=CARTESIAN_POINT('Ctrl Pts',(6.92130149020988,29.1131900028269,53.1451014027384));
#89582=CARTESIAN_POINT('Ctrl Pts',(6.92516026670296,29.1785411559669,53.1165980434172));
#89583=CARTESIAN_POINT('Ctrl Pts',(6.92901661229134,29.2438511399886,53.088112640293));
#89584=CARTESIAN_POINT('Ctrl Pts',(6.93287295787971,29.3106917213013,53.0630077278986));
#89585=CARTESIAN_POINT('Ctrl Pts',(6.93672930346809,29.3786787344817,53.0414399556014));
#89586=CARTESIAN_POINT('Ctrl Pts',(6.94058450971359,29.4466456611536,53.0198785554217));
#89587=CARTESIAN_POINT('Ctrl Pts',(6.9444397159591,29.5157578844699,53.0018523674691));
#89588=CARTESIAN_POINT('Ctrl Pts',(6.9482949222046,29.5856144232053,52.9874687191886));
#89589=CARTESIAN_POINT('Ctrl Pts',(6.95215027905601,29.6554736909276,52.9730845090023));
#89590=CARTESIAN_POINT('Ctrl Pts',(6.95600563590742,29.7260768555491,52.9623432168142));
#89591=CARTESIAN_POINT('Ctrl Pts',(6.95986099275883,29.7970127471481,52.9553010642934));
#89592=CARTESIAN_POINT('Ctrl Pts',(6.96372038522755,29.8680228913061,52.9482515403584));
#89593=CARTESIAN_POINT('Ctrl Pts',(6.96757977769628,29.9393659732943,52.9449089337533));
#89594=CARTESIAN_POINT('Ctrl Pts',(6.971439170165,30.0106266036311,52.9452774791239));
#89595=CARTESIAN_POINT('Ctrl Pts',(6.9753007477686,30.0819275807557,52.9456462331599));
#89596=CARTESIAN_POINT('Ctrl Pts',(6.9791623253722,30.1531455280784,52.9497302941936));
#89597=CARTESIAN_POINT('Ctrl Pts',(6.9830239029758,30.2238687213579,52.9574818585634));
#89598=CARTESIAN_POINT('Ctrl Pts',(6.98689223709084,30.294715657344,52.9652469856629));
#89599=CARTESIAN_POINT('Ctrl Pts',(6.99076057120587,30.3650656313385,52.9766923496815));
#89600=CARTESIAN_POINT('Ctrl Pts',(6.9946289053209,30.4345163633338,52.99171887115));
#89601=CARTESIAN_POINT('Ctrl Pts',(6.99692662449035,30.4757688181354,53.0006443479577));
#89602=CARTESIAN_POINT('Ctrl Pts',(6.9992243436598,30.5167042642628,53.0108323415111));
#89603=CARTESIAN_POINT('Ctrl Pts',(7.00152206282925,30.5572413556216,53.0222539005006));
#89604=CARTESIAN_POINT('Ctrl Pts',(7.00539113617725,30.6255007764713,53.0414863855086));
#89605=CARTESIAN_POINT('Ctrl Pts',(7.00926020952525,30.692897053114,53.0642945225908));
#89606=CARTESIAN_POINT('Ctrl Pts',(7.01312928287326,30.7590285452664,53.0905830130716));
#89607=CARTESIAN_POINT('Ctrl Pts',(7.01699259126884,30.8250615009292,53.1168323334765));
#89608=CARTESIAN_POINT('Ctrl Pts',(7.02085589966442,30.889832965112,53.146551535711));
#89609=CARTESIAN_POINT('Ctrl Pts',(7.02471920806,30.952955563574,53.1795953042377));
#89610=CARTESIAN_POINT('Ctrl Pts',(7.02857798455271,31.0160041152719,53.2126003103529));
#89611=CARTESIAN_POINT('Ctrl Pts',(7.03243676104541,31.0774072149769,53.2489219119856));
#89612=CARTESIAN_POINT('Ctrl Pts',(7.03629553753811,31.1367982471061,53.2883670639192));
#89613=CARTESIAN_POINT('Ctrl Pts',(7.04015188312611,31.196151864801,53.3277873666796));
#89614=CARTESIAN_POINT('Ctrl Pts',(7.04400822871411,31.2534955259851,53.3703270476572));
#89615=CARTESIAN_POINT('Ctrl Pts',(7.04786457430211,31.3084892651732,53.4157483137372));
#89616=CARTESIAN_POINT('Ctrl Pts',(7.05171978054724,31.3634667566669,53.4611561602741));
#89617=CARTESIAN_POINT('Ctrl Pts',(7.05557498679237,31.4160953301477,53.5094435925552));
#89618=CARTESIAN_POINT('Ctrl Pts',(7.0594301930375,31.4660673373388,53.5603319393387));
#89619=CARTESIAN_POINT('Ctrl Pts',(7.06328554988854,31.516041296716,53.6112222741056));
#89620=CARTESIAN_POINT('Ctrl Pts',(7.06714090673959,31.563358144965,53.6647133769486));
#89621=CARTESIAN_POINT('Ctrl Pts',(7.07099626359064,31.607747644014,53.7204902987208));
#89622=CARTESIAN_POINT('Ctrl Pts',(7.074855656059,31.6521836080304,53.7763256053117));
#89623=CARTESIAN_POINT('Ctrl Pts',(7.07871504852737,31.6936858028527,53.8344511263032));
#89624=CARTESIAN_POINT('Ctrl Pts',(7.08257444099573,31.7320253784342,53.8945201716178));
#89625=CARTESIAN_POINT('Ctrl Pts',(7.08643601859897,31.7703866613556,53.954623227199));
#89626=CARTESIAN_POINT('Ctrl Pts',(7.09029759620222,31.8055815206531,54.0166715749086));
#89627=CARTESIAN_POINT('Ctrl Pts',(7.09415917380546,31.8374268138238,54.0802933802883));
#89628=CARTESIAN_POINT('Ctrl Pts',(7.09802750792014,31.8693278259543,54.1440265032434));
#89629=CARTESIAN_POINT('Ctrl Pts',(7.10189584203482,31.8978673764082,54.2093381351131));
#89630=CARTESIAN_POINT('Ctrl Pts',(7.1057641761495,31.922910523935,54.2758365657946));
#89631=CARTESIAN_POINT('Ctrl Pts',(7.10806189532227,31.9377856920338,54.3153354080884));
#89632=CARTESIAN_POINT('Ctrl Pts',(7.11035961449504,31.9514282306982,54.355252661328));
#89633=CARTESIAN_POINT('Ctrl Pts',(7.1126573336678,31.9638183439841,54.3955042809652));
#89634=CARTESIAN_POINT('Ctrl Pts',(7.11737359945988,31.9892501148215,54.4781241846597));
#89635=CARTESIAN_POINT('Ctrl Pts',(7.12208986525197,32.0094837420675,54.562414597967));
#89636=CARTESIAN_POINT('Ctrl Pts',(7.12680613104405,32.024337058198,54.647782684545));
#89637=CARTESIAN_POINT('Ctrl Pts',(7.13145774528214,32.0389867619766,54.7319805276077));
#89638=CARTESIAN_POINT('Ctrl Pts',(7.13610935952022,32.0484026072855,54.8172267077028));
#89639=CARTESIAN_POINT('Ctrl Pts',(7.1407609737583,32.0524559155886,54.9029315856441));
#89640=CARTESIAN_POINT('Ctrl Pts',(7.14248240933913,32.0539559344585,54.9346486238136));
#89641=CARTESIAN_POINT('Ctrl Pts',(7.14420384491996,32.0547219964682,54.966428274309));
#89642=CARTESIAN_POINT('Ctrl Pts',(7.1459252805008,32.0547492461588,54.9982399120147));
#89643=CARTESIAN_POINT('Origin',(-1.54592528053767,30.,55.));
#89644=CARTESIAN_POINT('',(5.99388650947633,28.7479524050421,56.6292250864936));
#89645=CARTESIAN_POINT('',(6.05208116311818,28.7479524050421,56.6292250864936));
#89646=CARTESIAN_POINT('',(-1.54592528053767,28.7479524050421,56.6292250864936));
#89647=CARTESIAN_POINT('',(6.50407471951138,32.0547499427048,55.0004852364685));
#89648=CARTESIAN_POINT('Ctrl Pts',(6.05208116311818,28.7479524050421,56.6292250864936));
#89649=CARTESIAN_POINT('Ctrl Pts',(6.05593629750659,28.6914020110631,56.5857665212147));
#89650=CARTESIAN_POINT('Ctrl Pts',(6.059791431895,28.6371119664565,56.5393564016427));
#89651=CARTESIAN_POINT('Ctrl Pts',(6.06364656628342,28.5853961878313,56.4902662906668));
#89652=CARTESIAN_POINT('Ctrl Pts',(6.06753147914733,28.5332809375167,56.4407969896238));
#89653=CARTESIAN_POINT('Ctrl Pts',(6.07141639201125,28.4837802730513,56.388606443096));
#89654=CARTESIAN_POINT('Ctrl Pts',(6.07530130487517,28.4371775409704,56.3340103163217));
#89655=CARTESIAN_POINT('Ctrl Pts',(6.07916181998135,28.3908674801041,56.2797570603196));
#89656=CARTESIAN_POINT('Ctrl Pts',(6.08302233508754,28.3474193099307,56.2231287771434));
#89657=CARTESIAN_POINT('Ctrl Pts',(6.08688285019373,28.3070691274068,56.1644666689608));
#89658=CARTESIAN_POINT('Ctrl Pts',(6.09077996193651,28.2663364360917,56.1052484598963));
#89659=CARTESIAN_POINT('Ctrl Pts',(6.09467707367929,28.2287610480401,56.0439580900017));
#89660=CARTESIAN_POINT('Ctrl Pts',(6.09857418542207,28.1945386894449,55.9809724861527));
#89661=CARTESIAN_POINT('Ctrl Pts',(6.10247129716486,28.1603163308497,55.9179868823037));
#89662=CARTESIAN_POINT('Ctrl Pts',(6.10636840890764,28.1294471595806,55.8533065255599));
#89663=CARTESIAN_POINT('Ctrl Pts',(6.11026552065042,28.1020766226353,55.7873273881637));
#89664=CARTESIAN_POINT('Ctrl Pts',(6.11413459399864,28.0749030074016,55.7218229482382));
#89665=CARTESIAN_POINT('Ctrl Pts',(6.11800366734685,28.0510713524173,55.6547817560974));
#89666=CARTESIAN_POINT('Ctrl Pts',(6.12187274069507,28.0307555752006,55.5865781771397));
#89667=CARTESIAN_POINT('Ctrl Pts',(6.12573604909085,28.010470068666,55.5184762220988));
#89668=CARTESIAN_POINT('Ctrl Pts',(6.12959935748664,27.9936901788,55.449215779923));
#89669=CARTESIAN_POINT('Ctrl Pts',(6.13346266588243,27.9805417175088,55.3791909911608));
#89670=CARTESIAN_POINT('Ctrl Pts',(6.13732144237534,27.9674086801867,55.3092483458646));
#89671=CARTESIAN_POINT('Ctrl Pts',(6.14118021886825,27.957898699064,55.2385436101104));
#89672=CARTESIAN_POINT('Ctrl Pts',(6.14503899536116,27.9520872552484,55.1674841854739));
#89673=CARTESIAN_POINT('Ctrl Pts',(6.14889534094936,27.9462794724548,55.0964695259824));
#89674=CARTESIAN_POINT('Ctrl Pts',(6.15275168653757,27.9441656438702,55.0251011039398));
#89675=CARTESIAN_POINT('Ctrl Pts',(6.15660803212577,27.9457696122914,54.9537931096617));
#89676=CARTESIAN_POINT('Ctrl Pts',(6.16046323837111,27.9473731068262,54.8825061830636));
#89677=CARTESIAN_POINT('Ctrl Pts',(6.16431844461644,27.9526922068022,54.811280134185));
#89678=CARTESIAN_POINT('Ctrl Pts',(6.16817365086178,27.9616986453253,54.7405290959828));
#89679=CARTESIAN_POINT('Ctrl Pts',(6.17202900771301,27.9707054356903,54.6697752938497));
#89680=CARTESIAN_POINT('Ctrl Pts',(6.17588436456425,27.9833997870615,54.5994970208538));
#89681=CARTESIAN_POINT('Ctrl Pts',(6.17973972141549,27.9997017805379,54.5301015048795));
#89682=CARTESIAN_POINT('Ctrl Pts',(6.18359911388405,28.0160208382212,54.4606333487431));
#89683=CARTESIAN_POINT('Ctrl Pts',(6.1874585063526,28.0359549650723,54.3920502680835));
#89684=CARTESIAN_POINT('Ctrl Pts',(6.19131789882116,28.0593736888521,54.3247466527438));
#89685=CARTESIAN_POINT('Ctrl Pts',(6.19517947642459,28.0828056719909,54.2574049310238));
#89686=CARTESIAN_POINT('Ctrl Pts',(6.19904105402803,28.1097259961425,54.1913445667913));
#89687=CARTESIAN_POINT('Ctrl Pts',(6.20290263163146,28.139956139845,54.1269396350769));
#89688=CARTESIAN_POINT('Ctrl Pts',(6.20677096574633,28.1702391765183,54.0624220155695));
#89689=CARTESIAN_POINT('Ctrl Pts',(6.2106392998612,28.2038433657608,53.9995660400105));
#89690=CARTESIAN_POINT('Ctrl Pts',(6.21450763397607,28.2405447292237,53.9387202477021));
#89691=CARTESIAN_POINT('Ctrl Pts',(6.21680535314704,28.2623446627159,53.9025789684567));
#89692=CARTESIAN_POINT('Ctrl Pts',(6.21910307231801,28.2852364919427,53.8671463546764));
#89693=CARTESIAN_POINT('Ctrl Pts',(6.22140079148898,28.3091664896412,53.832489998866));
#89694=CARTESIAN_POINT('Ctrl Pts',(6.22526986483719,28.3494616299212,53.7741330054152));
#89695=CARTESIAN_POINT('Ctrl Pts',(6.2291389381854,28.3928604218901,53.7177502591308));
#89696=CARTESIAN_POINT('Ctrl Pts',(6.23300801153361,28.4391426714855,53.6636909180423));
#89697=CARTESIAN_POINT('Ctrl Pts',(6.23687131992938,28.4853559601326,53.6097121258351));
#89698=CARTESIAN_POINT('Ctrl Pts',(6.24073462832516,28.534443864862,53.5580502330751));
#89699=CARTESIAN_POINT('Ctrl Pts',(6.24459793672093,28.5861434868901,53.5090247075029));
#89700=CARTESIAN_POINT('Ctrl Pts',(6.24845671321384,28.6377824620215,53.4600566919447));
#89701=CARTESIAN_POINT('Ctrl Pts',(6.25231548970675,28.6920267181043,53.4137192332201));
#89702=CARTESIAN_POINT('Ctrl Pts',(6.25617426619966,28.7485749175707,53.3702967062784));
#89703=CARTESIAN_POINT('Ctrl Pts',(6.26003061178786,28.8050874934958,53.3269015341279));
#89704=CARTESIAN_POINT('Ctrl Pts',(6.26388695737606,28.8639007488455,53.2864179457088));
#89705=CARTESIAN_POINT('Ctrl Pts',(6.26774330296426,28.9246796357711,53.249090614345));
#89706=CARTESIAN_POINT('Ctrl Pts',(6.27159850920958,28.985440565802,53.2117743112017));
#89707=CARTESIAN_POINT('Ctrl Pts',(6.2754537154549,29.0481655607558,53.1776126679242));
#89708=CARTESIAN_POINT('Ctrl Pts',(6.27930892170022,29.1124913585484,53.1468065471061));
#89709=CARTESIAN_POINT('Ctrl Pts',(6.28316427855145,29.1768196692663,53.1159992228287));
#89710=CARTESIAN_POINT('Ctrl Pts',(6.28701963540268,29.2427484678953,53.0885478891027));
#89711=CARTESIAN_POINT('Ctrl Pts',(6.29087499225391,29.3098922794099,53.0646062683573));
#89712=CARTESIAN_POINT('Ctrl Pts',(6.29473438472246,29.3771063741018,53.0406395865804));
#89713=CARTESIAN_POINT('Ctrl Pts',(6.29859377719101,29.4455375620161,53.0201901150297));
#89714=CARTESIAN_POINT('Ctrl Pts',(6.30245316965956,29.5147837356099,53.0033621411805));
#89715=CARTESIAN_POINT('Ctrl Pts',(6.306314747263,29.584069115434,52.9865246395642));
#89716=CARTESIAN_POINT('Ctrl Pts',(6.31017632486643,29.6541699219019,52.9733128074614));
#89717=CARTESIAN_POINT('Ctrl Pts',(6.31403790246987,29.7246750546569,52.9637795460776));
#89718=CARTESIAN_POINT('Ctrl Pts',(6.31790623658473,29.7953035485829,52.9542296045709));
#89719=CARTESIAN_POINT('Ctrl Pts',(6.3217745706996,29.8663372969251,52.9483711240021));
#89720=CARTESIAN_POINT('Ctrl Pts',(6.32564290481447,29.9373619988214,52.9462049656043));
#89721=CARTESIAN_POINT('Ctrl Pts',(6.32794062398549,29.9795493627661,52.9449183074382));
#89722=CARTESIAN_POINT('Ctrl Pts',(6.33023834315651,30.0217335510167,52.9449333531371));
#89723=CARTESIAN_POINT('Ctrl Pts',(6.33253606232754,30.0638286364279,52.9462416238341));
#89724=CARTESIAN_POINT('Ctrl Pts',(6.33640513567577,30.1347115254729,52.948444588996));
#89725=CARTESIAN_POINT('Ctrl Pts',(6.34027420902401,30.205619072688,52.9543258278911));
#89726=CARTESIAN_POINT('Ctrl Pts',(6.34414328237225,30.2761385098526,52.9638897166714));
#89727=CARTESIAN_POINT('Ctrl Pts',(6.34800659076804,30.3465528724515,52.9734393551755));
#89728=CARTESIAN_POINT('Ctrl Pts',(6.35186989916384,30.4165797954267,52.986660686914));
#89729=CARTESIAN_POINT('Ctrl Pts',(6.35573320755963,30.4858082931554,53.0035061069962));
#89730=CARTESIAN_POINT('Ctrl Pts',(6.35959198405257,30.5549555815178,53.020331766345));
#89731=CARTESIAN_POINT('Ctrl Pts',(6.3634507605455,30.6233058353217,53.0407729552543));
#89732=CARTESIAN_POINT('Ctrl Pts',(6.36730953703843,30.690456704111,53.0647307416672));
#89733=CARTESIAN_POINT('Ctrl Pts',(6.37116588262667,30.7575652700194,53.0886734354475));
#89734=CARTESIAN_POINT('Ctrl Pts',(6.3750222282149,30.8234754935029,53.1161281686742));
#89735=CARTESIAN_POINT('Ctrl Pts',(6.37887857380313,30.8878000959244,53.146946155079));
#89736=CARTESIAN_POINT('Ctrl Pts',(6.38273378004849,30.9521056938828,53.177755036425));
#89737=CARTESIAN_POINT('Ctrl Pts',(6.38658898629385,31.0148261629514,53.2119249884776));
#89738=CARTESIAN_POINT('Ctrl Pts',(6.3904441925392,31.0755957294081,53.2492597595934));
#89739=CARTESIAN_POINT('Ctrl Pts',(6.39429954939046,31.1363676698636,53.286595989214));
#89740=CARTESIAN_POINT('Ctrl Pts',(6.39815490624172,31.1951881436373,53.3270970271897));
#89741=CARTESIAN_POINT('Ctrl Pts',(6.40201026309298,31.2517189340107,53.3705223926856));
#89742=CARTESIAN_POINT('Ctrl Pts',(6.40586965556155,31.3083088983194,53.4139932139367));
#89743=CARTESIAN_POINT('Ctrl Pts',(6.40972904803013,31.3626040087653,53.4603941767263));
#89744=CARTESIAN_POINT('Ctrl Pts',(6.41358844049871,31.4142985602079,53.5094440147737));
#89745=CARTESIAN_POINT('Ctrl Pts',(6.41745001810216,31.4660223803936,53.5585216241639));
#89746=CARTESIAN_POINT('Ctrl Pts',(6.4213115957056,31.5151423758184,53.6102507419261));
#89747=CARTESIAN_POINT('Ctrl Pts',(6.42517317330905,31.5613911358061,53.6643146764577));
#89748=CARTESIAN_POINT('Ctrl Pts',(6.42904150742394,31.6077208161606,53.7184732053831));
#89749=CARTESIAN_POINT('Ctrl Pts',(6.43290984153884,31.6511689348274,53.7749743220313));
#89750=CARTESIAN_POINT('Ctrl Pts',(6.43677817565373,31.6915100663392,53.8334704213038));
#89751=CARTESIAN_POINT('Ctrl Pts',(6.43907589482452,31.7154719549696,53.8682160261877));
#89752=CARTESIAN_POINT('Ctrl Pts',(6.44137361399532,31.7383385031005,53.9036649604587));
#89753=CARTESIAN_POINT('Ctrl Pts',(6.44367133316611,31.7600702303999,53.9397404343464));
#89754=CARTESIAN_POINT('Ctrl Pts',(6.44766818401097,31.7978722706671,54.0024932242084));
#89755=CARTESIAN_POINT('Ctrl Pts',(6.45166503485583,31.8323780045915,54.067375195746));
#89756=CARTESIAN_POINT('Ctrl Pts',(6.4556618857007,31.863350142198,54.134018585609));
#89757=CARTESIAN_POINT('Ctrl Pts',(6.45969628851417,31.8946132750867,54.2012881160465));
#89758=CARTESIAN_POINT('Ctrl Pts',(6.46373069132764,31.9222757546574,54.2703519944482));
#89759=CARTESIAN_POINT('Ctrl Pts',(6.46776509414111,31.9461388143958,54.3408025503675));
#89760=CARTESIAN_POINT('Ctrl Pts',(6.47174648699992,31.9696883259406,54.4103274226236));
#89761=CARTESIAN_POINT('Ctrl Pts',(6.47572787985874,31.9895374936084,54.4812023266619));
#89762=CARTESIAN_POINT('Ctrl Pts',(6.47970927271755,32.0055423268114,54.5530128213608));
#89763=CARTESIAN_POINT('Ctrl Pts',(6.48377018050835,32.0218668027296,54.6262574891754));
#89764=CARTESIAN_POINT('Ctrl Pts',(6.48783108829915,32.0341915119555,54.7004751038008));
#89765=CARTESIAN_POINT('Ctrl Pts',(6.49189199608994,32.0424167700165,54.7752083185361));
#89766=CARTESIAN_POINT('Ctrl Pts',(6.49595290388074,32.0506420280775,54.8499415332714));
#89767=CARTESIAN_POINT('Ctrl Pts',(6.50001381167153,32.0547677239393,54.9251898673997));
#89768=CARTESIAN_POINT('Ctrl Pts',(6.50407471946233,32.0547499427051,55.0004852355591));
#89769=CARTESIAN_POINT('Ctrl Pts',(6.50407471951138,32.0547499427048,55.0004852364685));
#89770=CARTESIAN_POINT('Ctrl Pts',(6.50830237655249,32.0547314313017,55.078872387755));
#89771=CARTESIAN_POINT('Ctrl Pts',(6.51253003359359,32.0502226030005,55.1571404354878));
#89772=CARTESIAN_POINT('Ctrl Pts',(6.51675769063469,32.0412922454997,55.2347840091714));
#89773=CARTESIAN_POINT('Ctrl Pts',(6.52089243721875,32.0325581488567,55.3107212240261));
#89774=CARTESIAN_POINT('Ctrl Pts',(6.52502718380281,32.0195950692558,55.3860607936641));
#89775=CARTESIAN_POINT('Ctrl Pts',(6.52916193038686,32.0025186272055,55.4603441214952));
#89776=CARTESIAN_POINT('Ctrl Pts',(6.53343604265649,31.9848666069413,55.5371312416868));
#89777=CARTESIAN_POINT('Ctrl Pts',(6.53771015492612,31.9628191668442,55.6127892221114));
#89778=CARTESIAN_POINT('Ctrl Pts',(6.54198426719576,31.9365582108483,55.6868332100999));
#89779=CARTESIAN_POINT('Ctrl Pts',(6.54625837946539,31.9102972548523,55.7608771980884));
#89780=CARTESIAN_POINT('Ctrl Pts',(6.55053249173502,31.8798230313502,55.833306828919));
#89781=CARTESIAN_POINT('Ctrl Pts',(6.55480660400465,31.8453691251967,55.9036649568678));
#89782=CARTESIAN_POINT('Ctrl Pts',(6.55867567735283,31.8141802650007,55.9673555528329));
#89783=CARTESIAN_POINT('Ctrl Pts',(6.56254475070101,31.7796291418862,56.029554339914));
#89784=CARTESIAN_POINT('Ctrl Pts',(6.56641382404918,31.7418816971565,56.0898833495431));
#89785=CARTESIAN_POINT('Ctrl Pts',(6.57027713244493,31.7041904964427,56.1501224684311));
#89786=CARTESIAN_POINT('Ctrl Pts',(6.57414044084068,31.6633126832068,56.2084969315057));
#89787=CARTESIAN_POINT('Ctrl Pts',(6.57800374923642,31.6194608366359,56.2646517944093));
#89788=CARTESIAN_POINT('Ctrl Pts',(6.58186252572929,31.5756604310293,56.3207407841393));
#89789=CARTESIAN_POINT('Ctrl Pts',(6.58572130222216,31.5288932194195,56.3746149645708));
#89790=CARTESIAN_POINT('Ctrl Pts',(6.58958007871504,31.4794150018997,56.4259483913011));
#89791=CARTESIAN_POINT('Ctrl Pts',(6.5934364243032,31.4299679540608,56.4772494796286));
#89792=CARTESIAN_POINT('Ctrl Pts',(6.59729276989137,31.3778136249783,56.5260126408673));
#89793=CARTESIAN_POINT('Ctrl Pts',(6.60114911547953,31.3232470434511,56.5719461900771));
#89794=CARTESIAN_POINT('Ctrl Pts',(6.60500432172482,31.2686965834163,56.6178661683916));
#89795=CARTESIAN_POINT('Ctrl Pts',(6.60885952797012,31.2117356572642,56.6609578816924));
#89796=CARTESIAN_POINT('Ctrl Pts',(6.61271473421541,31.1526936970947,56.7009687837166));
#89797=CARTESIAN_POINT('Ctrl Pts',(6.61657009106661,31.0936494304161,56.7409812487903));
#89798=CARTESIAN_POINT('Ctrl Pts',(6.62042544791781,31.0325243716964,56.7779123929433));
#89799=CARTESIAN_POINT('Ctrl Pts',(6.62428080476902,30.9696769155757,56.8115529917448));
#89800=CARTESIAN_POINT('Ctrl Pts',(6.62814019723753,30.906763673513,56.8452288040397));
#89801=CARTESIAN_POINT('Ctrl Pts',(6.63199958970605,30.8421248641636,56.8756069654698));
#89802=CARTESIAN_POINT('Ctrl Pts',(6.63585898217457,30.7761426666169,56.9025246709457));
#89803=CARTESIAN_POINT('Ctrl Pts',(6.63972055977796,30.7101231108584,56.9294576168557));
#89804=CARTESIAN_POINT('Ctrl Pts',(6.64358213738136,30.6427591117286,56.9529260466303));
#89805=CARTESIAN_POINT('Ctrl Pts',(6.64744371498475,30.5744493672258,56.9728166379555));
#89806=CARTESIAN_POINT('Ctrl Pts',(6.65131204909958,30.5060201027709,56.9927420313801));
#89807=CARTESIAN_POINT('Ctrl Pts',(6.65518038321441,30.4366422621961,57.0090769765954));
#89808=CARTESIAN_POINT('Ctrl Pts',(6.65904871732924,30.3667254312438,57.0217591401003));
#89809=CARTESIAN_POINT('Ctrl Pts',(6.66134643650057,30.325196122216,57.0292921114916));
#89810=CARTESIAN_POINT('Ctrl Pts',(6.66364415567189,30.2834767822597,57.0355373207603));
#89811=CARTESIAN_POINT('Ctrl Pts',(6.66594187484322,30.2416536453535,57.0404904013956));
#89812=CARTESIAN_POINT('Ctrl Pts',(6.6698098468366,30.1712487306679,57.0488283991009));
#89813=CARTESIAN_POINT('Ctrl Pts',(6.67367781882998,30.1002739040565,57.053534580653));
#89814=CARTESIAN_POINT('Ctrl Pts',(6.67754579082335,30.029136364528,57.0545434127227));
#89815=CARTESIAN_POINT('Ctrl Pts',(6.68140849503884,29.9580957069726,57.0555508708674));
#89816=CARTESIAN_POINT('Ctrl Pts',(6.68527119925432,29.8868932572574,57.0528709610102));
#89817=CARTESIAN_POINT('Ctrl Pts',(6.68913390346981,29.8159423194845,57.0464897587682));
#89818=CARTESIAN_POINT('Ctrl Pts',(6.69299263966132,29.7450642671841,57.0401151117171));
#89819=CARTESIAN_POINT('Ctrl Pts',(6.69685137585284,29.6744376953771,57.0300467605922));
#89820=CARTESIAN_POINT('Ctrl Pts',(6.70071011204435,29.6044751694042,57.0163228091955));
#89821=CARTESIAN_POINT('Ctrl Pts',(6.70456617531102,29.5345611060793,57.0026083643027));
#89822=CARTESIAN_POINT('Ctrl Pts',(6.70842223857769,29.4653106507555,56.9852434401794));
#89823=CARTESIAN_POINT('Ctrl Pts',(6.71227830184436,29.3971287898033,56.9643176592435));
#89824=CARTESIAN_POINT('Ctrl Pts',(6.71613400849578,29.328953234425,56.9433938135593));
#89825=CARTESIAN_POINT('Ctrl Pts',(6.71998971514719,29.2618465451175,56.9189098952704));
#89826=CARTESIAN_POINT('Ctrl Pts',(6.72384542179861,29.1961997293143,56.8910057343503));
#89827=CARTESIAN_POINT('Ctrl Pts',(6.72770090164963,29.1305567749884,56.8631032148088));
#89828=CARTESIAN_POINT('Ctrl Pts',(6.73155638150064,29.0663739676047,56.8317810498464));
#89829=CARTESIAN_POINT('Ctrl Pts',(6.73541186135166,29.0040215106627,56.7972268669474));
#89830=CARTESIAN_POINT('Ctrl Pts',(6.73927005832253,28.941625111305,56.762648332253));
#89831=CARTESIAN_POINT('Ctrl Pts',(6.7431282552934,28.8810620577117,56.7248334770607));
#89832=CARTESIAN_POINT('Ctrl Pts',(6.74698645226427,28.8226761059155,56.6840148487818));
#89833=CARTESIAN_POINT('Ctrl Pts',(6.74866000889936,28.7973502353695,56.6663090948487));
#89834=CARTESIAN_POINT('Ctrl Pts',(6.75033356553446,28.7724336105351,56.6480387143424));
#89835=CARTESIAN_POINT('Ctrl Pts',(6.75200712216955,28.7479524050421,56.6292250864936));
#89836=CARTESIAN_POINT('',(6.44592528053626,32.0547499999799,54.9999909154181));
#89837=CARTESIAN_POINT('Ctrl Pts',(6.44592528053768,32.0547499999799,54.9999909154441));
#89838=CARTESIAN_POINT('Ctrl Pts',(6.44979385259827,32.0547503134813,55.0708988474441));
#89839=CARTESIAN_POINT('Ctrl Pts',(6.45366242465885,32.0510758456684,55.1419458653844));
#89840=CARTESIAN_POINT('Ctrl Pts',(6.45753099671943,32.0437093535415,55.2127196294353));
#89841=CARTESIAN_POINT('Ctrl Pts',(6.46139380423281,32.0363538382016,55.2833879337203));
#89842=CARTESIAN_POINT('Ctrl Pts',(6.46525661174618,32.0253172686326,55.353783312964));
#89843=CARTESIAN_POINT('Ctrl Pts',(6.46911941925955,32.0106344132235,55.4234935877453));
#89844=CARTESIAN_POINT('Ctrl Pts',(6.47297769671015,31.9959687769631,55.4931221106092));
#89845=CARTESIAN_POINT('Ctrl Pts',(6.47683597416075,31.9776654483257,55.5620666517314));
#89846=CARTESIAN_POINT('Ctrl Pts',(6.48069425161135,31.9558107670499,55.6299220634268));
#89847=CARTESIAN_POINT('Ctrl Pts',(6.48455010010935,31.9339698442415,55.6977347572043));
#89848=CARTESIAN_POINT('Ctrl Pts',(6.48840594860734,31.9085821530333,55.7644592204329));
#89849=CARTESIAN_POINT('Ctrl Pts',(6.49226179710534,31.8797843322488,55.8297038186798));
#89850=CARTESIAN_POINT('Ctrl Pts',(6.49611650897051,31.8509950005293,55.8949291840257));
#89851=CARTESIAN_POINT('Ctrl Pts',(6.49997122083568,31.8187977310234,55.9586751061272));
#89852=CARTESIAN_POINT('Ctrl Pts',(6.50382593270085,31.7833772733351,56.0205699698953));
#89853=CARTESIAN_POINT('Ctrl Pts',(6.50768079864212,31.7479553998611,56.0824673076534));
#89854=CARTESIAN_POINT('Ctrl Pts',(6.51153566458339,31.7093103257034,56.1425130195337));
#89855=CARTESIAN_POINT('Ctrl Pts',(6.51539053052465,31.6676718636708,56.2003616611758));
#89856=CARTESIAN_POINT('Ctrl Pts',(6.51924943297202,31.6259898011841,56.2582708772706));
#89857=CARTESIAN_POINT('Ctrl Pts',(6.52310833541939,31.5813083783211,56.3139780354879));
#89858=CARTESIAN_POINT('Ctrl Pts',(6.52696723786676,31.5338991807724,56.367168923625));
#89859=CARTESIAN_POINT('Ctrl Pts',(6.53082833001041,31.4864630813403,56.4203899944089));
#89860=CARTESIAN_POINT('Ctrl Pts',(6.53468942215406,31.4362964679263,56.4710916072193));
#89861=CARTESIAN_POINT('Ctrl Pts',(6.53855051429771,31.3837075199634,56.5189967286656));
#89862=CARTESIAN_POINT('Ctrl Pts',(6.54241835505558,31.3310266543489,56.5669855811321));
#89863=CARTESIAN_POINT('Ctrl Pts',(6.54628619581346,31.2759153771656,56.612167875523));
#89864=CARTESIAN_POINT('Ctrl Pts',(6.55015403657133,31.2187140609575,56.6543075893329));
#89865=CARTESIAN_POINT('Ctrl Pts',(6.55242968420589,31.1850596144405,56.6791005283538));
#89866=CARTESIAN_POINT('Ctrl Pts',(6.55470533184045,31.1506822350117,56.7028410824422));
#89867=CARTESIAN_POINT('Ctrl Pts',(6.556980979475,31.1156552945759,56.7254885760806));
#89868=CARTESIAN_POINT('Ctrl Pts',(6.56085005282324,31.0561022250882,56.7639940163387));
#89869=CARTESIAN_POINT('Ctrl Pts',(6.56471912617149,30.9944367163045,56.7994881602145));
#89870=CARTESIAN_POINT('Ctrl Pts',(6.56858819951973,30.9309957744197,56.8317326307386));
#89871=CARTESIAN_POINT('Ctrl Pts',(6.57245150791554,30.8676493600817,56.8639290567255));
#89872=CARTESIAN_POINT('Ctrl Pts',(6.57631481631135,30.8025331932397,56.8928852023628));
#89873=CARTESIAN_POINT('Ctrl Pts',(6.58017812470716,30.7360123801288,56.9184064581827));
#89874=CARTESIAN_POINT('Ctrl Pts',(6.58403690120009,30.6695696001007,56.9438977759701));
#89875=CARTESIAN_POINT('Ctrl Pts',(6.58789567769302,30.6017258981191,56.9659620344101));
#89876=CARTESIAN_POINT('Ctrl Pts',(6.59175445418596,30.5328684724132,56.9844517513933));
#89877=CARTESIAN_POINT('Ctrl Pts',(6.59561079977419,30.4640544246641,57.0029298204514));
#89878=CARTESIAN_POINT('Ctrl Pts',(6.59946714536242,30.394228388246,57.0178376899948));
#89879=CARTESIAN_POINT('Ctrl Pts',(6.60332349095064,30.3237935215392,57.0290774548817));
#89880=CARTESIAN_POINT('Ctrl Pts',(6.607178697196,30.2533794645501,57.0403138990221));
#89881=CARTESIAN_POINT('Ctrl Pts',(6.61103390344136,30.1823574138323,57.0478843134958));
#89882=CARTESIAN_POINT('Ctrl Pts',(6.61488910968672,30.1111398380561,57.0517420644167));
#89883=CARTESIAN_POINT('Ctrl Pts',(6.61874446653799,30.0399194801232,57.0555999660429));
#89884=CARTESIAN_POINT('Ctrl Pts',(6.62259982338926,29.9685040671611,57.0557448920874));
#89885=CARTESIAN_POINT('Ctrl Pts',(6.62645518024052,29.8973085596809,57.0521822605668));
#89886=CARTESIAN_POINT('Ctrl Pts',(6.63031457270911,29.8260385278871,57.0486158998409));
#89887=CARTESIAN_POINT('Ctrl Pts',(6.63417396517768,29.7549893472539,57.0413342587147));
#89888=CARTESIAN_POINT('Ctrl Pts',(6.63803335764626,29.6845724363127,57.0303947927845));
#89889=CARTESIAN_POINT('Ctrl Pts',(6.64189493524972,29.6141156562862,57.0194491330793));
#89890=CARTESIAN_POINT('Ctrl Pts',(6.64575651285318,29.5442923343014,57.0048416253512));
#89891=CARTESIAN_POINT('Ctrl Pts',(6.64961809045664,29.4755025418036,56.9866806433963));
#89892=CARTESIAN_POINT('Ctrl Pts',(6.65348642457153,29.406592389425,56.9684878855987));
#89893=CARTESIAN_POINT('Ctrl Pts',(6.65735475868643,29.3387198396845,56.94672938864));
#89894=CARTESIAN_POINT('Ctrl Pts',(6.66122309280132,29.2722680150892,56.9215628328623));
#89895=CARTESIAN_POINT('Ctrl Pts',(6.66352081197207,29.2327968559886,56.9066143625506));
#89896=CARTESIAN_POINT('Ctrl Pts',(6.66581853114281,29.1938265516427,56.8904643983559));
#89897=CARTESIAN_POINT('Ctrl Pts',(6.66811625031356,29.1554332511048,56.8731536427001));
#89898=CARTESIAN_POINT('Ctrl Pts',(6.67198550519559,29.0907806741342,56.844003115218));
#89899=CARTESIAN_POINT('Ctrl Pts',(6.67585476007762,29.0275124372444,56.8114442962693));
#89900=CARTESIAN_POINT('Ctrl Pts',(6.67972401495966,28.9660116448843,56.7756310551421));
#89901=CARTESIAN_POINT('Ctrl Pts',(6.68358710202818,28.9046088883035,56.7398749023689));
#89902=CARTESIAN_POINT('Ctrl Pts',(6.6874501890967,28.8449683975511,56.7008748722515));
#89903=CARTESIAN_POINT('Ctrl Pts',(6.69131327616523,28.7874516304901,56.6588321235432));
#89904=CARTESIAN_POINT('Ctrl Pts',(6.69220528576216,28.7741706696179,56.6491242048077));
#89905=CARTESIAN_POINT('Ctrl Pts',(6.6930972953591,28.7610028408573,56.6392542512241));
#89906=CARTESIAN_POINT('Ctrl Pts',(6.69398930495604,28.7479524050421,56.6292250864936));
#89907=CARTESIAN_POINT('Ctrl Pts',(5.99388650947633,28.7479524050421,56.6292250864936));
#89908=CARTESIAN_POINT('Ctrl Pts',(5.99635921474496,28.7119320134646,56.6015436783089));
#89909=CARTESIAN_POINT('Ctrl Pts',(5.99883192001359,28.6768690092049,56.5726970773672));
#89910=CARTESIAN_POINT('Ctrl Pts',(6.00130462528221,28.6428394576484,56.5427614283434));
#89911=CARTESIAN_POINT('Ctrl Pts',(6.00517369863043,28.5895929860008,56.4959207379994));
#89912=CARTESIAN_POINT('Ctrl Pts',(6.00904277197864,28.5386700366479,56.4462284604087));
#89913=CARTESIAN_POINT('Ctrl Pts',(6.01291184532686,28.490391633517,56.3939440958463));
#89914=CARTESIAN_POINT('Ctrl Pts',(6.01677515372265,28.4421851656204,56.3417376354349));
#89915=CARTESIAN_POINT('Ctrl Pts',(6.02063846211843,28.3966157492419,56.2869471084689));
#89916=CARTESIAN_POINT('Ctrl Pts',(6.02450177051421,28.3539699294818,56.2298709564218));
#89917=CARTESIAN_POINT('Ctrl Pts',(6.02836054700713,28.3113741359411,56.1728617582783));
#89918=CARTESIAN_POINT('Ctrl Pts',(6.03221932350004,28.2716954161044,56.1135726480542));
#89919=CARTESIAN_POINT('Ctrl Pts',(6.03607809999295,28.2351809694622,56.0523361401907));
#89920=CARTESIAN_POINT('Ctrl Pts',(6.03993444558116,28.1986895257433,55.9911382093516));
#89921=CARTESIAN_POINT('Ctrl Pts',(6.04379079116937,28.1653586485714,55.9279957310736));
#89922=CARTESIAN_POINT('Ctrl Pts',(6.04764713675757,28.1353921673438,55.8632700579176));
#89923=CARTESIAN_POINT('Ctrl Pts',(6.05150234300291,28.1054345396009,55.7985635077194));
#89924=CARTESIAN_POINT('Ctrl Pts',(6.05535754924824,28.0788395384246,55.7322751318467));
#89925=CARTESIAN_POINT('Ctrl Pts',(6.05921275549357,28.0557641846634,55.6647891822695));
#89926=CARTESIAN_POINT('Ctrl Pts',(6.06306811234482,28.0326879294499,55.5973005963137));
#89927=CARTESIAN_POINT('Ctrl Pts',(6.06692346919607,28.0131317497197,55.5286148041409));
#89928=CARTESIAN_POINT('Ctrl Pts',(6.07077882604731,27.9972032527049,55.4591326077772));
#89929=CARTESIAN_POINT('Ctrl Pts',(6.07463821851587,27.9812580824428,55.3895776805184));
#89930=CARTESIAN_POINT('Ctrl Pts',(6.07849761098443,27.9689482839272,55.319225159408));
#89931=CARTESIAN_POINT('Ctrl Pts',(6.08235700345299,27.9603304240577,55.2484865861078));
#89932=CARTESIAN_POINT('Ctrl Pts',(6.08621858105643,27.9517076848747,55.1777079616014));
#89933=CARTESIAN_POINT('Ctrl Pts',(6.09008015865986,27.9467810790953,55.1065433346407));
#89934=CARTESIAN_POINT('Ctrl Pts',(6.0939417362633,27.9455550884156,55.0354071710931));
#89935=CARTESIAN_POINT('Ctrl Pts',(6.09781007037817,27.9443269526488,54.9641465422746));
#89936=CARTESIAN_POINT('Ctrl Pts',(6.10167840449304,27.9468123423208,54.8929149619447));
#89937=CARTESIAN_POINT('Ctrl Pts',(6.10554673860792,27.9529636818121,54.8221239911635));
#89938=CARTESIAN_POINT('Ctrl Pts',(6.10784445777887,27.9566174641009,54.7800754591949));
#89939=CARTESIAN_POINT('Ctrl Pts',(6.11014217694982,27.9615636544422,54.7381822477433));
#89940=CARTESIAN_POINT('Ctrl Pts',(6.11243989612077,27.9677837873881,54.6965287036682));
#89941=CARTESIAN_POINT('Ctrl Pts',(6.11630896946899,27.9782577177568,54.626389315323));
#89942=CARTESIAN_POINT('Ctrl Pts',(6.1201780428172,27.9923875858267,54.5566554207574));
#89943=CARTESIAN_POINT('Ctrl Pts',(6.12404711616542,28.0101294859619,54.4877374697856));
#89944=CARTESIAN_POINT('Ctrl Pts',(6.1279104245612,28.0278449505139,54.4189222071511));
#89945=CARTESIAN_POINT('Ctrl Pts',(6.13177373295699,28.0491616439714,54.3509209414692));
#89946=CARTESIAN_POINT('Ctrl Pts',(6.13563704135277,28.0739842444239,54.2841362756972));
#89947=CARTESIAN_POINT('Ctrl Pts',(6.13949581784568,28.0987777264104,54.2174299525237));
#89948=CARTESIAN_POINT('Ctrl Pts',(6.14335459433859,28.1270687778568,54.151937847602));
#89949=CARTESIAN_POINT('Ctrl Pts',(6.14721337083151,28.1587121110229,54.0880479878819));
#89950=CARTESIAN_POINT('Ctrl Pts',(6.15106971641971,28.1903355099099,54.0241983767124));
#89951=CARTESIAN_POINT('Ctrl Pts',(6.15492606200792,28.2253067855866,53.9619494424751));
#89952=CARTESIAN_POINT('Ctrl Pts',(6.15878240759612,28.2634328997712,53.9016684157764));
#89953=CARTESIAN_POINT('Ctrl Pts',(6.16263761384145,28.3015477497381,53.8414051988815));
#89954=CARTESIAN_POINT('Ctrl Pts',(6.16649282008678,28.3428153282386,53.7831091456008));
#89955=CARTESIAN_POINT('Ctrl Pts',(6.17034802633211,28.3869979709239,53.7271205804568));
#89956=CARTESIAN_POINT('Ctrl Pts',(6.17420338318336,28.4311823396304,53.6711298280865));
#89957=CARTESIAN_POINT('Ctrl Pts',(6.17805874003461,28.4782816959485,53.6174471228038));
#89958=CARTESIAN_POINT('Ctrl Pts',(6.18191409688585,28.5280176709357,53.566380250756));
#89959=CARTESIAN_POINT('Ctrl Pts',(6.18577348935441,28.5778057073453,53.5152599241615));
#89960=CARTESIAN_POINT('Ctrl Pts',(6.18963288182297,28.6302355321642,53.4667612454625));
#89961=CARTESIAN_POINT('Ctrl Pts',(6.19349227429153,28.6849920711708,53.4211549443925));
#89962=CARTESIAN_POINT('Ctrl Pts',(6.19735385189496,28.7397796125759,53.3755228216627));
#89963=CARTESIAN_POINT('Ctrl Pts',(6.20121542949839,28.7968961014696,53.3327866277352));
#89964=CARTESIAN_POINT('Ctrl Pts',(6.20507700710183,28.8559957577342,53.2931749192791));
#89965=CARTESIAN_POINT('Ctrl Pts',(6.2089453412167,28.9151988192763,53.2534939031491));
#89966=CARTESIAN_POINT('Ctrl Pts',(6.21281367533157,28.9763915587461,53.2169485363525));
#89967=CARTESIAN_POINT('Ctrl Pts',(6.21668200944644,29.0392024024628,53.1837220644773));
#89968=CARTESIAN_POINT('Ctrl Pts',(6.2189797286174,29.0765108860287,53.1639861525462));
#89969=CARTESIAN_POINT('Ctrl Pts',(6.22127744778836,29.1143898337741,53.1454202891854));
#89970=CARTESIAN_POINT('Ctrl Pts',(6.22357516695932,29.1527583672327,53.1280547074752));
#89971=CARTESIAN_POINT('Ctrl Pts',(6.22744424030754,29.2173662062111,53.0988132273934));
#89972=CARTESIAN_POINT('Ctrl Pts',(6.23131331365576,29.2836162215101,53.0728631850844));
#89973=CARTESIAN_POINT('Ctrl Pts',(6.23518238700398,29.3511397635225,53.050390306749));
#89974=CARTESIAN_POINT('Ctrl Pts',(6.23904569539977,29.4185626948788,53.0279509131948));
#89975=CARTESIAN_POINT('Ctrl Pts',(6.24290900379556,29.4872549291605,53.008978551621));
#89976=CARTESIAN_POINT('Ctrl Pts',(6.24677231219134,29.5568265229057,52.993611495323));
#89977=CARTESIAN_POINT('Ctrl Pts',(6.25063108868426,29.6263165048112,52.9782624655451));
#89978=CARTESIAN_POINT('Ctrl Pts',(6.25448986517717,29.6966833251353,52.9665104445909));
#89979=CARTESIAN_POINT('Ctrl Pts',(6.25834864167009,29.7675221866831,52.9584438217831));
#89980=CARTESIAN_POINT('Ctrl Pts',(6.26220498725829,29.8383164220334,52.9503822806875));
#89981=CARTESIAN_POINT('Ctrl Pts',(6.2660613328465,29.9095816271032,52.9460015863917));
#89982=CARTESIAN_POINT('Ctrl Pts',(6.26991767843471,29.9809045784327,52.9453387317187));
#89983=CARTESIAN_POINT('Ctrl Pts',(6.27377288468005,30.0522064576632,52.9446760728837));
#89984=CARTESIAN_POINT('Ctrl Pts',(6.27762809092538,30.1235655637825,52.9477290775123));
#89985=CARTESIAN_POINT('Ctrl Pts',(6.28148329717072,30.1945670747281,52.9544826532313));
#89986=CARTESIAN_POINT('Ctrl Pts',(6.28533865402196,30.2655713593897,52.9612364927827));
#89987=CARTESIAN_POINT('Ctrl Pts',(6.28919401087321,30.3362175377481,52.971691142247));
#89988=CARTESIAN_POINT('Ctrl Pts',(6.29304936772446,30.4060960479372,52.9857796639022));
#89989=CARTESIAN_POINT('Ctrl Pts',(6.29690876019302,30.4760477038651,52.9998829327998));
#89990=CARTESIAN_POINT('Ctrl Pts',(6.30076815266158,30.5452296103556,53.0176275708755));
#89991=CARTESIAN_POINT('Ctrl Pts',(6.30462754513014,30.6132434306249,53.0388957046359));
#89992=CARTESIAN_POINT('Ctrl Pts',(6.30848912273358,30.6812957593829,53.0601758801208));
#89993=CARTESIAN_POINT('Ctrl Pts',(6.31235070033702,30.7481782296865,53.0849833536127));
#89994=CARTESIAN_POINT('Ctrl Pts',(6.31621227794046,30.8135112824052,53.1131515811016));
#89995=CARTESIAN_POINT('Ctrl Pts',(6.32008061205533,30.8789586468285,53.1413690938751));
#89996=CARTESIAN_POINT('Ctrl Pts',(6.3239489461702,30.9428507455122,53.1729588853261));
#89997=CARTESIAN_POINT('Ctrl Pts',(6.32781728028508,31.0048320976366,53.2077081660457));
#89998=CARTESIAN_POINT('Ctrl Pts',(6.33011499945601,31.0416478784836,53.2283485983647));
#89999=CARTESIAN_POINT('Ctrl Pts',(6.33241271862695,31.0777900498443,53.2501028948123));
#90000=CARTESIAN_POINT('Ctrl Pts',(6.33471043779788,31.1131893460155,53.2729195032027));
#90001=CARTESIAN_POINT('Ctrl Pts',(6.3385795111461,31.1727973586455,53.3113398343453));
#90002=CARTESIAN_POINT('Ctrl Pts',(6.34244858449431,31.230530748491,53.352924986983));
#90003=CARTESIAN_POINT('Ctrl Pts',(6.34631765784252,31.2860335365734,53.3974659737439));
#90004=CARTESIAN_POINT('Ctrl Pts',(6.35018096623831,31.3414536250262,53.441940594053));
#90005=CARTESIAN_POINT('Ctrl Pts',(6.3540442746341,31.394649333214,53.4893620046678));
#90006=CARTESIAN_POINT('Ctrl Pts',(6.35790758302988,31.4452930003892,53.53947759157));
#90007=CARTESIAN_POINT('Ctrl Pts',(6.36176635952279,31.4958772593688,53.5895343897479));
#90008=CARTESIAN_POINT('Ctrl Pts',(6.3656251360157,31.5439150802224,53.642278746476));
#90009=CARTESIAN_POINT('Ctrl Pts',(6.36948391250862,31.5891126557695,53.6974185131927));
#90010=CARTESIAN_POINT('Ctrl Pts',(6.37334025809682,31.6342817583021,53.7525235436352));
#90011=CARTESIAN_POINT('Ctrl Pts',(6.37719660368503,31.6766138581673,53.8100206153618));
#90012=CARTESIAN_POINT('Ctrl Pts',(6.38105294927323,31.7158537585194,53.8695826249235));
#90013=CARTESIAN_POINT('Ctrl Pts',(6.38490815551856,31.7550820655897,53.9291270371123));
#90014=CARTESIAN_POINT('Ctrl Pts',(6.38876336176389,31.7912197197449,53.9907347705194));
#90015=CARTESIAN_POINT('Ctrl Pts',(6.39261856800922,31.8240544161565,54.0540491294998));
#90016=CARTESIAN_POINT('Ctrl Pts',(6.39647392486046,31.8568903952749,54.1173659618931));
#90017=CARTESIAN_POINT('Ctrl Pts',(6.40032928171171,31.8864229387863,54.1823891199662));
#90018=CARTESIAN_POINT('Ctrl Pts',(6.40418463856296,31.9124861523396,54.2487382083393));
#90019=CARTESIAN_POINT('Ctrl Pts',(6.40804403103151,31.938576647714,54.3151567480083));
#90020=CARTESIAN_POINT('Ctrl Pts',(6.41190342350007,31.9611903857798,54.3829035355099));
#90021=CARTESIAN_POINT('Ctrl Pts',(6.41576281596863,31.9802103536278,54.4515799804116));
#90022=CARTESIAN_POINT('Ctrl Pts',(6.41962439357206,31.9992410903197,54.5202953089708));
#90023=CARTESIAN_POINT('Ctrl Pts',(6.4234859711755,32.0146739011016,54.5899408682429));
#90024=CARTESIAN_POINT('Ctrl Pts',(6.42734754877893,32.0264428476099,54.6601074465797));
#90025=CARTESIAN_POINT('Ctrl Pts',(6.4312158828938,32.0382323859669,54.7303967937269));
#90026=CARTESIAN_POINT('Ctrl Pts',(6.43508421700867,32.0463452058353,54.8012084972222));
#90027=CARTESIAN_POINT('Ctrl Pts',(6.43895255112354,32.0507672808364,54.8721284928113));
#90028=CARTESIAN_POINT('Ctrl Pts',(6.44125027029451,32.0533939118884,54.9142536631382));
#90029=CARTESIAN_POINT('Ctrl Pts',(6.44354798946548,32.0547193955748,54.9564170246935));
#90030=CARTESIAN_POINT('Ctrl Pts',(6.44584570863644,32.0547494759025,54.9985324242889));
#90031=CARTESIAN_POINT('Ctrl Pts',(6.44587223260258,32.054749823138,54.9990185878927));
#90032=CARTESIAN_POINT('Ctrl Pts',(6.44589875656871,32.0547499978305,54.9995047516197));
#90033=CARTESIAN_POINT('Ctrl Pts',(6.44592528053485,32.0547499999799,54.9999909153921));
#90034=CARTESIAN_POINT('Origin',(-1.54592528053767,30.,55.));
#90035=CARTESIAN_POINT('',(5.29388070767824,28.7479524050421,56.6292250864936));
#90036=CARTESIAN_POINT('',(5.35213793390276,28.7479524050421,56.6292250864936));
#90037=CARTESIAN_POINT('',(-1.54592528053767,28.7479524050421,56.6292250864936));
#90038=CARTESIAN_POINT('',(5.80407471943462,32.0547491412314,54.9981214077884));
#90039=CARTESIAN_POINT('Ctrl Pts',(5.35213793390276,28.7479524050421,56.6292250864936));
#90040=CARTESIAN_POINT('Ctrl Pts',(5.35599766292863,28.6915503629408,56.5858805285507));
#90041=CARTESIAN_POINT('Ctrl Pts',(5.35985739195449,28.6373313286563,56.5395495273057));
#90042=CARTESIAN_POINT('Ctrl Pts',(5.36371712098035,28.5856246526876,56.4904831228213));
#90043=CARTESIAN_POINT('Ctrl Pts',(5.36757404196294,28.5339555945369,56.4414524152955));
#90044=CARTESIAN_POINT('Ctrl Pts',(5.37143096294552,28.484795620045,56.3896905857117));
#90045=CARTESIAN_POINT('Ctrl Pts',(5.3752878839281,28.4384404564927,56.3354884329642));
#90046=CARTESIAN_POINT('Ctrl Pts',(5.37914328914527,28.3921035104651,56.281307581599));
#90047=CARTESIAN_POINT('Ctrl Pts',(5.38299869436244,28.3485695030702,56.2246886793533));
#90048=CARTESIAN_POINT('Ctrl Pts',(5.38685409957961,28.3080955784032,56.1659575424007));
#90049=CARTESIAN_POINT('Ctrl Pts',(5.39070927931651,28.267624020821,56.1072298402915));
#90050=CARTESIAN_POINT('Ctrl Pts',(5.39456445905341,28.2302124649732,56.0463905496428));
#90051=CARTESIAN_POINT('Ctrl Pts',(5.39841963879031,28.196075196942,55.9837951348793));
#90052=CARTESIAN_POINT('Ctrl Pts',(5.40227861260071,28.161904332733,55.921138116865));
#90053=CARTESIAN_POINT('Ctrl Pts',(5.40613758641111,28.1310144263927,55.8567219499077));
#90054=CARTESIAN_POINT('Ctrl Pts',(5.40999656022151,28.1035737355695,55.7909266628949));
#90055=CARTESIAN_POINT('Ctrl Pts',(5.41385738135562,28.0761199086532,55.7250998791164));
#90056=CARTESIAN_POINT('Ctrl Pts',(5.41771820248974,28.0521187503223,55.6578931182441));
#90057=CARTESIAN_POINT('Ctrl Pts',(5.42157902362385,28.0316892851007,55.5897037324901));
#90058=CARTESIAN_POINT('Ctrl Pts',(5.42544695903229,28.0112221748252,55.5213886952283));
#90059=CARTESIAN_POINT('Ctrl Pts',(5.42931489444074,27.9943400227808,55.4520878885795));
#90060=CARTESIAN_POINT('Ctrl Pts',(5.43318282984919,27.9811110440717,55.3822106044194));
#90061=CARTESIAN_POINT('Ctrl Pts',(5.43660651843915,27.9694014629437,55.3203589871577));
#90062=CARTESIAN_POINT('Ctrl Pts',(5.44003020702911,27.9605533501439,55.2580560670572));
#90063=CARTESIAN_POINT('Ctrl Pts',(5.44345389561907,27.9545799673091,55.1955874545234));
#90064=CARTESIAN_POINT('Ctrl Pts',(5.44732296896728,27.9478295121444,55.1249923529236));
#90065=CARTESIAN_POINT('Ctrl Pts',(5.45119204231549,27.9447248768961,55.053909088628));
#90066=CARTESIAN_POINT('Ctrl Pts',(5.45506111566371,27.9453224383922,54.9827465851109));
#90067=CARTESIAN_POINT('Ctrl Pts',(5.4589244240595,27.9459191095165,54.9116901143336));
#90068=CARTESIAN_POINT('Ctrl Pts',(5.46278773245528,27.9502070236293,54.8405551205059));
#90069=CARTESIAN_POINT('Ctrl Pts',(5.46665104085107,27.9581907664978,54.7697553117116));
#90070=CARTESIAN_POINT('Ctrl Pts',(5.47050981734398,27.9661651439355,54.6990385555302));
#90071=CARTESIAN_POINT('Ctrl Pts',(5.47436859383689,27.9778266843106,54.6286566837512));
#90072=CARTESIAN_POINT('Ctrl Pts',(5.47822737032981,27.9931279671208,54.5590213087377));
#90073=CARTESIAN_POINT('Ctrl Pts',(5.48208371591801,28.0084196106165,54.489429801764));
#90074=CARTESIAN_POINT('Ctrl Pts',(5.48594006150622,28.0273463434204,54.4205843318948));
#90075=CARTESIAN_POINT('Ctrl Pts',(5.48979640709442,28.0498093885285,54.352887844784));
#90076=CARTESIAN_POINT('Ctrl Pts',(5.49365161333976,28.0722657970139,54.285211358347));
#90077=CARTESIAN_POINT('Ctrl Pts',(5.49750681958509,28.0982562906982,54.2186836415558));
#90078=CARTESIAN_POINT('Ctrl Pts',(5.50136202583042,28.127632294866,54.1536922904337));
#90079=CARTESIAN_POINT('Ctrl Pts',(5.50521738268167,28.1570094466249,54.0886984003861));
#90080=CARTESIAN_POINT('Ctrl Pts',(5.50907273953292,28.1897721693541,54.0252414369272));
#90081=CARTESIAN_POINT('Ctrl Pts',(5.51292809638416,28.2257245380364,53.9636872346758));
#90082=CARTESIAN_POINT('Ctrl Pts',(5.51678748885272,28.2617145400707,53.9020686002035));
#90083=CARTESIAN_POINT('Ctrl Pts',(5.52064688132128,28.3009006075061,53.8423571232076));
#90084=CARTESIAN_POINT('Ctrl Pts',(5.52450627378984,28.3430422566967,53.7848915277198));
#90085=CARTESIAN_POINT('Ctrl Pts',(5.52836785139328,28.3852077659088,53.727393396003));
#90086=CARTESIAN_POINT('Ctrl Pts',(5.53222942899671,28.4303318806809,53.6721440535545));
#90087=CARTESIAN_POINT('Ctrl Pts',(5.53609100660015,28.4781341470806,53.6194487013451));
#90088=CARTESIAN_POINT('Ctrl Pts',(5.53995934071502,28.5260200519805,53.5666611493183));
#90089=CARTESIAN_POINT('Ctrl Pts',(5.54382767482989,28.5765931192425,53.5164368517539));
#90090=CARTESIAN_POINT('Ctrl Pts',(5.54769600894476,28.6295369352046,53.4690432564793));
#90091=CARTESIAN_POINT('Ctrl Pts',(5.54999372811572,28.6609845861332,53.4408923343487));
#90092=CARTESIAN_POINT('Ctrl Pts',(5.55229144728667,28.6932680392855,53.4137393489293));
#90093=CARTESIAN_POINT('Ctrl Pts',(5.55458916645763,28.7263160946049,53.3876331460745));
#90094=CARTESIAN_POINT('Ctrl Pts',(5.55845823980585,28.7819649100315,53.3436735469358));
#90095=CARTESIAN_POINT('Ctrl Pts',(5.56232731315406,28.8400012139871,53.302512198001));
#90096=CARTESIAN_POINT('Ctrl Pts',(5.56619638650228,28.9001120288156,53.2644182493055));
#90097=CARTESIAN_POINT('Ctrl Pts',(5.57005969489807,28.9601332780151,53.2263810609198));
#90098=CARTESIAN_POINT('Ctrl Pts',(5.57392300329385,29.022222495477,53.1914024584711));
#90099=CARTESIAN_POINT('Ctrl Pts',(5.57778631168964,29.0860345941754,53.1597106750688));
#90100=CARTESIAN_POINT('Ctrl Pts',(5.58164508818255,29.1497718372826,53.1280560681146));
#90101=CARTESIAN_POINT('Ctrl Pts',(5.58550386467546,29.2152275141708,53.0996808366239));
#90102=CARTESIAN_POINT('Ctrl Pts',(5.58936264116837,29.282030092187,53.0747683843301));
#90103=CARTESIAN_POINT('Ctrl Pts',(5.59321898675658,29.3487905867342,53.0498716260775));
#90104=CARTESIAN_POINT('Ctrl Pts',(5.59707533234478,29.4168958449017,53.0284334884235));
#90105=CARTESIAN_POINT('Ctrl Pts',(5.60093167793299,29.4859537613947,53.0105895277556));
#90106=CARTESIAN_POINT('Ctrl Pts',(5.60478688417832,29.5549912749846,52.9927508390191));
#90107=CARTESIAN_POINT('Ctrl Pts',(5.60864209042365,29.6249804180432,52.9785043405957));
#90108=CARTESIAN_POINT('Ctrl Pts',(5.61249729666899,29.6955149726785,52.9679354265582));
#90109=CARTESIAN_POINT('Ctrl Pts',(5.61635265352023,29.766052282788,52.9573660996399));
#90110=CARTESIAN_POINT('Ctrl Pts',(5.62020801037148,29.8371345660271,52.9504747121478));
#90111=CARTESIAN_POINT('Ctrl Pts',(5.62406336722272,29.9083482061046,52.9472950744991));
#90112=CARTESIAN_POINT('Ctrl Pts',(5.62792275969128,29.9796363894761,52.944112108546));
#90113=CARTESIAN_POINT('Ctrl Pts',(5.63178215215984,30.051055717867,52.9446486700726));
#90114=CARTESIAN_POINT('Ctrl Pts',(5.6356415446284,30.1221911847715,52.9488864300424));
#90115=CARTESIAN_POINT('Ctrl Pts',(5.63950312223183,30.1933669275979,52.9531265893736));
#90116=CARTESIAN_POINT('Ctrl Pts',(5.64336469983527,30.2642580060049,52.9610720646429));
#90117=CARTESIAN_POINT('Ctrl Pts',(5.6472262774387,30.3344558992222,52.9726527643308));
#90118=CARTESIAN_POINT('Ctrl Pts',(5.65109461155358,30.4047766160409,52.9842537264964));
#90119=CARTESIAN_POINT('Ctrl Pts',(5.65496294566845,30.4744012514912,52.9995025079733));
#90120=CARTESIAN_POINT('Ctrl Pts',(5.65883127978332,30.5429334995974,53.0182783299578));
#90121=CARTESIAN_POINT('Ctrl Pts',(5.66112899895427,30.5836403919252,53.0294308221787));
#90122=CARTESIAN_POINT('Ctrl Pts',(5.66342671812523,30.623962183262,53.0418267532859));
#90123=CARTESIAN_POINT('Ctrl Pts',(5.66572443729618,30.6638192197251,53.0554327972468));
#90124=CARTESIAN_POINT('Ctrl Pts',(5.6695935106444,30.7309335126586,53.0783436832806));
#90125=CARTESIAN_POINT('Ctrl Pts',(5.67346258399261,30.7969917617407,53.1047780728358));
#90126=CARTESIAN_POINT('Ctrl Pts',(5.67733165734083,30.861598094463,53.1346189970631));
#90127=CARTESIAN_POINT('Ctrl Pts',(5.68119496573661,30.9261081631961,53.1644154580578));
#90128=CARTESIAN_POINT('Ctrl Pts',(5.6850582741324,30.9891701723715,53.1976081764317));
#90129=CARTESIAN_POINT('Ctrl Pts',(5.68892158252818,31.0504052106035,53.2340310149844));
#90130=CARTESIAN_POINT('Ctrl Pts',(5.69278035902109,31.1115684162978,53.2704111272648));
#90131=CARTESIAN_POINT('Ctrl Pts',(5.69663913551401,31.1709084925866,53.3100135860908));
#90132=CARTESIAN_POINT('Ctrl Pts',(5.70049791200692,31.2280698480373,53.3526257222958));
#90133=CARTESIAN_POINT('Ctrl Pts',(5.70435425759513,31.2851951936782,53.3952110142295));
#90134=CARTESIAN_POINT('Ctrl Pts',(5.70821060318333,31.340144152993,53.4408019322545));
#90135=CARTESIAN_POINT('Ctrl Pts',(5.71206694877154,31.3925901753264,53.4891425725489));
#90136=CARTESIAN_POINT('Ctrl Pts',(5.71592215501687,31.4450207026788,53.537468930782));
#90137=CARTESIAN_POINT('Ctrl Pts',(5.71977736126221,31.4949494041253,53.5885430693971));
#90138=CARTESIAN_POINT('Ctrl Pts',(5.72363256750754,31.5420842183902,53.6420700217273));
#90139=CARTESIAN_POINT('Ctrl Pts',(5.72748792435879,31.5892208740046,53.6955990651195));
#90140=CARTESIAN_POINT('Ctrl Pts',(5.73134328121004,31.6335631063546,53.7515807464294));
#90141=CARTESIAN_POINT('Ctrl Pts',(5.73519863806129,31.6748581792146,53.80968590615));
#90142=CARTESIAN_POINT('Ctrl Pts',(5.73905803052985,31.7161964779335,53.8678518877861));
#90143=CARTESIAN_POINT('Ctrl Pts',(5.74291742299841,31.7544809679483,53.9281453881853));
#90144=CARTESIAN_POINT('Ctrl Pts',(5.74677681546697,31.789501963657,53.9902078012939));
#90145=CARTESIAN_POINT('Ctrl Pts',(5.75063839307041,31.8245427877712,54.0523053532862));
#90146=CARTESIAN_POINT('Ctrl Pts',(5.75449997067384,31.8563162228105,54.1161733765902));
#90147=CARTESIAN_POINT('Ctrl Pts',(5.75836154827727,31.8846595887194,54.1814306399895));
#90148=CARTESIAN_POINT('Ctrl Pts',(5.76222988239215,31.9130525463485,54.2468020824865));
#90149=CARTESIAN_POINT('Ctrl Pts',(5.76609821650702,31.938003282546,54.3135671628902));
#90150=CARTESIAN_POINT('Ctrl Pts',(5.76996655062189,31.9593983267177,54.3813274212027));
#90151=CARTESIAN_POINT('Ctrl Pts',(5.77226426979284,31.9721065886457,54.4215757658208));
#90152=CARTESIAN_POINT('Ctrl Pts',(5.77456198896379,31.9835613184563,54.4621749669161));
#90153=CARTESIAN_POINT('Ctrl Pts',(5.77685970813474,31.9937473133959,54.5030400289493));
#90154=CARTESIAN_POINT('Ctrl Pts',(5.78191177765076,32.0161435901798,54.5928913636023));
#90155=CARTESIAN_POINT('Ctrl Pts',(5.78696384716678,32.0324751044773,54.6843103064811));
#90156=CARTESIAN_POINT('Ctrl Pts',(5.79201591668279,32.0425683991214,54.7765902924879));
#90157=CARTESIAN_POINT('Ctrl Pts',(5.79603551760007,32.0505989727865,54.8500114350955));
#90158=CARTESIAN_POINT('Ctrl Pts',(5.80005511851734,32.0546813537135,54.9239774059945));
#90159=CARTESIAN_POINT('Ctrl Pts',(5.80407471943462,32.0547491412314,54.9981214077884));
#90160=CARTESIAN_POINT('Ctrl Pts',(5.80407471946232,32.0547491412319,54.9981214082994));
#90161=CARTESIAN_POINT('Ctrl Pts',(5.80788808427067,32.0548134507169,55.0684612587007));
#90162=CARTESIAN_POINT('Ctrl Pts',(5.81170144907902,32.0512616122162,55.1388965966684));
#90163=CARTESIAN_POINT('Ctrl Pts',(5.81551481388736,32.0440909046793,55.2090213766761));
#90164=CARTESIAN_POINT('Ctrl Pts',(5.81932566294072,32.0369249278052,55.2790998939279));
#90165=CARTESIAN_POINT('Ctrl Pts',(5.82313651199408,32.0261448653966,55.3488677648101));
#90166=CARTESIAN_POINT('Ctrl Pts',(5.82694736104743,32.0118000195855,55.4179213367317));
#90167=CARTESIAN_POINT('Ctrl Pts',(5.83075704398262,31.9974595632911,55.4869537782901));
#90168=CARTESIAN_POINT('Ctrl Pts',(5.83456672691781,31.9795565892295,55.5552718667561));
#90169=CARTESIAN_POINT('Ctrl Pts',(5.838376409853,31.9581916522916,55.6224813373874));
#90170=CARTESIAN_POINT('Ctrl Pts',(5.84218627454133,31.9368256960708,55.6896940144621));
#90171=CARTESIAN_POINT('Ctrl Pts',(5.84599613922967,31.9119976032424,55.7557974946331));
#90172=CARTESIAN_POINT('Ctrl Pts',(5.849806003918,31.8838574485778,55.8204137224217));
#90173=CARTESIAN_POINT('Ctrl Pts',(5.85361981396675,31.8556881529696,55.8850968644785));
#90174=CARTESIAN_POINT('Ctrl Pts',(5.8574336240155,31.8242001532049,55.9482892241745));
#90175=CARTESIAN_POINT('Ctrl Pts',(5.86124743406425,31.7895907717139,56.0096348014487));
#90176=CARTESIAN_POINT('Ctrl Pts',(5.86506356527389,31.7549603262628,56.0710177148652));
#90177=CARTESIAN_POINT('Ctrl Pts',(5.86887969648353,31.7172049893169,56.130551190873));
#90178=CARTESIAN_POINT('Ctrl Pts',(5.87269582769317,31.6765654040821,56.1879082491232));
#90179=CARTESIAN_POINT('Ctrl Pts',(5.87651830066253,31.6358582827825,56.2453606250294));
#90180=CARTESIAN_POINT('Ctrl Pts',(5.88034077363189,31.5922576630937,56.3006289805395));
#90181=CARTESIAN_POINT('Ctrl Pts',(5.88416324660125,31.5460437137662,56.3534202590563));
#90182=CARTESIAN_POINT('Ctrl Pts',(5.88544049072526,31.5306017483947,56.3710599783756));
#90183=CARTESIAN_POINT('Ctrl Pts',(5.88671773484928,31.5148682976371,56.3884234488371));
#90184=CARTESIAN_POINT('Ctrl Pts',(5.8879949789733,31.4988546567116,56.4055007223598));
#90185=CARTESIAN_POINT('Ctrl Pts',(5.89186405232151,31.450345565812,56.4572318069697));
#90186=CARTESIAN_POINT('Ctrl Pts',(5.89573312566973,31.3990601643256,56.5065499255199));
#90187=CARTESIAN_POINT('Ctrl Pts',(5.89960219901794,31.3452680229111,56.5531424625683));
#90188=CARTESIAN_POINT('Ctrl Pts',(5.90346550741372,31.2915560322483,56.5996655763374));
#90189=CARTESIAN_POINT('Ctrl Pts',(5.9073288158095,31.2353450798583,56.6434708543948));
#90190=CARTESIAN_POINT('Ctrl Pts',(5.91119212420528,31.1769425622696,56.6842813801791));
#90191=CARTESIAN_POINT('Ctrl Pts',(5.91505090069819,31.1186085544943,56.725044032659));
#90192=CARTESIAN_POINT('Ctrl Pts',(5.9189096771911,31.0580884843514,56.7628186340324));
#90193=CARTESIAN_POINT('Ctrl Pts',(5.92276845368401,30.9957225538102,56.7973686762414));
#90194=CARTESIAN_POINT('Ctrl Pts',(5.92662479927221,30.9333959117934,56.8318969530383));
#90195=CARTESIAN_POINT('Ctrl Pts',(5.93048114486042,30.8692261403501,56.8632044660194));
#90196=CARTESIAN_POINT('Ctrl Pts',(5.93433749044863,30.8035808867981,56.8910989717285));
#90197=CARTESIAN_POINT('Ctrl Pts',(5.93819269669395,30.7379550278906,56.9189852361103));
#90198=CARTESIAN_POINT('Ctrl Pts',(5.94204790293928,30.6708549991593,56.9434603052145));
#90199=CARTESIAN_POINT('Ctrl Pts',(5.94590310918461,30.6026698482918,56.9643794481871));
#90200=CARTESIAN_POINT('Ctrl Pts',(5.94975846603586,30.534482033731,56.9852994083784));
#90201=CARTESIAN_POINT('Ctrl Pts',(5.9536138228871,30.4652094779389,57.0026630262639));
#90202=CARTESIAN_POINT('Ctrl Pts',(5.95746917973835,30.3952562000434,57.0163754855748));
#90203=CARTESIAN_POINT('Ctrl Pts',(5.9613285722069,30.3252296981456,57.0301022984827));
#90204=CARTESIAN_POINT('Ctrl Pts',(5.96518796467546,30.2545215294252,57.0401702298633));
#90205=CARTESIAN_POINT('Ctrl Pts',(5.96904735714402,30.1835448252711,57.0465358192849));
#90206=CARTESIAN_POINT('Ctrl Pts',(5.97290893474745,30.1125279350842,57.0529050128157));
#90207=CARTESIAN_POINT('Ctrl Pts',(5.97677051235089,30.0412426924744,57.0555676733289));
#90208=CARTESIAN_POINT('Ctrl Pts',(5.98063208995432,29.9701034964045,57.0545324922164));
#90209=CARTESIAN_POINT('Ctrl Pts',(5.98450042406919,29.8988398297577,57.0534954998718));
#90210=CARTESIAN_POINT('Ctrl Pts',(5.98836875818406,29.8277232046934,57.048747780675));
#90211=CARTESIAN_POINT('Ctrl Pts',(5.99223709229893,29.757163462566,57.0403499647333));
#90212=CARTESIAN_POINT('Ctrl Pts',(5.99453481146991,29.7152522761558,57.0353618168353));
#90213=CARTESIAN_POINT('Ctrl Pts',(5.99683253064088,29.673537401737,57.0290868493545));
#90214=CARTESIAN_POINT('Ctrl Pts',(5.99913024981186,29.6321025567787,57.0215461987724));
#90215=CARTESIAN_POINT('Ctrl Pts',(6.00299944641644,29.5623292078643,57.0088482764167));
#90216=CARTESIAN_POINT('Ctrl Pts',(6.00686864302101,29.4930773589399,56.992508916201));
#90217=CARTESIAN_POINT('Ctrl Pts',(6.01073783962559,29.424755896298,56.9725850510576));
#90218=CARTESIAN_POINT('Ctrl Pts',(6.01460043061965,29.3565510741421,56.9526952005449));
#90219=CARTESIAN_POINT('Ctrl Pts',(6.0184630216137,29.2892739449733,56.9292331382224));
#90220=CARTESIAN_POINT('Ctrl Pts',(6.02232561260776,29.2233236576029,56.902306868426));
#90221=CARTESIAN_POINT('Ctrl Pts',(6.02618437399501,29.1574387573444,56.8754072949653));
#90222=CARTESIAN_POINT('Ctrl Pts',(6.03004313538226,29.0928785364837,56.8450505102895));
#90223=CARTESIAN_POINT('Ctrl Pts',(6.03390189676951,29.0300262074176,56.8113940499525));
#90224=CARTESIAN_POINT('Ctrl Pts',(6.03775817547493,28.9672143168031,56.7777592437875));
#90225=CARTESIAN_POINT('Ctrl Pts',(6.04161445418034,28.9061085647321,56.7408292034265));
#90226=CARTESIAN_POINT('Ctrl Pts',(6.04547073288576,28.8470698473807,56.7008085211691));
#90227=CARTESIAN_POINT('Ctrl Pts',(6.0476742096299,28.8133351381894,56.6779407127518));
#90228=CARTESIAN_POINT('Ctrl Pts',(6.04987768637404,28.7802748782558,56.6540646713894));
#90229=CARTESIAN_POINT('Ctrl Pts',(6.05208116311818,28.7479524050421,56.6292250864936));
#90230=CARTESIAN_POINT('',(5.74592528057397,32.0547492412561,55.0017658022556));
#90231=CARTESIAN_POINT('Ctrl Pts',(5.74592528057397,32.0547492412561,55.0017658022556));
#90232=CARTESIAN_POINT('Ctrl Pts',(5.75057817989353,32.0546753518278,55.0877461243741));
#90233=CARTESIAN_POINT('Ctrl Pts',(5.7552310792131,32.0492009128718,55.1734909003204));
#90234=CARTESIAN_POINT('Ctrl Pts',(5.75988397853267,32.0384370230129,55.25840291351));
#90235=CARTESIAN_POINT('Ctrl Pts',(5.76460377517735,32.027518374714,55.3445357540079));
#90236=CARTESIAN_POINT('Ctrl Pts',(5.76932357182203,32.0111571571895,55.4298117228975));
#90237=CARTESIAN_POINT('Ctrl Pts',(5.77404336846671,31.9895181111646,55.5136294849872));
#90238=CARTESIAN_POINT('Ctrl Pts',(5.7757069401795,31.9818910654317,55.543172465022));
#90239=CARTESIAN_POINT('Ctrl Pts',(5.7773705118923,31.9736087726772,55.5725344842986));
#90240=CARTESIAN_POINT('Ctrl Pts',(5.77903408360509,31.9646798449385,55.6016898448475));
#90241=CARTESIAN_POINT('Ctrl Pts',(5.78290315695331,31.9439132761899,55.669498300347));
#90242=CARTESIAN_POINT('Ctrl Pts',(5.78677223030153,31.919591424662,55.7363632146236));
#90243=CARTESIAN_POINT('Ctrl Pts',(5.79064130364974,31.891818620162,55.8018851980854));
#90244=CARTESIAN_POINT('Ctrl Pts',(5.79450461204553,31.8640871973786,55.8673095532306));
#90245=CARTESIAN_POINT('Ctrl Pts',(5.79836792044131,31.8329152162863,55.9313945058254));
#90246=CARTESIAN_POINT('Ctrl Pts',(5.80223122883709,31.7984566891992,55.9937560563713));
#90247=CARTESIAN_POINT('Ctrl Pts',(5.80609000533,31.764038584124,56.05604445291));
#90248=CARTESIAN_POINT('Ctrl Pts',(5.80994878182292,31.7263418248368,56.1166130399686));
#90249=CARTESIAN_POINT('Ctrl Pts',(5.81380755831583,31.6855676731749,56.1750996475396));
#90250=CARTESIAN_POINT('Ctrl Pts',(5.81766390390404,31.6448192079132,56.2335494104346));
#90251=CARTESIAN_POINT('Ctrl Pts',(5.82152024949224,31.600997473704,56.2899193984339));
#90252=CARTESIAN_POINT('Ctrl Pts',(5.82537659508045,31.554347868057,56.3438750937371));
#90253=CARTESIAN_POINT('Ctrl Pts',(5.82923180132578,31.5077120448613,56.3978148480319));
#90254=CARTESIAN_POINT('Ctrl Pts',(5.83308700757112,31.4582503264421,56.449341358436));
#90255=CARTESIAN_POINT('Ctrl Pts',(5.83694221381645,31.4062482494231,56.4981533377777));
#90256=CARTESIAN_POINT('Ctrl Pts',(5.8407975706677,31.3542441409122,56.5469672239883));
#90257=CARTESIAN_POINT('Ctrl Pts',(5.84465292751894,31.2996998324747,56.5930660377379));
#90258=CARTESIAN_POINT('Ctrl Pts',(5.84850828437019,31.2429362859699,56.6361867104702));
#90259=CARTESIAN_POINT('Ctrl Pts',(5.85236767683875,31.1861133218912,56.6793525200186));
#90260=CARTESIAN_POINT('Ctrl Pts',(5.85622706930731,31.127066870136,56.7195336710873));
#90261=CARTESIAN_POINT('Ctrl Pts',(5.86008646177587,31.0661486922942,56.7565091882536));
#90262=CARTESIAN_POINT('Ctrl Pts',(5.86394803937931,31.0051960234189,56.7935056404486));
#90263=CARTESIAN_POINT('Ctrl Pts',(5.86780961698274,30.9423699468744,56.8272926154684));
#90264=CARTESIAN_POINT('Ctrl Pts',(5.87167119458618,30.8780463317208,56.8576954007188));
#90265=CARTESIAN_POINT('Ctrl Pts',(5.87553952870105,30.8136101710518,56.8881513810069));
#90266=CARTESIAN_POINT('Ctrl Pts',(5.87940786281593,30.7476716900095,56.9152111651147));
#90267=CARTESIAN_POINT('Ctrl Pts',(5.8832761969308,30.6806255415039,56.938748677563));
#90268=CARTESIAN_POINT('Ctrl Pts',(5.88557391610175,30.6408013649502,56.9527295261617));
#90269=CARTESIAN_POINT('Ctrl Pts',(5.8878716352727,30.6005866745913,56.9654686251862));
#90270=CARTESIAN_POINT('Ctrl Pts',(5.89016935444365,30.5600659399301,56.9769480785873));
#90271=CARTESIAN_POINT('Ctrl Pts',(5.89403860384475,30.4918309570381,56.9962789301375));
#90272=CARTESIAN_POINT('Ctrl Pts',(5.89790785324585,30.4224603230496,57.0121107721138));
#90273=CARTESIAN_POINT('Ctrl Pts',(5.90177710264696,30.352346221252,57.0243146254645));
#90274=CARTESIAN_POINT('Ctrl Pts',(5.90563962090602,30.2823540934936,57.0364972483744));
#90275=CARTESIAN_POINT('Ctrl Pts',(5.90950213916508,30.2116215424782,57.0450643409051));
#90276=CARTESIAN_POINT('Ctrl Pts',(5.91336465742414,30.1405544638856,57.0499370734688));
#90277=CARTESIAN_POINT('Ctrl Pts',(5.91722337851842,30.0695572499225,57.0548050157462));
#90278=CARTESIAN_POINT('Ctrl Pts',(5.9210820996127,29.9982266427402,57.0559857693842));
#90279=CARTESIAN_POINT('Ctrl Pts',(5.92494082070698,29.9269760556761,57.0534519877648));
#90280=CARTESIAN_POINT('Ctrl Pts',(5.92879703927701,29.8557716772699,57.0509198493972));
#90281=CARTESIAN_POINT('Ctrl Pts',(5.93265325784704,29.7846477002684,57.0446779736162));
#90282=CARTESIAN_POINT('Ctrl Pts',(5.93650947641706,29.7140182219434,57.0347510867719));
#90283=CARTESIAN_POINT('Ctrl Pts',(5.94036448407722,29.6434109223231,57.0248273171175));
#90284=CARTESIAN_POINT('Ctrl Pts',(5.94421949173738,29.5732982936435,57.0112209023425));
#90285=CARTESIAN_POINT('Ctrl Pts',(5.94807449939753,29.5040882643472,56.9940083031276));
#90286=CARTESIAN_POINT('Ctrl Pts',(5.95193183773653,29.4348363917225,56.9767852974377));
#90287=CARTESIAN_POINT('Ctrl Pts',(5.95578917607553,29.3664886826125,56.9559518624032));
#90288=CARTESIAN_POINT('Ctrl Pts',(5.95964651441454,29.2994408398931,56.9316351688894));
#90289=CARTESIAN_POINT('Ctrl Pts',(5.96350485094092,29.2323756467872,56.9073121827938));
#90290=CARTESIAN_POINT('Ctrl Pts',(5.96736318746731,29.1666114412787,56.8795043250355));
#90291=CARTESIAN_POINT('Ctrl Pts',(5.97122152399369,29.1025243457336,56.8483871381556));
#90292=CARTESIAN_POINT('Ctrl Pts',(5.97508578920756,29.038338774496,56.8172221368678));
#90293=CARTESIAN_POINT('Ctrl Pts',(5.97895005442143,28.9758358925275,56.7827378749951));
#90294=CARTESIAN_POINT('Ctrl Pts',(5.98281431963531,28.9153670640459,56.745155854571));
#90295=CARTESIAN_POINT('Ctrl Pts',(5.98650504958231,28.8576137516344,56.7092615562837));
#90296=CARTESIAN_POINT('Ctrl Pts',(5.99019577952932,28.8017160054131,56.6705420212124));
#90297=CARTESIAN_POINT('Ctrl Pts',(5.99388650947633,28.7479524050421,56.6292250864936));
#90298=CARTESIAN_POINT('Ctrl Pts',(5.29388070767824,28.7479524050421,56.6292250864936));
#90299=CARTESIAN_POINT('Ctrl Pts',(5.29774025035993,28.6913741458772,56.5857451070227));
#90300=CARTESIAN_POINT('Ctrl Pts',(5.30159979304163,28.6370931697353,56.5393373503055));
#90301=CARTESIAN_POINT('Ctrl Pts',(5.30545933572333,28.5854145236434,56.4902836953348));
#90302=CARTESIAN_POINT('Ctrl Pts',(5.30932116858873,28.5337052123657,56.4412009328013));
#90303=CARTESIAN_POINT('Ctrl Pts',(5.31318300145413,28.4846016390198,56.3894694995279));
#90304=CARTESIAN_POINT('Ctrl Pts',(5.31704483431953,28.4383704634804,56.3354065872121));
#90305=CARTESIAN_POINT('Ctrl Pts',(5.32091331711177,28.3920596796446,56.2812505806521));
#90306=CARTESIAN_POINT('Ctrl Pts',(5.32478179990401,28.3486314623212,56.2247554664636));
#90307=CARTESIAN_POINT('Ctrl Pts',(5.32865028269625,28.3083103737035,56.1662691673799));
#90308=CARTESIAN_POINT('Ctrl Pts',(5.33059785521445,28.2880108794798,56.1368244690565));
#90309=CARTESIAN_POINT('Ctrl Pts',(5.33254542773266,28.2684982009073,56.1068755093954));
#90310=CARTESIAN_POINT('Ctrl Pts',(5.33449300025086,28.2497965371344,56.0764689503526));
#90311=CARTESIAN_POINT('Ctrl Pts',(5.33836207359907,28.2126435642953,56.0160628776113));
#90312=CARTESIAN_POINT('Ctrl Pts',(5.34223114694728,28.1785487493108,55.9536127950323));
#90313=CARTESIAN_POINT('Ctrl Pts',(5.3461002202955,28.147742810437,55.8894609975778));
#90314=CARTESIAN_POINT('Ctrl Pts',(5.34996352869129,28.1169827726758,55.8254047868508));
#90315=CARTESIAN_POINT('Ctrl Pts',(5.35382683708707,28.0895020923366,55.7596523286275));
#90316=CARTESIAN_POINT('Ctrl Pts',(5.35769014548286,28.0654870977573,55.6925730239884));
#90317=CARTESIAN_POINT('Ctrl Pts',(5.36154892197578,28.0415002742717,55.6255724075777));
#90318=CARTESIAN_POINT('Ctrl Pts',(5.36540769846869,28.0209712240983,55.5572484915745));
#90319=CARTESIAN_POINT('Ctrl Pts',(5.3692664749616,28.0040386621116,55.4879917009076));
#90320=CARTESIAN_POINT('Ctrl Pts',(5.37312282054981,27.9871167670927,55.4187785397847));
#90321=CARTESIAN_POINT('Ctrl Pts',(5.37697916613801,27.9737869803035,55.348634140719));
#90322=CARTESIAN_POINT('Ctrl Pts',(5.38083551172622,27.9641380924165,55.2779637669743));
#90323=CARTESIAN_POINT('Ctrl Pts',(5.38469071797155,27.9544920552574,55.2073142725271));
#90324=CARTESIAN_POINT('Ctrl Pts',(5.38854592421688,27.9485248236772,55.1361395929656));
#90325=CARTESIAN_POINT('Ctrl Pts',(5.39240113046221,27.9462737202159,55.0648531435187));
#90326=CARTESIAN_POINT('Ctrl Pts',(5.39625648731345,27.944022528814,54.9935639092246));
#90327=CARTESIAN_POINT('Ctrl Pts',(5.40011184416469,27.9454877668835,54.9221633819897));
#90328=CARTESIAN_POINT('Ctrl Pts',(5.40396720101593,27.9506546621121,54.851066294691));
#90329=CARTESIAN_POINT('Ctrl Pts',(5.40782659348449,27.9558269658185,54.7798947861007));
#90330=CARTESIAN_POINT('Ctrl Pts',(5.41168598595305,27.9647086262349,54.7090278370035));
#90331=CARTESIAN_POINT('Ctrl Pts',(5.41554537842161,27.9772329265544,54.6388754659617));
#90332=CARTESIAN_POINT('Ctrl Pts',(5.41940695602504,27.9897643179602,54.5686833756135));
#90333=CARTESIAN_POINT('Ctrl Pts',(5.42326853362847,28.0059423446728,54.4992071420754));
#90334=CARTESIAN_POINT('Ctrl Pts',(5.4271301112319,28.0256496404589,54.4308442917092));
#90335=CARTESIAN_POINT('Ctrl Pts',(5.43099844534677,28.0453914176367,54.3623618284728));
#90336=CARTESIAN_POINT('Ctrl Pts',(5.43486677946164,28.0686746338715,54.2949970970483));
#90337=CARTESIAN_POINT('Ctrl Pts',(5.43873511357652,28.0953330110473,54.2291295675058));
#90338=CARTESIAN_POINT('Ctrl Pts',(5.44103283274748,28.1111675957767,54.1900054688939));
#90339=CARTESIAN_POINT('Ctrl Pts',(5.44333055191844,28.1281920767405,54.151409186527));
#90340=CARTESIAN_POINT('Ctrl Pts',(5.44562827108941,28.1463640450114,54.1134159324275));
#90341=CARTESIAN_POINT('Ctrl Pts',(5.44949734443762,28.1769633797821,54.0494400172219));
#90342=CARTESIAN_POINT('Ctrl Pts',(5.45336641778584,28.2109386112393,53.9869247961123));
#90343=CARTESIAN_POINT('Ctrl Pts',(5.45723549113405,28.2481272957714,53.9262497540495));
#90344=CARTESIAN_POINT('Ctrl Pts',(5.46109879952983,28.285260568845,53.8656651183191));
#90345=CARTESIAN_POINT('Ctrl Pts',(5.46496210792562,28.3255975390151,53.8069156298805));
#90346=CARTESIAN_POINT('Ctrl Pts',(5.4688254163214,28.3689289141422,53.750358181166));
#90347=CARTESIAN_POINT('Ctrl Pts',(5.47268419281431,28.4122094588506,53.6938670778834));
#90348=CARTESIAN_POINT('Ctrl Pts',(5.47654296930722,28.4584771372476,53.6395632904025));
#90349=CARTESIAN_POINT('Ctrl Pts',(5.48040174580014,28.5074791703103,53.5877751115908));
#90350=CARTESIAN_POINT('Ctrl Pts',(5.48425809138834,28.556450333673,53.5360195576611));
#90351=CARTESIAN_POINT('Ctrl Pts',(5.48811443697655,28.6081521010895,53.4867768203067));
#90352=CARTESIAN_POINT('Ctrl Pts',(5.49197078256476,28.6622921501111,53.4403412966788));
#90353=CARTESIAN_POINT('Ctrl Pts',(5.49582598881009,28.716416203658,53.3939194922524));
#90354=CARTESIAN_POINT('Ctrl Pts',(5.49968119505543,28.7729767401188,53.3503035710919));
#90355=CARTESIAN_POINT('Ctrl Pts',(5.50353640130077,28.8316466737575,53.3097491110613));
#90356=CARTESIAN_POINT('Ctrl Pts',(5.50739175815202,28.8903188993719,53.2691930667466));
#90357=CARTESIAN_POINT('Ctrl Pts',(5.51124711500326,28.9511002849051,53.2316989954189));
#90358=CARTESIAN_POINT('Ctrl Pts',(5.51510247185451,29.01363438323,53.1974794224326));
#90359=CARTESIAN_POINT('Ctrl Pts',(5.51896186432308,29.0762339394878,53.1632240299083));
#90360=CARTESIAN_POINT('Ctrl Pts',(5.52282125679163,29.1405894439088,53.132250211661));
#90361=CARTESIAN_POINT('Ctrl Pts',(5.5266806492602,29.2063202372391,53.1047242953375));
#90362=CARTESIAN_POINT('Ctrl Pts',(5.53054222686363,29.2720882464395,53.0771827942192));
#90363=CARTESIAN_POINT('Ctrl Pts',(5.53440380446706,29.3392326371751,53.0530932452881));
#90364=CARTESIAN_POINT('Ctrl Pts',(5.53826538207049,29.4073557750041,53.032572648081));
#90365=CARTESIAN_POINT('Ctrl Pts',(5.54213371618536,29.4755981062838,53.012016146468));
#90366=CARTESIAN_POINT('Ctrl Pts',(5.54600205030023,29.5448221317369,52.9950411796585));
#90367=CARTESIAN_POINT('Ctrl Pts',(5.5498703844151,29.6146188587501,52.9817138611017));
#90368=CARTESIAN_POINT('Ctrl Pts',(5.55216810358606,29.6560768282445,52.973797679501));
#90369=CARTESIAN_POINT('Ctrl Pts',(5.55446582275701,29.6977367133036,52.9671674501319));
#90370=CARTESIAN_POINT('Ctrl Pts',(5.55676354192797,29.739512323952,52.9618283357069));
#90371=CARTESIAN_POINT('Ctrl Pts',(5.56063261527619,29.8098572572268,52.9528379309675));
#90372=CARTESIAN_POINT('Ctrl Pts',(5.5645016886244,29.8808059628848,52.9474759921008));
#90373=CARTESIAN_POINT('Ctrl Pts',(5.56837076197262,29.9519515155083,52.9458118621611));
#90374=CARTESIAN_POINT('Ctrl Pts',(5.57223407036841,30.0229910606491,52.9441502117893));
#90375=CARTESIAN_POINT('Ctrl Pts',(5.5760973787642,30.0942263888595,52.946175444879));
#90376=CARTESIAN_POINT('Ctrl Pts',(5.57996068715999,30.1652441467217,52.9519052916249));
#90377=CARTESIAN_POINT('Ctrl Pts',(5.5838194636529,30.2361785963031,52.9576284169014));
#90378=CARTESIAN_POINT('Ctrl Pts',(5.58767824014582,30.3068955006345,52.9670474848391));
#90379=CARTESIAN_POINT('Ctrl Pts',(5.59153701663873,30.3769819483143,52.9801281790309));
#90380=CARTESIAN_POINT('Ctrl Pts',(5.59539336222694,30.4470242437931,52.9932006328073));
#90381=CARTESIAN_POINT('Ctrl Pts',(5.59924970781515,30.5164363941828,53.0099300474541));
#90382=CARTESIAN_POINT('Ctrl Pts',(5.60310605340336,30.5848125184159,53.0302305005905));
#90383=CARTESIAN_POINT('Ctrl Pts',(5.60696125964869,30.6531684411789,53.0505249560339));
#90384=CARTESIAN_POINT('Ctrl Pts',(5.61081646589403,30.7204884800177,53.0743882172142));
#90385=CARTESIAN_POINT('Ctrl Pts',(5.61467167213936,30.7863805132799,53.1016841014116));
#90386=CARTESIAN_POINT('Ctrl Pts',(5.61852702899061,30.8522751206535,53.1289810519388));
#90387=CARTESIAN_POINT('Ctrl Pts',(5.62238238584187,30.9167411637363,53.1597107037642));
#90388=CARTESIAN_POINT('Ctrl Pts',(5.62623774269312,30.9794067666008,53.1936888562497));
#90389=CARTESIAN_POINT('Ctrl Pts',(5.63009713516168,31.0421379650511,53.2277025755648));
#90390=CARTESIAN_POINT('Ctrl Pts',(5.63395652763024,31.1030645332306,53.2649713514497));
#90391=CARTESIAN_POINT('Ctrl Pts',(5.6378159200988,31.1618402761301,53.3052655856265));
#90392=CARTESIAN_POINT('Ctrl Pts',(5.64167749770225,31.2206492970461,53.3455826338439));
#90393=CARTESIAN_POINT('Ctrl Pts',(5.64553907530569,31.2773046824805,53.388928255033));
#90394=CARTESIAN_POINT('Ctrl Pts',(5.64940065290914,31.3314924733856,53.4350318355259));
#90395=CARTESIAN_POINT('Ctrl Pts',(5.65326898702401,31.3857750753928,53.4812160823682));
#90396=CARTESIAN_POINT('Ctrl Pts',(5.65713732113888,31.437581109668,53.5301675890948));
#90397=CARTESIAN_POINT('Ctrl Pts',(5.66100565525375,31.486633208518,53.5815786007566));
#90398=CARTESIAN_POINT('Ctrl Pts',(5.66330337442468,31.5157692512058,53.61211579418));
#90399=CARTESIAN_POINT('Ctrl Pts',(5.66560109359561,31.5439344211605,53.6435200799704));
#90400=CARTESIAN_POINT('Ctrl Pts',(5.66789881276654,31.571077634615,53.6757218462451));
#90401=CARTESIAN_POINT('Ctrl Pts',(5.67174314546748,31.6164911666132,53.7295988842593));
#90402=CARTESIAN_POINT('Ctrl Pts',(5.67558747816843,31.6592258384195,53.7859284481417));
#90403=CARTESIAN_POINT('Ctrl Pts',(5.67943181086938,31.6990035717013,53.8444116538117));
#90404=CARTESIAN_POINT('Ctrl Pts',(5.68327073565045,31.7387253486413,53.9028125896796));
#90405=CARTESIAN_POINT('Ctrl Pts',(5.68710966043152,31.7754981613696,53.9633607567449));
#90406=CARTESIAN_POINT('Ctrl Pts',(5.69094858521259,31.8090834220944,54.02572348155));
#90407=CARTESIAN_POINT('Ctrl Pts',(5.69478343427784,31.8426330259658,54.0880199969972));
#90408=CARTESIAN_POINT('Ctrl Pts',(5.69861828334308,31.8730015594206,54.1521268173281));
#90409=CARTESIAN_POINT('Ctrl Pts',(5.70245313240832,31.899994128269,54.2176830085934));
#90410=CARTESIAN_POINT('Ctrl Pts',(5.7062858215248,31.9269714937639,54.2832022758464));
#90411=CARTESIAN_POINT('Ctrl Pts',(5.71011851064129,31.9505764742473,54.3501688427883));
#90412=CARTESIAN_POINT('Ctrl Pts',(5.71395119975777,31.970661212502,54.4181993915093));
#90413=CARTESIAN_POINT('Ctrl Pts',(5.71778249936705,31.9907386692143,54.4862052763627));
#90414=CARTESIAN_POINT('Ctrl Pts',(5.72161379897633,32.007298281549,54.555273904177));
#90415=CARTESIAN_POINT('Ctrl Pts',(5.72544509858562,32.0202418689665,54.6250061955517));
#90416=CARTESIAN_POINT('Ctrl Pts',(5.72927810286536,32.0331912154093,54.6947695131027));
#90417=CARTESIAN_POINT('Ctrl Pts',(5.7331111071451,32.0425212306723,54.7651965997985));
#90418=CARTESIAN_POINT('Ctrl Pts',(5.73694411142483,32.048185000157,54.8358788020031));
#90419=CARTESIAN_POINT('Ctrl Pts',(5.73993783446245,32.0526086208859,54.8910843070446));
#90420=CARTESIAN_POINT('Ctrl Pts',(5.74293155750006,32.0547967824529,54.9464451824544));
#90421=CARTESIAN_POINT('Ctrl Pts',(5.74592528053768,32.0547492412566,55.0017658015851));
#90422=CARTESIAN_POINT('Origin',(-1.54592528053767,30.,55.));
#90423=CARTESIAN_POINT('',(4.59397380484682,28.7479524050421,56.6292250864936));
#90424=CARTESIAN_POINT('',(4.6520175253044,28.7479524050421,56.6292250864936));
#90425=CARTESIAN_POINT('',(-1.54592528053767,28.7479524050421,56.6292250864936));
#90426=CARTESIAN_POINT('',(5.10407471942445,32.0547498925786,55.0006644157262));
#90427=CARTESIAN_POINT('Ctrl Pts',(4.6520175253044,28.7479524050421,56.6292250864936));
#90428=CARTESIAN_POINT('Ctrl Pts',(4.65588667393895,28.6914965352496,56.5858391623626));
#90429=CARTESIAN_POINT('Ctrl Pts',(4.6597558225735,28.6373821256713,56.5395797426843));
#90430=CARTESIAN_POINT('Ctrl Pts',(4.66362497120805,28.5858980096712,56.4907424738862));
#90431=CARTESIAN_POINT('Ctrl Pts',(4.66425231405508,28.577550387246,56.482824010642));
#90432=CARTESIAN_POINT('Ctrl Pts',(4.66487965690211,28.5692718285588,56.474837849469));
#90433=CARTESIAN_POINT('Ctrl Pts',(4.66550699974914,28.5610634645336,56.4667853317374));
#90434=CARTESIAN_POINT('Ctrl Pts',(4.66937607309736,28.5104392123682,56.417122245773));
#90435=CARTESIAN_POINT('Ctrl Pts',(4.67324514644557,28.4622899074248,56.3647379575138));
#90436=CARTESIAN_POINT('Ctrl Pts',(4.67711421979379,28.4169220079584,56.3099090173037));
#90437=CARTESIAN_POINT('Ctrl Pts',(4.68097752818958,28.3716217070508,56.2551617726841));
#90438=CARTESIAN_POINT('Ctrl Pts',(4.68484083658536,28.3290948924322,56.1979774777012));
#90439=CARTESIAN_POINT('Ctrl Pts',(4.68870414498115,28.289611479732,56.1386696940885));
#90440=CARTESIAN_POINT('Ctrl Pts',(4.69256292147406,28.2501743835495,56.0794314822229));
#90441=CARTESIAN_POINT('Ctrl Pts',(4.69642169796697,28.2137738657556,56.0180751320759));
#90442=CARTESIAN_POINT('Ctrl Pts',(4.70028047445989,28.1806387041183,55.9549460914354));
#90443=CARTESIAN_POINT('Ctrl Pts',(4.70413682004809,28.1475244165639,55.891856820054));
#90444=CARTESIAN_POINT('Ctrl Pts',(4.7079931656363,28.11767162921,55.8269975028873));
#90445=CARTESIAN_POINT('Ctrl Pts',(4.71184951122451,28.0912642476933,55.7607400281082));
#90446=CARTESIAN_POINT('Ctrl Pts',(4.71570471746984,28.0648646681386,55.6945021288521));
#90447=CARTESIAN_POINT('Ctrl Pts',(4.71955992371517,28.0419086533007,55.626867343082));
#90448=CARTESIAN_POINT('Ctrl Pts',(4.7234151299605,28.0225321258001,55.5582278826853));
#90449=CARTESIAN_POINT('Ctrl Pts',(4.72727048681175,28.003154841344,55.4895857408473));
#90450=CARTESIAN_POINT('Ctrl Pts',(4.731125843663,27.9873574517059,55.4199393145738));
#90451=CARTESIAN_POINT('Ctrl Pts',(4.73498120051424,27.9752256400638,55.3496946580158));
#90452=CARTESIAN_POINT('Ctrl Pts',(4.7388405929828,27.9630811293769,55.279376472453));
#90453=CARTESIAN_POINT('Ctrl Pts',(4.74269998545136,27.9546099389754,55.2084592862478));
#90454=CARTESIAN_POINT('Ctrl Pts',(4.74655937791992,27.9498462038099,55.1373571056304));
#90455=CARTESIAN_POINT('Ctrl Pts',(4.75042095552336,27.9450797714831,55.0662146679373));
#90456=CARTESIAN_POINT('Ctrl Pts',(4.75428253312679,27.9440249802595,54.9948875132875));
#90457=CARTESIAN_POINT('Ctrl Pts',(4.75814411073023,27.9466637979444,54.9237897393517));
#90458=CARTESIAN_POINT('Ctrl Pts',(4.7620124448451,27.9493072327066,54.8525675673143));
#90459=CARTESIAN_POINT('Ctrl Pts',(4.76588077895997,27.9556571358943,54.7815760612898));
#90460=CARTESIAN_POINT('Ctrl Pts',(4.76974911307484,27.9656436525551,54.7112235914919));
#90461=CARTESIAN_POINT('Ctrl Pts',(4.7720468322458,27.9715754594005,54.6694355210258));
#90462=CARTESIAN_POINT('Ctrl Pts',(4.77434455141675,27.9787893326922,54.6278727252012));
#90463=CARTESIAN_POINT('Ctrl Pts',(4.77664227058771,27.9872622538327,54.586618423665));
#90464=CARTESIAN_POINT('Ctrl Pts',(4.78051134393593,28.0015295993727,54.5171513101072));
#90465=CARTESIAN_POINT('Ctrl Pts',(4.78438041728414,28.0194254679784,54.4482876251215));
#90466=CARTESIAN_POINT('Ctrl Pts',(4.78824949063236,28.0408837296112,54.3804348286113));
#90467=CARTESIAN_POINT('Ctrl Pts',(4.79211279902815,28.0623100182504,54.312683133349));
#90468=CARTESIAN_POINT('Ctrl Pts',(4.79597610742393,28.0872880184086,54.2459397961355));
#90469=CARTESIAN_POINT('Ctrl Pts',(4.79983941581972,28.1157006857587,54.1806016494709));
#90470=CARTESIAN_POINT('Ctrl Pts',(4.80369819231263,28.1440800232693,54.1153401485473));
#90471=CARTESIAN_POINT('Ctrl Pts',(4.80755696880555,28.1758858320737,54.0514810072649));
#90472=CARTESIAN_POINT('Ctrl Pts',(4.81141574529846,28.2109519672827,53.9894037902653));
#90473=CARTESIAN_POINT('Ctrl Pts',(4.81527209088667,28.2459960119577,53.9273656799098));
#90474=CARTESIAN_POINT('Ctrl Pts',(4.81912843647487,28.2842960697709,53.867107688675));
#90475=CARTESIAN_POINT('Ctrl Pts',(4.82298478206308,28.3256394450817,53.808986022486));
#90476=CARTESIAN_POINT('Ctrl Pts',(4.82683998830841,28.3669706056469,53.7508815281258));
#90477=CARTESIAN_POINT('Ctrl Pts',(4.83069519455375,28.411343017247,53.6949125014039));
#90478=CARTESIAN_POINT('Ctrl Pts',(4.83455040079908,28.4585008851392,53.641405858476));
#90479=CARTESIAN_POINT('Ctrl Pts',(4.83840575765033,28.5056605952813,53.5878971252795));
#90480=CARTESIAN_POINT('Ctrl Pts',(4.84226111450158,28.5556056549018,53.5368513298448));
#90481=CARTESIAN_POINT('Ctrl Pts',(4.84611647135282,28.6080413916997,53.4885606875304));
#90482=CARTESIAN_POINT('Ctrl Pts',(4.84997586382138,28.6605320159115,53.4402194967039));
#90483=CARTESIAN_POINT('Ctrl Pts',(4.85383525628994,28.7155181636516,53.3946395458177));
#90484=CARTESIAN_POINT('Ctrl Pts',(4.8576946487585,28.7726705238238,53.3520740552412));
#90485=CARTESIAN_POINT('Ctrl Pts',(4.86155622636194,28.8298552428755,53.30948446467));
#90486=CARTESIAN_POINT('Ctrl Pts',(4.86541780396537,28.8892082115208,53.2699130016197));
#90487=CARTESIAN_POINT('Ctrl Pts',(4.86927938156881,28.9503717482546,53.2335691081625));
#90488=CARTESIAN_POINT('Ctrl Pts',(4.87314771568368,29.0116423013889,53.1971616246504));
#90489=CARTESIAN_POINT('Ctrl Pts',(4.87701604979855,29.0747293173161,53.1639932116718));
#90490=CARTESIAN_POINT('Ctrl Pts',(4.88088438391342,29.1392518196144,53.1342266663759));
#90491=CARTESIAN_POINT('Ctrl Pts',(4.88318210308437,29.1775769968317,53.1165458870667));
#90492=CARTESIAN_POINT('Ctrl Pts',(4.88547982225532,29.2164082578056,53.1000644084989));
#90493=CARTESIAN_POINT('Ctrl Pts',(4.88777754142626,29.2556632016253,53.0848080270935));
#90494=CARTESIAN_POINT('Ctrl Pts',(4.89164661477447,29.3217636454215,53.0591181780328));
#90495=CARTESIAN_POINT('Ctrl Pts',(4.89551568812269,29.3893251031837,53.0368040872381));
#90496=CARTESIAN_POINT('Ctrl Pts',(4.8993847614709,29.4579693835411,53.0180311876013));
#90497=CARTESIAN_POINT('Ctrl Pts',(4.90324806986669,29.5265113833328,52.9992862597457));
#90498=CARTESIAN_POINT('Ctrl Pts',(4.90711137826247,29.596132538375,52.9840721766353));
#90499=CARTESIAN_POINT('Ctrl Pts',(4.91097468665826,29.6664359717593,52.9725058319285));
#90500=CARTESIAN_POINT('Ctrl Pts',(4.91483346315117,29.7366569348102,52.960953055269));
#90501=CARTESIAN_POINT('Ctrl Pts',(4.91869223964408,29.8075581094114,52.9530395958994));
#90502=CARTESIAN_POINT('Ctrl Pts',(4.922551016137,29.8787304957534,52.9488317304912));
#90503=CARTESIAN_POINT('Ctrl Pts',(4.9264073617252,29.9498580457881,52.9446265159024));
#90504=CARTESIAN_POINT('Ctrl Pts',(4.93026370731341,30.0212559847979,52.9441222924568));
#90505=CARTESIAN_POINT('Ctrl Pts',(4.93412005290161,30.0925096901931,52.9473335585828));
#90506=CARTESIAN_POINT('Ctrl Pts',(4.93797525914695,30.1637423439476,52.9505438759522));
#90507=CARTESIAN_POINT('Ctrl Pts',(4.94183046539228,30.2348303636575,52.9574674817409));
#90508=CARTESIAN_POINT('Ctrl Pts',(4.94568567163761,30.3053603589388,52.9680667792251));
#90509=CARTESIAN_POINT('Ctrl Pts',(4.94954102848885,30.3758931095161,52.9786664907771));
#90510=CARTESIAN_POINT('Ctrl Pts',(4.9533963853401,30.4458673123203,52.9929421047382));
#90511=CARTESIAN_POINT('Ctrl Pts',(4.95725174219134,30.5148776448274,53.0108045411883));
#90512=CARTESIAN_POINT('Ctrl Pts',(4.9611111346599,30.5839602143033,53.0286856752482));
#90513=CARTESIAN_POINT('Ctrl Pts',(4.96497052712846,30.6520764281661,53.0501610047003));
#90514=CARTESIAN_POINT('Ctrl Pts',(4.96882991959702,30.7188349384421,53.0750911985824));
#90515=CARTESIAN_POINT('Ctrl Pts',(4.97269149720045,30.7856312464675,53.1000355075971));
#90516=CARTESIAN_POINT('Ctrl Pts',(4.97655307480389,30.8510678748055,53.1284383815136));
#90517=CARTESIAN_POINT('Ctrl Pts',(4.98041465240732,30.9147748684456,53.1601129103773));
#90518=CARTESIAN_POINT('Ctrl Pts',(4.98428298652219,30.978593328713,53.1918428594186));
#90519=CARTESIAN_POINT('Ctrl Pts',(4.98815132063707,31.0406756889177,53.2268556535021));
#90520=CARTESIAN_POINT('Ctrl Pts',(4.99201965475194,31.1006785481548,53.2649195130681));
#90521=CARTESIAN_POINT('Ctrl Pts',(4.9943173739229,31.1363191406909,53.2875287441346));
#90522=CARTESIAN_POINT('Ctrl Pts',(4.99661509309386,31.1712266300883,53.311213615859));
#90523=CARTESIAN_POINT('Ctrl Pts',(4.99891281226483,31.2053346523553,53.3359188906993));
#90524=CARTESIAN_POINT('Ctrl Pts',(5.00275064676246,31.26230460158,53.3771836184579));
#90525=CARTESIAN_POINT('Ctrl Pts',(5.00658848126009,31.3172734889281,53.4214646825556));
#90526=CARTESIAN_POINT('Ctrl Pts',(5.01042631575773,31.3699002709869,53.4685396479014));
#90527=CARTESIAN_POINT('Ctrl Pts',(5.01432833257717,31.4234071611025,53.5164018750681));
#90528=CARTESIAN_POINT('Ctrl Pts',(5.01823034939662,31.4744924192996,53.5671520862871));
#90529=CARTESIAN_POINT('Ctrl Pts',(5.02213236621606,31.522828336926,53.6205104499289));
#90530=CARTESIAN_POINT('Ctrl Pts',(5.02595997436977,31.5702425232262,53.6728513077966));
#90531=CARTESIAN_POINT('Ctrl Pts',(5.02978758252348,31.6150109502794,53.7277013416823));
#90532=CARTESIAN_POINT('Ctrl Pts',(5.03361519067719,31.6568593683213,53.7847573920792));
#90533=CARTESIAN_POINT('Ctrl Pts',(5.03744050268938,31.6986826819412,53.8417792151569));
#90534=CARTESIAN_POINT('Ctrl Pts',(5.04126581470158,31.7375891686526,53.901004032373));
#90535=CARTESIAN_POINT('Ctrl Pts',(5.04509112671377,31.7733450235497,53.9620958666853));
#90536=CARTESIAN_POINT('Ctrl Pts',(5.04891547573736,31.8090918772253,54.0231723216665));
#90537=CARTESIAN_POINT('Ctrl Pts',(5.05273982476095,31.8416894240058,54.0861144340417));
#90538=CARTESIAN_POINT('Ctrl Pts',(5.05656417378454,31.8709483479536,54.1505591004728));
#90539=CARTESIAN_POINT('Ctrl Pts',(5.0605233859212,31.901239068305,54.2172763650066));
#90540=CARTESIAN_POINT('Ctrl Pts',(5.06448259805786,31.9279510192921,54.2856036450338));
#90541=CARTESIAN_POINT('Ctrl Pts',(5.06844181019452,31.9509280911055,54.3551146258167));
#90542=CARTESIAN_POINT('Ctrl Pts',(5.07227054686683,31.9731479556739,54.4223348787524));
#90543=CARTESIAN_POINT('Ctrl Pts',(5.07609928353915,31.9918752129524,54.490661515234));
#90544=CARTESIAN_POINT('Ctrl Pts',(5.07992802021147,32.0070199603936,54.5596950589858));
#90545=CARTESIAN_POINT('Ctrl Pts',(5.0839524700803,32.0229388605609,54.6322573843359));
#90546=CARTESIAN_POINT('Ctrl Pts',(5.08797691994912,32.0348990846252,54.7056002068221));
#90547=CARTESIAN_POINT('Ctrl Pts',(5.09200136981795,32.0428577974627,54.779252221198));
#90548=CARTESIAN_POINT('Ctrl Pts',(5.09602581968678,32.0508165103001,54.8529042355738));
#90549=CARTESIAN_POINT('Ctrl Pts',(5.10005026955561,32.0547737561238,54.9268648126138));
#90550=CARTESIAN_POINT('Ctrl Pts',(5.10407471942444,32.0547498925786,55.0006644157262));
#90551=CARTESIAN_POINT('Ctrl Pts',(5.10407471946233,32.0547498925784,55.0006644164209));
#90552=CARTESIAN_POINT('Ctrl Pts',(5.10606584067601,32.0547380859309,55.0371772219239));
#90553=CARTESIAN_POINT('Ctrl Pts',(5.1080569618897,32.0537530962652,55.0736730530944));
#90554=CARTESIAN_POINT('Ctrl Pts',(5.11004808310338,32.0517972511101,55.1101163150356));
#90555=CARTESIAN_POINT('Ctrl Pts',(5.1139171564516,32.0479967248986,55.1809315183137));
#90556=CARTESIAN_POINT('Ctrl Pts',(5.11778622979981,32.040518304,55.2516884433728));
#90557=CARTESIAN_POINT('Ctrl Pts',(5.12165530314803,32.02936691962,55.3219743282499));
#90558=CARTESIAN_POINT('Ctrl Pts',(5.12551861154381,32.0182321508982,55.3921554865566));
#90559=CARTESIAN_POINT('Ctrl Pts',(5.1293819199396,32.0034353574455,55.4618665219658));
#90560=CARTESIAN_POINT('Ctrl Pts',(5.13324522833539,31.9850333981067,55.5306976266206));
#90561=CARTESIAN_POINT('Ctrl Pts',(5.1371040048283,31.9666530254196,55.5994479880758));
#90562=CARTESIAN_POINT('Ctrl Pts',(5.14096278132121,31.9446760120999,55.667320002077));
#90563=CARTESIAN_POINT('Ctrl Pts',(5.14482155781412,31.9192103364242,55.733913650958));
#90564=CARTESIAN_POINT('Ctrl Pts',(5.14867790340233,31.8937607033027,55.8004653479885));
#90565=CARTESIAN_POINT('Ctrl Pts',(5.15253424899053,31.8648269412174,55.8657398249892));
#90566=CARTESIAN_POINT('Ctrl Pts',(5.15639059457873,31.8325665301756,55.9293532562918));
#90567=CARTESIAN_POINT('Ctrl Pts',(5.16024580082406,31.8003156503515,55.9929478932441));
#90568=CARTESIAN_POINT('Ctrl Pts',(5.1641010070694,31.7647402923912,56.054882025751));
#90569=CARTESIAN_POINT('Ctrl Pts',(5.16795621331473,31.726044904763,56.1147943977442));
#90570=CARTESIAN_POINT('Ctrl Pts',(5.17181157016597,31.6873480054765,56.1747091102496));
#90571=CARTESIAN_POINT('Ctrl Pts',(5.17566692701722,31.645531099945,56.232601498556));
#90572=CARTESIAN_POINT('Ctrl Pts',(5.17952228386847,31.6008422332874,56.2881388537823));
#90573=CARTESIAN_POINT('Ctrl Pts',(5.18338167633703,31.5561065882974,56.3437343430597));
#90574=CARTESIAN_POINT('Ctrl Pts',(5.18724106880558,31.5084932862138,56.3969694990261));
#90575=CARTESIAN_POINT('Ctrl Pts',(5.19110046127414,31.45829041423,56.4475450356604));
#90576=CARTESIAN_POINT('Ctrl Pts',(5.19496203887757,31.4080591180712,56.4981492074672));
#90577=CARTESIAN_POINT('Ctrl Pts',(5.198823616481,31.3552356931969,56.5460904356481));
#90578=CARTESIAN_POINT('Ctrl Pts',(5.20268519408444,31.3001427797329,56.5911085176092));
#90579=CARTESIAN_POINT('Ctrl Pts',(5.20655352819931,31.244953471495,56.6362053666486));
#90580=CARTESIAN_POINT('Ctrl Pts',(5.21042186231418,31.1874871385044,56.6783685706389));
#90581=CARTESIAN_POINT('Ctrl Pts',(5.21429019642905,31.1280963799291,56.7173805984961));
#90582=CARTESIAN_POINT('Ctrl Pts',(5.21658791560001,31.0928193639051,56.7405530240529));
#90583=CARTESIAN_POINT('Ctrl Pts',(5.21888563477098,31.0568638927504,56.762614530318));
#90584=CARTESIAN_POINT('Ctrl Pts',(5.22118335394194,31.0203076268373,56.7835273782921));
#90585=CARTESIAN_POINT('Ctrl Pts',(5.22505242729016,30.9587514210389,56.8187420136377));
#90586=CARTESIAN_POINT('Ctrl Pts',(5.22892150063837,30.8952494193225,56.8508350814401));
#90587=CARTESIAN_POINT('Ctrl Pts',(5.23279057398659,30.8301510755014,56.8795868573556));
#90588=CARTESIAN_POINT('Ctrl Pts',(5.23665388238237,30.7651497287701,56.9082957928788));
#90589=CARTESIAN_POINT('Ctrl Pts',(5.24051719077816,30.6985572020688,56.9336731241379));
#90590=CARTESIAN_POINT('Ctrl Pts',(5.24438049917394,30.6307486310241,56.9555443556619));
#90591=CARTESIAN_POINT('Ctrl Pts',(5.24823927566685,30.563019603683,56.9773899308606));
#90592=CARTESIAN_POINT('Ctrl Pts',(5.25209805215977,30.4940778255901,56.9957374274862));
#90593=CARTESIAN_POINT('Ctrl Pts',(5.25595682865268,30.4243179325502,57.0104606075764));
#90594=CARTESIAN_POINT('Ctrl Pts',(5.25981317424089,30.3546019859924,57.0251745125381));
#90595=CARTESIAN_POINT('Ctrl Pts',(5.26366951982909,30.2840694211964,57.0362685307208));
#90596=CARTESIAN_POINT('Ctrl Pts',(5.2675258654173,30.2131281183253,57.0436667946804));
#90597=CARTESIAN_POINT('Ctrl Pts',(5.27138107166263,30.1422077747966,57.0510628728505));
#90598=CARTESIAN_POINT('Ctrl Pts',(5.27523627790797,30.0708794158375,57.0547653141544));
#90599=CARTESIAN_POINT('Ctrl Pts',(5.2790914841533,29.9995574339136,57.0547499523385));
#90600=CARTESIAN_POINT('Ctrl Pts',(5.28294684100455,29.9282326657542,57.0547345899226));
#90601=CARTESIAN_POINT('Ctrl Pts',(5.28680219785579,29.8569147609101,57.0510011383427));
#90602=CARTESIAN_POINT('Ctrl Pts',(5.29065755470704,29.7860177733686,57.04357754176));
#90603=CARTESIAN_POINT('Ctrl Pts',(5.2945169471756,29.7150465739912,57.0361461744842));
#90604=CARTESIAN_POINT('Ctrl Pts',(5.29837633964416,29.6444976555829,57.02501700212));
#90605=CARTESIAN_POINT('Ctrl Pts',(5.30223573211272,29.5747787095139,57.0102697372784));
#90606=CARTESIAN_POINT('Ctrl Pts',(5.30609730971616,29.5050202895377,56.9955141227385));
#90607=CARTESIAN_POINT('Ctrl Pts',(5.30995888731959,29.436093246975,56.9771364629712));
#90608=CARTESIAN_POINT('Ctrl Pts',(5.31382046492302,29.3683911777761,56.9552666974582));
#90609=CARTESIAN_POINT('Ctrl Pts',(5.3176887990379,29.3005706518603,56.9333586669312));
#90610=CARTESIAN_POINT('Ctrl Pts',(5.32155713315277,29.2339798324878,56.9079465050117));
#90611=CARTESIAN_POINT('Ctrl Pts',(5.32542546726764,29.168992714123,56.8792084645721));
#90612=CARTESIAN_POINT('Ctrl Pts',(5.32772318643859,29.1303915635248,56.8621385981921));
#90613=CARTESIAN_POINT('Ctrl Pts',(5.33002090560955,29.0923557749171,56.8438962093788));
#90614=CARTESIAN_POINT('Ctrl Pts',(5.33231862478051,29.0549591746737,56.8245260757157));
#90615=CARTESIAN_POINT('Ctrl Pts',(5.33618678846678,28.9920027555951,56.7919168480168));
#90616=CARTESIAN_POINT('Ctrl Pts',(5.34005495215306,28.930612833919,56.7559814127838));
#90617=CARTESIAN_POINT('Ctrl Pts',(5.34392311583933,28.8711632793371,56.7168940621317));
#90618=CARTESIAN_POINT('Ctrl Pts',(5.34666138852714,28.8290789455763,56.6892241305025));
#90619=CARTESIAN_POINT('Ctrl Pts',(5.34939966121495,28.7879666574385,56.6599757475854));
#90620=CARTESIAN_POINT('Ctrl Pts',(5.35213793390276,28.7479524050421,56.6292250864936));
#90621=CARTESIAN_POINT('',(5.04592528049196,32.0547497417017,54.9989697199742));
#90622=CARTESIAN_POINT('Ctrl Pts',(5.04592528053768,32.0547497417021,54.9989697208213));
#90623=CARTESIAN_POINT('Ctrl Pts',(5.04983580638859,32.0547860725486,55.0714265840048));
#90624=CARTESIAN_POINT('Ctrl Pts',(5.0537463322395,32.0509854787254,55.1438783326772));
#90625=CARTESIAN_POINT('Ctrl Pts',(5.05765685809041,32.0433759542005,55.2158987547329));
#90626=CARTESIAN_POINT('Ctrl Pts',(5.06156889758461,32.0357634842646,55.2879470536605));
#90627=CARTESIAN_POINT('Ctrl Pts',(5.0654809370788,32.0243392038328,55.3595632307956));
#90628=CARTESIAN_POINT('Ctrl Pts',(5.069392976573,32.0091827682212,55.4303279753663));
#90629=CARTESIAN_POINT('Ctrl Pts',(5.07331083119321,31.9940038030357,55.5011979095466));
#90630=CARTESIAN_POINT('Ctrl Pts',(5.07722868581341,31.9750817055291,55.5712134277556));
#90631=CARTESIAN_POINT('Ctrl Pts',(5.08114654043362,31.9525468000705,55.6399676210829));
#90632=CARTESIAN_POINT('Ctrl Pts',(5.08506751736912,31.9299939355279,55.708776607732));
#90633=CARTESIAN_POINT('Ctrl Pts',(5.08898849430461,31.9038226982931,55.7763218332456));
#90634=CARTESIAN_POINT('Ctrl Pts',(5.09290947124011,31.8742116465852,55.8422162823791));
#90635=CARTESIAN_POINT('Ctrl Pts',(5.0968384919827,31.8445398483868,55.9082459126795));
#90636=CARTESIAN_POINT('Ctrl Pts',(5.10076751272528,31.8114143545489,55.9726175877549));
#90637=CARTESIAN_POINT('Ctrl Pts',(5.10469653346786,31.7750596081185,56.0349690575694));
#90638=CARTESIAN_POINT('Ctrl Pts',(5.10720517516982,31.7518474545224,56.0747798673368));
#90639=CARTESIAN_POINT('Ctrl Pts',(5.10971381687178,31.7273197264889,56.1137676684778));
#90640=CARTESIAN_POINT('Ctrl Pts',(5.11222245857374,31.7015435920207,56.1518450273163));
#90641=CARTESIAN_POINT('Ctrl Pts',(5.11609153192196,31.6617891086231,56.2105716657746));
#90642=CARTESIAN_POINT('Ctrl Pts',(5.11996060527018,31.6189128733263,56.2673528041018));
#90643=CARTESIAN_POINT('Ctrl Pts',(5.12382967861839,31.5731318462584,56.3218372656223));
#90644=CARTESIAN_POINT('Ctrl Pts',(5.12769298701418,31.5274190333129,56.3762405448283));
#90645=CARTESIAN_POINT('Ctrl Pts',(5.13155629540997,31.4788103298453,56.4283535710454));
#90646=CARTESIAN_POINT('Ctrl Pts',(5.13541960380576,31.4275656730795,56.477854462234));
#90647=CARTESIAN_POINT('Ctrl Pts',(5.13927838029867,31.3763811295078,56.5272972857749));
#90648=CARTESIAN_POINT('Ctrl Pts',(5.14313715679158,31.3225671223705,56.5741337249527));
#90649=CARTESIAN_POINT('Ctrl Pts',(5.1469959332845,31.2664223501252,56.6180766340329));
#90650=CARTESIAN_POINT('Ctrl Pts',(5.1508522788727,31.2103129472751,56.6619918604981));
#90651=CARTESIAN_POINT('Ctrl Pts',(5.15470862446091,31.1518760740568,56.7030168746311));
#90652=CARTESIAN_POINT('Ctrl Pts',(5.15856497004912,31.0914445044239,56.7409039193083));
#90653=CARTESIAN_POINT('Ctrl Pts',(5.16242017629445,31.0310307890721,56.7787797703999));
#90654=CARTESIAN_POINT('Ctrl Pts',(5.16627538253979,30.968623958642,56.8135192346888));
#90655=CARTESIAN_POINT('Ctrl Pts',(5.17013058878512,30.9045854047204,56.8449181033495));
#90656=CARTESIAN_POINT('Ctrl Pts',(5.17398594563637,30.8405443490947,56.8763181986257));
#90657=CARTESIAN_POINT('Ctrl Pts',(5.17784130248762,30.7748718805687,56.9043772272931));
#90658=CARTESIAN_POINT('Ctrl Pts',(5.18169665933887,30.7079520380719,56.9289379135394));
#90659=CARTESIAN_POINT('Ctrl Pts',(5.18555605180743,30.640962146839,56.9535243088276));
#90660=CARTESIAN_POINT('Ctrl Pts',(5.18941544427599,30.5727227321486,56.974604883981));
#90661=CARTESIAN_POINT('Ctrl Pts',(5.19327483674455,30.5036349212799,56.9920716424284));
#90662=CARTESIAN_POINT('Ctrl Pts',(5.19713641434798,30.4345079938441,57.0095482903139));
#90663=CARTESIAN_POINT('Ctrl Pts',(5.20099799195142,30.364532190757,57.0234069539317));
#90664=CARTESIAN_POINT('Ctrl Pts',(5.20485956955485,30.2941181062907,57.0335909377385));
#90665=CARTESIAN_POINT('Ctrl Pts',(5.20872790366972,30.2235808199582,57.0437927402219));
#90666=CARTESIAN_POINT('Ctrl Pts',(5.21259623778459,30.1526042051134,57.0503069817965));
#90667=CARTESIAN_POINT('Ctrl Pts',(5.21646457189946,30.0816025369965,57.0531289751147));
#90668=CARTESIAN_POINT('Ctrl Pts',(5.21876229107041,30.0394288546937,57.0548051871365));
#90669=CARTESIAN_POINT('Ctrl Pts',(5.22106001024135,29.9972463264547,57.0551797214769));
#90670=CARTESIAN_POINT('Ctrl Pts',(5.2233577294123,29.9551409540643,57.0542602630869));
#90671=CARTESIAN_POINT('Ctrl Pts',(5.2272261855104,29.8842520540425,57.052712256498));
#90672=CARTESIAN_POINT('Ctrl Pts',(5.23109464160851,29.8133045461066,57.0474875355493));
#90673=CARTESIAN_POINT('Ctrl Pts',(5.23496309770662,29.7427109426911,57.0385779120478));
#90674=CARTESIAN_POINT('Ctrl Pts',(5.23882613522175,29.6722162204024,57.02968076834));
#90675=CARTESIAN_POINT('Ctrl Pts',(5.24268917273688,29.6020748968272,57.0171090230153));
#90676=CARTESIAN_POINT('Ctrl Pts',(5.24655221025201,29.5326982937989,57.0009064640511));
#90677=CARTESIAN_POINT('Ctrl Pts',(5.2504962517042,29.4618669345165,56.9843641540332));
#90678=CARTESIAN_POINT('Ctrl Pts',(5.25444029315638,29.3918332494984,56.9640370254787));
#90679=CARTESIAN_POINT('Ctrl Pts',(5.25838433460857,29.323027683322,56.9400273309806));
#90680=CARTESIAN_POINT('Ctrl Pts',(5.26224054865168,29.2557543055571,56.9165522934546));
#90681=CARTESIAN_POINT('Ctrl Pts',(5.26609676269479,29.1896553918124,56.8895571900547));
#90682=CARTESIAN_POINT('Ctrl Pts',(5.26995297673789,29.1251191575739,56.8591882836485));
#90683=CARTESIAN_POINT('Ctrl Pts',(5.27394093189462,29.0583781506563,56.8277818742655));
#90684=CARTESIAN_POINT('Ctrl Pts',(5.27792888705134,28.9933090523761,56.7927671232011));
#90685=CARTESIAN_POINT('Ctrl Pts',(5.28191684220807,28.9303176686924,56.7543595049443));
#90686=CARTESIAN_POINT('Ctrl Pts',(5.28590479736479,28.8673262850087,56.7159518866875));
#90687=CARTESIAN_POINT('Ctrl Pts',(5.28989275252152,28.8064131033691,56.6741517067297));
#90688=CARTESIAN_POINT('Ctrl Pts',(5.29388070767824,28.7479524050421,56.6292250864936));
#90689=CARTESIAN_POINT('Ctrl Pts',(4.59397380484682,28.7479524050421,56.6292250864936));
#90690=CARTESIAN_POINT('Ctrl Pts',(4.5978297750184,28.6914443882701,56.5857990877893));
#90691=CARTESIAN_POINT('Ctrl Pts',(4.60168574518998,28.6371627163018,56.5394024137685));
#90692=CARTESIAN_POINT('Ctrl Pts',(4.60554171536156,28.5854289256007,56.4902973656196));
#90693=CARTESIAN_POINT('Ctrl Pts',(4.60939684217606,28.5337064498362,56.441203057463));
#90694=CARTESIAN_POINT('Ctrl Pts',(4.61325196899057,28.4845311008614,56.3894018859296));
#90695=CARTESIAN_POINT('Ctrl Pts',(4.61710709580507,28.4381891114174,56.3351944842624));
#90696=CARTESIAN_POINT('Ctrl Pts',(4.62096266902407,28.3918417558017,56.280980805648));
#90697=CARTESIAN_POINT('Ctrl Pts',(4.62481824224307,28.3483287247538,56.2243607146393));
#90698=CARTESIAN_POINT('Ctrl Pts',(4.62867381546206,28.3078962192091,56.1656682021626));
#90699=CARTESIAN_POINT('Ctrl Pts',(4.63253360638861,28.2674194835398,56.1069114844851));
#90700=CARTESIAN_POINT('Ctrl Pts',(4.63639339731515,28.2300302732144,56.0460782226223));
#90701=CARTESIAN_POINT('Ctrl Pts',(4.6402531882417,28.1959311208761,55.9835309053999));
#90702=CARTESIAN_POINT('Ctrl Pts',(4.64411543010531,28.1618103158427,55.9209438711201));
#90703=CARTESIAN_POINT('Ctrl Pts',(4.64797767196891,28.1309839357524,55.8566410535872));
#90704=CARTESIAN_POINT('Ctrl Pts',(4.65183991383252,28.1036070581878,55.7910065567016));
#90705=CARTESIAN_POINT('Ctrl Pts',(4.65570864680383,28.0761841694549,55.7252617506735));
#90706=CARTESIAN_POINT('Ctrl Pts',(4.65957737977513,28.0522225139632,55.6581812563938));
#90707=CARTESIAN_POINT('Ctrl Pts',(4.66344611274644,28.0318275943512,55.5901651837772));
#90708=CARTESIAN_POINT('Ctrl Pts',(4.66485786690413,28.024385206166,55.56534517836));
#90709=CARTESIAN_POINT('Ctrl Pts',(4.66626962106181,28.0174172795207,55.5404006892119));
#90710=CARTESIAN_POINT('Ctrl Pts',(4.66768137521949,28.0109272352027,55.515351432366));
#90711=CARTESIAN_POINT('Ctrl Pts',(4.67155044856771,27.9931405282447,55.4467010858963));
#90712=CARTESIAN_POINT('Ctrl Pts',(4.67541952191593,27.9788772247288,55.3769943617172));
#90713=CARTESIAN_POINT('Ctrl Pts',(4.67928859526415,27.9682574135064,55.3066261970675));
#90714=CARTESIAN_POINT('Ctrl Pts',(4.68315190365994,27.9576534258936,55.2363628815859));
#90715=CARTESIAN_POINT('Ctrl Pts',(4.68701521205573,27.9506822263921,55.1654405583595));
#90716=CARTESIAN_POINT('Ctrl Pts',(4.69087852045152,27.9474135131066,55.0942670479151));
#90717=CARTESIAN_POINT('Ctrl Pts',(4.69473729694444,27.9441486342267,55.0231770284592));
#90718=CARTESIAN_POINT('Ctrl Pts',(4.69859607343735,27.9445776365808,54.9518368899955));
#90719=CARTESIAN_POINT('Ctrl Pts',(4.70245484993026,27.9487185311776,54.8806605758113));
#90720=CARTESIAN_POINT('Ctrl Pts',(4.70631119551847,27.9528568171443,54.8095291004089));
#90721=CARTESIAN_POINT('Ctrl Pts',(4.71016754110668,27.960702327913,54.7385617283502));
#90722=CARTESIAN_POINT('Ctrl Pts',(4.71402388669489,27.9722209939527,54.6681719343788));
#90723=CARTESIAN_POINT('Ctrl Pts',(4.71787909294022,27.9837362568457,54.5978029368086));
#90724=CARTESIAN_POINT('Ctrl Pts',(4.72173429918555,27.9989224421392,54.5280116576999));
#90725=CARTESIAN_POINT('Ctrl Pts',(4.72558950543088,28.0176938863608,54.4592042582187));
#90726=CARTESIAN_POINT('Ctrl Pts',(4.72944486228214,28.0364660639002,54.3903941707354));
#90727=CARTESIAN_POINT('Ctrl Pts',(4.73330021913339,28.0588236484586,54.3225685072681));
#90728=CARTESIAN_POINT('Ctrl Pts',(4.73715557598465,28.0846307894571,54.2561193981531));
#90729=CARTESIAN_POINT('Ctrl Pts',(4.74101496845321,28.1104649442312,54.1896007330449));
#90730=CARTESIAN_POINT('Ctrl Pts',(4.74487436092177,28.1397556872707,54.1244619524432));
#90731=CARTESIAN_POINT('Ctrl Pts',(4.74873375339033,28.1723188950766,54.0610754336977));
#90732=CARTESIAN_POINT('Ctrl Pts',(4.75259533099376,28.2049005397224,53.9976530263781));
#90733=CARTESIAN_POINT('Ctrl Pts',(4.7564569085972,28.2407580932333,53.9359852760448));
#90734=CARTESIAN_POINT('Ctrl Pts',(4.76031848620064,28.2796626801179,53.8764177518664));
#90735=CARTESIAN_POINT('Ctrl Pts',(4.76418682031551,28.3186353374425,53.816746003793));
#90736=CARTESIAN_POINT('Ctrl Pts',(4.76805515443038,28.3606653857271,53.7591822110122));
#90737=CARTESIAN_POINT('Ctrl Pts',(4.77192348854526,28.4054824916269,53.7040403254763));
#90738=CARTESIAN_POINT('Ctrl Pts',(4.77422120771619,28.4321030265532,53.6712870617315));
#90739=CARTESIAN_POINT('Ctrl Pts',(4.77651892688712,28.4597061291633,53.6393876151707));
#90740=CARTESIAN_POINT('Ctrl Pts',(4.77881664605806,28.4882291828091,53.6084014376301));
#90741=CARTESIAN_POINT('Ctrl Pts',(4.78268571940627,28.5362584581298,53.5562245679752));
#90742=CARTESIAN_POINT('Ctrl Pts',(4.78655479275449,28.5870862098638,53.5064349216959));
#90743=CARTESIAN_POINT('Ctrl Pts',(4.79042386610271,28.6404457659141,53.4593475904412));
#90744=CARTESIAN_POINT('Ctrl Pts',(4.79428717449849,28.6937258157687,53.4123304197136));
#90745=CARTESIAN_POINT('Ctrl Pts',(4.79815048289427,28.7495298205365,53.3680078903842));
#90746=CARTESIAN_POINT('Ctrl Pts',(4.80201379129005,28.8075529541779,53.3266597460737));
#90747=CARTESIAN_POINT('Ctrl Pts',(4.80587256778296,28.8655080230471,53.2853601057278));
#90748=CARTESIAN_POINT('Ctrl Pts',(4.80973134427587,28.9256766563068,53.2470282003395));
#90749=CARTESIAN_POINT('Ctrl Pts',(4.81359012076878,28.9877208506948,53.2119036697141));
#90750=CARTESIAN_POINT('Ctrl Pts',(4.81744646635699,29.0497259592418,53.1768012664098));
#90751=CARTESIAN_POINT('Ctrl Pts',(4.82130281194519,29.1136038630109,53.1449024679027));
#90752=CARTESIAN_POINT('Ctrl Pts',(4.8251591575334,29.1789887057697,53.1164029047468));
#90753=CARTESIAN_POINT('Ctrl Pts',(4.82901436377873,29.2443542308214,53.0879117616802));
#90754=CARTESIAN_POINT('Ctrl Pts',(4.83286957002406,29.3112253658996,53.062818054167));
#90755=CARTESIAN_POINT('Ctrl Pts',(4.83672477626939,29.379214416526,53.0412700998221));
#90756=CARTESIAN_POINT('Ctrl Pts',(4.84058013312063,29.4472061231849,53.0197213036937));
#90757=CARTESIAN_POINT('Ctrl Pts',(4.84443548997187,29.5163153683469,53.0017186804078));
#90758=CARTESIAN_POINT('Ctrl Pts',(4.84829084682311,29.5861390257607,52.9873607733869));
#90759=CARTESIAN_POINT('Ctrl Pts',(4.85215023929167,29.6560357714959,52.972987837143));
#90760=CARTESIAN_POINT('Ctrl Pts',(4.85600963176022,29.726647945485,52.9622673310629));
#90761=CARTESIAN_POINT('Ctrl Pts',(4.85986902422878,29.7975628353229,52.9552465290756));
#90762=CARTESIAN_POINT('Ctrl Pts',(4.86373060183221,29.868517876195,52.9482217520069));
#90763=CARTESIAN_POINT('Ctrl Pts',(4.86759217943564,29.9397754886184,52.944900871601));
#90764=CARTESIAN_POINT('Ctrl Pts',(4.87145375703907,30.0109212110354,52.9452790238941));
#90765=CARTESIAN_POINT('Ctrl Pts',(4.87532209115394,30.0821914154484,52.9456578378314));
#90766=CARTESIAN_POINT('Ctrl Pts',(4.87919042526881,30.1533488538527,52.9497485783339));
#90767=CARTESIAN_POINT('Ctrl Pts',(4.88305875938368,30.2239831424404,52.9574944028467));
#90768=CARTESIAN_POINT('Ctrl Pts',(4.88535647855466,30.2659386080742,52.962095279852));
#90769=CARTESIAN_POINT('Ctrl Pts',(4.88765419772564,30.307709654124,52.9679847345438));
#90770=CARTESIAN_POINT('Ctrl Pts',(4.88995191689661,30.3492123714913,52.9751424044893));
#90771=CARTESIAN_POINT('Ctrl Pts',(4.89382099024483,30.4190977864161,52.9871950305765));
#90772=CARTESIAN_POINT('Ctrl Pts',(4.89769006359304,30.4884953840999,53.0028935228187));
#90773=CARTESIAN_POINT('Ctrl Pts',(4.90155913694125,30.5569958089551,53.0221847327654));
#90774=CARTESIAN_POINT('Ctrl Pts',(4.90542244533704,30.6253941675906,53.041447198644));
#90775=CARTESIAN_POINT('Ctrl Pts',(4.90928575373283,30.6928975431113,53.0642916257024));
#90776=CARTESIAN_POINT('Ctrl Pts',(4.91314906212862,30.7591055840198,53.0906136391998));
#90777=CARTESIAN_POINT('Ctrl Pts',(4.91700783862153,30.8252359587469,53.1169047753256));
#90778=CARTESIAN_POINT('Ctrl Pts',(4.92086661511444,30.8900735678922,53.1466652161715));
#90779=CARTESIAN_POINT('Ctrl Pts',(4.92472539160735,30.953233758787,53.1797409624977));
#90780=CARTESIAN_POINT('Ctrl Pts',(4.92858173719555,31.0163541607992,53.2127958721708));
#90781=CARTESIAN_POINT('Ctrl Pts',(4.93243808278376,31.0777988117451,53.2491617188719));
#90782=CARTESIAN_POINT('Ctrl Pts',(4.93629442837197,31.1372049265938,53.2886372338306));
#90783=CARTESIAN_POINT('Ctrl Pts',(4.94014963461732,31.1965934901283,53.3281010858963));
#90784=CARTESIAN_POINT('Ctrl Pts',(4.94400484086266,31.2539443088724,53.3706725135541));
#90785=CARTESIAN_POINT('Ctrl Pts',(4.947860047108,31.3089225031761,53.416106239933));
#90786=CARTESIAN_POINT('Ctrl Pts',(4.95171540395928,31.3639028452357,53.4615417412075));
#90787=CARTESIAN_POINT('Ctrl Pts',(4.95557076081055,31.4165100057726,53.5098394520472));
#90788=CARTESIAN_POINT('Ctrl Pts',(4.95942611766182,31.4664425529645,53.5607141349422));
#90789=CARTESIAN_POINT('Ctrl Pts',(4.96328551013038,31.5164273673416,53.6116420712085));
#90790=CARTESIAN_POINT('Ctrl Pts',(4.96714490259894,31.5637316386344,53.6651520168592));
#90791=CARTESIAN_POINT('Ctrl Pts',(4.9710042950675,31.6080918095699,53.7209228739071));
#90792=CARTESIAN_POINT('Ctrl Pts',(4.97486587267093,31.6524770966234,53.7767253076463));
#90793=CARTESIAN_POINT('Ctrl Pts',(4.97872745027436,31.693914682697,53.8347908054513));
#90794=CARTESIAN_POINT('Ctrl Pts',(4.9825890278778,31.7321838651551,53.894768522075));
#90795=CARTESIAN_POINT('Ctrl Pts',(4.98645736199267,31.770520006301,53.9548511802977));
#90796=CARTESIAN_POINT('Ctrl Pts',(4.99032569610754,31.8056764360204,54.0168523145415));
#90797=CARTESIAN_POINT('Ctrl Pts',(4.99419403022242,31.8374783327811,54.0803963141331));
#90798=CARTESIAN_POINT('Ctrl Pts',(4.99649174939334,31.8563680733487,54.118140278776));
#90799=CARTESIAN_POINT('Ctrl Pts',(4.99878946856425,31.8740752011145,54.1564281827517));
#90800=CARTESIAN_POINT('Ctrl Pts',(5.00108718773517,31.8905713141638,54.1951784865195));
#90801=CARTESIAN_POINT('Ctrl Pts',(5.00537446195649,31.9213511244745,54.2674820040749));
#90802=CARTESIAN_POINT('Ctrl Pts',(5.00966173617781,31.9480150746282,54.3416372137357));
#90803=CARTESIAN_POINT('Ctrl Pts',(5.01394901039913,31.9703612656978,54.4171843815255));
#90804=CARTESIAN_POINT('Ctrl Pts',(5.01822262075583,31.9926362377798,54.4924907748231));
#90805=CARTESIAN_POINT('Ctrl Pts',(5.02249623111252,32.0106207692059,54.5691800046967));
#90806=CARTESIAN_POINT('Ctrl Pts',(5.02676984146922,32.024161307071,54.6467740589132));
#90807=CARTESIAN_POINT('Ctrl Pts',(5.03102083155032,32.0376301746917,54.7239574067843));
#90808=CARTESIAN_POINT('Ctrl Pts',(5.03527182163142,32.0467018415724,54.8020357440816));
#90809=CARTESIAN_POINT('Ctrl Pts',(5.03952281171252,32.0512732988444,54.8805202278706));
#90810=CARTESIAN_POINT('Ctrl Pts',(5.04165696797233,32.0535683416385,54.9199223787064));
#90811=CARTESIAN_POINT('Ctrl Pts',(5.04379112423215,32.0547299142487,54.9594266319029));
#90812=CARTESIAN_POINT('Ctrl Pts',(5.04592528049197,32.0547497417017,54.9989697199742));
#90813=CARTESIAN_POINT('Origin',(-1.54592528053767,30.,55.));
#90814=CARTESIAN_POINT('',(3.89394682837563,28.7479524050421,56.6292250864936));
#90815=CARTESIAN_POINT('',(3.95204618956481,28.7479524050421,56.6292250864936));
#90816=CARTESIAN_POINT('',(-1.54592528053767,28.7479524050421,56.6292250864936));
#90817=CARTESIAN_POINT('',(4.40407471951261,32.0547494817011,55.0014594345582));
#90818=CARTESIAN_POINT('Ctrl Pts',(3.95204618956481,28.7479524050421,56.6292250864936));
#90819=CARTESIAN_POINT('Ctrl Pts',(3.95593362166089,28.6909406676674,56.5854119821803));
#90820=CARTESIAN_POINT('Ctrl Pts',(3.95982105375698,28.6362494734195,56.5386166933452));
#90821=CARTESIAN_POINT('Ctrl Pts',(3.96370848585306,28.5841940618756,56.4891242755632));
#90822=CARTESIAN_POINT('Ctrl Pts',(3.96756899650448,28.5324991471446,56.4399746052181));
#90823=CARTESIAN_POINT('Ctrl Pts',(3.9714295071559,28.4834039172625,56.3881654430581));
#90824=CARTESIAN_POINT('Ctrl Pts',(3.97529001780731,28.4371786472169,56.3340116123127));
#90825=CARTESIAN_POINT('Ctrl Pts',(3.97919091062573,28.3904698461716,56.2792913153057));
#90826=CARTESIAN_POINT('Ctrl Pts',(3.98309180344414,28.3466917103696,56.2221774112299));
#90827=CARTESIAN_POINT('Ctrl Pts',(3.98699269626255,28.3060787348042,56.1630254983523));
#90828=CARTESIAN_POINT('Ctrl Pts',(3.99089358908096,28.2654657592389,56.1038735854746));
#90829=CARTESIAN_POINT('Ctrl Pts',(3.99479448189937,28.2280181518745,56.0426841281137));
#90830=CARTESIAN_POINT('Ctrl Pts',(3.99869537471779,28.1939221902578,55.9798369801436));
#90831=CARTESIAN_POINT('Ctrl Pts',(4.002564448066,28.1601043484166,55.9175024745467));
#90832=CARTESIAN_POINT('Ctrl Pts',(4.00643352141422,28.12945115043,55.8532930462971));
#90833=CARTESIAN_POINT('Ctrl Pts',(4.01030259476243,28.1021743860266,55.7875630142703));
#90834=CARTESIAN_POINT('Ctrl Pts',(4.01416590315822,28.0749382642358,55.7219309205542));
#90835=CARTESIAN_POINT('Ctrl Pts',(4.01802921155401,28.0510687744827,55.6547831654671));
#90836=CARTESIAN_POINT('Ctrl Pts',(4.02189251994979,28.0307319100996,55.5864987234428));
#90837=CARTESIAN_POINT('Ctrl Pts',(4.02575129644271,28.010418902133,55.5182943833486));
#90838=CARTESIAN_POINT('Ctrl Pts',(4.02961007293562,27.9936304261562,55.448956468227));
#90839=CARTESIAN_POINT('Ctrl Pts',(4.03346884942853,27.9804837906095,55.3788823597224));
#90840=CARTESIAN_POINT('Ctrl Pts',(4.03732519501674,27.967345437019,55.3088523956456));
#90841=CARTESIAN_POINT('Ctrl Pts',(4.04118154060495,27.9578444614835,55.2380876346411));
#90842=CARTESIAN_POINT('Ctrl Pts',(4.04503788619316,27.9520475161225,55.1669975636947));
#90843=CARTESIAN_POINT('Ctrl Pts',(4.0488930924385,27.9462522834473,55.0959284960438));
#90844=CARTESIAN_POINT('Ctrl Pts',(4.05274829868383,27.9441589478354,55.0245347931742));
#90845=CARTESIAN_POINT('Ctrl Pts',(4.05660350492917,27.9457823265314,54.9532312870671));
#90846=CARTESIAN_POINT('Ctrl Pts',(4.06045886178042,27.9474057686458,54.8819249954463));
#90847=CARTESIAN_POINT('Ctrl Pts',(4.06431421863168,27.9527462000759,54.8107093931937));
#90848=CARTESIAN_POINT('Ctrl Pts',(4.06816957548293,27.9617663485298,54.7399977990202));
#90849=CARTESIAN_POINT('Ctrl Pts',(4.07202896795149,27.9707959388767,54.6692121870724));
#90850=CARTESIAN_POINT('Ctrl Pts',(4.07588836042004,27.9835128736404,54.5989321192273));
#90851=CARTESIAN_POINT('Ctrl Pts',(4.0797477528886,27.9998282686893,54.529563386028));
#90852=CARTESIAN_POINT('Ctrl Pts',(4.08360933049203,28.0161529012901,54.4601553772072));
#90853=CARTESIAN_POINT('Ctrl Pts',(4.08747090809547,28.0360799142424,54.3916601968676));
#90854=CARTESIAN_POINT('Ctrl Pts',(4.0913324856989,28.0594705271053,54.3244684113035));
#90855=CARTESIAN_POINT('Ctrl Pts',(4.09520081981377,28.0829020659729,54.2571590618537));
#90856=CARTESIAN_POINT('Ctrl Pts',(4.09906915392864,28.1098091206272,54.1911581102851));
#90857=CARTESIAN_POINT('Ctrl Pts',(4.10293748804351,28.1400050514512,54.1268354371181));
#90858=CARTESIAN_POINT('Ctrl Pts',(4.10523520721446,28.1579408778505,54.0886289547219));
#90859=CARTESIAN_POINT('Ctrl Pts',(4.1075329263854,28.1770361820226,54.0510141262206));
#90860=CARTESIAN_POINT('Ctrl Pts',(4.10983064555635,28.1972445332813,54.0140637496694));
#90861=CARTESIAN_POINT('Ctrl Pts',(4.11369971890457,28.2312728837671,53.9518439105661));
#90862=CARTESIAN_POINT('Ctrl Pts',(4.11756879225278,28.2685928276122,53.8912659359023));
#90863=CARTESIAN_POINT('Ctrl Pts',(4.121437865601,28.3090215532379,53.8326999292872));
#90864=CARTESIAN_POINT('Ctrl Pts',(4.12530117399678,28.3493900397161,53.7742211865238));
#90865=CARTESIAN_POINT('Ctrl Pts',(4.12916448239255,28.3928578396379,53.7177488576873));
#90866=CARTESIAN_POINT('Ctrl Pts',(4.13302779078832,28.4391965888961,53.6636279431287));
#90867=CARTESIAN_POINT('Ctrl Pts',(4.13688656728124,28.4854809798974,53.6095705157946));
#90868=CARTESIAN_POINT('Ctrl Pts',(4.14074534377415,28.5346293162252,53.5578593909253));
#90869=CARTESIAN_POINT('Ctrl Pts',(4.14460412026706,28.5863713641356,53.5088086499834));
#90870=CARTESIAN_POINT('Ctrl Pts',(4.14846046585527,28.6380808162251,53.459788809426));
#90871=CARTESIAN_POINT('Ctrl Pts',(4.15231681144348,28.6923803864422,53.4134263611475));
#90872=CARTESIAN_POINT('Ctrl Pts',(4.15617315703168,28.7489621966495,53.3699993935314));
#90873=CARTESIAN_POINT('Ctrl Pts',(4.16002836327702,28.8055272899728,53.3265852562503));
#90874=CARTESIAN_POINT('Ctrl Pts',(4.16388356952235,28.8643728994989,53.2861051734575));
#90875=CARTESIAN_POINT('Ctrl Pts',(4.16773877576769,28.9251585431525,53.2487965837339));
#90876=CARTESIAN_POINT('Ctrl Pts',(4.17159413261893,28.9859465614332,53.2114865365282));
#90877=CARTESIAN_POINT('Ctrl Pts',(4.17544948947017,29.0486743491362,53.1773484806093));
#90878=CARTESIAN_POINT('Ctrl Pts',(4.17930484632141,29.1129744440563,53.1465752711257));
#90879=CARTESIAN_POINT('Ctrl Pts',(4.18316423878997,29.1773418454766,53.1157698496052));
#90880=CARTESIAN_POINT('Ctrl Pts',(4.18702363125853,29.2432844004578,53.0883365157092));
#90881=CARTESIAN_POINT('Ctrl Pts',(4.19088302372709,29.3104129791282,53.0644206802238));
#90882=CARTESIAN_POINT('Ctrl Pts',(4.19474460133053,29.3775795650757,53.0404913039216));
#90883=CARTESIAN_POINT('Ctrl Pts',(4.19860617893397,29.4459330457793,53.0200835296513));
#90884=CARTESIAN_POINT('Ctrl Pts',(4.20246775653741,29.5150700199561,53.0032925910503));
#90885=CARTESIAN_POINT('Ctrl Pts',(4.20633609065228,29.5843279614691,52.9864722737393));
#90886=CARTESIAN_POINT('Ctrl Pts',(4.21020442476715,29.6543716558712,52.973281516649));
#90887=CARTESIAN_POINT('Ctrl Pts',(4.21407275888202,29.724789123801,52.9637641256176));
#90888=CARTESIAN_POINT('Ctrl Pts',(4.21637047805298,29.7666158019596,52.9581109707502));
#90889=CARTESIAN_POINT('Ctrl Pts',(4.21866819722395,29.8085742650115,52.9537528354883));
#90890=CARTESIAN_POINT('Ctrl Pts',(4.22096591639491,29.8505781698028,52.9506901944409));
#90891=CARTESIAN_POINT('Ctrl Pts',(4.22483498974313,29.9213075220241,52.9455330877756));
#90892=CARTESIAN_POINT('Ctrl Pts',(4.22870406309134,29.9924427144347,52.9440318803733));
#90893=CARTESIAN_POINT('Ctrl Pts',(4.23257313643955,30.0635736564367,52.9462337151693));
#90894=CARTESIAN_POINT('Ctrl Pts',(4.23643644483534,30.1345986127257,52.9484322692126));
#90895=CARTESIAN_POINT('Ctrl Pts',(4.24029975323112,30.2056188495799,52.9543228983359));
#90896=CARTESIAN_POINT('Ctrl Pts',(4.2441630616269,30.2762206606864,52.963900859705));
#90897=CARTESIAN_POINT('Ctrl Pts',(4.24802183811981,30.3467396514436,52.9734675855252));
#90898=CARTESIAN_POINT('Ctrl Pts',(4.25188061461272,30.4168407123865,52.9867129867538));
#90899=CARTESIAN_POINT('Ctrl Pts',(4.25573939110564,30.4861134049202,53.0035803747566));
#90900=CARTESIAN_POINT('Ctrl Pts',(4.25959573669384,30.5553424578924,53.0204371368492));
#90901=CARTESIAN_POINT('Ctrl Pts',(4.26345208228205,30.6237437069085,53.0409112441355));
#90902=CARTESIAN_POINT('Ctrl Pts',(4.26730842787026,30.6909165357602,53.0648948599332));
#90903=CARTESIAN_POINT('Ctrl Pts',(4.27116363411559,30.7580695186511,53.0888713898613));
#90904=CARTESIAN_POINT('Ctrl Pts',(4.27501884036093,30.8239943446481,53.1163552065664));
#90905=CARTESIAN_POINT('Ctrl Pts',(4.27887404660627,30.8883068660076,53.1471890343849));
#90906=CARTESIAN_POINT('Ctrl Pts',(4.28272940345752,30.9526218997738,53.178024066745));
#90907=CARTESIAN_POINT('Ctrl Pts',(4.28658476030876,31.0153240667616,53.2122091580435));
#90908=CARTESIAN_POINT('Ctrl Pts',(4.29044011716001,31.0760520426574,53.249540184982));
#90909=CARTESIAN_POINT('Ctrl Pts',(4.29429950962857,31.1368435859168,53.286910288391));
#90910=CARTESIAN_POINT('Ctrl Pts',(4.29815890209713,31.1956563982002,53.3274326461382));
#90911=CARTESIAN_POINT('Ctrl Pts',(4.30201829456569,31.2521572635057,53.3708591988567));
#90912=CARTESIAN_POINT('Ctrl Pts',(4.30587987216913,31.3086901188233,53.4143103390915));
#90913=CARTESIAN_POINT('Ctrl Pts',(4.30974144977257,31.3629080519673,53.4606686317754));
#90914=CARTESIAN_POINT('Ctrl Pts',(4.31360302737602,31.4145122626426,53.5096468132239));
#90915=CARTESIAN_POINT('Ctrl Pts',(4.31747136149089,31.4662067639906,53.5587106906435));
#90916=CARTESIAN_POINT('Ctrl Pts',(4.32133969560576,31.5152780778462,53.6104032564012));
#90917=CARTESIAN_POINT('Ctrl Pts',(4.32520802972063,31.5614659582069,53.6644021474033));
#90918=CARTESIAN_POINT('Ctrl Pts',(4.32750574889158,31.5889007078999,53.6964764934606));
#90919=CARTESIAN_POINT('Ctrl Pts',(4.32980346806252,31.6153189306063,53.729363929871));
#90920=CARTESIAN_POINT('Ctrl Pts',(4.33210118723347,31.6406733981608,53.7629921734008));
#90921=CARTESIAN_POINT('Ctrl Pts',(4.33598223894954,31.6834993453246,53.8197932628943));
#90922=CARTESIAN_POINT('Ctrl Pts',(4.3398632906656,31.723457290319,53.8789338902988));
#90923=CARTESIAN_POINT('Ctrl Pts',(4.34374434238167,31.7602831217971,53.9400939222665));
#90924=CARTESIAN_POINT('Ctrl Pts',(4.34761960540842,31.7970540265922,54.0011627324601));
#90925=CARTESIAN_POINT('Ctrl Pts',(4.35149486843518,31.8307018422724,54.0642445616435));
#90926=CARTESIAN_POINT('Ctrl Pts',(4.35537013146193,31.8610038890175,54.1289878947099));
#90927=CARTESIAN_POINT('Ctrl Pts',(4.35942884712863,31.8927404165791,54.1967961385419));
#90928=CARTESIAN_POINT('Ctrl Pts',(4.36348756279533,31.920806196447,54.2664266821933));
#90929=CARTESIAN_POINT('Ctrl Pts',(4.36754627846203,31.9449979565058,54.3374439558133));
#90930=CARTESIAN_POINT('Ctrl Pts',(4.37141366678506,31.9680493200522,54.4051134841285));
#90931=CARTESIAN_POINT('Ctrl Pts',(4.37528105510808,31.9875834868991,54.4740414408063));
#90932=CARTESIAN_POINT('Ctrl Pts',(4.3791484434311,32.0034736409941,54.543830149679));
#90933=CARTESIAN_POINT('Ctrl Pts',(4.38301406018565,32.0193565161468,54.6135868898258));
#90934=CARTESIAN_POINT('Ctrl Pts',(4.38687967694019,32.0315985897945,54.6842031295411));
#90935=CARTESIAN_POINT('Ctrl Pts',(4.39074529369473,32.040123513712,54.7552682870991));
#90936=CARTESIAN_POINT('Ctrl Pts',(4.39461092103566,32.0486484609759,54.8263336392762));
#90937=CARTESIAN_POINT('Ctrl Pts',(4.39847654837658,32.0534561785917,54.8978474341116));
#90938=CARTESIAN_POINT('Ctrl Pts',(4.40234217571751,32.0545220261428,54.9693927035783));
#90939=CARTESIAN_POINT('Ctrl Pts',(4.40291969029912,32.0546812609702,54.980081379107));
#90940=CARTESIAN_POINT('Ctrl Pts',(4.40349720488072,32.0547570735857,54.9907707532352));
#90941=CARTESIAN_POINT('Ctrl Pts',(4.40407471946233,32.0547494817017,55.0014594336275));
#90942=CARTESIAN_POINT('Ctrl Pts',(4.40407471951261,32.0547494817011,55.0014594345582));
#90943=CARTESIAN_POINT('Ctrl Pts',(4.40849095806831,32.0546914267306,55.0831954875701));
#90944=CARTESIAN_POINT('Ctrl Pts',(4.41290719662402,32.0497522762913,55.1647368982365));
#90945=CARTESIAN_POINT('Ctrl Pts',(4.41732343517972,32.0400254037017,55.2455481923201));
#90946=CARTESIAN_POINT('Ctrl Pts',(4.4217797159885,32.030210337078,55.327092206398));
#90947=CARTESIAN_POINT('Ctrl Pts',(4.42623599679728,32.0155204432684,55.4078926142023));
#90948=CARTESIAN_POINT('Ctrl Pts',(4.43069227760607,31.9961013728872,55.4874185795163));
#90949=CARTESIAN_POINT('Ctrl Pts',(4.43487367109472,31.9778801750024,55.5620389564206));
#90950=CARTESIAN_POINT('Ctrl Pts',(4.43905506458338,31.9554957935063,55.6355373428861));
#90951=CARTESIAN_POINT('Ctrl Pts',(4.44323645807203,31.9291064843791,55.7074925684604));
#90952=CARTESIAN_POINT('Ctrl Pts',(4.44710553142025,31.9046882676053,55.7740732541313));
#90953=CARTESIAN_POINT('Ctrl Pts',(4.45097460476847,31.8767712524526,55.8395187237066));
#90954=CARTESIAN_POINT('Ctrl Pts',(4.45484367811669,31.8454813033535,55.9034358424772));
#90955=CARTESIAN_POINT('Ctrl Pts',(4.45870698651247,31.8142379765466,55.9672577241934));
#90956=CARTESIAN_POINT('Ctrl Pts',(4.46257029490826,31.7796319035185,56.029555342638));
#90957=CARTESIAN_POINT('Ctrl Pts',(4.46643360330405,31.7418377221506,56.08995362846));
#90958=CARTESIAN_POINT('Ctrl Pts',(4.47029237979696,31.7040878757261,56.1502810633074));
#90959=CARTESIAN_POINT('Ctrl Pts',(4.47415115628987,31.6631576060078,56.2087131813575));
#90960=CARTESIAN_POINT('Ctrl Pts',(4.47800993278278,31.6192675452452,56.2648992763914));
#90961=CARTESIAN_POINT('Ctrl Pts',(4.48186627837099,31.575405133805,56.3210499759981));
#90962=CARTESIAN_POINT('Ctrl Pts',(4.48572262395919,31.5285869289446,56.3749570778473));
#90963=CARTESIAN_POINT('Ctrl Pts',(4.4895789695474,31.4790761318269,56.4262998838813));
#90964=CARTESIAN_POINT('Ctrl Pts',(4.49343417579273,31.429579962489,56.4776275208754));
#90965=CARTESIAN_POINT('Ctrl Pts',(4.49728938203806,31.3773931172375,56.5263920166289));
#90966=CARTESIAN_POINT('Ctrl Pts',(4.5011445882834,31.3228170725557,56.5723080344052));
#90967=CARTESIAN_POINT('Ctrl Pts',(4.50499994513464,31.2682388958285,56.6182258459179));
#90968=CARTESIAN_POINT('Ctrl Pts',(4.50885530198588,31.2112717075104,56.6612946474703));
#90969=CARTESIAN_POINT('Ctrl Pts',(4.51271065883712,31.152250281613,56.7012691882894));
#90970=CARTESIAN_POINT('Ctrl Pts',(4.51657005130568,31.0931670746931,56.7412855726927));
#90971=CARTESIAN_POINT('Ctrl Pts',(4.52042944377424,31.0320257407813,56.7782009577452));
#90972=CARTESIAN_POINT('Ctrl Pts',(4.52428883624279,30.9691895223348,56.811813796254));
#90973=CARTESIAN_POINT('Ctrl Pts',(4.52815041384623,30.9063177268866,56.8454456658892));
#90974=CARTESIAN_POINT('Ctrl Pts',(4.53201199144966,30.8417495765086,56.8757710600617));
#90975=CARTESIAN_POINT('Ctrl Pts',(4.5358735690531,30.7758698732853,56.9026359352825));
#90976=CARTESIAN_POINT('Ctrl Pts',(4.53974190316797,30.7098749018961,56.929547815343));
#90977=CARTESIAN_POINT('Ctrl Pts',(4.54361023728284,30.6425642549529,56.9529869280869));
#90978=CARTESIAN_POINT('Ctrl Pts',(4.54747857139771,30.5743388494694,56.9728488154165));
#90979=CARTESIAN_POINT('Ctrl Pts',(4.54977629056867,30.5338142160043,56.9846464104362));
#90980=CARTESIAN_POINT('Ctrl Pts',(4.55207400973963,30.4929670773006,56.995182881589));
#90981=CARTESIAN_POINT('Ctrl Pts',(4.55437172891059,30.4518827500531,57.0044449462892));
#90982=CARTESIAN_POINT('Ctrl Pts',(4.55844030376033,30.3791346689688,57.0208452984178));
#90983=CARTESIAN_POINT('Ctrl Pts',(4.56250887861007,30.3053427076324,57.0333138865847));
#90984=CARTESIAN_POINT('Ctrl Pts',(4.56657745345982,30.2309707793399,57.0417272250698));
#90985=CARTESIAN_POINT('Ctrl Pts',(4.57043978118483,30.1603689663671,57.0497140685447));
#90986=CARTESIAN_POINT('Ctrl Pts',(4.57430210890985,30.0892451145857,57.0540466922945));
#90987=CARTESIAN_POINT('Ctrl Pts',(4.57816443663487,30.01800922301,57.05467107596));
#90988=CARTESIAN_POINT('Ctrl Pts',(4.58202297547393,29.9468432127825,57.0552948471144));
#90989=CARTESIAN_POINT('Ctrl Pts',(4.585881514313,29.8755658640219,57.052217591045));
#90990=CARTESIAN_POINT('Ctrl Pts',(4.58974005315206,29.8045915154746,57.045437138285));
#90991=CARTESIAN_POINT('Ctrl Pts',(4.59359609769486,29.7336630472617,57.0386610686499));
#90992=CARTESIAN_POINT('Ctrl Pts',(4.59745214223766,29.6630376728841,57.0281866000545));
#90993=CARTESIAN_POINT('Ctrl Pts',(4.60130818678046,29.5931272137334,57.0140635785137));
#90994=CARTESIAN_POINT('Ctrl Pts',(4.60516302857667,29.5232385604942,56.999944962113));
#90995=CARTESIAN_POINT('Ctrl Pts',(4.60901787037287,29.4540648551168,56.9821801503313));
#90996=CARTESIAN_POINT('Ctrl Pts',(4.61287271216908,29.3860085838065,56.9608702413318));
#90997=CARTESIAN_POINT('Ctrl Pts',(4.61672933980179,29.3179207839976,56.9395504600689));
#90998=CARTESIAN_POINT('Ctrl Pts',(4.62058596743451,29.2509519173612,56.9146824432169));
#90999=CARTESIAN_POINT('Ctrl Pts',(4.62444259506723,29.1854889899216,56.8864170739688));
#91000=CARTESIAN_POINT('Ctrl Pts',(4.62830025698201,29.1200085064361,56.8581441244286));
#91001=CARTESIAN_POINT('Ctrl Pts',(4.63215791889679,29.0560352053134,56.8264722170175));
#91002=CARTESIAN_POINT('Ctrl Pts',(4.63601558081158,28.9939336051439,56.7915992776403));
#91003=CARTESIAN_POINT('Ctrl Pts',(4.63987770210721,28.9317602167531,56.7566860258351));
#91004=CARTESIAN_POINT('Ctrl Pts',(4.64373982340285,28.8714632614709,56.718564611389));
#91005=CARTESIAN_POINT('Ctrl Pts',(4.64760194469848,28.813379370413,56.6774769876033));
#91006=CARTESIAN_POINT('Ctrl Pts',(4.64907380490046,28.7912435126604,56.6618184327277));
#91007=CARTESIAN_POINT('Ctrl Pts',(4.65054566510243,28.7694287440933,56.6457294964002));
#91008=CARTESIAN_POINT('Ctrl Pts',(4.6520175253044,28.7479524050421,56.6292250864936));
#91009=CARTESIAN_POINT('',(4.34592528058805,32.054749644159,54.9987907322124));
#91010=CARTESIAN_POINT('Ctrl Pts',(4.34592528058805,32.054749644159,54.9987907322123));
#91011=CARTESIAN_POINT('Ctrl Pts',(4.34974237135586,32.0547908859483,55.0688674784532));
#91012=CARTESIAN_POINT('Ctrl Pts',(4.35355946212367,32.0512429716119,55.1390874484566));
#91013=CARTESIAN_POINT('Ctrl Pts',(4.35737655289148,32.0440883161928,55.2090466888139));
#91014=CARTESIAN_POINT('Ctrl Pts',(4.36118805254388,32.0369441406146,55.2789034557928));
#91015=CARTESIAN_POINT('Ctrl Pts',(4.36499955219628,32.0262037618752,55.3484997581352));
#91016=CARTESIAN_POINT('Ctrl Pts',(4.36881105184869,32.0119016127208,55.4174319863538));
#91017=CARTESIAN_POINT('Ctrl Pts',(4.37261948474162,31.9976109711765,55.4863087512158));
#91018=CARTESIAN_POINT('Ctrl Pts',(4.37642791763454,31.9797643402277,55.554522013904));
#91019=CARTESIAN_POINT('Ctrl Pts',(4.38023635052747,31.958447737978,55.6216751725047));
#91020=CARTESIAN_POINT('Ctrl Pts',(4.38404307118795,31.9371407194545,55.6887981397326));
#91021=CARTESIAN_POINT('Ctrl Pts',(4.38784979184843,31.9123669743003,55.754861472588));
#91022=CARTESIAN_POINT('Ctrl Pts',(4.39165651250891,31.8842627237978,55.8194824892614));
#91023=CARTESIAN_POINT('Ctrl Pts',(4.39546287300827,31.8561611322921,55.884097392017));
#91024=CARTESIAN_POINT('Ctrl Pts',(4.39926923350764,31.82472986167,55.9472697921498));
#91025=CARTESIAN_POINT('Ctrl Pts',(4.403075594007,31.7901530068413,56.0086375833753));
#91026=CARTESIAN_POINT('Ctrl Pts',(4.40688551322988,31.755543824684,56.0700627498813));
#91027=CARTESIAN_POINT('Ctrl Pts',(4.41069543245276,31.7177834317607,56.129679502477));
#91028=CARTESIAN_POINT('Ctrl Pts',(4.41450535167564,31.6771010428824,56.1871519087558));
#91029=CARTESIAN_POINT('Ctrl Pts',(4.41831711300166,31.6363989839922,56.2446521030517));
#91030=CARTESIAN_POINT('Ctrl Pts',(4.42212887432769,31.5927724276063,56.3000054956356));
#91031=CARTESIAN_POINT('Ctrl Pts',(4.42594063565372,31.546491159843,56.3529089603619));
#91032=CARTESIAN_POINT('Ctrl Pts',(4.42975910316213,31.5001284676157,56.405905500245));
#91033=CARTESIAN_POINT('Ctrl Pts',(4.43357757067055,31.4511020881627,56.4564431490457));
#91034=CARTESIAN_POINT('Ctrl Pts',(4.43739603817897,31.3997183644062,56.5042559831505));
#91035=CARTESIAN_POINT('Ctrl Pts',(4.44006763663344,31.3637676389724,56.5377083284741));
#91036=CARTESIAN_POINT('Ctrl Pts',(4.44273923508791,31.3266637077791,56.5698276548949));
#91037=CARTESIAN_POINT('Ctrl Pts',(4.44541083354238,31.288520118375,56.6005353688822));
#91038=CARTESIAN_POINT('Ctrl Pts',(4.44927990689059,31.2332796517841,56.6450070212647));
#91039=CARTESIAN_POINT('Ctrl Pts',(4.45314898023881,31.1756259560803,56.6867025917087));
#91040=CARTESIAN_POINT('Ctrl Pts',(4.45701805358702,31.1158695099185,56.7253500512459));
#91041=CARTESIAN_POINT('Ctrl Pts',(4.46088136198281,31.0562021013733,56.7639399257374));
#91042=CARTESIAN_POINT('Ctrl Pts',(4.46474467037861,30.9944385661033,56.7994904428259));
#91043=CARTESIAN_POINT('Ctrl Pts',(4.4686079787744,30.93092186864,56.8317701921878));
#91044=CARTESIAN_POINT('Ctrl Pts',(4.47246675526731,30.8674796802436,56.8640120753806));
#91045=CARTESIAN_POINT('Ctrl Pts',(4.47632553176022,30.8022888456627,56.892990593039));
#91046=CARTESIAN_POINT('Ctrl Pts',(4.48018430825314,30.7357191879358,56.9185189180728));
#91047=CARTESIAN_POINT('Ctrl Pts',(4.48404065384134,30.6691914669457,56.9440311610853));
#91048=CARTESIAN_POINT('Ctrl Pts',(4.48789699942955,30.6012870986316,56.9660973501538));
#91049=CARTESIAN_POINT('Ctrl Pts',(4.49175334501776,30.5323969196768,56.984578313501));
#91050=CARTESIAN_POINT('Ctrl Pts',(4.49560855126309,30.4635270940676,57.0030538167168));
#91051=CARTESIAN_POINT('Ctrl Pts',(4.49946375750842,30.3936725049778,57.0179460712978));
#91052=CARTESIAN_POINT('Ctrl Pts',(4.50331896375375,30.3232385643448,57.0291659353095));
#91053=CARTESIAN_POINT('Ctrl Pts',(4.50717432060499,30.2528018721683,57.0403862376318));
#91054=CARTESIAN_POINT('Ctrl Pts',(4.51102967745623,30.1817862635981,57.0479337903105));
#91055=CARTESIAN_POINT('Ctrl Pts',(4.51488503430747,30.1106050250406,57.0517709645415));
#91056=CARTESIAN_POINT('Ctrl Pts',(4.51874442677603,30.0393492771056,57.0556121553571));
#91057=CARTESIAN_POINT('Ctrl Pts',(4.52260381924459,29.9679280391652,57.0557351884641));
#91058=CARTESIAN_POINT('Ctrl Pts',(4.52646321171315,29.8967564692996,57.0521545594493));
#91059=CARTESIAN_POINT('Ctrl Pts',(4.53032478931658,29.8255446030712,57.0485719031317));
#91060=CARTESIAN_POINT('Ctrl Pts',(4.53418636692,29.7545831697904,57.0412814599578));
#91061=CARTESIAN_POINT('Ctrl Pts',(4.53804794452343,29.6842813201151,57.0303495456871));
#91062=CARTESIAN_POINT('Ctrl Pts',(4.5419162786383,29.6138564649481,57.0193985041033));
#91063=CARTESIAN_POINT('Ctrl Pts',(4.54578461275318,29.5440939731254,57.0047933703205));
#91064=CARTESIAN_POINT('Ctrl Pts',(4.54965294686805,29.4753912491385,56.9866512580268));
#91065=CARTESIAN_POINT('Ctrl Pts',(4.55195066603901,29.4345830972794,56.9758751776829));
#91066=CARTESIAN_POINT('Ctrl Pts',(4.55424838520997,29.3941485465822,56.9638521549952));
#91067=CARTESIAN_POINT('Ctrl Pts',(4.55654610438093,29.3541675553053,56.9506147789555));
#91068=CARTESIAN_POINT('Ctrl Pts',(4.56041440940474,29.2868579069515,56.9283291102439));
#91069=CARTESIAN_POINT('Ctrl Pts',(4.56428271442855,29.2205713103213,56.9025117402514));
#91070=CARTESIAN_POINT('Ctrl Pts',(4.56815101945236,29.1557044660339,56.8732759043518));
#91071=CARTESIAN_POINT('Ctrl Pts',(4.57201426849238,29.0909224045418,56.8440782805144));
#91072=CARTESIAN_POINT('Ctrl Pts',(4.57587751753241,29.0275568547142,56.8114712484247));
#91073=CARTESIAN_POINT('Ctrl Pts',(4.57974076657243,28.9659882323256,56.7756174212963));
#91074=CARTESIAN_POINT('Ctrl Pts',(4.58359955333986,28.9044907252013,56.7398050073796));
#91075=CARTESIAN_POINT('Ctrl Pts',(4.58745834010729,28.844786440948,56.7007534901179));
#91076=CARTESIAN_POINT('Ctrl Pts',(4.59131712687472,28.7872329280312,56.6586722375587));
#91077=CARTESIAN_POINT('Ctrl Pts',(4.59220268619875,28.7740248776604,56.6490149416736));
#91078=CARTESIAN_POINT('Ctrl Pts',(4.59308824552279,28.7609299953523,56.6391982699849));
#91079=CARTESIAN_POINT('Ctrl Pts',(4.59397380484682,28.7479524050421,56.6292250864936));
#91080=CARTESIAN_POINT('Ctrl Pts',(3.89394682837563,28.7479524050421,56.6292250864936));
#91081=CARTESIAN_POINT('Ctrl Pts',(3.89781364428523,28.6916779684571,56.5859785924591));
#91082=CARTESIAN_POINT('Ctrl Pts',(3.90168046019482,28.6375451445928,56.539734920853));
#91083=CARTESIAN_POINT('Ctrl Pts',(3.90554727610442,28.5858898030596,56.4907346891413));
#91084=CARTESIAN_POINT('Ctrl Pts',(3.90951904585791,28.5328324225418,56.4404044839347));
#91085=CARTESIAN_POINT('Ctrl Pts',(3.91349081561139,28.4823894318975,56.3871661480069));
#91086=CARTESIAN_POINT('Ctrl Pts',(3.91746258536488,28.434890663223,56.3313265288551));
#91087=CARTESIAN_POINT('Ctrl Pts',(3.92132025666669,28.3887564086816,56.2770910344343));
#91088=CARTESIAN_POINT('Ctrl Pts',(3.9251779279685,28.3453998344527,56.2204020964724));
#91089=CARTESIAN_POINT('Ctrl Pts',(3.9290355992703,28.3050860971334,56.16157841938));
#91090=CARTESIAN_POINT('Ctrl Pts',(3.93289134533374,28.2647924790902,56.1027840992732));
#91091=CARTESIAN_POINT('Ctrl Pts',(3.93674709139717,28.227538958787,56.04185755422));
#91092=CARTESIAN_POINT('Ctrl Pts',(3.9406028374606,28.1935488776755,55.979148561329));
#91093=CARTESIAN_POINT('Ctrl Pts',(3.94445794906157,28.1595643896271,55.9164498871939));
#91094=CARTESIAN_POINT('Ctrl Pts',(3.94831306066253,28.1288425052922,55.8519697749701));
#91095=CARTESIAN_POINT('Ctrl Pts',(3.9521681722635,28.1015610149185,55.786083317736));
#91096=CARTESIAN_POINT('Ctrl Pts',(3.95622663709055,28.0728404536037,55.7167214167221));
#91097=CARTESIAN_POINT('Ctrl Pts',(3.96028510191761,28.0479335052111,55.6458012472298));
#91098=CARTESIAN_POINT('Ctrl Pts',(3.96434356674466,28.0269894365152,55.5737829545024));
#91099=CARTESIAN_POINT('Ctrl Pts',(3.96820378534732,28.0070684350922,55.505282581784));
#91100=CARTESIAN_POINT('Ctrl Pts',(3.97206400394997,27.9907322761517,55.4357893650098));
#91101=CARTESIAN_POINT('Ctrl Pts',(3.97592422255263,27.9780571691284,55.3657112948582));
#91102=CARTESIAN_POINT('Ctrl Pts',(3.97978714071035,27.9653731980606,55.2955842172206));
#91103=CARTESIAN_POINT('Ctrl Pts',(3.98365005886806,27.9563554330937,55.2248719538347));
#91104=CARTESIAN_POINT('Ctrl Pts',(3.98751297702578,27.9510282251341,55.1539877537434));
#91105=CARTESIAN_POINT('Ctrl Pts',(3.99138215086262,27.9456923901982,55.0829887625039));
#91106=CARTESIAN_POINT('Ctrl Pts',(3.99525132469946,27.944059041005,55.0118177633292));
#91107=CARTESIAN_POINT('Ctrl Pts',(3.9991204985363,27.9461004820823,54.940887118177));
#91108=CARTESIAN_POINT('Ctrl Pts',(3.99970358242024,27.9464081269291,54.9301978811951));
#91109=CARTESIAN_POINT('Ctrl Pts',(4.00028666630419,27.9467991323694,54.9195140894891));
#91110=CARTESIAN_POINT('Ctrl Pts',(4.00086975018814,27.947273302386,54.9088371380301));
#91111=CARTESIAN_POINT('Ctrl Pts',(4.00473882353635,27.9504196739869,54.8379898560741));
#91112=CARTESIAN_POINT('Ctrl Pts',(4.00860789688457,27.9572443216408,54.7671668837603));
#91113=CARTESIAN_POINT('Ctrl Pts',(4.01247697023278,27.9677461262914,54.69678101099));
#91114=CARTESIAN_POINT('Ctrl Pts',(4.01634027862857,27.978232283163,54.6265000137731));
#91115=CARTESIAN_POINT('Ctrl Pts',(4.02020358702435,27.992384650276,54.5566552998758));
#91116=CARTESIAN_POINT('Ctrl Pts',(4.02406689542013,28.0101501558676,54.4876571847814));
#91117=CARTESIAN_POINT('Ctrl Pts',(4.02792567191305,28.0278948214076,54.4187400088003));
#91118=CARTESIAN_POINT('Ctrl Pts',(4.03178444840596,28.0492440859143,54.3506679271217));
#91119=CARTESIAN_POINT('Ctrl Pts',(4.03564322489887,28.0740936699586,54.2838419375538));
#91120=CARTESIAN_POINT('Ctrl Pts',(4.03949957048707,28.0989275995667,54.2170580462036));
#91121=CARTESIAN_POINT('Ctrl Pts',(4.04335591607528,28.1272573049385,54.1515191437892));
#91122=CARTESIAN_POINT('Ctrl Pts',(4.04721226166348,28.1589288574891,54.0876104939701));
#91123=CARTESIAN_POINT('Ctrl Pts',(4.05106746790881,28.190591052798,54.0237207257224));
#91124=CARTESIAN_POINT('Ctrl Pts',(4.05492267415414,28.2255929195596,53.9614606888882));
#91125=CARTESIAN_POINT('Ctrl Pts',(4.05877788039947,28.2637333542961,53.9011935122524));
#91126=CARTESIAN_POINT('Ctrl Pts',(4.06263323725072,28.3018752790113,53.8409239812437));
#91127=CARTESIAN_POINT('Ctrl Pts',(4.06648859410196,28.3431557534853,53.7826478743109));
#91128=CARTESIAN_POINT('Ctrl Pts',(4.07034395095321,28.3873298158101,53.7267001768927));
#91129=CARTESIAN_POINT('Ctrl Pts',(4.07420334342177,28.4315501175928,53.6706939158954));
#91130=CARTESIAN_POINT('Ctrl Pts',(4.07806273589032,28.4786697518997,53.6170213118141));
#91131=CARTESIAN_POINT('Ctrl Pts',(4.08192212835888,28.528403407789,53.5659842984497));
#91132=CARTESIAN_POINT('Ctrl Pts',(4.08578370596231,28.5781652221894,53.514918388631));
#91133=CARTESIAN_POINT('Ctrl Pts',(4.08964528356575,28.6305436475791,53.4664913700499));
#91134=CARTESIAN_POINT('Ctrl Pts',(4.09350686116918,28.685218460614,53.42096641385));
#91135=CARTESIAN_POINT('Ctrl Pts',(4.09737519528405,28.7399889368823,53.3753618037058));
#91136=CARTESIAN_POINT('Ctrl Pts',(4.10124352939892,28.7970634335964,53.3326696847263));
#91137=CARTESIAN_POINT('Ctrl Pts',(4.10511186351379,28.8560913755677,53.2931108350425));
#91138=CARTESIAN_POINT('Ctrl Pts',(4.10740958268476,28.8911528852157,53.2696136073985));
#91139=CARTESIAN_POINT('Ctrl Pts',(4.10970730185573,28.9269030806228,53.2472209860022));
#91140=CARTESIAN_POINT('Ctrl Pts',(4.1120050210267,28.9632646532559,53.2259714254524));
#91141=CARTESIAN_POINT('Ctrl Pts',(4.11587409437492,29.0244930197819,53.1901898080018));
#91142=CARTESIAN_POINT('Ctrl Pts',(4.11974316772313,29.0876959275459,53.1575116551603));
#91143=CARTESIAN_POINT('Ctrl Pts',(4.12361224107135,29.1525259668356,53.1281599091771));
#91144=CARTESIAN_POINT('Ctrl Pts',(4.12747554946714,29.2172594088114,53.0988518975468));
#91145=CARTESIAN_POINT('Ctrl Pts',(4.13133885786292,29.2836147309311,53.0728606532385));
#91146=CARTESIAN_POINT('Ctrl Pts',(4.13520216625871,29.3512184250663,53.0503641287341));
#91147=CARTESIAN_POINT('Ctrl Pts',(4.13906094275162,29.4187428158314,53.027893994063));
#91148=CARTESIAN_POINT('Ctrl Pts',(4.14291971924454,29.4875122110839,53.008910588793));
#91149=CARTESIAN_POINT('Ctrl Pts',(4.14677849573745,29.5571331576811,52.9935437900431));
#91150=CARTESIAN_POINT('Ctrl Pts',(4.15063484132565,29.6267102453279,52.9781866718808));
#91151=CARTESIAN_POINT('Ctrl Pts',(4.15449118691386,29.6971373467649,52.9664417444936));
#91152=CARTESIAN_POINT('Ctrl Pts',(4.15834753250207,29.768007299874,52.9583886389451));
#91153=CARTESIAN_POINT('Ctrl Pts',(4.1622027387474,29.8388563147208,52.9503379126565));
#91154=CARTESIAN_POINT('Ctrl Pts',(4.16605794499273,29.9101474390716,52.9459768976138));
#91155=CARTESIAN_POINT('Ctrl Pts',(4.16991315123806,29.981466521313,52.945333586037));
#91156=CARTESIAN_POINT('Ctrl Pts',(4.17376850808931,30.0527883896766,52.9446902493287));
#91157=CARTESIAN_POINT('Ctrl Pts',(4.17762386494056,30.1241377323131,52.9477649066092));
#91158=CARTESIAN_POINT('Ctrl Pts',(4.18147922179181,30.1951002548227,52.9545334387803));
#91159=CARTESIAN_POINT('Ctrl Pts',(4.18533861426037,30.2661370577674,52.9613090559519));
#91160=CARTESIAN_POINT('Ctrl Pts',(4.18919800672893,30.3367857477192,52.9717862203667));
#91161=CARTESIAN_POINT('Ctrl Pts',(4.19305739919749,30.4066379145324,52.9858889879243));
#91162=CARTESIAN_POINT('Ctrl Pts',(4.19691897680092,30.4765296306807,52.9999997402747));
#91163=CARTESIAN_POINT('Ctrl Pts',(4.20078055440436,30.5456234551803,53.0177400613253));
#91164=CARTESIAN_POINT('Ctrl Pts',(4.20464213200779,30.613524608849,53.0389836520731));
#91165=CARTESIAN_POINT('Ctrl Pts',(4.20851046612266,30.6815445675681,53.0602644122315));
#91166=CARTESIAN_POINT('Ctrl Pts',(4.21237880023754,30.7483672335379,53.0850605109329));
#91167=CARTESIAN_POINT('Ctrl Pts',(4.21624713435241,30.8136169820425,53.11319715682));
#91168=CARTESIAN_POINT('Ctrl Pts',(4.21854485352336,30.8523741301032,53.1299098059194));
#91169=CARTESIAN_POINT('Ctrl Pts',(4.2208425726943,30.8905767687622,53.1478001486802));
#91170=CARTESIAN_POINT('Ctrl Pts',(4.22314029186525,30.9281506612641,53.1668240912299));
#91171=CARTESIAN_POINT('Ctrl Pts',(4.22700936521347,30.9914204236902,53.1988580447381));
#91172=CARTESIAN_POINT('Ctrl Pts',(4.23087843856169,31.0531537505688,53.2342341040927));
#91173=CARTESIAN_POINT('Ctrl Pts',(4.2347475119099,31.1129749158544,53.2727813111308));
#91174=CARTESIAN_POINT('Ctrl Pts',(4.23861082030568,31.1727069470912,53.3112710825002));
#91175=CARTESIAN_POINT('Ctrl Pts',(4.24247412870147,31.2305320671684,53.3529223615003));
#91176=CARTESIAN_POINT('Ctrl Pts',(4.24633743709725,31.2860981930602,53.3975178627182));
#91177=CARTESIAN_POINT('Ctrl Pts',(4.25019621359016,31.3415991364039,53.4420610506182));
#91178=CARTESIAN_POINT('Ctrl Pts',(4.25405499008307,31.3948459722212,53.4895412978214));
#91179=CARTESIAN_POINT('Ctrl Pts',(4.25791376657599,31.4455161902335,53.5396984878892));
#91180=CARTESIAN_POINT('Ctrl Pts',(4.26177011216419,31.496154487643,53.5898240805454));
#91181=CARTESIAN_POINT('Ctrl Pts',(4.2656264577524,31.5442190431926,53.6426229293582));
#91182=CARTESIAN_POINT('Ctrl Pts',(4.26948280334061,31.5894221252477,53.6977961487259));
#91183=CARTESIAN_POINT('Ctrl Pts',(4.27333800958594,31.6346118522213,53.7529530673723));
#91184=CARTESIAN_POINT('Ctrl Pts',(4.27719321583127,31.676941476376,53.8104825883361));
#91185=CARTESIAN_POINT('Ctrl Pts',(4.2810484220766,31.7161628592673,53.8700519467818));
#91186=CARTESIAN_POINT('Ctrl Pts',(4.28490377892785,31.7553857743651,53.9296236323398));
#91187=CARTESIAN_POINT('Ctrl Pts',(4.28875913577909,31.7914999418219,53.9912349066404));
#91188=CARTESIAN_POINT('Ctrl Pts',(4.29261449263034,31.8243009267392,54.05452462158));
#91189=CARTESIAN_POINT('Ctrl Pts',(4.2964738850989,31.8571362462791,54.1178805853985));
#91190=CARTESIAN_POINT('Ctrl Pts',(4.30033327756746,31.886651236198,54.1829180648712));
#91191=CARTESIAN_POINT('Ctrl Pts',(4.30419267003602,31.9126881934473,54.2492527474926));
#91192=CARTESIAN_POINT('Ctrl Pts',(4.30805424763945,31.9387398924632,54.3156249878979));
#91193=CARTESIAN_POINT('Ctrl Pts',(4.31191582524288,31.9613094849413,54.3832954324829));
#91194=CARTESIAN_POINT('Ctrl Pts',(4.31577740284632,31.9802889661255,54.4518639100173));
#91195=CARTESIAN_POINT('Ctrl Pts',(4.31964573696119,31.9993016552611,54.5205523602028));
#91196=CARTESIAN_POINT('Ctrl Pts',(4.32351407107606,32.0147115867772,54.5901415059713));
#91197=CARTESIAN_POINT('Ctrl Pts',(4.32738240519093,32.0264618851509,54.6602209680826));
#91198=CARTESIAN_POINT('Ctrl Pts',(4.32968012436189,32.0334413458272,54.7018468770145));
#91199=CARTESIAN_POINT('Ctrl Pts',(4.33197784353285,32.0391306287755,54.7436456571901));
#91200=CARTESIAN_POINT('Ctrl Pts',(4.33427556270382,32.0435265158288,54.7855310241446));
#91201=CARTESIAN_POINT('Ctrl Pts',(4.33815880198177,32.0509557445539,54.8563190056285));
#91202=CARTESIAN_POINT('Ctrl Pts',(4.34204204125973,32.0547076876349,54.9274995857473));
#91203=CARTESIAN_POINT('Ctrl Pts',(4.34592528053768,32.0547496441584,54.9987907312877));
#91204=CARTESIAN_POINT('Origin',(-1.54592528053767,30.,55.));
#91205=CARTESIAN_POINT('',(3.19386027176893,28.7479524050421,56.6292250864936));
#91206=CARTESIAN_POINT('',(3.25213375383374,28.7479524050421,56.6292250864936));
#91207=CARTESIAN_POINT('',(-1.54592528053767,28.7479524050421,56.6292250864936));
#91208=CARTESIAN_POINT('',(3.70407471941232,32.0547494644754,54.9985165115458));
#91209=CARTESIAN_POINT('Ctrl Pts',(3.25213375383374,28.7479524050421,56.6292250864936));
#91210=CARTESIAN_POINT('Ctrl Pts',(3.25599067728616,28.6914737930115,56.5858216851185));
#91211=CARTESIAN_POINT('Ctrl Pts',(3.25984760073858,28.6372072335646,56.5394414926044));
#91212=CARTESIAN_POINT('Ctrl Pts',(3.263704524191,28.5854770435146,56.4903430370475));
#91213=CARTESIAN_POINT('Ctrl Pts',(3.26755993040323,28.5337672031355,56.4412638958872));
#91214=CARTESIAN_POINT('Ctrl Pts',(3.27141533661547,28.484592103884,56.3894689480892));
#91215=CARTESIAN_POINT('Ctrl Pts',(3.2752707428277,28.4382413232633,56.3352555553667));
#91216=CARTESIAN_POINT('Ctrl Pts',(3.27912592208643,28.3918932711416,56.2810453539862));
#91217=CARTESIAN_POINT('Ctrl Pts',(3.28298110134515,28.3483695220187,56.2244173606011));
#91218=CARTESIAN_POINT('Ctrl Pts',(3.28683628060388,28.3079201049453,56.1657028743431));
#91219=CARTESIAN_POINT('Ctrl Pts',(3.29069525296784,28.2674308897497,56.106930618988));
#91220=CARTESIAN_POINT('Ctrl Pts',(3.2945542253318,28.2300223251508,56.0460681709911));
#91221=CARTESIAN_POINT('Ctrl Pts',(3.29841319769576,28.1959012107259,55.983476039891));
#91222=CARTESIAN_POINT('Ctrl Pts',(3.30227401606044,28.1617637739239,55.9208539668508));
#91223=CARTESIAN_POINT('Ctrl Pts',(3.30613483442512,28.1309171305301,55.856501001065));
#91224=CARTESIAN_POINT('Ctrl Pts',(3.30999565278981,28.1035209114166,55.7907999930867));
#91225=CARTESIAN_POINT('Ctrl Pts',(3.313863586875,28.0760741994231,55.7249778941981));
#91226=CARTESIAN_POINT('Ctrl Pts',(3.3177315209602,28.0520907814756,55.6578032477188));
#91227=CARTESIAN_POINT('Ctrl Pts',(3.3215994550454,28.0316809932176,55.5896760551685));
#91228=CARTESIAN_POINT('Ctrl Pts',(3.32502755325908,28.0135920710364,55.5292958361833));
#91229=CARTESIAN_POINT('Ctrl Pts',(3.32845565147276,27.9983095611418,55.4681678213857));
#91230=CARTESIAN_POINT('Ctrl Pts',(3.33188374968643,27.985876448174,55.4065757991813));
#91231=CARTESIAN_POINT('Ctrl Pts',(3.33575282303467,27.9718439954784,55.3370608562825));
#91232=CARTESIAN_POINT('Ctrl Pts',(3.33962189638291,27.9613871130557,55.2666824303764));
#91233=CARTESIAN_POINT('Ctrl Pts',(3.34349096973115,27.9546042657693,55.195841397286));
#91234=CARTESIAN_POINT('Ctrl Pts',(3.34735427812696,27.9478315249834,55.1251059179417));
#91235=CARTESIAN_POINT('Ctrl Pts',(3.35121758652277,27.9447219988389,55.0539096792663));
#91236=CARTESIAN_POINT('Ctrl Pts',(3.35508089491858,27.9453231361891,54.9826636849266));
#91237=CARTESIAN_POINT('Ctrl Pts',(3.35893967141151,27.9459235683676,54.9115012666035));
#91238=CARTESIAN_POINT('Ctrl Pts',(3.36279844790444,27.950226013748,54.8402896919626));
#91239=CARTESIAN_POINT('Ctrl Pts',(3.36665722439738,27.958225977863,54.7694432715653));
#91240=CARTESIAN_POINT('Ctrl Pts',(3.37051356998561,27.9662209022587,54.6986414821272));
#91241=CARTESIAN_POINT('Ctrl Pts',(3.37436991557383,27.9779086696814,54.6282048721231));
#91242=CARTESIAN_POINT('Ctrl Pts',(3.37822626116206,27.9932328074166,54.558544456065));
#91243=CARTESIAN_POINT('Ctrl Pts',(3.38208146740741,28.0085524176927,54.4889046209161));
#91244=CARTESIAN_POINT('Ctrl Pts',(3.38593667365277,28.0275061610827,54.4200409986257));
#91245=CARTESIAN_POINT('Ctrl Pts',(3.38979187989812,28.0499864442201,54.3523544991473));
#91246=CARTESIAN_POINT('Ctrl Pts',(3.39364723674939,28.0724676055632,54.2846653554555));
#91247=CARTESIAN_POINT('Ctrl Pts',(3.39750259360066,28.0984754249632,54.2181538862027));
#91248=CARTESIAN_POINT('Ctrl Pts',(3.40135795045193,28.1278529579359,54.1532042658406));
#91249=CARTESIAN_POINT('Ctrl Pts',(3.40521734292052,28.1572612420128,54.088186659084));
#91250=CARTESIAN_POINT('Ctrl Pts',(3.4090767353891,28.19004608027,54.0247346083166));
#91251=CARTESIAN_POINT('Ctrl Pts',(3.41293612785768,28.2260033992049,53.9632099427235));
#91252=CARTESIAN_POINT('Ctrl Pts',(3.41679770546114,28.2619810766787,53.9016504427119));
#91253=CARTESIAN_POINT('Ctrl Pts',(3.42065928306459,28.3011345437811,53.8420209064998));
#91254=CARTESIAN_POINT('Ctrl Pts',(3.42452086066805,28.343216496851,53.7846539644227));
#91255=CARTESIAN_POINT('Ctrl Pts',(3.42838919478294,28.3853720797237,53.7271866487574));
#91256=CARTESIAN_POINT('Ctrl Pts',(3.43225752889784,28.4304660711418,53.6719902074214));
#91257=CARTESIAN_POINT('Ctrl Pts',(3.43612586301273,28.4782114877151,53.6193634488477));
#91258=CARTESIAN_POINT('Ctrl Pts',(3.43842358218348,28.5065713852105,53.5881041241673));
#91259=CARTESIAN_POINT('Ctrl Pts',(3.44072130135424,28.5358660346034,53.5577507144534));
#91260=CARTESIAN_POINT('Ctrl Pts',(3.44301902052499,28.5660296831505,53.528359183464));
#91261=CARTESIAN_POINT('Ctrl Pts',(3.4468880938732,28.6168215162709,53.4788675002934));
#91262=CARTESIAN_POINT('Ctrl Pts',(3.45075716722141,28.6702780599787,53.4319114872838));
#91263=CARTESIAN_POINT('Ctrl Pts',(3.45462624056962,28.726115924839,53.387791289705));
#91264=CARTESIAN_POINT('Ctrl Pts',(3.4584895489654,28.7818705908022,53.3437368315986));
#91265=CARTESIAN_POINT('Ctrl Pts',(3.46235285736117,28.8399991568081,53.302510100363));
#91266=CARTESIAN_POINT('Ctrl Pts',(3.46621616575694,28.9001820553276,53.2643738734749));
#91267=CARTESIAN_POINT('Ctrl Pts',(3.47007494224985,28.9602943555354,53.2262823827709));
#91268=CARTESIAN_POINT('Ctrl Pts',(3.47393371874276,29.0224557931115,53.1912744539904));
#91269=CARTESIAN_POINT('Ctrl Pts',(3.47779249523567,29.0863158500689,53.1595710183045));
#91270=CARTESIAN_POINT('Ctrl Pts',(3.48164884082387,29.1501356772506,53.1278875547603));
#91271=CARTESIAN_POINT('Ctrl Pts',(3.48550518641207,29.215651566714,53.0995046697073));
#91272=CARTESIAN_POINT('Ctrl Pts',(3.48936153200027,29.2824875784926,53.0745978374681));
#91273=CARTESIAN_POINT('Ctrl Pts',(3.49321673824559,29.3493038438215,53.0496983638593));
#91274=CARTESIAN_POINT('Ctrl Pts',(3.49707194449091,29.4174390022002,53.0282730737539));
#91275=CARTESIAN_POINT('Ctrl Pts',(3.50092715073624,29.4864978769356,53.0104490124381));
#91276=CARTESIAN_POINT('Ctrl Pts',(3.50478250758748,29.555559449497,52.9926242548149));
#91277=CARTESIAN_POINT('Ctrl Pts',(3.50863786443872,29.6255443391362,52.9784011245611));
#91278=CARTESIAN_POINT('Ctrl Pts',(3.51249322128996,29.6960446631106,52.9678561282044));
#91279=CARTESIAN_POINT('Ctrl Pts',(3.51635261375851,29.7666187837111,52.9573000938111));
#91280=CARTESIAN_POINT('Ctrl Pts',(3.52021200622706,29.8377089342517,52.9504299510045));
#91281=CARTESIAN_POINT('Ctrl Pts',(3.52407139869561,29.9089004441347,52.9472704919008));
#91282=CARTESIAN_POINT('Ctrl Pts',(3.52793297629904,29.9801322616705,52.9441092439549));
#91283=CARTESIAN_POINT('Ctrl Pts',(3.53179455390247,30.0514650667895,52.9446628582596));
#91284=CARTESIAN_POINT('Ctrl Pts',(3.5356561315059,30.122485273634,52.9489039709846));
#91285=CARTESIAN_POINT('Ctrl Pts',(3.53952446562076,30.1936297428628,52.9531525042847));
#91286=CARTESIAN_POINT('Ctrl Pts',(3.54339279973563,30.2644600389151,52.9611013632751));
#91287=CARTESIAN_POINT('Ctrl Pts',(3.54726113385049,30.3345694703267,52.9726715036716));
#91288=CARTESIAN_POINT('Ctrl Pts',(3.54955885302151,30.3762131804719,52.97954395383));
#91289=CARTESIAN_POINT('Ctrl Pts',(3.55185657219254,30.4176027678515,52.9876930655164));
#91290=CARTESIAN_POINT('Ctrl Pts',(3.55415429136356,30.4586555529481,52.9970939497196));
#91291=CARTESIAN_POINT('Ctrl Pts',(3.55802336471177,30.5277833378795,53.0129238696588));
#91292=CARTESIAN_POINT('Ctrl Pts',(3.56189243805998,30.5962260391793,53.0323677854611));
#91293=CARTESIAN_POINT('Ctrl Pts',(3.56576151140819,30.6635777914809,53.0553503973329));
#91294=CARTESIAN_POINT('Ctrl Pts',(3.56962481980397,30.7308291890946,53.0782987649161));
#91295=CARTESIAN_POINT('Ctrl Pts',(3.57348812819975,30.7969924083183,53.1047752068268));
#91296=CARTESIAN_POINT('Ctrl Pts',(3.57735143659553,30.8616733563969,53.1346537615296));
#91297=CARTESIAN_POINT('Ctrl Pts',(3.58121021308843,30.9262784296698,53.1644972668152));
#91298=CARTESIAN_POINT('Ctrl Pts',(3.58506898958134,30.9894042467702,53.1977347549037));
#91299=CARTESIAN_POINT('Ctrl Pts',(3.58892776607425,31.0506750854305,53.2341915654988));
#91300=CARTESIAN_POINT('Ctrl Pts',(3.59278411166246,31.111907325439,53.2706254094793));
#91301=CARTESIAN_POINT('Ctrl Pts',(3.59664045725066,31.1712864889574,53.3102743044954));
#91302=CARTESIAN_POINT('Ctrl Pts',(3.60049680283886,31.2284612560273,53.3529175779762));
#91303=CARTESIAN_POINT('Ctrl Pts',(3.60435200908419,31.2856191310263,53.3955482526614));
#91304=CARTESIAN_POINT('Ctrl Pts',(3.60820721532952,31.3405735133567,53.4411712592051));
#91305=CARTESIAN_POINT('Ctrl Pts',(3.61206242157485,31.3930033370939,53.4895234972549));
#91306=CARTESIAN_POINT('Ctrl Pts',(3.6159177784261,31.4454352090333,53.5378776242134));
#91307=CARTESIAN_POINT('Ctrl Pts',(3.61977313527734,31.4953419709606,53.5889608634017));
#91308=CARTESIAN_POINT('Ctrl Pts',(3.62362849212858,31.542438125459,53.6424720291536));
#91309=CARTESIAN_POINT('Ctrl Pts',(3.62748788459715,31.5895835781324,53.696039208031));
#91310=CARTESIAN_POINT('Ctrl Pts',(3.63134727706571,31.6339122288386,53.7520390213581));
#91311=CARTESIAN_POINT('Ctrl Pts',(3.63520666953427,31.6751783462013,53.8101365326567));
#91312=CARTESIAN_POINT('Ctrl Pts',(3.6390682471377,31.7164678278714,53.8682669379662));
#91313=CARTESIAN_POINT('Ctrl Pts',(3.64292982474114,31.7546910639894,53.9284969952103));
#91314=CARTESIAN_POINT('Ctrl Pts',(3.64679140234457,31.7896467299854,53.9904643917361));
#91315=CARTESIAN_POINT('Ctrl Pts',(3.65065973645944,31.8246635570874,54.052540211157));
#91316=CARTESIAN_POINT('Ctrl Pts',(3.65452807057431,31.8564011831489,54.1163590037662));
#91317=CARTESIAN_POINT('Ctrl Pts',(3.65839640468919,31.8847054418722,54.1815362195691));
#91318=CARTESIAN_POINT('Ctrl Pts',(3.66069412386016,31.9015176499074,54.2202502845423));
#91319=CARTESIAN_POINT('Ctrl Pts',(3.66299184303114,31.9171194519221,54.2594432652729));
#91320=CARTESIAN_POINT('Ctrl Pts',(3.66528956220212,31.9314869158582,54.2990322001912));
#91321=CARTESIAN_POINT('Ctrl Pts',(3.66976608681323,31.9594782851783,54.3761612261088));
#91322=CARTESIAN_POINT('Ctrl Pts',(3.67424261142434,31.982872578991,54.4550424288438));
#91323=CARTESIAN_POINT('Ctrl Pts',(3.67871913603545,32.0014795158374,54.5351588333815));
#91324=CARTESIAN_POINT('Ctrl Pts',(3.68315616207688,32.0199222745645,54.6145683316331));
#91325=CARTESIAN_POINT('Ctrl Pts',(3.6875931881183,32.033661696059,54.6951911642588));
#91326=CARTESIAN_POINT('Ctrl Pts',(3.69203021415973,32.0425588387469,54.7765029021285));
#91327=CARTESIAN_POINT('Ctrl Pts',(3.69604504924393,32.050609402408,54.850077682828));
#91328=CARTESIAN_POINT('Ctrl Pts',(3.70005988432813,32.0546958210966,54.9242161665668));
#91329=CARTESIAN_POINT('Ctrl Pts',(3.70407471941232,32.0547494644754,54.9985165115458));
#91330=CARTESIAN_POINT('Ctrl Pts',(3.70407471946232,32.0547494644761,54.998516512471));
#91331=CARTESIAN_POINT('Ctrl Pts',(3.70793830290605,32.0548010869056,55.0700177265207));
#91332=CARTESIAN_POINT('Ctrl Pts',(3.71180188634978,32.05111623467,55.1415522381299));
#91333=CARTESIAN_POINT('Ctrl Pts',(3.71566546979351,32.0437110737994,55.2127031013635));
#91334=CARTESIAN_POINT('Ctrl Pts',(3.71952882663495,32.0363063472475,55.2838497915415));
#91335=CARTESIAN_POINT('Ctrl Pts',(3.7233921834764,32.0251817962441,55.3546123983532));
#91336=CARTESIAN_POINT('Ctrl Pts',(3.72725554031784,32.0104054413667,55.4245792315022));
#91337=CARTESIAN_POINT('Ctrl Pts',(3.73111993974999,31.9956250988457,55.4945649463577));
#91338=CARTESIAN_POINT('Ctrl Pts',(3.73498433918215,31.9771910976799,55.563753989815));
#91339=CARTESIAN_POINT('Ctrl Pts',(3.7388487386143,31.9552221704314,55.6317466475999));
#91340=CARTESIAN_POINT('Ctrl Pts',(3.74271803189463,31.9332254218883,55.699825410807));
#91341=CARTESIAN_POINT('Ctrl Pts',(3.74658732517497,31.9076849661807,55.7667043065627));
#91342=CARTESIAN_POINT('Ctrl Pts',(3.7504566184553,31.87876856606,55.8320013447615));
#91343=CARTESIAN_POINT('Ctrl Pts',(3.75432884727622,31.8498302277557,55.897347922267));
#91344=CARTESIAN_POINT('Ctrl Pts',(3.75820107609715,31.8175110677505,55.9611098252564));
#91345=CARTESIAN_POINT('Ctrl Pts',(3.76207330491807,31.7820246506315,56.0229299619434));
#91346=CARTESIAN_POINT('Ctrl Pts',(3.76595231070725,31.7464761270789,56.0848582929349));
#91347=CARTESIAN_POINT('Ctrl Pts',(3.76983131649643,31.7077495507213,56.1448376751856));
#91348=CARTESIAN_POINT('Ctrl Pts',(3.7737103222856,31.6661010629529,56.2025409808098));
#91349=CARTESIAN_POINT('Ctrl Pts',(3.77461515920396,31.6563859216578,56.2160011518118));
#91350=CARTESIAN_POINT('Ctrl Pts',(3.77551999612232,31.6465119574723,56.2293376254161));
#91351=CARTESIAN_POINT('Ctrl Pts',(3.77642483304068,31.6364827163498,56.242546530955));
#91352=CARTESIAN_POINT('Ctrl Pts',(3.78029390638889,31.5935977845543,56.2990276750626));
#91353=CARTESIAN_POINT('Ctrl Pts',(3.7841629797371,31.5477013562299,56.3533966652134));
#91354=CARTESIAN_POINT('Ctrl Pts',(3.78803205308531,31.499029141768,56.4053146247835));
#91355=CARTESIAN_POINT('Ctrl Pts',(3.7918953614811,31.4504294493225,56.4571552261492));
#91356=CARTESIAN_POINT('Ctrl Pts',(3.79575866987688,31.3990625100132,56.5065516946494));
#91357=CARTESIAN_POINT('Ctrl Pts',(3.79962197827267,31.3452053570871,56.5531967389112));
#91358=CARTESIAN_POINT('Ctrl Pts',(3.80348075476558,31.2914113819766,56.5997870656127));
#91359=CARTESIAN_POINT('Ctrl Pts',(3.80733953125849,31.2351333611201,56.6436320626762));
#91360=CARTESIAN_POINT('Ctrl Pts',(3.8111983077514,31.1766851454725,56.6844612286795));
#91361=CARTESIAN_POINT('Ctrl Pts',(3.81505465333961,31.1182737503153,56.7252646736253));
#91362=CARTESIAN_POINT('Ctrl Pts',(3.81891099892781,31.0576952700763,56.7630557792994));
#91363=CARTESIAN_POINT('Ctrl Pts',(3.82276734451602,30.9952954419552,56.7976052252158));
#91364=CARTESIAN_POINT('Ctrl Pts',(3.82662255076135,30.9329140496299,56.8321444636277));
#91365=CARTESIAN_POINT('Ctrl Pts',(3.83047775700668,30.8687128024807,56.863443708473));
#91366=CARTESIAN_POINT('Ctrl Pts',(3.83433296325201,30.8030636482535,56.8913186773661));
#91367=CARTESIAN_POINT('Ctrl Pts',(3.83818832010326,30.7374119294031,56.9191947352114));
#91368=CARTESIAN_POINT('Ctrl Pts',(3.84204367695451,30.6703126391839,56.9436460636852));
#91369=CARTESIAN_POINT('Ctrl Pts',(3.84589903380576,30.6021577906026,56.9645364740102));
#91370=CARTESIAN_POINT('Ctrl Pts',(3.84975842627431,30.5339316005354,56.9854487514943));
#91371=CARTESIAN_POINT('Ctrl Pts',(3.85361781874287,30.4646481118632,57.0027925274235));
#91372=CARTESIAN_POINT('Ctrl Pts',(3.85747721121143,30.3947137246528,57.0164817475174));
#91373=CARTESIAN_POINT('Ctrl Pts',(3.86133878881486,30.3247397415552,57.0301787182592));
#91374=CARTESIAN_POINT('Ctrl Pts',(3.8652003664183,30.2541146074705,57.0402169457162));
#91375=CARTESIAN_POINT('Ctrl Pts',(3.86906194402173,30.183251389623,57.0465621150362));
#91376=CARTESIAN_POINT('Ctrl Pts',(3.8729302781366,30.1122641840712,57.0529183863495));
#91377=CARTESIAN_POINT('Ctrl Pts',(3.87679861225147,30.0410385486675,57.0555686805711));
#91378=CARTESIAN_POINT('Ctrl Pts',(3.88066694636634,29.9699884019044,57.0545308141957));
#91379=CARTESIAN_POINT('Ctrl Pts',(3.88296466553731,29.9277859241789,57.0539143406966));
#91380=CARTESIAN_POINT('Ctrl Pts',(3.88526238470827,29.885645300261,57.0519976298562));
#91381=CARTESIAN_POINT('Ctrl Pts',(3.88756010387923,29.8436519877082,57.0487930255525));
#91382=CARTESIAN_POINT('Ctrl Pts',(3.89142879126944,29.7729475253008,57.0433974087089));
#91383=CARTESIAN_POINT('Ctrl Pts',(3.89529747865965,29.7023842197183,57.0343268801619));
#91384=CARTESIAN_POINT('Ctrl Pts',(3.89916616604986,29.6323744933448,57.0215956691081));
#91385=CARTESIAN_POINT('Ctrl Pts',(3.90302937622933,29.5624638853508,57.0088824826499));
#91386=CARTESIAN_POINT('Ctrl Pts',(3.9068925864088,29.4931057753174,56.9925189834931));
#91387=CARTESIAN_POINT('Ctrl Pts',(3.91075579658827,29.424708554523,56.9725712446604));
#91388=CARTESIAN_POINT('Ctrl Pts',(3.91461452942191,29.3563906040755,56.9526466246644));
#91389=CARTESIAN_POINT('Ctrl Pts',(3.91847326225554,29.2890317950303,56.9291461509425));
#91390=CARTESIAN_POINT('Ctrl Pts',(3.92233199508918,29.2230295971289,56.9021867825117));
#91391=CARTESIAN_POINT('Ctrl Pts',(3.92618810381818,29.1570722835668,56.8752457476135));
#91392=CARTESIAN_POINT('Ctrl Pts',(3.93004421254717,29.0924701982269,56.8448506709057));
#91393=CARTESIAN_POINT('Ctrl Pts',(3.93390032127617,29.0296034520015,56.8111676074103));
#91394=CARTESIAN_POINT('Ctrl Pts',(3.93775577559101,28.9667473747926,56.7774902602148));
#91395=CARTESIAN_POINT('Ctrl Pts',(3.94161122990586,28.9056264836543,56.7405262564653));
#91396=CARTESIAN_POINT('Ctrl Pts',(3.9454666842207,28.8465974065651,56.7004881710725));
#91397=CARTESIAN_POINT('Ctrl Pts',(3.94765985266874,28.81301881924,56.6777125761796));
#91398=CARTESIAN_POINT('Ctrl Pts',(3.94985302111678,28.7801166565293,56.6539430791467));
#91399=CARTESIAN_POINT('Ctrl Pts',(3.95204618956481,28.7479524050421,56.6292250864936));
#91400=CARTESIAN_POINT('',(3.64592528049244,32.0547492155205,55.0017954993351));
#91401=CARTESIAN_POINT('Ctrl Pts',(3.64592528053768,32.0547492155198,55.001795500168));
#91402=CARTESIAN_POINT('Ctrl Pts',(3.65155534725615,32.0546586344092,55.1054554547564));
#91403=CARTESIAN_POINT('Ctrl Pts',(3.65718541397462,32.0467203700807,55.2087840266247));
#91404=CARTESIAN_POINT('Ctrl Pts',(3.66281548069309,32.0311035472159,55.3108310521601));
#91405=CARTESIAN_POINT('Ctrl Pts',(3.66436496635288,32.0268055443164,55.3389160484129));
#91406=CARTESIAN_POINT('Ctrl Pts',(3.66591445201267,32.0219261885247,55.3669041565549));
#91407=CARTESIAN_POINT('Ctrl Pts',(3.66746393767245,32.0164695735925,55.394775912735));
#91408=CARTESIAN_POINT('Ctrl Pts',(3.67133301102066,32.0028443791468,55.4643718256258));
#91409=CARTESIAN_POINT('Ctrl Pts',(3.67520208436887,31.9855852435917,55.5333978458126));
#91410=CARTESIAN_POINT('Ctrl Pts',(3.67907115771708,31.9647545311723,55.6014459200443));
#91411=CARTESIAN_POINT('Ctrl Pts',(3.68293446611286,31.9439548566929,55.6693926020625));
#91412=CARTESIAN_POINT('Ctrl Pts',(3.68679777450863,31.9195943097706,55.7363637697985));
#91413=CARTESIAN_POINT('Ctrl Pts',(3.69066108290441,31.8917862649139,55.8019615267474));
#91414=CARTESIAN_POINT('Ctrl Pts',(3.69451985939732,31.8640108406366,55.8674823334163));
#91415=CARTESIAN_POINT('Ctrl Pts',(3.69837863589022,31.8327961401176,55.9316324843945));
#91416=CARTESIAN_POINT('Ctrl Pts',(3.70223741238313,31.7983047958053,55.9940308968456));
#91417=CARTESIAN_POINT('Ctrl Pts',(3.70609375797133,31.7638351799272,56.0563900003099));
#91418=CARTESIAN_POINT('Ctrl Pts',(3.70995010355953,31.7260932500095,56.1169991304984));
#91419=CARTESIAN_POINT('Ctrl Pts',(3.71380644914773,31.6852884029895,56.1755001323901));
#91420=CARTESIAN_POINT('Ctrl Pts',(3.71766165539305,31.6444956116089,56.2339838503796));
#91421=CARTESIAN_POINT('Ctrl Pts',(3.72151686163838,31.6006419774188,56.2903602783589));
#91422=CARTESIAN_POINT('Ctrl Pts',(3.7253720678837,31.5539802651177,56.3443001517983));
#91423=CARTESIAN_POINT('Ctrl Pts',(3.72922742473494,31.5073167299491,56.3982421324307));
#91424=CARTESIAN_POINT('Ctrl Pts',(3.73308278158618,31.4578452183628,56.4497470035925));
#91425=CARTESIAN_POINT('Ctrl Pts',(3.73693813843742,31.4058576914259,56.4985198410294));
#91426=CARTESIAN_POINT('Ctrl Pts',(3.74079753090597,31.3538157462414,56.5473437317188));
#91427=CARTESIAN_POINT('Ctrl Pts',(3.74465692337453,31.2992528833491,56.59342954688));
#91428=CARTESIAN_POINT('Ctrl Pts',(3.74851631584308,31.2424960612611,56.6365210356884));
#91429=CARTESIAN_POINT('Ctrl Pts',(3.75237789344651,31.1857071042418,56.6796369223045));
#91430=CARTESIAN_POINT('Ctrl Pts',(3.75623947104993,31.1267221170847,56.7197548343266));
#91431=CARTESIAN_POINT('Ctrl Pts',(3.76010104865336,31.0658968318021,56.7566620353541));
#91432=CARTESIAN_POINT('Ctrl Pts',(3.76396938276822,31.0049651219496,56.7936338120424));
#91433=CARTESIAN_POINT('Ctrl Pts',(3.76783771688309,30.942187113305,56.8273834317251));
#91434=CARTESIAN_POINT('Ctrl Pts',(3.77170605099795,30.8779422625793,56.8577445858021));
#91435=CARTESIAN_POINT('Ctrl Pts',(3.77400377016897,30.8397820052776,56.8757785517693));
#91436=CARTESIAN_POINT('Ctrl Pts',(3.77630148934,30.8011046100197,56.8926179419242));
#91437=CARTESIAN_POINT('Ctrl Pts',(3.77859920851102,30.7619922359673,56.9082361999568));
#91438=CARTESIAN_POINT('Ctrl Pts',(3.78246828185923,30.696131861932,56.9345354042555));
#91439=CARTESIAN_POINT('Ctrl Pts',(3.78633735520744,30.6287793604348,56.957472487004));
#91440=CARTESIAN_POINT('Ctrl Pts',(3.79020642855566,30.5603113789127,56.976878529693));
#91441=CARTESIAN_POINT('Ctrl Pts',(3.79406973695144,30.4919454152695,56.996255657212));
#91442=CARTESIAN_POINT('Ctrl Pts',(3.79793304534723,30.4224677343409,57.0121120567743));
#91443=CARTESIAN_POINT('Ctrl Pts',(3.80179635374301,30.3522741165739,57.0243271744686));
#91444=CARTESIAN_POINT('Ctrl Pts',(3.80565513023592,30.2821628403199,57.0365279630643));
#91445=CARTESIAN_POINT('Ctrl Pts',(3.80951390672883,30.2113377717017,57.0450958714596));
#91446=CARTESIAN_POINT('Ctrl Pts',(3.81337268322174,30.140207281009,57.0499608486144));
#91447=CARTESIAN_POINT('Ctrl Pts',(3.81722902880995,30.0691216002307,57.0548227609906));
#91448=CARTESIAN_POINT('Ctrl Pts',(3.82108537439815,29.9977313626162,57.0559863371499));
#91449=CARTESIAN_POINT('Ctrl Pts',(3.82494171998636,29.9264510391778,57.0534332501598));
#91450=CARTESIAN_POINT('Ctrl Pts',(3.82879692623169,29.8551917752442,57.0508809174698));
#91451=CARTESIAN_POINT('Ctrl Pts',(3.83265213247702,29.7840428462275,57.0446141189907));
#91452=CARTESIAN_POINT('Ctrl Pts',(3.83650733872235,29.7134179720959,57.0346666321003));
#91453=CARTESIAN_POINT('Ctrl Pts',(3.8403626955736,29.6427903389618,57.0247187566055));
#91454=CARTESIAN_POINT('Ctrl Pts',(3.84421805242484,29.5726872820889,57.0110899771617));
#91455=CARTESIAN_POINT('Ctrl Pts',(3.84807340927609,29.503514929387,56.9938656266555));
#91456=CARTESIAN_POINT('Ctrl Pts',(3.85193280174465,29.4342701701207,56.9766232464598));
#91457=CARTESIAN_POINT('Ctrl Pts',(3.8557921942132,29.3659585321451,56.9557778996608));
#91458=CARTESIAN_POINT('Ctrl Pts',(3.85965158668176,29.298972633494,56.9314652971021));
#91459=CARTESIAN_POINT('Ctrl Pts',(3.8635131642852,29.2319488083494,56.9071389290825));
#91460=CARTESIAN_POINT('Ctrl Pts',(3.86737474188863,29.166252664371,56.8793415867396));
#91461=CARTESIAN_POINT('Ctrl Pts',(3.87123631949207,29.1022558669431,56.8482567554488));
#91462=CARTESIAN_POINT('Ctrl Pts',(3.87510465360694,29.0381470958252,56.8171175357603));
#91463=CARTESIAN_POINT('Ctrl Pts',(3.87897298772181,28.9757440330042,56.7826795777972));
#91464=CARTESIAN_POINT('Ctrl Pts',(3.88284132183667,28.915392205271,56.7451714798589));
#91465=CARTESIAN_POINT('Ctrl Pts',(3.88513904100764,28.8795443318796,56.7228923609566));
#91466=CARTESIAN_POINT('Ctrl Pts',(3.88743676017861,28.8444195966072,56.6995308769136));
#91467=CARTESIAN_POINT('Ctrl Pts',(3.88973447934958,28.8100848707453,56.6751416500317));
#91468=CARTESIAN_POINT('Ctrl Pts',(3.8911385956916,28.7891032162897,56.6602376041123));
#91469=CARTESIAN_POINT('Ctrl Pts',(3.89254271203362,28.7683867515158,56.644928732705));
#91470=CARTESIAN_POINT('Ctrl Pts',(3.89394682837563,28.7479524050421,56.6292250864936));
#91471=CARTESIAN_POINT('Ctrl Pts',(3.19386027176893,28.7479524050421,56.6292250864936));
#91472=CARTESIAN_POINT('Ctrl Pts',(3.19772209747134,28.6914220012474,56.5857818835256));
#91473=CARTESIAN_POINT('Ctrl Pts',(3.20158392317375,28.6372079170157,56.5394334898166));
#91474=CARTESIAN_POINT('Ctrl Pts',(3.20544574887617,28.5856083501764,56.4904676525874));
#91475=CARTESIAN_POINT('Ctrl Pts',(3.20931422741344,28.5339198918585,56.4414174610517));
#91476=CARTESIAN_POINT('Ctrl Pts',(3.21318270595072,28.4848552756939,56.3897411776724));
#91477=CARTESIAN_POINT('Ctrl Pts',(3.217051184488,28.4386740269193,56.3357614937868));
#91478=CARTESIAN_POINT('Ctrl Pts',(3.21900840776474,28.4153090232932,56.3084509393261));
#91479=CARTESIAN_POINT('Ctrl Pts',(3.22096563104148,28.3926814269665,56.2805512636196));
#91480=CARTESIAN_POINT('Ctrl Pts',(3.22292285431822,28.3708205831157,56.2521070202265));
#91481=CARTESIAN_POINT('Ctrl Pts',(3.2267919276666,28.3276056830472,56.195877940318));
#91482=CARTESIAN_POINT('Ctrl Pts',(3.23066100101498,28.2872205677673,56.1372988340834));
#91483=CARTESIAN_POINT('Ctrl Pts',(3.23453007436335,28.249930197065,56.076686234404));
#91484=CARTESIAN_POINT('Ctrl Pts',(3.2383933827593,28.2126953893345,56.0161639480173));
#91485=CARTESIAN_POINT('Ctrl Pts',(3.24225669115525,28.1785464255646,55.9536145928793));
#91486=CARTESIAN_POINT('Ctrl Pts',(3.2461199995512,28.1477069248002,55.8893862637049));
#91487=CARTESIAN_POINT('Ctrl Pts',(3.24997877604428,28.116903600703,55.8252332783859));
#91488=CARTESIAN_POINT('Ctrl Pts',(3.25383755253736,28.0894022374831,55.759405667002));
#91489=CARTESIAN_POINT('Ctrl Pts',(3.25769632903044,28.0653812767344,55.6922773707773));
#91490=CARTESIAN_POINT('Ctrl Pts',(3.26155267461882,28.0413754484161,55.6251913632135));
#91491=CARTESIAN_POINT('Ctrl Pts',(3.26540902020719,28.0208458358845,55.5568067527675));
#91492=CARTESIAN_POINT('Ctrl Pts',(3.26926536579557,28.003922763762,55.4875174145327));
#91493=CARTESIAN_POINT('Ctrl Pts',(3.27312057204107,27.9870046914979,55.4182485475735));
#91494=CARTESIAN_POINT('Ctrl Pts',(3.27697577828658,27.9736911594497,55.3480759551445));
#91495=CARTESIAN_POINT('Ctrl Pts',(3.28083098453208,27.9640621465015,55.2774069559186));
#91496=CARTESIAN_POINT('Ctrl Pts',(3.2846863413835,27.9544327573902,55.2067351959664));
#91497=CARTESIAN_POINT('Ctrl Pts',(3.28854169823492,27.9484882365511,55.135567472352));
#91498=CARTESIAN_POINT('Ctrl Pts',(3.29239705508633,27.9462568852949,55.0643178148045));
#91499=CARTESIAN_POINT('Ctrl Pts',(3.29625644755507,27.9440231983586,54.9929935762615));
#91500=CARTESIAN_POINT('Ctrl Pts',(3.3001158400238,27.9455104551327,54.9215877191223));
#91501=CARTESIAN_POINT('Ctrl Pts',(3.30397523249253,27.9506948035876,54.8505149691208));
#91502=CARTESIAN_POINT('Ctrl Pts',(3.30783681009614,27.9558820873492,54.7794019787068));
#91503=CARTESIAN_POINT('Ctrl Pts',(3.31169838769975,27.9647705692329,54.7086229531048));
#91504=CARTESIAN_POINT('Ctrl Pts',(3.31555996530335,27.977284725652,54.6385854438191));
#91505=CARTESIAN_POINT('Ctrl Pts',(3.3194282994184,27.989820777796,54.5684253915521));
#91506=CARTESIAN_POINT('Ctrl Pts',(3.32329663353344,28.0059950596976,54.4990099191882));
#91507=CARTESIAN_POINT('Ctrl Pts',(3.32716496764848,28.0256815275821,54.4307336897643));
#91508=CARTESIAN_POINT('Ctrl Pts',(3.32946268681792,28.0373749266762,54.3901788678441));
#91509=CARTESIAN_POINT('Ctrl Pts',(3.33176040598735,28.0503065279621,54.3500256656002));
#91510=CARTESIAN_POINT('Ctrl Pts',(3.33405812515678,28.0644419479984,54.310353286217));
#91511=CARTESIAN_POINT('Ctrl Pts',(3.33792719850495,28.0882442375276,54.2435499327991));
#91512=CARTESIAN_POINT('Ctrl Pts',(3.34179627185313,28.1155556601753,54.1778494349638));
#91513=CARTESIAN_POINT('Ctrl Pts',(3.34566534520131,28.1462539875542,54.1136460730379));
#91514=CARTESIAN_POINT('Ctrl Pts',(3.34952865359705,28.1769065741622,54.0495383746711));
#91515=CARTESIAN_POINT('Ctrl Pts',(3.35339196199279,28.2109358404614,53.9869238189406));
#91516=CARTESIAN_POINT('Ctrl Pts',(3.35725527038854,28.2481706198582,53.9261790720181));
#91517=CARTESIAN_POINT('Ctrl Pts',(3.36111404688141,28.2853617205251,53.8655055824908));
#91518=CARTESIAN_POINT('Ctrl Pts',(3.36497282337429,28.3257506124843,53.8066979570904));
#91519=CARTESIAN_POINT('Ctrl Pts',(3.36883159986716,28.3691199117373,53.7501089246625));
#91520=CARTESIAN_POINT('Ctrl Pts',(3.37268794545533,28.4124618897308,53.6935555414996));
#91521=CARTESIAN_POINT('Ctrl Pts',(3.37654429104349,28.4587802551666,53.6392183630728));
#91522=CARTESIAN_POINT('Ctrl Pts',(3.38040063663166,28.5078147798167,53.5874205044789));
#91523=CARTESIAN_POINT('Ctrl Pts',(3.38425584287695,28.5568348174,53.5356379493685));
#91524=CARTESIAN_POINT('Ctrl Pts',(3.38811104912224,28.608569087273,53.4863935772635));
#91525=CARTESIAN_POINT('Ctrl Pts',(3.39196625536753,28.6627187609505,53.4399754969277));
#91526=CARTESIAN_POINT('Ctrl Pts',(3.39582161221874,28.716870550017,53.393555603242));
#91527=CARTESIAN_POINT('Ctrl Pts',(3.39967696906994,28.7734375599698,53.3499625350206));
#91528=CARTESIAN_POINT('Ctrl Pts',(3.40353232592115,28.8320872960135,53.3094446242826));
#91529=CARTESIAN_POINT('Ctrl Pts',(3.40739171838967,28.8907984240112,53.2688843011848));
#91530=CARTESIAN_POINT('Ctrl Pts',(3.41125111085819,28.951596229579,53.2314058379809));
#91531=CARTESIAN_POINT('Ctrl Pts',(3.41511050332671,29.014119347079,53.1972141278854));
#91532=CARTESIAN_POINT('Ctrl Pts',(3.4189720809301,29.0766778643073,53.1630030589144));
#91533=CARTESIAN_POINT('Ctrl Pts',(3.4228336585335,29.1409632000845,53.1320826582238));
#91534=CARTESIAN_POINT('Ctrl Pts',(3.42669523613689,29.2065919913585,53.1046105164575));
#91535=CARTESIAN_POINT('Ctrl Pts',(3.43056357025173,29.2723356117837,53.0770903073314));
#91536=CARTESIAN_POINT('Ctrl Pts',(3.43443190436656,29.3394269233546,53.0530305668982));
#91537=CARTESIAN_POINT('Ctrl Pts',(3.43830023848139,29.4074659908464,53.0325394513495));
#91538=CARTESIAN_POINT('Ctrl Pts',(3.44059795765271,29.4478799429853,53.0203681063621));
#91539=CARTESIAN_POINT('Ctrl Pts',(3.44289567682402,29.4886280333401,53.0094548530609));
#91540=CARTESIAN_POINT('Ctrl Pts',(3.44519339599534,29.5296250715218,52.9998137613814));
#91541=CARTESIAN_POINT('Ctrl Pts',(3.44906246934354,29.5986589855718,52.9835793619256));
#91542=CARTESIAN_POINT('Ctrl Pts',(3.45293154269173,29.6686695703827,52.9708912873145));
#91543=CARTESIAN_POINT('Ctrl Pts',(3.45680061603993,29.7392592815901,52.9618606916447));
#91544=CARTESIAN_POINT('Ctrl Pts',(3.46066392443569,29.8097438135233,52.9528435516397));
#91545=CARTESIAN_POINT('Ctrl Pts',(3.46452723283146,29.8808052810812,52.9474731342666));
#91546=CARTESIAN_POINT('Ctrl Pts',(3.46839054122722,29.9520343959929,52.9458099252182));
#91547=CARTESIAN_POINT('Ctrl Pts',(3.47224931772011,30.0231799546887,52.9441486672182));
#91548=CARTESIAN_POINT('Ctrl Pts',(3.47610809421301,30.094492286807,52.9461859906645));
#91549=CARTESIAN_POINT('Ctrl Pts',(3.4799668707059,30.1655571482066,52.9519305692488));
#91550=CARTESIAN_POINT('Ctrl Pts',(3.48382321629408,30.2365772410361,52.9576715289339));
#91551=CARTESIAN_POINT('Ctrl Pts',(3.48767956188226,30.3073496893853,52.967115071211));
#91552=CARTESIAN_POINT('Ctrl Pts',(3.49153590747045,30.3774618917421,52.9802178130347));
#91553=CARTESIAN_POINT('Ctrl Pts',(3.49539111371576,30.4475533797111,52.9933166837023));
#91554=CARTESIAN_POINT('Ctrl Pts',(3.49924631996107,30.5169845316913,53.0100725184486));
#91555=CARTESIAN_POINT('Ctrl Pts',(3.50310152620637,30.5853512211227,53.030390518293));
#91556=CARTESIAN_POINT('Ctrl Pts',(3.5069568830576,30.6537205813393,53.050709311872));
#91557=CARTESIAN_POINT('Ctrl Pts',(3.51081223990882,30.7210249314183,53.0745904063286));
#91558=CARTESIAN_POINT('Ctrl Pts',(3.51466759676005,30.7868753035779,53.1018891446706));
#91559=CARTESIAN_POINT('Ctrl Pts',(3.51852698922858,30.8527946049993,53.1292164581265));
#91560=CARTESIAN_POINT('Ctrl Pts',(3.52238638169712,30.9172564406547,53.1599683704244));
#91561=CARTESIAN_POINT('Ctrl Pts',(3.52624577416566,30.9798926790859,53.1939524092722));
#91562=CARTESIAN_POINT('Ctrl Pts',(3.53010735176907,31.042564381293,53.2279556894149));
#91563=CARTESIAN_POINT('Ctrl Pts',(3.53396892937248,31.1034080141042,53.2651944853304));
#91564=CARTESIAN_POINT('Ctrl Pts',(3.53783050697589,31.162083256404,53.3054321885255));
#91565=CARTESIAN_POINT('Ctrl Pts',(3.54169884109074,31.2208611613942,53.3457402946828));
#91566=CARTESIAN_POINT('Ctrl Pts',(3.54556717520559,31.2774627151784,53.3890574888126));
#91567=CARTESIAN_POINT('Ctrl Pts',(3.54943550932044,31.3315801405265,53.4351064279462));
#91568=CARTESIAN_POINT('Ctrl Pts',(3.55173322849159,31.3637248938038,53.4624586491135));
#91569=CARTESIAN_POINT('Ctrl Pts',(3.55403094766275,31.3949938940229,53.4907739380971));
#91570=CARTESIAN_POINT('Ctrl Pts',(3.5563286668339,31.4253291162108,53.5199883537682));
#91571=CARTESIAN_POINT('Ctrl Pts',(3.56013990426076,31.4756462896958,53.5684464402949));
#91572=CARTESIAN_POINT('Ctrl Pts',(3.56395114168762,31.5236017843575,53.6195819833469));
#91573=CARTESIAN_POINT('Ctrl Pts',(3.56776237911448,31.5688910656209,53.6731321140691));
#91574=CARTESIAN_POINT('Ctrl Pts',(3.5715685505651,31.6141201474276,53.7266110648411));
#91575=CARTESIAN_POINT('Ctrl Pts',(3.57537472201571,31.6566897173767,53.7824978653989));
#91576=CARTESIAN_POINT('Ctrl Pts',(3.57918089346633,31.6963307948588,53.8404917434905));
#91577=CARTESIAN_POINT('Ctrl Pts',(3.58298336737587,31.7359333626432,53.8984292828836));
#91578=CARTESIAN_POINT('Ctrl Pts',(3.58678584128542,31.7726127957148,53.9584694309203));
#91579=CARTESIAN_POINT('Ctrl Pts',(3.59058831519496,31.8061405313258,54.0202786398154));
#91580=CARTESIAN_POINT('Ctrl Pts',(3.5943884546426,31.8396476831739,54.0820499020349));
#91581=CARTESIAN_POINT('Ctrl Pts',(3.59818859409023,31.870006736961,54.145587631284));
#91582=CARTESIAN_POINT('Ctrl Pts',(3.60198873353787,31.8970336522008,54.2105312641291));
#91583=CARTESIAN_POINT('Ctrl Pts',(3.60578956781207,31.9240655091063,54.275486771423));
#91584=CARTESIAN_POINT('Ctrl Pts',(3.60959040208628,31.9477638020177,54.3418482392775));
#91585=CARTESIAN_POINT('Ctrl Pts',(3.61339123636048,31.9679921061031,54.4092338594539));
#91586=CARTESIAN_POINT('Ctrl Pts',(3.61719222217702,31.9882212167074,54.4766221663494));
#91587=CARTESIAN_POINT('Ctrl Pts',(3.62099320799356,32.0049799299312,54.5450342228552));
#91588=CARTESIAN_POINT('Ctrl Pts',(3.62479419381009,32.0181820637142,54.6140742037614));
#91589=CARTESIAN_POINT('Ctrl Pts',(3.62859963984799,32.0313996893832,54.6831951988078));
#91590=CARTESIAN_POINT('Ctrl Pts',(3.63240508588588,32.0410523192832,54.7529450939127));
#91591=CARTESIAN_POINT('Ctrl Pts',(3.63621053192378,32.0471053357224,54.8229200548993));
#91592=CARTESIAN_POINT('Ctrl Pts',(3.63944878144667,32.0522561583595,54.8824653438806));
#91593=CARTESIAN_POINT('Ctrl Pts',(3.64268703096955,32.0548013150988,54.9421733287147));
#91594=CARTESIAN_POINT('Ctrl Pts',(3.64592528049244,32.0547492155205,55.0017954993351));
#91595=CARTESIAN_POINT('Origin',(-1.54592528053767,30.,55.));
#91596=CARTESIAN_POINT('',(2.49394378209486,28.7479524050421,56.6292250864936));
#91597=CARTESIAN_POINT('',(2.55206205739628,28.7479524050421,56.6292250864936));
#91598=CARTESIAN_POINT('',(-1.54592528053767,28.7479524050421,56.6292250864936));
#91599=CARTESIAN_POINT('',(3.00407471949931,32.0547499051081,54.9993755336174));
#91600=CARTESIAN_POINT('Ctrl Pts',(2.55206205739628,28.7479524050421,56.6292250864936));
#91601=CARTESIAN_POINT('Ctrl Pts',(2.55268698953636,28.7388644085502,56.6222410274799));
#91602=CARTESIAN_POINT('Ctrl Pts',(2.55331192167644,28.729837617433,56.615183051692));
#91603=CARTESIAN_POINT('Ctrl Pts',(2.55393685381652,28.720873281012,56.6080523621048));
#91604=CARTESIAN_POINT('Ctrl Pts',(2.55780592716298,28.6653733748771,56.5639049111191));
#91605=CARTESIAN_POINT('Ctrl Pts',(2.56167500050944,28.6120529828087,56.516794349591));
#91606=CARTESIAN_POINT('Ctrl Pts',(2.5655440738559,28.5612455809797,56.466963968286));
#91607=CARTESIAN_POINT('Ctrl Pts',(2.56940738224989,28.5105138826151,56.4172078346765));
#91608=CARTESIAN_POINT('Ctrl Pts',(2.57327069064389,28.4622880860022,56.3647402628779));
#91609=CARTESIAN_POINT('Ctrl Pts',(2.57713399903788,28.4168691584292,56.3098451438882));
#91610=CARTESIAN_POINT('Ctrl Pts',(2.58099277552896,28.3715035101054,56.2550144203142));
#91611=CARTESIAN_POINT('Ctrl Pts',(2.58485155202003,28.3289384987099,56.1977621784438));
#91612=CARTESIAN_POINT('Ctrl Pts',(2.58871032851111,28.2894374808424,56.1384082881608));
#91613=CARTESIAN_POINT('Ctrl Pts',(2.59256667409745,28.2499613473421,56.0790917889143));
#91614=CARTESIAN_POINT('Ctrl Pts',(2.59642301968379,28.2135456463576,56.0176766714484));
#91615=CARTESIAN_POINT('Ctrl Pts',(2.60027936527013,28.1804118451149,55.9545137553235));
#91616=CARTESIAN_POINT('Ctrl Pts',(2.60413457151358,28.14728783313,55.8913695004463));
#91617=CARTESIAN_POINT('Ctrl Pts',(2.60798977775702,28.117444021457,55.8264789020229));
#91618=CARTESIAN_POINT('Ctrl Pts',(2.61184498400046,28.0910562597286,55.7602179680715));
#91619=CARTESIAN_POINT('Ctrl Pts',(2.6157003408498,28.0646674671469,55.6939544455979));
#91620=CARTESIAN_POINT('Ctrl Pts',(2.61955569769913,28.0417351702449,55.6263209334428));
#91621=CARTESIAN_POINT('Ctrl Pts',(2.62341105454847,28.0223866848822,55.5577124154696));
#91622=CARTESIAN_POINT('Ctrl Pts',(2.62727044701509,28.0030179463795,55.4890320811296));
#91623=CARTESIAN_POINT('Ctrl Pts',(2.63112983948172,27.9872406401299,55.4193751721457));
#91624=CARTESIAN_POINT('Ctrl Pts',(2.63498923194835,27.97513163587,55.3491499254552));
#91625=CARTESIAN_POINT('Ctrl Pts',(2.63885080954984,27.9630157756586,55.2788849181971));
#91626=CARTESIAN_POINT('Ctrl Pts',(2.64271238715133,27.9545724095138,55.2080514152575));
#91627=CARTESIAN_POINT('Ctrl Pts',(2.64657396475282,27.9498265305783,55.1370631525225));
#91628=CARTESIAN_POINT('Ctrl Pts',(2.65044229886574,27.9450723478902,55.065950683295));
#91629=CARTESIAN_POINT('Ctrl Pts',(2.65431063297867,27.9440285758852,54.994683399541));
#91630=CARTESIAN_POINT('Ctrl Pts',(2.65817896709159,27.9466680704179,54.9236747128482));
#91631=CARTESIAN_POINT('Ctrl Pts',(2.66047668627942,27.9482358815369,54.8814968613096));
#91632=CARTESIAN_POINT('Ctrl Pts',(2.66277440546725,27.9511022049546,54.8394101629236));
#91633=CARTESIAN_POINT('Ctrl Pts',(2.66507212465507,27.95525277321,54.7974997752229));
#91634=CARTESIAN_POINT('Ctrl Pts',(2.66894119800453,27.9622418139541,54.726927894648));
#91635=CARTESIAN_POINT('Ctrl Pts',(2.67281027135398,27.972902383093,54.6565800340402));
#91636=CARTESIAN_POINT('Ctrl Pts',(2.67667934470343,27.987210946956,54.5868683134322));
#91637=CARTESIAN_POINT('Ctrl Pts',(2.68054265310047,28.0014981909364,54.5172604638847));
#91638=CARTESIAN_POINT('Ctrl Pts',(2.68440596149751,28.0194225433629,54.4482873448617));
#91639=CARTESIAN_POINT('Ctrl Pts',(2.68826926989455,28.0409087288895,54.3803557843741));
#91640=CARTESIAN_POINT('Ctrl Pts',(2.69212804638874,28.062369709774,54.312503911864));
#91641=CARTESIAN_POINT('Ctrl Pts',(2.69598682288293,28.0873840785482,54.2456916318765));
#91642=CARTESIAN_POINT('Ctrl Pts',(2.69984559937711,28.1158259337503,54.1803136876999));
#91643=CARTESIAN_POINT('Ctrl Pts',(2.70370194496661,28.1442498715013,54.1149769295188));
#91644=CARTESIAN_POINT('Ctrl Pts',(2.70755829055611,28.1760968185179,54.0510731588551));
#91645=CARTESIAN_POINT('Ctrl Pts',(2.7114146361456,28.211192151875,53.9889787119025));
#91646=CARTESIAN_POINT('Ctrl Pts',(2.71526984239223,28.2462771164472,53.9269026105218));
#91647=CARTESIAN_POINT('Ctrl Pts',(2.71912504863886,28.2846083231466,53.866635194288));
#91648=CARTESIAN_POINT('Ctrl Pts',(2.72298025488549,28.3259652457834,53.8085281353825));
#91649=CARTESIAN_POINT('Ctrl Pts',(2.72683561173805,28.367323784053,53.7504188064904));
#91650=CARTESIAN_POINT('Ctrl Pts',(2.7306909685906,28.4117079894499,53.6944703969827));
#91651=CARTESIAN_POINT('Ctrl Pts',(2.73454632544316,28.4588550703749,53.641004095521));
#91652=CARTESIAN_POINT('Ctrl Pts',(2.73840571791303,28.5060515027824,53.5874818278957));
#91653=CARTESIAN_POINT('Ctrl Pts',(2.7422651103829,28.5560162619583,53.5364472199352));
#91654=CARTESIAN_POINT('Ctrl Pts',(2.74612450285277,28.6084480616532,53.4881862663068));
#91655=CARTESIAN_POINT('Ctrl Pts',(2.74998608045752,28.6609095475113,53.439897987991));
#91656=CARTESIAN_POINT('Ctrl Pts',(2.75384765806227,28.7158404802419,53.3943868002737));
#91657=CARTESIAN_POINT('Ctrl Pts',(2.75770923566703,28.7729068176881,53.3518980964687));
#91658=CARTESIAN_POINT('Ctrl Pts',(2.76157756978321,28.8300730027615,53.3093350511788));
#91659=CARTESIAN_POINT('Ctrl Pts',(2.76544590389939,28.8893816477604,53.2698053176901));
#91660=CARTESIAN_POINT('Ctrl Pts',(2.76931423801557,28.9504707055922,53.2335103106217));
#91661=CARTESIAN_POINT('Ctrl Pts',(2.77161195717492,28.9867564798794,53.211951745455));
#91662=CARTESIAN_POINT('Ctrl Pts',(2.77390967633428,29.0236699388517,53.1915335551998));
#91663=CARTESIAN_POINT('Ctrl Pts',(2.77620739549364,29.0611317998012,53.1722899395267));
#91664=CARTESIAN_POINT('Ctrl Pts',(2.78007646884162,29.1242129153393,53.1398860836347));
#91665=CARTESIAN_POINT('Ctrl Pts',(2.78394554218961,29.1890971270844,53.1106883390549));
#91666=CARTESIAN_POINT('Ctrl Pts',(2.78781461553759,29.2554254312286,53.0849004532299));
#91667=CARTESIAN_POINT('Ctrl Pts',(2.79167792393314,29.3216549056314,53.0591509915758));
#91668=CARTESIAN_POINT('Ctrl Pts',(2.7955412323287,29.3893237522684,53.0368014781914));
#91669=CARTESIAN_POINT('Ctrl Pts',(2.79940454072425,29.4580493505633,53.0180093198819));
#91670=CARTESIAN_POINT('Ctrl Pts',(2.80326331721693,29.5266943294242,52.9992392059518));
#91671=CARTESIAN_POINT('Ctrl Pts',(2.80712209370961,29.5963931312968,52.9840182856127));
#91672=CARTESIAN_POINT('Ctrl Pts',(2.8109808702023,29.6667458307197,52.9724548781452));
#91673=CARTESIAN_POINT('Ctrl Pts',(2.81483721579027,29.7370542102115,52.9608987552513));
#91674=CARTESIAN_POINT('Ctrl Pts',(2.81869356137825,29.8080151917614,52.952995652504));
#91675=CARTESIAN_POINT('Ctrl Pts',(2.82254990696622,29.8792178897378,52.948802972813));
#91676=CARTESIAN_POINT('Ctrl Pts',(2.82640511321133,29.9503995511435,52.9446115318337));
#91677=CARTESIAN_POINT('Ctrl Pts',(2.83026031945643,30.0218223025168,52.9441283661294));
#91678=CARTESIAN_POINT('Ctrl Pts',(2.83411552570153,30.093071083255,52.9473589364037));
#91679=CARTESIAN_POINT('Ctrl Pts',(2.83797088255255,30.164322647369,52.9505896328822));
#91680=CARTESIAN_POINT('Ctrl Pts',(2.84182623940357,30.2353997421671,52.9575343291708));
#91681=CARTESIAN_POINT('Ctrl Pts',(2.84568159625458,30.3058899943393,52.968146443795));
#91682=CARTESIAN_POINT('Ctrl Pts',(2.84954098872291,30.376454032595,52.9787696667121));
#91683=CARTESIAN_POINT('Ctrl Pts',(2.85340038119125,30.4464295206248,52.9930678987879));
#91684=CARTESIAN_POINT('Ctrl Pts',(2.85725977365958,30.5154127750105,53.0109431295571));
#91685=CARTESIAN_POINT('Ctrl Pts',(2.86112135126279,30.5844350867651,53.0288284810359));
#91686=CARTESIAN_POINT('Ctrl Pts',(2.864982928866,30.6524635830381,53.0502947165979));
#91687=CARTESIAN_POINT('Ctrl Pts',(2.86884450646921,30.7191109257491,53.075194285397));
#91688=CARTESIAN_POINT('Ctrl Pts',(2.87271284058386,30.7858748797468,53.1001374203855));
#91689=CARTESIAN_POINT('Ctrl Pts',(2.87658117469851,30.8512524096939,53.1285256886584));
#91690=CARTESIAN_POINT('Ctrl Pts',(2.88044950881317,30.9148779370555,53.1601641587389));
#91691=CARTESIAN_POINT('Ctrl Pts',(2.88274722798618,30.9526703277277,53.1789568268885));
#91692=CARTESIAN_POINT('Ctrl Pts',(2.88504494715919,30.9898450733868,53.1988953386927));
#91693=CARTESIAN_POINT('Ctrl Pts',(2.8873426663322,31.0263304413053,53.2199316339674));
#91694=CARTESIAN_POINT('Ctrl Pts',(2.89121173968022,31.0877672636396,53.2553541391823));
#91695=CARTESIAN_POINT('Ctrl Pts',(2.89508081302825,31.1474884268327,53.2940303836905));
#91696=CARTESIAN_POINT('Ctrl Pts',(2.89894988637627,31.2051280430109,53.3357692580508));
#91697=CARTESIAN_POINT('Ctrl Pts',(2.90281319477187,31.2626817756671,53.3774459411307));
#91698=CARTESIAN_POINT('Ctrl Pts',(2.90667650316746,31.3181597274908,53.4221759133552));
#91699=CARTESIAN_POINT('Ctrl Pts',(2.91053981156305,31.3712221345096,53.4697230903099));
#91700=CARTESIAN_POINT('Ctrl Pts',(2.91439858805577,31.4242222959994,53.517214491446));
#91701=CARTESIAN_POINT('Ctrl Pts',(2.91825736454848,31.47481218111,53.5675162103333));
#91702=CARTESIAN_POINT('Ctrl Pts',(2.9221161410412,31.5226838808883,53.6203510006589));
#91703=CARTESIAN_POINT('Ctrl Pts',(2.9259724866292,31.5705254230401,53.673152506771));
#91704=CARTESIAN_POINT('Ctrl Pts',(2.92982883221721,31.6156518517652,53.7284835592295));
#91705=CARTESIAN_POINT('Ctrl Pts',(2.93368517780522,31.6577920907689,53.7860300883942));
#91706=CARTESIAN_POINT('Ctrl Pts',(2.93754038405034,31.6999198795965,53.8435596156521));
#91707=CARTESIAN_POINT('Ctrl Pts',(2.94139559029547,31.7390629433785,53.9033029284216));
#91708=CARTESIAN_POINT('Ctrl Pts',(2.94525079654059,31.7749915803759,53.9649142779002));
#91709=CARTESIAN_POINT('Ctrl Pts',(2.94910615339163,31.8109216209466,54.0265280342627));
#91710=CARTESIAN_POINT('Ctrl Pts',(2.95296151024267,31.8436367426098,54.0900095514636));
#91711=CARTESIAN_POINT('Ctrl Pts',(2.95681686709371,31.872952424018,54.1549871126042));
#91712=CARTESIAN_POINT('Ctrl Pts',(2.96067625956206,31.9022987917871,54.2200326893865));
#91713=CARTESIAN_POINT('Ctrl Pts',(2.96453565203041,31.9282384157792,54.2865769924692));
#91714=CARTESIAN_POINT('Ctrl Pts',(2.96839504449875,31.9506346954674,54.3542277124723));
#91715=CARTESIAN_POINT('Ctrl Pts',(2.97225662210198,31.9730436556208,54.4219167353815));
#91716=CARTESIAN_POINT('Ctrl Pts',(2.9761181997052,31.9919051492532,54.4907129535365));
#91717=CARTESIAN_POINT('Ctrl Pts',(2.97997977730842,32.0071330619939,54.5602109210643));
#91718=CARTESIAN_POINT('Ctrl Pts',(2.98384811142308,32.022387618655,54.6298304875501));
#91719=CARTESIAN_POINT('Ctrl Pts',(2.98771644553774,32.0339958221669,54.7001537753634));
#91720=CARTESIAN_POINT('Ctrl Pts',(2.9915847796524,32.0419231662864,54.770767922221));
#91721=CARTESIAN_POINT('Ctrl Pts',(2.99388249882518,32.0466318625967,54.8127114240735));
#91722=CARTESIAN_POINT('Ctrl Pts',(2.99618021799797,32.0500428972691,54.8547574798927));
#91723=CARTESIAN_POINT('Ctrl Pts',(2.99847793717075,32.0521577425027,54.8968197577717));
#91724=CARTESIAN_POINT('Ctrl Pts',(3.00034353126794,32.0538748552077,54.9309715106294));
#91725=CARTESIAN_POINT('Ctrl Pts',(3.00220912536513,32.054739508502,54.9651664828388));
#91726=CARTESIAN_POINT('Ctrl Pts',(3.00407471946232,32.0547499051079,54.9993755329391));
#91727=CARTESIAN_POINT('Ctrl Pts',(3.00407471949931,32.0547499051081,54.9993755336174));
#91728=CARTESIAN_POINT('Ctrl Pts',(3.00791348792943,32.0547712978211,55.0697663124845));
#91729=CARTESIAN_POINT('Ctrl Pts',(3.01175225635954,32.0511712983844,55.1403032604116));
#91730=CARTESIAN_POINT('Ctrl Pts',(3.01559102478966,32.0439310014567,55.2105792577257));
#91731=CARTESIAN_POINT('Ctrl Pts',(3.01950861575714,32.0365420374276,55.2822982523253));
#91732=CARTESIAN_POINT('Ctrl Pts',(3.02342620672463,32.0253615175388,55.3537449447917));
#91733=CARTESIAN_POINT('Ctrl Pts',(3.02734379769211,32.0104254036403,55.4244846980724));
#91734=CARTESIAN_POINT('Ctrl Pts',(3.03117271153814,31.9958273780204,55.4936232127998));
#91735=CARTESIAN_POINT('Ctrl Pts',(3.03500162538417,31.9776420962988,55.5620859435654));
#91736=CARTESIAN_POINT('Ctrl Pts',(3.03883053923019,31.9559553954488,55.6294728377895));
#91737=CARTESIAN_POINT('Ctrl Pts',(3.04265730106963,31.934280883414,55.6968218578157));
#91738=CARTESIAN_POINT('Ctrl Pts',(3.04648406290907,31.9091090062367,55.7630957710834));
#91739=CARTESIAN_POINT('Ctrl Pts',(3.05031082474851,31.8805758631093,55.8279081987701));
#91740=CARTESIAN_POINT('Ctrl Pts',(3.05413676563536,31.8520488411774,55.8927067222914));
#91741=CARTESIAN_POINT('Ctrl Pts',(3.05796270652221,31.8201621840695,55.9560439306865));
#91742=CARTESIAN_POINT('Ctrl Pts',(3.06178864740907,31.7850999946472,56.0175537192751));
#91743=CARTESIAN_POINT('Ctrl Pts',(3.06577402745909,31.7485766519281,56.081626816997));
#91744=CARTESIAN_POINT('Ctrl Pts',(3.06975940750911,31.7086075443476,56.1437163194024));
#91745=CARTESIAN_POINT('Ctrl Pts',(3.07374478755913,31.6654523582068,56.203439240279));
#91746=CARTESIAN_POINT('Ctrl Pts',(3.07757550004278,31.623971970337,56.2608443900239));
#91747=CARTESIAN_POINT('Ctrl Pts',(3.08140621252642,31.579548618677,56.3160629059919));
#91748=CARTESIAN_POINT('Ctrl Pts',(3.08523692501007,31.5324542627966,56.368788330947));
#91749=CARTESIAN_POINT('Ctrl Pts',(3.08907026922274,31.4853275527304,56.4215499786756));
#91750=CARTESIAN_POINT('Ctrl Pts',(3.0929036134354,31.4355265377711,56.4718147802392));
#91751=CARTESIAN_POINT('Ctrl Pts',(3.09673695764807,31.3833590795809,56.5193140621482));
#91752=CARTESIAN_POINT('Ctrl Pts',(3.10057644985484,31.3311079541779,56.5668895243553));
#91753=CARTESIAN_POINT('Ctrl Pts',(3.10441594206161,31.2764832012901,56.6116903146892));
#91754=CARTESIAN_POINT('Ctrl Pts',(3.10825543426838,31.2198237246292,56.6534895352955));
#91755=CARTESIAN_POINT('Ctrl Pts',(3.10870802551535,31.213144824969,56.6584167393001));
#91756=CARTESIAN_POINT('Ctrl Pts',(3.10916061676233,31.2064376818367,56.6633022876482));
#91757=CARTESIAN_POINT('Ctrl Pts',(3.10961320800931,31.1997028730535,56.6681458506039));
#91758=CARTESIAN_POINT('Ctrl Pts',(3.11348228135748,31.1421289156642,56.7095520873955));
#91759=CARTESIAN_POINT('Ctrl Pts',(3.11735135470566,31.0822960432207,56.7480552898336));
#91760=CARTESIAN_POINT('Ctrl Pts',(3.12122042805383,31.0205290485874,56.783400690672));
#91761=CARTESIAN_POINT('Ctrl Pts',(3.12508373644957,30.9588540873052,56.8186934265603));
#91762=CARTESIAN_POINT('Ctrl Pts',(3.12894704484532,30.8952511424399,56.8508374611336));
#91763=CARTESIAN_POINT('Ctrl Pts',(3.13281035324106,30.8300752390306,56.8796203499772));
#91764=CARTESIAN_POINT('Ctrl Pts',(3.13666912973393,30.7649757910408,56.9083694746882));
#91765=CARTESIAN_POINT('Ctrl Pts',(3.1405279062268,30.6983074918813,56.933765090178));
#91766=CARTESIAN_POINT('Ctrl Pts',(3.14438668271967,30.6304497644057,56.9556407280124));
#91767=CARTESIAN_POINT('Ctrl Pts',(3.14824302830784,30.5626347851093,56.9775025849006));
#91768=CARTESIAN_POINT('Ctrl Pts',(3.15209937389601,30.4936323253602,56.9958487148634));
#91769=CARTESIAN_POINT('Ctrl Pts',(3.15595571948418,30.4238402027613,57.0105613755922));
#91770=CARTESIAN_POINT('Ctrl Pts',(3.15981092572947,30.3540686999839,57.0252696895204));
#91771=CARTESIAN_POINT('Ctrl Pts',(3.16366613197476,30.2835084726075,57.0363465652489));
#91772=CARTESIAN_POINT('Ctrl Pts',(3.16752133822006,30.2125691751471,57.0437250079884));
#91773=CARTESIAN_POINT('Ctrl Pts',(3.17137669507126,30.141627106401,57.0511037389711));
#91774=CARTESIAN_POINT('Ctrl Pts',(3.17523205192246,30.0703064215777,57.0547837020508));
#91775=CARTESIAN_POINT('Ctrl Pts',(3.17908740877366,29.9990218406574,57.0547497671747));
#91776=CARTESIAN_POINT('Ctrl Pts',(3.18294680124218,29.9276626421854,57.054715796777));
#91777=CARTESIAN_POINT('Ctrl Pts',(3.1868061937107,29.856340109839,57.0509601682432));
#91778=CARTESIAN_POINT('Ctrl Pts',(3.19066558617921,29.7854680019323,57.0435199006384));
#91779=CARTESIAN_POINT('Ctrl Pts',(3.19452716378261,29.7145557672138,57.0360754204565));
#91780=CARTESIAN_POINT('Ctrl Pts',(3.198388741386,29.64409494467,57.0249422240913));
#91781=CARTESIAN_POINT('Ctrl Pts',(3.2022503189894,29.5744904799988,57.0102087480877));
#91782=CARTESIAN_POINT('Ctrl Pts',(3.20611865310423,29.5047642300343,56.995449493268));
#91783=CARTESIAN_POINT('Ctrl Pts',(3.20998698721906,29.4358977989596,56.9770775072826));
#91784=CARTESIAN_POINT('Ctrl Pts',(3.21385532133389,29.3682816450929,56.9552313117822));
#91785=CARTESIAN_POINT('Ctrl Pts',(3.21615304050522,29.3281188958527,56.9422550742774));
#91786=CARTESIAN_POINT('Ctrl Pts',(3.21845075967655,29.2883969108282,56.9280540225236));
#91787=CARTESIAN_POINT('Ctrl Pts',(3.22074847884788,29.2491937605716,56.9126650395026));
#91788=CARTESIAN_POINT('Ctrl Pts',(3.22461723637989,29.1831859190886,56.8867540209954));
#91789=CARTESIAN_POINT('Ctrl Pts',(3.2284859939119,29.1183916904716,56.8573712555023));
#91790=CARTESIAN_POINT('Ctrl Pts',(3.23235475144391,29.0552011768238,56.824651404029));
#91791=CARTESIAN_POINT('Ctrl Pts',(3.23621738593897,28.9921106740573,56.791983337879));
#91792=CARTESIAN_POINT('Ctrl Pts',(3.24008002043403,28.9306192735358,56.7559888953893));
#91793=CARTESIAN_POINT('Ctrl Pts',(3.24394265492909,28.8710978213459,56.7168510225206));
#91794=CARTESIAN_POINT('Ctrl Pts',(3.24667302123064,28.8290241103887,56.6891857776388));
#91795=CARTESIAN_POINT('Ctrl Pts',(3.24940338753219,28.7879343494465,56.6599509191292));
#91796=CARTESIAN_POINT('Ctrl Pts',(3.25213375383374,28.7479524050421,56.6292250864936));
#91797=CARTESIAN_POINT('',(2.94592528057331,32.0547499982312,55.000085258463));
#91798=CARTESIAN_POINT('Ctrl Pts',(2.94592528057331,32.0547499982312,55.000085258463));
#91799=CARTESIAN_POINT('Ctrl Pts',(2.94997591064043,32.0547468813369,55.0752031797358));
#91800=CARTESIAN_POINT('Ctrl Pts',(2.95402654070755,32.0506202133317,55.1502363805521));
#91801=CARTESIAN_POINT('Ctrl Pts',(2.95807717077467,32.0424234247646,55.2247312093873));
#91802=CARTESIAN_POINT('Ctrl Pts',(2.96213971867067,32.0342025194745,55.2994452181052));
#91803=CARTESIAN_POINT('Ctrl Pts',(2.96620226656668,32.0218876070698,55.3736172816528));
#91804=CARTESIAN_POINT('Ctrl Pts',(2.97026481446268,32.0055836153857,55.446801884728));
#91805=CARTESIAN_POINT('Ctrl Pts',(2.97433371205498,31.9892541408277,55.5201008741474));
#91806=CARTESIAN_POINT('Ctrl Pts',(2.97840260964727,31.9689232661609,55.5924089327683));
#91807=CARTESIAN_POINT('Ctrl Pts',(2.98247150723956,31.9447455641139,55.6632965048598));
#91808=CARTESIAN_POINT('Ctrl Pts',(2.98655160384017,31.9205013166993,55.7343791839775));
#91809=CARTESIAN_POINT('Ctrl Pts',(2.99063170044077,31.8923892324745,55.8040331824788));
#91810=CARTESIAN_POINT('Ctrl Pts',(2.99471179704137,31.8606118986411,55.8718491412711));
#91811=CARTESIAN_POINT('Ctrl Pts',(2.99669196890795,31.8451895720123,55.904761904583));
#91812=CARTESIAN_POINT('Ctrl Pts',(2.99867214077452,31.8289046141135,55.9372421261628));
#91813=CARTESIAN_POINT('Ctrl Pts',(3.0006523126411,31.8117839056032,55.9692453981822));
#91814=CARTESIAN_POINT('Ctrl Pts',(3.00452138598909,31.7783316189031,56.0317768425022));
#91815=CARTESIAN_POINT('Ctrl Pts',(3.00839045933708,31.7415727162695,56.0926968909224));
#91816=CARTESIAN_POINT('Ctrl Pts',(3.01225953268507,31.7016865835042,56.1516337673158));
#91817=CARTESIAN_POINT('Ctrl Pts',(3.01612284108062,31.6618598814184,56.2104828272583));
#91818=CARTESIAN_POINT('Ctrl Pts',(3.01998614947618,31.6189154684274,56.2673541816167));
#91819=CARTESIAN_POINT('Ctrl Pts',(3.02384945787173,31.5730785127529,56.3219007357647));
#91820=CARTESIAN_POINT('Ctrl Pts',(3.02770823436442,31.5272953267001,56.376383303386));
#91821=CARTESIAN_POINT('Ctrl Pts',(3.0315670108571,31.4786266488835,56.4285461177085));
#91822=CARTESIAN_POINT('Ctrl Pts',(3.03542578734978,31.4273398009177,56.4780726150012));
#91823=CARTESIAN_POINT('Ctrl Pts',(3.03928213293776,31.3760852620116,56.5275679121982));
#91824=CARTESIAN_POINT('Ctrl Pts',(3.04313847852574,31.3222161738864,56.5744298507));
#91825=CARTESIAN_POINT('Ctrl Pts',(3.04699482411372,31.2660378333485,56.6183775106662));
#91826=CARTESIAN_POINT('Ctrl Pts',(3.05085003035883,31.209876090491,56.6623121864608));
#91827=CARTESIAN_POINT('Ctrl Pts',(3.05470523660393,31.1514068321055,56.7033339939137));
#91828=CARTESIAN_POINT('Ctrl Pts',(3.05856044284904,31.0909683329546,56.7412023601495));
#91829=CARTESIAN_POINT('Ctrl Pts',(3.06241579970006,31.030527472738,56.7790722057355));
#91830=CARTESIAN_POINT('Ctrl Pts',(3.06627115655108,30.9681176318487,56.8137881094637));
#91831=CARTESIAN_POINT('Ctrl Pts',(3.0701265134021,30.9041044757656,56.845153830823));
#91832=CARTESIAN_POINT('Ctrl Pts',(3.07398590587044,30.8400243135373,56.8765523844344));
#91833=CARTESIAN_POINT('Ctrl Pts',(3.07784529833877,30.774337923019,56.9045935410831));
#91834=CARTESIAN_POINT('Ctrl Pts',(3.08170469080711,30.70743307459,56.9291283024921));
#91835=CARTESIAN_POINT('Ctrl Pts',(3.08556626841032,30.640490345557,56.9536769551453));
#91836=CARTESIAN_POINT('Ctrl Pts',(3.08942784601353,30.5723282496859,56.974715117157));
#91837=CARTESIAN_POINT('Ctrl Pts',(3.09328942361675,30.5033492915548,56.9921438334597));
#91838=CARTESIAN_POINT('Ctrl Pts',(3.0971577577314,30.4342496425641,57.009603044377));
#91839=CARTESIAN_POINT('Ctrl Pts',(3.10102609184606,30.36433075448,57.0234401064428));
#91840=CARTESIAN_POINT('Ctrl Pts',(3.10489442596071,30.2940041845394,57.0336074109752));
#91841=CARTESIAN_POINT('Ctrl Pts',(3.1071921451337,30.2522314980719,57.0396466024901));
#91842=CARTESIAN_POINT('Ctrl Pts',(3.10948986430668,30.2103150725664,57.0443920466834));
#91843=CARTESIAN_POINT('Ctrl Pts',(3.11178758347967,30.1683412431117,57.0478424715704));
#91844=CARTESIAN_POINT('Ctrl Pts',(3.11565566451447,30.0976806612701,57.053651067862));
#91845=CARTESIAN_POINT('Ctrl Pts',(3.11952374554928,30.0265807194194,57.0558095440457));
#91846=CARTESIAN_POINT('Ctrl Pts',(3.12339182658408,29.95545073906,57.0542670045176));
#91847=CARTESIAN_POINT('Ctrl Pts',(3.12725460112043,29.8844183396786,57.0527265811509));
#91848=CARTESIAN_POINT('Ctrl Pts',(3.13111737565678,29.8133564647233,57.0474952245098));
#91849=CARTESIAN_POINT('Ctrl Pts',(3.13498015019314,29.7426786744688,57.0385738392138));
#91850=CARTESIAN_POINT('Ctrl Pts',(3.13883891816641,29.6720741929262,57.0296617073942));
#91851=CARTESIAN_POINT('Ctrl Pts',(3.14269768613968,29.6018534849097,57.0170672030055));
#91852=CARTESIAN_POINT('Ctrl Pts',(3.14655645411294,29.5324274942923,57.0008432008546));
#91853=CARTESIAN_POINT('Ctrl Pts',(3.15049843891761,29.4615042872069,56.984269317586));
#91854=CARTESIAN_POINT('Ctrl Pts',(3.15444042372228,29.3914109959895,56.9639075844468));
#91855=CARTESIAN_POINT('Ctrl Pts',(3.15838240852694,29.322576421289,56.9398698042669));
#91856=CARTESIAN_POINT('Ctrl Pts',(3.16223780698054,29.2552538094563,56.9163600179216));
#91857=CARTESIAN_POINT('Ctrl Pts',(3.16609320543414,29.1891356459562,56.8893342362753));
#91858=CARTESIAN_POINT('Ctrl Pts',(3.16994860388774,29.1246071532437,56.8589472629281));
#91859=CARTESIAN_POINT('Ctrl Pts',(3.17393388186794,29.0579048436906,56.8275366221803));
#91860=CARTESIAN_POINT('Ctrl Pts',(3.17791915984814,28.9929017427155,56.7925344658481));
#91861=CARTESIAN_POINT('Ctrl Pts',(3.18190443782834,28.9299978980659,56.7541644918184));
#91862=CARTESIAN_POINT('Ctrl Pts',(3.18588971580853,28.8670940534163,56.7157945177888));
#91863=CARTESIAN_POINT('Ctrl Pts',(3.18987499378873,28.8062899352195,56.6740570529051));
#91864=CARTESIAN_POINT('Ctrl Pts',(3.19386027176893,28.7479524050421,56.6292250864936));
#91865=CARTESIAN_POINT('Ctrl Pts',(2.49394378209486,28.7479524050421,56.6292250864936));
#91866=CARTESIAN_POINT('Ctrl Pts',(2.49779890937301,28.6914083389449,56.5857713841458));
#91867=CARTESIAN_POINT('Ctrl Pts',(2.50165403665116,28.6371162652407,56.5393607504666));
#91868=CARTESIAN_POINT('Ctrl Pts',(2.50550916392931,28.5853921214667,56.4902624307455));
#91869=CARTESIAN_POINT('Ctrl Pts',(2.50936473451369,28.5336620298643,56.441158465143));
#91870=CARTESIAN_POINT('Ctrl Pts',(2.51322030509808,28.48450080496,56.3893665362161));
#91871=CARTESIAN_POINT('Ctrl Pts',(2.51707587568247,28.438188038051,56.3351932287175));
#91872=CARTESIAN_POINT('Ctrl Pts',(2.52093566210309,28.3918246308965,56.2809606859415));
#91873=CARTESIAN_POINT('Ctrl Pts',(2.52479544852371,28.3483162124722,56.2243419389469));
#91874=CARTESIAN_POINT('Ctrl Pts',(2.52865523494433,28.3079019058973,56.1656764570129));
#91875=CARTESIAN_POINT('Ctrl Pts',(2.5325174695175,28.2674619656793,56.1069737652352));
#91876=CARTESIAN_POINT('Ctrl Pts',(2.53637970409067,28.2301202966293,56.0462221690235));
#91877=CARTESIAN_POINT('Ctrl Pts',(2.54024193866385,28.1960710714782,55.9837875702315));
#91878=CARTESIAN_POINT('Ctrl Pts',(2.54411066705154,28.161964597253,55.9212479962764));
#91879=CARTESIAN_POINT('Ctrl Pts',(2.54797939543923,28.1311618222452,55.8570202108948));
#91880=CARTESIAN_POINT('Ctrl Pts',(2.55184812382693,28.103809277651,55.7914911919774));
#91881=CARTESIAN_POINT('Ctrl Pts',(2.55326915898024,28.0937623259125,55.7674215158171));
#91882=CARTESIAN_POINT('Ctrl Pts',(2.55469019413355,28.0841803910862,55.743176430814));
#91883=CARTESIAN_POINT('Ctrl Pts',(2.55611122928687,28.0750690305662,55.7187755737466));
#91884=CARTESIAN_POINT('Ctrl Pts',(2.55998030264427,28.0502613949809,55.6523390005508));
#91885=CARTESIAN_POINT('Ctrl Pts',(2.56384937600167,28.0288486677511,55.5844864813534));
#91886=CARTESIAN_POINT('Ctrl Pts',(2.56771844935906,28.0109912325788,55.5155983762792));
#91887=CARTESIAN_POINT('Ctrl Pts',(2.57158175776416,27.9931604051373,55.4468129150691));
#91888=CARTESIAN_POINT('Ctrl Pts',(2.57544506616926,27.9788744754376,55.3769953972689));
#91889=CARTESIAN_POINT('Ctrl Pts',(2.57930837457436,27.9682450435054,55.3065442207244));
#91890=CARTESIAN_POINT('Ctrl Pts',(2.58316715107673,27.9576280805626,55.2361756878225));
#91891=CARTESIAN_POINT('Ctrl Pts',(2.5870259275791,27.9506591675067,55.1651754506821));
#91892=CARTESIAN_POINT('Ctrl Pts',(2.59088470408147,27.9473991304798,55.0939533551561));
#91893=CARTESIAN_POINT('Ctrl Pts',(2.59474104967922,27.9441411471711,55.022776127251));
#91894=CARTESIAN_POINT('Ctrl Pts',(2.59859739527697,27.9445874265286,54.9513778023797));
#91895=CARTESIAN_POINT('Ctrl Pts',(2.60245374087473,27.9487469461884,54.880173159399));
#91896=CARTESIAN_POINT('Ctrl Pts',(2.60630894712967,27.9529052369337,54.8089895535622));
#91897=CARTESIAN_POINT('Ctrl Pts',(2.61016415338462,27.9607745616937,54.7380000007084));
#91898=CARTESIAN_POINT('Ctrl Pts',(2.61401935963957,27.9723118239717,54.6676173541004));
#91899=CARTESIAN_POINT('Ctrl Pts',(2.61787471650049,27.98384953696,54.5972319579517));
#91900=CARTESIAN_POINT('Ctrl Pts',(2.6217300733614,27.9990553911943,54.5274539941519));
#91901=CARTESIAN_POINT('Ctrl Pts',(2.62558543022232,28.0178349189445,54.458687563468));
#91902=CARTESIAN_POINT('Ctrl Pts',(2.62944482270057,28.0366341042751,54.3898491511208));
#91903=CARTESIAN_POINT('Ctrl Pts',(2.63330421517883,28.0590143022865,54.3220248551342));
#91904=CARTESIAN_POINT('Ctrl Pts',(2.63716360765709,28.0848309846897,54.2556041340152));
#91905=CARTESIAN_POINT('Ctrl Pts',(2.64102518527025,28.1106622841431,54.1891458063981));
#91906=CARTESIAN_POINT('Ctrl Pts',(2.64488676288341,28.1399337418262,54.1240930788353));
#91907=CARTESIAN_POINT('Ctrl Pts',(2.64874834049657,28.1724535394593,54.0608133853887));
#91908=CARTESIAN_POINT('Ctrl Pts',(2.6526166746211,28.2050302362161,53.9974229729533));
#91909=CARTESIAN_POINT('Ctrl Pts',(2.65648500874563,28.2408663759584,53.9358122083899));
#91910=CARTESIAN_POINT('Ctrl Pts',(2.66035334287016,28.2797256282689,53.8763213766983));
#91911=CARTESIAN_POINT('Ctrl Pts',(2.66265106195524,28.3028073070463,53.8409849204964));
#91912=CARTESIAN_POINT('Ctrl Pts',(2.66494878104033,28.3269547719297,53.8063958214775));
#91913=CARTESIAN_POINT('Ctrl Pts',(2.66724650012542,28.3521119068325,53.7726197024163));
#91914=CARTESIAN_POINT('Ctrl Pts',(2.67111557347256,28.3944733951337,53.7157449160783));
#91915=CARTESIAN_POINT('Ctrl Pts',(2.67498464681969,28.4398657576993,53.6609543818507));
#91916=CARTESIAN_POINT('Ctrl Pts',(2.67885372016682,28.4880564237835,53.6085891387381));
#91917=CARTESIAN_POINT('Ctrl Pts',(2.68271702856152,28.5361752853624,53.5563019202862));
#91918=CARTESIAN_POINT('Ctrl Pts',(2.68658033695623,28.5870838478484,53.5064331743903));
#91919=CARTESIAN_POINT('Ctrl Pts',(2.69044364535093,28.6405079277061,53.4592927377759));
#91920=CARTESIAN_POINT('Ctrl Pts',(2.69430242184279,28.6938693377704,53.4122075998477));
#91921=CARTESIAN_POINT('Ctrl Pts',(2.69816119833464,28.7497400413137,53.3678447338221));
#91922=CARTESIAN_POINT('Ctrl Pts',(2.7020199748265,28.8078086989003,53.3264775280618));
#91923=CARTESIAN_POINT('Ctrl Pts',(2.70587632041366,28.8658407751059,53.2851363823065));
#91924=CARTESIAN_POINT('Ctrl Pts',(2.70973266600082,28.9260676635307,53.2467874338958));
#91925=CARTESIAN_POINT('Ctrl Pts',(2.71358901158797,28.9881457595397,53.211663186488));
#91926=CARTESIAN_POINT('Ctrl Pts',(2.71744421783227,29.0502055148076,53.1765493164075));
#91927=CARTESIAN_POINT('Ctrl Pts',(2.72129942407657,29.1141149692776,53.1446584949986));
#91928=CARTESIAN_POINT('Ctrl Pts',(2.72515463032086,29.1795038929504,53.1161784317997));
#91929=CARTESIAN_POINT('Ctrl Pts',(2.72900998717109,29.2448953710806,53.0876972560102));
#91930=CARTESIAN_POINT('Ctrl Pts',(2.73286534402132,29.3117659869061,53.0626272949309));
#91931=CARTESIAN_POINT('Ctrl Pts',(2.73672070087155,29.3797250018685,53.0411083518497));
#91932=CARTESIAN_POINT('Ctrl Pts',(2.74058009333911,29.4477551533273,53.019566883689));
#91933=CARTESIAN_POINT('Ctrl Pts',(2.74443948580667,29.516875514126,53.0015840005375));
#91934=CARTESIAN_POINT('Ctrl Pts',(2.74829887827424,29.5866804962575,52.9872495061916));
#91935=CARTESIAN_POINT('Ctrl Pts',(2.7521604558767,29.656525001009,52.9729068958522));
#91936=CARTESIAN_POINT('Ctrl Pts',(2.75602203347916,29.7270544182035,52.962216859258));
#91937=CARTESIAN_POINT('Ctrl Pts',(2.75988361108161,29.7978560151366,52.9552175245558));
#91938=CARTESIAN_POINT('Ctrl Pts',(2.76375194519554,29.8687814919579,52.9482059432824));
#91939=CARTESIAN_POINT('Ctrl Pts',(2.76762027930946,29.9399796139013,52.9448979791088));
#91940=CARTESIAN_POINT('Ctrl Pts',(2.77148861342339,30.0110363155874,52.9452796389196));
#91941=CARTESIAN_POINT('Ctrl Pts',(2.77378633260359,30.0532426869962,52.9455063378143));
#91942=CARTESIAN_POINT('Ctrl Pts',(2.77608405178379,30.0953992151863,52.9470337898436));
#91943=CARTESIAN_POINT('Ctrl Pts',(2.77838177096398,30.1374203322452,52.9498504408737));
#91944=CARTESIAN_POINT('Ctrl Pts',(2.78225084431045,30.2081786674685,52.9545933309191));
#91945=CARTESIAN_POINT('Ctrl Pts',(2.78611991765693,30.2788297690568,52.9630130139421));
#91946=CARTESIAN_POINT('Ctrl Pts',(2.7899889910034,30.3489609772674,52.9750990644368));
#91947=CARTESIAN_POINT('Ctrl Pts',(2.7938522993974,30.4189876893763,52.9871671066127));
#91948=CARTESIAN_POINT('Ctrl Pts',(2.7977156077914,30.4884955709285,53.0028905906901));
#91949=CARTESIAN_POINT('Ctrl Pts',(2.80157891618539,30.5570756072926,53.0222072074508));
#91950=CARTESIAN_POINT('Ctrl Pts',(2.80543769267648,30.6255751949752,53.0415011646092));
#91951=CARTESIAN_POINT('Ctrl Pts',(2.80929646916757,30.6931486341189,53.0643797510298));
#91952=CARTESIAN_POINT('Ctrl Pts',(2.81315524565865,30.7593973799234,53.0907296729207));
#91953=CARTESIAN_POINT('Ctrl Pts',(2.817011591245,30.8256043911547,53.1170629952106));
#91954=CARTESIAN_POINT('Ctrl Pts',(2.82086793683135,30.8904879143848,53.1468631352238));
#91955=CARTESIAN_POINT('Ctrl Pts',(2.8247242824177,30.9536662543494,53.1799675173736));
#91956=CARTESIAN_POINT('Ctrl Pts',(2.82857948866116,31.0168259285095,53.2130621189575));
#91957=CARTESIAN_POINT('Ctrl Pts',(2.83243469490461,31.0782809895073,53.2494587992554));
#91958=CARTESIAN_POINT('Ctrl Pts',(2.83628990114807,31.1376729349282,53.2889483188308));
#91959=CARTESIAN_POINT('Ctrl Pts',(2.84014525799743,31.1970672005305,53.3284393810876));
#91960=CARTESIAN_POINT('Ctrl Pts',(2.8440006148468,31.2543977872325,53.3710232516974));
#91961=CARTESIAN_POINT('Ctrl Pts',(2.84785597169616,31.3093353176415,53.4164474784597));
#91962=CARTESIAN_POINT('Ctrl Pts',(2.8517153641628,31.3643303542309,53.4619192532963));
#91963=CARTESIAN_POINT('Ctrl Pts',(2.85557475662944,31.4169269589407,53.5102370091911));
#91964=CARTESIAN_POINT('Ctrl Pts',(2.85943414909608,31.4668297073214,53.5611087003462));
#91965=CARTESIAN_POINT('Ctrl Pts',(2.86329572669758,31.5167607099511,53.6120091943524));
#91966=CARTESIAN_POINT('Ctrl Pts',(2.86715730429908,31.5639944981892,53.6654661379542));
#91967=CARTESIAN_POINT('Ctrl Pts',(2.87101888190058,31.6082751875232,53.7211534557667));
#91968=CARTESIAN_POINT('Ctrl Pts',(2.87488721601352,31.6526333537369,53.7769382083685));
#91969=CARTESIAN_POINT('Ctrl Pts',(2.87875555012646,31.6940278228252,53.8349607309145));
#91970=CARTESIAN_POINT('Ctrl Pts',(2.8826238842394,31.7322457768227,53.8948655596807));
#91971=CARTESIAN_POINT('Ctrl Pts',(2.88492160342711,31.7549465373184,53.930447924201));
#91972=CARTESIAN_POINT('Ctrl Pts',(2.88721932261482,31.7765274452677,53.9666938950511));
#91973=CARTESIAN_POINT('Ctrl Pts',(2.88951704180254,31.7969517988388,54.0035253163527));
#91974=CARTESIAN_POINT('Ctrl Pts',(2.89357123056584,31.8329893552072,54.068512167303));
#91975=CARTESIAN_POINT('Ctrl Pts',(2.89762541932915,31.865553742363,54.1355570099445));
#91976=CARTESIAN_POINT('Ctrl Pts',(2.90167960809246,31.8944168444321,54.2042724197114));
#91977=CARTESIAN_POINT('Ctrl Pts',(2.90572241802795,31.9231989368867,54.2727949670188));
#91978=CARTESIAN_POINT('Ctrl Pts',(2.90976522796344,31.9483002686522,54.3429783611878));
#91979=CARTESIAN_POINT('Ctrl Pts',(2.91380803789893,31.9695390126303,54.4144117144042));
#91980=CARTESIAN_POINT('Ctrl Pts',(2.91784402707856,31.9907419240342,54.4857245500916));
#91981=CARTESIAN_POINT('Ctrl Pts',(2.92188001625818,32.0080950853209,54.5582827532557));
#91982=CARTESIAN_POINT('Ctrl Pts',(2.92591600543781,32.0214649404899,54.631656333202));
#91983=CARTESIAN_POINT('Ctrl Pts',(2.92994364806252,32.0348071463701,54.7048781742343));
#91984=CARTESIAN_POINT('Ctrl Pts',(2.93397129068723,32.0441823724226,54.778911624555));
#91985=CARTESIAN_POINT('Ctrl Pts',(2.93799893331194,32.0495074524647,54.853314060689));
#91986=CARTESIAN_POINT('Ctrl Pts',(2.94064104905385,32.0530006814121,54.902121729607));
#91987=CARTESIAN_POINT('Ctrl Pts',(2.94328316479577,32.0547520312807,54.9510878823305));
#91988=CARTESIAN_POINT('Ctrl Pts',(2.94592528053768,32.0547499982312,55.0000852578023));
#91989=CARTESIAN_POINT('Origin',(-1.54592528053767,30.,55.));
#91990=CARTESIAN_POINT('',(1.79398372125809,28.7479524050421,56.6292250864936));
#91991=CARTESIAN_POINT('',(1.85198267906976,28.7489102161968,56.6279533026672));
#91992=CARTESIAN_POINT('',(-1.54592528053767,28.7479524050421,56.6292250864936));
#91993=CARTESIAN_POINT('',(2.30407472893336,32.05474914222,55.0018775106353));
#91994=CARTESIAN_POINT('Ctrl Pts',(1.85198267906975,28.748910216197,56.6279533026674));
#91995=CARTESIAN_POINT('Ctrl Pts',(1.86369686230822,28.5761851337391,56.4975417835351));
#91996=CARTESIAN_POINT('Ctrl Pts',(1.91245613582621,27.9428459579379,55.8463605828614));
#91997=CARTESIAN_POINT('Ctrl Pts',(1.99826049962372,27.759896125161,54.0618362182718));
#91998=CARTESIAN_POINT('Ctrl Pts',(2.10939577046228,29.5732403634016,52.6091648250566));
#91999=CARTESIAN_POINT('Ctrl Pts',(2.21133384374181,31.5947942490703,53.2838822194413));
#92000=CARTESIAN_POINT('Ctrl Pts',(2.27622682674183,32.0498098766772,54.4882110177461));
#92001=CARTESIAN_POINT('Ctrl Pts',(2.30407471946232,32.0544624073133,55.0018770739377));
#92002=CARTESIAN_POINT('Ctrl Pts',(2.30407472893336,32.05474914222,55.0018775106353));
#92003=CARTESIAN_POINT('Ctrl Pts',(2.30909837625834,32.0546644608409,55.0945528797447));
#92004=CARTESIAN_POINT('Ctrl Pts',(2.31412202358331,32.0483061176117,55.1869490612125));
#92005=CARTESIAN_POINT('Ctrl Pts',(2.31914567090828,32.0358091112648,55.2783501841048));
#92006=CARTESIAN_POINT('Ctrl Pts',(2.32331921798532,32.0254268449677,55.3542844335871));
#92007=CARTESIAN_POINT('Ctrl Pts',(2.32749276506236,32.0108086115702,55.4295325551524));
#92008=CARTESIAN_POINT('Ctrl Pts',(2.3316663121394,31.992056109336,55.5036963567041));
#92009=CARTESIAN_POINT('Ctrl Pts',(2.33553538549684,31.9746716626195,55.5724496697432));
#92010=CARTESIAN_POINT('Ctrl Pts',(2.33940445885429,31.9536895845222,55.6404365923658));
#92011=CARTESIAN_POINT('Ctrl Pts',(2.34327353221173,31.9291943063137,55.7072530600759));
#92012=CARTESIAN_POINT('Ctrl Pts',(2.34713684061688,31.9047355262786,55.7739699706794));
#92013=CARTESIAN_POINT('Ctrl Pts',(2.35100014902202,31.8767741027081,55.8395194357512));
#92014=CARTESIAN_POINT('Ctrl Pts',(2.35486345742717,31.8454448503109,55.9035103026313));
#92015=CARTESIAN_POINT('Ctrl Pts',(2.35872223392959,31.814152349089,55.9674261042166));
#92016=CARTESIAN_POINT('Ctrl Pts',(2.36258101043202,31.7795000789876,56.0297865051145));
#92017=CARTESIAN_POINT('Ctrl Pts',(2.36643978693444,31.7416711269176,56.0902198164414));
#92018=CARTESIAN_POINT('Ctrl Pts',(2.37029613253224,31.7038660058662,56.1506150567333));
#92019=CARTESIAN_POINT('Ctrl Pts',(2.37415247813005,31.6628884303501,56.2090852052249));
#92020=CARTESIAN_POINT('Ctrl Pts',(2.37800882372785,31.6189669376859,56.2652840065297));
#92021=CARTESIAN_POINT('Ctrl Pts',(2.38186402998285,31.5750584214616,56.32146620411));
#92022=CARTESIAN_POINT('Ctrl Pts',(2.38571923623786,31.5282080137986,56.375378004196));
#92023=CARTESIAN_POINT('Ctrl Pts',(2.38957444249286,31.4786859869049,56.4267043543184));
#92024=CARTESIAN_POINT('Ctrl Pts',(2.39342979935383,31.4291620254032,56.4780327095358));
#92025=CARTESIAN_POINT('Ctrl Pts',(2.3972851562148,31.3769665763488,56.5267750662));
#92026=CARTESIAN_POINT('Ctrl Pts',(2.40114051307577,31.3224071856569,56.5726527899772));
#92027=CARTESIAN_POINT('Ctrl Pts',(2.40499990555408,31.2677906846039,56.6185785365299));
#92028=CARTESIAN_POINT('Ctrl Pts',(2.40885929803238,31.2108056748858,56.6616333510883));
#92029=CARTESIAN_POINT('Ctrl Pts',(2.41271869051069,31.1517925480879,56.7015791161945));
#92030=CARTESIAN_POINT('Ctrl Pts',(2.4165802681239,31.0927460088698,56.7415474980431));
#92031=CARTESIAN_POINT('Ctrl Pts',(2.42044184573711,31.0316694828008,56.7784030751206));
#92032=CARTESIAN_POINT('Ctrl Pts',(2.42430342335032,30.9689297294892,56.8119527427094));
#92033=CARTESIAN_POINT('Ctrl Pts',(2.42817175747491,30.9060802019094,56.8455611113611));
#92034=CARTESIAN_POINT('Ctrl Pts',(2.43204009159949,30.8415620768424,56.8758518155404));
#92035=CARTESIAN_POINT('Ctrl Pts',(2.43590842572407,30.7757632823584,56.9026793981763));
#92036=CARTESIAN_POINT('Ctrl Pts',(2.4382061448087,30.7366800126712,56.9186144871918));
#92037=CARTESIAN_POINT('Ctrl Pts',(2.44050386389333,30.6971452387346,56.9333286803501));
#92038=CARTESIAN_POINT('Ctrl Pts',(2.44280158297796,30.6572424405911,56.946799922125));
#92039=CARTESIAN_POINT('Ctrl Pts',(2.4466706999575,30.590050330441,56.9694840746985));
#92040=CARTESIAN_POINT('Ctrl Pts',(2.45053981693705,30.5215508426835,56.9887299601902));
#92041=CARTESIAN_POINT('Ctrl Pts',(2.45440893391659,30.4521292551403,57.0043893581703));
#92042=CARTESIAN_POINT('Ctrl Pts',(2.45827227321803,30.382811333521,57.020025372272));
#92043=CARTESIAN_POINT('Ctrl Pts',(2.46213561251947,30.3125745154167,57.0320854237826));
#92044=CARTESIAN_POINT('Ctrl Pts',(2.46599895182091,30.2418205537346,57.0404706276473));
#92045=CARTESIAN_POINT('Ctrl Pts',(2.46985771066873,30.1711504793881,57.0488458898439));
#92046=CARTESIAN_POINT('Ctrl Pts',(2.47371646951655,30.099964959523,57.0535549025544));
#92047=CARTESIAN_POINT('Ctrl Pts',(2.47757522836436,30.0286755604101,57.0545498958982));
#92048=CARTESIAN_POINT('Ctrl Pts',(2.48143153828633,29.9574314044596,57.0555442577785));
#92049=CARTESIAN_POINT('Ctrl Pts',(2.48528784820829,29.8860839846391,57.0528292702121));
#92050=CARTESIAN_POINT('Ctrl Pts',(2.48914415813026,29.8150481441099,57.0464091412772));
#92051=CARTESIAN_POINT('Ctrl Pts',(2.49299931069921,29.7440336228069,57.0399909391468));
#92052=CARTESIAN_POINT('Ctrl Pts',(2.49685446326816,29.6733309786471,57.0298698472307));
#92053=CARTESIAN_POINT('Ctrl Pts',(2.50070961583712,29.6033514697071,57.0161020574159));
#92054=CARTESIAN_POINT('Ctrl Pts',(2.50456490098847,29.5333695541045,57.0023337941135));
#92055=CARTESIAN_POINT('Ctrl Pts',(2.50842018613982,29.4641112992215,56.9849186801397));
#92056=CARTESIAN_POINT('Ctrl Pts',(2.51227547129117,29.3959775776441,56.9639639700848));
#92057=CARTESIAN_POINT('Ctrl Pts',(2.5161345829473,29.3277762309751,56.9429884617504));
#92058=CARTESIAN_POINT('Ctrl Pts',(2.51999369460343,29.2607021103072,56.9184664888628));
#92059=CARTESIAN_POINT('Ctrl Pts',(2.52385280625956,29.1951398020452,56.890554845607));
#92060=CARTESIAN_POINT('Ctrl Pts',(2.52771409566082,29.1295404961499,56.8626274514607));
#92061=CARTESIAN_POINT('Ctrl Pts',(2.53157538506208,29.0654551374486,56.83130679249));
#92062=CARTESIAN_POINT('Ctrl Pts',(2.53543667446335,29.0032448017733,56.7967962147411));
#92063=CARTESIAN_POINT('Ctrl Pts',(2.53930424364821,28.9409332907121,56.7622295109324));
#92064=CARTESIAN_POINT('Ctrl Pts',(2.54317181283307,28.8805033005149,56.7244627914188));
#92065=CARTESIAN_POINT('Ctrl Pts',(2.54703938201794,28.8222872461249,56.6837429233289));
#92066=CARTESIAN_POINT('Ctrl Pts',(2.54871360714405,28.7970862021761,56.6661157722607));
#92067=CARTESIAN_POINT('Ctrl Pts',(2.55038783227017,28.7722996118778,56.6479357373517));
#92068=CARTESIAN_POINT('Ctrl Pts',(2.55206205739628,28.7479524050421,56.6292250864936));
#92069=CARTESIAN_POINT('',(2.24592528056623,32.0547491760433,54.9981598779361));
#92070=CARTESIAN_POINT('Ctrl Pts',(2.24592528056623,32.0547491760433,54.9981598779361));
#92071=CARTESIAN_POINT('Ctrl Pts',(2.24973199312511,32.0548119776976,55.0682865558832));
#92072=CARTESIAN_POINT('Ctrl Pts',(2.25353870568399,32.0512805113251,55.1385255805531));
#92073=CARTESIAN_POINT('Ctrl Pts',(2.25734541824288,32.044146919601,55.2084728605491));
#92074=CARTESIAN_POINT('Ctrl Pts',(2.26114901960424,32.0370191581078,55.2783629731596));
#92075=CARTESIAN_POINT('Ctrl Pts',(2.26495262096559,32.0262951561432,55.3479613175541));
#92076=CARTESIAN_POINT('Ctrl Pts',(2.26875622232695,32.0120190898361,55.4168653795114));
#92077=CARTESIAN_POINT('Ctrl Pts',(2.27255807195707,31.9977495983061,55.4857377080177));
#92078=CARTESIAN_POINT('Ctrl Pts',(2.27635992158718,31.9799313876817,55.5539158984091));
#92079=CARTESIAN_POINT('Ctrl Pts',(2.2801617712173,31.9586600131765,55.6210060509233));
#92080=CARTESIAN_POINT('Ctrl Pts',(2.28396322602705,31.9373908476939,55.6880892361555));
#92081=CARTESIAN_POINT('Ctrl Pts',(2.28776468083681,31.9126693830407,55.7540841309633));
#92082=CARTESIAN_POINT('Ctrl Pts',(2.29156613564656,31.8846409249957,55.8186123296965));
#92083=CARTESIAN_POINT('Ctrl Pts',(2.29537111074416,31.8565865115612,55.8832002839301));
#92084=CARTESIAN_POINT('Ctrl Pts',(2.29917608584177,31.8252191898369,55.9463183697466));
#92085=CARTESIAN_POINT('Ctrl Pts',(2.30298106093937,31.7907318497726,56.0076095497314));
#92086=CARTESIAN_POINT('Ctrl Pts',(2.30678785585504,31.7562280153338,56.0689300436522));
#92087=CARTESIAN_POINT('Ctrl Pts',(2.3105946507707,31.7186014616975,56.1284214698961));
#92088=CARTESIAN_POINT('Ctrl Pts',(2.31440144568637,31.6780888169565,56.1857552381945));
#92089=CARTESIAN_POINT('Ctrl Pts',(2.31821492477416,31.6375050379683,56.2431896761596));
#92090=CARTESIAN_POINT('Ctrl Pts',(2.32202840386194,31.5940253617011,56.2984584997057));
#92091=CARTESIAN_POINT('Ctrl Pts',(2.32584188294973,31.5479266015151,56.3512663685676));
#92092=CARTESIAN_POINT('Ctrl Pts',(2.32850815116974,31.5156957549742,56.3881880191841));
#92093=CARTESIAN_POINT('Ctrl Pts',(2.33117441938974,31.4821854249881,56.4239073940361));
#92094=CARTESIAN_POINT('Ctrl Pts',(2.33384068760975,31.44750006139,56.4583350557317));
#92095=CARTESIAN_POINT('Ctrl Pts',(2.33770976095523,31.3971674599028,56.5082937010076));
#92096=CARTESIAN_POINT('Ctrl Pts',(2.34157883430071,31.3441468440493,56.5557413933921));
#92097=CARTESIAN_POINT('Ctrl Pts',(2.34544790764619,31.2887188192779,56.6003753832582));
#92098=CARTESIAN_POINT('Ctrl Pts',(2.34931121603938,31.2333733827363,56.6449428680987));
#92099=CARTESIAN_POINT('Ctrl Pts',(2.35317452443257,31.1756280327693,56.6867046701));
#92100=CARTESIAN_POINT('Ctrl Pts',(2.35703783282577,31.1157998964758,56.7253950717226));
#92101=CARTESIAN_POINT('Ctrl Pts',(2.36089660931632,31.0560419423322,56.7640400870816));
#92102=CARTESIAN_POINT('Ctrl Pts',(2.36475538580687,30.9942064609002,56.7996205962112));
#92103=CARTESIAN_POINT('Ctrl Pts',(2.36861416229742,30.9306419148754,56.8319124402594));
#92104=CARTESIAN_POINT('Ctrl Pts',(2.3724705078834,30.8671174124616,56.8641839414887));
#92105=CARTESIAN_POINT('Ctrl Pts',(2.37632685346939,30.8018664385975,56.8931706684575));
#92106=CARTESIAN_POINT('Ctrl Pts',(2.38018319905538,30.7352632966772,56.9186936824463));
#92107=CARTESIAN_POINT('Ctrl Pts',(2.38403840529864,30.6686798324034,56.9442091557572));
#92108=CARTESIAN_POINT('Ctrl Pts',(2.3878936115419,30.6007454465498,56.9662627739661));
#92109=CARTESIAN_POINT('Ctrl Pts',(2.39174881778516,30.531854125668,56.98472384767));
#92110=CARTESIAN_POINT('Ctrl Pts',(2.39560417463449,30.4629601135034,57.0031856425673));
#92111=CARTESIAN_POINT('Ctrl Pts',(2.39945953148381,30.3931095618915,57.0180544907091));
#92112=CARTESIAN_POINT('Ctrl Pts',(2.40331488833313,30.3227096296274,57.0292501219529));
#92113=CARTESIAN_POINT('Ctrl Pts',(2.40717428080002,30.2522360058182,57.0404574722898));
#92114=CARTESIAN_POINT('Ctrl Pts',(2.41103367326691,30.1812123341334,57.0479838538699));
#92115=CARTESIAN_POINT('Ctrl Pts',(2.41489306573379,30.1100530385263,57.0518006460695));
#92116=CARTESIAN_POINT('Ctrl Pts',(2.41875464333569,30.0388534535032,57.0556195992844));
#92117=CARTESIAN_POINT('Ctrl Pts',(2.4226162209376,29.9675185777114,57.0557247813157));
#92118=CARTESIAN_POINT('Ctrl Pts',(2.4264777985395,29.896462232081,57.0521397352798));
#92119=CARTESIAN_POINT('Ctrl Pts',(2.43034613265307,29.8252815608309,57.0485484165731));
#92120=CARTESIAN_POINT('Ctrl Pts',(2.43421446676664,29.7543808761147,57.0412540285312));
#92121=CARTESIAN_POINT('Ctrl Pts',(2.43808280088021,29.684167582042,57.0303318561917));
#92122=CARTESIAN_POINT('Ctrl Pts',(2.44038052006958,29.6424621790435,57.0238442870631));
#92123=CARTESIAN_POINT('Ctrl Pts',(2.44267823925894,29.6009990977538,57.0160777639568));
#92124=CARTESIAN_POINT('Ctrl Pts',(2.44497595844831,29.5598612440212,57.0070564112614));
#92125=CARTESIAN_POINT('Ctrl Pts',(2.4488453513732,29.4905844930089,56.9918643205769));
#92126=CARTESIAN_POINT('Ctrl Pts',(2.45271474429808,29.4219595281757,56.9730514624946));
#92127=CARTESIAN_POINT('Ctrl Pts',(2.45658413722297,29.3543929934636,56.9506894052132));
#92128=CARTESIAN_POINT('Ctrl Pts',(2.46044683546966,29.2869433598302,56.9283660379228));
#92129=CARTESIAN_POINT('Ctrl Pts',(2.46430953371635,29.2205489751626,56.9025058240117));
#92130=CARTESIAN_POINT('Ctrl Pts',(2.46817223196304,29.1556048914633,56.8732310223727));
#92131=CARTESIAN_POINT('Ctrl Pts',(2.47203108508053,29.090725456457,56.8439853623822));
#92132=CARTESIAN_POINT('Ctrl Pts',(2.47588993819801,29.0272938988342,56.8113320565347));
#92133=CARTESIAN_POINT('Ctrl Pts',(2.4797487913155,28.9656875616429,56.7754422948549));
#92134=CARTESIAN_POINT('Ctrl Pts',(2.48360488003521,28.9041253578811,56.7395782438137));
#92135=CARTESIAN_POINT('Ctrl Pts',(2.48746096875492,28.8443861964193,56.7004825855419));
#92136=CARTESIAN_POINT('Ctrl Pts',(2.49131705747463,28.7868233519627,56.6583726912721));
#92137=CARTESIAN_POINT('Ctrl Pts',(2.49219263234804,28.7737529627907,56.6488110945287));
#92138=CARTESIAN_POINT('Ctrl Pts',(2.49306820722145,28.7607946693678,56.6390942729529));
#92139=CARTESIAN_POINT('Ctrl Pts',(2.49394378209486,28.7479524050421,56.6292250864936));
#92140=CARTESIAN_POINT('Ctrl Pts',(1.79398372125809,28.7479524050421,56.6292250864936));
#92141=CARTESIAN_POINT('Ctrl Pts',(1.79795521638298,28.689969871642,56.5846659325161));
#92142=CARTESIAN_POINT('Ctrl Pts',(1.80192671150787,28.6342860545768,56.5369438653214));
#92143=CARTESIAN_POINT('Ctrl Pts',(1.80589820663276,28.5812607271816,56.486329855134));
#92144=CARTESIAN_POINT('Ctrl Pts',(1.80975587549361,28.5297551485781,56.4371664834359));
#92145=CARTESIAN_POINT('Ctrl Pts',(1.81361354435446,28.4807580968254,56.3852750716134));
#92146=CARTESIAN_POINT('Ctrl Pts',(1.81747121321531,28.4345663209761,56.3309451375161));
#92147=CARTESIAN_POINT('Ctrl Pts',(1.82132695746882,28.3883975903995,56.2766423088531));
#92148=CARTESIAN_POINT('Ctrl Pts',(1.82518270172232,28.3450316727083,56.2199037415867));
#92149=CARTESIAN_POINT('Ctrl Pts',(1.82903844597583,28.304726946003,56.1610541911951));
#92150=CARTESIAN_POINT('Ctrl Pts',(1.83289355639876,28.2644288448327,56.1022143148487));
#92151=CARTESIAN_POINT('Ctrl Pts',(1.83674866682168,28.2271912092852,56.04126454557));
#92152=CARTESIAN_POINT('Ctrl Pts',(1.84060377724461,28.1932297341536,55.9785595377663));
#92153=CARTESIAN_POINT('Ctrl Pts',(1.84466176282885,28.1574810366108,55.9125546793286));
#92154=CARTESIAN_POINT('Ctrl Pts',(1.84871974841309,28.125363111767,55.844605265604));
#92155=CARTESIAN_POINT('Ctrl Pts',(1.85277773399733,28.0970720302535,55.7751533425434));
#92156=CARTESIAN_POINT('Ctrl Pts',(1.85663795219314,28.0701597247831,55.7090861839579));
#92157=CARTESIAN_POINT('Ctrl Pts',(1.86049817038895,28.0467100748932,55.6416600474042));
#92158=CARTESIAN_POINT('Ctrl Pts',(1.86435838858476,28.026841155681,55.5732728299735));
#92159=CARTESIAN_POINT('Ctrl Pts',(1.86822130676439,28.006958339389,55.5048377799148));
#92160=CARTESIAN_POINT('Ctrl Pts',(1.87208422494403,27.9906613465503,55.4354407840832));
#92161=CARTESIAN_POINT('Ctrl Pts',(1.87594714312366,27.9780172177736,55.3654903430737));
#92162=CARTESIAN_POINT('Ctrl Pts',(1.87981631658485,27.9653526141689,55.2954266302621));
#92163=CARTESIAN_POINT('Ctrl Pts',(1.88368549004604,27.9563527309751,55.2248081654246));
#92164=CARTESIAN_POINT('Ctrl Pts',(1.88755466350723,27.9510327507063,55.1540479594862));
#92165=CARTESIAN_POINT('Ctrl Pts',(1.88813631042332,27.9502330062265,55.1434106861825));
#92166=CARTESIAN_POINT('Ctrl Pts',(1.88871795733942,27.9495163266622,55.132770206435));
#92167=CARTESIAN_POINT('Ctrl Pts',(1.88929960425551,27.9488826620024,55.1221279176341));
#92168=CARTESIAN_POINT('Ctrl Pts',(1.89316867807688,27.9446675698584,55.0513361711988));
#92169=CARTESIAN_POINT('Ctrl Pts',(1.89703775189826,27.9441134566244,54.9801872885577));
#92170=CARTESIAN_POINT('Ctrl Pts',(1.90090682571963,27.9472620018025,54.9090919516438));
#92171=CARTESIAN_POINT('Ctrl Pts',(1.90477013459435,27.9504058556265,54.8381025472719));
#92172=CARTESIAN_POINT('Ctrl Pts',(1.90863344346907,27.9572413954818,54.7671670116155));
#92173=CARTESIAN_POINT('Ctrl Pts',(1.91249675234378,27.9677583715647,54.69669895128));
#92174=CARTESIAN_POINT('Ctrl Pts',(1.91635552932186,27.9782630105941,54.6263135542717));
#92175=CARTESIAN_POINT('Ctrl Pts',(1.92021430629993,27.9924404363935,54.5563950214545));
#92176=CARTESIAN_POINT('Ctrl Pts',(1.92407308327801,28.0102285014632,54.4873530004859));
#92177=CARTESIAN_POINT('Ctrl Pts',(1.92792942935496,28.0280053606438,54.4183544736937));
#92178=CARTESIAN_POINT('Ctrl Pts',(1.93178577543191,28.0493882254456,54.3502318325588));
#92179=CARTESIAN_POINT('Ctrl Pts',(1.93564212150886,28.0742639356115,54.2833842223245));
#92180=CARTESIAN_POINT('Ctrl Pts',(1.93949732824578,28.0991322963613,54.2165563619146));
#92181=CARTESIAN_POINT('Ctrl Pts',(1.94335253498271,28.1274912844472,54.1510032395835));
#92182=CARTESIAN_POINT('Ctrl Pts',(1.94720774171963,28.1591785242444,54.0871068754246));
#92183=CARTESIAN_POINT('Ctrl Pts',(1.95106309906459,28.1908670019396,54.0232080150816));
#92184=CARTESIAN_POINT('Ctrl Pts',(1.95491845640955,28.2258837716872,53.9609664756402));
#92185=CARTESIAN_POINT('Ctrl Pts',(1.9587738137545,28.2640199182091,53.9007408321395));
#92186=CARTESIAN_POINT('Ctrl Pts',(1.9626332067166,28.3021959839585,53.8404521471054));
#92187=CARTESIAN_POINT('Ctrl Pts',(1.9664925996787,28.3434976841852,53.7821839816096));
#92188=CARTESIAN_POINT('Ctrl Pts',(1.97035199264079,28.3876725456196,53.726266219985));
#92189=CARTESIAN_POINT('Ctrl Pts',(1.97421357073841,28.4318724182566,53.6703167984883));
#92190=CARTESIAN_POINT('Ctrl Pts',(1.97807514883603,28.4789483697121,53.6167207951661));
#92191=CARTESIAN_POINT('Ctrl Pts',(1.98193672693366,28.5286091840201,53.5657731598));
#92192=CARTESIAN_POINT('Ctrl Pts',(1.98580506153836,28.5783568886189,53.5147363826243));
#92193=CARTESIAN_POINT('Ctrl Pts',(1.98967339614307,28.630698128859,53.4663575547262));
#92194=CARTESIAN_POINT('Ctrl Pts',(1.99354173074778,28.6853071057159,53.4208926077626));
#92195=CARTESIAN_POINT('Ctrl Pts',(1.99583944552988,28.7177437654626,53.3938873221861));
#92196=CARTESIAN_POINT('Ctrl Pts',(1.99813716031198,28.7509799082505,53.367909293596));
#92197=CARTESIAN_POINT('Ctrl Pts',(2.00043487509407,28.7849426289779,53.3430047834635));
#92198=CARTESIAN_POINT('Ctrl Pts',(2.00430394846558,28.8421317367879,53.3010686050767));
#92199=CARTESIAN_POINT('Ctrl Pts',(2.00817302183709,28.9016064734258,53.2620144757941));
#92200=CARTESIAN_POINT('Ctrl Pts',(2.01204209520859,28.9630444126907,53.226100151517));
#92201=CARTESIAN_POINT('Ctrl Pts',(2.01590540362951,29.0243908089297,53.1902393398732));
#92202=CARTESIAN_POINT('Ctrl Pts',(2.01976871205043,29.08769418541,53.1575092900324));
#92203=CARTESIAN_POINT('Ctrl Pts',(2.02363202047135,29.1526014941873,53.1281257160679));
#92204=CARTESIAN_POINT('Ctrl Pts',(2.02749079699203,29.2174326626681,53.098776610857));
#92205=CARTESIAN_POINT('Ctrl Pts',(2.03134957351271,29.2838635857244,53.0727663832764));
#92206=CARTESIAN_POINT('Ctrl Pts',(2.03520835003339,29.3515163940419,53.0502649986976));
#92207=CARTESIAN_POINT('Ctrl Pts',(2.03906469565097,29.4191265833013,53.0277777892558));
#92208=CARTESIAN_POINT('Ctrl Pts',(2.04292104126856,29.4879566707864,53.0087951902587));
#92209=CARTESIAN_POINT('Ctrl Pts',(2.04677738688614,29.5576099432245,52.9934386129086));
#92210=CARTESIAN_POINT('Ctrl Pts',(2.05063259316243,29.6272426368925,52.9780865725956));
#92211=CARTESIAN_POINT('Ctrl Pts',(2.05448779943871,29.6976975585464,52.9663585316496));
#92212=CARTESIAN_POINT('Ctrl Pts',(2.05834300571499,29.7685656898447,52.9583252652337));
#92213=CARTESIAN_POINT('Ctrl Pts',(2.06219836259872,29.8394365896767,52.9502916849903));
#92214=CARTESIAN_POINT('Ctrl Pts',(2.06605371948246,29.9107202482591,52.9459532183724));
#92215=CARTESIAN_POINT('Ctrl Pts',(2.06990907636619,29.9820021030213,52.9453288247984));
#92216=CARTESIAN_POINT('Ctrl Pts',(2.07376846886937,30.0533585725203,52.9447037776364));
#92217=CARTESIAN_POINT('Ctrl Pts',(2.07762786137254,30.1247127476673,52.9478005685642));
#92218=CARTESIAN_POINT('Ctrl Pts',(2.08148725387572,30.195650545911,52.954586001225));
#92219=CARTESIAN_POINT('Ctrl Pts',(2.08534883151504,30.2666285081821,52.9613752757065));
#92220=CARTESIAN_POINT('Ctrl Pts',(2.08921040915435,30.3371891435098,52.9718572779838));
#92221=CARTESIAN_POINT('Ctrl Pts',(2.09307198679367,30.4069267067339,52.9859473150271));
#92222=CARTESIAN_POINT('Ctrl Pts',(2.09694032094603,30.4767862881588,53.0000620050822));
#92223=CARTESIAN_POINT('Ctrl Pts',(2.1008086550984,30.5458194516021,53.0177972128657));
#92224=CARTESIAN_POINT('Ctrl Pts',(2.10467698925076,30.6136344761209,53.0390180285847));
#92225=CARTESIAN_POINT('Ctrl Pts',(2.10697470814472,30.6539153456098,53.0516228003811));
#92226=CARTESIAN_POINT('Ctrl Pts',(2.10927242703867,30.693766781177,53.0654564044256));
#92227=CARTESIAN_POINT('Ctrl Pts',(2.11157014593263,30.7331103750084,53.0804826803191));
#92228=CARTESIAN_POINT('Ctrl Pts',(2.11543921914776,30.7993601001079,53.1057850624929));
#92229=CARTESIAN_POINT('Ctrl Pts',(2.1193082923629,30.8644281334726,53.1345708206484));
#92230=CARTESIAN_POINT('Ctrl Pts',(2.12317736557803,30.9279230507677,53.1667088680862));
#92231=CARTESIAN_POINT('Ctrl Pts',(2.12704067383826,30.9913233600482,53.1987990295357));
#92232=CARTESIAN_POINT('Ctrl Pts',(2.13090398209848,31.0531547760517,53.2342313478549));
#92233=CARTESIAN_POINT('Ctrl Pts',(2.13476729035871,31.1130445874744,53.2728262077041));
#92234=CARTESIAN_POINT('Ctrl Pts',(2.13862606671304,31.1728641443455,53.311375793332));
#92235=CARTESIAN_POINT('Ctrl Pts',(2.14248484306737,31.2307462144121,53.3530802895793));
#92236=CARTESIAN_POINT('Ctrl Pts',(2.1463436194217,31.2863430596233,53.3977144151373));
#92237=CARTESIAN_POINT('Ctrl Pts',(2.15019996486953,31.3419048805885,53.4423204226142));
#92238=CARTESIAN_POINT('Ctrl Pts',(2.15405631031736,31.3951839549608,53.4898520944146));
#92239=CARTESIAN_POINT('Ctrl Pts',(2.15791265576519,31.445863116871,53.5400419835584));
#92240=CARTESIAN_POINT('Ctrl Pts',(2.16176786186857,31.4965273057911,53.5902170442662));
#92241=CARTESIAN_POINT('Ctrl Pts',(2.16562306797194,31.5445927622341,53.6430484215114));
#92242=CARTESIAN_POINT('Ctrl Pts',(2.16947827407531,31.5897781880421,53.6982308671175));
#92243=CARTESIAN_POINT('Ctrl Pts',(2.17333363078323,31.6349653790295,53.7534154684389));
#92244=CARTESIAN_POINT('Ctrl Pts',(2.17718898749114,31.6772720099486,53.8109509432151));
#92245=CARTESIAN_POINT('Ctrl Pts',(2.18104434419906,31.7164573083123,53.8704992823193));
#92246=CARTESIAN_POINT('Ctrl Pts',(2.18490373652315,31.7556836241061,53.9301099539802));
#92247=CARTESIAN_POINT('Ctrl Pts',(2.18876312884725,31.79178181755,53.9917372893305));
#92248=CARTESIAN_POINT('Ctrl Pts',(2.19262252117135,31.8245551948391,54.0550153951065));
#92249=CARTESIAN_POINT('Ctrl Pts',(2.19648409862947,31.8573471279565,54.118329328062));
#92250=CARTESIAN_POINT('Ctrl Pts',(2.20034567608759,31.8868102967758,54.1832954494049));
#92251=CARTESIAN_POINT('Ctrl Pts',(2.20420725354571,31.9127957939903,54.2495269405282));
#92252=CARTESIAN_POINT('Ctrl Pts',(2.20807558751549,31.9388267574208,54.3158743153406));
#92253=CARTESIAN_POINT('Ctrl Pts',(2.21194392148527,31.961367747085,54.3834910192252));
#92254=CARTESIAN_POINT('Ctrl Pts',(2.21581225545505,31.9803196511975,54.4519747801598));
#92255=CARTESIAN_POINT('Ctrl Pts',(2.21810997589376,31.9915767395906,54.4926528959711));
#92256=CARTESIAN_POINT('Ctrl Pts',(2.22040769633247,32.0015685212364,54.5336367005789));
#92257=CARTESIAN_POINT('Ctrl Pts',(2.22270541677119,32.0102828504532,54.5748407078828));
#92258=CARTESIAN_POINT('Ctrl Pts',(2.22812785170467,32.0308479646294,54.6720788421834));
#92259=CARTESIAN_POINT('Ctrl Pts',(2.23355028663815,32.044363796373,54.7708559975936));
#92260=CARTESIAN_POINT('Ctrl Pts',(2.23897272157163,32.0506537445644,54.870320462662));
#92261=CARTESIAN_POINT('Ctrl Pts',(2.24129024122698,32.0533420347409,54.9128310424351));
#92262=CARTESIAN_POINT('Ctrl Pts',(2.24360776088233,32.0547109424995,54.9554668839174));
#92263=CARTESIAN_POINT('Ctrl Pts',(2.24592528053768,32.0547491760429,54.9981598774102));
#92264=CARTESIAN_POINT('Origin',(-1.54592528053767,30.,55.));
#92265=CARTESIAN_POINT('',(1.0938611646792,28.7479524050421,56.6292250864936));
#92266=CARTESIAN_POINT('',(1.15211015888001,28.7479524050421,56.6292250864936));
#92267=CARTESIAN_POINT('',(-1.54592528053767,28.7479524050421,56.6292250864936));
#92268=CARTESIAN_POINT('',(1.60407469463907,32.0544744411595,54.9994775005687));
#92269=CARTESIAN_POINT('Ctrl Pts',(1.15211015888001,28.7479524050421,56.6292250864936));
#92270=CARTESIAN_POINT('Ctrl Pts',(1.15596557431626,28.6914238068245,56.5857832710984));
#92271=CARTESIAN_POINT('Ctrl Pts',(1.15982098975252,28.637134064618,56.5393769881983));
#92272=CARTESIAN_POINT('Ctrl Pts',(1.16367640518878,28.5854020922282,56.4902718952686));
#92273=CARTESIAN_POINT('Ctrl Pts',(1.16753159109547,28.5336731996664,56.4411697257776));
#92274=CARTESIAN_POINT('Ctrl Pts',(1.17138677700217,28.4845021258141,56.3893694008486));
#92275=CARTESIAN_POINT('Ctrl Pts',(1.17524196290887,28.4381719776294,56.3351744421752));
#92276=CARTESIAN_POINT('Ctrl Pts',(1.17910094029473,28.3917962648997,56.280926184112));
#92277=CARTESIAN_POINT('Ctrl Pts',(1.18295991768059,28.3482673754369,56.224278958049));
#92278=CARTESIAN_POINT('Ctrl Pts',(1.18681889506645,28.307828457096,56.1655698314069));
#92279=CARTESIAN_POINT('Ctrl Pts',(1.19067971611772,28.2673702186535,56.1068326558866));
#92280=CARTESIAN_POINT('Ctrl Pts',(1.194540537169,28.2300051471003,56.0460320317991));
#92281=CARTESIAN_POINT('Ctrl Pts',(1.19840135822027,28.1959317990882,55.9835321494282));
#92282=CARTESIAN_POINT('Ctrl Pts',(1.20226929772362,28.1617956277824,55.9209170318751));
#92283=CARTESIAN_POINT('Ctrl Pts',(1.20613723722698,28.1309635168494,55.856596835388));
#92284=CARTESIAN_POINT('Ctrl Pts',(1.21000517673033,28.1035867777666,55.7909579337982));
#92285=CARTESIAN_POINT('Ctrl Pts',(1.21344131907149,28.0792662390809,55.7326466265028));
#92286=CARTESIAN_POINT('Ctrl Pts',(1.21687746141264,28.0576720240531,55.6732951092148));
#92287=CARTESIAN_POINT('Ctrl Pts',(1.2203136037538,28.0388768515798,55.6131831367794));
#92288=CARTESIAN_POINT('Ctrl Pts',(1.22418266805922,28.0177136622499,55.545497615114));
#92289=CARTESIAN_POINT('Ctrl Pts',(1.22805173236463,28.0000172432589,55.4765825943095));
#92290=CARTESIAN_POINT('Ctrl Pts',(1.23192079667004,27.9859270877188,55.4068265803942));
#92291=CARTESIAN_POINT('Ctrl Pts',(1.23578409586991,27.9718579272379,55.3371745065406));
#92292=CARTESIAN_POINT('Ctrl Pts',(1.23964739506977,27.9613844593252,55.2666843992818));
#92293=CARTESIAN_POINT('Ctrl Pts',(1.24351069426964,27.9545964859637,55.1957601268589));
#92294=CARTESIAN_POINT('Ctrl Pts',(1.24736946138368,27.9478164756607,55.1249190566094));
#92295=CARTESIAN_POINT('Ctrl Pts',(1.25122822849772,27.944713418032,55.0536453141185));
#92296=CARTESIAN_POINT('Ctrl Pts',(1.25508699561175,27.9453257944649,54.982351441733));
#92297=CARTESIAN_POINT('Ctrl Pts',(1.25894333171321,27.9459377851025,54.9111024842893));
#92298=CARTESIAN_POINT('Ctrl Pts',(1.26279966781467,27.9502605617029,54.8398339067335));
#92299=CARTESIAN_POINT('Ctrl Pts',(1.26665600391613,27.9582805657826,54.7689603617579));
#92300=CARTESIAN_POINT('Ctrl Pts',(1.27051120058094,27.9662982001813,54.6981077578807));
#92301=CARTESIAN_POINT('Ctrl Pts',(1.27436639724576,27.9780108387014,54.6276504373054));
#92302=CARTESIAN_POINT('Ctrl Pts',(1.27822159391058,27.9933530301187,54.5579983023039));
#92303=CARTESIAN_POINT('Ctrl Pts',(1.28207694110156,28.0086958205719,54.4883434477345));
#92304=CARTESIAN_POINT('Ctrl Pts',(1.28593228829254,28.0276683386305,54.419494315098));
#92305=CARTESIAN_POINT('Ctrl Pts',(1.28978763548352,28.0501543129043,54.3518492775485));
#92306=CARTESIAN_POINT('Ctrl Pts',(1.29364701823621,28.0726638242378,54.2841334329587));
#92307=CARTESIAN_POINT('Ctrl Pts',(1.2975064009889,28.0986939797298,54.217624661388));
#92308=CARTESIAN_POINT('Ctrl Pts',(1.30136578374159,28.1280793163987,54.1527039969375));
#92309=CARTESIAN_POINT('Ctrl Pts',(1.30522735158312,28.157481290332,54.0877465759825));
#92310=CARTESIAN_POINT('Ctrl Pts',(1.30908891942465,28.1902420037978,54.0243794838064));
#92311=CARTESIAN_POINT('Ctrl Pts',(1.31295048726618,28.2261499695875,53.9629591945804));
#92312=CARTESIAN_POINT('Ctrl Pts',(1.31681881165199,28.2621207631639,53.9014314389258));
#92313=CARTESIAN_POINT('Ctrl Pts',(1.32068713603781,28.3012495366031,53.8418576931656));
#92314=CARTESIAN_POINT('Ctrl Pts',(1.32455546042362,28.343281830513,53.7845649053151));
#92315=CARTESIAN_POINT('Ctrl Pts',(1.32685326514654,28.3682492308209,53.7505326925579));
#92316=CARTESIAN_POINT('Ctrl Pts',(1.32915106986945,28.3942403379088,53.7173046697533));
#92317=CARTESIAN_POINT('Ctrl Pts',(1.33144887459236,28.4211955479515,53.6849433226313));
#92318=CARTESIAN_POINT('Ctrl Pts',(1.33531795118427,28.4665831177334,53.6304528215963));
#92319=CARTESIAN_POINT('Ctrl Pts',(1.33918702777618,28.5148839095463,53.5782080925501));
#92320=CARTESIAN_POINT('Ctrl Pts',(1.34305610436809,28.565847175084,53.5285370418235));
#92321=CARTESIAN_POINT('Ctrl Pts',(1.34691941604287,28.6167345054482,53.4789400008727));
#92322=CARTESIAN_POINT('Ctrl Pts',(1.35078272771764,28.6702760899426,53.4319093626192));
#92323=CARTESIAN_POINT('Ctrl Pts',(1.35464603939242,28.7261813233442,53.3877396173376));
#92324=CARTESIAN_POINT('Ctrl Pts',(1.35850481920069,28.7820209769852,53.3436216854757));
#92325=CARTESIAN_POINT('Ctrl Pts',(1.36236359900897,28.8402183927242,53.3023582801752));
#92326=CARTESIAN_POINT('Ctrl Pts',(1.36622237881724,28.9004478436164,53.2642054793576));
#92327=CARTESIAN_POINT('Ctrl Pts',(1.37007872774143,28.9606393522521,53.2260767133492));
#92328=CARTESIAN_POINT('Ctrl Pts',(1.37393507666562,29.0228599469266,53.1910549234259));
#92329=CARTESIAN_POINT('Ctrl Pts',(1.3777914255898,29.0867539033691,53.1593536109594));
#92330=CARTESIAN_POINT('Ctrl Pts',(1.38164663518673,29.1506289828561,53.1276616643905));
#92331=CARTESIAN_POINT('Ctrl Pts',(1.38550184478365,29.2161760076978,53.0992884634977));
#92332=CARTESIAN_POINT('Ctrl Pts',(1.38935705438057,29.2830151001007,53.0744013357357));
#92333=CARTESIAN_POINT('Ctrl Pts',(1.39321241459403,29.3498568037942,53.0495132356756));
#92334=CARTESIAN_POINT('Ctrl Pts',(1.39706777480749,29.4179902192486,53.0281116465895));
#92335=CARTESIAN_POINT('Ctrl Pts',(1.40092313502095,29.4870175919196,53.0103149466561));
#92336=CARTESIAN_POINT('Ctrl Pts',(1.40478253084469,29.5561172192072,52.9924996179719));
#92337=CARTESIAN_POINT('Ctrl Pts',(1.40864192666842,29.6261122003175,52.9782968325805));
#92338=CARTESIAN_POINT('Ctrl Pts',(1.41250132249215,29.6965926683802,52.9677742365526));
#92339=CARTESIAN_POINT('Ctrl Pts',(1.41636290345185,29.7671130414986,52.9572456827779));
#92340=CARTESIAN_POINT('Ctrl Pts',(1.42022448441154,29.8381189649896,52.9504015129451));
#92341=CARTESIAN_POINT('Ctrl Pts',(1.42408606537124,29.9091962440461,52.9472573857386));
#92342=CARTESIAN_POINT('Ctrl Pts',(1.42795440280756,29.9803978845959,52.9441077573599));
#92343=CARTESIAN_POINT('Ctrl Pts',(1.43182274024388,30.0516706440507,52.9446710929736));
#92344=CARTESIAN_POINT('Ctrl Pts',(1.4356910776802,30.122601827308,52.9489109345422));
#92345=CARTESIAN_POINT('Ctrl Pts',(1.43798876693044,30.1647330580912,52.9514292873371));
#92346=CARTESIAN_POINT('Ctrl Pts',(1.44028645618068,30.2067438852967,52.955243733322));
#92347=CARTESIAN_POINT('Ctrl Pts',(1.44258414543092,30.2485494981069,52.9603380894151));
#92348=CARTESIAN_POINT('Ctrl Pts',(1.4464532193052,30.3189458775589,52.9689164644343));
#92349=CARTESIAN_POINT('Ctrl Pts',(1.45032229317949,30.3890355151986,52.9811603850249));
#92350=CARTESIAN_POINT('Ctrl Pts',(1.45419136705377,30.4584069262394,52.9970370316764));
#92351=CARTESIAN_POINT('Ctrl Pts',(1.45805467599527,30.5276749736498,53.0128900220722));
#92352=CARTESIAN_POINT('Ctrl Pts',(1.46191798493676,30.5962264490148,53.0323648868309));
#92353=CARTESIAN_POINT('Ctrl Pts',(1.46578129387826,30.6636563248155,53.0553771972353));
#92354=CARTESIAN_POINT('Ctrl Pts',(1.46964007094354,30.7310071016223,53.0783625129199));
#92355=CARTESIAN_POINT('Ctrl Pts',(1.47349884800882,30.7972384347695,53.1048768755598));
#92356=CARTESIAN_POINT('Ctrl Pts',(1.4773576250741,30.8619585198236,53.1347855156568));
#92357=CARTESIAN_POINT('Ctrl Pts',(1.48121397125084,30.9266378335891,53.1646753144036));
#92358=CARTESIAN_POINT('Ctrl Pts',(1.48507031742757,30.9898073481427,53.1979549450098));
#92359=CARTESIAN_POINT('Ctrl Pts',(1.48892666360431,31.0510947599586,53.2344413439119));
#92360=CARTESIAN_POINT('Ctrl Pts',(1.49278187045349,31.1123640648841,53.2709169631905));
#92361=CARTESIAN_POINT('Ctrl Pts',(1.49663707730267,31.1717519538029,53.310597221519));
#92362=CARTESIAN_POINT('Ctrl Pts',(1.50049228415185,31.2289118158825,53.3532537198207));
#92363=CARTESIAN_POINT('Ctrl Pts',(1.50434764162142,31.2860739111603,53.3959118846837));
#92364=CARTESIAN_POINT('Ctrl Pts',(1.508202999091,31.3410074187695,53.4415462280725));
#92365=CARTESIAN_POINT('Ctrl Pts',(1.51205835656057,31.3933971565771,53.4898867835348));
#92366=CARTESIAN_POINT('Ctrl Pts',(1.51591774966546,31.4458417338846,53.5382779399735));
#92367=CARTESIAN_POINT('Ctrl Pts',(1.51977714277035,31.4957368682545,53.589380633199));
#92368=CARTESIAN_POINT('Ctrl Pts',(1.52363653587523,31.5428034305105,53.6428872053859));
#92369=CARTESIAN_POINT('Ctrl Pts',(1.52749811412611,31.5898966413371,53.6964240724064));
#92370=CARTESIAN_POINT('Ctrl Pts',(1.53135969237699,31.6341577903864,53.75236714667));
#92371=CARTESIAN_POINT('Ctrl Pts',(1.53522127062787,31.675349078037,53.8103769381772));
#92372=CARTESIAN_POINT('Ctrl Pts',(1.53908960540088,31.7166124372159,53.8684882281948));
#92373=CARTESIAN_POINT('Ctrl Pts',(1.54295794017389,31.7547949507744,53.9286730447583));
#92374=CARTESIAN_POINT('Ctrl Pts',(1.5468262749469,31.7897034180098,53.9905648916032));
#92375=CARTESIAN_POINT('Ctrl Pts',(1.54912398872109,31.8104383519567,54.0273274153636));
#92376=CARTESIAN_POINT('Ctrl Pts',(1.55142170249528,31.8300190545549,54.0646917503932));
#92377=CARTESIAN_POINT('Ctrl Pts',(1.55371941626948,31.8484131225733,54.1025778636568));
#92378=CARTESIAN_POINT('Ctrl Pts',(1.55791568927328,31.8820058754753,54.1717685853616));
#92379=CARTESIAN_POINT('Ctrl Pts',(1.56211196227709,31.9117555147201,54.2429419085303));
#92380=CARTESIAN_POINT('Ctrl Pts',(1.5663082352809,31.9374425894471,54.3156654508967));
#92381=CARTESIAN_POINT('Ctrl Pts',(1.57045671771888,31.9628371189002,54.3875607584855));
#92382=CARTESIAN_POINT('Ctrl Pts',(1.57460520015686,31.9842609658738,54.4609708157442));
#92383=CARTESIAN_POINT('Ctrl Pts',(1.57875368259484,32.0015478850653,54.5354533109678));
#92384=CARTESIAN_POINT('Ctrl Pts',(1.58297385088156,32.0191335225213,54.6112228650054));
#92385=CARTESIAN_POINT('Ctrl Pts',(1.58719401916828,32.0324376878795,54.6881019450392));
#92386=CARTESIAN_POINT('Ctrl Pts',(1.591414187455,32.0413368548877,54.7656041651877));
#92387=CARTESIAN_POINT('Ctrl Pts',(1.59563435574172,32.0502360218958,54.8431063853363));
#92388=CARTESIAN_POINT('Ctrl Pts',(1.59985452402844,32.0547300321603,54.9212313568403));
#92389=CARTESIAN_POINT('Ctrl Pts',(1.60407469231516,32.0547499335384,54.9994773874789));
#92390=CARTESIAN_POINT('Ctrl Pts',(1.60407471946232,32.0515317218955,54.9994787085569));
#92391=CARTESIAN_POINT('Ctrl Pts',(1.62433470867756,32.0506800991794,55.3745305470031));
#92392=CARTESIAN_POINT('Ctrl Pts',(1.68163978817232,31.7726765815566,56.4365344554507));
#92393=CARTESIAN_POINT('Ctrl Pts',(1.76427577470813,30.2789783374865,57.3046346940974));
#92394=CARTESIAN_POINT('Ctrl Pts',(1.8266517720287,29.1224132525016,56.909956921782));
#92395=CARTESIAN_POINT('Ctrl Pts',(1.85198267906975,28.748910216197,56.6279533026674));
#92396=CARTESIAN_POINT('',(1.54592528048776,32.0547497261996,55.0010607463466));
#92397=CARTESIAN_POINT('Ctrl Pts',(1.54592528053768,32.0547497261991,55.0010607472628));
#92398=CARTESIAN_POINT('Ctrl Pts',(1.54924811760506,32.0547182463142,55.0620397260944));
#92399=CARTESIAN_POINT('Ctrl Pts',(1.55257095467244,32.0519724929102,55.1229466291482));
#92400=CARTESIAN_POINT('Ctrl Pts',(1.55589379173983,32.0465301511204,55.1836080146816));
#92401=CARTESIAN_POINT('Ctrl Pts',(1.55976286831917,32.0401931455047,55.2542414948306));
#92402=CARTESIAN_POINT('Ctrl Pts',(1.56363194489852,32.030182692726,55.3246848692759));
#92403=CARTESIAN_POINT('Ctrl Pts',(1.56750102147786,32.016518520056,55.3945258176229));
#92404=CARTESIAN_POINT('Ctrl Pts',(1.57136433313993,32.0028747069793,55.4642627030801));
#92405=CARTESIAN_POINT('Ctrl Pts',(1.575227644802,31.985588072785,55.5333984713152));
#92406=CARTESIAN_POINT('Ctrl Pts',(1.57909095646407,31.9647301330804,55.6015256159682));
#92407=CARTESIAN_POINT('Ctrl Pts',(1.58294973625947,31.9438966608302,55.6695728439167));
#92408=CARTESIAN_POINT('Ctrl Pts',(1.58680851605488,31.9195003460157,55.7366133362076));
#92409=CARTESIAN_POINT('Ctrl Pts',(1.59066729585028,31.8916634397915,55.8022512032126));
#92410=CARTESIAN_POINT('Ctrl Pts',(1.5945236447615,31.8638440697572,55.8678477208634));
#92411=CARTESIAN_POINT('Ctrl Pts',(1.59837999367272,31.8325885977026,55.9320429201068));
#92412=CARTESIAN_POINT('Ctrl Pts',(1.60223634258394,31.7980681641413,55.9944588677273));
#92413=CARTESIAN_POINT('Ctrl Pts',(1.60609155216783,31.7635579293651,56.0568563750571));
#92414=CARTESIAN_POINT('Ctrl Pts',(1.60994676175171,31.7257848830761,56.1174752494872));
#92415=CARTESIAN_POINT('Ctrl Pts',(1.6138019713356,31.6849662948508,56.1759617968781));
#92416=CARTESIAN_POINT('Ctrl Pts',(1.61765733153597,31.6441461119126,56.234450629239));
#92417=CARTESIAN_POINT('Ctrl Pts',(1.62151269173635,31.6002804306385,56.2908065720668));
#92418=CARTESIAN_POINT('Ctrl Pts',(1.62536805193672,31.553629065714,56.3447060231398));
#92419=CARTESIAN_POINT('Ctrl Pts',(1.62922744774737,31.5069288683283,56.3986618936309));
#92420=CARTESIAN_POINT('Ctrl Pts',(1.63308684355802,31.4574374850222,56.4501557713316));
#92421=CARTESIAN_POINT('Ctrl Pts',(1.63694623936868,31.4054535484968,56.4988988910256));
#92422=CARTESIAN_POINT('Ctrl Pts',(1.64080782031528,31.3534401793933,56.5476696083925));
#92423=CARTESIAN_POINT('Ctrl Pts',(1.64466940126188,31.2989318190824,56.5936861538513));
#92424=CARTESIAN_POINT('Ctrl Pts',(1.64853098220848,31.2422602297307,56.6367000593052));
#92425=CARTESIAN_POINT('Ctrl Pts',(1.65239931963182,31.1854894840281,56.6797892247252));
#92426=CARTESIAN_POINT('Ctrl Pts',(1.65626765705516,31.1265483544151,56.7198649879123));
#92427=CARTESIAN_POINT('Ctrl Pts',(1.6601359944785,31.0657970129473,56.7567225989588));
#92428=CARTESIAN_POINT('Ctrl Pts',(1.66243368384513,31.0297123346933,56.7786150379353));
#92429=CARTESIAN_POINT('Ctrl Pts',(1.66473137321176,30.9929894840122,56.7993729766357));
#92430=CARTESIAN_POINT('Ctrl Pts',(1.66702906257839,30.9557074212098,56.8189614859981));
#92431=CARTESIAN_POINT('Ctrl Pts',(1.67089813645219,30.8929282408536,56.8519465321499));
#92432=CARTESIAN_POINT('Ctrl Pts',(1.67476721032598,30.8283164320441,56.881742254264));
#92433=CARTESIAN_POINT('Ctrl Pts',(1.67863628419978,30.7622291018219,56.9081415982143));
#92434=CARTESIAN_POINT('Ctrl Pts',(1.68249959314074,30.6962402419397,56.934501607055));
#92435=CARTESIAN_POINT('Ctrl Pts',(1.6863629020817,30.6287806721178,56.9574751041712));
#92436=CARTESIAN_POINT('Ctrl Pts',(1.69022621102266,30.5602315430996,56.9769011560056));
#92437=CARTESIAN_POINT('Ctrl Pts',(1.69408498808734,30.4917628260228,56.9963044200006));
#92438=CARTESIAN_POINT('Ctrl Pts',(1.69794376515202,30.4222075536278,57.0121683727561));
#92439=CARTESIAN_POINT('Ctrl Pts',(1.7018025422167,30.351964634118,57.02438100634));
#92440=CARTESIAN_POINT('Ctrl Pts',(1.7056588883928,30.2817659650812,57.0365859464109));
#92441=CARTESIAN_POINT('Ctrl Pts',(1.70951523456889,30.2108809858512,57.0451440478502));
#92442=CARTESIAN_POINT('Ctrl Pts',(1.71337158074499,30.1397200345346,57.049994115711));
#92443=CARTESIAN_POINT('Ctrl Pts',(1.71722678759349,30.0685801071696,57.0548427506568));
#92444=CARTESIAN_POINT('Ctrl Pts',(1.72108199444199,29.9971648539827,57.0559854938997));
#92445=CARTESIAN_POINT('Ctrl Pts',(1.7249372012905,29.9258892675496,57.0534130519298));
#92446=CARTESIAN_POINT('Ctrl Pts',(1.72879255875936,29.854610896427,57.0508405094563));
#92447=CARTESIAN_POINT('Ctrl Pts',(1.73264791622821,29.7834726882822,57.0445525133166));
#92448=CARTESIAN_POINT('Ctrl Pts',(1.73650327369707,29.7128874291141,57.0345918347765));
#92449=CARTESIAN_POINT('Ctrl Pts',(1.74036266680119,29.6422282840968,57.0246207297933));
#92450=CARTESIAN_POINT('Ctrl Pts',(1.7442220599053,29.572123725487,57.0109693361057));
#92451=CARTESIAN_POINT('Ctrl Pts',(1.74808145300941,29.5029783247046,56.9937319320276));
#92452=CARTESIAN_POINT('Ctrl Pts',(1.75194303125949,29.4337937745563,56.9764847683208));
#92453=CARTESIAN_POINT('Ctrl Pts',(1.75580460950957,29.3655699281291,56.9556476943698));
#92454=CARTESIAN_POINT('Ctrl Pts',(1.75966618775964,29.2986954697037,56.9313646777048));
#92455=CARTESIAN_POINT('Ctrl Pts',(1.7635345225318,29.2317040024477,56.9070391735573));
#92456=CARTESIAN_POINT('Ctrl Pts',(1.76740285730397,29.166067084491,56.8792558784584));
#92457=CARTESIAN_POINT('Ctrl Pts',(1.77127119207613,29.1021520790547,56.8482063394963));
#92458=CARTESIAN_POINT('Ctrl Pts',(1.7735689058564,29.0641878392959,56.8297635319973));
#92459=CARTESIAN_POINT('Ctrl Pts',(1.77586661963668,29.0268306333798,56.8101692312318));
#92460=CARTESIAN_POINT('Ctrl Pts',(1.77816433341695,28.9901526342878,56.7894708325268));
#92461=CARTESIAN_POINT('Ctrl Pts',(1.78203306890535,28.9283966932524,56.7546202648405));
#92462=CARTESIAN_POINT('Ctrl Pts',(1.78590180439376,28.8683259936513,56.7165008236237));
#92463=CARTESIAN_POINT('Ctrl Pts',(1.78977053988216,28.8103080775549,56.6753001797197));
#92464=CARTESIAN_POINT('Ctrl Pts',(1.79117493367413,28.7892469320117,56.6603438900747));
#92465=CARTESIAN_POINT('Ctrl Pts',(1.79257932746611,28.7684560963194,56.6449820236807));
#92466=CARTESIAN_POINT('Ctrl Pts',(1.79398372125809,28.7479524050421,56.6292250864936));
#92467=CARTESIAN_POINT('Ctrl Pts',(1.0938611646792,28.7479524050421,56.6292250864936));
#92468=CARTESIAN_POINT('Ctrl Pts',(1.0977297220774,28.6914507587339,56.5858039834442));
#92469=CARTESIAN_POINT('Ctrl Pts',(1.1015982794756,28.637286265427,56.5394984821215));
#92470=CARTESIAN_POINT('Ctrl Pts',(1.10546683687381,28.5857505639064,56.4906025945936));
#92471=CARTESIAN_POINT('Ctrl Pts',(1.1074287940444,28.5596139892786,56.4658048141101));
#92472=CARTESIAN_POINT('Ctrl Pts',(1.109390751215,28.53415294125,56.4403413350234));
#92473=CARTESIAN_POINT('Ctrl Pts',(1.1113527083856,28.509401474378,56.4142537247303));
#92474=CARTESIAN_POINT('Ctrl Pts',(1.11522171013032,28.4605913015836,56.3628086619877));
#92475=CARTESIAN_POINT('Ctrl Pts',(1.11909071187505,28.4143519004918,56.3087329477492));
#92476=CARTESIAN_POINT('Ctrl Pts',(1.12295971361977,28.3709796177163,56.2523139209496));
#92477=CARTESIAN_POINT('Ctrl Pts',(1.12682294925331,28.3276719741995,56.1959789774364));
#92478=CARTESIAN_POINT('Ctrl Pts',(1.13068618488685,28.2872232609604,56.1373080355254));
#92479=CARTESIAN_POINT('Ctrl Pts',(1.13454942052039,28.2498919800653,56.0766241131706));
#92480=CARTESIAN_POINT('Ctrl Pts',(1.13840812288228,28.2126045051539,56.0160113997015));
#92481=CARTESIAN_POINT('Ctrl Pts',(1.14226682524417,28.1784274496466,55.9533908095042));
#92482=CARTESIAN_POINT('Ctrl Pts',(1.14612552760606,28.1475770620854,55.8891157526373));
#92483=CARTESIAN_POINT('Ctrl Pts',(1.14998179825842,28.1167461160811,55.8248812011668));
#92484=CARTESIAN_POINT('Ctrl Pts',(1.15383806891078,28.0892378884678,55.7589946885105));
#92485=CARTESIAN_POINT('Ctrl Pts',(1.15769433956313,28.0652228373674,55.6918344407842));
#92486=CARTESIAN_POINT('Ctrl Pts',(1.16154947017932,28.0412148858793,55.6246940477617));
#92487=CARTESIAN_POINT('Ctrl Pts',(1.1654046007955,28.0206982242059,55.5562811244291));
#92488=CARTESIAN_POINT('Ctrl Pts',(1.16925973141168,28.0037946301486,55.4869924885217));
#92489=CARTESIAN_POINT('Ctrl Pts',(1.17311501205124,27.9868903782838,55.4177011562296));
#92490=CARTESIAN_POINT('Ctrl Pts',(1.17697029269079,27.9735995861848,55.3475345161915));
#92491=CARTESIAN_POINT('Ctrl Pts',(1.18082557333034,27.9639933284843,55.2769014193601));
#92492=CARTESIAN_POINT('Ctrl Pts',(1.18468488922055,27.9543770160923,55.2061943921779));
#92493=CARTESIAN_POINT('Ctrl Pts',(1.18854420511077,27.9484530022102,55.1350204159442));
#92494=CARTESIAN_POINT('Ctrl Pts',(1.19240352100098,27.9462405613698,55.0637944412743));
#92495=CARTESIAN_POINT('Ctrl Pts',(1.19626502170354,27.944026868036,54.9925281445905));
#92496=CARTESIAN_POINT('Ctrl Pts',(1.20012652240609,27.9455289202923,54.9212102767999));
#92497=CARTESIAN_POINT('Ctrl Pts',(1.20398802310865,27.9507138557503,54.8502540101159));
#92498=CARTESIAN_POINT('Ctrl Pts',(1.20785628064545,27.9559078637821,54.7791735845182));
#92499=CARTESIAN_POINT('Ctrl Pts',(1.21172453818225,27.9647975606131,54.7084565054525));
#92500=CARTESIAN_POINT('Ctrl Pts',(1.21559279571905,27.9772984996671,54.6385083637885));
#92501=CARTESIAN_POINT('Ctrl Pts',(1.21789119022075,27.9847261565163,54.5969474225441));
#92502=CARTESIAN_POINT('Ctrl Pts',(1.22018958472245,27.9934277350247,54.5556577220521));
#92503=CARTESIAN_POINT('Ctrl Pts',(1.22248797922415,28.0033772232959,54.5147216777495));
#92504=CARTESIAN_POINT('Ctrl Pts',(1.2263570736365,28.0201260927555,54.44581034849));
#92505=CARTESIAN_POINT('Ctrl Pts',(1.23022616804885,28.0404795568516,54.3776321742186));
#92506=CARTESIAN_POINT('Ctrl Pts',(1.2340952624612,28.0643569152215,54.3105919852154));
#92507=CARTESIAN_POINT('Ctrl Pts',(1.23795859211244,28.0881986974973,54.2436516828094));
#92508=CARTESIAN_POINT('Ctrl Pts',(1.24182192176367,28.1155537904264,54.1778464539593));
#92509=CARTESIAN_POINT('Ctrl Pts',(1.24568525141491,28.1462909932252,54.1135686824677));
#92510=CARTESIAN_POINT('Ctrl Pts',(1.24954404934275,28.1769921409852,54.0493663094295));
#92511=CARTESIAN_POINT('Ctrl Pts',(1.25340284727059,28.2110673097648,53.9866882709052));
#92512=CARTESIAN_POINT('Ctrl Pts',(1.25726164519843,28.2483368490322,53.9259079331634));
#92513=CARTESIAN_POINT('Ctrl Pts',(1.26111801232047,28.2855829107777,53.8651658833031));
#92514=CARTESIAN_POINT('Ctrl Pts',(1.2649743794425,28.3260190973889,53.8063195756463));
#92515=CARTESIAN_POINT('Ctrl Pts',(1.26883074656453,28.3694200751477,53.7497173634859));
#92516=CARTESIAN_POINT('Ctrl Pts',(1.27268597441018,28.41280823107,53.6931318731679));
#92517=CARTESIAN_POINT('Ctrl Pts',(1.27654120225583,28.4591591438457,53.6387895474606));
#92518=CARTESIAN_POINT('Ctrl Pts',(1.28039643010148,28.508205458637,53.587007923285));
#92519=CARTESIAN_POINT('Ctrl Pts',(1.28425180858722,28.5572536898756,53.5352242757819));
#92520=CARTESIAN_POINT('Ctrl Pts',(1.28810718707295,28.6089971965746,53.4860018796339));
#92521=CARTESIAN_POINT('Ctrl Pts',(1.29196256555869,28.6631310155764,53.439622199278));
#92522=CARTESIAN_POINT('Ctrl Pts',(1.29582197956375,28.7173214977758,53.3931939721718));
#92523=CARTESIAN_POINT('Ctrl Pts',(1.29968139356882,28.7739069171724,53.3496147174127));
#92524=CARTESIAN_POINT('Ctrl Pts',(1.30354080757388,28.8325490922598,53.3091256875461));
#92525=CARTESIAN_POINT('Ctrl Pts',(1.30740240669101,28.8912244692073,53.2686137337156));
#92526=CARTESIAN_POINT('Ctrl Pts',(1.31126400580813,28.9519585062001,53.2311957426527));
#92527=CARTESIAN_POINT('Ctrl Pts',(1.31512560492525,29.0143862391476,53.1970681995931));
#92528=CARTESIAN_POINT('Ctrl Pts',(1.31899396028313,29.0769231954454,53.1628809470997));
#92529=CARTESIAN_POINT('Ctrl Pts',(1.32286231564101,29.1411593260394,53.1319958471076));
#92530=CARTESIAN_POINT('Ctrl Pts',(1.32673067099888,29.2067080592444,53.1045619347411));
#92531=CARTESIAN_POINT('Ctrl Pts',(1.32902819735349,29.245639317652,53.0882681533171));
#92532=CARTESIAN_POINT('Ctrl Pts',(1.3313257237081,29.285033255374,53.073190842872));
#92533=CARTESIAN_POINT('Ctrl Pts',(1.33362325006271,29.32480662124,53.0593528234688));
#92534=CARTESIAN_POINT('Ctrl Pts',(1.33749233009983,29.3917857597262,53.0360493238075));
#92535=CARTESIAN_POINT('Ctrl Pts',(1.34136141013695,29.4601039418764,53.0161718100105));
#92536=CARTESIAN_POINT('Ctrl Pts',(1.34523049017407,29.5293772862274,52.9998720481476));
#92537=CARTESIAN_POINT('Ctrl Pts',(1.3490938054489,29.5985474162846,52.9835965722265));
#92538=CARTESIAN_POINT('Ctrl Pts',(1.35295712072372,29.6686694146107,52.9708883773142));
#92539=CARTESIAN_POINT('Ctrl Pts',(1.35682043599855,29.7393424667455,52.9618500514296));
#92540=CARTESIAN_POINT('Ctrl Pts',(1.36067921962054,29.8099326196826,52.9528223274637));
#92541=CARTESIAN_POINT('Ctrl Pts',(1.36453800324253,29.8810720629707,52.9474559831786));
#92542=CARTESIAN_POINT('Ctrl Pts',(1.36839678686451,29.9523496820247,52.9458025874574));
#92543=CARTESIAN_POINT('Ctrl Pts',(1.37225313973244,30.0235824013435,52.9441502332556));
#92544=CARTESIAN_POINT('Ctrl Pts',(1.37610949260036,30.0949526392354,52.9462061985391));
#92545=CARTESIAN_POINT('Ctrl Pts',(1.37996584546828,30.1660455185716,52.9519701056229));
#92546=CARTESIAN_POINT('Ctrl Pts',(1.38382105913332,30.2371173964031,52.9577323099944));
#92547=CARTESIAN_POINT('Ctrl Pts',(1.38767627279836,30.3079115944096,52.9672002423364));
#92548=CARTESIAN_POINT('Ctrl Pts',(1.3915314864634,30.3780163348335,52.9803215074921));
#92549=CARTESIAN_POINT('Ctrl Pts',(1.39538685086384,30.4481238162901,52.9934432856775));
#92550=CARTESIAN_POINT('Ctrl Pts',(1.39924221526429,30.5175413095568,53.0102185887353));
#92551=CARTESIAN_POINT('Ctrl Pts',(1.40309757966473,30.5858669455365,53.0305438606997));
#92552=CARTESIAN_POINT('Ctrl Pts',(1.40695697982935,30.6542641042375,53.0508904089938));
#92553=CARTESIAN_POINT('Ctrl Pts',(1.41081637999396,30.7215666574989,53.0747942055277));
#92554=CARTESIAN_POINT('Ctrl Pts',(1.41467578015858,30.7873885035599,53.1021019766695));
#92555=CARTESIAN_POINT('Ctrl Pts',(1.41853736555258,30.8532476185814,53.1294252097332));
#92556=CARTESIAN_POINT('Ctrl Pts',(1.42239895094658,30.9176239188223,53.1601560448173));
#92557=CARTESIAN_POINT('Ctrl Pts',(1.42626053634058,30.9801543876826,53.1940944269408));
#92558=CARTESIAN_POINT('Ctrl Pts',(1.43012887831197,31.0427942654798,53.2280921907124));
#92559=CARTESIAN_POINT('Ctrl Pts',(1.43399722028336,31.1035814494069,53.2653084527368));
#92560=CARTESIAN_POINT('Ctrl Pts',(1.43786556225475,31.1621810686832,53.3054992693733));
#92561=CARTESIAN_POINT('Ctrl Pts',(1.44016321513692,31.1969870876753,53.3293711365362));
#92562=CARTESIAN_POINT('Ctrl Pts',(1.4424608680191,31.2310219537611,53.3542916065651));
#92563=CARTESIAN_POINT('Ctrl Pts',(1.44475852090127,31.2642213318106,53.380203103258));
#92564=CARTESIAN_POINT('Ctrl Pts',(1.4485823544001,31.3194728865213,53.4233259134211));
#92565=CARTESIAN_POINT('Ctrl Pts',(1.45240618789893,31.3726360605504,53.4693732485111));
#92566=CARTESIAN_POINT('Ctrl Pts',(1.45623002139776,31.4233792996943,53.5181130502964));
#92567=CARTESIAN_POINT('Ctrl Pts',(1.46004734993108,31.4740362162981,53.566769937716));
#92568=CARTESIAN_POINT('Ctrl Pts',(1.4638646784644,31.5222810158461,53.618109855358));
#92569=CARTESIAN_POINT('Ctrl Pts',(1.46768200699772,31.5678140408072,53.6718596851432));
#92570=CARTESIAN_POINT('Ctrl Pts',(1.47149570170064,31.6133037215056,53.7255583488409));
#92571=CARTESIAN_POINT('Ctrl Pts',(1.47530939640356,31.6560864236995,53.7816619997429));
#92572=CARTESIAN_POINT('Ctrl Pts',(1.47912309110647,31.6958993234528,53.8398607638683));
#92573=CARTESIAN_POINT('Ctrl Pts',(1.48293450363163,31.7356883985107,53.898024700894));
#92574=CARTESIAN_POINT('Ctrl Pts',(1.48674591615678,31.7725109144556,53.9582808546584));
#92575=CARTESIAN_POINT('Ctrl Pts',(1.49055732868193,31.8061455356611,54.0202878654873));
#92576=CARTESIAN_POINT('Ctrl Pts',(1.49436780754815,31.8397719175946,54.0822796868295));
#92577=CARTESIAN_POINT('Ctrl Pts',(1.49817828641437,31.8702117178646,54.1460210758164));
#92578=CARTESIAN_POINT('Ctrl Pts',(1.50198876528059,31.8972889701406,54.2111450537121));
#92579=CARTESIAN_POINT('Ctrl Pts',(1.50580205921379,31.9243862262747,54.2763171432405));
#92580=CARTESIAN_POINT('Ctrl Pts',(1.509615353147,31.9481157772653,54.3428734022453));
#92581=CARTESIAN_POINT('Ctrl Pts',(1.5134286470802,31.968349831146,54.410426845313));
#92582=CARTESIAN_POINT('Ctrl Pts',(1.51724327663821,31.9885909721027,54.4780039493037));
#92583=CARTESIAN_POINT('Ctrl Pts',(1.52105790619622,32.00533405718,54.5465784486412));
#92584=CARTESIAN_POINT('Ctrl Pts',(1.52487253575423,32.0185019668706,54.6157508981929));
#92585=CARTESIAN_POINT('Ctrl Pts',(1.52869346797487,32.0316916330361,54.6850376368532));
#92586=CARTESIAN_POINT('Ctrl Pts',(1.5325144001955,32.0412942558452,54.7549238045444));
#92587=CARTESIAN_POINT('Ctrl Pts',(1.53633533241613,32.047284473777,54.8250032973687));
#92588=CARTESIAN_POINT('Ctrl Pts',(1.53953198177334,32.0522959801831,54.8836328549622));
#92589=CARTESIAN_POINT('Ctrl Pts',(1.54272863113055,32.0547800105815,54.9423974987856));
#92590=CARTESIAN_POINT('Ctrl Pts',(1.54592528048776,32.0547497261996,55.0010607463466));
#92591=CARTESIAN_POINT('Origin',(-1.54592528053767,30.,55.));
#92592=CARTESIAN_POINT('',(0.393903217269906,28.7479524050421,56.6292250864936));
#92593=CARTESIAN_POINT('',(0.452117494115148,28.7479524050421,56.6292250864936));
#92594=CARTESIAN_POINT('',(-1.54592528053767,28.7479524050421,56.6292250864936));
#92595=CARTESIAN_POINT('',(0.145925152720326,32.0544673062769,54.9976428107105));
#92596=CARTESIAN_POINT('Ctrl Pts',(0.145925280537679,32.0547486502654,54.9976448497734));
#92597=CARTESIAN_POINT('Ctrl Pts',(0.149739546941021,32.0548295065906,55.0681878763859));
#92598=CARTESIAN_POINT('Ctrl Pts',(0.153553813344363,32.0512732959282,55.1387966811012));
#92599=CARTESIAN_POINT('Ctrl Pts',(0.157368079747704,32.0440865851276,55.2090636147235));
#92600=CARTESIAN_POINT('Ctrl Pts',(0.16118104386731,32.0369023280457,55.2793065574979));
#92601=CARTESIAN_POINT('Ctrl Pts',(0.164994007986915,32.0260900801542,55.3492073667697));
#92602=CARTESIAN_POINT('Ctrl Pts',(0.168806972106521,32.0117083701161,55.4183622785397));
#92603=CARTESIAN_POINT('Ctrl Pts',(0.17261997446274,31.9973265158574,55.4875178837989));
#92604=CARTESIAN_POINT('Ctrl Pts',(0.17643297681896,31.9793752318499,55.5559270906845));
#92605=CARTESIAN_POINT('Ctrl Pts',(0.18024597917518,31.9579640201056,55.6231969660323));
#92606=CARTESIAN_POINT('Ctrl Pts',(0.184063075019275,31.9365298221349,55.6905390596463));
#92607=CARTESIAN_POINT('Ctrl Pts',(0.187880170863369,31.9116284331976,55.7567389057323));
#92608=CARTESIAN_POINT('Ctrl Pts',(0.191697266707464,31.8834187459821,55.8214203490195));
#92609=CARTESIAN_POINT('Ctrl Pts',(0.195516531191688,31.8551930317496,55.8861385403422));
#92610=CARTESIAN_POINT('Ctrl Pts',(0.199335795675912,31.8236555029915,55.9493361684856));
#92611=CARTESIAN_POINT('Ctrl Pts',(0.203155060160136,31.7890112742995,56.0106612800189));
#92612=CARTESIAN_POINT('Ctrl Pts',(0.206981404197841,31.7543028275699,56.0721000664256));
#92613=CARTESIAN_POINT('Ctrl Pts',(0.210807748235547,31.7164764527575,56.1316589887038));
#92614=CARTESIAN_POINT('Ctrl Pts',(0.214634092273253,31.6757804376753,56.1890153435531));
#92615=CARTESIAN_POINT('Ctrl Pts',(0.217179575407875,31.6487073310709,56.2271717749909));
#92616=CARTESIAN_POINT('Ctrl Pts',(0.219725058542498,31.6203650995654,56.2643540944347));
#92617=CARTESIAN_POINT('Ctrl Pts',(0.22227054167712,31.5908360390092,56.3004761664443));
#92618=CARTESIAN_POINT('Ctrl Pts',(0.226143011689853,31.5459131715374,56.355429050929));
#92619=CARTESIAN_POINT('Ctrl Pts',(0.230015481702586,31.4980521337605,56.4081584923707));
#92620=CARTESIAN_POINT('Ctrl Pts',(0.233887951715319,31.4475011920355,56.4583339334856));
#92621=CARTESIAN_POINT('Ctrl Pts',(0.237754632281614,31.397025825323,56.5084343609716));
#92622=CARTESIAN_POINT('Ctrl Pts',(0.241621312847911,31.3438688788997,56.5559880289897));
#92623=CARTESIAN_POINT('Ctrl Pts',(0.245487993414207,31.2883187640707,56.6006974494399));
#92624=CARTESIAN_POINT('Ctrl Pts',(0.249350087975477,31.2328345334288,56.6453538431081));
#92625=CARTESIAN_POINT('Ctrl Pts',(0.253212182536747,31.1749631486356,56.6871723879026));
#92626=CARTESIAN_POINT('Ctrl Pts',(0.257074277098017,31.1150284775513,56.7258936979865));
#92627=CARTESIAN_POINT('Ctrl Pts',(0.260933905263996,31.0551320817056,56.7645902800231));
#92628=CARTESIAN_POINT('Ctrl Pts',(0.264793533429976,30.9931754201667,56.8001932893774));
#92629=CARTESIAN_POINT('Ctrl Pts',(0.268653161595956,30.9295127465629,56.8324856388188));
#92630=CARTESIAN_POINT('Ctrl Pts',(0.272511609673873,30.8658695379329,56.8647681148178));
#92631=CARTESIAN_POINT('Ctrl Pts',(0.276370057751791,30.8005217849537,56.8937417214125));
#92632=CARTESIAN_POINT('Ctrl Pts',(0.280228505829709,30.7338483284433,56.9192353147389));
#92633=CARTESIAN_POINT('Ctrl Pts',(0.284087058474176,30.6671730650373,56.9447295989589));
#92634=CARTESIAN_POINT('Ctrl Pts',(0.287945611118644,30.59917248037,56.9667435115671));
#92635=CARTESIAN_POINT('Ctrl Pts',(0.291804163763111,30.5302437648765,56.9851546822124));
#92636=CARTESIAN_POINT('Ctrl Pts',(0.295666658520141,30.4612446279632,57.0035846627363));
#92637=CARTESIAN_POINT('Ctrl Pts',(0.299529153277172,30.3913159365964,57.0184044280303));
#92638=CARTESIAN_POINT('Ctrl Pts',(0.303391648034202,30.3208674842945,57.029542219325));
#92639=CARTESIAN_POINT('Ctrl Pts',(0.307256279705638,30.2503800565838,57.0406861725715));
#92640=CARTESIAN_POINT('Ctrl Pts',(0.311120911377074,30.1793727778278,57.0481440453768));
#92641=CARTESIAN_POINT('Ctrl Pts',(0.31498554304851,30.1082603018613,57.0518960182087));
#92642=CARTESIAN_POINT('Ctrl Pts',(0.31885682091095,30.0370255303856,57.0556544434869));
#92643=CARTESIAN_POINT('Ctrl Pts',(0.32272809877339,29.9656856854891,57.0556942436997));
#92644=CARTESIAN_POINT('Ctrl Pts',(0.326599376635829,29.8946544516291,57.0520477279874));
#92645=CARTESIAN_POINT('Ctrl Pts',(0.32886818859578,29.8530256875264,57.0499106407635));
#92646=CARTESIAN_POINT('Ctrl Pts',(0.331137000555731,29.8115028259049,57.0465083981366));
#92647=CARTESIAN_POINT('Ctrl Pts',(0.333405812515682,29.7701676343163,57.0418556869143));
#92648=CARTESIAN_POINT('Ctrl Pts',(0.337281013011975,29.699565857798,57.0339087132752));
#92649=CARTESIAN_POINT('Ctrl Pts',(0.341156213508268,29.6292435862739,57.0222806428858));
#92650=CARTESIAN_POINT('Ctrl Pts',(0.345031414004561,29.5596137015207,57.0070021102659));
#92651=CARTESIAN_POINT('Ctrl Pts',(0.349104064276673,29.4864360248151,56.9909451036435));
#92652=CARTESIAN_POINT('Ctrl Pts',(0.353176714548785,29.4140237118823,56.9708556847076));
#92653=CARTESIAN_POINT('Ctrl Pts',(0.357249364820897,29.3428506238397,56.9468313383321));
#92654=CARTESIAN_POINT('Ctrl Pts',(0.361114530947594,29.2753035007984,56.9240309298458));
#92655=CARTESIAN_POINT('Ctrl Pts',(0.364979697074291,29.2088729566203,56.8976868836698));
#92656=CARTESIAN_POINT('Ctrl Pts',(0.368844863200987,29.1439519288621,56.8679344909287));
#92657=CARTESIAN_POINT('Ctrl Pts',(0.372707539625806,29.0790727192302,56.838201262846));
#92658=CARTESIAN_POINT('Ctrl Pts',(0.376570216050625,29.0157015340332,56.8050642490638));
#92659=CARTESIAN_POINT('Ctrl Pts',(0.380432892475445,28.9542116974909,56.7687069821865));
#92660=CARTESIAN_POINT('Ctrl Pts',(0.384294627206833,28.8927368517396,56.7323585789559));
#92661=CARTESIAN_POINT('Ctrl Pts',(0.388156361938221,28.8331428604117,56.6927917271036));
#92662=CARTESIAN_POINT('Ctrl Pts',(0.39201809666961,28.7757773515059,56.6502352769875));
#92663=CARTESIAN_POINT('Ctrl Pts',(0.392646470203042,28.7664429538749,56.6433105789464));
#92664=CARTESIAN_POINT('Ctrl Pts',(0.393274843736474,28.7571674975787,56.6363068178906));
#92665=CARTESIAN_POINT('Ctrl Pts',(0.393903217269906,28.7479524050421,56.6292250864936));
#92666=CARTESIAN_POINT('',(0.,30.5301702171886,53.0148256743283));
#92667=CARTESIAN_POINT('Ctrl Pts',(-8.32667268468867E-16,30.5301702171886,
53.0148256743283));
#92668=CARTESIAN_POINT('Ctrl Pts',(0.037045090279519,31.1902723495278,53.1911157292334));
#92669=CARTESIAN_POINT('Ctrl Pts',(0.0856865365995149,31.9249421915379,
53.8871678923641));
#92670=CARTESIAN_POINT('Ctrl Pts',(0.13432798291951,32.0542927425914,54.7833750251074));
#92671=CARTESIAN_POINT('Ctrl Pts',(0.145924338959986,32.0526761052044,54.9976298288387));
#92672=CARTESIAN_POINT('',(5.304521544236E-9,29.4696598908744,53.0148710542757));
#92673=CARTESIAN_POINT('Origin',(0.,30.,55.));
#92674=CARTESIAN_POINT('',(0.204074719418398,32.0547494571313,55.0014936260708));
#92675=CARTESIAN_POINT('Ctrl Pts',(5.30452171076945E-9,29.4696598908744,
53.0148710542757));
#92676=CARTESIAN_POINT('Ctrl Pts',(0.00385890399912051,29.5379947425062,
52.9966149542125));
#92677=CARTESIAN_POINT('Ctrl Pts',(0.00771780269371889,29.6074108442032,
52.9818547624561));
#92678=CARTESIAN_POINT('Ctrl Pts',(0.0115767013883177,29.6775162317845,
52.9707139724185));
#92679=CARTESIAN_POINT('Ctrl Pts',(0.0154298333236881,29.7475168534927,
52.9595898312383));
#92680=CARTESIAN_POINT('Ctrl Pts',(0.0192829652590586,29.8182042381468,
52.9520744330023));
#92681=CARTESIAN_POINT('Ctrl Pts',(0.023136097194429,29.8891730296929,52.9482410119235));
#92682=CARTESIAN_POINT('Ctrl Pts',(0.0269847084857915,29.9600585578971,
52.9444120883633));
#92683=CARTESIAN_POINT('Ctrl Pts',(0.0308333197771542,30.0312243517176,
52.9442565885634));
#92684=CARTESIAN_POINT('Ctrl Pts',(0.0346819310685167,30.1022584494044,
52.9477961183095));
#92685=CARTESIAN_POINT('Ctrl Pts',(0.0385281380490834,30.1732481705524,
52.9513334368348));
#92686=CARTESIAN_POINT('Ctrl Pts',(0.0423743450296501,30.2441058718704,
52.9585611814656));
#92687=CARTESIAN_POINT('Ctrl Pts',(0.0462205520102168,30.3144196125068,
52.9694488753614));
#92688=CARTESIAN_POINT('Ctrl Pts',(0.0500656609004903,30.3847132786032,
52.9803334608257));
#92689=CARTESIAN_POINT('Ctrl Pts',(0.053910769790764,30.4544628096774,52.994875846421));
#92690=CARTESIAN_POINT('Ctrl Pts',(0.0577558786810375,30.5232631732663,
53.0129939069033));
#92691=CARTESIAN_POINT('Ctrl Pts',(0.0616011941145184,30.5920672325237,
53.0311129406122));
#92692=CARTESIAN_POINT('Ctrl Pts',(0.0654465095479991,30.6599215512192,
53.0528079035498));
#92693=CARTESIAN_POINT('Ctrl Pts',(0.06929182498148,30.7264347704545,53.0779463881633));
#92694=CARTESIAN_POINT('Ctrl Pts',(0.0731411148383938,30.793016736117,53.103110855296));
#92695=CARTESIAN_POINT('Ctrl Pts',(0.076990404695308,30.8582543783197,53.1317257734965));
#92696=CARTESIAN_POINT('Ctrl Pts',(0.0808396945522218,30.9217758215303,
53.163610363419));
#92697=CARTESIAN_POINT('Ctrl Pts',(0.084691250721741,30.9853346637036,53.1955137257517));
#92698=CARTESIAN_POINT('Ctrl Pts',(0.08854280689126,31.047174871546,53.2306903488843));
#92699=CARTESIAN_POINT('Ctrl Pts',(0.0923943630607791,31.1069511199342,
53.2689145657778));
#92700=CARTESIAN_POINT('Ctrl Pts',(0.0962523586056887,31.1668273075901,
53.3072026893289));
#92701=CARTESIAN_POINT('Ctrl Pts',(0.100110354150598,31.2246322528145,53.3485482903));
#92702=CARTESIAN_POINT('Ctrl Pts',(0.103968349695508,31.2800521355636,53.3926841963263));
#92703=CARTESIAN_POINT('Ctrl Pts',(0.105632531586408,31.3039580121239,53.411722625659));
#92704=CARTESIAN_POINT('Ctrl Pts',(0.107296713477309,31.3274205505818,53.4312797685466));
#92705=CARTESIAN_POINT('Ctrl Pts',(0.108960895368209,31.3504167214721,53.4513321076265));
#92706=CARTESIAN_POINT('Ctrl Pts',(0.1129239713703,31.4051797095168,53.4990846665434));
#92707=CARTESIAN_POINT('Ctrl Pts',(0.116887047372392,31.4575298680422,53.5498532961102));
#92708=CARTESIAN_POINT('Ctrl Pts',(0.120850123374483,31.5071127270913,53.6033580307253));
#92709=CARTESIAN_POINT('Ctrl Pts',(0.124661299696715,31.5547951380006,53.6548119966813));
#92710=CARTESIAN_POINT('Ctrl Pts',(0.128472476018948,31.5999181155289,53.7087957560177));
#92711=CARTESIAN_POINT('Ctrl Pts',(0.13228365234118,31.6421997492177,53.7650192122266));
#92712=CARTESIAN_POINT('Ctrl Pts',(0.136091341570936,31.6844426966968,53.8211912259479));
#92713=CARTESIAN_POINT('Ctrl Pts',(0.139899030800692,31.7238491543833,53.8795984771563));
#92714=CARTESIAN_POINT('Ctrl Pts',(0.143706720030447,31.7601762542011,53.9399164577041));
#92715=CARTESIAN_POINT('Ctrl Pts',(0.147512279769376,31.7964830377006,54.0002007047776));
#92716=CARTESIAN_POINT('Ctrl Pts',(0.151317839508305,31.8297136215381,54.062393134388));
#92717=CARTESIAN_POINT('Ctrl Pts',(0.155123399247234,31.8596685075762,54.1261403977586));
#92718=CARTESIAN_POINT('Ctrl Pts',(0.158928184040522,31.8896172937472,54.1898746799472));
#92719=CARTESIAN_POINT('Ctrl Pts',(0.162732968833809,31.9162914953339,54.2551627143676));
#92720=CARTESIAN_POINT('Ctrl Pts',(0.166537753627097,31.9395384961683,54.3216284319187));
#92721=CARTESIAN_POINT('Ctrl Pts',(0.170345033965938,31.9628007446324,54.3881377441104));
#92722=CARTESIAN_POINT('Ctrl Pts',(0.174152314304778,31.9826311393778,54.455825808995));
#92723=CARTESIAN_POINT('Ctrl Pts',(0.177959594643619,31.9989264298968,54.5242997894053));
#92724=CARTESIAN_POINT('Ctrl Pts',(0.18176838555138,32.0152281857027,54.5928009374148));
#92725=CARTESIAN_POINT('Ctrl Pts',(0.185577176459142,32.0279919539674,54.6620881300336));
#92726=CARTESIAN_POINT('Ctrl Pts',(0.189385967366902,32.0371658013398,54.7317593238308));
#92727=CARTESIAN_POINT('Ctrl Pts',(0.193199808432185,32.046351812513,54.8015228961576));
#92728=CARTESIAN_POINT('Ctrl Pts',(0.197013649497467,32.0519383688091,54.8716709875907));
#92729=CARTESIAN_POINT('Ctrl Pts',(0.20082749056275,32.0539255509878,54.9417986812918));
#92730=CARTESIAN_POINT('Ctrl Pts',(0.201909900181299,32.0544895349261,54.9617016842984));
#92731=CARTESIAN_POINT('Ctrl Pts',(0.202992309799848,32.0547639158599,54.9816030621975));
#92732=CARTESIAN_POINT('Ctrl Pts',(0.204074719418398,32.0547494571313,55.0014936260708));
#92733=CARTESIAN_POINT('Ctrl Pts',(0.204074719462323,32.0547494571307,55.001493626878));
#92734=CARTESIAN_POINT('Ctrl Pts',(0.209415201710472,32.0546781194191,55.099631338747));
#92735=CARTESIAN_POINT('Ctrl Pts',(0.214755683958621,32.0475753669382,55.1975148182993));
#92736=CARTESIAN_POINT('Ctrl Pts',(0.22009616620677,32.0335530902504,55.2943796725878));
#92737=CARTESIAN_POINT('Ctrl Pts',(0.223961018827296,32.0234053114012,55.3644797812556));
#92738=CARTESIAN_POINT('Ctrl Pts',(0.227825871447822,32.0096082627772,55.4341947647113));
#92739=CARTESIAN_POINT('Ctrl Pts',(0.231690724068348,31.9922030861659,55.5031147244626));
#92740=CARTESIAN_POINT('Ctrl Pts',(0.235549750404866,31.9748241479425,55.5719307870415));
#92741=CARTESIAN_POINT('Ctrl Pts',(0.239408776741384,31.9538479958985,55.6399537365013));
#92742=CARTESIAN_POINT('Ctrl Pts',(0.243267803077902,31.9293672381135,55.7067811705148));
#92743=CARTESIAN_POINT('Ctrl Pts',(0.247122226949458,31.9049156772866,55.7735289028375));
#92744=CARTESIAN_POINT('Ctrl Pts',(0.250976650821015,31.8769679793644,55.8390834967379));
#92745=CARTESIAN_POINT('Ctrl Pts',(0.254831074692571,31.8456668085387,55.9030568057207));
#92746=CARTESIAN_POINT('Ctrl Pts',(0.258683026364569,31.8143857140574,55.9669890826863));
#92747=CARTESIAN_POINT('Ctrl Pts',(0.262534978036566,31.7797556271541,56.0293416503832));
#92748=CARTESIAN_POINT('Ctrl Pts',(0.266386929708563,31.7419670894156,56.0897468613825));
#92749=CARTESIAN_POINT('Ctrl Pts',(0.270237707179487,31.7041900708614,56.1501336588944));
#92750=CARTESIAN_POINT('Ctrl Pts',(0.27408848465041,31.6632567708552,56.2085738654515));
#92751=CARTESIAN_POINT('Ctrl Pts',(0.277939262121334,31.6194025140626,56.264726476337));
#92752=CARTESIAN_POINT('Ctrl Pts',(0.28179016173665,31.5755468662387,56.3208808683503));
#92753=CARTESIAN_POINT('Ctrl Pts',(0.285641061351966,31.5287703791993,56.3747471381674));
#92754=CARTESIAN_POINT('Ctrl Pts',(0.289491960967283,31.4793492625247,56.4260165924588));
#92755=CARTESIAN_POINT('Ctrl Pts',(0.293346883174129,31.4298765212986,56.4773396020471));
#92756=CARTESIAN_POINT('Ctrl Pts',(0.297201805380976,31.377753974451,56.5260600297737));
#92757=CARTESIAN_POINT('Ctrl Pts',(0.301056727587822,31.3232947326731,56.5719060445776));
#92758=CARTESIAN_POINT('Ctrl Pts',(0.30491382072567,31.2688048217274,56.61777787794));
#92759=CARTESIAN_POINT('Ctrl Pts',(0.308770913863518,31.2119759850091,56.6607717822148));
#92760=CARTESIAN_POINT('Ctrl Pts',(0.312628007001366,31.153152247426,56.7006579481943));
#92761=CARTESIAN_POINT('Ctrl Pts',(0.316491882785907,31.0942250690871,56.7406142534632));
#92762=CARTESIAN_POINT('Ctrl Pts',(0.320355758570448,31.0332964030478,56.7774516576836));
#92763=CARTESIAN_POINT('Ctrl Pts',(0.324219634354988,30.9707362862754,56.8109855397016));
#92764=CARTESIAN_POINT('Ctrl Pts',(0.326556901918436,30.9328935242791,56.8312702639235));
#92765=CARTESIAN_POINT('Ctrl Pts',(0.328894169481882,30.8944542432968,56.8503471227924));
#92766=CARTESIAN_POINT('Ctrl Pts',(0.331231437045329,30.8555035810296,56.8681839270654));
#92767=CARTESIAN_POINT('Ctrl Pts',(0.335101212782371,30.7910136055811,56.8977160326239));
#92768=CARTESIAN_POINT('Ctrl Pts',(0.338970988519412,30.7248666075646,56.9239626367947));
#92769=CARTESIAN_POINT('Ctrl Pts',(0.342840764256454,30.6574305658347,56.9467364006476));
#92770=CARTESIAN_POINT('Ctrl Pts',(0.346704775982027,30.5900949697494,56.9694762430939));
#92771=CARTESIAN_POINT('Ctrl Pts',(0.3505687877076,30.52147459751,56.9887533590595));
#92772=CARTESIAN_POINT('Ctrl Pts',(0.354432799433173,30.4519589210478,57.0044277727534));
#92773=CARTESIAN_POINT('Ctrl Pts',(0.358292277119959,30.3825248144139,57.0200837940602));
#92774=CARTESIAN_POINT('Ctrl Pts',(0.362151754806745,30.3121979617338,57.0321454040004));
#92775=CARTESIAN_POINT('Ctrl Pts',(0.366011232493531,30.2413829000894,57.0405224473268));
#92776=CARTESIAN_POINT('Ctrl Pts',(0.369868277554051,30.1706124731322,57.0488942106082));
#92777=CARTESIAN_POINT('Ctrl Pts',(0.373725322614572,30.0993549288082,57.0535859579957));
#92778=CARTESIAN_POINT('Ctrl Pts',(0.377582367675092,30.0280234515252,57.0545588939392));
#92779=CARTESIAN_POINT('Ctrl Pts',(0.381438270602589,29.9567130966389,57.0555315417807));
#92780=CARTESIAN_POINT('Ctrl Pts',(0.385294173530085,29.8853293375297,57.0527875577745));
#92781=CARTESIAN_POINT('Ctrl Pts',(0.389150076457581,29.8142871840368,57.0463402240309));
#92782=CARTESIAN_POINT('Ctrl Pts',(0.393006126129889,29.7432423268796,57.03989264492));
#92783=CARTESIAN_POINT('Ctrl Pts',(0.396862175802196,29.6725395845461,57.0297414823329));
#92784=CARTESIAN_POINT('Ctrl Pts',(0.400718225474503,29.6025889352621,57.0159518863614));
#92785=CARTESIAN_POINT('Ctrl Pts',(0.40457829999136,29.5325652733063,57.0021478971675));
#92786=CARTESIAN_POINT('Ctrl Pts',(0.408438374508216,29.4632957488624,56.9846979875983));
#92787=CARTESIAN_POINT('Ctrl Pts',(0.412298449025072,29.3951793406887,56.963718292569));
#92788=CARTESIAN_POINT('Ctrl Pts',(0.416160703621026,29.3270244619733,56.9427267487025));
#92789=CARTESIAN_POINT('Ctrl Pts',(0.420022958216979,29.2600244522189,56.9182016177523));
#92790=CARTESIAN_POINT('Ctrl Pts',(0.423885212812933,29.1945597327353,56.8903077893212));
#92791=CARTESIAN_POINT('Ctrl Pts',(0.42775420848448,29.1289807528859,56.86236527575));
#92792=CARTESIAN_POINT('Ctrl Pts',(0.431623204156027,29.0649428496908,56.8310425391956));
#92793=CARTESIAN_POINT('Ctrl Pts',(0.435492199827575,29.002802575406,56.7965508227944));
#92794=CARTESIAN_POINT('Ctrl Pts',(0.437783702513013,28.9659985524797,56.7761223014238));
#92795=CARTESIAN_POINT('Ctrl Pts',(0.440075205198452,28.929859670375,56.754582989294));
#92796=CARTESIAN_POINT('Ctrl Pts',(0.44236670788389,28.894454859707,56.7319836908223));
#92797=CARTESIAN_POINT('Ctrl Pts',(0.445616969960976,28.8442367586366,56.6999288984549));
#92798=CARTESIAN_POINT('Ctrl Pts',(0.448867232038062,28.7953317342127,56.6656357553635));
#92799=CARTESIAN_POINT('Ctrl Pts',(0.452117494115148,28.7479524050421,56.6292250864936));
#92800=CARTESIAN_POINT('Origin',(-1.54592528053767,30.,125.));
#92801=CARTESIAN_POINT('',(9.49394826790656,28.7479590808042,126.629230216746));
#92802=CARTESIAN_POINT('',(9.55204643235015,28.7459520887588,126.631857121398));
#92803=CARTESIAN_POINT('',(-1.54592528053767,28.7479590808042,126.629230216746));
#92804=CARTESIAN_POINT('',(10.,32.0533758325287,124.92486510207));
#92805=CARTESIAN_POINT('Ctrl Pts',(9.55204643235015,28.7459520887588,126.631857121398));
#92806=CARTESIAN_POINT('Ctrl Pts',(9.55318392711536,28.7293562993152,126.619178672138));
#92807=CARTESIAN_POINT('Ctrl Pts',(9.59136651216008,28.1793709776662,126.184464664884));
#92808=CARTESIAN_POINT('Ctrl Pts',(9.66659418748432,27.5870688000586,124.728220627396));
#92809=CARTESIAN_POINT('Ctrl Pts',(9.77772945832287,28.9190809534992,122.823596121193));
#92810=CARTESIAN_POINT('Ctrl Pts',(9.88886472916145,31.2434480688362,122.91515608673));
#92811=CARTESIAN_POINT('Ctrl Pts',(9.96295490972048,32.0283922803563,124.242084880697));
#92812=CARTESIAN_POINT('Ctrl Pts',(10.,32.0533758325287,124.92486510207));
#92813=CARTESIAN_POINT('',(9.99999184700732,31.8181879239729,125.959175310784));
#92814=CARTESIAN_POINT('Origin',(10.,30.,125.));
#92815=CARTESIAN_POINT('',(9.94592528057841,32.0547499998285,125.000026545906));
#92816=CARTESIAN_POINT('Ctrl Pts',(9.94592528057841,32.0547499998285,125.000026545906));
#92817=CARTESIAN_POINT('Ctrl Pts',(9.94992641744506,32.054749041194,125.074228358377));
#92818=CARTESIAN_POINT('Ctrl Pts',(9.9539275543117,32.0507243787667,125.148359152486));
#92819=CARTESIAN_POINT('Ctrl Pts',(9.95792869117834,32.0427247640096,125.221975451349));
#92820=CARTESIAN_POINT('Ctrl Pts',(9.96193973980718,32.0347053323151,125.295774115194));
#92821=CARTESIAN_POINT('Ctrl Pts',(9.96595078843603,32.0226913261354,125.369055309329));
#92822=CARTESIAN_POINT('Ctrl Pts',(9.96996183706487,32.0067830122535,125.441383624788));
#92823=CARTESIAN_POINT('Ctrl Pts',(9.97397827600221,31.9908533197428,125.513809139749));
#92824=CARTESIAN_POINT('Ctrl Pts',(9.97799471493955,31.9710190057058,125.585278810454));
#92825=CARTESIAN_POINT('Ctrl Pts',(9.98201115387689,31.9474300268147,125.65537306411));
#92826=CARTESIAN_POINT('Ctrl Pts',(9.98603789130173,31.9237805637962,125.725647045331));
#92827=CARTESIAN_POINT('Ctrl Pts',(9.99006462872657,31.8963573593182,125.794538163325));
#92828=CARTESIAN_POINT('Ctrl Pts',(9.99409136615141,31.8653583165232,125.861647209406));
#92829=CARTESIAN_POINT('Ctrl Pts',(9.99605728180693,31.8502241031124,125.894410886398));
#92830=CARTESIAN_POINT('Ctrl Pts',(9.99802319746244,31.8342382610577,125.926750191666));
#92831=CARTESIAN_POINT('Ctrl Pts',(9.99998911311796,31.8174276116447,125.958621113335));
#92832=CARTESIAN_POINT('Ctrl Pts',(9.49394826790656,28.7479590808042,126.629230216746));
#92833=CARTESIAN_POINT('Ctrl Pts',(9.49780412631023,28.6914091793736,126.585772398545));
#92834=CARTESIAN_POINT('Ctrl Pts',(9.50165998471389,28.6371086349064,126.539354686076));
#92835=CARTESIAN_POINT('Ctrl Pts',(9.50551584311756,28.5853742599313,126.490245475764));
#92836=CARTESIAN_POINT('Ctrl Pts',(9.50937196777623,28.5336363125906,126.441132874359));
#92837=CARTESIAN_POINT('Ctrl Pts',(9.5132280924349,28.4844652370948,126.389328742153));
#92838=CARTESIAN_POINT('Ctrl Pts',(9.51708421709357,28.4381416398565,126.335138953574));
#92839=CARTESIAN_POINT('Ctrl Pts',(9.52094443867069,28.3917688263668,126.280891591351));
#92840=CARTESIAN_POINT('Ctrl Pts',(9.52480466024782,28.3482498452297,126.224253883872));
#92841=CARTESIAN_POINT('Ctrl Pts',(9.52866488182495,28.3078249672196,126.165564764796));
#92842=CARTESIAN_POINT('Ctrl Pts',(9.53252739110166,28.2673761320416,126.106840864537));
#92843=CARTESIAN_POINT('Ctrl Pts',(9.53638990037837,28.2300253039295,126.046063546692));
#92844=CARTESIAN_POINT('Ctrl Pts',(9.54025240965508,28.1959678988961,125.983598363503));
#92845=CARTESIAN_POINT('Ctrl Pts',(9.54412154523635,28.1618520668863,125.921026018545));
#92846=CARTESIAN_POINT('Ctrl Pts',(9.54799068081762,28.1310411454322,125.856760466181));
#92847=CARTESIAN_POINT('Ctrl Pts',(9.55185981639889,28.1036830108545,125.791188624272));
#92848=CARTESIAN_POINT('Ctrl Pts',(9.55378430830463,28.0900751887854,125.758573463509));
#92849=CARTESIAN_POINT('Ctrl Pts',(9.55570880021036,28.077320825225,125.725635382705));
#92850=CARTESIAN_POINT('Ctrl Pts',(9.5576332921161,28.0654334809787,125.692423241942));
#92851=CARTESIAN_POINT('Ctrl Pts',(9.56150282286142,28.0415318766622,125.625644369338));
#92852=CARTESIAN_POINT('Ctrl Pts',(9.56537235360673,28.0210453328819,125.557496028693));
#92853=CARTESIAN_POINT('Ctrl Pts',(9.56924188435204,28.0041289561955,125.488360869648));
#92854=CARTESIAN_POINT('Ctrl Pts',(9.57310565989046,27.9872377394715,125.419328536286));
#92855=CARTESIAN_POINT('Ctrl Pts',(9.57696943542886,27.973906264106,125.349312765815));
#92856=CARTESIAN_POINT('Ctrl Pts',(9.58083321096727,27.9642406054079,125.278713562336));
#92857=CARTESIAN_POINT('Ctrl Pts',(9.58469246665209,27.9545862536197,125.208196945969));
#92858=CARTESIAN_POINT('Ctrl Pts',(9.58855172233691,27.9485892660344,125.13709873111));
#92859=CARTESIAN_POINT('Ctrl Pts',(9.59241097802173,27.9463047893954,125.06582966231));
#92860=CARTESIAN_POINT('Ctrl Pts',(9.59626780995489,27.9440217474901,124.994605353054));
#92861=CARTESIAN_POINT('Ctrl Pts',(9.60012464188805,27.9454466061684,124.923210886997));
#92862=CARTESIAN_POINT('Ctrl Pts',(9.60398147382121,27.9505825998578,124.852061220452));
#92863=CARTESIAN_POINT('Ctrl Pts',(9.6078371727826,27.9557170848125,124.780932454626));
#92864=CARTESIAN_POINT('Ctrl Pts',(9.61169287174399,27.9645605055126,124.710048829665));
#92865=CARTESIAN_POINT('Ctrl Pts',(9.61554857070539,27.9770640538327,124.63982265451));
#92866=CARTESIAN_POINT('Ctrl Pts',(9.61940442586884,27.9895681086965,124.569593634352));
#92867=CARTESIAN_POINT('Ctrl Pts',(9.6232602810323,28.0057324982751,124.500022594616));
#92868=CARTESIAN_POINT('Ctrl Pts',(9.62711613619576,28.0254571691084,124.431512382303));
#92869=CARTESIAN_POINT('Ctrl Pts',(9.63097603195377,28.045202509649,124.362930377358));
#92870=CARTESIAN_POINT('Ctrl Pts',(9.63483592771178,28.068515444427,124.295411886582));
#92871=CARTESIAN_POINT('Ctrl Pts',(9.6386958234698,28.0952460660982,124.229344425969));
#92872=CARTESIAN_POINT('Ctrl Pts',(9.64255790792351,28.1219918449655,124.163239502798));
#92873=CARTESIAN_POINT('Ctrl Pts',(9.64641999237723,28.1521589631565,124.098587688006));
#92874=CARTESIAN_POINT('Ctrl Pts',(9.65028207683095,28.1855505308414,124.035753824809));
#92875=CARTESIAN_POINT('Ctrl Pts',(9.65415091781318,28.2190005154465,123.972810036831));
#92876=CARTESIAN_POINT('Ctrl Pts',(9.65801975879542,28.2556859620026,123.911690966773));
#92877=CARTESIAN_POINT('Ctrl Pts',(9.66188859977765,28.2953658457551,123.852733700189));
#92878=CARTESIAN_POINT('Ctrl Pts',(9.66418192083665,28.31888676932,123.817785781249));
#92879=CARTESIAN_POINT('Ctrl Pts',(9.66647524189564,28.3434590555142,123.783596865762));
#92880=CARTESIAN_POINT('Ctrl Pts',(9.66876856295463,28.3690260367847,123.750231423897));
#92881=CARTESIAN_POINT('Ctrl Pts',(9.6726337119706,28.4121164676299,123.693997516183));
#92882=CARTESIAN_POINT('Ctrl Pts',(9.67649886098656,28.4582040821038,123.63988326682));
#92883=CARTESIAN_POINT('Ctrl Pts',(9.68036401000252,28.5070524760954,123.588226203187));
#92884=CARTESIAN_POINT('Ctrl Pts',(9.68422338351675,28.5558278783387,123.53664632816));
#92885=CARTESIAN_POINT('Ctrl Pts',(9.68808275703098,28.6073555402847,123.48751670204));
#92886=CARTESIAN_POINT('Ctrl Pts',(9.69194213054521,28.6613578349713,123.441143137903));
#92887=CARTESIAN_POINT('Ctrl Pts',(9.69579697527658,28.7152967606512,123.394823990836));
#92888=CARTESIAN_POINT('Ctrl Pts',(9.69965182000794,28.7717041838798,123.351254797824));
#92889=CARTESIAN_POINT('Ctrl Pts',(9.70350666473931,28.8302657844179,123.310704458244));
#92890=CARTESIAN_POINT('Ctrl Pts',(9.70735908251337,28.8887905153765,123.270179648601));
#92891=CARTESIAN_POINT('Ctrl Pts',(9.71121150028743,28.9494663337615,123.232670198377));
#92892=CARTESIAN_POINT('Ctrl Pts',(9.71506391806149,29.0119471850551,123.198403708546));
#92893=CARTESIAN_POINT('Ctrl Pts',(9.71891520608934,29.0744097134385,123.164147267583));
#92894=CARTESIAN_POINT('Ctrl Pts',(9.72276649411718,29.1386757972613,123.133132133113));
#92895=CARTESIAN_POINT('Ctrl Pts',(9.72661778214502,29.2043733503988,123.105540763979));
#92896=CARTESIAN_POINT('Ctrl Pts',(9.73046923603155,29.2700737328518,123.077948206602));
#92897=CARTESIAN_POINT('Ctrl Pts',(9.73432068991807,29.3372052572478,123.053779893772));
#92898=CARTESIAN_POINT('Ctrl Pts',(9.7381721438046,29.4053759770119,123.033170105529));
#92899=CARTESIAN_POINT('Ctrl Pts',(9.74202768323323,29.4736190108565,123.012538454851));
#92900=CARTESIAN_POINT('Ctrl Pts',(9.74588322266187,29.5429029735657,122.995473005168));
#92901=CARTESIAN_POINT('Ctrl Pts',(9.7497387620905,29.6128217507138,122.982057838842));
#92902=CARTESIAN_POINT('Ctrl Pts',(9.75359650888248,29.6827805575773,122.9686349921));
#92903=CARTESIAN_POINT('Ctrl Pts',(9.75745425567446,29.7533744198051,122.95886665521));
#92904=CARTESIAN_POINT('Ctrl Pts',(9.76131200246644,29.8241908068457,122.952785138267));
#92905=CARTESIAN_POINT('Ctrl Pts',(9.76517658251364,29.8951326314726,122.946692849088));
#92906=CARTESIAN_POINT('Ctrl Pts',(9.76904116256084,29.9662972811123,122.944300434156));
#92907=CARTESIAN_POINT('Ctrl Pts',(9.77290574260804,30.0372716269973,122.945588067519));
#92908=CARTESIAN_POINT('Ctrl Pts',(9.77523843966978,30.0801124133396,122.946365295193));
#92909=CARTESIAN_POINT('Ctrl Pts',(9.77757113673153,30.1228839281888,122.94848231543));
#92910=CARTESIAN_POINT('Ctrl Pts',(9.77990383379327,30.1654967268378,122.951925685942));
#92911=CARTESIAN_POINT('Ctrl Pts',(9.7837796915926,30.2362993830008,122.957646966545));
#92912=CARTESIAN_POINT('Ctrl Pts',(9.78765554939193,30.3069415042382,122.967055082892));
#92913=CARTESIAN_POINT('Ctrl Pts',(9.79153140719126,30.3770094735591,122.980133316442));
#92914=CARTESIAN_POINT('Ctrl Pts',(9.79540148372107,30.4469729287734,122.993192042364));
#92915=CARTESIAN_POINT('Ctrl Pts',(9.79927156025088,30.5163634602671,123.009909929784));
#92916=CARTESIAN_POINT('Ctrl Pts',(9.80314163678069,30.5847718858269,123.030218437479));
#92917=CARTESIAN_POINT('Ctrl Pts',(9.8070071246871,30.6530992017497,123.05050286604));
#92918=CARTESIAN_POINT('Ctrl Pts',(9.8108726125935,30.7204462633365,123.074369320275));
#92919=CARTESIAN_POINT('Ctrl Pts',(9.8147381004999,30.7864151190072,123.101698437261));
#92920=CARTESIAN_POINT('Ctrl Pts',(9.81860111864384,30.8523418254312,123.129010092952));
#92921=CARTESIAN_POINT('Ctrl Pts',(9.82246413678777,30.916891627173,123.159779836718));
#92922=CARTESIAN_POINT('Ctrl Pts',(9.82632715493171,30.9796841247431,123.193839271209));
#92923=CARTESIAN_POINT('Ctrl Pts',(9.83018898513618,31.0424573126224,123.227888231883));
#92924=CARTESIAN_POINT('Ctrl Pts',(9.83405081534065,31.1034738441465,123.265224644079));
#92925=CARTESIAN_POINT('Ctrl Pts',(9.83791264554513,31.1623771550894,123.305633772815));
#92926=CARTESIAN_POINT('Ctrl Pts',(9.84177456797417,31.2212818727055,123.346043866563));
#92927=CARTESIAN_POINT('Ctrl Pts',(9.84563649040322,31.278072871718,123.389526546977));
#92928=CARTESIAN_POINT('Ctrl Pts',(9.84949841283227,31.3324232868658,123.435824259516));
#92929=CARTESIAN_POINT('Ctrl Pts',(9.85336423707635,31.3868286138537,123.482168748011));
#92930=CARTESIAN_POINT('Ctrl Pts',(9.85723006132043,31.4387880652972,123.531333631963));
#92931=CARTESIAN_POINT('Ctrl Pts',(9.86109588556451,31.4880092499235,123.583022218014));
#92932=CARTESIAN_POINT('Ctrl Pts',(9.86496382883615,31.5372574148367,123.634739136842));
#92933=CARTESIAN_POINT('Ctrl Pts',(9.86883177210779,31.5837640090157,123.68898214469));
#92934=CARTESIAN_POINT('Ctrl Pts',(9.87269971537943,31.6272765958774,123.745421009657));
#92935=CARTESIAN_POINT('Ctrl Pts',(9.87657424252348,31.6708632482824,123.801955942808));
#92936=CARTESIAN_POINT('Ctrl Pts',(9.88044876966754,31.7114454426296,123.860693797643));
#92937=CARTESIAN_POINT('Ctrl Pts',(9.88432329681159,31.7488141688587,123.921275491472));
#92938=CARTESIAN_POINT('Ctrl Pts',(9.88656189941833,31.7704048623388,123.956278043444));
#92939=CARTESIAN_POINT('Ctrl Pts',(9.88880050202507,31.7909236763886,123.991895640431));
#92940=CARTESIAN_POINT('Ctrl Pts',(9.89103910463182,31.8103375264705,124.0280557615));
#92941=CARTESIAN_POINT('Ctrl Pts',(9.89510077167261,31.8455615518402,124.093663820517));
#92942=CARTESIAN_POINT('Ctrl Pts',(9.8991624387134,31.8772691212244,124.161289087594));
#92943=CARTESIAN_POINT('Ctrl Pts',(9.90322410575419,31.9052369260509,124.230539267986));
#92944=CARTESIAN_POINT('Ctrl Pts',(9.90727424704382,31.9331253669229,124.299592937846));
#92945=CARTESIAN_POINT('Ctrl Pts',(9.91132438833347,31.9572950211504,124.370261955961));
#92946=CARTESIAN_POINT('Ctrl Pts',(9.9153745296231,31.9775692252997,124.442131268444));
#92947=CARTESIAN_POINT('Ctrl Pts',(9.91941770625547,31.9978085657558,124.513876993849));
#92948=CARTESIAN_POINT('Ctrl Pts',(9.92346088288783,32.0141656631297,124.586818512363));
#92949=CARTESIAN_POINT('Ctrl Pts',(9.9275040595202,32.0265123954516,124.660522351868));
#92950=CARTESIAN_POINT('Ctrl Pts',(9.93153868618936,32.0388330185734,124.73407033246));
#92951=CARTESIAN_POINT('Ctrl Pts',(9.93557331285852,32.047160093344,124.808377016412));
#92952=CARTESIAN_POINT('Ctrl Pts',(9.93960793952768,32.0514160614572,124.882996985956));
#92953=CARTESIAN_POINT('Ctrl Pts',(9.94171371986435,32.0536373658557,124.921943158049));
#92954=CARTESIAN_POINT('Ctrl Pts',(9.94381950020102,32.0547505043392,124.96097446499));
#92955=CARTESIAN_POINT('Ctrl Pts',(9.94592528053769,32.0547499998285,125.00002654515));
#92956=CARTESIAN_POINT('Origin',(-1.54592528053767,30.,125.));
#92957=CARTESIAN_POINT('',(8.79398045138579,28.7479590808042,126.629230216746));
#92958=CARTESIAN_POINT('',(8.852020734751,28.7479590808042,126.629230216746));
#92959=CARTESIAN_POINT('',(-1.54592528053767,28.7479590808042,126.629230216746));
#92960=CARTESIAN_POINT('',(9.30407471946232,32.0547491738536,125.001842565591));
#92961=CARTESIAN_POINT('Ctrl Pts',(8.85202073475099,28.7479590808042,126.629230216746));
#92962=CARTESIAN_POINT('Ctrl Pts',(8.85588087637188,28.6913947464198,126.585761307019));
#92963=CARTESIAN_POINT('Ctrl Pts',(8.85974101799276,28.6371344517981,126.539372158411));
#92964=CARTESIAN_POINT('Ctrl Pts',(8.86360115961365,28.5854809162024,126.490346712706));
#92965=CARTESIAN_POINT('Ctrl Pts',(8.86746399129527,28.5337913842206,126.441287102081));
#92966=CARTESIAN_POINT('Ctrl Pts',(8.8713268229769,28.4847125588429,126.389587891694));
#92967=CARTESIAN_POINT('Ctrl Pts',(8.87518965465852,28.4385084505345,126.335567932921));
#92968=CARTESIAN_POINT('Ctrl Pts',(8.87905875237596,28.3922293929087,126.281460346464));
#92969=CARTESIAN_POINT('Ctrl Pts',(8.88292785009341,28.3488346463894,126.225024888472));
#92970=CARTESIAN_POINT('Ctrl Pts',(8.88679694781086,28.3085457296492,126.166610480757));
#92971=CARTESIAN_POINT('Ctrl Pts',(8.88741372907871,28.302123185955,126.157298513192));
#92972=CARTESIAN_POINT('Ctrl Pts',(8.88803051034656,28.2957794736538,126.147936307201));
#92973=CARTESIAN_POINT('Ctrl Pts',(8.8886472916144,28.2895153812363,126.138525331942));
#92974=CARTESIAN_POINT('Ctrl Pts',(8.89251643699301,28.2502199527083,126.079489117112));
#92975=CARTESIAN_POINT('Ctrl Pts',(8.89638558237161,28.2139075453724,126.01830051077));
#92976=CARTESIAN_POINT('Ctrl Pts',(8.90025472775021,28.1808210041849,125.955293328609));
#92977=CARTESIAN_POINT('Ctrl Pts',(8.90411810779598,28.1477837645623,125.892380032136));
#92978=CARTESIAN_POINT('Ctrl Pts',(8.90798148784175,28.1179630737262,125.827653965344));
#92979=CARTESIAN_POINT('Ctrl Pts',(8.91184486788753,28.0915583867166,125.761477623564));
#92980=CARTESIAN_POINT('Ctrl Pts',(8.91570371513117,28.0651846796314,125.695378924744));
#92981=CARTESIAN_POINT('Ctrl Pts',(8.91956256237482,28.0422191944493,125.627833779822));
#92982=CARTESIAN_POINT('Ctrl Pts',(8.92342140961847,28.0228145568944,125.559227401038));
#92983=CARTESIAN_POINT('Ctrl Pts',(8.92727782536573,28.0034221463863,125.490664251785));
#92984=CARTESIAN_POINT('Ctrl Pts',(8.93113424111299,27.9875862638826,125.421041661673));
#92985=CARTESIAN_POINT('Ctrl Pts',(8.93499065686025,27.9754101749661,125.350761461494));
#92986=CARTESIAN_POINT('Ctrl Pts',(8.93884593257506,27.9632376855413,125.280502037526));
#92987=CARTESIAN_POINT('Ctrl Pts',(8.94270120828986,27.9547229246952,125.209585867809));
#92988=CARTESIAN_POINT('Ctrl Pts',(8.94655648400467,27.9499180152724,125.138424775222));
#92989=CARTESIAN_POINT('Ctrl Pts',(8.95041190953726,27.9451129191286,125.067260917283));
#92990=CARTESIAN_POINT('Ctrl Pts',(8.95426733506985,27.94401799116,124.995852602389));
#92991=CARTESIAN_POINT('Ctrl Pts',(8.95812276060244,27.9466333401222,124.924614838314));
#92992=CARTESIAN_POINT('Ctrl Pts',(8.96198222008824,27.9492514255386,124.853302537769));
#92993=CARTESIAN_POINT('Ctrl Pts',(8.96584167957404,27.9555875195432,124.782161630701));
#92994=CARTESIAN_POINT('Ctrl Pts',(8.96970113905983,27.9655896507679,124.711604276319));
#92995=CARTESIAN_POINT('Ctrl Pts',(8.97356278284336,27.9755974427937,124.641006989333));
#92996=CARTESIAN_POINT('Ctrl Pts',(8.97742442662689,27.9892753092108,124.570994389477));
#92997=CARTESIAN_POINT('Ctrl Pts',(8.98128607041042,28.006520213743,124.501967968616));
#92998=CARTESIAN_POINT('Ctrl Pts',(8.98515446867269,28.0237952816842,124.432820812255));
#92999=CARTESIAN_POINT('Ctrl Pts',(8.98902286693495,28.0446497022752,124.364663743452));
#93000=CARTESIAN_POINT('Ctrl Pts',(8.99289126519722,28.0689309111879,124.297881963816));
#93001=CARTESIAN_POINT('Ctrl Pts',(8.99518836428247,28.0833493704573,124.258226180076));
#93002=CARTESIAN_POINT('Ctrl Pts',(8.99748546336772,28.0989752341499,124.219054955029));
#93003=CARTESIAN_POINT('Ctrl Pts',(8.99978256245297,28.1157688523033,124.180444910607));
#93004=CARTESIAN_POINT('Ctrl Pts',(9.00365172648552,28.1440555134024,124.115411322753));
#93005=CARTESIAN_POINT('Ctrl Pts',(9.00752089051807,28.1757684267354,124.051716582142));
#93006=CARTESIAN_POINT('Ctrl Pts',(9.01139005455062,28.2107588361673,123.989745764599));
#93007=CARTESIAN_POINT('Ctrl Pts',(9.01525345479223,28.2456971213151,123.927867263337));
#93008=CARTESIAN_POINT('Ctrl Pts',(9.01911685503385,28.2839029742327,123.867708007108));
#93009=CARTESIAN_POINT('Ctrl Pts',(9.02298025527546,28.3251800113167,123.809632171131));
#93010=CARTESIAN_POINT('Ctrl Pts',(9.02683912487806,28.3664086425036,123.751624441131));
#93011=CARTESIAN_POINT('Ctrl Pts',(9.03069799448066,28.4107010238021,123.695695672289));
#93012=CARTESIAN_POINT('Ctrl Pts',(9.03455686408325,28.4578162883206,123.64218301604));
#93013=CARTESIAN_POINT('Ctrl Pts',(9.03841330350832,28.504901881337,123.58870406014));
#93014=CARTESIAN_POINT('Ctrl Pts',(9.04226974293338,28.5548065102983,123.537638561759));
#93015=CARTESIAN_POINT('Ctrl Pts',(9.04612618235844,28.6072485761315,123.489291214756));
#93016=CARTESIAN_POINT('Ctrl Pts',(9.04998148302309,28.6596751564503,123.440958144147));
#93017=CARTESIAN_POINT('Ctrl Pts',(9.05383678368775,28.7146373291714,123.395341960534));
#93018=CARTESIAN_POINT('Ctrl Pts',(9.05769208435241,28.7718173635003,123.352709808837));
#93019=CARTESIAN_POINT('Ctrl Pts',(9.06154753606142,28.8289996380491,123.310075986883));
#93020=CARTESIAN_POINT('Ctrl Pts',(9.06540298777042,28.8883995559704,123.270426717542));
#93021=CARTESIAN_POINT('Ctrl Pts',(9.06925843947943,28.9496685012271,123.233987172984));
#93022=CARTESIAN_POINT('Ctrl Pts',(9.07311792680895,29.0110015785831,123.197509486028));
#93023=CARTESIAN_POINT('Ctrl Pts',(9.07697741413847,29.0742071702716,123.164248479424));
#93024=CARTESIAN_POINT('Ctrl Pts',(9.08083690146798,29.1389108080243,123.134384025057));
#93025=CARTESIAN_POINT('Ctrl Pts',(9.08469857407678,29.2036510816062,123.104502661145));
#93026=CARTESIAN_POINT('Ctrl Pts',(9.08856024668558,29.2698906385116,123.078021858301));
#93027=CARTESIAN_POINT('Ctrl Pts',(9.09242191929437,29.3372362779288,123.055072800538));
#93028=CARTESIAN_POINT('Ctrl Pts',(9.09629034760057,29.4046997333308,123.032083595174));
#93029=CARTESIAN_POINT('Ctrl Pts',(9.10015877590678,29.47327266706,123.012638603043));
#93030=CARTESIAN_POINT('Ctrl Pts',(9.10402720421298,29.5425487032,122.996818561998));
#93031=CARTESIAN_POINT('Ctrl Pts',(9.10632408057249,29.5836812968778,122.987425424681));
#93032=CARTESIAN_POINT('Ctrl Pts',(9.10862095693201,29.6250615840998,122.979309237482));
#93033=CARTESIAN_POINT('Ctrl Pts',(9.11091783329152,29.6666037127054,122.972478242258));
#93034=CARTESIAN_POINT('Ctrl Pts',(9.11478641228267,29.7365722181084,122.960972945291));
#93035=CARTESIAN_POINT('Ctrl Pts',(9.11865499127382,29.8072742400406,122.953071185289));
#93036=CARTESIAN_POINT('Ctrl Pts',(9.12252357026497,29.8783056996825,122.948856889495));
#93037=CARTESIAN_POINT('Ctrl Pts',(9.12638638331592,29.9492312901799,122.944648874918));
#93038=CARTESIAN_POINT('Ctrl Pts',(9.13024919636687,30.0204848626401,122.944117443783));
#93039=CARTESIAN_POINT('Ctrl Pts',(9.13411200941782,30.0916540559551,122.9472951755));
#93040=CARTESIAN_POINT('Ctrl Pts',(9.13797029147812,30.1627397694472,122.950469179811));
#93041=CARTESIAN_POINT('Ctrl Pts',(9.14182857353843,30.2337408173102,122.957343683396));
#93042=CARTESIAN_POINT('Ctrl Pts',(9.14568685559873,30.3042434075366,122.967899236881));
#93043=CARTESIAN_POINT('Ctrl Pts',(9.14954270758185,30.3747015928353,122.978448142119));
#93044=CARTESIAN_POINT('Ctrl Pts',(9.15339855956497,30.4446614639241,122.992673425752));
#93045=CARTESIAN_POINT('Ctrl Pts',(9.15725441154809,30.5137143999239,123.01050381307));
#93046=CARTESIAN_POINT('Ctrl Pts',(9.16110912573307,30.5827469595445,123.028328938935));
#93047=CARTESIAN_POINT('Ctrl Pts',(9.16496383991805,30.650872645138,123.049756935133));
#93048=CARTESIAN_POINT('Ctrl Pts',(9.16881855410303,30.717694781864,123.074665804961));
#93049=CARTESIAN_POINT('Ctrl Pts',(9.17267342115715,30.7845195686029,123.099575662619));
#93050=CARTESIAN_POINT('Ctrl Pts',(9.17652828821127,30.8500402492908,123.127966496182));
#93051=CARTESIAN_POINT('Ctrl Pts',(9.18038315526539,30.9138786595047,123.159667595731));
#93052=CARTESIAN_POINT('Ctrl Pts',(9.18424206474163,30.977784014129,123.191401938768));
#93053=CARTESIAN_POINT('Ctrl Pts',(9.18810097421787,31.0400031405998,123.226453260751));
#93054=CARTESIAN_POINT('Ctrl Pts',(9.19195988369411,31.1001819112534,123.264604562455));
#93055=CARTESIAN_POINT('Ctrl Pts',(9.19582098141221,31.1603948070156,123.302777498323));
#93056=CARTESIAN_POINT('Ctrl Pts',(9.19968207913031,31.218564647273,123.344053631923));
#93057=CARTESIAN_POINT('Ctrl Pts',(9.20354317684842,31.2743680517039,123.388173821004));
#93058=CARTESIAN_POINT('Ctrl Pts',(9.20741104118738,31.3302692522818,123.432371331255));
#93059=CARTESIAN_POINT('Ctrl Pts',(9.21127890552634,31.383795371967,123.479422527217));
#93060=CARTESIAN_POINT('Ctrl Pts',(9.2151467698653,31.4346582690326,123.529029839325));
#93061=CARTESIAN_POINT('Ctrl Pts',(9.2174488812869,31.4649313205176,123.558555580093));
#93062=CARTESIAN_POINT('Ctrl Pts',(9.21975099270849,31.4942616564072,123.588986141993));
#93063=CARTESIAN_POINT('Ctrl Pts',(9.22205310413008,31.5225954262331,123.620253381771));
#93064=CARTESIAN_POINT('Ctrl Pts',(9.22588174244541,31.5697172795699,123.67225388492));
#93065=CARTESIAN_POINT('Ctrl Pts',(9.22971038076074,31.6142741301639,123.726783950541));
#93066=CARTESIAN_POINT('Ctrl Pts',(9.23353901907606,31.6559786780319,123.783557572097));
#93067=CARTESIAN_POINT('Ctrl Pts',(9.23736240814987,31.6976260470216,123.840253354372));
#93068=CARTESIAN_POINT('Ctrl Pts',(9.24118579722367,31.7364285742198,123.899186198871));
#93069=CARTESIAN_POINT('Ctrl Pts',(9.24500918629747,31.7721371255726,123.960034822378));
#93070=CARTESIAN_POINT('Ctrl Pts',(9.24882867712127,31.8078092692101,124.02082140586));
#93071=CARTESIAN_POINT('Ctrl Pts',(9.25264816794507,31.8403934429899,124.083519468726));
#93072=CARTESIAN_POINT('Ctrl Pts',(9.25646765876886,31.8696831258354,124.147777862605));
#93073=CARTESIAN_POINT('Ctrl Pts',(9.26043491382665,31.9001059355162,124.214522214112));
#93074=CARTESIAN_POINT('Ctrl Pts',(9.26440216888444,31.9269738125268,124.282949638816));
#93075=CARTESIAN_POINT('Ctrl Pts',(9.26836942394223,31.9501078793459,124.352638569721));
#93076=CARTESIAN_POINT('Ctrl Pts',(9.27218609766135,31.9723638683253,124.419682383951));
#93077=CARTESIAN_POINT('Ctrl Pts',(9.27600277138047,31.9911642561016,124.48789314573));
#93078=CARTESIAN_POINT('Ctrl Pts',(9.2798194450996,32.0063997648491,124.556877504392));
#93079=CARTESIAN_POINT('Ctrl Pts',(9.28363614006936,32.0216353584255,124.625862247149));
#93080=CARTESIAN_POINT('Ctrl Pts',(9.28745283503914,32.03330593664,124.69562010812));
#93081=CARTESIAN_POINT('Ctrl Pts',(9.2912695300089,32.0413532894075,124.765747336568));
#93082=CARTESIAN_POINT('Ctrl Pts',(9.29508879757109,32.0494060663859,124.835921833339));
#93083=CARTESIAN_POINT('Ctrl Pts',(9.29890806513328,32.0538307059046,124.906465699354));
#93084=CARTESIAN_POINT('Ctrl Pts',(9.30272733269546,32.0546209489418,124.976971351112));
#93085=CARTESIAN_POINT('Ctrl Pts',(9.30317646161775,32.0547138780173,124.985262502981));
#93086=CARTESIAN_POINT('Ctrl Pts',(9.30362559054003,32.0547566072828,124.993553127999));
#93087=CARTESIAN_POINT('Ctrl Pts',(9.30407471946232,32.0547491738536,125.001842565591));
#93088=CARTESIAN_POINT('Ctrl Pts',(9.30407499487673,32.0541926768234,125.001847148429));
#93089=CARTESIAN_POINT('Ctrl Pts',(9.31377945490737,32.0557826428579,125.180912501179));
#93090=CARTESIAN_POINT('Ctrl Pts',(9.36052900521752,31.9523516367539,126.041729875259));
#93091=CARTESIAN_POINT('Ctrl Pts',(9.443186151042,30.7618134898646,127.294355624062));
#93092=CARTESIAN_POINT('Ctrl Pts',(9.51613883683583,29.2698357256828,127.032081053584));
#93093=CARTESIAN_POINT('Ctrl Pts',(9.55204643235015,28.7459520887588,126.631857121398));
#93094=CARTESIAN_POINT('',(9.24592528058239,32.0547492111101,124.998199460483));
#93095=CARTESIAN_POINT('Ctrl Pts',(9.24592528058239,32.0547492111101,124.998199460483));
#93096=CARTESIAN_POINT('Ctrl Pts',(9.24973097260797,32.0548106153326,125.068273055967));
#93097=CARTESIAN_POINT('Ctrl Pts',(9.25353666463355,32.0512831902227,125.138464586469));
#93098=CARTESIAN_POINT('Ctrl Pts',(9.25734235665914,32.0441573624556,125.208370439407));
#93099=CARTESIAN_POINT('Ctrl Pts',(9.26114473195258,32.0370377449812,125.27821536808));
#93100=CARTESIAN_POINT('Ctrl Pts',(9.26494710724602,32.0263259898409,125.347774616338));
#93101=CARTESIAN_POINT('Ctrl Pts',(9.26874948253946,32.0120645565245,125.416645872268));
#93102=CARTESIAN_POINT('Ctrl Pts',(9.27254990270275,31.9978104562451,125.485481715525));
#93103=CARTESIAN_POINT('Ctrl Pts',(9.27635032286603,31.9800103979003,125.553629777835));
#93104=CARTESIAN_POINT('Ctrl Pts',(9.28015074302932,31.9587582599149,125.62069609449));
#93105=CARTESIAN_POINT('Ctrl Pts',(9.28395056682591,31.9375094568417,125.687751887014));
#93106=CARTESIAN_POINT('Ctrl Pts',(9.2877503906225,31.912809801656,125.753725793385));
#93107=CARTESIAN_POINT('Ctrl Pts',(9.29155021441908,31.8848030010516,125.818239090808));
#93108=CARTESIAN_POINT('Ctrl Pts',(9.29535341054954,31.8567713444835,125.882809643618));
#93109=CARTESIAN_POINT('Ctrl Pts',(9.29915660668,31.8254268793358,125.945916537134));
#93110=CARTESIAN_POINT('Ctrl Pts',(9.30295980281046,31.7909610139902,126.007202168816));
#93111=CARTESIAN_POINT('Ctrl Pts',(9.30676464085467,31.7564802690602,126.068514258697));
#93112=CARTESIAN_POINT('Ctrl Pts',(9.31056947889889,31.7188757098795,126.128003097546));
#93113=CARTESIAN_POINT('Ctrl Pts',(9.3143743169431,31.6783826326264,126.185339318929));
#93114=CARTESIAN_POINT('Ctrl Pts',(9.31818598583954,31.6378168578698,126.242778476428));
#93115=CARTESIAN_POINT('Ctrl Pts',(9.32199765473598,31.5943525193413,126.298056904219));
#93116=CARTESIAN_POINT('Ctrl Pts',(9.32580932363243,31.5482653438227,126.350878228271));
#93117=CARTESIAN_POINT('Ctrl Pts',(9.32899379923462,31.5097616096317,126.395008036575));
#93118=CARTESIAN_POINT('Ctrl Pts',(9.33217827483681,31.4694279859487,126.4374233548));
#93119=CARTESIAN_POINT('Ctrl Pts',(9.335362750439,31.4274433973735,126.477972567335));
#93120=CARTESIAN_POINT('Ctrl Pts',(9.33923133005976,31.3764394821177,126.527232752322));
#93121=CARTESIAN_POINT('Ctrl Pts',(9.34309990968052,31.3227826115909,126.573946299928));
#93122=CARTESIAN_POINT('Ctrl Pts',(9.34696848930128,31.2667573975064,126.617814346074));
#93123=CARTESIAN_POINT('Ctrl Pts',(9.35083130298269,31.2108156864174,126.661617008922));
#93124=CARTESIAN_POINT('Ctrl Pts',(9.35469411666409,31.1525130179493,126.702582291555));
#93125=CARTESIAN_POINT('Ctrl Pts',(9.3585569303455,31.0921700218974,126.740448851811));
#93126=CARTESIAN_POINT('Ctrl Pts',(9.36241521303453,31.0318978068041,126.778270995455));
#93127=CARTESIAN_POINT('Ctrl Pts',(9.36627349572356,30.9695904274972,126.813001379431));
#93128=CARTESIAN_POINT('Ctrl Pts',(9.37013177841259,30.9055992840115,126.844420640553));
#93129=CARTESIAN_POINT('Ctrl Pts',(9.37398763102304,30.8416484443396,126.875820112748));
#93130=CARTESIAN_POINT('Ctrl Pts',(9.37784348363349,30.7760163796195,126.903912385907));
#93131=CARTESIAN_POINT('Ctrl Pts',(9.38169933624394,30.7090797143445,126.928523663636));
#93132=CARTESIAN_POINT('Ctrl Pts',(9.38555405105399,30.6421628010084,126.953127678971));
#93133=CARTESIAN_POINT('Ctrl Pts',(9.38940876586403,30.5739425072005,126.974252570507));
#93134=CARTESIAN_POINT('Ctrl Pts',(9.39326348067407,30.504814482049,126.991773054646));
#93135=CARTESIAN_POINT('Ctrl Pts',(9.39711834835005,30.4356837154963,127.009294233592));
#93136=CARTESIAN_POINT('Ctrl Pts',(9.40097321602602,30.3656456177036,127.023210604109));
#93137=CARTESIAN_POINT('Ctrl Pts',(9.404828083702,30.2951083207736,127.033447476949));
#93138=CARTESIAN_POINT('Ctrl Pts',(9.40868699379105,30.2244970547956,127.043695084702));
#93139=CARTESIAN_POINT('Ctrl Pts',(9.41254590388011,30.1533860265598,127.050255422412));
#93140=CARTESIAN_POINT('Ctrl Pts',(9.41640481396917,30.0821899271222,127.053105544871));
#93141=CARTESIAN_POINT('Ctrl Pts',(9.42026591229591,30.0109534551483,127.055957283523));
#93142=CARTESIAN_POINT('Ctrl Pts',(9.42412701062264,29.9396323020567,127.055094624619));
#93143=CARTESIAN_POINT('Ctrl Pts',(9.42798810894938,29.8686398401611,127.050546773645));
#93144=CARTESIAN_POINT('Ctrl Pts',(9.43185597388382,29.7975229633716,127.045990952524));
#93145=CARTESIAN_POINT('Ctrl Pts',(9.43572383881826,29.7267364106452,127.037737101432));
#93146=CARTESIAN_POINT('Ctrl Pts',(9.43959170375269,29.6566864281149,127.025866075006));
#93147=CARTESIAN_POINT('Ctrl Pts',(9.44189380959432,29.6149935363716,127.018800585454));
#93148=CARTESIAN_POINT('Ctrl Pts',(9.44419591543594,29.5735613605143,127.010454695704));
#93149=CARTESIAN_POINT('Ctrl Pts',(9.44649802127757,29.5324729501561,127.000853822788));
#93150=CARTESIAN_POINT('Ctrl Pts',(9.45045220849665,29.4618978861634,126.984362987183));
#93151=CARTESIAN_POINT('Ctrl Pts',(9.45440639571573,29.3920553464406,126.964100580526));
#93152=CARTESIAN_POINT('Ctrl Pts',(9.45836058293481,29.3233780040058,126.940149539865));
#93153=CARTESIAN_POINT('Ctrl Pts',(9.4622239475365,29.2562780921907,126.91674862394));
#93154=CARTESIAN_POINT('Ctrl Pts',(9.4660873121382,29.1902909208563,126.889826853226));
#93155=CARTESIAN_POINT('Ctrl Pts',(9.46995067673989,29.1258096198384,126.859513038871));
#93156=CARTESIAN_POINT('Ctrl Pts',(9.47395027526767,29.0590545130314,126.828130267696));
#93157=CARTESIAN_POINT('Ctrl Pts',(9.47794987379545,28.9939139882292,126.793111859723));
#93158=CARTESIAN_POINT('Ctrl Pts',(9.48194947232322,28.9308044976357,126.7546562456));
#93159=CARTESIAN_POINT('Ctrl Pts',(9.485949070851,28.8676950070421,126.716200631477));
#93160=CARTESIAN_POINT('Ctrl Pts',(9.48994866937878,28.8066170704991,126.674308071663));
#93161=CARTESIAN_POINT('Ctrl Pts',(9.49394826790656,28.7479590808042,126.629230216746));
#93162=CARTESIAN_POINT('Ctrl Pts',(8.79398045138579,28.7479590808042,126.629230216746));
#93163=CARTESIAN_POINT('Ctrl Pts',(8.79801550203991,28.6890704171239,126.583975092058));
#93164=CARTESIAN_POINT('Ctrl Pts',(8.80205055269404,28.6325495847743,126.535454723247));
#93165=CARTESIAN_POINT('Ctrl Pts',(8.80608560334816,28.5787741825237,126.483952404304));
#93166=CARTESIAN_POINT('Ctrl Pts',(8.80994358492291,28.5273585922768,126.43471014824));
#93167=CARTESIAN_POINT('Ctrl Pts',(8.81380156649766,28.4784529275307,126.382742540837));
#93168=CARTESIAN_POINT('Ctrl Pts',(8.81765954807242,28.4323541291087,126.328338806923));
#93169=CARTESIAN_POINT('Ctrl Pts',(8.82151545604507,28.3862801080382,126.273964314128));
#93170=CARTESIAN_POINT('Ctrl Pts',(8.82537136401772,28.3430102733044,126.217156662901));
#93171=CARTESIAN_POINT('Ctrl Pts',(8.82922727199037,28.3028032515543,126.158240372101));
#93172=CARTESIAN_POINT('Ctrl Pts',(8.83308239733767,28.2626043905369,126.099336039414));
#93173=CARTESIAN_POINT('Ctrl Pts',(8.83693752268498,28.2254673815428,126.038324318359));
#93174=CARTESIAN_POINT('Ctrl Pts',(8.84079264803228,28.1916082143369,125.975559691688));
#93175=CARTESIAN_POINT('Ctrl Pts',(8.84464828047665,28.1577445933498,125.912786809057));
#93176=CARTESIAN_POINT('Ctrl Pts',(8.84850391292102,28.1271598984163,125.848260991818));
#93177=CARTESIAN_POINT('Ctrl Pts',(8.85235954536539,28.1000239191649,125.782360821331));
#93178=CARTESIAN_POINT('Ctrl Pts',(8.85621943189836,28.0728579995958,125.716387940293));
#93179=CARTESIAN_POINT('Ctrl Pts',(8.86007931843133,28.0491485725025,125.649038130586));
#93180=CARTESIAN_POINT('Ctrl Pts',(8.8639392049643,28.0290167046793,125.580708543132));
#93181=CARTESIAN_POINT('Ctrl Pts',(8.86780159697256,28.0088717691411,125.512334602537));
#93182=CARTESIAN_POINT('Ctrl Pts',(8.87166398898081,27.992309126067,125.442980090994));
#93183=CARTESIAN_POINT('Ctrl Pts',(8.87552638098906,27.9793988842256,125.373053204558));
#93184=CARTESIAN_POINT('Ctrl Pts',(8.87939521111159,27.9664671226595,125.303009758932));
#93185=CARTESIAN_POINT('Ctrl Pts',(8.88326404123413,27.9571999712989,125.232392515708));
#93186=CARTESIAN_POINT('Ctrl Pts',(8.88713287135666,27.9516157013587,125.161614750502));
#93187=CARTESIAN_POINT('Ctrl Pts',(8.88836246993269,27.949840898602,125.13912003335));
#93188=CARTESIAN_POINT('Ctrl Pts',(8.88959206850872,27.9484377112274,125.116609094769));
#93189=CARTESIAN_POINT('Ctrl Pts',(8.89082166708475,27.9474056254475,125.094095143633));
#93190=CARTESIAN_POINT('Ctrl Pts',(8.89469075534478,27.9441580363138,125.02325213379));
#93191=CARTESIAN_POINT('Ctrl Pts',(8.89855984360481,27.9445759933657,124.952102042037));
#93192=CARTESIAN_POINT('Ctrl Pts',(8.90242893186485,27.9486955595437,124.881056084375));
#93193=CARTESIAN_POINT('Ctrl Pts',(8.90629225530753,27.9528089877002,124.810115982911));
#93194=CARTESIAN_POINT('Ctrl Pts',(8.91015557875022,27.9606130494148,124.739280188572));
#93195=CARTESIAN_POINT('Ctrl Pts',(8.9140189021929,27.9720918431932,124.66896213199));
#93196=CARTESIAN_POINT('Ctrl Pts',(8.91787769385889,27.9835571720544,124.598726560278));
#93197=CARTESIAN_POINT('Ctrl Pts',(8.92173648552489,27.998688592875,124.529007997088));
#93198=CARTESIAN_POINT('Ctrl Pts',(8.92559527719088,28.0174183654138,124.460215205196));
#93199=CARTESIAN_POINT('Ctrl Pts',(8.92945163802158,28.0361363391835,124.391465749136));
#93200=CARTESIAN_POINT('Ctrl Pts',(8.93330799885228,28.0584480401178,124.32364137495));
#93201=CARTESIAN_POINT('Ctrl Pts',(8.93716435968298,28.0842348635052,124.257139646844));
#93202=CARTESIAN_POINT('Ctrl Pts',(8.94101958121716,28.1100140686122,124.190657565548));
#93203=CARTESIAN_POINT('Ctrl Pts',(8.94487480275135,28.1392661824246,124.125497807253));
#93204=CARTESIAN_POINT('Ctrl Pts',(8.94873002428554,28.1718236234698,124.062040140093));
#93205=CARTESIAN_POINT('Ctrl Pts',(8.952585396449,28.2043823365829,123.998579993547));
#93206=CARTESIAN_POINT('Ctrl Pts',(8.95644076861247,28.2402464096163,123.93682250138));
#93207=CARTESIAN_POINT('Ctrl Pts',(8.96029614077593,28.2792020461361,123.877123352956));
#93208=CARTESIAN_POINT('Ctrl Pts',(8.96415554848578,28.3181984588174,123.817361715445));
#93209=CARTESIAN_POINT('Ctrl Pts',(8.96801495619562,28.3602926288398,123.759663130279));
#93210=CARTESIAN_POINT('Ctrl Pts',(8.97187436390547,28.4052275978471,123.70435400366));
#93211=CARTESIAN_POINT('Ctrl Pts',(8.97573595673313,28.4501880081161,123.649013562144));
#93212=CARTESIAN_POINT('Ctrl Pts',(8.9795975495608,28.4979920935116,123.596065633046));
#93213=CARTESIAN_POINT('Ctrl Pts',(8.98345914238846,28.5483446338577,123.545801161997));
#93214=CARTESIAN_POINT('Ctrl Pts',(8.98732749153428,28.5987852719909,123.495448747248));
#93215=CARTESIAN_POINT('Ctrl Pts',(8.99119584068009,28.6517829059278,123.447789489243));
#93216=CARTESIAN_POINT('Ctrl Pts',(8.99506418982591,28.7070082687023,123.403074846683));
#93217=CARTESIAN_POINT('Ctrl Pts',(8.99736177252505,28.7398090406287,123.376516853785));
#93218=CARTESIAN_POINT('Ctrl Pts',(8.99965935522418,28.7733950950642,123.350996826026));
#93219=CARTESIAN_POINT('Ctrl Pts',(9.00195693792331,28.8076929148876,123.326560016824));
#93220=CARTESIAN_POINT('Ctrl Pts',(9.00582595067416,28.8654487041671,123.285409669363));
#93221=CARTESIAN_POINT('Ctrl Pts',(9.00969496342501,28.9254504889425,123.24717222179));
#93222=CARTESIAN_POINT('Ctrl Pts',(9.01356397617586,28.987372364539,123.212100999944));
#93223=CARTESIAN_POINT('Ctrl Pts',(9.01742722389497,29.0492019732962,123.177082036057));
#93224=CARTESIAN_POINT('Ctrl Pts',(9.02129047161409,29.1129455745374,123.145220170585));
#93225=CARTESIAN_POINT('Ctrl Pts',(9.0251537193332,29.1782472182896,123.116726273679));
#93226=CARTESIAN_POINT('Ctrl Pts',(9.02901243532262,29.243472260845,123.088265801148));
#93227=CARTESIAN_POINT('Ctrl Pts',(9.03287115131202,29.3102512725042,123.063165643009));
#93228=CARTESIAN_POINT('Ctrl Pts',(9.03672986730144,29.3782041085501,123.041590586247));
#93229=CARTESIAN_POINT('Ctrl Pts',(9.04058615252545,29.4461141382834,123.020029120509));
#93230=CARTESIAN_POINT('Ctrl Pts',(9.04444243774945,29.5151960634365,123.001988497164));
#93231=CARTESIAN_POINT('Ctrl Pts',(9.04829872297347,29.5850515599355,122.987584696295));
#93232=CARTESIAN_POINT('Ctrl Pts',(9.05215386908144,29.6548864216754,122.973185150193));
#93233=CARTESIAN_POINT('Ctrl Pts',(9.05600901518941,29.725493925578,122.962420391861));
#93234=CARTESIAN_POINT('Ctrl Pts',(9.05986416129738,29.7964641351358,122.955355602014));
#93235=CARTESIAN_POINT('Ctrl Pts',(9.06371945832583,29.8674371230208,122.948290535597));
#93236=CARTESIAN_POINT('Ctrl Pts',(9.06757475535427,29.9387723611197,122.944925771168));
#93237=CARTESIAN_POINT('Ctrl Pts',(9.07143005238271,30.0100550770384,122.945274602793));
#93238=CARTESIAN_POINT('Ctrl Pts',(9.07528938591728,30.081412426148,122.945623799646));
#93239=CARTESIAN_POINT('Ctrl Pts',(9.07914871945184,30.1527166565108,122.94969435178));
#93240=CARTESIAN_POINT('Ctrl Pts',(9.08300805298641,30.2235541882578,122.957447408899));
#93241=CARTESIAN_POINT('Ctrl Pts',(9.08686957206813,30.2944318354196,122.965204856588));
#93242=CARTESIAN_POINT('Ctrl Pts',(9.09073109114985,30.3648417781052,122.976648882686));
#93243=CARTESIAN_POINT('Ctrl Pts',(9.09459261023157,30.4343794770015,122.991689258989));
#93244=CARTESIAN_POINT('Ctrl Pts',(9.0984608871096,30.5040388693545,123.006755956488));
#93245=CARTESIAN_POINT('Ctrl Pts',(9.10232916398764,30.5728225013246,123.025431442491));
#93246=CARTESIAN_POINT('Ctrl Pts',(9.10619744086568,30.6403405429456,123.047575468409));
#93247=CARTESIAN_POINT('Ctrl Pts',(9.10849569683108,30.6804549780857,123.0607318792));
#93248=CARTESIAN_POINT('Ctrl Pts',(9.11079395279648,30.7201230286415,123.075111713347));
#93249=CARTESIAN_POINT('Ctrl Pts',(9.11309220876188,30.7592667329505,123.090677714283));
#93250=CARTESIAN_POINT('Ctrl Pts',(9.11696135407878,30.8251656939425,123.116883289524));
#93251=CARTESIAN_POINT('Ctrl Pts',(9.12083049939568,30.8898354221716,123.146555879442));
#93252=CARTESIAN_POINT('Ctrl Pts',(9.12469964471258,30.952886311134,123.179559053264));
#93253=CARTESIAN_POINT('Ctrl Pts',(9.1285630246973,31.0158432492909,123.212513049749));
#93254=CARTESIAN_POINT('Ctrl Pts',(9.13242640468201,31.0771857094646,123.248787555605));
#93255=CARTESIAN_POINT('Ctrl Pts',(9.13628978466673,31.1365434600309,123.288197871844));
#93256=CARTESIAN_POINT('Ctrl Pts',(9.14014863185054,31.1958315677284,123.327561949007));
#93257=CARTESIAN_POINT('Ctrl Pts',(9.14400747903436,31.2531391885007,123.370054261092));
#93258=CARTESIAN_POINT('Ctrl Pts',(9.14786632621817,31.3081216859858,123.415444788859));
#93259=CARTESIAN_POINT('Ctrl Pts',(9.15172274190637,31.3630695384864,123.460806715631));
#93260=CARTESIAN_POINT('Ctrl Pts',(9.15557915759458,31.4156948006809,123.50906292642));
#93261=CARTESIAN_POINT('Ctrl Pts',(9.15943557328279,31.4656839817026,123.559941658029));
#93262=CARTESIAN_POINT('Ctrl Pts',(9.1632908489394,31.5156583849488,123.610805348894));
#93263=CARTESIAN_POINT('Ctrl Pts',(9.16714612459602,31.5629979138436,123.664289675139));
#93264=CARTESIAN_POINT('Ctrl Pts',(9.17100140025264,31.6074254582294,123.720085565854));
#93265=CARTESIAN_POINT('Ctrl Pts',(9.17485682572797,31.6518547291008,123.775883624836));
#93266=CARTESIAN_POINT('Ctrl Pts',(9.17871225120331,31.6933714899315,123.833993045247));
#93267=CARTESIAN_POINT('Ctrl Pts',(9.18256767667864,31.7317395997958,123.894072551657));
#93268=CARTESIAN_POINT('Ctrl Pts',(9.186427136109,31.7701478544457,123.954214919618));
#93269=CARTESIAN_POINT('Ctrl Pts',(9.19028659553936,31.8054006196676,124.016331078181));
#93270=CARTESIAN_POINT('Ctrl Pts',(9.19414605496972,31.8373062098376,124.080052472261));
#93271=CARTESIAN_POINT('Ctrl Pts',(9.19800769869874,31.8692298572872,124.143809930085));
#93272=CARTESIAN_POINT('Ctrl Pts',(9.20186934242776,31.8978023639166,124.209173986659));
#93273=CARTESIAN_POINT('Ctrl Pts',(9.20573098615679,31.9228801116375,124.275755815509));
#93274=CARTESIAN_POINT('Ctrl Pts',(9.20959938436661,31.9480017233648,124.342454104011));
#93275=CARTESIAN_POINT('Ctrl Pts',(9.21346778257643,31.9696162245264,124.410373954418));
#93276=CARTESIAN_POINT('Ctrl Pts',(9.21733618078625,31.9876299987723,124.479111767766));
#93277=CARTESIAN_POINT('Ctrl Pts',(9.21963328039098,31.9983267862941,124.519929076457));
#93278=CARTESIAN_POINT('Ctrl Pts',(9.22193037999571,32.0077548910856,124.561034600731));
#93279=CARTESIAN_POINT('Ctrl Pts',(9.22422747960044,32.0159033429618,124.602342767782));
#93280=CARTESIAN_POINT('Ctrl Pts',(9.22983481554542,32.0357941248016,124.703178086132));
#93281=CARTESIAN_POINT('Ctrl Pts',(9.23544215149041,32.0481241011246,124.805550423609));
#93282=CARTESIAN_POINT('Ctrl Pts',(9.24104948743539,32.0527129388303,124.908527855286));
#93283=CARTESIAN_POINT('Ctrl Pts',(9.24267475180283,32.0540429954711,124.938375460636));
#93284=CARTESIAN_POINT('Ctrl Pts',(9.24430001617026,32.0547229877209,124.968273728132));
#93285=CARTESIAN_POINT('Ctrl Pts',(9.24592528053769,32.0547492111093,124.99819945966));
#93286=CARTESIAN_POINT('Origin',(-1.54592528053767,30.,125.));
#93287=CARTESIAN_POINT('',(8.09385900549202,28.7479590808042,126.629230216746));
#93288=CARTESIAN_POINT('',(8.1521135920327,28.7479590808041,126.629230216746));
#93289=CARTESIAN_POINT('',(-1.54592528053767,28.7479590808042,126.629230216746));
#93290=CARTESIAN_POINT('',(8.60407471942971,32.0547498911252,124.999331104703));
#93291=CARTESIAN_POINT('Ctrl Pts',(8.1521135920327,28.7479590808041,126.629230216746));
#93292=CARTESIAN_POINT('Ctrl Pts',(8.15596912515558,28.6914354667109,126.585792600001));
#93293=CARTESIAN_POINT('Ctrl Pts',(8.15982465827847,28.6371472850519,126.539388739369));
#93294=CARTESIAN_POINT('Ctrl Pts',(8.16368019140134,28.5854141825686,126.490283371585));
#93295=CARTESIAN_POINT('Ctrl Pts',(8.16753532555932,28.5336864333507,126.441183085152));
#93296=CARTESIAN_POINT('Ctrl Pts',(8.17139045971729,28.484513589786,126.389382181945));
#93297=CARTESIAN_POINT('Ctrl Pts',(8.17524559387527,28.4381796297543,126.335183393241));
#93298=CARTESIAN_POINT('Ctrl Pts',(8.17912809993425,28.3915166932162,126.280599786832));
#93299=CARTESIAN_POINT('Ctrl Pts',(8.18301060599323,28.3477334539812,126.223584474127));
#93300=CARTESIAN_POINT('Ctrl Pts',(8.18689311205222,28.3070784500729,126.164480222371));
#93301=CARTESIAN_POINT('Ctrl Pts',(8.19075363060142,28.2666536846453,126.105710691357));
#93302=CARTESIAN_POINT('Ctrl Pts',(8.19461414915062,28.2293220239667,126.04487626749));
#93303=CARTESIAN_POINT('Ctrl Pts',(8.19847466769982,28.1952828349408,125.982340835271));
#93304=CARTESIAN_POINT('Ctrl Pts',(8.20236816751369,28.1609528415868,125.919271149009));
#93305=CARTESIAN_POINT('Ctrl Pts',(8.20626166732756,28.1299720655184,125.854471704079));
#93306=CARTESIAN_POINT('Ctrl Pts',(8.21015516714143,28.1024956005184,125.788336613667));
#93307=CARTESIAN_POINT('Ctrl Pts',(8.21404866695531,28.0750191355185,125.722201523256));
#93308=CARTESIAN_POINT('Ctrl Pts',(8.21794216676918,28.0510470881701,125.654731279922));
#93309=CARTESIAN_POINT('Ctrl Pts',(8.22183566658305,28.0306827603615,125.586333669648));
#93310=CARTESIAN_POINT('Ctrl Pts',(8.22570474050518,28.0104461882713,125.518365152144));
#93311=CARTESIAN_POINT('Ctrl Pts',(8.22957381442732,27.9936928812771,125.449214612468));
#93312=CARTESIAN_POINT('Ctrl Pts',(8.23344288834945,27.9805570105946,125.379272428528));
#93313=CARTESIAN_POINT('Ctrl Pts',(8.23730619731202,27.9674407124932,125.309434459154));
#93314=CARTESIAN_POINT('Ctrl Pts',(8.24116950627459,27.9579312406085,125.238807660454));
#93315=CARTESIAN_POINT('Ctrl Pts',(8.24503281523716,27.9521128697065,125.167797091983));
#93316=CARTESIAN_POINT('Ctrl Pts',(8.24889159228369,27.946301324137,125.09686982359));
#93317=CARTESIAN_POINT('Ctrl Pts',(8.25275036933023,27.944172318373,125.025560161463));
#93318=CARTESIAN_POINT('Ctrl Pts',(8.25660914637676,27.945758692832,124.954281137102));
#93319=CARTESIAN_POINT('Ctrl Pts',(8.26046549251019,27.9473440679229,124.883047016375));
#93320=CARTESIAN_POINT('Ctrl Pts',(8.26432183864362,27.9526401687858,124.81184397964));
#93321=CARTESIAN_POINT('Ctrl Pts',(8.26817818477705,27.9616277719837,124.74108645738));
#93322=CARTESIAN_POINT('Ctrl Pts',(8.27203339155849,27.970612719807,124.670349840331));
#93323=CARTESIAN_POINT('Ctrl Pts',(8.27588859833991,27.9832869435458,124.600058958094));
#93324=CARTESIAN_POINT('Ctrl Pts',(8.27974380512135,27.9995793967808,124.530622782065));
#93325=CARTESIAN_POINT('Ctrl Pts',(8.28359916249883,28.0158724864484,124.461183893649));
#93326=CARTESIAN_POINT('Ctrl Pts',(8.28745451987631,28.0357839731073,124.392600250166));
#93327=CARTESIAN_POINT('Ctrl Pts',(8.29130987725379,28.0591921524534,124.325268600552));
#93328=CARTESIAN_POINT('Ctrl Pts',(8.29516927023008,28.0826248343324,124.257866471472));
#93329=CARTESIAN_POINT('Ctrl Pts',(8.29902866320638,28.1095613555654,124.191719412152));
#93330=CARTESIAN_POINT('Ctrl Pts',(8.30288805618267,28.1398310617643,124.127206161959));
#93331=CARTESIAN_POINT('Ctrl Pts',(8.30674963428417,28.1701179061759,124.062656385418));
#93332=CARTESIAN_POINT('Ctrl Pts',(8.31061121238567,28.2037414632937,123.999742688106));
#93333=CARTESIAN_POINT('Ctrl Pts',(8.31447279048717,28.2404853943586,123.938818622933));
#93334=CARTESIAN_POINT('Ctrl Pts',(8.31834112507955,28.2772936152109,123.877787960694));
#93335=CARTESIAN_POINT('Ctrl Pts',(8.32220945967192,28.3172328380164,123.818754283396));
#93336=CARTESIAN_POINT('Ctrl Pts',(8.3260777942643,28.360044159249,123.76204103344));
#93337=CARTESIAN_POINT('Ctrl Pts',(8.32837550865007,28.3854732389526,123.728354482503));
#93338=CARTESIAN_POINT('Ctrl Pts',(8.33067322303584,28.4119148620755,123.695485968757));
#93339=CARTESIAN_POINT('Ctrl Pts',(8.33297093742161,28.4393085841369,123.663497150414));
#93340=CARTESIAN_POINT('Ctrl Pts',(8.3368400130158,28.48543632835,123.609631814886));
#93341=CARTESIAN_POINT('Ctrl Pts',(8.34070908860998,28.5344463408364,123.558051838837));
#93342=CARTESIAN_POINT('Ctrl Pts',(8.34457816420417,28.5860834172975,123.509081672371));
#93343=CARTESIAN_POINT('Ctrl Pts',(8.34844147486131,28.6376435543222,123.460184471636));
#93344=CARTESIAN_POINT('Ctrl Pts',(8.35230478551845,28.691822635864,123.413889693227));
#93345=CARTESIAN_POINT('Ctrl Pts',(8.35616809617559,28.74832606092,123.370487829831));
#93346=CARTESIAN_POINT('Ctrl Pts',(8.36002687494163,28.8047632041282,123.327136879379));
#93347=CARTESIAN_POINT('Ctrl Pts',(8.36388565370767,28.8635188915363,123.286672397668));
#93348=CARTESIAN_POINT('Ctrl Pts',(8.36774443247371,28.9242639284487,123.249345988819));
#93349=CARTESIAN_POINT('Ctrl Pts',(8.37160078034105,28.9849706980646,123.212043094332));
#93350=CARTESIAN_POINT('Ctrl Pts',(8.3754571282084,29.0476639178999,123.177874604336));
#93351=CARTESIAN_POINT('Ctrl Pts',(8.37931347607574,29.1119849803721,123.147049140583));
#93352=CARTESIAN_POINT('Ctrl Pts',(8.3831686846028,29.1762870394816,123.116232784071));
#93353=CARTESIAN_POINT('Ctrl Pts',(8.38702389312987,29.2422155485944,123.088757702811));
#93354=CARTESIAN_POINT('Ctrl Pts',(8.39087910165693,29.3093883796462,123.064786018981));
#93355=CARTESIAN_POINT('Ctrl Pts',(8.39473446078913,29.3765638348293,123.040813398688));
#93356=CARTESIAN_POINT('Ctrl Pts',(8.39858981992133,29.4449832501951,123.020344608747));
#93357=CARTESIAN_POINT('Ctrl Pts',(8.40244517905353,29.5142472913024,123.00349258241));
#93358=CARTESIAN_POINT('Ctrl Pts',(8.406304573786,29.5835838346004,122.986622916201));
#93359=CARTESIAN_POINT('Ctrl Pts',(8.41016396851848,29.6537662955446,122.973377686081));
#93360=CARTESIAN_POINT('Ctrl Pts',(8.41402336325095,29.7243839215627,122.96381893246));
#93361=CARTESIAN_POINT('Ctrl Pts',(8.41788494311211,29.7950415301716,122.954254766824));
#93362=CARTESIAN_POINT('Ctrl Pts',(8.42174652297327,29.8661343099628,122.948381272724));
#93363=CARTESIAN_POINT('Ctrl Pts',(8.42560810283443,29.9372478910485,122.946208448912));
#93364=CARTESIAN_POINT('Ctrl Pts',(8.42947643917265,30.0084858971871,122.944031823382));
#93365=CARTESIAN_POINT('Ctrl Pts',(8.43334477551087,30.0797442914579,122.945568785064));
#93366=CARTESIAN_POINT('Ctrl Pts',(8.43721311184909,30.1506109155235,122.950777241336));
#93367=CARTESIAN_POINT('Ctrl Pts',(8.43951081065278,30.192703986834,122.953870939169));
#93368=CARTESIAN_POINT('Ctrl Pts',(8.44180850945647,30.2346589582454,122.958258975204));
#93369=CARTESIAN_POINT('Ctrl Pts',(8.44410620826017,30.2763912468542,122.963924008991));
#93370=CARTESIAN_POINT('Ctrl Pts',(8.44797527432202,30.346663721767,122.973463288));
#93371=CARTESIAN_POINT('Ctrl Pts',(8.45184434038386,30.4165794115984,122.986663565757));
#93372=CARTESIAN_POINT('Ctrl Pts',(8.45571340644571,30.4857273196364,123.003486405391));
#93373=CARTESIAN_POINT('Ctrl Pts',(8.45957670755058,30.5547721964238,123.020284178783));
#93374=CARTESIAN_POINT('Ctrl Pts',(8.46344000865546,30.6230510940604,123.040693685944));
#93375=CARTESIAN_POINT('Ctrl Pts',(8.46730330976033,30.6901601774277,123.064624973812));
#93376=CARTESIAN_POINT('Ctrl Pts',(8.47116207899044,30.7571905379739,123.0885281889));
#93377=CARTESIAN_POINT('Ctrl Pts',(8.47502084822055,30.8230533546779,123.115944816256));
#93378=CARTESIAN_POINT('Ctrl Pts',(8.47887961745066,30.8873587018988,123.146734747354));
#93379=CARTESIAN_POINT('Ctrl Pts',(8.4827359557973,30.9516235391031,123.177505281922));
#93380=CARTESIAN_POINT('Ctrl Pts',(8.48659229414393,31.0143324162908,123.211644694856));
#93381=CARTESIAN_POINT('Ctrl Pts',(8.49044863249057,31.0751155666091,123.248964854455));
#93382=CARTESIAN_POINT('Ctrl Pts',(8.49430383152602,31.1358807592387,123.286273988238));
#93383=CARTESIAN_POINT('Ctrl Pts',(8.49815903056147,31.1947209407328,123.326761749048));
#93384=CARTESIAN_POINT('Ctrl Pts',(8.50201422959692,31.2512926538453,123.370195024878));
#93385=CARTESIAN_POINT('Ctrl Pts',(8.50586957928047,31.3078665775885,123.413629997933));
#93386=CARTESIAN_POINT('Ctrl Pts',(8.50972492896403,31.3621714729788,123.460010416944));
#93387=CARTESIAN_POINT('Ctrl Pts',(8.51358027864759,31.413895876396,123.509062035761));
#93388=CARTESIAN_POINT('Ctrl Pts',(8.51743966406173,31.465674424255,123.558165001182));
#93389=CARTESIAN_POINT('Ctrl Pts',(8.52129904947586,31.5148667346747,123.609944413246));
#93390=CARTESIAN_POINT('Ctrl Pts',(8.52515843489,31.5611979085457,123.664088830478));
#93391=CARTESIAN_POINT('Ctrl Pts',(8.52902000549224,31.6075553151763,123.718263904337));
#93392=CARTESIAN_POINT('Ctrl Pts',(8.53288157609448,31.651048064057,123.774806263801));
#93393=CARTESIAN_POINT('Ctrl Pts',(8.53674314669673,31.6914430166796,123.833373202851));
#93394=CARTESIAN_POINT('Ctrl Pts',(8.54061147397022,31.7319086491999,123.892042617705));
#93395=CARTESIAN_POINT('Ctrl Pts',(8.54447980124372,31.7692654090247,123.952743270899));
#93396=CARTESIAN_POINT('Ctrl Pts',(8.54834812851722,31.8033251213736,124.015106061993));
#93397=CARTESIAN_POINT('Ctrl Pts',(8.55064591204439,31.8235565652103,124.052149513581));
#93398=CARTESIAN_POINT('Ctrl Pts',(8.55294369557156,31.842625593561,124.089778987952));
#93399=CARTESIAN_POINT('Ctrl Pts',(8.55524147909873,31.8605008968746,124.127914009269));
#93400=CARTESIAN_POINT('Ctrl Pts',(8.559432104139,31.8931013106136,124.197463456967));
#93401=CARTESIAN_POINT('Ctrl Pts',(8.56362272917927,31.9218404086957,124.268933251934));
#93402=CARTESIAN_POINT('Ctrl Pts',(8.56781335421954,31.9465077850154,124.341892861781));
#93403=CARTESIAN_POINT('Ctrl Pts',(8.57199336345927,31.9711126732947,124.414667648444));
#93404=CARTESIAN_POINT('Ctrl Pts',(8.57617337269901,31.9916662582748,124.488924405375));
#93405=CARTESIAN_POINT('Ctrl Pts',(8.58035338193875,32.0080055595422,124.56421193758));
#93406=CARTESIAN_POINT('Ctrl Pts',(8.58451634367378,32.0242782235609,124.639192421526));
#93407=CARTESIAN_POINT('Ctrl Pts',(8.58867930540881,32.0363707665731,124.715194962654));
#93408=CARTESIAN_POINT('Ctrl Pts',(8.59284226714384,32.0441701294669,124.791754845686));
#93409=CARTESIAN_POINT('Ctrl Pts',(8.5965864179058,32.0511848445616,124.860612491428));
#93410=CARTESIAN_POINT('Ctrl Pts',(8.60033056866774,32.0547272954872,124.929920563126));
#93411=CARTESIAN_POINT('Ctrl Pts',(8.6040747194297,32.0547498911252,124.999331104703));
#93412=CARTESIAN_POINT('Ctrl Pts',(8.60407471946233,32.0547498911254,124.999331105308));
#93413=CARTESIAN_POINT('Ctrl Pts',(8.60802536883305,32.0547737329438,125.07256979943));
#93414=CARTESIAN_POINT('Ctrl Pts',(8.61197601820377,32.0508774975988,125.145776561394));
#93415=CARTESIAN_POINT('Ctrl Pts',(8.61592666757449,32.0430975791866,125.218517377849));
#93416=CARTESIAN_POINT('Ctrl Pts',(8.61988033452302,32.0353117183313,125.291313755061));
#93417=CARTESIAN_POINT('Ctrl Pts',(8.62383400147154,32.0236363229151,125.363643030758));
#93418=CARTESIAN_POINT('Ctrl Pts',(8.62778766842007,32.0081592793619,125.435079155112));
#93419=CARTESIAN_POINT('Ctrl Pts',(8.63174857351,31.9926539013458,125.506646060529));
#93420=CARTESIAN_POINT('Ctrl Pts',(8.63570947859993,31.9733330790047,125.57731610935));
#93421=CARTESIAN_POINT('Ctrl Pts',(8.63967038368986,31.950335120339,125.646676488572));
#93422=CARTESIAN_POINT('Ctrl Pts',(8.64363548345035,31.9273128064167,125.716110321699));
#93423=CARTESIAN_POINT('Ctrl Pts',(8.64760058321084,31.9006057650142,125.784231303702));
#93424=CARTESIAN_POINT('Ctrl Pts',(8.65156568297133,31.87040019397,125.850647210597));
#93425=CARTESIAN_POINT('Ctrl Pts',(8.65553895286672,31.8401323839897,125.917199968254));
#93426=CARTESIAN_POINT('Ctrl Pts',(8.65951222276212,31.8063518609842,125.982040237618));
#93427=CARTESIAN_POINT('Ctrl Pts',(8.66348549265752,31.7692902203559,126.044801262754));
#93428=CARTESIAN_POINT('Ctrl Pts',(8.66444924508411,31.7603005853628,126.060024515104));
#93429=CARTESIAN_POINT('Ctrl Pts',(8.6654129975107,31.7511180998049,126.075125578529));
#93430=CARTESIAN_POINT('Ctrl Pts',(8.66637674993729,31.7417464325632,126.090099503327));
#93431=CARTESIAN_POINT('Ctrl Pts',(8.67024583823578,31.7041228613408,126.150213943116));
#93432=CARTESIAN_POINT('Ctrl Pts',(8.67411492653427,31.663309772076,126.208496033772));
#93433=CARTESIAN_POINT('Ctrl Pts',(8.67798401483276,31.6195113983516,126.264587044497));
#93434=CARTESIAN_POINT('Ctrl Pts',(8.68184733831414,31.5757782827953,126.32059448142));
#93435=CARTESIAN_POINT('Ctrl Pts',(8.68571066179551,31.5290690084294,126.374416938867));
#93436=CARTESIAN_POINT('Ctrl Pts',(8.68957398527689,31.4796318084124,126.425723421297));
#93437=CARTESIAN_POINT('Ctrl Pts',(8.69343277698174,31.4302525994862,126.47696971992));
#93438=CARTESIAN_POINT('Ctrl Pts',(8.69729156868659,31.3781521564779,126.525705557696));
#93439=CARTESIAN_POINT('Ctrl Pts',(8.70115036039145,31.3236186940698,126.571633263586));
#93440=CARTESIAN_POINT('Ctrl Pts',(8.70500672126109,31.2691195848661,126.617532037443));
#93441=CARTESIAN_POINT('Ctrl Pts',(8.70886308213074,31.212190867749,126.660625876843));
#93442=CARTESIAN_POINT('Ctrl Pts',(8.71271944300038,31.1531562230052,126.700655252497));
#93443=CARTESIAN_POINT('Ctrl Pts',(8.71657466457353,31.0941390190471,126.740672802149));
#93444=CARTESIAN_POINT('Ctrl Pts',(8.72042988614668,31.0330175244716,126.777627412935));
#93445=CARTESIAN_POINT('Ctrl Pts',(8.72428510771983,30.9701455799791,126.811302049948));
#93446=CARTESIAN_POINT('Ctrl Pts',(8.72814047992222,30.9072711789862,126.84497800268));
#93447=CARTESIAN_POINT('Ctrl Pts',(8.73199585212462,30.8426466215573,126.875373499789));
#93448=CARTESIAN_POINT('Ctrl Pts',(8.73585122432701,30.7766500637452,126.902317597297));
#93449=CARTESIAN_POINT('Ctrl Pts',(8.73971063207546,30.7105844251453,126.929289898085));
#93450=CARTESIAN_POINT('Ctrl Pts',(8.74357003982391,30.6431443700123,126.952803403531));
#93451=CARTESIAN_POINT('Ctrl Pts',(8.74742944757237,30.5747268984803,126.972735804578));
#93452=CARTESIAN_POINT('Ctrl Pts',(8.75129104043852,30.5062706903758,126.992679490942));
#93453=CARTESIAN_POINT('Ctrl Pts',(8.75515263330467,30.4368364372972,127.009037925231));
#93454=CARTESIAN_POINT('Ctrl Pts',(8.75901422617082,30.3668324395648,127.021739727013));
#93455=CARTESIAN_POINT('Ctrl Pts',(8.76288257535451,30.2967059614845,127.034463752113));
#93456=CARTESIAN_POINT('Ctrl Pts',(8.76675092453821,30.2260082305367,127.04351830975));
#93457=CARTESIAN_POINT('Ctrl Pts',(8.77061927372191,30.1551530902908,127.048883862271));
#93458=CARTESIAN_POINT('Ctrl Pts',(8.77291685607322,30.1130691128632,127.052070699392));
#93459=CARTESIAN_POINT('Ctrl Pts',(8.77521443842453,30.0709296353044,127.053957167735));
#93460=CARTESIAN_POINT('Ctrl Pts',(8.77751202077585,30.0288208638428,127.054547862744));
#93461=CARTESIAN_POINT('Ctrl Pts',(8.78138027673787,29.9579256873689,127.055542368769));
#93462=CARTESIAN_POINT('Ctrl Pts',(8.78524853269989,29.8868401127541,127.052865003996));
#93463=CARTESIAN_POINT('Ctrl Pts',(8.78911678866191,29.8159760378281,127.046492791057));
#93464=CARTESIAN_POINT('Ctrl Pts',(8.79297966466309,29.7452105204824,127.040129440575));
#93465=CARTESIAN_POINT('Ctrl Pts',(8.79684254066427,29.6746663711641,127.030081480092));
#93466=CARTESIAN_POINT('Ctrl Pts',(8.80070541666546,29.604756174732,127.016377911277));
#93467=CARTESIAN_POINT('Ctrl Pts',(8.8045642130925,29.5349198102917,127.002688814769));
#93468=CARTESIAN_POINT('Ctrl Pts',(8.80842300951955,29.4657165441792,126.985351865614));
#93469=CARTESIAN_POINT('Ctrl Pts',(8.8122818059466,29.3975527960711,126.964447741473));
#93470=CARTESIAN_POINT('Ctrl Pts',(8.81613815589117,29.3294322638773,126.943556870576));
#93471=CARTESIAN_POINT('Ctrl Pts',(8.81999450583573,29.2623504054606,126.919103454006));
#93472=CARTESIAN_POINT('Ctrl Pts',(8.8238508557803,29.1967008280559,126.891218655485));
#93473=CARTESIAN_POINT('Ctrl Pts',(8.82770577827881,29.1310755511508,126.863344178653));
#93474=CARTESIAN_POINT('Ctrl Pts',(8.83156070077733,29.0668819478089,126.832041035445));
#93475=CARTESIAN_POINT('Ctrl Pts',(8.83541562327585,29.0044941995705,126.79748873816));
#93476=CARTESIAN_POINT('Ctrl Pts',(8.83927149035687,28.9420911642866,126.762927974428));
#93477=CARTESIAN_POINT('Ctrl Pts',(8.8431273574379,28.8814952931375,126.725116701829));
#93478=CARTESIAN_POINT('Ctrl Pts',(8.84698322451892,28.8230554528631,126.684279993191));
#93479=CARTESIAN_POINT('Ctrl Pts',(8.84866239459628,28.7976058123407,126.666496242413));
#93480=CARTESIAN_POINT('Ctrl Pts',(8.85034156467364,28.7725646904092,126.648139287884));
#93481=CARTESIAN_POINT('Ctrl Pts',(8.85202073475099,28.7479590808042,126.629230216746));
#93482=CARTESIAN_POINT('',(8.54592528048629,32.0547496520905,125.001195714812));
#93483=CARTESIAN_POINT('Ctrl Pts',(8.54592528053769,32.05474965209,125.001195715756));
#93484=CARTESIAN_POINT('Ctrl Pts',(8.54975547188149,32.0547087341196,125.071510240684));
#93485=CARTESIAN_POINT('Ctrl Pts',(8.55358566322529,32.0510587896527,125.141718266712));
#93486=CARTESIAN_POINT('Ctrl Pts',(8.55741585456908,32.0438307944864,125.211549630132));
#93487=CARTESIAN_POINT('Ctrl Pts',(8.56128493015697,32.0365294204461,125.282089924135));
#93488=CARTESIAN_POINT('Ctrl Pts',(8.56515400574485,32.02555754131,125.352389946217));
#93489=CARTESIAN_POINT('Ctrl Pts',(8.56902308133273,32.0109405151941,125.42203768416));
#93490=CARTESIAN_POINT('Ctrl Pts',(8.57288639198354,31.9963452685017,125.491581646712));
#93491=CARTESIAN_POINT('Ctrl Pts',(8.57674970263436,31.9781157547389,125.560474782776));
#93492=CARTESIAN_POINT('Ctrl Pts',(8.58061301328517,31.9563290497598,125.628310601189));
#93493=CARTESIAN_POINT('Ctrl Pts',(8.58447179204486,31.9345679018699,125.696066844188));
#93494=CARTESIAN_POINT('Ctrl Pts',(8.58833057080455,31.909257999171,125.762767772912));
#93495=CARTESIAN_POINT('Ctrl Pts',(8.59218934956424,31.8805269896333,125.828019204947));
#93496=CARTESIAN_POINT('Ctrl Pts',(8.59604569742522,31.8518140796495,125.89322953081));
#93497=CARTESIAN_POINT('Ctrl Pts',(8.5999020452862,31.8196845339681,125.956991728081));
#93498=CARTESIAN_POINT('Ctrl Pts',(8.60375839314718,31.7843146400526,126.018930236961));
#93499=CARTESIAN_POINT('Ctrl Pts',(8.60761360166789,31.7489551960099,126.080850446393));
#93500=CARTESIAN_POINT('Ctrl Pts',(8.6114688101886,31.7103575450951,126.140947615484));
#93501=CARTESIAN_POINT('Ctrl Pts',(8.61532401870931,31.6687437683968,126.198871051422));
#93502=CARTESIAN_POINT('Ctrl Pts',(8.61917937783514,31.6271283660412,126.25679675016));
#93503=CARTESIAN_POINT('Ctrl Pts',(8.62303473696097,31.5824968892007,126.312548153912));
#93504=CARTESIAN_POINT('Ctrl Pts',(8.6268900960868,31.5351135490116,126.365805240194));
#93505=CARTESIAN_POINT('Ctrl Pts',(8.63074949081298,31.487680610272,126.419118073375));
#93506=CARTESIAN_POINT('Ctrl Pts',(8.63460888553917,31.4374903815943,126.46993101341));
#93507=CARTESIAN_POINT('Ctrl Pts',(8.63846828026535,31.38484541259,126.517959401871));
#93508=CARTESIAN_POINT('Ctrl Pts',(8.64232986012025,31.3321706368306,126.566014983252));
#93509=CARTESIAN_POINT('Ctrl Pts',(8.64619143997515,31.2770387296325,126.611282566182));
#93510=CARTESIAN_POINT('Ctrl Pts',(8.65005301983005,31.2197848164688,126.653518238185));
#93511=CARTESIAN_POINT('Ctrl Pts',(8.65392135616211,31.1624307280476,126.695827808533));
#93512=CARTESIAN_POINT('Ctrl Pts',(8.65778969249417,31.102947626487,126.735094608986));
#93513=CARTESIAN_POINT('Ctrl Pts',(8.66165802882622,31.0416984472471,126.771118829301));
#93514=CARTESIAN_POINT('Ctrl Pts',(8.66395572768669,31.0053179060367,126.792516350834));
#93515=CARTESIAN_POINT('Ctrl Pts',(8.66625342654716,30.9683147455938,126.812770750143));
#93516=CARTESIAN_POINT('Ctrl Pts',(8.66855112540763,30.9307683970591,126.831848179718));
#93517=CARTESIAN_POINT('Ctrl Pts',(8.67242019148436,30.8675445752087,126.863972422311));
#93518=CARTESIAN_POINT('Ctrl Pts',(8.67628925756109,30.8025318708695,126.892882616512));
#93519=CARTESIAN_POINT('Ctrl Pts',(8.68015832363782,30.7360901847401,126.918376605995));
#93520=CARTESIAN_POINT('Ctrl Pts',(8.68402162475757,30.6697474975563,126.943832609114));
#93521=CARTESIAN_POINT('Ctrl Pts',(8.68788492587733,30.6019805048365,126.965882338784));
#93522=CARTESIAN_POINT('Ctrl Pts',(8.69174822699708,30.5331725187789,126.984370083356));
#93523=CARTESIAN_POINT('Ctrl Pts',(8.69560699624201,30.4644452484538,127.002836140739));
#93524=CARTESIAN_POINT('Ctrl Pts',(8.69946576548694,30.3946798772693,127.017748387325));
#93525=CARTESIAN_POINT('Ctrl Pts',(8.70332453473188,30.3242768049301,127.029000275082));
#93526=CARTESIAN_POINT('Ctrl Pts',(8.70718087309328,30.253918083952,127.040245074562));
#93527=CARTESIAN_POINT('Ctrl Pts',(8.71103721145469,30.1829229374078,127.047834013581));
#93528=CARTESIAN_POINT('Ctrl Pts',(8.7148935498161,30.1117024997309,127.051711508486));
#93529=CARTESIAN_POINT('Ctrl Pts',(8.71874874886626,30.0405031033212,127.055587857829));
#93530=CARTESIAN_POINT('Ctrl Pts',(8.72260394791642,29.9690790327236,127.055754913527));
#93531=CARTESIAN_POINT('Ctrl Pts',(8.72645914696657,29.8978453674011,127.052209052104));
#93532=CARTESIAN_POINT('Ctrl Pts',(8.73031449666474,29.8266089185103,127.048663052121));
#93533=CARTESIAN_POINT('Ctrl Pts',(8.73416984636291,29.7555633747443,127.041403873315));
#93534=CARTESIAN_POINT('Ctrl Pts',(8.73802519606107,29.6851208979289,127.030479921984));
#93535=CARTESIAN_POINT('Ctrl Pts',(8.74188458148958,29.6146046828372,127.019544535601));
#93536=CARTESIAN_POINT('Ctrl Pts',(8.7457439669181,29.5446932759119,127.004936793299));
#93537=CARTESIAN_POINT('Ctrl Pts',(8.74960335234661,29.4757899215076,126.986756491397));
#93538=CARTESIAN_POINT('Ctrl Pts',(8.75346492296311,29.4068475539533,126.968565895788));
#93539=CARTESIAN_POINT('Ctrl Pts',(8.75732649357962,29.3389148379663,126.946798862138));
#93540=CARTESIAN_POINT('Ctrl Pts',(8.76118806419612,29.2723784533722,126.921604654288));
#93541=CARTESIAN_POINT('Ctrl Pts',(8.76505639148356,29.2057256486734,126.896366363606));
#93542=CARTESIAN_POINT('Ctrl Pts',(8.76892471877099,29.1404744981413,126.867689121859));
#93543=CARTESIAN_POINT('Ctrl Pts',(8.77279304605842,29.076989712482,126.835769476714));
#93544=CARTESIAN_POINT('Ctrl Pts',(8.77509082945434,29.0392797992448,126.816809232359));
#93545=CARTESIAN_POINT('Ctrl Pts',(8.77738861285027,29.0021926314037,126.796705825613));
#93546=CARTESIAN_POINT('Ctrl Pts',(8.7796863962462,28.9657997342526,126.775507638065));
#93547=CARTESIAN_POINT('Ctrl Pts',(8.78355540286644,28.9045213908469,126.739814139667));
#93548=CARTESIAN_POINT('Ctrl Pts',(8.78742440948668,28.8449730340153,126.700874643057));
#93549=CARTESIAN_POINT('Ctrl Pts',(8.79129341610692,28.7875196822617,126.658881864871));
#93550=CARTESIAN_POINT('Ctrl Pts',(8.79218909453321,28.7742191809355,126.649160499887));
#93551=CARTESIAN_POINT('Ctrl Pts',(8.7930847729595,28.7610308635729,126.639275701261));
#93552=CARTESIAN_POINT('Ctrl Pts',(8.79398045138579,28.7479590808042,126.629230216746));
#93553=CARTESIAN_POINT('Ctrl Pts',(8.09385900549202,28.7479590808042,126.629230216746));
#93554=CARTESIAN_POINT('Ctrl Pts',(8.09772727053521,28.6914420071518,126.585797626239));
#93555=CARTESIAN_POINT('Ctrl Pts',(8.1015955355784,28.6372602689121,126.539476708772));
#93556=CARTESIAN_POINT('Ctrl Pts',(8.10546380062159,28.5857065484924,126.490560832547));
#93557=CARTESIAN_POINT('Ctrl Pts',(8.10793412415267,28.5527836832683,126.459322528363));
#93558=CARTESIAN_POINT('Ctrl Pts',(8.11040444768375,28.5209318401603,126.427026677829));
#93559=CARTESIAN_POINT('Ctrl Pts',(8.11287477121484,28.490218582045,126.393756661867));
#93560=CARTESIAN_POINT('Ctrl Pts',(8.11674384460118,28.4421148223202,126.341648453488));
#93561=CARTESIAN_POINT('Ctrl Pts',(8.12061291798752,28.3966176809064,126.28694489407));
#93562=CARTESIAN_POINT('Ctrl Pts',(8.12448199137386,28.3540195505217,126.229937365249));
#93563=CARTESIAN_POINT('Ctrl Pts',(8.12834529980684,28.3114848917257,126.173014778147));
#93564=CARTESIAN_POINT('Ctrl Pts',(8.13220860823982,28.2718409581833,126.113795421894));
#93565=CARTESIAN_POINT('Ctrl Pts',(8.13607191667281,28.2353418126453,126.052605835202));
#93566=CARTESIAN_POINT('Ctrl Pts',(8.13993069320138,28.1988854829067,125.991488027755));
#93567=CARTESIAN_POINT('Ctrl Pts',(8.14378946972996,28.165566861152,125.92840499588));
#93568=CARTESIAN_POINT('Ctrl Pts',(8.14764824625854,28.1355973442775,125.863713088841));
#93569=CARTESIAN_POINT('Ctrl Pts',(8.15150459188144,28.1056467072391,125.799061935632));
#93570=CARTESIAN_POINT('Ctrl Pts',(8.15536093750435,28.0790411929319,125.732804357848));
#93571=CARTESIAN_POINT('Ctrl Pts',(8.15921728312725,28.0559460722781,125.665320891457));
#93572=CARTESIAN_POINT('Ctrl Pts',(8.16307248940628,28.0328577749974,125.597857362821));
#93573=CARTESIAN_POINT('Ctrl Pts',(8.1669276956853,28.0132779695831,125.529169123978));
#93574=CARTESIAN_POINT('Ctrl Pts',(8.17078290196433,27.997322996701,125.459654634435));
#93575=CARTESIAN_POINT('Ctrl Pts',(8.17463825884822,27.9813674005329,125.390137429286));
#93576=CARTESIAN_POINT('Ctrl Pts',(8.17849361573211,27.9690370245609,125.31979438332));
#93577=CARTESIAN_POINT('Ctrl Pts',(8.182348972616,27.9603973463798,125.249035294377));
#93578=CARTESIAN_POINT('Ctrl Pts',(8.18620836511539,27.9517486245691,125.178202137978));
#93579=CARTESIAN_POINT('Ctrl Pts',(8.19006775761479,27.9467983714776,125.106952552449));
#93580=CARTESIAN_POINT('Ctrl Pts',(8.19392715011418,27.9455601860251,125.035701726213));
#93581=CARTESIAN_POINT('Ctrl Pts',(8.19778872774748,27.9443212995293,124.96441055876));
#93582=CARTESIAN_POINT('Ctrl Pts',(8.20165030538077,27.9467986476714,124.893118634925));
#93583=CARTESIAN_POINT('Ctrl Pts',(8.20551188301407,27.9529537216554,124.822238652077));
#93584=CARTESIAN_POINT('Ctrl Pts',(8.20938021715695,27.9591195650244,124.751234652226));
#93585=CARTESIAN_POINT('Ctrl Pts',(8.21324855129984,27.9689759143582,124.68064451366));
#93586=CARTESIAN_POINT('Ctrl Pts',(8.21711688544273,27.9824327851579,124.610872647974));
#93587=CARTESIAN_POINT('Ctrl Pts',(8.21941460431295,27.9904259172992,124.569429451375));
#93588=CARTESIAN_POINT('Ctrl Pts',(8.22171232318318,27.9996883921957,124.528274718171));
#93589=CARTESIAN_POINT('Ctrl Pts',(8.2240100420534,28.0101930999335,124.487490426482));
#93590=CARTESIAN_POINT('Ctrl Pts',(8.22787911571879,28.0278817252034,124.418814736439));
#93591=CARTESIAN_POINT('Ctrl Pts',(8.23174818938418,28.0491645546055,124.350921355076));
#93592=CARTESIAN_POINT('Ctrl Pts',(8.23561726304956,28.0739553689881,124.284213969227));
#93593=CARTESIAN_POINT('Ctrl Pts',(8.23948057176422,28.0987092448589,124.217605977916));
#93594=CARTESIAN_POINT('Ctrl Pts',(8.24334388047887,28.1269605625616,124.152180926039));
#93595=CARTESIAN_POINT('Ctrl Pts',(8.24720718919353,28.1585727771566,124.088329365686));
#93596=CARTESIAN_POINT('Ctrl Pts',(8.25106596600628,28.1901479086537,124.024552707192));
#93597=CARTESIAN_POINT('Ctrl Pts',(8.25492474281903,28.2250758913303,123.96234630707));
#93598=CARTESIAN_POINT('Ctrl Pts',(8.25878351963178,28.2631719946789,123.902081040134));
#93599=CARTESIAN_POINT('Ctrl Pts',(8.26263986554025,28.3012440987176,123.841853738363));
#93600=CARTESIAN_POINT('Ctrl Pts',(8.26649621144872,28.3424801048097,123.783565553315));
#93601=CARTESIAN_POINT('Ctrl Pts',(8.27035255735718,28.3866499450746,123.727561725359));
#93602=CARTESIAN_POINT('Ctrl Pts',(8.27420776392272,28.4308067355261,123.671574443523));
#93603=CARTESIAN_POINT('Ctrl Pts',(8.27806297048826,28.4778953386646,123.617870560131));
#93604=CARTESIAN_POINT('Ctrl Pts',(8.2819181770538,28.5276440902535,123.566763928191));
#93605=CARTESIAN_POINT('Ctrl Pts',(8.28577353422473,28.5773947852999,123.515655299748));
#93606=CARTESIAN_POINT('Ctrl Pts',(8.28962889139566,28.6298054946908,123.467144470758));
#93607=CARTESIAN_POINT('Ctrl Pts',(8.29348424856659,28.6845674420588,123.421508711456));
#93608=CARTESIAN_POINT('Ctrl Pts',(8.29734364135182,28.7393867117677,123.375825182696));
#93609=CARTESIAN_POINT('Ctrl Pts',(8.30120303413705,28.7965617585492,123.333023042882));
#93610=CARTESIAN_POINT('Ctrl Pts',(8.30506242692227,28.8557511400428,123.293338900371));
#93611=CARTESIAN_POINT('Ctrl Pts',(8.30892400484116,28.9149740337277,123.253632289259));
#93612=CARTESIAN_POINT('Ctrl Pts',(8.31278558276005,28.9762131152528,123.217047439008));
#93613=CARTESIAN_POINT('Ctrl Pts',(8.31664716067893,29.039100773748,123.183775828955));
#93614=CARTESIAN_POINT('Ctrl Pts',(8.3205154951039,29.1020984652027,123.150446004399));
#93615=CARTESIAN_POINT('Ctrl Pts',(8.32438382952886,29.1667500517798,123.120441198674));
#93616=CARTESIAN_POINT('Ctrl Pts',(8.32825216395382,29.2326669652735,123.093905150231));
#93617=CARTESIAN_POINT('Ctrl Pts',(8.33054988026653,29.2718203451986,123.078143247384));
#93618=CARTESIAN_POINT('Ctrl Pts',(8.33284759657924,29.311419819351,123.063604224152));
#93619=CARTESIAN_POINT('Ctrl Pts',(8.33514531289195,29.3513818111861,123.050309766235));
#93620=CARTESIAN_POINT('Ctrl Pts',(8.33901438538704,29.4186729047829,123.027923529439));
#93621=CARTESIAN_POINT('Ctrl Pts',(8.34288345788212,29.4872561137565,123.008981234008));
#93622=CARTESIAN_POINT('Ctrl Pts',(8.3467525303772,29.5567455212836,122.993629388772));
#93623=CARTESIAN_POINT('Ctrl Pts',(8.35061583791992,29.6261313889768,122.978300417922));
#93624=CARTESIAN_POINT('Ctrl Pts',(8.35447914546264,29.6964203045437,122.966551381999));
#93625=CARTESIAN_POINT('Ctrl Pts',(8.35834245300537,29.7672100913159,122.958479385136));
#93626=CARTESIAN_POINT('Ctrl Pts',(8.36220122864938,29.8379168372896,122.950416857225));
#93627=CARTESIAN_POINT('Ctrl Pts',(8.3660600042934,29.9091228070739,122.946022855284));
#93628=CARTESIAN_POINT('Ctrl Pts',(8.36991877993741,29.9804162215998,122.945343328407));
#93629=CARTESIAN_POINT('Ctrl Pts',(8.37377512467975,30.0516647236204,122.944664229609));
#93630=CARTESIAN_POINT('Ctrl Pts',(8.37763146942208,30.1230000764747,122.947694967979));
#93631=CARTESIAN_POINT('Ctrl Pts',(8.38148781416442,30.1940074483337,122.954429499506));
#93632=CARTESIAN_POINT('Ctrl Pts',(8.38534301956812,30.264993841404,122.961162041348));
#93633=CARTESIAN_POINT('Ctrl Pts',(8.38919822497183,30.3356519625006,122.971596158081));
#93634=CARTESIAN_POINT('Ctrl Pts',(8.39305343037553,30.4055707893079,122.985673835408));
#93635=CARTESIAN_POINT('Ctrl Pts',(8.39690878639061,30.4754923476351,122.999752062707));
#93636=CARTESIAN_POINT('Ctrl Pts',(8.4007641424057,30.544674078537,123.017474035159));
#93637=CARTESIAN_POINT('Ctrl Pts',(8.40461949842078,30.6127155661947,123.038730717764));
#93638=CARTESIAN_POINT('Ctrl Pts',(8.4084788900672,30.6808282769402,123.060009651008));
#93639=CARTESIAN_POINT('Ctrl Pts',(8.41233828171362,30.7477978971905,123.084830535264));
#93640=CARTESIAN_POINT('Ctrl Pts',(8.41619767336005,30.8132404560791,123.113034837869));
#93641=CARTESIAN_POINT('Ctrl Pts',(8.42005925014802,30.8787200677644,123.141255109414));
#93642=CARTESIAN_POINT('Ctrl Pts',(8.42392082693599,30.9426704612239,123.172862397432));
#93643=CARTESIAN_POINT('Ctrl Pts',(8.42778240372396,31.0047313875944,123.207651707596));
#93644=CARTESIAN_POINT('Ctrl Pts',(8.43165073704272,31.0669009008409,123.242501887985));
#93645=CARTESIAN_POINT('Ctrl Pts',(8.43551907036148,31.1271739356095,123.280544946878));
#93646=CARTESIAN_POINT('Ctrl Pts',(8.43938740368024,31.1852189857341,123.32153238984));
#93647=CARTESIAN_POINT('Ctrl Pts',(8.44168513036367,31.2196967955612,123.345878260172));
#93648=CARTESIAN_POINT('Ctrl Pts',(8.44398285704709,31.253389149455,123.371262169097));
#93649=CARTESIAN_POINT('Ctrl Pts',(8.44628058373052,31.2862324985407,123.397625661027));
#93650=CARTESIAN_POINT('Ctrl Pts',(8.45010049336537,31.3408336948092,123.441454266736));
#93651=CARTESIAN_POINT('Ctrl Pts',(8.45392040300023,31.3933122556876,123.488173581411));
#93652=CARTESIAN_POINT('Ctrl Pts',(8.45774031263508,31.4433401853721,123.537547719825));
#93653=CARTESIAN_POINT('Ctrl Pts',(8.46155371406939,31.493282879585,123.586837736669));
#93654=CARTESIAN_POINT('Ctrl Pts',(8.4653671155037,31.5407828803758,123.63877324907));
#93655=CARTESIAN_POINT('Ctrl Pts',(8.46918051693801,31.5855446175212,123.693077726738));
#93656=CARTESIAN_POINT('Ctrl Pts',(8.4729902881967,31.6302637436357,123.747330509142));
#93657=CARTESIAN_POINT('Ctrl Pts',(8.4768000594554,31.6722494565306,123.803947404127));
#93658=CARTESIAN_POINT('Ctrl Pts',(8.48060983071409,31.7112435016815,123.862615614468));
#93659=CARTESIAN_POINT('Ctrl Pts',(8.48441732747834,31.750214266763,123.921248798947));
#93660=CARTESIAN_POINT('Ctrl Pts',(8.48822482424259,31.7861966299445,123.981930455412));
#93661=CARTESIAN_POINT('Ctrl Pts',(8.49203232100684,31.8189742451768,124.044316863242));
#93662=CARTESIAN_POINT('Ctrl Pts',(8.49583889577238,31.8517439231946,124.106688163984));
#93663=CARTESIAN_POINT('Ctrl Pts',(8.49964547053792,31.8813101621532,124.170762954494));
#93664=CARTESIAN_POINT('Ctrl Pts',(8.50345204530346,31.9075023321529,124.236172522534));
#93665=CARTESIAN_POINT('Ctrl Pts',(8.50726133137383,31.9337131580207,124.301628679776));
#93666=CARTESIAN_POINT('Ctrl Pts',(8.51107061744421,31.9565449262708,124.368421050014));
#93667=CARTESIAN_POINT('Ctrl Pts',(8.51487990351458,31.9758754657729,124.436161631088));
#93668=CARTESIAN_POINT('Ctrl Pts',(8.51869054789537,31.9952128981343,124.503926367014));
#93669=CARTESIAN_POINT('Ctrl Pts',(8.52250119227616,32.0110465016042,124.572639500276));
#93670=CARTESIAN_POINT('Ctrl Pts',(8.52631183665695,32.0233049403347,124.641901297242));
#93671=CARTESIAN_POINT('Ctrl Pts',(8.53012846309201,32.0355826226992,124.71127182328));
#93672=CARTESIAN_POINT('Ctrl Pts',(8.53394508952706,32.0442738707611,124.781192236842));
#93673=CARTESIAN_POINT('Ctrl Pts',(8.53776171596212,32.0493591892279,124.85125701352));
#93674=CARTESIAN_POINT('Ctrl Pts',(8.54048290413684,32.0529849327247,124.901211978985));
#93675=CARTESIAN_POINT('Ctrl Pts',(8.54320409231157,32.0547787225466,124.951240233068));
#93676=CARTESIAN_POINT('Ctrl Pts',(8.54592528048629,32.0547496520905,125.001195714812));
#93677=CARTESIAN_POINT('Origin',(-1.54592528053767,30.,125.));
#93678=CARTESIAN_POINT('',(7.39391265022091,28.7479590808041,126.629230216746));
#93679=CARTESIAN_POINT('',(7.45211278982742,28.7479590808042,126.629230216746));
#93680=CARTESIAN_POINT('',(-1.54592528053767,28.7479590808042,126.629230216746));
#93681=CARTESIAN_POINT('',(7.90407471950836,32.0547494456331,124.998490639097));
#93682=CARTESIAN_POINT('Ctrl Pts',(7.45211278982742,28.7479590808042,126.629230216746));
#93683=CARTESIAN_POINT('Ctrl Pts',(7.45597763088531,28.6916459119271,126.585954324243));
#93684=CARTESIAN_POINT('Ctrl Pts',(7.4598424719432,28.6374854701366,126.539683431744));
#93685=CARTESIAN_POINT('Ctrl Pts',(7.46370731300109,28.5858120325335,126.490660912204));
#93686=CARTESIAN_POINT('Ctrl Pts',(7.46756704224479,28.5342069405642,126.441703232073));
#93687=CARTESIAN_POINT('Ctrl Pts',(7.47142677148849,28.4850826687522,126.390001486985));
#93688=CARTESIAN_POINT('Ctrl Pts',(7.47528650073219,28.4387407708862,126.335839504584));
#93689=CARTESIAN_POINT('Ctrl Pts',(7.47914342184703,28.3924325888621,126.281716927492));
#93690=CARTESIAN_POINT('Ctrl Pts',(7.48300034296188,28.348903079861,126.225138031865));
#93691=CARTESIAN_POINT('Ctrl Pts',(7.48685726407672,28.3084162342584,126.166422704674));
#93692=CARTESIAN_POINT('Ctrl Pts',(7.49071266934076,28.2679453008343,126.107730453837));
#93693=CARTESIAN_POINT('Ctrl Pts',(7.4945680746048,28.230514932911,126.046903837491));
#93694=CARTESIAN_POINT('Ctrl Pts',(7.49842347986884,28.196347115702,125.984293571788));
#93695=CARTESIAN_POINT('Ctrl Pts',(7.50227865956733,28.162181297526,125.921686969181));
#93696=CARTESIAN_POINT('Ctrl Pts',(7.50613383926581,28.1312778823822,125.857297351586));
#93697=CARTESIAN_POINT('Ctrl Pts',(7.5099890189643,28.1038131550659,125.791500481111));
#93698=CARTESIAN_POINT('Ctrl Pts',(7.51384799268039,28.0763213987479,125.725638857627));
#93699=CARTESIAN_POINT('Ctrl Pts',(7.51770696639648,28.0522752778304,125.658367664183));
#93700=CARTESIAN_POINT('Ctrl Pts',(7.52156594011256,28.031802750325,125.590082323809));
#93701=CARTESIAN_POINT('Ctrl Pts',(7.5254267610758,28.0113204228518,125.521764296013));
#93702=CARTESIAN_POINT('Ctrl Pts',(7.52928758203904,27.9944152119565,125.452431626849));
#93703=CARTESIAN_POINT('Ctrl Pts',(7.53314840300228,27.9811643120378,125.38249186594));
#93704=CARTESIAN_POINT('Ctrl Pts',(7.53701633832392,27.9678889946048,125.312423226606));
#93705=CARTESIAN_POINT('Ctrl Pts',(7.54088427364555,27.958281507931,125.241745742989));
#93706=CARTESIAN_POINT('Ctrl Pts',(7.54475220896719,27.9523672730575,125.170873573305));
#93707=CARTESIAN_POINT('Ctrl Pts',(7.54817615316203,27.9471319191857,125.108136651979));
#93708=CARTESIAN_POINT('Ctrl Pts',(7.55160009735686,27.9447898338038,125.045247454545));
#93709=CARTESIAN_POINT('Ctrl Pts',(7.5550240415517,27.945324596286,124.982491491417));
#93710=CARTESIAN_POINT('Ctrl Pts',(7.55889311490067,27.9459288804537,124.911576952333));
#93711=CARTESIAN_POINT('Ctrl Pts',(7.56276218824965,27.9502099474241,124.840554831223));
#93712=CARTESIAN_POINT('Ctrl Pts',(7.56663126159862,27.9581814784833,124.769837692722));
#93713=CARTESIAN_POINT('Ctrl Pts',(7.57049456999505,27.9661411318927,124.699225923365));
#93714=CARTESIAN_POINT('Ctrl Pts',(7.57435787839147,27.9777802804095,124.628918713388));
#93715=CARTESIAN_POINT('Ctrl Pts',(7.5782211867879,27.9930605972998,124.55932801724));
#93716=CARTESIAN_POINT('Ctrl Pts',(7.58207996328128,28.00832298942,124.489818955344));
#93717=CARTESIAN_POINT('Ctrl Pts',(7.58593873977465,28.0272179619513,124.421025209909));
#93718=CARTESIAN_POINT('Ctrl Pts',(7.58979751626803,28.0496556793524,124.353351259633));
#93719=CARTESIAN_POINT('Ctrl Pts',(7.59365386185659,28.0720792617147,124.285719941765));
#93720=CARTESIAN_POINT('Ctrl Pts',(7.59751020744516,28.0980410085421,124.219207479496));
#93721=CARTESIAN_POINT('Ctrl Pts',(7.60136655303372,28.127400902946,124.154204407547));
#93722=CARTESIAN_POINT('Ctrl Pts',(7.6052217592793,28.1567521230781,124.089220540514));
#93723=CARTESIAN_POINT('Ctrl Pts',(7.60907696552488,28.1894992977735,124.02574562096));
#93724=CARTESIAN_POINT('Ctrl Pts',(7.61293217177046,28.2254544719855,123.964149754306));
#93725=CARTESIAN_POINT('Ctrl Pts',(7.61678752862185,28.2614110508067,123.902551481375));
#93726=CARTESIAN_POINT('Ctrl Pts',(7.62064288547323,28.3005756311566,123.842832825513));
#93727=CARTESIAN_POINT('Ctrl Pts',(7.62449824232462,28.3427154187412,123.785337339332));
#93728=CARTESIAN_POINT('Ctrl Pts',(7.62835763479315,28.3848993163929,123.727781669417));
#93729=CARTESIAN_POINT('Ctrl Pts',(7.63221702726169,28.4300643503926,123.672454207248));
#93730=CARTESIAN_POINT('Ctrl Pts',(7.63607641973023,28.4779362183637,123.61966692167));
#93731=CARTESIAN_POINT('Ctrl Pts',(7.63993799733355,28.5258351907262,123.56684974866));
#93732=CARTESIAN_POINT('Ctrl Pts',(7.64379957493687,28.5764437031346,123.516575957801));
#93733=CARTESIAN_POINT('Ctrl Pts',(7.6476611525402,28.629451173511,123.469120031907));
#93734=CARTESIAN_POINT('Ctrl Pts',(7.65152948665481,28.6825513898086,123.421581073497));
#93735=CARTESIAN_POINT('Ctrl Pts',(7.65539782076942,28.738058565867,123.376870128474));
#93736=CARTESIAN_POINT('Ctrl Pts',(7.65926615488404,28.7956302673745,123.335220402085));
#93737=CARTESIAN_POINT('Ctrl Pts',(7.66156387405278,28.8298267969945,123.310481232235));
#93738=CARTESIAN_POINT('Ctrl Pts',(7.66386159322151,28.8647511726965,123.286821267237));
#93739=CARTESIAN_POINT('Ctrl Pts',(7.66615931239025,28.9003275143506,123.264281708685));
#93740=CARTESIAN_POINT('Ctrl Pts',(7.67002838578168,28.9602336502836,123.226327894557));
#93741=CARTESIAN_POINT('Ctrl Pts',(7.67389745917311,29.0222243255323,123.191404757273));
#93742=CARTESIAN_POINT('Ctrl Pts',(7.67776653256454,29.0859603468053,123.159747551316));
#93743=CARTESIAN_POINT('Ctrl Pts',(7.68162984100372,29.1496014008647,123.128137514865));
#93744=CARTESIAN_POINT('Ctrl Pts',(7.6854931494429,29.2149822073397,123.099783964679));
#93745=CARTESIAN_POINT('Ctrl Pts',(7.68935645788208,29.2817358782989,123.074878130097));
#93746=CARTESIAN_POINT('Ctrl Pts',(7.69321523441845,29.3484112430204,123.05000151162));
#93747=CARTESIAN_POINT('Ctrl Pts',(7.69707401095481,29.4164558203857,123.028564744215));
#93748=CARTESIAN_POINT('Ctrl Pts',(7.70093278749118,29.4854810666423,123.010711727849));
#93749=CARTESIAN_POINT('Ctrl Pts',(7.70478913312285,29.5544628292212,122.992869958308));
#93750=CARTESIAN_POINT('Ctrl Pts',(7.70864547875453,29.6244235658091,122.978607582025));
#93751=CARTESIAN_POINT('Ctrl Pts',(7.7125018243862,29.6949592310368,122.968018776718));
#93752=CARTESIAN_POINT('Ctrl Pts',(7.71635703067495,29.7654740567655,122.957433099834));
#93753=CARTESIAN_POINT('Ctrl Pts',(7.7202122369637,29.8365629937725,122.950518911299));
#93754=CARTESIAN_POINT('Ctrl Pts',(7.72406744325245,29.9078131602965,122.947319033779));
#93755=CARTESIAN_POINT('Ctrl Pts',(7.727922800147,29.9790661102483,122.944119031254));
#93756=CARTESIAN_POINT('Ctrl Pts',(7.73177815704155,30.0504798168263,122.944633647418));
#93757=CARTESIAN_POINT('Ctrl Pts',(7.7356335139361,30.1216393872444,122.948853632241));
#93758=CARTESIAN_POINT('Ctrl Pts',(7.73949290644749,30.1928734443492,122.953078034358));
#93759=CARTESIAN_POINT('Ctrl Pts',(7.74335229895888,30.2638523483338,122.961015518905));
#93760=CARTESIAN_POINT('Ctrl Pts',(7.74721169147027,30.3341652288182,122.972604833204));
#93761=CARTESIAN_POINT('Ctrl Pts',(7.75107326911633,30.4045179194833,122.984200709212));
#93762=CARTESIAN_POINT('Ctrl Pts',(7.7549348467624,30.4742033611939,122.999452427044));
#93763=CARTESIAN_POINT('Ctrl Pts',(7.75879642440846,30.5428225004122,123.018247922785));
#93764=CARTESIAN_POINT('Ctrl Pts',(7.76266475856518,30.6115617009079,123.037076304558));
#93765=CARTESIAN_POINT('Ctrl Pts',(7.7665330927219,30.679230412665,123.059460691033));
#93766=CARTESIAN_POINT('Ctrl Pts',(7.77040142687861,30.7454469857162,123.085239870379));
#93767=CARTESIAN_POINT('Ctrl Pts',(7.77269914566201,30.7847784026796,123.100552225052));
#93768=CARTESIAN_POINT('Ctrl Pts',(7.77499686444541,30.8235978903797,123.117061396472));
#93769=CARTESIAN_POINT('Ctrl Pts',(7.77729458322881,30.8618296789442,123.134725980723));
#93770=CARTESIAN_POINT('Ctrl Pts',(7.781163656479,30.9262072657535,123.164470948163));
#93771=CARTESIAN_POINT('Ctrl Pts',(7.78503272972918,30.9891692283516,123.197610957942));
#93772=CARTESIAN_POINT('Ctrl Pts',(7.78890180297937,31.050333952957,123.233988632606));
#93773=CARTESIAN_POINT('Ctrl Pts',(7.79276511127721,31.1114075415978,123.270312104222));
#93774=CARTESIAN_POINT('Ctrl Pts',(7.79662841957505,31.1706887936818,123.309863418628));
#93775=CARTESIAN_POINT('Ctrl Pts',(7.80049172787288,31.2278180622896,123.352438053239));
#93776=CARTESIAN_POINT('Ctrl Pts',(7.80435050426844,31.2848803146919,123.39496274514));
#93777=CARTESIAN_POINT('Ctrl Pts',(7.80820928066399,31.3397952103248,123.440503423738));
#93778=CARTESIAN_POINT('Ctrl Pts',(7.81206805705954,31.3922311203958,123.488811702698));
#93779=CARTESIAN_POINT('Ctrl Pts',(7.81592440255081,31.4446339975397,123.537089549005));
#93780=CARTESIAN_POINT('Ctrl Pts',(7.81978074804207,31.4945606310389,123.588131208226));
#93781=CARTESIAN_POINT('Ctrl Pts',(7.82363709353333,31.5417127584062,123.64164830288));
#93782=CARTESIAN_POINT('Ctrl Pts',(7.82749229968227,31.5888509548604,123.695149586116));
#93783=CARTESIAN_POINT('Ctrl Pts',(7.83134750583121,31.6332159515802,123.751124488543));
#93784=CARTESIAN_POINT('Ctrl Pts',(7.83520271198014,31.6745478391525,123.809249355705));
#93785=CARTESIAN_POINT('Ctrl Pts',(7.83905806873569,31.715881341387,123.867376493559));
#93786=CARTESIAN_POINT('Ctrl Pts',(7.84291342549123,31.7541812195027,123.927653365725));
#93787=CARTESIAN_POINT('Ctrl Pts',(7.84676878224677,31.7892302219191,123.989726385838));
#93788=CARTESIAN_POINT('Ctrl Pts',(7.85062817462134,31.8243159121,124.051864381277));
#93789=CARTESIAN_POINT('Ctrl Pts',(7.85448756699591,31.8561436943397,124.115801853944));
#93790=CARTESIAN_POINT('Ctrl Pts',(7.85834695937048,31.8845421883571,124.181160392505));
#93791=CARTESIAN_POINT('Ctrl Pts',(7.86220853688075,31.9129567612171,124.246555936185));
#93792=CARTESIAN_POINT('Ctrl Pts',(7.86607011439102,31.9379380104941,124.313373692206));
#93793=CARTESIAN_POINT('Ctrl Pts',(7.86993169190128,31.95936365367,124.381217618886));
#93794=CARTESIAN_POINT('Ctrl Pts',(7.87380002592529,31.9808267848032,124.449180250532));
#93795=CARTESIAN_POINT('Ctrl Pts',(7.8776683599493,31.9987217670988,124.518172167164));
#93796=CARTESIAN_POINT('Ctrl Pts',(7.8815366939733,32.0129770484167,124.587785292538));
#93797=CARTESIAN_POINT('Ctrl Pts',(7.88383441400466,32.0214444261647,124.629134222498));
#93798=CARTESIAN_POINT('Ctrl Pts',(7.88613213403602,32.0286286525971,124.670702169053));
#93799=CARTESIAN_POINT('Ctrl Pts',(7.88842985406737,32.0345234180833,124.712403018495));
#93800=CARTESIAN_POINT('Ctrl Pts',(7.89364480919903,32.0479023054596,124.807048169263));
#93801=CARTESIAN_POINT('Ctrl Pts',(7.89885976433068,32.0546790423352,124.90264805037));
#93802=CARTESIAN_POINT('Ctrl Pts',(7.90407471946233,32.0547494456325,124.998490638251));
#93803=CARTESIAN_POINT('Ctrl Pts',(7.90407471950836,32.0547494456331,124.998490639097));
#93804=CARTESIAN_POINT('Ctrl Pts',(7.90805348639992,32.0548031600265,125.071614051636));
#93805=CARTESIAN_POINT('Ctrl Pts',(7.91203225329149,32.0509484181439,125.144885851501));
#93806=CARTESIAN_POINT('Ctrl Pts',(7.91601102018305,32.0431692286218,125.2178464269));
#93807=CARTESIAN_POINT('Ctrl Pts',(7.91981486837858,32.0357320359355,125.287599433457));
#93808=CARTESIAN_POINT('Ctrl Pts',(7.92361871657411,32.0247082535841,125.357067439174));
#93809=CARTESIAN_POINT('Ctrl Pts',(7.92742256476964,32.0101370400902,125.42584814495));
#93810=CARTESIAN_POINT('Ctrl Pts',(7.93122379847059,31.9955758418117,125.494581575763));
#93811=CARTESIAN_POINT('Ctrl Pts',(7.93502503217154,31.9774721486446,125.562628154096));
#93812=CARTESIAN_POINT('Ctrl Pts',(7.93882626587248,31.9559166138979,125.629593330634));
#93813=CARTESIAN_POINT('Ctrl Pts',(7.94262624496905,31.9343681935962,125.696536405188));
#93814=CARTESIAN_POINT('Ctrl Pts',(7.94642622406562,31.9093703451663,125.762398309188));
#93815=CARTESIAN_POINT('Ctrl Pts',(7.95022620316219,31.8810637191461,125.826799157602));
#93816=CARTESIAN_POINT('Ctrl Pts',(7.9540262856104,31.8527563232437,125.891201757588));
#93817=CARTESIAN_POINT('Ctrl Pts',(7.95782636805862,31.8211401758106,125.954142765617));
#93818=CARTESIAN_POINT('Ctrl Pts',(7.96162645050683,31.7864034775327,126.015263600233));
#93819=CARTESIAN_POINT('Ctrl Pts',(7.96543037574972,31.7516316521226,126.076446242671));
#93820=CARTESIAN_POINT('Ctrl Pts',(7.9692343009926,31.7137332295808,126.13580460387));
#93821=CARTESIAN_POINT('Ctrl Pts',(7.97303822623548,31.672941063085,126.193007025102));
#93822=CARTESIAN_POINT('Ctrl Pts',(7.97684442188819,31.6321245493875,126.250243588157));
#93823=CARTESIAN_POINT('Ctrl Pts',(7.98065061754089,31.5884111702421,126.305321261529));
#93824=CARTESIAN_POINT('Ctrl Pts',(7.9844568131936,31.5420737759433,126.357941836769));
#93825=CARTESIAN_POINT('Ctrl Pts',(7.98826926353303,31.4956602358255,126.410648882923));
#93826=CARTESIAN_POINT('Ctrl Pts',(7.99208171387245,31.4466144322414,126.460890422923));
#93827=CARTESIAN_POINT('Ctrl Pts',(7.99589416421188,31.3952448791565,126.508406208449));
#93828=CARTESIAN_POINT('Ctrl Pts',(7.99711781777657,31.3787571793434,126.52365699342));
#93829=CARTESIAN_POINT('Ctrl Pts',(7.99834147134126,31.3620303335553,126.538627302503));
#93830=CARTESIAN_POINT('Ctrl Pts',(7.99956512490594,31.3450751861379,126.553309468888));
#93831=CARTESIAN_POINT('Ctrl Pts',(8.00343419857232,31.2914646575736,126.599733052296));
#93832=CARTESIAN_POINT('Ctrl Pts',(8.0073032722387,31.2353429211326,126.643468858699));
#93833=CARTESIAN_POINT('Ctrl Pts',(8.01117234590508,31.177010502966,126.684233902523));
#93834=CARTESIAN_POINT('Ctrl Pts',(8.01503565462073,31.1187650005694,126.724938206105));
#93835=CARTESIAN_POINT('Ctrl Pts',(8.01889896333638,31.0583157497566,126.762680257503));
#93836=CARTESIAN_POINT('Ctrl Pts',(8.02276227205203,30.9959971979523,126.79721649897));
#93837=CARTESIAN_POINT('Ctrl Pts',(8.02662104886578,30.9337517496933,126.831712227274));
#93838=CARTESIAN_POINT('Ctrl Pts',(8.03047982567953,30.8696417789356,126.863009381168));
#93839=CARTESIAN_POINT('Ctrl Pts',(8.03433860249328,30.8040301727672,126.890907994531));
#93840=CARTESIAN_POINT('Ctrl Pts',(8.03819494840275,30.7384598997835,126.918789032671));
#93841=CARTESIAN_POINT('Ctrl Pts',(8.04205129431221,30.6713903141947,126.94327558829));
#93842=CARTESIAN_POINT('Ctrl Pts',(8.04590764022167,30.6032070117903,126.964214566545));
#93843=CARTESIAN_POINT('Ctrl Pts',(8.04976284678821,30.5350438538867,126.985147358457));
#93844=CARTESIAN_POINT('Ctrl Pts',(8.05361805335475,30.4657680965384,127.002534511279));
#93845=CARTESIAN_POINT('Ctrl Pts',(8.05747325992129,30.3957816951196,127.016272405284));
#93846=CARTESIAN_POINT('Ctrl Pts',(8.0613286170932,30.3257925596506,127.030010835966));
#93847=CARTESIAN_POINT('Ctrl Pts',(8.06518397426512,30.2550932021072,127.040099633387));
#93848=CARTESIAN_POINT('Ctrl Pts',(8.06903933143703,30.1840952941523,127.046486375516));
#93849=CARTESIAN_POINT('Ctrl Pts',(8.07289872422324,30.113023068784,127.052879802998));
#93850=CARTESIAN_POINT('Ctrl Pts',(8.07675811700946,30.0416521539894,127.055563395913));
#93851=CARTESIAN_POINT('Ctrl Pts',(8.08061750979567,29.9703979606998,127.054536756003));
#93852=CARTESIAN_POINT('Ctrl Pts',(8.08447908771554,29.8991034242929,127.053509534825));
#93853=CARTESIAN_POINT('Ctrl Pts',(8.08834066563541,29.8279262258892,127.048767931317));
#93854=CARTESIAN_POINT('Ctrl Pts',(8.09220224355529,29.7572776307531,127.040363549461));
#93855=CARTESIAN_POINT('Ctrl Pts',(8.09607057798121,29.6865054235418,127.031944462668));
#93856=CARTESIAN_POINT('Ctrl Pts',(8.09993891240713,29.6162641450483,127.019849884887));
#93857=CARTESIAN_POINT('Ctrl Pts',(8.10380724683306,29.5469551431653,127.0041826065));
#93858=CARTESIAN_POINT('Ctrl Pts',(8.10610496313687,29.5057869280907,126.994876544246));
#93859=CARTESIAN_POINT('Ctrl Pts',(8.10840267944068,29.4649473669824,126.984310949874));
#93860=CARTESIAN_POINT('Ctrl Pts',(8.11070039574449,29.4245175347868,126.972515524586));
#93861=CARTESIAN_POINT('Ctrl Pts',(8.1145684545292,29.3564564920335,126.952658678756));
#93862=CARTESIAN_POINT('Ctrl Pts',(8.11843651331391,29.2892911078502,126.929236177456));
#93863=CARTESIAN_POINT('Ctrl Pts',(8.12230457209862,29.2234218115874,126.902346939909));
#93864=CARTESIAN_POINT('Ctrl Pts',(8.12616759077854,29.1576383434297,126.875492739207));
#93865=CARTESIAN_POINT('Ctrl Pts',(8.13003060945846,29.0931480601149,126.845180941222));
#93866=CARTESIAN_POINT('Ctrl Pts',(8.13389362813838,29.0303368956155,126.811560384446));
#93867=CARTESIAN_POINT('Ctrl Pts',(8.13775232965377,28.9675959265135,126.777977400741));
#93868=CARTESIAN_POINT('Ctrl Pts',(8.14161103116916,28.9065307762037,126.741093228774));
#93869=CARTESIAN_POINT('Ctrl Pts',(8.14546973268454,28.8475062487581,126.701104263662));
#93870=CARTESIAN_POINT('Ctrl Pts',(8.14768435246726,28.8136303748079,126.678153446431));
#93871=CARTESIAN_POINT('Ctrl Pts',(8.14989897224998,28.7804262675646,126.654180801346));
#93872=CARTESIAN_POINT('Ctrl Pts',(8.1521135920327,28.7479590808041,126.629230216746));
#93873=CARTESIAN_POINT('',(7.8459252805834,32.0547497348706,125.001043814792));
#93874=CARTESIAN_POINT('Ctrl Pts',(7.8459252805834,32.0547497348706,125.001043814792));
#93875=CARTESIAN_POINT('Ctrl Pts',(7.85018308156599,32.0547096589831,125.079933211422));
#93876=CARTESIAN_POINT('Ctrl Pts',(7.85444088254858,32.0501221476059,125.158666320287));
#93877=CARTESIAN_POINT('Ctrl Pts',(7.85869868353118,32.041065772293,125.236744747933));
#93878=CARTESIAN_POINT('Ctrl Pts',(7.86297170281514,32.0319770275365,125.315102244763));
#93879=CARTESIAN_POINT('Ctrl Pts',(7.8672447220991,32.0183875520912,125.392800086567));
#93880=CARTESIAN_POINT('Ctrl Pts',(7.87151774138306,32.0004267208688,125.469351144596));
#93881=CARTESIAN_POINT('Ctrl Pts',(7.87581130795464,31.9823795229954,125.546270306888));
#93882=CARTESIAN_POINT('Ctrl Pts',(7.88010487452622,31.9599189696943,125.62203135299));
#93883=CARTESIAN_POINT('Ctrl Pts',(7.8843984410978,31.9332245829694,125.696161097953));
#93884=CARTESIAN_POINT('Ctrl Pts',(7.88646703724444,31.9203635024212,125.731876045474));
#93885=CARTESIAN_POINT('Ctrl Pts',(7.88853563339108,31.9065203606893,125.767212670556));
#93886=CARTESIAN_POINT('Ctrl Pts',(7.89060422953772,31.8917190494166,125.802120066183));
#93887=CARTESIAN_POINT('Ctrl Pts',(7.894473302929,31.8640348831796,125.867410372268));
#93888=CARTESIAN_POINT('Ctrl Pts',(7.89834237632028,31.8329124035663,125.931393656006));
#93889=CARTESIAN_POINT('Ctrl Pts',(7.90221144971156,31.7984967817137,125.993683495216));
#93890=CARTESIAN_POINT('Ctrl Pts',(7.90607475815059,31.7641324394302,126.055880522036));
#93891=CARTESIAN_POINT('Ctrl Pts',(7.90993806658963,31.7264849278007,126.116388691164));
#93892=CARTESIAN_POINT('Ctrl Pts',(7.91380137502866,31.6857472373416,126.174842038018));
#93893=CARTESIAN_POINT('Ctrl Pts',(7.91766015156488,31.6450573347453,126.233226815435));
#93894=CARTESIAN_POINT('Ctrl Pts',(7.9215189281011,31.6012847301518,126.289561161906));
#93895=CARTESIAN_POINT('Ctrl Pts',(7.92537770463731,31.5546671460301,126.343505722933));
#93896=CARTESIAN_POINT('Ctrl Pts',(7.92923405026884,31.508078929482,126.397416300628));
#93897=CARTESIAN_POINT('Ctrl Pts',(7.93309039590037,31.4586496060732,126.448939713055));
#93898=CARTESIAN_POINT('Ctrl Pts',(7.93694674153189,31.4066579295296,126.497768684341));
#93899=CARTESIAN_POINT('Ctrl Pts',(7.9408019478205,31.3546816137329,126.546583229288));
#93900=CARTESIAN_POINT('Ctrl Pts',(7.9446571541091,31.3001448016416,126.592704581117));
#93901=CARTESIAN_POINT('Ctrl Pts',(7.9485123603977,31.2433627249165,126.635862676629));
#93902=CARTESIAN_POINT('Ctrl Pts',(7.9523677172921,31.1865784299676,126.679022458137));
#93903=CARTESIAN_POINT('Ctrl Pts',(7.95622307418651,31.1275490843282,126.719218461297));
#93904=CARTESIAN_POINT('Ctrl Pts',(7.96007843108091,31.0666211920245,126.756222308031));
#93905=CARTESIAN_POINT('Ctrl Pts',(7.96393782359215,31.0056295231018,126.793264888752));
#93906=CARTESIAN_POINT('Ctrl Pts',(7.9677972161034,30.9427357564469,126.827108390158));
#93907=CARTESIAN_POINT('Ctrl Pts',(7.97165660861464,30.8783126662094,126.857569493418));
#93908=CARTESIAN_POINT('Ctrl Pts',(7.97551818626056,30.813853100509,126.888047843333));
#93909=CARTESIAN_POINT('Ctrl Pts',(7.97937976390648,30.7478629371237,126.915139798214));
#93910=CARTESIAN_POINT('Ctrl Pts',(7.9832413415524,30.6807341318648,126.938710551943));
#93911=CARTESIAN_POINT('Ctrl Pts',(7.98710967570898,30.6134878729303,126.962322546859));
#93912=CARTESIAN_POINT('Ctrl Pts',(7.99097800986555,30.5450994607886,126.982400903193));
#93913=CARTESIAN_POINT('Ctrl Pts',(7.99484634402213,30.4759744918409,126.998861137152));
#93914=CARTESIAN_POINT('Ctrl Pts',(7.99714406280685,30.4349155416016,127.008638211013));
#93915=CARTESIAN_POINT('Ctrl Pts',(7.99944178159156,30.3935969099127,127.017139742854));
#93916=CARTESIAN_POINT('Ctrl Pts',(8.00173950037628,30.3521044663438,127.024356689736));
#93917=CARTESIAN_POINT('Ctrl Pts',(8.00560732713476,30.2822588505194,127.03650521742));
#93918=CARTESIAN_POINT('Ctrl Pts',(8.00947515389324,30.2116469980773,127.045058506921));
#93919=CARTESIAN_POINT('Ctrl Pts',(8.01334298065171,30.1406719027978,127.04992901786));
#93920=CARTESIAN_POINT('Ctrl Pts',(8.01720559832235,30.0697923949189,127.054792969321));
#93921=CARTESIAN_POINT('Ctrl Pts',(8.02106821599298,29.9985510945436,127.055983946858));
#93922=CARTESIAN_POINT('Ctrl Pts',(8.02493083366361,29.927359911755,127.053465602361));
#93923=CARTESIAN_POINT('Ctrl Pts',(8.02878954173858,29.8562407859919,127.050949806837));
#93924=CARTESIAN_POINT('Ctrl Pts',(8.03264824981354,29.7851721600219,127.044732155691));
#93925=CARTESIAN_POINT('Ctrl Pts',(8.0365069578885,29.7145680506028,127.034828288766));
#93926=CARTESIAN_POINT('Ctrl Pts',(8.04036305129555,29.644011782662,127.02493113272));
#93927=CARTESIAN_POINT('Ctrl Pts',(8.04421914470261,29.5739198862576,127.011352786759));
#93928=CARTESIAN_POINT('Ctrl Pts',(8.04807523810967,29.5047016271448,126.994160746867));
#93929=CARTESIAN_POINT('Ctrl Pts',(8.0519314655949,29.4354809612807,126.976968109201));
#93930=CARTESIAN_POINT('Ctrl Pts',(8.05578769308013,29.3671344693989,126.956161625204));
#93931=CARTESIAN_POINT('Ctrl Pts',(8.05964392056537,29.3000603365109,126.931859733515));
#93932=CARTESIAN_POINT('Ctrl Pts',(8.0634999444501,29.2329897449925,126.907559124913));
#93933=CARTESIAN_POINT('Ctrl Pts',(8.06735596833484,29.1671918335515,126.879763648173));
#93934=CARTESIAN_POINT('Ctrl Pts',(8.07121199221957,29.1030466060486,126.848640628023));
#93935=CARTESIAN_POINT('Ctrl Pts',(8.07507195470925,29.0388358595764,126.81748581832));
#93936=CARTESIAN_POINT('Ctrl Pts',(8.07893191719892,28.9762816047668,126.782996893776));
#93937=CARTESIAN_POINT('Ctrl Pts',(8.0827918796886,28.9157401949308,126.745387704097));
#93938=CARTESIAN_POINT('Ctrl Pts',(8.08648092162307,28.857879580934,126.709443863134));
#93939=CARTESIAN_POINT('Ctrl Pts',(8.09016996355755,28.8018576250842,126.670650503597));
#93940=CARTESIAN_POINT('Ctrl Pts',(8.09385900549202,28.7479590808042,126.629230216746));
#93941=CARTESIAN_POINT('Ctrl Pts',(7.39391265022091,28.7479590808041,126.629230216746));
#93942=CARTESIAN_POINT('Ctrl Pts',(7.39776808670206,28.6914048962311,126.585769107009));
#93943=CARTESIAN_POINT('Ctrl Pts',(7.40162352318322,28.6371232308455,126.539365203168));
#93944=CARTESIAN_POINT('Ctrl Pts',(7.40547895966437,28.5854248540264,126.490293500923));
#93945=CARTESIAN_POINT('Ctrl Pts',(7.40933850650131,28.5336713605626,126.441169482382));
#93946=CARTESIAN_POINT('Ctrl Pts',(7.41319805333826,28.4845070053736,126.389372323985));
#93947=CARTESIAN_POINT('Ctrl Pts',(7.4170576001752,28.4382058739118,126.335214091528));
#93948=CARTESIAN_POINT('Ctrl Pts',(7.42091944001119,28.3918772344406,126.281023683073));
#93949=CARTESIAN_POINT('Ctrl Pts',(7.42478127984718,28.3484155004047,126.224469793889));
#93950=CARTESIAN_POINT('Ctrl Pts',(7.42864311968317,28.3080529063201,126.165895619122));
#93951=CARTESIAN_POINT('Ctrl Pts',(7.43251160661999,28.2676208390714,126.107220624937));
#93952=CARTESIAN_POINT('Ctrl Pts',(7.43638009355682,28.2302988135901,126.046518817859));
#93953=CARTESIAN_POINT('Ctrl Pts',(7.44024858049364,28.1962739987851,125.984159578037));
#93954=CARTESIAN_POINT('Ctrl Pts',(7.44218676905692,28.1792268927718,125.952916363981));
#93955=CARTESIAN_POINT('Ctrl Pts',(7.4441249576202,28.1630067093441,125.921257441353));
#93956=CARTESIAN_POINT('Ctrl Pts',(7.44606314618348,28.1476323957825,125.889231028106));
#93957=CARTESIAN_POINT('Ctrl Pts',(7.44993221953134,28.1169417045001,125.825298888441));
#93958=CARTESIAN_POINT('Ctrl Pts',(7.45380129287919,28.0895045899316,125.759650781342));
#93959=CARTESIAN_POINT('Ctrl Pts',(7.45767036622704,28.065515042618,125.692651075335));
#93960=CARTESIAN_POINT('Ctrl Pts',(7.46153367462244,28.0415612399355,125.625751199465));
#93961=CARTESIAN_POINT('Ctrl Pts',(7.46539698301783,28.0210449703193,125.557504175837));
#93962=CARTESIAN_POINT('Ctrl Pts',(7.46926029141322,28.004113263557,125.488296731293));
#93963=CARTESIAN_POINT('Ctrl Pts',(7.47311906790573,27.987201418748,125.419170471418));
#93964=CARTESIAN_POINT('Ctrl Pts',(7.47697784439825,27.9738658992889,125.349086498082));
#93965=CARTESIAN_POINT('Ctrl Pts',(7.48083662089076,27.9642041985661,125.278447512763));
#93966=CARTESIAN_POINT('Ctrl Pts',(7.48469296647855,27.9545485844031,125.207853027727));
#93967=CARTESIAN_POINT('Ctrl Pts',(7.48854931206635,27.9485622629447,125.136704704553));
#93968=CARTESIAN_POINT('Ctrl Pts',(7.49240565765414,27.9462915341202,125.065414827627));
#93969=CARTESIAN_POINT('Ctrl Pts',(7.49626086389906,27.944021476174,124.994146013029));
#93970=CARTESIAN_POINT('Ctrl Pts',(7.50011607014396,27.9454648469652,124.92273621298));
#93971=CARTESIAN_POINT('Ctrl Pts',(7.50397127638888,27.9506159105085,124.85160048437));
#93972=CARTESIAN_POINT('Ctrl Pts',(7.50782663323969,27.9557671752812,124.780461976801));
#93973=CARTESIAN_POINT('Ctrl Pts',(7.5116819900905,27.9646263830915,124.709598046287));
#93974=CARTESIAN_POINT('Ctrl Pts',(7.51553734694131,27.9771358471879,124.639419659759));
#93975=CARTESIAN_POINT('Ctrl Pts',(7.51939673940942,27.989658405639,124.569167813596));
#93976=CARTESIAN_POINT('Ctrl Pts',(7.52325613187754,28.0058387623819,124.499603423131));
#93977=CARTESIAN_POINT('Ctrl Pts',(7.52711552434565,28.0255680547611,124.431127381464));
#93978=CARTESIAN_POINT('Ctrl Pts',(7.53097710194864,28.0453085175939,124.362612569605));
#93979=CARTESIAN_POINT('Ctrl Pts',(7.53483867955163,28.0686017573754,124.295187792598));
#93980=CARTESIAN_POINT('Ctrl Pts',(7.53870025715462,28.0952898299455,124.229236267984));
#93981=CARTESIAN_POINT('Ctrl Pts',(7.54256859126903,28.1220245980078,124.163169349541));
#93982=CARTESIAN_POINT('Ctrl Pts',(7.54643692538344,28.1521658524618,124.098581270323));
#93983=CARTESIAN_POINT('Ctrl Pts',(7.55030525949785,28.1855088726354,124.035832218328));
#93984=CARTESIAN_POINT('Ctrl Pts',(7.55260297867259,28.2053140121426,123.99856043784));
#93985=CARTESIAN_POINT('Ctrl Pts',(7.55490069784731,28.2262479198027,123.961936982506));
#93986=CARTESIAN_POINT('Ctrl Pts',(7.55719841702205,28.2482606181941,123.926032262714));
#93987=CARTESIAN_POINT('Ctrl Pts',(7.56106749037592,28.2853272648625,123.865573179572));
#93988=CARTESIAN_POINT('Ctrl Pts',(7.56493656372979,28.3256001936858,123.806916888848));
#93989=CARTESIAN_POINT('Ctrl Pts',(7.56880563708366,28.368878496293,123.750423990849));
#93990=CARTESIAN_POINT('Ctrl Pts',(7.57266894548512,28.4120923138589,123.694015267752));
#93991=CARTESIAN_POINT('Ctrl Pts',(7.57653225388659,28.4583023234205,123.639763921366));
#93992=CARTESIAN_POINT('Ctrl Pts',(7.58039556228805,28.5072633625889,123.588003224568));
#93993=CARTESIAN_POINT('Ctrl Pts',(7.58425433878664,28.5561669673899,123.536303246312));
#93994=CARTESIAN_POINT('Ctrl Pts',(7.58811311528523,28.6078148594203,123.487088465385));
#93995=CARTESIAN_POINT('Ctrl Pts',(7.59197189178381,28.661921588537,123.440659201048));
#93996=CARTESIAN_POINT('Ctrl Pts',(7.59582823737769,28.7159942321598,123.39425918565));
#93997=CARTESIAN_POINT('Ctrl Pts',(7.59968458297157,28.7725222719124,123.350641520977));
#93998=CARTESIAN_POINT('Ctrl Pts',(7.60354092856544,28.8311844411433,123.31006871386));
#93999=CARTESIAN_POINT('Ctrl Pts',(7.60739613481643,28.8898292788556,123.269507893827));
#94000=CARTESIAN_POINT('Ctrl Pts',(7.61125134106742,28.9506065949708,123.231990421594));
#94001=CARTESIAN_POINT('Ctrl Pts',(7.61510654731841,29.013164571123,123.197736590059));
#94002=CARTESIAN_POINT('Ctrl Pts',(7.61896190417531,29.0757249911396,123.163481420378));
#94003=CARTESIAN_POINT('Ctrl Pts',(7.62281726103221,29.1400657821498,123.132490375898));
#94004=CARTESIAN_POINT('Ctrl Pts',(7.62667261788911,29.2058103857097,123.104937885173));
#94005=CARTESIAN_POINT('Ctrl Pts',(7.63053201036323,29.271623807816,123.077356553717));
#94006=CARTESIAN_POINT('Ctrl Pts',(7.63439140283736,29.3388435268718,123.053221149227));
#94007=CARTESIAN_POINT('Ctrl Pts',(7.63825079531149,29.4070736919278,123.032657641463));
#94008=CARTESIAN_POINT('Ctrl Pts',(7.64211237292047,29.4753424879634,123.012082490923));
#94009=CARTESIAN_POINT('Ctrl Pts',(7.64597395052945,29.5446223968602,122.995083378818));
#94010=CARTESIAN_POINT('Ctrl Pts',(7.64983552813843,29.6145057976293,122.981735452811));
#94011=CARTESIAN_POINT('Ctrl Pts',(7.65370386225874,29.6845114717375,122.968364172253));
#94012=CARTESIAN_POINT('Ctrl Pts',(7.65757219637904,29.7551222644717,122.958656898589));
#94013=CARTESIAN_POINT('Ctrl Pts',(7.66144053049935,29.8259245330664,122.952636990099));
#94014=CARTESIAN_POINT('Ctrl Pts',(7.66373824961977,29.867979774744,122.949061275486));
#94015=CARTESIAN_POINT('Ctrl Pts',(7.66603596874018,29.9101025335228,122.946785516384));
#94016=CARTESIAN_POINT('Ctrl Pts',(7.6683336878606,29.9522065486158,122.94580591265));
#94017=CARTESIAN_POINT('Ctrl Pts',(7.6722027611979,30.0231044754954,122.94415638175));
#94018=CARTESIAN_POINT('Ctrl Pts',(7.6760718345352,30.0942267702318,122.946178357979));
#94019=CARTESIAN_POINT('Ctrl Pts',(7.6799409078725,30.1651615113171,122.951898626122));
#94020=CARTESIAN_POINT('Ctrl Pts',(7.68380421625738,30.2359905590305,122.957610371017));
#94021=CARTESIAN_POINT('Ctrl Pts',(7.68766752464226,30.3066321275373,122.967009430934));
#94022=CARTESIAN_POINT('Ctrl Pts',(7.69153083302714,30.3766732525031,122.980070589513));
#94023=CARTESIAN_POINT('Ctrl Pts',(7.69538960950924,30.4466322148411,122.993116426536));
#94024=CARTESIAN_POINT('Ctrl Pts',(7.69924838599134,30.5159916574953,123.009815740546));
#94025=CARTESIAN_POINT('Ctrl Pts',(7.70310716247344,30.5843444512707,123.030091594828));
#94026=CARTESIAN_POINT('Ctrl Pts',(7.70696350805088,30.6526541849918,123.050354675975));
#94027=CARTESIAN_POINT('Ctrl Pts',(7.71081985362832,30.7199580633634,123.074189689446));
#94028=CARTESIAN_POINT('Ctrl Pts',(7.71467619920577,30.7858612994716,123.101469099411));
#94029=CARTESIAN_POINT('Ctrl Pts',(7.7185314054404,30.8517450647164,123.128740449776));
#94030=CARTESIAN_POINT('Ctrl Pts',(7.72238661167505,30.9162285606263,123.159453990657));
#94031=CARTESIAN_POINT('Ctrl Pts',(7.72624181790968,30.9789358958969,123.193433623078));
#94032=CARTESIAN_POINT('Ctrl Pts',(7.73009717475033,31.0416456808683,123.227414582935));
#94033=CARTESIAN_POINT('Ctrl Pts',(7.73395253159098,31.1025787413811,123.264661654271));
#94034=CARTESIAN_POINT('Ctrl Pts',(7.73780788843163,31.1613843006375,123.304953077719));
#94035=CARTESIAN_POINT('Ctrl Pts',(7.74166728088979,31.2202514149598,123.345286676453));
#94036=CARTESIAN_POINT('Ctrl Pts',(7.74552667334794,31.2769861809183,123.388670713517));
#94037=CARTESIAN_POINT('Ctrl Pts',(7.7493860658061,31.3312680704952,123.434840938761));
#94038=CARTESIAN_POINT('Ctrl Pts',(7.75324764339922,31.385580693732,123.481037304951));
#94039=CARTESIAN_POINT('Ctrl Pts',(7.75710922099235,31.4374373226377,123.530022665896));
#94040=CARTESIAN_POINT('Ctrl Pts',(7.76097079858548,31.4865537434053,123.581495318842));
#94041=CARTESIAN_POINT('Ctrl Pts',(7.76483913269032,31.5357561020219,123.63305803228));
#94042=CARTESIAN_POINT('Ctrl Pts',(7.76870746679515,31.5822083634828,123.687116357967));
#94043=CARTESIAN_POINT('Ctrl Pts',(7.77257580089999,31.6256665585024,123.743335445289));
#94044=CARTESIAN_POINT('Ctrl Pts',(7.77487352016638,31.65147992655,123.776728548516));
#94045=CARTESIAN_POINT('Ctrl Pts',(7.77717123943277,31.676237764067,123.81088342508));
#94046=CARTESIAN_POINT('Ctrl Pts',(7.77946895869917,31.6998964789576,123.845725542461));
#94047=CARTESIAN_POINT('Ctrl Pts',(7.78339694507706,31.740341415451,123.905288677283));
#94048=CARTESIAN_POINT('Ctrl Pts',(7.78732493145496,31.7777270929251,123.967090244454));
#94049=CARTESIAN_POINT('Ctrl Pts',(7.79125291783286,31.8118021955754,124.030788791538));
#94050=CARTESIAN_POINT('Ctrl Pts',(7.79517455591723,31.8458222270689,124.094384390945));
#94051=CARTESIAN_POINT('Ctrl Pts',(7.7990961940016,31.8765420914259,124.159870473948));
#94052=CARTESIAN_POINT('Ctrl Pts',(7.80301783208597,31.9037535790036,124.226876547419));
#94053=CARTESIAN_POINT('Ctrl Pts',(7.80693336836421,31.9309227273297,124.293778363929));
#94054=CARTESIAN_POINT('Ctrl Pts',(7.81084890464245,31.9545941797125,124.362195038262));
#94055=CARTESIAN_POINT('Ctrl Pts',(7.81476444092069,31.9746063344711,124.431732997292));
#94056=CARTESIAN_POINT('Ctrl Pts',(7.81867638559684,31.99460013269,124.501207171272));
#94057=CARTESIAN_POINT('Ctrl Pts',(7.822588330273,32.010941171143,124.571800140764));
#94058=CARTESIAN_POINT('Ctrl Pts',(7.82650027494915,32.0235168923249,124.643100926065));
#94059=CARTESIAN_POINT('Ctrl Pts',(7.83040988896528,32.0360851211384,124.714359231754));
#94060=CARTESIAN_POINT('Ctrl Pts',(7.8343195029814,32.0448924075045,124.786324057116));
#94061=CARTESIAN_POINT('Ctrl Pts',(7.83822911699753,32.0498770839559,124.858573329346));
#94062=CARTESIAN_POINT('Ctrl Pts',(7.84079450484425,32.0531479000354,124.905981437704));
#94063=CARTESIAN_POINT('Ctrl Pts',(7.84335989269096,32.0547738811643,124.953511789743));
#94064=CARTESIAN_POINT('Ctrl Pts',(7.84592528053768,32.054749734871,125.001043813945));
#94065=CARTESIAN_POINT('Origin',(-1.54592528053767,30.,125.));
#94066=CARTESIAN_POINT('',(6.69398884866211,28.7479590808042,126.629230216746));
#94067=CARTESIAN_POINT('',(6.75200666580924,28.7479590808042,126.629230216746));
#94068=CARTESIAN_POINT('',(-1.54592528053767,28.7479590808042,126.629230216746));
#94069=CARTESIAN_POINT('',(7.20407471942241,32.054749359036,125.001622972929));
#94070=CARTESIAN_POINT('Ctrl Pts',(6.75200666580924,28.7479590808042,126.629230216746));
#94071=CARTESIAN_POINT('Ctrl Pts',(6.75586954865699,28.6914516806324,126.585805060175));
#94072=CARTESIAN_POINT('Ctrl Pts',(6.75973243150475,28.637266657374,126.539483217538));
#94073=CARTESIAN_POINT('Ctrl Pts',(6.7635953143525,28.5856997459588,126.490554378048));
#94074=CARTESIAN_POINT('Ctrl Pts',(6.76746446443362,28.5340491711553,126.441546155241));
#94075=CARTESIAN_POINT('Ctrl Pts',(6.77133361451474,28.4850255120238,126.389922852198));
#94076=CARTESIAN_POINT('Ctrl Pts',(6.77520276459586,28.438885369153,126.336008484949));
#94077=CARTESIAN_POINT('Ctrl Pts',(6.77582755829117,28.4314346190498,126.327302346382));
#94078=CARTESIAN_POINT('Ctrl Pts',(6.77645235198647,28.4240589685884,126.318536528105));
#94079=CARTESIAN_POINT('Ctrl Pts',(6.77707714568178,28.4167593915136,126.309712463917));
#94080=CARTESIAN_POINT('Ctrl Pts',(6.78094621902987,28.3715563119621,126.255068904245));
#94081=CARTESIAN_POINT('Ctrl Pts',(6.78481529237797,28.32909694316,126.197975373757));
#94082=CARTESIAN_POINT('Ctrl Pts',(6.78868436572606,28.2896574231008,126.138738702313));
#94083=CARTESIAN_POINT('Ctrl Pts',(6.79254767412172,28.2502766682644,126.079590294017));
#94084=CARTESIAN_POINT('Ctrl Pts',(6.79641098251739,28.2139070976185,126.018305484439));
#94085=CARTESIAN_POINT('Ctrl Pts',(6.80027429091305,28.1807846665672,125.955224127157));
#94086=CARTESIAN_POINT('Ctrl Pts',(6.80413306740584,28.1477010902034,125.892216768261));
#94087=CARTESIAN_POINT('Ctrl Pts',(6.80799184389864,28.1178573120154,125.827417475809));
#94088=CARTESIAN_POINT('Ctrl Pts',(6.81185062039143,28.0914450656681,125.761193553006));
#94089=CARTESIAN_POINT('Ctrl Pts',(6.81570696597952,28.0650494581839,125.695011349137));
#94090=CARTESIAN_POINT('Ctrl Pts',(6.81956331156761,28.0420812731913,125.62740674564));
#94091=CARTESIAN_POINT('Ctrl Pts',(6.82341965715569,28.0226848730009,125.558768691894));
#94092=CARTESIAN_POINT('Ctrl Pts',(6.82727486340091,28.0032942034043,125.490150917004));
#94093=CARTESIAN_POINT('Ctrl Pts',(6.83113006964612,27.9874733556387,125.420500765251));
#94094=CARTESIAN_POINT('Ctrl Pts',(6.83498527589134,27.9753168606325,125.350222425982));
#94095=CARTESIAN_POINT('Ctrl Pts',(6.83884063274247,27.9631598907256,125.279941341248));
#94096=CARTESIAN_POINT('Ctrl Pts',(6.8426959895936,27.9546676384135,125.209032499328));
#94097=CARTESIAN_POINT('Ctrl Pts',(6.84655134644473,27.9498832308849,125.137908649088));
#94098=CARTESIAN_POINT('Ctrl Pts',(6.85041073891317,27.9450938152499,125.066710349542));
#94099=CARTESIAN_POINT('Ctrl Pts',(6.85427013138162,27.9440200248333,124.995297078087));
#94100=CARTESIAN_POINT('Ctrl Pts',(6.85812952385006,27.9466528919678,124.924084148982));
#94101=CARTESIAN_POINT('Ctrl Pts',(6.86199110145338,27.9492872497954,124.852830900098));
#94102=CARTESIAN_POINT('Ctrl Pts',(6.86585267905671,27.9556323997252,124.78177870346));
#94103=CARTESIAN_POINT('Ctrl Pts',(6.86971425666003,27.9656274785372,124.711337556276));
#94104=CARTESIAN_POINT('Ctrl Pts',(6.87358259077479,27.9756400455033,124.640773159874));
#94105=CARTESIAN_POINT('Ctrl Pts',(6.87745092488956,27.9893151983398,124.570822424404));
#94106=CARTESIAN_POINT('Ctrl Pts',(6.88131925900432,28.0065411240329,124.501884278176));
#94107=CARTESIAN_POINT('Ctrl Pts',(6.88361697817632,28.0167730064263,124.460936289825));
#94108=CARTESIAN_POINT('Ctrl Pts',(6.88591469734833,28.0282566940969,124.420345270082));
#94109=CARTESIAN_POINT('Ctrl Pts',(6.88821241652033,28.0409606653547,124.380191603951));
#94110=CARTESIAN_POINT('Ctrl Pts',(6.89208148986845,28.0623525731246,124.312577823577));
#94111=CARTESIAN_POINT('Ctrl Pts',(6.89595056321656,28.0872908982659,124.245940377934));
#94112=CARTESIAN_POINT('Ctrl Pts',(6.89981963656468,28.1156676269778,124.180677676076));
#94113=CARTESIAN_POINT('Ctrl Pts',(6.90368294496036,28.1440020741209,124.115512216202));
#94114=CARTESIAN_POINT('Ctrl Pts',(6.90754625335605,28.1757645631989,124.051717876002));
#94115=CARTESIAN_POINT('Ctrl Pts',(6.91140956175174,28.2107975421538,123.989677216263));
#94116=CARTESIAN_POINT('Ctrl Pts',(6.91526833824455,28.2457894252287,123.927709334107));
#94117=CARTESIAN_POINT('Ctrl Pts',(6.91912711473736,28.2840439399123,123.867491467115));
#94118=CARTESIAN_POINT('Ctrl Pts',(6.92298589123017,28.3253564882379,123.809383911156));
#94119=CARTESIAN_POINT('Ctrl Pts',(6.92684223681827,28.3666430109907,123.751312961084));
#94120=CARTESIAN_POINT('Ctrl Pts',(6.93069858240637,28.4109834644939,123.695350079465));
#94121=CARTESIAN_POINT('Ctrl Pts',(6.93455492799447,28.4581293723644,123.641827503542));
#94122=CARTESIAN_POINT('Ctrl Pts',(6.9384101342397,28.5052613511528,123.588320740664));
#94123=CARTESIAN_POINT('Ctrl Pts',(6.94226534048493,28.5551968178644,123.537253216468));
#94124=CARTESIAN_POINT('Ctrl Pts',(6.94612054673015,28.6076474656051,123.488923568292));
#94125=CARTESIAN_POINT('Ctrl Pts',(6.94997590358129,28.6601001623613,123.440592032089));
#94126=CARTESIAN_POINT('Ctrl Pts',(6.95383126043243,28.7150678764803,123.394998911815));
#94127=CARTESIAN_POINT('Ctrl Pts',(6.95768661728358,28.7722272302995,123.352404300661));
#94128=CARTESIAN_POINT('Ctrl Pts',(6.96154600975203,28.8294464160063,123.309765103348));
#94129=CARTESIAN_POINT('Ctrl Pts',(6.96540540222048,28.8888614306513,123.270130971586));
#94130=CARTESIAN_POINT('Ctrl Pts',(6.96926479468893,28.9501184868936,123.233719622784));
#94131=CARTESIAN_POINT('Ctrl Pts',(6.97312637229226,29.0114102260377,123.197287658378));
#94132=CARTESIAN_POINT('Ctrl Pts',(6.97698794989559,29.0745456527964,123.164082335572));
#94133=CARTESIAN_POINT('Ctrl Pts',(6.98084952749892,29.1391473006333,123.134274888283));
#94134=CARTESIAN_POINT('Ctrl Pts',(6.98471786161368,29.2038619804528,123.104415287604));
#94135=CARTESIAN_POINT('Ctrl Pts',(6.98858619572845,29.270047552029,123.077965612503));
#94136=CARTESIAN_POINT('Ctrl Pts',(6.99245452984321,29.3373082149498,123.055048288382));
#94137=CARTESIAN_POINT('Ctrl Pts',(6.99475224901511,29.3772598091303,123.041435820214));
#94138=CARTESIAN_POINT('Ctrl Pts',(6.997049968187,29.4175904326575,123.029068655139));
#94139=CARTESIAN_POINT('Ctrl Pts',(6.99934768735889,29.4582154543571,123.01796390835));
#94140=CARTESIAN_POINT('Ctrl Pts',(7.00321676070783,29.5266229389101,122.999264895707));
#94141=CARTESIAN_POINT('Ctrl Pts',(7.00708583405677,29.596133611542,122.984074911669));
#94142=CARTESIAN_POINT('Ctrl Pts',(7.01095490740571,29.6663541686468,122.972519291899));
#94143=CARTESIAN_POINT('Ctrl Pts',(7.01481821580223,29.7364700965202,122.960980890102));
#94144=CARTESIAN_POINT('Ctrl Pts',(7.01868152419874,29.8072933338607,122.953066181724));
#94145=CARTESIAN_POINT('Ctrl Pts',(7.02254483259525,29.8784170241083,122.94885028765));
#94146=CARTESIAN_POINT('Ctrl Pts',(7.02640360908889,29.9494572818097,122.944639339084));
#94147=CARTESIAN_POINT('Ctrl Pts',(7.03026238558253,30.020796809752,122.944118614824));
#94148=CARTESIAN_POINT('Ctrl Pts',(7.03412116207617,30.0920219410923,122.947311634744));
#94149=CARTESIAN_POINT('Ctrl Pts',(7.03797750766511,30.1632022028975,122.950502643165));
#94150=CARTESIAN_POINT('Ctrl Pts',(7.04183385325404,30.2342677269276,122.957402732454));
#94151=CARTESIAN_POINT('Ctrl Pts',(7.04569019884297,30.3048046215392,122.967983340327));
#94152=CARTESIAN_POINT('Ctrl Pts',(7.04954540508902,30.3753206762891,122.978560822199));
#94153=CARTESIAN_POINT('Ctrl Pts',(7.05340061133508,30.4453079315347,122.992816591849));
#94154=CARTESIAN_POINT('Ctrl Pts',(7.05725581758114,30.5143591217371,123.010670400264));
#94155=CARTESIAN_POINT('Ctrl Pts',(7.06111117443311,30.583413009465,123.028524906148));
#94156=CARTESIAN_POINT('Ctrl Pts',(7.06496653128508,30.6515302897811,123.049977606121));
#94157=CARTESIAN_POINT('Ctrl Pts',(7.06882188813704,30.718317058636,123.074897881729));
#94158=CARTESIAN_POINT('Ctrl Pts',(7.07268128060632,30.7851737369313,123.09984424278));
#94159=CARTESIAN_POINT('Ctrl Pts',(7.07654067307558,30.850696667515,123.128265255));
#94160=CARTESIAN_POINT('Ctrl Pts',(7.08040006554485,30.9145110549591,123.159981768336));
#94161=CARTESIAN_POINT('Ctrl Pts',(7.08426164314899,30.9783615732306,123.191716239125));
#94162=CARTESIAN_POINT('Ctrl Pts',(7.08812322075314,31.0405011992929,123.226749686708));
#94163=CARTESIAN_POINT('Ctrl Pts',(7.09198479835728,31.10058134778,123.264857856134));
#94164=CARTESIAN_POINT('Ctrl Pts',(7.09585313247284,31.1607666170885,123.303032702527));
#94165=CARTESIAN_POINT('Ctrl Pts',(7.09972146658841,31.2188848182504,123.344292730323));
#94166=CARTESIAN_POINT('Ctrl Pts',(7.10358980070397,31.2746184284222,123.388371809496));
#94167=CARTESIAN_POINT('Ctrl Pts',(7.10588751986847,31.3077231655965,123.414553970071));
#94168=CARTESIAN_POINT('Ctrl Pts',(7.10818523903296,31.339987241309,123.441729977376));
#94169=CARTESIAN_POINT('Ctrl Pts',(7.11048295819745,31.3713503754315,123.469838011744));
#94170=CARTESIAN_POINT('Ctrl Pts',(7.11438261491516,31.4245794464856,123.517542573179));
#94171=CARTESIAN_POINT('Ctrl Pts',(7.11828227163287,31.4754382086281,123.568137518425));
#94172=CARTESIAN_POINT('Ctrl Pts',(7.12218192835057,31.5235907696476,123.621352572575));
#94173=CARTESIAN_POINT('Ctrl Pts',(7.12598698948198,31.5705752740736,123.673276767142));
#94174=CARTESIAN_POINT('Ctrl Pts',(7.1297920506134,31.6149830001644,123.727695018052));
#94175=CARTESIAN_POINT('Ctrl Pts',(7.13359711174481,31.6565353095317,123.784315694444));
#94176=CARTESIAN_POINT('Ctrl Pts',(7.13739855500656,31.6980481107719,123.840882535636));
#94177=CARTESIAN_POINT('Ctrl Pts',(7.14119999826832,31.7367105810086,123.89964724987));
#94178=CARTESIAN_POINT('Ctrl Pts',(7.14500144153007,31.7722833964744,123.960284113288));
#94179=CARTESIAN_POINT('Ctrl Pts',(7.14880063066542,31.807835118472,124.020885021111));
#94180=CARTESIAN_POINT('Ctrl Pts',(7.15259981980078,31.8403005657239,124.083355444928));
#94181=CARTESIAN_POINT('Ctrl Pts',(7.15639900893613,31.8694840247516,124.147341191508));
#94182=CARTESIAN_POINT('Ctrl Pts',(7.16037198480999,31.9000024260477,124.214253845334));
#94183=CARTESIAN_POINT('Ctrl Pts',(7.16434496068385,31.9269310579514,124.282823287038));
#94184=CARTESIAN_POINT('Ctrl Pts',(7.1683179365577,31.9501011080216,124.352618172179));
#94185=CARTESIAN_POINT('Ctrl Pts',(7.17211850690861,31.9722657040629,124.419384339287));
#94186=CARTESIAN_POINT('Ctrl Pts',(7.17591907725952,31.9909910752724,124.487271268715));
#94187=CARTESIAN_POINT('Ctrl Pts',(7.17971964761043,32.0061804532505,124.555885654932));
#94188=CARTESIAN_POINT('Ctrl Pts',(7.1835216969548,32.0213757421811,124.624526742464));
#94189=CARTESIAN_POINT('Ctrl Pts',(7.18732374629917,32.0330322152424,124.693895355795));
#94190=CARTESIAN_POINT('Ctrl Pts',(7.19112579564354,32.0411045496223,124.763589805611));
#94191=CARTESIAN_POINT('Ctrl Pts',(7.19493249874043,32.0491867646331,124.833369562242));
#94192=CARTESIAN_POINT('Ctrl Pts',(7.19873920183731,32.0536760627127,124.9034754511));
#94193=CARTESIAN_POINT('Ctrl Pts',(7.2025459049342,32.0545791584134,124.973503881167));
#94194=CARTESIAN_POINT('Ctrl Pts',(7.2030555097636,32.0547000561874,124.982878614434));
#94195=CARTESIAN_POINT('Ctrl Pts',(7.20356511459301,32.0547567608592,124.992251965448));
#94196=CARTESIAN_POINT('Ctrl Pts',(7.20407471942241,32.054749359036,125.001622972929));
#94197=CARTESIAN_POINT('Ctrl Pts',(7.20407471946233,32.0547493590354,125.001622973663));
#94198=CARTESIAN_POINT('Ctrl Pts',(7.20992255598689,32.0546644213169,125.109157511514));
#94199=CARTESIAN_POINT('Ctrl Pts',(7.21577039251145,32.0461359067699,125.216366166843));
#94200=CARTESIAN_POINT('Ctrl Pts',(7.22161822903602,32.0293269300174,125.322226277026));
#94201=CARTESIAN_POINT('Ctrl Pts',(7.22548730238386,32.0182056950642,125.392265945404));
#94202=CARTESIAN_POINT('Ctrl Pts',(7.22935637573169,32.0034324231356,125.461866373981));
#94203=CARTESIAN_POINT('Ctrl Pts',(7.23322544907953,31.9850548085808,125.530617535924));
#94204=CARTESIAN_POINT('Ctrl Pts',(7.23708875747492,31.9667045768292,125.599266258047));
#94205=CARTESIAN_POINT('Ctrl Pts',(7.24095206587031,31.944760787173,125.667067759863));
#94206=CARTESIAN_POINT('Ctrl Pts',(7.2448153742657,31.9193224755762,125.733620335901));
#94207=CARTESIAN_POINT('Ctrl Pts',(7.2486741507582,31.8939140047133,125.800094841597));
#94208=CARTESIAN_POINT('Ctrl Pts',(7.25253292725071,31.8650193270942,125.86532288007));
#94209=CARTESIAN_POINT('Ctrl Pts',(7.25639170374321,31.8327873077696,125.92891778268));
#94210=CARTESIAN_POINT('Ctrl Pts',(7.26024804933099,31.8005755935773,125.992472622552));
#94211=CARTESIAN_POINT('Ctrl Pts',(7.26410439491877,31.7650309279384,126.054395935445));
#94212=CARTESIAN_POINT('Ctrl Pts',(7.26796074050655,31.7263497323502,126.114322289158));
#94213=CARTESIAN_POINT('Ctrl Pts',(7.27181594675145,31.6876799649766,126.174230937854));
#94214=CARTESIAN_POINT('Ctrl Pts',(7.27567115299635,31.6458757706677,126.23214339075));
#94215=CARTESIAN_POINT('Ctrl Pts',(7.27952635924124,31.6011779466017,126.287721532714));
#94216=CARTESIAN_POINT('Ctrl Pts',(7.28338171609205,31.5564783763889,126.343301845871));
#94217=CARTESIAN_POINT('Ctrl Pts',(7.28723707294285,31.508885258151,126.396547289877));
#94218=CARTESIAN_POINT('Ctrl Pts',(7.29109242979365,31.4586797914259,126.447152662502));
#94219=CARTESIAN_POINT('Ctrl Pts',(7.29495182226175,31.4084217718353,126.497811006596));
#94220=CARTESIAN_POINT('Ctrl Pts',(7.29881121472986,31.3555462879374,126.545823417153));
#94221=CARTESIAN_POINT('Ctrl Pts',(7.30267060719796,31.3003709007601,126.590922085759));
#94222=CARTESIAN_POINT('Ctrl Pts',(7.30653218480093,31.2451642740384,126.63604628861));
#94223=CARTESIAN_POINT('Ctrl Pts',(7.31039376240389,31.1876555436276,126.678253177863));
#94224=CARTESIAN_POINT('Ctrl Pts',(7.31425534000686,31.1281925856658,126.717317399944));
#94225=CARTESIAN_POINT('Ctrl Pts',(7.31812367412126,31.0686255867662,126.756449971774));
#94226=CARTESIAN_POINT('Ctrl Pts',(7.32199200823566,31.0070979531369,126.79242865292));
#94227=CARTESIAN_POINT('Ctrl Pts',(7.32586034235006,30.9439829349224,126.825073637165));
#94228=CARTESIAN_POINT('Ctrl Pts',(7.32815806152489,30.9064937772428,126.844464156196));
#94229=CARTESIAN_POINT('Ctrl Pts',(7.33045578069973,30.8684449853415,126.862679408199));
#94230=CARTESIAN_POINT('Ctrl Pts',(7.33275349987457,30.8299177134446,126.879689908312));
#94231=CARTESIAN_POINT('Ctrl Pts',(7.33662257322846,30.7650425786904,126.908333475135));
#94232=CARTESIAN_POINT('Ctrl Pts',(7.34049164658236,30.6985557347294,126.933670578712));
#94233=CARTESIAN_POINT('Ctrl Pts',(7.34436071993625,30.6308275306673,126.955518905317));
#94234=CARTESIAN_POINT('Ctrl Pts',(7.34822402833774,30.563200242209,126.977334677728));
#94235=CARTESIAN_POINT('Ctrl Pts',(7.35208733673922,30.4943357236864,126.995671843735));
#94236=CARTESIAN_POINT('Ctrl Pts',(7.35595064514071,30.424625178915,127.010395737145));
#94237=CARTESIAN_POINT('Ctrl Pts',(7.35980942163932,30.3549964089815,127.025102358506));
#94238=CARTESIAN_POINT('Ctrl Pts',(7.36366819813793,30.2845240571169,127.03620402665));
#94239=CARTESIAN_POINT('Ctrl Pts',(7.36752697463654,30.2136137195477,127.043616094407));
#94240=CARTESIAN_POINT('Ctrl Pts',(7.37138332023044,30.1427480532036,127.051023492802));
#94241=CARTESIAN_POINT('Ctrl Pts',(7.37523966582434,30.0714454305808,127.054745851857));
#94242=CARTESIAN_POINT('Ctrl Pts',(7.37909601141824,30.000119399154,127.054749996531));
#94243=CARTESIAN_POINT('Ctrl Pts',(7.38295121766926,29.9288144407364,127.05475413998));
#94244=CARTESIAN_POINT('Ctrl Pts',(7.38680642392028,29.8574865727665,127.051042249909));
#94245=CARTESIAN_POINT('Ctrl Pts',(7.39066163017129,29.7865504602363,127.043633249014));
#94246=CARTESIAN_POINT('Ctrl Pts',(7.3945169870282,29.7156115765452,127.036223958681));
#94247=CARTESIAN_POINT('Ctrl Pts',(7.39837234388512,29.6450649616074,127.025117323432));
#94248=CARTESIAN_POINT('Ctrl Pts',(7.40222770074203,29.5753195416403,127.010384060519));
#94249=CARTESIAN_POINT('Ctrl Pts',(7.40608709321618,29.5055011152488,126.995635375477));
#94250=CARTESIAN_POINT('Ctrl Pts',(7.40994648569033,29.4364860342437,126.977252585325));
#94251=CARTESIAN_POINT('Ctrl Pts',(7.41380587816449,29.3686715298374,126.955357237249));
#94252=CARTESIAN_POINT('Ctrl Pts',(7.41766745577349,29.3008186297929,126.933449492329));
#94253=CARTESIAN_POINT('Ctrl Pts',(7.42152903338249,29.2341681136199,126.908025403692));
#94254=CARTESIAN_POINT('Ctrl Pts',(7.4253906109915,29.1690979861963,126.879255013551));
#94255=CARTESIAN_POINT('Ctrl Pts',(7.42925894511183,29.1039140071045,126.850434284536));
#94256=CARTESIAN_POINT('Ctrl Pts',(7.43312727923216,29.0403163711,126.818255783837));
#94257=CARTESIAN_POINT('Ctrl Pts',(7.43699561335248,28.9786585786913,126.782935574725));
#94258=CARTESIAN_POINT('Ctrl Pts',(7.4392933324727,28.9420349872122,126.761956021955));
#94259=CARTESIAN_POINT('Ctrl Pts',(7.44159105159292,28.9060952632211,126.739868873525));
#94260=CARTESIAN_POINT('Ctrl Pts',(7.44388877071313,28.8709081933679,126.716726319102));
#94261=CARTESIAN_POINT('Ctrl Pts',(7.44663011041789,28.8289275566425,126.689115632158));
#94262=CARTESIAN_POINT('Ctrl Pts',(7.44937145012266,28.7879021272144,126.659925896233));
#94263=CARTESIAN_POINT('Ctrl Pts',(7.45211278982742,28.7479590808042,126.629230216746));
#94264=CARTESIAN_POINT('',(7.14592528050144,32.0547492461588,124.998239912027));
#94265=CARTESIAN_POINT('Ctrl Pts',(7.14592528053768,32.0547492461594,124.998239912697));
#94266=CARTESIAN_POINT('Ctrl Pts',(7.14975890798153,32.0548099310451,125.069084252562));
#94267=CARTESIAN_POINT('Ctrl Pts',(7.15359253542538,32.0512024328575,125.139993721177));
#94268=CARTESIAN_POINT('Ctrl Pts',(7.15742616286923,32.0439332342781,125.210557584317));
#94269=CARTESIAN_POINT('Ctrl Pts',(7.1612583463496,32.036666773695,125.281094869068));
#94270=CARTESIAN_POINT('Ctrl Pts',(7.16509052982997,32.0257413995742,125.351286317587));
#94271=CARTESIAN_POINT('Ctrl Pts',(7.16892271331034,32.0112155594126,125.420725012421));
#94272=CARTESIAN_POINT('Ctrl Pts',(7.17275477350104,31.9966901865788,125.490161473262));
#94273=CARTESIAN_POINT('Ctrl Pts',(7.17658683369175,31.9785646802636,125.558844747243));
#94274=CARTESIAN_POINT('Ctrl Pts',(7.18041889388246,31.9569484900836,125.626378615264));
#94275=CARTESIAN_POINT('Ctrl Pts',(7.18425485641164,31.935310287282,125.693981255694));
#94276=CARTESIAN_POINT('Ctrl Pts',(7.18809081894083,31.910174452894,125.760431683198));
#94277=CARTESIAN_POINT('Ctrl Pts',(7.19192678147001,31.8816998964671,125.825350266333));
#94278=CARTESIAN_POINT('Ctrl Pts',(7.19576473620573,31.8532105517838,125.890302564924));
#94279=CARTESIAN_POINT('Ctrl Pts',(7.19960269094144,31.8213792546822,125.953720995477));
#94280=CARTESIAN_POINT('Ctrl Pts',(7.20344064567716,31.7864112720226,126.015249885344));
#94281=CARTESIAN_POINT('Ctrl Pts',(7.20728565488989,31.7513790153299,126.07689187038));
#94282=CARTESIAN_POINT('Ctrl Pts',(7.21113066410261,31.7131988248325,126.136636963837));
#94283=CARTESIAN_POINT('Ctrl Pts',(7.21497567331534,31.672119382862,126.194158419958));
#94284=CARTESIAN_POINT('Ctrl Pts',(7.21791465037902,31.640719838398,126.238125607254));
#94285=CARTESIAN_POINT('Ctrl Pts',(7.22085362744269,31.6076273167987,126.280794230264));
#94286=CARTESIAN_POINT('Ctrl Pts',(7.22379260450636,31.572967724563,126.322032563889));
#94287=CARTESIAN_POINT('Ctrl Pts',(7.2276616778553,31.5273394322359,126.376321567895));
#94288=CARTESIAN_POINT('Ctrl Pts',(7.23153075120424,31.4788078915284,126.428351931928));
#94289=CARTESIAN_POINT('Ctrl Pts',(7.23539982455317,31.4276252989682,126.477796862984));
#94290=CARTESIAN_POINT('Ctrl Pts',(7.23926313294969,31.3765189689092,126.52716812067));
#94291=CARTESIAN_POINT('Ctrl Pts',(7.2431264413462,31.3227697743507,126.573961257351));
#94292=CARTESIAN_POINT('Ctrl Pts',(7.24698974974272,31.2666696204782,126.617883072122));
#94293=CARTESIAN_POINT('Ctrl Pts',(7.25084852623635,31.2106352756022,126.661753363851));
#94294=CARTESIAN_POINT('Ctrl Pts',(7.25470730272998,31.1522558300256,126.702758726121));
#94295=CARTESIAN_POINT('Ctrl Pts',(7.25856607922361,31.0918581403232,126.74064452543));
#94296=CARTESIAN_POINT('Ctrl Pts',(7.26242242481254,31.0314984992169,126.778506457907));
#94297=CARTESIAN_POINT('Ctrl Pts',(7.26627877040147,30.9691235470309,126.813252468868));
#94298=CARTESIAN_POINT('Ctrl Pts',(7.2701351159904,30.9050899489487,126.844670633694));
#94299=CARTESIAN_POINT('Ctrl Pts',(7.27399032223645,30.8410752693535,126.876079516141));
#94300=CARTESIAN_POINT('Ctrl Pts',(7.2778455284825,30.77540335261,126.904162290511));
#94301=CARTESIAN_POINT('Ctrl Pts',(7.28170073472854,30.7084548128327,126.92875331255));
#94302=CARTESIAN_POINT('Ctrl Pts',(7.2855560915805,30.6415036576711,126.953345295253));
#94303=CARTESIAN_POINT('Ctrl Pts',(7.28941144843246,30.5732762372185,126.974445089379));
#94304=CARTESIAN_POINT('Ctrl Pts',(7.29326680528442,30.5041708255149,126.991936078593));
#94305=CARTESIAN_POINT('Ctrl Pts',(7.29712619775369,30.434993077318,127.009445376602));
#94306=CARTESIAN_POINT('Ctrl Pts',(7.30098559022295,30.3649359751554,127.023338209445));
#94307=CARTESIAN_POINT('Ctrl Pts',(7.30484498269221,30.2944096807248,127.033548746009));
#94308=CARTESIAN_POINT('Ctrl Pts',(7.30870656029635,30.2238434552775,127.043765063638));
#94309=CARTESIAN_POINT('Ctrl Pts',(7.31256813790048,30.1528079927104,127.050294890176));
#94310=CARTESIAN_POINT('Ctrl Pts',(7.31642971550461,30.0817175524931,127.053124400545));
#94311=CARTESIAN_POINT('Ctrl Pts',(7.32029804962017,30.0105027270062,127.055958861642));
#94312=CARTESIAN_POINT('Ctrl Pts',(7.32416638373573,29.93923321772,127.055080086321));
#94313=CARTESIAN_POINT('Ctrl Pts',(7.32803471785129,29.8683215537164,127.050526359081));
#94314=CARTESIAN_POINT('Ctrl Pts',(7.33033243701584,29.826201332323,127.047821529033));
#94315=CARTESIAN_POINT('Ctrl Pts',(7.33263015618038,29.7842072534164,127.043821117613));
#94316=CARTESIAN_POINT('Ctrl Pts',(7.33492787534493,29.742424058736,127.038541683896));
#94317=CARTESIAN_POINT('Ctrl Pts',(7.33879679457315,29.6720691573147,127.029652128142));
#94318=CARTESIAN_POINT('Ctrl Pts',(7.34266571380137,29.6020371943226,127.017098714014));
#94319=CARTESIAN_POINT('Ctrl Pts',(7.3465346330296,29.5327394560202,127.000916076836));
#94320=CARTESIAN_POINT('Ctrl Pts',(7.35048280112887,29.4620222599304,126.984401963177));
#94321=CARTESIAN_POINT('Ctrl Pts',(7.35443096922814,29.3920702167941,126.964108264813));
#94322=CARTESIAN_POINT('Ctrl Pts',(7.35837913732742,29.323315123349,126.94012760926));
#94323=CARTESIAN_POINT('Ctrl Pts',(7.36223776870244,29.2561192608404,126.916690788034));
#94324=CARTESIAN_POINT('Ctrl Pts',(7.36609640007746,29.1900671186566,126.889732637857));
#94325=CARTESIAN_POINT('Ctrl Pts',(7.36995503145248,29.1255495136279,126.85939073607));
#94326=CARTESIAN_POINT('Ctrl Pts',(7.37394796791389,29.058786282709,126.827992741761));
#94327=CARTESIAN_POINT('Ctrl Pts',(7.37794090437529,28.993666907158,126.792971229341));
#94328=CARTESIAN_POINT('Ctrl Pts',(7.3819338408367,28.9306027627195,126.754533303017));
#94329=CARTESIAN_POINT('Ctrl Pts',(7.3859267772981,28.8675386182809,126.716095376693));
#94330=CARTESIAN_POINT('Ctrl Pts',(7.3899197137595,28.806530209321,126.674241320047));
#94331=CARTESIAN_POINT('Ctrl Pts',(7.39391265022091,28.7479590808041,126.629230216746));
#94332=CARTESIAN_POINT('Ctrl Pts',(6.69398884866211,28.7479590808042,126.629230216746));
#94333=CARTESIAN_POINT('Ctrl Pts',(6.6978469486556,28.6915134540401,126.585852532186));
#94334=CARTESIAN_POINT('Ctrl Pts',(6.70170504864909,28.6372663028371,126.539493111356));
#94335=CARTESIAN_POINT('Ctrl Pts',(6.70556314864259,28.5855443913852,126.490406955753));
#94336=CARTESIAN_POINT('Ctrl Pts',(6.70941911634607,28.5338510655364,126.441347929027));
#94337=CARTESIAN_POINT('Ctrl Pts',(6.71327508404956,28.4846805619422,126.389565491501));
#94338=CARTESIAN_POINT('Ctrl Pts',(6.71713105175305,28.4383254317381,126.335353925124));
#94339=CARTESIAN_POINT('Ctrl Pts',(6.7209861782402,28.3919804143504,126.281154185521));
#94340=CARTESIAN_POINT('Ctrl Pts',(6.72484130472734,28.3484498661655,126.224526738619));
#94341=CARTESIAN_POINT('Ctrl Pts',(6.72869643121448,28.3079872435019,126.165800323532));
#94342=CARTESIAN_POINT('Ctrl Pts',(6.73255200624573,28.2675199130106,126.107067075625));
#94343=CARTESIAN_POINT('Ctrl Pts',(6.73640758127698,28.2301214901697,126.046234776163));
#94344=CARTESIAN_POINT('Ctrl Pts',(6.74026315630823,28.196002150772,125.983661182766));
#94345=CARTESIAN_POINT('Ctrl Pts',(6.74412295033885,28.161845475965,125.921019117624));
#94346=CARTESIAN_POINT('Ctrl Pts',(6.74798274436946,28.1309752768927,125.856632383921));
#94347=CARTESIAN_POINT('Ctrl Pts',(6.75184253840008,28.1035553368084,125.790882546243));
#94348=CARTESIAN_POINT('Ctrl Pts',(6.75570478529074,28.0761179716298,125.725090925209));
#94349=CARTESIAN_POINT('Ctrl Pts',(6.7595670321814,28.0521353916157,125.65793493382));
#94350=CARTESIAN_POINT('Ctrl Pts',(6.76342927907205,28.0317219363814,125.589812704829));
#94351=CARTESIAN_POINT('Ctrl Pts',(6.76729801520192,28.0112741830305,125.521576018774));
#94352=CARTESIAN_POINT('Ctrl Pts',(6.77116675133179,27.994407634488,125.452370327107));
#94353=CARTESIAN_POINT('Ctrl Pts',(6.77503548746166,27.981185660923,125.382604530602));
#94354=CARTESIAN_POINT('Ctrl Pts',(6.77644083202515,27.9763826896051,125.357261633194));
#94355=CARTESIAN_POINT('Ctrl Pts',(6.77784617658864,27.9720601435449,125.331844874585));
#94356=CARTESIAN_POINT('Ctrl Pts',(6.77925152115213,27.9682193607167,125.306373948523));
#94357=CARTESIAN_POINT('Ctrl Pts',(6.78312059450033,27.9576452489559,125.236249593444));
#94358=CARTESIAN_POINT('Ctrl Pts',(6.78698966784853,27.9506850681282,125.165439812299));
#94359=CARTESIAN_POINT('Ctrl Pts',(6.79085874119674,27.9474173181754,125.094349863665));
#94360=CARTESIAN_POINT('Ctrl Pts',(6.79472204959251,27.944154437198,125.023365839664));
#94361=CARTESIAN_POINT('Ctrl Pts',(6.79858535798829,27.9445730883938,124.952102958123));
#94362=CARTESIAN_POINT('Ctrl Pts',(6.80244866638406,27.9487003168899,124.880974067647));
#94363=CARTESIAN_POINT('Ctrl Pts',(6.80630744287696,27.9528227038883,124.809928615817));
#94364=CARTESIAN_POINT('Ctrl Pts',(6.81016621936986,27.9606449988303,124.739017325455));
#94365=CARTESIAN_POINT('Ctrl Pts',(6.81402499586275,27.9721422035054,124.668653776699));
#94366=CARTESIAN_POINT('Ctrl Pts',(6.81788134145095,27.9836321653125,124.598334554709));
#94367=CARTESIAN_POINT('Ctrl Pts',(6.82173768703914,27.9987923656303,124.528562868027));
#94368=CARTESIAN_POINT('Ctrl Pts',(6.82559403262733,28.0175460548874,124.45974643175));
#94369=CARTESIAN_POINT('Ctrl Pts',(6.82944923887265,28.036294203437,124.390950327031));
#94370=CARTESIAN_POINT('Ctrl Pts',(6.83330444511796,28.0586336055338,124.323109380861));
#94371=CARTESIAN_POINT('Ctrl Pts',(6.83715965136327,28.0844369538239,124.256618685583));
#94372=CARTESIAN_POINT('Ctrl Pts',(6.84101500821451,28.1102413101371,124.190125392807));
#94373=CARTESIAN_POINT('Ctrl Pts',(6.84487036506575,28.1395097035015,124.124982907731));
#94374=CARTESIAN_POINT('Ctrl Pts',(6.84872572191698,28.172066364392,124.06156716473));
#94375=CARTESIAN_POINT('Ctrl Pts',(6.85258511438553,28.2046571041575,123.99808504093));
#94376=CARTESIAN_POINT('Ctrl Pts',(6.85644450685407,28.2405427601609,123.936333700384));
#94377=CARTESIAN_POINT('Ctrl Pts',(6.86030389932261,28.2795015977766,123.876664426608));
#94378=CARTESIAN_POINT('Ctrl Pts',(6.86416547692604,28.3184824933498,123.816961368912));
#94379=CARTESIAN_POINT('Ctrl Pts',(6.86802705452946,28.360539747782,123.75934311725));
#94380=CARTESIAN_POINT('Ctrl Pts',(6.87188863213289,28.4054098946934,123.704129652103));
#94381=CARTESIAN_POINT('Ctrl Pts',(6.87575696624774,28.4503585498446,123.648819581256));
#94382=CARTESIAN_POINT('Ctrl Pts',(6.8796253003626,28.4981295980007,123.595923058155));
#94383=CARTESIAN_POINT('Ctrl Pts',(6.88349363447745,28.5484216159555,123.545724318613));
#94384=CARTESIAN_POINT('Ctrl Pts',(6.88579135364853,28.5782941477421,123.515907192484));
#94385=CARTESIAN_POINT('Ctrl Pts',(6.88808907281961,28.6090554407216,123.487041142892));
#94386=CARTESIAN_POINT('Ctrl Pts',(6.89038679199069,28.6406370524375,123.459178810084));
#94387=CARTESIAN_POINT('Ctrl Pts',(6.89425586533899,28.6938165591956,123.412262106491));
#94388=CARTESIAN_POINT('Ctrl Pts',(6.89812493868729,28.7495319885931,123.368009873212));
#94389=CARTESIAN_POINT('Ctrl Pts',(6.9019940120356,28.8074854407965,123.326707859163));
#94390=CARTESIAN_POINT('Ctrl Pts',(6.90585732043149,28.8653525418598,123.285467385469));
#94391=CARTESIAN_POINT('Ctrl Pts',(6.90972062882737,28.9254506541184,123.247168685001));
#94392=CARTESIAN_POINT('Ctrl Pts',(6.91358393722326,28.9874475937836,123.212058393804));
#94393=CARTESIAN_POINT('Ctrl Pts',(6.91744271371626,29.0493718071528,123.17698928918));
#94394=CARTESIAN_POINT('Ctrl Pts',(6.92130149020926,29.113190002817,123.145101402743));
#94395=CARTESIAN_POINT('Ctrl Pts',(6.92516026670227,29.1785411559556,123.116598043422));
#94396=CARTESIAN_POINT('Ctrl Pts',(6.92901661229056,29.2438511399759,123.088112640298));
#94397=CARTESIAN_POINT('Ctrl Pts',(6.93287295787886,29.3106917212872,123.063007727904));
#94398=CARTESIAN_POINT('Ctrl Pts',(6.93672930346716,29.3786787344663,123.041439955606));
#94399=CARTESIAN_POINT('Ctrl Pts',(6.94058450971258,29.4466456611367,123.019878555426));
#94400=CARTESIAN_POINT('Ctrl Pts',(6.944439715958,29.5157578844515,123.001852367474));
#94401=CARTESIAN_POINT('Ctrl Pts',(6.94829492220343,29.5856144231854,122.987468719193));
#94402=CARTESIAN_POINT('Ctrl Pts',(6.95215027905476,29.6554736909063,122.973084509006));
#94403=CARTESIAN_POINT('Ctrl Pts',(6.95600563590609,29.7260768555264,122.962343216817));
#94404=CARTESIAN_POINT('Ctrl Pts',(6.95986099275742,29.7970127471239,122.955301064296));
#94405=CARTESIAN_POINT('Ctrl Pts',(6.96372038522607,29.8680228912806,122.94825154036));
#94406=CARTESIAN_POINT('Ctrl Pts',(6.96757977769471,29.9393659732674,122.944908933754));
#94407=CARTESIAN_POINT('Ctrl Pts',(6.97143917016336,30.0106266036029,122.945277479124));
#94408=CARTESIAN_POINT('Ctrl Pts',(6.97530074776688,30.081927580726,122.945646233159));
#94409=CARTESIAN_POINT('Ctrl Pts',(6.9791623253704,30.1531455280473,122.949730294191));
#94410=CARTESIAN_POINT('Ctrl Pts',(6.98302390297392,30.2238687213255,122.95748185856));
#94411=CARTESIAN_POINT('Ctrl Pts',(6.98689223708888,30.2947156573103,122.965246985658));
#94412=CARTESIAN_POINT('Ctrl Pts',(6.99076057120383,30.3650656313036,122.976692349675));
#94413=CARTESIAN_POINT('Ctrl Pts',(6.99462890531879,30.4345163632976,122.991718871142));
#94414=CARTESIAN_POINT('Ctrl Pts',(6.99692662448894,30.475768818112,123.000644347952));
#94415=CARTESIAN_POINT('Ctrl Pts',(6.9992243436591,30.5167042642521,123.010832341508));
#94416=CARTESIAN_POINT('Ctrl Pts',(7.00152206282925,30.5572413556232,123.022253900501));
#94417=CARTESIAN_POINT('Ctrl Pts',(7.00539113617735,30.6255007764743,123.04148638551));
#94418=CARTESIAN_POINT('Ctrl Pts',(7.00926020952544,30.6928970531184,123.064294522592));
#94419=CARTESIAN_POINT('Ctrl Pts',(7.01312928287354,30.7590285452722,123.090583013074));
#94420=CARTESIAN_POINT('Ctrl Pts',(7.0169925912692,30.8250615009361,123.116832333479));
#94421=CARTESIAN_POINT('Ctrl Pts',(7.02085589966486,30.8898329651199,123.146551535715));
#94422=CARTESIAN_POINT('Ctrl Pts',(7.02471920806053,30.9529555635828,123.179595304242));
#94423=CARTESIAN_POINT('Ctrl Pts',(7.02857798455332,31.0160041152818,123.212600310359));
#94424=CARTESIAN_POINT('Ctrl Pts',(7.03243676104611,31.0774072149879,123.248921911992));
#94425=CARTESIAN_POINT('Ctrl Pts',(7.0362955375389,31.1367982471179,123.288367063927));
#94426=CARTESIAN_POINT('Ctrl Pts',(7.04015188312699,31.1961518648137,123.327787366689));
#94427=CARTESIAN_POINT('Ctrl Pts',(7.04400822871507,31.2534955259985,123.370327047667));
#94428=CARTESIAN_POINT('Ctrl Pts',(7.04786457430316,31.3084892651872,123.415748313749));
#94429=CARTESIAN_POINT('Ctrl Pts',(7.05171978054837,31.3634667566816,123.461156160287));
#94430=CARTESIAN_POINT('Ctrl Pts',(7.05557498679359,31.4160953301631,123.50944359257));
#94431=CARTESIAN_POINT('Ctrl Pts',(7.05943019303881,31.4660673373546,123.560331939355));
#94432=CARTESIAN_POINT('Ctrl Pts',(7.06328554988996,31.5160412967324,123.611222274123));
#94433=CARTESIAN_POINT('Ctrl Pts',(7.0671409067411,31.5633581449818,123.664713376968));
#94434=CARTESIAN_POINT('Ctrl Pts',(7.07099626359225,31.6077476440311,123.720490298742));
#94435=CARTESIAN_POINT('Ctrl Pts',(7.07485565606069,31.6521836080477,123.776325605335));
#94436=CARTESIAN_POINT('Ctrl Pts',(7.07871504852913,31.6936858028699,123.834451126328));
#94437=CARTESIAN_POINT('Ctrl Pts',(7.08257444099757,31.7320253784512,123.894520171645));
#94438=CARTESIAN_POINT('Ctrl Pts',(7.08643601860089,31.7703866613724,123.954623227227));
#94439=CARTESIAN_POINT('Ctrl Pts',(7.09029759620421,31.8055815206696,124.016671574939));
#94440=CARTESIAN_POINT('Ctrl Pts',(7.09415917380753,31.8374268138397,124.08029338032));
#94441=CARTESIAN_POINT('Ctrl Pts',(7.09802750792229,31.8693278259698,124.144026503277));
#94442=CARTESIAN_POINT('Ctrl Pts',(7.10189584203705,31.8978673764232,124.209338135149));
#94443=CARTESIAN_POINT('Ctrl Pts',(7.10576417615181,31.9229105239492,124.275836565832));
#94444=CARTESIAN_POINT('Ctrl Pts',(7.10806189532381,31.9377856920423,124.315335408113));
#94445=CARTESIAN_POINT('Ctrl Pts',(7.1103596144958,31.9514282307018,124.35525266134));
#94446=CARTESIAN_POINT('Ctrl Pts',(7.1126573336678,31.9638183439836,124.395504280964));
#94447=CARTESIAN_POINT('Ctrl Pts',(7.11737359945938,31.9892501148184,124.478124184649));
#94448=CARTESIAN_POINT('Ctrl Pts',(7.12208986525095,32.0094837420629,124.562414597948));
#94449=CARTESIAN_POINT('Ctrl Pts',(7.12680613104252,32.024337058193,124.647782684517));
#94450=CARTESIAN_POINT('Ctrl Pts',(7.1314577452802,32.0389867619716,124.731980527572));
#94451=CARTESIAN_POINT('Ctrl Pts',(7.13610935951787,32.0484026072813,124.81722670766));
#94452=CARTESIAN_POINT('Ctrl Pts',(7.14076097375554,32.0524559155862,124.902931585593));
#94453=CARTESIAN_POINT('Ctrl Pts',(7.14248240933751,32.0539559344579,124.934648623784));
#94454=CARTESIAN_POINT('Ctrl Pts',(7.14420384491947,32.0547219964684,124.9664282743));
#94455=CARTESIAN_POINT('Ctrl Pts',(7.14592528050144,32.0547492461588,124.998239912027));
#94456=CARTESIAN_POINT('Origin',(-1.54592528053767,30.,125.));
#94457=CARTESIAN_POINT('',(5.99388605120356,28.7479590808042,126.629230216746));
#94458=CARTESIAN_POINT('',(6.05208070802109,28.7479590808042,126.629230216746));
#94459=CARTESIAN_POINT('',(-1.54592528053767,28.7479590808042,126.629230216746));
#94460=CARTESIAN_POINT('',(6.50407471951103,32.0547499427048,125.000485236461));
#94461=CARTESIAN_POINT('Ctrl Pts',(6.05208070802109,28.7479590808042,126.629230216746));
#94462=CARTESIAN_POINT('Ctrl Pts',(6.05593584239997,28.6914085092978,126.585771883601));
#94463=CARTESIAN_POINT('Ctrl Pts',(6.05979097677885,28.6371182741293,126.539361986267));
#94464=CARTESIAN_POINT('Ctrl Pts',(6.06364611115773,28.585402293254,126.490272086087));
#94465=CARTESIAN_POINT('Ctrl Pts',(6.06753106194879,28.533286330212,126.440802514394));
#94466=CARTESIAN_POINT('Ctrl Pts',(6.07141601273984,28.4837849922821,126.38861163239));
#94467=CARTESIAN_POINT('Ctrl Pts',(6.0753009635309,28.4371816356836,126.334015113353));
#94468=CARTESIAN_POINT('Ctrl Pts',(6.07916147856999,28.3908714071385,126.279761998151));
#94469=CARTESIAN_POINT('Ctrl Pts',(6.08302199360908,28.3474230615833,126.223133846222));
#94470=CARTESIAN_POINT('Ctrl Pts',(6.08688250864816,28.307072697256,126.16447185888));
#94471=CARTESIAN_POINT('Ctrl Pts',(6.09077967731521,28.2663392267299,126.105252905787));
#94472=CARTESIAN_POINT('Ctrl Pts',(6.09467684598224,28.2287631453916,126.043961720597));
#94473=CARTESIAN_POINT('Ctrl Pts',(6.09857401464929,28.1945401890826,125.980975246202));
#94474=CARTESIAN_POINT('Ctrl Pts',(6.10247118331633,28.1603172327736,125.917988771808));
#94475=CARTESIAN_POINT('Ctrl Pts',(6.10636835198337,28.129447559376,125.853307489303));
#94476=CARTESIAN_POINT('Ctrl Pts',(6.11026552065042,28.1020766226353,125.787327388164));
#94477=CARTESIAN_POINT('Ctrl Pts',(6.11413459399863,28.0749030074016,125.721822948238));
#94478=CARTESIAN_POINT('Ctrl Pts',(6.11800366734684,28.0510713524173,125.654781756097));
#94479=CARTESIAN_POINT('Ctrl Pts',(6.12187274069505,28.0307555752007,125.58657817714));
#94480=CARTESIAN_POINT('Ctrl Pts',(6.12573604909084,28.010470068666,125.518476222099));
#94481=CARTESIAN_POINT('Ctrl Pts',(6.12959935748662,27.9936901788,125.449215779923));
#94482=CARTESIAN_POINT('Ctrl Pts',(6.13346266588241,27.9805417175088,125.379190991161));
#94483=CARTESIAN_POINT('Ctrl Pts',(6.13732144237532,27.9674086801868,125.309248345865));
#94484=CARTESIAN_POINT('Ctrl Pts',(6.14118021886823,27.9578986990641,125.238543610111));
#94485=CARTESIAN_POINT('Ctrl Pts',(6.14503899536114,27.9520872552484,125.167484185474));
#94486=CARTESIAN_POINT('Ctrl Pts',(6.14889534094935,27.9462794724548,125.096469525983));
#94487=CARTESIAN_POINT('Ctrl Pts',(6.15275168653755,27.9441656438702,125.02510110394));
#94488=CARTESIAN_POINT('Ctrl Pts',(6.15660803212576,27.9457696122914,124.953793109662));
#94489=CARTESIAN_POINT('Ctrl Pts',(6.16046323837109,27.9473731068262,124.882506183064));
#94490=CARTESIAN_POINT('Ctrl Pts',(6.16431844461642,27.9526922068022,124.811280134185));
#94491=CARTESIAN_POINT('Ctrl Pts',(6.16817365086174,27.9616986453253,124.740529095983));
#94492=CARTESIAN_POINT('Ctrl Pts',(6.172029007713,27.9707054356902,124.66977529385));
#94493=CARTESIAN_POINT('Ctrl Pts',(6.17588436456425,27.9833997870615,124.599497020854));
#94494=CARTESIAN_POINT('Ctrl Pts',(6.1797397214155,27.9997017805379,124.530101504879));
#94495=CARTESIAN_POINT('Ctrl Pts',(6.18359911388406,28.0160208382212,124.460633348743));
#94496=CARTESIAN_POINT('Ctrl Pts',(6.18745850635261,28.0359549650724,124.392050268083));
#94497=CARTESIAN_POINT('Ctrl Pts',(6.19131789882117,28.0593736888523,124.324746652744));
#94498=CARTESIAN_POINT('Ctrl Pts',(6.19517947642461,28.082805671991,124.257404931023));
#94499=CARTESIAN_POINT('Ctrl Pts',(6.19904105402804,28.1097259961427,124.191344566791));
#94500=CARTESIAN_POINT('Ctrl Pts',(6.20290263163148,28.1399561398452,124.126939635076));
#94501=CARTESIAN_POINT('Ctrl Pts',(6.20677096574635,28.1702391765186,124.062422015569));
#94502=CARTESIAN_POINT('Ctrl Pts',(6.21063929986123,28.2038433657611,123.99956604001));
#94503=CARTESIAN_POINT('Ctrl Pts',(6.2145076339761,28.240544729224,123.938720247702));
#94504=CARTESIAN_POINT('Ctrl Pts',(6.21680535314706,28.2623446627161,123.902578968456));
#94505=CARTESIAN_POINT('Ctrl Pts',(6.21910307231802,28.2852364919428,123.867146354676));
#94506=CARTESIAN_POINT('Ctrl Pts',(6.22140079148898,28.3091664896413,123.832489998866));
#94507=CARTESIAN_POINT('Ctrl Pts',(6.22526986483719,28.3494616299212,123.774133005415));
#94508=CARTESIAN_POINT('Ctrl Pts',(6.2291389381854,28.3928604218902,123.717750259131));
#94509=CARTESIAN_POINT('Ctrl Pts',(6.23300801153361,28.4391426714857,123.663690918042));
#94510=CARTESIAN_POINT('Ctrl Pts',(6.23687131992939,28.4853559601328,123.609712125835));
#94511=CARTESIAN_POINT('Ctrl Pts',(6.24073462832517,28.5344438648622,123.558050233075));
#94512=CARTESIAN_POINT('Ctrl Pts',(6.24459793672094,28.5861434868903,123.509024707503));
#94513=CARTESIAN_POINT('Ctrl Pts',(6.24845671321385,28.6377824620217,123.460056691945));
#94514=CARTESIAN_POINT('Ctrl Pts',(6.25231548970676,28.6920267181045,123.41371923322));
#94515=CARTESIAN_POINT('Ctrl Pts',(6.25617426619967,28.748574917571,123.370296706278));
#94516=CARTESIAN_POINT('Ctrl Pts',(6.26003061178788,28.8050874934961,123.326901534128));
#94517=CARTESIAN_POINT('Ctrl Pts',(6.26388695737608,28.8639007488459,123.286417945709));
#94518=CARTESIAN_POINT('Ctrl Pts',(6.26774330296429,28.9246796357716,123.249090614345));
#94519=CARTESIAN_POINT('Ctrl Pts',(6.27159850920962,28.9854405658025,123.211774311201));
#94520=CARTESIAN_POINT('Ctrl Pts',(6.27545371545495,29.0481655607565,123.177612667924));
#94521=CARTESIAN_POINT('Ctrl Pts',(6.27930892170027,29.1124913585492,123.146806547106));
#94522=CARTESIAN_POINT('Ctrl Pts',(6.28316427855152,29.1768196692674,123.115999222828));
#94523=CARTESIAN_POINT('Ctrl Pts',(6.28701963540277,29.2427484678968,123.088547889102));
#94524=CARTESIAN_POINT('Ctrl Pts',(6.29087499225402,29.3098922794118,123.064606268357));
#94525=CARTESIAN_POINT('Ctrl Pts',(6.29473438472258,29.3771063741038,123.04063958658));
#94526=CARTESIAN_POINT('Ctrl Pts',(6.29859377719114,29.4455375620182,123.020190115029));
#94527=CARTESIAN_POINT('Ctrl Pts',(6.30245316965969,29.5147837356122,123.00336214118));
#94528=CARTESIAN_POINT('Ctrl Pts',(6.30631474726314,29.5840691154363,122.986524639564));
#94529=CARTESIAN_POINT('Ctrl Pts',(6.31017632486658,29.6541699219043,122.973312807461));
#94530=CARTESIAN_POINT('Ctrl Pts',(6.31403790247002,29.7246750546594,122.963779546077));
#94531=CARTESIAN_POINT('Ctrl Pts',(6.31790623658489,29.7953035485856,122.954229604571));
#94532=CARTESIAN_POINT('Ctrl Pts',(6.32177457069976,29.8663372969278,122.948371124002));
#94533=CARTESIAN_POINT('Ctrl Pts',(6.32564290481463,29.9373619988242,122.946204965604));
#94534=CARTESIAN_POINT('Ctrl Pts',(6.3279406239856,29.9795493627679,122.944918307438));
#94535=CARTESIAN_POINT('Ctrl Pts',(6.33023834315657,30.0217335510174,122.944933353137));
#94536=CARTESIAN_POINT('Ctrl Pts',(6.33253606232754,30.0638286364277,122.946241623834));
#94537=CARTESIAN_POINT('Ctrl Pts',(6.33640513567576,30.1347115254724,122.948444588996));
#94538=CARTESIAN_POINT('Ctrl Pts',(6.34027420902399,30.2056190726874,122.954325827891));
#94539=CARTESIAN_POINT('Ctrl Pts',(6.34414328237221,30.2761385098518,122.963889716671));
#94540=CARTESIAN_POINT('Ctrl Pts',(6.348006590768,30.3465528724506,122.973439355175));
#94541=CARTESIAN_POINT('Ctrl Pts',(6.35186989916379,30.4165797954258,122.986660686914));
#94542=CARTESIAN_POINT('Ctrl Pts',(6.35573320755958,30.4858082931544,123.003506106996));
#94543=CARTESIAN_POINT('Ctrl Pts',(6.3595919840525,30.5549555815166,123.020331766345));
#94544=CARTESIAN_POINT('Ctrl Pts',(6.36345076054542,30.6233058353202,123.040772955254));
#94545=CARTESIAN_POINT('Ctrl Pts',(6.36730953703834,30.6904567041093,123.064730741667));
#94546=CARTESIAN_POINT('Ctrl Pts',(6.37116588262656,30.7575652700174,123.088673435447));
#94547=CARTESIAN_POINT('Ctrl Pts',(6.37502222821477,30.8234754935007,123.116128168673));
#94548=CARTESIAN_POINT('Ctrl Pts',(6.37887857380298,30.887800095922,123.146946155078));
#94549=CARTESIAN_POINT('Ctrl Pts',(6.38273378004833,30.9521056938803,123.177755036424));
#94550=CARTESIAN_POINT('Ctrl Pts',(6.38658898629367,31.0148261629487,123.211924988476));
#94551=CARTESIAN_POINT('Ctrl Pts',(6.39044419253901,31.0755957294053,123.249259759592));
#94552=CARTESIAN_POINT('Ctrl Pts',(6.39429954939027,31.1363676698609,123.286595989212));
#94553=CARTESIAN_POINT('Ctrl Pts',(6.39815490624154,31.1951881436347,123.327097027188));
#94554=CARTESIAN_POINT('Ctrl Pts',(6.4020102630928,31.2517189340083,123.370522392684));
#94555=CARTESIAN_POINT('Ctrl Pts',(6.40586965556137,31.308308898317,123.413993213935));
#94556=CARTESIAN_POINT('Ctrl Pts',(6.40972904802994,31.3626040087628,123.460394176724));
#94557=CARTESIAN_POINT('Ctrl Pts',(6.41358844049851,31.4142985602054,123.509444014771));
#94558=CARTESIAN_POINT('Ctrl Pts',(6.41745001810195,31.4660223803912,123.558521624161));
#94559=CARTESIAN_POINT('Ctrl Pts',(6.42131159570539,31.515142375816,123.610250741924));
#94560=CARTESIAN_POINT('Ctrl Pts',(6.42517317330884,31.5613911358037,123.664314676455));
#94561=CARTESIAN_POINT('Ctrl Pts',(6.42904150742372,31.6077208161582,123.71847320538));
#94562=CARTESIAN_POINT('Ctrl Pts',(6.4329098415386,31.651168934825,123.774974322028));
#94563=CARTESIAN_POINT('Ctrl Pts',(6.43677817565348,31.6915100663368,123.8334704213));
#94564=CARTESIAN_POINT('Ctrl Pts',(6.43907589482435,31.715471954968,123.868216026185));
#94565=CARTESIAN_POINT('Ctrl Pts',(6.44137361399522,31.7383385030997,123.903664960457));
#94566=CARTESIAN_POINT('Ctrl Pts',(6.44367133316609,31.7600702303999,123.939740434346));
#94567=CARTESIAN_POINT('Ctrl Pts',(6.447668184011,31.7978722706675,124.002493224209));
#94568=CARTESIAN_POINT('Ctrl Pts',(6.4516650348559,31.8323780045921,124.067375195747));
#94569=CARTESIAN_POINT('Ctrl Pts',(6.4556618857008,31.8633501421989,124.134018585611));
#94570=CARTESIAN_POINT('Ctrl Pts',(6.45969628851426,31.8946132750874,124.201288116048));
#94571=CARTESIAN_POINT('Ctrl Pts',(6.46373069132772,31.922275754658,124.27035199445));
#94572=CARTESIAN_POINT('Ctrl Pts',(6.46776509414118,31.9461388143962,124.340802550369));
#94573=CARTESIAN_POINT('Ctrl Pts',(6.47174648700002,31.9696883259411,124.410327422625));
#94574=CARTESIAN_POINT('Ctrl Pts',(6.47572787985886,31.989537493609,124.481202326664));
#94575=CARTESIAN_POINT('Ctrl Pts',(6.4797092727177,32.005542326812,124.553012821363));
#94576=CARTESIAN_POINT('Ctrl Pts',(6.48377018050848,32.0218668027299,124.626257489177));
#94577=CARTESIAN_POINT('Ctrl Pts',(6.48783108829924,32.0341915119557,124.700475103802));
#94578=CARTESIAN_POINT('Ctrl Pts',(6.49189199609001,32.0424167700166,124.775208318537));
#94579=CARTESIAN_POINT('Ctrl Pts',(6.49595290388078,32.0506420280775,124.849941533272));
#94580=CARTESIAN_POINT('Ctrl Pts',(6.50001381167156,32.0547677239393,124.9251898674));
#94581=CARTESIAN_POINT('Ctrl Pts',(6.50407471946233,32.0547499427051,125.000485235558));
#94582=CARTESIAN_POINT('Ctrl Pts',(6.50407471951103,32.0547499427048,125.000485236461));
#94583=CARTESIAN_POINT('Ctrl Pts',(6.50830237655217,32.054731431302,125.078872387748));
#94584=CARTESIAN_POINT('Ctrl Pts',(6.5125300335933,32.050222603001,125.157140435482));
#94585=CARTESIAN_POINT('Ctrl Pts',(6.51675769063444,32.0412922455004,125.234784009166));
#94586=CARTESIAN_POINT('Ctrl Pts',(6.52089243721851,32.0325581488575,125.310721224021));
#94587=CARTESIAN_POINT('Ctrl Pts',(6.52502718380259,32.0195950692566,125.38606079366));
#94588=CARTESIAN_POINT('Ctrl Pts',(6.52916193038667,32.0025186272063,125.460344121491));
#94589=CARTESIAN_POINT('Ctrl Pts',(6.53343604265633,31.9848666069422,125.537131241684));
#94590=CARTESIAN_POINT('Ctrl Pts',(6.537710154926,31.9628191668451,125.612789222109));
#94591=CARTESIAN_POINT('Ctrl Pts',(6.54198426719566,31.936558210849,125.686833210098));
#94592=CARTESIAN_POINT('Ctrl Pts',(6.54625837946533,31.9102972548528,125.760877198087));
#94593=CARTESIAN_POINT('Ctrl Pts',(6.55053249173499,31.8798230313505,125.833306828918));
#94594=CARTESIAN_POINT('Ctrl Pts',(6.55480660400465,31.8453691251967,125.903664956868));
#94595=CARTESIAN_POINT('Ctrl Pts',(6.55867567735285,31.8141802650006,125.967355552833));
#94596=CARTESIAN_POINT('Ctrl Pts',(6.56254475070105,31.7796291418859,126.029554339915));
#94597=CARTESIAN_POINT('Ctrl Pts',(6.56641382404924,31.7418816971559,126.089883349544));
#94598=CARTESIAN_POINT('Ctrl Pts',(6.570277132445,31.704190496442,126.150122468432));
#94599=CARTESIAN_POINT('Ctrl Pts',(6.57414044084076,31.6633126832059,126.208496931507));
#94600=CARTESIAN_POINT('Ctrl Pts',(6.57800374923652,31.6194608366348,126.264651794411));
#94601=CARTESIAN_POINT('Ctrl Pts',(6.58186252572942,31.5756604310279,126.320740784141));
#94602=CARTESIAN_POINT('Ctrl Pts',(6.58572130222231,31.5288932194177,126.374614964573));
#94603=CARTESIAN_POINT('Ctrl Pts',(6.5895800787152,31.4794150018976,126.425948391303));
#94604=CARTESIAN_POINT('Ctrl Pts',(6.59343642430339,31.4299679540584,126.477249479631));
#94605=CARTESIAN_POINT('Ctrl Pts',(6.59729276989158,31.3778136249756,126.52601264087));
#94606=CARTESIAN_POINT('Ctrl Pts',(6.60114911547976,31.323247043448,126.57194619008));
#94607=CARTESIAN_POINT('Ctrl Pts',(6.60500432172508,31.2686965834128,126.617866168394));
#94608=CARTESIAN_POINT('Ctrl Pts',(6.60885952797039,31.2117356572602,126.660957881695));
#94609=CARTESIAN_POINT('Ctrl Pts',(6.61271473421571,31.1526936970903,126.70096878372));
#94610=CARTESIAN_POINT('Ctrl Pts',(6.61657009106693,31.0936494304113,126.740981248793));
#94611=CARTESIAN_POINT('Ctrl Pts',(6.62042544791816,31.0325243716912,126.777912392946));
#94612=CARTESIAN_POINT('Ctrl Pts',(6.62428080476939,30.96967691557,126.811552991748));
#94613=CARTESIAN_POINT('Ctrl Pts',(6.62814019723793,30.9067636735069,126.845228804043));
#94614=CARTESIAN_POINT('Ctrl Pts',(6.63199958970647,30.842124864157,126.875606965473));
#94615=CARTESIAN_POINT('Ctrl Pts',(6.63585898217501,30.7761426666099,126.902524670949));
#94616=CARTESIAN_POINT('Ctrl Pts',(6.63972055977842,30.710123110851,126.929457616859));
#94617=CARTESIAN_POINT('Ctrl Pts',(6.64358213738184,30.6427591117206,126.952926046633));
#94618=CARTESIAN_POINT('Ctrl Pts',(6.64744371498526,30.5744493672173,126.972816637958));
#94619=CARTESIAN_POINT('Ctrl Pts',(6.65131204910011,30.506020102762,126.992742031382));
#94620=CARTESIAN_POINT('Ctrl Pts',(6.65518038321497,30.4366422621867,127.009076976597));
#94621=CARTESIAN_POINT('Ctrl Pts',(6.65904871732982,30.3667254312339,127.021759140102));
#94622=CARTESIAN_POINT('Ctrl Pts',(6.66134643650095,30.3251961222096,127.029292111493));
#94623=CARTESIAN_POINT('Ctrl Pts',(6.66364415567209,30.2834767822568,127.035537320761));
#94624=CARTESIAN_POINT('Ctrl Pts',(6.66594187484322,30.241653645354,127.040490401395));
#94625=CARTESIAN_POINT('Ctrl Pts',(6.66980984684837,30.1712487304541,127.048828399126));
#94626=CARTESIAN_POINT('Ctrl Pts',(6.67367781885353,30.1002739036248,127.053534580682));
#94627=CARTESIAN_POINT('Ctrl Pts',(6.67754579085868,30.0291363638787,127.054543412732));
#94628=CARTESIAN_POINT('Ctrl Pts',(6.68140849508152,29.958095706187,127.055550870856));
#94629=CARTESIAN_POINT('Ctrl Pts',(6.68527119930435,29.8868932563362,127.052870960964));
#94630=CARTESIAN_POINT('Ctrl Pts',(6.68913390352719,29.8159423184307,127.046489758673));
#94631=CARTESIAN_POINT('Ctrl Pts',(6.69299263972165,29.7450642660785,127.040115111581));
#94632=CARTESIAN_POINT('Ctrl Pts',(6.69685137591611,29.6744376942221,127.030046760409));
#94633=CARTESIAN_POINT('Ctrl Pts',(6.70071011211057,29.6044751682032,127.01632280896));
#94634=CARTESIAN_POINT('Ctrl Pts',(6.70456617537579,29.534561104912,127.00260836403));
#94635=CARTESIAN_POINT('Ctrl Pts',(6.70842223864102,29.4653106496237,126.985243439874));
#94636=CARTESIAN_POINT('Ctrl Pts',(6.71227830190625,29.3971287887083,126.964317658907));
#94637=CARTESIAN_POINT('Ctrl Pts',(6.71613400852199,29.3289532339721,126.943393813379));
#94638=CARTESIAN_POINT('Ctrl Pts',(6.71998971513772,29.261846545289,126.918909895312));
#94639=CARTESIAN_POINT('Ctrl Pts',(6.72384542175346,29.1961997300817,126.891005734676));
#94640=CARTESIAN_POINT('Ctrl Pts',(6.72770090156705,29.1305567763815,126.863103215432));
#94641=CARTESIAN_POINT('Ctrl Pts',(6.73155638138065,29.0663739695936,126.831781050833));
#94642=CARTESIAN_POINT('Ctrl Pts',(6.73541186119425,29.004021513207,126.797226868357));
#94643=CARTESIAN_POINT('Ctrl Pts',(6.73927005804661,28.9416251157159,126.762648334813));
#94644=CARTESIAN_POINT('Ctrl Pts',(6.74312825489898,28.8810620638715,126.724833480967));
#94645=CARTESIAN_POINT('Ctrl Pts',(6.74698645175134,28.8226761136759,126.684014854207));
#94646=CARTESIAN_POINT('Ctrl Pts',(6.74865985643731,28.7973525424869,126.666310707968));
#94647=CARTESIAN_POINT('Ctrl Pts',(6.75033326112327,28.7724381426773,126.648042037699));
#94648=CARTESIAN_POINT('Ctrl Pts',(6.75200666580924,28.7479590808042,126.629230216746));
#94649=CARTESIAN_POINT('',(6.44592528053627,32.0547499999799,124.999990915418));
#94650=CARTESIAN_POINT('Ctrl Pts',(6.44592528053768,32.0547499999799,124.999990915444));
#94651=CARTESIAN_POINT('Ctrl Pts',(6.44979385259826,32.0547503134814,125.070898847444));
#94652=CARTESIAN_POINT('Ctrl Pts',(6.45366242465885,32.0510758456684,125.141945865384));
#94653=CARTESIAN_POINT('Ctrl Pts',(6.45753099671943,32.0437093535415,125.212719629435));
#94654=CARTESIAN_POINT('Ctrl Pts',(6.4613938042328,32.0363538382016,125.28338793372));
#94655=CARTESIAN_POINT('Ctrl Pts',(6.46525661174617,32.0253172686326,125.353783312964));
#94656=CARTESIAN_POINT('Ctrl Pts',(6.46911941925955,32.0106344132236,125.423493587745));
#94657=CARTESIAN_POINT('Ctrl Pts',(6.47297769671014,31.9959687769632,125.493122110609));
#94658=CARTESIAN_POINT('Ctrl Pts',(6.47683597416074,31.9776654483258,125.562066651731));
#94659=CARTESIAN_POINT('Ctrl Pts',(6.48069425161134,31.95581076705,125.629922063426));
#94660=CARTESIAN_POINT('Ctrl Pts',(6.48455010010933,31.9339698442417,125.697734757204));
#94661=CARTESIAN_POINT('Ctrl Pts',(6.48840594860733,31.9085821530335,125.764459220432));
#94662=CARTESIAN_POINT('Ctrl Pts',(6.49226179710532,31.8797843322491,125.829703818679));
#94663=CARTESIAN_POINT('Ctrl Pts',(6.49611650897049,31.8509950005295,125.894929184025));
#94664=CARTESIAN_POINT('Ctrl Pts',(6.49997122083567,31.8187977310236,125.958675106127));
#94665=CARTESIAN_POINT('Ctrl Pts',(6.50382593270084,31.7833772733353,126.020569969895));
#94666=CARTESIAN_POINT('Ctrl Pts',(6.5076807986421,31.7479553998615,126.082467307653));
#94667=CARTESIAN_POINT('Ctrl Pts',(6.51153566458336,31.7093103257038,126.142513019533));
#94668=CARTESIAN_POINT('Ctrl Pts',(6.51539053052462,31.6676718636714,126.200361661175));
#94669=CARTESIAN_POINT('Ctrl Pts',(6.51924943297198,31.6259898011847,126.25827087727));
#94670=CARTESIAN_POINT('Ctrl Pts',(6.52310833541935,31.5813083783217,126.313978035487));
#94671=CARTESIAN_POINT('Ctrl Pts',(6.52696723786672,31.5338991807731,126.367168923624));
#94672=CARTESIAN_POINT('Ctrl Pts',(6.53082833001037,31.486463081341,126.420389994408));
#94673=CARTESIAN_POINT('Ctrl Pts',(6.53468942215402,31.436296467927,126.471091607219));
#94674=CARTESIAN_POINT('Ctrl Pts',(6.53855051429767,31.3837075199641,126.518996728665));
#94675=CARTESIAN_POINT('Ctrl Pts',(6.54241835505554,31.3310266543496,126.566985581131));
#94676=CARTESIAN_POINT('Ctrl Pts',(6.54628619581342,31.2759153771664,126.612167875522));
#94677=CARTESIAN_POINT('Ctrl Pts',(6.55015403657129,31.2187140609584,126.654307589332));
#94678=CARTESIAN_POINT('Ctrl Pts',(6.55242968420586,31.1850596144411,126.679100528353));
#94679=CARTESIAN_POINT('Ctrl Pts',(6.55470533184043,31.1506822350121,126.702841082442));
#94680=CARTESIAN_POINT('Ctrl Pts',(6.556980979475,31.1156552945761,126.72548857608));
#94681=CARTESIAN_POINT('Ctrl Pts',(6.56085005282323,31.0561022250886,126.763994016338));
#94682=CARTESIAN_POINT('Ctrl Pts',(6.56471912617146,30.9944367163052,126.799488160214));
#94683=CARTESIAN_POINT('Ctrl Pts',(6.56858819951969,30.9309957744205,126.831732630738));
#94684=CARTESIAN_POINT('Ctrl Pts',(6.57245150791549,30.8676493600825,126.863929056725));
#94685=CARTESIAN_POINT('Ctrl Pts',(6.5763148163113,30.8025331932406,126.892885202362));
#94686=CARTESIAN_POINT('Ctrl Pts',(6.58017812470711,30.7360123801297,126.918406458182));
#94687=CARTESIAN_POINT('Ctrl Pts',(6.58403690120003,30.6695696001018,126.94389777597));
#94688=CARTESIAN_POINT('Ctrl Pts',(6.58789567769296,30.6017258981203,126.96596203441));
#94689=CARTESIAN_POINT('Ctrl Pts',(6.59175445418588,30.5328684724145,126.984451751393));
#94690=CARTESIAN_POINT('Ctrl Pts',(6.5956107997741,30.4640544246657,127.002929820451));
#94691=CARTESIAN_POINT('Ctrl Pts',(6.59946714536232,30.3942283882477,127.017837689994));
#94692=CARTESIAN_POINT('Ctrl Pts',(6.60332349095054,30.3237935215411,127.029077454881));
#94693=CARTESIAN_POINT('Ctrl Pts',(6.60717869719588,30.2533794645522,127.040313899022));
#94694=CARTESIAN_POINT('Ctrl Pts',(6.61103390344123,30.1823574138346,127.047884313496));
#94695=CARTESIAN_POINT('Ctrl Pts',(6.61488910968657,30.1111398380587,127.051742064417));
#94696=CARTESIAN_POINT('Ctrl Pts',(6.61874446653784,30.0399194801259,127.055599966043));
#94697=CARTESIAN_POINT('Ctrl Pts',(6.6225998233891,29.9685040671639,127.055744892087));
#94698=CARTESIAN_POINT('Ctrl Pts',(6.62645518024037,29.8973085596836,127.052182260567));
#94699=CARTESIAN_POINT('Ctrl Pts',(6.63031457270894,29.82603852789,127.048615899841));
#94700=CARTESIAN_POINT('Ctrl Pts',(6.63417396517751,29.754989347257,127.041334258715));
#94701=CARTESIAN_POINT('Ctrl Pts',(6.63803335764608,29.6845724363159,127.030394792785));
#94702=CARTESIAN_POINT('Ctrl Pts',(6.64189493524953,29.6141156562895,127.01944913308));
#94703=CARTESIAN_POINT('Ctrl Pts',(6.64575651285299,29.5442923343048,127.004841625352));
#94704=CARTESIAN_POINT('Ctrl Pts',(6.64961809045644,29.475502541807,126.986680643397));
#94705=CARTESIAN_POINT('Ctrl Pts',(6.65348642457132,29.4065923894286,126.9684878856));
#94706=CARTESIAN_POINT('Ctrl Pts',(6.6573547586862,29.3387198396882,126.946729388641));
#94707=CARTESIAN_POINT('Ctrl Pts',(6.66122309280108,29.2722680150932,126.921562832864));
#94708=CARTESIAN_POINT('Ctrl Pts',(6.66352081197191,29.2327968559911,126.906614362552));
#94709=CARTESIAN_POINT('Ctrl Pts',(6.66581853114274,29.1938265516438,126.890464398356));
#94710=CARTESIAN_POINT('Ctrl Pts',(6.66811625031357,29.1554332511046,126.8731536427));
#94711=CARTESIAN_POINT('Ctrl Pts',(6.67198550524007,29.0907806733909,126.844003114883));
#94712=CARTESIAN_POINT('Ctrl Pts',(6.67585476016658,29.0275124357899,126.811444295521));
#94713=CARTESIAN_POINT('Ctrl Pts',(6.67972401509308,28.9660116427636,126.775631053907));
#94714=CARTESIAN_POINT('Ctrl Pts',(6.68358710221244,28.9046088854154,126.739874900589));
#94715=CARTESIAN_POINT('Ctrl Pts',(6.6874501893318,28.8449683939462,126.700874869843));
#94716=CARTESIAN_POINT('Ctrl Pts',(6.69131327645116,28.787451626233,126.658832120431));
#94717=CARTESIAN_POINT('Ctrl Pts',(6.69220513385481,28.7741729313617,126.649125858011));
#94718=CARTESIAN_POINT('Ctrl Pts',(6.69309699125846,28.7610073299989,126.639257616034));
#94719=CARTESIAN_POINT('Ctrl Pts',(6.69398884866211,28.7479590808042,126.629230216746));
#94720=CARTESIAN_POINT('Ctrl Pts',(5.99388605120356,28.7479590808042,126.629230216746));
#94721=CARTESIAN_POINT('Ctrl Pts',(5.99635890922978,28.711936345746,126.601547242388));
#94722=CARTESIAN_POINT('Ctrl Pts',(5.998831767256,28.6768711114662,126.572698926717));
#94723=CARTESIAN_POINT('Ctrl Pts',(6.00130462528222,28.6428394576485,126.542761428343));
#94724=CARTESIAN_POINT('Ctrl Pts',(6.00517369863043,28.589592986001,126.495920738));
#94725=CARTESIAN_POINT('Ctrl Pts',(6.00904277197863,28.5386700366482,126.446228460409));
#94726=CARTESIAN_POINT('Ctrl Pts',(6.01291184532684,28.4903916335173,126.393944095847));
#94727=CARTESIAN_POINT('Ctrl Pts',(6.01677515372263,28.4421851656207,126.341737635435));
#94728=CARTESIAN_POINT('Ctrl Pts',(6.02063846211841,28.3966157492422,126.286947108469));
#94729=CARTESIAN_POINT('Ctrl Pts',(6.02450177051419,28.3539699294822,126.229870956422));
#94730=CARTESIAN_POINT('Ctrl Pts',(6.0283605470071,28.3113741359415,126.172861758279));
#94731=CARTESIAN_POINT('Ctrl Pts',(6.03221932350001,28.2716954161049,126.113572648055));
#94732=CARTESIAN_POINT('Ctrl Pts',(6.03607809999291,28.2351809694626,126.052336140191));
#94733=CARTESIAN_POINT('Ctrl Pts',(6.03993444558111,28.1986895257437,125.991138209352));
#94734=CARTESIAN_POINT('Ctrl Pts',(6.04379079116931,28.1653586485718,125.927995731075));
#94735=CARTESIAN_POINT('Ctrl Pts',(6.04764713675752,28.1353921673442,125.863270057919));
#94736=CARTESIAN_POINT('Ctrl Pts',(6.05150234300284,28.1054345396013,125.798563507721));
#94737=CARTESIAN_POINT('Ctrl Pts',(6.05535754924817,28.0788395384251,125.732275131848));
#94738=CARTESIAN_POINT('Ctrl Pts',(6.0592127554935,28.0557641846639,125.664789182271));
#94739=CARTESIAN_POINT('Ctrl Pts',(6.06306811234474,28.0326879294503,125.597300596315));
#94740=CARTESIAN_POINT('Ctrl Pts',(6.06692346919598,28.0131317497201,125.528614804142));
#94741=CARTESIAN_POINT('Ctrl Pts',(6.07077882604722,27.9972032527053,125.459132607779));
#94742=CARTESIAN_POINT('Ctrl Pts',(6.07463821851578,27.9812580824431,125.38957768052));
#94743=CARTESIAN_POINT('Ctrl Pts',(6.07849761098433,27.9689482839275,125.31922515941));
#94744=CARTESIAN_POINT('Ctrl Pts',(6.08235700345289,27.9603304240579,125.24848658611));
#94745=CARTESIAN_POINT('Ctrl Pts',(6.08621858105632,27.9517076848748,125.177707961603));
#94746=CARTESIAN_POINT('Ctrl Pts',(6.09008015865975,27.9467810790954,125.106543334643));
#94747=CARTESIAN_POINT('Ctrl Pts',(6.09394173626318,27.9455550884156,125.035407171095));
#94748=CARTESIAN_POINT('Ctrl Pts',(6.09781007037804,27.9443269526488,124.964146542277));
#94749=CARTESIAN_POINT('Ctrl Pts',(6.10167840449291,27.9468123423206,124.892914961947));
#94750=CARTESIAN_POINT('Ctrl Pts',(6.10554673860778,27.9529636818119,124.822123991166));
#94751=CARTESIAN_POINT('Ctrl Pts',(6.10784445777877,27.9566174641007,124.780075459196));
#94752=CARTESIAN_POINT('Ctrl Pts',(6.11014217694977,27.9615636544421,124.738182247744));
#94753=CARTESIAN_POINT('Ctrl Pts',(6.11243989612077,27.9677837873881,124.696528703668));
#94754=CARTESIAN_POINT('Ctrl Pts',(6.11630896946898,27.9782577177568,124.626389315323));
#94755=CARTESIAN_POINT('Ctrl Pts',(6.1201780428172,27.9923875858268,124.556655420757));
#94756=CARTESIAN_POINT('Ctrl Pts',(6.12404711616542,28.010129485962,124.487737469785));
#94757=CARTESIAN_POINT('Ctrl Pts',(6.12791042456121,28.027844950514,124.418922207151));
#94758=CARTESIAN_POINT('Ctrl Pts',(6.13177373295699,28.0491616439716,124.350920941469));
#94759=CARTESIAN_POINT('Ctrl Pts',(6.13563704135278,28.0739842444241,124.284136275697));
#94760=CARTESIAN_POINT('Ctrl Pts',(6.1394958178457,28.0987777264106,124.217429952523));
#94761=CARTESIAN_POINT('Ctrl Pts',(6.14335459433861,28.1270687778571,124.151937847601));
#94762=CARTESIAN_POINT('Ctrl Pts',(6.14721337083153,28.1587121110232,124.088047987881));
#94763=CARTESIAN_POINT('Ctrl Pts',(6.15106971641973,28.1903355099103,124.024198376712));
#94764=CARTESIAN_POINT('Ctrl Pts',(6.15492606200794,28.225306785587,123.961949442474));
#94765=CARTESIAN_POINT('Ctrl Pts',(6.15878240759615,28.2634328997717,123.901668415776));
#94766=CARTESIAN_POINT('Ctrl Pts',(6.16263761384149,28.3015477497386,123.841405198881));
#94767=CARTESIAN_POINT('Ctrl Pts',(6.16649282008682,28.3428153282392,123.7831091456));
#94768=CARTESIAN_POINT('Ctrl Pts',(6.17034802633216,28.3869979709246,123.727120580456));
#94769=CARTESIAN_POINT('Ctrl Pts',(6.17420338318341,28.4311823396311,123.671129828086));
#94770=CARTESIAN_POINT('Ctrl Pts',(6.17805874003466,28.4782816959494,123.617447122803));
#94771=CARTESIAN_POINT('Ctrl Pts',(6.18191409688591,28.5280176709366,123.566380250755));
#94772=CARTESIAN_POINT('Ctrl Pts',(6.18577348935447,28.5778057073463,123.515259924161));
#94773=CARTESIAN_POINT('Ctrl Pts',(6.18963288182303,28.6302355321652,123.466761245462));
#94774=CARTESIAN_POINT('Ctrl Pts',(6.19349227429159,28.6849920711719,123.421154944392));
#94775=CARTESIAN_POINT('Ctrl Pts',(6.19735385189503,28.7397796125771,123.375522821662));
#94776=CARTESIAN_POINT('Ctrl Pts',(6.20121542949847,28.7968961014709,123.332786627734));
#94777=CARTESIAN_POINT('Ctrl Pts',(6.20507700710191,28.8559957577356,123.293174919278));
#94778=CARTESIAN_POINT('Ctrl Pts',(6.20894534121678,28.9151988192777,123.253493903148));
#94779=CARTESIAN_POINT('Ctrl Pts',(6.21281367533165,28.9763915587476,123.216948536352));
#94780=CARTESIAN_POINT('Ctrl Pts',(6.21668200944653,29.0392024024643,123.183722064476));
#94781=CARTESIAN_POINT('Ctrl Pts',(6.21897972861746,29.0765108860298,123.163986152546));
#94782=CARTESIAN_POINT('Ctrl Pts',(6.2212774477884,29.1143898337748,123.145420289185));
#94783=CARTESIAN_POINT('Ctrl Pts',(6.22357516695933,29.152758367233,123.128054707475));
#94784=CARTESIAN_POINT('Ctrl Pts',(6.22744424030755,29.2173662062113,123.098813227393));
#94785=CARTESIAN_POINT('Ctrl Pts',(6.23131331365577,29.2836162215103,123.072863185084));
#94786=CARTESIAN_POINT('Ctrl Pts',(6.23518238700398,29.3511397635226,123.050390306749));
#94787=CARTESIAN_POINT('Ctrl Pts',(6.23904569539977,29.4185626948789,123.027950913195));
#94788=CARTESIAN_POINT('Ctrl Pts',(6.24290900379556,29.4872549291607,123.008978551621));
#94789=CARTESIAN_POINT('Ctrl Pts',(6.24677231219135,29.5568265229058,122.993611495323));
#94790=CARTESIAN_POINT('Ctrl Pts',(6.25063108868426,29.6263165048113,122.978262465545));
#94791=CARTESIAN_POINT('Ctrl Pts',(6.25448986517718,29.6966833251354,122.966510444591));
#94792=CARTESIAN_POINT('Ctrl Pts',(6.25834864167009,29.7675221866832,122.958443821783));
#94793=CARTESIAN_POINT('Ctrl Pts',(6.2622049872583,29.8383164220336,122.950382280688));
#94794=CARTESIAN_POINT('Ctrl Pts',(6.26606133284651,29.9095816271033,122.946001586392));
#94795=CARTESIAN_POINT('Ctrl Pts',(6.26991767843472,29.9809045784329,122.945338731719));
#94796=CARTESIAN_POINT('Ctrl Pts',(6.27377288468005,30.0522064576634,122.944676072884));
#94797=CARTESIAN_POINT('Ctrl Pts',(6.27762809092539,30.1235655637827,122.947729077512));
#94798=CARTESIAN_POINT('Ctrl Pts',(6.28148329717073,30.1945670747283,122.954482653231));
#94799=CARTESIAN_POINT('Ctrl Pts',(6.28533865402197,30.2655713593899,122.961236492783));
#94800=CARTESIAN_POINT('Ctrl Pts',(6.28919401087323,30.3362175377482,122.971691142247));
#94801=CARTESIAN_POINT('Ctrl Pts',(6.29304936772447,30.4060960479373,122.985779663902));
#94802=CARTESIAN_POINT('Ctrl Pts',(6.29690876019304,30.4760477038653,122.9998829328));
#94803=CARTESIAN_POINT('Ctrl Pts',(6.3007681526616,30.5452296103558,123.017627570876));
#94804=CARTESIAN_POINT('Ctrl Pts',(6.30462754513016,30.6132434306251,123.038895704636));
#94805=CARTESIAN_POINT('Ctrl Pts',(6.3084891227336,30.6812957593831,123.060175880121));
#94806=CARTESIAN_POINT('Ctrl Pts',(6.31235070033704,30.7481782296867,123.084983353613));
#94807=CARTESIAN_POINT('Ctrl Pts',(6.31621227794047,30.8135112824055,123.113151581102));
#94808=CARTESIAN_POINT('Ctrl Pts',(6.32008061205535,30.8789586468287,123.141369093875));
#94809=CARTESIAN_POINT('Ctrl Pts',(6.32394894617022,30.9428507455124,123.172958885326));
#94810=CARTESIAN_POINT('Ctrl Pts',(6.3278172802851,31.0048320976367,123.207708166046));
#94811=CARTESIAN_POINT('Ctrl Pts',(6.33011499945603,31.0416478784838,123.228348598365));
#94812=CARTESIAN_POINT('Ctrl Pts',(6.33241271862696,31.0777900498444,123.250102894812));
#94813=CARTESIAN_POINT('Ctrl Pts',(6.33471043779789,31.1131893460155,123.272919503203));
#94814=CARTESIAN_POINT('Ctrl Pts',(6.33857951114609,31.1727973586454,123.311339834345));
#94815=CARTESIAN_POINT('Ctrl Pts',(6.3424485844943,31.2305307484908,123.352924986983));
#94816=CARTESIAN_POINT('Ctrl Pts',(6.34631765784251,31.2860335365731,123.397465973744));
#94817=CARTESIAN_POINT('Ctrl Pts',(6.35018096623829,31.3414536250258,123.441940594053));
#94818=CARTESIAN_POINT('Ctrl Pts',(6.35404427463407,31.3946493332136,123.489362004667));
#94819=CARTESIAN_POINT('Ctrl Pts',(6.35790758302985,31.4452930003888,123.53947759157));
#94820=CARTESIAN_POINT('Ctrl Pts',(6.36176635952276,31.4958772593683,123.589534389747));
#94821=CARTESIAN_POINT('Ctrl Pts',(6.36562513601567,31.5439150802219,123.642278746475));
#94822=CARTESIAN_POINT('Ctrl Pts',(6.36948391250857,31.589112655769,123.697418513192));
#94823=CARTESIAN_POINT('Ctrl Pts',(6.37334025809677,31.6342817583016,123.752523543634));
#94824=CARTESIAN_POINT('Ctrl Pts',(6.37719660368497,31.6766138581668,123.810020615361));
#94825=CARTESIAN_POINT('Ctrl Pts',(6.38105294927317,31.7158537585188,123.869582624923));
#94826=CARTESIAN_POINT('Ctrl Pts',(6.3849081555185,31.7550820655891,123.929127037111));
#94827=CARTESIAN_POINT('Ctrl Pts',(6.38876336176383,31.7912197197443,123.990734770518));
#94828=CARTESIAN_POINT('Ctrl Pts',(6.39261856800916,31.8240544161559,124.054049129499));
#94829=CARTESIAN_POINT('Ctrl Pts',(6.3964739248604,31.8568903952743,124.117365961892));
#94830=CARTESIAN_POINT('Ctrl Pts',(6.40032928171164,31.8864229387857,124.182389119965));
#94831=CARTESIAN_POINT('Ctrl Pts',(6.40418463856289,31.9124861523391,124.248738208338));
#94832=CARTESIAN_POINT('Ctrl Pts',(6.40804403103144,31.9385766477135,124.315156748007));
#94833=CARTESIAN_POINT('Ctrl Pts',(6.41190342349999,31.9611903857793,124.382903535508));
#94834=CARTESIAN_POINT('Ctrl Pts',(6.41576281596854,31.9802103536273,124.45157998041));
#94835=CARTESIAN_POINT('Ctrl Pts',(6.41962439357197,31.9992410903193,124.520295308969));
#94836=CARTESIAN_POINT('Ctrl Pts',(6.4234859711754,32.0146739011013,124.589940868241));
#94837=CARTESIAN_POINT('Ctrl Pts',(6.42734754877883,32.0264428476096,124.660107446578));
#94838=CARTESIAN_POINT('Ctrl Pts',(6.43121588289369,32.0382323859666,124.730396793725));
#94839=CARTESIAN_POINT('Ctrl Pts',(6.43508421700856,32.0463452058351,124.80120849722));
#94840=CARTESIAN_POINT('Ctrl Pts',(6.43895255112342,32.0507672808363,124.872128492809));
#94841=CARTESIAN_POINT('Ctrl Pts',(6.44125027029443,32.0533939118884,124.914253663137));
#94842=CARTESIAN_POINT('Ctrl Pts',(6.44354798946544,32.0547193955748,124.956417024693));
#94843=CARTESIAN_POINT('Ctrl Pts',(6.44584570863644,32.0547494759025,124.998532424289));
#94844=CARTESIAN_POINT('Ctrl Pts',(6.44587223260258,32.054749823138,124.999018587893));
#94845=CARTESIAN_POINT('Ctrl Pts',(6.44589875656872,32.0547499978305,124.99950475162));
#94846=CARTESIAN_POINT('Ctrl Pts',(6.44592528053486,32.0547499999799,124.999990915392));
#94847=CARTESIAN_POINT('Origin',(-1.54592528053767,30.,125.));
#94848=CARTESIAN_POINT('',(5.29388025228517,28.7479590808042,126.629230216746));
#94849=CARTESIAN_POINT('',(5.35213747706482,28.7479590808042,126.629230216746));
#94850=CARTESIAN_POINT('',(-1.54592528053767,28.7479590808042,126.629230216746));
#94851=CARTESIAN_POINT('',(5.80407471941277,32.0547491412311,124.998121407385));
#94852=CARTESIAN_POINT('Ctrl Pts',(5.35213747706482,28.7479590808042,126.629230216746));
#94853=CARTESIAN_POINT('Ctrl Pts',(5.35599720622694,28.6915568646519,126.585885892641));
#94854=CARTESIAN_POINT('Ctrl Pts',(5.35985693538906,28.6373376428878,126.539555115962));
#94855=CARTESIAN_POINT('Ctrl Pts',(5.36371666455118,28.5856307672311,126.490488925117));
#94856=CARTESIAN_POINT('Ctrl Pts',(5.36757358561901,28.5339615102197,126.441458431723));
#94857=CARTESIAN_POINT('Ctrl Pts',(5.37143050668683,28.4848013246118,126.389696805431));
#94858=CARTESIAN_POINT('Ctrl Pts',(5.37528742775466,28.4384459391161,126.335494843658));
#94859=CARTESIAN_POINT('Ctrl Pts',(5.37914283300616,28.3921087718439,126.281314183907));
#94860=CARTESIAN_POINT('Ctrl Pts',(5.38299823825766,28.3485745323137,126.224695461029));
#94861=CARTESIAN_POINT('Ctrl Pts',(5.38685364350916,28.3081003662311,126.165964489919));
#94862=CARTESIAN_POINT('Ctrl Pts',(5.39070882322953,28.2676285677814,126.107236954418));
#94863=CARTESIAN_POINT('Ctrl Pts',(5.39456400294989,28.2302167617084,126.046397816908));
#94864=CARTESIAN_POINT('Ctrl Pts',(5.39841918267026,28.1960792358592,125.983802540758));
#94865=CARTESIAN_POINT('Ctrl Pts',(5.40227815643071,28.1619081138742,125.921145662036));
#94866=CARTESIAN_POINT('Ctrl Pts',(5.40613713019115,28.1310179420956,125.856729619846));
#94867=CARTESIAN_POINT('Ctrl Pts',(5.4099961039516,28.1035769800651,125.790934442265));
#94868=CARTESIAN_POINT('Ctrl Pts',(5.41385692499008,28.0761228821365,125.725107768749));
#94869=CARTESIAN_POINT('Ctrl Pts',(5.41771774602856,28.0521214469396,125.657901102821));
#94870=CARTESIAN_POINT('Ctrl Pts',(5.42157856706705,28.0316917009795,125.58971179614));
#94871=CARTESIAN_POINT('Ctrl Pts',(5.42544650242978,28.0112243091829,125.521396837213));
#94872=CARTESIAN_POINT('Ctrl Pts',(5.42931443779252,27.9943418718265,125.452096092942));
#94873=CARTESIAN_POINT('Ctrl Pts',(5.43318237315526,27.9811126060574,125.382218854951));
#94874=CARTESIAN_POINT('Ctrl Pts',(5.43660621397653,27.9694022500334,125.320364527648));
#94875=CARTESIAN_POINT('Ctrl Pts',(5.4400300547978,27.9605536157451,125.258058844669));
#94876=CARTESIAN_POINT('Ctrl Pts',(5.44345389561907,27.9545799673092,125.195587454524));
#94877=CARTESIAN_POINT('Ctrl Pts',(5.44732296896728,27.9478295121444,125.124992352924));
#94878=CARTESIAN_POINT('Ctrl Pts',(5.45119204231549,27.9447248768961,125.053909088628));
#94879=CARTESIAN_POINT('Ctrl Pts',(5.4550611156637,27.9453224383922,124.982746585111));
#94880=CARTESIAN_POINT('Ctrl Pts',(5.45892442405948,27.9459191095165,124.911690114334));
#94881=CARTESIAN_POINT('Ctrl Pts',(5.46278773245526,27.9502070236293,124.840555120507));
#94882=CARTESIAN_POINT('Ctrl Pts',(5.46665104085104,27.9581907664977,124.769755311712));
#94883=CARTESIAN_POINT('Ctrl Pts',(5.47050981734395,27.9661651439354,124.699038555531));
#94884=CARTESIAN_POINT('Ctrl Pts',(5.47436859383686,27.9778266843104,124.628656683752));
#94885=CARTESIAN_POINT('Ctrl Pts',(5.47822737032977,27.9931279671206,124.559021308739));
#94886=CARTESIAN_POINT('Ctrl Pts',(5.48208371591797,28.0084196106162,124.489429801765));
#94887=CARTESIAN_POINT('Ctrl Pts',(5.48594006150617,28.0273463434201,124.420584331896));
#94888=CARTESIAN_POINT('Ctrl Pts',(5.48979640709437,28.0498093885281,124.352887844785));
#94889=CARTESIAN_POINT('Ctrl Pts',(5.4936516133397,28.0722657970135,124.285211358348));
#94890=CARTESIAN_POINT('Ctrl Pts',(5.49750681958503,28.0982562906977,124.218683641557));
#94891=CARTESIAN_POINT('Ctrl Pts',(5.50136202583035,28.1276322948654,124.153692290435));
#94892=CARTESIAN_POINT('Ctrl Pts',(5.5052173826816,28.1570094466242,124.088698400387));
#94893=CARTESIAN_POINT('Ctrl Pts',(5.50907273953284,28.1897721693534,124.025241436929));
#94894=CARTESIAN_POINT('Ctrl Pts',(5.51292809638408,28.2257245380356,123.963687234677));
#94895=CARTESIAN_POINT('Ctrl Pts',(5.51678748885264,28.2617145400699,123.902068600205));
#94896=CARTESIAN_POINT('Ctrl Pts',(5.52064688132119,28.3009006075052,123.842357123209));
#94897=CARTESIAN_POINT('Ctrl Pts',(5.52450627378975,28.3430422566957,123.784891527721));
#94898=CARTESIAN_POINT('Ctrl Pts',(5.52836785139318,28.3852077659077,123.727393396004));
#94899=CARTESIAN_POINT('Ctrl Pts',(5.53222942899661,28.4303318806798,123.672144053556));
#94900=CARTESIAN_POINT('Ctrl Pts',(5.53609100660004,28.4781341470793,123.619448701346));
#94901=CARTESIAN_POINT('Ctrl Pts',(5.53995934071491,28.5260200519791,123.56666114932));
#94902=CARTESIAN_POINT('Ctrl Pts',(5.54382767482978,28.576593119241,123.516436851755));
#94903=CARTESIAN_POINT('Ctrl Pts',(5.54769600894465,28.629536935203,123.469043256481));
#94904=CARTESIAN_POINT('Ctrl Pts',(5.54999372811564,28.6609845861321,123.44089233435));
#94905=CARTESIAN_POINT('Ctrl Pts',(5.55229144728663,28.6932680392849,123.41373934893));
#94906=CARTESIAN_POINT('Ctrl Pts',(5.55458916645762,28.7263160946048,123.387633146075));
#94907=CARTESIAN_POINT('Ctrl Pts',(5.55845823980583,28.7819649100314,123.343673546936));
#94908=CARTESIAN_POINT('Ctrl Pts',(5.56232731315405,28.840001213987,123.302512198001));
#94909=CARTESIAN_POINT('Ctrl Pts',(5.56619638650227,28.9001120288155,123.264418249306));
#94910=CARTESIAN_POINT('Ctrl Pts',(5.57005969489806,28.960133278015,123.22638106092));
#94911=CARTESIAN_POINT('Ctrl Pts',(5.57392300329384,29.0222224954769,123.191402458471));
#94912=CARTESIAN_POINT('Ctrl Pts',(5.57778631168963,29.0860345941753,123.159710675069));
#94913=CARTESIAN_POINT('Ctrl Pts',(5.58164508818254,29.1497718372826,123.128056068115));
#94914=CARTESIAN_POINT('Ctrl Pts',(5.58550386467546,29.2152275141707,123.099680836624));
#94915=CARTESIAN_POINT('Ctrl Pts',(5.58936264116837,29.282030092187,123.07476838433));
#94916=CARTESIAN_POINT('Ctrl Pts',(5.59321898675658,29.3487905867342,123.049871626077));
#94917=CARTESIAN_POINT('Ctrl Pts',(5.59707533234479,29.4168958449018,123.028433488424));
#94918=CARTESIAN_POINT('Ctrl Pts',(5.600931677933,29.4859537613948,123.010589527756));
#94919=CARTESIAN_POINT('Ctrl Pts',(5.60478688417833,29.5549912749848,122.992750839019));
#94920=CARTESIAN_POINT('Ctrl Pts',(5.60864209042367,29.6249804180435,122.978504340596));
#94921=CARTESIAN_POINT('Ctrl Pts',(5.612497296669,29.6955149726789,122.967935426558));
#94922=CARTESIAN_POINT('Ctrl Pts',(5.61635265352025,29.7660522827885,122.95736609964));
#94923=CARTESIAN_POINT('Ctrl Pts',(5.62020801037151,29.8371345660277,122.950474712148));
#94924=CARTESIAN_POINT('Ctrl Pts',(5.62406336722276,29.9083482061054,122.947295074499));
#94925=CARTESIAN_POINT('Ctrl Pts',(5.62792275969132,29.9796363894768,122.944112108546));
#94926=CARTESIAN_POINT('Ctrl Pts',(5.63178215215988,30.0510557178678,122.944648670073));
#94927=CARTESIAN_POINT('Ctrl Pts',(5.63564154462844,30.1221911847723,122.948886430042));
#94928=CARTESIAN_POINT('Ctrl Pts',(5.63950312223188,30.1933669275988,122.953126589374));
#94929=CARTESIAN_POINT('Ctrl Pts',(5.64336469983532,30.2642580060058,122.961072064643));
#94930=CARTESIAN_POINT('Ctrl Pts',(5.64722627743876,30.3344558992232,122.972652764331));
#94931=CARTESIAN_POINT('Ctrl Pts',(5.65109461155363,30.4047766160419,122.984253726497));
#94932=CARTESIAN_POINT('Ctrl Pts',(5.65496294566851,30.4744012514923,122.999502507974));
#94933=CARTESIAN_POINT('Ctrl Pts',(5.65883127978338,30.5429334995985,123.018278329958));
#94934=CARTESIAN_POINT('Ctrl Pts',(5.66112899895431,30.583640391926,123.029430822179));
#94935=CARTESIAN_POINT('Ctrl Pts',(5.66342671812525,30.6239621832624,123.041826753286));
#94936=CARTESIAN_POINT('Ctrl Pts',(5.66572443729618,30.6638192197252,123.055432797247));
#94937=CARTESIAN_POINT('Ctrl Pts',(5.66959351064439,30.7309335126585,123.078343683281));
#94938=CARTESIAN_POINT('Ctrl Pts',(5.6734625839926,30.7969917617406,123.104778072836));
#94939=CARTESIAN_POINT('Ctrl Pts',(5.67733165734081,30.8615980944628,123.134618997063));
#94940=CARTESIAN_POINT('Ctrl Pts',(5.68119496573659,30.9261081631958,123.164415458058));
#94941=CARTESIAN_POINT('Ctrl Pts',(5.68505827413237,30.9891701723712,123.197608176431));
#94942=CARTESIAN_POINT('Ctrl Pts',(5.68892158252814,31.050405210603,123.234031014984));
#94943=CARTESIAN_POINT('Ctrl Pts',(5.69278035902105,31.1115684162972,123.270411127264));
#94944=CARTESIAN_POINT('Ctrl Pts',(5.69663913551396,31.170908492586,123.31001358609));
#94945=CARTESIAN_POINT('Ctrl Pts',(5.70049791200686,31.2280698480367,123.352625722295));
#94946=CARTESIAN_POINT('Ctrl Pts',(5.70435425759507,31.2851951936774,123.395211014229));
#94947=CARTESIAN_POINT('Ctrl Pts',(5.70821060318327,31.3401441529922,123.440801932254));
#94948=CARTESIAN_POINT('Ctrl Pts',(5.71206694877147,31.3925901753256,123.489142572548));
#94949=CARTESIAN_POINT('Ctrl Pts',(5.71592215501679,31.445020702678,123.537468930781));
#94950=CARTESIAN_POINT('Ctrl Pts',(5.71977736126212,31.4949494041244,123.588543069396));
#94951=CARTESIAN_POINT('Ctrl Pts',(5.72363256750745,31.5420842183893,123.642070021726));
#94952=CARTESIAN_POINT('Ctrl Pts',(5.72748792435869,31.5892208740036,123.695599065118));
#94953=CARTESIAN_POINT('Ctrl Pts',(5.73134328120994,31.6335631063536,123.751580746428));
#94954=CARTESIAN_POINT('Ctrl Pts',(5.73519863806119,31.6748581792137,123.809685906149));
#94955=CARTESIAN_POINT('Ctrl Pts',(5.73905803052974,31.7161964779325,123.867851887785));
#94956=CARTESIAN_POINT('Ctrl Pts',(5.74291742299829,31.7544809679474,123.928145388184));
#94957=CARTESIAN_POINT('Ctrl Pts',(5.74677681546684,31.7895019636561,123.990207801292));
#94958=CARTESIAN_POINT('Ctrl Pts',(5.75063839307027,31.8245427877703,124.052305353284));
#94959=CARTESIAN_POINT('Ctrl Pts',(5.7544999706737,31.8563162228096,124.116173376588));
#94960=CARTESIAN_POINT('Ctrl Pts',(5.75836154827713,31.8846595887185,124.181430639987));
#94961=CARTESIAN_POINT('Ctrl Pts',(5.762229882392,31.9130525463476,124.246802082484));
#94962=CARTESIAN_POINT('Ctrl Pts',(5.76609821650687,31.9380032825452,124.313567162888));
#94963=CARTESIAN_POINT('Ctrl Pts',(5.76996655062173,31.959398326717,124.3813274212));
#94964=CARTESIAN_POINT('Ctrl Pts',(5.77226426979273,31.9721065886453,124.421575765819));
#94965=CARTESIAN_POINT('Ctrl Pts',(5.77456198896374,31.9835613184562,124.462174966916));
#94966=CARTESIAN_POINT('Ctrl Pts',(5.77685970813474,31.993747313396,124.50304002895));
#94967=CARTESIAN_POINT('Ctrl Pts',(5.78191177765028,32.0161435901778,124.592891363594));
#94968=CARTESIAN_POINT('Ctrl Pts',(5.78696384716583,32.0324751044743,124.684310306464));
#94969=CARTESIAN_POINT('Ctrl Pts',(5.79201591668137,32.0425683991186,124.776590292462));
#94970=CARTESIAN_POINT('Ctrl Pts',(5.79603551759184,32.050598972771,124.850011434945));
#94971=CARTESIAN_POINT('Ctrl Pts',(5.80005511850231,32.0546813536987,124.923977405718));
#94972=CARTESIAN_POINT('Ctrl Pts',(5.80407471941277,32.0547491412311,124.998121407385));
#94973=CARTESIAN_POINT('Ctrl Pts',(5.80407471946232,32.0547491412319,124.998121408299));
#94974=CARTESIAN_POINT('Ctrl Pts',(5.80788808427068,32.0548134507169,125.068461258701));
#94975=CARTESIAN_POINT('Ctrl Pts',(5.81170144907905,32.0512616122161,125.138896596669));
#94976=CARTESIAN_POINT('Ctrl Pts',(5.81551481388741,32.0440909046791,125.209021376677));
#94977=CARTESIAN_POINT('Ctrl Pts',(5.81932566294079,32.036924927805,125.279099893929));
#94978=CARTESIAN_POINT('Ctrl Pts',(5.82313651199416,32.0261448653963,125.348867764812));
#94979=CARTESIAN_POINT('Ctrl Pts',(5.82694736104754,32.0118000195851,125.417921336734));
#94980=CARTESIAN_POINT('Ctrl Pts',(5.83075704398274,31.9974595632906,125.486953778293));
#94981=CARTESIAN_POINT('Ctrl Pts',(5.83456672691795,31.9795565892288,125.555271866759));
#94982=CARTESIAN_POINT('Ctrl Pts',(5.83837640985316,31.9581916522906,125.62248133739));
#94983=CARTESIAN_POINT('Ctrl Pts',(5.84218627454151,31.9368256960695,125.689694014466));
#94984=CARTESIAN_POINT('Ctrl Pts',(5.84599613922986,31.9119976032409,125.755797494637));
#94985=CARTESIAN_POINT('Ctrl Pts',(5.84980600391822,31.8838574485761,125.820413722426));
#94986=CARTESIAN_POINT('Ctrl Pts',(5.85361981396699,31.8556881529677,125.885096864483));
#94987=CARTESIAN_POINT('Ctrl Pts',(5.85743362401575,31.8242001532027,125.948289224179));
#94988=CARTESIAN_POINT('Ctrl Pts',(5.86124743406452,31.7895907717114,126.009634801453));
#94989=CARTESIAN_POINT('Ctrl Pts',(5.86506356527418,31.75496032626,126.07101771487));
#94990=CARTESIAN_POINT('Ctrl Pts',(5.86887969648384,31.7172049893137,126.130551190878));
#94991=CARTESIAN_POINT('Ctrl Pts',(5.8726958276935,31.6765654040786,126.187908249128));
#94992=CARTESIAN_POINT('Ctrl Pts',(5.87651830066288,31.6358582827786,126.245360625035));
#94993=CARTESIAN_POINT('Ctrl Pts',(5.88034077363226,31.5922576630893,126.300628980545));
#94994=CARTESIAN_POINT('Ctrl Pts',(5.88416324660164,31.5460437137614,126.353420259062));
#94995=CARTESIAN_POINT('Ctrl Pts',(5.88544049072553,31.5306017483915,126.371059978379));
#94996=CARTESIAN_POINT('Ctrl Pts',(5.88671773484941,31.5148682976354,126.388423448839));
#94997=CARTESIAN_POINT('Ctrl Pts',(5.88799497897329,31.4988546567116,126.40550072236));
#94998=CARTESIAN_POINT('Ctrl Pts',(5.89186405232151,31.4503455658121,126.45723180697));
#94999=CARTESIAN_POINT('Ctrl Pts',(5.89573312566972,31.3990601643257,126.50654992552));
#95000=CARTESIAN_POINT('Ctrl Pts',(5.89960219901793,31.3452680229113,126.553142462568));
#95001=CARTESIAN_POINT('Ctrl Pts',(5.90346550741372,31.2915560322484,126.599665576337));
#95002=CARTESIAN_POINT('Ctrl Pts',(5.9073288158095,31.2353450798584,126.643470854395));
#95003=CARTESIAN_POINT('Ctrl Pts',(5.91119212420528,31.1769425622697,126.684281380179));
#95004=CARTESIAN_POINT('Ctrl Pts',(5.91505090069819,31.1186085544943,126.725044032659));
#95005=CARTESIAN_POINT('Ctrl Pts',(5.9189096771911,31.0580884843514,126.762818634032));
#95006=CARTESIAN_POINT('Ctrl Pts',(5.92276845368401,30.9957225538103,126.797368676241));
#95007=CARTESIAN_POINT('Ctrl Pts',(5.92662479927221,30.9333959117936,126.831896953038));
#95008=CARTESIAN_POINT('Ctrl Pts',(5.9304811448604,30.8692261403504,126.863204466019));
#95009=CARTESIAN_POINT('Ctrl Pts',(5.93433749044861,30.8035808867985,126.891098971728));
#95010=CARTESIAN_POINT('Ctrl Pts',(5.93819269669394,30.737955027891,126.91898523611));
#95011=CARTESIAN_POINT('Ctrl Pts',(5.94204790293927,30.6708549991597,126.943460305214));
#95012=CARTESIAN_POINT('Ctrl Pts',(5.9459031091846,30.6026698482921,126.964379448187));
#95013=CARTESIAN_POINT('Ctrl Pts',(5.94975846603584,30.5344820337313,126.985299408378));
#95014=CARTESIAN_POINT('Ctrl Pts',(5.95361382288709,30.4652094779392,127.002663026264));
#95015=CARTESIAN_POINT('Ctrl Pts',(5.95746917973834,30.3952562000437,127.016375485575));
#95016=CARTESIAN_POINT('Ctrl Pts',(5.96132857220689,30.325229698146,127.030102298483));
#95017=CARTESIAN_POINT('Ctrl Pts',(5.96518796467544,30.2545215294256,127.040170229863));
#95018=CARTESIAN_POINT('Ctrl Pts',(5.969047357144,30.1835448252715,127.046535819285));
#95019=CARTESIAN_POINT('Ctrl Pts',(5.97290893474743,30.1125279350846,127.052905012816));
#95020=CARTESIAN_POINT('Ctrl Pts',(5.97677051235087,30.0412426924747,127.055567673329));
#95021=CARTESIAN_POINT('Ctrl Pts',(5.98063208995431,29.9701034964048,127.054532492216));
#95022=CARTESIAN_POINT('Ctrl Pts',(5.98450042406917,29.8988398297581,127.053495499872));
#95023=CARTESIAN_POINT('Ctrl Pts',(5.98836875818404,29.8277232046938,127.048747780675));
#95024=CARTESIAN_POINT('Ctrl Pts',(5.99223709229891,29.7571634625664,127.040349964733));
#95025=CARTESIAN_POINT('Ctrl Pts',(5.99453481146989,29.7152522761561,127.035361816835));
#95026=CARTESIAN_POINT('Ctrl Pts',(5.99683253064088,29.6735374017371,127.029086849354));
#95027=CARTESIAN_POINT('Ctrl Pts',(5.99913024981186,29.6321025567787,127.021546198772));
#95028=CARTESIAN_POINT('Ctrl Pts',(6.00299944643827,29.5623292074706,127.008848276345));
#95029=CARTESIAN_POINT('Ctrl Pts',(6.00686864306468,29.4930773581584,126.992508916017));
#95030=CARTESIAN_POINT('Ctrl Pts',(6.01073783969108,29.4247558951416,126.97258505072));
#95031=CARTESIAN_POINT('Ctrl Pts',(6.01460043069499,29.3565510728223,126.952695200117));
#95032=CARTESIAN_POINT('Ctrl Pts',(6.01846302169889,29.2892739434971,126.929233137685));
#95033=CARTESIAN_POINT('Ctrl Pts',(6.02232561270279,29.2233236559803,126.902306867764));
#95034=CARTESIAN_POINT('Ctrl Pts',(6.02618437409812,29.1574387556056,126.87540729419));
#95035=CARTESIAN_POINT('Ctrl Pts',(6.03004313549344,29.0928785346375,126.845050509388));
#95036=CARTESIAN_POINT('Ctrl Pts',(6.03390189688877,29.030026205475,126.811394048912));
#95037=CARTESIAN_POINT('Ctrl Pts',(6.03775817556283,28.9672143154064,126.777759242953));
#95038=CARTESIAN_POINT('Ctrl Pts',(6.0416144542369,28.9061085638573,126.740829202853));
#95039=CARTESIAN_POINT('Ctrl Pts',(6.04547073291096,28.8470698469948,126.700808520907));
#95040=CARTESIAN_POINT('Ctrl Pts',(6.04767405794767,28.8133374604137,126.677942286911));
#95041=CARTESIAN_POINT('Ctrl Pts',(6.04987738298438,28.7802794301862,126.654067958849));
#95042=CARTESIAN_POINT('Ctrl Pts',(6.05208070802109,28.7479590808042,126.629230216746));
#95043=CARTESIAN_POINT('',(5.74592528057331,32.0547492412561,125.001765802243));
#95044=CARTESIAN_POINT('Ctrl Pts',(5.74592528057331,32.0547492412561,125.001765802243));
#95045=CARTESIAN_POINT('Ctrl Pts',(5.75057817989322,32.0546753518283,125.087746124368));
#95046=CARTESIAN_POINT('Ctrl Pts',(5.75523107921313,32.0492009128721,125.173490900321));
#95047=CARTESIAN_POINT('Ctrl Pts',(5.75988397853304,32.038437023012,125.258402913517));
#95048=CARTESIAN_POINT('Ctrl Pts',(5.76460377517814,32.0275183747119,125.344535754023));
#95049=CARTESIAN_POINT('Ctrl Pts',(5.76932357182325,32.011157157185,125.42981172292));
#95050=CARTESIAN_POINT('Ctrl Pts',(5.77404336846835,31.9895181111569,125.513629485017));
#95051=CARTESIAN_POINT('Ctrl Pts',(5.7757069401806,31.9818910654261,125.543172465042));
#95052=CARTESIAN_POINT('Ctrl Pts',(5.77737051189285,31.9736087726741,125.572534484309));
#95053=CARTESIAN_POINT('Ctrl Pts',(5.77903408360509,31.9646798449384,125.601689844848));
#95054=CARTESIAN_POINT('Ctrl Pts',(5.78290315695331,31.9439132761898,125.669498300347));
#95055=CARTESIAN_POINT('Ctrl Pts',(5.78677223030153,31.9195914246618,125.736363214624));
#95056=CARTESIAN_POINT('Ctrl Pts',(5.79064130364975,31.8918186201618,125.801885198086));
#95057=CARTESIAN_POINT('Ctrl Pts',(5.79450461204554,31.8640871973784,125.867309553231));
#95058=CARTESIAN_POINT('Ctrl Pts',(5.79836792044133,31.8329152162861,125.931394505826));
#95059=CARTESIAN_POINT('Ctrl Pts',(5.80223122883712,31.7984566891989,125.993756056372));
#95060=CARTESIAN_POINT('Ctrl Pts',(5.80609000533003,31.7640385841237,126.056044452911));
#95061=CARTESIAN_POINT('Ctrl Pts',(5.80994878182295,31.7263418248365,126.116613039969));
#95062=CARTESIAN_POINT('Ctrl Pts',(5.81380755831586,31.6855676731745,126.17509964754));
#95063=CARTESIAN_POINT('Ctrl Pts',(5.81766390390407,31.6448192079127,126.233549410435));
#95064=CARTESIAN_POINT('Ctrl Pts',(5.82152024949228,31.6009974737035,126.289919398434));
#95065=CARTESIAN_POINT('Ctrl Pts',(5.82537659508049,31.5543478680564,126.343875093738));
#95066=CARTESIAN_POINT('Ctrl Pts',(5.82923180132582,31.5077120448608,126.397814848033));
#95067=CARTESIAN_POINT('Ctrl Pts',(5.83308700757116,31.4582503264415,126.449341358437));
#95068=CARTESIAN_POINT('Ctrl Pts',(5.83694221381649,31.4062482494225,126.498153337778));
#95069=CARTESIAN_POINT('Ctrl Pts',(5.84079757066774,31.3542441409115,126.546967223989));
#95070=CARTESIAN_POINT('Ctrl Pts',(5.84465292751899,31.2996998324739,126.593066037739));
#95071=CARTESIAN_POINT('Ctrl Pts',(5.84850828437024,31.2429362859692,126.636186710471));
#95072=CARTESIAN_POINT('Ctrl Pts',(5.8523676768388,31.1861133218904,126.679352520019));
#95073=CARTESIAN_POINT('Ctrl Pts',(5.85622706930737,31.1270668701352,126.719533671088));
#95074=CARTESIAN_POINT('Ctrl Pts',(5.86008646177593,31.0661486922933,126.756509188254));
#95075=CARTESIAN_POINT('Ctrl Pts',(5.86394803937936,31.005196023418,126.793505640449));
#95076=CARTESIAN_POINT('Ctrl Pts',(5.8678096169828,30.9423699468735,126.827292615469));
#95077=CARTESIAN_POINT('Ctrl Pts',(5.87167119458624,30.8780463317198,126.857695400719));
#95078=CARTESIAN_POINT('Ctrl Pts',(5.87553952870111,30.8136101710508,126.888151381007));
#95079=CARTESIAN_POINT('Ctrl Pts',(5.87940786281599,30.7476716900085,126.915211165115));
#95080=CARTESIAN_POINT('Ctrl Pts',(5.88327619693086,30.6806255415029,126.938748677563));
#95081=CARTESIAN_POINT('Ctrl Pts',(5.88557391610179,30.6408013649495,126.952729526162));
#95082=CARTESIAN_POINT('Ctrl Pts',(5.88787163527272,30.600586674591,126.965468625186));
#95083=CARTESIAN_POINT('Ctrl Pts',(5.89016935444365,30.5600659399301,126.976948078587));
#95084=CARTESIAN_POINT('Ctrl Pts',(5.89403860385591,30.4918309568413,126.996278930193));
#95085=CARTESIAN_POINT('Ctrl Pts',(5.89790785326818,30.4224603226495,127.012110772205));
#95086=CARTESIAN_POINT('Ctrl Pts',(5.90177710268044,30.3523462206453,127.02431462557));
#95087=CARTESIAN_POINT('Ctrl Pts',(5.90563962094158,30.2823540928449,127.036497248466));
#95088=CARTESIAN_POINT('Ctrl Pts',(5.90950213920273,30.2116215417877,127.045064340978));
#95089=CARTESIAN_POINT('Ctrl Pts',(5.91336465746388,30.1405544631544,127.049937073519));
#95090=CARTESIAN_POINT('Ctrl Pts',(5.91722337855583,30.069557249232,127.054805015768));
#95091=CARTESIAN_POINT('Ctrl Pts',(5.92108209964779,29.998226642092,127.055985769382));
#95092=CARTESIAN_POINT('Ctrl Pts',(5.92494082073974,29.9269760550714,127.053451987743));
#95093=CARTESIAN_POINT('Ctrl Pts',(5.92879703930303,29.8557716767901,127.050919849359));
#95094=CARTESIAN_POINT('Ctrl Pts',(5.93265325786631,29.7846476999144,127.044677973575));
#95095=CARTESIAN_POINT('Ctrl Pts',(5.9365094764296,29.7140182217139,127.03475108674));
#95096=CARTESIAN_POINT('Ctrl Pts',(5.94036448407861,29.6434109222987,127.024827317106));
#95097=CARTESIAN_POINT('Ctrl Pts',(5.94421949172763,29.5732982938219,127.011220902373));
#95098=CARTESIAN_POINT('Ctrl Pts',(5.94807449937664,29.5040882647224,126.994008303221));
#95099=CARTESIAN_POINT('Ctrl Pts',(5.95193183765665,29.4348363931536,126.976785297807));
#95100=CARTESIAN_POINT('Ctrl Pts',(5.95578917593665,29.3664886850711,126.95595186316));
#95101=CARTESIAN_POINT('Ctrl Pts',(5.95964651421665,29.2994408433327,126.931635170137));
#95102=CARTESIAN_POINT('Ctrl Pts',(5.96350485068227,29.2323756512388,126.907312184543));
#95103=CARTESIAN_POINT('Ctrl Pts',(5.96736318714789,29.1666114466945,126.879504327395));
#95104=CARTESIAN_POINT('Ctrl Pts',(5.9712215236135,29.1025243520487,126.848387141222));
#95105=CARTESIAN_POINT('Ctrl Pts',(5.97508578864727,29.0383387836925,126.817222141604));
#95106=CARTESIAN_POINT('Ctrl Pts',(5.97895005368104,28.9758359044361,126.782737881705));
#95107=CARTESIAN_POINT('Ctrl Pts',(5.98281431871481,28.9153670784502,126.745155863523));
#95108=CARTESIAN_POINT('Ctrl Pts',(5.98650489621106,28.8576161513119,126.70926304837));
#95109=CARTESIAN_POINT('Ctrl Pts',(5.99019547370731,28.8017206368457,126.670545230028));
#95110=CARTESIAN_POINT('Ctrl Pts',(5.99388605120356,28.7479590808042,126.629230216746));
#95111=CARTESIAN_POINT('Ctrl Pts',(5.29388025228516,28.7479590808042,126.629230216746));
#95112=CARTESIAN_POINT('Ctrl Pts',(5.29773979489958,28.691380642155,126.585750468087));
#95113=CARTESIAN_POINT('Ctrl Pts',(5.30159933751399,28.637099473738,126.539342931937));
#95114=CARTESIAN_POINT('Ctrl Pts',(5.30545888012841,28.5854206239971,126.4902894858));
#95115=CARTESIAN_POINT('Ctrl Pts',(5.30932071288091,28.5337111095598,126.441206932804));
#95116=CARTESIAN_POINT('Ctrl Pts',(5.31318254563342,28.4846073216076,126.389475697383));
#95117=CARTESIAN_POINT('Ctrl Pts',(5.31704437838592,28.4383759216136,126.335412969947));
#95118=CARTESIAN_POINT('Ctrl Pts',(5.32091286111107,28.3920649123862,126.281257147942));
#95119=CARTESIAN_POINT('Ctrl Pts',(5.32478134383621,28.3486364598602,126.224762205235));
#95120=CARTESIAN_POINT('Ctrl Pts',(5.32864982656136,28.3083151279993,126.166276063522));
#95121=CARTESIAN_POINT('Ctrl Pts',(5.33059755112453,28.2880139261936,126.136829145204));
#95122=CARTESIAN_POINT('Ctrl Pts',(5.33254527568769,28.2684996609268,126.106877883204));
#95123=CARTESIAN_POINT('Ctrl Pts',(5.33449300025086,28.2497965371345,126.076468950353));
#95124=CARTESIAN_POINT('Ctrl Pts',(5.33836207359907,28.2126435642954,126.016062877611));
#95125=CARTESIAN_POINT('Ctrl Pts',(5.34223114694728,28.1785487493109,125.953612795032));
#95126=CARTESIAN_POINT('Ctrl Pts',(5.3461002202955,28.147742810437,125.889460997578));
#95127=CARTESIAN_POINT('Ctrl Pts',(5.34996352869128,28.1169827726759,125.825404786851));
#95128=CARTESIAN_POINT('Ctrl Pts',(5.35382683708706,28.0895020923367,125.759652328628));
#95129=CARTESIAN_POINT('Ctrl Pts',(5.35769014548284,28.0654870977575,125.692573023989));
#95130=CARTESIAN_POINT('Ctrl Pts',(5.36154892197575,28.0415002742719,125.625572407578));
#95131=CARTESIAN_POINT('Ctrl Pts',(5.36540769846866,28.0209712240985,125.557248491575));
#95132=CARTESIAN_POINT('Ctrl Pts',(5.36926647496157,28.0040386621117,125.487991700908));
#95133=CARTESIAN_POINT('Ctrl Pts',(5.37312282054977,27.9871167670928,125.418778539785));
#95134=CARTESIAN_POINT('Ctrl Pts',(5.37697916613798,27.9737869803036,125.34863414072));
#95135=CARTESIAN_POINT('Ctrl Pts',(5.38083551172618,27.9641380924166,125.277963766975));
#95136=CARTESIAN_POINT('Ctrl Pts',(5.38469071797151,27.9544920552575,125.207314272528));
#95137=CARTESIAN_POINT('Ctrl Pts',(5.38854592421683,27.9485248236773,125.136139592967));
#95138=CARTESIAN_POINT('Ctrl Pts',(5.39240113046216,27.946273720216,125.06485314352));
#95139=CARTESIAN_POINT('Ctrl Pts',(5.3962564873134,27.944022528814,124.993563909226));
#95140=CARTESIAN_POINT('Ctrl Pts',(5.40011184416465,27.9454877668835,124.922163381991));
#95141=CARTESIAN_POINT('Ctrl Pts',(5.40396720101589,27.950654662112,124.851066294692));
#95142=CARTESIAN_POINT('Ctrl Pts',(5.40782659348445,27.9558269658184,124.779894786101));
#95143=CARTESIAN_POINT('Ctrl Pts',(5.411685985953,27.9647086262348,124.709027837004));
#95144=CARTESIAN_POINT('Ctrl Pts',(5.41554537842156,27.9772329265542,124.638875465963));
#95145=CARTESIAN_POINT('Ctrl Pts',(5.41940695602499,27.9897643179601,124.568683375614));
#95146=CARTESIAN_POINT('Ctrl Pts',(5.42326853362842,28.0059423446726,124.499207142076));
#95147=CARTESIAN_POINT('Ctrl Pts',(5.42713011123186,28.0256496404587,124.43084429171));
#95148=CARTESIAN_POINT('Ctrl Pts',(5.43099844534672,28.0453914176364,124.362361828474));
#95149=CARTESIAN_POINT('Ctrl Pts',(5.43486677946159,28.0686746338712,124.294997097049));
#95150=CARTESIAN_POINT('Ctrl Pts',(5.43873511357646,28.0953330110469,124.229129567507));
#95151=CARTESIAN_POINT('Ctrl Pts',(5.44103283274744,28.1111675957764,124.190005468895));
#95152=CARTESIAN_POINT('Ctrl Pts',(5.44333055191843,28.1281920767404,124.151409186527));
#95153=CARTESIAN_POINT('Ctrl Pts',(5.44562827108941,28.1463640450114,124.113415932427));
#95154=CARTESIAN_POINT('Ctrl Pts',(5.44949734443763,28.1769633797821,124.049440017222));
#95155=CARTESIAN_POINT('Ctrl Pts',(5.45336641778585,28.2109386112394,123.986924796112));
#95156=CARTESIAN_POINT('Ctrl Pts',(5.45723549113407,28.2481272957716,123.926249754049));
#95157=CARTESIAN_POINT('Ctrl Pts',(5.46109879952985,28.2852605688453,123.865665118319));
#95158=CARTESIAN_POINT('Ctrl Pts',(5.46496210792564,28.3255975390154,123.80691562988));
#95159=CARTESIAN_POINT('Ctrl Pts',(5.46882541632142,28.3689289141425,123.750358181166));
#95160=CARTESIAN_POINT('Ctrl Pts',(5.47268419281434,28.4122094588509,123.693867077883));
#95161=CARTESIAN_POINT('Ctrl Pts',(5.47654296930725,28.458477137248,123.639563290402));
#95162=CARTESIAN_POINT('Ctrl Pts',(5.48040174580017,28.5074791703107,123.58777511159));
#95163=CARTESIAN_POINT('Ctrl Pts',(5.48425809138837,28.5564503336734,123.536019557661));
#95164=CARTESIAN_POINT('Ctrl Pts',(5.48811443697657,28.6081521010899,123.486776820306));
#95165=CARTESIAN_POINT('Ctrl Pts',(5.49197078256478,28.6622921501115,123.440341296678));
#95166=CARTESIAN_POINT('Ctrl Pts',(5.49582598881011,28.7164162036583,123.393919492252));
#95167=CARTESIAN_POINT('Ctrl Pts',(5.49968119505544,28.7729767401191,123.350303571092));
#95168=CARTESIAN_POINT('Ctrl Pts',(5.50353640130078,28.8316466737578,123.309749111061));
#95169=CARTESIAN_POINT('Ctrl Pts',(5.50739175815202,28.8903188993721,123.269193066747));
#95170=CARTESIAN_POINT('Ctrl Pts',(5.51124711500327,28.9511002849052,123.231698995419));
#95171=CARTESIAN_POINT('Ctrl Pts',(5.51510247185452,29.0136343832301,123.197479422433));
#95172=CARTESIAN_POINT('Ctrl Pts',(5.51896186432308,29.0762339394879,123.163224029908));
#95173=CARTESIAN_POINT('Ctrl Pts',(5.52282125679164,29.1405894439089,123.132250211661));
#95174=CARTESIAN_POINT('Ctrl Pts',(5.5266806492602,29.2063202372392,123.104724295337));
#95175=CARTESIAN_POINT('Ctrl Pts',(5.53054222686364,29.2720882464397,123.077182794219));
#95176=CARTESIAN_POINT('Ctrl Pts',(5.53440380446707,29.3392326371753,123.053093245288));
#95177=CARTESIAN_POINT('Ctrl Pts',(5.53826538207051,29.4073557750043,123.032572648081));
#95178=CARTESIAN_POINT('Ctrl Pts',(5.54213371618538,29.4755981062841,123.012016146468));
#95179=CARTESIAN_POINT('Ctrl Pts',(5.54600205030026,29.5448221317373,122.995041179658));
#95180=CARTESIAN_POINT('Ctrl Pts',(5.54987038441513,29.6146188587507,122.981713861102));
#95181=CARTESIAN_POINT('Ctrl Pts',(5.55216810358608,29.6560768282449,122.973797679501));
#95182=CARTESIAN_POINT('Ctrl Pts',(5.55446582275702,29.6977367133038,122.967167450132));
#95183=CARTESIAN_POINT('Ctrl Pts',(5.55676354192797,29.739512323952,122.961828335707));
#95184=CARTESIAN_POINT('Ctrl Pts',(5.56063261527618,29.8098572572268,122.952837930967));
#95185=CARTESIAN_POINT('Ctrl Pts',(5.5645016886244,29.8808059628848,122.947475992101));
#95186=CARTESIAN_POINT('Ctrl Pts',(5.56837076197261,29.9519515155082,122.945811862161));
#95187=CARTESIAN_POINT('Ctrl Pts',(5.57223407036839,30.0229910606489,122.944150211789));
#95188=CARTESIAN_POINT('Ctrl Pts',(5.57609737876418,30.0942263888592,122.946175444879));
#95189=CARTESIAN_POINT('Ctrl Pts',(5.57996068715996,30.1652441467213,122.951905291625));
#95190=CARTESIAN_POINT('Ctrl Pts',(5.58381946365287,30.2361785963026,122.957628416901));
#95191=CARTESIAN_POINT('Ctrl Pts',(5.58767824014578,30.306895500634,122.967047484839));
#95192=CARTESIAN_POINT('Ctrl Pts',(5.59153701663869,30.3769819483138,122.980128179031));
#95193=CARTESIAN_POINT('Ctrl Pts',(5.5953933622269,30.4470242437925,122.993200632807));
#95194=CARTESIAN_POINT('Ctrl Pts',(5.5992497078151,30.516436394182,123.009930047454));
#95195=CARTESIAN_POINT('Ctrl Pts',(5.6031060534033,30.584812518415,123.03023050059));
#95196=CARTESIAN_POINT('Ctrl Pts',(5.60696125964862,30.6531684411778,123.050524956034));
#95197=CARTESIAN_POINT('Ctrl Pts',(5.61081646589394,30.7204884800164,123.074388217214));
#95198=CARTESIAN_POINT('Ctrl Pts',(5.61467167213927,30.7863805132784,123.101684101411));
#95199=CARTESIAN_POINT('Ctrl Pts',(5.61852702899051,30.8522751206518,123.128981051938));
#95200=CARTESIAN_POINT('Ctrl Pts',(5.62238238584174,30.9167411637344,123.159710703763));
#95201=CARTESIAN_POINT('Ctrl Pts',(5.62623774269298,30.9794067665987,123.193688856249));
#95202=CARTESIAN_POINT('Ctrl Pts',(5.63009713516154,31.042137965049,123.227702575564));
#95203=CARTESIAN_POINT('Ctrl Pts',(5.6339565276301,31.1030645332285,123.264971351448));
#95204=CARTESIAN_POINT('Ctrl Pts',(5.63781592009865,31.161840276128,123.305265585625));
#95205=CARTESIAN_POINT('Ctrl Pts',(5.64167749770208,31.2206492970438,123.345582633842));
#95206=CARTESIAN_POINT('Ctrl Pts',(5.6455390753055,31.2773046824779,123.388928255031));
#95207=CARTESIAN_POINT('Ctrl Pts',(5.64940065290893,31.3314924733828,123.435031835524));
#95208=CARTESIAN_POINT('Ctrl Pts',(5.6532689870238,31.3857750753901,123.481216082366));
#95209=CARTESIAN_POINT('Ctrl Pts',(5.65713732113867,31.4375811096654,123.530167589092));
#95210=CARTESIAN_POINT('Ctrl Pts',(5.66100565525355,31.4866332085155,123.581578600754));
#95211=CARTESIAN_POINT('Ctrl Pts',(5.66330337442454,31.5157692512043,123.612115794178));
#95212=CARTESIAN_POINT('Ctrl Pts',(5.66560109359554,31.5439344211598,123.64352007997));
#95213=CARTESIAN_POINT('Ctrl Pts',(5.66789881276654,31.5710776346151,123.675721846245));
#95214=CARTESIAN_POINT('Ctrl Pts',(5.67174314546748,31.6164911666133,123.729598884259));
#95215=CARTESIAN_POINT('Ctrl Pts',(5.67558747816843,31.6592258384196,123.785928448142));
#95216=CARTESIAN_POINT('Ctrl Pts',(5.67943181086938,31.6990035717014,123.844411653812));
#95217=CARTESIAN_POINT('Ctrl Pts',(5.68327073565044,31.7387253486413,123.90281258968));
#95218=CARTESIAN_POINT('Ctrl Pts',(5.6871096604315,31.7754981613695,123.963360756745));
#95219=CARTESIAN_POINT('Ctrl Pts',(5.69094858521257,31.8090834220943,124.02572348155));
#95220=CARTESIAN_POINT('Ctrl Pts',(5.69478343427781,31.8426330259657,124.088019996997));
#95221=CARTESIAN_POINT('Ctrl Pts',(5.69861828334306,31.8730015594205,124.152126817328));
#95222=CARTESIAN_POINT('Ctrl Pts',(5.70245313240831,31.8999941282689,124.217683008593));
#95223=CARTESIAN_POINT('Ctrl Pts',(5.70628582152479,31.9269714937638,124.283202275846));
#95224=CARTESIAN_POINT('Ctrl Pts',(5.71011851064127,31.9505764742472,124.350168842788));
#95225=CARTESIAN_POINT('Ctrl Pts',(5.71395119975776,31.970661212502,124.418199391509));
#95226=CARTESIAN_POINT('Ctrl Pts',(5.71778249936704,31.9907386692143,124.486205276363));
#95227=CARTESIAN_POINT('Ctrl Pts',(5.72161379897631,32.0072982815489,124.555273904177));
#95228=CARTESIAN_POINT('Ctrl Pts',(5.72544509858559,32.0202418689665,124.625006195551));
#95229=CARTESIAN_POINT('Ctrl Pts',(5.72927810286533,32.0331912154092,124.694769513102));
#95230=CARTESIAN_POINT('Ctrl Pts',(5.73311110714508,32.0425212306723,124.765196599798));
#95231=CARTESIAN_POINT('Ctrl Pts',(5.73694411142483,32.048185000157,124.835878802003));
#95232=CARTESIAN_POINT('Ctrl Pts',(5.73993783446244,32.0526086208859,124.891084307044));
#95233=CARTESIAN_POINT('Ctrl Pts',(5.74293155750006,32.0547967824529,124.946445182454));
#95234=CARTESIAN_POINT('Ctrl Pts',(5.74592528053768,32.0547492412566,125.001765801585));
#95235=CARTESIAN_POINT('Origin',(-1.54592528053767,30.,125.));
#95236=CARTESIAN_POINT('',(4.59397334930969,28.7479590808042,126.629230216746));
#95237=CARTESIAN_POINT('',(4.65201706778823,28.7479590808042,126.629230216746));
#95238=CARTESIAN_POINT('',(-1.54592528053767,28.7479590808042,126.629230216746));
#95239=CARTESIAN_POINT('',(5.10407471942417,32.0547498925786,125.000664415722));
#95240=CARTESIAN_POINT('Ctrl Pts',(4.65201706778823,28.7479590808042,126.629230216746));
#95241=CARTESIAN_POINT('Ctrl Pts',(4.65588621633621,28.6915030279502,126.58584451988));
#95242=CARTESIAN_POINT('Ctrl Pts',(4.6597553648842,28.6373884230477,126.53958531662));
#95243=CARTESIAN_POINT('Ctrl Pts',(4.66362451343219,28.5859041009941,126.490748252025));
#95244=CARTESIAN_POINT('Ctrl Pts',(4.66425200887117,28.5775544145276,126.482827895671));
#95245=CARTESIAN_POINT('Ctrl Pts',(4.66487950431016,28.5692738251231,126.474839808126));
#95246=CARTESIAN_POINT('Ctrl Pts',(4.66550699974915,28.5610634645336,126.466785331737));
#95247=CARTESIAN_POINT('Ctrl Pts',(4.66937607309736,28.5104392123683,126.417122245773));
#95248=CARTESIAN_POINT('Ctrl Pts',(4.67324514644557,28.4622899074249,126.364737957514));
#95249=CARTESIAN_POINT('Ctrl Pts',(4.67711421979379,28.4169220079585,126.309909017304));
#95250=CARTESIAN_POINT('Ctrl Pts',(4.68097752818957,28.3716217070509,126.255161772684));
#95251=CARTESIAN_POINT('Ctrl Pts',(4.68484083658536,28.3290948924323,126.197977477701));
#95252=CARTESIAN_POINT('Ctrl Pts',(4.68870414498114,28.2896114797321,126.138669694089));
#95253=CARTESIAN_POINT('Ctrl Pts',(4.69256292147405,28.2501743835496,126.079431482223));
#95254=CARTESIAN_POINT('Ctrl Pts',(4.69642169796697,28.2137738657557,126.018075132076));
#95255=CARTESIAN_POINT('Ctrl Pts',(4.70028047445988,28.1806387041184,125.954946091436));
#95256=CARTESIAN_POINT('Ctrl Pts',(4.70413682004808,28.147524416564,125.891856820054));
#95257=CARTESIAN_POINT('Ctrl Pts',(4.70799316563629,28.1176716292101,125.826997502888));
#95258=CARTESIAN_POINT('Ctrl Pts',(4.7118495112245,28.0912642476934,125.760740028108));
#95259=CARTESIAN_POINT('Ctrl Pts',(4.71570471746983,28.0648646681387,125.694502128852));
#95260=CARTESIAN_POINT('Ctrl Pts',(4.71955992371516,28.0419086533008,125.626867343082));
#95261=CARTESIAN_POINT('Ctrl Pts',(4.72341512996049,28.0225321258002,125.558227882686));
#95262=CARTESIAN_POINT('Ctrl Pts',(4.72727048681174,28.0031548413441,125.489585740848));
#95263=CARTESIAN_POINT('Ctrl Pts',(4.73112584366298,27.9873574517059,125.419939314574));
#95264=CARTESIAN_POINT('Ctrl Pts',(4.73498120051423,27.9752256400638,125.349694658016));
#95265=CARTESIAN_POINT('Ctrl Pts',(4.73884059298279,27.963081129377,125.279376472453));
#95266=CARTESIAN_POINT('Ctrl Pts',(4.74269998545134,27.9546099389754,125.208459286248));
#95267=CARTESIAN_POINT('Ctrl Pts',(4.7465593779199,27.9498462038099,125.137357105631));
#95268=CARTESIAN_POINT('Ctrl Pts',(4.75042095552334,27.9450797714831,125.066214667938));
#95269=CARTESIAN_POINT('Ctrl Pts',(4.75428253312677,27.9440249802595,124.994887513288));
#95270=CARTESIAN_POINT('Ctrl Pts',(4.75814411073021,27.9466637979444,124.923789739352));
#95271=CARTESIAN_POINT('Ctrl Pts',(4.76201244484508,27.9493072327066,124.852567567315));
#95272=CARTESIAN_POINT('Ctrl Pts',(4.76588077895995,27.9556571358942,124.78157606129));
#95273=CARTESIAN_POINT('Ctrl Pts',(4.76974911307482,27.9656436525551,124.711223591492));
#95274=CARTESIAN_POINT('Ctrl Pts',(4.77204683224578,27.9715754594005,124.669435521026));
#95275=CARTESIAN_POINT('Ctrl Pts',(4.77434455141674,27.9787893326922,124.627872725201));
#95276=CARTESIAN_POINT('Ctrl Pts',(4.7766422705877,27.9872622538326,124.586618423665));
#95277=CARTESIAN_POINT('Ctrl Pts',(4.78051134393592,28.0015295993726,124.517151310107));
#95278=CARTESIAN_POINT('Ctrl Pts',(4.78438041728413,28.0194254679784,124.448287625122));
#95279=CARTESIAN_POINT('Ctrl Pts',(4.78824949063234,28.0408837296111,124.380434828612));
#95280=CARTESIAN_POINT('Ctrl Pts',(4.79211279902813,28.0623100182503,124.312683133349));
#95281=CARTESIAN_POINT('Ctrl Pts',(4.79597610742391,28.0872880184085,124.245939796136));
#95282=CARTESIAN_POINT('Ctrl Pts',(4.79983941581969,28.1157006857585,124.180601649471));
#95283=CARTESIAN_POINT('Ctrl Pts',(4.8036981923126,28.1440800232691,124.115340148548));
#95284=CARTESIAN_POINT('Ctrl Pts',(4.80755696880551,28.1758858320734,124.051481007265));
#95285=CARTESIAN_POINT('Ctrl Pts',(4.81141574529843,28.2109519672824,123.989403790266));
#95286=CARTESIAN_POINT('Ctrl Pts',(4.81527209088663,28.2459960119574,123.92736567991));
#95287=CARTESIAN_POINT('Ctrl Pts',(4.81912843647484,28.2842960697706,123.867107688676));
#95288=CARTESIAN_POINT('Ctrl Pts',(4.82298478206304,28.3256394450813,123.808986022487));
#95289=CARTESIAN_POINT('Ctrl Pts',(4.82683998830837,28.3669706056465,123.750881528126));
#95290=CARTESIAN_POINT('Ctrl Pts',(4.8306951945537,28.4113430172466,123.694912501404));
#95291=CARTESIAN_POINT('Ctrl Pts',(4.83455040079903,28.4585008851387,123.641405858477));
#95292=CARTESIAN_POINT('Ctrl Pts',(4.83840575765028,28.5056605952808,123.58789712528));
#95293=CARTESIAN_POINT('Ctrl Pts',(4.84226111450152,28.5556056549012,123.536851329845));
#95294=CARTESIAN_POINT('Ctrl Pts',(4.84611647135276,28.608041391699,123.488560687531));
#95295=CARTESIAN_POINT('Ctrl Pts',(4.84997586382132,28.6605320159108,123.440219496705));
#95296=CARTESIAN_POINT('Ctrl Pts',(4.85383525628988,28.7155181636508,123.394639545818));
#95297=CARTESIAN_POINT('Ctrl Pts',(4.85769464875844,28.772670523823,123.352074055242));
#95298=CARTESIAN_POINT('Ctrl Pts',(4.86155622636187,28.8298552428746,123.309484464671));
#95299=CARTESIAN_POINT('Ctrl Pts',(4.8654178039653,28.8892082115199,123.26991300162));
#95300=CARTESIAN_POINT('Ctrl Pts',(4.86927938156873,28.9503717482536,123.233569108163));
#95301=CARTESIAN_POINT('Ctrl Pts',(4.8731477156836,29.0116423013879,123.197161624651));
#95302=CARTESIAN_POINT('Ctrl Pts',(4.87701604979848,29.074729317315,123.163993211672));
#95303=CARTESIAN_POINT('Ctrl Pts',(4.88088438391335,29.1392518196133,123.134226666376));
#95304=CARTESIAN_POINT('Ctrl Pts',(4.88318210308432,29.177576996831,123.116545887067));
#95305=CARTESIAN_POINT('Ctrl Pts',(4.88547982225529,29.2164082578054,123.100064408499));
#95306=CARTESIAN_POINT('Ctrl Pts',(4.88777754142626,29.2556632016255,123.084808027093));
#95307=CARTESIAN_POINT('Ctrl Pts',(4.89164661477448,29.3217636454217,123.059118178033));
#95308=CARTESIAN_POINT('Ctrl Pts',(4.8955156881227,29.389325103184,123.036804087238));
#95309=CARTESIAN_POINT('Ctrl Pts',(4.89938476147091,29.4579693835414,123.018031187601));
#95310=CARTESIAN_POINT('Ctrl Pts',(4.9032480698667,29.5265113833331,122.999286259746));
#95311=CARTESIAN_POINT('Ctrl Pts',(4.90711137826249,29.5961325383754,122.984072176635));
#95312=CARTESIAN_POINT('Ctrl Pts',(4.91097468665828,29.6664359717598,122.972505831928));
#95313=CARTESIAN_POINT('Ctrl Pts',(4.9148334631512,29.7366569348108,122.960953055269));
#95314=CARTESIAN_POINT('Ctrl Pts',(4.91869223964411,29.807558109412,122.953039595899));
#95315=CARTESIAN_POINT('Ctrl Pts',(4.92255101613703,29.8787304957541,122.948831730491));
#95316=CARTESIAN_POINT('Ctrl Pts',(4.92640736172524,29.9498580457888,122.944626515902));
#95317=CARTESIAN_POINT('Ctrl Pts',(4.93026370731345,30.0212559847986,122.944122292457));
#95318=CARTESIAN_POINT('Ctrl Pts',(4.93412005290166,30.0925096901938,122.947333558583));
#95319=CARTESIAN_POINT('Ctrl Pts',(4.93797525914699,30.1637423439484,122.950543875952));
#95320=CARTESIAN_POINT('Ctrl Pts',(4.94183046539232,30.2348303636584,122.957467481741));
#95321=CARTESIAN_POINT('Ctrl Pts',(4.94568567163766,30.3053603589397,122.968066779225));
#95322=CARTESIAN_POINT('Ctrl Pts',(4.94954102848891,30.3758931095171,122.978666490777));
#95323=CARTESIAN_POINT('Ctrl Pts',(4.95339638534016,30.4458673123213,122.992942104738));
#95324=CARTESIAN_POINT('Ctrl Pts',(4.95725174219141,30.5148776448284,123.010804541189));
#95325=CARTESIAN_POINT('Ctrl Pts',(4.96111113465997,30.5839602143043,123.028685675249));
#95326=CARTESIAN_POINT('Ctrl Pts',(4.96497052712853,30.6520764281672,123.050161004701));
#95327=CARTESIAN_POINT('Ctrl Pts',(4.96882991959709,30.7188349384432,123.075091198583));
#95328=CARTESIAN_POINT('Ctrl Pts',(4.97269149720053,30.7856312464686,123.100035507598));
#95329=CARTESIAN_POINT('Ctrl Pts',(4.97655307480396,30.8510678748066,123.128438381514));
#95330=CARTESIAN_POINT('Ctrl Pts',(4.9804146524074,30.9147748684468,123.160112910378));
#95331=CARTESIAN_POINT('Ctrl Pts',(4.98428298652227,30.9785933287141,123.191842859419));
#95332=CARTESIAN_POINT('Ctrl Pts',(4.98815132063715,31.0406756889188,123.226855653503));
#95333=CARTESIAN_POINT('Ctrl Pts',(4.99201965475202,31.1006785481559,123.264919513069));
#95334=CARTESIAN_POINT('Ctrl Pts',(4.99431737392296,31.1363191406915,123.287528744135));
#95335=CARTESIAN_POINT('Ctrl Pts',(4.99661509309389,31.1712266300885,123.311213615859));
#95336=CARTESIAN_POINT('Ctrl Pts',(4.99891281226483,31.2053346523551,123.335918890699));
#95337=CARTESIAN_POINT('Ctrl Pts',(5.00275064676246,31.2623046015798,123.377183618458));
#95338=CARTESIAN_POINT('Ctrl Pts',(5.00658848126009,31.3172734889279,123.421464682555));
#95339=CARTESIAN_POINT('Ctrl Pts',(5.01042631575773,31.3699002709867,123.468539647901));
#95340=CARTESIAN_POINT('Ctrl Pts',(5.01432833257716,31.4234071611021,123.516401875068));
#95341=CARTESIAN_POINT('Ctrl Pts',(5.0182303493966,31.4744924192991,123.567152086287));
#95342=CARTESIAN_POINT('Ctrl Pts',(5.02213236621603,31.5228283369254,123.620510449928));
#95343=CARTESIAN_POINT('Ctrl Pts',(5.02595997436975,31.5702425232257,123.672851307796));
#95344=CARTESIAN_POINT('Ctrl Pts',(5.02978758252347,31.615010950279,123.727701341682));
#95345=CARTESIAN_POINT('Ctrl Pts',(5.03361519067718,31.656859368321,123.784757392079));
#95346=CARTESIAN_POINT('Ctrl Pts',(5.03744050268938,31.6986826819409,123.841779215157));
#95347=CARTESIAN_POINT('Ctrl Pts',(5.04126581470157,31.7375891686524,123.901004032373));
#95348=CARTESIAN_POINT('Ctrl Pts',(5.04509112671377,31.7733450235495,123.962095866685));
#95349=CARTESIAN_POINT('Ctrl Pts',(5.04891547573736,31.8090918772252,124.023172321666));
#95350=CARTESIAN_POINT('Ctrl Pts',(5.05273982476096,31.8416894240058,124.086114434042));
#95351=CARTESIAN_POINT('Ctrl Pts',(5.05656417378455,31.8709483479536,124.150559100473));
#95352=CARTESIAN_POINT('Ctrl Pts',(5.06052338592119,31.9012390683048,124.217276365006));
#95353=CARTESIAN_POINT('Ctrl Pts',(5.06448259805782,31.9279510192918,124.285603645033));
#95354=CARTESIAN_POINT('Ctrl Pts',(5.06844181019445,31.9509280911051,124.355114625816));
#95355=CARTESIAN_POINT('Ctrl Pts',(5.07227054686677,31.9731479556736,124.422334878751));
#95356=CARTESIAN_POINT('Ctrl Pts',(5.07609928353909,31.9918752129522,124.490661515233));
#95357=CARTESIAN_POINT('Ctrl Pts',(5.07992802021141,32.0070199603934,124.559695058985));
#95358=CARTESIAN_POINT('Ctrl Pts',(5.08395247008021,32.0229388605606,124.632257384334));
#95359=CARTESIAN_POINT('Ctrl Pts',(5.087976919949,32.0348990846249,124.70560020682));
#95360=CARTESIAN_POINT('Ctrl Pts',(5.09200136981779,32.0428577974624,124.779252221195));
#95361=CARTESIAN_POINT('Ctrl Pts',(5.09602581968658,32.0508165102998,124.85290423557));
#95362=CARTESIAN_POINT('Ctrl Pts',(5.10005026955538,32.0547737561236,124.92686481261));
#95363=CARTESIAN_POINT('Ctrl Pts',(5.10407471942417,32.0547498925786,125.000664415722));
#95364=CARTESIAN_POINT('Ctrl Pts',(5.10407471946233,32.0547498925784,125.000664416421));
#95365=CARTESIAN_POINT('Ctrl Pts',(5.10606584067601,32.0547380859309,125.037177221924));
#95366=CARTESIAN_POINT('Ctrl Pts',(5.1080569618897,32.0537530962652,125.073673053094));
#95367=CARTESIAN_POINT('Ctrl Pts',(5.11004808310338,32.0517972511101,125.110116315035));
#95368=CARTESIAN_POINT('Ctrl Pts',(5.11391715645159,32.0479967248987,125.180931518313));
#95369=CARTESIAN_POINT('Ctrl Pts',(5.1177862297998,32.0405183040001,125.251688443372));
#95370=CARTESIAN_POINT('Ctrl Pts',(5.12165530314801,32.0293669196201,125.321974328249));
#95371=CARTESIAN_POINT('Ctrl Pts',(5.12551861154379,32.0182321508984,125.392155486556));
#95372=CARTESIAN_POINT('Ctrl Pts',(5.12938191993958,32.0034353574457,125.461866521965));
#95373=CARTESIAN_POINT('Ctrl Pts',(5.13324522833536,31.985033398107,125.53069762662));
#95374=CARTESIAN_POINT('Ctrl Pts',(5.13710400482826,31.9666530254199,125.599447988075));
#95375=CARTESIAN_POINT('Ctrl Pts',(5.14096278132117,31.9446760121003,125.667320002076));
#95376=CARTESIAN_POINT('Ctrl Pts',(5.14482155781407,31.9192103364247,125.733913650957));
#95377=CARTESIAN_POINT('Ctrl Pts',(5.14867790340227,31.8937607033032,125.800465347987));
#95378=CARTESIAN_POINT('Ctrl Pts',(5.15253424899047,31.864826941218,125.865739824988));
#95379=CARTESIAN_POINT('Ctrl Pts',(5.15639059457868,31.8325665301762,125.929353256291));
#95380=CARTESIAN_POINT('Ctrl Pts',(5.160245800824,31.8003156503523,125.992947893243));
#95381=CARTESIAN_POINT('Ctrl Pts',(5.16410100706933,31.764740292392,126.05488202575));
#95382=CARTESIAN_POINT('Ctrl Pts',(5.16795621331465,31.7260449047639,126.114794397743));
#95383=CARTESIAN_POINT('Ctrl Pts',(5.17181157016589,31.6873480054775,126.174709110248));
#95384=CARTESIAN_POINT('Ctrl Pts',(5.17566692701713,31.6455310999461,126.232601498554));
#95385=CARTESIAN_POINT('Ctrl Pts',(5.17952228386837,31.6008422332886,126.288138853781));
#95386=CARTESIAN_POINT('Ctrl Pts',(5.18338167633693,31.5561065882988,126.343734343058));
#95387=CARTESIAN_POINT('Ctrl Pts',(5.18724106880548,31.5084932862153,126.396969499024));
#95388=CARTESIAN_POINT('Ctrl Pts',(5.19110046127403,31.4582904142315,126.447545035659));
#95389=CARTESIAN_POINT('Ctrl Pts',(5.19496203887746,31.4080591180729,126.498149207466));
#95390=CARTESIAN_POINT('Ctrl Pts',(5.19882361648089,31.3552356931987,126.546090435647));
#95391=CARTESIAN_POINT('Ctrl Pts',(5.20268519408432,31.3001427797347,126.591108517608));
#95392=CARTESIAN_POINT('Ctrl Pts',(5.20655352819918,31.244953471497,126.636205366647));
#95393=CARTESIAN_POINT('Ctrl Pts',(5.21042186231405,31.1874871385065,126.678368570637));
#95394=CARTESIAN_POINT('Ctrl Pts',(5.21429019642891,31.1280963799313,126.717380598495));
#95395=CARTESIAN_POINT('Ctrl Pts',(5.21658791559992,31.0928193639066,126.740553024052));
#95396=CARTESIAN_POINT('Ctrl Pts',(5.21888563477093,31.0568638927513,126.762614530318));
#95397=CARTESIAN_POINT('Ctrl Pts',(5.22118335394194,31.0203076268374,126.783527378292));
#95398=CARTESIAN_POINT('Ctrl Pts',(5.22505242729016,30.958751421039,126.818742013638));
#95399=CARTESIAN_POINT('Ctrl Pts',(5.22892150063837,30.8952494193226,126.85083508144));
#95400=CARTESIAN_POINT('Ctrl Pts',(5.23279057398659,30.8301510755014,126.879586857356));
#95401=CARTESIAN_POINT('Ctrl Pts',(5.23665388238237,30.7651497287701,126.908295792879));
#95402=CARTESIAN_POINT('Ctrl Pts',(5.24051719077816,30.6985572020688,126.933673124138));
#95403=CARTESIAN_POINT('Ctrl Pts',(5.24438049917394,30.6307486310241,126.955544355662));
#95404=CARTESIAN_POINT('Ctrl Pts',(5.24823927566686,30.563019603683,126.977389930861));
#95405=CARTESIAN_POINT('Ctrl Pts',(5.25209805215977,30.4940778255901,126.995737427486));
#95406=CARTESIAN_POINT('Ctrl Pts',(5.25595682865268,30.4243179325502,127.010460607576));
#95407=CARTESIAN_POINT('Ctrl Pts',(5.25981317424089,30.3546019859924,127.025174512538));
#95408=CARTESIAN_POINT('Ctrl Pts',(5.26366951982909,30.2840694211964,127.036268530721));
#95409=CARTESIAN_POINT('Ctrl Pts',(5.2675258654173,30.2131281183253,127.04366679468));
#95410=CARTESIAN_POINT('Ctrl Pts',(5.27138107166263,30.1422077747966,127.051062872851));
#95411=CARTESIAN_POINT('Ctrl Pts',(5.27523627790796,30.0708794158375,127.054765314154));
#95412=CARTESIAN_POINT('Ctrl Pts',(5.2790914841533,29.9995574339136,127.054749952339));
#95413=CARTESIAN_POINT('Ctrl Pts',(5.28294684100454,29.9282326657543,127.054734589923));
#95414=CARTESIAN_POINT('Ctrl Pts',(5.28680219785578,29.8569147609102,127.051001138343));
#95415=CARTESIAN_POINT('Ctrl Pts',(5.29065755470703,29.7860177733689,127.04357754176));
#95416=CARTESIAN_POINT('Ctrl Pts',(5.29451694717559,29.7150465739914,127.036146174484));
#95417=CARTESIAN_POINT('Ctrl Pts',(5.29837633964415,29.6444976555832,127.02501700212));
#95418=CARTESIAN_POINT('Ctrl Pts',(5.30223573211271,29.5747787095142,127.010269737278));
#95419=CARTESIAN_POINT('Ctrl Pts',(5.30609730971614,29.5050202895379,126.995514122739));
#95420=CARTESIAN_POINT('Ctrl Pts',(5.30995888731958,29.4360932469752,126.977136462971));
#95421=CARTESIAN_POINT('Ctrl Pts',(5.31382046492301,29.3683911777763,126.955266697458));
#95422=CARTESIAN_POINT('Ctrl Pts',(5.31768879903788,29.3005706518605,126.933358666931));
#95423=CARTESIAN_POINT('Ctrl Pts',(5.32155713315276,29.2339798324881,126.907946505012));
#95424=CARTESIAN_POINT('Ctrl Pts',(5.32542546726763,29.1689927141232,126.879208464572));
#95425=CARTESIAN_POINT('Ctrl Pts',(5.32772318643859,29.130391563525,126.862138598192));
#95426=CARTESIAN_POINT('Ctrl Pts',(5.33002090560955,29.0923557749172,126.843896209379));
#95427=CARTESIAN_POINT('Ctrl Pts',(5.33231862478051,29.0549591746737,126.824526075716));
#95428=CARTESIAN_POINT('Ctrl Pts',(5.33618678852251,28.9920027546881,126.791916847547));
#95429=CARTESIAN_POINT('Ctrl Pts',(5.34005495226452,28.9306128321502,126.755981411748));
#95430=CARTESIAN_POINT('Ctrl Pts',(5.34392311600652,28.8711632767676,126.716894060442));
#95431=CARTESIAN_POINT('Ctrl Pts',(5.34666123635929,28.8290812842738,126.689225668077));
#95432=CARTESIAN_POINT('Ctrl Pts',(5.34939935671205,28.7879712291961,126.659979000151));
#95433=CARTESIAN_POINT('Ctrl Pts',(5.35213747706482,28.7479590808042,126.629230216746));
#95434=CARTESIAN_POINT('',(5.04592528049233,32.0547497417017,124.998969719981));
#95435=CARTESIAN_POINT('Ctrl Pts',(5.04592528053768,32.0547497417021,124.998969720821));
#95436=CARTESIAN_POINT('Ctrl Pts',(5.04983580638861,32.0547860725486,125.071426584005));
#95437=CARTESIAN_POINT('Ctrl Pts',(5.05374633223954,32.0509854787254,125.143878332678));
#95438=CARTESIAN_POINT('Ctrl Pts',(5.05765685809047,32.0433759542004,125.215898754734));
#95439=CARTESIAN_POINT('Ctrl Pts',(5.06156889758468,32.0357634842644,125.287947053662));
#95440=CARTESIAN_POINT('Ctrl Pts',(5.06548093707889,32.0243392038325,125.359563230797));
#95441=CARTESIAN_POINT('Ctrl Pts',(5.0693929765731,32.0091827682208,125.430327975368));
#95442=CARTESIAN_POINT('Ctrl Pts',(5.07331083119333,31.9940038030351,125.501197909549));
#95443=CARTESIAN_POINT('Ctrl Pts',(5.07722868581356,31.9750817055283,125.571213427758));
#95444=CARTESIAN_POINT('Ctrl Pts',(5.08114654043379,31.9525468000694,125.639967621086));
#95445=CARTESIAN_POINT('Ctrl Pts',(5.0850675173693,31.9299939355267,125.708776607735));
#95446=CARTESIAN_POINT('Ctrl Pts',(5.08898849430482,31.9038226982916,125.776321833249));
#95447=CARTESIAN_POINT('Ctrl Pts',(5.09290947124033,31.8742116465834,125.842216282383));
#95448=CARTESIAN_POINT('Ctrl Pts',(5.09683849198294,31.8445398483848,125.908245912684));
#95449=CARTESIAN_POINT('Ctrl Pts',(5.10076751272554,31.8114143545465,125.972617587759));
#95450=CARTESIAN_POINT('Ctrl Pts',(5.10469653346815,31.7750596081158,126.034969057574));
#95451=CARTESIAN_POINT('Ctrl Pts',(5.10720517517001,31.7518474545204,126.07477986734));
#95452=CARTESIAN_POINT('Ctrl Pts',(5.10971381687188,31.7273197264878,126.113767668479));
#95453=CARTESIAN_POINT('Ctrl Pts',(5.11222245857374,31.7015435920206,126.151845027316));
#95454=CARTESIAN_POINT('Ctrl Pts',(5.11609153192196,31.661789108623,126.210571665775));
#95455=CARTESIAN_POINT('Ctrl Pts',(5.11996060527018,31.6189128733263,126.267352804102));
#95456=CARTESIAN_POINT('Ctrl Pts',(5.12382967861839,31.5731318462583,126.321837265622));
#95457=CARTESIAN_POINT('Ctrl Pts',(5.12769298701418,31.5274190333129,126.376240544828));
#95458=CARTESIAN_POINT('Ctrl Pts',(5.13155629540996,31.4788103298453,126.428353571045));
#95459=CARTESIAN_POINT('Ctrl Pts',(5.13541960380575,31.4275656730796,126.477854462234));
#95460=CARTESIAN_POINT('Ctrl Pts',(5.13927838029866,31.3763811295078,126.527297285775));
#95461=CARTESIAN_POINT('Ctrl Pts',(5.14313715679157,31.3225671223705,126.574133724953));
#95462=CARTESIAN_POINT('Ctrl Pts',(5.14699593328449,31.2664223501252,126.618076634033));
#95463=CARTESIAN_POINT('Ctrl Pts',(5.15085227887269,31.2103129472752,126.661991860498));
#95464=CARTESIAN_POINT('Ctrl Pts',(5.1547086244609,31.151876074057,126.703016874631));
#95465=CARTESIAN_POINT('Ctrl Pts',(5.15856497004911,31.0914445044241,126.740903919308));
#95466=CARTESIAN_POINT('Ctrl Pts',(5.16242017629444,31.0310307890723,126.7787797704));
#95467=CARTESIAN_POINT('Ctrl Pts',(5.16627538253977,30.9686239586422,126.813519234689));
#95468=CARTESIAN_POINT('Ctrl Pts',(5.1701305887851,30.9045854047206,126.844918103349));
#95469=CARTESIAN_POINT('Ctrl Pts',(5.17398594563635,30.840544349095,126.876318198626));
#95470=CARTESIAN_POINT('Ctrl Pts',(5.17784130248759,30.7748718805691,126.904377227293));
#95471=CARTESIAN_POINT('Ctrl Pts',(5.18169665933884,30.7079520380723,126.928937913539));
#95472=CARTESIAN_POINT('Ctrl Pts',(5.1855560518074,30.6409621468395,126.953524308827));
#95473=CARTESIAN_POINT('Ctrl Pts',(5.18941544427596,30.5727227321491,126.974604883981));
#95474=CARTESIAN_POINT('Ctrl Pts',(5.19327483674452,30.5036349212805,126.992071642428));
#95475=CARTESIAN_POINT('Ctrl Pts',(5.19713641434795,30.4345079938446,127.009548290314));
#95476=CARTESIAN_POINT('Ctrl Pts',(5.20099799195139,30.3645321907575,127.023406953932));
#95477=CARTESIAN_POINT('Ctrl Pts',(5.20485956955482,30.2941181062911,127.033590937738));
#95478=CARTESIAN_POINT('Ctrl Pts',(5.2087279036697,30.2235808199586,127.043792740222));
#95479=CARTESIAN_POINT('Ctrl Pts',(5.21259623778457,30.1526042051138,127.050306981796));
#95480=CARTESIAN_POINT('Ctrl Pts',(5.21646457189944,30.0816025369967,127.053128975115));
#95481=CARTESIAN_POINT('Ctrl Pts',(5.21876229107039,30.0394288546939,127.054805187137));
#95482=CARTESIAN_POINT('Ctrl Pts',(5.22106001024135,29.9972463264548,127.055179721477));
#95483=CARTESIAN_POINT('Ctrl Pts',(5.2233577294123,29.9551409540642,127.054260263087));
#95484=CARTESIAN_POINT('Ctrl Pts',(5.22722618552694,29.8842520537394,127.052712256491));
#95485=CARTESIAN_POINT('Ctrl Pts',(5.23109464164159,29.8133045455,127.047487535505));
#95486=CARTESIAN_POINT('Ctrl Pts',(5.23496309775624,29.7427109417857,127.038577911934));
#95487=CARTESIAN_POINT('Ctrl Pts',(5.23882613528347,29.6722162192791,127.029680768166));
#95488=CARTESIAN_POINT('Ctrl Pts',(5.24268917281071,29.6020748954899,127.017109022759));
#95489=CARTESIAN_POINT('Ctrl Pts',(5.24655221033795,29.5326982922555,127.000906463691));
#95490=CARTESIAN_POINT('Ctrl Pts',(5.25049621383355,29.46186761465,126.984364312817));
#95491=CARTESIAN_POINT('Ctrl Pts',(5.25444021732915,29.3918345959394,126.964037416345));
#95492=CARTESIAN_POINT('Ctrl Pts',(5.25838422082475,29.3230296683319,126.940028023648));
#95493=CARTESIAN_POINT('Ctrl Pts',(5.26224043487251,29.2557562674104,126.916553055257));
#95494=CARTESIAN_POINT('Ctrl Pts',(5.26609664892028,29.1896573266088,126.889558019786));
#95495=CARTESIAN_POINT('Ctrl Pts',(5.26995286296804,29.1251210615865,126.859189179621));
#95496=CARTESIAN_POINT('Ctrl Pts',(5.27394076118756,29.0583809757952,126.827783287178));
#95497=CARTESIAN_POINT('Ctrl Pts',(5.27792865940708,28.9933127468431,126.792769154415));
#95498=CARTESIAN_POINT('Ctrl Pts',(5.2819165576266,28.9303221637766,126.754362245716));
#95499=CARTESIAN_POINT('Ctrl Pts',(5.28590445584612,28.8673315807101,126.715955337016));
#95500=CARTESIAN_POINT('Ctrl Pts',(5.28989235406564,28.8064191309432,126.674155957848));
#95501=CARTESIAN_POINT('Ctrl Pts',(5.29388025228516,28.7479590808042,126.629230216746));
#95502=CARTESIAN_POINT('Ctrl Pts',(4.59397334930969,28.7479590808042,126.629230216746));
#95503=CARTESIAN_POINT('Ctrl Pts',(4.59782931953988,28.6914508880382,126.585804451078));
#95504=CARTESIAN_POINT('Ctrl Pts',(4.60168528977007,28.6371690268486,126.539408000481));
#95505=CARTESIAN_POINT('Ctrl Pts',(4.60554126000026,28.5854350349871,126.490303164547));
#95506=CARTESIAN_POINT('Ctrl Pts',(4.60939638682258,28.5337123587876,126.441209069205));
#95507=CARTESIAN_POINT('Ctrl Pts',(4.6132515136449,28.4845367973786,126.389408099351));
#95508=CARTESIAN_POINT('Ctrl Pts',(4.61710664046723,28.4381945849889,126.335200886811));
#95509=CARTESIAN_POINT('Ctrl Pts',(4.62096221364327,28.391847007012,126.280987398061));
#95510=CARTESIAN_POINT('Ctrl Pts',(4.62481778681932,28.3483337430163,126.224367484424));
#95511=CARTESIAN_POINT('Ctrl Pts',(4.62867335999537,28.3079009955974,126.165675135619));
#95512=CARTESIAN_POINT('Ctrl Pts',(4.6325331508483,28.2674240181103,126.106918582258));
#95513=CARTESIAN_POINT('Ctrl Pts',(4.63639294170124,28.2300345569746,126.046085471014));
#95514=CARTESIAN_POINT('Ctrl Pts',(4.64025273255417,28.1959351466428,125.983538289738));
#95515=CARTESIAN_POINT('Ctrl Pts',(4.64411497429854,28.1618140838547,125.92095139223));
#95516=CARTESIAN_POINT('Ctrl Pts',(4.6479772160429,28.1309874387423,125.856648696817));
#95517=CARTESIAN_POINT('Ctrl Pts',(4.65183945778726,28.103610290807,125.791014306677));
#95518=CARTESIAN_POINT('Ctrl Pts',(4.65570819068367,28.0761871309332,125.725269606815));
#95519=CARTESIAN_POINT('Ctrl Pts',(4.65957692358008,28.0522251990167,125.658189203244));
#95520=CARTESIAN_POINT('Ctrl Pts',(4.66344565647649,28.0318299997003,125.590173205441));
#95521=CARTESIAN_POINT('Ctrl Pts',(4.66485756272416,28.0243867075143,125.565350552957));
#95522=CARTESIAN_POINT('Ctrl Pts',(4.66626946897183,28.017417978701,125.540403387799));
#95523=CARTESIAN_POINT('Ctrl Pts',(4.6676813752195,28.0109272352027,125.515351432366));
#95524=CARTESIAN_POINT('Ctrl Pts',(4.67155044856771,27.9931405282447,125.446701085896));
#95525=CARTESIAN_POINT('Ctrl Pts',(4.67541952191593,27.9788772247288,125.376994361717));
#95526=CARTESIAN_POINT('Ctrl Pts',(4.67928859526414,27.9682574135064,125.306626197068));
#95527=CARTESIAN_POINT('Ctrl Pts',(4.68315190365993,27.9576534258936,125.236362881586));
#95528=CARTESIAN_POINT('Ctrl Pts',(4.68701521205572,27.9506822263921,125.16544055836));
#95529=CARTESIAN_POINT('Ctrl Pts',(4.69087852045151,27.9474135131066,125.094267047915));
#95530=CARTESIAN_POINT('Ctrl Pts',(4.69473729694442,27.9441486342267,125.02317702846));
#95531=CARTESIAN_POINT('Ctrl Pts',(4.69859607343734,27.9445776365808,124.951836889996));
#95532=CARTESIAN_POINT('Ctrl Pts',(4.70245484993025,27.9487185311775,124.880660575812));
#95533=CARTESIAN_POINT('Ctrl Pts',(4.70631119551846,27.9528568171443,124.809529100409));
#95534=CARTESIAN_POINT('Ctrl Pts',(4.71016754110667,27.960702327913,124.73856172835));
#95535=CARTESIAN_POINT('Ctrl Pts',(4.71402388669488,27.9722209939527,124.668171934379));
#95536=CARTESIAN_POINT('Ctrl Pts',(4.71787909294022,27.9837362568456,124.597802936809));
#95537=CARTESIAN_POINT('Ctrl Pts',(4.72173429918555,27.9989224421391,124.5280116577));
#95538=CARTESIAN_POINT('Ctrl Pts',(4.72558950543088,28.0176938863608,124.459204258219));
#95539=CARTESIAN_POINT('Ctrl Pts',(4.72944486228212,28.0364660639001,124.390394170736));
#95540=CARTESIAN_POINT('Ctrl Pts',(4.73330021913336,28.0588236484584,124.322568507269));
#95541=CARTESIAN_POINT('Ctrl Pts',(4.73715557598461,28.0846307894568,124.256119398154));
#95542=CARTESIAN_POINT('Ctrl Pts',(4.74101496845316,28.1104649442308,124.189600733046));
#95543=CARTESIAN_POINT('Ctrl Pts',(4.74487436092172,28.1397556872703,124.124461952444));
#95544=CARTESIAN_POINT('Ctrl Pts',(4.74873375339028,28.1723188950762,124.061075433698));
#95545=CARTESIAN_POINT('Ctrl Pts',(4.75259533099371,28.2049005397219,123.997653026379));
#95546=CARTESIAN_POINT('Ctrl Pts',(4.75645690859714,28.2407580932328,123.935985276046));
#95547=CARTESIAN_POINT('Ctrl Pts',(4.76031848620058,28.2796626801174,123.876417751867));
#95548=CARTESIAN_POINT('Ctrl Pts',(4.76418682031545,28.3186353374418,123.816746003794));
#95549=CARTESIAN_POINT('Ctrl Pts',(4.76805515443032,28.3606653857265,123.759182211013));
#95550=CARTESIAN_POINT('Ctrl Pts',(4.77192348854519,28.4054824916262,123.704040325477));
#95551=CARTESIAN_POINT('Ctrl Pts',(4.77422120771614,28.4321030265527,123.671287061732));
#95552=CARTESIAN_POINT('Ctrl Pts',(4.7765189268871,28.4597061291631,123.639387615171));
#95553=CARTESIAN_POINT('Ctrl Pts',(4.77881664605805,28.4882291828091,123.60840143763));
#95554=CARTESIAN_POINT('Ctrl Pts',(4.78268571940627,28.5362584581298,123.556224567975));
#95555=CARTESIAN_POINT('Ctrl Pts',(4.78655479275448,28.5870862098637,123.506434921696));
#95556=CARTESIAN_POINT('Ctrl Pts',(4.79042386610269,28.6404457659139,123.459347590441));
#95557=CARTESIAN_POINT('Ctrl Pts',(4.79428717449847,28.6937258157686,123.412330419714));
#95558=CARTESIAN_POINT('Ctrl Pts',(4.79815048289426,28.7495298205365,123.368007890384));
#95559=CARTESIAN_POINT('Ctrl Pts',(4.80201379129004,28.807552954178,123.326659746074));
#95560=CARTESIAN_POINT('Ctrl Pts',(4.80587256778296,28.8655080230472,123.285360105728));
#95561=CARTESIAN_POINT('Ctrl Pts',(4.80973134427587,28.9256766563069,123.24702820034));
#95562=CARTESIAN_POINT('Ctrl Pts',(4.81359012076878,28.9877208506948,123.211903669714));
#95563=CARTESIAN_POINT('Ctrl Pts',(4.81744646635699,29.0497259592419,123.17680126641));
#95564=CARTESIAN_POINT('Ctrl Pts',(4.82130281194519,29.113603863011,123.144902467903));
#95565=CARTESIAN_POINT('Ctrl Pts',(4.8251591575334,29.1789887057697,123.116402904747));
#95566=CARTESIAN_POINT('Ctrl Pts',(4.82901436377873,29.2443542308214,123.08791176168));
#95567=CARTESIAN_POINT('Ctrl Pts',(4.83286957002406,29.3112253658995,123.062818054167));
#95568=CARTESIAN_POINT('Ctrl Pts',(4.83672477626939,29.379214416526,123.041270099822));
#95569=CARTESIAN_POINT('Ctrl Pts',(4.84058013312064,29.4472061231851,123.019721303694));
#95570=CARTESIAN_POINT('Ctrl Pts',(4.84443548997189,29.5163153683473,123.001718680408));
#95571=CARTESIAN_POINT('Ctrl Pts',(4.84829084682315,29.5861390257614,122.987360773387));
#95572=CARTESIAN_POINT('Ctrl Pts',(4.8521502392917,29.6560357714966,122.972987837143));
#95573=CARTESIAN_POINT('Ctrl Pts',(4.85600963176026,29.7266479454857,122.962267331063));
#95574=CARTESIAN_POINT('Ctrl Pts',(4.85986902422882,29.7975628353236,122.955246529075));
#95575=CARTESIAN_POINT('Ctrl Pts',(4.86373060183225,29.8685178761958,122.948221752007));
#95576=CARTESIAN_POINT('Ctrl Pts',(4.86759217943569,29.9397754886193,122.944900871601));
#95577=CARTESIAN_POINT('Ctrl Pts',(4.87145375703912,30.0109212110364,122.945279023894));
#95578=CARTESIAN_POINT('Ctrl Pts',(4.875322091154,30.0821914154493,122.945657837831));
#95579=CARTESIAN_POINT('Ctrl Pts',(4.87919042526887,30.1533488538536,122.949748578334));
#95580=CARTESIAN_POINT('Ctrl Pts',(4.88305875938374,30.2239831424414,122.957494402847));
#95581=CARTESIAN_POINT('Ctrl Pts',(4.8853564785547,30.2659386080748,122.962095279852));
#95582=CARTESIAN_POINT('Ctrl Pts',(4.88765419772566,30.3077096541242,122.967984734544));
#95583=CARTESIAN_POINT('Ctrl Pts',(4.88995191689662,30.3492123714913,122.975142404489));
#95584=CARTESIAN_POINT('Ctrl Pts',(4.89382099024483,30.4190977864161,122.987195030576));
#95585=CARTESIAN_POINT('Ctrl Pts',(4.89769006359304,30.4884953840998,123.002893522819));
#95586=CARTESIAN_POINT('Ctrl Pts',(4.90155913694126,30.556995808955,123.022184732765));
#95587=CARTESIAN_POINT('Ctrl Pts',(4.90542244533704,30.6253941675905,123.041447198644));
#95588=CARTESIAN_POINT('Ctrl Pts',(4.90928575373283,30.6928975431111,123.064291625702));
#95589=CARTESIAN_POINT('Ctrl Pts',(4.91314906212862,30.7591055840197,123.0906136392));
#95590=CARTESIAN_POINT('Ctrl Pts',(4.91700783862153,30.8252359587468,123.116904775326));
#95591=CARTESIAN_POINT('Ctrl Pts',(4.92086661511444,30.8900735678922,123.146665216172));
#95592=CARTESIAN_POINT('Ctrl Pts',(4.92472539160736,30.9532337587871,123.179740962498));
#95593=CARTESIAN_POINT('Ctrl Pts',(4.92858173719556,31.0163541607992,123.212795872171));
#95594=CARTESIAN_POINT('Ctrl Pts',(4.93243808278376,31.0777988117449,123.249161718872));
#95595=CARTESIAN_POINT('Ctrl Pts',(4.93629442837197,31.1372049265935,123.28863723383));
#95596=CARTESIAN_POINT('Ctrl Pts',(4.9401496346173,31.1965934901279,123.328101085896));
#95597=CARTESIAN_POINT('Ctrl Pts',(4.94400484086263,31.2539443088718,123.370672513554));
#95598=CARTESIAN_POINT('Ctrl Pts',(4.94786004710797,31.3089225031754,123.416106239932));
#95599=CARTESIAN_POINT('Ctrl Pts',(4.95171540395921,31.3639028452346,123.461541741206));
#95600=CARTESIAN_POINT('Ctrl Pts',(4.95557076081045,31.4165100057711,123.509839452046));
#95601=CARTESIAN_POINT('Ctrl Pts',(4.95942611766169,31.4664425529626,123.56071413494));
#95602=CARTESIAN_POINT('Ctrl Pts',(4.96328551013024,31.5164273673398,123.611642071207));
#95603=CARTESIAN_POINT('Ctrl Pts',(4.9671449025988,31.5637316386327,123.665152016857));
#95604=CARTESIAN_POINT('Ctrl Pts',(4.97100429506736,31.6080918095682,123.720922873905));
#95605=CARTESIAN_POINT('Ctrl Pts',(4.97486587267079,31.6524770966218,123.776725307644));
#95606=CARTESIAN_POINT('Ctrl Pts',(4.97872745027423,31.6939146826955,123.834790805449));
#95607=CARTESIAN_POINT('Ctrl Pts',(4.98258902787766,31.7321838651537,123.894768522073));
#95608=CARTESIAN_POINT('Ctrl Pts',(4.98645736199253,31.7705200062996,123.954851180295));
#95609=CARTESIAN_POINT('Ctrl Pts',(4.99032569610741,31.8056764360191,124.016852314539));
#95610=CARTESIAN_POINT('Ctrl Pts',(4.99419403022228,31.8374783327799,124.080396314131));
#95611=CARTESIAN_POINT('Ctrl Pts',(4.99649174939324,31.8563680733479,124.118140278774));
#95612=CARTESIAN_POINT('Ctrl Pts',(4.99878946856421,31.8740752011141,124.156428182751));
#95613=CARTESIAN_POINT('Ctrl Pts',(5.00108718773517,31.8905713141637,124.195178486519));
#95614=CARTESIAN_POINT('Ctrl Pts',(5.00537446195653,31.9213511244747,124.267482004075));
#95615=CARTESIAN_POINT('Ctrl Pts',(5.00966173617788,31.9480150746286,124.341637213737));
#95616=CARTESIAN_POINT('Ctrl Pts',(5.01394901039923,31.9703612656983,124.417184381527));
#95617=CARTESIAN_POINT('Ctrl Pts',(5.01822262075598,31.9926362377804,124.492490774826));
#95618=CARTESIAN_POINT('Ctrl Pts',(5.02249623111273,32.0106207692067,124.5691800047));
#95619=CARTESIAN_POINT('Ctrl Pts',(5.02676984146948,32.0241613070718,124.646774058918));
#95620=CARTESIAN_POINT('Ctrl Pts',(5.03102083155061,32.0376301746924,124.723957406789));
#95621=CARTESIAN_POINT('Ctrl Pts',(5.03527182163173,32.046701841573,124.802035744087));
#95622=CARTESIAN_POINT('Ctrl Pts',(5.03952281171286,32.0512732988447,124.880520227877));
#95623=CARTESIAN_POINT('Ctrl Pts',(5.04165696797268,32.0535683416387,124.919922378713));
#95624=CARTESIAN_POINT('Ctrl Pts',(5.04379112423251,32.0547299142489,124.959426631909));
#95625=CARTESIAN_POINT('Ctrl Pts',(5.04592528049234,32.0547497417017,124.998969719981));
#95626=CARTESIAN_POINT('Origin',(-1.54592528053767,30.,125.));
#95627=CARTESIAN_POINT('',(3.89394636966105,28.7479590808042,126.629230216746));
#95628=CARTESIAN_POINT('',(3.95204573436854,28.7479590808042,126.629230216746));
#95629=CARTESIAN_POINT('',(-1.54592528053767,28.7479590808042,126.629230216746));
#95630=CARTESIAN_POINT('',(4.40407471951208,32.0547494817011,125.001459434548));
#95631=CARTESIAN_POINT('Ctrl Pts',(3.95204573436854,28.7479590808042,126.629230216746));
#95632=CARTESIAN_POINT('Ctrl Pts',(3.95593320439764,28.6909466062034,126.585416917452));
#95633=CARTESIAN_POINT('Ctrl Pts',(3.95982067442675,28.6362547070576,126.538621365018));
#95634=CARTESIAN_POINT('Ctrl Pts',(3.96370814445585,28.5841986334277,126.489128622018));
#95635=CARTESIAN_POINT('Ctrl Pts',(3.96756865504022,28.5325035665271,126.439979109154));
#95636=CARTESIAN_POINT('Ctrl Pts',(3.97142916562458,28.4834081758202,126.388170095774));
#95637=CARTESIAN_POINT('Ctrl Pts',(3.97528967620894,28.4371827374804,126.334016404124));
#95638=CARTESIAN_POINT('Ctrl Pts',(3.97919062596042,28.3904730838574,126.279295448082));
#95639=CARTESIAN_POINT('Ctrl Pts',(3.98309157571189,28.346694173615,126.222180805065));
#95640=CARTESIAN_POINT('Ctrl Pts',(3.98699252546337,28.3060805130307,126.163028088296));
#95641=CARTESIAN_POINT('Ctrl Pts',(3.99089347521484,28.2654668524464,126.103875371528));
#95642=CARTESIAN_POINT('Ctrl Pts',(3.99479442496632,28.2280186495009,126.04268504536));
#95643=CARTESIAN_POINT('Ctrl Pts',(3.99869537471779,28.1939221902578,125.979836980144));
#95644=CARTESIAN_POINT('Ctrl Pts',(4.002564448066,28.1601043484165,125.917502474547));
#95645=CARTESIAN_POINT('Ctrl Pts',(4.00643352141422,28.1294511504299,125.853293046297));
#95646=CARTESIAN_POINT('Ctrl Pts',(4.01030259476243,28.1021743860266,125.78756301427));
#95647=CARTESIAN_POINT('Ctrl Pts',(4.01416590315821,28.0749382642358,125.721930920554));
#95648=CARTESIAN_POINT('Ctrl Pts',(4.01802921155399,28.0510687744828,125.654783165467));
#95649=CARTESIAN_POINT('Ctrl Pts',(4.02189251994977,28.0307319100997,125.586498723443));
#95650=CARTESIAN_POINT('Ctrl Pts',(4.02575129644268,28.0104189021331,125.518294383349));
#95651=CARTESIAN_POINT('Ctrl Pts',(4.02961007293559,27.9936304261563,125.448956468227));
#95652=CARTESIAN_POINT('Ctrl Pts',(4.0334688494285,27.9804837906095,125.378882359723));
#95653=CARTESIAN_POINT('Ctrl Pts',(4.03732519501671,27.967345437019,125.308852395646));
#95654=CARTESIAN_POINT('Ctrl Pts',(4.04118154060491,27.9578444614835,125.238087634642));
#95655=CARTESIAN_POINT('Ctrl Pts',(4.04503788619312,27.9520475161225,125.166997563695));
#95656=CARTESIAN_POINT('Ctrl Pts',(4.04889309243845,27.9462522834474,125.095928496044));
#95657=CARTESIAN_POINT('Ctrl Pts',(4.05274829868378,27.9441589478354,125.024534793175));
#95658=CARTESIAN_POINT('Ctrl Pts',(4.05660350492912,27.9457823265314,124.953231287068));
#95659=CARTESIAN_POINT('Ctrl Pts',(4.06045886178037,27.9474057686457,124.881924995447));
#95660=CARTESIAN_POINT('Ctrl Pts',(4.06431421863162,27.9527462000759,124.810709393194));
#95661=CARTESIAN_POINT('Ctrl Pts',(4.06816957548287,27.9617663485297,124.739997799021));
#95662=CARTESIAN_POINT('Ctrl Pts',(4.07202896795143,27.9707959388766,124.669212187073));
#95663=CARTESIAN_POINT('Ctrl Pts',(4.07588836041999,27.9835128736403,124.598932119228));
#95664=CARTESIAN_POINT('Ctrl Pts',(4.07974775288854,27.9998282686891,124.529563386029));
#95665=CARTESIAN_POINT('Ctrl Pts',(4.08360933049198,28.0161529012899,124.460155377208));
#95666=CARTESIAN_POINT('Ctrl Pts',(4.08747090809541,28.0360799142421,124.391660196868));
#95667=CARTESIAN_POINT('Ctrl Pts',(4.09133248569884,28.059470527105,124.324468411304));
#95668=CARTESIAN_POINT('Ctrl Pts',(4.09520081981371,28.0829020659726,124.257159061854));
#95669=CARTESIAN_POINT('Ctrl Pts',(4.09906915392858,28.1098091206268,124.191158110286));
#95670=CARTESIAN_POINT('Ctrl Pts',(4.10293748804345,28.1400050514508,124.126835437119));
#95671=CARTESIAN_POINT('Ctrl Pts',(4.10523520721442,28.1579408778502,124.088628954722));
#95672=CARTESIAN_POINT('Ctrl Pts',(4.10753292638539,28.1770361820225,124.051014126221));
#95673=CARTESIAN_POINT('Ctrl Pts',(4.10983064555635,28.1972445332815,124.014063749669));
#95674=CARTESIAN_POINT('Ctrl Pts',(4.11369971890457,28.2312728837673,123.951843910566));
#95675=CARTESIAN_POINT('Ctrl Pts',(4.11756879225279,28.2685928276123,123.891265935902));
#95676=CARTESIAN_POINT('Ctrl Pts',(4.12143786560101,28.3090215532381,123.832699929287));
#95677=CARTESIAN_POINT('Ctrl Pts',(4.1253011739968,28.3493900397164,123.774221186523));
#95678=CARTESIAN_POINT('Ctrl Pts',(4.1291644823926,28.3928578396386,123.717748857686));
#95679=CARTESIAN_POINT('Ctrl Pts',(4.13302779078839,28.439196588897,123.663627943128));
#95680=CARTESIAN_POINT('Ctrl Pts',(4.13688656728131,28.4854809798984,123.609570515794));
#95681=CARTESIAN_POINT('Ctrl Pts',(4.14074534377422,28.5346293162262,123.557859390924));
#95682=CARTESIAN_POINT('Ctrl Pts',(4.14460412026714,28.5863713641367,123.508808649982));
#95683=CARTESIAN_POINT('Ctrl Pts',(4.14846046585534,28.6380808162262,123.459788809425));
#95684=CARTESIAN_POINT('Ctrl Pts',(4.15231681144355,28.6923803864433,123.413426361147));
#95685=CARTESIAN_POINT('Ctrl Pts',(4.15617315703175,28.7489621966506,123.369999393531));
#95686=CARTESIAN_POINT('Ctrl Pts',(4.16002836327709,28.8055272899739,123.32658525625));
#95687=CARTESIAN_POINT('Ctrl Pts',(4.16388356952242,28.8643728995,123.286105173457));
#95688=CARTESIAN_POINT('Ctrl Pts',(4.16773877576775,28.9251585431536,123.248796583733));
#95689=CARTESIAN_POINT('Ctrl Pts',(4.17159413261901,28.9859465614344,123.211486536528));
#95690=CARTESIAN_POINT('Ctrl Pts',(4.17544948947026,29.0486743491377,123.177348480609));
#95691=CARTESIAN_POINT('Ctrl Pts',(4.17930484632152,29.1129744440581,123.146575271125));
#95692=CARTESIAN_POINT('Ctrl Pts',(4.18316423879008,29.1773418454784,123.115769849604));
#95693=CARTESIAN_POINT('Ctrl Pts',(4.18702363125864,29.2432844004596,123.088336515709));
#95694=CARTESIAN_POINT('Ctrl Pts',(4.1908830237272,29.3104129791301,123.064420680223));
#95695=CARTESIAN_POINT('Ctrl Pts',(4.19474460133064,29.3775795650775,123.040491303921));
#95696=CARTESIAN_POINT('Ctrl Pts',(4.19860617893407,29.4459330457811,123.020083529651));
#95697=CARTESIAN_POINT('Ctrl Pts',(4.20246775653751,29.5150700199579,123.00329259105));
#95698=CARTESIAN_POINT('Ctrl Pts',(4.20633609065238,29.5843279614709,122.986472273739));
#95699=CARTESIAN_POINT('Ctrl Pts',(4.21020442476726,29.6543716558731,122.973281516649));
#95700=CARTESIAN_POINT('Ctrl Pts',(4.21407275888213,29.7247891238029,122.963764125617));
#95701=CARTESIAN_POINT('Ctrl Pts',(4.21637047805306,29.7666158019609,122.95811097075));
#95702=CARTESIAN_POINT('Ctrl Pts',(4.21866819722398,29.8085742650121,122.953752835488));
#95703=CARTESIAN_POINT('Ctrl Pts',(4.22096591639491,29.8505781698027,122.950690194441));
#95704=CARTESIAN_POINT('Ctrl Pts',(4.22483498974313,29.9213075220243,122.945533087776));
#95705=CARTESIAN_POINT('Ctrl Pts',(4.22870406309136,29.992442714435,122.944031880373));
#95706=CARTESIAN_POINT('Ctrl Pts',(4.23257313643958,30.0635736564372,122.946233715169));
#95707=CARTESIAN_POINT('Ctrl Pts',(4.23643644483536,30.1345986127262,122.948432269213));
#95708=CARTESIAN_POINT('Ctrl Pts',(4.24029975323114,30.2056188495803,122.954322898336));
#95709=CARTESIAN_POINT('Ctrl Pts',(4.24416306162692,30.2762206606867,122.963900859705));
#95710=CARTESIAN_POINT('Ctrl Pts',(4.24802183811984,30.3467396514441,122.973467585525));
#95711=CARTESIAN_POINT('Ctrl Pts',(4.25188061461276,30.4168407123872,122.986712986754));
#95712=CARTESIAN_POINT('Ctrl Pts',(4.25573939110568,30.486113404921,123.003580374757));
#95713=CARTESIAN_POINT('Ctrl Pts',(4.25959573669389,30.5553424578932,123.020437136849));
#95714=CARTESIAN_POINT('Ctrl Pts',(4.2634520822821,30.6237437069094,123.040911244136));
#95715=CARTESIAN_POINT('Ctrl Pts',(4.26730842787031,30.6909165357611,123.064894859933));
#95716=CARTESIAN_POINT('Ctrl Pts',(4.27116363411565,30.758069518652,123.088871389862));
#95717=CARTESIAN_POINT('Ctrl Pts',(4.27501884036099,30.823994344649,123.116355206567));
#95718=CARTESIAN_POINT('Ctrl Pts',(4.27887404660633,30.8883068660086,123.147189034385));
#95719=CARTESIAN_POINT('Ctrl Pts',(4.28272940345757,30.9526218997746,123.178024066745));
#95720=CARTESIAN_POINT('Ctrl Pts',(4.28658476030882,31.0153240667623,123.212209158044));
#95721=CARTESIAN_POINT('Ctrl Pts',(4.29044011716006,31.076052042658,123.249540184982));
#95722=CARTESIAN_POINT('Ctrl Pts',(4.29429950962863,31.1368435859175,123.286910288391));
#95723=CARTESIAN_POINT('Ctrl Pts',(4.2981589020972,31.1956563982011,123.327432646139));
#95724=CARTESIAN_POINT('Ctrl Pts',(4.30201829456576,31.2521572635066,123.370859198857));
#95725=CARTESIAN_POINT('Ctrl Pts',(4.30587987216921,31.3086901188242,123.414310339092));
#95726=CARTESIAN_POINT('Ctrl Pts',(4.30974144977265,31.3629080519682,123.460668631776));
#95727=CARTESIAN_POINT('Ctrl Pts',(4.31360302737609,31.4145122626436,123.509646813225));
#95728=CARTESIAN_POINT('Ctrl Pts',(4.31747136149097,31.4662067639916,123.558710690645));
#95729=CARTESIAN_POINT('Ctrl Pts',(4.32133969560585,31.5152780778472,123.610403256402));
#95730=CARTESIAN_POINT('Ctrl Pts',(4.32520802972072,31.5614659582079,123.664402147404));
#95731=CARTESIAN_POINT('Ctrl Pts',(4.32750574889164,31.5889007079005,123.696476493461));
#95732=CARTESIAN_POINT('Ctrl Pts',(4.32980346806255,31.6153189306065,123.729363929871));
#95733=CARTESIAN_POINT('Ctrl Pts',(4.33210118723347,31.6406733981607,123.762992173401));
#95734=CARTESIAN_POINT('Ctrl Pts',(4.33598223894951,31.6834993453242,123.819793262894));
#95735=CARTESIAN_POINT('Ctrl Pts',(4.33986329066555,31.7234572903184,123.878933890298));
#95736=CARTESIAN_POINT('Ctrl Pts',(4.34374434238158,31.7602831217962,123.940093922265));
#95737=CARTESIAN_POINT('Ctrl Pts',(4.34761960540831,31.7970540265912,124.001162732458));
#95738=CARTESIAN_POINT('Ctrl Pts',(4.35149486843504,31.8307018422713,124.064244561641));
#95739=CARTESIAN_POINT('Ctrl Pts',(4.35537013146177,31.8610038890162,124.128987894707));
#95740=CARTESIAN_POINT('Ctrl Pts',(4.35942884712848,31.892740416578,124.196796138539));
#95741=CARTESIAN_POINT('Ctrl Pts',(4.36348756279519,31.9208061964461,124.266426682191));
#95742=CARTESIAN_POINT('Ctrl Pts',(4.3675462784619,31.9449979565051,124.337443955811));
#95743=CARTESIAN_POINT('Ctrl Pts',(4.3714136667849,31.9680493200514,124.405113484126));
#95744=CARTESIAN_POINT('Ctrl Pts',(4.3752810551079,31.9875834868983,124.474041440803));
#95745=CARTESIAN_POINT('Ctrl Pts',(4.3791484434309,32.0034736409933,124.543830149675));
#95746=CARTESIAN_POINT('Ctrl Pts',(4.38301406018542,32.019356516146,124.613586889822));
#95747=CARTESIAN_POINT('Ctrl Pts',(4.38687967693995,32.0315985897938,124.684203129537));
#95748=CARTESIAN_POINT('Ctrl Pts',(4.39074529369447,32.0401235137114,124.755268287094));
#95749=CARTESIAN_POINT('Ctrl Pts',(4.39461092103537,32.0486484609754,124.826333639271));
#95750=CARTESIAN_POINT('Ctrl Pts',(4.39847654837627,32.0534561785914,124.897847434106));
#95751=CARTESIAN_POINT('Ctrl Pts',(4.40234217571717,32.0545220261427,124.969392703572));
#95752=CARTESIAN_POINT('Ctrl Pts',(4.40291969029889,32.0546812609701,124.980081379103));
#95753=CARTESIAN_POINT('Ctrl Pts',(4.4034972048806,32.0547570735857,124.990770753233));
#95754=CARTESIAN_POINT('Ctrl Pts',(4.40407471946232,32.0547494817017,125.001459433627));
#95755=CARTESIAN_POINT('Ctrl Pts',(4.40407471951208,32.0547494817011,125.001459434548));
#95756=CARTESIAN_POINT('Ctrl Pts',(4.40849095806784,32.054691426731,125.083195487561));
#95757=CARTESIAN_POINT('Ctrl Pts',(4.41290719662359,32.0497522762919,125.164736898229));
#95758=CARTESIAN_POINT('Ctrl Pts',(4.41732343517935,32.0400254037025,125.245548192314));
#95759=CARTESIAN_POINT('Ctrl Pts',(4.4217797159882,32.0302103370789,125.327092206393));
#95760=CARTESIAN_POINT('Ctrl Pts',(4.42623599679705,32.0155204432693,125.407892614198));
#95761=CARTESIAN_POINT('Ctrl Pts',(4.4306922776059,31.9961013728879,125.487418579513));
#95762=CARTESIAN_POINT('Ctrl Pts',(4.43487367109461,31.9778801750029,125.562038956419));
#95763=CARTESIAN_POINT('Ctrl Pts',(4.43905506458332,31.9554957935067,125.635537342885));
#95764=CARTESIAN_POINT('Ctrl Pts',(4.44323645807203,31.929106484379,125.70749256846));
#95765=CARTESIAN_POINT('Ctrl Pts',(4.44710553142024,31.9046882676053,125.774073254131));
#95766=CARTESIAN_POINT('Ctrl Pts',(4.45097460476846,31.8767712524526,125.839518723707));
#95767=CARTESIAN_POINT('Ctrl Pts',(4.45484367811667,31.8454813033536,125.903435842477));
#95768=CARTESIAN_POINT('Ctrl Pts',(4.45870698651246,31.8142379765467,125.967257724193));
#95769=CARTESIAN_POINT('Ctrl Pts',(4.46257029490824,31.7796319035186,126.029555342638));
#95770=CARTESIAN_POINT('Ctrl Pts',(4.46643360330402,31.7418377221508,126.08995362846));
#95771=CARTESIAN_POINT('Ctrl Pts',(4.47029237979693,31.7040878757263,126.150281063307));
#95772=CARTESIAN_POINT('Ctrl Pts',(4.47415115628985,31.663157606008,126.208713181357));
#95773=CARTESIAN_POINT('Ctrl Pts',(4.47800993278276,31.6192675452454,126.264899276391));
#95774=CARTESIAN_POINT('Ctrl Pts',(4.48186627837097,31.5754051338052,126.321049975998));
#95775=CARTESIAN_POINT('Ctrl Pts',(4.48572262395917,31.5285869289447,126.374957077847));
#95776=CARTESIAN_POINT('Ctrl Pts',(4.48957896954738,31.4790761318271,126.426299883881));
#95777=CARTESIAN_POINT('Ctrl Pts',(4.49343417579271,31.4295799624892,126.477627520875));
#95778=CARTESIAN_POINT('Ctrl Pts',(4.49728938203805,31.3773931172376,126.526392016629));
#95779=CARTESIAN_POINT('Ctrl Pts',(4.50114458828338,31.3228170725558,126.572308034405));
#95780=CARTESIAN_POINT('Ctrl Pts',(4.50499994513463,31.2682388958286,126.618225845918));
#95781=CARTESIAN_POINT('Ctrl Pts',(4.50885530198588,31.2112717075103,126.66129464747));
#95782=CARTESIAN_POINT('Ctrl Pts',(4.51271065883712,31.1522502816128,126.701269188289));
#95783=CARTESIAN_POINT('Ctrl Pts',(4.51657005130568,31.0931670746929,126.741285572693));
#95784=CARTESIAN_POINT('Ctrl Pts',(4.52042944377424,31.0320257407811,126.778200957745));
#95785=CARTESIAN_POINT('Ctrl Pts',(4.5242888362428,30.9691895223346,126.811813796254));
#95786=CARTESIAN_POINT('Ctrl Pts',(4.52815041384624,30.9063177268864,126.845445665889));
#95787=CARTESIAN_POINT('Ctrl Pts',(4.53201199144967,30.8417495765083,126.875771060062));
#95788=CARTESIAN_POINT('Ctrl Pts',(4.53587356905311,30.7758698732851,126.902635935283));
#95789=CARTESIAN_POINT('Ctrl Pts',(4.53974190316798,30.7098749018958,126.929547815343));
#95790=CARTESIAN_POINT('Ctrl Pts',(4.54361023728285,30.6425642549527,126.952986928087));
#95791=CARTESIAN_POINT('Ctrl Pts',(4.54747857139773,30.5743388494691,126.972848815417));
#95792=CARTESIAN_POINT('Ctrl Pts',(4.54977629056868,30.533814216004,126.984646410436));
#95793=CARTESIAN_POINT('Ctrl Pts',(4.55207400973964,30.4929670773005,126.995182881589));
#95794=CARTESIAN_POINT('Ctrl Pts',(4.55437172891059,30.451882750053,127.004444946289));
#95795=CARTESIAN_POINT('Ctrl Pts',(4.55844028469716,30.3791350098275,127.020845221574));
#95796=CARTESIAN_POINT('Ctrl Pts',(4.56250884048373,30.3053433991469,127.03331376979));
#95797=CARTESIAN_POINT('Ctrl Pts',(4.56657739627029,30.2309718247415,127.041727106808));
#95798=CARTESIAN_POINT('Ctrl Pts',(4.57043972402091,30.1603700164458,127.049713986366));
#95799=CARTESIAN_POINT('Ctrl Pts',(4.57430205177154,30.0892461673342,127.054046646543));
#95800=CARTESIAN_POINT('Ctrl Pts',(4.57816437952216,30.0180102763838,127.054671066727));
#95801=CARTESIAN_POINT('Ctrl Pts',(4.58202291837601,29.9468442669799,127.055294874362));
#95802=CARTESIAN_POINT('Ctrl Pts',(4.58588145722987,29.8755669170033,127.052217654884));
#95803=CARTESIAN_POINT('Ctrl Pts',(4.58973999608372,29.8045925651953,127.045437238569));
#95804=CARTESIAN_POINT('Ctrl Pts',(4.59359604063054,29.733664093922,127.038661205374));
#95805=CARTESIAN_POINT('Ctrl Pts',(4.59745208517735,29.6630387144404,127.028186773093));
#95806=CARTESIAN_POINT('Ctrl Pts',(4.60130812972416,29.5931282481697,127.014063787486));
#95807=CARTESIAN_POINT('Ctrl Pts',(4.6051629715136,29.5232395880081,126.999945207047));
#95808=CARTESIAN_POINT('Ctrl Pts',(4.60901781330305,29.4540658736896,126.982180430866));
#95809=CARTESIAN_POINT('Ctrl Pts',(4.6128726550925,29.3860095914793,126.960870556856));
#95810=CARTESIAN_POINT('Ctrl Pts',(4.61672928267136,29.3179217815969,126.939550810859));
#95811=CARTESIAN_POINT('Ctrl Pts',(4.62058591025023,29.2509529028989,126.914682828748));
#95812=CARTESIAN_POINT('Ctrl Pts',(4.62444253782909,29.1854899614899,126.886417493469));
#95813=CARTESIAN_POINT('Ctrl Pts',(4.62830019968253,29.1200094641579,126.858144577962));
#95814=CARTESIAN_POINT('Ctrl Pts',(4.63215786153597,29.0560361472741,126.826472703826));
#95815=CARTESIAN_POINT('Ctrl Pts',(4.63601552338942,28.9939345295402,126.791599796732));
#95816=CARTESIAN_POINT('Ctrl Pts',(4.63987764453128,28.9317611250517,126.756686578081));
#95817=CARTESIAN_POINT('Ctrl Pts',(4.64373976567315,28.8714641517747,126.718565195949));
#95818=CARTESIAN_POINT('Ctrl Pts',(4.64760188681501,28.8133802409445,126.677477603403));
#95819=CARTESIAN_POINT('Ctrl Pts',(4.64907361380609,28.7912463781847,126.661820476988));
#95820=CARTESIAN_POINT('Ctrl Pts',(4.65054534079716,28.769433546249,126.645733046843));
#95821=CARTESIAN_POINT('Ctrl Pts',(4.65201706778823,28.7479590808042,126.629230216746));
#95822=CARTESIAN_POINT('',(4.34592528058851,32.054749644159,124.998790732221));
#95823=CARTESIAN_POINT('Ctrl Pts',(4.34592528058851,32.054749644159,124.998790732221));
#95824=CARTESIAN_POINT('Ctrl Pts',(4.34974237135631,32.054790885948,125.068867478462));
#95825=CARTESIAN_POINT('Ctrl Pts',(4.35355946212412,32.0512429716114,125.139087448465));
#95826=CARTESIAN_POINT('Ctrl Pts',(4.35737655289193,32.0440883161919,125.209046688822));
#95827=CARTESIAN_POINT('Ctrl Pts',(4.36118805254433,32.0369441406135,125.278903455801));
#95828=CARTESIAN_POINT('Ctrl Pts',(4.36499955219674,32.0262037618738,125.348499758144));
#95829=CARTESIAN_POINT('Ctrl Pts',(4.36881105184914,32.0119016127191,125.417431986362));
#95830=CARTESIAN_POINT('Ctrl Pts',(4.37261948474207,31.9976109711744,125.486308751224));
#95831=CARTESIAN_POINT('Ctrl Pts',(4.37642791763499,31.9797643402254,125.554522013912));
#95832=CARTESIAN_POINT('Ctrl Pts',(4.38023635052792,31.9584477379755,125.621675172513));
#95833=CARTESIAN_POINT('Ctrl Pts',(4.3840430711884,31.9371407194517,125.688798139741));
#95834=CARTESIAN_POINT('Ctrl Pts',(4.38784979184888,31.9123669742972,125.754861472596));
#95835=CARTESIAN_POINT('Ctrl Pts',(4.39165651250936,31.8842627237944,125.819482489269));
#95836=CARTESIAN_POINT('Ctrl Pts',(4.39546287300873,31.8561611322884,125.884097392025));
#95837=CARTESIAN_POINT('Ctrl Pts',(4.3992692335081,31.824729861666,125.947269792158));
#95838=CARTESIAN_POINT('Ctrl Pts',(4.40307559400747,31.790153006837,126.008637583383));
#95839=CARTESIAN_POINT('Ctrl Pts',(4.40688551323035,31.7555438246795,126.070062749889));
#95840=CARTESIAN_POINT('Ctrl Pts',(4.41069543245322,31.7177834317559,126.129679502484));
#95841=CARTESIAN_POINT('Ctrl Pts',(4.4145053516761,31.6771010428774,126.187151908763));
#95842=CARTESIAN_POINT('Ctrl Pts',(4.41831711300213,31.636398983987,126.244652103059));
#95843=CARTESIAN_POINT('Ctrl Pts',(4.42212887432815,31.5927724276009,126.300005495642));
#95844=CARTESIAN_POINT('Ctrl Pts',(4.42594063565417,31.5464911598374,126.352908960368));
#95845=CARTESIAN_POINT('Ctrl Pts',(4.42975910316259,31.5001284676098,126.405905500251));
#95846=CARTESIAN_POINT('Ctrl Pts',(4.43357757067101,31.4511020881567,126.456443149052));
#95847=CARTESIAN_POINT('Ctrl Pts',(4.43739603817942,31.3997183644,126.504255983156));
#95848=CARTESIAN_POINT('Ctrl Pts',(4.44006763663374,31.3637676389681,126.537708328478));
#95849=CARTESIAN_POINT('Ctrl Pts',(4.44273923508806,31.3266637077768,126.569827654897));
#95850=CARTESIAN_POINT('Ctrl Pts',(4.44541083354239,31.2885201183749,126.600535368882));
#95851=CARTESIAN_POINT('Ctrl Pts',(4.4492799068906,31.233279651784,126.645007021265));
#95852=CARTESIAN_POINT('Ctrl Pts',(4.45314898023881,31.1756259560803,126.686702591709));
#95853=CARTESIAN_POINT('Ctrl Pts',(4.45701805358702,31.1158695099186,126.725350051246));
#95854=CARTESIAN_POINT('Ctrl Pts',(4.46088136198281,31.0562021013734,126.763939925737));
#95855=CARTESIAN_POINT('Ctrl Pts',(4.4647446703786,30.9944385661034,126.799490442826));
#95856=CARTESIAN_POINT('Ctrl Pts',(4.4686079787744,30.93092186864,126.831770192188));
#95857=CARTESIAN_POINT('Ctrl Pts',(4.47246675526731,30.8674796802436,126.864012075381));
#95858=CARTESIAN_POINT('Ctrl Pts',(4.47632553176023,30.8022888456627,126.892990593039));
#95859=CARTESIAN_POINT('Ctrl Pts',(4.48018430825314,30.7357191879357,126.918518918073));
#95860=CARTESIAN_POINT('Ctrl Pts',(4.48404065384135,30.6691914669456,126.944031161085));
#95861=CARTESIAN_POINT('Ctrl Pts',(4.48789699942955,30.6012870986315,126.966097350154));
#95862=CARTESIAN_POINT('Ctrl Pts',(4.49175334501776,30.5323969196767,126.984578313501));
#95863=CARTESIAN_POINT('Ctrl Pts',(4.4956085512631,30.4635270940674,127.003053816717));
#95864=CARTESIAN_POINT('Ctrl Pts',(4.49946375750843,30.3936725049776,127.017946071298));
#95865=CARTESIAN_POINT('Ctrl Pts',(4.50331896375376,30.3232385643445,127.02916593531));
#95866=CARTESIAN_POINT('Ctrl Pts',(4.50717432060501,30.252801872168,127.040386237632));
#95867=CARTESIAN_POINT('Ctrl Pts',(4.51102967745625,30.1817862635977,127.047933790311));
#95868=CARTESIAN_POINT('Ctrl Pts',(4.51488503430749,30.1106050250402,127.051770964542));
#95869=CARTESIAN_POINT('Ctrl Pts',(4.51874442677605,30.0393492771052,127.055612155357));
#95870=CARTESIAN_POINT('Ctrl Pts',(4.52260381924461,29.9679280391648,127.055735188464));
#95871=CARTESIAN_POINT('Ctrl Pts',(4.52646321171317,29.8967564692991,127.052154559449));
#95872=CARTESIAN_POINT('Ctrl Pts',(4.53032478931661,29.8255446030706,127.048571903132));
#95873=CARTESIAN_POINT('Ctrl Pts',(4.53418636692004,29.7545831697897,127.041281459958));
#95874=CARTESIAN_POINT('Ctrl Pts',(4.53804794452347,29.6842813201143,127.030349545687));
#95875=CARTESIAN_POINT('Ctrl Pts',(4.54191627863834,29.6138564649473,127.019398504103));
#95876=CARTESIAN_POINT('Ctrl Pts',(4.54578461275322,29.5440939731246,127.00479337032));
#95877=CARTESIAN_POINT('Ctrl Pts',(4.54965294686809,29.4753912491378,126.986651258027));
#95878=CARTESIAN_POINT('Ctrl Pts',(4.55195066603904,29.4345830972788,126.975875177683));
#95879=CARTESIAN_POINT('Ctrl Pts',(4.55424838520999,29.3941485465819,126.963852154995));
#95880=CARTESIAN_POINT('Ctrl Pts',(4.55654610438094,29.3541675553052,126.950614778955));
#95881=CARTESIAN_POINT('Ctrl Pts',(4.56041440943521,29.2868579064214,126.928329110068));
#95882=CARTESIAN_POINT('Ctrl Pts',(4.56428271448948,29.2205713092772,126.902511739845));
#95883=CARTESIAN_POINT('Ctrl Pts',(4.56815101954375,29.1557044645014,126.873275903661));
#95884=CARTESIAN_POINT('Ctrl Pts',(4.57201426861242,29.0909224025513,126.844078279553));
#95885=CARTESIAN_POINT('Ctrl Pts',(4.57587751768109,29.0275568522896,126.811471247144));
#95886=CARTESIAN_POINT('Ctrl Pts',(4.57974076674976,28.9659882294994,126.77561741965));
#95887=CARTESIAN_POINT('Ctrl Pts',(4.5835995535365,28.9044907221223,126.739805005455));
#95888=CARTESIAN_POINT('Ctrl Pts',(4.58745834032323,28.8447864376399,126.700753487886));
#95889=CARTESIAN_POINT('Ctrl Pts',(4.59131712710997,28.7872329245225,126.658672234993));
#95890=CARTESIAN_POINT('Ctrl Pts',(4.59220253450987,28.7740271401086,126.649016595859));
#95891=CARTESIAN_POINT('Ctrl Pts',(4.59308794190978,28.7609344849291,126.639201635604));
#95892=CARTESIAN_POINT('Ctrl Pts',(4.59397334930969,28.7479590808042,126.629230216746));
#95893=CARTESIAN_POINT('Ctrl Pts',(3.89394636966105,28.7479590808042,126.629230216746));
#95894=CARTESIAN_POINT('Ctrl Pts',(3.89781318580622,28.6916844716005,126.585983956819));
#95895=CARTESIAN_POINT('Ctrl Pts',(3.9016800019514,28.6375514615491,126.539740510312));
#95896=CARTESIAN_POINT('Ctrl Pts',(3.90554681809657,28.585895921426,126.490740492997));
#95897=CARTESIAN_POINT('Ctrl Pts',(3.90951860693371,28.5328380852282,126.440410269246));
#95898=CARTESIAN_POINT('Ctrl Pts',(3.91349039577086,28.4823946506547,126.387171875852));
#95899=CARTESIAN_POINT('Ctrl Pts',(3.91746218460801,28.434895455922,126.331332163138));
#95900=CARTESIAN_POINT('Ctrl Pts',(3.92131985599883,28.3887610081656,126.277096837183));
#95901=CARTESIAN_POINT('Ctrl Pts',(3.92517752738964,28.3454042309927,126.220408057136));
#95902=CARTESIAN_POINT('Ctrl Pts',(3.92903519878045,28.3050902823745,126.161584526239));
#95903=CARTESIAN_POINT('Ctrl Pts',(3.93289094488817,28.2647964536047,126.102790352936));
#95904=CARTESIAN_POINT('Ctrl Pts',(3.93674669099589,28.2275427141598,126.041863943026));
#95905=CARTESIAN_POINT('Ctrl Pts',(3.94060243710361,28.1935524070084,125.979155072639));
#95906=CARTESIAN_POINT('Ctrl Pts',(3.94445754870422,28.1595676933507,125.916456521714));
#95907=CARTESIAN_POINT('Ctrl Pts',(3.94831266030482,28.1288455764369,125.851976520105));
#95908=CARTESIAN_POINT('Ctrl Pts',(3.95216777190542,28.1015638481471,125.78609016012));
#95909=CARTESIAN_POINT('Ctrl Pts',(3.95622627009564,28.0728428002602,125.71672779128));
#95910=CARTESIAN_POINT('Ctrl Pts',(3.96028476828587,28.0479354221679,125.6458071135));
#95911=CARTESIAN_POINT('Ctrl Pts',(3.9643432664761,28.026990986085,125.573788282828));
#95912=CARTESIAN_POINT('Ctrl Pts',(3.96820348502378,28.0070697992694,125.505287962533));
#95913=CARTESIAN_POINT('Ctrl Pts',(3.97206370357146,27.9907334521896,125.43579478774));
#95914=CARTESIAN_POINT('Ctrl Pts',(3.97592392211914,27.9780581556152,125.3657167489));
#95915=CARTESIAN_POINT('Ctrl Pts',(3.97978684019179,27.9653739949625,125.295589703142));
#95916=CARTESIAN_POINT('Ctrl Pts',(3.98364975826444,27.9563560389418,125.224877460961));
#95917=CARTESIAN_POINT('Ctrl Pts',(3.98751267633709,27.9510286398102,125.153993271353));
#95918=CARTESIAN_POINT('Ctrl Pts',(3.99138185011661,27.9456926133542,125.082994290102));
#95919=CARTESIAN_POINT('Ctrl Pts',(3.99525102389613,27.9440590725777,125.011823290158));
#95920=CARTESIAN_POINT('Ctrl Pts',(3.99912019767565,27.9461003233506,124.940892633628));
#95921=CARTESIAN_POINT('Ctrl Pts',(3.99970338184648,27.9464079924312,124.93020155629));
#95922=CARTESIAN_POINT('Ctrl Pts',(4.00028656601731,27.9467990508151,124.919515925859));
#95923=CARTESIAN_POINT('Ctrl Pts',(4.00086975018814,27.947273302386,124.90883713803));
#95924=CARTESIAN_POINT('Ctrl Pts',(4.00473882353636,27.9504196739869,124.837989856074));
#95925=CARTESIAN_POINT('Ctrl Pts',(4.00860789688458,27.9572443216409,124.76716688376));
#95926=CARTESIAN_POINT('Ctrl Pts',(4.01247697023279,27.9677461262914,124.696781010989));
#95927=CARTESIAN_POINT('Ctrl Pts',(4.01634027862858,27.9782322831631,124.626500013772));
#95928=CARTESIAN_POINT('Ctrl Pts',(4.02020358702437,27.9923846502762,124.556655299875));
#95929=CARTESIAN_POINT('Ctrl Pts',(4.02406689542016,28.0101501558678,124.487657184781));
#95930=CARTESIAN_POINT('Ctrl Pts',(4.02792567191308,28.0278948214079,124.4187400088));
#95931=CARTESIAN_POINT('Ctrl Pts',(4.03178444840599,28.0492440859145,124.350667927121));
#95932=CARTESIAN_POINT('Ctrl Pts',(4.03564322489891,28.074093669959,124.283841937553));
#95933=CARTESIAN_POINT('Ctrl Pts',(4.03949957048712,28.0989275995671,124.217058046203));
#95934=CARTESIAN_POINT('Ctrl Pts',(4.04335591607532,28.1272573049389,124.151519143788));
#95935=CARTESIAN_POINT('Ctrl Pts',(4.04721226166353,28.1589288574896,124.087610493969));
#95936=CARTESIAN_POINT('Ctrl Pts',(4.05106746790887,28.1905910527986,124.023720725721));
#95937=CARTESIAN_POINT('Ctrl Pts',(4.0549226741542,28.2255929195603,123.961460688887));
#95938=CARTESIAN_POINT('Ctrl Pts',(4.05877788039954,28.2637333542969,123.901193512251));
#95939=CARTESIAN_POINT('Ctrl Pts',(4.06263323725079,28.3018752790121,123.840923981242));
#95940=CARTESIAN_POINT('Ctrl Pts',(4.06648859410204,28.3431557534862,123.78264787431));
#95941=CARTESIAN_POINT('Ctrl Pts',(4.07034395095329,28.3873298158111,123.726700176891));
#95942=CARTESIAN_POINT('Ctrl Pts',(4.07420334342185,28.4315501175939,123.670693915894));
#95943=CARTESIAN_POINT('Ctrl Pts',(4.07806273589041,28.4786697519009,123.617021311813));
#95944=CARTESIAN_POINT('Ctrl Pts',(4.08192212835897,28.5284034077903,123.565984298448));
#95945=CARTESIAN_POINT('Ctrl Pts',(4.08578370596241,28.5781652221908,123.51491838863));
#95946=CARTESIAN_POINT('Ctrl Pts',(4.08964528356585,28.6305436475806,123.466491370049));
#95947=CARTESIAN_POINT('Ctrl Pts',(4.09350686116929,28.6852184606156,123.420966413849));
#95948=CARTESIAN_POINT('Ctrl Pts',(4.09737519528416,28.739988936884,123.375361803704));
#95949=CARTESIAN_POINT('Ctrl Pts',(4.10124352939904,28.7970634335981,123.332669684725));
#95950=CARTESIAN_POINT('Ctrl Pts',(4.10511186351391,28.8560913755696,123.293110835041));
#95951=CARTESIAN_POINT('Ctrl Pts',(4.10740958268484,28.891152885217,123.269613607398));
#95952=CARTESIAN_POINT('Ctrl Pts',(4.10970730185577,28.9269030806235,123.247220986002));
#95953=CARTESIAN_POINT('Ctrl Pts',(4.1120050210267,28.963264653256,123.225971425452));
#95954=CARTESIAN_POINT('Ctrl Pts',(4.11587409437491,29.0244930197819,123.190189808002));
#95955=CARTESIAN_POINT('Ctrl Pts',(4.11974316772313,29.0876959275458,123.15751165516));
#95956=CARTESIAN_POINT('Ctrl Pts',(4.12361224107134,29.1525259668354,123.128159909177));
#95957=CARTESIAN_POINT('Ctrl Pts',(4.12747554946713,29.2172594088112,123.098851897547));
#95958=CARTESIAN_POINT('Ctrl Pts',(4.13133885786291,29.2836147309308,123.072860653239));
#95959=CARTESIAN_POINT('Ctrl Pts',(4.1352021662587,29.3512184250661,123.050364128734));
#95960=CARTESIAN_POINT('Ctrl Pts',(4.13906094275161,29.4187428158311,123.027893994063));
#95961=CARTESIAN_POINT('Ctrl Pts',(4.14291971924452,29.4875122110835,123.008910588793));
#95962=CARTESIAN_POINT('Ctrl Pts',(4.14677849573743,29.5571331576807,122.993543790043));
#95963=CARTESIAN_POINT('Ctrl Pts',(4.15063484132563,29.6267102453275,122.978186671881));
#95964=CARTESIAN_POINT('Ctrl Pts',(4.15449118691384,29.6971373467644,122.966441744494));
#95965=CARTESIAN_POINT('Ctrl Pts',(4.15834753250204,29.7680072998736,122.958388638945));
#95966=CARTESIAN_POINT('Ctrl Pts',(4.16220273874737,29.8388563147202,122.950337912657));
#95967=CARTESIAN_POINT('Ctrl Pts',(4.1660579449927,29.910147439071,122.945976897614));
#95968=CARTESIAN_POINT('Ctrl Pts',(4.16991315123804,29.9814665213124,122.945333586037));
#95969=CARTESIAN_POINT('Ctrl Pts',(4.17376850808928,30.052788389676,122.944690249329));
#95970=CARTESIAN_POINT('Ctrl Pts',(4.17762386494053,30.1241377323125,122.947764906609));
#95971=CARTESIAN_POINT('Ctrl Pts',(4.18147922179178,30.1951002548221,122.95453343878));
#95972=CARTESIAN_POINT('Ctrl Pts',(4.18533861426034,30.2661370577668,122.961309055952));
#95973=CARTESIAN_POINT('Ctrl Pts',(4.18919800672889,30.3367857477186,122.971786220367));
#95974=CARTESIAN_POINT('Ctrl Pts',(4.19305739919745,30.4066379145317,122.985888987924));
#95975=CARTESIAN_POINT('Ctrl Pts',(4.19691897680088,30.47652963068,122.999999740275));
#95976=CARTESIAN_POINT('Ctrl Pts',(4.20078055440432,30.5456234551795,123.017740061325));
#95977=CARTESIAN_POINT('Ctrl Pts',(4.20464213200775,30.6135246088483,123.038983652073));
#95978=CARTESIAN_POINT('Ctrl Pts',(4.20851046612262,30.6815445675673,123.060264412231));
#95979=CARTESIAN_POINT('Ctrl Pts',(4.21237880023749,30.7483672335371,123.085060510933));
#95980=CARTESIAN_POINT('Ctrl Pts',(4.21624713435236,30.8136169820417,123.11319715682));
#95981=CARTESIAN_POINT('Ctrl Pts',(4.21854485352333,30.8523741301027,123.129909805919));
#95982=CARTESIAN_POINT('Ctrl Pts',(4.22084257269429,30.890576768762,123.14780014868));
#95983=CARTESIAN_POINT('Ctrl Pts',(4.22314029186526,30.9281506612642,123.16682409123));
#95984=CARTESIAN_POINT('Ctrl Pts',(4.22700936521348,30.9914204236903,123.198858044738));
#95985=CARTESIAN_POINT('Ctrl Pts',(4.2308784385617,31.053153750569,123.234234104093));
#95986=CARTESIAN_POINT('Ctrl Pts',(4.23474751190992,31.1129749158546,123.272781311131));
#95987=CARTESIAN_POINT('Ctrl Pts',(4.23861082030571,31.1727069470915,123.3112710825));
#95988=CARTESIAN_POINT('Ctrl Pts',(4.24247412870151,31.2305320671689,123.352922361501));
#95989=CARTESIAN_POINT('Ctrl Pts',(4.2463374370973,31.2860981930608,123.397517862719));
#95990=CARTESIAN_POINT('Ctrl Pts',(4.25019621359021,31.3415991364045,123.442061050619));
#95991=CARTESIAN_POINT('Ctrl Pts',(4.25405499008313,31.3948459722219,123.489541297822));
#95992=CARTESIAN_POINT('Ctrl Pts',(4.25791376657605,31.4455161902342,123.53969848789));
#95993=CARTESIAN_POINT('Ctrl Pts',(4.26177011216426,31.4961544876437,123.589824080546));
#95994=CARTESIAN_POINT('Ctrl Pts',(4.26562645775247,31.5442190431934,123.642622929359));
#95995=CARTESIAN_POINT('Ctrl Pts',(4.26948280334068,31.5894221252485,123.697796148727));
#95996=CARTESIAN_POINT('Ctrl Pts',(4.27333800958602,31.6346118522222,123.752953067373));
#95997=CARTESIAN_POINT('Ctrl Pts',(4.27719321583136,31.6769414763768,123.810482588337));
#95998=CARTESIAN_POINT('Ctrl Pts',(4.28104842207669,31.7161628592682,123.870051946783));
#95999=CARTESIAN_POINT('Ctrl Pts',(4.28490377892795,31.7553857743661,123.929623632341));
#96000=CARTESIAN_POINT('Ctrl Pts',(4.28875913577921,31.7914999418229,123.991234906642));
#96001=CARTESIAN_POINT('Ctrl Pts',(4.29261449263046,31.8243009267402,124.054524621582));
#96002=CARTESIAN_POINT('Ctrl Pts',(4.29647388509903,31.8571362462801,124.117880585401));
#96003=CARTESIAN_POINT('Ctrl Pts',(4.30033327756759,31.886651236199,124.182918064873));
#96004=CARTESIAN_POINT('Ctrl Pts',(4.30419267003616,31.9126881934482,124.249252747495));
#96005=CARTESIAN_POINT('Ctrl Pts',(4.3080542476396,31.9387398924641,124.3156249879));
#96006=CARTESIAN_POINT('Ctrl Pts',(4.31191582524304,31.9613094849422,124.383295432486));
#96007=CARTESIAN_POINT('Ctrl Pts',(4.31577740284648,31.9802889661263,124.45186391002));
#96008=CARTESIAN_POINT('Ctrl Pts',(4.31964573696136,31.9993016552619,124.520552360206));
#96009=CARTESIAN_POINT('Ctrl Pts',(4.32351407107624,32.0147115867778,124.590141505974));
#96010=CARTESIAN_POINT('Ctrl Pts',(4.32738240519111,32.0264618851514,124.660220968086));
#96011=CARTESIAN_POINT('Ctrl Pts',(4.32968012436202,32.0334413458276,124.701846877017));
#96012=CARTESIAN_POINT('Ctrl Pts',(4.33197784353292,32.0391306287757,124.743645657191));
#96013=CARTESIAN_POINT('Ctrl Pts',(4.33427556270382,32.0435265158289,124.785531024145));
#96014=CARTESIAN_POINT('Ctrl Pts',(4.33815880198178,32.0509557445539,124.856319005629));
#96015=CARTESIAN_POINT('Ctrl Pts',(4.34204204125973,32.0547076876349,124.927499585747));
#96016=CARTESIAN_POINT('Ctrl Pts',(4.34592528053768,32.0547496441584,124.998790731288));
#96017=CARTESIAN_POINT('Origin',(-1.54592528053767,30.,125.));
#96018=CARTESIAN_POINT('',(3.19385981572075,28.7479590808042,126.629230216746));
#96019=CARTESIAN_POINT('',(3.25213329794676,28.7479590808042,126.629230216746));
#96020=CARTESIAN_POINT('',(-1.54592528053767,28.7479590808042,126.629230216746));
#96021=CARTESIAN_POINT('',(3.70407471941286,32.0547494644754,124.998516511556));
#96022=CARTESIAN_POINT('Ctrl Pts',(3.25213329794676,28.7479590808042,126.629230216746));
#96023=CARTESIAN_POINT('Ctrl Pts',(3.25599022148438,28.6914802934207,126.585827048708));
#96024=CARTESIAN_POINT('Ctrl Pts',(3.259847145022,28.6372135453225,126.539447080033));
#96025=CARTESIAN_POINT('Ctrl Pts',(3.26370406855962,28.5854831545881,126.490348837201));
#96026=CARTESIAN_POINT('Ctrl Pts',(3.26755947480621,28.533773114285,126.441269909328));
#96027=CARTESIAN_POINT('Ctrl Pts',(3.2714148810528,28.4845978030209,126.389475163782));
#96028=CARTESIAN_POINT('Ctrl Pts',(3.27527028729939,28.4382467997662,126.335261960837));
#96029=CARTESIAN_POINT('Ctrl Pts',(3.27912546654167,28.3918985256343,126.281051949938));
#96030=CARTESIAN_POINT('Ctrl Pts',(3.28298064578395,28.3483745438087,126.224424134623));
#96031=CARTESIAN_POINT('Ctrl Pts',(3.28683582502624,28.3079248849838,126.165709812793));
#96032=CARTESIAN_POINT('Ctrl Pts',(3.29069479734036,28.2674354281489,126.106937722537));
#96033=CARTESIAN_POINT('Ctrl Pts',(3.29455376965448,28.2300266127931,126.046075426003));
#96034=CARTESIAN_POINT('Ctrl Pts',(3.29841274196861,28.1959052402902,125.98348343173));
#96035=CARTESIAN_POINT('Ctrl Pts',(3.30227356023783,28.16176754569,125.920861496322));
#96036=CARTESIAN_POINT('Ctrl Pts',(3.30613437850706,28.1309206370948,125.856508653557));
#96037=CARTESIAN_POINT('Ctrl Pts',(3.30999519677628,28.1035241472872,125.790807753235));
#96038=CARTESIAN_POINT('Ctrl Pts',(3.3138631308159,28.0760771637456,125.72498576135));
#96039=CARTESIAN_POINT('Ctrl Pts',(3.31773106485551,28.0520934688296,125.657811206416));
#96040=CARTESIAN_POINT('Ctrl Pts',(3.32159899889512,28.0316834001859,125.589684089489));
#96041=CARTESIAN_POINT('Ctrl Pts',(3.32502724915889,28.0135934269613,125.529301258711));
#96042=CARTESIAN_POINT('Ctrl Pts',(3.32845549942266,27.998310112601,125.468170553243));
#96043=CARTESIAN_POINT('Ctrl Pts',(3.33188374968643,27.9858764481741,125.406575799182));
#96044=CARTESIAN_POINT('Ctrl Pts',(3.33575282303466,27.9718439954785,125.337060856283));
#96045=CARTESIAN_POINT('Ctrl Pts',(3.33962189638289,27.9613871130559,125.266682430377));
#96046=CARTESIAN_POINT('Ctrl Pts',(3.34349096973111,27.9546042657694,125.195841397287));
#96047=CARTESIAN_POINT('Ctrl Pts',(3.34735427812691,27.9478315249835,125.125105917943));
#96048=CARTESIAN_POINT('Ctrl Pts',(3.35121758652271,27.9447219988389,125.053909679268));
#96049=CARTESIAN_POINT('Ctrl Pts',(3.35508089491851,27.9453231361891,124.982663684928));
#96050=CARTESIAN_POINT('Ctrl Pts',(3.35893967141143,27.9459235683675,124.911501266606));
#96051=CARTESIAN_POINT('Ctrl Pts',(3.36279844790435,27.9502260137478,124.840289691965));
#96052=CARTESIAN_POINT('Ctrl Pts',(3.36665722439727,27.9582259778627,124.769443271568));
#96053=CARTESIAN_POINT('Ctrl Pts',(3.37051356998549,27.9662209022584,124.69864148213));
#96054=CARTESIAN_POINT('Ctrl Pts',(3.37436991557371,27.9779086696809,124.628204872126));
#96055=CARTESIAN_POINT('Ctrl Pts',(3.37822626116192,27.9932328074159,124.558544456068));
#96056=CARTESIAN_POINT('Ctrl Pts',(3.38208146740726,28.0085524176919,124.488904620919));
#96057=CARTESIAN_POINT('Ctrl Pts',(3.3859366736526,28.0275061610818,124.420040998629));
#96058=CARTESIAN_POINT('Ctrl Pts',(3.38979187989794,28.049986444219,124.352354499151));
#96059=CARTESIAN_POINT('Ctrl Pts',(3.39364723674921,28.0724676055618,124.284665355459));
#96060=CARTESIAN_POINT('Ctrl Pts',(3.39750259360047,28.0984754249617,124.218153886206));
#96061=CARTESIAN_POINT('Ctrl Pts',(3.40135795045173,28.1278529579342,124.153204265844));
#96062=CARTESIAN_POINT('Ctrl Pts',(3.4052173429203,28.1572612420109,124.088186659088));
#96063=CARTESIAN_POINT('Ctrl Pts',(3.40907673538887,28.1900460802679,124.024734608321));
#96064=CARTESIAN_POINT('Ctrl Pts',(3.41293612785744,28.2260033992025,123.963209942728));
#96065=CARTESIAN_POINT('Ctrl Pts',(3.41679770546088,28.261981076676,123.901650442716));
#96066=CARTESIAN_POINT('Ctrl Pts',(3.42065928306432,28.3011345437782,123.842020906504));
#96067=CARTESIAN_POINT('Ctrl Pts',(3.42452086066776,28.3432164968478,123.784653964427));
#96068=CARTESIAN_POINT('Ctrl Pts',(3.42838919478264,28.3853720797202,123.727186648762));
#96069=CARTESIAN_POINT('Ctrl Pts',(3.43225752889752,28.430466071138,123.671990207426));
#96070=CARTESIAN_POINT('Ctrl Pts',(3.4361258630124,28.478211487711,123.619363448852));
#96071=CARTESIAN_POINT('Ctrl Pts',(3.43842358218327,28.5065713852076,123.58810412417));
#96072=CARTESIAN_POINT('Ctrl Pts',(3.44072130135413,28.5358660346019,123.557750714455));
#96073=CARTESIAN_POINT('Ctrl Pts',(3.44301902052499,28.5660296831504,123.528359183464));
#96074=CARTESIAN_POINT('Ctrl Pts',(3.4468880938732,28.6168215162709,123.478867500293));
#96075=CARTESIAN_POINT('Ctrl Pts',(3.45075716722141,28.6702780599787,123.431911487284));
#96076=CARTESIAN_POINT('Ctrl Pts',(3.45462624056962,28.726115924839,123.387791289705));
#96077=CARTESIAN_POINT('Ctrl Pts',(3.4584895489654,28.7818705908023,123.343736831598));
#96078=CARTESIAN_POINT('Ctrl Pts',(3.46235285736118,28.8399991568083,123.302510100363));
#96079=CARTESIAN_POINT('Ctrl Pts',(3.46621616575696,28.9001820553279,123.264373873475));
#96080=CARTESIAN_POINT('Ctrl Pts',(3.47007494224987,28.9602943555357,123.226282382771));
#96081=CARTESIAN_POINT('Ctrl Pts',(3.47393371874278,29.0224557931118,123.19127445399));
#96082=CARTESIAN_POINT('Ctrl Pts',(3.47779249523568,29.0863158500692,123.159571018304));
#96083=CARTESIAN_POINT('Ctrl Pts',(3.48164884082389,29.1501356772509,123.12788755476));
#96084=CARTESIAN_POINT('Ctrl Pts',(3.48550518641209,29.2156515667144,123.099504669707));
#96085=CARTESIAN_POINT('Ctrl Pts',(3.48936153200029,29.282487578493,123.074597837468));
#96086=CARTESIAN_POINT('Ctrl Pts',(3.49321673824562,29.3493038438221,123.049698363859));
#96087=CARTESIAN_POINT('Ctrl Pts',(3.49707194449095,29.4174390022008,123.028273073754));
#96088=CARTESIAN_POINT('Ctrl Pts',(3.50092715073628,29.4864978769364,123.010449012438));
#96089=CARTESIAN_POINT('Ctrl Pts',(3.50478250758752,29.5555594494978,122.992624254815));
#96090=CARTESIAN_POINT('Ctrl Pts',(3.50863786443876,29.6255443391371,122.978401124561));
#96091=CARTESIAN_POINT('Ctrl Pts',(3.51249322129,29.6960446631114,122.967856128204));
#96092=CARTESIAN_POINT('Ctrl Pts',(3.51635261375855,29.766618783712,122.957300093811));
#96093=CARTESIAN_POINT('Ctrl Pts',(3.52021200622711,29.8377089342526,122.950429951004));
#96094=CARTESIAN_POINT('Ctrl Pts',(3.52407139869566,29.9089004441357,122.947270491901));
#96095=CARTESIAN_POINT('Ctrl Pts',(3.52793297629909,29.9801322616715,122.944109243955));
#96096=CARTESIAN_POINT('Ctrl Pts',(3.53179455390252,30.0514650667905,122.94466285826));
#96097=CARTESIAN_POINT('Ctrl Pts',(3.53565613150595,30.1224852736351,122.948903970985));
#96098=CARTESIAN_POINT('Ctrl Pts',(3.53952446562081,30.1936297428639,122.953152504285));
#96099=CARTESIAN_POINT('Ctrl Pts',(3.54339279973568,30.2644600389161,122.961101363275));
#96100=CARTESIAN_POINT('Ctrl Pts',(3.54726113385054,30.3345694703278,122.972671503672));
#96101=CARTESIAN_POINT('Ctrl Pts',(3.54955885302155,30.3762131804726,122.97954395383));
#96102=CARTESIAN_POINT('Ctrl Pts',(3.55185657219255,30.4176027678518,122.987693065516));
#96103=CARTESIAN_POINT('Ctrl Pts',(3.55415429136355,30.4586555529481,122.99709394972));
#96104=CARTESIAN_POINT('Ctrl Pts',(3.55802336471178,30.5277833378797,123.012923869659));
#96105=CARTESIAN_POINT('Ctrl Pts',(3.56189243806,30.5962260391797,123.032367785461));
#96106=CARTESIAN_POINT('Ctrl Pts',(3.56576151140822,30.6635777914816,123.055350397333));
#96107=CARTESIAN_POINT('Ctrl Pts',(3.569624819804,30.7308291890953,123.078298764916));
#96108=CARTESIAN_POINT('Ctrl Pts',(3.57348812819978,30.7969924083189,123.104775206827));
#96109=CARTESIAN_POINT('Ctrl Pts',(3.57735143659556,30.8616733563976,123.13465376153));
#96110=CARTESIAN_POINT('Ctrl Pts',(3.58121021308847,30.9262784296706,123.164497266816));
#96111=CARTESIAN_POINT('Ctrl Pts',(3.58506898958139,30.989404246771,123.197734754904));
#96112=CARTESIAN_POINT('Ctrl Pts',(3.5889277660743,31.0506750854314,123.234191565499));
#96113=CARTESIAN_POINT('Ctrl Pts',(3.59278411166251,31.11190732544,123.27062540948));
#96114=CARTESIAN_POINT('Ctrl Pts',(3.59664045725072,31.1712864889583,123.310274304496));
#96115=CARTESIAN_POINT('Ctrl Pts',(3.60049680283892,31.2284612560282,123.352917577977));
#96116=CARTESIAN_POINT('Ctrl Pts',(3.60435200908425,31.2856191310272,123.395548252662));
#96117=CARTESIAN_POINT('Ctrl Pts',(3.60820721532958,31.3405735133575,123.441171259206));
#96118=CARTESIAN_POINT('Ctrl Pts',(3.61206242157491,31.3930033370947,123.489523497256));
#96119=CARTESIAN_POINT('Ctrl Pts',(3.61591777842617,31.4454352090343,123.537877624214));
#96120=CARTESIAN_POINT('Ctrl Pts',(3.61977313527743,31.4953419709618,123.588960863403));
#96121=CARTESIAN_POINT('Ctrl Pts',(3.62362849212869,31.5424381254604,123.642472029155));
#96122=CARTESIAN_POINT('Ctrl Pts',(3.62748788459725,31.5895835781337,123.696039208033));
#96123=CARTESIAN_POINT('Ctrl Pts',(3.63134727706582,31.6339122288398,123.75203902136));
#96124=CARTESIAN_POINT('Ctrl Pts',(3.63520666953438,31.6751783462025,123.810136532658));
#96125=CARTESIAN_POINT('Ctrl Pts',(3.63906824713783,31.7164678278727,123.868266937968));
#96126=CARTESIAN_POINT('Ctrl Pts',(3.64292982474127,31.7546910639906,123.928496995212));
#96127=CARTESIAN_POINT('Ctrl Pts',(3.64679140234471,31.7896467299866,123.990464391738));
#96128=CARTESIAN_POINT('Ctrl Pts',(3.65065973645959,31.8246635570886,124.052540211159));
#96129=CARTESIAN_POINT('Ctrl Pts',(3.65452807057446,31.8564011831501,124.116359003769));
#96130=CARTESIAN_POINT('Ctrl Pts',(3.65839640468934,31.8847054418733,124.181536219572));
#96131=CARTESIAN_POINT('Ctrl Pts',(3.66069412386026,31.9015176499081,124.220250284544));
#96132=CARTESIAN_POINT('Ctrl Pts',(3.66299184303119,31.9171194519224,124.259443265274));
#96133=CARTESIAN_POINT('Ctrl Pts',(3.66528956220212,31.9314869158582,124.299032200191));
#96134=CARTESIAN_POINT('Ctrl Pts',(3.66976608681316,31.9594782851779,124.376161226108));
#96135=CARTESIAN_POINT('Ctrl Pts',(3.67424261142421,31.9828725789903,124.455042428842));
#96136=CARTESIAN_POINT('Ctrl Pts',(3.67871913603526,32.0014795158366,124.535158833378));
#96137=CARTESIAN_POINT('Ctrl Pts',(3.68315616207663,32.0199222745636,124.614568331629));
#96138=CARTESIAN_POINT('Ctrl Pts',(3.687593188118,32.0336616960581,124.695191164253));
#96139=CARTESIAN_POINT('Ctrl Pts',(3.69203021415936,32.0425588387462,124.776502902122));
#96140=CARTESIAN_POINT('Ctrl Pts',(3.69604504924386,32.0506094024081,124.850077682827));
#96141=CARTESIAN_POINT('Ctrl Pts',(3.70005988432836,32.0546958210969,124.924216166571));
#96142=CARTESIAN_POINT('Ctrl Pts',(3.70407471941286,32.0547494644754,124.998516511556));
#96143=CARTESIAN_POINT('Ctrl Pts',(3.70407471946232,32.0547494644761,124.998516512471));
#96144=CARTESIAN_POINT('Ctrl Pts',(3.70793830290603,32.0548010869056,125.07001772652));
#96145=CARTESIAN_POINT('Ctrl Pts',(3.71180188634973,32.05111623467,125.141552238129));
#96146=CARTESIAN_POINT('Ctrl Pts',(3.71566546979344,32.0437110737996,125.212703101362));
#96147=CARTESIAN_POINT('Ctrl Pts',(3.71952882663486,32.0363063472477,125.28384979154));
#96148=CARTESIAN_POINT('Ctrl Pts',(3.72339218347628,32.0251817962445,125.354612398351));
#96149=CARTESIAN_POINT('Ctrl Pts',(3.72725554031771,32.0104054413673,125.4245792315));
#96150=CARTESIAN_POINT('Ctrl Pts',(3.73111993974985,31.9956250988464,125.494564946355));
#96151=CARTESIAN_POINT('Ctrl Pts',(3.73498433918199,31.9771910976808,125.563753989812));
#96152=CARTESIAN_POINT('Ctrl Pts',(3.73884873861412,31.9552221704324,125.631746647597));
#96153=CARTESIAN_POINT('Ctrl Pts',(3.74271803189443,31.9332254218896,125.699825410803));
#96154=CARTESIAN_POINT('Ctrl Pts',(3.74658732517474,31.9076849661823,125.766704306559));
#96155=CARTESIAN_POINT('Ctrl Pts',(3.75045661845505,31.8787685660619,125.832001344757));
#96156=CARTESIAN_POINT('Ctrl Pts',(3.75432884727595,31.849830227758,125.897347922262));
#96157=CARTESIAN_POINT('Ctrl Pts',(3.75820107609685,31.8175110677532,125.961109825251));
#96158=CARTESIAN_POINT('Ctrl Pts',(3.76207330491775,31.7820246506346,126.022929961938));
#96159=CARTESIAN_POINT('Ctrl Pts',(3.7659523107069,31.7464761270824,126.084858292929));
#96160=CARTESIAN_POINT('Ctrl Pts',(3.76983131649604,31.7077495507253,126.14483767518));
#96161=CARTESIAN_POINT('Ctrl Pts',(3.77371032228519,31.6661010629575,126.202540980804));
#96162=CARTESIAN_POINT('Ctrl Pts',(3.77461515920368,31.6563859216609,126.216001151808));
#96163=CARTESIAN_POINT('Ctrl Pts',(3.77551999612218,31.6465119574739,126.229337625414));
#96164=CARTESIAN_POINT('Ctrl Pts',(3.77642483304067,31.6364827163499,126.242546530955));
#96165=CARTESIAN_POINT('Ctrl Pts',(3.78029390638889,31.5935977845543,126.299027675063));
#96166=CARTESIAN_POINT('Ctrl Pts',(3.7841629797371,31.5477013562299,126.353396665213));
#96167=CARTESIAN_POINT('Ctrl Pts',(3.78803205308531,31.499029141768,126.405314624783));
#96168=CARTESIAN_POINT('Ctrl Pts',(3.79189536148109,31.4504294493225,126.457155226149));
#96169=CARTESIAN_POINT('Ctrl Pts',(3.79575866987688,31.3990625100133,126.506551694649));
#96170=CARTESIAN_POINT('Ctrl Pts',(3.79962197827266,31.3452053570871,126.553196738911));
#96171=CARTESIAN_POINT('Ctrl Pts',(3.80348075476557,31.2914113819767,126.599787065613));
#96172=CARTESIAN_POINT('Ctrl Pts',(3.80733953125848,31.2351333611201,126.643632062676));
#96173=CARTESIAN_POINT('Ctrl Pts',(3.8111983077514,31.1766851454725,126.684461228679));
#96174=CARTESIAN_POINT('Ctrl Pts',(3.8150546533396,31.1182737503153,126.725264673625));
#96175=CARTESIAN_POINT('Ctrl Pts',(3.81891099892781,31.0576952700762,126.763055779299));
#96176=CARTESIAN_POINT('Ctrl Pts',(3.82276734451601,30.9952954419552,126.797605225216));
#96177=CARTESIAN_POINT('Ctrl Pts',(3.82662255076135,30.9329140496297,126.832144463628));
#96178=CARTESIAN_POINT('Ctrl Pts',(3.83047775700669,30.8687128024804,126.863443708473));
#96179=CARTESIAN_POINT('Ctrl Pts',(3.83433296325203,30.8030636482531,126.891318677366));
#96180=CARTESIAN_POINT('Ctrl Pts',(3.83818832010328,30.7374119294027,126.919194735212));
#96181=CARTESIAN_POINT('Ctrl Pts',(3.84204367695452,30.6703126391835,126.943646063685));
#96182=CARTESIAN_POINT('Ctrl Pts',(3.84589903380577,30.6021577906023,126.96453647401));
#96183=CARTESIAN_POINT('Ctrl Pts',(3.84975842627433,30.5339316005351,126.985448751494));
#96184=CARTESIAN_POINT('Ctrl Pts',(3.85361781874289,30.4646481118627,127.002792527424));
#96185=CARTESIAN_POINT('Ctrl Pts',(3.85747721121145,30.3947137246523,127.016481747517));
#96186=CARTESIAN_POINT('Ctrl Pts',(3.86133878881489,30.3247397415547,127.030178718259));
#96187=CARTESIAN_POINT('Ctrl Pts',(3.86520036641832,30.2541146074701,127.040216945716));
#96188=CARTESIAN_POINT('Ctrl Pts',(3.86906194402176,30.1832513896225,127.046562115036));
#96189=CARTESIAN_POINT('Ctrl Pts',(3.87293027813663,30.1122641840707,127.05291838635));
#96190=CARTESIAN_POINT('Ctrl Pts',(3.8767986122515,30.041038548667,127.055568680571));
#96191=CARTESIAN_POINT('Ctrl Pts',(3.88066694636638,29.9699884019038,127.054530814196));
#96192=CARTESIAN_POINT('Ctrl Pts',(3.88296466553733,29.9277859241786,127.053914340697));
#96193=CARTESIAN_POINT('Ctrl Pts',(3.88526238470828,29.8856453002609,127.051997629856));
#96194=CARTESIAN_POINT('Ctrl Pts',(3.88756010387923,29.8436519877084,127.048793025552));
#96195=CARTESIAN_POINT('Ctrl Pts',(3.89142879128779,29.7729475249656,127.043397408683));
#96196=CARTESIAN_POINT('Ctrl Pts',(3.89529747869635,29.7023842190489,127.034326880076));
#96197=CARTESIAN_POINT('Ctrl Pts',(3.89916616610492,29.6323744923485,127.021595668927));
#96198=CARTESIAN_POINT('Ctrl Pts',(3.90302937629832,29.5624638841077,127.008882482388));
#96199=CARTESIAN_POINT('Ctrl Pts',(3.90689258649171,29.4931057738335,126.992518983125));
#96200=CARTESIAN_POINT('Ctrl Pts',(3.91075579668511,29.4247085528086,126.97257124416));
#96201=CARTESIAN_POINT('Ctrl Pts',(3.91461452951286,29.3563906024815,126.952646624135));
#96202=CARTESIAN_POINT('Ctrl Pts',(3.9184732623406,29.289031793557,126.929146150395));
#96203=CARTESIAN_POINT('Ctrl Pts',(3.92233199516835,29.2230295957748,126.902186781959));
#96204=CARTESIAN_POINT('Ctrl Pts',(3.9261881038897,29.157072282362,126.875245747067));
#96205=CARTESIAN_POINT('Ctrl Pts',(3.93004421261106,29.0924701971686,126.84485067038));
#96206=CARTESIAN_POINT('Ctrl Pts',(3.93390032133241,29.0296034510846,126.811167606919));
#96207=CARTESIAN_POINT('Ctrl Pts',(3.93775577558456,28.9667473749147,126.777490260239));
#96208=CARTESIAN_POINT('Ctrl Pts',(3.94161122983672,28.9056264847606,126.740526257113));
#96209=CARTESIAN_POINT('Ctrl Pts',(3.94546668408887,28.8465974085836,126.700488172442));
#96210=CARTESIAN_POINT('Ctrl Pts',(3.94765970084876,28.8130211436585,126.677714152838));
#96211=CARTESIAN_POINT('Ctrl Pts',(3.94985271760865,28.7801212097431,126.653946368624));
#96212=CARTESIAN_POINT('Ctrl Pts',(3.95204573436854,28.7479590808042,126.629230216746));
#96213=CARTESIAN_POINT('',(3.64592528049121,32.0547492155205,125.001795499313));
#96214=CARTESIAN_POINT('Ctrl Pts',(3.64592528053768,32.0547492155198,125.001795500168));
#96215=CARTESIAN_POINT('Ctrl Pts',(3.65155534725559,32.0546586344092,125.105455454746));
#96216=CARTESIAN_POINT('Ctrl Pts',(3.65718541397351,32.0467203700823,125.208784026605));
#96217=CARTESIAN_POINT('Ctrl Pts',(3.66281548069143,32.0311035472205,125.31083105213));
#96218=CARTESIAN_POINT('Ctrl Pts',(3.66436496635177,32.0268055443198,125.338916048393));
#96219=CARTESIAN_POINT('Ctrl Pts',(3.66591445201212,32.0219261885265,125.366904156545));
#96220=CARTESIAN_POINT('Ctrl Pts',(3.66746393767247,32.0164695735924,125.394775912736));
#96221=CARTESIAN_POINT('Ctrl Pts',(3.67133301102069,32.0028443791466,125.464371825627));
#96222=CARTESIAN_POINT('Ctrl Pts',(3.67520208436891,31.9855852435914,125.533397845814));
#96223=CARTESIAN_POINT('Ctrl Pts',(3.67907115771713,31.964754531172,125.601445920045));
#96224=CARTESIAN_POINT('Ctrl Pts',(3.68293446611291,31.9439548566924,125.669392602064));
#96225=CARTESIAN_POINT('Ctrl Pts',(3.6867977745087,31.91959430977,125.7363637698));
#96226=CARTESIAN_POINT('Ctrl Pts',(3.69066108290449,31.8917862649132,125.801961526749));
#96227=CARTESIAN_POINT('Ctrl Pts',(3.69451985939741,31.8640108406358,125.867482333418));
#96228=CARTESIAN_POINT('Ctrl Pts',(3.69837863589032,31.8327961401166,125.931632484396));
#96229=CARTESIAN_POINT('Ctrl Pts',(3.70223741238324,31.7983047958042,125.994030896848));
#96230=CARTESIAN_POINT('Ctrl Pts',(3.70609375797145,31.7638351799259,126.056390000312));
#96231=CARTESIAN_POINT('Ctrl Pts',(3.70995010355966,31.726093250008,126.116999130501));
#96232=CARTESIAN_POINT('Ctrl Pts',(3.71380644914788,31.6852884029878,126.175500132392));
#96233=CARTESIAN_POINT('Ctrl Pts',(3.71766165539321,31.644495611607,126.233983850382));
#96234=CARTESIAN_POINT('Ctrl Pts',(3.72151686163855,31.6006419774167,126.290360278362));
#96235=CARTESIAN_POINT('Ctrl Pts',(3.72537206788388,31.5539802651154,126.344300151801));
#96236=CARTESIAN_POINT('Ctrl Pts',(3.72922742473514,31.5073167299466,126.398242132433));
#96237=CARTESIAN_POINT('Ctrl Pts',(3.73308278158639,31.45784521836,126.449747003595));
#96238=CARTESIAN_POINT('Ctrl Pts',(3.73693813843765,31.4058576914228,126.498519841032));
#96239=CARTESIAN_POINT('Ctrl Pts',(3.74079753090621,31.3538157462381,126.547343731722));
#96240=CARTESIAN_POINT('Ctrl Pts',(3.74465692337477,31.2992528833456,126.593429546883));
#96241=CARTESIAN_POINT('Ctrl Pts',(3.74851631584333,31.2424960612573,126.636521035691));
#96242=CARTESIAN_POINT('Ctrl Pts',(3.75237789344677,31.1857071042378,126.679636922307));
#96243=CARTESIAN_POINT('Ctrl Pts',(3.75623947105021,31.1267221170804,126.719754834329));
#96244=CARTESIAN_POINT('Ctrl Pts',(3.76010104865366,31.0658968317975,126.756662035357));
#96245=CARTESIAN_POINT('Ctrl Pts',(3.76396938276853,31.0049651219447,126.793633812045));
#96246=CARTESIAN_POINT('Ctrl Pts',(3.7678377168834,30.9421871132999,126.827383431728));
#96247=CARTESIAN_POINT('Ctrl Pts',(3.77170605099828,30.8779422625739,126.857744585805));
#96248=CARTESIAN_POINT('Ctrl Pts',(3.77400377016919,30.839782005274,126.875778551771));
#96249=CARTESIAN_POINT('Ctrl Pts',(3.7763014893401,30.8011046100179,126.892617941925));
#96250=CARTESIAN_POINT('Ctrl Pts',(3.77859920851102,30.7619922359674,126.908236199957));
#96251=CARTESIAN_POINT('Ctrl Pts',(3.78246828185923,30.6961318619321,126.934535404255));
#96252=CARTESIAN_POINT('Ctrl Pts',(3.78633735520744,30.6287793604349,126.957472487004));
#96253=CARTESIAN_POINT('Ctrl Pts',(3.79020642855566,30.5603113789128,126.976878529693));
#96254=CARTESIAN_POINT('Ctrl Pts',(3.79406973695144,30.4919454152697,126.996255657212));
#96255=CARTESIAN_POINT('Ctrl Pts',(3.79793304534722,30.4224677343411,127.012112056774));
#96256=CARTESIAN_POINT('Ctrl Pts',(3.801796353743,30.3522741165742,127.024327174469));
#96257=CARTESIAN_POINT('Ctrl Pts',(3.80565513023591,30.2821628403201,127.036527963064));
#96258=CARTESIAN_POINT('Ctrl Pts',(3.80951390672882,30.211337771702,127.04509587146));
#96259=CARTESIAN_POINT('Ctrl Pts',(3.81337268322173,30.1402072810093,127.049960848614));
#96260=CARTESIAN_POINT('Ctrl Pts',(3.81722902880993,30.069121600231,127.054822760991));
#96261=CARTESIAN_POINT('Ctrl Pts',(3.82108537439814,29.9977313626166,127.05598633715));
#96262=CARTESIAN_POINT('Ctrl Pts',(3.82494171998634,29.9264510391781,127.05343325016));
#96263=CARTESIAN_POINT('Ctrl Pts',(3.82879692623167,29.8551917752445,127.05088091747));
#96264=CARTESIAN_POINT('Ctrl Pts',(3.832652132477,29.7840428462279,127.044614118991));
#96265=CARTESIAN_POINT('Ctrl Pts',(3.83650733872233,29.7134179720963,127.0346666321));
#96266=CARTESIAN_POINT('Ctrl Pts',(3.84036269557357,29.6427903389622,127.024718756606));
#96267=CARTESIAN_POINT('Ctrl Pts',(3.84421805242482,29.5726872820893,127.011089977162));
#96268=CARTESIAN_POINT('Ctrl Pts',(3.84807340927606,29.5035149293875,126.993865626656));
#96269=CARTESIAN_POINT('Ctrl Pts',(3.85193280174462,29.4342701701212,126.97662324646));
#96270=CARTESIAN_POINT('Ctrl Pts',(3.85579219421317,29.3659585321456,126.955777899661));
#96271=CARTESIAN_POINT('Ctrl Pts',(3.85965158668173,29.2989726334945,126.931465297102));
#96272=CARTESIAN_POINT('Ctrl Pts',(3.86351316428516,29.2319488083499,126.907138929083));
#96273=CARTESIAN_POINT('Ctrl Pts',(3.8673747418886,29.1662526643715,126.87934158674));
#96274=CARTESIAN_POINT('Ctrl Pts',(3.87123631949203,29.1022558669436,126.848256755449));
#96275=CARTESIAN_POINT('Ctrl Pts',(3.8751046536069,29.0381470958257,126.817117535761));
#96276=CARTESIAN_POINT('Ctrl Pts',(3.87897298772177,28.9757440330046,126.782679577797));
#96277=CARTESIAN_POINT('Ctrl Pts',(3.88284132183664,28.9153922052714,126.745171479859));
#96278=CARTESIAN_POINT('Ctrl Pts',(3.88513904100762,28.8795443318798,126.722892360957));
#96279=CARTESIAN_POINT('Ctrl Pts',(3.8874367601786,28.8444195966073,126.699530876914));
#96280=CARTESIAN_POINT('Ctrl Pts',(3.88973447934958,28.8100848707453,126.675141650032));
#96281=CARTESIAN_POINT('Ctrl Pts',(3.89113844278674,28.7891055011408,126.660239227127));
#96282=CARTESIAN_POINT('Ctrl Pts',(3.8925424062239,28.7683912634568,126.644932066913));
#96283=CARTESIAN_POINT('Ctrl Pts',(3.89394636966105,28.7479590808042,126.629230216746));
#96284=CARTESIAN_POINT('Ctrl Pts',(3.19385981572075,28.7479590808042,126.629230216746));
#96285=CARTESIAN_POINT('Ctrl Pts',(3.19772164131035,28.6914284965474,126.585787243526));
#96286=CARTESIAN_POINT('Ctrl Pts',(3.20158346689996,28.6372142192413,126.539439069122));
#96287=CARTESIAN_POINT('Ctrl Pts',(3.20544529248956,28.5856144481732,126.490473439308));
#96288=CARTESIAN_POINT('Ctrl Pts',(3.2093137709599,28.5339257846591,126.441423454961));
#96289=CARTESIAN_POINT('Ctrl Pts',(3.21318224943023,28.4848609521703,126.389747366776));
#96290=CARTESIAN_POINT('Ctrl Pts',(3.21705072790057,28.4386794775978,126.335767864872));
#96291=CARTESIAN_POINT('Ctrl Pts',(3.21900810337312,28.41531254243,126.30845527832));
#96292=CARTESIAN_POINT('Ctrl Pts',(3.22096547884567,28.3926831268905,126.280553475476));
#96293=CARTESIAN_POINT('Ctrl Pts',(3.22292285431822,28.3708205831168,126.252107020228));
#96294=CARTESIAN_POINT('Ctrl Pts',(3.22679192766653,28.3276056830492,126.195877940321));
#96295=CARTESIAN_POINT('Ctrl Pts',(3.23066100101483,28.28722056777,126.137298834087));
#96296=CARTESIAN_POINT('Ctrl Pts',(3.23453007436313,28.2499301970683,126.076686234409));
#96297=CARTESIAN_POINT('Ctrl Pts',(3.238393382759,28.2126953893384,126.016163948024));
#96298=CARTESIAN_POINT('Ctrl Pts',(3.24225669115488,28.1785464255689,125.953614592887));
#96299=CARTESIAN_POINT('Ctrl Pts',(3.24611999955075,28.1477069248048,125.889386263714));
#96300=CARTESIAN_POINT('Ctrl Pts',(3.24997877604375,28.1169036007079,125.825233278397));
#96301=CARTESIAN_POINT('Ctrl Pts',(3.25383755253675,28.0894022374881,125.759405667014));
#96302=CARTESIAN_POINT('Ctrl Pts',(3.25769632902976,28.0653812767394,125.692277370791));
#96303=CARTESIAN_POINT('Ctrl Pts',(3.26155267461805,28.041375448421,125.625191363229));
#96304=CARTESIAN_POINT('Ctrl Pts',(3.26540902020635,28.0208458358893,125.556806752784));
#96305=CARTESIAN_POINT('Ctrl Pts',(3.26926536579465,28.0039227637665,125.487517414551));
#96306=CARTESIAN_POINT('Ctrl Pts',(3.27312057204007,27.987004691502,125.418248547593));
#96307=CARTESIAN_POINT('Ctrl Pts',(3.27697577828549,27.9736911594534,125.348075955166));
#96308=CARTESIAN_POINT('Ctrl Pts',(3.28083098453091,27.9640621465046,125.277406955941));
#96309=CARTESIAN_POINT('Ctrl Pts',(3.28468634138225,27.9544327573927,125.20673519599));
#96310=CARTESIAN_POINT('Ctrl Pts',(3.28854169823359,27.9484882365528,125.135567472377));
#96311=CARTESIAN_POINT('Ctrl Pts',(3.29239705508493,27.9462568852957,125.064317814831));
#96312=CARTESIAN_POINT('Ctrl Pts',(3.29625644755358,27.9440231983586,124.99299357629));
#96313=CARTESIAN_POINT('Ctrl Pts',(3.30011584002223,27.9455104551316,124.921587719152));
#96314=CARTESIAN_POINT('Ctrl Pts',(3.30397523249088,27.9506948035853,124.850514969151));
#96315=CARTESIAN_POINT('Ctrl Pts',(3.30783681009441,27.9558820873458,124.779401978739));
#96316=CARTESIAN_POINT('Ctrl Pts',(3.31169838769794,27.9647705692282,124.708622953138));
#96317=CARTESIAN_POINT('Ctrl Pts',(3.31555996530147,27.9772847256459,124.638585443853));
#96318=CARTESIAN_POINT('Ctrl Pts',(3.31942829941643,27.9898207777885,124.568425391587));
#96319=CARTESIAN_POINT('Ctrl Pts',(3.32329663353139,28.0059950596886,124.499009919224));
#96320=CARTESIAN_POINT('Ctrl Pts',(3.32716496764636,28.0256815275713,124.430733689802));
#96321=CARTESIAN_POINT('Ctrl Pts',(3.3294626868165,28.0373749266683,124.390178867869));
#96322=CARTESIAN_POINT('Ctrl Pts',(3.33176040598664,28.0503065279579,124.350025665612));
#96323=CARTESIAN_POINT('Ctrl Pts',(3.33405812515678,28.0644419479985,124.310353286217));
#96324=CARTESIAN_POINT('Ctrl Pts',(3.33792719850497,28.0882442375279,124.243549932798));
#96325=CARTESIAN_POINT('Ctrl Pts',(3.34179627185317,28.1155556601758,124.177849434963));
#96326=CARTESIAN_POINT('Ctrl Pts',(3.34566534520137,28.1462539875549,124.113646073036));
#96327=CARTESIAN_POINT('Ctrl Pts',(3.34952865359713,28.1769065741631,124.049538374669));
#96328=CARTESIAN_POINT('Ctrl Pts',(3.3533919619929,28.2109358404626,123.986923818939));
#96329=CARTESIAN_POINT('Ctrl Pts',(3.35725527038866,28.2481706198596,123.926179072016));
#96330=CARTESIAN_POINT('Ctrl Pts',(3.36111404688156,28.2853617205268,123.865505582488));
#96331=CARTESIAN_POINT('Ctrl Pts',(3.36497282337445,28.3257506124864,123.806697957088));
#96332=CARTESIAN_POINT('Ctrl Pts',(3.36883159986734,28.3691199117396,123.75010892466));
#96333=CARTESIAN_POINT('Ctrl Pts',(3.37268794545553,28.4124618897335,123.693555541496));
#96334=CARTESIAN_POINT('Ctrl Pts',(3.37654429104372,28.4587802551696,123.639218363069));
#96335=CARTESIAN_POINT('Ctrl Pts',(3.3804006366319,28.5078147798201,123.587420504475));
#96336=CARTESIAN_POINT('Ctrl Pts',(3.38425584287721,28.5568348174038,123.535637949365));
#96337=CARTESIAN_POINT('Ctrl Pts',(3.38811104912253,28.6085690872771,123.48639357726));
#96338=CARTESIAN_POINT('Ctrl Pts',(3.39196625536784,28.662718760955,123.439975496924));
#96339=CARTESIAN_POINT('Ctrl Pts',(3.39582161221907,28.7168705500219,123.393555603238));
#96340=CARTESIAN_POINT('Ctrl Pts',(3.3996769690703,28.7734375599752,123.349962535017));
#96341=CARTESIAN_POINT('Ctrl Pts',(3.40353232592153,28.8320872960194,123.309444624279));
#96342=CARTESIAN_POINT('Ctrl Pts',(3.40739171839007,28.8907984240175,123.268884301181));
#96343=CARTESIAN_POINT('Ctrl Pts',(3.41125111085861,28.9515962295857,123.231405837977));
#96344=CARTESIAN_POINT('Ctrl Pts',(3.41511050332715,29.0141193470862,123.197214127881));
#96345=CARTESIAN_POINT('Ctrl Pts',(3.41897208093056,29.076677864315,123.163003058911));
#96346=CARTESIAN_POINT('Ctrl Pts',(3.42283365853398,29.1409632000927,123.13208265822));
#96347=CARTESIAN_POINT('Ctrl Pts',(3.4266952361374,29.2065919913672,123.104610516454));
#96348=CARTESIAN_POINT('Ctrl Pts',(3.43056357025225,29.2723356117929,123.077090307328));
#96349=CARTESIAN_POINT('Ctrl Pts',(3.4344319043671,29.3394269233642,123.053030566895));
#96350=CARTESIAN_POINT('Ctrl Pts',(3.43830023848196,29.4074659908564,123.032539451346));
#96351=CARTESIAN_POINT('Ctrl Pts',(3.44059795765308,29.4478799429921,123.02036810636));
#96352=CARTESIAN_POINT('Ctrl Pts',(3.44289567682421,29.4886280333437,123.00945485306));
#96353=CARTESIAN_POINT('Ctrl Pts',(3.44519339599534,29.529625071522,122.999813761381));
#96354=CARTESIAN_POINT('Ctrl Pts',(3.44906246934355,29.5986589855722,122.983579361925));
#96355=CARTESIAN_POINT('Ctrl Pts',(3.45293154269175,29.6686695703833,122.970891287314));
#96356=CARTESIAN_POINT('Ctrl Pts',(3.45680061603996,29.7392592815909,122.961860691645));
#96357=CARTESIAN_POINT('Ctrl Pts',(3.46066392443573,29.8097438135242,122.95284355164));
#96358=CARTESIAN_POINT('Ctrl Pts',(3.46452723283151,29.8808052810823,122.947473134267));
#96359=CARTESIAN_POINT('Ctrl Pts',(3.46839054122728,29.9520343959943,122.945809925218));
#96360=CARTESIAN_POINT('Ctrl Pts',(3.47224931772019,30.0231799546903,122.944148667218));
#96361=CARTESIAN_POINT('Ctrl Pts',(3.47610809421309,30.0944922868088,122.946185990665));
#96362=CARTESIAN_POINT('Ctrl Pts',(3.47996687070599,30.1655571482086,122.951930569249));
#96363=CARTESIAN_POINT('Ctrl Pts',(3.48382321629418,30.2365772410383,122.957671528934));
#96364=CARTESIAN_POINT('Ctrl Pts',(3.48767956188238,30.3073496893877,122.967115071211));
#96365=CARTESIAN_POINT('Ctrl Pts',(3.49153590747058,30.3774618917446,122.980217813035));
#96366=CARTESIAN_POINT('Ctrl Pts',(3.4953911137159,30.4475533797138,122.993316683703));
#96367=CARTESIAN_POINT('Ctrl Pts',(3.49924631996122,30.5169845316942,123.010072518449));
#96368=CARTESIAN_POINT('Ctrl Pts',(3.50310152620654,30.5853512211257,123.030390518294));
#96369=CARTESIAN_POINT('Ctrl Pts',(3.50695688305778,30.6537205813425,123.050709311873));
#96370=CARTESIAN_POINT('Ctrl Pts',(3.51081223990901,30.7210249314217,123.07459040633));
#96371=CARTESIAN_POINT('Ctrl Pts',(3.51466759676025,30.7868753035814,123.101889144672));
#96372=CARTESIAN_POINT('Ctrl Pts',(3.51852698922879,30.8527946050029,123.129216458128));
#96373=CARTESIAN_POINT('Ctrl Pts',(3.52238638169734,30.9172564406584,123.159968370426));
#96374=CARTESIAN_POINT('Ctrl Pts',(3.52624577416589,30.9798926790898,123.193952409274));
#96375=CARTESIAN_POINT('Ctrl Pts',(3.53010735176932,31.0425643812969,123.227955689417));
#96376=CARTESIAN_POINT('Ctrl Pts',(3.53396892937274,31.1034080141082,123.265194485333));
#96377=CARTESIAN_POINT('Ctrl Pts',(3.53783050697616,31.1620832564081,123.305432188528));
#96378=CARTESIAN_POINT('Ctrl Pts',(3.54169884109102,31.2208611613983,123.345740294686));
#96379=CARTESIAN_POINT('Ctrl Pts',(3.54556717520588,31.2774627151825,123.389057488816));
#96380=CARTESIAN_POINT('Ctrl Pts',(3.54943550932074,31.3315801405306,123.43510642795));
#96381=CARTESIAN_POINT('Ctrl Pts',(3.5517332284918,31.3637248938064,123.462458649116));
#96382=CARTESIAN_POINT('Ctrl Pts',(3.55403094766285,31.3949938940242,123.490773938098));
#96383=CARTESIAN_POINT('Ctrl Pts',(3.5563286668339,31.4253291162108,123.519988353768));
#96384=CARTESIAN_POINT('Ctrl Pts',(3.56013990426075,31.4756462896956,123.568446440295));
#96385=CARTESIAN_POINT('Ctrl Pts',(3.5639511416876,31.5236017843571,123.619581983346));
#96386=CARTESIAN_POINT('Ctrl Pts',(3.56776237911445,31.5688910656204,123.673132114068));
#96387=CARTESIAN_POINT('Ctrl Pts',(3.57156855056505,31.6141201474269,123.72661106484));
#96388=CARTESIAN_POINT('Ctrl Pts',(3.57537472201566,31.656689717376,123.782497865398));
#96389=CARTESIAN_POINT('Ctrl Pts',(3.57918089346626,31.696330794858,123.840491743489));
#96390=CARTESIAN_POINT('Ctrl Pts',(3.58298336737579,31.7359333626423,123.898429282882));
#96391=CARTESIAN_POINT('Ctrl Pts',(3.58678584128533,31.7726127957139,123.958469430919));
#96392=CARTESIAN_POINT('Ctrl Pts',(3.59058831519486,31.8061405313248,124.020278639814));
#96393=CARTESIAN_POINT('Ctrl Pts',(3.59438845464248,31.8396476831728,124.082049902033));
#96394=CARTESIAN_POINT('Ctrl Pts',(3.5981885940901,31.8700067369599,124.145587631282));
#96395=CARTESIAN_POINT('Ctrl Pts',(3.60198873353771,31.8970336521997,124.210531264126));
#96396=CARTESIAN_POINT('Ctrl Pts',(3.60578956781191,31.9240655091052,124.27548677142));
#96397=CARTESIAN_POINT('Ctrl Pts',(3.6095904020861,31.9477638020166,124.341848239274));
#96398=CARTESIAN_POINT('Ctrl Pts',(3.61339123636029,31.9679921061021,124.40923385945));
#96399=CARTESIAN_POINT('Ctrl Pts',(3.61719222217681,31.9882212167064,124.476622166346));
#96400=CARTESIAN_POINT('Ctrl Pts',(3.62099320799334,32.0049799299303,124.545034222851));
#96401=CARTESIAN_POINT('Ctrl Pts',(3.62479419380986,32.0181820637134,124.614074203757));
#96402=CARTESIAN_POINT('Ctrl Pts',(3.62859963984775,32.0313996893825,124.683195198803));
#96403=CARTESIAN_POINT('Ctrl Pts',(3.63240508588563,32.0410523192826,124.752945093908));
#96404=CARTESIAN_POINT('Ctrl Pts',(3.63621053192351,32.047105335722,124.822920054895));
#96405=CARTESIAN_POINT('Ctrl Pts',(3.63944878144608,32.0522561583587,124.88246534387));
#96406=CARTESIAN_POINT('Ctrl Pts',(3.64268703096864,32.0548013150982,124.942173328698));
#96407=CARTESIAN_POINT('Ctrl Pts',(3.6459252804912,32.0547492155205,125.001795499313));
#96408=CARTESIAN_POINT('Origin',(-1.54592528053767,30.,125.));
#96409=CARTESIAN_POINT('',(2.49394332694137,28.7479590808042,126.629230216746));
#96410=CARTESIAN_POINT('',(2.55206159834044,28.7479590808042,126.629230216746));
#96411=CARTESIAN_POINT('',(-1.54592528053767,28.7479590808042,126.629230216746));
#96412=CARTESIAN_POINT('',(3.00407471949958,32.0547499051081,124.999375533621));
#96413=CARTESIAN_POINT('Ctrl Pts',(2.55206159834044,28.7479590808042,126.629230216746));
#96414=CARTESIAN_POINT('Ctrl Pts',(2.55268668349913,28.738868829079,126.622244483847));
#96415=CARTESIAN_POINT('Ctrl Pts',(2.55331176865783,28.729839812397,126.615184797678));
#96416=CARTESIAN_POINT('Ctrl Pts',(2.55393685381652,28.720873281001,126.608052362096));
#96417=CARTESIAN_POINT('Ctrl Pts',(2.55780592716366,28.665373374855,126.563904911101));
#96418=CARTESIAN_POINT('Ctrl Pts',(2.5616750005108,28.612052982777,126.516794349563));
#96419=CARTESIAN_POINT('Ctrl Pts',(2.56554407385794,28.5612455809398,126.466963968247));
#96420=CARTESIAN_POINT('Ctrl Pts',(2.56940738225263,28.5105138825668,126.417207834626));
#96421=CARTESIAN_POINT('Ctrl Pts',(2.57327069064732,28.4622880859468,126.364740262816));
#96422=CARTESIAN_POINT('Ctrl Pts',(2.57713399904201,28.4168691583682,126.309845143814));
#96423=CARTESIAN_POINT('Ctrl Pts',(2.5809927755338,28.3715035100386,126.255014420228));
#96424=CARTESIAN_POINT('Ctrl Pts',(2.58485155202558,28.3289384986386,126.197762178345));
#96425=CARTESIAN_POINT('Ctrl Pts',(2.58871032851737,28.289437480768,126.138408288049));
#96426=CARTESIAN_POINT('Ctrl Pts',(2.59256667410444,28.2499613472646,126.079091788789));
#96427=CARTESIAN_POINT('Ctrl Pts',(2.5964230196915,28.2135456462783,126.01767667131));
#96428=CARTESIAN_POINT('Ctrl Pts',(2.60027936527857,28.1804118450352,125.954513755172));
#96429=CARTESIAN_POINT('Ctrl Pts',(2.60413457152274,28.1472878330499,125.891369500281));
#96430=CARTESIAN_POINT('Ctrl Pts',(2.60798977776692,28.1174440213778,125.826478901844));
#96431=CARTESIAN_POINT('Ctrl Pts',(2.6118449840111,28.0910562596518,125.760217967879));
#96432=CARTESIAN_POINT('Ctrl Pts',(2.61570034086117,28.0646674670723,125.693954445391));
#96433=CARTESIAN_POINT('Ctrl Pts',(2.61955569771125,28.0417351701739,125.626320933222));
#96434=CARTESIAN_POINT('Ctrl Pts',(2.62341105456133,28.0223866848161,125.557712415235));
#96435=CARTESIAN_POINT('Ctrl Pts',(2.62727044702871,28.0030179463183,125.489032080881));
#96436=CARTESIAN_POINT('Ctrl Pts',(2.63112983949609,27.9872406400749,125.419375171884));
#96437=CARTESIAN_POINT('Ctrl Pts',(2.63498923196346,27.9751316358225,125.34914992518));
#96438=CARTESIAN_POINT('Ctrl Pts',(2.63885080956571,27.9630157756187,125.278884917909));
#96439=CARTESIAN_POINT('Ctrl Pts',(2.64271238716795,27.9545724094827,125.208051414956));
#96440=CARTESIAN_POINT('Ctrl Pts',(2.6465739647702,27.9498265305573,125.137063152208));
#96441=CARTESIAN_POINT('Ctrl Pts',(2.65044229888388,27.9450723478793,125.065950682968));
#96442=CARTESIAN_POINT('Ctrl Pts',(2.65431063299756,27.9440285758856,124.994683399202));
#96443=CARTESIAN_POINT('Ctrl Pts',(2.65817896711124,27.946668070431,124.923674712498));
#96444=CARTESIAN_POINT('Ctrl Pts',(2.66047668629252,27.9482358815526,124.881496861081));
#96445=CARTESIAN_POINT('Ctrl Pts',(2.6627744054738,27.9511022049655,124.839410162816));
#96446=CARTESIAN_POINT('Ctrl Pts',(2.66507212465508,27.9552527732088,124.797499775235));
#96447=CARTESIAN_POINT('Ctrl Pts',(2.66894119800399,27.9622418139514,124.726927894671));
#96448=CARTESIAN_POINT('Ctrl Pts',(2.67281027135289,27.9729023830876,124.656580034074));
#96449=CARTESIAN_POINT('Ctrl Pts',(2.6766793447018,27.987210946947,124.586868313476));
#96450=CARTESIAN_POINT('Ctrl Pts',(2.68054265309829,28.0014981909238,124.517260463939));
#96451=CARTESIAN_POINT('Ctrl Pts',(2.68440596149477,28.0194225433456,124.448287344925));
#96452=CARTESIAN_POINT('Ctrl Pts',(2.68826926989126,28.0409087288666,124.380355784446));
#96453=CARTESIAN_POINT('Ctrl Pts',(2.69212804638489,28.0623697097455,124.312503911945));
#96454=CARTESIAN_POINT('Ctrl Pts',(2.69598682287851,28.0873840785132,124.245691631966));
#96455=CARTESIAN_POINT('Ctrl Pts',(2.69984559937214,28.115825933708,124.180313687797));
#96456=CARTESIAN_POINT('Ctrl Pts',(2.70370194496106,28.1442498714517,124.114976929624));
#96457=CARTESIAN_POINT('Ctrl Pts',(2.70755829054999,28.1760968184601,124.051073158967));
#96458=CARTESIAN_POINT('Ctrl Pts',(2.71141463613892,28.2111921518084,123.98897871202));
#96459=CARTESIAN_POINT('Ctrl Pts',(2.71526984238497,28.2462771163718,123.926902610646));
#96460=CARTESIAN_POINT('Ctrl Pts',(2.71912504863103,28.2846083230616,123.866635194417));
#96461=CARTESIAN_POINT('Ctrl Pts',(2.72298025487709,28.3259652456882,123.808528135516));
#96462=CARTESIAN_POINT('Ctrl Pts',(2.72683561172907,28.3673237839476,123.750418806629));
#96463=CARTESIAN_POINT('Ctrl Pts',(2.73069096858105,28.4117079893338,123.694470397125));
#96464=CARTESIAN_POINT('Ctrl Pts',(2.73454632543302,28.4588550702475,123.641004095665));
#96465=CARTESIAN_POINT('Ctrl Pts',(2.73840571790231,28.5060515026436,123.587481828043));
#96466=CARTESIAN_POINT('Ctrl Pts',(2.74226511037161,28.5560162618077,123.536447220084));
#96467=CARTESIAN_POINT('Ctrl Pts',(2.7461245028409,28.6084480614904,123.488186266457));
#96468=CARTESIAN_POINT('Ctrl Pts',(2.74998608044507,28.6609095473362,123.439897988142));
#96469=CARTESIAN_POINT('Ctrl Pts',(2.75384765804924,28.7158404800542,123.394386800424));
#96470=CARTESIAN_POINT('Ctrl Pts',(2.75770923565341,28.7729068174874,123.351898096618));
#96471=CARTESIAN_POINT('Ctrl Pts',(2.76157756976901,28.8300730025479,123.309335051327));
#96472=CARTESIAN_POINT('Ctrl Pts',(2.76544590388462,28.8893816475336,123.269805317836));
#96473=CARTESIAN_POINT('Ctrl Pts',(2.76931423800022,28.950470705352,123.233510310764));
#96474=CARTESIAN_POINT('Ctrl Pts',(2.77161195716469,28.9867564797174,123.211951745545));
#96475=CARTESIAN_POINT('Ctrl Pts',(2.77390967632917,29.0236699387709,123.191533555241));
#96476=CARTESIAN_POINT('Ctrl Pts',(2.77620739549364,29.0611317998039,123.172289939525));
#96477=CARTESIAN_POINT('Ctrl Pts',(2.78007646884175,29.1242129153441,123.139886083632));
#96478=CARTESIAN_POINT('Ctrl Pts',(2.78394554218985,29.1890971270914,123.110688339052));
#96479=CARTESIAN_POINT('Ctrl Pts',(2.78781461553796,29.2554254312378,123.084900453226));
#96480=CARTESIAN_POINT('Ctrl Pts',(2.79167792393363,29.3216549056429,123.059150991572));
#96481=CARTESIAN_POINT('Ctrl Pts',(2.79554123232931,29.3893237522822,123.036801478187));
#96482=CARTESIAN_POINT('Ctrl Pts',(2.79940454072499,29.4580493505793,123.018009319877));
#96483=CARTESIAN_POINT('Ctrl Pts',(2.80326331721779,29.5266943294424,122.999239205947));
#96484=CARTESIAN_POINT('Ctrl Pts',(2.80712209371059,29.5963931313173,122.984018285609));
#96485=CARTESIAN_POINT('Ctrl Pts',(2.8109808702034,29.6667458307424,122.972454878141));
#96486=CARTESIAN_POINT('Ctrl Pts',(2.81483721579149,29.7370542102364,122.960898755248));
#96487=CARTESIAN_POINT('Ctrl Pts',(2.81869356137959,29.8080151917885,122.952995652501));
#96488=CARTESIAN_POINT('Ctrl Pts',(2.82254990696769,29.879217889767,122.948802972811));
#96489=CARTESIAN_POINT('Ctrl Pts',(2.82640511321291,29.9503995511748,122.944611531833));
#96490=CARTESIAN_POINT('Ctrl Pts',(2.83026031945813,30.0218223025503,122.94412836613));
#96491=CARTESIAN_POINT('Ctrl Pts',(2.83411552570336,30.0930710832905,122.947358936405));
#96492=CARTESIAN_POINT('Ctrl Pts',(2.8379708825545,30.1643226474065,122.950589632885));
#96493=CARTESIAN_POINT('Ctrl Pts',(2.84182623940563,30.2353997422065,122.957534329175));
#96494=CARTESIAN_POINT('Ctrl Pts',(2.84568159625677,30.3058899943805,122.968146443801));
#96495=CARTESIAN_POINT('Ctrl Pts',(2.84954098872522,30.376454032638,122.97876966672));
#96496=CARTESIAN_POINT('Ctrl Pts',(2.85340038119368,30.4464295206696,122.993067898798));
#96497=CARTESIAN_POINT('Ctrl Pts',(2.85725977366213,30.515412775057,123.010943129569));
#96498=CARTESIAN_POINT('Ctrl Pts',(2.86112135126546,30.5844350868131,123.02882848105));
#96499=CARTESIAN_POINT('Ctrl Pts',(2.86498292886879,30.6524635830876,123.050294716614));
#96500=CARTESIAN_POINT('Ctrl Pts',(2.86884450647211,30.7191109257999,123.075194285416));
#96501=CARTESIAN_POINT('Ctrl Pts',(2.87271284058688,30.7858748797991,123.100137420407));
#96502=CARTESIAN_POINT('Ctrl Pts',(2.87658117470165,30.8512524097474,123.128525688683));
#96503=CARTESIAN_POINT('Ctrl Pts',(2.88044950881642,30.91487793711,123.160164158766));
#96504=CARTESIAN_POINT('Ctrl Pts',(2.88274722798835,30.9526703277639,123.178956826908));
#96505=CARTESIAN_POINT('Ctrl Pts',(2.88504494716027,30.9898450734053,123.198895338703));
#96506=CARTESIAN_POINT('Ctrl Pts',(2.8873426663322,31.0263304413067,123.219931633968));
#96507=CARTESIAN_POINT('Ctrl Pts',(2.89121173968032,31.0877672636426,123.255354139184));
#96508=CARTESIAN_POINT('Ctrl Pts',(2.89508081302843,31.1474884268371,123.294030383693));
#96509=CARTESIAN_POINT('Ctrl Pts',(2.89894988637655,31.2051280430165,123.335769258055));
#96510=CARTESIAN_POINT('Ctrl Pts',(2.90281319477223,31.262681775674,123.377445941136));
#96511=CARTESIAN_POINT('Ctrl Pts',(2.90667650316791,31.3181597274988,123.422175913362));
#96512=CARTESIAN_POINT('Ctrl Pts',(2.91053981156359,31.3712221345186,123.469723090318));
#96513=CARTESIAN_POINT('Ctrl Pts',(2.91439858805639,31.4242222960094,123.517214491455));
#96514=CARTESIAN_POINT('Ctrl Pts',(2.9182573645492,31.4748121811208,123.567516210344));
#96515=CARTESIAN_POINT('Ctrl Pts',(2.92211614104201,31.5226838808997,123.620351000671));
#96516=CARTESIAN_POINT('Ctrl Pts',(2.92597248663011,31.5705254230521,123.673152506785));
#96517=CARTESIAN_POINT('Ctrl Pts',(2.92982883221821,31.6156518517778,123.728483559245));
#96518=CARTESIAN_POINT('Ctrl Pts',(2.93368517780631,31.6577920907818,123.786030088412));
#96519=CARTESIAN_POINT('Ctrl Pts',(2.93754038405153,31.6999198796098,123.843559615672));
#96520=CARTESIAN_POINT('Ctrl Pts',(2.94139559029676,31.739062943392,123.903302928443));
#96521=CARTESIAN_POINT('Ctrl Pts',(2.94525079654198,31.7749915803893,123.964914277923));
#96522=CARTESIAN_POINT('Ctrl Pts',(2.94910615339311,31.81092162096,124.026528034287));
#96523=CARTESIAN_POINT('Ctrl Pts',(2.95296151024424,31.843636742623,124.09000955149));
#96524=CARTESIAN_POINT('Ctrl Pts',(2.95681686709537,31.8729524240308,124.154987112633));
#96525=CARTESIAN_POINT('Ctrl Pts',(2.96067625956382,31.9022987917995,124.220032689417));
#96526=CARTESIAN_POINT('Ctrl Pts',(2.96453565203227,31.9282384157911,124.286576992501));
#96527=CARTESIAN_POINT('Ctrl Pts',(2.96839504450071,31.9506346954787,124.354227712506));
#96528=CARTESIAN_POINT('Ctrl Pts',(2.97225662210403,31.9730436556314,124.421916735417));
#96529=CARTESIAN_POINT('Ctrl Pts',(2.97611819970736,31.991905149263,124.490712953574));
#96530=CARTESIAN_POINT('Ctrl Pts',(2.97997977731068,32.0071330620026,124.560210921104));
#96531=CARTESIAN_POINT('Ctrl Pts',(2.98384811142543,32.0223876186627,124.629830487592));
#96532=CARTESIAN_POINT('Ctrl Pts',(2.98771644554019,32.0339958221734,124.700153775407));
#96533=CARTESIAN_POINT('Ctrl Pts',(2.99158477965495,32.0419231662915,124.770767922266));
#96534=CARTESIAN_POINT('Ctrl Pts',(2.99388249882688,32.0466318625991,124.812711424103));
#96535=CARTESIAN_POINT('Ctrl Pts',(2.99618021799882,32.0500428972698,124.854757479907));
#96536=CARTESIAN_POINT('Ctrl Pts',(2.99847793717076,32.0521577425026,124.89681975777));
#96537=CARTESIAN_POINT('Ctrl Pts',(3.00034353126794,32.0538748552077,124.930971510628));
#96538=CARTESIAN_POINT('Ctrl Pts',(3.00220912536513,32.054739508502,124.965166482837));
#96539=CARTESIAN_POINT('Ctrl Pts',(3.00407471946232,32.0547499051079,124.999375532937));
#96540=CARTESIAN_POINT('Ctrl Pts',(3.00407471949959,32.0547499051081,124.999375533621));
#96541=CARTESIAN_POINT('Ctrl Pts',(3.00791348792961,32.054771297821,125.069766312486));
#96542=CARTESIAN_POINT('Ctrl Pts',(3.01175225635963,32.0511712983844,125.140303260411));
#96543=CARTESIAN_POINT('Ctrl Pts',(3.01559102478966,32.0439310014569,125.210579257724));
#96544=CARTESIAN_POINT('Ctrl Pts',(3.01950861575714,32.0365420374279,125.282298252323));
#96545=CARTESIAN_POINT('Ctrl Pts',(3.02342620672463,32.0253615175391,125.35374494479));
#96546=CARTESIAN_POINT('Ctrl Pts',(3.02734379769211,32.0104254036408,125.42448469807));
#96547=CARTESIAN_POINT('Ctrl Pts',(3.03117271153805,31.9958273780213,125.493623212796));
#96548=CARTESIAN_POINT('Ctrl Pts',(3.03500162538399,31.9776420963002,125.56208594356));
#96549=CARTESIAN_POINT('Ctrl Pts',(3.03883053922993,31.9559553954509,125.629472837783));
#96550=CARTESIAN_POINT('Ctrl Pts',(3.04265730106928,31.9342808834168,125.696821857808));
#96551=CARTESIAN_POINT('Ctrl Pts',(3.04648406290863,31.9091090062404,125.763095771074));
#96552=CARTESIAN_POINT('Ctrl Pts',(3.05031082474797,31.8805758631139,125.82790819876));
#96553=CARTESIAN_POINT('Ctrl Pts',(3.05413676563474,31.8520488411831,125.89270672228));
#96554=CARTESIAN_POINT('Ctrl Pts',(3.0579627065215,31.8201621840763,125.956043930674));
#96555=CARTESIAN_POINT('Ctrl Pts',(3.06178864740826,31.7850999946552,126.017553719261));
#96556=CARTESIAN_POINT('Ctrl Pts',(3.06577402745835,31.7485766519359,126.081626816984));
#96557=CARTESIAN_POINT('Ctrl Pts',(3.06975940750843,31.7086075443551,126.143716319391));
#96558=CARTESIAN_POINT('Ctrl Pts',(3.07374478755852,31.6654523582138,126.203439240269));
#96559=CARTESIAN_POINT('Ctrl Pts',(3.07757550004208,31.6239719703452,126.260844390013));
#96560=CARTESIAN_POINT('Ctrl Pts',(3.08140621252563,31.5795486186866,126.31606290598));
#96561=CARTESIAN_POINT('Ctrl Pts',(3.08523692500919,31.5324542628075,126.368788330935));
#96562=CARTESIAN_POINT('Ctrl Pts',(3.08907026922176,31.4853275527429,126.421549978663));
#96563=CARTESIAN_POINT('Ctrl Pts',(3.09290361343433,31.4355265377851,126.471814780226));
#96564=CARTESIAN_POINT('Ctrl Pts',(3.09673695764691,31.3833590795965,126.519314062134));
#96565=CARTESIAN_POINT('Ctrl Pts',(3.10057644985358,31.3311079541952,126.566889524341));
#96566=CARTESIAN_POINT('Ctrl Pts',(3.10441594206026,31.2764832013092,126.611690314674));
#96567=CARTESIAN_POINT('Ctrl Pts',(3.10825543426693,31.2198237246501,126.65348953528));
#96568=CARTESIAN_POINT('Ctrl Pts',(3.10870802551439,31.2131448249829,126.65841673929));
#96569=CARTESIAN_POINT('Ctrl Pts',(3.10916061676185,31.2064376818435,126.663302287643));
#96570=CARTESIAN_POINT('Ctrl Pts',(3.10961320800931,31.1997028730531,126.668145850604));
#96571=CARTESIAN_POINT('Ctrl Pts',(3.11348228135751,31.1421289156634,126.709552087396));
#96572=CARTESIAN_POINT('Ctrl Pts',(3.1173513547057,31.0822960432195,126.748055289834));
#96573=CARTESIAN_POINT('Ctrl Pts',(3.1212204280539,31.0205290485858,126.783400690673));
#96574=CARTESIAN_POINT('Ctrl Pts',(3.12508373644967,30.9588540873032,126.818693426561));
#96575=CARTESIAN_POINT('Ctrl Pts',(3.12894704484544,30.8952511424374,126.850837461135));
#96576=CARTESIAN_POINT('Ctrl Pts',(3.13281035324121,30.8300752390276,126.879620349978));
#96577=CARTESIAN_POINT('Ctrl Pts',(3.1366691297341,30.7649757910374,126.90836947469));
#96578=CARTESIAN_POINT('Ctrl Pts',(3.140527906227,30.6983074918774,126.933765090179));
#96579=CARTESIAN_POINT('Ctrl Pts',(3.14438668271989,30.6304497644014,126.955640728014));
#96580=CARTESIAN_POINT('Ctrl Pts',(3.14824302830808,30.5626347851046,126.977502584902));
#96581=CARTESIAN_POINT('Ctrl Pts',(3.15209937389627,30.4936323253551,126.995848714865));
#96582=CARTESIAN_POINT('Ctrl Pts',(3.15595571948446,30.4238402027558,127.010561375593));
#96583=CARTESIAN_POINT('Ctrl Pts',(3.15981092572978,30.3540686999779,127.025269689521));
#96584=CARTESIAN_POINT('Ctrl Pts',(3.16366613197509,30.2835084726011,127.03634656525));
#96585=CARTESIAN_POINT('Ctrl Pts',(3.16752133822041,30.2125691751402,127.043725007989));
#96586=CARTESIAN_POINT('Ctrl Pts',(3.17137669507164,30.1416271063936,127.051103738972));
#96587=CARTESIAN_POINT('Ctrl Pts',(3.17523205192287,30.0703064215698,127.054783702051));
#96588=CARTESIAN_POINT('Ctrl Pts',(3.17908740877411,29.9990218406489,127.054749767175));
#96589=CARTESIAN_POINT('Ctrl Pts',(3.18294680124265,29.9276626421765,127.054715796777));
#96590=CARTESIAN_POINT('Ctrl Pts',(3.18680619371119,29.8563401098298,127.050960168243));
#96591=CARTESIAN_POINT('Ctrl Pts',(3.19066558617973,29.7854680019227,127.043519900637));
#96592=CARTESIAN_POINT('Ctrl Pts',(3.19452716378315,29.7145557672039,127.036075420455));
#96593=CARTESIAN_POINT('Ctrl Pts',(3.19838874138656,29.6440949446598,127.02494222409));
#96594=CARTESIAN_POINT('Ctrl Pts',(3.20225031898998,29.5744904799883,127.010208748085));
#96595=CARTESIAN_POINT('Ctrl Pts',(3.20611865310484,29.5047642300233,126.995449493265));
#96596=CARTESIAN_POINT('Ctrl Pts',(3.20998698721969,29.4358977989483,126.977077507279));
#96597=CARTESIAN_POINT('Ctrl Pts',(3.21385532133455,29.3682816450813,126.955231311778));
#96598=CARTESIAN_POINT('Ctrl Pts',(3.21615304050566,29.328118895845,126.942255074275));
#96599=CARTESIAN_POINT('Ctrl Pts',(3.21845075967677,29.2883969108243,126.928054022522));
#96600=CARTESIAN_POINT('Ctrl Pts',(3.22074847884788,29.2491937605714,126.912665039503));
#96601=CARTESIAN_POINT('Ctrl Pts',(3.22461723641768,29.1831859184435,126.886754020742));
#96602=CARTESIAN_POINT('Ctrl Pts',(3.22848599398749,29.1183916892054,126.857371254928));
#96603=CARTESIAN_POINT('Ctrl Pts',(3.2323547515573,29.0552011749716,126.82465140307));
#96604=CARTESIAN_POINT('Ctrl Pts',(3.23621738607644,28.992110671843,126.791983336651));
#96605=CARTESIAN_POINT('Ctrl Pts',(3.24008002059558,28.9306192709831,126.755988893853));
#96606=CARTESIAN_POINT('Ctrl Pts',(3.24394265511472,28.8710978184853,126.71685102064));
#96607=CARTESIAN_POINT('Ctrl Pts',(3.24667286939206,28.8290264501969,126.689187316061));
#96608=CARTESIAN_POINT('Ctrl Pts',(3.24940308366941,28.7879389222963,126.659954172745));
#96609=CARTESIAN_POINT('Ctrl Pts',(3.25213329794676,28.7479590808042,126.629230216746));
#96610=CARTESIAN_POINT('',(2.94592528057306,32.0547499982312,125.000085258451));
#96611=CARTESIAN_POINT('Ctrl Pts',(2.94592528057306,32.0547499982312,125.000085258451));
#96612=CARTESIAN_POINT('Ctrl Pts',(2.94997591063978,32.0547468813374,125.075203179717));
#96613=CARTESIAN_POINT('Ctrl Pts',(2.9540265407065,32.0506202133333,125.150236380527));
#96614=CARTESIAN_POINT('Ctrl Pts',(2.95807717077322,32.042423424768,125.224731209357));
#96615=CARTESIAN_POINT('Ctrl Pts',(2.96213971866882,32.0342025194797,125.299445218068));
#96616=CARTESIAN_POINT('Ctrl Pts',(2.96620226656442,32.0218876070775,125.37361728161));
#96617=CARTESIAN_POINT('Ctrl Pts',(2.97026481446001,32.0055836153966,125.446801884679));
#96618=CARTESIAN_POINT('Ctrl Pts',(2.9743337120519,31.9892541408419,125.520100874092));
#96619=CARTESIAN_POINT('Ctrl Pts',(2.97840260964378,31.968923266179,125.592408932707));
#96620=CARTESIAN_POINT('Ctrl Pts',(2.98247150723566,31.9447455641367,125.663296504793));
#96621=CARTESIAN_POINT('Ctrl Pts',(2.98655160383586,31.9205013167266,125.734379183905));
#96622=CARTESIAN_POINT('Ctrl Pts',(2.99063170043607,31.8923892325071,125.804033182401));
#96623=CARTESIAN_POINT('Ctrl Pts',(2.99471179703627,31.8606118986796,125.871849141189));
#96624=CARTESIAN_POINT('Ctrl Pts',(2.99669196890455,31.8451895720389,125.90476190453));
#96625=CARTESIAN_POINT('Ctrl Pts',(2.99867214077283,31.8289046141268,125.937242126138));
#96626=CARTESIAN_POINT('Ctrl Pts',(3.0006523126411,31.8117839056016,125.969245398185));
#96627=CARTESIAN_POINT('Ctrl Pts',(3.00452138598921,31.7783316189004,126.031776842507));
#96628=CARTESIAN_POINT('Ctrl Pts',(3.00839045933732,31.7415727162655,126.092696890929));
#96629=CARTESIAN_POINT('Ctrl Pts',(3.01225953268542,31.7016865834987,126.151633767324));
#96630=CARTESIAN_POINT('Ctrl Pts',(3.0161228410811,31.6618598814113,126.210482827268));
#96631=CARTESIAN_POINT('Ctrl Pts',(3.01998614947678,31.6189154684186,126.267354181628));
#96632=CARTESIAN_POINT('Ctrl Pts',(3.02384945787245,31.5730785127423,126.321900735777));
#96633=CARTESIAN_POINT('Ctrl Pts',(3.02770823436526,31.5272953266877,126.3763833034));
#96634=CARTESIAN_POINT('Ctrl Pts',(3.03156701085806,31.4786266488691,126.428546117723));
#96635=CARTESIAN_POINT('Ctrl Pts',(3.03542578735086,31.4273398009013,126.478072615017));
#96636=CARTESIAN_POINT('Ctrl Pts',(3.03928213293896,31.3760852619932,126.527567912215));
#96637=CARTESIAN_POINT('Ctrl Pts',(3.04313847852706,31.3222161738659,126.574429850717));
#96638=CARTESIAN_POINT('Ctrl Pts',(3.04699482411516,31.2660378333257,126.618377510684));
#96639=CARTESIAN_POINT('Ctrl Pts',(3.05085003036038,31.209876090466,126.662312186479));
#96640=CARTESIAN_POINT('Ctrl Pts',(3.05470523660561,31.1514068320782,126.703333993932));
#96641=CARTESIAN_POINT('Ctrl Pts',(3.05856044285083,31.090968332925,126.741202360168));
#96642=CARTESIAN_POINT('Ctrl Pts',(3.06241579970197,31.030527472706,126.779072205754));
#96643=CARTESIAN_POINT('Ctrl Pts',(3.0662711565531,30.9681176318143,126.813788109482));
#96644=CARTESIAN_POINT('Ctrl Pts',(3.07012651340424,30.9041044757288,126.845153830841));
#96645=CARTESIAN_POINT('Ctrl Pts',(3.0739859058727,30.840024313498,126.876552384452));
#96646=CARTESIAN_POINT('Ctrl Pts',(3.07784529834115,30.7743379229772,126.9045935411));
#96647=CARTESIAN_POINT('Ctrl Pts',(3.0817046908096,30.7074330745457,126.929128302508));
#96648=CARTESIAN_POINT('Ctrl Pts',(3.08556626841293,30.6404903455103,126.953676955161));
#96649=CARTESIAN_POINT('Ctrl Pts',(3.08942784601626,30.5723282496367,126.974715117171));
#96650=CARTESIAN_POINT('Ctrl Pts',(3.09328942361959,30.5033492915031,126.992143833473));
#96651=CARTESIAN_POINT('Ctrl Pts',(3.09715775773435,30.43424964251,127.009603044389));
#96652=CARTESIAN_POINT('Ctrl Pts',(3.10102609184912,30.3643307544234,127.023440106453));
#96653=CARTESIAN_POINT('Ctrl Pts',(3.10489442596389,30.2940041844803,127.033607410984));
#96654=CARTESIAN_POINT('Ctrl Pts',(3.10719214513581,30.2522314980318,127.039646602495));
#96655=CARTESIAN_POINT('Ctrl Pts',(3.10948986430774,30.2103150725455,127.044392046685));
#96656=CARTESIAN_POINT('Ctrl Pts',(3.11178758347967,30.16834124311,127.047842471571));
#96657=CARTESIAN_POINT('Ctrl Pts',(3.11565566452761,30.0976806610281,127.053651067882));
#96658=CARTESIAN_POINT('Ctrl Pts',(3.11952374557556,30.0265807189343,127.05580954406));
#96659=CARTESIAN_POINT('Ctrl Pts',(3.1233918266235,29.9554507383329,127.054267004502));
#96660=CARTESIAN_POINT('Ctrl Pts',(3.12725460116857,29.8844183387909,127.052726581106));
#96661=CARTESIAN_POINT('Ctrl Pts',(3.13111737571364,29.8133564636762,127.04749522442));
#96662=CARTESIAN_POINT('Ctrl Pts',(3.13498015025872,29.7426786732666,127.038573839062));
#96663=CARTESIAN_POINT('Ctrl Pts',(3.1388389182363,29.6720741916493,127.029661707191));
#96664=CARTESIAN_POINT('Ctrl Pts',(3.14269768621389,29.6018534835615,127.017067202742));
#96665=CARTESIAN_POINT('Ctrl Pts',(3.14655645419147,29.5324274928773,127.000843200524));
#96666=CARTESIAN_POINT('Ctrl Pts',(3.15049840098558,29.4615049696795,126.984269477019));
#96667=CARTESIAN_POINT('Ctrl Pts',(3.15444034777968,29.3914123463251,126.96390797678));
#96668=CARTESIAN_POINT('Ctrl Pts',(3.15838229457379,29.322578411127,126.939870499139));
#96669=CARTESIAN_POINT('Ctrl Pts',(3.16223769300454,29.2552557759909,126.916360782134));
#96670=CARTESIAN_POINT('Ctrl Pts',(3.1660930914353,29.1891375852841,126.889335068584));
#96671=CARTESIAN_POINT('Ctrl Pts',(3.16994848986605,29.1246090616445,126.858948161608));
#96672=CARTESIAN_POINT('Ctrl Pts',(3.17393371084183,29.0579076738206,126.82753803857));
#96673=CARTESIAN_POINT('Ctrl Pts',(3.17791893181762,28.9929054419377,126.792536500927));
#96674=CARTESIAN_POINT('Ctrl Pts',(3.1819041527934,28.9300023970759,126.754167236109));
#96675=CARTESIAN_POINT('Ctrl Pts',(3.18588937376918,28.8670993522142,126.71579797129));
#96676=CARTESIAN_POINT('Ctrl Pts',(3.18987459474497,28.8062959644687,126.674061306113));
#96677=CARTESIAN_POINT('Ctrl Pts',(3.19385981572075,28.7479590808042,126.629230216746));
#96678=CARTESIAN_POINT('Ctrl Pts',(2.49394332694137,28.7479590808042,126.629230216746));
#96679=CARTESIAN_POINT('Ctrl Pts',(2.49779845423341,28.6914148374794,126.585776746721));
#96680=CARTESIAN_POINT('Ctrl Pts',(2.50165358152545,28.6371225734697,126.539366335534));
#96681=CARTESIAN_POINT('Ctrl Pts',(2.50550870881748,28.5853982276444,126.490268226914));
#96682=CARTESIAN_POINT('Ctrl Pts',(2.50936427936507,28.5336679346476,126.441164473082));
#96683=CARTESIAN_POINT('Ctrl Pts',(2.51321984991265,28.4845064965347,126.3893727446));
#96684=CARTESIAN_POINT('Ctrl Pts',(2.51707542046023,28.4381935061283,126.33519962485));
#96685=CARTESIAN_POINT('Ctrl Pts',(2.52093520681344,28.391829875599,126.280967270457));
#96686=CARTESIAN_POINT('Ctrl Pts',(2.52479499316666,28.3483212234455,126.224348699157));
#96687=CARTESIAN_POINT('Ctrl Pts',(2.52865477951988,28.3079066744851,126.165683379073));
#96688=CARTESIAN_POINT('Ctrl Pts',(2.53251701398007,28.2674664922046,126.106980849941));
#96689=CARTESIAN_POINT('Ctrl Pts',(2.53637924844027,28.2301245723542,126.04622940256));
#96690=CARTESIAN_POINT('Ctrl Pts',(2.54024148290046,28.1960750894974,125.983794937865));
#96691=CARTESIAN_POINT('Ctrl Pts',(2.54411021121953,28.1619683567407,125.921255497512));
#96692=CARTESIAN_POINT('Ctrl Pts',(2.54797893953859,28.1311653163517,125.85702783091));
#96693=CARTESIAN_POINT('Ctrl Pts',(2.55184766785766,28.1038125014745,125.791498915309));
#96694=CARTESIAN_POINT('Ctrl Pts',(2.55326885500073,28.093764375676,125.767426702253));
#96695=CARTESIAN_POINT('Ctrl Pts',(2.5546900421438,28.0841813656411,125.743179040737));
#96696=CARTESIAN_POINT('Ctrl Pts',(2.55611122928687,28.0750690305967,125.718775573828));
#96697=CARTESIAN_POINT('Ctrl Pts',(2.55998030264048,28.0502613950355,125.652339000705));
#96698=CARTESIAN_POINT('Ctrl Pts',(2.56384937599409,28.0288486678213,125.584486481582));
#96699=CARTESIAN_POINT('Ctrl Pts',(2.56771844934771,28.0109912326569,125.51559837658));
#96700=CARTESIAN_POINT('Ctrl Pts',(2.57158175774896,27.9931604052234,125.446812915444));
#96701=CARTESIAN_POINT('Ctrl Pts',(2.57544506615021,27.9788744755237,125.376995397717));
#96702=CARTESIAN_POINT('Ctrl Pts',(2.57930837455146,27.9682450435839,125.306544221245));
#96703=CARTESIAN_POINT('Ctrl Pts',(2.58316715104994,27.9576280806337,125.236175688416));
#96704=CARTESIAN_POINT('Ctrl Pts',(2.58702592754841,27.9506591675626,125.165175451347));
#96705=CARTESIAN_POINT('Ctrl Pts',(2.59088470404688,27.9473991305134,125.09395335589));
#96706=CARTESIAN_POINT('Ctrl Pts',(2.5947410496407,27.9441411471824,125.022776128055));
#96707=CARTESIAN_POINT('Ctrl Pts',(2.59859739523451,27.9445874265103,124.951377803251));
#96708=CARTESIAN_POINT('Ctrl Pts',(2.60245374082833,27.9487469461337,124.880173160335));
#96709=CARTESIAN_POINT('Ctrl Pts',(2.60630894707931,27.9529052368426,124.808989554563));
#96710=CARTESIAN_POINT('Ctrl Pts',(2.6101641533303,27.9607745615594,124.738000001772));
#96711=CARTESIAN_POINT('Ctrl Pts',(2.61401935958128,27.9723118237879,124.667617355222));
#96712=CARTESIAN_POINT('Ctrl Pts',(2.6178747164382,27.9838495367264,124.597231959133));
#96713=CARTESIAN_POINT('Ctrl Pts',(2.62173007329512,27.9990553909046,124.527453995389));
#96714=CARTESIAN_POINT('Ctrl Pts',(2.62558543015203,28.0178349185927,124.458687564756));
#96715=CARTESIAN_POINT('Ctrl Pts',(2.62944482262629,28.0366341038612,124.38984915246));
#96716=CARTESIAN_POINT('Ctrl Pts',(2.63330421510055,28.0590143018045,124.322024856521));
#96717=CARTESIAN_POINT('Ctrl Pts',(2.6371636075748,28.0848309841341,124.255604135445));
#96718=CARTESIAN_POINT('Ctrl Pts',(2.64102518518395,28.1106622835139,124.18914580787));
#96719=CARTESIAN_POINT('Ctrl Pts',(2.64488676279309,28.1399337411178,124.124093080345));
#96720=CARTESIAN_POINT('Ctrl Pts',(2.64874834040224,28.1724535386666,124.060813386931));
#96721=CARTESIAN_POINT('Ctrl Pts',(2.65261667452279,28.2050302353393,123.997422974528));
#96722=CARTESIAN_POINT('Ctrl Pts',(2.65648500864334,28.2408663749926,123.935812209991));
#96723=CARTESIAN_POINT('Ctrl Pts',(2.66035334276388,28.2797256272094,123.87632137832));
#96724=CARTESIAN_POINT('Ctrl Pts',(2.6626510618844,28.3028073063108,123.84098492155));
#96725=CARTESIAN_POINT('Ctrl Pts',(2.66494878100491,28.3269547715516,123.806395821985));
#96726=CARTESIAN_POINT('Ctrl Pts',(2.66724650012542,28.3521119068426,123.772619702403));
#96727=CARTESIAN_POINT('Ctrl Pts',(2.67111557347318,28.3944733951511,123.715744916056));
#96728=CARTESIAN_POINT('Ctrl Pts',(2.67498464682093,28.4398657577249,123.66095438182));
#96729=CARTESIAN_POINT('Ctrl Pts',(2.67885372016868,28.4880564238179,123.608589138701));
#96730=CARTESIAN_POINT('Ctrl Pts',(2.68271702856402,28.5361752854058,123.556301920242));
#96731=CARTESIAN_POINT('Ctrl Pts',(2.68658033695935,28.5870838479015,123.506433174339));
#96732=CARTESIAN_POINT('Ctrl Pts',(2.69044364535469,28.6405079277696,123.45929273772));
#96733=CARTESIAN_POINT('Ctrl Pts',(2.69430242184716,28.6938693378438,123.412207599787));
#96734=CARTESIAN_POINT('Ctrl Pts',(2.69816119833963,28.7497400413977,123.367844733757));
#96735=CARTESIAN_POINT('Ctrl Pts',(2.7020199748321,28.8078086989951,123.326477527994));
#96736=CARTESIAN_POINT('Ctrl Pts',(2.70587632041987,28.8658407752118,123.285136382236));
#96737=CARTESIAN_POINT('Ctrl Pts',(2.70973266600764,28.9260676636479,123.246787433824));
#96738=CARTESIAN_POINT('Ctrl Pts',(2.71358901159541,28.9881457596686,123.211663186415));
#96739=CARTESIAN_POINT('Ctrl Pts',(2.71744421784032,29.0502055149483,123.176549316334));
#96740=CARTESIAN_POINT('Ctrl Pts',(2.72129942408523,29.1141149694304,123.144658494925));
#96741=CARTESIAN_POINT('Ctrl Pts',(2.72515463033013,29.1795038931155,123.116178431728));
#96742=CARTESIAN_POINT('Ctrl Pts',(2.72900998718095,29.2448953712576,123.08769725594));
#96743=CARTESIAN_POINT('Ctrl Pts',(2.73286534403177,29.3117659870952,123.062627294863));
#96744=CARTESIAN_POINT('Ctrl Pts',(2.73672070088259,29.3797250020698,123.041108351786));
#96745=CARTESIAN_POINT('Ctrl Pts',(2.74058009335075,29.4477551535409,123.019566883629));
#96746=CARTESIAN_POINT('Ctrl Pts',(2.74443948581891,29.5168755143521,123.001584000482));
#96747=CARTESIAN_POINT('Ctrl Pts',(2.74829887828707,29.586680496496,122.987249506143));
#96748=CARTESIAN_POINT('Ctrl Pts',(2.75216045589011,29.6565250012597,122.972906895809));
#96749=CARTESIAN_POINT('Ctrl Pts',(2.75602203349315,29.7270544184664,122.962216859222));
#96750=CARTESIAN_POINT('Ctrl Pts',(2.7598836110962,29.7978560154116,122.955217524529));
#96751=CARTESIAN_POINT('Ctrl Pts',(2.7637519452107,29.8687814922449,122.948205943264));
#96752=CARTESIAN_POINT('Ctrl Pts',(2.7676202793252,29.9399796142001,122.9448979791));
#96753=CARTESIAN_POINT('Ctrl Pts',(2.7714886134397,30.0110363158979,122.945279638921));
#96754=CARTESIAN_POINT('Ctrl Pts',(2.77378633261446,30.0532426872075,122.945506337822));
#96755=CARTESIAN_POINT('Ctrl Pts',(2.77608405178923,30.0953992152986,122.947033789851));
#96756=CARTESIAN_POINT('Ctrl Pts',(2.77838177096399,30.1374203322592,122.949850440875));
#96757=CARTESIAN_POINT('Ctrl Pts',(2.78225084431114,30.2081786674968,122.954593330921));
#96758=CARTESIAN_POINT('Ctrl Pts',(2.78611991765828,30.2788297690987,122.963013013947));
#96759=CARTESIAN_POINT('Ctrl Pts',(2.78998899100542,30.3489609773221,122.975099064446));
#96760=CARTESIAN_POINT('Ctrl Pts',(2.79385229940011,30.4189876894441,122.987167106626));
#96761=CARTESIAN_POINT('Ctrl Pts',(2.79771560779481,30.4884955710087,123.002890590709));
#96762=CARTESIAN_POINT('Ctrl Pts',(2.8015789161895,30.5570756073842,123.022207207477));
#96763=CARTESIAN_POINT('Ctrl Pts',(2.80543769268129,30.6255751950785,123.041501164642));
#96764=CARTESIAN_POINT('Ctrl Pts',(2.80929646917308,30.6931486342329,123.06437975107));
#96765=CARTESIAN_POINT('Ctrl Pts',(2.81315524566487,30.7593973800472,123.09072967297));
#96766=CARTESIAN_POINT('Ctrl Pts',(2.81701159125195,30.8256043912887,123.117062995269));
#96767=CARTESIAN_POINT('Ctrl Pts',(2.82086793683902,30.8904879145281,123.146863135292));
#96768=CARTESIAN_POINT('Ctrl Pts',(2.8247242824261,30.9536662545008,123.179967517453));
#96769=CARTESIAN_POINT('Ctrl Pts',(2.82857948867028,31.0168259286689,123.213062119048));
#96770=CARTESIAN_POINT('Ctrl Pts',(2.83243469491446,31.0782809896736,123.249458799357));
#96771=CARTESIAN_POINT('Ctrl Pts',(2.83628990115864,31.1376729351003,123.288948318945));
#96772=CARTESIAN_POINT('Ctrl Pts',(2.84014525800872,31.1970672007082,123.328439381214));
#96773=CARTESIAN_POINT('Ctrl Pts',(2.84400061485879,31.2543977874148,123.371023251837));
#96774=CARTESIAN_POINT('Ctrl Pts',(2.84785597170887,31.3093353178271,123.416447478613));
#96775=CARTESIAN_POINT('Ctrl Pts',(2.85171536417625,31.3643303544203,123.461919253464));
#96776=CARTESIAN_POINT('Ctrl Pts',(2.85557475664364,31.4169269591328,123.510237009373));
#96777=CARTESIAN_POINT('Ctrl Pts',(2.85943414911102,31.4668297075149,123.561108700543));
#96778=CARTESIAN_POINT('Ctrl Pts',(2.86329572671327,31.5167607101459,123.612009194565));
#96779=CARTESIAN_POINT('Ctrl Pts',(2.86715730431552,31.5639944983842,123.665466138182));
#96780=CARTESIAN_POINT('Ctrl Pts',(2.87101888191777,31.608275187717,123.721153456011));
#96781=CARTESIAN_POINT('Ctrl Pts',(2.87488721603145,31.6526333539297,123.776938208628));
#96782=CARTESIAN_POINT('Ctrl Pts',(2.87875555014514,31.6940278230156,123.834960731191));
#96783=CARTESIAN_POINT('Ctrl Pts',(2.88262388425883,31.7322457770094,123.894865559973));
#96784=CARTESIAN_POINT('Ctrl Pts',(2.88492160344006,31.7549465374345,123.930447924396));
#96785=CARTESIAN_POINT('Ctrl Pts',(2.8872193226213,31.7765274453195,123.966693895145));
#96786=CARTESIAN_POINT('Ctrl Pts',(2.88951704180254,31.796951798833,124.003525316342));
#96787=CARTESIAN_POINT('Ctrl Pts',(2.89357123056498,31.8329893551935,124.068512167277));
#96788=CARTESIAN_POINT('Ctrl Pts',(2.89762541932743,31.8655537423432,124.135557009903));
#96789=CARTESIAN_POINT('Ctrl Pts',(2.90167960808987,31.8944168444081,124.204272419654));
#96790=CARTESIAN_POINT('Ctrl Pts',(2.90572241802451,31.9231989368586,124.272794966946));
#96791=CARTESIAN_POINT('Ctrl Pts',(2.90976522795915,31.9483002686216,124.342978361099));
#96792=CARTESIAN_POINT('Ctrl Pts',(2.91380803789379,31.9695390125992,124.414411714299));
#96793=CARTESIAN_POINT('Ctrl Pts',(2.91784402707256,31.9907419240024,124.485724549971));
#96794=CARTESIAN_POINT('Ctrl Pts',(2.92188001625134,32.0080950852903,124.558282753119));
#96795=CARTESIAN_POINT('Ctrl Pts',(2.92591600543012,32.0214649404621,124.63165633305));
#96796=CARTESIAN_POINT('Ctrl Pts',(2.92994364805396,32.0348071463451,124.704878174066));
#96797=CARTESIAN_POINT('Ctrl Pts',(2.9339712906778,32.0441823724021,124.778911624371));
#96798=CARTESIAN_POINT('Ctrl Pts',(2.93799893330165,32.0495074524504,124.853314060489));
#96799=CARTESIAN_POINT('Ctrl Pts',(2.94064104904699,32.0530006814071,124.902121729471));
#96800=CARTESIAN_POINT('Ctrl Pts',(2.94328316479234,32.0547520312806,124.951087882258));
#96801=CARTESIAN_POINT('Ctrl Pts',(2.94592528053768,32.0547499982312,125.000085257794));
#96802=CARTESIAN_POINT('Origin',(-1.54592528053767,30.,125.));
#96803=CARTESIAN_POINT('',(1.79398326352072,28.7479590808042,126.629230216746));
#96804=CARTESIAN_POINT('',(1.85201788434095,28.7479590808042,126.629230216746));
#96805=CARTESIAN_POINT('',(-1.54592528053767,28.7479590808042,126.629230216746));
#96806=CARTESIAN_POINT('',(2.30407471949582,32.0547491423791,125.001877336539));
#96807=CARTESIAN_POINT('Ctrl Pts',(1.85201788434095,28.7479590808042,126.629230216746));
#96808=CARTESIAN_POINT('Ctrl Pts',(1.85587837143644,28.6913998975434,126.585765265587));
#96809=CARTESIAN_POINT('Ctrl Pts',(1.85973885853193,28.6371473338627,126.5393829153));
#96810=CARTESIAN_POINT('Ctrl Pts',(1.86359934562742,28.585503225249,126.490367886369));
#96811=CARTESIAN_POINT('Ctrl Pts',(1.86752032615371,28.5330498588311,126.440584797038));
#96812=CARTESIAN_POINT('Ctrl Pts',(1.87144130668,28.4832877655838,126.388086181911));
#96813=CARTESIAN_POINT('Ctrl Pts',(1.87536228720629,28.4364915744155,126.333206272722));
#96814=CARTESIAN_POINT('Ctrl Pts',(1.87928326773258,28.3896953832472,126.278326363534));
#96815=CARTESIAN_POINT('Ctrl Pts',(1.88320424825887,28.3458653561315,126.221065611797));
#96816=CARTESIAN_POINT('Ctrl Pts',(1.88712522878516,28.3052297563666,126.161788011556));
#96817=CARTESIAN_POINT('Ctrl Pts',(1.89099430204314,28.2651321044353,126.103295148265));
#96818=CARTESIAN_POINT('Ctrl Pts',(1.89486337530113,28.2279876780811,126.042609395796));
#96819=CARTESIAN_POINT('Ctrl Pts',(1.89873244855911,28.1940438570375,125.980061208393));
#96820=CARTESIAN_POINT('Ctrl Pts',(1.902595756863,28.1601506125936,125.917606218353));
#96821=CARTESIAN_POINT('Ctrl Pts',(1.90645906516689,28.1294487370859,125.853294725252));
#96822=CARTESIAN_POINT('Ctrl Pts',(1.91032237347079,28.1021426165629,125.787486453619));
#96823=CARTESIAN_POINT('Ctrl Pts',(1.91418114986976,28.0748685278459,125.721755379249));
#96824=CARTESIAN_POINT('Ctrl Pts',(1.91803992626874,28.0509824669386,125.654531460506));
#96825=CARTESIAN_POINT('Ctrl Pts',(1.92189870266772,28.0306423055256,125.586197776961));
#96826=CARTESIAN_POINT('Ctrl Pts',(1.92575504816078,28.0103149577648,125.517907141455));
#96827=CARTESIAN_POINT('Ctrl Pts',(1.92961139365385,27.9935292159303,125.44850859268));
#96828=CARTESIAN_POINT('Ctrl Pts',(1.93346773914691,27.9803938232411,125.378402501706));
#96829=CARTESIAN_POINT('Ctrl Pts',(1.93732294529604,27.9672623113582,125.308317123334));
#96830=CARTESIAN_POINT('Ctrl Pts',(1.94117815144516,27.9577790969468,125.237525094986));
#96831=CARTESIAN_POINT('Ctrl Pts',(1.94503335759429,27.9520019217323,125.166437477486));
#96832=CARTESIAN_POINT('Ctrl Pts',(1.9488887143484,27.9462245208304,125.095347082923));
#96833=CARTESIAN_POINT('Ctrl Pts',(1.95274407110252,27.9441534837165,125.023961560652));
#96834=CARTESIAN_POINT('Ctrl Pts',(1.95659942785664,27.9457945863574,124.952695866338));
#96835=CARTESIAN_POINT('Ctrl Pts',(1.96045882022731,27.9474374068318,124.881355574254));
#96836=CARTESIAN_POINT('Ctrl Pts',(1.96431821259799,27.9528001125915,124.810135847169));
#96837=CARTESIAN_POINT('Ctrl Pts',(1.96817760496867,27.9618363654228,124.739449503576));
#96838=CARTESIAN_POINT('Ctrl Pts',(1.97203918247366,27.9708777344548,124.668723138357));
#96839=CARTESIAN_POINT('Ctrl Pts',(1.97590075997865,27.9835967043639,124.598531236038));
#96840=CARTESIAN_POINT('Ctrl Pts',(1.97976233748364,27.9998957312151,124.529276645482));
#96841=CARTESIAN_POINT('Ctrl Pts',(1.98363067150023,28.0162232760913,124.459900881794));
#96842=CARTESIAN_POINT('Ctrl Pts',(1.98749900551682,28.03614324824,124.391466170738));
#96843=CARTESIAN_POINT('Ctrl Pts',(1.99136733953341,28.0595083579832,124.324359748266));
#96844=CARTESIAN_POINT('Ctrl Pts',(1.99366505956351,28.0733868080943,124.284499754171));
#96845=CARTESIAN_POINT('Ctrl Pts',(1.99596277959362,28.0884798245971,124.245108027168));
#96846=CARTESIAN_POINT('Ctrl Pts',(1.99826049962372,28.1047487736662,124.206261786494));
#96847=CARTESIAN_POINT('Ctrl Pts',(2.00212957301354,28.1321436508049,124.140849571725));
#96848=CARTESIAN_POINT('Ctrl Pts',(2.00599864640336,28.1629825933744,124.076729146266));
#96849=CARTESIAN_POINT('Ctrl Pts',(2.00986771979318,28.1971221422172,124.014287571136));
#96850=CARTESIAN_POINT('Ctrl Pts',(2.01373102823112,28.2312108228451,123.951939034478));
#96851=CARTESIAN_POINT('Ctrl Pts',(2.01759433666905,28.2685901166468,123.891264805505));
#96852=CARTESIAN_POINT('Ctrl Pts',(2.02145764510699,28.3090686549949,123.832631699514));
#96853=CARTESIAN_POINT('Ctrl Pts',(2.02531642164265,28.3494997094873,123.774067373822));
#96854=CARTESIAN_POINT('Ctrl Pts',(2.02917519817831,28.393022512329,123.717539812924));
#96855=CARTESIAN_POINT('Ctrl Pts',(2.03303397471397,28.4394008455845,123.663389420311));
#96856=CARTESIAN_POINT('Ctrl Pts',(2.03689032034528,28.4857499619907,123.609273140692));
#96857=CARTESIAN_POINT('Ctrl Pts',(2.04074666597658,28.5349507245829,123.55753142635));
#96858=CARTESIAN_POINT('Ctrl Pts',(2.04460301160788,28.58672574257,123.508472784095));
#96859=CARTESIAN_POINT('Ctrl Pts',(2.04845821789659,28.6384854638258,123.459428636028));
#96860=CARTESIAN_POINT('Ctrl Pts',(2.0523134241853,28.6928175781301,123.413066320258));
#96861=CARTESIAN_POINT('Ctrl Pts',(2.05616863047401,28.7494080523871,123.369657292755));
#96862=CARTESIAN_POINT('Ctrl Pts',(2.06002398736886,28.8060007373877,123.326246569451));
#96863=CARTESIAN_POINT('Ctrl Pts',(2.06387934426371,28.8648515707109,123.285789657389));
#96864=CARTESIAN_POINT('Ctrl Pts',(2.06773470115855,28.9256150626758,123.248516466263));
#96865=CARTESIAN_POINT('Ctrl Pts',(2.07159409367074,28.9864421591807,123.211204259207));
#96866=CARTESIAN_POINT('Ctrl Pts',(2.07545348618293,29.0491854960062,123.177082680191));
#96867=CARTESIAN_POINT('Ctrl Pts',(2.07931287869512,29.1134731141439,123.146336696389));
#96868=CARTESIAN_POINT('Ctrl Pts',(2.08317445634226,29.1777971310468,123.115573304634));
#96869=CARTESIAN_POINT('Ctrl Pts',(2.08703603398941,29.2436667210448,123.088189499305));
#96870=CARTESIAN_POINT('Ctrl Pts',(2.09089761163656,29.3106905289069,123.06432182025));
#96871=CARTESIAN_POINT('Ctrl Pts',(2.0947659457948,29.3778316067407,123.040412380481));
#96872=CARTESIAN_POINT('Ctrl Pts',(2.09863427995304,29.4461304687944,123.020031488752));
#96873=CARTESIAN_POINT('Ctrl Pts',(2.10250261411128,29.515181896621,123.003265423464));
#96874=CARTESIAN_POINT('Ctrl Pts',(2.10480033289494,29.5561971647612,122.99330669147));
#96875=CARTESIAN_POINT('Ctrl Pts',(2.10709805167861,29.5974777581921,122.984622339476));
#96876=CARTESIAN_POINT('Ctrl Pts',(2.10939577046228,29.6389378482157,122.977221790445));
#96877=CARTESIAN_POINT('Ctrl Pts',(2.11326484381022,29.7087514957575,122.964760184083));
#96878=CARTESIAN_POINT('Ctrl Pts',(2.11713391715816,29.7793477922384,122.955892707146));
#96879=CARTESIAN_POINT('Ctrl Pts',(2.12100299050609,29.8503237437522,122.950708761348));
#96880=CARTESIAN_POINT('Ctrl Pts',(2.12486629890171,29.9211939404924,122.945532539673));
#96881=CARTESIAN_POINT('Ctrl Pts',(2.12872960729733,29.9924421888402,122.944028989731));
#96882=CARTESIAN_POINT('Ctrl Pts',(2.13259291569295,30.0636565198238,122.946236281851));
#96883=CARTESIAN_POINT('Ctrl Pts',(2.13645169218588,30.1347873119372,122.94844098468));
#96884=CARTESIAN_POINT('Ctrl Pts',(2.14031046867881,30.2058837825211,122.954347867964));
#96885=CARTESIAN_POINT('Ctrl Pts',(2.14416924517173,30.2765318276607,122.963943097359));
#96886=CARTESIAN_POINT('Ctrl Pts',(2.14802559076006,30.3471353668129,122.97353228207));
#96887=CARTESIAN_POINT('Ctrl Pts',(2.15188193634839,30.4172905607548,122.986805137805));
#96888=CARTESIAN_POINT('Ctrl Pts',(2.15573828193672,30.4865877726813,123.003695939498));
#96889=CARTESIAN_POINT('Ctrl Pts',(2.15959348818228,30.5558645110076,123.020581750867));
#96890=CARTESIAN_POINT('Ctrl Pts',(2.16344869442784,30.6242832988505,123.041083271137));
#96891=CARTESIAN_POINT('Ctrl Pts',(2.16730390067339,30.6914457539578,123.065083895402));
#96892=CARTESIAN_POINT('Ctrl Pts',(2.17115925752498,30.7586108328083,123.089085457265));
#96893=CARTESIAN_POINT('Ctrl Pts',(2.17501461437657,30.8245190247689,123.116586228966));
#96894=CARTESIAN_POINT('Ctrl Pts',(2.17886997122817,30.8887897915024,123.147420644339));
#96895=CARTESIAN_POINT('Ctrl Pts',(2.18272936369722,30.953127834039,123.178287335818));
#96896=CARTESIAN_POINT('Ctrl Pts',(2.18658875616628,31.0158245909643,123.21249442626));
#96897=CARTESIAN_POINT('Ctrl Pts',(2.19044814863534,31.0765229260956,123.249829736257));
#96898=CARTESIAN_POINT('Ctrl Pts',(2.19430972623936,31.1372556277899,123.287186184993));
#96899=CARTESIAN_POINT('Ctrl Pts',(2.19817130384338,31.195987255117,123.327674103258));
#96900=CARTESIAN_POINT('Ctrl Pts',(2.2020328814474,31.2523908379861,123.37103875079));
#96901=CARTESIAN_POINT('Ctrl Pts',(2.20590121556301,31.3088931088786,123.414479272426));
#96902=CARTESIAN_POINT('Ctrl Pts',(2.20976954967862,31.3630588335097,123.460806256701));
#96903=CARTESIAN_POINT('Ctrl Pts',(2.21363788379424,31.4145957497104,123.509726056256));
#96904=CARTESIAN_POINT('Ctrl Pts',(2.2159356029631,31.4452077280762,123.53878351557));
#96905=CARTESIAN_POINT('Ctrl Pts',(2.21823332213197,31.4748929468977,123.568755064472));
#96906=CARTESIAN_POINT('Ctrl Pts',(2.22053104130084,31.5035969390997,123.599573705178));
#96907=CARTESIAN_POINT('Ctrl Pts',(2.22435385578604,31.5513530089709,123.650848006972));
#96908=CARTESIAN_POINT('Ctrl Pts',(2.22817667027124,31.5965877387593,123.704680314487));
#96909=CARTESIAN_POINT('Ctrl Pts',(2.23199948475644,31.6390104049229,123.760789584028));
#96910=CARTESIAN_POINT('Ctrl Pts',(2.23581710151328,31.6813753906795,123.816822564032));
#96911=CARTESIAN_POINT('Ctrl Pts',(2.23963471827012,31.7209355935308,123.875125976649));
#96912=CARTESIAN_POINT('Ctrl Pts',(2.24345233502696,31.7574379329582,123.935382944764));
#96913=CARTESIAN_POINT('Ctrl Pts',(2.24726611122817,31.793903550715,123.995579293845));
#96914=CARTESIAN_POINT('Ctrl Pts',(2.25107988742938,31.8273171481452,124.057724877735));
#96915=CARTESIAN_POINT('Ctrl Pts',(2.25489366363059,31.857467826878,124.121472348407));
#96916=CARTESIAN_POINT('Ctrl Pts',(2.25870495117365,31.8875988309556,124.185178221027));
#96917=CARTESIAN_POINT('Ctrl Pts',(2.26251623871672,31.9144709287458,124.250483456992));
#96918=CARTESIAN_POINT('Ctrl Pts',(2.26632752625978,31.9379191584348,124.317016180374));
#96919=CARTESIAN_POINT('Ctrl Pts',(2.27013878558036,31.9613672144904,124.383548411083));
#96920=CARTESIAN_POINT('Ctrl Pts',(2.27395004490095,31.9813912732469,124.451307646262));
#96921=CARTESIAN_POINT('Ctrl Pts',(2.27776130422154,31.9978751103787,124.519903545286));
#96922=CARTESIAN_POINT('Ctrl Pts',(2.28157259449264,32.0143590813727,124.588500001364));
#96923=CARTESIAN_POINT('Ctrl Pts',(2.28538388476374,32.0273026673966,124.657932647783));
#96924=CARTESIAN_POINT('Ctrl Pts',(2.28919517503484,32.036640523058,124.727799812017));
#96925=CARTESIAN_POINT('Ctrl Pts',(2.29300941452528,32.0459856044573,124.79772104025));
#96926=CARTESIAN_POINT('Ctrl Pts',(2.29682365401572,32.0517193372988,124.868076961445));
#96927=CARTESIAN_POINT('Ctrl Pts',(2.30063789350616,32.0538282590476,124.938461029929));
#96928=CARTESIAN_POINT('Ctrl Pts',(2.30178350215821,32.0544616747018,124.959600918503));
#96929=CARTESIAN_POINT('Ctrl Pts',(2.30292911081027,32.054768451596,124.980743347368));
#96930=CARTESIAN_POINT('Ctrl Pts',(2.30407471946232,32.0547491423796,125.001877335921));
#96931=CARTESIAN_POINT('Ctrl Pts',(2.30407471949582,32.0547491423791,125.001877336539));
#96932=CARTESIAN_POINT('Ctrl Pts',(2.30909836680698,32.0546644688522,125.094552705719));
#96933=CARTESIAN_POINT('Ctrl Pts',(2.31412201411815,32.0483061334431,125.186948887716));
#96934=CARTESIAN_POINT('Ctrl Pts',(2.31914566142931,32.0358091348523,125.27835001159));
#96935=CARTESIAN_POINT('Ctrl Pts',(2.32331921166601,32.0254268671101,125.354284319583));
#96936=CARTESIAN_POINT('Ctrl Pts',(2.3274927619027,32.0108086257834,125.429532498928));
#96937=CARTESIAN_POINT('Ctrl Pts',(2.3316663121394,31.9920561093575,125.503696356619));
#96938=CARTESIAN_POINT('Ctrl Pts',(2.33553538549304,31.9746716626628,125.572449669584));
#96939=CARTESIAN_POINT('Ctrl Pts',(2.33940445884669,31.9536895845946,125.640436592137));
#96940=CARTESIAN_POINT('Ctrl Pts',(2.34327353220033,31.9291943064212,125.707253059783));
#96941=CARTESIAN_POINT('Ctrl Pts',(2.34713684060162,31.9047355264217,125.773969970321));
#96942=CARTESIAN_POINT('Ctrl Pts',(2.35100014900292,31.876774102893,125.839519435332));
#96943=CARTESIAN_POINT('Ctrl Pts',(2.35486345740421,31.8454448505431,125.903510302157));
#96944=CARTESIAN_POINT('Ctrl Pts',(2.35872223390271,31.814152349369,125.967426103686));
#96945=CARTESIAN_POINT('Ctrl Pts',(2.36258101040121,31.7795000793208,126.029786504534));
#96946=CARTESIAN_POINT('Ctrl Pts',(2.36643978689972,31.7416711273088,126.090219815816));
#96947=CARTESIAN_POINT('Ctrl Pts',(2.37029613249356,31.7038660063157,126.150615056063));
#96948=CARTESIAN_POINT('Ctrl Pts',(2.37415247808741,31.6628884308627,126.209085204516));
#96949=CARTESIAN_POINT('Ctrl Pts',(2.37800882368126,31.6189669382656,126.265284005788));
#96950=CARTESIAN_POINT('Ctrl Pts',(2.38186402993228,31.5750584221086,126.321466203335));
#96951=CARTESIAN_POINT('Ctrl Pts',(2.38571923618329,31.5282080145169,126.375378003394));
#96952=CARTESIAN_POINT('Ctrl Pts',(2.38957444243431,31.4786859876977,126.426704353497));
#96953=CARTESIAN_POINT('Ctrl Pts',(2.39342979929127,31.4291620262708,126.478032708694));
#96954=CARTESIAN_POINT('Ctrl Pts',(2.39728515614824,31.3769665772944,126.526775065344));
#96955=CARTESIAN_POINT('Ctrl Pts',(2.4011405130052,31.3224071866831,126.572652789114));
#96956=CARTESIAN_POINT('Ctrl Pts',(2.40499990547949,31.2677906857108,126.61857853566));
#96957=CARTESIAN_POINT('Ctrl Pts',(2.40885929795377,31.2108056760759,126.661633350218));
#96958=CARTESIAN_POINT('Ctrl Pts',(2.41271869042806,31.1517925493631,126.701579115331));
#96959=CARTESIAN_POINT('Ctrl Pts',(2.41658026803724,31.0927460102302,126.741547497187));
#96960=CARTESIAN_POINT('Ctrl Pts',(2.42044184564642,31.0316694842483,126.778403074278));
#96961=CARTESIAN_POINT('Ctrl Pts',(2.4243034232556,30.9689297310249,126.811952741888));
#96962=CARTESIAN_POINT('Ctrl Pts',(2.42817175737618,30.9060802035329,126.845561110561));
#96963=CARTESIAN_POINT('Ctrl Pts',(2.43204009149675,30.8415620785549,126.87585181477));
#96964=CARTESIAN_POINT('Ctrl Pts',(2.43590842561733,30.7757632841604,126.902679397442));
#96965=CARTESIAN_POINT('Ctrl Pts',(2.43820614473754,30.7366800138806,126.918614486742));
#96966=CARTESIAN_POINT('Ctrl Pts',(2.44050386385775,30.6971452393366,126.933328680147));
#96967=CARTESIAN_POINT('Ctrl Pts',(2.44280158297796,30.657242440575,126.94679992213));
#96968=CARTESIAN_POINT('Ctrl Pts',(2.44667069996888,30.590050330227,126.96948407477));
#96969=CARTESIAN_POINT('Ctrl Pts',(2.45053981695979,30.5215508422643,126.988729960308));
#96970=CARTESIAN_POINT('Ctrl Pts',(2.45440893395071,30.4521292545118,127.004389358312));
#96971=CARTESIAN_POINT('Ctrl Pts',(2.45827227326041,30.3828113327391,127.020025372426));
#96972=CARTESIAN_POINT('Ctrl Pts',(2.46213561257011,30.3125745144788,127.032085423932));
#96973=CARTESIAN_POINT('Ctrl Pts',(2.46599895187981,30.2418205526408,127.040470627777));
#96974=CARTESIAN_POINT('Ctrl Pts',(2.46985771072421,30.1711504783521,127.048845889928));
#96975=CARTESIAN_POINT('Ctrl Pts',(2.47371646956861,30.099964958548,127.0535549026));
#96976=CARTESIAN_POINT('Ctrl Pts',(2.47757522841301,30.0286755594982,127.054549895911));
#96977=CARTESIAN_POINT('Ctrl Pts',(2.48143153832715,29.9574314036922,127.055544257758));
#96978=CARTESIAN_POINT('Ctrl Pts',(2.48528784824128,29.8860839840186,127.052829270173));
#96979=CARTESIAN_POINT('Ctrl Pts',(2.48914415815541,29.8150481436358,127.046409141234));
#96980=CARTESIAN_POINT('Ctrl Pts',(2.49299931071212,29.7440336225606,127.039990939108));
#96981=CARTESIAN_POINT('Ctrl Pts',(2.49685446326883,29.6733309786274,127.02986984722));
#96982=CARTESIAN_POINT('Ctrl Pts',(2.50070961582553,29.6033514699089,127.016102057456));
#96983=CARTESIAN_POINT('Ctrl Pts',(2.50456490096022,29.533369554608,127.00233379422));
#96984=CARTESIAN_POINT('Ctrl Pts',(2.50842018609492,29.4641113000198,126.984918680344));
#96985=CARTESIAN_POINT('Ctrl Pts',(2.51227547122961,29.3959775787253,126.963963970417));
#96986=CARTESIAN_POINT('Ctrl Pts',(2.51613458281872,29.3277762332291,126.942988462485));
#96987=CARTESIAN_POINT('Ctrl Pts',(2.51999369440783,29.2607021136925,126.918466490122));
#96988=CARTESIAN_POINT('Ctrl Pts',(2.52385280599695,29.1951398065005,126.890554847504));
#96989=CARTESIAN_POINT('Ctrl Pts',(2.52771409532938,29.1295405017061,126.862627454009));
#96990=CARTESIAN_POINT('Ctrl Pts',(2.53157538466181,29.0654551440428,126.831306795806));
#96991=CARTESIAN_POINT('Ctrl Pts',(2.53543667399424,29.0032448093244,126.79679621893));
#96992=CARTESIAN_POINT('Ctrl Pts',(2.53930424299694,28.9409333010456,126.762229517007));
#96993=CARTESIAN_POINT('Ctrl Pts',(2.54317181199964,28.880503313439,126.724462799672));
#96994=CARTESIAN_POINT('Ctrl Pts',(2.54703938100235,28.822287261403,126.683742934015));
#96995=CARTESIAN_POINT('Ctrl Pts',(2.54871345344838,28.7970885154822,126.666117390669));
#96996=CARTESIAN_POINT('Ctrl Pts',(2.55038752589441,28.7723041475986,126.647939064332));
#96997=CARTESIAN_POINT('Ctrl Pts',(2.55206159834044,28.7479590808042,126.629230216746));
#96998=CARTESIAN_POINT('',(2.24592528056747,32.0547491760428,124.998159877295));
#96999=CARTESIAN_POINT('Ctrl Pts',(2.24592528056747,32.0547491760428,124.998159877295));
#97000=CARTESIAN_POINT('Ctrl Pts',(2.24973199310623,32.0548119777186,125.06828655489));
#97001=CARTESIAN_POINT('Ctrl Pts',(2.25353870564499,32.0512805114038,125.138525579216));
#97002=CARTESIAN_POINT('Ctrl Pts',(2.25734541818375,32.0441469197713,125.208472858879));
#97003=CARTESIAN_POINT('Ctrl Pts',(2.26114901952491,32.0370191583699,125.278362971156));
#97004=CARTESIAN_POINT('Ctrl Pts',(2.26495262086607,32.0262951565311,125.347961315228));
#97005=CARTESIAN_POINT('Ctrl Pts',(2.26875622220723,32.0120190903817,125.416865376878));
#97006=CARTESIAN_POINT('Ctrl Pts',(2.2725580718171,31.9977495990097,125.485737705075));
#97007=CARTESIAN_POINT('Ctrl Pts',(2.27635992142697,31.9799313885755,125.553915895173));
#97008=CARTESIAN_POINT('Ctrl Pts',(2.28016177103684,31.9586600142903,125.62100604741));
#97009=CARTESIAN_POINT('Ctrl Pts',(2.28396322582631,31.937390849028,125.688089232365));
#97010=CARTESIAN_POINT('Ctrl Pts',(2.28776468061578,31.9126693846252,125.754084126914));
#97011=CARTESIAN_POINT('Ctrl Pts',(2.29156613540525,31.8846409268587,125.818612325408));
#97012=CARTESIAN_POINT('Ctrl Pts',(2.29537111048262,31.8565865137025,125.883200279403));
#97013=CARTESIAN_POINT('Ctrl Pts',(2.29917608555998,31.8252191922844,125.946318365001));
#97014=CARTESIAN_POINT('Ctrl Pts',(2.30298106063735,31.7907318525525,126.007609544791));
#97015=CARTESIAN_POINT('Ctrl Pts',(2.30678785553278,31.7562280184462,126.068930038517));
#97016=CARTESIAN_POINT('Ctrl Pts',(2.3105946504282,31.7186014651685,126.128421464589));
#97017=CARTESIAN_POINT('Ctrl Pts',(2.31440144532363,31.6780888208102,126.185755232741));
#97018=CARTESIAN_POINT('Ctrl Pts',(2.31821492439134,31.6375050422032,126.243189670562));
#97019=CARTESIAN_POINT('Ctrl Pts',(2.32202840345906,31.5940253663411,126.298458493991));
#97020=CARTESIAN_POINT('Ctrl Pts',(2.32584188252678,31.5479266065822,126.351266362763));
#97021=CARTESIAN_POINT('Ctrl Pts',(2.32850815088777,31.515695758466,126.388188015464));
#97022=CARTESIAN_POINT('Ctrl Pts',(2.33117441924876,31.4821854267664,126.423907392274));
#97023=CARTESIAN_POINT('Ctrl Pts',(2.33384068760975,31.4475000613344,126.458335055787));
#97024=CARTESIAN_POINT('Ctrl Pts',(2.3377097609577,31.3971674598155,126.50829370109));
#97025=CARTESIAN_POINT('Ctrl Pts',(2.34157883430565,31.3441468439275,126.555741393499));
#97026=CARTESIAN_POINT('Ctrl Pts',(2.34544790765359,31.2887188191192,126.600375383386));
#97027=CARTESIAN_POINT('Ctrl Pts',(2.34931121604922,31.2333733825411,126.644942868247));
#97028=CARTESIAN_POINT('Ctrl Pts',(2.35317452444486,31.1756280325353,126.686704670265));
#97029=CARTESIAN_POINT('Ctrl Pts',(2.35703783284049,31.1157998962009,126.7253950719));
#97030=CARTESIAN_POINT('Ctrl Pts',(2.36089660933342,31.0560419420173,126.764040087272));
#97031=CARTESIAN_POINT('Ctrl Pts',(2.36475538582635,30.9942064605435,126.79962059641));
#97032=CARTESIAN_POINT('Ctrl Pts',(2.36861416231929,30.9306419144751,126.831912440463));
#97033=CARTESIAN_POINT('Ctrl Pts',(2.37247050790762,30.8671174120184,126.864183941696));
#97034=CARTESIAN_POINT('Ctrl Pts',(2.37632685349596,30.8018664381098,126.893170668666));
#97035=CARTESIAN_POINT('Ctrl Pts',(2.38018319908429,30.7352632961439,126.918693682651));
#97036=CARTESIAN_POINT('Ctrl Pts',(2.38403840532987,30.668679831825,126.944209155958));
#97037=CARTESIAN_POINT('Ctrl Pts',(2.38789361157544,30.6007454459252,126.966262774158));
#97038=CARTESIAN_POINT('Ctrl Pts',(2.39174881782102,30.5318541249963,126.98472384785));
#97039=CARTESIAN_POINT('Ctrl Pts',(2.39560417467261,30.4629601127853,127.003185642735));
#97040=CARTESIAN_POINT('Ctrl Pts',(2.39945953152421,30.3931095611263,127.01805449086));
#97041=CARTESIAN_POINT('Ctrl Pts',(2.40331488837581,30.3227096288147,127.029250122082));
#97042=CARTESIAN_POINT('Ctrl Pts',(2.40717428084488,30.2522360049596,127.040457472397));
#97043=CARTESIAN_POINT('Ctrl Pts',(2.41103367331395,30.1812123332285,127.047983853952));
#97044=CARTESIAN_POINT('Ctrl Pts',(2.41489306578302,30.1100530375752,127.05180064612));
#97045=CARTESIAN_POINT('Ctrl Pts',(2.41875464338706,30.0388534525067,127.055619599305));
#97046=CARTESIAN_POINT('Ctrl Pts',(2.4226162209911,29.9675185766697,127.055724781301));
#97047=CARTESIAN_POINT('Ctrl Pts',(2.42647779859514,29.8964622309945,127.052139735225));
#97048=CARTESIAN_POINT('Ctrl Pts',(2.43034613271076,29.8252815597013,127.048548416478));
#97049=CARTESIAN_POINT('Ctrl Pts',(2.43421446682637,29.7543808749425,127.041254028392));
#97050=CARTESIAN_POINT('Ctrl Pts',(2.43808280094199,29.6841675808283,127.030331856003));
#97051=CARTESIAN_POINT('Ctrl Pts',(2.44038052011077,29.642462178201,127.023844286907));
#97052=CARTESIAN_POINT('Ctrl Pts',(2.44267823927954,29.6009990972783,127.016077763855));
#97053=CARTESIAN_POINT('Ctrl Pts',(2.44497595844831,29.5598612439062,127.007056411236));
#97054=CARTESIAN_POINT('Ctrl Pts',(2.44884535140177,29.4905844923686,126.991864320432));
#97055=CARTESIAN_POINT('Ctrl Pts',(2.45271474435522,29.4219595270247,126.973051462177));
#97056=CARTESIAN_POINT('Ctrl Pts',(2.45658413730868,29.3543929918247,126.950689404671));
#97057=CARTESIAN_POINT('Ctrl Pts',(2.46044683557572,29.2869433578469,126.928366037204));
#97058=CARTESIAN_POINT('Ctrl Pts',(2.46430953384276,29.2205489728531,126.90250582308));
#97059=CARTESIAN_POINT('Ctrl Pts',(2.46817223210981,29.155604888851,126.873231021195));
#97060=CARTESIAN_POINT('Ctrl Pts',(2.47203108524594,29.0907254535705,126.843985360972));
#97061=CARTESIAN_POINT('Ctrl Pts',(2.47588993838208,29.0272938956955,126.811332054863));
#97062=CARTESIAN_POINT('Ctrl Pts',(2.47974879151821,28.9656875582782,126.775442292895));
#97063=CARTESIAN_POINT('Ctrl Pts',(2.48360488023173,28.9041253546868,126.739578241797));
#97064=CARTESIAN_POINT('Ctrl Pts',(2.48746096894525,28.8443861933981,126.700482583483));
#97065=CARTESIAN_POINT('Ctrl Pts',(2.49131705765877,28.7868233491138,126.658372689188));
#97066=CARTESIAN_POINT('Ctrl Pts',(2.49219248075297,28.7737552256867,126.648812749908));
#97067=CARTESIAN_POINT('Ctrl Pts',(2.49306790384717,28.7607991591468,126.63909763961));
#97068=CARTESIAN_POINT('Ctrl Pts',(2.49394332694137,28.7479590808042,126.629230216746));
#97069=CARTESIAN_POINT('Ctrl Pts',(1.79398326352072,28.7479590808042,126.629230216746));
#97070=CARTESIAN_POINT('Ctrl Pts',(1.797954777718,28.6899760925928,126.584671091147));
#97071=CARTESIAN_POINT('Ctrl Pts',(1.80192629191528,28.6342918285549,126.536949012551));
#97072=CARTESIAN_POINT('Ctrl Pts',(1.80589780611257,28.5812660683278,126.486334953374));
#97073=CARTESIAN_POINT('Ctrl Pts',(1.8097554753957,28.5297603110066,126.437171764806));
#97074=CARTESIAN_POINT('Ctrl Pts',(1.81361314467883,28.4807630703145,126.385280526293));
#97075=CARTESIAN_POINT('Ctrl Pts',(1.81747081396196,28.4345710965617,126.330950754453));
#97076=CARTESIAN_POINT('Ctrl Pts',(1.8213265585967,28.3884021686694,126.276648088542));
#97077=CARTESIAN_POINT('Ctrl Pts',(1.82518230323143,28.3450360446497,126.219909673037));
#97078=CARTESIAN_POINT('Ctrl Pts',(1.82903804786617,28.3047311040181,126.161060262353));
#97079=CARTESIAN_POINT('Ctrl Pts',(1.83289315862884,28.2644327893895,126.102220526325));
#97080=CARTESIAN_POINT('Ctrl Pts',(1.83674826939151,28.2271949327246,126.041270885359));
#97081=CARTESIAN_POINT('Ctrl Pts',(1.84060338015418,28.193233230365,125.978565992993));
#97082=CARTESIAN_POINT('Ctrl Pts',(1.84466139882929,28.1574840052718,125.912560723649));
#97083=CARTESIAN_POINT('Ctrl Pts',(1.8487194175044,28.1253656047626,125.844610853344));
#97084=CARTESIAN_POINT('Ctrl Pts',(1.85277743617951,28.097074105914,125.775158438074));
#97085=CARTESIAN_POINT('Ctrl Pts',(1.85663765466487,28.0701616208867,125.709091345055));
#97086=CARTESIAN_POINT('Ctrl Pts',(1.86049787315022,28.0467117881968,125.641665263829));
#97087=CARTESIAN_POINT('Ctrl Pts',(1.86435809163558,28.0268426842568,125.573278091182));
#97088=CARTESIAN_POINT('Ctrl Pts',(1.86822101007597,28.0069596832569,125.504843086451));
#97089=CARTESIAN_POINT('Ctrl Pts',(1.87208392851635,27.9906625037277,125.435446125403));
#97090=CARTESIAN_POINT('Ctrl Pts',(1.87594684695674,27.9780181876272,125.365495708502));
#97091=CARTESIAN_POINT('Ctrl Pts',(1.87981602070602,27.9653533963072,125.295432019351));
#97092=CARTESIAN_POINT('Ctrl Pts',(1.8836851944553,27.9563533248157,125.224813567457));
#97093=CARTESIAN_POINT('Ctrl Pts',(1.88755436820458,27.9510331570283,125.154053363815));
#97094=CARTESIAN_POINT('Ctrl Pts',(1.88813611355489,27.9502332490703,125.143414291464));
#97095=CARTESIAN_POINT('Ctrl Pts',(1.8887178589052,27.9495164341508,125.132772011345));
#97096=CARTESIAN_POINT('Ctrl Pts',(1.88929960425551,27.9488826622359,125.122127921556));
#97097=CARTESIAN_POINT('Ctrl Pts',(1.89316867791212,27.9446675701536,125.051336178438));
#97098=CARTESIAN_POINT('Ctrl Pts',(1.89703775156872,27.9441134566319,124.980187299026));
#97099=CARTESIAN_POINT('Ctrl Pts',(1.90090682522533,27.9472620012012,124.909091965219));
#97100=CARTESIAN_POINT('Ctrl Pts',(1.90477013393318,27.9504058544156,124.838102563993));
#97101=CARTESIAN_POINT('Ctrl Pts',(1.90863344264103,27.9572413933367,124.767167031359));
#97102=CARTESIAN_POINT('Ctrl Pts',(1.91249675134888,27.9677583681898,124.696698973893));
#97103=CARTESIAN_POINT('Ctrl Pts',(1.91635552815778,27.9782630059839,124.626313579797));
#97104=CARTESIAN_POINT('Ctrl Pts',(1.92021430496668,27.9924404302484,124.556395049738));
#97105=CARTESIAN_POINT('Ctrl Pts',(1.92407308177558,28.0102284935119,124.487353031348));
#97106=CARTESIAN_POINT('Ctrl Pts',(1.92792942768202,28.0280053508806,124.418354507159));
#97107=CARTESIAN_POINT('Ctrl Pts',(1.93178577358846,28.0493882135971,124.350231868445));
#97108=CARTESIAN_POINT('Ctrl Pts',(1.9356421194949,28.074263921432,124.283384260429));
#97109=CARTESIAN_POINT('Ctrl Pts',(1.93949732606024,28.0991322798441,124.216556402255));
#97110=CARTESIAN_POINT('Ctrl Pts',(1.94335253262557,28.1274912653449,124.151003281955));
#97111=CARTESIAN_POINT('Ctrl Pts',(1.94720773919091,28.1591785023363,124.087106919602));
#97112=CARTESIAN_POINT('Ctrl Pts',(1.95106309636345,28.1908669772189,124.023208061078));
#97113=CARTESIAN_POINT('Ctrl Pts',(1.954918453536,28.2258837439318,123.960966523228));
#97114=CARTESIAN_POINT('Ctrl Pts',(1.95877381070854,28.2640198872233,123.900740881073));
#97115=CARTESIAN_POINT('Ctrl Pts',(1.96263320349815,28.3021959497398,123.840452197385));
#97116=CARTESIAN_POINT('Ctrl Pts',(1.96649259628776,28.3434976465376,123.782184032988));
#97117=CARTESIAN_POINT('Ctrl Pts',(1.97035198907737,28.3876725043722,123.726266272197));
#97118=CARTESIAN_POINT('Ctrl Pts',(1.9742135670022,28.431872373405,123.670316851538));
#97119=CARTESIAN_POINT('Ctrl Pts',(1.97807514492703,28.478948321085,123.616720848788));
#97120=CARTESIAN_POINT('Ctrl Pts',(1.98193672285186,28.5286091314708,123.565773213711));
#97121=CARTESIAN_POINT('Ctrl Pts',(1.98580505728517,28.5783568321624,123.514736436803));
#97122=CARTESIAN_POINT('Ctrl Pts',(1.98967339171848,28.6306980683504,123.46635760889));
#97123=CARTESIAN_POINT('Ctrl Pts',(1.9935417261518,28.6853070410347,123.420892661613));
#97124=CARTESIAN_POINT('Ctrl Pts',(1.99583944246589,28.7177437213672,123.393887356648));
#97125=CARTESIAN_POINT('Ctrl Pts',(1.99813715877998,28.7509798858357,123.367909310026));
#97126=CARTESIAN_POINT('Ctrl Pts',(2.00043487509407,28.7849426291869,123.34300478331));
#97127=CARTESIAN_POINT('Ctrl Pts',(2.0043039484699,28.8421317370261,123.301068604913));
#97128=CARTESIAN_POINT('Ctrl Pts',(2.00817302184573,28.9016064736999,123.262014475619));
#97129=CARTESIAN_POINT('Ctrl Pts',(2.01204209522156,28.9630444130083,123.226100151331));
#97130=CARTESIAN_POINT('Ctrl Pts',(2.01590540364639,29.0243908092844,123.190239339681));
#97131=CARTESIAN_POINT('Ctrl Pts',(2.01976871207123,29.087694185809,123.157509289833));
#97132=CARTESIAN_POINT('Ctrl Pts',(2.02363202049606,29.1526014946385,123.128125715864));
#97133=CARTESIAN_POINT('Ctrl Pts',(2.02749079702003,29.2174326631611,123.098776610653));
#97134=CARTESIAN_POINT('Ctrl Pts',(2.03134957354399,29.2838635862665,123.072766383073));
#97135=CARTESIAN_POINT('Ctrl Pts',(2.03520835006796,29.351516394641,123.050264998498));
#97136=CARTESIAN_POINT('Ctrl Pts',(2.03906469568844,29.4191265839505,123.027777789063));
#97137=CARTESIAN_POINT('Ctrl Pts',(2.04292104130893,29.4879566714932,123.008795190075));
#97138=CARTESIAN_POINT('Ctrl Pts',(2.04677738692941,29.5576099439968,122.993438612738));
#97139=CARTESIAN_POINT('Ctrl Pts',(2.0506325932082,29.627242637723,122.978086572441));
#97140=CARTESIAN_POINT('Ctrl Pts',(2.05448779948698,29.6976975594426,122.966358531514));
#97141=CARTESIAN_POINT('Ctrl Pts',(2.05834300576577,29.768565690814,122.958325265124));
#97142=CARTESIAN_POINT('Ctrl Pts',(2.0621983626516,29.8394365907116,122.950291684907));
#97143=CARTESIAN_POINT('Ctrl Pts',(2.06605371953743,29.9107202493668,122.945953218321));
#97144=CARTESIAN_POINT('Ctrl Pts',(2.06990907642327,29.9820021042085,122.945328824788));
#97145=CARTESIAN_POINT('Ctrl Pts',(2.07376846892791,30.0533585737753,122.944703777667));
#97146=CARTESIAN_POINT('Ctrl Pts',(2.07762786143256,30.1247127489968,122.947800568642));
#97147=CARTESIAN_POINT('Ctrl Pts',(2.08148725393721,30.1956505473206,122.95458600136));
#97148=CARTESIAN_POINT('Ctrl Pts',(2.08534883157763,30.2666285096654,122.961375275898));
#97149=CARTESIAN_POINT('Ctrl Pts',(2.08921040921806,30.3371891450725,122.97185727824));
#97150=CARTESIAN_POINT('Ctrl Pts',(2.09307198685849,30.4069267083804,122.98594731536));
#97151=CARTESIAN_POINT('Ctrl Pts',(2.09694032101139,30.4767862898788,123.000062005489));
#97152=CARTESIAN_POINT('Ctrl Pts',(2.10080865516429,30.5458194534001,123.017797213357));
#97153=CARTESIAN_POINT('Ctrl Pts',(2.10467698931718,30.6136344780001,123.039018029173));
#97154=CARTESIAN_POINT('Ctrl Pts',(2.106974708189,30.6539153471434,123.051622800903));
#97155=CARTESIAN_POINT('Ctrl Pts',(2.10927242706081,30.6937667823746,123.065456404862));
#97156=CARTESIAN_POINT('Ctrl Pts',(2.11157014593263,30.7331103758812,123.080482680652));
#97157=CARTESIAN_POINT('Ctrl Pts',(2.11543921919087,30.7993601018102,123.105785063178));
#97158=CARTESIAN_POINT('Ctrl Pts',(2.11930829244911,30.86442813594,123.13457082176));
#97159=CARTESIAN_POINT('Ctrl Pts',(2.12317736570736,30.9279230539306,123.166708869687));
#97160=CARTESIAN_POINT('Ctrl Pts',(2.1270406740115,30.99132336392,123.198799031633));
#97161=CARTESIAN_POINT('Ctrl Pts',(2.13090398231565,31.0531547805624,123.234231350513));
#97162=CARTESIAN_POINT('Ctrl Pts',(2.13476729061979,31.1130445925503,123.272826210975));
#97163=CARTESIAN_POINT('Ctrl Pts',(2.13862606701903,31.1728641500021,123.311375797226));
#97164=CARTESIAN_POINT('Ctrl Pts',(2.14248484341828,31.2307462205748,123.353080294151));
#97165=CARTESIAN_POINT('Ctrl Pts',(2.14634361981752,31.286343066215,123.397714420429));
#97166=CARTESIAN_POINT('Ctrl Pts',(2.15019996531085,31.3419048876177,123.442320428633));
#97167=CARTESIAN_POINT('Ctrl Pts',(2.15405631080419,31.3951839623497,123.489852101205));
#97168=CARTESIAN_POINT('Ctrl Pts',(2.15791265629752,31.4458631245401,123.540041991153));
#97169=CARTESIAN_POINT('Ctrl Pts',(2.16176786244692,31.4965273137473,123.590217052673));
#97170=CARTESIAN_POINT('Ctrl Pts',(2.16562306859632,31.5445927703971,123.643048430764));
#97171=CARTESIAN_POINT('Ctrl Pts',(2.16947827474572,31.5897781963307,123.69823087724));
#97172=CARTESIAN_POINT('Ctrl Pts',(2.17333363150011,31.6349653874489,123.753415479438));
#97173=CARTESIAN_POINT('Ctrl Pts',(2.17718898825451,31.6772720184169,123.810950955116));
#97174=CARTESIAN_POINT('Ctrl Pts',(2.1810443450089,31.716457316747,123.870499295137));
#97175=CARTESIAN_POINT('Ctrl Pts',(2.18490373737986,31.7556836325105,123.930109967721));
#97176=CARTESIAN_POINT('Ctrl Pts',(2.18876312975082,31.7917818258409,123.991737304011));
#97177=CARTESIAN_POINT('Ctrl Pts',(2.19262252212177,31.8245552029329,124.055015410734));
#97178=CARTESIAN_POINT('Ctrl Pts',(2.19648409962704,31.8573471358554,124.118329344641));
#97179=CARTESIAN_POINT('Ctrl Pts',(2.20034567713231,31.8868103043958,124.183295466943));
#97180=CARTESIAN_POINT('Ctrl Pts',(2.20420725463758,31.9127958012473,124.249526959025));
#97181=CARTESIAN_POINT('Ctrl Pts',(2.20807558865445,31.9388267643132,124.315874334795));
#97182=CARTESIAN_POINT('Ctrl Pts',(2.21194392267132,31.9613677535286,124.383491039636));
#97183=CARTESIAN_POINT('Ctrl Pts',(2.21581225668819,31.9803196571083,124.451974801519));
#97184=CARTESIAN_POINT('Ctrl Pts',(2.21810997671586,31.991576743034,124.492652910121));
#97185=CARTESIAN_POINT('Ctrl Pts',(2.22040769674352,32.0015685226665,124.533636707399));
#97186=CARTESIAN_POINT('Ctrl Pts',(2.22270541677119,32.0102828503303,124.574840707302));
#97187=CARTESIAN_POINT('Ctrl Pts',(2.22812785149402,32.0308479637217,124.672078837752));
#97188=CARTESIAN_POINT('Ctrl Pts',(2.23355028621685,32.0443637952467,124.770855989235));
#97189=CARTESIAN_POINT('Ctrl Pts',(2.23897272093967,32.0506537437881,124.870320450387));
#97190=CARTESIAN_POINT('Ctrl Pts',(2.24129024080568,32.0533420344631,124.912831034002));
#97191=CARTESIAN_POINT('Ctrl Pts',(2.24360776067168,32.0547109424816,124.955466879361));
#97192=CARTESIAN_POINT('Ctrl Pts',(2.24592528053768,32.0547491760423,124.998159876746));
#97193=CARTESIAN_POINT('Origin',(-1.54592528053767,30.,125.));
#97194=CARTESIAN_POINT('',(1.09386069726047,28.7479590808042,126.629230216746));
#97195=CARTESIAN_POINT('',(1.15210970476697,28.7479590808042,126.629230216746));
#97196=CARTESIAN_POINT('',(-1.54592528053767,28.7479590808042,126.629230216746));
#97197=CARTESIAN_POINT('',(1.60407471941017,32.0547499336679,124.999477896888));
#97198=CARTESIAN_POINT('Ctrl Pts',(1.15210970476697,28.7479590808042,126.629230216746));
#97199=CARTESIAN_POINT('Ctrl Pts',(1.15596511927351,28.6914303187086,126.585788643832));
#97200=CARTESIAN_POINT('Ctrl Pts',(1.15982053378006,28.637140397984,126.539382594661));
#97201=CARTESIAN_POINT('Ctrl Pts',(1.16367594828661,28.5854082337326,126.490277724892));
#97202=CARTESIAN_POINT('Ctrl Pts',(1.16753113318894,28.5336791503234,126.441175779499));
#97203=CARTESIAN_POINT('Ctrl Pts',(1.17138631809126,28.484507872185,126.389375668203));
#97204=CARTESIAN_POINT('Ctrl Pts',(1.17524150299359,28.4381775077876,126.335180911083));
#97205=CARTESIAN_POINT('Ctrl Pts',(1.17910047930994,28.3918015794037,126.280932855672));
#97206=CARTESIAN_POINT('Ctrl Pts',(1.18295945562628,28.3482724622444,126.224285820236));
#97207=CARTESIAN_POINT('Ctrl Pts',(1.18681843194263,28.3078333058655,126.165576870808));
#97208=CARTESIAN_POINT('Ctrl Pts',(1.19067925186039,28.2673748299366,126.106839873552));
#97209=CARTESIAN_POINT('Ctrl Pts',(1.19454007177816,28.2300095104467,126.046039414369));
#97210=CARTESIAN_POINT('Ctrl Pts',(1.19840089169592,28.1959359058974,125.983539682407));
#97211=CARTESIAN_POINT('Ctrl Pts',(1.20226883009373,28.1617994773162,125.920924715054));
#97212=CARTESIAN_POINT('Ctrl Pts',(1.20613676849153,28.13096710053,125.856604654191));
#97213=CARTESIAN_POINT('Ctrl Pts',(1.21000470688934,28.1035900889946,125.790965872804));
#97214=CARTESIAN_POINT('Ctrl Pts',(1.21344100584417,28.0792681928189,125.732651997897));
#97215=CARTESIAN_POINT('Ctrl Pts',(1.21687730479899,28.057672865426,125.673297805368));
#97216=CARTESIAN_POINT('Ctrl Pts',(1.22031360375381,28.0388768364194,125.613183088292));
#97217=CARTESIAN_POINT('Ctrl Pts',(1.22418267030568,28.0177136349363,125.545497521882));
#97218=CARTESIAN_POINT('Ctrl Pts',(1.22805173685754,28.0000172088715,125.476582456488));
#97219=CARTESIAN_POINT('Ctrl Pts',(1.23192080340941,27.9859270510232,125.406826398726));
#97220=CARTESIAN_POINT('Ctrl Pts',(1.23578410489414,27.9718578880855,125.337174280337));
#97221=CARTESIAN_POINT('Ctrl Pts',(1.23964740637886,27.9613844225443,125.266684129265));
#97222=CARTESIAN_POINT('Ctrl Pts',(1.24351070786359,27.9545964560466,125.19575981427));
#97223=CARTESIAN_POINT('Ctrl Pts',(1.24736947730855,27.9478164525138,125.124918700603));
#97224=CARTESIAN_POINT('Ctrl Pts',(1.25122824675351,27.9447134062291,125.053644915922));
#97225=CARTESIAN_POINT('Ctrl Pts',(1.25508701619847,27.9453257982332,124.982351003036));
#97226=CARTESIAN_POINT('Ctrl Pts',(1.25894335465805,27.9459378044365,124.911102004587));
#97227=CARTESIAN_POINT('Ctrl Pts',(1.26279969311762,27.950260600879,124.839833387712));
#97228=CARTESIAN_POINT('Ctrl Pts',(1.2666560315772,27.9582806287272,124.768959805511));
#97229=CARTESIAN_POINT('Ctrl Pts',(1.27051123062385,27.966298286938,124.698107163972));
#97230=CARTESIAN_POINT('Ctrl Pts',(1.27436642967051,27.9780109532406,124.627649807831));
#97231=CARTESIAN_POINT('Ctrl Pts',(1.27822162871716,27.9933531760644,124.557997639724));
#97232=CARTESIAN_POINT('Ctrl Pts',(1.28207697831025,28.0086959980057,124.488342751684));
#97233=CARTESIAN_POINT('Ctrl Pts',(1.28593232790333,28.0276685512144,124.419493588044));
#97234=CARTESIAN_POINT('Ctrl Pts',(1.28978767749641,28.0501545639622,124.351848522286));
#97235=CARTESIAN_POINT('Ctrl Pts',(1.29364706266578,28.0726641138803,124.284132649247));
#97236=CARTESIAN_POINT('Ctrl Pts',(1.29750644783515,28.0986943113096,124.217623852034));
#97237=CARTESIAN_POINT('Ctrl Pts',(1.30136583300452,28.1280796929401,124.15270316505));
#97238=CARTESIAN_POINT('Ctrl Pts',(1.30522740327461,28.1574817119403,124.087745721371));
#97239=CARTESIAN_POINT('Ctrl Pts',(1.30908897354469,28.190242473519,124.024378609592));
#97240=CARTESIAN_POINT('Ctrl Pts',(1.31295054381478,28.2261504901487,123.962958304165));
#97241=CARTESIAN_POINT('Ctrl Pts',(1.31681887062171,28.2621213345455,123.901430532467));
#97242=CARTESIAN_POINT('Ctrl Pts',(1.32068719742865,28.3012501615227,123.841856774067));
#97243=CARTESIAN_POINT('Ctrl Pts',(1.32455552423558,28.3432825113791,123.78456397725));
#97244=CARTESIAN_POINT('Ctrl Pts',(1.32685330768785,28.3682496981706,123.750532095502));
#97245=CARTESIAN_POINT('Ctrl Pts',(1.3291510911401,28.3942405723508,123.717304389099));
#97246=CARTESIAN_POINT('Ctrl Pts',(1.33144887459237,28.421195531819,123.684943341999));
#97247=CARTESIAN_POINT('Ctrl Pts',(1.33531795015252,28.4665830877268,123.630452856262));
#97248=CARTESIAN_POINT('Ctrl Pts',(1.33918702571268,28.5148838644452,123.578208140637));
#97249=CARTESIAN_POINT('Ctrl Pts',(1.34305610127283,28.5658471139435,123.528537101414));
#97250=CARTESIAN_POINT('Ctrl Pts',(1.34691941190361,28.6167344281107,123.478940072126));
#97251=CARTESIAN_POINT('Ctrl Pts',(1.35078272253439,28.6702759954471,123.431909443606));
#97252=CARTESIAN_POINT('Ctrl Pts',(1.35464603316517,28.7261812109882,123.387739706108));
#97253=CARTESIAN_POINT('Ctrl Pts',(1.35850481191629,28.7820208465816,123.343621782185));
#97254=CARTESIAN_POINT('Ctrl Pts',(1.3623635906674,28.8402182435544,123.302358382856));
#97255=CARTESIAN_POINT('Ctrl Pts',(1.36622236941852,28.9004476752037,123.26420558604));
#97256=CARTESIAN_POINT('Ctrl Pts',(1.37007871727802,28.9606391644807,123.226076824111));
#97257=CARTESIAN_POINT('Ctrl Pts',(1.37393506513752,29.0228597393117,123.191055036286));
#97258=CARTESIAN_POINT('Ctrl Pts',(1.37779141299703,29.0867536756516,123.159353723943));
#97259=CARTESIAN_POINT('Ctrl Pts',(1.38164662152332,29.1506287349384,123.127661777548));
#97260=CARTESIAN_POINT('Ctrl Pts',(1.38550183004962,29.2161757393154,123.099288574846));
#97261=CARTESIAN_POINT('Ctrl Pts',(1.38935703857592,29.2830148112008,123.074401443306));
#97262=CARTESIAN_POINT('Ctrl Pts',(1.39321239771438,29.3498564943008,123.049513339495));
#97263=CARTESIAN_POINT('Ctrl Pts',(1.39706775685283,29.4179898891058,123.028111744681));
#97264=CARTESIAN_POINT('Ctrl Pts',(1.40092311599129,29.4870172412722,123.01031503706));
#97265=CARTESIAN_POINT('Ctrl Pts',(1.40478251074077,29.5561168480673,122.992499700672));
#97266=CARTESIAN_POINT('Ctrl Pts',(1.40864190549024,29.6261118088308,122.978296905618));
#97267=CARTESIAN_POINT('Ctrl Pts',(1.41250130023971,29.6965922568846,122.967774297988));
#97268=CARTESIAN_POINT('Ctrl Pts',(1.41636288012395,29.767112609972,122.957245732606));
#97269=CARTESIAN_POINT('Ctrl Pts',(1.42022446000818,29.8381185137698,122.950401549224));
#97270=CARTESIAN_POINT('Ctrl Pts',(1.42408603989241,29.9091957736597,122.947257406546));
#97271=CARTESIAN_POINT('Ctrl Pts',(1.42795437626303,29.9803973952236,122.94410776266));
#97272=CARTESIAN_POINT('Ctrl Pts',(1.43182271263365,30.051670136221,122.944671080859));
#97273=CARTESIAN_POINT('Ctrl Pts',(1.43569104900427,30.1226013017354,122.948910903127));
#97274=CARTESIAN_POINT('Ctrl Pts',(1.43798874781315,30.1647327088573,122.951429255628));
#97275=CARTESIAN_POINT('Ctrl Pts',(1.44028644662203,30.2067437115844,122.955243712156));
#97276=CARTESIAN_POINT('Ctrl Pts',(1.44258414543092,30.2485494980138,122.960338089404));
#97277=CARTESIAN_POINT('Ctrl Pts',(1.44645321925177,30.3189458759938,122.96891646424));
#97278=CARTESIAN_POINT('Ctrl Pts',(1.45032229307263,30.3890355122788,122.981160384508));
#97279=CARTESIAN_POINT('Ctrl Pts',(1.45419136689349,30.4584069220931,122.997037030727));
#97280=CARTESIAN_POINT('Ctrl Pts',(1.45805467577754,30.5276749682054,123.012890020675));
#97281=CARTESIAN_POINT('Ctrl Pts',(1.4619179846616,30.5962264424015,123.03236488487));
#97282=CARTESIAN_POINT('Ctrl Pts',(1.46578129354566,30.6636563171689,123.055377194626));
#97283=CARTESIAN_POINT('Ctrl Pts',(1.46964007054779,30.7310070928427,123.078362509628));
#97284=CARTESIAN_POINT('Ctrl Pts',(1.47349884754992,30.7972384249955,123.10487687149));
#97285=CARTESIAN_POINT('Ctrl Pts',(1.47735762455205,30.8619585091962,123.134785510746));
#97286=CARTESIAN_POINT('Ctrl Pts',(1.48121397066214,30.9266378220495,123.164675308624));
#97287=CARTESIAN_POINT('Ctrl Pts',(1.48507031677223,30.9898073358345,123.19795493829));
#97288=CARTESIAN_POINT('Ctrl Pts',(1.48892666288232,31.051094747024,123.234441336212));
#97289=CARTESIAN_POINT('Ctrl Pts',(1.49278186966143,31.1123640512688,123.270916954477));
#97290=CARTESIAN_POINT('Ctrl Pts',(1.49663707644054,31.1717519396523,123.310597211745));
#97291=CARTESIAN_POINT('Ctrl Pts',(1.50049228321965,31.228911801337,123.353253708966));
#97292=CARTESIAN_POINT('Ctrl Pts',(1.50434764061583,31.2860738961709,123.395911872712));
#97293=CARTESIAN_POINT('Ctrl Pts',(1.50820299801202,31.3410074034804,123.441546214958));
#97294=CARTESIAN_POINT('Ctrl Pts',(1.51205835540821,31.3933971411248,123.489886769277));
#97295=CARTESIAN_POINT('Ctrl Pts',(1.5159177484351,31.4458417182073,123.538277924514));
#97296=CARTESIAN_POINT('Ctrl Pts',(1.51977714146198,31.4957368524949,123.589380616532));
#97297=CARTESIAN_POINT('Ctrl Pts',(1.52363653448887,31.542803414801,123.642887187527));
#97298=CARTESIAN_POINT('Ctrl Pts',(1.52749811265903,31.5898966256451,123.696424053318));
#97299=CARTESIAN_POINT('Ctrl Pts',(1.53135969082919,31.6341577748484,123.752367126364));
#97300=CARTESIAN_POINT('Ctrl Pts',(1.53522126899934,31.6753490627772,123.810376916687));
#97301=CARTESIAN_POINT('Ctrl Pts',(1.53908960368816,31.7166124221993,123.868488205468));
#97302=CARTESIAN_POINT('Ctrl Pts',(1.54295793837697,31.7547949361307,123.928673020824));
#97303=CARTESIAN_POINT('Ctrl Pts',(1.54682627306579,31.7897034038552,123.990564866507));
#97304=CARTESIAN_POINT('Ctrl Pts',(1.54912398746702,31.8104383442023,124.027327400411));
#97305=CARTESIAN_POINT('Ctrl Pts',(1.55142170186825,31.8300190525612,124.064691745954));
#97306=CARTESIAN_POINT('Ctrl Pts',(1.55371941626948,31.8484131256698,124.102577870035));
#97307=CARTESIAN_POINT('Ctrl Pts',(1.5579156915312,31.8820058967761,124.171768629842));
#97308=CARTESIAN_POINT('Ctrl Pts',(1.56211196679292,31.9117555498864,124.242941993056));
#97309=CARTESIAN_POINT('Ctrl Pts',(1.56630824205465,31.9374426338775,124.315665576685));
#97310=CARTESIAN_POINT('Ctrl Pts',(1.57045672473028,31.9628371602797,124.3875608905));
#97311=CARTESIAN_POINT('Ctrl Pts',(1.57460520740591,31.9842610035269,124.460970953717));
#97312=CARTESIAN_POINT('Ctrl Pts',(1.57875369008154,32.001547918388,124.535453454542));
#97313=CARTESIAN_POINT('Ctrl Pts',(1.58297386163631,32.0191335640494,124.611223068613));
#97314=CARTESIAN_POINT('Ctrl Pts',(1.58719403319109,32.0324377308413,124.688102209905));
#97315=CARTESIAN_POINT('Ctrl Pts',(1.59141420474586,32.0413368923456,124.765604491407));
#97316=CARTESIAN_POINT('Ctrl Pts',(1.59563437630063,32.05023605385,124.843106772909));
#97317=CARTESIAN_POINT('Ctrl Pts',(1.5998545478554,32.0547300516731,124.921231805861));
#97318=CARTESIAN_POINT('Ctrl Pts',(1.60407471941017,32.0547499336679,124.999477896888));
#97319=CARTESIAN_POINT('Ctrl Pts',(1.60407471946232,32.0547499336682,124.999477897855));
#97320=CARTESIAN_POINT('Ctrl Pts',(1.60804279144016,32.0547686279415,125.073049817185));
#97321=CARTESIAN_POINT('Ctrl Pts',(1.61201086341801,32.0508315372123,125.146579353464));
#97322=CARTESIAN_POINT('Ctrl Pts',(1.61597893539585,32.0429783696597,125.219629104635));
#97323=CARTESIAN_POINT('Ctrl Pts',(1.6200519147052,32.0349175811625,125.294610134902));
#97324=CARTESIAN_POINT('Ctrl Pts',(1.62412489401455,32.0227307791439,125.369085155989));
#97325=CARTESIAN_POINT('Ctrl Pts',(1.6281978733239,32.0065169291057,125.442591657978));
#97326=CARTESIAN_POINT('Ctrl Pts',(1.63217761780328,31.9906742313461,125.514415517928));
#97327=CARTESIAN_POINT('Ctrl Pts',(1.63615736228266,31.9709871018473,125.585314321767));
#97328=CARTESIAN_POINT('Ctrl Pts',(1.64013710676205,31.9475982431018,125.654872999876));
#97329=CARTESIAN_POINT('Ctrl Pts',(1.64425670348638,31.9233874762115,125.726876040265));
#97330=CARTESIAN_POINT('Ctrl Pts',(1.64837630021071,31.8952101842859,125.79744252895));
#97331=CARTESIAN_POINT('Ctrl Pts',(1.65249589693504,31.8632776562454,125.86613736684));
#97332=CARTESIAN_POINT('Ctrl Pts',(1.65661549365937,31.831345128205,125.93483220473));
#97333=CARTESIAN_POINT('Ctrl Pts',(1.66073509038371,31.7956576771194,126.001654970645));
#97334=CARTESIAN_POINT('Ctrl Pts',(1.66485468710804,31.7564763038383,126.066202868386));
#97335=CARTESIAN_POINT('Ctrl Pts',(1.66872376076561,31.719677648685,126.126825445671));
#97336=CARTESIAN_POINT('Ctrl Pts',(1.67259283442317,31.6796647620033,126.185659440821));
#97337=CARTESIAN_POINT('Ctrl Pts',(1.67646190808074,31.6366369540205,126.242343367686));
#97338=CARTESIAN_POINT('Ctrl Pts',(1.68032521678957,31.593673257794,126.298942835076));
#97339=CARTESIAN_POINT('Ctrl Pts',(1.68418852549839,31.5477038485901,126.353398209488));
#97340=CARTESIAN_POINT('Ctrl Pts',(1.68805183420721,31.4989724111852,126.405375136042));
#97341=CARTESIAN_POINT('Ctrl Pts',(1.6919106110171,31.4502981387562,126.457291090462));
#97342=CARTESIAN_POINT('Ctrl Pts',(1.69576938782699,31.3988686045674,126.50673401938));
#97343=CARTESIAN_POINT('Ctrl Pts',(1.69962816463688,31.3449679266251,126.553402342875));
#97344=CARTESIAN_POINT('Ctrl Pts',(1.70348451054431,31.2911012043367,126.600041266862));
#97345=CARTESIAN_POINT('Ctrl Pts',(1.70734085645174,31.234766793229,126.643908736025));
#97346=CARTESIAN_POINT('Ctrl Pts',(1.71119720235918,31.176284794844,126.68474082396));
#97347=CARTESIAN_POINT('Ctrl Pts',(1.71505240892552,31.1178200747181,126.725560848228));
#97348=CARTESIAN_POINT('Ctrl Pts',(1.71890761549186,31.0572094250554,126.763346993699));
#97349=CARTESIAN_POINT('Ctrl Pts',(1.7227628220582,30.9948036856758,126.797877412246));
#97350=CARTESIAN_POINT('Ctrl Pts',(1.72661817923176,30.9323955083583,126.832409179757));
#97351=CARTESIAN_POINT('Ctrl Pts',(1.73047353640531,30.8681925282185,126.863684734564));
#97352=CARTESIAN_POINT('Ctrl Pts',(1.73432889357887,30.8025705279352,126.891527982925));
#97353=CARTESIAN_POINT('Ctrl Pts',(1.73818828636949,30.7368798374496,126.919400376366));
#97354=CARTESIAN_POINT('Ctrl Pts',(1.7420476791601,30.6697676098064,126.943833101219));
#97355=CARTESIAN_POINT('Ctrl Pts',(1.74590707195072,30.6016291345085,126.964698436659));
#97356=CARTESIAN_POINT('Ctrl Pts',(1.74976864987655,30.5334520801414,126.985575585766));
#97357=CARTESIAN_POINT('Ctrl Pts',(1.75363022780239,30.4642480929311,127.002881206742));
#97358=CARTESIAN_POINT('Ctrl Pts',(1.75749180572823,30.3944244572758,127.01653834826));
#97359=CARTESIAN_POINT('Ctrl Pts',(1.76136014016254,30.3244786529126,127.030219385344));
#97360=CARTESIAN_POINT('Ctrl Pts',(1.76522847459685,30.2539115166146,127.040239129505));
#97361=CARTESIAN_POINT('Ctrl Pts',(1.76909680903117,30.183136583751,127.046572391632));
#97362=CARTESIAN_POINT('Ctrl Pts',(1.77139452533631,30.1410976339142,127.050334227612));
#97363=CARTESIAN_POINT('Ctrl Pts',(1.77369224164145,30.0989854134141,127.052796422884));
#97364=CARTESIAN_POINT('Ctrl Pts',(1.7759899579466,30.0568861986886,127.053962395688));
#97365=CARTESIAN_POINT('Ctrl Pts',(1.77985822425496,29.986011054718,127.055925341811));
#97366=CARTESIAN_POINT('Ctrl Pts',(1.78372649056332,29.914895393203,127.054219342807));
#97367=CARTESIAN_POINT('Ctrl Pts',(1.78759475687167,29.8439507547856,127.048815803231));
#97368=CARTESIAN_POINT('Ctrl Pts',(1.79145765803481,29.7731045140113,127.043419758168));
#97369=CARTESIAN_POINT('Ctrl Pts',(1.79532055919795,29.7024293057619,127.034336383239));
#97370=CARTESIAN_POINT('Ctrl Pts',(1.79918346036109,29.6323380715102,127.021589045489));
#97371=CARTESIAN_POINT('Ctrl Pts',(1.8030422966023,29.5623205941017,127.008855121732));
#97372=CARTESIAN_POINT('Ctrl Pts',(1.8069011328435,29.4928863465248,126.992464974017));
#97373=CARTESIAN_POINT('Ctrl Pts',(1.81075996908471,29.4244428158648,126.972493723765));
#97374=CARTESIAN_POINT('Ctrl Pts',(1.81461644855455,29.3560410868629,126.952534670886));
#97375=CARTESIAN_POINT('Ctrl Pts',(1.81847292802439,29.2886293399383,126.928998989315));
#97376=CARTESIAN_POINT('Ctrl Pts',(1.82232940749423,29.2226029680551,126.902012465055));
#97377=CARTESIAN_POINT('Ctrl Pts',(1.8261844651669,29.1566009386091,126.875035890118));
#97378=CARTESIAN_POINT('Ctrl Pts',(1.83003952283957,29.0919837179562,126.844611186077));
#97379=CARTESIAN_POINT('Ctrl Pts',(1.83389458051224,29.0291279358746,126.81091275262));
#97380=CARTESIAN_POINT('Ctrl Pts',(1.83775080895684,28.9662530646401,126.777204085027));
#97381=CARTESIAN_POINT('Ctrl Pts',(1.84160703740144,28.9051411295302,126.740219930772));
#97382=CARTESIAN_POINT('Ctrl Pts',(1.84546326584604,28.8461441294545,126.700180635258));
#97383=CARTESIAN_POINT('Ctrl Pts',(1.84764813867768,28.8127174420926,126.677495057829));
#97384=CARTESIAN_POINT('Ctrl Pts',(1.84983301150931,28.7799691924376,126.653829545424));
#97385=CARTESIAN_POINT('Ctrl Pts',(1.85201788434095,28.7479590808042,126.629230216746));
#97386=CARTESIAN_POINT('',(1.54592528048733,32.0547497262092,125.0010607277));
#97387=CARTESIAN_POINT('Ctrl Pts',(1.54592528053768,32.0547497262087,125.001060728624));
#97388=CARTESIAN_POINT('Ctrl Pts',(1.54924811760506,32.0547182468784,125.062039704689));
#97389=CARTESIAN_POINT('Ctrl Pts',(1.55257095467244,32.0519724942774,125.122946605602));
#97390=CARTESIAN_POINT('Ctrl Pts',(1.55589379173983,32.0465301533583,125.183607989737));
#97391=CARTESIAN_POINT('Ctrl Pts',(1.55976286729383,32.0401931504359,125.25424144954));
#97392=CARTESIAN_POINT('Ctrl Pts',(1.56363194284784,32.0301827024085,125.324684804482));
#97393=CARTESIAN_POINT('Ctrl Pts',(1.56750101840185,32.0165185363462,125.39452573436));
#97394=CARTESIAN_POINT('Ctrl Pts',(1.5713643290264,32.0028747299156,125.464262601128));
#97395=CARTESIAN_POINT('Ctrl Pts',(1.57522763965095,31.9855881042439,125.533398351708));
#97396=CARTESIAN_POINT('Ctrl Pts',(1.5790909502755,31.9647301747385,125.601525479903));
#97397=CARTESIAN_POINT('Ctrl Pts',(1.58294972902032,31.9438967127526,125.669572691161));
#97398=CARTESIAN_POINT('Ctrl Pts',(1.58680850776514,31.9195004099013,125.736613167962));
#97399=CARTESIAN_POINT('Ctrl Pts',(1.59066728650996,31.8916635171442,125.802251020819));
#97400=CARTESIAN_POINT('Ctrl Pts',(1.59452363436312,31.8638441606273,125.867847524193));
#97401=CARTESIAN_POINT('Ctrl Pts',(1.59837998221628,31.8325887036063,125.932042710504));
#97402=CARTESIAN_POINT('Ctrl Pts',(1.60223633006943,31.7980682864068,125.994458646661));
#97403=CARTESIAN_POINT('Ctrl Pts',(1.60609153858935,31.7635580680431,126.056856142429));
#97404=CARTESIAN_POINT('Ctrl Pts',(1.60994674710926,31.7257850395042,126.11747500677));
#97405=CARTESIAN_POINT('Ctrl Pts',(1.61380195562917,31.6849664701856,126.175961545651));
#97406=CARTESIAN_POINT('Ctrl Pts',(1.61765731476124,31.6441463062003,126.234450369437));
#97407=CARTESIAN_POINT('Ctrl Pts',(1.6215126738933,31.6002806450424,126.290806305275));
#97408=CARTESIAN_POINT('Ctrl Pts',(1.62536803302536,31.5536293012231,126.34470575104));
#97409=CARTESIAN_POINT('Ctrl Pts',(1.62922742776844,31.5069291249422,126.398661616244));
#97410=CARTESIAN_POINT('Ctrl Pts',(1.63308682251151,31.4574377637294,126.450155490342));
#97411=CARTESIAN_POINT('Ctrl Pts',(1.63694621725458,31.4054538501172,126.498898608209));
#97412=CARTESIAN_POINT('Ctrl Pts',(1.64080779713241,31.3534405039478,126.54766932374));
#97413=CARTESIAN_POINT('Ctrl Pts',(1.64466937701023,31.2989321673928,126.593685869142));
#97414=CARTESIAN_POINT('Ctrl Pts',(1.64853095688806,31.2422606024531,126.636699776408));
#97415=CARTESIAN_POINT('Ctrl Pts',(1.65239929325233,31.1854898810355,126.679788943771));
#97416=CARTESIAN_POINT('Ctrl Pts',(1.6562676296166,31.126548776353,126.719864710759));
#97417=CARTESIAN_POINT('Ctrl Pts',(1.66013596598087,31.065797460298,126.756722327553));
#97418=CARTESIAN_POINT('Ctrl Pts',(1.66243366484671,31.0297126380765,126.778614866445));
#97419=CARTESIAN_POINT('Ctrl Pts',(1.66473136371255,30.9929896379703,126.799372895742));
#97420=CARTESIAN_POINT('Ctrl Pts',(1.66702906257839,30.9557074212992,126.818961485951));
#97421=CARTESIAN_POINT('Ctrl Pts',(1.67089813639883,30.8929282422543,126.851946531418));
#97422=CARTESIAN_POINT('Ctrl Pts',(1.67476721021927,30.8283164347397,126.881742253029));
#97423=CARTESIAN_POINT('Ctrl Pts',(1.67863628403971,30.7622291057691,126.908141596638));
#97424=CARTESIAN_POINT('Ctrl Pts',(1.68249959292333,30.6962402472061,126.93450160511));
#97425=CARTESIAN_POINT('Ctrl Pts',(1.68636290180695,30.6287806786634,126.957475102026));
#97426=CARTESIAN_POINT('Ctrl Pts',(1.69022621069057,30.5602315508614,126.976901153806));
#97427=CARTESIAN_POINT('Ctrl Pts',(1.69408498769223,30.4917628351015,126.996304417718));
#97428=CARTESIAN_POINT('Ctrl Pts',(1.69794376469388,30.4222075639637,127.012168370547));
#97429=CARTESIAN_POINT('Ctrl Pts',(1.70180254169554,30.3519646456321,127.024381004338));
#97430=CARTESIAN_POINT('Ctrl Pts',(1.70565888780513,30.2817659778371,127.036585944604));
#97431=CARTESIAN_POINT('Ctrl Pts',(1.70951523391472,30.2108809997711,127.045144046379));
#97432=CARTESIAN_POINT('Ctrl Pts',(1.71337158002432,30.1397200495256,127.049994114689));
#97433=CARTESIAN_POINT('Ctrl Pts',(1.71722678680292,30.0685801232945,127.05484275008));
#97434=CARTESIAN_POINT('Ctrl Pts',(1.72108199358152,29.997164871149,127.05598549389));
#97435=CARTESIAN_POINT('Ctrl Pts',(1.72493720036013,29.9258892856538,127.053413052583));
#97436=CARTESIAN_POINT('Ctrl Pts',(1.72879255775578,29.8546109155301,127.050840510775));
#97437=CARTESIAN_POINT('Ctrl Pts',(1.73264791515144,29.7834727082802,127.044552515403));
#97438=CARTESIAN_POINT('Ctrl Pts',(1.73650327254709,29.7128874498955,127.034591837709));
#97439=CARTESIAN_POINT('Ctrl Pts',(1.74036266557341,29.6422283057451,127.024620733584));
#97440=CARTESIAN_POINT('Ctrl Pts',(1.74422205859973,29.5721237478891,127.010969340842));
#97441=CARTESIAN_POINT('Ctrl Pts',(1.74808145162605,29.5029783477431,126.993731937771));
#97442=CARTESIAN_POINT('Ctrl Pts',(1.75194302979563,29.4337937982791,126.976484775084));
#97443=CARTESIAN_POINT('Ctrl Pts',(1.7558046079652,29.3655699524173,126.95564770222));
#97444=CARTESIAN_POINT('Ctrl Pts',(1.75966618613478,29.298695494437,126.931364686686));
#97445=CARTESIAN_POINT('Ctrl Pts',(1.76353452082299,29.2317040276841,126.907039183692));
#97446=CARTESIAN_POINT('Ctrl Pts',(1.7674028555112,29.1660671101076,126.879255889797));
#97447=CARTESIAN_POINT('Ctrl Pts',(1.77127119019941,29.10215210493,126.848206352066));
#97448=CARTESIAN_POINT('Ctrl Pts',(1.77356890460526,29.064187854165,126.829763539878));
#97449=CARTESIAN_POINT('Ctrl Pts',(1.7758666190111,29.0268306375569,126.810169233755));
#97450=CARTESIAN_POINT('Ctrl Pts',(1.77816433341695,28.9901526281511,126.789470829064));
#97451=CARTESIAN_POINT('Ctrl Pts',(1.78203306929966,28.9283966802693,126.754620257234));
#97452=CARTESIAN_POINT('Ctrl Pts',(1.78590180518237,28.8683259744342,126.716500811269));
#97453=CARTESIAN_POINT('Ctrl Pts',(1.78977054106508,28.8103080527618,126.675300162113));
#97454=CARTESIAN_POINT('Ctrl Pts',(1.79117478188363,28.7892492014239,126.660345501199));
#97455=CARTESIAN_POINT('Ctrl Pts',(1.79257902270217,28.7684606010765,126.644985351916));
#97456=CARTESIAN_POINT('Ctrl Pts',(1.79398326352072,28.7479590808042,126.629230216746));
#97457=CARTESIAN_POINT('Ctrl Pts',(1.09386069726047,28.7479590808042,126.629230216746));
#97458=CARTESIAN_POINT('Ctrl Pts',(1.09772924549863,28.6914573570451,126.58580942242));
#97459=CARTESIAN_POINT('Ctrl Pts',(1.1015977937368,28.6372927651895,126.539504229736));
#97460=CARTESIAN_POINT('Ctrl Pts',(1.10546634197497,28.5857569445798,126.490608648404));
#97461=CARTESIAN_POINT('Ctrl Pts',(1.10742846411185,28.5596180500294,126.465808879441));
#97462=CARTESIAN_POINT('Ctrl Pts',(1.10939058624872,28.5341547936423,126.440343296117));
#97463=CARTESIAN_POINT('Ctrl Pts',(1.1113527083856,28.5094012387782,126.414253476412));
#97464=CARTESIAN_POINT('Ctrl Pts',(1.11522172486416,28.460590866645,126.362808186406));
#97465=CARTESIAN_POINT('Ctrl Pts',(1.11909074134271,28.4143512962968,126.308732231128));
#97466=CARTESIAN_POINT('Ctrl Pts',(1.12295975782127,28.3709788742317,126.252312953818));
#97467=CARTESIAN_POINT('Ctrl Pts',(1.12682300843003,28.3276710886807,126.195977756328));
#97468=CARTESIAN_POINT('Ctrl Pts',(1.13068625903878,28.2872222636681,126.13730655068));
#97469=CARTESIAN_POINT('Ctrl Pts',(1.13454950964754,28.249890900826,126.076622358809));
#97470=CARTESIAN_POINT('Ctrl Pts',(1.13840822727143,28.2126033411229,126.01600937136));
#97471=CARTESIAN_POINT('Ctrl Pts',(1.14226694489532,28.1784262310649,125.953388501099));
#97472=CARTESIAN_POINT('Ctrl Pts',(1.14612566251921,28.1475758185352,125.889113161765));
#97473=CARTESIAN_POINT('Ctrl Pts',(1.14998194860246,28.1167448461508,125.824878325033));
#97474=CARTESIAN_POINT('Ctrl Pts',(1.15383823468571,28.0892366220044,125.75899152456));
#97475=CARTESIAN_POINT('Ctrl Pts',(1.15769452076896,28.0652216033881,125.691830989841));
#97476=CARTESIAN_POINT('Ctrl Pts',(1.16154966696221,28.0412136834359,125.624690307285));
#97477=CARTESIAN_POINT('Ctrl Pts',(1.16540481315546,28.0206970825669,125.55627709514));
#97478=CARTESIAN_POINT('Ctrl Pts',(1.16925995934871,28.0037935776479,125.486988174251));
#97479=CARTESIAN_POINT('Ctrl Pts',(1.17311525568896,27.9868894143853,125.417696554755));
#97480=CARTESIAN_POINT('Ctrl Pts',(1.17697055202921,27.9735987394515,125.347529631285));
#97481=CARTESIAN_POINT('Ctrl Pts',(1.18082584836946,27.9639926264908,125.276896257678));
#97482=CARTESIAN_POINT('Ctrl Pts',(1.18468518004213,27.9543764588272,125.206188952234));
#97483=CARTESIAN_POINT('Ctrl Pts',(1.1885445117148,27.9484526174281,125.135014704389));
#97484=CARTESIAN_POINT('Ctrl Pts',(1.19240384338747,27.9462403758186,125.063788467469));
#97485=CARTESIAN_POINT('Ctrl Pts',(1.19626535994249,27.9440268817932,124.99252190726));
#97486=CARTESIAN_POINT('Ctrl Pts',(1.2001268764975,27.9455291602523,124.921203785309));
#97487=CARTESIAN_POINT('Ctrl Pts',(1.20398839305252,27.9507143478077,124.850247276423));
#97488=CARTESIAN_POINT('Ctrl Pts',(1.2078566663814,27.9559086082595,124.779166609818));
#97489=CARTESIAN_POINT('Ctrl Pts',(1.21172493971028,27.9647985833273,124.708449301724));
#97490=CARTESIAN_POINT('Ctrl Pts',(1.21559321303916,27.977299825455,124.638500945512));
#97491=CARTESIAN_POINT('Ctrl Pts',(1.21789146843416,27.9847271825007,124.59694256187));
#97492=CARTESIAN_POINT('Ctrl Pts',(1.22018972382915,27.9934283053086,124.555655389018));
#97493=CARTESIAN_POINT('Ctrl Pts',(1.22248797922415,28.0033771870154,124.514721827021));
#97494=CARTESIAN_POINT('Ctrl Pts',(1.22635706753339,28.0201260226695,124.445810614402));
#97495=CARTESIAN_POINT('Ctrl Pts',(1.23022615584263,28.0404794416406,124.3776325501));
#97496=CARTESIAN_POINT('Ctrl Pts',(1.23409524415187,28.0643567448886,124.310592463458));
#97497=CARTESIAN_POINT('Ctrl Pts',(1.2379585676327,28.0881984716531,124.243652264583));
#97498=CARTESIAN_POINT('Ctrl Pts',(1.24182189111353,28.1155534989662,124.177847131634));
#97499=CARTESIAN_POINT('Ctrl Pts',(1.24568521459436,28.1462906273317,124.113569447626));
#97500=CARTESIAN_POINT('Ctrl Pts',(1.24954400628193,28.1769917001321,124.049367163252));
#97501=CARTESIAN_POINT('Ctrl Pts',(1.25340279796949,28.2110667850215,123.986689204937));
#97502=CARTESIAN_POINT('Ctrl Pts',(1.25726158965706,28.2483362327094,123.925908938283));
#97503=CARTESIAN_POINT('Ctrl Pts',(1.2611179504991,28.2855822025117,123.865166960153));
#97504=CARTESIAN_POINT('Ctrl Pts',(1.26497431134114,28.3260182894283,123.806320715076));
#97505=CARTESIAN_POINT('Ctrl Pts',(1.26883067218318,28.36941916093,123.749718555781));
#97506=CARTESIAN_POINT('Ctrl Pts',(1.27268589371849,28.4128072102641,123.693133118785));
#97507=CARTESIAN_POINT('Ctrl Pts',(1.2765411152538,28.4591580098432,123.638790836655));
#97508=CARTESIAN_POINT('Ctrl Pts',(1.28039633678911,28.5082042059661,123.587009245818));
#97509=CARTESIAN_POINT('Ctrl Pts',(1.28425170894349,28.5572523182675,123.535225631934));
#97510=CARTESIAN_POINT('Ctrl Pts',(1.28810708109787,28.6089957005272,123.48600325914));
#97511=CARTESIAN_POINT('Ctrl Pts',(1.29196245325224,28.6631293906798,123.439623591425));
#97512=CARTESIAN_POINT('Ctrl Pts',(1.2958218609375,28.7173197441505,123.393195376755));
#97513=CARTESIAN_POINT('Ctrl Pts',(1.29968126862277,28.7739050304206,123.349616123726));
#97514=CARTESIAN_POINT('Ctrl Pts',(1.30354067630803,28.8325470690385,123.309127084465));
#97515=CARTESIAN_POINT('Ctrl Pts',(1.30740226910233,28.8912223094478,123.268615121229));
#97516=CARTESIAN_POINT('Ctrl Pts',(1.31126386189663,28.9519562065549,123.231197109626));
#97517=CARTESIAN_POINT('Ctrl Pts',(1.31512545469094,29.0143837973087,123.197069534482));
#97518=CARTESIAN_POINT('Ctrl Pts',(1.3189938037899,29.0769206123762,123.162882249185));
#97519=CARTESIAN_POINT('Ctrl Pts',(1.32286215288887,29.1411565994881,123.131997104933));
#97520=CARTESIAN_POINT('Ctrl Pts',(1.32673050198783,29.2067051879891,123.104563136441));
#97521=CARTESIAN_POINT('Ctrl Pts',(1.32902808467946,29.2456373780649,123.088268895783));
#97522=CARTESIAN_POINT('Ctrl Pts',(1.33132566737108,29.2850322712179,123.073191185541));
#97523=CARTESIAN_POINT('Ctrl Pts',(1.33362325006271,29.3248066099531,123.059352827396));
#97524=CARTESIAN_POINT('Ctrl Pts',(1.33749232926375,29.3917857299198,123.036049333741));
#97525=CARTESIAN_POINT('Ctrl Pts',(1.34136140846479,29.4601038938102,123.016171823725));
#97526=CARTESIAN_POINT('Ctrl Pts',(1.34523048766583,29.5293772204397,122.999872063627));
#97527=CARTESIAN_POINT('Ctrl Pts',(1.34909380207173,29.5985473321916,122.983596589612));
#97528=CARTESIAN_POINT('Ctrl Pts',(1.35295711647764,29.668669312732,122.970888394534));
#97529=CARTESIAN_POINT('Ctrl Pts',(1.35682043088354,29.7393423478386,122.961850066636));
#97530=CARTESIAN_POINT('Ctrl Pts',(1.36067921359172,29.8099324829276,122.952822340768));
#97531=CARTESIAN_POINT('Ctrl Pts',(1.36453799629991,29.88107190911,122.94745599265));
#97532=CARTESIAN_POINT('Ctrl Pts',(1.36839677900809,29.9523495120027,122.945802591401));
#97533=CARTESIAN_POINT('Ctrl Pts',(1.37225313093495,30.0235822146564,122.944150231687));
#97534=CARTESIAN_POINT('Ctrl Pts',(1.37610948286181,30.0949524368243,122.946206189712));
#97535=CARTESIAN_POINT('Ctrl Pts',(1.37996583478866,30.1660453015422,122.951970088027));
#97536=CARTESIAN_POINT('Ctrl Pts',(1.38382104748671,30.2371171642766,122.957732283594));
#97537=CARTESIAN_POINT('Ctrl Pts',(1.38767626018475,30.3079113482947,122.967200205572));
#97538=CARTESIAN_POINT('Ctrl Pts',(1.3915314728828,30.3780160759691,122.980321459041));
#97539=CARTESIAN_POINT('Ctrl Pts',(1.39538683629162,30.4481235442284,122.993443225456));
#97540=CARTESIAN_POINT('Ctrl Pts',(1.39924219970043,30.5175410255454,123.010218515374));
#97541=CARTESIAN_POINT('Ctrl Pts',(1.40309756310925,30.5858666509226,123.030543773059));
#97542=CARTESIAN_POINT('Ctrl Pts',(1.40695696225114,30.6542637984771,123.0508903069));
#97543=CARTESIAN_POINT('Ctrl Pts',(1.41081636139302,30.7215663419588,123.074794087784));
#97544=CARTESIAN_POINT('Ctrl Pts',(1.41467576053491,30.7873881796827,123.102101842301));
#97545=CARTESIAN_POINT('Ctrl Pts',(1.41853734488708,30.8532472860464,123.1294250586));
#97546=CARTESIAN_POINT('Ctrl Pts',(1.42239892923925,30.9176235790874,123.16015587591));
#97547=CARTESIAN_POINT('Ctrl Pts',(1.42626051359142,30.9801540422591,123.194094239462));
#97548=CARTESIAN_POINT('Ctrl Pts',(1.43012885450178,31.0427939140761,123.228091984477));
#97549=CARTESIAN_POINT('Ctrl Pts',(1.43399719541214,31.1035810935558,123.265308226916));
#97550=CARTESIAN_POINT('Ctrl Pts',(1.4378655363225,31.1621807099525,123.305499023336));
#97551=CARTESIAN_POINT('Ctrl Pts',(1.44016319784876,31.1969868677261,123.329370974848));
#97552=CARTESIAN_POINT('Ctrl Pts',(1.44246085937501,31.2310218669175,123.354291537472));
#97553=CARTESIAN_POINT('Ctrl Pts',(1.44475852090127,31.2642213716314,123.380203134337));
#97554=CARTESIAN_POINT('Ctrl Pts',(1.44858235651171,31.3194729597889,123.423325972791));
#97555=CARTESIAN_POINT('Ctrl Pts',(1.45240619212214,31.3726361632414,123.469373338719));
#97556=CARTESIAN_POINT('Ctrl Pts',(1.45623002773257,31.4233794277243,123.518113173272));
#97557=CARTESIAN_POINT('Ctrl Pts',(1.4600473584239,31.4740363702874,123.56677009404));
#97558=CARTESIAN_POINT('Ctrl Pts',(1.46386468911523,31.522281191662,123.618110047023));
#97559=CARTESIAN_POINT('Ctrl Pts',(1.46768201980656,31.5678142343074,123.671859913562));
#97560=CARTESIAN_POINT('Ctrl Pts',(1.47149571669541,31.6133039330309,123.725558614401));
#97561=CARTESIAN_POINT('Ctrl Pts',(1.47530941358426,31.6560866490738,123.78166230389));
#97562=CARTESIAN_POINT('Ctrl Pts',(1.47912311047312,31.6958995585341,123.839861107512));
#97563=CARTESIAN_POINT('Ctrl Pts',(1.4829345252099,31.735688643575,123.898025084422));
#97564=CARTESIAN_POINT('Ctrl Pts',(1.48674593994668,31.7725111653249,123.958281279008));
#97565=CARTESIAN_POINT('Ctrl Pts',(1.49055735468346,31.8061457882238,124.020288331099));
#97566=CARTESIAN_POINT('Ctrl Pts',(1.49436783578483,31.8397721720627,124.082280194084));
#97567=CARTESIAN_POINT('Ctrl Pts',(1.4981783168862,31.8702119700892,124.146021625177));
#97568=CARTESIAN_POINT('Ctrl Pts',(1.50198879798757,31.8972892160619,124.211145645182));
#97569=CARTESIAN_POINT('Ctrl Pts',(1.50580209417981,31.9243864660461,124.276317777232));
#97570=CARTESIAN_POINT('Ctrl Pts',(1.50961539037206,31.9481160067823,124.342874078778));
#97571=CARTESIAN_POINT('Ctrl Pts',(1.5134286865643,31.9683500464069,124.410427563984));
#97572=CARTESIAN_POINT('Ctrl Pts',(1.51724331839847,31.9885911731893,124.478004710417));
#97573=CARTESIAN_POINT('Ctrl Pts',(1.52105795023265,32.0053342400584,124.546579251802));
#97574=CARTESIAN_POINT('Ctrl Pts',(1.52487258206682,32.0185021276165,124.615751742609));
#97575=CARTESIAN_POINT('Ctrl Pts',(1.52869351656884,32.031691771618,124.685038522621));
#97576=CARTESIAN_POINT('Ctrl Pts',(1.53251445107087,32.0412943683235,124.75492473087));
#97577=CARTESIAN_POINT('Ctrl Pts',(1.53633538557289,32.0472845563241,124.825004263089));
#97578=CARTESIAN_POINT('Ctrl Pts',(1.53953201721104,32.0522960069184,124.88363349365));
#97579=CARTESIAN_POINT('Ctrl Pts',(1.54272864884919,32.0547800098895,124.942397807972));
#97580=CARTESIAN_POINT('Ctrl Pts',(1.54592528048733,32.0547497262092,125.0010607277));
#97581=CARTESIAN_POINT('Origin',(-1.54592528053767,30.,125.));
#97582=CARTESIAN_POINT('',(0.393902765004298,28.7479590808042,126.629230216746));
#97583=CARTESIAN_POINT('',(0.45211710701879,28.7479590808042,126.629230216746));
#97584=CARTESIAN_POINT('',(-1.54592528053767,28.7479590808042,126.629230216746));
#97585=CARTESIAN_POINT('',(0.145925136815139,32.0544293158457,124.997774677963));
#97586=CARTESIAN_POINT('Ctrl Pts',(0.145925280537677,32.0547487974726,124.997776987473));
#97587=CARTESIAN_POINT('Ctrl Pts',(0.149742847505049,32.0548251766857,125.068374923493));
#97588=CARTESIAN_POINT('Ctrl Pts',(0.153560414472421,32.0512588264106,125.139037406976));
#97589=CARTESIAN_POINT('Ctrl Pts',(0.157377981439792,32.0440566342328,125.209356247934));
#97590=CARTESIAN_POINT('Ctrl Pts',(0.161194267518903,32.0368568585688,125.27965149518));
#97591=CARTESIAN_POINT('Ctrl Pts',(0.165010553598014,32.0260237115458,125.349602835495));
#97592=CARTESIAN_POINT('Ctrl Pts',(0.168826839677125,32.011616039834,125.418806006144));
#97593=CARTESIAN_POINT('Ctrl Pts',(0.172643182166181,31.997208155157,125.488010199712));
#97594=CARTESIAN_POINT('Ctrl Pts',(0.176459524655237,31.9792257443085,125.556465716465));
#97595=CARTESIAN_POINT('Ctrl Pts',(0.180275867144293,31.9577786210231,125.623779154481));
#97596=CARTESIAN_POINT('Ctrl Pts',(0.184096314207838,31.9363084308052,125.69116498983));
#97597=CARTESIAN_POINT('Ctrl Pts',(0.187916761271383,31.9113662409764,125.757405820921));
#97598=CARTESIAN_POINT('Ctrl Pts',(0.191737208334928,31.8831112492071,125.822125042563));
#97599=CARTESIAN_POINT('Ctrl Pts',(0.195559834797493,31.8548401391929,125.886881183709));
#97600=CARTESIAN_POINT('Ctrl Pts',(0.199382461260057,31.8232526902279,125.950113545109));
#97601=CARTESIAN_POINT('Ctrl Pts',(0.203205087722621,31.7885543176414,126.011469730316));
#97602=CARTESIAN_POINT('Ctrl Pts',(0.207034783311059,31.7537917778742,126.072939380598));
#97603=CARTESIAN_POINT('Ctrl Pts',(0.210864478899498,31.7159070973764,126.132525510666));
#97604=CARTESIAN_POINT('Ctrl Pts',(0.214694174487936,31.6751488627916,126.189904975193));
#97605=CARTESIAN_POINT('Ctrl Pts',(0.217219630217664,31.6482712390514,126.227743308321));
#97606=CARTESIAN_POINT('Ctrl Pts',(0.219745085947392,31.6201448756126,126.264622703573));
#97607=CARTESIAN_POINT('Ctrl Pts',(0.22227054167712,31.5908499886023,126.300459102111));
#97608=CARTESIAN_POINT('Ctrl Pts',(0.226141676453319,31.5459454375006,126.355390783156));
#97609=CARTESIAN_POINT('Ctrl Pts',(0.230012811229518,31.4981043722261,126.408101583541));
#97610=CARTESIAN_POINT('Ctrl Pts',(0.233883946005718,31.4475746723825,126.458260995287));
#97611=CARTESIAN_POINT('Ctrl Pts',(0.237749271054588,31.397120806576,126.508345128718));
#97612=CARTESIAN_POINT('Ctrl Pts',(0.241614596103459,31.3439866574102,126.555885135297));
#97613=CARTESIAN_POINT('Ctrl Pts',(0.245479921152329,31.2884602743133,126.600583544841));
#97614=CARTESIAN_POINT('Ctrl Pts',(0.249340636948719,31.2330001043073,126.645228653239));
#97615=CARTESIAN_POINT('Ctrl Pts',(0.253201352745109,31.1751537431435,126.687038592961));
#97616=CARTESIAN_POINT('Ctrl Pts',(0.257062068541499,31.1152447204755,126.725753973181));
#97617=CARTESIAN_POINT('Ctrl Pts',(0.260920304427269,31.0553741800551,126.76444448478));
#97618=CARTESIAN_POINT('Ctrl Pts',(0.264778540313038,30.9934440134148,126.80004411804));
#97619=CARTESIAN_POINT('Ctrl Pts',(0.268636776198808,30.9298081599305,126.832335762961));
#97620=CARTESIAN_POINT('Ctrl Pts',(0.272493820670667,30.8661919570439,126.8646174363));
#97621=CARTESIAN_POINT('Ctrl Pts',(0.276350865142527,30.8008715454328,126.89359292988));
#97622=CARTESIAN_POINT('Ctrl Pts',(0.280207909614387,30.7342254730604,126.919091065377));
#97623=CARTESIAN_POINT('Ctrl Pts',(0.284065049503794,30.6675777519632,126.944589831659));
#97624=CARTESIAN_POINT('Ctrl Pts',(0.287922189393201,30.5996047589391,126.966610897738));
#97625=CARTESIAN_POINT('Ctrl Pts',(0.291779329282608,30.5307034092699,126.98503185211));
#97626=CARTESIAN_POINT('Ctrl Pts',(0.295640407261538,30.4617317122214,127.003471614035));
#97627=CARTESIAN_POINT('Ctrl Pts',(0.299501485240468,30.3918302360401,127.01830380093));
#97628=CARTESIAN_POINT('Ctrl Pts',(0.303362563219398,30.3214085129597,127.029456609612));
#97629=CARTESIAN_POINT('Ctrl Pts',(0.307225773774024,30.2509478940953,127.040615578286));
#97630=CARTESIAN_POINT('Ctrl Pts',(0.31108898432865,30.1799669390398,127.048091071826));
#97631=CARTESIAN_POINT('Ctrl Pts',(0.314952194883276,30.1088800485825,127.051863225832));
#97632=CARTESIAN_POINT('Ctrl Pts',(0.318822060279675,30.0376707024626,127.055641877823));
#97633=CARTESIAN_POINT('Ctrl Pts',(0.322691925676074,29.9663555419922,127.055704452657));
#97634=CARTESIAN_POINT('Ctrl Pts',(0.326561791072473,29.8953480046004,127.052083215262));
#97635=CARTESIAN_POINT('Ctrl Pts',(0.328843131553543,29.853488055243,127.04994844451));
#97636=CARTESIAN_POINT('Ctrl Pts',(0.331124472034613,29.8117349175731,127.046534437514));
#97637=CARTESIAN_POINT('Ctrl Pts',(0.333405812515682,29.7701717568777,127.041856150948));
#97638=CARTESIAN_POINT('Ctrl Pts',(0.337280820487943,29.699573974397,127.033909771224));
#97639=CARTESIAN_POINT('Ctrl Pts',(0.341155828460203,29.6292554674172,127.022282690525));
#97640=CARTESIAN_POINT('Ctrl Pts',(0.345030836432464,29.5596290834691,127.007005485387));
#97641=CARTESIAN_POINT('Ctrl Pts',(0.349103497146784,29.4864512627742,126.990949035017));
#97642=CARTESIAN_POINT('Ctrl Pts',(0.353176157861103,29.414038594576,126.970860123394));
#97643=CARTESIAN_POINT('Ctrl Pts',(0.357248818575423,29.3428649859014,126.946836186161));
#97644=CARTESIAN_POINT('Ctrl Pts',(0.36111377939119,29.2753211299458,126.924037435526));
#97645=CARTESIAN_POINT('Ctrl Pts',(0.364978740206958,29.2088935797027,126.897695353925));
#97646=CARTESIAN_POINT('Ctrl Pts',(0.368843701022725,29.1439752527045,126.867945179741));
#97647=CARTESIAN_POINT('Ctrl Pts',(0.372706168135226,29.0790988115239,126.838214200604));
#97648=CARTESIAN_POINT('Ctrl Pts',(0.376568635247727,29.015730098834,126.805079696651));
#97649=CARTESIAN_POINT('Ctrl Pts',(0.380431102360228,28.954242424875,126.768725150092));
#97650=CARTESIAN_POINT('Ctrl Pts',(0.384292622927454,28.89276981923,126.732379512664));
#97651=CARTESIAN_POINT('Ctrl Pts',(0.38815414349468,28.8331777535429,126.692815645137));
#97652=CARTESIAN_POINT('Ctrl Pts',(0.392015664061906,28.7758138465268,126.650262350096));
#97653=CARTESIAN_POINT('Ctrl Pts',(0.39264469770937,28.7664693857023,126.643330507076));
#97654=CARTESIAN_POINT('Ctrl Pts',(0.393273731356834,28.7571839880914,126.636319430585));
#97655=CARTESIAN_POINT('Ctrl Pts',(0.393902765004298,28.7479590808042,126.629230216746));
#97656=CARTESIAN_POINT('',(0.,30.5301702171886,123.014825674328));
#97657=CARTESIAN_POINT('Ctrl Pts',(-2.77555756156289E-16,30.5301702171886,
123.014825674328));
#97658=CARTESIAN_POINT('Ctrl Pts',(0.0370450902795195,31.1902723495278,
123.191115729233));
#97659=CARTESIAN_POINT('Ctrl Pts',(0.0856865378388906,31.9249100643917,
123.887375341273));
#97660=CARTESIAN_POINT('Ctrl Pts',(0.134327985398261,32.0542758854422,124.783527116577));
#97661=CARTESIAN_POINT('Ctrl Pts',(0.145924342678113,32.0526640242463,124.997761916792));
#97662=CARTESIAN_POINT('',(7.76557151915824E-9,29.4696366853849,123.014877253918));
#97663=CARTESIAN_POINT('Origin',(0.,30.,125.));
#97664=CARTESIAN_POINT('',(0.20407471941795,32.054749451866,125.001500851857));
#97665=CARTESIAN_POINT('Ctrl Pts',(7.76557151915824E-9,29.4696366853849,
123.014877253918));
#97666=CARTESIAN_POINT('Ctrl Pts',(0.00385761022877746,29.5379454299378,
122.996627273029));
#97667=CARTESIAN_POINT('Ctrl Pts',(0.00771521269198336,29.6073355558211,
122.981870298801));
#97668=CARTESIAN_POINT('Ctrl Pts',(0.0115728151551893,29.6774154225185,
122.970729995079));
#97669=CARTESIAN_POINT('Ctrl Pts',(0.0154246336215809,29.747390213141,122.959606394862));
#97670=CARTESIAN_POINT('Ctrl Pts',(0.0192764520879721,29.8180522132104,
122.952088779147));
#97671=CARTESIAN_POINT('Ctrl Pts',(0.0231282705543638,29.8889963546714,
122.948250562758));
#97672=CARTESIAN_POINT('Ctrl Pts',(0.0269755489459578,29.9598568754449,
122.944416870411));
#97673=CARTESIAN_POINT('Ctrl Pts',(0.030822827337552,30.0309983912348,122.94425399043));
#97674=CARTESIAN_POINT('Ctrl Pts',(0.0346701057291459,30.1020091979917,
122.947783713634));
#97675=CARTESIAN_POINT('Ctrl Pts',(0.0385149683480649,30.1729754158344,
122.951311220464));
#97676=CARTESIAN_POINT('Ctrl Pts',(0.0423598309669836,30.2438106001824,
122.958526706804));
#97677=CARTESIAN_POINT('Ctrl Pts',(0.0462046935859026,30.3141030405584,
122.969399881214));
#97678=CARTESIAN_POINT('Ctrl Pts',(0.0500484485266476,30.3843752301713,
122.980269923139));
#97679=CARTESIAN_POINT('Ctrl Pts',(0.0538922034673924,30.4541045031858,
122.994795486533));
#97680=CARTESIAN_POINT('Ctrl Pts',(0.0577359584081374,30.5228860355374,
123.012894628778));
#97681=CARTESIAN_POINT('Ctrl Pts',(0.0615799121663579,30.5916711256003,
123.030994707197));
#97682=CARTESIAN_POINT('Ctrl Pts',(0.0654238659245789,30.6595079054338,
123.052668604445));
#97683=CARTESIAN_POINT('Ctrl Pts',(0.0692678196827994,30.726005208168,123.077784091156));
#97684=CARTESIAN_POINT('Ctrl Pts',(0.0731157450116613,30.7925712158741,
123.102925527172));
#97685=CARTESIAN_POINT('Ctrl Pts',(0.0769636703405231,30.8577945264371,
123.131515475442));
#97686=CARTESIAN_POINT('Ctrl Pts',(0.0808115956693851,30.9213034447518,
123.163373329937));
#97687=CARTESIAN_POINT('Ctrl Pts',(0.0846617836232696,30.984849707052,123.195249917222));
#97688=CARTESIAN_POINT('Ctrl Pts',(0.0885119715771539,31.0466791460969,
123.230397992699));
#97689=CARTESIAN_POINT('Ctrl Pts',(0.0923621595310384,31.1064466115173,
123.268592058941));
#97690=CARTESIAN_POINT('Ctrl Pts',(0.0962187949191377,31.16631416213,123.306850084069));
#97691=CARTESIAN_POINT('Ctrl Pts',(0.100075430307237,31.2241124513603,123.348163994447));
#97692=CARTESIAN_POINT('Ctrl Pts',(0.103932065695336,31.279527830583,123.392266784176));
#97693=CARTESIAN_POINT('Ctrl Pts',(0.105608342252961,31.3036139812752,123.411435947218));
#97694=CARTESIAN_POINT('Ctrl Pts',(0.107284618810585,31.3272504139545,123.431131494297));
#97695=CARTESIAN_POINT('Ctrl Pts',(0.10896089536821,31.350413588026,123.451329375311));
#97696=CARTESIAN_POINT('Ctrl Pts',(0.112923971370282,31.405176281495,123.499081482311));
#97697=CARTESIAN_POINT('Ctrl Pts',(0.116887047372355,31.4575262780038,123.549849701845));
#97698=CARTESIAN_POINT('Ctrl Pts',(0.120850123374427,31.507109086759,123.603354102462));
#97699=CARTESIAN_POINT('Ctrl Pts',(0.124661304975432,31.5547915153461,123.65480781849));
#97700=CARTESIAN_POINT('Ctrl Pts',(0.128472486576437,31.5999146066877,123.708791405287));
#97701=CARTESIAN_POINT('Ctrl Pts',(0.132283668177441,31.6421964245354,123.765014791286));
#97702=CARTESIAN_POINT('Ctrl Pts',(0.136091357626874,31.684439499932,123.821186660299));
#97703=CARTESIAN_POINT('Ctrl Pts',(0.139899047076306,31.7238461632285,123.879593863066));
#97704=CARTESIAN_POINT('Ctrl Pts',(0.143706736525739,31.7601735166201,123.939911912203));
#97705=CARTESIAN_POINT('Ctrl Pts',(0.147512291410529,31.7964805051461,124.000196147454));
#97706=CARTESIAN_POINT('Ctrl Pts',(0.151317846295318,31.8297113500592,124.062388677103));
#97707=CARTESIAN_POINT('Ctrl Pts',(0.155123401180107,31.8596665201771,124.126136168369));
#97708=CARTESIAN_POINT('Ctrl Pts',(0.158928176024214,31.8896155502571,124.189870593042));
#97709=CARTESIAN_POINT('Ctrl Pts',(0.16273295086832,31.9162900274481,124.255158893629));
#97710=CARTESIAN_POINT('Ctrl Pts',(0.166537725712426,31.9395372999307,124.321625011754));
#97711=CARTESIAN_POINT('Ctrl Pts',(0.17034498854872,31.9627997741097,124.388134592945));
#97712=CARTESIAN_POINT('Ctrl Pts',(0.174152251385013,31.9826304041421,124.455823056767));
#97713=CARTESIAN_POINT('Ctrl Pts',(0.177959514221306,31.9989259021712,124.52429757187));
#97714=CARTESIAN_POINT('Ctrl Pts',(0.18176828320523,32.0152278466756,124.59279917539));
#97715=CARTESIAN_POINT('Ctrl Pts',(0.185577052189154,32.0279917839574,124.662086957578));
#97716=CARTESIAN_POINT('Ctrl Pts',(0.189385821173078,32.0371657421938,124.731758874644));
#97717=CARTESIAN_POINT('Ctrl Pts',(0.193199633965217,32.0463518491549,124.801523055586));
#97718=CARTESIAN_POINT('Ctrl Pts',(0.197013446757356,32.0519384547796,124.871671888419));
#97719=CARTESIAN_POINT('Ctrl Pts',(0.200827259549495,32.0539256011114,124.94180045018));
#97720=CARTESIAN_POINT('Ctrl Pts',(0.201909746172313,32.0544896191791,124.961705263059));
#97721=CARTESIAN_POINT('Ctrl Pts',(0.202992232795132,32.054763981877,124.98160846073));
#97722=CARTESIAN_POINT('Ctrl Pts',(0.20407471941795,32.054749451866,125.001500851857));
#97723=CARTESIAN_POINT('Ctrl Pts',(0.204074719462323,32.0547494518654,125.001500852673));
#97724=CARTESIAN_POINT('Ctrl Pts',(0.209415201710472,32.0546777675541,125.099640598186));
#97725=CARTESIAN_POINT('Ctrl Pts',(0.214755683958621,32.0475743595618,125.197525900642));
#97726=CARTESIAN_POINT('Ctrl Pts',(0.22009616620677,32.0335513132822,125.294391947492));
#97727=CARTESIAN_POINT('Ctrl Pts',(0.223961505002541,32.0234017008875,125.364501737486));
#97728=CARTESIAN_POINT('Ctrl Pts',(0.227826843798313,32.0096018595663,125.434225914476));
#97729=CARTESIAN_POINT('Ctrl Pts',(0.231692182594084,31.9921930417871,125.503154495911));
#97730=CARTESIAN_POINT('Ctrl Pts',(0.235551702466996,31.9748104314305,125.571979311513));
#97731=CARTESIAN_POINT('Ctrl Pts',(0.239411222339908,31.9538297464012,125.640010440692));
#97732=CARTESIAN_POINT('Ctrl Pts',(0.243270742212821,31.9293437036226,125.706845411523));
#97733=CARTESIAN_POINT('Ctrl Pts',(0.247125668264792,31.9048868055304,125.773600831556));
#97734=CARTESIAN_POINT('Ctrl Pts',(0.250980594316762,31.8769330034826,125.839162466248));
#97735=CARTESIAN_POINT('Ctrl Pts',(0.254835520368733,31.8456250674413,125.90314211115));
#97736=CARTESIAN_POINT('Ctrl Pts',(0.258687979313753,31.8143371681078,125.967080809838));
#97737=CARTESIAN_POINT('Ctrl Pts',(0.262540438258773,31.7796996067612,126.029439091024));
#97738=CARTESIAN_POINT('Ctrl Pts',(0.266392897203793,31.7419030265743,126.089849259536));
#97739=CARTESIAN_POINT('Ctrl Pts',(0.270244186324789,31.704117923563,126.150241084111));
#97740=CARTESIAN_POINT('Ctrl Pts',(0.274095475445786,31.6631759640342,126.208685557808));
#97741=CARTESIAN_POINT('Ctrl Pts',(0.277946764566783,31.6193125696332,126.264841636067));
#97742=CARTESIAN_POINT('Ctrl Pts',(0.281798179498721,31.5754477423367,126.320999548789));
#97743=CARTESIAN_POINT('Ctrl Pts',(0.285649594430659,31.5286615921515,126.374868535323));
#97744=CARTESIAN_POINT('Ctrl Pts',(0.289501009362597,31.4792304211519,126.426139868189));
#97745=CARTESIAN_POINT('Ctrl Pts',(0.293356449034519,31.4297475944326,126.47746477975));
#97746=CARTESIAN_POINT('Ctrl Pts',(0.297211888706441,31.3776145678265,126.526186267525));
#97747=CARTESIAN_POINT('Ctrl Pts',(0.301067328378363,31.323144540542,126.572032470191));
#97748=CARTESIAN_POINT('Ctrl Pts',(0.304924940998853,31.2686438136283,126.617904512047));
#97749=CARTESIAN_POINT('Ctrl Pts',(0.308782553619344,31.2118038526668,126.660897749185));
#97750=CARTESIAN_POINT('Ctrl Pts',(0.312640166239834,31.1529687681419,126.700782344155));
#97751=CARTESIAN_POINT('Ctrl Pts',(0.316504559112776,31.0940302733564,126.740737041452));
#97752=CARTESIAN_POINT('Ctrl Pts',(0.320368951985719,31.0330900707049,126.777571936079));
#97753=CARTESIAN_POINT('Ctrl Pts',(0.324233344858661,30.9705182802118,126.811102379843));
#97754=CARTESIAN_POINT('Ctrl Pts',(0.326566042254217,30.9327475209962,126.831342655978));
#97755=CARTESIAN_POINT('Ctrl Pts',(0.328898739649774,30.8943826830153,126.850379771625));
#97756=CARTESIAN_POINT('Ctrl Pts',(0.33123143704533,30.855508387678,126.868181725934));
#97757=CARTESIAN_POINT('Ctrl Pts',(0.335101017398882,30.7910220081836,126.897712385496));
#97758=CARTESIAN_POINT('Ctrl Pts',(0.338970597752434,30.7248786638559,126.923957958651));
#97759=CARTESIAN_POINT('Ctrl Pts',(0.342840178105986,30.6574462840317,126.946731092399));
#97760=CARTESIAN_POINT('Ctrl Pts',(0.346703992403464,30.5901143850989,126.969470291934));
#97761=CARTESIAN_POINT('Ctrl Pts',(0.350567806700942,30.5214977197823,126.988747168817));
#97762=CARTESIAN_POINT('Ctrl Pts',(0.35443162099842,30.4519857149758,127.004421731063));
#97763=CARTESIAN_POINT('Ctrl Pts',(0.358290899187939,30.3825553170826,127.020077891414));
#97764=CARTESIAN_POINT('Ctrl Pts',(0.362150177377457,30.3122321390617,127.032140031349));
#97765=CARTESIAN_POINT('Ctrl Pts',(0.366009455566976,30.2414206768526,127.040517978183));
#97766=CARTESIAN_POINT('Ctrl Pts',(0.369866299964003,30.1706538707674,127.048890641598));
#97767=CARTESIAN_POINT('Ctrl Pts',(0.37372314436103,30.0993998725611,127.053583664579));
#97768=CARTESIAN_POINT('Ctrl Pts',(0.377579988758057,30.0280718289488,127.054558233519));
#97769=CARTESIAN_POINT('Ctrl Pts',(0.381435690157131,29.9567649238112,127.055532513639));
#97770=CARTESIAN_POINT('Ctrl Pts',(0.385291391556204,29.8853845021612,127.052790520854));
#97771=CARTESIAN_POINT('Ctrl Pts',(0.389147092955278,29.8143455388811,127.046345519106));
#97772=CARTESIAN_POINT('Ctrl Pts',(0.393002940534494,29.7433038823205,127.039900273011));
#97773=CARTESIAN_POINT('Ctrl Pts',(0.39685878811371,29.672604193286,127.029751785297));
#97774=CARTESIAN_POINT('Ctrl Pts',(0.400714635692925,29.6026564170064,127.015965188081));
#97775=CARTESIAN_POINT('Ctrl Pts',(0.404574508651722,29.5326356175212,127.002164198105));
#97776=CARTESIAN_POINT('Ctrl Pts',(0.408434381610518,29.463368775227,126.984717610905));
#97777=CARTESIAN_POINT('Ctrl Pts',(0.412294254569315,29.3952548372765,126.963741543753));
#97778=CARTESIAN_POINT('Ctrl Pts',(0.416156307606727,29.3271024281792,126.942753629198));
#97779=CARTESIAN_POINT('Ctrl Pts',(0.420018360644138,29.2601046759995,126.918232433224));
#97780=CARTESIAN_POINT('Ctrl Pts',(0.42388041368155,29.1946419708229,126.890342827992));
#97781=CARTESIAN_POINT('Ctrl Pts',(0.427749209984033,29.1290649657211,126.862404526639));
#97782=CARTESIAN_POINT('Ctrl Pts',(0.431618006286515,29.0650287952297,126.831086287122));
#97783=CARTESIAN_POINT('Ctrl Pts',(0.435486802588998,29.0028899805489,126.796599335303));
#97784=CARTESIAN_POINT('Ctrl Pts',(0.437780104353962,28.966056029563,126.77615654605));
#97785=CARTESIAN_POINT('Ctrl Pts',(0.440073406118926,28.9298882374949,126.754601199828));
#97786=CARTESIAN_POINT('Ctrl Pts',(0.44236670788389,28.8944556997489,126.73198422703));
#97787=CARTESIAN_POINT('Ctrl Pts',(0.445616840928857,28.8442396908682,126.699930804411));
#97788=CARTESIAN_POINT('Ctrl Pts',(0.448866973973823,28.795336617669,126.665639199464));
#97789=CARTESIAN_POINT('Ctrl Pts',(0.452117107018789,28.7479590808042,126.629230216746));
#97790=CARTESIAN_POINT('Origin',(-1.54592528053767,-30.,125.));
#97791=CARTESIAN_POINT('',(9.49394826732427,-31.2520409112987,126.629230222815));
#97792=CARTESIAN_POINT('',(9.55204643304504,-31.2540479291372,126.631857161249));
#97793=CARTESIAN_POINT('',(-1.54592528053767,-31.2520409112987,126.629230222815));
#97794=CARTESIAN_POINT('',(10.,-27.9466241674713,124.92486510207));
#97795=CARTESIAN_POINT('Ctrl Pts',(9.55204643304504,-31.2540479291372,126.631857161249));
#97796=CARTESIAN_POINT('Ctrl Pts',(9.55318392757862,-31.2706437159061,126.619178714129));
#97797=CARTESIAN_POINT('Ctrl Pts',(9.59136651239171,-31.8206290607534,126.184464695852));
#97798=CARTESIAN_POINT('Ctrl Pts',(9.66659418748432,-32.4129313959741,124.728220591155));
#97799=CARTESIAN_POINT('Ctrl Pts',(9.77772945832288,-31.0809188200307,122.823596089609));
#97800=CARTESIAN_POINT('Ctrl Pts',(9.88886472916144,-28.7565525546702,122.915156040329));
#97801=CARTESIAN_POINT('Ctrl Pts',(9.96295490972048,-27.9716077196437,124.242084880697));
#97802=CARTESIAN_POINT('Ctrl Pts',(10.,-27.9466241674713,124.92486510207));
#97803=CARTESIAN_POINT('',(9.99999184526219,-28.1818120683087,125.959175316415));
#97804=CARTESIAN_POINT('Origin',(10.,-30.,125.));
#97805=CARTESIAN_POINT('',(9.94592528057839,-27.9452500001719,125.000026582061));
#97806=CARTESIAN_POINT('Ctrl Pts',(9.94592528057839,-27.9452500001719,125.000026582061));
#97807=CARTESIAN_POINT('Ctrl Pts',(9.94992641061459,-27.9452509601105,125.074228272518));
#97808=CARTESIAN_POINT('Ctrl Pts',(9.95392754065078,-27.9492756106224,125.14835894506));
#97809=CARTESIAN_POINT('Ctrl Pts',(9.95792867068697,-27.9572752004394,125.221975124192));
#97810=CARTESIAN_POINT('Ctrl Pts',(9.96193971239158,-27.9652946069784,125.295773666595));
#97811=CARTESIAN_POINT('Ctrl Pts',(9.96595075409619,-27.9773085747598,125.369054741152));
#97812=CARTESIAN_POINT('Ctrl Pts',(9.9699617958008,-27.9932168371984,125.441382940309));
#97813=CARTESIAN_POINT('Ctrl Pts',(9.97397822777386,-28.0091464780746,125.513808338258));
#97814=CARTESIAN_POINT('Ctrl Pts',(9.97799465974692,-28.0289807273363,125.58527789525));
#97815=CARTESIAN_POINT('Ctrl Pts',(9.98201109171998,-28.0525696285214,125.655372039946));
#97816=CARTESIAN_POINT('Ctrl Pts',(9.9860378222072,-28.0762190138961,125.725645912706));
#97817=CARTESIAN_POINT('Ctrl Pts',(9.99006455269442,-28.1036421278151,125.794536926984));
#97818=CARTESIAN_POINT('Ctrl Pts',(9.99409128318165,-28.1346410673708,125.861645875613));
#97819=CARTESIAN_POINT('Ctrl Pts',(9.99605722571572,-28.1497754633721,125.894410009429));
#97820=CARTESIAN_POINT('Ctrl Pts',(9.99802316824979,-28.1657615112236,125.926749759945));
#97821=CARTESIAN_POINT('Ctrl Pts',(9.99998911078386,-28.1825723884147,125.958621113448));
#97822=CARTESIAN_POINT('Ctrl Pts',(9.49394826732428,-31.2520409112987,126.629230222815));
#97823=CARTESIAN_POINT('Ctrl Pts',(9.4978041255961,-31.3085908113369,126.58577240612));
#97824=CARTESIAN_POINT('Ctrl Pts',(9.50165998386792,-31.3628913545301,126.539354695332));
#97825=CARTESIAN_POINT('Ctrl Pts',(9.50551584213974,-31.4146257283712,126.490245486868));
#97826=CARTESIAN_POINT('Ctrl Pts',(9.50937196666856,-31.4663636746049,126.441132887286));
#97827=CARTESIAN_POINT('Ctrl Pts',(9.51322809119738,-31.5155347491312,126.389328757068));
#97828=CARTESIAN_POINT('Ctrl Pts',(9.5170842157262,-31.5618583455608,126.335138970633));
#97829=CARTESIAN_POINT('Ctrl Pts',(9.52094443717721,-31.6082311582875,126.280891610502));
#97830=CARTESIAN_POINT('Ctrl Pts',(9.52480465862823,-31.6517501388171,126.224253905268));
#97831=CARTESIAN_POINT('Ctrl Pts',(9.52866488007924,-31.6921750163993,126.165564788579));
#97832=CARTESIAN_POINT('Ctrl Pts',(9.53252738923184,-31.732623851171,126.106840890676));
#97833=CARTESIAN_POINT('Ctrl Pts',(9.53638989838445,-31.7699746790533,126.046063575328));
#97834=CARTESIAN_POINT('Ctrl Pts',(9.54025240753705,-31.8040320840594,125.983598394765));
#97835=CARTESIAN_POINT('Ctrl Pts',(9.54412154299831,-31.8381479160798,125.921026052367));
#97836=CARTESIAN_POINT('Ctrl Pts',(9.54799067845958,-31.8689588377403,125.856760502689));
#97837=CARTESIAN_POINT('Ctrl Pts',(9.55185981392084,-31.8963169727468,125.791188663577));
#97838=CARTESIAN_POINT('Ctrl Pts',(9.55378430665259,-31.9099248012919,125.758573489194));
#97839=CARTESIAN_POINT('Ctrl Pts',(9.55570879938434,-31.9226791705976,125.725635394501));
#97840=CARTESIAN_POINT('Ctrl Pts',(9.5576332921161,-31.9345665198439,125.692423239644));
#97841=CARTESIAN_POINT('Ctrl Pts',(9.56150282241141,-31.9584681211752,125.62564437513));
#97842=CARTESIAN_POINT('Ctrl Pts',(9.56537235270673,-31.9789546628836,125.557496042673));
#97843=CARTESIAN_POINT('Ctrl Pts',(9.56924188300204,-31.9958710383814,125.488360891811));
#97844=CARTESIAN_POINT('Ctrl Pts',(9.57310565808745,-32.0127622539026,125.419328566686));
#97845=CARTESIAN_POINT('Ctrl Pts',(9.57696943317286,-32.0260937289525,125.349312804447));
#97846=CARTESIAN_POINT('Ctrl Pts',(9.58083320825827,-32.0357593881892,125.278713609104));
#97847=CARTESIAN_POINT('Ctrl Pts',(9.58469246348782,-32.0454137405083,125.208197000913));
#97848=CARTESIAN_POINT('Ctrl Pts',(9.58855171871737,-32.0514107294817,125.137098794134));
#97849=CARTESIAN_POINT('Ctrl Pts',(9.59241097394691,-32.0536952083313,125.06582973323));
#97850=CARTESIAN_POINT('Ctrl Pts',(9.59626780542365,-32.0559782524449,124.994605431891));
#97851=CARTESIAN_POINT('Ctrl Pts',(9.60012463690039,-32.054553396799,124.923210973568));
#97852=CARTESIAN_POINT('Ctrl Pts',(9.60398146837713,-32.0494174069306,124.852061314492));
#97853=CARTESIAN_POINT('Ctrl Pts',(9.60783716688164,-32.0442829257965,124.780932556144));
#97854=CARTESIAN_POINT('Ctrl Pts',(9.61169286538615,-32.0354395097063,124.710048938397));
#97855=CARTESIAN_POINT('Ctrl Pts',(9.61554856389066,-32.0229359667501,124.639822770114));
#97856=CARTESIAN_POINT('Ctrl Pts',(9.61940441859746,-32.0104319172498,124.569593756824));
#97857=CARTESIAN_POINT('Ctrl Pts',(9.62326027330426,-31.9942675337882,124.500022723614));
#97858=CARTESIAN_POINT('Ctrl Pts',(9.62711612801105,-31.9745428697909,124.431512517413));
#97859=CARTESIAN_POINT('Ctrl Pts',(9.63097602331588,-31.9547975360732,124.362930518516));
#97860=CARTESIAN_POINT('Ctrl Pts',(9.63483591862072,-31.9314846088313,124.295412033373));
#97861=CARTESIAN_POINT('Ctrl Pts',(9.63869581392555,-31.9047539953752,124.229344577906));
#97862=CARTESIAN_POINT('Ctrl Pts',(9.64255789792737,-31.878008224717,124.163239659859));
#97863=CARTESIAN_POINT('Ctrl Pts',(9.64641998192919,-31.8478411154121,124.098587849704));
#97864=CARTESIAN_POINT('Ctrl Pts',(9.65028206593101,-31.814449557256,124.035753990585));
#97865=CARTESIAN_POINT('Ctrl Pts',(9.6541509064683,-31.7809995821294,123.972810206565));
#97866=CARTESIAN_POINT('Ctrl Pts',(9.65801974700559,-31.7443141456839,123.911691139911));
#97867=CARTESIAN_POINT('Ctrl Pts',(9.66188858754287,-31.7046342726389,123.852733876102));
#97868=CARTESIAN_POINT('Ctrl Pts',(9.66418191268013,-31.6811133108882,123.817785892639));
#97869=CARTESIAN_POINT('Ctrl Pts',(9.66647523781738,-31.6565409827353,123.783596915282));
#97870=CARTESIAN_POINT('Ctrl Pts',(9.66876856295464,-31.6309739560517,123.750231414549));
#97871=CARTESIAN_POINT('Ctrl Pts',(9.67263371316888,-31.587883511937,123.693997490185));
#97872=CARTESIAN_POINT('Ctrl Pts',(9.67649886338311,-31.5417958827293,123.639883225883));
#97873=CARTESIAN_POINT('Ctrl Pts',(9.68036401359735,-31.4929474727728,123.588226149115));
#97874=CARTESIAN_POINT('Ctrl Pts',(9.68422338831157,-31.4441720545441,123.536646260926));
#97875=CARTESIAN_POINT('Ctrl Pts',(9.6880827630258,-31.3926443753802,123.487516623446));
#97876=CARTESIAN_POINT('Ctrl Pts',(9.69194213774002,-31.3386420624652,123.441143049828));
#97877=CARTESIAN_POINT('Ctrl Pts',(9.69579698366837,-31.2847031186007,123.394823893312));
#97878=CARTESIAN_POINT('Ctrl Pts',(9.69965182959673,-31.2282956761813,123.351254692722));
#97879=CARTESIAN_POINT('Ctrl Pts',(9.70350667552509,-31.1697340556572,123.310704347506));
#97880=CARTESIAN_POINT('Ctrl Pts',(9.70735909449371,-31.1112093047505,123.270179532247));
#97881=CARTESIAN_POINT('Ctrl Pts',(9.71121151346233,-31.0505334656249,123.232670078342));
#97882=CARTESIAN_POINT('Ctrl Pts',(9.71506393243095,-30.9880525930008,123.198403586825));
#97883=CARTESIAN_POINT('Ctrl Pts',(9.71891522164929,-30.9255900433535,123.16414714421));
#97884=CARTESIAN_POINT('Ctrl Pts',(9.72276651086764,-30.8613239376804,123.133132010075));
#97885=CARTESIAN_POINT('Ctrl Pts',(9.72661780008598,-30.7956263623038,123.105540643321));
#97886=CARTESIAN_POINT('Ctrl Pts',(9.7304692551573,-30.7299259577087,123.077948088366));
#97887=CARTESIAN_POINT('Ctrl Pts',(9.73432071022861,-30.6627944107858,123.053779779993));
#97888=CARTESIAN_POINT('Ctrl Pts',(9.73817216529993,-30.5946236683056,123.033169998299));
#97889=CARTESIAN_POINT('Ctrl Pts',(9.7420277058967,-30.5263806120378,123.012538354273));
#97890=CARTESIAN_POINT('Ctrl Pts',(9.74588324649348,-30.4570966267253,122.995472913306));
#97891=CARTESIAN_POINT('Ctrl Pts',(9.74973878709025,-30.3871778269895,122.982057757817));
#97892=CARTESIAN_POINT('Ctrl Pts',(9.75359653504282,-30.3172189976746,122.968634921946));
#97893=CARTESIAN_POINT('Ctrl Pts',(9.75745428299538,-30.2466251130133,122.958866598036));
#97894=CARTESIAN_POINT('Ctrl Pts',(9.76131203094795,-30.1758087037608,122.952785096239));
#97895=CARTESIAN_POINT('Ctrl Pts',(9.76517661213126,-30.1048668573695,122.946692822275));
#97896=CARTESIAN_POINT('Ctrl Pts',(9.76904119331458,-30.0337021861904,122.944300424681));
#97897=CARTESIAN_POINT('Ctrl Pts',(9.7729057744979,-29.962727819202,122.945588077566));
#97898=CARTESIAN_POINT('Ctrl Pts',(9.77523846092969,-29.9198872279385,122.946365313254));
#97899=CARTESIAN_POINT('Ctrl Pts',(9.77757114736148,-29.8771159076542,122.948482329295));
#97900=CARTESIAN_POINT('Ctrl Pts',(9.77990383379327,-29.8345033018076,122.951925683627));
#97901=CARTESIAN_POINT('Ctrl Pts',(9.78377969104042,-29.7637006534364,122.957646962603));
#97902=CARTESIAN_POINT('Ctrl Pts',(9.78765554828756,-29.693058539817,122.967055076515));
#97903=CARTESIAN_POINT('Ctrl Pts',(9.79153140553471,-29.6229905778606,122.980133306845));
#97904=CARTESIAN_POINT('Ctrl Pts',(9.79540148151799,-29.5530271299125,122.993192029567));
#97905=CARTESIAN_POINT('Ctrl Pts',(9.79927155750128,-29.4836366054338,123.009909913015));
#97906=CARTESIAN_POINT('Ctrl Pts',(9.80314163348456,-29.4152281865604,123.03021841599));
#97907=CARTESIAN_POINT('Ctrl Pts',(9.80700712085521,-29.3469008771373,123.050502839889));
#97908=CARTESIAN_POINT('Ctrl Pts',(9.81087260822585,-29.2795538217276,123.074369288734));
#97909=CARTESIAN_POINT('Ctrl Pts',(9.8147380955965,-29.2135849718361,123.101698399627));
#97910=CARTESIAN_POINT('Ctrl Pts',(9.81860111321162,-29.147658271075,123.129010049275));
#97911=CARTESIAN_POINT('Ctrl Pts',(9.82246413082675,-29.0831084746034,123.159779786309));
#97912=CARTESIAN_POINT('Ctrl Pts',(9.82632714844188,-29.0203159818345,123.1938392134));
#97913=CARTESIAN_POINT('Ctrl Pts',(9.83018897812518,-28.9575427986333,123.227888166742));
#97914=CARTESIAN_POINT('Ctrl Pts',(9.83405080780849,-28.8965262713254,123.265224570954));
#97915=CARTESIAN_POINT('Ctrl Pts',(9.83791263749179,-28.8376229640577,123.305633691077));
#97916=CARTESIAN_POINT('Ctrl Pts',(9.84177455940801,-28.7787182499896,123.346043776299));
#97917=CARTESIAN_POINT('Ctrl Pts',(9.84563648132423,-28.721927253993,123.389526447573));
#97918=CARTESIAN_POINT('Ctrl Pts',(9.84949840324045,-28.6675768412463,123.435824150386));
#97919=CARTESIAN_POINT('Ctrl Pts',(9.85336422698768,-28.6131715164297,123.482168629341));
#97920=CARTESIAN_POINT('Ctrl Pts',(9.85723005073492,-28.5612120665622,123.531333503191));
#97921=CARTESIAN_POINT('Ctrl Pts',(9.86109587448215,-28.5119908828302,123.583022078605));
#97922=CARTESIAN_POINT('Ctrl Pts',(9.86496381726527,-28.4627427187025,123.634738986907));
#97923=CARTESIAN_POINT('Ctrl Pts',(9.86883176004839,-28.4162361246387,123.688981983705));
#97924=CARTESIAN_POINT('Ctrl Pts',(9.8726997028315,-28.3727235371298,123.745420837138));
#97925=CARTESIAN_POINT('Ctrl Pts',(9.87657422950515,-28.3291368838632,123.801955759011));
#97926=CARTESIAN_POINT('Ctrl Pts',(9.8804487561788,-28.2885546879188,123.860693602102));
#97927=CARTESIAN_POINT('Ctrl Pts',(9.88432328285245,-28.2511859592603,123.921275283767));
#97928=CARTESIAN_POINT('Ctrl Pts',(9.88656189011224,-28.229595216878,123.956277905715));
#97929=CARTESIAN_POINT('Ctrl Pts',(9.88880049737203,-28.2090763583662,123.991895575244));
#97930=CARTESIAN_POINT('Ctrl Pts',(9.89103910463182,-28.1896624684553,124.028055770952));
#97931=CARTESIAN_POINT('Ctrl Pts',(9.89510077117281,-28.1544384483701,124.093663820947));
#97932=CARTESIAN_POINT('Ctrl Pts',(9.89916243771379,-28.122730882925,124.161289079108));
#97933=CARTESIAN_POINT('Ctrl Pts',(9.90322410425478,-28.094763080848,124.230539250903));
#97934=CARTESIAN_POINT('Ctrl Pts',(9.90727424497689,-28.0668746431938,124.299592911014));
#97935=CARTESIAN_POINT('Ctrl Pts',(9.91132438569901,-28.0427049908748,124.370261919641));
#97936=CARTESIAN_POINT('Ctrl Pts',(9.91537452642113,-28.022430787494,124.442131223092));
#97937=CARTESIAN_POINT('Ctrl Pts',(9.91941770244941,-28.002191447993,124.513876938815));
#97938=CARTESIAN_POINT('Ctrl Pts',(9.92346087847769,-27.9858343503665,124.586818448078));
#97939=CARTESIAN_POINT('Ctrl Pts',(9.92750405450597,-27.9734876167677,124.660522278925));
#97940=CARTESIAN_POINT('Ctrl Pts',(9.93153868051992,-27.9611669925315,124.734070249922));
#97941=CARTESIAN_POINT('Ctrl Pts',(9.93557330653388,-27.9528399155232,124.80837692485));
#97942=CARTESIAN_POINT('Ctrl Pts',(9.93960793254784,-27.9485839442394,124.882996886077));
#97943=CARTESIAN_POINT('Ctrl Pts',(9.94171371521112,-27.9463626353712,124.921943103184));
#97944=CARTESIAN_POINT('Ctrl Pts',(9.9438194978744,-27.9452494949735,124.960974455546));
#97945=CARTESIAN_POINT('Ctrl Pts',(9.94592528053769,-27.9452500001719,125.000026581306));
#97946=CARTESIAN_POINT('Origin',(-1.54592528053767,-30.,125.));
#97947=CARTESIAN_POINT('',(8.79398045084826,-31.2520409112987,126.629230222815));
#97948=CARTESIAN_POINT('',(8.85202073424513,-31.2520409112987,126.629230222815));
#97949=CARTESIAN_POINT('',(-1.54592528053767,-31.2520409112987,126.629230222815));
#97950=CARTESIAN_POINT('',(9.30407471946233,-27.9452508261495,125.001842569092));
#97951=CARTESIAN_POINT('Ctrl Pts',(8.85202073424513,-31.2520409112987,126.629230222815));
#97952=CARTESIAN_POINT('Ctrl Pts',(8.85588087589068,-31.3086052462336,126.585761313101));
#97953=CARTESIAN_POINT('Ctrl Pts',(8.85974101753623,-31.3628655414002,126.539372164453));
#97954=CARTESIAN_POINT('Ctrl Pts',(8.86360115918179,-31.4145190775282,126.490346718656));
#97955=CARTESIAN_POINT('Ctrl Pts',(8.86746399088779,-31.4662086100386,126.441287107943));
#97956=CARTESIAN_POINT('Ctrl Pts',(8.8713268225938,-31.5152874359326,126.389587897415));
#97957=CARTESIAN_POINT('Ctrl Pts',(8.8751896542998,-31.5614915447377,126.335567938449));
#97958=CARTESIAN_POINT('Ctrl Pts',(8.8790587520412,-31.6077706028556,126.281460351804));
#97959=CARTESIAN_POINT('Ctrl Pts',(8.88292784978261,-31.6511653498478,126.225024893573));
#97960=CARTESIAN_POINT('Ctrl Pts',(8.88679694752401,-31.691454267034,126.166610485566));
#97961=CARTESIAN_POINT('Ctrl Pts',(8.88741372888748,-31.6978768117552,126.157298516568));
#97962=CARTESIAN_POINT('Ctrl Pts',(8.88803051025094,-31.7042205250594,126.147936309128));
#97963=CARTESIAN_POINT('Ctrl Pts',(8.88864729161441,-31.7104846184552,126.138525332405));
#97964=CARTESIAN_POINT('Ctrl Pts',(8.89251643697727,-31.7497800468686,126.079489117783));
#97965=CARTESIAN_POINT('Ctrl Pts',(8.89638558234013,-31.7860924541118,126.018300511658));
#97966=CARTESIAN_POINT('Ctrl Pts',(8.90025472770299,-31.8191789952293,125.955293329725));
#97967=CARTESIAN_POINT('Ctrl Pts',(8.90411810773317,-31.8522162347832,125.892380033477));
#97968=CARTESIAN_POINT('Ctrl Pts',(8.90798148776336,-31.8820369255731,125.827653966917));
#97969=CARTESIAN_POINT('Ctrl Pts',(8.91184486779355,-31.9084416125598,125.761477625377));
#97970=CARTESIAN_POINT('Ctrl Pts',(8.91570371502192,-31.9348153196242,125.695378926792));
#97971=CARTESIAN_POINT('Ctrl Pts',(8.9195625622503,-31.9577808048082,125.627833782111));
#97972=CARTESIAN_POINT('Ctrl Pts',(8.92342140947868,-31.9771854423888,125.559227403572));
#97973=CARTESIAN_POINT('Ctrl Pts',(8.92727782521086,-31.9965778529234,125.490664254561));
#97974=CARTESIAN_POINT('Ctrl Pts',(8.93113424094305,-32.012413735477,125.421041664695));
#97975=CARTESIAN_POINT('Ctrl Pts',(8.93499065667524,-32.0245898244675,125.350761464763));
#97976=CARTESIAN_POINT('Ctrl Pts',(8.9388459323752,-32.036762313967,125.280502041038));
#97977=CARTESIAN_POINT('Ctrl Pts',(8.94270120807515,-32.0452770749115,125.209585871567));
#97978=CARTESIAN_POINT('Ctrl Pts',(8.9465564837751,-32.0500819844574,125.138424779225));
#97979=CARTESIAN_POINT('Ctrl Pts',(8.95041190929307,-32.0548870807244,125.067260921526));
#97980=CARTESIAN_POINT('Ctrl Pts',(8.95426733481105,-32.0559820088406,124.995852606872));
#97981=CARTESIAN_POINT('Ctrl Pts',(8.95812276032902,-32.053366660051,124.924614843033));
#97982=CARTESIAN_POINT('Ctrl Pts',(8.96198221980066,-32.0507485748071,124.853302542717));
#97983=CARTESIAN_POINT('Ctrl Pts',(8.9658416792723,-32.0444124809993,124.782161635874));
#97984=CARTESIAN_POINT('Ctrl Pts',(8.96970113874394,-32.0344103499965,124.711604281712));
#97985=CARTESIAN_POINT('Ctrl Pts',(8.97356278251356,-32.0244025581922,124.641006994941));
#97986=CARTESIAN_POINT('Ctrl Pts',(8.97742442628316,-32.0107246920212,124.570994395295));
#97987=CARTESIAN_POINT('Ctrl Pts',(8.98128607005277,-31.9934797877607,124.501967974635));
#97988=CARTESIAN_POINT('Ctrl Pts',(8.98515446830165,-31.9762047200892,124.432820818465));
#97989=CARTESIAN_POINT('Ctrl Pts',(8.98902286655053,-31.9553502997926,124.364663749846));
#97990=CARTESIAN_POINT('Ctrl Pts',(8.9928912647994,-31.9310690911997,124.297881970383));
#97991=CARTESIAN_POINT('Ctrl Pts',(8.99518836401726,-31.9166506312381,124.258226184318));
#97992=CARTESIAN_POINT('Ctrl Pts',(8.99748546323511,-31.9010247667144,124.219054957003));
#97993=CARTESIAN_POINT('Ctrl Pts',(8.99978256245296,-31.8842311475986,124.180444910382));
#97994=CARTESIAN_POINT('Ctrl Pts',(9.00365172642783,-31.855944486933,124.115411323546));
#97995=CARTESIAN_POINT('Ctrl Pts',(9.00752089040269,-31.8242315741275,124.051716583882));
#97996=CARTESIAN_POINT('Ctrl Pts',(9.01139005437756,-31.7892411653051,123.989745767206));
#97997=CARTESIAN_POINT('Ctrl Pts',(9.01525345456108,-31.7543028807703,123.927867266819));
#97998=CARTESIAN_POINT('Ctrl Pts',(9.01911685474461,-31.7160970285483,123.867708011387));
#97999=CARTESIAN_POINT('Ctrl Pts',(9.02298025492813,-31.6748199922309,123.809632176122));
#98000=CARTESIAN_POINT('Ctrl Pts',(9.02683912447235,-31.6335913618136,123.751624446839));
#98001=CARTESIAN_POINT('Ctrl Pts',(9.03069799401657,-31.5892989813561,123.695695678629));
#98002=CARTESIAN_POINT('Ctrl Pts',(9.03455686356078,-31.5421837177392,123.642183022922));
#98003=CARTESIAN_POINT('Ctrl Pts',(9.0384133029273,-31.4950981256261,123.588704067568));
#98004=CARTESIAN_POINT('Ctrl Pts',(9.04226974229383,-31.445193497629,123.537638569641));
#98005=CARTESIAN_POINT('Ctrl Pts',(9.04612618166035,-31.3927514328102,123.489291223));
#98006=CARTESIAN_POINT('Ctrl Pts',(9.04998148226639,-31.3403248535067,123.440958152752));
#98007=CARTESIAN_POINT('Ctrl Pts',(9.05383678287242,-31.2853626818514,123.395341969407));
#98008=CARTESIAN_POINT('Ctrl Pts',(9.05769208347846,-31.2281826486284,123.35270981788));
#98009=CARTESIAN_POINT('Ctrl Pts',(9.06154753512888,-31.1710003751851,123.310075996096));
#98010=CARTESIAN_POINT('Ctrl Pts',(9.0654029867793,-31.1116004584095,123.270426726825));
#98011=CARTESIAN_POINT('Ctrl Pts',(9.06925843842972,-31.050331514329,123.233987182236));
#98012=CARTESIAN_POINT('Ctrl Pts',(9.07311792570109,-30.9889984381425,123.197509495244));
#98013=CARTESIAN_POINT('Ctrl Pts',(9.07697741297245,-30.9257928476536,123.164248488503));
#98014=CARTESIAN_POINT('Ctrl Pts',(9.08083690024381,-30.8610892111209,123.134384033894));
#98015=CARTESIAN_POINT('Ctrl Pts',(9.08469857279461,-30.7963489387564,123.104502669738));
#98016=CARTESIAN_POINT('Ctrl Pts',(9.08856024534542,-30.7301093830888,123.078021866545));
#98017=CARTESIAN_POINT('Ctrl Pts',(9.09242191789622,-30.6627637449199,123.055072808324));
#98018=CARTESIAN_POINT('Ctrl Pts',(9.09629034614531,-30.5953002907513,123.032083602496));
#98019=CARTESIAN_POINT('Ctrl Pts',(9.10015877439439,-30.5267273582656,123.012638609793));
#98020=CARTESIAN_POINT('Ctrl Pts',(9.10402720264347,-30.4574513233694,122.996818568065));
#98021=CARTESIAN_POINT('Ctrl Pts',(9.10632407952615,-30.4163187204538,122.987425428064));
#98022=CARTESIAN_POINT('Ctrl Pts',(9.10862095640884,-30.374938423874,122.979309238762));
#98023=CARTESIAN_POINT('Ctrl Pts',(9.11091783329152,-30.3333962858509,122.97247824202));
#98024=CARTESIAN_POINT('Ctrl Pts',(9.11478641244339,-30.2634277776161,122.960972944639));
#98025=CARTESIAN_POINT('Ctrl Pts',(9.11865499159526,-30.1927257528652,122.953071184525));
#98026=CARTESIAN_POINT('Ctrl Pts',(9.12252357074712,-30.1216942904492,122.94885688891));
#98027=CARTESIAN_POINT('Ctrl Pts',(9.12638638395902,-30.0507686971733,122.94464887451));
#98028=CARTESIAN_POINT('Ctrl Pts',(9.13024919717092,-29.9795151219791,122.944117443843));
#98029=CARTESIAN_POINT('Ctrl Pts',(9.13411201038282,-29.9083459260032,122.947295176305));
#98030=CARTESIAN_POINT('Ctrl Pts',(9.13797029260362,-29.8372602098581,122.950469181361));
#98031=CARTESIAN_POINT('Ctrl Pts',(9.14182857482442,-29.7662591594153,122.957343685967));
#98032=CARTESIAN_POINT('Ctrl Pts',(9.14568685704522,-29.6957565667091,122.967899240736));
#98033=CARTESIAN_POINT('Ctrl Pts',(9.14954270918848,-29.6252983789367,122.978448147258));
#98034=CARTESIAN_POINT('Ctrl Pts',(9.15339856133174,-29.5553385054741,122.992673432437));
#98035=CARTESIAN_POINT('Ctrl Pts',(9.157254413475,-29.4862855672259,123.010503821552));
#98036=CARTESIAN_POINT('Ctrl Pts',(9.16110912781955,-29.4172530053669,123.028328949211));
#98037=CARTESIAN_POINT('Ctrl Pts',(9.16496384216409,-29.3491273176599,123.049756947452));
#98038=CARTESIAN_POINT('Ctrl Pts',(9.16881855650864,-29.2823051789703,123.074665819561));
#98039=CARTESIAN_POINT('Ctrl Pts',(9.17267342372151,-29.2154803902819,123.099575679493));
#98040=CARTESIAN_POINT('Ctrl Pts',(9.17652829093437,-29.1499597077937,123.127966515567));
#98041=CARTESIAN_POINT('Ctrl Pts',(9.18038315814724,-29.0861212959532,123.15966761785));
#98042=CARTESIAN_POINT('Ctrl Pts',(9.18424206777992,-29.0222159397417,123.191401963603));
#98043=CARTESIAN_POINT('Ctrl Pts',(9.18810097741259,-28.9599968118557,123.226453288522));
#98044=CARTESIAN_POINT('Ctrl Pts',(9.19195988704527,-28.8998180399836,123.264604593369));
#98045=CARTESIAN_POINT('Ctrl Pts',(9.19582098491875,-28.83960514302,123.30277753237));
#98046=CARTESIAN_POINT('Ctrl Pts',(9.19968208279223,-28.781435301757,123.34405366931));
#98047=CARTESIAN_POINT('Ctrl Pts',(9.20354318066571,-28.7256318965417,123.388173861923));
#98048=CARTESIAN_POINT('Ctrl Pts',(9.20741104515668,-28.6697306952305,123.43237137567));
#98049=CARTESIAN_POINT('Ctrl Pts',(9.21127890964764,-28.6162045750296,123.479422575318));
#98050=CARTESIAN_POINT('Ctrl Pts',(9.21514677413861,-28.5653416776921,123.529029891285));
#98051=CARTESIAN_POINT('Ctrl Pts',(9.21744888413577,-28.5350686459666,123.558555614921));
#98052=CARTESIAN_POINT('Ctrl Pts',(9.21975099413293,-28.5057383286815,123.588986158559));
#98053=CARTESIAN_POINT('Ctrl Pts',(9.22205310413008,-28.4774045762066,123.620253379079));
#98054=CARTESIAN_POINT('Ctrl Pts',(9.22588174222822,-28.4302827252427,123.672253879425));
#98055=CARTESIAN_POINT('Ctrl Pts',(9.22971038032636,-28.3857258767059,123.726783942029));
#98056=CARTESIAN_POINT('Ctrl Pts',(9.2335390184245,-28.3440213305649,123.783557560393));
#98057=CARTESIAN_POINT('Ctrl Pts',(9.23736240728238,-28.3023739632892,123.840253339496));
#98058=CARTESIAN_POINT('Ctrl Pts',(9.24118579614027,-28.2635714374772,123.899186180647));
#98059=CARTESIAN_POINT('Ctrl Pts',(9.24500918499815,-28.2278628871692,123.960034800665));
#98060=CARTESIAN_POINT('Ctrl Pts',(9.24882867560751,-28.1921907445636,124.020821380683));
#98061=CARTESIAN_POINT('Ctrl Pts',(9.25264816621688,-28.1596065714772,124.083519439945));
#98062=CARTESIAN_POINT('Ctrl Pts',(9.25646765682624,-28.1303168889735,124.147777830116));
#98063=CARTESIAN_POINT('Ctrl Pts',(9.26043491204592,-28.0998940766984,124.214522184242));
#98064=CARTESIAN_POINT('Ctrl Pts',(9.26440216726559,-28.0730261974045,124.282949611777));
#98065=CARTESIAN_POINT('Ctrl Pts',(9.26836942248526,-28.0498921286478,124.352638545641));
#98066=CARTESIAN_POINT('Ctrl Pts',(9.27218609599499,-28.0276361399335,124.419682356304));
#98067=CARTESIAN_POINT('Ctrl Pts',(9.27600276950471,-28.0088357520803,124.487893114409));
#98068=CARTESIAN_POINT('Ctrl Pts',(9.27981944301444,-27.9936002428959,124.556877469324));
#98069=CARTESIAN_POINT('Ctrl Pts',(9.28363613777674,-27.9783646488747,124.625862208369));
#98070=CARTESIAN_POINT('Ctrl Pts',(9.28745283253905,-27.9666940698592,124.695620065554));
#98071=CARTESIAN_POINT('Ctrl Pts',(9.29126952730136,-27.958646715916,124.765747290177));
#98072=CARTESIAN_POINT('Ctrl Pts',(9.29508879465965,-27.9505939377532,124.835921783189));
#98073=CARTESIAN_POINT('Ctrl Pts',(9.29890806201793,-27.946169296682,124.906465645406));
#98074=CARTESIAN_POINT('Ctrl Pts',(9.30272732937622,-27.9453790517055,124.976971293364));
#98075=CARTESIAN_POINT('Ctrl Pts',(9.30317645940493,-27.945286122168,124.985262465654));
#98076=CARTESIAN_POINT('Ctrl Pts',(9.30362558943363,-27.9452433926879,124.99355311109));
#98077=CARTESIAN_POINT('Ctrl Pts',(9.30407471946233,-27.9452508261495,125.001842569092));
#98078=CARTESIAN_POINT('Ctrl Pts',(9.30407499484945,-27.9458072677851,125.001847151475));
#98079=CARTESIAN_POINT('Ctrl Pts',(9.31377945488918,-27.9442173011669,125.180912509003));
#98080=CARTESIAN_POINT('Ctrl Pts',(9.36052900520844,-28.047648310415,126.041729903938));
#98081=CARTESIAN_POINT('Ctrl Pts',(9.44318615127363,-29.2381865360278,127.294355664252));
#98082=CARTESIAN_POINT('Ctrl Pts',(9.5161388372991,-30.7301642665838,127.03208110996));
#98083=CARTESIAN_POINT('Ctrl Pts',(9.55204643304504,-31.2540479291372,126.631857161249));
#98084=CARTESIAN_POINT('',(9.24592528058238,-27.9452507888899,124.998199460575));
#98085=CARTESIAN_POINT('Ctrl Pts',(9.24592528058238,-27.9452507888899,124.998199460575));
#98086=CARTESIAN_POINT('Ctrl Pts',(9.24973097250201,-27.9451893846722,125.068273054101));
#98087=CARTESIAN_POINT('Ctrl Pts',(9.25353666442164,-27.9487168095866,125.138464582685));
#98088=CARTESIAN_POINT('Ctrl Pts',(9.25734235634127,-27.9558426369693,125.208370433764));
#98089=CARTESIAN_POINT('Ctrl Pts',(9.26114473152835,-27.9629622540585,125.278215360571));
#98090=CARTESIAN_POINT('Ctrl Pts',(9.26494710671543,-27.9736740086242,125.347774607021));
#98091=CARTESIAN_POINT('Ctrl Pts',(9.26874948190251,-27.9879354411875,125.416645861219));
#98092=CARTESIAN_POINT('Ctrl Pts',(9.27254990195913,-28.002189540713,125.485481702739));
#98093=CARTESIAN_POINT('Ctrl Pts',(9.27635032201574,-28.0199895981251,125.553629763388));
#98094=CARTESIAN_POINT('Ctrl Pts',(9.28015074207236,-28.04124173501,125.620696078474));
#98095=CARTESIAN_POINT('Ctrl Pts',(9.28395056576206,-28.0624905369817,125.687751869427));
#98096=CARTESIAN_POINT('Ctrl Pts',(9.28775038945177,-28.0871901908978,125.753725774317));
#98097=CARTESIAN_POINT('Ctrl Pts',(9.29155021314147,-28.1151969900754,125.81823907037));
#98098=CARTESIAN_POINT('Ctrl Pts',(9.29535340916529,-28.1432286452179,125.882809621812));
#98099=CARTESIAN_POINT('Ctrl Pts',(9.29915660518911,-28.1745731087831,125.945916514069));
#98100=CARTESIAN_POINT('Ctrl Pts',(9.30295980121293,-28.2090389723999,126.007202144615));
#98101=CARTESIAN_POINT('Ctrl Pts',(9.30676463915046,-28.2435197156005,126.06851423336));
#98102=CARTESIAN_POINT('Ctrl Pts',(9.31056947708799,-28.2811242729052,126.128003071197));
#98103=CARTESIAN_POINT('Ctrl Pts',(9.31437431502552,-28.3216173481466,126.185339291704));
#98104=CARTESIAN_POINT('Ctrl Pts',(9.31818598381621,-28.3621831209,126.242778448345));
#98105=CARTESIAN_POINT('Ctrl Pts',(9.32199765260691,-28.4056474572905,126.298056875414));
#98106=CARTESIAN_POINT('Ctrl Pts',(9.32580932139761,-28.4517346305472,126.350878198896));
#98107=CARTESIAN_POINT('Ctrl Pts',(9.32899379774474,-28.4902383729238,126.395008018272));
#98108=CARTESIAN_POINT('Ctrl Pts',(9.33217827409187,-28.5305720056642,126.437423346777));
#98109=CARTESIAN_POINT('Ctrl Pts',(9.335362750439,-28.5725566040327,126.477972568693));
#98110=CARTESIAN_POINT('Ctrl Pts',(9.33923133027462,-28.623560522087,126.527232756289));
#98111=CARTESIAN_POINT('Ctrl Pts',(9.34309991011025,-28.677217395628,126.573946306162));
#98112=CARTESIAN_POINT('Ctrl Pts',(9.34696848994588,-28.7332426128984,126.617814354221));
#98113=CARTESIAN_POINT('Ctrl Pts',(9.35083130384245,-28.7891843271776,126.661617018986));
#98114=CARTESIAN_POINT('Ctrl Pts',(9.35469411773903,-28.8474869990078,126.702582303184));
#98115=CARTESIAN_POINT('Ctrl Pts',(9.3585569316356,-28.9078299985523,126.740448864643));
#98116=CARTESIAN_POINT('Ctrl Pts',(9.3624152145392,-28.9681022171288,126.778271009486));
#98117=CARTESIAN_POINT('Ctrl Pts',(9.3662734974428,-29.0304096000489,126.813001394302));
#98118=CARTESIAN_POINT('Ctrl Pts',(9.3701317803464,-29.0944007472384,126.844420655896));
#98119=CARTESIAN_POINT('Ctrl Pts',(9.37398763317096,-29.1583515906063,126.875820128561));
#98120=CARTESIAN_POINT('Ctrl Pts',(9.37784348599552,-29.2239836591128,126.903912401826));
#98121=CARTESIAN_POINT('Ctrl Pts',(9.38169933882007,-29.2909203282268,126.928523679289));
#98122=CARTESIAN_POINT('Ctrl Pts',(9.38555405384343,-29.3578372453881,126.953127694353));
#98123=CARTESIAN_POINT('Ctrl Pts',(9.3894087688668,-29.4260575430735,126.97425258525));
#98124=CARTESIAN_POINT('Ctrl Pts',(9.39326348389015,-29.495185572118,126.991773068375));
#98125=CARTESIAN_POINT('Ctrl Pts',(9.39711835177837,-29.5643163425443,127.009294246302));
#98126=CARTESIAN_POINT('Ctrl Pts',(9.40097321966658,-29.6343544442259,127.023210615427));
#98127=CARTESIAN_POINT('Ctrl Pts',(9.40482808755479,-29.7048917450234,127.033447486498));
#98128=CARTESIAN_POINT('Ctrl Pts',(9.40868699785299,-29.7755030148122,127.043695092471));
#98129=CARTESIAN_POINT('Ctrl Pts',(9.41254590815119,-29.8466140468367,127.050255428029));
#98130=CARTESIAN_POINT('Ctrl Pts',(9.41640481844939,-29.9178101500043,127.053105547958));
#98131=CARTESIAN_POINT('Ctrl Pts',(9.42026591698384,-29.989046625682,127.055957284079));
#98132=CARTESIAN_POINT('Ctrl Pts',(9.4241270155183,-30.0603677824187,127.055094622268));
#98133=CARTESIAN_POINT('Ctrl Pts',(9.42798811405276,-30.1313602478627,127.050546768006));
#98134=CARTESIAN_POINT('Ctrl Pts',(9.43185597919042,-30.2024771281176,127.045990943597));
#98135=CARTESIAN_POINT('Ctrl Pts',(9.43572384432809,-30.2732636842133,127.037737088846));
#98136=CARTESIAN_POINT('Ctrl Pts',(9.43959170946575,-30.3433136699777,127.025866058383));
#98137=CARTESIAN_POINT('Ctrl Pts',(9.44189381340302,-30.3850065269659,127.018800572644));
#98138=CARTESIAN_POINT('Ctrl Pts',(9.4441959173403,-30.4264386684793,127.010454688827));
#98139=CARTESIAN_POINT('Ctrl Pts',(9.44649802127757,-30.467527045114,127.000853823893));
#98140=CARTESIAN_POINT('Ctrl Pts',(9.45045220844813,-30.5381021086969,126.98436298856));
#98141=CARTESIAN_POINT('Ctrl Pts',(9.45440639561869,-30.6079446480582,126.964100582213));
#98142=CARTESIAN_POINT('Ctrl Pts',(9.45836058278925,-30.6766219901702,126.940149541896));
#98143=CARTESIAN_POINT('Ctrl Pts',(9.46222394725379,-30.7437219001114,126.916748626851));
#98144=CARTESIAN_POINT('Ctrl Pts',(9.46608731171834,-30.8097090696607,126.889826857212));
#98145=CARTESIAN_POINT('Ctrl Pts',(9.46995067618289,-30.8741903690013,126.859513044118));
#98146=CARTESIAN_POINT('Ctrl Pts',(9.47395027470645,-30.9409454763712,126.828130273167));
#98147=CARTESIAN_POINT('Ctrl Pts',(9.47794987323002,-31.0060860017405,126.793111865367));
#98148=CARTESIAN_POINT('Ctrl Pts',(9.48194947175358,-31.0691954928842,126.754656251377));
#98149=CARTESIAN_POINT('Ctrl Pts',(9.48594907027715,-31.1323049840279,126.716200637386));
#98150=CARTESIAN_POINT('Ctrl Pts',(9.48994866880071,-31.193382921104,126.674308077663));
#98151=CARTESIAN_POINT('Ctrl Pts',(9.49394826732428,-31.2520409112987,126.629230222815));
#98152=CARTESIAN_POINT('Ctrl Pts',(8.79398045084826,-31.2520409112987,126.629230222815));
#98153=CARTESIAN_POINT('Ctrl Pts',(8.79801550152478,-31.3109295755264,126.58397509816));
#98154=CARTESIAN_POINT('Ctrl Pts',(8.8020505522013,-31.3674504084139,126.535454729334));
#98155=CARTESIAN_POINT('Ctrl Pts',(8.80608560287782,-31.4212258111848,126.483952410329));
#98156=CARTESIAN_POINT('Ctrl Pts',(8.80994358445035,-31.472641401614,126.434710154509));
#98157=CARTESIAN_POINT('Ctrl Pts',(8.81380156602287,-31.5215470665571,126.382742547341));
#98158=CARTESIAN_POINT('Ctrl Pts',(8.81765954759539,-31.5676458651896,126.328338813652));
#98159=CARTESIAN_POINT('Ctrl Pts',(8.8215154555658,-31.6137198864705,126.273964321082));
#98160=CARTESIAN_POINT('Ctrl Pts',(8.82537136353622,-31.6569897214282,126.21715667007));
#98161=CARTESIAN_POINT('Ctrl Pts',(8.82922727150664,-31.6971967434146,126.158240379473));
#98162=CARTESIAN_POINT('Ctrl Pts',(8.8330823968517,-31.7373956046681,126.09933604699));
#98163=CARTESIAN_POINT('Ctrl Pts',(8.83693752219675,-31.7745326139107,126.038324326127));
#98164=CARTESIAN_POINT('Ctrl Pts',(8.84079264754181,-31.808391781376,125.975559699635));
#98165=CARTESIAN_POINT('Ctrl Pts',(8.84464827998394,-31.8422554026225,125.912786817183));
#98166=CARTESIAN_POINT('Ctrl Pts',(8.84850391242607,-31.8728400978263,125.848261000111));
#98167=CARTESIAN_POINT('Ctrl Pts',(8.8523595448682,-31.8999760773574,125.782360829777));
#98168=CARTESIAN_POINT('Ctrl Pts',(8.85621943139899,-31.9271419972069,125.71638794889));
#98169=CARTESIAN_POINT('Ctrl Pts',(8.86007931792977,-31.95085142459,125.649038139322));
#98170=CARTESIAN_POINT('Ctrl Pts',(8.86393920446055,-31.9709832927106,125.580708551991));
#98171=CARTESIAN_POINT('Ctrl Pts',(8.86780159646662,-31.9911282285465,125.51233461152));
#98172=CARTESIAN_POINT('Ctrl Pts',(8.87166398847269,-32.007690871926,125.442980100085));
#98173=CARTESIAN_POINT('Ctrl Pts',(8.87552638047876,-32.0206011140789,125.373053213742));
#98174=CARTESIAN_POINT('Ctrl Pts',(8.87939521059924,-32.0335328759573,125.303009768206));
#98175=CARTESIAN_POINT('Ctrl Pts',(8.88326404071972,-32.0428000276362,125.232392525058));
#98176=CARTESIAN_POINT('Ctrl Pts',(8.88713287084019,-32.0483842978989,125.161614759911));
#98177=CARTESIAN_POINT('Ctrl Pts',(8.88836246958838,-32.0501591010075,125.139120039617));
#98178=CARTESIAN_POINT('Ctrl Pts',(8.88959206833657,-32.05156228863,125.116609097887));
#98179=CARTESIAN_POINT('Ctrl Pts',(8.89082166708476,-32.0525943745539,125.094095143603));
#98180=CARTESIAN_POINT('Ctrl Pts',(8.89469075533167,-32.0558419636751,125.023252134009));
#98181=CARTESIAN_POINT('Ctrl Pts',(8.89855984357858,-32.0554240066368,124.9521020425));
#98182=CARTESIAN_POINT('Ctrl Pts',(8.90242893182549,-32.0513044404969,124.881056085075));
#98183=CARTESIAN_POINT('Ctrl Pts',(8.90629225525498,-32.0471910123784,124.810115983849));
#98184=CARTESIAN_POINT('Ctrl Pts',(8.91015557868447,-32.0393869507265,124.739280189741));
#98185=CARTESIAN_POINT('Ctrl Pts',(8.91401890211395,-32.0279081570336,124.66896213338));
#98186=CARTESIAN_POINT('Ctrl Pts',(8.91787769376668,-32.016442828258,124.598726561889));
#98187=CARTESIAN_POINT('Ctrl Pts',(8.92173648541941,-32.0013114075459,124.529007998911));
#98188=CARTESIAN_POINT('Ctrl Pts',(8.92559527707215,-31.9825816351369,124.460215207219));
#98189=CARTESIAN_POINT('Ctrl Pts',(8.92945163788956,-31.963863661497,124.391465751358));
#98190=CARTESIAN_POINT('Ctrl Pts',(8.93330799870698,-31.9415519607138,124.323641377361));
#98191=CARTESIAN_POINT('Ctrl Pts',(8.93716435952439,-31.9157651374972,124.257139649429));
#98192=CARTESIAN_POINT('Ctrl Pts',(8.94101958104529,-31.8899859325611,124.190657568307));
#98193=CARTESIAN_POINT('Ctrl Pts',(8.94487480256618,-31.8607338189391,124.125497810172));
#98194=CARTESIAN_POINT('Ctrl Pts',(8.94873002408707,-31.8281763781024,124.062040143157));
#98195=CARTESIAN_POINT('Ctrl Pts',(8.95258539623725,-31.7956176651977,123.998579996756));
#98196=CARTESIAN_POINT('Ctrl Pts',(8.95644076838744,-31.7597535923906,123.936822504717));
#98197=CARTESIAN_POINT('Ctrl Pts',(8.96029614053762,-31.7207979561137,123.877123356403));
#98198=CARTESIAN_POINT('Ctrl Pts',(8.96415554823429,-31.6818015436743,123.817361719002));
#98199=CARTESIAN_POINT('Ctrl Pts',(8.96801495593096,-31.63970737391,123.759663133927));
#98200=CARTESIAN_POINT('Ctrl Pts',(8.97187436362763,-31.5947724051756,123.704354007381));
#98201=CARTESIAN_POINT('Ctrl Pts',(8.97573595644216,-31.549811995179,123.649013565936));
#98202=CARTESIAN_POINT('Ctrl Pts',(8.9795975492567,-31.5020079100707,123.59606563689));
#98203=CARTESIAN_POINT('Ctrl Pts',(8.98345914207123,-31.4516553700248,123.545801165872));
#98204=CARTESIAN_POINT('Ctrl Pts',(8.98732749120413,-31.4012147321894,123.495448751152));
#98205=CARTESIAN_POINT('Ctrl Pts',(8.99119584033703,-31.3482170985631,123.447789493155));
#98206=CARTESIAN_POINT('Ctrl Pts',(8.99506418946993,-31.2929917361105,123.40307485058));
#98207=CARTESIAN_POINT('Ctrl Pts',(8.99736177228772,-31.2601909625717,123.376516856212));
#98208=CARTESIAN_POINT('Ctrl Pts',(8.99965935510552,-31.2266049064413,123.350996827091));
#98209=CARTESIAN_POINT('Ctrl Pts',(9.00195693792331,-31.1923070848524,123.326560016639));
#98210=CARTESIAN_POINT('Ctrl Pts',(9.00582595070848,-31.1345512950706,123.285409668833));
#98211=CARTESIAN_POINT('Ctrl Pts',(9.00969496349365,-31.0745495097668,123.247172220975));
#98212=CARTESIAN_POINT('Ctrl Pts',(9.01356397627882,-31.0126276336229,123.212100998903));
#98213=CARTESIAN_POINT('Ctrl Pts',(9.01742722403229,-30.9507980243179,123.177082034789));
#98214=CARTESIAN_POINT('Ctrl Pts',(9.02129047178576,-30.8870544225097,123.145220169151));
#98215=CARTESIAN_POINT('Ctrl Pts',(9.02515371953923,-30.8217527781783,123.116726272138));
#98216=CARTESIAN_POINT('Ctrl Pts',(9.02901243556288,-30.7565277350457,123.0882657995));
#98217=CARTESIAN_POINT('Ctrl Pts',(9.03287115158653,-30.6897487227971,123.063165641315));
#98218=CARTESIAN_POINT('Ctrl Pts',(9.03672986761017,-30.6217958861558,123.041590584566));
#98219=CARTESIAN_POINT('Ctrl Pts',(9.04058615286833,-30.5538858558287,123.020029118841));
#98220=CARTESIAN_POINT('Ctrl Pts',(9.04444243812649,-30.4848039300759,123.00198849557));
#98221=CARTESIAN_POINT('Ctrl Pts',(9.04829872338465,-30.4149484329774,122.987584694833));
#98222=CARTESIAN_POINT('Ctrl Pts',(9.05215386952663,-30.3451135706405,122.973185148865));
#98223=CARTESIAN_POINT('Ctrl Pts',(9.05600901566861,-30.2745060661412,122.962420390725));
#98224=CARTESIAN_POINT('Ctrl Pts',(9.05986416181059,-30.2035358559927,122.955355601131));
#98225=CARTESIAN_POINT('Ctrl Pts',(9.06371945887285,-30.1325628675205,122.948290534967));
#98226=CARTESIAN_POINT('Ctrl Pts',(9.06757475593511,-30.0612276288406,122.944925770849));
#98227=CARTESIAN_POINT('Ctrl Pts',(9.07143005299737,-29.9899449123528,122.945274602845));
#98228=CARTESIAN_POINT('Ctrl Pts',(9.07528938656523,-29.9185875626837,122.94562380007));
#98229=CARTESIAN_POINT('Ctrl Pts',(9.0791487201331,-29.8472833317735,122.949694352633));
#98230=CARTESIAN_POINT('Ctrl Pts',(9.08300805370096,-29.776445799497,122.957447410239));
#98231=CARTESIAN_POINT('Ctrl Pts',(9.08686957281574,-29.7055681518101,122.965204858416));
#98232=CARTESIAN_POINT('Ctrl Pts',(9.09073109193052,-29.6351582086173,122.976648885059));
#98233=CARTESIAN_POINT('Ctrl Pts',(9.09459261104529,-29.5656205092378,122.991689261965));
#98234=CARTESIAN_POINT('Ctrl Pts',(9.09846088795565,-29.495961116415,123.006755960065));
#98235=CARTESIAN_POINT('Ctrl Pts',(9.10232916486601,-29.4271774839988,123.025431446726));
#98236=CARTESIAN_POINT('Ctrl Pts',(9.10619744177637,-29.3596594419617,123.047575473359));
#98237=CARTESIAN_POINT('Ctrl Pts',(9.1084956974382,-29.3195450122081,123.060731882727));
#98238=CARTESIAN_POINT('Ctrl Pts',(9.11079395310004,-29.279876966924,123.075111715127));
#98239=CARTESIAN_POINT('Ctrl Pts',(9.11309220876188,-29.2407332677406,123.090677714008));
#98240=CARTESIAN_POINT('Ctrl Pts',(9.11696135405773,-29.174834307032,123.116883289109));
#98241=CARTESIAN_POINT('Ctrl Pts',(9.12083049935358,-29.1101645790708,123.146555878858));
#98242=CARTESIAN_POINT('Ctrl Pts',(9.12469964464943,-29.047113690358,123.179559052483));
#98243=CARTESIAN_POINT('Ctrl Pts',(9.12856302461331,-28.9841567524474,123.212513048774));
#98244=CARTESIAN_POINT('Ctrl Pts',(9.1324264045772,-28.9228142925019,123.248787554408));
#98245=CARTESIAN_POINT('Ctrl Pts',(9.13628978454108,-28.8634565421432,123.2881978704));
#98246=CARTESIAN_POINT('Ctrl Pts',(9.14014863170448,-28.804168434647,123.327561947321));
#98247=CARTESIAN_POINT('Ctrl Pts',(9.14400747886788,-28.7468608140558,123.37005425914));
#98248=CARTESIAN_POINT('Ctrl Pts',(9.14786632603128,-28.6918783167288,123.415444786618));
#98249=CARTESIAN_POINT('Ctrl Pts',(9.15172274169934,-28.6369304643827,123.460806713105));
#98250=CARTESIAN_POINT('Ctrl Pts',(9.1555791573674,-28.5843052023202,123.509062923585));
#98251=CARTESIAN_POINT('Ctrl Pts',(9.15943557303546,-28.5343160214053,123.559941654866));
#98252=CARTESIAN_POINT('Ctrl Pts',(9.16329084867223,-28.4843416182621,123.610805345406));
#98253=CARTESIAN_POINT('Ctrl Pts',(9.167146124309,-28.4370020894456,123.664289671307));
#98254=CARTESIAN_POINT('Ctrl Pts',(9.17100139994577,-28.3925745451105,123.720085561659));
#98255=CARTESIAN_POINT('Ctrl Pts',(9.17485682540158,-28.3481452742862,123.775883620284));
#98256=CARTESIAN_POINT('Ctrl Pts',(9.17871225085739,-28.3066285134754,123.833993040319));
#98257=CARTESIAN_POINT('Ctrl Pts',(9.1825676763132,-28.2682604036012,123.894072546337));
#98258=CARTESIAN_POINT('Ctrl Pts',(9.18642713572464,-28.2298521489351,123.954214913916));
#98259=CARTESIAN_POINT('Ctrl Pts',(9.19028659513609,-28.1945993836681,124.016331072083));
#98260=CARTESIAN_POINT('Ctrl Pts',(9.19414605454754,-28.1626937934211,124.080052465753));
#98261=CARTESIAN_POINT('Ctrl Pts',(9.19800769825797,-28.1307701458917,124.143809923172));
#98262=CARTESIAN_POINT('Ctrl Pts',(9.20186934196841,-28.1021976391511,124.209173979329));
#98263=CARTESIAN_POINT('Ctrl Pts',(9.20573098567884,-28.0771198912845,124.275755807751));
#98264=CARTESIAN_POINT('Ctrl Pts',(9.20959938387077,-28.0519982794066,124.342454095837));
#98265=CARTESIAN_POINT('Ctrl Pts',(9.2134677820627,-28.0303837780611,124.410373945818));
#98266=CARTESIAN_POINT('Ctrl Pts',(9.21733618025462,-28.0123700035947,124.479111758733));
#98267=CARTESIAN_POINT('Ctrl Pts',(9.21963328003656,-28.0016732150674,124.519929070505));
#98268=CARTESIAN_POINT('Ctrl Pts',(9.2219303798185,-27.9922451094651,124.561034597905));
#98269=CARTESIAN_POINT('Ctrl Pts',(9.22422747960044,-27.9840966569744,124.602342768105));
#98270=CARTESIAN_POINT('Ctrl Pts',(9.22983481597178,-27.9642058736569,124.703178094032));
#98271=CARTESIAN_POINT('Ctrl Pts',(9.23544215234312,-27.9518758969885,124.805550439328));
#98272=CARTESIAN_POINT('Ctrl Pts',(9.24104948871445,-27.9472870601179,124.908527878888));
#98273=CARTESIAN_POINT('Ctrl Pts',(9.24267475265553,-27.9459570041692,124.938375476424));
#98274=CARTESIAN_POINT('Ctrl Pts',(9.2443000165966,-27.9452770122708,124.968273736077));
#98275=CARTESIAN_POINT('Ctrl Pts',(9.24592528053768,-27.9452507888906,124.998199459752));
#98276=CARTESIAN_POINT('Origin',(-1.54592528053767,-30.,125.));
#98277=CARTESIAN_POINT('',(8.09385900495164,-31.2520409112987,126.629230222815));
#98278=CARTESIAN_POINT('',(8.15211359149425,-31.2520409112987,126.629230222815));
#98279=CARTESIAN_POINT('',(-1.54592528053767,-31.2520409112987,126.629230222815));
#98280=CARTESIAN_POINT('',(8.60407471942971,-27.9452501088748,124.999331104759));
#98281=CARTESIAN_POINT('Ctrl Pts',(8.15211359149425,-31.2520409112987,126.629230222815));
#98282=CARTESIAN_POINT('Ctrl Pts',(8.15596912461769,-31.3085645256072,126.58579260634));
#98283=CARTESIAN_POINT('Ctrl Pts',(8.15982465774113,-31.3628527074967,126.539388745966));
#98284=CARTESIAN_POINT('Ctrl Pts',(8.16368019086458,-31.4145858102238,126.490283378426));
#98285=CARTESIAN_POINT('Ctrl Pts',(8.16753532502306,-31.4663135596848,126.441183092238));
#98286=CARTESIAN_POINT('Ctrl Pts',(8.17139045918155,-31.5154864035061,126.389382189262));
#98287=CARTESIAN_POINT('Ctrl Pts',(8.17524559334003,-31.561820363806,126.335183400773));
#98288=CARTESIAN_POINT('Ctrl Pts',(8.17912809944362,-31.6084833011442,126.280599793961));
#98289=CARTESIAN_POINT('Ctrl Pts',(8.1830106055472,-31.6522665411257,126.223584480783));
#98290=CARTESIAN_POINT('Ctrl Pts',(8.18689311165078,-31.6929215457164,126.164480228492));
#98291=CARTESIAN_POINT('Ctrl Pts',(8.19075363020041,-31.7333463113627,126.105710697616));
#98292=CARTESIAN_POINT('Ctrl Pts',(8.19461414875003,-31.7706779722671,126.044876273873));
#98293=CARTESIAN_POINT('Ctrl Pts',(8.19847466729966,-31.8047171615244,125.982340841765));
#98294=CARTESIAN_POINT('Ctrl Pts',(8.20236816718022,-31.839047155696,125.919271154542));
#98295=CARTESIAN_POINT('Ctrl Pts',(8.20626166706079,-31.8700279324735,125.854471708577));
#98296=CARTESIAN_POINT('Ctrl Pts',(8.21015516694136,-31.8975043980646,125.788336617078));
#98297=CARTESIAN_POINT('Ctrl Pts',(8.21404866682192,-31.9249808636556,125.722201525579));
#98298=CARTESIAN_POINT('Ctrl Pts',(8.21794216670249,-31.9489529114773,125.654731281105));
#98299=CARTESIAN_POINT('Ctrl Pts',(8.22183566658305,-31.9693172396355,125.586333669658));
#98300=CARTESIAN_POINT('Ctrl Pts',(8.22570474050503,-31.9895538117255,125.518365152156));
#98301=CARTESIAN_POINT('Ctrl Pts',(8.22957381442702,-32.0063071187198,125.449214612482));
#98302=CARTESIAN_POINT('Ctrl Pts',(8.233442888349,-32.0194429894025,125.379272428543));
#98303=CARTESIAN_POINT('Ctrl Pts',(8.23730619731142,-32.0325592875042,125.309434459171));
#98304=CARTESIAN_POINT('Ctrl Pts',(8.24116950627384,-32.0420687593893,125.238807660473));
#98305=CARTESIAN_POINT('Ctrl Pts',(8.24503281523626,-32.0478871302918,125.167797092004));
#98306=CARTESIAN_POINT('Ctrl Pts',(8.24889159228266,-32.0536986758619,125.096869823612));
#98307=CARTESIAN_POINT('Ctrl Pts',(8.25275036932905,-32.0558276816266,125.025560161487));
#98308=CARTESIAN_POINT('Ctrl Pts',(8.25660914637545,-32.0542413071686,124.954281137128));
#98309=CARTESIAN_POINT('Ctrl Pts',(8.26046549250875,-32.0526559320786,124.883047016403));
#98310=CARTESIAN_POINT('Ctrl Pts',(8.26432183864205,-32.0473598312168,124.811843979669));
#98311=CARTESIAN_POINT('Ctrl Pts',(8.26817818477534,-32.0383722280202,124.741086457411));
#98312=CARTESIAN_POINT('Ctrl Pts',(8.27203339155665,-32.0293872801981,124.670349840363));
#98313=CARTESIAN_POINT('Ctrl Pts',(8.27588859833795,-32.0167130564608,124.600058958127));
#98314=CARTESIAN_POINT('Ctrl Pts',(8.27974380511925,-32.0004206032274,124.5306227821));
#98315=CARTESIAN_POINT('Ctrl Pts',(8.28359916249661,-31.9841275135615,124.461183893686));
#98316=CARTESIAN_POINT('Ctrl Pts',(8.28745451987398,-31.9642160269044,124.392600250205));
#98317=CARTESIAN_POINT('Ctrl Pts',(8.29130987725134,-31.9408078475603,124.325268600591));
#98318=CARTESIAN_POINT('Ctrl Pts',(8.29516927022752,-31.9173751656833,124.257866471513));
#98319=CARTESIAN_POINT('Ctrl Pts',(8.2990286632037,-31.8904386444525,124.191719412194));
#98320=CARTESIAN_POINT('Ctrl Pts',(8.30288805617987,-31.860168938256,124.127206162002));
#98321=CARTESIAN_POINT('Ctrl Pts',(8.30674963428127,-31.8298820938467,124.062656385462));
#98322=CARTESIAN_POINT('Ctrl Pts',(8.31061121238265,-31.7962585367315,123.999742688151));
#98323=CARTESIAN_POINT('Ctrl Pts',(8.31447279048405,-31.7595146056693,123.938818622979));
#98324=CARTESIAN_POINT('Ctrl Pts',(8.31834112507632,-31.7227063848198,123.877787960742));
#98325=CARTESIAN_POINT('Ctrl Pts',(8.3222094596686,-31.6827671620172,123.818754283444));
#98326=CARTESIAN_POINT('Ctrl Pts',(8.32607779426087,-31.6399558407878,123.762041033489));
#98327=CARTESIAN_POINT('Ctrl Pts',(8.32837550864778,-31.6145267610728,123.728354482534));
#98328=CARTESIAN_POINT('Ctrl Pts',(8.33067322303469,-31.5880851379374,123.695485968772));
#98329=CARTESIAN_POINT('Ctrl Pts',(8.3329709374216,-31.5606914158628,123.663497150414));
#98330=CARTESIAN_POINT('Ctrl Pts',(8.33684001301417,-31.5145636716695,123.609631814909));
#98331=CARTESIAN_POINT('Ctrl Pts',(8.34070908860674,-31.4655536592048,123.55805183888));
#98332=CARTESIAN_POINT('Ctrl Pts',(8.34457816419931,-31.4139165827671,123.509081672433));
#98333=CARTESIAN_POINT('Ctrl Pts',(8.34844147485484,-31.3623564457655,123.460184471715));
#98334=CARTESIAN_POINT('Ctrl Pts',(8.35230478551036,-31.3081773642485,123.413889693321));
#98335=CARTESIAN_POINT('Ctrl Pts',(8.35616809616589,-31.2516739392184,123.370487829938));
#98336=CARTESIAN_POINT('Ctrl Pts',(8.3600268749303,-31.1952367960364,123.327136879498));
#98337=CARTESIAN_POINT('Ctrl Pts',(8.36388565369471,-31.1364811086558,123.286672397797));
#98338=CARTESIAN_POINT('Ctrl Pts',(8.36774443245912,-31.0757360717717,123.249345988955));
#98339=CARTESIAN_POINT('Ctrl Pts',(8.37160078032483,-31.0150293021842,123.212043094474));
#98340=CARTESIAN_POINT('Ctrl Pts',(8.37545712819055,-30.952336082378,123.177874604482));
#98341=CARTESIAN_POINT('Ctrl Pts',(8.37931347605626,-30.8880150199357,123.14704914073));
#98342=CARTESIAN_POINT('Ctrl Pts',(8.3831686845817,-30.8237129608559,123.11623278422));
#98343=CARTESIAN_POINT('Ctrl Pts',(8.38702389310713,-30.7577844517736,123.088757702958));
#98344=CARTESIAN_POINT('Ctrl Pts',(8.39087910163257,-30.6906116207524,123.064786019123));
#98345=CARTESIAN_POINT('Ctrl Pts',(8.39473446076312,-30.6234361656004,123.040813398826));
#98346=CARTESIAN_POINT('Ctrl Pts',(8.39858981989367,-30.555016750266,123.020344608877));
#98347=CARTESIAN_POINT('Ctrl Pts',(8.40244517902421,-30.4857527091902,123.00349258253));
#98348=CARTESIAN_POINT('Ctrl Pts',(8.40630457375508,-30.4164161659229,122.98662291631));
#98349=CARTESIAN_POINT('Ctrl Pts',(8.41016396848594,-30.3462337050095,122.973377686177));
#98350=CARTESIAN_POINT('Ctrl Pts',(8.4140233632168,-30.2756160790219,122.963818932539));
#98351=CARTESIAN_POINT('Ctrl Pts',(8.41788494307635,-30.2049584704434,122.954254766886));
#98352=CARTESIAN_POINT('Ctrl Pts',(8.4217465229359,-30.1338656906824,122.948381272767));
#98353=CARTESIAN_POINT('Ctrl Pts',(8.42560810279545,-30.0627521096263,122.946208448932));
#98354=CARTESIAN_POINT('Ctrl Pts',(8.42947643913209,-29.9915141035166,122.94403182338));
#98355=CARTESIAN_POINT('Ctrl Pts',(8.43334477546873,-29.9202557092741,122.945568785037));
#98356=CARTESIAN_POINT('Ctrl Pts',(8.43721311180537,-29.849389085236,122.950777241281));
#98357=CARTESIAN_POINT('Ctrl Pts',(8.43951081062364,-29.8072960136578,122.953870939117));
#98358=CARTESIAN_POINT('Ctrl Pts',(8.4418085094419,-29.7653410419802,122.958258975172));
#98359=CARTESIAN_POINT('Ctrl Pts',(8.44410620826017,-29.7236087531083,122.963924008996));
#98360=CARTESIAN_POINT('Ctrl Pts',(8.44797527432581,-29.6533362781294,122.973463288015));
#98361=CARTESIAN_POINT('Ctrl Pts',(8.45184434039146,-29.5834205882342,122.986663565789));
#98362=CARTESIAN_POINT('Ctrl Pts',(8.4557134064571,-29.5142726801353,123.003486405446));
#98363=CARTESIAN_POINT('Ctrl Pts',(8.45957670756576,-29.4452278032871,123.020284178862));
#98364=CARTESIAN_POINT('Ctrl Pts',(8.46344000867443,-29.3769489055926,123.040693686052));
#98365=CARTESIAN_POINT('Ctrl Pts',(8.46730330978309,-29.3098398221709,123.064624973955));
#98366=CARTESIAN_POINT('Ctrl Pts',(8.47116207901698,-29.2428094615703,123.088528189078));
#98367=CARTESIAN_POINT('Ctrl Pts',(8.47502084825087,-29.1769466448156,123.115944816475));
#98368=CARTESIAN_POINT('Ctrl Pts',(8.47887961748476,-29.1126412975478,123.146734747619));
#98369=CARTESIAN_POINT('Ctrl Pts',(8.48273595583517,-29.0483764602968,123.177505282233));
#98370=CARTESIAN_POINT('Ctrl Pts',(8.48659229418558,-28.9856675830665,123.211644695218));
#98371=CARTESIAN_POINT('Ctrl Pts',(8.49044863253599,-28.92488443271,123.248964854873));
#98372=CARTESIAN_POINT('Ctrl Pts',(8.49430383157519,-28.8641192400424,123.286273988712));
#98373=CARTESIAN_POINT('Ctrl Pts',(8.4981590306144,-28.805279058515,123.326761749583));
#98374=CARTESIAN_POINT('Ctrl Pts',(8.5020142296536,-28.748707345374,123.370195025477));
#98375=CARTESIAN_POINT('Ctrl Pts',(8.50586957934089,-28.6921334216027,123.413629998597));
#98376=CARTESIAN_POINT('Ctrl Pts',(8.50972492902817,-28.6378285261893,123.460010417677));
#98377=CARTESIAN_POINT('Ctrl Pts',(8.51358027871546,-28.5861041227543,123.509062036566));
#98378=CARTESIAN_POINT('Ctrl Pts',(8.51743966413327,-28.5343255748783,123.55816500206));
#98379=CARTESIAN_POINT('Ctrl Pts',(8.52129904955107,-28.4851332644469,123.6099444142));
#98380=CARTESIAN_POINT('Ctrl Pts',(8.52515843496888,-28.4388020905701,123.664088831512));
#98381=CARTESIAN_POINT('Ctrl Pts',(8.52902000557476,-28.392444683934,123.718263905449));
#98382=CARTESIAN_POINT('Ctrl Pts',(8.53288157618065,-28.3489519350537,123.774806264996));
#98383=CARTESIAN_POINT('Ctrl Pts',(8.53674314678653,-28.3085569824377,123.833373204131));
#98384=CARTESIAN_POINT('Ctrl Pts',(8.54061147406359,-28.268091349925,123.892042619069));
#98385=CARTESIAN_POINT('Ctrl Pts',(8.54447980134064,-28.2307345901141,123.95274327235));
#98386=CARTESIAN_POINT('Ctrl Pts',(8.5483481286177,-28.1966748777856,124.015106063533));
#98387=CARTESIAN_POINT('Ctrl Pts',(8.55064591211137,-28.1764434342746,124.0521495146));
#98388=CARTESIAN_POINT('Ctrl Pts',(8.55294369560505,-28.1573744062158,124.089778988432));
#98389=CARTESIAN_POINT('Ctrl Pts',(8.55524147909873,-28.1394991031592,124.127914009197));
#98390=CARTESIAN_POINT('Ctrl Pts',(8.55943210412707,-28.1068986895066,124.197463456703));
#98391=CARTESIAN_POINT('Ctrl Pts',(8.56362272915541,-28.0781595914887,124.268933251471));
#98392=CARTESIAN_POINT('Ctrl Pts',(8.56781335418376,-28.0534922152104,124.341892861113));
#98393=CARTESIAN_POINT('Ctrl Pts',(8.57199336341184,-28.0288873269709,124.414667647576));
#98394=CARTESIAN_POINT('Ctrl Pts',(8.57617337263993,-28.0083337420086,124.488924404301));
#98395=CARTESIAN_POINT('Ctrl Pts',(8.58035338186801,-27.9919944407361,124.564211936298));
#98396=CARTESIAN_POINT('Ctrl Pts',(8.58451634359201,-27.9757217767101,124.639192420046));
#98397=CARTESIAN_POINT('Ctrl Pts',(8.58867930531602,-27.9636292336692,124.715194960974));
#98398=CARTESIAN_POINT('Ctrl Pts',(8.59284226704002,-27.9558298707247,124.791754843805));
#98399=CARTESIAN_POINT('Ctrl Pts',(8.59658641783658,-27.948815155501,124.860612490186));
#98400=CARTESIAN_POINT('Ctrl Pts',(8.60033056863314,-27.9452727045111,124.929920562533));
#98401=CARTESIAN_POINT('Ctrl Pts',(8.6040747194297,-27.9452501088748,124.999331104759));
#98402=CARTESIAN_POINT('Ctrl Pts',(8.60407471946233,-27.9452501088746,124.999331105364));
#98403=CARTESIAN_POINT('Ctrl Pts',(8.60802536883708,-27.9452262670581,125.072569799569));
#98404=CARTESIAN_POINT('Ctrl Pts',(8.61197601821182,-27.9491225024139,125.145776561612));
#98405=CARTESIAN_POINT('Ctrl Pts',(8.61592666758657,-27.9569024208448,125.218517378142));
#98406=CARTESIAN_POINT('Ctrl Pts',(8.61988033453931,-27.9646882817192,125.291313755434));
#98407=CARTESIAN_POINT('Ctrl Pts',(8.62383400149206,-27.9763636771627,125.363643031206));
#98408=CARTESIAN_POINT('Ctrl Pts',(8.62778766844481,-27.9918407207505,125.43507915563));
#98409=CARTESIAN_POINT('Ctrl Pts',(8.63174857353918,-28.0073460988021,125.506646061123));
#98410=CARTESIAN_POINT('Ctrl Pts',(8.63570947863356,-28.0266669211867,125.577316110013));
#98411=CARTESIAN_POINT('Ctrl Pts',(8.63967038372794,-28.0496648799025,125.646676489301));
#98412=CARTESIAN_POINT('Ctrl Pts',(8.643635483493,-28.0726871938758,125.716110322494));
#98413=CARTESIAN_POINT('Ctrl Pts',(8.64760058325807,-28.0993942353363,125.784231304558));
#98414=CARTESIAN_POINT('Ctrl Pts',(8.65156568302313,-28.1295998064449,125.850647211509));
#98415=CARTESIAN_POINT('Ctrl Pts',(8.65553895292325,-28.1598676164907,125.917199969224));
#98416=CARTESIAN_POINT('Ctrl Pts',(8.65951222282338,-28.1936481395682,125.98204023864));
#98417=CARTESIAN_POINT('Ctrl Pts',(8.6634854927235,-28.2307097802741,126.044801263821));
#98418=CARTESIAN_POINT('Ctrl Pts',(8.6644492451281,-28.2396994150702,126.060024515816));
#98419=CARTESIAN_POINT('Ctrl Pts',(8.66541299753269,-28.2488819004221,126.075125578892));
#98420=CARTESIAN_POINT('Ctrl Pts',(8.66637674993729,-28.2582535674493,126.090099503347));
#98421=CARTESIAN_POINT('Ctrl Pts',(8.67024583822596,-28.2958771385732,126.150213942977));
#98422=CARTESIAN_POINT('Ctrl Pts',(8.67411492651463,-28.3366902277256,126.208496033488));
#98423=CARTESIAN_POINT('Ctrl Pts',(8.6779840148033,-28.3804886013258,126.264587044084));
#98424=CARTESIAN_POINT('Ctrl Pts',(8.6818473382748,-28.4242217167573,126.320594480877));
#98425=CARTESIAN_POINT('Ctrl Pts',(8.6857106617463,-28.4709309909865,126.374416938209));
#98426=CARTESIAN_POINT('Ctrl Pts',(8.6895739852178,-28.520368190857,126.425723420539));
#98427=CARTESIAN_POINT('Ctrl Pts',(8.69343277691273,-28.5697473996361,126.476969719061));
#98428=CARTESIAN_POINT('Ctrl Pts',(8.69729156860766,-28.6218478424875,126.525705556754));
#98429=CARTESIAN_POINT('Ctrl Pts',(8.70115036030259,-28.6763813047308,126.571633262576));
#98430=CARTESIAN_POINT('Ctrl Pts',(8.70500672116229,-28.7308804137692,126.617532036365));
#98431=CARTESIAN_POINT('Ctrl Pts',(8.70886308202199,-28.7878091307132,126.660625875713));
#98432=CARTESIAN_POINT('Ctrl Pts',(8.71271944288169,-28.8468437752777,126.700655251332));
#98433=CARTESIAN_POINT('Ctrl Pts',(8.7165746644449,-28.9058609790565,126.74067280095));
#98434=CARTESIAN_POINT('Ctrl Pts',(8.7204298860081,-28.9669824734465,126.777627411718));
#98435=CARTESIAN_POINT('Ctrl Pts',(8.7242851075713,-29.0298544177493,126.811302048732));
#98436=CARTESIAN_POINT('Ctrl Pts',(8.72814047976376,-29.0927288185526,126.844978001463));
#98437=CARTESIAN_POINT('Ctrl Pts',(8.73199585195621,-29.1573533757876,126.87537349859));
#98438=CARTESIAN_POINT('Ctrl Pts',(8.73585122414867,-29.2233499334031,126.902317596132));
#98439=CARTESIAN_POINT('Ctrl Pts',(8.73971063188726,-29.2894155718077,126.929289896957));
#98440=CARTESIAN_POINT('Ctrl Pts',(8.74357003962586,-29.3568556267428,126.952803402456));
#98441=CARTESIAN_POINT('Ctrl Pts',(8.74742944736446,-29.4252730980761,126.972735803575));
#98442=CARTESIAN_POINT('Ctrl Pts',(8.75129104022078,-29.4937293059824,126.992679490011));
#98443=CARTESIAN_POINT('Ctrl Pts',(8.7551526330771,-29.563163558862,127.00903792439));
#98444=CARTESIAN_POINT('Ctrl Pts',(8.75901422593343,-29.6331675563962,127.02173972628));
#98445=CARTESIAN_POINT('Ctrl Pts',(8.76288257510745,-29.7032940342811,127.03446375149));
#98446=CARTESIAN_POINT('Ctrl Pts',(8.76675092428148,-29.7739917650344,127.043518309254));
#98447=CARTESIAN_POINT('Ctrl Pts',(8.7706192734555,-29.8448469050885,127.048883861921));
#98448=CARTESIAN_POINT('Ctrl Pts',(8.77291685589562,-29.8869308841339,127.05207069926));
#98449=CARTESIAN_POINT('Ctrl Pts',(8.77521443833573,-29.9290703633161,127.053957167721));
#98450=CARTESIAN_POINT('Ctrl Pts',(8.77751202077585,-29.9711791363964,127.054547862748));
#98451=CARTESIAN_POINT('Ctrl Pts',(8.78138027676357,-30.0420743133264,127.055542368771));
#98452=CARTESIAN_POINT('Ctrl Pts',(8.78524853275129,-30.1131598883882,127.052865003948));
#98453=CARTESIAN_POINT('Ctrl Pts',(8.78911678873902,-30.1840239637477,127.046492790915));
#98454=CARTESIAN_POINT('Ctrl Pts',(8.79297966476592,-30.2547894815271,127.04012944034));
#98455=CARTESIAN_POINT('Ctrl Pts',(8.79684254079282,-30.3253336312653,127.030081479718));
#98456=CARTESIAN_POINT('Ctrl Pts',(8.80070541681972,-30.3952438280996,127.016377910722));
#98457=CARTESIAN_POINT('Ctrl Pts',(8.80456421327246,-30.4650801929417,127.002688814034));
#98458=CARTESIAN_POINT('Ctrl Pts',(8.8084230097252,-30.5342834594381,126.985351864656));
#98459=CARTESIAN_POINT('Ctrl Pts',(8.81228180617794,-30.6024472079082,126.964447740253));
#98460=CARTESIAN_POINT('Ctrl Pts',(8.81613815614803,-30.6705677404611,126.943556869095));
#98461=CARTESIAN_POINT('Ctrl Pts',(8.81999450611811,-30.7376495992151,126.919103452224));
#98462=CARTESIAN_POINT('Ctrl Pts',(8.82385085608819,-30.8032991769315,126.891218653366));
#98463=CARTESIAN_POINT('Ctrl Pts',(8.82770577861216,-30.8689244541473,126.863344176198));
#98464=CARTESIAN_POINT('Ctrl Pts',(8.83156070113612,-30.9331180577745,126.832041032617));
#98465=CARTESIAN_POINT('Ctrl Pts',(8.83541562366009,-30.995505806269,126.797488734926));
#98466=CARTESIAN_POINT('Ctrl Pts',(8.83927149076623,-31.0579088418036,126.76292797079));
#98467=CARTESIAN_POINT('Ctrl Pts',(8.84312735787237,-31.1185047131747,126.725116697754));
#98468=CARTESIAN_POINT('Ctrl Pts',(8.8469832249785,-31.1769445536386,126.684279988648));
#98469=CARTESIAN_POINT('Ctrl Pts',(8.84866239473405,-31.2023941892003,126.66649624119));
#98470=CARTESIAN_POINT('Ctrl Pts',(8.85034156448959,-31.227435306327,126.648139290202));
#98471=CARTESIAN_POINT('Ctrl Pts',(8.85202073424513,-31.2520409112987,126.629230222815));
#98472=CARTESIAN_POINT('',(8.54592528048628,-27.9452503479095,125.001195714817));
#98473=CARTESIAN_POINT('Ctrl Pts',(8.54592528053768,-27.94525034791,125.001195715761));
#98474=CARTESIAN_POINT('Ctrl Pts',(8.54975547188148,-27.9452912658805,125.071510240688));
#98475=CARTESIAN_POINT('Ctrl Pts',(8.55358566322528,-27.9489412103475,125.141718266714));
#98476=CARTESIAN_POINT('Ctrl Pts',(8.55741585456908,-27.9561692055137,125.211549630133));
#98477=CARTESIAN_POINT('Ctrl Pts',(8.56128493015481,-27.9634705795499,125.282089924095));
#98478=CARTESIAN_POINT('Ctrl Pts',(8.56515400574055,-27.9744424586778,125.352389946139));
#98479=CARTESIAN_POINT('Ctrl Pts',(8.56902308132629,-27.9890594847817,125.422037684045));
#98480=CARTESIAN_POINT('Ctrl Pts',(8.57288639197494,-28.0036547314622,125.49158164656));
#98481=CARTESIAN_POINT('Ctrl Pts',(8.57674970262359,-28.0218842452092,125.560474782588));
#98482=CARTESIAN_POINT('Ctrl Pts',(8.58061301327225,-28.0436709501691,125.628310600967));
#98483=CARTESIAN_POINT('Ctrl Pts',(8.58447179202976,-28.0654320980398,125.696066843933));
#98484=CARTESIAN_POINT('Ctrl Pts',(8.58833057078728,-28.090742000716,125.762767772626));
#98485=CARTESIAN_POINT('Ctrl Pts',(8.5921893495448,-28.1194730102278,125.828019204631));
#98486=CARTESIAN_POINT('Ctrl Pts',(8.59604569740361,-28.1481859201858,125.893229530466));
#98487=CARTESIAN_POINT('Ctrl Pts',(8.59990204526242,-28.1803154658383,125.95699172771));
#98488=CARTESIAN_POINT('Ctrl Pts',(8.60375839312123,-28.2156853597219,126.018930236566));
#98489=CARTESIAN_POINT('Ctrl Pts',(8.60761360163977,-28.2510448037328,126.080850445975));
#98490=CARTESIAN_POINT('Ctrl Pts',(8.61146881015831,-28.2896424546131,126.140947615044));
#98491=CARTESIAN_POINT('Ctrl Pts',(8.61532401867685,-28.3312562312742,126.198871050964));
#98492=CARTESIAN_POINT('Ctrl Pts',(8.61917937780052,-28.3728716335927,126.256796749683));
#98493=CARTESIAN_POINT('Ctrl Pts',(8.62303473692418,-28.4175031103935,126.31254815342));
#98494=CARTESIAN_POINT('Ctrl Pts',(8.62689009604785,-28.4648864505407,126.365805239691));
#98495=CARTESIAN_POINT('Ctrl Pts',(8.63074949077188,-28.5123193892386,126.41911807286));
#98496=CARTESIAN_POINT('Ctrl Pts',(8.63460888549592,-28.5625096178725,126.469931012886));
#98497=CARTESIAN_POINT('Ctrl Pts',(8.63846828021996,-28.6151545868309,126.517959401343));
#98498=CARTESIAN_POINT('Ctrl Pts',(8.64232986007272,-28.6678293625445,126.566014982719));
#98499=CARTESIAN_POINT('Ctrl Pts',(8.64619143992547,-28.7229612696949,126.611282565647));
#98500=CARTESIAN_POINT('Ctrl Pts',(8.65005301977823,-28.7802151828092,126.653518237653));
#98501=CARTESIAN_POINT('Ctrl Pts',(8.65392135610818,-28.8375692711816,126.695827808003));
#98502=CARTESIAN_POINT('Ctrl Pts',(8.65778969243814,-28.8970523726919,126.735094608463));
#98503=CARTESIAN_POINT('Ctrl Pts',(8.66165802876809,-28.9583015518801,126.771118828787));
#98504=CARTESIAN_POINT('Ctrl Pts',(8.66395572764794,-28.9946820933864,126.792516350519));
#98505=CARTESIAN_POINT('Ctrl Pts',(8.66625342652779,-29.0316852541359,126.812770750007));
#98506=CARTESIAN_POINT('Ctrl Pts',(8.66855112540763,-29.0692316029857,126.831848179741));
#98507=CARTESIAN_POINT('Ctrl Pts',(8.67242019148944,-29.1324554249167,126.863972422373));
#98508=CARTESIAN_POINT('Ctrl Pts',(8.67628925757124,-29.197468129339,126.892882616604));
#98509=CARTESIAN_POINT('Ctrl Pts',(8.68015832365304,-29.2639098155531,126.918376606108));
#98510=CARTESIAN_POINT('Ctrl Pts',(8.68402162477788,-29.3302525028216,126.943832609247));
#98511=CARTESIAN_POINT('Ctrl Pts',(8.68788492590271,-29.3980194956275,126.965882338929));
#98512=CARTESIAN_POINT('Ctrl Pts',(8.69174822702754,-29.4668274817719,126.984370083504));
#98513=CARTESIAN_POINT('Ctrl Pts',(8.69560699627753,-29.5355547521833,127.00283614089));
#98514=CARTESIAN_POINT('Ctrl Pts',(8.69946576552751,-29.6053201234546,127.017748387469));
#98515=CARTESIAN_POINT('Ctrl Pts',(8.7033245347775,-29.6757231958804,127.029000275212));
#98516=CARTESIAN_POINT('Ctrl Pts',(8.70718087314394,-29.7460819169446,127.040245074677));
#98517=CARTESIAN_POINT('Ctrl Pts',(8.71103721151039,-29.8170770635746,127.047834013672));
#98518=CARTESIAN_POINT('Ctrl Pts',(8.71489354987684,-29.888297501336,127.051711508544));
#98519=CARTESIAN_POINT('Ctrl Pts',(8.71874874893201,-29.9594968978298,127.055587857855));
#98520=CARTESIAN_POINT('Ctrl Pts',(8.72260394798719,-30.0309209685101,127.055754913512));
#98521=CARTESIAN_POINT('Ctrl Pts',(8.72645914704236,-30.1021546339133,127.052209052039));
#98522=CARTESIAN_POINT('Ctrl Pts',(8.73031449674551,-30.1733910828842,127.048663052006));
#98523=CARTESIAN_POINT('Ctrl Pts',(8.73416984644866,-30.2444366267281,127.041403873142));
#98524=CARTESIAN_POINT('Ctrl Pts',(8.73802519615181,-30.3148791036184,127.030479921744));
#98525=CARTESIAN_POINT('Ctrl Pts',(8.74188458158523,-30.3853953187836,127.019544535294));
#98526=CARTESIAN_POINT('Ctrl Pts',(8.74574396701865,-30.4553067257793,127.004936792918));
#98527=CARTESIAN_POINT('Ctrl Pts',(8.74960335245206,-30.5242100802503,126.986756490933));
#98528=CARTESIAN_POINT('Ctrl Pts',(8.75346492307344,-30.5931524478707,126.968565895242));
#98529=CARTESIAN_POINT('Ctrl Pts',(8.75732649369481,-30.6610851639198,126.946798861501));
#98530=CARTESIAN_POINT('Ctrl Pts',(8.76118806431618,-30.7276215485713,126.921604653553));
#98531=CARTESIAN_POINT('Ctrl Pts',(8.76505639160837,-30.7942743533256,126.896366362772));
#98532=CARTESIAN_POINT('Ctrl Pts',(8.76892471890055,-30.8595255039085,126.867689120919));
#98533=CARTESIAN_POINT('Ctrl Pts',(8.77279304619274,-30.923010289613,126.835769475661));
#98534=CARTESIAN_POINT('Ctrl Pts',(8.77509082954389,-30.9607202020959,126.816809231631));
#98535=CARTESIAN_POINT('Ctrl Pts',(8.77738861289505,-30.9978073692065,126.796705825255));
#98536=CARTESIAN_POINT('Ctrl Pts',(8.7796863962462,-31.0342002656552,126.775507638119));
#98537=CARTESIAN_POINT('Ctrl Pts',(8.78355540286408,-31.0954786090349,126.73981413974));
#98538=CARTESIAN_POINT('Ctrl Pts',(8.78742440948197,-31.1550269658424,126.700874643153));
#98539=CARTESIAN_POINT('Ctrl Pts',(8.79129341609986,-31.212480317574,126.658881864991));
#98540=CARTESIAN_POINT('Ctrl Pts',(8.79218909434932,-31.2257808162775,126.649160501926));
#98541=CARTESIAN_POINT('Ctrl Pts',(8.79308477259879,-31.2389691310616,126.639275705284));
#98542=CARTESIAN_POINT('Ctrl Pts',(8.79398045084826,-31.2520409112987,126.629230222815));
#98543=CARTESIAN_POINT('Ctrl Pts',(8.09385900495164,-31.2520409112987,126.629230222815));
#98544=CARTESIAN_POINT('Ctrl Pts',(8.09772726999485,-31.3085579851685,126.585797632577));
#98545=CARTESIAN_POINT('Ctrl Pts',(8.10159553503806,-31.3627397236403,126.539476715365));
#98546=CARTESIAN_POINT('Ctrl Pts',(8.10546380008126,-31.4142934443049,126.490560839381));
#98547=CARTESIAN_POINT('Ctrl Pts',(8.10793412379246,-31.4472163120855,126.459322533074));
#98548=CARTESIAN_POINT('Ctrl Pts',(8.11040444750365,-31.4790681575991,126.427026680256));
#98549=CARTESIAN_POINT('Ctrl Pts',(8.11287477121484,-31.5097814179538,126.393756661868));
#98550=CARTESIAN_POINT('Ctrl Pts',(8.11674384460118,-31.5578851776787,126.341648453489));
#98551=CARTESIAN_POINT('Ctrl Pts',(8.12061291798751,-31.6033823190926,126.286944894071));
#98552=CARTESIAN_POINT('Ctrl Pts',(8.12448199137385,-31.6459804494774,126.22993736525));
#98553=CARTESIAN_POINT('Ctrl Pts',(8.12834529980683,-31.6885151082736,126.173014778148));
#98554=CARTESIAN_POINT('Ctrl Pts',(8.13220860823981,-31.728159041816,126.113795421895));
#98555=CARTESIAN_POINT('Ctrl Pts',(8.13607191667279,-31.7646581873541,126.052605835203));
#98556=CARTESIAN_POINT('Ctrl Pts',(8.13993069320136,-31.8011145170929,125.991488027756));
#98557=CARTESIAN_POINT('Ctrl Pts',(8.14378946972994,-31.8344331388476,125.92840499588));
#98558=CARTESIAN_POINT('Ctrl Pts',(8.14764824625851,-31.8644026557222,125.863713088841));
#98559=CARTESIAN_POINT('Ctrl Pts',(8.15150459188142,-31.8943532927606,125.799061935633));
#98560=CARTESIAN_POINT('Ctrl Pts',(8.15536093750432,-31.9209588070679,125.732804357849));
#98561=CARTESIAN_POINT('Ctrl Pts',(8.15921728312723,-31.9440539277217,125.665320891458));
#98562=CARTESIAN_POINT('Ctrl Pts',(8.16307248940625,-31.9671422250025,125.597857362821));
#98563=CARTESIAN_POINT('Ctrl Pts',(8.16692769568528,-31.9867220304168,125.529169123979));
#98564=CARTESIAN_POINT('Ctrl Pts',(8.17078290196431,-32.0026770032989,125.459654634435));
#98565=CARTESIAN_POINT('Ctrl Pts',(8.1746382588482,-32.018632599467,125.390137429286));
#98566=CARTESIAN_POINT('Ctrl Pts',(8.17849361573209,-32.0309629754391,125.31979438332));
#98567=CARTESIAN_POINT('Ctrl Pts',(8.18234897261598,-32.0396026536202,125.249035294377));
#98568=CARTESIAN_POINT('Ctrl Pts',(8.18620836511537,-32.0482513754309,125.178202137978));
#98569=CARTESIAN_POINT('Ctrl Pts',(8.19006775761477,-32.0532016285224,125.106952552449));
#98570=CARTESIAN_POINT('Ctrl Pts',(8.19392715011417,-32.0544398139749,125.035701726213));
#98571=CARTESIAN_POINT('Ctrl Pts',(8.19778872774747,-32.0556787004707,124.96441055876));
#98572=CARTESIAN_POINT('Ctrl Pts',(8.20165030538077,-32.0532013523286,124.893118634925));
#98573=CARTESIAN_POINT('Ctrl Pts',(8.20551188301407,-32.0470462783446,124.822238652077));
#98574=CARTESIAN_POINT('Ctrl Pts',(8.20938021715696,-32.0408804349756,124.751234652226));
#98575=CARTESIAN_POINT('Ctrl Pts',(8.21324855129985,-32.0310240856418,124.68064451366));
#98576=CARTESIAN_POINT('Ctrl Pts',(8.21711688544274,-32.0175672148421,124.610872647974));
#98577=CARTESIAN_POINT('Ctrl Pts',(8.21941460431296,-32.0095740827008,124.569429451375));
#98578=CARTESIAN_POINT('Ctrl Pts',(8.22171232318319,-32.0003116078043,124.528274718171));
#98579=CARTESIAN_POINT('Ctrl Pts',(8.22401004205341,-31.9898069000665,124.487490426482));
#98580=CARTESIAN_POINT('Ctrl Pts',(8.22787911571846,-31.9721182747982,124.418814736446));
#98581=CARTESIAN_POINT('Ctrl Pts',(8.23174818938351,-31.9508354453984,124.350921355088));
#98582=CARTESIAN_POINT('Ctrl Pts',(8.23561726304855,-31.9260446310184,124.284213969244));
#98583=CARTESIAN_POINT('Ctrl Pts',(8.23948057176287,-31.9012907551503,124.217605977939));
#98584=CARTESIAN_POINT('Ctrl Pts',(8.24334388047719,-31.873039437451,124.152180926067));
#98585=CARTESIAN_POINT('Ctrl Pts',(8.2472071891915,-31.8414272228597,124.088329365718));
#98586=CARTESIAN_POINT('Ctrl Pts',(8.25106596600391,-31.8098520913663,124.024552707229));
#98587=CARTESIAN_POINT('Ctrl Pts',(8.25492474281632,-31.774924108694,123.962346307112));
#98588=CARTESIAN_POINT('Ctrl Pts',(8.25878351962873,-31.73682800535,123.90208104018));
#98589=CARTESIAN_POINT('Ctrl Pts',(8.26263986553686,-31.698755901316,123.841853738413));
#98590=CARTESIAN_POINT('Ctrl Pts',(8.26649621144499,-31.6575198952291,123.783565553368));
#98591=CARTESIAN_POINT('Ctrl Pts',(8.27035255735312,-31.6133500549696,123.727561725415));
#98592=CARTESIAN_POINT('Ctrl Pts',(8.27420776391832,-31.5691932645236,123.671574443582));
#98593=CARTESIAN_POINT('Ctrl Pts',(8.27806297048352,-31.5221046613909,123.617870560192));
#98594=CARTESIAN_POINT('Ctrl Pts',(8.28191817704872,-31.4723559098081,123.566763928254));
#98595=CARTESIAN_POINT('Ctrl Pts',(8.28577353421931,-31.4226052147679,123.515655299813));
#98596=CARTESIAN_POINT('Ctrl Pts',(8.2896288913899,-31.3701945053835,123.467144470825));
#98597=CARTESIAN_POINT('Ctrl Pts',(8.29348424856049,-31.3154325580222,123.421508711524));
#98598=CARTESIAN_POINT('Ctrl Pts',(8.29734364134539,-31.26061328832,123.375825182765));
#98599=CARTESIAN_POINT('Ctrl Pts',(8.30120303413028,-31.2034382415455,123.333023042951));
#98600=CARTESIAN_POINT('Ctrl Pts',(8.30506242691517,-31.1442488600592,123.293338900439));
#98601=CARTESIAN_POINT('Ctrl Pts',(8.30892400483373,-31.0850259663815,123.253632289327));
#98602=CARTESIAN_POINT('Ctrl Pts',(8.31278558275228,-31.0237868848638,123.217047439076));
#98603=CARTESIAN_POINT('Ctrl Pts',(8.31664716067083,-30.9608992263762,123.183775829021));
#98604=CARTESIAN_POINT('Ctrl Pts',(8.32051549509547,-30.897901534929,123.150446004464));
#98605=CARTESIAN_POINT('Ctrl Pts',(8.3243838295201,-30.8332499483595,123.120441198736));
#98606=CARTESIAN_POINT('Ctrl Pts',(8.32825216394474,-30.7673330348737,123.09390515029));
#98607=CARTESIAN_POINT('Ctrl Pts',(8.33054988026048,-30.7281796548982,123.07814324742));
#98608=CARTESIAN_POINT('Ctrl Pts',(8.33284759657622,-30.6885801806942,123.063604224167));
#98609=CARTESIAN_POINT('Ctrl Pts',(8.33514531289196,-30.6486181888067,123.050309766232));
#98610=CARTESIAN_POINT('Ctrl Pts',(8.33901438538775,-30.5813270951981,123.027923529433));
#98611=CARTESIAN_POINT('Ctrl Pts',(8.34288345788354,-30.5127438862126,123.008981234));
#98612=CARTESIAN_POINT('Ctrl Pts',(8.34675253037932,-30.4432544786734,122.993629388763));
#98613=CARTESIAN_POINT('Ctrl Pts',(8.35061583792275,-30.3738686109683,122.978300417911));
#98614=CARTESIAN_POINT('Ctrl Pts',(8.35447914546617,-30.3035796953893,122.966551381988));
#98615=CARTESIAN_POINT('Ctrl Pts',(8.3583424530096,-30.2327899086053,122.958479385127));
#98616=CARTESIAN_POINT('Ctrl Pts',(8.36220122865432,-30.1620831626198,122.950416857217));
#98617=CARTESIAN_POINT('Ctrl Pts',(8.36606000429903,-30.0908771928238,122.946022855279));
#98618=CARTESIAN_POINT('Ctrl Pts',(8.36991877994375,-30.0195837782864,122.945343328405));
#98619=CARTESIAN_POINT('Ctrl Pts',(8.37377512468678,-29.9483352762543,122.944664229612));
#98620=CARTESIAN_POINT('Ctrl Pts',(8.37763146942982,-29.8769999233888,122.947694967986));
#98621=CARTESIAN_POINT('Ctrl Pts',(8.38148781417285,-29.8059925515189,122.95442949952));
#98622=CARTESIAN_POINT('Ctrl Pts',(8.38534301957725,-29.7350061584378,122.961162041369));
#98623=CARTESIAN_POINT('Ctrl Pts',(8.38919822498165,-29.6643480373307,122.971596158109));
#98624=CARTESIAN_POINT('Ctrl Pts',(8.39305343038605,-29.5944292105134,122.985673835444));
#98625=CARTESIAN_POINT('Ctrl Pts',(8.39690878640181,-29.5245076521763,122.999752062752));
#98626=CARTESIAN_POINT('Ctrl Pts',(8.40076414241759,-29.4553259212649,123.017474035213));
#98627=CARTESIAN_POINT('Ctrl Pts',(8.40461949843336,-29.3872844335983,123.038730717829));
#98628=CARTESIAN_POINT('Ctrl Pts',(8.40847889008046,-29.3191717228442,123.060009651083));
#98629=CARTESIAN_POINT('Ctrl Pts',(8.41233828172756,-29.2522021025857,123.084830535351));
#98630=CARTESIAN_POINT('Ctrl Pts',(8.41619767337466,-29.1867595436897,123.113034837969));
#98631=CARTESIAN_POINT('Ctrl Pts',(8.4200592501633,-29.1212799319971,123.141255109526));
#98632=CARTESIAN_POINT('Ctrl Pts',(8.42392082695194,-29.0573295385309,123.172862397558));
#98633=CARTESIAN_POINT('Ctrl Pts',(8.42778240374059,-28.9952686121545,123.207651707737));
#98634=CARTESIAN_POINT('Ctrl Pts',(8.43165073706,-28.9330990989024,123.242501888141));
#98635=CARTESIAN_POINT('Ctrl Pts',(8.43551907037942,-28.8728260641291,123.280544947049));
#98636=CARTESIAN_POINT('Ctrl Pts',(8.43938740369884,-28.8147810140006,123.321532390028));
#98637=CARTESIAN_POINT('Ctrl Pts',(8.44168513037607,-28.78030320427,123.3458782603));
#98638=CARTESIAN_POINT('Ctrl Pts',(8.44398285705329,-28.7466108504686,123.371262169159));
#98639=CARTESIAN_POINT('Ctrl Pts',(8.44628058373051,-28.7137675014706,123.397625661018));
#98640=CARTESIAN_POINT('Ctrl Pts',(8.45010049336493,-28.6591663052068,123.441454266722));
#98641=CARTESIAN_POINT('Ctrl Pts',(8.45392040299934,-28.6066877443327,123.488173581393));
#98642=CARTESIAN_POINT('Ctrl Pts',(8.45774031263375,-28.5566598146521,123.537547719801));
#98643=CARTESIAN_POINT('Ctrl Pts',(8.46155371406763,-28.5067171204429,123.586837736639));
#98644=CARTESIAN_POINT('Ctrl Pts',(8.46536711550151,-28.4592171196553,123.638773249035));
#98645=CARTESIAN_POINT('Ctrl Pts',(8.46918051693538,-28.4144553825126,123.693077726697));
#98646=CARTESIAN_POINT('Ctrl Pts',(8.47299028819365,-28.3697362564007,123.747330509095));
#98647=CARTESIAN_POINT('Ctrl Pts',(8.47680005945192,-28.3277505435078,123.803947404073));
#98648=CARTESIAN_POINT('Ctrl Pts',(8.48060983071019,-28.2887564983585,123.862615614407));
#98649=CARTESIAN_POINT('Ctrl Pts',(8.48441732747402,-28.2497857332784,123.921248798881));
#98650=CARTESIAN_POINT('Ctrl Pts',(8.48822482423785,-28.2138033700979,123.981930455338));
#98651=CARTESIAN_POINT('Ctrl Pts',(8.49203232100168,-28.1810257548658,124.044316863161));
#98652=CARTESIAN_POINT('Ctrl Pts',(8.49583889576681,-28.1482560768483,124.106688163896));
#98653=CARTESIAN_POINT('Ctrl Pts',(8.49964547053193,-28.1186898378894,124.170762954398));
#98654=CARTESIAN_POINT('Ctrl Pts',(8.50345204529706,-28.0924976678887,124.236172522431));
#98655=CARTESIAN_POINT('Ctrl Pts',(8.50726133136703,-28.0662868420197,124.301628679665));
#98656=CARTESIAN_POINT('Ctrl Pts',(8.511070617437,-28.0434550737678,124.368421049895));
#98657=CARTESIAN_POINT('Ctrl Pts',(8.51487990350697,-28.0241245342633,124.436161630962));
#98658=CARTESIAN_POINT('Ctrl Pts',(8.51869054788737,-28.0047871018994,124.503926366879));
#98659=CARTESIAN_POINT('Ctrl Pts',(8.52250119226777,-27.9889534984263,124.572639500133));
#98660=CARTESIAN_POINT('Ctrl Pts',(8.52631183664817,-27.9766950596919,124.641901297091));
#98661=CARTESIAN_POINT('Ctrl Pts',(8.53012846308285,-27.9644173773235,124.711271823122));
#98662=CARTESIAN_POINT('Ctrl Pts',(8.53394508951753,-27.955726129257,124.781192236676));
#98663=CARTESIAN_POINT('Ctrl Pts',(8.53776171595221,-27.9506408107848,124.851257013345));
#98664=CARTESIAN_POINT('Ctrl Pts',(8.54048290413023,-27.9470150672793,124.901211978871));
#98665=CARTESIAN_POINT('Ctrl Pts',(8.54320409230826,-27.9452212774533,124.951240233013));
#98666=CARTESIAN_POINT('Ctrl Pts',(8.54592528048628,-27.9452503479095,125.001195714817));
#98667=CARTESIAN_POINT('Origin',(-1.54592528053767,-30.,125.));
#98668=CARTESIAN_POINT('',(7.39391264968254,-31.2520409112987,126.629230222815));
#98669=CARTESIAN_POINT('',(7.45211278928543,-31.2520409112987,126.629230222815));
#98670=CARTESIAN_POINT('',(-1.54592528053767,-31.2520409112987,126.629230222815));
#98671=CARTESIAN_POINT('',(7.90407471950836,-27.9452505543669,124.998490639097));
#98672=CARTESIAN_POINT('Ctrl Pts',(7.45211278928543,-31.2520409112987,126.629230222815));
#98673=CARTESIAN_POINT('Ctrl Pts',(7.45597763034358,-31.3083540803805,126.585954330588));
#98674=CARTESIAN_POINT('Ctrl Pts',(7.45984247140173,-31.3625145223919,126.539683438356));
#98675=CARTESIAN_POINT('Ctrl Pts',(7.46370731245988,-31.4141879602304,126.490660919069));
#98676=CARTESIAN_POINT('Ctrl Pts',(7.46756704170375,-31.4657930524336,126.441703239192));
#98677=CARTESIAN_POINT('Ctrl Pts',(7.47142677094762,-31.5149173244941,126.390001494346));
#98678=CARTESIAN_POINT('Ctrl Pts',(7.47528650019149,-31.5612592226217,126.335839512172));
#98679=CARTESIAN_POINT('Ctrl Pts',(7.47914342130644,-31.6075674049065,126.281716935308));
#98680=CARTESIAN_POINT('Ctrl Pts',(7.48300034242139,-31.6510969141813,126.225138039894));
#98681=CARTESIAN_POINT('Ctrl Pts',(7.48685726353634,-31.691583760069,126.166422712901));
#98682=CARTESIAN_POINT('Ctrl Pts',(7.49071266880043,-31.7320546937773,126.107730462262));
#98683=CARTESIAN_POINT('Ctrl Pts',(7.49456807406451,-31.7694850619962,126.046903846099));
#98684=CARTESIAN_POINT('Ctrl Pts',(7.4984234793286,-31.8036528795101,125.984293580562));
#98685=CARTESIAN_POINT('Ctrl Pts',(7.50227865902707,-31.8378186979904,125.921686978121));
#98686=CARTESIAN_POINT('Ctrl Pts',(7.50613383872555,-31.8687221134478,125.857297360676));
#98687=CARTESIAN_POINT('Ctrl Pts',(7.50998901842402,-31.8961868410849,125.791500490332));
#98688=CARTESIAN_POINT('Ctrl Pts',(7.51384799214005,-31.9236785977238,125.725638866981));
#98689=CARTESIAN_POINT('Ctrl Pts',(7.51770696585608,-31.9477247189694,125.658367673651));
#98690=CARTESIAN_POINT('Ctrl Pts',(7.52156593957212,-31.9681972468078,125.590082333372));
#98691=CARTESIAN_POINT('Ctrl Pts',(7.52542676053524,-31.9886795746138,125.521764305673));
#98692=CARTESIAN_POINT('Ctrl Pts',(7.52928758149837,-32.0055847858469,125.452431636587));
#98693=CARTESIAN_POINT('Ctrl Pts',(7.5331484024615,-32.0188356861061,125.382491875737));
#98694=CARTESIAN_POINT('Ctrl Pts',(7.53701633778309,-32.0321110038805,125.31242323646));
#98695=CARTESIAN_POINT('Ctrl Pts',(7.54088427310468,-32.041718490898,125.241745752882));
#98696=CARTESIAN_POINT('Ctrl Pts',(7.54475220842627,-32.0476327261154,125.170873583216));
#98697=CARTESIAN_POINT('Ctrl Pts',(7.54817615280141,-32.0528680805674,125.108136658603));
#98698=CARTESIAN_POINT('Ctrl Pts',(7.55160009717655,-32.0552101662244,125.04524745785));
#98699=CARTESIAN_POINT('Ctrl Pts',(7.55502404155169,-32.054675403714,124.982491491417));
#98700=CARTESIAN_POINT('Ctrl Pts',(7.55889311490067,-32.0540711195463,124.911576952333));
#98701=CARTESIAN_POINT('Ctrl Pts',(7.56276218824965,-32.0497900525759,124.840554831224));
#98702=CARTESIAN_POINT('Ctrl Pts',(7.56663126159862,-32.0418185215167,124.769837692722));
#98703=CARTESIAN_POINT('Ctrl Pts',(7.57049456999505,-32.0338588681072,124.699225923365));
#98704=CARTESIAN_POINT('Ctrl Pts',(7.57435787839148,-32.0222197195905,124.628918713387));
#98705=CARTESIAN_POINT('Ctrl Pts',(7.57822118678791,-32.0069394027001,124.55932801724));
#98706=CARTESIAN_POINT('Ctrl Pts',(7.5820799632813,-31.9916770105799,124.489818955344));
#98707=CARTESIAN_POINT('Ctrl Pts',(7.58593873977468,-31.9727820380486,124.421025209909));
#98708=CARTESIAN_POINT('Ctrl Pts',(7.58979751626806,-31.9503443206474,124.353351259633));
#98709=CARTESIAN_POINT('Ctrl Pts',(7.59365386185663,-31.927920738285,124.285719941764));
#98710=CARTESIAN_POINT('Ctrl Pts',(7.59751020744519,-31.9019589914577,124.219207479496));
#98711=CARTESIAN_POINT('Ctrl Pts',(7.60136655303376,-31.8725990970537,124.154204407547));
#98712=CARTESIAN_POINT('Ctrl Pts',(7.60522175927935,-31.8432478769215,124.089220540514));
#98713=CARTESIAN_POINT('Ctrl Pts',(7.60907696552493,-31.810500702226,124.025745620959));
#98714=CARTESIAN_POINT('Ctrl Pts',(7.61293217177052,-31.7745455280139,123.964149754305));
#98715=CARTESIAN_POINT('Ctrl Pts',(7.61678752862191,-31.7385889491926,123.902551481374));
#98716=CARTESIAN_POINT('Ctrl Pts',(7.6206428854733,-31.6994243688427,123.842832825512));
#98717=CARTESIAN_POINT('Ctrl Pts',(7.62449824232469,-31.657284581258,123.785337339331));
#98718=CARTESIAN_POINT('Ctrl Pts',(7.62835763479323,-31.6151006836062,123.727781669415));
#98719=CARTESIAN_POINT('Ctrl Pts',(7.63221702726178,-31.5699356496064,123.672454207247));
#98720=CARTESIAN_POINT('Ctrl Pts',(7.63607641973032,-31.5220637816352,123.619666921669));
#98721=CARTESIAN_POINT('Ctrl Pts',(7.63993799733364,-31.4741648092726,123.566849748658));
#98722=CARTESIAN_POINT('Ctrl Pts',(7.64379957493697,-31.4235562968641,123.5165759578));
#98723=CARTESIAN_POINT('Ctrl Pts',(7.64766115254029,-31.3705488264876,123.469120031905));
#98724=CARTESIAN_POINT('Ctrl Pts',(7.65152948665491,-31.3174486101899,123.421581073496));
#98725=CARTESIAN_POINT('Ctrl Pts',(7.65539782076953,-31.2619414341314,123.376870128472));
#98726=CARTESIAN_POINT('Ctrl Pts',(7.65926615488415,-31.2043697326239,123.335220402083));
#98727=CARTESIAN_POINT('Ctrl Pts',(7.66156387405285,-31.1701732030044,123.310481232234));
#98728=CARTESIAN_POINT('Ctrl Pts',(7.66386159322155,-31.135248827303,123.286821267237));
#98729=CARTESIAN_POINT('Ctrl Pts',(7.66615931239025,-31.0996724856495,123.264281708685));
#98730=CARTESIAN_POINT('Ctrl Pts',(7.67002838578164,-31.0397663497171,123.226327894557));
#98731=CARTESIAN_POINT('Ctrl Pts',(7.67389745917303,-30.977775674469,123.191404757273));
#98732=CARTESIAN_POINT('Ctrl Pts',(7.67776653256441,-30.9140396531967,123.159747551317));
#98733=CARTESIAN_POINT('Ctrl Pts',(7.68162984100355,-30.850398599138,123.128137514866));
#98734=CARTESIAN_POINT('Ctrl Pts',(7.68549314944269,-30.7850177926637,123.099783964681));
#98735=CARTESIAN_POINT('Ctrl Pts',(7.68935645788183,-30.7182641217052,123.074878130099));
#98736=CARTESIAN_POINT('Ctrl Pts',(7.69321523441816,-30.6515887569844,123.050001511621));
#98737=CARTESIAN_POINT('Ctrl Pts',(7.69707401095449,-30.5835441796199,123.028564744217));
#98738=CARTESIAN_POINT('Ctrl Pts',(7.70093278749081,-30.514518933364,123.010711727851));
#98739=CARTESIAN_POINT('Ctrl Pts',(7.70478913312245,-30.4455371707857,122.992869958309));
#98740=CARTESIAN_POINT('Ctrl Pts',(7.70864547875409,-30.3755764341985,122.978607582026));
#98741=CARTESIAN_POINT('Ctrl Pts',(7.71250182438572,-30.3050407689715,122.968018776719));
#98742=CARTESIAN_POINT('Ctrl Pts',(7.71635703067443,-30.2345259432436,122.957433099835));
#98743=CARTESIAN_POINT('Ctrl Pts',(7.72021223696314,-30.1634370062372,122.9505189113));
#98744=CARTESIAN_POINT('Ctrl Pts',(7.72406744325185,-30.0921868397139,122.94731903378));
#98745=CARTESIAN_POINT('Ctrl Pts',(7.72792280014636,-30.0209338897628,122.944119031254));
#98746=CARTESIAN_POINT('Ctrl Pts',(7.73177815704087,-29.9495201831855,122.944633647418));
#98747=CARTESIAN_POINT('Ctrl Pts',(7.73563351393538,-29.878360612768,122.94885363224));
#98748=CARTESIAN_POINT('Ctrl Pts',(7.73949290644673,-29.8071265556639,122.953078034356));
#98749=CARTESIAN_POINT('Ctrl Pts',(7.74335229895808,-29.73614765168,122.961015518903));
#98750=CARTESIAN_POINT('Ctrl Pts',(7.74721169146943,-29.6658347711962,122.972604833201));
#98751=CARTESIAN_POINT('Ctrl Pts',(7.75107326911546,-29.5954820805316,122.984200709209));
#98752=CARTESIAN_POINT('Ctrl Pts',(7.75493484676149,-29.5257966388214,122.999452427041));
#98753=CARTESIAN_POINT('Ctrl Pts',(7.75879642440752,-29.4571774996037,123.018247922781));
#98754=CARTESIAN_POINT('Ctrl Pts',(7.7626647585642,-29.3884382991085,123.037076304553));
#98755=CARTESIAN_POINT('Ctrl Pts',(7.76653309272088,-29.3207695873519,123.059460691027));
#98756=CARTESIAN_POINT('Ctrl Pts',(7.77040142687756,-29.2545530143012,123.085239870372));
#98757=CARTESIAN_POINT('Ctrl Pts',(7.77269914566131,-29.2152215973316,123.100552225048));
#98758=CARTESIAN_POINT('Ctrl Pts',(7.77499686444506,-29.1764021096255,123.11706139647));
#98759=CARTESIAN_POINT('Ctrl Pts',(7.77729458322881,-29.1381703210552,123.134725980723));
#98760=CARTESIAN_POINT('Ctrl Pts',(7.78116365647907,-29.0737927342447,123.164470948164));
#98761=CARTESIAN_POINT('Ctrl Pts',(7.78503272972934,-29.0108307716454,123.197610957943));
#98762=CARTESIAN_POINT('Ctrl Pts',(7.7889018029796,-28.949666047039,123.233988632608));
#98763=CARTESIAN_POINT('Ctrl Pts',(7.79276511127752,-28.8885924583971,123.270312104226));
#98764=CARTESIAN_POINT('Ctrl Pts',(7.79662841957544,-28.8293112063121,123.309863418632));
#98765=CARTESIAN_POINT('Ctrl Pts',(7.80049172787336,-28.7721819377034,123.352438053244));
#98766=CARTESIAN_POINT('Ctrl Pts',(7.80435050426899,-28.7151196853003,123.394962745146));
#98767=CARTESIAN_POINT('Ctrl Pts',(7.80820928066463,-28.6602047896665,123.440503423746));
#98768=CARTESIAN_POINT('Ctrl Pts',(7.81206805706026,-28.6077688795949,123.488811702707));
#98769=CARTESIAN_POINT('Ctrl Pts',(7.8159244025516,-28.5553660024503,123.537089549015));
#98770=CARTESIAN_POINT('Ctrl Pts',(7.81978074804294,-28.5054393689506,123.588131208238));
#98771=CARTESIAN_POINT('Ctrl Pts',(7.82363709353428,-28.4582872415828,123.641648302893));
#98772=CARTESIAN_POINT('Ctrl Pts',(7.8274922996833,-28.4111490451282,123.69514958613));
#98773=CARTESIAN_POINT('Ctrl Pts',(7.83134750583233,-28.3667840484081,123.751124488558));
#98774=CARTESIAN_POINT('Ctrl Pts',(7.83520271198135,-28.3254521608355,123.809249355722));
#98775=CARTESIAN_POINT('Ctrl Pts',(7.83905806873697,-28.2841186586008,123.867376493578));
#98776=CARTESIAN_POINT('Ctrl Pts',(7.8429134254926,-28.2458187804849,123.927653365745));
#98777=CARTESIAN_POINT('Ctrl Pts',(7.84676878224822,-28.2107697780686,123.98972638586));
#98778=CARTESIAN_POINT('Ctrl Pts',(7.85062817462287,-28.1756840878878,124.0518643813));
#98779=CARTESIAN_POINT('Ctrl Pts',(7.85448756699751,-28.1438563056484,124.115801853969));
#98780=CARTESIAN_POINT('Ctrl Pts',(7.85834695937215,-28.1154578116314,124.181160392532));
#98781=CARTESIAN_POINT('Ctrl Pts',(7.86220853688249,-28.0870432387717,124.246555936213));
#98782=CARTESIAN_POINT('Ctrl Pts',(7.86607011439284,-28.0620619894954,124.313373692235));
#98783=CARTESIAN_POINT('Ctrl Pts',(7.86993169190318,-28.0406363463201,124.381217618918));
#98784=CARTESIAN_POINT('Ctrl Pts',(7.87380002592726,-28.0191732151876,124.449180250565));
#98785=CARTESIAN_POINT('Ctrl Pts',(7.87766835995134,-28.0012782328927,124.518172167199));
#98786=CARTESIAN_POINT('Ctrl Pts',(7.88153669397541,-27.9870229515759,124.587785292575));
#98787=CARTESIAN_POINT('Ctrl Pts',(7.88383441400607,-27.9785555738312,124.629134222522));
#98788=CARTESIAN_POINT('Ctrl Pts',(7.88613213403672,-27.9713713474013,124.670702169065));
#98789=CARTESIAN_POINT('Ctrl Pts',(7.88842985406737,-27.9654765819169,124.712403018494));
#98790=CARTESIAN_POINT('Ctrl Pts',(7.89364480919903,-27.9520976945405,124.807048169262));
#98791=CARTESIAN_POINT('Ctrl Pts',(7.89885976433068,-27.9453209576648,124.90264805037));
#98792=CARTESIAN_POINT('Ctrl Pts',(7.90407471946233,-27.9452505543675,124.998490638251));
#98793=CARTESIAN_POINT('Ctrl Pts',(7.90407471950836,-27.9452505543669,124.998490639097));
#98794=CARTESIAN_POINT('Ctrl Pts',(7.90805348639992,-27.9451968399735,125.071614051636));
#98795=CARTESIAN_POINT('Ctrl Pts',(7.91203225329149,-27.9490515818561,125.144885851501));
#98796=CARTESIAN_POINT('Ctrl Pts',(7.91601102018306,-27.9568307713783,125.2178464269));
#98797=CARTESIAN_POINT('Ctrl Pts',(7.91981486837864,-27.9642679640647,125.287599433458));
#98798=CARTESIAN_POINT('Ctrl Pts',(7.92361871657422,-27.9752917464163,125.357067439177));
#98799=CARTESIAN_POINT('Ctrl Pts',(7.9274225647698,-27.9898629599105,125.425848144953));
#98800=CARTESIAN_POINT('Ctrl Pts',(7.93122379847079,-28.0044241581893,125.494581575767));
#98801=CARTESIAN_POINT('Ctrl Pts',(7.93502503217179,-28.0225278513569,125.562628154102));
#98802=CARTESIAN_POINT('Ctrl Pts',(7.93882626587279,-28.0440833861041,125.62959333064));
#98803=CARTESIAN_POINT('Ctrl Pts',(7.94262624496941,-28.0656318064063,125.696536405195));
#98804=CARTESIAN_POINT('Ctrl Pts',(7.94642622406603,-28.0906296548367,125.762398309196));
#98805=CARTESIAN_POINT('Ctrl Pts',(7.95022620316264,-28.1189362808575,125.826799157611));
#98806=CARTESIAN_POINT('Ctrl Pts',(7.95402628561092,-28.1472436767607,125.891201757597));
#98807=CARTESIAN_POINT('Ctrl Pts',(7.95782636805919,-28.1788598241947,125.954142765628));
#98808=CARTESIAN_POINT('Ctrl Pts',(7.96162645050747,-28.2135965224734,126.015263600244));
#98809=CARTESIAN_POINT('Ctrl Pts',(7.96543037575041,-28.2483683478844,126.076446242682));
#98810=CARTESIAN_POINT('Ctrl Pts',(7.96923430099335,-28.2862667704271,126.135804603882));
#98811=CARTESIAN_POINT('Ctrl Pts',(7.97303822623629,-28.3270589369239,126.193007025115));
#98812=CARTESIAN_POINT('Ctrl Pts',(7.97684442188905,-28.3678754506224,126.25024358817));
#98813=CARTESIAN_POINT('Ctrl Pts',(7.98065061754181,-28.4115888297688,126.305321261542));
#98814=CARTESIAN_POINT('Ctrl Pts',(7.98445681319456,-28.4579262240686,126.357941836783));
#98815=CARTESIAN_POINT('Ctrl Pts',(7.98826926353405,-28.5043397641874,126.410648882936));
#98816=CARTESIAN_POINT('Ctrl Pts',(7.99208171387354,-28.5533855677727,126.460890422937));
#98817=CARTESIAN_POINT('Ctrl Pts',(7.99589416421303,-28.6047551208587,126.508406208463));
#98818=CARTESIAN_POINT('Ctrl Pts',(7.99711781777733,-28.6212428206668,126.523656993429));
#98819=CARTESIAN_POINT('Ctrl Pts',(7.99834147134164,-28.6379696664498,126.538627302508));
#98820=CARTESIAN_POINT('Ctrl Pts',(7.99956512490594,-28.6549248138619,126.553309468887));
#98821=CARTESIAN_POINT('Ctrl Pts',(8.00343419857207,-28.7085353424225,126.599733052292));
#98822=CARTESIAN_POINT('Ctrl Pts',(8.00730327223819,-28.7646570788596,126.643468858693));
#98823=CARTESIAN_POINT('Ctrl Pts',(8.01117234590431,-28.8229894970222,126.684233902515));
#98824=CARTESIAN_POINT('Ctrl Pts',(8.01503565461971,-28.8812349994148,126.724938206094));
#98825=CARTESIAN_POINT('Ctrl Pts',(8.0188989633351,-28.9416842502233,126.762680257491));
#98826=CARTESIAN_POINT('Ctrl Pts',(8.0227622720505,-29.0040028020232,126.797216498957));
#98827=CARTESIAN_POINT('Ctrl Pts',(8.02662104886399,-29.0662482502779,126.831712227259));
#98828=CARTESIAN_POINT('Ctrl Pts',(8.03047982567748,-29.130358221031,126.863009381153));
#98829=CARTESIAN_POINT('Ctrl Pts',(8.03433860249097,-29.1959698271948,126.890907994514));
#98830=CARTESIAN_POINT('Ctrl Pts',(8.03819494840018,-29.2615401001739,126.918789032655));
#98831=CARTESIAN_POINT('Ctrl Pts',(8.04205129430939,-29.3286096857582,126.943275588273));
#98832=CARTESIAN_POINT('Ctrl Pts',(8.04590764021859,-29.3967929881579,126.964214566529));
#98833=CARTESIAN_POINT('Ctrl Pts',(8.04976284678488,-29.4649561460568,126.985147358442));
#98834=CARTESIAN_POINT('Ctrl Pts',(8.05361805335116,-29.5342319034004,127.002534511264));
#98835=CARTESIAN_POINT('Ctrl Pts',(8.05747325991744,-29.6042183048147,127.016272405271));
#98836=CARTESIAN_POINT('Ctrl Pts',(8.0613286170891,-29.6742074402792,127.030010835954));
#98837=CARTESIAN_POINT('Ctrl Pts',(8.06518397426077,-29.744906797818,127.040099633378));
#98838=CARTESIAN_POINT('Ctrl Pts',(8.06903933143243,-29.8159047057685,127.046486375508));
#98839=CARTESIAN_POINT('Ctrl Pts',(8.07289872421839,-29.8869769311322,127.052879802993));
#98840=CARTESIAN_POINT('Ctrl Pts',(8.07675811700435,-29.9583478459224,127.055563395911));
#98841=CARTESIAN_POINT('Ctrl Pts',(8.08061750979031,-30.0296020392076,127.054536756005));
#98842=CARTESIAN_POINT('Ctrl Pts',(8.08447908770992,-30.10089657561,127.053509534829));
#98843=CARTESIAN_POINT('Ctrl Pts',(8.08834066562953,-30.1720737740093,127.048767931325));
#98844=CARTESIAN_POINT('Ctrl Pts',(8.09220224354914,-30.2427223691411,127.040363549473));
#98845=CARTESIAN_POINT('Ctrl Pts',(8.09607057797482,-30.3134945763485,127.031944462685));
#98846=CARTESIAN_POINT('Ctrl Pts',(8.09993891240049,-30.3837358548381,127.019849884909));
#98847=CARTESIAN_POINT('Ctrl Pts',(8.10380724682617,-30.4530448567175,127.004182606526));
#98848=CARTESIAN_POINT('Ctrl Pts',(8.10610496313228,-30.4942130718339,126.994876544265));
#98849=CARTESIAN_POINT('Ctrl Pts',(8.10840267943838,-30.5350526329831,126.984310949884));
#98850=CARTESIAN_POINT('Ctrl Pts',(8.11070039574449,-30.5754824652189,126.972515524584));
#98851=CARTESIAN_POINT('Ctrl Pts',(8.11456845452976,-30.6435435079816,126.952658678751));
#98852=CARTESIAN_POINT('Ctrl Pts',(8.11843651331503,-30.7107088921738,126.929236177448));
#98853=CARTESIAN_POINT('Ctrl Pts',(8.1223045721003,-30.776578188445,126.902346939896));
#98854=CARTESIAN_POINT('Ctrl Pts',(8.12616759078078,-30.8423616566109,126.875492739189));
#98855=CARTESIAN_POINT('Ctrl Pts',(8.13003060946125,-30.9068519399335,126.845180941199));
#98856=CARTESIAN_POINT('Ctrl Pts',(8.13389362814173,-30.96966310444,126.811560384417));
#98857=CARTESIAN_POINT('Ctrl Pts',(8.13775232965764,-31.0324040735486,126.777977400706));
#98858=CARTESIAN_POINT('Ctrl Pts',(8.14161103117355,-31.0934692238645,126.741093228731));
#98859=CARTESIAN_POINT('Ctrl Pts',(8.14546973268947,-31.1524937513155,126.701104263612));
#98860=CARTESIAN_POINT('Ctrl Pts',(8.14768435229106,-31.1863696224936,126.678153448257));
#98861=CARTESIAN_POINT('Ctrl Pts',(8.14989897189265,-31.2195737270747,126.654180805215));
#98862=CARTESIAN_POINT('Ctrl Pts',(8.15211359149425,-31.2520409112987,126.629230222815));
#98863=CARTESIAN_POINT('',(7.8459252805834,-27.9452502651294,125.001043814792));
#98864=CARTESIAN_POINT('Ctrl Pts',(7.8459252805834,-27.9452502651294,125.001043814792));
#98865=CARTESIAN_POINT('Ctrl Pts',(7.85018308156602,-27.9452903410169,125.079933211422));
#98866=CARTESIAN_POINT('Ctrl Pts',(7.85444088254865,-27.9498778523941,125.158666320287));
#98867=CARTESIAN_POINT('Ctrl Pts',(7.85869868353127,-27.9589342277071,125.236744747935));
#98868=CARTESIAN_POINT('Ctrl Pts',(7.86297170281527,-27.9680229724638,125.315102244765));
#98869=CARTESIAN_POINT('Ctrl Pts',(7.86724472209928,-27.9816124479092,125.392800086569));
#98870=CARTESIAN_POINT('Ctrl Pts',(7.87151774138328,-27.999573279132,125.4693511446));
#98871=CARTESIAN_POINT('Ctrl Pts',(7.87581130795489,-28.0176204770056,125.546270306891));
#98872=CARTESIAN_POINT('Ctrl Pts',(7.88010487452649,-28.0400810303069,125.622031352994));
#98873=CARTESIAN_POINT('Ctrl Pts',(7.8843984410981,-28.0667754170322,125.696161097957));
#98874=CARTESIAN_POINT('Ctrl Pts',(7.88646703724464,-28.0796364975799,125.731876045476));
#98875=CARTESIAN_POINT('Ctrl Pts',(7.88853563339119,-28.0934796393112,125.767212670557));
#98876=CARTESIAN_POINT('Ctrl Pts',(7.89060422953773,-28.1082809505831,125.802120066183));
#98877=CARTESIAN_POINT('Ctrl Pts',(7.89447330292895,-28.1359651168198,125.867410372267));
#98878=CARTESIAN_POINT('Ctrl Pts',(7.89834237632017,-28.1670875964325,125.931393656004));
#98879=CARTESIAN_POINT('Ctrl Pts',(7.90221144971139,-28.2015032182845,125.993683495213));
#98880=CARTESIAN_POINT('Ctrl Pts',(7.90607475815036,-28.2358675605674,126.055880522032));
#98881=CARTESIAN_POINT('Ctrl Pts',(7.90993806658933,-28.2735150721962,126.116388691159));
#98882=CARTESIAN_POINT('Ctrl Pts',(7.91380137502831,-28.3142527626546,126.174842038013));
#98883=CARTESIAN_POINT('Ctrl Pts',(7.91766015156447,-28.35494266525,126.233226815429));
#98884=CARTESIAN_POINT('Ctrl Pts',(7.92151892810063,-28.3987152698427,126.289561161899));
#98885=CARTESIAN_POINT('Ctrl Pts',(7.92537770463679,-28.4453328539635,126.343505722926));
#98886=CARTESIAN_POINT('Ctrl Pts',(7.92923405026826,-28.4919210705108,126.39741630062));
#98887=CARTESIAN_POINT('Ctrl Pts',(7.93309039589973,-28.5413503939185,126.448939713047));
#98888=CARTESIAN_POINT('Ctrl Pts',(7.93694674153119,-28.5933420704611,126.497768684332));
#98889=CARTESIAN_POINT('Ctrl Pts',(7.94080194781973,-28.6453183862568,126.546583229279));
#98890=CARTESIAN_POINT('Ctrl Pts',(7.94465715410827,-28.699855198347,126.592704581107));
#98891=CARTESIAN_POINT('Ctrl Pts',(7.94851236039682,-28.756637275071,126.63586267662));
#98892=CARTESIAN_POINT('Ctrl Pts',(7.95236771729116,-28.8134215700188,126.679022458127));
#98893=CARTESIAN_POINT('Ctrl Pts',(7.95622307418551,-28.872450915657,126.719218461287));
#98894=CARTESIAN_POINT('Ctrl Pts',(7.96007843107985,-28.9333788079595,126.756222308021));
#98895=CARTESIAN_POINT('Ctrl Pts',(7.96393782359104,-28.9943704768811,126.793264888742));
#98896=CARTESIAN_POINT('Ctrl Pts',(7.96779721610223,-29.0572642435349,126.827108390148));
#98897=CARTESIAN_POINT('Ctrl Pts',(7.97165660861341,-29.1216873337711,126.857569493409));
#98898=CARTESIAN_POINT('Ctrl Pts',(7.97551818625927,-29.1861468994703,126.888047843324));
#98899=CARTESIAN_POINT('Ctrl Pts',(7.97937976390514,-29.2521370628543,126.915139798205));
#98900=CARTESIAN_POINT('Ctrl Pts',(7.983241341551,-29.319265868112,126.938710551935));
#98901=CARTESIAN_POINT('Ctrl Pts',(7.98710967570752,-29.3865121270452,126.962322546852));
#98902=CARTESIAN_POINT('Ctrl Pts',(7.99097800986404,-29.4549005391858,126.982400903186));
#98903=CARTESIAN_POINT('Ctrl Pts',(7.99484634402056,-29.5240255081322,126.998861137146));
#98904=CARTESIAN_POINT('Ctrl Pts',(7.9971440628058,-29.5650844583808,127.008638211009));
#98905=CARTESIAN_POINT('Ctrl Pts',(7.99944178159104,-29.606403090079,127.017139742853));
#98906=CARTESIAN_POINT('Ctrl Pts',(8.00173950037628,-29.6478955336573,127.024356689737));
#98907=CARTESIAN_POINT('Ctrl Pts',(8.00560732713487,-29.7177411494836,127.03650521742));
#98908=CARTESIAN_POINT('Ctrl Pts',(8.00947515389345,-29.7883530019275,127.045058506922));
#98909=CARTESIAN_POINT('Ctrl Pts',(8.01334298065203,-29.8593280972088,127.04992901786));
#98910=CARTESIAN_POINT('Ctrl Pts',(8.01720559832277,-29.9302076050894,127.054792969322));
#98911=CARTESIAN_POINT('Ctrl Pts',(8.0210682159935,-30.0014489054664,127.055983946858));
#98912=CARTESIAN_POINT('Ctrl Pts',(8.02493083366424,-30.0726400882567,127.053465602361));
#98913=CARTESIAN_POINT('Ctrl Pts',(8.0287895417393,-30.1437592140213,127.050949806836));
#98914=CARTESIAN_POINT('Ctrl Pts',(8.03264824981435,-30.2148278399929,127.04473215569));
#98915=CARTESIAN_POINT('Ctrl Pts',(8.03650695788941,-30.2854319494135,127.034828288764));
#98916=CARTESIAN_POINT('Ctrl Pts',(8.04036305129656,-30.3559882173556,127.024931132717));
#98917=CARTESIAN_POINT('Ctrl Pts',(8.0442191447037,-30.4260801137613,127.011352786755));
#98918=CARTESIAN_POINT('Ctrl Pts',(8.04807523811084,-30.4952983728753,126.994160746862));
#98919=CARTESIAN_POINT('Ctrl Pts',(8.05193146559612,-30.5645190387397,126.976968109195));
#98920=CARTESIAN_POINT('Ctrl Pts',(8.05578769308139,-30.6328655306219,126.956161625197));
#98921=CARTESIAN_POINT('Ctrl Pts',(8.05964392056666,-30.6999396635101,126.931859733507));
#98922=CARTESIAN_POINT('Ctrl Pts',(8.06349994445144,-30.7670102550287,126.907559124904));
#98923=CARTESIAN_POINT('Ctrl Pts',(8.06735596833621,-30.8328081664699,126.879763648163));
#98924=CARTESIAN_POINT('Ctrl Pts',(8.07121199222098,-30.896953393973,126.848640628013));
#98925=CARTESIAN_POINT('Ctrl Pts',(8.07507195471058,-30.9611641404433,126.817485818309));
#98926=CARTESIAN_POINT('Ctrl Pts',(8.07893191720017,-31.0237183952511,126.782996893766));
#98927=CARTESIAN_POINT('Ctrl Pts',(8.08279187968976,-31.0842598050853,126.745387704087));
#98928=CARTESIAN_POINT('Ctrl Pts',(8.08648092144372,-31.1421204162504,126.709443864883));
#98929=CARTESIAN_POINT('Ctrl Pts',(8.09016996319768,-31.1981423694488,126.670650507383));
#98930=CARTESIAN_POINT('Ctrl Pts',(8.09385900495164,-31.2520409112987,126.629230222815));
#98931=CARTESIAN_POINT('Ctrl Pts',(7.39391264968254,-31.2520409112987,126.629230222815));
#98932=CARTESIAN_POINT('Ctrl Pts',(7.39776808616367,-31.3085950960826,126.585769113352));
#98933=CARTESIAN_POINT('Ctrl Pts',(7.4016235226448,-31.3628767616946,126.539365209773));
#98934=CARTESIAN_POINT('Ctrl Pts',(7.40547895912594,-31.4145751387537,126.490293507776));
#98935=CARTESIAN_POINT('Ctrl Pts',(7.40933850596281,-31.4663286324569,126.441169489484));
#98936=CARTESIAN_POINT('Ctrl Pts',(7.41319805279968,-31.5154929878992,126.389372331323));
#98937=CARTESIAN_POINT('Ctrl Pts',(7.41705759963655,-31.5617941196262,126.335214099087));
#98938=CARTESIAN_POINT('Ctrl Pts',(7.42091943947241,-31.608122759362,126.281023690853));
#98939=CARTESIAN_POINT('Ctrl Pts',(7.42478127930827,-31.6515844936747,126.224469801876));
#98940=CARTESIAN_POINT('Ctrl Pts',(7.42864311914413,-31.6919470880459,126.165895627298));
#98941=CARTESIAN_POINT('Ctrl Pts',(7.43251160608088,-31.7323791555825,126.107220633302));
#98942=CARTESIAN_POINT('Ctrl Pts',(7.43638009301764,-31.7697011813615,126.046518826397));
#98943=CARTESIAN_POINT('Ctrl Pts',(7.44024857995439,-31.803725996472,125.984159586729));
#98944=CARTESIAN_POINT('Ctrl Pts',(7.44218676869742,-31.8207731042195,125.952916369853));
#98945=CARTESIAN_POINT('Ctrl Pts',(7.44412495744045,-31.83699328923,125.921257444323));
#98946=CARTESIAN_POINT('Ctrl Pts',(7.44606314618348,-31.8523676042174,125.889231028106));
#98947=CARTESIAN_POINT('Ctrl Pts',(7.44993221953132,-31.8830582954997,125.825298888442));
#98948=CARTESIAN_POINT('Ctrl Pts',(7.45380129287916,-31.9104954100681,125.759650781342));
#98949=CARTESIAN_POINT('Ctrl Pts',(7.457670366227,-31.9344849573817,125.692651075336));
#98950=CARTESIAN_POINT('Ctrl Pts',(7.4615336746224,-31.9584387600643,125.625751199465));
#98951=CARTESIAN_POINT('Ctrl Pts',(7.4653969830178,-31.9789550296805,125.557504175838));
#98952=CARTESIAN_POINT('Ctrl Pts',(7.4692602914132,-31.9958867364429,125.488296731293));
#98953=CARTESIAN_POINT('Ctrl Pts',(7.47311906790571,-32.0127985812519,125.419170471419));
#98954=CARTESIAN_POINT('Ctrl Pts',(7.47697784439821,-32.026134100711,125.349086498083));
#98955=CARTESIAN_POINT('Ctrl Pts',(7.48083662089072,-32.0357958014338,125.278447512764));
#98956=CARTESIAN_POINT('Ctrl Pts',(7.48469296647851,-32.0454514155968,125.207853027727));
#98957=CARTESIAN_POINT('Ctrl Pts',(7.4885493120663,-32.0514377370552,125.136704704554));
#98958=CARTESIAN_POINT('Ctrl Pts',(7.49240565765409,-32.0537084658798,125.065414827628));
#98959=CARTESIAN_POINT('Ctrl Pts',(7.49626086389899,-32.055978523826,124.99414601303));
#98960=CARTESIAN_POINT('Ctrl Pts',(7.5001160701439,-32.0545351530348,124.922736212981));
#98961=CARTESIAN_POINT('Ctrl Pts',(7.5039712763888,-32.0493840894916,124.851600484371));
#98962=CARTESIAN_POINT('Ctrl Pts',(7.50782663323961,-32.0442328247189,124.780461976803));
#98963=CARTESIAN_POINT('Ctrl Pts',(7.51168199009042,-32.0353736169087,124.709598046288));
#98964=CARTESIAN_POINT('Ctrl Pts',(7.51553734694123,-32.0228641528123,124.639419659761));
#98965=CARTESIAN_POINT('Ctrl Pts',(7.51939673940933,-32.0103415943612,124.569167813597));
#98966=CARTESIAN_POINT('Ctrl Pts',(7.52325613187744,-31.9941612376184,124.499603423133));
#98967=CARTESIAN_POINT('Ctrl Pts',(7.52711552434555,-31.9744319452394,124.431127381466));
#98968=CARTESIAN_POINT('Ctrl Pts',(7.53097710194852,-31.9546914824067,124.362612569607));
#98969=CARTESIAN_POINT('Ctrl Pts',(7.53483867955149,-31.9313982426254,124.2951877926));
#98970=CARTESIAN_POINT('Ctrl Pts',(7.53870025715446,-31.9047101700555,124.229236267987));
#98971=CARTESIAN_POINT('Ctrl Pts',(7.54256859126887,-31.8779754019933,124.163169349543));
#98972=CARTESIAN_POINT('Ctrl Pts',(7.54643692538327,-31.8478341475395,124.098581270326));
#98973=CARTESIAN_POINT('Ctrl Pts',(7.55030525949767,-31.8144911273661,124.03583221833));
#98974=CARTESIAN_POINT('Ctrl Pts',(7.55260297867246,-31.7946859878584,123.998560437841));
#98975=CARTESIAN_POINT('Ctrl Pts',(7.55490069784725,-31.7737520801978,123.961936982506));
#98976=CARTESIAN_POINT('Ctrl Pts',(7.55719841702204,-31.7517393818058,123.926032262714));
#98977=CARTESIAN_POINT('Ctrl Pts',(7.5610674903759,-31.7146727351375,123.865573179572));
#98978=CARTESIAN_POINT('Ctrl Pts',(7.56493656372977,-31.6743998063143,123.806916888848));
#98979=CARTESIAN_POINT('Ctrl Pts',(7.56880563708363,-31.6311215037072,123.75042399085));
#98980=CARTESIAN_POINT('Ctrl Pts',(7.57266894548509,-31.5879076861414,123.694015267753));
#98981=CARTESIAN_POINT('Ctrl Pts',(7.57653225388655,-31.5416976765799,123.639763921366));
#98982=CARTESIAN_POINT('Ctrl Pts',(7.58039556228801,-31.4927366374115,123.588003224568));
#98983=CARTESIAN_POINT('Ctrl Pts',(7.58425433878659,-31.4438330326106,123.536303246312));
#98984=CARTESIAN_POINT('Ctrl Pts',(7.58811311528517,-31.3921851405803,123.487088465385));
#98985=CARTESIAN_POINT('Ctrl Pts',(7.59197189178375,-31.3380784114637,123.440659201048));
#98986=CARTESIAN_POINT('Ctrl Pts',(7.59582823737763,-31.2840057678409,123.39425918565));
#98987=CARTESIAN_POINT('Ctrl Pts',(7.5996845829715,-31.2274777280884,123.350641520978));
#98988=CARTESIAN_POINT('Ctrl Pts',(7.60354092856538,-31.1688155588575,123.310068713861));
#98989=CARTESIAN_POINT('Ctrl Pts',(7.60739613481637,-31.1101707211453,123.269507893828));
#98990=CARTESIAN_POINT('Ctrl Pts',(7.61125134106735,-31.0493934050301,123.231990421594));
#98991=CARTESIAN_POINT('Ctrl Pts',(7.61510654731834,-30.9868354288779,123.197736590059));
#98992=CARTESIAN_POINT('Ctrl Pts',(7.61896190417522,-30.9242750088616,123.163481420378));
#98993=CARTESIAN_POINT('Ctrl Pts',(7.6228172610321,-30.8599342178517,123.132490375899));
#98994=CARTESIAN_POINT('Ctrl Pts',(7.62667261788899,-30.7941896142922,123.104937885174));
#98995=CARTESIAN_POINT('Ctrl Pts',(7.63053201036311,-30.7283761921859,123.077356553718));
#98996=CARTESIAN_POINT('Ctrl Pts',(7.63439140283724,-30.6611564731301,123.053221149228));
#98997=CARTESIAN_POINT('Ctrl Pts',(7.63825079531137,-30.5929263080741,123.032657641463));
#98998=CARTESIAN_POINT('Ctrl Pts',(7.64211237292035,-30.5246575120386,123.012082490923));
#98999=CARTESIAN_POINT('Ctrl Pts',(7.64597395052932,-30.455377603142,122.995083378819));
#99000=CARTESIAN_POINT('Ctrl Pts',(7.6498355281383,-30.385494202373,122.981735452812));
#99001=CARTESIAN_POINT('Ctrl Pts',(7.6537038622586,-30.3154885282649,122.968364172253));
#99002=CARTESIAN_POINT('Ctrl Pts',(7.6575721963789,-30.2448777355307,122.958656898589));
#99003=CARTESIAN_POINT('Ctrl Pts',(7.6614405304992,-30.1740754669361,122.952636990099));
#99004=CARTESIAN_POINT('Ctrl Pts',(7.66373824961967,-30.1320202252576,122.949061275486));
#99005=CARTESIAN_POINT('Ctrl Pts',(7.66603596874013,-30.0898974664779,122.946785516384));
#99006=CARTESIAN_POINT('Ctrl Pts',(7.6683336878606,-30.0477934513841,122.94580591265));
#99007=CARTESIAN_POINT('Ctrl Pts',(7.67220276119791,-29.9768955245042,122.94415638175));
#99008=CARTESIAN_POINT('Ctrl Pts',(7.67607183453523,-29.9057732297676,122.946178357979));
#99009=CARTESIAN_POINT('Ctrl Pts',(7.67994090787254,-29.8348384886821,122.951898626122));
#99010=CARTESIAN_POINT('Ctrl Pts',(7.68380421625744,-29.7640094409683,122.957610371017));
#99011=CARTESIAN_POINT('Ctrl Pts',(7.68766752464235,-29.6933678724612,122.967009430934));
#99012=CARTESIAN_POINT('Ctrl Pts',(7.69153083302725,-29.623326747495,122.980070589514));
#99013=CARTESIAN_POINT('Ctrl Pts',(7.69538960950936,-29.5533677851569,122.993116426536));
#99014=CARTESIAN_POINT('Ctrl Pts',(7.69924838599147,-29.4840083425025,123.009815740546));
#99015=CARTESIAN_POINT('Ctrl Pts',(7.70310716247358,-29.415655548727,123.030091594828));
#99016=CARTESIAN_POINT('Ctrl Pts',(7.70696350805104,-29.3473458150056,123.050354675976));
#99017=CARTESIAN_POINT('Ctrl Pts',(7.7108198536285,-29.2800419366338,123.074189689447));
#99018=CARTESIAN_POINT('Ctrl Pts',(7.71467619920596,-29.2141387005253,123.101469099412));
#99019=CARTESIAN_POINT('Ctrl Pts',(7.71853140544062,-29.1482549352802,123.128740449777));
#99020=CARTESIAN_POINT('Ctrl Pts',(7.72238661167528,-29.08377143937,123.159453990659));
#99021=CARTESIAN_POINT('Ctrl Pts',(7.72624181790994,-29.0210641040991,123.19343362308));
#99022=CARTESIAN_POINT('Ctrl Pts',(7.7300971747506,-28.9583543191277,123.227414582937));
#99023=CARTESIAN_POINT('Ctrl Pts',(7.73395253159126,-28.8974212586147,123.264661654274));
#99024=CARTESIAN_POINT('Ctrl Pts',(7.73780788843192,-28.8386156993583,123.304953077722));
#99025=CARTESIAN_POINT('Ctrl Pts',(7.74166728089009,-28.779748585036,123.345286676456));
#99026=CARTESIAN_POINT('Ctrl Pts',(7.74552667334827,-28.7230138190774,123.38867071352));
#99027=CARTESIAN_POINT('Ctrl Pts',(7.74938606580644,-28.6687319295004,123.434840938764));
#99028=CARTESIAN_POINT('Ctrl Pts',(7.75324764339958,-28.6144193062634,123.481037304956));
#99029=CARTESIAN_POINT('Ctrl Pts',(7.75710922099272,-28.5625626773577,123.530022665901));
#99030=CARTESIAN_POINT('Ctrl Pts',(7.76097079858587,-28.51344625659,123.581495318847));
#99031=CARTESIAN_POINT('Ctrl Pts',(7.76483913269071,-28.4642438979735,123.633058032286));
#99032=CARTESIAN_POINT('Ctrl Pts',(7.76870746679556,-28.4177916365127,123.687116357972));
#99033=CARTESIAN_POINT('Ctrl Pts',(7.7725758009004,-28.3743334414932,123.743335445295));
#99034=CARTESIAN_POINT('Ctrl Pts',(7.77487352016666,-28.3485200734473,123.77672854852));
#99035=CARTESIAN_POINT('Ctrl Pts',(7.77717123943291,-28.3237622359318,123.810883425082));
#99036=CARTESIAN_POINT('Ctrl Pts',(7.77946895869917,-28.3001035210426,123.84572554246));
#99037=CARTESIAN_POINT('Ctrl Pts',(7.78339694507704,-28.2596585845495,123.905288677283));
#99038=CARTESIAN_POINT('Ctrl Pts',(7.78732493145491,-28.2222729070755,123.967090244453));
#99039=CARTESIAN_POINT('Ctrl Pts',(7.79125291783279,-28.1881978044253,124.030788791537));
#99040=CARTESIAN_POINT('Ctrl Pts',(7.79517455591714,-28.1541777729319,124.094384390943));
#99041=CARTESIAN_POINT('Ctrl Pts',(7.79909619400149,-28.123457908575,124.159870473946));
#99042=CARTESIAN_POINT('Ctrl Pts',(7.80301783208584,-28.0962464209973,124.226876547417));
#99043=CARTESIAN_POINT('Ctrl Pts',(7.80693336836405,-28.0690772726713,124.293778363926));
#99044=CARTESIAN_POINT('Ctrl Pts',(7.81084890464227,-28.0454058202885,124.362195038258));
#99045=CARTESIAN_POINT('Ctrl Pts',(7.81476444092048,-28.02539366553,124.431732997288));
#99046=CARTESIAN_POINT('Ctrl Pts',(7.8186763855966,-28.0053998673111,124.501207171268));
#99047=CARTESIAN_POINT('Ctrl Pts',(7.82258833027271,-27.9890588288581,124.571800140759));
#99048=CARTESIAN_POINT('Ctrl Pts',(7.82650027494883,-27.9764831076761,124.643100926059));
#99049=CARTESIAN_POINT('Ctrl Pts',(7.83040988896492,-27.9639148788626,124.714359231747));
#99050=CARTESIAN_POINT('Ctrl Pts',(7.834319502981,-27.9551075924963,124.786324057108));
#99051=CARTESIAN_POINT('Ctrl Pts',(7.83822911699709,-27.9501229160446,124.858573329338));
#99052=CARTESIAN_POINT('Ctrl Pts',(7.84079450484395,-27.9468520999648,124.905981437698));
#99053=CARTESIAN_POINT('Ctrl Pts',(7.84335989269082,-27.9452261188357,124.95351178974));
#99054=CARTESIAN_POINT('Ctrl Pts',(7.84592528053768,-27.945250265129,125.001043813945));
#99055=CARTESIAN_POINT('Origin',(-1.54592528053767,-30.,125.));
#99056=CARTESIAN_POINT('',(6.69398884812234,-31.2520409112987,126.629230222815));
#99057=CARTESIAN_POINT('',(6.75200666526939,-31.2520409112987,126.629230222815));
#99058=CARTESIAN_POINT('',(-1.54592528053767,-31.2520409112987,126.629230222815));
#99059=CARTESIAN_POINT('',(7.20407471942241,-27.945250640964,125.001622972929));
#99060=CARTESIAN_POINT('Ctrl Pts',(6.75200666526939,-31.2520409112987,126.629230222815));
#99061=CARTESIAN_POINT('Ctrl Pts',(6.755869548117,-31.3085483116843,126.585805066515));
#99062=CARTESIAN_POINT('Ctrl Pts',(6.75973243096461,-31.3627333351714,126.539483224137));
#99063=CARTESIAN_POINT('Ctrl Pts',(6.76359531381222,-31.4143002468284,126.490554384892));
#99064=CARTESIAN_POINT('Ctrl Pts',(6.76746446389324,-31.4659508218749,126.441546162329));
#99065=CARTESIAN_POINT('Ctrl Pts',(6.77133361397426,-31.5149744812624,126.389922859516));
#99066=CARTESIAN_POINT('Ctrl Pts',(6.77520276405529,-31.5611146244003,126.336008492482));
#99067=CARTESIAN_POINT('Ctrl Pts',(6.77582755793078,-31.5685653766956,126.327302351438));
#99068=CARTESIAN_POINT('Ctrl Pts',(6.77645235180628,-31.5759410293061,126.31853653065));
#99069=CARTESIAN_POINT('Ctrl Pts',(6.77707714568177,-31.583240608486,126.309712463917));
#99070=CARTESIAN_POINT('Ctrl Pts',(6.78094621902986,-31.6284436880375,126.255068904246));
#99071=CARTESIAN_POINT('Ctrl Pts',(6.78481529237795,-31.6709030568395,126.197975373758));
#99072=CARTESIAN_POINT('Ctrl Pts',(6.78868436572603,-31.7103425768986,126.138738702314));
#99073=CARTESIAN_POINT('Ctrl Pts',(6.79254767412169,-31.749723331735,126.079590294018));
#99074=CARTESIAN_POINT('Ctrl Pts',(6.79641098251735,-31.7860929023809,126.01830548444));
#99075=CARTESIAN_POINT('Ctrl Pts',(6.800274290913,-31.8192153334322,125.955224127158));
#99076=CARTESIAN_POINT('Ctrl Pts',(6.80413306740579,-31.852298909796,125.892216768262));
#99077=CARTESIAN_POINT('Ctrl Pts',(6.80799184389858,-31.8821426879839,125.827417475811));
#99078=CARTESIAN_POINT('Ctrl Pts',(6.81185062039136,-31.9085549343313,125.761193553007));
#99079=CARTESIAN_POINT('Ctrl Pts',(6.81570696597944,-31.9349505418155,125.695011349139));
#99080=CARTESIAN_POINT('Ctrl Pts',(6.81956331156752,-31.9579187268081,125.627406745642));
#99081=CARTESIAN_POINT('Ctrl Pts',(6.8234196571556,-31.9773151269986,125.558768691896));
#99082=CARTESIAN_POINT('Ctrl Pts',(6.82727486340081,-31.9967057965952,125.490150917006));
#99083=CARTESIAN_POINT('Ctrl Pts',(6.83113006964602,-32.0125266443608,125.420500765254));
#99084=CARTESIAN_POINT('Ctrl Pts',(6.83498527589122,-32.0246831393671,125.350222425985));
#99085=CARTESIAN_POINT('Ctrl Pts',(6.83884063274235,-32.036840109274,125.279941341251));
#99086=CARTESIAN_POINT('Ctrl Pts',(6.84269598959347,-32.0453323615862,125.209032499331));
#99087=CARTESIAN_POINT('Ctrl Pts',(6.8465513464446,-32.0501167691149,125.137908649091));
#99088=CARTESIAN_POINT('Ctrl Pts',(6.85041073891303,-32.05490618475,125.066710349545));
#99089=CARTESIAN_POINT('Ctrl Pts',(6.85427013138147,-32.0559799751667,124.995297078089));
#99090=CARTESIAN_POINT('Ctrl Pts',(6.85812952384991,-32.0533471080323,124.924084148985));
#99091=CARTESIAN_POINT('Ctrl Pts',(6.86199110145323,-32.0507127502048,124.852830900101));
#99092=CARTESIAN_POINT('Ctrl Pts',(6.86585267905654,-32.0443676002752,124.781778703463));
#99093=CARTESIAN_POINT('Ctrl Pts',(6.86971425665986,-32.0343725214633,124.711337556279));
#99094=CARTESIAN_POINT('Ctrl Pts',(6.87358259077461,-32.0243599544973,124.640773159877));
#99095=CARTESIAN_POINT('Ctrl Pts',(6.87745092488936,-32.010684801661,124.570822424408));
#99096=CARTESIAN_POINT('Ctrl Pts',(6.88131925900412,-31.993458875968,124.50188427818));
#99097=CARTESIAN_POINT('Ctrl Pts',(6.88361697817619,-31.9832269935744,124.460936289827));
#99098=CARTESIAN_POINT('Ctrl Pts',(6.88591469734826,-31.9717433059035,124.420345270084));
#99099=CARTESIAN_POINT('Ctrl Pts',(6.88821241652033,-31.9590393346454,124.380191603951));
#99100=CARTESIAN_POINT('Ctrl Pts',(6.89208148986845,-31.9376474268754,124.312577823577));
#99101=CARTESIAN_POINT('Ctrl Pts',(6.89595056321657,-31.9127091017341,124.245940377934));
#99102=CARTESIAN_POINT('Ctrl Pts',(6.89981963656469,-31.8843323730222,124.180677676076));
#99103=CARTESIAN_POINT('Ctrl Pts',(6.90368294496038,-31.8559979258791,124.115512216202));
#99104=CARTESIAN_POINT('Ctrl Pts',(6.90754625335606,-31.824235436801,124.051717876002));
#99105=CARTESIAN_POINT('Ctrl Pts',(6.91140956175175,-31.7892024578461,123.989677216263));
#99106=CARTESIAN_POINT('Ctrl Pts',(6.91526833824456,-31.7542105747712,123.927709334107));
#99107=CARTESIAN_POINT('Ctrl Pts',(6.91912711473738,-31.7159560600875,123.867491467115));
#99108=CARTESIAN_POINT('Ctrl Pts',(6.92298589123019,-31.6746435117619,123.809383911156));
#99109=CARTESIAN_POINT('Ctrl Pts',(6.9268422368183,-31.6333569890091,123.751312961083));
#99110=CARTESIAN_POINT('Ctrl Pts',(6.9306985824064,-31.5890165355058,123.695350079465));
#99111=CARTESIAN_POINT('Ctrl Pts',(6.93455492799451,-31.5418706276353,123.641827503542));
#99112=CARTESIAN_POINT('Ctrl Pts',(6.93841013423974,-31.4947386488468,123.588320740663));
#99113=CARTESIAN_POINT('Ctrl Pts',(6.94226534048497,-31.4448031821351,123.537253216468));
#99114=CARTESIAN_POINT('Ctrl Pts',(6.9461205467302,-31.3923525343944,123.488923568291));
#99115=CARTESIAN_POINT('Ctrl Pts',(6.94997590358134,-31.3398998376382,123.440592032088));
#99116=CARTESIAN_POINT('Ctrl Pts',(6.95383126043248,-31.2849321235192,123.394998911814));
#99117=CARTESIAN_POINT('Ctrl Pts',(6.95768661728363,-31.2277727696999,123.35240430066));
#99118=CARTESIAN_POINT('Ctrl Pts',(6.96154600975208,-31.1705535839931,123.309765103348));
#99119=CARTESIAN_POINT('Ctrl Pts',(6.96540540222054,-31.111138569348,123.270130971585));
#99120=CARTESIAN_POINT('Ctrl Pts',(6.96926479468899,-31.0498815131056,123.233719622784));
#99121=CARTESIAN_POINT('Ctrl Pts',(6.97312637229232,-30.9885897739615,123.197287658378));
#99122=CARTESIAN_POINT('Ctrl Pts',(6.97698794989566,-30.9254543472026,123.164082335571));
#99123=CARTESIAN_POINT('Ctrl Pts',(6.98084952749899,-30.8608526993657,123.134274888282));
#99124=CARTESIAN_POINT('Ctrl Pts',(6.98471786161376,-30.7961380195462,123.104415287604));
#99125=CARTESIAN_POINT('Ctrl Pts',(6.98858619572852,-30.7299524479699,123.077965612502));
#99126=CARTESIAN_POINT('Ctrl Pts',(6.99245452984329,-30.662691785049,123.055048288381));
#99127=CARTESIAN_POINT('Ctrl Pts',(6.99475224901516,-30.6227401908689,123.041435820213));
#99128=CARTESIAN_POINT('Ctrl Pts',(6.99704996818703,-30.5824095673422,123.029068655138));
#99129=CARTESIAN_POINT('Ctrl Pts',(6.9993476873589,-30.5417845456429,123.01796390835));
#99130=CARTESIAN_POINT('Ctrl Pts',(7.00321676070784,-30.47337706109,122.999264895707));
#99131=CARTESIAN_POINT('Ctrl Pts',(7.00708583405677,-30.4038663884582,122.984074911669));
#99132=CARTESIAN_POINT('Ctrl Pts',(7.01095490740571,-30.3336458313534,122.972519291899));
#99133=CARTESIAN_POINT('Ctrl Pts',(7.01481821580221,-30.2635299034802,122.960980890102));
#99134=CARTESIAN_POINT('Ctrl Pts',(7.01868152419872,-30.1927066661399,122.953066181724));
#99135=CARTESIAN_POINT('Ctrl Pts',(7.02254483259522,-30.1215829758924,122.94885028765));
#99136=CARTESIAN_POINT('Ctrl Pts',(7.02640360908886,-30.0505427181911,122.944639339084));
#99137=CARTESIAN_POINT('Ctrl Pts',(7.03026238558249,-29.9792031902488,122.944118614824));
#99138=CARTESIAN_POINT('Ctrl Pts',(7.03412116207613,-29.9079780589086,122.947311634744));
#99139=CARTESIAN_POINT('Ctrl Pts',(7.03797750766506,-29.8367977971034,122.950502643165));
#99140=CARTESIAN_POINT('Ctrl Pts',(7.04183385325398,-29.7657322730734,122.957402732454));
#99141=CARTESIAN_POINT('Ctrl Pts',(7.04569019884291,-29.6951953784619,122.967983340327));
#99142=CARTESIAN_POINT('Ctrl Pts',(7.04954540508896,-29.624679323712,122.978560822198));
#99143=CARTESIAN_POINT('Ctrl Pts',(7.05340061133501,-29.5546920684666,122.992816591849));
#99144=CARTESIAN_POINT('Ctrl Pts',(7.05725581758106,-29.4856408782643,123.010670400264));
#99145=CARTESIAN_POINT('Ctrl Pts',(7.06111117443302,-29.4165869905364,123.028524906148));
#99146=CARTESIAN_POINT('Ctrl Pts',(7.06496653128498,-29.3484697102204,123.049977606121));
#99147=CARTESIAN_POINT('Ctrl Pts',(7.06882188813695,-29.2816829413656,123.074897881728));
#99148=CARTESIAN_POINT('Ctrl Pts',(7.07268128060621,-29.2148262630703,123.099844242779));
#99149=CARTESIAN_POINT('Ctrl Pts',(7.07654067307548,-29.1493033324867,123.128265254999));
#99150=CARTESIAN_POINT('Ctrl Pts',(7.08040006554475,-29.0854889450426,123.159981768335));
#99151=CARTESIAN_POINT('Ctrl Pts',(7.08426164314888,-29.0216384267712,123.191716239124));
#99152=CARTESIAN_POINT('Ctrl Pts',(7.08812322075302,-28.9594988007089,123.226749686707));
#99153=CARTESIAN_POINT('Ctrl Pts',(7.09198479835716,-28.8994186522218,123.264857856133));
#99154=CARTESIAN_POINT('Ctrl Pts',(7.09585313247272,-28.8392333829133,123.303032702526));
#99155=CARTESIAN_POINT('Ctrl Pts',(7.09972146658828,-28.7811151817515,123.344292730321));
#99156=CARTESIAN_POINT('Ctrl Pts',(7.10358980070384,-28.7253815715797,123.388371809495));
#99157=CARTESIAN_POINT('Ctrl Pts',(7.10588751986837,-28.6922768344048,123.41455397007));
#99158=CARTESIAN_POINT('Ctrl Pts',(7.10818523903291,-28.6600127586917,123.441729977376));
#99159=CARTESIAN_POINT('Ctrl Pts',(7.11048295819744,-28.6286496245686,123.469838011744));
#99160=CARTESIAN_POINT('Ctrl Pts',(7.11438261491515,-28.5754205535146,123.517542573179));
#99161=CARTESIAN_POINT('Ctrl Pts',(7.11828227163285,-28.524561791372,123.568137518425));
#99162=CARTESIAN_POINT('Ctrl Pts',(7.12218192835056,-28.4764092303526,123.621352572575));
#99163=CARTESIAN_POINT('Ctrl Pts',(7.12598698948199,-28.4294247259264,123.673276767142));
#99164=CARTESIAN_POINT('Ctrl Pts',(7.12979205061342,-28.3850169998354,123.727695018053));
#99165=CARTESIAN_POINT('Ctrl Pts',(7.13359711174485,-28.3434646904679,123.784315694445));
#99166=CARTESIAN_POINT('Ctrl Pts',(7.13739855500662,-28.3019518892276,123.840882535637));
#99167=CARTESIAN_POINT('Ctrl Pts',(7.1411999982684,-28.2632894189908,123.899647249871));
#99168=CARTESIAN_POINT('Ctrl Pts',(7.14500144153017,-28.2277166035248,123.960284113289));
#99169=CARTESIAN_POINT('Ctrl Pts',(7.14880063066554,-28.1921648815271,124.020885021112));
#99170=CARTESIAN_POINT('Ctrl Pts',(7.15259981980092,-28.1596994342751,124.08335544493));
#99171=CARTESIAN_POINT('Ctrl Pts',(7.15639900893629,-28.1305159752474,124.147341191511));
#99172=CARTESIAN_POINT('Ctrl Pts',(7.16037198481014,-28.0999975739514,124.214253845336));
#99173=CARTESIAN_POINT('Ctrl Pts',(7.16434496068397,-28.0730689420479,124.28282328704));
#99174=CARTESIAN_POINT('Ctrl Pts',(7.16831793655782,-28.0498988919779,124.352618172181));
#99175=CARTESIAN_POINT('Ctrl Pts',(7.17211850690874,-28.0277342959365,124.419384339289));
#99176=CARTESIAN_POINT('Ctrl Pts',(7.17591907725967,-28.009008924727,124.487271268717));
#99177=CARTESIAN_POINT('Ctrl Pts',(7.17971964761059,-27.9938195467489,124.555885654934));
#99178=CARTESIAN_POINT('Ctrl Pts',(7.18352169695498,-27.9786242578183,124.624526742467));
#99179=CARTESIAN_POINT('Ctrl Pts',(7.18732374629936,-27.9669677847571,124.693895355798));
#99180=CARTESIAN_POINT('Ctrl Pts',(7.19112579564375,-27.9588954503773,124.763589805614));
#99181=CARTESIAN_POINT('Ctrl Pts',(7.19493249874065,-27.9508132353665,124.833369562246));
#99182=CARTESIAN_POINT('Ctrl Pts',(7.19873920183755,-27.9463239372871,124.903475451104));
#99183=CARTESIAN_POINT('Ctrl Pts',(7.20254590493445,-27.9454208415865,124.973503881172));
#99184=CARTESIAN_POINT('Ctrl Pts',(7.20305550976377,-27.9452999438126,124.982878614437));
#99185=CARTESIAN_POINT('Ctrl Pts',(7.20356511459309,-27.9452432391408,124.992251965449));
#99186=CARTESIAN_POINT('Ctrl Pts',(7.20407471942241,-27.945250640964,125.001622972929));
#99187=CARTESIAN_POINT('Ctrl Pts',(7.20407471946233,-27.9452506409646,125.001622973663));
#99188=CARTESIAN_POINT('Ctrl Pts',(7.20992255598689,-27.9453355786831,125.109157511513));
#99189=CARTESIAN_POINT('Ctrl Pts',(7.21577039251146,-27.95386409323,125.216366166843));
#99190=CARTESIAN_POINT('Ctrl Pts',(7.22161822903602,-27.9706730699826,125.322226277026));
#99191=CARTESIAN_POINT('Ctrl Pts',(7.22548730238386,-27.9817943049358,125.392265945404));
#99192=CARTESIAN_POINT('Ctrl Pts',(7.2293563757317,-27.9965675768644,125.461866373981));
#99193=CARTESIAN_POINT('Ctrl Pts',(7.23322544907954,-28.0149451914192,125.530617535924));
#99194=CARTESIAN_POINT('Ctrl Pts',(7.23708875747494,-28.0332954231708,125.599266258047));
#99195=CARTESIAN_POINT('Ctrl Pts',(7.24095206587034,-28.055239212827,125.667067759863));
#99196=CARTESIAN_POINT('Ctrl Pts',(7.24481537426573,-28.0806775244239,125.733620335902));
#99197=CARTESIAN_POINT('Ctrl Pts',(7.24867415075823,-28.1060859952868,125.800094841597));
#99198=CARTESIAN_POINT('Ctrl Pts',(7.25253292725074,-28.1349806729059,125.86532288007));
#99199=CARTESIAN_POINT('Ctrl Pts',(7.25639170374324,-28.1672126922306,125.92891778268));
#99200=CARTESIAN_POINT('Ctrl Pts',(7.26024804933102,-28.1994244064229,125.992472622553));
#99201=CARTESIAN_POINT('Ctrl Pts',(7.26410439491881,-28.2349690720618,126.054395935445));
#99202=CARTESIAN_POINT('Ctrl Pts',(7.26796074050659,-28.2736502676501,126.114322289158));
#99203=CARTESIAN_POINT('Ctrl Pts',(7.27181594675149,-28.3123200350238,126.174230937855));
#99204=CARTESIAN_POINT('Ctrl Pts',(7.27567115299639,-28.3541242293327,126.232143390751));
#99205=CARTESIAN_POINT('Ctrl Pts',(7.27952635924128,-28.3988220533987,126.287721532715));
#99206=CARTESIAN_POINT('Ctrl Pts',(7.28338171609209,-28.4435216236116,126.343301845872));
#99207=CARTESIAN_POINT('Ctrl Pts',(7.28723707294289,-28.4911147418495,126.396547289877));
#99208=CARTESIAN_POINT('Ctrl Pts',(7.2910924297937,-28.5413202085746,126.447152662502));
#99209=CARTESIAN_POINT('Ctrl Pts',(7.2949518222618,-28.5915782281652,126.497811006596));
#99210=CARTESIAN_POINT('Ctrl Pts',(7.2988112147299,-28.6444537120632,126.545823417154));
#99211=CARTESIAN_POINT('Ctrl Pts',(7.302670607198,-28.6996290992405,126.59092208576));
#99212=CARTESIAN_POINT('Ctrl Pts',(7.30653218480097,-28.7548357259622,126.636046288611));
#99213=CARTESIAN_POINT('Ctrl Pts',(7.31039376240394,-28.8123444563731,126.678253177863));
#99214=CARTESIAN_POINT('Ctrl Pts',(7.31425534000691,-28.871807414335,126.717317399944));
#99215=CARTESIAN_POINT('Ctrl Pts',(7.31812367412132,-28.9313744132346,126.756449971774));
#99216=CARTESIAN_POINT('Ctrl Pts',(7.32199200823571,-28.992902046864,126.79242865292));
#99217=CARTESIAN_POINT('Ctrl Pts',(7.32586034235011,-29.0560170650786,126.825073637166));
#99218=CARTESIAN_POINT('Ctrl Pts',(7.32815806152493,-29.0935062227578,126.844464156196));
#99219=CARTESIAN_POINT('Ctrl Pts',(7.33045578069975,-29.1315550146588,126.862679408199));
#99220=CARTESIAN_POINT('Ctrl Pts',(7.33275349987457,-29.1700822865554,126.879689908312));
#99221=CARTESIAN_POINT('Ctrl Pts',(7.33662257322846,-29.2349574213094,126.908333475135));
#99222=CARTESIAN_POINT('Ctrl Pts',(7.34049164658234,-29.3014442652705,126.933670578712));
#99223=CARTESIAN_POINT('Ctrl Pts',(7.34436071993624,-29.3691724693324,126.955518905317));
#99224=CARTESIAN_POINT('Ctrl Pts',(7.34822402833771,-29.4367997577907,126.977334677728));
#99225=CARTESIAN_POINT('Ctrl Pts',(7.35208733673919,-29.5056642763131,126.995671843735));
#99226=CARTESIAN_POINT('Ctrl Pts',(7.35595064514066,-29.5753748210843,127.010395737145));
#99227=CARTESIAN_POINT('Ctrl Pts',(7.35980942163927,-29.6450035910178,127.025102358505));
#99228=CARTESIAN_POINT('Ctrl Pts',(7.36366819813788,-29.7154759428823,127.03620402665));
#99229=CARTESIAN_POINT('Ctrl Pts',(7.36752697463649,-29.7863862804515,127.043616094407));
#99230=CARTESIAN_POINT('Ctrl Pts',(7.37138332023038,-29.8572519467955,127.051023492802));
#99231=CARTESIAN_POINT('Ctrl Pts',(7.37523966582429,-29.9285545694183,127.054745851857));
#99232=CARTESIAN_POINT('Ctrl Pts',(7.37909601141819,-29.999880600845,127.054749996531));
#99233=CARTESIAN_POINT('Ctrl Pts',(7.3829512176692,-30.0711855592625,127.05475413998));
#99234=CARTESIAN_POINT('Ctrl Pts',(7.38680642392021,-30.1425134272324,127.051042249909));
#99235=CARTESIAN_POINT('Ctrl Pts',(7.39066163017122,-30.2134495397625,127.043633249014));
#99236=CARTESIAN_POINT('Ctrl Pts',(7.39451698702813,-30.2843884234535,127.036223958681));
#99237=CARTESIAN_POINT('Ctrl Pts',(7.39837234388504,-30.3549350383914,127.025117323432));
#99238=CARTESIAN_POINT('Ctrl Pts',(7.40222770074195,-30.4246804583584,127.010384060519));
#99239=CARTESIAN_POINT('Ctrl Pts',(7.4060870932161,-30.4944988847499,126.995635375477));
#99240=CARTESIAN_POINT('Ctrl Pts',(7.40994648569025,-30.5635139657549,126.977252585325));
#99241=CARTESIAN_POINT('Ctrl Pts',(7.41380587816441,-30.6313284701612,126.955357237249));
#99242=CARTESIAN_POINT('Ctrl Pts',(7.4176674557734,-30.6991813702056,126.93344949233));
#99243=CARTESIAN_POINT('Ctrl Pts',(7.4215290333824,-30.7658318863786,126.908025403693));
#99244=CARTESIAN_POINT('Ctrl Pts',(7.4253906109914,-30.830902013802,126.879255013552));
#99245=CARTESIAN_POINT('Ctrl Pts',(7.42925894511172,-30.8960859928938,126.850434284537));
#99246=CARTESIAN_POINT('Ctrl Pts',(7.43312727923205,-30.9596836288983,126.818255783838));
#99247=CARTESIAN_POINT('Ctrl Pts',(7.43699561335237,-31.0213414213069,126.782935574726));
#99248=CARTESIAN_POINT('Ctrl Pts',(7.43929333247263,-31.0579650127866,126.761956021956));
#99249=CARTESIAN_POINT('Ctrl Pts',(7.44159105159288,-31.0939047367783,126.739868873526));
#99250=CARTESIAN_POINT('Ctrl Pts',(7.44388877071314,-31.1290918066321,126.716726319102));
#99251=CARTESIAN_POINT('Ctrl Pts',(7.44663011023724,-31.1710724405908,126.689115633978));
#99252=CARTESIAN_POINT('Ctrl Pts',(7.44937144976133,-31.2120978673782,126.65992590008));
#99253=CARTESIAN_POINT('Ctrl Pts',(7.45211278928543,-31.2520409112987,126.629230222815));
#99254=CARTESIAN_POINT('',(7.14592528050144,-27.9452507538412,124.998239912027));
#99255=CARTESIAN_POINT('Ctrl Pts',(7.14592528053768,-27.9452507538406,124.998239912696));
#99256=CARTESIAN_POINT('Ctrl Pts',(7.14975890798157,-27.9451900689549,125.069084252562));
#99257=CARTESIAN_POINT('Ctrl Pts',(7.15359253542545,-27.9487975671426,125.139993721178));
#99258=CARTESIAN_POINT('Ctrl Pts',(7.15742616286934,-27.9560667657221,125.210557584319));
#99259=CARTESIAN_POINT('Ctrl Pts',(7.16125834634974,-27.9633332263054,125.281094869071));
#99260=CARTESIAN_POINT('Ctrl Pts',(7.16509052983015,-27.9742586004264,125.35128631759));
#99261=CARTESIAN_POINT('Ctrl Pts',(7.16892271331055,-27.9887844405883,125.420725012425));
#99262=CARTESIAN_POINT('Ctrl Pts',(7.17275477350129,-28.0033098134223,125.490161473266));
#99263=CARTESIAN_POINT('Ctrl Pts',(7.17658683369203,-28.0214353197379,125.558844747248));
#99264=CARTESIAN_POINT('Ctrl Pts',(7.18041889388276,-28.0430515099182,125.626378615269));
#99265=CARTESIAN_POINT('Ctrl Pts',(7.18425485641198,-28.0646897127202,125.6939812557));
#99266=CARTESIAN_POINT('Ctrl Pts',(7.1880908189412,-28.0898255471087,125.760431683205));
#99267=CARTESIAN_POINT('Ctrl Pts',(7.19192678147043,-28.1183001035361,125.82535026634));
#99268=CARTESIAN_POINT('Ctrl Pts',(7.19576473620619,-28.14678944822,125.890302564932));
#99269=CARTESIAN_POINT('Ctrl Pts',(7.19960269094194,-28.1786207453222,125.953720995485));
#99270=CARTESIAN_POINT('Ctrl Pts',(7.2034406456777,-28.2135887279824,126.015249885353));
#99271=CARTESIAN_POINT('Ctrl Pts',(7.20728565489047,-28.2486209846758,126.076891870389));
#99272=CARTESIAN_POINT('Ctrl Pts',(7.21113066410324,-28.2868011751739,126.136636963846));
#99273=CARTESIAN_POINT('Ctrl Pts',(7.21497567331601,-28.3278806171451,126.194158419968));
#99274=CARTESIAN_POINT('Ctrl Pts',(7.21791465037946,-28.3592801616071,126.238125607261));
#99275=CARTESIAN_POINT('Ctrl Pts',(7.22085362744291,-28.392372683204,126.280794230267));
#99276=CARTESIAN_POINT('Ctrl Pts',(7.22379260450636,-28.427032275437,126.322032563889));
#99277=CARTESIAN_POINT('Ctrl Pts',(7.22766167785529,-28.472660567764,126.376321567895));
#99278=CARTESIAN_POINT('Ctrl Pts',(7.23153075120422,-28.5211921084715,126.428351931928));
#99279=CARTESIAN_POINT('Ctrl Pts',(7.23539982455315,-28.5723747010316,126.477796862984));
#99280=CARTESIAN_POINT('Ctrl Pts',(7.23926313294966,-28.6234810310905,126.52716812067));
#99281=CARTESIAN_POINT('Ctrl Pts',(7.24312644134617,-28.6772302256488,126.57396125735));
#99282=CARTESIAN_POINT('Ctrl Pts',(7.24698974974267,-28.7333303795212,126.617883072121));
#99283=CARTESIAN_POINT('Ctrl Pts',(7.2508485262363,-28.7893647243971,126.66175336385));
#99284=CARTESIAN_POINT('Ctrl Pts',(7.25470730272993,-28.8477441699736,126.702758726121));
#99285=CARTESIAN_POINT('Ctrl Pts',(7.25856607922356,-28.9081418596759,126.74064452543));
#99286=CARTESIAN_POINT('Ctrl Pts',(7.26242242481248,-28.968501500782,126.778506457907));
#99287=CARTESIAN_POINT('Ctrl Pts',(7.2662787704014,-29.0308764529679,126.813252468867));
#99288=CARTESIAN_POINT('Ctrl Pts',(7.27013511599032,-29.09491005105,126.844670633693));
#99289=CARTESIAN_POINT('Ctrl Pts',(7.27399032223637,-29.1589247306451,126.87607951614));
#99290=CARTESIAN_POINT('Ctrl Pts',(7.27784552848242,-29.2245966473887,126.904162290511));
#99291=CARTESIAN_POINT('Ctrl Pts',(7.28170073472847,-29.291545187166,126.92875331255));
#99292=CARTESIAN_POINT('Ctrl Pts',(7.28555609158043,-29.3584963423276,126.953345295252));
#99293=CARTESIAN_POINT('Ctrl Pts',(7.28941144843239,-29.4267237627802,126.974445089378));
#99294=CARTESIAN_POINT('Ctrl Pts',(7.29326680528435,-29.4958291744837,126.991936078592));
#99295=CARTESIAN_POINT('Ctrl Pts',(7.29712619775361,-29.5650069226805,127.009445376602));
#99296=CARTESIAN_POINT('Ctrl Pts',(7.30098559022287,-29.6350640248431,127.023338209445));
#99297=CARTESIAN_POINT('Ctrl Pts',(7.30484498269213,-29.7055903192736,127.033548746009));
#99298=CARTESIAN_POINT('Ctrl Pts',(7.30870656029626,-29.7761565447209,127.043765063638));
#99299=CARTESIAN_POINT('Ctrl Pts',(7.31256813790039,-29.8471920072879,127.050294890176));
#99300=CARTESIAN_POINT('Ctrl Pts',(7.31642971550451,-29.9182824475051,127.053124400545));
#99301=CARTESIAN_POINT('Ctrl Pts',(7.32029804962007,-29.989497272992,127.055958861642));
#99302=CARTESIAN_POINT('Ctrl Pts',(7.32416638373562,-30.0607667822781,127.055080086321));
#99303=CARTESIAN_POINT('Ctrl Pts',(7.32803471785117,-30.1316784462816,127.050526359081));
#99304=CARTESIAN_POINT('Ctrl Pts',(7.33033243701576,-30.1737986676757,127.047821529033));
#99305=CARTESIAN_POINT('Ctrl Pts',(7.33263015618034,-30.2157927465829,127.043821117613));
#99306=CARTESIAN_POINT('Ctrl Pts',(7.33492787534492,-30.257575941264,127.038541683896));
#99307=CARTESIAN_POINT('Ctrl Pts',(7.33879679457318,-30.327930842686,127.029652128142));
#99308=CARTESIAN_POINT('Ctrl Pts',(7.34266571380144,-30.3979628056788,127.017098714014));
#99309=CARTESIAN_POINT('Ctrl Pts',(7.34653463302971,-30.4672605439819,127.000916076835));
#99310=CARTESIAN_POINT('Ctrl Pts',(7.35048280108411,-30.537977739268,126.984401963365));
#99311=CARTESIAN_POINT('Ctrl Pts',(7.35443096913851,-30.6079297816178,126.964108265274));
#99312=CARTESIAN_POINT('Ctrl Pts',(7.35837913719291,-30.6766848743087,126.940127610077));
#99313=CARTESIAN_POINT('Ctrl Pts',(7.36223776856797,-30.7438807368446,126.916690788933));
#99314=CARTESIAN_POINT('Ctrl Pts',(7.36609639994304,-30.8099328790602,126.889732638835));
#99315=CARTESIAN_POINT('Ctrl Pts',(7.3699550313181,-30.8744504841252,126.859390737127));
#99316=CARTESIAN_POINT('Ctrl Pts',(7.37394796771217,-30.9412137139551,126.827992743429));
#99317=CARTESIAN_POINT('Ctrl Pts',(7.37794090410625,-31.0063330884774,126.792971231739));
#99318=CARTESIAN_POINT('Ctrl Pts',(7.38193384050032,-31.0693972319678,126.754533306255));
#99319=CARTESIAN_POINT('Ctrl Pts',(7.38592677689439,-31.1324613754582,126.716095380771));
#99320=CARTESIAN_POINT('Ctrl Pts',(7.38991971328846,-31.1934697835506,126.674241325073));
#99321=CARTESIAN_POINT('Ctrl Pts',(7.39391264968254,-31.2520409112987,126.629230222815));
#99322=CARTESIAN_POINT('Ctrl Pts',(6.69398884812234,-31.2520409112987,126.629230222815));
#99323=CARTESIAN_POINT('Ctrl Pts',(6.69784694811596,-31.3084865382694,126.585852538531));
#99324=CARTESIAN_POINT('Ctrl Pts',(6.70170504810959,-31.362733689695,126.539493117966));
#99325=CARTESIAN_POINT('Ctrl Pts',(6.70556314810321,-31.4144556013838,126.490406962616));
#99326=CARTESIAN_POINT('Ctrl Pts',(6.70941911580678,-31.4661489274686,126.441347936143));
#99327=CARTESIAN_POINT('Ctrl Pts',(6.71327508351035,-31.5153194313132,126.389565498856));
#99328=CARTESIAN_POINT('Ctrl Pts',(6.71713105121391,-31.5616745617803,126.335353932704));
#99329=CARTESIAN_POINT('Ctrl Pts',(6.72098617770107,-31.6080195794303,126.281154193327));
#99330=CARTESIAN_POINT('Ctrl Pts',(6.72484130418823,-31.6515501278902,126.224526746636));
#99331=CARTESIAN_POINT('Ctrl Pts',(6.72869643067539,-31.6920127508397,126.165800331745));
#99332=CARTESIAN_POINT('Ctrl Pts',(6.7325520057066,-31.7324800816163,126.107067084033));
#99333=CARTESIAN_POINT('Ctrl Pts',(6.73640758073781,-31.7698785047534,126.046234784751));
#99334=CARTESIAN_POINT('Ctrl Pts',(6.74026315576902,-31.8039978444562,125.983661191517));
#99335=CARTESIAN_POINT('Ctrl Pts',(6.74412294979956,-31.8381545195681,125.921019126539));
#99336=CARTESIAN_POINT('Ctrl Pts',(6.74798274383009,-31.8690247189543,125.856632392983));
#99337=CARTESIAN_POINT('Ctrl Pts',(6.75184253786063,-31.8964446593591,125.790882555433));
#99338=CARTESIAN_POINT('Ctrl Pts',(6.75570478475116,-31.9238820248582,125.725090934528));
#99339=CARTESIAN_POINT('Ctrl Pts',(6.75956703164169,-31.9478646051994,125.65793494325));
#99340=CARTESIAN_POINT('Ctrl Pts',(6.76342927853222,-31.9682780607652,125.589812714351));
#99341=CARTESIAN_POINT('Ctrl Pts',(6.76729801466201,-31.9887258144484,125.521576028388));
#99342=CARTESIAN_POINT('Ctrl Pts',(6.77116675079179,-32.0055923633275,125.452370336794));
#99343=CARTESIAN_POINT('Ctrl Pts',(6.77503548692158,-32.0188143372311,125.382604540342));
#99344=CARTESIAN_POINT('Ctrl Pts',(6.7764408316651,-32.0236173092873,125.357261639707));
#99345=CARTESIAN_POINT('Ctrl Pts',(6.77784617640862,-32.027939855963,125.331844877848));
#99346=CARTESIAN_POINT('Ctrl Pts',(6.77925152115213,-32.0317806392832,125.306373948524));
#99347=CARTESIAN_POINT('Ctrl Pts',(6.78312059450033,-32.042354751044,125.236249593445));
#99348=CARTESIAN_POINT('Ctrl Pts',(6.78698966784852,-32.0493149318718,125.1654398123));
#99349=CARTESIAN_POINT('Ctrl Pts',(6.79085874119672,-32.0525826818246,125.094349863666));
#99350=CARTESIAN_POINT('Ctrl Pts',(6.79472204959248,-32.0558455628019,125.023365839665));
#99351=CARTESIAN_POINT('Ctrl Pts',(6.79858535798824,-32.0554269116062,124.952102958125));
#99352=CARTESIAN_POINT('Ctrl Pts',(6.80244866638399,-32.0512996831102,124.880974067649));
#99353=CARTESIAN_POINT('Ctrl Pts',(6.80630744287689,-32.0471772961118,124.809928615819));
#99354=CARTESIAN_POINT('Ctrl Pts',(6.81016621936978,-32.03935500117,124.739017325457));
#99355=CARTESIAN_POINT('Ctrl Pts',(6.81402499586267,-32.027857796495,124.668653776701));
#99356=CARTESIAN_POINT('Ctrl Pts',(6.81788134145086,-32.016367834688,124.598334554711));
#99357=CARTESIAN_POINT('Ctrl Pts',(6.82173768703904,-32.0012076343702,124.528562868029));
#99358=CARTESIAN_POINT('Ctrl Pts',(6.82559403262723,-31.9824539451133,124.459746431752));
#99359=CARTESIAN_POINT('Ctrl Pts',(6.82944923887254,-31.9637057965637,124.390950327033));
#99360=CARTESIAN_POINT('Ctrl Pts',(6.83330444511785,-31.941366394467,124.323109380863));
#99361=CARTESIAN_POINT('Ctrl Pts',(6.83715965136317,-31.915563046177,124.256618685585));
#99362=CARTESIAN_POINT('Ctrl Pts',(6.84101500821439,-31.8897586898639,124.190125392809));
#99363=CARTESIAN_POINT('Ctrl Pts',(6.84487036506562,-31.8604902964996,124.124982907733));
#99364=CARTESIAN_POINT('Ctrl Pts',(6.84872572191684,-31.8279336356094,124.061567164733));
#99365=CARTESIAN_POINT('Ctrl Pts',(6.85258511438538,-31.795342895844,123.998085040933));
#99366=CARTESIAN_POINT('Ctrl Pts',(6.85644450685392,-31.7594572398407,123.936333700387));
#99367=CARTESIAN_POINT('Ctrl Pts',(6.86030389932245,-31.7204984022252,123.876664426611));
#99368=CARTESIAN_POINT('Ctrl Pts',(6.86416547692587,-31.6815175066521,123.816961368915));
#99369=CARTESIAN_POINT('Ctrl Pts',(6.86802705452929,-31.6394602522201,123.759343117253));
#99370=CARTESIAN_POINT('Ctrl Pts',(6.87188863213271,-31.5945901053088,123.704129652106));
#99371=CARTESIAN_POINT('Ctrl Pts',(6.87575696624757,-31.5496414501577,123.648819581259));
#99372=CARTESIAN_POINT('Ctrl Pts',(6.87962530036242,-31.5018704020018,123.595923058158));
#99373=CARTESIAN_POINT('Ctrl Pts',(6.88349363447727,-31.4515783840471,123.545724318615));
#99374=CARTESIAN_POINT('Ctrl Pts',(6.88579135364841,-31.4217058522598,123.515907192485));
#99375=CARTESIAN_POINT('Ctrl Pts',(6.88808907281955,-31.3909445592794,123.487041142893));
#99376=CARTESIAN_POINT('Ctrl Pts',(6.89038679199069,-31.3593629475626,123.459178810084));
#99377=CARTESIAN_POINT('Ctrl Pts',(6.89425586533899,-31.3061834408045,123.412262106491));
#99378=CARTESIAN_POINT('Ctrl Pts',(6.8981249386873,-31.2504680114071,123.368009873212));
#99379=CARTESIAN_POINT('Ctrl Pts',(6.9019940120356,-31.1925145592037,123.326707859163));
#99380=CARTESIAN_POINT('Ctrl Pts',(6.90585732043148,-31.1346474581404,123.285467385469));
#99381=CARTESIAN_POINT('Ctrl Pts',(6.90972062882735,-31.074549345882,123.247168685001));
#99382=CARTESIAN_POINT('Ctrl Pts',(6.91358393722323,-31.0125524062171,123.212058393805));
#99383=CARTESIAN_POINT('Ctrl Pts',(6.91744271371623,-30.9506281928479,123.17698928918));
#99384=CARTESIAN_POINT('Ctrl Pts',(6.92130149020923,-30.8868099971837,123.145101402743));
#99385=CARTESIAN_POINT('Ctrl Pts',(6.92516026670223,-30.8214588440452,123.116598043422));
#99386=CARTESIAN_POINT('Ctrl Pts',(6.92901661229052,-30.7561488600249,123.088112640298));
#99387=CARTESIAN_POINT('Ctrl Pts',(6.93287295787882,-30.6893082787137,123.063007727904));
#99388=CARTESIAN_POINT('Ctrl Pts',(6.93672930346711,-30.6213212655347,123.041439955607));
#99389=CARTESIAN_POINT('Ctrl Pts',(6.94058450971253,-30.5533543388642,123.019878555427));
#99390=CARTESIAN_POINT('Ctrl Pts',(6.94443971595795,-30.4842421155495,123.001852367474));
#99391=CARTESIAN_POINT('Ctrl Pts',(6.94829492220338,-30.4143855768155,122.987468719193));
#99392=CARTESIAN_POINT('Ctrl Pts',(6.95215027905471,-30.3445263090946,122.973084509006));
#99393=CARTESIAN_POINT('Ctrl Pts',(6.95600563590605,-30.2739231444744,122.962343216817));
#99394=CARTESIAN_POINT('Ctrl Pts',(6.95986099275738,-30.2029872528767,122.955301064296));
#99395=CARTESIAN_POINT('Ctrl Pts',(6.96372038522603,-30.13197710872,122.94825154036));
#99396=CARTESIAN_POINT('Ctrl Pts',(6.96757977769468,-30.0606340267332,122.944908933754));
#99397=CARTESIAN_POINT('Ctrl Pts',(6.97143917016332,-29.9893733963977,122.945277479124));
#99398=CARTESIAN_POINT('Ctrl Pts',(6.97530074776684,-29.9180724192746,122.945646233159));
#99399=CARTESIAN_POINT('Ctrl Pts',(6.97916232537037,-29.8468544719533,122.949730294191));
#99400=CARTESIAN_POINT('Ctrl Pts',(6.98302390297389,-29.776131278675,122.95748185856));
#99401=CARTESIAN_POINT('Ctrl Pts',(6.98689223708884,-29.7052843426903,122.965246985658));
#99402=CARTESIAN_POINT('Ctrl Pts',(6.9907605712038,-29.634934368697,122.976692349675));
#99403=CARTESIAN_POINT('Ctrl Pts',(6.99462890531875,-29.5654836367029,122.991718871142));
#99404=CARTESIAN_POINT('Ctrl Pts',(6.99692662448891,-29.5242311818884,123.000644347952));
#99405=CARTESIAN_POINT('Ctrl Pts',(6.99922434365908,-29.4832957357481,123.010832341508));
#99406=CARTESIAN_POINT('Ctrl Pts',(7.00152206282925,-29.4427586443768,123.022253900501));
#99407=CARTESIAN_POINT('Ctrl Pts',(7.00539113617734,-29.3744992235256,123.04148638551));
#99408=CARTESIAN_POINT('Ctrl Pts',(7.00926020952544,-29.3071029468815,123.064294522592));
#99409=CARTESIAN_POINT('Ctrl Pts',(7.01312928287354,-29.2409714547277,123.090583013074));
#99410=CARTESIAN_POINT('Ctrl Pts',(7.01699259126921,-29.1749384990637,123.11683233348));
#99411=CARTESIAN_POINT('Ctrl Pts',(7.02085589966487,-29.1101670348799,123.146551535715));
#99412=CARTESIAN_POINT('Ctrl Pts',(7.02471920806054,-29.0470444364168,123.179595304243));
#99413=CARTESIAN_POINT('Ctrl Pts',(7.02857798455334,-28.9839958847178,123.212600310359));
#99414=CARTESIAN_POINT('Ctrl Pts',(7.03243676104614,-28.9225927850117,123.248921911993));
#99415=CARTESIAN_POINT('Ctrl Pts',(7.03629553753893,-28.8632017528815,123.288367063927));
#99416=CARTESIAN_POINT('Ctrl Pts',(7.04015188312703,-28.8038481351857,123.327787366689));
#99417=CARTESIAN_POINT('Ctrl Pts',(7.04400822871512,-28.7465044740008,123.370327047668));
#99418=CARTESIAN_POINT('Ctrl Pts',(7.04786457430321,-28.6915107348119,123.415748313749));
#99419=CARTESIAN_POINT('Ctrl Pts',(7.05171978054843,-28.6365332433176,123.461156160288));
#99420=CARTESIAN_POINT('Ctrl Pts',(7.05557498679364,-28.5839046698362,123.50944359257));
#99421=CARTESIAN_POINT('Ctrl Pts',(7.05943019303886,-28.5339326626447,123.560331939355));
#99422=CARTESIAN_POINT('Ctrl Pts',(7.06328554989,-28.483958703267,123.611222274124));
#99423=CARTESIAN_POINT('Ctrl Pts',(7.06714090674115,-28.4366418550176,123.664713376969));
#99424=CARTESIAN_POINT('Ctrl Pts',(7.07099626359229,-28.3922523559684,123.720490298743));
#99425=CARTESIAN_POINT('Ctrl Pts',(7.07485565606074,-28.3478163919517,123.776325605336));
#99426=CARTESIAN_POINT('Ctrl Pts',(7.07871504852919,-28.3063141971294,123.834451126329));
#99427=CARTESIAN_POINT('Ctrl Pts',(7.08257444099764,-28.267974621548,123.894520171646));
#99428=CARTESIAN_POINT('Ctrl Pts',(7.08643601860097,-28.2296133386268,123.954623227229));
#99429=CARTESIAN_POINT('Ctrl Pts',(7.0902975962043,-28.1944184793295,124.01667157494));
#99430=CARTESIAN_POINT('Ctrl Pts',(7.09415917380763,-28.1625731861594,124.080293380322));
#99431=CARTESIAN_POINT('Ctrl Pts',(7.0980275079224,-28.1306721740293,124.144026503279));
#99432=CARTESIAN_POINT('Ctrl Pts',(7.10189584203717,-28.1021326235759,124.209338135151));
#99433=CARTESIAN_POINT('Ctrl Pts',(7.10576417615195,-28.0770894760499,124.275836565835));
#99434=CARTESIAN_POINT('Ctrl Pts',(7.1080618953239,-28.0622143079571,124.315335408115));
#99435=CARTESIAN_POINT('Ctrl Pts',(7.11035961449585,-28.0485717692979,124.355252661341));
#99436=CARTESIAN_POINT('Ctrl Pts',(7.1126573336678,-28.0361816560163,124.395504280964));
#99437=CARTESIAN_POINT('Ctrl Pts',(7.11737359945866,-28.0107498851854,124.478124184637));
#99438=CARTESIAN_POINT('Ctrl Pts',(7.12208986524952,-27.9905162579432,124.562414597922));
#99439=CARTESIAN_POINT('Ctrl Pts',(7.12680613104038,-27.9756629418137,124.647782684478));
#99440=CARTESIAN_POINT('Ctrl Pts',(7.13145774527747,-27.9610132380354,124.731980527522));
#99441=CARTESIAN_POINT('Ctrl Pts',(7.13610935951457,-27.9515973927245,124.817226707599));
#99442=CARTESIAN_POINT('Ctrl Pts',(7.14076097375166,-27.9475440844172,124.902931585522));
#99443=CARTESIAN_POINT('Ctrl Pts',(7.14248240933492,-27.9460440655433,124.934648623736));
#99444=CARTESIAN_POINT('Ctrl Pts',(7.14420384491818,-27.9452780035317,124.966428274276));
#99445=CARTESIAN_POINT('Ctrl Pts',(7.14592528050144,-27.9452507538412,124.998239912027));
#99446=CARTESIAN_POINT('Origin',(-1.54592528053767,-30.,125.));
#99447=CARTESIAN_POINT('',(5.99388605066143,-31.2520409112987,126.629230222815));
#99448=CARTESIAN_POINT('',(6.05208070748271,-31.2520409112987,126.629230222815));
#99449=CARTESIAN_POINT('',(-1.54592528053767,-31.2520409112987,126.629230222815));
#99450=CARTESIAN_POINT('',(6.50407471951103,-27.9452500572952,125.000485236462));
#99451=CARTESIAN_POINT('Ctrl Pts',(6.05208070748271,-31.2520409112986,126.629230222815));
#99452=CARTESIAN_POINT('Ctrl Pts',(6.05593584186157,-31.3085914830148,126.585771889945));
#99453=CARTESIAN_POINT('Ctrl Pts',(6.05979097624043,-31.3628817184085,126.539361992874));
#99454=CARTESIAN_POINT('Ctrl Pts',(6.06364611061928,-31.4145976995229,126.490272092943));
#99455=CARTESIAN_POINT('Ctrl Pts',(6.06753106145521,-31.4667136634081,126.44080252093));
#99456=CARTESIAN_POINT('Ctrl Pts',(6.07141601229114,-31.5162150021348,126.388611638529));
#99457=CARTESIAN_POINT('Ctrl Pts',(6.07530096312706,-31.5628183594721,126.334015119029));
#99458=CARTESIAN_POINT('Ctrl Pts',(6.07916147816606,-31.6091285882156,126.279762003993));
#99459=CARTESIAN_POINT('Ctrl Pts',(6.08302199320507,-31.6525769339782,126.223133852219));
#99460=CARTESIAN_POINT('Ctrl Pts',(6.08688250824407,-31.6929272985205,126.16447186502));
#99461=CARTESIAN_POINT('Ctrl Pts',(6.09077967697846,-31.7336607699686,126.105252911047));
#99462=CARTESIAN_POINT('Ctrl Pts',(6.09467684571285,-31.7712368521271,126.043961724892));
#99463=CARTESIAN_POINT('Ctrl Pts',(6.09857401444724,-31.8054598091433,125.980975249468));
#99464=CARTESIAN_POINT('Ctrl Pts',(6.10247118318163,-31.8396827661595,125.917988774043));
#99465=CARTESIAN_POINT('Ctrl Pts',(6.10636835191603,-31.8705524401511,125.853307490443));
#99466=CARTESIAN_POINT('Ctrl Pts',(6.11026552065042,-31.8979233773648,125.787327388163));
#99467=CARTESIAN_POINT('Ctrl Pts',(6.11413459399864,-31.9250969925986,125.721822948238));
#99468=CARTESIAN_POINT('Ctrl Pts',(6.11800366734686,-31.9489286475829,125.654781756097));
#99469=CARTESIAN_POINT('Ctrl Pts',(6.12187274069508,-31.9692444247995,125.586578177139));
#99470=CARTESIAN_POINT('Ctrl Pts',(6.12573604909087,-31.9895299313342,125.518476222098));
#99471=CARTESIAN_POINT('Ctrl Pts',(6.12959935748666,-32.0063098212002,125.449215779922));
#99472=CARTESIAN_POINT('Ctrl Pts',(6.13346266588246,-32.0194582824914,125.37919099116));
#99473=CARTESIAN_POINT('Ctrl Pts',(6.13732144237538,-32.0325913198134,125.309248345864));
#99474=CARTESIAN_POINT('Ctrl Pts',(6.1411802188683,-32.0421013009361,125.238543610109));
#99475=CARTESIAN_POINT('Ctrl Pts',(6.14503899536122,-32.0479127447517,125.167484185473));
#99476=CARTESIAN_POINT('Ctrl Pts',(6.14889534094943,-32.0537205275452,125.096469525981));
#99477=CARTESIAN_POINT('Ctrl Pts',(6.15275168653764,-32.0558343561298,125.025101103938));
#99478=CARTESIAN_POINT('Ctrl Pts',(6.15660803212585,-32.0542303877085,124.95379310966));
#99479=CARTESIAN_POINT('Ctrl Pts',(6.16046323837119,-32.0526268931737,124.882506183062));
#99480=CARTESIAN_POINT('Ctrl Pts',(6.16431844461653,-32.0473077931976,124.811280134183));
#99481=CARTESIAN_POINT('Ctrl Pts',(6.16817365086187,-32.0383013546744,124.740529095981));
#99482=CARTESIAN_POINT('Ctrl Pts',(6.17202900771313,-32.0292945643094,124.669775293847));
#99483=CARTESIAN_POINT('Ctrl Pts',(6.1758843645644,-32.016600212938,124.599497020851));
#99484=CARTESIAN_POINT('Ctrl Pts',(6.17973972141566,-32.0002982194614,124.530101504876));
#99485=CARTESIAN_POINT('Ctrl Pts',(6.18359911388422,-31.983979161778,124.46063334874));
#99486=CARTESIAN_POINT('Ctrl Pts',(6.18745850635279,-31.9640450349266,124.39205026808));
#99487=CARTESIAN_POINT('Ctrl Pts',(6.19131789882135,-31.9406263111467,124.32474665274));
#99488=CARTESIAN_POINT('Ctrl Pts',(6.1951794764248,-31.9171943280077,124.25740493102));
#99489=CARTESIAN_POINT('Ctrl Pts',(6.19904105402824,-31.890274003856,124.191344566788));
#99490=CARTESIAN_POINT('Ctrl Pts',(6.20290263163169,-31.8600438601533,124.126939635073));
#99491=CARTESIAN_POINT('Ctrl Pts',(6.20677096574656,-31.8297608234797,124.062422015566));
#99492=CARTESIAN_POINT('Ctrl Pts',(6.21063929986144,-31.7961566342371,123.999566040007));
#99493=CARTESIAN_POINT('Ctrl Pts',(6.21450763397632,-31.7594552707739,123.938720247698));
#99494=CARTESIAN_POINT('Ctrl Pts',(6.21680535314721,-31.7376553372826,123.902578968454));
#99495=CARTESIAN_POINT('Ctrl Pts',(6.21910307231809,-31.7147635080566,123.867146354675));
#99496=CARTESIAN_POINT('Ctrl Pts',(6.22140079148898,-31.6908335103589,123.832489998866));
#99497=CARTESIAN_POINT('Ctrl Pts',(6.22526986483719,-31.650538370079,123.774133005415));
#99498=CARTESIAN_POINT('Ctrl Pts',(6.2291389381854,-31.60713957811,123.717750259131));
#99499=CARTESIAN_POINT('Ctrl Pts',(6.23300801153361,-31.5608573285145,123.663690918042));
#99500=CARTESIAN_POINT('Ctrl Pts',(6.23687131992939,-31.5146440398673,123.609712125835));
#99501=CARTESIAN_POINT('Ctrl Pts',(6.24073462832518,-31.4655561351378,123.558050233075));
#99502=CARTESIAN_POINT('Ctrl Pts',(6.24459793672096,-31.4138565131096,123.509024707503));
#99503=CARTESIAN_POINT('Ctrl Pts',(6.24845671321387,-31.3622175379782,123.460056691944));
#99504=CARTESIAN_POINT('Ctrl Pts',(6.25231548970678,-31.3079732818954,123.41371923322));
#99505=CARTESIAN_POINT('Ctrl Pts',(6.25617426619968,-31.2514250824289,123.370296706278));
#99506=CARTESIAN_POINT('Ctrl Pts',(6.26003061178788,-31.1949125065039,123.326901534128));
#99507=CARTESIAN_POINT('Ctrl Pts',(6.26388695737608,-31.1360992511542,123.286417945709));
#99508=CARTESIAN_POINT('Ctrl Pts',(6.26774330296428,-31.0753203642286,123.249090614345));
#99509=CARTESIAN_POINT('Ctrl Pts',(6.27159850920961,-31.0145594341977,123.211774311201));
#99510=CARTESIAN_POINT('Ctrl Pts',(6.27545371545494,-30.9518344392437,123.177612667924));
#99511=CARTESIAN_POINT('Ctrl Pts',(6.27930892170026,-30.887508641451,123.146806547106));
#99512=CARTESIAN_POINT('Ctrl Pts',(6.2831642785515,-30.8231803307329,123.115999222828));
#99513=CARTESIAN_POINT('Ctrl Pts',(6.28701963540274,-30.7572515321037,123.088547889102));
#99514=CARTESIAN_POINT('Ctrl Pts',(6.29087499225398,-30.6901077205889,123.064606268357));
#99515=CARTESIAN_POINT('Ctrl Pts',(6.29473438472254,-30.622893625897,123.04063958658));
#99516=CARTESIAN_POINT('Ctrl Pts',(6.29859377719109,-30.5544624379827,123.020190115029));
#99517=CARTESIAN_POINT('Ctrl Pts',(6.30245316965964,-30.4852162643888,123.00336214118));
#99518=CARTESIAN_POINT('Ctrl Pts',(6.30631474726306,-30.415930884565,122.986524639564));
#99519=CARTESIAN_POINT('Ctrl Pts',(6.31017632486648,-30.3458300780973,122.973312807461));
#99520=CARTESIAN_POINT('Ctrl Pts',(6.31403790246991,-30.2753249453426,122.963779546078));
#99521=CARTESIAN_POINT('Ctrl Pts',(6.31790623658477,-30.2046964514165,122.954229604571));
#99522=CARTESIAN_POINT('Ctrl Pts',(6.32177457069963,-30.1336627030745,122.948371124002));
#99523=CARTESIAN_POINT('Ctrl Pts',(6.3256429048145,-30.0626380011782,122.946204965604));
#99524=CARTESIAN_POINT('Ctrl Pts',(6.32794062398551,-30.0204506372337,122.944918307438));
#99525=CARTESIAN_POINT('Ctrl Pts',(6.33023834315652,-29.9782664489834,122.944933353137));
#99526=CARTESIAN_POINT('Ctrl Pts',(6.33253606232753,-29.9361713635724,122.946241623834));
#99527=CARTESIAN_POINT('Ctrl Pts',(6.33640513567575,-29.8652884745277,122.948444588996));
#99528=CARTESIAN_POINT('Ctrl Pts',(6.34027420902398,-29.7943809273128,122.954325827891));
#99529=CARTESIAN_POINT('Ctrl Pts',(6.3441432823722,-29.7238614901485,122.963889716671));
#99530=CARTESIAN_POINT('Ctrl Pts',(6.34800659076799,-29.6534471275495,122.973439355175));
#99531=CARTESIAN_POINT('Ctrl Pts',(6.35186989916379,-29.5834202045742,122.986660686914));
#99532=CARTESIAN_POINT('Ctrl Pts',(6.35573320755959,-29.5141917068454,123.003506106996));
#99533=CARTESIAN_POINT('Ctrl Pts',(6.35959198405251,-29.4450444184832,123.020331766345));
#99534=CARTESIAN_POINT('Ctrl Pts',(6.36345076054543,-29.3766941646795,123.040772955254));
#99535=CARTESIAN_POINT('Ctrl Pts',(6.36730953703836,-29.3095432958903,123.064730741667));
#99536=CARTESIAN_POINT('Ctrl Pts',(6.37116588262657,-29.2424347299823,123.088673435447));
#99537=CARTESIAN_POINT('Ctrl Pts',(6.37502222821478,-29.176524506499,123.116128168673));
#99538=CARTESIAN_POINT('Ctrl Pts',(6.37887857380299,-29.1121999040778,123.146946155078));
#99539=CARTESIAN_POINT('Ctrl Pts',(6.38273378004833,-29.0478943061196,123.177755036424));
#99540=CARTESIAN_POINT('Ctrl Pts',(6.38658898629367,-28.9851738370512,123.211924988476));
#99541=CARTESIAN_POINT('Ctrl Pts',(6.39044419253901,-28.9244042705948,123.249259759592));
#99542=CARTESIAN_POINT('Ctrl Pts',(6.39429954939025,-28.8636323301393,123.286595989212));
#99543=CARTESIAN_POINT('Ctrl Pts',(6.3981549062415,-28.8048118563657,123.327097027188));
#99544=CARTESIAN_POINT('Ctrl Pts',(6.40201026309274,-28.7482810659924,123.370522392683));
#99545=CARTESIAN_POINT('Ctrl Pts',(6.40586965556131,-28.6916911016837,123.413993213934));
#99546=CARTESIAN_POINT('Ctrl Pts',(6.40972904802988,-28.6373959912379,123.460394176724));
#99547=CARTESIAN_POINT('Ctrl Pts',(6.41358844049845,-28.5857014397953,123.509444014771));
#99548=CARTESIAN_POINT('Ctrl Pts',(6.4174500181019,-28.5339776196093,123.558521624161));
#99549=CARTESIAN_POINT('Ctrl Pts',(6.42131159570535,-28.4848576241844,123.610250741923));
#99550=CARTESIAN_POINT('Ctrl Pts',(6.42517317330881,-28.4386088641965,123.664314676455));
#99551=CARTESIAN_POINT('Ctrl Pts',(6.42904150742369,-28.392279183842,123.71847320538));
#99552=CARTESIAN_POINT('Ctrl Pts',(6.43290984153857,-28.3488310651752,123.774974322028));
#99553=CARTESIAN_POINT('Ctrl Pts',(6.43677817565345,-28.3084899336634,123.8334704213));
#99554=CARTESIAN_POINT('Ctrl Pts',(6.43907589482433,-28.284528045032,123.868216026185));
#99555=CARTESIAN_POINT('Ctrl Pts',(6.44137361399521,-28.2616614969002,123.903664960458));
#99556=CARTESIAN_POINT('Ctrl Pts',(6.44367133316609,-28.2399297695999,123.939740434347));
#99557=CARTESIAN_POINT('Ctrl Pts',(6.44766818401098,-28.2021277293325,124.002493224209));
#99558=CARTESIAN_POINT('Ctrl Pts',(6.45166503485587,-28.167621995408,124.067375195747));
#99559=CARTESIAN_POINT('Ctrl Pts',(6.45566188570075,-28.1366498578013,124.13401858561));
#99560=CARTESIAN_POINT('Ctrl Pts',(6.45969628851421,-28.1053867249128,124.201288116048));
#99561=CARTESIAN_POINT('Ctrl Pts',(6.46373069132768,-28.0777242453421,124.270351994449));
#99562=CARTESIAN_POINT('Ctrl Pts',(6.46776509414114,-28.0538611856038,124.340802550369));
#99563=CARTESIAN_POINT('Ctrl Pts',(6.47174648699997,-28.0303116740591,124.410327422625));
#99564=CARTESIAN_POINT('Ctrl Pts',(6.47572787985879,-28.0104625063912,124.481202326663));
#99565=CARTESIAN_POINT('Ctrl Pts',(6.47970927271762,-27.9944576731882,124.553012821362));
#99566=CARTESIAN_POINT('Ctrl Pts',(6.48377018050841,-27.9781331972702,124.626257489177));
#99567=CARTESIAN_POINT('Ctrl Pts',(6.48783108829919,-27.9658084880444,124.700475103802));
#99568=CARTESIAN_POINT('Ctrl Pts',(6.49189199608997,-27.9575832299834,124.775208318537));
#99569=CARTESIAN_POINT('Ctrl Pts',(6.49595290388076,-27.9493579719225,124.849941533272));
#99570=CARTESIAN_POINT('Ctrl Pts',(6.50001381167155,-27.9452322760607,124.9251898674));
#99571=CARTESIAN_POINT('Ctrl Pts',(6.50407471946233,-27.9452500572949,125.000485235559));
#99572=CARTESIAN_POINT('Ctrl Pts',(6.50407471951103,-27.9452500572952,125.000485236462));
#99573=CARTESIAN_POINT('Ctrl Pts',(6.50830237655216,-27.945268568698,125.078872387749));
#99574=CARTESIAN_POINT('Ctrl Pts',(6.5125300335933,-27.9497773969991,125.157140435482));
#99575=CARTESIAN_POINT('Ctrl Pts',(6.51675769063443,-27.9587077544997,125.234784009167));
#99576=CARTESIAN_POINT('Ctrl Pts',(6.52089243721856,-27.9674418511427,125.310721224023));
#99577=CARTESIAN_POINT('Ctrl Pts',(6.52502718380269,-27.9804049307438,125.386060793662));
#99578=CARTESIAN_POINT('Ctrl Pts',(6.52916193038682,-27.9974813727944,125.460344121494));
#99579=CARTESIAN_POINT('Ctrl Pts',(6.53343604265646,-28.0151333930585,125.537131241686));
#99580=CARTESIAN_POINT('Ctrl Pts',(6.5377101549261,-28.0371808331556,125.612789222111));
#99581=CARTESIAN_POINT('Ctrl Pts',(6.54198426719574,-28.0634417891516,125.686833210099));
#99582=CARTESIAN_POINT('Ctrl Pts',(6.54625837946537,-28.0897027451476,125.760877198088));
#99583=CARTESIAN_POINT('Ctrl Pts',(6.55053249173501,-28.1201769686497,125.833306828919));
#99584=CARTESIAN_POINT('Ctrl Pts',(6.55480660400465,-28.1546308748033,125.903664956868));
#99585=CARTESIAN_POINT('Ctrl Pts',(6.55867567735284,-28.1858197349993,125.967355552833));
#99586=CARTESIAN_POINT('Ctrl Pts',(6.56254475070102,-28.2203708581139,126.029554339914));
#99587=CARTESIAN_POINT('Ctrl Pts',(6.56641382404921,-28.2581183028438,126.089883349544));
#99588=CARTESIAN_POINT('Ctrl Pts',(6.57027713244497,-28.2958095035577,126.150122468432));
#99589=CARTESIAN_POINT('Ctrl Pts',(6.57414044084073,-28.3366873167936,126.208496931506));
#99590=CARTESIAN_POINT('Ctrl Pts',(6.57800374923648,-28.3805391633647,126.26465179441));
#99591=CARTESIAN_POINT('Ctrl Pts',(6.58186252572937,-28.4243395689715,126.32074078414));
#99592=CARTESIAN_POINT('Ctrl Pts',(6.58572130222225,-28.4711067805815,126.374614964572));
#99593=CARTESIAN_POINT('Ctrl Pts',(6.58958007871514,-28.5205849981015,126.425948391302));
#99594=CARTESIAN_POINT('Ctrl Pts',(6.59343642430332,-28.5700320459406,126.47724947963));
#99595=CARTESIAN_POINT('Ctrl Pts',(6.5972927698915,-28.6221863750233,126.526012640869));
#99596=CARTESIAN_POINT('Ctrl Pts',(6.60114911547968,-28.6767529565507,126.571946190079));
#99597=CARTESIAN_POINT('Ctrl Pts',(6.60500432172498,-28.7313034165857,126.617866168393));
#99598=CARTESIAN_POINT('Ctrl Pts',(6.60885952797029,-28.7882643427381,126.660957881694));
#99599=CARTESIAN_POINT('Ctrl Pts',(6.6127147342156,-28.8473063029079,126.700968783718));
#99600=CARTESIAN_POINT('Ctrl Pts',(6.61657009106682,-28.9063505695867,126.740981248792));
#99601=CARTESIAN_POINT('Ctrl Pts',(6.62042544791804,-28.9674756283068,126.777912392945));
#99602=CARTESIAN_POINT('Ctrl Pts',(6.62428080476926,-29.0303230844278,126.811552991747));
#99603=CARTESIAN_POINT('Ctrl Pts',(6.62814019723779,-29.0932363264908,126.845228804042));
#99604=CARTESIAN_POINT('Ctrl Pts',(6.63199958970633,-29.1578751358405,126.875606965472));
#99605=CARTESIAN_POINT('Ctrl Pts',(6.63585898217486,-29.2238573333875,126.902524670947));
#99606=CARTESIAN_POINT('Ctrl Pts',(6.63972055977826,-29.2898768891462,126.929457616857));
#99607=CARTESIAN_POINT('Ctrl Pts',(6.64358213738167,-29.3572408882763,126.952926046632));
#99608=CARTESIAN_POINT('Ctrl Pts',(6.64744371498507,-29.4255506327794,126.972816637957));
#99609=CARTESIAN_POINT('Ctrl Pts',(6.65131204909992,-29.4939798972346,126.992742031381));
#99610=CARTESIAN_POINT('Ctrl Pts',(6.65518038321476,-29.5633577378097,127.009076976597));
#99611=CARTESIAN_POINT('Ctrl Pts',(6.65904871732961,-29.6332745687623,127.021759140101));
#99612=CARTESIAN_POINT('Ctrl Pts',(6.66134643650081,-29.6748038777878,127.029292111492));
#99613=CARTESIAN_POINT('Ctrl Pts',(6.66364415567202,-29.7165232177419,127.035537320761));
#99614=CARTESIAN_POINT('Ctrl Pts',(6.66594187484322,-29.758346354646,127.040490401395));
#99615=CARTESIAN_POINT('Ctrl Pts',(6.66980984684839,-29.8287512695462,127.048828399126));
#99616=CARTESIAN_POINT('Ctrl Pts',(6.67367781885357,-29.899726096376,127.053534580682));
#99617=CARTESIAN_POINT('Ctrl Pts',(6.67754579085874,-29.9708636361224,127.054543412732));
#99618=CARTESIAN_POINT('Ctrl Pts',(6.6814084950816,-30.0419042938144,127.055550870856));
#99619=CARTESIAN_POINT('Ctrl Pts',(6.68527119930445,-30.1131067436655,127.052870960964));
#99620=CARTESIAN_POINT('Ctrl Pts',(6.6891339035273,-30.1840576815714,127.046489758673));
#99621=CARTESIAN_POINT('Ctrl Pts',(6.69299263972177,-30.2549357339238,127.040115111581));
#99622=CARTESIAN_POINT('Ctrl Pts',(6.69685137591624,-30.3255623057803,127.030046760409));
#99623=CARTESIAN_POINT('Ctrl Pts',(6.70071011211071,-30.3955248317993,127.016322808959));
#99624=CARTESIAN_POINT('Ctrl Pts',(6.70456617537594,-30.4654388950907,127.00260836403));
#99625=CARTESIAN_POINT('Ctrl Pts',(6.70842223864117,-30.534689350379,126.985243439873));
#99626=CARTESIAN_POINT('Ctrl Pts',(6.7122783019064,-30.6028712112944,126.964317658907));
#99627=CARTESIAN_POINT('Ctrl Pts',(6.71613400852211,-30.67104676603,126.943393813378));
#99628=CARTESIAN_POINT('Ctrl Pts',(6.71998971513781,-30.7381534547125,126.918909895311));
#99629=CARTESIAN_POINT('Ctrl Pts',(6.72384542175351,-30.8038002699191,126.891005734676));
#99630=CARTESIAN_POINT('Ctrl Pts',(6.72770090156707,-30.8694432236187,126.863103215432));
#99631=CARTESIAN_POINT('Ctrl Pts',(6.73155638138064,-30.9336260304061,126.831781050833));
#99632=CARTESIAN_POINT('Ctrl Pts',(6.7354118611942,-30.9959784867921,126.797226868358));
#99633=CARTESIAN_POINT('Ctrl Pts',(6.73927005804643,-31.058374884281,126.762648334815));
#99634=CARTESIAN_POINT('Ctrl Pts',(6.74312825489866,-31.1189379361233,126.72483348097));
#99635=CARTESIAN_POINT('Ctrl Pts',(6.74698645175089,-31.1773238863171,126.684014854212));
#99636=CARTESIAN_POINT('Ctrl Pts',(6.74865985625706,-31.2026474547853,126.666310709875));
#99637=CARTESIAN_POINT('Ctrl Pts',(6.75033326076323,-31.227561851962,126.64804204163));
#99638=CARTESIAN_POINT('Ctrl Pts',(6.75200666526939,-31.2520409112987,126.629230222815));
#99639=CARTESIAN_POINT('',(6.44592528055971,-27.9452500000201,124.999990915848));
#99640=CARTESIAN_POINT('Ctrl Pts',(6.44592528055971,-27.9452500000201,124.999990915848));
#99641=CARTESIAN_POINT('Ctrl Pts',(6.44979385262029,-27.9452496865326,125.070898847849));
#99642=CARTESIAN_POINT('Ctrl Pts',(6.45366242468087,-27.9489241543595,125.141945865788));
#99643=CARTESIAN_POINT('Ctrl Pts',(6.45753099674145,-27.9562906465005,125.212719629838));
#99644=CARTESIAN_POINT('Ctrl Pts',(6.46139380425482,-27.9636461618544,125.283387934122));
#99645=CARTESIAN_POINT('Ctrl Pts',(6.4652566117682,-27.9746827314373,125.353783313364));
#99646=CARTESIAN_POINT('Ctrl Pts',(6.46911941928157,-27.9893655868602,125.423493588143));
#99647=CARTESIAN_POINT('Ctrl Pts',(6.47297769673217,-28.0040312231345,125.493122111004));
#99648=CARTESIAN_POINT('Ctrl Pts',(6.47683597418277,-28.0223345517855,125.562066652123));
#99649=CARTESIAN_POINT('Ctrl Pts',(6.48069425163337,-28.0441892330749,125.629922063814));
#99650=CARTESIAN_POINT('Ctrl Pts',(6.48455010013137,-28.0660301558968,125.697734757588));
#99651=CARTESIAN_POINT('Ctrl Pts',(6.48840594862937,-28.0914178471182,125.764459220811));
#99652=CARTESIAN_POINT('Ctrl Pts',(6.49226179712736,-28.1202156679157,125.829703819053));
#99653=CARTESIAN_POINT('Ctrl Pts',(6.49611650899254,-28.1490049996483,125.894929184393));
#99654=CARTESIAN_POINT('Ctrl Pts',(6.49997122085771,-28.1812022691669,125.958675106488));
#99655=CARTESIAN_POINT('Ctrl Pts',(6.50382593272288,-28.2166227268674,126.020569970249));
#99656=CARTESIAN_POINT('Ctrl Pts',(6.50768079866415,-28.2520446003537,126.082467308));
#99657=CARTESIAN_POINT('Ctrl Pts',(6.51153566460542,-28.2906896745233,126.142513019873));
#99658=CARTESIAN_POINT('Ctrl Pts',(6.51539053054669,-28.3323281365673,126.200361661507));
#99659=CARTESIAN_POINT('Ctrl Pts',(6.51924943299407,-28.3740101990655,126.258270877593));
#99660=CARTESIAN_POINT('Ctrl Pts',(6.52310833544145,-28.4186916219396,126.313978035802));
#99661=CARTESIAN_POINT('Ctrl Pts',(6.52696723788883,-28.4661008194988,126.367168923929));
#99662=CARTESIAN_POINT('Ctrl Pts',(6.53082833003249,-28.5135369189414,126.420389994704));
#99663=CARTESIAN_POINT('Ctrl Pts',(6.53468942217615,-28.5637035323654,126.471091607504));
#99664=CARTESIAN_POINT('Ctrl Pts',(6.53855051431981,-28.6162924803377,126.51899672894));
#99665=CARTESIAN_POINT('Ctrl Pts',(6.5424183550777,-28.6689733459616,126.566985581396));
#99666=CARTESIAN_POINT('Ctrl Pts',(6.54628619583559,-28.7240846231536,126.612167875776));
#99667=CARTESIAN_POINT('Ctrl Pts',(6.55015403659347,-28.7812859393698,126.654307589574));
#99668=CARTESIAN_POINT('Ctrl Pts',(6.55242968422065,-28.8149403857824,126.679100528508));
#99669=CARTESIAN_POINT('Ctrl Pts',(6.55470533184783,-28.8493177651018,126.702841082516));
#99670=CARTESIAN_POINT('Ctrl Pts',(6.556980979475,-28.884344705424,126.725488576081));
#99671=CARTESIAN_POINT('Ctrl Pts',(6.56085005282323,-28.9438977749115,126.763994016338));
#99672=CARTESIAN_POINT('Ctrl Pts',(6.56471912617145,-29.0055632836948,126.799488160214));
#99673=CARTESIAN_POINT('Ctrl Pts',(6.56858819951967,-29.0690042255794,126.831732630738));
#99674=CARTESIAN_POINT('Ctrl Pts',(6.57245150791546,-29.1323506399171,126.863929056725));
#99675=CARTESIAN_POINT('Ctrl Pts',(6.57631481631125,-29.1974668067587,126.892885202362));
#99676=CARTESIAN_POINT('Ctrl Pts',(6.58017812470704,-29.2639876198692,126.918406458182));
#99677=CARTESIAN_POINT('Ctrl Pts',(6.58403690119997,-29.3304303998971,126.943897775969));
#99678=CARTESIAN_POINT('Ctrl Pts',(6.58789567769289,-29.3982741018786,126.965962034409));
#99679=CARTESIAN_POINT('Ctrl Pts',(6.59175445418582,-29.4671315275843,126.984451751393));
#99680=CARTESIAN_POINT('Ctrl Pts',(6.59561079977403,-29.535945575333,127.002929820451));
#99681=CARTESIAN_POINT('Ctrl Pts',(6.59946714536224,-29.6057716117509,127.017837689994));
#99682=CARTESIAN_POINT('Ctrl Pts',(6.60332349095046,-29.6762064784574,127.029077454881));
#99683=CARTESIAN_POINT('Ctrl Pts',(6.6071786971958,-29.7466205354462,127.040313899022));
#99684=CARTESIAN_POINT('Ctrl Pts',(6.61103390344114,-29.8176425861638,127.047884313495));
#99685=CARTESIAN_POINT('Ctrl Pts',(6.61488910968649,-29.8888601619396,127.051742064416));
#99686=CARTESIAN_POINT('Ctrl Pts',(6.61874446653774,-29.9600805198723,127.055599966043));
#99687=CARTESIAN_POINT('Ctrl Pts',(6.622599823389,-30.0314959328342,127.055744892087));
#99688=CARTESIAN_POINT('Ctrl Pts',(6.62645518024026,-30.1026914403144,127.052182260567));
#99689=CARTESIAN_POINT('Ctrl Pts',(6.63031457270883,-30.1739614721079,127.048615899841));
#99690=CARTESIAN_POINT('Ctrl Pts',(6.6341739651774,-30.245010652741,127.041334258715));
#99691=CARTESIAN_POINT('Ctrl Pts',(6.63803335764597,-30.315427563682,127.030394792785));
#99692=CARTESIAN_POINT('Ctrl Pts',(6.64189493524942,-30.3858843437084,127.01944913308));
#99693=CARTESIAN_POINT('Ctrl Pts',(6.64575651285287,-30.455707665693,127.004841625352));
#99694=CARTESIAN_POINT('Ctrl Pts',(6.64961809045631,-30.5244974581908,126.986680643398));
#99695=CARTESIAN_POINT('Ctrl Pts',(6.6534864245712,-30.5934076105692,126.9684878856));
#99696=CARTESIAN_POINT('Ctrl Pts',(6.65735475868608,-30.6612801603096,126.946729388642));
#99697=CARTESIAN_POINT('Ctrl Pts',(6.66122309280097,-30.7277319849047,126.921562832865));
#99698=CARTESIAN_POINT('Ctrl Pts',(6.66352081197183,-30.7672031440075,126.906614362552));
#99699=CARTESIAN_POINT('Ctrl Pts',(6.6658185311427,-30.8061734483555,126.890464398357));
#99700=CARTESIAN_POINT('Ctrl Pts',(6.66811625031357,-30.8445667488954,126.8731536427));
#99701=CARTESIAN_POINT('Ctrl Pts',(6.67198550524012,-30.9092193266097,126.844003114883));
#99702=CARTESIAN_POINT('Ctrl Pts',(6.67585476016666,-30.9724875642114,126.81144429552));
#99703=CARTESIAN_POINT('Ctrl Pts',(6.6797240150932,-31.0339883572384,126.775631053906));
#99704=CARTESIAN_POINT('Ctrl Pts',(6.68358710221264,-31.0953911145877,126.739874900587));
#99705=CARTESIAN_POINT('Ctrl Pts',(6.68745018933207,-31.1550316060579,126.70087486984));
#99706=CARTESIAN_POINT('Ctrl Pts',(6.6913132764515,-31.212548373772,126.658832120428));
#99707=CARTESIAN_POINT('Ctrl Pts',(6.69220513367511,-31.2258270659627,126.649125859967));
#99708=CARTESIAN_POINT('Ctrl Pts',(6.69309699089873,-31.2389926646906,126.639257620015));
#99709=CARTESIAN_POINT('Ctrl Pts',(6.69398884812234,-31.2520409112987,126.629230222815));
#99710=CARTESIAN_POINT('Ctrl Pts',(5.99388605066143,-31.2520409112987,126.629230222815));
#99711=CARTESIAN_POINT('Ctrl Pts',(5.99635890886836,-31.2880636491292,126.601547246604));
#99712=CARTESIAN_POINT('Ctrl Pts',(5.99883176707529,-31.323128886047,126.572698928905));
#99713=CARTESIAN_POINT('Ctrl Pts',(6.00130462528221,-31.3571605423516,126.542761428343));
#99714=CARTESIAN_POINT('Ctrl Pts',(6.00517369863043,-31.4104070139993,126.495920737999));
#99715=CARTESIAN_POINT('Ctrl Pts',(6.00904277197865,-31.4613299633522,126.446228460409));
#99716=CARTESIAN_POINT('Ctrl Pts',(6.01291184532687,-31.5096083664831,126.393944095846));
#99717=CARTESIAN_POINT('Ctrl Pts',(6.01677515372265,-31.5578148343798,126.341737635435));
#99718=CARTESIAN_POINT('Ctrl Pts',(6.02063846211844,-31.6033842507583,126.286947108469));
#99719=CARTESIAN_POINT('Ctrl Pts',(6.02450177051423,-31.6460300705184,126.229870956422));
#99720=CARTESIAN_POINT('Ctrl Pts',(6.02836054700715,-31.6886258640592,126.172861758278));
#99721=CARTESIAN_POINT('Ctrl Pts',(6.03221932350006,-31.7283045838958,126.113572648054));
#99722=CARTESIAN_POINT('Ctrl Pts',(6.03607809999298,-31.7648190305381,126.05233614019));
#99723=CARTESIAN_POINT('Ctrl Pts',(6.03993444558119,-31.801310474257,125.991138209351));
#99724=CARTESIAN_POINT('Ctrl Pts',(6.04379079116939,-31.8346413514289,125.927995731073));
#99725=CARTESIAN_POINT('Ctrl Pts',(6.0476471367576,-31.8646078326565,125.863270057917));
#99726=CARTESIAN_POINT('Ctrl Pts',(6.05150234300294,-31.8945654603994,125.798563507719));
#99727=CARTESIAN_POINT('Ctrl Pts',(6.05535754924827,-31.9211604615756,125.732275131846));
#99728=CARTESIAN_POINT('Ctrl Pts',(6.05921275549361,-31.9442358153368,125.664789182269));
#99729=CARTESIAN_POINT('Ctrl Pts',(6.06306811234486,-31.9673120705504,125.597300596313));
#99730=CARTESIAN_POINT('Ctrl Pts',(6.06692346919611,-31.9868682502805,125.52861480414));
#99731=CARTESIAN_POINT('Ctrl Pts',(6.07077882604736,-32.0027967472953,125.459132607776));
#99732=CARTESIAN_POINT('Ctrl Pts',(6.07463821851592,-32.0187419175574,125.389577680518));
#99733=CARTESIAN_POINT('Ctrl Pts',(6.07849761098448,-32.0310517160729,125.319225159407));
#99734=CARTESIAN_POINT('Ctrl Pts',(6.08235700345304,-32.0396695759424,125.248486586107));
#99735=CARTESIAN_POINT('Ctrl Pts',(6.08621858105648,-32.0482923151254,125.1777079616));
#99736=CARTESIAN_POINT('Ctrl Pts',(6.09008015865992,-32.0532189209048,125.10654333464));
#99737=CARTESIAN_POINT('Ctrl Pts',(6.09394173626336,-32.0544449115845,125.035407171092));
#99738=CARTESIAN_POINT('Ctrl Pts',(6.09781007037823,-32.0556730473512,124.964146542274));
#99739=CARTESIAN_POINT('Ctrl Pts',(6.10167840449311,-32.0531876576792,124.892914961944));
#99740=CARTESIAN_POINT('Ctrl Pts',(6.10554673860798,-32.0470363181878,124.822123991162));
#99741=CARTESIAN_POINT('Ctrl Pts',(6.10784445777891,-32.043382535899,124.780075459194));
#99742=CARTESIAN_POINT('Ctrl Pts',(6.11014217694984,-32.0384363455578,124.738182247743));
#99743=CARTESIAN_POINT('Ctrl Pts',(6.11243989612077,-32.0322162126119,124.696528703668));
#99744=CARTESIAN_POINT('Ctrl Pts',(6.11630896946898,-32.0217422822432,124.626389315323));
#99745=CARTESIAN_POINT('Ctrl Pts',(6.1201780428172,-32.0076124141733,124.556655420757));
#99746=CARTESIAN_POINT('Ctrl Pts',(6.12404711616541,-31.9898705140382,124.487737469786));
#99747=CARTESIAN_POINT('Ctrl Pts',(6.12791042456119,-31.9721550494862,124.418922207151));
#99748=CARTESIAN_POINT('Ctrl Pts',(6.13177373295697,-31.9508383560286,124.350920941469));
#99749=CARTESIAN_POINT('Ctrl Pts',(6.13563704135276,-31.9260157555762,124.284136275697));
#99750=CARTESIAN_POINT('Ctrl Pts',(6.13949581784567,-31.9012222735897,124.217429952524));
#99751=CARTESIAN_POINT('Ctrl Pts',(6.14335459433857,-31.8729312221434,124.151937847602));
#99752=CARTESIAN_POINT('Ctrl Pts',(6.14721337083148,-31.8412878889773,124.088047987882));
#99753=CARTESIAN_POINT('Ctrl Pts',(6.15106971641969,-31.8096644900903,124.024198376713));
#99754=CARTESIAN_POINT('Ctrl Pts',(6.15492606200789,-31.7746932144136,123.961949442476));
#99755=CARTESIAN_POINT('Ctrl Pts',(6.15878240759609,-31.736567100229,123.901668415777));
#99756=CARTESIAN_POINT('Ctrl Pts',(6.16263761384142,-31.6984522502622,123.841405198882));
#99757=CARTESIAN_POINT('Ctrl Pts',(6.16649282008675,-31.6571846717618,123.783109145601));
#99758=CARTESIAN_POINT('Ctrl Pts',(6.17034802633208,-31.6130020290764,123.727120580457));
#99759=CARTESIAN_POINT('Ctrl Pts',(6.17420338318332,-31.56881766037,123.671129828087));
#99760=CARTESIAN_POINT('Ctrl Pts',(6.17805874003457,-31.5217183040519,123.617447122804));
#99761=CARTESIAN_POINT('Ctrl Pts',(6.18191409688581,-31.4719823290648,123.566380250757));
#99762=CARTESIAN_POINT('Ctrl Pts',(6.18577348935437,-31.4221942926552,123.515259924162));
#99763=CARTESIAN_POINT('Ctrl Pts',(6.18963288182292,-31.3697644678364,123.466761245463));
#99764=CARTESIAN_POINT('Ctrl Pts',(6.19349227429148,-31.3150079288298,123.421154944393));
#99765=CARTESIAN_POINT('Ctrl Pts',(6.19735385189491,-31.2602203874248,123.375522821663));
#99766=CARTESIAN_POINT('Ctrl Pts',(6.20121542949834,-31.2031038985311,123.332786627736));
#99767=CARTESIAN_POINT('Ctrl Pts',(6.20507700710177,-31.1440042422665,123.29317491928));
#99768=CARTESIAN_POINT('Ctrl Pts',(6.20894534121664,-31.0848011807245,123.25349390315));
#99769=CARTESIAN_POINT('Ctrl Pts',(6.21281367533151,-31.0236084412548,123.216948536353));
#99770=CARTESIAN_POINT('Ctrl Pts',(6.21668200944638,-30.9607975975381,123.183722064478));
#99771=CARTESIAN_POINT('Ctrl Pts',(6.21897972861736,-30.9234891139718,123.163986152546));
#99772=CARTESIAN_POINT('Ctrl Pts',(6.22127744778835,-30.885610166226,123.145420289185));
#99773=CARTESIAN_POINT('Ctrl Pts',(6.22357516695933,-30.847241632767,123.128054707475));
#99774=CARTESIAN_POINT('Ctrl Pts',(6.22744424030755,-30.7826337937887,123.098813227393));
#99775=CARTESIAN_POINT('Ctrl Pts',(6.23131331365577,-30.7163837784896,123.072863185084));
#99776=CARTESIAN_POINT('Ctrl Pts',(6.23518238700399,-30.6488602364773,123.050390306749));
#99777=CARTESIAN_POINT('Ctrl Pts',(6.23904569539978,-30.5814373051209,123.027950913195));
#99778=CARTESIAN_POINT('Ctrl Pts',(6.24290900379558,-30.5127450708391,123.008978551621));
#99779=CARTESIAN_POINT('Ctrl Pts',(6.24677231219137,-30.4431734770939,122.993611495323));
#99780=CARTESIAN_POINT('Ctrl Pts',(6.25063108868428,-30.3736834951884,122.978262465545));
#99781=CARTESIAN_POINT('Ctrl Pts',(6.2544898651772,-30.3033166748642,122.966510444591));
#99782=CARTESIAN_POINT('Ctrl Pts',(6.25834864167012,-30.2324778133163,122.958443821783));
#99783=CARTESIAN_POINT('Ctrl Pts',(6.26220498725833,-30.1616835779659,122.950382280687));
#99784=CARTESIAN_POINT('Ctrl Pts',(6.26606133284654,-30.0904183728962,122.946001586392));
#99785=CARTESIAN_POINT('Ctrl Pts',(6.26991767843475,-30.0190954215666,122.945338731719));
#99786=CARTESIAN_POINT('Ctrl Pts',(6.27377288468009,-29.947793542336,122.944676072884));
#99787=CARTESIAN_POINT('Ctrl Pts',(6.27762809092543,-29.8764344362167,122.947729077512));
#99788=CARTESIAN_POINT('Ctrl Pts',(6.28148329717076,-29.8054329252711,122.954482653231));
#99789=CARTESIAN_POINT('Ctrl Pts',(6.28533865402201,-29.7344286406094,122.961236492783));
#99790=CARTESIAN_POINT('Ctrl Pts',(6.28919401087327,-29.6637824622511,122.971691142247));
#99791=CARTESIAN_POINT('Ctrl Pts',(6.29304936772452,-29.5939039520619,122.985779663902));
#99792=CARTESIAN_POINT('Ctrl Pts',(6.29690876019308,-29.5239522961339,122.9998829328));
#99793=CARTESIAN_POINT('Ctrl Pts',(6.30076815266165,-29.4547703896434,123.017627570876));
#99794=CARTESIAN_POINT('Ctrl Pts',(6.30462754513021,-29.386756569374,123.038895704636));
#99795=CARTESIAN_POINT('Ctrl Pts',(6.30848912273365,-29.3187042406161,123.060175880121));
#99796=CARTESIAN_POINT('Ctrl Pts',(6.31235070033709,-29.2518217703124,123.084983353613));
#99797=CARTESIAN_POINT('Ctrl Pts',(6.31621227794053,-29.1864887175937,123.113151581102));
#99798=CARTESIAN_POINT('Ctrl Pts',(6.32008061205541,-29.1210413531704,123.141369093876));
#99799=CARTESIAN_POINT('Ctrl Pts',(6.32394894617028,-29.0571492544867,123.172958885327));
#99800=CARTESIAN_POINT('Ctrl Pts',(6.32781728028516,-28.9951679023623,123.207708166046));
#99801=CARTESIAN_POINT('Ctrl Pts',(6.33011499945607,-28.9583521215156,123.228348598365));
#99802=CARTESIAN_POINT('Ctrl Pts',(6.33241271862698,-28.9222099501554,123.250102894812));
#99803=CARTESIAN_POINT('Ctrl Pts',(6.33471043779789,-28.8868106539846,123.272919503203));
#99804=CARTESIAN_POINT('Ctrl Pts',(6.33857951114609,-28.8272026413547,123.311339834345));
#99805=CARTESIAN_POINT('Ctrl Pts',(6.34244858449429,-28.7694692515095,123.352924986983));
#99806=CARTESIAN_POINT('Ctrl Pts',(6.34631765784249,-28.7139664634272,123.397465973743));
#99807=CARTESIAN_POINT('Ctrl Pts',(6.35018096623826,-28.6585463749746,123.441940594052));
#99808=CARTESIAN_POINT('Ctrl Pts',(6.35404427463404,-28.6053506667869,123.489362004667));
#99809=CARTESIAN_POINT('Ctrl Pts',(6.35790758302981,-28.5547069996118,123.539477591569));
#99810=CARTESIAN_POINT('Ctrl Pts',(6.36176635952271,-28.5041227406324,123.589534389747));
#99811=CARTESIAN_POINT('Ctrl Pts',(6.36562513601561,-28.4560849197788,123.642278746475));
#99812=CARTESIAN_POINT('Ctrl Pts',(6.3694839125085,-28.4108873442318,123.697418513191));
#99813=CARTESIAN_POINT('Ctrl Pts',(6.3733402580967,-28.3657182416993,123.752523543633));
#99814=CARTESIAN_POINT('Ctrl Pts',(6.37719660368489,-28.3233861418341,123.81002061536));
#99815=CARTESIAN_POINT('Ctrl Pts',(6.38105294927308,-28.2841462414821,123.869582624921));
#99816=CARTESIAN_POINT('Ctrl Pts',(6.3849081555184,-28.2449179344118,123.92912703711));
#99817=CARTESIAN_POINT('Ctrl Pts',(6.38876336176371,-28.2087802802567,123.990734770517));
#99818=CARTESIAN_POINT('Ctrl Pts',(6.39261856800903,-28.1759455838451,124.054049129497));
#99819=CARTESIAN_POINT('Ctrl Pts',(6.39647392486026,-28.1431096047267,124.11736596189));
#99820=CARTESIAN_POINT('Ctrl Pts',(6.40032928171149,-28.1135770612153,124.182389119962));
#99821=CARTESIAN_POINT('Ctrl Pts',(6.40418463856272,-28.087513847662,124.248738208335));
#99822=CARTESIAN_POINT('Ctrl Pts',(6.40804403103126,-28.0614233522875,124.315156748004));
#99823=CARTESIAN_POINT('Ctrl Pts',(6.41190342349981,-28.0388096142217,124.382903535505));
#99824=CARTESIAN_POINT('Ctrl Pts',(6.41576281596836,-28.0197896463736,124.451579980407));
#99825=CARTESIAN_POINT('Ctrl Pts',(6.41962439357178,-28.0007589096816,124.520295308966));
#99826=CARTESIAN_POINT('Ctrl Pts',(6.4234859711752,-27.9853260988995,124.589940868237));
#99827=CARTESIAN_POINT('Ctrl Pts',(6.42734754877862,-27.973557152391,124.660107446574));
#99828=CARTESIAN_POINT('Ctrl Pts',(6.43121588289348,-27.9617676140339,124.730396793721));
#99829=CARTESIAN_POINT('Ctrl Pts',(6.43508421700834,-27.9536547941653,124.801208497216));
#99830=CARTESIAN_POINT('Ctrl Pts',(6.43895255112319,-27.949232719164,124.872128492805));
#99831=CARTESIAN_POINT('Ctrl Pts',(6.44125027029428,-27.9466060881117,124.914253663134));
#99832=CARTESIAN_POINT('Ctrl Pts',(6.44354798946536,-27.9452806044252,124.956417024691));
#99833=CARTESIAN_POINT('Ctrl Pts',(6.44584570863644,-27.9452505240975,124.998532424289));
#99834=CARTESIAN_POINT('Ctrl Pts',(6.44587223260258,-27.9452501768621,124.999018587892));
#99835=CARTESIAN_POINT('Ctrl Pts',(6.44589875656872,-27.9452500021695,124.999504751619));
#99836=CARTESIAN_POINT('Ctrl Pts',(6.44592528053486,-27.9452500000201,124.999990915393));
#99837=CARTESIAN_POINT('Origin',(-1.54592528053767,-30.,125.));
#99838=CARTESIAN_POINT('',(5.29388025174645,-31.2520409112987,126.629230222815));
#99839=CARTESIAN_POINT('',(5.35213747652439,-31.2520409112987,126.629230222815));
#99840=CARTESIAN_POINT('',(-1.54592528053767,-31.2520409112987,126.629230222815));
#99841=CARTESIAN_POINT('',(5.80407471941279,-27.9452508587689,124.998121407386));
#99842=CARTESIAN_POINT('Ctrl Pts',(5.35213747652439,-31.2520409112987,126.629230222815));
#99843=CARTESIAN_POINT('Ctrl Pts',(5.35599720568668,-31.3084431276569,126.585885898987));
#99844=CARTESIAN_POINT('Ctrl Pts',(5.35985693484896,-31.3626623496427,126.539555122573));
#99845=CARTESIAN_POINT('Ctrl Pts',(5.36371666401124,-31.4143692255357,126.490488931981));
#99846=CARTESIAN_POINT('Ctrl Pts',(5.36757358507917,-31.4660384827823,126.44145843884));
#99847=CARTESIAN_POINT('Ctrl Pts',(5.3714305061471,-31.5151986686399,126.389696812789));
#99848=CARTESIAN_POINT('Ctrl Pts',(5.37528742721503,-31.5615540543982,126.335494851241));
#99849=CARTESIAN_POINT('Ctrl Pts',(5.37914283246657,-31.6078912219321,126.281314191717));
#99850=CARTESIAN_POINT('Ctrl Pts',(5.38299823771811,-31.6514254617369,126.224695469051));
#99851=CARTESIAN_POINT('Ctrl Pts',(5.38685364296964,-31.6918996281051,126.165964498138));
#99852=CARTESIAN_POINT('Ctrl Pts',(5.39070882268999,-31.7323714268398,126.107236962834));
#99853=CARTESIAN_POINT('Ctrl Pts',(5.39456400241034,-31.7697832332088,126.046397825505));
#99854=CARTESIAN_POINT('Ctrl Pts',(5.39841918213069,-31.803920759363,125.983802549519));
#99855=CARTESIAN_POINT('Ctrl Pts',(5.40227815589108,-31.8380918816529,125.921145670961));
#99856=CARTESIAN_POINT('Ctrl Pts',(5.40613712965147,-31.8689820537455,125.856729628919));
#99857=CARTESIAN_POINT('Ctrl Pts',(5.40999610341185,-31.8964230160968,125.790934451468));
#99858=CARTESIAN_POINT('Ctrl Pts',(5.41385692445022,-31.923877114346,125.725107778082));
#99859=CARTESIAN_POINT('Ctrl Pts',(5.4177177454886,-31.9478785498704,125.657901112266));
#99860=CARTESIAN_POINT('Ctrl Pts',(5.42157856652697,-31.9683082961627,125.589711805679));
#99861=CARTESIAN_POINT('Ctrl Pts',(5.42544650188966,-31.9887756882923,125.521396846844));
#99862=CARTESIAN_POINT('Ctrl Pts',(5.42931443725234,-32.0056581259862,125.452096102648));
#99863=CARTESIAN_POINT('Ctrl Pts',(5.43318237261502,-32.0188873920948,125.38221886471));
#99864=CARTESIAN_POINT('Ctrl Pts',(5.43660621361637,-32.0305977490355,125.320364534202));
#99865=CARTESIAN_POINT('Ctrl Pts',(5.44003005461772,-32.0394463839407,125.258058847955));
#99866=CARTESIAN_POINT('Ctrl Pts',(5.44345389561906,-32.0454200326908,125.195587454524));
#99867=CARTESIAN_POINT('Ctrl Pts',(5.44732296896727,-32.0521704878556,125.124992352924));
#99868=CARTESIAN_POINT('Ctrl Pts',(5.45119204231548,-32.0552751231039,125.053909088628));
#99869=CARTESIAN_POINT('Ctrl Pts',(5.45506111566369,-32.0546775616078,124.982746585111));
#99870=CARTESIAN_POINT('Ctrl Pts',(5.45892442405947,-32.0540808904835,124.911690114334));
#99871=CARTESIAN_POINT('Ctrl Pts',(5.46278773245525,-32.0497929763708,124.840555120507));
#99872=CARTESIAN_POINT('Ctrl Pts',(5.46665104085102,-32.0418092335023,124.769755311713));
#99873=CARTESIAN_POINT('Ctrl Pts',(5.47050981734393,-32.0338348560647,124.699038555531));
#99874=CARTESIAN_POINT('Ctrl Pts',(5.47436859383683,-32.0221733156896,124.628656683752));
#99875=CARTESIAN_POINT('Ctrl Pts',(5.47822737032974,-32.0068720328795,124.559021308739));
#99876=CARTESIAN_POINT('Ctrl Pts',(5.48208371591794,-31.9915803893839,124.489429801765));
#99877=CARTESIAN_POINT('Ctrl Pts',(5.48594006150614,-31.9726536565801,124.420584331896));
#99878=CARTESIAN_POINT('Ctrl Pts',(5.48979640709434,-31.9501906114721,124.352887844786));
#99879=CARTESIAN_POINT('Ctrl Pts',(5.49365161333966,-31.9277342029867,124.285211358349));
#99880=CARTESIAN_POINT('Ctrl Pts',(5.49750681958499,-31.9017437093025,124.218683641558));
#99881=CARTESIAN_POINT('Ctrl Pts',(5.50136202583031,-31.8723677051348,124.153692290436));
#99882=CARTESIAN_POINT('Ctrl Pts',(5.50521738268155,-31.8429905533761,124.088698400388));
#99883=CARTESIAN_POINT('Ctrl Pts',(5.50907273953279,-31.8102278306469,124.025241436929));
#99884=CARTESIAN_POINT('Ctrl Pts',(5.51292809638403,-31.7742754619648,123.963687234678));
#99885=CARTESIAN_POINT('Ctrl Pts',(5.51678748885258,-31.7382854599306,123.902068600206));
#99886=CARTESIAN_POINT('Ctrl Pts',(5.52064688132113,-31.6990993924953,123.84235712321));
#99887=CARTESIAN_POINT('Ctrl Pts',(5.52450627378969,-31.6569577433049,123.784891527722));
#99888=CARTESIAN_POINT('Ctrl Pts',(5.52836785139311,-31.6147922340929,123.727393396005));
#99889=CARTESIAN_POINT('Ctrl Pts',(5.53222942899655,-31.5696681193209,123.672144053557));
#99890=CARTESIAN_POINT('Ctrl Pts',(5.53609100659997,-31.5218658529214,123.619448701347));
#99891=CARTESIAN_POINT('Ctrl Pts',(5.53995934071484,-31.4739799480217,123.566661149321));
#99892=CARTESIAN_POINT('Ctrl Pts',(5.5438276748297,-31.4234068807599,123.516436851756));
#99893=CARTESIAN_POINT('Ctrl Pts',(5.54769600894457,-31.3704630647979,123.469043256482));
#99894=CARTESIAN_POINT('Ctrl Pts',(5.54999372811558,-31.3390154138685,123.44089233435));
#99895=CARTESIAN_POINT('Ctrl Pts',(5.5522914472866,-31.3067319607153,123.41373934893));
#99896=CARTESIAN_POINT('Ctrl Pts',(5.55458916645762,-31.2736839053951,123.387633146075));
#99897=CARTESIAN_POINT('Ctrl Pts',(5.55845823980584,-31.2180350899684,123.343673546936));
#99898=CARTESIAN_POINT('Ctrl Pts',(5.56232731315406,-31.1599987860128,123.302512198001));
#99899=CARTESIAN_POINT('Ctrl Pts',(5.56619638650228,-31.0998879711842,123.264418249305));
#99900=CARTESIAN_POINT('Ctrl Pts',(5.57005969489807,-31.0398667219847,123.22638106092));
#99901=CARTESIAN_POINT('Ctrl Pts',(5.57392300329386,-30.9777775045226,123.191402458471));
#99902=CARTESIAN_POINT('Ctrl Pts',(5.57778631168965,-30.9139654058242,123.159710675069));
#99903=CARTESIAN_POINT('Ctrl Pts',(5.58164508818257,-30.8502281627168,123.128056068114));
#99904=CARTESIAN_POINT('Ctrl Pts',(5.58550386467549,-30.7847724858286,123.099680836624));
#99905=CARTESIAN_POINT('Ctrl Pts',(5.58936264116841,-30.7179699078123,123.07476838433));
#99906=CARTESIAN_POINT('Ctrl Pts',(5.59321898675662,-30.651209413265,123.049871626077));
#99907=CARTESIAN_POINT('Ctrl Pts',(5.59707533234483,-30.5831041550974,123.028433488423));
#99908=CARTESIAN_POINT('Ctrl Pts',(5.60093167793304,-30.5140462386043,123.010589527755));
#99909=CARTESIAN_POINT('Ctrl Pts',(5.60478688417838,-30.4450087250143,122.992750839019));
#99910=CARTESIAN_POINT('Ctrl Pts',(5.60864209042371,-30.3750195819556,122.978504340595));
#99911=CARTESIAN_POINT('Ctrl Pts',(5.61249729666905,-30.3044850273202,122.967935426558));
#99912=CARTESIAN_POINT('Ctrl Pts',(5.6163526535203,-30.2339477172106,122.95736609964));
#99913=CARTESIAN_POINT('Ctrl Pts',(5.62020801037156,-30.1628654339714,122.950474712148));
#99914=CARTESIAN_POINT('Ctrl Pts',(5.62406336722281,-30.0916517938937,122.947295074499));
#99915=CARTESIAN_POINT('Ctrl Pts',(5.62792275969137,-30.0203636105222,122.944112108546));
#99916=CARTESIAN_POINT('Ctrl Pts',(5.63178215215993,-29.9489442821312,122.944648670073));
#99917=CARTESIAN_POINT('Ctrl Pts',(5.6356415446285,-29.8778088152267,122.948886430043));
#99918=CARTESIAN_POINT('Ctrl Pts',(5.63950312223194,-29.8066330724002,122.953126589374));
#99919=CARTESIAN_POINT('Ctrl Pts',(5.64336469983538,-29.7357419939932,122.961072064643));
#99920=CARTESIAN_POINT('Ctrl Pts',(5.64722627743882,-29.6655441007758,122.972652764331));
#99921=CARTESIAN_POINT('Ctrl Pts',(5.6510946115537,-29.595223383957,122.984253726497));
#99922=CARTESIAN_POINT('Ctrl Pts',(5.65496294566857,-29.5255987485067,122.999502507974));
#99923=CARTESIAN_POINT('Ctrl Pts',(5.65883127978345,-29.4570665004004,123.018278329958));
#99924=CARTESIAN_POINT('Ctrl Pts',(5.66112899895436,-29.4163596080734,123.029430822179));
#99925=CARTESIAN_POINT('Ctrl Pts',(5.66342671812527,-29.3760378167373,123.041826753286));
#99926=CARTESIAN_POINT('Ctrl Pts',(5.66572443729618,-29.336180780275,123.055432797247));
#99927=CARTESIAN_POINT('Ctrl Pts',(5.66959351064439,-29.2690664873416,123.078343683281));
#99928=CARTESIAN_POINT('Ctrl Pts',(5.6734625839926,-29.2030082382595,123.104778072836));
#99929=CARTESIAN_POINT('Ctrl Pts',(5.67733165734081,-29.1384019055373,123.134618997063));
#99930=CARTESIAN_POINT('Ctrl Pts',(5.68119496573659,-29.0738918368044,123.164415458058));
#99931=CARTESIAN_POINT('Ctrl Pts',(5.68505827413237,-29.010829827629,123.197608176431));
#99932=CARTESIAN_POINT('Ctrl Pts',(5.68892158252814,-28.9495947893972,123.234031014984));
#99933=CARTESIAN_POINT('Ctrl Pts',(5.69278035902105,-28.8884315837029,123.270411127264));
#99934=CARTESIAN_POINT('Ctrl Pts',(5.69663913551396,-28.8290915074142,123.31001358609));
#99935=CARTESIAN_POINT('Ctrl Pts',(5.70049791200687,-28.7719301519635,123.352625722295));
#99936=CARTESIAN_POINT('Ctrl Pts',(5.70435425759507,-28.7148048063227,123.395211014229));
#99937=CARTESIAN_POINT('Ctrl Pts',(5.70821060318327,-28.6598558470079,123.440801932254));
#99938=CARTESIAN_POINT('Ctrl Pts',(5.71206694877147,-28.6074098246745,123.489142572548));
#99939=CARTESIAN_POINT('Ctrl Pts',(5.7159221550168,-28.5549792973221,123.537468930781));
#99940=CARTESIAN_POINT('Ctrl Pts',(5.71977736126213,-28.5050505958757,123.588543069396));
#99941=CARTESIAN_POINT('Ctrl Pts',(5.72363256750745,-28.4579157816108,123.642070021726));
#99942=CARTESIAN_POINT('Ctrl Pts',(5.7274879243587,-28.4107791259965,123.695599065118));
#99943=CARTESIAN_POINT('Ctrl Pts',(5.73134328120994,-28.3664368936465,123.751580746428));
#99944=CARTESIAN_POINT('Ctrl Pts',(5.73519863806118,-28.3251418207865,123.809685906148));
#99945=CARTESIAN_POINT('Ctrl Pts',(5.73905803052974,-28.2838035220677,123.867851887784));
#99946=CARTESIAN_POINT('Ctrl Pts',(5.74291742299829,-28.2455190320528,123.928145388184));
#99947=CARTESIAN_POINT('Ctrl Pts',(5.74677681546684,-28.2104980363441,123.990207801292));
#99948=CARTESIAN_POINT('Ctrl Pts',(5.75063839307027,-28.1754572122299,124.052305353284));
#99949=CARTESIAN_POINT('Ctrl Pts',(5.7544999706737,-28.1436837771905,124.116173376588));
#99950=CARTESIAN_POINT('Ctrl Pts',(5.75836154827713,-28.1153404112816,124.181430639987));
#99951=CARTESIAN_POINT('Ctrl Pts',(5.762229882392,-28.0869474536525,124.246802082484));
#99952=CARTESIAN_POINT('Ctrl Pts',(5.76609821650687,-28.0619967174549,124.313567162888));
#99953=CARTESIAN_POINT('Ctrl Pts',(5.76996655062174,-28.0406016732831,124.3813274212));
#99954=CARTESIAN_POINT('Ctrl Pts',(5.77226426979274,-28.0278934113548,124.421575765819));
#99955=CARTESIAN_POINT('Ctrl Pts',(5.77456198896374,-28.0164386815439,124.462174966915));
#99956=CARTESIAN_POINT('Ctrl Pts',(5.77685970813474,-28.0062526866041,124.503040028949));
#99957=CARTESIAN_POINT('Ctrl Pts',(5.78191177765178,-27.9838564098157,124.592891363621));
#99958=CARTESIAN_POINT('Ctrl Pts',(5.78696384716883,-27.9675248955161,124.684310306518));
#99959=CARTESIAN_POINT('Ctrl Pts',(5.79201591668587,-27.9574316008725,124.776590292544));
#99960=CARTESIAN_POINT('Ctrl Pts',(5.79603551759484,-27.9494010272259,124.850011435));
#99961=CARTESIAN_POINT('Ctrl Pts',(5.80005511850382,-27.9453186463013,124.923977405746));
#99962=CARTESIAN_POINT('Ctrl Pts',(5.80407471941279,-27.9452508587689,124.998121407386));
#99963=CARTESIAN_POINT('Ctrl Pts',(5.80407471946233,-27.9452508587681,124.9981214083));
#99964=CARTESIAN_POINT('Ctrl Pts',(5.80788808427067,-27.9451865492831,125.068461258701));
#99965=CARTESIAN_POINT('Ctrl Pts',(5.81170144907901,-27.9487383877838,125.138896596668));
#99966=CARTESIAN_POINT('Ctrl Pts',(5.81551481388736,-27.9559090953207,125.209021376676));
#99967=CARTESIAN_POINT('Ctrl Pts',(5.81932566294071,-27.9630750721948,125.279099893928));
#99968=CARTESIAN_POINT('Ctrl Pts',(5.82313651199406,-27.9738551346033,125.34886776481));
#99969=CARTESIAN_POINT('Ctrl Pts',(5.82694736104741,-27.9881999804143,125.417921336731));
#99970=CARTESIAN_POINT('Ctrl Pts',(5.83075704398259,-28.0025404367087,125.486953778289));
#99971=CARTESIAN_POINT('Ctrl Pts',(5.83456672691777,-28.0204434107702,125.555271866755));
#99972=CARTESIAN_POINT('Ctrl Pts',(5.83837640985295,-28.0418083477081,125.622481337386));
#99973=CARTESIAN_POINT('Ctrl Pts',(5.84218627454128,-28.0631743039288,125.689694014461));
#99974=CARTESIAN_POINT('Ctrl Pts',(5.84599613922961,-28.0880023967571,125.755797494632));
#99975=CARTESIAN_POINT('Ctrl Pts',(5.84980600391794,-28.1161425514216,125.82041372242));
#99976=CARTESIAN_POINT('Ctrl Pts',(5.85361981396668,-28.1443118470297,125.885096864477));
#99977=CARTESIAN_POINT('Ctrl Pts',(5.85743362401542,-28.1757998467943,125.948289224173));
#99978=CARTESIAN_POINT('Ctrl Pts',(5.86124743406417,-28.2104092282852,126.009634801447));
#99979=CARTESIAN_POINT('Ctrl Pts',(5.8650635652738,-28.2450396737361,126.071017714863));
#99980=CARTESIAN_POINT('Ctrl Pts',(5.86887969648342,-28.2827950106818,126.130551190871));
#99981=CARTESIAN_POINT('Ctrl Pts',(5.87269582769305,-28.3234345959164,126.187908249121));
#99982=CARTESIAN_POINT('Ctrl Pts',(5.8765183006624,-28.3641417172158,126.245360625027));
#99983=CARTESIAN_POINT('Ctrl Pts',(5.88034077363176,-28.4077423369046,126.300628980537));
#99984=CARTESIAN_POINT('Ctrl Pts',(5.88416324660111,-28.4539562862319,126.353420259054));
#99985=CARTESIAN_POINT('Ctrl Pts',(5.88544049072517,-28.4693982516039,126.371059978374));
#99986=CARTESIAN_POINT('Ctrl Pts',(5.88671773484924,-28.4851317023621,126.388423448836));
#99987=CARTESIAN_POINT('Ctrl Pts',(5.8879949789733,-28.5011453432883,126.40550072236));
#99988=CARTESIAN_POINT('Ctrl Pts',(5.89186405232152,-28.5496544341878,126.45723180697));
#99989=CARTESIAN_POINT('Ctrl Pts',(5.89573312566973,-28.6009398356742,126.50654992552));
#99990=CARTESIAN_POINT('Ctrl Pts',(5.89960219901794,-28.6547319770886,126.553142462568));
#99991=CARTESIAN_POINT('Ctrl Pts',(5.90346550741373,-28.7084439677515,126.599665576337));
#99992=CARTESIAN_POINT('Ctrl Pts',(5.90732881580952,-28.7646549201417,126.643470854395));
#99993=CARTESIAN_POINT('Ctrl Pts',(5.9111921242053,-28.8230574377305,126.684281380179));
#99994=CARTESIAN_POINT('Ctrl Pts',(5.91505090069822,-28.8813914455059,126.725044032659));
#99995=CARTESIAN_POINT('Ctrl Pts',(5.91890967719113,-28.9419115156489,126.762818634033));
#99996=CARTESIAN_POINT('Ctrl Pts',(5.92276845368404,-29.0042774461901,126.797368676242));
#99997=CARTESIAN_POINT('Ctrl Pts',(5.92662479927225,-29.066604088207,126.831896953038));
#99998=CARTESIAN_POINT('Ctrl Pts',(5.93048114486046,-29.1307738596502,126.86320446602));
#99999=CARTESIAN_POINT('Ctrl Pts',(5.93433749044866,-29.1964191132023,126.891098971729));
#100000=CARTESIAN_POINT('Ctrl Pts',(5.93819269669399,-29.2620449721098,
126.918985236111));
#100001=CARTESIAN_POINT('Ctrl Pts',(5.94204790293932,-29.3291450008412,
126.943460305215));
#100002=CARTESIAN_POINT('Ctrl Pts',(5.94590310918465,-29.3973301517087,
126.964379448187));
#100003=CARTESIAN_POINT('Ctrl Pts',(5.9497584660359,-29.4655179662695,126.985299408379));
#100004=CARTESIAN_POINT('Ctrl Pts',(5.95361382288714,-29.5347905220617,
127.002663026264));
#100005=CARTESIAN_POINT('Ctrl Pts',(5.95746917973839,-29.6047437999571,
127.016375485575));
#100006=CARTESIAN_POINT('Ctrl Pts',(5.96132857220694,-29.674770301855,127.030102298483));
#100007=CARTESIAN_POINT('Ctrl Pts',(5.9651879646755,-29.7454784705754,127.040170229863));
#100008=CARTESIAN_POINT('Ctrl Pts',(5.96904735714406,-29.8164551747296,
127.046535819285));
#100009=CARTESIAN_POINT('Ctrl Pts',(5.97290893474749,-29.8874720649164,
127.052905012816));
#100010=CARTESIAN_POINT('Ctrl Pts',(5.97677051235093,-29.9587573075263,
127.055567673329));
#100011=CARTESIAN_POINT('Ctrl Pts',(5.98063208995436,-30.0298965035962,
127.054532492216));
#100012=CARTESIAN_POINT('Ctrl Pts',(5.98450042406923,-30.101160170243,127.053495499872));
#100013=CARTESIAN_POINT('Ctrl Pts',(5.9883687581841,-30.1722767953073,127.048747780675));
#100014=CARTESIAN_POINT('Ctrl Pts',(5.99223709229897,-30.2428365374347,
127.040349964733));
#100015=CARTESIAN_POINT('Ctrl Pts',(5.99453481146993,-30.2847477238447,
127.035361816835));
#100016=CARTESIAN_POINT('Ctrl Pts',(5.9968325306409,-30.3264625982632,127.029086849354));
#100017=CARTESIAN_POINT('Ctrl Pts',(5.99913024981186,-30.3678974432213,
127.021546198772));
#100018=CARTESIAN_POINT('Ctrl Pts',(6.00299944643829,-30.4376707925297,
127.008848276345));
#100019=CARTESIAN_POINT('Ctrl Pts',(6.00686864306471,-30.5069226418422,
126.992508916016));
#100020=CARTESIAN_POINT('Ctrl Pts',(6.01073783969114,-30.5752441048594,
126.97258505072));
#100021=CARTESIAN_POINT('Ctrl Pts',(6.01460043069505,-30.6434489271788,
126.952695200116));
#100022=CARTESIAN_POINT('Ctrl Pts',(6.01846302169896,-30.7107260565041,
126.929233137685));
#100023=CARTESIAN_POINT('Ctrl Pts',(6.02232561270287,-30.776676344021,126.902306867763));
#100024=CARTESIAN_POINT('Ctrl Pts',(6.0261843740982,-30.8425612443958,126.875407294189));
#100025=CARTESIAN_POINT('Ctrl Pts',(6.03004313549353,-30.907121465364,126.845050509387));
#100026=CARTESIAN_POINT('Ctrl Pts',(6.03390189688886,-30.9699737945266,
126.811394048911));
#100027=CARTESIAN_POINT('Ctrl Pts',(6.03775817556289,-31.0327856845946,
126.777759242952));
#100028=CARTESIAN_POINT('Ctrl Pts',(6.04161445423691,-31.0938914361431,
126.740829202853));
#100029=CARTESIAN_POINT('Ctrl Pts',(6.04547073291094,-31.1529301530049,
126.700808520908));
#100030=CARTESIAN_POINT('Ctrl Pts',(6.04767405776819,-31.1866625368388,
126.677942288774));
#100031=CARTESIAN_POINT('Ctrl Pts',(6.04987738262545,-31.2197205644288,
126.654067962738));
#100032=CARTESIAN_POINT('Ctrl Pts',(6.05208070748271,-31.2520409112986,
126.629230222815));
#100033=CARTESIAN_POINT('',(5.7459252805733,-27.9452507587439,125.001765802243));
#100034=CARTESIAN_POINT('Ctrl Pts',(5.7459252805733,-27.9452507587439,125.001765802243));
#100035=CARTESIAN_POINT('Ctrl Pts',(5.75057817989281,-27.9453246481717,
125.087746124361));
#100036=CARTESIAN_POINT('Ctrl Pts',(5.75523107921231,-27.950799087127,125.173490900306));
#100037=CARTESIAN_POINT('Ctrl Pts',(5.75988397853181,-27.9615629769852,
125.258402913494));
#100038=CARTESIAN_POINT('Ctrl Pts',(5.76460377517644,-27.9724816252832,
125.344535753992));
#100039=CARTESIAN_POINT('Ctrl Pts',(5.76932357182106,-27.9888428428069,
125.42981172288));
#100040=CARTESIAN_POINT('Ctrl Pts',(5.77404336846569,-28.0104818888308,
125.513629484969));
#100041=CARTESIAN_POINT('Ctrl Pts',(5.77570694017882,-28.018108934565,125.54317246501));
#100042=CARTESIAN_POINT('Ctrl Pts',(5.77737051189196,-28.0263912273211,
125.572534484293));
#100043=CARTESIAN_POINT('Ctrl Pts',(5.77903408360509,-28.0353201550616,
125.601689844848));
#100044=CARTESIAN_POINT('Ctrl Pts',(5.78290315695331,-28.0560867238102,
125.669498300347));
#100045=CARTESIAN_POINT('Ctrl Pts',(5.78677223030153,-28.0804085753381,
125.736363214624));
#100046=CARTESIAN_POINT('Ctrl Pts',(5.79064130364974,-28.1081813798381,
125.801885198086));
#100047=CARTESIAN_POINT('Ctrl Pts',(5.79450461204553,-28.1359128026216,
125.867309553231));
#100048=CARTESIAN_POINT('Ctrl Pts',(5.79836792044132,-28.1670847837139,
125.931394505826));
#100049=CARTESIAN_POINT('Ctrl Pts',(5.80223122883711,-28.2015433108011,
125.993756056372));
#100050=CARTESIAN_POINT('Ctrl Pts',(5.80609000533003,-28.2359614158763,
126.056044452911));
#100051=CARTESIAN_POINT('Ctrl Pts',(5.80994878182294,-28.2736581751636,
126.116613039969));
#100052=CARTESIAN_POINT('Ctrl Pts',(5.81380755831586,-28.3144323268255,
126.17509964754));
#100053=CARTESIAN_POINT('Ctrl Pts',(5.81766390390407,-28.3551807920873,
126.233549410435));
#100054=CARTESIAN_POINT('Ctrl Pts',(5.82152024949228,-28.3990025262966,
126.289919398435));
#100055=CARTESIAN_POINT('Ctrl Pts',(5.82537659508049,-28.4456521319437,
126.343875093738));
#100056=CARTESIAN_POINT('Ctrl Pts',(5.82923180132583,-28.4922879551394,
126.397814848033));
#100057=CARTESIAN_POINT('Ctrl Pts',(5.83308700757117,-28.5417496735587,
126.449341358437));
#100058=CARTESIAN_POINT('Ctrl Pts',(5.8369422138165,-28.5937517505778,126.498153337779));
#100059=CARTESIAN_POINT('Ctrl Pts',(5.84079757066776,-28.6457558590888,
126.546967223989));
#100060=CARTESIAN_POINT('Ctrl Pts',(5.84465292751901,-28.7003001675264,
126.593066037739));
#100061=CARTESIAN_POINT('Ctrl Pts',(5.84850828437026,-28.7570637140312,
126.636186710471));
#100062=CARTESIAN_POINT('Ctrl Pts',(5.85236767683882,-28.81388667811,126.679352520019));
#100063=CARTESIAN_POINT('Ctrl Pts',(5.85622706930739,-28.8729331298652,
126.719533671088));
#100064=CARTESIAN_POINT('Ctrl Pts',(5.86008646177595,-28.9338513077071,
126.756509188254));
#100065=CARTESIAN_POINT('Ctrl Pts',(5.86394803937939,-28.9948039765826,
126.793505640449));
#100066=CARTESIAN_POINT('Ctrl Pts',(5.86780961698283,-29.0576300531272,
126.827292615469));
#100067=CARTESIAN_POINT('Ctrl Pts',(5.87167119458628,-29.1219536682809,
126.85769540072));
#100068=CARTESIAN_POINT('Ctrl Pts',(5.87553952870115,-29.1863898289499,
126.888151381008));
#100069=CARTESIAN_POINT('Ctrl Pts',(5.87940786281603,-29.2523283099923,
126.915211165115));
#100070=CARTESIAN_POINT('Ctrl Pts',(5.8832761969309,-29.3193744584979,126.938748677564));
#100071=CARTESIAN_POINT('Ctrl Pts',(5.88557391610182,-29.3591986350511,
126.952729526162));
#100072=CARTESIAN_POINT('Ctrl Pts',(5.88787163527273,-29.3994133254093,
126.965468625186));
#100073=CARTESIAN_POINT('Ctrl Pts',(5.89016935444365,-29.43993406007,126.976948078587));
#100074=CARTESIAN_POINT('Ctrl Pts',(5.89403860385592,-29.5081690431589,
126.996278930193));
#100075=CARTESIAN_POINT('Ctrl Pts',(5.89790785326819,-29.5775396773508,
127.012110772205));
#100076=CARTESIAN_POINT('Ctrl Pts',(5.90177710268046,-29.6476537793551,
127.02431462557));
#100077=CARTESIAN_POINT('Ctrl Pts',(5.9056396209416,-29.7176459071555,127.036497248466));
#100078=CARTESIAN_POINT('Ctrl Pts',(5.90950213920275,-29.7883784582127,
127.045064340978));
#100079=CARTESIAN_POINT('Ctrl Pts',(5.9133646574639,-29.859445536846,127.049937073519));
#100080=CARTESIAN_POINT('Ctrl Pts',(5.91722337855584,-29.9304427507683,
127.054805015768));
#100081=CARTESIAN_POINT('Ctrl Pts',(5.92108209964779,-30.0017733579082,
127.055985769382));
#100082=CARTESIAN_POINT('Ctrl Pts',(5.92494082073974,-30.0730239449286,
127.053451987743));
#100083=CARTESIAN_POINT('Ctrl Pts',(5.92879703930301,-30.1442283232098,
127.050919849359));
#100084=CARTESIAN_POINT('Ctrl Pts',(5.93265325786629,-30.2153523000852,
127.044677973575));
#100085=CARTESIAN_POINT('Ctrl Pts',(5.93650947642956,-30.2859817782854,
127.03475108674));
#100086=CARTESIAN_POINT('Ctrl Pts',(5.94036448407856,-30.3565890777004,
127.024827317106));
#100087=CARTESIAN_POINT('Ctrl Pts',(5.94421949172756,-30.426701706177,127.011220902373));
#100088=CARTESIAN_POINT('Ctrl Pts',(5.94807449937655,-30.4959117352762,
126.994008303221));
#100089=CARTESIAN_POINT('Ctrl Pts',(5.95193183765649,-30.5651636068437,
126.976785297808));
#100090=CARTESIAN_POINT('Ctrl Pts',(5.95578917593642,-30.6335113149249,
126.955951863161));
#100091=CARTESIAN_POINT('Ctrl Pts',(5.95964651421635,-30.7005591566621,
126.931635170139));
#100092=CARTESIAN_POINT('Ctrl Pts',(5.96350485068189,-30.7676243487548,
126.907312184546));
#100093=CARTESIAN_POINT('Ctrl Pts',(5.96736318714743,-30.8333885532979,
126.879504327398));
#100094=CARTESIAN_POINT('Ctrl Pts',(5.97122152361297,-30.8974756479425,
126.848387141226));
#100095=CARTESIAN_POINT('Ctrl Pts',(5.97508578864652,-30.9616612162953,
126.81722214161));
#100096=CARTESIAN_POINT('Ctrl Pts',(5.97895005368007,-31.0241640955484,
126.782737881713));
#100097=CARTESIAN_POINT('Ctrl Pts',(5.98281431871362,-31.0846329215314,
126.745155863535));
#100098=CARTESIAN_POINT('Ctrl Pts',(5.98650489602956,-31.1423838458485,
126.709263050135));
#100099=CARTESIAN_POINT('Ctrl Pts',(5.99019547334549,-31.1982793576751,
126.670545233824));
#100100=CARTESIAN_POINT('Ctrl Pts',(5.99388605066143,-31.2520409112987,
126.629230222815));
#100101=CARTESIAN_POINT('Ctrl Pts',(5.29388025174645,-31.2520409112987,
126.629230222815));
#100102=CARTESIAN_POINT('Ctrl Pts',(5.29773979436079,-31.3086193501602,
126.585750474428));
#100103=CARTESIAN_POINT('Ctrl Pts',(5.30159933697512,-31.3629005188046,
126.539342938539));
#100104=CARTESIAN_POINT('Ctrl Pts',(5.30545887958946,-31.4145793687864,
126.49028949265));
#100105=CARTESIAN_POINT('Ctrl Pts',(5.30932071234183,-31.4662888834641,
126.441206939902));
#100106=CARTESIAN_POINT('Ctrl Pts',(5.31318254509421,-31.5153926716702,
126.389475704715));
#100107=CARTESIAN_POINT('Ctrl Pts',(5.31704437784659,-31.5616240719298,
126.335412977498));
#100108=CARTESIAN_POINT('Ctrl Pts',(5.32091286057165,-31.6079350814237,
126.281257155711));
#100109=CARTESIAN_POINT('Ctrl Pts',(5.32478134329671,-31.651363534228,126.224762213207));
#100110=CARTESIAN_POINT('Ctrl Pts',(5.32864982602178,-31.6916848663766,
126.16627607168));
#100111=CARTESIAN_POINT('Ctrl Pts',(5.3305975507648,-31.7119860702023,126.136829150736));
#100112=CARTESIAN_POINT('Ctrl Pts',(5.33254527550783,-31.731500337346,126.106877886012));
#100113=CARTESIAN_POINT('Ctrl Pts',(5.33449300025086,-31.7502034628655,
126.076468950353));
#100114=CARTESIAN_POINT('Ctrl Pts',(5.33836207359907,-31.7873564357046,
126.016062877612));
#100115=CARTESIAN_POINT('Ctrl Pts',(5.34223114694728,-31.8214512506891,
125.953612795033));
#100116=CARTESIAN_POINT('Ctrl Pts',(5.34610022029549,-31.8522571895629,
125.889460997578));
#100117=CARTESIAN_POINT('Ctrl Pts',(5.34996352869127,-31.883017227324,125.825404786851));
#100118=CARTESIAN_POINT('Ctrl Pts',(5.35382683708705,-31.9104979076632,
125.759652328628));
#100119=CARTESIAN_POINT('Ctrl Pts',(5.35769014548283,-31.9345129022425,
125.692573023989));
#100120=CARTESIAN_POINT('Ctrl Pts',(5.36154892197574,-31.958499725728,125.625572407579));
#100121=CARTESIAN_POINT('Ctrl Pts',(5.36540769846865,-31.9790287759014,
125.557248491575));
#100122=CARTESIAN_POINT('Ctrl Pts',(5.36926647496156,-31.9959613378882,
125.487991700909));
#100123=CARTESIAN_POINT('Ctrl Pts',(5.37312282054977,-32.0128832329071,
125.418778539786));
#100124=CARTESIAN_POINT('Ctrl Pts',(5.37697916613797,-32.0262130196964,
125.34863414072));
#100125=CARTESIAN_POINT('Ctrl Pts',(5.38083551172617,-32.0358619075833,
125.277963766975));
#100126=CARTESIAN_POINT('Ctrl Pts',(5.3846907179715,-32.0455079447425,125.207314272528));
#100127=CARTESIAN_POINT('Ctrl Pts',(5.38854592421683,-32.0514751763227,
125.136139592967));
#100128=CARTESIAN_POINT('Ctrl Pts',(5.39240113046216,-32.053726279784,125.06485314352));
#100129=CARTESIAN_POINT('Ctrl Pts',(5.3962564873134,-32.055977471186,124.993563909226));
#100130=CARTESIAN_POINT('Ctrl Pts',(5.40011184416465,-32.0545122331165,
124.922163381991));
#100131=CARTESIAN_POINT('Ctrl Pts',(5.40396720101589,-32.049345337888,124.851066294692));
#100132=CARTESIAN_POINT('Ctrl Pts',(5.40782659348445,-32.0441730341816,
124.779894786102));
#100133=CARTESIAN_POINT('Ctrl Pts',(5.411685985953,-32.0352913737652,124.709027837005));
#100134=CARTESIAN_POINT('Ctrl Pts',(5.41554537842156,-32.0227670734458,
124.638875465963));
#100135=CARTESIAN_POINT('Ctrl Pts',(5.41940695602499,-32.01023568204,124.568683375614));
#100136=CARTESIAN_POINT('Ctrl Pts',(5.42326853362843,-31.9940576553275,
124.499207142076));
#100137=CARTESIAN_POINT('Ctrl Pts',(5.42713011123186,-31.9743503595413,
124.43084429171));
#100138=CARTESIAN_POINT('Ctrl Pts',(5.43099844534673,-31.9546085823636,
124.362361828474));
#100139=CARTESIAN_POINT('Ctrl Pts',(5.4348667794616,-31.9313253661288,124.294997097049));
#100140=CARTESIAN_POINT('Ctrl Pts',(5.43873511357647,-31.9046669889531,
124.229129567507));
#100141=CARTESIAN_POINT('Ctrl Pts',(5.44103283274745,-31.8888324042236,
124.190005468895));
#100142=CARTESIAN_POINT('Ctrl Pts',(5.44333055191843,-31.8718079232597,
124.151409186527));
#100143=CARTESIAN_POINT('Ctrl Pts',(5.44562827108941,-31.8536359549887,
124.113415932428));
#100144=CARTESIAN_POINT('Ctrl Pts',(5.44949734443762,-31.823036620218,124.049440017222));
#100145=CARTESIAN_POINT('Ctrl Pts',(5.45336641778584,-31.7890613887607,
123.986924796112));
#100146=CARTESIAN_POINT('Ctrl Pts',(5.45723549113406,-31.7518727042285,
123.926249754049));
#100147=CARTESIAN_POINT('Ctrl Pts',(5.46109879952985,-31.7147394311548,
123.865665118319));
#100148=CARTESIAN_POINT('Ctrl Pts',(5.46496210792564,-31.6744024609846,
123.80691562988));
#100149=CARTESIAN_POINT('Ctrl Pts',(5.46882541632144,-31.6310710858574,
123.750358181165));
#100150=CARTESIAN_POINT('Ctrl Pts',(5.47268419281435,-31.587790541149,123.693867077883));
#100151=CARTESIAN_POINT('Ctrl Pts',(5.47654296930726,-31.5415228627519,
123.639563290402));
#100152=CARTESIAN_POINT('Ctrl Pts',(5.48040174580018,-31.4925208296892,
123.58777511159));
#100153=CARTESIAN_POINT('Ctrl Pts',(5.48425809138838,-31.4435496663265,
123.536019557661));
#100154=CARTESIAN_POINT('Ctrl Pts',(5.48811443697659,-31.3918478989099,
123.486776820306));
#100155=CARTESIAN_POINT('Ctrl Pts',(5.4919707825648,-31.3377078498883,123.440341296678));
#100156=CARTESIAN_POINT('Ctrl Pts',(5.49582598881013,-31.2835837963415,
123.393919492252));
#100157=CARTESIAN_POINT('Ctrl Pts',(5.49968119505546,-31.2270232598807,
123.350303571092));
#100158=CARTESIAN_POINT('Ctrl Pts',(5.5035364013008,-31.168353326242,123.309749111061));
#100159=CARTESIAN_POINT('Ctrl Pts',(5.50739175815204,-31.1096811006276,
123.269193066746));
#100160=CARTESIAN_POINT('Ctrl Pts',(5.51124711500329,-31.0488997150945,
123.231698995419));
#100161=CARTESIAN_POINT('Ctrl Pts',(5.51510247185453,-30.9863656167697,
123.197479422432));
#100162=CARTESIAN_POINT('Ctrl Pts',(5.51896186432309,-30.923766060512,123.163224029908));
#100163=CARTESIAN_POINT('Ctrl Pts',(5.52282125679164,-30.859410556091,123.132250211661));
#100164=CARTESIAN_POINT('Ctrl Pts',(5.5266806492602,-30.7936797627607,123.104724295337));
#100165=CARTESIAN_POINT('Ctrl Pts',(5.53054222686363,-30.7279117535604,
123.077182794219));
#100166=CARTESIAN_POINT('Ctrl Pts',(5.53440380446706,-30.6607673628248,
123.053093245288));
#100167=CARTESIAN_POINT('Ctrl Pts',(5.5382653820705,-30.5926442249959,123.032572648081));
#100168=CARTESIAN_POINT('Ctrl Pts',(5.54213371618537,-30.5244018937161,
123.012016146468));
#100169=CARTESIAN_POINT('Ctrl Pts',(5.54600205030024,-30.4551778682629,
122.995041179658));
#100170=CARTESIAN_POINT('Ctrl Pts',(5.54987038441511,-30.3853811412496,
122.981713861102));
#100171=CARTESIAN_POINT('Ctrl Pts',(5.55216810358607,-30.3439231717553,
122.973797679501));
#100172=CARTESIAN_POINT('Ctrl Pts',(5.55446582275702,-30.3022632866963,
122.967167450132));
#100173=CARTESIAN_POINT('Ctrl Pts',(5.55676354192797,-30.260487676048,122.961828335707));
#100174=CARTESIAN_POINT('Ctrl Pts',(5.56063261527619,-30.1901427427731,
122.952837930967));
#100175=CARTESIAN_POINT('Ctrl Pts',(5.56450168862441,-30.1191940371151,
122.947475992101));
#100176=CARTESIAN_POINT('Ctrl Pts',(5.56837076197263,-30.0480484844915,
122.945811862161));
#100177=CARTESIAN_POINT('Ctrl Pts',(5.57223407036841,-29.9770089393508,
122.944150211789));
#100178=CARTESIAN_POINT('Ctrl Pts',(5.5760973787642,-29.9057736111404,122.946175444879));
#100179=CARTESIAN_POINT('Ctrl Pts',(5.57996068715999,-29.8347558532781,
122.951905291625));
#100180=CARTESIAN_POINT('Ctrl Pts',(5.5838194636529,-29.7638214036968,122.957628416901));
#100181=CARTESIAN_POINT('Ctrl Pts',(5.58767824014582,-29.6931044993654,
122.967047484839));
#100182=CARTESIAN_POINT('Ctrl Pts',(5.59153701663873,-29.6230180516856,
122.980128179031));
#100183=CARTESIAN_POINT('Ctrl Pts',(5.59539336222694,-29.5529757562069,
122.993200632807));
#100184=CARTESIAN_POINT('Ctrl Pts',(5.59924970781514,-29.4835636058172,
123.009930047454));
#100185=CARTESIAN_POINT('Ctrl Pts',(5.60310605340335,-29.4151874815842,
123.03023050059));
#100186=CARTESIAN_POINT('Ctrl Pts',(5.60696125964868,-29.3468315588213,
123.050524956034));
#100187=CARTESIAN_POINT('Ctrl Pts',(5.61081646589401,-29.2795115199826,
123.074388217214));
#100188=CARTESIAN_POINT('Ctrl Pts',(5.61467167213934,-29.2136194867204,
123.101684101411));
#100189=CARTESIAN_POINT('Ctrl Pts',(5.61852702899058,-29.147724879347,123.128981051939));
#100190=CARTESIAN_POINT('Ctrl Pts',(5.62238238584182,-29.0832588362644,
123.159710703764));
#100191=CARTESIAN_POINT('Ctrl Pts',(5.62623774269306,-29.0205932334001,
123.193688856249));
#100192=CARTESIAN_POINT('Ctrl Pts',(5.63009713516162,-28.9578620349498,
123.227702575564));
#100193=CARTESIAN_POINT('Ctrl Pts',(5.63395652763018,-28.8969354667703,
123.264971351449));
#100194=CARTESIAN_POINT('Ctrl Pts',(5.63781592009874,-28.8381597238708,
123.305265585626));
#100195=CARTESIAN_POINT('Ctrl Pts',(5.64167749770218,-28.7793507029549,
123.345582633843));
#100196=CARTESIAN_POINT('Ctrl Pts',(5.64553907530561,-28.7226953175207,
123.388928255032));
#100197=CARTESIAN_POINT('Ctrl Pts',(5.64940065290904,-28.6685075266158,
123.435031835525));
#100198=CARTESIAN_POINT('Ctrl Pts',(5.65326898702391,-28.6142249246086,
123.481216082367));
#100199=CARTESIAN_POINT('Ctrl Pts',(5.65713732113878,-28.5624188903334,
123.530167589093));
#100200=CARTESIAN_POINT('Ctrl Pts',(5.66100565525365,-28.5133667914834,
123.581578600755));
#100201=CARTESIAN_POINT('Ctrl Pts',(5.66330337442461,-28.4842307487951,
123.612115794179));
#100202=CARTESIAN_POINT('Ctrl Pts',(5.66560109359557,-28.4560655788399,
123.64352007997));
#100203=CARTESIAN_POINT('Ctrl Pts',(5.66789881276654,-28.428922365385,123.675721846245));
#100204=CARTESIAN_POINT('Ctrl Pts',(5.6717431454675,-28.3835088333867,123.729598884259));
#100205=CARTESIAN_POINT('Ctrl Pts',(5.67558747816845,-28.3407741615803,
123.785928448142));
#100206=CARTESIAN_POINT('Ctrl Pts',(5.67943181086941,-28.3009964282984,
123.844411653812));
#100207=CARTESIAN_POINT('Ctrl Pts',(5.68327073565049,-28.2612746513583,
123.90281258968));
#100208=CARTESIAN_POINT('Ctrl Pts',(5.68710966043156,-28.2245018386301,
123.963360756745));
#100209=CARTESIAN_POINT('Ctrl Pts',(5.69094858521263,-28.1909165779052,
124.025723481551));
#100210=CARTESIAN_POINT('Ctrl Pts',(5.69478343427791,-28.1573669740336,
124.088019996998));
#100211=CARTESIAN_POINT('Ctrl Pts',(5.69861828334319,-28.1269984405786,
124.15212681733));
#100212=CARTESIAN_POINT('Ctrl Pts',(5.70245313240846,-28.1000058717301,
124.217683008596));
#100213=CARTESIAN_POINT('Ctrl Pts',(5.70628582152496,-28.0730285062352,
124.283202275849));
#100214=CARTESIAN_POINT('Ctrl Pts',(5.71011851064145,-28.0494235257518,
124.350168842791));
#100215=CARTESIAN_POINT('Ctrl Pts',(5.71395119975794,-28.0293387874971,
124.418199391512));
#100216=CARTESIAN_POINT('Ctrl Pts',(5.71778249936723,-28.0092613307849,
124.486205276366));
#100217=CARTESIAN_POINT('Ctrl Pts',(5.72161379897651,-27.9927017184503,
124.55527390418));
#100218=CARTESIAN_POINT('Ctrl Pts',(5.7254450985858,-27.9797581310329,124.625006195555));
#100219=CARTESIAN_POINT('Ctrl Pts',(5.72927810286555,-27.9668087845902,
124.694769513106));
#100220=CARTESIAN_POINT('Ctrl Pts',(5.73311110714531,-27.9574787693273,
124.765196599802));
#100221=CARTESIAN_POINT('Ctrl Pts',(5.73694411142506,-27.9518149998427,
124.835878802007));
#100222=CARTESIAN_POINT('Ctrl Pts',(5.7399378344626,-27.947391379114,124.891084307047));
#100223=CARTESIAN_POINT('Ctrl Pts',(5.74293155750014,-27.9452032175471,
124.946445182456));
#100224=CARTESIAN_POINT('Ctrl Pts',(5.74592528053768,-27.9452507587434,
125.001765801585));
#100225=CARTESIAN_POINT('Origin',(-1.54592528053767,-30.,125.));
#100226=CARTESIAN_POINT('',(4.59397334877082,-31.2520409112987,126.629230222815));
#100227=CARTESIAN_POINT('',(4.65201706724701,-31.2520409112987,126.629230222815));
#100228=CARTESIAN_POINT('',(-1.54592528053767,-31.2520409112987,126.629230222815));
#100229=CARTESIAN_POINT('',(5.10407471942417,-27.9452501074214,125.000664415721));
#100230=CARTESIAN_POINT('Ctrl Pts',(4.65201706724701,-31.2520409112987,
126.629230222815));
#100231=CARTESIAN_POINT('Ctrl Pts',(4.6558862157949,-31.3084969643693,126.585844526217));
#100232=CARTESIAN_POINT('Ctrl Pts',(4.65975536434279,-31.3626115695028,
126.539585323213));
#100233=CARTESIAN_POINT('Ctrl Pts',(4.66362451289068,-31.4140958918003,
126.49074825886));
#100234=CARTESIAN_POINT('Ctrl Pts',(4.66425200851017,-31.4224455807083,
126.482827900266));
#100235=CARTESIAN_POINT('Ctrl Pts',(4.66487950412965,-31.430726172515,126.474839810443));
#100236=CARTESIAN_POINT('Ctrl Pts',(4.66550699974914,-31.4389365354662,
126.466785331738));
#100237=CARTESIAN_POINT('Ctrl Pts',(4.66937607309736,-31.4895607876316,
126.417122245773));
#100238=CARTESIAN_POINT('Ctrl Pts',(4.67324514644558,-31.5377100925751,
126.364737957514));
#100239=CARTESIAN_POINT('Ctrl Pts',(4.6771142197938,-31.5830779920416,126.309909017304));
#100240=CARTESIAN_POINT('Ctrl Pts',(4.68097752818959,-31.6283782929492,
126.255161772684));
#100241=CARTESIAN_POINT('Ctrl Pts',(4.68484083658538,-31.6709051075679,
126.197977477701));
#100242=CARTESIAN_POINT('Ctrl Pts',(4.68870414498117,-31.7103885202681,
126.138669694088));
#100243=CARTESIAN_POINT('Ctrl Pts',(4.69256292147409,-31.7498256164506,
126.079431482223));
#100244=CARTESIAN_POINT('Ctrl Pts',(4.696421697967,-31.7862261342446,126.018075132076));
#100245=CARTESIAN_POINT('Ctrl Pts',(4.70028047445992,-31.8193612958819,
125.954946091435));
#100246=CARTESIAN_POINT('Ctrl Pts',(4.70413682004813,-31.8524755834363,
125.891856820054));
#100247=CARTESIAN_POINT('Ctrl Pts',(4.70799316563634,-31.8823283707902,
125.826997502887));
#100248=CARTESIAN_POINT('Ctrl Pts',(4.71184951122455,-31.908735752307,125.760740028108));
#100249=CARTESIAN_POINT('Ctrl Pts',(4.71570471746989,-31.9351353318617,
125.694502128851));
#100250=CARTESIAN_POINT('Ctrl Pts',(4.71955992371522,-31.9580913466996,
125.626867343081));
#100251=CARTESIAN_POINT('Ctrl Pts',(4.72341512996056,-31.9774678742001,
125.558227882684));
#100252=CARTESIAN_POINT('Ctrl Pts',(4.72727048681181,-31.9968451586562,
125.489585740846));
#100253=CARTESIAN_POINT('Ctrl Pts',(4.73112584366306,-32.0126425482943,
125.419939314573));
#100254=CARTESIAN_POINT('Ctrl Pts',(4.73498120051431,-32.0247743599364,
125.349694658015));
#100255=CARTESIAN_POINT('Ctrl Pts',(4.73884059298288,-32.0369188706232,
125.279376472452));
#100256=CARTESIAN_POINT('Ctrl Pts',(4.74269998545144,-32.0453900610247,
125.208459286247));
#100257=CARTESIAN_POINT('Ctrl Pts',(4.74655937792,-32.0501537961902,125.137357105629));
#100258=CARTESIAN_POINT('Ctrl Pts',(4.75042095552344,-32.054920228517,125.066214667936));
#100259=CARTESIAN_POINT('Ctrl Pts',(4.75428253312688,-32.0559750197405,
124.994887513286));
#100260=CARTESIAN_POINT('Ctrl Pts',(4.75814411073032,-32.0533362020555,
124.92378973935));
#100261=CARTESIAN_POINT('Ctrl Pts',(4.7620124448452,-32.0506927672933,124.852567567313));
#100262=CARTESIAN_POINT('Ctrl Pts',(4.76588077896007,-32.0443428641056,
124.781576061288));
#100263=CARTESIAN_POINT('Ctrl Pts',(4.76974911307495,-32.0343563474446,
124.71122359149));
#100264=CARTESIAN_POINT('Ctrl Pts',(4.77204683224587,-32.0284245405993,
124.669435521025));
#100265=CARTESIAN_POINT('Ctrl Pts',(4.77434455141679,-32.0212106673077,
124.627872725201));
#100266=CARTESIAN_POINT('Ctrl Pts',(4.7766422705877,-32.0127377461674,124.586618423665));
#100267=CARTESIAN_POINT('Ctrl Pts',(4.78051134393591,-31.9984704006274,
124.517151310108));
#100268=CARTESIAN_POINT('Ctrl Pts',(4.78438041728412,-31.9805745320217,
124.448287625122));
#100269=CARTESIAN_POINT('Ctrl Pts',(4.78824949063234,-31.959116270389,124.380434828612));
#100270=CARTESIAN_POINT('Ctrl Pts',(4.79211279902812,-31.9376899817499,
124.31268313335));
#100271=CARTESIAN_POINT('Ctrl Pts',(4.7959761074239,-31.9127119815917,124.245939796136));
#100272=CARTESIAN_POINT('Ctrl Pts',(4.79983941581968,-31.8842993142417,
124.180601649472));
#100273=CARTESIAN_POINT('Ctrl Pts',(4.80369819231259,-31.8559199767311,
124.115340148548));
#100274=CARTESIAN_POINT('Ctrl Pts',(4.8075569688055,-31.8241141679269,124.051481007266));
#100275=CARTESIAN_POINT('Ctrl Pts',(4.8114157452984,-31.7890480327179,123.989403790266));
#100276=CARTESIAN_POINT('Ctrl Pts',(4.81527209088661,-31.7540039880429,
123.927365679911));
#100277=CARTESIAN_POINT('Ctrl Pts',(4.81912843647481,-31.7157039302298,
123.867107688676));
#100278=CARTESIAN_POINT('Ctrl Pts',(4.82298478206301,-31.6743605549191,
123.808986022487));
#100279=CARTESIAN_POINT('Ctrl Pts',(4.82683998830834,-31.633029394354,123.750881528127));
#100280=CARTESIAN_POINT('Ctrl Pts',(4.83069519455367,-31.588656982754,123.694912501405));
#100281=CARTESIAN_POINT('Ctrl Pts',(4.834550400799,-31.5414991148619,123.641405858477));
#100282=CARTESIAN_POINT('Ctrl Pts',(4.83840575765024,-31.4943394047199,
123.587897125281));
#100283=CARTESIAN_POINT('Ctrl Pts',(4.84226111450148,-31.4443943450995,
123.536851329846));
#100284=CARTESIAN_POINT('Ctrl Pts',(4.84611647135272,-31.3919586083017,
123.488560687532));
#100285=CARTESIAN_POINT('Ctrl Pts',(4.84997586382128,-31.33946798409,123.440219496705));
#100286=CARTESIAN_POINT('Ctrl Pts',(4.85383525628983,-31.28448183635,123.394639545819));
#100287=CARTESIAN_POINT('Ctrl Pts',(4.85769464875839,-31.2273294761779,
123.352074055242));
#100288=CARTESIAN_POINT('Ctrl Pts',(4.86155622636182,-31.1701447571263,
123.309484464671));
#100289=CARTESIAN_POINT('Ctrl Pts',(4.86541780396525,-31.1107917884811,
123.269913001621));
#100290=CARTESIAN_POINT('Ctrl Pts',(4.86927938156868,-31.0496282517474,
123.233569108164));
#100291=CARTESIAN_POINT('Ctrl Pts',(4.87314771568355,-30.9883576986132,
123.197161624652));
#100292=CARTESIAN_POINT('Ctrl Pts',(4.87701604979842,-30.9252706826861,
123.163993211673));
#100293=CARTESIAN_POINT('Ctrl Pts',(4.88088438391328,-30.8607481803879,
123.134226666377));
#100294=CARTESIAN_POINT('Ctrl Pts',(4.88318210308428,-30.8224230031699,
123.116545887067));
#100295=CARTESIAN_POINT('Ctrl Pts',(4.88547982225527,-30.7835917421951,
123.100064408499));
#100296=CARTESIAN_POINT('Ctrl Pts',(4.88777754142627,-30.7443367983746,
123.084808027094));
#100297=CARTESIAN_POINT('Ctrl Pts',(4.89164661477449,-30.6782363545784,
123.059118178033));
#100298=CARTESIAN_POINT('Ctrl Pts',(4.8955156881227,-30.6106748968161,123.036804087238));
#100299=CARTESIAN_POINT('Ctrl Pts',(4.89938476147092,-30.5420306164587,
123.018031187601));
#100300=CARTESIAN_POINT('Ctrl Pts',(4.90324806986671,-30.473488616667,122.999286259746));
#100301=CARTESIAN_POINT('Ctrl Pts',(4.90711137826249,-30.4038674616248,
122.984072176635));
#100302=CARTESIAN_POINT('Ctrl Pts',(4.91097468665827,-30.3335640282405,
122.972505831928));
#100303=CARTESIAN_POINT('Ctrl Pts',(4.91483346315119,-30.2633430651896,
122.960953055269));
#100304=CARTESIAN_POINT('Ctrl Pts',(4.9186922396441,-30.1924418905883,122.953039595899));
#100305=CARTESIAN_POINT('Ctrl Pts',(4.92255101613702,-30.1212695042463,
122.948831730491));
#100306=CARTESIAN_POINT('Ctrl Pts',(4.92640736172523,-30.0501419542116,
122.944626515902));
#100307=CARTESIAN_POINT('Ctrl Pts',(4.93026370731343,-29.9787440152017,
122.944122292457));
#100308=CARTESIAN_POINT('Ctrl Pts',(4.93412005290164,-29.9074903098065,
122.947333558583));
#100309=CARTESIAN_POINT('Ctrl Pts',(4.93797525914697,-29.836257656052,122.950543875952));
#100310=CARTESIAN_POINT('Ctrl Pts',(4.94183046539231,-29.765169636342,122.957467481741));
#100311=CARTESIAN_POINT('Ctrl Pts',(4.94568567163765,-29.6946396410606,
122.968066779225));
#100312=CARTESIAN_POINT('Ctrl Pts',(4.94954102848889,-29.6241068904833,
122.978666490777));
#100313=CARTESIAN_POINT('Ctrl Pts',(4.95339638534014,-29.5541326876791,
122.992942104738));
#100314=CARTESIAN_POINT('Ctrl Pts',(4.95725174219139,-29.485122355172,123.010804541188));
#100315=CARTESIAN_POINT('Ctrl Pts',(4.96111113465995,-29.4160397856961,
123.028685675248));
#100316=CARTESIAN_POINT('Ctrl Pts',(4.96497052712851,-29.3479235718333,
123.0501610047));
#100317=CARTESIAN_POINT('Ctrl Pts',(4.96882991959707,-29.2811650615572,
123.075091198583));
#100318=CARTESIAN_POINT('Ctrl Pts',(4.97269149720051,-29.2143687535318,
123.100035507597));
#100319=CARTESIAN_POINT('Ctrl Pts',(4.97655307480395,-29.1489321251938,
123.128438381514));
#100320=CARTESIAN_POINT('Ctrl Pts',(4.98041465240738,-29.0852251315536,
123.160112910378));
#100321=CARTESIAN_POINT('Ctrl Pts',(4.98428298652226,-29.0214066712862,
123.191842859419));
#100322=CARTESIAN_POINT('Ctrl Pts',(4.98815132063713,-28.9593243110815,
123.226855653503));
#100323=CARTESIAN_POINT('Ctrl Pts',(4.992019654752,-28.8993214518444,123.264919513069));
#100324=CARTESIAN_POINT('Ctrl Pts',(4.99431737392295,-28.8636808593086,
123.287528744135));
#100325=CARTESIAN_POINT('Ctrl Pts',(4.99661509309389,-28.8287733699115,
123.311213615859));
#100326=CARTESIAN_POINT('Ctrl Pts',(4.99891281226483,-28.7946653476448,
123.335918890699));
#100327=CARTESIAN_POINT('Ctrl Pts',(5.00275064676246,-28.7376953984201,
123.377183618458));
#100328=CARTESIAN_POINT('Ctrl Pts',(5.00658848126009,-28.6827265110721,
123.421464682555));
#100329=CARTESIAN_POINT('Ctrl Pts',(5.01042631575773,-28.6300997290133,
123.468539647901));
#100330=CARTESIAN_POINT('Ctrl Pts',(5.01432833257716,-28.5765928388979,
123.516401875068));
#100331=CARTESIAN_POINT('Ctrl Pts',(5.0182303493966,-28.5255075807009,123.567152086287));
#100332=CARTESIAN_POINT('Ctrl Pts',(5.02213236621603,-28.4771716630746,
123.620510449928));
#100333=CARTESIAN_POINT('Ctrl Pts',(5.02595997436974,-28.4297574767744,
123.672851307796));
#100334=CARTESIAN_POINT('Ctrl Pts',(5.02978758252346,-28.3849890497211,
123.727701341682));
#100335=CARTESIAN_POINT('Ctrl Pts',(5.03361519067717,-28.3431406316792,
123.784757392079));
#100336=CARTESIAN_POINT('Ctrl Pts',(5.03744050268937,-28.3013173180592,
123.841779215156));
#100337=CARTESIAN_POINT('Ctrl Pts',(5.04126581470156,-28.2624108313477,
123.901004032373));
#100338=CARTESIAN_POINT('Ctrl Pts',(5.04509112671375,-28.2266549764506,
123.962095866685));
#100339=CARTESIAN_POINT('Ctrl Pts',(5.04891547573735,-28.190908122775,124.023172321666));
#100340=CARTESIAN_POINT('Ctrl Pts',(5.05273982476093,-28.1583105759944,
124.086114434041));
#100341=CARTESIAN_POINT('Ctrl Pts',(5.05656417378453,-28.1290516520466,
124.150559100472));
#100342=CARTESIAN_POINT('Ctrl Pts',(5.06052338592116,-28.0987609316954,
124.217276365006));
#100343=CARTESIAN_POINT('Ctrl Pts',(5.0644825980578,-28.0720489807084,124.285603645032));
#100344=CARTESIAN_POINT('Ctrl Pts',(5.06844181019444,-28.0490719088951,
124.355114625815));
#100345=CARTESIAN_POINT('Ctrl Pts',(5.07227054686676,-28.0268520443266,
124.422334878751));
#100346=CARTESIAN_POINT('Ctrl Pts',(5.07609928353908,-28.008124787048,124.490661515232));
#100347=CARTESIAN_POINT('Ctrl Pts',(5.0799280202114,-27.9929800396067,124.559695058984));
#100348=CARTESIAN_POINT('Ctrl Pts',(5.08395247008019,-27.9770611394396,
124.632257384334));
#100349=CARTESIAN_POINT('Ctrl Pts',(5.08797691994899,-27.9651009153752,
124.705600206819));
#100350=CARTESIAN_POINT('Ctrl Pts',(5.09200136981778,-27.9571422025377,
124.779252221195));
#100351=CARTESIAN_POINT('Ctrl Pts',(5.09602581968658,-27.9491834897002,
124.85290423557));
#100352=CARTESIAN_POINT('Ctrl Pts',(5.10005026955537,-27.9452262438764,
124.926864812609));
#100353=CARTESIAN_POINT('Ctrl Pts',(5.10407471942417,-27.9452501074214,
125.000664415721));
#100354=CARTESIAN_POINT('Ctrl Pts',(5.10407471946233,-27.9452501074216,
125.000664416421));
#100355=CARTESIAN_POINT('Ctrl Pts',(5.10606584067601,-27.9452619140691,
125.037177221924));
#100356=CARTESIAN_POINT('Ctrl Pts',(5.1080569618897,-27.9462469037348,125.073673053094));
#100357=CARTESIAN_POINT('Ctrl Pts',(5.11004808310338,-27.9482027488899,
125.110116315035));
#100358=CARTESIAN_POINT('Ctrl Pts',(5.1139171564516,-27.9520032751013,125.180931518313));
#100359=CARTESIAN_POINT('Ctrl Pts',(5.11778622979981,-27.9594816959999,
125.251688443372));
#100360=CARTESIAN_POINT('Ctrl Pts',(5.12165530314802,-27.9706330803799,
125.32197432825));
#100361=CARTESIAN_POINT('Ctrl Pts',(5.1255186115438,-27.9817678491017,125.392155486556));
#100362=CARTESIAN_POINT('Ctrl Pts',(5.12938191993959,-27.9965646425544,
125.461866521965));
#100363=CARTESIAN_POINT('Ctrl Pts',(5.13324522833537,-28.0149666018931,
125.53069762662));
#100364=CARTESIAN_POINT('Ctrl Pts',(5.13710400482828,-28.0333469745802,
125.599447988075));
#100365=CARTESIAN_POINT('Ctrl Pts',(5.14096278132119,-28.0553239878999,
125.667320002076));
#100366=CARTESIAN_POINT('Ctrl Pts',(5.1448215578141,-28.0807896635756,125.733913650957));
#100367=CARTESIAN_POINT('Ctrl Pts',(5.1486779034023,-28.1062392966971,125.800465347988));
#100368=CARTESIAN_POINT('Ctrl Pts',(5.15253424899051,-28.1351730587823,
125.865739824989));
#100369=CARTESIAN_POINT('Ctrl Pts',(5.15639059457871,-28.1674334698241,
125.929353256291));
#100370=CARTESIAN_POINT('Ctrl Pts',(5.16024580082404,-28.1996843496481,
125.992947893243));
#100371=CARTESIAN_POINT('Ctrl Pts',(5.16410100706936,-28.2352597076084,
126.05488202575));
#100372=CARTESIAN_POINT('Ctrl Pts',(5.16795621331469,-28.2739550952365,
126.114794397743));
#100373=CARTESIAN_POINT('Ctrl Pts',(5.17181157016593,-28.3126519945229,
126.174709110249));
#100374=CARTESIAN_POINT('Ctrl Pts',(5.17566692701717,-28.3544689000543,
126.232601498555));
#100375=CARTESIAN_POINT('Ctrl Pts',(5.17952228386841,-28.3991577667119,
126.288138853781));
#100376=CARTESIAN_POINT('Ctrl Pts',(5.18338167633697,-28.4438934117017,
126.343734343059));
#100377=CARTESIAN_POINT('Ctrl Pts',(5.18724106880552,-28.4915067137853,
126.396969499025));
#100378=CARTESIAN_POINT('Ctrl Pts',(5.19110046127408,-28.5417095857691,
126.447545035659));
#100379=CARTESIAN_POINT('Ctrl Pts',(5.19496203887751,-28.5919408819278,
126.498149207466));
#100380=CARTESIAN_POINT('Ctrl Pts',(5.19882361648094,-28.6447643068021,
126.546090435647));
#100381=CARTESIAN_POINT('Ctrl Pts',(5.20268519408437,-28.699857220266,126.591108517608));
#100382=CARTESIAN_POINT('Ctrl Pts',(5.20655352819924,-28.7550465285039,
126.636205366648));
#100383=CARTESIAN_POINT('Ctrl Pts',(5.2104218623141,-28.8125128614944,126.678368570638));
#100384=CARTESIAN_POINT('Ctrl Pts',(5.21429019642897,-28.8719036200696,
126.717380598495));
#100385=CARTESIAN_POINT('Ctrl Pts',(5.21658791559996,-28.907180636094,126.740553024052));
#100386=CARTESIAN_POINT('Ctrl Pts',(5.21888563477095,-28.9431361072491,
126.762614530318));
#100387=CARTESIAN_POINT('Ctrl Pts',(5.22118335394194,-28.9796923731626,
126.783527378292));
#100388=CARTESIAN_POINT('Ctrl Pts',(5.22505242729016,-29.0412485789611,
126.818742013638));
#100389=CARTESIAN_POINT('Ctrl Pts',(5.22892150063837,-29.1047505806774,
126.85083508144));
#100390=CARTESIAN_POINT('Ctrl Pts',(5.23279057398659,-29.1698489244986,
126.879586857356));
#100391=CARTESIAN_POINT('Ctrl Pts',(5.23665388238237,-29.2348502712299,
126.908295792879));
#100392=CARTESIAN_POINT('Ctrl Pts',(5.24051719077816,-29.3014427979312,
126.933673124138));
#100393=CARTESIAN_POINT('Ctrl Pts',(5.24438049917394,-29.3692513689759,
126.955544355662));
#100394=CARTESIAN_POINT('Ctrl Pts',(5.24823927566686,-29.4369803963171,
126.977389930861));
#100395=CARTESIAN_POINT('Ctrl Pts',(5.25209805215977,-29.50592217441,126.995737427486));
#100396=CARTESIAN_POINT('Ctrl Pts',(5.25595682865268,-29.5756820674499,
127.010460607576));
#100397=CARTESIAN_POINT('Ctrl Pts',(5.25981317424089,-29.6453980140077,
127.025174512538));
#100398=CARTESIAN_POINT('Ctrl Pts',(5.2636695198291,-29.7159305788037,127.036268530721));
#100399=CARTESIAN_POINT('Ctrl Pts',(5.2675258654173,-29.7868718816748,127.04366679468));
#100400=CARTESIAN_POINT('Ctrl Pts',(5.27138107166264,-29.8577922252035,
127.051062872851));
#100401=CARTESIAN_POINT('Ctrl Pts',(5.27523627790797,-29.9291205841626,
127.054765314154));
#100402=CARTESIAN_POINT('Ctrl Pts',(5.2790914841533,-30.0004425660865,127.054749952339));
#100403=CARTESIAN_POINT('Ctrl Pts',(5.28294684100455,-30.0717673342459,
127.054734589923));
#100404=CARTESIAN_POINT('Ctrl Pts',(5.28680219785579,-30.14308523909,127.051001138343));
#100405=CARTESIAN_POINT('Ctrl Pts',(5.29065755470704,-30.2139822266315,
127.04357754176));
#100406=CARTESIAN_POINT('Ctrl Pts',(5.2945169471756,-30.2849534260089,127.036146174484));
#100407=CARTESIAN_POINT('Ctrl Pts',(5.29837633964416,-30.3555023444172,
127.02501700212));
#100408=CARTESIAN_POINT('Ctrl Pts',(5.30223573211272,-30.4252212904861,
127.010269737278));
#100409=CARTESIAN_POINT('Ctrl Pts',(5.30609730971616,-30.4949797104624,
126.995514122738));
#100410=CARTESIAN_POINT('Ctrl Pts',(5.30995888731959,-30.5639067530251,
126.977136462971));
#100411=CARTESIAN_POINT('Ctrl Pts',(5.31382046492303,-30.631608822224,126.955266697458));
#100412=CARTESIAN_POINT('Ctrl Pts',(5.3176887990379,-30.6994293481398,126.933358666931));
#100413=CARTESIAN_POINT('Ctrl Pts',(5.32155713315277,-30.7660201675122,
126.907946505012));
#100414=CARTESIAN_POINT('Ctrl Pts',(5.32542546726764,-30.8310072858771,
126.879208464572));
#100415=CARTESIAN_POINT('Ctrl Pts',(5.32772318643859,-30.8696084364752,
126.862138598192));
#100416=CARTESIAN_POINT('Ctrl Pts',(5.33002090560955,-30.9076442250829,
126.843896209379));
#100417=CARTESIAN_POINT('Ctrl Pts',(5.3323186247805,-30.9450408253262,126.824526075716));
#100418=CARTESIAN_POINT('Ctrl Pts',(5.33618678852257,-31.0079972453129,
126.791916847547));
#100419=CARTESIAN_POINT('Ctrl Pts',(5.34005495226464,-31.0693871678518,
126.755981411747));
#100420=CARTESIAN_POINT('Ctrl Pts',(5.34392311600671,-31.1288367232353,
126.71689406044));
#100421=CARTESIAN_POINT('Ctrl Pts',(5.34666123617927,-31.1709187129596,
126.689225669896));
#100422=CARTESIAN_POINT('Ctrl Pts',(5.34939935635183,-31.2120287653956,
126.659979003999));
#100423=CARTESIAN_POINT('Ctrl Pts',(5.35213747652439,-31.2520409112987,
126.629230222815));
#100424=CARTESIAN_POINT('',(5.04592528049234,-27.9452502582983,124.998969719981));
#100425=CARTESIAN_POINT('Ctrl Pts',(5.04592528053768,-27.9452502582979,
124.998969720821));
#100426=CARTESIAN_POINT('Ctrl Pts',(5.04983580638859,-27.9452139274514,
125.071426584004));
#100427=CARTESIAN_POINT('Ctrl Pts',(5.0537463322395,-27.9490145212745,125.143878332677));
#100428=CARTESIAN_POINT('Ctrl Pts',(5.05765685809041,-27.9566240457995,
125.215898754732));
#100429=CARTESIAN_POINT('Ctrl Pts',(5.0615688975846,-27.9642365157353,125.28794705366));
#100430=CARTESIAN_POINT('Ctrl Pts',(5.0654809370788,-27.9756607961671,125.359563230795));
#100431=CARTESIAN_POINT('Ctrl Pts',(5.06939297657299,-27.9908172317787,
125.430327975366));
#100432=CARTESIAN_POINT('Ctrl Pts',(5.0733108311932,-28.0059961969642,125.501197909546));
#100433=CARTESIAN_POINT('Ctrl Pts',(5.07722868581341,-28.0249182944708,
125.571213427755));
#100434=CARTESIAN_POINT('Ctrl Pts',(5.08114654043362,-28.0474531999294,
125.639967621083));
#100435=CARTESIAN_POINT('Ctrl Pts',(5.08506751736911,-28.070006064472,125.708776607732));
#100436=CARTESIAN_POINT('Ctrl Pts',(5.08898849430461,-28.0961773017068,
125.776321833245));
#100437=CARTESIAN_POINT('Ctrl Pts',(5.09290947124011,-28.1257883534147,
125.842216282379));
#100438=CARTESIAN_POINT('Ctrl Pts',(5.09683849198269,-28.1554601516131,
125.908245912679));
#100439=CARTESIAN_POINT('Ctrl Pts',(5.10076751272527,-28.188585645451,125.972617587755));
#100440=CARTESIAN_POINT('Ctrl Pts',(5.10469653346786,-28.2249403918814,
126.034969057569));
#100441=CARTESIAN_POINT('Ctrl Pts',(5.10720517516982,-28.2481525454776,
126.074779867337));
#100442=CARTESIAN_POINT('Ctrl Pts',(5.10971381687178,-28.272680273511,126.113767668478));
#100443=CARTESIAN_POINT('Ctrl Pts',(5.11222245857374,-28.2984564079792,
126.151845027316));
#100444=CARTESIAN_POINT('Ctrl Pts',(5.11609153192196,-28.3382108913768,
126.210571665775));
#100445=CARTESIAN_POINT('Ctrl Pts',(5.11996060527017,-28.3810871266736,
126.267352804102));
#100446=CARTESIAN_POINT('Ctrl Pts',(5.12382967861839,-28.4268681537416,
126.321837265622));
#100447=CARTESIAN_POINT('Ctrl Pts',(5.12769298701418,-28.472580966687,126.376240544828));
#100448=CARTESIAN_POINT('Ctrl Pts',(5.13155629540996,-28.5211896701545,
126.428353571045));
#100449=CARTESIAN_POINT('Ctrl Pts',(5.13541960380575,-28.5724343269203,
126.477854462234));
#100450=CARTESIAN_POINT('Ctrl Pts',(5.13927838029866,-28.623618870492,126.527297285775));
#100451=CARTESIAN_POINT('Ctrl Pts',(5.14313715679158,-28.6774328776293,
126.574133724953));
#100452=CARTESIAN_POINT('Ctrl Pts',(5.14699593328449,-28.7335776498747,
126.618076634033));
#100453=CARTESIAN_POINT('Ctrl Pts',(5.1508522788727,-28.7896870527247,126.661991860498));
#100454=CARTESIAN_POINT('Ctrl Pts',(5.1547086244609,-28.848123925943,126.703016874631));
#100455=CARTESIAN_POINT('Ctrl Pts',(5.15856497004911,-28.9085554955759,
126.740903919308));
#100456=CARTESIAN_POINT('Ctrl Pts',(5.16242017629445,-28.9689692109278,
126.7787797704));
#100457=CARTESIAN_POINT('Ctrl Pts',(5.16627538253979,-29.0313760413579,
126.813519234689));
#100458=CARTESIAN_POINT('Ctrl Pts',(5.17013058878512,-29.0954145952796,
126.84491810335));
#100459=CARTESIAN_POINT('Ctrl Pts',(5.17398594563638,-29.1594556509053,
126.876318198626));
#100460=CARTESIAN_POINT('Ctrl Pts',(5.17784130248763,-29.2251281194314,
126.904377227293));
#100461=CARTESIAN_POINT('Ctrl Pts',(5.18169665933888,-29.2920479619282,
126.928937913539));
#100462=CARTESIAN_POINT('Ctrl Pts',(5.18555605180745,-29.3590378531612,
126.953524308828));
#100463=CARTESIAN_POINT('Ctrl Pts',(5.18941544427601,-29.4272772678516,
126.974604883981));
#100464=CARTESIAN_POINT('Ctrl Pts',(5.19327483674457,-29.4963650787203,
126.992071642428));
#100465=CARTESIAN_POINT('Ctrl Pts',(5.19713641434801,-29.5654920061563,
127.009548290314));
#100466=CARTESIAN_POINT('Ctrl Pts',(5.20099799195145,-29.6354678092435,
127.023406953932));
#100467=CARTESIAN_POINT('Ctrl Pts',(5.20485956955489,-29.7058818937099,
127.033590937739));
#100468=CARTESIAN_POINT('Ctrl Pts',(5.20872790366976,-29.7764191800424,
127.043792740222));
#100469=CARTESIAN_POINT('Ctrl Pts',(5.21259623778464,-29.8473957948873,
127.050306981797));
#100470=CARTESIAN_POINT('Ctrl Pts',(5.21646457189951,-29.9183974630044,
127.053128975115));
#100471=CARTESIAN_POINT('Ctrl Pts',(5.21876229107044,-29.9605711453068,
127.054805187137));
#100472=CARTESIAN_POINT('Ctrl Pts',(5.22106001024137,-30.0027536735455,
127.055179721477));
#100473=CARTESIAN_POINT('Ctrl Pts',(5.2233577294123,-30.0448590459357,127.054260263087));
#100474=CARTESIAN_POINT('Ctrl Pts',(5.22722618552696,-30.1157479462608,
127.052712256491));
#100475=CARTESIAN_POINT('Ctrl Pts',(5.23109464164162,-30.1866954545005,
127.047487535505));
#100476=CARTESIAN_POINT('Ctrl Pts',(5.23496309775628,-30.2572890582151,
127.038577911933));
#100477=CARTESIAN_POINT('Ctrl Pts',(5.23882613528354,-30.327783780722,127.029680768166));
#100478=CARTESIAN_POINT('Ctrl Pts',(5.2426891728108,-30.3979251045115,127.017109022759));
#100479=CARTESIAN_POINT('Ctrl Pts',(5.24655221033805,-30.4673017077463,
127.00090646369));
#100480=CARTESIAN_POINT('Ctrl Pts',(5.25049621378875,-30.5381323845454,
126.984364313005));
#100481=CARTESIAN_POINT('Ctrl Pts',(5.25444021723945,-30.6081654024678,
126.964037416808));
#100482=CARTESIAN_POINT('Ctrl Pts',(5.25838422069015,-30.6769703293199,
126.940028024468));
#100483=CARTESIAN_POINT('Ctrl Pts',(5.26224043473793,-30.7442437302688,
126.916553056158));
#100484=CARTESIAN_POINT('Ctrl Pts',(5.2660966487857,-30.8103426711026,126.889558020767));
#100485=CARTESIAN_POINT('Ctrl Pts',(5.26995286283347,-30.8748789361614,
126.859189180681));
#100486=CARTESIAN_POINT('Ctrl Pts',(5.27394076098563,-30.9416190208629,
126.827783288849));
#100487=CARTESIAN_POINT('Ctrl Pts',(5.2779286591378,-31.0066872487866,126.792769156818));
#100488=CARTESIAN_POINT('Ctrl Pts',(5.28191655728996,-31.069677830906,126.754362248958));
#100489=CARTESIAN_POINT('Ctrl Pts',(5.28590445544213,-31.1326684130254,
126.715955341098));
#100490=CARTESIAN_POINT('Ctrl Pts',(5.28989235359429,-31.1935808619265,
126.674155962877));
#100491=CARTESIAN_POINT('Ctrl Pts',(5.29388025174645,-31.2520409112987,
126.629230222815));
#100492=CARTESIAN_POINT('Ctrl Pts',(4.59397334877082,-31.2520409112987,
126.629230222815));
#100493=CARTESIAN_POINT('Ctrl Pts',(4.59782931900108,-31.3085491042728,
126.585804457422));
#100494=CARTESIAN_POINT('Ctrl Pts',(4.60168528923134,-31.3628309656863,
126.53940800709));
#100495=CARTESIAN_POINT('Ctrl Pts',(4.6055412594616,-31.4145649577858,126.490303171407));
#100496=CARTESIAN_POINT('Ctrl Pts',(4.60939638628394,-31.4662876342226,
126.441209076316));
#100497=CARTESIAN_POINT('Ctrl Pts',(4.61325151310627,-31.5154631958829,
126.389408106701));
#100498=CARTESIAN_POINT('Ctrl Pts',(4.61710663992861,-31.5618054085364,
126.335200894385));
#100499=CARTESIAN_POINT('Ctrl Pts',(4.62096221310461,-31.6081529867762,
126.280987405859));
#100500=CARTESIAN_POINT('Ctrl Pts',(4.6248177862806,-31.6516662510474,126.224367492432));
#100501=CARTESIAN_POINT('Ctrl Pts',(4.6286733594566,-31.6920989987525,126.16567514382));
#100502=CARTESIAN_POINT('Ctrl Pts',(4.63253315030944,-31.7325759765256,
126.106918590654));
#100503=CARTESIAN_POINT('Ctrl Pts',(4.63639294116229,-31.769965437958,126.046085479588));
#100504=CARTESIAN_POINT('Ctrl Pts',(4.64025273201513,-31.804064848595,125.983538298473));
#100505=CARTESIAN_POINT('Ctrl Pts',(4.64411497375936,-31.838185911688,125.920951401127));
#100506=CARTESIAN_POINT('Ctrl Pts',(4.64797721550358,-31.869012557114,125.856648705859));
#100507=CARTESIAN_POINT('Ctrl Pts',(4.65183945724781,-31.8963897053691,
125.791014315844));
#100508=CARTESIAN_POINT('Ctrl Pts',(4.65570819014413,-31.9238128655636,
125.725269616109));
#100509=CARTESIAN_POINT('Ctrl Pts',(4.65957692304045,-31.9477747978071,
125.658189212644));
#100510=CARTESIAN_POINT('Ctrl Pts',(4.66344565593677,-31.9681699974544,
125.59017321493));
#100511=CARTESIAN_POINT('Ctrl Pts',(4.66485756236435,-31.9756132907097,
125.565350559315));
#100512=CARTESIAN_POINT('Ctrl Pts',(4.66626946879192,-31.9825820204718,
125.540403390991));
#100513=CARTESIAN_POINT('Ctrl Pts',(4.66768137521949,-31.9890727647972,
125.515351432366));
#100514=CARTESIAN_POINT('Ctrl Pts',(4.6715504485677,-32.0068594717552,125.446701085897));
#100515=CARTESIAN_POINT('Ctrl Pts',(4.67541952191591,-32.0211227752711,
125.376994361718));
#100516=CARTESIAN_POINT('Ctrl Pts',(4.67928859526412,-32.0317425864935,
125.306626197068));
#100517=CARTESIAN_POINT('Ctrl Pts',(4.6831519036599,-32.0423465741063,125.236362881587));
#100518=CARTESIAN_POINT('Ctrl Pts',(4.68701521205567,-32.0493177736078,
125.165440558361));
#100519=CARTESIAN_POINT('Ctrl Pts',(4.69087852045145,-32.0525864868933,
125.094267047917));
#100520=CARTESIAN_POINT('Ctrl Pts',(4.69473729694436,-32.0558513657733,
125.023177028461));
#100521=CARTESIAN_POINT('Ctrl Pts',(4.69859607343727,-32.0554223634192,
124.951836889997));
#100522=CARTESIAN_POINT('Ctrl Pts',(4.70245484993018,-32.0512814688225,
124.880660575813));
#100523=CARTESIAN_POINT('Ctrl Pts',(4.70631119551838,-32.0471431828559,
124.809529100411));
#100524=CARTESIAN_POINT('Ctrl Pts',(4.71016754110659,-32.0392976720872,
124.738561728352));
#100525=CARTESIAN_POINT('Ctrl Pts',(4.71402388669479,-32.0277790060476,
124.668171934381));
#100526=CARTESIAN_POINT('Ctrl Pts',(4.71787909294012,-32.0162637431547,
124.597802936811));
#100527=CARTESIAN_POINT('Ctrl Pts',(4.72173429918545,-32.0010775578613,
124.528011657702));
#100528=CARTESIAN_POINT('Ctrl Pts',(4.72558950543078,-31.9823061136397,
124.459204258221));
#100529=CARTESIAN_POINT('Ctrl Pts',(4.72944486228203,-31.9635339361005,
124.390394170738));
#100530=CARTESIAN_POINT('Ctrl Pts',(4.73330021913327,-31.9411763515422,
124.32256850727));
#100531=CARTESIAN_POINT('Ctrl Pts',(4.73715557598452,-31.9153692105439,
124.256119398155));
#100532=CARTESIAN_POINT('Ctrl Pts',(4.74101496845307,-31.8895350557699,
124.189600733047));
#100533=CARTESIAN_POINT('Ctrl Pts',(4.74487436092163,-31.8602443127305,
124.124461952446));
#100534=CARTESIAN_POINT('Ctrl Pts',(4.74873375339018,-31.8276811049247,
124.0610754337));
#100535=CARTESIAN_POINT('Ctrl Pts',(4.75259533099361,-31.795099460279,123.997653026381));
#100536=CARTESIAN_POINT('Ctrl Pts',(4.75645690859704,-31.7592419067682,
123.935985276047));
#100537=CARTESIAN_POINT('Ctrl Pts',(4.76031848620047,-31.7203373198838,
123.876417751869));
#100538=CARTESIAN_POINT('Ctrl Pts',(4.76418682031534,-31.6813646625594,
123.816746003796));
#100539=CARTESIAN_POINT('Ctrl Pts',(4.76805515443021,-31.6393346142748,
123.759182211015));
#100540=CARTESIAN_POINT('Ctrl Pts',(4.77192348854507,-31.5945175083752,
123.704040325479));
#100541=CARTESIAN_POINT('Ctrl Pts',(4.77422120771607,-31.5678969734483,
123.671287061733));
#100542=CARTESIAN_POINT('Ctrl Pts',(4.77651892688706,-31.5402938708374,
123.639387615172));
#100543=CARTESIAN_POINT('Ctrl Pts',(4.77881664605806,-31.5117708171909,
123.60840143763));
#100544=CARTESIAN_POINT('Ctrl Pts',(4.78268571940627,-31.4637415418702,
123.556224567975));
#100545=CARTESIAN_POINT('Ctrl Pts',(4.78655479275449,-31.4129137901362,
123.506434921696));
#100546=CARTESIAN_POINT('Ctrl Pts',(4.7904238661027,-31.359554234086,123.459347590441));
#100547=CARTESIAN_POINT('Ctrl Pts',(4.79428717449849,-31.3062741842313,
123.412330419714));
#100548=CARTESIAN_POINT('Ctrl Pts',(4.79815048289428,-31.2504701794633,
123.368007890384));
#100549=CARTESIAN_POINT('Ctrl Pts',(4.80201379129007,-31.1924470458218,
123.326659746073));
#100550=CARTESIAN_POINT('Ctrl Pts',(4.80587256778298,-31.1344919769526,
123.285360105728));
#100551=CARTESIAN_POINT('Ctrl Pts',(4.8097313442759,-31.0743233436928,123.247028200339));
#100552=CARTESIAN_POINT('Ctrl Pts',(4.81359012076881,-31.0122791493048,
123.211903669714));
#100553=CARTESIAN_POINT('Ctrl Pts',(4.81744646635702,-30.9502740407578,
123.17680126641));
#100554=CARTESIAN_POINT('Ctrl Pts',(4.82130281194522,-30.8863961369886,
123.144902467902));
#100555=CARTESIAN_POINT('Ctrl Pts',(4.82515915753343,-30.8210112942298,
123.116402904747));
#100556=CARTESIAN_POINT('Ctrl Pts',(4.82901436377876,-30.7556457691782,
123.08791176168));
#100557=CARTESIAN_POINT('Ctrl Pts',(4.83286957002409,-30.6887746341,123.062818054167));
#100558=CARTESIAN_POINT('Ctrl Pts',(4.83672477626942,-30.6207855834735,
123.041270099822));
#100559=CARTESIAN_POINT('Ctrl Pts',(4.84058013312067,-30.5527938768144,
123.019721303693));
#100560=CARTESIAN_POINT('Ctrl Pts',(4.84443548997193,-30.4836846316522,
123.001718680408));
#100561=CARTESIAN_POINT('Ctrl Pts',(4.84829084682318,-30.4138609742382,
122.987360773387));
#100562=CARTESIAN_POINT('Ctrl Pts',(4.85215023929174,-30.3439642285028,
122.972987837143));
#100563=CARTESIAN_POINT('Ctrl Pts',(4.8560096317603,-30.2733520545136,122.962267331063));
#100564=CARTESIAN_POINT('Ctrl Pts',(4.85986902422886,-30.2024371646756,
122.955246529075));
#100565=CARTESIAN_POINT('Ctrl Pts',(4.86373060183231,-30.1314821238033,
122.948221752007));
#100566=CARTESIAN_POINT('Ctrl Pts',(4.86759217943575,-30.0602245113797,
122.944900871601));
#100567=CARTESIAN_POINT('Ctrl Pts',(4.87145375703919,-29.9890787889625,
122.945279023894));
#100568=CARTESIAN_POINT('Ctrl Pts',(4.87532209115406,-29.9178085845495,
122.945657837831));
#100569=CARTESIAN_POINT('Ctrl Pts',(4.87919042526894,-29.8466511461452,
122.949748578334));
#100570=CARTESIAN_POINT('Ctrl Pts',(4.88305875938381,-29.7760168575574,
122.957494402847));
#100571=CARTESIAN_POINT('Ctrl Pts',(4.88535647855474,-29.7340613919243,
122.962095279852));
#100572=CARTESIAN_POINT('Ctrl Pts',(4.88765419772568,-29.6922903458753,
122.967984734544));
#100573=CARTESIAN_POINT('Ctrl Pts',(4.88995191689662,-29.6507876285087,
122.975142404489));
#100574=CARTESIAN_POINT('Ctrl Pts',(4.89382099024483,-29.580902213584,122.987195030576));
#100575=CARTESIAN_POINT('Ctrl Pts',(4.89769006359304,-29.5115046159004,
123.002893522819));
#100576=CARTESIAN_POINT('Ctrl Pts',(4.90155913694124,-29.4430041910452,
123.022184732765));
#100577=CARTESIAN_POINT('Ctrl Pts',(4.90542244533703,-29.3746058324097,
123.041447198644));
#100578=CARTESIAN_POINT('Ctrl Pts',(4.90928575373282,-29.307102456889,123.064291625702));
#100579=CARTESIAN_POINT('Ctrl Pts',(4.91314906212861,-29.2408944159804,
123.0906136392));
#100580=CARTESIAN_POINT('Ctrl Pts',(4.91700783862152,-29.1747640412533,
123.116904775326));
#100581=CARTESIAN_POINT('Ctrl Pts',(4.92086661511442,-29.109926432108,123.146665216171));
#100582=CARTESIAN_POINT('Ctrl Pts',(4.92472539160733,-29.0467662412132,
123.179740962498));
#100583=CARTESIAN_POINT('Ctrl Pts',(4.92858173719554,-28.9836458392011,
123.212795872171));
#100584=CARTESIAN_POINT('Ctrl Pts',(4.93243808278374,-28.9222011882553,
123.249161718872));
#100585=CARTESIAN_POINT('Ctrl Pts',(4.93629442837195,-28.8627950734066,
123.28863723383));
#100586=CARTESIAN_POINT('Ctrl Pts',(4.94014963461728,-28.8034065098723,
123.328101085896));
#100587=CARTESIAN_POINT('Ctrl Pts',(4.94400484086261,-28.7460556911284,
123.370672513553));
#100588=CARTESIAN_POINT('Ctrl Pts',(4.94786004710794,-28.6910774968249,
123.416106239932));
#100589=CARTESIAN_POINT('Ctrl Pts',(4.95171540395919,-28.6360971547655,
123.461541741206));
#100590=CARTESIAN_POINT('Ctrl Pts',(4.95557076081044,-28.5834899942288,
123.509839452046));
#100591=CARTESIAN_POINT('Ctrl Pts',(4.9594261176617,-28.5335574470371,123.560714134941));
#100592=CARTESIAN_POINT('Ctrl Pts',(4.96328551013025,-28.48357263266,123.611642071207));
#100593=CARTESIAN_POINT('Ctrl Pts',(4.9671449025988,-28.4362683613671,123.665152016857));
#100594=CARTESIAN_POINT('Ctrl Pts',(4.97100429506736,-28.3919081904316,
123.720922873905));
#100595=CARTESIAN_POINT('Ctrl Pts',(4.97486587267079,-28.3475229033782,
123.776725307644));
#100596=CARTESIAN_POINT('Ctrl Pts',(4.97872745027421,-28.3060853173045,
123.834790805449));
#100597=CARTESIAN_POINT('Ctrl Pts',(4.98258902787764,-28.2678161348464,
123.894768522073));
#100598=CARTESIAN_POINT('Ctrl Pts',(4.9864573619925,-28.2294799937006,123.954851180295));
#100599=CARTESIAN_POINT('Ctrl Pts',(4.99032569610737,-28.1943235639811,
124.016852314539));
#100600=CARTESIAN_POINT('Ctrl Pts',(4.99419403022223,-28.1625216672204,
124.08039631413));
#100601=CARTESIAN_POINT('Ctrl Pts',(4.99649174939321,-28.1436319266522,
124.118140278774));
#100602=CARTESIAN_POINT('Ctrl Pts',(4.99878946856419,-28.1259247988859,
124.156428182751));
#100603=CARTESIAN_POINT('Ctrl Pts',(5.00108718773517,-28.1094286858362,
124.19517848652));
#100604=CARTESIAN_POINT('Ctrl Pts',(5.00537446195644,-28.0786488755259,
124.267482004074));
#100605=CARTESIAN_POINT('Ctrl Pts',(5.0096617361777,-28.0519849253725,124.341637213734));
#100606=CARTESIAN_POINT('Ctrl Pts',(5.01394901039897,-28.0296387343031,
124.417184381523));
#100607=CARTESIAN_POINT('Ctrl Pts',(5.0182226207556,-28.0073637622213,124.492490774819));
#100608=CARTESIAN_POINT('Ctrl Pts',(5.02249623111224,-27.9893792307952,
124.569180004692));
#100609=CARTESIAN_POINT('Ctrl Pts',(5.02676984146888,-27.9758386929301,
124.646774058907));
#100610=CARTESIAN_POINT('Ctrl Pts',(5.03102083154993,-27.9623698253093,
124.723957406777));
#100611=CARTESIAN_POINT('Ctrl Pts',(5.03527182163098,-27.9532981584284,
124.802035744073));
#100612=CARTESIAN_POINT('Ctrl Pts',(5.03952281171203,-27.9487267011562,
124.880520227861));
#100613=CARTESIAN_POINT('Ctrl Pts',(5.04165696797213,-27.9464316583616,
124.919922378702));
#100614=CARTESIAN_POINT('Ctrl Pts',(5.04379112423223,-27.9452700857511,
124.959426631904));
#100615=CARTESIAN_POINT('Ctrl Pts',(5.04592528049234,-27.9452502582983,
124.998969719981));
#100616=CARTESIAN_POINT('Origin',(-1.54592528053767,-30.,125.));
#100617=CARTESIAN_POINT('',(3.89394636911841,-31.2520409112987,126.629230222815));
#100618=CARTESIAN_POINT('',(3.95204573383007,-31.2520409112987,126.629230222815));
#100619=CARTESIAN_POINT('',(-1.54592528053767,-31.2520409112987,126.629230222815));
#100620=CARTESIAN_POINT('',(4.40407471951209,-27.9452505182989,125.001459434549));
#100621=CARTESIAN_POINT('Ctrl Pts',(3.95204573383007,-31.2520409112987,
126.629230222815));
#100622=CARTESIAN_POINT('Ctrl Pts',(3.95593320390404,-31.3090533867716,
126.585416923291));
#100623=CARTESIAN_POINT('Ctrl Pts',(3.95982067397802,-31.3637452867511,
126.538621370544));
#100624=CARTESIAN_POINT('Ctrl Pts',(3.963708144052,-31.4158013611643,126.489128627159));
#100625=CARTESIAN_POINT('Ctrl Pts',(3.96756865463629,-31.467496428245,126.439979114482));
#100626=CARTESIAN_POINT('Ctrl Pts',(3.97142916522058,-31.5165918191422,
126.388170101277));
#100627=CARTESIAN_POINT('Ctrl Pts',(3.97528967580487,-31.5628172576812,
126.334016409792));
#100628=CARTESIAN_POINT('Ctrl Pts',(3.97919062562369,-31.6095269123127,
126.279295452971));
#100629=CARTESIAN_POINT('Ctrl Pts',(3.98309157544251,-31.6533058234712,
126.222180809079));
#100630=CARTESIAN_POINT('Ctrl Pts',(3.98699252526133,-31.6939194848657,
126.16302809136));
#100631=CARTESIAN_POINT('Ctrl Pts',(3.99089347508015,-31.7345331462603,
126.10387537364));
#100632=CARTESIAN_POINT('Ctrl Pts',(3.99479442489897,-31.7719813499103,
126.042685046445));
#100633=CARTESIAN_POINT('Ctrl Pts',(3.99869537471779,-31.8060778097421,
125.979836980144));
#100634=CARTESIAN_POINT('Ctrl Pts',(4.002564448066,-31.8398956515833,125.917502474547));
#100635=CARTESIAN_POINT('Ctrl Pts',(4.00643352141422,-31.8705488495699,
125.853293046297));
#100636=CARTESIAN_POINT('Ctrl Pts',(4.01030259476243,-31.8978256139733,
125.78756301427));
#100637=CARTESIAN_POINT('Ctrl Pts',(4.01416590315822,-31.9250617357641,
125.721930920554));
#100638=CARTESIAN_POINT('Ctrl Pts',(4.01802921155401,-31.9489312255172,
125.654783165467));
#100639=CARTESIAN_POINT('Ctrl Pts',(4.0218925199498,-31.9692680899003,125.586498723443));
#100640=CARTESIAN_POINT('Ctrl Pts',(4.02575129644272,-31.989581097867,125.518294383349));
#100641=CARTESIAN_POINT('Ctrl Pts',(4.02961007293563,-32.0063695738438,
125.448956468227));
#100642=CARTESIAN_POINT('Ctrl Pts',(4.03346884942855,-32.0195162093905,
125.378882359722));
#100643=CARTESIAN_POINT('Ctrl Pts',(4.03732519501675,-32.032654562981,125.308852395646));
#100644=CARTESIAN_POINT('Ctrl Pts',(4.04118154060496,-32.0421555385165,
125.238087634641));
#100645=CARTESIAN_POINT('Ctrl Pts',(4.04503788619317,-32.0479524838775,
125.166997563695));
#100646=CARTESIAN_POINT('Ctrl Pts',(4.04889309243851,-32.0537477165527,
125.095928496044));
#100647=CARTESIAN_POINT('Ctrl Pts',(4.05274829868384,-32.0558410521646,
125.024534793174));
#100648=CARTESIAN_POINT('Ctrl Pts',(4.05660350492917,-32.0542176734686,
124.953231287067));
#100649=CARTESIAN_POINT('Ctrl Pts',(4.06045886178043,-32.0525942313542,
124.881924995447));
#100650=CARTESIAN_POINT('Ctrl Pts',(4.06431421863168,-32.0472537999241,
124.810709393194));
#100651=CARTESIAN_POINT('Ctrl Pts',(4.06816957548293,-32.0382336514703,
124.73999779902));
#100652=CARTESIAN_POINT('Ctrl Pts',(4.07202896795149,-32.0292040611233,
124.669212187073));
#100653=CARTESIAN_POINT('Ctrl Pts',(4.07588836042005,-32.0164871263596,
124.598932119228));
#100654=CARTESIAN_POINT('Ctrl Pts',(4.07974775288861,-32.0001717313108,
124.529563386028));
#100655=CARTESIAN_POINT('Ctrl Pts',(4.08360933049205,-31.9838470987099,
124.460155377207));
#100656=CARTESIAN_POINT('Ctrl Pts',(4.08747090809549,-31.9639200857576,
124.391660196868));
#100657=CARTESIAN_POINT('Ctrl Pts',(4.09133248569893,-31.9405294728947,
124.324468411303));
#100658=CARTESIAN_POINT('Ctrl Pts',(4.0952008198138,-31.917097934027,124.257159061853));
#100659=CARTESIAN_POINT('Ctrl Pts',(4.09906915392867,-31.8901908793727,
124.191158110285));
#100660=CARTESIAN_POINT('Ctrl Pts',(4.10293748804354,-31.8599949485487,
124.126835437118));
#100661=CARTESIAN_POINT('Ctrl Pts',(4.10523520721448,-31.8420591221495,
124.088628954722));
#100662=CARTESIAN_POINT('Ctrl Pts',(4.10753292638542,-31.8229638179775,
124.051014126221));
#100663=CARTESIAN_POINT('Ctrl Pts',(4.10983064555635,-31.8027554667188,
124.01406374967));
#100664=CARTESIAN_POINT('Ctrl Pts',(4.11369971890456,-31.768727116233,123.951843910566));
#100665=CARTESIAN_POINT('Ctrl Pts',(4.11756879225278,-31.731407172388,123.891265935903));
#100666=CARTESIAN_POINT('Ctrl Pts',(4.12143786560099,-31.6909784467623,
123.832699929288));
#100667=CARTESIAN_POINT('Ctrl Pts',(4.12530117399678,-31.6506099602841,
123.774221186524));
#100668=CARTESIAN_POINT('Ctrl Pts',(4.12916448239257,-31.607142160362,123.717748857687));
#100669=CARTESIAN_POINT('Ctrl Pts',(4.13302779078836,-31.5608034111036,
123.663627943128));
#100670=CARTESIAN_POINT('Ctrl Pts',(4.13688656728126,-31.5145190201024,
123.609570515794));
#100671=CARTESIAN_POINT('Ctrl Pts',(4.14074534377418,-31.4653706837746,
123.557859390925));
#100672=CARTESIAN_POINT('Ctrl Pts',(4.14460412026708,-31.4136286358643,
123.508808649983));
#100673=CARTESIAN_POINT('Ctrl Pts',(4.14846046585529,-31.3619191837748,
123.459788809426));
#100674=CARTESIAN_POINT('Ctrl Pts',(4.1523168114435,-31.3076196135577,123.413426361147));
#100675=CARTESIAN_POINT('Ctrl Pts',(4.1561731570317,-31.2510378033503,123.369999393531));
#100676=CARTESIAN_POINT('Ctrl Pts',(4.16002836327703,-31.1944727100272,
123.32658525625));
#100677=CARTESIAN_POINT('Ctrl Pts',(4.16388356952235,-31.1356271005012,
123.286105173458));
#100678=CARTESIAN_POINT('Ctrl Pts',(4.16773877576768,-31.0748414568478,
123.248796583734));
#100679=CARTESIAN_POINT('Ctrl Pts',(4.17159413261893,-31.014053438567,123.211486536528));
#100680=CARTESIAN_POINT('Ctrl Pts',(4.17544948947017,-30.9513256508639,
123.177348480609));
#100681=CARTESIAN_POINT('Ctrl Pts',(4.17930484632142,-30.8870255559437,
123.146575271126));
#100682=CARTESIAN_POINT('Ctrl Pts',(4.18316423878998,-30.8226581545234,
123.115769849605));
#100683=CARTESIAN_POINT('Ctrl Pts',(4.18702363125854,-30.7567155995423,
123.088336515709));
#100684=CARTESIAN_POINT('Ctrl Pts',(4.1908830237271,-30.6895870208718,123.064420680224));
#100685=CARTESIAN_POINT('Ctrl Pts',(4.19474460133053,-30.6224204349244,
123.040491303922));
#100686=CARTESIAN_POINT('Ctrl Pts',(4.19860617893397,-30.5540669542209,
123.020083529651));
#100687=CARTESIAN_POINT('Ctrl Pts',(4.2024677565374,-30.4849299800442,123.00329259105));
#100688=CARTESIAN_POINT('Ctrl Pts',(4.20633609065227,-30.4156720385312,
122.986472273739));
#100689=CARTESIAN_POINT('Ctrl Pts',(4.21020442476714,-30.3456283441291,
122.973281516649));
#100690=CARTESIAN_POINT('Ctrl Pts',(4.21407275888201,-30.2752108761994,
122.963764125618));
#100691=CARTESIAN_POINT('Ctrl Pts',(4.21637047805297,-30.2333841980406,
122.95811097075));
#100692=CARTESIAN_POINT('Ctrl Pts',(4.21866819722394,-30.1914257349887,
122.953752835488));
#100693=CARTESIAN_POINT('Ctrl Pts',(4.22096591639491,-30.1494218301973,
122.950690194441));
#100694=CARTESIAN_POINT('Ctrl Pts',(4.22483498974313,-30.0786924779759,
122.945533087776));
#100695=CARTESIAN_POINT('Ctrl Pts',(4.22870406309134,-30.0075572855653,
122.944031880373));
#100696=CARTESIAN_POINT('Ctrl Pts',(4.23257313643955,-29.9364263435634,
122.946233715169));
#100697=CARTESIAN_POINT('Ctrl Pts',(4.23643644483533,-29.8654013872744,
122.948432269213));
#100698=CARTESIAN_POINT('Ctrl Pts',(4.2402997532311,-29.7943811504204,122.954322898336));
#100699=CARTESIAN_POINT('Ctrl Pts',(4.24416306162688,-29.7237793393141,
122.963900859705));
#100700=CARTESIAN_POINT('Ctrl Pts',(4.24802183811979,-29.6532603485569,
122.973467585525));
#100701=CARTESIAN_POINT('Ctrl Pts',(4.2518806146127,-29.5831592876139,122.986712986754));
#100702=CARTESIAN_POINT('Ctrl Pts',(4.25573939110561,-29.5138865950802,
123.003580374757));
#100703=CARTESIAN_POINT('Ctrl Pts',(4.25959573669382,-29.4446575421081,
123.020437136849));
#100704=CARTESIAN_POINT('Ctrl Pts',(4.26345208228203,-29.3762562930919,
123.040911244135));
#100705=CARTESIAN_POINT('Ctrl Pts',(4.26730842787023,-29.3090834642402,
123.064894859933));
#100706=CARTESIAN_POINT('Ctrl Pts',(4.27116363411556,-29.2419304813494,
123.088871389861));
#100707=CARTESIAN_POINT('Ctrl Pts',(4.2750188403609,-29.1760056553525,123.116355206566));
#100708=CARTESIAN_POINT('Ctrl Pts',(4.27887404660623,-29.1116931339931,
123.147189034385));
#100709=CARTESIAN_POINT('Ctrl Pts',(4.28272940345749,-29.0473781002267,
123.178024066745));
#100710=CARTESIAN_POINT('Ctrl Pts',(4.28658476030875,-28.9846759332387,
123.212209158043));
#100711=CARTESIAN_POINT('Ctrl Pts',(4.29044011716001,-28.9239479573427,
123.249540184982));
#100712=CARTESIAN_POINT('Ctrl Pts',(4.29429950962857,-28.8631564140833,
123.286910288391));
#100713=CARTESIAN_POINT('Ctrl Pts',(4.29815890209712,-28.8043436017998,
123.327432646138));
#100714=CARTESIAN_POINT('Ctrl Pts',(4.30201829456568,-28.7478427364944,
123.370859198857));
#100715=CARTESIAN_POINT('Ctrl Pts',(4.30587987216911,-28.691309881177,123.414310339091));
#100716=CARTESIAN_POINT('Ctrl Pts',(4.30974144977254,-28.6370919480332,
123.460668631775));
#100717=CARTESIAN_POINT('Ctrl Pts',(4.31360302737596,-28.5854877373581,
123.509646813223));
#100718=CARTESIAN_POINT('Ctrl Pts',(4.31747136149083,-28.5337932360101,
123.558710690643));
#100719=CARTESIAN_POINT('Ctrl Pts',(4.3213396956057,-28.4847219221545,123.6104032564));
#100720=CARTESIAN_POINT('Ctrl Pts',(4.32520802972057,-28.4385340417937,
123.664402147403));
#100721=CARTESIAN_POINT('Ctrl Pts',(4.32750574889154,-28.4110992921005,
123.69647649346));
#100722=CARTESIAN_POINT('Ctrl Pts',(4.32980346806251,-28.3846810693939,
123.729363929871));
#100723=CARTESIAN_POINT('Ctrl Pts',(4.33210118723347,-28.3593266018392,
123.762992173401));
#100724=CARTESIAN_POINT('Ctrl Pts',(4.33598223894955,-28.3165006546752,
123.819793262895));
#100725=CARTESIAN_POINT('Ctrl Pts',(4.33986329066564,-28.2765427096807,
123.878933890299));
#100726=CARTESIAN_POINT('Ctrl Pts',(4.34374434238172,-28.2397168782025,
123.940093922267));
#100727=CARTESIAN_POINT('Ctrl Pts',(4.34761960540849,-28.2029459734072,
124.001162732461));
#100728=CARTESIAN_POINT('Ctrl Pts',(4.35149486843527,-28.1692981577268,
124.064244561645));
#100729=CARTESIAN_POINT('Ctrl Pts',(4.35537013146204,-28.1389961109817,
124.128987894712));
#100730=CARTESIAN_POINT('Ctrl Pts',(4.35942884712873,-28.1072595834202,
124.196796138544));
#100731=CARTESIAN_POINT('Ctrl Pts',(4.36348756279542,-28.0791938035524,
124.266426682195));
#100732=CARTESIAN_POINT('Ctrl Pts',(4.36754627846211,-28.0550020434937,
124.337443955815));
#100733=CARTESIAN_POINT('Ctrl Pts',(4.37141366678514,-28.0319506799473,
124.40511348413));
#100734=CARTESIAN_POINT('Ctrl Pts',(4.37528105510817,-28.0124165131004,
124.474041440808));
#100735=CARTESIAN_POINT('Ctrl Pts',(4.3791484434312,-27.9965263590055,124.543830149681));
#100736=CARTESIAN_POINT('Ctrl Pts',(4.38301406018575,-27.9806434838528,
124.613586889828));
#100737=CARTESIAN_POINT('Ctrl Pts',(4.38687967694029,-27.9684014102052,
124.684203129543));
#100738=CARTESIAN_POINT('Ctrl Pts',(4.39074529369484,-27.9598764862877,
124.755268287101));
#100739=CARTESIAN_POINT('Ctrl Pts',(4.39461092103577,-27.9513515390239,
124.826333639279));
#100740=CARTESIAN_POINT('Ctrl Pts',(4.3984765483767,-27.9465438214082,124.897847434114));
#100741=CARTESIAN_POINT('Ctrl Pts',(4.40234217571764,-27.9454779738572,
124.969392703581));
#100742=CARTESIAN_POINT('Ctrl Pts',(4.4029196902992,-27.9453187390298,124.980081379109));
#100743=CARTESIAN_POINT('Ctrl Pts',(4.40349720488077,-27.9452429264143,
124.990770753236));
#100744=CARTESIAN_POINT('Ctrl Pts',(4.40407471946233,-27.9452505182983,
125.001459433628));
#100745=CARTESIAN_POINT('Ctrl Pts',(4.40407471951209,-27.9452505182989,
125.001459434549));
#100746=CARTESIAN_POINT('Ctrl Pts',(4.40849095806752,-27.945308573269,125.083195487555));
#100747=CARTESIAN_POINT('Ctrl Pts',(4.41290719662295,-27.9502477237073,
125.164736898217));
#100748=CARTESIAN_POINT('Ctrl Pts',(4.41732343517838,-27.9599745962953,
125.245548192295));
#100749=CARTESIAN_POINT('Ctrl Pts',(4.42177971598686,-27.9697896629173,
125.327092206368));
#100750=CARTESIAN_POINT('Ctrl Pts',(4.42623599679533,-27.9844795567246,
125.407892614167));
#100751=CARTESIAN_POINT('Ctrl Pts',(4.43069227760381,-28.0038986271028,
125.487418579475));
#100752=CARTESIAN_POINT('Ctrl Pts',(4.43487367109322,-28.0221198249895,
125.562038956394));
#100753=CARTESIAN_POINT('Ctrl Pts',(4.43905506458263,-28.0445042064888,
125.635537342873));
#100754=CARTESIAN_POINT('Ctrl Pts',(4.44323645807204,-28.0708935156208,
125.70749256846));
#100755=CARTESIAN_POINT('Ctrl Pts',(4.44710553142024,-28.0953117323945,
125.774073254131));
#100756=CARTESIAN_POINT('Ctrl Pts',(4.45097460476845,-28.1232287475471,
125.839518723706));
#100757=CARTESIAN_POINT('Ctrl Pts',(4.45484367811666,-28.1545186966461,
125.903435842476));
#100758=CARTESIAN_POINT('Ctrl Pts',(4.45870698651244,-28.1857620234529,
125.967257724192));
#100759=CARTESIAN_POINT('Ctrl Pts',(4.46257029490822,-28.2203680964809,
126.029555342637));
#100760=CARTESIAN_POINT('Ctrl Pts',(4.466433603304,-28.2581622778487,126.089953628459));
#100761=CARTESIAN_POINT('Ctrl Pts',(4.4702923797969,-28.2959121242731,126.150281063306));
#100762=CARTESIAN_POINT('Ctrl Pts',(4.47415115628981,-28.3368423939913,
126.208713181356));
#100763=CARTESIAN_POINT('Ctrl Pts',(4.47800993278271,-28.3807324547538,
126.26489927639));
#100764=CARTESIAN_POINT('Ctrl Pts',(4.48186627837091,-28.4245948661939,
126.321049975997));
#100765=CARTESIAN_POINT('Ctrl Pts',(4.48572262395911,-28.4714130710542,
126.374957077846));
#100766=CARTESIAN_POINT('Ctrl Pts',(4.48957896954731,-28.5209238681718,
126.42629988388));
#100767=CARTESIAN_POINT('Ctrl Pts',(4.49343417579264,-28.5704200375096,
126.477627520874));
#100768=CARTESIAN_POINT('Ctrl Pts',(4.49728938203796,-28.622606882761,126.526392016628));
#100769=CARTESIAN_POINT('Ctrl Pts',(4.50114458828329,-28.6771829274427,
126.572308034404));
#100770=CARTESIAN_POINT('Ctrl Pts',(4.50499994513453,-28.7317611041698,
126.618225845917));
#100771=CARTESIAN_POINT('Ctrl Pts',(4.50885530198577,-28.7887282924879,
126.661294647469));
#100772=CARTESIAN_POINT('Ctrl Pts',(4.51271065883701,-28.8477497183853,
126.701269188288));
#100773=CARTESIAN_POINT('Ctrl Pts',(4.51657005130556,-28.9068329253051,
126.741285572692));
#100774=CARTESIAN_POINT('Ctrl Pts',(4.52042944377412,-28.9679742592167,
126.778200957744));
#100775=CARTESIAN_POINT('Ctrl Pts',(4.52428883624267,-29.0308104776631,
126.811813796253));
#100776=CARTESIAN_POINT('Ctrl Pts',(4.5281504138461,-29.0936822731112,126.845445665888));
#100777=CARTESIAN_POINT('Ctrl Pts',(4.53201199144952,-29.1582504234891,
126.875771060061));
#100778=CARTESIAN_POINT('Ctrl Pts',(4.53587356905295,-29.2241301267122,
126.902635935281));
#100779=CARTESIAN_POINT('Ctrl Pts',(4.53974190316782,-29.2901250981013,
126.929547815342));
#100780=CARTESIAN_POINT('Ctrl Pts',(4.54361023728269,-29.3574357450443,
126.952986928086));
#100781=CARTESIAN_POINT('Ctrl Pts',(4.54747857139755,-29.4256611505277,
126.972848815416));
#100782=CARTESIAN_POINT('Ctrl Pts',(4.54977629056857,-29.4661857839938,
126.984646410436));
#100783=CARTESIAN_POINT('Ctrl Pts',(4.55207400973958,-29.5070329226985,
126.995182881589));
#100784=CARTESIAN_POINT('Ctrl Pts',(4.55437172891059,-29.548117249947,127.004444946289));
#100785=CARTESIAN_POINT('Ctrl Pts',(4.55844028467461,-29.6208649897693,
127.020845221484));
#100786=CARTESIAN_POINT('Ctrl Pts',(4.56250884043863,-29.694656600035,127.033313769652));
#100787=CARTESIAN_POINT('Ctrl Pts',(4.56657739620265,-29.7690281740219,
127.041727106668));
#100788=CARTESIAN_POINT('Ctrl Pts',(4.5704397239533,-29.839629982312,127.049713986269));
#100789=CARTESIAN_POINT('Ctrl Pts',(4.57430205170395,-29.9107538314205,
127.054046646489));
#100790=CARTESIAN_POINT('Ctrl Pts',(4.5781643794546,-29.9819897223702,127.054671066716));
#100791=CARTESIAN_POINT('Ctrl Pts',(4.58202291830848,-30.0531557317731,
127.055294874394));
#100792=CARTESIAN_POINT('Ctrl Pts',(4.58588145716235,-30.1244330817512,
127.052217654959));
#100793=CARTESIAN_POINT('Ctrl Pts',(4.58973999601623,-30.195407433563,127.045437238687));
#100794=CARTESIAN_POINT('Ctrl Pts',(4.59359604056304,-30.26633590484,127.038661205536));
#100795=CARTESIAN_POINT('Ctrl Pts',(4.59745208510986,-30.3369612843276,
127.028186773298));
#100796=CARTESIAN_POINT('Ctrl Pts',(4.60130812965668,-30.4068717506067,
127.014063787733));
#100797=CARTESIAN_POINT('Ctrl Pts',(4.60516297144612,-30.4767604107765,
126.999945207337));
#100798=CARTESIAN_POINT('Ctrl Pts',(4.60901781323556,-30.5459341251056,
126.982180431198));
#100799=CARTESIAN_POINT('Ctrl Pts',(4.612872655025,-30.6139904073288,126.960870557229));
#100800=CARTESIAN_POINT('Ctrl Pts',(4.6167292826038,-30.6820782172232,126.939550811274));
#100801=CARTESIAN_POINT('Ctrl Pts',(4.6205859101826,-30.7490470959354,126.914682829204));
#100802=CARTESIAN_POINT('Ctrl Pts',(4.6244425377614,-30.814510037361,126.886417493965));
#100803=CARTESIAN_POINT('Ctrl Pts',(4.62830019961477,-30.8799905347093,
126.858144578499));
#100804=CARTESIAN_POINT('Ctrl Pts',(4.63215786146814,-30.9439638516118,
126.826472704402));
#100805=CARTESIAN_POINT('Ctrl Pts',(4.63601552332152,-31.0060654693665,
126.791599797345));
#100806=CARTESIAN_POINT('Ctrl Pts',(4.6398776444632,-31.068238873874,126.756686578735));
#100807=CARTESIAN_POINT('Ctrl Pts',(4.64373976560488,-31.1285358471724,
126.718565196641));
#100808=CARTESIAN_POINT('Ctrl Pts',(4.64760188674656,-31.1866197580259,
126.677477604131));
#100809=CARTESIAN_POINT('Ctrl Pts',(4.64907361358005,-31.2087536184256,
126.661820479406));
#100810=CARTESIAN_POINT('Ctrl Pts',(4.65054534041353,-31.2305664480703,
126.645733051043));
#100811=CARTESIAN_POINT('Ctrl Pts',(4.65201706724701,-31.2520409112987,
126.629230222815));
#100812=CARTESIAN_POINT('',(4.34592528058851,-27.945250355841,124.99879073222));
#100813=CARTESIAN_POINT('Ctrl Pts',(4.34592528058851,-27.945250355841,124.99879073222));
#100814=CARTESIAN_POINT('Ctrl Pts',(4.34974237135632,-27.945209114052,125.068867478461));
#100815=CARTESIAN_POINT('Ctrl Pts',(4.35355946212413,-27.9487570283886,
125.139087448465));
#100816=CARTESIAN_POINT('Ctrl Pts',(4.35737655289194,-27.955911683808,125.209046688822));
#100817=CARTESIAN_POINT('Ctrl Pts',(4.36118805254435,-27.9630558593865,
125.278903455801));
#100818=CARTESIAN_POINT('Ctrl Pts',(4.36499955219676,-27.9737962381263,
125.348499758144));
#100819=CARTESIAN_POINT('Ctrl Pts',(4.36881105184917,-27.988098387281,125.417431986363));
#100820=CARTESIAN_POINT('Ctrl Pts',(4.37261948474211,-28.0023890288257,
125.486308751225));
#100821=CARTESIAN_POINT('Ctrl Pts',(4.37642791763504,-28.0202356597748,
125.554522013913));
#100822=CARTESIAN_POINT('Ctrl Pts',(4.38023635052798,-28.0415522620249,
125.621675172514));
#100823=CARTESIAN_POINT('Ctrl Pts',(4.38404307118847,-28.0628592805488,
125.688798139742));
#100824=CARTESIAN_POINT('Ctrl Pts',(4.38784979184896,-28.0876330257033,
125.754861472597));
#100825=CARTESIAN_POINT('Ctrl Pts',(4.39165651250945,-28.1157372762062,
125.819482489271));
#100826=CARTESIAN_POINT('Ctrl Pts',(4.39546287300883,-28.1438388677124,
125.884097392026));
#100827=CARTESIAN_POINT('Ctrl Pts',(4.39926923350821,-28.1752701383349,
125.947269792159));
#100828=CARTESIAN_POINT('Ctrl Pts',(4.40307559400758,-28.2098469931641,
126.008637583385));
#100829=CARTESIAN_POINT('Ctrl Pts',(4.40688551323047,-28.2444561753217,
126.070062749891));
#100830=CARTESIAN_POINT('Ctrl Pts',(4.41069543245336,-28.2822165682454,
126.129679502486));
#100831=CARTESIAN_POINT('Ctrl Pts',(4.41450535167624,-28.3228989571241,
126.187151908765));
#100832=CARTESIAN_POINT('Ctrl Pts',(4.41831711300228,-28.3636010160147,
126.244652103061));
#100833=CARTESIAN_POINT('Ctrl Pts',(4.42212887432831,-28.407227572401,126.300005495645));
#100834=CARTESIAN_POINT('Ctrl Pts',(4.42594063565434,-28.4535088401647,
126.352908960371));
#100835=CARTESIAN_POINT('Ctrl Pts',(4.42975910316277,-28.4998715323924,
126.405905500254));
#100836=CARTESIAN_POINT('Ctrl Pts',(4.43357757067119,-28.5488979118458,
126.456443149054));
#100837=CARTESIAN_POINT('Ctrl Pts',(4.43739603817962,-28.6002816356027,
126.504255983159));
#100838=CARTESIAN_POINT('Ctrl Pts',(4.44006763663388,-28.6362323610338,
126.537708328479));
#100839=CARTESIAN_POINT('Ctrl Pts',(4.44273923508813,-28.6733362922242,
126.569827654898));
#100840=CARTESIAN_POINT('Ctrl Pts',(4.44541083354239,-28.7114798816252,
126.600535368882));
#100841=CARTESIAN_POINT('Ctrl Pts',(4.4492799068906,-28.7667203482161,126.645007021265));
#100842=CARTESIAN_POINT('Ctrl Pts',(4.45314898023881,-28.8243740439198,
126.686702591709));
#100843=CARTESIAN_POINT('Ctrl Pts',(4.45701805358702,-28.8841304900815,
126.725350051246));
#100844=CARTESIAN_POINT('Ctrl Pts',(4.46088136198282,-28.9437978986267,
126.763939925737));
#100845=CARTESIAN_POINT('Ctrl Pts',(4.46474467037861,-29.0055614338967,
126.799490442826));
#100846=CARTESIAN_POINT('Ctrl Pts',(4.4686079787744,-29.0690781313601,126.831770192188));
#100847=CARTESIAN_POINT('Ctrl Pts',(4.47246675526731,-29.1325203197564,
126.864012075381));
#100848=CARTESIAN_POINT('Ctrl Pts',(4.47632553176022,-29.1977111543373,
126.892990593039));
#100849=CARTESIAN_POINT('Ctrl Pts',(4.48018430825314,-29.2642808120643,
126.918518918073));
#100850=CARTESIAN_POINT('Ctrl Pts',(4.48404065384134,-29.3308085330544,
126.944031161085));
#100851=CARTESIAN_POINT('Ctrl Pts',(4.48789699942955,-29.3987129013685,
126.966097350154));
#100852=CARTESIAN_POINT('Ctrl Pts',(4.49175334501776,-29.4676030803233,
126.984578313501));
#100853=CARTESIAN_POINT('Ctrl Pts',(4.49560855126309,-29.5364729059325,
127.003053816717));
#100854=CARTESIAN_POINT('Ctrl Pts',(4.49946375750842,-29.6063274950223,
127.017946071298));
#100855=CARTESIAN_POINT('Ctrl Pts',(4.50331896375375,-29.6767614356553,
127.029165935309));
#100856=CARTESIAN_POINT('Ctrl Pts',(4.507174320605,-29.7471981278319,127.040386237632));
#100857=CARTESIAN_POINT('Ctrl Pts',(4.51102967745624,-29.8182137364021,
127.047933790311));
#100858=CARTESIAN_POINT('Ctrl Pts',(4.51488503430748,-29.8893949749596,
127.051770964542));
#100859=CARTESIAN_POINT('Ctrl Pts',(4.51874442677604,-29.9606507228947,
127.055612155357));
#100860=CARTESIAN_POINT('Ctrl Pts',(4.5226038192446,-30.0320719608351,127.055735188464));
#100861=CARTESIAN_POINT('Ctrl Pts',(4.52646321171316,-30.1032435307007,
127.052154559449));
#100862=CARTESIAN_POINT('Ctrl Pts',(4.5303247893166,-30.1744553969292,127.048571903132));
#100863=CARTESIAN_POINT('Ctrl Pts',(4.53418636692004,-30.2454168302102,
127.041281459958));
#100864=CARTESIAN_POINT('Ctrl Pts',(4.53804794452347,-30.3157186798857,
127.030349545687));
#100865=CARTESIAN_POINT('Ctrl Pts',(4.54191627863834,-30.3861435350527,
127.019398504103));
#100866=CARTESIAN_POINT('Ctrl Pts',(4.54578461275322,-30.4559060268753,
127.00479337032));
#100867=CARTESIAN_POINT('Ctrl Pts',(4.54965294686809,-30.5246087508621,
126.986651258027));
#100868=CARTESIAN_POINT('Ctrl Pts',(4.55195066603904,-30.5654169027211,
126.975875177683));
#100869=CARTESIAN_POINT('Ctrl Pts',(4.55424838520999,-30.605851453418,126.963852154995));
#100870=CARTESIAN_POINT('Ctrl Pts',(4.55654610438093,-30.6458324446947,
126.950614778956));
#100871=CARTESIAN_POINT('Ctrl Pts',(4.56041440943523,-30.7131420935789,
126.928329110068));
#100872=CARTESIAN_POINT('Ctrl Pts',(4.56428271448952,-30.7794286907234,
126.902511739844));
#100873=CARTESIAN_POINT('Ctrl Pts',(4.56815101954381,-30.8442955354996,
126.873275903661));
#100874=CARTESIAN_POINT('Ctrl Pts',(4.57201426861251,-30.9090775974502,
126.844078279553));
#100875=CARTESIAN_POINT('Ctrl Pts',(4.57587751768122,-30.9724431477123,
126.811471247143));
#100876=CARTESIAN_POINT('Ctrl Pts',(4.57974076674992,-31.0340117705029,
126.775617419649));
#100877=CARTESIAN_POINT('Ctrl Pts',(4.58359955353666,-31.0955092778802,
126.739805005454));
#100878=CARTESIAN_POINT('Ctrl Pts',(4.58745834032341,-31.1552135623627,
126.700753487884));
#100879=CARTESIAN_POINT('Ctrl Pts',(4.59131712711015,-31.2127670754802,
126.658672234991));
#100880=CARTESIAN_POINT('Ctrl Pts',(4.59220253433037,-31.2259728572141,
126.649016597817));
#100881=CARTESIAN_POINT('Ctrl Pts',(4.59308794155059,-31.2390655097594,
126.639201639586));
#100882=CARTESIAN_POINT('Ctrl Pts',(4.59397334877082,-31.2520409112987,
126.629230222815));
#100883=CARTESIAN_POINT('Ctrl Pts',(3.89394636911841,-31.2520409112987,
126.629230222815));
#100884=CARTESIAN_POINT('Ctrl Pts',(3.89781318526386,-31.3083155207066,
126.585983963165));
#100885=CARTESIAN_POINT('Ctrl Pts',(3.90168000140932,-31.3624485309783,
126.539740516924));
#100886=CARTESIAN_POINT('Ctrl Pts',(3.90554681755477,-31.4141040713363,
126.490740499862));
#100887=CARTESIAN_POINT('Ctrl Pts',(3.90951860641449,-31.4671619080732,
126.440410276089));
#100888=CARTESIAN_POINT('Ctrl Pts',(3.91349039527422,-31.5176053431718,
126.387171882628));
#100889=CARTESIAN_POINT('Ctrl Pts',(3.91746218413394,-31.5651045384085,
126.331332169803));
#100890=CARTESIAN_POINT('Ctrl Pts',(3.92131985552486,-31.6112389863935,
126.277096844048));
#100891=CARTESIAN_POINT('Ctrl Pts',(3.92517752691578,-31.6545957638065,
126.220408064187));
#100892=CARTESIAN_POINT('Ctrl Pts',(3.92903519830671,-31.6949097126747,
126.161584533463));
#100893=CARTESIAN_POINT('Ctrl Pts',(3.93289094441448,-31.7352035416938,
126.102790360333));
#100894=CARTESIAN_POINT('Ctrl Pts',(3.93674669052226,-31.7724572813979,
126.041863950583));
#100895=CARTESIAN_POINT('Ctrl Pts',(3.94060243663004,-31.8064475888168,
125.979155080341));
#100896=CARTESIAN_POINT('Ctrl Pts',(3.94445754823064,-31.8404323027414,
125.916456529562));
#100897=CARTESIAN_POINT('Ctrl Pts',(3.94831265983124,-31.8711544199303,
125.851976528084));
#100898=CARTESIAN_POINT('Ctrl Pts',(3.95216777143185,-31.8984361485015,
125.786090168214));
#100899=CARTESIAN_POINT('Ctrl Pts',(3.95622626966154,-31.927157196964,125.716727798821));
#100900=CARTESIAN_POINT('Ctrl Pts',(3.96028476789123,-31.9520645755645,
125.645807120439));
#100901=CARTESIAN_POINT('Ctrl Pts',(3.96434326612092,-31.973009012082,125.57378828913));
#100902=CARTESIAN_POINT('Ctrl Pts',(3.96820348466854,-31.9929301991169,
125.505287968898));
#100903=CARTESIAN_POINT('Ctrl Pts',(3.97206370321616,-32.0092665464193,
125.435794794154));
#100904=CARTESIAN_POINT('Ctrl Pts',(3.97592392176378,-32.0219418432179,
125.365716755351));
#100905=CARTESIAN_POINT('Ctrl Pts',(3.97978683983634,-32.0346260040949,
125.295589709631));
#100906=CARTESIAN_POINT('Ctrl Pts',(3.98364975790889,-32.0436439603416,
125.224877467475));
#100907=CARTESIAN_POINT('Ctrl Pts',(3.98751267598145,-32.0489713596993,
125.153993277879));
#100908=CARTESIAN_POINT('Ctrl Pts',(3.9913818497609,-32.0543073863818,125.08299429664));
#100909=CARTESIAN_POINT('Ctrl Pts',(3.99525102354035,-32.055940927385,125.011823296695));
#100910=CARTESIAN_POINT('Ctrl Pts',(3.9991201973198,-32.0538996768372,124.940892640152));
#100911=CARTESIAN_POINT('Ctrl Pts',(3.99970338160925,-32.0535920077279,
124.930201560636));
#100912=CARTESIAN_POINT('Ctrl Pts',(4.00028656589869,-32.0532009492814,
124.919515928032));
#100913=CARTESIAN_POINT('Ctrl Pts',(4.00086975018814,-32.052726697614,124.90883713803));
#100914=CARTESIAN_POINT('Ctrl Pts',(4.00473882353635,-32.0495803260131,
124.837989856074));
#100915=CARTESIAN_POINT('Ctrl Pts',(4.00860789688457,-32.0427556783592,
124.76716688376));
#100916=CARTESIAN_POINT('Ctrl Pts',(4.01247697023278,-32.0322538737086,
124.69678101099));
#100917=CARTESIAN_POINT('Ctrl Pts',(4.01634027862857,-32.0217677168369,
124.626500013773));
#100918=CARTESIAN_POINT('Ctrl Pts',(4.02020358702436,-32.0076153497239,
124.556655299875));
#100919=CARTESIAN_POINT('Ctrl Pts',(4.02406689542014,-31.9898498441324,
124.487657184781));
#100920=CARTESIAN_POINT('Ctrl Pts',(4.02792567191305,-31.9721051785923,
124.4187400088));
#100921=CARTESIAN_POINT('Ctrl Pts',(4.03178444840596,-31.9507559140856,
124.350667927121));
#100922=CARTESIAN_POINT('Ctrl Pts',(4.03564322489888,-31.9259063300412,
124.283841937554));
#100923=CARTESIAN_POINT('Ctrl Pts',(4.03949957048708,-31.9010724004331,
124.217058046203));
#100924=CARTESIAN_POINT('Ctrl Pts',(4.04335591607529,-31.8727426950614,
124.151519143789));
#100925=CARTESIAN_POINT('Ctrl Pts',(4.04721226166349,-31.8410711425107,
124.08761049397));
#100926=CARTESIAN_POINT('Ctrl Pts',(4.05106746790882,-31.8094089472018,
124.023720725722));
#100927=CARTESIAN_POINT('Ctrl Pts',(4.05492267415416,-31.7744070804402,
123.961460688888));
#100928=CARTESIAN_POINT('Ctrl Pts',(4.05877788039949,-31.7362666457037,
123.901193512252));
#100929=CARTESIAN_POINT('Ctrl Pts',(4.06263323725073,-31.6981247209885,
123.840923981243));
#100930=CARTESIAN_POINT('Ctrl Pts',(4.06648859410198,-31.6568442465144,
123.782647874311));
#100931=CARTESIAN_POINT('Ctrl Pts',(4.07034395095322,-31.6126701841896,
123.726700176892));
#100932=CARTESIAN_POINT('Ctrl Pts',(4.07420334342178,-31.5684498824069,
123.670693915895));
#100933=CARTESIAN_POINT('Ctrl Pts',(4.07806273589034,-31.5213302481,123.617021311814));
#100934=CARTESIAN_POINT('Ctrl Pts',(4.0819221283589,-31.4715965922107,123.565984298449));
#100935=CARTESIAN_POINT('Ctrl Pts',(4.08578370596233,-31.4218347778102,
123.514918388631));
#100936=CARTESIAN_POINT('Ctrl Pts',(4.08964528356577,-31.3694563524205,
123.46649137005));
#100937=CARTESIAN_POINT('Ctrl Pts',(4.0935068611692,-31.3147815393856,123.42096641385));
#100938=CARTESIAN_POINT('Ctrl Pts',(4.09737519528408,-31.2600110631173,
123.375361803705));
#100939=CARTESIAN_POINT('Ctrl Pts',(4.10124352939895,-31.2029365664032,
123.332669684726));
#100940=CARTESIAN_POINT('Ctrl Pts',(4.10511186351382,-31.1439086244318,
123.293110835042));
#100941=CARTESIAN_POINT('Ctrl Pts',(4.10740958268478,-31.1088471147839,
123.269613607398));
#100942=CARTESIAN_POINT('Ctrl Pts',(4.10970730185574,-31.073096919377,123.247220986002));
#100943=CARTESIAN_POINT('Ctrl Pts',(4.1120050210267,-31.036735346744,123.225971425452));
#100944=CARTESIAN_POINT('Ctrl Pts',(4.11587409437491,-30.9755069802181,
123.190189808002));
#100945=CARTESIAN_POINT('Ctrl Pts',(4.11974316772313,-30.9123040724542,
123.15751165516));
#100946=CARTESIAN_POINT('Ctrl Pts',(4.12361224107134,-30.8474740331646,
123.128159909177));
#100947=CARTESIAN_POINT('Ctrl Pts',(4.12747554946713,-30.7827405911888,
123.098851897547));
#100948=CARTESIAN_POINT('Ctrl Pts',(4.13133885786291,-30.7163852690692,
123.072860653239));
#100949=CARTESIAN_POINT('Ctrl Pts',(4.13520216625869,-30.648781574934,123.050364128734));
#100950=CARTESIAN_POINT('Ctrl Pts',(4.1390609427516,-30.5812571841689,123.027893994063));
#100951=CARTESIAN_POINT('Ctrl Pts',(4.14291971924451,-30.5124877889165,
123.008910588793));
#100952=CARTESIAN_POINT('Ctrl Pts',(4.14677849573742,-30.4428668423194,
122.993543790043));
#100953=CARTESIAN_POINT('Ctrl Pts',(4.15063484132563,-30.3732897546726,
122.978186671881));
#100954=CARTESIAN_POINT('Ctrl Pts',(4.15449118691383,-30.3028626532357,
122.966441744494));
#100955=CARTESIAN_POINT('Ctrl Pts',(4.15834753250204,-30.2319927001266,
122.958388638945));
#100956=CARTESIAN_POINT('Ctrl Pts',(4.16220273874737,-30.1611436852799,
122.950337912657));
#100957=CARTESIAN_POINT('Ctrl Pts',(4.1660579449927,-30.0898525609291,122.945976897614));
#100958=CARTESIAN_POINT('Ctrl Pts',(4.16991315123803,-30.0185334786877,
122.945333586037));
#100959=CARTESIAN_POINT('Ctrl Pts',(4.17376850808927,-29.9472116103242,
122.944690249329));
#100960=CARTESIAN_POINT('Ctrl Pts',(4.17762386494052,-29.8758622676878,
122.947764906609));
#100961=CARTESIAN_POINT('Ctrl Pts',(4.18147922179176,-29.8048997451783,
122.95453343878));
#100962=CARTESIAN_POINT('Ctrl Pts',(4.18533861426031,-29.7338629422336,
122.961309055952));
#100963=CARTESIAN_POINT('Ctrl Pts',(4.18919800672887,-29.6632142522818,
122.971786220367));
#100964=CARTESIAN_POINT('Ctrl Pts',(4.19305739919743,-29.5933620854687,
122.985888987924));
#100965=CARTESIAN_POINT('Ctrl Pts',(4.19691897680086,-29.5234703693204,
122.999999740274));
#100966=CARTESIAN_POINT('Ctrl Pts',(4.20078055440429,-29.4543765448209,
123.017740061325));
#100967=CARTESIAN_POINT('Ctrl Pts',(4.20464213200773,-29.3864753911521,
123.038983652073));
#100968=CARTESIAN_POINT('Ctrl Pts',(4.2085104661226,-29.3184554324331,123.060264412231));
#100969=CARTESIAN_POINT('Ctrl Pts',(4.21237880023747,-29.2516327664633,
123.085060510932));
#100970=CARTESIAN_POINT('Ctrl Pts',(4.21624713435234,-29.1863830179587,
123.113197156819));
#100971=CARTESIAN_POINT('Ctrl Pts',(4.21854485352331,-29.1476258698976,
123.129909805919));
#100972=CARTESIAN_POINT('Ctrl Pts',(4.22084257269429,-29.1094232312381,
123.14780014868));
#100973=CARTESIAN_POINT('Ctrl Pts',(4.22314029186526,-29.0718493387358,
123.16682409123));
#100974=CARTESIAN_POINT('Ctrl Pts',(4.22700936521348,-29.0085795763096,
123.198858044738));
#100975=CARTESIAN_POINT('Ctrl Pts',(4.2308784385617,-28.946846249431,123.234234104093));
#100976=CARTESIAN_POINT('Ctrl Pts',(4.23474751190992,-28.8870250841454,
123.272781311131));
#100977=CARTESIAN_POINT('Ctrl Pts',(4.23861082030572,-28.8272930529084,
123.311271082501));
#100978=CARTESIAN_POINT('Ctrl Pts',(4.24247412870151,-28.769467932831,123.352922361501));
#100979=CARTESIAN_POINT('Ctrl Pts',(4.2463374370973,-28.7139018069391,123.397517862719));
#100980=CARTESIAN_POINT('Ctrl Pts',(4.25019621359022,-28.6584008635953,
123.442061050619));
#100981=CARTESIAN_POINT('Ctrl Pts',(4.25405499008314,-28.6051540277779,
123.489541297822));
#100982=CARTESIAN_POINT('Ctrl Pts',(4.25791376657606,-28.5544838097656,
123.53969848789));
#100983=CARTESIAN_POINT('Ctrl Pts',(4.26177011216428,-28.503845512356,123.589824080546));
#100984=CARTESIAN_POINT('Ctrl Pts',(4.26562645775249,-28.4557809568064,
123.642622929359));
#100985=CARTESIAN_POINT('Ctrl Pts',(4.26948280334071,-28.4105778747512,
123.697796148727));
#100986=CARTESIAN_POINT('Ctrl Pts',(4.27333800958605,-28.3653881477776,
123.752953067374));
#100987=CARTESIAN_POINT('Ctrl Pts',(4.27719321583139,-28.3230585236229,
123.810482588338));
#100988=CARTESIAN_POINT('Ctrl Pts',(4.28104842207672,-28.2838371407315,
123.870051946784));
#100989=CARTESIAN_POINT('Ctrl Pts',(4.28490377892798,-28.2446142256337,
123.929623632342));
#100990=CARTESIAN_POINT('Ctrl Pts',(4.28875913577923,-28.208500058177,123.991234906642));
#100991=CARTESIAN_POINT('Ctrl Pts',(4.29261449263048,-28.1756990732597,
124.054524621582));
#100992=CARTESIAN_POINT('Ctrl Pts',(4.29647388509905,-28.1428637537198,
124.117880585401));
#100993=CARTESIAN_POINT('Ctrl Pts',(4.30033327756761,-28.1133487638009,
124.182918064874));
#100994=CARTESIAN_POINT('Ctrl Pts',(4.30419267003618,-28.0873118065517,
124.249252747495));
#100995=CARTESIAN_POINT('Ctrl Pts',(4.30805424763962,-28.0612601075358,
124.315624987901));
#100996=CARTESIAN_POINT('Ctrl Pts',(4.31191582524307,-28.0386905150577,
124.383295432486));
#100997=CARTESIAN_POINT('Ctrl Pts',(4.31577740284651,-28.0197110338736,
124.45186391002));
#100998=CARTESIAN_POINT('Ctrl Pts',(4.31964573696139,-28.0006983447381,
124.520552360206));
#100999=CARTESIAN_POINT('Ctrl Pts',(4.32351407107627,-27.9852884132221,
124.590141505975));
#101000=CARTESIAN_POINT('Ctrl Pts',(4.32738240519115,-27.9735381148485,
124.660220968086));
#101001=CARTESIAN_POINT('Ctrl Pts',(4.32968012436204,-27.9665586541724,
124.701846877017));
#101002=CARTESIAN_POINT('Ctrl Pts',(4.33197784353293,-27.9608693712244,
124.743645657191));
#101003=CARTESIAN_POINT('Ctrl Pts',(4.33427556270382,-27.9564734841712,
124.785531024144));
#101004=CARTESIAN_POINT('Ctrl Pts',(4.33815880198178,-27.9490442554462,
124.856319005628));
#101005=CARTESIAN_POINT('Ctrl Pts',(4.34204204125973,-27.9452923123651,
124.927499585747));
#101006=CARTESIAN_POINT('Ctrl Pts',(4.34592528053768,-27.9452503558416,
124.998790731287));
#101007=CARTESIAN_POINT('Origin',(-1.54592528053767,-30.,125.));
#101008=CARTESIAN_POINT('',(3.19385981518126,-31.2520409112986,126.629230222815));
#101009=CARTESIAN_POINT('',(3.25213329740746,-31.2520409112987,126.629230222815));
#101010=CARTESIAN_POINT('',(-1.54592528053767,-31.2520409112987,126.629230222815));
#101011=CARTESIAN_POINT('',(3.70407471941287,-27.9452505355246,124.998516511556));
#101012=CARTESIAN_POINT('Ctrl Pts',(3.25213329740746,-31.2520409112987,
126.629230222815));
#101013=CARTESIAN_POINT('Ctrl Pts',(3.25599022094518,-31.3085196988896,
126.585827055053));
#101014=CARTESIAN_POINT('Ctrl Pts',(3.2598471444829,-31.3627864472108,126.539447086643));
#101015=CARTESIAN_POINT('Ctrl Pts',(3.26370406802062,-31.4145168381827,
126.490348844062));
#101016=CARTESIAN_POINT('Ctrl Pts',(3.26755947426724,-31.4662268787221,
126.441269916442));
#101017=CARTESIAN_POINT('Ctrl Pts',(3.27141488051386,-31.515402190237,126.389475171135));
#101018=CARTESIAN_POINT('Ctrl Pts',(3.27527028676049,-31.561753193755,126.335261968415));
#101019=CARTESIAN_POINT('Ctrl Pts',(3.27912546600276,-31.6081014681496,
126.281051957741));
#101020=CARTESIAN_POINT('Ctrl Pts',(3.28298064524503,-31.6516254502506,
126.224424142637));
#101021=CARTESIAN_POINT('Ctrl Pts',(3.2868358244873,-31.6920751093616,126.165709821001));
#101022=CARTESIAN_POINT('Ctrl Pts',(3.29069479680136,-31.7325645664823,
126.10693773094));
#101023=CARTESIAN_POINT('Ctrl Pts',(3.29455376911542,-31.7699733821347,
126.046075434586));
#101024=CARTESIAN_POINT('Ctrl Pts',(3.29841274142948,-31.8040947549429,
125.983483440474));
#101025=CARTESIAN_POINT('Ctrl Pts',(3.30227355969859,-31.838232449848,125.920861505229));
#101026=CARTESIAN_POINT('Ctrl Pts',(3.30613437796769,-31.8690793587569,
125.85650866261));
#101027=CARTESIAN_POINT('Ctrl Pts',(3.3099951962368,-31.8964758488847,125.790807762416));
#101028=CARTESIAN_POINT('Ctrl Pts',(3.31386313027636,-31.9239228327476,
125.724985770657));
#101029=CARTESIAN_POINT('Ctrl Pts',(3.31773106431591,-31.9479065279911,
125.657811215831));
#101030=CARTESIAN_POINT('Ctrl Pts',(3.32159899835547,-31.9683165969665,
125.589684098994));
#101031=CARTESIAN_POINT('Ctrl Pts',(3.32502724879912,-31.9864065714346,
125.529301265126));
#101032=CARTESIAN_POINT('Ctrl Pts',(3.32845549924278,-32.0016898867466,
125.468170556474));
#101033=CARTESIAN_POINT('Ctrl Pts',(3.33188374968643,-32.014123551826,125.406575799181));
#101034=CARTESIAN_POINT('Ctrl Pts',(3.33575282303466,-32.0281560045215,
125.337060856283));
#101035=CARTESIAN_POINT('Ctrl Pts',(3.33962189638288,-32.0386128869442,
125.266682430377));
#101036=CARTESIAN_POINT('Ctrl Pts',(3.34349096973111,-32.0453957342306,
125.195841397287));
#101037=CARTESIAN_POINT('Ctrl Pts',(3.3473542781269,-32.0521684750165,125.125105917943));
#101038=CARTESIAN_POINT('Ctrl Pts',(3.35121758652268,-32.0552780011611,
125.053909679268));
#101039=CARTESIAN_POINT('Ctrl Pts',(3.35508089491847,-32.0546768638109,
124.982663684929));
#101040=CARTESIAN_POINT('Ctrl Pts',(3.35893967141139,-32.0540764316325,
124.911501266606));
#101041=CARTESIAN_POINT('Ctrl Pts',(3.36279844790432,-32.0497739862522,
124.840289691965));
#101042=CARTESIAN_POINT('Ctrl Pts',(3.36665722439724,-32.0417740221373,
124.769443271568));
#101043=CARTESIAN_POINT('Ctrl Pts',(3.37051356998546,-32.0337790977417,
124.69864148213));
#101044=CARTESIAN_POINT('Ctrl Pts',(3.37436991557368,-32.0220913303191,
124.628204872126));
#101045=CARTESIAN_POINT('Ctrl Pts',(3.3782262611619,-32.0067671925841,124.558544456068));
#101046=CARTESIAN_POINT('Ctrl Pts',(3.38208146740724,-31.9914475823081,
124.488904620919));
#101047=CARTESIAN_POINT('Ctrl Pts',(3.38593667365259,-31.9724938389182,
124.420040998629));
#101048=CARTESIAN_POINT('Ctrl Pts',(3.38979187989793,-31.9500135557809,
124.35235449915));
#101049=CARTESIAN_POINT('Ctrl Pts',(3.39364723674919,-31.9275323944381,
124.284665355459));
#101050=CARTESIAN_POINT('Ctrl Pts',(3.39750259360046,-31.9015245750382,
124.218153886206));
#101051=CARTESIAN_POINT('Ctrl Pts',(3.40135795045172,-31.8721470420658,
124.153204265844));
#101052=CARTESIAN_POINT('Ctrl Pts',(3.40521734292029,-31.842738757989,124.088186659088));
#101053=CARTESIAN_POINT('Ctrl Pts',(3.40907673538886,-31.809953919732,124.02473460832));
#101054=CARTESIAN_POINT('Ctrl Pts',(3.41293612785744,-31.7739966007973,
123.963209942727));
#101055=CARTESIAN_POINT('Ctrl Pts',(3.41679770546088,-31.7380189233238,
123.901650442716));
#101056=CARTESIAN_POINT('Ctrl Pts',(3.42065928306433,-31.6988654562216,
123.842020906504));
#101057=CARTESIAN_POINT('Ctrl Pts',(3.42452086066778,-31.6567835031518,
123.784653964427));
#101058=CARTESIAN_POINT('Ctrl Pts',(3.42838919478266,-31.6146279202794,
123.727186648761));
#101059=CARTESIAN_POINT('Ctrl Pts',(3.43225752889754,-31.5695339288615,
123.671990207425));
#101060=CARTESIAN_POINT('Ctrl Pts',(3.43612586301243,-31.5217885122885,
123.619363448852));
#101061=CARTESIAN_POINT('Ctrl Pts',(3.43842358218328,-31.493428614792,123.58810412417));
#101062=CARTESIAN_POINT('Ctrl Pts',(3.44072130135414,-31.4641339653978,
123.557750714455));
#101063=CARTESIAN_POINT('Ctrl Pts',(3.44301902052499,-31.4339703168494,
123.528359183464));
#101064=CARTESIAN_POINT('Ctrl Pts',(3.4468880938732,-31.3831784837289,123.478867500293));
#101065=CARTESIAN_POINT('Ctrl Pts',(3.45075716722142,-31.3297219400211,
123.431911487284));
#101066=CARTESIAN_POINT('Ctrl Pts',(3.45462624056963,-31.2738840751607,
123.387791289705));
#101067=CARTESIAN_POINT('Ctrl Pts',(3.4584895489654,-31.2181294091975,123.343736831598));
#101068=CARTESIAN_POINT('Ctrl Pts',(3.46235285736118,-31.1600008431917,
123.302510100363));
#101069=CARTESIAN_POINT('Ctrl Pts',(3.46621616575695,-31.0998179446722,
123.264373873475));
#101070=CARTESIAN_POINT('Ctrl Pts',(3.47007494224986,-31.0397056444643,
123.226282382771));
#101071=CARTESIAN_POINT('Ctrl Pts',(3.47393371874277,-30.9775442068882,
123.19127445399));
#101072=CARTESIAN_POINT('Ctrl Pts',(3.47779249523568,-30.9136841499307,
123.159571018304));
#101073=CARTESIAN_POINT('Ctrl Pts',(3.48164884082389,-30.849864322749,123.12788755476));
#101074=CARTESIAN_POINT('Ctrl Pts',(3.48550518641209,-30.7843484332854,
123.099504669707));
#101075=CARTESIAN_POINT('Ctrl Pts',(3.4893615320003,-30.7175124215067,123.074597837468));
#101076=CARTESIAN_POINT('Ctrl Pts',(3.49321673824563,-30.6506961561776,
123.049698363859));
#101077=CARTESIAN_POINT('Ctrl Pts',(3.49707194449096,-30.5825609977989,
123.028273073754));
#101078=CARTESIAN_POINT('Ctrl Pts',(3.50092715073629,-30.5135021230633,
123.010449012438));
#101079=CARTESIAN_POINT('Ctrl Pts',(3.50478250758755,-30.4444405505017,
122.992624254815));
#101080=CARTESIAN_POINT('Ctrl Pts',(3.5086378644388,-30.3744556608622,122.978401124561));
#101081=CARTESIAN_POINT('Ctrl Pts',(3.51249322129005,-30.3039553368876,
122.967856128204));
#101082=CARTESIAN_POINT('Ctrl Pts',(3.51635261375861,-30.233381216287,122.957300093811));
#101083=CARTESIAN_POINT('Ctrl Pts',(3.52021200622717,-30.1622910657463,
122.950429951004));
#101084=CARTESIAN_POINT('Ctrl Pts',(3.52407139869572,-30.0910995558632,
122.947270491901));
#101085=CARTESIAN_POINT('Ctrl Pts',(3.52793297629916,-30.0198677383272,
122.944109243955));
#101086=CARTESIAN_POINT('Ctrl Pts',(3.5317945539026,-29.9485349332081,122.94466285826));
#101087=CARTESIAN_POINT('Ctrl Pts',(3.53565613150604,-29.8775147263634,
122.948903970985));
#101088=CARTESIAN_POINT('Ctrl Pts',(3.53952446562091,-29.8063702571345,
122.953152504285));
#101089=CARTESIAN_POINT('Ctrl Pts',(3.54339279973578,-29.7355399610821,
122.961101363275));
#101090=CARTESIAN_POINT('Ctrl Pts',(3.54726113385065,-29.6654305296703,
122.972671503672));
#101091=CARTESIAN_POINT('Ctrl Pts',(3.54955885302162,-29.6237868195261,
122.97954395383));
#101092=CARTESIAN_POINT('Ctrl Pts',(3.55185657219259,-29.5823972321476,
122.987693065517));
#101093=CARTESIAN_POINT('Ctrl Pts',(3.55415429136355,-29.541344447052,122.99709394972));
#101094=CARTESIAN_POINT('Ctrl Pts',(3.55802336471178,-29.4722166621203,
123.012923869659));
#101095=CARTESIAN_POINT('Ctrl Pts',(3.56189243806001,-29.4037739608203,
123.032367785461));
#101096=CARTESIAN_POINT('Ctrl Pts',(3.56576151140823,-29.3364222085184,
123.055350397333));
#101097=CARTESIAN_POINT('Ctrl Pts',(3.56962481980402,-29.2691708109044,
123.078298764916));
#101098=CARTESIAN_POINT('Ctrl Pts',(3.57348812819982,-29.2030075916806,
123.104775206827));
#101099=CARTESIAN_POINT('Ctrl Pts',(3.57735143659561,-29.1383266436017,
123.13465376153));
#101100=CARTESIAN_POINT('Ctrl Pts',(3.58121021308853,-29.0737215703287,
123.164497266816));
#101101=CARTESIAN_POINT('Ctrl Pts',(3.58506898958144,-29.0105957532282,
123.197734754905));
#101102=CARTESIAN_POINT('Ctrl Pts',(3.58892776607436,-28.9493249145678,
123.2341915655));
#101103=CARTESIAN_POINT('Ctrl Pts',(3.59278411166257,-28.8880926745592,
123.27062540948));
#101104=CARTESIAN_POINT('Ctrl Pts',(3.59664045725078,-28.8287135110409,
123.310274304497));
#101105=CARTESIAN_POINT('Ctrl Pts',(3.60049680283899,-28.771538743971,123.352917577977));
#101106=CARTESIAN_POINT('Ctrl Pts',(3.60435200908432,-28.714380868972,123.395548252663));
#101107=CARTESIAN_POINT('Ctrl Pts',(3.60820721532965,-28.6594264866417,
123.441171259207));
#101108=CARTESIAN_POINT('Ctrl Pts',(3.61206242157498,-28.6069966629045,
123.489523497256));
#101109=CARTESIAN_POINT('Ctrl Pts',(3.61591777842622,-28.5545647909652,
123.537877624215));
#101110=CARTESIAN_POINT('Ctrl Pts',(3.61977313527747,-28.5046580290379,
123.588960863403));
#101111=CARTESIAN_POINT('Ctrl Pts',(3.62362849212871,-28.4575618745395,
123.642472029155));
#101112=CARTESIAN_POINT('Ctrl Pts',(3.62748788459728,-28.4104164218662,
123.696039208033));
#101113=CARTESIAN_POINT('Ctrl Pts',(3.63134727706584,-28.36608777116,123.75203902136));
#101114=CARTESIAN_POINT('Ctrl Pts',(3.63520666953441,-28.3248216537974,
123.810136532659));
#101115=CARTESIAN_POINT('Ctrl Pts',(3.63906824713785,-28.2835321721272,
123.868266937968));
#101116=CARTESIAN_POINT('Ctrl Pts',(3.64292982474129,-28.2453089360093,
123.928496995213));
#101117=CARTESIAN_POINT('Ctrl Pts',(3.64679140234473,-28.2103532700133,
123.990464391739));
#101118=CARTESIAN_POINT('Ctrl Pts',(3.65065973645961,-28.1753364429113,
124.05254021116));
#101119=CARTESIAN_POINT('Ctrl Pts',(3.65452807057448,-28.1435988168498,
124.116359003769));
#101120=CARTESIAN_POINT('Ctrl Pts',(3.65839640468936,-28.1152945581266,
124.181536219572));
#101121=CARTESIAN_POINT('Ctrl Pts',(3.66069412386027,-28.0984823500919,
124.220250284544));
#101122=CARTESIAN_POINT('Ctrl Pts',(3.66299184303119,-28.0828805480776,
124.259443265274));
#101123=CARTESIAN_POINT('Ctrl Pts',(3.66528956220211,-28.0685130841419,
124.299032200191));
#101124=CARTESIAN_POINT('Ctrl Pts',(3.66976608681314,-28.0405217148223,
124.376161226107));
#101125=CARTESIAN_POINT('Ctrl Pts',(3.67424261142417,-28.01712742101,124.455042428841));
#101126=CARTESIAN_POINT('Ctrl Pts',(3.67871913603519,-27.9985204841637,
124.535158833377));
#101127=CARTESIAN_POINT('Ctrl Pts',(3.68315616207655,-27.9800777254367,
124.614568331627));
#101128=CARTESIAN_POINT('Ctrl Pts',(3.68759318811791,-27.9663383039422,
124.695191164252));
#101129=CARTESIAN_POINT('Ctrl Pts',(3.69203021415927,-27.957441161254,124.77650290212));
#101130=CARTESIAN_POINT('Ctrl Pts',(3.69604504924381,-27.949390597592,124.850077682826));
#101131=CARTESIAN_POINT('Ctrl Pts',(3.70005988432834,-27.945304178903,124.924216166571));
#101132=CARTESIAN_POINT('Ctrl Pts',(3.70407471941287,-27.9452505355246,
124.998516511556));
#101133=CARTESIAN_POINT('Ctrl Pts',(3.70407471946233,-27.9452505355239,
124.998516512471));
#101134=CARTESIAN_POINT('Ctrl Pts',(3.70793830290607,-27.9451989130944,
125.070017726521));
#101135=CARTESIAN_POINT('Ctrl Pts',(3.71180188634981,-27.94888376533,125.14155223813));
#101136=CARTESIAN_POINT('Ctrl Pts',(3.71566546979354,-27.9562889262007,
125.212703101364));
#101137=CARTESIAN_POINT('Ctrl Pts',(3.719528826635,-27.9636936527526,125.283849791542));
#101138=CARTESIAN_POINT('Ctrl Pts',(3.72339218347645,-27.9748182037561,
125.354612398354));
#101139=CARTESIAN_POINT('Ctrl Pts',(3.7272555403179,-27.9895945586335,125.424579231503));
#101140=CARTESIAN_POINT('Ctrl Pts',(3.73111993975008,-28.0043749011546,
125.494564946359));
#101141=CARTESIAN_POINT('Ctrl Pts',(3.73498433918225,-28.0228089023206,
125.563753989817));
#101142=CARTESIAN_POINT('Ctrl Pts',(3.73884873861442,-28.0447778295693,
125.631746647602));
#101143=CARTESIAN_POINT('Ctrl Pts',(3.74271803189476,-28.0667745781126,
125.699825410809));
#101144=CARTESIAN_POINT('Ctrl Pts',(3.7465873251751,-28.0923150338203,125.766704306565));
#101145=CARTESIAN_POINT('Ctrl Pts',(3.75045661845545,-28.1212314339412,
125.832001344764));
#101146=CARTESIAN_POINT('Ctrl Pts',(3.75432884727638,-28.1501697722456,
125.89734792227));
#101147=CARTESIAN_POINT('Ctrl Pts',(3.75820107609731,-28.1824889322509,
125.961109825259));
#101148=CARTESIAN_POINT('Ctrl Pts',(3.76207330491825,-28.2179753493701,
126.022929961946));
#101149=CARTESIAN_POINT('Ctrl Pts',(3.76595231070743,-28.2535238729228,
126.084858292938));
#101150=CARTESIAN_POINT('Ctrl Pts',(3.76983131649661,-28.2922504492806,
126.144837675188));
#101151=CARTESIAN_POINT('Ctrl Pts',(3.77371032228579,-28.3338989370491,
126.202540980813));
#101152=CARTESIAN_POINT('Ctrl Pts',(3.77461515920409,-28.3436140783436,
126.216001151814));
#101153=CARTESIAN_POINT('Ctrl Pts',(3.77551999612238,-28.3534880425284,
126.229337625417));
#101154=CARTESIAN_POINT('Ctrl Pts',(3.77642483304068,-28.3635172836502,
126.242546530955));
#101155=CARTESIAN_POINT('Ctrl Pts',(3.78029390638889,-28.4064022154457,
126.299027675063));
#101156=CARTESIAN_POINT('Ctrl Pts',(3.7841629797371,-28.4522986437701,126.353396665213));
#101157=CARTESIAN_POINT('Ctrl Pts',(3.78803205308531,-28.500970858232,126.405314624784));
#101158=CARTESIAN_POINT('Ctrl Pts',(3.7918953614811,-28.5495705506775,126.457155226149));
#101159=CARTESIAN_POINT('Ctrl Pts',(3.79575866987688,-28.6009374899867,
126.506551694649));
#101160=CARTESIAN_POINT('Ctrl Pts',(3.79962197827266,-28.6547946429129,
126.553196738911));
#101161=CARTESIAN_POINT('Ctrl Pts',(3.80348075476557,-28.7085886180233,
126.599787065613));
#101162=CARTESIAN_POINT('Ctrl Pts',(3.80733953125848,-28.7648666388798,
126.643632062676));
#101163=CARTESIAN_POINT('Ctrl Pts',(3.81119830775139,-28.8233148545274,
126.684461228679));
#101164=CARTESIAN_POINT('Ctrl Pts',(3.81505465333959,-28.8817262496846,
126.725264673625));
#101165=CARTESIAN_POINT('Ctrl Pts',(3.8189109989278,-28.9423047299235,126.763055779299));
#101166=CARTESIAN_POINT('Ctrl Pts',(3.822767344516,-29.0047045580445,126.797605225216));
#101167=CARTESIAN_POINT('Ctrl Pts',(3.82662255076133,-29.0670859503699,
126.832144463628));
#101168=CARTESIAN_POINT('Ctrl Pts',(3.83047775700666,-29.1312871975191,
126.863443708473));
#101169=CARTESIAN_POINT('Ctrl Pts',(3.834332963252,-29.1969363517463,126.891318677366));
#101170=CARTESIAN_POINT('Ctrl Pts',(3.83818832010324,-29.2625880705965,
126.919194735211));
#101171=CARTESIAN_POINT('Ctrl Pts',(3.84204367695448,-29.3296873608155,
126.943646063685));
#101172=CARTESIAN_POINT('Ctrl Pts',(3.84589903380572,-29.3978422093966,
126.96453647401));
#101173=CARTESIAN_POINT('Ctrl Pts',(3.84975842627427,-29.4660683994638,
126.985448751494));
#101174=CARTESIAN_POINT('Ctrl Pts',(3.85361781874282,-29.535351888136,127.002792527423));
#101175=CARTESIAN_POINT('Ctrl Pts',(3.85747721121138,-29.6052862753463,
127.016481747517));
#101176=CARTESIAN_POINT('Ctrl Pts',(3.86133878881481,-29.6752602584438,
127.030178718259));
#101177=CARTESIAN_POINT('Ctrl Pts',(3.86520036641824,-29.7458853925284,
127.040216945716));
#101178=CARTESIAN_POINT('Ctrl Pts',(3.86906194402167,-29.8167486103759,
127.046562115036));
#101179=CARTESIAN_POINT('Ctrl Pts',(3.87293027813654,-29.8877358159276,
127.052918386349));
#101180=CARTESIAN_POINT('Ctrl Pts',(3.87679861225141,-29.9589614513313,
127.055568680571));
#101181=CARTESIAN_POINT('Ctrl Pts',(3.88066694636628,-30.0300115980944,
127.054530814196));
#101182=CARTESIAN_POINT('Ctrl Pts',(3.88296466553726,-30.0722140758202,
127.053914340697));
#101183=CARTESIAN_POINT('Ctrl Pts',(3.88526238470825,-30.1143546997385,
127.051997629856));
#101184=CARTESIAN_POINT('Ctrl Pts',(3.88756010387923,-30.1563480122916,
127.048793025552));
#101185=CARTESIAN_POINT('Ctrl Pts',(3.89142879128781,-30.2270524750349,
127.043397408683));
#101186=CARTESIAN_POINT('Ctrl Pts',(3.8952974786964,-30.2976157809519,127.034326880076));
#101187=CARTESIAN_POINT('Ctrl Pts',(3.89916616610498,-30.3676255076527,
127.021595668927));
#101188=CARTESIAN_POINT('Ctrl Pts',(3.90302937629839,-30.4375361158937,
127.008882482388));
#101189=CARTESIAN_POINT('Ctrl Pts',(3.9068925864918,-30.506894226168,126.992518983124));
#101190=CARTESIAN_POINT('Ctrl Pts',(3.91075579668521,-30.5752914471932,
126.97257124416));
#101191=CARTESIAN_POINT('Ctrl Pts',(3.91461452951295,-30.6436093975202,
126.952646624134));
#101192=CARTESIAN_POINT('Ctrl Pts',(3.91847326234069,-30.7109682064446,
126.929146150395));
#101193=CARTESIAN_POINT('Ctrl Pts',(3.92233199516844,-30.7769704042266,
126.902186781958));
#101194=CARTESIAN_POINT('Ctrl Pts',(3.92618810388979,-30.8429277176394,
126.875245747066));
#101195=CARTESIAN_POINT('Ctrl Pts',(3.93004421261113,-30.9075298028326,
126.844850670379));
#101196=CARTESIAN_POINT('Ctrl Pts',(3.93390032133248,-30.9703965489165,
126.811167606919));
#101197=CARTESIAN_POINT('Ctrl Pts',(3.93775577558456,-31.0332526250852,
126.777490260239));
#101198=CARTESIAN_POINT('Ctrl Pts',(3.94161122983664,-31.0943735152382,
126.740526257114));
#101199=CARTESIAN_POINT('Ctrl Pts',(3.94546668408872,-31.1534025914141,
126.700488172443));
#101200=CARTESIAN_POINT('Ctrl Pts',(3.94765970066917,-31.1869788535919,
126.677714154703));
#101201=CARTESIAN_POINT('Ctrl Pts',(3.94985271724962,-31.2198787848706,
126.653946372515));
#101202=CARTESIAN_POINT('Ctrl Pts',(3.95204573383007,-31.2520409112987,
126.629230222815));
#101203=CARTESIAN_POINT('',(3.6459252804912,-27.9452507844795,125.001795499313));
#101204=CARTESIAN_POINT('Ctrl Pts',(3.64592528053768,-27.9452507844802,
125.001795500168));
#101205=CARTESIAN_POINT('Ctrl Pts',(3.65155534725441,-27.9453413655908,
125.105455454725));
#101206=CARTESIAN_POINT('Ctrl Pts',(3.65718541397115,-27.9532796299144,
125.208784026561));
#101207=CARTESIAN_POINT('Ctrl Pts',(3.66281548068789,-27.9688964527697,
125.310831052066));
#101208=CARTESIAN_POINT('Ctrl Pts',(3.66436496634941,-27.9731944556727,
125.33891604835));
#101209=CARTESIAN_POINT('Ctrl Pts',(3.66591445201094,-27.9780738114693,
125.366904156524));
#101210=CARTESIAN_POINT('Ctrl Pts',(3.66746393767247,-27.9835304264076,
125.394775912735));
#101211=CARTESIAN_POINT('Ctrl Pts',(3.67133301102068,-27.9971556208534,
125.464371825626));
#101212=CARTESIAN_POINT('Ctrl Pts',(3.6752020843689,-28.0144147564085,125.533397845813));
#101213=CARTESIAN_POINT('Ctrl Pts',(3.67907115771711,-28.0352454688279,
125.601445920045));
#101214=CARTESIAN_POINT('Ctrl Pts',(3.6829344661129,-28.0560451433074,125.669392602063));
#101215=CARTESIAN_POINT('Ctrl Pts',(3.68679777450868,-28.0804056902298,
125.736363769799));
#101216=CARTESIAN_POINT('Ctrl Pts',(3.69066108290446,-28.1082137350865,
125.801961526748));
#101217=CARTESIAN_POINT('Ctrl Pts',(3.69451985939738,-28.1359891593639,
125.867482333417));
#101218=CARTESIAN_POINT('Ctrl Pts',(3.69837863589029,-28.167203859883,125.931632484396));
#101219=CARTESIAN_POINT('Ctrl Pts',(3.7022374123832,-28.2016952041954,125.994030896847));
#101220=CARTESIAN_POINT('Ctrl Pts',(3.70609375797141,-28.2361648200736,
126.056390000311));
#101221=CARTESIAN_POINT('Ctrl Pts',(3.70995010355962,-28.2739067499914,
126.1169991305));
#101222=CARTESIAN_POINT('Ctrl Pts',(3.71380644914783,-28.3147115970116,
126.175500132392));
#101223=CARTESIAN_POINT('Ctrl Pts',(3.71766165539316,-28.3555043883924,
126.233983850381));
#101224=CARTESIAN_POINT('Ctrl Pts',(3.72151686163849,-28.3993580225826,
126.290360278361));
#101225=CARTESIAN_POINT('Ctrl Pts',(3.72537206788382,-28.4460197348839,
126.3443001518));
#101226=CARTESIAN_POINT('Ctrl Pts',(3.72922742473507,-28.4926832700525,
126.398242132433));
#101227=CARTESIAN_POINT('Ctrl Pts',(3.73308278158632,-28.5421547816391,
126.449747003594));
#101228=CARTESIAN_POINT('Ctrl Pts',(3.73693813843757,-28.5941423085762,
126.498519841031));
#101229=CARTESIAN_POINT('Ctrl Pts',(3.74079753090613,-28.6461842537608,
126.547343731721));
#101230=CARTESIAN_POINT('Ctrl Pts',(3.74465692337469,-28.7007471166532,
126.593429546882));
#101231=CARTESIAN_POINT('Ctrl Pts',(3.74851631584325,-28.7575039387415,
126.63652103569));
#101232=CARTESIAN_POINT('Ctrl Pts',(3.75237789344669,-28.8142928957609,
126.679636922306));
#101233=CARTESIAN_POINT('Ctrl Pts',(3.75623947105013,-28.8732778829183,
126.719754834329));
#101234=CARTESIAN_POINT('Ctrl Pts',(3.76010104865356,-28.9341031682011,
126.756662035356));
#101235=CARTESIAN_POINT('Ctrl Pts',(3.76396938276844,-28.9950348780537,
126.793633812044));
#101236=CARTESIAN_POINT('Ctrl Pts',(3.76783771688331,-29.0578128866984,
126.827383431727));
#101237=CARTESIAN_POINT('Ctrl Pts',(3.77170605099818,-29.1220577374244,
126.857744585804));
#101238=CARTESIAN_POINT('Ctrl Pts',(3.77400377016912,-29.1602179947248,
126.87577855177));
#101239=CARTESIAN_POINT('Ctrl Pts',(3.77630148934007,-29.1988953899815,
126.892617941925));
#101240=CARTESIAN_POINT('Ctrl Pts',(3.77859920851102,-29.2380077640326,
126.908236199957));
#101241=CARTESIAN_POINT('Ctrl Pts',(3.78246828185923,-29.3038681380679,
126.934535404255));
#101242=CARTESIAN_POINT('Ctrl Pts',(3.78633735520744,-29.3712206395651,
126.957472487004));
#101243=CARTESIAN_POINT('Ctrl Pts',(3.79020642855565,-29.4396886210872,
126.976878529693));
#101244=CARTESIAN_POINT('Ctrl Pts',(3.79406973695143,-29.5080545847303,
126.996255657212));
#101245=CARTESIAN_POINT('Ctrl Pts',(3.79793304534722,-29.5775322656589,
127.012112056774));
#101246=CARTESIAN_POINT('Ctrl Pts',(3.801796353743,-29.6477258834258,127.024327174469));
#101247=CARTESIAN_POINT('Ctrl Pts',(3.80565513023591,-29.7178371596798,
127.036527963064));
#101248=CARTESIAN_POINT('Ctrl Pts',(3.80951390672882,-29.7886622282979,
127.04509587146));
#101249=CARTESIAN_POINT('Ctrl Pts',(3.81337268322173,-29.8597927189906,
127.049960848614));
#101250=CARTESIAN_POINT('Ctrl Pts',(3.81722902880993,-29.9308783997689,
127.054822760991));
#101251=CARTESIAN_POINT('Ctrl Pts',(3.82108537439813,-30.0022686373834,
127.05598633715));
#101252=CARTESIAN_POINT('Ctrl Pts',(3.82494171998634,-30.0735489608218,
127.05343325016));
#101253=CARTESIAN_POINT('Ctrl Pts',(3.82879692623166,-30.1448082247554,
127.05088091747));
#101254=CARTESIAN_POINT('Ctrl Pts',(3.83265213247699,-30.215957153772,127.044614118991));
#101255=CARTESIAN_POINT('Ctrl Pts',(3.83650733872232,-30.2865820279036,
127.0346666321));
#101256=CARTESIAN_POINT('Ctrl Pts',(3.84036269557357,-30.3572096610377,
127.024718756606));
#101257=CARTESIAN_POINT('Ctrl Pts',(3.84421805242481,-30.4273127179105,
127.011089977162));
#101258=CARTESIAN_POINT('Ctrl Pts',(3.84807340927605,-30.4964850706124,
126.993865626656));
#101259=CARTESIAN_POINT('Ctrl Pts',(3.85193280174461,-30.5657298298786,
126.97662324646));
#101260=CARTESIAN_POINT('Ctrl Pts',(3.85579219421316,-30.6340414678542,
126.955777899661));
#101261=CARTESIAN_POINT('Ctrl Pts',(3.85965158668172,-30.7010273665053,
126.931465297102));
#101262=CARTESIAN_POINT('Ctrl Pts',(3.86351316428515,-30.7680511916499,
126.907138929083));
#101263=CARTESIAN_POINT('Ctrl Pts',(3.86737474188858,-30.8337473356283,
126.87934158674));
#101264=CARTESIAN_POINT('Ctrl Pts',(3.87123631949202,-30.8977441330561,
126.848256755449));
#101265=CARTESIAN_POINT('Ctrl Pts',(3.87510465360688,-30.9618529041741,
126.817117535761));
#101266=CARTESIAN_POINT('Ctrl Pts',(3.87897298772175,-31.0242559669951,
126.782679577798));
#101267=CARTESIAN_POINT('Ctrl Pts',(3.88284132183662,-31.0846077947283,
126.745171479859));
#101268=CARTESIAN_POINT('Ctrl Pts',(3.88513904100761,-31.12045566812,126.722892360957));
#101269=CARTESIAN_POINT('Ctrl Pts',(3.88743676017859,-31.1555804033926,
126.699530876914));
#101270=CARTESIAN_POINT('Ctrl Pts',(3.88973447934958,-31.1899151292548,
126.675141650032));
#101271=CARTESIAN_POINT('Ctrl Pts',(3.89113844260586,-31.2108944961563,
126.660239229047));
#101272=CARTESIAN_POINT('Ctrl Pts',(3.89254240586213,-31.2316087312057,
126.644932070857));
#101273=CARTESIAN_POINT('Ctrl Pts',(3.89394636911841,-31.2520409112987,
126.629230222815));
#101274=CARTESIAN_POINT('Ctrl Pts',(3.19385981518126,-31.2520409112986,
126.629230222815));
#101275=CARTESIAN_POINT('Ctrl Pts',(3.19772164077073,-31.3085714957689,
126.585787249867));
#101276=CARTESIAN_POINT('Ctrl Pts',(3.2015834663602,-31.3627857733034,126.539439075722));
#101277=CARTESIAN_POINT('Ctrl Pts',(3.20544529194967,-31.414385544613,126.490473446154));
#101278=CARTESIAN_POINT('Ctrl Pts',(3.20931377041992,-31.4660742083699,
126.441423462052));
#101279=CARTESIAN_POINT('Ctrl Pts',(3.21318224889018,-31.5151390411146,
126.389747374098));
#101280=CARTESIAN_POINT('Ctrl Pts',(3.21705072736043,-31.5613205159542,
126.335767872409));
#101281=CARTESIAN_POINT('Ctrl Pts',(3.21900810301303,-31.5846874534069,
126.308455283453));
#101282=CARTESIAN_POINT('Ctrl Pts',(3.22096547866562,-31.6073168710985,
126.280553478093));
#101283=CARTESIAN_POINT('Ctrl Pts',(3.22292285431822,-31.6291794168833,
126.252107020228));
#101284=CARTESIAN_POINT('Ctrl Pts',(3.22679192766652,-31.6723943169508,
126.195877940321));
#101285=CARTESIAN_POINT('Ctrl Pts',(3.23066100101482,-31.71277943223,126.137298834087));
#101286=CARTESIAN_POINT('Ctrl Pts',(3.23453007436312,-31.7500698029317,
126.076686234409));
#101287=CARTESIAN_POINT('Ctrl Pts',(3.23839338275899,-31.7873046106615,
126.016163948024));
#101288=CARTESIAN_POINT('Ctrl Pts',(3.24225669115486,-31.821453574431,125.953614592888));
#101289=CARTESIAN_POINT('Ctrl Pts',(3.24611999955073,-31.8522930751951,
125.889386263715));
#101290=CARTESIAN_POINT('Ctrl Pts',(3.24997877604373,-31.883096399292,125.825233278397));
#101291=CARTESIAN_POINT('Ctrl Pts',(3.25383755253673,-31.9105977625118,
125.759405667015));
#101292=CARTESIAN_POINT('Ctrl Pts',(3.25769632902973,-31.9346187232605,
125.692277370791));
#101293=CARTESIAN_POINT('Ctrl Pts',(3.26155267461802,-31.9586245515789,
125.625191363229));
#101294=CARTESIAN_POINT('Ctrl Pts',(3.26540902020632,-31.9791541641106,
125.556806752785));
#101295=CARTESIAN_POINT('Ctrl Pts',(3.26926536579461,-31.9960772362334,
125.487517414551));
#101296=CARTESIAN_POINT('Ctrl Pts',(3.27312057204003,-32.0129953084979,
125.418248547594));
#101297=CARTESIAN_POINT('Ctrl Pts',(3.27697577828545,-32.0263088405465,
125.348075955166));
#101298=CARTESIAN_POINT('Ctrl Pts',(3.28083098453088,-32.0359378534953,
125.277406955942));
#101299=CARTESIAN_POINT('Ctrl Pts',(3.28468634138221,-32.0455672426072,
125.206735195991));
#101300=CARTESIAN_POINT('Ctrl Pts',(3.28854169823355,-32.0515117634471,
125.135567472378));
#101301=CARTESIAN_POINT('Ctrl Pts',(3.29239705508489,-32.0537431147043,
125.064317814832));
#101302=CARTESIAN_POINT('Ctrl Pts',(3.29625644755354,-32.0559768016414,
124.99299357629));
#101303=CARTESIAN_POINT('Ctrl Pts',(3.30011584002218,-32.0544895448684,
124.921587719152));
#101304=CARTESIAN_POINT('Ctrl Pts',(3.30397523249083,-32.0493051964147,
124.850514969152));
#101305=CARTESIAN_POINT('Ctrl Pts',(3.30783681009436,-32.0441179126543,
124.779401978739));
#101306=CARTESIAN_POINT('Ctrl Pts',(3.31169838769789,-32.0352294307718,
124.708622953139));
#101307=CARTESIAN_POINT('Ctrl Pts',(3.31555996530141,-32.0227152743542,
124.638585443854));
#101308=CARTESIAN_POINT('Ctrl Pts',(3.31942829941637,-32.0101792222116,
124.568425391588));
#101309=CARTESIAN_POINT('Ctrl Pts',(3.32329663353133,-31.9940049403116,
124.499009919225));
#101310=CARTESIAN_POINT('Ctrl Pts',(3.3271649676463,-31.9743184724289,124.430733689802));
#101311=CARTESIAN_POINT('Ctrl Pts',(3.32946268681646,-31.9626250733319,
124.390178867869));
#101312=CARTESIAN_POINT('Ctrl Pts',(3.33176040598662,-31.9496934720421,
124.350025665612));
#101313=CARTESIAN_POINT('Ctrl Pts',(3.33405812515678,-31.9355580520013,
124.310353286216));
#101314=CARTESIAN_POINT('Ctrl Pts',(3.33792719850498,-31.911755762472,124.243549932798));
#101315=CARTESIAN_POINT('Ctrl Pts',(3.34179627185318,-31.884444339824,124.177849434962));
#101316=CARTESIAN_POINT('Ctrl Pts',(3.34566534520138,-31.8537460124449,
124.113646073036));
#101317=CARTESIAN_POINT('Ctrl Pts',(3.34952865359714,-31.8230934258366,
124.049538374669));
#101318=CARTESIAN_POINT('Ctrl Pts',(3.35339196199291,-31.7890641595371,
123.986923818938));
#101319=CARTESIAN_POINT('Ctrl Pts',(3.35725527038868,-31.7518293801401,
123.926179072015));
#101320=CARTESIAN_POINT('Ctrl Pts',(3.36111404688158,-31.7146382794729,
123.865505582488));
#101321=CARTESIAN_POINT('Ctrl Pts',(3.36497282337447,-31.6742493875133,
123.806697957087));
#101322=CARTESIAN_POINT('Ctrl Pts',(3.36883159986737,-31.6308800882599,
123.750108924659));
#101323=CARTESIAN_POINT('Ctrl Pts',(3.37268794545556,-31.5875381102661,
123.693555541496));
#101324=CARTESIAN_POINT('Ctrl Pts',(3.37654429104375,-31.5412197448298,
123.639218363069));
#101325=CARTESIAN_POINT('Ctrl Pts',(3.38040063663193,-31.4921852201793,
123.587420504475));
#101326=CARTESIAN_POINT('Ctrl Pts',(3.38425584287725,-31.4431651825956,
123.535637949364));
#101327=CARTESIAN_POINT('Ctrl Pts',(3.38811104912256,-31.3914309127222,
123.486393577259));
#101328=CARTESIAN_POINT('Ctrl Pts',(3.39196625536788,-31.3372812390443,
123.439975496923));
#101329=CARTESIAN_POINT('Ctrl Pts',(3.39582161221911,-31.2831294499774,
123.393555603237));
#101330=CARTESIAN_POINT('Ctrl Pts',(3.39967696907034,-31.2265624400241,
123.349962535016));
#101331=CARTESIAN_POINT('Ctrl Pts',(3.40353232592156,-31.1679127039799,
123.309444624278));
#101332=CARTESIAN_POINT('Ctrl Pts',(3.40739171839011,-31.1092015759818,
123.26888430118));
#101333=CARTESIAN_POINT('Ctrl Pts',(3.41125111085865,-31.0484037704135,
123.231405837976));
#101334=CARTESIAN_POINT('Ctrl Pts',(3.41511050332719,-30.985880652913,123.197214127881));
#101335=CARTESIAN_POINT('Ctrl Pts',(3.41897208093061,-30.9233221356842,
123.16300305891));
#101336=CARTESIAN_POINT('Ctrl Pts',(3.42283365853403,-30.8590367999064,
123.13208265822));
#101337=CARTESIAN_POINT('Ctrl Pts',(3.42669523613745,-30.793408008632,123.104610516454));
#101338=CARTESIAN_POINT('Ctrl Pts',(3.4305635702523,-30.7276643882062,123.077090307328));
#101339=CARTESIAN_POINT('Ctrl Pts',(3.43443190436716,-30.6605730766348,
123.053030566895));
#101340=CARTESIAN_POINT('Ctrl Pts',(3.43830023848201,-30.5925340091425,
123.032539451346));
#101341=CARTESIAN_POINT('Ctrl Pts',(3.44059795765313,-30.5521200570071,
123.02036810636));
#101342=CARTESIAN_POINT('Ctrl Pts',(3.44289567682424,-30.5113719666559,
123.00945485306));
#101343=CARTESIAN_POINT('Ctrl Pts',(3.44519339599535,-30.4703749284779,
122.999813761381));
#101344=CARTESIAN_POINT('Ctrl Pts',(3.44906246934355,-30.4013410144278,
122.983579361925));
#101345=CARTESIAN_POINT('Ctrl Pts',(3.45293154269175,-30.3313304296167,
122.970891287314));
#101346=CARTESIAN_POINT('Ctrl Pts',(3.45680061603996,-30.2607407184091,
122.961860691645));
#101347=CARTESIAN_POINT('Ctrl Pts',(3.46066392443573,-30.1902561864759,
122.95284355164));
#101348=CARTESIAN_POINT('Ctrl Pts',(3.4645272328315,-30.1191947189178,122.947473134267));
#101349=CARTESIAN_POINT('Ctrl Pts',(3.46839054122728,-30.0479656040059,
122.945809925218));
#101350=CARTESIAN_POINT('Ctrl Pts',(3.47224931772018,-29.97682004531,122.944148667218));
#101351=CARTESIAN_POINT('Ctrl Pts',(3.47610809421308,-29.9055077131915,
122.946185990665));
#101352=CARTESIAN_POINT('Ctrl Pts',(3.47996687070598,-29.8344428517917,
122.951930569249));
#101353=CARTESIAN_POINT('Ctrl Pts',(3.48382321629417,-29.7634227589621,
122.957671528934));
#101354=CARTESIAN_POINT('Ctrl Pts',(3.48767956188236,-29.6926503106128,
122.967115071211));
#101355=CARTESIAN_POINT('Ctrl Pts',(3.49153590747056,-29.6225381082558,
122.980217813035));
#101356=CARTESIAN_POINT('Ctrl Pts',(3.49539111371587,-29.5524466202867,
122.993316683703));
#101357=CARTESIAN_POINT('Ctrl Pts',(3.49924631996119,-29.4830154683063,
123.010072518449));
#101358=CARTESIAN_POINT('Ctrl Pts',(3.50310152620651,-29.4146487788748,
123.030390518294));
#101359=CARTESIAN_POINT('Ctrl Pts',(3.50695688305774,-29.3462794186581,
123.050709311873));
#101360=CARTESIAN_POINT('Ctrl Pts',(3.51081223990897,-29.278975068579,123.07459040633));
#101361=CARTESIAN_POINT('Ctrl Pts',(3.5146675967602,-29.2131246964193,123.101889144672));
#101362=CARTESIAN_POINT('Ctrl Pts',(3.51852698922875,-29.1472053949978,
123.129216458128));
#101363=CARTESIAN_POINT('Ctrl Pts',(3.52238638169729,-29.0827435593424,
123.159968370426));
#101364=CARTESIAN_POINT('Ctrl Pts',(3.52624577416584,-29.020107320911,123.193952409274));
#101365=CARTESIAN_POINT('Ctrl Pts',(3.53010735176926,-28.9574356187039,
123.227955689417));
#101366=CARTESIAN_POINT('Ctrl Pts',(3.53396892937268,-28.8965919858927,
123.265194485332));
#101367=CARTESIAN_POINT('Ctrl Pts',(3.5378305069761,-28.8379167435928,123.305432188528));
#101368=CARTESIAN_POINT('Ctrl Pts',(3.54169884109096,-28.7791388386026,
123.345740294685));
#101369=CARTESIAN_POINT('Ctrl Pts',(3.54556717520581,-28.7225372848184,
123.389057488815));
#101370=CARTESIAN_POINT('Ctrl Pts',(3.54943550932067,-28.6684198594702,
123.435106427949));
#101371=CARTESIAN_POINT('Ctrl Pts',(3.55173322849175,-28.6362751061941,
123.462458649115));
#101372=CARTESIAN_POINT('Ctrl Pts',(3.55403094766283,-28.605006105976,123.490773938098));
#101373=CARTESIAN_POINT('Ctrl Pts',(3.55632866683391,-28.5746708837891,
123.519988353768));
#101374=CARTESIAN_POINT('Ctrl Pts',(3.56013990426075,-28.5243537103043,
123.568446440295));
#101375=CARTESIAN_POINT('Ctrl Pts',(3.5639511416876,-28.4763982156428,123.619581983347));
#101376=CARTESIAN_POINT('Ctrl Pts',(3.56776237911444,-28.4311089343795,
123.673132114069));
#101377=CARTESIAN_POINT('Ctrl Pts',(3.57156855056504,-28.3858798525731,
123.72661106484));
#101378=CARTESIAN_POINT('Ctrl Pts',(3.57537472201564,-28.343310282624,123.782497865398));
#101379=CARTESIAN_POINT('Ctrl Pts',(3.57918089346624,-28.303669205142,123.840491743489));
#101380=CARTESIAN_POINT('Ctrl Pts',(3.58298336737577,-28.2640666373578,
123.898429282882));
#101381=CARTESIAN_POINT('Ctrl Pts',(3.5867858412853,-28.2273872042862,123.958469430919));
#101382=CARTESIAN_POINT('Ctrl Pts',(3.59058831519483,-28.1938594686753,
124.020278639813));
#101383=CARTESIAN_POINT('Ctrl Pts',(3.59438845464245,-28.1603523168273,
124.082049902033));
#101384=CARTESIAN_POINT('Ctrl Pts',(3.59818859409007,-28.1299932630402,
124.145587631281));
#101385=CARTESIAN_POINT('Ctrl Pts',(3.60198873353769,-28.1029663478004,
124.210531264126));
#101386=CARTESIAN_POINT('Ctrl Pts',(3.60578956781187,-28.0759344908949,
124.27548677142));
#101387=CARTESIAN_POINT('Ctrl Pts',(3.60959040208607,-28.0522361979834,
124.341848239274));
#101388=CARTESIAN_POINT('Ctrl Pts',(3.61339123636026,-28.032007893898,124.40923385945));
#101389=CARTESIAN_POINT('Ctrl Pts',(3.61719222217678,-28.0117787832937,
124.476622166345));
#101390=CARTESIAN_POINT('Ctrl Pts',(3.6209932079933,-27.9950200700698,124.545034222851));
#101391=CARTESIAN_POINT('Ctrl Pts',(3.62479419380982,-27.9818179362867,
124.614074203757));
#101392=CARTESIAN_POINT('Ctrl Pts',(3.6285996398477,-27.9686003106176,124.683195198803));
#101393=CARTESIAN_POINT('Ctrl Pts',(3.63240508588558,-27.9589476807175,
124.752945093907));
#101394=CARTESIAN_POINT('Ctrl Pts',(3.63621053192346,-27.9528946642781,
124.822920054894));
#101395=CARTESIAN_POINT('Ctrl Pts',(3.63944878144604,-27.9477438416413,
124.882465343869));
#101396=CARTESIAN_POINT('Ctrl Pts',(3.64268703096862,-27.9451986849018,
124.942173328698));
#101397=CARTESIAN_POINT('Ctrl Pts',(3.6459252804912,-27.9452507844795,125.001795499313));
#101398=CARTESIAN_POINT('Origin',(-1.54592528053767,-30.,125.));
#101399=CARTESIAN_POINT('',(2.49394332640294,-31.2520409112987,126.629230222815));
#101400=CARTESIAN_POINT('',(2.55206159779739,-31.2520409112987,126.629230222815));
#101401=CARTESIAN_POINT('',(-1.54592528053767,-31.2520409112987,126.629230222815));
#101402=CARTESIAN_POINT('',(3.00407471949958,-27.9452500948919,124.999375533621));
#101403=CARTESIAN_POINT('Ctrl Pts',(2.55206159779739,-31.2520409112987,
126.629230222815));
#101404=CARTESIAN_POINT('Ctrl Pts',(2.5526866831371,-31.2611311656917,126.622244487936));
#101405=CARTESIAN_POINT('Ctrl Pts',(2.55331176847681,-31.2701601850064,
126.615184799744));
#101406=CARTESIAN_POINT('Ctrl Pts',(2.55393685381652,-31.2791267189991,
126.608052362096));
#101407=CARTESIAN_POINT('Ctrl Pts',(2.55780592716366,-31.334626625145,126.563904911101));
#101408=CARTESIAN_POINT('Ctrl Pts',(2.5616750005108,-31.3879470172231,126.516794349563));
#101409=CARTESIAN_POINT('Ctrl Pts',(2.56554407385794,-31.4387544190603,
126.466963968247));
#101410=CARTESIAN_POINT('Ctrl Pts',(2.56940738225263,-31.4894861174333,
126.417207834626));
#101411=CARTESIAN_POINT('Ctrl Pts',(2.57327069064732,-31.5377119140533,
126.364740262816));
#101412=CARTESIAN_POINT('Ctrl Pts',(2.57713399904201,-31.5831308416319,
126.309845143814));
#101413=CARTESIAN_POINT('Ctrl Pts',(2.5809927755338,-31.6284964899615,126.255014420228));
#101414=CARTESIAN_POINT('Ctrl Pts',(2.58485155202558,-31.6710615013615,
126.197762178345));
#101415=CARTESIAN_POINT('Ctrl Pts',(2.58871032851737,-31.7105625192321,
126.138408288049));
#101416=CARTESIAN_POINT('Ctrl Pts',(2.59256667410444,-31.7500386527355,
126.079091788789));
#101417=CARTESIAN_POINT('Ctrl Pts',(2.5964230196915,-31.7864543537217,126.01767667131));
#101418=CARTESIAN_POINT('Ctrl Pts',(2.60027936527857,-31.8195881549648,
125.954513755172));
#101419=CARTESIAN_POINT('Ctrl Pts',(2.60413457152274,-31.8527121669502,
125.891369500281));
#101420=CARTESIAN_POINT('Ctrl Pts',(2.60798977776692,-31.8825559786222,
125.826478901844));
#101421=CARTESIAN_POINT('Ctrl Pts',(2.61184498401109,-31.9089437403483,
125.760217967878));
#101422=CARTESIAN_POINT('Ctrl Pts',(2.61570034086117,-31.9353325329277,
125.693954445391));
#101423=CARTESIAN_POINT('Ctrl Pts',(2.61955569771125,-31.9582648298261,
125.626320933222));
#101424=CARTESIAN_POINT('Ctrl Pts',(2.62341105456133,-31.9776133151839,
125.557712415235));
#101425=CARTESIAN_POINT('Ctrl Pts',(2.62727044702871,-31.9969820536817,
125.489032080881));
#101426=CARTESIAN_POINT('Ctrl Pts',(2.63112983949608,-32.0127593599251,
125.419375171884));
#101427=CARTESIAN_POINT('Ctrl Pts',(2.63498923196346,-32.0248683641775,
125.34914992518));
#101428=CARTESIAN_POINT('Ctrl Pts',(2.63885080956571,-32.0369842243814,
125.278884917908));
#101429=CARTESIAN_POINT('Ctrl Pts',(2.64271238716795,-32.0454275905173,
125.208051414956));
#101430=CARTESIAN_POINT('Ctrl Pts',(2.6465739647702,-32.0501734694427,125.137063152208));
#101431=CARTESIAN_POINT('Ctrl Pts',(2.65044229888388,-32.0549276521207,
125.065950682968));
#101432=CARTESIAN_POINT('Ctrl Pts',(2.65431063299756,-32.0559714241144,
124.994683399202));
#101433=CARTESIAN_POINT('Ctrl Pts',(2.65817896711124,-32.053331929569,124.923674712497));
#101434=CARTESIAN_POINT('Ctrl Pts',(2.66047668629252,-32.0517641184474,
124.88149686108));
#101435=CARTESIAN_POINT('Ctrl Pts',(2.6627744054738,-32.0488977950344,124.839410162816));
#101436=CARTESIAN_POINT('Ctrl Pts',(2.66507212465508,-32.0447472267912,
124.797499775235));
#101437=CARTESIAN_POINT('Ctrl Pts',(2.66894119800399,-32.0377581860486,
124.726927894671));
#101438=CARTESIAN_POINT('Ctrl Pts',(2.67281027135289,-32.0270976169124,
124.656580034074));
#101439=CARTESIAN_POINT('Ctrl Pts',(2.6766793447018,-32.0127890530529,124.586868313476));
#101440=CARTESIAN_POINT('Ctrl Pts',(2.68054265309829,-31.9985018090762,
124.517260463938));
#101441=CARTESIAN_POINT('Ctrl Pts',(2.68440596149478,-31.9805774566544,
124.448287344925));
#101442=CARTESIAN_POINT('Ctrl Pts',(2.68826926989126,-31.9590912711333,
124.380355784446));
#101443=CARTESIAN_POINT('Ctrl Pts',(2.69212804638489,-31.9376302902544,
124.312503911945));
#101444=CARTESIAN_POINT('Ctrl Pts',(2.69598682287852,-31.9126159214867,
124.245691631966));
#101445=CARTESIAN_POINT('Ctrl Pts',(2.69984559937214,-31.8841740662919,
124.180313687797));
#101446=CARTESIAN_POINT('Ctrl Pts',(2.70370194496107,-31.8557501285482,
124.114976929623));
#101447=CARTESIAN_POINT('Ctrl Pts',(2.70755829055,-31.8239031815397,124.051073158967));
#101448=CARTESIAN_POINT('Ctrl Pts',(2.71141463613892,-31.7888078481915,
123.98897871202));
#101449=CARTESIAN_POINT('Ctrl Pts',(2.71526984238498,-31.7537228836281,
123.926902610645));
#101450=CARTESIAN_POINT('Ctrl Pts',(2.71912504863104,-31.7153916769383,
123.866635194417));
#101451=CARTESIAN_POINT('Ctrl Pts',(2.7229802548771,-31.6740347543116,123.808528135516));
#101452=CARTESIAN_POINT('Ctrl Pts',(2.72683561172908,-31.6326762160522,
123.750418806628));
#101453=CARTESIAN_POINT('Ctrl Pts',(2.73069096858106,-31.5882920106661,
123.694470397124));
#101454=CARTESIAN_POINT('Ctrl Pts',(2.73454632543303,-31.5411449297523,
123.641004095665));
#101455=CARTESIAN_POINT('Ctrl Pts',(2.73840571790233,-31.4939484973562,
123.587481828043));
#101456=CARTESIAN_POINT('Ctrl Pts',(2.74226511037162,-31.4439837381921,
123.536447220084));
#101457=CARTESIAN_POINT('Ctrl Pts',(2.74612450284091,-31.3915519385093,
123.488186266456));
#101458=CARTESIAN_POINT('Ctrl Pts',(2.74998608044508,-31.3390904526635,
123.439897988141));
#101459=CARTESIAN_POINT('Ctrl Pts',(2.75384765804925,-31.2841595199455,
123.394386800424));
#101460=CARTESIAN_POINT('Ctrl Pts',(2.75770923565342,-31.2270931825123,
123.351898096618));
#101461=CARTESIAN_POINT('Ctrl Pts',(2.76157756976903,-31.1699269974518,
123.309335051327));
#101462=CARTESIAN_POINT('Ctrl Pts',(2.76544590388463,-31.1106183524661,
123.269805317836));
#101463=CARTESIAN_POINT('Ctrl Pts',(2.76931423800023,-31.0495292946477,
123.233510310764));
#101464=CARTESIAN_POINT('Ctrl Pts',(2.7716119571647,-31.0132435202823,123.211951745544));
#101465=CARTESIAN_POINT('Ctrl Pts',(2.77390967632917,-30.976330061229,123.191533555241));
#101466=CARTESIAN_POINT('Ctrl Pts',(2.77620739549364,-30.9388682001961,
123.172289939525));
#101467=CARTESIAN_POINT('Ctrl Pts',(2.78007646884175,-30.8757870846558,
123.139886083632));
#101468=CARTESIAN_POINT('Ctrl Pts',(2.78394554218985,-30.8109028729085,
123.110688339052));
#101469=CARTESIAN_POINT('Ctrl Pts',(2.78781461553796,-30.7445745687621,
123.084900453226));
#101470=CARTESIAN_POINT('Ctrl Pts',(2.79167792393363,-30.6783450943571,
123.059150991572));
#101471=CARTESIAN_POINT('Ctrl Pts',(2.79554123232931,-30.6106762477178,
123.036801478187));
#101472=CARTESIAN_POINT('Ctrl Pts',(2.79940454072498,-30.5419506494207,
123.018009319877));
#101473=CARTESIAN_POINT('Ctrl Pts',(2.80326331721779,-30.4733056705576,
122.999239205947));
#101474=CARTESIAN_POINT('Ctrl Pts',(2.80712209371059,-30.4036068686827,
122.984018285609));
#101475=CARTESIAN_POINT('Ctrl Pts',(2.8109808702034,-30.3332541692576,122.972454878141));
#101476=CARTESIAN_POINT('Ctrl Pts',(2.8148372157915,-30.2629457897636,122.960898755248));
#101477=CARTESIAN_POINT('Ctrl Pts',(2.81869356137959,-30.1919848082115,
122.952995652501));
#101478=CARTESIAN_POINT('Ctrl Pts',(2.82254990696769,-30.1207821102329,
122.948802972811));
#101479=CARTESIAN_POINT('Ctrl Pts',(2.82640511321291,-30.0496004488251,
122.944611531833));
#101480=CARTESIAN_POINT('Ctrl Pts',(2.83026031945814,-29.9781776974497,
122.94412836613));
#101481=CARTESIAN_POINT('Ctrl Pts',(2.83411552570336,-29.9069289167095,
122.947358936405));
#101482=CARTESIAN_POINT('Ctrl Pts',(2.8379708825545,-29.8356773525935,122.950589632885));
#101483=CARTESIAN_POINT('Ctrl Pts',(2.84182623940564,-29.7646002577934,
122.957534329175));
#101484=CARTESIAN_POINT('Ctrl Pts',(2.84568159625677,-29.6941100056194,
122.968146443801));
#101485=CARTESIAN_POINT('Ctrl Pts',(2.84954098872523,-29.6235459673619,
122.97876966672));
#101486=CARTESIAN_POINT('Ctrl Pts',(2.85340038119368,-29.5535704793302,
122.993067898798));
#101487=CARTESIAN_POINT('Ctrl Pts',(2.85725977366213,-29.4845872249428,
123.010943129569));
#101488=CARTESIAN_POINT('Ctrl Pts',(2.86112135126546,-29.4155649131867,
123.02882848105));
#101489=CARTESIAN_POINT('Ctrl Pts',(2.86498292886879,-29.3475364169122,
123.050294716615));
#101490=CARTESIAN_POINT('Ctrl Pts',(2.86884450647212,-29.2808890741998,
123.075194285416));
#101491=CARTESIAN_POINT('Ctrl Pts',(2.87271284058689,-29.2141251202007,
123.100137420407));
#101492=CARTESIAN_POINT('Ctrl Pts',(2.87658117470166,-29.1487475902524,
123.128525688683));
#101493=CARTESIAN_POINT('Ctrl Pts',(2.88044950881643,-29.0851220628897,
123.160164158766));
#101494=CARTESIAN_POINT('Ctrl Pts',(2.88274722798835,-29.0473296722359,
123.178956826908));
#101495=CARTESIAN_POINT('Ctrl Pts',(2.88504494716027,-29.0101549265945,
123.198895338703));
#101496=CARTESIAN_POINT('Ctrl Pts',(2.8873426663322,-28.9736695586932,123.219931633968));
#101497=CARTESIAN_POINT('Ctrl Pts',(2.8912117396803,-28.9122327363575,123.255354139184));
#101498=CARTESIAN_POINT('Ctrl Pts',(2.8950808130284,-28.8525115731632,123.294030383693));
#101499=CARTESIAN_POINT('Ctrl Pts',(2.8989498863765,-28.794871956984,123.335769258055));
#101500=CARTESIAN_POINT('Ctrl Pts',(2.90281319477217,-28.7373182243266,
123.377445941135));
#101501=CARTESIAN_POINT('Ctrl Pts',(2.90667650316783,-28.6818402725019,
123.422175913361));
#101502=CARTESIAN_POINT('Ctrl Pts',(2.9105398115635,-28.6287778654823,123.469723090317));
#101503=CARTESIAN_POINT('Ctrl Pts',(2.91439858805629,-28.5757777039916,
123.517214491454));
#101504=CARTESIAN_POINT('Ctrl Pts',(2.91825736454909,-28.5251878188804,
123.567516210343));
#101505=CARTESIAN_POINT('Ctrl Pts',(2.92211614104188,-28.4773161191015,
123.62035100067));
#101506=CARTESIAN_POINT('Ctrl Pts',(2.92597248662997,-28.4294745769492,
123.673152506784));
#101507=CARTESIAN_POINT('Ctrl Pts',(2.92982883221806,-28.3843481482237,
123.728483559244));
#101508=CARTESIAN_POINT('Ctrl Pts',(2.93368517780614,-28.3422079092198,
123.78603008841));
#101509=CARTESIAN_POINT('Ctrl Pts',(2.93754038405135,-28.3000801203918,
123.843559615669));
#101510=CARTESIAN_POINT('Ctrl Pts',(2.94139559029656,-28.2609370566097,
123.90330292844));
#101511=CARTESIAN_POINT('Ctrl Pts',(2.94525079654177,-28.2250084196124,
123.96491427792));
#101512=CARTESIAN_POINT('Ctrl Pts',(2.94910615339289,-28.1890783790417,
124.026528034284));
#101513=CARTESIAN_POINT('Ctrl Pts',(2.952961510244,-28.1563632573787,124.090009551487));
#101514=CARTESIAN_POINT('Ctrl Pts',(2.95681686709512,-28.1270475759708,
124.154987112629));
#101515=CARTESIAN_POINT('Ctrl Pts',(2.96067625956356,-28.0977012082021,
124.220032689413));
#101516=CARTESIAN_POINT('Ctrl Pts',(2.96453565203199,-28.0717615842105,
124.286576992497));
#101517=CARTESIAN_POINT('Ctrl Pts',(2.96839504450043,-28.0493653045228,
124.354227712502));
#101518=CARTESIAN_POINT('Ctrl Pts',(2.97225662210374,-28.02695634437,124.421916735413));
#101519=CARTESIAN_POINT('Ctrl Pts',(2.97611819970705,-28.0080948507384,
124.490712953569));
#101520=CARTESIAN_POINT('Ctrl Pts',(2.97997977731036,-27.9928669379986,
124.560210921099));
#101521=CARTESIAN_POINT('Ctrl Pts',(2.98384811142511,-27.9776123813384,
124.629830487586));
#101522=CARTESIAN_POINT('Ctrl Pts',(2.98771644553985,-27.9660041778276,
124.700153775401));
#101523=CARTESIAN_POINT('Ctrl Pts',(2.9915847796546,-27.9580768337092,124.77076792226));
#101524=CARTESIAN_POINT('Ctrl Pts',(2.99388249882665,-27.9533681374013,
124.812711424099));
#101525=CARTESIAN_POINT('Ctrl Pts',(2.9961802179987,-27.9499571027303,124.854757479904));
#101526=CARTESIAN_POINT('Ctrl Pts',(2.99847793717075,-27.9478422574974,
124.89681975777));
#101527=CARTESIAN_POINT('Ctrl Pts',(3.00034353126794,-27.9461251447924,
124.930971510627));
#101528=CARTESIAN_POINT('Ctrl Pts',(3.00220912536513,-27.945260491498,124.965166482837));
#101529=CARTESIAN_POINT('Ctrl Pts',(3.00407471946232,-27.9452500948921,
124.999375532937));
#101530=CARTESIAN_POINT('Ctrl Pts',(3.00407471949959,-27.9452500948919,
124.999375533621));
#101531=CARTESIAN_POINT('Ctrl Pts',(3.00791348792962,-27.945228702179,125.069766312486));
#101532=CARTESIAN_POINT('Ctrl Pts',(3.01175225635965,-27.9488287016156,
125.140303260411));
#101533=CARTESIAN_POINT('Ctrl Pts',(3.01559102478968,-27.9560689985432,
125.210579257724));
#101534=CARTESIAN_POINT('Ctrl Pts',(3.01950861575716,-27.9634579625721,
125.282298252324));
#101535=CARTESIAN_POINT('Ctrl Pts',(3.02342620672465,-27.9746384824609,
125.35374494479));
#101536=CARTESIAN_POINT('Ctrl Pts',(3.02734379769213,-27.9895745963593,
125.424484698071));
#101537=CARTESIAN_POINT('Ctrl Pts',(3.03117271153808,-28.0041726219789,
125.493623212797));
#101538=CARTESIAN_POINT('Ctrl Pts',(3.03500162538402,-28.0223579037,125.562085943561));
#101539=CARTESIAN_POINT('Ctrl Pts',(3.03883053922997,-28.0440446045493,
125.629472837784));
#101540=CARTESIAN_POINT('Ctrl Pts',(3.04265730106932,-28.0657191165835,
125.696821857809));
#101541=CARTESIAN_POINT('Ctrl Pts',(3.04648406290868,-28.0908909937601,
125.763095771075));
#101542=CARTESIAN_POINT('Ctrl Pts',(3.05031082474803,-28.1194241368866,
125.827908198761));
#101543=CARTESIAN_POINT('Ctrl Pts',(3.0541367656348,-28.1479511588175,125.892706722281));
#101544=CARTESIAN_POINT('Ctrl Pts',(3.05796270652157,-28.1798378159244,
125.956043930675));
#101545=CARTESIAN_POINT('Ctrl Pts',(3.06178864740834,-28.2149000053456,
126.017553719262));
#101546=CARTESIAN_POINT('Ctrl Pts',(3.06577402745842,-28.2514233480649,
126.081626816986));
#101547=CARTESIAN_POINT('Ctrl Pts',(3.0697594075085,-28.2913924556458,126.143716319393));
#101548=CARTESIAN_POINT('Ctrl Pts',(3.07374478755858,-28.334547641787,126.20343924027));
#101549=CARTESIAN_POINT('Ctrl Pts',(3.07757550004214,-28.3760280296557,
126.260844390014));
#101550=CARTESIAN_POINT('Ctrl Pts',(3.08140621252571,-28.4204513813144,
126.316062905982));
#101551=CARTESIAN_POINT('Ctrl Pts',(3.08523692500927,-28.4675457371936,
126.368788330936));
#101552=CARTESIAN_POINT('Ctrl Pts',(3.08907026922185,-28.5146724472584,
126.421549978664));
#101553=CARTESIAN_POINT('Ctrl Pts',(3.09290361343443,-28.5644734622162,
126.471814780227));
#101554=CARTESIAN_POINT('Ctrl Pts',(3.096736957647,-28.616640920405,126.519314062135));
#101555=CARTESIAN_POINT('Ctrl Pts',(3.10057644985369,-28.6688920458064,
126.566889524342));
#101556=CARTESIAN_POINT('Ctrl Pts',(3.10441594206038,-28.7235167986926,
126.611690314675));
#101557=CARTESIAN_POINT('Ctrl Pts',(3.10825543426707,-28.7801762753519,
126.653489535282));
#101558=CARTESIAN_POINT('Ctrl Pts',(3.10870802551448,-28.7868551750185,
126.658416739291));
#101559=CARTESIAN_POINT('Ctrl Pts',(3.10916061676189,-28.7935623181573,
126.663302287644));
#101560=CARTESIAN_POINT('Ctrl Pts',(3.10961320800931,-28.800297126947,126.668145850604));
#101561=CARTESIAN_POINT('Ctrl Pts',(3.11348228135751,-28.8578710843367,
126.709552087396));
#101562=CARTESIAN_POINT('Ctrl Pts',(3.11735135470571,-28.9177039567807,
126.748055289834));
#101563=CARTESIAN_POINT('Ctrl Pts',(3.12122042805391,-28.9794709514144,
126.783400690673));
#101564=CARTESIAN_POINT('Ctrl Pts',(3.12508373644968,-29.041145912697,126.818693426562));
#101565=CARTESIAN_POINT('Ctrl Pts',(3.12894704484544,-29.1047488575628,
126.850837461135));
#101566=CARTESIAN_POINT('Ctrl Pts',(3.13281035324121,-29.1699247609725,
126.879620349979));
#101567=CARTESIAN_POINT('Ctrl Pts',(3.13666912973411,-29.2350242089628,
126.90836947469));
#101568=CARTESIAN_POINT('Ctrl Pts',(3.140527906227,-29.3016925081228,126.93376509018));
#101569=CARTESIAN_POINT('Ctrl Pts',(3.1443866827199,-29.3695502355988,126.955640728014));
#101570=CARTESIAN_POINT('Ctrl Pts',(3.14824302830809,-29.4373652148956,
126.977502584902));
#101571=CARTESIAN_POINT('Ctrl Pts',(3.15209937389628,-29.5063676746451,
126.995848714865));
#101572=CARTESIAN_POINT('Ctrl Pts',(3.15595571948447,-29.5761597972444,
127.010561375593));
#101573=CARTESIAN_POINT('Ctrl Pts',(3.15981092572979,-29.6459313000223,
127.025269689522));
#101574=CARTESIAN_POINT('Ctrl Pts',(3.16366613197511,-29.7164915273992,
127.03634656525));
#101575=CARTESIAN_POINT('Ctrl Pts',(3.16752133822043,-29.7874308248601,
127.043725007989));
#101576=CARTESIAN_POINT('Ctrl Pts',(3.17137669507166,-29.8583728936066,
127.051103738972));
#101577=CARTESIAN_POINT('Ctrl Pts',(3.17523205192289,-29.9296935784304,
127.054783702051));
#101578=CARTESIAN_POINT('Ctrl Pts',(3.17908740877412,-30.0009781593512,
127.054749767175));
#101579=CARTESIAN_POINT('Ctrl Pts',(3.18294680124266,-30.0723373578237,
127.054715796777));
#101580=CARTESIAN_POINT('Ctrl Pts',(3.18680619371121,-30.1436598901705,
127.050960168243));
#101581=CARTESIAN_POINT('Ctrl Pts',(3.19066558617975,-30.2145319980777,
127.043519900637));
#101582=CARTESIAN_POINT('Ctrl Pts',(3.19452716378317,-30.2854442327965,
127.036075420455));
#101583=CARTESIAN_POINT('Ctrl Pts',(3.19838874138659,-30.3559050553407,
127.024942224089));
#101584=CARTESIAN_POINT('Ctrl Pts',(3.20225031899001,-30.4255095200121,
127.010208748085));
#101585=CARTESIAN_POINT('Ctrl Pts',(3.20611865310487,-30.4952357699771,
126.995449493265));
#101586=CARTESIAN_POINT('Ctrl Pts',(3.20998698721973,-30.5641022010522,
126.977077507279));
#101587=CARTESIAN_POINT('Ctrl Pts',(3.21385532133458,-30.6317183549193,
126.955231311778));
#101588=CARTESIAN_POINT('Ctrl Pts',(3.21615304050568,-30.6718811041553,
126.942255074274));
#101589=CARTESIAN_POINT('Ctrl Pts',(3.21845075967678,-30.7116030891758,
126.928054022522));
#101590=CARTESIAN_POINT('Ctrl Pts',(3.22074847884788,-30.7508062394284,
126.912665039503));
#101591=CARTESIAN_POINT('Ctrl Pts',(3.22461723641773,-30.8168140815572,
126.886754020742));
#101592=CARTESIAN_POINT('Ctrl Pts',(3.22848599398759,-30.8816083107962,
126.857371254927));
#101593=CARTESIAN_POINT('Ctrl Pts',(3.23235475155745,-30.9447988250308,
126.824651403069));
#101594=CARTESIAN_POINT('Ctrl Pts',(3.23621738607661,-31.0078893281598,
126.79198333665));
#101595=CARTESIAN_POINT('Ctrl Pts',(3.24008002059578,-31.0693807290199,
126.755988893851));
#101596=CARTESIAN_POINT('Ctrl Pts',(3.24394265511494,-31.1289021815181,
126.716851020637));
#101597=CARTESIAN_POINT('Ctrl Pts',(3.24667286921245,-31.1709735470352,
126.689187317881));
#101598=CARTESIAN_POINT('Ctrl Pts',(3.24940308330995,-31.2120610722941,
126.659954176594));
#101599=CARTESIAN_POINT('Ctrl Pts',(3.25213329740746,-31.2520409112987,
126.629230222815));
#101600=CARTESIAN_POINT('',(2.94592528057306,-27.9452500017688,125.000085258451));
#101601=CARTESIAN_POINT('Ctrl Pts',(2.94592528057306,-27.9452500017688,
125.000085258451));
#101602=CARTESIAN_POINT('Ctrl Pts',(2.94997591063975,-27.9452531186627,
125.075203179717));
#101603=CARTESIAN_POINT('Ctrl Pts',(2.95402654070645,-27.9493797866667,
125.150236380527));
#101604=CARTESIAN_POINT('Ctrl Pts',(2.95807717077314,-27.9575765752318,
125.224731209355));
#101605=CARTESIAN_POINT('Ctrl Pts',(2.96213971866872,-27.9657974805201,
125.299445218067));
#101606=CARTESIAN_POINT('Ctrl Pts',(2.96620226656431,-27.9781123929221,
125.373617281608));
#101607=CARTESIAN_POINT('Ctrl Pts',(2.97026481445989,-27.9944163846029,
125.446801884677));
#101608=CARTESIAN_POINT('Ctrl Pts',(2.97433371205176,-28.0107458591575,
125.52010087409));
#101609=CARTESIAN_POINT('Ctrl Pts',(2.97840260964364,-28.0310767338203,
125.592408932705));
#101610=CARTESIAN_POINT('Ctrl Pts',(2.98247150723551,-28.0552544358625,
125.663296504791));
#101611=CARTESIAN_POINT('Ctrl Pts',(2.9865516038357,-28.0794986832723,125.734379183903));
#101612=CARTESIAN_POINT('Ctrl Pts',(2.99063170043589,-28.1076107674917,
125.804033182399));
#101613=CARTESIAN_POINT('Ctrl Pts',(2.99471179703608,-28.1393881013189,
125.871849141186));
#101614=CARTESIAN_POINT('Ctrl Pts',(2.99669196890442,-28.1548104279601,
125.904761904528));
#101615=CARTESIAN_POINT('Ctrl Pts',(2.99867214077276,-28.1710953858727,
125.937242126137));
#101616=CARTESIAN_POINT('Ctrl Pts',(3.0006523126411,-28.1882160943984,125.969245398185));
#101617=CARTESIAN_POINT('Ctrl Pts',(3.00452138598921,-28.2216683810996,
126.031776842507));
#101618=CARTESIAN_POINT('Ctrl Pts',(3.00839045933732,-28.2584272837346,
126.092696890929));
#101619=CARTESIAN_POINT('Ctrl Pts',(3.01225953268542,-28.2983134165014,
126.151633767324));
#101620=CARTESIAN_POINT('Ctrl Pts',(3.0161228410811,-28.3381401185887,126.210482827268));
#101621=CARTESIAN_POINT('Ctrl Pts',(3.01998614947677,-28.3810845315813,
126.267354181628));
#101622=CARTESIAN_POINT('Ctrl Pts',(3.02384945787244,-28.4269214872576,
126.321900735777));
#101623=CARTESIAN_POINT('Ctrl Pts',(3.02770823436524,-28.4727046733122,
126.3763833034));
#101624=CARTESIAN_POINT('Ctrl Pts',(3.03156701085805,-28.5213733511308,
126.428546117723));
#101625=CARTESIAN_POINT('Ctrl Pts',(3.03542578735085,-28.5726601990986,
126.478072615017));
#101626=CARTESIAN_POINT('Ctrl Pts',(3.03928213293895,-28.6239147380067,
126.527567912215));
#101627=CARTESIAN_POINT('Ctrl Pts',(3.04313847852704,-28.677783826134,126.574429850717));
#101628=CARTESIAN_POINT('Ctrl Pts',(3.04699482411514,-28.7339621666742,
126.618377510684));
#101629=CARTESIAN_POINT('Ctrl Pts',(3.05085003036037,-28.7901239095339,
126.662312186479));
#101630=CARTESIAN_POINT('Ctrl Pts',(3.05470523660559,-28.8485931679217,
126.703333993932));
#101631=CARTESIAN_POINT('Ctrl Pts',(3.05856044285081,-28.9090316670749,
126.741202360168));
#101632=CARTESIAN_POINT('Ctrl Pts',(3.06241579970195,-28.9694725272939,
126.779072205754));
#101633=CARTESIAN_POINT('Ctrl Pts',(3.06627115655309,-29.0318823681856,
126.813788109482));
#101634=CARTESIAN_POINT('Ctrl Pts',(3.07012651340423,-29.0958955242712,
126.845153830841));
#101635=CARTESIAN_POINT('Ctrl Pts',(3.07398590587269,-29.159975686502,126.876552384452));
#101636=CARTESIAN_POINT('Ctrl Pts',(3.07784529834114,-29.2256620770228,
126.9045935411));
#101637=CARTESIAN_POINT('Ctrl Pts',(3.08170469080959,-29.2925669254543,
126.929128302508));
#101638=CARTESIAN_POINT('Ctrl Pts',(3.08556626841292,-29.3595096544898,
126.953676955161));
#101639=CARTESIAN_POINT('Ctrl Pts',(3.08942784601626,-29.4276717503634,
126.974715117171));
#101640=CARTESIAN_POINT('Ctrl Pts',(3.09328942361959,-29.4966507084971,
126.992143833473));
#101641=CARTESIAN_POINT('Ctrl Pts',(3.09715775773436,-29.5657503574902,
127.009603044389));
#101642=CARTESIAN_POINT('Ctrl Pts',(3.10102609184912,-29.6356692455768,
127.023440106453));
#101643=CARTESIAN_POINT('Ctrl Pts',(3.10489442596389,-29.7059958155199,
127.033607410984));
#101644=CARTESIAN_POINT('Ctrl Pts',(3.10719214513581,-29.7477685019683,
127.039646602495));
#101645=CARTESIAN_POINT('Ctrl Pts',(3.10948986430774,-29.7896849274545,
127.044392046685));
#101646=CARTESIAN_POINT('Ctrl Pts',(3.11178758347966,-29.83165875689,127.047842471571));
#101647=CARTESIAN_POINT('Ctrl Pts',(3.11565566452762,-29.9023193389722,
127.053651067882));
#101648=CARTESIAN_POINT('Ctrl Pts',(3.11952374557558,-29.9734192810663,
127.05580954406));
#101649=CARTESIAN_POINT('Ctrl Pts',(3.12339182662354,-30.0445492616679,
127.054267004502));
#101650=CARTESIAN_POINT('Ctrl Pts',(3.12725460116862,-30.1155816612101,
127.052726581106));
#101651=CARTESIAN_POINT('Ctrl Pts',(3.1311173757137,-30.186643536325,127.04749522442));
#101652=CARTESIAN_POINT('Ctrl Pts',(3.13498015025878,-30.2573213267348,
127.038573839062));
#101653=CARTESIAN_POINT('Ctrl Pts',(3.13883891823638,-30.3279258083522,
127.029661707191));
#101654=CARTESIAN_POINT('Ctrl Pts',(3.14269768621397,-30.3981465164401,
127.017067202742));
#101655=CARTESIAN_POINT('Ctrl Pts',(3.14655645419157,-30.4675725071244,
127.000843200524));
#101656=CARTESIAN_POINT('Ctrl Pts',(3.15049840094071,-30.5384950295132,
126.984269477207));
#101657=CARTESIAN_POINT('Ctrl Pts',(3.15444034768985,-30.6085876520776,
126.963907977244));
#101658=CARTESIAN_POINT('Ctrl Pts',(3.15838229443899,-30.6774215865192,
126.939870499961));
#101659=CARTESIAN_POINT('Ctrl Pts',(3.16223769286971,-30.7447442216828,
126.916360783038));
#101660=CARTESIAN_POINT('Ctrl Pts',(3.16609309130044,-30.8108624124218,
126.889335069568));
#101661=CARTESIAN_POINT('Ctrl Pts',(3.16994848973117,-30.875390936098,126.858948162671));
#101662=CARTESIAN_POINT('Ctrl Pts',(3.17393371063952,-30.9420923228315,
126.827538040246));
#101663=CARTESIAN_POINT('Ctrl Pts',(3.17791893154787,-31.0070945536863,
126.792536503335));
#101664=CARTESIAN_POINT('Ctrl Pts',(3.18190415245621,-31.0699975976019,
126.754167239355));
#101665=CARTESIAN_POINT('Ctrl Pts',(3.18588937336456,-31.1329006415176,
126.715797975375));
#101666=CARTESIAN_POINT('Ctrl Pts',(3.18987459427291,-31.1937040283989,
126.674061311145));
#101667=CARTESIAN_POINT('Ctrl Pts',(3.19385981518126,-31.2520409112986,
126.629230222815));
#101668=CARTESIAN_POINT('Ctrl Pts',(2.49394332640294,-31.2520409112987,
126.629230222815));
#101669=CARTESIAN_POINT('Ctrl Pts',(2.49779845369501,-31.3085851548333,
126.585776753065));
#101670=CARTESIAN_POINT('Ctrl Pts',(2.50165358098708,-31.3628774190682,
126.539366342141));
#101671=CARTESIAN_POINT('Ctrl Pts',(2.50550870827915,-31.4146017651328,
126.49026823377));
#101672=CARTESIAN_POINT('Ctrl Pts',(2.50936427882671,-31.4663320583681,
126.441164480188));
#101673=CARTESIAN_POINT('Ctrl Pts',(2.51321984937427,-31.5154934967334,
126.389372751944));
#101674=CARTESIAN_POINT('Ctrl Pts',(2.51707541992182,-31.5618064874044,
126.335199632415));
#101675=CARTESIAN_POINT('Ctrl Pts',(2.52093520627497,-31.6081701181979,
126.280967278245));
#101676=CARTESIAN_POINT('Ctrl Pts',(2.52479499262811,-31.6516787706278,
126.224348707153));
#101677=CARTESIAN_POINT('Ctrl Pts',(2.52865477898125,-31.6920933198749,
126.16568338726));
#101678=CARTESIAN_POINT('Ctrl Pts',(2.53251701344132,-31.7325335024418,
126.10698085832));
#101679=CARTESIAN_POINT('Ctrl Pts',(2.53637924790139,-31.7698754225889,
126.046229411115));
#101680=CARTESIAN_POINT('Ctrl Pts',(2.54024148236146,-31.8039249057506,
125.983794946578));
#101681=CARTESIAN_POINT('Ctrl Pts',(2.54411021068045,-31.8380316388132,
125.921255506383));
#101682=CARTESIAN_POINT('Ctrl Pts',(2.54797893899944,-31.868834679516,125.857027839922));
#101683=CARTESIAN_POINT('Ctrl Pts',(2.55184766731844,-31.8961874947129,
125.791498924443));
#101684=CARTESIAN_POINT('Ctrl Pts',(2.55326885464125,-31.9062356218998,
125.767426708387));
#101685=CARTESIAN_POINT('Ctrl Pts',(2.55469004196406,-31.9158186332063,
125.743179043823));
#101686=CARTESIAN_POINT('Ctrl Pts',(2.55611122928687,-31.9249309694032,
125.718775573829));
#101687=CARTESIAN_POINT('Ctrl Pts',(2.55998030264048,-31.9497386049644,
125.652339000706));
#101688=CARTESIAN_POINT('Ctrl Pts',(2.56384937599409,-31.9711513321785,
125.584486481582));
#101689=CARTESIAN_POINT('Ctrl Pts',(2.5677184493477,-31.989008767343,125.515598376581));
#101690=CARTESIAN_POINT('Ctrl Pts',(2.57158175774896,-32.0068395947765,
125.446812915445));
#101691=CARTESIAN_POINT('Ctrl Pts',(2.57544506615022,-32.0211255244763,
125.376995397718));
#101692=CARTESIAN_POINT('Ctrl Pts',(2.57930837455148,-32.0317549564161,
125.306544221245));
#101693=CARTESIAN_POINT('Ctrl Pts',(2.58316715104994,-32.0423719193663,
125.236175688416));
#101694=CARTESIAN_POINT('Ctrl Pts',(2.58702592754841,-32.0493408324374,
125.165175451347));
#101695=CARTESIAN_POINT('Ctrl Pts',(2.59088470404687,-32.0526008694865,
125.09395335589));
#101696=CARTESIAN_POINT('Ctrl Pts',(2.59474104964069,-32.0558588528176,
125.022776128055));
#101697=CARTESIAN_POINT('Ctrl Pts',(2.5985973952345,-32.0554125734897,124.951377803252));
#101698=CARTESIAN_POINT('Ctrl Pts',(2.60245374082832,-32.0512530538663,
124.880173160335));
#101699=CARTESIAN_POINT('Ctrl Pts',(2.6063089470793,-32.0470947631574,124.808989554564));
#101700=CARTESIAN_POINT('Ctrl Pts',(2.61016415333028,-32.0392254384407,
124.738000001772));
#101701=CARTESIAN_POINT('Ctrl Pts',(2.61401935958127,-32.0276881762123,
124.667617355223));
#101702=CARTESIAN_POINT('Ctrl Pts',(2.61787471643819,-32.0161504632737,
124.597231959133));
#101703=CARTESIAN_POINT('Ctrl Pts',(2.62173007329512,-32.0009446090955,
124.527453995389));
#101704=CARTESIAN_POINT('Ctrl Pts',(2.62558543015205,-31.9821650814073,
124.458687564756));
#101705=CARTESIAN_POINT('Ctrl Pts',(2.6294448226263,-31.9633658961389,124.389849152461));
#101706=CARTESIAN_POINT('Ctrl Pts',(2.63330421510055,-31.9409856981956,
124.322024856521));
#101707=CARTESIAN_POINT('Ctrl Pts',(2.6371636075748,-31.915169015866,124.255604135445));
#101708=CARTESIAN_POINT('Ctrl Pts',(2.64102518518395,-31.8893377164863,
124.18914580787));
#101709=CARTESIAN_POINT('Ctrl Pts',(2.64488676279309,-31.8600662588824,
124.124093080346));
#101710=CARTESIAN_POINT('Ctrl Pts',(2.64874834040224,-31.8275464613336,
124.060813386931));
#101711=CARTESIAN_POINT('Ctrl Pts',(2.65261667452278,-31.7949697646609,
123.997422974528));
#101712=CARTESIAN_POINT('Ctrl Pts',(2.65648500864332,-31.7591336250078,
123.935812209992));
#101713=CARTESIAN_POINT('Ctrl Pts',(2.66035334276386,-31.720274372791,123.876321378321));
#101714=CARTESIAN_POINT('Ctrl Pts',(2.66265106188438,-31.6971926936896,
123.84098492155));
#101715=CARTESIAN_POINT('Ctrl Pts',(2.6649487810049,-31.6730452284487,123.806395821985));
#101716=CARTESIAN_POINT('Ctrl Pts',(2.66724650012542,-31.6478880931576,
123.772619702403));
#101717=CARTESIAN_POINT('Ctrl Pts',(2.67111557347318,-31.605526604849,123.715744916056));
#101718=CARTESIAN_POINT('Ctrl Pts',(2.67498464682093,-31.5601342422752,
123.66095438182));
#101719=CARTESIAN_POINT('Ctrl Pts',(2.67885372016868,-31.5119435761822,
123.608589138701));
#101720=CARTESIAN_POINT('Ctrl Pts',(2.68271702856402,-31.4638247145944,
123.556301920242));
#101721=CARTESIAN_POINT('Ctrl Pts',(2.68658033695935,-31.4129161520987,
123.50643317434));
#101722=CARTESIAN_POINT('Ctrl Pts',(2.69044364535468,-31.3594920722307,
123.45929273772));
#101723=CARTESIAN_POINT('Ctrl Pts',(2.69430242184715,-31.3061306621565,
123.412207599787));
#101724=CARTESIAN_POINT('Ctrl Pts',(2.69816119833963,-31.2502599586026,
123.367844733758));
#101725=CARTESIAN_POINT('Ctrl Pts',(2.7020199748321,-31.192191301005,123.326477527994));
#101726=CARTESIAN_POINT('Ctrl Pts',(2.70587632041987,-31.1341592247884,
123.285136382236));
#101727=CARTESIAN_POINT('Ctrl Pts',(2.70973266600764,-31.0739323363522,
123.246787433824));
#101728=CARTESIAN_POINT('Ctrl Pts',(2.71358901159541,-31.0118542403315,
123.211663186415));
#101729=CARTESIAN_POINT('Ctrl Pts',(2.71744421784031,-30.9497944850519,
123.176549316334));
#101730=CARTESIAN_POINT('Ctrl Pts',(2.72129942408521,-30.8858850305699,
123.144658494925));
#101731=CARTESIAN_POINT('Ctrl Pts',(2.72515463033012,-30.8204961068849,
123.116178431728));
#101732=CARTESIAN_POINT('Ctrl Pts',(2.72900998718095,-30.7551046287427,
123.08769725594));
#101733=CARTESIAN_POINT('Ctrl Pts',(2.73286534403177,-30.6882340129049,
123.062627294863));
#101734=CARTESIAN_POINT('Ctrl Pts',(2.7367207008826,-30.6202749979301,123.041108351786));
#101735=CARTESIAN_POINT('Ctrl Pts',(2.74058009335076,-30.5522448464589,
123.019566883629));
#101736=CARTESIAN_POINT('Ctrl Pts',(2.74443948581892,-30.4831244856478,
123.001584000482));
#101737=CARTESIAN_POINT('Ctrl Pts',(2.74829887828708,-30.4133195035039,
122.987249506143));
#101738=CARTESIAN_POINT('Ctrl Pts',(2.75216045589012,-30.3434749987401,
122.972906895809));
#101739=CARTESIAN_POINT('Ctrl Pts',(2.75602203349316,-30.2729455815335,
122.962216859222));
#101740=CARTESIAN_POINT('Ctrl Pts',(2.7598836110962,-30.2021439845883,122.955217524529));
#101741=CARTESIAN_POINT('Ctrl Pts',(2.7637519452107,-30.1312185077551,122.948205943264));
#101742=CARTESIAN_POINT('Ctrl Pts',(2.7676202793252,-30.0600203857999,122.9448979791));
#101743=CARTESIAN_POINT('Ctrl Pts',(2.7714886134397,-29.9889636841022,122.945279638921));
#101744=CARTESIAN_POINT('Ctrl Pts',(2.77378633261446,-29.9467573127925,
122.945506337822));
#101745=CARTESIAN_POINT('Ctrl Pts',(2.77608405178923,-29.9046007847015,
122.947033789851));
#101746=CARTESIAN_POINT('Ctrl Pts',(2.77838177096399,-29.8625796677408,
122.949850440875));
#101747=CARTESIAN_POINT('Ctrl Pts',(2.78225084431114,-29.7918213325031,
122.954593330921));
#101748=CARTESIAN_POINT('Ctrl Pts',(2.78611991765829,-29.7211702309011,
122.963013013947));
#101749=CARTESIAN_POINT('Ctrl Pts',(2.78998899100544,-29.6510390226777,
122.975099064446));
#101750=CARTESIAN_POINT('Ctrl Pts',(2.79385229940014,-29.5810123105554,
122.987167106626));
#101751=CARTESIAN_POINT('Ctrl Pts',(2.79771560779484,-29.5115044289906,
123.002890590709));
#101752=CARTESIAN_POINT('Ctrl Pts',(2.80157891618955,-29.4429243926149,
123.022207207477));
#101753=CARTESIAN_POINT('Ctrl Pts',(2.80543769268135,-29.3744248049205,
123.041501164642));
#101754=CARTESIAN_POINT('Ctrl Pts',(2.80929646917315,-29.3068513657659,
123.064379751071));
#101755=CARTESIAN_POINT('Ctrl Pts',(2.81315524566495,-29.2406026199514,
123.09072967297));
#101756=CARTESIAN_POINT('Ctrl Pts',(2.81701159125203,-29.1743956087099,
123.11706299527));
#101757=CARTESIAN_POINT('Ctrl Pts',(2.82086793683911,-29.1095120854706,
123.146863135293));
#101758=CARTESIAN_POINT('Ctrl Pts',(2.82472428242619,-29.0463337454979,
123.179967517454));
#101759=CARTESIAN_POINT('Ctrl Pts',(2.82857948867037,-28.9831740713298,
123.213062119048));
#101760=CARTESIAN_POINT('Ctrl Pts',(2.83243469491455,-28.9217190103251,
123.249458799358));
#101761=CARTESIAN_POINT('Ctrl Pts',(2.83628990115873,-28.8623270648984,
123.288948318946));
#101762=CARTESIAN_POINT('Ctrl Pts',(2.84014525800883,-28.8029327992902,
123.328439381216));
#101763=CARTESIAN_POINT('Ctrl Pts',(2.84400061485893,-28.7456022125833,
123.371023251839));
#101764=CARTESIAN_POINT('Ctrl Pts',(2.84785597170903,-28.6906646821707,
123.416447478615));
#101765=CARTESIAN_POINT('Ctrl Pts',(2.85171536417643,-28.6356696455774,
123.461919253466));
#101766=CARTESIAN_POINT('Ctrl Pts',(2.85557475664382,-28.5830730408649,
123.510237009375));
#101767=CARTESIAN_POINT('Ctrl Pts',(2.85943414911121,-28.5331702924828,
123.561108700546));
#101768=CARTESIAN_POINT('Ctrl Pts',(2.86329572671347,-28.4832392898516,
123.612009194567));
#101769=CARTESIAN_POINT('Ctrl Pts',(2.86715730431574,-28.4360055016132,
123.665466138185));
#101770=CARTESIAN_POINT('Ctrl Pts',(2.871018881918,-28.3917248122804,123.721153456014));
#101771=CARTESIAN_POINT('Ctrl Pts',(2.8748872160317,-28.3473666460677,123.776938208632));
#101772=CARTESIAN_POINT('Ctrl Pts',(2.87875555014539,-28.3059721769819,
123.834960731194));
#101773=CARTESIAN_POINT('Ctrl Pts',(2.88262388425909,-28.2677542229881,
123.894865559977));
#101774=CARTESIAN_POINT('Ctrl Pts',(2.88492160344024,-28.2450534625639,
123.930447924399));
#101775=CARTESIAN_POINT('Ctrl Pts',(2.88721932262139,-28.2234725546798,
123.966693895146));
#101776=CARTESIAN_POINT('Ctrl Pts',(2.88951704180254,-28.2030482011671,
124.003525316342));
#101777=CARTESIAN_POINT('Ctrl Pts',(2.89357123056495,-28.1670106448069,
124.068512167277));
#101778=CARTESIAN_POINT('Ctrl Pts',(2.89762541932736,-28.1344462576574,
124.135557009902));
#101779=CARTESIAN_POINT('Ctrl Pts',(2.90167960808977,-28.1055831555926,
124.204272419653));
#101780=CARTESIAN_POINT('Ctrl Pts',(2.90572241802439,-28.0768010631422,
124.272794966944));
#101781=CARTESIAN_POINT('Ctrl Pts',(2.909765227959,-28.0516997313792,124.342978361097));
#101782=CARTESIAN_POINT('Ctrl Pts',(2.91380803789362,-28.0304609874017,
124.414411714297));
#101783=CARTESIAN_POINT('Ctrl Pts',(2.91784402707238,-28.0092580759984,
124.485724549968));
#101784=CARTESIAN_POINT('Ctrl Pts',(2.92188001625114,-27.9919049147105,
124.558282753116));
#101785=CARTESIAN_POINT('Ctrl Pts',(2.9259160054299,-27.9785350595386,124.631656333046));
#101786=CARTESIAN_POINT('Ctrl Pts',(2.92994364805372,-27.9651928536556,
124.704878174062));
#101787=CARTESIAN_POINT('Ctrl Pts',(2.93397129067754,-27.9558176275984,
124.778911624366));
#101788=CARTESIAN_POINT('Ctrl Pts',(2.93799893330136,-27.9504925475499,
124.853314060484));
#101789=CARTESIAN_POINT('Ctrl Pts',(2.9406410490468,-27.946999318593,124.902121729467));
#101790=CARTESIAN_POINT('Ctrl Pts',(2.94328316479224,-27.9452479687194,
124.951087882257));
#101791=CARTESIAN_POINT('Ctrl Pts',(2.94592528053768,-27.9452500017688,
125.000085257795));
#101792=CARTESIAN_POINT('Origin',(-1.54592528053767,-30.,125.));
#101793=CARTESIAN_POINT('',(1.79398326297881,-31.2520409112987,126.629230222815));
#101794=CARTESIAN_POINT('',(1.85201788380192,-31.2520409112987,126.629230222815));
#101795=CARTESIAN_POINT('',(-1.54592528053767,-31.2520409112987,126.629230222815));
#101796=CARTESIAN_POINT('',(2.30407471949582,-27.9452508576209,125.001877336539));
#101797=CARTESIAN_POINT('Ctrl Pts',(1.85201788380192,-31.2520409112987,
126.629230222815));
#101798=CARTESIAN_POINT('Ctrl Pts',(1.85587837089731,-31.3086000947725,
126.585765271928));
#101799=CARTESIAN_POINT('Ctrl Pts',(1.85973885799271,-31.3628526586814,
126.539382921901));
#101800=CARTESIAN_POINT('Ctrl Pts',(1.86359934508811,-31.4144967675365,
126.490367893216));
#101801=CARTESIAN_POINT('Ctrl Pts',(1.86752032570428,-31.4669501354034,
126.440584802992));
#101802=CARTESIAN_POINT('Ctrl Pts',(1.87144130632046,-31.5167122299897,
126.388086186834));
#101803=CARTESIAN_POINT('Ctrl Pts',(1.87536228693663,-31.5635084223667,
126.333206276496));
#101804=CARTESIAN_POINT('Ctrl Pts',(1.87928326755281,-31.6103046147436,
126.278326366158));
#101805=CARTESIAN_POINT('Ctrl Pts',(1.88320424816899,-31.6541346429375,
126.221065613155));
#101806=CARTESIAN_POINT('Ctrl Pts',(1.88712522878516,-31.694770243634,126.161788011555));
#101807=CARTESIAN_POINT('Ctrl Pts',(1.8909943020432,-31.734867895566,126.103295148263));
#101808=CARTESIAN_POINT('Ctrl Pts',(1.89486337530124,-31.7720123219207,
126.042609395793));
#101809=CARTESIAN_POINT('Ctrl Pts',(1.89873244855929,-31.8059561429648,
125.980061208388));
#101810=CARTESIAN_POINT('Ctrl Pts',(1.90259575686323,-31.8398493874089,
125.917606218348));
#101811=CARTESIAN_POINT('Ctrl Pts',(1.90645906516718,-31.8705512629169,
125.853294725246));
#101812=CARTESIAN_POINT('Ctrl Pts',(1.91032237347112,-31.89785738344,125.787486453612));
#101813=CARTESIAN_POINT('Ctrl Pts',(1.91418114987016,-31.9251314721572,
125.721755379241));
#101814=CARTESIAN_POINT('Ctrl Pts',(1.9180399262692,-31.9490175330646,125.654531460497));
#101815=CARTESIAN_POINT('Ctrl Pts',(1.92189870266824,-31.9693576944775,
125.586197776951));
#101816=CARTESIAN_POINT('Ctrl Pts',(1.92575504816137,-31.9896850422383,
125.517907141443));
#101817=CARTESIAN_POINT('Ctrl Pts',(1.9296113936545,-32.0064707840726,125.448508592667));
#101818=CARTESIAN_POINT('Ctrl Pts',(1.93346773914762,-32.0196061767615,
125.378402501692));
#101819=CARTESIAN_POINT('Ctrl Pts',(1.93732294529681,-32.0327376886441,
125.308317123319));
#101820=CARTESIAN_POINT('Ctrl Pts',(1.941178151446,-32.0422209030551,125.237525094969));
#101821=CARTESIAN_POINT('Ctrl Pts',(1.94503335759519,-32.0479980782691,
125.166437477468));
#101822=CARTESIAN_POINT('Ctrl Pts',(1.94888871434936,-32.0537754791705,
125.095347082905));
#101823=CARTESIAN_POINT('Ctrl Pts',(1.95274407110353,-32.0558465162838,
125.023961560633));
#101824=CARTESIAN_POINT('Ctrl Pts',(1.9565994278577,-32.0542054136421,124.952695866318));
#101825=CARTESIAN_POINT('Ctrl Pts',(1.96045882022845,-32.052562593167,124.881355574233));
#101826=CARTESIAN_POINT('Ctrl Pts',(1.96431821259919,-32.0471998874065,
124.810135847147));
#101827=CARTESIAN_POINT('Ctrl Pts',(1.96817760496994,-32.0381636345743,
124.739449503553));
#101828=CARTESIAN_POINT('Ctrl Pts',(1.97203918247499,-32.0291222655413,
124.668723138333));
#101829=CARTESIAN_POINT('Ctrl Pts',(1.97590075998004,-32.0164032956312,
124.598531236013));
#101830=CARTESIAN_POINT('Ctrl Pts',(1.97976233748509,-32.0001042687789,
124.529276645457));
#101831=CARTESIAN_POINT('Ctrl Pts',(1.98363067150175,-31.9837767239016,
124.459900881767));
#101832=CARTESIAN_POINT('Ctrl Pts',(1.9874990055184,-31.9638567517517,124.39146617071));
#101833=CARTESIAN_POINT('Ctrl Pts',(1.99136733953506,-31.9404916420071,
124.324359748238));
#101834=CARTESIAN_POINT('Ctrl Pts',(1.99366505956461,-31.9266131918988,
124.284499754153));
#101835=CARTESIAN_POINT('Ctrl Pts',(1.99596277959417,-31.9115201753994,
124.24510802716));
#101836=CARTESIAN_POINT('Ctrl Pts',(1.99826049962372,-31.8952512263342,
124.206261786495));
#101837=CARTESIAN_POINT('Ctrl Pts',(2.00212957301351,-31.8678563491958,
124.140849571726));
#101838=CARTESIAN_POINT('Ctrl Pts',(2.00599864640329,-31.8370174066266,
124.076729146268));
#101839=CARTESIAN_POINT('Ctrl Pts',(2.00986771979308,-31.8028778577843,
124.014287571139));
#101840=CARTESIAN_POINT('Ctrl Pts',(2.01373102823097,-31.7687891771568,
123.951939034482));
#101841=CARTESIAN_POINT('Ctrl Pts',(2.01759433666887,-31.7314098833556,
123.891264805509));
#101842=CARTESIAN_POINT('Ctrl Pts',(2.02145764510676,-31.6909313450081,
123.832631699519));
#101843=CARTESIAN_POINT('Ctrl Pts',(2.02531642164239,-31.6505002905162,
123.774067373826));
#101844=CARTESIAN_POINT('Ctrl Pts',(2.02917519817801,-31.6069774876751,
123.717539812929));
#101845=CARTESIAN_POINT('Ctrl Pts',(2.03303397471363,-31.5605991544203,
123.663389420316));
#101846=CARTESIAN_POINT('Ctrl Pts',(2.0368903203449,-31.5142500380146,123.609273140698));
#101847=CARTESIAN_POINT('Ctrl Pts',(2.04074666597617,-31.4650492754231,
123.557531426356));
#101848=CARTESIAN_POINT('Ctrl Pts',(2.04460301160743,-31.4132742574366,
123.508472784101));
#101849=CARTESIAN_POINT('Ctrl Pts',(2.04845821789611,-31.3615145361815,
123.459428636035));
#101850=CARTESIAN_POINT('Ctrl Pts',(2.05231342418478,-31.3071824218778,
123.413066320264));
#101851=CARTESIAN_POINT('Ctrl Pts',(2.05616863047345,-31.2505919476215,
123.369657292762));
#101852=CARTESIAN_POINT('Ctrl Pts',(2.06002398736825,-31.1939992626219,
123.326246569458));
#101853=CARTESIAN_POINT('Ctrl Pts',(2.06387934426304,-31.1351484292998,
123.285789657396));
#101854=CARTESIAN_POINT('Ctrl Pts',(2.06773470115783,-31.074384937336,123.248516466271));
#101855=CARTESIAN_POINT('Ctrl Pts',(2.07159409366998,-31.0135578408318,
123.211204259214));
#101856=CARTESIAN_POINT('Ctrl Pts',(2.07545348618213,-30.9508145040071,
123.177082680198));
#101857=CARTESIAN_POINT('Ctrl Pts',(2.07931287869428,-30.8865268858702,
123.146336696396));
#101858=CARTESIAN_POINT('Ctrl Pts',(2.08317445634139,-30.8222028689681,
123.115573304641));
#101859=CARTESIAN_POINT('Ctrl Pts',(2.0870360339885,-30.7563332789708,123.088189499311));
#101860=CARTESIAN_POINT('Ctrl Pts',(2.09089761163561,-30.6893094711095,
123.064321820256));
#101861=CARTESIAN_POINT('Ctrl Pts',(2.09476594579382,-30.6221683932764,
123.040412380487));
#101862=CARTESIAN_POINT('Ctrl Pts',(2.09863427995202,-30.5538695312235,
123.020031488757));
#101863=CARTESIAN_POINT('Ctrl Pts',(2.10250261411023,-30.4848181033976,
123.003265423468));
#101864=CARTESIAN_POINT('Ctrl Pts',(2.10480033289425,-30.4438028352512,
122.993306691473));
#101865=CARTESIAN_POINT('Ctrl Pts',(2.10709805167827,-30.4025222418141,
122.984622339477));
#101866=CARTESIAN_POINT('Ctrl Pts',(2.10939577046228,-30.3610621517842,
122.977221790445));
#101867=CARTESIAN_POINT('Ctrl Pts',(2.11326484381022,-30.2912485042424,
122.964760184083));
#101868=CARTESIAN_POINT('Ctrl Pts',(2.11713391715816,-30.2206522077615,
122.955892707146));
#101869=CARTESIAN_POINT('Ctrl Pts',(2.1210029905061,-30.1496762562476,122.950708761348));
#101870=CARTESIAN_POINT('Ctrl Pts',(2.12486629890172,-30.0788060595074,
122.945532539673));
#101871=CARTESIAN_POINT('Ctrl Pts',(2.12872960729734,-30.0075578111597,
122.944028989731));
#101872=CARTESIAN_POINT('Ctrl Pts',(2.13259291569296,-29.9363434801761,
122.946236281851));
#101873=CARTESIAN_POINT('Ctrl Pts',(2.13645169218589,-29.8652126880627,
122.94844098468));
#101874=CARTESIAN_POINT('Ctrl Pts',(2.14031046867881,-29.7941162174787,
122.954347867964));
#101875=CARTESIAN_POINT('Ctrl Pts',(2.14416924517174,-29.7234681723392,
122.963943097359));
#101876=CARTESIAN_POINT('Ctrl Pts',(2.14802559076006,-29.6528646331871,
122.97353228207));
#101877=CARTESIAN_POINT('Ctrl Pts',(2.15188193634839,-29.5827094392452,
122.986805137805));
#101878=CARTESIAN_POINT('Ctrl Pts',(2.15573828193672,-29.5134122273188,
123.003695939498));
#101879=CARTESIAN_POINT('Ctrl Pts',(2.15959348818228,-29.4441354889923,
123.020581750867));
#101880=CARTESIAN_POINT('Ctrl Pts',(2.16344869442785,-29.3757167011493,
123.041083271138));
#101881=CARTESIAN_POINT('Ctrl Pts',(2.16730390067341,-29.3085542460418,
123.065083895402));
#101882=CARTESIAN_POINT('Ctrl Pts',(2.17115925752499,-29.2413891671916,
123.089085457265));
#101883=CARTESIAN_POINT('Ctrl Pts',(2.17501461437657,-29.1754809752312,
123.116586228966));
#101884=CARTESIAN_POINT('Ctrl Pts',(2.17886997122815,-29.1112102084979,
123.147420644339));
#101885=CARTESIAN_POINT('Ctrl Pts',(2.18272936369721,-29.0468721659611,
123.178287335818));
#101886=CARTESIAN_POINT('Ctrl Pts',(2.18658875616628,-28.9841754090357,
123.21249442626));
#101887=CARTESIAN_POINT('Ctrl Pts',(2.19044814863534,-28.9234770739043,
123.249829736257));
#101888=CARTESIAN_POINT('Ctrl Pts',(2.19430972623937,-28.8627443722099,
123.287186184994));
#101889=CARTESIAN_POINT('Ctrl Pts',(2.1981713038434,-28.8040127448828,123.327674103258));
#101890=CARTESIAN_POINT('Ctrl Pts',(2.20203288144743,-28.7476091620136,
123.37103875079));
#101891=CARTESIAN_POINT('Ctrl Pts',(2.20590121556304,-28.691106891121,123.414479272427));
#101892=CARTESIAN_POINT('Ctrl Pts',(2.20976954967865,-28.6369411664899,
123.460806256701));
#101893=CARTESIAN_POINT('Ctrl Pts',(2.21363788379427,-28.5854042502891,
123.509726056257));
#101894=CARTESIAN_POINT('Ctrl Pts',(2.21593560296312,-28.5547922719235,
123.53878351557));
#101895=CARTESIAN_POINT('Ctrl Pts',(2.21823332213197,-28.5251070531022,
123.568755064472));
#101896=CARTESIAN_POINT('Ctrl Pts',(2.22053104130083,-28.4964030609004,
123.599573705178));
#101897=CARTESIAN_POINT('Ctrl Pts',(2.22435385578605,-28.4486469910289,
123.650848006972));
#101898=CARTESIAN_POINT('Ctrl Pts',(2.22817667027127,-28.4034122612403,
123.704680314488));
#101899=CARTESIAN_POINT('Ctrl Pts',(2.23199948475649,-28.3609895950765,
123.760789584028));
#101900=CARTESIAN_POINT('Ctrl Pts',(2.23581710151335,-28.3186246093197,
123.816822564033));
#101901=CARTESIAN_POINT('Ctrl Pts',(2.23963471827021,-28.2790644064682,
123.875125976651));
#101902=CARTESIAN_POINT('Ctrl Pts',(2.24345233502707,-28.2425620670407,
123.935382944766));
#101903=CARTESIAN_POINT('Ctrl Pts',(2.2472661112283,-28.2060964492838,123.995579293847));
#101904=CARTESIAN_POINT('Ctrl Pts',(2.25107988742953,-28.1726828518535,
124.057724877737));
#101905=CARTESIAN_POINT('Ctrl Pts',(2.25489366363075,-28.1425321731206,
124.12147234841));
#101906=CARTESIAN_POINT('Ctrl Pts',(2.25870495117383,-28.112401169043,124.185178221031));
#101907=CARTESIAN_POINT('Ctrl Pts',(2.26251623871691,-28.0855290712528,
124.250483456995));
#101908=CARTESIAN_POINT('Ctrl Pts',(2.26632752625999,-28.0620808415638,
124.317016180378));
#101909=CARTESIAN_POINT('Ctrl Pts',(2.27013878558059,-28.0386327855083,
124.383548411087));
#101910=CARTESIAN_POINT('Ctrl Pts',(2.2739500449012,-28.0186087267518,124.451307646267));
#101911=CARTESIAN_POINT('Ctrl Pts',(2.27776130422181,-28.00212488962,124.519903545291));
#101912=CARTESIAN_POINT('Ctrl Pts',(2.28157259449292,-27.9856409186262,
124.588500001369));
#101913=CARTESIAN_POINT('Ctrl Pts',(2.28538388476404,-27.9726973326024,
124.657932647788));
#101914=CARTESIAN_POINT('Ctrl Pts',(2.28919517503516,-27.9633594769412,
124.727799812023));
#101915=CARTESIAN_POINT('Ctrl Pts',(2.29300941452562,-27.9540143955421,
124.797721040257));
#101916=CARTESIAN_POINT('Ctrl Pts',(2.29682365401607,-27.9482806627008,
124.868076961452));
#101917=CARTESIAN_POINT('Ctrl Pts',(2.30063789350653,-27.9461717409522,
124.938461029936));
#101918=CARTESIAN_POINT('Ctrl Pts',(2.30178350215846,-27.9455383252981,
124.959600918508));
#101919=CARTESIAN_POINT('Ctrl Pts',(2.3029291108104,-27.9452315484039,124.980743347371));
#101920=CARTESIAN_POINT('Ctrl Pts',(2.30407471946233,-27.9452508576204,
125.001877335921));
#101921=CARTESIAN_POINT('Ctrl Pts',(2.30407471949582,-27.9452508576209,
125.001877336539));
#101922=CARTESIAN_POINT('Ctrl Pts',(2.30909836680706,-27.9453355311479,
125.094552705721));
#101923=CARTESIAN_POINT('Ctrl Pts',(2.31412201411831,-27.9516938665571,
125.18694888772));
#101924=CARTESIAN_POINT('Ctrl Pts',(2.31914566142955,-27.9641908651484,
125.278350011594));
#101925=CARTESIAN_POINT('Ctrl Pts',(2.32331921166617,-27.9745731328905,
125.354284319586));
#101926=CARTESIAN_POINT('Ctrl Pts',(2.32749276190278,-27.989191374217,125.429532498929));
#101927=CARTESIAN_POINT('Ctrl Pts',(2.33166631213939,-28.0079438906425,
125.503696356619));
#101928=CARTESIAN_POINT('Ctrl Pts',(2.33553538549303,-28.0253283373371,
125.572449669584));
#101929=CARTESIAN_POINT('Ctrl Pts',(2.33940445884667,-28.0463104154053,
125.640436592137));
#101930=CARTESIAN_POINT('Ctrl Pts',(2.3432735322003,-28.0708056935786,125.707253059782));
#101931=CARTESIAN_POINT('Ctrl Pts',(2.34713684060158,-28.095264473578,125.77396997032));
#101932=CARTESIAN_POINT('Ctrl Pts',(2.35100014900287,-28.1232258971066,
125.839519435331));
#101933=CARTESIAN_POINT('Ctrl Pts',(2.35486345740415,-28.1545551494563,
125.903510302156));
#101934=CARTESIAN_POINT('Ctrl Pts',(2.35872223390264,-28.1858476506304,
125.967426103685));
#101935=CARTESIAN_POINT('Ctrl Pts',(2.36258101040114,-28.2204999206784,
126.029786504532));
#101936=CARTESIAN_POINT('Ctrl Pts',(2.36643978689963,-28.2583288726902,
126.090219815815));
#101937=CARTESIAN_POINT('Ctrl Pts',(2.37029613249347,-28.2961339936832,
126.150615056062));
#101938=CARTESIAN_POINT('Ctrl Pts',(2.37415247808731,-28.3371115691361,
126.209085204514));
#101939=CARTESIAN_POINT('Ctrl Pts',(2.37800882368115,-28.381033061733,126.265284005786));
#101940=CARTESIAN_POINT('Ctrl Pts',(2.38186402993216,-28.4249415778899,
126.321466203333));
#101941=CARTESIAN_POINT('Ctrl Pts',(2.38571923618317,-28.4717919854813,
126.375378003393));
#101942=CARTESIAN_POINT('Ctrl Pts',(2.38957444243417,-28.5213140123004,
126.426704353495));
#101943=CARTESIAN_POINT('Ctrl Pts',(2.39342979929112,-28.5708379737271,
126.478032708692));
#101944=CARTESIAN_POINT('Ctrl Pts',(2.39728515614807,-28.6230334227032,
126.526775065342));
#101945=CARTESIAN_POINT('Ctrl Pts',(2.40114051300502,-28.6775928133142,
126.572652789112));
#101946=CARTESIAN_POINT('Ctrl Pts',(2.4049999054793,-28.7322093142863,126.618578535658));
#101947=CARTESIAN_POINT('Ctrl Pts',(2.40885929795358,-28.789194323921,126.661633350216));
#101948=CARTESIAN_POINT('Ctrl Pts',(2.41271869042785,-28.8482074506336,
126.701579115329));
#101949=CARTESIAN_POINT('Ctrl Pts',(2.41658026803702,-28.9072539897662,
126.741547497185));
#101950=CARTESIAN_POINT('Ctrl Pts',(2.42044184564619,-28.9683305157479,
126.778403074276));
#101951=CARTESIAN_POINT('Ctrl Pts',(2.42430342325536,-29.031070268971,126.811952741886));
#101952=CARTESIAN_POINT('Ctrl Pts',(2.42817175737592,-29.0939197964628,
126.845561110559));
#101953=CARTESIAN_POINT('Ctrl Pts',(2.43204009149649,-29.1584379214406,
126.875851814768));
#101954=CARTESIAN_POINT('Ctrl Pts',(2.43590842561706,-29.2242367158349,
126.90267939744));
#101955=CARTESIAN_POINT('Ctrl Pts',(2.43820614473736,-29.2633199861162,
126.918614486741));
#101956=CARTESIAN_POINT('Ctrl Pts',(2.44050386385766,-29.3028547606617,
126.933328680147));
#101957=CARTESIAN_POINT('Ctrl Pts',(2.44280158297796,-29.3427575594249,
126.94679992213));
#101958=CARTESIAN_POINT('Ctrl Pts',(2.44667069996889,-29.4099496697731,
126.96948407477));
#101959=CARTESIAN_POINT('Ctrl Pts',(2.45053981695982,-29.4784491577362,
126.988729960308));
#101960=CARTESIAN_POINT('Ctrl Pts',(2.45440893395075,-29.5478707454889,
127.004389358312));
#101961=CARTESIAN_POINT('Ctrl Pts',(2.45827227326046,-29.6171886672618,
127.020025372426));
#101962=CARTESIAN_POINT('Ctrl Pts',(2.46213561257017,-29.6874254855223,
127.032085423932));
#101963=CARTESIAN_POINT('Ctrl Pts',(2.46599895187988,-29.7581794473605,
127.040470627777));
#101964=CARTESIAN_POINT('Ctrl Pts',(2.46985771072428,-29.8288495216491,
127.048845889928));
#101965=CARTESIAN_POINT('Ctrl Pts',(2.47371646956868,-29.9000350414532,
127.0535549026));
#101966=CARTESIAN_POINT('Ctrl Pts',(2.47757522841307,-29.9713244405029,
127.054549895911));
#101967=CARTESIAN_POINT('Ctrl Pts',(2.4814315383272,-30.0425685963087,127.055544257758));
#101968=CARTESIAN_POINT('Ctrl Pts',(2.48528784824132,-30.1139160159822,
127.052829270173));
#101969=CARTESIAN_POINT('Ctrl Pts',(2.48914415815545,-30.1849518563648,
127.046409141234));
#101970=CARTESIAN_POINT('Ctrl Pts',(2.49299931071214,-30.2559663774397,
127.039990939108));
#101971=CARTESIAN_POINT('Ctrl Pts',(2.49685446326883,-30.3266690213727,
127.029869847219));
#101972=CARTESIAN_POINT('Ctrl Pts',(2.50070961582552,-30.3966485300909,
127.016102057456));
#101973=CARTESIAN_POINT('Ctrl Pts',(2.5045649009602,-30.4666304453915,127.00233379422));
#101974=CARTESIAN_POINT('Ctrl Pts',(2.50842018609487,-30.5358886999794,
126.984918680344));
#101975=CARTESIAN_POINT('Ctrl Pts',(2.51227547122954,-30.6040224212736,
126.963963970418));
#101976=CARTESIAN_POINT('Ctrl Pts',(2.51613458281858,-30.6722237667684,
126.942988462486));
#101977=CARTESIAN_POINT('Ctrl Pts',(2.51999369440761,-30.7392978863037,
126.918466490123));
#101978=CARTESIAN_POINT('Ctrl Pts',(2.52385280599665,-30.8048601934944,
126.890554847506));
#101979=CARTESIAN_POINT('Ctrl Pts',(2.527714095329,-30.8704594982875,126.862627454012));
#101980=CARTESIAN_POINT('Ctrl Pts',(2.53157538466135,-30.9345448559496,
126.83130679581));
#101981=CARTESIAN_POINT('Ctrl Pts',(2.5354366739937,-30.9967551906669,126.796796218935));
#101982=CARTESIAN_POINT('Ctrl Pts',(2.53930424299619,-31.0590666989424,
126.762229517014));
#101983=CARTESIAN_POINT('Ctrl Pts',(2.54317181199867,-31.119496686546,126.724462799682));
#101984=CARTESIAN_POINT('Ctrl Pts',(2.54703938100116,-31.1777127385792,
126.683742934028));
#101985=CARTESIAN_POINT('Ctrl Pts',(2.54871345326657,-31.2029114817815,
126.666117392583));
#101986=CARTESIAN_POINT('Ctrl Pts',(2.55038752553198,-31.2276958470359,
126.647939068268));
#101987=CARTESIAN_POINT('Ctrl Pts',(2.55206159779739,-31.2520409112987,
126.629230222815));
#101988=CARTESIAN_POINT('',(2.24592528056747,-27.9452508239572,124.998159877293));
#101989=CARTESIAN_POINT('Ctrl Pts',(2.24592528056747,-27.9452508239572,
124.998159877293));
#101990=CARTESIAN_POINT('Ctrl Pts',(2.24973199310619,-27.9451880222813,
125.068286554887));
#101991=CARTESIAN_POINT('Ctrl Pts',(2.25353870564491,-27.9487194885961,
125.138525579213));
#101992=CARTESIAN_POINT('Ctrl Pts',(2.25734541818363,-27.9558530802283,
125.208472858876));
#101993=CARTESIAN_POINT('Ctrl Pts',(2.26114901952475,-27.9629808416296,
125.278362971152));
#101994=CARTESIAN_POINT('Ctrl Pts',(2.26495262086587,-27.9737048434681,
125.347961315223));
#101995=CARTESIAN_POINT('Ctrl Pts',(2.268756222207,-27.9879809096171,125.416865376872));
#101996=CARTESIAN_POINT('Ctrl Pts',(2.27255807181682,-28.0022504009888,
125.485737705069));
#101997=CARTESIAN_POINT('Ctrl Pts',(2.27635992142664,-28.0200686114227,
125.553915895166));
#101998=CARTESIAN_POINT('Ctrl Pts',(2.28016177103647,-28.0413399857073,
125.621006047403));
#101999=CARTESIAN_POINT('Ctrl Pts',(2.28396322582589,-28.0626091509691,
125.688089232357));
#102000=CARTESIAN_POINT('Ctrl Pts',(2.28776468061532,-28.0873306153714,
125.754084126905));
#102001=CARTESIAN_POINT('Ctrl Pts',(2.29156613540474,-28.1153590731372,
125.818612325398));
#102002=CARTESIAN_POINT('Ctrl Pts',(2.29537111048207,-28.1434134862929,
125.883200279393));
#102003=CARTESIAN_POINT('Ctrl Pts',(2.2991760855594,-28.1747808077104,125.946318364991));
#102004=CARTESIAN_POINT('Ctrl Pts',(2.30298106063673,-28.2092681474416,
126.00760954478));
#102005=CARTESIAN_POINT('Ctrl Pts',(2.30678785553211,-28.2437719815472,
126.068930038506));
#102006=CARTESIAN_POINT('Ctrl Pts',(2.3105946504275,-28.2813985348242,126.128421464577));
#102007=CARTESIAN_POINT('Ctrl Pts',(2.31440144532288,-28.3219111791817,
126.185755232729));
#102008=CARTESIAN_POINT('Ctrl Pts',(2.31821492439056,-28.3624949577879,
126.243189670551));
#102009=CARTESIAN_POINT('Ctrl Pts',(2.32202840345824,-28.4059746336492,
126.298458493979));
#102010=CARTESIAN_POINT('Ctrl Pts',(2.32584188252591,-28.4520733934073,
126.351266362751));
#102011=CARTESIAN_POINT('Ctrl Pts',(2.32850815088719,-28.4843042415268,
126.388188015456));
#102012=CARTESIAN_POINT('Ctrl Pts',(2.33117441924847,-28.5178145732298,
126.42390739227));
#102013=CARTESIAN_POINT('Ctrl Pts',(2.33384068760975,-28.5524999386655,
126.458335055787));
#102014=CARTESIAN_POINT('Ctrl Pts',(2.3377097609577,-28.6028325401845,126.50829370109));
#102015=CARTESIAN_POINT('Ctrl Pts',(2.34157883430565,-28.6558531560725,
126.555741393499));
#102016=CARTESIAN_POINT('Ctrl Pts',(2.3454479076536,-28.7112811808808,126.600375383386));
#102017=CARTESIAN_POINT('Ctrl Pts',(2.34931121604923,-28.766626617459,126.644942868247));
#102018=CARTESIAN_POINT('Ctrl Pts',(2.35317452444486,-28.8243719674648,
126.686704670265));
#102019=CARTESIAN_POINT('Ctrl Pts',(2.3570378328405,-28.8842001037992,126.7253950719));
#102020=CARTESIAN_POINT('Ctrl Pts',(2.36089660933343,-28.9439580579829,
126.764040087272));
#102021=CARTESIAN_POINT('Ctrl Pts',(2.36475538582637,-29.0057935394568,
126.79962059641));
#102022=CARTESIAN_POINT('Ctrl Pts',(2.36861416231931,-29.0693580855252,
126.831912440463));
#102023=CARTESIAN_POINT('Ctrl Pts',(2.37247050790765,-29.132882587982,126.864183941697));
#102024=CARTESIAN_POINT('Ctrl Pts',(2.37632685349599,-29.1981335618907,
126.893170668666));
#102025=CARTESIAN_POINT('Ctrl Pts',(2.38018319908433,-29.2647367038568,
126.918693682651));
#102026=CARTESIAN_POINT('Ctrl Pts',(2.3840384053299,-29.3313201681756,126.944209155958));
#102027=CARTESIAN_POINT('Ctrl Pts',(2.38789361157548,-29.3992545540755,
126.966262774159));
#102028=CARTESIAN_POINT('Ctrl Pts',(2.39174881782105,-29.4681458750043,
126.98472384785));
#102029=CARTESIAN_POINT('Ctrl Pts',(2.39560417467265,-29.5370398872153,
127.003185642735));
#102030=CARTESIAN_POINT('Ctrl Pts',(2.39945953152424,-29.6068904388744,
127.01805449086));
#102031=CARTESIAN_POINT('Ctrl Pts',(2.40331488837584,-29.677290371186,127.029250122082));
#102032=CARTESIAN_POINT('Ctrl Pts',(2.40717428084491,-29.7477639950412,
127.040457472397));
#102033=CARTESIAN_POINT('Ctrl Pts',(2.41103367331399,-29.8187876667723,
127.047983853952));
#102034=CARTESIAN_POINT('Ctrl Pts',(2.41489306578306,-29.8899469624257,
127.051800646121));
#102035=CARTESIAN_POINT('Ctrl Pts',(2.4187546433871,-29.9611465474941,127.055619599305));
#102036=CARTESIAN_POINT('Ctrl Pts',(2.42261622099113,-30.0324814233311,
127.055724781301));
#102037=CARTESIAN_POINT('Ctrl Pts',(2.42647779859517,-30.1035377690062,
127.052139735225));
#102038=CARTESIAN_POINT('Ctrl Pts',(2.43034613271079,-30.1747184402994,
127.048548416478));
#102039=CARTESIAN_POINT('Ctrl Pts',(2.43421446682641,-30.2456191250582,
127.041254028392));
#102040=CARTESIAN_POINT('Ctrl Pts',(2.43808280094203,-30.3158324191724,
127.030331856003));
#102041=CARTESIAN_POINT('Ctrl Pts',(2.44038052011079,-30.3575378217996,
127.023844286906));
#102042=CARTESIAN_POINT('Ctrl Pts',(2.44267823927955,-30.3990009027221,
127.016077763855));
#102043=CARTESIAN_POINT('Ctrl Pts',(2.44497595844831,-30.440138756094,127.007056411236));
#102044=CARTESIAN_POINT('Ctrl Pts',(2.44884535140181,-30.5094155076324,
126.991864320432));
#102045=CARTESIAN_POINT('Ctrl Pts',(2.45271474435532,-30.5780404729772,
126.973051462176));
#102046=CARTESIAN_POINT('Ctrl Pts',(2.45658413730882,-30.645607008178,126.95068940467));
#102047=CARTESIAN_POINT('Ctrl Pts',(2.46044683557589,-30.7130566421563,
126.928366037202));
#102048=CARTESIAN_POINT('Ctrl Pts',(2.46430953384297,-30.7794510271505,
126.902505823078));
#102049=CARTESIAN_POINT('Ctrl Pts',(2.46817223211004,-30.8443951111531,
126.873231021193));
#102050=CARTESIAN_POINT('Ctrl Pts',(2.47203108524621,-30.9092745464342,
126.84398536097));
#102051=CARTESIAN_POINT('Ctrl Pts',(2.47588993838239,-30.9727061043097,
126.81133205486));
#102052=CARTESIAN_POINT('Ctrl Pts',(2.47974879151856,-31.0343124417274,
126.775442292891));
#102053=CARTESIAN_POINT('Ctrl Pts',(2.48360488023206,-31.0958746453184,
126.739578241793));
#102054=CARTESIAN_POINT('Ctrl Pts',(2.48746096894557,-31.1556138066068,
126.70048258348));
#102055=CARTESIAN_POINT('Ctrl Pts',(2.49131705765907,-31.2131766508907,
126.658372689185));
#102056=CARTESIAN_POINT('Ctrl Pts',(2.49219248057369,-31.2262447716371,
126.648812751865));
#102057=CARTESIAN_POINT('Ctrl Pts',(2.49306790348832,-31.2392008355424,
126.639097643592));
#102058=CARTESIAN_POINT('Ctrl Pts',(2.49394332640294,-31.2520409112987,
126.629230222815));
#102059=CARTESIAN_POINT('Ctrl Pts',(1.79398326297881,-31.2520409112987,
126.629230222815));
#102060=CARTESIAN_POINT('Ctrl Pts',(1.79795477719867,-31.3100239000484,
126.584671097249));
#102061=CARTESIAN_POINT('Ctrl Pts',(1.80192629141854,-31.3657081646153,
126.53694901864));
#102062=CARTESIAN_POINT('Ctrl Pts',(1.8058978056384,-31.4187339253545,126.486334959405));
#102063=CARTESIAN_POINT('Ctrl Pts',(1.80975547492232,-31.4702396828908,
126.43717177105));
#102064=CARTESIAN_POINT('Ctrl Pts',(1.81361314420623,-31.5192369238096,
126.385280532738));
#102065=CARTESIAN_POINT('Ctrl Pts',(1.81747081349015,-31.5654288977993,
126.330950761086));
#102066=CARTESIAN_POINT('Ctrl Pts',(1.82132655812563,-31.6115978259278,
126.276648095363));
#102067=CARTESIAN_POINT('Ctrl Pts',(1.8251823027611,-31.6549639501939,126.219909680033));
#102068=CARTESIAN_POINT('Ctrl Pts',(1.82903804739658,-31.6952688910805,
126.16106026951));
#102069=CARTESIAN_POINT('Ctrl Pts',(1.83289315815994,-31.7355672059634,
126.102220533643));
#102070=CARTESIAN_POINT('Ctrl Pts',(1.83674826892331,-31.7728050628913,
126.041270892824));
#102071=CARTESIAN_POINT('Ctrl Pts',(1.84060337968667,-31.8067667655206,
125.97856600059));
#102072=CARTESIAN_POINT('Ctrl Pts',(1.84466139840074,-31.8425159912344,
125.912560730762));
#102073=CARTESIAN_POINT('Ctrl Pts',(1.84871941711481,-31.8746343923033,
125.844610859921));
#102074=CARTESIAN_POINT('Ctrl Pts',(1.85277743582888,-31.902925891643,125.775158444071));
#102075=CARTESIAN_POINT('Ctrl Pts',(1.85663765431487,-31.9298383768834,
125.709091351125));
#102076=CARTESIAN_POINT('Ctrl Pts',(1.86049787280086,-31.9532882097898,
125.64166526996));
#102077=CARTESIAN_POINT('Ctrl Pts',(1.86435809128686,-31.9731573139482,
125.57327809736));
#102078=CARTESIAN_POINT('Ctrl Pts',(1.86822100972785,-31.9930403151663,
125.504843092678));
#102079=CARTESIAN_POINT('Ctrl Pts',(1.87208392816884,-32.0093374949156,
125.435446131666));
#102080=CARTESIAN_POINT('Ctrl Pts',(1.87594684660983,-32.0219818112365,
125.365495714789));
#102081=CARTESIAN_POINT('Ctrl Pts',(1.87981602035975,-32.0346466027773,
125.29543202566));
#102082=CARTESIAN_POINT('Ctrl Pts',(1.88368519410967,-32.0436466744898,
125.224813573776));
#102083=CARTESIAN_POINT('Ctrl Pts',(1.88755436785959,-32.0489668424968,
125.154053370131));
#102084=CARTESIAN_POINT('Ctrl Pts',(1.88813611332489,-32.0497667506458,
125.143414295679));
#102085=CARTESIAN_POINT('Ctrl Pts',(1.8887178587902,-32.0504835657235,125.132772013456));
#102086=CARTESIAN_POINT('Ctrl Pts',(1.88929960425551,-32.0511173377636,
125.122127921564));
#102087=CARTESIAN_POINT('Ctrl Pts',(1.8931686779118,-32.0553324298458,125.051336178452));
#102088=CARTESIAN_POINT('Ctrl Pts',(1.89703775156808,-32.0558865433681,
124.980187299047));
#102089=CARTESIAN_POINT('Ctrl Pts',(1.90090682522436,-32.0527379987999,
124.909091965246));
#102090=CARTESIAN_POINT('Ctrl Pts',(1.90477013393189,-32.0495941455867,
124.838102564025));
#102091=CARTESIAN_POINT('Ctrl Pts',(1.90863344263941,-32.0427586066674,
124.767167031397));
#102092=CARTESIAN_POINT('Ctrl Pts',(1.91249675134693,-32.0322416318168,
124.696698973937));
#102093=CARTESIAN_POINT('Ctrl Pts',(1.9163555281555,-32.021736994025,124.626313579847));
#102094=CARTESIAN_POINT('Ctrl Pts',(1.92021430496407,-32.0075595697636,
124.556395049793));
#102095=CARTESIAN_POINT('Ctrl Pts',(1.92407308177264,-31.9897715065036,
124.487353031408));
#102096=CARTESIAN_POINT('Ctrl Pts',(1.92792942767875,-31.9719946491384,
124.418354507224));
#102097=CARTESIAN_POINT('Ctrl Pts',(1.93178577358485,-31.950611786426,124.350231868515));
#102098=CARTESIAN_POINT('Ctrl Pts',(1.93564211949096,-31.9257360785957,
124.283384260503));
#102099=CARTESIAN_POINT('Ctrl Pts',(1.93949732605596,-31.9008677201881,
124.216556402334));
#102100=CARTESIAN_POINT('Ctrl Pts',(1.94335253262096,-31.8725087346924,
124.151003282038));
#102101=CARTESIAN_POINT('Ctrl Pts',(1.94720773918597,-31.8408214977065,
124.087106919688));
#102102=CARTESIAN_POINT('Ctrl Pts',(1.95106309635817,-31.8091330228294,
124.023208061167));
#102103=CARTESIAN_POINT('Ctrl Pts',(1.95491845353038,-31.7741162561223,
123.960966523321));
#102104=CARTESIAN_POINT('Ctrl Pts',(1.95877381070259,-31.7359801128372,
123.900740881169));
#102105=CARTESIAN_POINT('Ctrl Pts',(1.96263320349186,-31.697804050327,123.840452197483));
#102106=CARTESIAN_POINT('Ctrl Pts',(1.96649259628114,-31.6565023535359,
123.782184033088));
#102107=CARTESIAN_POINT('Ctrl Pts',(1.97035198907041,-31.6123274957083,
123.726266272299));
#102108=CARTESIAN_POINT('Ctrl Pts',(1.9742135669949,-31.5681276266825,123.670316851641));
#102109=CARTESIAN_POINT('Ctrl Pts',(1.97807514491939,-31.5210516790099,
123.616720848893));
#102110=CARTESIAN_POINT('Ctrl Pts',(1.98193672284388,-31.4713908686318,
123.565773213816));
#102111=CARTESIAN_POINT('Ctrl Pts',(1.98580505727686,-31.4216431679479,
123.514736436908));
#102112=CARTESIAN_POINT('Ctrl Pts',(1.98967339170984,-31.3693019317678,
123.466357608996));
#102113=CARTESIAN_POINT('Ctrl Pts',(1.99354172614282,-31.3146929590917,
123.420892661718));
#102114=CARTESIAN_POINT('Ctrl Pts',(1.9958394424599,-31.282256278719,123.393887356716));
#102115=CARTESIAN_POINT('Ctrl Pts',(1.99813715877699,-31.2490201142081,
123.367909310058));
#102116=CARTESIAN_POINT('Ctrl Pts',(2.00043487509407,-31.2150573708127,
123.34300478331));
#102117=CARTESIAN_POINT('Ctrl Pts',(2.00430394846991,-31.1578682629736,
123.301068604913));
#102118=CARTESIAN_POINT('Ctrl Pts',(2.00817302184574,-31.0983935262999,
123.262014475619));
#102119=CARTESIAN_POINT('Ctrl Pts',(2.01204209522157,-31.0369555869914,
123.226100151331));
#102120=CARTESIAN_POINT('Ctrl Pts',(2.01590540364641,-30.9756091907153,
123.19023933968));
#102121=CARTESIAN_POINT('Ctrl Pts',(2.01976871207125,-30.9123058141906,
123.157509289833));
#102122=CARTESIAN_POINT('Ctrl Pts',(2.02363202049609,-30.8473985053611,
123.128125715863));
#102123=CARTESIAN_POINT('Ctrl Pts',(2.02749079702005,-30.7825673368385,
123.098776610652));
#102124=CARTESIAN_POINT('Ctrl Pts',(2.03134957354402,-30.7161364137331,
123.072766383073));
#102125=CARTESIAN_POINT('Ctrl Pts',(2.03520835006799,-30.6484836053586,
123.050264998498));
#102126=CARTESIAN_POINT('Ctrl Pts',(2.03906469568848,-30.5808734160492,
123.027777789063));
#102127=CARTESIAN_POINT('Ctrl Pts',(2.04292104130896,-30.5120433285063,
123.008795190075));
#102128=CARTESIAN_POINT('Ctrl Pts',(2.04677738692944,-30.4423900560028,
122.993438612738));
#102129=CARTESIAN_POINT('Ctrl Pts',(2.05063259320823,-30.3727573622766,
122.97808657244));
#102130=CARTESIAN_POINT('Ctrl Pts',(2.05448779948702,-30.3023024405569,
122.966358531514));
#102131=CARTESIAN_POINT('Ctrl Pts',(2.0583430057658,-30.2314343091854,122.958325265124));
#102132=CARTESIAN_POINT('Ctrl Pts',(2.06219836265164,-30.1605634092877,
122.950291684907));
#102133=CARTESIAN_POINT('Ctrl Pts',(2.06605371953747,-30.0892797506324,
122.945953218321));
#102134=CARTESIAN_POINT('Ctrl Pts',(2.0699090764233,-30.0179978957906,122.945328824788));
#102135=CARTESIAN_POINT('Ctrl Pts',(2.07376846892795,-29.9466414262238,
122.944703777667));
#102136=CARTESIAN_POINT('Ctrl Pts',(2.07762786143259,-29.8752872510023,
122.947800568642));
#102137=CARTESIAN_POINT('Ctrl Pts',(2.08148725393723,-29.8043494526783,
122.95458600136));
#102138=CARTESIAN_POINT('Ctrl Pts',(2.08534883157766,-29.7333714903335,
122.961375275898));
#102139=CARTESIAN_POINT('Ctrl Pts',(2.08921040921808,-29.6628108549264,
122.97185727824));
#102140=CARTESIAN_POINT('Ctrl Pts',(2.0930719868585,-29.5930732916184,122.98594731536));
#102141=CARTESIAN_POINT('Ctrl Pts',(2.09694032101139,-29.52321371012,123.000062005489));
#102142=CARTESIAN_POINT('Ctrl Pts',(2.10080865516429,-29.4541805465985,
123.017797213357));
#102143=CARTESIAN_POINT('Ctrl Pts',(2.10467698931718,-29.3863655219985,
123.039018029173));
#102144=CARTESIAN_POINT('Ctrl Pts',(2.106974708189,-29.346084652855,123.051622800904));
#102145=CARTESIAN_POINT('Ctrl Pts',(2.10927242706081,-29.3062332176237,
123.065456404863));
#102146=CARTESIAN_POINT('Ctrl Pts',(2.11157014593263,-29.266889624117,123.080482680653));
#102147=CARTESIAN_POINT('Ctrl Pts',(2.11543921919095,-29.2006398981864,
123.105785063179));
#102148=CARTESIAN_POINT('Ctrl Pts',(2.11930829244926,-29.1355718640553,
123.134570821762));
#102149=CARTESIAN_POINT('Ctrl Pts',(2.12317736570758,-29.0720769460634,
123.16670886969));
#102150=CARTESIAN_POINT('Ctrl Pts',(2.12704067401181,-29.0086766360726,
123.198799031637));
#102151=CARTESIAN_POINT('Ctrl Pts',(2.13090398231604,-28.946845219429,123.234231350518));
#102152=CARTESIAN_POINT('Ctrl Pts',(2.13476729062027,-28.88695540744,123.272826210981));
#102153=CARTESIAN_POINT('Ctrl Pts',(2.1386260670196,-28.8271358499872,123.311375797234));
#102154=CARTESIAN_POINT('Ctrl Pts',(2.14248484341893,-28.7692537794135,
123.353080294159));
#102155=CARTESIAN_POINT('Ctrl Pts',(2.14634361981825,-28.7136569337726,
123.397714420439));
#102156=CARTESIAN_POINT('Ctrl Pts',(2.15019996531167,-28.658095112369,123.442320428645));
#102157=CARTESIAN_POINT('Ctrl Pts',(2.15405631080509,-28.6048160376363,
123.489852101218));
#102158=CARTESIAN_POINT('Ctrl Pts',(2.15791265629851,-28.5541368754454,
123.540041991168));
#102159=CARTESIAN_POINT('Ctrl Pts',(2.16176786244799,-28.5034726862377,
123.590217052689));
#102160=CARTESIAN_POINT('Ctrl Pts',(2.16562306859748,-28.4554072295875,
123.643048430781));
#102161=CARTESIAN_POINT('Ctrl Pts',(2.16947827474696,-28.4102218036538,
123.698230877259));
#102162=CARTESIAN_POINT('Ctrl Pts',(2.17333363150144,-28.3650346125353,
123.753415479459));
#102163=CARTESIAN_POINT('Ctrl Pts',(2.17718898825592,-28.3227279815673,
123.810950955138));
#102164=CARTESIAN_POINT('Ctrl Pts',(2.1810443450104,-28.2835426832373,123.870499295161));
#102165=CARTESIAN_POINT('Ctrl Pts',(2.18490373738144,-28.2443163674738,
123.930109967747));
#102166=CARTESIAN_POINT('Ctrl Pts',(2.18876312975249,-28.2082181741437,
123.991737304038));
#102167=CARTESIAN_POINT('Ctrl Pts',(2.19262252212353,-28.175444797052,124.055015410763));
#102168=CARTESIAN_POINT('Ctrl Pts',(2.19648409962889,-28.1426528641299,
124.118329344672));
#102169=CARTESIAN_POINT('Ctrl Pts',(2.20034567713425,-28.11318969559,124.183295466976));
#102170=CARTESIAN_POINT('Ctrl Pts',(2.20420725463961,-28.0872041987393,
124.249526959059));
#102171=CARTESIAN_POINT('Ctrl Pts',(2.20807558865656,-28.061173235674,124.315874334831));
#102172=CARTESIAN_POINT('Ctrl Pts',(2.21194392267352,-28.0386322464595,
124.383491039674));
#102173=CARTESIAN_POINT('Ctrl Pts',(2.21581225669047,-28.0196803428808,
124.451974801558));
#102174=CARTESIAN_POINT('Ctrl Pts',(2.21810997671738,-28.0084232569597,
124.492652910147));
#102175=CARTESIAN_POINT('Ctrl Pts',(2.22040769674429,-27.9984314773309,
124.533636707412));
#102176=CARTESIAN_POINT('Ctrl Pts',(2.22270541677119,-27.98971714967,124.5748407073));
#102177=CARTESIAN_POINT('Ctrl Pts',(2.22812785149404,-27.9691520362785,
124.672078837751));
#102178=CARTESIAN_POINT('Ctrl Pts',(2.23355028621689,-27.9556362047534,
124.770855989234));
#102179=CARTESIAN_POINT('Ctrl Pts',(2.23897272093974,-27.9493462562119,
124.870320450387));
#102180=CARTESIAN_POINT('Ctrl Pts',(2.24129024080572,-27.946657965537,124.912831034001));
#102181=CARTESIAN_POINT('Ctrl Pts',(2.2436077606717,-27.9452890575184,124.95546687936));
#102182=CARTESIAN_POINT('Ctrl Pts',(2.24592528053768,-27.9452508239577,
124.998159876744));
#102183=CARTESIAN_POINT('Origin',(-1.54592528053767,-30.,125.));
#102184=CARTESIAN_POINT('',(1.09386069669771,-31.2520409112987,126.629230222815));
#102185=CARTESIAN_POINT('',(1.15210970423049,-31.2520409112987,126.629230222815));
#102186=CARTESIAN_POINT('',(-1.54592528053767,-31.2520409112987,126.629230222815));
#102187=CARTESIAN_POINT('',(1.60407471941018,-27.9452500663321,124.999477896899));
#102188=CARTESIAN_POINT('Ctrl Pts',(1.15210970423049,-31.2520409112987,
126.629230222815));
#102189=CARTESIAN_POINT('Ctrl Pts',(1.1559651187354,-31.308569673581,126.585788650193));
#102190=CARTESIAN_POINT('Ctrl Pts',(1.15982053324031,-31.3628595945105,
126.539382601305));
#102191=CARTESIAN_POINT('Ctrl Pts',(1.16367594774522,-31.4145917589832,
126.490277731806));
#102192=CARTESIAN_POINT('Ctrl Pts',(1.16753113264579,-31.4663208426124,
126.441175786685));
#102193=CARTESIAN_POINT('Ctrl Pts',(1.17138631754637,-31.5154921209874,
126.389375675649));
#102194=CARTESIAN_POINT('Ctrl Pts',(1.17524150244695,-31.5618224856364,
126.335180918775));
#102195=CARTESIAN_POINT('Ctrl Pts',(1.17910047876147,-31.6081984142713,
126.280932863612));
#102196=CARTESIAN_POINT('Ctrl Pts',(1.18295945507599,-31.6517275316966,
126.224285828409));
#102197=CARTESIAN_POINT('Ctrl Pts',(1.18681843139052,-31.6921666883546,
126.165576879199));
#102198=CARTESIAN_POINT('Ctrl Pts',(1.19067925130637,-31.7326251645619,
126.106839882162));
#102199=CARTESIAN_POINT('Ctrl Pts',(1.19454007122222,-31.7699904843435,
126.046039423183));
#102200=CARTESIAN_POINT('Ctrl Pts',(1.19840089113807,-31.8040640891954,
125.983539691408));
#102201=CARTESIAN_POINT('Ctrl Pts',(1.202268829534,-31.8382005180801,125.920924724242));
#102202=CARTESIAN_POINT('Ctrl Pts',(1.20613676792992,-31.8690328951808,
125.856604663548));
#102203=CARTESIAN_POINT('Ctrl Pts',(1.21000470632584,-31.8964099070394,
125.790965882313));
#102204=CARTESIAN_POINT('Ctrl Pts',(1.2134410054685,-31.9207318048435,125.732652004325));
#102205=CARTESIAN_POINT('Ctrl Pts',(1.21687730461115,-31.9423271335707,
125.673297808585));
#102206=CARTESIAN_POINT('Ctrl Pts',(1.2203136037538,-31.9611231636045,125.613183088216));
#102207=CARTESIAN_POINT('Ctrl Pts',(1.22418267030921,-31.9822863651068,
125.545497521735));
#102208=CARTESIAN_POINT('Ctrl Pts',(1.22805173686462,-31.9999827911828,
125.476582456271));
#102209=CARTESIAN_POINT('Ctrl Pts',(1.23192080342002,-32.0140729490346,
125.406826398439));
#102210=CARTESIAN_POINT('Ctrl Pts',(1.23578410490835,-32.0281421119762,
125.33717427998));
#102211=CARTESIAN_POINT('Ctrl Pts',(1.23964740639668,-32.0386155775137,
125.266684128839));
#102212=CARTESIAN_POINT('Ctrl Pts',(1.24351070788501,-32.0454035440006,
125.195759813777));
#102213=CARTESIAN_POINT('Ctrl Pts',(1.24736947733365,-32.0521835475227,
125.124918700042));
#102214=CARTESIAN_POINT('Ctrl Pts',(1.25122824678228,-32.0552865937895,
125.053644915294));
#102215=CARTESIAN_POINT('Ctrl Pts',(1.25508701623091,-32.0546742017609,
124.982351002343));
#102216=CARTESIAN_POINT('Ctrl Pts',(1.25894335469421,-32.054062195533,124.91110200383));
#102217=CARTESIAN_POINT('Ctrl Pts',(1.2627996931575,-32.0497393990592,124.839833386893));
#102218=CARTESIAN_POINT('Ctrl Pts',(1.2666560316208,-32.0417193711735,124.768959804634));
#102219=CARTESIAN_POINT('Ctrl Pts',(1.2705112306712,-32.0337017129251,124.698107163035));
#102220=CARTESIAN_POINT('Ctrl Pts',(1.27436642972161,-32.0219890465787,
124.627649806838));
#102221=CARTESIAN_POINT('Ctrl Pts',(1.27822162877202,-32.0066468237053,
124.557997638679));
#102222=CARTESIAN_POINT('Ctrl Pts',(1.28207697836888,-31.9913040017144,
124.488342750586));
#102223=CARTESIAN_POINT('Ctrl Pts',(1.28593232796574,-31.9723314484503,
124.419493586897));
#102224=CARTESIAN_POINT('Ctrl Pts',(1.2897876775626,-31.9498454356419,124.351848521095));
#102225=CARTESIAN_POINT('Ctrl Pts',(1.29364706273577,-31.9273358856629,
124.284132648011));
#102226=CARTESIAN_POINT('Ctrl Pts',(1.29750644790895,-31.9013056881675,
124.217623850758));
#102227=CARTESIAN_POINT('Ctrl Pts',(1.30136583308213,-31.8719203064661,
124.152703163738));
#102228=CARTESIAN_POINT('Ctrl Pts',(1.30522740335605,-31.8425182873948,
124.087745720024));
#102229=CARTESIAN_POINT('Ctrl Pts',(1.30908897362996,-31.8097575257402,
124.024378608213));
#102230=CARTESIAN_POINT('Ctrl Pts',(1.31295054390387,-31.7738495090303,
123.962958302761));
#102231=CARTESIAN_POINT('Ctrl Pts',(1.31681887071462,-31.7378786645533,
123.901430531038));
#102232=CARTESIAN_POINT('Ctrl Pts',(1.32068719752537,-31.6987498374917,
123.841856772617));
#102233=CARTESIAN_POINT('Ctrl Pts',(1.32455552433612,-31.6567174875471,
123.784563975787));
#102234=CARTESIAN_POINT('Ctrl Pts',(1.32685330775487,-31.6317503010919,
123.75053209456));
#102235=CARTESIAN_POINT('Ctrl Pts',(1.32915109117362,-31.6057594272786,
123.717304388655));
#102236=CARTESIAN_POINT('Ctrl Pts',(1.33144887459236,-31.5788044682051,
123.684943342028));
#102237=CARTESIAN_POINT('Ctrl Pts',(1.33531795015095,-31.5334169123184,
123.630452856314));
#102238=CARTESIAN_POINT('Ctrl Pts',(1.33918702570954,-31.485116135623,123.578208140709));
#102239=CARTESIAN_POINT('Ctrl Pts',(1.34305610126813,-31.434152886149,123.528537101504));
#102240=CARTESIAN_POINT('Ctrl Pts',(1.34691941189731,-31.3832655720066,
123.478940072234));
#102241=CARTESIAN_POINT('Ctrl Pts',(1.35078272252649,-31.3297240046965,
123.431909443729));
#102242=CARTESIAN_POINT('Ctrl Pts',(1.35464603315567,-31.2738187891828,
123.387739706243));
#102243=CARTESIAN_POINT('Ctrl Pts',(1.35850481190518,-31.2179791536169,
123.343621782332));
#102244=CARTESIAN_POINT('Ctrl Pts',(1.36236359065469,-31.1597817566726,
123.302358383013));
#102245=CARTESIAN_POINT('Ctrl Pts',(1.36622236940421,-31.0995523250525,
123.264205586202));
#102246=CARTESIAN_POINT('Ctrl Pts',(1.37007871726209,-31.039360835805,123.226076824279));
#102247=CARTESIAN_POINT('Ctrl Pts',(1.37393506511997,-30.9771402610041,
123.191055036457));
#102248=CARTESIAN_POINT('Ctrl Pts',(1.37779141297786,-30.9132463246948,
123.159353724114));
#102249=CARTESIAN_POINT('Ctrl Pts',(1.38164662150252,-30.8493712654389,
123.127661777721));
#102250=CARTESIAN_POINT('Ctrl Pts',(1.38550183002718,-30.7838242610932,
123.099288575016));
#102251=CARTESIAN_POINT('Ctrl Pts',(1.38935703855185,-30.7169851892392,
123.07440144347));
#102252=CARTESIAN_POINT('Ctrl Pts',(1.39321239768867,-30.6501435061704,
123.049513339653));
#102253=CARTESIAN_POINT('Ctrl Pts',(1.3970677568255,-30.5820101113969,123.02811174483));
#102254=CARTESIAN_POINT('Ctrl Pts',(1.40092311596233,-30.5129827592616,
123.010315037198));
#102255=CARTESIAN_POINT('Ctrl Pts',(1.40478251071016,-30.4438831524978,
122.992499700798));
#102256=CARTESIAN_POINT('Ctrl Pts',(1.40864190545801,-30.3738881917653,
122.978296905729));
#102257=CARTESIAN_POINT('Ctrl Pts',(1.41250130020584,-30.3034077437419,
122.967774298082));
#102258=CARTESIAN_POINT('Ctrl Pts',(1.41636288008844,-30.2328873906851,
122.957245732682));
#102259=CARTESIAN_POINT('Ctrl Pts',(1.42022445997104,-30.1618814869173,
122.950401549279));
#102260=CARTESIAN_POINT('Ctrl Pts',(1.42408603985364,-30.0908042270566,
122.947257406578));
#102261=CARTESIAN_POINT('Ctrl Pts',(1.42795437622264,-30.0196026055215,
122.944107762668));
#102262=CARTESIAN_POINT('Ctrl Pts',(1.43182271259164,-29.9483298645522,
122.944671080841));
#102263=CARTESIAN_POINT('Ctrl Pts',(1.43569104896064,-29.8773986990648,
122.948910903079));
#102264=CARTESIAN_POINT('Ctrl Pts',(1.43798874778407,-29.8352672916747,
122.951429255579));
#102265=CARTESIAN_POINT('Ctrl Pts',(1.44028644660749,-29.7932562886806,
122.955243712123));
#102266=CARTESIAN_POINT('Ctrl Pts',(1.44258414543092,-29.7514505019871,
122.960338089404));
#102267=CARTESIAN_POINT('Ctrl Pts',(1.44645321925166,-29.68105412401,122.96891646424));
#102268=CARTESIAN_POINT('Ctrl Pts',(1.45032229307241,-29.6109644877276,
122.981160384507));
#102269=CARTESIAN_POINT('Ctrl Pts',(1.45419136689315,-29.5415930779158,
122.997037030725));
#102270=CARTESIAN_POINT('Ctrl Pts',(1.45805467577709,-29.472325031806,123.012890020672));
#102271=CARTESIAN_POINT('Ctrl Pts',(1.46191798466102,-29.4037735576123,
123.032364884866));
#102272=CARTESIAN_POINT('Ctrl Pts',(1.46578129354496,-29.336343682847,123.05537719462));
#102273=CARTESIAN_POINT('Ctrl Pts',(1.46964007054697,-29.2689929071752,
123.078362509621));
#102274=CARTESIAN_POINT('Ctrl Pts',(1.47349884754898,-29.2027615750243,
123.104876871482));
#102275=CARTESIAN_POINT('Ctrl Pts',(1.47735762455099,-29.1380414908253,
123.134785510736));
#102276=CARTESIAN_POINT('Ctrl Pts',(1.48121397066095,-29.0733621779736,
123.164675308612));
#102277=CARTESIAN_POINT('Ctrl Pts',(1.48507031677091,-29.0101926641901,
123.197954938277));
#102278=CARTESIAN_POINT('Ctrl Pts',(1.48892666288088,-28.9489052530017,
123.234441336196));
#102279=CARTESIAN_POINT('Ctrl Pts',(1.49278186965987,-28.887635948758,123.27091695446));
#102280=CARTESIAN_POINT('Ctrl Pts',(1.49663707643886,-28.8282480603753,
123.310597211726));
#102281=CARTESIAN_POINT('Ctrl Pts',(1.50049228321786,-28.7710881986911,
123.353253708945));
#102282=CARTESIAN_POINT('Ctrl Pts',(1.50434764061392,-28.713926103858,123.395911872688));
#102283=CARTESIAN_POINT('Ctrl Pts',(1.50820299800997,-28.6589925965489,
123.441546214932));
#102284=CARTESIAN_POINT('Ctrl Pts',(1.51205835540603,-28.6066028589048,
123.489886769249));
#102285=CARTESIAN_POINT('Ctrl Pts',(1.51591774843277,-28.5541582818228,
123.538277924485));
#102286=CARTESIAN_POINT('Ctrl Pts',(1.51977714145951,-28.5042631475354,
123.5893806165));
#102287=CARTESIAN_POINT('Ctrl Pts',(1.52363653448625,-28.4571965852293,
123.642887187493));
#102288=CARTESIAN_POINT('Ctrl Pts',(1.52749811265627,-28.410103374385,123.696424053281));
#102289=CARTESIAN_POINT('Ctrl Pts',(1.53135969082629,-28.3658422251813,
123.752367126325));
#102290=CARTESIAN_POINT('Ctrl Pts',(1.53522126899631,-28.324650937252,123.810376916646));
#102291=CARTESIAN_POINT('Ctrl Pts',(1.53908960368497,-28.2833875778295,
123.868488205424));
#102292=CARTESIAN_POINT('Ctrl Pts',(1.54295793837363,-28.2452050638975,
123.928673020778));
#102293=CARTESIAN_POINT('Ctrl Pts',(1.54682627306229,-28.2102965961721,
123.990564866459));
#102294=CARTESIAN_POINT('Ctrl Pts',(1.54912398746468,-28.1895616558131,
124.027327400381));
#102295=CARTESIAN_POINT('Ctrl Pts',(1.55142170186708,-28.1699809474435,
124.064691745944));
#102296=CARTESIAN_POINT('Ctrl Pts',(1.55371941626948,-28.1515868743254,
124.102577870044));
#102297=CARTESIAN_POINT('Ctrl Pts',(1.5579156915312,-28.1179941032189,124.171768629853));
#102298=CARTESIAN_POINT('Ctrl Pts',(1.56211196679293,-28.0882444501088,
124.242941993068));
#102299=CARTESIAN_POINT('Ctrl Pts',(1.56630824205465,-28.0625573661179,
124.315665576698));
#102300=CARTESIAN_POINT('Ctrl Pts',(1.57045672473061,-28.037162839714,124.38756089052));
#102301=CARTESIAN_POINT('Ctrl Pts',(1.57460520740658,-28.0157389964659,
124.460970953742));
#102302=CARTESIAN_POINT('Ctrl Pts',(1.57875369008254,-27.9984520816046,
124.535453454574));
#102303=CARTESIAN_POINT('Ctrl Pts',(1.58297386163715,-27.9808664359451,
124.611223068642));
#102304=CARTESIAN_POINT('Ctrl Pts',(1.58719403319175,-27.9675622691549,
124.688102209931));
#102305=CARTESIAN_POINT('Ctrl Pts',(1.59141420474636,-27.9586631076518,
124.765604491429));
#102306=CARTESIAN_POINT('Ctrl Pts',(1.59563437630097,-27.9497639461487,
124.843106772928));
#102307=CARTESIAN_POINT('Ctrl Pts',(1.59985454785558,-27.9452699483265,
124.921231805876));
#102308=CARTESIAN_POINT('Ctrl Pts',(1.60407471941018,-27.9452500663321,
124.999477896899));
#102309=CARTESIAN_POINT('Ctrl Pts',(1.60407471946233,-27.9452500663318,
124.999477897865));
#102310=CARTESIAN_POINT('Ctrl Pts',(1.60804279144092,-27.9452313720589,
125.073049817208));
#102311=CARTESIAN_POINT('Ctrl Pts',(1.6120108634195,-27.9491684627898,125.1465793535));
#102312=CARTESIAN_POINT('Ctrl Pts',(1.61597893539809,-27.9570216303455,
125.219629104683));
#102313=CARTESIAN_POINT('Ctrl Pts',(1.62005191470725,-27.9650824188439,
125.294610134945));
#102314=CARTESIAN_POINT('Ctrl Pts',(1.62412489401641,-27.9772692208633,
125.369085156028));
#102315=CARTESIAN_POINT('Ctrl Pts',(1.62819787332558,-27.9934830709017,
125.442591658012));
#102316=CARTESIAN_POINT('Ctrl Pts',(1.63217761780573,-28.0093257686653,
125.514415517974));
#102317=CARTESIAN_POINT('Ctrl Pts',(1.63615736228589,-28.0290128981694,
125.585314321825));
#102318=CARTESIAN_POINT('Ctrl Pts',(1.64013710676604,-28.0524017569215,
125.654872999945));
#102319=CARTESIAN_POINT('Ctrl Pts',(1.64425670348971,-28.0766125238101,
125.726876040321));
#102320=CARTESIAN_POINT('Ctrl Pts',(1.64837630021338,-28.1047898157325,
125.797442528993));
#102321=CARTESIAN_POINT('Ctrl Pts',(1.65249589693704,-28.1367223437685,
125.86613736687));
#102322=CARTESIAN_POINT('Ctrl Pts',(1.65661549366071,-28.1686548718044,
125.934832204747));
#102323=CARTESIAN_POINT('Ctrl Pts',(1.66073509038437,-28.2043423228842,
126.00165497065));
#102324=CARTESIAN_POINT('Ctrl Pts',(1.66485468710804,-28.2435236961586,
126.066202868381));
#102325=CARTESIAN_POINT('Ctrl Pts',(1.66872376076535,-28.280322351309,126.126825445661));
#102326=CARTESIAN_POINT('Ctrl Pts',(1.67259283442267,-28.3203352379876,
126.185659440808));
#102327=CARTESIAN_POINT('Ctrl Pts',(1.67646190807999,-28.3633630459669,
126.24234336767));
#102328=CARTESIAN_POINT('Ctrl Pts',(1.68032521678857,-28.40632674219,126.298942835056));
#102329=CARTESIAN_POINT('Ctrl Pts',(1.68418852549714,-28.4522961513903,
126.353398209465));
#102330=CARTESIAN_POINT('Ctrl Pts',(1.68805183420572,-28.5010275887913,
126.405375136017));
#102331=CARTESIAN_POINT('Ctrl Pts',(1.69191061101535,-28.5497018612162,
126.457291090434));
#102332=CARTESIAN_POINT('Ctrl Pts',(1.69576938782498,-28.6011313954007,
126.50673401935));
#102333=CARTESIAN_POINT('Ctrl Pts',(1.69962816463461,-28.6550320733385,
126.553402342844));
#102334=CARTESIAN_POINT('Ctrl Pts',(1.70348451054179,-28.7088987956224,
126.600041266829));
#102335=CARTESIAN_POINT('Ctrl Pts',(1.70734085644897,-28.7652332067255,
126.643908735991));
#102336=CARTESIAN_POINT('Ctrl Pts',(1.71119720235615,-28.8237152051057,
126.684740823925));
#102337=CARTESIAN_POINT('Ctrl Pts',(1.71505240892223,-28.8821799252267,
126.725560848192));
#102338=CARTESIAN_POINT('Ctrl Pts',(1.71890761548831,-28.9427905748845,
126.763346993663));
#102339=CARTESIAN_POINT('Ctrl Pts',(1.72276282205439,-29.0051963142589,
126.79787741221));
#102340=CARTESIAN_POINT('Ctrl Pts',(1.72661817922768,-29.0676044915714,
126.832409179721));
#102341=CARTESIAN_POINT('Ctrl Pts',(1.73047353640098,-29.131807471706,126.863684734528));
#102342=CARTESIAN_POINT('Ctrl Pts',(1.73432889357427,-29.1974294719842,
126.891527982891));
#102343=CARTESIAN_POINT('Ctrl Pts',(1.73818828636462,-29.2631201624646,
126.919400376333));
#102344=CARTESIAN_POINT('Ctrl Pts',(1.74204767915498,-29.3302323901025,
126.943833101187));
#102345=CARTESIAN_POINT('Ctrl Pts',(1.74590707194533,-29.3983708653951,
126.96469843663));
#102346=CARTESIAN_POINT('Ctrl Pts',(1.74976864987091,-29.4665479197571,
126.985575585739));
#102347=CARTESIAN_POINT('Ctrl Pts',(1.75363022779649,-29.5357519069623,
127.002881206717));
#102348=CARTESIAN_POINT('Ctrl Pts',(1.75749180572206,-29.6055755426125,
127.016538348238));
#102349=CARTESIAN_POINT('Ctrl Pts',(1.76136014015612,-29.6755213469706,
127.030219385325));
#102350=CARTESIAN_POINT('Ctrl Pts',(1.76522847459017,-29.7460884832636,
127.040239129489));
#102351=CARTESIAN_POINT('Ctrl Pts',(1.76909680902422,-29.8168634161222,
127.046572391621));
#102352=CARTESIAN_POINT('Ctrl Pts',(1.77139452533168,-29.8589023660013,
127.050334227607));
#102353=CARTESIAN_POINT('Ctrl Pts',(1.77369224163914,-29.9010145865438,
127.052796422883));
#102354=CARTESIAN_POINT('Ctrl Pts',(1.7759899579466,-29.9431138013116,127.053962395688));
#102355=CARTESIAN_POINT('Ctrl Pts',(1.77985822425498,-30.0139889452827,
127.055925341811));
#102356=CARTESIAN_POINT('Ctrl Pts',(1.78372649056337,-30.0851046067981,
127.054219342807));
#102357=CARTESIAN_POINT('Ctrl Pts',(1.78759475687176,-30.156049245216,127.048815803231));
#102358=CARTESIAN_POINT('Ctrl Pts',(1.79145765803492,-30.2268954859906,
127.043419758168));
#102359=CARTESIAN_POINT('Ctrl Pts',(1.79532055919808,-30.2975706942403,
127.034336383239));
#102360=CARTESIAN_POINT('Ctrl Pts',(1.79918346036124,-30.3676619284924,
127.021589045488));
#102361=CARTESIAN_POINT('Ctrl Pts',(1.80304229660246,-30.4376794059011,
127.008855121732));
#102362=CARTESIAN_POINT('Ctrl Pts',(1.80690113284367,-30.5071136534782,
126.992464974016));
#102363=CARTESIAN_POINT('Ctrl Pts',(1.81075996908489,-30.5755571841383,
126.972493723764));
#102364=CARTESIAN_POINT('Ctrl Pts',(1.81461644855471,-30.6439589131398,
126.952534670886));
#102365=CARTESIAN_POINT('Ctrl Pts',(1.81847292802453,-30.711370660064,126.928998989314));
#102366=CARTESIAN_POINT('Ctrl Pts',(1.82232940749435,-30.7773970319467,
126.902012465054));
#102367=CARTESIAN_POINT('Ctrl Pts',(1.826184465167,-30.8433990613924,126.875035890117));
#102368=CARTESIAN_POINT('Ctrl Pts',(1.83003952283965,-30.9080162820449,
126.844611186077));
#102369=CARTESIAN_POINT('Ctrl Pts',(1.83389458051229,-30.9708720641262,
126.810912752619));
#102370=CARTESIAN_POINT('Ctrl Pts',(1.83775080895679,-31.0337469353589,
126.777204085028));
#102371=CARTESIAN_POINT('Ctrl Pts',(1.84160703740129,-31.0948588704673,
126.740219930774));
#102372=CARTESIAN_POINT('Ctrl Pts',(1.84546326584578,-31.1538558705416,
126.700180635261));
#102373=CARTESIAN_POINT('Ctrl Pts',(1.84764813849783,-31.1872825551559,
126.677495059696));
#102374=CARTESIAN_POINT('Ctrl Pts',(1.84983301114987,-31.220030802175,126.653829549317));
#102375=CARTESIAN_POINT('Ctrl Pts',(1.85201788380192,-31.2520409112987,
126.629230222815));
#102376=CARTESIAN_POINT('',(1.54592528048733,-27.9452502737908,125.001060727663));
#102377=CARTESIAN_POINT('Ctrl Pts',(1.54592528053768,-27.9452502737913,
125.001060728586));
#102378=CARTESIAN_POINT('Ctrl Pts',(1.54924811760506,-27.9452817531205,
125.062039704646));
#102379=CARTESIAN_POINT('Ctrl Pts',(1.55257095467244,-27.9480275057199,
125.122946605554));
#102380=CARTESIAN_POINT('Ctrl Pts',(1.55589379173983,-27.9534698466372,
125.183607989687));
#102381=CARTESIAN_POINT('Ctrl Pts',(1.55976286729176,-27.9598068495541,
125.254241449448));
#102382=CARTESIAN_POINT('Ctrl Pts',(1.56363194284369,-27.9698172975719,
125.324684804351));
#102383=CARTESIAN_POINT('Ctrl Pts',(1.56750101839562,-27.9834814636208,
125.394525734191));
#102384=CARTESIAN_POINT('Ctrl Pts',(1.57136432901806,-27.9971252700379,
125.464262600921));
#102385=CARTESIAN_POINT('Ctrl Pts',(1.57522763964051,-28.0144118956924,
125.533398351465));
#102386=CARTESIAN_POINT('Ctrl Pts',(1.57909095026296,-28.0352698251771,
125.601525479627));
#102387=CARTESIAN_POINT('Ctrl Pts',(1.58294972900565,-28.0561032871422,
125.669572690851));
#102388=CARTESIAN_POINT('Ctrl Pts',(1.58680850774834,-28.0804995899692,
125.736613167621));
#102389=CARTESIAN_POINT('Ctrl Pts',(1.59066728649103,-28.108336482699,125.80225102045));
#102390=CARTESIAN_POINT('Ctrl Pts',(1.59452363434205,-28.1361558391885,
125.867847523794));
#102391=CARTESIAN_POINT('Ctrl Pts',(1.59837998219306,-28.167411296179,125.932042710079));
#102392=CARTESIAN_POINT('Ctrl Pts',(1.60223633004407,-28.2019317133454,
125.994458646213));
#102393=CARTESIAN_POINT('Ctrl Pts',(1.60609153856183,-28.2364419316758,
126.056856141957));
#102394=CARTESIAN_POINT('Ctrl Pts',(1.60994674707959,-28.2742149601786,
126.117475006278));
#102395=CARTESIAN_POINT('Ctrl Pts',(1.61380195559734,-28.3150335294589,
126.175961545142));
#102396=CARTESIAN_POINT('Ctrl Pts',(1.61765731472724,-28.3558536934058,
126.23445036891));
#102397=CARTESIAN_POINT('Ctrl Pts',(1.62151267385714,-28.3997193545229,
126.290806304734));
#102398=CARTESIAN_POINT('Ctrl Pts',(1.62536803298704,-28.4463706982994,
126.344705750489));
#102399=CARTESIAN_POINT('Ctrl Pts',(1.62922742772796,-28.4930708745375,
126.398661615682));
#102400=CARTESIAN_POINT('Ctrl Pts',(1.63308682246887,-28.5425622357055,
126.450155489772));
#102401=CARTESIAN_POINT('Ctrl Pts',(1.63694621720978,-28.5945461492713,
126.498898607636));
#102402=CARTESIAN_POINT('Ctrl Pts',(1.64080779708544,-28.6465594953941,
126.547669323163));
#102403=CARTESIAN_POINT('Ctrl Pts',(1.6446693769611,-28.7010678319009,126.593685868565));
#102404=CARTESIAN_POINT('Ctrl Pts',(1.64853095683675,-28.757739396791,126.636699775834));
#102405=CARTESIAN_POINT('Ctrl Pts',(1.65239929319888,-28.8145101181594,
126.679788943202));
#102406=CARTESIAN_POINT('Ctrl Pts',(1.65626762956101,-28.8734512227913,
126.719864710197));
#102407=CARTESIAN_POINT('Ctrl Pts',(1.66013596592313,-28.9342025387947,
126.756722327002));
#102408=CARTESIAN_POINT('Ctrl Pts',(1.66243366480822,-28.9702873613079,
126.778614866097));
#102409=CARTESIAN_POINT('Ctrl Pts',(1.6647313636933,-29.0070103617168,126.799372895577));
#102410=CARTESIAN_POINT('Ctrl Pts',(1.66702906257839,-29.0442925786996,
126.81896148595));
#102411=CARTESIAN_POINT('Ctrl Pts',(1.67089813639869,-29.1070717577412,
126.851946531416));
#102412=CARTESIAN_POINT('Ctrl Pts',(1.67476721021898,-29.1716835652525,
126.881742253025));
#102413=CARTESIAN_POINT('Ctrl Pts',(1.67863628403928,-29.2377708942199,
126.908141596633));
#102414=CARTESIAN_POINT('Ctrl Pts',(1.68249959292275,-29.3037597527794,
126.934501605104));
#102415=CARTESIAN_POINT('Ctrl Pts',(1.68636290180621,-29.3712193213189,
126.95747510202));
#102416=CARTESIAN_POINT('Ctrl Pts',(1.69022621068968,-29.4397684491177,
126.9769011538));
#102417=CARTESIAN_POINT('Ctrl Pts',(1.69408498769117,-29.5082371648743,
126.996304417712));
#102418=CARTESIAN_POINT('Ctrl Pts',(1.69794376469266,-29.5777924360088,
127.012168370542));
#102419=CARTESIAN_POINT('Ctrl Pts',(1.70180254169415,-29.6480353543373,
127.024381004333));
#102420=CARTESIAN_POINT('Ctrl Pts',(1.70565888780357,-29.7182340221292,
127.0365859446));
#102421=CARTESIAN_POINT('Ctrl Pts',(1.70951523391299,-29.7891190001922,
127.045144046375));
#102422=CARTESIAN_POINT('Ctrl Pts',(1.71337158002241,-29.8602799504348,
127.049994114687));
#102423=CARTESIAN_POINT('Ctrl Pts',(1.71722678680084,-29.931419876663,127.054842750079));
#102424=CARTESIAN_POINT('Ctrl Pts',(1.72108199357926,-30.0028351288057,
127.05598549389));
#102425=CARTESIAN_POINT('Ctrl Pts',(1.72493720035769,-30.0741107142985,
127.053413052585));
#102426=CARTESIAN_POINT('Ctrl Pts',(1.72879255775315,-30.1453890844195,
127.050840510778));
#102427=CARTESIAN_POINT('Ctrl Pts',(1.73264791514862,-30.216527291667,127.044552515409));
#102428=CARTESIAN_POINT('Ctrl Pts',(1.73650327254409,-30.2871125500495,
127.034591837717));
#102429=CARTESIAN_POINT('Ctrl Pts',(1.74036266557021,-30.3577716941975,
127.024620733594));
#102430=CARTESIAN_POINT('Ctrl Pts',(1.74422205859634,-30.4278762520515,
127.010969340854));
#102431=CARTESIAN_POINT('Ctrl Pts',(1.74808145162246,-30.4970216521958,
126.993731937786));
#102432=CARTESIAN_POINT('Ctrl Pts',(1.75194302979184,-30.566206201658,126.976484775102));
#102433=CARTESIAN_POINT('Ctrl Pts',(1.75580460796121,-30.6344300475182,
126.955647702241));
#102434=CARTESIAN_POINT('Ctrl Pts',(1.75966618613059,-30.7013045054973,
126.93136468671));
#102435=CARTESIAN_POINT('Ctrl Pts',(1.76353452081859,-30.7682959722487,
126.907039183719));
#102436=CARTESIAN_POINT('Ctrl Pts',(1.76740285550659,-30.833932889824,126.879255889827));
#102437=CARTESIAN_POINT('Ctrl Pts',(1.77127119019459,-30.8978478950008,
126.8482063521));
#102438=CARTESIAN_POINT('Ctrl Pts',(1.77356890460204,-30.9358121457939,
126.829763539899));
#102439=CARTESIAN_POINT('Ctrl Pts',(1.7758666190095,-30.9731693624293,126.810169233763));
#102440=CARTESIAN_POINT('Ctrl Pts',(1.77816433341695,-31.0098473718615,
126.789470829057));
#102441=CARTESIAN_POINT('Ctrl Pts',(1.78203306930039,-31.0716033197561,
126.75462025722));
#102442=CARTESIAN_POINT('Ctrl Pts',(1.78590180518384,-31.1316740256028,
126.716500811245));
#102443=CARTESIAN_POINT('Ctrl Pts',(1.78977054106728,-31.1896919472856,
126.67530016208));
#102444=CARTESIAN_POINT('Ctrl Pts',(1.79117478170446,-31.2107507959034,
126.660345503096));
#102445=CARTESIAN_POINT('Ctrl Pts',(1.79257902234163,-31.2315393936004,
126.644985355848));
#102446=CARTESIAN_POINT('Ctrl Pts',(1.79398326297881,-31.2520409112987,
126.629230222815));
#102447=CARTESIAN_POINT('Ctrl Pts',(1.09386069669771,-31.2520409112987,
126.629230222815));
#102448=CARTESIAN_POINT('Ctrl Pts',(1.09772924491478,-31.3085426350283,
126.585809428947));
#102449=CARTESIAN_POINT('Ctrl Pts',(1.10159779313184,-31.3627072268892,
126.539504236734));
#102450=CARTESIAN_POINT('Ctrl Pts',(1.1054663413489,-31.4142430475397,126.49060865588));
#102451=CARTESIAN_POINT('Ctrl Pts',(1.10742846369447,-31.4403819450334,
126.465808884388));
#102452=CARTESIAN_POINT('Ctrl Pts',(1.10939058604003,-31.4658452042217,
126.440343298387));
#102453=CARTESIAN_POINT('Ctrl Pts',(1.1113527083856,-31.4905987617337,126.414253475873));
#102454=CARTESIAN_POINT('Ctrl Pts',(1.11522172489627,-31.5394091343021,
126.36280818537));
#102455=CARTESIAN_POINT('Ctrl Pts',(1.11909074140694,-31.5856487050198,
126.308732229566));
#102456=CARTESIAN_POINT('Ctrl Pts',(1.12295975791762,-31.6290211273891,
126.25231295171));
#102457=CARTESIAN_POINT('Ctrl Pts',(1.12682300855902,-31.6723289132502,
126.195977753665));
#102458=CARTESIAN_POINT('Ctrl Pts',(1.13068625920042,-31.7127777385068,
126.137306547442));
#102459=CARTESIAN_POINT('Ctrl Pts',(1.13454950984182,-31.7501091015278,
126.076622354983));
#102460=CARTESIAN_POINT('Ctrl Pts',(1.13840822749898,-31.7873966614162,
126.016009366936));
#102461=CARTESIAN_POINT('Ctrl Pts',(1.14226694515614,-31.8215737715933,
125.953388496063));
#102462=CARTESIAN_POINT('Ctrl Pts',(1.1461256628133,-31.8524241841776,125.889113156113));
#102463=CARTESIAN_POINT('Ctrl Pts',(1.14998194893019,-31.8832551566196,
125.824878318758));
#102464=CARTESIAN_POINT('Ctrl Pts',(1.15383823504708,-31.9107633807586,
125.758991517657));
#102465=CARTESIAN_POINT('Ctrl Pts',(1.15769452116397,-31.9347783993041,
125.691830982312));
#102466=CARTESIAN_POINT('Ctrl Pts',(1.16154966739118,-31.9587863191875,
125.624690299124));
#102467=CARTESIAN_POINT('Ctrl Pts',(1.1654048136184,-31.9793029199239,125.556277086349));
#102468=CARTESIAN_POINT('Ctrl Pts',(1.16925995984561,-31.9962064246485,
125.486988164838));
#102469=CARTESIAN_POINT('Ctrl Pts',(1.17311525622009,-32.0131105877178,
125.417696544715));
#102470=CARTESIAN_POINT('Ctrl Pts',(1.17697055259457,-32.026401262396,125.347529620626));
#102471=CARTESIAN_POINT('Ctrl Pts',(1.18082584896905,-32.0360073750409,
125.276896246415));
#102472=CARTESIAN_POINT('Ctrl Pts',(1.18468518067613,-32.0456235423888,
125.206188940364));
#102473=CARTESIAN_POINT('Ctrl Pts',(1.18854451238321,-32.0515473834114,
125.135014691927));
#102474=CARTESIAN_POINT('Ctrl Pts',(1.19240384409029,-32.0537596245863,
125.063788454434));
#102475=CARTESIAN_POINT('Ctrl Pts',(1.19626536067988,-32.0559731181767,
124.99252189365));
#102476=CARTESIAN_POINT('Ctrl Pts',(1.20012687726946,-32.0544708392241,
124.921203771145));
#102477=CARTESIAN_POINT('Ctrl Pts',(1.20398839385904,-32.0492856511186,
124.85024726173));
#102478=CARTESIAN_POINT('Ctrl Pts',(1.20785666722236,-32.044091390116,124.779166594599));
#102479=CARTESIAN_POINT('Ctrl Pts',(1.21172494058567,-32.035201414441,124.708449286005));
#102480=CARTESIAN_POINT('Ctrl Pts',(1.21559321394899,-32.022700171652,124.638500929325));
#102481=CARTESIAN_POINT('Ctrl Pts',(1.21789146904071,-32.0152728152596,
124.596942551259));
#102482=CARTESIAN_POINT('Ctrl Pts',(1.22018972413243,-32.0065716934448,
124.555655383917));
#102483=CARTESIAN_POINT('Ctrl Pts',(1.22248797922415,-31.9966228130601,
124.514721827332));
#102484=CARTESIAN_POINT('Ctrl Pts',(1.22635706752053,-31.9798739774771,
124.445810614958));
#102485=CARTESIAN_POINT('Ctrl Pts',(1.23022615581692,-31.959520558601,124.377632550889));
#102486=CARTESIAN_POINT('Ctrl Pts',(1.23409524411331,-31.9356432554691,
124.310592464462));
#102487=CARTESIAN_POINT('Ctrl Pts',(1.23795856758115,-31.9118015288215,
124.243652265805));
#102488=CARTESIAN_POINT('Ctrl Pts',(1.24182189104898,-31.8844465016466,
124.177847133058));
#102489=CARTESIAN_POINT('Ctrl Pts',(1.24568521451682,-31.8537093734378,
124.113569449235));
#102490=CARTESIAN_POINT('Ctrl Pts',(1.24954400619125,-31.8230083007953,
124.049367165049));
#102491=CARTESIAN_POINT('Ctrl Pts',(1.25340279786567,-31.7889332160827,
123.986689206902));
#102492=CARTESIAN_POINT('Ctrl Pts',(1.2572615895401,-31.7516637685877,123.925908940398));
#102493=CARTESIAN_POINT('Ctrl Pts',(1.26111795036892,-31.7144177989791,
123.865166962419));
#102494=CARTESIAN_POINT('Ctrl Pts',(1.26497431119774,-31.6739817122725,
123.806320717475));
#102495=CARTESIAN_POINT('Ctrl Pts',(1.26883067202656,-31.6305808409948,
123.749718558291));
#102496=CARTESIAN_POINT('Ctrl Pts',(1.27268589354858,-31.5871927918853,
123.693133121408));
#102497=CARTESIAN_POINT('Ctrl Pts',(1.2765411150706,-31.5408419925447,123.63879083937));
#102498=CARTESIAN_POINT('Ctrl Pts',(1.28039633659263,-31.4917957966719,
123.587009248603));
#102499=CARTESIAN_POINT('Ctrl Pts',(1.28425170873368,-31.4427476846212,
123.53522563479));
#102500=CARTESIAN_POINT('Ctrl Pts',(1.28810708087473,-31.3910043026237,
123.486003262045));
#102501=CARTESIAN_POINT('Ctrl Pts',(1.29196245301577,-31.3368706127427,
123.439623594358));
#102502=CARTESIAN_POINT('Ctrl Pts',(1.29582186068773,-31.2826802595433,
123.393195379714));
#102503=CARTESIAN_POINT('Ctrl Pts',(1.29968126835969,-31.2260949735539,
123.349616126688));
#102504=CARTESIAN_POINT('Ctrl Pts',(1.30354067603165,-31.1674529352236,
123.309127087408));
#102505=CARTESIAN_POINT('Ctrl Pts',(1.30740226881264,-31.1087776951022,
123.268615124152));
#102506=CARTESIAN_POINT('Ctrl Pts',(1.31126386159363,-31.04804379829,123.231197112506));
#102507=CARTESIAN_POINT('Ctrl Pts',(1.31512545437463,-30.9856162078359,
123.197069537295));
#102508=CARTESIAN_POINT('Ctrl Pts',(1.31899380346042,-30.9230793930662,
123.162882251929));
#102509=CARTESIAN_POINT('Ctrl Pts',(1.32286215254621,-30.8588434062568,
123.131997107583));
#102510=CARTESIAN_POINT('Ctrl Pts',(1.326730501632,-30.793294818061,123.104563138974));
#102511=CARTESIAN_POINT('Ctrl Pts',(1.32902808444224,-30.7543626260239,
123.088268897348));
#102512=CARTESIAN_POINT('Ctrl Pts',(1.33132566725247,-30.7149677308598,
123.073191186264));
#102513=CARTESIAN_POINT('Ctrl Pts',(1.33362325006271,-30.6751933900766,
123.059352827406));
#102514=CARTESIAN_POINT('Ctrl Pts',(1.33749232926178,-30.608214270153,123.036049333765));
#102515=CARTESIAN_POINT('Ctrl Pts',(1.34136140846086,-30.5398961063051,
123.016171823758));
#102516=CARTESIAN_POINT('Ctrl Pts',(1.34523048765993,-30.470622779717,122.999872063664));
#102517=CARTESIAN_POINT('Ctrl Pts',(1.3490938020638,-30.4014526680079,122.983596589653));
#102518=CARTESIAN_POINT('Ctrl Pts',(1.35295711646766,-30.3313306875089,
122.970888394575));
#102519=CARTESIAN_POINT('Ctrl Pts',(1.35682043087152,-30.2606576524422,
122.961850066672));
#102520=CARTESIAN_POINT('Ctrl Pts',(1.36067921357757,-30.1900675173948,
122.952822340799));
#102521=CARTESIAN_POINT('Ctrl Pts',(1.36453799628361,-30.1189280912524,
122.947455992673));
#102522=CARTESIAN_POINT('Ctrl Pts',(1.36839677898966,-30.0476504883975,
122.945802591411));
#102523=CARTESIAN_POINT('Ctrl Pts',(1.37225313091432,-29.9764177857827,
122.944150231683));
#102524=CARTESIAN_POINT('Ctrl Pts',(1.37610948283898,-29.9050475636516,
122.946206189691));
#102525=CARTESIAN_POINT('Ctrl Pts',(1.37996583476364,-29.8339546989679,
122.951970087986));
#102526=CARTESIAN_POINT('Ctrl Pts',(1.38382104745943,-29.7628828362689,
122.957732283532));
#102527=CARTESIAN_POINT('Ctrl Pts',(1.38767626015522,-29.6920886522836,
122.967200205486));
#102528=CARTESIAN_POINT('Ctrl Pts',(1.39153147285101,-29.6219839246391,
122.980321458927));
#102529=CARTESIAN_POINT('Ctrl Pts',(1.39538683625752,-29.5518764564108,
122.993443225315));
#102530=CARTESIAN_POINT('Ctrl Pts',(1.39924219966403,-29.4824589751218,
123.010218515202));
#102531=CARTESIAN_POINT('Ctrl Pts',(1.40309756307054,-29.4141333497697,
123.030543772853));
#102532=CARTESIAN_POINT('Ctrl Pts',(1.40695696221005,-29.3457362022413,
123.05089030666));
#102533=CARTESIAN_POINT('Ctrl Pts',(1.41081636134956,-29.2784336587827,
123.074794087508));
#102534=CARTESIAN_POINT('Ctrl Pts',(1.41467576048908,-29.2126118210786,
123.102101841986));
#102535=CARTESIAN_POINT('Ctrl Pts',(1.41853734483883,-29.1467527147353,
123.129425058245));
#102536=CARTESIAN_POINT('Ctrl Pts',(1.42239892918858,-29.0823764217114,
123.160155875513));
#102537=CARTESIAN_POINT('Ctrl Pts',(1.42626051353833,-29.0198459585534,
123.194094239021));
#102538=CARTESIAN_POINT('Ctrl Pts',(1.43012885444623,-28.9572060867505,
123.228091983992));
#102539=CARTESIAN_POINT('Ctrl Pts',(1.43399719535414,-28.8964189072815,
123.265308226385));
#102540=CARTESIAN_POINT('Ctrl Pts',(1.43786553626204,-28.8378192908918,
123.305499022757));
#102541=CARTESIAN_POINT('Ctrl Pts',(1.44016319780845,-28.8030131327949,
123.329370974465));
#102542=CARTESIAN_POINT('Ctrl Pts',(1.44246085935486,-28.7689781332935,
123.354291537304));
#102543=CARTESIAN_POINT('Ctrl Pts',(1.44475852090127,-28.7357786282846,
123.380203134403));
#102544=CARTESIAN_POINT('Ctrl Pts',(1.44858235651619,-28.680527040056,123.423325972916));
#102545=CARTESIAN_POINT('Ctrl Pts',(1.45240619213111,-28.6273638365409,
123.46937333891));
#102546=CARTESIAN_POINT('Ctrl Pts',(1.45623002774603,-28.5766205720042,
123.518113173532));
#102547=CARTESIAN_POINT('Ctrl Pts',(1.46004735844195,-28.5259636293858,
123.566770094372));
#102548=CARTESIAN_POINT('Ctrl Pts',(1.46386468913786,-28.4777188079647,
123.61811004743));
#102549=CARTESIAN_POINT('Ctrl Pts',(1.46768201983378,-28.4321857652817,
123.671859914047));
#102550=CARTESIAN_POINT('Ctrl Pts',(1.47149571672727,-28.3866960665198,
123.725558614965));
#102551=CARTESIAN_POINT('Ctrl Pts',(1.47530941362077,-28.3439133504474,
123.781662304536));
#102552=CARTESIAN_POINT('Ctrl Pts',(1.47912311051427,-28.3041004409665,
123.839861108242));
#102553=CARTESIAN_POINT('Ctrl Pts',(1.48293452525575,-28.2643113559042,
123.898025085237));
#102554=CARTESIAN_POINT('Ctrl Pts',(1.48674593999724,-28.227488834142,123.95828127991));
#102555=CARTESIAN_POINT('Ctrl Pts',(1.49055735473872,-28.1938542112394,
124.020288332088));
#102556=CARTESIAN_POINT('Ctrl Pts',(1.49436783584484,-28.1602278273964,
124.082280195162));
#102557=CARTESIAN_POINT('Ctrl Pts',(1.49817831695096,-28.1297880293746,
124.146021626344));
#102558=CARTESIAN_POINT('Ctrl Pts',(1.50198879805707,-28.1027107834153,
124.211145646439));
#102559=CARTESIAN_POINT('Ctrl Pts',(1.50580209425412,-28.0756135334441,
124.276317778579));
#102560=CARTESIAN_POINT('Ctrl Pts',(1.50961539045116,-28.0518839927297,
124.342874080217));
#102561=CARTESIAN_POINT('Ctrl Pts',(1.51342868664821,-28.0316499531354,
124.410427565512));
#102562=CARTESIAN_POINT('Ctrl Pts',(1.51724331848722,-28.0114088263831,
124.478004712035));
#102563=CARTESIAN_POINT('Ctrl Pts',(1.52105795032623,-27.9946657595528,
124.546579253509));
#102564=CARTESIAN_POINT('Ctrl Pts',(1.52487258216524,-27.9814978720417,
124.615751744405));
#102565=CARTESIAN_POINT('Ctrl Pts',(1.52869351667211,-27.9683082280873,
124.685038524504));
#102566=CARTESIAN_POINT('Ctrl Pts',(1.53251445117898,-27.9587056314373,
124.75492473284));
#102567=CARTESIAN_POINT('Ctrl Pts',(1.53633538568585,-27.9527154435004,
124.825004265143));
#102568=CARTESIAN_POINT('Ctrl Pts',(1.53953201728634,-27.9477039930247,
124.883633495009));
#102569=CARTESIAN_POINT('Ctrl Pts',(1.54272864888684,-27.9452199901119,
124.942397808631));
#102570=CARTESIAN_POINT('Ctrl Pts',(1.54592528048734,-27.9452502737908,
125.001060727663));
#102571=CARTESIAN_POINT('Origin',(-1.54592528053767,-30.,125.));
#102572=CARTESIAN_POINT('',(0.39390276451725,-31.2520409112987,126.629230222815));
#102573=CARTESIAN_POINT('',(0.452117106605179,-31.2520409112987,126.629230222815));
#102574=CARTESIAN_POINT('',(-1.54592528053767,-31.2520409112987,126.629230222815));
#102575=CARTESIAN_POINT('',(0.145925136774057,-27.9455707835906,124.9977750384));
#102576=CARTESIAN_POINT('Ctrl Pts',(0.145925280537678,-27.9452512021367,
124.997777348617));
#102577=CARTESIAN_POINT('Ctrl Pts',(0.149742855972762,-27.945174835179,
125.068375426051));
#102578=CARTESIAN_POINT('Ctrl Pts',(0.153560431407846,-27.948741212299,
125.13903804764));
#102579=CARTESIAN_POINT('Ctrl Pts',(0.15737800684293,-27.955943445049,125.209357022003));
#102580=CARTESIAN_POINT('Ctrl Pts',(0.161194301449952,-27.9631432613905,
125.27965240377));
#102581=CARTESIAN_POINT('Ctrl Pts',(0.165010596056974,-27.9739764629279,
125.349603873899));
#102582=CARTESIAN_POINT('Ctrl Pts',(0.168826890663996,-27.9883842021359,
125.418807168377));
#102583=CARTESIAN_POINT('Ctrl Pts',(0.17264324173275,-28.0027921545051,
125.48801148671));
#102584=CARTESIAN_POINT('Ctrl Pts',(0.176459592801504,-28.0207746461243,
125.556467122227));
#102585=CARTESIAN_POINT('Ctrl Pts',(0.180275943870259,-28.0422218624211,
125.623780671806));
#102586=CARTESIAN_POINT('Ctrl Pts',(0.184096399549484,-28.063692145901,
125.69116661931));
#102587=CARTESIAN_POINT('Ctrl Pts',(0.187916855228711,-28.0886344413074,
125.757407555328));
#102588=CARTESIAN_POINT('Ctrl Pts',(0.191737310907937,-28.1168895501514,
125.822126873524));
#102589=CARTESIAN_POINT('Ctrl Pts',(0.195559946017952,-28.1451607775057,
125.886883111735));
#102590=CARTESIAN_POINT('Ctrl Pts',(0.199382581127968,-28.1767483553683,
125.9501155618));
#102591=CARTESIAN_POINT('Ctrl Pts',(0.203205216237984,-28.2114468676046,
126.011471826152));
#102592=CARTESIAN_POINT('Ctrl Pts',(0.207034920453413,-28.2462095469491,
126.072941555139));
#102593=CARTESIAN_POINT('Ctrl Pts',(0.210864624668841,-28.2840943777579,
126.132527754396));
#102594=CARTESIAN_POINT('Ctrl Pts',(0.214694328884269,-28.3248527725902,
126.189907277481));
#102595=CARTESIAN_POINT('Ctrl Pts',(0.217219733148553,-28.3517298937267,
126.227744792894));
#102596=CARTESIAN_POINT('Ctrl Pts',(0.219745137412836,-28.3798557023373,
126.264623409239));
#102597=CARTESIAN_POINT('Ctrl Pts',(0.22227054167712,-28.4091499875841,
126.30045907298));
#102598=CARTESIAN_POINT('Ctrl Pts',(0.226141673197727,-28.4540544936058,
126.355390700931));
#102599=CARTESIAN_POINT('Ctrl Pts',(0.230012804718335,-28.5018955096994,
126.40810145461));
#102600=CARTESIAN_POINT('Ctrl Pts',(0.233883936238942,-28.5524251572329,
126.458260826151));
#102601=CARTESIAN_POINT('Ctrl Pts',(0.237749257978822,-28.602878970047,
126.508344918682));
#102602=CARTESIAN_POINT('Ctrl Pts',(0.241614579718701,-28.6560130630199,
126.555884890918));
#102603=CARTESIAN_POINT('Ctrl Pts',(0.245479901458581,-28.7115393876318,
126.600583272709));
#102604=CARTESIAN_POINT('Ctrl Pts',(0.249340613883586,-28.7669994982696,
126.64522835262));
#102605=CARTESIAN_POINT('Ctrl Pts',(0.25320132630859,-28.8248457976965,
126.687038270525));
#102606=CARTESIAN_POINT('Ctrl Pts',(0.257062038733595,-28.8847547571072,
126.725753635576));
#102607=CARTESIAN_POINT('Ctrl Pts',(0.260920271211504,-28.9446252337112,
126.764444131627));
#102608=CARTESIAN_POINT('Ctrl Pts',(0.264778503689414,-29.0065553349753,
126.800043756038));
#102609=CARTESIAN_POINT('Ctrl Pts',(0.268636736167323,-29.0701911223101,
126.832335398738));
#102610=CARTESIAN_POINT('Ctrl Pts',(0.272493777200255,-29.1338072585379,
126.864617069588));
#102611=CARTESIAN_POINT('Ctrl Pts',(0.276350818233187,-29.1991276026886,
126.893592567357));
#102612=CARTESIAN_POINT('Ctrl Pts',(0.280207859266119,-29.2657736075305,
126.91909071362));
#102613=CARTESIAN_POINT('Ctrl Pts',(0.284064995690883,-29.3324212606527,
126.944589490499));
#102614=CARTESIAN_POINT('Ctrl Pts',(0.287922132115646,-29.4003941856134,
126.966610573799));
#102615=CARTESIAN_POINT('Ctrl Pts',(0.291779268540409,-29.4692954678159,
126.985031551895));
#102616=CARTESIAN_POINT('Ctrl Pts',(0.295640343039968,-29.538267097129,
127.003471337517));
#102617=CARTESIAN_POINT('Ctrl Pts',(0.299501417539527,-29.6081685061665,
127.018303554646));
#102618=CARTESIAN_POINT('Ctrl Pts',(0.303362492039085,-29.6785901633433,
127.029456399975));
#102619=CARTESIAN_POINT('Ctrl Pts',(0.307225699100924,-29.7490507160582,
127.040615405283));
#102620=CARTESIAN_POINT('Ctrl Pts',(0.311088906162763,-29.8200316062018,
127.048090941898));
#102621=CARTESIAN_POINT('Ctrl Pts',(0.314952113224602,-29.8911184336103,
127.05186314529));
#102622=CARTESIAN_POINT('Ctrl Pts',(0.318821975145273,-29.9623277169973,
127.055641846777));
#102623=CARTESIAN_POINT('Ctrl Pts',(0.322691837065945,-30.0336428166044,
127.055704477394));
#102624=CARTESIAN_POINT('Ctrl Pts',(0.326561698986616,-30.1046502956107,
127.052083301947));
#102625=CARTESIAN_POINT('Ctrl Pts',(0.328843070162972,-30.1465108113685,
127.049948537074));
#102626=CARTESIAN_POINT('Ctrl Pts',(0.331124441339327,-30.1882645132298,
127.046534501362));
#102627=CARTESIAN_POINT('Ctrl Pts',(0.333405812515682,-30.2298282324623,
127.041856152148));
#102628=CARTESIAN_POINT('Ctrl Pts',(0.337280820021117,-30.3004260052618,
127.033909773887));
#102629=CARTESIAN_POINT('Ctrl Pts',(0.341155827526552,-30.370744503116,
127.022282695611));
#102630=CARTESIAN_POINT('Ctrl Pts',(0.345030835031987,-30.4403708785773,
127.007005493715));
#102631=CARTESIAN_POINT('Ctrl Pts',(0.349103495822425,-30.5135487005361,
126.990949044517));
#102632=CARTESIAN_POINT('Ctrl Pts',(0.353176156612864,-30.5859613704907,
126.970860133849));
#102633=CARTESIAN_POINT('Ctrl Pts',(0.357248817403303,-30.6571349812852,
126.946836197237));
#102634=CARTESIAN_POINT('Ctrl Pts',(0.361113777721505,-30.7246788292949,
126.924037450552));
#102635=CARTESIAN_POINT('Ctrl Pts',(0.364978738039707,-30.7911063722484,
126.897695373647));
#102636=CARTESIAN_POINT('Ctrl Pts',(0.368843698357909,-30.8560246926624,
126.867945204778));
#102637=CARTESIAN_POINT('Ctrl Pts',(0.372706164963254,-30.9209011270965,
126.838214231029));
#102638=CARTESIAN_POINT('Ctrl Pts',(0.376568631568599,-30.9842698337519,
126.805079733099));
#102639=CARTESIAN_POINT('Ctrl Pts',(0.380431098173944,-31.0457575024229,
126.768725193077));
#102640=CARTESIAN_POINT('Ctrl Pts',(0.384292618222436,-31.1072301025949,
126.732379562295));
#102641=CARTESIAN_POINT('Ctrl Pts',(0.388154138270928,-31.1668221635663,
126.692815701947));
#102642=CARTESIAN_POINT('Ctrl Pts',(0.392015658319421,-31.2241860666473,
126.650262414505));
#102643=CARTESIAN_POINT('Ctrl Pts',(0.392644693718697,-31.2335305541096,
126.643330552486));
#102644=CARTESIAN_POINT('Ctrl Pts',(0.393273729117974,-31.2428159780343,
126.636319456546));
#102645=CARTESIAN_POINT('Ctrl Pts',(0.393902764517251,-31.2520409112987,
126.629230222815));
#102646=CARTESIAN_POINT('',(0.,-29.4698297828114,123.014825674328));
#102647=CARTESIAN_POINT('Ctrl Pts',(-2.77555756156289E-16,-29.4698297828114,
123.014825674328));
#102648=CARTESIAN_POINT('Ctrl Pts',(0.0370450902795195,-28.8097276504723,
123.191115729233));
#102649=CARTESIAN_POINT('Ctrl Pts',(0.0856865378424994,-28.0750900177817,
123.887375885199));
#102650=CARTESIAN_POINT('Ctrl Pts',(0.134327985405479,-27.9457241577746,
124.783527527238));
#102651=CARTESIAN_POINT('Ctrl Pts',(0.145924342688939,-27.9473360067712,
124.997762277807));
#102652=CARTESIAN_POINT('',(7.76923664291829E-9,-30.530363345704,123.014877262224));
#102653=CARTESIAN_POINT('Origin',(0.,-30.,125.));
#102654=CARTESIAN_POINT('',(0.20407471941795,-27.945250548143,125.001500864184));
#102655=CARTESIAN_POINT('Ctrl Pts',(7.76923658740714E-9,-30.530363345704,
123.014877262224));
#102656=CARTESIAN_POINT('Ctrl Pts',(0.00385760787619837,-30.4620546494468,
122.996627293092));
#102657=CARTESIAN_POINT('Ctrl Pts',(0.00771520798316006,-30.3926645715971,
122.981870325238));
#102658=CARTESIAN_POINT('Ctrl Pts',(0.0115728080901218,-30.3225847520692,
122.970730022833));
#102659=CARTESIAN_POINT('Ctrl Pts',(0.0154246241661233,-30.25261000923,
122.959606424039));
#102660=CARTESIAN_POINT('Ctrl Pts',(0.0192764402421246,-30.1819480560963,
122.952088804636));
#102661=CARTESIAN_POINT('Ctrl Pts',(0.0231282563181261,-30.1110039601888,
122.948250579792));
#102662=CARTESIAN_POINT('Ctrl Pts',(0.0269755322799582,-30.0401434856922,
122.944416879043));
#102663=CARTESIAN_POINT('Ctrl Pts',(0.0308228082417903,-29.9690020148071,
122.944253985825));
#102664=CARTESIAN_POINT('Ctrl Pts',(0.0346700842036225,-29.8979912511057,
122.947783691311));
#102665=CARTESIAN_POINT('Ctrl Pts',(0.0385149443694312,-29.8270250767507,
122.951311180411));
#102666=CARTESIAN_POINT('Ctrl Pts',(0.0423598045352404,-29.7561899340426,
122.958526644498));
#102667=CARTESIAN_POINT('Ctrl Pts',(0.046204664701049,-29.6858975330341,
122.969399792488));
#102668=CARTESIAN_POINT('Ctrl Pts',(0.0500484171687816,-29.6156253831542,
122.980269807942));
#102669=CARTESIAN_POINT('Ctrl Pts',(0.0538921696365139,-29.5458961475966,
122.99479534066));
#102670=CARTESIAN_POINT('Ctrl Pts',(0.0577359221042466,-29.4771146500438,
123.012894448374));
#102671=CARTESIAN_POINT('Ctrl Pts',(0.0615798733729778,-29.4083295950741,
123.030994492184));
#102672=CARTESIAN_POINT('Ctrl Pts',(0.0654238246417088,-29.3404928476682,
123.052668350937));
#102673=CARTESIAN_POINT('Ctrl Pts',(0.0692677759104399,-29.2739955743463,
123.077783795607));
#102674=CARTESIAN_POINT('Ctrl Pts',(0.0731156987411403,-29.2074295961883,
123.102925189499));
#102675=CARTESIAN_POINT('Ctrl Pts',(0.0769636215718412,-29.1422063121485,
123.131515092081));
#102676=CARTESIAN_POINT('Ctrl Pts',(0.0808115444025417,-29.0786974170051,
123.163372897655));
#102677=CARTESIAN_POINT('Ctrl Pts',(0.0846617298495252,-29.0151511780099,
123.195249435931));
#102678=CARTESIAN_POINT('Ctrl Pts',(0.0885119152965084,-28.9533217589085,
123.23039745915));
#102679=CARTESIAN_POINT('Ctrl Pts',(0.0923621007434918,-28.8935543097556,
123.268591470207));
#102680=CARTESIAN_POINT('Ctrl Pts',(0.0962187336365197,-28.833686775189,
123.306849440216));
#102681=CARTESIAN_POINT('Ctrl Pts',(0.100075366529548,-28.7758884983343,
123.348163292566));
#102682=CARTESIAN_POINT('Ctrl Pts',(0.103931999422576,-28.7204731275101,
123.39226602167));
#102683=CARTESIAN_POINT('Ctrl Pts',(0.105608298071121,-28.6963866474645,
123.411435423386));
#102684=CARTESIAN_POINT('Ctrl Pts',(0.107284596719665,-28.6727498971189,
123.431131223205));
#102685=CARTESIAN_POINT('Ctrl Pts',(0.10896089536821,-28.6495864180097,
123.451329370048));
#102686=CARTESIAN_POINT('Ctrl Pts',(0.112923971370282,-28.5948237250601,
123.499081476219));
#102687=CARTESIAN_POINT('Ctrl Pts',(0.116887047372355,-28.5424737288281,
123.549849695004));
#102688=CARTESIAN_POINT('Ctrl Pts',(0.120850123374427,-28.4928909201467,
123.603354095011));
#102689=CARTESIAN_POINT('Ctrl Pts',(0.12466130497301,-28.4452084916609,
123.654807810418));
#102690=CARTESIAN_POINT('Ctrl Pts',(0.128472486571594,-28.4000854002298,
123.708791396722));
#102691=CARTESIAN_POINT('Ctrl Pts',(0.132283668170177,-28.3578035821471,
123.7650147824));
#102692=CARTESIAN_POINT('Ctrl Pts',(0.136091357608174,-28.3155605066157,
123.82118665096));
#102693=CARTESIAN_POINT('Ctrl Pts',(0.139899047046172,-28.2761538430259,
123.879593853435));
#102694=CARTESIAN_POINT('Ctrl Pts',(0.143706736484169,-28.2398264892347,
123.939911902482));
#102695=CARTESIAN_POINT('Ctrl Pts',(0.147512291348494,-28.2035195003957,
124.000196137499));
#102696=CARTESIAN_POINT('Ctrl Pts',(0.151317846212819,-28.1702886550489,
124.062388667107));
#102697=CARTESIAN_POINT('Ctrl Pts',(0.155123401077145,-28.1403334844351,
124.126136158554));
#102698=CARTESIAN_POINT('Ctrl Pts',(0.158928175891731,-28.1103844539307,
124.189870583256));
#102699=CARTESIAN_POINT('Ctrl Pts',(0.162732950706317,-28.0837099762376,
124.255158884088));
#102700=CARTESIAN_POINT('Ctrl Pts',(0.166537725520903,-28.0604627032384,
124.321625002693));
#102701=CARTESIAN_POINT('Ctrl Pts',(0.170344988314308,-28.037200228624,
124.388134584133));
#102702=CARTESIAN_POINT('Ctrl Pts',(0.174152251107713,-28.0173695981176,
124.455823048431));
#102703=CARTESIAN_POINT('Ctrl Pts',(0.177959513901117,-28.001074099642,
124.524297564251));
#102704=CARTESIAN_POINT('Ctrl Pts',(0.181768282834312,-27.9847721547245,
124.592799168348));
#102705=CARTESIAN_POINT('Ctrl Pts',(0.185577051767507,-27.9720082170426,
124.662086951351));
#102706=CARTESIAN_POINT('Ctrl Pts',(0.189385820700702,-27.9628342584875,
124.731758869471));
#102707=CARTESIAN_POINT('Ctrl Pts',(0.193199633430934,-27.9536481512339,
124.801523051264));
#102708=CARTESIAN_POINT('Ctrl Pts',(0.197013446161167,-27.9480615453774,
124.871671885187));
#102709=CARTESIAN_POINT('Ctrl Pts',(0.200827258891399,-27.9460743989428,
124.941800448267));
#102710=CARTESIAN_POINT('Ctrl Pts',(0.201909745733583,-27.9455103807225,
124.961705265877));
#102711=CARTESIAN_POINT('Ctrl Pts',(0.202992232575767,-27.9452360180092,
124.981608468297));
#102712=CARTESIAN_POINT('Ctrl Pts',(0.20407471941795,-27.945250548143,125.001500864184));
#102713=CARTESIAN_POINT('Ctrl Pts',(0.204074719462324,-27.9452505481436,
125.001500864999));
#102714=CARTESIAN_POINT('Ctrl Pts',(0.209415201710473,-27.9453222330462,
125.099640614109));
#102715=CARTESIAN_POINT('Ctrl Pts',(0.214755683958622,-27.9524256421758,
125.197525919788));
#102716=CARTESIAN_POINT('Ctrl Pts',(0.220096166206771,-27.9664486897963,
125.294391968757));
#102717=CARTESIAN_POINT('Ctrl Pts',(0.223961505846526,-27.9765983053776,
125.364501775592));
#102718=CARTESIAN_POINT('Ctrl Pts',(0.227826845486281,-27.9903981515537,
125.434225968574));
#102719=CARTESIAN_POINT('Ctrl Pts',(0.231692185126037,-28.0078069756633,
125.503154565004));
#102720=CARTESIAN_POINT('Ctrl Pts',(0.235551705855852,-28.0251895924046,
125.571979395832));
#102721=CARTESIAN_POINT('Ctrl Pts',(0.239411226585667,-28.0461702853158,
125.640010539238));
#102722=CARTESIAN_POINT('Ctrl Pts',(0.243270747315482,-28.0706563372835,
125.706845523177));
#102723=CARTESIAN_POINT('Ctrl Pts',(0.247125674239539,-28.0951132446568,
125.773600956583));
#102724=CARTESIAN_POINT('Ctrl Pts',(0.250980601163595,-28.1230670573192,
125.83916260352));
#102725=CARTESIAN_POINT('Ctrl Pts',(0.254835528087652,-28.1543750051239,
125.903142259441));
#102726=CARTESIAN_POINT('Ctrl Pts',(0.25868798791371,-28.1856629162906,
125.967080969299));
#102727=CARTESIAN_POINT('Ctrl Pts',(0.262540447739768,-28.2203004906343,
126.029439260421));
#102728=CARTESIAN_POINT('Ctrl Pts',(0.266392907565826,-28.258097084805,
126.089849437553));
#102729=CARTESIAN_POINT('Ctrl Pts',(0.270244197575565,-28.2958822018742,
126.150241270871));
#102730=CARTESIAN_POINT('Ctrl Pts',(0.274095487585303,-28.3368241764601,
126.208685751987));
#102731=CARTESIAN_POINT('Ctrl Pts',(0.277946777595041,-28.3806875867483,
126.264841836274));
#102732=CARTESIAN_POINT('Ctrl Pts',(0.281798193422183,-28.4245524300058,
126.320999755118));
#102733=CARTESIAN_POINT('Ctrl Pts',(0.285649609249325,-28.4713385969919,
126.374868746374));
#102734=CARTESIAN_POINT('Ctrl Pts',(0.289501025076467,-28.5207697854712,
126.426140082504));
#102735=CARTESIAN_POINT('Ctrl Pts',(0.293356465647466,-28.5702526297261,
126.477464997371));
#102736=CARTESIAN_POINT('Ctrl Pts',(0.297211906218466,-28.6223856745522,
126.526186486988));
#102737=CARTESIAN_POINT('Ctrl Pts',(0.301067346789465,-28.6768557205867,
126.572032689977));
#102738=CARTESIAN_POINT('Ctrl Pts',(0.304924960312611,-28.7313564663043,
126.617904732193));
#102739=CARTESIAN_POINT('Ctrl Pts',(0.308782573835757,-28.7881964466043,
126.660897968169));
#102740=CARTESIAN_POINT('Ctrl Pts',(0.312640187358902,-28.8470315508531,
126.700782560403));
#102741=CARTESIAN_POINT('Ctrl Pts',(0.316504581130456,-28.9059700653112,
126.740737254902));
#102742=CARTESIAN_POINT('Ctrl Pts',(0.320368974902009,-28.9669102880165,
126.777572145162));
#102743=CARTESIAN_POINT('Ctrl Pts',(0.324233368673562,-29.0294820987998,
126.811102582945));
#102744=CARTESIAN_POINT('Ctrl Pts',(0.326566058130818,-29.0672527329443,
126.831342781884));
#102745=CARTESIAN_POINT('Ctrl Pts',(0.328898747588075,-29.1056174416194,
126.850379828498));
#102746=CARTESIAN_POINT('Ctrl Pts',(0.331231437045331,-29.1444916043112,
126.868181722265));
#102747=CARTESIAN_POINT('Ctrl Pts',(0.335101017067839,-29.2089779777015,
126.897712379366));
#102748=CARTESIAN_POINT('Ctrl Pts',(0.338970597090347,-29.275121315827,
126.923957950765));
#102749=CARTESIAN_POINT('Ctrl Pts',(0.342840177112856,-29.3425536894351,
126.946731083438));
#102750=CARTESIAN_POINT('Ctrl Pts',(0.346703991075797,-29.4098855820916,
126.969470281876));
#102751=CARTESIAN_POINT('Ctrl Pts',(0.350567805038738,-29.4785022411153,
126.988747158347));
#102752=CARTESIAN_POINT('Ctrl Pts',(0.354431619001679,-29.5480142396889,
127.00442172084));
#102753=CARTESIAN_POINT('Ctrl Pts',(0.358290896853122,-29.6174446312858,
127.020077881422));
#102754=CARTESIAN_POINT('Ctrl Pts',(0.362150174704567,-29.6877678030683,
127.032140022251));
#102755=CARTESIAN_POINT('Ctrl Pts',(0.36600945255601,-29.7585792591669,
127.040517970613));
#102756=CARTESIAN_POINT('Ctrl Pts',(0.369866296612965,-29.8293460591048,
127.048890635551));
#102757=CARTESIAN_POINT('Ctrl Pts',(0.37372314066992,-29.9006000512908,
127.053583660692));
#102758=CARTESIAN_POINT('Ctrl Pts',(0.377579984726875,-29.9719280890738,
127.054558232399));
#102759=CARTESIAN_POINT('Ctrl Pts',(0.38143568578439,-30.0432349883545,
127.055532515285));
#102760=CARTESIAN_POINT('Ctrl Pts',(0.385291386841906,-30.1146154043383,
127.052790525874));
#102761=CARTESIAN_POINT('Ctrl Pts',(0.389147087899421,-30.1856543622022,
127.046345528081));
#102762=CARTESIAN_POINT('Ctrl Pts',(0.393002935136099,-30.2566960133287,
127.039900285941));
#102763=CARTESIAN_POINT('Ctrl Pts',(0.396858782372778,-30.3273956971792,
127.029751802762));
#102764=CARTESIAN_POINT('Ctrl Pts',(0.400714629609457,-30.397343468581,
127.015965210631));
#102765=CARTESIAN_POINT('Ctrl Pts',(0.404574502226595,-30.4673642632056,
127.002164225742));
#102766=CARTESIAN_POINT('Ctrl Pts',(0.408434374843733,-30.5366311009456,
126.984717644176));
#102767=CARTESIAN_POINT('Ctrl Pts',(0.412294247460872,-30.6047450347016,
126.963741583178));
#102768=CARTESIAN_POINT('Ctrl Pts',(0.416156300156607,-30.6728974396053,
126.942753674779));
#102769=CARTESIAN_POINT('Ctrl Pts',(0.420018352852343,-30.7398951879513,
126.918232485479));
#102770=CARTESIAN_POINT('Ctrl Pts',(0.423880405548079,-30.8053578897072,
126.890342887411));
#102771=CARTESIAN_POINT('Ctrl Pts',(0.427749201512576,-30.870934891455,
126.862404593204));
#102772=CARTESIAN_POINT('Ctrl Pts',(0.431617997477072,-30.9349710590033,
126.831086361316));
#102773=CARTESIAN_POINT('Ctrl Pts',(0.435486793441568,-30.9971098712046,
126.796599417579));
#102774=CARTESIAN_POINT('Ctrl Pts',(0.437780098255676,-31.0339438729126,
126.776156604151));
#102775=CARTESIAN_POINT('Ctrl Pts',(0.440073403069785,-31.0701117139769,
126.75460123076));
#102776=CARTESIAN_POINT('Ctrl Pts',(0.442366707883893,-31.1055442987138,
126.731984228012));
#102777=CARTESIAN_POINT('Ctrl Pts',(0.445616840790988,-31.1557603052944,
126.699930806923));
#102778=CARTESIAN_POINT('Ctrl Pts',(0.448866973698083,-31.204663376369,
126.665639203681));
#102779=CARTESIAN_POINT('Ctrl Pts',(0.452117106605179,-31.2520409112987,
126.629230222815));
#102780=CARTESIAN_POINT('Origin',(5.,30.,55.));
#102781=CARTESIAN_POINT('',(9.56912139758663,31.5634376777551,55.575515966569));
#102782=CARTESIAN_POINT('',(9.76070772053754,31.5634376782623,55.5755159651912));
#102783=CARTESIAN_POINT('',(5.,31.5634376782623,55.5755159651912));
#102784=CARTESIAN_POINT('',(10.,28.6653082844465,55.9970727277551));
#102785=CARTESIAN_POINT('Ctrl Pts',(9.76070772053754,31.5634376782623,55.5755159651912));
#102786=CARTESIAN_POINT('Ctrl Pts',(9.76500822046156,31.5412735069596,55.6357268066236));
#102787=CARTESIAN_POINT('Ctrl Pts',(9.76930872038559,31.5156588479085,55.6945694832879));
#102788=CARTESIAN_POINT('Ctrl Pts',(9.77360922030962,31.4867958201399,55.7516609536318));
#102789=CARTESIAN_POINT('Ctrl Pts',(9.7749826329807,31.4775780899309,55.7698937521823));
#102790=CARTESIAN_POINT('Ctrl Pts',(9.77635604565179,31.4680293913545,55.7879481540697));
#102791=CARTESIAN_POINT('Ctrl Pts',(9.77772945832288,31.4581572365982,55.8058123065306));
#102792=CARTESIAN_POINT('Ctrl Pts',(9.78176791912768,31.4291285907429,55.8583410774113));
#102793=CARTESIAN_POINT('Ctrl Pts',(9.78580637993247,31.3971912918331,55.9094193856562));
#102794=CARTESIAN_POINT('Ctrl Pts',(9.78984484073727,31.3625153003126,55.9587012341778));
#102795=CARTESIAN_POINT('Ctrl Pts',(9.79397066942161,31.3270891299501,56.0090492439953));
#102796=CARTESIAN_POINT('Ctrl Pts',(9.79809649810595,31.2888045450285,56.0575216187083));
#102797=CARTESIAN_POINT('Ctrl Pts',(9.80222232679029,31.2478929598246,56.1037749593193));
#102798=CARTESIAN_POINT('Ctrl Pts',(9.80624967600004,31.2079578939394,56.1489242781614));
#102799=CARTESIAN_POINT('Ctrl Pts',(9.81027702520978,31.1655202145113,56.1919589071941));
#102800=CARTESIAN_POINT('Ctrl Pts',(9.81430437441952,31.1208378861853,56.2325901317517));
#102801=CARTESIAN_POINT('Ctrl Pts',(9.81832937588719,31.0761816054098,56.2731976703486));
#102802=CARTESIAN_POINT('Ctrl Pts',(9.82235437735485,31.0292836539648,56.3114042292453));
#102803=CARTESIAN_POINT('Ctrl Pts',(9.82637937882252,30.9804387670977,56.346957988941));
#102804=CARTESIAN_POINT('Ctrl Pts',(9.83040359871507,30.9316033649346,56.3825048448048));
#102805=CARTESIAN_POINT('Ctrl Pts',(9.83442781860763,30.8808221998901,56.4153996160489));
#102806=CARTESIAN_POINT('Ctrl Pts',(9.83845203850019,30.8284212102314,56.4454322185557));
#102807=CARTESIAN_POINT('Ctrl Pts',(9.8426530960553,30.7737175460733,56.4767845539223));
#102808=CARTESIAN_POINT('Ctrl Pts',(9.8468541536104,30.717248904141,56.505016989362));
#102809=CARTESIAN_POINT('Ctrl Pts',(9.85105521116551,30.6594148160633,56.5299438226145));
#102810=CARTESIAN_POINT('Ctrl Pts',(9.85508552229091,30.6039313180275,56.5538575376876));
#102811=CARTESIAN_POINT('Ctrl Pts',(9.85911583341631,30.5471917684168,56.574729072882));
#102812=CARTESIAN_POINT('Ctrl Pts',(9.86314614454171,30.4895667884119,56.5924447744534));
#102813=CARTESIAN_POINT('Ctrl Pts',(9.86717971472583,30.4318952107157,56.6101748015968));
#102814=CARTESIAN_POINT('Ctrl Pts',(9.87121328490995,30.3733372865983,56.62474380153));
#102815=CARTESIAN_POINT('Ctrl Pts',(9.87524685509407,30.3142743232612,56.6360891325777));
#102816=CARTESIAN_POINT('Ctrl Pts',(9.87928790344763,30.2551018582104,56.6474554976731));
#102817=CARTESIAN_POINT('Ctrl Pts',(9.8833289518012,30.1954230035822,56.6555862179572));
#102818=CARTESIAN_POINT('Ctrl Pts',(9.88737000015477,30.1356231791982,56.6604705216487));
#102819=CARTESIAN_POINT('Ctrl Pts',(9.88786824315699,30.1282501310614,56.6610727342237));
#102820=CARTESIAN_POINT('Ctrl Pts',(9.88836648615922,30.1208752406347,56.6616256604532));
#102821=CARTESIAN_POINT('Ctrl Pts',(9.88886472916144,30.1134992263197,56.6621293348067));
#102822=CARTESIAN_POINT('Ctrl Pts',(9.89305224182562,30.0515070794814,56.6663624955822));
#102823=CARTESIAN_POINT('Ctrl Pts',(9.89723975448979,29.9891721256139,56.6671303991492));
#102824=CARTESIAN_POINT('Ctrl Pts',(9.90142726715397,29.9269022972419,56.6643956037708));
#102825=CARTESIAN_POINT('Ctrl Pts',(9.90560583628048,29.8647654625107,56.6616666492691));
#102826=CARTESIAN_POINT('Ctrl Pts',(9.90978440540699,29.8026939512104,56.6554498951321));
#102827=CARTESIAN_POINT('Ctrl Pts',(9.91396297453351,29.7410974011908,56.6457598379866));
#102828=CARTESIAN_POINT('Ctrl Pts',(9.91813627185461,29.679578563186,56.6360820061016));
#102829=CARTESIAN_POINT('Ctrl Pts',(9.92230956917571,29.6185339664344,56.622939646519));
#102830=CARTESIAN_POINT('Ctrl Pts',(9.92648286649681,29.5583688605115,56.606399058962));
#102831=CARTESIAN_POINT('Ctrl Pts',(9.93065213828524,29.4982617894182,56.5898744263372));
#102832=CARTESIAN_POINT('Ctrl Pts',(9.93482141007368,29.4390329837869,56.56995820315));
#102833=CARTESIAN_POINT('Ctrl Pts',(9.93899068186211,29.3810765727086,56.5467675297697));
#102834=CARTESIAN_POINT('Ctrl Pts',(9.94315716884789,29.3231588727472,56.5235923462524));
#102835=CARTESIAN_POINT('Ctrl Pts',(9.94732365583366,29.2665123218583,56.497147236304));
#102836=CARTESIAN_POINT('Ctrl Pts',(9.95149014281944,29.2115133833492,56.4675983290269));
#102837=CARTESIAN_POINT('Ctrl Pts',(9.95565639117634,29.1565175948163,56.4380511141162));
#102838=CARTESIAN_POINT('Ctrl Pts',(9.95982263953323,29.1031696592298,56.4054006693019));
#102839=CARTESIAN_POINT('Ctrl Pts',(9.96398888789013,29.0518224621395,56.3698596120394));
#102840=CARTESIAN_POINT('Ctrl Pts',(9.96815464396323,29.0004813322328,56.3343227543074));
#102841=CARTESIAN_POINT('Ctrl Pts',(9.97232040003632,28.9511408610854,56.2958962407257));
#102842=CARTESIAN_POINT('Ctrl Pts',(9.97648615610942,28.9041241251909,56.2548354740807));
#102843=CARTESIAN_POINT('Ctrl Pts',(9.98065518728645,28.8570704248908,56.2137424255939));
#102844=CARTESIAN_POINT('Ctrl Pts',(9.98482421846348,28.8123444693646,56.1700113037728));
#102845=CARTESIAN_POINT('Ctrl Pts',(9.98899324964051,28.7702347417616,56.1239365683302));
#102846=CARTESIAN_POINT('Ctrl Pts',(9.99266216642701,28.7331764709268,56.0833889295335));
#102847=CARTESIAN_POINT('Ctrl Pts',(9.9963310832135,28.6981440032315,56.0410269555827));
#102848=CARTESIAN_POINT('Ctrl Pts',(10.,28.6653082844465,55.9970727277551));
#102849=CARTESIAN_POINT('',(10.,29.207701741744,53.534455913333));
#102850=CARTESIAN_POINT('Origin',(10.,30.,55.));
#102851=CARTESIAN_POINT('Ctrl Pts',(10.,29.207701741744,53.534455913333));
#102852=CARTESIAN_POINT('Ctrl Pts',(9.9999921334966,29.2076011593475,53.5345102899009));
#102853=CARTESIAN_POINT('Ctrl Pts',(9.99998428041792,29.2075007614304,53.5345645801173));
#102854=CARTESIAN_POINT('Ctrl Pts',(9.99924409863901,29.1980390851774,53.5396822377603));
#102855=CARTESIAN_POINT('Ctrl Pts',(9.99850690240549,29.1887266307341,53.5448351356371));
#102856=CARTESIAN_POINT('Ctrl Pts',(9.98871049730391,29.0663555033177,53.6140869791279));
#102857=CARTESIAN_POINT('Ctrl Pts',(9.97908838697546,28.9611311285857,53.6911087323511));
#102858=CARTESIAN_POINT('Ctrl Pts',(9.96547087946054,28.8230334408968,53.8194344968611));
#102859=CARTESIAN_POINT('Ctrl Pts',(9.96129063692594,28.7822640983707,53.8615336559987));
#102860=CARTESIAN_POINT('Ctrl Pts',(9.95536217401458,28.7265932318676,53.92544106697));
#102861=CARTESIAN_POINT('Ctrl Pts',(9.95354765844531,28.7098603486707,53.9455894979658));
#102862=CARTESIAN_POINT('Ctrl Pts',(9.9502902850344,28.6803877058669,53.982830757882));
#102863=CARTESIAN_POINT('Ctrl Pts',(9.94884150801389,28.6674879769311,53.9997891949158));
#102864=CARTESIAN_POINT('Ctrl Pts',(9.94657711500799,28.6476679566286,54.0269095813354));
#102865=CARTESIAN_POINT('Ctrl Pts',(9.94575320398035,28.6405291332994,54.0369081586646));
#102866=CARTESIAN_POINT('Ctrl Pts',(9.94421115893203,28.6273090069964,54.0558640875259));
#102867=CARTESIAN_POINT('Ctrl Pts',(9.94349212969346,28.6212031894676,54.0648034708836));
#102868=CARTESIAN_POINT('Ctrl Pts',(9.94187407736825,28.6075992945117,54.0851434830152));
#102869=CARTESIAN_POINT('Ctrl Pts',(9.94097700410683,28.6001532151457,54.0965780784546));
#102870=CARTESIAN_POINT('Ctrl Pts',(9.93865937760413,28.581176216018,54.1265182189766));
#102871=CARTESIAN_POINT('Ctrl Pts',(9.93724674340839,28.5698663821802,54.1451612691884));
#102872=CARTESIAN_POINT('Ctrl Pts',(9.92880290084574,28.5039289990767,54.2588253280436));
#102873=CARTESIAN_POINT('Ctrl Pts',(9.92209637357502,28.4584200902975,54.3588269039648));
#102874=CARTESIAN_POINT('Ctrl Pts',(9.90957491399275,28.3925433534241,54.5521284972471));
#102875=CARTESIAN_POINT('Ctrl Pts',(9.90377823975221,28.369712852453,54.6440997978177));
#102876=CARTESIAN_POINT('Ctrl Pts',(9.89667275096164,28.3525038873702,54.7519538800272));
#102877=CARTESIAN_POINT('Ctrl Pts',(9.89571196948037,28.3503879452385,54.7664398308436));
#102878=CARTESIAN_POINT('Ctrl Pts',(9.8942461764201,28.3474812667112,54.7883549751589));
#102879=CARTESIAN_POINT('Ctrl Pts',(9.89374843852431,28.3465490980117,54.7957651110021));
#102880=CARTESIAN_POINT('Ctrl Pts',(9.89283834932606,28.34494466509,54.8092509423548));
#102881=CARTESIAN_POINT('Ctrl Pts',(9.89242689546626,28.3442559718041,54.8153244055713));
#102882=CARTESIAN_POINT('Ctrl Pts',(9.89148437809254,28.3427617626,54.829182354735));
#102883=CARTESIAN_POINT('Ctrl Pts',(9.89095220180115,28.3419776746004,54.8369686968788));
#102884=CARTESIAN_POINT('Ctrl Pts',(9.88930777585709,28.3397361169874,54.860919926778));
#102885=CARTESIAN_POINT('Ctrl Pts',(9.88818650237146,28.3384600395756,54.8771002860524));
#102886=CARTESIAN_POINT('Ctrl Pts',(9.88143658466501,28.3322568641657,54.973753328602));
#102887=CARTESIAN_POINT('Ctrl Pts',(9.87558979249202,28.3329407862813,55.0544720596489));
#102888=CARTESIAN_POINT('Ctrl Pts',(9.86438828937606,28.3454057313998,55.208003988834));
#102889=CARTESIAN_POINT('Ctrl Pts',(9.85904784155947,28.3561803189986,55.2807240357849));
#102890=CARTESIAN_POINT('Ctrl Pts',(9.85078615767219,28.3806875041675,55.3939287792899));
#102891=CARTESIAN_POINT('Ctrl Pts',(9.84779849883295,28.3912348448639,55.4350034609071));
#102892=CARTESIAN_POINT('Ctrl Pts',(9.84273624168451,28.4120610560996,55.5049152269595));
#102893=CARTESIAN_POINT('Ctrl Pts',(9.84064051823436,28.4215880117049,55.533952509169));
#102894=CARTESIAN_POINT('Ctrl Pts',(9.83762117921648,28.4366419197326,55.5759026667076));
#102895=CARTESIAN_POINT('Ctrl Pts',(9.83667736323895,28.4415413894456,55.5890323832796));
#102896=CARTESIAN_POINT('Ctrl Pts',(9.83501642720591,28.4505062074001,55.6121612908367));
#102897=CARTESIAN_POINT('Ctrl Pts',(9.83429711970387,28.4545040982892,55.6221855723715));
#102898=CARTESIAN_POINT('Ctrl Pts',(9.83279079984806,28.4631184296286,55.6431896166631));
#102899=CARTESIAN_POINT('Ctrl Pts',(9.8320045368151,28.4677557923953,55.6541601829281));
#102900=CARTESIAN_POINT('Ctrl Pts',(9.82992068834927,28.480419579384,55.6832450934806));
#102901=CARTESIAN_POINT('Ctrl Pts',(9.82863012633181,28.4886523055433,55.7012679323898));
#102902=CARTESIAN_POINT('Ctrl Pts',(9.82166564186228,28.5351693697122,55.7984751409863));
#102903=CARTESIAN_POINT('Ctrl Pts',(9.81620162899176,28.5793586830698,55.8746841845705));
#102904=CARTESIAN_POINT('Ctrl Pts',(9.80490794400726,28.6840408201953,56.026186466088));
#102905=CARTESIAN_POINT('Ctrl Pts',(9.79911265478617,28.7454635057324,56.1004286345801));
#102906=CARTESIAN_POINT('Ctrl Pts',(9.79133331747189,28.8324496410791,56.1887619974792));
#102907=CARTESIAN_POINT('Ctrl Pts',(9.78956928065937,28.8524484059355,56.2080786786343));
#102908=CARTESIAN_POINT('Ctrl Pts',(9.78654535833426,28.8869700316724,56.2397920352963));
#102909=CARTESIAN_POINT('Ctrl Pts',(9.78530112692813,28.9012401155837,56.2524562436854));
#102910=CARTESIAN_POINT('Ctrl Pts',(9.78349882617448,28.9219422404081,56.2702025633031));
#102911=CARTESIAN_POINT('Ctrl Pts',(9.78295440190788,28.9281997786776,56.2754871083198));
#102912=CARTESIAN_POINT('Ctrl Pts',(9.78200208682903,28.9391465516507,56.2845943174286));
#102913=CARTESIAN_POINT('Ctrl Pts',(9.78159570555835,28.9438180690526,56.2884379406307));
#102914=CARTESIAN_POINT('Ctrl Pts',(9.78071919834293,28.9538921187521,56.2966350437827));
#102915=CARTESIAN_POINT('Ctrl Pts',(9.78024854822626,28.9593008614875,56.3009801822757));
#102916=CARTESIAN_POINT('Ctrl Pts',(9.7789359381167,28.9743880307589,56.3129462438892));
#102917=CARTESIAN_POINT('Ctrl Pts',(9.7780891580952,28.9841238541162,56.320493613994));
#102918=CARTESIAN_POINT('Ctrl Pts',(9.77161173858368,29.0586842643619,56.3769815114018));
#102919=CARTESIAN_POINT('Ctrl Pts',(9.76573180447678,29.1269198814428,56.4212253838409));
#102920=CARTESIAN_POINT('Ctrl Pts',(9.75291363113925,29.2813131213122,56.5060071409655));
#102921=CARTESIAN_POINT('Ctrl Pts',(9.74599280184867,29.3682876933211,56.5445100250906));
#102922=CARTESIAN_POINT('Ctrl Pts',(9.7356583718456,29.5064217705223,56.5920271868783));
#102923=CARTESIAN_POINT('Ctrl Pts',(9.73210263381972,29.5555127458148,56.606425246884));
#102924=CARTESIAN_POINT('Ctrl Pts',(9.72747810644054,29.6214674384418,56.6225133937519));
#102925=CARTESIAN_POINT('Ctrl Pts',(9.72634490236115,29.6378012218125,56.6262375884116));
#102926=CARTESIAN_POINT('Ctrl Pts',(9.72446881266807,29.6651226433057,56.632034952004));
#102927=CARTESIAN_POINT('Ctrl Pts',(9.7237215868202,29.6760796489352,56.6342449465537));
#102928=CARTESIAN_POINT('Ctrl Pts',(9.72225894172217,29.6976712846713,56.6383742255235));
#102929=CARTESIAN_POINT('Ctrl Pts',(9.72154332754521,29.7083039696301,56.6403006402005));
#102930=CARTESIAN_POINT('Ctrl Pts',(9.71981549057166,29.7341376432104,56.6447220057654));
#102931=CARTESIAN_POINT('Ctrl Pts',(9.71880671242831,29.7493561355462,56.6471098774975));
#102932=CARTESIAN_POINT('Ctrl Pts',(9.71537206282122,29.8016080993668,56.6545675266043));
#102933=CARTESIAN_POINT('Ctrl Pts',(9.71297862446614,29.8387794100014,56.6586022123196));
#102934=CARTESIAN_POINT('Ctrl Pts',(9.702975055107,29.9966288627798,56.6703781122689));
#102935=CARTESIAN_POINT('Ctrl Pts',(9.69571902315179,30.1178188968901,56.6662215698574));
#102936=CARTESIAN_POINT('Ctrl Pts',(9.685218760115,30.2871537633829,56.6418330608564));
#102937=CARTESIAN_POINT('Ctrl Pts',(9.68211195186999,30.3364601418657,56.6324420203433));
#102938=CARTESIAN_POINT('Ctrl Pts',(9.6771040355738,30.4130889463502,56.6142278331624));
#102939=CARTESIAN_POINT('Ctrl Pts',(9.67525946604597,30.4407370908712,56.6068990504903));
#102940=CARTESIAN_POINT('Ctrl Pts',(9.6727539684467,30.4772828515812,56.5961976784617));
#102941=CARTESIAN_POINT('Ctrl Pts',(9.67212594439946,30.4863616153848,56.5934548370253));
#102942=CARTESIAN_POINT('Ctrl Pts',(9.67107703854111,30.5013788504092,56.58877759629));
#102943=CARTESIAN_POINT('Ctrl Pts',(9.67065865726054,30.5073309349506,56.5868869912357));
#102944=CARTESIAN_POINT('Ctrl Pts',(9.66980524836908,30.5193917341402,56.5829812388149));
#102945=CARTESIAN_POINT('Ctrl Pts',(9.66937013269844,30.5254996044484,56.5809641166416));
#102946=CARTESIAN_POINT('Ctrl Pts',(9.66823795423821,30.541289573384,56.5756478747855));
#102947=CARTESIAN_POINT('Ctrl Pts',(9.66753789391651,30.5509530713428,56.5722949238469));
#102948=CARTESIAN_POINT('Ctrl Pts',(9.66462500577775,30.590776069752,56.558065316548));
#102949=CARTESIAN_POINT('Ctrl Pts',(9.66237347034805,30.6206474170141,56.5464088600235));
#102950=CARTESIAN_POINT('Ctrl Pts',(9.6531773800464,30.7397117547678,56.4959420103337));
#102951=CARTESIAN_POINT('Ctrl Pts',(9.64603165138362,30.8257630429656,56.4502174096908));
#102952=CARTESIAN_POINT('Ctrl Pts',(9.63431974001052,30.9613407943762,56.3621772499679));
#102953=CARTESIAN_POINT('Ctrl Pts',(9.62970407341772,31.0132751120928,56.3240007484282));
#102954=CARTESIAN_POINT('Ctrl Pts',(9.62232836234123,31.094278698707,56.2568903873615));
#102955=CARTESIAN_POINT('Ctrl Pts',(9.61951036125195,31.1247205053202,56.2297250084522));
#102956=CARTESIAN_POINT('Ctrl Pts',(9.6156798326698,31.1653669870621,56.1906797535968));
#102957=CARTESIAN_POINT('Ctrl Pts',(9.61462830541647,31.1764456152332,56.1797348147418));
#102958=CARTESIAN_POINT('Ctrl Pts',(9.61284485989911,31.1950932890359,56.1607882117486));
#102959=CARTESIAN_POINT('Ctrl Pts',(9.61210959425413,31.2027392501759,56.1528640631639));
#102960=CARTESIAN_POINT('Ctrl Pts',(9.61071538918272,31.2171540195357,56.1376253296534));
#102961=CARTESIAN_POINT('Ctrl Pts',(9.61005586610363,31.2239368255041,56.1303247110512));
#102962=CARTESIAN_POINT('Ctrl Pts',(9.60835166070601,31.2413658924711,56.1112242259723));
#102963=CARTESIAN_POINT('Ctrl Pts',(9.60731129854455,31.2519097063717,56.0993319221415));
#102964=CARTESIAN_POINT('Ctrl Pts',(9.60367941479996,31.2883535708544,56.0570226703431));
#102965=CARTESIAN_POINT('Ctrl Pts',(9.60112506719479,31.3133294369489,56.0258255369275));
#102966=CARTESIAN_POINT('Ctrl Pts',(9.59049652839227,31.413827073112,55.8905999988086));
#102967=CARTESIAN_POINT('Ctrl Pts',(9.5828136701822,31.4782952439529,55.7789212372678));
#102968=CARTESIAN_POINT('Ctrl Pts',(9.57297165895243,31.5414547301015,55.6327830043088));
#102969=CARTESIAN_POINT('Ctrl Pts',(9.57106030652439,31.5528431753127,55.6042968262802));
#102970=CARTESIAN_POINT('Ctrl Pts',(9.56912139758663,31.5634376777551,55.575515966569));
#102971=CARTESIAN_POINT('Origin',(5.,30.,55.));
#102972=CARTESIAN_POINT('',(8.86797183897061,31.5634375186471,55.575516398799));
#102973=CARTESIAN_POINT('',(9.06224863102698,31.5634376784282,55.5755159647402));
#102974=CARTESIAN_POINT('',(5.,31.5634376782623,55.5755159651912));
#102975=CARTESIAN_POINT('',(9.72158833090148,31.6659999998112,55.0000015226055));
#102976=CARTESIAN_POINT('Ctrl Pts',(9.06224863102697,31.5634376784283,55.5755159647401));
#102977=CARTESIAN_POINT('Ctrl Pts',(9.06293928128569,31.5597675361453,55.5854862159268));
#102978=CARTESIAN_POINT('Ctrl Pts',(9.06362691885452,31.5560019522037,55.5954215478723));
#102979=CARTESIAN_POINT('Ctrl Pts',(9.07227369261313,31.5072540733995,55.7204191142712));
#102980=CARTESIAN_POINT('Ctrl Pts',(9.07977931942399,31.4497036442719,55.8301699251228));
#102981=CARTESIAN_POINT('Ctrl Pts',(9.09272378845509,31.3311181141229,56.0057216985928));
#102982=CARTESIAN_POINT('Ctrl Pts',(9.09813272625667,31.2759635575033,56.0748324046651));
#102983=CARTESIAN_POINT('Ctrl Pts',(9.10491873848209,31.2043377353272,56.1512593088233));
#102984=CARTESIAN_POINT('Ctrl Pts',(9.10599655431006,31.19289571438,56.1631109755843));
#102985=CARTESIAN_POINT('Ctrl Pts',(9.10759798742486,31.1758371962787,56.1802637300698));
#102986=CARTESIAN_POINT('Ctrl Pts',(9.10811173698039,31.1703561771518,56.1856989488918));
#102987=CARTESIAN_POINT('Ctrl Pts',(9.10903052724184,31.1605435552389,56.195295248907));
#102988=CARTESIAN_POINT('Ctrl Pts',(9.10943440023325,31.1562269354538,56.1994712781793));
#102989=CARTESIAN_POINT('Ctrl Pts',(9.11033221764584,31.1466246925319,56.2086607810446));
#102990=CARTESIAN_POINT('Ctrl Pts',(9.1108269550082,31.1413287935606,56.2136629058821));
#102991=CARTESIAN_POINT('Ctrl Pts',(9.11229679390002,31.1255764231085,56.2283471813861));
#102992=CARTESIAN_POINT('Ctrl Pts',(9.11327876789436,31.1150286382456,56.2379297978141));
#102993=CARTESIAN_POINT('Ctrl Pts',(9.11557758347753,31.0902529116233,56.2598649031498));
#102994=CARTESIAN_POINT('Ctrl Pts',(9.1169002135782,31.0759359162082,56.2721135269541));
#102995=CARTESIAN_POINT('Ctrl Pts',(9.1216112363507,31.0246277780649,56.3145234173586));
#102996=CARTESIAN_POINT('Ctrl Pts',(9.12505479880484,30.9865531261056,56.3433340096796));
#102997=CARTESIAN_POINT('Ctrl Pts',(9.13668862231103,30.8547290214093,56.4344536269194));
#102998=CARTESIAN_POINT('Ctrl Pts',(9.14492219155174,30.755904048157,56.4889034494751));
#102999=CARTESIAN_POINT('Ctrl Pts',(9.1560675588748,30.6103743046556,56.5508316952402));
#103000=CARTESIAN_POINT('Ctrl Pts',(9.15923110531494,30.5676929085884,56.566959216064));
#103001=CARTESIAN_POINT('Ctrl Pts',(9.16347228959737,30.5085835509555,56.5865611973252));
#103002=CARTESIAN_POINT('Ctrl Pts',(9.16459934446256,30.492689104707,56.5915687677051));
#103003=CARTESIAN_POINT('Ctrl Pts',(9.16639595110731,30.4670590358538,56.5992227957994));
#103004=CARTESIAN_POINT('Ctrl Pts',(9.16707039746375,30.4573702030699,56.602020661119));
#103005=CARTESIAN_POINT('Ctrl Pts',(9.16846536848271,30.4371936504265,56.6076491219757));
#103006=CARTESIAN_POINT('Ctrl Pts',(9.16918540206304,30.4267024257003,56.6104654720852));
#103007=CARTESIAN_POINT('Ctrl Pts',(9.17088149007747,30.4018130523105,56.616886683418));
#103008=CARTESIAN_POINT('Ctrl Pts',(9.17185462937672,30.3873926425779,56.6204021846428));
#103009=CARTESIAN_POINT('Ctrl Pts',(9.17516181891229,30.3379309813643,56.6317622257666));
#103010=CARTESIAN_POINT('Ctrl Pts',(9.17746609259214,30.302682675301,56.6386667761133));
#103011=CARTESIAN_POINT('Ctrl Pts',(9.18311688138339,30.2146517914985,56.6529727156887));
#103012=CARTESIAN_POINT('Ctrl Pts',(9.18642450480134,30.1616849501031,56.6589914994885));
#103013=CARTESIAN_POINT('Ctrl Pts',(9.1931045230721,30.0532834277847,56.6660674302036));
#103014=CARTESIAN_POINT('Ctrl Pts',(9.19647019781724,29.9979034581181,56.6669179602142));
#103015=CARTESIAN_POINT('Ctrl Pts',(9.20070013024026,29.9287972729098,56.6645349114707));
#103016=CARTESIAN_POINT('Ctrl Pts',(9.20154517656372,29.9150170858926,56.6638882770147));
#103017=CARTESIAN_POINT('Ctrl Pts',(9.20691140084649,29.8278006458662,56.658709352287));
#103018=CARTESIAN_POINT('Ctrl Pts',(9.2114851009775,29.7547331623437,56.6494880319336));
#103019=CARTESIAN_POINT('Ctrl Pts',(9.2170916499667,29.6704756082838,56.6331320577941));
#103020=CARTESIAN_POINT('Ctrl Pts',(9.21789968334496,29.6584535006396,56.6306601761097));
#103021=CARTESIAN_POINT('Ctrl Pts',(9.21917627988038,29.6396719364905,56.6265816735425));
#103022=CARTESIAN_POINT('Ctrl Pts',(9.21963996527995,29.6328930736158,56.6250651538587));
#103023=CARTESIAN_POINT('Ctrl Pts',(9.22051226721762,29.6202254395123,56.62214793468));
#103024=CARTESIAN_POINT('Ctrl Pts',(9.22092031075189,29.6143345610657,56.6207574782435));
#103025=CARTESIAN_POINT('Ctrl Pts',(9.22188648273589,29.6004660433869,56.6174041279162));
#103026=CARTESIAN_POINT('Ctrl Pts',(9.22244609695882,29.5924951987902,56.6154142890924));
#103027=CARTESIAN_POINT('Ctrl Pts',(9.22433020439821,29.5658544997367,56.6085539996208));
#103028=CARTESIAN_POINT('Ctrl Pts',(9.22566823457467,29.5472553652699,56.6034183800581));
#103029=CARTESIAN_POINT('Ctrl Pts',(9.22899864395205,29.5016456753128,56.589967779792));
#103030=CARTESIAN_POINT('Ctrl Pts',(9.23100558775403,29.4747499649182,56.5812864364313));
#103031=CARTESIAN_POINT('Ctrl Pts',(9.24019387779678,29.3537610240141,56.5388066657188));
#103032=CARTESIAN_POINT('Ctrl Pts',(9.24754721382004,29.2626056634811,56.497264435469));
#103033=CARTESIAN_POINT('Ctrl Pts',(9.26073727958948,29.1036603813908,56.4067720877262));
#103034=CARTESIAN_POINT('Ctrl Pts',(9.26660347042933,29.0347520069989,56.360416286323));
#103035=CARTESIAN_POINT('Ctrl Pts',(9.27362333424604,28.9541520129957,56.2969746240103));
#103036=CARTESIAN_POINT('Ctrl Pts',(9.27495582875827,28.9389452618019,56.2845637730119));
#103037=CARTESIAN_POINT('Ctrl Pts',(9.27707452383162,28.914925732336,56.2642428144208));
#103038=CARTESIAN_POINT('Ctrl Pts',(9.27786751495595,28.9059721887577,56.2565027739306));
#103039=CARTESIAN_POINT('Ctrl Pts',(9.27937300013986,28.8890479467531,56.241554268009));
#103040=CARTESIAN_POINT('Ctrl Pts',(9.28008614719488,28.8810630694573,56.234362839572));
#103041=CARTESIAN_POINT('Ctrl Pts',(9.2817198949902,28.862849079093,56.2176367698139));
#103042=CARTESIAN_POINT('Ctrl Pts',(9.28263820707428,28.8526692186604,56.2080495097675));
#103043=CARTESIAN_POINT('Ctrl Pts',(9.28554909999279,28.8206026065786,56.1770785836723));
#103044=CARTESIAN_POINT('Ctrl Pts',(9.2875210425452,28.7991829570915,56.1552189495418));
#103045=CARTESIAN_POINT('Ctrl Pts',(9.29217893993317,28.7494800660016,56.1016179042624));
#103046=CARTESIAN_POINT('Ctrl Pts',(9.29484235655604,28.7217853574685,56.069359536966));
#103047=CARTESIAN_POINT('Ctrl Pts',(9.30204530464079,28.6495387928007,55.9783852237224));
#103048=CARTESIAN_POINT('Ctrl Pts',(9.30651745083815,28.6076004530641,55.9177183576028));
#103049=CARTESIAN_POINT('Ctrl Pts',(9.31186054882374,28.5628111182578,55.8427518034916));
#103050=CARTESIAN_POINT('Ctrl Pts',(9.31269722941317,28.5559515872971,55.8309432352984));
#103051=CARTESIAN_POINT('Ctrl Pts',(9.31805984532966,28.5130327468991,55.754922374555));
#103052=CARTESIAN_POINT('Ctrl Pts',(9.32263808235209,28.4811238448674,55.6884706863783));
#103053=CARTESIAN_POINT('Ctrl Pts',(9.32824990129537,28.4491448636682,55.608732541227));
#103054=CARTESIAN_POINT('Ctrl Pts',(9.32905877137347,28.4446978697281,55.5972790155644));
#103055=CARTESIAN_POINT('Ctrl Pts',(9.3303368815668,28.4379320189691,55.5792650700017));
#103056=CARTESIAN_POINT('Ctrl Pts',(9.33080124643702,28.4355267895186,55.5727372591254));
#103057=CARTESIAN_POINT('Ctrl Pts',(9.33167549849056,28.4310989439311,55.5604840290776));
#103058=CARTESIAN_POINT('Ctrl Pts',(9.33208481850921,28.4290666513074,55.5547623633094));
#103059=CARTESIAN_POINT('Ctrl Pts',(9.33305483032973,28.4243457156412,55.5412371935046));
#103060=CARTESIAN_POINT('Ctrl Pts',(9.3336170225781,28.4216837310813,55.53342466345));
#103061=CARTESIAN_POINT('Ctrl Pts',(9.33551298120203,28.4129499800598,55.5071545934103));
#103062=CARTESIAN_POINT('Ctrl Pts',(9.33686042197716,28.4071433423331,55.4886114356529));
#103063=CARTESIAN_POINT('Ctrl Pts',(9.34021857972493,28.3936172014157,55.4426101064415));
#103064=CARTESIAN_POINT('Ctrl Pts',(9.34224406405335,28.3862761427188,55.4150476252237));
#103065=CARTESIAN_POINT('Ctrl Pts',(9.35160860557777,28.3558912858513,55.2879299189499));
#103066=CARTESIAN_POINT('Ctrl Pts',(9.35912300282084,28.3413294135802,55.186573554496));
#103067=CARTESIAN_POINT('Ctrl Pts',(9.37220621381704,28.3321092200796,55.0050654559412));
#103068=CARTESIAN_POINT('Ctrl Pts',(9.37782459907529,28.3337690258278,54.9254146775234));
#103069=CARTESIAN_POINT('Ctrl Pts',(9.38460402308866,28.3429177027656,54.8267521393244));
#103070=CARTESIAN_POINT('Ctrl Pts',(9.38592822619664,28.3450599923048,54.8073599523512));
#103071=CARTESIAN_POINT('Ctrl Pts',(9.38803771301508,28.3490465822965,54.7762846959257));
#103072=CARTESIAN_POINT('Ctrl Pts',(9.38882965584497,28.3506754590439,54.7645763483789));
#103073=CARTESIAN_POINT('Ctrl Pts',(9.39033565813448,28.3540263238609,54.7422352846733));
#103074=CARTESIAN_POINT('Ctrl Pts',(9.39105034530193,28.3557270719483,54.7316000403139));
#103075=CARTESIAN_POINT('Ctrl Pts',(9.39269122752458,28.3598871765332,54.7071111580265));
#103076=CARTESIAN_POINT('Ctrl Pts',(9.39361508286203,28.3624191561991,54.6932705629591));
#103077=CARTESIAN_POINT('Ctrl Pts',(9.39655903638998,28.3710954800286,54.649017607785));
#103078=CARTESIAN_POINT('Ctrl Pts',(9.39855784591758,28.3779143118231,54.6187431433732));
#103079=CARTESIAN_POINT('Ctrl Pts',(9.4099350245357,28.4220179381688,54.4456390954479));
#103080=CARTESIAN_POINT('Ctrl Pts',(9.41870203428594,28.477304108859,54.3080897440184));
#103081=CARTESIAN_POINT('Ctrl Pts',(9.43134065343489,28.5777528360631,54.130547089414));
#103082=CARTESIAN_POINT('Ctrl Pts',(9.43488985288649,28.6079891438743,54.0829178102258));
#103083=CARTESIAN_POINT('Ctrl Pts',(9.43935430827129,28.6474654603177,54.0271956565969));
#103084=CARTESIAN_POINT('Ctrl Pts',(9.44013925237602,28.654457255636,54.0175476221827));
#103085=CARTESIAN_POINT('Ctrl Pts',(9.44138741222215,28.6656420234885,54.0024570296437));
#103086=CARTESIAN_POINT('Ctrl Pts',(9.44184610499773,28.6697663642701,53.9969637806512));
#103087=CARTESIAN_POINT('Ctrl Pts',(9.44271278265618,28.6775822968313,53.9866866570922));
#103088=CARTESIAN_POINT('Ctrl Pts',(9.44312024102352,28.6812660848524,53.9818971716314));
#103089=CARTESIAN_POINT('Ctrl Pts',(9.44409173264595,28.6900717686854,53.9705764139777));
#103090=CARTESIAN_POINT('Ctrl Pts',(9.44465732957572,28.6952164879157,53.9640632886545));
#103091=CARTESIAN_POINT('Ctrl Pts',(9.44659809780187,28.7129383854756,53.9419691141793));
#103092=CARTESIAN_POINT('Ctrl Pts',(9.44798808105683,28.7257471612771,53.9265771712717));
#103093=CARTESIAN_POINT('Ctrl Pts',(9.45148133423516,28.758294527602,53.888869511172));
#103094=CARTESIAN_POINT('Ctrl Pts',(9.45360111481002,28.7783598370672,53.8668457524919));
#103095=CARTESIAN_POINT('Ctrl Pts',(9.46387144260097,28.8774946323081,53.763729723926));
#103096=CARTESIAN_POINT('Ctrl Pts',(9.47222581443075,28.9641069803916,53.6903014162346));
#103097=CARTESIAN_POINT('Ctrl Pts',(9.48531563202135,29.1147225511038,53.5869696312445));
#103098=CARTESIAN_POINT('Ctrl Pts',(9.49019306822294,29.1743438227994,53.5513229644445));
#103099=CARTESIAN_POINT('Ctrl Pts',(9.49622371898402,29.2527443836546,53.5108663189698));
#103100=CARTESIAN_POINT('Ctrl Pts',(9.49750006791159,29.2696117482676,53.5025210757432));
#103101=CARTESIAN_POINT('Ctrl Pts',(9.49954793400567,29.2971115278384,53.4894906005289));
#103102=CARTESIAN_POINT('Ctrl Pts',(9.50032556481102,29.3076574818053,53.484627867628));
#103103=CARTESIAN_POINT('Ctrl Pts',(9.50181338288449,29.3280303158158,53.4754910456978));
#103104=CARTESIAN_POINT('Ctrl Pts',(9.50252409959971,29.3378492395932,53.4712007365601));
#103105=CARTESIAN_POINT('Ctrl Pts',(9.50416871529685,29.3607683112844,53.4614486459508));
#103106=CARTESIAN_POINT('Ctrl Pts',(9.50510012806694,29.3738983459009,53.4560588870174));
#103107=CARTESIAN_POINT('Ctrl Pts',(9.50812329622769,29.4169869333384,53.4390115039924));
#103108=CARTESIAN_POINT('Ctrl Pts',(9.51019175471155,29.447215307859,53.4280526019688));
#103109=CARTESIAN_POINT('Ctrl Pts',(9.51513454339689,29.5210272682812,53.4036858791511));
#103110=CARTESIAN_POINT('Ctrl Pts',(9.51798193817156,29.5648811646825,53.3911787860515));
#103111=CARTESIAN_POINT('Ctrl Pts',(9.52509598764719,29.6767720585325,53.3641784262859));
#103112=CARTESIAN_POINT('Ctrl Pts',(9.52931399503807,29.7453043411834,53.3521168466163));
#103113=CARTESIAN_POINT('Ctrl Pts',(9.53434103965144,29.8269811132401,53.3429601687225));
#103114=CARTESIAN_POINT('Ctrl Pts',(9.53511708763151,29.839588182171,53.3416922536186));
#103115=CARTESIAN_POINT('Ctrl Pts',(9.54041152767559,29.9254787169282,53.3340427070248));
#103116=CARTESIAN_POINT('Ctrl Pts',(9.54498322551238,29.999091844044,53.3323778784447));
#103117=CARTESIAN_POINT('Ctrl Pts',(9.5505868677634,30.0847941746212,53.3361142412321));
#103118=CARTESIAN_POINT('Ctrl Pts',(9.55139286450664,30.0970180179242,53.3367822292992));
#103119=CARTESIAN_POINT('Ctrl Pts',(9.55266584410028,30.1161402967374,53.33803870412));
#103120=CARTESIAN_POINT('Ctrl Pts',(9.55312794535591,30.1230445979865,53.3385356037256));
#103121=CARTESIAN_POINT('Ctrl Pts',(9.55399890063669,30.1359830999371,53.339547870928));
#103122=CARTESIAN_POINT('Ctrl Pts',(9.55440719738167,30.1420178669402,53.3400531342943));
#103123=CARTESIAN_POINT('Ctrl Pts',(9.55537431830951,30.1562422845859,53.3413222125061));
#103124=CARTESIAN_POINT('Ctrl Pts',(9.5559346382882,30.1644292226808,53.342113792247));
#103125=CARTESIAN_POINT('Ctrl Pts',(9.55781829539099,30.1917821508138,53.3449630891386));
#103126=CARTESIAN_POINT('Ctrl Pts',(9.55915511183033,30.2109174498649,53.347292730092));
#103127=CARTESIAN_POINT('Ctrl Pts',(9.56247984889537,30.2579316078467,53.3538462335772));
#103128=CARTESIAN_POINT('Ctrl Pts',(9.56448223031771,30.2857514051568,53.3584468049578));
#103129=CARTESIAN_POINT('Ctrl Pts',(9.57360822445225,30.4108354900165,53.3824078746661));
#103130=CARTESIAN_POINT('Ctrl Pts',(9.58090199874208,30.5063703582634,53.4097234631507));
#103131=CARTESIAN_POINT('Ctrl Pts',(9.59414466477184,30.6776067192957,53.4756911215899));
#103132=CARTESIAN_POINT('Ctrl Pts',(9.60011509632396,30.7538980002194,53.5119441748055));
#103133=CARTESIAN_POINT('Ctrl Pts',(9.6072444541771,30.8442980617198,53.5636476236931));
#103134=CARTESIAN_POINT('Ctrl Pts',(9.60858795697425,30.8612950058578,53.5737747943839));
#103135=CARTESIAN_POINT('Ctrl Pts',(9.61072253968059,30.8882262619261,53.5904781433869));
#103136=CARTESIAN_POINT('Ctrl Pts',(9.61152050508331,30.8982769915131,53.5968620111175));
#103137=CARTESIAN_POINT('Ctrl Pts',(9.61303453680375,30.9173100591049,53.6092394773106));
#103138=CARTESIAN_POINT('Ctrl Pts',(9.61375126878156,30.9263042080106,53.6152136989617));
#103139=CARTESIAN_POINT('Ctrl Pts',(9.61539209895532,30.9468529024029,53.629152633958));
#103140=CARTESIAN_POINT('Ctrl Pts',(9.61631391074184,30.9583662676364,53.6371768138606));
#103141=CARTESIAN_POINT('Ctrl Pts',(9.61923223901578,30.9946993618172,53.6631871440359));
#103142=CARTESIAN_POINT('Ctrl Pts',(9.6212081772296,31.0191255948057,53.6817137479796));
#103143=CARTESIAN_POINT('Ctrl Pts',(9.62587587064451,31.0762244665977,53.7275577481859));
#103144=CARTESIAN_POINT('Ctrl Pts',(9.62854516136255,31.1083886019676,53.7554745998401));
#103145=CARTESIAN_POINT('Ctrl Pts',(9.63571344019281,31.1926820468283,53.8345001976203));
#103146=CARTESIAN_POINT('Ctrl Pts',(9.64014781064916,31.2425793870167,53.8878502460746));
#103147=CARTESIAN_POINT('Ctrl Pts',(9.64532676979143,31.2961694168032,53.9532739545163));
#103148=CARTESIAN_POINT('Ctrl Pts',(9.6460379820886,31.3034263651314,53.9623245792557));
#103149=CARTESIAN_POINT('Ctrl Pts',(9.65139201868645,31.3572323658479,54.0308847082958));
#103150=CARTESIAN_POINT('Ctrl Pts',(9.65608516034864,31.3997738872444,54.0934161255742));
#103151=CARTESIAN_POINT('Ctrl Pts',(9.6618257008195,31.4441601149845,54.1692712942414));
#103152=CARTESIAN_POINT('Ctrl Pts',(9.66263892300595,31.4502803016499,54.1800026554667));
#103153=CARTESIAN_POINT('Ctrl Pts',(9.6639246942477,31.4596841040202,54.1969262645773));
#103154=CARTESIAN_POINT('Ctrl Pts',(9.66439237439429,31.4630490880941,54.203073109093));
#103155=CARTESIAN_POINT('Ctrl Pts',(9.66527785028223,31.4693135982272,54.2146899483029));
#103156=CARTESIAN_POINT('Ctrl Pts',(9.66569511987698,31.4722215700353,54.220155162289));
#103157=CARTESIAN_POINT('Ctrl Pts',(9.666688503862,31.4790417852602,54.233147109499));
#103158=CARTESIAN_POINT('Ctrl Pts',(9.66726620417077,31.4829271100746,54.2406877211072));
#103159=CARTESIAN_POINT('Ctrl Pts',(9.66923214447231,31.4958821909095,54.2663095598047));
#103160=CARTESIAN_POINT('Ctrl Pts',(9.67063484700283,31.5046797883318,54.2845254454026));
#103161=CARTESIAN_POINT('Ctrl Pts',(9.68050126631705,31.5636329629896,54.4124899746156));
#103162=CARTESIAN_POINT('Ctrl Pts',(9.6893817068692,31.6020652382261,54.5272401423611));
#103163=CARTESIAN_POINT('Ctrl Pts',(9.70405552931875,31.6455025616253,54.7264852314741));
#103164=CARTESIAN_POINT('Ctrl Pts',(9.7099398458228,31.6571167822441,54.8090637802794));
#103165=CARTESIAN_POINT('Ctrl Pts',(9.71695427045445,31.6637537404347,54.9113969690014));
#103166=CARTESIAN_POINT('Ctrl Pts',(9.71826169886316,31.6646669638397,54.9306389267541));
#103167=CARTESIAN_POINT('Ctrl Pts',(9.72022163497542,31.6655422914515,54.9597294550104));
#103168=CARTESIAN_POINT('Ctrl Pts',(9.7208816490184,31.665751111934,54.9695684112151));
#103169=CARTESIAN_POINT('Ctrl Pts',(9.72199553663507,31.6659572261724,54.9862435190925));
#103170=CARTESIAN_POINT('Ctrl Pts',(9.72245078595099,31.6659996453322,54.99307873824));
#103171=CARTESIAN_POINT('Ctrl Pts',(9.72290474287967,31.6659999977852,54.9999140956723));
#103172=CARTESIAN_POINT('Ctrl Pts',(9.72148036344425,31.6659999999773,55.0000086930536));
#103173=CARTESIAN_POINT('Ctrl Pts',(9.72575162903862,31.6659996648664,55.0642317834644));
#103174=CARTESIAN_POINT('Ctrl Pts',(9.73002289463299,31.6622813967003,55.128381221177));
#103175=CARTESIAN_POINT('Ctrl Pts',(9.73429416022736,31.6548963909707,55.192025871049));
#103176=CARTESIAN_POINT('Ctrl Pts',(9.73869642027905,31.6472848962072,55.2576224239783));
#103177=CARTESIAN_POINT('Ctrl Pts',(9.74309868033075,31.6357781724688,55.3226822259613));
#103178=CARTESIAN_POINT('Ctrl Pts',(9.74750094038244,31.6204884723869,55.3867468304473));
#103179=CARTESIAN_POINT('Ctrl Pts',(9.75190320043414,31.6051987723051,55.4508114349334));
#103180=CARTESIAN_POINT('Ctrl Pts',(9.75630546048584,31.5861263069399,55.5138803910486));
#103181=CARTESIAN_POINT('Ctrl Pts',(9.76070772053754,31.5634376782623,55.5755159651912));
#103182=CARTESIAN_POINT('Ctrl Pts',(9.56912139758663,31.5634376777551,55.575515966569));
#103183=CARTESIAN_POINT('Ctrl Pts',(9.56843888003858,31.5671670606512,55.5653847832946));
#103184=CARTESIAN_POINT('Ctrl Pts',(9.56775294050477,31.5707980645885,55.5552170859515));
#103185=CARTESIAN_POINT('Ctrl Pts',(9.56544857079703,31.5825951755981,55.5211399118735));
#103186=CARTESIAN_POINT('Ctrl Pts',(9.56381286286895,31.5903155367117,55.497082113429));
#103187=CARTESIAN_POINT('Ctrl Pts',(9.56154741322078,31.6000746418027,55.4641124419768));
#103188=CARTESIAN_POINT('Ctrl Pts',(9.56094266118142,31.60259188435,55.4553443323174));
#103189=CARTESIAN_POINT('Ctrl Pts',(9.55991911091215,31.6067025944225,55.4405693928223));
#103190=CARTESIAN_POINT('Ctrl Pts',(9.55950248788842,31.608334734456,55.4345733506667));
#103191=CARTESIAN_POINT('Ctrl Pts',(9.55864070723962,31.6116256346078,55.4222109598002));
#103192=CARTESIAN_POINT('Ctrl Pts',(9.55819534445324,31.613280284311,55.4158437220623));
#103193=CARTESIAN_POINT('Ctrl Pts',(9.55700795882038,31.6175712483432,55.3989205861298));
#103194=CARTESIAN_POINT('Ctrl Pts',(9.55626240405005,31.620141888435,55.3883485845622));
#103195=CARTESIAN_POINT('Ctrl Pts',(9.55284758840529,31.6313657656347,55.3401372294056));
#103196=CARTESIAN_POINT('Ctrl Pts',(9.55012186546077,31.6388114398416,55.3022319369514));
#103197=CARTESIAN_POINT('Ctrl Pts',(9.54075737098301,31.6595734472879,55.1729196813758));
#103198=CARTESIAN_POINT('Ctrl Pts',(9.53397689092433,31.6666062158077,55.0806761496393));
#103199=CARTESIAN_POINT('Ctrl Pts',(9.52052986714115,31.665304347461,54.8948864531111));
#103200=CARTESIAN_POINT('Ctrl Pts',(9.51389078321266,31.6567896110581,54.8016547613869));
#103201=CARTESIAN_POINT('Ctrl Pts',(9.50615114195072,31.637077577199,54.6902936245822));
#103202=CARTESIAN_POINT('Ctrl Pts',(9.50481893139739,31.6333161965664,54.6710329927547));
#103203=CARTESIAN_POINT('Ctrl Pts',(9.50270074440271,31.6267427763886,54.6402724353493));
#103204=CARTESIAN_POINT('Ctrl Pts',(9.50190798132002,31.6241470459172,54.6287287150432));
#103205=CARTESIAN_POINT('Ctrl Pts',(9.50040296692266,31.6189604179501,54.6067589135398));
#103206=CARTESIAN_POINT('Ctrl Pts',(9.49969006264807,31.6163912322436,54.5963283753965));
#103207=CARTESIAN_POINT('Ctrl Pts',(9.49807234840389,31.6103053245132,54.5726106520954));
#103208=CARTESIAN_POINT('Ctrl Pts',(9.4971696425408,31.6067246720497,54.5593405625229));
#103209=CARTESIAN_POINT('Ctrl Pts',(9.49430651218749,31.5947806685594,54.5171579812168));
#103210=CARTESIAN_POINT('Ctrl Pts',(9.49236607054106,31.585797656029,54.4884261834884));
#103211=CARTESIAN_POINT('Ctrl Pts',(9.48140346894314,31.5300586917328,54.3257612329878));
#103212=CARTESIAN_POINT('Ctrl Pts',(9.47294360003098,31.4671304458004,54.1979985341477));
#103213=CARTESIAN_POINT('Ctrl Pts',(9.4615268026904,31.3649473971391,54.0437911004344));
#103214=CARTESIAN_POINT('Ctrl Pts',(9.45883671393636,31.3397333148186,54.0087729812608));
#103215=CARTESIAN_POINT('Ctrl Pts',(9.45442793195575,31.2972308252152,53.9543323593697));
#103216=CARTESIAN_POINT('Ctrl Pts',(9.45275013384337,31.280796721428,53.9342663512118));
#103217=CARTESIAN_POINT('Ctrl Pts',(9.45043645746936,31.257912358809,53.9076186461381));
#103218=CARTESIAN_POINT('Ctrl Pts',(9.44982710834959,31.2518651386115,53.9006937688619));
#103219=CARTESIAN_POINT('Ctrl Pts',(9.44879894430112,31.2416349493708,53.8891727091354));
#103220=CARTESIAN_POINT('Ctrl Pts',(9.44838237362555,31.2374828987417,53.8845491085432));
#103221=CARTESIAN_POINT('Ctrl Pts',(9.44752388156461,31.2289139827507,53.8751137463673));
#103222=CARTESIAN_POINT('Ctrl Pts',(9.44708178493124,31.2244945505675,53.8703045753224));
#103223=CARTESIAN_POINT('Ctrl Pts',(9.44591017285661,31.2127619320424,53.8576870174266));
#103224=CARTESIAN_POINT('Ctrl Pts',(9.44517726954991,31.205401752765,53.8499230228377));
#103225=CARTESIAN_POINT('Ctrl Pts',(9.4419086217738,31.1724632434546,53.815840873813));
#103226=CARTESIAN_POINT('Ctrl Pts',(9.43932186275907,31.146095950254,53.790303131795));
#103227=CARTESIAN_POINT('Ctrl Pts',(9.4291357477657,31.040401505385,53.6944928888983));
#103228=CARTESIAN_POINT('Ctrl Pts',(9.42133169317932,30.9552842901963,53.6309797720966));
#103229=CARTESIAN_POINT('Ctrl Pts',(9.40776036305137,30.7943870075803,53.5332777156577));
#103230=CARTESIAN_POINT('Ctrl Pts',(9.40194190944326,30.7209881840826,53.49583754913));
#103231=CARTESIAN_POINT('Ctrl Pts',(9.39496986376498,30.6270551730021,53.456386905623));
#103232=CARTESIAN_POINT('Ctrl Pts',(9.39364024069968,30.6088650410454,53.4491218636671));
#103233=CARTESIAN_POINT('Ctrl Pts',(9.39152582848276,30.5795035616891,53.4379912964515));
#103234=CARTESIAN_POINT('Ctrl Pts',(9.39073427172936,30.5684123186592,53.4339211333964));
#103235=CARTESIAN_POINT('Ctrl Pts',(9.3892313680882,30.5471678441394,53.4263804608205));
#103236=CARTESIAN_POINT('Ctrl Pts',(9.38851937083619,30.5370225952394,53.4228893998384));
#103237=CARTESIAN_POINT('Ctrl Pts',(9.38688810182456,30.5135974057995,53.4150808606403));
#103238=CARTESIAN_POINT('Ctrl Pts',(9.38597111633698,30.5002953753401,53.4108318117179));
#103239=CARTESIAN_POINT('Ctrl Pts',(9.38306412352662,30.4577162315701,53.397818447542));
#103240=CARTESIAN_POINT('Ctrl Pts',(9.38109473540321,30.4282497422575,53.3896918860816));
#103241=CARTESIAN_POINT('Ctrl Pts',(9.37644358074709,30.3573718268691,53.3722278625199));
#103242=CARTESIAN_POINT('Ctrl Pts',(9.37378431901489,30.3157941132131,53.3636530896065));
#103243=CARTESIAN_POINT('Ctrl Pts',(9.36657904545865,30.2011535168197,53.3445432215242));
#103244=CARTESIAN_POINT('Ctrl Pts',(9.3621011029355,30.1276478641984,53.3372594080665));
#103245=CARTESIAN_POINT('Ctrl Pts',(9.35677683137713,30.0406492200486,53.3344432033744));
#103246=CARTESIAN_POINT('Ctrl Pts',(9.35596473417298,30.0273925757854,53.3341724448094));
#103247=CARTESIAN_POINT('Ctrl Pts',(9.35059047955145,29.9398679825883,53.3334298663247));
#103248=CARTESIAN_POINT('Ctrl Pts',(9.34597604659209,29.8656518036035,53.3377666764457));
#103249=CARTESIAN_POINT('Ctrl Pts',(9.34032435664034,29.7798052221407,53.3485700427747));
#103250=CARTESIAN_POINT('Ctrl Pts',(9.33951634068205,29.7676453136079,53.350237010425));
#103251=CARTESIAN_POINT('Ctrl Pts',(9.3382399143794,29.7486362021598,53.3530572367882));
#103252=CARTESIAN_POINT('Ctrl Pts',(9.33777638380629,29.7417736231372,53.3541192758634));
#103253=CARTESIAN_POINT('Ctrl Pts',(9.3369044207251,29.7289446926024,53.3561868634161));
#103254=CARTESIAN_POINT('Ctrl Pts',(9.33649656133541,29.7229769187949,53.3571820504258));
#103255=CARTESIAN_POINT('Ctrl Pts',(9.33553096125169,29.7089239966555,53.3596042653874));
#103256=CARTESIAN_POINT('Ctrl Pts',(9.33497173761227,29.7008438253787,53.3610585788428));
#103257=CARTESIAN_POINT('Ctrl Pts',(9.33308971579237,29.6738347132591,53.3661262083867));
#103258=CARTESIAN_POINT('Ctrl Pts',(9.33175341910263,29.654958551408,53.3700080733511));
#103259=CARTESIAN_POINT('Ctrl Pts',(9.32842800910045,29.6086213823301,53.3803781777075));
#103260=CARTESIAN_POINT('Ctrl Pts',(9.32642438356216,29.5812502419328,53.3872382289343));
#103261=CARTESIAN_POINT('Ctrl Pts',(9.31726138820989,29.4580283564345,53.4214696076344));
#103262=CARTESIAN_POINT('Ctrl Pts',(9.30993080677071,29.3645774991331,53.4567145074392));
#103263=CARTESIAN_POINT('Ctrl Pts',(9.29674505771154,29.1999744623092,53.536295961376));
#103264=CARTESIAN_POINT('Ctrl Pts',(9.29086227013496,29.1279178614349,53.5780482122596));
#103265=CARTESIAN_POINT('Ctrl Pts',(9.28382707217414,29.0430754109903,53.6360951543477));
#103266=CARTESIAN_POINT('Ctrl Pts',(9.28249476205126,29.0270758684549,53.6474617238605));
#103267=CARTESIAN_POINT('Ctrl Pts',(9.2803765684037,29.0017586477555,53.6661296327067));
#103268=CARTESIAN_POINT('Ctrl Pts',(9.27958389327735,28.9923118638365,53.6732518751466));
#103269=CARTESIAN_POINT('Ctrl Pts',(9.27807914126751,28.9744356032813,53.6870304640742));
#103270=CARTESIAN_POINT('Ctrl Pts',(9.27736641054238,28.9659931027749,53.6936688475787));
#103271=CARTESIAN_POINT('Ctrl Pts',(9.275733813904,28.9467160331359,53.7091304872602));
#103272=CARTESIAN_POINT('Ctrl Pts',(9.27481623204606,28.9359269925767,53.7180094117578));
#103273=CARTESIAN_POINT('Ctrl Pts',(9.27190856507873,28.9019004751943,53.7467373341465));
#103274=CARTESIAN_POINT('Ctrl Pts',(9.26993906691906,28.8790960704118,53.7670910641118));
#103275=CARTESIAN_POINT('Ctrl Pts',(9.26528794143432,28.8259978657113,53.8171748896573));
#103276=CARTESIAN_POINT('Ctrl Pts',(9.2626287733219,28.7962544587725,53.8474578953481));
#103277=CARTESIAN_POINT('Ctrl Pts',(9.25542782535457,28.718098548194,53.9333618940862));
#103278=CARTESIAN_POINT('Ctrl Pts',(9.25095375909464,28.6721702728705,53.9911111238162));
#103279=CARTESIAN_POINT('Ctrl Pts',(9.24560870912098,28.6224417280865,54.0629430129494));
#103280=CARTESIAN_POINT('Ctrl Pts',(9.24477185811805,28.6148050548724,54.0742691817106));
#103281=CARTESIAN_POINT('Ctrl Pts',(9.23940295840345,28.5668343355864,54.1473387693496));
#103282=CARTESIAN_POINT('Ctrl Pts',(9.23481861962066,28.5305033768844,54.2116016775694));
#103283=CARTESIAN_POINT('Ctrl Pts',(9.22920030444782,28.4932316031709,54.2891162044358));
#103284=CARTESIAN_POINT('Ctrl Pts',(9.22839192343974,28.4880333004404,54.3002404340435));
#103285=CARTESIAN_POINT('Ctrl Pts',(9.22711468537034,28.4800856671172,54.3177502381017));
#103286=CARTESIAN_POINT('Ctrl Pts',(9.22665070295415,28.477252420096,54.3240975510956));
#103287=CARTESIAN_POINT('Ctrl Pts',(9.22577804538881,28.4720260580494,54.3360058109906));
#103288=CARTESIAN_POINT('Ctrl Pts',(9.22536994515191,28.4696234271096,54.3415623106149));
#103289=CARTESIAN_POINT('Ctrl Pts',(9.22440363460769,28.4640311513545,54.3546913813091));
#103290=CARTESIAN_POINT('Ctrl Pts',(9.22384393950127,28.4608671887328,54.3622745892069));
#103291=CARTESIAN_POINT('Ctrl Pts',(9.22195873761799,28.4504561077155,54.3877560975347));
#103292=CARTESIAN_POINT('Ctrl Pts',(9.22061967377745,28.443464393955,54.405756196596));
#103293=CARTESIAN_POINT('Ctrl Pts',(9.21728584882126,28.427003252466,54.4504203963385));
#103294=CARTESIAN_POINT('Ctrl Pts',(9.21527648876348,28.4178974297132,54.4772115295083));
#103295=CARTESIAN_POINT('Ctrl Pts',(9.20606239155674,28.3796302092884,54.5999773096793));
#103296=CARTESIAN_POINT('Ctrl Pts',(9.19868506082896,28.3584903070569,54.6982338519756));
#103297=CARTESIAN_POINT('Ctrl Pts',(9.18551250193248,28.3363151657845,54.8795889060205));
#103298=CARTESIAN_POINT('Ctrl Pts',(9.17968479460354,28.3323947406802,54.9620206181944));
#103299=CARTESIAN_POINT('Ctrl Pts',(9.17270303743105,28.335114636498,55.0640062432877));
#103300=CARTESIAN_POINT('Ctrl Pts',(9.1713725345938,28.3359827694484,55.0835869972811));
#103301=CARTESIAN_POINT('Ctrl Pts',(9.16925664323324,28.3379282236735,55.1149486240861));
#103302=CARTESIAN_POINT('Ctrl Pts',(9.16846448496528,28.3387858146876,55.1267407544119));
#103303=CARTESIAN_POINT('Ctrl Pts',(9.16696037153546,28.3406616825418,55.1492234730349));
#103304=CARTESIAN_POINT('Ctrl Pts',(9.16624776626329,28.3416579304798,55.1599152474169));
#103305=CARTESIAN_POINT('Ctrl Pts',(9.16461498515638,28.3441887078215,55.1845001768978));
#103306=CARTESIAN_POINT('Ctrl Pts',(9.16369709896174,28.3457948571069,55.1983852704428));
#103307=CARTESIAN_POINT('Ctrl Pts',(9.16078658377417,28.3514739313462,55.2425986556928));
#103308=CARTESIAN_POINT('Ctrl Pts',(9.15881461336789,28.3562078475767,55.2728366814595));
#103309=CARTESIAN_POINT('Ctrl Pts',(9.15415646784814,28.3695008319836,55.3447246616848));
#103310=CARTESIAN_POINT('Ctrl Pts',(9.1514928616421,28.3788264265774,55.386211411117));
#103311=CARTESIAN_POINT('Ctrl Pts',(9.14428667114999,28.4086385240908,55.4985580819379));
#103312=CARTESIAN_POINT('Ctrl Pts',(9.13981172065586,28.432257672762,55.5684855928086));
#103313=CARTESIAN_POINT('Ctrl Pts',(9.13445242938353,28.4657334458135,55.6494418264753));
#103314=CARTESIAN_POINT('Ctrl Pts',(9.1336023629126,28.4711957836392,55.6621980122535));
#103315=CARTESIAN_POINT('Ctrl Pts',(9.12823491606235,28.5065940840286,55.7420903600135));
#103316=CARTESIAN_POINT('Ctrl Pts',(9.12366503966482,28.5407830448044,55.8072437517862));
#103317=CARTESIAN_POINT('Ctrl Pts',(9.11806275655161,28.5855660190547,55.8803881055));
#103318=CARTESIAN_POINT('Ctrl Pts',(9.11725456451468,28.5920914028662,55.8907862050594));
#103319=CARTESIAN_POINT('Ctrl Pts',(9.11597769365475,28.6024891000288,55.9069551058199));
#103320=CARTESIAN_POINT('Ctrl Pts',(9.11551389048466,28.6062837810931,55.9127756440087));
#103321=CARTESIAN_POINT('Ctrl Pts',(9.11464155862745,28.6134514022043,55.923620923263));
#103322=CARTESIAN_POINT('Ctrl Pts',(9.11423360457744,28.6168154536837,55.9286512424472));
#103323=CARTESIAN_POINT('Ctrl Pts',(9.11326772223332,28.6248093842379,55.9404648953807));
#103324=CARTESIAN_POINT('Ctrl Pts',(9.11270831054794,28.6294620984284,55.9472324437079));
#103325=CARTESIAN_POINT('Ctrl Pts',(9.11082467040578,28.6452108640997,55.9697806709638));
#103326=CARTESIAN_POINT('Ctrl Pts',(9.10948690974453,28.6565304853925,55.9854023221984));
#103327=CARTESIAN_POINT('Ctrl Pts',(9.1061569511322,28.6850933062422,56.0234133393425));
#103328=CARTESIAN_POINT('Ctrl Pts',(9.10415019034259,28.7026395100741,56.0455668584097));
#103329=CARTESIAN_POINT('Ctrl Pts',(9.09495878113625,28.7848160281203,56.1440667175974));
#103330=CARTESIAN_POINT('Ctrl Pts',(9.08760211413387,28.8556785008973,56.2149442318511));
#103331=CARTESIAN_POINT('Ctrl Pts',(9.07442321463585,28.9959932289217,56.332055660511));
#103332=CARTESIAN_POINT('Ctrl Pts',(9.06857067622661,29.0633839453631,56.3802738727036));
#103333=CARTESIAN_POINT('Ctrl Pts',(9.06156504909387,29.1508395707369,56.4334807276759));
#103334=CARTESIAN_POINT('Ctrl Pts',(9.06023391260802,29.1677692533702,56.4433753748076));
#103335=CARTESIAN_POINT('Ctrl Pts',(9.05811732988295,29.1951820795511,56.4587542335006));
#103336=CARTESIAN_POINT('Ctrl Pts',(9.05732510356771,29.2055553641059,56.4644294219276));
#103337=CARTESIAN_POINT('Ctrl Pts',(9.05582105718531,29.2254609657391,56.4750459441564));
#103338=CARTESIAN_POINT('Ctrl Pts',(9.05510858502812,29.2349823040467,56.4800064820965));
#103339=CARTESIAN_POINT('Ctrl Pts',(9.05347638824164,29.2570022340538,56.4912094011162));
#103340=CARTESIAN_POINT('Ctrl Pts',(9.05255894933391,29.2695328345439,56.4973873573875));
#103341=CARTESIAN_POINT('Ctrl Pts',(9.04965103860313,29.3097227232626,56.5165775777828));
#103342=CARTESIAN_POINT('Ctrl Pts',(9.04768117630316,29.33766395817,56.52898705805));
#103343=CARTESIAN_POINT('Ctrl Pts',(9.04302895226361,29.4051809371577,56.5567747655664));
#103344=CARTESIAN_POINT('Ctrl Pts',(9.04036908224021,29.4450343113215,56.5714231929296));
#103345=CARTESIAN_POINT('Ctrl Pts',(9.03316538820894,29.5555417829254,56.6073116505606));
#103346=CARTESIAN_POINT('Ctrl Pts',(9.02868941773754,29.6271141542294,56.6254077529749));
#103347=CARTESIAN_POINT('Ctrl Pts',(9.02334928855865,29.7129769827958,56.6411451365426));
#103348=CARTESIAN_POINT('Ctrl Pts',(9.02251931711529,29.7263330487208,56.6434250716013));
#103349=CARTESIAN_POINT('Ctrl Pts',(9.01714811733028,29.8127171604241,56.6570889356044));
#103350=CARTESIAN_POINT('Ctrl Pts',(9.01255456462187,29.8863976007119,56.6637639027963));
#103351=CARTESIAN_POINT('Ctrl Pts',(9.00692601924097,29.9725405802788,56.6658189279834));
#103352=CARTESIAN_POINT('Ctrl Pts',(9.00611778419574,29.9848163379132,56.665976036805));
#103353=CARTESIAN_POINT('Ctrl Pts',(9.0048408787324,30.0040404844589,56.6660095895311));
#103354=CARTESIAN_POINT('Ctrl Pts',(9.00437708521899,30.0109885561357,56.6659782487136));
#103355=CARTESIAN_POINT('Ctrl Pts',(9.00350474681917,30.0239877560037,56.6658382918829));
#103356=CARTESIAN_POINT('Ctrl Pts',(9.00309677635804,30.0300387503311,56.6657401645936));
#103357=CARTESIAN_POINT('Ctrl Pts',(9.00213085668382,30.0443001382684,56.6654311611487));
#103358=CARTESIAN_POINT('Ctrl Pts',(9.00157142392235,30.0525096553228,56.6651925365575));
#103359=CARTESIAN_POINT('Ctrl Pts',(8.99968783654224,30.0799943028688,56.6641902011967));
#103360=CARTESIAN_POINT('Ctrl Pts',(8.99835015287118,30.0992570805142,56.6631524485093));
#103361=CARTESIAN_POINT('Ctrl Pts',(8.99502048223286,30.1466794286389,56.6597709073216));
#103362=CARTESIAN_POINT('Ctrl Pts',(8.99301393749694,30.1748051958208,56.6570447437967));
#103363=CARTESIAN_POINT('Ctrl Pts',(8.9838247306023,30.3020994262158,56.6414296646917));
#103364=CARTESIAN_POINT('Ctrl Pts',(8.9764701309106,30.4000540267934,56.6203433649102));
#103365=CARTESIAN_POINT('Ctrl Pts',(8.96328635188567,30.5746117732985,56.5659625293287));
#103366=CARTESIAN_POINT('Ctrl Pts',(8.95742726746579,30.6517580524963,56.5354584023196));
#103367=CARTESIAN_POINT('Ctrl Pts',(8.9504177634592,30.7439419965077,56.4908016294299));
#103368=CARTESIAN_POINT('Ctrl Pts',(8.94908882301312,30.7614078520939,56.4819572638775));
#103369=CARTESIAN_POINT('Ctrl Pts',(8.94697480182236,30.7891619710384,56.4672828793185));
#103370=CARTESIAN_POINT('Ctrl Pts',(8.94618297255658,30.799550657379,56.4616478451445));
#103371=CARTESIAN_POINT('Ctrl Pts',(8.94467910690707,30.8192634211448,56.4506821747156));
#103372=CARTESIAN_POINT('Ctrl Pts',(8.94396642434882,30.8285975896672,56.4453710142629));
#103373=CARTESIAN_POINT('Ctrl Pts',(8.94233293297492,30.8499689450331,56.432935594311));
#103374=CARTESIAN_POINT('Ctrl Pts',(8.94141442063563,30.8619691818833,56.4257491975129));
#103375=CARTESIAN_POINT('Ctrl Pts',(8.93849966168582,30.8999774049968,56.4023324931049));
#103376=CARTESIAN_POINT('Ctrl Pts',(8.93652416040779,30.925629419124,56.385534596638));
#103377=CARTESIAN_POINT('Ctrl Pts',(8.93185579651994,30.9857963952058,56.3437177313079));
#103378=CARTESIAN_POINT('Ctrl Pts',(8.92918564263991,31.0198438113091,56.3180632977824));
#103379=CARTESIAN_POINT('Ctrl Pts',(8.92197730699959,31.1099594331494,56.2445771229049));
#103380=CARTESIAN_POINT('Ctrl Pts',(8.91750625392741,31.1638978437474,56.1942882093984));
#103381=CARTESIAN_POINT('Ctrl Pts',(8.91212697571873,31.2240950862085,56.1301993700254));
#103382=CARTESIAN_POINT('Ctrl Pts',(8.9112531958362,31.2337251221126,56.1196792901001));
#103383=CARTESIAN_POINT('Ctrl Pts',(8.90589476105488,31.2917844259517,56.0545954180717));
#103384=CARTESIAN_POINT('Ctrl Pts',(8.90135742289196,31.3367156392568,55.9970291447507));
#103385=CARTESIAN_POINT('Ctrl Pts',(8.8957912748277,31.3846258643009,55.9265623944582));
#103386=CARTESIAN_POINT('Ctrl Pts',(8.89498320837052,31.3914144077802,55.9163364987807));
#103387=CARTESIAN_POINT('Ctrl Pts',(8.89370646796057,31.4018678646251,55.9002059592704));
#103388=CARTESIAN_POINT('Ctrl Pts',(8.89324266701334,31.4056100290262,55.8943515644891));
#103389=CARTESIAN_POINT('Ctrl Pts',(8.89237028226156,31.4125432127131,55.883354009506));
#103390=CARTESIAN_POINT('Ctrl Pts',(8.89196227251172,31.4157429668173,55.8782166481709));
#103391=CARTESIAN_POINT('Ctrl Pts',(8.89099617160445,31.4232197242359,55.8660653006766));
#103392=CARTESIAN_POINT('Ctrl Pts',(8.8904365957617,31.4274729184495,55.859036989024));
#103393=CARTESIAN_POINT('Ctrl Pts',(8.88855200720881,31.4415450468792,55.835390010543));
#103394=CARTESIAN_POINT('Ctrl Pts',(8.88721344657906,31.451126702301,55.8186328886552));
#103395=CARTESIAN_POINT('Ctrl Pts',(8.88388110120536,31.4740232419693,55.7769242005239));
#103396=CARTESIAN_POINT('Ctrl Pts',(8.88187273069933,31.4869977951015,55.7517932615117));
#103397=CARTESIAN_POINT('Ctrl Pts',(8.87592640617201,31.523178718102,55.6771084654667));
#103398=CARTESIAN_POINT('Ctrl Pts',(8.87194751235138,31.544570813737,55.6267693507067));
#103399=CARTESIAN_POINT('Ctrl Pts',(8.86797183897061,31.5634375186471,55.575516398799));
#103400=CARTESIAN_POINT('Origin',(5.,30.,55.));
#103401=CARTESIAN_POINT('',(8.16625307517082,31.5634376782623,55.5755159651912));
#103402=CARTESIAN_POINT('',(8.36103882979909,31.5634376856231,55.5755159451947));
#103403=CARTESIAN_POINT('',(5.,31.5634376782623,55.5755159651912));
#103404=CARTESIAN_POINT('Ctrl Pts',(8.36103882979909,31.5634376856231,55.5755159451947));
#103405=CARTESIAN_POINT('Ctrl Pts',(8.36205627649009,31.5585956668143,55.5886696983504));
#103406=CARTESIAN_POINT('Ctrl Pts',(8.36307222991977,31.5535870872764,55.6017638659151));
#103407=CARTESIAN_POINT('Ctrl Pts',(8.36843576746039,31.5262117404169,55.6707109554684));
#103408=CARTESIAN_POINT('Ctrl Pts',(8.37273595310039,31.5009962748264,55.7253873979175));
#103409=CARTESIAN_POINT('Ctrl Pts',(8.3788042038508,31.4604844203644,55.8020251027462));
#103410=CARTESIAN_POINT('Ctrl Pts',(8.38064270991459,31.4475349235036,55.8251677328212));
#103411=CARTESIAN_POINT('Ctrl Pts',(8.38393356177099,31.4231244565934,55.8664482070297));
#103412=CARTESIAN_POINT('Ctrl Pts',(8.38539217101872,31.4118553526886,55.8846921791763));
#103413=CARTESIAN_POINT('Ctrl Pts',(8.3876615210663,31.3936183896671,55.9129802718727));
#103414=CARTESIAN_POINT('Ctrl Pts',(8.38848086408679,31.3868871992046,55.9231733874505));
#103415=CARTESIAN_POINT('Ctrl Pts',(8.39000823057807,31.3740658124173,55.942132176784));
#103416=CARTESIAN_POINT('Ctrl Pts',(8.39071720763343,31.3680023442971,55.9509150805632));
#103417=CARTESIAN_POINT('Ctrl Pts',(8.3923041953239,31.3541798214715,55.9705310642995));
#103418=CARTESIAN_POINT('Ctrl Pts',(8.39318037718018,31.3463742998671,55.9813306259722));
#103419=CARTESIAN_POINT('Ctrl Pts',(8.39542499448463,31.325935616332,56.0089061962745));
#103420=CARTESIAN_POINT('Ctrl Pts',(8.39678606958796,31.3131130949825,56.0255393870726));
#103421=CARTESIAN_POINT('Ctrl Pts',(8.4063894878014,31.2196827289862,56.1421095478402));
#103422=CARTESIAN_POINT('Ctrl Pts',(8.41415207298269,31.128075389506,56.2326758698676));
#103423=CARTESIAN_POINT('Ctrl Pts',(8.42714731700296,30.9608330099099,56.3636019305316));
#103424=CARTESIAN_POINT('Ctrl Pts',(8.43232045910536,30.8908860865237,56.4102938096875));
#103425=CARTESIAN_POINT('Ctrl Pts',(8.43870216532561,30.8054625641133,56.4584184117172));
#103426=CARTESIAN_POINT('Ctrl Pts',(8.43962655498679,30.7931099673625,56.4651726019063));
#103427=CARTESIAN_POINT('Ctrl Pts',(8.44104140069344,30.7742656185709,56.4751682514421));
#103428=CARTESIAN_POINT('Ctrl Pts',(8.44152498915339,30.767835489199,56.4785253716999));
#103429=CARTESIAN_POINT('Ctrl Pts',(8.44241414991067,30.7560372658783,56.4845874122119));
#103430=CARTESIAN_POINT('Ctrl Pts',(8.44281890556004,30.7506761896033,56.4873054113144));
#103431=CARTESIAN_POINT('Ctrl Pts',(8.4437507378028,30.7383554763966,56.4934682763078));
#103432=CARTESIAN_POINT('Ctrl Pts',(8.44427896811244,30.7313864012709,56.4968935258967));
#103433=CARTESIAN_POINT('Ctrl Pts',(8.44591343049007,30.7098614556466,56.5072866811455));
#103434=CARTESIAN_POINT('Ctrl Pts',(8.44702867678168,30.6952285709147,56.5140916787555));
#103435=CARTESIAN_POINT('Ctrl Pts',(8.45379903316783,30.6065904147532,56.5537569224189));
#103436=CARTESIAN_POINT('Ctrl Pts',(8.45967662653935,30.5303749060301,56.5813957418237));
#103437=CARTESIAN_POINT('Ctrl Pts',(8.47093284823899,30.3815331505376,56.6233976049849));
#103438=CARTESIAN_POINT('Ctrl Pts',(8.47629712669906,30.3093511513442,56.6386856027348));
#103439=CARTESIAN_POINT('Ctrl Pts',(8.48459249075474,30.1942878553428,56.6551789267522));
#103440=CARTESIAN_POINT('Ctrl Pts',(8.48759132509216,30.1519669194229,56.6595998339502));
#103441=CARTESIAN_POINT('Ctrl Pts',(8.49266871781459,30.0789710662695,56.6644088632391));
#103442=CARTESIAN_POINT('Ctrl Pts',(8.49476880563511,30.0483707606269,56.6655791114978));
#103443=CARTESIAN_POINT('Ctrl Pts',(8.49779003535032,30.0037726874795,56.6660543987042));
#103444=CARTESIAN_POINT('Ctrl Pts',(8.49873164972401,29.9897899359217,56.6660273911016));
#103445=CARTESIAN_POINT('Ctrl Pts',(8.50038688120911,29.9650691642587,56.6656683946309));
#103446=CARTESIAN_POINT('Ctrl Pts',(8.50110270600235,29.9543310751578,56.6654085753201));
#103447=CARTESIAN_POINT('Ctrl Pts',(8.50259985222612,29.9317773424905,56.664644559856));
#103448=CARTESIAN_POINT('Ctrl Pts',(8.50338044663311,29.9199630046799,56.6641183651334));
#103449=CARTESIAN_POINT('Ctrl Pts',(8.50544465656957,29.8885837964544,56.6623858245411));
#103450=CARTESIAN_POINT('Ctrl Pts',(8.50672139226859,29.8690325433054,56.6609598965471));
#103451=CARTESIAN_POINT('Ctrl Pts',(8.51331372961258,29.7674414121054,56.651745506146));
#103452=CARTESIAN_POINT('Ctrl Pts',(8.51844679840904,29.686032601836,56.6382227151438));
#103453=CARTESIAN_POINT('Ctrl Pts',(8.52967070183395,29.5084836991051,56.5950017036998));
#103454=CARTESIAN_POINT('Ctrl Pts',(8.53570216748055,29.4133655981144,56.5625224609065));
#103455=CARTESIAN_POINT('Ctrl Pts',(8.54376391854017,29.2959083315333,56.5101693734412));
#103456=CARTESIAN_POINT('Ctrl Pts',(8.545557656361,29.2703632579819,56.4979942116819));
#103457=CARTESIAN_POINT('Ctrl Pts',(8.54862650761194,29.2279266813487,56.4764253187738));
#103458=CARTESIAN_POINT('Ctrl Pts',(8.54988527641027,29.2108656149202,56.467377175633));
#103459=CARTESIAN_POINT('Ctrl Pts',(8.55170421024368,29.1867743938961,56.4540590254996));
#103460=CARTESIAN_POINT('Ctrl Pts',(8.55225031257358,29.1796119134909,56.4500299709209));
#103461=CARTESIAN_POINT('Ctrl Pts',(8.55320454506792,29.167225112612,56.4429409694294));
#103462=CARTESIAN_POINT('Ctrl Pts',(8.55361114476291,29.1619871883431,56.4399052678831));
#103463=CARTESIAN_POINT('Ctrl Pts',(8.5544885743513,29.1507717538263,56.4333233020826));
#103464=CARTESIAN_POINT('Ctrl Pts',(8.55495992992316,29.1447999424607,56.4297682188284));
#103465=CARTESIAN_POINT('Ctrl Pts',(8.55627020811848,29.1283409314513,56.419829987886));
#103466=CARTESIAN_POINT('Ctrl Pts',(8.5571138777114,29.1179020249927,56.4133682700058));
#103467=CARTESIAN_POINT('Ctrl Pts',(8.56302674093423,29.0457739172337,56.3676104409821));
#103468=CARTESIAN_POINT('Ctrl Pts',(8.56829783249204,28.986665831434,56.3244082556172));
#103469=CARTESIAN_POINT('Ctrl Pts',(8.57463991073829,28.9197268208185,56.2683716770691));
#103470=CARTESIAN_POINT('Ctrl Pts',(8.57567095620926,28.9089762791907,56.2591362474495));
#103471=CARTESIAN_POINT('Ctrl Pts',(8.58206622320197,28.8430616759172,56.2010331907677));
#103472=CARTESIAN_POINT('Ctrl Pts',(8.58743037033348,28.7910693122629,56.1486839919751));
#103473=CARTESIAN_POINT('Ctrl Pts',(8.59572623647197,28.7148007825884,56.0609565121179));
#103474=CARTESIAN_POINT('Ctrl Pts',(8.5987256730966,28.6881277174367,56.0277924725809));
#103475=CARTESIAN_POINT('Ctrl Pts',(8.60380396940839,28.6444893757952,55.9690637294101));
#103476=CARTESIAN_POINT('Ctrl Pts',(8.60590436855001,28.6269071670899,55.9439861493138));
#103477=CARTESIAN_POINT('Ctrl Pts',(8.60892596337948,28.602316716161,55.906770618742));
#103478=CARTESIAN_POINT('Ctrl Pts',(8.60986763814666,28.5947552561777,55.895007680189));
#103479=CARTESIAN_POINT('Ctrl Pts',(8.61152294507793,28.581648757723,55.8740429751129));
#103480=CARTESIAN_POINT('Ctrl Pts',(8.61223878544998,28.576043033867,55.8648803019511));
#103481=CARTESIAN_POINT('Ctrl Pts',(8.61373593447631,28.5644527037283,55.8455174728347));
#103482=CARTESIAN_POINT('Ctrl Pts',(8.61451651638392,28.5584872802521,55.8353064872514));
#103483=CARTESIAN_POINT('Ctrl Pts',(8.61658062428933,28.5429248722342,55.8080050848434));
#103484=CARTESIAN_POINT('Ctrl Pts',(8.61785727193711,28.5335197151259,55.7908070382551));
#103485=CARTESIAN_POINT('Ctrl Pts',(8.62444643346127,28.4861850338615,55.7005019933978));
#103486=CARTESIAN_POINT('Ctrl Pts',(8.62957665226229,28.4534090839173,55.6248182193147));
#103487=CARTESIAN_POINT('Ctrl Pts',(8.64080026141045,28.3934132303803,55.4522229888109));
#103488=CARTESIAN_POINT('Ctrl Pts',(8.64683403084159,28.3690975507752,55.3546569237867));
#103489=CARTESIAN_POINT('Ctrl Pts',(8.65489854654159,28.3493687251707,55.227537462718));
#103490=CARTESIAN_POINT('Ctrl Pts',(8.65669259725022,28.3457420320228,55.1994675340614));
#103491=CARTESIAN_POINT('Ctrl Pts',(8.65976193398912,28.3408460214315,55.1521088679756));
#103492=CARTESIAN_POINT('Ctrl Pts',(8.66102086942313,28.3391942281276,55.1328651286049));
#103493=CARTESIAN_POINT('Ctrl Pts',(8.66284000985164,28.3373170226287,55.1053985864034));
#103494=CARTESIAN_POINT('Ctrl Pts',(8.66338614849168,28.336817324566,55.0971953002256));
#103495=CARTESIAN_POINT('Ctrl Pts',(8.66434043647391,28.3360549507858,55.0829429384075));
#103496=CARTESIAN_POINT('Ctrl Pts',(8.6647470551388,28.3357645221633,55.0768955837515));
#103497=CARTESIAN_POINT('Ctrl Pts',(8.66562452871365,28.3352114920588,55.0639025155719));
#103498=CARTESIAN_POINT('Ctrl Pts',(8.66609590933853,28.3349593922591,55.0569568067692));
#103499=CARTESIAN_POINT('Ctrl Pts',(8.6674062362673,28.3343822228256,55.0377379867326));
#103500=CARTESIAN_POINT('Ctrl Pts',(8.66824992930461,28.3341493592813,55.0254628354024));
#103501=CARTESIAN_POINT('Ctrl Pts',(8.67416389953594,28.333473131712,54.9400312543727));
#103502=CARTESIAN_POINT('Ctrl Pts',(8.67943614048649,28.3377134140135,54.8669248783947));
#103503=CARTESIAN_POINT('Ctrl Pts',(8.68577826874258,28.3484899467498,54.780293416415));
#103504=CARTESIAN_POINT('Ctrl Pts',(8.68680824145774,28.3504166264213,54.7662669714259));
#103505=CARTESIAN_POINT('Ctrl Pts',(8.6932021576332,28.3634798461617,54.6793937769295));
#103506=CARTESIAN_POINT('Ctrl Pts',(8.69856601264265,28.379261587988,54.6073234484704));
#103507=CARTESIAN_POINT('Ctrl Pts',(8.70686093306862,28.4115969197425,54.4956780143239));
#103508=CARTESIAN_POINT('Ctrl Pts',(8.70985972455127,28.4249899914488,54.4552899976558));
#103509=CARTESIAN_POINT('Ctrl Pts',(8.71493706540982,28.4506571189974,54.3867872130853));
#103510=CARTESIAN_POINT('Ctrl Pts',(8.71703714167927,28.4621877079846,54.3584184749675));
#103511=CARTESIAN_POINT('Ctrl Pts',(8.72005838896884,28.4801142091657,54.3175788054269));
#103512=CARTESIAN_POINT('Ctrl Pts',(8.72100003067838,28.485895227142,54.3048465913996));
#103513=CARTESIAN_POINT('Ctrl Pts',(8.72265532552244,28.496399527294,54.2824646390722));
#103514=CARTESIAN_POINT('Ctrl Pts',(8.72337118620915,28.5010570673973,54.2727851281822));
#103515=CARTESIAN_POINT('Ctrl Pts',(8.72486842380179,28.5110386027274,54.2525444368429));
#103516=CARTESIAN_POINT('Ctrl Pts',(8.72564907347848,28.5163821150826,54.2419935058615));
#103517=CARTESIAN_POINT('Ctrl Pts',(8.72771347101432,28.5308802208721,54.2141072885434));
#103518=CARTESIAN_POINT('Ctrl Pts',(8.72899033767368,28.5402293682744,54.1968748324737));
#103519=CARTESIAN_POINT('Ctrl Pts',(8.7355856539571,28.5904717925098,54.1080447156981));
#103520=CARTESIAN_POINT('Ctrl Pts',(8.74072136238261,28.6363367066296,54.0393861859714));
#103521=CARTESIAN_POINT('Ctrl Pts',(8.75194552477794,28.7488329683305,53.8953768822272));
#103522=CARTESIAN_POINT('Ctrl Pts',(8.75797484606344,28.8175673694881,53.8220942727128));
#103523=CARTESIAN_POINT('Ctrl Pts',(8.76603401967559,28.9136019400408,53.7366332231265));
#103524=CARTESIAN_POINT('Ctrl Pts',(8.76782748247126,28.9352104450464,53.7183684691837));
#103525=CARTESIAN_POINT('Ctrl Pts',(8.77089591604756,28.9723317549512,53.6885783185242));
#103526=CARTESIAN_POINT('Ctrl Pts',(8.77215454880021,28.9875995200781,53.6767562436189));
#103527=CARTESIAN_POINT('Ctrl Pts',(8.77397332815621,29.0096525779383,53.6602852855893));
#103528=CARTESIAN_POINT('Ctrl Pts',(8.77451941604781,29.0162728008566,53.6554166730715));
#103529=CARTESIAN_POINT('Ctrl Pts',(8.77547362680052,29.0278322707947,53.6470467268552));
#103530=CARTESIAN_POINT('Ctrl Pts',(8.77588021930316,29.0327550240435,53.6435230159822));
#103531=CARTESIAN_POINT('Ctrl Pts',(8.77675761398086,29.0433700381244,53.6360119455495));
#103532=CARTESIAN_POINT('Ctrl Pts',(8.77722894166771,29.0490679875311,53.6320334068777));
#103533=CARTESIAN_POINT('Ctrl Pts',(8.77853918054754,29.0649002422733,53.6211253990517));
#103534=CARTESIAN_POINT('Ctrl Pts',(8.77938283919927,29.0750862709956,53.6142722872705));
#103535=CARTESIAN_POINT('Ctrl Pts',(8.78530376321517,29.1465771447837,53.5673129378853));
#103536=CARTESIAN_POINT('Ctrl Pts',(8.79058358863294,29.2103872518454,53.5311800256463));
#103537=CARTESIAN_POINT('Ctrl Pts',(8.79692823295547,29.2890494401745,53.4932472709247));
#103538=CARTESIAN_POINT('Ctrl Pts',(8.79795319720536,29.3018165494048,53.4872890723419));
#103539=CARTESIAN_POINT('Ctrl Pts',(8.80434326283068,29.3818391817626,53.4511727286867));
#103540=CARTESIAN_POINT('Ctrl Pts',(8.80970823356939,29.4509631091155,53.4253417773784));
#103541=CARTESIAN_POINT('Ctrl Pts',(8.81800323613674,29.5623025569032,53.3919624209005));
#103542=CARTESIAN_POINT('Ctrl Pts',(8.82100109501396,29.6034862089017,53.3813149708069));
#103543=CARTESIAN_POINT('Ctrl Pts',(8.82607700920438,29.6749402197358,53.3657328917174));
#103544=CARTESIAN_POINT('Ctrl Pts',(8.82817657985738,29.7050208974012,53.3600364684965));
#103545=CARTESIAN_POINT('Ctrl Pts',(8.83119716665653,29.7490454986412,53.3529501294377));
#103546=CARTESIAN_POINT('Ctrl Pts',(8.8321386461157,29.7628755183767,53.3509022349246));
#103547=CARTESIAN_POINT('Ctrl Pts',(8.83379367495203,29.7873729445972,53.3475893131375));
#103548=CARTESIAN_POINT('Ctrl Pts',(8.83450943126546,29.7980297143815,53.346252934769));
#103549=CARTESIAN_POINT('Ctrl Pts',(8.83600646603725,29.8204455117738,53.3436618664201));
#103550=CARTESIAN_POINT('Ctrl Pts',(8.83678701723942,29.8322065133456,53.3424291312385));
#103551=CARTESIAN_POINT('Ctrl Pts',(8.83885118222315,29.8634948138343,53.3394860628645));
#103552=CARTESIAN_POINT('Ctrl Pts',(8.8401279152448,29.8830412323286,53.3379949156085));
#103553=CARTESIAN_POINT('Ctrl Pts',(8.8467222078802,29.984905580873,53.3320299982524));
#103554=CARTESIAN_POINT('Ctrl Pts',(8.85185707068511,30.06745050934,53.3333252636355));
#103555=CARTESIAN_POINT('Ctrl Pts',(8.86308118628233,30.2494532078754,53.3497312312895));
#103556=CARTESIAN_POINT('Ctrl Pts',(8.86911122386991,30.3483136382028,53.367734955653));
#103557=CARTESIAN_POINT('Ctrl Pts',(8.8771712662145,30.4722125859457,53.4020726878313));
#103558=CARTESIAN_POINT('Ctrl Pts',(8.87896479071521,30.4992782165408,53.4103215723689));
#103559=CARTESIAN_POINT('Ctrl Pts',(8.88203330015515,30.5444404486352,53.4253529115653));
#103560=CARTESIAN_POINT('Ctrl Pts',(8.88329194289921,30.562653424005,53.4317685433296));
#103561=CARTESIAN_POINT('Ctrl Pts',(8.88511070348003,30.5884517182196,53.4413633842885));
#103562=CARTESIAN_POINT('Ctrl Pts',(8.88565676015999,30.5961321227428,53.4442847272902));
#103563=CARTESIAN_POINT('Ctrl Pts',(8.88661092159961,30.6094327224263,53.4494567382818));
#103564=CARTESIAN_POINT('Ctrl Pts',(8.88701749610584,30.6150627705936,53.4516814163397));
#103565=CARTESIAN_POINT('Ctrl Pts',(8.88789488641821,30.6271301870447,53.456525987319));
#103566=CARTESIAN_POINT('Ctrl Pts',(8.88836622801419,30.6335632277531,53.4591554486718));
#103567=CARTESIAN_POINT('Ctrl Pts',(8.8896764567769,30.6513140726288,53.4665409390363));
#103568=CARTESIAN_POINT('Ctrl Pts',(8.89052009068216,30.6625957812576,53.4713818261564));
#103569=CARTESIAN_POINT('Ctrl Pts',(8.89642020845009,30.7405469393167,53.5058550554763));
#103570=CARTESIAN_POINT('Ctrl Pts',(8.90167759448997,30.8052538295571,53.5397113998074));
#103571=CARTESIAN_POINT('Ctrl Pts',(8.90801559435536,30.8797364771311,53.5851416012652));
#103572=CARTESIAN_POINT('Ctrl Pts',(8.90905610408381,30.891850295866,53.5927460771268));
#103573=CARTESIAN_POINT('Ctrl Pts',(8.91545986324786,30.9657593255029,53.6404802841695));
#103574=CARTESIAN_POINT('Ctrl Pts',(8.92082315572547,31.0249378234739,53.6845195943871));
#103575=CARTESIAN_POINT('Ctrl Pts',(8.92912216116893,31.1134180458005,53.7599716080982));
#103576=CARTESIAN_POINT('Ctrl Pts',(8.93212539735323,31.1447574534946,53.7888431005033));
#103577=CARTESIAN_POINT('Ctrl Pts',(8.93720937597408,31.1966854596676,53.8405004664004));
#103578=CARTESIAN_POINT('Ctrl Pts',(8.93931172232874,31.2178135270761,53.862711256745));
#103579=CARTESIAN_POINT('Ctrl Pts',(8.94233557728322,31.2476755165954,53.8958906461361));
#103580=CARTESIAN_POINT('Ctrl Pts',(8.94327760729109,31.2569019163401,53.9064053523242));
#103581=CARTESIAN_POINT('Ctrl Pts',(8.94493333658898,31.2729777268657,53.9251981129967));
#103582=CARTESIAN_POINT('Ctrl Pts',(8.94564924744788,31.2798814345576,53.9334284308271));
#103583=CARTESIAN_POINT('Ctrl Pts',(8.94714634714123,31.2942156155117,53.9508566674604));
#103584=CARTESIAN_POINT('Ctrl Pts',(8.9479268110971,31.3016287706111,53.9600681044917));
#103585=CARTESIAN_POINT('Ctrl Pts',(8.94999014895215,31.3210620786838,53.984748932016));
#103586=CARTESIAN_POINT('Ctrl Pts',(8.95126615464385,31.3329087470012,54.0003530265854));
#103587=CARTESIAN_POINT('Ctrl Pts',(8.95783371841241,31.392920719157,54.0823633260575));
#103588=CARTESIAN_POINT('Ctrl Pts',(8.9629445804669,31.4364112935496,54.1520552825639));
#103589=CARTESIAN_POINT('Ctrl Pts',(8.97416638327103,31.5214237126474,54.3137409249979));
#103590=CARTESIAN_POINT('Ctrl Pts',(8.98021596675857,31.5600845942449,54.4068597668906));
#103591=CARTESIAN_POINT('Ctrl Pts',(8.98829946599533,31.5985611533171,54.5299349960784));
#103592=CARTESIAN_POINT('Ctrl Pts',(8.99009564512755,31.6063240843312,54.5571889525425));
#103593=CARTESIAN_POINT('Ctrl Pts',(8.99316827400936,31.6182077206386,54.6033471469372));
#103594=CARTESIAN_POINT('Ctrl Pts',(8.99442833093867,31.6227011031554,54.6221498119952));
#103595=CARTESIAN_POINT('Ctrl Pts',(8.99624884499023,31.6286376972994,54.6490543438868));
#103596=CARTESIAN_POINT('Ctrl Pts',(8.99679520997813,31.6303498096392,54.6570960866291));
#103597=CARTESIAN_POINT('Ctrl Pts',(8.9977498283048,31.633219510297,54.6710825208833));
#103598=CARTESIAN_POINT('Ctrl Pts',(8.99815654944529,31.634404322585,54.6770213848546));
#103599=CARTESIAN_POINT('Ctrl Pts',(8.99903423950952,31.6368797218294,54.689791830915));
#103600=CARTESIAN_POINT('Ctrl Pts',(8.99950573412987,31.6381599180794,54.6966249675829));
#103601=CARTESIAN_POINT('Ctrl Pts',(9.00081619383511,31.6415826321533,54.7155475315672));
#103602=CARTESIAN_POINT('Ctrl Pts',(9.0016599028148,31.643634280061,54.727652655071));
#103603=CARTESIAN_POINT('Ctrl Pts',(9.00754905743618,31.6569229221559,54.8116856160863));
#103604=CARTESIAN_POINT('Ctrl Pts',(9.0127943932279,31.6635672820153,54.8842527319199));
#103605=CARTESIAN_POINT('Ctrl Pts',(9.01908762315329,31.6658027503877,54.9708607651056));
#103606=CARTESIAN_POINT('Ctrl Pts',(9.02009528315077,31.6659874532099,54.9847127389741));
#103607=CARTESIAN_POINT('Ctrl Pts',(9.03044946508363,31.6661099731375,55.1269885512871));
#103608=CARTESIAN_POINT('Ctrl Pts',(9.03975371819533,31.6513708722469,55.2550189113104));
#103609=CARTESIAN_POINT('Ctrl Pts',(9.05003537295159,31.6172724846976,55.4005322823692));
#103610=CARTESIAN_POINT('Ctrl Pts',(9.05146704967117,31.6120987630031,55.4208729580537));
#103611=CARTESIAN_POINT('Ctrl Pts',(9.05378749781389,31.6030145318558,55.4539580287628));
#103612=CARTESIAN_POINT('Ctrl Pts',(9.05468350440069,31.5993331225526,55.4667623187593));
#103613=CARTESIAN_POINT('Ctrl Pts',(9.05628847251154,31.5924259068171,55.4897445084674));
#103614=CARTESIAN_POINT('Ctrl Pts',(9.05699917740378,31.5892551434346,55.4999380466049));
#103615=CARTESIAN_POINT('Ctrl Pts',(9.05851677195906,31.5822442987145,55.5217359139965));
#103616=CARTESIAN_POINT('Ctrl Pts',(9.05932262640994,31.5783740304096,55.5333299337659));
#103617=CARTESIAN_POINT('Ctrl Pts',(9.06083570059036,31.5708299486596,55.5551277827587));
#103618=CARTESIAN_POINT('Ctrl Pts',(9.06154373499386,31.5671835233094,55.5653400610581));
#103619=CARTESIAN_POINT('Ctrl Pts',(9.06224863102697,31.5634376784283,55.5755159647401));
#103620=CARTESIAN_POINT('',(8.82705497355655,31.6659999398532,54.9995523290613));
#103621=CARTESIAN_POINT('Ctrl Pts',(8.86797183897061,31.5634375186471,55.575516398799));
#103622=CARTESIAN_POINT('Ctrl Pts',(8.86184835557125,31.5924967353516,55.4965746523031));
#103623=CARTESIAN_POINT('Ctrl Pts',(8.85573816968857,31.6155646837455,55.4154644668671));
#103624=CARTESIAN_POINT('Ctrl Pts',(8.84631919559105,31.6421995656765,55.28484965997));
#103625=CARTESIAN_POINT('Ctrl Pts',(8.84291221592427,31.6498699883968,55.2364077125598));
#103626=CARTESIAN_POINT('Ctrl Pts',(8.83841122193728,31.6573110519839,55.1707800307525));
#103627=CARTESIAN_POINT('Ctrl Pts',(8.83725933668326,31.658969484026,55.1538376753291));
#103628=CARTESIAN_POINT('Ctrl Pts',(8.83535763833246,31.661294759191,55.125630272975));
#103629=CARTESIAN_POINT('Ctrl Pts',(8.83460332395891,31.6621073148942,55.1143788747463));
#103630=CARTESIAN_POINT('Ctrl Pts',(8.83317998162107,31.6634310863907,55.0930330850496));
#103631=CARTESIAN_POINT('Ctrl Pts',(8.83251028085413,31.6639648402148,55.082940655086));
#103632=CARTESIAN_POINT('Ctrl Pts',(8.83105713180266,31.6649277509197,55.0609391251755));
#103633=CARTESIAN_POINT('Ctrl Pts',(8.83027483098005,31.6653210400976,55.0490289545022));
#103634=CARTESIAN_POINT('Ctrl Pts',(8.82867835061849,31.665865484226,55.0245964937025));
#103635=CARTESIAN_POINT('Ctrl Pts',(8.82786462710371,31.6660033047414,55.0120747044674));
#103636=CARTESIAN_POINT('Ctrl Pts',(8.82705497355655,31.6659999398532,54.9995523290613));
#103637=CARTESIAN_POINT('Ctrl Pts',(8.82705505845663,31.6659999402055,54.9995536421544));
#103638=CARTESIAN_POINT('Ctrl Pts',(8.82553610359139,31.6659936460075,54.9760609811571));
#103639=CARTESIAN_POINT('Ctrl Pts',(8.82403175635443,31.6654904404392,54.9525700214294));
#103640=CARTESIAN_POINT('Ctrl Pts',(8.81396003855586,31.6587392066447,54.7940820609814));
#103641=CARTESIAN_POINT('Ctrl Pts',(8.80588759280819,31.6365833860729,54.6602746920782));
#103642=CARTESIAN_POINT('Ctrl Pts',(8.79388677069296,31.5817697377278,54.4736064599062));
#103643=CARTESIAN_POINT('Ctrl Pts',(8.79017179395581,31.5619953544911,54.4175442576192));
#103644=CARTESIAN_POINT('Ctrl Pts',(8.78533510573124,31.5335120722739,54.3487523994713));
#103645=CARTESIAN_POINT('Ctrl Pts',(8.78434795440504,31.5275638649981,54.3349200705605));
#103646=CARTESIAN_POINT('Ctrl Pts',(8.78285664760139,31.5183948032396,54.3143698643188));
#103647=CARTESIAN_POINT('Ctrl Pts',(8.78236052743893,31.515314849947,54.3075894558272));
#103648=CARTESIAN_POINT('Ctrl Pts',(8.78145963817243,31.5096713422155,54.2953834760889));
#103649=CARTESIAN_POINT('Ctrl Pts',(8.78105583435059,31.5071237951953,54.2899507973767));
#103650=CARTESIAN_POINT('Ctrl Pts',(8.78014062095601,31.5013096242896,54.2777242654838));
#103651=CARTESIAN_POINT('Ctrl Pts',(8.7796282258575,31.4980262302407,54.2709388004939));
#103652=CARTESIAN_POINT('Ctrl Pts',(8.77805247463645,31.4878396145204,54.2502464825534));
#103653=CARTESIAN_POINT('Ctrl Pts',(8.77698075865629,31.4807881631426,54.2364140989553));
#103654=CARTESIAN_POINT('Ctrl Pts',(8.76869598900977,31.4252696380621,54.1311687196831));
#103655=CARTESIAN_POINT('Ctrl Pts',(8.76111592793846,31.3685784785411,54.0443583821508));
#103656=CARTESIAN_POINT('Ctrl Pts',(8.74555632899655,31.2354270282251,53.8768367646623));
#103657=CARTESIAN_POINT('Ctrl Pts',(8.73763023200618,31.1581918838061,53.7973465458893));
#103658=CARTESIAN_POINT('Ctrl Pts',(8.72900065786744,31.0619743711026,53.7162558433822));
#103659=CARTESIAN_POINT('Ctrl Pts',(8.72796105483216,31.0501770810135,53.7065871696235));
#103660=CARTESIAN_POINT('Ctrl Pts',(8.72598363199649,31.0273454410484,53.6883934655784));
#103661=CARTESIAN_POINT('Ctrl Pts',(8.72504482586285,31.0163336496218,53.6798423239843));
#103662=CARTESIAN_POINT('Ctrl Pts',(8.72339295013933,30.9966566009004,53.6649543786674));
#103663=CARTESIAN_POINT('Ctrl Pts',(8.72267769972337,30.9880351360616,53.658561305787));
#103664=CARTESIAN_POINT('Ctrl Pts',(8.72118021452816,30.9697742945875,53.6452919144908));
#103665=CARTESIAN_POINT('Ctrl Pts',(8.72039872111644,30.9601221502674,53.6384341190626));
#103666=CARTESIAN_POINT('Ctrl Pts',(8.71832853385494,30.934234190799,53.6204530577542));
#103667=CARTESIAN_POINT('Ctrl Pts',(8.71704679639953,30.9178726980463,53.6095133756436));
#103668=CARTESIAN_POINT('Ctrl Pts',(8.71044161629415,30.8319045157143,53.5542118242739));
#103669=CARTESIAN_POINT('Ctrl Pts',(8.7053011840619,30.7592616308765,53.5147751583784));
#103670=CARTESIAN_POINT('Ctrl Pts',(8.69408423991596,30.5927258897614,53.439792016934));
#103671=CARTESIAN_POINT('Ctrl Pts',(8.68806591503792,30.4979543025982,53.4070115811314));
#103672=CARTESIAN_POINT('Ctrl Pts',(8.68002004403746,30.3733864048549,53.3761350176207));
#103673=CARTESIAN_POINT('Ctrl Pts',(8.6782281655632,30.3457849104645,53.3700345083538));
#103674=CARTESIAN_POINT('Ctrl Pts',(8.67516224622675,30.2991029521632,53.3609558497359));
#103675=CARTESIAN_POINT('Ctrl Pts',(8.67390451237128,30.280101087901,53.3576018737098));
#103676=CARTESIAN_POINT('Ctrl Pts',(8.67208691732575,30.2529339655181,53.353291806335));
#103677=CARTESIAN_POINT('Ctrl Pts',(8.67154109405221,30.2448124584464,53.3520648316177));
#103678=CARTESIAN_POINT('Ctrl Pts',(8.67058728555508,30.2306916733415,53.3500381882641));
#103679=CARTESIAN_POINT('Ctrl Pts',(8.6701808286422,30.2246965726348,53.3492110742926));
#103680=CARTESIAN_POINT('Ctrl Pts',(8.66930364431018,30.2118085646209,53.347504489152));
#103681=CARTESIAN_POINT('Ctrl Pts',(8.6688323909263,30.2049147267133,53.3466354812707));
#103682=CARTESIAN_POINT('Ctrl Pts',(8.66752228513739,30.185826776063,53.3443505471011));
#103683=CARTESIAN_POINT('Ctrl Pts',(8.66667868599297,30.1736224257632,53.3430262727635));
#103684=CARTESIAN_POINT('Ctrl Pts',(8.6607400783166,30.0882358483373,53.3347147727091));
#103685=CARTESIAN_POINT('Ctrl Pts',(8.65544110967738,30.0146832630126,53.3324441660386));
#103686=CARTESIAN_POINT('Ctrl Pts',(8.64909088675572,29.9273340514737,53.3355274088435));
#103687=CARTESIAN_POINT('Ctrl Pts',(8.6480792702371,29.9134445347966,53.336191869634));
#103688=CARTESIAN_POINT('Ctrl Pts',(8.64170115626646,29.8259723798899,53.3414747452173));
#103689=CARTESIAN_POINT('Ctrl Pts',(8.63633492771701,29.7527512672942,53.3507998868397));
#103690=CARTESIAN_POINT('Ctrl Pts',(8.62804290047012,29.6387091217188,53.3730924525723));
#103691=CARTESIAN_POINT('Ctrl Pts',(8.6250490546401,29.5973570852291,53.3828301107252));
#103692=CARTESIAN_POINT('Ctrl Pts',(8.61997918816134,29.5269451683638,53.4022797052534));
#103693=CARTESIAN_POINT('Ctrl Pts',(8.61788172043162,29.497699133649,53.4112315880915));
#103694=CARTESIAN_POINT('Ctrl Pts',(8.61486367308045,29.4554710290015,53.4254399215573));
#103695=CARTESIAN_POINT('Ctrl Pts',(8.61392267684296,29.44228395252,53.430062398717));
#103696=CARTESIAN_POINT('Ctrl Pts',(8.61226832343055,29.4190693113459,53.4385292780688));
#103697=CARTESIAN_POINT('Ctrl Pts',(8.61155276327038,29.4090179904489,53.4423056929766));
#103698=CARTESIAN_POINT('Ctrl Pts',(8.61005597357871,29.3879757368174,53.4504445441467));
#103699=CARTESIAN_POINT('Ctrl Pts',(8.60927547247432,29.3769932900719,53.4548273685418));
#103700=CARTESIAN_POINT('Ctrl Pts',(8.60721106582747,29.3479275418711,53.466787071259));
#103701=CARTESIAN_POINT('Ctrl Pts',(8.60593404573643,29.3299294045247,53.4745670040198));
#103702=CARTESIAN_POINT('Ctrl Pts',(8.59932454190857,29.2367812274761,53.5167983797557));
#103703=CARTESIAN_POINT('Ctrl Pts',(8.59417587667596,29.1641305092543,53.5564922479013));
#103704=CARTESIAN_POINT('Ctrl Pts',(8.58295044249539,29.0106939113296,53.6558095623349));
#103705=CARTESIAN_POINT('Ctrl Pts',(8.57693165756953,28.9317460849413,53.7176561685824));
#103706=CARTESIAN_POINT('Ctrl Pts',(8.5688852400486,28.8382373814483,53.8055701933716));
#103707=CARTESIAN_POINT('Ctrl Pts',(8.56709329829167,28.8181412185335,53.825451326926));
#103708=CARTESIAN_POINT('Ctrl Pts',(8.56402727886024,28.785194025901,53.8597479361411));
#103709=CARTESIAN_POINT('Ctrl Pts',(8.5627695090207,28.7720698560035,53.8738935185878));
#103710=CARTESIAN_POINT('Ctrl Pts',(8.56095186516394,28.7537137636402,53.8943806775853));
#103711=CARTESIAN_POINT('Ctrl Pts',(8.56040602957827,28.7482779775385,53.9005385679675));
#103712=CARTESIAN_POINT('Ctrl Pts',(8.55945220306337,28.7389164986006,53.9113030578484));
#103713=CARTESIAN_POINT('Ctrl Pts',(8.5590457405223,28.7349700120069,53.9158912612256));
#103714=CARTESIAN_POINT('Ctrl Pts',(8.55816855126101,28.7265461748394,53.9257934851969));
#103715=CARTESIAN_POINT('Ctrl Pts',(8.55769729863433,28.7220771094003,53.9311139618555));
#103716=CARTESIAN_POINT('Ctrl Pts',(8.55638719524231,28.7098048090319,53.9459112607604));
#103717=CARTESIAN_POINT('Ctrl Pts',(8.55554359775215,28.702073021989,53.9554463926474));
#103718=CARTESIAN_POINT('Ctrl Pts',(8.54960515949182,28.6487809308619,54.022673481444));
#103719=CARTESIAN_POINT('Ctrl Pts',(8.54430637170586,28.6069821324187,54.0832345327938));
#103720=CARTESIAN_POINT('Ctrl Pts',(8.53795623954585,28.5621975538289,54.1582913174384));
#103721=CARTESIAN_POINT('Ctrl Pts',(8.5369445349373,28.5552219473771,54.1703218963868));
#103722=CARTESIAN_POINT('Ctrl Pts',(8.53056636141165,28.512217831074,54.2466768334407));
#103723=CARTESIAN_POINT('Ctrl Pts',(8.52520015924222,28.4803396438246,54.3132501962001));
#103724=CARTESIAN_POINT('Ctrl Pts',(8.51690810723396,28.4372155934243,54.4211526794455));
#103725=CARTESIAN_POINT('Ctrl Pts',(8.51391421336267,28.4229683669556,54.4611762335098));
#103726=CARTESIAN_POINT('Ctrl Pts',(8.50884427917112,28.4011193705922,54.5308819288071));
#103727=CARTESIAN_POINT('Ctrl Pts',(8.50674679078772,28.3927780522181,54.5603082267925));
#103728=CARTESIAN_POINT('Ctrl Pts',(8.50372872344318,28.3818118683094,54.6034922304952));
#103729=CARTESIAN_POINT('Ctrl Pts',(8.50278772726036,28.3785431708655,54.6170783203686));
#103730=CARTESIAN_POINT('Ctrl Pts',(8.50113337778597,28.3730657096828,54.6411740056661));
#103731=CARTESIAN_POINT('Ctrl Pts',(8.50041782146082,28.370786941366,54.6516666853801));
#103732=CARTESIAN_POINT('Ctrl Pts',(8.49892104370957,28.3662121421728,54.6737592266454));
#103733=CARTESIAN_POINT('Ctrl Pts',(8.49814055066797,28.3639378412726,54.6853630163244));
#103734=CARTESIAN_POINT('Ctrl Pts',(8.4960761750838,28.3582214629008,54.7162684423323));
#103735=CARTESIAN_POINT('Ctrl Pts',(8.49479917774291,28.3549961604493,54.7356086571121));
#103736=CARTESIAN_POINT('Ctrl Pts',(8.48819039339495,28.3399575555467,54.8367601825694));
#103737=CARTESIAN_POINT('Ctrl Pts',(8.48304237366808,28.3339025974047,54.9193148422241));
#103738=CARTESIAN_POINT('Ctrl Pts',(8.47181688524308,28.3341205591325,55.1020901699696));
#103739=CARTESIAN_POINT('Ctrl Pts',(8.4657974650397,28.3432617835874,55.2019724125215));
#103740=CARTESIAN_POINT('Ctrl Pts',(8.45775027725041,28.3664082481482,55.3282270770604));
#103741=CARTESIAN_POINT('Ctrl Pts',(8.45595824904168,28.3722120477668,55.3558949680674));
#103742=CARTESIAN_POINT('Ctrl Pts',(8.45289209763865,28.3831571896435,55.4021786629869));
#103743=CARTESIAN_POINT('Ctrl Pts',(8.45163428439331,28.3879235934513,55.4208775736203));
#103744=CARTESIAN_POINT('Ctrl Pts',(8.44981659164693,28.3951802673527,55.447411550849));
#103745=CARTESIAN_POINT('Ctrl Pts',(8.44927075186763,28.397405624294,55.4553182733951));
#103746=CARTESIAN_POINT('Ctrl Pts',(8.44831692322422,28.4013720257761,55.4690215656168));
#103747=CARTESIAN_POINT('Ctrl Pts',(8.44791046283195,28.4030863358875,55.474825628007));
#103748=CARTESIAN_POINT('Ctrl Pts',(8.4470332836435,28.4068368002712,55.487273330573));
#103749=CARTESIAN_POINT('Ctrl Pts',(8.44656203899971,28.4088828710595,55.4939135119102));
#103750=CARTESIAN_POINT('Ctrl Pts',(8.44525197541004,28.4146584994855,55.5122489789224));
#103751=CARTESIAN_POINT('Ctrl Pts',(8.44440841015877,28.418475788029,55.5239158658659));
#103752=CARTESIAN_POINT('Ctrl Pts',(8.43847834899337,28.4460135369473,55.6050359240063));
#103753=CARTESIAN_POINT('Ctrl Pts',(8.43318856979112,28.4741696063173,55.6728904955669));
#103754=CARTESIAN_POINT('Ctrl Pts',(8.42684061355435,28.5129091604143,55.7512075613265));
#103755=CARTESIAN_POINT('Ctrl Pts',(8.42582217631955,28.5192737127025,55.7636763868469));
#103756=CARTESIAN_POINT('Ctrl Pts',(8.41943779376698,28.560134796905,55.8412958516943));
#103757=CARTESIAN_POINT('Ctrl Pts',(8.41407206409622,28.5987690156022,55.9041811520905));
#103758=CARTESIAN_POINT('Ctrl Pts',(8.40577891398666,28.6660352119208,55.9989489437549));
#103759=CARTESIAN_POINT('Ctrl Pts',(8.4027835333492,28.6919444326111,56.0326432986966));
#103760=CARTESIAN_POINT('Ctrl Pts',(8.39771139040445,28.7386753921521,56.0888305268553));
#103761=CARTESIAN_POINT('Ctrl Pts',(8.39561315459719,28.7588803043475,56.1118065465268));
#103762=CARTESIAN_POINT('Ctrl Pts',(8.39259422869578,28.7892216466417,56.1444505543991));
#103763=CARTESIAN_POINT('Ctrl Pts',(8.39165310491,28.7988642995752,56.1545667335652));
#103764=CARTESIAN_POINT('Ctrl Pts',(8.38999861211679,28.8161387251966,56.1722387837488));
#103765=CARTESIAN_POINT('Ctrl Pts',(8.38928303876903,28.8237182877485,56.1798443231228));
#103766=CARTESIAN_POINT('Ctrl Pts',(8.38778630448792,28.8397974140994,56.1956695797933));
#103767=CARTESIAN_POINT('Ctrl Pts',(8.38700587117656,28.8483120466164,56.2038731887268));
#103768=CARTESIAN_POINT('Ctrl Pts',(8.38494183873673,28.8711726813434,56.2254342390859));
#103769=CARTESIAN_POINT('Ctrl Pts',(8.38366512064124,28.8856685750143,56.2386305815535));
#103770=CARTESIAN_POINT('Ctrl Pts',(8.37706593008509,28.9623810134926,56.3060287464395));
#103771=CARTESIAN_POINT('Ctrl Pts',(8.37192651587782,29.0283316036291,56.3558123985024));
#103772=CARTESIAN_POINT('Ctrl Pts',(8.36070163156955,29.1819640516161,56.4547917565012));
#103773=CARTESIAN_POINT('Ctrl Pts',(8.35467498637628,29.2709417606716,56.5013572548453));
#103774=CARTESIAN_POINT('Ctrl Pts',(8.34661911115974,29.3896958950261,56.5504466517915));
#103775=CARTESIAN_POINT('Ctrl Pts',(8.3448261167064,29.4161030991972,56.5605832722019));
#103776=CARTESIAN_POINT('Ctrl Pts',(8.34175847907943,29.4609462904271,56.5764992076295));
#103777=CARTESIAN_POINT('Ctrl Pts',(8.3405001664206,29.4792485523437,56.5826390950878));
#103778=CARTESIAN_POINT('Ctrl Pts',(8.33868187673522,29.5054853486663,56.5909364384793));
#103779=CARTESIAN_POINT('Ctrl Pts',(8.33813595197105,29.5133363259476,56.5933555639042));
#103780=CARTESIAN_POINT('Ctrl Pts',(8.33718202714467,29.5270016971516,56.5974558637262));
#103781=CARTESIAN_POINT('Ctrl Pts',(8.33677555650413,29.5328078811856,56.5991635794459));
#103782=CARTESIAN_POINT('Ctrl Pts',(8.3358984170954,29.5452993124806,56.6027637238111));
#103783=CARTESIAN_POINT('Ctrl Pts',(8.33542722307885,29.5519870291935,56.6046459557121));
#103784=CARTESIAN_POINT('Ctrl Pts',(8.33411743648922,29.5705200713913,56.6097371214792));
#103785=CARTESIAN_POINT('Ctrl Pts',(8.3332741007402,29.5823891040885,56.6128570075721));
#103786=CARTESIAN_POINT('Ctrl Pts',(8.32739914873105,29.6647052897696,56.6335250811979));
#103787=CARTESIAN_POINT('Ctrl Pts',(8.32216859223985,29.736192395319,56.6465812906607));
#103788=CARTESIAN_POINT('Ctrl Pts',(8.31584409808381,29.8226801139109,56.656599950404));
#103789=CARTESIAN_POINT('Ctrl Pts',(8.31479054129817,29.837087283724,56.6580787617991));
#103790=CARTESIAN_POINT('Ctrl Pts',(8.30828554897284,29.9261080965898,56.666044762055));
#103791=CARTESIAN_POINT('Ctrl Pts',(8.30283399774223,30.0010744490843,56.6676826436863));
#103792=CARTESIAN_POINT('Ctrl Pts',(8.29449542297255,30.1178583240142,56.6623566260043));
#103793=CARTESIAN_POINT('Ctrl Pts',(8.29153546152786,30.1597316104884,56.6588569665739));
#103794=CARTESIAN_POINT('Ctrl Pts',(8.28651598891549,30.2315431115093,56.6501102955644));
#103795=CARTESIAN_POINT('Ctrl Pts',(8.2844356050796,30.261551155552,56.6456206735221));
#103796=CARTESIAN_POINT('Ctrl Pts',(8.28143720769942,30.3051371854474,56.6378770869985));
#103797=CARTESIAN_POINT('Ctrl Pts',(8.28049915137323,30.3188219848497,56.6352683622274));
#103798=CARTESIAN_POINT('Ctrl Pts',(8.27884811207615,30.3429884248197,56.6303466210606));
#103799=CARTESIAN_POINT('Ctrl Pts',(8.27813295600121,30.353483293679,56.6281034164687));
#103800=CARTESIAN_POINT('Ctrl Pts',(8.27663519437453,30.3755153415698,56.6231711382093));
#103801=CARTESIAN_POINT('Ctrl Pts',(8.27585333477465,30.3870470287705,56.6204600968204));
#103802=CARTESIAN_POINT('Ctrl Pts',(8.27378105964955,30.4176832014621,56.6129119883268));
#103803=CARTESIAN_POINT('Ctrl Pts',(8.27249762586325,30.4367328000111,56.6078584681774));
#103804=CARTESIAN_POINT('Ctrl Pts',(8.26561050712643,30.5392549450564,56.5787045584924));
#103805=CARTESIAN_POINT('Ctrl Pts',(8.26021198918261,30.6208393787416,56.548439607445));
#103806=CARTESIAN_POINT('Ctrl Pts',(8.24896487390345,30.7872638936493,56.4714215111499));
#103807=CARTESIAN_POINT('Ctrl Pts',(8.24315368639412,30.8711368192315,56.4233706845726));
#103808=CARTESIAN_POINT('Ctrl Pts',(8.2345134171551,30.9842578537331,56.3448027210113));
#103809=CARTESIAN_POINT('Ctrl Pts',(8.23188284765405,31.0172520705503,56.3200210167398));
#103810=CARTESIAN_POINT('Ctrl Pts',(8.22847293717646,31.0576364318827,56.2872748949067));
#103811=CARTESIAN_POINT('Ctrl Pts',(8.22776317725223,31.0659173145016,56.2804263902247));
#103812=CARTESIAN_POINT('Ctrl Pts',(8.22661217809893,31.0791339109638,56.2692788643662));
#103813=CARTESIAN_POINT('Ctrl Pts',(8.22617444525673,31.0841117080983,56.2650298945001));
#103814=CARTESIAN_POINT('Ctrl Pts',(8.22532202885754,31.0937081824508,56.2567402557315));
#103815=CARTESIAN_POINT('Ctrl Pts',(8.22490760163971,31.0983297747668,56.2527032210022));
#103816=CARTESIAN_POINT('Ctrl Pts',(8.22397306221718,31.1086553385317,56.2435826145211));
#103817=CARTESIAN_POINT('Ctrl Pts',(8.22345195668135,31.1143468473354,56.2384851541254));
#103818=CARTESIAN_POINT('Ctrl Pts',(8.22160692658806,31.1342735092486,56.2203897708179));
#103819=CARTESIAN_POINT('Ctrl Pts',(8.22026919250675,31.1483173356322,56.2071846605633));
#103820=CARTESIAN_POINT('Ctrl Pts',(8.2113606105704,31.2394020687851,56.1185119452913));
#103821=CARTESIAN_POINT('Ctrl Pts',(8.20343273451831,31.3091840589787,56.035963837881));
#103822=CARTESIAN_POINT('Ctrl Pts',(8.18941145024412,31.4190509845364,55.8770079186528));
#103823=CARTESIAN_POINT('Ctrl Pts',(8.18329625522762,31.4621384129286,55.8031210712222));
#103824=CARTESIAN_POINT('Ctrl Pts',(8.17529348338707,31.5124376277498,55.699275698788));
#103825=CARTESIAN_POINT('Ctrl Pts',(8.1732388582997,31.5247719209036,55.6719560035575));
#103826=CARTESIAN_POINT('Ctrl Pts',(8.17027012358035,31.5417257004153,55.6315299870337));
#103827=CARTESIAN_POINT('Ctrl Pts',(8.16933652897778,31.5469285119554,55.6186763765713));
#103828=CARTESIAN_POINT('Ctrl Pts',(8.16769050166197,31.5558694711451,55.5957694041656));
#103829=CARTESIAN_POINT('Ctrl Pts',(8.16697594118911,31.5596720925595,55.5857422360674));
#103830=CARTESIAN_POINT('Ctrl Pts',(8.16626075047351,31.5633977026734,55.5756245535268));
#103831=CARTESIAN_POINT('Ctrl Pts',(8.166256912775,31.5634176918823,55.5755702598786));
#103832=CARTESIAN_POINT('Ctrl Pts',(8.16625307517082,31.5634376782623,55.5755159651912));
#103833=CARTESIAN_POINT('Origin',(5.,30.,55.));
#103834=CARTESIAN_POINT('',(7.46827878691259,31.5634376230276,55.5755161152408));
#103835=CARTESIAN_POINT('',(7.65925614416276,31.563437678903,55.5755159634506));
#103836=CARTESIAN_POINT('',(5.,31.5634376782623,55.5755159651912));
#103837=CARTESIAN_POINT('',(8.32030902926138,31.665999673445,55.0010431112818));
#103838=CARTESIAN_POINT('Ctrl Pts',(7.65925614416276,31.563437678903,55.5755159634506));
#103839=CARTESIAN_POINT('Ctrl Pts',(7.65963159048,31.5614376460338,55.5809492215099));
#103840=CARTESIAN_POINT('Ctrl Pts',(7.66000838851873,31.559409165902,55.5863723927665));
#103841=CARTESIAN_POINT('Ctrl Pts',(7.66118870360561,31.5529906532224,55.6032634618152));
#103842=CARTESIAN_POINT('Ctrl Pts',(7.66199708032709,31.5485023898747,55.6146926875642));
#103843=CARTESIAN_POINT('Ctrl Pts',(7.66327427744762,31.5412764375556,55.6325118591142));
#103844=CARTESIAN_POINT('Ctrl Pts',(7.66373822044195,31.5386242822467,55.6389363212319));
#103845=CARTESIAN_POINT('Ctrl Pts',(7.66461086647291,31.5335868428309,55.6509255339244));
#103846=CARTESIAN_POINT('Ctrl Pts',(7.66501899500722,31.5312113248434,55.6564941197066));
#103847=CARTESIAN_POINT('Ctrl Pts',(7.66598537297125,31.5255400249626,55.6695902916737));
#103848=CARTESIAN_POINT('Ctrl Pts',(7.66654510793023,31.5222188419567,55.6771065769736));
#103849=CARTESIAN_POINT('Ctrl Pts',(7.66843020185025,31.5109083480086,55.7021999336251));
#103850=CARTESIAN_POINT('Ctrl Pts',(7.66976911520282,31.5026694377293,55.7196619097496));
#103851=CARTESIAN_POINT('Ctrl Pts',(7.6731023784322,31.4816161755155,55.762344854778));
#103852=CARTESIAN_POINT('Ctrl Pts',(7.67511132091524,31.4684595478875,55.7873897032115));
#103853=CARTESIAN_POINT('Ctrl Pts',(7.68432087457773,31.405809189489,55.8996139705159));
#103854=CARTESIAN_POINT('Ctrl Pts',(7.69169395322286,31.3491462429622,55.9825526201571));
#103855=CARTESIAN_POINT('Ctrl Pts',(7.70486795675479,31.2329021130264,56.1235257660179));
#103856=CARTESIAN_POINT('Ctrl Pts',(7.71070090930999,31.1757749373198,56.1831799307067));
#103857=CARTESIAN_POINT('Ctrl Pts',(7.71768797249666,31.099883362438,56.2514778811915));
#103858=CARTESIAN_POINT('Ctrl Pts',(7.71901887146961,31.0850809177853,56.2643337205403));
#103859=CARTESIAN_POINT('Ctrl Pts',(7.72113538275762,31.0609902010117,56.2845215645147));
#103860=CARTESIAN_POINT('Ctrl Pts',(7.72192776914359,31.0518451368708,56.2920207726157));
#103861=CARTESIAN_POINT('Ctrl Pts',(7.72343231646594,31.0342433609175,56.3061439562762));
#103862=CARTESIAN_POINT('Ctrl Pts',(7.72414512787151,31.0258009637973,56.3127847333081));
#103863=CARTESIAN_POINT('Ctrl Pts',(7.72577839130045,31.0062228416963,56.3278806659074));
#103864=CARTESIAN_POINT('Ctrl Pts',(7.7266965521399,30.9950436246061,56.3362782924647));
#103865=CARTESIAN_POINT('Ctrl Pts',(7.7296080445694,30.9590559778833,56.3626094873501));
#103866=CARTESIAN_POINT('Ctrl Pts',(7.73158070212546,30.933857630097,56.3800011228142));
#103867=CARTESIAN_POINT('Ctrl Pts',(7.73624069398871,30.8725434888767,56.4198704547853));
#103868=CARTESIAN_POINT('Ctrl Pts',(7.73890543768339,30.8360178803313,56.4416791364344));
#103869=CARTESIAN_POINT('Ctrl Pts',(7.746111352965,30.7340132570919,56.4974020469629));
#103870=CARTESIAN_POINT('Ctrl Pts',(7.75058501916957,30.6670558228482,56.5284061126924));
#103871=CARTESIAN_POINT('Ctrl Pts',(7.75594783055933,30.5852424146112,56.5598852581263));
#103872=CARTESIAN_POINT('Ctrl Pts',(7.75680266838987,30.5721572274757,56.564732182654));
#103873=CARTESIAN_POINT('Ctrl Pts',(7.7621675047063,30.4898843024883,56.5940371430003));
#103874=CARTESIAN_POINT('Ctrl Pts',(7.76673002896838,30.4192128321675,56.6140628616324));
#103875=CARTESIAN_POINT('Ctrl Pts',(7.77232427557083,30.3354539449594,56.6319244461285));
#103876=CARTESIAN_POINT('Ctrl Pts',(7.77313258334213,30.3234185255547,56.6343522211045));
#103877=CARTESIAN_POINT('Ctrl Pts',(7.77440969496384,30.3045300481083,56.6379455898641));
#103878=CARTESIAN_POINT('Ctrl Pts',(7.77487362246632,30.2976943777533,56.6392017443362));
#103879=CARTESIAN_POINT('Ctrl Pts',(7.77574625672221,30.2848897735902,56.6414720444637));
#103880=CARTESIAN_POINT('Ctrl Pts',(7.77615438917134,30.2789229137948,56.6424964716342));
#103881=CARTESIAN_POINT('Ctrl Pts',(7.77712080008715,30.2648438704207,56.6448347204768));
#103882=CARTESIAN_POINT('Ctrl Pts',(7.77768056439062,30.2567274036312,56.6461210667904));
#103883=CARTESIAN_POINT('Ctrl Pts',(7.77956586335291,30.2295080461111,56.6502287530831));
#103884=CARTESIAN_POINT('Ctrl Pts',(7.78090495626985,30.2103664672671,56.6527778891059));
#103885=CARTESIAN_POINT('Ctrl Pts',(7.78423876687398,30.1630805058365,56.6582403947546));
#103886=CARTESIAN_POINT('Ctrl Pts',(7.78624808290117,30.1348984375856,56.6607705106326));
#103887=CARTESIAN_POINT('Ctrl Pts',(7.79546095714804,30.0065889503532,56.669002543238));
#103888=CARTESIAN_POINT('Ctrl Pts',(7.80283707374235,29.906135983675,56.666374182863));
#103889=CARTESIAN_POINT('Ctrl Pts',(7.81601039326826,29.7246594348859,56.6451558201465));
#103890=CARTESIAN_POINT('Ctrl Pts',(7.82183993394843,29.6436042322961,56.6295201240762));
#103891=CARTESIAN_POINT('Ctrl Pts',(7.82882370036997,29.5451096955661,56.6028147282216));
#103892=CARTESIAN_POINT('Ctrl Pts',(7.83015450015074,29.5262820226596,56.5973514256298));
#103893=CARTESIAN_POINT('Ctrl Pts',(7.83227089236381,29.4962570743077,56.5880613697007));
#103894=CARTESIAN_POINT('Ctrl Pts',(7.83306325751763,29.4849970068625,56.5844455745345));
#103895=CARTESIAN_POINT('Ctrl Pts',(7.83456778818429,29.4635851656586,56.5773174985461));
#103896=CARTESIAN_POINT('Ctrl Pts',(7.83528060391883,29.4534270424619,56.5738263490694));
#103897=CARTESIAN_POINT('Ctrl Pts',(7.83691391060792,29.4301251991416,56.565565137015));
#103898=CARTESIAN_POINT('Ctrl Pts',(7.83783210995017,29.417006227852,56.5607273202801));
#103899=CARTESIAN_POINT('Ctrl Pts',(7.84074386437779,29.3753620795096,56.5447720429243));
#103900=CARTESIAN_POINT('Ctrl Pts',(7.84271673999939,29.3470807928504,56.5330329069656));
#103901=CARTESIAN_POINT('Ctrl Pts',(7.84737735812253,29.2803212895614,56.5031391707893));
#103902=CARTESIAN_POINT('Ctrl Pts',(7.85004250136094,29.2421830169955,56.4842771350868));
#103903=CARTESIAN_POINT('Ctrl Pts',(7.85724861653753,29.1400418520056,56.4287966740701));
#103904=CARTESIAN_POINT('Ctrl Pts',(7.8617221095835,29.0776817179599,56.3893585939889));
#103905=CARTESIAN_POINT('Ctrl Pts',(7.8670863453393,29.0068442276365,56.3376819636178));
#103906=CARTESIAN_POINT('Ctrl Pts',(7.8679427701454,28.9956548321545,56.3293013961326));
#103907=CARTESIAN_POINT('Ctrl Pts',(7.87330713273971,28.9264229477285,56.276075336891));
#103908=CARTESIAN_POINT('Ctrl Pts',(7.8778676100798,28.8712964649854,56.2275836275946));
#103909=CARTESIAN_POINT('Ctrl Pts',(7.88345958440012,28.8108869492878,56.1669262600644));
#103910=CARTESIAN_POINT('Ctrl Pts',(7.88426788362659,28.8023197858966,56.1581316103053));
#103911=CARTESIAN_POINT('Ctrl Pts',(7.88554498458273,28.7890565239385,56.1442116075763));
#103912=CARTESIAN_POINT('Ctrl Pts',(7.88600891009339,28.7842937736759,56.1391499778476));
#103913=CARTESIAN_POINT('Ctrl Pts',(7.88688154272525,28.7754416570285,56.1296236189867));
#103914=CARTESIAN_POINT('Ctrl Pts',(7.88728967556645,28.7713447778844,56.1251662083443));
#103915=CARTESIAN_POINT('Ctrl Pts',(7.88825609025736,28.7617443109088,56.1146059315397));
#103916=CARTESIAN_POINT('Ctrl Pts',(7.88881585798119,28.7562614837534,56.1084845647622));
#103917=CARTESIAN_POINT('Ctrl Pts',(7.89070118111609,28.7380474101835,56.0878439931072));
#103918=CARTESIAN_POINT('Ctrl Pts',(7.89204029524548,28.7255238784898,56.0731446447318));
#103919=CARTESIAN_POINT('Ctrl Pts',(7.89537417052015,28.6952878378115,56.0363795955823));
#103920=CARTESIAN_POINT('Ctrl Pts',(7.89738353068785,28.6778768937669,56.0140743579871));
#103921=CARTESIAN_POINT('Ctrl Pts',(7.90659679602378,28.6013673418907,55.9107362670062));
#103922=CARTESIAN_POINT('Ctrl Pts',(7.91397327037209,28.5490914909691,55.8249114052757));
#103923=CARTESIAN_POINT('Ctrl Pts',(7.92714651609673,28.4684935822616,55.6609366863721));
#103924=CARTESIAN_POINT('Ctrl Pts',(7.93297566143948,28.4376708299431,55.5843632888298));
#103925=CARTESIAN_POINT('Ctrl Pts',(7.93995904599438,28.4066890555883,55.4871349608446));
#103926=CARTESIAN_POINT('Ctrl Pts',(7.94128983442738,28.4010676185352,55.4683540670327));
#103927=CARTESIAN_POINT('Ctrl Pts',(7.94340621305111,28.392588212488,55.4380903944065));
#103928=CARTESIAN_POINT('Ctrl Pts',(7.94419857580865,28.3895189570306,55.4266692759289));
#103929=CARTESIAN_POINT('Ctrl Pts',(7.94570310465096,28.3838945651968,55.4048142654578));
#103930=CARTESIAN_POINT('Ctrl Pts',(7.94641592092891,28.3813182326309,55.3943864996689));
#103931=CARTESIAN_POINT('Ctrl Pts',(7.94804923270478,28.3756207451255,55.3703289418695));
#103932=CARTESIAN_POINT('Ctrl Pts',(7.94896743654092,28.3725699378383,55.3566831946801));
#103933=CARTESIAN_POINT('Ctrl Pts',(7.95187922135973,28.3633882966704,55.3130420953412));
#103934=CARTESIAN_POINT('Ctrl Pts',(7.95385212225296,28.357912056782,55.2829144681088));
#103935=CARTESIAN_POINT('Ctrl Pts',(7.95851281304256,28.3468190423902,55.210612440084));
#103936=CARTESIAN_POINT('Ctrl Pts',(7.96117800267659,28.3419810253693,55.1683399499645));
#103937=CARTESIAN_POINT('Ctrl Pts',(7.96838413995461,28.3331951505188,55.0524356415399));
#103938=CARTESIAN_POINT('Ctrl Pts',(7.97285761186704,28.332507077862,54.9786547129672));
#103939=CARTESIAN_POINT('Ctrl Pts',(7.97822200202179,28.3375034759265,54.8911110165375));
#103940=CARTESIAN_POINT('Ctrl Pts',(7.97907860112277,28.338475890721,54.8771621738888));
#103941=CARTESIAN_POINT('Ctrl Pts',(7.98444290711716,28.3456450689222,54.7901306500289));
#103942=CARTESIAN_POINT('Ctrl Pts',(7.98900315506913,28.3564861301249,54.7175202272039));
#103943=CARTESIAN_POINT('Ctrl Pts',(7.99459487478488,28.3746822581407,54.6338729981434));
#103944=CARTESIAN_POINT('Ctrl Pts',(7.99540317319719,28.377424503538,54.6219054615397));
#103945=CARTESIAN_POINT('Ctrl Pts',(7.99668027322735,28.38192578622,54.6032127222205));
#103946=CARTESIAN_POINT('Ctrl Pts',(7.99714419864135,28.3835951376044,54.5964660837598));
#103947=CARTESIAN_POINT('Ctrl Pts',(7.99801683169108,28.3867975795262,54.5838622745005));
#103948=CARTESIAN_POINT('Ctrl Pts',(7.99842496505287,28.3883204469311,54.5780027612128));
#103949=CARTESIAN_POINT('Ctrl Pts',(7.99939138163754,28.3919856559909,54.5642094494099));
#103950=CARTESIAN_POINT('Ctrl Pts',(7.99995115074493,28.3941548008729,54.5562830588268));
#103951=CARTESIAN_POINT('Ctrl Pts',(8.00183648090793,28.4016172170938,54.5297858203319));
#103952=CARTESIAN_POINT('Ctrl Pts',(8.0031756007797,28.4071744942746,54.5112917800015));
#103953=CARTESIAN_POINT('Ctrl Pts',(8.00650949305517,28.4216635586059,54.4659488984786));
#103954=CARTESIAN_POINT('Ctrl Pts',(8.00851886462424,28.430960153971,54.4392235007593));
#103955=CARTESIAN_POINT('Ctrl Pts',(8.01773223287277,28.4762835290226,54.3188963137295));
#103956=CARTESIAN_POINT('Ctrl Pts',(8.0251088010293,28.5200369046607,54.2284276963778));
#103957=CARTESIAN_POINT('Ctrl Pts',(8.03828200312867,28.6140860174395,54.0717805433387));
#103958=CARTESIAN_POINT('Ctrl Pts',(8.04411102165076,28.6617006017761,54.0043558239765));
#103959=CARTESIAN_POINT('Ctrl Pts',(8.05109428420104,28.7265818096801,53.9255948872316));
#103960=CARTESIAN_POINT('Ctrl Pts',(8.05242506928609,28.7393115561493,53.9106860240202));
#103961=CARTESIAN_POINT('Ctrl Pts',(8.0545414443727,28.7601384195485,53.8871482086335));
#103962=CARTESIAN_POINT('Ctrl Pts',(8.05533380688427,28.7680691399381,53.8783751889618));
#103963=CARTESIAN_POINT('Ctrl Pts',(8.05683833638183,28.783380020198,53.8617965072268));
#103964=CARTESIAN_POINT('Ctrl Pts',(8.05755115354964,28.7907435373651,53.8539763601888));
#103965=CARTESIAN_POINT('Ctrl Pts',(8.05918446897586,28.8078652608931,53.8361416521534));
#103966=CARTESIAN_POINT('Ctrl Pts',(8.06010267554918,28.8176750265233,53.8261775403098));
#103967=CARTESIAN_POINT('Ctrl Pts',(8.06301447597311,28.8493601880155,53.7947941021487));
#103968=CARTESIAN_POINT('Ctrl Pts',(8.06498738944223,28.8717017492147,53.7738529945338));
#103969=CARTESIAN_POINT('Ctrl Pts',(8.06964811551408,28.92642981198,53.7253188786076));
#103970=CARTESIAN_POINT('Ctrl Pts',(8.07231332739492,28.9593211036829,53.6983269515445));
#103971=CARTESIAN_POINT('Ctrl Pts',(8.07951947700207,29.051932462727,53.6280831556815));
#103972=CARTESIAN_POINT('Ctrl Pts',(8.08399294042461,29.1135457644703,53.5874890672456));
#103973=CARTESIAN_POINT('Ctrl Pts',(8.08935742332851,29.1898062382662,53.5442055029688));
#103974=CARTESIAN_POINT('Ctrl Pts',(8.09021412316998,29.2020541217334,53.5374563533158));
#103975=CARTESIAN_POINT('Ctrl Pts',(8.09557840540333,29.2790611418513,53.4962772073723));
#103976=CARTESIAN_POINT('Ctrl Pts',(8.100138529637,29.3459422554202,53.4660049473089));
#103977=CARTESIAN_POINT('Ctrl Pts',(8.10573011210905,29.4260848868553,53.4359257734126));
#103978=CARTESIAN_POINT('Ctrl Pts',(8.10653841020586,29.4376266254109,53.4317388899915));
#103979=CARTESIAN_POINT('Ctrl Pts',(8.10781550993127,29.4557725380248,53.42538234014));
#103980=CARTESIAN_POINT('Ctrl Pts',(8.10827943536346,29.462346078788,53.4231256988139));
#103981=CARTESIAN_POINT('Ctrl Pts',(8.10915206783548,29.474671968237,53.4189803559276));
#103982=CARTESIAN_POINT('Ctrl Pts',(8.10956020059574,29.4804207402492,53.4170817948946));
#103983=CARTESIAN_POINT('Ctrl Pts',(8.1105266154132,29.4939969540745,53.4126801041525));
#103984=CARTESIAN_POINT('Ctrl Pts',(8.11108638334695,29.5018327092095,53.4102035106509));
#103985=CARTESIAN_POINT('Ctrl Pts',(8.11297170966746,29.5281414838758,53.4021018697337));
#103986=CARTESIAN_POINT('Ctrl Pts',(8.11431082685165,29.5466931610663,53.3967402817212));
#103987=CARTESIAN_POINT('Ctrl Pts',(8.11764471193652,29.5926459342696,53.3843208354584));
#103988=CARTESIAN_POINT('Ctrl Pts',(8.11965407898041,29.6201411785841,53.3776364178605));
#103989=CARTESIAN_POINT('Ctrl Pts',(8.12886740901152,29.7458145175515,53.3504534683223));
#103990=CARTESIAN_POINT('Ctrl Pts',(8.13624394312168,29.845550915368,53.3381456237804));
#103991=CARTESIAN_POINT('Ctrl Pts',(8.14941717408802,30.0281661795857,53.3322003346614));
#103992=CARTESIAN_POINT('Ctrl Pts',(8.15524625111241,30.1106378609247,53.3356346558013));
#103993=CARTESIAN_POINT('Ctrl Pts',(8.16222956843385,30.2119983827531,53.347427181732));
#103994=CARTESIAN_POINT('Ctrl Pts',(8.1635603538566,30.2314281299664,53.3500359665824));
#103995=CARTESIAN_POINT('Ctrl Pts',(8.16567672825,30.2624990063343,53.3547674573025));
#103996=CARTESIAN_POINT('Ctrl Pts',(8.16646908975953,30.2741709254493,53.3566722286782));
#103997=CARTESIAN_POINT('Ctrl Pts',(8.16797361654901,30.2964034297831,53.3605438790621));
#103998=CARTESIAN_POINT('Ctrl Pts',(8.16868643201802,30.306967158092,53.3624889195073));
#103999=CARTESIAN_POINT('Ctrl Pts',(8.17031974235481,30.3312370056854,53.3672007059445));
#104000=CARTESIAN_POINT('Ctrl Pts',(8.17123794555848,30.3449287044924,53.3700381301506));
#104001=CARTESIAN_POINT('Ctrl Pts',(8.17414972987248,30.3884799510167,53.3796369083406));
#104002=CARTESIAN_POINT('Ctrl Pts',(8.17612263085626,30.4181905599041,53.3870492675355));
#104003=CARTESIAN_POINT('Ctrl Pts',(8.18078332244457,30.4886482006191,53.4067053581101));
#104004=CARTESIAN_POINT('Ctrl Pts',(8.18344851273002,30.5291640231085,53.4196991751695));
#104005=CARTESIAN_POINT('Ctrl Pts',(8.19065465245124,30.6384078458108,53.4594081231101));
#104006=CARTESIAN_POINT('Ctrl Pts',(8.19512812596855,30.7059297372772,53.489155375738));
#104007=CARTESIAN_POINT('Ctrl Pts',(8.20459019166356,30.8430245666284,53.5607569553848));
#104008=CARTESIAN_POINT('Ctrl Pts',(8.20957425962665,30.9119530789412,53.6034150939223));
#104009=CARTESIAN_POINT('Ctrl Pts',(8.21586588284626,30.9905750436725,53.6603814656874));
#104010=CARTESIAN_POINT('Ctrl Pts',(8.21692241484219,31.0035117618374,53.6700448009833));
#104011=CARTESIAN_POINT('Ctrl Pts',(8.21850515162858,31.02246010189,53.6846324954647));
#104012=CARTESIAN_POINT('Ctrl Pts',(8.21902203001787,31.0285814445675,53.6894136663841));
#104013=CARTESIAN_POINT('Ctrl Pts',(8.21994425270688,31.0393802837109,53.6979705230566));
#104014=CARTESIAN_POINT('Ctrl Pts',(8.2203483954664,31.0440711053927,53.7017289737103));
#104015=CARTESIAN_POINT('Ctrl Pts',(8.22122422841557,31.0541465867422,53.7098917244783));
#104016=CARTESIAN_POINT('Ctrl Pts',(8.22169647569926,31.059523986063,53.7143043488144));
#104017=CARTESIAN_POINT('Ctrl Pts',(8.22301300035022,31.074366712232,53.7266404506612));
#104018=CARTESIAN_POINT('Ctrl Pts',(8.2238620600468,31.0837716269391,53.7346354625719));
#104019=CARTESIAN_POINT('Ctrl Pts',(8.22585941747524,31.1055272088131,53.7535501006916));
#104020=CARTESIAN_POINT('Ctrl Pts',(8.22701241427171,31.1178062031414,53.7645498763099));
#104021=CARTESIAN_POINT('Ctrl Pts',(8.23090037176596,31.1583448860011,53.80196435963));
#104022=CARTESIAN_POINT('Ctrl Pts',(8.23367346168671,31.1858463297726,53.8291796121029));
#104023=CARTESIAN_POINT('Ctrl Pts',(8.24157338291223,31.260819089416,53.9087254589146));
#104024=CARTESIAN_POINT('Ctrl Pts',(8.24674141994125,31.3059463004509,53.9631541828364));
#104025=CARTESIAN_POINT('Ctrl Pts',(8.25869915466466,31.4030484747042,54.0967065416247));
#104026=CARTESIAN_POINT('Ctrl Pts',(8.2654185770515,31.4520193026704,54.177729112473));
#104027=CARTESIAN_POINT('Ctrl Pts',(8.27325583122943,31.5026906660689,54.2803649597529));
#104028=CARTESIAN_POINT('Ctrl Pts',(8.2746104905053,31.5111988111378,54.2984074955985));
#104029=CARTESIAN_POINT('Ctrl Pts',(8.27675548501441,31.5242621508798,54.3274507632539));
#104030=CARTESIAN_POINT('Ctrl Pts',(8.27755292125273,31.5290267873699,54.3383545687644));
#104031=CARTESIAN_POINT('Ctrl Pts',(8.27906145396482,31.5378625644788,54.3591804274129));
#104032=CARTESIAN_POINT('Ctrl Pts',(8.27977325974764,31.5419554960087,54.3690925191919));
#104033=CARTESIAN_POINT('Ctrl Pts',(8.28139642352814,31.5511111355222,54.3918866878254));
#104034=CARTESIAN_POINT('Ctrl Pts',(8.28230558977907,31.5561096327392,54.404793829628));
#104035=CARTESIAN_POINT('Ctrl Pts',(8.28515654498737,31.5713647523713,54.4456919408238));
#104036=CARTESIAN_POINT('Ctrl Pts',(8.2870788921486,31.5810316497581,54.4738976270498));
#104037=CARTESIAN_POINT('Ctrl Pts',(8.29851342700332,31.6345903129926,54.6450113106569));
#104038=CARTESIAN_POINT('Ctrl Pts',(8.30738782332018,31.6598381214884,54.7930240966322));
#104039=CARTESIAN_POINT('Ctrl Pts',(8.3178623416834,31.6656802062543,54.9619538784274));
#104040=CARTESIAN_POINT('Ctrl Pts',(8.31908056412801,31.6660119108601,54.9814981883682));
#104041=CARTESIAN_POINT('Ctrl Pts',(8.32030902926138,31.665999673445,55.0010431112818));
#104042=CARTESIAN_POINT('Ctrl Pts',(8.32030918176878,31.665999671924,55.0010455376788));
#104043=CARTESIAN_POINT('Ctrl Pts',(8.32194772557573,31.6659833115337,55.0271148085817));
#104044=CARTESIAN_POINT('Ctrl Pts',(8.32360410126614,31.6653550622253,55.0531790328534));
#104045=CARTESIAN_POINT('Ctrl Pts',(8.32632096570275,31.663353304605,55.0952302538716));
#104046=CARTESIAN_POINT('Ctrl Pts',(8.32736521618276,31.6623599366694,55.1112313530609));
#104047=CARTESIAN_POINT('Ctrl Pts',(8.32888514943137,31.6605977381666,55.1342416336321));
#104048=CARTESIAN_POINT('Ctrl Pts',(8.32935150877709,31.6600150430196,55.1412647049778));
#104049=CARTESIAN_POINT('Ctrl Pts',(8.3301984943843,31.6588816762545,55.1539477901932));
#104050=CARTESIAN_POINT('Ctrl Pts',(8.33057828611858,31.6583465443042,55.1596091304013));
#104051=CARTESIAN_POINT('Ctrl Pts',(8.331364323057,31.6571840392508,55.1712701061304));
#104052=CARTESIAN_POINT('Ctrl Pts',(8.33177078463885,31.6565530628952,55.1772691024171));
#104053=CARTESIAN_POINT('Ctrl Pts',(8.33271294974264,31.655021827187,55.1911046102106));
#104054=CARTESIAN_POINT('Ctrl Pts',(8.33324989138303,31.6540984780162,55.1989382799917));
#104055=CARTESIAN_POINT('Ctrl Pts',(8.33496704599849,31.6509841690874,55.2238376950734));
#104056=CARTESIAN_POINT('Ctrl Pts',(8.33615772225577,31.6485845261539,55.2408755760136));
#104057=CARTESIAN_POINT('Ctrl Pts',(8.34123780411159,31.6373256422381,55.3127376313061));
#104058=CARTESIAN_POINT('Ctrl Pts',(8.34522559574536,31.6259924777415,55.367134109977));
#104059=CARTESIAN_POINT('Ctrl Pts',(8.35316770311035,31.5983070033082,55.4731747447218));
#104060=CARTESIAN_POINT('Ctrl Pts',(8.35711503915216,31.5821109667713,55.5247883994072));
#104061=CARTESIAN_POINT('Ctrl Pts',(8.36103882979909,31.5634376856231,55.5755159451947));
#104062=CARTESIAN_POINT('Ctrl Pts',(8.16625307517082,31.5634376782623,55.5755159651912));
#104063=CARTESIAN_POINT('Ctrl Pts',(8.1654689857109,31.5675212442298,55.5644226136918));
#104064=CARTESIAN_POINT('Ctrl Pts',(8.16468883772099,31.5714867118766,55.5532858795883));
#104065=CARTESIAN_POINT('Ctrl Pts',(8.16260806743168,31.5817969750552,55.5233248517541));
#104066=CARTESIAN_POINT('Ctrl Pts',(8.16131461585613,31.5879243263064,55.5044273578505));
#104067=CARTESIAN_POINT('Ctrl Pts',(8.15400399036986,31.6208982766069,55.3961694593425));
#104068=CARTESIAN_POINT('Ctrl Pts',(8.14822701968199,31.6405400220761,55.3047836819981));
#104069=CARTESIAN_POINT('Ctrl Pts',(8.13814300282262,31.6615214613163,55.1414169030305));
#104070=CARTESIAN_POINT('Ctrl Pts',(8.13381644262068,31.6660544910231,55.0701010364573));
#104071=CARTESIAN_POINT('Ctrl Pts',(8.12585887029341,31.6659555137899,54.9416043706985));
#104072=CARTESIAN_POINT('Ctrl Pts',(8.12226599904631,31.6629747266091,54.8845381260349));
#104073=CARTESIAN_POINT('Ctrl Pts',(8.11775192226371,31.6558348957875,54.8158541241578));
#104074=CARTESIAN_POINT('Ctrl Pts',(8.116964457239,31.6544709846876,54.8039779442338));
#104075=CARTESIAN_POINT('Ctrl Pts',(8.1157132948838,31.6521214343764,54.7852954399317));
#104076=CARTESIAN_POINT('Ctrl Pts',(8.11525415990859,31.6512212179353,54.7784785174439));
#104077=CARTESIAN_POINT('Ctrl Pts',(8.11438520856184,31.6494469295648,54.7656548029881));
#104078=CARTESIAN_POINT('Ctrl Pts',(8.11397590597296,31.6485821958361,54.7596469606278));
#104079=CARTESIAN_POINT('Ctrl Pts',(8.11299940032779,31.6464503390475,54.745388614632));
#104080=CARTESIAN_POINT('Ctrl Pts',(8.11243061602187,31.6451540150343,54.7371427461048));
#104081=CARTESIAN_POINT('Ctrl Pts',(8.1104809578297,31.6405237814545,54.709066905393));
#104082=CARTESIAN_POINT('Ctrl Pts',(8.10908528283463,31.6368929876308,54.6892885564858));
#104083=CARTESIAN_POINT('Ctrl Pts',(8.10557742183999,31.6269706917297,54.6402531997301));
#104084=CARTESIAN_POINT('Ctrl Pts',(8.10344875669529,31.6202472823083,54.611091361287));
#104085=CARTESIAN_POINT('Ctrl Pts',(8.09308104129543,31.5840151716182,54.4712564451794));
#104086=CARTESIAN_POINT('Ctrl Pts',(8.08463859021491,31.5439310907534,54.3636407458044));
#104087=CARTESIAN_POINT('Ctrl Pts',(8.07164485655367,31.4633667547676,54.2008673942762));
#104088=CARTESIAN_POINT('Ctrl Pts',(8.06693618237087,31.4300063988784,54.1425975605253));
#104089=CARTESIAN_POINT('Ctrl Pts',(8.06106914896445,31.3829351224479,54.0708077848959));
#104090=CARTESIAN_POINT('Ctrl Pts',(8.05979718372886,31.3723872133398,54.0552984005117));
#104091=CARTESIAN_POINT('Ctrl Pts',(8.0577515382181,31.3548699013491,54.0304541709546));
#104092=CARTESIAN_POINT('Ctrl Pts',(8.05697186744231,31.3480608094352,54.0210088712497));
#104093=CARTESIAN_POINT('Ctrl Pts',(8.05547689974625,31.3347509474218,54.0029481627606));
#104094=CARTESIAN_POINT('Ctrl Pts',(8.05476110354745,31.3282644069587,53.9943230477293));
#104095=CARTESIAN_POINT('Ctrl Pts',(8.05309976503262,31.3129465568645,53.9743617523121));
#104096=CARTESIAN_POINT('Ctrl Pts',(8.05215679196557,31.3040513940417,53.9630754803865));
#104097=CARTESIAN_POINT('Ctrl Pts',(8.04907205991135,31.2743030595855,53.9263188524834));
#104098=CARTESIAN_POINT('Ctrl Pts',(8.04695473140637,31.2528402793171,53.9013503924657));
#104099=CARTESIAN_POINT('Ctrl Pts',(8.04187226920585,31.1989388084011,53.8422802082121));
#104100=CARTESIAN_POINT('Ctrl Pts',(8.03893601871442,31.1657677515346,53.8088848029491));
#104101=CARTESIAN_POINT('Ctrl Pts',(8.03183109530371,31.0813128232839,53.7307714702887));
#104102=CARTESIAN_POINT('Ctrl Pts',(8.02770383043196,31.0286208109519,53.6877051010575));
#104103=CARTESIAN_POINT('Ctrl Pts',(8.02330839097962,30.9703415362762,53.6457445147084));
#104104=CARTESIAN_POINT('Ctrl Pts',(8.02307428604218,30.9672312328613,53.6435213387096));
#104105=CARTESIAN_POINT('Ctrl Pts',(8.01786325416568,30.8978654754573,53.5943001068665));
#104106=CARTESIAN_POINT('Ctrl Pts',(8.01284055411631,30.828276649342,53.5522055090314));
#104107=CARTESIAN_POINT('Ctrl Pts',(8.00673014466067,30.7449018940282,53.5097551631353));
#104108=CARTESIAN_POINT('Ctrl Pts',(8.0059172404046,30.7338353469973,53.5042747020569));
#104109=CARTESIAN_POINT('Ctrl Pts',(8.00463451755969,30.7164339056545,53.4958966232369));
#104110=CARTESIAN_POINT('Ctrl Pts',(8.00416964681807,30.7101397647097,53.4929147272504));
#104111=CARTESIAN_POINT('Ctrl Pts',(8.00329646715863,30.6983448255102,53.4874170794146));
#104112=CARTESIAN_POINT('Ctrl Pts',(8.00288874618628,30.6928487860687,53.4848917061889));
#104113=CARTESIAN_POINT('Ctrl Pts',(8.00192499500437,30.6798830351813,53.4790193765771));
#104114=CARTESIAN_POINT('Ctrl Pts',(8.0013675017544,30.6724022788147,53.4756974818622));
#104115=CARTESIAN_POINT('Ctrl Pts',(7.99949736146867,30.6473623553941,53.4647984763812));
#104116=CARTESIAN_POINT('Ctrl Pts',(7.99817143679796,30.6296979525992,53.4574689149167));
#104117=CARTESIAN_POINT('Ctrl Pts',(7.99487752301475,30.58594264874,53.4401901383625));
#104118=CARTESIAN_POINT('Ctrl Pts',(7.99289534718539,30.5597207339902,53.4305898824676));
#104119=CARTESIAN_POINT('Ctrl Pts',(7.98391876482938,30.4409895401603,53.3904745019434));
#104120=CARTESIAN_POINT('Ctrl Pts',(7.97675825528527,30.3461520196638,53.3674489068411));
#104121=CARTESIAN_POINT('Ctrl Pts',(7.96353282865088,30.1650345494987,53.3399764974163));
#104122=CARTESIAN_POINT('Ctrl Pts',(7.95745689652306,30.0793459343204,53.3336798727251));
#104123=CARTESIAN_POINT('Ctrl Pts',(7.95023686437213,29.9738569247563,53.3340888317368));
#104124=CARTESIAN_POINT('Ctrl Pts',(7.94890033864265,29.9541747406982,53.3345140096057));
#104125=CARTESIAN_POINT('Ctrl Pts',(7.94677724438336,29.9226722503671,53.3357534361846));
#104126=CARTESIAN_POINT('Ctrl Pts',(7.94598382328304,29.9108455841279,53.3363450752348));
#104127=CARTESIAN_POINT('Ctrl Pts',(7.94447876027205,29.8883130992987,53.3377132543517));
#104128=CARTESIAN_POINT('Ctrl Pts',(7.94376645311238,29.8776065655324,53.3384672603463));
#104129=CARTESIAN_POINT('Ctrl Pts',(7.94213638941917,29.8530130060767,53.3404382716168));
#104130=CARTESIAN_POINT('Ctrl Pts',(7.94122089630504,29.8391323503871,53.3417262211645));
#104131=CARTESIAN_POINT('Ctrl Pts',(7.93832645307775,29.7950500179682,53.3463752370039));
#104132=CARTESIAN_POINT('Ctrl Pts',(7.93636783144652,29.7649223644249,53.3503885179102));
#104133=CARTESIAN_POINT('Ctrl Pts',(7.93174786958889,29.6933554502602,53.361922594837));
#104134=CARTESIAN_POINT('Ctrl Pts',(7.92910857597325,29.6520580891277,53.3701947161593));
#104135=CARTESIAN_POINT('Ctrl Pts',(7.92182834702889,29.537915408683,53.3975952555952));
#104136=CARTESIAN_POINT('Ctrl Pts',(7.91726069360868,29.465989456128,53.4201087851613));
#104137=CARTESIAN_POINT('Ctrl Pts',(7.91182546623245,29.3832075900958,53.4523221870205));
#104138=CARTESIAN_POINT('Ctrl Pts',(7.91099544123318,29.3706443366304,53.457388275337));
#104139=CARTESIAN_POINT('Ctrl Pts',(7.90567968819271,29.2907998741095,53.4907230292039));
#104140=CARTESIAN_POINT('Ctrl Pts',(7.90114104059178,29.2253837157161,53.5232303091945));
#104141=CARTESIAN_POINT('Ctrl Pts',(7.89557344041552,29.1517081007515,53.5660866471952));
#104142=CARTESIAN_POINT('Ctrl Pts',(7.89476538875152,29.1411674520313,53.5723749503135));
#104143=CARTESIAN_POINT('Ctrl Pts',(7.89348868359969,29.1247704703638,53.5824043082926));
#104144=CARTESIAN_POINT('Ctrl Pts',(7.89302490339176,29.1188661852279,53.5860666667806));
#104145=CARTESIAN_POINT('Ctrl Pts',(7.89215255437734,29.1078619074573,53.5929881823327));
#104146=CARTESIAN_POINT('Ctrl Pts',(7.89174455957917,29.1027565440904,53.5962383366924));
#104147=CARTESIAN_POINT('Ctrl Pts',(7.89077850427102,29.0907635966205,53.6039653858493));
#104148=CARTESIAN_POINT('Ctrl Pts',(7.89021895922887,29.0838912910393,53.6084654846419));
#104149=CARTESIAN_POINT('Ctrl Pts',(7.88833455896171,29.0609847291038,53.6237083067728));
#104150=CARTESIAN_POINT('Ctrl Pts',(7.8869961590687,29.0451045840916,53.6346783642134));
#104151=CARTESIAN_POINT('Ctrl Pts',(7.88366429711673,29.0064383045922,53.6623936924725));
#104152=CARTESIAN_POINT('Ctrl Pts',(7.8816562540726,28.9838814840546,53.6794476694942));
#104153=CARTESIAN_POINT('Ctrl Pts',(7.87245368498565,28.883438273511,53.7594847953962));
#104154=CARTESIAN_POINT('Ctrl Pts',(7.86508685287616,28.8108946114786,53.8288395110735));
#104155=CARTESIAN_POINT('Ctrl Pts',(7.85191064759957,28.6907075943827,53.9664968781553));
#104156=CARTESIAN_POINT('Ctrl Pts',(7.8460699207212,28.6410898827901,54.0326622629877));
#104157=CARTESIAN_POINT('Ctrl Pts',(7.83907560558779,28.586015027664,54.1187583868265));
#104158=CARTESIAN_POINT('Ctrl Pts',(7.83774473231254,28.5757434266787,54.1354576048071));
#104159=CARTESIAN_POINT('Ctrl Pts',(7.83562841568059,28.5597527033934,54.1625135695074));
#104160=CARTESIAN_POINT('Ctrl Pts',(7.83483619698365,28.5538452411562,54.1727562495912));
#104161=CARTESIAN_POINT('Ctrl Pts',(7.83333206963248,28.5427822325502,54.1924186357606));
#104162=CARTESIAN_POINT('Ctrl Pts',(7.83261950983348,28.5376077585574,54.2018269467011));
#104163=CARTESIAN_POINT('Ctrl Pts',(7.83098697502548,28.5259090781151,54.2235933933471));
#104164=CARTESIAN_POINT('Ctrl Pts',(7.83006928771538,28.5194486209281,54.235985014234));
#104165=CARTESIAN_POINT('Ctrl Pts',(7.82715999420424,28.499348342297,54.2757514645404));
#104166=CARTESIAN_POINT('Ctrl Pts',(7.82518902217089,28.4863055795109,54.3034221304657));
#104167=CARTESIAN_POINT('Ctrl Pts',(7.82053366010357,28.4569860168231,54.3703429413191));
#104168=CARTESIAN_POINT('Ctrl Pts',(7.81787180120431,28.4414340112721,54.4098876361963));
#104169=CARTESIAN_POINT('Ctrl Pts',(7.81066718054126,28.4030696126762,54.519578403903));
#104170=CARTESIAN_POINT('Ctrl Pts',(7.80619212603821,28.3833754575499,54.5907115595036));
#104171=CARTESIAN_POINT('Ctrl Pts',(7.80083999972846,28.365674043276,54.6763891874583));
#104172=CARTESIAN_POINT('Ctrl Pts',(7.79999715780075,28.3630573359335,54.6898967919067));
#104173=CARTESIAN_POINT('Ctrl Pts',(7.79462855671414,28.3474981570939,54.7759069487567));
#104174=CARTESIAN_POINT('Ctrl Pts',(7.79005037509517,28.3392096945153,54.849159523034));
#104175=CARTESIAN_POINT('Ctrl Pts',(7.78443889153302,28.3352242827534,54.9349729039652));
#104176=CARTESIAN_POINT('Ctrl Pts',(7.7836306765562,28.3347903296891,54.94724164423));
#104177=CARTESIAN_POINT('Ctrl Pts',(7.78235376890748,28.3343231527469,54.9664601267501));
#104178=CARTESIAN_POINT('Ctrl Pts',(7.78188995201852,28.3341977561378,54.9734074720215));
#104179=CARTESIAN_POINT('Ctrl Pts',(7.78101757531465,28.334044459824,54.9864070663611));
#104180=CARTESIAN_POINT('Ctrl Pts',(7.78060958997865,28.3340060751918,54.9924589446918));
#104181=CARTESIAN_POINT('Ctrl Pts',(7.77964361330082,28.3339933235609,55.0067244867441));
#104182=CARTESIAN_POINT('Ctrl Pts',(7.7790841381583,28.3340467243174,55.0149378993074));
#104183=CARTESIAN_POINT('Ctrl Pts',(7.77720022499056,28.3344289637405,55.0424428408602));
#104184=CARTESIAN_POINT('Ctrl Pts',(7.77586225146258,28.335032185937,55.0617281979107));
#104185=CARTESIAN_POINT('Ctrl Pts',(7.77253168870701,28.3373442259207,55.1092271396294));
#104186=CARTESIAN_POINT('Ctrl Pts',(7.77052453208001,28.3394363660621,55.1374155321467));
#104187=CARTESIAN_POINT('Ctrl Pts',(7.76132982801723,28.352186751437,55.2651043857725));
#104188=CARTESIAN_POINT('Ctrl Pts',(7.75397018978691,28.3710792193116,55.3635744377672));
#104189=CARTESIAN_POINT('Ctrl Pts',(7.74079234931782,28.4215131404336,55.5392335084213));
#104190=CARTESIAN_POINT('Ctrl Pts',(7.73494352531683,28.450220534493,55.6169123619868));
#104191=CARTESIAN_POINT('Ctrl Pts',(7.7279413928737,28.4927292041249,55.7099825073175));
#104192=CARTESIAN_POINT('Ctrl Pts',(7.72661028936251,28.5011892805688,55.7276722456543));
#104193=CARTESIAN_POINT('Ctrl Pts',(7.72449369664643,28.5152490291249,55.7557846040994));
#104194=CARTESIAN_POINT('Ctrl Pts',(7.72370142896215,28.520650627779,55.7663036347916));
#104195=CARTESIAN_POINT('Ctrl Pts',(7.72219726366893,28.5311698397171,55.7862628301204));
#104196=CARTESIAN_POINT('Ctrl Pts',(7.72148471433916,28.5362675973549,55.7957127248184));
#104197=CARTESIAN_POINT('Ctrl Pts',(7.71985228109367,28.5482087299234,55.8173452964194));
#104198=CARTESIAN_POINT('Ctrl Pts',(7.71893468387943,28.5551147847291,55.8294925917958));
#104199=CARTESIAN_POINT('Ctrl Pts',(7.71602600126338,28.5776175765787,55.8679395633482));
#104200=CARTESIAN_POINT('Ctrl Pts',(7.7140555374062,28.5937863325539,55.8938982903509));
#104201=CARTESIAN_POINT('Ctrl Pts',(7.70940163380587,28.6340932381776,55.9548076085145));
#104202=CARTESIAN_POINT('Ctrl Pts',(7.70674070511053,28.6588713621722,55.9893094596976));
#104203=CARTESIAN_POINT('Ctrl Pts',(7.69953660422257,28.7302092053187,56.0810290057603));
#104204=CARTESIAN_POINT('Ctrl Pts',(7.69506119862694,28.7792910431705,56.136161249065));
#104205=CARTESIAN_POINT('Ctrl Pts',(7.68971384706615,28.8416141478796,56.1974494682131));
#104206=CARTESIAN_POINT('Ctrl Pts',(7.68887610742027,28.8514822141496,56.2069175205105));
#104207=CARTESIAN_POINT('Ctrl Pts',(7.68350640208746,28.9153086857956,56.266664988286));
#104208=CARTESIAN_POINT('Ctrl Pts',(7.67892205798069,28.9724326667835,56.3134298829397));
#104209=CARTESIAN_POINT('Ctrl Pts',(7.67330373076348,29.0424519722074,56.3633812731262));
#104210=CARTESIAN_POINT('Ctrl Pts',(7.67249549090482,29.0525244255663,56.3704002099891));
#104211=CARTESIAN_POINT('Ctrl Pts',(7.67121855238707,29.0684177150572,56.3812163951233));
#104212=CARTESIAN_POINT('Ctrl Pts',(7.67075472989186,29.074186541949,56.3850897878103));
#104213=CARTESIAN_POINT('Ctrl Pts',(7.66988234892712,29.0850249786524,56.3922691333822));
#104214=CARTESIAN_POINT('Ctrl Pts',(7.66947436500813,29.0900885896202,56.3955836951057));
#104215=CARTESIAN_POINT('Ctrl Pts',(7.66850840022717,29.1020666301471,56.4033314382105));
#104216=CARTESIAN_POINT('Ctrl Pts',(7.66794893567573,29.1089959078184,56.4077411561836));
#104217=CARTESIAN_POINT('Ctrl Pts',(7.66606509637627,29.1323104077254,56.4223371638982));
#104218=CARTESIAN_POINT('Ctrl Pts',(7.66472718751596,29.148839245191,56.432289609872));
#104219=CARTESIAN_POINT('Ctrl Pts',(7.66139682181687,29.1899967056376,56.4561076025831));
#104220=CARTESIAN_POINT('Ctrl Pts',(7.65938979963948,29.2148120346619,56.4696374947641));
#104221=CARTESIAN_POINT('Ctrl Pts',(7.65019628783019,29.3289894363844,56.5281723556831));
#104222=CARTESIAN_POINT('Ctrl Pts',(7.64283774004886,29.4219507307493,56.5657028485786));
#104223=CARTESIAN_POINT('Ctrl Pts',(7.62965965141574,29.5968835102083,56.6186084781));
#104224=CARTESIAN_POINT('Ctrl Pts',(7.62380959960134,29.6777308583614,56.636625376748));
#104225=CARTESIAN_POINT('Ctrl Pts',(7.6168062820679,29.7789953504499,56.651392556983));
#104226=CARTESIAN_POINT('Ctrl Pts',(7.61547514387438,29.7984462042601,56.6538792449243));
#104227=CARTESIAN_POINT('Ctrl Pts',(7.61335850955488,29.8296907233105,56.6573142629258));
#104228=CARTESIAN_POINT('Ctrl Pts',(7.61256623447685,29.8414579573358,56.6584813080072));
#104229=CARTESIAN_POINT('Ctrl Pts',(7.61106206342974,29.8639318676572,56.6604688315574));
#104230=CARTESIAN_POINT('Ctrl Pts',(7.61034951565319,29.8746359493407,56.6613112716227));
#104231=CARTESIAN_POINT('Ctrl Pts',(7.60871709763415,29.8992866176447,56.6630117360234));
#104232=CARTESIAN_POINT('Ctrl Pts',(7.60779951394328,29.9132374737514,56.6637979153967));
#104233=CARTESIAN_POINT('Ctrl Pts',(7.60489092310531,29.9577417273879,56.6657445807025));
#104234=CARTESIAN_POINT('Ctrl Pts',(7.60292053560572,29.9883189198263,56.6662396316288));
#104235=CARTESIAN_POINT('Ctrl Pts',(7.59826685115947,30.0613489739135,56.6654113478274));
#104236=CARTESIAN_POINT('Ctrl Pts',(7.59560606224221,30.1037719356854,56.6633070727821));
#104237=CARTESIAN_POINT('Ctrl Pts',(7.5884020407577,30.2195191601238,56.6531194237627));
#104238=CARTESIAN_POINT('Ctrl Pts',(7.5839265836452,30.2924592504376,56.6417857489463));
#104239=CARTESIAN_POINT('Ctrl Pts',(7.57445467251241,30.443540894953,56.6079191556948));
#104240=CARTESIAN_POINT('Ctrl Pts',(7.56946273537542,30.521263070193,56.5844286638284));
#104241=CARTESIAN_POINT('Ctrl Pts',(7.56316349761809,30.6120132481413,56.5495986261994));
#104242=CARTESIAN_POINT('Ctrl Pts',(7.56210818590097,30.6269851299292,56.543601541247));
#104243=CARTESIAN_POINT('Ctrl Pts',(7.5605270334629,30.6490298464412,56.5343977677214));
#104244=CARTESIAN_POINT('Ctrl Pts',(7.56001049509019,30.6561716210186,56.5313572571304));
#104245=CARTESIAN_POINT('Ctrl Pts',(7.55908875504542,30.6688038841038,56.5258746580552));
#104246=CARTESIAN_POINT('Ctrl Pts',(7.55868475218502,30.6743027874232,56.5234526104147));
#104247=CARTESIAN_POINT('Ctrl Pts',(7.55778909175074,30.6864092545777,56.5180418058125));
#104248=CARTESIAN_POINT('Ctrl Pts',(7.55729666711525,30.6930103757568,56.515039670468));
#104249=CARTESIAN_POINT('Ctrl Pts',(7.55584127124922,30.712365933217,56.5060839612423));
#104250=CARTESIAN_POINT('Ctrl Pts',(7.55487163049218,30.7250643985567,56.5000119020881));
#104251=CARTESIAN_POINT('Ctrl Pts',(7.54806868534156,30.812897954201,56.4566364384869));
#104252=CARTESIAN_POINT('Ctrl Pts',(7.5419820788777,30.8851917534359,56.4138689761082));
#104253=CARTESIAN_POINT('Ctrl Pts',(7.52652525687139,31.059306011282,56.2922620594852));
#104254=CARTESIAN_POINT('Ctrl Pts',(7.51721420295268,31.1558146621214,56.2067206892762));
#104255=CARTESIAN_POINT('Ctrl Pts',(7.50692676486953,31.2555294624945,56.0952817309755));
#104256=CARTESIAN_POINT('Ctrl Pts',(7.50549524115868,31.2692253941626,56.0793809659869));
#104257=CARTESIAN_POINT('Ctrl Pts',(7.50317527755965,31.2911168019607,56.0529723425865));
#104258=CARTESIAN_POINT('Ctrl Pts',(7.50227959898613,31.2994927431455,56.0426178489473));
#104259=CARTESIAN_POINT('Ctrl Pts',(7.50067538230539,31.3143534398637,56.0237894563849));
#104260=CARTESIAN_POINT('Ctrl Pts',(7.49996510007983,31.3208825747504,56.0153516871969));
#104261=CARTESIAN_POINT('Ctrl Pts',(7.49844859792349,31.3347107506058,55.99712203234));
#104262=CARTESIAN_POINT('Ctrl Pts',(7.49764341020147,31.3419841177594,55.9873113876414));
#104263=CARTESIAN_POINT('Ctrl Pts',(7.49543578745122,31.3617286385748,55.9600577363322));
#104264=CARTESIAN_POINT('Ctrl Pts',(7.49404207498355,31.373972216678,55.9424522047077));
#104265=CARTESIAN_POINT('Ctrl Pts',(7.48818256773555,31.4244297145494,55.8668231942112));
#104266=CARTESIAN_POINT('Ctrl Pts',(7.48383762888856,31.4593363503408,55.8066730894563));
#104267=CARTESIAN_POINT('Ctrl Pts',(7.47576622236848,31.5178498003253,55.6895391775552));
#104268=CARTESIAN_POINT('Ctrl Pts',(7.47203390583422,31.5422332525998,55.6331195595607));
#104269=CARTESIAN_POINT('Ctrl Pts',(7.46827878691259,31.5634376230276,55.5755161152408));
#104270=CARTESIAN_POINT('Origin',(5.,30.,55.));
#104271=CARTESIAN_POINT('',(6.76892549910492,31.5634376526692,55.5755160347169));
#104272=CARTESIAN_POINT('',(6.9616842973919,31.5634376940719,55.5755159222429));
#104273=CARTESIAN_POINT('',(5.,31.5634376782623,55.5755159651912));
#104274=CARTESIAN_POINT('Ctrl Pts',(6.9616842973919,31.5634376940719,55.5755159222429));
#104275=CARTESIAN_POINT('Ctrl Pts',(6.96605878096345,31.5391991836305,55.6413618865466));
#104276=CARTESIAN_POINT('Ctrl Pts',(6.97033680726182,31.510818319282,55.7056294995728));
#104277=CARTESIAN_POINT('Ctrl Pts',(6.97960774088078,31.4408418132267,55.8403512155861));
#104278=CARTESIAN_POINT('Ctrl Pts',(6.984589699559,31.3979601620666,55.9099011867989));
#104279=CARTESIAN_POINT('Ctrl Pts',(6.99144683607502,31.335035920585,55.9969461669099));
#104280=CARTESIAN_POINT('Ctrl Pts',(6.99311723203387,31.3194271468703,56.0175138320948));
#104281=CARTESIAN_POINT('Ctrl Pts',(6.99542234375112,31.2976299855697,56.0448907550862));
#104282=CARTESIAN_POINT('Ctrl Pts',(6.99603078389574,31.2918529972518,56.0520247589419));
#104283=CARTESIAN_POINT('Ctrl Pts',(6.99705796587303,31.282067579129,56.0639066349479));
#104284=CARTESIAN_POINT('Ctrl Pts',(6.9974744751748,31.2780908961335,56.0686806187769));
#104285=CARTESIAN_POINT('Ctrl Pts',(6.99833373373159,31.2698713889729,56.0784365887687));
#104286=CARTESIAN_POINT('Ctrl Pts',(6.99877666510884,31.2656257893292,56.0834159765248));
#104287=CARTESIAN_POINT('Ctrl Pts',(6.99995165755948,31.2543377663635,56.0964980701339));
#104288=CARTESIAN_POINT('Ctrl Pts',(7.00068713337997,31.247246302718,56.1045577826216));
#104289=CARTESIAN_POINT('Ctrl Pts',(7.00398200111639,31.2153421053471,56.1401191053309));
#104290=CARTESIAN_POINT('Ctrl Pts',(7.00659333309507,31.189695929694,56.1668552344542));
#104291=CARTESIAN_POINT('Ctrl Pts',(7.0159177694808,31.0962272142633,56.2580098117355));
#104292=CARTESIAN_POINT('Ctrl Pts',(7.02278600539818,31.0238941437296,56.3175519507439));
#104293=CARTESIAN_POINT('Ctrl Pts',(7.0341056887045,30.8952550118401,56.4064217150446));
#104294=CARTESIAN_POINT('Ctrl Pts',(7.03860457923511,30.8415786141611,56.439183928949));
#104295=CARTESIAN_POINT('Ctrl Pts',(7.04581928682043,30.7508075133655,56.4877678797704));
#104296=CARTESIAN_POINT('Ctrl Pts',(7.04858991700207,30.7147656914341,56.5054154459738));
#104297=CARTESIAN_POINT('Ctrl Pts',(7.05236697558147,30.6639937743315,56.5280403830164));
#104298=CARTESIAN_POINT('Ctrl Pts',(7.05341107596881,30.6497811328394,56.5341380811063));
#104299=CARTESIAN_POINT('Ctrl Pts',(7.05518486167894,30.6253375094143,56.5442245657764));
#104300=CARTESIAN_POINT('Ctrl Pts',(7.05591782820855,30.6151484536999,56.5483116288662));
#104301=CARTESIAN_POINT('Ctrl Pts',(7.05739747670118,30.5944038861428,56.5563956410507));
#104302=CARTESIAN_POINT('Ctrl Pts',(7.05814392764579,30.5838466606964,56.5603866375819));
#104303=CARTESIAN_POINT('Ctrl Pts',(7.06000839099854,30.5572523199332,56.5701325193655));
#104304=CARTESIAN_POINT('Ctrl Pts',(7.0611217945913,30.5411657210251,56.5757493372613));
#104305=CARTESIAN_POINT('Ctrl Pts',(7.06539707030997,30.4786449668356,56.5965087553796));
#104306=CARTESIAN_POINT('Ctrl Pts',(7.06850073577216,30.4316374986171,56.6098543291492));
#104307=CARTESIAN_POINT('Ctrl Pts',(7.07842143390615,30.2774277896715,56.6463928384726));
#104308=CARTESIAN_POINT('Ctrl Pts',(7.08501078287782,30.1685156231981,56.6610774527979));
#104309=CARTESIAN_POINT('Ctrl Pts',(7.09464516483473,30.0120876145971,56.6666159316788));
#104310=CARTESIAN_POINT('Ctrl Pts',(7.09755918558406,29.9651798272095,56.6662958103886));
#104311=CARTESIAN_POINT('Ctrl Pts',(7.10229181881558,29.8909824314054,56.6626551172728));
#104312=CARTESIAN_POINT('Ctrl Pts',(7.10406177420637,29.8636525155922,56.660637235264));
#104313=CARTESIAN_POINT('Ctrl Pts',(7.10648301761513,29.8270506616555,56.6570252071521));
#104314=CARTESIAN_POINT('Ctrl Pts',(7.10710451205596,29.8177228245269,56.6560250698242));
#104315=CARTESIAN_POINT('Ctrl Pts',(7.10814743850237,29.8021924527981,56.6542270936239));
#104316=CARTESIAN_POINT('Ctrl Pts',(7.10856648284714,29.7959848885515,56.6534729920111));
#104317=CARTESIAN_POINT('Ctrl Pts',(7.10937087599066,29.7841343500284,56.6519656263791));
#104318=CARTESIAN_POINT('Ctrl Pts',(7.10975585986795,29.7784907378013,56.6512183543889));
#104319=CARTESIAN_POINT('Ctrl Pts',(7.11080105572772,29.7632414859407,56.6491196140163));
#104320=CARTESIAN_POINT('Ctrl Pts',(7.11146421154153,29.7536438187596,56.6477131776893));
#104321=CARTESIAN_POINT('Ctrl Pts',(7.11403693553516,29.7166867423936,56.6419674065242));
#104322=CARTESIAN_POINT('Ctrl Pts',(7.11597515316308,29.6894264594142,56.6370300022833));
#104323=CARTESIAN_POINT('Ctrl Pts',(7.12580958903916,29.5534118974173,56.6088755691168));
#104324=CARTESIAN_POINT('Ctrl Pts',(7.13400651215752,29.4470536890573,56.5754907915846));
#104325=CARTESIAN_POINT('Ctrl Pts',(7.1462941521345,29.2906872324615,56.5086077636068));
#104326=CARTESIAN_POINT('Ctrl Pts',(7.15049845842193,29.2378194372421,56.482600399395));
#104327=CARTESIAN_POINT('Ctrl Pts',(7.15730693364231,29.1528992881794,56.4350795179289));
#104328=CARTESIAN_POINT('Ctrl Pts',(7.15995817737944,29.1200206041347,56.4151570649151));
#104329=CARTESIAN_POINT('Ctrl Pts',(7.16360271723309,29.0751177173069,56.3857779630177));
#104330=CARTESIAN_POINT('Ctrl Pts',(7.16463026714366,29.0624919315407,56.3772677473651));
#104331=CARTESIAN_POINT('Ctrl Pts',(7.16638460604484,29.041001669676,56.362350089912));
#104332=CARTESIAN_POINT('Ctrl Pts',(7.1671144980028,29.0320805579173,56.3560263745625));
#104333=CARTESIAN_POINT('Ctrl Pts',(7.168595283171,29.014026257364,56.3429596565791));
#104334=CARTESIAN_POINT('Ctrl Pts',(7.16934587683821,29.0048984257147,56.3362102110101));
#104335=CARTESIAN_POINT('Ctrl Pts',(7.17123509513117,28.9819906784605,56.3189064668498));
#104336=CARTESIAN_POINT('Ctrl Pts',(7.17236884621399,28.9683051799836,56.3082289869823));
#104337=CARTESIAN_POINT('Ctrl Pts',(7.17685749519357,28.9144154583463,56.2648123164017));
#104338=CARTESIAN_POINT('Ctrl Pts',(7.18014600508872,28.8755801182253,56.2304164826193));
#104339=CARTESIAN_POINT('Ctrl Pts',(7.19151845194387,28.7450558894532,56.1034630283681));
#104340=CARTESIAN_POINT('Ctrl Pts',(7.19926377393868,28.6626774574071,56.0020383521461));
#104341=CARTESIAN_POINT('Ctrl Pts',(7.20935364639527,28.5761500002311,55.8655587257811));
#104342=CARTESIAN_POINT('Ctrl Pts',(7.21133530491899,28.5601004609697,55.8385879878787));
#104343=CARTESIAN_POINT('Ctrl Pts',(7.21469136474507,28.5346917797679,55.7930074224237));
#104344=CARTESIAN_POINT('Ctrl Pts',(7.21604517200548,28.5249024562239,55.774645785246));
#104345=CARTESIAN_POINT('Ctrl Pts',(7.21797734270721,28.5116204247047,55.7485678440223));
#104346=CARTESIAN_POINT('Ctrl Pts',(7.21853915511936,28.5078383231723,55.7410000673838));
#104347=CARTESIAN_POINT('Ctrl Pts',(7.21951131419237,28.5014341441487,55.7279377978301));
#104348=CARTESIAN_POINT('Ctrl Pts',(7.21991995363518,28.4987842643689,55.7224571791995));
#104349=CARTESIAN_POINT('Ctrl Pts',(7.22079069355832,28.4932278908324,55.7108026252196));
#104350=CARTESIAN_POINT('Ctrl Pts',(7.22125321463698,28.4903293103046,55.7046254079117));
#104351=CARTESIAN_POINT('Ctrl Pts',(7.22253673186184,28.482428658832,55.6875156478742));
#104352=CARTESIAN_POINT('Ctrl Pts',(7.22336229199063,28.4775069727751,55.6765467483983));
#104353=CARTESIAN_POINT('Ctrl Pts',(7.22805529647081,28.4504016172849,55.6143434870941));
#104354=CARTESIAN_POINT('Ctrl Pts',(7.23204072404014,28.4306877802332,55.5620773311299));
#104355=CARTESIAN_POINT('Ctrl Pts',(7.24439011190475,28.3784717475078,55.3993158572814));
#104356=CARTESIAN_POINT('Ctrl Pts',(7.25285272177008,28.3547585893054,55.2863426391698));
#104357=CARTESIAN_POINT('Ctrl Pts',(7.26500701822658,28.3371014018802,55.1160525750548));
#104358=CARTESIAN_POINT('Ctrl Pts',(7.26891717713879,28.3341372015599,55.0600194059551));
#104359=CARTESIAN_POINT('Ctrl Pts',(7.27392176472738,28.3339637216004,54.9866192144537));
#104360=CARTESIAN_POINT('Ctrl Pts',(7.27509418772777,28.3341928317121,54.9693007528494));
#104361=CARTESIAN_POINT('Ctrl Pts',(7.27702062649477,28.3350188641001,54.9406493602572));
#104362=CARTESIAN_POINT('Ctrl Pts',(7.27777938644573,28.33546158406,54.929313691585));
#104363=CARTESIAN_POINT('Ctrl Pts',(7.27925453116482,28.3365525225946,54.907180428105));
#104364=CARTESIAN_POINT('Ctrl Pts',(7.27997120774794,28.337190182243,54.8963829050674));
#104365=CARTESIAN_POINT('Ctrl Pts',(7.28168499835746,28.3389744470515,54.8704618918199));
#104366=CARTESIAN_POINT('Ctrl Pts',(7.28267889926956,28.340222513103,54.8553461787118));
#104367=CARTESIAN_POINT('Ctrl Pts',(7.28596061648191,28.345054365208,54.8051882331202));
#104368=CARTESIAN_POINT('Ctrl Pts',(7.288220365409,28.3495431062944,54.7702414336188));
#104369=CARTESIAN_POINT('Ctrl Pts',(7.29820377937337,28.3745634184298,54.6146688501553));
#104370=CARTESIAN_POINT('Ctrl Pts',(7.30555594387433,28.4072355480808,54.4963860829649));
#104371=CARTESIAN_POINT('Ctrl Pts',(7.31616835007085,28.4712510215176,54.3359023028214));
#104372=CARTESIAN_POINT('Ctrl Pts',(7.31929271379768,28.4920514171192,54.2899369352619));
#104373=CARTESIAN_POINT('Ctrl Pts',(7.32432615251511,28.5279176976066,54.2193883910628));
#104374=CARTESIAN_POINT('Ctrl Pts',(7.32617870871891,28.5415917477417,54.1941303300494));
#104375=CARTESIAN_POINT('Ctrl Pts',(7.32869595031607,28.5606681658887,54.1609702656021));
#104376=CARTESIAN_POINT('Ctrl Pts',(7.32932775507096,28.5654964703236,54.1527416943151));
#104377=CARTESIAN_POINT('Ctrl Pts',(7.33038319056283,28.5736226210392,54.1391614065089));
#104378=CARTESIAN_POINT('Ctrl Pts',(7.33080430929422,28.5768806536416,54.1337859185545));
#104379=CARTESIAN_POINT('Ctrl Pts',(7.33166108525565,28.5835387476352,54.1229395627342));
#104380=CARTESIAN_POINT('Ctrl Pts',(7.33209682305247,28.5869402500874,54.1174697570728));
#104381=CARTESIAN_POINT('Ctrl Pts',(7.33323220332089,28.5958451431336,54.1033336572343));
#104382=CARTESIAN_POINT('Ctrl Pts',(7.33393487326718,28.6013969746332,54.0946984168727));
#104383=CARTESIAN_POINT('Ctrl Pts',(7.33687296088697,28.6247929819851,54.0590374830235));
#104384=CARTESIAN_POINT('Ctrl Pts',(7.33914789212967,28.6433423261855,54.0324854359747));
#104385=CARTESIAN_POINT('Ctrl Pts',(7.34834777601949,28.7204685121623,53.9286668015828));
#104386=CARTESIAN_POINT('Ctrl Pts',(7.35547038268582,28.7849661406488,53.856038653126));
#104387=CARTESIAN_POINT('Ctrl Pts',(7.36714653526506,28.9020787083574,53.7453089585798));
#104388=CARTESIAN_POINT('Ctrl Pts',(7.37174946631868,28.9512622934629,53.7039168865007));
#104389=CARTESIAN_POINT('Ctrl Pts',(7.37910617768451,29.0353124021925,53.6411072341496));
#104390=CARTESIAN_POINT('Ctrl Pts',(7.38191764461866,29.0687907301478,53.617950254636));
#104391=CARTESIAN_POINT('Ctrl Pts',(7.38573984266054,29.1161852243322,53.5876724686091));
#104392=CARTESIAN_POINT('Ctrl Pts',(7.38678945020077,29.1294011300752,53.5794876805362));
#104393=CARTESIAN_POINT('Ctrl Pts',(7.38856972450322,29.1521554437231,53.5658324922275));
#104394=CARTESIAN_POINT('Ctrl Pts',(7.3893037322654,29.1616367778829,53.5602694871104));
#104395=CARTESIAN_POINT('Ctrl Pts',(7.39069557057181,29.1798024914372,53.5498513815655));
#104396=CARTESIAN_POINT('Ctrl Pts',(7.39135398399864,29.1884766182542,53.5449794583038));
#104397=CARTESIAN_POINT('Ctrl Pts',(7.39288876624656,29.208881895304,53.533757842432));
#104398=CARTESIAN_POINT('Ctrl Pts',(7.39376289455994,29.2206468049796,53.5274707016041));
#104399=CARTESIAN_POINT('Ctrl Pts',(7.39679048882461,29.2618781161244,53.506069374918));
#104400=CARTESIAN_POINT('Ctrl Pts',(7.39891846956236,29.291719745271,53.4916923580391));
#104401=CARTESIAN_POINT('Ctrl Pts',(7.408925649166,29.4356832938722,53.4275497492198));
#104402=CARTESIAN_POINT('Ctrl Pts',(7.41640732848865,29.5547127289888,53.3897906887562));
#104403=CARTESIAN_POINT('Ctrl Pts',(7.42718355791543,29.7268812733978,53.3557482091025));
#104404=CARTESIAN_POINT('Ctrl Pts',(7.43034218624413,29.7773448750178,53.3481580698023));
#104405=CARTESIAN_POINT('Ctrl Pts',(7.43483335889778,29.8476023668032,53.3408687653566));
#104406=CARTESIAN_POINT('Ctrl Pts',(7.43609392040169,29.8671649106243,53.3391880717044));
#104407=CARTESIAN_POINT('Ctrl Pts',(7.43832620579238,29.901425354632,53.3368537779799));
#104408=CARTESIAN_POINT('Ctrl Pts',(7.4392909648623,29.9161110195968,53.3360484023967));
#104409=CARTESIAN_POINT('Ctrl Pts',(7.44075509085872,29.938178340151,53.3351310725891));
#104410=CARTESIAN_POINT('Ctrl Pts',(7.44124684945115,29.9455536630292,53.3348735620677));
#104411=CARTESIAN_POINT('Ctrl Pts',(7.44214365629856,29.9589321079609,53.3344954281089));
#104412=CARTESIAN_POINT('Ctrl Pts',(7.4425477914177,29.9649344951484,53.3343582444591));
#104413=CARTESIAN_POINT('Ctrl Pts',(7.44346871877992,29.9785526676406,53.3341206466661));
#104414=CARTESIAN_POINT('Ctrl Pts',(7.44398655380007,29.9861684379261,53.3340400094495));
#104415=CARTESIAN_POINT('Ctrl Pts',(7.44559552250121,30.0097113275793,53.3339521724374));
#104416=CARTESIAN_POINT('Ctrl Pts',(7.44669551210689,30.0256376692242,53.3341211516941));
#104417=CARTESIAN_POINT('Ctrl Pts',(7.4547521473933,30.1412379710788,53.3370057005297));
#104418=CARTESIAN_POINT('Ctrl Pts',(7.46204710573607,30.2404844424247,53.3484364400081));
#104419=CARTESIAN_POINT('Ctrl Pts',(7.47209091130659,30.375687687993,53.3764582060482));
#104420=CARTESIAN_POINT('Ctrl Pts',(7.47487542062039,30.4129918543761,53.3855443343301));
#104421=CARTESIAN_POINT('Ctrl Pts',(7.48142394225165,30.5006069290069,53.41012052554));
#104422=CARTESIAN_POINT('Ctrl Pts',(7.48516417682383,30.5505660896669,53.4267225604054));
#104423=CARTESIAN_POINT('Ctrl Pts',(7.49131977273814,30.6328770553442,53.4584779438754));
#104424=CARTESIAN_POINT('Ctrl Pts',(7.49377120946707,30.6656770074748,53.4723553843643));
#104425=CARTESIAN_POINT('Ctrl Pts',(7.49719204794729,30.7114491227021,53.4934757773371));
#104426=CARTESIAN_POINT('Ctrl Pts',(7.49819032687666,30.7248060840215,53.4998562559568));
#104427=CARTESIAN_POINT('Ctrl Pts',(7.49991050409725,30.7478145783698,53.5112262290877));
#104428=CARTESIAN_POINT('Ctrl Pts',(7.50063519516233,30.7575054332946,53.5161335933682));
#104429=CARTESIAN_POINT('Ctrl Pts',(7.50202767702168,30.776117710957,53.5257885467199));
#104430=CARTESIAN_POINT('Ctrl Pts',(7.50269588195686,30.7850452631518,53.530523204451));
#104431=CARTESIAN_POINT('Ctrl Pts',(7.50446396467172,30.808652193802,53.5433194991129));
#104432=CARTESIAN_POINT('Ctrl Pts',(7.50555881244014,30.8232542824333,53.5515218772777));
#104433=CARTESIAN_POINT('Ctrl Pts',(7.50964783892518,30.877688395064,53.5831880779939));
#104434=CARTESIAN_POINT('Ctrl Pts',(7.51259047533527,30.9166637316682,53.608087239961));
#104435=CARTESIAN_POINT('Ctrl Pts',(7.52375852737322,31.0625812368592,53.7100969648281));
#104436=CARTESIAN_POINT('Ctrl Pts',(7.53160205882745,31.1612562487365,53.798163654094));
#104437=CARTESIAN_POINT('Ctrl Pts',(7.54195588990297,31.2714675064711,53.9229078164203));
#104438=CARTESIAN_POINT('Ctrl Pts',(7.54413620160729,31.2935973853703,53.9495892715032));
#104439=CARTESIAN_POINT('Ctrl Pts',(7.54779202977871,31.3285865406652,53.9945587194966));
#104440=CARTESIAN_POINT('Ctrl Pts',(7.54924193474332,31.3419390328605,54.0124505683885));
#104441=CARTESIAN_POINT('Ctrl Pts',(7.55128795984955,31.3599850376022,54.0376735199897));
#104442=CARTESIAN_POINT('Ctrl Pts',(7.55186481112744,31.3649873057471,54.0447821172259));
#104443=CARTESIAN_POINT('Ctrl Pts',(7.5528544600751,31.3734189482748,54.0569655870034));
#104444=CARTESIAN_POINT('Ctrl Pts',(7.55326539092743,31.3768764612798,54.0620209379647));
#104445=CARTESIAN_POINT('Ctrl Pts',(7.55413123934494,31.3840688521163,54.0726626463423));
#104446=CARTESIAN_POINT('Ctrl Pts',(7.55458649931756,31.3877978816186,54.0782526427193));
#104447=CARTESIAN_POINT('Ctrl Pts',(7.55582957068282,31.3978400775973,54.0935054638303));
#104448=CARTESIAN_POINT('Ctrl Pts',(7.55662150217171,31.4040866684626,54.1032113763642));
#104449=CARTESIAN_POINT('Ctrl Pts',(7.56067180433702,31.4352978770733,54.1528326793087));
#104450=CARTESIAN_POINT('Ctrl Pts',(7.56401422468317,31.4586612315519,54.1937252209994));
#104451=CARTESIAN_POINT('Ctrl Pts',(7.57465828076498,31.5265704721966,54.3252223764167));
#104452=CARTESIAN_POINT('Ctrl Pts',(7.58207951644744,31.5646372979801,54.4189203581647));
#104453=CARTESIAN_POINT('Ctrl Pts',(7.59484875179544,31.6162990247435,54.5888825997773));
#104454=CARTESIAN_POINT('Ctrl Pts',(7.60025566188861,31.6335144953173,54.6637360100342));
#104455=CARTESIAN_POINT('Ctrl Pts',(7.60679056684221,31.6484616321655,54.758160325794));
#104456=CARTESIAN_POINT('Ctrl Pts',(7.6080707447755,31.6510955416035,54.7768503997537));
#104457=CARTESIAN_POINT('Ctrl Pts',(7.61012640958847,31.6548433975342,54.807164482254));
#104458=CARTESIAN_POINT('Ctrl Pts',(7.61090799260652,31.6561536847005,54.8187620571968));
#104459=CARTESIAN_POINT('Ctrl Pts',(7.61240458861309,31.658440303052,54.8411034419004));
#104460=CARTESIAN_POINT('Ctrl Pts',(7.61312012179271,31.6594343619786,54.8518448024095));
#104461=CARTESIAN_POINT('Ctrl Pts',(7.6147616322004,31.6614846358644,54.8766191989005));
#104462=CARTESIAN_POINT('Ctrl Pts',(7.61568527563044,31.6624675267487,54.8906576025065));
#104463=CARTESIAN_POINT('Ctrl Pts',(7.61869408056788,31.6651048252023,54.9366898637379));
#104464=CARTESIAN_POINT('Ctrl Pts',(7.62075616911904,31.6660144207487,54.9687203207882));
#104465=CARTESIAN_POINT('Ctrl Pts',(7.62567552230028,31.6659791981065,55.0460479865259));
#104466=CARTESIAN_POINT('Ctrl Pts',(7.62850644731632,31.6641118616799,55.09131954637));
#104467=CARTESIAN_POINT('Ctrl Pts',(7.63562981808123,31.6546777507552,55.2061096596105));
#104468=CARTESIAN_POINT('Ctrl Pts',(7.63987218161648,31.6445769255838,55.2753300566623));
#104469=CARTESIAN_POINT('Ctrl Pts',(7.64492146248019,31.6275528375619,55.3560720941749));
#104470=CARTESIAN_POINT('Ctrl Pts',(7.64569548756865,31.6248061902719,55.3684025174323));
#104471=CARTESIAN_POINT('Ctrl Pts',(7.65064046933885,31.6064087226453,55.4467822927442));
#104472=CARTESIAN_POINT('Ctrl Pts',(7.65485616124645,31.5868767434299,55.5118417667872));
#104473=CARTESIAN_POINT('Ctrl Pts',(7.65925614416276,31.563437678903,55.5755159634506));
#104474=CARTESIAN_POINT('',(7.42924477180836,31.6659997297127,55.0012652267279));
#104475=CARTESIAN_POINT('Ctrl Pts',(7.46827878691259,31.5634376230276,55.5755161152408));
#104476=CARTESIAN_POINT('Ctrl Pts',(7.4656539658509,31.5782594380647,55.535251416031));
#104477=CARTESIAN_POINT('Ctrl Pts',(7.46301743683412,31.5915279306235,55.494408327742));
#104478=CARTESIAN_POINT('Ctrl Pts',(7.45745227979136,31.6157720974862,55.4086205039906));
#104479=CARTESIAN_POINT('Ctrl Pts',(7.45452076845838,31.6264799160976,55.3636652849397));
#104480=CARTESIAN_POINT('Ctrl Pts',(7.45074649398307,31.6374954372626,55.3070766712269));
#104481=CARTESIAN_POINT('Ctrl Pts',(7.44999047643321,31.6395693643978,55.2958034320809));
#104482=CARTESIAN_POINT('Ctrl Pts',(7.44878249270745,31.642671099076,55.2779074742279));
#104483=CARTESIAN_POINT('Ctrl Pts',(7.44833467699693,31.6437755938566,55.2712981700257));
#104484=CARTESIAN_POINT('Ctrl Pts',(7.4474728606743,31.645813982304,55.2586308315242));
#104485=CARTESIAN_POINT('Ctrl Pts',(7.44705921983653,31.6467543571502,55.2525740554654));
#104486=CARTESIAN_POINT('Ctrl Pts',(7.44622483485821,31.6485756845497,55.2404005066046));
#104487=CARTESIAN_POINT('Ctrl Pts',(7.44580407019775,31.6494560722221,55.2342837042026));
#104488=CARTESIAN_POINT('Ctrl Pts',(7.44479672650825,31.6514738932723,55.2196887628783));
#104489=CARTESIAN_POINT('Ctrl Pts',(7.44420856977113,31.652580088181,55.2112065751816));
#104490=CARTESIAN_POINT('Ctrl Pts',(7.44212392557101,31.6562502390306,55.1812680196867));
#104491=CARTESIAN_POINT('Ctrl Pts',(7.44061140200932,31.6584619054565,55.1597715769524));
#104492=CARTESIAN_POINT('Ctrl Pts',(7.43585342418317,31.6640485999887,55.0926753967592));
#104493=CARTESIAN_POINT('Ctrl Pts',(7.43256029705638,31.6659648561359,55.0469779281573));
#104494=CARTESIAN_POINT('Ctrl Pts',(7.4292449970585,31.6659995210235,55.0012633089186));
#104495=CARTESIAN_POINT('Ctrl Pts',(7.42924513422323,31.6659995195882,55.0012652002811));
#104496=CARTESIAN_POINT('Ctrl Pts',(7.41936135371292,31.6661030194695,54.8649778827319));
#104497=CARTESIAN_POINT('Ctrl Pts',(7.40938169123781,31.6494818328085,54.7291573370653));
#104498=CARTESIAN_POINT('Ctrl Pts',(7.39771728103842,31.6088565340369,54.56625860823));
#104499=CARTESIAN_POINT('Ctrl Pts',(7.39555200428979,31.6003558274504,54.5358745847821));
#104500=CARTESIAN_POINT('Ctrl Pts',(7.39245617925532,31.5868023520165,54.4922459184446));
#104501=CARTESIAN_POINT('Ctrl Pts',(7.3915036984892,31.5824359088968,54.4787970382474));
#104502=CARTESIAN_POINT('Ctrl Pts',(7.38983635145403,31.5744463334028,54.4552151853474));
#104503=CARTESIAN_POINT('Ctrl Pts',(7.38911916494136,31.5708953101027,54.4450588453925));
#104504=CARTESIAN_POINT('Ctrl Pts',(7.38762589435441,31.5632627843851,54.4238894277458));
#104505=CARTESIAN_POINT('Ctrl Pts',(7.38685047238517,31.5591626986701,54.4128836440023));
#104506=CARTESIAN_POINT('Ctrl Pts',(7.3848154294815,31.5480432973963,54.3839742527801));
#104507=CARTESIAN_POINT('Ctrl Pts',(7.38356233987784,31.5408296700018,54.3661469021415));
#104508=CARTESIAN_POINT('Ctrl Pts',(7.3775013159638,31.5041719301216,54.2798796232642));
#104509=CARTESIAN_POINT('Ctrl Pts',(7.37283973460155,31.470466657887,54.2133384866256));
#104510=CARTESIAN_POINT('Ctrl Pts',(7.36163437503957,31.377608980505,54.0569893057153));
#104511=CARTESIAN_POINT('Ctrl Pts',(7.35519975023623,31.3140164567546,53.9702262801732));
#104512=CARTESIAN_POINT('Ctrl Pts',(7.34664975305962,31.2230466447546,53.8683781648411));
#104513=CARTESIAN_POINT('Ctrl Pts',(7.34479825774764,31.2029974935462,53.8470872073387));
#104514=CARTESIAN_POINT('Ctrl Pts',(7.34166016428255,31.1686790866063,53.8125133616532));
#104515=CARTESIAN_POINT('Ctrl Pts',(7.34039159863371,31.1547178449358,53.7989329981939));
#104516=CARTESIAN_POINT('Ctrl Pts',(7.33858416214926,31.1347654542844,53.7801943838589));
#104517=CARTESIAN_POINT('Ctrl Pts',(7.33805981535908,31.1289701718512,53.7748286967522));
#104518=CARTESIAN_POINT('Ctrl Pts',(7.33752869710769,31.1230960305806,53.7694670629413));
#104519=CARTESIAN_POINT('Ctrl Pts',(7.33752498343876,31.1230549573915,53.7694295770779));
#104520=CARTESIAN_POINT('Ctrl Pts',(7.33751748310661,31.1229720033011,53.7693538757969));
#104521=CARTESIAN_POINT('Ctrl Pts',(7.33751369643611,31.1229301223116,53.7693156604476));
#104522=CARTESIAN_POINT('Ctrl Pts',(7.33750604627074,31.1228455102381,53.7692384619741));
#104523=CARTESIAN_POINT('Ctrl Pts',(7.33750218276933,31.1228027790735,53.7691994789364));
#104524=CARTESIAN_POINT('Ctrl Pts',(7.33749437487349,31.1227164216271,53.769120704498));
#104525=CARTESIAN_POINT('Ctrl Pts',(7.33749043047031,31.1226727952395,53.7690809131727));
#104526=CARTESIAN_POINT('Ctrl Pts',(7.33748245644921,31.122584599523,53.769000479061));
#104527=CARTESIAN_POINT('Ctrl Pts',(7.33747842681846,31.1225400300429,53.7689598363215));
#104528=CARTESIAN_POINT('Ctrl Pts',(7.33747027774098,31.1224498972236,53.7688776535111));
#104529=CARTESIAN_POINT('Ctrl Pts',(7.3374661582819,31.1224043337378,53.7688361135055));
#104530=CARTESIAN_POINT('Ctrl Pts',(7.33745782463336,31.1223121585232,53.768752087186));
#104531=CARTESIAN_POINT('Ctrl Pts',(7.33745361044804,31.1222655468294,53.7687096011187));
#104532=CARTESIAN_POINT('Ctrl Pts',(7.337445082118,31.1221712173329,53.7686236305835));
#104533=CARTESIAN_POINT('Ctrl Pts',(7.33744076796644,31.1221234994429,53.7685801462677));
#104534=CARTESIAN_POINT('Ctrl Pts',(7.33743203411954,31.122026895754,53.7684921236232));
#104535=CARTESIAN_POINT('Ctrl Pts',(7.33742761441807,31.1219780098749,53.7684475854716));
#104536=CARTESIAN_POINT('Ctrl Pts',(7.3374186635088,31.1218790042225,53.7683573957999));
#104537=CARTESIAN_POINT('Ctrl Pts',(7.33741413227305,31.1218288841266,53.7683117442569));
#104538=CARTESIAN_POINT('Ctrl Pts',(7.33740495188074,31.1217273390527,53.7682192639682));
#104539=CARTESIAN_POINT('Ctrl Pts',(7.33740030272578,31.121675914078,53.7681724355192));
#104540=CARTESIAN_POINT('Ctrl Pts',(7.33739087962831,31.1215716832527,53.7680775331113));
#104541=CARTESIAN_POINT('Ctrl Pts',(7.33738610567137,31.1215188772269,53.7680294593119));
#104542=CARTESIAN_POINT('Ctrl Pts',(7.33737642560051,31.1214118027413,53.7679319929252));
#104543=CARTESIAN_POINT('Ctrl Pts',(7.33737151946792,31.1213575340581,53.7678826004817));
#104544=CARTESIAN_POINT('Ctrl Pts',(7.3373615671032,31.1212474463556,53.7677824178594));
#104545=CARTESIAN_POINT('Ctrl Pts',(7.33735652086198,31.1211916272173,53.7677316279506));
#104546=CARTESIAN_POINT('Ctrl Pts',(7.33734627972727,31.1210783439482,53.7676285654216));
#104547=CARTESIAN_POINT('Ctrl Pts',(7.33734108481863,31.1210208796301,53.7675762930437));
#104548=CARTESIAN_POINT('Ctrl Pts',(7.33733053712263,31.1209042038868,53.7674701739453));
#104549=CARTESIAN_POINT('Ctrl Pts',(7.33732518431461,31.120844992212,53.7674163274492));
#104550=CARTESIAN_POINT('Ctrl Pts',(7.33731431084044,31.1207247113062,53.7673069610485));
#104551=CARTESIAN_POINT('Ctrl Pts',(7.33730879015368,31.1206636418241,53.7672514414102));
#104552=CARTESIAN_POINT('Ctrl Pts',(7.33729757011571,31.1205395257016,53.7671386214993));
#104553=CARTESIAN_POINT('Ctrl Pts',(7.33729187073861,31.1204764787494,53.7670813214864));
#104554=CARTESIAN_POINT('Ctrl Pts',(7.33728028158943,31.1203482778526,53.7669648244831));
#104555=CARTESIAN_POINT('Ctrl Pts',(7.33727439179787,31.1202831236652,53.7669056278693));
#104556=CARTESIAN_POINT('Ctrl Pts',(7.337262409071,31.1201505671927,53.7667852112836));
#104557=CARTESIAN_POINT('Ctrl Pts',(7.33725631611415,31.1200831646392,53.7667239917266));
#104558=CARTESIAN_POINT('Ctrl Pts',(7.33724391318314,31.1199459578779,53.7665993917941));
#104559=CARTESIAN_POINT('Ctrl Pts',(7.33723760317389,31.1198761532488,53.7665360117643));
#104560=CARTESIAN_POINT('Ctrl Pts',(7.33722475099225,31.1197339746944,53.7664069408965));
#104561=CARTESIAN_POINT('Ctrl Pts',(7.33721820878539,31.1196616003518,53.7663412504866));
#104562=CARTESIAN_POINT('Ctrl Pts',(7.33720487564038,31.1195140989835,53.7662073948723));
#104563=CARTESIAN_POINT('Ctrl Pts',(7.33719808466971,31.1194389715584,53.7661392302019));
#104564=CARTESIAN_POINT('Ctrl Pts',(7.33718423584509,31.1192857631039,53.7660002465054));
#104565=CARTESIAN_POINT('Ctrl Pts',(7.3371771779531,31.1192076816101,53.7659294280565));
#104566=CARTESIAN_POINT('Ctrl Pts',(7.33716277536024,31.119048344462,53.7657849398154));
#104567=CARTESIAN_POINT('Ctrl Pts',(7.33715543060139,31.1189670881182,53.7657112705133));
#104568=CARTESIAN_POINT('Ctrl Pts',(7.33714043232229,31.1188011582741,53.7655608636701));
#104569=CARTESIAN_POINT('Ctrl Pts',(7.33713277875259,31.1187164841733,53.7654841268347));
#104570=CARTESIAN_POINT('Ctrl Pts',(7.3371171386195,31.1185434505803,53.7653273456586));
#104571=CARTESIAN_POINT('Ctrl Pts',(7.33710915200722,31.1184550904877,53.7652473021788));
#104572=CARTESIAN_POINT('Ctrl Pts',(7.33709281899485,31.1182743883132,53.765083643334));
#104573=CARTESIAN_POINT('Ctrl Pts',(7.33708447252312,31.1181820453727,53.7650000287754));
#104574=CARTESIAN_POINT('Ctrl Pts',(7.33706739005771,31.1179930483544,53.76482893459));
#104575=CARTESIAN_POINT('Ctrl Pts',(7.33705865398962,31.1178963933797,53.764741455944));
#104576=CARTESIAN_POINT('Ctrl Pts',(7.33704075924674,31.1176984060491,53.7645623076064));
#104577=CARTESIAN_POINT('Ctrl Pts',(7.3370316004879,31.117597072681,53.764470639035));
#104578=CARTESIAN_POINT('Ctrl Pts',(7.33661963579285,31.1130390161951,53.7603483324531));
#104579=CARTESIAN_POINT('Ctrl Pts',(7.33621501173573,31.1085607628729,53.756342032666));
#104580=CARTESIAN_POINT('Ctrl Pts',(7.33528349452633,31.0982475395454,53.7472156601709));
#104581=CARTESIAN_POINT('Ctrl Pts',(7.33475544850223,31.0923984060726,53.7421120969548));
#104582=CARTESIAN_POINT('Ctrl Pts',(7.33312162651768,31.074285378687,53.7265294903765));
#104583=CARTESIAN_POINT('Ctrl Pts',(7.33200684366963,31.061905192542,53.7161878922637));
#104584=CARTESIAN_POINT('Ctrl Pts',(7.32522946465763,30.9864025441923,53.6549572148642));
#104585=CARTESIAN_POINT('Ctrl Pts',(7.31934375050404,30.9197892594001,53.6085563923883));
#104586=CARTESIAN_POINT('Ctrl Pts',(7.30807741906914,30.7866631560088,53.5295739389255));
#104587=CARTESIAN_POINT('Ctrl Pts',(7.30271115037753,30.7208242667557,53.4962030009142));
#104588=CARTESIAN_POINT('Ctrl Pts',(7.29441923114099,30.6139225091634,53.4506587670401));
#104589=CARTESIAN_POINT('Ctrl Pts',(7.29142552549945,30.5742326464151,53.435513991074));
#104590=CARTESIAN_POINT('Ctrl Pts',(7.28635587043202,30.5050408717769,53.4121005485957));
#104591=CARTESIAN_POINT('Ctrl Pts',(7.28425847615295,30.4758113654081,53.4030984039399));
#104592=CARTESIAN_POINT('Ctrl Pts',(7.28124051673948,30.432887065572,53.3911619028423));
#104593=CARTESIAN_POINT('Ctrl Pts',(7.28029953645357,30.4193783395296,53.3875878121911));
#104594=CARTESIAN_POINT('Ctrl Pts',(7.27864520465512,30.3954125095825,53.3815685909063));
#104595=CARTESIAN_POINT('Ctrl Pts',(7.27792965027376,30.384973893948,53.3790538599535));
#104596=CARTESIAN_POINT('Ctrl Pts',(7.27643286654219,30.3629900068715,53.3739821451141));
#104597=CARTESIAN_POINT('Ctrl Pts',(7.27565236567342,30.3514403177188,53.3714468001591));
#104598=CARTESIAN_POINT('Ctrl Pts',(7.2735879457731,30.3206709415822,53.3650350061602));
#104599=CARTESIAN_POINT('Ctrl Pts',(7.2723109124728,30.3014077955811,53.3613744243243));
#104600=CARTESIAN_POINT('Ctrl Pts',(7.26570085748255,30.2006015240896,53.3440560529881));
#104601=CARTESIAN_POINT('Ctrl Pts',(7.26055169692385,30.1181850272333,53.3361411953126));
#104602=CARTESIAN_POINT('Ctrl Pts',(7.24932615985716,29.9354491086202,53.3322450857504));
#104603=CARTESIAN_POINT('Ctrl Pts',(7.24330772727876,29.8354035698146,53.3391330739407));
#104604=CARTESIAN_POINT('Ctrl Pts',(7.23526172914461,29.7086784113402,53.3594249074209));
#104605=CARTESIAN_POINT('Ctrl Pts',(7.23346983411112,29.6808888727648,53.3646031641164));
#104606=CARTESIAN_POINT('Ctrl Pts',(7.2304038875109,29.6343733939767,53.3745014630549));
#104607=CARTESIAN_POINT('Ctrl Pts',(7.22914614300898,29.6155728345928,53.3788448608118));
#104608=CARTESIAN_POINT('Ctrl Pts',(7.2273285319046,29.5888832143918,53.3855011750096));
#104609=CARTESIAN_POINT('Ctrl Pts',(7.22678270326308,29.5809284966649,53.3875476641457));
#104610=CARTESIAN_POINT('Ctrl Pts',(7.2258288866033,29.5671394418894,53.3912040632634));
#104611=CARTESIAN_POINT('Ctrl Pts',(7.22542242692411,29.5612982173978,53.392787079001));
#104612=CARTESIAN_POINT('Ctrl Pts',(7.22454524027695,29.5487690208073,53.3962559790522));
#104613=CARTESIAN_POINT('Ctrl Pts',(7.22407398737323,29.5420842835327,53.3981518569107));
#104614=CARTESIAN_POINT('Ctrl Pts',(7.22276388077397,29.5236226667169,53.4035128129715));
#104615=CARTESIAN_POINT('Ctrl Pts',(7.22192028030396,29.5118722035352,53.4070662492671));
#104616=CARTESIAN_POINT('Ctrl Pts',(7.21598088644478,29.4300234107072,53.4328086249645));
#104617=CARTESIAN_POINT('Ctrl Pts',(7.21068106986272,29.3614290365905,53.4594848761912));
#104618=CARTESIAN_POINT('Ctrl Pts',(7.2043306767875,29.2822392106961,53.4964812803225));
#104619=CARTESIAN_POINT('Ctrl Pts',(7.20331972864838,29.2697237864708,53.5025202039802));
#104620=CARTESIAN_POINT('Ctrl Pts',(7.1969422456024,29.1912900315833,53.541583086263));
#104621=CARTESIAN_POINT('Ctrl Pts',(7.19157598349826,29.1275450601664,53.5787979027861));
#104622=CARTESIAN_POINT('Ctrl Pts',(7.18328404853701,29.0313014756086,53.6439091856491));
#104623=CARTESIAN_POINT('Ctrl Pts',(7.18029032177354,28.9970510838288,53.6690405338959));
#104624=CARTESIAN_POINT('Ctrl Pts',(7.17522063532679,28.9398529346135,53.714473197895));
#104625=CARTESIAN_POINT('Ctrl Pts',(7.17312323042974,28.9164366852389,53.7341478304714));
#104626=CARTESIAN_POINT('Ctrl Pts',(7.17010525881311,28.8831275755497,53.763736588488));
#104627=CARTESIAN_POINT('Ctrl Pts',(7.16916427670842,28.8727981580041,53.7731474158654));
#104628=CARTESIAN_POINT('Ctrl Pts',(7.16750994286101,28.854742919506,53.790017562803));
#104629=CARTESIAN_POINT('Ctrl Pts',(7.16679438823088,28.8469686512666,53.7974236004051));
#104630=CARTESIAN_POINT('Ctrl Pts',(7.1652976051002,28.8307844177705,53.8131424974093));
#104631=CARTESIAN_POINT('Ctrl Pts',(7.16451710507027,28.8223902360731,53.8214708042556));
#104632=CARTESIAN_POINT('Ctrl Pts',(7.16245269001489,28.800315254679,53.8438439148331));
#104633=CARTESIAN_POINT('Ctrl Pts',(7.16117566066175,28.786792242434,53.858042307682));
#104634=CARTESIAN_POINT('Ctrl Pts',(7.15456574329001,28.7175700548323,53.9333395950971));
#104635=CARTESIAN_POINT('Ctrl Pts',(7.14941670621357,28.6662218487224,53.998286806429));
#104636=CARTESIAN_POINT('Ctrl Pts',(7.13819117751702,28.563838711539,54.1496974733098));
#104637=CARTESIAN_POINT('Ctrl Pts',(7.13217264094968,28.5153634203465,54.2374873646948));
#104638=CARTESIAN_POINT('Ctrl Pts',(7.12412651774114,28.4636793968143,54.3549620789907));
#104639=CARTESIAN_POINT('Ctrl Pts',(7.1223346087697,28.4529577285925,54.3811179872377));
#104640=CARTESIAN_POINT('Ctrl Pts',(7.11926864072834,28.4360452612514,54.4255664632346));
#104641=CARTESIAN_POINT('Ctrl Pts',(7.11801088902014,28.4294975488458,54.4437174404057));
#104642=CARTESIAN_POINT('Ctrl Pts',(7.1161932693053,28.4206142719863,54.4697508229514));
#104643=CARTESIAN_POINT('Ctrl Pts',(7.11564743944051,28.4180192569503,54.4775438877387));
#104644=CARTESIAN_POINT('Ctrl Pts',(7.11469362140238,28.4136124617742,54.4911117928085));
#104645=CARTESIAN_POINT('Ctrl Pts',(7.11428716158187,28.4117743508658,54.4968778329816));
#104646=CARTESIAN_POINT('Ctrl Pts',(7.11340997553306,28.4078933405523,54.5092855554374));
#104647=CARTESIAN_POINT('Ctrl Pts',(7.11293872337768,28.4058605914589,54.5159299400975));
#104648=CARTESIAN_POINT('Ctrl Pts',(7.11162862083806,28.4003516617981,54.5343478820785));
#104649=CARTESIAN_POINT('Ctrl Pts',(7.11078502372491,28.3969640411088,54.5461471678704));
#104650=CARTESIAN_POINT('Ctrl Pts',(7.10484654088162,28.3742029633798,54.6288609597439));
#104651=CARTESIAN_POINT('Ctrl Pts',(7.09954770427299,28.3594135002388,54.700945267841));
#104652=CARTESIAN_POINT('Ctrl Pts',(7.09319754130338,28.3475444176817,54.7875384218401));
#104653=CARTESIAN_POINT('Ctrl Pts',(7.09218585424388,28.345828608473,54.8013385351312));
#104654=CARTESIAN_POINT('Ctrl Pts',(7.08580768599559,28.3361058679432,54.8884297715622));
#104655=CARTESIAN_POINT('Ctrl Pts',(7.0804414722535,28.3327982581748,54.9621679190801));
#104656=CARTESIAN_POINT('Ctrl Pts',(7.07214942250059,28.3353012656139,55.0783417573029));
#104657=CARTESIAN_POINT('Ctrl Pts',(7.06915554129466,28.3378389444276,55.1207494660266));
#104658=CARTESIAN_POINT('Ctrl Pts',(7.06408562539641,28.3449867833987,55.1934483901222));
#104659=CARTESIAN_POINT('Ctrl Pts',(7.06198814285379,28.3488162459197,55.223793319982));
#104660=CARTESIAN_POINT('Ctrl Pts',(7.05897008198878,28.3556095415329,55.2678269228894));
#104661=CARTESIAN_POINT('Ctrl Pts',(7.05802908657451,28.3579137034547,55.2816094030332));
#104662=CARTESIAN_POINT('Ctrl Pts',(7.05637473772187,28.3622945595824,55.3059283734798));
#104663=CARTESIAN_POINT('Ctrl Pts',(7.05565918126057,28.3643002089105,55.3164766689362));
#104664=CARTESIAN_POINT('Ctrl Pts',(7.05416240249325,28.3687285654756,55.3385990457935));
#104665=CARTESIAN_POINT('Ctrl Pts',(7.05338190857903,28.371172808747,55.350168245385));
#104666=CARTESIAN_POINT('Ctrl Pts',(7.05131752889043,28.377996614594,55.3808482393211));
#104667=CARTESIAN_POINT('Ctrl Pts',(7.05004052835716,28.3825907787712,55.3999097740509));
#104668=CARTESIAN_POINT('Ctrl Pts',(7.04343161517723,28.4083036029674,55.4988898249042));
#104669=CARTESIAN_POINT('Ctrl Pts',(7.03828347913053,28.4350130610867,55.5772407237078));
#104670=CARTESIAN_POINT('Ctrl Pts',(7.02705801160689,28.5066852030141,55.7453772133003));
#104671=CARTESIAN_POINT('Ctrl Pts',(7.02103871636445,28.5541548375283,55.8337299911078));
#104672=CARTESIAN_POINT('Ctrl Pts',(7.01299168066608,28.6248265325165,55.9408788146017));
#104673=CARTESIAN_POINT('Ctrl Pts',(7.01119967001764,28.6409870709111,55.9640740054108));
#104674=CARTESIAN_POINT('Ctrl Pts',(7.0081335455616,28.6691588513973,56.0023922296672));
#104675=CARTESIAN_POINT('Ctrl Pts',(7.0068757412808,28.6808575139882,56.0177383596366));
#104676=CARTESIAN_POINT('Ctrl Pts',(7.00505805874144,28.6979119064701,56.0393219263367));
#104677=CARTESIAN_POINT('Ctrl Pts',(7.0045122199458,28.7030518396532,56.0457288999806));
#104678=CARTESIAN_POINT('Ctrl Pts',(7.00355839183945,28.7120608339707,56.0567901086185));
#104679=CARTESIAN_POINT('Ctrl Pts',(7.00315193098186,28.7159082194527,56.0614616935405));
#104680=CARTESIAN_POINT('Ctrl Pts',(7.00227474928508,28.7242275245877,56.0714517586226));
#104681=CARTESIAN_POINT('Ctrl Pts',(7.00180350258308,28.7287072188928,56.0767631774803));
#104682=CARTESIAN_POINT('Ctrl Pts',(7.00049342962972,28.7411928041527,56.0913803809645));
#104683=CARTESIAN_POINT('Ctrl Pts',(6.9996498569816,28.7492683373594,56.1006257212308));
#104684=CARTESIAN_POINT('Ctrl Pts',(6.99371799094271,28.8063513016481,56.164538102448));
#104685=CARTESIAN_POINT('Ctrl Pts',(6.98842627154945,28.8588185625995,56.2159970168365));
#104686=CARTESIAN_POINT('Ctrl Pts',(6.98207783193072,28.9251053585262,56.2729308396778));
#104687=CARTESIAN_POINT('Ctrl Pts',(6.9810608300407,28.9358239663894,56.2819051363999));
#104688=CARTESIAN_POINT('Ctrl Pts',(6.97467776353723,29.0037698176388,56.3373541713216));
#104689=CARTESIAN_POINT('Ctrl Pts',(6.96931192600109,29.0639198853448,56.3801253889907));
#104690=CARTESIAN_POINT('Ctrl Pts',(6.96101902013396,29.162885727613,56.4410414137333));
#104691=CARTESIAN_POINT('Ctrl Pts',(6.95802397280665,29.1999037731808,56.4619190095447));
#104692=CARTESIAN_POINT('Ctrl Pts',(6.95295232449897,29.2648788890727,56.4953556397664));
#104693=CARTESIAN_POINT('Ctrl Pts',(6.95085425575586,29.2924572810486,56.5086003616544));
#104694=CARTESIAN_POINT('Ctrl Pts',(6.94783552110862,29.3331450845323,56.5267795528042));
#104695=CARTESIAN_POINT('Ctrl Pts',(6.94689442522416,29.3459753432158,56.5323195000149));
#104696=CARTESIAN_POINT('Ctrl Pts',(6.9452399630988,29.3687842577523,56.5418294231166));
#104697=CARTESIAN_POINT('Ctrl Pts',(6.94452439281197,29.3787342861965,56.5458655198237));
#104698=CARTESIAN_POINT('Ctrl Pts',(6.94302764696574,29.3997215015171,56.5541433376583));
#104699=CARTESIAN_POINT('Ctrl Pts',(6.94224719920249,29.4107662604548,56.5583643354625));
#104700=CARTESIAN_POINT('Ctrl Pts',(6.9401830863956,29.4402388992497,56.5692698110047));
#104701=CARTESIAN_POINT('Ctrl Pts',(6.93890630334014,29.4587417514493,56.5757473752566));
#104702=CARTESIAN_POINT('Ctrl Pts',(6.93230491513963,29.5557334685815,56.6077925756956));
#104703=CARTESIAN_POINT('Ctrl Pts',(6.92716353017965,29.635932808174,56.6278290094954));
#104704=CARTESIAN_POINT('Ctrl Pts',(6.91593851664298,29.8160427756509,56.6588417077554));
#104705=CARTESIAN_POINT('Ctrl Pts',(6.90991353420581,29.9161157124277,56.6669004632127));
#104706=CARTESIAN_POINT('Ctrl Pts',(6.9018596587187,30.0445772531729,56.6656435942839));
#104707=CARTESIAN_POINT('Ctrl Pts',(6.90006688643726,30.0728419352257,56.6646469856563));
#104708=CARTESIAN_POINT('Ctrl Pts',(6.89699959035963,30.1203327782595,56.6617606946654));
#104709=CARTESIAN_POINT('Ctrl Pts',(6.89574139231349,30.1395768529188,56.6602550430834));
#104710=CARTESIAN_POINT('Ctrl Pts',(6.89392323923254,30.1669670377126,56.6576324970088));
#104711=CARTESIAN_POINT('Ctrl Pts',(6.89337733355555,30.175138559673,56.6567890525774));
#104712=CARTESIAN_POINT('Ctrl Pts',(6.89242343004667,30.1893188763338,56.6552193189123));
#104713=CARTESIAN_POINT('Ctrl Pts',(6.89201696141894,30.1953304928817,56.6545206640732));
#104714=CARTESIAN_POINT('Ctrl Pts',(6.89113981230245,30.2082352267473,56.6529495946015));
#104715=CARTESIAN_POINT('Ctrl Pts',(6.89066860642839,30.2151266293412,56.6520668270076));
#104716=CARTESIAN_POINT('Ctrl Pts',(6.88935875496266,30.2341757532931,56.6495054849027));
#104717=CARTESIAN_POINT('Ctrl Pts',(6.88851536546236,30.2463204716164,56.647735667917));
#104718=CARTESIAN_POINT('Ctrl Pts',(6.88262969400869,30.3303171094864,56.6345457222853));
#104719=CARTESIAN_POINT('Ctrl Pts',(6.87738763181497,30.401366034414,56.6185648188023));
#104720=CARTESIAN_POINT('Ctrl Pts',(6.87109326932466,30.4844775195886,56.5940611789448));
#104721=CARTESIAN_POINT('Ctrl Pts',(6.87008132834552,30.4977705925252,56.5899603588245));
#104722=CARTESIAN_POINT('Ctrl Pts',(6.86359730198435,30.5825668622907,56.5626336417741));
#104723=CARTESIAN_POINT('Ctrl Pts',(6.85812428195912,30.6524847319064,56.5347550690545));
#104724=CARTESIAN_POINT('Ctrl Pts',(6.84975947777016,30.7582232870142,56.484056524513));
#104725=CARTESIAN_POINT('Ctrl Pts',(6.84679413727263,30.7954625197656,56.4644337435514));
#104726=CARTESIAN_POINT('Ctrl Pts',(6.84176665891241,30.8582369938003,56.4282534127869));
#104727=CARTESIAN_POINT('Ctrl Pts',(6.83968355767121,30.884134231174,56.4123687262163));
#104728=CARTESIAN_POINT('Ctrl Pts',(6.83668203430711,30.9212607597868,56.3881746486524));
#104729=CARTESIAN_POINT('Ctrl Pts',(6.8357435101111,30.9328416894826,56.3804190108606));
#104730=CARTESIAN_POINT('Ctrl Pts',(6.83409194485034,30.9531659548508,56.3664354521437));
#104731=CARTESIAN_POINT('Ctrl Pts',(6.83337672591566,30.9619488489477,56.3602667398843));
#104732=CARTESIAN_POINT('Ctrl Pts',(6.83187912442134,30.9802961078255,56.3471138684557));
#104733=CARTESIAN_POINT('Ctrl Pts',(6.8310974849964,30.9898468808998,56.3401117110762));
#104734=CARTESIAN_POINT('Ctrl Pts',(6.82902648110482,31.0150768851456,56.3211974170714));
#104735=CARTESIAN_POINT('Ctrl Pts',(6.82774408281731,31.0306212690898,56.3091079216888));
#104736=CARTESIAN_POINT('Ctrl Pts',(6.82091056443519,31.1129362713106,56.2427130537237));
#104737=CARTESIAN_POINT('Ctrl Pts',(6.81556036864427,31.1756411298718,56.1835681352485));
#104738=CARTESIAN_POINT('Ctrl Pts',(6.80431808609745,31.2988208924428,56.0478854006752));
#104739=CARTESIAN_POINT('Ctrl Pts',(6.7984670929878,31.3577160787612,55.9703629809232));
#104740=CARTESIAN_POINT('Ctrl Pts',(6.7906228232605,31.4243845589283,55.8645591368767));
#104741=CARTESIAN_POINT('Ctrl Pts',(6.78885380496981,31.4386573981902,55.8405941882899));
#104742=CARTESIAN_POINT('Ctrl Pts',(6.78582307910406,31.4616839088293,55.7996257246469));
#104743=CARTESIAN_POINT('Ctrl Pts',(6.78457719509404,31.4707588344152,55.7828087404315));
#104744=CARTESIAN_POINT('Ctrl Pts',(6.78277376261574,31.4833035174229,55.7585734185253));
#104745=CARTESIAN_POINT('Ctrl Pts',(6.78222995566122,31.4870113073347,55.7512791232499));
#104746=CARTESIAN_POINT('Ctrl Pts',(6.7812784142699,31.4933660117108,55.7385462322214));
#104747=CARTESIAN_POINT('Ctrl Pts',(6.78087218547185,31.4960372853206,55.7331200594789));
#104748=CARTESIAN_POINT('Ctrl Pts',(6.77999399613911,31.5017218074526,55.721412602477));
#104749=CARTESIAN_POINT('Ctrl Pts',(6.77952149508007,31.5047251793298,55.7151270238548));
#104750=CARTESIAN_POINT('Ctrl Pts',(6.77820461129838,31.5129460086804,55.6976410579305));
#104751=CARTESIAN_POINT('Ctrl Pts',(6.77735540540176,31.5180782928327,55.6864014460978));
#104752=CARTESIAN_POINT('Ctrl Pts',(6.77401858093961,31.5376086796873,55.6423395834222));
#104753=CARTESIAN_POINT('Ctrl Pts',(6.7714867893049,31.5510657685036,55.6091252973127));
#104754=CARTESIAN_POINT('Ctrl Pts',(6.76892549910492,31.5634376526692,55.5755160347169));
#104755=CARTESIAN_POINT('Origin',(5.,30.,55.));
#104756=CARTESIAN_POINT('',(6.06643882015546,31.5634376718251,55.5755159826781));
#104757=CARTESIAN_POINT('',(6.26189397015589,31.5634377553307,55.5755157558283));
#104758=CARTESIAN_POINT('',(5.,31.5634376782623,55.5755159651912));
#104759=CARTESIAN_POINT('',(6.92208051667986,31.665999351236,54.9985297343455));
#104760=CARTESIAN_POINT('Ctrl Pts',(6.26189397015589,31.5634377553307,55.5755157558282));
#104761=CARTESIAN_POINT('Ctrl Pts',(6.26454446910789,31.5505005284184,55.6106608388241));
#104762=CARTESIAN_POINT('Ctrl Pts',(6.26716434398739,31.5363749856231,55.6453785376556));
#104763=CARTESIAN_POINT('Ctrl Pts',(6.27128114969912,31.5120082168646,55.6999156178218));
#104764=CARTESIAN_POINT('Ctrl Pts',(6.27280066409409,31.5025288324042,55.7200402144111));
#104765=CARTESIAN_POINT('Ctrl Pts',(6.27523278931301,31.4865707133745,55.7522305388054));
#104766=CARTESIAN_POINT('Ctrl Pts',(6.27615385824067,31.4803415632221,55.7644162118716));
#104767=CARTESIAN_POINT('Ctrl Pts',(6.27778610711501,31.4689728440355,55.7859957995209));
#104768=CARTESIAN_POINT('Ctrl Pts',(6.27849928604317,31.4638915984733,55.7954193928292));
#104769=CARTESIAN_POINT('Ctrl Pts',(6.28000407604947,31.4529300348091,55.8152876555579));
#104770=CARTESIAN_POINT('Ctrl Pts',(6.28079483181936,31.4470271076433,55.8257192075521));
#104771=CARTESIAN_POINT('Ctrl Pts',(6.28291780609597,31.430797396761,55.8536914463546));
#104772=CARTESIAN_POINT('Ctrl Pts',(6.28424241371186,31.4202606939117,55.8711084296106));
#104773=CARTESIAN_POINT('Ctrl Pts',(6.29309777851616,31.3471139573512,55.9871618018824));
#104774=CARTESIAN_POINT('Ctrl Pts',(6.30023260538611,31.2745965825394,56.0791720623636));
#104775=CARTESIAN_POINT('Ctrl Pts',(6.31334400596743,31.1247264743723,56.2329336508886));
#104776=CARTESIAN_POINT('Ctrl Pts',(6.31930587690848,31.0503782129085,56.296856046941));
#104777=CARTESIAN_POINT('Ctrl Pts',(6.32668323572236,30.9579381238079,56.3631447112663));
#104778=CARTESIAN_POINT('Ctrl Pts',(6.32772465881346,30.9448818417876,56.3722270995284));
#104779=CARTESIAN_POINT('Ctrl Pts',(6.32928199749853,30.9253877519606,56.3853777286699));
#104780=CARTESIAN_POINT('Ctrl Pts',(6.32978880196477,30.9190484240044,56.3895912820912));
#104781=CARTESIAN_POINT('Ctrl Pts',(6.33070053847853,30.9076576361282,56.3970503443272));
#104782=CARTESIAN_POINT('Ctrl Pts',(6.33110438354637,30.9026171944378,56.4003121961606));
#104783=CARTESIAN_POINT('Ctrl Pts',(6.33200898553347,30.8913385735679,56.4075248017062));
#104784=CARTESIAN_POINT('Ctrl Pts',(6.33251060968784,30.8850917710684,56.4114613249073));
#104785=CARTESIAN_POINT('Ctrl Pts',(6.33402030053552,30.8663076021315,56.4231247413204));
#104786=CARTESIAN_POINT('Ctrl Pts',(6.33503577436208,30.8536941119497,56.4307268142366));
#104787=CARTESIAN_POINT('Ctrl Pts',(6.33742713999119,30.8240036485659,56.4480886800526));
#104788=CARTESIAN_POINT('Ctrl Pts',(6.33880943489345,30.8068515265934,56.4577151231761));
#104789=CARTESIAN_POINT('Ctrl Pts',(6.34382784273806,30.7444902529549,56.4912769187487));
#104790=CARTESIAN_POINT('Ctrl Pts',(6.34752594371102,30.6983567311009,56.5134298214047));
#104791=CARTESIAN_POINT('Ctrl Pts',(6.3603275807005,30.5362156595595,56.5822948592716));
#104792=CARTESIAN_POINT('Ctrl Pts',(6.36944846596878,30.415995421047,56.6180671883888));
#104793=CARTESIAN_POINT('Ctrl Pts',(6.38042235669413,30.2608017692666,56.6457828247175));
#104794=CARTESIAN_POINT('Ctrl Pts',(6.38266379850855,30.2285478146143,56.6505710594049));
#104795=CARTESIAN_POINT('Ctrl Pts',(6.38577515583164,30.1830098682816,56.6559707327709));
#104796=CARTESIAN_POINT('Ctrl Pts',(6.38666951785534,30.1698291795518,56.6573743533363));
#104797=CARTESIAN_POINT('Ctrl Pts',(6.38829176844728,30.1457602698896,56.6596473149358));
#104798=CARTESIAN_POINT('Ctrl Pts',(6.38902119924368,30.134877684636,56.6605671580019));
#104799=CARTESIAN_POINT('Ctrl Pts',(6.390491444365,30.1128247724441,56.6622129380143));
#104800=CARTESIAN_POINT('Ctrl Pts',(6.39123205219052,30.1016545961667,56.662933442449));
#104801=CARTESIAN_POINT('Ctrl Pts',(6.39306106574678,30.0739228494996,56.6644417347846));
#104802=CARTESIAN_POINT('Ctrl Pts',(6.39414523447107,30.0573549430988,56.665094988));
#104803=CARTESIAN_POINT('Ctrl Pts',(6.39840371105517,29.9918098899949,56.6666998490327));
#104804=CARTESIAN_POINT('Ctrl Pts',(6.40151881609411,29.9428081657521,56.6657386500724));
#104805=CARTESIAN_POINT('Ctrl Pts',(6.41006368516231,29.8066567670543,56.6570514779924));
#104806=CARTESIAN_POINT('Ctrl Pts',(6.41537171933191,29.7199699196642,56.6446231657939));
#104807=CARTESIAN_POINT('Ctrl Pts',(6.42592259687318,29.5515755374984,56.6067739525485));
#104808=CARTESIAN_POINT('Ctrl Pts',(6.43115064643243,29.470059040529,56.5817604281636));
#104809=CARTESIAN_POINT('Ctrl Pts',(6.43771151061711,29.3758321436095,56.5447426549644));
#104810=CARTESIAN_POINT('Ctrl Pts',(6.43876536389152,29.3609289023786,56.538636886488));
#104811=CARTESIAN_POINT('Ctrl Pts',(6.44034482983503,29.3389807224503,56.5292709760042));
#104812=CARTESIAN_POINT('Ctrl Pts',(6.44086117112911,29.3318657861061,56.5261758973357));
#104813=CARTESIAN_POINT('Ctrl Pts',(6.44178282691114,29.319278120031,56.5205952286167));
#104814=CARTESIAN_POINT('Ctrl Pts',(6.44218694594865,29.3137968439858,56.5181295575934));
#104815=CARTESIAN_POINT('Ctrl Pts',(6.44308321191695,29.3017251270598,56.5126205387022));
#104816=CARTESIAN_POINT('Ctrl Pts',(6.44357613005769,29.2951412642526,56.5095637945923));
#104817=CARTESIAN_POINT('Ctrl Pts',(6.44503397754371,29.2758244845402,56.5004415153977));
#104818=CARTESIAN_POINT('Ctrl Pts',(6.44600560684886,29.2631487373168,56.4942573748045));
#104819=CARTESIAN_POINT('Ctrl Pts',(6.44827568555491,29.2339561352245,56.4795533652609));
#104820=CARTESIAN_POINT('Ctrl Pts',(6.44957972780327,29.217500477524,56.4709166525838));
#104821=CARTESIAN_POINT('Ctrl Pts',(6.45419605412011,29.1602319945494,56.4396264876734));
#104822=CARTESIAN_POINT('Ctrl Pts',(6.45756136787187,29.1202316004384,56.415535851681));
#104823=CARTESIAN_POINT('Ctrl Pts',(6.46884788794875,28.990478027427,56.3297645834281));
#104824=CARTESIAN_POINT('Ctrl Pts',(6.47681751322673,28.9057507187853,56.2609645375228));
#104825=CARTESIAN_POINT('Ctrl Pts',(6.48803071237488,28.7929972894757,56.1494223992228));
#104826=CARTESIAN_POINT('Ctrl Pts',(6.49148758115324,28.7592352638556,56.1128931405395));
#104827=CARTESIAN_POINT('Ctrl Pts',(6.49604405202577,28.7161035616119,56.0618188669129));
#104828=CARTESIAN_POINT('Ctrl Pts',(6.49720329321096,28.7052546358374,56.0485627547598));
#104829=CARTESIAN_POINT('Ctrl Pts',(6.49911395594621,28.6875878488317,56.0262836533291));
#104830=CARTESIAN_POINT('Ctrl Pts',(6.49986996430184,28.6806541798109,56.0173546133259));
#104831=CARTESIAN_POINT('Ctrl Pts',(6.50135219851044,28.6671751897656,55.9996270580687));
#104832=CARTESIAN_POINT('Ctrl Pts',(6.50207859914733,28.6606247995773,55.9908331404722));
#104833=CARTESIAN_POINT('Ctrl Pts',(6.50381679899227,28.6450878940491,55.9695391520569));
#104834=CARTESIAN_POINT('Ctrl Pts',(6.50482527981346,28.6361867781769,55.9569777971918));
#104835=CARTESIAN_POINT('Ctrl Pts',(6.50840621747789,28.6050070847161,55.9116578775794));
#104836=CARTESIAN_POINT('Ctrl Pts',(6.51094160109677,28.5837233407896,55.878228974684));
#104837=CARTESIAN_POINT('Ctrl Pts',(6.51733465407905,28.5324220010151,55.7909298246603));
#104838=CARTESIAN_POINT('Ctrl Pts',(6.52113766321207,28.5041652730762,55.7360940590507));
#104839=CARTESIAN_POINT('Ctrl Pts',(6.53046096434747,28.4420461664146,55.597111564984));
#104840=CARTESIAN_POINT('Ctrl Pts',(6.53592963512186,28.4118905269714,55.5115356666956));
#104841=CARTESIAN_POINT('Ctrl Pts',(6.5441871821628,28.3783803045492,55.3841817741611));
#104842=CARTESIAN_POINT('Ctrl Pts',(6.54680688343859,28.3693952104421,55.3440544764472));
#104843=CARTESIAN_POINT('Ctrl Pts',(6.55022846062596,28.3598779541345,55.2927101588169));
#104844=CARTESIAN_POINT('Ctrl Pts',(6.55096210681504,28.3579615179349,55.281760837159));
#104845=CARTESIAN_POINT('Ctrl Pts',(6.55214261794786,28.3550777166994,55.2642547958385));
#104846=CARTESIAN_POINT('Ctrl Pts',(6.55258565012885,28.3540396268147,55.2577098393394));
#104847=CARTESIAN_POINT('Ctrl Pts',(6.55344528518027,28.3521109466256,55.2450626405104));
#104848=CARTESIAN_POINT('Ctrl Pts',(6.55386159937029,28.3512151508746,55.2389613907362));
#104849=CARTESIAN_POINT('Ctrl Pts',(6.55488547629687,28.3491048139549,55.224010871304));
#104850=CARTESIAN_POINT('Ctrl Pts',(6.55549504762872,28.347927541058,55.2151566108729));
#104851=CARTESIAN_POINT('Ctrl Pts',(6.55775468789567,28.343851205502,55.1824900073672));
#104852=CARTESIAN_POINT('Ctrl Pts',(6.55942630127973,28.3413954934318,55.1586265363298));
#104853=CARTESIAN_POINT('Ctrl Pts',(6.56382548643563,28.3363473855281,55.0964040797225));
#104854=CARTESIAN_POINT('Ctrl Pts',(6.56658085768375,28.3345661070411,55.057994391017));
#104855=CARTESIAN_POINT('Ctrl Pts',(6.57445564284476,28.3332866279909,54.9490241308927));
#104856=CARTESIAN_POINT('Ctrl Pts',(6.57961695443758,28.336939103798,54.8785070727554));
#104857=CARTESIAN_POINT('Ctrl Pts',(6.59159850107301,28.3559608983907,54.714176993236));
#104858=CARTESIAN_POINT('Ctrl Pts',(6.59834763788879,28.3749053093943,54.6210118211431));
#104859=CARTESIAN_POINT('Ctrl Pts',(6.60621506602963,28.4073224590016,54.5107827219602));
#104860=CARTESIAN_POINT('Ctrl Pts',(6.60757227508838,28.4133049482404,54.4917144820485));
#104861=CARTESIAN_POINT('Ctrl Pts',(6.60972032538783,28.4233973722518,54.4614631672848));
#104862=CARTESIAN_POINT('Ctrl Pts',(6.61051830306708,28.4272865159286,54.4502090617554));
#104863=CARTESIAN_POINT('Ctrl Pts',(6.61202727250786,28.4349064538417,54.4289018062784));
#104864=CARTESIAN_POINT('Ctrl Pts',(6.61273897981658,28.4386142852798,54.4188411455231));
#104865=CARTESIAN_POINT('Ctrl Pts',(6.61436110699777,28.4473251782979,54.3958906956219));
#104866=CARTESIAN_POINT('Ctrl Pts',(6.61526934536675,28.4523921346682,54.3830258774828));
#104867=CARTESIAN_POINT('Ctrl Pts',(6.61811410739145,28.4688563564685,54.3427033520321));
#104868=CARTESIAN_POINT('Ctrl Pts',(6.62003131306179,28.4808290646567,54.3154858779349));
#104869=CARTESIAN_POINT('Ctrl Pts',(6.62754512384627,28.5311349856975,54.2089567012364));
#104870=CARTESIAN_POINT('Ctrl Pts',(6.63295707053892,28.5750038857815,54.1324158898279));
#104871=CARTESIAN_POINT('Ctrl Pts',(6.64524356702567,28.6884929689743,53.9664280889392));
#104872=CARTESIAN_POINT('Ctrl Pts',(6.6520649630289,28.7615759199393,53.8799017507475));
#104873=CARTESIAN_POINT('Ctrl Pts',(6.66036616825373,28.8534552610495,53.7911952029906));
#104874=CARTESIAN_POINT('Ctrl Pts',(6.66133432016541,28.8642096675191,53.7810848431364));
#104875=CARTESIAN_POINT('Ctrl Pts',(6.66280258186005,28.8805478499893,53.7661290579411));
#104876=CARTESIAN_POINT('Ctrl Pts',(6.6632950194684,28.8860321876878,53.7611754257529));
#104877=CARTESIAN_POINT('Ctrl Pts',(6.6641924778081,28.8960313416976,53.7522639508771));
#104878=CARTESIAN_POINT('Ctrl Pts',(6.66459657746125,28.9005348362815,53.7482938055264));
#104879=CARTESIAN_POINT('Ctrl Pts',(6.66551666969061,28.91079132902,53.7393500475988));
#104880=CARTESIAN_POINT('Ctrl Pts',(6.66603369637194,28.9165569479355,53.7343914591472));
#104881=CARTESIAN_POINT('Ctrl Pts',(6.66763762445608,28.9344559307134,53.7192097881502));
#104882=CARTESIAN_POINT('Ctrl Pts',(6.66873330520163,28.9467011399438,53.7091207663099));
#104883=CARTESIAN_POINT('Ctrl Pts',(6.67447905426606,29.0110979182744,53.6575895359064));
#104884=CARTESIAN_POINT('Ctrl Pts',(6.67928051055774,29.065552294662,53.6191310925398));
#104885=CARTESIAN_POINT('Ctrl Pts',(6.69275118747356,29.2231754402455,53.5214105296857));
#104886=CARTESIAN_POINT('Ctrl Pts',(6.70143597850424,29.3306226233818,53.4697632686658));
#104887=CARTESIAN_POINT('Ctrl Pts',(6.71247881518522,29.4792055752419,53.4170177042953));
#104888=CARTESIAN_POINT('Ctrl Pts',(6.71515692767405,29.5161940289344,53.4053238602658));
#104889=CARTESIAN_POINT('Ctrl Pts',(6.71886141760123,29.5686923505188,53.3907217689671));
#104890=CARTESIAN_POINT('Ctrl Pts',(6.71992231224148,29.5838842042955,53.3867268094654));
#104891=CARTESIAN_POINT('Ctrl Pts',(6.72170853920639,29.6097230589536,53.3803213277282));
#104892=CARTESIAN_POINT('Ctrl Pts',(6.72243740440672,29.6203411259396,53.3777995681036));
#104893=CARTESIAN_POINT('Ctrl Pts',(6.72390771829576,29.6419079726874,53.3729008625591));
#104894=CARTESIAN_POINT('Ctrl Pts',(6.72464894932268,29.6528574887926,53.3705296595572));
#104895=CARTESIAN_POINT('Ctrl Pts',(6.72648177991336,29.6801170785309,53.3649136311013));
#104896=CARTESIAN_POINT('Ctrl Pts',(6.72756910283182,29.6964536197185,53.3618021655201));
#104897=CARTESIAN_POINT('Ctrl Pts',(6.73185891907859,29.7615180864653,53.3504167066448));
#104898=CARTESIAN_POINT('Ctrl Pts',(6.73500104308888,29.810559647094,53.3440677170322));
#104899=CARTESIAN_POINT('Ctrl Pts',(6.74366052336572,29.948374881642,53.3324300146838));
#104900=CARTESIAN_POINT('Ctrl Pts',(6.74905156999228,30.0373922657802,53.3320498827654));
#104901=CARTESIAN_POINT('Ctrl Pts',(6.75955273346603,30.2086239896618,53.3450392765063));
#104902=CARTESIAN_POINT('Ctrl Pts',(6.76464545837968,30.2906376243938,53.3574576335264));
#104903=CARTESIAN_POINT('Ctrl Pts',(6.77108085283034,30.3874783324586,53.3796020973636));
#104904=CARTESIAN_POINT('Ctrl Pts',(6.77216146633097,30.4035236290371,53.383523136123));
#104905=CARTESIAN_POINT('Ctrl Pts',(6.77376626251121,30.42698514929,53.3896275625658));
#104906=CARTESIAN_POINT('Ctrl Pts',(6.77428051695907,30.4344492606985,53.3916251870434));
#104907=CARTESIAN_POINT('Ctrl Pts',(6.7751999762385,30.4476925808438,53.395268415404));
#104908=CARTESIAN_POINT('Ctrl Pts',(6.77560400927407,30.4534771725202,53.3968934666513));
#104909=CARTESIAN_POINT('Ctrl Pts',(6.77650198477888,30.4662556828926,53.4005580007246));
#104910=CARTESIAN_POINT('Ctrl Pts',(6.77699671860619,30.4732449875346,53.4026120547537));
#104911=CARTESIAN_POINT('Ctrl Pts',(6.77846529892519,30.4938490503898,53.4088143773793));
#104912=CARTESIAN_POINT('Ctrl Pts',(6.77944598902457,30.5074239810572,53.4130912313705));
#104913=CARTESIAN_POINT('Ctrl Pts',(6.78611282510082,30.5985838192819,53.4431008466858));
#104914=CARTESIAN_POINT('Ctrl Pts',(6.79203860541199,30.6742316553096,53.4743373562673));
#104915=CARTESIAN_POINT('Ctrl Pts',(6.80751906645864,30.8643624055347,53.5697565017614));
#104916=CARTESIAN_POINT('Ctrl Pts',(6.81701846628112,30.9741349591643,53.6421367851628));
#104917=CARTESIAN_POINT('Ctrl Pts',(6.82745087359127,31.0900955840493,53.7399704108144));
#104918=CARTESIAN_POINT('Ctrl Pts',(6.82886000950821,31.1056398069442,53.7535876959437));
#104919=CARTESIAN_POINT('Ctrl Pts',(6.83115152309085,31.1307114469955,53.7763895496966));
#104920=CARTESIAN_POINT('Ctrl Pts',(6.83204083996111,31.1403895244257,53.7854043221947));
#104921=CARTESIAN_POINT('Ctrl Pts',(6.83363841356968,31.1576763151014,53.8018951252541));
#104922=CARTESIAN_POINT('Ctrl Pts',(6.83434834825031,31.1653224387397,53.8093307074249));
#104923=CARTESIAN_POINT('Ctrl Pts',(6.83516741448436,31.1741003032443,53.8180324243905));
#104924=CARTESIAN_POINT('Ctrl Pts',(6.83527963444615,31.1753019998948,53.8192273373126));
#104925=CARTESIAN_POINT('Ctrl Pts',(6.83544884750548,31.1771125480504,53.8210331670805));
#104926=CARTESIAN_POINT('Ctrl Pts',(6.83550589996095,31.1777227489705,53.8216427237616));
#104927=CARTESIAN_POINT('Ctrl Pts',(6.83560860012256,31.1788207204448,53.8227412408269));
#104928=CARTESIAN_POINT('Ctrl Pts',(6.83565425526253,31.179308660484,53.823230030843));
#104929=CARTESIAN_POINT('Ctrl Pts',(6.83573741773183,31.1801971665912,53.8241211923311));
#104930=CARTESIAN_POINT('Ctrl Pts',(6.8357749293641,31.1805978309797,53.8245234652099));
#104931=CARTESIAN_POINT('Ctrl Pts',(6.83584390436646,31.181334356579,53.8252637040641));
#104932=CARTESIAN_POINT('Ctrl Pts',(6.83587537038675,31.1816702784592,53.8256016093207));
#104933=CARTESIAN_POINT('Ctrl Pts',(6.83593367511896,31.1822925792425,53.826228121663));
#104934=CARTESIAN_POINT('Ctrl Pts',(6.83596051554893,31.1825789974935,53.8265166895118));
#104935=CARTESIAN_POINT('Ctrl Pts',(6.83601056864273,31.1831130163785,53.8270551103278));
#104936=CARTESIAN_POINT('Ctrl Pts',(6.83603378245821,31.1833606434847,53.8273049368296));
#104937=CARTESIAN_POINT('Ctrl Pts',(6.83607730787514,31.1838248598031,53.8277735730241));
#104938=CARTESIAN_POINT('Ctrl Pts',(6.83609762027836,31.1840414674615,53.8279923643081));
#104939=CARTESIAN_POINT('Ctrl Pts',(6.83613588347032,31.1844494378197,53.8284046759575));
#104940=CARTESIAN_POINT('Ctrl Pts',(6.83615383483775,31.1846408137845,53.8285981832071));
#104941=CARTESIAN_POINT('Ctrl Pts',(6.83618778774809,31.1850027309763,53.8289643103386));
#104942=CARTESIAN_POINT('Ctrl Pts',(6.83620378971336,31.1851732819139,53.8291369205926));
#104943=CARTESIAN_POINT('Ctrl Pts',(6.83623416348085,31.1854969709265,53.8294646611739));
#104944=CARTESIAN_POINT('Ctrl Pts',(6.83624853559594,31.1856501162387,53.8296197842668));
#104945=CARTESIAN_POINT('Ctrl Pts',(6.83627590190537,31.185941693009,53.8299152425401));
#104946=CARTESIAN_POINT('Ctrl Pts',(6.8362888963381,31.1860801299844,53.8300555722115));
#104947=CARTESIAN_POINT('Ctrl Pts',(6.83631370920196,31.1863444497915,53.8303236009039));
#104948=CARTESIAN_POINT('Ctrl Pts',(6.83632552782,31.1864703369218,53.8304512956879));
#104949=CARTESIAN_POINT('Ctrl Pts',(6.8363481527537,31.1867113073393,53.8306958052231));
#104950=CARTESIAN_POINT('Ctrl Pts',(6.83635895921926,31.1868263940369,53.8308126166831));
#104951=CARTESIAN_POINT('Ctrl Pts',(6.83637969407458,31.1870471983068,53.8310367962609));
#104952=CARTESIAN_POINT('Ctrl Pts',(6.83638962257781,31.1871529185312,53.8311441617004));
#104953=CARTESIAN_POINT('Ctrl Pts',(6.83640871267701,31.1873561777663,53.8313506400732));
#104954=CARTESIAN_POINT('Ctrl Pts',(6.83641787437143,31.1874537189872,53.8314497509304));
#104955=CARTESIAN_POINT('Ctrl Pts',(6.83646162549998,31.1879194894079,53.8319231350813));
#104956=CARTESIAN_POINT('Ctrl Pts',(6.83649620782555,31.1882875543859,53.8322975705405));
#104957=CARTESIAN_POINT('Ctrl Pts',(6.83656536217928,31.1890233837649,53.8330468438649));
#104958=CARTESIAN_POINT('Ctrl Pts',(6.83659993420023,31.1893911480616,53.8334216817259));
#104959=CARTESIAN_POINT('Ctrl Pts',(6.83771236570147,31.2012216974717,53.8454911891868));
#104960=CARTESIAN_POINT('Ctrl Pts',(6.83878273897157,31.2125119319482,53.8573543826887));
#104961=CARTESIAN_POINT('Ctrl Pts',(6.84310574479034,31.2576969066564,53.9062564182439));
#104962=CARTESIAN_POINT('Ctrl Pts',(6.84629563101873,31.2900859938941,53.9446538966336));
#104963=CARTESIAN_POINT('Ctrl Pts',(6.85518459504228,31.3766862732671,54.0572760669948));
#104964=CARTESIAN_POINT('Ctrl Pts',(6.86074737879746,31.4265610848228,54.1345995941727));
#104965=CARTESIAN_POINT('Ctrl Pts',(6.86673819339692,31.4726450709742,54.2209565011216));
#104966=CARTESIAN_POINT('Ctrl Pts',(6.8671070829813,31.4754519351859,54.2262856698189));
#104967=CARTESIAN_POINT('Ctrl Pts',(6.87233807994812,31.5148072795536,54.3019995035082));
#104968=CARTESIAN_POINT('Ctrl Pts',(6.8772486017718,31.5463086025132,54.3748822613228));
#104969=CARTESIAN_POINT('Ctrl Pts',(6.88323164472075,31.5765647727414,54.4613431812816));
#104970=CARTESIAN_POINT('Ctrl Pts',(6.88404231908957,31.5805031617025,54.4730110201292));
#104971=CARTESIAN_POINT('Ctrl Pts',(6.88532236569692,31.5864638871805,54.4913382709559));
#104972=CARTESIAN_POINT('Ctrl Pts',(6.88578682527168,31.5885745438602,54.4979687916753));
#104973=CARTESIAN_POINT('Ctrl Pts',(6.88665986328564,31.5924433051095,54.5103910192878));
#104974=CARTESIAN_POINT('Ctrl Pts',(6.88706786060929,31.5942114644677,54.5161793349988));
#104975=CARTESIAN_POINT('Ctrl Pts',(6.88803314046332,31.5983018160076,54.5298355594006));
#104976=CARTESIAN_POINT('Ctrl Pts',(6.88859189828572,31.6005974776023,54.5377111250451));
#104977=CARTESIAN_POINT('Ctrl Pts',(6.89047019066464,31.6080779994046,54.5640978394452));
#104978=CARTESIAN_POINT('Ctrl Pts',(6.89180315187381,31.6130004002564,54.5826809661126));
#104979=CARTESIAN_POINT('Ctrl Pts',(6.90252368276676,31.6496326427416,54.7313212070418));
#104980=CARTESIAN_POINT('Ctrl Pts',(6.91245003382505,31.6658812228862,54.8646751798091));
#104981=CARTESIAN_POINT('Ctrl Pts',(6.92208051667986,31.665999351236,54.9985297343455));
#104982=CARTESIAN_POINT('Ctrl Pts',(6.92208062419127,31.6659993525541,54.998531228652));
#104983=CARTESIAN_POINT('Ctrl Pts',(6.92752430250826,31.6660660573411,55.0741931974836));
#104984=CARTESIAN_POINT('Ctrl Pts',(6.93286713313332,31.6609784705008,55.1497823894655));
#104985=CARTESIAN_POINT('Ctrl Pts',(6.9390761915014,31.6487537501628,55.2395615832835));
#104986=CARTESIAN_POINT('Ctrl Pts',(6.94009265401845,31.6465417946736,55.2543203183327));
#104987=CARTESIAN_POINT('Ctrl Pts',(6.94184206420286,31.6423685301795,55.2798228409888));
#104988=CARTESIAN_POINT('Ctrl Pts',(6.94257785034269,31.640499366719,55.2905805377481));
#104989=CARTESIAN_POINT('Ctrl Pts',(6.94404681408289,31.6365387213767,55.3121178717952));
#104990=CARTESIAN_POINT('Ctrl Pts',(6.94477991743677,31.6344461590539,55.3228967568165));
#104991=CARTESIAN_POINT('Ctrl Pts',(6.9461716460916,31.630252263745,55.3434134165066));
#104992=CARTESIAN_POINT('Ctrl Pts',(6.94683083937543,31.6281698637739,55.3531545272042));
#104993=CARTESIAN_POINT('Ctrl Pts',(6.94853761732648,31.622528699819,55.3784318107188));
#104994=CARTESIAN_POINT('Ctrl Pts',(6.94958082868873,31.6188340829349,55.3939368704649));
#104995=CARTESIAN_POINT('Ctrl Pts',(6.95324032441697,31.6050054202772,55.4484870871939));
#104996=CARTESIAN_POINT('Ctrl Pts',(6.95581850255506,31.5936761217487,55.4872164720534));
#104997=CARTESIAN_POINT('Ctrl Pts',(6.9594761742502,31.5753775740763,55.5422672213609));
#104998=CARTESIAN_POINT('Ctrl Pts',(6.96058317929051,31.5695388628525,55.5589415810635));
#104999=CARTESIAN_POINT('Ctrl Pts',(6.9616842973919,31.5634376940719,55.5755159222429));
#105000=CARTESIAN_POINT('Ctrl Pts',(6.76892549910492,31.5634376526692,55.5755160347169));
#105001=CARTESIAN_POINT('Ctrl Pts',(6.76565911937185,31.5792153539615,55.5326545838016));
#105002=CARTESIAN_POINT('Ctrl Pts',(6.76234507064774,31.5932281209808,55.4891507352691));
#105003=CARTESIAN_POINT('Ctrl Pts',(6.75469116315526,31.6213380402814,55.3877638984053));
#105004=CARTESIAN_POINT('Ctrl Pts',(6.75035204169247,31.6341546959461,55.3296008909939));
#105005=CARTESIAN_POINT('Ctrl Pts',(6.74215950402389,31.6526440596059,55.21739656209));
#105006=CARTESIAN_POINT('Ctrl Pts',(6.73830181290237,31.6588421481276,55.1635155351563));
#105007=CARTESIAN_POINT('Ctrl Pts',(6.731979587325,31.6647892737022,55.073164757906));
#105008=CARTESIAN_POINT('Ctrl Pts',(6.729476324338,31.665989175487,55.0368351927104));
#105009=CARTESIAN_POINT('Ctrl Pts',(6.72609830067245,31.6660038990593,54.9870677159392));
#105010=CARTESIAN_POINT('Ctrl Pts',(6.72519211718745,31.6658455943011,54.9736426591224));
#105011=CARTESIAN_POINT('Ctrl Pts',(6.72362203442421,31.665287049257,54.95025689691));
#105012=CARTESIAN_POINT('Ctrl Pts',(6.72295589879717,31.6649596662987,54.9402953119165));
#105013=CARTESIAN_POINT('Ctrl Pts',(6.72156261528189,31.6640843147945,54.9193794498966));
#105014=CARTESIAN_POINT('Ctrl Pts',(6.72083608895692,31.6635175280787,54.9084264045131));
#105015=CARTESIAN_POINT('Ctrl Pts',(6.71909601998206,31.66189363788,54.8820875302484));
#105016=CARTESIAN_POINT('Ctrl Pts',(6.71808581757055,31.6607309719811,54.8667090434471));
#105017=CARTESIAN_POINT('Ctrl Pts',(6.71448946446047,31.6558012336014,54.8116797662985));
#105018=CARTESIAN_POINT('Ctrl Pts',(6.71194083465546,31.6508260289116,54.7721490582995));
#105019=CARTESIAN_POINT('Ctrl Pts',(6.70550331699152,31.634471834921,54.6714877923803));
#105020=CARTESIAN_POINT('Ctrl Pts',(6.70167015351356,31.6210801107925,54.6107461511771));
#105021=CARTESIAN_POINT('Ctrl Pts',(6.6922398465037,31.5795632922062,54.4624378796174));
#105022=CARTESIAN_POINT('Ctrl Pts',(6.68669531528131,31.5475306897353,54.3761892385126));
#105023=CARTESIAN_POINT('Ctrl Pts',(6.6784524895859,31.4918423034467,54.2573601384714));
#105024=CARTESIAN_POINT('Ctrl Pts',(6.67593864523918,31.4738696561359,54.2223013987281));
#105025=CARTESIAN_POINT('Ctrl Pts',(6.67263998774119,31.4493409894124,54.1783636009939));
#105026=CARTESIAN_POINT('Ctrl Pts',(6.6719177215886,31.4439147299853,54.168864684572));
#105027=CARTESIAN_POINT('Ctrl Pts',(6.67075131951546,31.4350720159899,54.1537330811792));
#105028=CARTESIAN_POINT('Ctrl Pts',(6.67031085987238,31.4317149046991,54.1480658377198));
#105029=CARTESIAN_POINT('Ctrl Pts',(6.66945254843252,31.4251407450083,54.1371163998416));
#105030=CARTESIAN_POINT('Ctrl Pts',(6.66903494887247,31.4219277565512,54.1318319859096));
#105031=CARTESIAN_POINT('Ctrl Pts',(6.66800257927938,31.4139478307814,54.1188705009532));
#105032=CARTESIAN_POINT('Ctrl Pts',(6.66738572271682,31.4091477495981,54.1112141580838));
#105033=CARTESIAN_POINT('Ctrl Pts',(6.66506535594283,31.3909645148401,54.0827286768571));
#105034=CARTESIAN_POINT('Ctrl Pts',(6.66333882225146,31.3771805728924,54.062160742341));
#105035=CARTESIAN_POINT('Ctrl Pts',(6.65875260611361,31.3397877795645,54.008967156546));
#105036=CARTESIAN_POINT('Ctrl Pts',(6.65586239213901,31.3154458447325,53.9768777123148));
#105037=CARTESIAN_POINT('Ctrl Pts',(6.64436139454279,31.2148356054583,53.8537776904426));
#105038=CARTESIAN_POINT('Ctrl Pts',(6.63564038080289,31.130082447412,53.7701340003028));
#105039=CARTESIAN_POINT('Ctrl Pts',(6.62373805248037,30.9983233553895,53.6653208906011));
#105040=CARTESIAN_POINT('Ctrl Pts',(6.62028806826645,30.9581301561778,53.6361798785766));
#105041=CARTESIAN_POINT('Ctrl Pts',(6.61573914320249,30.902401031623,53.599456784676));
#105042=CARTESIAN_POINT('Ctrl Pts',(6.61458081120952,30.8879652151375,53.5902600471949));
#105043=CARTESIAN_POINT('Ctrl Pts',(6.612671402862,30.8637676441831,53.5753635092416));
#105044=CARTESIAN_POINT('Ctrl Pts',(6.61191574892079,30.8540853141077,53.5695378505429));
#105045=CARTESIAN_POINT('Ctrl Pts',(6.61043403987332,30.8348940315954,53.5582551785704));
#105046=CARTESIAN_POINT('Ctrl Pts',(6.60970781168411,30.8253890158533,53.5527926353211));
#105047=CARTESIAN_POINT('Ctrl Pts',(6.60796975446231,30.8024080148902,53.5398854925403));
#105048=CARTESIAN_POINT('Ctrl Pts',(6.6069612457587,30.7888812495336,53.5325329995176));
#105049=CARTESIAN_POINT('Ctrl Pts',(6.60337871521551,30.7401684892407,53.5069233623563));
#105050=CARTESIAN_POINT('Ctrl Pts',(6.60084181978597,30.7044338006731,53.4897349082269));
#105051=CARTESIAN_POINT('Ctrl Pts',(6.59444342688585,30.6115965395116,53.4490929936117));
#105052=CARTESIAN_POINT('Ctrl Pts',(6.59063672421522,30.5537417353607,53.4275071431035));
#105053=CARTESIAN_POINT('Ctrl Pts',(6.58130056451441,30.4081745374395,53.3822289141359));
#105054=CARTESIAN_POINT('Ctrl Pts',(6.57582285166048,30.3194778677749,53.3624036892467));
#105055=CARTESIAN_POINT('Ctrl Pts',(6.56756727858888,30.1891027090245,53.3442617500192));
#105056=CARTESIAN_POINT('Ctrl Pts',(6.56496038142273,30.1484005818776,53.3401187835617));
#105057=CARTESIAN_POINT('Ctrl Pts',(6.56155351888063,30.0965170860123,53.3367611114426));
#105058=CARTESIAN_POINT('Ctrl Pts',(6.56082107744078,30.085436514906,53.3361551352871));
#105059=CARTESIAN_POINT('Ctrl Pts',(6.55964214016954,30.0677362383127,53.3353644105716));
#105060=CARTESIAN_POINT('Ctrl Pts',(6.55919946114745,30.0611198290855,53.3351083499998));
#105061=CARTESIAN_POINT('Ctrl Pts',(6.55834020611756,30.048339109485,53.3346900123259));
#105062=CARTESIAN_POINT('Ctrl Pts',(6.55792391555715,30.042175165848,53.3345225084346));
#105063=CARTESIAN_POINT('Ctrl Pts',(6.55689967433441,30.0270748031653,53.3341960376499));
#105064=CARTESIAN_POINT('Ctrl Pts',(6.55628971008174,30.0181378367476,53.3340747628306));
#105065=CARTESIAN_POINT('Ctrl Pts',(6.55402604735073,29.9851604253147,53.3338926403799));
#105066=CARTESIAN_POINT('Ctrl Pts',(6.55235070368922,29.9611216913236,53.3342802522857));
#105067=CARTESIAN_POINT('Ctrl Pts',(6.54793869623674,29.8985613394167,53.336643859521));
#105068=CARTESIAN_POINT('Ctrl Pts',(6.54517404443425,29.8600858198119,53.3394377143644));
#105069=CARTESIAN_POINT('Ctrl Pts',(6.53729996037453,29.7517517887729,53.3510959588226));
#105070=CARTESIAN_POINT('Ctrl Pts',(6.53214929795718,29.6823071173561,53.363056806371));
#105071=CARTESIAN_POINT('Ctrl Pts',(6.5201809781779,29.5215606120598,53.4013605059429));
#105072=CARTESIAN_POINT('Ctrl Pts',(6.51343458450082,29.4313275791278,53.4311884795724));
#105073=CARTESIAN_POINT('Ctrl Pts',(6.50557024582169,29.3257496561618,53.4764050854349));
#105074=CARTESIAN_POINT('Ctrl Pts',(6.50421356553821,29.3075302802036,53.4845988196997));
#105075=CARTESIAN_POINT('Ctrl Pts',(6.50206631270421,29.2786962642302,53.4981948894288));
#105076=CARTESIAN_POINT('Ctrl Pts',(6.50126860944032,29.267985044698,53.5033865604917));
#105077=CARTESIAN_POINT('Ctrl Pts',(6.4997601429042,29.2477357702683,53.5134706831928));
#105078=CARTESIAN_POINT('Ctrl Pts',(6.4990486646831,29.2381875488748,53.5183412405233));
#105079=CARTESIAN_POINT('Ctrl Pts',(6.49742704632043,29.216435768787,53.5297027067191));
#105080=CARTESIAN_POINT('Ctrl Pts',(6.49651908639284,29.2042645461572,53.536254072028));
#105081=CARTESIAN_POINT('Ctrl Pts',(6.49367519742556,29.1661848905766,53.5573664530873));
#105082=CARTESIAN_POINT('Ctrl Pts',(6.4917585743462,29.1405828876277,53.572470109689));
#105083=CARTESIAN_POINT('Ctrl Pts',(6.4842386787959,29.0406725829616,53.6350739762306));
#105084=CARTESIAN_POINT('Ctrl Pts',(6.47882060970477,28.9697799096292,53.6877573026117));
#105085=CARTESIAN_POINT('Ctrl Pts',(6.46653434034759,28.8184077546284,53.8201111708132));
#105086=CARTESIAN_POINT('Ctrl Pts',(6.45971886838307,28.7412135004261,53.9028458848058));
#105087=CARTESIAN_POINT('Ctrl Pts',(6.45142396345215,28.6640547366363,54.004497893463));
#105088=CARTESIAN_POINT('Ctrl Pts',(6.45045512728118,28.6552812290801,54.0163813842829));
#105089=CARTESIAN_POINT('Ctrl Pts',(6.44898612506668,28.6423567356201,54.034383412082));
#105090=CARTESIAN_POINT('Ctrl Pts',(6.4484936450737,28.6380863162184,54.0404158500107));
#105091=CARTESIAN_POINT('Ctrl Pts',(6.44759628634361,28.6304211764548,54.0513979401307));
#105092=CARTESIAN_POINT('Ctrl Pts',(6.4471923304685,28.6270128742458,54.056337787586));
#105093=CARTESIAN_POINT('Ctrl Pts',(6.44627281039241,28.6193499759925,54.0675734624939));
#105094=CARTESIAN_POINT('Ctrl Pts',(6.44575621553459,28.6151117398446,54.0738800089329));
#105095=CARTESIAN_POINT('Ctrl Pts',(6.44415446716409,28.6021713282531,54.0934229569121));
#105096=CARTESIAN_POINT('Ctrl Pts',(6.44306056479699,28.5936149701943,54.1067542146976));
#105097=CARTESIAN_POINT('Ctrl Pts',(6.43733185489244,28.5501872798413,54.1765878640327));
#105098=CARTESIAN_POINT('Ctrl Pts',(6.43254655963957,28.5185294192158,54.2350113267309));
#105099=CARTESIAN_POINT('Ctrl Pts',(6.41913802495707,28.4404252015248,54.4022873427279));
#105100=CARTESIAN_POINT('Ctrl Pts',(6.41049803460797,28.4019441682706,54.5144501612296));
#105101=CARTESIAN_POINT('Ctrl Pts',(6.39944598388614,28.3668968193069,54.668208240349));
#105102=CARTESIAN_POINT('Ctrl Pts',(6.39672077394952,28.3594989288619,54.7069668026118));
#105103=CARTESIAN_POINT('Ctrl Pts',(6.39296414188989,28.3510742048676,54.761568999204));
#105104=CARTESIAN_POINT('Ctrl Pts',(6.3918968625506,28.3488871573478,54.7772175260533));
#105105=CARTESIAN_POINT('Ctrl Pts',(6.39010327499326,28.3455645516379,54.8037380373539));
#105106=CARTESIAN_POINT('Ctrl Pts',(6.38937336182883,28.3443128076106,54.8145941167331));
#105107=CARTESIAN_POINT('Ctrl Pts',(6.38790366461216,28.3419970009609,54.8365773047733));
#105108=CARTESIAN_POINT('Ctrl Pts',(6.38716407286781,28.340937922559,54.8477043807266));
#105109=CARTESIAN_POINT('Ctrl Pts',(6.3853404269031,28.3385918278208,54.8752942094089));
#105110=CARTESIAN_POINT('Ctrl Pts',(6.38426055741512,28.3374374129943,54.8917672642455));
#105111=CARTESIAN_POINT('Ctrl Pts',(6.38004253353108,28.3338615649757,54.9566028351024));
#105112=CARTESIAN_POINT('Ctrl Pts',(6.37696210588774,28.3333039267688,55.0050466381535));
#105113=CARTESIAN_POINT('Ctrl Pts',(6.368561479618,28.3376050930823,55.1390428267351));
#105114=CARTESIAN_POINT('Ctrl Pts',(6.36335742185344,28.3469479333945,55.2242980747015));
#105115=CARTESIAN_POINT('Ctrl Pts',(6.35276793898048,28.3790327232282,55.3945923478807));
#105116=CARTESIAN_POINT('Ctrl Pts',(6.34739549126449,28.4020304205631,55.479298902742));
#105117=CARTESIAN_POINT('Ctrl Pts',(6.34067251035354,28.4370129153623,55.5769636757493));
#105118=CARTESIAN_POINT('Ctrl Pts',(6.33961800815994,28.4426668373582,55.5920549666972));
#105119=CARTESIAN_POINT('Ctrl Pts',(6.33803784431309,28.4513660024572,55.614287354525));
#105120=CARTESIAN_POINT('Ctrl Pts',(6.33752146838993,28.4542438664272,55.621493509088));
#105121=CARTESIAN_POINT('Ctrl Pts',(6.33659990001523,28.4594393648644,55.6342436717513));
#105122=CARTESIAN_POINT('Ctrl Pts',(6.33619590453659,28.4617368048074,55.6397956281614));
#105123=CARTESIAN_POINT('Ctrl Pts',(6.3353001140434,28.4668740894821,55.6520226685981));
#105124=CARTESIAN_POINT('Ctrl Pts',(6.33480755042212,28.4697274800136,55.6586916027032));
#105125=CARTESIAN_POINT('Ctrl Pts',(6.33335133501082,28.4782494672888,55.6782549036394));
#105126=CARTESIAN_POINT('Ctrl Pts',(6.33238100279907,28.4840379845453,55.6910958928343));
#105127=CARTESIAN_POINT('Ctrl Pts',(6.32545203338066,28.52619062429,55.7815270143243));
#105128=CARTESIAN_POINT('Ctrl Pts',(6.31922931046621,28.5683272794901,55.8562761213077));
#105129=CARTESIAN_POINT('Ctrl Pts',(6.3038021595715,28.6863168726329,56.0323461573861));
#105130=CARTESIAN_POINT('Ctrl Pts',(6.29465972233035,28.7683263673373,56.1289345966134));
#105131=CARTESIAN_POINT('Ctrl Pts',(6.28450763392295,28.8759438515739,56.2298387186755));
#105132=CARTESIAN_POINT('Ctrl Pts',(6.28306088197729,28.8916861289083,56.2440441847461));
#105133=CARTESIAN_POINT('Ctrl Pts',(6.28072148724295,28.9177995605363,56.266719093448));
#105134=CARTESIAN_POINT('Ctrl Pts',(6.27982140021284,28.9280087725843,56.2753704870971));
#105135=CARTESIAN_POINT('Ctrl Pts',(6.27821240442564,28.9465469255068,56.290700021231));
#105136=CARTESIAN_POINT('Ctrl Pts',(6.27750170701223,28.9548378129768,56.297422805751));
#105137=CARTESIAN_POINT('Ctrl Pts',(6.27598761537083,28.9727176351743,56.3116382921029));
#105138=CARTESIAN_POINT('Ctrl Pts',(6.27518522019695,28.9823252497917,56.3191065849153));
#105139=CARTESIAN_POINT('Ctrl Pts',(6.2729938780674,29.0089194431084,56.3393155540326));
#105140=CARTESIAN_POINT('Ctrl Pts',(6.27161343546043,29.0260694672255,56.35183808465));
#105141=CARTESIAN_POINT('Ctrl Pts',(6.26855642918643,29.064892904632,56.3790635678446));
#105142=CARTESIAN_POINT('Ctrl Pts',(6.26688632111294,29.0866832011447,56.3935903768461));
#105143=CARTESIAN_POINT('Ctrl Pts',(6.2615042687905,29.158628006576,56.4391407726055));
#105144=CARTESIAN_POINT('Ctrl Pts',(6.25785899503546,29.2100902538788,56.4680178304589));
#105145=CARTESIAN_POINT('Ctrl Pts',(6.24742248065099,29.3627474015405,56.543321458361));
#105146=CARTESIAN_POINT('Ctrl Pts',(6.24074553007785,29.4671848368141,56.5824143597914));
#105147=CARTESIAN_POINT('Ctrl Pts',(6.23191086951282,29.6013760188719,56.6178425926378));
#105148=CARTESIAN_POINT('Ctrl Pts',(6.23013206342855,29.6281948301113,56.6242156387382));
#105149=CARTESIAN_POINT('Ctrl Pts',(6.22768265384676,29.6646282298012,56.6319238603171));
#105150=CARTESIAN_POINT('Ctrl Pts',(6.22704180413422,29.674115987311,56.633844946517));
#105151=CARTESIAN_POINT('Ctrl Pts',(6.2260171602238,29.6892040773609,56.6367633448034));
#105152=CARTESIAN_POINT('Ctrl Pts',(6.22563635378028,29.6947938804587,56.6378148779908));
#105153=CARTESIAN_POINT('Ctrl Pts',(6.22483333731474,29.7065412603464,56.6399625255993));
#105154=CARTESIAN_POINT('Ctrl Pts',(6.22441077834105,29.7126997680553,56.6410526162936));
#105155=CARTESIAN_POINT('Ctrl Pts',(6.22334882668066,29.7281228583254,56.6436931152702));
#105156=CARTESIAN_POINT('Ctrl Pts',(6.22270708178892,29.7373945923247,56.64519987444));
#105157=CARTESIAN_POINT('Ctrl Pts',(6.22017041484111,29.7738727907375,56.6508117787616));
#105158=CARTESIAN_POINT('Ctrl Pts',(6.21824680728647,29.8011649110137,56.654320839445));
#105159=CARTESIAN_POINT('Ctrl Pts',(6.21296146290074,29.8754694158971,56.6620093530622));
#105160=CARTESIAN_POINT('Ctrl Pts',(6.20955799413574,29.9225918069228,56.6648694765281));
#105161=CARTESIAN_POINT('Ctrl Pts',(6.19810119341712,30.0804216959721,56.6677339254671));
#105162=CARTESIAN_POINT('Ctrl Pts',(6.19000189333466,30.1910132467543,56.6587112659582));
#105163=CARTESIAN_POINT('Ctrl Pts',(6.17882658687335,30.3467522340408,56.6302109205204));
#105164=CARTESIAN_POINT('Ctrl Pts',(6.17551844198579,30.3932199502535,56.6196306997463));
#105165=CARTESIAN_POINT('Ctrl Pts',(6.17112079763952,30.4554817863482,56.602616026593));
#105166=CARTESIAN_POINT('Ctrl Pts',(6.16997698582802,30.4717207796462,56.597911552317));
#105167=CARTESIAN_POINT('Ctrl Pts',(6.1681604924861,30.4975734324719,56.5899935003967));
#105168=CARTESIAN_POINT('Ctrl Pts',(6.16748272079862,30.5072338900197,56.5869380708327));
#105169=CARTESIAN_POINT('Ctrl Pts',(6.16608581986091,30.527170545936,56.5804318101603));
#105170=CARTESIAN_POINT('Ctrl Pts',(6.16536714054307,30.5374421681683,56.576968425935));
#105171=CARTESIAN_POINT('Ctrl Pts',(6.16368292459527,30.5615422396621,56.5685795403138));
#105172=CARTESIAN_POINT('Ctrl Pts',(6.16272018016313,30.5753409844888,56.5635709883225));
#105173=CARTESIAN_POINT('Ctrl Pts',(6.15949230060128,30.6216562736052,56.5460636829091));
#105174=CARTESIAN_POINT('Ctrl Pts',(6.15725495077937,30.6538477697883,56.5327272423187));
#105175=CARTESIAN_POINT('Ctrl Pts',(6.15181098270919,30.7320684874088,56.4974082162702));
#105176=CARTESIAN_POINT('Ctrl Pts',(6.1486393830375,30.77755207393,56.4743028799099));
#105177=CARTESIAN_POINT('Ctrl Pts',(6.13929137637149,30.9095844175477,56.3994185827939));
#105178=CARTESIAN_POINT('Ctrl Pts',(6.133235355052,30.992563141032,56.3418393336228));
#105179=CARTESIAN_POINT('Ctrl Pts',(6.12399828956644,31.1060969094595,56.246733504011));
#105180=CARTESIAN_POINT('Ctrl Pts',(6.12099855308623,31.1410539128376,56.214820928005));
#105181=CARTESIAN_POINT('Ctrl Pts',(6.11714665268529,31.1827865586526,56.1733307935841));
#105182=CARTESIAN_POINT('Ctrl Pts',(6.11638557168548,31.1908859652968,56.1651093484501));
#105183=CARTESIAN_POINT('Ctrl Pts',(6.11517135017654,31.2035638049652,56.151970181987));
#105184=CARTESIAN_POINT('Ctrl Pts',(6.11472243326801,31.2081991974774,56.1471075921828));
#105185=CARTESIAN_POINT('Ctrl Pts',(6.11386000623778,31.2170025944169,56.1377601551767));
#105186=CARTESIAN_POINT('Ctrl Pts',(6.11344687141477,31.221175460885,56.1332801834442));
#105187=CARTESIAN_POINT('Ctrl Pts',(6.11244304877632,31.2312096707202,56.1223877328082));
#105188=CARTESIAN_POINT('Ctrl Pts',(6.11185053108079,31.2370456781989,56.1159522650149));
#105189=CARTESIAN_POINT('Ctrl Pts',(6.1098116416017,31.2568414084029,56.0937770736268));
#105190=CARTESIAN_POINT('Ctrl Pts',(6.10834919186775,31.2705525696277,56.0778194097897));
#105191=CARTESIAN_POINT('Ctrl Pts',(6.10181417219437,31.329841177883,56.0061130208916));
#105192=CARTESIAN_POINT('Ctrl Pts',(6.09658992949722,31.3720755896651,55.947706645059));
#105193=CARTESIAN_POINT('Ctrl Pts',(6.08493504205352,31.4573181988525,55.8121274161216));
#105194=CARTESIAN_POINT('Ctrl Pts',(6.07851905786425,31.4982468554402,55.7338843670799));
#105195=CARTESIAN_POINT('Ctrl Pts',(6.07031018813179,31.5436497110356,55.6272713353825));
#105196=CARTESIAN_POINT('Ctrl Pts',(6.06836462738581,31.5538675993448,55.6015138911432));
#105197=CARTESIAN_POINT('Ctrl Pts',(6.06643882015545,31.5634376718252,55.5755159826781));
#105198=CARTESIAN_POINT('Origin',(5.,30.,55.));
#105199=CARTESIAN_POINT('',(5.36787289354565,31.5634376782623,55.5755159651912));
#105200=CARTESIAN_POINT('',(5.55935725065089,31.5634376826058,55.5755159533916));
#105201=CARTESIAN_POINT('',(5.,31.5634376782623,55.5755159651912));
#105202=CARTESIAN_POINT('Ctrl Pts',(5.55935725065089,31.5634376826058,55.5755159533915));
#105203=CARTESIAN_POINT('Ctrl Pts',(5.56438142617607,31.5386334334857,55.642898790539));
#105204=CARTESIAN_POINT('Ctrl Pts',(5.56958176175285,31.5094976695741,55.7086108847468));
#105205=CARTESIAN_POINT('Ctrl Pts',(5.57506597430681,31.474553496052,55.7754100768546));
#105206=CARTESIAN_POINT('Ctrl Pts',(5.57532629573884,31.4728849165893,55.7785748663058));
#105207=CARTESIAN_POINT('Ctrl Pts',(5.58228131114254,31.428039808155,55.8629723445646));
#105208=CARTESIAN_POINT('Ctrl Pts',(5.58897634642658,31.3782145606548,55.9405034253079));
#105209=CARTESIAN_POINT('Ctrl Pts',(5.59903261293475,31.2916697514238,56.0534087962369));
#105210=CARTESIAN_POINT('Ctrl Pts',(5.60252539582477,31.259310001581,56.0918883030689));
#105211=CARTESIAN_POINT('Ctrl Pts',(5.6070645053916,31.2141584933073,56.1408958946897));
#105212=CARTESIAN_POINT('Ctrl Pts',(5.60817273521232,31.20288265202,56.1527782302515));
#105213=CARTESIAN_POINT('Ctrl Pts',(5.60930874773144,31.1910659530328,56.1648683064411));
#105214=CARTESIAN_POINT('Ctrl Pts',(5.60934403107992,31.1906986800897,56.1652437208836));
#105215=CARTESIAN_POINT('Ctrl Pts',(5.60941457768895,31.1899638260067,56.1659941545953));
#105216=CARTESIAN_POINT('Ctrl Pts',(5.60944984094736,31.1895962449558,56.1663691738652));
#105217=CARTESIAN_POINT('Ctrl Pts',(5.60949443673807,31.1891310553628,56.1668433281837));
#105218=CARTESIAN_POINT('Ctrl Pts',(5.609503776488,31.1890336119965,56.1669426245097));
#105219=CARTESIAN_POINT('Ctrl Pts',(5.60952323637707,31.1888305454974,56.1671495006305));
#105220=CARTESIAN_POINT('Ctrl Pts',(5.60953335642456,31.1887249201563,56.1672570783376));
#105221=CARTESIAN_POINT('Ctrl Pts',(5.60955448972941,31.1885043023187,56.1674817130455));
#105222=CARTESIAN_POINT('Ctrl Pts',(5.60956550287016,31.1883893071048,56.1675987674217));
#105223=CARTESIAN_POINT('Ctrl Pts',(5.60958855851705,31.1881485155607,56.1678437982768));
#105224=CARTESIAN_POINT('Ctrl Pts',(5.60960060087439,31.188022715836,56.1679717714313));
#105225=CARTESIAN_POINT('Ctrl Pts',(5.60962588093001,31.1877585659453,56.1682403981834));
#105226=CARTESIAN_POINT('Ctrl Pts',(5.60963911843756,31.1876202114697,56.1683810475324));
#105227=CARTESIAN_POINT('Ctrl Pts',(5.6096669934003,31.1873287938332,56.1686771936434));
#105228=CARTESIAN_POINT('Ctrl Pts',(5.60968163061705,31.1871757250234,56.1688326849994));
#105229=CARTESIAN_POINT('Ctrl Pts',(5.60971256045189,31.1868521817154,56.1691612197481));
#105230=CARTESIAN_POINT('Ctrl Pts',(5.60972885273997,31.1866816999834,56.169334255861));
#105231=CARTESIAN_POINT('Ctrl Pts',(5.60976341621427,31.1863199120729,56.1697013039481));
#105232=CARTESIAN_POINT('Ctrl Pts',(5.6097816869726,31.186128596093,56.1698953063284));
#105233=CARTESIAN_POINT('Ctrl Pts',(5.60982062380237,31.1857207341308,56.1703086924712));
#105234=CARTESIAN_POINT('Ctrl Pts',(5.60984128928755,31.1855041748085,56.1705280631122));
#105235=CARTESIAN_POINT('Ctrl Pts',(5.60988556177281,31.1850400404178,56.1709979618531));
#105236=CARTESIAN_POINT('Ctrl Pts',(5.609909167954,31.1847924467195,56.1712484716124));
#105237=CARTESIAN_POINT('Ctrl Pts',(5.60996005416152,31.1842584755389,56.1717883891228));
#105238=CARTESIAN_POINT('Ctrl Pts',(5.60998733301112,31.183972071315,56.1720777705064));
#105239=CARTESIAN_POINT('Ctrl Pts',(5.61004657226197,31.1833497733272,56.172706076415));
#105240=CARTESIAN_POINT('Ctrl Pts',(5.61007853091724,31.1830138398797,56.173044961776));
#105241=CARTESIAN_POINT('Ctrl Pts',(5.61014856038942,31.1822772575612,56.1737873783654));
#105242=CARTESIAN_POINT('Ctrl Pts',(5.61018662850561,31.1818765474767,56.174190849003));
#105243=CARTESIAN_POINT('Ctrl Pts',(5.61027098724686,31.1809879049234,56.1750846977867));
#105244=CARTESIAN_POINT('Ctrl Pts',(5.61031727349049,31.1804998732521,56.1755749775331));
#105245=CARTESIAN_POINT('Ctrl Pts',(5.6104213355967,31.1794016585379,56.1766768775831));
#105246=CARTESIAN_POINT('Ctrl Pts',(5.61047910390184,31.1787913044448,56.1772883278837));
#105247=CARTESIAN_POINT('Ctrl Pts',(5.61068048993553,31.1766611140632,56.1794190267513));
#105248=CARTESIAN_POINT('Ctrl Pts',(5.6108239984544,31.1751388090333,56.1809358143395));
#105249=CARTESIAN_POINT('Ctrl Pts',(5.61168020060985,31.1660306523415,56.1899759085126));
#105250=CARTESIAN_POINT('Ctrl Pts',(5.61238979142832,31.1583753687793,56.1974291875225));
#105251=CARTESIAN_POINT('Ctrl Pts',(5.61398643714876,31.1409117657192,56.2141077500461));
#105252=CARTESIAN_POINT('Ctrl Pts',(5.61487156491238,31.1310621662562,56.2232888782436));
#105253=CARTESIAN_POINT('Ctrl Pts',(5.61756513883188,31.1005834127957,56.2510162280415));
#105254=CARTESIAN_POINT('Ctrl Pts',(5.61935716118375,31.0796008549319,56.2691680692193));
#105255=CARTESIAN_POINT('Ctrl Pts',(5.62950549158411,30.9569847370767,56.3699998499438));
#105256=CARTESIAN_POINT('Ctrl Pts',(5.63738327934517,30.8463360884268,56.4409847635265));
#105257=CARTESIAN_POINT('Ctrl Pts',(5.64865786447829,30.68105782887,56.5213480949747));
#105258=CARTESIAN_POINT('Ctrl Pts',(5.65192040425943,30.6325418896573,56.5421510212462));
#105259=CARTESIAN_POINT('Ctrl Pts',(5.65714970409301,30.5554406712294,56.5709599175612));
#105260=CARTESIAN_POINT('Ctrl Pts',(5.6590544903043,30.5274883564841,56.5805648302918));
#105261=CARTESIAN_POINT('Ctrl Pts',(5.66163228132368,30.4901027419031,56.5923090746656));
#105262=CARTESIAN_POINT('Ctrl Pts',(5.66227037439265,30.4808833488748,56.5951175758118));
#105263=CARTESIAN_POINT('Ctrl Pts',(5.6633334671081,30.4655923155106,56.5996310705523));
#105264=CARTESIAN_POINT('Ctrl Pts',(5.66375587808909,30.4595342638098,56.6013819106883));
#105265=CARTESIAN_POINT('Ctrl Pts',(5.66461225681819,30.4472919072846,56.6048448916062));
#105266=CARTESIAN_POINT('Ctrl Pts',(5.66504627975323,30.4411073892707,56.6065557705979));
#105267=CARTESIAN_POINT('Ctrl Pts',(5.66617220095384,30.4251114320976,56.6108815514161));
#105268=CARTESIAN_POINT('Ctrl Pts',(5.66686703662255,30.415285864413,56.6134425122357));
#105269=CARTESIAN_POINT('Ctrl Pts',(5.66972852073009,30.3749847753909,56.6235541836016));
#105270=CARTESIAN_POINT('Ctrl Pts',(5.67193225510594,30.3443240648373,56.6303319931451));
#105271=CARTESIAN_POINT('Ctrl Pts',(5.68190384758507,30.2065197041298,56.6567344030723));
#105272=CARTESIAN_POINT('Ctrl Pts',(5.6899298328273,30.0977973217312,56.6666897565582));
#105273=CARTESIAN_POINT('Ctrl Pts',(5.701935769797,29.9314878439444,56.6655798774498));
#105274=CARTESIAN_POINT('Ctrl Pts',(5.70603035474739,29.874147400891,56.6622311703427));
#105275=CARTESIAN_POINT('Ctrl Pts',(5.71268592042958,29.7795369284339,56.6517806833118));
#105276=CARTESIAN_POINT('Ctrl Pts',(5.71529124385533,29.7421340745683,56.6463562654311));
#105277=CARTESIAN_POINT('Ctrl Pts',(5.71888458789381,29.6900542301858,56.6369845888825));
#105278=CARTESIAN_POINT('Ctrl Pts',(5.71990558846127,29.675199940804,56.634102160897));
#105279=CARTESIAN_POINT('Ctrl Pts',(5.72165225607404,29.6496978885732,56.6287920774072));
#105280=CARTESIAN_POINT('Ctrl Pts',(5.72238095613864,29.6390311566344,56.6264614058104));
#105281=CARTESIAN_POINT('Ctrl Pts',(5.72377262678835,29.6186113271342,56.6217889091472));
#105282=CARTESIAN_POINT('Ctrl Pts',(5.72443608874799,29.6088549940349,56.6194635461721));
#105283=CARTESIAN_POINT('Ctrl Pts',(5.72617229731467,29.5832727184829,56.6131214913951));
#105284=CARTESIAN_POINT('Ctrl Pts',(5.72724035843151,29.5674835349375,56.6089599471674));
#105285=CARTESIAN_POINT('Ctrl Pts',(5.73109742565772,29.5103151782821,56.5929897300078));
#105286=CARTESIAN_POINT('Ctrl Pts',(5.73384244620543,29.469334450681,56.5798107680502));
#105287=CARTESIAN_POINT('Ctrl Pts',(5.74377246347529,29.3210246398426,56.5256922428114));
#105288=CARTESIAN_POINT('Ctrl Pts',(5.75067322552188,29.2175036662022,56.4752777756366));
#105289=CARTESIAN_POINT('Ctrl Pts',(5.76070931432902,29.0789266853458,56.3890711197075));
#105290=CARTESIAN_POINT('Ctrl Pts',(5.76371069612895,29.0389987543043,56.3617527631369));
#105291=CARTESIAN_POINT('Ctrl Pts',(5.76799841422418,28.9851201218553,56.3213386331694));
#105292=CARTESIAN_POINT('Ctrl Pts',(5.76921949673666,28.9701186509693,56.3096798437433));
#105293=CARTESIAN_POINT('Ctrl Pts',(5.77138841407432,28.9441472004133,56.2887732951251));
#105294=CARTESIAN_POINT('Ctrl Pts',(5.77232981992269,28.9330909685501,56.2796354267453));
#105295=CARTESIAN_POINT('Ctrl Pts',(5.77376545365181,28.9165826084727,56.2656287576805));
#105296=CARTESIAN_POINT('Ctrl Pts',(5.77425250593635,28.9110419553616,56.260864690804));
#105297=CARTESIAN_POINT('Ctrl Pts',(5.77514486379189,28.9010036773915,56.2521178748903));
#105298=CARTESIAN_POINT('Ctrl Pts',(5.77554931159352,28.8964960184456,56.248147046171));
#105299=CARTESIAN_POINT('Ctrl Pts',(5.77647632172216,28.8862596628727,56.2390309725505));
#105300=CARTESIAN_POINT('Ctrl Pts',(5.77699998919003,28.8805451189608,56.2338703549874));
#105301=CARTESIAN_POINT('Ctrl Pts',(5.77864562373789,28.8627921127189,56.217613352367));
#105302=CARTESIAN_POINT('Ctrl Pts',(5.77977701361075,28.8508817321547,56.2063793811396));
#105303=CARTESIAN_POINT('Ctrl Pts',(5.78634064111896,28.783359353779,56.1407844956635));
#105304=CARTESIAN_POINT('Ctrl Pts',(5.79197758969326,28.7314470682383,56.0827626165985));
#105305=CARTESIAN_POINT('Ctrl Pts',(5.80248998111074,28.6428816280932,55.9686261851671));
#105306=CARTESIAN_POINT('Ctrl Pts',(5.80735135535522,28.6051830279587,55.9135060851548));
#105307=CARTESIAN_POINT('Ctrl Pts',(5.81560742853956,28.5460286048384,55.8147779025804));
#105308=CARTESIAN_POINT('Ctrl Pts',(5.81903484700217,28.5229841407807,55.7722180445302));
#105309=CARTESIAN_POINT('Ctrl Pts',(5.82474099980228,28.4871379370471,55.698520964106));
#105310=CARTESIAN_POINT('Ctrl Pts',(5.82704921748487,28.4733680782871,55.6678910202404));
#105311=CARTESIAN_POINT('Ctrl Pts',(5.83030816087445,28.4549973061191,55.6234840279199));
#105312=CARTESIAN_POINT('Ctrl Pts',(5.83128417573571,28.4496367125943,55.610032259169));
#105313=CARTESIAN_POINT('Ctrl Pts',(5.83297861701718,28.4405811674031,55.5864177526218));
#105314=CARTESIAN_POINT('Ctrl Pts',(5.83369960416216,28.4368085817856,55.5762859321121));
#105315=CARTESIAN_POINT('Ctrl Pts',(5.83518768648709,28.4291916236937,55.5552041988846));
#105316=CARTESIAN_POINT('Ctrl Pts',(5.83595424319227,28.4253624900285,55.544249374108));
#105317=CARTESIAN_POINT('Ctrl Pts',(5.83793710918573,28.4157076973509,55.5156726982956));
#105318=CARTESIAN_POINT('Ctrl Pts',(5.83914750209038,28.4100613779089,55.4979916213125));
#105319=CARTESIAN_POINT('Ctrl Pts',(5.84448122561573,28.3863106233631,55.4190916139728));
#105320=CARTESIAN_POINT('Ctrl Pts',(5.84850014935065,28.3714370626358,55.3569528054532));
#105321=CARTESIAN_POINT('Ctrl Pts',(5.86142117325569,28.3346224186023,55.1516881745476));
#105322=CARTESIAN_POINT('Ctrl Pts',(5.86996417475767,28.3277445217982,55.0065688996762));
#105323=CARTESIAN_POINT('Ctrl Pts',(5.88069467302052,28.3415639148894,54.8398135534096));
#105324=CARTESIAN_POINT('Ctrl Pts',(5.88216648745376,28.343897092926,54.8172625233612));
#105325=CARTESIAN_POINT('Ctrl Pts',(5.8842383858517,28.3477665979335,54.7860905946412));
#105326=CARTESIAN_POINT('Ctrl Pts',(5.88481855284784,28.3489119586705,54.7774225527197));
#105327=CARTESIAN_POINT('Ctrl Pts',(5.88581209580855,28.3509767504594,54.7626902020593));
#105328=CARTESIAN_POINT('Ctrl Pts',(5.88622356714983,28.3518615602632,54.7566210772582));
#105329=CARTESIAN_POINT('Ctrl Pts',(5.88708850889559,28.3537828453135,54.7439336931603));
#105330=CARTESIAN_POINT('Ctrl Pts',(5.88754230336582,28.3548257434434,54.7373166631237));
#105331=CARTESIAN_POINT('Ctrl Pts',(5.88877725004576,28.3577586396373,54.7194107528596));
#105332=CARTESIAN_POINT('Ctrl Pts',(5.88956243544875,28.3597250777891,54.7081350094737));
#105333=CARTESIAN_POINT('Ctrl Pts',(5.89352306029839,28.3701568976936,54.6517567576427));
#105334=CARTESIAN_POINT('Ctrl Pts',(5.89677840882485,28.3803664221921,54.6070010649619));
#105335=CARTESIAN_POINT('Ctrl Pts',(5.90634436388976,28.4153022520344,54.4785625148006));
#105336=CARTESIAN_POINT('Ctrl Pts',(5.91274379238227,28.4447698051571,54.3963253200586));
#105337=CARTESIAN_POINT('Ctrl Pts',(5.92341360657095,28.5052842518092,54.261744454002));
#105338=CARTESIAN_POINT('Ctrl Pts',(5.92772673531838,28.5330010181555,54.2080961884032));
#105339=CARTESIAN_POINT('Ctrl Pts',(5.9346860010844,28.5833573841249,54.1223864666511));
#105340=CARTESIAN_POINT('Ctrl Pts',(5.93738200309132,28.6043242335547,54.0894115050606));
#105341=CARTESIAN_POINT('Ctrl Pts',(5.94107632232717,28.6350999362334,54.0445742356365));
#105342=CARTESIAN_POINT('Ctrl Pts',(5.94211015684279,28.6439412168671,54.0320665419653));
#105343=CARTESIAN_POINT('Ctrl Pts',(5.94387187026964,28.659397719978,54.0108278983088));
#105344=CARTESIAN_POINT('Ctrl Pts',(5.94460291957702,28.6659287268419,54.00203719109));
#105345=CARTESIAN_POINT('Ctrl Pts',(5.94599451631321,28.6785832486332,53.985350508075));
#105346=CARTESIAN_POINT('Ctrl Pts',(5.9466555968881,28.6846920237563,53.977444007766));
#105347=CARTESIAN_POINT('Ctrl Pts',(5.94820463325613,28.6992327173627,53.9589701133856));
#105348=CARTESIAN_POINT('Ctrl Pts',(5.94909023768516,28.7077229435511,53.948449347169));
#105349=CARTESIAN_POINT('Ctrl Pts',(5.95220101933214,28.7381609783025,53.9116571810827));
#105350=CARTESIAN_POINT('Ctrl Pts',(5.95439877066066,28.7607902713254,53.8859590163247));
#105351=CARTESIAN_POINT('Ctrl Pts',(5.96517498497581,28.8769610361903,53.7619575309283));
#105352=CARTESIAN_POINT('Ctrl Pts',(5.97327247946438,28.9814689877015,53.6746470661402));
#105353=CARTESIAN_POINT('Ctrl Pts',(5.98427000393146,29.1310246177015,53.577946344057));
#105354=CARTESIAN_POINT('Ctrl Pts',(5.98691667608192,29.1675046059302,53.556287509775));
#105355=CARTESIAN_POINT('Ctrl Pts',(5.99126211897766,29.2273006583769,53.5238058271616));
#105356=CARTESIAN_POINT('Ctrl Pts',(5.99292143313435,29.2501109620411,53.512088790314));
#105357=CARTESIAN_POINT('Ctrl Pts',(5.99521358779847,29.2814204052399,53.4969087813291));
#105358=CARTESIAN_POINT('Ctrl Pts',(5.9958205305972,29.2896923519451,53.4929821231137));
#105359=CARTESIAN_POINT('Ctrl Pts',(5.99684591417611,29.3036267402538,53.4865077361036));
#105360=CARTESIAN_POINT('Ctrl Pts',(5.99726214006056,29.3092719775985,53.4839230404561));
#105361=CARTESIAN_POINT('Ctrl Pts',(5.99812161867224,29.3209030209689,53.4786761656712));
#105362=CARTESIAN_POINT('Ctrl Pts',(5.99856506046589,29.3268902601006,53.4760176542543));
#105363=CARTESIAN_POINT('Ctrl Pts',(5.99974286314159,29.3427606139052,53.4690825119363));
#105364=CARTESIAN_POINT('Ctrl Pts',(6.00048066687747,29.3526695918747,53.4648663597796));
#105365=CARTESIAN_POINT('Ctrl Pts',(6.00380368503843,29.3971838991493,53.4464336561704));
#105366=CARTESIAN_POINT('Ctrl Pts',(6.00644190064862,29.4322188698263,53.4332901519454));
#105367=CARTESIAN_POINT('Ctrl Pts',(6.01665735794077,29.5677149746606,53.3875998441156));
#105368=CARTESIAN_POINT('Ctrl Pts',(6.02443255821359,29.6707462143277,53.3634496752657));
#105369=CARTESIAN_POINT('Ctrl Pts',(6.03600598498834,29.8298438700515,53.341800635542));
#105370=CARTESIAN_POINT('Ctrl Pts',(6.03992106520626,29.8846543195539,53.3370885173216));
#105371=CARTESIAN_POINT('Ctrl Pts',(6.04632454628363,29.9762716849743,53.3337649026414));
#105372=CARTESIAN_POINT('Ctrl Pts',(6.04885299567858,30.0129775326438,53.333646381974));
#105373=CARTESIAN_POINT('Ctrl Pts',(6.05236034792536,30.0646215755687,53.335186466547));
#105374=CARTESIAN_POINT('Ctrl Pts',(6.0533701491903,30.0795769124824,53.3358342661861));
#105375=CARTESIAN_POINT('Ctrl Pts',(6.05510373452009,30.1053943551225,53.3373014039075));
#105376=CARTESIAN_POINT('Ctrl Pts',(6.05583043273052,30.1162606846872,53.3380258562676));
#105377=CARTESIAN_POINT('Ctrl Pts',(6.05722238753816,30.1371551828384,53.3396248124423));
#105378=CARTESIAN_POINT('Ctrl Pts',(6.0578880980002,30.147184025289,53.3404837518537));
#105379=CARTESIAN_POINT('Ctrl Pts',(6.05963950851647,30.1736583288824,53.3429930777817));
#105380=CARTESIAN_POINT('Ctrl Pts',(6.0607203596329,30.190088344681,53.3447974115597));
#105381=CARTESIAN_POINT('Ctrl Pts',(6.06468452423232,30.2506454151043,53.3523613688104));
#105382=CARTESIAN_POINT('Ctrl Pts',(6.06752045822625,30.2945654122062,53.3596439621735));
#105383=CARTESIAN_POINT('Ctrl Pts',(6.07744498142532,30.4492649245558,53.3917104224484));
#105384=CARTESIAN_POINT('Ctrl Pts',(6.08426439881451,30.5577391625354,53.4260362396723));
#105385=CARTESIAN_POINT('Ctrl Pts',(6.09419585415679,30.7059133693824,53.4901840333163));
#105386=CARTESIAN_POINT('Ctrl Pts',(6.09717458968547,30.7490960585087,53.5111372124569));
#105387=CARTESIAN_POINT('Ctrl Pts',(6.10143292372959,30.8079481485887,53.5429024705863));
#105388=CARTESIAN_POINT('Ctrl Pts',(6.1026482146318,30.8244302406474,53.5521643270762));
#105389=CARTESIAN_POINT('Ctrl Pts',(6.10480781772517,30.8530872632819,53.5689156823011));
#105390=CARTESIAN_POINT('Ctrl Pts',(6.10574577770904,30.8653303183613,53.5762852779555));
#105391=CARTESIAN_POINT('Ctrl Pts',(6.10717720349427,30.883678972499,53.5876541809736));
#105392=CARTESIAN_POINT('Ctrl Pts',(6.10766355656535,30.8898559296141,53.5915378391746));
#105393=CARTESIAN_POINT('Ctrl Pts',(6.10855526382174,30.9010722246558,53.5986931302238));
#105394=CARTESIAN_POINT('Ctrl Pts',(6.10895976851424,30.9061196373273,53.6019516115001));
#105395=CARTESIAN_POINT('Ctrl Pts',(6.10988772833993,30.9176065205782,53.6094555877559));
#105396=CARTESIAN_POINT('Ctrl Pts',(6.11041229823292,30.9240341830352,53.6137185308529));
#105397=CARTESIAN_POINT('Ctrl Pts',(6.11206365320363,30.9440707129814,53.6272083820125));
#105398=CARTESIAN_POINT('Ctrl Pts',(6.1131999510721,30.9575722628004,53.6365918995358));
#105399=CARTESIAN_POINT('Ctrl Pts',(6.12047552777701,31.0423588623688,53.6973988153171));
#105400=CARTESIAN_POINT('Ctrl Pts',(6.12687573452939,31.1096132770386,53.7541920552121));
#105401=CARTESIAN_POINT('Ctrl Pts',(6.13683136810198,31.2068083295225,53.8504090807581));
#105402=CARTESIAN_POINT('Ctrl Pts',(6.14038599273035,31.2400193819456,53.8863133897986));
#105403=CARTESIAN_POINT('Ctrl Pts',(6.14771407543596,31.3057951880298,53.9640195562467));
#105404=CARTESIAN_POINT('Ctrl Pts',(6.15147708698704,31.3380445123024,54.0060209611816));
#105405=CARTESIAN_POINT('Ctrl Pts',(6.15766510767683,31.3886372630467,54.0788483141074));
#105406=CARTESIAN_POINT('Ctrl Pts',(6.16012669806253,31.4080834187329,54.10885730668));
#105407=CARTESIAN_POINT('Ctrl Pts',(6.16355896420394,31.4342071195242,54.1521641169793));
#105408=CARTESIAN_POINT('Ctrl Pts',(6.16455877995208,31.4416944415924,54.1649593375249));
#105409=CARTESIAN_POINT('Ctrl Pts',(6.16628074228329,31.4543722876095,54.1873036770456));
#105410=CARTESIAN_POINT('Ctrl Pts',(6.16700569777559,31.459641895636,54.1968066170301));
#105411=CARTESIAN_POINT('Ctrl Pts',(6.16839809479899,31.4696293959761,54.2152405222175));
#105412=CARTESIAN_POINT('Ctrl Pts',(6.16906595583971,31.4743597685916,54.2241641411716));
#105413=CARTESIAN_POINT('Ctrl Pts',(6.17083175085771,31.4867035600154,54.2479707647085));
#105414=CARTESIAN_POINT('Ctrl Pts',(6.17192467978531,31.4941747486084,54.262926530197));
#105415=CARTESIAN_POINT('Ctrl Pts',(6.17599588874745,31.521346224349,54.3194298229548));
#105416=CARTESIAN_POINT('Ctrl Pts',(6.17892323530642,31.5395498953674,54.3616765719644));
#105417=CARTESIAN_POINT('Ctrl Pts',(6.18884425669667,31.5960594324387,54.5093616280592));
#105418=CARTESIAN_POINT('Ctrl Pts',(6.1955834187822,31.6254574578055,54.6178740724291));
#105419=CARTESIAN_POINT('Ctrl Pts',(6.20541143011197,31.6514884380471,54.7754832350751));
#105420=CARTESIAN_POINT('Ctrl Pts',(6.20836769698654,31.6572282965008,54.8227555652822));
#105421=CARTESIAN_POINT('Ctrl Pts',(6.21316100842611,31.6630920843164,54.8977922958354));
#105422=CARTESIAN_POINT('Ctrl Pts',(6.21494786037152,31.6645601052876,54.9254269459025));
#105423=CARTESIAN_POINT('Ctrl Pts',(6.21738876580524,31.6656043790455,54.9624941829058));
#105424=CARTESIAN_POINT('Ctrl Pts',(6.2180124066811,31.6657897214408,54.9719068075026));
#105425=CARTESIAN_POINT('Ctrl Pts',(6.21905793229511,31.665965463337,54.9875797775692));
#105426=CARTESIAN_POINT('Ctrl Pts',(6.21947740362127,31.6660003704114,54.9938395883496));
#105427=CARTESIAN_POINT('Ctrl Pts',(6.22033485673021,31.6659996108333,55.006574221476));
#105428=CARTESIAN_POINT('Ctrl Pts',(6.22077295319821,31.6659614782214,55.0130488755287));
#105429=CARTESIAN_POINT('Ctrl Pts',(6.22192132873125,31.6657634983231,55.029942377));
#105430=CARTESIAN_POINT('Ctrl Pts',(6.22263476050851,31.6655436442829,55.0403600466417));
#105431=CARTESIAN_POINT('Ctrl Pts',(6.22592344924527,31.6640892228774,55.0880598623975));
#105432=CARTESIAN_POINT('Ctrl Pts',(6.2285521248893,31.6617005110438,55.1252933180455));
#105433=CARTESIAN_POINT('Ctrl Pts',(6.23683766796736,31.650388174945,55.2407811107911));
#105434=CARTESIAN_POINT('Ctrl Pts',(6.24259887178799,31.6371654375801,55.3185046605562));
#105435=CARTESIAN_POINT('Ctrl Pts',(6.25289734072264,31.603563647212,55.4561870396466));
#105436=CARTESIAN_POINT('Ctrl Pts',(6.25743983383605,31.5851786325435,55.5164548041091));
#105437=CARTESIAN_POINT('Ctrl Pts',(6.26189397015589,31.5634377553307,55.5755157558282));
#105438=CARTESIAN_POINT('',(6.02851963656332,31.6659993037065,54.9984768292001));
#105439=CARTESIAN_POINT('Ctrl Pts',(6.06643882015545,31.5634376718252,55.5755159826781));
#105440=CARTESIAN_POINT('Ctrl Pts',(6.06472934739696,31.571932695597,55.5524385346354));
#105441=CARTESIAN_POINT('Ctrl Pts',(6.06303542075663,31.5799172711098,55.5291716135343));
#105442=CARTESIAN_POINT('Ctrl Pts',(6.06017046701639,31.5926705752753,55.4891417128373));
#105443=CARTESIAN_POINT('Ctrl Pts',(6.0589915588576,31.5976959179968,55.4724690150401));
#105444=CARTESIAN_POINT('Ctrl Pts',(6.05705752028612,31.6055667482191,55.4447926286377));
#105445=CARTESIAN_POINT('Ctrl Pts',(6.0562975660611,31.608562580033,55.4338334964505));
#105446=CARTESIAN_POINT('Ctrl Pts',(6.05481403277105,31.614218559563,55.4122787407976));
#105447=CARTESIAN_POINT('Ctrl Pts',(6.05409021742884,31.6168870540454,55.4016859249121));
#105448=CARTESIAN_POINT('Ctrl Pts',(6.05265582349213,31.6219917817132,55.3805467114568));
#105449=CARTESIAN_POINT('Ctrl Pts',(6.05194521956491,31.6244298025128,55.3700013046029));
#105450=CARTESIAN_POINT('Ctrl Pts',(6.05027908981712,31.6299294334358,55.3451103938039));
#105451=CARTESIAN_POINT('Ctrl Pts',(6.04932629407405,31.6329047289416,55.3307465946524));
#105452=CARTESIAN_POINT('Ctrl Pts',(6.04149014513026,31.6559460428788,55.2116094284625));
#105453=CARTESIAN_POINT('Ctrl Pts',(6.03493536642089,31.6660964531918,55.1051698531878));
#105454=CARTESIAN_POINT('Ctrl Pts',(6.02841825655256,31.665999309357,54.9984830221305));
#105455=CARTESIAN_POINT('Ctrl Pts',(6.02851963656332,31.6659993037066,54.9984768292001));
#105456=CARTESIAN_POINT('Ctrl Pts',(6.02319560874737,31.6659265050777,54.9188518357291));
#105457=CARTESIAN_POINT('Ctrl Pts',(6.01787158093143,31.6601415384276,54.8394810237068));
#105458=CARTESIAN_POINT('Ctrl Pts',(6.01254755311548,31.6487752899906,54.7610522167576));
#105459=CARTESIAN_POINT('Ctrl Pts',(6.00879991050439,31.6407744608358,54.7058453040553));
#105460=CARTESIAN_POINT('Ctrl Pts',(6.0050522678933,31.6300091693766,54.651104499668));
#105461=CARTESIAN_POINT('Ctrl Pts',(6.00130462528222,31.6165387634104,54.597062751298));
#105462=CARTESIAN_POINT('Ctrl Pts',(5.99722727558211,31.6018832688966,54.5382665614325));
#105463=CARTESIAN_POINT('Ctrl Pts',(5.993149925882,31.5839855577694,54.4801495795245));
#105464=CARTESIAN_POINT('Ctrl Pts',(5.98907257618189,31.5629257672557,54.4230952885891));
#105465=CARTESIAN_POINT('Ctrl Pts',(5.98495160860947,31.5416406874435,54.3654306534447));
#105466=CARTESIAN_POINT('Ctrl Pts',(5.98083064103704,31.5171255131336,54.3088521143315));
#105467=CARTESIAN_POINT('Ctrl Pts',(5.97670967346462,31.4895158984509,54.2537437516095));
#105468=CARTESIAN_POINT('Ctrl Pts',(5.97264355643921,31.4622737708795,54.1993688874622));
#105469=CARTESIAN_POINT('Ctrl Pts',(5.96857743941381,31.4320193111664,54.1464257733204));
#105470=CARTESIAN_POINT('Ctrl Pts',(5.96451132238841,31.3989316336097,54.095264522368));
#105471=CARTESIAN_POINT('Ctrl Pts',(5.96044769316903,31.3658642003606,54.0441345738271));
#105472=CARTESIAN_POINT('Ctrl Pts',(5.95638406394966,31.3299672636836,53.994784755908));
#105473=CARTESIAN_POINT('Ctrl Pts',(5.95232043473028,31.2914648767165,53.9475388500246));
#105474=CARTESIAN_POINT('Ctrl Pts',(5.9482577821136,31.2529717429399,53.9003042986414));
#105475=CARTESIAN_POINT('Ctrl Pts',(5.94419512949692,31.21187472517,53.8551730522363));
#105476=CARTESIAN_POINT('Ctrl Pts',(5.94013247688024,31.1684387532835,53.8124365786093));
#105477=CARTESIAN_POINT('Ctrl Pts',(5.93596888334386,31.1239235685369,53.7686382718994));
#105478=CARTESIAN_POINT('Ctrl Pts',(5.93180528980747,31.0769520072831,53.7273557654103));
#105479=CARTESIAN_POINT('Ctrl Pts',(5.92764169627109,31.0278483005124,53.6888616125162));
#105480=CARTESIAN_POINT('Ctrl Pts',(5.92357385644512,30.9798738735519,53.6512527424761));
#105481=CARTESIAN_POINT('Ctrl Pts',(5.91950601661914,30.9298648035666,53.6163055754419));
#105482=CARTESIAN_POINT('Ctrl Pts',(5.91543817679317,30.8781537564999,53.5842309581202));
#105483=CARTESIAN_POINT('Ctrl Pts',(5.91122670640158,30.8246168541251,53.551023824371));
#105484=CARTESIAN_POINT('Ctrl Pts',(5.90701523600999,30.769256040786,53.520896213991));
#105485=CARTESIAN_POINT('Ctrl Pts',(5.9028037656184,30.7124665881183,53.4940294289678));
#105486=CARTESIAN_POINT('Ctrl Pts',(5.89859229522682,30.6556771354505,53.4671626439445));
#105487=CARTESIAN_POINT('Ctrl Pts',(5.89438082483523,30.5974596275331,53.4435568429065));
#105488=CARTESIAN_POINT('Ctrl Pts',(5.89016935444364,30.5382274340246,53.4233366785318));
#105489=CARTESIAN_POINT('Ctrl Pts',(5.88609200474353,30.4808815799681,53.4037604561002));
#105490=CARTESIAN_POINT('Ctrl Pts',(5.88201465504341,30.4223478962537,53.3872765390741));
#105491=CARTESIAN_POINT('Ctrl Pts',(5.87793730534329,30.36299202722,53.3740255880935));
#105492=CARTESIAN_POINT('Ctrl Pts',(5.87381633777087,30.3030011926064,53.3606328836871));
#105493=CARTESIAN_POINT('Ctrl Pts',(5.86969537019844,30.2421709473292,53.3505429818469));
#105494=CARTESIAN_POINT('Ctrl Pts',(5.86557440262602,30.1808975479542,53.3438502250267));
#105495=CARTESIAN_POINT('Ctrl Pts',(5.86150828560061,30.1204397044928,53.3372465495608));
#105496=CARTESIAN_POINT('Ctrl Pts',(5.8574421685752,30.0595509558089,53.3339501953221));
#105497=CARTESIAN_POINT('Ctrl Pts',(5.85337605154979,29.9986225924009,53.3340005694034));
#105498=CARTESIAN_POINT('Ctrl Pts',(5.84931242233042,29.9377315072978,53.3340509126639));
#105499=CARTESIAN_POINT('Ctrl Pts',(5.84524879311104,29.8768013664309,53.3374439239197));
#105500=CARTESIAN_POINT('Ctrl Pts',(5.84118516389166,29.8162257110446,53.3441669737806));
#105501=CARTESIAN_POINT('Ctrl Pts',(5.83712251127498,29.7556646136666,53.3508884079063));
#105502=CARTESIAN_POINT('Ctrl Pts',(5.8330598586583,29.6954583412569,53.3609382354768));
#105503=CARTESIAN_POINT('Ctrl Pts',(5.82899720604162,29.6359954570605,53.3742519590295));
#105504=CARTESIAN_POINT('Ctrl Pts',(5.82483361250524,29.5750551543435,53.387896476186));
#105505=CARTESIAN_POINT('Ctrl Pts',(5.82067001896886,29.5148962345786,53.404969181928));
#105506=CARTESIAN_POINT('Ctrl Pts',(5.81650642543249,29.455923532972,53.4253454988391));
#105507=CARTESIAN_POINT('Ctrl Pts',(5.81243858560651,29.3983070768638,53.4452532042176));
#105508=CARTESIAN_POINT('Ctrl Pts',(5.80837074578053,29.3418233160874,53.4683139139436));
#105509=CARTESIAN_POINT('Ctrl Pts',(5.80430290595455,29.2868298182051,53.4943624965489));
#105510=CARTESIAN_POINT('Ctrl Pts',(5.80009143556298,29.2298945655972,53.5213308234933));
#105511=CARTESIAN_POINT('Ctrl Pts',(5.7958799651714,29.1745573309091,53.5515017203615));
#105512=CARTESIAN_POINT('Ctrl Pts',(5.79166849477982,29.1211848149767,53.5846414339212));
#105513=CARTESIAN_POINT('Ctrl Pts',(5.78745702438825,29.0678122990444,53.617781147481));
#105514=CARTESIAN_POINT('Ctrl Pts',(5.78324555399667,29.0164049519221,53.6538892730567));
#105515=CARTESIAN_POINT('Ctrl Pts',(5.7790340836051,28.9672916966112,53.6926861279281));
#105516=CARTESIAN_POINT('Ctrl Pts',(5.77495673390498,28.9197425277474,53.7302474378429));
#105517=CARTESIAN_POINT('Ctrl Pts',(5.77087938420487,28.8741471032048,53.7704838505866));
#105518=CARTESIAN_POINT('Ctrl Pts',(5.76680203450475,28.8308219104712,53.8131644617026));
#105519=CARTESIAN_POINT('Ctrl Pts',(5.76268106693233,28.7870332419841,53.8563016530932));
#105520=CARTESIAN_POINT('Ctrl Pts',(5.7585600993599,28.745564135601,53.901935391439));
#105521=CARTESIAN_POINT('Ctrl Pts',(5.75443913178748,28.7067087678565,53.9497839322973));
#105522=CARTESIAN_POINT('Ctrl Pts',(5.75037301476207,28.6683705694754,53.9969956036356));
#105523=CARTESIAN_POINT('Ctrl Pts',(5.74630689773666,28.6325772882021,54.0463630694733));
#105524=CARTESIAN_POINT('Ctrl Pts',(5.74224078071126,28.5995742535652,54.0975789626109));
#105525=CARTESIAN_POINT('Ctrl Pts',(5.73817715149188,28.5665914114481,54.1487635199047));
#105526=CARTESIAN_POINT('Ctrl Pts',(5.7341135222725,28.5363957078717,54.201793832717));
#105527=CARTESIAN_POINT('Ctrl Pts',(5.73004989305313,28.5091899749724,54.2563324201787));
#105528=CARTESIAN_POINT('Ctrl Pts',(5.72598724043645,28.4819907803645,54.3108579005067));
#105529=CARTESIAN_POINT('Ctrl Pts',(5.72192458781976,28.4577803583886,54.36689047799));
#105530=CARTESIAN_POINT('Ctrl Pts',(5.71786193520308,28.436715264666,54.4240687226137));
#105531=CARTESIAN_POINT('Ctrl Pts',(5.7136983416667,28.4151267863141,54.4826676214611));
#105532=CARTESIAN_POINT('Ctrl Pts',(5.70953474813032,28.3968422725698,54.5424693728215));
#105533=CARTESIAN_POINT('Ctrl Pts',(5.70537115459394,28.3819766285954,54.6030662906876));
#105534=CARTESIAN_POINT('Ctrl Pts',(5.70130331476797,28.3674528625098,54.6622696095691));
#105535=CARTESIAN_POINT('Ctrl Pts',(5.69723547494199,28.3561924059843,54.7222313780833));
#105536=CARTESIAN_POINT('Ctrl Pts',(5.69316763511601,28.3482504566835,54.7825616267682));
#105537=CARTESIAN_POINT('Ctrl Pts',(5.68895616472443,28.3400280866387,54.8450220644753));
#105538=CARTESIAN_POINT('Ctrl Pts',(5.68474469433285,28.3353630426135,54.9078768966285));
#105539=CARTESIAN_POINT('Ctrl Pts',(5.68053322394127,28.3342578236991,54.9706912625246));
#105540=CARTESIAN_POINT('Ctrl Pts',(5.67632175354969,28.3331526047847,55.0335056284206));
#105541=CARTESIAN_POINT('Ctrl Pts',(5.67211028315811,28.3356071150888,55.0962789304679));
#105542=CARTESIAN_POINT('Ctrl Pts',(5.66789881276653,28.3415647769982,55.1585831362628));
#105543=CARTESIAN_POINT('Ctrl Pts',(5.66382146306642,28.3473327080867,55.2189031696937));
#105544=CARTESIAN_POINT('Ctrl Pts',(5.6597441133663,28.3564077503369,55.2790326571175));
#105545=CARTESIAN_POINT('Ctrl Pts',(5.65566676366619,28.3687675623041,55.3385804693256));
#105546=CARTESIAN_POINT('Ctrl Pts',(5.65154579609376,28.3812595946448,55.3987653004457));
#105547=CARTESIAN_POINT('Ctrl Pts',(5.64742482852134,28.3971071320074,55.4583554038117));
#105548=CARTESIAN_POINT('Ctrl Pts',(5.64330386094891,28.4162330194006,55.5169508208359));
#105549=CARTESIAN_POINT('Ctrl Pts',(5.63923774392351,28.4351043390575,55.5747663261962));
#105550=CARTESIAN_POINT('Ctrl Pts',(5.6351716268981,28.4571671072163,55.6316129613537));
#105551=CARTESIAN_POINT('Ctrl Pts',(5.6311055098727,28.4822961492295,55.6871179093549));
#105552=CARTESIAN_POINT('Ctrl Pts',(5.62704188065332,28.5074098163328,55.7425888973045));
#105553=CARTESIAN_POINT('Ctrl Pts',(5.62297825143395,28.5355858268912,55.7967193602662));
#105554=CARTESIAN_POINT('Ctrl Pts',(5.61891462221457,28.5666506573924,55.8491558526245));
#105555=CARTESIAN_POINT('Ctrl Pts',(5.61485196959789,28.5977080221541,55.9015797430408));
#105556=CARTESIAN_POINT('Ctrl Pts',(5.61078931698121,28.6316525678179,55.9523100307528));
#105557=CARTESIAN_POINT('Ctrl Pts',(5.60672666436454,28.6682655514314,56.0010191599044));
#105558=CARTESIAN_POINT('Ctrl Pts',(5.60256307082815,28.7057882235139,56.0509385191097));
#105559=CARTESIAN_POINT('Ctrl Pts',(5.59839947729177,28.7461134161297,56.0987344577357));
#105560=CARTESIAN_POINT('Ctrl Pts',(5.59423588375539,28.7889609349392,56.1440893247018));
#105561=CARTESIAN_POINT('Ctrl Pts',(5.59016804392942,28.8308230528272,56.1884011271232));
#105562=CARTESIAN_POINT('Ctrl Pts',(5.58610020410344,28.8750922791935,56.2303826368797));
#105563=CARTESIAN_POINT('Ctrl Pts',(5.58203236427747,28.9214709209376,56.2697759745785));
#105564=CARTESIAN_POINT('Ctrl Pts',(5.57782089388588,28.9694871371267,56.3105602439798));
#105565=CARTESIAN_POINT('Ctrl Pts',(5.5736094234943,29.0197640671424,56.3485697542235));
#105566=CARTESIAN_POINT('Ctrl Pts',(5.56939795310272,29.0719377209833,56.3835665528866));
#105567=CARTESIAN_POINT('Ctrl Pts',(5.56518648271114,29.1241113748243,56.4185633515496));
#105568=CARTESIAN_POINT('Ctrl Pts',(5.56097501231955,29.1781811984192,56.4505471950831));
#105569=CARTESIAN_POINT('Ctrl Pts',(5.55676354192797,29.2337568974359,56.4793334674011));
#105570=CARTESIAN_POINT('Ctrl Pts',(5.55268619222786,29.287562703639,56.5072029970166));
#105571=CARTESIAN_POINT('Ctrl Pts',(5.54860884252774,29.3430020821623,56.5321907331816));
#105572=CARTESIAN_POINT('Ctrl Pts',(5.54453149282763,29.3997343111234,56.5541033114814));
#105573=CARTESIAN_POINT('Ctrl Pts',(5.5404105252552,29.4570734390018,56.5762503018657));
#105574=CARTESIAN_POINT('Ctrl Pts',(5.53628955768277,29.5157328156011,56.595255627346));
#105575=CARTESIAN_POINT('Ctrl Pts',(5.53216859011035,29.5753345721937,56.6109671860178));
#105576=CARTESIAN_POINT('Ctrl Pts',(5.52810247308494,29.6341430226283,56.626469622057));
#105577=CARTESIAN_POINT('Ctrl Pts',(5.52403635605954,29.6938684100509,56.6387653027937));
#105578=CARTESIAN_POINT('Ctrl Pts',(5.51997023903413,29.7541296244664,56.6477571903757));
#105579=CARTESIAN_POINT('Ctrl Pts',(5.51590660981475,29.8143539687644,56.6567435763768));
#105580=CARTESIAN_POINT('Ctrl Pts',(5.51184298059538,29.8751129847361,56.6624301016414));
#105581=CARTESIAN_POINT('Ctrl Pts',(5.507779351376,29.9360156144035,56.6647708546223));
#105582=CARTESIAN_POINT('Ctrl Pts',(5.50371669875932,29.9969036074814,56.6671110450554));
#105583=CARTESIAN_POINT('Ctrl Pts',(5.49965404614264,30.0579346343862,56.6661070397697));
#105584=CARTESIAN_POINT('Ctrl Pts',(5.49559139352596,30.1187148628539,56.6617649597153));
#105585=CARTESIAN_POINT('Ctrl Pts',(5.49142779998958,30.18100524066,56.6573149960696));
#105586=CARTESIAN_POINT('Ctrl Pts',(5.4872642064532,30.2430316268305,56.64935884579));
#105587=CARTESIAN_POINT('Ctrl Pts',(5.48310061291682,30.3043751815094,56.6379596298081));
#105588=CARTESIAN_POINT('Ctrl Pts',(5.47903277309084,30.3643079661603,56.626822571315));
#105589=CARTESIAN_POINT('Ctrl Pts',(5.47496493326487,30.423588499628,56.6123993290894));
#105590=CARTESIAN_POINT('Ctrl Pts',(5.47089709343889,30.4818386681553,56.594800143551));
#105591=CARTESIAN_POINT('Ctrl Pts',(5.46668562304731,30.5421455805589,56.5765795517918));
#105592=CARTESIAN_POINT('Ctrl Pts',(5.46247415265573,30.601347426917,56.5549547061609));
#105593=CARTESIAN_POINT('Ctrl Pts',(5.45826268226415,30.6590468779299,56.5301023536649));
#105594=CARTESIAN_POINT('Ctrl Pts',(5.45405121187257,30.7167463289428,56.5052500011689));
#105595=CARTESIAN_POINT('Ctrl Pts',(5.44983974148099,30.772942879486,56.477170475215));
#105596=CARTESIAN_POINT('Ctrl Pts',(5.44562827108941,30.8272697439158,56.4460915499378));
#105597=CARTESIAN_POINT('Ctrl Pts',(5.44155183030141,30.879854761844,56.4160090877886));
#105598=CARTESIAN_POINT('Ctrl Pts',(5.43747538951342,30.9309053356807,56.3829925194285));
#105599=CARTESIAN_POINT('Ctrl Pts',(5.43339894872543,30.9800744459655,56.3472230997001));
#105600=CARTESIAN_POINT('Ctrl Pts',(5.42932840892906,31.0291723798188,56.3115054592216));
#105601=CARTESIAN_POINT('Ctrl Pts',(5.4252578691327,31.0763938387612,56.2730431653455));
#105602=CARTESIAN_POINT('Ctrl Pts',(5.42118732933634,31.1214179744792,56.2320623874281));
#105603=CARTESIAN_POINT('Ctrl Pts',(5.41712116909536,31.1663936680481,56.1911257013499));
#105604=CARTESIAN_POINT('Ctrl Pts',(5.41305500885438,31.2091763505024,56.1476762483517));
#105605=CARTESIAN_POINT('Ctrl Pts',(5.4089888486134,31.2494773543157,56.101981098319));
#105606=CARTESIAN_POINT('Ctrl Pts',(5.40492500374107,31.2897554097759,56.0563119681949));
#105607=CARTESIAN_POINT('Ctrl Pts',(5.40086115886875,31.3275542482263,56.0084000576379));
#105608=CARTESIAN_POINT('Ctrl Pts',(5.39679731399643,31.3626226620096,55.9585486325575));
#105609=CARTESIAN_POINT('Ctrl Pts',(5.39273479857776,31.3976796034478,55.9087135159637));
#105610=CARTESIAN_POINT('Ctrl Pts',(5.38867228315909,31.4300076027422,55.8569405655971));
#105611=CARTESIAN_POINT('Ctrl Pts',(5.38460976774043,31.4593976665616,55.8035635947668));
#105612=CARTESIAN_POINT('Ctrl Pts',(5.38054576406626,31.4887984970907,55.7501670699011));
#105613=CARTESIAN_POINT('Ctrl Pts',(5.37648176039209,31.5152589994234,55.6951658017929));
#105614=CARTESIAN_POINT('Ctrl Pts',(5.37241775671792,31.5386160469458,55.6389183516546));
#105615=CARTESIAN_POINT('Ctrl Pts',(5.37090280232716,31.5473229440197,55.6179507718028));
#105616=CARTESIAN_POINT('Ctrl Pts',(5.3693878479364,31.555599061099,55.5968102300939));
#105617=CARTESIAN_POINT('Ctrl Pts',(5.36787289354565,31.5634376782623,55.5755159651912));
#105618=CARTESIAN_POINT('Origin',(5.,30.,55.));
#105619=CARTESIAN_POINT('',(4.66781602428403,31.5660238537031,55.5764683070372));
#105620=CARTESIAN_POINT('',(4.86076605062571,31.563437683379,55.5755159512911));
#105621=CARTESIAN_POINT('',(5.,31.5634376782623,55.5755159651912));
#105622=CARTESIAN_POINT('',(5.52206895547911,31.6659994155302,55.0013955117896));
#105623=CARTESIAN_POINT('Ctrl Pts',(4.86076605062571,31.563437683379,55.575515951291));
#105624=CARTESIAN_POINT('Ctrl Pts',(4.86235663650181,31.5544423538878,55.5999525234998));
#105625=CARTESIAN_POINT('Ctrl Pts',(4.86394540308067,31.5448739300461,55.6241786808564));
#105626=CARTESIAN_POINT('Ctrl Pts',(4.86634047276108,31.5296416355314,55.6602455418293));
#105627=CARTESIAN_POINT('Ctrl Pts',(4.86714313447064,31.5244012764948,55.6722562398718));
#105628=CARTESIAN_POINT('Ctrl Pts',(4.87251833492517,31.4884500562448,55.7520725425401));
#105629=CARTESIAN_POINT('Ctrl Pts',(4.87714293081916,31.4533698782181,55.8178079565178));
#105630=CARTESIAN_POINT('Ctrl Pts',(4.88280612972829,31.4075242765575,55.8913934335003));
#105631=CARTESIAN_POINT('Ctrl Pts',(4.88361468741238,31.4009149122755,55.9017451021056));
#105632=CARTESIAN_POINT('Ctrl Pts',(4.88489210896611,31.3903866965534,55.9178393931811));
#105633=CARTESIAN_POINT('Ctrl Pts',(4.88535609265786,31.3865451634237,55.923632406879));
#105634=CARTESIAN_POINT('Ctrl Pts',(4.88622876943183,31.3792901511753,55.9344256698058));
#105635=CARTESIAN_POINT('Ctrl Pts',(4.88663688748976,31.3758855231996,55.9394315706274));
#105636=CARTESIAN_POINT('Ctrl Pts',(4.88760317836795,31.3677960797829,55.9511873592213));
#105637=CARTESIAN_POINT('Ctrl Pts',(4.88816283590673,31.3630885313786,55.9579212685606));
#105638=CARTESIAN_POINT('Ctrl Pts',(4.89004739048439,31.3471561890903,55.9803564289671));
#105639=CARTESIAN_POINT('Ctrl Pts',(4.89138583176619,31.335708847404,55.9958967422528));
#105640=CARTESIAN_POINT('Ctrl Pts',(4.89471765645642,31.3068330198224,56.0337034720899));
#105641=CARTESIAN_POINT('Ctrl Pts',(4.89672561742635,31.2891029932193,56.0557313589832));
#105642=CARTESIAN_POINT('Ctrl Pts',(4.90592645439317,31.2060698470409,56.1536806195336));
#105643=CARTESIAN_POINT('Ctrl Pts',(4.91329155941284,31.134563286062,56.2240710967319));
#105644=CARTESIAN_POINT('Ctrl Pts',(4.92646737058855,30.9933318201047,56.3400260584977));
#105645=CARTESIAN_POINT('Ctrl Pts',(4.93230929159736,30.9256791495063,56.3876237797659));
#105646=CARTESIAN_POINT('Ctrl Pts',(4.93930501687842,30.8379345535513,56.4400715703094));
#105647=CARTESIAN_POINT('Ctrl Pts',(4.94063617362945,30.8209278042958,56.4498337976376));
#105648=CARTESIAN_POINT('Ctrl Pts',(4.94275299396792,30.7933925546242,56.4649997028176));
#105649=CARTESIAN_POINT('Ctrl Pts',(4.94354543514238,30.7829723901156,56.4705951597197));
#105650=CARTESIAN_POINT('Ctrl Pts',(4.94505002476253,30.7629771240952,56.4810595085514));
#105651=CARTESIAN_POINT('Ctrl Pts',(4.94576282432307,30.7534128385819,56.4859476651747));
#105652=CARTESIAN_POINT('Ctrl Pts',(4.94739597361152,30.7312928664252,56.4969843584031));
#105653=CARTESIAN_POINT('Ctrl Pts',(4.94831403327499,30.7187056127938,56.5030680914914));
#105654=CARTESIAN_POINT('Ctrl Pts',(4.9512248397847,30.6783257533892,56.5219614318327));
#105655=CARTESIAN_POINT('Ctrl Pts',(4.95319692678012,30.6502552341312,56.5341645109156));
#105656=CARTESIAN_POINT('Ctrl Pts',(4.95785528068165,30.5824290333054,56.5614541919447));
#105657=CARTESIAN_POINT('Ctrl Pts',(4.96051897956434,30.5424005024078,56.5758060944509));
#105658=CARTESIAN_POINT('Ctrl Pts',(4.96772435997881,30.4315771743691,56.6108167218702));
#105659=CARTESIAN_POINT('Ctrl Pts',(4.97219846733111,30.3598920182885,56.6283327268158));
#105660=CARTESIAN_POINT('Ctrl Pts',(4.97755725133607,30.2736090208458,56.6434374930756));
#105661=CARTESIAN_POINT('Ctrl Pts',(4.97840764802541,30.259906398373,56.6456601557228));
#105662=CARTESIAN_POINT('Ctrl Pts',(4.98377372505517,30.1735058138186,56.6585689086929));
#105663=CARTESIAN_POINT('Ctrl Pts',(4.98834189284911,30.1002040276405,56.6646055127479));
#105664=CARTESIAN_POINT('Ctrl Pts',(4.99394240468856,30.0144768926542,56.6659823454786));
#105665=CARTESIAN_POINT('Ctrl Pts',(4.99475073555195,30.0021988454305,56.666043786695));
#105666=CARTESIAN_POINT('Ctrl Pts',(4.99602787579493,29.9829715155292,56.6659274706254));
#105667=CARTESIAN_POINT('Ctrl Pts',(4.99649180847242,29.9760218314703,56.6658419341962));
#105668=CARTESIAN_POINT('Ctrl Pts',(4.99736444665823,29.9630196971493,56.665600526189));
#105669=CARTESIAN_POINT('Ctrl Pts',(4.99777257779605,29.9569672993867,56.6654551442883));
#105670=CARTESIAN_POINT('Ctrl Pts',(4.99873897767125,29.9427017624914,56.6650346672203));
#105671=CARTESIAN_POINT('Ctrl Pts',(4.99929873214277,29.9344897185266,56.66473178831));
#105672=CARTESIAN_POINT('Ctrl Pts',(5.00118396234252,29.9069901123561,56.6635137536867));
#105673=CARTESIAN_POINT('Ctrl Pts',(5.00252299503156,29.8877170753713,56.6623240698753));
#105674=CARTESIAN_POINT('Ctrl Pts',(5.00585662201406,29.8402677783128,56.6585662418381));
#105675=CARTESIAN_POINT('Ctrl Pts',(5.00786581272343,29.81212843595,56.6556148271649));
#105676=CARTESIAN_POINT('Ctrl Pts',(5.01707757252619,29.6846547490511,56.6389531863565));
#105677=CARTESIAN_POINT('Ctrl Pts',(5.0244526694838,29.5866068564928,56.6170085804126));
#105678=CARTESIAN_POINT('Ctrl Pts',(5.03762621900644,29.4126241659588,56.5611989952842));
#105679=CARTESIAN_POINT('Ctrl Pts',(5.04345690518757,29.3360901828385,56.5302222415589));
#105680=CARTESIAN_POINT('Ctrl Pts',(5.05044177860603,29.2445792350055,56.4850184270763));
#105681=CARTESIAN_POINT('Ctrl Pts',(5.05177261180772,29.2271579603793,56.4760269305421));
#105682=CARTESIAN_POINT('Ctrl Pts',(5.05388904417198,29.19948737997,56.4611212806397));
#105683=CARTESIAN_POINT('Ctrl Pts',(5.05468141651019,29.1891357749937,56.4554020312796));
#105684=CARTESIAN_POINT('Ctrl Pts',(5.05618595286663,29.1695002115588,56.4442788742467));
#105685=CARTESIAN_POINT('Ctrl Pts',(5.05689876718966,29.1602059467897,56.4388944793154));
#105686=CARTESIAN_POINT('Ctrl Pts',(5.05853205943992,29.1389346158975,56.4262951607404));
#105687=CARTESIAN_POINT('Ctrl Pts',(5.05945024589866,29.1269948967195,56.4190185307593));
#105688=CARTESIAN_POINT('Ctrl Pts',(5.0623619124653,29.0892100928351,56.3953332469326));
#105689=CARTESIAN_POINT('Ctrl Pts',(5.06433471493293,29.0637241660238,56.3783616638133));
#105690=CARTESIAN_POINT('Ctrl Pts',(5.06899512294395,29.0039846144587,56.3361579155534));
#105691=CARTESIAN_POINT('Ctrl Pts',(5.07166013212919,28.9702009022567,56.3102972266712));
#105692=CARTESIAN_POINT('Ctrl Pts',(5.07886618036332,28.880675439424,56.2361636681823));
#105693=CARTESIAN_POINT('Ctrl Pts',(5.08333973163574,28.8270894971359,56.1854405943642));
#105694=CARTESIAN_POINT('Ctrl Pts',(5.08870349548183,28.7675510834482,56.1210802167872));
#105695=CARTESIAN_POINT('Ctrl Pts',(5.08955939369601,28.758193311437,56.1107057785937));
#105696=CARTESIAN_POINT('Ctrl Pts',(5.09492391492343,28.7005209677286,56.0451276905725));
#105697=CARTESIAN_POINT('Ctrl Pts',(5.09948507290607,28.6557720421935,55.986907351982));
#105698=CARTESIAN_POINT('Ctrl Pts',(5.10507780280791,28.6081863491954,55.9157300400978));
#105699=CARTESIAN_POINT('Ctrl Pts',(5.10588610492336,28.6014758125052,55.905448408324));
#105700=CARTESIAN_POINT('Ctrl Pts',(5.10716320951199,28.5911456251963,55.8892320596307));
#105701=CARTESIAN_POINT('Ctrl Pts',(5.10762713572351,28.5874482853521,55.883347018079));
#105702=CARTESIAN_POINT('Ctrl Pts',(5.10849976902017,28.5805992579069,55.8722924906557));
#105703=CARTESIAN_POINT('Ctrl Pts',(5.10890790181771,28.577438787206,55.8671287373172));
#105704=CARTESIAN_POINT('Ctrl Pts',(5.1098743155168,28.5700548366442,55.85491541322));
#105705=CARTESIAN_POINT('Ctrl Pts',(5.11043408228111,28.5658552951224,55.8478516924311));
#105706=CARTESIAN_POINT('Ctrl Pts',(5.11231939817491,28.551963216115,55.8240863797617));
#105707=CARTESIAN_POINT('Ctrl Pts',(5.11365850587876,28.5425092294102,55.8072480801908));
#105708=CARTESIAN_POINT('Ctrl Pts',(5.11699236148828,28.5199301492602,55.7653428766653));
#105709=CARTESIAN_POINT('Ctrl Pts',(5.11900170820245,28.5071471452543,55.7400990847667));
#105710=CARTESIAN_POINT('Ctrl Pts',(5.12821485489357,28.452000748355,55.6239486258526));
#105711=CARTESIAN_POINT('Ctrl Pts',(5.13559122067235,28.4172558720462,55.5296556087123));
#105712=CARTESIAN_POINT('Ctrl Pts',(5.14876448388332,28.3697891449328,55.3532167014955));
#105713=CARTESIAN_POINT('Ctrl Pts',(5.15459374451775,28.3543100239748,55.2721353545114));
#105714=CARTESIAN_POINT('Ctrl Pts',(5.1615772404742,28.3426579610005,55.1707559758881));
#105715=CARTESIAN_POINT('Ctrl Pts',(5.16290803222408,28.3407635223316,55.1512435309539));
#105716=CARTESIAN_POINT('Ctrl Pts',(5.16502441488257,28.3382789666538,55.1199127011607));
#105717=CARTESIAN_POINT('Ctrl Pts',(5.16581677840161,28.3374696371733,55.1081140773727));
#105718=CARTESIAN_POINT('Ctrl Pts',(5.1673213079361,28.3361650836573,55.0855846776702));
#105719=CARTESIAN_POINT('Ctrl Pts',(5.1680341241527,28.3356478796665,55.074855825759));
#105720=CARTESIAN_POINT('Ctrl Pts',(5.16966743472992,28.3346963188003,55.0501511489765));
#105721=CARTESIAN_POINT('Ctrl Pts',(5.17058563744198,28.3343340655208,55.0361732334579));
#105722=CARTESIAN_POINT('Ctrl Pts',(5.17349741426955,28.3337400167845,54.991580811281));
#105723=CARTESIAN_POINT('Ctrl Pts',(5.17547030846364,28.3341760311844,54.960962736805));
#105724=CARTESIAN_POINT('Ctrl Pts',(5.18013097984319,28.3372331129386,54.8878789036314));
#105725=CARTESIAN_POINT('Ctrl Pts',(5.18279615703603,28.3406372269072,54.845467062748));
#105726=CARTESIAN_POINT('Ctrl Pts',(5.19000228883895,28.3543658854286,54.7300439330904));
#105727=CARTESIAN_POINT('Ctrl Pts',(5.19447576684108,28.3679178182753,54.6575149154913));
#105728=CARTESIAN_POINT('Ctrl Pts',(5.19984011989559,28.3897012342677,54.5725782307036));
#105729=CARTESIAN_POINT('Ctrl Pts',(5.20069667615469,28.3933449462772,54.5590793539671));
#105730=CARTESIAN_POINT('Ctrl Pts',(5.20606099815161,28.4171617269136,54.4750633097786));
#105731=CARTESIAN_POINT('Ctrl Pts',(5.21062130456655,28.4418010098706,54.4059051296081));
#105732=CARTESIAN_POINT('Ctrl Pts',(5.21621308917605,28.475785663444,54.3273355964502));
#105733=CARTESIAN_POINT('Ctrl Pts',(5.21702138778401,28.4807841352829,54.3161214448463));
#105734=CARTESIAN_POINT('Ctrl Pts',(5.21829848802258,28.4888054471132,54.2986475005859));
#105735=CARTESIAN_POINT('Ctrl Pts',(5.21876241344514,28.4917444177771,54.2923493803947));
#105736=CARTESIAN_POINT('Ctrl Pts',(5.21963504614521,28.4973171378532,54.2805996443204));
#105737=CARTESIAN_POINT('Ctrl Pts',(5.22004317914523,28.4999413076421,54.275143758569));
#105738=CARTESIAN_POINT('Ctrl Pts',(5.22100959453115,28.5061974749979,54.2623160903091));
#105739=CARTESIAN_POINT('Ctrl Pts',(5.2215693627954,28.5098543441761,54.2549567451017));
#105740=CARTESIAN_POINT('Ctrl Pts',(5.22345468914561,28.5222861242735,54.2303958190944));
#105741=CARTESIAN_POINT('Ctrl Pts',(5.22479380600284,28.5313052743471,54.2133205118007));
#105742=CARTESIAN_POINT('Ctrl Pts',(5.22812768950991,28.5542657806628,54.1716226320691));
#105743=CARTESIAN_POINT('Ctrl Pts',(5.23013705526025,28.5685412927402,54.1471915306869));
#105744=CARTESIAN_POINT('Ctrl Pts',(5.23935037120251,28.6362162396475,54.0378628786241));
#105745=CARTESIAN_POINT('Ctrl Pts',(5.24672689182591,28.6965930003308,53.9575295465222));
#105746=CARTESIAN_POINT('Ctrl Pts',(5.2599001201097,28.8190831724509,53.8219573327791));
#105747=CARTESIAN_POINT('Ctrl Pts',(5.26572920679015,28.8788062375034,53.7649788243938));
#105748=CARTESIAN_POINT('Ctrl Pts',(5.27271253465233,28.9576579358876,53.7002064563712));
#105749=CARTESIAN_POINT('Ctrl Pts',(5.27404332133784,28.9730236603695,53.6880320547133));
#105750=CARTESIAN_POINT('Ctrl Pts',(5.27615969792345,28.9979984534086,53.668952011073));
#105751=CARTESIAN_POINT('Ctrl Pts',(5.27695206036505,29.0074720282609,53.6618729185927));
#105752=CARTESIAN_POINT('Ctrl Pts',(5.27845658906621,29.0256924072131,53.6485577775517));
#105753=CARTESIAN_POINT('Ctrl Pts',(5.27916940551415,29.0344256739778,53.6423043065102));
#105754=CARTESIAN_POINT('Ctrl Pts',(5.28080271833059,29.0546650866662,53.6281059112081));
#105755=CARTESIAN_POINT('Ctrl Pts',(5.28172092302855,29.0662120958323,53.62022043101));
#105756=CARTESIAN_POINT('Ctrl Pts',(5.28463271332843,29.1033541196631,53.5955359062602));
#105757=CARTESIAN_POINT('Ctrl Pts',(5.28660561873014,29.1293143327372,53.5792959904505));
#105758=CARTESIAN_POINT('Ctrl Pts',(5.29126632228987,29.1923737612445,53.5422260983115));
#105759=CARTESIAN_POINT('Ctrl Pts',(5.29393152001118,29.2298523818477,53.5220832510944));
#105760=CARTESIAN_POINT('Ctrl Pts',(5.30113766199339,29.3342705475308,53.4710159606947));
#105761=CARTESIAN_POINT('Ctrl Pts',(5.3056111310124,29.402555312167,53.4430645147566));
#105762=CARTESIAN_POINT('Ctrl Pts',(5.31097555531217,29.4857299830408,53.4152988074354));
#105763=CARTESIAN_POINT('Ctrl Pts',(5.31183219125765,29.4990484399682,53.4110383741189));
#105764=CARTESIAN_POINT('Ctrl Pts',(5.31719648891537,29.5825509913188,53.3854810017439));
#105765=CARTESIAN_POINT('Ctrl Pts',(5.32175669199643,29.6540155697621,53.3686731396946));
#105766=CARTESIAN_POINT('Ctrl Pts',(5.32734836190012,29.7384555793296,53.3546121249323));
#105767=CARTESIAN_POINT('Ctrl Pts',(5.32815666008225,29.7505880616639,53.3527294069703));
#105768=CARTESIAN_POINT('Ctrl Pts',(5.32943375979257,29.7696191468434,53.3499912219665));
#105769=CARTESIAN_POINT('Ctrl Pts',(5.32989768511939,29.7765044626304,53.3490445052972));
#105770=CARTESIAN_POINT('Ctrl Pts',(5.33077031774719,29.7893983698063,53.3473537555467));
#105771=CARTESIAN_POINT('Ctrl Pts',(5.3311784507719,29.795405352857,53.3465993584057));
#105772=CARTESIAN_POINT('Ctrl Pts',(5.33214486636234,29.8095755591308,53.3448981702983));
#105773=CARTESIAN_POINT('Ctrl Pts',(5.33270463480862,29.8177418227126,53.3439790206355));
#105774=CARTESIAN_POINT('Ctrl Pts',(5.33458996242873,29.8451190957674,53.3411025348467));
#105775=CARTESIAN_POINT('Ctrl Pts',(5.33592908039743,29.8643564839536,53.339418881393));
#105776=CARTESIAN_POINT('Ctrl Pts',(5.33926296729188,29.9118416903326,53.3360935690707));
#105777=CARTESIAN_POINT('Ctrl Pts',(5.34127233535368,29.9401098795163,53.3348364971635));
#105778=CARTESIAN_POINT('Ctrl Pts',(5.35048567184742,30.0686663857335,53.3323972406065));
#105779=CARTESIAN_POINT('Ctrl Pts',(5.35786221127302,30.1689043533885,53.339552523285));
#105780=CARTESIAN_POINT('Ctrl Pts',(5.37103725007931,30.3492635363559,53.368936493002));
#105781=CARTESIAN_POINT('Ctrl Pts',(5.37686805330178,30.4295491680146,53.3882170197411));
#105782=CARTESIAN_POINT('Ctrl Pts',(5.38385203872933,30.5267432920322,53.4193415230747));
#105783=CARTESIAN_POINT('Ctrl Pts',(5.38518190713605,30.5452926178412,53.4256443431887));
#105784=CARTESIAN_POINT('Ctrl Pts',(5.38729718258022,30.5748527040983,53.4362736331698));
#105785=CARTESIAN_POINT('Ctrl Pts',(5.38808934964544,30.5859355717253,53.4403925814524));
#105786=CARTESIAN_POINT('Ctrl Pts',(5.38959372734781,30.6070021964862,53.4484782583155));
#105787=CARTESIAN_POINT('Ctrl Pts',(5.39030658587293,30.6169932230632,53.4524242333991));
#105788=CARTESIAN_POINT('Ctrl Pts',(5.39194030534308,30.6399047730358,53.4617303459898));
#105789=CARTESIAN_POINT('Ctrl Pts',(5.39285887062399,30.6527974677927,53.4671571728283));
#105790=CARTESIAN_POINT('Ctrl Pts',(5.39577310790037,30.6937148995898,53.4849901488772));
#105791=CARTESIAN_POINT('Ctrl Pts',(5.39774804903468,30.7214672687489,53.4980078628039));
#105792=CARTESIAN_POINT('Ctrl Pts',(5.40241459905559,30.7868939522836,53.5309295206623));
#105793=CARTESIAN_POINT('Ctrl Pts',(5.40508352673329,30.8241952869313,53.55152746792));
#105794=CARTESIAN_POINT('Ctrl Pts',(5.41233927746679,30.9244107189907,53.611993133956));
#105795=CARTESIAN_POINT('Ctrl Pts',(5.41685664461958,30.9855040234186,53.6546820401439));
#105796=CARTESIAN_POINT('Ctrl Pts',(5.4222283522364,31.0539381406431,53.7096712117875));
#105797=CARTESIAN_POINT('Ctrl Pts',(5.42304582824291,31.0642370360891,53.7181523055947));
#105798=CARTESIAN_POINT('Ctrl Pts',(5.42835820140213,31.1303248987084,53.7739208609916));
#105799=CARTESIAN_POINT('Ctrl Pts',(5.43290598065822,31.183043878114,53.8247090086364));
#105800=CARTESIAN_POINT('Ctrl Pts',(5.43848386119012,31.2405120390993,53.8878684409762));
#105801=CARTESIAN_POINT('Ctrl Pts',(5.43929210777578,31.2486734655022,53.8970397656657));
#105802=CARTESIAN_POINT('Ctrl Pts',(5.44056914349405,31.2612950510678,53.9115427905758));
#105803=CARTESIAN_POINT('Ctrl Pts',(5.44103305721563,31.265824655015,53.9168138474957));
#105804=CARTESIAN_POINT('Ctrl Pts',(5.44190568106951,31.2742382215263,53.9267294790082));
#105805=CARTESIAN_POINT('Ctrl Pts',(5.44231381707429,31.2781300170575,53.9313670830248));
#105806=CARTESIAN_POINT('Ctrl Pts',(5.44328025748123,31.2872448883106,53.9423497094576));
#105807=CARTESIAN_POINT('Ctrl Pts',(5.44384004799494,31.2924463870803,53.9487122805771));
#105808=CARTESIAN_POINT('Ctrl Pts',(5.44572552945688,31.3097128574698,53.9701547695029));
#105809=CARTESIAN_POINT('Ctrl Pts',(5.44706478209705,31.3215621547659,53.9854053226042));
#105810=CARTESIAN_POINT('Ctrl Pts',(5.45451787189272,31.3853822330601,54.0705596400865));
#105811=CARTESIAN_POINT('Ctrl Pts',(5.46086903257902,31.4320703266873,54.144245665123));
#105812=CARTESIAN_POINT('Ctrl Pts',(5.47371934623301,31.5145970471616,54.3003183880402));
#105813=CARTESIAN_POINT('Ctrl Pts',(5.48019534484159,31.5499802940644,54.382648356998));
#105814=CARTESIAN_POINT('Ctrl Pts',(5.48939999497811,31.5918823640378,54.5068495656644));
#105815=CARTESIAN_POINT('Ctrl Pts',(5.49227859868952,31.6037012827997,54.5467566533317));
#105816=CARTESIAN_POINT('Ctrl Pts',(5.49620663499285,31.6180111360496,54.6026890801662));
#105817=CARTESIAN_POINT('Ctrl Pts',(5.49729641366454,31.6217808763644,54.6183682085881));
#105818=CARTESIAN_POINT('Ctrl Pts',(5.4990497623105,31.6275173367581,54.6438494887592));
#105819=CARTESIAN_POINT('Ctrl Pts',(5.49971778261907,31.6296244398868,54.6536186198092));
#105820=CARTESIAN_POINT('Ctrl Pts',(5.50111179637471,31.6338555992209,54.6741292353459));
#105821=CARTESIAN_POINT('Ctrl Pts',(5.50183719467011,31.6359619306563,54.6848739212149));
#105822=CARTESIAN_POINT('Ctrl Pts',(5.50327581299805,31.6399471560584,54.7063209682102));
#105823=CARTESIAN_POINT('Ctrl Pts',(5.50398904821198,31.6418275749237,54.7170224887864));
#105824=CARTESIAN_POINT('Ctrl Pts',(5.50566479121968,31.6460181664571,54.7423207939145));
#105825=CARTESIAN_POINT('Ctrl Pts',(5.50662450582426,31.6482391033695,54.756931577679));
#105826=CARTESIAN_POINT('Ctrl Pts',(5.51254171926052,31.6608060215381,54.8477199279824));
#105827=CARTESIAN_POINT('Ctrl Pts',(5.5173393256724,31.6660638176322,54.9245105544638));
#105828=CARTESIAN_POINT('Ctrl Pts',(5.52206895547911,31.6659994155302,55.0013955117896));
#105829=CARTESIAN_POINT('Ctrl Pts',(5.5220688677794,31.6659994167237,55.0013940861415));
#105830=CARTESIAN_POINT('Ctrl Pts',(5.53026528752143,31.6658879223103,55.1346352268217));
#105831=CARTESIAN_POINT('Ctrl Pts',(5.53818966990361,31.6497930141248,55.2673674871747));
#105832=CARTESIAN_POINT('Ctrl Pts',(5.54801370322328,31.6135136075547,55.4153259430768));
#105833=CARTESIAN_POINT('Ctrl Pts',(5.54926067071279,31.6086395532938,55.4338208298432));
#105834=CARTESIAN_POINT('Ctrl Pts',(5.55106550065771,31.6012261259723,55.4601064243879));
#105835=CARTESIAN_POINT('Ctrl Pts',(5.55160959587991,31.5989457914207,55.4679694193285));
#105836=CARTESIAN_POINT('Ctrl Pts',(5.55256157280845,31.5948796144338,55.4816135628806));
#105837=CARTESIAN_POINT('Ctrl Pts',(5.55296794664354,31.5931200835991,55.487402304405));
#105838=CARTESIAN_POINT('Ctrl Pts',(5.55384638297178,31.5892663307709,55.4998370543067));
#105839=CARTESIAN_POINT('Ctrl Pts',(5.55431898567185,31.5871619689062,55.506479447757));
#105840=CARTESIAN_POINT('Ctrl Pts',(5.55563602444341,31.581210309918,55.5248644069739));
#105841=CARTESIAN_POINT('Ctrl Pts',(5.55648528359108,31.5772740324032,55.5365773887186));
#105842=CARTESIAN_POINT('Ctrl Pts',(5.55800937646137,31.5700298200513,55.5573649041467));
#105843=CARTESIAN_POINT('Ctrl Pts',(5.55868169084271,31.5667729072001,55.5664555341626));
#105844=CARTESIAN_POINT('Ctrl Pts',(5.55935725065089,31.5634376826058,55.5755159533915));
#105845=CARTESIAN_POINT('',(5.3285190759848,31.667962423648,55.0005309979303));
#105846=CARTESIAN_POINT('Ctrl Pts',(5.36787289354565,31.5634376782623,55.5755159651912));
#105847=CARTESIAN_POINT('Ctrl Pts',(5.36380422315238,31.5844896318861,55.5183265569258));
#105848=CARTESIAN_POINT('Ctrl Pts',(5.3597355527591,31.6023823060254,55.4600275789832));
#105849=CARTESIAN_POINT('Ctrl Pts',(5.35566688236583,31.6170202081189,55.4010008061526));
#105850=CARTESIAN_POINT('Ctrl Pts',(5.35159065514323,31.6316852975039,55.341864401623));
#105851=CARTESIAN_POINT('Ctrl Pts',(5.34751442792064,31.6430834450864,55.2819980062784));
#105852=CARTESIAN_POINT('Ctrl Pts',(5.34343820069804,31.6511704975579,55.2217926689373));
#105853=CARTESIAN_POINT('Ctrl Pts',(5.34045646721565,31.6570861234078,55.1777528594847));
#105854=CARTESIAN_POINT('Ctrl Pts',(5.33747473373325,31.6612311284502,55.1335318674855));
#105855=CARTESIAN_POINT('Ctrl Pts',(5.33449300025085,31.6636058986979,55.0892827744734));
#105856=CARTESIAN_POINT('Ctrl Pts',(5.33250187903717,31.6651917062309,55.0597344233873));
#105857=CARTESIAN_POINT('Ctrl Pts',(5.33051075782348,31.6659903400224,55.0301434489476));
#105858=CARTESIAN_POINT('Ctrl Pts',(5.32851963660979,31.6659999129021,55.0005387116472));
#105859=CARTESIAN_POINT('Ctrl Pts',(5.32851891017001,31.6685428710302,55.0005287164616));
#105860=CARTESIAN_POINT('Ctrl Pts',(5.29346518325078,31.6663312333053,54.4785404025847));
#105861=CARTESIAN_POINT('Ctrl Pts',(5.22136636605202,31.1216350812794,53.4009406959792));
#105862=CARTESIAN_POINT('Ctrl Pts',(5.11222245857373,29.2866759464458,53.1646043774385));
#105863=CARTESIAN_POINT('Ctrl Pts',(5.00108718773517,28.0711228425453,54.60384194045));
#105864=CARTESIAN_POINT('Ctrl Pts',(4.88995191689661,28.6210166627157,56.4056718152503));
#105865=CARTESIAN_POINT('Ctrl Pts',(4.77886152907957,30.4323232756296,56.9207217847491));
#105866=CARTESIAN_POINT('Ctrl Pts',(4.70481623154204,31.3756950548499,56.0933234118257));
#105867=CARTESIAN_POINT('Ctrl Pts',(4.66781602428403,31.5660238537031,55.5764683070371));
#105868=CARTESIAN_POINT('Origin',(5.,30.,55.));
#105869=CARTESIAN_POINT('',(3.96712534830139,31.5634376767977,55.5755159691697));
#105870=CARTESIAN_POINT('',(4.16232242021249,31.5634376783907,55.5755159648424));
#105871=CARTESIAN_POINT('',(5.,31.5634376782623,55.5755159651912));
#105872=CARTESIAN_POINT('Ctrl Pts',(4.16232242021249,31.5634376783906,55.5755159648424));
#105873=CARTESIAN_POINT('Ctrl Pts',(4.16283813385309,31.5608103487311,55.5826533275469));
#105874=CARTESIAN_POINT('Ctrl Pts',(4.16335223587354,31.558134084724,55.5897728603756));
#105875=CARTESIAN_POINT('Ctrl Pts',(4.16467335641337,31.5511094127128,55.6080786290433));
#105876=CARTESIAN_POINT('Ctrl Pts',(4.16547790768569,31.5466887235781,55.6192366548532));
#105877=CARTESIAN_POINT('Ctrl Pts',(4.1669923035432,31.5380982316544,55.640253372118));
#105878=CARTESIAN_POINT('Ctrl Pts',(4.16770293852686,31.533953262297,55.6501214878334));
#105879=CARTESIAN_POINT('Ctrl Pts',(4.16931310081107,31.5243033729042,55.6724892180871));
#105880=CARTESIAN_POINT('Ctrl Pts',(4.17021056532531,31.5187392231987,55.6849625620775));
#105881=CARTESIAN_POINT('Ctrl Pts',(4.17255011010829,31.503751708711,55.7174798186707));
#105882=CARTESIAN_POINT('Ctrl Pts',(4.1739837145369,31.4940807657592,55.7374070995912));
#105883=CARTESIAN_POINT('Ctrl Pts',(4.18231018932071,31.4351168494857,55.8529785284581));
#105884=CARTESIAN_POINT('Ctrl Pts',(4.18888569401557,31.3770479724169,55.9438617677663));
#105885=CARTESIAN_POINT('Ctrl Pts',(4.19994051564531,31.2652800543895,56.0862847435557));
#105886=CARTESIAN_POINT('Ctrl Pts',(4.20441636953415,31.2161800806057,56.1409875951416));
#105887=CARTESIAN_POINT('Ctrl Pts',(4.21057609909438,31.1462864271764,56.209202703844));
#105888=CARTESIAN_POINT('Ctrl Pts',(4.21212154010923,31.1285698790687,56.225754322193));
#105889=CARTESIAN_POINT('Ctrl Pts',(4.21447114938599,31.1014974278408,56.2499620983466));
#105890=CARTESIAN_POINT('Ctrl Pts',(4.21525804145268,31.0924084289675,56.2579132069522));
#105891=CARTESIAN_POINT('Ctrl Pts',(4.21668095986283,31.0759529832811,56.27199568374));
#105892=CARTESIAN_POINT('Ctrl Pts',(4.2173145811575,31.0686184508188,56.2781636974812));
#105893=CARTESIAN_POINT('Ctrl Pts',(4.21837162823822,31.0563802200761,56.2882765359056));
#105894=CARTESIAN_POINT('Ctrl Pts',(4.21879252918983,31.0515065381851,56.2922575591554));
#105895=CARTESIAN_POINT('Ctrl Pts',(4.21962651068774,31.0418516552295,56.3000532835367));
#105896=CARTESIAN_POINT('Ctrl Pts',(4.22003948862542,31.0370718359291,56.3038694006139));
#105897=CARTESIAN_POINT('Ctrl Pts',(4.22096668045426,31.0263409611412,56.3123403960948));
#105898=CARTESIAN_POINT('Ctrl Pts',(4.22148183785593,31.0203790381539,56.3169812818609));
#105899=CARTESIAN_POINT('Ctrl Pts',(4.22330440495648,30.9992803693504,56.333175663116));
#105900=CARTESIAN_POINT('Ctrl Pts',(4.22462532274783,30.9839779421821,56.3445095531925));
#105901=CARTESIAN_POINT('Ctrl Pts',(4.23352540274032,30.8805947515072,56.4183711170017));
#105902=CARTESIAN_POINT('Ctrl Pts',(4.24146563824476,30.7868113674687,56.4724636038578));
#105903=CARTESIAN_POINT('Ctrl Pts',(4.25552570786375,30.6103777985771,56.5525292819306));
#105904=CARTESIAN_POINT('Ctrl Pts',(4.26166650033521,30.5296684763962,56.5818859575669));
#105905=CARTESIAN_POINT('Ctrl Pts',(4.26969064508329,30.418213223528,56.6129319967477));
#105906=CARTESIAN_POINT('Ctrl Pts',(4.27174274776361,30.3891662298304,56.6201857214714));
#105907=CARTESIAN_POINT('Ctrl Pts',(4.27470875501087,30.3464031821576,56.6296481191194));
#105908=CARTESIAN_POINT('Ctrl Pts',(4.2756420881411,30.3328313138985,56.6324740406557));
#105909=CARTESIAN_POINT('Ctrl Pts',(4.27728801600493,30.3086981128824,56.6371855492519));
#105910=CARTESIAN_POINT('Ctrl Pts',(4.27800273409458,30.2981510264143,56.6391391101038));
#105911=CARTESIAN_POINT('Ctrl Pts',(4.27950274847185,30.2758768179673,56.6430426918769));
#105912=CARTESIAN_POINT('Ctrl Pts',(4.28028726759658,30.264146169273,56.6449693369796));
#105913=CARTESIAN_POINT('Ctrl Pts',(4.28237414750275,30.2327339204768,56.649783800005));
#105914=CARTESIAN_POINT('Ctrl Pts',(4.28366935014773,30.2130191597457,56.6524450238862));
#105915=CARTESIAN_POINT('Ctrl Pts',(4.29126959631204,30.0961570901069,56.6660935004305));
#105916=CARTESIAN_POINT('Ctrl Pts',(4.29730806518718,29.998238368268,56.6688661167145));
#105917=CARTESIAN_POINT('Ctrl Pts',(4.30780756501426,29.8268872674085,56.6586276046746));
#105918=CARTESIAN_POINT('Ctrl Pts',(4.31228607655116,29.7535214093718,56.6493213728924));
#105919=CARTESIAN_POINT('Ctrl Pts',(4.3190359910938,29.6470136912755,56.6285444440918));
#105920=CARTESIAN_POINT('Ctrl Pts',(4.32121556005548,29.6132259851334,56.6208522154244));
#105921=CARTESIAN_POINT('Ctrl Pts',(4.32487027445901,29.5581082088159,56.6064824187245));
#105922=CARTESIAN_POINT('Ctrl Pts',(4.32631982815338,29.5366281545712,56.6004188617187));
#105923=CARTESIAN_POINT('Ctrl Pts',(4.3283654381972,29.5069621656253,56.5913972590653));
#105924=CARTESIAN_POINT('Ctrl Pts',(4.32894223598817,29.4986668103672,56.5888035017117));
#105925=CARTESIAN_POINT('Ctrl Pts',(4.32993182223119,29.4845613866193,56.5842716136195));
#105926=CARTESIAN_POINT('Ctrl Pts',(4.330342744475,29.4787408835318,56.582366089832));
#105927=CARTESIAN_POINT('Ctrl Pts',(4.3312086080303,29.4665561011166,56.5783024951669));
#105928=CARTESIAN_POINT('Ctrl Pts',(4.33166389204858,29.4601942478669,56.5761379715815));
#105929=CARTESIAN_POINT('Ctrl Pts',(4.33290709675902,29.4429397718215,56.5701506823678));
#105930=CARTESIAN_POINT('Ctrl Pts',(4.33369913897965,29.4320737424715,56.5662531757526));
#105931=CARTESIAN_POINT('Ctrl Pts',(4.33776675198897,29.3768689185041,56.5458019294094));
#105932=CARTESIAN_POINT('Ctrl Pts',(4.341127303514,29.3332132351503,56.5274784747139));
#105933=CARTESIAN_POINT('Ctrl Pts',(4.35178349107516,29.1991770843532,56.4643786347515));
#105934=CARTESIAN_POINT('Ctrl Pts',(4.35919710277712,29.112039175885,56.4132405648925));
#105935=CARTESIAN_POINT('Ctrl Pts',(4.37010694540066,28.9886320596101,56.324872385041));
#105936=CARTESIAN_POINT('Ctrl Pts',(4.37372443638217,28.9485865934312,56.2933223135008));
#105937=CARTESIAN_POINT('Ctrl Pts',(4.37970460196693,28.8837135110756,56.2372036460356));
#105938=CARTESIAN_POINT('Ctrl Pts',(4.38210068635491,28.8580989567626,56.2136023676452));
#105939=CARTESIAN_POINT('Ctrl Pts',(4.38545911184596,28.8227631202627,56.1789337568608));
#105940=CARTESIAN_POINT('Ctrl Pts',(4.38644891703554,28.8124210657607,56.1685152001527));
#105941=CARTESIAN_POINT('Ctrl Pts',(4.388159270635,28.7946818832143,56.1501659834469));
#105942=CARTESIAN_POINT('Ctrl Pts',(4.38888252313148,28.7872221238133,56.1422974151812));
#105943=CARTESIAN_POINT('Ctrl Pts',(4.3902755579086,28.7729379533952,56.1269327736997));
#105944=CARTESIAN_POINT('Ctrl Pts',(4.3909457243175,28.7661041192247,56.1194461602688));
#105945=CARTESIAN_POINT('Ctrl Pts',(4.39272679567373,28.7480482258861,56.0992992993217));
#105946=CARTESIAN_POINT('Ctrl Pts',(4.39383252817931,28.7369497667524,56.0865294919277));
#105947=CARTESIAN_POINT('Ctrl Pts',(4.39802779174855,28.6953009920132,56.0371079776084));
#105948=CARTESIAN_POINT('Ctrl Pts',(4.4010620449907,28.6661342113754,55.9993173451037));
#105949=CARTESIAN_POINT('Ctrl Pts',(4.41161197917421,28.5690732551866,55.8617219988201));
#105950=CARTESIAN_POINT('Ctrl Pts',(4.41882941762728,28.51043930039,55.7558600777894));
#105951=CARTESIAN_POINT('Ctrl Pts',(4.42879877015058,28.4480718271118,55.6072212452058));
#105952=CARTESIAN_POINT('Ctrl Pts',(4.43133266424086,28.4337602849347,55.5692902751069));
#105953=CARTESIAN_POINT('Ctrl Pts',(4.43551305552126,28.4129221615758,55.5073050537952));
#105954=CARTESIAN_POINT('Ctrl Pts',(4.43712370485106,28.4055267713564,55.4835591468595));
#105955=CARTESIAN_POINT('Ctrl Pts',(4.43935888308449,28.3961681492935,55.450956052531));
#105956=CARTESIAN_POINT('Ctrl Pts',(4.4399591414771,28.3937412754614,55.4422339508539));
#105957=CARTESIAN_POINT('Ctrl Pts',(4.44097651753335,28.3897752590063,55.4275167707363));
#105958=CARTESIAN_POINT('Ctrl Pts',(4.44139149864227,28.3881981742691,55.4215319429374));
#105959=CARTESIAN_POINT('Ctrl Pts',(4.44219695605938,28.3852161284823,55.409954026074));
#105960=CARTESIAN_POINT('Ctrl Pts',(4.44258714227081,28.383806805956,55.4043622289235));
#105961=CARTESIAN_POINT('Ctrl Pts',(4.4436638038028,28.3800137041978,55.3889756071637));
#105962=CARTESIAN_POINT('Ctrl Pts',(4.4443535275396,28.3776897991491,55.3791664820515));
#105963=CARTESIAN_POINT('Ctrl Pts',(4.44716620852365,28.3686339095457,55.3393337770422));
#105964=CARTESIAN_POINT('Ctrl Pts',(4.44932474667618,28.3626456894253,55.3091493350984));
#105965=CARTESIAN_POINT('Ctrl Pts',(4.45927229540769,28.3392059774649,55.1710675564686));
#105966=CARTESIAN_POINT('Ctrl Pts',(4.467326343228,28.331562481225,55.0617807114785));
#105967=CARTESIAN_POINT('Ctrl Pts',(4.47937924976396,28.3363187689734,54.8949095859488));
#105968=CARTESIAN_POINT('Ctrl Pts',(4.48349254313625,28.3409510942873,54.8374051946401));
#105969=CARTESIAN_POINT('Ctrl Pts',(4.49017424374649,28.353554219054,54.7426906207558));
#105970=CARTESIAN_POINT('Ctrl Pts',(4.49278745376725,28.3598325925154,54.7053084635835));
#105971=CARTESIAN_POINT('Ctrl Pts',(4.49638959945624,28.3703978054925,54.6533270880344));
#105972=CARTESIAN_POINT('Ctrl Pts',(4.49741173223651,28.3736170374182,54.6385253735316));
#105973=CARTESIAN_POINT('Ctrl Pts',(4.49915972496514,28.3795040031089,54.6131305293424));
#105974=CARTESIAN_POINT('Ctrl Pts',(4.49988863000191,28.3820748236023,54.602516168089));
#105975=CARTESIAN_POINT('Ctrl Pts',(4.50128028366652,28.3872056032259,54.5822072890153));
#105976=CARTESIAN_POINT('Ctrl Pts',(4.50194352740437,28.3897490614654,54.5725091369312));
#105977=CARTESIAN_POINT('Ctrl Pts',(4.50367825069259,28.3966591101202,54.5470983280366));
#105978=CARTESIAN_POINT('Ctrl Pts',(4.50474506063968,28.4011691949799,54.531425543359));
#105979=CARTESIAN_POINT('Ctrl Pts',(4.5085918602712,28.4183732362959,54.4747836548872));
#105980=CARTESIAN_POINT('Ctrl Pts',(4.5113281820529,28.4324183756111,54.4342405467219));
#105981=CARTESIAN_POINT('Ctrl Pts',(4.5212588097925,28.4898145665806,54.2871785699899));
#105982=CARTESIAN_POINT('Ctrl Pts',(4.52816741711857,28.5425886254987,54.184691960459));
#105983=CARTESIAN_POINT('Ctrl Pts',(4.53821358558086,28.6319761328701,54.047944923547));
#105984=CARTESIAN_POINT('Ctrl Pts',(4.54121714447261,28.6602066222092,54.0086114641782));
#105985=CARTESIAN_POINT('Ctrl Pts',(4.54550768627988,28.7018517190081,53.9556206002979));
#105986=CARTESIAN_POINT('Ctrl Pts',(4.54672932414605,28.7138510657058,53.9408785979324));
#105987=CARTESIAN_POINT('Ctrl Pts',(4.54889913437573,28.7353465380309,53.9153740232821));
#105988=CARTESIAN_POINT('Ctrl Pts',(4.54984087037637,28.7447346106193,53.9045226352961));
#105989=CARTESIAN_POINT('Ctrl Pts',(4.55127690722263,28.7591139242739,53.8883295638116));
#105990=CARTESIAN_POINT('Ctrl Pts',(4.55176402643552,28.7640023640918,53.8828969382277));
#105991=CARTESIAN_POINT('Ctrl Pts',(4.55265644671194,28.7729738973071,53.8730576623736));
#105992=CARTESIAN_POINT('Ctrl Pts',(4.55306088921458,28.7770452890834,53.8686407022879));
#105993=CARTESIAN_POINT('Ctrl Pts',(4.55398780908502,28.7863889142307,53.8586133858283));
#105994=CARTESIAN_POINT('Ctrl Pts',(4.55451139067789,28.7916761851476,53.8530175140435));
#105995=CARTESIAN_POINT('Ctrl Pts',(4.5561564815387,28.808323780469,53.8356411093869));
#105996=CARTESIAN_POINT('Ctrl Pts',(4.5572874050676,28.8198186419073,53.8239916027553));
#105997=CARTESIAN_POINT('Ctrl Pts',(4.56382731770072,28.88667630101,53.7582019232234));
#105998=CARTESIAN_POINT('Ctrl Pts',(4.56943929196914,28.9455842249568,53.707809143538));
#105999=CARTESIAN_POINT('Ctrl Pts',(4.5818394987114,29.0824801690206,53.6063136056006));
#106000=CARTESIAN_POINT('Ctrl Pts',(4.58861071367887,29.1616984072832,53.5572741027483));
#106001=CARTESIAN_POINT('Ctrl Pts',(4.59876767631203,29.2897341042386,53.4921397667207));
#106002=CARTESIAN_POINT('Ctrl Pts',(4.60228799551275,29.3358938115403,53.4712475593601));
#106003=CARTESIAN_POINT('Ctrl Pts',(4.60687963580261,29.3985088147929,53.4462801574541));
#106004=CARTESIAN_POINT('Ctrl Pts',(4.60801359176219,29.4141728045458,53.4403065917489));
#106005=CARTESIAN_POINT('Ctrl Pts',(4.60989403373137,29.4404767928441,53.4307275917063));
#106006=CARTESIAN_POINT('Ctrl Pts',(4.6106448093776,29.4510675902408,53.4269916303602));
#106007=CARTESIAN_POINT('Ctrl Pts',(4.61211679218591,29.4720033701583,53.4198436168642));
#106008=CARTESIAN_POINT('Ctrl Pts',(4.61283817238461,29.4823456260084,53.4164253743687));
#106009=CARTESIAN_POINT('Ctrl Pts',(4.61458430228583,29.5075739706603,53.4083606676544));
#106010=CARTESIAN_POINT('Ctrl Pts',(4.61560551709185,29.5224933943488,53.403821242057));
#106011=CARTESIAN_POINT('Ctrl Pts',(4.61910123917343,29.5741032202546,53.3889067002341));
#106012=CARTESIAN_POINT('Ctrl Pts',(4.62154214149323,29.6110861792708,53.3795815125446));
#106013=CARTESIAN_POINT('Ctrl Pts',(4.63224061350549,29.7766003060196,53.3438414151382));
#106014=CARTESIAN_POINT('Ctrl Pts',(4.64007488303997,29.9076578018976,53.3313953490188));
#106015=CARTESIAN_POINT('Ctrl Pts',(4.65076679503384,30.0806818671835,53.3354280125569));
#106016=CARTESIAN_POINT('Ctrl Pts',(4.65338125590551,30.1224905347588,53.3379816282574));
#106017=CARTESIAN_POINT('Ctrl Pts',(4.65767966430228,30.1894550353858,53.3446120923456));
#106018=CARTESIAN_POINT('Ctrl Pts',(4.65932520263956,30.2146921705761,53.3476957181483));
#106019=CARTESIAN_POINT('Ctrl Pts',(4.66160124143916,30.2488799056959,53.3526693989337));
#106020=CARTESIAN_POINT('Ctrl Pts',(4.66220631015672,30.2579014071987,53.3540576646166));
#106021=CARTESIAN_POINT('Ctrl Pts',(4.66322944520891,30.2730339393776,53.3565137820419));
#106022=CARTESIAN_POINT('Ctrl Pts',(4.66364531867461,30.2791514112839,53.3575417908756));
#106023=CARTESIAN_POINT('Ctrl Pts',(4.664505084181,30.2917263325982,53.3597272227256));
#106024=CARTESIAN_POINT('Ctrl Pts',(4.66494917406099,30.2981828767792,53.3608886537988));
#106025=CARTESIAN_POINT('Ctrl Pts',(4.66613054539578,30.3152610073173,53.3640649843135));
#106026=CARTESIAN_POINT('Ctrl Pts',(4.66687130551921,30.3258699218904,53.3661451542912));
#106027=CARTESIAN_POINT('Ctrl Pts',(4.67023045957177,30.3735652898927,53.3759801376771));
#106028=CARTESIAN_POINT('Ctrl Pts',(4.67290323259024,30.4103982062694,53.3848949387347));
#106029=CARTESIAN_POINT('Ctrl Pts',(4.68225111857294,30.5364039318481,53.4199808700875));
#106030=CARTESIAN_POINT('Ctrl Pts',(4.68907425729419,30.6236718886279,53.4523493183181));
#106031=CARTESIAN_POINT('Ctrl Pts',(4.70033061720281,30.7644370784319,53.518410230628));
#106032=CARTESIAN_POINT('Ctrl Pts',(4.70481090948164,30.8195504984283,53.5481699040625));
#106033=CARTESIAN_POINT('Ctrl Pts',(4.71200015265218,30.9069428990667,53.6019258126873));
#106034=CARTESIAN_POINT('Ctrl Pts',(4.71476341073818,30.9402585659378,53.6241107771918));
#106035=CARTESIAN_POINT('Ctrl Pts',(4.71853231031078,30.9852883320304,53.6564965206022));
#106036=CARTESIAN_POINT('Ctrl Pts',(4.71957540826618,30.9977053512757,53.66569165619));
#106037=CARTESIAN_POINT('Ctrl Pts',(4.72134801380106,31.0187213183329,53.6817119709214));
#106038=CARTESIAN_POINT('Ctrl Pts',(4.72208079173014,31.0273838158864,53.6884516948168));
#106039=CARTESIAN_POINT('Ctrl Pts',(4.72356049512437,31.0448207568923,53.7022970127118));
#106040=CARTESIAN_POINT('Ctrl Pts',(4.72430718551478,31.0535908417358,53.7094071881195));
#106041=CARTESIAN_POINT('Ctrl Pts',(4.72617308716575,31.0754271947817,53.7274815295486));
#106042=CARTESIAN_POINT('Ctrl Pts',(4.72728767434761,31.0883988252924,53.7385583877239));
#106043=CARTESIAN_POINT('Ctrl Pts',(4.73157557281459,31.1379806346987,53.7822320773032));
#106044=CARTESIAN_POINT('Ctrl Pts',(4.73469020703579,31.1733172842122,53.816240785988));
#106045=CARTESIAN_POINT('Ctrl Pts',(4.74610174471999,31.2989754937157,53.9483410807389));
#106046=CARTESIAN_POINT('Ctrl Pts',(4.75402222409377,31.3789162251238,54.0555896581443));
#106047=CARTESIAN_POINT('Ctrl Pts',(4.76431596960786,31.4609555750366,54.1986479453005));
#106048=CARTESIAN_POINT('Ctrl Pts',(4.76631264686039,31.4759040505895,54.2265251762463));
#106049=CARTESIAN_POINT('Ctrl Pts',(4.76969150464396,31.499408569833,54.2735237283791));
#106050=CARTESIAN_POINT('Ctrl Pts',(4.77105273055319,31.5084140153461,54.2924119183667));
#106051=CARTESIAN_POINT('Ctrl Pts',(4.77299371296883,31.5205649939473,54.319184321938));
#106052=CARTESIAN_POINT('Ctrl Pts',(4.77355671586167,31.5240100474343,54.326931462642));
#106053=CARTESIAN_POINT('Ctrl Pts',(4.77453024877183,31.5298279311554,54.3402882473822));
#106054=CARTESIAN_POINT('Ctrl Pts',(4.7749390581352,31.5322293897791,54.3458851848185));
#106055=CARTESIAN_POINT('Ctrl Pts',(4.77580936103992,31.5372528818615,54.3577726116578));
#106056=CARTESIAN_POINT('Ctrl Pts',(4.77627126775305,31.5398669901336,54.364065970673));
#106057=CARTESIAN_POINT('Ctrl Pts',(4.77755134910518,31.5469705624184,54.3814681570488));
#106058=CARTESIAN_POINT('Ctrl Pts',(4.77837404928239,31.5513788054187,54.3926093982103));
#106059=CARTESIAN_POINT('Ctrl Pts',(4.78299495638825,31.5752898401613,54.4550001942932));
#106060=CARTESIAN_POINT('Ctrl Pts',(4.78690699088596,31.5923714556087,54.5071361526437));
#106061=CARTESIAN_POINT('Ctrl Pts',(4.80157606841262,31.6460178008095,54.7030548853134));
#106062=CARTESIAN_POINT('Ctrl Pts',(4.81249360620914,31.6659176429962,54.8507206310839));
#106063=CARTESIAN_POINT('Ctrl Pts',(4.82499129265967,31.6660171922899,55.0306050153185));
#106064=CARTESIAN_POINT('Ctrl Pts',(4.82715546894155,31.6651397279086,55.0621278657168));
#106065=CARTESIAN_POINT('Ctrl Pts',(4.8302399093024,31.6625821967124,55.1075735692989));
#106066=CARTESIAN_POINT('Ctrl Pts',(4.83118219986254,31.6616204529125,55.1215282881547));
#106067=CARTESIAN_POINT('Ctrl Pts',(4.83284059726982,31.6596069630516,55.1462081081664));
#106068=CARTESIAN_POINT('Ctrl Pts',(4.83355889530278,31.6586267024974,55.1569380573531));
#106069=CARTESIAN_POINT('Ctrl Pts',(4.83505103387841,31.6563640485858,55.1793076766305));
#106070=CARTESIAN_POINT('Ctrl Pts',(4.83582424471099,31.6550628889343,55.1909448868516));
#106071=CARTESIAN_POINT('Ctrl Pts',(4.83784570684523,31.6513224308644,55.2214797094866));
#106072=CARTESIAN_POINT('Ctrl Pts',(4.8390875916497,31.6486814045713,55.2403512160899));
#106073=CARTESIAN_POINT('Ctrl Pts',(4.84549601455918,31.6332682194872,55.338222727906));
#106074=CARTESIAN_POINT('Ctrl Pts',(4.8504904266267,31.6151394352568,55.4162771223049));
#106075=CARTESIAN_POINT('Ctrl Pts',(4.85720460833585,31.5828485078716,55.5205726360054));
#106076=CARTESIAN_POINT('Ctrl Pts',(4.85898648174111,31.5735017790748,55.5481759854316));
#106077=CARTESIAN_POINT('Ctrl Pts',(4.86076605062571,31.563437683379,55.575515951291));
#106078=CARTESIAN_POINT('',(4.62852046321459,31.6642316419507,55.0011944504675));
#106079=CARTESIAN_POINT('Ctrl Pts',(4.66781602428403,31.5660238537031,55.5764683070371));
#106080=CARTESIAN_POINT('Ctrl Pts',(4.66777114126252,31.5662547316415,55.5758413370685));
#106081=CARTESIAN_POINT('Ctrl Pts',(4.65467262090604,31.6335127243303,55.3928239797156));
#106082=CARTESIAN_POINT('Ctrl Pts',(4.64157410054956,31.6655128862826,55.1968759451668));
#106083=CARTESIAN_POINT('Ctrl Pts',(4.62852046321459,31.6642316419507,55.0011944504675));
#106084=CARTESIAN_POINT('Ctrl Pts',(4.62750288773491,31.6659995270476,55.0012553395138));
#106085=CARTESIAN_POINT('Ctrl Pts',(4.62392608253606,31.6660375735313,54.9507626853719));
#106086=CARTESIAN_POINT('Ctrl Pts',(4.62040756350042,31.6637801570908,54.9002895119885));
#106087=CARTESIAN_POINT('Ctrl Pts',(4.61603290565177,31.6580121437699,54.8364900498272));
#106088=CARTESIAN_POINT('Ctrl Pts',(4.61511224377004,31.6566267453367,54.8230039035159));
#106089=CARTESIAN_POINT('Ctrl Pts',(4.6134917819864,31.653883489832,54.7991658327399));
#106090=CARTESIAN_POINT('Ctrl Pts',(4.61278992858583,31.6525926679084,54.7888070946701));
#106091=CARTESIAN_POINT('Ctrl Pts',(4.61140045450403,31.6498325545355,54.7682350462989));
#106092=CARTESIAN_POINT('Ctrl Pts',(4.61071279398538,31.6483655722525,54.7580219013712));
#106093=CARTESIAN_POINT('Ctrl Pts',(4.60924923531365,31.6450271562619,54.7362208940149));
#106094=CARTESIAN_POINT('Ctrl Pts',(4.6084742537118,31.6431279418675,54.7246378019317));
#106095=CARTESIAN_POINT('Ctrl Pts',(4.60644175916033,31.6378002899008,54.6941655218651));
#106096=CARTESIAN_POINT('Ctrl Pts',(4.60519074714566,31.6341674474727,54.6753135038796));
#106097=CARTESIAN_POINT('Ctrl Pts',(4.59879713054056,31.6137835864916,54.5785663258725));
#106098=CARTESIAN_POINT('Ctrl Pts',(4.59382466559208,31.5917854667709,54.5018783785038));
#106099=CARTESIAN_POINT('Ctrl Pts',(4.58406222880871,31.5371924023319,54.3528173416392));
#106100=CARTESIAN_POINT('Ctrl Pts',(4.57928269727814,31.5047557353687,54.280614389318));
#106101=CARTESIAN_POINT('Ctrl Pts',(4.57074277749213,31.4391902586471,54.1586829738244));
#106102=CARTESIAN_POINT('Ctrl Pts',(4.56702916256826,31.4082904411514,54.107924055398));
#106103=CARTESIAN_POINT('Ctrl Pts',(4.56219410992613,31.3662473081641,54.0465059381401));
#106104=CARTESIAN_POINT('Ctrl Pts',(4.56120712878124,31.3575759560073,54.0341997525652));
#106105=CARTESIAN_POINT('Ctrl Pts',(4.55971602666297,31.3443679615188,54.0159846351031));
#106106=CARTESIAN_POINT('Ctrl Pts',(4.55921993762499,31.3399562435075,54.0099854978386));
#106107=CARTESIAN_POINT('Ctrl Pts',(4.55831907440673,31.3319171794065,53.9992059975433));
#106108=CARTESIAN_POINT('Ctrl Pts',(4.55791526509758,31.3283040251912,53.9944153831105));
#106109=CARTESIAN_POINT('Ctrl Pts',(4.55699999935006,31.320093024641,53.9836500399698));
#106110=CARTESIAN_POINT('Ctrl Pts',(4.55648755692153,31.3154804915835,53.9776869825341));
#106111=CARTESIAN_POINT('Ctrl Pts',(4.55491153162744,31.3012432123387,53.9595369974291));
#106112=CARTESIAN_POINT('Ctrl Pts',(4.55383958501061,31.2914887151701,53.947453557862));
#106113=CARTESIAN_POINT('Ctrl Pts',(4.54555837142807,31.215492287527,53.8559595870152));
#106114=CARTESIAN_POINT('Ctrl Pts',(4.53798250483419,31.1421599526536,53.7827419212522));
#106115=CARTESIAN_POINT('Ctrl Pts',(4.52242343743735,30.9773435228809,53.6462697939842));
#106116=CARTESIAN_POINT('Ctrl Pts',(4.51449384916197,30.8853404804869,53.5843848509661));
#106117=CARTESIAN_POINT('Ctrl Pts',(4.5054639809538,30.7693265223364,53.5221179080577));
#106118=CARTESIAN_POINT('Ctrl Pts',(4.50403310547343,30.7505984152836,53.5125186169315));
#106119=CARTESIAN_POINT('Ctrl Pts',(4.50179705062597,30.7207967755109,53.4979497003995));
#106120=CARTESIAN_POINT('Ctrl Pts',(4.50098367920247,30.7098427638429,53.4927421062698));
#106121=CARTESIAN_POINT('Ctrl Pts',(4.49946192721021,30.6891387653193,53.4831750933216));
#106122=CARTESIAN_POINT('Ctrl Pts',(4.49875265578805,30.6794018941504,53.478788932895));
#106123=CARTESIAN_POINT('Ctrl Pts',(4.49715781781391,30.6573155951919,53.4690940996785));
#106124=CARTESIAN_POINT('Ctrl Pts',(4.49627416406383,30.644942645305,53.4638406107462));
#106125=CARTESIAN_POINT('Ctrl Pts',(4.49399584933292,30.6127020940637,53.4506096542735));
#106126=CARTESIAN_POINT('Ctrl Pts',(4.49260893958195,30.5927415276213,53.4428642167012));
#106127=CARTESIAN_POINT('Ctrl Pts',(4.48326972852482,30.4562294387731,53.3928980497413));
#106128=CARTESIAN_POINT('Ctrl Pts',(4.47575849343676,30.3354299973551,53.3634144047361));
#106129=CARTESIAN_POINT('Ctrl Pts',(4.46282136053429,30.1255626529175,53.3364293276458));
#106130=CARTESIAN_POINT('Ctrl Pts',(4.45743786002316,30.0379224568773,53.3321297403098));
#106131=CARTESIAN_POINT('Ctrl Pts',(4.45081904007182,29.9362743243497,53.3351595481324));
#106132=CARTESIAN_POINT('Ctrl Pts',(4.44989354294296,29.9221912371156,53.3357582939663));
#106133=CARTESIAN_POINT('Ctrl Pts',(4.44847743663394,29.900873134756,53.3369358060815));
#106134=CARTESIAN_POINT('Ctrl Pts',(4.44799371586475,29.8936311105201,53.3373832964499));
#106135=CARTESIAN_POINT('Ctrl Pts',(4.44710458076348,29.8803977120386,53.3382878116181));
#106136=CARTESIAN_POINT('Ctrl Pts',(4.44669998600041,29.874405586259,53.3387299605948));
#106137=CARTESIAN_POINT('Ctrl Pts',(4.44576889385398,29.8606832045598,53.3398171782372));
#106138=CARTESIAN_POINT('Ctrl Pts',(4.44524124784759,29.8529549944233,53.3404838260823));
#106139=CARTESIAN_POINT('Ctrl Pts',(4.44360983622891,29.8291994143394,53.3427002568481));
#106140=CARTESIAN_POINT('Ctrl Pts',(4.44249710017374,29.8131901648763,53.3444284018405));
#106141=CARTESIAN_POINT('Ctrl Pts',(4.43541681984961,29.7123855200508,53.3567905848384));
#106142=CARTESIAN_POINT('Ctrl Pts',(4.42920132067106,29.6284956954561,53.3737032468747));
#106143=CARTESIAN_POINT('Ctrl Pts',(4.41663266173739,29.4623614360909,53.420725604156));
#106144=CARTESIAN_POINT('Ctrl Pts',(4.41030008263312,29.3804277776422,53.4510339207596));
#106145=CARTESIAN_POINT('Ctrl Pts',(4.40068671476945,29.256833463031,53.50813800948));
#106146=CARTESIAN_POINT('Ctrl Pts',(4.39728956770065,29.2133503121205,53.5306015484871));
#106147=CARTESIAN_POINT('Ctrl Pts',(4.39283004687733,29.1565437583529,53.5631937910363));
#106148=CARTESIAN_POINT('Ctrl Pts',(4.39170954924573,29.1422960154746,53.5716532553097));
#106149=CARTESIAN_POINT('Ctrl Pts',(4.38984533407847,29.1186424326813,53.5861789316156));
#106150=CARTESIAN_POINT('Ctrl Pts',(4.38909748101786,29.1091675090358,53.5921297437398));
#106151=CARTESIAN_POINT('Ctrl Pts',(4.38762676660182,29.0905661171268,53.6040754962339));
#106152=CARTESIAN_POINT('Ctrl Pts',(4.38690377456692,29.0814372252639,53.6100655964997));
#106153=CARTESIAN_POINT('Ctrl Pts',(4.38531048022611,29.0613587925301,53.6235246689107));
#106154=CARTESIAN_POINT('Ctrl Pts',(4.38444179719749,29.0504380916647,53.6310354816876));
#106155=CARTESIAN_POINT('Ctrl Pts',(4.38142986492495,29.0126826937431,53.657671304738));
#106156=CARTESIAN_POINT('Ctrl Pts',(4.37931187430215,28.9863256488539,53.6774621630467));
#106157=CARTESIAN_POINT('Ctrl Pts',(4.36929390308862,28.863059580359,53.7758711637061));
#106158=CARTESIAN_POINT('Ctrl Pts',(4.36179479820369,28.7746031192559,53.8644256573008));
#106159=CARTESIAN_POINT('Ctrl Pts',(4.35099642222793,28.6650308349105,54.0019903543665));
#106160=CARTESIAN_POINT('Ctrl Pts',(4.34783306114754,28.6350588214409,54.0433910007479));
#106161=CARTESIAN_POINT('Ctrl Pts',(4.34333586572791,28.596258330771,54.1025305024615));
#106162=CARTESIAN_POINT('Ctrl Pts',(4.34207422642964,28.5857704738276,54.1191498709518));
#106163=CARTESIAN_POINT('Ctrl Pts',(4.33984026983917,28.5679468775651,54.1485327745743));
#106164=CARTESIAN_POINT('Ctrl Pts',(4.33887493339831,28.5604816227675,54.1612155302659));
#106165=CARTESIAN_POINT('Ctrl Pts',(4.33741019689928,28.5495265170467,54.18040428022));
#106166=CARTESIAN_POINT('Ctrl Pts',(4.3369184169902,28.5459100776486,54.1868376784591));
#106167=CARTESIAN_POINT('Ctrl Pts',(4.33602173067697,28.5394302446526,54.1985463110036));
#106168=CARTESIAN_POINT('Ctrl Pts',(4.33561773895219,28.536552454398,54.2038132732765));
#106169=CARTESIAN_POINT('Ctrl Pts',(4.33469736098629,28.5300902719843,54.2157938348754));
#106170=CARTESIAN_POINT('Ctrl Pts',(4.33417993517464,28.526523402679,54.2225164764516));
#106171=CARTESIAN_POINT('Ctrl Pts',(4.3325730084847,28.5156453803827,54.2433625128973));
#106172=CARTESIAN_POINT('Ctrl Pts',(4.33147468020476,28.5084905503534,54.2575658687918));
#106173=CARTESIAN_POINT('Ctrl Pts',(4.32340649147518,28.4578768202241,54.3617265292075));
#106174=CARTESIAN_POINT('Ctrl Pts',(4.31609683987139,28.4223880497606,54.455321923888));
#106175=CARTESIAN_POINT('Ctrl Pts',(4.30052825652344,28.3647719229351,54.6614532026222));
#106176=CARTESIAN_POINT('Ctrl Pts',(4.29233432248276,28.3454187492353,54.774268640264));
#106177=CARTESIAN_POINT('Ctrl Pts',(4.28308877247625,28.3363668961022,54.9088448001041));
#106178=CARTESIAN_POINT('Ctrl Pts',(4.28168188633582,28.3353627898426,54.9295202129776));
#106179=CARTESIAN_POINT('Ctrl Pts',(4.27947451735669,28.3343838914722,54.962259914996));
#106180=CARTESIAN_POINT('Ctrl Pts',(4.27866619208725,28.3341543979604,54.9743138480727));
#106181=CARTESIAN_POINT('Ctrl Pts',(4.27714884811469,28.3339683038534,54.9970585883093));
#106182=CARTESIAN_POINT('Ctrl Pts',(4.27643899431975,28.3339837232162,55.0077484873008));
#106183=CARTESIAN_POINT('Ctrl Pts',(4.27483616983301,28.334252052041,55.0319927317074));
#106184=CARTESIAN_POINT('Ctrl Pts',(4.27394519241046,28.33456751408,55.0455457341369));
#106185=CARTESIAN_POINT('Ctrl Pts',(4.27163420195255,28.335821732058,55.0808830319278));
#106186=CARTESIAN_POINT('Ctrl Pts',(4.27022232481575,28.3370227829073,55.1026558232917));
#106187=CARTESIAN_POINT('Ctrl Pts',(4.25945157065493,28.3495484657367,55.2699355554147));
#106188=CARTESIAN_POINT('Ctrl Pts',(4.25073123579656,28.3795199573312,55.4134026828032));
#106189=CARTESIAN_POINT('Ctrl Pts',(4.23888477965579,28.4431716993595,55.5949791414188));
#106190=CARTESIAN_POINT('Ctrl Pts',(4.23599642303174,28.4603676042876,55.638158313174));
#106191=CARTESIAN_POINT('Ctrl Pts',(4.23130081349718,28.4904696140823,55.70541887716));
#106192=CARTESIAN_POINT('Ctrl Pts',(4.22954130058974,28.5022025123248,55.7300001794339));
#106193=CARTESIAN_POINT('Ctrl Pts',(4.22713233276354,28.5187690120197,55.7626259570023));
#106194=CARTESIAN_POINT('Ctrl Pts',(4.22651229393094,28.5230763965082,55.7709346596035));
#106195=CARTESIAN_POINT('Ctrl Pts',(4.22547122306904,28.5303753668707,55.7847282756772));
#106196=CARTESIAN_POINT('Ctrl Pts',(4.22505256213403,28.5333283000348,55.7902336056585));
#106197=CARTESIAN_POINT('Ctrl Pts',(4.22419505914448,28.5394105582043,55.801421591165));
#106198=CARTESIAN_POINT('Ctrl Pts',(4.22375608795675,28.5425422181252,55.8071027782687));
#106199=CARTESIAN_POINT('Ctrl Pts',(4.222602492518,28.5508210851472,55.8219162767302));
#106200=CARTESIAN_POINT('Ctrl Pts',(4.22188466310825,28.5560213541198,55.8310183808447));
#106201=CARTESIAN_POINT('Ctrl Pts',(4.21879032494597,28.5786592927831,55.8697877979095));
#106202=CARTESIAN_POINT('Ctrl Pts',(4.21636909449108,28.5969268202498,55.8989580020446));
#106203=CARTESIAN_POINT('Ctrl Pts',(4.20627824297224,28.6757617551641,56.0165821637736));
#106204=CARTESIAN_POINT('Ctrl Pts',(4.19838199190649,28.7438938263939,56.0996561404667));
#106205=CARTESIAN_POINT('Ctrl Pts',(4.18659668922015,28.8591809156105,56.2154194875824));
#106206=CARTESIAN_POINT('Ctrl Pts',(4.18259195852655,28.9008189178275,56.2532017804535));
#106207=CARTESIAN_POINT('Ctrl Pts',(4.17688945201212,28.9639432052222,56.3049090825147));
#106208=CARTESIAN_POINT('Ctrl Pts',(4.1751303495383,28.9839626288232,56.3205565398546));
#106209=CARTESIAN_POINT('Ctrl Pts',(4.17196686941235,29.0209624903413,56.3481363969568));
#106210=CARTESIAN_POINT('Ctrl Pts',(4.17055693786601,29.0378225686264,56.3602208820861));
#106211=CARTESIAN_POINT('Ctrl Pts',(4.16834592575701,29.0648401846509,56.3788319976896));
#106212=CARTESIAN_POINT('Ctrl Pts',(4.16753695872247,29.0748500411115,56.385568159611));
#106213=CARTESIAN_POINT('Ctrl Pts',(4.16601906048028,29.0938638582634,56.3980656371764));
#106214=CARTESIAN_POINT('Ctrl Pts',(4.1653092870467,29.1028517526657,56.4038501574643));
#106215=CARTESIAN_POINT('Ctrl Pts',(4.16370750953633,29.123351374253,56.4167662272335));
#106216=CARTESIAN_POINT('Ctrl Pts',(4.16281748822097,29.1348957235678,56.4238447824599));
#106217=CARTESIAN_POINT('Ctrl Pts',(4.16051077259799,29.1652056817379,56.4419249514623));
#106218=CARTESIAN_POINT('Ctrl Pts',(4.15910216336266,29.1841030626167,56.4527014066301));
#106219=CARTESIAN_POINT('Ctrl Pts',(4.14831717175063,29.3316054957921,56.5330298376717));
#106220=CARTESIAN_POINT('Ctrl Pts',(4.13958228448592,29.4686438069036,56.5857471895375));
#106221=CARTESIAN_POINT('Ctrl Pts',(4.12772570974535,29.6558758464832,56.6307307658874));
#106222=CARTESIAN_POINT('Ctrl Pts',(4.12484394740102,29.7013720150023,56.6396722244861));
#106223=CARTESIAN_POINT('Ctrl Pts',(4.12015783416611,29.7740565259787,56.6508316127432));
#106224=CARTESIAN_POINT('Ctrl Pts',(4.11840098765949,29.8010299262758,56.6542993004619));
#106225=CARTESIAN_POINT('Ctrl Pts',(4.11599512508008,29.8373779317457,56.6580704309633));
#106226=CARTESIAN_POINT('Ctrl Pts',(4.11537542860821,29.8466893566352,56.6589573013335));
#106227=CARTESIAN_POINT('Ctrl Pts',(4.11433477180292,29.8622303635508,56.6603055571012));
#106228=CARTESIAN_POINT('Ctrl Pts',(4.1139161784708,29.8684561419605,56.6608104127609));
#106229=CARTESIAN_POINT('Ctrl Pts',(4.11305863934986,29.8811548986549,56.6617683188711));
#106230=CARTESIAN_POINT('Ctrl Pts',(4.11261956294185,29.8876279111249,56.6622185818125));
#106231=CARTESIAN_POINT('Ctrl Pts',(4.11146538821747,29.9045718950883,56.6632977827065));
#106232=CARTESIAN_POINT('Ctrl Pts',(4.11074707908674,29.9150462725682,56.6638656457732));
#106233=CARTESIAN_POINT('Ctrl Pts',(4.10764767817032,29.9599688341473,56.6658758240063));
#106234=CARTESIAN_POINT('Ctrl Pts',(4.10522169057012,29.9944495579494,56.6663473718565));
#106235=CARTESIAN_POINT('Ctrl Pts',(4.09512817233281,30.1360569264897,56.6638890916981));
#106236=CARTESIAN_POINT('Ctrl Pts',(4.08723467045153,30.242765518535,56.6516971358001));
#106237=CARTESIAN_POINT('Ctrl Pts',(4.07545411476279,30.4024865823204,56.6176261236222));
#106238=CARTESIAN_POINT('Ctrl Pts',(4.07145135730114,30.4567855538752,56.6031399568175));
#106239=CARTESIAN_POINT('Ctrl Pts',(4.06492459590977,30.5456914129049,56.5745357146169));
#106240=CARTESIAN_POINT('Ctrl Pts',(4.06235846771108,30.5807393178021,56.5619488017357));
#106241=CARTESIAN_POINT('Ctrl Pts',(4.05880911804395,30.6293200576447,56.5426401485739));
#106242=CARTESIAN_POINT('Ctrl Pts',(4.05779398319049,30.6432260278243,56.5368938368909));
#106243=CARTESIAN_POINT('Ctrl Pts',(4.05605435132113,30.6670695858688,56.5266607312253));
#106244=CARTESIAN_POINT('Ctrl Pts',(4.05532688203491,30.6770442841548,56.5222634028574));
#106245=CARTESIAN_POINT('Ctrl Pts',(4.05393555121215,30.6961250642125,56.5136270227263));
#106246=CARTESIAN_POINT('Ctrl Pts',(4.05327121696123,30.7052373440137,56.5094029167318));
#106247=CARTESIAN_POINT('Ctrl Pts',(4.05152820542748,30.729144118317,56.4980568855487));
#106248=CARTESIAN_POINT('Ctrl Pts',(4.05045428949456,30.7438727333469,56.4907980968879));
#106249=CARTESIAN_POINT('Ctrl Pts',(4.04654723815605,30.7974153589723,56.4634192523556));
#106250=CARTESIAN_POINT('Ctrl Pts',(4.04375966293906,30.8355423989993,56.4419904879222));
#106251=CARTESIAN_POINT('Ctrl Pts',(4.03383220710234,30.9700645711245,56.3592548342384));
#106252=CARTESIAN_POINT('Ctrl Pts',(4.02696948416452,31.0609325213869,56.2895820159823));
#106253=CARTESIAN_POINT('Ctrl Pts',(4.01698214615392,31.1789897627733,56.1780750529946));
#106254=CARTESIAN_POINT('Ctrl Pts',(4.0139911860069,31.2125646951688,56.1434876089795));
#106255=CARTESIAN_POINT('Ctrl Pts',(4.00914824256803,31.2631306896512,56.0866621582956));
#106256=CARTESIAN_POINT('Ctrl Pts',(4.00734773464094,31.2811428128532,56.0653669145895));
#106257=CARTESIAN_POINT('Ctrl Pts',(4.00489106618436,31.3045238026577,56.0362734911865));
#106258=CARTESIAN_POINT('Ctrl Pts',(4.00426582520555,31.3103740416305,56.0288658614668));
#106259=CARTESIAN_POINT('Ctrl Pts',(4.00321845409541,31.3200009941074,56.016460824661));
#106260=CARTESIAN_POINT('Ctrl Pts',(4.00279875747084,31.3238131480955,56.0114909684755));
#106261=CARTESIAN_POINT('Ctrl Pts',(4.00194175962675,31.3315029012076,56.0013480014726));
#106262=CARTESIAN_POINT('Ctrl Pts',(4.0015043515384,31.3353785602897,55.9961736259792));
#106263=CARTESIAN_POINT('Ctrl Pts',(4.00035936345872,31.3453987905753,55.9826321079127));
#106264=CARTESIAN_POINT('Ctrl Pts',(3.99964866193045,31.3514953338419,55.9742300108421));
#106265=CARTESIAN_POINT('Ctrl Pts',(3.99662839559915,31.3769039654457,55.9385150075283));
#106266=CARTESIAN_POINT('Ctrl Pts',(3.99427661623603,31.395468372566,55.9106825001384));
#106267=CARTESIAN_POINT('Ctrl Pts',(3.98422441648481,31.4702356091155,55.790929419651));
#106268=CARTESIAN_POINT('Ctrl Pts',(3.97628760402876,31.5182909273427,55.6942296257175));
#106269=CARTESIAN_POINT('Ctrl Pts',(3.96805081481214,31.55896341148,55.5875630831849));
#106270=CARTESIAN_POINT('Ctrl Pts',(3.96758775221476,31.5612180395373,55.5815458010209));
#106271=CARTESIAN_POINT('Ctrl Pts',(3.96712534830139,31.5634376767977,55.5755159691697));
#106272=CARTESIAN_POINT('Origin',(5.,30.,55.));
#106273=CARTESIAN_POINT('',(3.26653908718979,31.5634376777881,55.5755159664792));
#106274=CARTESIAN_POINT('',(3.46016014030872,31.5634377287949,55.5755158279149));
#106275=CARTESIAN_POINT('',(5.,31.5634376782623,55.5755159651912));
#106276=CARTESIAN_POINT('',(4.12032061737785,31.6659997582528,54.999102502649));
#106277=CARTESIAN_POINT('Ctrl Pts',(3.46016014030872,31.5634377287949,55.5755158279149));
#106278=CARTESIAN_POINT('Ctrl Pts',(3.46533508665415,31.5387976594635,55.6424526733747));
#106279=CARTESIAN_POINT('Ctrl Pts',(3.47055209472285,31.5098738865113,55.7077663328729));
#106280=CARTESIAN_POINT('Ctrl Pts',(3.48167284141879,31.43849959412,55.8444735671295));
#106281=CARTESIAN_POINT('Ctrl Pts',(3.48753195065647,31.3947381704652,55.914945819601));
#106282=CARTESIAN_POINT('Ctrl Pts',(3.49454426464309,31.3343484856101,55.9977248299006));
#106283=CARTESIAN_POINT('Ctrl Pts',(3.49587590576348,31.3225092538315,56.0133657029079));
#106284=CARTESIAN_POINT('Ctrl Pts',(3.49799330691346,31.3030918251546,56.0380980711248));
#106285=CARTESIAN_POINT('Ctrl Pts',(3.49878585113611,31.2956885016182,56.0473238416662));
#106286=CARTESIAN_POINT('Ctrl Pts',(3.5002905205491,31.2813766440671,56.0647747403505));
#106287=CARTESIAN_POINT('Ctrl Pts',(3.50100329806649,31.2744856282455,56.0730133942589));
#106288=CARTESIAN_POINT('Ctrl Pts',(3.50263623362298,31.2584449385539,56.0918185194894));
#106289=CARTESIAN_POINT('Ctrl Pts',(3.50355410369704,31.249240921583,56.1023377351952));
#106290=CARTESIAN_POINT('Ctrl Pts',(3.50646362457264,31.2194779302772,56.1355020755035));
#106291=CARTESIAN_POINT('Ctrl Pts',(3.50843464210021,31.1984266293029,56.1576982284507));
#106292=CARTESIAN_POINT('Ctrl Pts',(3.51308992617994,31.1467094549826,56.2093045248518));
#106293=CARTESIAN_POINT('Ctrl Pts',(3.51575166701474,31.1155062043054,56.2381463142057));
#106294=CARTESIAN_POINT('Ctrl Pts',(3.52295599516635,31.0272205083045,56.3137005683529));
#106295=CARTESIAN_POINT('Ctrl Pts',(3.52743088156339,30.9680867638358,56.3578658035549));
#106296=CARTESIAN_POINT('Ctrl Pts',(3.53278087428709,30.8947040643059,56.4054355367462));
#106297=CARTESIAN_POINT('Ctrl Pts',(3.53362175135898,30.8830943621304,56.4127592691422));
#106298=CARTESIAN_POINT('Ctrl Pts',(3.53899015858684,30.8085994909791,56.4584756820157));
#106299=CARTESIAN_POINT('Ctrl Pts',(3.54357009394533,30.7433237598665,56.4927998824545));
#106300=CARTESIAN_POINT('Ctrl Pts',(3.54918367207347,30.6647779423351,56.5276704688808));
#106301=CARTESIAN_POINT('Ctrl Pts',(3.54999205075681,30.6535008555704,56.5325284284833));
#106302=CARTESIAN_POINT('Ctrl Pts',(3.55126925030795,30.6357581397266,56.5399402250574));
#106303=CARTESIAN_POINT('Ctrl Pts',(3.55173319374091,30.6293282080846,56.5425791101632));
#106304=CARTESIAN_POINT('Ctrl Pts',(3.55260584006009,30.6172668219132,56.5474412188377));
#106305=CARTESIAN_POINT('Ctrl Pts',(3.55301396843795,30.6116395184423,56.5496740786344));
#106306=CARTESIAN_POINT('Ctrl Pts',(3.55398034532309,30.5983457314973,56.5548652391269));
#106307=CARTESIAN_POINT('Ctrl Pts',(3.55454007935012,30.5906693931238,56.557797543712));
#106308=CARTESIAN_POINT('Ctrl Pts',(3.55642516703632,30.5648850221224,56.5674290069065));
#106309=CARTESIAN_POINT('Ctrl Pts',(3.55776407497309,30.5466830282125,56.5738698698242));
#106310=CARTESIAN_POINT('Ctrl Pts',(3.56109732175184,30.5015474379016,56.5889639165221));
#106311=CARTESIAN_POINT('Ctrl Pts',(3.56310625303131,30.4744979832408,56.5972500254272));
#106312=CARTESIAN_POINT('Ctrl Pts',(3.5723157071,30.3506897651624,56.6317540310309));
#106313=CARTESIAN_POINT('Ctrl Pts',(3.57968869467792,30.2518961893848,56.6498949366246));
#106314=CARTESIAN_POINT('Ctrl Pts',(3.5928627206271,30.0699400603664,56.6665732474566));
#106315=CARTESIAN_POINT('Ctrl Pts',(3.59869577729024,29.9873546364215,56.6679933394905));
#106316=CARTESIAN_POINT('Ctrl Pts',(3.60568294097849,29.8854206476869,56.6621708311039));
#106317=CARTESIAN_POINT('Ctrl Pts',(3.60701384290961,29.8658695534124,56.6607074938125));
#106318=CARTESIAN_POINT('Ctrl Pts',(3.60913035768893,29.8345724024207,56.6578086640202));
#106319=CARTESIAN_POINT('Ctrl Pts',(3.60992274464965,29.8228084032032,56.6565925893377));
#106320=CARTESIAN_POINT('Ctrl Pts',(3.61142729231794,29.8003866142317,56.6540332101452));
#106321=CARTESIAN_POINT('Ctrl Pts',(3.61214010350258,29.7897269682926,56.6527119003));
#106322=CARTESIAN_POINT('Ctrl Pts',(3.61377336537157,29.7652230562985,56.6494336167819));
#106323=CARTESIAN_POINT('Ctrl Pts',(3.61469152488574,29.7513890330395,56.6474052556401));
#106324=CARTESIAN_POINT('Ctrl Pts',(3.61760300867053,29.7073538613577,56.6403814234232));
#106325=CARTESIAN_POINT('Ctrl Pts',(3.61957565908218,29.6772631290063,56.6347275239019));
#106326=CARTESIAN_POINT('Ctrl Pts',(3.62423563051579,29.605784004053,56.6192461142565));
#106327=CARTESIAN_POINT('Ctrl Pts',(3.62690036120363,29.564582278122,56.6086565878944));
#106328=CARTESIAN_POINT('Ctrl Pts',(3.63410626988643,29.4531986702559,56.5754353907735));
#106329=CARTESIAN_POINT('Ctrl Pts',(3.63857994163612,29.38404296712,56.5497050243978));
#106330=CARTESIAN_POINT('Ctrl Pts',(3.64394270453551,29.3040926545885,56.513758119578));
#106331=CARTESIAN_POINT('Ctrl Pts',(3.64479748866411,29.2914395285092,56.5078768949202));
#106332=CARTESIAN_POINT('Ctrl Pts',(3.65016234028007,29.2127088940172,56.4700727628586));
#106333=CARTESIAN_POINT('Ctrl Pts',(3.65472493308989,29.1487349860253,56.4339757202959));
#106334=CARTESIAN_POINT('Ctrl Pts',(3.66031925577431,29.0770852193275,56.3870598598369));
#106335=CARTESIAN_POINT('Ctrl Pts',(3.661127563792,29.0668884777912,56.3802208564271));
#106336=CARTESIAN_POINT('Ctrl Pts',(3.66240467570083,29.0510396165593,56.3693350562313));
#106337=CARTESIAN_POINT('Ctrl Pts',(3.66286860323989,29.0453354170697,56.3653643599008));
#106338=CARTESIAN_POINT('Ctrl Pts',(3.66374123754035,29.0347090494322,56.357868195594));
#106339=CARTESIAN_POINT('Ctrl Pts',(3.66414936999714,29.029781038941,56.3543514384286));
#106340=CARTESIAN_POINT('Ctrl Pts',(3.66511578085771,29.018209260603,56.3459979485143));
#106341=CARTESIAN_POINT('Ctrl Pts',(3.665675545098,29.0115819916774,56.3411388321555));
#106342=CARTESIAN_POINT('Ctrl Pts',(3.66756084339686,28.9895032609136,56.3246981621082));
#106343=CARTESIAN_POINT('Ctrl Pts',(3.66889993569834,28.9742178946141,56.312897510548));
#106344=CARTESIAN_POINT('Ctrl Pts',(3.67223374436468,28.9370508779154,56.2831584551422));
#106345=CARTESIAN_POINT('Ctrl Pts',(3.6742430590468,28.9154149006627,56.2649234912472));
#106346=CARTESIAN_POINT('Ctrl Pts',(3.6834559209495,28.8192437790371,56.179587902602));
#106347=CARTESIAN_POINT('Ctrl Pts',(3.69083202618176,28.750395952079,56.1063919124717));
#106348=CARTESIAN_POINT('Ctrl Pts',(3.70400534816922,28.637714151063,55.9625629296919));
#106349=CARTESIAN_POINT('Ctrl Pts',(3.70983490151272,28.5917596889583,55.893987154749));
#106350=CARTESIAN_POINT('Ctrl Pts',(3.71681868031431,28.5413908424466,55.8052326172279));
#106351=CARTESIAN_POINT('Ctrl Pts',(3.71814948058291,28.5320172084058,55.7880144813866));
#106352=CARTESIAN_POINT('Ctrl Pts',(3.72026587345646,28.5174790784654,55.7601496999893));
#106353=CARTESIAN_POINT('Ctrl Pts',(3.72105823878788,28.5121205482233,55.7496069627771));
#106354=CARTESIAN_POINT('Ctrl Pts',(3.72256276972427,28.5021101606159,55.7293815152714));
#106355=CARTESIAN_POINT('Ctrl Pts',(3.72327558555169,28.4974388251294,55.7197091709414));
#106356=CARTESIAN_POINT('Ctrl Pts',(3.72490889236232,28.4869027563188,55.6973436871903));
#106357=CARTESIAN_POINT('Ctrl Pts',(3.72582709173406,28.4811035669327,55.6846204293308));
#106358=CARTESIAN_POINT('Ctrl Pts',(3.72873884590078,28.4631199289388,55.643811185987));
#106359=CARTESIAN_POINT('Ctrl Pts',(3.73071172124312,28.4515487083012,55.615460788233));
#106360=CARTESIAN_POINT('Ctrl Pts',(3.73537233849443,28.4257845846137,55.5470014973659));
#106361=CARTESIAN_POINT('Ctrl Pts',(3.73803748115778,28.4123334374677,55.5066360417781));
#106362=CARTESIAN_POINT('Ctrl Pts',(3.7452435958232,28.3798348511975,55.3950352422274));
#106363=CARTESIAN_POINT('Ctrl Pts',(3.74971708892027,28.3639464814892,55.3229817340117));
#106364=CARTESIAN_POINT('Ctrl Pts',(3.75508132177096,28.3507827396229,55.236291876073));
#106365=CARTESIAN_POINT('Ctrl Pts',(3.75593774364295,28.348858105026,55.22244518258));
#106366=CARTESIAN_POINT('Ctrl Pts',(3.76130210658127,28.3379250955385,55.1358049058926));
#106367=CARTESIAN_POINT('Ctrl Pts',(3.76586258715842,28.3335591700475,55.0625156050565));
#106368=CARTESIAN_POINT('Ctrl Pts',(3.77145456509739,28.3341147717062,54.976909959023));
#106369=CARTESIAN_POINT('Ctrl Pts',(3.772262864423,28.334330171417,54.9646341375197));
#106370=CARTESIAN_POINT('Ctrl Pts',(3.77353996555152,28.334879952118,54.945414917008));
#106371=CARTESIAN_POINT('Ctrl Pts',(3.77400389113555,28.3351221541964,54.9384690377012));
#106372=CARTESIAN_POINT('Ctrl Pts',(3.77487652395781,28.3356566489741,54.9254757366308));
#106373=CARTESIAN_POINT('Ctrl Pts',(3.77528465691647,28.3359384551154,54.9194281309053));
#106374=CARTESIAN_POINT('Ctrl Pts',(3.77625107195705,28.336680474099,54.9051754831087));
#106375=CARTESIAN_POINT('Ctrl Pts',(3.77681083991436,28.3371684415244,54.8969721624713));
#106376=CARTESIAN_POINT('Ctrl Pts',(3.77869616412535,28.3390062855521,54.8695056578784));
#106377=CARTESIAN_POINT('Ctrl Pts',(3.78003527910983,28.3406303303832,54.8502631880619));
#106378=CARTESIAN_POINT('Ctrl Pts',(3.7833691569091,28.345457487882,54.8029072065176));
#106379=CARTESIAN_POINT('Ctrl Pts',(3.78537851876467,28.349043019405,54.7748392549013));
#106380=CARTESIAN_POINT('Ctrl Pts',(3.79459180007811,28.3685785299282,54.6477530873025));
#106381=CARTESIAN_POINT('Ctrl Pts',(3.80196828902024,28.3927349615413,54.5502073094739));
#106382=CARTESIAN_POINT('Ctrl Pts',(3.81514152444983,28.4524590790366,54.3775321234921));
#106383=CARTESIAN_POINT('Ctrl Pts',(3.82097064672097,28.4851466357642,54.3017363519848));
#106384=CARTESIAN_POINT('Ctrl Pts',(3.82795400897509,28.5323921862791,54.2112874158683));
#106385=CARTESIAN_POINT('Ctrl Pts',(3.82928479669688,28.5417738910934,54.1940738821026));
#106386=CARTESIAN_POINT('Ctrl Pts',(3.83140117452513,28.5572992479177,54.1667471042869));
#106387=CARTESIAN_POINT('Ctrl Pts',(3.83219353718721,28.5632503696404,54.1565272023256));
#106388=CARTESIAN_POINT('Ctrl Pts',(3.8336980660589,28.5748133640607,54.1371475104627));
#106389=CARTESIAN_POINT('Ctrl Pts',(3.83441088245948,28.5804059644971,54.127976978778));
#106390=CARTESIAN_POINT('Ctrl Pts',(3.83604419481766,28.593481847257,54.1069948628052));
#106391=CARTESIAN_POINT('Ctrl Pts',(3.83696239910928,28.6010259835407,54.0952220106202));
#106392=CARTESIAN_POINT('Ctrl Pts',(3.83987418665241,28.6255582267854,54.0579792809409));
#106393=CARTESIAN_POINT('Ctrl Pts',(3.84184708976075,28.6431010893036,54.0328812079989));
#106394=CARTESIAN_POINT('Ctrl Pts',(3.84650778673558,28.6866440214969,53.9741048017639));
#106395=CARTESIAN_POINT('Ctrl Pts',(3.84917298025618,28.7132619733805,53.940910525331));
#106396=CARTESIAN_POINT('Ctrl Pts',(3.85637912015602,28.7893971622503,53.8530786121888));
#106397=CARTESIAN_POINT('Ctrl Pts',(3.86085259101378,28.8413150506234,53.800651238141));
#106398=CARTESIAN_POINT('Ctrl Pts',(3.8662170007479,28.9070097061631,53.7425725745712));
#106399=CARTESIAN_POINT('Ctrl Pts',(3.86707362039982,28.9176015479757,53.7334436066009));
#106400=CARTESIAN_POINT('Ctrl Pts',(3.87243792303791,28.9844617265538,53.6772689849089));
#106401=CARTESIAN_POINT('Ctrl Pts',(3.87699814725148,29.0436639965253,53.6338543078848));
#106402=CARTESIAN_POINT('Ctrl Pts',(3.88258984061333,29.1158826912752,53.5878940096969));
#106403=CARTESIAN_POINT('Ctrl Pts',(3.88339813888248,29.1263129550086,53.5814170207238));
#106404=CARTESIAN_POINT('Ctrl Pts',(3.88467523870082,29.1427580236849,53.5714551112631));
#106405=CARTESIAN_POINT('Ctrl Pts',(3.8851391640472,29.1487249180685,53.5678914023021));
#106406=CARTESIAN_POINT('Ctrl Pts',(3.88601179668975,29.1599310446839,53.5612933564278));
#106407=CARTESIAN_POINT('Ctrl Pts',(3.8864199297094,29.1651647439661,53.5582501095731));
#106408=CARTESIAN_POINT('Ctrl Pts',(3.88738634525808,29.1775414651067,53.5511433843424));
#106409=CARTESIAN_POINT('Ctrl Pts',(3.88794611366717,29.1846980938452,53.5471041575202));
#106410=CARTESIAN_POINT('Ctrl Pts',(3.88983144102737,29.208770721434,53.5337513433923));
#106411=CARTESIAN_POINT('Ctrl Pts',(3.89117055876866,29.2258180170275,53.5246793324716));
#106412=CARTESIAN_POINT('Ctrl Pts',(3.89450444497027,29.2682220233958,53.5030506050495));
#106413=CARTESIAN_POINT('Ctrl Pts',(3.89651381255923,29.2937478685106,53.4908398878478));
#106414=CARTESIAN_POINT('Ctrl Pts',(3.90572714484882,29.4111145052723,53.4383252901231));
#106415=CARTESIAN_POINT('Ctrl Pts',(3.91310368042812,29.5061691616486,53.4057147067374));
#106416=CARTESIAN_POINT('Ctrl Pts',(3.92627690533863,29.6836332936735,53.3622389830126));
#106417=CARTESIAN_POINT('Ctrl Pts',(3.93210597521771,29.7650404821818,53.348592495939));
#106418=CARTESIAN_POINT('Ctrl Pts',(3.93908928684428,29.8666541304664,53.3392293615676));
#106419=CARTESIAN_POINT('Ctrl Pts',(3.94042007304057,29.8862042478938,53.3377753406513));
#106420=CARTESIAN_POINT('Ctrl Pts',(3.94253644903959,29.9175830336683,53.3359978089487));
#106421=CARTESIAN_POINT('Ctrl Pts',(3.94332881137708,29.9293968885114,53.3354546983357));
#106422=CARTESIAN_POINT('Ctrl Pts',(3.94483333999774,29.9519499612372,53.3346584254991));
#106423=CARTESIAN_POINT('Ctrl Pts',(3.94554615646801,29.962687751182,53.3343832459746));
#106424=CARTESIAN_POINT('Ctrl Pts',(3.94717946950067,29.9874076405158,53.3339889190656));
#106425=CARTESIAN_POINT('Ctrl Pts',(3.94809767439053,30.0013902043818,53.3339419048581));
#106426=CARTESIAN_POINT('Ctrl Pts',(3.95100946599199,30.0459849145829,53.3343533946195));
#106427=CARTESIAN_POINT('Ctrl Pts',(3.95298237247646,30.0765855711247,53.3354796290588));
#106428=CARTESIAN_POINT('Ctrl Pts',(3.9576430791451,30.1495824683159,53.3401837517527));
#106429=CARTESIAN_POINT('Ctrl Pts',(3.9603082788496,30.1919071482605,53.3445432896958));
#106430=CARTESIAN_POINT('Ctrl Pts',(3.96751442181486,30.3069916107435,53.3608709491741));
#106431=CARTESIAN_POINT('Ctrl Pts',(3.9719878899657,30.379196483283,53.3760547160427));
#106432=CARTESIAN_POINT('Ctrl Pts',(3.98145089247296,30.5281247722577,53.4178502988029));
#106433=CARTESIAN_POINT('Ctrl Pts',(3.98643591211819,30.6043826998837,53.4453836941138));
#106434=CARTESIAN_POINT('Ctrl Pts',(3.99272799625555,30.6930659031125,53.4849171433578));
#106435=CARTESIAN_POINT('Ctrl Pts',(3.99378388267648,30.7077080098458,53.4917010460959));
#106436=CARTESIAN_POINT('Ctrl Pts',(3.9953658315541,30.7292463088972,53.5020627109277));
#106437=CARTESIAN_POINT('Ctrl Pts',(3.99588258090173,30.7362202232012,53.505477976739));
#106438=CARTESIAN_POINT('Ctrl Pts',(3.99680466777476,30.7485496024603,53.5116231578253));
#106439=CARTESIAN_POINT('Ctrl Pts',(3.99720880522894,30.75391454024,53.5143334844259));
#106440=CARTESIAN_POINT('Ctrl Pts',(3.99810474396323,30.7657216264186,53.5203787611708));
#106441=CARTESIAN_POINT('Ctrl Pts',(3.9985973125665,30.7721566307778,53.5237267352773));
#106442=CARTESIAN_POINT('Ctrl Pts',(4.000053098539,30.7910165133656,53.5336961104309));
#106443=CARTESIAN_POINT('Ctrl Pts',(4.00102298844109,30.8033792035477,53.540432925965));
#106444=CARTESIAN_POINT('Ctrl Pts',(4.00784036257214,30.8889764114697,53.5884944430012));
#106445=CARTESIAN_POINT('Ctrl Pts',(4.01394234123824,30.9590688230319,53.6351516189576));
#106446=CARTESIAN_POINT('Ctrl Pts',(4.02939497361657,31.1264124677434,53.7658210616265));
#106447=CARTESIAN_POINT('Ctrl Pts',(4.0386861009998,31.218060330235,53.8561715340597));
#106448=CARTESIAN_POINT('Ctrl Pts',(4.04895779111851,31.3116069335795,53.9725347874851));
#106449=CARTESIAN_POINT('Ctrl Pts',(4.05039132668525,31.3244617220503,53.989159395468));
#106450=CARTESIAN_POINT('Ctrl Pts',(4.05271401000041,31.3449508888141,54.0167193982816));
#106451=CARTESIAN_POINT('Ctrl Pts',(4.05361042175633,31.352774245051,54.0275106710706));
#106452=CARTESIAN_POINT('Ctrl Pts',(4.05521563714506,31.3666275113448,54.0471101083771));
#106453=CARTESIAN_POINT('Ctrl Pts',(4.05592619045449,31.3727037942888,54.0558844336824));
#106454=CARTESIAN_POINT('Ctrl Pts',(4.05744294394216,31.3855510569989,54.074822506494));
#106455=CARTESIAN_POINT('Ctrl Pts',(4.05824811450683,31.3922954767459,54.0850035820852));
#106456=CARTESIAN_POINT('Ctrl Pts',(4.06045485056925,31.4105643138374,54.1132511732276));
#106457=CARTESIAN_POINT('Ctrl Pts',(4.06184770924882,31.4218533139321,54.1314676822671));
#106458=CARTESIAN_POINT('Ctrl Pts',(4.0649364367016,31.4463071040002,54.1726828364681));
#106459=CARTESIAN_POINT('Ctrl Pts',(4.06662563888547,31.4592811039789,54.195788149299));
#106460=CARTESIAN_POINT('Ctrl Pts',(4.0720956847489,31.4998607068951,54.2722744549125));
#106461=CARTESIAN_POINT('Ctrl Pts',(4.07580726781239,31.5251314898594,54.3268422649182));
#106462=CARTESIAN_POINT('Ctrl Pts',(4.08363158950441,31.5724428485431,54.4454308566849));
#106463=CARTESIAN_POINT('Ctrl Pts',(4.08772902335711,31.5936425456686,54.5096668983709));
#106464=CARTESIAN_POINT('Ctrl Pts',(4.0953320080324,31.6250899440977,54.6288655270577));
#106465=CARTESIAN_POINT('Ctrl Pts',(4.09881093912048,31.6365870327772,54.6833932552034));
#106466=CARTESIAN_POINT('Ctrl Pts',(4.10355714718408,31.6481170479877,54.7559080333767));
#106467=CARTESIAN_POINT('Ctrl Pts',(4.10471580038967,31.6506225513418,54.7734700383525));
#106468=CARTESIAN_POINT('Ctrl Pts',(4.10640913186407,31.6538332404562,54.7988695636052));
#106469=CARTESIAN_POINT('Ctrl Pts',(4.1069320946566,31.6547641626954,54.8066779904675));
#106470=CARTESIAN_POINT('Ctrl Pts',(4.10786147985884,31.656311152587,54.8204847541879));
#106471=CARTESIAN_POINT('Ctrl Pts',(4.10826663774894,31.656949988806,54.8264802876139));
#106472=CARTESIAN_POINT('Ctrl Pts',(4.10905780292853,31.6581284720227,54.8381409510528));
#106473=CARTESIAN_POINT('Ctrl Pts',(4.10944355608575,31.6586716421921,54.8438053700639));
#106474=CARTESIAN_POINT('Ctrl Pts',(4.11031154180718,31.6598239276151,54.856506396263));
#106475=CARTESIAN_POINT('Ctrl Pts',(4.11079459211428,31.6604173316357,54.8635442729869));
#106476=CARTESIAN_POINT('Ctrl Pts',(4.11238837719785,31.6622193504549,54.8866722313403));
#106477=CARTESIAN_POINT('Ctrl Pts',(4.11350821152835,31.6632389234635,54.9027755704834));
#106478=CARTESIAN_POINT('Ctrl Pts',(4.11650950326211,31.6653267889015,54.9456097238552));
#106479=CARTESIAN_POINT('Ctrl Pts',(4.11840677441157,31.665985348925,54.9723548619076));
#106480=CARTESIAN_POINT('Ctrl Pts',(4.12032061737785,31.6659997582528,54.999102502649));
#106481=CARTESIAN_POINT('Ctrl Pts',(4.12032044382387,31.6659997569444,54.9991000770787));
#106482=CARTESIAN_POINT('Ctrl Pts',(4.1277658568908,31.6660559650028,55.1031563350326));
#106483=CARTESIAN_POINT('Ctrl Pts',(4.13542588510684,31.6563635124353,55.2069926789193));
#106484=CARTESIAN_POINT('Ctrl Pts',(4.14684877837074,31.6269365538621,55.3627664368907));
#106485=CARTESIAN_POINT('Ctrl Pts',(4.15072582248182,31.6142084265747,55.4157573269186));
#106486=CARTESIAN_POINT('Ctrl Pts',(4.15626917939867,31.5919075112809,55.4919421309294));
#106487=CARTESIAN_POINT('Ctrl Pts',(4.15799304522444,31.5843733837398,55.5156914561716));
#106488=CARTESIAN_POINT('Ctrl Pts',(4.16057877508544,31.5721582975419,55.5513970694736));
#106489=CARTESIAN_POINT('Ctrl Pts',(4.16145289012264,31.5678675441439,55.5634818607482));
#106490=CARTESIAN_POINT('Ctrl Pts',(4.16232242021249,31.5634376783906,55.5755159648424));
#106491=CARTESIAN_POINT('Ctrl Pts',(3.96712534830139,31.5634376767977,55.5755159691697));
#106492=CARTESIAN_POINT('Ctrl Pts',(3.96351693599737,31.5807588243258,55.5284616108175));
#106493=CARTESIAN_POINT('Ctrl Pts',(3.95994981330664,31.5959492132535,55.4806429514429));
#106494=CARTESIAN_POINT('Ctrl Pts',(3.95382910339297,31.6186666688434,55.3960731365343));
#106495=CARTESIAN_POINT('Ctrl Pts',(3.95124982411429,31.6271533038374,55.3596223372666));
#106496=CARTESIAN_POINT('Ctrl Pts',(3.94768576870063,31.6373274053918,55.3081268621989));
#106497=CARTESIAN_POINT('Ctrl Pts',(3.94666872224283,31.6400482132038,55.2933003238372));
#106498=CARTESIAN_POINT('Ctrl Pts',(3.94492685658813,31.6443901052209,55.2676865830567));
#106499=CARTESIAN_POINT('Ctrl Pts',(3.94419904482276,31.6461071253268,55.2569168476138));
#106500=CARTESIAN_POINT('Ctrl Pts',(3.94271778550572,31.6494012813139,55.2348641787326));
#106501=CARTESIAN_POINT('Ctrl Pts',(3.94196468106963,31.6509686863954,55.2235803584588));
#106502=CARTESIAN_POINT('Ctrl Pts',(3.94005976102336,31.6546578326869,55.1948636245157));
#106503=CARTESIAN_POINT('Ctrl Pts',(3.93891299250075,31.6566199416375,55.1774113374755));
#106504=CARTESIAN_POINT('Ctrl Pts',(3.93428740746794,31.663468325158,55.1064011320388));
#106505=CARTESIAN_POINT('Ctrl Pts',(3.93088051265922,31.6660363066166,55.0526495522779));
#106506=CARTESIAN_POINT('Ctrl Pts',(3.92156614302989,31.6659344230191,54.9033095725002));
#106507=CARTESIAN_POINT('Ctrl Pts',(3.9157973412044,31.6576488346749,54.8079391668846));
#106508=CARTESIAN_POINT('Ctrl Pts',(3.90524392672487,31.6281028549061,54.6385037627577));
#106509=CARTESIAN_POINT('Ctrl Pts',(3.90050166830427,31.6098072576345,54.564206456795));
#106510=CARTESIAN_POINT('Ctrl Pts',(3.89470757655666,31.5827296226805,54.4797366760682));
#106511=CARTESIAN_POINT('Ctrl Pts',(3.89389864654783,31.5788495192567,54.4680778642752));
#106512=CARTESIAN_POINT('Ctrl Pts',(3.89262085209436,31.5725731570898,54.4498927534408));
#106513=CARTESIAN_POINT('Ctrl Pts',(3.89215687439136,31.5702643108389,54.4433364509457));
#106514=CARTESIAN_POINT('Ctrl Pts',(3.8912843758664,31.5658687305618,54.4310995327023));
#106515=CARTESIAN_POINT('Ctrl Pts',(3.89087643158248,31.5637919861012,54.4254155914231));
#106516=CARTESIAN_POINT('Ctrl Pts',(3.88991079769832,31.5588251046717,54.4120478881272));
#106517=CARTESIAN_POINT('Ctrl Pts',(3.88935162749118,31.5559090901205,54.4043740359645));
#106518=CARTESIAN_POINT('Ctrl Pts',(3.88746983846932,31.5459593591221,54.3787617851433));
#106519=CARTESIAN_POINT('Ctrl Pts',(3.88613372408595,31.5386714650072,54.360924649634));
#106520=CARTESIAN_POINT('Ctrl Pts',(3.8828088246177,31.5199551331978,54.3172934742659));
#106521=CARTESIAN_POINT('Ctrl Pts',(3.88080553128511,31.5081778997748,54.2916561213737));
#106522=CARTESIAN_POINT('Ctrl Pts',(3.87164500323877,31.451873921206,54.176867164766));
#106523=CARTESIAN_POINT('Ctrl Pts',(3.86431661374217,31.4000540829402,54.0915207684663));
#106524=CARTESIAN_POINT('Ctrl Pts',(3.85113159956565,31.2915605416186,53.9443747845352));
#106525=CARTESIAN_POINT('Ctrl Pts',(3.84524751388157,31.2372542570995,53.8812154346461));
#106526=CARTESIAN_POINT('Ctrl Pts',(3.83821138036139,31.1645797457592,53.808490463106));
#106527=CARTESIAN_POINT('Ctrl Pts',(3.8368793069299,31.1504662557193,53.794857513695));
#106528=CARTESIAN_POINT('Ctrl Pts',(3.8347615511707,31.1274641692756,53.7734110588611));
#106529=CARTESIAN_POINT('Ctrl Pts',(3.83396907713306,31.1187278207651,53.7654377459773));
#106530=CARTESIAN_POINT('Ctrl Pts',(3.83246475185865,31.1019005912223,53.7504055263115));
#106531=CARTESIAN_POINT('Ctrl Pts',(3.83175224647607,31.093824971513,53.7433305118262));
#106532=CARTESIAN_POINT('Ctrl Pts',(3.83012024026566,31.0750878167344,53.7272324461413));
#106533=CARTESIAN_POINT('Ctrl Pts',(3.82920302194552,31.0643799857062,53.7182643308571));
#106534=CARTESIAN_POINT('Ctrl Pts',(3.82629690733746,31.0299015933912,53.6901177634513));
#106535=CARTESIAN_POINT('Ctrl Pts',(3.82432857957748,31.0057151105571,53.6714571631206));
#106536=CARTESIAN_POINT('Ctrl Pts',(3.81968080490962,30.9467625665421,53.6285066590519));
#106537=CARTESIAN_POINT('Ctrl Pts',(3.81702378475737,30.9115551663822,53.6048581083218));
#106538=CARTESIAN_POINT('Ctrl Pts',(3.80982203774112,30.8127342678802,53.5438206336987));
#106539=CARTESIAN_POINT('Ctrl Pts',(3.8053453193444,30.7474808736292,53.5092726434648));
#106540=CARTESIAN_POINT('Ctrl Pts',(3.80002286597666,30.6680575399765,53.4737527458333));
#106541=CARTESIAN_POINT('Ctrl Pts',(3.79921124124492,30.6558981942765,53.4684879656685));
#106542=CARTESIAN_POINT('Ctrl Pts',(3.79383689466949,30.5751743500369,53.4346736595079));
#106543=CARTESIAN_POINT('Ctrl Pts',(3.78922202893699,30.5048374316564,53.4105949396591));
#106544=CARTESIAN_POINT('Ctrl Pts',(3.7835697924003,30.4212828203044,53.3880981564157));
#106545=CARTESIAN_POINT('Ctrl Pts',(3.78276143036741,30.4093917966758,53.3850371202145));
#106546=CARTESIAN_POINT('Ctrl Pts',(3.78148434032301,30.3907200450586,53.3804500205093));
#106547=CARTESIAN_POINT('Ctrl Pts',(3.7810204903474,30.3839614771555,53.3788344102571));
#106548=CARTESIAN_POINT('Ctrl Pts',(3.78014808858631,30.371298176158,53.3758909233979));
#106549=CARTESIAN_POINT('Ctrl Pts',(3.77974011170337,30.3653960601807,53.3745528790974));
#106550=CARTESIAN_POINT('Ctrl Pts',(3.77877420558863,30.3514675648094,53.3714749001763));
#106551=CARTESIAN_POINT('Ctrl Pts',(3.77821479321375,30.3434354659475,53.369762126703));
#106552=CARTESIAN_POINT('Ctrl Pts',(3.77633131746291,30.31649722076,53.3642256964015));
#106553=CARTESIAN_POINT('Ctrl Pts',(3.77499372681293,30.2975381686213,53.3606711671988));
#106554=CARTESIAN_POINT('Ctrl Pts',(3.77166433063021,30.2506683260128,53.3527235914143));
#106555=CARTESIAN_POINT('Ctrl Pts',(3.7696579698927,30.2226998111734,53.3487099618955));
#106556=CARTESIAN_POINT('Ctrl Pts',(3.76047032018012,30.0953510883449,53.333728778789));
#106557=CARTESIAN_POINT('Ctrl Pts',(3.75311713354603,29.9952086114025,53.3310095594829));
#106558=CARTESIAN_POINT('Ctrl Pts',(3.73993782178608,29.8128003182597,53.3424819126742));
#106559=CARTESIAN_POINT('Ctrl Pts',(3.73408172994153,29.7306674360097,53.3538306208928));
#106560=CARTESIAN_POINT('Ctrl Pts',(3.7270725839085,29.630536633256,53.3753654722435));
#106561=CARTESIAN_POINT('Ctrl Pts',(3.72574127616074,29.611439214048,53.3798268300046));
#106562=CARTESIAN_POINT('Ctrl Pts',(3.72362443853387,29.5809587112737,53.387517371741));
#106563=CARTESIAN_POINT('Ctrl Pts',(3.72283212739023,29.569524016104,53.3905323029453));
#106564=CARTESIAN_POINT('Ctrl Pts',(3.72132792841555,29.547770076989,53.3965164886697));
#106565=CARTESIAN_POINT('Ctrl Pts',(3.72061538835289,29.537445593168,53.3994642446043));
#106566=CARTESIAN_POINT('Ctrl Pts',(3.7189830451154,29.5137535946439,53.4064769773177));
#106567=CARTESIAN_POINT('Ctrl Pts',(3.71806552775814,29.5004071562692,53.4106107459998));
#106568=CARTESIAN_POINT('Ctrl Pts',(3.71515738656525,29.4580304898693,53.4243225406966));
#106569=CARTESIAN_POINT('Ctrl Pts',(3.71318737309003,29.4292101969342,53.4345321484676));
#106570=CARTESIAN_POINT('Ctrl Pts',(3.70853476198478,29.3610808902053,53.4607988891379));
#106571=CARTESIAN_POINT('Ctrl Pts',(3.70587465761056,29.32207233312,53.4775768834822));
#106572=CARTESIAN_POINT('Ctrl Pts',(3.69867102988447,29.217171069946,53.527528635154));
#106573=CARTESIAN_POINT('Ctrl Pts',(3.69419532516638,29.1527736619489,53.5636153180848));
#106574=CARTESIAN_POINT('Ctrl Pts',(3.68885255439594,29.0795847512065,53.6112679801964));
#106575=CARTESIAN_POINT('Ctrl Pts',(3.6880196739884,29.0682822220925,53.6188255613811));
#106576=CARTESIAN_POINT('Ctrl Pts',(3.68264898927925,28.9961896184221,53.6683188567357));
#106577=CARTESIAN_POINT('Ctrl Pts',(3.67805884893528,28.938159744,53.71411413687));
#106578=CARTESIAN_POINT('Ctrl Pts',(3.67243408395006,28.8742548214744,53.7718287890703));
#106579=CARTESIAN_POINT('Ctrl Pts',(3.67162582078034,28.8652350049933,53.7801577500834));
#106580=CARTESIAN_POINT('Ctrl Pts',(3.67034885334892,28.8512556898266,53.7933555640755));
#106581=CARTESIAN_POINT('Ctrl Pts',(3.66988502560803,28.8462329980052,53.7981572541971));
#106582=CARTESIAN_POINT('Ctrl Pts',(3.66901264067446,28.8368921328437,53.8071996317067));
#106583=CARTESIAN_POINT('Ctrl Pts',(3.6686046580995,28.8325668401442,53.8114326094681));
#106584=CARTESIAN_POINT('Ctrl Pts',(3.66763870451816,28.8224261124351,53.8214656563581));
#106585=CARTESIAN_POINT('Ctrl Pts',(3.66707924992637,28.8166304003645,53.8272852676762));
#106586=CARTESIAN_POINT('Ctrl Pts',(3.6651954800106,28.7973657520686,53.846917579279));
#106587=CARTESIAN_POINT('Ctrl Pts',(3.66385763187953,28.7840943125196,53.8609207739745));
#106588=CARTESIAN_POINT('Ctrl Pts',(3.66052745121167,28.7519896194922,53.8959960689645));
#106589=CARTESIAN_POINT('Ctrl Pts',(3.65852055527039,28.7334440102807,53.9173226084009));
#106590=CARTESIAN_POINT('Ctrl Pts',(3.64932816259986,28.6517489897376,54.0162406772163));
#106591=CARTESIAN_POINT('Ctrl Pts',(3.64197063835687,28.5951240229557,54.0989522087406));
#106592=CARTESIAN_POINT('Ctrl Pts',(3.62879231646135,28.5058551570325,54.2584272815812));
#106593=CARTESIAN_POINT('Ctrl Pts',(3.622941111821,28.4708770270296,54.333527526658));
#106594=CARTESIAN_POINT('Ctrl Pts',(3.61593668169071,28.4346869464832,54.4292675800241));
#106595=CARTESIAN_POINT('Ctrl Pts',(3.61460551102319,28.4280781306889,54.4477300076102));
#106596=CARTESIAN_POINT('Ctrl Pts',(3.61248883777089,28.4180086221042,54.4775068436473));
#106597=CARTESIAN_POINT('Ctrl Pts',(3.61169655579118,28.4143399910984,54.4887484309854));
#106598=CARTESIAN_POINT('Ctrl Pts',(3.6101923794108,28.4075691574767,54.5102701883214));
#106599=CARTESIAN_POINT('Ctrl Pts',(3.60947983312135,28.4044460615004,54.5205431039082));
#106600=CARTESIAN_POINT('Ctrl Pts',(3.60784742945471,28.3974878709704,54.5442521637048));
#106601=CARTESIAN_POINT('Ctrl Pts',(3.60692985848848,28.3937220208725,54.5577079161389));
#106602=CARTESIAN_POINT('Ctrl Pts',(3.60402135387329,28.3822570389804,54.6007526931826));
#106603=CARTESIAN_POINT('Ctrl Pts',(3.60205103809121,28.3752026247366,54.6305079471121));
#106604=CARTESIAN_POINT('Ctrl Pts',(3.59739755945635,28.3603176302196,54.7020063840521));
#106605=CARTESIAN_POINT('Ctrl Pts',(3.5947369018002,28.3532560667696,54.74388817644));
#106606=CARTESIAN_POINT('Ctrl Pts',(3.5875329551255,28.338330628906,54.8591188383726));
#106607=CARTESIAN_POINT('Ctrl Pts',(3.58305744987355,28.3337239340639,54.9327910685991));
#106608=CARTESIAN_POINT('Ctrl Pts',(3.57771156749899,28.3340662538672,55.0201759678629));
#106609=CARTESIAN_POINT('Ctrl Pts',(3.57687538987544,28.3342874727752,55.0338243592471));
#106610=CARTESIAN_POINT('Ctrl Pts',(3.57150536251012,28.3367786751581,55.1212227054904));
#106611=CARTESIAN_POINT('Ctrl Pts',(3.56691914791976,28.3437780972681,55.194746932433));
#106612=CARTESIAN_POINT('Ctrl Pts',(3.56129874328014,28.3575962943456,55.2796726514467));
#106613=CARTESIAN_POINT('Ctrl Pts',(3.56049049588562,28.3597017575764,55.2917676789191));
#106614=CARTESIAN_POINT('Ctrl Pts',(3.55921354801901,28.3632078893186,55.3106700348482));
#106615=CARTESIAN_POINT('Ctrl Pts',(3.55874972382617,28.3645178623578,55.317494027066));
#106616=CARTESIAN_POINT('Ctrl Pts',(3.55787734157736,28.3670486025996,55.3302459130961));
#106617=CARTESIAN_POINT('Ctrl Pts',(3.55746935809367,28.3682590321286,55.3361756066161));
#106618=CARTESIAN_POINT('Ctrl Pts',(3.55650339693592,28.3711882914034,55.3501369437018));
#106619=CARTESIAN_POINT('Ctrl Pts',(3.55594393560588,28.3729342376776,55.3581626158835));
#106620=CARTESIAN_POINT('Ctrl Pts',(3.55406011873552,28.3789799050259,55.3849962043276));
#106621=CARTESIAN_POINT('Ctrl Pts',(3.55272222950467,28.3835468020544,55.4037415079455));
#106622=CARTESIAN_POINT('Ctrl Pts',(3.54939192360981,28.3956031643451,55.4497393126902));
#106623=CARTESIAN_POINT('Ctrl Pts',(3.54738494223224,28.4034624406231,55.4768881387664));
#106624=CARTESIAN_POINT('Ctrl Pts',(3.53819179213125,28.4422629619782,55.599183078923));
#106625=CARTESIAN_POINT('Ctrl Pts',(3.53083357515847,28.4810458725131,55.691624061468));
#106626=CARTESIAN_POINT('Ctrl Pts',(3.51765541113551,28.5666142170721,55.8531133259261));
#106627=CARTESIAN_POINT('Ctrl Pts',(3.51180498673131,28.6107333819444,55.923222144402));
#106628=CARTESIAN_POINT('Ctrl Pts',(3.50480130961133,28.6715341526858,56.0055440969087));
#106629=CARTESIAN_POINT('Ctrl Pts',(3.50347016092373,28.6834606778057,56.0211095477042));
#106630=CARTESIAN_POINT('Ctrl Pts',(3.50135351402786,28.7030159288008,56.0457189563342));
#106631=CARTESIAN_POINT('Ctrl Pts',(3.50056123672444,28.7104707040302,56.0548981106696));
#106632=CARTESIAN_POINT('Ctrl Pts',(3.49905706396646,28.7248797876153,56.0722591669003));
#106633=CARTESIAN_POINT('Ctrl Pts',(3.49834451667812,28.7318166707834,56.0804546865723));
#106634=CARTESIAN_POINT('Ctrl Pts',(3.49671210331965,28.7479619189958,56.0991596160014));
#106635=CARTESIAN_POINT('Ctrl Pts',(3.49579452375558,28.7572243157534,56.1096214832458));
#106636=CARTESIAN_POINT('Ctrl Pts',(3.49288596085128,28.7871705448035,56.1426003062044));
#106637=CARTESIAN_POINT('Ctrl Pts',(3.49091559658207,28.8083437336193,56.1646657365186));
#106638=CARTESIAN_POINT('Ctrl Pts',(3.48626197879834,28.8603413031889,56.2159509237159));
#106639=CARTESIAN_POINT('Ctrl Pts',(3.48360123239604,28.8916992694844,56.2445997202942));
#106640=CARTESIAN_POINT('Ctrl Pts',(3.47639723507272,28.9804156426917,56.3196364139072));
#106641=CARTESIAN_POINT('Ctrl Pts',(3.47192176230318,29.0398121681107,56.3634633188437));
#106642=CARTESIAN_POINT('Ctrl Pts',(3.46657539492045,29.113420514866,56.4105741249164));
#106643=CARTESIAN_POINT('Ctrl Pts',(3.46573870203686,29.1250143099819,56.4177949717942));
#106644=CARTESIAN_POINT('Ctrl Pts',(3.46036878010049,29.1997917024351,56.4631012467367));
#106645=CARTESIAN_POINT('Ctrl Pts',(3.45578318171749,29.265349860318,56.4970921781871));
#106646=CARTESIAN_POINT('Ctrl Pts',(3.45016346146697,29.3441845464325,56.5315393609799));
#106647=CARTESIAN_POINT('Ctrl Pts',(3.44935521655202,29.3554879984601,56.5363303620918));
#106648=CARTESIAN_POINT('Ctrl Pts',(3.44807827176066,29.3732702477765,56.5436366482108));
#106649=CARTESIAN_POINT('Ctrl Pts',(3.44761444812548,29.379713855339,56.5462371675752));
#106650=CARTESIAN_POINT('Ctrl Pts',(3.44674206629878,29.3917998468096,56.5510271445306));
#106651=CARTESIAN_POINT('Ctrl Pts',(3.44633408267239,29.397438135996,56.5532262632292));
#106652=CARTESIAN_POINT('Ctrl Pts',(3.44536812032378,29.4107564046268,56.5583373983087));
#106653=CARTESIAN_POINT('Ctrl Pts',(3.44480865793477,29.4184460743518,56.5612233940571));
#106654=CARTESIAN_POINT('Ctrl Pts',(3.4429248336845,29.4442691941899,56.5706977750823));
#106655=CARTESIAN_POINT('Ctrl Pts',(3.44158693799392,29.4624949483031,56.5770277325728));
#106656=CARTESIAN_POINT('Ctrl Pts',(3.43825661241683,29.5076789101521,56.5918462898501));
#106657=CARTESIAN_POINT('Ctrl Pts',(3.43624961761092,29.5347505899071,56.5999679597363));
#106658=CARTESIAN_POINT('Ctrl Pts',(3.42705634845486,29.6585415037072,56.6336986955327));
#106659=CARTESIAN_POINT('Ctrl Pts',(3.41969802259601,29.7572411300288,56.6512522235544));
#106660=CARTESIAN_POINT('Ctrl Pts',(3.40651988337975,29.9393243258093,56.6669479103152));
#106661=CARTESIAN_POINT('Ctrl Pts',(3.40066958160671,30.0221527718848,56.6679058252841));
#106662=CARTESIAN_POINT('Ctrl Pts',(3.39366602284187,30.1242894650576,56.661473010684));
#106663=CARTESIAN_POINT('Ctrl Pts',(3.39233487761129,30.1438351473273,56.6598951604656));
#106664=CARTESIAN_POINT('Ctrl Pts',(3.39021823486088,30.1751165889508,56.6568132051034));
#106665=CARTESIAN_POINT('Ctrl Pts',(3.38942595829297,30.1868715880752,56.6555285676722));
#106666=CARTESIAN_POINT('Ctrl Pts',(3.38792178610482,30.209272329075,56.652838881856));
#106667=CARTESIAN_POINT('Ctrl Pts',(3.3872092386594,30.219920061012,56.6514558586476));
#106668=CARTESIAN_POINT('Ctrl Pts',(3.38557682377657,30.2443915131544,56.648036409374));
#106669=CARTESIAN_POINT('Ctrl Pts',(3.38465924286035,30.2582045956096,56.6459288030873));
#106670=CARTESIAN_POINT('Ctrl Pts',(3.38175067078847,30.3021534403055,56.6386561729252));
#106671=CARTESIAN_POINT('Ctrl Pts',(3.37978029889314,30.3321752646589,56.6328351221111));
#106672=CARTESIAN_POINT('Ctrl Pts',(3.37512665922375,30.4034641383369,56.6169648428055));
#106673=CARTESIAN_POINT('Ctrl Pts',(3.37246589886321,30.4445408937129,56.6061576468486));
#106674=CARTESIAN_POINT('Ctrl Pts',(3.36526189358678,30.5556991842574,56.5723202382245));
#106675=CARTESIAN_POINT('Ctrl Pts',(3.36078642593863,30.6247345265697,56.5461887510835));
#106676=CARTESIAN_POINT('Ctrl Pts',(3.35132894064446,30.7653706120716,56.4819926279907));
#106677=CARTESIAN_POINT('Ctrl Pts',(3.34635158199632,30.8363787465844,56.443108378759));
#106678=CARTESIAN_POINT('Ctrl Pts',(3.34004640934146,30.9181186591092,56.3902826448104));
#106679=CARTESIAN_POINT('Ctrl Pts',(3.33896795752298,30.9318285094974,56.3811311608567));
#106680=CARTESIAN_POINT('Ctrl Pts',(3.33736587219883,30.9517556144202,56.3673978338083));
#106681=CARTESIAN_POINT('Ctrl Pts',(3.33685212205673,30.9580808678511,56.3629734517851));
#106682=CARTESIAN_POINT('Ctrl Pts',(3.3359333169489,30.9692729037333,56.3550284560361));
#106683=CARTESIAN_POINT('Ctrl Pts',(3.33552942920174,30.9741517222669,56.351525248855));
#106684=CARTESIAN_POINT('Ctrl Pts',(3.33463148557265,30.9849073268589,56.3437137537299));
#106685=CARTESIAN_POINT('Ctrl Pts',(3.33413663572504,30.9907747699822,56.3393933121366));
#106686=CARTESIAN_POINT('Ctrl Pts',(3.33266690514873,31.008030792598,56.3265115594664));
#106687=CARTESIAN_POINT('Ctrl Pts',(3.33168516312223,31.0193377699553,56.3178427346103));
#106688=CARTESIAN_POINT('Ctrl Pts',(3.32938713765778,31.0453300263599,56.2973803790608));
#106689=CARTESIAN_POINT('Ctrl Pts',(3.32806507818891,31.0599290851682,56.2854808369965));
#106690=CARTESIAN_POINT('Ctrl Pts',(3.32335736215911,31.1107736650876,56.2425829360346));
#106691=CARTESIAN_POINT('Ctrl Pts',(3.31991667456228,31.1458851744092,56.2102797571266));
#106692=CARTESIAN_POINT('Ctrl Pts',(3.30829275845901,31.2589670846898,56.096905358102));
#106693=CARTESIAN_POINT('Ctrl Pts',(3.30006621409789,31.3301201011451,56.0094481072516));
#106694=CARTESIAN_POINT('Ctrl Pts',(3.28892506433188,31.4169972062571,55.8773580650816));
#106695=CARTESIAN_POINT('Ctrl Pts',(3.28575959374229,31.4404972149207,55.8382163896087));
#106696=CARTESIAN_POINT('Ctrl Pts',(3.28151599394438,31.4703489322232,55.7835227668013));
#106697=CARTESIAN_POINT('Ctrl Pts',(3.28038842618937,31.4781157212353,55.7687703547314));
#106698=CARTESIAN_POINT('Ctrl Pts',(3.27859099704444,31.4902254515667,55.7449066303861));
#106699=CARTESIAN_POINT('Ctrl Pts',(3.27791624043787,31.4947091471847,55.7358684376632));
#106700=CARTESIAN_POINT('Ctrl Pts',(3.27652061557265,31.5038513541364,55.7170112976197));
#106701=CARTESIAN_POINT('Ctrl Pts',(3.2758002386179,31.5084964591263,55.7071863534999));
#106702=CARTESIAN_POINT('Ctrl Pts',(3.27410330459937,31.51926038285,55.6838306692777));
#106703=CARTESIAN_POINT('Ctrl Pts',(3.27312966385485,31.5252951562397,55.6702620420479));
#106704=CARTESIAN_POINT('Ctrl Pts',(3.27026542530456,31.5426175643117,55.6298682013147));
#106705=CARTESIAN_POINT('Ctrl Pts',(3.26839227694276,31.5533845038351,55.6028262616837));
#106706=CARTESIAN_POINT('Ctrl Pts',(3.26653908718979,31.5634376777881,55.5755159664792));
#106707=CARTESIAN_POINT('Origin',(5.,30.,55.));
#106708=CARTESIAN_POINT('',(2.56903902087732,31.5634376730794,55.5755159792709));
#106709=CARTESIAN_POINT('',(2.75980447732861,31.5634376782628,55.5755159651897));
#106710=CARTESIAN_POINT('',(5.,31.5634376782623,55.5755159651912));
#106711=CARTESIAN_POINT('Ctrl Pts',(2.75980447732862,31.5634376782628,55.5755159651897));
#106712=CARTESIAN_POINT('Ctrl Pts',(2.762192831449,31.5501199861041,55.6116945996113));
#106713=CARTESIAN_POINT('Ctrl Pts',(2.76460760539681,31.5355513221819,55.6473978851748));
#106714=CARTESIAN_POINT('Ctrl Pts',(2.76861985484581,31.5098628697695,55.7045945635996));
#106715=CARTESIAN_POINT('Ctrl Pts',(2.77018535434155,31.4994898538802,55.7264085747185));
#106716=CARTESIAN_POINT('Ctrl Pts',(2.77236755591098,31.4846263241562,55.7559899968398));
#106717=CARTESIAN_POINT('Ctrl Pts',(2.77296145010307,31.4805412912738,55.7639592093834));
#106718=CARTESIAN_POINT('Ctrl Pts',(2.77397123613029,31.4735332071027,55.7773634720219));
#106719=CARTESIAN_POINT('Ctrl Pts',(2.77438506543448,31.4706437663534,55.7828160647602));
#106720=CARTESIAN_POINT('Ctrl Pts',(2.77524682266853,31.4645925727568,55.7940833721435));
#106721=CARTESIAN_POINT('Ctrl Pts',(2.77569500274132,31.4614263844038,55.7998954464275));
#106722=CARTESIAN_POINT('Ctrl Pts',(2.77689891593948,31.4528682672194,55.8153848924919));
#106723=CARTESIAN_POINT('Ctrl Pts',(2.77765835717101,31.4474144115905,55.8250274112784));
#106724=CARTESIAN_POINT('Ctrl Pts',(2.7812277508218,31.4215069847876,55.8697846158843));
#106725=CARTESIAN_POINT('Ctrl Pts',(2.78410026247713,31.3998707259214,55.9041950820981));
#106726=CARTESIAN_POINT('Ctrl Pts',(2.79352160172908,31.325822373065,56.0129252103728));
#106727=CARTESIAN_POINT('Ctrl Pts',(2.8001962293002,31.2685795415418,56.083756522839));
#106728=CARTESIAN_POINT('Ctrl Pts',(2.81124499199724,31.1632224067688,56.1942717860872));
#106729=CARTESIAN_POINT('Ctrl Pts',(2.81566486019702,31.1181438060857,56.2365788324746));
#106730=CARTESIAN_POINT('Ctrl Pts',(2.8218800493281,31.050170696569,56.2936088005877));
#106731=CARTESIAN_POINT('Ctrl Pts',(2.82374966321167,31.029107863017,56.3104271700733));
#106732=CARTESIAN_POINT('Ctrl Pts',(2.82709019006151,30.9903547873915,56.3398599940553));
#106733=CARTESIAN_POINT('Ctrl Pts',(2.82856765666853,30.9728086357885,56.3526532607957));
#106734=CARTESIAN_POINT('Ctrl Pts',(2.83085950494593,30.9449618921524,56.372134687948));
#106735=CARTESIAN_POINT('Ctrl Pts',(2.83168277375302,30.934829477541,56.3790578092931));
#106736=CARTESIAN_POINT('Ctrl Pts',(2.83321372702154,30.9157484639601,56.3917882455475));
#106737=CARTESIAN_POINT('Ctrl Pts',(2.83392240747059,30.9068188547276,56.3976227471841));
#106738=CARTESIAN_POINT('Ctrl Pts',(2.83550396357362,30.8866767929159,56.4105090175721));
#106739=CARTESIAN_POINT('Ctrl Pts',(2.83637506625521,30.8754349580437,56.4175136947662));
#106740=CARTESIAN_POINT('Ctrl Pts',(2.83859722948818,30.8463880922487,56.4351351413961));
#106741=CARTESIAN_POINT('Ctrl Pts',(2.83994118263824,30.8284659718062,56.4455552120685));
#106742=CARTESIAN_POINT('Ctrl Pts',(2.85099728879109,30.6782536221692,56.5291783711156));
#106743=CARTESIAN_POINT('Ctrl Pts',(2.86000964392068,30.5367660063161,56.5843920509653));
#106744=CARTESIAN_POINT('Ctrl Pts',(2.87303656083141,30.3313639210802,56.6338183443995));
#106745=CARTESIAN_POINT('Ctrl Pts',(2.87679073185298,30.272249373356,56.6447015492948));
#106746=CARTESIAN_POINT('Ctrl Pts',(2.88167460469858,30.1976711930005,56.6543008174358));
#106747=CARTESIAN_POINT('Ctrl Pts',(2.88266681174194,30.1826341565861,56.6560283272249));
#106748=CARTESIAN_POINT('Ctrl Pts',(2.88416436774143,30.1601500610783,56.6583014415473));
#106749=CARTESIAN_POINT('Ctrl Pts',(2.88466158482524,30.1527190117687,56.6590022939116));
#106750=CARTESIAN_POINT('Ctrl Pts',(2.88556369250385,30.1393040470891,56.6601766208769));
#106751=CARTESIAN_POINT('Ctrl Pts',(2.8859676064051,30.1333219425452,56.6606677231264));
#106752=CARTESIAN_POINT('Ctrl Pts',(2.88688210129736,30.1198330423465,56.6617017440049));
#106753=CARTESIAN_POINT('Ctrl Pts',(2.8873936575018,30.1123252029223,56.6622261240094));
#106754=CARTESIAN_POINT('Ctrl Pts',(2.88896372817565,30.0893888561556,56.6636719991686));
#106755=CARTESIAN_POINT('Ctrl Pts',(2.89003051600365,30.073951350422,56.6644296451507));
#106756=CARTESIAN_POINT('Ctrl Pts',(2.89841483180061,29.953590291132,56.6686590687371));
#106757=CARTESIAN_POINT('Ctrl Pts',(2.90611038012386,29.8485695373917,56.6624206311296));
#106758=CARTESIAN_POINT('Ctrl Pts',(2.92159852329018,29.6380276938933,56.6297900808525));
#106759=CARTESIAN_POINT('Ctrl Pts',(2.92934586780103,29.5330599040482,56.6028768622299));
#106760=CARTESIAN_POINT('Ctrl Pts',(2.93825155730654,29.411100299962,56.558595750202));
#106761=CARTESIAN_POINT('Ctrl Pts',(2.93972285830505,29.3909200051703,56.5508208166785));
#106762=CARTESIAN_POINT('Ctrl Pts',(2.94200735171948,29.3595505069973,56.5380281442608));
#106763=CARTESIAN_POINT('Ctrl Pts',(2.94282933771966,29.3482562028332,56.5332762837722));
#106764=CARTESIAN_POINT('Ctrl Pts',(2.94435911114239,29.3272281004076,56.5241547753734));
#106765=CARTESIAN_POINT('Ctrl Pts',(2.9450678807507,29.3174819320897,56.5198154178061));
#106766=CARTESIAN_POINT('Ctrl Pts',(2.94665117543704,29.2957073454677,56.5098688544217));
#106767=CARTESIAN_POINT('Ctrl Pts',(2.94752390959784,29.2837028001406,56.5042109025053));
#106768=CARTESIAN_POINT('Ctrl Pts',(2.95013865196282,29.2477457558812,56.4867356372854));
#106769=CARTESIAN_POINT('Ctrl Pts',(2.95186564912727,29.2240078698965,56.4744848744385));
#106770=CARTESIAN_POINT('Ctrl Pts',(2.96293133879509,29.0723255020617,56.3915256328562));
#106771=CARTESIAN_POINT('Ctrl Pts',(2.97164640739505,28.9538721806745,56.3048145778868));
#106772=CARTESIAN_POINT('Ctrl Pts',(2.98431526781305,28.8054976525151,56.1628505146025));
#106773=CARTESIAN_POINT('Ctrl Pts',(2.98801594309327,28.7649582031302,56.1196997227499));
#106774=CARTESIAN_POINT('Ctrl Pts',(2.99283557954543,28.717109766335,56.0630026220432));
#106775=CARTESIAN_POINT('Ctrl Pts',(2.99382105457645,28.7075719127845,56.0513855272244));
#106776=CARTESIAN_POINT('Ctrl Pts',(2.99531041724624,28.6935479008493,56.0338250913653));
#106777=CARTESIAN_POINT('Ctrl Pts',(2.9958063029131,28.6889419930898,56.027977774141));
#106778=CARTESIAN_POINT('Ctrl Pts',(2.99670710456393,28.680692824441,56.0173596263555));
#106779=CARTESIAN_POINT('Ctrl Pts',(2.99711105929862,28.6770359548356,56.0125997061588));
#106780=CARTESIAN_POINT('Ctrl Pts',(2.99802706545986,28.6688390849313,56.0018101535062));
#106781=CARTESIAN_POINT('Ctrl Pts',(2.9985401081394,28.6643143205601,55.9957694138972));
#106782=CARTESIAN_POINT('Ctrl Pts',(3.00011933530606,28.650583307638,55.9771759901348));
#106783=CARTESIAN_POINT('Ctrl Pts',(3.00119392854953,28.6415121174535,55.964525248448));
#106784=CARTESIAN_POINT('Ctrl Pts',(3.00944127222337,28.5738467964191,55.867310405856));
#106785=CARTESIAN_POINT('Ctrl Pts',(3.01697666831238,28.5230264519377,55.7776156329591));
#106786=CARTESIAN_POINT('Ctrl Pts',(3.03262326792838,28.434707796143,55.5814032477442));
#106787=CARTESIAN_POINT('Ctrl Pts',(3.04067575700009,28.3990762155491,55.4745746203949));
#106788=CARTESIAN_POINT('Ctrl Pts',(3.04976801332803,28.3700047520245,55.3450885213731));
#106789=CARTESIAN_POINT('Ctrl Pts',(3.05115157336887,28.3659087435678,55.3251406240996));
#106790=CARTESIAN_POINT('Ctrl Pts',(3.05333118837893,28.3599839285205,55.2933376427417));
#106791=CARTESIAN_POINT('Ctrl Pts',(3.05413475010823,28.3579157569915,55.2815298194306));
#106792=CARTESIAN_POINT('Ctrl Pts',(3.055648314555,28.3542421066987,55.2591361868749));
#106793=CARTESIAN_POINT('Ctrl Pts',(3.05635909650707,28.3526108872717,55.2485552797859));
#106794=CARTESIAN_POINT('Ctrl Pts',(3.0579709878513,28.3491275371512,55.2244176950384));
#106795=CARTESIAN_POINT('Ctrl Pts',(3.0588700172328,28.3473401740332,55.2108523384027));
#106796=CARTESIAN_POINT('Ctrl Pts',(3.06121659479051,28.3430876175583,55.1751902723923));
#106797=CARTESIAN_POINT('Ctrl Pts',(3.06265558152968,28.3408972216891,55.1530631240404));
#106798=CARTESIAN_POINT('Ctrl Pts',(3.07364340595797,28.32744332101,54.9823582686439));
#106799=CARTESIAN_POINT('Ctrl Pts',(3.0825251144406,28.3357148773882,54.8329272952165));
#106800=CARTESIAN_POINT('Ctrl Pts',(3.0953890685054,28.3749502571241,54.6280911057452));
#106801=CARTESIAN_POINT('Ctrl Pts',(3.09911265225977,28.3892814806941,54.5702474521909));
#106802=CARTESIAN_POINT('Ctrl Pts',(3.10395979775142,28.4110804312326,54.4988833585535));
#106803=CARTESIAN_POINT('Ctrl Pts',(3.10494816403895,28.4156799775532,54.4845261288192));
#106804=CARTESIAN_POINT('Ctrl Pts',(3.10644104603881,28.4228432903786,54.4631683208464));
#106805=CARTESIAN_POINT('Ctrl Pts',(3.1069375041088,28.4252603851029,54.456118874751));
#106806=CARTESIAN_POINT('Ctrl Pts',(3.10783886624866,28.429709585898,54.4434211225431));
#106807=CARTESIAN_POINT('Ctrl Pts',(3.1082428024251,28.4317250317328,54.4377672614678));
#106808=CARTESIAN_POINT('Ctrl Pts',(3.10915815445181,28.4363405364721,54.4250374720399));
#106809=CARTESIAN_POINT('Ctrl Pts',(3.10967055462556,28.4389580734989,54.417968278697));
#106810=CARTESIAN_POINT('Ctrl Pts',(3.11124582010558,28.4471107606551,54.3964009233395));
#106811=CARTESIAN_POINT('Ctrl Pts',(3.11231703545546,28.4528004126447,54.3819625991251));
#106812=CARTESIAN_POINT('Ctrl Pts',(3.12061211693978,28.4980248061075,54.2717388502146));
#106813=CARTESIAN_POINT('Ctrl Pts',(3.12820411794129,28.5462140142126,54.1797581401613));
#106814=CARTESIAN_POINT('Ctrl Pts',(3.14383534850046,28.6632727544579,53.9994397683538));
#106815=CARTESIAN_POINT('Ctrl Pts',(3.15181898770457,28.7331417194772,53.9123240341774));
#106816=CARTESIAN_POINT('Ctrl Pts',(3.16085896318759,28.8255619578962,53.8181913236632));
#106817=CARTESIAN_POINT('Ctrl Pts',(3.16225249928016,28.840197038981,53.8038254228799));
#106818=CARTESIAN_POINT('Ctrl Pts',(3.1644440570885,28.8638242082639,53.7814742567735));
#106819=CARTESIAN_POINT('Ctrl Pts',(3.16524972770047,28.8726435140325,53.7733102334799));
#106820=CARTESIAN_POINT('Ctrl Pts',(3.16676506993478,28.8894808849447,53.7580588643268));
#106821=CARTESIAN_POINT('Ctrl Pts',(3.16747554454272,28.8974803529654,53.7509519919538));
#106822=CARTESIAN_POINT('Ctrl Pts',(3.16908378019546,28.9158241625205,53.7349685661392));
#106823=CARTESIAN_POINT('Ctrl Pts',(3.16997949767706,28.926210167351,53.7261408284813));
#106824=CARTESIAN_POINT('Ctrl Pts',(3.17231120001677,28.9536802011014,53.7033669870436));
#106825=CARTESIAN_POINT('Ctrl Pts',(3.17373880401777,28.970935165951,53.6896306124683));
#106826=CARTESIAN_POINT('Ctrl Pts',(3.18230574952777,29.0769891874961,53.6085901835577));
#106827=CARTESIAN_POINT('Ctrl Pts',(3.18910123354758,29.1720852095538,53.5499893559828));
#106828=CARTESIAN_POINT('Ctrl Pts',(3.20022244779849,29.3359103095552,53.470445641023));
#106829=CARTESIAN_POINT('Ctrl Pts',(3.2045378348824,29.4013876629973,53.4436537849391));
#106830=CARTESIAN_POINT('Ctrl Pts',(3.21049743224233,29.490866766143,53.4135249184435));
#106831=CARTESIAN_POINT('Ctrl Pts',(3.21201219932955,29.5135287978645,53.4064299550166));
#106832=CARTESIAN_POINT('Ctrl Pts',(3.21464760816669,29.5526355101684,53.3950984199941));
#106833=CARTESIAN_POINT('Ctrl Pts',(3.21575731031687,29.5690079807562,53.3906243778192));
#106834=CARTESIAN_POINT('Ctrl Pts',(3.21739724754887,29.5930100407439,53.3844579306685));
#106835=CARTESIAN_POINT('Ctrl Pts',(3.21791692644899,29.6005883092084,53.3825676830527));
#106836=CARTESIAN_POINT('Ctrl Pts',(3.2188038607759,29.6134689097773,53.3794509160738));
#106837=CARTESIAN_POINT('Ctrl Pts',(3.21916955387508,29.618764420622,53.3781969759039));
#106838=CARTESIAN_POINT('Ctrl Pts',(3.220007119421,29.6308567066252,53.3753961051972));
#106839=CARTESIAN_POINT('Ctrl Pts',(3.22047989784708,29.6376569484175,53.373865905105));
#106840=CARTESIAN_POINT('Ctrl Pts',(3.22179789165491,29.6565495628262,53.3697390498291));
#106841=CARTESIAN_POINT('Ctrl Pts',(3.2226479409213,29.6686612668371,53.3672343739002));
#106842=CARTESIAN_POINT('Ctrl Pts',(3.22917445446895,29.7611800149765,53.349173449974));
#106843=CARTESIAN_POINT('Ctrl Pts',(3.23510297296059,29.842599846584,53.3394321656467));
#106844=CARTESIAN_POINT('Ctrl Pts',(3.2453972073933,29.9839539088188,53.3330107847476));
#106845=CARTESIAN_POINT('Ctrl Pts',(3.2497437502269,30.04361661882,53.3335041080862));
#106846=CARTESIAN_POINT('Ctrl Pts',(3.25792115360078,30.1569285241922,53.3405316204381));
#106847=CARTESIAN_POINT('Ctrl Pts',(3.26175709224196,30.2105415118794,53.346477979323));
#106848=CARTESIAN_POINT('Ctrl Pts',(3.26804866122616,30.2995237469021,53.3607464292378));
#106849=CARTESIAN_POINT('Ctrl Pts',(3.27054251608933,30.3350771148501,53.3676426796411));
#106850=CARTESIAN_POINT('Ctrl Pts',(3.27401105181878,30.3849012283676,53.3790037401622));
#106851=CARTESIAN_POINT('Ctrl Pts',(3.27501571520984,30.3993777957766,53.3825095885063));
#106852=CARTESIAN_POINT('Ctrl Pts',(3.27674331498653,30.4243423652611,53.3889109660382));
#106853=CARTESIAN_POINT('Ctrl Pts',(3.27746911128389,30.4348524062334,53.3917159104296));
#106854=CARTESIAN_POINT('Ctrl Pts',(3.27895236015647,30.4563716396816,53.3976853865388));
#106855=CARTESIAN_POINT('Ctrl Pts',(3.27970941238696,30.4673771962034,53.4008609311399));
#106856=CARTESIAN_POINT('Ctrl Pts',(3.28163677980139,30.4954448162457,53.4092740817893));
#106857=CARTESIAN_POINT('Ctrl Pts',(3.2828018047602,30.5124573361096,53.4146728944527));
#106858=CARTESIAN_POINT('Ctrl Pts',(3.28761811353891,30.5829226736348,53.4382875114647));
#106859=CARTESIAN_POINT('Ctrl Pts',(3.29118940451463,30.6355215500645,53.4589425391526));
#106860=CARTESIAN_POINT('Ctrl Pts',(3.30250392432469,30.8011028190942,53.5338881184471));
#106861=CARTESIAN_POINT('Ctrl Pts',(3.30996626207958,30.909032617586,53.5982487361089));
#106862=CARTESIAN_POINT('Ctrl Pts',(3.32066125008828,31.0452831200364,53.701905535497));
#106863=CARTESIAN_POINT('Ctrl Pts',(3.32357878701688,31.0806717960673,53.7312156670767));
#106864=CARTESIAN_POINT('Ctrl Pts',(3.32731472610871,31.1230393696455,53.7693654162959));
#106865=CARTESIAN_POINT('Ctrl Pts',(3.32804645879156,31.1312033393007,53.7768655457425));
#106866=CARTESIAN_POINT('Ctrl Pts',(3.3292246124801,31.1441219706879,53.7889736808378));
#106867=CARTESIAN_POINT('Ctrl Pts',(3.32966722735544,31.1489252291285,53.7935296756392));
#106868=CARTESIAN_POINT('Ctrl Pts',(3.33052191820137,31.1581012955926,53.8023378643225));
#106869=CARTESIAN_POINT('Ctrl Pts',(3.33093366719485,31.1624780971939,53.8065856248699));
#106870=CARTESIAN_POINT('Ctrl Pts',(3.33195040009536,31.1731806683872,53.8170873877078));
#106871=CARTESIAN_POINT('Ctrl Pts',(3.33255740227154,31.1794798064217,53.8233681517258));
#106872=CARTESIAN_POINT('Ctrl Pts',(3.33468528086541,31.2012587371824,53.8454341749122));
#106873=CARTESIAN_POINT('Ctrl Pts',(3.33622399157413,31.2164736499495,53.8614761565749));
#106874=CARTESIAN_POINT('Ctrl Pts',(3.34518700790741,31.3023029519025,53.9556559223591));
#106875=CARTESIAN_POINT('Ctrl Pts',(3.35292833181909,31.3656971655209,54.040043359502));
#106876=CARTESIAN_POINT('Ctrl Pts',(3.3676544003265,31.4717278134838,54.2131591836692));
#106877=CARTESIAN_POINT('Ctrl Pts',(3.37462543029682,31.5153361751184,54.3008124080588));
#106878=CARTESIAN_POINT('Ctrl Pts',(3.38281218895757,31.5588838560674,54.41186580207));
#106879=CARTESIAN_POINT('Ctrl Pts',(3.38427888458028,31.5663637237997,54.4320867391528));
#106880=CARTESIAN_POINT('Ctrl Pts',(3.38655788291962,31.5774717521726,54.464006849123));
#106881=CARTESIAN_POINT('Ctrl Pts',(3.3873789096106,31.5813667661031,54.4756099241933));
#106882=CARTESIAN_POINT('Ctrl Pts',(3.38890780464844,31.5884174094386,54.4974067532732));
#106883=CARTESIAN_POINT('Ctrl Pts',(3.389616644836,31.5916036295338,54.5075898723917));
#106884=CARTESIAN_POINT('Ctrl Pts',(3.39120125897616,31.5985383373874,54.5305239109813));
#106885=CARTESIAN_POINT('Ctrl Pts',(3.39207522842764,31.6022325485948,54.5432905830679));
#106886=CARTESIAN_POINT('Ctrl Pts',(3.39431006211169,31.6113374570936,54.5762269109505));
#106887=CARTESIAN_POINT('Ctrl Pts',(3.39566367665842,31.6165225243874,54.5964569144616));
#106888=CARTESIAN_POINT('Ctrl Pts',(3.40533445059828,31.6511211387637,54.7428365560153));
#106889=CARTESIAN_POINT('Ctrl Pts',(3.41316151932202,31.6661145849942,54.8719377554898));
#106890=CARTESIAN_POINT('Ctrl Pts',(3.42170261966234,31.6659904235466,55.0115057965245));
#106891=CARTESIAN_POINT('Ctrl Pts',(3.42231671609912,31.6658910431593,55.0215291638363));
#106892=CARTESIAN_POINT('Ctrl Pts',(3.42758549390243,31.6642652244521,55.1073626089405));
#106893=CARTESIAN_POINT('Ctrl Pts',(3.43229186060158,31.6576553938596,55.1829784297439));
#106894=CARTESIAN_POINT('Ctrl Pts',(3.4380460691107,31.6440199935811,55.2700096958341));
#106895=CARTESIAN_POINT('Ctrl Pts',(3.43885497469513,31.6419839622348,55.2821269591806));
#106896=CARTESIAN_POINT('Ctrl Pts',(3.44013282772137,31.6385863721852,55.3010631749777));
#106897=CARTESIAN_POINT('Ctrl Pts',(3.44059688965219,31.6373157829344,55.3078982900468));
#106898=CARTESIAN_POINT('Ctrl Pts',(3.44146962565931,31.6348588246095,55.3206700389454));
#106899=CARTESIAN_POINT('Ctrl Pts',(3.4418777237089,31.633682829636,55.3266084165438));
#106900=CARTESIAN_POINT('Ctrl Pts',(3.44284384765443,31.6308349267368,55.340589070502));
#106901=CARTESIAN_POINT('Ctrl Pts',(3.44340335671327,31.6291358758658,55.3486255356502));
#106902=CARTESIAN_POINT('Ctrl Pts',(3.44528687674318,31.623248403358,55.3754898845752));
#106903=CARTESIAN_POINT('Ctrl Pts',(3.44662441249491,31.6187926235885,55.3942567628162));
#106904=CARTESIAN_POINT('Ctrl Pts',(3.44995347821207,31.6070106220397,55.4403076373684));
#106905=CARTESIAN_POINT('Ctrl Pts',(3.45195955689978,31.5993144282699,55.4674902505505));
#106906=CARTESIAN_POINT('Ctrl Pts',(3.45602872890287,31.5824589863616,55.5217225823812));
#106907=CARTESIAN_POINT('Ctrl Pts',(3.45809077358494,31.573290843425,55.5487490034217));
#106908=CARTESIAN_POINT('Ctrl Pts',(3.46016014030872,31.5634377287949,55.5755158279149));
#106909=CARTESIAN_POINT('',(3.22999287141707,31.6660003168857,54.9993964881822));
#106910=CARTESIAN_POINT('Ctrl Pts',(3.26653908718979,31.5634376777881,55.5755159664792));
#106911=CARTESIAN_POINT('Ctrl Pts',(3.26610426703045,31.5657964878847,55.569108059845));
#106912=CARTESIAN_POINT('Ctrl Pts',(3.2656705388314,31.5681160028208,55.5626853798124));
#106913=CARTESIAN_POINT('Ctrl Pts',(3.26185959025895,31.5881978274955,55.5059905195));
#106914=CARTESIAN_POINT('Ctrl Pts',(3.25854924041725,31.6035775375029,55.4549048857212));
#106915=CARTESIAN_POINT('Ctrl Pts',(3.25151260756041,31.631268582732,55.3438786386606));
#106916=CARTESIAN_POINT('Ctrl Pts',(3.24780193291552,31.6427825896574,55.2838223117538));
#106917=CARTESIAN_POINT('Ctrl Pts',(3.23947063478459,31.6610074929674,55.1490576405224));
#106918=CARTESIAN_POINT('Ctrl Pts',(3.23484348653673,31.6660269351427,55.0742640495692));
#106919=CARTESIAN_POINT('Ctrl Pts',(3.22999372004333,31.6659998913039,54.9993981898735));
#106920=CARTESIAN_POINT('Ctrl Pts',(3.22999360673357,31.6659998906711,54.9993964407109));
#106921=CARTESIAN_POINT('Ctrl Pts',(3.22944625435921,31.6659968295913,54.9909469664633));
#106922=CARTESIAN_POINT('Ctrl Pts',(3.22889611782431,31.665929488637,54.9824977945502));
#106923=CARTESIAN_POINT('Ctrl Pts',(3.22781975627913,31.6656734189151,54.9660602298663));
#106924=CARTESIAN_POINT('Ctrl Pts',(3.22729387167398,31.6654914836522,54.9580719856899));
#106925=CARTESIAN_POINT('Ctrl Pts',(3.22635465675499,31.6650663378729,54.9438882199871));
#106926=CARTESIAN_POINT('Ctrl Pts',(3.22594251123523,31.6648459880331,54.9376920993005));
#106927=CARTESIAN_POINT('Ctrl Pts',(3.22514987919618,31.6643579486853,54.9258328877708));
#106928=CARTESIAN_POINT('Ctrl Pts',(3.22476970234351,31.6640959248837,54.9201695956893));
#106929=CARTESIAN_POINT('Ctrl Pts',(3.22394833587324,31.6634701117978,54.9079903461829));
#106930=CARTESIAN_POINT('Ctrl Pts',(3.22350664129181,31.6630969373089,54.9014750657985));
#106931=CARTESIAN_POINT('Ctrl Pts',(3.22233805425277,31.6620133732046,54.8843228801411));
#106932=CARTESIAN_POINT('Ctrl Pts',(3.22160780912958,31.6612391601384,54.8736905120352));
#106933=CARTESIAN_POINT('Ctrl Pts',(3.21836849965964,31.6573778981183,54.8268714064288));
#106934=CARTESIAN_POINT('Ctrl Pts',(3.2158095147202,31.6532102762678,54.7907863561573));
#106935=CARTESIAN_POINT('Ctrl Pts',(3.20797664671837,31.6370635512358,54.6822414682852));
#106936=CARTESIAN_POINT('Ctrl Pts',(3.20261267191694,31.621470453918,54.6104100660507));
#106937=CARTESIAN_POINT('Ctrl Pts',(3.18901679655734,31.5698386859,54.4307483437689));
#106938=CARTESIAN_POINT('Ctrl Pts',(3.18087215203561,31.5274134839663,54.3251238290562));
#106939=CARTESIAN_POINT('Ctrl Pts',(3.17168389567752,31.4650118142507,54.206452432826));
#106940=CARTESIAN_POINT('Ctrl Pts',(3.17028884243349,31.4551229572515,54.1884615832385));
#106941=CARTESIAN_POINT('Ctrl Pts',(3.16809563275909,31.438920359593,54.16023296824));
#106942=CARTESIAN_POINT('Ctrl Pts',(3.16728980407335,31.4328242176489,54.1498733957147));
#106943=CARTESIAN_POINT('Ctrl Pts',(3.16577459790435,31.4210926113148,54.1304218365937));
#106944=CARTESIAN_POINT('Ctrl Pts',(3.16506441320801,31.4154806941634,54.1213164359299));
#106945=CARTESIAN_POINT('Ctrl Pts',(3.16345742492406,31.4025264738042,54.1007442727398));
#106946=CARTESIAN_POINT('Ctrl Pts',(3.16256265628449,31.3951304473644,54.0893121139253));
#106947=CARTESIAN_POINT('Ctrl Pts',(3.16023468771261,31.3754145265064,54.0596408888545));
#106948=CARTESIAN_POINT('Ctrl Pts',(3.15880982704021,31.3628716677318,54.0415526790033));
#106949=CARTESIAN_POINT('Ctrl Pts',(3.15015445315678,31.283853656419,53.9322889758917));
#106950=CARTESIAN_POINT('Ctrl Pts',(3.14327792943381,31.2086154424092,53.8478110738396));
#106951=CARTESIAN_POINT('Ctrl Pts',(3.13044718459681,31.0537023702456,53.7058885608238));
#106952=CARTESIAN_POINT('Ctrl Pts',(3.12451208724406,30.9763924990241,53.6466095846522));
#106953=CARTESIAN_POINT('Ctrl Pts',(3.11725516956851,30.882278959991,53.5867253749865));
#106954=CARTESIAN_POINT('Ctrl Pts',(3.11631468519567,30.870091269779,53.5791894998109));
#106955=CARTESIAN_POINT('Ctrl Pts',(3.11488026934627,30.8515478539379,53.5680518213126));
#106956=CARTESIAN_POINT('Ctrl Pts',(3.11439349757838,30.845262795309,53.5643328603626));
#106957=CARTESIAN_POINT('Ctrl Pts',(3.11350154655221,30.8337650922628,53.5576311712793));
#106958=CARTESIAN_POINT('Ctrl Pts',(3.11309722308082,30.8285605044065,53.5546351484413));
#106959=CARTESIAN_POINT('Ctrl Pts',(3.11217037658896,30.8166463855088,53.5478622787772));
#106960=CARTESIAN_POINT('Ctrl Pts',(3.11164674768942,30.8099268230292,53.544103775739));
#106961=CARTESIAN_POINT('Ctrl Pts',(3.11000083133167,30.7888334572667,53.5324966835846));
#106962=CARTESIAN_POINT('Ctrl Pts',(3.1088691140153,30.7743703147326,53.5248136481837));
#106963=CARTESIAN_POINT('Ctrl Pts',(3.10208074778319,30.687724397871,53.4804113270766));
#106964=CARTESIAN_POINT('Ctrl Pts',(3.09620202750226,30.6130613270886,53.4487850172177));
#106965=CARTESIAN_POINT('Ctrl Pts',(3.08494313061414,30.4666078721951,53.3989791149915));
#106966=CARTESIAN_POINT('Ctrl Pts',(3.07957728196145,30.3953096316626,53.3799004998563));
#106967=CARTESIAN_POINT('Ctrl Pts',(3.07128440049202,30.2813036242831,53.3573713465668));
#106968=CARTESIAN_POINT('Ctrl Pts',(3.06828938676094,30.2393263287214,53.3507322740104));
#106969=CARTESIAN_POINT('Ctrl Pts',(3.06321778836286,30.1667666607243,53.3420855259456));
#106970=CARTESIAN_POINT('Ctrl Pts',(3.06111973650694,30.1362997298789,53.3393031224058));
#106971=CARTESIAN_POINT('Ctrl Pts',(3.05810102127006,30.091825577335,53.3364738224719));
#106972=CARTESIAN_POINT('Ctrl Pts',(3.05715992828005,30.0778685421131,53.3357620991018));
#106973=CARTESIAN_POINT('Ctrl Pts',(3.05550546941852,30.0531747294682,53.3348142051769));
#106974=CARTESIAN_POINT('Ctrl Pts',(3.05478989953064,30.0424416922831,53.3345060807169));
#106975=CARTESIAN_POINT('Ctrl Pts',(3.05329315273818,30.0198850563073,53.3340767200262));
#106976=CARTESIAN_POINT('Ctrl Pts',(3.05251270364678,30.0080615973514,53.3339775472694));
#106977=CARTESIAN_POINT('Ctrl Pts',(3.05044858315771,29.9766359979648,53.3340485130381));
#106978=CARTESIAN_POINT('Ctrl Pts',(3.04917179384185,29.9570358455797,53.3344387229689));
#106979=CARTESIAN_POINT('Ctrl Pts',(3.04257019029153,29.8549561663917,53.3382742283473));
#106980=CARTESIAN_POINT('Ctrl Pts',(3.0374286121493,29.7728050168556,53.3475003235681));
#106981=CARTESIAN_POINT('Ctrl Pts',(3.02620358572786,29.5932013787038,53.3813244962504));
#106982=CARTESIAN_POINT('Ctrl Pts',(3.02017876609559,29.4966152516834,53.4087121705521));
#106983=CARTESIAN_POINT('Ctrl Pts',(3.01212508639738,29.3766796929032,53.4547403165617));
#106984=CARTESIAN_POINT('Ctrl Pts',(3.01033233590518,29.3505420139992,53.4655424937043));
#106985=CARTESIAN_POINT('Ctrl Pts',(3.00726507334515,29.3070480101583,53.4848280240195));
#106986=CARTESIAN_POINT('Ctrl Pts',(3.00600688656322,29.2895408219206,53.4929577791572));
#106987=CARTESIAN_POINT('Ctrl Pts',(3.00418874694282,29.2647901408738,53.5049782779568));
#106988=CARTESIAN_POINT('Ctrl Pts',(3.00364284317889,29.257427364817,53.5086216573862));
#106989=CARTESIAN_POINT('Ctrl Pts',(3.00268894182674,29.2446875114186,53.5150435443472));
#106990=CARTESIAN_POINT('Ctrl Pts',(3.00228247342119,29.2392981416458,53.517797142107));
#106991=CARTESIAN_POINT('Ctrl Pts',(3.00140532337214,29.2277540232609,53.5237749414149));
#106992=CARTESIAN_POINT('Ctrl Pts',(3.00093411632965,29.2216044962385,53.5270082459475));
#106993=CARTESIAN_POINT('Ctrl Pts',(2.9996242585279,29.2046483340678,53.5360593053381));
#106994=CARTESIAN_POINT('Ctrl Pts',(2.99878086378888,29.1938857409914,53.5419580220997));
#106995=CARTESIAN_POINT('Ctrl Pts',(2.99289408307777,29.1197662669068,53.5836525831057));
#106996=CARTESIAN_POINT('Ctrl Pts',(2.98765082980358,29.0587552784197,53.6234436232251));
#106997=CARTESIAN_POINT('Ctrl Pts',(2.98135709746304,28.9894379669817,53.6754196156919));
#106998=CARTESIAN_POINT('Ctrl Pts',(2.98034696811561,28.9784329928107,53.6838884305932));
#106999=CARTESIAN_POINT('Ctrl Pts',(2.97386431526517,28.9085277927202,53.7390886700488));
#107000=CARTESIAN_POINT('Ctrl Pts',(2.96839083863729,28.8527384250328,53.7896276440894));
#107001=CARTESIAN_POINT('Ctrl Pts',(2.9600254768904,28.7713493275451,53.8740586261583));
#107002=CARTESIAN_POINT('Ctrl Pts',(2.95706002226077,28.7433035656484,53.9054494014103));
#107003=CARTESIAN_POINT('Ctrl Pts',(2.95203237405372,28.697109961684,53.9612718610856));
#107004=CARTESIAN_POINT('Ctrl Pts',(2.94994921517149,28.678387924918,53.9851993642137));
#107005=CARTESIAN_POINT('Ctrl Pts',(2.94694762549407,28.6520443636831,54.0208341053681));
#107006=CARTESIAN_POINT('Ctrl Pts',(2.94600909136777,28.6438999581359,54.0321451846255));
#107007=CARTESIAN_POINT('Ctrl Pts',(2.9443575149301,28.6297368585232,54.0523449436327));
#107008=CARTESIAN_POINT('Ctrl Pts',(2.9436422946478,28.6236604205636,54.0611919503485));
#107009=CARTESIAN_POINT('Ctrl Pts',(2.94214469650621,28.611060010307,54.0799228636113));
#107010=CARTESIAN_POINT('Ctrl Pts',(2.94136306172215,28.6045550567397,54.0898188892371));
#107011=CARTESIAN_POINT('Ctrl Pts',(2.93929208467216,28.5875167798997,54.1163514063674));
#107012=CARTESIAN_POINT('Ctrl Pts',(2.93800970825652,28.5771717322979,54.1331070089019));
#107013=CARTESIAN_POINT('Ctrl Pts',(2.93117728150452,28.5232266526374,54.2240486481736));
#107014=CARTESIAN_POINT('Ctrl Pts',(2.92582806964664,28.4851239674327,54.3013489112153));
#107015=CARTESIAN_POINT('Ctrl Pts',(2.91458588276082,28.4170642128829,54.4714959253409));
#107016=CARTESIAN_POINT('Ctrl Pts',(2.90873407783388,28.3889358859035,54.5647156968043));
#107017=CARTESIAN_POINT('Ctrl Pts',(2.90088882838858,28.3633995412924,54.6871535286934));
#107018=CARTESIAN_POINT('Ctrl Pts',(2.89911969706786,28.3583916357568,54.7145954093701));
#107019=CARTESIAN_POINT('Ctrl Pts',(2.89608879704332,28.351117483773,54.7610279685365));
#107020=CARTESIAN_POINT('Ctrl Pts',(2.8948428542756,28.3484850138574,54.7799560068179));
#107021=CARTESIAN_POINT('Ctrl Pts',(2.89303935152854,28.3451912035126,54.8070471412584));
#107022=CARTESIAN_POINT('Ctrl Pts',(2.89249553452392,28.3442634723556,54.8151771044148));
#107023=CARTESIAN_POINT('Ctrl Pts',(2.89154398184076,28.3427542405423,54.8293275797033));
#107024=CARTESIAN_POINT('Ctrl Pts',(2.89113775191381,28.3421455742041,54.8353449552002));
#107025=CARTESIAN_POINT('Ctrl Pts',(2.89025956765069,28.3409063533848,54.8483002949875));
#107026=CARTESIAN_POINT('Ctrl Pts',(2.88978707286325,28.340286552025,54.8552388349163));
#107027=CARTESIAN_POINT('Ctrl Pts',(2.88847022316319,28.3386881860321,54.8744941526137));
#107028=CARTESIAN_POINT('Ctrl Pts',(2.88762104546219,28.3378031218823,54.8868179483406));
#107029=CARTESIAN_POINT('Ctrl Pts',(2.88112077333767,28.3321196560862,54.9805342419203));
#107030=CARTESIAN_POINT('Ctrl Pts',(2.87521974773726,28.3331656720694,55.0621623683281));
#107031=CARTESIAN_POINT('Ctrl Pts',(2.86495103515304,28.3453134726731,55.2027938404641));
#107032=CARTESIAN_POINT('Ctrl Pts',(2.86060273911687,28.3536330663101,55.2618954082176));
#107033=CARTESIAN_POINT('Ctrl Pts',(2.85240635342677,28.375515817583,55.3735472215677));
#107034=CARTESIAN_POINT('Ctrl Pts',(2.84855362817948,28.3885110195655,55.4261344838264));
#107035=CARTESIAN_POINT('Ctrl Pts',(2.84223842724568,28.4144620106634,55.5127801267044));
#107036=CARTESIAN_POINT('Ctrl Pts',(2.83973733851493,28.4260137041177,55.5472126344215));
#107037=CARTESIAN_POINT('Ctrl Pts',(2.83626087343051,28.4438829990229,55.5952126432583));
#107038=CARTESIAN_POINT('Ctrl Pts',(2.83525532147062,28.4492711499528,55.6091126908437));
#107039=CARTESIAN_POINT('Ctrl Pts',(2.8335268665955,28.458912294769,55.6330268485495));
#107040=CARTESIAN_POINT('Ctrl Pts',(2.83280109276724,28.4630780702189,55.6430748771489));
#107041=CARTESIAN_POINT('Ctrl Pts',(2.83140944006814,28.4712915149809,55.6623502656591));
#107042=CARTESIAN_POINT('Ctrl Pts',(2.83074312094827,28.4753250595583,55.6715830850484));
#107043=CARTESIAN_POINT('Ctrl Pts',(2.82898675566258,28.4862232765387,55.6959248624893));
#107044=CARTESIAN_POINT('Ctrl Pts',(2.82790161495484,28.4932304757536,55.7109690682439));
#107045=CARTESIAN_POINT('Ctrl Pts',(2.82389877873612,28.5200840665376,55.7664417663029));
#107046=CARTESIAN_POINT('Ctrl Pts',(2.82102973601192,28.5413433076273,55.8061670747001));
#107047=CARTESIAN_POINT('Ctrl Pts',(2.81110653575018,28.6214991568649,55.9423691996979));
#107048=CARTESIAN_POINT('Ctrl Pts',(2.80431620736474,28.688567738787,56.0336683329275));
#107049=CARTESIAN_POINT('Ctrl Pts',(2.79442207206462,28.7964541714676,56.1529624923979));
#107050=CARTESIAN_POINT('Ctrl Pts',(2.79145131585022,28.8300574893814,56.1870463186561));
#107051=CARTESIAN_POINT('Ctrl Pts',(2.78720342425234,28.8788932887346,56.2324901074083));
#107052=CARTESIAN_POINT('Ctrl Pts',(2.78599026920631,28.8929252320497,56.2451094401012));
#107053=CARTESIAN_POINT('Ctrl Pts',(2.783834156443,28.9179382289738,56.2668472426611));
#107054=CARTESIAN_POINT('Ctrl Pts',(2.78289752377072,28.9288279736686,56.2760682071113));
#107055=CARTESIAN_POINT('Ctrl Pts',(2.78146781171153,28.9454585764189,56.28978740258));
#107056=CARTESIAN_POINT('Ctrl Pts',(2.78098182185311,28.9511130561891,56.2943899458835));
#107057=CARTESIAN_POINT('Ctrl Pts',(2.780090597682,28.9614804595104,56.3027161009907));
#107058=CARTESIAN_POINT('Ctrl Pts',(2.77968620990052,28.966183547632,56.3064515356395));
#107059=CARTESIAN_POINT('Ctrl Pts',(2.77875829834379,28.976973031557,56.314926357589));
#107060=CARTESIAN_POINT('Ctrl Pts',(2.77823365791272,28.9830721907153,56.3196489415116));
#107061=CARTESIAN_POINT('Ctrl Pts',(2.77658132671932,29.0022841383563,56.3343124925949));
#107062=CARTESIAN_POINT('Ctrl Pts',(2.77544410510628,29.0155110958333,56.3441013039572));
#107063=CARTESIAN_POINT('Ctrl Pts',(2.76848716838464,29.0965746376666,56.4022551531613));
#107064=CARTESIAN_POINT('Ctrl Pts',(2.76243293500468,29.1678102502294,56.4456675084561));
#107065=CARTESIAN_POINT('Ctrl Pts',(2.74992033862268,29.3208844366412,56.5238793235253));
#107066=CARTESIAN_POINT('Ctrl Pts',(2.74348287288277,29.4028809997553,56.5578375837998));
#107067=CARTESIAN_POINT('Ctrl Pts',(2.73373856018003,29.5341394610491,56.6003013130221));
#107068=CARTESIAN_POINT('Ctrl Pts',(2.73031112311749,29.5817381565389,56.6133964875471));
#107069=CARTESIAN_POINT('Ctrl Pts',(2.72581910047962,29.64605340353,56.6280521815794));
#107070=CARTESIAN_POINT('Ctrl Pts',(2.72469529579295,29.6623091435252,56.6315014616292));
#107071=CARTESIAN_POINT('Ctrl Pts',(2.72282713652296,29.6896017220355,56.6368672209045));
#107072=CARTESIAN_POINT('Ctrl Pts',(2.72207860831648,29.7006108758323,56.6389165789433));
#107073=CARTESIAN_POINT('Ctrl Pts',(2.72060770965235,29.7223859096299,56.6427432713776));
#107074=CARTESIAN_POINT('Ctrl Pts',(2.71988519772299,29.7331502299482,56.6445261471513));
#107075=CARTESIAN_POINT('Ctrl Pts',(2.71829434589841,29.7569973567743,56.6482355906932));
#107076=CARTESIAN_POINT('Ctrl Pts',(2.71742760742161,29.7700872368508,56.6501124158597));
#107077=CARTESIAN_POINT('Ctrl Pts',(2.71487975612785,29.8088381245535,56.655198434563));
#107078=CARTESIAN_POINT('Ctrl Pts',(2.71321229972178,29.8345537499226,56.6579663365107));
#107079=CARTESIAN_POINT('Ctrl Pts',(2.70239519965883,30.0033581612133,56.672168699889));
#107080=CARTESIAN_POINT('Ctrl Pts',(2.69383560305068,30.1473400697987,56.6656683525366));
#107081=CARTESIAN_POINT('Ctrl Pts',(2.68230533942275,30.3313663860346,56.633287556543));
#107082=CARTESIAN_POINT('Ctrl Pts',(2.67960485524833,30.373711324652,56.6241216907912));
#107083=CARTESIAN_POINT('Ctrl Pts',(2.67518111768609,30.4408283217483,56.6068299612183));
#107084=CARTESIAN_POINT('Ctrl Pts',(2.67349910458422,30.4658516583023,56.5997544148883));
#107085=CARTESIAN_POINT('Ctrl Pts',(2.67118053179044,30.4994914333947,56.5893863556519));
#107086=CARTESIAN_POINT('Ctrl Pts',(2.67057064858865,30.5082625215215,56.5866032519627));
#107087=CARTESIAN_POINT('Ctrl Pts',(2.66954182784076,30.5229191861294,56.5818186262539));
#107088=CARTESIAN_POINT('Ctrl Pts',(2.66912514071762,30.5288175982171,56.5798565085947));
#107089=CARTESIAN_POINT('Ctrl Pts',(2.6683206113678,30.5401305370615,56.5760227859248));
#107090=CARTESIAN_POINT('Ctrl Pts',(2.66793309463653,30.5455466087627,56.5741561911006));
#107091=CARTESIAN_POINT('Ctrl Pts',(2.66687209972316,30.5602886939326,56.5689902613267));
#107092=CARTESIAN_POINT('Ctrl Pts',(2.66619552454134,30.569594939344,56.5656357985697));
#107093=CARTESIAN_POINT('Ctrl Pts',(2.6635033370614,30.6062756534328,56.5520438135286));
#107094=CARTESIAN_POINT('Ctrl Pts',(2.6614557153734,30.6334069519871,56.5411701896093));
#107095=CARTESIAN_POINT('Ctrl Pts',(2.6515659254076,30.7614462791947,56.4859029450022));
#107096=CARTESIAN_POINT('Ctrl Pts',(2.64344117357296,30.8580676792771,56.4322804830139));
#107097=CARTESIAN_POINT('Ctrl Pts',(2.63127095580434,30.996582925341,56.3363284610601));
#107098=CARTESIAN_POINT('Ctrl Pts',(2.62711151325164,31.0427120272375,56.300655238638));
#107099=CARTESIAN_POINT('Ctrl Pts',(2.62036560635973,31.1158043504782,56.2377370993233));
#107100=CARTESIAN_POINT('Ctrl Pts',(2.61773318828583,31.1438658827417,56.2118513631203));
#107101=CARTESIAN_POINT('Ctrl Pts',(2.61410981907972,31.1818154865199,56.1743503280618));
#107102=CARTESIAN_POINT('Ctrl Pts',(2.6130851363498,31.1924693439305,56.1635305872637));
#107103=CARTESIAN_POINT('Ctrl Pts',(2.61133433434729,31.2105319151769,56.1446780458907));
#107104=CARTESIAN_POINT('Ctrl Pts',(2.61060514115145,31.218012096855,56.1367153945103));
#107105=CARTESIAN_POINT('Ctrl Pts',(2.60921397460609,31.2321976134097,56.1213141018225));
#107106=CARTESIAN_POINT('Ctrl Pts',(2.60855149694907,31.238915234735,56.113887481748));
#107107=CARTESIAN_POINT('Ctrl Pts',(2.606821103123,31.2563589197377,56.0942496994622));
#107108=CARTESIAN_POINT('Ctrl Pts',(2.60575781323695,31.2669741422331,56.08194116913));
#107109=CARTESIAN_POINT('Ctrl Pts',(2.60193832302589,31.3047017734345,56.0368785012215));
#107110=CARTESIAN_POINT('Ctrl Pts',(2.59922496084412,31.3307392569159,56.003243361325));
#107111=CARTESIAN_POINT('Ctrl Pts',(2.58929244575557,31.4225128198616,55.8748211975686));
#107112=CARTESIAN_POINT('Ctrl Pts',(2.58236290164678,31.4796386600055,55.7742899947083));
#107113=CARTESIAN_POINT('Ctrl Pts',(2.57321247415541,31.5393658010715,55.6379893698703));
#107114=CARTESIAN_POINT('Ctrl Pts',(2.5711402764649,31.5518752793647,55.6069261964945));
#107115=CARTESIAN_POINT('Ctrl Pts',(2.56903902087732,31.5634376730794,55.5755159792709));
#107116=CARTESIAN_POINT('Origin',(5.,30.,55.));
#107117=CARTESIAN_POINT('',(1.86810672180998,31.5634374966623,55.5755164585225));
#107118=CARTESIAN_POINT('',(2.06220431895159,31.5634376782779,55.5755159651488));
#107119=CARTESIAN_POINT('',(5.,31.5634376782623,55.5755159651912));
#107120=CARTESIAN_POINT('',(2.72303746985885,31.6659995411549,54.9999657602353));
#107121=CARTESIAN_POINT('Ctrl Pts',(2.06220431895159,31.5634376782779,55.5755159651488));
#107122=CARTESIAN_POINT('Ctrl Pts',(2.06232540429763,31.5627902658092,55.5772747157451));
#107123=CARTESIAN_POINT('Ctrl Pts',(2.06244639919516,31.5621398792575,55.5790323912606));
#107124=CARTESIAN_POINT('Ctrl Pts',(2.0692563660251,31.5253396178637,55.6779721330753));
#107125=CARTESIAN_POINT('Ctrl Pts',(2.07563303263128,31.4801978116672,55.7715732829012));
#107126=CARTESIAN_POINT('Ctrl Pts',(2.08880065368226,31.368895752159,55.956129126645));
#107127=CARTESIAN_POINT('Ctrl Pts',(2.09555586961352,31.3016663470947,56.0458088321837));
#107128=CARTESIAN_POINT('Ctrl Pts',(2.10378745721772,31.2158931193864,56.1390266486023));
#107129=CARTESIAN_POINT('Ctrl Pts',(2.10476405948136,31.2056632308649,56.1498495206366));
#107130=CARTESIAN_POINT('Ctrl Pts',(2.10624261757951,31.1901238226439,56.1658543175442));
#107131=CARTESIAN_POINT('Ctrl Pts',(2.10673674116683,31.1849222201491,56.1711406106491));
#107132=CARTESIAN_POINT('Ctrl Pts',(2.10763582711352,31.175446637847,56.180642723389));
#107133=CARTESIAN_POINT('Ctrl Pts',(2.10803984872027,31.1711849345059,56.1848704084022));
#107134=CARTESIAN_POINT('Ctrl Pts',(2.1089579113828,31.1614929324864,56.1943816683135));
#107135=CARTESIAN_POINT('Ctrl Pts',(2.10947296534857,31.1560494206872,56.1996512547932));
#107136=CARTESIAN_POINT('Ctrl Pts',(2.11106463315109,31.1392031375439,56.2157381499317));
#107137=CARTESIAN_POINT('Ctrl Pts',(2.11214984141663,31.1276834487795,56.2264310141797));
#107138=CARTESIAN_POINT('Ctrl Pts',(2.11778809318652,31.0675774153764,56.2806601597612));
#107139=CARTESIAN_POINT('Ctrl Pts',(2.12248677020479,31.0166194999587,56.3214745987046));
#107140=CARTESIAN_POINT('Ctrl Pts',(2.13556736520961,30.8696443067331,56.4256517293417));
#107141=CARTESIAN_POINT('Ctrl Pts',(2.14397173822651,30.7692440274854,56.4822394713103));
#107142=CARTESIAN_POINT('Ctrl Pts',(2.15507110839096,30.624442798128,56.5451438230635));
#107143=CARTESIAN_POINT('Ctrl Pts',(2.1580434821902,30.5844267309309,56.5607191329328));
#107144=CARTESIAN_POINT('Ctrl Pts',(2.16207539005294,30.5284319188495,56.5800575279464));
#107145=CARTESIAN_POINT('Ctrl Pts',(2.16317814180095,30.512935607371,56.5851558850938));
#107146=CARTESIAN_POINT('Ctrl Pts',(2.16494665405738,30.4877970899146,56.5930193128866));
#107147=CARTESIAN_POINT('Ctrl Pts',(2.16561701565783,30.4782007523768,56.5959262452181));
#107148=CARTESIAN_POINT('Ctrl Pts',(2.16701157104049,30.4580993054746,56.6018178032274));
#107149=CARTESIAN_POINT('Ctrl Pts',(2.16773520592432,30.4475898883431,56.6047861383744));
#107150=CARTESIAN_POINT('Ctrl Pts',(2.1694543836726,30.4224394307187,56.6116234765641));
#107151=CARTESIAN_POINT('Ctrl Pts',(2.17044679570398,30.4077731709646,56.6153966598869));
#107152=CARTESIAN_POINT('Ctrl Pts',(2.17389927620722,30.3562599329835,56.6279031612635));
#107153=CARTESIAN_POINT('Ctrl Pts',(2.17632582431559,30.3191669303792,56.6355802197411));
#107154=CARTESIAN_POINT('Ctrl Pts',(2.182362810349,30.225083285305,56.6517293966722));
#107155=CARTESIAN_POINT('Ctrl Pts',(2.18592659607798,30.1678545427402,56.6585228573174));
#107156=CARTESIAN_POINT('Ctrl Pts',(2.19615443991781,30.0015118365955,56.6695686655818));
#107157=CARTESIAN_POINT('Ctrl Pts',(2.20270356128101,29.8922012011302,56.6660843688747));
#107158=CARTESIAN_POINT('Ctrl Pts',(2.21158303835314,29.7532908855624,56.6479233778603));
#107159=CARTESIAN_POINT('Ctrl Pts',(2.21357661494237,29.7226753163071,56.6430482587471));
#107160=CARTESIAN_POINT('Ctrl Pts',(2.21627674049872,29.6822823236471,56.6354551784842));
#107161=CARTESIAN_POINT('Ctrl Pts',(2.21694522979157,29.6723662571569,56.6334975606553));
#107162=CARTESIAN_POINT('Ctrl Pts',(2.21800325380079,29.6568166465546,56.6302804978471));
#107163=CARTESIAN_POINT('Ctrl Pts',(2.21838944968555,29.6511705922984,56.6290817528651));
#107164=CARTESIAN_POINT('Ctrl Pts',(2.21919302385363,29.6394872564652,56.6265376787553));
#107165=CARTESIAN_POINT('Ctrl Pts',(2.21961066290857,29.6334511193051,56.6251880419655));
#107166=CARTESIAN_POINT('Ctrl Pts',(2.22064278062039,29.6186190682315,56.6217848720257));
#107167=CARTESIAN_POINT('Ctrl Pts',(2.22125934184864,29.6098321469426,56.6196933732738));
#107168=CARTESIAN_POINT('Ctrl Pts',(2.22357638913647,29.5770675073683,56.6116125185774));
#107169=CARTESIAN_POINT('Ctrl Pts',(2.22529981193475,29.553208261852,56.6051616082514));
#107170=CARTESIAN_POINT('Ctrl Pts',(2.22987510543446,29.4909791340074,56.5868416629499));
#107171=CARTESIAN_POINT('Ctrl Pts',(2.23275733939101,29.4528803159673,56.5741119254505));
#107172=CARTESIAN_POINT('Ctrl Pts',(2.24419459540176,29.3048255743947,56.5186187630342));
#107173=CARTESIAN_POINT('Ctrl Pts',(2.25285973217857,29.1990648359915,56.4655984032174));
#107174=CARTESIAN_POINT('Ctrl Pts',(2.26476836567766,29.0574037426249,56.3746292807991));
#107175=CARTESIAN_POINT('Ctrl Pts',(2.26827238203317,29.0162710885428,56.345500540494));
#107176=CARTESIAN_POINT('Ctrl Pts',(2.2728789672711,28.9629495293853,56.3039854385422));
#107177=CARTESIAN_POINT('Ctrl Pts',(2.2740429137102,28.9495450536394,56.2932115630105));
#107178=CARTESIAN_POINT('Ctrl Pts',(2.2759592062457,28.9275981007034,56.2750052057164));
#107179=CARTESIAN_POINT('Ctrl Pts',(2.27671619512917,28.9189605493326,56.2676899562755));
#107180=CARTESIAN_POINT('Ctrl Pts',(2.27819882052242,28.9021103634607,56.2531218504513));
#107181=CARTESIAN_POINT('Ctrl Pts',(2.27892464645223,28.8938934120145,56.2458748941433));
#107182=CARTESIAN_POINT('Ctrl Pts',(2.28065894651848,28.8743421507444,56.2282857190393));
#107183=CARTESIAN_POINT('Ctrl Pts',(2.28166414082456,28.8630779233587,56.2178668312642));
#107184=CARTESIAN_POINT('Ctrl Pts',(2.28521842693762,28.8235149853102,56.1802455923551));
#107185=CARTESIAN_POINT('Ctrl Pts',(2.28773119898034,28.7960342589038,56.1521994274092));
#107186=CARTESIAN_POINT('Ctrl Pts',(2.29404930433798,28.7285906386371,56.0783174165078));
#107187=CARTESIAN_POINT('Ctrl Pts',(2.29780172839346,28.6900982352185,56.0312169440984));
#107188=CARTESIAN_POINT('Ctrl Pts',(2.30694124963367,28.6021546988718,55.9107130399362));
#107189=CARTESIAN_POINT('Ctrl Pts',(2.31227860491102,28.5558135544345,55.8352805588255));
#107190=CARTESIAN_POINT('Ctrl Pts',(2.32057073070602,28.4955949243702,55.7171312077826));
#107191=CARTESIAN_POINT('Ctrl Pts',(2.32338154721156,28.4770912611605,55.6769490630186));
#107192=CARTESIAN_POINT('Ctrl Pts',(2.32701979222787,28.4558797041877,55.6256014025907));
#107193=CARTESIAN_POINT('Ctrl Pts',(2.32776792652735,28.4516572204354,55.6150765988106));
#107194=CARTESIAN_POINT('Ctrl Pts',(2.32896628765358,28.4451203323608,55.5982890483825));
#107195=CARTESIAN_POINT('Ctrl Pts',(2.32941247766674,28.4427354787605,55.592053860074));
#107196=CARTESIAN_POINT('Ctrl Pts',(2.33027364152953,28.4382280083915,55.5800534364318));
#107197=CARTESIAN_POINT('Ctrl Pts',(2.33068828068522,28.436099716354,55.574290554183));
#107198=CARTESIAN_POINT('Ctrl Pts',(2.33170146322498,28.4309999000106,55.5602429418544));
#107199=CARTESIAN_POINT('Ctrl Pts',(2.33230191906718,28.4280620889743,55.5519462500468));
#107200=CARTESIAN_POINT('Ctrl Pts',(2.33448864828343,28.4176626624701,55.5218205916539));
#107201=CARTESIAN_POINT('Ctrl Pts',(2.33609476245566,28.4105892768647,55.4998615833911));
#107202=CARTESIAN_POINT('Ctrl Pts',(2.34689949531901,28.3665701099992,55.3528105654454));
#107203=CARTESIAN_POINT('Ctrl Pts',(2.3565633048541,28.3439692621466,55.2238999392736));
#107204=CARTESIAN_POINT('Ctrl Pts',(2.37140380373618,28.3323620291091,55.0177874383956));
#107205=CARTESIAN_POINT('Ctrl Pts',(2.37676301517307,28.3332859493035,54.9416904755232));
#107206=CARTESIAN_POINT('Ctrl Pts',(2.38328526312079,28.3409599723459,54.846652124405));
#107207=CARTESIAN_POINT('Ctrl Pts',(2.3845966977376,28.3428502146688,54.8274195032873));
#107208=CARTESIAN_POINT('Ctrl Pts',(2.38668986434178,28.3464291687937,54.7965351221572));
#107209=CARTESIAN_POINT('Ctrl Pts',(2.38747810704083,28.3479074508192,54.7848612736721));
#107210=CARTESIAN_POINT('Ctrl Pts',(2.38897950539198,28.3509736779068,54.7625470581729));
#107211=CARTESIAN_POINT('Ctrl Pts',(2.38969326231711,28.3525412411101,54.7519045394426));
#107212=CARTESIAN_POINT('Ctrl Pts',(2.39133541711911,28.3564020907914,54.7273448410855));
#107213=CARTESIAN_POINT('Ctrl Pts',(2.39226143663871,28.358769272765,54.713439983484));
#107214=CARTESIAN_POINT('Ctrl Pts',(2.39522661232573,28.3669611969427,54.6687578782081));
#107215=CARTESIAN_POINT('Ctrl Pts',(2.3972439680344,28.3734775612873,54.6381132316702));
#107216=CARTESIAN_POINT('Ctrl Pts',(2.40866426114851,28.4157197191725,54.4637803802679));
#107217=CARTESIAN_POINT('Ctrl Pts',(2.41745314600417,28.4696054994871,54.3251910621148));
#107218=CARTESIAN_POINT('Ctrl Pts',(2.43006580999499,28.5678372695841,54.147044230671));
#107219=CARTESIAN_POINT('Ctrl Pts',(2.43355478808953,28.5969805827967,54.0999117734772));
#107220=CARTESIAN_POINT('Ctrl Pts',(2.43796010627278,28.6352253575784,54.0444424581536));
#107221=CARTESIAN_POINT('Ctrl Pts',(2.43875089438252,28.6421442394223,54.0346359477472));
#107222=CARTESIAN_POINT('Ctrl Pts',(2.44000179015747,28.6531593556398,54.0193763319056));
#107223=CARTESIAN_POINT('Ctrl Pts',(2.44045723538463,28.6571843152702,54.0138719492775));
#107224=CARTESIAN_POINT('Ctrl Pts',(2.44132385619027,28.6648672601333,54.0034992989771));
#107225=CARTESIAN_POINT('Ctrl Pts',(2.4417345686675,28.6685182948526,53.9986261716564));
#107226=CARTESIAN_POINT('Ctrl Pts',(2.44272092878818,28.6773113839332,53.9870229219868));
#107227=CARTESIAN_POINT('Ctrl Pts',(2.44329824605438,28.6824781531593,53.9803118559885));
#107228=CARTESIAN_POINT('Ctrl Pts',(2.4453090611323,28.7005511090837,53.9572037530578));
#107229=CARTESIAN_POINT('Ctrl Pts',(2.44675858528434,28.7137134583588,53.9410107333393));
#107230=CARTESIAN_POINT('Ctrl Pts',(2.45043444918533,28.7475038916599,53.9009994854796));
#107231=CARTESIAN_POINT('Ctrl Pts',(2.45267918224455,28.7685096749546,53.8775117026402));
#107232=CARTESIAN_POINT('Ctrl Pts',(2.46441336530542,28.880742763951,53.7589614976529));
#107233=CARTESIAN_POINT('Ctrl Pts',(2.47414013539612,28.9823624478311,53.674355286441));
#107234=CARTESIAN_POINT('Ctrl Pts',(2.48702869590481,29.135186787656,53.5751501738372));
#107235=CARTESIAN_POINT('Ctrl Pts',(2.49053665606153,29.1787119961823,53.5496256177514));
#107236=CARTESIAN_POINT('Ctrl Pts',(2.49514743340021,29.2385505214296,53.5180935960251));
#107237=CARTESIAN_POINT('Ctrl Pts',(2.49631177454217,29.2538923896594,53.510310310537));
#107238=CARTESIAN_POINT('Ctrl Pts',(2.49822853941949,29.2795255501322,53.4978013773415));
#107239=CARTESIAN_POINT('Ctrl Pts',(2.49898561064752,29.2897490759343,53.4929406877568));
#107240=CARTESIAN_POINT('Ctrl Pts',(2.50046826964479,29.309962594973,53.4835817236322));
#107241=CARTESIAN_POINT('Ctrl Pts',(2.50119404805641,29.3199489719083,53.4790770505477));
#107242=CARTESIAN_POINT('Ctrl Pts',(2.50292802448296,29.3440226492828,53.4685023717036));
#107243=CARTESIAN_POINT('Ctrl Pts',(2.50393294586499,29.3581509286866,53.462527702485));
#107244=CARTESIAN_POINT('Ctrl Pts',(2.50748502761936,29.4086913844414,53.4419729106831));
#107245=CARTESIAN_POINT('Ctrl Pts',(2.50999593016234,29.4455350909037,53.4284837475064));
#107246=CARTESIAN_POINT('Ctrl Pts',(2.5163078623732,29.540533303779,53.397460763133));
#107247=CARTESIAN_POINT('Ctrl Pts',(2.52005612543067,29.5992335025666,53.3817822557363));
#107248=CARTESIAN_POINT('Ctrl Pts',(2.52918028931319,29.7450012008427,53.3512693465073));
#107249=CARTESIAN_POINT('Ctrl Pts',(2.53450661555806,29.8326348764367,53.3400829932201));
#107250=CARTESIAN_POINT('Ctrl Pts',(2.54280178006679,29.9651737470456,53.3337700469263));
#107251=CARTESIAN_POINT('Ctrl Pts',(2.54562869825601,30.0096735549496,53.3334344312139));
#107252=CARTESIAN_POINT('Ctrl Pts',(2.54928513062462,30.0654805395876,53.3352485791749));
#107253=CARTESIAN_POINT('Ctrl Pts',(2.55003437755436,30.0768276500641,53.3357336484546));
#107254=CARTESIAN_POINT('Ctrl Pts',(2.55123410948158,30.094838715699,53.3366881728324));
#107255=CARTESIAN_POINT('Ctrl Pts',(2.55168054181886,30.1015065726278,53.3370817734519));
#107256=CARTESIAN_POINT('Ctrl Pts',(2.55254183077088,30.1143006228662,53.3379142350946));
#107257=CARTESIAN_POINT('Ctrl Pts',(2.55295634921271,30.1204270113956,53.3383468917561));
#107258=CARTESIAN_POINT('Ctrl Pts',(2.55396874729597,30.1353172514732,53.3394812437472));
#107259=CARTESIAN_POINT('Ctrl Pts',(2.55456853233412,30.1440781362252,53.340218453983));
#107260=CARTESIAN_POINT('Ctrl Pts',(2.55674998041512,30.1757381218518,53.3431351197193));
#107261=CARTESIAN_POINT('Ctrl Pts',(2.55835136365921,30.198596189258,53.3457193275088));
#107262=CARTESIAN_POINT('Ctrl Pts',(2.57021060639035,30.3655949302287,53.3681100971558));
#107263=CARTESIAN_POINT('Ctrl Pts',(2.58103335778621,30.5066440734105,53.4062496758576));
#107264=CARTESIAN_POINT('Ctrl Pts',(2.59589384632307,30.698864366677,53.4863682291498));
#107265=CARTESIAN_POINT('Ctrl Pts',(2.60028874690668,30.7553727954231,53.5137610596324));
#107266=CARTESIAN_POINT('Ctrl Pts',(2.6058376094995,30.8263475215815,53.5532633359977));
#107267=CARTESIAN_POINT('Ctrl Pts',(2.60708996396829,30.8423377164095,53.5625145494312));
#107268=CARTESIAN_POINT('Ctrl Pts',(2.60911224063516,30.8681017366143,53.5779980295346));
#107269=CARTESIAN_POINT('Ctrl Pts',(2.60988789851,30.8779698390797,53.5840694923429));
#107270=CARTESIAN_POINT('Ctrl Pts',(2.61138052753846,30.8969282597795,53.5960082873435));
#107271=CARTESIAN_POINT('Ctrl Pts',(2.61209794429056,30.9060263082142,53.6018621775289));
#107272=CARTESIAN_POINT('Ctrl Pts',(2.6137710775707,30.927206093141,53.615783295755));
#107273=CARTESIAN_POINT('Ctrl Pts',(2.61472411340977,30.9392407372461,53.6239208296653));
#107274=CARTESIAN_POINT('Ctrl Pts',(2.61787987952028,30.9789702972248,53.6515490562528));
#107275=CARTESIAN_POINT('Ctrl Pts',(2.62005655018282,31.0061782815751,53.6717273221006));
#107276=CARTESIAN_POINT('Ctrl Pts',(2.62531616961249,31.0711782562362,53.7230775159884));
#107277=CARTESIAN_POINT('Ctrl Pts',(2.62836732340689,31.1082474357985,53.7551136465377));
#107278=CARTESIAN_POINT('Ctrl Pts',(2.6374473329851,31.21529249259,53.8562015181109));
#107279=CARTESIAN_POINT('Ctrl Pts',(2.64335522083053,31.2806198628961,53.9298493947642));
#107280=CARTESIAN_POINT('Ctrl Pts',(2.65273274339902,31.3704383735152,54.0511935192407));
#107281=CARTESIAN_POINT('Ctrl Pts',(2.65606072062755,31.3997700024202,54.0950260547638));
#107282=CARTESIAN_POINT('Ctrl Pts',(2.66028177518287,31.433074748508,54.1502985224751));
#107283=CARTESIAN_POINT('Ctrl Pts',(2.66106118743689,31.4390695697947,54.1604914596091));
#107284=CARTESIAN_POINT('Ctrl Pts',(2.6622980768278,31.4483304220239,54.1766282912769));
#107285=CARTESIAN_POINT('Ctrl Pts',(2.66275106203928,31.4516696616105,54.1825300179458));
#107286=CARTESIAN_POINT('Ctrl Pts',(2.66361610631598,31.4579450949911,54.1937808403398));
#107287=CARTESIAN_POINT('Ctrl Pts',(2.66402773558948,31.4608880549701,54.1991259030078));
#107288=CARTESIAN_POINT('Ctrl Pts',(2.66502064479975,31.4678847725331,54.212000368039));
#107289=CARTESIAN_POINT('Ctrl Pts',(2.66560365398541,31.4719100086226,54.2195449763146));
#107290=CARTESIAN_POINT('Ctrl Pts',(2.66765658815592,31.4858009951762,54.2460709397786));
#107291=CARTESIAN_POINT('Ctrl Pts',(2.66914341484772,31.4953586259579,54.2652101666436));
#107292=CARTESIAN_POINT('Ctrl Pts',(2.67293736702885,31.5185557684826,54.3139906685801));
#107293=CARTESIAN_POINT('Ctrl Pts',(2.67526429493369,31.5316976635665,54.343857912993));
#107294=CARTESIAN_POINT('Ctrl Pts',(2.68304221476275,31.5723114456568,54.4440412753233));
#107295=CARTESIAN_POINT('Ctrl Pts',(2.68856836627649,31.5958823139534,54.5158380075733));
#107296=CARTESIAN_POINT('Ctrl Pts',(2.70125404883385,31.6390406682402,54.6853677622887));
#107297=CARTESIAN_POINT('Ctrl Pts',(2.7083411534123,31.65490114175,54.7837682524219));
#107298=CARTESIAN_POINT('Ctrl Pts',(2.71648668243657,31.6632558801577,54.9024516376962));
#107299=CARTESIAN_POINT('Ctrl Pts',(2.7178104124869,31.6642832231064,54.921915333777));
#107300=CARTESIAN_POINT('Ctrl Pts',(2.71989468522261,31.6653714860199,54.9528320087661));
#107301=CARTESIAN_POINT('Ctrl Pts',(2.72066212585408,31.6656562449746,54.9642747883555));
#107302=CARTESIAN_POINT('Ctrl Pts',(2.72196519519543,31.6659408519501,54.9838012238661));
#107303=CARTESIAN_POINT('Ctrl Pts',(2.72250264605235,31.6659998341427,54.9918834489475));
#107304=CARTESIAN_POINT('Ctrl Pts',(2.72303827374538,31.6659999996507,54.9999658845042));
#107305=CARTESIAN_POINT('Ctrl Pts',(2.72303826203026,31.6659999996471,54.9999657077272));
#107306=CARTESIAN_POINT('Ctrl Pts',(2.72365866824712,31.6660001923448,55.0093274212484));
#107307=CARTESIAN_POINT('Ctrl Pts',(2.72427661150426,31.6659214760123,55.0186891663787));
#107308=CARTESIAN_POINT('Ctrl Pts',(2.72592145939162,31.6655002618234,55.0437032318179));
#107309=CARTESIAN_POINT('Ctrl Pts',(2.72694394157471,31.6650160391201,55.05935243227));
#107310=CARTESIAN_POINT('Ctrl Pts',(2.73099403122546,31.6622067581869,55.1216985516583));
#107311=CARTESIAN_POINT('Ctrl Pts',(2.73396789704877,31.6581370098067,55.1682976661332));
#107312=CARTESIAN_POINT('Ctrl Pts',(2.74466954164758,31.6361375639892,55.3376086933545));
#107313=CARTESIAN_POINT('Ctrl Pts',(2.75207414576663,31.6064916702442,55.4583768259009));
#107314=CARTESIAN_POINT('Ctrl Pts',(2.75977020846451,31.5636287079815,55.5749968174508));
#107315=CARTESIAN_POINT('Ctrl Pts',(2.7597873422125,31.5635332253174,55.5752564035542));
#107316=CARTESIAN_POINT('Ctrl Pts',(2.75980447732862,31.5634376782628,55.5755159651897));
#107317=CARTESIAN_POINT('Ctrl Pts',(2.56903902087732,31.5634376730794,55.5755159792709));
#107318=CARTESIAN_POINT('Ctrl Pts',(2.56703832709278,31.5744467142337,55.5456089909248));
#107319=CARTESIAN_POINT('Ctrl Pts',(2.56501125490043,31.584597150557,55.5153873830606));
#107320=CARTESIAN_POINT('Ctrl Pts',(2.56192251703097,31.5984538539087,55.4698390336222));
#107321=CARTESIAN_POINT('Ctrl Pts',(2.56089224524731,31.6028185591783,55.4547263606249));
#107322=CARTESIAN_POINT('Ctrl Pts',(2.55934852915817,31.6089676453066,55.4322459177972));
#107323=CARTESIAN_POINT('Ctrl Pts',(2.55884397055743,31.6109169204052,55.4249236249913));
#107324=CARTESIAN_POINT('Ctrl Pts',(2.55793465409424,31.6143203786623,55.4117787400294));
#107325=CARTESIAN_POINT('Ctrl Pts',(2.55753095870801,31.6157931457939,55.4059612334005));
#107326=CARTESIAN_POINT('Ctrl Pts',(2.55662466577699,31.6190142929406,55.3929422780383));
#107327=CARTESIAN_POINT('Ctrl Pts',(2.55612117936977,31.6207460562079,55.3857371263221));
#107328=CARTESIAN_POINT('Ctrl Pts',(2.55459979059657,31.6258080166508,55.3640403690167));
#107329=CARTESIAN_POINT('Ctrl Pts',(2.55357431454301,31.628992224923,55.3495159370959));
#107330=CARTESIAN_POINT('Ctrl Pts',(2.54475053051766,31.6545010834067,55.2252293240228));
#107331=CARTESIAN_POINT('Ctrl Pts',(2.53651828560861,31.6658963723887,55.1135246429918));
#107332=CARTESIAN_POINT('Ctrl Pts',(2.52138067042813,31.6660879584933,54.9050563313741));
#107333=CARTESIAN_POINT('Ctrl Pts',(2.51447540910696,31.6577966079625,54.8087432123935));
#107334=CARTESIAN_POINT('Ctrl Pts',(2.50627876799148,31.6373615881475,54.6916093219608));
#107335=CARTESIAN_POINT('Ctrl Pts',(2.50474819009306,31.6330669601417,54.6696211739158));
#107336=CARTESIAN_POINT('Ctrl Pts',(2.50230218166022,31.6254272867301,54.634308073459));
#107337=CARTESIAN_POINT('Ctrl Pts',(2.50137813197071,31.6223587769904,54.6209268304253));
#107338=CARTESIAN_POINT('Ctrl Pts',(2.49974276754146,31.6166030602353,54.5971784561518));
#107339=CARTESIAN_POINT('Ctrl Pts',(2.49902942185785,31.6139806664587,54.5867965778889));
#107340=CARTESIAN_POINT('Ctrl Pts',(2.49752647213994,31.6082191044489,54.5648790799132));
#107341=CARTESIAN_POINT('Ctrl Pts',(2.49673770137291,31.6050554856787,54.5533504691269));
#107342=CARTESIAN_POINT('Ctrl Pts',(2.49462544257866,31.5962079662301,54.522417632488));
#107343=CARTESIAN_POINT('Ctrl Pts',(2.49330943344632,31.5902943589723,54.5030807927141));
#107344=CARTESIAN_POINT('Ctrl Pts',(2.48464646038119,31.5487257399475,54.3755080608609));
#107345=CARTESIAN_POINT('Ctrl Pts',(2.47767428538728,31.5023976900992,54.2710644312253));
#107346=CARTESIAN_POINT('Ctrl Pts',(2.4645313593107,31.3954452534932,54.0842800468393));
#107347=CARTESIAN_POINT('Ctrl Pts',(2.45837550547428,31.3372257074833,54.0011844958416));
#107348=CARTESIAN_POINT('Ctrl Pts',(2.4507870835654,31.2616745700886,53.9118912286464));
#107349=CARTESIAN_POINT('Ctrl Pts',(2.44975685549702,31.2513454478176,53.90002820698));
#107350=CARTESIAN_POINT('Ctrl Pts',(2.44821319246676,31.2357942230931,53.8826701233351));
#107351=CARTESIAN_POINT('Ctrl Pts',(2.44770864232784,31.2306997473911,53.8770612032184));
#107352=CARTESIAN_POINT('Ctrl Pts',(2.44679933447179,31.2215021565176,53.8670725984019));
#107353=CARTESIAN_POINT('Ctrl Pts',(2.44639563913415,31.2174133919079,53.8626800598839));
#107354=CARTESIAN_POINT('Ctrl Pts',(2.44548933794259,31.208222550221,53.8529127384811));
#107355=CARTESIAN_POINT('Ctrl Pts',(2.44498584313436,31.2031083485751,53.8475499087982));
#107356=CARTESIAN_POINT('Ctrl Pts',(2.4434644035796,31.1876248635897,53.8315290765823));
#107357=CARTESIAN_POINT('Ctrl Pts',(2.44243888442806,31.1771488118049,53.8209759323005));
#107358=CARTESIAN_POINT('Ctrl Pts',(2.44001941682391,31.1523109414172,53.7966162976543));
#107359=CARTESIAN_POINT('Ctrl Pts',(2.4386188679723,31.1378401207268,53.7829245602019));
#107360=CARTESIAN_POINT('Ctrl Pts',(2.43350353001001,31.0845441051653,53.7342792419828));
#107361=CARTESIAN_POINT('Ctrl Pts',(2.42972451406117,31.0443274033177,53.7008985532057));
#107362=CARTESIAN_POINT('Ctrl Pts',(2.41654038897413,30.8994768408192,53.5917478557784));
#107363=CARTESIAN_POINT('Ctrl Pts',(2.4071292340123,30.7876355721483,53.5262721418095));
#107364=CARTESIAN_POINT('Ctrl Pts',(2.39613397636486,30.6423752199784,53.4625420018965));
#107365=CARTESIAN_POINT('Ctrl Pts',(2.39411604863357,30.615100729484,53.4514283024843));
#107366=CARTESIAN_POINT('Ctrl Pts',(2.39118965336059,30.5746564907069,53.4361855580708));
#107367=CARTESIAN_POINT('Ctrl Pts',(2.39026248305905,30.5617085149661,53.4314882037128));
#107368=CARTESIAN_POINT('Ctrl Pts',(2.38862364152204,30.5385885245693,53.4234235949403));
#107369=CARTESIAN_POINT('Ctrl Pts',(2.38790990771771,30.5284396251308,53.4199929330566));
#107370=CARTESIAN_POINT('Ctrl Pts',(2.38640819107006,30.5069209778355,53.412949457667));
#107371=CARTESIAN_POINT('Ctrl Pts',(2.3856210214882,30.4955440524567,53.4093603782715));
#107372=CARTESIAN_POINT('Ctrl Pts',(2.38351802995604,30.464896883769,53.4000528479526));
#107373=CARTESIAN_POINT('Ctrl Pts',(2.38220957042046,30.4455596983682,53.394560305201));
#107374=CARTESIAN_POINT('Ctrl Pts',(2.37933594228214,30.4025404061344,53.3831782717954));
#107375=CARTESIAN_POINT('Ctrl Pts',(2.3777760734263,30.3788185833725,53.3774563640163));
#107376=CARTESIAN_POINT('Ctrl Pts',(2.37288859520862,30.3034742800915,53.3610252513701));
#107377=CARTESIAN_POINT('Ctrl Pts',(2.36961407675322,30.251463441224,53.3522434593206));
#107378=CARTESIAN_POINT('Ctrl Pts',(2.36376389457143,30.1570463585992,53.3408772389344));
#107379=CARTESIAN_POINT('Ctrl Pts',(2.3611790268356,30.114793663017,53.3374193562994));
#107380=CARTESIAN_POINT('Ctrl Pts',(2.35276587877904,29.9771579868969,53.3314278794156));
#107381=CARTESIAN_POINT('Ctrl Pts',(2.34694670894351,29.8816930190841,53.3354720126228));
#107382=CARTESIAN_POINT('Ctrl Pts',(2.33972386028802,29.7712103413333,53.3497065808873));
#107383=CARTESIAN_POINT('Ctrl Pts',(2.33867417491907,29.7553392796416,53.3519847808123));
#107384=CARTESIAN_POINT('Ctrl Pts',(2.33710691593126,29.7319632171216,53.3556853780243));
#107385=CARTESIAN_POINT('Ctrl Pts',(2.33659862398766,29.7244306196399,53.3569309801671));
#107386=CARTESIAN_POINT('Ctrl Pts',(2.33568548985234,29.7109914235352,53.3592483193188));
#107387=CARTESIAN_POINT('Ctrl Pts',(2.33528175280421,29.7050816801383,53.3603002662017));
#107388=CARTESIAN_POINT('Ctrl Pts',(2.33437901140455,29.6919402558563,53.3627128110156));
#107389=CARTESIAN_POINT('Ctrl Pts',(2.33387915794543,29.6847119187796,53.3640893771848));
#107390=CARTESIAN_POINT('Ctrl Pts',(2.33237961804386,29.6631632595541,53.3683412275828));
#107391=CARTESIAN_POINT('Ctrl Pts',(2.33137266330465,29.6488718101618,53.3713569152939));
#107392=CARTESIAN_POINT('Ctrl Pts',(2.32347606220776,29.5380388992977,53.3962706947691));
#107393=CARTESIAN_POINT('Ctrl Pts',(2.31624123179921,29.4435914353407,53.4265446369797));
#107394=CARTESIAN_POINT('Ctrl Pts',(2.30099907038259,29.2505860335259,53.5079726290602));
#107395=CARTESIAN_POINT('Ctrl Pts',(2.29304595366654,29.1532831835809,53.5609567768923));
#107396=CARTESIAN_POINT('Ctrl Pts',(2.28390852586352,29.0436911163339,53.635625948877));
#107397=CARTESIAN_POINT('Ctrl Pts',(2.28240082919366,29.0256975327826,53.6484164785268));
#107398=CARTESIAN_POINT('Ctrl Pts',(2.27998386290921,28.9970094800734,53.6696797761203));
#107399=CARTESIAN_POINT('Ctrl Pts',(2.27906630214358,28.9861560739729,53.6779325304779));
#107400=CARTESIAN_POINT('Ctrl Pts',(2.2774381380777,28.966969774949,53.6928967187799));
#107401=CARTESIAN_POINT('Ctrl Pts',(2.27672556952316,28.9585980332496,53.6995568499692));
#107402=CARTESIAN_POINT('Ctrl Pts',(2.27521990454015,28.9409659160703,53.71386353309));
#107403=CARTESIAN_POINT('Ctrl Pts',(2.27442768406975,28.9317228609004,53.7215305364587));
#107404=CARTESIAN_POINT('Ctrl Pts',(2.27229544511293,28.9069467837972,53.7425383205256));
#107405=CARTESIAN_POINT('Ctrl Pts',(2.27096315925479,28.8915751630459,53.7560668630174));
#107406=CARTESIAN_POINT('Ctrl Pts',(2.26238190380118,28.793401970359,53.8457341321196));
#107407=CARTESIAN_POINT('Ctrl Pts',(2.25549600707798,28.718240184404,53.9298110173004));
#107408=CARTESIAN_POINT('Ctrl Pts',(2.24236958218581,28.5918981527878,54.1037279383149));
#107409=CARTESIAN_POINT('Ctrl Pts',(2.23614509653355,28.539461417703,54.1919926911794));
#107410=CARTESIAN_POINT('Ctrl Pts',(2.22848555235427,28.4887690525829,54.2985868698199));
#107411=CARTESIAN_POINT('Ctrl Pts',(2.22746362733322,28.4822678394983,54.3127675780948));
#107412=CARTESIAN_POINT('Ctrl Pts',(2.22593004321559,28.4729162592118,54.3339457317402));
#107413=CARTESIAN_POINT('Ctrl Pts',(2.22542710207359,28.469912611736,54.3408751116811));
#107414=CARTESIAN_POINT('Ctrl Pts',(2.22451942302356,28.4646071489452,54.3533464581515));
#107415=CARTESIAN_POINT('Ctrl Pts',(2.2241157290447,28.4622880178096,54.358880769807));
#107416=CARTESIAN_POINT('Ctrl Pts',(2.22320782431244,28.4571628260129,54.3712991837081));
#107417=CARTESIAN_POINT('Ctrl Pts',(2.22270270691986,28.4543729410728,54.3781895375374));
#107418=CARTESIAN_POINT('Ctrl Pts',(2.22117145138896,28.4460973068399,54.3990282284693));
#107419=CARTESIAN_POINT('Ctrl Pts',(2.22013759968003,28.4407537570065,54.4130317174724));
#107420=CARTESIAN_POINT('Ctrl Pts',(2.21087348919067,28.3949562074735,54.5380906778809));
#107421=CARTESIAN_POINT('Ctrl Pts',(2.20216477450047,28.3662411647657,54.6530784275947));
#107422=CARTESIAN_POINT('Ctrl Pts',(2.18703014679514,28.337439096311,54.8598252212338));
#107423=CARTESIAN_POINT('Ctrl Pts',(2.18056557021985,28.3322762760155,54.9504032813295));
#107424=CARTESIAN_POINT('Ctrl Pts',(2.17279666076356,28.3350483283738,55.0631074250266));
#107425=CARTESIAN_POINT('Ctrl Pts',(2.17128361314673,28.3360345210605,55.0852383860907));
#107426=CARTESIAN_POINT('Ctrl Pts',(2.16885985122805,28.3383416784113,55.1209715001071));
#107427=CARTESIAN_POINT('Ctrl Pts',(2.16794076955702,28.339389093405,55.1345879553264));
#107428=CARTESIAN_POINT('Ctrl Pts',(2.16631092169266,28.3415555733005,55.1588476210601));
#107429=CARTESIAN_POINT('Ctrl Pts',(2.16559817485443,28.3426099715321,55.1694956809977));
#107430=CARTESIAN_POINT('Ctrl Pts',(2.16409316554087,28.3450638891817,55.1920582223113));
#107431=CARTESIAN_POINT('Ctrl Pts',(2.16330176887972,28.3464896624196,55.2039692815413));
#107432=CARTESIAN_POINT('Ctrl Pts',(2.16117430280529,28.350688962815,55.2361055065412));
#107433=CARTESIAN_POINT('Ctrl Pts',(2.15984590508754,28.353705824445,55.256297199131));
#107434=CARTESIAN_POINT('Ctrl Pts',(2.15126733036294,28.3757580586625,55.3873607116074));
#107435=CARTESIAN_POINT('Ctrl Pts',(2.1443804974883,28.4056103303477,55.4961209340929));
#107436=CARTESIAN_POINT('Ctrl Pts',(2.1312461149849,28.4832109679758,55.6967284291529));
#107437=CARTESIAN_POINT('Ctrl Pts',(2.12501464617572,28.5289736279465,55.7887681582714));
#107438=CARTESIAN_POINT('Ctrl Pts',(2.11734771545702,28.5910959131991,55.8892627822139));
#107439=CARTESIAN_POINT('Ctrl Pts',(2.11632647603932,28.5994782285968,55.9024066415216));
#107440=CARTESIAN_POINT('Ctrl Pts',(2.1147937244984,28.6121921510527,55.9217387824128));
#107441=CARTESIAN_POINT('Ctrl Pts',(2.114290916621,28.6163836689581,55.9280187775906));
#107442=CARTESIAN_POINT('Ctrl Pts',(2.11338337210674,28.6239828058318,55.9392383569808));
#107443=CARTESIAN_POINT('Ctrl Pts',(2.11297967787029,28.627374625035,55.9441883218439));
#107444=CARTESIAN_POINT('Ctrl Pts',(2.11207163863731,28.6350293224486,55.9552310402254));
#107445=CARTESIAN_POINT('Ctrl Pts',(2.11156638552315,28.6393062478497,55.9613135795951));
#107446=CARTESIAN_POINT('Ctrl Pts',(2.11003430704773,28.6523324186776,55.9795779897269));
#107447=CARTESIAN_POINT('Ctrl Pts',(2.10899975639033,28.6612053183635,55.9916701614192));
#107448=CARTESIAN_POINT('Ctrl Pts',(2.10655505230234,28.6823772340039,56.0197216135052));
#107449=CARTESIAN_POINT('Ctrl Pts',(2.10513812012677,28.6948047644001,56.0355806308413));
#107450=CARTESIAN_POINT('Ctrl Pts',(2.09993527430348,28.7410978032091,56.0924988718621));
#107451=CARTESIAN_POINT('Ctrl Pts',(2.09608309853945,28.776636689922,56.1321528427651));
#107452=CARTESIAN_POINT('Ctrl Pts',(2.08254317607198,28.9074212941199,56.2647208324352));
#107453=CARTESIAN_POINT('Ctrl Pts',(2.07286121941079,29.0118549316054,56.3478979244634));
#107454=CARTESIAN_POINT('Ctrl Pts',(2.06189989286676,29.146972301534,56.4312795825947));
#107455=CARTESIAN_POINT('Ctrl Pts',(2.06014216595753,29.1691706150017,56.4442784214195));
#107456=CARTESIAN_POINT('Ctrl Pts',(2.05750725913073,29.2032428107282,56.4631846727804));
#107457=CARTESIAN_POINT('Ctrl Pts',(2.05661664438505,29.2148999834214,56.4694724859158));
#107458=CARTESIAN_POINT('Ctrl Pts',(2.05501788598772,29.2360757654427,56.4805706551836));
#107459=CARTESIAN_POINT('Ctrl Pts',(2.0543080493953,29.2455678220526,56.4854298364726));
#107460=CARTESIAN_POINT('Ctrl Pts',(2.05278862245614,29.2660762589244,56.4956812351074));
#107461=CARTESIAN_POINT('Ctrl Pts',(2.05198010356523,29.2771069031143,56.5010436365183));
#107462=CARTESIAN_POINT('Ctrl Pts',(2.04975301920599,29.3078080386062,56.5155516527618));
#107463=CARTESIAN_POINT('Ctrl Pts',(2.04834344038275,29.327599889755,56.5244358582175));
#107464=CARTESIAN_POINT('Ctrl Pts',(2.04521158281744,29.3723282421418,56.5434729467122));
#107465=CARTESIAN_POINT('Ctrl Pts',(2.04349626842317,29.3973488938929,56.5534131244396));
#107466=CARTESIAN_POINT('Ctrl Pts',(2.03790339842026,29.4804422881466,56.5841143230176));
#107467=CARTESIAN_POINT('Ctrl Pts',(2.03409883039588,29.5394289221737,56.6022588775444));
#107468=CARTESIAN_POINT('Ctrl Pts',(2.02477031179079,29.6872769446932,56.6388952322896));
#107469=CARTESIAN_POINT('Ctrl Pts',(2.019298032406,29.7768921739977,56.6534794371085));
#107470=CARTESIAN_POINT('Ctrl Pts',(2.01104110948433,29.9081421314178,56.6639716345134));
#107471=CARTESIAN_POINT('Ctrl Pts',(2.00842634409198,29.9491449704016,56.6657288578313));
#107472=CARTESIAN_POINT('Ctrl Pts',(2.00501052258785,30.001274131753,56.6660365392934));
#107473=CARTESIAN_POINT('Ctrl Pts',(2.00427742585355,30.012381316934,56.6659910144505));
#107474=CARTESIAN_POINT('Ctrl Pts',(2.0030976812207,30.0301098493991,56.665741057276));
#107475=CARTESIAN_POINT('Ctrl Pts',(2.00265485925248,30.0367320948796,56.6656081839085));
#107476=CARTESIAN_POINT('Ctrl Pts',(2.00179553940694,30.0495164249859,56.6652753929621));
#107477=CARTESIAN_POINT('Ctrl Pts',(2.00137932908808,30.0556784508741,56.6650807535451));
#107478=CARTESIAN_POINT('Ctrl Pts',(2.00035559313652,30.0707646597869,56.6645203930283));
#107479=CARTESIAN_POINT('Ctrl Pts',(1.99974605845575,30.0796871799554,56.6641170993239));
#107480=CARTESIAN_POINT('Ctrl Pts',(1.99748588980919,30.1125681851058,56.6623658531569));
#107481=CARTESIAN_POINT('Ctrl Pts',(1.99581369419722,30.1364987544499,56.6605721215487));
#107482=CARTESIAN_POINT('Ctrl Pts',(1.99141230716418,30.1986662884355,56.6545595200941));
#107483=CARTESIAN_POINT('Ctrl Pts',(1.98865527953901,30.2368099072141,56.6495321154896));
#107484=CARTESIAN_POINT('Ctrl Pts',(1.98078049732849,30.3442941709518,56.6315606482647));
#107485=CARTESIAN_POINT('Ctrl Pts',(1.97562095791853,30.413036767812,56.6155275690231));
#107486=CARTESIAN_POINT('Ctrl Pts',(1.96362254397682,30.5716560136923,56.5677428501653));
#107487=CARTESIAN_POINT('Ctrl Pts',(1.95685560119414,30.6602494140888,56.532541822499));
#107488=CARTESIAN_POINT('Ctrl Pts',(1.94898191140086,30.7631094854507,56.4810852682087));
#107489=CARTESIAN_POINT('Ctrl Pts',(1.94763453161505,30.7806944746662,56.4718919303925));
#107490=CARTESIAN_POINT('Ctrl Pts',(1.94549842501006,30.8085345767801,56.4566979205397));
#107491=CARTESIAN_POINT('Ctrl Pts',(1.94470269637493,30.8188965471971,56.450898153276));
#107492=CARTESIAN_POINT('Ctrl Pts',(1.94319581221635,30.8384977918962,56.4396501212028));
#107493=CARTESIAN_POINT('Ctrl Pts',(1.94248396456794,30.8477481428783,56.4342224771344));
#107494=CARTESIAN_POINT('Ctrl Pts',(1.94085851683372,30.8688444294752,56.421568807772));
#107495=CARTESIAN_POINT('Ctrl Pts',(1.93994713472802,30.8806538975934,56.4142832989968));
#107496=CARTESIAN_POINT('Ctrl Pts',(1.9370803637487,30.9177222215727,56.3907707099766));
#107497=CARTESIAN_POINT('Ctrl Pts',(1.93514474017117,30.9426350508713,56.3740074901538));
#107498=CARTESIAN_POINT('Ctrl Pts',(1.92370972981544,31.0886747386681,56.2698982545292));
#107499=CARTESIAN_POINT('Ctrl Pts',(1.91484519344245,31.1980536579125,56.1672706669635));
#107500=CARTESIAN_POINT('Ctrl Pts',(1.90212103745279,31.3276316898167,56.0080105142467));
#107501=CARTESIAN_POINT('Ctrl Pts',(1.89859554197249,31.3607534859795,55.96282899989));
#107502=CARTESIAN_POINT('Ctrl Pts',(1.89414911264204,31.3981491541458,55.9060240876121));
#107503=CARTESIAN_POINT('Ctrl Pts',(1.89335654397829,31.4046543808281,55.8959055499316));
#107504=CARTESIAN_POINT('Ctrl Pts',(1.8921035461101,31.4146769956061,55.8799383845685));
#107505=CARTESIAN_POINT('Ctrl Pts',(1.89164780712139,31.4182691340537,55.8741368438452));
#107506=CARTESIAN_POINT('Ctrl Pts',(1.89078118143745,31.4249970225,55.8631202205903));
#107507=CARTESIAN_POINT('Ctrl Pts',(1.89037076350753,31.4281399738144,55.8579098085268));
#107508=CARTESIAN_POINT('Ctrl Pts',(1.88938589843034,31.4355802337925,55.8454210981417));
#107509=CARTESIAN_POINT('Ctrl Pts',(1.88880979341608,31.4398507874121,55.8381271640748));
#107510=CARTESIAN_POINT('Ctrl Pts',(1.88680716602338,31.4544213841984,55.8128011348444));
#107511=CARTESIAN_POINT('Ctrl Pts',(1.88536478096997,31.4644391965092,55.7946099609426));
#107512=CARTESIAN_POINT('Ctrl Pts',(1.88171118202069,31.4886957518609,55.7485455421434));
#107513=CARTESIAN_POINT('Ctrl Pts',(1.87948183114997,31.5024936600626,55.7204498882326));
#107514=CARTESIAN_POINT('Ctrl Pts',(1.87421257502843,31.532948237739,55.6537523329074));
#107515=CARTESIAN_POINT('Ctrl Pts',(1.87116107209707,31.5489395752854,55.6149012468612));
#107516=CARTESIAN_POINT('Ctrl Pts',(1.86810672180998,31.5634374966623,55.5755164585225));
#107517=CARTESIAN_POINT('Origin',(5.,30.,55.));
#107518=CARTESIAN_POINT('',(1.16624544379888,31.5634376782622,55.5755159651913));
#107519=CARTESIAN_POINT('',(1.36116735710803,31.5634376788384,55.575515963626));
#107520=CARTESIAN_POINT('',(5.,31.5634376782623,55.5755159651912));
#107521=CARTESIAN_POINT('Ctrl Pts',(1.36116735710803,31.5634376788384,55.575515963626));
#107522=CARTESIAN_POINT('Ctrl Pts',(1.3613845116336,31.5624022301552,55.578328847348));
#107523=CARTESIAN_POINT('Ctrl Pts',(1.36160158161901,31.5613591468225,55.5811390545062));
#107524=CARTESIAN_POINT('Ctrl Pts',(1.36633196778185,31.538452467193,55.6423458298376));
#107525=CARTESIAN_POINT('Ctrl Pts',(1.37079547469062,31.5133333770567,55.699476656108));
#107526=CARTESIAN_POINT('Ctrl Pts',(1.37796171917311,31.4669765940998,55.790651004218));
#107527=CARTESIAN_POINT('Ctrl Pts',(1.38071830898915,31.447611335838,55.8255732699834));
#107528=CARTESIAN_POINT('Ctrl Pts',(1.38447982978756,31.4190422483487,55.8729910592628));
#107529=CARTESIAN_POINT('Ctrl Pts',(1.38552202255295,31.4108922490538,55.8861023538935));
#107530=CARTESIAN_POINT('Ctrl Pts',(1.38729356594832,31.396639243336,55.9083365150875));
#107531=CARTESIAN_POINT('Ctrl Pts',(1.38802617708115,31.3906263001302,55.9175156151169));
#107532=CARTESIAN_POINT('Ctrl Pts',(1.38941786703856,31.3789787627736,55.9349186768279));
#107533=CARTESIAN_POINT('Ctrl Pts',(1.39007750555529,31.3733602099005,55.9431527456587));
#107534=CARTESIAN_POINT('Ctrl Pts',(1.39161885991712,31.360003835093,55.9623542532146));
#107535=CARTESIAN_POINT('Ctrl Pts',(1.39249828427459,31.3522066363019,55.9732796978327));
#107536=CARTESIAN_POINT('Ctrl Pts',(1.39556426922443,31.3244124818949,56.0112460557422));
#107537=CARTESIAN_POINT('Ctrl Pts',(1.3977244576177,31.3037288181165,56.0377757082481));
#107538=CARTESIAN_POINT('Ctrl Pts',(1.40772469980558,31.2031196223636,56.1590610238801));
#107539=CARTESIAN_POINT('Ctrl Pts',(1.4151738033165,31.1135871821581,56.2453290536538));
#107540=CARTESIAN_POINT('Ctrl Pts',(1.42590888589875,30.9749844173835,56.3518684976956));
#107541=CARTESIAN_POINT('Ctrl Pts',(1.4290589355703,30.9332624940005,56.3810008860487));
#107542=CARTESIAN_POINT('Ctrl Pts',(1.43353903457282,30.8737101246704,56.4186510391869));
#107543=CARTESIAN_POINT('Ctrl Pts',(1.43479747631727,30.8569606918965,56.4288311501258));
#107544=CARTESIAN_POINT('Ctrl Pts',(1.43702636567507,30.8273519677758,56.4461191051649));
#107545=CARTESIAN_POINT('Ctrl Pts',(1.43798987789507,30.8145707229978,56.4533568887049));
#107546=CARTESIAN_POINT('Ctrl Pts',(1.43945248612774,30.795230077515,56.4639738831506));
#107547=CARTESIAN_POINT('Ctrl Pts',(1.43994399730035,30.7887408087137,56.4674802684311));
#107548=CARTESIAN_POINT('Ctrl Pts',(1.44084056948911,30.7769272363381,56.473762573178));
#107549=CARTESIAN_POINT('Ctrl Pts',(1.44124472029134,30.7716109256635,56.4765529549372));
#107550=CARTESIAN_POINT('Ctrl Pts',(1.44216596302616,30.7595129121344,56.4828196823788));
#107551=CARTESIAN_POINT('Ctrl Pts',(1.44268410095706,30.7527224067631,56.486278253488));
#107552=CARTESIAN_POINT('Ctrl Pts',(1.44429495887164,30.7316465041888,56.4968312519475));
#107553=CARTESIAN_POINT('Ctrl Pts',(1.44539656354536,30.717283249439,56.5037669691452));
#107554=CARTESIAN_POINT('Ctrl Pts',(1.45323504987242,30.6152832017317,56.5512269124238));
#107555=CARTESIAN_POINT('Ctrl Pts',(1.46028962061975,30.5243756124098,56.5842680973235));
#107556=CARTESIAN_POINT('Ctrl Pts',(1.47571355515163,30.3196248322529,56.639122111583));
#107557=CARTESIAN_POINT('Ctrl Pts',(1.48401553333094,30.205299966021,56.657329888676));
#107558=CARTESIAN_POINT('Ctrl Pts',(1.49344027156436,30.0682231815618,56.6647453082959));
#107559=CARTESIAN_POINT('Ctrl Pts',(1.49492403274362,30.0464307622696,56.6654956038666));
#107560=CARTESIAN_POINT('Ctrl Pts',(1.49722338728746,30.0123403598309,56.6659996273685));
#107561=CARTESIAN_POINT('Ctrl Pts',(1.49804796372593,30.0000498425013,56.6660453338416));
#107562=CARTESIAN_POINT('Ctrl Pts',(1.49958012541974,29.9770954033315,56.6658766796563));
#107563=CARTESIAN_POINT('Ctrl Pts',(1.50028872069814,29.9664319453511,56.6656959287701));
#107564=CARTESIAN_POINT('Ctrl Pts',(1.50186853324321,29.9425563120589,56.6650618508168));
#107565=CARTESIAN_POINT('Ctrl Pts',(1.50273799558165,29.9293462208004,56.6645536352387));
#107566=CARTESIAN_POINT('Ctrl Pts',(1.50495291904238,29.8955279958919,56.6628492621613));
#107567=CARTESIAN_POINT('Ctrl Pts',(1.50629135347019,29.8749331415438,56.6614272205867));
#107568=CARTESIAN_POINT('Ctrl Pts',(1.51736969143367,29.7033490444511,56.646370837997));
#107569=CARTESIAN_POINT('Ctrl Pts',(1.52640483462278,29.5548521132859,56.6125704629521));
#107570=CARTESIAN_POINT('Ctrl Pts',(1.53944594997554,29.356944332807,56.5380569741244));
#107571=CARTESIAN_POINT('Ctrl Pts',(1.54318793533599,29.3021019400113,56.5139605787668));
#107572=CARTESIAN_POINT('Ctrl Pts',(1.54805717667697,29.2351931073914,56.4801536376115));
#107573=CARTESIAN_POINT('Ctrl Pts',(1.54904785588184,29.2217989583892,56.4731556175565));
#107574=CARTESIAN_POINT('Ctrl Pts',(1.5505435522493,29.201938576557,56.4624327703978));
#107575=CARTESIAN_POINT('Ctrl Pts',(1.55104046708579,29.1953987485923,56.4588449075971));
#107576=CARTESIAN_POINT('Ctrl Pts',(1.5519422768732,29.183640314036,56.4522909121648));
#107577=CARTESIAN_POINT('Ctrl Pts',(1.55234619862556,29.1784133446259,56.4493403310046));
#107578=CARTESIAN_POINT('Ctrl Pts',(1.55326103080455,29.1666642339802,56.442624073368));
#107579=CARTESIAN_POINT('Ctrl Pts',(1.55377292004837,29.1601516635725,56.4388424105032));
#107580=CARTESIAN_POINT('Ctrl Pts',(1.55534504166852,29.1403306326248,56.4271524918029));
#107581=CARTESIAN_POINT('Ctrl Pts',(1.55641357765907,29.1271069975175,56.4191030334511));
#107582=CARTESIAN_POINT('Ctrl Pts',(1.56476075036911,29.0255711178278,56.3553402961769));
#107583=CARTESIAN_POINT('Ctrl Pts',(1.57241330265993,28.9425679890345,56.2916242129417));
#107584=CARTESIAN_POINT('Ctrl Pts',(1.58792565713245,28.7862453544414,56.1463987663533));
#107585=CARTESIAN_POINT('Ctrl Pts',(1.59573718666305,28.7138669473411,56.0645656690184));
#107586=CARTESIAN_POINT('Ctrl Pts',(1.60468710956191,28.6374377502348,55.9588738902445));
#107587=CARTESIAN_POINT('Ctrl Pts',(1.60614459488135,28.6252189309845,55.9412715380698));
#107588=CARTESIAN_POINT('Ctrl Pts',(1.60841259941169,28.6065741700207,55.9132740909396));
#107589=CARTESIAN_POINT('Ctrl Pts',(1.60923170409134,28.5999175919399,55.903036197077));
#107590=CARTESIAN_POINT('Ctrl Pts',(1.6107588485616,28.5876551787815,55.8837148904707));
#107591=CARTESIAN_POINT('Ctrl Pts',(1.61146783941328,28.5820229444001,55.8746490613466));
#107592=CARTESIAN_POINT('Ctrl Pts',(1.6130551443398,28.5695533716093,55.854140564694));
#107593=CARTESIAN_POINT('Ctrl Pts',(1.61393162628132,28.5627654065791,55.8426686190815));
#107594=CARTESIAN_POINT('Ctrl Pts',(1.61657005535108,28.5426376325992,55.8077009712989));
#107595=CARTESIAN_POINT('Ctrl Pts',(1.61831657374723,28.529730589903,55.7839604090271));
#107596=CARTESIAN_POINT('Ctrl Pts',(1.62848372593572,28.4572477316185,55.6425464302532));
#107597=CARTESIAN_POINT('Ctrl Pts',(1.63641476948454,28.4112391723817,55.5184516451336));
#107598=CARTESIAN_POINT('Ctrl Pts',(1.64775293039193,28.3679465253655,55.3387616204373));
#107599=CARTESIAN_POINT('Ctrl Pts',(1.65102565499799,28.3580084947632,55.2867422065955));
#107600=CARTESIAN_POINT('Ctrl Pts',(1.65566383450378,28.3477389281926,55.214459010337));
#107601=CARTESIAN_POINT('Ctrl Pts',(1.65695225245788,28.345273939358,55.1945273919168));
#107602=CARTESIAN_POINT('Ctrl Pts',(1.65922912249614,28.3416022271565,55.1596768735656));
#107603=CARTESIAN_POINT('Ctrl Pts',(1.66021021849415,28.3402351105793,55.144776899537));
#107604=CARTESIAN_POINT('Ctrl Pts',(1.66169424919326,28.3384897467637,55.1224536071972));
#107605=CARTESIAN_POINT('Ctrl Pts',(1.66218926588359,28.3379601559401,55.115042422648));
#107606=CARTESIAN_POINT('Ctrl Pts',(1.66308921941328,28.3370923625884,55.1016377135591));
#107607=CARTESIAN_POINT('Ctrl Pts',(1.66349320510095,28.3367369549213,55.0956455702197));
#107608=CARTESIAN_POINT('Ctrl Pts',(1.6644102166037,28.3360070230248,55.082100861987));
#107609=CARTESIAN_POINT('Ctrl Pts',(1.66492424428685,28.3356515321349,55.0745476417261));
#107610=CARTESIAN_POINT('Ctrl Pts',(1.66650955598791,28.3347185531049,55.0513646427978));
#107611=CARTESIAN_POINT('Ctrl Pts',(1.66758933931891,28.3343097566956,55.0357294455583));
#107612=CARTESIAN_POINT('Ctrl Pts',(1.6757861888573,28.3328902581874,54.9180324692068));
#107613=CARTESIAN_POINT('Ctrl Pts',(1.68325974279632,28.3410408456804,54.8160849339055));
#107614=CARTESIAN_POINT('Ctrl Pts',(1.69884571307632,28.3776353914028,54.6049135283959));
#107615=CARTESIAN_POINT('Ctrl Pts',(1.70689902126361,28.4079406611171,54.4964964104152));
#107616=CARTESIAN_POINT('Ctrl Pts',(1.71602137160445,28.4565090893896,54.3726062413552));
#107617=CARTESIAN_POINT('Ctrl Pts',(1.71743285902179,28.4644484000797,54.35341785432));
#107618=CARTESIAN_POINT('Ctrl Pts',(1.71964589679254,28.4775677706495,54.3233155548683));
#107619=CARTESIAN_POINT('Ctrl Pts',(1.72045535448743,28.4825111185041,54.3123014911524));
#107620=CARTESIAN_POINT('Ctrl Pts',(1.72197394412251,28.4920572586976,54.2916364026767));
#107621=CARTESIAN_POINT('Ctrl Pts',(1.72268392131808,28.4966340612578,54.2819741227576));
#107622=CARTESIAN_POINT('Ctrl Pts',(1.72428586243481,28.5072174880883,54.2601758927125));
#107623=CARTESIAN_POINT('Ctrl Pts',(1.72517584585647,28.5132797400498,54.2480676731046));
#107624=CARTESIAN_POINT('Ctrl Pts',(1.7279007153697,28.5323973828499,54.2110190430211));
#107625=CARTESIAN_POINT('Ctrl Pts',(1.72971859866416,28.5459381668397,54.1863337746199));
#107626=CARTESIAN_POINT('Ctrl Pts',(1.73986196903656,28.6257893369015,54.049128380564));
#107627=CARTESIAN_POINT('Ctrl Pts',(1.74771443297892,28.7045222853212,53.9443714226131));
#107628=CARTESIAN_POINT('Ctrl Pts',(1.75895510742115,28.8310035613843,53.8118203862827));
#107629=CARTESIAN_POINT('Ctrl Pts',(1.7622084757703,28.8691003975332,53.7755046818852));
#107630=CARTESIAN_POINT('Ctrl Pts',(1.76742481691253,28.9311394508808,53.7217342598243));
#107631=CARTESIAN_POINT('Ctrl Pts',(1.76932618509085,28.9539383697286,53.703010798017));
#107632=CARTESIAN_POINT('Ctrl Pts',(1.77190001742731,28.9848233937124,53.6789908311738));
#107633=CARTESIAN_POINT('Ctrl Pts',(1.77253770469505,28.9924771643754,53.6731441333751));
#107634=CARTESIAN_POINT('Ctrl Pts',(1.77360030297302,29.0052241327182,53.6635806333742));
#107635=CARTESIAN_POINT('Ctrl Pts',(1.77402263028919,29.0102886472361,53.6598256885007));
#107636=CARTESIAN_POINT('Ctrl Pts',(1.7748790321333,29.0205517785922,53.6523062744813));
#107637=CARTESIAN_POINT('Ctrl Pts',(1.77531316346494,29.025751054369,53.6485429401458));
#107638=CARTESIAN_POINT('Ctrl Pts',(1.77643968277249,29.0392372137466,53.6388996675455));
#107639=CARTESIAN_POINT('Ctrl Pts',(1.77713501381907,29.0475562336769,53.6330654348135));
#107640=CARTESIAN_POINT('Ctrl Pts',(1.78000127547812,29.081847900978,53.6094812622407));
#107641=CARTESIAN_POINT('Ctrl Pts',(1.78220944109247,29.1082657825847,53.5923937263753));
#107642=CARTESIAN_POINT('Ctrl Pts',(1.7921834047149,29.2282112954471,53.5195427930953));
#107643=CARTESIAN_POINT('Ctrl Pts',(1.80020665929339,29.3265877951364,53.4722804099938));
#107644=CARTESIAN_POINT('Ctrl Pts',(1.81220800968084,29.4827655406637,53.4152868022079));
#107645=CARTESIAN_POINT('Ctrl Pts',(1.81630075860788,29.5376438405063,53.3984147595423));
#107646=CARTESIAN_POINT('Ctrl Pts',(1.82295375790556,29.6299151533283,53.3751862352941));
#107647=CARTESIAN_POINT('Ctrl Pts',(1.82555830594628,29.6668475383269,53.3672133032159));
#107648=CARTESIAN_POINT('Ctrl Pts',(1.82915078435788,29.7189097200391,53.3578145262619));
#107649=CARTESIAN_POINT('Ctrl Pts',(1.83017167337182,29.7338340236791,53.3553296455147));
#107650=CARTESIAN_POINT('Ctrl Pts',(1.83191821038516,29.7595833396045,53.3514021036281));
#107651=CARTESIAN_POINT('Ctrl Pts',(1.83264689021625,29.77039227256,53.3498619767445));
#107652=CARTESIAN_POINT('Ctrl Pts',(1.8340385624863,29.7911585120793,53.3471110668164));
#107653=CARTESIAN_POINT('Ctrl Pts',(1.83470204593146,29.8011131045779,53.3458837396373));
#107654=CARTESIAN_POINT('Ctrl Pts',(1.83643840095637,29.8273020336422,53.3428946778498));
#107655=CARTESIAN_POINT('Ctrl Pts',(1.83750658547659,29.8435525035648,53.3412815645414));
#107656=CARTESIAN_POINT('Ctrl Pts',(1.84136466773641,29.9027149308821,53.3362859872617));
#107657=CARTESIAN_POINT('Ctrl Pts',(1.84411054842524,29.9457320033905,53.3343277124911));
#107658=CARTESIAN_POINT('Ctrl Pts',(1.85404050963707,30.1036047654424,53.3332644314698));
#107659=CARTESIAN_POINT('Ctrl Pts',(1.86094049954242,30.2181998099546,53.3443638947905));
#107660=CARTESIAN_POINT('Ctrl Pts',(1.87097559680838,30.378138044721,53.3767606775331));
#107661=CARTESIAN_POINT('Ctrl Pts',(1.87397676478242,30.4250877286833,53.388418771063));
#107662=CARTESIAN_POINT('Ctrl Pts',(1.87883442126873,30.4982724912221,53.4100119522052));
#107663=CARTESIAN_POINT('Ctrl Pts',(1.88063906103567,30.5248793281929,53.418595895637));
#107664=CARTESIAN_POINT('Ctrl Pts',(1.88310065145339,30.5601726003448,53.4309710188183));
#107665=CARTESIAN_POINT('Ctrl Pts',(1.88372653088112,30.5690624433048,53.4341733138086));
#107666=CARTESIAN_POINT('Ctrl Pts',(1.88477477000892,30.5838021380773,53.4396249365411));
#107667=CARTESIAN_POINT('Ctrl Pts',(1.88519468936442,30.5896675709933,53.4418320281007));
#107668=CARTESIAN_POINT('Ctrl Pts',(1.88599902327518,30.6008246053475,53.4461023037309));
#107669=CARTESIAN_POINT('Ctrl Pts',(1.88638305838771,30.6061183576474,53.4481595472037));
#107670=CARTESIAN_POINT('Ctrl Pts',(1.88742242905564,30.6203591087152,53.4537777307764));
#107671=CARTESIAN_POINT('Ctrl Pts',(1.88808065298119,30.6292857570461,53.4573891759503));
#107672=CARTESIAN_POINT('Ctrl Pts',(1.89061116502186,30.6632735111864,53.4714836600468));
#107673=CARTESIAN_POINT('Ctrl Pts',(1.8925109634703,30.6881067549831,53.4825011224374));
#107674=CARTESIAN_POINT('Ctrl Pts',(1.90232643874191,30.8134854672589,53.5418366013268));
#107675=CARTESIAN_POINT('Ctrl Pts',(1.91054940359927,30.9092625715218,53.5995572370022));
#107676=CARTESIAN_POINT('Ctrl Pts',(1.92287904315784,31.0458478202143,53.7018284200254));
#107677=CARTESIAN_POINT('Ctrl Pts',(1.92709918374005,31.0912304092289,53.7397363424899));
#107678=CARTESIAN_POINT('Ctrl Pts',(1.93306878782953,31.1537069462699,53.7978337343026));
#107679=CARTESIAN_POINT('Ctrl Pts',(1.93488616758742,31.1724841225784,53.8161399741545));
#107680=CARTESIAN_POINT('Ctrl Pts',(1.93814322064888,31.2056876787681,53.8500760723677));
#107681=CARTESIAN_POINT('Ctrl Pts',(1.93958896415238,31.2202615054464,53.8655531088244));
#107682=CARTESIAN_POINT('Ctrl Pts',(1.94184294799629,31.2427114999154,53.8903278080177));
#107683=CARTESIAN_POINT('Ctrl Pts',(1.9426595985208,31.2507882782727,53.8994397143947));
#107684=CARTESIAN_POINT('Ctrl Pts',(1.94418453071952,31.2657586511735,53.9167063984218));
#107685=CARTESIAN_POINT('Ctrl Pts',(1.94489373676881,31.2726751026927,53.924840438681));
#107686=CARTESIAN_POINT('Ctrl Pts',(1.94648458733679,31.2880823222194,53.9433169969082));
#107687=CARTESIAN_POINT('Ctrl Pts',(1.94736436352499,31.2965277084127,53.9536965275173));
#107688=CARTESIAN_POINT('Ctrl Pts',(1.94962492938421,31.3180231906617,53.9807748228198));
#107689=CARTESIAN_POINT('Ctrl Pts',(1.95099817639356,31.3308815990393,53.9976231611595));
#107690=CARTESIAN_POINT('Ctrl Pts',(1.96048457186252,31.4181813568334,54.1166543017011));
#107691=CARTESIAN_POINT('Ctrl Pts',(1.96813546344748,31.4811022622504,54.2267744266908));
#107692=CARTESIAN_POINT('Ctrl Pts',(1.98110323404326,31.5647173877109,54.421605940013));
#107693=CARTESIAN_POINT('Ctrl Pts',(1.98636871638347,31.5923547647007,54.5027247491917));
#107694=CARTESIAN_POINT('Ctrl Pts',(1.9928544280686,31.6171410703874,54.5992392132915));
#107695=CARTESIAN_POINT('Ctrl Pts',(1.99377937361443,31.6204718191115,54.6129270081891));
#107696=CARTESIAN_POINT('Ctrl Pts',(1.99519489801449,31.6252544143446,54.6337258784986));
#107697=CARTESIAN_POINT('Ctrl Pts',(1.9956785992869,31.6268341179498,54.6408073063535));
#107698=CARTESIAN_POINT('Ctrl Pts',(1.99656786505943,31.6296378505498,54.6537737636451));
#107699=CARTESIAN_POINT('Ctrl Pts',(1.99697261158695,31.6308763519442,54.6596553928348));
#107700=CARTESIAN_POINT('Ctrl Pts',(1.99790428819096,31.6336415143507,54.6731488542433));
#107701=CARTESIAN_POINT('Ctrl Pts',(1.99843237039652,31.6351468131204,54.6807647224817));
#107702=CARTESIAN_POINT('Ctrl Pts',(2.00006592327948,31.6396151401567,54.7042327551615));
#107703=CARTESIAN_POINT('Ctrl Pts',(2.00118039423116,31.6424011672701,54.7201171157184));
#107704=CARTESIAN_POINT('Ctrl Pts',(2.00843434240002,31.6588863359117,54.8228495023147));
#107705=CARTESIAN_POINT('Ctrl Pts',(2.0148359334606,31.6659214902038,54.9106190018576));
#107706=CARTESIAN_POINT('Ctrl Pts',(2.02993617082025,31.6661052143905,55.118056849621));
#107707=CARTESIAN_POINT('Ctrl Pts',(2.03856946052953,31.6533464665299,55.2372744191505));
#107708=CARTESIAN_POINT('Ctrl Pts',(2.04830036998259,31.6233134415598,55.3753416569323));
#107709=CARTESIAN_POINT('Ctrl Pts',(2.04978357248641,31.6182812322145,55.3964767578125));
#107710=CARTESIAN_POINT('Ctrl Pts',(2.05216955248848,31.6094449571812,55.430611338695));
#107711=CARTESIAN_POINT('Ctrl Pts',(2.05308027434977,31.6058933891001,55.4436728939457));
#107712=CARTESIAN_POINT('Ctrl Pts',(2.054701096337,31.5992524351727,55.466971021231));
#107713=CARTESIAN_POINT('Ctrl Pts',(2.05541309076138,31.5962229790226,55.47722373837));
#107714=CARTESIAN_POINT('Ctrl Pts',(2.05692248619468,31.5895619642043,55.4989935590384));
#107715=CARTESIAN_POINT('Ctrl Pts',(2.0577189617956,31.5859034382728,55.5105018191712));
#107716=CARTESIAN_POINT('Ctrl Pts',(2.05975211463279,31.576196994763,55.5399226136569));
#107717=CARTESIAN_POINT('Ctrl Pts',(2.06098283076197,31.5699686641503,55.5577739909768));
#107718=CARTESIAN_POINT('Ctrl Pts',(2.06220431895159,31.5634376782779,55.5755159651488));
#107719=CARTESIAN_POINT('',(1.82701796270648,31.6659995261751,54.9996754260968));
#107720=CARTESIAN_POINT('Ctrl Pts',(1.86810672180998,31.5634374966623,55.5755164585225));
#107721=CARTESIAN_POINT('Ctrl Pts',(1.86162124916867,31.5942217432641,55.4918885366255));
#107722=CARTESIAN_POINT('Ctrl Pts',(1.85513196704194,31.6182725433958,55.4058535797404));
#107723=CARTESIAN_POINT('Ctrl Pts',(1.84519623197039,31.6450887968234,55.2680535911724));
#107724=CARTESIAN_POINT('Ctrl Pts',(1.8416383236559,31.652540421337,55.217441910937));
#107725=CARTESIAN_POINT('Ctrl Pts',(1.83699844869998,31.6593446954984,55.1497249313236));
#107726=CARTESIAN_POINT('Ctrl Pts',(1.83585274662337,31.660779980928,55.132861827411));
#107727=CARTESIAN_POINT('Ctrl Pts',(1.8339491592536,31.6627512610417,55.1046137945673));
#107728=CARTESIAN_POINT('Ctrl Pts',(1.83318694045077,31.6634278047983,55.0932402889168));
#107729=CARTESIAN_POINT('Ctrl Pts',(1.83175227031401,31.6644865851243,55.0717183387098));
#107730=CARTESIAN_POINT('Ctrl Pts',(1.83107910221284,31.6648928048197,55.0615716525277));
#107731=CARTESIAN_POINT('Ctrl Pts',(1.82982340625863,31.6654799565435,55.0425577175188));
#107732=CARTESIAN_POINT('Ctrl Pts',(1.82924022080164,31.6656829016532,55.0336915593658));
#107733=CARTESIAN_POINT('Ctrl Pts',(1.82810991512576,31.6659399624236,55.0164415316275));
#107734=CARTESIAN_POINT('Ctrl Pts',(1.82756258501001,31.6660016065409,55.0080580840373));
#107735=CARTESIAN_POINT('Ctrl Pts',(1.82701713034439,31.6659999681879,54.9996744265695));
#107736=CARTESIAN_POINT('Ctrl Pts',(1.8270171986045,31.6659999683926,54.9996754757297));
#107737=CARTESIAN_POINT('Ctrl Pts',(1.82545459450402,31.6659952900083,54.9756582024739));
#107738=CARTESIAN_POINT('Ctrl Pts',(1.82390766287911,31.6654712595334,54.9516426944095));
#107739=CARTESIAN_POINT('Ctrl Pts',(1.81315015462543,31.6581516881125,54.7832643755715));
#107740=CARTESIAN_POINT('Ctrl Pts',(1.80453959996092,31.6331175236017,54.6403210644769));
#107741=CARTESIAN_POINT('Ctrl Pts',(1.79300163391142,31.5773144908242,54.4620173072672));
#107742=CARTESIAN_POINT('Ctrl Pts',(1.79036091279522,31.5631434602999,54.4221345953644));
#107743=CARTESIAN_POINT('Ctrl Pts',(1.78602424539879,31.5379874958443,54.3590586422362));
#107744=CARTESIAN_POINT('Ctrl Pts',(1.78436756545193,31.5279578624559,54.3355032268822));
#107745=CARTESIAN_POINT('Ctrl Pts',(1.78207860655124,31.5136128755519,54.3038564981124));
#107746=CARTESIAN_POINT('Ctrl Pts',(1.7814721376765,31.5097670407183,54.2955546965675));
#107747=CARTESIAN_POINT('Ctrl Pts',(1.78044741990471,31.5031982042695,54.2816757882732));
#107748=CARTESIAN_POINT('Ctrl Pts',(1.78003138120708,31.5005119884205,54.2760812991001));
#107749=CARTESIAN_POINT('Ctrl Pts',(1.77922665751888,31.4952808050423,54.2653407102399));
#107750=CARTESIAN_POINT('Ctrl Pts',(1.77883828585564,31.4927404000865,54.2601925565485));
#107751=CARTESIAN_POINT('Ctrl Pts',(1.77777213454489,31.4857222691937,54.2461535724902));
#107752=CARTESIAN_POINT('Ctrl Pts',(1.77709120786874,31.4811914696723,54.2372897565894));
#107753=CARTESIAN_POINT('Ctrl Pts',(1.7743593978341,31.4628120778357,54.2021147411864));
#107754=CARTESIAN_POINT('Ctrl Pts',(1.77227534997809,31.4483404714248,54.1761373406294));
#107755=CARTESIAN_POINT('Ctrl Pts',(1.76236674633126,31.3771367907041,54.0560014286126));
#107756=CARTESIAN_POINT('Ctrl Pts',(1.75426545387636,31.3118715025401,53.967221323938));
#107757=CARTESIAN_POINT('Ctrl Pts',(1.74213386481641,31.1994948296562,53.8423558831478));
#107758=CARTESIAN_POINT('Ctrl Pts',(1.73798944924613,31.1584177609886,53.8012518331443));
#107759=CARTESIAN_POINT('Ctrl Pts',(1.73211358199466,31.0960080514969,53.7450119661342));
#107760=CARTESIAN_POINT('Ctrl Pts',(1.73031656073776,31.0763381613991,53.7281018505269));
#107761=CARTESIAN_POINT('Ctrl Pts',(1.72749013393833,31.0444689505283,53.7019730726805));
#107762=CARTESIAN_POINT('Ctrl Pts',(1.7264489937337,31.0325244545265,53.6924516948419));
#107763=CARTESIAN_POINT('Ctrl Pts',(1.72446897629792,31.0094182648121,53.6745470387924));
#107764=CARTESIAN_POINT('Ctrl Pts',(1.72352910642904,30.9982789087764,53.6661371784974));
#107765=CARTESIAN_POINT('Ctrl Pts',(1.7218760262348,30.9783869572933,53.6515081770223));
#107766=CARTESIAN_POINT('Ctrl Pts',(1.72116062434236,30.9696775921364,53.6452318975485));
#107767=CARTESIAN_POINT('Ctrl Pts',(1.7196634746959,30.9512422684978,53.6322156066511));
#107768=CARTESIAN_POINT('Ctrl Pts',(1.71888246202362,30.9415039114763,53.6254941262773));
#107769=CARTESIAN_POINT('Ctrl Pts',(1.7168150815245,30.9154098789987,53.6078913024881));
#107770=CARTESIAN_POINT('Ctrl Pts',(1.71553563556124,30.8989316521528,53.597194307843));
#107771=CARTESIAN_POINT('Ctrl Pts',(1.70892845913668,30.8122012453888,53.5430484505212));
#107772=CARTESIAN_POINT('Ctrl Pts',(1.70378412295184,30.7389745377882,53.5045743745793));
#107773=CARTESIAN_POINT('Ctrl Pts',(1.69256306151661,30.5713699875706,53.4318449418227));
#107774=CARTESIAN_POINT('Ctrl Pts',(1.68654443308458,30.4761547902633,53.4003599704506));
#107775=CARTESIAN_POINT('Ctrl Pts',(1.67849819986473,30.3511711655311,53.3711864013255));
#107776=CARTESIAN_POINT('Ctrl Pts',(1.67670627845677,30.3234882523873,53.3654633386732));
#107777=CARTESIAN_POINT('Ctrl Pts',(1.67364029107188,30.2766855969896,53.3570230076238));
#107778=CARTESIAN_POINT('Ctrl Pts',(1.67238253268194,30.2576393175246,53.353928852905));
#107779=CARTESIAN_POINT('Ctrl Pts',(1.6705649045693,30.2304153576684,53.3499902330701));
#107780=CARTESIAN_POINT('Ctrl Pts',(1.67001907312608,30.2222777255236,53.3488743010434));
#107781=CARTESIAN_POINT('Ctrl Pts',(1.66906525194994,30.2081303849035,53.3470407228183));
#107782=CARTESIAN_POINT('Ctrl Pts',(1.66865879056953,30.2021244785667,53.3462955756964));
#107783=CARTESIAN_POINT('Ctrl Pts',(1.66778159904653,30.1892142541833,53.3447651985333));
#107784=CARTESIAN_POINT('Ctrl Pts',(1.66731034295626,30.1823091485964,53.343990443292));
#107785=CARTESIAN_POINT('Ctrl Pts',(1.66600022926708,30.1631916496731,53.341966469299));
#107786=CARTESIAN_POINT('Ctrl Pts',(1.6651566249039,30.150970271677,53.3408090349767));
#107787=CARTESIAN_POINT('Ctrl Pts',(1.6592168991312,30.0654620199834,53.3336634369441));
#107788=CARTESIAN_POINT('Ctrl Pts',(1.65391673065422,29.9918691341066,53.3323986358104));
#107789=CARTESIAN_POINT('Ctrl Pts',(1.64756627910136,29.9045673928382,53.3366775421322));
#107790=CARTESIAN_POINT('Ctrl Pts',(1.64655561902706,29.8907013871527,53.3375311157672));
#107791=CARTESIAN_POINT('Ctrl Pts',(1.64017844236694,29.8033223804976,53.3440079722916));
#107792=CARTESIAN_POINT('Ctrl Pts',(1.63481220114361,29.7302352218971,53.3543329734595));
#107793=CARTESIAN_POINT('Ctrl Pts',(1.62652038347741,29.6165109170415,53.3781815319759));
#107794=CARTESIAN_POINT('Ctrl Pts',(1.62352675071475,29.5752986202062,53.3884826222272));
#107795=CARTESIAN_POINT('Ctrl Pts',(1.61845720268266,29.505163266743,53.4088911016016));
#107796=CARTESIAN_POINT('Ctrl Pts',(1.61635984400561,29.4760437236068,53.4182411838164));
#107797=CARTESIAN_POINT('Ctrl Pts',(1.61334192209568,29.4340153478832,53.4330243757939));
#107798=CARTESIAN_POINT('Ctrl Pts',(1.61240094466489,29.4208928935409,53.43782644588));
#107799=CARTESIAN_POINT('Ctrl Pts',(1.61074661247312,29.3977963482315,53.4466095012775));
#107800=CARTESIAN_POINT('Ctrl Pts',(1.61003105491761,29.3877975768246,53.4505228359022));
#107801=CARTESIAN_POINT('Ctrl Pts',(1.60853425910978,29.3668683551399,53.4589483678406));
#107802=CARTESIAN_POINT('Ctrl Pts',(1.60775374939678,29.3559466698598,53.4634808387872));
#107803=CARTESIAN_POINT('Ctrl Pts',(1.60568929300342,29.3270462736511,53.4758367270113));
#107804=CARTESIAN_POINT('Ctrl Pts',(1.60441223239766,29.3091555001576,53.4838620345714));
#107805=CARTESIAN_POINT('Ctrl Pts',(1.59780139379085,29.2165740891088,53.5273706809531));
#107806=CARTESIAN_POINT('Ctrl Pts',(1.5926515337153,29.1444554901765,53.5680644717262));
#107807=CARTESIAN_POINT('Ctrl Pts',(1.58142593811846,28.9923901465746,53.6694761797207));
#107808=CARTESIAN_POINT('Ctrl Pts',(1.57540808406082,28.9143084514867,53.7323869777593));
#107809=CARTESIAN_POINT('Ctrl Pts',(1.56736278156584,28.8220230030647,53.8215582210736));
#107810=CARTESIAN_POINT('Ctrl Pts',(1.56557096281884,28.8022018018608,53.8417106889399));
#107811=CARTESIAN_POINT('Ctrl Pts',(1.56250513301176,28.7697283474813,53.876452072187));
#107812=CARTESIAN_POINT('Ctrl Pts',(1.56124742731583,28.7567993401324,53.8907748981509));
#107813=CARTESIAN_POINT('Ctrl Pts',(1.55942986174889,28.7387256357218,53.9115100166402));
#107814=CARTESIAN_POINT('Ctrl Pts',(1.55888403880474,28.7333746086386,53.9177414464075));
#107815=CARTESIAN_POINT('Ctrl Pts',(1.55793022935023,28.7241612274403,53.9286326237052));
#107816=CARTESIAN_POINT('Ctrl Pts',(1.55752377112301,28.7202778318203,53.9332742622951));
#107817=CARTESIAN_POINT('Ctrl Pts',(1.55664658713342,28.7119901085546,53.9432905789275));
#107818=CARTESIAN_POINT('Ctrl Pts',(1.55617533542854,28.7075941538739,53.9486715995747));
#107819=CARTESIAN_POINT('Ctrl Pts',(1.55486522167967,28.6955250552195,53.9636352845701));
#107820=CARTESIAN_POINT('Ctrl Pts',(1.55402161266648,28.6879241519822,53.9732752794011));
#107821=CARTESIAN_POINT('Ctrl Pts',(1.54807856574748,28.6355148457625,54.0412768276282));
#107822=CARTESIAN_POINT('Ctrl Pts',(1.54277481148151,28.5945138895433,54.1024610031834));
#107823=CARTESIAN_POINT('Ctrl Pts',(1.53642350898985,28.5507604716399,54.1781406808692));
#107824=CARTESIAN_POINT('Ctrl Pts',(1.53541554604558,28.5439759738917,54.190221028372));
#107825=CARTESIAN_POINT('Ctrl Pts',(1.52904081938915,28.5020437887612,54.2671157321701));
#107826=CARTESIAN_POINT('Ctrl Pts',(1.52367434873561,28.471078415021,54.3341229360585));
#107827=CARTESIAN_POINT('Ctrl Pts',(1.51538281450795,28.4294383682575,54.44260012493));
#107828=CARTESIAN_POINT('Ctrl Pts',(1.51238966252254,28.4157435181653,54.4828052975065));
#107829=CARTESIAN_POINT('Ctrl Pts',(1.50732083444693,28.3948543619303,54.5527884341238));
#107830=CARTESIAN_POINT('Ctrl Pts',(1.50522372261267,28.3869175343474,54.5823208456159));
#107831=CARTESIAN_POINT('Ctrl Pts',(1.50220609444681,28.3765440683641,54.6256444867381));
#107832=CARTESIAN_POINT('Ctrl Pts',(1.5012651688785,28.3734615738662,54.6392729823871));
#107833=CARTESIAN_POINT('Ctrl Pts',(1.49961090561002,28.3683141622381,54.6634400481494));
#107834=CARTESIAN_POINT('Ctrl Pts',(1.49889536551323,28.3661790367167,54.6739626653955));
#107835=CARTESIAN_POINT('Ctrl Pts',(1.49739858490073,28.361906545279,54.6961157336074));
#107836=CARTESIAN_POINT('Ctrl Pts',(1.4966180731144,28.3597909716438,54.707749817461));
#107837=CARTESIAN_POINT('Ctrl Pts',(1.49455356233962,28.3544971109928,54.738732560366));
#107838=CARTESIAN_POINT('Ctrl Pts',(1.49327645039224,28.3515361626938,54.7581168412506));
#107839=CARTESIAN_POINT('Ctrl Pts',(1.48666336828763,28.3378726599678,54.8595307272466));
#107840=CARTESIAN_POINT('Ctrl Pts',(1.48151148629976,28.3329476417354,54.9422259193693));
#107841=CARTESIAN_POINT('Ctrl Pts',(1.47028574270696,28.3356854107449,55.1249893805996));
#107842=CARTESIAN_POINT('Ctrl Pts',(1.4642695819662,28.3461916918903,55.2246800784204));
#107843=CARTESIAN_POINT('Ctrl Pts',(1.45622631486988,28.3710513278489,55.3505436374686));
#107844=CARTESIAN_POINT('Ctrl Pts',(1.45443472761848,28.3772314402018,55.378122519316));
#107845=CARTESIAN_POINT('Ctrl Pts',(1.45136925654467,28.3888056774827,55.4242417539828));
#107846=CARTESIAN_POINT('Ctrl Pts',(1.45011167355326,28.39382627003,55.4428702768221));
#107847=CARTESIAN_POINT('Ctrl Pts',(1.44829425887694,28.4014436626229,55.4692985144436));
#107848=CARTESIAN_POINT('Ctrl Pts',(1.44774846134071,28.4037766650638,55.4771734668222));
#107849=CARTESIAN_POINT('Ctrl Pts',(1.44679468340232,28.4079297042952,55.4908205384443));
#107850=CARTESIAN_POINT('Ctrl Pts',(1.44638823104354,28.4097231193882,55.496600512557));
#107851=CARTESIAN_POINT('Ctrl Pts',(1.44551104208058,28.4136433481497,55.5089959295817));
#107852=CARTESIAN_POINT('Ctrl Pts',(1.44503977937014,28.4157800345318,55.515607777103));
#107853=CARTESIAN_POINT('Ctrl Pts',(1.44372960885209,28.4218061357239,55.5338640724257));
#107854=CARTESIAN_POINT('Ctrl Pts',(1.44288595344469,28.4257829089762,55.5454789173592));
#107855=CARTESIAN_POINT('Ctrl Pts',(1.4369315645855,28.4545440905291,55.6265460139007));
#107856=CARTESIAN_POINT('Ctrl Pts',(1.43161561287307,28.4837851026776,55.694322583514));
#107857=CARTESIAN_POINT('Ctrl Pts',(1.42526155549592,28.5236756656456,55.7721469283415));
#107858=CARTESIAN_POINT('Ctrl Pts',(1.42426289883446,28.5300876309351,55.7842844146353));
#107859=CARTESIAN_POINT('Ctrl Pts',(1.41789682521329,28.5718958598099,55.861110930057));
#107860=CARTESIAN_POINT('Ctrl Pts',(1.41252976239839,28.6114064343231,55.9234731705136));
#107861=CARTESIAN_POINT('Ctrl Pts',(1.40423943834486,28.6799580098698,56.0172736240694));
#107862=CARTESIAN_POINT('Ctrl Pts',(1.40124798970957,28.706296106715,56.050565189975));
#107863=CARTESIAN_POINT('Ctrl Pts',(1.39618168343564,28.7537417114864,56.1060426049515));
#107864=CARTESIAN_POINT('Ctrl Pts',(1.39408541939701,28.7742410938291,56.1287184247126));
#107865=CARTESIAN_POINT('Ctrl Pts',(1.3910687584268,28.8050038513502,56.1609200493473));
#107866=CARTESIAN_POINT('Ctrl Pts',(1.39012797114075,28.8147806762966,56.1708997957246));
#107867=CARTESIAN_POINT('Ctrl Pts',(1.38847385639718,28.8322914476585,56.188329923855));
#107868=CARTESIAN_POINT('Ctrl Pts',(1.38775832804057,28.8399739474269,56.1958306058005));
#107869=CARTESIAN_POINT('Ctrl Pts',(1.38626147944064,28.8562694708485,56.2114356439742));
#107870=CARTESIAN_POINT('Ctrl Pts',(1.38548088882809,28.8648973858091,56.219523640689));
#107871=CARTESIAN_POINT('Ctrl Pts',(1.38341595200232,28.8880613567772,56.2407792296484));
#107872=CARTESIAN_POINT('Ctrl Pts',(1.38213849778741,28.9027453236686,56.2537834226763));
#107873=CARTESIAN_POINT('Ctrl Pts',(1.37551350721059,28.9806793800562,56.3203840874707));
#107874=CARTESIAN_POINT('Ctrl Pts',(1.37035093906019,29.0476387778234,56.3694667858024));
#107875=CARTESIAN_POINT('Ctrl Pts',(1.35912456372117,29.2027232024081,56.4662480885993));
#107876=CARTESIAN_POINT('Ctrl Pts',(1.35311749275381,29.2920432085326,56.5113995486379));
#107877=CARTESIAN_POINT('Ctrl Pts',(1.34508516528203,29.4111071176862,56.5587041622979));
#107878=CARTESIAN_POINT('Ctrl Pts',(1.34329479314591,29.437610964459,56.568461630211));
#107879=CARTESIAN_POINT('Ctrl Pts',(1.34023118724796,29.4826074929771,56.583740138446));
#107880=CARTESIAN_POINT('Ctrl Pts',(1.33897422775287,29.5009718970461,56.5896221900902));
#107881=CARTESIAN_POINT('Ctrl Pts',(1.33715755068577,29.5272960708878,56.5975526376363));
#107882=CARTESIAN_POINT('Ctrl Pts',(1.33661185106327,29.5351760729126,56.5998631642844));
#107883=CARTESIAN_POINT('Ctrl Pts',(1.33565816888094,29.5488926446665,56.6037751655902));
#107884=CARTESIAN_POINT('Ctrl Pts',(1.33525171306428,29.5547213811644,56.6054032446893));
#107885=CARTESIAN_POINT('Ctrl Pts',(1.33437441443045,29.5672630641948,56.6088328220225));
#107886=CARTESIAN_POINT('Ctrl Pts',(1.33390304450917,29.5739783496648,56.6106240572732));
#107887=CARTESIAN_POINT('Ctrl Pts',(1.3325923797577,29.5925916017846,56.6154644088117));
#107888=CARTESIAN_POINT('Ctrl Pts',(1.33174833256043,29.6045121023447,56.618423974039));
#107889=CARTESIAN_POINT('Ctrl Pts',(1.32569160292859,29.6896575730394,56.6385666687387));
#107890=CARTESIAN_POINT('Ctrl Pts',(1.3202655089478,29.7639321438001,56.6509035733368));
#107891=CARTESIAN_POINT('Ctrl Pts',(1.31070997068137,29.894793894958,56.6636271464996));
#107892=CARTESIAN_POINT('Ctrl Pts',(1.30660272508455,29.9510524710172,56.6662316696808));
#107893=CARTESIAN_POINT('Ctrl Pts',(1.29817811186969,30.0675683411384,56.665718640139));
#107894=CARTESIAN_POINT('Ctrl Pts',(1.29387263590671,30.1277471969581,56.662187100707));
#107895=CARTESIAN_POINT('Ctrl Pts',(1.28692410013935,30.2263751524321,56.6510095420821));
#107896=CARTESIAN_POINT('Ctrl Pts',(1.28423137128154,30.2649788139003,56.6452552633158));
#107897=CARTESIAN_POINT('Ctrl Pts',(1.28054086101679,30.318398556562,56.6353631569457));
#107898=CARTESIAN_POINT('Ctrl Pts',(1.27950765465472,30.3334107026459,56.6323687164494));
#107899=CARTESIAN_POINT('Ctrl Pts',(1.27774683097975,30.359084741412,56.6268786009717));
#107900=CARTESIAN_POINT('Ctrl Pts',(1.27701604876348,30.369766981032,56.6244839868125));
#107901=CARTESIAN_POINT('Ctrl Pts',(1.27562484554485,30.3901503610339,56.6197032074149));
#107902=CARTESIAN_POINT('Ctrl Pts',(1.27496389274934,30.3998551189811,56.6173347444214));
#107903=CARTESIAN_POINT('Ctrl Pts',(1.27341498931098,30.4226417428048,56.6115559884474));
#107904=CARTESIAN_POINT('Ctrl Pts',(1.27252939093446,30.4357046894401,56.6080734398498));
#107905=CARTESIAN_POINT('Ctrl Pts',(1.26941772926448,30.481703914959,56.5952084759964));
#107906=CARTESIAN_POINT('Ctrl Pts',(1.2672191170551,30.5143931039393,56.5849696322846));
#107907=CARTESIAN_POINT('Ctrl Pts',(1.25644277347106,30.6749036518491,56.529205044749));
#107908=CARTESIAN_POINT('Ctrl Pts',(1.24834585110935,30.797137664849,56.4691952569685));
#107909=CARTESIAN_POINT('Ctrl Pts',(1.2373489311958,30.9462572848193,56.3718425264055));
#107910=CARTESIAN_POINT('Ctrl Pts',(1.23470228392069,30.980870334512,56.3473112755981));
#107911=CARTESIAN_POINT('Ctrl Pts',(1.23035696506312,31.0348454794541,56.3058745178396));
#107912=CARTESIAN_POINT('Ctrl Pts',(1.22869775243213,31.0548191214636,56.2897945078219));
#107913=CARTESIAN_POINT('Ctrl Pts',(1.22640582586112,31.0814091491183,56.2673571174912));
#107914=CARTESIAN_POINT('Ctrl Pts',(1.22579900734392,31.0883568653186,56.2613957092289));
#107915=CARTESIAN_POINT('Ctrl Pts',(1.22477387015729,31.0999320792366,56.2512969065872));
#107916=CARTESIAN_POINT('Ctrl Pts',(1.22435776580286,31.1045863560583,56.2471902452294));
#107917=CARTESIAN_POINT('Ctrl Pts',(1.22349863386286,31.1141030028915,56.2386982568206));
#107918=CARTESIAN_POINT('Ctrl Pts',(1.22305541799609,31.1189626173108,56.2343101432923));
#107919=CARTESIAN_POINT('Ctrl Pts',(1.22187833058131,31.1317407156787,56.2226343547589));
#107920=CARTESIAN_POINT('Ctrl Pts',(1.22114102080575,31.1396145163202,56.2152985443536));
#107921=CARTESIAN_POINT('Ctrl Pts',(1.21782195287873,31.1745048246528,56.1821549588813));
#107922=CARTESIAN_POINT('Ctrl Pts',(1.21518732554207,31.2007177114103,56.1555208490829));
#107923=CARTESIAN_POINT('Ctrl Pts',(1.20585337135115,31.2891848315141,56.0593695155096));
#107924=CARTESIAN_POINT('Ctrl Pts',(1.19900156327357,31.3464777613659,55.9855244947298));
#107925=CARTESIAN_POINT('Ctrl Pts',(1.18770469930283,31.4314555064802,55.8546506428026));
#107926=CARTESIAN_POINT('Ctrl Pts',(1.1832123278711,31.4626265737974,55.8001358997034));
#107927=CARTESIAN_POINT('Ctrl Pts',(1.17690862871526,31.5027993434716,55.7196459222719));
#107928=CARTESIAN_POINT('Ctrl Pts',(1.17502061616985,31.5143508787191,55.6950091230303));
#107929=CARTESIAN_POINT('Ctrl Pts',(1.17165087375399,31.5340909334462,55.6500763802735));
#107930=CARTESIAN_POINT('Ctrl Pts',(1.17016241288042,31.5424926772205,55.629881506246));
#107931=CARTESIAN_POINT('Ctrl Pts',(1.16786919232177,31.5549326156587,55.598237158764));
#107932=CARTESIAN_POINT('Ctrl Pts',(1.16705525638087,31.5592472018856,55.5868997478374));
#107933=CARTESIAN_POINT('Ctrl Pts',(1.16624544379888,31.5634376782622,55.5755159651914));
#107934=CARTESIAN_POINT('Origin',(5.,30.,55.));
#107935=CARTESIAN_POINT('',(0.468131466136091,31.5634376737814,55.5755159773639));
#107936=CARTESIAN_POINT('',(0.659214778542432,31.5634376782623,55.5755159651912));
#107937=CARTESIAN_POINT('',(5.,31.5634376782623,55.5755159651912));
#107938=CARTESIAN_POINT('',(0.428519636557294,31.6659995598398,55.0012110382147));
#107939=CARTESIAN_POINT('Ctrl Pts',(0.468131466136093,31.5634376737814,
55.5755159773639));
#107940=CARTESIAN_POINT('Ctrl Pts',(0.464345120637409,31.5848558755545,
55.5173316264964));
#107941=CARTESIAN_POINT('Ctrl Pts',(0.460549326597193,31.60301167801,55.4579905871979));
#107942=CARTESIAN_POINT('Ctrl Pts',(0.454337482247741,31.6265637629815,
55.3621989390725));
#107943=CARTESIAN_POINT('Ctrl Pts',(0.451994271554866,31.6341331843492,
55.3263526177191));
#107944=CARTESIAN_POINT('Ctrl Pts',(0.448892310075098,31.6423730132732,
55.2797867743918));
#107945=CARTESIAN_POINT('Ctrl Pts',(0.448187753916178,31.6441304562902,
55.2692671198243));
#107946=CARTESIAN_POINT('Ctrl Pts',(0.447044451267056,31.6467972710023,
55.2523035667945));
#107947=CARTESIAN_POINT('Ctrl Pts',(0.44660917319137,31.6477701312234,55.2458697471883));
#107948=CARTESIAN_POINT('Ctrl Pts',(0.445791850431163,31.6495173148384,
55.2338387385693));
#107949=CARTESIAN_POINT('Ctrl Pts',(0.445410339313308,31.6503009011882,
55.2282429847506));
#107950=CARTESIAN_POINT('Ctrl Pts',(0.44460714387084,31.6518841620995,55.2165020060958));
#107951=CARTESIAN_POINT('Ctrl Pts',(0.444185149393181,31.6526780456202,
55.2103560746072));
#107952=CARTESIAN_POINT('Ctrl Pts',(0.443174754118641,31.65448920107,55.1956913104553));
#107953=CARTESIAN_POINT('Ctrl Pts',(0.442584768285556,31.655474981912,55.1871688601511));
#107954=CARTESIAN_POINT('Ctrl Pts',(0.440597126672424,31.6585582222188,
55.1585801863687));
#107955=CARTESIAN_POINT('Ctrl Pts',(0.439185907728137,31.6603569074475,
55.1384843286982));
#107956=CARTESIAN_POINT('Ctrl Pts',(0.435001096303271,31.6645687872148,
55.0793498872961));
#107957=CARTESIAN_POINT('Ctrl Pts',(0.432193622589638,31.6659726121579,
55.0402549587981));
#107958=CARTESIAN_POINT('Ctrl Pts',(0.429364752169372,31.6659996031586,
55.0011499023514));
#107959=CARTESIAN_POINT('',(0.,28.7309291201476,56.0793586530485));
#107960=CARTESIAN_POINT('Ctrl Pts',(0.428519636557294,31.6659995598398,
55.0012110382147));
#107961=CARTESIAN_POINT('Ctrl Pts',(0.424501125348764,31.6660430829186,
54.9413372627796));
#107962=CARTESIAN_POINT('Ctrl Pts',(0.420482614140233,31.6628547021932,
54.8813422492068));
#107963=CARTESIAN_POINT('Ctrl Pts',(0.416464102931704,31.6564216609204,
54.8216091896046));
#107964=CARTESIAN_POINT('Ctrl Pts',(0.412450057222996,31.6499957682515,
54.761942507313));
#107965=CARTESIAN_POINT('Ctrl Pts',(0.408436011514289,31.6403324089542,
54.7025377229252));
#107966=CARTESIAN_POINT('Ctrl Pts',(0.404421965805581,31.6274708361703,
54.6437772081757));
#107967=CARTESIAN_POINT('Ctrl Pts',(0.400410794811274,31.6146184743798,
54.5850587755822));
#107968=CARTESIAN_POINT('Ctrl Pts',(0.396399623816967,31.5985725481162,
54.5269842119095));
#107969=CARTESIAN_POINT('Ctrl Pts',(0.39238845282266,31.5794237286546,54.469927660255));
#107970=CARTESIAN_POINT('Ctrl Pts',(0.38837857024516,31.5602810599308,54.4128894355728));
#107971=CARTESIAN_POINT('Ctrl Pts',(0.384368687667659,31.5380376421222,
54.3568690735601));
#107972=CARTESIAN_POINT('Ctrl Pts',(0.380358805090159,31.5128338933948,
54.3022252433659));
#107973=CARTESIAN_POINT('Ctrl Pts',(0.376345830822693,31.4876107121341,
54.2475392818179));
#107974=CARTESIAN_POINT('Ctrl Pts',(0.372332856555225,31.4594228570205,
54.1942324538898));
#107975=CARTESIAN_POINT('Ctrl Pts',(0.368319882287759,31.4284581866362,
54.1426417265623));
#107976=CARTESIAN_POINT('Ctrl Pts',(0.364305504855201,31.3974826892339,
54.0910329601688));
#107977=CARTESIAN_POINT('Ctrl Pts',(0.360291127422645,31.3637287366319,
54.0411419279943));
#107978=CARTESIAN_POINT('Ctrl Pts',(0.356276749990087,31.3274275547484,
53.9932765588829));
#107979=CARTESIAN_POINT('Ctrl Pts',(0.352255018940661,31.2910598756338,
53.945323509031));
#107980=CARTESIAN_POINT('Ctrl Pts',(0.348233287891235,31.2521359874029,
53.8994039381293));
#107981=CARTESIAN_POINT('Ctrl Pts',(0.344211556841809,31.2109267358645,
53.8557917845215));
#107982=CARTESIAN_POINT('Ctrl Pts',(0.340609642066431,31.1740191927757,
53.8167321710029));
#107983=CARTESIAN_POINT('Ctrl Pts',(0.337007727291054,31.13527922971,53.779523063681));
#107984=CARTESIAN_POINT('Ctrl Pts',(0.333405812515677,31.094923595558,53.7443335156617));
#107985=CARTESIAN_POINT('Ctrl Pts',(0.329325373458233,31.0492066044432,
53.7044689394277));
#107986=CARTESIAN_POINT('Ctrl Pts',(0.325244934400788,31.0012172877576,
53.6670237995497));
#107987=CARTESIAN_POINT('Ctrl Pts',(0.321164495343345,30.9512418930247,
53.6322665241522));
#107988=CARTESIAN_POINT('Ctrl Pts',(0.317043913940585,30.900774852779,53.5971673153177));
#107989=CARTESIAN_POINT('Ctrl Pts',(0.312923332537826,30.8482827832112,
53.5648095557538));
#107990=CARTESIAN_POINT('Ctrl Pts',(0.308802751135066,30.7940968522758,
53.5354296912727));
#107991=CARTESIAN_POINT('Ctrl Pts',(0.304733332277322,30.7405837123521,
53.5064146172161));
#107992=CARTESIAN_POINT('Ctrl Pts',(0.30066391341958,30.6854189962044,53.4803041598103));
#107993=CARTESIAN_POINT('Ctrl Pts',(0.296594494561836,30.6289508082089,
53.4572826309225));
#107994=CARTESIAN_POINT('Ctrl Pts',(0.292527494313683,30.572516181394,53.4342747846004));
#107995=CARTESIAN_POINT('Ctrl Pts',(0.288460494065529,30.514780091052,53.4143524190334));
#107996=CARTESIAN_POINT('Ctrl Pts',(0.284393493817376,30.4561123350777,
53.3976524915644));
#107997=CARTESIAN_POINT('Ctrl Pts',(0.280327407330037,30.3974577603903,
53.3809563161824));
#107998=CARTESIAN_POINT('Ctrl Pts',(0.2762613208427,30.3378724268665,53.3674812812633));
#107999=CARTESIAN_POINT('Ctrl Pts',(0.272195234355361,30.2777410795449,
53.3573144266984));
#108000=CARTESIAN_POINT('Ctrl Pts',(0.268034843298841,30.2162151084686,
53.3469117727124));
#108001=CARTESIAN_POINT('Ctrl Pts',(0.26387445224232,30.1541180189296,53.3399728205527));
#108002=CARTESIAN_POINT('Ctrl Pts',(0.259714061185799,30.0918702755418,
53.3365349860992));
#108003=CARTESIAN_POINT('Ctrl Pts',(0.255642675296597,30.030954226877,53.333170698826));
#108004=CARTESIAN_POINT('Ctrl Pts',(0.251571289407394,29.9698944311992,
53.3331591269708));
#108005=CARTESIAN_POINT('Ctrl Pts',(0.247499903518191,29.9090849219344,
53.3364825072815));
#108006=CARTESIAN_POINT('Ctrl Pts',(0.243295009878012,29.8462813641954,
53.3399148669529));
#108007=CARTESIAN_POINT('Ctrl Pts',(0.239090116237834,29.7837453854805,
53.3469046841571));
#108008=CARTESIAN_POINT('Ctrl Pts',(0.234885222597655,29.7219023645269,
53.3573747520678));
#108009=CARTESIAN_POINT('Ctrl Pts',(0.230680328957476,29.6600593435732,
53.3678448199785));
#108010=CARTESIAN_POINT('Ctrl Pts',(0.226475435317296,29.5989098420213,
53.3817949370555));
#108011=CARTESIAN_POINT('Ctrl Pts',(0.222270541677116,29.5388618222693,
53.3990916387753));
#108012=CARTESIAN_POINT('Ctrl Pts',(0.218232113312067,29.4811910113088,
53.4157035906638));
#108013=CARTESIAN_POINT('Ctrl Pts',(0.214193684947017,29.4242870361325,
53.4354739837199));
#108014=CARTESIAN_POINT('Ctrl Pts',(0.210155256581968,29.3685250348176,
53.4583141148899));
#108015=CARTESIAN_POINT('Ctrl Pts',(0.206029423842659,29.3115561672686,
53.4816485788033));
#108016=CARTESIAN_POINT('Ctrl Pts',(0.20190359110335,29.2557798435259,53.5081871754044));
#108017=CARTESIAN_POINT('Ctrl Pts',(0.197777758364041,29.2015823541271,
53.5377807063375));
#108018=CARTESIAN_POINT('Ctrl Pts',(0.193750441684768,29.1486789848385,
53.566667607057));
#108019=CARTESIAN_POINT('Ctrl Pts',(0.189723125005496,29.097280373175,53.5984649015941));
#108020=CARTESIAN_POINT('Ctrl Pts',(0.185695808326223,29.0477253943993,
53.6329853418752));
#108021=CARTESIAN_POINT('Ctrl Pts',(0.181670839359022,28.9981993035486,
53.6674856585701));
#108022=CARTESIAN_POINT('Ctrl Pts',(0.177645870391821,28.9505151443782,
53.7047056779388));
#108023=CARTESIAN_POINT('Ctrl Pts',(0.17362090142462,28.9049840044379,53.7444140931568));
#108024=CARTESIAN_POINT('Ctrl Pts',(0.169596713967543,28.8594617050743,
53.7841147983704));
#108025=CARTESIAN_POINT('Ctrl Pts',(0.165572526510465,28.8160919892732,
53.8263025973608));
#108026=CARTESIAN_POINT('Ctrl Pts',(0.161548339053389,28.7751521989994,
53.8707064755415));
#108027=CARTESIAN_POINT('Ctrl Pts',(0.157347250035486,28.7324127130412,
53.9170623292305));
#108028=CARTESIAN_POINT('Ctrl Pts',(0.153146161017584,28.6923222014449,
53.9658331994606));
#108029=CARTESIAN_POINT('Ctrl Pts',(0.148945071999681,28.6551506234517,
54.0166708819537));
#108030=CARTESIAN_POINT('Ctrl Pts',(0.144914792838728,28.6194903849928,
54.0654415819959));
#108031=CARTESIAN_POINT('Ctrl Pts',(0.140884513677775,28.5865165179998,
54.1161137639525));
#108032=CARTESIAN_POINT('Ctrl Pts',(0.136854234516822,28.5564222938698,
54.1683513924956));
#108033=CARTESIAN_POINT('Ctrl Pts',(0.13282069613264,28.5263037330152,54.2206312647855));
#108034=CARTESIAN_POINT('Ctrl Pts',(0.128787157748456,28.4990696747672,
54.2744786325056));
#108035=CARTESIAN_POINT('Ctrl Pts',(0.124753619364273,28.4748660351428,
54.3295356913013));
#108036=CARTESIAN_POINT('Ctrl Pts',(0.120712602360063,28.450617519331,54.3846948318881));
#108037=CARTESIAN_POINT('Ctrl Pts',(0.116671585355855,28.4294107979235,
54.4410676451706));
#108038=CARTESIAN_POINT('Ctrl Pts',(0.112630568351645,28.411342132553,54.4982807755341));
#108039=CARTESIAN_POINT('Ctrl Pts',(0.112132135847282,28.4091134831507,
54.5053376337012));
#108040=CARTESIAN_POINT('Ctrl Pts',(0.11163370334292,28.4069325106936,54.5124072648878));
#108041=CARTESIAN_POINT('Ctrl Pts',(0.111135270838558,28.4047993415728,
54.5194889602171));
#108042=CARTESIAN_POINT('Ctrl Pts',(0.10694773358615,28.3868777070868,54.5789852064324));
#108043=CARTESIAN_POINT('Ctrl Pts',(0.102760196333741,28.3722582064485,
54.6395867581065));
#108044=CARTESIAN_POINT('Ctrl Pts',(0.0985726590813334,28.361068114678,
54.7009042372838));
#108045=CARTESIAN_POINT('Ctrl Pts',(0.094394065281421,28.3499019219317,
54.7620907588291));
#108046=CARTESIAN_POINT('Ctrl Pts',(0.0902154714815101,28.3421506564006,
54.823989699565));
#108047=CARTESIAN_POINT('Ctrl Pts',(0.0860368776815976,28.3378913362989,
54.8861984620064));
#108048=CARTESIAN_POINT('Ctrl Pts',(0.081863555698731,28.3336373898605,
54.9483287403381));
#108049=CARTESIAN_POINT('Ctrl Pts',(0.0776902337158637,28.3328666732709,
55.0107675896895));
#108050=CARTESIAN_POINT('Ctrl Pts',(0.0735169117329972,28.3356047239275,
55.0731051638905));
#108051=CARTESIAN_POINT('Ctrl Pts',(0.0693476153733081,28.3383401334363,
55.1353826067179));
#108052=CARTESIAN_POINT('Ctrl Pts',(0.0651783190136198,28.344577566342,
55.1975584921095));
#108053=CARTESIAN_POINT('Ctrl Pts',(0.0610090226539306,28.3542905195358,
55.2592225027079));
#108054=CARTESIAN_POINT('Ctrl Pts',(0.0568425112665161,28.363996984751,
55.3208453234878));
#108055=CARTESIAN_POINT('Ctrl Pts',(0.0526759998791017,28.3771742824678,
55.3819564771624));
#108056=CARTESIAN_POINT('Ctrl Pts',(0.0485094884916872,28.3937442181091,
55.4421519683798));
#108057=CARTESIAN_POINT('Ctrl Pts',(0.0443432162434608,28.4103132027099,
55.5023440046443));
#108058=CARTESIAN_POINT('Ctrl Pts',(0.0401769439952331,28.4302743247372,
55.5616200178857));
#108059=CARTESIAN_POINT('Ctrl Pts',(0.0360106717470066,28.4534988203197,
55.6195886548731));
#108060=CARTESIAN_POINT('Ctrl Pts',(0.0318448920729993,28.4767205700933,
55.6775504382863));
#108061=CARTESIAN_POINT('Ctrl Pts',(0.0276791123989913,28.5032047426116,
55.7342047105123));
#108062=CARTESIAN_POINT('Ctrl Pts',(0.0235133327249839,28.5327742282485,
55.789179659335));
#108063=CARTESIAN_POINT('Ctrl Pts',(0.0193442787315363,28.562366955619,
55.8441978186868));
#108064=CARTESIAN_POINT('Ctrl Pts',(0.0151752247380916,28.5950496116564,
55.8975335963454));
#108065=CARTESIAN_POINT('Ctrl Pts',(0.0110061707446443,28.6305993113128,
55.9488402151169));
#108066=CARTESIAN_POINT('Ctrl Pts',(0.0073374471630959,28.6618826723945,
55.9939894989765));
#108067=CARTESIAN_POINT('Ctrl Pts',(0.00366872358154585,28.6953854232188,
56.0375676592882));
#108068=CARTESIAN_POINT('Ctrl Pts',(-2.66453525910038E-15,28.7309291201476,
56.0793586530485));
#108069=CARTESIAN_POINT('',(0.,31.2524971005285,56.0985476836113));
#108070=CARTESIAN_POINT('Origin',(0.,30.,55.));
#108071=CARTESIAN_POINT('Ctrl Pts',(2.67147415300428E-15,31.2524971005285,
56.0985476836113));
#108072=CARTESIAN_POINT('Ctrl Pts',(1.83597981159629E-5,31.2523211353076,
56.0987483084291));
#108073=CARTESIAN_POINT('Ctrl Pts',(3.6656070824688E-5,31.2521457602486,
56.0989481631351));
#108074=CARTESIAN_POINT('Ctrl Pts',(0.000824856977073492,31.2445898311209,
56.1075546572744));
#108075=CARTESIAN_POINT('Ctrl Pts',(0.00160018034423123,31.2371243889807,
56.1158872690425));
#108076=CARTESIAN_POINT('Ctrl Pts',(0.0110976438791952,31.1452132458219,
56.2164186425925));
#108077=CARTESIAN_POINT('Ctrl Pts',(0.0203386739047423,31.0507368921928,
56.2988984721567));
#108078=CARTESIAN_POINT('Ctrl Pts',(0.0338113421918995,30.8975843292538,
56.4048652618427));
#108079=CARTESIAN_POINT('Ctrl Pts',(0.0381896109813574,30.8453534875539,
56.4369004143079));
#108080=CARTESIAN_POINT('Ctrl Pts',(0.0452509386994067,30.7566195219529,
56.4848069695065));
#108081=CARTESIAN_POINT('Ctrl Pts',(0.0479850563921831,30.7211038969048,
56.5023762710287));
#108082=CARTESIAN_POINT('Ctrl Pts',(0.0517303998707915,30.6708493560734,
56.5250435672022));
#108083=CARTESIAN_POINT('Ctrl Pts',(0.0527777899603529,30.656616890892,
56.5312253351431));
#108084=CARTESIAN_POINT('Ctrl Pts',(0.0545628029434932,30.632060782159,
56.5414857464113));
#108085=CARTESIAN_POINT('Ctrl Pts',(0.0553036355238125,30.6217791529212,
56.5456616168665));
#108086=CARTESIAN_POINT('Ctrl Pts',(0.056804276582878,30.6007730323576,
56.5539496981985));
#108087=CARTESIAN_POINT('Ctrl Pts',(0.0575638025458454,30.5900461949569,
56.5580543635409));
#108088=CARTESIAN_POINT('Ctrl Pts',(0.0594718706053218,30.5628657219638,
56.568134104341));
#108089=CARTESIAN_POINT('Ctrl Pts',(0.060615561867242,30.5463585282036,
56.5739614944509));
#108090=CARTESIAN_POINT('Ctrl Pts',(0.0651444211712528,30.4801836818865,
56.5961560523604));
#108091=CARTESIAN_POINT('Ctrl Pts',(0.0684634539763917,30.4298469161307,
56.6104418433936));
#108092=CARTESIAN_POINT('Ctrl Pts',(0.0791568788711061,30.2633513629574,
56.6493290014665));
#108093=CARTESIAN_POINT('Ctrl Pts',(0.0862781617391556,30.1452383291482,
56.663894336486));
#108094=CARTESIAN_POINT('Ctrl Pts',(0.0968562652397831,29.9756139385913,
56.6666012978211));
#108095=CARTESIAN_POINT('Ctrl Pts',(0.100084655815293,29.924638792038,56.66507483552));
#108096=CARTESIAN_POINT('Ctrl Pts',(0.104178676525356,29.8623061231741,
56.6603402406218));
#108097=CARTESIAN_POINT('Ctrl Pts',(0.104940381370858,29.8508027193609,
56.659346097684));
#108098=CARTESIAN_POINT('Ctrl Pts',(0.106161960988369,29.832522341434,56.6575746595812));
#108099=CARTESIAN_POINT('Ctrl Pts',(0.106617769261076,29.8257379675249,
56.6568751486365));
#108100=CARTESIAN_POINT('Ctrl Pts',(0.107490412906336,29.8128235478706,
56.6554633973033));
#108101=CARTESIAN_POINT('Ctrl Pts',(0.107906844171426,29.8066929315724,
56.6547587305746));
#108102=CARTESIAN_POINT('Ctrl Pts',(0.108834943345581,29.7930992167291,
56.6531196679365));
#108103=CARTESIAN_POINT('Ctrl Pts',(0.109347476754292,29.7856383144847,
56.6521687665214));
#108104=CARTESIAN_POINT('Ctrl Pts',(0.110874759711977,29.7635344966901,
56.6491993679362));
#108105=CARTESIAN_POINT('Ctrl Pts',(0.11189662808557,29.7489121464357,56.647036533615));
#108106=CARTESIAN_POINT('Ctrl Pts',(0.118448471979047,29.6560969241584,
56.6320433127101));
#108107=CARTESIAN_POINT('Ctrl Pts',(0.124191073859531,29.5788810749015,
56.6138436072384));
#108108=CARTESIAN_POINT('Ctrl Pts',(0.135432551178239,29.4313115670386,
56.5677472179664));
#108109=CARTESIAN_POINT('Ctrl Pts',(0.140916869769389,29.3609656178965,
56.5404136788341));
#108110=CARTESIAN_POINT('Ctrl Pts',(0.149296156777252,29.2545748905735,
56.4905272177693));
#108111=CARTESIAN_POINT('Ctrl Pts',(0.15226404725487,29.2171297806641,56.4712051811317));
#108112=CARTESIAN_POINT('Ctrl Pts',(0.157297029857244,29.1539762159922,
56.4355224445658));
#108113=CARTESIAN_POINT('Ctrl Pts',(0.159382911851385,29.127911008596,56.4198386989598));
#108114=CARTESIAN_POINT('Ctrl Pts',(0.1623911100197,29.0905019115551,56.3959100915562));
#108115=CARTESIAN_POINT('Ctrl Pts',(0.163333410471777,29.0788106865775,
56.3882226140059));
#108116=CARTESIAN_POINT('Ctrl Pts',(0.164992836773618,29.0582756200063,
56.3743462651356));
#108117=CARTESIAN_POINT('Ctrl Pts',(0.165712132913501,29.0493926091652,
56.3682171107777));
#108118=CARTESIAN_POINT('Ctrl Pts',(0.167219573811755,29.0308186496625,
56.3551331196595));
#108119=CARTESIAN_POINT('Ctrl Pts',(0.168006957659973,29.0211415386663,
56.348159629608));
#108120=CARTESIAN_POINT('Ctrl Pts',(0.170096504076276,28.9955348448932,
56.329285927887));
#108121=CARTESIAN_POINT('Ctrl Pts',(0.171391576806219,28.9797416927699,
56.3172032368028));
#108122=CARTESIAN_POINT('Ctrl Pts',(0.178581572859988,28.8925967655724,
56.2480242730929));
#108123=CARTESIAN_POINT('Ctrl Pts',(0.184248021750184,28.8258168839281,
56.1854128375601));
#108124=CARTESIAN_POINT('Ctrl Pts',(0.195563713904977,28.7019202403468,
56.0484501502279));
#108125=CARTESIAN_POINT('Ctrl Pts',(0.201192073634327,28.6452632852692,
55.9741381166266));
#108126=CARTESIAN_POINT('Ctrl Pts',(0.209602091530792,28.5732648357742,
55.8611835014227));
#108127=CARTESIAN_POINT('Ctrl Pts',(0.212197524231318,28.5526684593564,
55.8260999130033));
#108128=CARTESIAN_POINT('Ctrl Pts',(0.215568687310567,28.5282918390693,
55.7808623779926));
#108129=CARTESIAN_POINT('Ctrl Pts',(0.216277043595974,28.5232969751751,
55.7713748284425));
#108130=CARTESIAN_POINT('Ctrl Pts',(0.217427156332468,28.5153981723771,
55.7560134513898));
#108131=CARTESIAN_POINT('Ctrl Pts',(0.217865444868287,28.5124366097955,
55.7501693686632));
#108132=CARTESIAN_POINT('Ctrl Pts',(0.218717502412834,28.5067745952872,
55.7388310828383));
#108133=CARTESIAN_POINT('Ctrl Pts',(0.219131006050289,28.5040698497753,
55.7333392522463));
#108134=CARTESIAN_POINT('Ctrl Pts',(0.220163695622516,28.4974202177336,
55.7196476893046));
#108135=CARTESIAN_POINT('Ctrl Pts',(0.220785064485526,28.4935121674317,
55.7114303898661));
#108136=CARTESIAN_POINT('Ctrl Pts',(0.2230250187394,28.4797485635398,55.681868245285));
#108137=CARTESIAN_POINT('Ctrl Pts',(0.224664018238215,28.4702782582574,
55.6603483852834));
#108138=CARTESIAN_POINT('Ctrl Pts',(0.233658549623416,28.4213621754429,
55.5424898549807));
#108139=CARTESIAN_POINT('Ctrl Pts',(0.241313474749086,28.3905586237278,
55.4428196748542));
#108140=CARTESIAN_POINT('Ctrl Pts',(0.255856475213649,28.349538573163,55.2466130624324));
#108141=CARTESIAN_POINT('Ctrl Pts',(0.262732574084232,28.3380368449464,
55.1507480538985));
#108142=CARTESIAN_POINT('Ctrl Pts',(0.270853560327245,28.334174254411,55.0325458625757));
#108143=CARTESIAN_POINT('Ctrl Pts',(0.272342630146473,28.3338904751538,
55.0106667020239));
#108144=CARTESIAN_POINT('Ctrl Pts',(0.274645055299875,28.3341202396614,
54.9765285345599));
#108145=CARTESIAN_POINT('Ctrl Pts',(0.275467564185079,28.3343380541171,
54.9642707172966));
#108146=CARTESIAN_POINT('Ctrl Pts',(0.276992962365944,28.3349962955883,
54.9414260544925));
#108147=CARTESIAN_POINT('Ctrl Pts',(0.27769688979855,28.335402451747,54.9308389266132));
#108148=CARTESIAN_POINT('Ctrl Pts',(0.279262445145711,28.3365353768146,
54.9071970979099));
#108149=CARTESIAN_POINT('Ctrl Pts',(0.280122373210363,28.3373148886055,
54.8941455342565));
#108150=CARTESIAN_POINT('Ctrl Pts',(0.282304998167148,28.3396961325095,
54.8608639867664));
#108151=CARTESIAN_POINT('Ctrl Pts',(0.283620911834001,28.3415140027721,
54.8406512717586));
#108152=CARTESIAN_POINT('Ctrl Pts',(0.293631048118927,28.3582822096851,
54.6859467139495));
#108153=CARTESIAN_POINT('Ctrl Pts',(0.301776924415256,28.389197942145,54.5536961079399));
#108154=CARTESIAN_POINT('Ctrl Pts',(0.314901330963546,28.4630105634767,
54.3523249702993));
#108155=CARTESIAN_POINT('Ctrl Pts',(0.319787514929989,28.4955049501309,
54.2800618458996));
#108156=CARTESIAN_POINT('Ctrl Pts',(0.325858242338115,28.5397332197106,
54.1978912546828));
#108157=CARTESIAN_POINT('Ctrl Pts',(0.32678994045868,28.5466204008419,54.1854785352419));
#108158=CARTESIAN_POINT('Ctrl Pts',(0.328211698808857,28.5572613786767,
54.166865090334));
#108159=CARTESIAN_POINT('Ctrl Pts',(0.328694681296393,28.5608986143964,
54.1605980080032));
#108160=CARTESIAN_POINT('Ctrl Pts',(0.329581771722879,28.5676169682787,
54.1491940703694));
#108161=CARTESIAN_POINT('Ctrl Pts',(0.329985051861543,28.5706850616466,
54.1440498365433));
#108162=CARTESIAN_POINT('Ctrl Pts',(0.330911122899019,28.5777624440121,
54.1323274350608));
#108163=CARTESIAN_POINT('Ctrl Pts',(0.331435040839736,28.5817896769313,
54.1257604337139));
#108164=CARTESIAN_POINT('Ctrl Pts',(0.333082024375022,28.5945263519232,
54.1053110030829));
#108165=CARTESIAN_POINT('Ctrl Pts',(0.33421453204808,28.6033948858236,54.0915294822928));
#108166=CARTESIAN_POINT('Ctrl Pts',(0.340824267351567,28.6558644839782,
54.0125771277401));
#108167=CARTESIAN_POINT('Ctrl Pts',(0.346509541133681,28.7038163245726,
53.9504240108421));
#108168=CARTESIAN_POINT('Ctrl Pts',(0.357115853067144,28.8007587007387,
53.841590449507));
#108169=CARTESIAN_POINT('Ctrl Pts',(0.362022899779359,28.8485682275159,
53.7940571768463));
#108170=CARTESIAN_POINT('Ctrl Pts',(0.370272839559134,28.9349387281348,
53.7180182855952));
#108171=CARTESIAN_POINT('Ctrl Pts',(0.373651723276434,28.9720919153647,
53.6880402897391));
#108172=CARTESIAN_POINT('Ctrl Pts',(0.379288772256287,29.037247746346,53.6399371948873));
#108173=CARTESIAN_POINT('Ctrl Pts',(0.381575400116662,29.0645990448363,
53.620982936451));
#108174=CARTESIAN_POINT('Ctrl Pts',(0.384811013073159,29.1046165366089,
53.5949899801629));
#108175=CARTESIAN_POINT('Ctrl Pts',(0.385784713883485,29.1168338497882,
53.5872784151604));
#108176=CARTESIAN_POINT('Ctrl Pts',(0.387477641220054,29.1383769427103,
53.5740691304188));
#108177=CARTESIAN_POINT('Ctrl Pts',(0.388199389372679,29.1476587105933,
53.5685016683409));
#108178=CARTESIAN_POINT('Ctrl Pts',(0.389691410715679,29.167045108487,53.5571285798178));
#108179=CARTESIAN_POINT('Ctrl Pts',(0.390461121931159,29.1771577455723,
53.5513377127813));
#108180=CARTESIAN_POINT('Ctrl Pts',(0.392457484151237,29.2036704560835,
53.5365227650024));
#108181=CARTESIAN_POINT('Ctrl Pts',(0.393678099810462,29.2201636067752,
53.5276679703333));
#108182=CARTESIAN_POINT('Ctrl Pts',(0.399163327670633,29.2954986011431,
53.4888435015911));
#108183=CARTESIAN_POINT('Ctrl Pts',(0.403315864424741,29.3559444883501,
53.4621085362646));
#108184=CARTESIAN_POINT('Ctrl Pts',(0.41451443773383,29.5254452944506,53.3988918496805));
#108185=CARTESIAN_POINT('Ctrl Pts',(0.421385131033552,29.6369217232387,
53.3699935622469));
#108186=CARTESIAN_POINT('Ctrl Pts',(0.431351459641604,29.7944101138259,
53.3461368985851));
#108187=CARTESIAN_POINT('Ctrl Pts',(0.4341776012236,29.8385872564153,53.3412427745767));
#108188=CARTESIAN_POINT('Ctrl Pts',(0.437810857550247,29.8938795668999,
53.3373468359415));
#108189=CARTESIAN_POINT('Ctrl Pts',(0.43853732886452,29.9048634872641,53.3366821956495));
#108190=CARTESIAN_POINT('Ctrl Pts',(0.439709907753333,29.9224606919825,
53.3357922511445));
#108191=CARTESIAN_POINT('Ctrl Pts',(0.440152303627195,29.9290703515636,
53.3354974446387));
#108192=CARTESIAN_POINT('Ctrl Pts',(0.441008403262815,29.9417999500566,
53.3350056317995));
#108193=CARTESIAN_POINT('Ctrl Pts',(0.441421798811537,29.9479194765934,
53.3348029827983));
#108194=CARTESIAN_POINT('Ctrl Pts',(0.442349261851213,29.961590530056,53.3344256938195));
#108195=CARTESIAN_POINT('Ctrl Pts',(0.442864265507579,29.9691424003378,
53.3342686711598));
#108196=CARTESIAN_POINT('Ctrl Pts',(0.444663580905068,29.9953994953719,
53.3339013336793));
#108197=CARTESIAN_POINT('Ctrl Pts',(0.445960831834122,30.0141062315033,
53.3339547206964));
#108198=CARTESIAN_POINT('Ctrl Pts',(0.454857550442134,30.1411447509441,
53.3364568664201));
#108199=CARTESIAN_POINT('Ctrl Pts',(0.462822343415812,30.2490086222056,
53.3491548485529));
#108200=CARTESIAN_POINT('Ctrl Pts',(0.47689960307504,30.4385638680515,53.3904797244061));
#108201=CARTESIAN_POINT('Ctrl Pts',(0.483033883756178,30.5207366015291,
53.4151559036246));
#108202=CARTESIAN_POINT('Ctrl Pts',(0.491051664193381,30.6285696140749,
53.4568370730676));
#108203=CARTESIAN_POINT('Ctrl Pts',(0.493103366587028,30.6561887941298,
53.4683773163695));
#108204=CARTESIAN_POINT('Ctrl Pts',(0.496069210098696,30.6961281892577,
53.4863442323496));
#108205=CARTESIAN_POINT('Ctrl Pts',(0.497002754327989,30.7087015074602,
53.4921901869558));
#108206=CARTESIAN_POINT('Ctrl Pts',(0.498649231103817,30.7308740344684,
53.5028379186073));
#108207=CARTESIAN_POINT('Ctrl Pts',(0.499364285110635,30.7405024325399,
53.507576699164));
#108208=CARTESIAN_POINT('Ctrl Pts',(0.500865187011454,30.7607060936868,
53.5177639395345));
#108209=CARTESIAN_POINT('Ctrl Pts',(0.501650255515002,30.7712701779175,
53.5232333207597));
#108210=CARTESIAN_POINT('Ctrl Pts',(0.503739044624494,30.7993584242877,
53.5381591775348));
#108211=CARTESIAN_POINT('Ctrl Pts',(0.505035592197242,30.8167734899739,
53.547817641679));
#108212=CARTESIAN_POINT('Ctrl Pts',(0.512569449201807,30.9177357515773,
53.6062026952636));
#108213=CARTESIAN_POINT('Ctrl Pts',(0.518546636043419,30.9970894914989,
53.6618199679902));
#108214=CARTESIAN_POINT('Ctrl Pts',(0.529871425488197,31.1388681621492,
53.7808418367603));
#108215=CARTESIAN_POINT('Ctrl Pts',(0.535214815243482,31.2019256108957,
53.8429606082419));
#108216=CARTESIAN_POINT('Ctrl Pts',(0.543254265624867,31.2856508676295,
53.939705758929));
#108217=CARTESIAN_POINT('Ctrl Pts',(0.545781372741443,31.3104705599105,
53.9705397596888));
#108218=CARTESIAN_POINT('Ctrl Pts',(0.549073637453976,31.3405238789814,
54.0107253184978));
#108219=CARTESIAN_POINT('Ctrl Pts',(0.549774907106035,31.3467993099269,
54.0192858367955));
#108220=CARTESIAN_POINT('Ctrl Pts',(0.550915557698269,31.3567951809981,
54.0331984102282));
#108221=CARTESIAN_POINT('Ctrl Pts',(0.551351547160664,31.3605668750842,
54.0385135196339));
#108222=CARTESIAN_POINT('Ctrl Pts',(0.552203363780374,31.3678384781535,
54.0488891988903));
#108223=CARTESIAN_POINT('Ctrl Pts',(0.552618961901155,31.371341695453,54.0539472488365));
#108224=CARTESIAN_POINT('Ctrl Pts',(0.553660460574954,31.3800120201602,
54.0666150670986));
#108225=CARTESIAN_POINT('Ctrl Pts',(0.554288606335351,31.3851442229303,
54.0742483698756));
#108226=CARTESIAN_POINT('Ctrl Pts',(0.556571975011686,31.4034611217988,
54.1019850442026));
#108227=CARTESIAN_POINT('Ctrl Pts',(0.55824850234757,31.4162728292788,54.1223297263369));
#108228=CARTESIAN_POINT('Ctrl Pts',(0.567250499211459,31.4819470958181,
54.2318030018032));
#108229=CARTESIAN_POINT('Ctrl Pts',(0.574867304558297,31.526845771178,54.3254378698075));
#108230=CARTESIAN_POINT('Ctrl Pts',(0.588424246287592,31.5916261467172,
54.5007779820069));
#108231=CARTESIAN_POINT('Ctrl Pts',(0.594384838700808,31.6145987734815,
54.5809885521008));
#108232=CARTESIAN_POINT('Ctrl Pts',(0.602235581992067,31.637525566472,54.6918466129138));
#108233=CARTESIAN_POINT('Ctrl Pts',(0.604283661190095,31.6427882680995,
54.721261061071));
#108234=CARTESIAN_POINT('Ctrl Pts',(0.607244579136839,31.6493283518256,
54.7644926987932));
#108235=CARTESIAN_POINT('Ctrl Pts',(0.60817678024153,31.6512286668053,54.7782081807424));
#108236=CARTESIAN_POINT('Ctrl Pts',(0.609820963984576,31.6542961946478,
54.8025792443031));
#108237=CARTESIAN_POINT('Ctrl Pts',(0.610535064463687,31.6555319541182,
54.8132252358287));
#108238=CARTESIAN_POINT('Ctrl Pts',(0.612034014795316,31.6579208692689,
54.8356967950003));
#108239=CARTESIAN_POINT('Ctrl Pts',(0.612818085869981,31.6590504294753,
54.8475243078358));
#108240=CARTESIAN_POINT('Ctrl Pts',(0.614904274286197,31.6617322708977,
54.8791803077942));
#108241=CARTESIAN_POINT('Ctrl Pts',(0.6161992268751,31.6630562114821,54.8990265850614));
#108242=CARTESIAN_POINT('Ctrl Pts',(0.623783185459972,31.6687721426706,
55.016296285606));
#108243=CARTESIAN_POINT('Ctrl Pts',(0.62980687651647,31.6649590129717,55.1139341390001));
#108244=CARTESIAN_POINT('Ctrl Pts',(0.640245327946243,31.6433754112351,
55.2832344436734));
#108245=CARTESIAN_POINT('Ctrl Pts',(0.644678555324356,31.6293602331118,
55.3550900063826));
#108246=CARTESIAN_POINT('Ctrl Pts',(0.652476622941987,31.5972936523927,
55.4763911004249));
#108247=CARTESIAN_POINT('Ctrl Pts',(0.655783593749164,31.5815409558817,
55.5263293049961));
#108248=CARTESIAN_POINT('Ctrl Pts',(0.659211143171056,31.5634568606164,
55.5754638529456));
#108249=CARTESIAN_POINT('Ctrl Pts',(0.659212960815814,31.5634472697237,
55.575489909177));
#108250=CARTESIAN_POINT('Ctrl Pts',(0.659214778542432,31.5634376782623,
55.5755159651912));
#108251=CARTESIAN_POINT('Origin',(5.,-30.,55.));
#108252=CARTESIAN_POINT('',(9.56912142374065,-28.4365623107092,55.5755159352313));
#108253=CARTESIAN_POINT('',(9.76070771184276,-28.4365623102018,55.5755159338528));
#108254=CARTESIAN_POINT('',(5.,-28.4365623102018,55.5755159338528));
#108255=CARTESIAN_POINT('',(10.,-31.3346917155535,55.9970727277551));
#108256=CARTESIAN_POINT('Ctrl Pts',(9.76070771184276,-28.4365623102018,
55.5755159338528));
#108257=CARTESIAN_POINT('Ctrl Pts',(9.76500820034434,-28.4587264214961,
55.6357266159905));
#108258=CARTESIAN_POINT('Ctrl Pts',(9.76930868884592,-28.4843410012575,
55.6945691379123));
#108259=CARTESIAN_POINT('Ctrl Pts',(9.7736091773475,-28.5132039305782,55.7516604605484));
#108260=CARTESIAN_POINT('Ctrl Pts',(9.77498260433929,-28.5224217499437,
55.7698934504696));
#108261=CARTESIAN_POINT('Ctrl Pts',(9.77635603133109,-28.5319705443847,
55.7879480397777));
#108262=CARTESIAN_POINT('Ctrl Pts',(9.77772945832288,-28.5418428014225,
55.8058123753309));
#108263=CARTESIAN_POINT('Ctrl Pts',(9.78176793020917,-28.5708715250019,
55.8583412810026));
#108264=CARTESIAN_POINT('Ctrl Pts',(9.78580640209546,-28.6028089144853,
55.9094197125127));
#108265=CARTESIAN_POINT('Ctrl Pts',(9.78984487398175,-28.637485007624,55.95870167182));
#108266=CARTESIAN_POINT('Ctrl Pts',(9.7939707012809,-28.6729111727002,56.0090496397621));
#108267=CARTESIAN_POINT('Ctrl Pts',(9.79809652858006,-28.7111957462312,
56.0575219711458));
#108268=CARTESIAN_POINT('Ctrl Pts',(9.80222235587921,-28.7521073143149,
56.1037752692526));
#108269=CARTESIAN_POINT('Ctrl Pts',(9.80624971620123,-28.7920424870852,
56.1489246863395));
#108270=CARTESIAN_POINT('Ctrl Pts',(9.81027707652325,-28.834480283458,56.1919594013044));
#108271=CARTESIAN_POINT('Ctrl Pts',(9.81430443684527,-28.8791627372751,
56.2325906986861));
#108272=CARTESIAN_POINT('Ctrl Pts',(9.81832944941489,-28.9238191434258,
56.2731983100256));
#108273=CARTESIAN_POINT('Ctrl Pts',(9.82235446198451,-28.9707172287795,
56.311404928579));
#108274=CARTESIAN_POINT('Ctrl Pts',(9.82637947455413,-29.0195622566284,
56.3469587341015));
#108275=CARTESIAN_POINT('Ctrl Pts',(9.83040370552636,-29.0683977995017,
56.3825056356055));
#108276=CARTESIAN_POINT('Ctrl Pts',(9.8344279364986,-29.1191791123094,56.4154004386937));
#108277=CARTESIAN_POINT('Ctrl Pts',(9.83845216747083,-29.1715802553535,
56.445433058526));
#108278=CARTESIAN_POINT('Ctrl Pts',(9.84265321427838,-29.2262837890762,
56.4767852454506));
#108279=CARTESIAN_POINT('Ctrl Pts',(9.84685426108594,-29.2827522879325,
56.5050175498202));
#108280=CARTESIAN_POINT('Ctrl Pts',(9.85105530789349,-29.3405862250839,
56.5299442713546));
#108281=CARTESIAN_POINT('Ctrl Pts',(9.85508562993745,-29.3960698705818,
56.5538580052134));
#108282=CARTESIAN_POINT('Ctrl Pts',(9.85911595198142,-29.4528095736924,
56.5747295449078));
#108283=CARTESIAN_POINT('Ctrl Pts',(9.86314627402539,-29.5104347118588,
56.5924452356823));
#108284=CARTESIAN_POINT('Ctrl Pts',(9.8671798550718,-29.5681064469136,56.6101752517337));
#108285=CARTESIAN_POINT('Ctrl Pts',(9.87121343611822,-29.6266645330332,
56.6247442253542));
#108286=CARTESIAN_POINT('Ctrl Pts',(9.87524701716463,-29.6857276615195,
56.6360895138305));
#108287=CARTESIAN_POINT('Ctrl Pts',(9.87928807622649,-29.7449002894757,
56.6474558357857));
#108288=CARTESIAN_POINT('Ctrl Pts',(9.88332913528834,-29.8045793101271,
56.6555864968878));
#108289=CARTESIAN_POINT('Ctrl Pts',(9.88737019435019,-29.8643793020183,
56.6604707243065));
#108290=CARTESIAN_POINT('Ctrl Pts',(9.88786837262061,-29.8717513933626,
56.6610728476436));
#108291=CARTESIAN_POINT('Ctrl Pts',(9.88836655089103,-29.8791253265308,
56.6616256974425));
#108292=CARTESIAN_POINT('Ctrl Pts',(9.88886472916145,-29.8865003834034,
56.6621293081564));
#108293=CARTESIAN_POINT('Ctrl Pts',(9.89305223342453,-29.9484924130206,
56.6663624755514));
#108294=CARTESIAN_POINT('Ctrl Pts',(9.8972397376876,-30.0108272523294,56.6671303990113));
#108295=CARTESIAN_POINT('Ctrl Pts',(9.90142724195068,-30.0730969702636,
56.6643956359407));
#108296=CARTESIAN_POINT('Ctrl Pts',(9.90560580264708,-30.1352336940947,
56.6616667137084));
#108297=CARTESIAN_POINT('Ctrl Pts',(9.90978436334349,-30.1973050985972,
56.6554500042795));
#108298=CARTESIAN_POINT('Ctrl Pts',(9.91396292403989,-30.2589015472335,
56.6457600034149));
#108299=CARTESIAN_POINT('Ctrl Pts',(9.91813621293491,-30.3204202838853,
56.636082227755));
#108300=CARTESIAN_POINT('Ctrl Pts',(9.92230950182992,-30.3814647846837,
56.6229399359512));
#108301=CARTESIAN_POINT('Ctrl Pts',(9.92648279072493,-30.4416298012493,
56.6063994268701));
#108302=CARTESIAN_POINT('Ctrl Pts',(9.93065205411825,-30.5017367834006,
56.5898748725549));
#108303=CARTESIAN_POINT('Ctrl Pts',(9.93482131751156,-30.5609655066609,
56.5699587383165));
#108304=CARTESIAN_POINT('Ctrl Pts',(9.93899058090487,-30.6189218430517,
56.5467681636863));
#108305=CARTESIAN_POINT('Ctrl Pts',(9.94315705955352,-30.6768394691037,
56.5235930785618));
#108306=CARTESIAN_POINT('Ctrl Pts',(9.94732353820217,-30.733485953722,56.4971480767127));
#108307=CARTESIAN_POINT('Ctrl Pts',(9.95149001685081,-30.7884848346613,
56.4675992864229));
#108308=CARTESIAN_POINT('Ctrl Pts',(9.95565625704499,-30.8434805679236,
56.4380521872593));
#108309=CARTESIAN_POINT('Ctrl Pts',(9.95982249723917,-30.8968284567992,
56.4054018668211));
#108310=CARTESIAN_POINT('Ctrl Pts',(9.96398873743335,-30.948175616757,56.3698609417702));
#108311=CARTESIAN_POINT('Ctrl Pts',(9.96815448544298,-30.999516710747,56.3343242153956));
#108312=CARTESIAN_POINT('Ctrl Pts',(9.9723202334526,-31.0488571554576,56.2958978408706));
#108313=CARTESIAN_POINT('Ctrl Pts',(9.97648598146223,-31.0958738754253,
56.2548372201845));
#108314=CARTESIAN_POINT('Ctrl Pts',(9.98065500484387,-31.1429275628832,
56.2137443150665));
#108315=CARTESIAN_POINT('Ctrl Pts',(9.98482402822551,-31.1876535157859,
56.1700133431822));
#108316=CARTESIAN_POINT('Ctrl Pts',(9.98899305160715,-31.2297632520183,
56.1239387634499));
#108317=CARTESIAN_POINT('Ctrl Pts',(9.99266203440477,-31.2668222664938,
56.0833904563356));
#108318=CARTESIAN_POINT('Ctrl Pts',(9.99633101720238,-31.3018554059886,
56.0410277464068));
#108319=CARTESIAN_POINT('Ctrl Pts',(10.,-31.3346917155535,55.997072727755));
#108320=CARTESIAN_POINT('',(10.,-30.7922981853442,53.5344558739157));
#108321=CARTESIAN_POINT('Origin',(10.,-30.,55.));
#108322=CARTESIAN_POINT('Ctrl Pts',(10.,-30.7922981853442,53.5344558739157));
#108323=CARTESIAN_POINT('Ctrl Pts',(9.9999895507263,-30.7924317913625,53.5345281036111));
#108324=CARTESIAN_POINT('Ctrl Pts',(9.99997912415357,-30.7925650844869,
53.5346001877614));
#108325=CARTESIAN_POINT('Ctrl Pts',(9.99922746147901,-30.8021727116768,
53.5397976234626));
#108326=CARTESIAN_POINT('Ctrl Pts',(9.99848123226477,-30.8115971491062,
53.5450147446011));
#108327=CARTESIAN_POINT('Ctrl Pts',(9.9887478481477,-30.9331383582474,53.6138450241866));
#108328=CARTESIAN_POINT('Ctrl Pts',(9.97920752635469,-31.0375491743558,
53.6901670441422));
#108329=CARTESIAN_POINT('Ctrl Pts',(9.96562194606746,-31.1754837971264,
53.8179303698092));
#108330=CARTESIAN_POINT('Ctrl Pts',(9.96140028395281,-31.2166884014272,
53.8603854672475));
#108331=CARTESIAN_POINT('Ctrl Pts',(9.95455608602756,-31.2809875574851,
53.9341086583401));
#108332=CARTESIAN_POINT('Ctrl Pts',(9.95188652061651,-31.3054008952533,
53.9641513625317));
#108333=CARTESIAN_POINT('Ctrl Pts',(9.94821315572095,-31.3380263903812,
54.007287561637));
#108334=CARTESIAN_POINT('Ctrl Pts',(9.94717501445229,-31.3471351882834,
54.0196840211513));
#108335=CARTESIAN_POINT('Ctrl Pts',(9.94540101462986,-31.3625022167179,
54.0412162572487));
#108336=CARTESIAN_POINT('Ctrl Pts',(9.9446620441781,-31.3688433226312,54.0502913477976));
#108337=CARTESIAN_POINT('Ctrl Pts',(9.94316113007218,-31.3815964603314,
54.0689361512455));
#108338=CARTESIAN_POINT('Ctrl Pts',(9.94239950637326,-31.3880006531753,
54.0785105168658));
#108339=CARTESIAN_POINT('Ctrl Pts',(9.94047814363316,-31.4039804294269,
54.1029451306809));
#108340=CARTESIAN_POINT('Ctrl Pts',(9.93932340119048,-31.4134198898699,
54.1178930121746));
#108341=CARTESIAN_POINT('Ctrl Pts',(9.93467599619422,-31.4507053135286,
54.1790721362612));
#108342=CARTESIAN_POINT('Ctrl Pts',(9.93125419284011,-31.476536662721,54.2264957622331));
#108343=CARTESIAN_POINT('Ctrl Pts',(9.91846158366147,-31.565638033155,54.4108699618767));
#108344=CARTESIAN_POINT('Ctrl Pts',(9.90954918582949,-31.6125064658418,
54.5549057966934));
#108345=CARTESIAN_POINT('Ctrl Pts',(9.89842211506384,-31.6433755242008,
54.7254437253278));
#108346=CARTESIAN_POINT('Ctrl Pts',(9.89695743171525,-31.6469401338778,
54.7477058456394));
#108347=CARTESIAN_POINT('Ctrl Pts',(9.89488686068027,-31.6512723519226,
54.7787901175801));
#108348=CARTESIAN_POINT('Ctrl Pts',(9.89430004866978,-31.6524231747233,
54.7875574536069));
#108349=CARTESIAN_POINT('Ctrl Pts',(9.89329214313155,-31.6542680176757,
54.8025351371788));
#108350=CARTESIAN_POINT('Ctrl Pts',(9.89287292972902,-31.6549970072383,
54.8087411424422));
#108351=CARTESIAN_POINT('Ctrl Pts',(9.89199136166798,-31.6564496852979,
54.8217387086142));
#108352=CARTESIAN_POINT('Ctrl Pts',(9.89152865629633,-31.6571665474248,
54.8285308253323));
#108353=CARTESIAN_POINT('Ctrl Pts',(9.8902558830858,-31.6590147704626,54.8471377684626));
#108354=CARTESIAN_POINT('Ctrl Pts',(9.88944145643934,-31.6600616429765,
54.8589603176703));
#108355=CARTESIAN_POINT('Ctrl Pts',(9.88501590135887,-31.6650282123523,
54.9228063800054));
#108356=CARTESIAN_POINT('Ctrl Pts',(9.88130256055543,-31.6666284927841,
54.9749765033606));
#108357=CARTESIAN_POINT('Ctrl Pts',(9.87047810674105,-31.6641825107861,
55.1251595544139));
#108358=CARTESIAN_POINT('Ctrl Pts',(9.86328280742476,-31.653935251428,55.222863017276));
#108359=CARTESIAN_POINT('Ctrl Pts',(9.8527376184587,-31.6257789510615,55.367144749838));
#108360=CARTESIAN_POINT('Ctrl Pts',(9.84926831083307,-31.6142888003592,
55.4147587925479));
#108361=CARTESIAN_POINT('Ctrl Pts',(9.84350003437192,-31.5913292520589,
55.494342247431));
#108362=CARTESIAN_POINT('Ctrl Pts',(9.84117104050136,-31.5809506733445,
55.5265912076722));
#108363=CARTESIAN_POINT('Ctrl Pts',(9.8378852659409,-31.5647108406881,55.5722309758614));
#108364=CARTESIAN_POINT('Ctrl Pts',(9.83690290765468,-31.5596462140594,
55.5858942011597));
#108365=CARTESIAN_POINT('Ctrl Pts',(9.83519807901544,-31.550491546665,55.609631128162));
#108366=CARTESIAN_POINT('Ctrl Pts',(9.83447302624096,-31.5464810124777,
55.6197343272185));
#108367=CARTESIAN_POINT('Ctrl Pts',(9.83297703475667,-31.5379640059224,
55.640592436894));
#108368=CARTESIAN_POINT('Ctrl Pts',(9.83220663305353,-31.5334429147084,
55.6513407653839));
#108369=CARTESIAN_POINT('Ctrl Pts',(9.83021468689445,-31.5214041070829,
55.6791412205976));
#108370=CARTESIAN_POINT('Ctrl Pts',(9.82899907408536,-31.5137123418511,
55.696116546252));
#108371=CARTESIAN_POINT('Ctrl Pts',(9.82364997459325,-31.4783569714157,
55.7707854021922));
#108372=CARTESIAN_POINT('Ctrl Pts',(9.8196209352178,-31.44766674586,55.8269896200116));
#108373=CARTESIAN_POINT('Ctrl Pts',(9.80666555862741,-31.337086300955,56.0043883113706));
#108374=CARTESIAN_POINT('Ctrl Pts',(9.7981000873514,-31.2446210532701,56.1169171280181));
#108375=CARTESIAN_POINT('Ctrl Pts',(9.78733159535497,-31.1220372754486,
56.2317118161577));
#108376=CARTESIAN_POINT('Ctrl Pts',(9.78584323162145,-31.1049817906408,
56.2470351889401));
#108377=CARTESIAN_POINT('Ctrl Pts',(9.78375101357186,-31.0809555234475,
56.2677414884306));
#108378=CARTESIAN_POINT('Ctrl Pts',(9.78316749508805,-31.0742492733071,
56.2734291560583));
#108379=CARTESIAN_POINT('Ctrl Pts',(9.7821697175137,-31.0627802015948,56.2830011738737));
#108380=CARTESIAN_POINT('Ctrl Pts',(9.78175739471841,-31.0580402140477,
56.2869128459267));
#108381=CARTESIAN_POINT('Ctrl Pts',(9.78089484030599,-31.0481262362839,
56.2950025551221));
#108382=CARTESIAN_POINT('Ctrl Pts',(9.78044431334554,-31.0429487327193,
56.2991759549698));
#108383=CARTESIAN_POINT('Ctrl Pts',(9.77922112279171,-31.0288899855247,
56.3103700104131));
#108384=CARTESIAN_POINT('Ctrl Pts',(9.77844450833406,-31.0199621259124,
56.3173311696475));
#108385=CARTESIAN_POINT('Ctrl Pts',(9.77459103245255,-30.9756214528343,
56.3511831708394));
#108386=CARTESIAN_POINT('Ctrl Pts',(9.77143878767359,-30.9392156813891,
56.376737570432));
#108387=CARTESIAN_POINT('Ctrl Pts',(9.7619054639744,-30.8276186391752,56.4485836171115));
#108388=CARTESIAN_POINT('Ctrl Pts',(9.75542554905745,-30.7497230379969,
56.4903900467147));
#108389=CARTESIAN_POINT('Ctrl Pts',(9.74464520482683,-30.6132492585995,
56.5502164831805));
#108390=CARTESIAN_POINT('Ctrl Pts',(9.74030073825637,-30.5563197766408,
56.5715455366727));
#108391=CARTESIAN_POINT('Ctrl Pts',(9.73330221244073,-30.4609531853645,
56.6014411947685));
#108392=CARTESIAN_POINT('Ctrl Pts',(9.73059706325198,-30.4231545833061,
56.6118413017412));
#108393=CARTESIAN_POINT('Ctrl Pts',(9.72689685990628,-30.3701592184003,
56.6244295927669));
#108394=CARTESIAN_POINT('Ctrl Pts',(9.72586575739022,-30.3552487260126,
56.6277554234771));
#108395=CARTESIAN_POINT('Ctrl Pts',(9.72411086194284,-30.3296332350201,
56.633100282859));
#108396=CARTESIAN_POINT('Ctrl Pts',(9.72338387492583,-30.3189505470272,
56.6352202181431));
#108397=CARTESIAN_POINT('Ctrl Pts',(9.72191376625709,-30.2972073622525,
56.6393138782821));
#108398=CARTESIAN_POINT('Ctrl Pts',(9.72117089719986,-30.2861461435036,
56.6412807812171));
#108399=CARTESIAN_POINT('Ctrl Pts',(9.71931079089906,-30.2582697916766,
56.6459473626901));
#108400=CARTESIAN_POINT('Ctrl Pts',(9.71819821761413,-30.2414313330276,
56.6485014263601));
#108401=CARTESIAN_POINT('Ctrl Pts',(9.71389173401649,-30.1756571723526,
56.6574486152894));
#108402=CARTESIAN_POINT('Ctrl Pts',(9.71075787729547,-30.1264837773524,
56.6619247621374));
#108403=CARTESIAN_POINT('Ctrl Pts',(9.70018132944217,-29.9575452347866,
56.6697595411296));
#108404=CARTESIAN_POINT('Ctrl Pts',(9.69302581855393,-29.8376659477646,
56.6623917367566));
#108405=CARTESIAN_POINT('Ctrl Pts',(9.6831214731309,-29.6796904926494,56.6354198625513));
#108406=CARTESIAN_POINT('Ctrl Pts',(9.68059085175588,-29.640031892613,56.6271505255885));
#108407=CARTESIAN_POINT('Ctrl Pts',(9.67641614440543,-29.5766079541128,
56.6114936648456));
#108408=CARTESIAN_POINT('Ctrl Pts',(9.67480824130579,-29.5526367319564,
56.6050042381909));
#108409=CARTESIAN_POINT('Ctrl Pts',(9.67257868960013,-29.5201803359578,
56.5954341864869));
#108410=CARTESIAN_POINT('Ctrl Pts',(9.67198146693663,-29.5115606595721,
56.59281642225));
#108411=CARTESIAN_POINT('Ctrl Pts',(9.67096952054722,-29.4970892778027,
56.5882930067925));
#108412=CARTESIAN_POINT('Ctrl Pts',(9.67055692859207,-29.4912259825609,
56.5864245547614));
#108413=CARTESIAN_POINT('Ctrl Pts',(9.66975456632122,-29.4798979011573,
56.5827453830793));
#108414=CARTESIAN_POINT('Ctrl Pts',(9.669365077656,-29.4744319869831,56.5809387723855));
#108415=CARTESIAN_POINT('Ctrl Pts',(9.66829238069286,-29.4594655189485,
56.5759058173555));
#108416=CARTESIAN_POINT('Ctrl Pts',(9.66760596238923,-29.4499847634579,
56.5726219817434));
#108417=CARTESIAN_POINT('Ctrl Pts',(9.66482384437344,-29.411921143772,56.559051650655));
#108418=CARTESIAN_POINT('Ctrl Pts',(9.66269348856463,-29.383594161389,56.5480705276859));
#108419=CARTESIAN_POINT('Ctrl Pts',(9.65353982683574,-29.2647002145217,
56.4982001288676));
#108420=CARTESIAN_POINT('Ctrl Pts',(9.64629819090916,-29.1773805179267,
56.4520900750812));
#108421=CARTESIAN_POINT('Ctrl Pts',(9.63445285251202,-29.0401627209945,
56.3632613643615));
#108422=CARTESIAN_POINT('Ctrl Pts',(9.62979898090483,-28.9877781664185,
56.3248311546177));
#108423=CARTESIAN_POINT('Ctrl Pts',(9.62237133318643,-28.9061861294285,
56.2573017133974));
#108424=CARTESIAN_POINT('Ctrl Pts',(9.61953852456733,-28.8755799817851,
56.2300067102434));
#108425=CARTESIAN_POINT('Ctrl Pts',(9.61569165448205,-28.8347575791015,
56.1908020327079));
#108426=CARTESIAN_POINT('Ctrl Pts',(9.61463815165872,-28.8236575723699,
56.1798380830576));
#108427=CARTESIAN_POINT('Ctrl Pts',(9.61285237687562,-28.8049848186099,
56.1608686724202));
#108428=CARTESIAN_POINT('Ctrl Pts',(9.6121167360181,-28.7973346690859,56.1529412258251));
#108429=CARTESIAN_POINT('Ctrl Pts',(9.61072247753064,-28.7829188287173,
56.1377032211147));
#108430=CARTESIAN_POINT('Ctrl Pts',(9.61006327013571,-28.7761389990831,
56.1304067650837));
#108431=CARTESIAN_POINT('Ctrl Pts',(9.60836128941283,-28.7587319146771,
56.1113330564206));
#108432=CARTESIAN_POINT('Ctrl Pts',(9.60732281296323,-28.7482065419591,
56.0994638642334));
#108433=CARTESIAN_POINT('Ctrl Pts',(9.60370527085614,-28.7119034297809,
56.0573285225653));
#108434=CARTESIAN_POINT('Ctrl Pts',(9.60116297775279,-28.6870397505686,
56.0262904803422));
#108435=CARTESIAN_POINT('Ctrl Pts',(9.59053082494693,-28.5864620714503,
55.8910907793065));
#108436=CARTESIAN_POINT('Ctrl Pts',(9.58283499485131,-28.5218515488968,
55.7792362877486));
#108437=CARTESIAN_POINT('Ctrl Pts',(9.57297692957263,-28.4585765100932,
55.6328611417994));
#108438=CARTESIAN_POINT('Ctrl Pts',(9.57106299303262,-28.4471713507646,
55.6043362893767));
#108439=CARTESIAN_POINT('Ctrl Pts',(9.56912142374065,-28.4365623107092,
55.5755159352313));
#108440=CARTESIAN_POINT('Origin',(5.,-30.,55.));
#108441=CARTESIAN_POINT('',(8.86797186106678,-28.4365624698124,55.5755163674483));
#108442=CARTESIAN_POINT('',(9.06224859760916,-28.4365623100358,55.5755159334019));
#108443=CARTESIAN_POINT('',(5.,-28.4365623102018,55.5755159338528));
#108444=CARTESIAN_POINT('',(9.72158590647257,-28.3340000001852,55.0000017306777));
#108445=CARTESIAN_POINT('Ctrl Pts',(9.06224859760915,-28.4365623100358,
55.5755159334018));
#108446=CARTESIAN_POINT('Ctrl Pts',(9.06293925223953,-28.4402324751857,
55.5854862473248));
#108447=CARTESIAN_POINT('Ctrl Pts',(9.06362689414098,-28.4439980831935,
55.5954216415668));
#108448=CARTESIAN_POINT('Ctrl Pts',(9.07227367572701,-28.4927460191911,
55.7204193176186));
#108449=CARTESIAN_POINT('Ctrl Pts',(9.0797793055815,-28.550296491161,55.8301701699813));
#108450=CARTESIAN_POINT('Ctrl Pts',(9.09272385742568,-28.6688828142423,
56.0057230412234));
#108451=CARTESIAN_POINT('Ctrl Pts',(9.09813287492223,-28.7240382781921,
56.0748346903343));
#108452=CARTESIAN_POINT('Ctrl Pts',(9.10491892357804,-28.7956645587084,
56.1512616956104));
#108453=CARTESIAN_POINT('Ctrl Pts',(9.10599668128744,-28.8071059684168,
56.1631126885977));
#108454=CARTESIAN_POINT('Ctrl Pts',(9.10759804419394,-28.8241637427529,
56.1802646644835));
#108455=CARTESIAN_POINT('Ctrl Pts',(9.10811178289267,-28.8296446470031,
56.1856997612915));
#108456=CARTESIAN_POINT('Ctrl Pts',(9.10903056196332,-28.8394571506665,
56.195295934259));
#108457=CARTESIAN_POINT('Ctrl Pts',(9.10943443474575,-28.8437737686655,
56.199471956883));
#108458=CARTESIAN_POINT('Ctrl Pts',(9.11033226203008,-28.8533761183069,
56.2086615511469));
#108459=CARTESIAN_POINT('Ctrl Pts',(9.11082700958379,-28.8586721271647,
56.2136637726093));
#108460=CARTESIAN_POINT('Ctrl Pts',(9.11229690775663,-28.8744251359664,
56.228348618249));
#108461=CARTESIAN_POINT('Ctrl Pts',(9.11327893163169,-28.8849734602126,
56.2379316961005));
#108462=CARTESIAN_POINT('Ctrl Pts',(9.12157709962656,-28.9744078912339,
56.3171118266752));
#108463=CARTESIAN_POINT('Ctrl Pts',(9.12928507060617,-29.0595936277881,
56.3792225741385));
#108464=CARTESIAN_POINT('Ctrl Pts',(9.14455037579019,-29.240137526273,56.486315778396));
#108465=CARTESIAN_POINT('Ctrl Pts',(9.15207139677135,-29.3350692252378,
56.5311431599763));
#108466=CARTESIAN_POINT('Ctrl Pts',(9.16082162778065,-29.4544741908131,
56.5743095113059));
#108467=CARTESIAN_POINT('Ctrl Pts',(9.16233819953936,-29.47550153301,56.5814393084298));
#108468=CARTESIAN_POINT('Ctrl Pts',(9.16476621371594,-29.5096945368631,
56.592276152332));
#108469=CARTESIAN_POINT('Ctrl Pts',(9.16568608273025,-29.5227737084982,
56.5962449306129));
#108470=CARTESIAN_POINT('Ctrl Pts',(9.16731651785406,-29.5461738849994,
56.6030322134154));
#108471=CARTESIAN_POINT('Ctrl Pts',(9.16802907659645,-29.5564758457131,
56.6059130591792));
#108472=CARTESIAN_POINT('Ctrl Pts',(9.16953285683048,-29.578372654003,56.6118095090994));
#108473=CARTESIAN_POINT('Ctrl Pts',(9.17032322088,-29.5899737673449,56.6147996822084));
#108474=CARTESIAN_POINT('Ctrl Pts',(9.17244582798156,-29.621370520841,56.6225319814092));
#108475=CARTESIAN_POINT('Ctrl Pts',(9.1737704504239,-29.6412228620489,56.6270369808837));
#108476=CARTESIAN_POINT('Ctrl Pts',(9.18237025923551,-29.7716661776567,
56.6541341353175));
#108477=CARTESIAN_POINT('Ctrl Pts',(9.18927890005292,-29.8842296768193,
56.6658023665987));
#108478=CARTESIAN_POINT('Ctrl Pts',(9.20241624195797,-30.0993869791171,
56.6661742910775));
#108479=CARTESIAN_POINT('Ctrl Pts',(9.20862919714916,-30.2014393774716,
56.6569342414695));
#108480=CARTESIAN_POINT('Ctrl Pts',(9.21627684966869,-30.3173428481181,
56.6355712725491));
#108481=CARTESIAN_POINT('Ctrl Pts',(9.21729982790151,-30.3326592857006,
56.6325249239855));
#108482=CARTESIAN_POINT('Ctrl Pts',(9.21883460208811,-30.3553174785965,
56.6276862577836));
#108483=CARTESIAN_POINT('Ctrl Pts',(9.21933765095702,-30.3626940090964,
56.6260584597764));
#108484=CARTESIAN_POINT('Ctrl Pts',(9.22024544229879,-30.3759099800456,
56.6230476570874));
#108485=CARTESIAN_POINT('Ctrl Pts',(9.22064913911115,-30.3817533713685,
56.6216831906735));
#108486=CARTESIAN_POINT('Ctrl Pts',(9.22155693640405,-30.3948175656427,
56.6185581011228));
#108487=CARTESIAN_POINT('Ctrl Pts',(9.22206194297282,-30.4020339628245,
56.6167807285658));
#108488=CARTESIAN_POINT('Ctrl Pts',(9.22359194301112,-30.4237508079991,
56.6112775669169));
#108489=CARTESIAN_POINT('Ctrl Pts',(9.22462463028459,-30.4382127126801,
56.607404654866));
#108490=CARTESIAN_POINT('Ctrl Pts',(9.22706393457485,-30.4719613889587,
56.5978774534785));
#108491=CARTESIAN_POINT('Ctrl Pts',(9.22847729085736,-30.4912016862202,
56.5920680690244));
#108492=CARTESIAN_POINT('Ctrl Pts',(9.23365984005963,-30.560772506691,56.5696808522721));
#108493=CARTESIAN_POINT('Ctrl Pts',(9.23749483522645,-30.6104077332117,
56.5510530316408));
#108494=CARTESIAN_POINT('Ctrl Pts',(9.25094771624656,-30.780338231835,56.4778576835971));
#108495=CARTESIAN_POINT('Ctrl Pts',(9.26056312309516,-30.8949926774089,
56.4113792041917));
#108496=CARTESIAN_POINT('Ctrl Pts',(9.27155611086018,-31.0221614749094,
56.3158529296848));
#108497=CARTESIAN_POINT('Ctrl Pts',(9.27340012341623,-31.0433245390844,
56.2991370468007));
#108498=CARTESIAN_POINT('Ctrl Pts',(9.27612501687463,-31.0743249503579,
56.2734046484244));
#108499=CARTESIAN_POINT('Ctrl Pts',(9.27702108322519,-31.0844740865783,
56.2647724977327));
#108500=CARTESIAN_POINT('Ctrl Pts',(9.27862625966872,-31.1025682513995,
56.249004902254));
#108501=CARTESIAN_POINT('Ctrl Pts',(9.27933711215892,-31.1105501999869,
56.2419131440087));
#108502=CARTESIAN_POINT('Ctrl Pts',(9.28085512987648,-31.1275249598017,
56.2265369726383));
#108503=CARTESIAN_POINT('Ctrl Pts',(9.28166125861218,-31.1364959033203,
56.2182292704265));
#108504=CARTESIAN_POINT('Ctrl Pts',(9.28387231140808,-31.1609728163527,
56.1950562688631));
#108505=CARTESIAN_POINT('Ctrl Pts',(9.2852684822894,-31.1762843504367,56.1799883734328));
#108506=CARTESIAN_POINT('Ctrl Pts',(9.29385695711891,-31.2694401842072,
56.0846990464278));
#108507=CARTESIAN_POINT('Ctrl Pts',(9.30069509648075,-31.3393403806675,
55.9971066837057));
#108508=CARTESIAN_POINT('Ctrl Pts',(9.31368930568585,-31.4546887899291,
55.8183111790544));
#108509=CARTESIAN_POINT('Ctrl Pts',(9.31982939229436,-31.5015957314056,
55.7286682986457));
#108510=CARTESIAN_POINT('Ctrl Pts',(9.32740139997794,-31.5461082135954,
55.6207689138374));
#108511=CARTESIAN_POINT('Ctrl Pts',(9.32843414023273,-31.5519142476679,
55.606107891618));
#108512=CARTESIAN_POINT('Ctrl Pts',(9.32998126384525,-31.5602056810896,
55.5842703660201));
#108513=CARTESIAN_POINT('Ctrl Pts',(9.33048672862475,-31.5628517048656,
55.5771552398773));
#108514=CARTESIAN_POINT('Ctrl Pts',(9.33139800273318,-31.5675077089459,
55.5643684862156));
#108515=CARTESIAN_POINT('Ctrl Pts',(9.33180275126667,-31.5695357181002,
55.5587037072991));
#108516=CARTESIAN_POINT('Ctrl Pts',(9.33271206263157,-31.574002648334,55.5460100851986));
#108517=CARTESIAN_POINT('Ctrl Pts',(9.33321752467188,-31.5764251792079,
55.5389758799242));
#108518=CARTESIAN_POINT('Ctrl Pts',(9.33474551486824,-31.5835697411635,
55.5177702221211));
#108519=CARTESIAN_POINT('Ctrl Pts',(9.33577565581616,-31.5881482262139,
55.5035516866736));
#108520=CARTESIAN_POINT('Ctrl Pts',(9.33820703864514,-31.5984160511905,
55.4701310205612));
#108521=CARTESIAN_POINT('Ctrl Pts',(9.33961492299902,-31.6039514758649,
55.4508842837714));
#108522=CARTESIAN_POINT('Ctrl Pts',(9.34476690521399,-31.6227780381693,
55.380683824411));
#108523=CARTESIAN_POINT('Ctrl Pts',(9.34857567270648,-31.6339979886334,
55.3292091247706));
#108524=CARTESIAN_POINT('Ctrl Pts',(9.36193004229679,-31.6645861375307,
55.147996405325));
#108525=CARTESIAN_POINT('Ctrl Pts',(9.37147470611721,-31.6710738317391,
55.0165497831416));
#108526=CARTESIAN_POINT('Ctrl Pts',(9.38242621515086,-31.6602043746123,
54.8585091856916));
#108527=CARTESIAN_POINT('Ctrl Pts',(9.3842897278416,-31.6576685808561,54.8313784026227));
#108528=CARTESIAN_POINT('Ctrl Pts',(9.38703814307414,-31.6528960294267,
54.7910265075426));
#108529=CARTESIAN_POINT('Ctrl Pts',(9.38793856963188,-31.651163482567,54.7777515430919));
#108530=CARTESIAN_POINT('Ctrl Pts',(9.38954939596825,-31.6477590895474,
54.753909791038));
#108531=CARTESIAN_POINT('Ctrl Pts',(9.39026157129356,-31.646145137778,54.7433356225638));
#108532=CARTESIAN_POINT('Ctrl Pts',(9.39178016933653,-31.6424702423539,
54.7207211101581));
#108533=CARTESIAN_POINT('Ctrl Pts',(9.3925855762082,-31.6403784834013,54.7086863548727));
#108534=CARTESIAN_POINT('Ctrl Pts',(9.3947888594805,-31.6342636490974,54.6756621820449));
#108535=CARTESIAN_POINT('Ctrl Pts',(9.39617811114267,-31.6299686970547,
54.6547250241144));
#108536=CARTESIAN_POINT('Ctrl Pts',(9.39925653958761,-31.6194733673752,
54.6081349580547));
#108537=CARTESIAN_POINT('Ctrl Pts',(9.40093914108252,-31.613063903461,54.5825348471223));
#108538=CARTESIAN_POINT('Ctrl Pts',(9.40637463139229,-31.5901957480408,
54.4996107091246));
#108539=CARTESIAN_POINT('Ctrl Pts',(9.41005936867706,-31.5712669266334,
54.4430143776762));
#108540=CARTESIAN_POINT('Ctrl Pts',(9.4205939150763,-31.5080853540179,54.2831805288463));
#108541=CARTESIAN_POINT('Ctrl Pts',(9.42732977788127,-31.4563915375526,
54.183256368342));
#108542=CARTESIAN_POINT('Ctrl Pts',(9.4361514317286,-31.3807813342478,54.0674332831621));
#108543=CARTESIAN_POINT('Ctrl Pts',(9.43783905729265,-31.3659970051774,
54.0459089260239));
#108544=CARTESIAN_POINT('Ctrl Pts',(9.44018158972882,-31.3451600439263,
54.0170501169487));
#108545=CARTESIAN_POINT('Ctrl Pts',(9.44080996623051,-31.339540607661,54.0094057509363));
#108546=CARTESIAN_POINT('Ctrl Pts',(9.44181972215474,-31.3304696530224,
53.9972844606632));
#108547=CARTESIAN_POINT('Ctrl Pts',(9.4421982689784,-31.3270600077186,53.992776249313));
#108548=CARTESIAN_POINT('Ctrl Pts',(9.44299895906726,-31.3198309374382,
53.9833184455798));
#108549=CARTESIAN_POINT('Ctrl Pts',(9.44342147455041,-31.3160065241504,
53.9783729105213));
#108550=CARTESIAN_POINT('Ctrl Pts',(9.44449150750472,-31.3062946332791,
53.9659590089201));
#108551=CARTESIAN_POINT('Ctrl Pts',(9.44514149752914,-31.300370935075,53.9585193902067));
#108552=CARTESIAN_POINT('Ctrl Pts',(9.44777621567138,-31.276249854754,53.9287521407785));
#108553=CARTESIAN_POINT('Ctrl Pts',(9.44979277863327,-31.2575396136645,
53.906848799934));
#108554=CARTESIAN_POINT('Ctrl Pts',(9.45542926711212,-31.2043369205143,
53.8477406187477));
#108555=CARTESIAN_POINT('Ctrl Pts',(9.45909768839969,-31.1686991170854,
53.8116099816927));
#108556=CARTESIAN_POINT('Ctrl Pts',(9.47172458057161,-31.0412385142775,
53.6936726870126));
#108557=CARTESIAN_POINT('Ctrl Pts',(9.48070688070601,-30.942026348135,53.620411760282));
#108558=CARTESIAN_POINT('Ctrl Pts',(9.49175140214039,-30.8051607615466,
53.5410572863816));
#108559=CARTESIAN_POINT('Ctrl Pts',(9.49417917103131,-30.7741215032174,
53.5243530514464));
#108560=CARTESIAN_POINT('Ctrl Pts',(9.49759843923497,-30.7290488303423,
53.5019105256419));
#108561=CARTESIAN_POINT('Ctrl Pts',(9.49861798839922,-30.7154326791235,
53.4953603826383));
#108562=CARTESIAN_POINT('Ctrl Pts',(9.50035228431299,-30.6919739828229,
53.4844658732685));
#108563=CARTESIAN_POINT('Ctrl Pts',(9.50107016476252,-30.6821752256601,
53.4800300486228));
#108564=CARTESIAN_POINT('Ctrl Pts',(9.50253301346504,-30.6620301972741,
53.4711445978106));
#108565=CARTESIAN_POINT('Ctrl Pts',(9.50327762984543,-30.6516803741721,
53.4667043587695));
#108566=CARTESIAN_POINT('Ctrl Pts',(9.50514731649012,-30.6254573448493,
53.4557677506344));
#108567=CARTESIAN_POINT('Ctrl Pts',(9.50626763091572,-30.6095271323434,
53.4494108084193));
#108568=CARTESIAN_POINT('Ctrl Pts',(9.51094699021412,-30.5421213952134,
53.4237119587478));
#108569=CARTESIAN_POINT('Ctrl Pts',(9.51442941034639,-30.4898000691273,
53.4066775493768));
#108570=CARTESIAN_POINT('Ctrl Pts',(9.52473473766321,-30.33024411988,53.3633356490567));
#108571=CARTESIAN_POINT('Ctrl Pts',(9.53135041530668,-30.2211543199084,
53.3450614276894));
#108572=CARTESIAN_POINT('Ctrl Pts',(9.54197303705375,-30.0494914689011,
53.3335924351692));
#108573=CARTESIAN_POINT('Ctrl Pts',(9.54584118843888,-29.9877490583328,
53.3329032054045));
#108574=CARTESIAN_POINT('Ctrl Pts',(9.55065742154364,-29.9141340963614,
53.3361709955755));
#108575=CARTESIAN_POINT('Ctrl Pts',(9.55144757943654,-29.9021561964138,
53.336832396005));
#108576=CARTESIAN_POINT('Ctrl Pts',(9.55270090921045,-29.8833347764164,
53.3380756989943));
#108577=CARTESIAN_POINT('Ctrl Pts',(9.55315944036612,-29.8764856576638,
53.3385706877353));
#108578=CARTESIAN_POINT('Ctrl Pts',(9.5540278250404,-29.863588304781,53.3395829748461));
#108579=CARTESIAN_POINT('Ctrl Pts',(9.55443716751813,-29.8575395593624,
53.3400910067401));
#108580=CARTESIAN_POINT('Ctrl Pts',(9.55541228837665,-29.8432010029824,
53.3413742444181));
#108581=CARTESIAN_POINT('Ctrl Pts',(9.55597963507766,-29.8349140293788,
53.3421785568071));
#108582=CARTESIAN_POINT('Ctrl Pts',(9.55791262463374,-29.80685538861,53.3451143177642));
#108583=CARTESIAN_POINT('Ctrl Pts',(9.55929268811388,-29.7871168162554,
53.3475375568392));
#108584=CARTESIAN_POINT('Ctrl Pts',(9.56274982125294,-29.7382834551279,
53.3544220758374));
#108585=CARTESIAN_POINT('Ctrl Pts',(9.56484276194549,-29.7092550692085,
53.3593021483128));
#108586=CARTESIAN_POINT('Ctrl Pts',(9.57273146158079,-29.6013457664813,
53.3803967296731));
#108587=CARTESIAN_POINT('Ctrl Pts',(9.57863170854992,-29.523544332806,53.4015540115763));
#108588=CARTESIAN_POINT('Ctrl Pts',(9.59116414568343,-29.360567195844,53.4588354995367));
#108589=CARTESIAN_POINT('Ctrl Pts',(9.59775266420647,-29.2762338746358,
53.4965939755112));
#108590=CARTESIAN_POINT('Ctrl Pts',(9.60564497624947,-29.1759671815406,
53.5518905768821));
#108591=CARTESIAN_POINT('Ctrl Pts',(9.60716507294531,-29.1567015847465,
53.5630244078401));
#108592=CARTESIAN_POINT('Ctrl Pts',(9.60960076574813,-29.1259198022432,
53.5816459506195));
#108593=CARTESIAN_POINT('Ctrl Pts',(9.61052475964601,-29.1142636027221,
53.5888956610034));
#108594=CARTESIAN_POINT('Ctrl Pts',(9.61216377771439,-29.0936307767483,
53.6020848949512));
#108595=CARTESIAN_POINT('Ctrl Pts',(9.61288078876066,-29.0846197267271,
53.6079688313926));
#108596=CARTESIAN_POINT('Ctrl Pts',(9.61439537966407,-29.0656213488485,
53.6206384425984));
#108597=CARTESIAN_POINT('Ctrl Pts',(9.61519208187553,-29.0556494602472,
53.627446233963));
#108598=CARTESIAN_POINT('Ctrl Pts',(9.61733564201717,-29.0288873985013,
53.6461463852554));
#108599=CARTESIAN_POINT('Ctrl Pts',(9.61867474065101,-29.0122417381222,
53.6582425810944));
#108600=CARTESIAN_POINT('Ctrl Pts',(9.62162446182995,-28.9757834746243,
53.6857826327796));
#108601=CARTESIAN_POINT('Ctrl Pts',(9.62322938883063,-28.9560873070933,
53.7013725838815));
#108602=CARTESIAN_POINT('Ctrl Pts',(9.62831039557595,-28.8943328442518,
53.7525658937851));
#108603=CARTESIAN_POINT('Ctrl Pts',(9.63172889701348,-28.8536836290377,
53.7898135885128));
#108604=CARTESIAN_POINT('Ctrl Pts',(9.64164017127283,-28.7403816030223,
53.9044756750137));
#108605=CARTESIAN_POINT('Ctrl Pts',(9.64801663953327,-28.6731954207139,
53.9868867254564));
#108606=CARTESIAN_POINT('Ctrl Pts',(9.65698296904393,-28.5942444095642,
54.1051743135878));
#108607=CARTESIAN_POINT('Ctrl Pts',(9.65929641099807,-28.575168431265,54.1358724844858));
#108608=CARTESIAN_POINT('Ctrl Pts',(9.66236915911345,-28.5517514234138,
54.1764425714994));
#108609=CARTESIAN_POINT('Ctrl Pts',(9.66307682217678,-28.5464855587735,
54.1857724322418));
#108610=CARTESIAN_POINT('Ctrl Pts',(9.66422796605379,-28.5381313958928,
54.2009133458744));
#108611=CARTESIAN_POINT('Ctrl Pts',(9.6646680359289,-28.5349867978189,54.2066932428746));
#108612=CARTESIAN_POINT('Ctrl Pts',(9.66553988730539,-28.5288553286742,
54.2181239178098));
#108613=CARTESIAN_POINT('Ctrl Pts',(9.66597152911856,-28.525866582324,54.2237735411965));
#108614=CARTESIAN_POINT('Ctrl Pts',(9.66705364139782,-28.5184884739654,
54.2379166682481));
#108615=CARTESIAN_POINT('Ctrl Pts',(9.66770646402914,-28.5141396418008,
54.2464308978936));
#108616=CARTESIAN_POINT('Ctrl Pts',(9.67027370243341,-28.4974259497794,
54.2798605076404));
#108617=CARTESIAN_POINT('Ctrl Pts',(9.67221643695832,-28.4856132568221,
54.3050451472343));
#108618=CARTESIAN_POINT('Ctrl Pts',(9.67756592902582,-28.4551879071138,
54.3743753946855));
#108619=CARTESIAN_POINT('Ctrl Pts',(9.68101367702895,-28.437840339896,54.4190462898142));
#108620=CARTESIAN_POINT('Ctrl Pts',(9.69456347867808,-28.3776483703072,
54.5963357292153));
#108621=CARTESIAN_POINT('Ctrl Pts',(9.7046919813584,-28.3495734734474,54.7333991472846));
#108622=CARTESIAN_POINT('Ctrl Pts',(9.71584768315985,-28.3371437734708,
54.8951754240954));
#108623=CARTESIAN_POINT('Ctrl Pts',(9.71740609096478,-28.3358614383319,
54.9180124536265));
#108624=CARTESIAN_POINT('Ctrl Pts',(9.71973947582919,-28.3346347042239,
54.9525539573496));
#108625=CARTESIAN_POINT('Ctrl Pts',(9.72052498555687,-28.3343427385083,
54.96424256035));
#108626=CARTESIAN_POINT('Ctrl Pts',(9.72184116965428,-28.3340583620148,
54.9839264509187));
#108627=CARTESIAN_POINT('Ctrl Pts',(9.72237383948339,-28.3340004141805,
54.9919201945016));
#108628=CARTESIAN_POINT('Ctrl Pts',(9.72290474247879,-28.3340000022123,
54.999914142671));
#108629=CARTESIAN_POINT('Ctrl Pts',(9.72148036344419,-28.3340000000229,
55.0000087401189));
#108630=CARTESIAN_POINT('Ctrl Pts',(9.72575161781573,-28.3340003369473,
55.0642316688592));
#108631=CARTESIAN_POINT('Ctrl Pts',(9.73002287218727,-28.3377185882288,
55.1283809457949));
#108632=CARTESIAN_POINT('Ctrl Pts',(9.73429412655882,-28.345103558767,55.1920254378838));
#108633=CARTESIAN_POINT('Ctrl Pts',(9.73869639077281,-28.3527150444557,
55.2576220625679));
#108634=CARTESIAN_POINT('Ctrl Pts',(9.7430986549868,-28.3642217675405,55.3226819356344));
#108635=CARTESIAN_POINT('Ctrl Pts',(9.74750091920079,-28.3795114745026,
55.3867466079117));
#108636=CARTESIAN_POINT('Ctrl Pts',(9.75190318341478,-28.3948011814646,
55.4508112801889));
#108637=CARTESIAN_POINT('Ctrl Pts',(9.75630544762877,-28.4138736612379,
55.5138803007899));
#108638=CARTESIAN_POINT('Ctrl Pts',(9.76070771184276,-28.4365623102018,
55.5755159338528));
#108639=CARTESIAN_POINT('Ctrl Pts',(9.56912142374065,-28.4365623107092,
55.5755159352313));
#108640=CARTESIAN_POINT('Ctrl Pts',(9.56843982933344,-28.4328379716411,
55.5653984533158));
#108641=CARTESIAN_POINT('Ctrl Pts',(9.56775482209394,-28.4292117451295,
55.5552445547067));
#108642=CARTESIAN_POINT('Ctrl Pts',(9.56545070081313,-28.4174148268356,
55.5211708329592));
#108643=CARTESIAN_POINT('Ctrl Pts',(9.56381428263611,-28.4096906314247,
55.4971024197191));
#108644=CARTESIAN_POINT('Ctrl Pts',(9.56154800177924,-28.3999277035981,
55.4641205574211));
#108645=CARTESIAN_POINT('Ctrl Pts',(9.56094315248967,-28.3974100062228,
55.4553510162443));
#108646=CARTESIAN_POINT('Ctrl Pts',(9.55991948585289,-28.3932987692135,
55.4405743698173));
#108647=CARTESIAN_POINT('Ctrl Pts',(9.55950284485447,-28.391666536423,55.4345780581646));
#108648=CARTESIAN_POINT('Ctrl Pts',(9.55864108061242,-28.3883756569633,
55.4222158820929));
#108649=CARTESIAN_POINT('Ctrl Pts',(9.55819575267008,-28.3867211118918,
55.4158491307793));
#108650=CARTESIAN_POINT('Ctrl Pts',(9.55700855891035,-28.3824307669899,
55.3989286959595));
#108651=CARTESIAN_POINT('Ctrl Pts',(9.55626316310687,-28.3798606038035,
55.3883589180524));
#108652=CARTESIAN_POINT('Ctrl Pts',(9.55285032949156,-28.3686428085694,
55.340175377312));
#108653=CARTESIAN_POINT('Ctrl Pts',(9.55012650698277,-28.3612010007808,
55.3022960426285));
#108654=CARTESIAN_POINT('Ctrl Pts',(9.54076273385981,-28.340433079154,55.1729923015376));
#108655=CARTESIAN_POINT('Ctrl Pts',(9.53398086220428,-28.3333953684809,
55.0807302803421));
#108656=CARTESIAN_POINT('Ctrl Pts',(9.52053162090534,-28.3346934974039,
54.89491061205));
#108657=CARTESIAN_POINT('Ctrl Pts',(9.51389170401175,-28.3432082207743,
54.8016675754));
#108658=CARTESIAN_POINT('Ctrl Pts',(9.50615126326317,-28.3629221622149,
54.6902949781091));
#108659=CARTESIAN_POINT('Ctrl Pts',(9.504819026515,-28.366683601444,54.6710339731172));
#108660=CARTESIAN_POINT('Ctrl Pts',(9.50270080794925,-28.3732571062508,
54.6402729633543));
#108661=CARTESIAN_POINT('Ctrl Pts',(9.50190803913437,-28.3758528513925,
54.6287291616344));
#108662=CARTESIAN_POINT('Ctrl Pts',(9.5004030200086,-28.3810394896025,54.6067592945939));
#108663=CARTESIAN_POINT('Ctrl Pts',(9.49969011667312,-28.3836086688535,
54.5963287718655));
#108664=CARTESIAN_POINT('Ctrl Pts',(9.49807241286668,-28.3896945298868,
54.5726112054111));
#108665=CARTESIAN_POINT('Ctrl Pts',(9.49716971639863,-28.3932751389009,
54.5593412564179));
#108666=CARTESIAN_POINT('Ctrl Pts',(9.49430665080666,-28.4052188461538,
54.5171596376686));
#108667=CARTESIAN_POINT('Ctrl Pts',(9.49236626320087,-28.4142015647743,
54.4884286494787));
#108668=CARTESIAN_POINT('Ctrl Pts',(9.48140364221558,-28.4699402372424,
54.325763453626));
#108669=CARTESIAN_POINT('Ctrl Pts',(9.47294371389912,-28.5328687792529,
54.1979997753101));
#108670=CARTESIAN_POINT('Ctrl Pts',(9.46152684923223,-28.6350523915768,
54.0437913974955));
#108671=CARTESIAN_POINT('Ctrl Pts',(9.45883675440065,-28.6602665261369,
54.0087731918474));
#108672=CARTESIAN_POINT('Ctrl Pts',(9.45442796353356,-28.7027690980143,
53.9543324535729));
#108673=CARTESIAN_POINT('Ctrl Pts',(9.45275016278633,-28.7192032270749,
53.9342664120844));
#108674=CARTESIAN_POINT('Ctrl Pts',(9.45043648313065,-28.7420876220084,
53.9076186681539));
#108675=CARTESIAN_POINT('Ctrl Pts',(9.44982713344136,-28.7481348478599,
53.9006937841948));
#108676=CARTESIAN_POINT('Ctrl Pts',(9.44879896852383,-28.7583650458036,
53.8891727145041));
#108677=CARTESIAN_POINT('Ctrl Pts',(9.44838239755285,-28.7625170994122,
53.8845491105663));
#108678=CARTESIAN_POINT('Ctrl Pts',(9.44752390494259,-28.7710860209794,
53.8751137422702));
#108679=CARTESIAN_POINT('Ctrl Pts',(9.44708180805566,-28.7755054557552,
53.8703045684471));
#108680=CARTESIAN_POINT('Ctrl Pts',(9.44591019537158,-28.7872380805656,
53.8576870039915));
#108681=CARTESIAN_POINT('Ctrl Pts',(9.44517729170724,-28.7945982635757,
53.8499230056618));
#108682=CARTESIAN_POINT('Ctrl Pts',(9.44190864263936,-28.8275367866623,
53.8158408435692));
#108683=CARTESIAN_POINT('Ctrl Pts',(9.43932188267386,-28.8539040904638,
53.7903030928028));
#108684=CARTESIAN_POINT('Ctrl Pts',(9.42913576754911,-28.9595985416822,
53.6944928522457));
#108685=CARTESIAN_POINT('Ctrl Pts',(9.42133171400559,-29.0447157504235,
53.6309797445694));
#108686=CARTESIAN_POINT('Ctrl Pts',(9.40776038693575,-29.2056130035749,
53.5332777111057));
#108687=CARTESIAN_POINT('Ctrl Pts',(9.4019419353104,-29.2790118032807,53.4958375566414));
#108688=CARTESIAN_POINT('Ctrl Pts',(9.39496989100612,-29.3729447943659,
53.4563869188035));
#108689=CARTESIAN_POINT('Ctrl Pts',(9.39364026752912,-29.3911349317075,
53.449121874289));
#108690=CARTESIAN_POINT('Ctrl Pts',(9.391525854498,-29.4204964220282,53.4379913024474));
#108691=CARTESIAN_POINT('Ctrl Pts',(9.39073429734198,-29.4315876706034,
53.4339211372488));
#108692=CARTESIAN_POINT('Ctrl Pts',(9.38923139282455,-29.4528321573832,
53.4263804602427));
#108693=CARTESIAN_POINT('Ctrl Pts',(9.38851939509967,-29.4629774129986,
53.4228893969851));
#108694=CARTESIAN_POINT('Ctrl Pts',(9.38688812482984,-29.4864026205342,
53.4150808520019));
#108695=CARTESIAN_POINT('Ctrl Pts',(9.38597113856145,-29.4997046624214,
53.4108317997254));
#108696=CARTESIAN_POINT('Ctrl Pts',(9.38306414242658,-29.5422838554441,
53.3978184219363));
#108697=CARTESIAN_POINT('Ctrl Pts',(9.38109475180961,-29.5717503830855,
53.3896918520039));
#108698=CARTESIAN_POINT('Ctrl Pts',(9.37644359037693,-29.6426284050969,
53.3722278097989));
#108699=CARTESIAN_POINT('Ctrl Pts',(9.37378432443822,-29.6842061876161,
53.3636530297656));
#108700=CARTESIAN_POINT('Ctrl Pts',(9.3665790489543,-29.7988468226766,53.3445431817866));
#108701=CARTESIAN_POINT('Ctrl Pts',(9.36210110838623,-29.872352442782,53.3372593860087));
#108702=CARTESIAN_POINT('Ctrl Pts',(9.35677680363508,-29.9593516241079,
53.3344431782267));
#108703=CARTESIAN_POINT('Ctrl Pts',(9.35596467135432,-29.9726088394847,
53.3341724169929));
#108704=CARTESIAN_POINT('Ctrl Pts',(9.35059042223113,-30.060133318606,53.3334299438422));
#108705=CARTESIAN_POINT('Ctrl Pts',(9.34597602956322,-30.1343488081574,
53.3377667565187));
#108706=CARTESIAN_POINT('Ctrl Pts',(9.34032438422154,-30.2201947115743,
53.348570033923));
#108707=CARTESIAN_POINT('Ctrl Pts',(9.33951636813612,-30.2323546219843,
53.3502370013402));
#108708=CARTESIAN_POINT('Ctrl Pts',(9.33823994150718,-30.2513637382742,
53.3530572276845));
#108709=CARTESIAN_POINT('Ctrl Pts',(9.33777641073297,-30.2582263202643,
53.354119266971));
#108710=CARTESIAN_POINT('Ctrl Pts',(9.33690444727359,-30.2710552563362,
53.3561868549869));
#108711=CARTESIAN_POINT('Ctrl Pts',(9.3364965877071,-30.2770230327132,53.3571820422393));
#108712=CARTESIAN_POINT('Ctrl Pts',(9.33553098709224,-30.2910759625075,
53.3596042581156));
#108713=CARTESIAN_POINT('Ctrl Pts',(9.33497176309603,-30.2991561388637,
53.3610585722903));
#108714=CARTESIAN_POINT('Ctrl Pts',(9.3330897392773,-30.3261652793219,53.3661262066272));
#108715=CARTESIAN_POINT('Ctrl Pts',(9.33175344091018,-30.3450414642944,
53.370008076396));
#108716=CARTESIAN_POINT('Ctrl Pts',(9.32842802591731,-30.3913787009429,
53.3803781970309));
#108717=CARTESIAN_POINT('Ctrl Pts',(9.32642439701582,-30.4187498854221,
53.3872382611992));
#108718=CARTESIAN_POINT('Ctrl Pts',(9.31726137253638,-30.5419721526149,
53.4214697600547));
#108719=CARTESIAN_POINT('Ctrl Pts',(9.30993076456218,-30.6354233282733,
53.4567148252314));
#108720=CARTESIAN_POINT('Ctrl Pts',(9.29674502322023,-30.8000262380954,
53.536296368608));
#108721=CARTESIAN_POINT('Ctrl Pts',(9.2908622671464,-30.8720824507001,53.5780484288349));
#108722=CARTESIAN_POINT('Ctrl Pts',(9.28382709947328,-30.9569245390145,
53.6360951194296));
#108723=CARTESIAN_POINT('Ctrl Pts',(9.28249479011752,-30.9729240730013,
53.6474616819082));
#108724=CARTESIAN_POINT('Ctrl Pts',(9.28037659732261,-30.9982412846925,
53.6661295821638));
#108725=CARTESIAN_POINT('Ctrl Pts',(9.27958392229206,-31.0076880679296,
53.6732518233335));
#108726=CARTESIAN_POINT('Ctrl Pts',(9.27807917023678,-31.0255643299315,
53.6870304118883));
#108727=CARTESIAN_POINT('Ctrl Pts',(9.27736643937243,-31.0340068325236,
53.6936687963469));
#108728=CARTESIAN_POINT('Ctrl Pts',(9.27573384209259,-31.0532839107511,
53.7091304413902));
#108729=CARTESIAN_POINT('Ctrl Pts',(9.27481625973758,-31.0640729577196,
53.7180093704176));
#108730=CARTESIAN_POINT('Ctrl Pts',(9.27190858983632,-31.0980995111877,
53.746737321285));
#108731=CARTESIAN_POINT('Ctrl Pts',(9.26993908930246,-31.1209039444224,
53.7670910766533));
#108732=CARTESIAN_POINT('Ctrl Pts',(9.26528795718768,-31.1740022260542,
53.8171749782271));
#108733=CARTESIAN_POINT('Ctrl Pts',(9.26262878491381,-31.2037456791508,
53.847458036821));
#108734=CARTESIAN_POINT('Ctrl Pts',(9.25542783362706,-31.2819016189352,
53.9333620953678));
#108735=CARTESIAN_POINT('Ctrl Pts',(9.25095376802016,-31.3278298814751,
53.9911113274041));
#108736=CARTESIAN_POINT('Ctrl Pts',(9.24560870097535,-31.377558575413,54.0629434549367));
#108737=CARTESIAN_POINT('Ctrl Pts',(9.244771832375,-31.385195404497,54.0742698648418));
#108738=CARTESIAN_POINT('Ctrl Pts',(9.23940293652337,-31.4331660357246,
54.1473394244863));
#108739=CARTESIAN_POINT('Ctrl Pts',(9.23481861900438,-31.4694967952229,
54.2116020319002));
#108740=CARTESIAN_POINT('Ctrl Pts',(9.22920032731129,-31.5067684117664,
54.2891162361011));
#108741=CARTESIAN_POINT('Ctrl Pts',(9.22839194632402,-31.5119667141518,
54.3002404655774));
#108742=CARTESIAN_POINT('Ctrl Pts',(9.22711470826635,-31.5199143470558,
54.3177502696748));
#108743=CARTESIAN_POINT('Ctrl Pts',(9.22665072584179,-31.5227475939977,
54.3240975828462));
#108744=CARTESIAN_POINT('Ctrl Pts',(9.22577806818685,-31.5279739563276,
54.336005844064));
#108745=CARTESIAN_POINT('Ctrl Pts',(9.2253699678682,-31.5303765876197,54.3415623448388));
#108746=CARTESIAN_POINT('Ctrl Pts',(9.22440365707393,-31.5359688645001,
54.3546914190152));
#108747=CARTESIAN_POINT('Ctrl Pts',(9.22384396179741,-31.5391328278752,
54.362274629258));
#108748=CARTESIAN_POINT('Ctrl Pts',(9.22195875922678,-31.5495439119172,
54.3877561469904));
#108749=CARTESIAN_POINT('Ctrl Pts',(9.22061969485834,-31.5565356277408,
54.4057562531847));
#108750=CARTESIAN_POINT('Ctrl Pts',(9.21728586842703,-31.572996774463,54.4504204727444));
#108751=CARTESIAN_POINT('Ctrl Pts',(9.21527650740867,-31.582102599997,54.4772116187155));
#108752=CARTESIAN_POINT('Ctrl Pts',(9.20606240262917,-31.6203698432869,
54.5999774999973));
#108753=CARTESIAN_POINT('Ctrl Pts',(9.19868506509942,-31.6415097503523,
54.6982341342242));
#108754=CARTESIAN_POINT('Ctrl Pts',(9.1855125076129,-31.6636848490288,54.8795891810071));
#108755=CARTESIAN_POINT('Ctrl Pts',(9.17968480780526,-31.6676052581658,
54.9620207906268));
#108756=CARTESIAN_POINT('Ctrl Pts',(9.17270305762754,-31.6648853608091,
55.0640063135525));
#108757=CARTESIAN_POINT('Ctrl Pts',(9.171372554744,-31.6640172269966,55.0835870682194));
#108758=CARTESIAN_POINT('Ctrl Pts',(9.16925666316464,-31.6620717712169,
55.1149486982338));
#108759=CARTESIAN_POINT('Ctrl Pts',(9.16846450472534,-31.6612141794798,
55.1267408311022));
#108760=CARTESIAN_POINT('Ctrl Pts',(9.16696039087394,-31.6593383100204,
55.1492235560166));
#108761=CARTESIAN_POINT('Ctrl Pts',(9.16624778535209,-31.6583420611814,
55.1599153341477));
#108762=CARTESIAN_POINT('Ctrl Pts',(9.16461500352786,-31.6558112813696,
55.1845002744488));
#108763=CARTESIAN_POINT('Ctrl Pts',(9.16369711686896,-31.654205130409,55.1983853750473));
#108764=CARTESIAN_POINT('Ctrl Pts',(9.16078659953252,-31.6485260489236,
55.2425987930737));
#108765=CARTESIAN_POINT('Ctrl Pts',(9.15881462747923,-31.6437921258762,
55.2728368443439));
#108766=CARTESIAN_POINT('Ctrl Pts',(9.15415647739166,-31.6304991198075,
55.3447248955641));
#108767=CARTESIAN_POINT('Ctrl Pts',(9.15149286832201,-31.6211735082459,
55.3862116899348));
#108768=CARTESIAN_POINT('Ctrl Pts',(9.14428667704628,-31.5913613838325,
55.4985583713471));
#108769=CARTESIAN_POINT('Ctrl Pts',(9.13981172839539,-31.5677422328208,
55.5684858492453));
#108770=CARTESIAN_POINT('Ctrl Pts',(9.13445242539774,-31.5342663757148,
55.6494422527935));
#108771=CARTESIAN_POINT('Ctrl Pts',(9.13360234543159,-31.5288039470944,
55.6621986385028));
#108772=CARTESIAN_POINT('Ctrl Pts',(9.12823490300193,-31.4934056370254,
55.7420908914308));
#108773=CARTESIAN_POINT('Ctrl Pts',(9.12366504441963,-31.4592167996161,
55.8072440055121));
#108774=CARTESIAN_POINT('Ctrl Pts',(9.11806278095909,-31.4144339826314,
55.88038810281));
#108775=CARTESIAN_POINT('Ctrl Pts',(9.1172545888331,-31.4079085981119,55.8907862035323));
#108776=CARTESIAN_POINT('Ctrl Pts',(9.11597771776019,-31.397510899214,55.906955107001));
#108777=CARTESIAN_POINT('Ctrl Pts',(9.1155139144663,-31.39371621713,55.9127756467359));
#108778=CARTESIAN_POINT('Ctrl Pts',(9.11464158231399,-31.386548593571,55.9236209296218));
#108779=CARTESIAN_POINT('Ctrl Pts',(9.11423362809236,-31.3831845406598,
55.9286512508888));
#108780=CARTESIAN_POINT('Ctrl Pts',(9.1132677452322,-31.3751906057792,55.9404649100221));
#108781=CARTESIAN_POINT('Ctrl Pts',(9.11270833320018,-31.3705378886568,
55.9472324624377));
#108782=CARTESIAN_POINT('Ctrl Pts',(9.11082469136427,-31.3547891085982,
55.9697807094916));
#108783=CARTESIAN_POINT('Ctrl Pts',(9.10948692932894,-31.3434694753646,
55.9854023760814));
#108784=CARTESIAN_POINT('Ctrl Pts',(9.1061569667178,-31.3149066189579,56.0234134364546));
#108785=CARTESIAN_POINT('Ctrl Pts',(9.104150203266,-31.2973603905905,56.0455669826529));
#108786=CARTESIAN_POINT('Ctrl Pts',(9.09495877155585,-31.2151836626063,
56.14406706998));
#108787=CARTESIAN_POINT('Ctrl Pts',(9.08760208414111,-31.1443209697658,
56.214944752921));
#108788=CARTESIAN_POINT('Ctrl Pts',(9.07442319040452,-31.0040062123244,
56.3320560612969));
#108789=CARTESIAN_POINT('Ctrl Pts',(9.06857067604743,-30.9366157485235,
56.380274060758));
#108790=CARTESIAN_POINT('Ctrl Pts',(9.0615650718232,-30.8491604071941,56.4334807406714));
#108791=CARTESIAN_POINT('Ctrl Pts',(9.06023393573327,-30.8322307293258,
56.4433753847078));
#108792=CARTESIAN_POINT('Ctrl Pts',(9.05811735329604,-30.804817906601,56.4587542411534));
#108793=CARTESIAN_POINT('Ctrl Pts',(9.05732512688044,-30.7944446206193,
56.4644294302267));
#108794=CARTESIAN_POINT('Ctrl Pts',(9.05582108009009,-30.7745390133528,
56.4750459551692));
#108795=CARTESIAN_POINT('Ctrl Pts',(9.05510860762732,-30.7650176708136,
56.4800064951252));
#108796=CARTESIAN_POINT('Ctrl Pts',(9.05347640982454,-30.7429977266769,
56.4912094207845));
#108797=CARTESIAN_POINT('Ctrl Pts',(9.05255897021153,-30.7304671162053,
56.4973873815154));
#108798=CARTESIAN_POINT('Ctrl Pts',(9.04965105585291,-30.690277175909,56.5165776245903));
#108799=CARTESIAN_POINT('Ctrl Pts',(9.04768119069732,-30.6623358984938,
56.528987121049));
#108800=CARTESIAN_POINT('Ctrl Pts',(9.04302895869763,-30.5948187974355,
56.5567748692359));
#108801=CARTESIAN_POINT('Ctrl Pts',(9.0403690836724,-30.5549653424431,56.5714233174479));
#108802=CARTESIAN_POINT('Ctrl Pts',(9.03316538696934,-30.4444578123017,
56.607311761038));
#108803=CARTESIAN_POINT('Ctrl Pts',(9.02868941849306,-30.3728854674023,
56.6254078383399));
#108804=CARTESIAN_POINT('Ctrl Pts',(9.02334926032758,-30.2870221723148,
56.6411452884556));
#108805=CARTESIAN_POINT('Ctrl Pts',(9.0225192580234,-30.2736656094489,56.6434252991884));
#108806=CARTESIAN_POINT('Ctrl Pts',(9.01714806449828,-30.187281603874,56.657089047366));
#108807=CARTESIAN_POINT('Ctrl Pts',(9.01255454864607,-30.113601784719,56.6637639169931));
#108808=CARTESIAN_POINT('Ctrl Pts',(9.00692604406243,-30.0274594297945,
56.6658189278203));
#108809=CARTESIAN_POINT('Ctrl Pts',(9.00611780898928,-30.0151836717667,
56.6659760367197));
#108810=CARTESIAN_POINT('Ctrl Pts',(9.00484090339151,-29.9959595232366,
56.6660095895564));
#108811=CARTESIAN_POINT('Ctrl Pts',(9.00437710977084,-29.9890114499722,
56.6659782487605));
#108812=CARTESIAN_POINT('Ctrl Pts',(9.0035047711123,-29.9760122462962,56.665838291924));
#108813=CARTESIAN_POINT('Ctrl Pts',(9.00309680049941,-29.9699612497489,
56.6657401646032));
#108814=CARTESIAN_POINT('Ctrl Pts',(9.00213088035454,-29.9556998549556,
56.6654311609913));
#108815=CARTESIAN_POINT('Ctrl Pts',(9.00157144727216,-29.9474903332707,
56.6651925362206));
#108816=CARTESIAN_POINT('Ctrl Pts',(8.99968785824294,-29.9200056619961,
56.6641901997295));
#108817=CARTESIAN_POINT('Ctrl Pts',(8.99835017321592,-29.9007428652824,
56.6631524454962));
#108818=CARTESIAN_POINT('Ctrl Pts',(8.99502049859785,-29.8533204619571,
56.6597708982724));
#108819=CARTESIAN_POINT('Ctrl Pts',(8.99301395119953,-29.8251946587656,
56.6570447290768));
#108820=CARTESIAN_POINT('Ctrl Pts',(8.98382472161351,-29.6979001206998,
56.6414295980765));
#108821=CARTESIAN_POINT('Ctrl Pts',(8.97647010130321,-29.5999452568105,
56.6203432050362));
#108822=CARTESIAN_POINT('Ctrl Pts',(8.9632863275333,-29.4253875891599,56.5659622782712));
#108823=CARTESIAN_POINT('Ctrl Pts',(8.95742726686729,-29.348241621807,56.5354582465984));
#108824=CARTESIAN_POINT('Ctrl Pts',(8.95041778574361,-29.2560579783346,
56.4908016167568));
#108825=CARTESIAN_POINT('Ctrl Pts',(8.94908884592761,-29.2385921309491,
56.4819572550457));
#108826=CARTESIAN_POINT('Ctrl Pts',(8.94697482534883,-29.2108380198982,
56.4672828744456));
#108827=CARTESIAN_POINT('Ctrl Pts',(8.94618299607484,-29.2004493333971,
56.4616478401007));
#108828=CARTESIAN_POINT('Ctrl Pts',(8.94467913016412,-29.1807365661083,
56.4506821675457));
#108829=CARTESIAN_POINT('Ctrl Pts',(8.943966447355,-29.1714023942565,56.4453710050757));
#108830=CARTESIAN_POINT('Ctrl Pts',(8.94233295505179,-29.1500310266431,
56.4329355776126));
#108831=CARTESIAN_POINT('Ctrl Pts',(8.94141444204003,-29.1380307809724,
56.4257491751591));
#108832=CARTESIAN_POINT('Ctrl Pts',(8.93849967941638,-29.1000225099225,
56.4023324395238));
#108833=CARTESIAN_POINT('Ctrl Pts',(8.93652417520848,-29.074370457933,56.3855345155379));
#108834=CARTESIAN_POINT('Ctrl Pts',(8.93185580310137,-29.014203377522,56.3437175673087));
#108835=CARTESIAN_POINT('Ctrl Pts',(8.92918564404222,-28.9801558974309,
56.3180630752109));
#108836=CARTESIAN_POINT('Ctrl Pts',(8.92197730625953,-28.8900402613201,
56.2445768479305));
#108837=CARTESIAN_POINT('Ctrl Pts',(8.91750625586159,-28.8361018933773,
56.1942879506145));
#108838=CARTESIAN_POINT('Ctrl Pts',(8.91212697057785,-28.7759045854073,
56.1301990163297));
#108839=CARTESIAN_POINT('Ctrl Pts',(8.91125318109112,-28.7662744476001,
56.1196788179742));
#108840=CARTESIAN_POINT('Ctrl Pts',(8.90589475245924,-28.7082152470863,
56.0545949992605));
#108841=CARTESIAN_POINT('Ctrl Pts',(8.90135742994437,-28.6632842109067,
55.997028924508));
#108842=CARTESIAN_POINT('Ctrl Pts',(8.8957912991061,-28.6153741340944,55.9265623920747));
#108843=CARTESIAN_POINT('Ctrl Pts',(8.89498323257773,-28.6085855900273,
55.9163364954661));
#108844=CARTESIAN_POINT('Ctrl Pts',(8.89370649200509,-28.5981321318931,
55.9002059538589));
#108845=CARTESIAN_POINT('Ctrl Pts',(8.8932426909668,-28.5943899667841,55.894351557915));
#108846=CARTESIAN_POINT('Ctrl Pts',(8.89237030599036,-28.5874567813836,
55.8833540000798));
#108847=CARTESIAN_POINT('Ctrl Pts',(8.89196229610667,-28.5842570262775,
55.8782166370528));
#108848=CARTESIAN_POINT('Ctrl Pts',(8.89099619480252,-28.5767802659301,
55.8660652845525));
#108849=CARTESIAN_POINT('Ctrl Pts',(8.89043661869484,-28.5725270698195,
55.8590369695671));
#108850=CARTESIAN_POINT('Ctrl Pts',(8.8885520288937,-28.5584549325702,55.8353899754078));
#108851=CARTESIAN_POINT('Ctrl Pts',(8.88721346726057,-28.5488732706043,
55.8186328409601));
#108852=CARTESIAN_POINT('Ctrl Pts',(8.88388111898545,-28.5259767132005,
55.7769241164269));
#108853=CARTESIAN_POINT('Ctrl Pts',(8.88187274655414,-28.5130021496351,
55.7517931531932));
#108854=CARTESIAN_POINT('Ctrl Pts',(8.87592642271712,-28.476821238482,55.6771083647092));
#108855=CARTESIAN_POINT('Ctrl Pts',(8.87194753167041,-28.4554291605364,
55.6267692839885));
#108856=CARTESIAN_POINT('Ctrl Pts',(8.86797186106679,-28.4365624698124,
55.5755163674484));
#108857=CARTESIAN_POINT('Origin',(5.,-30.,55.));
#108858=CARTESIAN_POINT('',(8.16625309736762,-28.4365623102018,55.5755159338529));
#108859=CARTESIAN_POINT('',(8.36103879467172,-28.436562302838,55.5755159138484));
#108860=CARTESIAN_POINT('',(5.,-28.4365623102018,55.5755159338528));
#108861=CARTESIAN_POINT('Ctrl Pts',(8.36103879467171,-28.436562302838,55.5755159138484));
#108862=CARTESIAN_POINT('Ctrl Pts',(8.36205644453806,-28.4414052882876,
55.588672293779));
#108863=CARTESIAN_POINT('Ctrl Pts',(8.36307260053714,-28.4464149009599,
55.6017690642261));
#108864=CARTESIAN_POINT('Ctrl Pts',(8.36843620734845,-28.4737909734731,
55.6707169719365));
#108865=CARTESIAN_POINT('Ctrl Pts',(8.37273626111417,-28.499005882396,55.7253917146297));
#108866=CARTESIAN_POINT('Ctrl Pts',(8.37880434975973,-28.5395168239628,
55.8020273527629));
#108867=CARTESIAN_POINT('Ctrl Pts',(8.38064282139152,-28.5524661183118,
55.825169544951));
#108868=CARTESIAN_POINT('Ctrl Pts',(8.38393361830657,-28.5768762279705,
55.8664493240042));
#108869=CARTESIAN_POINT('Ctrl Pts',(8.38539220672554,-28.5881451872141,
55.8846930335348));
#108870=CARTESIAN_POINT('Ctrl Pts',(8.38766153209908,-28.6063819676379,
55.9129808164793));
#108871=CARTESIAN_POINT('Ctrl Pts',(8.38848087095959,-28.6131131288968,
55.923173879566));
#108872=CARTESIAN_POINT('Ctrl Pts',(8.39000823397003,-28.6259344944288,
55.9421326244342));
#108873=CARTESIAN_POINT('Ctrl Pts',(8.39071721165674,-28.6319979717759,
55.9509155353961));
#108874=CARTESIAN_POINT('Ctrl Pts',(8.39230420627689,-28.6458205638035,
55.9705316032104));
#108875=CARTESIAN_POINT('Ctrl Pts',(8.39318039436532,-28.6536261471042,
55.9813312405345));
#108876=CARTESIAN_POINT('Ctrl Pts',(8.39542503868652,-28.6740650956907,
56.0089071387764));
#108877=CARTESIAN_POINT('Ctrl Pts',(8.3967861342715,-28.6868878282321,56.0255405757992));
#108878=CARTESIAN_POINT('Ctrl Pts',(8.40638936492191,-28.7803165422586,
56.1421084132425));
#108879=CARTESIAN_POINT('Ctrl Pts',(8.41415177060872,-28.8719214473129,
56.2326726449401));
#108880=CARTESIAN_POINT('Ctrl Pts',(8.42714696822361,-29.0391627200592,
56.3635990773941));
#108881=CARTESIAN_POINT('Ctrl Pts',(8.43232025710095,-29.1091116456632,
56.4102925275115));
#108882=CARTESIAN_POINT('Ctrl Pts',(8.43870212862059,-29.1945373812508,
56.4584183817035));
#108883=CARTESIAN_POINT('Ctrl Pts',(8.43962651935254,-29.206889992403,56.4651725802872));
#108884=CARTESIAN_POINT('Ctrl Pts',(8.44104136647557,-29.2257343601534,
56.4751682402998));
#108885=CARTESIAN_POINT('Ctrl Pts',(8.44152495526307,-29.23216449391,56.4785253629525));
#108886=CARTESIAN_POINT('Ctrl Pts',(8.44241411649535,-29.2439627235751,
56.4845874068499));
#108887=CARTESIAN_POINT('Ctrl Pts',(8.44281887228989,-29.2493238017906,
56.4873054069796));
#108888=CARTESIAN_POINT('Ctrl Pts',(8.44375070472134,-29.2616445175238,
56.4934682733055));
#108889=CARTESIAN_POINT('Ctrl Pts',(8.44427893507324,-29.2686135932243,
56.4968935232104));
#108890=CARTESIAN_POINT('Ctrl Pts',(8.44591339711864,-29.2901385345245,
56.5072866764585));
#108891=CARTESIAN_POINT('Ctrl Pts',(8.44702864302743,-29.3047714142887,
56.5140916719036));
#108892=CARTESIAN_POINT('Ctrl Pts',(8.45379899117702,-29.393409462981,56.553756868862));
#108893=CARTESIAN_POINT('Ctrl Pts',(8.45967657610195,-29.4696248630934,
56.5813956586708));
#108894=CARTESIAN_POINT('Ctrl Pts',(8.47093278662194,-29.6184664632564,
56.6233975123883));
#108895=CARTESIAN_POINT('Ctrl Pts',(8.47629706234238,-29.6906484190402,
56.6386855198168));
#108896=CARTESIAN_POINT('Ctrl Pts',(8.48459243043702,-29.8057117566777,
56.6551788834509));
#108897=CARTESIAN_POINT('Ctrl Pts',(8.48759127115807,-29.8480327784988,
56.6595998085246));
#108898=CARTESIAN_POINT('Ctrl Pts',(8.4926686735133,-29.921028765655,56.664408856142));
#108899=CARTESIAN_POINT('Ctrl Pts',(8.49476876468717,-29.9516291189015,
56.6655791088764));
#108900=CARTESIAN_POINT('Ctrl Pts',(8.49778999847616,-29.9962272512632,
56.6660543986621));
#108901=CARTESIAN_POINT('Ctrl Pts',(8.49873161364051,-30.0102100143427,
56.6660273915031));
#108902=CARTESIAN_POINT('Ctrl Pts',(8.50038684624884,-30.0349308025088,
56.6656683953599));
#108903=CARTESIAN_POINT('Ctrl Pts',(8.5011026713807,-30.0456688965927,56.6654085761269));
#108904=CARTESIAN_POINT('Ctrl Pts',(8.50259981806097,-30.0682226359772,
56.6646445607507));
#108905=CARTESIAN_POINT('Ctrl Pts',(8.50338041258762,-30.0800369755225,
56.6641183660979));
#108906=CARTESIAN_POINT('Ctrl Pts',(8.50544462227414,-30.1114161797634,
56.6623858260673));
#108907=CARTESIAN_POINT('Ctrl Pts',(8.5067213576112,-30.1309674272096,56.6609598988043));
#108908=CARTESIAN_POINT('Ctrl Pts',(8.51331367343572,-30.2325582257957,
56.6517455407422));
#108909=CARTESIAN_POINT('Ctrl Pts',(8.51844672269567,-30.3139667150035,
56.6382228295446));
#108910=CARTESIAN_POINT('Ctrl Pts',(8.5296706241596,-30.4915155920471,56.5950019394245));
#108911=CARTESIAN_POINT('Ctrl Pts',(8.53570210564608,-30.5866339665642,
56.562522641987));
#108912=CARTESIAN_POINT('Ctrl Pts',(8.54376387583394,-30.7040915238797,
56.51016944154));
#108913=CARTESIAN_POINT('Ctrl Pts',(8.54555761589486,-30.7296366316034,
56.4979942661551));
#108914=CARTESIAN_POINT('Ctrl Pts',(8.54862647067718,-30.7720732595398,
56.4764253499417));
#108915=CARTESIAN_POINT('Ctrl Pts',(8.54988524072237,-30.7891343436007,
56.4673771981978));
#108916=CARTESIAN_POINT('Ctrl Pts',(8.55170417616894,-30.81322558651,56.4540590364872));
#108917=CARTESIAN_POINT('Ctrl Pts',(8.55225027883618,-30.8203880714563,
56.4500299794666));
#108918=CARTESIAN_POINT('Ctrl Pts',(8.55320451184597,-30.8327748791546,
56.4429409741923));
#108919=CARTESIAN_POINT('Ctrl Pts',(8.55361111171659,-30.8380128057251,
56.4399052713465));
#108920=CARTESIAN_POINT('Ctrl Pts',(8.55448854161612,-30.8492282442665,
56.4333233032224));
#108921=CARTESIAN_POINT('Ctrl Pts',(8.5549598973233,-30.855200057358,56.4297682189466));
#108922=CARTESIAN_POINT('Ctrl Pts',(8.55627017576744,-30.8716590714876,
56.419829986096));
#108923=CARTESIAN_POINT('Ctrl Pts',(8.55711384547436,-30.8820979793374,
56.4133682673177));
#108924=CARTESIAN_POINT('Ctrl Pts',(8.56302668609428,-30.9542258111416,
56.3676106129489));
#108925=CARTESIAN_POINT('Ctrl Pts',(8.56829775310585,-31.0133336436953,
56.3244086390886));
#108926=CARTESIAN_POINT('Ctrl Pts',(8.57463982260552,-31.0802725996905,
56.2683721730138));
#108927=CARTESIAN_POINT('Ctrl Pts',(8.575670883623,-31.0910233073556,56.2591366081106));
#108928=CARTESIAN_POINT('Ctrl Pts',(8.58206616323697,-31.1569380531708,
56.2010334493029));
#108929=CARTESIAN_POINT('Ctrl Pts',(8.5874303076493,-31.2089304011858,56.1486842910115));
#108930=CARTESIAN_POINT('Ctrl Pts',(8.59572617725535,-31.2851989808541,
56.0609568018601));
#108931=CARTESIAN_POINT('Ctrl Pts',(8.59872561969606,-31.3118721025196,
56.0277927056786));
#108932=CARTESIAN_POINT('Ctrl Pts',(8.60380392478917,-31.3555105251157,
55.9690638693902));
#108933=CARTESIAN_POINT('Ctrl Pts',(8.60590432699071,-31.3730927610895,
55.9439862551947));
#108934=CARTESIAN_POINT('Ctrl Pts',(8.60892592555243,-31.3976832438337,
55.9067706805712));
#108935=CARTESIAN_POINT('Ctrl Pts',(8.60986760105582,-31.4052447101054,
55.8950077332954));
#108936=CARTESIAN_POINT('Ctrl Pts',(8.61152290904499,-31.4183512174646,
55.8740430154364));
#108937=CARTESIAN_POINT('Ctrl Pts',(8.61223874974407,-31.4239569440843,
55.8648803383123));
#108938=CARTESIAN_POINT('Ctrl Pts',(8.6137358992321,-31.4355472781651,55.8455175036047));
#108939=CARTESIAN_POINT('Ctrl Pts',(8.61451648127609,-31.4415127028641,
55.8353065164166));
#108940=CARTESIAN_POINT('Ctrl Pts',(8.61658058904433,-31.4570751102941,
55.8080051162473));
#108941=CARTESIAN_POINT('Ctrl Pts',(8.61785723642462,-31.4664802657605,
55.7908070735944));
#108942=CARTESIAN_POINT('Ctrl Pts',(8.62444637975549,-31.5138148183353,
55.7005022801057));
#108943=CARTESIAN_POINT('Ctrl Pts',(8.62957658200243,-31.5465906782297,
55.6248187713869));
#108944=CARTESIAN_POINT('Ctrl Pts',(8.64080018953408,-31.6065866081312,
55.45222361441));
#108945=CARTESIAN_POINT('Ctrl Pts',(8.64683397242618,-31.6309023755291,
55.3546573288335));
#108946=CARTESIAN_POINT('Ctrl Pts',(8.65489850440016,-31.6506312553793,
55.2275376077274));
#108947=CARTESIAN_POINT('Ctrl Pts',(8.65669255702701,-31.654257954759,55.1994676481461));
#108948=CARTESIAN_POINT('Ctrl Pts',(8.65976189679851,-31.6591539726957,
55.1521089341842));
#108949=CARTESIAN_POINT('Ctrl Pts',(8.66102083330871,-31.6608057681174,
55.1328651780026));
#108950=CARTESIAN_POINT('Ctrl Pts',(8.66283997513964,-31.6626829756213,
55.1053986143683));
#108951=CARTESIAN_POINT('Ctrl Pts',(8.66338611408049,-31.6631826740899,
55.0971953236136));
#108952=CARTESIAN_POINT('Ctrl Pts',(8.66434040252225,-31.6639450484021,
55.0829429548707));
#108953=CARTESIAN_POINT('Ctrl Pts',(8.66474702134359,-31.6642354771929,
55.0768955978695));
#108954=CARTESIAN_POINT('Ctrl Pts',(8.66562449518401,-31.6647885075575,
55.0639025257418));
#108955=CARTESIAN_POINT('Ctrl Pts',(8.66609587591762,-31.6650406074545,
55.0569568153376));
#108956=CARTESIAN_POINT('Ctrl Pts',(8.66740620304431,-31.6656177770549,
55.0377379924225));
#108957=CARTESIAN_POINT('Ctrl Pts',(8.66824989617126,-31.6658506406607,
55.0254628398163));
#108958=CARTESIAN_POINT('Ctrl Pts',(8.67416384317432,-31.6665268657327,
54.9400315946026));
#108959=CARTESIAN_POINT('Ctrl Pts',(8.67943605895062,-31.6622866253168,
54.8669255549198));
#108960=CARTESIAN_POINT('Ctrl Pts',(8.68577817864848,-31.6515101591123,
54.7802941976796));
#108961=CARTESIAN_POINT('Ctrl Pts',(8.68680816770537,-31.6495834545274,
54.7662675291058));
#108962=CARTESIAN_POINT('Ctrl Pts',(8.69320209769039,-31.6365202242126,
54.6793941441958));
#108963=CARTESIAN_POINT('Ctrl Pts',(8.69856595038103,-31.6207385068172,
54.607323846346));
#108964=CARTESIAN_POINT('Ctrl Pts',(8.70686087509572,-31.5884031908434,
54.4956783554412));
#108965=CARTESIAN_POINT('Ctrl Pts',(8.70985967282089,-31.5750100999582,
54.455290255304));
#108966=CARTESIAN_POINT('Ctrl Pts',(8.7149370230895,-31.5493429339376,54.3867873445081));
#108967=CARTESIAN_POINT('Ctrl Pts',(8.71703710263003,-31.5378123294387,
54.3584185624472));
#108968=CARTESIAN_POINT('Ctrl Pts',(8.72005835386869,-31.5198858063695,
54.3175788398036));
#108969=CARTESIAN_POINT('Ctrl Pts',(8.72099999632613,-31.5141047841358,
54.3048466157444));
#108970=CARTESIAN_POINT('Ctrl Pts',(8.72265529221371,-31.5036004776881,
54.2824646494459));
#108971=CARTESIAN_POINT('Ctrl Pts',(8.72337115320179,-31.4989429357188,
54.2727851345396));
#108972=CARTESIAN_POINT('Ctrl Pts',(8.72486839116716,-31.4889613980052,
54.2525444382857));
#108973=CARTESIAN_POINT('Ctrl Pts',(8.72564904091723,-31.483617885189,54.241993506377));
#108974=CARTESIAN_POINT('Ctrl Pts',(8.72771343806372,-31.469119782213,54.2141072944889));
#108975=CARTESIAN_POINT('Ctrl Pts',(8.72899030426879,-31.459770638328,54.196874844649));
#108976=CARTESIAN_POINT('Ctrl Pts',(8.73558559721569,-31.4095283935687,
54.1080450425794));
#108977=CARTESIAN_POINT('Ctrl Pts',(8.74072128450398,-31.3636637003218,
54.0393867941631));
#108978=CARTESIAN_POINT('Ctrl Pts',(8.75194544474392,-31.2511675681152,
53.8953774628601));
#108979=CARTESIAN_POINT('Ctrl Pts',(8.75797478313652,-31.1824329905659,
53.8220946088521));
#108980=CARTESIAN_POINT('Ctrl Pts',(8.76603397739983,-31.0863981786469,
53.7366333243088));
#108981=CARTESIAN_POINT('Ctrl Pts',(8.76782744259251,-31.0647896451103,
53.7183685432193));
#108982=CARTESIAN_POINT('Ctrl Pts',(8.77089587993537,-31.0276682897423,
53.6885783532414));
#108983=CARTESIAN_POINT('Ctrl Pts',(8.77215451400889,-31.0124005085154,
53.6767562651925));
#108984=CARTESIAN_POINT('Ctrl Pts',(8.77397329505741,-30.9903474299995,
53.6602852914252));
#108985=CARTESIAN_POINT('Ctrl Pts',(8.77451938328889,-30.9837272029174,
53.655416675801));
#108986=CARTESIAN_POINT('Ctrl Pts',(8.7754735945591,-30.9721677266366,53.6470467249977));
#108987=CARTESIAN_POINT('Ctrl Pts',(8.77588018723681,-30.9672449712374,
53.6435230126054));
#108988=CARTESIAN_POINT('Ctrl Pts',(8.77675758223686,-30.956629953191,53.6360119394475));
#108989=CARTESIAN_POINT('Ctrl Pts',(8.77722891007052,-30.9509320019738,
53.6320333995711));
#108990=CARTESIAN_POINT('Ctrl Pts',(8.77853914920168,-30.9350997440919,
53.6211253897916));
#108991=CARTESIAN_POINT('Ctrl Pts',(8.77938280795775,-30.9249137140377,
53.6142722772674));
#108992=CARTESIAN_POINT('Ctrl Pts',(8.78530369925469,-30.8534232347532,
53.5673131882141));
#108993=CARTESIAN_POINT('Ctrl Pts',(8.79058348920429,-30.7896135565884,
53.5311804838857));
#108994=CARTESIAN_POINT('Ctrl Pts',(8.79692812260266,-30.7109515274574,
53.4932477243841));
#108995=CARTESIAN_POINT('Ctrl Pts',(8.79795311102322,-30.6981841198993,
53.4872893781569));
#108996=CARTESIAN_POINT('Ctrl Pts',(8.80434319745441,-30.6181612345226,
53.4511728970002));
#108997=CARTESIAN_POINT('Ctrl Pts',(8.80970816508356,-30.5490373573055,
53.4253419421403));
#108998=CARTESIAN_POINT('Ctrl Pts',(8.81800317227188,-30.4376978687496,
53.391962534131));
#108999=CARTESIAN_POINT('Ctrl Pts',(8.82100103842605,-30.3965141228512,
53.3813150494601));
#109000=CARTESIAN_POINT('Ctrl Pts',(8.82607696360062,-30.3250599639222,
53.3657329272283));
#109001=CARTESIAN_POINT('Ctrl Pts',(8.82817653807854,-30.2949792333003,
53.3600364909898));
#109002=CARTESIAN_POINT('Ctrl Pts',(8.83119712952773,-30.2509545656604,
53.3529501391233));
#109003=CARTESIAN_POINT('Ctrl Pts',(8.83213860989103,-30.2371245329765,
53.3509022421972));
#109004=CARTESIAN_POINT('Ctrl Pts',(8.83379364001393,-30.2126270881354,
53.3475893173124));
#109005=CARTESIAN_POINT('Ctrl Pts',(8.83450939671646,-30.2019703127115,
53.3462529380408));
#109006=CARTESIAN_POINT('Ctrl Pts',(8.8360064320162,-30.1795545076767,53.3436618685142));
#109007=CARTESIAN_POINT('Ctrl Pts',(8.83678698335938,-30.1677935041096,
53.3424291329911));
#109008=CARTESIAN_POINT('Ctrl Pts',(8.83885114807321,-30.1365052080355,
53.3394860647382));
#109009=CARTESIAN_POINT('Ctrl Pts',(8.84012788069282,-30.1169587959746,
53.3379949176761));
#109010=CARTESIAN_POINT('Ctrl Pts',(8.84672214900402,-30.0150948249356,
53.3320300202904));
#109011=CARTESIAN_POINT('Ctrl Pts',(8.85185698973024,-29.9325502691058,
53.3333252505191));
#109012=CARTESIAN_POINT('Ctrl Pts',(8.86308110306673,-29.7505476214336,
53.3497310871379));
#109013=CARTESIAN_POINT('Ctrl Pts',(8.86911115851816,-29.6516868776118,
53.3677348265827));
#109014=CARTESIAN_POINT('Ctrl Pts',(8.87717122241691,-29.5277875874255,
53.4020726358655));
#109015=CARTESIAN_POINT('Ctrl Pts',(8.8789647494459,-29.5007219164786,53.4103215298553));
#109016=CARTESIAN_POINT('Ctrl Pts',(8.88203326287157,-29.4555596232797,
53.425352886429));
#109017=CARTESIAN_POINT('Ctrl Pts',(8.8832919070243,-29.4373466267782,53.431768524837));
#109018=CARTESIAN_POINT('Ctrl Pts',(8.88511066943044,-29.4115483061215,
53.4413633750677));
#109019=CARTESIAN_POINT('Ctrl Pts',(8.885656726495,-29.4038678960609,53.4442847200538));
#109020=CARTESIAN_POINT('Ctrl Pts',(8.88661088852498,-29.390567287998,53.4494567341726));
#109021=CARTESIAN_POINT('Ctrl Pts',(8.88701746323427,-29.3849372369696,
53.4516814133233));
#109022=CARTESIAN_POINT('Ctrl Pts',(8.88789485391384,-29.3728698153983,
53.4565259863154));
#109023=CARTESIAN_POINT('Ctrl Pts',(8.8883661956736,-29.3664367724308,53.4591554485851));
#109024=CARTESIAN_POINT('Ctrl Pts',(8.88967642476368,-29.348685923088,53.4665409408362));
#109025=CARTESIAN_POINT('Ctrl Pts',(8.89052005883307,-29.3374042122592,
53.4713818289472));
#109026=CARTESIAN_POINT('Ctrl Pts',(8.89642016612353,-29.2594531926701,
53.5058549975597));
#109027=CARTESIAN_POINT('Ctrl Pts',(8.90167754063202,-29.1947464344649,
53.539711261887));
#109028=CARTESIAN_POINT('Ctrl Pts',(8.90801553430914,-29.1202638437203,
53.5851414010311));
#109029=CARTESIAN_POINT('Ctrl Pts',(8.90905604928723,-29.1081499619329,
53.5927459130084));
#109030=CARTESIAN_POINT('Ctrl Pts',(8.91545981092512,-29.0342408953424,
53.6404801292691));
#109031=CARTESIAN_POINT('Ctrl Pts',(8.92082310075635,-28.9750624191942,
53.6845194073648));
#109032=CARTESIAN_POINT('Ctrl Pts',(8.92912210705646,-28.8865821753877,
53.7599714079682));
#109033=CARTESIAN_POINT('Ctrl Pts',(8.93212534648026,-28.8552427302041,
53.788842925313));
#109034=CARTESIAN_POINT('Ctrl Pts',(8.93720933003145,-28.8033146684374,
53.8405003335306));
#109035=CARTESIAN_POINT('Ctrl Pts',(8.93931167812699,-28.7821865816071,
53.8627111396972));
#109036=CARTESIAN_POINT('Ctrl Pts',(8.94233553529857,-28.7523245677706,
53.8958905507051));
#109037=CARTESIAN_POINT('Ctrl Pts',(8.94327756581707,-28.7430981623012,
53.9064052618435));
#109038=CARTESIAN_POINT('Ctrl Pts',(8.94493329592076,-28.7270223427386,
53.925198030514));
#109039=CARTESIAN_POINT('Ctrl Pts',(8.94564920707794,-28.7201186316598,
53.9334283513217));
#109040=CARTESIAN_POINT('Ctrl Pts',(8.94714630731439,-28.7057844444699,
53.9508565934256));
#109041=CARTESIAN_POINT('Ctrl Pts',(8.94792677151531,-28.6983712865154,
53.960068032947));
#109042=CARTESIAN_POINT('Ctrl Pts',(8.94999010985199,-28.6789379725493,
53.9847488652794));
#109043=CARTESIAN_POINT('Ctrl Pts',(8.95126611577876,-28.6670913012273,
54.0003529622062));
#109044=CARTESIAN_POINT('Ctrl Pts',(8.95783367769749,-28.607079341856,54.0823632362805));
#109045=CARTESIAN_POINT('Ctrl Pts',(8.96294453783008,-28.563588779137,54.1520551625051));
#109046=CARTESIAN_POINT('Ctrl Pts',(8.97416634056554,-28.4785763442164,
54.313740794546));
#109047=CARTESIAN_POINT('Ctrl Pts',(8.98021592572293,-28.4399154439783,
54.406859661282));
#109048=CARTESIAN_POINT('Ctrl Pts',(8.98829942708434,-28.4014388681968,
54.5299349225709));
#109049=CARTESIAN_POINT('Ctrl Pts',(8.99009560655676,-28.3936759344107,
54.5571888841898));
#109050=CARTESIAN_POINT('Ctrl Pts',(8.99316823603421,-28.3817922938904,
54.6033470874716));
#109051=CARTESIAN_POINT('Ctrl Pts',(8.99442829321239,-28.3772989097884,
54.6221497562056));
#109052=CARTESIAN_POINT('Ctrl Pts',(8.99624880765714,-28.3713623134828,
54.6490542938006));
#109053=CARTESIAN_POINT('Ctrl Pts',(8.9967951727833,-28.3696502004651,54.6570960385376));
#109054=CARTESIAN_POINT('Ctrl Pts',(8.99774979133304,-28.3667804987433,
54.6710824759717));
#109055=CARTESIAN_POINT('Ctrl Pts',(8.99815651255716,-28.365595686052,54.6770213411244));
#109056=CARTESIAN_POINT('Ctrl Pts',(8.99903420273079,-28.363120286176,54.6897917886652));
#109057=CARTESIAN_POINT('Ctrl Pts',(8.99950569737639,-28.361840089689,54.6966249256274));
#109058=CARTESIAN_POINT('Ctrl Pts',(9.00081615719047,-28.3584173748759,
54.7155474909531));
#109059=CARTESIAN_POINT('Ctrl Pts',(9.00165986625656,-28.3563657264857,
54.7276526155108));
#109060=CARTESIAN_POINT('Ctrl Pts',(9.0075490219938,-28.3430770800997,54.8116855909185));
#109061=CARTESIAN_POINT('Ctrl Pts',(9.01279435896811,-28.3364327181828,
54.8842527204255));
#109062=CARTESIAN_POINT('Ctrl Pts',(9.01908759015743,-28.3341972495725,
54.9708607673746));
#109063=CARTESIAN_POINT('Ctrl Pts',(9.02009525019884,-28.334012546769,54.9847127412555));
#109064=CARTESIAN_POINT('Ctrl Pts',(9.0304494357485,-28.3338900269998,55.1269885971));
#109065=CARTESIAN_POINT('Ctrl Pts',(9.03975369241362,-28.348629138094,55.2550190002214));
#109066=CARTESIAN_POINT('Ctrl Pts',(9.05003535051255,-28.3827275479487,
55.4005324143705));
#109067=CARTESIAN_POINT('Ctrl Pts',(9.05146702747879,-28.3879012721811,
55.4208730929955));
#109068=CARTESIAN_POINT('Ctrl Pts',(9.05378747600319,-28.3969855076301,
55.4539581682557));
#109069=CARTESIAN_POINT('Ctrl Pts',(9.05468348272912,-28.4006669186226,
55.4667624599023));
#109070=CARTESIAN_POINT('Ctrl Pts',(9.05628845107866,-28.4075741374467,
55.4897446524266));
#109071=CARTESIAN_POINT('Ctrl Pts',(9.05699915607152,-28.4107449022115,
55.4999381917423));
#109072=CARTESIAN_POINT('Ctrl Pts',(9.05851675083272,-28.4177557499196,
55.5217360615256));
#109073=CARTESIAN_POINT('Ctrl Pts',(9.0593226053885,-28.4216260198357,55.5333300825033));
#109074=CARTESIAN_POINT('Ctrl Pts',(9.06083567546823,-28.4291700832666,
55.5551278718492));
#109075=CARTESIAN_POINT('Ctrl Pts',(9.06154370570593,-28.4328164874729,
55.5653400897199));
#109076=CARTESIAN_POINT('Ctrl Pts',(9.06224859760915,-28.4365623100358,
55.5755159334018));
#109077=CARTESIAN_POINT('',(8.82705499792788,-28.3340000601472,54.9995523275645));
#109078=CARTESIAN_POINT('Ctrl Pts',(8.86797186106679,-28.4365624698124,
55.5755163674484));
#109079=CARTESIAN_POINT('Ctrl Pts',(8.86184838023776,-28.4075032668568,
55.4965746534193));
#109080=CARTESIAN_POINT('Ctrl Pts',(8.85573819692927,-28.3844353272406,
55.4154645023934));
#109081=CARTESIAN_POINT('Ctrl Pts',(8.84631922382268,-28.3578004428699,
55.284849712552));
#109082=CARTESIAN_POINT('Ctrl Pts',(8.84291224277331,-28.3501300158674,
55.2364077463103));
#109083=CARTESIAN_POINT('Ctrl Pts',(8.83841124708172,-28.3426889489288,
55.1707800401415));
#109084=CARTESIAN_POINT('Ctrl Pts',(8.83725936146111,-28.3410305162976,
55.1538376794101));
#109085=CARTESIAN_POINT('Ctrl Pts',(8.83535766250728,-28.3387052404224,
55.1256302681827));
#109086=CARTESIAN_POINT('Ctrl Pts',(8.83460334789464,-28.3378926845071,
55.1143788663979));
#109087=CARTESIAN_POINT('Ctrl Pts',(8.83318000510604,-28.3365689127441,
55.0930330699288));
#109088=CARTESIAN_POINT('Ctrl Pts',(8.8325103041271,-28.3360351588518,55.0829406367506));
#109089=CARTESIAN_POINT('Ctrl Pts',(8.83105715513884,-28.3350722484711,
55.0609391077272));
#109090=CARTESIAN_POINT('Ctrl Pts',(8.8302748545869,-28.3346789595391,55.0490289411635));
#109091=CARTESIAN_POINT('Ctrl Pts',(8.82867837466067,-28.3341345156952,
55.024596487052));
#109092=CARTESIAN_POINT('Ctrl Pts',(8.82786465131135,-28.3339966952485,
55.0120747003937));
#109093=CARTESIAN_POINT('Ctrl Pts',(8.82705499792788,-28.3340000601472,
54.9995523275645));
#109094=CARTESIAN_POINT('Ctrl Pts',(8.82705508282654,-28.3340000597949,
54.9995536406356));
#109095=CARTESIAN_POINT('Ctrl Pts',(8.82553617924465,-28.3340063538018,
54.9760617728887));
#109096=CARTESIAN_POINT('Ctrl Pts',(8.82403188229458,-28.3345095256223,
54.9525716062054));
#109097=CARTESIAN_POINT('Ctrl Pts',(8.81396006572755,-28.3412605954388,
54.7940821744825));
#109098=CARTESIAN_POINT('Ctrl Pts',(8.80588749310837,-28.3634168684129,
54.6602725688371));
#109099=CARTESIAN_POINT('Ctrl Pts',(8.79388659909176,-28.4182312943844,
54.4736034974832));
#109100=CARTESIAN_POINT('Ctrl Pts',(8.79017169561399,-28.4380053519377,
54.4175424887028));
#109101=CARTESIAN_POINT('Ctrl Pts',(8.78533509524416,-28.46648813663,54.3487519108468));
#109102=CARTESIAN_POINT('Ctrl Pts',(8.7843479530302,-28.4724362915505,54.3349197142162));
#109103=CARTESIAN_POINT('Ctrl Pts',(8.78285665722318,-28.4816052876738,
54.3143696632688));
#109104=CARTESIAN_POINT('Ctrl Pts',(8.78236053876815,-28.4846852308977,
54.3075892791853));
#109105=CARTESIAN_POINT('Ctrl Pts',(8.7814596510359,-28.4903287297755,54.2953833218251));
#109106=CARTESIAN_POINT('Ctrl Pts',(8.78105584701978,-28.4928762783555,
54.2899506412407));
#109107=CARTESIAN_POINT('Ctrl Pts',(8.78014063116624,-28.4986904656686,
54.2777240781553));
#109108=CARTESIAN_POINT('Ctrl Pts',(8.77962823377947,-28.5019738749475,
54.2709385840204));
#109109=CARTESIAN_POINT('Ctrl Pts',(8.77805246895655,-28.512160580754,54.2502460916597));
#109110=CARTESIAN_POINT('Ctrl Pts',(8.77698074146401,-28.5192121106592,
54.2364135646621));
#109111=CARTESIAN_POINT('Ctrl Pts',(8.76869615160337,-28.5747294637855,
54.1311705239456));
#109112=CARTESIAN_POINT('Ctrl Pts',(8.76111630225965,-28.6314189173206,
54.0443624123599));
#109113=CARTESIAN_POINT('Ctrl Pts',(8.74555672798814,-28.7645693483943,
53.8768405178082));
#109114=CARTESIAN_POINT('Ctrl Pts',(8.73763045269787,-28.8418059592626,
53.7973484058349));
#109115=CARTESIAN_POINT('Ctrl Pts',(8.72900071158429,-28.9380252977885,
53.7162561166272));
#109116=CARTESIAN_POINT('Ctrl Pts',(8.72796110462585,-28.9498226287945,
53.7065874045834));
#109117=CARTESIAN_POINT('Ctrl Pts',(8.72598367510743,-28.9726543404673,
53.6883936362838));
#109118=CARTESIAN_POINT('Ctrl Pts',(8.72504486619891,-28.9836661623395,
53.6798424683227));
#109119=CARTESIAN_POINT('Ctrl Pts',(8.72339298715939,-29.0033432477191,
53.6649544916141));
#109120=CARTESIAN_POINT('Ctrl Pts',(8.72267773617592,-29.011964718241,53.6585614130366));
#109121=CARTESIAN_POINT('Ctrl Pts',(8.72118025132079,-29.0302255532999,
53.6452920235054));
#109122=CARTESIAN_POINT('Ctrl Pts',(8.72039875880233,-29.0398776852558,
53.6384342351684));
#109123=CARTESIAN_POINT('Ctrl Pts',(8.7183285774858,-29.0657655664845,53.6204532232389));
#109124=CARTESIAN_POINT('Ctrl Pts',(8.71704684500549,-29.0821269919892,
53.6095135813616));
#109125=CARTESIAN_POINT('Ctrl Pts',(8.71044167823371,-29.1680949753429,
53.5542121251439));
#109126=CARTESIAN_POINT('Ctrl Pts',(8.70530125383583,-29.2407377204961,
53.5147754977768));
#109127=CARTESIAN_POINT('Ctrl Pts',(8.69408430280294,-29.4072735079882,
53.439792230691));
#109128=CARTESIAN_POINT('Ctrl Pts',(8.6880659644171,-29.5020453078056,53.407011688188));
#109129=CARTESIAN_POINT('Ctrl Pts',(8.68002007710013,-29.626613460373,53.3761350480645));
#109130=CARTESIAN_POINT('Ctrl Pts',(8.67822819671343,-29.6542149849184,
53.3700345300044));
#109131=CARTESIAN_POINT('Ctrl Pts',(8.67516227436431,-29.7008969899472,
53.3609558601034));
#109132=CARTESIAN_POINT('Ctrl Pts',(8.67390453944673,-29.719898870554,53.3576018805989));
#109133=CARTESIAN_POINT('Ctrl Pts',(8.67208694303045,-29.7470660136405,
53.3532918095146));
#109134=CARTESIAN_POINT('Ctrl Pts',(8.67154111947347,-29.7551875249804,
53.3520648340582));
#109135=CARTESIAN_POINT('Ctrl Pts',(8.67058731054735,-29.7693083164924,
53.3500381896775));
#109136=CARTESIAN_POINT('Ctrl Pts',(8.67018085349109,-29.7753034193322,
53.3492110753782));
#109137=CARTESIAN_POINT('Ctrl Pts',(8.66930366891522,-29.7881914309504,
53.3475044897134));
#109138=CARTESIAN_POINT('Ctrl Pts',(8.66883241543114,-29.7950852703291,
53.346635481631));
#109139=CARTESIAN_POINT('Ctrl Pts',(8.66752230948051,-29.8141732233366,
53.3443505471619));
#109140=CARTESIAN_POINT('Ctrl Pts',(8.66667871027514,-29.8263775745153,
53.3430262727278));
#109141=CARTESIAN_POINT('Ctrl Pts',(8.66074013012445,-29.9117637561331,
53.3347148112614));
#109142=CARTESIAN_POINT('Ctrl Pts',(8.65544119128776,-29.9853159410088,
53.3324441906106));
#109143=CARTESIAN_POINT('Ctrl Pts',(8.64909097603331,-30.0726650564518,
53.3355273673913));
#109144=CARTESIAN_POINT('Ctrl Pts',(8.64807933770529,-30.0865548732217,
53.3361918363297));
#109145=CARTESIAN_POINT('Ctrl Pts',(8.6417012039095,-30.174027301581,53.341474712998));
#109146=CARTESIAN_POINT('Ctrl Pts',(8.63633497716954,-30.2472483890798,
53.3507998365353));
#109147=CARTESIAN_POINT('Ctrl Pts',(8.62804294649771,-30.3612905792742,
53.3730923844101));
#109148=CARTESIAN_POINT('Ctrl Pts',(8.62504909572653,-30.4026426831145,
53.382830051275));
#109149=CARTESIAN_POINT('Ctrl Pts',(8.61997922178802,-30.4730547026799,
53.4022796663642));
#109150=CARTESIAN_POINT('Ctrl Pts',(8.61788175145896,-30.5023007734022,
53.411231557993));
#109151=CARTESIAN_POINT('Ctrl Pts',(8.61486370094582,-30.5445289221495,
53.4254399045841));
#109152=CARTESIAN_POINT('Ctrl Pts',(8.61392270409118,-30.5577160072512,
53.4300623843458));
#109153=CARTESIAN_POINT('Ctrl Pts',(8.61226834979894,-30.5809306607443,
53.4385292676582));
#109154=CARTESIAN_POINT('Ctrl Pts',(8.61155278937163,-30.5909819853868,
53.4423056837817));
#109155=CARTESIAN_POINT('Ctrl Pts',(8.61005599931498,-30.6120242441422,
53.4504445366153));
#109156=CARTESIAN_POINT('Ctrl Pts',(8.60927549811119,-30.6230066922844,
53.4548273614169));
#109157=CARTESIAN_POINT('Ctrl Pts',(8.60721109163747,-30.652072438047,53.4667870627722));
#109158=CARTESIAN_POINT('Ctrl Pts',(8.60593407181327,-30.6700705716299,
53.4745669935996));
#109159=CARTESIAN_POINT('Ctrl Pts',(8.59932458490185,-30.7632185103023,
53.5167982592224));
#109160=CARTESIAN_POINT('Ctrl Pts',(8.59417593504113,-30.8358690107976,
53.5564919847867));
#109161=CARTESIAN_POINT('Ctrl Pts',(8.58295050239305,-30.9893056217987,
53.655809202575));
#109162=CARTESIAN_POINT('Ctrl Pts',(8.57693170498292,-31.0682536377392,
53.7176559206365));
#109163=CARTESIAN_POINT('Ctrl Pts',(8.56888527237285,-31.1617625285975,
53.8055701051896));
#109164=CARTESIAN_POINT('Ctrl Pts',(8.56709332884275,-31.18185871352,53.8254512578571));
#109165=CARTESIAN_POINT('Ctrl Pts',(8.56402730661505,-31.214805938451,53.8597478978994));
#109166=CARTESIAN_POINT('Ctrl Pts',(8.5627695357879,-31.227930119295,53.8738934913865));
#109167=CARTESIAN_POINT('Ctrl Pts',(8.56095189065356,-31.2462862250038,
53.8943806647541));
#109168=CARTESIAN_POINT('Ctrl Pts',(8.56040605480154,-31.2517220138551,
53.9005385581389));
#109169=CARTESIAN_POINT('Ctrl Pts',(8.55945222787983,-31.2610834968888,
53.911303052612));
#109170=CARTESIAN_POINT('Ctrl Pts',(8.55904576520032,-31.2650299848567,
53.9158912575542));
#109171=CARTESIAN_POINT('Ctrl Pts',(8.55816857569379,-31.2734538244118,
53.925793484299));
#109172=CARTESIAN_POINT('Ctrl Pts',(8.55769732296065,-31.2779228908654,
53.9311139621629));
#109173=CARTESIAN_POINT('Ctrl Pts',(8.55638721937728,-31.2901951930068,
53.9459112632415));
#109174=CARTESIAN_POINT('Ctrl Pts',(8.55554362180173,-31.2979269808047,
53.9554463961042));
#109175=CARTESIAN_POINT('Ctrl Pts',(8.54960520472496,-31.3512188815377,
54.0226732451926));
#109176=CARTESIAN_POINT('Ctrl Pts',(8.54430643992107,-31.3930175213769,
54.0832340313737));
#109177=CARTESIAN_POINT('Ctrl Pts',(8.53795631379941,-31.4378021014612,
54.1582907248116));
#109178=CARTESIAN_POINT('Ctrl Pts',(8.53694459249697,-31.4447778272773,
54.1703215001261));
#109179=CARTESIAN_POINT('Ctrl Pts',(8.53056640387706,-31.4877820559782,
54.2466766125069));
#109180=CARTESIAN_POINT('Ctrl Pts',(8.52520020317049,-31.5196602441179,
54.3132499505791));
#109181=CARTESIAN_POINT('Ctrl Pts',(8.51690814852958,-31.5627843248727,
54.4211524549926));
#109182=CARTESIAN_POINT('Ctrl Pts',(8.51391425079502,-31.5770315741539,
54.4611760569905));
#109183=CARTESIAN_POINT('Ctrl Pts',(8.50884431074162,-31.5988806006418,
54.5308818288539));
#109184=CARTESIAN_POINT('Ctrl Pts',(8.50674682029753,-31.6072219285935,
54.5603081546132));
#109185=CARTESIAN_POINT('Ctrl Pts',(8.50372875040669,-31.6181881227919,
54.6034921939073));
#109186=CARTESIAN_POINT('Ctrl Pts',(8.50278775369559,-31.6214568223152,
54.6170782912113));
#109187=CARTESIAN_POINT('Ctrl Pts',(8.50113340343795,-31.6269342863765,
54.6411739876842));
#109188=CARTESIAN_POINT('Ctrl Pts',(8.50041784685424,-31.629213055609,54.6516666711136));
#109189=CARTESIAN_POINT('Ctrl Pts',(8.4989210686974,-31.6337878561679,54.6737592182554));
#109190=CARTESIAN_POINT('Ctrl Pts',(8.49814057550794,-31.6360621575444,
54.68536301009));
#109191=CARTESIAN_POINT('Ctrl Pts',(8.49607619983112,-31.641778536238,54.7162684374084));
#109192=CARTESIAN_POINT('Ctrl Pts',(8.49479920254292,-31.645003838611,54.7356086513292));
#109193=CARTESIAN_POINT('Ctrl Pts',(8.48819042771245,-31.6600424222173,
54.8367600307408));
#109194=CARTESIAN_POINT('Ctrl Pts',(8.48304241671865,-31.666097380804,54.9193145426247));
#109195=CARTESIAN_POINT('Ctrl Pts',(8.47181692945927,-31.6658794680774,
55.1020898418589));
#109196=CARTESIAN_POINT('Ctrl Pts',(8.46579750244033,-31.6567382489378,
55.2019722042967));
#109197=CARTESIAN_POINT('Ctrl Pts',(8.4577503063853,-31.6335917670788,55.3282270027051));
#109198=CARTESIAN_POINT('Ctrl Pts',(8.45595827716415,-31.6277879651729,
55.3558949102023));
#109199=CARTESIAN_POINT('Ctrl Pts',(8.45289212413416,-31.6168428185066,
55.4021786306713));
#109200=CARTESIAN_POINT('Ctrl Pts',(8.45163431029328,-31.612076412706,55.4208775504655));
#109201=CARTESIAN_POINT('Ctrl Pts',(8.4498166167352,-31.6048197357512,55.4474115397722));
#109202=CARTESIAN_POINT('Ctrl Pts',(8.44927077675313,-31.6025943780206,
55.4553182653044));
#109203=CARTESIAN_POINT('Ctrl Pts',(8.44831694777217,-31.5986279751689,
55.4690215624216));
#109204=CARTESIAN_POINT('Ctrl Pts',(8.44791048724636,-31.5969136645005,
55.4748256267276));
#109205=CARTESIAN_POINT('Ctrl Pts',(8.44703330777454,-31.5931631989013,
55.4872733333099));
#109206=CARTESIAN_POINT('Ctrl Pts',(8.44656206298062,-31.591117127449,55.493913516746));
#109207=CARTESIAN_POINT('Ctrl Pts',(8.44525199896465,-31.5853414970811,
55.5122489896442));
#109208=CARTESIAN_POINT('Ctrl Pts',(8.44440843343443,-31.5815242072024,
55.5239158803544));
#109209=CARTESIAN_POINT('Ctrl Pts',(8.43847834147419,-31.5539863145305,
55.6050363588819));
#109210=CARTESIAN_POINT('Ctrl Pts',(8.43318852934751,-31.5258300482248,
55.6728913269193));
#109211=CARTESIAN_POINT('Ctrl Pts',(8.42684056546539,-31.4870903879816,
55.7512084489353));
#109212=CARTESIAN_POINT('Ctrl Pts',(8.4258221531402,-31.4807259853443,55.7636769660354));
#109213=CARTESIAN_POINT('Ctrl Pts',(8.4194377937421,-31.4398650350181,55.8412961414796));
#109214=CARTESIAN_POINT('Ctrl Pts',(8.41407206250087,-31.4012307904917,
55.9041814545707));
#109215=CARTESIAN_POINT('Ctrl Pts',(8.40577891656175,-31.3339646014261,
55.9989491898386));
#109216=CARTESIAN_POINT('Ctrl Pts',(8.40278354136814,-31.3080554206888,
56.0326434814578));
#109217=CARTESIAN_POINT('Ctrl Pts',(8.39771140638847,-31.261324527223,56.0888306192055));
#109218=CARTESIAN_POINT('Ctrl Pts',(8.39561317319922,-31.2411196382306,
56.1118066096013));
#109219=CARTESIAN_POINT('Ctrl Pts',(8.39259425012894,-31.2107783230305,
56.144450586437));
#109220=CARTESIAN_POINT('Ctrl Pts',(8.39165312661661,-31.2011356725252,
56.154566762543));
#109221=CARTESIAN_POINT('Ctrl Pts',(8.38999863394394,-31.1838612475959,
56.1722388112475));
#109222=CARTESIAN_POINT('Ctrl Pts',(8.38928306044775,-31.1762816832033,
56.1798443521048));
#109223=CARTESIAN_POINT('Ctrl Pts',(8.38778632549781,-31.1602025490578,
56.1956696156224));
#109224=CARTESIAN_POINT('Ctrl Pts',(8.38700589167017,-31.1516879105022,
56.2038732298281));
#109225=CARTESIAN_POINT('Ctrl Pts',(8.38494185700755,-31.1288272498575,
56.2254343028839));
#109226=CARTESIAN_POINT('Ctrl Pts',(8.38366513722902,-31.1143313357955,
56.2386306622115));
#109227=CARTESIAN_POINT('Ctrl Pts',(8.37706589660129,-31.0376183063484,
56.3060293343457));
#109228=CARTESIAN_POINT('Ctrl Pts',(8.37192643767452,-30.9716670751973,
56.3558133911492));
#109229=CARTESIAN_POINT('Ctrl Pts',(8.36070155094149,-30.8180344104257,
56.4547925755347));
#109230=CARTESIAN_POINT('Ctrl Pts',(8.35467494395419,-30.7290572541563,
56.5013576889035));
#109231=CARTESIAN_POINT('Ctrl Pts',(8.34661911461226,-30.6103037973624,
56.5504467713805));
#109232=CARTESIAN_POINT('Ctrl Pts',(8.34482612517006,-30.583896668051,56.5605833578003));
#109233=CARTESIAN_POINT('Ctrl Pts',(8.3417584951817,-30.5390535898384,56.5764992480857));
#109234=CARTESIAN_POINT('Ctrl Pts',(8.34050018504127,-30.5207513650662,
56.5826391217805));
#109235=CARTESIAN_POINT('Ctrl Pts',(8.3386818982657,-30.4945146110847,56.5909364509638));
#109236=CARTESIAN_POINT('Ctrl Pts',(8.33813597382793,-30.4866636385935,
56.5933555747084));
#109237=CARTESIAN_POINT('Ctrl Pts',(8.3371820492612,-30.47299827125,56.5974558730859));
#109238=CARTESIAN_POINT('Ctrl Pts',(8.33677557854923,-30.4671920862621,
56.5991635889597));
#109239=CARTESIAN_POINT('Ctrl Pts',(8.33589843860159,-30.4547006474348,
56.6027637352125));
#109240=CARTESIAN_POINT('Ctrl Pts',(8.33542724411356,-30.4480129241238,
56.6046459687753));
#109241=CARTESIAN_POINT('Ctrl Pts',(8.33411745535199,-30.4294798514906,
56.6097371422419));
#109242=CARTESIAN_POINT('Ctrl Pts',(8.33327411788015,-30.4176107948431,
56.6128570339284));
#109243=CARTESIAN_POINT('Ctrl Pts',(8.32739887247102,-30.3352905007319,
56.6335261323278));
#109244=CARTESIAN_POINT('Ctrl Pts',(8.32216800137943,-30.2637991907535,
56.6465828242112));
#109245=CARTESIAN_POINT('Ctrl Pts',(8.31584324417443,-30.1773078760519,
56.656601230076));
#109246=CARTESIAN_POINT('Ctrl Pts',(8.31478973529396,-30.1629013581077,
56.6580798719303));
#109247=CARTESIAN_POINT('Ctrl Pts',(8.30828496922489,-30.0738836088459,
56.666045019249));
#109248=CARTESIAN_POINT('Ctrl Pts',(8.30283360293201,-29.9989197191716,
56.6676825293435));
#109249=CARTESIAN_POINT('Ctrl Pts',(8.29449525406011,-29.8821389467974,
56.6623564165119));
#109250=CARTESIAN_POINT('Ctrl Pts',(8.2915353389042,-29.8402662970178,56.6588567490511));
#109251=CARTESIAN_POINT('Ctrl Pts',(8.2865159350786,-29.7684557613351,56.650110131308));
#109252=CARTESIAN_POINT('Ctrl Pts',(8.28443557452401,-29.7384480479612,
56.6456205408177));
#109253=CARTESIAN_POINT('Ctrl Pts',(8.2814372037558,-29.6948624013613,56.6378770095487));
#109254=CARTESIAN_POINT('Ctrl Pts',(8.28049915127017,-29.6811776570974,
56.6352682919464));
#109255=CARTESIAN_POINT('Ctrl Pts',(8.27884811610634,-29.6570112764264,
56.6303465581826));
#109256=CARTESIAN_POINT('Ctrl Pts',(8.2781329603651,-29.6465164119705,56.6281033525343));
#109257=CARTESIAN_POINT('Ctrl Pts',(8.27663519685349,-29.6244843353795,
56.6231710637236));
#109258=CARTESIAN_POINT('Ctrl Pts',(8.27585333506021,-29.6129526152548,
56.6204600120473));
#109259=CARTESIAN_POINT('Ctrl Pts',(8.27378104800953,-29.5823162646349,
56.6129118519075));
#109260=CARTESIAN_POINT('Ctrl Pts',(8.27249760463375,-29.5632665222696,
56.6078582859401));
#109261=CARTESIAN_POINT('Ctrl Pts',(8.26560998383705,-29.4607368949674,
56.5787021918441));
#109262=CARTESIAN_POINT('Ctrl Pts',(8.26021101340171,-29.3791454853494,
56.5484339677419));
#109263=CARTESIAN_POINT('Ctrl Pts',(8.24896385204374,-29.2127209986545,
56.4714130038672));
#109264=CARTESIAN_POINT('Ctrl Pts',(8.24315303708851,-29.1288541209504,
56.4233647014439));
#109265=CARTESIAN_POINT('Ctrl Pts',(8.23451324305029,-29.015739650852,56.344800855531));
#109266=CARTESIAN_POINT('Ctrl Pts',(8.23188275192659,-28.9827464906395,
56.3200198681405));
#109267=CARTESIAN_POINT('Ctrl Pts',(8.22847293050118,-28.9423632052686,
56.2872745959769));
#109268=CARTESIAN_POINT('Ctrl Pts',(8.22776317684413,-28.9340823991569,
56.2804261510396));
#109269=CARTESIAN_POINT('Ctrl Pts',(8.22661218532108,-28.9208658939211,
56.2692786983777));
#109270=CARTESIAN_POINT('Ctrl Pts',(8.22617445375682,-28.915888112556,56.2650297407005));
#109271=CARTESIAN_POINT('Ctrl Pts',(8.22532203759895,-28.9062916430472,
56.2567401039398));
#109272=CARTESIAN_POINT('Ctrl Pts',(8.22490760932303,-28.9016700400614,
56.2527030587226));
#109273=CARTESIAN_POINT('Ctrl Pts',(8.22397306517343,-28.8913444267807,
56.2435824056227));
#109274=CARTESIAN_POINT('Ctrl Pts',(8.22345195593882,-28.8856528795086,
56.2384849086761));
#109275=CARTESIAN_POINT('Ctrl Pts',(8.22160690026736,-28.865725949537,56.2203892727729));
#109276=CARTESIAN_POINT('Ctrl Pts',(8.22026914383081,-28.8516819005572,
56.2071839390308));
#109277=CARTESIAN_POINT('Ctrl Pts',(8.21136055728577,-28.7605972343528,
56.1185111434971));
#109278=CARTESIAN_POINT('Ctrl Pts',(8.20343270390961,-28.6908154886555,
56.0359632342641));
#109279=CARTESIAN_POINT('Ctrl Pts',(8.18941145534872,-28.5809488814632,
55.8770076844964));
#109280=CARTESIAN_POINT('Ctrl Pts',(8.18329627340985,-28.5378615511692,
55.8031209869155));
#109281=CARTESIAN_POINT('Ctrl Pts',(8.17529351248492,-28.4875624006019,
55.6992757608946));
#109282=CARTESIAN_POINT('Ctrl Pts',(8.17323888610889,-28.4752280989282,
55.6719560493771));
#109283=CARTESIAN_POINT('Ctrl Pts',(8.17027014972838,-28.4582743093055,
55.6315300108923));
#109284=CARTESIAN_POINT('Ctrl Pts',(8.16933655472817,-28.4530714954049,
55.6186763951053));
#109285=CARTESIAN_POINT('Ctrl Pts',(8.16769052677727,-28.4441305326062,
55.5957694140264));
#109286=CARTESIAN_POINT('Ctrl Pts',(8.16697596606473,-28.4403279098729,
55.5857422426098));
#109287=CARTESIAN_POINT('Ctrl Pts',(8.16626077429774,-28.4366022942655,
55.5756245452141));
#109288=CARTESIAN_POINT('Ctrl Pts',(8.16625693578549,-28.4365823008186,
55.5755702400533));
#109289=CARTESIAN_POINT('Ctrl Pts',(8.16625309736762,-28.4365623102018,
55.5755159338529));
#109290=CARTESIAN_POINT('Origin',(5.,-30.,55.));
#109291=CARTESIAN_POINT('',(7.4682788092303,-28.4365623654365,55.5755160839024));
#109292=CARTESIAN_POINT('',(7.65925610934961,-28.4365623095611,55.5755159321123));
#109293=CARTESIAN_POINT('',(5.,-28.4365623102018,55.5755159338528));
#109294=CARTESIAN_POINT('',(8.32030899669651,-28.3340003265563,55.0010431133336));
#109295=CARTESIAN_POINT('Ctrl Pts',(7.65925610934961,-28.4365623095611,
55.5755159321123));
#109296=CARTESIAN_POINT('Ctrl Pts',(7.6596315560846,-28.4385623445714,55.5809491963241));
#109297=CARTESIAN_POINT('Ctrl Pts',(7.66000835454394,-28.4405908269087,
55.5863723737114));
#109298=CARTESIAN_POINT('Ctrl Pts',(7.66118867024847,-28.4470093428382,
55.6032634517357));
#109299=CARTESIAN_POINT('Ctrl Pts',(7.66199704716634,-28.4514976072287,
55.6146926803279));
#109300=CARTESIAN_POINT('Ctrl Pts',(7.66327424463479,-28.4587235614784,
55.632511856785));
#109301=CARTESIAN_POINT('Ctrl Pts',(7.66373818777893,-28.4613757176395,
55.6389363209823));
#109302=CARTESIAN_POINT('Ctrl Pts',(7.6646108341278,-28.4664131588991,55.6509255380234));
#109303=CARTESIAN_POINT('Ctrl Pts',(7.6650189628302,-28.4687886778772,55.6564941260748));
#109304=CARTESIAN_POINT('Ctrl Pts',(7.66598534126336,-28.4744599805603,
55.6695903043105));
#109305=CARTESIAN_POINT('Ctrl Pts',(7.66654507652535,-28.4777811654128,
55.6771065935943));
#109306=CARTESIAN_POINT('Ctrl Pts',(7.66843017181659,-28.489091667823,55.7021999681124));
#109307=CARTESIAN_POINT('Ctrl Pts',(7.66976908625898,-28.4973305851432,
55.7196619579204));
#109308=CARTESIAN_POINT('Ctrl Pts',(7.67310235261717,-28.5183838684203,
55.7623449412159));
#109309=CARTESIAN_POINT('Ctrl Pts',(7.67511129716783,-28.5315405108667,
55.7873898138015));
#109310=CARTESIAN_POINT('Ctrl Pts',(7.68432086803433,-28.5941909948013,
55.8996142816884));
#109311=CARTESIAN_POINT('Ctrl Pts',(7.69169396224523,-28.6508540825793,
55.9825530883988));
#109312=CARTESIAN_POINT('Ctrl Pts',(7.70486796129938,-28.7670982509054,
56.123526146945));
#109313=CARTESIAN_POINT('Ctrl Pts',(7.71070089544379,-28.8242252665084,
56.1831801157415));
#109314=CARTESIAN_POINT('Ctrl Pts',(7.71768794115089,-28.9001166530769,
56.2514778947734));
#109315=CARTESIAN_POINT('Ctrl Pts',(7.7190188398837,-28.9149190952913,56.2643337317098));
#109316=CARTESIAN_POINT('Ctrl Pts',(7.72113535107662,-28.939009811252,56.284521574664));
#109317=CARTESIAN_POINT('Ctrl Pts',(7.72192773760227,-28.9481548771276,
56.2920207840315));
#109318=CARTESIAN_POINT('Ctrl Pts',(7.72343228537405,-28.9657566586118,
56.3061439717789));
#109319=CARTESIAN_POINT('Ctrl Pts',(7.72414509708789,-28.9741990595568,
56.3127847515955));
#109320=CARTESIAN_POINT('Ctrl Pts',(7.72577836149336,-28.9937771938607,
56.3278806929596));
#109321=CARTESIAN_POINT('Ctrl Pts',(7.72669652299578,-29.0049564194279,
56.3362783253617));
#109322=CARTESIAN_POINT('Ctrl Pts',(7.72960801873068,-29.0409441086675,
56.3626095491915));
#109323=CARTESIAN_POINT('Ctrl Pts',(7.73158067886816,-29.0661424916406,
56.3800012061073));
#109324=CARTESIAN_POINT('Ctrl Pts',(7.73624067789816,-29.1274567344713,
56.4198705942748));
#109325=CARTESIAN_POINT('Ctrl Pts',(7.73890542608523,-29.1639824111575,
56.44167930767));
#109326=CARTESIAN_POINT('Ctrl Pts',(7.74611134338234,-29.2659870836606,
56.4974022123086));
#109327=CARTESIAN_POINT('Ctrl Pts',(7.75058500742547,-29.332944493393,56.5284062490572));
#109328=CARTESIAN_POINT('Ctrl Pts',(7.75594783319387,-29.4147581248127,
56.5598854628989));
#109329=CARTESIAN_POINT('Ctrl Pts',(7.7568026874433,-29.4278435645864,56.5647324746603));
#109330=CARTESIAN_POINT('Ctrl Pts',(7.76216751804569,-29.5101164097297,
56.5940373447245));
#109331=CARTESIAN_POINT('Ctrl Pts',(7.76673002031649,-29.5807875270263,
56.6140629379912));
#109332=CARTESIAN_POINT('Ctrl Pts',(7.77232424267155,-29.6645460512457,
56.6319244453593));
#109333=CARTESIAN_POINT('Ctrl Pts',(7.77313255053717,-29.6765814720595,
56.6343522206432));
#109334=CARTESIAN_POINT('Ctrl Pts',(7.77440966238008,-29.6954699527762,
56.6379455900366));
#109335=CARTESIAN_POINT('Ctrl Pts',(7.77487359000941,-29.702305624994,56.6392017448432));
#109336=CARTESIAN_POINT('Ctrl Pts',(7.77574622456606,-29.7151102335457,
56.6414720457116));
#109337=CARTESIAN_POINT('Ctrl Pts',(7.77615435718938,-29.7210770958674,
56.6424964732844));
#109338=CARTESIAN_POINT('Ctrl Pts',(7.77712076862338,-29.7351561467272,
56.6448347232629));
#109339=CARTESIAN_POINT('Ctrl Pts',(7.77768053327363,-29.7432726184884,
56.6461210702653));
#109340=CARTESIAN_POINT('Ctrl Pts',(7.77956583391251,-29.7704919999724,
56.6502287597163));
#109341=CARTESIAN_POINT('Ctrl Pts',(7.78090492818634,-29.7896335978844,
56.6527778976221));
#109342=CARTESIAN_POINT('Ctrl Pts',(7.784238742733,-29.8369196142278,56.6582404071742));
#109343=CARTESIAN_POINT('Ctrl Pts',(7.78624806138309,-29.8651017184155,
56.6607705239147));
#109344=CARTESIAN_POINT('Ctrl Pts',(7.79546095777827,-29.9934115102855,
56.6690025611873));
#109345=CARTESIAN_POINT('Ctrl Pts',(7.8028370944624,-30.0938647460717,56.6663741579223));
#109346=CARTESIAN_POINT('Ctrl Pts',(7.81601040849399,-30.2753412307959,
56.645155692686));
#109347=CARTESIAN_POINT('Ctrl Pts',(7.82183992568639,-30.3563961126456,
56.629520032418));
#109348=CARTESIAN_POINT('Ctrl Pts',(7.82882366971938,-30.4548903340898,
56.6028147197367));
#109349=CARTESIAN_POINT('Ctrl Pts',(7.83015446910984,-30.4737180015393,
56.5973514183847));
#109350=CARTESIAN_POINT('Ctrl Pts',(7.83227086104797,-30.503742946058,56.5880613632532));
#109351=CARTESIAN_POINT('Ctrl Pts',(7.83306322630967,-30.5150030150613,
56.5844455674211));
#109352=CARTESIAN_POINT('Ctrl Pts',(7.83456775740151,-30.536414862361,56.5773174890502));
#109353=CARTESIAN_POINT('Ctrl Pts',(7.8352805734515,-30.5465729900774,56.5738263378019));
#109354=CARTESIAN_POINT('Ctrl Pts',(7.83691388118452,-30.5698748483488,
56.5655651198284));
#109355=CARTESIAN_POINT('Ctrl Pts',(7.83783208124924,-30.5829938300014,
56.5607272987701));
#109356=CARTESIAN_POINT('Ctrl Pts',(7.84074383938508,-30.6246380314961,
56.5447719989589));
#109357=CARTESIAN_POINT('Ctrl Pts',(7.84271671792307,-30.6529193600798,
56.5330328427604));
#109358=CARTESIAN_POINT('Ctrl Pts',(7.84737734417492,-30.7196789794392,
56.503139044398));
#109359=CARTESIAN_POINT('Ctrl Pts',(7.85004249251946,-30.757817324341,56.4842769632459));
#109360=CARTESIAN_POINT('Ctrl Pts',(7.85724860998728,-30.8599585141434,
56.4287964516835));
#109361=CARTESIAN_POINT('Ctrl Pts',(7.86172210057593,-30.922318605461,56.3893583772187));
#109362=CARTESIAN_POINT('Ctrl Pts',(7.86708635212909,-30.9931562915815,
56.3376815812076));
#109363=CARTESIAN_POINT('Ctrl Pts',(7.86794279505195,-31.0043459190581,
56.3293008316584));
#109364=CARTESIAN_POINT('Ctrl Pts',(7.87330715120606,-31.0735776699446,
56.2760747934682));
#109365=CARTESIAN_POINT('Ctrl Pts',(7.87786760414623,-31.1287038233733,
56.2275833377726));
#109366=CARTESIAN_POINT('Ctrl Pts',(7.88345955154642,-31.1891130484753,
56.1669262623574));
#109367=CARTESIAN_POINT('Ctrl Pts',(7.88426785085735,-31.1976802127793,
56.1581316116883));
#109368=CARTESIAN_POINT('Ctrl Pts',(7.88554495202271,-31.2109434769139,
56.1442116066855));
#109369=CARTESIAN_POINT('Ctrl Pts',(7.88600887765798,-31.2157062284432,
56.1391499755974));
#109370=CARTESIAN_POINT('Ctrl Pts',(7.88688151058901,-31.2245583480746,
56.1296236134685));
#109371=CARTESIAN_POINT('Ctrl Pts',(7.88728964360507,-31.2286552289323,
56.1251662009145));
#109372=CARTESIAN_POINT('Ctrl Pts',(7.88825605881983,-31.2382557009753,
56.1146059183747));
#109373=CARTESIAN_POINT('Ctrl Pts',(7.8888158268952,-31.2437385314501,56.1084845477414));
#109374=CARTESIAN_POINT('Ctrl Pts',(7.89070115173866,-31.2619526209694,
56.0878439573151));
#109375=CARTESIAN_POINT('Ctrl Pts',(7.89204026725288,-31.2744761648335,
56.0731445936323));
#109376=CARTESIAN_POINT('Ctrl Pts',(7.89537414655539,-31.3047122392942,
56.0363794995134));
#109377=CARTESIAN_POINT('Ctrl Pts',(7.89738350940413,-31.3221232040059,
56.0140742315358));
#109378=CARTESIAN_POINT('Ctrl Pts',(7.90659679740837,-31.3986329290325,
55.9107358812078));
#109379=CARTESIAN_POINT('Ctrl Pts',(7.91397329232241,-31.4509088925012,
55.8249107642318));
#109380=CARTESIAN_POINT('Ctrl Pts',(7.9271465324345,-31.5315066775885,55.6609360433827));
#109381=CARTESIAN_POINT('Ctrl Pts',(7.93297565374477,-31.5623292826959,
55.5843629414212));
#109382=CARTESIAN_POINT('Ctrl Pts',(7.93995901538397,-31.5933109535508,
55.4871349307183));
#109383=CARTESIAN_POINT('Ctrl Pts',(7.94128980341016,-31.598932388612,55.4683540423891));
#109384=CARTESIAN_POINT('Ctrl Pts',(7.94340618173923,-31.6074117931698,
55.4380903736915));
#109385=CARTESIAN_POINT('Ctrl Pts',(7.94419854460112,-31.6104810488991,
55.4266692535922));
#109386=CARTESIAN_POINT('Ctrl Pts',(7.9457030738659,-31.616105442028,55.4048142367437));
#109387=CARTESIAN_POINT('Ctrl Pts',(7.94641589046009,-31.61868177556,55.3943864661833));
#109388=CARTESIAN_POINT('Ctrl Pts',(7.94804920328722,-31.6243792662271,
55.3703288925008));
#109389=CARTESIAN_POINT('Ctrl Pts',(7.94896740785243,-31.6274300755234,
55.3566831341589));
#109390=CARTESIAN_POINT('Ctrl Pts',(7.95187919642386,-31.6366117267863,
55.3130419773073));
#109391=CARTESIAN_POINT('Ctrl Pts',(7.95385210027032,-31.6420879724912,
55.282914303293));
#109392=CARTESIAN_POINT('Ctrl Pts',(7.95851279929422,-31.6531809977565,
55.2106121423244));
#109393=CARTESIAN_POINT('Ctrl Pts',(7.96117799410164,-31.6580190158564,
55.1683395656584));
#109394=CARTESIAN_POINT('Ctrl Pts',(7.96838413370204,-31.6668048613645,
55.0524352083223));
#109395=CARTESIAN_POINT('Ctrl Pts',(7.97285760312556,-31.6674929153515,
54.9786543191881));
#109396=CARTESIAN_POINT('Ctrl Pts',(7.97822200922568,-31.6624964839714,
54.8911103660414));
#109397=CARTESIAN_POINT('Ctrl Pts',(7.97907862662128,-31.661524041769,54.8771612268574));
#109398=CARTESIAN_POINT('Ctrl Pts',(7.98444292609883,-31.6543548082804,
54.7901298280449));
#109399=CARTESIAN_POINT('Ctrl Pts',(7.98900314939803,-31.6435137818949,
54.7175198237225));
#109400=CARTESIAN_POINT('Ctrl Pts',(7.99459484191308,-31.6253177426105,
54.6338730014353));
#109401=CARTESIAN_POINT('Ctrl Pts',(7.99540314040856,-31.6225754969494,
54.6219054635903));
#109402=CARTESIAN_POINT('Ctrl Pts',(7.99668024064619,-31.6180742135462,
54.6032127212348));
#109403=CARTESIAN_POINT('Ctrl Pts',(7.99714416618442,-31.6164048617091,
54.5964660809779));
#109404=CARTESIAN_POINT('Ctrl Pts',(7.99801679953228,-31.6132024186657,
54.5838622674543));
#109405=CARTESIAN_POINT('Ctrl Pts',(7.99842493306825,-31.6116795505877,
54.5780027516996));
#109406=CARTESIAN_POINT('Ctrl Pts',(7.99939135017537,-31.6080143394654,
54.5642094325487));
#109407=CARTESIAN_POINT('Ctrl Pts',(7.99995111963336,-31.6058451931492,
54.5562830370985));
#109408=CARTESIAN_POINT('Ctrl Pts',(8.00183645150218,-31.5983827698241,
54.5297857750607));
#109409=CARTESIAN_POINT('Ctrl Pts',(8.00317557275699,-31.5928254863949,
54.5112917162276));
#109410=CARTESIAN_POINT('Ctrl Pts',(8.00650946905542,-31.5783364026377,
54.4659487819985));
#109411=CARTESIAN_POINT('Ctrl Pts',(8.00851884330254,-31.5690397929779,
54.4392233504771));
#109412=CARTESIAN_POINT('Ctrl Pts',(8.01773223419145,-31.5237162941274,
54.31889587768));
#109413=CARTESIAN_POINT('Ctrl Pts',(8.02510882288873,-31.4799627653021,
54.2284270276355));
#109414=CARTESIAN_POINT('Ctrl Pts',(8.03828201941204,-31.3859135837764,
54.0717799769512));
#109415=CARTESIAN_POINT('Ctrl Pts',(8.04411101395925,-31.3382991674952,
54.0043555409284));
#109416=CARTESIAN_POINT('Ctrl Pts',(8.05109425364852,-31.2734181694795,
53.9255948626369));
#109417=CARTESIAN_POINT('Ctrl Pts',(8.05242503832777,-31.2606884265202,
53.9106860040677));
#109418=CARTESIAN_POINT('Ctrl Pts',(8.05454141312019,-31.2398615655984,
53.8871481920678));
#109419=CARTESIAN_POINT('Ctrl Pts',(8.05533377573571,-31.2319308439942,
53.8783751712968));
#109420=CARTESIAN_POINT('Ctrl Pts',(8.05683830565413,-31.2166199590876,
53.8617964850396));
#109421=CARTESIAN_POINT('Ctrl Pts',(8.05755112313711,-31.2092564384435,
53.8539763346173));
#109422=CARTESIAN_POINT('Ctrl Pts',(8.05918443961101,-31.1921347033163,
53.8361416153578));
#109423=CARTESIAN_POINT('Ctrl Pts',(8.06010264691097,-31.1823249294284,
53.8261774958079));
#109424=CARTESIAN_POINT('Ctrl Pts',(8.06301445107528,-31.1506397252153,
53.7947940181171));
#109425=CARTESIAN_POINT('Ctrl Pts',(8.06498736748796,-31.1282981279739,
53.7738528803521));
#109426=CARTESIAN_POINT('Ctrl Pts',(8.0696481017676,-31.0735699597277,53.7253186834731));
#109427=CARTESIAN_POINT('Ctrl Pts',(8.07231331880534,-31.040678596113,53.6983267087313));
#109428=CARTESIAN_POINT('Ctrl Pts',(8.07951947072292,-30.948067180262,53.6280829110851));
#109429=CARTESIAN_POINT('Ctrl Pts',(8.08399293166016,-30.8864539014938,
53.5874888596716));
#109430=CARTESIAN_POINT('Ctrl Pts',(8.08935743038982,-30.8101931956547,
53.5442051850884));
#109431=CARTESIAN_POINT('Ctrl Pts',(8.09021414840303,-30.7979450499567,
53.5374558985732));
#109432=CARTESIAN_POINT('Ctrl Pts',(8.09557842413529,-30.7209381047754,
53.4962768664403));
#109433=CARTESIAN_POINT('Ctrl Pts',(8.10013852385392,-30.6540573596111,
53.4660048030172));
#109434=CARTESIAN_POINT('Ctrl Pts',(8.10573007927809,-30.5739151158481,
53.4359257743946));
#109435=CARTESIAN_POINT('Ctrl Pts',(8.10653837745834,-30.5623733761013,
53.4317388905237));
#109436=CARTESIAN_POINT('Ctrl Pts',(8.10781547739135,-30.5442274605415,
53.4253823396363));
#109437=CARTESIAN_POINT('Ctrl Pts',(8.10827940294775,-30.5376539180235,
53.4231256977185));
#109438=CARTESIAN_POINT('Ctrl Pts',(8.10915203571862,-30.5253280243721,
53.4189803534619));
#109439=CARTESIAN_POINT('Ctrl Pts',(8.10956016865383,-30.5195792499108,
53.4170817916549));
#109440=CARTESIAN_POINT('Ctrl Pts',(8.11052658399545,-30.5060030287681,
53.4126800986567));
#109441=CARTESIAN_POINT('Ctrl Pts',(8.11108635228107,-30.4981672687478,
53.4102035037174));
#109442=CARTESIAN_POINT('Ctrl Pts',(8.11297168031135,-30.471858470391,53.4021018559924));
#109443=CARTESIAN_POINT('Ctrl Pts',(8.11431079888123,-30.4533067742275,
53.3967402631907));
#109444=CARTESIAN_POINT('Ctrl Pts',(8.11764468799606,-30.4073539461049,
53.3843208046556));
#109445=CARTESIAN_POINT('Ctrl Pts',(8.1196540577223,-30.3798586655754,53.3776363807328));
#109446=CARTESIAN_POINT('Ctrl Pts',(8.12886741042828,-30.2541850188842,
53.3504533801769));
#109447=CARTESIAN_POINT('Ctrl Pts',(8.13624396510959,-30.1544483420492,
53.3381455381687));
#109448=CARTESIAN_POINT('Ctrl Pts',(8.1494171904731,-29.9718331268217,53.3322003625689));
#109449=CARTESIAN_POINT('Ctrl Pts',(8.15524624346938,-29.8893617754007,
53.3356346962159));
#109450=CARTESIAN_POINT('Ctrl Pts',(8.16222953788076,-29.7880015852572,
53.3474271859046));
#109451=CARTESIAN_POINT('Ctrl Pts',(8.16356032289799,-29.7685718438436,
53.3500359703248));
#109452=CARTESIAN_POINT('Ctrl Pts',(8.16567669699883,-29.737500971642,53.3547674608046));
#109453=CARTESIAN_POINT('Ctrl Pts',(8.16646905861369,-29.7258290509246,
53.3566722326081));
#109454=CARTESIAN_POINT('Ctrl Pts',(8.16797358582743,-29.703596540222,53.3605438844531));
#109455=CARTESIAN_POINT('Ctrl Pts',(8.16868640161362,-29.6930328071546,
53.3624889259901));
#109456=CARTESIAN_POINT('Ctrl Pts',(8.170319713004,-29.6687629437538,53.3672007161043));
#109457=CARTESIAN_POINT('Ctrl Pts',(8.17123791693804,-29.6550712339391,
53.3700381430823));
#109458=CARTESIAN_POINT('Ctrl Pts',(8.17414970500974,-29.6115199307771,
53.3796369357906));
#109459=CARTESIAN_POINT('Ctrl Pts',(8.17612260895051,-29.5818092768106,
53.3870493089765));
#109460=CARTESIAN_POINT('Ctrl Pts',(8.18078330878355,-29.5113515103222,
53.406705444463));
#109461=CARTESIAN_POINT('Ctrl Pts',(8.18344850424901,-29.4708356084273,
53.4196992962317));
#109462=CARTESIAN_POINT('Ctrl Pts',(8.19065464629215,-29.3615917532791,
53.4594082911376));
#109463=CARTESIAN_POINT('Ctrl Pts',(8.19512811731426,-29.294069905572,53.4891555445464));
#109464=CARTESIAN_POINT('Ctrl Pts',(8.20459017312364,-29.1569752385731,
53.5607570765928));
#109465=CARTESIAN_POINT('Ctrl Pts',(8.20957423370653,-29.0880468383341,
53.6034151552594));
#109466=CARTESIAN_POINT('Ctrl Pts',(8.21586584900291,-29.0094249711747,
53.6603814546508));
#109467=CARTESIAN_POINT('Ctrl Pts',(8.21692238130636,-28.9964882490675,
53.6700447926968));
#109468=CARTESIAN_POINT('Ctrl Pts',(8.21850511857984,-28.977539903036,53.68463249162));
#109469=CARTESIAN_POINT('Ctrl Pts',(8.219021997144,-28.9714185582601,53.6894136641493));
#109470=CARTESIAN_POINT('Ctrl Pts',(8.21994422016446,-28.9606197152262,
53.6979705238945));
#109471=CARTESIAN_POINT('Ctrl Pts',(8.22034836307997,-28.9559288917451,
53.7017289760014));
#109472=CARTESIAN_POINT('Ctrl Pts',(8.22122419628099,-28.9458534075547,
53.7098917291308));
#109473=CARTESIAN_POINT('Ctrl Pts',(8.22169644366011,-28.9404760071868,
53.7143043543697));
#109474=CARTESIAN_POINT('Ctrl Pts',(8.22301296868687,-28.9256332769151,
53.7266404597789));
#109475=CARTESIAN_POINT('Ctrl Pts',(8.22386202866696,-28.9162283592018,
53.7346354744026));
#109476=CARTESIAN_POINT('Ctrl Pts',(8.22585938682102,-28.8944727698386,
53.7535501195441));
#109477=CARTESIAN_POINT('Ctrl Pts',(8.2270123840631,-28.8821937710913,53.7645498995407));
#109478=CARTESIAN_POINT('Ctrl Pts',(8.23090034323011,-28.841655072139,53.8019643995563));
#109479=CARTESIAN_POINT('Ctrl Pts',(8.23367343440232,-28.8141536174004,
53.8291796650484));
#109480=CARTESIAN_POINT('Ctrl Pts',(8.24157336144965,-28.7391808075946,
53.9087255738542));
#109481=CARTESIAN_POINT('Ctrl Pts',(8.2467414030818,-28.6940535625495,53.963154351128));
#109482=CARTESIAN_POINT('Ctrl Pts',(8.25869913563055,-28.5969514253275,
54.0967067060545));
#109483=CARTESIAN_POINT('Ctrl Pts',(8.26541855150029,-28.5479806500927,
54.1777292059504));
#109484=CARTESIAN_POINT('Ctrl Pts',(8.27325579944305,-28.4973093277464,
54.2803649727449));
#109485=CARTESIAN_POINT('Ctrl Pts',(8.27461045852226,-28.4888011840107,
54.2984075061279));
#109486=CARTESIAN_POINT('Ctrl Pts',(8.27675545298924,-28.4757378446312,
54.3274507733873));
#109487=CARTESIAN_POINT('Ctrl Pts',(8.2775528893772,-28.4709732073057,54.3383545810277));
#109488=CARTESIAN_POINT('Ctrl Pts',(8.27906142254259,-28.4621374276909,
54.3591804461267));
#109489=CARTESIAN_POINT('Ctrl Pts',(8.27977322862785,-28.4580444945273,
54.3690925422433));
#109490=CARTESIAN_POINT('Ctrl Pts',(8.28139639334399,-28.4488888500594,
54.3918867243803));
#109491=CARTESIAN_POINT('Ctrl Pts',(8.28230556022336,-28.4438903496652,
54.4047938754036));
#109492=CARTESIAN_POINT('Ctrl Pts',(8.28515651846395,-28.428635215,54.4456920313092));
#109493=CARTESIAN_POINT('Ctrl Pts',(8.28707886797538,-28.4189683074252,
54.4738977536022));
#109494=CARTESIAN_POINT('Ctrl Pts',(8.2985133530453,-28.3654098926784,54.6450107049187));
#109495=CARTESIAN_POINT('Ctrl Pts',(8.3073877056156,-28.340162129873,54.793022665805));
#109496=CARTESIAN_POINT('Ctrl Pts',(8.31786221559161,-28.3343198191641,
54.961952380141));
#109497=CARTESIAN_POINT('Ctrl Pts',(8.3190804844051,-28.3339880886474,54.9814974401968));
#109498=CARTESIAN_POINT('Ctrl Pts',(8.32030899669651,-28.3340003265563,
55.0010431133336));
#109499=CARTESIAN_POINT('Ctrl Pts',(8.32030914920813,-28.3340003280773,
55.0010455397981));
#109500=CARTESIAN_POINT('Ctrl Pts',(8.32194769227677,-28.3340166884934,
55.0271147988701));
#109501=CARTESIAN_POINT('Ctrl Pts',(8.32360406721264,-28.3346449372721,
55.0531790113172));
#109502=CARTESIAN_POINT('Ctrl Pts',(8.32632093082785,-28.3366466934674,
55.09523022013));
#109503=CARTESIAN_POINT('Ctrl Pts',(8.3273651812665,-28.3376400610496,55.1112313189089));
#109504=CARTESIAN_POINT('Ctrl Pts',(8.32888511474766,-28.3394022593687,
55.1342416033686));
#109505=CARTESIAN_POINT('Ctrl Pts',(8.32935147437191,-28.3399849547518,
55.1412646790038));
#109506=CARTESIAN_POINT('Ctrl Pts',(8.33019846042677,-28.3411183219608,
55.1539477710566));
#109507=CARTESIAN_POINT('Ctrl Pts',(8.33057825232876,-28.3416534540907,
55.1596091138152));
#109508=CARTESIAN_POINT('Ctrl Pts',(8.33136428957251,-28.3428159595042,
55.1712700941568));
#109509=CARTESIAN_POINT('Ctrl Pts',(8.33177075129179,-28.3434469360366,
55.1772690925057));
#109510=CARTESIAN_POINT('Ctrl Pts',(8.33271291659901,-28.3449781720149,
55.1911046033392));
#109511=CARTESIAN_POINT('Ctrl Pts',(8.333249858305,-28.3459015212706,55.198938274101));
#109512=CARTESIAN_POINT('Ctrl Pts',(8.33496701273572,-28.3490158297965,
55.2238376865618));
#109513=CARTESIAN_POINT('Ctrl Pts',(8.3361576887361,-28.3514154721163,55.2408755639152));
#109514=CARTESIAN_POINT('Ctrl Pts',(8.34123777236479,-28.3626743593439,
55.3127376448182));
#109515=CARTESIAN_POINT('Ctrl Pts',(8.34522556615071,-28.3740075307818,
55.367134152179));
#109516=CARTESIAN_POINT('Ctrl Pts',(8.35316767324996,-28.4016930087281,
55.4731747815175));
#109517=CARTESIAN_POINT('Ctrl Pts',(8.35711500669199,-28.4178890354192,
55.5247884022205));
#109518=CARTESIAN_POINT('Ctrl Pts',(8.36103879467171,-28.436562302838,55.5755159138484));
#109519=CARTESIAN_POINT('Ctrl Pts',(8.16625309736762,-28.4365623102018,
55.5755159338529));
#109520=CARTESIAN_POINT('Ctrl Pts',(8.16546900852282,-28.4324787476223,
55.5644225908714));
#109521=CARTESIAN_POINT('Ctrl Pts',(8.1646888611418,-28.4285132831813,55.5532858653556));
#109522=CARTESIAN_POINT('Ctrl Pts',(8.16260809123437,-28.4182030219882,
55.5233248429461));
#109523=CARTESIAN_POINT('Ctrl Pts',(8.16131463944129,-28.4120756698158,
55.5044273457766));
#109524=CARTESIAN_POINT('Ctrl Pts',(8.15400401417909,-28.3791017214555,
55.396169449892));
#109525=CARTESIAN_POINT('Ctrl Pts',(8.14822704388146,-28.3594599777026,
55.3047836788268));
#109526=CARTESIAN_POINT('Ctrl Pts',(8.13814302729113,-28.3384785387546,
55.1414169046907));
#109527=CARTESIAN_POINT('Ctrl Pts',(8.13381646698004,-28.3339455089076,
55.0701010364793));
#109528=CARTESIAN_POINT('Ctrl Pts',(8.12585889475046,-28.3340444862641,
54.9416043726171));
#109529=CARTESIAN_POINT('Ctrl Pts',(8.12226602372084,-28.3370252731339,
54.8845381314829));
#109530=CARTESIAN_POINT('Ctrl Pts',(8.1177519470481,-28.344165103434,54.8158541310242));
#109531=CARTESIAN_POINT('Ctrl Pts',(8.11696448188888,-28.3455290147279,
54.8039779490404));
#109532=CARTESIAN_POINT('Ctrl Pts',(8.11571331928025,-28.3478785654863,
54.7852954409316));
#109533=CARTESIAN_POINT('Ctrl Pts',(8.11525418418712,-28.348778782158,54.7784785166936));
#109534=CARTESIAN_POINT('Ctrl Pts',(8.11438523257934,-28.3505530710785,
54.7656547984055));
#109535=CARTESIAN_POINT('Ctrl Pts',(8.11397592984726,-28.3514178051278,
54.7596469539634));
#109536=CARTESIAN_POINT('Ctrl Pts',(8.11299942379024,-28.3535496628824,
54.7453886020238));
#109537=CARTESIAN_POINT('Ctrl Pts',(8.11243063921369,-28.3548459875767,
54.7371427296385));
#109538=CARTESIAN_POINT('Ctrl Pts',(8.11048097973005,-28.3594762245311,
54.7090668706257));
#109539=CARTESIAN_POINT('Ctrl Pts',(8.10908530369263,-28.3631070215134,
54.6892885073624));
#109540=CARTESIAN_POINT('Ctrl Pts',(8.10557743963958,-28.3730293277662,
54.6402531092369));
#109541=CARTESIAN_POINT('Ctrl Pts',(8.10344877244855,-28.3797527453266,
54.611091244009));
#109542=CARTESIAN_POINT('Ctrl Pts',(8.09308103662054,-28.4159849388838,
54.4712560593727));
#109543=CARTESIAN_POINT('Ctrl Pts',(8.08463856667436,-28.4560691427194,
54.3636401338143));
#109544=CARTESIAN_POINT('Ctrl Pts',(8.0716448370268,-28.536633554827,54.200866850913));
#109545=CARTESIAN_POINT('Ctrl Pts',(8.06693618316653,-28.5699937877662,
54.1425972712099));
#109546=CARTESIAN_POINT('Ctrl Pts',(8.06106916973828,-28.6170649074812,
54.0708077405523));
#109547=CARTESIAN_POINT('Ctrl Pts',(8.05979720519407,-28.6276128114538,
54.0552983646907));
#109548=CARTESIAN_POINT('Ctrl Pts',(8.05775156035253,-28.6451301183857,
54.0304541433732));
#109549=CARTESIAN_POINT('Ctrl Pts',(8.0569718895653,-28.6519392106594,54.0210088435764));
#109550=CARTESIAN_POINT('Ctrl Pts',(8.05547692155473,-28.6652490759773,
54.002948131386));
#109551=CARTESIAN_POINT('Ctrl Pts',(8.05476112505549,-28.6717356194537,
53.9943230127946));
#109552=CARTESIAN_POINT('Ctrl Pts',(8.05309978540135,-28.68705348084,53.9743617038643));
#109553=CARTESIAN_POINT('Ctrl Pts',(8.05215681150299,-28.6959486521331,
53.9630754221371));
#109554=CARTESIAN_POINT('Ctrl Pts',(8.04907207461392,-28.7256970358459,
53.9263187373103));
#109555=CARTESIAN_POINT('Ctrl Pts',(8.04695474220814,-28.74715985946,53.901350232345));
#109556=CARTESIAN_POINT('Ctrl Pts',(8.04187226865597,-28.8010614640508,
53.8422799211189));
#109557=CARTESIAN_POINT('Ctrl Pts',(8.0389360108893,-28.8342326158722,53.8088844385573));
#109558=CARTESIAN_POINT('Ctrl Pts',(8.03183109091855,-28.9186875411587,
53.7307711687195));
#109559=CARTESIAN_POINT('Ctrl Pts',(8.02770383609716,-28.9713794343182,
53.6877049174311));
#109560=CARTESIAN_POINT('Ctrl Pts',(8.02330844259633,-29.0296581024667,
53.6457447752059));
#109561=CARTESIAN_POINT('Ctrl Pts',(8.0230743735086,-29.0327679287627,53.6435219381598));
#109562=CARTESIAN_POINT('Ctrl Pts',(8.01786334683111,-29.102133579534,53.5943006808269));
#109563=CARTESIAN_POINT('Ctrl Pts',(8.01284061693164,-29.171722824896,53.5522057810508));
#109564=CARTESIAN_POINT('Ctrl Pts',(8.00673017319034,-29.2550980487812,
53.509755191596));
#109565=CARTESIAN_POINT('Ctrl Pts',(8.00591726795293,-29.2661646092712,
53.5042747233868));
#109566=CARTESIAN_POINT('Ctrl Pts',(8.0046345438046,-29.2835660683993,53.4958966355738));
#109567=CARTESIAN_POINT('Ctrl Pts',(8.00416967275482,-29.2898602135499,
53.4929147374727));
#109568=CARTESIAN_POINT('Ctrl Pts',(8.00329649269078,-29.3016551582643,
53.4874170868999));
#109569=CARTESIAN_POINT('Ctrl Pts',(8.00288877162436,-29.3071511989961,
53.4848917130128));
#109570=CARTESIAN_POINT('Ctrl Pts',(8.00192502043843,-29.3201169499807,
53.4790193832166));
#109571=CARTESIAN_POINT('Ctrl Pts',(8.00136752728035,-29.3275977051412,
53.4756974889465));
#109572=CARTESIAN_POINT('Ctrl Pts',(7.99949738824004,-29.3526376119806,
53.4647984903462));
#109573=CARTESIAN_POINT('Ctrl Pts',(7.9981714647494,-29.3703019991891,53.4574689348044));
#109574=CARTESIAN_POINT('Ctrl Pts',(7.99487755470649,-29.4140572537097,
53.4401901756449));
#109575=CARTESIAN_POINT('Ctrl Pts',(7.99289538147933,-29.4402791342934,
53.430589930077));
#109576=CARTESIAN_POINT('Ctrl Pts',(7.98391882243183,-29.5590100201079,
53.3904746396749));
#109577=CARTESIAN_POINT('Ctrl Pts',(7.97675833426756,-29.6538472536567,
53.3674490779349));
#109578=CARTESIAN_POINT('Ctrl Pts',(7.96353290311014,-29.8349647461463,
53.3399765506513));
#109579=CARTESIAN_POINT('Ctrl Pts',(7.9574569470784,-29.9206536848369,53.3336798741204));
#109580=CARTESIAN_POINT('Ctrl Pts',(7.95023689186184,-30.0261430299179,
53.3340888309023));
#109581=CARTESIAN_POINT('Ctrl Pts',(7.94890036541021,-30.0458252244153,
53.3345140085225));
#109582=CARTESIAN_POINT('Ctrl Pts',(7.94677727012515,-30.0773277297797,
53.3357534352295));
#109583=CARTESIAN_POINT('Ctrl Pts',(7.94598384871292,-30.0891544006187,
53.3363450743846));
#109584=CARTESIAN_POINT('Ctrl Pts',(7.94447878517693,-30.1116868932502,
53.3377132538303));
#109585=CARTESIAN_POINT('Ctrl Pts',(7.94376647780302,-30.1223934302214,
53.3384672600128));
#109586=CARTESIAN_POINT('Ctrl Pts',(7.9421364137043,-30.1469869957855,53.3404382717573));
#109587=CARTESIAN_POINT('Ctrl Pts',(7.94122092039929,-30.1608676543762,
53.341726221602));
#109588=CARTESIAN_POINT('Ctrl Pts',(7.93832647686448,-30.2049499915313,
53.346375238147));
#109589=CARTESIAN_POINT('Ctrl Pts',(7.93636785511698,-30.2350776469022,
53.3503885194899));
#109590=CARTESIAN_POINT('Ctrl Pts',(7.93174789312771,-30.3066445631736,
53.3619225973425));
#109591=CARTESIAN_POINT('Ctrl Pts',(7.92910859949375,-30.347941924589,53.3701947190784));
#109592=CARTESIAN_POINT('Ctrl Pts',(7.92182837098411,-30.4620845980504,
53.3975952578798));
#109593=CARTESIAN_POINT('Ctrl Pts',(7.91726071798911,-30.5340105435723,
53.4201087854077));
#109594=CARTESIAN_POINT('Ctrl Pts',(7.9118254931315,-30.6167923712374,53.4523221719086));
#109595=CARTESIAN_POINT('Ctrl Pts',(7.91099547021895,-30.6293555933179,
53.457388247056));
#109596=CARTESIAN_POINT('Ctrl Pts',(7.90567971731644,-30.7092000568921,
53.4907229951963));
#109597=CARTESIAN_POINT('Ctrl Pts',(7.90114106778398,-30.7746162459226,
53.523230287453));
#109598=CARTESIAN_POINT('Ctrl Pts',(7.89557346532666,-30.848291891667,53.5660866426888));
#109599=CARTESIAN_POINT('Ctrl Pts',(7.89476541350128,-30.8588325425529,
53.572374947034));
#109600=CARTESIAN_POINT('Ctrl Pts',(7.89348870806266,-30.8752295279517,
53.5824043072435));
#109601=CARTESIAN_POINT('Ctrl Pts',(7.89302492773093,-30.8811338146683,
53.5860666667068));
#109602=CARTESIAN_POINT('Ctrl Pts',(7.89215257845308,-30.8921380957446,
53.592988184354));
#109603=CARTESIAN_POINT('Ctrl Pts',(7.8917445835153,-30.8972434608367,53.5962383398328));
#109604=CARTESIAN_POINT('Ctrl Pts',(7.8907785278172,-30.9092364130671,53.6039653921374));
#109605=CARTESIAN_POINT('Ctrl Pts',(7.89021898252295,-30.9161087216678,
53.608465492986));
#109606=CARTESIAN_POINT('Ctrl Pts',(7.88833458111314,-30.9390152971421,
53.6237083245001));
#109607=CARTESIAN_POINT('Ctrl Pts',(7.88699618031173,-30.9548954524501,
53.6346783895893));
#109608=CARTESIAN_POINT('Ctrl Pts',(7.88366431575138,-30.9935617605602,
53.6623937403691));
#109609=CARTESIAN_POINT('Ctrl Pts',(7.88165627098331,-31.0161185989506,
53.6794477328594));
#109610=CARTESIAN_POINT('Ctrl Pts',(7.87245368756215,-31.1165619573282,
53.7594849891748));
#109611=CARTESIAN_POINT('Ctrl Pts',(7.86508684248383,-31.1891057293026,
53.8288398422448));
#109612=CARTESIAN_POINT('Ctrl Pts',(7.85191064094459,-31.309292669304,53.9664972289344));
#109613=CARTESIAN_POINT('Ctrl Pts',(7.84606992941473,-31.3589102415018,
54.0326624554777));
#109614=CARTESIAN_POINT('Ctrl Pts',(7.83907562884825,-31.4139849812364,
54.1187584011698));
#109615=CARTESIAN_POINT('Ctrl Pts',(7.83774475576899,-31.4242565806027,
54.135457616866));
#109616=CARTESIAN_POINT('Ctrl Pts',(7.83562843921193,-31.4402473031941,
54.1625135808108));
#109617=CARTESIAN_POINT('Ctrl Pts',(7.83483622039832,-31.4461547662397,
54.172756262495));
#109618=CARTESIAN_POINT('Ctrl Pts',(7.8333320926736,-31.4572177774492,54.1924186537517));
#109619=CARTESIAN_POINT('Ctrl Pts',(7.8326195326189,-31.4623922532045,54.2018269681982));
#109620=CARTESIAN_POINT('Ctrl Pts',(7.83098699700206,-31.4740909391633,
54.2235934259987));
#109621=CARTESIAN_POINT('Ctrl Pts',(7.83006930914324,-31.4805513999805,
54.235985054596));
#109622=CARTESIAN_POINT('Ctrl Pts',(7.82716001290008,-31.5006516964904,
54.2757515434737));
#109623=CARTESIAN_POINT('Ctrl Pts',(7.82518903873379,-31.5136944720293,
54.3034222409728));
#109624=CARTESIAN_POINT('Ctrl Pts',(7.82053367074762,-31.543014066843,54.3703431421876));
#109625=CARTESIAN_POINT('Ctrl Pts',(7.81787180813912,-31.5585660890979,
54.4098878968463));
#109626=CARTESIAN_POINT('Ctrl Pts',(7.81066718564559,-31.5969304771628,
54.519578706459));
#109627=CARTESIAN_POINT('Ctrl Pts',(7.80619213276827,-31.6166246125156,
54.5907118408678));
#109628=CARTESIAN_POINT('Ctrl Pts',(7.80083998974719,-31.6343260681113,
54.67638973737));
#109629=CARTESIAN_POINT('Ctrl Pts',(7.79999712957875,-31.6369428261872,
54.6898976345195));
#109630=CARTESIAN_POINT('Ctrl Pts',(7.79462853320518,-31.6525019294607,
54.7759077140508));
#109631=CARTESIAN_POINT('Ctrl Pts',(7.79005037438479,-31.6607903231339,
54.8491599059464));
#109632=CARTESIAN_POINT('Ctrl Pts',(7.78443891600197,-31.6647757171713,
54.9349729018631));
#109633=CARTESIAN_POINT('Ctrl Pts',(7.78363070096398,-31.6652096702806,
54.9472416430588));
#109634=CARTESIAN_POINT('Ctrl Pts',(7.78235379315276,-31.665676847285,54.9664601280206));
#109635=CARTESIAN_POINT('Ctrl Pts',(7.78188997616242,-31.6658022439129,
54.9734074748025));
#109636=CARTESIAN_POINT('Ctrl Pts',(7.78101759921209,-31.6659555402362,
54.9864070727862));
#109637=CARTESIAN_POINT('Ctrl Pts',(7.78060961373072,-31.6659939248547,
54.9924589532505));
#109638=CARTESIAN_POINT('Ctrl Pts',(7.77964363661456,-31.6660066763997,
55.0067245017045));
#109639=CARTESIAN_POINT('Ctrl Pts',(7.77908416117705,-31.6659532755312,
55.014937918535));
#109640=CARTESIAN_POINT('Ctrl Pts',(7.77720024656801,-31.6655710354316,
55.0424428808545));
#109641=CARTESIAN_POINT('Ctrl Pts',(7.77586227187023,-31.6649678121603,
55.0617282543878));
#109642=CARTESIAN_POINT('Ctrl Pts',(7.77253170571016,-31.6626557677863,
55.1092272434393));
#109643=CARTESIAN_POINT('Ctrl Pts',(7.77052454681614,-31.6605636233287,
55.1374156667221));
#109644=CARTESIAN_POINT('Ctrl Pts',(7.76132982361888,-31.6478131991142,
55.2651047806643));
#109645=CARTESIAN_POINT('Ctrl Pts',(7.75397016803103,-31.6289206569506,
55.3635750560071));
#109646=CARTESIAN_POINT('Ctrl Pts',(7.740792332311,-31.5784866574934,55.5392340574848));
#109647=CARTESIAN_POINT('Ctrl Pts',(7.73494352861573,-31.5497793390555,
55.6169126425103));
#109648=CARTESIAN_POINT('Ctrl Pts',(7.72794141551738,-31.5072707847691,
55.7099825307644));
#109649=CARTESIAN_POINT('Ctrl Pts',(7.72661031233688,-31.4988107101176,
55.7276722647103));
#109650=CARTESIAN_POINT('Ctrl Pts',(7.72449371985725,-31.484750962785,55.7557846200141));
#109651=CARTESIAN_POINT('Ctrl Pts',(7.72370145208496,-31.4793493633843,
55.7663036518721));
#109652=CARTESIAN_POINT('Ctrl Pts',(7.72219728644031,-31.4688301486798,
55.7862628518513));
#109653=CARTESIAN_POINT('Ctrl Pts',(7.72148473684885,-31.4637323889801,
55.7957127500098));
#109654=CARTESIAN_POINT('Ctrl Pts',(7.71985230273546,-31.4517912495304,
55.8173453330737));
#109655=CARTESIAN_POINT('Ctrl Pts',(7.71893470491997,-31.4448851897696,
55.8294926363736));
#109656=CARTESIAN_POINT('Ctrl Pts',(7.71602601921615,-31.4223823722624,
55.8679396485503));
#109657=CARTESIAN_POINT('Ctrl Pts',(7.71405555293017,-31.4062135939717,
55.893898407259));
#109658=CARTESIAN_POINT('Ctrl Pts',(7.70940164256252,-31.3659066215379,
55.9548078123419));
#109659=CARTESIAN_POINT('Ctrl Pts',(7.70674070961701,-31.341128450423,55.9893097167809));
#109660=CARTESIAN_POINT('Ctrl Pts',(7.69953660653275,-31.2697905595201,
56.0810292800917));
#109661=CARTESIAN_POINT('Ctrl Pts',(7.69506120270623,-31.2207087286931,
56.1361614923766));
#109662=CARTESIAN_POINT('Ctrl Pts',(7.68971382987555,-31.1583853663143,
56.1974499424351));
#109663=CARTESIAN_POINT('Ctrl Pts',(7.68887606729939,-31.1485170256714,
56.2069182481364));
#109664=CARTESIAN_POINT('Ctrl Pts',(7.68350636732053,-31.0846905780033,
56.2666655909917));
#109665=CARTESIAN_POINT('Ctrl Pts',(7.67892205130089,-31.0275669466909,
56.3134301586142));
#109666=CARTESIAN_POINT('Ctrl Pts',(7.67330375513987,-30.9575480283627,
56.3633812727313));
#109667=CARTESIAN_POINT('Ctrl Pts',(7.67249551524096,-30.9474755745075,
56.3704002099435));
#109668=CARTESIAN_POINT('Ctrl Pts',(7.67121857658665,-30.9315822833227,
56.3812163962233));
#109669=CARTESIAN_POINT('Ctrl Pts',(7.67075475399479,-30.9258134552311,
56.3850897897023));
#109670=CARTESIAN_POINT('Ctrl Pts',(7.66988237278712,-30.9149750155157,
56.3922691372242));
#109671=CARTESIAN_POINT('Ctrl Pts',(7.66947438872151,-30.9099114027328,
56.3955837001008));
#109672=CARTESIAN_POINT('Ctrl Pts',(7.66850842349245,-30.8979333566605,
56.4033314466776));
#109673=CARTESIAN_POINT('Ctrl Pts',(7.66794895863715,-30.891004075234,56.407741166936));
#109674=CARTESIAN_POINT('Ctrl Pts',(7.66606511783465,-30.8676895567504,
56.4223371858038));
#109675=CARTESIAN_POINT('Ctrl Pts',(7.66472720775049,-30.8511607041876,
56.4322896401871));
#109676=CARTESIAN_POINT('Ctrl Pts',(7.66139683848214,-30.810003199556,56.4561076559533));
#109677=CARTESIAN_POINT('Ctrl Pts',(7.65938981392534,-30.7851878409481,
56.4696375618476));
#109678=CARTESIAN_POINT('Ctrl Pts',(7.65019628198844,-30.6710101870318,
56.5281725370147));
#109679=CARTESIAN_POINT('Ctrl Pts',(7.64283771594158,-30.5780486528418,
56.5657030917546));
#109680=CARTESIAN_POINT('Ctrl Pts',(7.62965963226652,-30.4031158893757,
56.6186086127721));
#109681=CARTESIAN_POINT('Ctrl Pts',(7.6238096017832,-30.3222688212911,56.636625425118));
#109682=CARTESIAN_POINT('Ctrl Pts',(7.61680630458279,-30.2210046219497,
56.6513925606158));
#109683=CARTESIAN_POINT('Ctrl Pts',(7.61547516674784,-30.2015537731965,
56.6538792476108));
#109684=CARTESIAN_POINT('Ctrl Pts',(7.61335853269813,-30.1703092579291,
56.6573142648629));
#109685=CARTESIAN_POINT('Ctrl Pts',(7.61256625753809,-30.1585420226049,
56.658481309934));
#109686=CARTESIAN_POINT('Ctrl Pts',(7.61106208614438,-30.1360681069418,
56.6604688336651));
#109687=CARTESIAN_POINT('Ctrl Pts',(7.61034953810482,-30.1253640212102,
56.6613112738711));
#109688=CARTESIAN_POINT('Ctrl Pts',(7.60871711920563,-30.1007133393514,
56.6630117387076));
#109689=CARTESIAN_POINT('Ctrl Pts',(7.60779953490273,-30.0867624737311,
56.6637979182151));
#109690=CARTESIAN_POINT('Ctrl Pts',(7.60489094090366,-30.0422581709076,
56.6657445840105));
#109691=CARTESIAN_POINT('Ctrl Pts',(7.6029205509142,-30.0116809387551,56.6662396333481));
#109692=CARTESIAN_POINT('Ctrl Pts',(7.59826685952555,-29.9386507725836,
56.6654113403378));
#109693=CARTESIAN_POINT('Ctrl Pts',(7.59560606624645,-29.8962277386669,
56.6633070543167));
#109694=CARTESIAN_POINT('Ctrl Pts',(7.58840204249181,-29.7804804725137,
56.6531193737223));
#109695=CARTESIAN_POINT('Ctrl Pts',(7.58392658717963,-29.7075404125967,
56.6417856876531));
#109696=CARTESIAN_POINT('Ctrl Pts',(7.57445468397707,-29.5564589046027,
56.6079190951));
#109697=CARTESIAN_POINT('Ctrl Pts',(7.56946275296196,-29.4787368325959,
56.5844286264686));
#109698=CARTESIAN_POINT('Ctrl Pts',(7.56316352201244,-29.3879867527561,
56.5495986265538));
#109699=CARTESIAN_POINT('Ctrl Pts',(7.56210821029538,-29.3730148709698,
56.5436015416121));
#109700=CARTESIAN_POINT('Ctrl Pts',(7.5605270577653,-29.3509701531688,56.5343977675635));
#109701=CARTESIAN_POINT('Ctrl Pts',(7.56001051929912,-29.3438283773067,
56.5313572564199));
#109702=CARTESIAN_POINT('Ctrl Pts',(7.55908877903474,-29.3311961112442,
56.5258746560235));
#109703=CARTESIAN_POINT('Ctrl Pts',(7.55868477604811,-29.3256972062326,
56.523452607614));
#109704=CARTESIAN_POINT('Ctrl Pts',(7.55778911525175,-29.3135907342639,
56.5180418007835));
#109705=CARTESIAN_POINT('Ctrl Pts',(7.55729669037934,-29.3069896099765,
56.5150396639586));
#109706=CARTESIAN_POINT('Ctrl Pts',(7.55584129356492,-29.2876340401669,
56.5060839487491));
#109707=CARTESIAN_POINT('Ctrl Pts',(7.55487165208585,-29.2749355656764,
56.5000118848959));
#109708=CARTESIAN_POINT('Ctrl Pts',(7.54806860581032,-29.1871007072822,
56.456635774672));
#109709=CARTESIAN_POINT('Ctrl Pts',(7.54198189040395,-29.1148057167452,
56.4138674778945));
#109710=CARTESIAN_POINT('Ctrl Pts',(7.52652509404827,-28.9406920829547,
56.292260316728));
#109711=CARTESIAN_POINT('Ctrl Pts',(7.51721417737031,-28.8441848903718,
56.2067200671039));
#109712=CARTESIAN_POINT('Ctrl Pts',(7.50692684856819,-28.744471106177,56.095282386431));
#109713=CARTESIAN_POINT('Ctrl Pts',(7.50549531179536,-28.7307750450062,
56.0793814860348));
#109714=CARTESIAN_POINT('Ctrl Pts',(7.50317533137304,-28.7088834736268,
56.0529726812225));
#109715=CARTESIAN_POINT('Ctrl Pts',(7.5022796488648,-28.7005074940628,56.0426181453256));
#109716=CARTESIAN_POINT('Ctrl Pts',(7.50067542772868,-28.6856467537763,
56.0237897050599));
#109717=CARTESIAN_POINT('Ctrl Pts',(7.49996514494438,-28.6791176127512,
56.0153519311982));
#109718=CARTESIAN_POINT('Ctrl Pts',(7.49844864434826,-28.6652894490124,
55.9971222991381));
#109719=CARTESIAN_POINT('Ctrl Pts',(7.4976434587183,-28.6580160994207,55.9873116824316));
#109720=CARTESIAN_POINT('Ctrl Pts',(7.49543584894414,-28.638271690347,55.9600581991023));
#109721=CARTESIAN_POINT('Ctrl Pts',(7.49404214718164,-28.6260282016741,
55.9424528107725));
#109722=CARTESIAN_POINT('Ctrl Pts',(7.48818262791022,-28.575570571396,55.8668236908045));
#109723=CARTESIAN_POINT('Ctrl Pts',(7.483837667993,-28.540663753194,55.8066733054715));
#109724=CARTESIAN_POINT('Ctrl Pts',(7.47576624225721,-28.4821501698588,
55.6895391101249));
#109725=CARTESIAN_POINT('Ctrl Pts',(7.47203392693749,-28.4577667277519,
55.6331195097459));
#109726=CARTESIAN_POINT('Ctrl Pts',(7.4682788092303,-28.4365623654365,55.5755160839024));
#109727=CARTESIAN_POINT('Origin',(5.,-30.,55.));
#109728=CARTESIAN_POINT('',(6.76892552105682,-28.4365623357949,55.5755160033788));
#109729=CARTESIAN_POINT('',(6.96168426276526,-28.4365622954254,55.5755158937115));
#109730=CARTESIAN_POINT('',(5.,-28.4365623102018,55.5755159338528));
#109731=CARTESIAN_POINT('Ctrl Pts',(6.96168426276526,-28.4365622954254,
55.5755158937115));
#109732=CARTESIAN_POINT('Ctrl Pts',(6.96621518142781,-28.4616675932655,
55.6437165631571));
#109733=CARTESIAN_POINT('Ctrl Pts',(6.97064208339495,-28.4912153733055,
55.7102200871842));
#109734=CARTESIAN_POINT('Ctrl Pts',(6.98045131201361,-28.5658855718998,
55.8524056583878));
#109735=CARTESIAN_POINT('Ctrl Pts',(6.98582286381548,-28.6128348680477,
55.9268489312456));
#109736=CARTESIAN_POINT('Ctrl Pts',(6.99273224835812,-28.6769889517844,
56.0127046830646));
#109737=CARTESIAN_POINT('Ctrl Pts',(6.9939911449183,-28.6888171338552,56.0279729676906));
#109738=CARTESIAN_POINT('Ctrl Pts',(6.99581023495253,-28.7060527208452,
56.0494398416683));
#109739=CARTESIAN_POINT('Ctrl Pts',(6.99635636275573,-28.7112452400216,
56.0558099753933));
#109740=CARTESIAN_POINT('Ctrl Pts',(6.99731062774461,-28.7203444544684,
56.0668056713412));
#109741=CARTESIAN_POINT('Ctrl Pts',(6.99771723422941,-28.7242295780451,
56.0714487784013));
#109742=CARTESIAN_POINT('Ctrl Pts',(6.99859466467693,-28.7326289929784,
56.0813764524015));
#109743=CARTESIAN_POINT('Ctrl Pts',(6.99906601418982,-28.7371509997338,
56.0866539004525));
#109744=CARTESIAN_POINT('Ctrl Pts',(7.00037624838465,-28.749751868468,56.1011749736396));
#109745=CARTESIAN_POINT('Ctrl Pts',(7.00121987943293,-28.7578998983068,
56.1103576127689));
#109746=CARTESIAN_POINT('Ctrl Pts',(7.00712258834165,-28.8151970859454,
56.173510313324));
#109747=CARTESIAN_POINT('Ctrl Pts',(7.01238275956817,-28.8677406511134,
56.2242837933754));
#109748=CARTESIAN_POINT('Ctrl Pts',(7.01866998297382,-28.9337897989067,
56.2802092961043));
#109749=CARTESIAN_POINT('Ctrl Pts',(7.01965683970123,-28.9442495711575,
56.2888487355971));
#109750=CARTESIAN_POINT('Ctrl Pts',(7.02605497037705,-29.0127083006775,
56.3440008618084));
#109751=CARTESIAN_POINT('Ctrl Pts',(7.03146755548613,-29.0736637822695,
56.3867176214096));
#109752=CARTESIAN_POINT('Ctrl Pts',(7.03981425682617,-29.1737129336764,
56.4472802831541));
#109753=CARTESIAN_POINT('Ctrl Pts',(7.04281780370092,-29.2109888247271,
56.4679347412167));
#109754=CARTESIAN_POINT('Ctrl Pts',(7.04790219938002,-29.2763767610055,
56.5009546190904));
#109755=CARTESIAN_POINT('Ctrl Pts',(7.05000465795058,-29.304112765303,56.5140133855634));
#109756=CARTESIAN_POINT('Ctrl Pts',(7.05302861890522,-29.3450098454189,
56.5319071632787));
#109757=CARTESIAN_POINT('Ctrl Pts',(7.05397064568387,-29.3578951848249,
56.5373526227106));
#109758=CARTESIAN_POINT('Ctrl Pts',(7.05562634932108,-29.3807941633213,
56.5466917968988));
#109759=CARTESIAN_POINT('Ctrl Pts',(7.05634223797634,-29.3907795927555,
56.5506520845949));
#109760=CARTESIAN_POINT('Ctrl Pts',(7.05783927153277,-29.4118344015886,
56.5587677843286));
#109761=CARTESIAN_POINT('Ctrl Pts',(7.05861969177156,-29.4229111546025,
56.5629025091999));
#109762=CARTESIAN_POINT('Ctrl Pts',(7.06068286589565,-29.452453973323,56.5735733301861));
#109763=CARTESIAN_POINT('Ctrl Pts',(7.06195875277496,-29.470993236278,56.5799023935795));
#109764=CARTESIAN_POINT('Ctrl Pts',(7.06855152141681,-29.5681014126966,
56.6111527766408));
#109765=CARTESIAN_POINT('Ctrl Pts',(7.07368575319151,-29.6483329508286,
56.6305466646248));
#109766=CARTESIAN_POINT('Ctrl Pts',(7.08491115739104,-29.828668763627,56.660200438404));
#109767=CARTESIAN_POINT('Ctrl Pts',(7.09094296923891,-29.9289195531927,
56.6675026571761));
#109768=CARTESIAN_POINT('Ctrl Pts',(7.09900513516252,-30.0575029425793,
56.6652477505995));
#109769=CARTESIAN_POINT('Ctrl Pts',(7.10079892255601,-30.0857757204209,
56.6640309505864));
#109770=CARTESIAN_POINT('Ctrl Pts',(7.10386785218044,-30.1332687369025,
56.6607734318758));
#109771=CARTESIAN_POINT('Ctrl Pts',(7.10512664904486,-30.1525099028869,
56.6591171145437));
#109772=CARTESIAN_POINT('Ctrl Pts',(7.1069456199482,-30.1798913003411,56.6562797644973));
#109773=CARTESIAN_POINT('Ctrl Pts',(7.10749173082356,-30.1880591027401,
56.6553722557459));
#109774=CARTESIAN_POINT('Ctrl Pts',(7.10844597672613,-30.2022318599154,
56.6536913043409));
#109775=CARTESIAN_POINT('Ctrl Pts',(7.1088525812426,-30.2082398547515,56.6529454972162));
#109776=CARTESIAN_POINT('Ctrl Pts',(7.1097300199277,-30.2211361800173,56.6512731733999));
#109777=CARTESIAN_POINT('Ctrl Pts',(7.11020137976753,-30.2280227138228,
56.6503363114462));
#109778=CARTESIAN_POINT('Ctrl Pts',(7.11151166998711,-30.2470575564767,
56.6476253497013));
#109779=CARTESIAN_POINT('Ctrl Pts',(7.11235534736275,-30.2591921405052,
56.6457600497577));
#109780=CARTESIAN_POINT('Ctrl Pts',(7.11827021345181,-30.3434985463762,
56.631845184428));
#109781=CARTESIAN_POINT('Ctrl Pts',(7.12354345524137,-30.414821449314,56.6151875278324));
#109782=CARTESIAN_POINT('Ctrl Pts',(7.12988609766378,-30.4983484276038,
56.5897814599893));
#109783=CARTESIAN_POINT('Ctrl Pts',(7.13091558348857,-30.5118337578577,
56.5854912318652));
#109784=CARTESIAN_POINT('Ctrl Pts',(7.13730938858278,-30.5952008931364,
56.5577943155168));
#109785=CARTESIAN_POINT('Ctrl Pts',(7.14267361662341,-30.6635246454671,
56.5299423479419));
#109786=CARTESIAN_POINT('Ctrl Pts',(7.15096898362861,-30.7680184096244,
56.4790242830641));
#109787=CARTESIAN_POINT('Ctrl Pts',(7.15396786626985,-30.8055290254171,
56.4589340628651));
#109788=CARTESIAN_POINT('Ctrl Pts',(7.15904533529387,-30.8686474719768,
56.421951084817));
#109789=CARTESIAN_POINT('Ctrl Pts',(7.1611454515922,-30.8946324639411,56.4057475898815));
#109790=CARTESIAN_POINT('Ctrl Pts',(7.16416672082881,-30.93181357247,56.3811136678013));
#109791=CARTESIAN_POINT('Ctrl Pts',(7.16510834657614,-30.943372104113,56.373244548908));
#109792=CARTESIAN_POINT('Ctrl Pts',(7.16676359793443,-30.9636323138791,
56.359074733226));
#109793=CARTESIAN_POINT('Ctrl Pts',(7.16747943125642,-30.9723745493317,
56.352833734036));
#109794=CARTESIAN_POINT('Ctrl Pts',(7.16897659545759,-30.9906137865963,
56.3395447625111));
#109795=CARTESIAN_POINT('Ctrl Pts',(7.16975719930146,-31.0000973623873,
56.3324793142298));
#109796=CARTESIAN_POINT('Ctrl Pts',(7.17182143522502,-31.025098045213,56.3134360309749));
#109797=CARTESIAN_POINT('Ctrl Pts',(7.17309818736336,-31.0404806551089,
56.3012840845532));
#109798=CARTESIAN_POINT('Ctrl Pts',(7.17969080504897,-31.119400282756,56.2366448120204));
#109799=CARTESIAN_POINT('Ctrl Pts',(7.18482411989755,-31.1791966486213,
56.1797648604262));
#109800=CARTESIAN_POINT('Ctrl Pts',(7.19604801789148,-31.301898830322,56.0443549800158));
#109801=CARTESIAN_POINT('Ctrl Pts',(7.20207925632942,-31.3623991066989,
55.9640976176675));
#109802=CARTESIAN_POINT('Ctrl Pts',(7.21014073276843,-31.4302373332694,
55.854855402271));
#109803=CARTESIAN_POINT('Ctrl Pts',(7.21193444353455,-31.4445484845188,
55.8304433054732));
#109804=CARTESIAN_POINT('Ctrl Pts',(7.2150032552912,-31.4675692333252,55.7887771989649));
#109805=CARTESIAN_POINT('Ctrl Pts',(7.21626201254865,-31.4766130971013,
55.7717140711922));
#109806=CARTESIAN_POINT('Ctrl Pts',(7.21808093612233,-31.4890796617931,
55.7471715314109));
#109807=CARTESIAN_POINT('Ctrl Pts',(7.21862704027083,-31.4927470977546,
55.7398172961326));
#109808=CARTESIAN_POINT('Ctrl Pts',(7.21958127858724,-31.4990215967239,
55.7269985609439));
#109809=CARTESIAN_POINT('Ctrl Pts',(7.21998788231997,-31.5016535251124,
55.7215464948521));
#109810=CARTESIAN_POINT('Ctrl Pts',(7.22086532427292,-31.507243053211,55.7098046792364));
#109811=CARTESIAN_POINT('Ctrl Pts',(7.22133668821244,-31.5101909861983,
55.7035108278614));
#109812=CARTESIAN_POINT('Ctrl Pts',(7.22264700068007,-31.518237332114,55.6860482045806));
#109813=CARTESIAN_POINT('Ctrl Pts',(7.22349069645405,-31.5232516753402,
55.6748414977552));
#109814=CARTESIAN_POINT('Ctrl Pts',(7.22941044138503,-31.5573139459685,
55.5964004568086));
#109815=CARTESIAN_POINT('Ctrl Pts',(7.2346889293594,-31.5820214166076,55.5273766125611));
#109816=CARTESIAN_POINT('Ctrl Pts',(7.24103312200397,-31.6059735451085,
55.44340027442));
#109817=CARTESIAN_POINT('Ctrl Pts',(7.24205896876814,-31.6096688516448,
55.4297918277798));
#109818=CARTESIAN_POINT('Ctrl Pts',(7.24844958324113,-31.6316006943965,
55.3447713906876));
#109819=CARTESIAN_POINT('Ctrl Pts',(7.25381422201391,-31.6452554597833,
55.2722570870789));
#109820=CARTESIAN_POINT('Ctrl Pts',(7.26210883717743,-31.6591440513098,
55.1568593254738));
#109821=CARTESIAN_POINT('Ctrl Pts',(7.26510662173684,-31.6626071101923,
55.1144636658827));
#109822=CARTESIAN_POINT('Ctrl Pts',(7.27018245977213,-31.6657667624,55.04139964646));
#109823=CARTESIAN_POINT('Ctrl Pts',(7.27228202438619,-31.6662462802018,
55.0107881790076));
#109824=CARTESIAN_POINT('Ctrl Pts',(7.27530265957547,-31.6657157551822,
54.96619937969));
#109825=CARTESIAN_POINT('Ctrl Pts',(7.27624419081851,-31.6653734541985,
54.9522219952471));
#109826=CARTESIAN_POINT('Ctrl Pts',(7.27789933561335,-31.6644571358084,
54.9275168560619));
#109827=CARTESIAN_POINT('Ctrl Pts',(7.27861515591332,-31.6639552387455,
54.9167874057729));
#109828=CARTESIAN_POINT('Ctrl Pts',(7.2801123509929,-31.6626827836571,54.8942558652585));
#109829=CARTESIAN_POINT('Ctrl Pts',(7.28089299817733,-31.66189024367,54.8824555776007));
#109830=CARTESIAN_POINT('Ctrl Pts',(7.28295748474491,-31.6594501587259,
54.8511191539172));
#109831=CARTESIAN_POINT('Ctrl Pts',(7.28423444113182,-31.6575832903937,
54.8316015924579));
#109832=CARTESIAN_POINT('Ctrl Pts',(7.2908340214254,-31.6460668721509,54.7301323310598));
#109833=CARTESIAN_POINT('Ctrl Pts',(7.29597358115768,-31.630682765215,54.6489431522947));
#109834=CARTESIAN_POINT('Ctrl Pts',(7.30719789076433,-31.5834295010451,
54.4724106234053));
#109835=CARTESIAN_POINT('Ctrl Pts',(7.31322386323513,-31.5488355934436,
54.3781435087354));
#109836=CARTESIAN_POINT('Ctrl Pts',(7.32127900734691,-31.4938894219803,
54.2619957108953));
#109837=CARTESIAN_POINT('Ctrl Pts',(7.32307201393636,-31.4811461754492,
54.236742663029));
#109838=CARTESIAN_POINT('Ctrl Pts',(7.32613974251045,-31.4586338393338,
54.1948192588194));
#109839=CARTESIAN_POINT('Ctrl Pts',(7.32739813576945,-31.4492060642606,
54.1779717714153));
#109840=CARTESIAN_POINT('Ctrl Pts',(7.3292166243775,-31.4353514814661,54.1541929029019));
#109841=CARTESIAN_POINT('Ctrl Pts',(7.32976266671018,-31.4311624149671,
54.1471238918628));
#109842=CARTESIAN_POINT('Ctrl Pts',(7.33071683533746,-31.4237964218145,
54.1349009288898));
#109843=CARTESIAN_POINT('Ctrl Pts',(7.33112343189134,-31.4206434164772,
54.1297328367203));
#109844=CARTESIAN_POINT('Ctrl Pts',(7.33200090396927,-31.413809917374,54.1186681503736));
#109845=CARTESIAN_POINT('Ctrl Pts',(7.3324723056546,-31.410120727729,54.1127774571996));
#109846=CARTESIAN_POINT('Ctrl Pts',(7.3337828228654,-31.3998120274257,54.096543812465));
#109847=CARTESIAN_POINT('Ctrl Pts',(7.33462668793699,-31.3931150106181,
54.086250942553));
#109848=CARTESIAN_POINT('Ctrl Pts',(7.34059242515841,-31.3453186346939,
54.0145380033295));
#109849=CARTESIAN_POINT('Ctrl Pts',(7.34592038894971,-31.3002901097811,
53.9558444632713));
#109850=CARTESIAN_POINT('Ctrl Pts',(7.35218794612908,-31.2433539942865,
53.8910455671176));
#109851=CARTESIAN_POINT('Ctrl Pts',(7.35308802366798,-31.2350838655923,
53.8818421704967));
#109852=CARTESIAN_POINT('Ctrl Pts',(7.36062545788623,-31.1650070666426,
53.8055834316504));
#109853=CARTESIAN_POINT('Ctrl Pts',(7.36725972676522,-31.097886844223,53.7436083656047));
#109854=CARTESIAN_POINT('Ctrl Pts',(7.37724821209399,-30.9865425254855,
53.6565710456839));
#109855=CARTESIAN_POINT('Ctrl Pts',(7.38073115976119,-30.9456835841416,
53.6275019235884));
#109856=CARTESIAN_POINT('Ctrl Pts',(7.38528285569322,-30.8895369049362,
53.5912561711071));
#109857=CARTESIAN_POINT('Ctrl Pts',(7.38641285185037,-30.875365759119,53.5824070034882));
#109858=CARTESIAN_POINT('Ctrl Pts',(7.38828856707251,-30.8514596660405,
53.5679740616524));
#109859=CARTESIAN_POINT('Ctrl Pts',(7.38903852978729,-30.8417973694629,
53.5622729569252));
#109860=CARTESIAN_POINT('Ctrl Pts',(7.3905102575756,-30.8226341482198,53.5512253846552));
#109861=CARTESIAN_POINT('Ctrl Pts',(7.39123218298962,-30.8131368882363,
53.5458737199049));
#109862=CARTESIAN_POINT('Ctrl Pts',(7.39281935311893,-30.7920466236917,
53.5342606902959));
#109863=CARTESIAN_POINT('Ctrl Pts',(7.39368302601269,-30.7804304172427,
53.5280428136756));
#109864=CARTESIAN_POINT('Ctrl Pts',(7.39663601617687,-30.7402478366114,
53.5071434600193));
#109865=CARTESIAN_POINT('Ctrl Pts',(7.39870152466308,-30.7113303486268,
53.4931500212548));
#109866=CARTESIAN_POINT('Ctrl Pts',(7.40872301150565,-30.5674845587046,
53.4286063155227));
#109867=CARTESIAN_POINT('Ctrl Pts',(7.41626853170064,-30.447504509216,53.390323535924));
#109868=CARTESIAN_POINT('Ctrl Pts',(7.42712522636434,-30.2740500514831,
53.3558944230957));
#109869=CARTESIAN_POINT('Ctrl Pts',(7.43030053923293,-30.2233114199783,
53.3482379541306));
#109870=CARTESIAN_POINT('Ctrl Pts',(7.43481324112559,-30.1527098241845,
53.3408966854821));
#109871=CARTESIAN_POINT('Ctrl Pts',(7.43607791719862,-30.133081537075,53.3392070170325));
#109872=CARTESIAN_POINT('Ctrl Pts',(7.43831679471423,-30.0987175930176,
53.336861922427));
#109873=CARTESIAN_POINT('Ctrl Pts',(7.43928397423673,-30.0839942976495,
53.3360533813809));
#109874=CARTESIAN_POINT('Ctrl Pts',(7.44075105084913,-30.0618818367307,
53.3351332750675));
#109875=CARTESIAN_POINT('Ctrl Pts',(7.4412432940879,-30.0544990499121,53.3348752533596));
#109876=CARTESIAN_POINT('Ctrl Pts',(7.44214056586419,-30.0411133774042,
53.3344965511557));
#109877=CARTESIAN_POINT('Ctrl Pts',(7.44254467559746,-30.0351112299551,
53.3343592085464));
#109878=CARTESIAN_POINT('Ctrl Pts',(7.44346500644764,-30.0215015784999,
53.3341213837841));
#109879=CARTESIAN_POINT('Ctrl Pts',(7.44398226414735,-30.0138940923868,
53.334040567615));
#109880=CARTESIAN_POINT('Ctrl Pts',(7.44558763121654,-29.9904031635162,
53.3339519259724));
#109881=CARTESIAN_POINT('Ctrl Pts',(7.44668454175472,-29.97452048513,53.3341191421271));
#109882=CARTESIAN_POINT('Ctrl Pts',(7.45476353841384,-29.8585905154747,
53.3369978642721));
#109883=CARTESIAN_POINT('Ctrl Pts',(7.46208676688197,-29.7589736460459,
53.3484928754846));
#109884=CARTESIAN_POINT('Ctrl Pts',(7.47213594336692,-29.6237086119743,
53.3766049502253));
#109885=CARTESIAN_POINT('Ctrl Pts',(7.47489892943558,-29.5866931442184,
53.3856319166404));
#109886=CARTESIAN_POINT('Ctrl Pts',(7.48142576930492,-29.499368230722,53.4101285660257));
#109887=CARTESIAN_POINT('Ctrl Pts',(7.48516551511177,-29.4494155830256,
53.4267291953293));
#109888=CARTESIAN_POINT('Ctrl Pts',(7.49132041496104,-29.3671139153554,
53.4584817222655));
#109889=CARTESIAN_POINT('Ctrl Pts',(7.49377163356675,-29.3343168795382,
53.4723581201619));
#109890=CARTESIAN_POINT('Ctrl Pts',(7.49719222671062,-29.2885480472576,
53.4934771184817));
#109891=CARTESIAN_POINT('Ctrl Pts',(7.49819047278937,-29.2751915258093,
53.4998574154764));
#109892=CARTESIAN_POINT('Ctrl Pts',(7.49991061207578,-29.2521835396078,
53.5112271749809));
#109893=CARTESIAN_POINT('Ctrl Pts',(7.50063529771064,-29.2424927577267,
53.5161345173923));
#109894=CARTESIAN_POINT('Ctrl Pts',(7.50202778199032,-29.2238804487528,
53.5257895147222));
#109895=CARTESIAN_POINT('Ctrl Pts',(7.50269599466004,-29.214952793889,53.530524241602));
#109896=CARTESIAN_POINT('Ctrl Pts',(7.50446412777975,-29.1913451926609,
53.5433209423904));
#109897=CARTESIAN_POINT('Ctrl Pts',(7.50555901767156,-29.1767425448151,
53.5515236729096));
#109898=CARTESIAN_POINT('Ctrl Pts',(7.50964843614083,-29.1223032317046,
53.5831930872221));
#109899=CARTESIAN_POINT('Ctrl Pts',(7.51259140897434,-29.083323481546,53.6080954798478));
#109900=CARTESIAN_POINT('Ctrl Pts',(7.52375930369471,-28.9374086499711,
53.7101060285925));
#109901=CARTESIAN_POINT('Ctrl Pts',(7.53160242487166,-28.8387395689174,
53.7981684816556));
#109902=CARTESIAN_POINT('Ctrl Pts',(7.54195581803577,-28.7285328946065,
53.9229073378102));
#109903=CARTESIAN_POINT('Ctrl Pts',(7.54413613941967,-28.706402904693,53.9495889090035));
#109904=CARTESIAN_POINT('Ctrl Pts',(7.54779198220074,-28.671413597476,53.9945585353159));
#109905=CARTESIAN_POINT('Ctrl Pts',(7.54924189184222,-28.6580610589869,
54.0124504419106));
#109906=CARTESIAN_POINT('Ctrl Pts',(7.55128792260117,-28.6400150024705,
54.0376734632412));
#109907=CARTESIAN_POINT('Ctrl Pts',(7.55186477472032,-28.6350127266119,
54.0447820708678));
#109908=CARTESIAN_POINT('Ctrl Pts',(7.5528544247746,-28.6265810741588,54.0569655543058));
#109909=CARTESIAN_POINT('Ctrl Pts',(7.5532653558838,-28.623123558812,54.0620209084459));
#109910=CARTESIAN_POINT('Ctrl Pts',(7.55413120447432,-28.6159311662204,
54.072662618983));
#109911=CARTESIAN_POINT('Ctrl Pts',(7.55458646436,-28.6122021372565,54.0782526143093));
#109912=CARTESIAN_POINT('Ctrl Pts',(7.55582953476184,-28.6021599485698,
54.0935054236412));
#109913=CARTESIAN_POINT('Ctrl Pts',(7.55662146536172,-28.5959133642476,
54.1032113253135));
#109914=CARTESIAN_POINT('Ctrl Pts',(7.5606717483727,-28.5647023001121,54.1528323937191));
#109915=CARTESIAN_POINT('Ctrl Pts',(7.56401414950227,-28.5413390646799,
54.1937247004124));
#109916=CARTESIAN_POINT('Ctrl Pts',(7.57465819325055,-28.4734298242484,
54.3252216886936));
#109917=CARTESIAN_POINT('Ctrl Pts',(7.58207943763155,-28.4353629164446,
54.4189197609928));
#109918=CARTESIAN_POINT('Ctrl Pts',(7.59484869291408,-28.3837010598797,
54.5888822390953));
#109919=CARTESIAN_POINT('Ctrl Pts',(7.60025561399403,-28.3664855423021,
54.6637357930428));
#109920=CARTESIAN_POINT('Ctrl Pts',(7.6067905302043,-28.351538376,54.7581602691291));
#109921=CARTESIAN_POINT('Ctrl Pts',(7.60807070902892,-28.3489044641932,
54.7768503557741));
#109922=CARTESIAN_POINT('Ctrl Pts',(7.61012637510473,-28.3451566054189,
54.8071644565715));
#109923=CARTESIAN_POINT('Ctrl Pts',(7.61090795850382,-28.3438463174616,
54.8187620370786));
#109924=CARTESIAN_POINT('Ctrl Pts',(7.61240455514058,-28.3415596979604,
54.8411034310793));
#109925=CARTESIAN_POINT('Ctrl Pts',(7.61312008857083,-28.3405656386302,
54.8518447953176));
#109926=CARTESIAN_POINT('Ctrl Pts',(7.61476159942384,-28.3385153641405,
54.8766191984961));
#109927=CARTESIAN_POINT('Ctrl Pts',(7.61568524304847,-28.3375324730583,
54.8906576050593));
#109928=CARTESIAN_POINT('Ctrl Pts',(7.61869404810372,-28.3348951746517,
54.9366898681428));
#109929=CARTESIAN_POINT('Ctrl Pts',(7.6207561365832,-28.333985579211,54.9687203240773));
#109930=CARTESIAN_POINT('Ctrl Pts',(7.62567548929244,-28.3340208019506,
55.0460479823162));
#109931=CARTESIAN_POINT('Ctrl Pts',(7.62850641392198,-28.3358881379129,
55.0913195357843));
#109932=CARTESIAN_POINT('Ctrl Pts',(7.63562978463511,-28.3453222475496,
55.2061096476721));
#109933=CARTESIAN_POINT('Ctrl Pts',(7.6398721484824,-28.3554230730368,55.2753300496743));
#109934=CARTESIAN_POINT('Ctrl Pts',(7.64492142645656,-28.372447151158,55.3560720407562));
#109935=CARTESIAN_POINT('Ctrl Pts',(7.64569544833211,-28.3751937864551,
55.3684024129919));
#109936=CARTESIAN_POINT('Ctrl Pts',(7.65064042938412,-28.3935912442189,
55.4467821799943));
#109937=CARTESIAN_POINT('Ctrl Pts',(7.65485612376256,-28.4131232317943,
55.5118416955448));
#109938=CARTESIAN_POINT('Ctrl Pts',(7.65925610934961,-28.4365623095611,
55.5755159321123));
#109939=CARTESIAN_POINT('',(7.4292447960249,-28.334000270279,55.0012652250353));
#109940=CARTESIAN_POINT('Ctrl Pts',(7.4682788092303,-28.4365623654365,55.5755160839024));
#109941=CARTESIAN_POINT('Ctrl Pts',(7.46565398779176,-28.4217405491484,
55.5352513788047));
#109942=CARTESIAN_POINT('Ctrl Pts',(7.46301745838831,-28.4084720557853,
55.4944082845082));
#109943=CARTESIAN_POINT('Ctrl Pts',(7.45745230202699,-28.3842278948838,
55.4086204717661));
#109944=CARTESIAN_POINT('Ctrl Pts',(7.45452079180897,-28.3735200811348,
55.3636652702551));
#109945=CARTESIAN_POINT('Ctrl Pts',(7.45074651845308,-28.3625045631199,
55.3070766733074));
#109946=CARTESIAN_POINT('Ctrl Pts',(7.44999050083058,-28.3604306357742,
55.2958034330771));
#109947=CARTESIAN_POINT('Ctrl Pts',(7.44878251692798,-28.357328900644,55.2779074726101));
#109948=CARTESIAN_POINT('Ctrl Pts',(7.44833470111328,-28.3562244056175,
55.2712981668777));
#109949=CARTESIAN_POINT('Ctrl Pts',(7.44747288453206,-28.3541860165994,
55.2586308246002));
#109950=CARTESIAN_POINT('Ctrl Pts',(7.44705924353949,-28.3532456414348,
55.2525740462948));
#109951=CARTESIAN_POINT('Ctrl Pts',(7.44622485822675,-28.3514243133995,
55.2404004926074));
#109952=CARTESIAN_POINT('Ctrl Pts',(7.44580409338623,-28.3505439254131,
55.2342836876218));
#109953=CARTESIAN_POINT('Ctrl Pts',(7.44479674920522,-28.3485261035645,
55.2196887392727));
#109954=CARTESIAN_POINT('Ctrl Pts',(7.44420859215493,-28.347419908211,55.2112065471316));
#109955=CARTESIAN_POINT('Ctrl Pts',(7.44212394764507,-28.34374975745,55.1812679874869));
#109956=CARTESIAN_POINT('Ctrl Pts',(7.44061142409316,-28.341538091476,55.1597715450636));
#109957=CARTESIAN_POINT('Ctrl Pts',(7.43585344695961,-28.3359513990773,
55.0926753750645));
#109958=CARTESIAN_POINT('Ctrl Pts',(7.4325603205512,-28.334035143807,55.0469779164252));
#109959=CARTESIAN_POINT('Ctrl Pts',(7.42924502128251,-28.3340004789752,
55.001263307162));
#109960=CARTESIAN_POINT('Ctrl Pts',(7.42924515845182,-28.3340004804105,
55.0012651985876));
#109961=CARTESIAN_POINT('Ctrl Pts',(7.41936138148925,-28.3338969807047,
54.8649779297204));
#109962=CARTESIAN_POINT('Ctrl Pts',(7.40938172257902,-28.3505181555921,
54.7291574322246));
#109963=CARTESIAN_POINT('Ctrl Pts',(7.39771731316611,-28.3911434361544,
54.5662587165018));
#109964=CARTESIAN_POINT('Ctrl Pts',(7.39555203419563,-28.3996441494935,
54.5358746621357));
#109965=CARTESIAN_POINT('Ctrl Pts',(7.39245620643845,-28.4131976353831,
54.4922459575998));
#109966=CARTESIAN_POINT('Ctrl Pts',(7.39150372512375,-28.4175640806743,
54.4787970696937));
#109967=CARTESIAN_POINT('Ctrl Pts',(7.38983637728091,-28.4255536596276,
54.455215205413));
#109968=CARTESIAN_POINT('Ctrl Pts',(7.3891191905053,-28.4291046840929,54.4450588617478));
#109969=CARTESIAN_POINT('Ctrl Pts',(7.38762591951027,-28.4367372116957,
54.4238894383361));
#109970=CARTESIAN_POINT('Ctrl Pts',(7.38685049739493,-28.4408372981033,
54.4128836525272));
#109971=CARTESIAN_POINT('Ctrl Pts',(7.38481545440832,-28.4519566996848,
54.3839742601459));
#109972=CARTESIAN_POINT('Ctrl Pts',(7.38356236486527,-28.4591703266196,
54.3661469103846));
#109973=CARTESIAN_POINT('Ctrl Pts',(7.37750134567894,-28.495828037269,54.2798796988732));
#109974=CARTESIAN_POINT('Ctrl Pts',(7.37283976866374,-28.529533271925,54.2133386246886));
#109975=CARTESIAN_POINT('Ctrl Pts',(7.36163441330213,-28.6223908901131,
54.056989494922));
#109976=CARTESIAN_POINT('Ctrl Pts',(7.35519978860848,-28.68598340088,53.9702264620119));
#109977=CARTESIAN_POINT('Ctrl Pts',(7.34664978927114,-28.7769532270693,
53.8683783022279));
#109978=CARTESIAN_POINT('Ctrl Pts',(7.34479829125985,-28.7970024065456,
53.8470873104637));
#109979=CARTESIAN_POINT('Ctrl Pts',(7.34166019357542,-28.8313208588417,
53.8125134149638));
#109980=CARTESIAN_POINT('Ctrl Pts',(7.34039162646372,-28.8452821164815,
53.7989330349147));
#109981=CARTESIAN_POINT('Ctrl Pts',(7.33858418817246,-28.8652345270069,
53.7801944012327));
#109982=CARTESIAN_POINT('Ctrl Pts',(7.33805984107423,-28.871029812833,53.774828710835));
#109983=CARTESIAN_POINT('Ctrl Pts',(7.33752872251798,-28.8769039574688,
53.7694670738485));
#109984=CARTESIAN_POINT('Ctrl Pts',(7.33752500883319,-28.8769450308333,
53.7694295878243));
#109985=CARTESIAN_POINT('Ctrl Pts',(7.33751750847075,-28.8770279852585,
53.7693538862362));
#109986=CARTESIAN_POINT('Ctrl Pts',(7.33751372179506,-28.8770698663054,
53.7693156708339));
#109987=CARTESIAN_POINT('Ctrl Pts',(7.33750607161743,-28.8771544785145,
53.7692384722354));
#109988=CARTESIAN_POINT('Ctrl Pts',(7.3375022081073,-28.8771972097754,53.769199489109));
#109989=CARTESIAN_POINT('Ctrl Pts',(7.33749440017999,-28.87728356757,53.7691207143516));
#109990=CARTESIAN_POINT('Ctrl Pts',(7.33749045577606,-28.8773271939658,
53.7690809230181));
#109991=CARTESIAN_POINT('Ctrl Pts',(7.33748248175057,-28.8774153897306,
53.7690004888609));
#109992=CARTESIAN_POINT('Ctrl Pts',(7.33747845210965,-28.8774599593233,
53.7689598460181));
#109993=CARTESIAN_POINT('Ctrl Pts',(7.33747030301537,-28.8775500923283,
53.768877663037));
#109994=CARTESIAN_POINT('Ctrl Pts',(7.33746618354772,-28.8775956559089,
53.7688361229442));
#109995=CARTESIAN_POINT('Ctrl Pts',(7.33745784989176,-28.8776878312054,
53.7687520965486));
#109996=CARTESIAN_POINT('Ctrl Pts',(7.3374536356941,-28.8777344430355,53.7687096103563));
#109997=CARTESIAN_POINT('Ctrl Pts',(7.33744510734816,-28.8778287727079,
53.7686236396594));
#109998=CARTESIAN_POINT('Ctrl Pts',(7.33744079318678,-28.8778764907065,
53.7685801552441));
#109999=CARTESIAN_POINT('Ctrl Pts',(7.33743205931893,-28.877973094627,53.7684921323871));
#110000=CARTESIAN_POINT('Ctrl Pts',(7.33742763961158,-28.8780219805711,
53.7684475941756));
#110001=CARTESIAN_POINT('Ctrl Pts',(7.33741868867015,-28.8781209865791,
53.7683574041785));
#110002=CARTESIAN_POINT('Ctrl Pts',(7.33741415743625,-28.8781711066546,
53.7683117526535));
#110003=CARTESIAN_POINT('Ctrl Pts',(7.33740497705346,-28.8782726516231,
53.7682192724593));
#110004=CARTESIAN_POINT('Ctrl Pts',(7.33740032788345,-28.8783240767642,
53.7681724438581));
#110005=CARTESIAN_POINT('Ctrl Pts',(7.33739090476232,-28.8784283078511,
53.7680775412106));
#110006=CARTESIAN_POINT('Ctrl Pts',(7.33738613079863,-28.8784811139514,
53.7680294673427));
#110007=CARTESIAN_POINT('Ctrl Pts',(7.33737645071386,-28.8785881885908,
53.7679320008146));
#110008=CARTESIAN_POINT('Ctrl Pts',(7.33737154457397,-28.8786424573547,
53.7678826082969));
#110009=CARTESIAN_POINT('Ctrl Pts',(7.33736159219885,-28.8787525451723,
53.7677824255685));
#110010=CARTESIAN_POINT('Ctrl Pts',(7.33735654594842,-28.8788083644123,
53.7677316355665));
#110011=CARTESIAN_POINT('Ctrl Pts',(7.337346304797,-28.8789216478662,53.7676285728679));
#110012=CARTESIAN_POINT('Ctrl Pts',(7.33734110988152,-28.87897911226,53.7675763004205));
#110013=CARTESIAN_POINT('Ctrl Pts',(7.33733056216958,-28.8790957881795,
53.7674701811605));
#110014=CARTESIAN_POINT('Ctrl Pts',(7.33732520935568,-28.8791549999193,
53.7674163346046));
#110015=CARTESIAN_POINT('Ctrl Pts',(7.33731433586652,-28.8792752809908,
53.7673069680517));
#110016=CARTESIAN_POINT('Ctrl Pts',(7.33730881517404,-28.8793363505361,
53.7672514483553));
#110017=CARTESIAN_POINT('Ctrl Pts',(7.3372975951219,-28.8794604668154,53.7671386283006));
#110018=CARTESIAN_POINT('Ctrl Pts',(7.33729189573896,-28.8795235138322,
53.7670813282284));
#110019=CARTESIAN_POINT('Ctrl Pts',(7.33728030657738,-28.879651714866,53.7669648310991));
#110020=CARTESIAN_POINT('Ctrl Pts',(7.33727441677917,-28.8797168691269,
53.7669056344178));
#110021=CARTESIAN_POINT('Ctrl Pts',(7.33726243404441,-28.8798494256865,
53.7667852177515));
#110022=CARTESIAN_POINT('Ctrl Pts',(7.33725634107848,-28.8799168283404,
53.7667239981026));
#110023=CARTESIAN_POINT('Ctrl Pts',(7.33724393813633,-28.880054035225,53.7665993980568));
#110024=CARTESIAN_POINT('Ctrl Pts',(7.3372376281186,-28.8801238399478,53.7665360179411));
#110025=CARTESIAN_POINT('Ctrl Pts',(7.33722477591552,-28.8802660187392,
53.7664069468568));
#110026=CARTESIAN_POINT('Ctrl Pts',(7.33721823370589,-28.8803383931125,
53.7663412564184));
#110027=CARTESIAN_POINT('Ctrl Pts',(7.33720490055903,-28.8804858945012,
53.7662074007842));
#110028=CARTESIAN_POINT('Ctrl Pts',(7.33719810957887,-28.8805610220313,
53.7661392360177));
#110029=CARTESIAN_POINT('Ctrl Pts',(7.33718426073402,-28.8807142307094,
53.7660002521169));
#110030=CARTESIAN_POINT('Ctrl Pts',(7.33717720283863,-28.8807923122409,
53.7659294336332));
#110031=CARTESIAN_POINT('Ctrl Pts',(7.3371628002295,-28.8809516495688,53.7657849452276));
#110032=CARTESIAN_POINT('Ctrl Pts',(7.33715545546863,-28.881032905935,53.7657112759044));
#110033=CARTESIAN_POINT('Ctrl Pts',(7.33714045718768,-28.8811988357995,
53.7655608690414));
#110034=CARTESIAN_POINT('Ctrl Pts',(7.33713280360971,-28.8812835099917,
53.7654841321223));
#110035=CARTESIAN_POINT('Ctrl Pts',(7.33711716346841,-28.8814565436755,
53.7653273508625));
#110036=CARTESIAN_POINT('Ctrl Pts',(7.33710917684828,-28.8815449038548,
53.7652473073035));
#110037=CARTESIAN_POINT('Ctrl Pts',(7.33709284381398,-28.8817256062719,
53.7650836482374));
#110038=CARTESIAN_POINT('Ctrl Pts',(7.33708449734189,-28.8818179492163,
53.7650000336746));
#110039=CARTESIAN_POINT('Ctrl Pts',(7.33706741487229,-28.882006946281,53.7648289394457));
#110040=CARTESIAN_POINT('Ctrl Pts',(7.33705867879913,-28.8821036013116,
53.7647414607483));
#110041=CARTESIAN_POINT('Ctrl Pts',(7.33704078404828,-28.8823015887304,
53.7645623123294));
#110042=CARTESIAN_POINT('Ctrl Pts',(7.33703162528436,-28.8824029221547,
53.7644706437065));
#110043=CARTESIAN_POINT('Ctrl Pts',(7.33661966045941,-28.886960980076,53.760348335792));
#110044=CARTESIAN_POINT('Ctrl Pts',(7.33621503627641,-28.8914392347911,
53.7563420347391));
#110045=CARTESIAN_POINT('Ctrl Pts',(7.33528351882049,-28.9017524608487,
53.7472156598144));
#110046=CARTESIAN_POINT('Ctrl Pts',(7.33475547267559,-28.9076015956614,
53.742112095438));
#110047=CARTESIAN_POINT('Ctrl Pts',(7.33312165043831,-28.9257146258615,
53.7265294865155));
#110048=CARTESIAN_POINT('Ctrl Pts',(7.33200686745723,-28.9380948134998,
53.7161878872425));
#110049=CARTESIAN_POINT('Ctrl Pts',(7.32522949568416,-29.0135973813667,
53.6549572758446));
#110050=CARTESIAN_POINT('Ctrl Pts',(7.31934378950463,-29.0802105747121,
53.6085565082187));
#110051=CARTESIAN_POINT('Ctrl Pts',(7.30807746792457,-29.2133365480952,
53.5295740986431));
#110052=CARTESIAN_POINT('Ctrl Pts',(7.30271120111838,-29.2791754050481,
53.4962031596171));
#110053=CARTESIAN_POINT('Ctrl Pts',(7.29441927823271,-29.3860771915527,
53.4506588836747));
#110054=CARTESIAN_POINT('Ctrl Pts',(7.29142556736562,-29.4257671184623,
53.4355140754363));
#110055=CARTESIAN_POINT('Ctrl Pts',(7.28635590441309,-29.4949589952015,
53.412100590152));
#110056=CARTESIAN_POINT('Ctrl Pts',(7.28425850738909,-29.5241885382703,
53.4030984318918));
#110057=CARTESIAN_POINT('Ctrl Pts',(7.28124054464323,-29.5671128843571,
53.3911619162331));
#110058=CARTESIAN_POINT('Ctrl Pts',(7.28029956371222,-29.5806216193866,
53.3875878227953));
#110059=CARTESIAN_POINT('Ctrl Pts',(7.27864523099934,-29.6045874622423,
53.3815685977633));
#110060=CARTESIAN_POINT('Ctrl Pts',(7.27792967634378,-29.6150260817573,
53.3790538656968));
#110061=CARTESIAN_POINT('Ctrl Pts',(7.2764328922464,-29.6370099740115,53.373982149372));
#110062=CARTESIAN_POINT('Ctrl Pts',(7.27565239128449,-29.64855966445,53.3714468039974));
#110063=CARTESIAN_POINT('Ctrl Pts',(7.27358797160599,-29.6793290370596,
53.3650350104078));
#110064=CARTESIAN_POINT('Ctrl Pts',(7.27231093861435,-29.6985921782093,
53.3613744292037));
#110065=CARTESIAN_POINT('Ctrl Pts',(7.26570090209875,-29.7993981666942,
53.3440561045228));
#110066=CARTESIAN_POINT('Ctrl Pts',(7.26055175831115,-29.8818143795768,
53.3361412514622));
#110067=CARTESIAN_POINT('Ctrl Pts',(7.24932622292816,-30.0645502504756,
53.3322450467618));
#110068=CARTESIAN_POINT('Ctrl Pts',(7.24330777673946,-30.1645960286204,
53.3391330199052));
#110069=CARTESIAN_POINT('Ctrl Pts',(7.23526176216511,-30.2913214536345,
53.3594248829007));
#110070=CARTESIAN_POINT('Ctrl Pts',(7.23346986520759,-30.3191110235992,
53.3646031433493));
#110071=CARTESIAN_POINT('Ctrl Pts',(7.2304039155781,-30.3656265500736,53.3745014502709));
#110072=CARTESIAN_POINT('Ctrl Pts',(7.22914617000949,-30.3844271259328,
53.3788448512516));
#110073=CARTESIAN_POINT('Ctrl Pts',(7.22732855753112,-30.4111167666871,
53.3855011701696));
#110074=CARTESIAN_POINT('Ctrl Pts',(7.22678272860742,-30.4190714886125,
53.3875476602974));
#110075=CARTESIAN_POINT('Ctrl Pts',(7.22582891152124,-30.4328605496481,
53.3912040609785));
#110076=CARTESIAN_POINT('Ctrl Pts',(7.22542245169999,-30.4387017762115,
53.3927870772486));
#110077=CARTESIAN_POINT('Ctrl Pts',(7.22454526481024,-30.451230976305,53.3962559782332));
#110078=CARTESIAN_POINT('Ctrl Pts',(7.22407401180635,-30.4579157150116,
53.3981518564881));
#110079=CARTESIAN_POINT('Ctrl Pts',(7.22276390505091,-30.4763773340345,
53.4035128131894));
#110080=CARTESIAN_POINT('Ctrl Pts',(7.22192030452483,-30.4881277979946,
53.4070662497296));
#110081=CARTESIAN_POINT('Ctrl Pts',(7.21598093992014,-30.56997618762,53.4328084987455));
#110082=CARTESIAN_POINT('Ctrl Pts',(7.21068115500295,-30.6385701759523,
53.4594845699778));
#110083=CARTESIAN_POINT('Ctrl Pts',(7.20433076996824,-30.7177599366058,
53.4964808702952));
#110084=CARTESIAN_POINT('Ctrl Pts',(7.20331979855189,-30.7302756521869,
53.5025199272583));
#110085=CARTESIAN_POINT('Ctrl Pts',(7.19694229428744,-30.8087096757976,
53.5415829254223));
#110086=CARTESIAN_POINT('Ctrl Pts',(7.19157603405899,-30.8724546306259,
53.5787977144274));
#110087=CARTESIAN_POINT('Ctrl Pts',(7.18328409547715,-30.9686982658194,
53.6439089987239));
#110088=CARTESIAN_POINT('Ctrl Pts',(7.18029036352442,-31.0029487190825,
53.6690403831172));
#110089=CARTESIAN_POINT('Ctrl Pts',(7.17522066924653,-31.0601469590131,
53.7144731092484));
#110090=CARTESIAN_POINT('Ctrl Pts',(7.17312326162279,-31.0835632395142,
53.734147765123));
#110091=CARTESIAN_POINT('Ctrl Pts',(7.17010528669471,-31.1168723862871,
53.7637365539046));
#110092=CARTESIAN_POINT('Ctrl Pts',(7.16916430394805,-31.127201811013,53.7731473872925));
#110093=CARTESIAN_POINT('Ctrl Pts',(7.1675099691897,-31.1452570596212,53.790017543011));
#110094=CARTESIAN_POINT('Ctrl Pts',(7.16679441428582,-31.1530313308955,
53.7974235832662));
#110095=CARTESIAN_POINT('Ctrl Pts',(7.16529763078826,-31.1692155684582,
53.8131424838291));
#110096=CARTESIAN_POINT('Ctrl Pts',(7.16451713066375,-31.1776097512204,
53.8214707915453));
#110097=CARTESIAN_POINT('Ctrl Pts',(7.16245271582189,-31.1996847304443,
53.8438438994774));
#110098=CARTESIAN_POINT('Ctrl Pts',(7.16117568677052,-31.213207739598,53.8580422886749));
#110099=CARTESIAN_POINT('Ctrl Pts',(7.15456578763205,-31.2824297370214,
53.9333393664157));
#110100=CARTESIAN_POINT('Ctrl Pts',(7.14941676711014,-31.3337777872687,
53.9982863447298));
#110101=CARTESIAN_POINT('Ctrl Pts',(7.13819124008231,-31.4361609777227,
54.1496969210285));
#110102=CARTESIAN_POINT('Ctrl Pts',(7.13217269008688,-31.4846364094691,
54.23748700274));
#110103=CARTESIAN_POINT('Ctrl Pts',(7.12412655065735,-31.5363205511849,
54.3549619537736));
#110104=CARTESIAN_POINT('Ctrl Pts',(7.12233463978635,-31.5470422331034,
54.3811178900663));
#110105=CARTESIAN_POINT('Ctrl Pts',(7.11926866875335,-31.5639547193652,
54.4255664099045));
#110106=CARTESIAN_POINT('Ctrl Pts',(7.1180109159911,-31.5705024379246,54.4437174024808));
#110107=CARTESIAN_POINT('Ctrl Pts',(7.1161932949173,-31.5793857218873,54.4697508046372));
#110108=CARTESIAN_POINT('Ctrl Pts',(7.11564746477252,-31.5819807383557,
54.477543873458));
#110109=CARTESIAN_POINT('Ctrl Pts',(7.11469364631046,-31.5863875356006,
54.4911117845995));
#110110=CARTESIAN_POINT('Ctrl Pts',(7.11428718634815,-31.5882256471835,
54.496877826798));
#110111=CARTESIAN_POINT('Ctrl Pts',(7.1134100000558,-31.5921066586156,54.5092855527162));
#110112=CARTESIAN_POINT('Ctrl Pts',(7.11293874779902,-31.594139408157,54.5159299388113));
#110113=CARTESIAN_POINT('Ctrl Pts',(7.11162864509591,-31.5996483385049,
54.5343478830958));
#110114=CARTESIAN_POINT('Ctrl Pts',(7.11078504792078,-31.603035959432,54.546147169756));
#110115=CARTESIAN_POINT('Ctrl Pts',(7.10484659272836,-31.6257969310291,
54.6288605765015));
#110116=CARTESIAN_POINT('Ctrl Pts',(7.09954778605901,-31.6405863392822,
54.7009444858452));
#110117=CARTESIAN_POINT('Ctrl Pts',(7.09319763078049,-31.6524554706508,
54.7875375335864));
#110118=CARTESIAN_POINT('Ctrl Pts',(7.09218592180018,-31.6541713232472,
54.8013379454803));
#110119=CARTESIAN_POINT('Ctrl Pts',(7.08580773362252,-31.6638941094912,
54.8884294529822));
#110120=CARTESIAN_POINT('Ctrl Pts',(7.08044152169657,-31.66720173276,54.9621675725987));
#110121=CARTESIAN_POINT('Ctrl Pts',(7.07214946850077,-31.6646987504846,
55.0783414519699));
#110122=CARTESIAN_POINT('Ctrl Pts',(7.06915558233061,-31.6621610745342,
55.120749228861));
#110123=CARTESIAN_POINT('Ctrl Pts',(7.06408565893557,-31.6550132327113,
55.1934482581732));
#110124=CARTESIAN_POINT('Ctrl Pts',(7.06198817377946,-31.6511837676141,
55.2237932252094));
#110125=CARTESIAN_POINT('Ctrl Pts',(7.05897010973319,-31.6443904664943,
55.2678268740775));
#110126=CARTESIAN_POINT('Ctrl Pts',(7.05802911369633,-31.6420863034479,
55.2816093632342));
#110127=CARTESIAN_POINT('Ctrl Pts',(7.05637476395455,-31.6377054454607,
55.305928346623));
#110128=CARTESIAN_POINT('Ctrl Pts',(7.05565920722219,-31.6356997955474,
55.3164766460311));
#110129=CARTESIAN_POINT('Ctrl Pts',(7.05416242808172,-31.6312714381596,
55.3385990283326));
#110130=CARTESIAN_POINT('Ctrl Pts',(7.05338193406396,-31.6288271946948,
55.350168229426));
#110131=CARTESIAN_POINT('Ctrl Pts',(7.05131755453722,-31.6220033896862,
55.3808482208801));
#110132=CARTESIAN_POINT('Ctrl Pts',(7.05004055426368,-31.6174092267133,
55.3999097516673));
#110133=CARTESIAN_POINT('Ctrl Pts',(7.04343165782151,-31.5916964694584,
55.4988895514643));
#110134=CARTESIAN_POINT('Ctrl Pts',(7.03828353698695,-31.5649871134795,
55.577240213801));
#110135=CARTESIAN_POINT('Ctrl Pts',(7.02705807103857,-31.4933150681704,
55.7453766986767));
#110136=CARTESIAN_POINT('Ctrl Pts',(7.02103876349687,-31.4458453571029,
55.8337296792155));
#110137=CARTESIAN_POINT('Ctrl Pts',(7.01299171293547,-31.3751735386733,
55.9408787114126));
#110138=CARTESIAN_POINT('Ctrl Pts',(7.01119970053903,-31.3590129854394,
55.9640739268158));
#110139=CARTESIAN_POINT('Ctrl Pts',(7.00813357332449,-31.3308411804608,
56.0023921876658));
#110140=CARTESIAN_POINT('Ctrl Pts',(7.00687576806807,-31.3191425089811,
56.0177383301558));
#110141=CARTESIAN_POINT('Ctrl Pts',(7.00505808426361,-31.3020881047485,
56.039321912314));
#110142=CARTESIAN_POINT('Ctrl Pts',(7.00451224520122,-31.2969481690766,
56.0457288891856));
#110143=CARTESIAN_POINT('Ctrl Pts',(7.0035584166858,-31.2879391709183,56.0567901026722));
#110144=CARTESIAN_POINT('Ctrl Pts',(7.00315195568784,-31.2840917841132,
56.0614616892386));
#110145=CARTESIAN_POINT('Ctrl Pts',(7.00227477374129,-31.2757724766153,
56.0714517572007));
#110146=CARTESIAN_POINT('Ctrl Pts',(7.0018035269298,-31.2712927812697,56.0767631772989));
#110147=CARTESIAN_POINT('Ctrl Pts',(7.00049345376872,-31.2588071940219,
56.0913803830859));
#110148=CARTESIAN_POINT('Ctrl Pts',(6.99964988102214,-31.2507316598614,
56.1006257244048));
#110149=CARTESIAN_POINT('Ctrl Pts',(6.99371803261137,-31.1936488650788,
56.1645379154008));
#110150=CARTESIAN_POINT('Ctrl Pts',(6.98842633237386,-31.1411817993022,
56.2159966617393));
#110151=CARTESIAN_POINT('Ctrl Pts',(6.9820778981905,-31.0748950826226,56.2729304692034));
#110152=CARTESIAN_POINT('Ctrl Pts',(6.98106088278504,-31.0641763347269,
56.2819048884559));
#110153=CARTESIAN_POINT('Ctrl Pts',(6.97467780430104,-30.9962303623445,
56.337354036096));
#110154=CARTESIAN_POINT('Ctrl Pts',(6.96931196817566,-30.9360803177665,
56.3801252501119));
#110155=CARTESIAN_POINT('Ctrl Pts',(6.96101906000775,-30.837114462397,56.4410413047622));
#110156=CARTESIAN_POINT('Ctrl Pts',(6.95802400918304,-30.8000963776383,
56.4619189283905));
#110157=CARTESIAN_POINT('Ctrl Pts',(6.95295235555819,-30.7351211980397,
56.4953555974874));
#110158=CARTESIAN_POINT('Ctrl Pts',(6.9508542849393,-30.7075427826604,56.5086003323156));
#110159=CARTESIAN_POINT('Ctrl Pts',(6.94783554795873,-30.6668549486714,
56.526779538368));
#110160=CARTESIAN_POINT('Ctrl Pts',(6.94689445157823,-30.6540246834458,
56.5323194887012));
#110161=CARTESIAN_POINT('Ctrl Pts',(6.94523998870642,-30.6312157588782,
56.5418294163343));
#110162=CARTESIAN_POINT('Ctrl Pts',(6.94452441816591,-30.6212657269899,
56.5458655145503));
#110163=CARTESIAN_POINT('Ctrl Pts',(6.94302767190505,-30.6002785059707,
56.5541433347846));
#110164=CARTESIAN_POINT('Ctrl Pts',(6.94224722398002,-30.5892337447838,
56.5583643335002));
#110165=CARTESIAN_POINT('Ctrl Pts',(6.94018311099836,-30.5597611035498,
56.5692698100086));
#110166=CARTESIAN_POINT('Ctrl Pts',(6.93890632792845,-30.5412582511765,
56.5757473743571));
#110167=CARTESIAN_POINT('Ctrl Pts',(6.93230494682998,-30.4442666385814,
56.6077925404246));
#110168=CARTESIAN_POINT('Ctrl Pts',(6.92716356843504,-30.3640674084027,
56.6278289554652));
#110169=CARTESIAN_POINT('Ctrl Pts',(6.91593855588035,-30.1839574699845,
56.6588416857747));
#110170=CARTESIAN_POINT('Ctrl Pts',(6.90991356842101,-30.0838844468811,
56.6669004604288));
#110171=CARTESIAN_POINT('Ctrl Pts',(6.90185968682402,-29.9554228063539,
56.6656435960921));
#110172=CARTESIAN_POINT('Ctrl Pts',(6.90006691377061,-29.9271581116038,
56.6646469879206));
#110173=CARTESIAN_POINT('Ctrl Pts',(6.89699961643601,-29.8796672484711,
56.6617606966871));
#110174=CARTESIAN_POINT('Ctrl Pts',(6.89574141791898,-29.8604231664034,
56.6602550447939));
#110175=CARTESIAN_POINT('Ctrl Pts',(6.893923264176,-29.8330329714778,56.6576324979482));
#110176=CARTESIAN_POINT('Ctrl Pts',(6.89337735831805,-29.8248614467759,
56.6567890532728));
#110177=CARTESIAN_POINT('Ctrl Pts',(6.89242345449698,-29.8106811254468,
56.6552193191231));
#110178=CARTESIAN_POINT('Ctrl Pts',(6.89201698573904,-29.8046695069703,
56.6545206640629));
#110179=CARTESIAN_POINT('Ctrl Pts',(6.89113983633043,-29.7917647688217,
56.6529495940533));
#110180=CARTESIAN_POINT('Ctrl Pts',(6.89066863029436,-29.7848733638788,
56.6520668261346));
#110181=CARTESIAN_POINT('Ctrl Pts',(6.88935877833707,-29.7658242328667,
56.6495054829733));
#110182=CARTESIAN_POINT('Ctrl Pts',(6.8885153885033,-29.7536795098386,56.6477356651802));
#110183=CARTESIAN_POINT('Ctrl Pts',(6.88262968131166,-29.6696823628383,
56.6345456383852));
#110184=CARTESIAN_POINT('Ctrl Pts',(6.87738758094027,-29.5986329456008,
56.6185645888189));
#110185=CARTESIAN_POINT('Ctrl Pts',(6.87109323771207,-29.5155217465157,
56.5940609490431));
#110186=CARTESIAN_POINT('Ctrl Pts',(6.87008135385466,-29.5022294248012,
56.5899603573803));
#110187=CARTESIAN_POINT('Ctrl Pts',(6.86359737181203,-29.417433719875,56.5626338673675));
#110188=CARTESIAN_POINT('Ctrl Pts',(6.8581243384229,-29.3475156755454,56.5347552509911));
#110189=CARTESIAN_POINT('Ctrl Pts',(6.84975951773613,-29.2417769087201,
56.4840566258741));
#110190=CARTESIAN_POINT('Ctrl Pts',(6.84679417373141,-29.2045376312284,
56.4644338269463));
#110191=CARTESIAN_POINT('Ctrl Pts',(6.84176669003119,-29.1417630897022,
56.4282534635349));
#110192=CARTESIAN_POINT('Ctrl Pts',(6.83968358690166,-29.1158658286087,
56.4123687642179));
#110193=CARTESIAN_POINT('Ctrl Pts',(6.83668206118834,-29.0787392707339,
56.3881746689807));
#110194=CARTESIAN_POINT('Ctrl Pts',(6.83574353649287,-29.067158334824,56.3804190273599));
#110195=CARTESIAN_POINT('Ctrl Pts',(6.83409197048213,-29.0468340601644,
56.3664354626472));
#110196=CARTESIAN_POINT('Ctrl Pts',(6.83337675129373,-29.0380511629309,
56.3602667483142));
#110197=CARTESIAN_POINT('Ctrl Pts',(6.8318791493878,-29.0197038989824,56.3471138734307));
#110198=CARTESIAN_POINT('Ctrl Pts',(6.83109750980437,-29.0101531239621,
56.3401117146883));
#110199=CARTESIAN_POINT('Ctrl Pts',(6.82902650575648,-28.9849231178045,
56.3211974193374));
#110200=CARTESIAN_POINT('Ctrl Pts',(6.82774410746935,-28.9693787338623,
56.3091079240124));
#110201=CARTESIAN_POINT('Ctrl Pts',(6.82091060019877,-28.8870638654833,
56.2427131643128));
#110202=CARTESIAN_POINT('Ctrl Pts',(6.81556041461678,-28.8243591234056,
56.1835683743095));
#110203=CARTESIAN_POINT('Ctrl Pts',(6.80431813359718,-28.701179341995,56.0478857039811));
#110204=CARTESIAN_POINT('Ctrl Pts',(6.7984671325709,-28.6422840575745,55.9703631854246));
#110205=CARTESIAN_POINT('Ctrl Pts',(6.79062285321755,-28.5756154868537,
55.8645592129393));
#110206=CARTESIAN_POINT('Ctrl Pts',(6.78885383372478,-28.5613426363736,
55.8405942480984));
#110207=CARTESIAN_POINT('Ctrl Pts',(6.78582310593807,-28.5383161095083,
55.7996257584288));
#110208=CARTESIAN_POINT('Ctrl Pts',(6.78457722123195,-28.529241178391,55.7828087647592));
#110209=CARTESIAN_POINT('Ctrl Pts',(6.78277378782216,-28.5166964885727,
55.7585734302852));
#110210=CARTESIAN_POINT('Ctrl Pts',(6.78222998064803,-28.5129886970933,
55.7512791320508));
#110211=CARTESIAN_POINT('Ctrl Pts',(6.78127843890094,-28.5066339902723,
55.7385462362477));
#110212=CARTESIAN_POINT('Ctrl Pts',(6.78087220996819,-28.5039627157606,
55.7331200617019));
#110213=CARTESIAN_POINT('Ctrl Pts',(6.77999402036308,-28.4982781918607,
55.721412601067));
#110214=CARTESIAN_POINT('Ctrl Pts',(6.77952151916618,-28.4952748191201,
55.7151270206129));
#110215=CARTESIAN_POINT('Ctrl Pts',(6.77820463502334,-28.4870539875925,
55.6976410499048));
#110216=CARTESIAN_POINT('Ctrl Pts',(6.77735542890128,-28.4819217021689,
55.6864014351012));
#110217=CARTESIAN_POINT('Ctrl Pts',(6.77401860377976,-28.4623913119626,
55.6423395637711));
#110218=CARTESIAN_POINT('Ctrl Pts',(6.77148681170204,-28.4489342213664,
55.6091252718719));
#110219=CARTESIAN_POINT('Ctrl Pts',(6.76892552105682,-28.4365623357949,
55.5755160033788));
#110220=CARTESIAN_POINT('Origin',(5.,-30.,55.));
#110221=CARTESIAN_POINT('',(6.06643884243078,-28.4365623175998,55.5755159539501));
#110222=CARTESIAN_POINT('',(6.26189393505974,-28.4365622331338,55.5755157244911));
#110223=CARTESIAN_POINT('',(5.,-28.4365623102018,55.5755159338528));
#110224=CARTESIAN_POINT('',(6.92208048413035,-28.3340006487619,54.9985297366875));
#110225=CARTESIAN_POINT('Ctrl Pts',(6.26189393505974,-28.4365622331338,
55.5755157244911));
#110226=CARTESIAN_POINT('Ctrl Pts',(6.26454443424848,-28.4494994604332,
55.6106608107115));
#110227=CARTESIAN_POINT('Ctrl Pts',(6.26716430935981,-28.4636250038082,
55.6453785126745));
#110228=CARTESIAN_POINT('Ctrl Pts',(6.27128111558779,-28.4879917747115,
55.6999155997547));
#110229=CARTESIAN_POINT('Ctrl Pts',(6.27280063026977,-28.4974711607094,
55.7200402001679));
#110230=CARTESIAN_POINT('Ctrl Pts',(6.27523275603405,-28.5134292830489,
55.7522305318072));
#110231=CARTESIAN_POINT('Ctrl Pts',(6.27615382522183,-28.5196584349094,
55.764416208322));
#110232=CARTESIAN_POINT('Ctrl Pts',(6.27778607461691,-28.5310271577228,
55.7859958028606));
#110233=CARTESIAN_POINT('Ctrl Pts',(6.27849925380626,-28.5361084051871,
55.7954193996187));
#110234=CARTESIAN_POINT('Ctrl Pts',(6.28000404443252,-28.5470699735413,
55.8152876705199));
#110235=CARTESIAN_POINT('Ctrl Pts',(6.28079480055977,-28.5529729035312,
55.8257192272144));
#110236=CARTESIAN_POINT('Ctrl Pts',(6.28291777598941,-28.5692026238206,
55.8536914811434));
#110237=CARTESIAN_POINT('Ctrl Pts',(6.28424238439093,-28.579739333538,55.8711084746527));
#110238=CARTESIAN_POINT('Ctrl Pts',(6.2930977839093,-28.6528863625755,55.9871623009155));
#110239=CARTESIAN_POINT('Ctrl Pts',(6.30023264072672,-28.7254041138658,
56.0791729420103));
#110240=CARTESIAN_POINT('Ctrl Pts',(6.31334404471934,-28.8752744103748,
56.2329344202666));
#110241=CARTESIAN_POINT('Ctrl Pts',(6.31930588883164,-28.9496223452665,
56.2968564631899));
#110242=CARTESIAN_POINT('Ctrl Pts',(6.32668321439504,-29.042062018077,56.3631448104139));
#110243=CARTESIAN_POINT('Ctrl Pts',(6.32772463441115,-29.055118261451,56.372227170059));
#110244=CARTESIAN_POINT('Ctrl Pts',(6.32928196947959,-29.0746123058996,
56.3853777672779));
#110245=CARTESIAN_POINT('Ctrl Pts',(6.32978877346842,-29.0809516278452,
56.3895913163429));
#110246=CARTESIAN_POINT('Ctrl Pts',(6.33070050964634,-29.092342411459,56.397050375253));
#110247=CARTESIAN_POINT('Ctrl Pts',(6.33110435486264,-29.0973828549652,
56.4003122280136));
#110248=CARTESIAN_POINT('Ctrl Pts',(6.33200895785928,-29.1086614883493,
56.407524840982));
#110249=CARTESIAN_POINT('Ctrl Pts',(6.33251058288281,-29.1149083016265,
56.411461370558));
#110250=CARTESIAN_POINT('Ctrl Pts',(6.33402027839573,-29.133692528476,56.4231248213934));
#110251=CARTESIAN_POINT('Ctrl Pts',(6.33503575608031,-29.1463060664516,
56.4307269212504));
#110252=CARTESIAN_POINT('Ctrl Pts',(6.33742713232091,-29.175996661458,56.4480888577481));
#110253=CARTESIAN_POINT('Ctrl Pts',(6.33880943404792,-29.1931488681659,
56.4577153429514));
#110254=CARTESIAN_POINT('Ctrl Pts',(6.34382787724757,-29.2555105829052,
56.4912773495486));
#110255=CARTESIAN_POINT('Ctrl Pts',(6.34752600754672,-29.3016444755732,
56.5134303915248));
#110256=CARTESIAN_POINT('Ctrl Pts',(6.36032778263557,-29.4637873504093,
56.5822959968397));
#110257=CARTESIAN_POINT('Ctrl Pts',(6.36944877284455,-29.5840091139911,
56.6180684694178));
#110258=CARTESIAN_POINT('Ctrl Pts',(6.38042265245481,-29.7392029462727,
56.6457835440303));
#110259=CARTESIAN_POINT('Ctrl Pts',(6.38266399484551,-29.7714555164209,
56.6505714927712));
#110260=CARTESIAN_POINT('Ctrl Pts',(6.38577523926507,-29.8169918410653,
56.6559709198486));
#110261=CARTESIAN_POINT('Ctrl Pts',(6.38666958545936,-29.8301723037498,
56.657374503499));
#110262=CARTESIAN_POINT('Ctrl Pts',(6.38829181642349,-29.8542409324696,
56.6596474201703));
#110263=CARTESIAN_POINT('Ctrl Pts',(6.38902124328637,-29.8651234633131,
56.6605672508789));
#110264=CARTESIAN_POINT('Ctrl Pts',(6.39049148943486,-29.8871763988337,
56.6622130180382));
#110265=CARTESIAN_POINT('Ctrl Pts',(6.39123210213837,-29.8983466530495,
56.6629335193349));
#110266=CARTESIAN_POINT('Ctrl Pts',(6.39306114458357,-29.9260788493085,
56.6644418139332));
#110267=CARTESIAN_POINT('Ctrl Pts',(6.39414533702312,-29.9426471277199,
56.6650950630284));
#110268=CARTESIAN_POINT('Ctrl Pts',(6.39840404599992,-30.0081958039325,
56.6666999165734));
#110269=CARTESIAN_POINT('Ctrl Pts',(6.40151935112882,-30.0572007786793,
56.6657384385704));
#110270=CARTESIAN_POINT('Ctrl Pts',(6.41006506225163,-30.1933658791567,
56.6570493918086));
#110271=CARTESIAN_POINT('Ctrl Pts',(6.41537370517354,-30.2800630003335,
56.6446181206207));
#110272=CARTESIAN_POINT('Ctrl Pts',(6.42592433737092,-30.4484520774009,
56.6067654527329));
#110273=CARTESIAN_POINT('Ctrl Pts',(6.43115151797511,-30.5299538928468,
56.5817552902691));
#110274=CARTESIAN_POINT('Ctrl Pts',(6.43771142480958,-30.6241671028476,
56.5447429617688));
#110275=CARTESIAN_POINT('Ctrl Pts',(6.43876529236094,-30.6390705533312,
56.5386371148954));
#110276=CARTESIAN_POINT('Ctrl Pts',(6.44034477585217,-30.6610189829191,
56.5292711035896));
#110277=CARTESIAN_POINT('Ctrl Pts',(6.44086112012565,-30.668133961902,56.5261760078868));
#110278=CARTESIAN_POINT('Ctrl Pts',(6.44178277919925,-30.68072167513,56.5205953203357));
#110279=CARTESIAN_POINT('Ctrl Pts',(6.44218689851657,-30.6862029559263,
56.5181296480535));
#110280=CARTESIAN_POINT('Ctrl Pts',(6.44308316261483,-30.6982746496565,
56.5126206416278));
#110281=CARTESIAN_POINT('Ctrl Pts',(6.44357607857959,-30.7048584846996,
56.509563911664));
#110282=CARTESIAN_POINT('Ctrl Pts',(6.44503391268635,-30.7241750915241,
56.5004417184846));
#110283=CARTESIAN_POINT('Ctrl Pts',(6.44600553060751,-30.7368506952597,
56.4942576530855));
#110284=CARTESIAN_POINT('Ctrl Pts',(6.4482755778935,-30.7660429090638,56.4795538565577));
#110285=CARTESIAN_POINT('Ctrl Pts',(6.44957959990121,-30.7824983244714,
56.470917286353));
#110286=CARTESIAN_POINT('Ctrl Pts',(6.45419582406069,-30.8397655975806,
56.4396278555028));
#110287=CARTESIAN_POINT('Ctrl Pts',(6.45756105367133,-30.8797650680921,
56.4155378848624));
#110288=CARTESIAN_POINT('Ctrl Pts',(6.46884719803039,-31.0095146381318,
56.3297698259801));
#110289=CARTESIAN_POINT('Ctrl Pts',(6.47681653686281,-31.0942392898449,
56.2609728641792));
#110290=CARTESIAN_POINT('Ctrl Pts',(6.48802982171822,-31.2069943132559,
56.149431417208));
#110291=CARTESIAN_POINT('Ctrl Pts',(6.49148702134616,-31.240759703818,56.1128989578508));
#110292=CARTESIAN_POINT('Ctrl Pts',(6.49604384421507,-31.2838947961095,
56.0618208604164));
#110293=CARTESIAN_POINT('Ctrl Pts',(6.49720311866262,-31.2947440448116,
56.0485643917151));
#110294=CARTESIAN_POINT('Ctrl Pts',(6.49911382138648,-31.3124112152241,
56.026284851335));
#110295=CARTESIAN_POINT('Ctrl Pts',(6.49986983686129,-31.3193449545432,
56.0173557370598));
#110296=CARTESIAN_POINT('Ctrl Pts',(6.50135207430642,-31.3328239830127,
55.9996281603467));
#110297=CARTESIAN_POINT('Ctrl Pts',(6.50207847116319,-31.3393743439319,
55.990834297567));
#110298=CARTESIAN_POINT('Ctrl Pts',(6.50381664423439,-31.3549110227476,
55.9695406601622));
#110299=CARTESIAN_POINT('Ctrl Pts',(6.50482510233097,-31.3638119482423,
55.956979606478));
#110300=CARTESIAN_POINT('Ctrl Pts',(6.5084058534178,-31.3949900649015,55.9116621283627));
#110301=CARTESIAN_POINT('Ctrl Pts',(6.51094107849887,-31.4162725664222,
55.8782354598566));
#110302=CARTESIAN_POINT('Ctrl Pts',(6.51733360379184,-31.4675700854227,
55.7909440369044));
#110303=CARTESIAN_POINT('Ctrl Pts',(6.52113625623734,-31.495824671124,55.736113986869));
#110304=CARTESIAN_POINT('Ctrl Pts',(6.53045827924483,-31.5579374823455,
55.5971519243775));
#110305=CARTESIAN_POINT('Ctrl Pts',(6.53592604086477,-31.58809067844,55.5115913280997));
#110306=CARTESIAN_POINT('Ctrl Pts',(6.54418381491401,-31.6216081323308,
55.384232870677));
#110307=CARTESIAN_POINT('Ctrl Pts',(6.546804833239,-31.6305989143249,55.3440848786691));
#110308=CARTESIAN_POINT('Ctrl Pts',(6.55022790961468,-31.6401206751567,
55.2927179031992));
#110309=CARTESIAN_POINT('Ctrl Pts',(6.55096166475799,-31.642037448462,55.2817669272673));
#110310=CARTESIAN_POINT('Ctrl Pts',(6.55214231022928,-31.6449216312794,
55.264258863758));
#110311=CARTESIAN_POINT('Ctrl Pts',(6.55258536627677,-31.6459597945717,
55.2577135443564));
#110312=CARTESIAN_POINT('Ctrl Pts',(6.55344501240524,-31.6478885285661,
55.2450661648734));
#110313=CARTESIAN_POINT('Ctrl Pts',(6.55386131345546,-31.648784311075,55.2389650984162));
#110314=CARTESIAN_POINT('Ctrl Pts',(6.55488510715645,-31.6508945156848,
55.2240157711139));
#110315=CARTESIAN_POINT('Ctrl Pts',(6.55549460765298,-31.6520716836945,
55.2151625213445));
#110316=CARTESIAN_POINT('Ctrl Pts',(6.55775367196738,-31.6561471291876,
55.1825041635758));
#110317=CARTESIAN_POINT('Ctrl Pts',(6.55942476648695,-31.6586023523677,
55.158647959365));
#110318=CARTESIAN_POINT('Ctrl Pts',(6.56382220246398,-31.6636495727199,
55.0964497839689));
#110319=CARTESIAN_POINT('Ctrl Pts',(6.56657631845046,-31.6654313142897,
55.0580571472878));
#110320=CARTESIAN_POINT('Ctrl Pts',(6.57445120362573,-31.6667160417164,
54.9490843839346));
#110321=CARTESIAN_POINT('Ctrl Pts',(6.57961396198102,-31.6630646877723,
54.8785476238241));
#110322=CARTESIAN_POINT('Ctrl Pts',(6.59159738118093,-31.6440420474533,
54.7141919616201));
#110323=CARTESIAN_POINT('Ctrl Pts',(6.59834696353943,-31.6250971284716,
54.6210207830579));
#110324=CARTESIAN_POINT('Ctrl Pts',(6.60621484709289,-31.5926783515014,
54.5107853364076));
#110325=CARTESIAN_POINT('Ctrl Pts',(6.6075720973104,-31.5866957127602,54.4917165221717));
#110326=CARTESIAN_POINT('Ctrl Pts',(6.60972019712478,-31.5766030886609,
54.4614645137954));
#110327=CARTESIAN_POINT('Ctrl Pts',(6.61051818373063,-31.5727139121417,
54.4502102834942));
#110328=CARTESIAN_POINT('Ctrl Pts',(6.6120271607111,-31.565093953576,54.4289029232398));
#110329=CARTESIAN_POINT('Ctrl Pts',(6.6127388667327,-31.5613861373545,54.4188422814309));
#110330=CARTESIAN_POINT('Ctrl Pts',(6.61436097808779,-31.552675349376,54.3958920569952));
#110331=CARTESIAN_POINT('Ctrl Pts',(6.61526920207865,-31.5476084876256,
54.3830274434801));
#110332=CARTESIAN_POINT('Ctrl Pts',(6.61811386707399,-31.5311448823686,
54.3427062959116));
#110333=CARTESIAN_POINT('Ctrl Pts',(6.62003099203653,-31.5191727540191,
54.3154899699754));
#110334=CARTESIAN_POINT('Ctrl Pts',(6.62754596938904,-31.4688594641646,
54.2089442347415));
#110335=CARTESIAN_POINT('Ctrl Pts',(6.6329590627278,-31.4249797997386,54.1323871235107));
#110336=CARTESIAN_POINT('Ctrl Pts',(6.64524540973922,-31.3114866432478,
53.9664045617817));
#110337=CARTESIAN_POINT('Ctrl Pts',(6.65206559460718,-31.2384165709876,
53.8798956084));
#110338=CARTESIAN_POINT('Ctrl Pts',(6.66036552659228,-31.1465515002008,
53.7912015860564));
#110339=CARTESIAN_POINT('Ctrl Pts',(6.66133383591659,-31.1357953540181,
53.7810894925221));
#110340=CARTESIAN_POINT('Ctrl Pts',(6.66280228957537,-31.1194550410455,
53.7661316779733));
#110341=CARTESIAN_POINT('Ctrl Pts',(6.66329475876906,-31.1139703526395,
53.7611777071479));
#110342=CARTESIAN_POINT('Ctrl Pts',(6.66419224763573,-31.1039708595749,
53.7522658985747));
#110343=CARTESIAN_POINT('Ctrl Pts',(6.66459634586287,-31.099467381068,53.7482957532474));
#110344=CARTESIAN_POINT('Ctrl Pts',(6.66551640010813,-31.0892113127656,
53.7393523333189));
#110345=CARTESIAN_POINT('Ctrl Pts',(6.66603338983346,-31.0834461069383,
53.7343940775085));
#110346=CARTESIAN_POINT('Ctrl Pts',(6.66763708710476,-31.0655497049758,
53.7192145114203));
#110347=CARTESIAN_POINT('Ctrl Pts',(6.66873257049119,-31.0533067096527,
53.709127205663));
#110348=CARTESIAN_POINT('Ctrl Pts',(6.67447627725844,-30.9889329192329,
53.6576135496223));
#110349=CARTESIAN_POINT('Ctrl Pts',(6.67927577834879,-30.9345011445328,
53.6191685166873));
#110350=CARTESIAN_POINT('Ctrl Pts',(6.69273899257741,-30.7769696367807,
53.5214928191034));
#110351=CARTESIAN_POINT('Ctrl Pts',(6.70141841924839,-30.669597349037,53.4698653735107));
#110352=CARTESIAN_POINT('Ctrl Pts',(6.71246226014045,-30.5210218901359,
53.417090640398));
#110353=CARTESIAN_POINT('Ctrl Pts',(6.71514591414966,-30.4839602232894,
53.4053687628767));
#110354=CARTESIAN_POINT('Ctrl Pts',(6.71885660419074,-30.4313759477885,
53.390739960444));
#110355=CARTESIAN_POINT('Ctrl Pts',(6.71991831292793,-30.4161728647477,
53.386741415857));
#110356=CARTESIAN_POINT('Ctrl Pts',(6.7217054999011,-30.3903206469363,53.3803318449864));
#110357=CARTESIAN_POINT('Ctrl Pts',(6.72243451998192,-30.3797005215353,
53.3778093011255));
#110358=CARTESIAN_POINT('Ctrl Pts',(6.72390481430653,-30.3581343286676,
53.3729101916273));
#110359=CARTESIAN_POINT('Ctrl Pts',(6.72464587395247,-30.347187546578,53.3705392733303));
#110360=CARTESIAN_POINT('Ctrl Pts',(6.72647765479427,-30.3199441082982,
53.364925740841));
#110361=CARTESIAN_POINT('Ctrl Pts',(6.72756411025945,-30.3036210497676,
53.3618161409262));
#110362=CARTESIAN_POINT('Ctrl Pts',(6.73184527654185,-30.2386899828942,
53.3504504281761));
#110363=CARTESIAN_POINT('Ctrl Pts',(6.7349799413163,-30.1897698543038,53.3441090603889));
#110364=CARTESIAN_POINT('Ctrl Pts',(6.74360761037585,-30.0524770583381,
53.3324778720197));
#110365=CARTESIAN_POINT('Ctrl Pts',(6.74897558756391,-29.9638616631134,
53.3320435002566));
#110366=CARTESIAN_POINT('Ctrl Pts',(6.7594938352577,-29.7923215208844,53.3448853630534));
#110367=CARTESIAN_POINT('Ctrl Pts',(6.76462755606351,-29.7096121550668,
53.3573782164383));
#110368=CARTESIAN_POINT('Ctrl Pts',(6.77110298398023,-29.6121919639257,
53.3796819447237));
#110369=CARTESIAN_POINT('Ctrl Pts',(6.7721774885088,-29.5962401927215,53.3835830854678));
#110370=CARTESIAN_POINT('Ctrl Pts',(6.77377489571398,-29.5728888557533,
53.3896610600392));
#110371=CARTESIAN_POINT('Ctrl Pts',(6.77428799971171,-29.5654420285151,
53.391654640737));
#110372=CARTESIAN_POINT('Ctrl Pts',(6.77520625420989,-29.552216891469,53.3952936772094));
#110373=CARTESIAN_POINT('Ctrl Pts',(6.77561024597358,-29.546433260931,53.3969188088018));
#110374=CARTESIAN_POINT('Ctrl Pts',(6.7765091908108,-29.5336417413808,53.4005878394914));
#110375=CARTESIAN_POINT('Ctrl Pts',(6.77700494655082,-29.5266385206989,
53.4026465045521));
#110376=CARTESIAN_POINT('Ctrl Pts',(6.77847958508031,-29.5059512434473,
53.4088757202914));
#110377=CARTESIAN_POINT('Ctrl Pts',(6.7794653931904,-29.4923075223388,53.4131764555359));
#110378=CARTESIAN_POINT('Ctrl Pts',(6.78632560307716,-29.3985226082869,
53.4440723573382));
#110379=CARTESIAN_POINT('Ctrl Pts',(6.79245505366984,-29.3204563505974,
53.4765488418306));
#110380=CARTESIAN_POINT('Ctrl Pts',(6.80788164753911,-29.1315073154385,
53.5725757407264));
#110381=CARTESIAN_POINT('Ctrl Pts',(6.81711789559479,-29.0248065886135,
53.6432284561324));
#110382=CARTESIAN_POINT('Ctrl Pts',(6.82734013490775,-28.9111276206617,
53.7389074687808));
#110383=CARTESIAN_POINT('Ctrl Pts',(6.82877353692025,-28.89530988061,53.7527401069981));
#110384=CARTESIAN_POINT('Ctrl Pts',(6.83109604993436,-28.869892769504,53.7758303762298));
#110385=CARTESIAN_POINT('Ctrl Pts',(6.83199242314646,-28.8601357967463,
53.7849101941681));
#110386=CARTESIAN_POINT('Ctrl Pts',(6.83359759708086,-28.8427636436285,
53.8014701025973));
#110387=CARTESIAN_POINT('Ctrl Pts',(6.83430814708804,-28.8351094944398,
53.8089080561819));
#110388=CARTESIAN_POINT('Ctrl Pts',(6.83507857929352,-28.8268512987124,
53.8170887481323));
#110389=CARTESIAN_POINT('Ctrl Pts',(6.83514161006157,-28.8261759781728,
53.8177588778444));
#110390=CARTESIAN_POINT('Ctrl Pts',(6.83526452264084,-28.8248596649576,
53.8190673129861));
#110391=CARTESIAN_POINT('Ctrl Pts',(6.83532440685726,-28.8242186175232,
53.8197055626126));
#110392=CARTESIAN_POINT('Ctrl Pts',(6.83544187066243,-28.8229617318725,
53.820959002801));
#110393=CARTESIAN_POINT('Ctrl Pts',(6.83549945192553,-28.8223458554046,
53.8215741544607));
#110394=CARTESIAN_POINT('Ctrl Pts',(6.83560305029199,-28.8212382498314,
53.8226821919843));
#110395=CARTESIAN_POINT('Ctrl Pts',(6.83564907499752,-28.8207463474032,
53.823174903577));
#110396=CARTESIAN_POINT('Ctrl Pts',(6.83573287662861,-28.8198509918158,
53.8240728570715));
#110397=CARTESIAN_POINT('Ctrl Pts',(6.83577065794308,-28.8194474383768,
53.8244779984022));
#110398=CARTESIAN_POINT('Ctrl Pts',(6.83584010609792,-28.818705846083,53.8252232757313));
#110399=CARTESIAN_POINT('Ctrl Pts',(6.83587177563708,-28.8183677454655,
53.8255633499389));
#110400=CARTESIAN_POINT('Ctrl Pts',(6.83593044164009,-28.8177415784931,
53.8261937161408));
#110401=CARTESIAN_POINT('Ctrl Pts',(6.83595743984718,-28.8174534721845,
53.8264839682376));
#110402=CARTESIAN_POINT('Ctrl Pts',(6.8360077757481,-28.8169164284342,53.8270254104384));
#110403=CARTESIAN_POINT('Ctrl Pts',(6.83603111461288,-28.8166674641071,
53.8272765737124));
#110404=CARTESIAN_POINT('Ctrl Pts',(6.83607486602183,-28.8162008317435,
53.8277476274427));
#110405=CARTESIAN_POINT('Ctrl Pts',(6.83609527937983,-28.8159831449993,
53.8279674992538));
#110406=CARTESIAN_POINT('Ctrl Pts',(6.83613372631143,-28.815573211118,53.8283817786788));
#110407=CARTESIAN_POINT('Ctrl Pts',(6.83615176046674,-28.8153809505954,
53.8285761729668));
#110408=CARTESIAN_POINT('Ctrl Pts',(6.8361858649719,-28.8150174139846,53.8289439252416));
#110409=CARTESIAN_POINT('Ctrl Pts',(6.83620193575106,-28.8148461280511,
53.8291172735098));
#110410=CARTESIAN_POINT('Ctrl Pts',(6.83623243619874,-28.814521086211,53.8294463733511));
#110411=CARTESIAN_POINT('Ctrl Pts',(6.83624686618403,-28.8143673229833,
53.8296021176157));
#110412=CARTESIAN_POINT('Ctrl Pts',(6.83627433952821,-28.8140746035144,
53.8298987252713));
#110413=CARTESIAN_POINT('Ctrl Pts',(6.836287383132,-28.8139356416561,53.8300395831406));
#110414=CARTESIAN_POINT('Ctrl Pts',(6.83631228732558,-28.8136703470738,
53.830308593273));
#110415=CARTESIAN_POINT('Ctrl Pts',(6.83632414810166,-28.8135440100357,
53.8304367412317));
#110416=CARTESIAN_POINT('Ctrl Pts',(6.83634685163478,-28.813302200916,53.8306820959549));
#110417=CARTESIAN_POINT('Ctrl Pts',(6.83635769454145,-28.8131867254108,
53.8307992993801));
#110418=CARTESIAN_POINT('Ctrl Pts',(6.83637849756472,-28.8129651939076,
53.8310242124088));
#110419=CARTESIAN_POINT('Ctrl Pts',(6.83638845779823,-28.8128591352087,
53.8311319193375));
#110420=CARTESIAN_POINT('Ctrl Pts',(6.83640760744377,-28.8126552408453,
53.8313390387445));
#110421=CARTESIAN_POINT('Ctrl Pts',(6.83641679694208,-28.8125574030905,
53.8314384489897));
#110422=CARTESIAN_POINT('Ctrl Pts',(6.83646057669842,-28.8120913255394,
53.8319121365132));
#110423=CARTESIAN_POINT('Ctrl Pts',(6.83649515985212,-28.8117232498803,
53.8322865759057));
#110424=CARTESIAN_POINT('Ctrl Pts',(6.83656431451738,-28.8109874134505,
53.8330358425514));
#110425=CARTESIAN_POINT('Ctrl Pts',(6.83659888602374,-28.8106196527552,
53.8334106698021));
#110426=CARTESIAN_POINT('Ctrl Pts',(6.83771103258841,-28.7987920731994,
53.8454769237986));
#110427=CARTESIAN_POINT('Ctrl Pts',(6.83878112541177,-28.7875047105982,
53.8573367857502));
#110428=CARTESIAN_POINT('Ctrl Pts',(6.84310129633435,-28.7423488813134,
53.90620559449));
#110429=CARTESIAN_POINT('Ctrl Pts',(6.84628873624599,-28.7099834588903,
53.9445708939718));
#110430=CARTESIAN_POINT('Ctrl Pts',(6.85516692072802,-28.6234808572727,
54.0570453664965));
#110431=CARTESIAN_POINT('Ctrl Pts',(6.8607218294409,-28.5736642265657,54.1342427942307));
#110432=CARTESIAN_POINT('Ctrl Pts',(6.86680934089025,-28.5268050245209,
54.2219816610238));
#110433=CARTESIAN_POINT('Ctrl Pts',(6.86728370050633,-28.5232044675888,
54.2288379378827));
#110434=CARTESIAN_POINT('Ctrl Pts',(6.8725302379048,-28.4839611774338,54.3048489007251));
#110435=CARTESIAN_POINT('Ctrl Pts',(6.8773524817932,-28.4531611918282,54.37638528604));
#110436=CARTESIAN_POINT('Ctrl Pts',(6.88323618885321,-28.4234128320027,
54.4614091006557));
#110437=CARTESIAN_POINT('Ctrl Pts',(6.8840458277414,-28.4194800173811,54.4730618462956));
#110438=CARTESIAN_POINT('Ctrl Pts',(6.88532459030823,-28.4135257891944,
54.4913705195861));
#110439=CARTESIAN_POINT('Ctrl Pts',(6.8857888172279,-28.411416350646,54.4979976548669));
#110440=CARTESIAN_POINT('Ctrl Pts',(6.88666167855222,-28.407548622983,54.5104172640336));
#110441=CARTESIAN_POINT('Ctrl Pts',(6.88706973481944,-28.4057803301274,
54.5162063631653));
#110442=CARTESIAN_POINT('Ctrl Pts',(6.88803550844753,-28.4016881818446,
54.5298694525105));
#110443=CARTESIAN_POINT('Ctrl Pts',(6.88859470570326,-28.3993909380068,
54.5377511240206));
#110444=CARTESIAN_POINT('Ctrl Pts',(6.89047605389359,-28.3918991639899,
54.5641804279561));
#110445=CARTESIAN_POINT('Ctrl Pts',(6.8918116887932,-28.3869682669896,54.5828003504918));
#110446=CARTESIAN_POINT('Ctrl Pts',(6.90253166792987,-28.3503542747171,
54.7314284138191));
#110447=CARTESIAN_POINT('Ctrl Pts',(6.91245387919625,-28.3341187293571,
54.8647290811869));
#110448=CARTESIAN_POINT('Ctrl Pts',(6.92208048413035,-28.3340006487619,
54.9985297366875));
#110449=CARTESIAN_POINT('Ctrl Pts',(6.92208059163593,-28.3340006474439,
54.9985312309128));
#110450=CARTESIAN_POINT('Ctrl Pts',(6.92754558400022,-28.3339336815855,
55.0744894450113));
#110451=CARTESIAN_POINT('Ctrl Pts',(6.9329088628046,-28.3390614478877,55.1503739691616));
#110452=CARTESIAN_POINT('Ctrl Pts',(6.93913001267378,-28.3513608312705,
55.240342760058));
#110453=CARTESIAN_POINT('Ctrl Pts',(6.94013956192787,-28.3535646995461,
55.2550030920907));
#110454=CARTESIAN_POINT('Ctrl Pts',(6.94187955803527,-28.3577252098531,
55.2803710625575));
#110455=CARTESIAN_POINT('Ctrl Pts',(6.94261278500586,-28.3595916142998,
55.2910923512533));
#110456=CARTESIAN_POINT('Ctrl Pts',(6.94407769604804,-28.3635481035932,
55.3125720400525));
#110457=CARTESIAN_POINT('Ctrl Pts',(6.94480929686973,-28.3656395611335,
55.3233296386573));
#110458=CARTESIAN_POINT('Ctrl Pts',(6.94620091272753,-28.3698387894156,
55.3438460153887));
#110459=CARTESIAN_POINT('Ctrl Pts',(6.9468614704027,-28.3719284220095,55.3536079737256));
#110460=CARTESIAN_POINT('Ctrl Pts',(6.94857774680902,-28.3776091700568,
55.3790277533253));
#110461=CARTESIAN_POINT('Ctrl Pts',(6.94962899207316,-28.3813392795987,
55.3946537021924));
#110462=CARTESIAN_POINT('Ctrl Pts',(6.95335095277997,-28.3954360792833,
55.4501409233542));
#110463=CARTESIAN_POINT('Ctrl Pts',(6.95598175595763,-28.4070544959849,
55.4896705798554));
#110464=CARTESIAN_POINT('Ctrl Pts',(6.95961845963333,-28.4253742592874,
55.5444108263045));
#110465=CARTESIAN_POINT('Ctrl Pts',(6.96065394412911,-28.4308534186706,
55.5600072461366));
#110466=CARTESIAN_POINT('Ctrl Pts',(6.96168426276526,-28.4365622954254,
55.5755158937115));
#110467=CARTESIAN_POINT('Ctrl Pts',(6.76892552105682,-28.4365623357949,
55.5755160033788));
#110468=CARTESIAN_POINT('Ctrl Pts',(6.76565913960721,-28.4207846271609,
55.5326545298688));
#110469=CARTESIAN_POINT('Ctrl Pts',(6.76234508913007,-28.4067718546495,
55.4891506581147));
#110470=CARTESIAN_POINT('Ctrl Pts',(6.75469118016146,-28.3786619363516,
55.3877638001349));
#110471=CARTESIAN_POINT('Ctrl Pts',(6.75035205900689,-28.3658452849425,
55.3296007955738));
#110472=CARTESIAN_POINT('Ctrl Pts',(6.74215952333329,-28.3473559318162,
55.2173964913116));
#110473=CARTESIAN_POINT('Ctrl Pts',(6.7383018338593,-28.3411578477954,55.1635154863884));
#110474=CARTESIAN_POINT('Ctrl Pts',(6.73197961047013,-28.3352107256762,
55.0731647396338));
#110475=CARTESIAN_POINT('Ctrl Pts',(6.72947634806754,-28.3340108244741,
55.0368351827447));
#110476=CARTESIAN_POINT('Ctrl Pts',(6.7260983248784,-28.3339961009531,54.9870677129444));
#110477=CARTESIAN_POINT('Ctrl Pts',(6.72519214130387,-28.3341544057567,
54.9736426547827));
#110478=CARTESIAN_POINT('Ctrl Pts',(6.72362205828857,-28.3347129509713,
54.9502568887751));
#110479=CARTESIAN_POINT('Ctrl Pts',(6.72295592249942,-28.3350403340662,
54.9402953013315));
#110480=CARTESIAN_POINT('Ctrl Pts',(6.72156263854722,-28.3359156860119,
54.9193794326819));
#110481=CARTESIAN_POINT('Ctrl Pts',(6.7208361119486,-28.3364824730713,54.90842638312));
#110482=CARTESIAN_POINT('Ctrl Pts',(6.71909604212404,-28.3381063644793,
54.8820874958341));
#110483=CARTESIAN_POINT('Ctrl Pts',(6.71808583914157,-28.3392690314072,
54.8667090002036));
#110484=CARTESIAN_POINT('Ctrl Pts',(6.71448948270676,-28.3441987761385,
54.8116796715743));
#110485=CARTESIAN_POINT('Ctrl Pts',(6.71194085023437,-28.349173988967,54.7721489212533));
#110486=CARTESIAN_POINT('Ctrl Pts',(6.7055033239652,-28.3655282164239,54.6714875184788));
#110487=CARTESIAN_POINT('Ctrl Pts',(6.70167015474496,-28.3789199735198,
54.6107457844851));
#110488=CARTESIAN_POINT('Ctrl Pts',(6.69223982706329,-28.4204369267072,
54.4624371944141));
#110489=CARTESIAN_POINT('Ctrl Pts',(6.68669528109406,-28.4524696586101,
54.3761883382278));
#110490=CARTESIAN_POINT('Ctrl Pts',(6.67845245895701,-28.5081580881101,
54.2573593702817));
#110491=CARTESIAN_POINT('Ctrl Pts',(6.67593863597083,-28.526130591661,54.2223009466579));
#110492=CARTESIAN_POINT('Ctrl Pts',(6.67264000283335,-28.5506590798549,
54.1783634791932));
#110493=CARTESIAN_POINT('Ctrl Pts',(6.67191773854498,-28.5560853256686,
54.1688645882659));
#110494=CARTESIAN_POINT('Ctrl Pts',(6.67075133868079,-28.564928023312,54.1537330145712));
#110495=CARTESIAN_POINT('Ctrl Pts',(6.67031087935598,-28.5682851323065,
54.148065775569));
#110496=CARTESIAN_POINT('Ctrl Pts',(6.66945256782083,-28.5748592929456,
54.1371163371139));
#110497=CARTESIAN_POINT('Ctrl Pts',(6.66903496784038,-28.5780722847564,
54.1318319182112));
#110498=CARTESIAN_POINT('Ctrl Pts',(6.66800259614495,-28.586052227117,54.1188704077936));
#110499=CARTESIAN_POINT('Ctrl Pts',(6.66738573788347,-28.5908523218151,
54.1112140446122));
#110500=CARTESIAN_POINT('Ctrl Pts',(6.66506535781466,-28.6090356622443,
54.0827284038169));
#110501=CARTESIAN_POINT('Ctrl Pts',(6.66333881220431,-28.6228197022216,
54.0621603339405));
#110502=CARTESIAN_POINT('Ctrl Pts',(6.65875255541449,-28.6602128406918,
54.0089663019004));
#110503=CARTESIAN_POINT('Ctrl Pts',(6.65586231210795,-28.6845550395998,
53.9768765597092));
#110504=CARTESIAN_POINT('Ctrl Pts',(6.64436107731688,-28.7851674674738,
53.8537741387872));
#110505=CARTESIAN_POINT('Ctrl Pts',(6.63563985538018,-28.8699229760116,
53.7701287418851));
#110506=CARTESIAN_POINT('Ctrl Pts',(6.62373755226918,-29.0016827291212,
53.6653164449545));
#110507=CARTESIAN_POINT('Ctrl Pts',(6.62028777090021,-29.0418737345012,
53.6361772485195));
#110508=CARTESIAN_POINT('Ctrl Pts',(6.61573906128677,-29.0976002886783,
53.599455937511));
#110509=CARTESIAN_POINT('Ctrl Pts',(6.61458074932236,-29.112035869094,53.5902593677723));
#110510=CARTESIAN_POINT('Ctrl Pts',(6.61267136477174,-29.1362331540602,
53.5753630257135));
#110511=CARTESIAN_POINT('Ctrl Pts',(6.61191571483802,-29.145915438421,53.5695374016819));
#110512=CARTESIAN_POINT('Ctrl Pts',(6.61043400696999,-29.1651067156508,
53.5582547455127));
#110513=CARTESIAN_POINT('Ctrl Pts',(6.60970777601657,-29.1746117728639,
53.5527921851536));
#110514=CARTESIAN_POINT('Ctrl Pts',(6.6079697011109,-29.1975930211952,53.5398849207254));
#110515=CARTESIAN_POINT('Ctrl Pts',(6.60696117765908,-29.2111199950772,
53.5325323280187));
#110516=CARTESIAN_POINT('Ctrl Pts',(6.60337852832171,-29.2598344180083,
53.5069218781544));
#110517=CARTESIAN_POINT('Ctrl Pts',(6.60084153221793,-29.2955706091488,
53.4897328088498));
#110518=CARTESIAN_POINT('Ctrl Pts',(6.59444280456623,-29.3884130256801,
53.4490890690541));
#110519=CARTESIAN_POINT('Ctrl Pts',(6.59063587572078,-29.446271590263,53.427502300134));
#110520=CARTESIAN_POINT('Ctrl Pts',(6.58129890638515,-29.5918521135978,
53.3822216512348));
#110521=CARTESIAN_POINT('Ctrl Pts',(6.57582061778002,-29.6805585883479,
53.3623960455244));
#110522=CARTESIAN_POINT('Ctrl Pts',(6.56756518769043,-29.8109303378142,
53.344258310898));
#110523=CARTESIAN_POINT('Ctrl Pts',(6.56495912441035,-29.8516190317749,
53.3401173639789));
#110524=CARTESIAN_POINT('Ctrl Pts',(6.56155321139184,-29.9034879401764,
53.3367608269718));
#110525=CARTESIAN_POINT('Ctrl Pts',(6.56082083952193,-29.9145674369421,
53.3361549395543));
#110526=CARTESIAN_POINT('Ctrl Pts',(6.55964198787364,-29.9322664048435,
53.3353643039506));
#110527=CARTESIAN_POINT('Ctrl Pts',(6.55919932393568,-29.9388825807096,
53.3351082624658));
#110528=CARTESIAN_POINT('Ctrl Pts',(6.55834007545749,-29.9516631893432,
53.3346899451462));
#110529=CARTESIAN_POINT('Ctrl Pts',(6.55792377613938,-29.9578272555728,
53.3345224466653));
#110530=CARTESIAN_POINT('Ctrl Pts',(6.55689948046678,-29.9729284031371,
53.3341959819868));
#110531=CARTESIAN_POINT('Ctrl Pts',(6.55628947003476,-29.9818660319469,
53.3340747171622));
#110532=CARTESIAN_POINT('Ctrl Pts',(6.55402543249386,-30.014848840184,53.3338926546128));
#110533=CARTESIAN_POINT('Ctrl Pts',(6.55234975124015,-30.0388923062775,
53.3342805107416));
#110534=CARTESIAN_POINT('Ctrl Pts',(6.54793660452432,-30.1014684288166,
53.3366454183497));
#110535=CARTESIAN_POINT('Ctrl Pts',(6.54517113475498,-30.1399549445576,
53.3394408923582));
#110536=CARTESIAN_POINT('Ctrl Pts',(6.53729713520417,-30.2482866903495,
53.3511023076848));
#110537=CARTESIAN_POINT('Ctrl Pts',(6.53214743478204,-30.3177182737567,
53.3630622936105));
#110538=CARTESIAN_POINT('Ctrl Pts',(6.52018033767066,-30.4784482649231,
53.4013633801534));
#110539=CARTESIAN_POINT('Ctrl Pts',(6.51343421824998,-30.5686776635636,
53.4311906017877));
#110540=CARTESIAN_POINT('Ctrl Pts',(6.50557015903207,-30.6742518370309,
53.4764057508554));
#110541=CARTESIAN_POINT('Ctrl Pts',(6.50421350324754,-30.6924708840814,
53.4845993563753));
#110542=CARTESIAN_POINT('Ctrl Pts',(6.50206627961172,-30.72130450789,53.498195260846));
#110543=CARTESIAN_POINT('Ctrl Pts',(6.50126858138943,-30.7320156596414,
53.5033869055708));
#110544=CARTESIAN_POINT('Ctrl Pts',(6.49976011864925,-30.7522648828816,
53.5134710135772));
#110545=CARTESIAN_POINT('Ctrl Pts',(6.49904863924309,-30.7618131200177,
53.5183415842971));
#110546=CARTESIAN_POINT('Ctrl Pts',(6.49742701024426,-30.7835650422488,
53.5297031375696));
#110547=CARTESIAN_POINT('Ctrl Pts',(6.49651904096685,-30.7957363897359,
53.5362545794267));
#110548=CARTESIAN_POINT('Ctrl Pts',(6.49367509061945,-30.8338168646511,
53.5573674509288));
#110549=CARTESIAN_POINT('Ctrl Pts',(6.49175841672865,-30.8594195421304,
53.5724715556519));
#110550=CARTESIAN_POINT('Ctrl Pts',(6.48423921188111,-30.9593206248306,
53.6350699472592));
#110551=CARTESIAN_POINT('Ctrl Pts',(6.47882182428877,-31.0302044313446,
53.6877457840761));
#110552=CARTESIAN_POINT('Ctrl Pts',(6.46653547230616,-31.181579873004,53.820097571756));
#110553=CARTESIAN_POINT('Ctrl Pts',(6.45971928616396,-31.2587834073888,
53.9028410379685));
#110554=CARTESIAN_POINT('Ctrl Pts',(6.45142363028504,-31.3359485144926,
54.004502277826));
#110555=CARTESIAN_POINT('Ctrl Pts',(6.45045488656884,-31.3447211317998,
54.01638463353));
#110556=CARTESIAN_POINT('Ctrl Pts',(6.44898599694043,-31.3576445911966,
54.0343852797418));
#110557=CARTESIAN_POINT('Ctrl Pts',(6.44849353533333,-31.3619148388974,
54.0404174916245));
#110558=CARTESIAN_POINT('Ctrl Pts',(6.44759619415702,-31.3695798107692,
54.0513993654085));
#110559=CARTESIAN_POINT('Ctrl Pts',(6.44719223723379,-31.3729881136117,
54.0563392248127));
#110560=CARTESIAN_POINT('Ctrl Pts',(6.4462726942587,-31.3806511842817,54.0675751779392));
#110561=CARTESIAN_POINT('Ctrl Pts',(6.4457560773142,-31.3848895887407,54.0738819930576));
#110562=CARTESIAN_POINT('Ctrl Pts',(6.44415419193571,-31.3978310598427,
54.0934266100667));
#110563=CARTESIAN_POINT('Ctrl Pts',(6.44306017257623,-31.4063882728738,
54.1067592913909));
#110564=CARTESIAN_POINT('Ctrl Pts',(6.43733025671541,-31.4498246622094,
54.1766076473768));
#110565=CARTESIAN_POINT('Ctrl Pts',(6.43254380757642,-31.4814888094224,
54.2350452908363));
#110566=CARTESIAN_POINT('Ctrl Pts',(6.41913087593009,-31.5596129183819,
54.4023780319856));
#110567=CARTESIAN_POINT('Ctrl Pts',(6.41048772483013,-31.5981003872293,
54.5145859991129));
#110568=CARTESIAN_POINT('Ctrl Pts',(6.39943625471713,-31.6331301734757,
54.6683465839482));
#110569=CARTESIAN_POINT('Ctrl Pts',(6.39671430126995,-31.6405167081928,
54.7070605367482));
#110570=CARTESIAN_POINT('Ctrl Pts',(6.3929613210461,-31.6489317475928,54.7616106358652));
#110571=CARTESIAN_POINT('Ctrl Pts',(6.39189452965546,-31.6511174567935,
54.7772522259164));
#110572=CARTESIAN_POINT('Ctrl Pts',(6.39010151789645,-31.654438577159,54.8037644873379));
#110573=CARTESIAN_POINT('Ctrl Pts',(6.38937169798392,-31.6556900011961,
54.8146192788589));
#110574=CARTESIAN_POINT('Ctrl Pts',(6.38790199257379,-31.6580055197637,
54.836602772055));
#110575=CARTESIAN_POINT('Ctrl Pts',(6.38716230119331,-31.6590645725183,
54.8477314471046));
#110576=CARTESIAN_POINT('Ctrl Pts',(6.38533804317809,-31.6614109970575,
54.875330799598));
#110577=CARTESIAN_POINT('Ctrl Pts',(6.38425766760158,-31.6625655640006,
54.8918117930393));
#110578=CARTESIAN_POINT('Ctrl Pts',(6.38003469447249,-31.6661436116671,
54.9567244872429));
#110579=CARTESIAN_POINT('Ctrl Pts',(6.37695000439576,-31.6666974965136,
55.0052376413418));
#110580=CARTESIAN_POINT('Ctrl Pts',(6.36853173401014,-31.6623660967111,
55.1395219713638));
#110581=CARTESIAN_POINT('Ctrl Pts',(6.3633149707635,-31.6529689842531,55.2249932908889));
#110582=CARTESIAN_POINT('Ctrl Pts',(6.35273130926609,-31.6208093352436,
55.3951693111171));
#110583=CARTESIAN_POINT('Ctrl Pts',(6.34737753893032,-31.5978743123499,
55.4795576963606));
#110584=CARTESIAN_POINT('Ctrl Pts',(6.34067490008158,-31.5629997112202,
55.5769297476035));
#110585=CARTESIAN_POINT('Ctrl Pts',(6.33961976133011,-31.5573425782077,
55.5920304706183));
#110586=CARTESIAN_POINT('Ctrl Pts',(6.33803882002499,-31.5486392841874,
55.6142740514982));
#110587=CARTESIAN_POINT('Ctrl Pts',(6.33752231626647,-31.5457607467596,
55.6214820598275));
#110588=CARTESIAN_POINT('Ctrl Pts',(6.3366006126894,-31.5405645387525,55.6342341910222));
#110589=CARTESIAN_POINT('Ctrl Pts',(6.33619661128963,-31.5382670870313,
55.6397862720448));
#110590=CARTESIAN_POINT('Ctrl Pts',(6.33530092274614,-31.5331304351076,
55.6520120122583));
#110591=CARTESIAN_POINT('Ctrl Pts',(6.3348084682096,-31.5302777091874,55.6586795298017));
#110592=CARTESIAN_POINT('Ctrl Pts',(6.33335289649635,-31.5217596048237,
55.6782343884176));
#110593=CARTESIAN_POINT('Ctrl Pts',(6.33238310745829,-31.5159744657094,
55.6910684243616));
#110594=CARTESIAN_POINT('Ctrl Pts',(6.32555324472647,-31.4744261789098,
55.780208305354));
#110595=CARTESIAN_POINT('Ctrl Pts',(6.31943758145037,-31.4330842354636,
55.8537705976458));
#110596=CARTESIAN_POINT('Ctrl Pts',(6.30398734668806,-31.3153632882223,
56.0304205842287));
#110597=CARTESIAN_POINT('Ctrl Pts',(6.29471262151449,-31.2323071698481,
56.1284405037142));
#110598=CARTESIAN_POINT('Ctrl Pts',(6.28445419227063,-31.1234770690454,
56.2303648311442));
#110599=CARTESIAN_POINT('Ctrl Pts',(6.28301927600217,-31.1078547368788,
56.2444501976226));
#110600=CARTESIAN_POINT('Ctrl Pts',(6.2806949817233,-31.0819006765262,56.2669746074155));
#110601=CARTESIAN_POINT('Ctrl Pts',(6.27979831944513,-31.0717273510327,
56.2755917186481));
#110602=CARTESIAN_POINT('Ctrl Pts',(6.2781930383006,-31.0532277523854,56.2908838604507));
#110603=CARTESIAN_POINT('Ctrl Pts',(6.27748266537849,-31.0449388083166,
56.2976026878558));
#110604=CARTESIAN_POINT('Ctrl Pts',(6.275966711171,-31.0270331436314,56.3118337604913));
#110605=CARTESIAN_POINT('Ctrl Pts',(6.27516215461958,-31.0173972371559,
56.3193209497322));
#110606=CARTESIAN_POINT('Ctrl Pts',(6.27295821498649,-30.9906425858215,
56.3396421102787));
#110607=CARTESIAN_POINT('Ctrl Pts',(6.27156750488079,-30.9733571736003,
56.3522535253417));
#110608=CARTESIAN_POINT('Ctrl Pts',(6.26848416334874,-30.9341758651185,
56.3796994699422));
#110609=CARTESIAN_POINT('Ctrl Pts',(6.26679816403113,-30.9121598520017,
56.394352785779));
#110610=CARTESIAN_POINT('Ctrl Pts',(6.2613425696314,-30.8391584250602,56.4404713568075));
#110611=CARTESIAN_POINT('Ctrl Pts',(6.25764181277045,-30.7868220310939,
56.4697130563502));
#110612=CARTESIAN_POINT('Ctrl Pts',(6.24705519159442,-30.631701448412,56.5457164832189));
#110613=CARTESIAN_POINT('Ctrl Pts',(6.24028335159298,-30.525611856789,56.5849331272356));
#110614=CARTESIAN_POINT('Ctrl Pts',(6.23147096204794,-30.391991959689,56.6194236928982));
#110615=CARTESIAN_POINT('Ctrl Pts',(6.22984092402359,-30.3674582929019,
56.6251661559635));
#110616=CARTESIAN_POINT('Ctrl Pts',(6.22756639512607,-30.333649021922,56.6322750618287));
#110617=CARTESIAN_POINT('Ctrl Pts',(6.22694650420925,-30.3244767785757,
56.6341231157266));
#110618=CARTESIAN_POINT('Ctrl Pts',(6.22594692689197,-30.3097638685522,
56.6369587701112));
#110619=CARTESIAN_POINT('Ctrl Pts',(6.22556997045007,-30.3042327582114,
56.63799575572));
#110620=CARTESIAN_POINT('Ctrl Pts',(6.2247659752807,-30.2924754111959,56.6401384461436));
#110621=CARTESIAN_POINT('Ctrl Pts',(6.22433851405639,-30.2862479628438,
56.6412367558021));
#110622=CARTESIAN_POINT('Ctrl Pts',(6.22324859214083,-30.2704253361429,
56.643934537624));
#110623=CARTESIAN_POINT('Ctrl Pts',(6.22258352627971,-30.2608222607942,
56.6454854491177));
#110624=CARTESIAN_POINT('Ctrl Pts',(6.21982557876068,-30.2211898667766,
56.6515305021562));
#110625=CARTESIAN_POINT('Ctrl Pts',(6.21769755102649,-30.1910559042534,
56.6552870815289));
#110626=CARTESIAN_POINT('Ctrl Pts',(6.21163307096178,-30.1059932103466,
56.6635377201471));
#110627=CARTESIAN_POINT('Ctrl Pts',(6.20764067030133,-30.0509208727521,
56.6661328452094));
#110628=CARTESIAN_POINT('Ctrl Pts',(6.19369668431815,-29.859214975582,56.6656524085174));
#110629=CARTESIAN_POINT('Ctrl Pts',(6.18377226498223,-29.7231363052639,
56.6485081443138));
#110630=CARTESIAN_POINT('Ctrl Pts',(6.17287212023248,-29.5693351443392,
56.6095241200098));
#110631=CARTESIAN_POINT('Ctrl Pts',(6.17137385763873,-29.5481154474207,
56.6036959008019));
#110632=CARTESIAN_POINT('Ctrl Pts',(6.16904845124402,-29.5150708146775,
56.593911821669));
#110633=CARTESIAN_POINT('Ctrl Pts',(6.16821220287055,-29.50316488592,56.5902408918359));
#110634=CARTESIAN_POINT('Ctrl Pts',(6.16667604723887,-29.4812574091198,
56.5832161473564));
#110635=CARTESIAN_POINT('Ctrl Pts',(6.16597494257161,-29.4712444664426,
56.579900262463));
#110636=CARTESIAN_POINT('Ctrl Pts',(6.16441998665112,-29.4490098870519,
56.5723020005301));
#110637=CARTESIAN_POINT('Ctrl Pts',(6.163567761031,-29.4368052453364,56.5679717374854));
#110638=CARTESIAN_POINT('Ctrl Pts',(6.16107954471644,-29.4011313341281,
56.5548441912792));
#110639=CARTESIAN_POINT('Ctrl Pts',(6.1594564367364,-29.3778080046413,56.5456588775443));
#110640=CARTESIAN_POINT('Ctrl Pts',(6.1557642500518,-29.324734250198,56.523360953281));
#110641=CARTESIAN_POINT('Ctrl Pts',(6.15370666320824,-29.2951423092575,
56.5098967703338));
#110642=CARTESIAN_POINT('Ctrl Pts',(6.14631411352556,-29.1892381060753,
56.4579182726777));
#110643=CARTESIAN_POINT('Ctrl Pts',(6.14111992281912,-29.1155245406598,
56.4144132103598));
#110644=CARTESIAN_POINT('Ctrl Pts',(6.13052716357668,-28.9734485739807,
56.3150933427554));
#110645=CARTESIAN_POINT('Ctrl Pts',(6.1251414737833,-28.9055305507484,56.2591310944306));
#110646=CARTESIAN_POINT('Ctrl Pts',(6.11840332696257,-28.8307574367917,
56.1868815102113));
#110647=CARTESIAN_POINT('Ctrl Pts',(6.11734846581929,-28.8193278486441,
56.1755122777082));
#110648=CARTESIAN_POINT('Ctrl Pts',(6.11576786352582,-28.8026433639619,
56.1584270869045));
#110649=CARTESIAN_POINT('Ctrl Pts',(6.11525141547136,-28.7972601671323,
56.1528369867466));
#110650=CARTESIAN_POINT('Ctrl Pts',(6.11432977076201,-28.7877786421232,
56.142852346549));
#110651=CARTESIAN_POINT('Ctrl Pts',(6.11392577189538,-28.7836647459912,
56.1384729483725));
#110652=CARTESIAN_POINT('Ctrl Pts',(6.11303003876439,-28.7746373588998,
56.1287581684698));
#110653=CARTESIAN_POINT('Ctrl Pts',(6.11253753657757,-28.7697350401914,
56.1234129822956));
#110654=CARTESIAN_POINT('Ctrl Pts',(6.1111662516064,-28.7562498899095,56.1085154827675));
#110655=CARTESIAN_POINT('Ctrl Pts',(6.11028232248432,-28.7477425734866,
56.0988959116583));
#110656=CARTESIAN_POINT('Ctrl Pts',(6.10386852958636,-28.6872780949533,
56.0289123142471));
#110657=CARTESIAN_POINT('Ctrl Pts',(6.09810499110205,-28.6396026750669,
55.9649952137625));
#110658=CARTESIAN_POINT('Ctrl Pts',(6.08576410893854,-28.5481673300027,
55.8220958458226));
#110659=CARTESIAN_POINT('Ctrl Pts',(6.07920231560819,-28.5058704460738,
55.7424548369521));
#110660=CARTESIAN_POINT('Ctrl Pts',(6.07066779044151,-28.458232716068,55.6320007499705));
#110661=CARTESIAN_POINT('Ctrl Pts',(6.06854154822013,-28.4470114662275,
55.6039019484675));
#110662=CARTESIAN_POINT('Ctrl Pts',(6.06643884243078,-28.4365623175998,
55.5755159539501));
#110663=CARTESIAN_POINT('Origin',(5.,-30.,55.));
#110664=CARTESIAN_POINT('',(5.36787289131612,-28.4365623102018,55.5755159338528));
#110665=CARTESIAN_POINT('',(5.55935721585159,-28.4365623067732,55.5755159245387));
#110666=CARTESIAN_POINT('',(5.,-28.4365623102018,55.5755159338528));
#110667=CARTESIAN_POINT('Ctrl Pts',(5.55935721585159,-28.4365623067732,
55.5755159245387));
#110668=CARTESIAN_POINT('Ctrl Pts',(5.56381476847205,-28.4585691496616,
55.6352993748544));
#110669=CARTESIAN_POINT('Ctrl Pts',(5.56841204010037,-28.4839877256715,
55.6937734764538));
#110670=CARTESIAN_POINT('Ctrl Pts',(5.57397509760752,-28.5184874138571,
55.7621298013789));
#110671=CARTESIAN_POINT('Ctrl Pts',(5.57491059573364,-28.5244144050035,
55.7735428404087));
#110672=CARTESIAN_POINT('Ctrl Pts',(5.58247805316143,-28.5734009825808,
55.8652594684437));
#110673=CARTESIAN_POINT('Ctrl Pts',(5.58910661587447,-28.6228547543361,
55.9419834019496));
#110674=CARTESIAN_POINT('Ctrl Pts',(5.59908095274396,-28.7087755324195,
56.0539424144225));
#110675=CARTESIAN_POINT('Ctrl Pts',(5.60255546273909,-28.7409836611449,
56.0922151764099));
#110676=CARTESIAN_POINT('Ctrl Pts',(5.60707502115421,-28.7859483278344,
56.1410091598792));
#110677=CARTESIAN_POINT('Ctrl Pts',(5.60818129790271,-28.7972057452019,
56.1528700617814));
#110678=CARTESIAN_POINT('Ctrl Pts',(5.60931537774297,-28.8090033880795,
56.1649392027702));
#110679=CARTESIAN_POINT('Ctrl Pts',(5.60935065576839,-28.8093706381696,
56.1653145491692));
#110680=CARTESIAN_POINT('Ctrl Pts',(5.60942120053917,-28.8101055381518,
56.1660649405104));
#110681=CARTESIAN_POINT('Ctrl Pts',(5.60945646727773,-28.8104731880354,
56.1664399853584));
#110682=CARTESIAN_POINT('Ctrl Pts',(5.60950124849403,-28.8109403532348,
56.1669160966205));
#110683=CARTESIAN_POINT('Ctrl Pts',(5.60951077018214,-28.8110397039575,
56.1670173240154));
#110684=CARTESIAN_POINT('Ctrl Pts',(5.60953061972351,-28.8112468563811,
56.1672283355068));
#110685=CARTESIAN_POINT('Ctrl Pts',(5.60954094747514,-28.8113546603562,
56.1673381173494));
#110686=CARTESIAN_POINT('Ctrl Pts',(5.60956252718555,-28.8115799618273,
56.1675674888317));
#110687=CARTESIAN_POINT('Ctrl Pts',(5.60957377901646,-28.811697462146,56.1676870756487));
#110688=CARTESIAN_POINT('Ctrl Pts',(5.60959734966741,-28.8119436603209,
56.1679375700131));
#110689=CARTESIAN_POINT('Ctrl Pts',(5.60960966833416,-28.8120723618202,
56.1680684740838));
#110690=CARTESIAN_POINT('Ctrl Pts',(5.60963554717833,-28.8123428021082,
56.1683434517053));
#110691=CARTESIAN_POINT('Ctrl Pts',(5.6096491071513,-28.8124845454619,56.1684875207208));
#110692=CARTESIAN_POINT('Ctrl Pts',(5.60967768438927,-28.8127833460569,
56.1687911133795));
#110693=CARTESIAN_POINT('Ctrl Pts',(5.60969270139474,-28.812940409274,56.1689506311989));
#110694=CARTESIAN_POINT('Ctrl Pts',(5.60972446299037,-28.8132727039299,
56.1692879829594));
#110695=CARTESIAN_POINT('Ctrl Pts',(5.60974120723446,-28.8134479432009,
56.1694658091782));
#110696=CARTESIAN_POINT('Ctrl Pts',(5.609776766907,-28.8138202221092,56.1698434139914));
#110697=CARTESIAN_POINT('Ctrl Pts',(5.60979558187417,-28.8140172722958,
56.1700431822474));
#110698=CARTESIAN_POINT('Ctrl Pts',(5.60983572721639,-28.8144378741486,
56.1704693703758));
#110699=CARTESIAN_POINT('Ctrl Pts',(5.60985705695728,-28.8146614402658,
56.1706957760446));
#110700=CARTESIAN_POINT('Ctrl Pts',(5.60990281747921,-28.8151412793974,
56.1711814313325));
#110701=CARTESIAN_POINT('Ctrl Pts',(5.60992724736499,-28.8153975726833,
56.1714406609307));
#110702=CARTESIAN_POINT('Ctrl Pts',(5.60997999805565,-28.8159512476809,
56.1720003117833));
#110703=CARTESIAN_POINT('Ctrl Pts',(5.61000831756943,-28.8162486587638,
56.1723007040903));
#110704=CARTESIAN_POINT('Ctrl Pts',(5.61006994216472,-28.8168962036133,
56.1729542421939));
#110705=CARTESIAN_POINT('Ctrl Pts',(5.61010324530987,-28.817246381325,56.1733073445681));
#110706=CARTESIAN_POINT('Ctrl Pts',(5.61085603759109,-28.8251671191855,
56.1812870866818));
#110707=CARTESIAN_POINT('Ctrl Pts',(5.61157226006442,-28.8328112839442,
56.1888406072384));
#110708=CARTESIAN_POINT('Ctrl Pts',(5.61306852499768,-28.849005497753,56.2045360216964));
#110709=CARTESIAN_POINT('Ctrl Pts',(5.6138478569042,-28.8575701104603,56.2126620845613));
#110710=CARTESIAN_POINT('Ctrl Pts',(5.61590473699746,-28.8805136005019,
56.2339719310193));
#110711=CARTESIAN_POINT('Ctrl Pts',(5.61717549465498,-28.8950391533021,
56.246995631246));
#110712=CARTESIAN_POINT('Ctrl Pts',(5.62377386703542,-28.9722329712203,
56.3137998748662));
#110713=CARTESIAN_POINT('Ctrl Pts',(5.62891788108628,-29.0386105406685,
56.3631243445983));
#110714=CARTESIAN_POINT('Ctrl Pts',(5.64015274367635,-29.1931222854185,
56.4610161214553));
#110715=CARTESIAN_POINT('Ctrl Pts',(5.64618451687078,-29.282534900663,56.5069377021184));
#110716=CARTESIAN_POINT('Ctrl Pts',(5.65424663631671,-29.4017612085817,
56.5551421166367));
#110717=CARTESIAN_POINT('Ctrl Pts',(5.65604041854473,-29.4282585662594,
56.5650776999504));
#110718=CARTESIAN_POINT('Ctrl Pts',(5.65910934022343,-29.4732437429048,
56.5806507496122));
#110719=CARTESIAN_POINT('Ctrl Pts',(5.6603681344177,-29.4916005110858,56.5866501909058));
#110720=CARTESIAN_POINT('Ctrl Pts',(5.66218710212996,-29.5179111785148,
56.5947457183845));
#110721=CARTESIAN_POINT('Ctrl Pts',(5.66273321255146,-29.5257834974828,
56.5971043296673));
#110722=CARTESIAN_POINT('Ctrl Pts',(5.66368745794205,-29.5394850809295,
56.6010992050839));
#110723=CARTESIAN_POINT('Ctrl Pts',(5.6640940624055,-29.5453063370879,56.6027620930042));
#110724=CARTESIAN_POINT('Ctrl Pts',(5.66497150131107,-29.5578297581885,
56.6062657876622));
#110725=CARTESIAN_POINT('Ctrl Pts',(5.66544286142756,-29.5645343148914,
56.6080963702605));
#110726=CARTESIAN_POINT('Ctrl Pts',(5.66675315314743,-29.5831136469388,
56.6130444811773));
#110727=CARTESIAN_POINT('Ctrl Pts',(5.66759683176353,-29.5950114524396,
56.6160727037659));
#110728=CARTESIAN_POINT('Ctrl Pts',(5.67351202571793,-29.6780509161312,
56.6362333069588));
#110729=CARTESIAN_POINT('Ctrl Pts',(5.67878562004379,-29.7502132858333,
56.6487919432388));
#110730=CARTESIAN_POINT('Ctrl Pts',(5.68512836949179,-29.8370256572337,
56.6580698161686));
#110731=CARTESIAN_POINT('Ctrl Pts',(5.68615761361952,-29.8511115592374,
56.6593939797661));
#110732=CARTESIAN_POINT('Ctrl Pts',(5.69255120868608,-29.9386682830437,
56.6665010402185));
#110733=CARTESIAN_POINT('Ctrl Pts',(5.69791546578073,-30.0124433489972,
56.6675832123819));
#110734=CARTESIAN_POINT('Ctrl Pts',(5.70621078107003,-30.1285269737078,
56.6615793197355));
#110735=CARTESIAN_POINT('Ctrl Pts',(5.70920958744079,-30.1709057512181,
56.6577565400483));
#110736=CARTESIAN_POINT('Ctrl Pts',(5.714286943184,-30.2434584523678,56.6483996077296));
#110737=CARTESIAN_POINT('Ctrl Pts',(5.7163870211675,-30.2737099797993,56.6436472692005));
#110738=CARTESIAN_POINT('Ctrl Pts',(5.71940824637081,-30.3175626297166,
56.6355138246984));
#110739=CARTESIAN_POINT('Ctrl Pts',(5.72034986555627,-30.3312778175844,
56.6327910224048));
#110740=CARTESIAN_POINT('Ctrl Pts',(5.72200510951612,-30.3554655900278,
56.6276718283769));
#110741=CARTESIAN_POINT('Ctrl Pts',(5.7227209419347,-30.3659521586349,56.6253462380257));
#110742=CARTESIAN_POINT('Ctrl Pts',(5.72421810828184,-30.3879355752872,
56.6202474611963));
#110743=CARTESIAN_POINT('Ctrl Pts',(5.72499871513617,-30.3994268996737,
56.6174529390502));
#110744=CARTESIAN_POINT('Ctrl Pts',(5.72706296846563,-30.4298837392738,
56.6097018945165));
#110745=CARTESIAN_POINT('Ctrl Pts',(5.72833973478736,-30.4487935475131,
56.6045325246997));
#110746=CARTESIAN_POINT('Ctrl Pts',(5.73493283338865,-30.5467125119296,
56.5758978421885));
#110747=CARTESIAN_POINT('Ctrl Pts',(5.74006657953628,-30.6239961763504,
56.5469259290523));
#110748=CARTESIAN_POINT('Ctrl Pts',(5.75129050574025,-30.7898777544275,
56.4702754004316));
#110749=CARTESIAN_POINT('Ctrl Pts',(5.75732138034986,-30.8769380467955,
56.4200682856675));
#110750=CARTESIAN_POINT('Ctrl Pts',(5.76538241930614,-30.9820859161215,
56.346054901022));
#110751=CARTESIAN_POINT('Ctrl Pts',(5.76717608144822,-31.00480279622,56.3291830962633));
#110752=CARTESIAN_POINT('Ctrl Pts',(5.77024481841223,-31.0422823480289,
56.2998370728428));
#110753=CARTESIAN_POINT('Ctrl Pts',(5.7715035505377,-31.0572780142117,56.2876692244578));
#110754=CARTESIAN_POINT('Ctrl Pts',(5.77332244408069,-31.0783484961954,
56.2699559268684));
#110755=CARTESIAN_POINT('Ctrl Pts',(5.77386854396232,-31.0845996045342,
56.2646213766478));
#110756=CARTESIAN_POINT('Ctrl Pts',(5.77482277746939,-31.0953869776575,
56.2552768715058));
#110757=CARTESIAN_POINT('Ctrl Pts',(5.77522938070761,-31.099941265392,56.2512880828584));
#110758=CARTESIAN_POINT('Ctrl Pts',(5.77610682474372,-31.1096771757829,
56.2426668379674));
#110759=CARTESIAN_POINT('Ctrl Pts',(5.77657819129145,-31.1148515049855,
56.2380268260678));
#110760=CARTESIAN_POINT('Ctrl Pts',(5.77788851790048,-31.1290857562103,
56.2251008508895));
#110761=CARTESIAN_POINT('Ctrl Pts',(5.77873222536627,-31.1380831339001,
56.2167470969534));
#110762=CARTESIAN_POINT('Ctrl Pts',(5.7846550842979,-31.200138735104,56.1578401489165));
#110763=CARTESIAN_POINT('Ctrl Pts',(5.78993692096085,-31.2498976765032,
56.1039385001513));
#110764=CARTESIAN_POINT('Ctrl Pts',(5.79628205926844,-31.3047821960186,
56.0360006440789));
#110765=CARTESIAN_POINT('Ctrl Pts',(5.79730553951035,-31.3134838791567,
56.0249458566415));
#110766=CARTESIAN_POINT('Ctrl Pts',(5.80369405025996,-31.3668958921132,
55.9552927763773));
#110767=CARTESIAN_POINT('Ctrl Pts',(5.80905892901138,-31.4078192001801,
55.8938876217719));
#110768=CARTESIAN_POINT('Ctrl Pts',(5.81735308261318,-31.4657204185634,
55.7931120445557));
#110769=CARTESIAN_POINT('Ctrl Pts',(5.82035020426002,-31.4854807608247,
55.7554538187264));
#110770=CARTESIAN_POINT('Ctrl Pts',(5.8254250576153,-31.5169523577242,55.6894549235681));
#110771=CARTESIAN_POINT('Ctrl Pts',(5.82752428912979,-31.5293615715799,
55.6614725573775));
#110772=CARTESIAN_POINT('Ctrl Pts',(5.83054454148244,-31.5463066077674,
55.6202316588876));
#110773=CARTESIAN_POINT('Ctrl Pts',(5.83148601565894,-31.5514568050176,
55.6072340889345));
#110774=CARTESIAN_POINT('Ctrl Pts',(5.8331410961117,-31.5602735301203,55.5841385726384));
#110775=CARTESIAN_POINT('Ctrl Pts',(5.83385690855483,-31.5640070815287,
55.5740672600437));
#110776=CARTESIAN_POINT('Ctrl Pts',(5.83535412230743,-31.5716465267158,
55.5528318604387));
#110777=CARTESIAN_POINT('Ctrl Pts',(5.83613479568354,-31.5755314737361,
55.5416608332368));
#110778=CARTESIAN_POINT('Ctrl Pts',(5.83819943370811,-31.5855398434333,
55.5118630838176));
#110779=CARTESIAN_POINT('Ctrl Pts',(5.83947651351413,-31.5914540856422,
55.4931676769893));
#110780=CARTESIAN_POINT('Ctrl Pts',(5.8460803395214,-31.6205504057329,55.3952109121176));
#110781=CARTESIAN_POINT('Ctrl Pts',(5.85122370793894,-31.6381472094588,
55.3144065706583));
#110782=CARTESIAN_POINT('Ctrl Pts',(5.86244827180834,-31.6636651722821,
55.1334411910619));
#110783=CARTESIAN_POINT('Ctrl Pts',(5.86847103463282,-31.6686770886506,
55.0332082588864));
#110784=CARTESIAN_POINT('Ctrl Pts',(5.87652231881853,-31.6635230087185,
54.9048856614526));
#110785=CARTESIAN_POINT('Ctrl Pts',(5.87831489579065,-31.6616691669251,
54.8766673709718));
#110786=CARTESIAN_POINT('Ctrl Pts',(5.88138196348994,-31.6573432045811,
54.8292895122289));
#110787=CARTESIAN_POINT('Ctrl Pts',(5.88264013464415,-31.6552542495464,
54.810100395298));
#110788=CARTESIAN_POINT('Ctrl Pts',(5.88445835783913,-31.6518015172962,
54.7828013380675));
#110789=CARTESIAN_POINT('Ctrl Pts',(5.88500436244594,-31.6507102573269,
54.7746577033895));
#110790=CARTESIAN_POINT('Ctrl Pts',(5.88595848854139,-31.6487103898355,
54.760528283153));
#110791=CARTESIAN_POINT('Ctrl Pts',(5.88636508071307,-31.6478293204928,
54.7545388383054));
#110792=CARTESIAN_POINT('Ctrl Pts',(5.88724257116995,-31.6458664996866,
54.741682789144));
#110793=CARTESIAN_POINT('Ctrl Pts',(5.8877139958863,-31.6447744323901,54.7348182163806));
#110794=CARTESIAN_POINT('Ctrl Pts',(5.88902463806697,-31.6416340616574,
54.7158443406801));
#110795=CARTESIAN_POINT('Ctrl Pts',(5.88986860648203,-31.639494811816,54.7037508295164));
#110796=CARTESIAN_POINT('Ctrl Pts',(5.89586299519639,-31.623469138227,54.6186515736115));
#110797=CARTESIAN_POINT('Ctrl Pts',(5.90122179749431,-31.604846489722,54.5466304369187));
#110798=CARTESIAN_POINT('Ctrl Pts',(5.90758332847298,-31.5773165755554,
54.4635264158598));
#110799=CARTESIAN_POINT('Ctrl Pts',(5.90854712647041,-31.5730010040137,
54.4510015260347));
#110800=CARTESIAN_POINT('Ctrl Pts',(5.91487932650507,-31.5436805226036,
54.369091174738));
#110801=CARTESIAN_POINT('Ctrl Pts',(5.920247202629,-31.5142393507344,54.3013756282619));
#110802=CARTESIAN_POINT('Ctrl Pts',(5.92853306006111,-31.4609744777292,
54.198186917614));
#110803=CARTESIAN_POINT('Ctrl Pts',(5.93151947819228,-31.440113129539,54.1612954539647));
#110804=CARTESIAN_POINT('Ctrl Pts',(5.93657842741133,-31.4018380147697,
54.0992569491608));
#110805=CARTESIAN_POINT('Ctrl Pts',(5.93867227575047,-31.3850977001122,
54.0737211886202));
#110806=CARTESIAN_POINT('Ctrl Pts',(5.94168634001977,-31.3596887748554,
54.0371929070712));
#110807=CARTESIAN_POINT('Ctrl Pts',(5.94262689100957,-31.3515693821288,
54.0258278958099));
#110808=CARTESIAN_POINT('Ctrl Pts',(5.94428093089611,-31.3369557741545,
54.0059071560768));
#110809=CARTESIAN_POINT('Ctrl Pts',(5.94499661655691,-31.330520038534,53.9973097383904));
#110810=CARTESIAN_POINT('Ctrl Pts',(5.94649413411054,-31.3168188840876,
53.9793707550318));
#110811=CARTESIAN_POINT('Ctrl Pts',(5.94727523258584,-31.3095361349709,
53.9700431307374));
#110812=CARTESIAN_POINT('Ctrl Pts',(5.94934232894496,-31.2899048585016,
53.945444594442));
#110813=CARTESIAN_POINT('Ctrl Pts',(5.95062141199184,-31.2773844271271,
53.9303127907655));
#110814=CARTESIAN_POINT('Ctrl Pts',(5.95729865268596,-31.2101163073132,
53.8518805455481));
#110815=CARTESIAN_POINT('Ctrl Pts',(5.96250795019032,-31.1509212589895,
53.7925470707537));
#110816=CARTESIAN_POINT('Ctrl Pts',(5.97373728748757,-31.0123609009764,
53.6731533349377));
#110817=CARTESIAN_POINT('Ctrl Pts',(5.97970471808478,-30.9315827223317,
53.6152444322808));
#110818=CARTESIAN_POINT('Ctrl Pts',(5.9876894205928,-30.8218868791671,53.550568867974));
#110819=CARTESIAN_POINT('Ctrl Pts',(5.98947454141996,-30.7972771096186,
53.5368876732036));
#110820=CARTESIAN_POINT('Ctrl Pts',(5.99253013626929,-30.755285132068,53.5149173087543));
#110821=CARTESIAN_POINT('Ctrl Pts',(5.99378444915729,-30.7380839028855,
53.5062937686262));
#110822=CARTESIAN_POINT('Ctrl Pts',(5.99559806116517,-30.7133393859499,
53.4944202892037));
#110823=CARTESIAN_POINT('Ctrl Pts',(5.99614340965538,-30.7059147286573,
53.4909248746346));
#110824=CARTESIAN_POINT('Ctrl Pts',(5.99709679651142,-30.6929694988752,
53.4849468949833));
#110825=CARTESIAN_POINT('Ctrl Pts',(5.99750331293053,-30.6874607307519,
53.4824393324454));
#110826=CARTESIAN_POINT('Ctrl Pts',(5.99838112511672,-30.6755910058959,
53.4771141904084));
#110827=CARTESIAN_POINT('Ctrl Pts',(5.9988529520233,-30.6692261260914,53.4743064580192));
#110828=CARTESIAN_POINT('Ctrl Pts',(6.00016577682306,-30.6515529495901,
53.4666421755225));
#110829=CARTESIAN_POINT('Ctrl Pts',(6.00101155022345,-30.6402084028865,
53.4618710578713));
#110830=CARTESIAN_POINT('Ctrl Pts',(6.00731587880736,-30.5558766721878,
53.4274986535648));
#110831=CARTESIAN_POINT('Ctrl Pts',(6.01300815964939,-30.4809323685515,
53.4029838221265));
#110832=CARTESIAN_POINT('Ctrl Pts',(6.01922058563892,-30.3980606676793,
53.3822397000027));
#110833=CARTESIAN_POINT('Ctrl Pts',(6.01970692183623,-30.3915664723031,
53.3806555706626));
#110834=CARTESIAN_POINT('Ctrl Pts',(6.02415494514287,-30.3321005371325,
53.3665286802304));
#110835=CARTESIAN_POINT('Ctrl Pts',(6.02812082550603,-30.278551673164,53.356549778747));
#110836=CARTESIAN_POINT('Ctrl Pts',(6.03600709162865,-30.1701402319231,
53.3417991408803));
#110837=CARTESIAN_POINT('Ctrl Pts',(6.03992186653345,-30.1153338575021,
53.3370878335869));
#110838=CARTESIAN_POINT('Ctrl Pts',(6.04551237462032,-30.0353478865128,
53.3341865434709));
#110839=CARTESIAN_POINT('Ctrl Pts',(6.04724676363678,-30.0102871466204,
53.3338432744814));
#110840=CARTESIAN_POINT('Ctrl Pts',(6.05037056930551,-29.9647050938863,
53.3342474817267));
#110841=CARTESIAN_POINT('Ctrl Pts',(6.05176532567895,-29.9441875297688,
53.33480865484));
#110842=CARTESIAN_POINT('Ctrl Pts',(6.05395834424886,-29.9116763066197,
53.3362994767213));
#110843=CARTESIAN_POINT('Ctrl Pts',(6.05476427279886,-29.8996739093941,
53.3369800979448));
#110844=CARTESIAN_POINT('Ctrl Pts',(6.05627983430849,-29.8770046672131,
53.3385119248834));
#110845=CARTESIAN_POINT('Ctrl Pts',(6.05699027314522,-29.8663366719089,
53.3393360967718));
#110846=CARTESIAN_POINT('Ctrl Pts',(6.05859807031123,-29.8421046495762,
53.3414431985336));
#110847=CARTESIAN_POINT('Ctrl Pts',(6.05949338946172,-29.8285468235387,
53.3427898648737));
#110848=CARTESIAN_POINT('Ctrl Pts',(6.06182330440288,-29.7931125650952,
53.3467489825772));
#110849=CARTESIAN_POINT('Ctrl Pts',(6.06324954091493,-29.7712683391104,
53.3496293637383));
#110850=CARTESIAN_POINT('Ctrl Pts',(6.07186433091572,-29.6385802226222,
53.3698108794264));
#110851=CARTESIAN_POINT('Ctrl Pts',(6.07870358396223,-29.5296578724719,
53.3978381298946));
#110852=CARTESIAN_POINT('Ctrl Pts',(6.09153487111977,-29.3324868948639,
53.4704349467432));
#110853=CARTESIAN_POINT('Ctrl Pts',(6.09750814091866,-29.2437774161109,
53.5122953460405));
#110854=CARTESIAN_POINT('Ctrl Pts',(6.10480659976119,-29.1469282496465,
53.5689063882489));
#110855=CARTESIAN_POINT('Ctrl Pts',(6.10574485994584,-29.13468111709,53.5762782806325));
#110856=CARTESIAN_POINT('Ctrl Pts',(6.10717665247066,-29.1163276266195,
53.5876500471782));
#110857=CARTESIAN_POINT('Ctrl Pts',(6.10766306661534,-29.110149854637,53.5915341798626));
#110858=CARTESIAN_POINT('Ctrl Pts',(6.10855483075937,-29.0989327856324,
53.5986899087401));
#110859=CARTESIAN_POINT('Ctrl Pts',(6.10895933054403,-29.0938854069513,
53.6019483423882));
#110860=CARTESIAN_POINT('Ctrl Pts',(6.10988720756494,-29.0823994873474,
53.6094516294687));
#110861=CARTESIAN_POINT('Ctrl Pts',(6.11041169872084,-29.0759727463843,
53.6137139183153));
#110862=CARTESIAN_POINT('Ctrl Pts',(6.11206255344805,-29.0559421252614,
53.6271996261016));
#110863=CARTESIAN_POINT('Ctrl Pts',(6.11319842191964,-29.0424454687913,
53.6365795195112));
#110864=CARTESIAN_POINT('Ctrl Pts',(6.12047377225749,-28.9576596554269,
53.6973837360031));
#110865=CARTESIAN_POINT('Ctrl Pts',(6.12687424672248,-28.8904015227084,
53.7541786006832));
#110866=CARTESIAN_POINT('Ctrl Pts',(6.13683052997786,-28.7931992036148,
53.8504009581148));
#110867=CARTESIAN_POINT('Ctrl Pts',(6.1403855256211,-28.7599845347559,53.886308807245));
#110868=CARTESIAN_POINT('Ctrl Pts',(6.1477139866559,-28.6942052960615,53.9640189361251));
#110869=CARTESIAN_POINT('Ctrl Pts',(6.15147701261901,-28.6619558355591,
54.0060204825314));
#110870=CARTESIAN_POINT('Ctrl Pts',(6.15766505398325,-28.6113629031833,
54.078848059903));
#110871=CARTESIAN_POINT('Ctrl Pts',(6.16012665094559,-28.5919166921978,
54.1088571276642));
#110872=CARTESIAN_POINT('Ctrl Pts',(6.16355892471389,-28.5657929311301,
54.1521640309832));
#110873=CARTESIAN_POINT('Ctrl Pts',(6.16455874167893,-28.5583055994359,
54.164959266376));
#110874=CARTESIAN_POINT('Ctrl Pts',(6.16628070563613,-28.5456277408097,
54.1873036261058));
#110875=CARTESIAN_POINT('Ctrl Pts',(6.16700566154838,-28.5403581294968,
54.1968065712734));
#110876=CARTESIAN_POINT('Ctrl Pts',(6.16839805906141,-28.5303706252655,
54.2152404824255));
#110877=CARTESIAN_POINT('Ctrl Pts',(6.16906592017479,-28.5256402519568,
54.2241641021098));
#110878=CARTESIAN_POINT('Ctrl Pts',(6.17083171466432,-28.5132964637648,
54.2479707179044));
#110879=CARTESIAN_POINT('Ctrl Pts',(6.17192464300019,-28.505825278829,54.2629264747883));
#110880=CARTESIAN_POINT('Ctrl Pts',(6.17599584452797,-28.4786538508444,
54.3194296620581));
#110881=CARTESIAN_POINT('Ctrl Pts',(6.17892318451078,-28.4604502161505,
54.3616763106675));
#110882=CARTESIAN_POINT('Ctrl Pts',(6.18884420582201,-28.4039406497918,
54.5093613396289));
#110883=CARTESIAN_POINT('Ctrl Pts',(6.19558337341051,-28.3745425837921,
54.6178738685986));
#110884=CARTESIAN_POINT('Ctrl Pts',(6.20541139166293,-28.3485115738653,
54.775483142563));
#110885=CARTESIAN_POINT('Ctrl Pts',(6.20836765990743,-28.3427717103106,
54.8227554954057));
#110886=CARTESIAN_POINT('Ctrl Pts',(6.21316097342454,-28.3369079177467,
54.8977922593837));
#110887=CARTESIAN_POINT('Ctrl Pts',(6.21494782603538,-28.3354398956936,
54.9254269200532));
#110888=CARTESIAN_POINT('Ctrl Pts',(6.21738873238108,-28.3343956212004,
54.9624941711237));
#110889=CARTESIAN_POINT('Ctrl Pts',(6.21801237348241,-28.3342102786804,
54.9719067991632));
#110890=CARTESIAN_POINT('Ctrl Pts',(6.21905789948024,-28.3340345366733,
54.9875797750158));
#110891=CARTESIAN_POINT('Ctrl Pts',(6.21947737096312,-28.3339996295805,
54.9938395881387));
#110892=CARTESIAN_POINT('Ctrl Pts',(6.22033482441398,-28.3340003891752,
55.0065742263296));
#110893=CARTESIAN_POINT('Ctrl Pts',(6.22077292106741,-28.3340385218274,
55.013048883104));
#110894=CARTESIAN_POINT('Ctrl Pts',(6.22192129714633,-28.3342365019233,
55.0299423925286));
#110895=CARTESIAN_POINT('Ctrl Pts',(6.22263472928739,-28.3344563561875,
55.0403600674017));
#110896=CARTESIAN_POINT('Ctrl Pts',(6.225923420595,-28.3359107794599,55.0880599199513));
#110897=CARTESIAN_POINT('Ctrl Pts',(6.22855209853136,-28.3382994949583,
55.1252934070511));
#110898=CARTESIAN_POINT('Ctrl Pts',(6.23683765239157,-28.3496118538595,
55.2407813463081));
#110899=CARTESIAN_POINT('Ctrl Pts',(6.24259886493134,-28.3628346246,55.3185050089652));
#110900=CARTESIAN_POINT('Ctrl Pts',(6.25289732980732,-28.3964364415772,
55.4561873285643));
#110901=CARTESIAN_POINT('Ctrl Pts',(6.25743981058664,-28.4148214150369,
55.5164549297136));
#110902=CARTESIAN_POINT('Ctrl Pts',(6.26189393505974,-28.4365622331338,
55.5755157244911));
#110903=CARTESIAN_POINT('',(6.02851963656333,-28.3340006962934,54.9984768292002));
#110904=CARTESIAN_POINT('Ctrl Pts',(6.06643884243078,-28.4365623175998,
55.5755159539501));
#110905=CARTESIAN_POINT('Ctrl Pts',(6.06476015297658,-28.4282202681816,
55.5528540723474));
#110906=CARTESIAN_POINT('Ctrl Pts',(6.06309642773074,-28.4203703265032,
55.5300091476633));
#110907=CARTESIAN_POINT('Ctrl Pts',(6.06024616305704,-28.4076552517071,
55.4902089456295));
#110908=CARTESIAN_POINT('Ctrl Pts',(6.05905255999884,-28.4025584563348,
55.4733362058938));
#110909=CARTESIAN_POINT('Ctrl Pts',(6.05710091519478,-28.394605925368,55.4454165873849));
#110910=CARTESIAN_POINT('Ctrl Pts',(6.05633787123136,-28.3915943141442,
55.4344159666343));
#110911=CARTESIAN_POINT('Ctrl Pts',(6.05485285341196,-28.3859263311193,
55.4128449529414));
#110912=CARTESIAN_POINT('Ctrl Pts',(6.05413059942039,-28.3832602559977,
55.402277731802));
#110913=CARTESIAN_POINT('Ctrl Pts',(6.05270061135005,-28.3781640856808,
55.3812091665214));
#110914=CARTESIAN_POINT('Ctrl Pts',(6.05199283979134,-28.3757318316159,
55.3707088990512));
#110915=CARTESIAN_POINT('Ctrl Pts',(6.0503374763543,-28.3702574687587,55.3459866700841));
#110916=CARTESIAN_POINT('Ctrl Pts',(6.0493925421128,-28.3672993157626,55.3317468778488));
#110917=CARTESIAN_POINT('Ctrl Pts',(6.04631836623588,-28.3582307013777,
55.2850291581921));
#110918=CARTESIAN_POINT('Ctrl Pts',(6.0442127279856,-28.3528998070025,55.2524068598318));
#110919=CARTESIAN_POINT('Ctrl Pts',(6.03746967039496,-28.3387916277564,
55.1463313002844));
#110920=CARTESIAN_POINT('Ctrl Pts',(6.03293646769578,-28.3339333426273,
55.0724469474433));
#110921=CARTESIAN_POINT('Ctrl Pts',(6.02841828083449,-28.3340006906443,
54.9984830206473));
#110922=CARTESIAN_POINT('Ctrl Pts',(6.02851963656333,-28.3340006962934,
54.9984768292002));
#110923=CARTESIAN_POINT('Ctrl Pts',(6.02319560874774,-28.3340734949223,
54.9188518357346));
#110924=CARTESIAN_POINT('Ctrl Pts',(6.01787158093214,-28.3398584615716,
54.8394810237176));
#110925=CARTESIAN_POINT('Ctrl Pts',(6.01254755311655,-28.3512247100071,
54.7610522167735));
#110926=CARTESIAN_POINT('Ctrl Pts',(6.0087999105051,-28.3592255391622,54.7058453040658));
#110927=CARTESIAN_POINT('Ctrl Pts',(6.00505226789365,-28.3699908306221,
54.6511044996732));
#110928=CARTESIAN_POINT('Ctrl Pts',(6.0013046252822,-28.3834612365896,54.597062751298));
#110929=CARTESIAN_POINT('Ctrl Pts',(5.99722727558209,-28.3981167311034,
54.5382665614325));
#110930=CARTESIAN_POINT('Ctrl Pts',(5.99314992588198,-28.4160144422306,
54.4801495795245));
#110931=CARTESIAN_POINT('Ctrl Pts',(5.98907257618187,-28.4370742327443,
54.423095288589));
#110932=CARTESIAN_POINT('Ctrl Pts',(5.98495160860944,-28.4583593125565,
54.3654306534446));
#110933=CARTESIAN_POINT('Ctrl Pts',(5.98083064103702,-28.4828744868665,
54.3088521143314));
#110934=CARTESIAN_POINT('Ctrl Pts',(5.97670967346459,-28.5104841015491,
54.2537437516094));
#110935=CARTESIAN_POINT('Ctrl Pts',(5.97264355643919,-28.5377262291206,
54.1993688874621));
#110936=CARTESIAN_POINT('Ctrl Pts',(5.96857743941378,-28.5679806888336,
54.1464257733204));
#110937=CARTESIAN_POINT('Ctrl Pts',(5.96451132238838,-28.6010683663903,
54.0952645223679));
#110938=CARTESIAN_POINT('Ctrl Pts',(5.96044769316901,-28.6341357996394,
54.044134573827));
#110939=CARTESIAN_POINT('Ctrl Pts',(5.95638406394963,-28.6700327363164,
53.994784755908));
#110940=CARTESIAN_POINT('Ctrl Pts',(5.95232043473026,-28.7085351232835,
53.9475388500246));
#110941=CARTESIAN_POINT('Ctrl Pts',(5.94825778211358,-28.7470282570601,
53.9003042986414));
#110942=CARTESIAN_POINT('Ctrl Pts',(5.94419512949691,-28.7881252748301,
53.8551730522363));
#110943=CARTESIAN_POINT('Ctrl Pts',(5.94013247688023,-28.8315612467165,
53.8124365786093));
#110944=CARTESIAN_POINT('Ctrl Pts',(5.93596888334385,-28.8760764314631,
53.7686382718994));
#110945=CARTESIAN_POINT('Ctrl Pts',(5.93180528980747,-28.9230479927169,
53.7273557654103));
#110946=CARTESIAN_POINT('Ctrl Pts',(5.92764169627109,-28.9721516994875,
53.6888616125162));
#110947=CARTESIAN_POINT('Ctrl Pts',(5.92357385644511,-29.0201261264481,
53.6512527424761));
#110948=CARTESIAN_POINT('Ctrl Pts',(5.91950601661914,-29.0701351964334,
53.6163055754419));
#110949=CARTESIAN_POINT('Ctrl Pts',(5.91543817679316,-29.1218462435001,
53.5842309581202));
#110950=CARTESIAN_POINT('Ctrl Pts',(5.91122670640158,-29.1753831458749,
53.551023824371));
#110951=CARTESIAN_POINT('Ctrl Pts',(5.90701523600999,-29.230743959214,53.520896213991));
#110952=CARTESIAN_POINT('Ctrl Pts',(5.90280376561841,-29.2875334118817,
53.4940294289678));
#110953=CARTESIAN_POINT('Ctrl Pts',(5.89859229522682,-29.3443228645495,
53.4671626439445));
#110954=CARTESIAN_POINT('Ctrl Pts',(5.89438082483524,-29.4025403724669,
53.4435568429065));
#110955=CARTESIAN_POINT('Ctrl Pts',(5.89016935444365,-29.4617725659754,
53.4233366785318));
#110956=CARTESIAN_POINT('Ctrl Pts',(5.88609200474354,-29.5191184200318,
53.4037604561002));
#110957=CARTESIAN_POINT('Ctrl Pts',(5.88201465504343,-29.5776521037462,
53.3872765390742));
#110958=CARTESIAN_POINT('Ctrl Pts',(5.87793730534331,-29.6370079727799,
53.3740255880935));
#110959=CARTESIAN_POINT('Ctrl Pts',(5.87381633777089,-29.6969988073934,
53.3606328836871));
#110960=CARTESIAN_POINT('Ctrl Pts',(5.86969537019846,-29.7578290526706,
53.3505429818469));
#110961=CARTESIAN_POINT('Ctrl Pts',(5.86557440262604,-29.8191024520456,
53.3438502250267));
#110962=CARTESIAN_POINT('Ctrl Pts',(5.86150828560063,-29.879560295507,53.3372465495609));
#110963=CARTESIAN_POINT('Ctrl Pts',(5.85744216857522,-29.9404490441909,
53.3339501953221));
#110964=CARTESIAN_POINT('Ctrl Pts',(5.85337605154982,-30.0013774075988,
53.3340005694034));
#110965=CARTESIAN_POINT('Ctrl Pts',(5.84931242233044,-30.062268492702,53.3340509126639));
#110966=CARTESIAN_POINT('Ctrl Pts',(5.84524879311107,-30.1231986335689,
53.3374439239197));
#110967=CARTESIAN_POINT('Ctrl Pts',(5.84118516389169,-30.1837742889552,
53.3441669737806));
#110968=CARTESIAN_POINT('Ctrl Pts',(5.83712251127501,-30.2443353863331,
53.3508884079063));
#110969=CARTESIAN_POINT('Ctrl Pts',(5.83305985865833,-30.3045416587428,
53.3609382354768));
#110970=CARTESIAN_POINT('Ctrl Pts',(5.82899720604165,-30.3640045429392,
53.3742519590294));
#110971=CARTESIAN_POINT('Ctrl Pts',(5.82483361250527,-30.4249448456562,
53.3878964761859));
#110972=CARTESIAN_POINT('Ctrl Pts',(5.82067001896889,-30.4851037654212,
53.4049691819279));
#110973=CARTESIAN_POINT('Ctrl Pts',(5.81650642543251,-30.5440764670278,
53.425345498839));
#110974=CARTESIAN_POINT('Ctrl Pts',(5.81243858560653,-30.6016929231359,
53.4452532042175));
#110975=CARTESIAN_POINT('Ctrl Pts',(5.80837074578055,-30.6581766839123,
53.4683139139434));
#110976=CARTESIAN_POINT('Ctrl Pts',(5.80430290595458,-30.7131701817946,
53.4943624965487));
#110977=CARTESIAN_POINT('Ctrl Pts',(5.800091435563,-30.7701054344026,53.5213308234932));
#110978=CARTESIAN_POINT('Ctrl Pts',(5.79587996517141,-30.8254426690907,
53.5515017203613));
#110979=CARTESIAN_POINT('Ctrl Pts',(5.79166849477983,-30.8788151850231,
53.5846414339211));
#110980=CARTESIAN_POINT('Ctrl Pts',(5.78745702438825,-30.9321877009555,
53.6177811474809));
#110981=CARTESIAN_POINT('Ctrl Pts',(5.78324555399667,-30.9835950480778,
53.6538892730566));
#110982=CARTESIAN_POINT('Ctrl Pts',(5.77903408360509,-31.0327083033889,
53.6926861279281));
#110983=CARTESIAN_POINT('Ctrl Pts',(5.77495673390497,-31.0802574722526,
53.7302474378429));
#110984=CARTESIAN_POINT('Ctrl Pts',(5.77087938420486,-31.1258528967952,
53.7704838505866));
#110985=CARTESIAN_POINT('Ctrl Pts',(5.76680203450474,-31.1691780895288,
53.8131644617026));
#110986=CARTESIAN_POINT('Ctrl Pts',(5.76268106693232,-31.2129667580159,
53.8563016530932));
#110987=CARTESIAN_POINT('Ctrl Pts',(5.75856009935989,-31.2544358643991,
53.901935391439));
#110988=CARTESIAN_POINT('Ctrl Pts',(5.75443913178747,-31.2932912321435,
53.9497839322974));
#110989=CARTESIAN_POINT('Ctrl Pts',(5.75037301476206,-31.3316294305246,
53.9969956036356));
#110990=CARTESIAN_POINT('Ctrl Pts',(5.74630689773665,-31.367422711798,54.0463630694734));
#110991=CARTESIAN_POINT('Ctrl Pts',(5.74224078071125,-31.4004257464349,
54.0975789626109));
#110992=CARTESIAN_POINT('Ctrl Pts',(5.73817715149187,-31.4334085885519,
54.1487635199047));
#110993=CARTESIAN_POINT('Ctrl Pts',(5.73411352227249,-31.4636042921283,
54.2017938327171));
#110994=CARTESIAN_POINT('Ctrl Pts',(5.73004989305312,-31.4908100250276,
54.2563324201788));
#110995=CARTESIAN_POINT('Ctrl Pts',(5.72598724043644,-31.5180092196355,
54.3108579005068));
#110996=CARTESIAN_POINT('Ctrl Pts',(5.72192458781976,-31.5422196416114,
54.3668904779901));
#110997=CARTESIAN_POINT('Ctrl Pts',(5.71786193520308,-31.563284735334,54.4240687226138));
#110998=CARTESIAN_POINT('Ctrl Pts',(5.7136983416667,-31.5848732136859,54.4826676214612));
#110999=CARTESIAN_POINT('Ctrl Pts',(5.70953474813032,-31.6031577274303,
54.5424693728216));
#111000=CARTESIAN_POINT('Ctrl Pts',(5.70537115459394,-31.6180233714046,
54.6030662906877));
#111001=CARTESIAN_POINT('Ctrl Pts',(5.70130331476796,-31.6325471374902,
54.6622696095692));
#111002=CARTESIAN_POINT('Ctrl Pts',(5.69723547494198,-31.6438075940157,
54.7222313780834));
#111003=CARTESIAN_POINT('Ctrl Pts',(5.69316763511601,-31.6517495433165,
54.7825616267683));
#111004=CARTESIAN_POINT('Ctrl Pts',(5.68895616472443,-31.6599719133613,
54.8450220644754));
#111005=CARTESIAN_POINT('Ctrl Pts',(5.68474469433285,-31.6646369573865,
54.9078768966285));
#111006=CARTESIAN_POINT('Ctrl Pts',(5.68053322394127,-31.6657421763009,
54.9706912625246));
#111007=CARTESIAN_POINT('Ctrl Pts',(5.67632175354969,-31.6668473952153,
55.0335056284207));
#111008=CARTESIAN_POINT('Ctrl Pts',(5.67211028315811,-31.6643928849112,
55.0962789304679));
#111009=CARTESIAN_POINT('Ctrl Pts',(5.66789881276653,-31.6584352230018,
55.1585831362628));
#111010=CARTESIAN_POINT('Ctrl Pts',(5.66382146306642,-31.6526672919133,
55.2189031696937));
#111011=CARTESIAN_POINT('Ctrl Pts',(5.6597441133663,-31.6435922496631,55.2790326571175));
#111012=CARTESIAN_POINT('Ctrl Pts',(5.65566676366619,-31.6312324376959,
55.3385804693257));
#111013=CARTESIAN_POINT('Ctrl Pts',(5.65154579609376,-31.6187404053552,
55.3987653004457));
#111014=CARTESIAN_POINT('Ctrl Pts',(5.64742482852134,-31.6028928679926,
55.4583554038117));
#111015=CARTESIAN_POINT('Ctrl Pts',(5.64330386094891,-31.5837669805994,
55.516950820836));
#111016=CARTESIAN_POINT('Ctrl Pts',(5.63923774392351,-31.5648956609425,
55.5747663261962));
#111017=CARTESIAN_POINT('Ctrl Pts',(5.6351716268981,-31.5428328927836,55.6316129613537));
#111018=CARTESIAN_POINT('Ctrl Pts',(5.6311055098727,-31.5177038507705,55.6871179093549));
#111019=CARTESIAN_POINT('Ctrl Pts',(5.62704188065332,-31.4925901836672,
55.7425888973045));
#111020=CARTESIAN_POINT('Ctrl Pts',(5.62297825143395,-31.4644141731088,
55.7967193602663));
#111021=CARTESIAN_POINT('Ctrl Pts',(5.61891462221457,-31.4333493426076,
55.8491558526245));
#111022=CARTESIAN_POINT('Ctrl Pts',(5.61485196959789,-31.4022919778458,
55.9015797430408));
#111023=CARTESIAN_POINT('Ctrl Pts',(5.61078931698121,-31.3683474321821,
55.9523100307528));
#111024=CARTESIAN_POINT('Ctrl Pts',(5.60672666436453,-31.3317344485686,
56.0010191599044));
#111025=CARTESIAN_POINT('Ctrl Pts',(5.60256307082815,-31.2942117764861,
56.0509385191097));
#111026=CARTESIAN_POINT('Ctrl Pts',(5.59839947729177,-31.2538865838703,
56.0987344577357));
#111027=CARTESIAN_POINT('Ctrl Pts',(5.59423588375539,-31.2110390650608,
56.1440893247019));
#111028=CARTESIAN_POINT('Ctrl Pts',(5.59016804392942,-31.1691769471728,
56.1884011271232));
#111029=CARTESIAN_POINT('Ctrl Pts',(5.58610020410344,-31.1249077208064,
56.2303826368797));
#111030=CARTESIAN_POINT('Ctrl Pts',(5.58203236427746,-31.0785290790624,
56.2697759745785));
#111031=CARTESIAN_POINT('Ctrl Pts',(5.57782089388588,-31.0305128628733,
56.3105602439798));
#111032=CARTESIAN_POINT('Ctrl Pts',(5.5736094234943,-30.9802359328576,56.3485697542235));
#111033=CARTESIAN_POINT('Ctrl Pts',(5.56939795310271,-30.9280622790166,
56.3835665528866));
#111034=CARTESIAN_POINT('Ctrl Pts',(5.56518648271113,-30.8758886251756,
56.4185633515496));
#111035=CARTESIAN_POINT('Ctrl Pts',(5.56097501231955,-30.8218188015808,
56.4505471950831));
#111036=CARTESIAN_POINT('Ctrl Pts',(5.55676354192797,-30.7662431025641,
56.4793334674011));
#111037=CARTESIAN_POINT('Ctrl Pts',(5.55268619222785,-30.712437296361,56.5072029970166));
#111038=CARTESIAN_POINT('Ctrl Pts',(5.54860884252774,-30.6569979178377,
56.5321907331816));
#111039=CARTESIAN_POINT('Ctrl Pts',(5.54453149282763,-30.6002656888766,
56.5541033114814));
#111040=CARTESIAN_POINT('Ctrl Pts',(5.5404105252552,-30.5429265609982,56.5762503018657));
#111041=CARTESIAN_POINT('Ctrl Pts',(5.53628955768277,-30.4842671843989,
56.595255627346));
#111042=CARTESIAN_POINT('Ctrl Pts',(5.53216859011035,-30.4246654278063,
56.6109671860178));
#111043=CARTESIAN_POINT('Ctrl Pts',(5.52810247308494,-30.3658569773717,
56.626469622057));
#111044=CARTESIAN_POINT('Ctrl Pts',(5.52403635605954,-30.3061315899491,
56.6387653027936));
#111045=CARTESIAN_POINT('Ctrl Pts',(5.51997023903413,-30.2458703755336,
56.6477571903757));
#111046=CARTESIAN_POINT('Ctrl Pts',(5.51590660981475,-30.1856460312356,
56.6567435763768));
#111047=CARTESIAN_POINT('Ctrl Pts',(5.51184298059538,-30.1248870152639,
56.6624301016414));
#111048=CARTESIAN_POINT('Ctrl Pts',(5.507779351376,-30.0639843855966,56.6647708546223));
#111049=CARTESIAN_POINT('Ctrl Pts',(5.50371669875932,-30.0030963925187,
56.6671110450554));
#111050=CARTESIAN_POINT('Ctrl Pts',(5.49965404614264,-29.9420653656139,
56.6661070397698));
#111051=CARTESIAN_POINT('Ctrl Pts',(5.49559139352596,-29.8812851371461,
56.6617649597153));
#111052=CARTESIAN_POINT('Ctrl Pts',(5.49142779998958,-29.81899475934,56.6573149960696));
#111053=CARTESIAN_POINT('Ctrl Pts',(5.4872642064532,-29.7569683731696,56.64935884579));
#111054=CARTESIAN_POINT('Ctrl Pts',(5.48310061291682,-29.6956248184907,
56.6379596298081));
#111055=CARTESIAN_POINT('Ctrl Pts',(5.47903277309084,-29.6356920338397,
56.626822571315));
#111056=CARTESIAN_POINT('Ctrl Pts',(5.47496493326487,-29.5764115003721,
56.6123993290894));
#111057=CARTESIAN_POINT('Ctrl Pts',(5.47089709343889,-29.5181613318447,
56.594800143551));
#111058=CARTESIAN_POINT('Ctrl Pts',(5.46668562304731,-29.4578544194411,
56.5765795517918));
#111059=CARTESIAN_POINT('Ctrl Pts',(5.46247415265573,-29.3986525730831,
56.554954706161));
#111060=CARTESIAN_POINT('Ctrl Pts',(5.45826268226415,-29.3409531220702,
56.5301023536649));
#111061=CARTESIAN_POINT('Ctrl Pts',(5.45405121187257,-29.2832536710573,
56.5052500011689));
#111062=CARTESIAN_POINT('Ctrl Pts',(5.44983974148099,-29.2270571205141,
56.4771704752151));
#111063=CARTESIAN_POINT('Ctrl Pts',(5.44562827108941,-29.1727302560843,
56.4460915499379));
#111064=CARTESIAN_POINT('Ctrl Pts',(5.44155183030149,-29.1201452381571,
56.4160090877892));
#111065=CARTESIAN_POINT('Ctrl Pts',(5.43747538951358,-29.0690946643213,
56.3829925194298));
#111066=CARTESIAN_POINT('Ctrl Pts',(5.43339894872566,-29.0199255540374,
56.3472230997021));
#111067=CARTESIAN_POINT('Ctrl Pts',(5.42932840892935,-28.9708276201846,
56.3115054592242));
#111068=CARTESIAN_POINT('Ctrl Pts',(5.42525786913304,-28.9236061612427,
56.2730431653487));
#111069=CARTESIAN_POINT('Ctrl Pts',(5.42118732933672,-28.8785820255251,
56.232062387432));
#111070=CARTESIAN_POINT('Ctrl Pts',(5.41712116909577,-28.8336063319563,
56.1911257013542));
#111071=CARTESIAN_POINT('Ctrl Pts',(5.41305500885481,-28.7908236495021,
56.1476762483564));
#111072=CARTESIAN_POINT('Ctrl Pts',(5.40898884861385,-28.7505226456888,
56.1019810983241));
#111073=CARTESIAN_POINT('Ctrl Pts',(5.4049250037414,-28.7102445902272,56.0563119681988));
#111074=CARTESIAN_POINT('Ctrl Pts',(5.40086115886896,-28.6724457517756,
56.0084000576405));
#111075=CARTESIAN_POINT('Ctrl Pts',(5.39679731399651,-28.6373773379912,
55.9585486325586));
#111076=CARTESIAN_POINT('Ctrl Pts',(5.39273479857771,-28.6023203965518,
55.9087135159632));
#111077=CARTESIAN_POINT('Ctrl Pts',(5.38867228315891,-28.5699923972564,
55.8569405655949));
#111078=CARTESIAN_POINT('Ctrl Pts',(5.38460976774011,-28.5406023334362,
55.8035635947628));
#111079=CARTESIAN_POINT('Ctrl Pts',(5.38054576406545,-28.5112015029036,
55.7501670698905));
#111080=CARTESIAN_POINT('Ctrl Pts',(5.37648176039079,-28.4847410005683,
55.6951658017754));
#111081=CARTESIAN_POINT('Ctrl Pts',(5.37241775671613,-28.461383953044,55.6389183516299));
#111082=CARTESIAN_POINT('Ctrl Pts',(5.37090280158279,-28.4526770517025,
55.6179507615004));
#111083=CARTESIAN_POINT('Ctrl Pts',(5.36938784644946,-28.4444009307782,
55.5968102093442));
#111084=CARTESIAN_POINT('Ctrl Pts',(5.36787289131612,-28.4365623102018,
55.5755159338528));
#111085=CARTESIAN_POINT('Origin',(5.,-30.,55.));
#111086=CARTESIAN_POINT('',(4.66781602203697,-28.4339760950611,55.5764682902535));
#111087=CARTESIAN_POINT('',(4.86076601588518,-28.4365623050844,55.575515919951));
#111088=CARTESIAN_POINT('',(5.,-28.4365623102018,55.5755159338528));
#111089=CARTESIAN_POINT('',(5.52206892288488,-28.3340005844715,55.0013955137945));
#111090=CARTESIAN_POINT('Ctrl Pts',(4.86076601588518,-28.4365623050844,
55.575515919951));
#111091=CARTESIAN_POINT('Ctrl Pts',(4.8623567140795,-28.4455582692477,55.5999542178111));
#111092=CARTESIAN_POINT('Ctrl Pts',(4.86394559269076,-28.4551274085992,
55.624182070837));
#111093=CARTESIAN_POINT('Ctrl Pts',(4.86634136946606,-28.4703643130818,
55.6602595159302));
#111094=CARTESIAN_POINT('Ctrl Pts',(4.86714462675909,-28.4756086977021,
55.672279046011));
#111095=CARTESIAN_POINT('Ctrl Pts',(4.87251974102098,-28.5115608474941,
55.7520929863859));
#111096=CARTESIAN_POINT('Ctrl Pts',(4.8771436608712,-28.546636291689,55.817817877537));
#111097=CARTESIAN_POINT('Ctrl Pts',(4.88280610841908,-28.5924758159412,
55.8913935790166));
#111098=CARTESIAN_POINT('Ctrl Pts',(4.8836146635785,-28.5990851600588,55.901745213947));
#111099=CARTESIAN_POINT('Ctrl Pts',(4.88489208210546,-28.6096133512663,
55.917839465566));
#111100=CARTESIAN_POINT('Ctrl Pts',(4.88535606533497,-28.6134548806998,
55.9236324730624));
#111101=CARTESIAN_POINT('Ctrl Pts',(4.88622874196377,-28.6207098919458,
55.9344257334858));
#111102=CARTESIAN_POINT('Ctrl Pts',(4.88663686034659,-28.6241145227322,
55.9394316379284));
#111103=CARTESIAN_POINT('Ctrl Pts',(4.88760315300092,-28.6322039812901,
55.9511874472255));
#111104=CARTESIAN_POINT('Ctrl Pts',(4.88816281200508,-28.6369115422406,
55.9579213734989));
#111105=CARTESIAN_POINT('Ctrl Pts',(4.89004737605434,-28.6528439655818,
55.9803566437827));
#111106=CARTESIAN_POINT('Ctrl Pts',(4.8913858255163,-28.6642913787573,55.9958970478198));
#111107=CARTESIAN_POINT('Ctrl Pts',(4.89471767494053,-28.6931674271695,
56.0337040434749));
#111108=CARTESIAN_POINT('Ctrl Pts',(4.89672565271892,-28.7108976090683,
56.0557321005616));
#111109=CARTESIAN_POINT('Ctrl Pts',(4.90592663770011,-28.7939321407047,
56.1536828542115));
#111110=CARTESIAN_POINT('Ctrl Pts',(4.91329187793459,-28.8654401602113,
56.224074438732));
#111111=CARTESIAN_POINT('Ctrl Pts',(4.92646765745908,-29.0066718683498,
56.3400286640871));
#111112=CARTESIAN_POINT('Ctrl Pts',(4.93230942541209,-29.07432292447,56.3876250390495));
#111113=CARTESIAN_POINT('Ctrl Pts',(4.93930500320949,-29.1620656893365,
56.4400717108394));
#111114=CARTESIAN_POINT('Ctrl Pts',(4.94063615588275,-29.1790723891478,
56.4498339063757));
#111115=CARTESIAN_POINT('Ctrl Pts',(4.94275297152449,-29.2066075804795,
56.4649997759076));
#111116=CARTESIAN_POINT('Ctrl Pts',(4.94354541202223,-29.2170277370284,
56.4705952273363));
#111117=CARTESIAN_POINT('Ctrl Pts',(4.94505000146004,-29.237023002231,56.4810595736852));
#111118=CARTESIAN_POINT('Ctrl Pts',(4.94576280150384,-29.2465872950526,
56.4859477329866));
#111119=CARTESIAN_POINT('Ctrl Pts',(4.94739595346363,-29.2687073054138,
56.496984442664));
#111120=CARTESIAN_POINT('Ctrl Pts',(4.94831401529336,-29.281294590246,56.5030681888911));
#111121=CARTESIAN_POINT('Ctrl Pts',(4.951224835303,-29.3216746427434,56.5219616119271));
#111122=CARTESIAN_POINT('Ctrl Pts',(4.95319693336021,-29.3497453274675,
56.5341647524631));
#111123=CARTESIAN_POINT('Ctrl Pts',(4.95785531877274,-29.4175720132559,
56.5614545913724));
#111124=CARTESIAN_POINT('Ctrl Pts',(4.96051903767616,-29.4576008687515,
56.5758065753862));
#111125=CARTESIAN_POINT('Ctrl Pts',(4.96772442826368,-29.5684244243163,
56.6108171440893));
#111126=CARTESIAN_POINT('Ctrl Pts',(4.9721985270971,-29.6401094669447,56.6283330490329));
#111127=CARTESIAN_POINT('Ctrl Pts',(4.97755739051451,-29.7263937469962,
56.643437965899));
#111128=CARTESIAN_POINT('Ctrl Pts',(4.97840787460967,-29.7400977788795,
56.6456608274519));
#111129=CARTESIAN_POINT('Ctrl Pts',(4.9837739274647,-29.8264979564302,56.6585692198715));
#111130=CARTESIAN_POINT('Ctrl Pts',(4.9883419844306,-29.8997978747434,56.6646055443897));
#111131=CARTESIAN_POINT('Ctrl Pts',(4.99394237339087,-29.9855231278391,
56.6659823456259));
#111132=CARTESIAN_POINT('Ctrl Pts',(4.99475070398619,-29.9978011708774,
56.6660437866857));
#111133=CARTESIAN_POINT('Ctrl Pts',(4.99602784400119,-30.0170284972259,
56.6659274704977));
#111134=CARTESIAN_POINT('Ctrl Pts',(4.99649177672391,-30.0239781819155,
56.6658419340061));
#111135=CARTESIAN_POINT('Ctrl Pts',(4.99736441514848,-30.0369803196991,
56.6656005258252));
#111136=CARTESIAN_POINT('Ctrl Pts',(4.99777254648116,-30.0430327202934,
56.6654551437902));
#111137=CARTESIAN_POINT('Ctrl Pts',(4.99873894704928,-30.0572982672592,
56.6650346662323));
#111138=CARTESIAN_POINT('Ctrl Pts',(4.99929870202256,-30.0655103184548,
56.6647317868905));
#111139=CARTESIAN_POINT('Ctrl Pts',(5.00118393497902,-30.0930099642885,
56.6635137497785));
#111140=CARTESIAN_POINT('Ctrl Pts',(5.00252296997056,-30.1122830336431,
56.6623240628892));
#111141=CARTESIAN_POINT('Ctrl Pts',(5.00585660377775,-30.159732425323,56.6585662232968));
#111142=CARTESIAN_POINT('Ctrl Pts',(5.00786579907666,-30.1878718297024,
56.6556147980918));
#111143=CARTESIAN_POINT('Ctrl Pts',(5.01707759850643,-30.3153460533314,
56.6389530614541));
#111144=CARTESIAN_POINT('Ctrl Pts',(5.02445273154417,-30.4133944052274,
56.6170082877466));
#111145=CARTESIAN_POINT('Ctrl Pts',(5.03762627195972,-30.587376957223,56.5611985428563));
#111146=CARTESIAN_POINT('Ctrl Pts',(5.04345691668225,-30.6639103968867,
56.5302219595604));
#111147=CARTESIAN_POINT('Ctrl Pts',(5.05044175034944,-30.7554208238062,
56.4850183969864));
#111148=CARTESIAN_POINT('Ctrl Pts',(5.05177258263981,-30.7728420864773,
56.4760269058343));
#111149=CARTESIAN_POINT('Ctrl Pts',(5.05388901410431,-30.8005126550865,
56.4611212614339));
#111150=CARTESIAN_POINT('Ctrl Pts',(5.05468138643945,-30.8108642600047,
56.4554020117813));
#111151=CARTESIAN_POINT('Ctrl Pts',(5.05618592313508,-30.8304998278226,
56.4442788516404));
#111152=CARTESIAN_POINT('Ctrl Pts',(5.05689873779717,-30.8397940969839,
56.4388944538067));
#111153=CARTESIAN_POINT('Ctrl Pts',(5.05853203132116,-30.8610654443726,
56.4262951244961));
#111154=CARTESIAN_POINT('Ctrl Pts',(5.05945021870636,-30.8730051755176,
56.4190184864598));
#111155=CARTESIAN_POINT('Ctrl Pts',(5.06236189036535,-30.9107900450925,
56.395333158323));
#111156=CARTESIAN_POINT('Ctrl Pts',(5.06433469690093,-30.936276023862,56.3783615362693));
#111157=CARTESIAN_POINT('Ctrl Pts',(5.06899511634689,-30.9960157188682,
56.3361576708979));
#111158=CARTESIAN_POINT('Ctrl Pts',(5.07166013274733,-31.0297995190664,
56.3102968994351));
#111159=CARTESIAN_POINT('Ctrl Pts',(5.07886618433584,-31.1193250042724,
56.2361632632531));
#111160=CARTESIAN_POINT('Ctrl Pts',(5.08333973224457,-31.1729108903475,
56.1854402076683));
#111161=CARTESIAN_POINT('Ctrl Pts',(5.08870351962095,-31.2324495439091,
56.1210795325227));
#111162=CARTESIAN_POINT('Ctrl Pts',(5.08955944453588,-31.2418075998604,
56.1107047651971));
#111163=CARTESIAN_POINT('Ctrl Pts',(5.09492395682153,-31.2994797634546,
56.0451267393175));
#111164=CARTESIAN_POINT('Ctrl Pts',(5.09948507939289,-31.3442282907643,
55.9869068538925));
#111165=CARTESIAN_POINT('Ctrl Pts',(5.10507777015086,-31.3918136507074,
55.9157300402534));
#111166=CARTESIAN_POINT('Ctrl Pts',(5.10588607230528,-31.3985241877153,
55.9054484079914));
#111167=CARTESIAN_POINT('Ctrl Pts',(5.10716317704671,-31.4088543762412,
55.8892320573665));
#111168=CARTESIAN_POINT('Ctrl Pts',(5.10762710337254,-31.4125517169767,
55.8833470143684));
#111169=CARTESIAN_POINT('Ctrl Pts',(5.1084997369603,-31.4194007466447,55.8722924832673));
#111170=CARTESIAN_POINT('Ctrl Pts',(5.10890786993506,-31.4225612186711,
55.8671287276937));
#111171=CARTESIAN_POINT('Ctrl Pts',(5.10987428417919,-31.4299451732476,
55.8549153967264));
#111172=CARTESIAN_POINT('Ctrl Pts',(5.11043405131392,-31.4341447174143,
55.8478516712772));
#111173=CARTESIAN_POINT('Ctrl Pts',(5.11231936904938,-31.4480368093912,
55.8240863354401));
#111174=CARTESIAN_POINT('Ctrl Pts',(5.11365847825465,-31.457490805846,55.8072480170422));
#111175=CARTESIAN_POINT('Ctrl Pts',(5.11699233824742,-31.4800699126507,
55.7653427584155));
#111176=CARTESIAN_POINT('Ctrl Pts',(5.11900168788523,-31.4928529323951,
55.7400989296676));
#111177=CARTESIAN_POINT('Ctrl Pts',(5.1282148593998,-31.5479994607116,55.6239481555645));
#111178=CARTESIAN_POINT('Ctrl Pts',(5.13559124771605,-31.5827444042041,
55.5296548402536));
#111179=CARTESIAN_POINT('Ctrl Pts',(5.14876450488049,-31.6302109985374,
55.3532159558411));
#111180=CARTESIAN_POINT('Ctrl Pts',(5.15459373927756,-31.6456900239156,
55.2721349564532));
#111181=CARTESIAN_POINT('Ctrl Pts',(5.16157721018784,-31.6573420426315,
55.170755939862));
#111182=CARTESIAN_POINT('Ctrl Pts',(5.16290800146684,-31.6592364802638,
55.1512435016055));
#111183=CARTESIAN_POINT('Ctrl Pts',(5.16502438375361,-31.6617210350949,
55.1199126770692));
#111184=CARTESIAN_POINT('Ctrl Pts',(5.16581674736336,-31.6625303644978,
55.1081140518327));
#111185=CARTESIAN_POINT('Ctrl Pts',(5.16732127730966,-31.6638349180154,
55.0855846457683));
#111186=CARTESIAN_POINT('Ctrl Pts',(5.16803409384519,-31.6643521220211,
55.0748557889417));
#111187=CARTESIAN_POINT('Ctrl Pts',(5.16966740550135,-31.6653036829076,
55.0501510955302));
#111188=CARTESIAN_POINT('Ctrl Pts',(5.17058560896727,-31.6656659359927,
55.0361731682925));
#111189=CARTESIAN_POINT('Ctrl Pts',(5.17349738971624,-31.6662599834833,
54.9915806851101));
#111190=CARTESIAN_POINT('Ctrl Pts',(5.17547028700397,-31.6658239656103,
54.9609625613734));
#111191=CARTESIAN_POINT('Ctrl Pts',(5.18013096702135,-31.6627668681661,
54.8878785891644));
#111192=CARTESIAN_POINT('Ctrl Pts',(5.18279614964513,-31.6593627377994,
54.8454666589146));
#111193=CARTESIAN_POINT('Ctrl Pts',(5.19000228389805,-31.6456340391557,
54.7300434846203));
#111194=CARTESIAN_POINT('Ctrl Pts',(5.19447575929849,-31.6320820950291,
54.6575145112323));
#111195=CARTESIAN_POINT('Ctrl Pts',(5.19984012921103,-31.6102985922564,
54.5725775668585));
#111196=CARTESIAN_POINT('Ctrl Pts',(5.20069670478339,-31.606654791506,54.5590783885206));
#111197=CARTESIAN_POINT('Ctrl Pts',(5.20606101995594,-31.5828379788928,
54.4750624841905));
#111198=CARTESIAN_POINT('Ctrl Pts',(5.21062130040077,-31.5581988168998,
54.4059047295577));
#111199=CARTESIAN_POINT('Ctrl Pts',(5.21621305634732,-31.5242143376925,
54.3273355990037));
#111200=CARTESIAN_POINT('Ctrl Pts',(5.21702135503304,-31.5192158653859,
54.3161214463109));
#111201=CARTESIAN_POINT('Ctrl Pts',(5.21829845547237,-31.5111945523011,
54.2986474993057));
#111202=CARTESIAN_POINT('Ctrl Pts',(5.21876238101803,-31.5082555808525,
54.292349377456));
#111203=CARTESIAN_POINT('Ctrl Pts',(5.21963501401595,-31.5026828588532,
54.2805996374192));
#111204=CARTESIAN_POINT('Ctrl Pts',(5.22004314719105,-31.5000586879212,
54.2751437493661));
#111205=CARTESIAN_POINT('Ctrl Pts',(5.22100956310321,-31.4938025170977,
54.2623160742457));
#111206=CARTESIAN_POINT('Ctrl Pts',(5.22156933172131,-31.4901456455509,
54.2549567244982));
#111207=CARTESIAN_POINT('Ctrl Pts',(5.22345465979769,-31.4777138538021,
54.2303957765015));
#111208=CARTESIAN_POINT('Ctrl Pts',(5.22479377805522,-31.4686946939059,
54.2133204520457));
#111209=CARTESIAN_POINT('Ctrl Pts',(5.22812766563737,-31.4457341579815,
54.1716225237206));
#111210=CARTESIAN_POINT('Ctrl Pts',(5.23013703410107,-31.4314586250855,
54.1471913915251));
#111211=CARTESIAN_POINT('Ctrl Pts',(5.23935037299783,-31.3637834991395,
54.0378624793571));
#111212=CARTESIAN_POINT('Ctrl Pts',(5.24672691444889,-31.3034065405392,
53.957528945681));
#111213=CARTESIAN_POINT('Ctrl Pts',(5.25990013707229,-31.1809163200732,
53.8219568472659));
#111214=CARTESIAN_POINT('Ctrl Pts',(5.26572919943675,-31.1211934776836,
53.7649785879782));
#111215=CARTESIAN_POINT('Ctrl Pts',(5.27271250410914,-31.042342038768,53.7002064361364));
#111216=CARTESIAN_POINT('Ctrl Pts',(5.27404329037955,-31.0269763187291,
53.688032038441));
#111217=CARTESIAN_POINT('Ctrl Pts',(5.27615966666045,-31.0020015288965,
53.6689519977381));
#111218=CARTESIAN_POINT('Ctrl Pts',(5.27695202920453,-30.9925279526575,
53.6618729044251));
#111219=CARTESIAN_POINT('Ctrl Pts',(5.27845655832646,-30.9743075682746,
53.6485577598412));
#111220=CARTESIAN_POINT('Ctrl Pts',(5.27916937509087,-30.9655742974295,
53.6423042861369));
#111221=CARTESIAN_POINT('Ctrl Pts',(5.28080268896172,-30.9453348711106,
53.6281058819975));
#111222=CARTESIAN_POINT('Ctrl Pts',(5.28172089439166,-30.9337878522869,
53.6202203957837));
#111223=CARTESIAN_POINT('Ctrl Pts',(5.28463268846466,-30.8966457784893,
53.5955358402068));
#111224=CARTESIAN_POINT('Ctrl Pts',(5.28660559683672,-30.870685523867,53.5792959015499));
#111225=CARTESIAN_POINT('Ctrl Pts',(5.29126630868025,-30.8076259751611,
53.542225949752));
#111226=CARTESIAN_POINT('Ctrl Pts',(5.29393151160667,-30.7701472740657,
53.5220830692988));
#111227=CARTESIAN_POINT('Ctrl Pts',(5.30113765592516,-30.6657290517363,
53.4710157881275));
#111228=CARTESIAN_POINT('Ctrl Pts',(5.30561112243963,-30.5974443170091,
53.4430643743414));
#111229=CARTESIAN_POINT('Ctrl Pts',(5.31097556277097,-30.5142693939606,
53.4152986026176));
#111230=CARTESIAN_POINT('Ctrl Pts',(5.31183221711195,-30.5009506498419,
53.4110380845298));
#111231=CARTESIAN_POINT('Ctrl Pts',(5.31719650821312,-30.4174481947714,
53.3854808103858));
#111232=CARTESIAN_POINT('Ctrl Pts',(5.32175668650177,-30.3459840202621,
53.3686730716207));
#111233=CARTESIAN_POINT('Ctrl Pts',(5.3273483290499,-30.2615444237552,53.3546121254132));
#111234=CARTESIAN_POINT('Ctrl Pts',(5.32815662731468,-30.2494119401777,
53.3527294072398));
#111235=CARTESIAN_POINT('Ctrl Pts',(5.32943372723195,-30.2303808519183,
53.3499912217858));
#111236=CARTESIAN_POINT('Ctrl Pts',(5.3298976526829,-30.2234955342965,53.3490445048733));
#111237=CARTESIAN_POINT('Ctrl Pts',(5.33077028560924,-30.2106016227377,
53.3473537545872));
#111238=CARTESIAN_POINT('Ctrl Pts',(5.33117841880865,-30.2045946371384,
53.3465993571583));
#111239=CARTESIAN_POINT('Ctrl Pts',(5.33214483492325,-30.1904244232498,
53.3448981682458));
#111240=CARTESIAN_POINT('Ctrl Pts',(5.33270460372141,-30.1822581545972,
53.343979018113));
#111241=CARTESIAN_POINT('Ctrl Pts',(5.334589933053,-30.1548808569597,53.3411025302052));
#111242=CARTESIAN_POINT('Ctrl Pts',(5.33592905240931,-30.1356434492066,
53.3394188757055));
#111243=CARTESIAN_POINT('Ctrl Pts',(5.33926294334032,-30.0881581864813,
53.3360935619194));
#111244=CARTESIAN_POINT('Ctrl Pts',(5.34127231408916,-30.0598899604796,
53.3348364907847));
#111245=CARTESIAN_POINT('Ctrl Pts',(5.35048567330346,-29.931333141851,53.3323972434933));
#111246=CARTESIAN_POINT('Ctrl Pts',(5.35786223334268,-29.8310949003424,
53.3395525825514));
#111247=CARTESIAN_POINT('Ctrl Pts',(5.37103726636608,-29.650735789786,53.3689366540128));
#111248=CARTESIAN_POINT('Ctrl Pts',(5.37686804534955,-29.570450487176,53.3882171285635));
#111249=CARTESIAN_POINT('Ctrl Pts',(5.3838520077568,-29.4732566832071,53.419341531383));
#111250=CARTESIAN_POINT('Ctrl Pts',(5.385181875842,-29.454707361839,53.4256443502839));
#111251=CARTESIAN_POINT('Ctrl Pts',(5.38729715109357,-29.425147278229,53.4362736396523));
#111252=CARTESIAN_POINT('Ctrl Pts',(5.38808931828124,-29.414064408873,53.4403925887271));
#111253=CARTESIAN_POINT('Ctrl Pts',(5.38959369642006,-29.3929977779737,
53.4484782682744));
#111254=CARTESIAN_POINT('Ctrl Pts',(5.39030655525759,-29.3830067470044,
53.4524242452993));
#111255=CARTESIAN_POINT('Ctrl Pts',(5.39194027574191,-29.3600951827815,
53.4617303642711));
#111256=CARTESIAN_POINT('Ctrl Pts',(5.39285884171903,-29.3472024782364,
53.4671571957145));
#111257=CARTESIAN_POINT('Ctrl Pts',(5.39577308252747,-29.3062849968276,
53.4849901954147));
#111258=CARTESIAN_POINT('Ctrl Pts',(5.39774802643174,-29.2785325887568,
53.4980079303492));
#111259=CARTESIAN_POINT('Ctrl Pts',(5.40241458416427,-29.2131057978863,
53.5309296521478));
#111260=CARTESIAN_POINT('Ctrl Pts',(5.40508351668301,-29.1758043966805,
53.5515276455805));
#111261=CARTESIAN_POINT('Ctrl Pts',(5.41233927071798,-29.0755889277856,
53.6119933702054));
#111262=CARTESIAN_POINT('Ctrl Pts',(5.41685663662433,-29.0144956493842,
53.6546822808664));
#111263=CARTESIAN_POINT('Ctrl Pts',(5.42222831087502,-28.9460619721675,
53.7096711251169));
#111264=CARTESIAN_POINT('Ctrl Pts',(5.42304575443613,-28.9357634833076,
53.7181518798815));
#111265=CARTESIAN_POINT('Ctrl Pts',(5.42835811847697,-28.8696756840611,
53.7739203002458));
#111266=CARTESIAN_POINT('Ctrl Pts',(5.43290592097097,-28.8169564015635,
53.8247087026248));
#111267=CARTESIAN_POINT('Ctrl Pts',(5.43848382745701,-28.7594879719249,
53.8878684286313));
#111268=CARTESIAN_POINT('Ctrl Pts',(5.43929207432471,-28.7513265425459,
53.8970397565057));
#111269=CARTESIAN_POINT('Ctrl Pts',(5.44056911049709,-28.7387049523823,
53.9115427865617));
#111270=CARTESIAN_POINT('Ctrl Pts',(5.44103302438772,-28.7341753467639,
53.9168138454005));
#111271=CARTESIAN_POINT('Ctrl Pts',(5.44190564857413,-28.7257617770451,
53.9267294806907));
#111272=CARTESIAN_POINT('Ctrl Pts',(5.44231378474214,-28.7218699799735,
53.9313670865621));
#111273=CARTESIAN_POINT('Ctrl Pts',(5.44328022557728,-28.7127551047572,
53.9423497178646));
#111274=CARTESIAN_POINT('Ctrl Pts',(5.44384001635758,-28.7075536035884,
53.9487122920186));
#111275=CARTESIAN_POINT('Ctrl Pts',(5.44572549893681,-28.6902871233375,
53.9701547936817));
#111276=CARTESIAN_POINT('Ctrl Pts',(5.4470647524444,-28.6784378188698,53.9854053567121));
#111277=CARTESIAN_POINT('Ctrl Pts',(5.45451784039417,-28.6146177603126,
54.0705596537538));
#111278=CARTESIAN_POINT('Ctrl Pts',(5.4608689980552,-28.5679296881899,54.1442456443403));
#111279=CARTESIAN_POINT('Ctrl Pts',(5.47371931183086,-28.4854029606339,
54.3003183657453));
#111280=CARTESIAN_POINT('Ctrl Pts',(5.48019531352583,-28.4500196967943,
54.3826483738021));
#111281=CARTESIAN_POINT('Ctrl Pts',(5.48939996520383,-28.4081176237134,
54.5068496067561));
#111282=CARTESIAN_POINT('Ctrl Pts',(5.49227856761209,-28.3962987109907,
54.5467566769934));
#111283=CARTESIAN_POINT('Ctrl Pts',(5.4962066027086,-28.3819888623059,54.6026890868305));
#111284=CARTESIAN_POINT('Ctrl Pts',(5.49729638143236,-28.3782191218697,
54.6183682160584));
#111285=CARTESIAN_POINT('Ctrl Pts',(5.49904973031991,-28.3724826607999,
54.6438494998385));
#111286=CARTESIAN_POINT('Ctrl Pts',(5.49971775081693,-28.3703755571437,
54.6536186336977));
#111287=CARTESIAN_POINT('Ctrl Pts',(5.50111176509432,-28.3661443964154,
54.674129257054));
#111288=CARTESIAN_POINT('Ctrl Pts',(5.50183716372146,-28.3640380641614,
54.6848739479423));
#111289=CARTESIAN_POINT('Ctrl Pts',(5.50327578275009,-28.360052837199,54.70632100565));
#111290=CARTESIAN_POINT('Ctrl Pts',(5.50398901833256,-28.3581724176039,
54.717022531921));
#111291=CARTESIAN_POINT('Ctrl Pts',(5.50566476235029,-28.3539818242413,
54.742320852755));
#111292=CARTESIAN_POINT('Ctrl Pts',(5.50662447759174,-28.3517608863835,
54.756931646552));
#111293=CARTESIAN_POINT('Ctrl Pts',(5.5125416898833,-28.3391939747328,54.8477199817409));
#111294=CARTESIAN_POINT('Ctrl Pts',(5.51733929466059,-28.3339361822987,
54.9245105823954));
#111295=CARTESIAN_POINT('Ctrl Pts',(5.52206892288488,-28.3340005844715,
55.0013955137945));
#111296=CARTESIAN_POINT('Ctrl Pts',(5.52206883519007,-28.334000583278,55.001394088226));
#111297=CARTESIAN_POINT('Ctrl Pts',(5.53024916938802,-28.3341118590488,
55.1343737416745));
#111298=CARTESIAN_POINT('Ctrl Pts',(5.53815870841351,-28.3501438770418,
55.2668475249079));
#111299=CARTESIAN_POINT('Ctrl Pts',(5.54797471152312,-28.3863352685772,
55.41474686797));
#111300=CARTESIAN_POINT('Ctrl Pts',(5.54923331350285,-28.3912502527335,
55.4334201225411));
#111301=CARTESIAN_POINT('Ctrl Pts',(5.55105205152663,-28.3987179130186,
55.459912173948));
#111302=CARTESIAN_POINT('Ctrl Pts',(5.55159812930721,-28.4010058783937,
55.4678047903748));
#111303=CARTESIAN_POINT('Ctrl Pts',(5.55255233789641,-28.4050807134963,
55.4814822156406));
#111304=CARTESIAN_POINT('Ctrl Pts',(5.55295893856606,-28.4068408784732,
55.4872747342021));
#111305=CARTESIAN_POINT('Ctrl Pts',(5.55383639336371,-28.4106896072668,
55.4996966908758));
#111306=CARTESIAN_POINT('Ctrl Pts',(5.55430777339972,-28.4127880620997,
55.5063225919339));
#111307=CARTESIAN_POINT('Ctrl Pts',(5.55561817318169,-28.4187082138394,
55.524617048843));
#111308=CARTESIAN_POINT('Ctrl Pts',(5.55646194115444,-28.4226174544054,
55.5362565091912));
#111309=CARTESIAN_POINT('Ctrl Pts',(5.55798998048575,-28.4298763917018,
55.5571030685315));
#111310=CARTESIAN_POINT('Ctrl Pts',(5.55867192322872,-28.4331790316067,
55.5663249713499));
#111311=CARTESIAN_POINT('Ctrl Pts',(5.55935721585159,-28.4365623067732,
55.5755159245387));
#111312=CARTESIAN_POINT('',(5.32851907597573,-28.3320375446013,55.0005309978053));
#111313=CARTESIAN_POINT('Ctrl Pts',(5.36787289131612,-28.4365623102018,
55.5755159338528));
#111314=CARTESIAN_POINT('Ctrl Pts',(5.36380422092234,-28.415510357728,55.5183265251754));
#111315=CARTESIAN_POINT('Ctrl Pts',(5.35973555052857,-28.3976176847615,
55.4600275468893));
#111316=CARTESIAN_POINT('Ctrl Pts',(5.3556668801348,-28.3829797838545,55.4010007737856));
#111317=CARTESIAN_POINT('Ctrl Pts',(5.35159065291195,-28.3683146956591,
55.3418643689861));
#111318=CARTESIAN_POINT('Ctrl Pts',(5.3475144256891,-28.3569165492793,55.2819979734425));
#111319=CARTESIAN_POINT('Ctrl Pts',(5.34343819846625,-28.3488294980143,
55.2217926359741));
#111320=CARTESIAN_POINT('Ctrl Pts',(5.34045646572778,-28.3429138745232,
55.1777528374188));
#111321=CARTESIAN_POINT('Ctrl Pts',(5.33747473298932,-28.3387688709573,
55.1335318564456));
#111322=CARTESIAN_POINT('Ctrl Pts',(5.33449300025085,-28.3363941013021,
55.0892827744734));
#111323=CARTESIAN_POINT('Ctrl Pts',(5.33250187903717,-28.3348082937692,
55.0597344233874));
#111324=CARTESIAN_POINT('Ctrl Pts',(5.33051075782348,-28.3340096599776,
55.0301434489476));
#111325=CARTESIAN_POINT('Ctrl Pts',(5.32851963660979,-28.3340000870979,
55.0005387116473));
#111326=CARTESIAN_POINT('Ctrl Pts',(5.32851891015794,-28.3314570866962,
55.0005287162952));
#111327=CARTESIAN_POINT('Ctrl Pts',(5.29346518324273,-28.3336687245373,
54.4785403892527));
#111328=CARTESIAN_POINT('Ctrl Pts',(5.221366366048,-28.8783648903703,53.4009406554565));
#111329=CARTESIAN_POINT('Ctrl Pts',(5.11222245857373,-30.7133240716271,
53.1646043309368));
#111330=CARTESIAN_POINT('Ctrl Pts',(5.00108718773517,-31.9288772063249,
54.6038419304127));
#111331=CARTESIAN_POINT('Ctrl Pts',(4.88995191689662,-31.3789833722224,
56.4056718508646));
#111332=CARTESIAN_POINT('Ctrl Pts',(4.77886152833055,-29.5676767012044,
56.9207218368853));
#111333=CARTESIAN_POINT('Ctrl Pts',(4.704816230044,-28.6243048912095,56.0933234227868));
#111334=CARTESIAN_POINT('Ctrl Pts',(4.66781602203697,-28.4339760950611,
55.5764682902535));
#111335=CARTESIAN_POINT('Origin',(5.,-30.,55.));
#111336=CARTESIAN_POINT('',(3.96712537028317,-28.4365623116664,55.5755159378315));
#111337=CARTESIAN_POINT('',(4.16232238521864,-28.4365623101738,55.5755159337767));
#111338=CARTESIAN_POINT('',(5.,-28.4365623102018,55.5755159338528));
#111339=CARTESIAN_POINT('Ctrl Pts',(4.16232238521864,-28.4365623101738,
55.5755159337767));
#111340=CARTESIAN_POINT('Ctrl Pts',(4.16243211065126,-28.4371213119974,
55.57703450949));
#111341=CARTESIAN_POINT('Ctrl Pts',(4.16254176393469,-28.4376825329798,
55.5785522888462));
#111342=CARTESIAN_POINT('Ctrl Pts',(4.16358804680715,-28.4430622566701,
55.5930364300062));
#111343=CARTESIAN_POINT('Ctrl Pts',(4.16451935117471,-28.4480399748959,
55.605943433365));
#111344=CARTESIAN_POINT('Ctrl Pts',(4.16616300711542,-28.4571605741507,
55.6287427762166));
#111345=CARTESIAN_POINT('Ctrl Pts',(4.1668774614397,-28.4612392419544,55.638659777453));
#111346=CARTESIAN_POINT('Ctrl Pts',(4.16837821887263,-28.4700469726591,
55.659500881152));
#111347=CARTESIAN_POINT('Ctrl Pts',(4.1691637322308,-28.4747979571576,55.6704151094574));
#111348=CARTESIAN_POINT('Ctrl Pts',(4.17125636230181,-28.4878298909142,
55.6994970775095));
#111349=CARTESIAN_POINT('Ctrl Pts',(4.17255624952594,-28.4963212858166,
55.717568798265));
#111350=CARTESIAN_POINT('Ctrl Pts',(4.17995993473596,-28.5469250244852,
55.8204203914948));
#111351=CARTESIAN_POINT('Ctrl Pts',(4.1858159223418,-28.5958792134244,55.9016454920731));
#111352=CARTESIAN_POINT('Ctrl Pts',(4.19592518127326,-28.6928722832729,
56.0353470365276));
#111353=CARTESIAN_POINT('Ctrl Pts',(4.20019943960676,-28.7378497637999,
56.0897259021831));
#111354=CARTESIAN_POINT('Ctrl Pts',(4.20696058789092,-28.8125992073484,
56.1692426038715));
#111355=CARTESIAN_POINT('Ctrl Pts',(4.20938085575127,-28.8400332859465,
56.1964638503042));
#111356=CARTESIAN_POINT('Ctrl Pts',(4.21290755393678,-28.8804767132497,
56.2338942312861));
#111357=CARTESIAN_POINT('Ctrl Pts',(4.2139711068955,-28.8927314107955,56.2449030447944));
#111358=CARTESIAN_POINT('Ctrl Pts',(4.21585137077576,-28.9144487382782,
56.2638381065356));
#111359=CARTESIAN_POINT('Ctrl Pts',(4.21666303688062,-28.9238401492346,
56.2718444303598));
#111360=CARTESIAN_POINT('Ctrl Pts',(4.21794280289821,-28.9386549214848,
56.2841926925827));
#111361=CARTESIAN_POINT('Ctrl Pts',(4.21840598100122,-28.9440181888169,
56.2886064789089));
#111362=CARTESIAN_POINT('Ctrl Pts',(4.21927452204453,-28.954074011514,56.2967771435341));
#111363=CARTESIAN_POINT('Ctrl Pts',(4.21967928766356,-28.9587594817694,
56.3005423148981));
#111364=CARTESIAN_POINT('Ctrl Pts',(4.22061123773838,-28.9695458685734,
56.3091144370171));
#111365=CARTESIAN_POINT('Ctrl Pts',(4.22113957705317,-28.9756600786149,
56.3139041234454));
#111366=CARTESIAN_POINT('Ctrl Pts',(4.22277467941608,-28.9945865701455,
56.3285181623988));
#111367=CARTESIAN_POINT('Ctrl Pts',(4.22389046619346,-29.007507924915,56.3381988289139));
#111368=CARTESIAN_POINT('Ctrl Pts',(4.23066062726888,-29.0860593549262,
56.3952860326472));
#111369=CARTESIAN_POINT('Ctrl Pts',(4.23653737146867,-29.1549277087525,
56.4380406696468));
#111370=CARTESIAN_POINT('Ctrl Pts',(4.24779272152279,-29.2918984796872,
56.509827652349));
#111371=CARTESIAN_POINT('Ctrl Pts',(4.25315698148687,-29.3593762754129,
56.5396719965527));
#111372=CARTESIAN_POINT('Ctrl Pts',(4.26145229165483,-29.468564696303,56.5795383907822));
#111373=CARTESIAN_POINT('Ctrl Pts',(4.26445109047989,-29.5090638997846,
56.5925913658569));
#111374=CARTESIAN_POINT('Ctrl Pts',(4.2695284350158,-29.5794984757368,56.612349760313));
#111375=CARTESIAN_POINT('Ctrl Pts',(4.27162850920852,-29.6091995610068,
56.6198050846228));
#111376=CARTESIAN_POINT('Ctrl Pts',(4.27464973005518,-29.6527409209396,
56.6294669761365));
#111377=CARTESIAN_POINT('Ctrl Pts',(4.27559134859135,-29.6664287623135,
56.6323240316784));
#111378=CARTESIAN_POINT('Ctrl Pts',(4.27724659181909,-29.690692397222,56.6370706073421));
#111379=CARTESIAN_POINT('Ctrl Pts',(4.27796242414816,-29.7012533758513,
56.6390307594453));
#111380=CARTESIAN_POINT('Ctrl Pts',(4.27945959070728,-29.7234802013295,
56.6429341578835));
#111381=CARTESIAN_POINT('Ctrl Pts',(4.28024019785937,-29.7351493072579,
56.6448556073072));
#111382=CARTESIAN_POINT('Ctrl Pts',(4.28230445291056,-29.7662120225624,
56.6496312924324));
#111383=CARTESIAN_POINT('Ctrl Pts',(4.28358122063522,-29.7856375905309,
56.6522678443218));
#111384=CARTESIAN_POINT('Ctrl Pts',(4.29017436683072,-29.8869577869544,
56.664202558619));
#111385=CARTESIAN_POINT('Ctrl Pts',(4.29530815566265,-29.9694175722315,
56.6677577436673));
#111386=CARTESIAN_POINT('Ctrl Pts',(4.30653208466127,-30.1520640630736,
56.6620749126426));
#111387=CARTESIAN_POINT('Ctrl Pts',(4.31256292326601,-30.2518243018729,
56.6499086851521));
#111388=CARTESIAN_POINT('Ctrl Pts',(4.32062391892838,-30.3775408688769,
56.6229046278441));
#111389=CARTESIAN_POINT('Ctrl Pts',(4.32241757625831,-30.4050462954552,
56.6162592170699));
#111390=CARTESIAN_POINT('Ctrl Pts',(4.3254863058203,-30.4510167220484,56.6039054909413));
#111391=CARTESIAN_POINT('Ctrl Pts',(4.32674503545846,-30.4695763640406,
56.5985702573787));
#111392=CARTESIAN_POINT('Ctrl Pts',(4.32856392602924,-30.4958955665614,
56.5905065615686));
#111393=CARTESIAN_POINT('Ctrl Pts',(4.32911002548848,-30.5037349143724,
56.5880411406401));
#111394=CARTESIAN_POINT('Ctrl Pts',(4.33006425851927,-30.517317354206,56.5836588679341));
#111395=CARTESIAN_POINT('Ctrl Pts',(4.33047086170832,-30.5230687574497,
56.5817685445683));
#111396=CARTESIAN_POINT('Ctrl Pts',(4.33134830595028,-30.5354006471635,
56.5776407866514));
#111397=CARTESIAN_POINT('Ctrl Pts',(4.33181967275585,-30.5419773753784,
56.5753935460262));
#111398=CARTESIAN_POINT('Ctrl Pts',(4.33313000076289,-30.5601327361099,
56.5690627960888));
#111399=CARTESIAN_POINT('Ctrl Pts',(4.33397370938485,-30.5716803123751,
56.5648924367061));
#111400=CARTESIAN_POINT('Ctrl Pts',(4.33989687688816,-30.6518335068084,
56.5349399088824));
#111401=CARTESIAN_POINT('Ctrl Pts',(4.34517904538841,-30.7187116703811,
56.5047852334948));
#111402=CARTESIAN_POINT('Ctrl Pts',(4.35152427570334,-30.7957926739051,
56.4637171319259));
#111403=CARTESIAN_POINT('Ctrl Pts',(4.35254751974055,-30.8081213881181,
56.456946684157));
#111404=CARTESIAN_POINT('Ctrl Pts',(4.35893581942883,-30.8845144947408,
56.4137265746421));
#111405=CARTESIAN_POINT('Ctrl Pts',(4.36430072111089,-30.9461908951115,
56.3732125915553));
#111406=CARTESIAN_POINT('Ctrl Pts',(4.37259482970425,-31.0388876293453,
56.3031022521645));
#111407=CARTESIAN_POINT('Ctrl Pts',(4.37559188714158,-31.07179940411,56.2761698655432));
#111408=CARTESIAN_POINT('Ctrl Pts',(4.38066664511901,-31.1265717084339,
56.2277331570357));
#111409=CARTESIAN_POINT('Ctrl Pts',(4.38276584436773,-31.1489344902655,
56.2068315001478));
#111410=CARTESIAN_POINT('Ctrl Pts',(4.38578605963622,-31.180656394891,56.175500706456));
#111411=CARTESIAN_POINT('Ctrl Pts',(4.3867275282844,-31.1904789142066,56.1655519761865));
#111412=CARTESIAN_POINT('Ctrl Pts',(4.38838260250387,-31.2076246259359,
56.1477430563729));
#111413=CARTESIAN_POINT('Ctrl Pts',(4.38909841418583,-31.2149990894154,
56.1399335869368));
#111414=CARTESIAN_POINT('Ctrl Pts',(4.39059562974747,-31.2303339792498,
56.1233762376435));
#111415=CARTESIAN_POINT('Ctrl Pts',(4.39137630566097,-31.2382778397364,
56.1146137786509));
#111416=CARTESIAN_POINT('Ctrl Pts',(4.39344095835931,-31.2591413065225,
56.0911020068116));
#111417=CARTESIAN_POINT('Ctrl Pts',(4.39471805012289,-31.2718952412442,
56.0762076783809));
#111418=CARTESIAN_POINT('Ctrl Pts',(4.40132228906001,-31.3369830112365,
55.9974230493677));
#111419=CARTESIAN_POINT('Ctrl Pts',(4.40646602792858,-31.3847789123154,
55.9299280429754));
#111420=CARTESIAN_POINT('Ctrl Pts',(4.41769061665509,-31.4790267099188,
55.7733480857006));
#111421=CARTESIAN_POINT('Ctrl Pts',(4.42371306737134,-31.5228307391293,
55.6830603693174));
#111422=CARTESIAN_POINT('Ctrl Pts',(4.43176397620187,-31.5682627428966,
55.5629453512309));
#111423=CARTESIAN_POINT('Ctrl Pts',(4.43355651138082,-31.5775904701257,
55.5362495944699));
#111424=CARTESIAN_POINT('Ctrl Pts',(4.43662351478916,-31.5921348118628,
55.4909534561919));
#111425=CARTESIAN_POINT('Ctrl Pts',(4.4378816643358,-31.5977156160317,55.47247570063));
#111426=CARTESIAN_POINT('Ctrl Pts',(4.43969986170973,-31.605212462451,55.4460005165346));
#111427=CARTESIAN_POINT('Ctrl Pts',(4.44024586264612,-31.6073924884716,
55.4380786360471));
#111428=CARTESIAN_POINT('Ctrl Pts',(4.44119998460395,-31.6110768784822,
55.4242922863489));
#111429=CARTESIAN_POINT('Ctrl Pts',(4.44160657634965,-31.6126080181545,
55.4184352172965));
#111430=CARTESIAN_POINT('Ctrl Pts',(4.44248406859626,-31.6158286004892,
55.4058352504433));
#111431=CARTESIAN_POINT('Ctrl Pts',(4.44295549555467,-31.6175077538273,
55.3990901885068));
#111432=CARTESIAN_POINT('Ctrl Pts',(4.44426614989972,-31.6220368388786,
55.3803989063622));
#111433=CARTESIAN_POINT('Ctrl Pts',(4.44511012837367,-31.6247968877908,
55.3684316570703));
#111434=CARTESIAN_POINT('Ctrl Pts',(4.45110730840338,-31.6433322501858,
55.2838023084108));
#111435=CARTESIAN_POINT('Ctrl Pts',(4.45646911568256,-31.6543581590369,
55.2101933988584));
#111436=CARTESIAN_POINT('Ctrl Pts',(4.46272943876652,-31.6613963162143,
55.1243295597897));
#111437=CARTESIAN_POINT('Ctrl Pts',(4.46358882770382,-31.6622361542528,
55.11254565401));
#111438=CARTESIAN_POINT('Ctrl Pts',(4.47401157832634,-31.6708972052907,
54.9695943126691));
#111439=CARTESIAN_POINT('Ctrl Pts',(4.48353089996228,-31.6633002424257,
54.8379284727486));
#111440=CARTESIAN_POINT('Ctrl Pts',(4.49406129198292,-31.6364677088518,
54.6869353601699));
#111441=CARTESIAN_POINT('Ctrl Pts',(4.49555251643617,-31.6322089684988,
54.6654405982236));
#111442=CARTESIAN_POINT('Ctrl Pts',(4.49786076861307,-31.6248965807297,
54.6320072085027));
#111443=CARTESIAN_POINT('Ctrl Pts',(4.4986868937088,-31.6221325673299,54.6200084990784));
#111444=CARTESIAN_POINT('Ctrl Pts',(4.5002204952924,-31.6167271428059,54.5976779439363));
#111445=CARTESIAN_POINT('Ctrl Pts',(4.50092899837004,-31.6141190791023,
54.5873387604858));
#111446=CARTESIAN_POINT('Ctrl Pts',(4.50250678748599,-31.6080633235219,
54.5642680843485));
#111447=CARTESIAN_POINT('Ctrl Pts',(4.50337433962746,-31.6045633168758,
54.5515509688137));
#111448=CARTESIAN_POINT('Ctrl Pts',(4.50558083920576,-31.5952274235107,
54.5191389417782));
#111449=CARTESIAN_POINT('Ctrl Pts',(4.50691285335141,-31.5891775592401,
54.4995076079731));
#111450=CARTESIAN_POINT('Ctrl Pts',(4.51676586711935,-31.541369031248,54.3539910411241));
#111451=CARTESIAN_POINT('Ctrl Pts',(4.52476790493922,-31.4850755979531,
54.233383937309));
#111452=CARTESIAN_POINT('Ctrl Pts',(4.53782898807933,-31.3724990106375,
54.052208504936));
#111453=CARTESIAN_POINT('Ctrl Pts',(4.54280835877174,-31.3250133922257,
53.9868867493938));
#111454=CARTESIAN_POINT('Ctrl Pts',(4.54897253594656,-31.2639220446676,
53.9145255623659));
#111455=CARTESIAN_POINT('Ctrl Pts',(4.54989574808572,-31.2547165702832,
53.9038978213636));
#111456=CARTESIAN_POINT('Ctrl Pts',(4.55130915368142,-31.2405623084587,
53.8879686502041));
#111457=CARTESIAN_POINT('Ctrl Pts',(4.55179250060612,-31.235711334333,53.8825806260069));
#111458=CARTESIAN_POINT('Ctrl Pts',(4.55268144352086,-31.2267742365302,
53.8727834687516));
#111459=CARTESIAN_POINT('Ctrl Pts',(4.55308622576839,-31.2226992165382,
53.8683645649483));
#111460=CARTESIAN_POINT('Ctrl Pts',(4.55401841394519,-31.2133019299071,
53.858284272262));
#111461=CARTESIAN_POINT('Ctrl Pts',(4.55454697711084,-31.2079639234371,
53.8526380127801));
#111462=CARTESIAN_POINT('Ctrl Pts',(4.55618342963906,-31.1914019573732,
53.8353633297176));
#111463=CARTESIAN_POINT('Ctrl Pts',(4.55730036319552,-31.1800485052258,
53.8238611157512));
#111464=CARTESIAN_POINT('Ctrl Pts',(4.56381289901495,-31.1134709966227,
53.758345703902));
#111465=CARTESIAN_POINT('Ctrl Pts',(4.56941075916856,-31.0547154314812,
53.7080649654478));
#111466=CARTESIAN_POINT('Ctrl Pts',(4.58180749125572,-30.9178907675277,
53.6065483117389));
#111467=CARTESIAN_POINT('Ctrl Pts',(4.58858959507342,-30.8385608835689,
53.5574155516046));
#111468=CARTESIAN_POINT('Ctrl Pts',(4.59875990850559,-30.7103669359251,
53.4921859887675));
#111469=CARTESIAN_POINT('Ctrl Pts',(4.60228315990653,-30.6641709818896,
53.4712743497823));
#111470=CARTESIAN_POINT('Ctrl Pts',(4.60687793181026,-30.6015142074444,
53.4462890221044));
#111471=CARTESIAN_POINT('Ctrl Pts',(4.6080121966321,-30.5858461287501,53.4403136553393));
#111472=CARTESIAN_POINT('Ctrl Pts',(4.60989300757114,-30.5595371860798,
53.4307325694619));
#111473=CARTESIAN_POINT('Ctrl Pts',(4.6106438469159,-30.5489455653351,53.4269962148431));
#111474=CARTESIAN_POINT('Ctrl Pts',(4.61211585078803,-30.5280096188241,
53.4198479617214));
#111475=CARTESIAN_POINT('Ctrl Pts',(4.6128371893371,-30.5176680300435,53.4164298430815));
#111476=CARTESIAN_POINT('Ctrl Pts',(4.61458303893485,-30.4924439150111,
53.4083662374511));
#111477=CARTESIAN_POINT('Ctrl Pts',(4.61560401789845,-30.4775280800389,
53.4038277024767));
#111478=CARTESIAN_POINT('Ctrl Pts',(4.61909824108944,-30.4259409882255,
53.3889188542871));
#111479=CARTESIAN_POINT('Ctrl Pts',(4.62153791870066,-30.3889774894569,
53.3795972591304));
#111480=CARTESIAN_POINT('Ctrl Pts',(4.63223687516057,-30.2234609931224,
53.3438477812189));
#111481=CARTESIAN_POINT('Ctrl Pts',(4.64007255399123,-30.0923796976781,
53.3313955347718));
#111482=CARTESIAN_POINT('Ctrl Pts',(4.6507661062621,-29.919328642491,53.3354274294738));
#111483=CARTESIAN_POINT('Ctrl Pts',(4.65338074260183,-29.877517033542,53.3379809966893));
#111484=CARTESIAN_POINT('Ctrl Pts',(4.65767940755035,-29.8105484071424,
53.3446116799654));
#111485=CARTESIAN_POINT('Ctrl Pts',(4.6593250213079,-29.7853100774154,53.3476954076343));
#111486=CARTESIAN_POINT('Ctrl Pts',(4.66160114849966,-29.7511209947354,
53.3526692620038));
#111487=CARTESIAN_POINT('Ctrl Pts',(4.66220622765236,-29.7420993333675,
53.3540575476851));
#111488=CARTESIAN_POINT('Ctrl Pts',(4.6632293753309,-29.7269666092213,53.3565136907798));
#111489=CARTESIAN_POINT('Ctrl Pts',(4.66364525086665,-29.7208491048592,
53.3575417030293));
#111490=CARTESIAN_POINT('Ctrl Pts',(4.66450501511909,-29.7082741981267,
53.359727128527));
#111491=CARTESIAN_POINT('Ctrl Pts',(4.66494910162733,-29.7018177008032,
53.3608885489187));
#111492=CARTESIAN_POINT('Ctrl Pts',(4.6661304539194,-29.6847398392727,53.3640648226665));
#111493=CARTESIAN_POINT('Ctrl Pts',(4.66687119817837,-29.6741311460916,
53.3661449427848));
#111494=CARTESIAN_POINT('Ctrl Pts',(4.6702301552907,-29.6264385410179,53.375979317183));
#111495=CARTESIAN_POINT('Ctrl Pts',(4.67290273966302,-29.5896081277386,
53.3848933902908));
#111496=CARTESIAN_POINT('Ctrl Pts',(4.6822505533842,-29.4636029282342,53.4199784320118));
#111497=CARTESIAN_POINT('Ctrl Pts',(4.68907383001019,-29.3763330994635,
53.4523471968534));
#111498=CARTESIAN_POINT('Ctrl Pts',(4.70033038323411,-29.2355654021857,
53.5184089186888));
#111499=CARTESIAN_POINT('Ctrl Pts',(4.70481073208242,-29.1804512695654,
53.5481688733211));
#111500=CARTESIAN_POINT('Ctrl Pts',(4.71200005293278,-29.0930579090775,
53.6019252793024));
#111501=CARTESIAN_POINT('Ctrl Pts',(4.71476333365495,-29.0597419654664,
53.6241104047534));
#111502=CARTESIAN_POINT('Ctrl Pts',(4.71853225852293,-29.014711894783,53.6564963537114));
#111503=CARTESIAN_POINT('Ctrl Pts',(4.71957535979378,-29.0022948355298,
53.6656915159536));
#111504=CARTESIAN_POINT('Ctrl Pts',(4.7213479694372,-28.9812788190681,53.6817118646445));
#111505=CARTESIAN_POINT('Ctrl Pts',(4.72208074819327,-28.9726163114684,
53.6884515949557));
#111506=CARTESIAN_POINT('Ctrl Pts',(4.72356045199374,-28.9551793651692,
53.7022969144946));
#111507=CARTESIAN_POINT('Ctrl Pts',(4.72430714197504,-28.9464092848474,
53.7094070848405));
#111508=CARTESIAN_POINT('Ctrl Pts',(4.72617304018116,-28.9245729713239,
53.7274813897998));
#111509=CARTESIAN_POINT('Ctrl Pts',(4.72728762436781,-28.9116013749652,
53.738558215573));
#111510=CARTESIAN_POINT('Ctrl Pts',(4.73157548840588,-28.862019959771,53.7822315414736));
#111511=CARTESIAN_POINT('Ctrl Pts',(4.73469009249451,-28.8266836419565,
53.8162398882538));
#111512=CARTESIAN_POINT('Ctrl Pts',(4.74610163635663,-28.7010252701647,
53.9483400712824));
#111513=CARTESIAN_POINT('Ctrl Pts',(4.75402214546896,-28.6210841601526,
54.0555890221869));
#111514=CARTESIAN_POINT('Ctrl Pts',(4.76431592560086,-28.5390445108868,
54.1986477869557));
#111515=CARTESIAN_POINT('Ctrl Pts',(4.76631260546256,-28.5240960123518,
54.2265250543874));
#111516=CARTESIAN_POINT('Ctrl Pts',(4.76969146729471,-28.5005914614878,
54.2735236631076));
#111517=CARTESIAN_POINT('Ctrl Pts',(4.77105269458402,-28.4915860059077,
54.2924118724151));
#111518=CARTESIAN_POINT('Ctrl Pts',(4.77299367876181,-28.4794350156575,
54.3191843004202));
#111519=CARTESIAN_POINT('Ctrl Pts',(4.77355668200135,-28.4759899599184,
54.3269314459267));
#111520=CARTESIAN_POINT('Ctrl Pts',(4.7745302154362,-28.4701720729221,54.3402882379023));
#111521=CARTESIAN_POINT('Ctrl Pts',(4.77493902497483,-28.4677706132277,
54.3458851777506));
#111522=CARTESIAN_POINT('Ctrl Pts',(4.77580932818307,-28.4627471193443,
54.3577726087513));
#111523=CARTESIAN_POINT('Ctrl Pts',(4.7762712350242,-28.4601330103361,54.3640659695152));
#111524=CARTESIAN_POINT('Ctrl Pts',(4.77755131660434,-28.4530294367921,
54.3814681589952));
#111525=CARTESIAN_POINT('Ctrl Pts',(4.77837401688177,-28.4486211932762,
54.3926094015151));
#111526=CARTESIAN_POINT('Ctrl Pts',(4.78299492143553,-28.4247101719522,
54.455000163146));
#111527=CARTESIAN_POINT('Ctrl Pts',(4.78690695310832,-28.4076285668422,
54.5071360843809));
#111528=CARTESIAN_POINT('Ctrl Pts',(4.80157603031304,-28.3539822088949,
54.7030548127338));
#111529=CARTESIAN_POINT('Ctrl Pts',(4.81249357102556,-28.334082356827,54.8507205956567));
#111530=CARTESIAN_POINT('Ctrl Pts',(4.82499125992332,-28.3339828077517,
55.0306050154698));
#111531=CARTESIAN_POINT('Ctrl Pts',(4.82715543606239,-28.3348602720593,
55.0621278638137));
#111532=CARTESIAN_POINT('Ctrl Pts',(4.83023987647433,-28.3374178031887,
55.1075735681334));
#111533=CARTESIAN_POINT('Ctrl Pts',(4.83118216722175,-28.3383795471822,
55.1215282897699));
#111534=CARTESIAN_POINT('Ctrl Pts',(4.83284056506335,-28.3403930376387,
55.1462081162762));
#111535=CARTESIAN_POINT('Ctrl Pts',(4.8335588633432,-28.3413732985971,55.1569380691767));
#111536=CARTESIAN_POINT('Ctrl Pts',(4.83505100254139,-28.3436359536721,
55.1793076978632));
#111537=CARTESIAN_POINT('Ctrl Pts',(4.8358242137481,-28.3449371141311,55.190944913774));
#111538=CARTESIAN_POINT('Ctrl Pts',(4.83784567712815,-28.3486775751411,
55.2214797554228));
#111539=CARTESIAN_POINT('Ctrl Pts',(4.83908756279389,-28.3513186039049,
55.2403512753014));
#111540=CARTESIAN_POINT('Ctrl Pts',(4.8454959978053,-28.3667318226923,55.3382229731083));
#111541=CARTESIAN_POINT('Ctrl Pts',(4.85049042030508,-28.3848606625276,
55.4162775354516));
#111542=CARTESIAN_POINT('Ctrl Pts',(4.85720459938426,-28.4171516170431,
55.5205730040301));
#111543=CARTESIAN_POINT('Ctrl Pts',(4.85898645989029,-28.4264982828747,
55.548176152032));
#111544=CARTESIAN_POINT('Ctrl Pts',(4.86076601588518,-28.4365623050844,
55.575515919951));
#111545=CARTESIAN_POINT('',(4.62852046319487,-28.3357683158861,55.0011944502022));
#111546=CARTESIAN_POINT('Ctrl Pts',(4.66781602203697,-28.4339760950611,
55.5764682902535));
#111547=CARTESIAN_POINT('Ctrl Pts',(4.66777113976448,-28.4337452209835,
55.5758413307269));
#111548=CARTESIAN_POINT('Ctrl Pts',(4.65467262015045,-28.3664872324192,
55.3928239783714));
#111549=CARTESIAN_POINT('Ctrl Pts',(4.64157410053641,-28.3344870714878,
55.1968759499582));
#111550=CARTESIAN_POINT('Ctrl Pts',(4.62852046319487,-28.3357683158861,
55.0011944502022));
#111551=CARTESIAN_POINT('Ctrl Pts',(4.6275029120089,-28.3340004729511,55.0012553377942));
#111552=CARTESIAN_POINT('Ctrl Pts',(4.62392610857778,-28.3339624265383,
54.9507627085131));
#111553=CARTESIAN_POINT('Ctrl Pts',(4.62040759124933,-28.3362198407892,
54.900289559962));
#111554=CARTESIAN_POINT('Ctrl Pts',(4.61603293442498,-28.3419878498603,
54.8364901137));
#111555=CARTESIAN_POINT('Ctrl Pts',(4.61511227194061,-28.3433732486938,
54.8230039587256));
#111556=CARTESIAN_POINT('Ctrl Pts',(4.61349180923425,-28.3461165050552,
54.7991658746005));
#111557=CARTESIAN_POINT('Ctrl Pts',(4.61278995550999,-28.3474073273124,
54.7888071318349));
#111558=CARTESIAN_POINT('Ctrl Pts',(4.61140048097976,-28.3501674411464,
54.7682350769568));
#111559=CARTESIAN_POINT('Ctrl Pts',(4.61071282033464,-28.3516344235026,
54.7580219302104));
#111560=CARTESIAN_POINT('Ctrl Pts',(4.60924926147721,-28.3549728395331,
54.736220920203));
#111561=CARTESIAN_POINT('Ctrl Pts',(4.60847427981564,-28.3568720538779,
54.7246378272849));
#111562=CARTESIAN_POINT('Ctrl Pts',(4.60644178568113,-28.3621997042574,
54.6941655536125));
#111563=CARTESIAN_POINT('Ctrl Pts',(4.60519077413458,-28.3658325448802,
54.6753135428048));
#111564=CARTESIAN_POINT('Ctrl Pts',(4.59879715589171,-28.3862164080763,
54.5785663407397));
#111565=CARTESIAN_POINT('Ctrl Pts',(4.59382468899969,-28.4082145364832,
54.5018783630823));
#111566=CARTESIAN_POINT('Ctrl Pts',(4.58411984082222,-28.462485560859,54.3536966381393));
#111567=CARTESIAN_POINT('Ctrl Pts',(4.57939577425797,-28.4944769933123,
54.2823240242972));
#111568=CARTESIAN_POINT('Ctrl Pts',(4.57086876488907,-28.5597682281909,
54.1604108765062));
#111569=CARTESIAN_POINT('Ctrl Pts',(4.56710814704191,-28.5910298677669,
54.1089449571422));
#111570=CARTESIAN_POINT('Ctrl Pts',(4.56221665598818,-28.6335551471678,
54.0467875999827));
#111571=CARTESIAN_POINT('Ctrl Pts',(4.56122377112638,-28.6422773535168,
54.0344045406386));
#111572=CARTESIAN_POINT('Ctrl Pts',(4.55972548438599,-28.6555482313965,
54.0160990067003));
#111573=CARTESIAN_POINT('Ctrl Pts',(4.55922822850234,-28.6599701338663,
54.0100850161533));
#111574=CARTESIAN_POINT('Ctrl Pts',(4.55832621899242,-28.6680191659258,
53.9992907197034));
#111575=CARTESIAN_POINT('Ctrl Pts',(4.55792244375978,-28.6716319077777,
53.9945000176292));
#111576=CARTESIAN_POINT('Ctrl Pts',(4.55700849506298,-28.6798308344944,
53.9837490815523));
#111577=CARTESIAN_POINT('Ctrl Pts',(4.55649734960544,-28.6844315057099,
53.9778003687513));
#111578=CARTESIAN_POINT('Ctrl Pts',(4.55492930737978,-28.6985959399777,
53.9597396288654));
#111579=CARTESIAN_POINT('Ctrl Pts',(4.5538641646634,-28.7082875573673,53.9477295545404));
#111580=CARTESIAN_POINT('Ctrl Pts',(4.54544931006988,-28.7854979288526,
53.854722779957));
#111581=CARTESIAN_POINT('Ctrl Pts',(4.53771813303804,-28.8603967164886,
53.7801737291206));
#111582=CARTESIAN_POINT('Ctrl Pts',(4.522227603577,-29.0249939948267,53.6448201398954));
#111583=CARTESIAN_POINT('Ctrl Pts',(4.51451177172979,-29.1146045093627,
53.5846443771792));
#111584=CARTESIAN_POINT('Ctrl Pts',(4.5056353911302,-29.2284394062949,53.5232747213344));
#111585=CARTESIAN_POINT('Ctrl Pts',(4.50416452543651,-29.2476660519554,
53.513387405793));
#111586=CARTESIAN_POINT('Ctrl Pts',(4.501880716072,-29.2780803446503,53.4984880803524));
#111587=CARTESIAN_POINT('Ctrl Pts',(4.50105898371458,-29.2891395320179,
53.4932208381553));
#111588=CARTESIAN_POINT('Ctrl Pts',(4.49952969482263,-29.309934375398,53.4835966343295));
#111589=CARTESIAN_POINT('Ctrl Pts',(4.49882115655741,-29.3196556590131,
53.4792102971145));
#111590=CARTESIAN_POINT('Ctrl Pts',(4.49723840278723,-29.3415620830002,
53.4695780044849));
#111591=CARTESIAN_POINT('Ctrl Pts',(4.49636597671586,-29.3537692006748,
53.4643835941725));
#111592=CARTESIAN_POINT('Ctrl Pts',(4.4941374604437,-29.3852789953532,53.4514177398141));
#111593=CARTESIAN_POINT('Ctrl Pts',(4.49278855206704,-29.4046679148364,
53.4438609638078));
#111594=CARTESIAN_POINT('Ctrl Pts',(4.483078113687,-29.5463746798032,53.3916675330745));
#111595=CARTESIAN_POINT('Ctrl Pts',(4.47521287643015,-29.6734091076345,
53.3611432843665));
#111596=CARTESIAN_POINT('Ctrl Pts',(4.4622135647754,-29.8843073632692,53.3359916571011));
#111597=CARTESIAN_POINT('Ctrl Pts',(4.45714744851914,-29.9665012394781,
53.3323120954081));
#111598=CARTESIAN_POINT('Ctrl Pts',(4.45087209574492,-30.0629173671654,
53.3351270271916));
#111599=CARTESIAN_POINT('Ctrl Pts',(4.44993322119866,-30.0772089392624,
53.3357285807938));
#111600=CARTESIAN_POINT('Ctrl Pts',(4.448500771071,-30.0987773611785,53.3369148267931));
#111601=CARTESIAN_POINT('Ctrl Pts',(4.44801432582664,-30.1060614384736,
53.3373634712672));
#111602=CARTESIAN_POINT('Ctrl Pts',(4.44712267861577,-30.119334133906,53.3382685430023));
#111603=CARTESIAN_POINT('Ctrl Pts',(4.44671832857179,-30.1253235398353,
53.3387095144197));
#111604=CARTESIAN_POINT('Ctrl Pts',(4.44579103866265,-30.1389918948557,
53.3397901859565));
#111605=CARTESIAN_POINT('Ctrl Pts',(4.44526698842956,-30.1466688473069,
53.340450779032));
#111606=CARTESIAN_POINT('Ctrl Pts',(4.44361840258863,-30.1706796672498,
53.3426847848211));
#111607=CARTESIAN_POINT('Ctrl Pts',(4.44248439516168,-30.1869944829755,
53.3444462303274));
#111608=CARTESIAN_POINT('Ctrl Pts',(4.43561061410905,-30.2848382865128,
53.3564746852698));
#111609=CARTESIAN_POINT('Ctrl Pts',(4.42964240513635,-30.3655356789864,
53.3725205216777));
#111610=CARTESIAN_POINT('Ctrl Pts',(4.41714937591296,-30.5309443749194,
53.4183361143562));
#111611=CARTESIAN_POINT('Ctrl Pts',(4.41064528395722,-30.6151209513739,
53.4491319388265));
#111612=CARTESIAN_POINT('Ctrl Pts',(4.4008181228388,-30.7414845882965,53.5072786049749));
#111613=CARTESIAN_POINT('Ctrl Pts',(4.3973717343108,-30.7856017552619,53.5300179202062));
#111614=CARTESIAN_POINT('Ctrl Pts',(4.39285939822965,-30.8430831877679,
53.5629739655451));
#111615=CARTESIAN_POINT('Ctrl Pts',(4.3917335413244,-30.857399528334,53.5714695771727));
#111616=CARTESIAN_POINT('Ctrl Pts',(4.38986293367065,-30.8811347994737,
53.5860399620916));
#111617=CARTESIAN_POINT('Ctrl Pts',(4.38911398560713,-30.8906238257837,
53.5919976082481));
#111618=CARTESIAN_POINT('Ctrl Pts',(4.38764296689,-30.9092295081736,53.603942466339));
#111619=CARTESIAN_POINT('Ctrl Pts',(4.38692074810337,-30.9183488878025,
53.6099243669145));
#111620=CARTESIAN_POINT('Ctrl Pts',(4.385168041037,-30.940436928269,53.6247253656872));
#111621=CARTESIAN_POINT('Ctrl Pts',(4.38414115693104,-30.9533412349638,
53.633638974095));
#111622=CARTESIAN_POINT('Ctrl Pts',(4.38060684533501,-30.9975984047242,
53.6651417489173));
#111623=CARTESIAN_POINT('Ctrl Pts',(4.37813403593957,-31.0282912511862,
53.6886394125771));
#111624=CARTESIAN_POINT('Ctrl Pts',(4.36817806968181,-31.1500651240415,
53.7887733989361));
#111625=CARTESIAN_POINT('Ctrl Pts',(4.36102682012918,-31.2336237046339,
53.8739923280919));
#111626=CARTESIAN_POINT('Ctrl Pts',(4.34961635713186,-31.3487101084422,
54.0197035987373));
#111627=CARTESIAN_POINT('Ctrl Pts',(4.34547200827575,-31.3868473824026,
54.0744448297454));
#111628=CARTESIAN_POINT('Ctrl Pts',(4.34011993749505,-31.4298737934105,
54.1448574557848));
#111629=CARTESIAN_POINT('Ctrl Pts',(4.33908076338134,-31.43795409721,54.1585157129639));
#111630=CARTESIAN_POINT('Ctrl Pts',(4.3375262473493,-31.4496155212339,54.1788857206626));
#111631=CARTESIAN_POINT('Ctrl Pts',(4.33701997170316,-31.4533480218838,
54.1855103801808));
#111632=CARTESIAN_POINT('Ctrl Pts',(4.33610890578113,-31.4599452860549,
54.1974093290067));
#111633=CARTESIAN_POINT('Ctrl Pts',(4.33570519762758,-31.4628270807533,
54.2026738730948));
#111634=CARTESIAN_POINT('Ctrl Pts',(4.3348005663061,-31.4691919254312,54.2144520118825));
#111635=CARTESIAN_POINT('Ctrl Pts',(4.33429877277393,-31.472660102355,54.2209731884658));
#111636=CARTESIAN_POINT('Ctrl Pts',(4.33278758738486,-31.4829222481296,
54.2405824194703));
#111637=CARTESIAN_POINT('Ctrl Pts',(4.33177076520623,-31.489585718095,54.2537374411038));
#111638=CARTESIAN_POINT('Ctrl Pts',(4.32288193049175,-31.5458341430318,
54.3685386905486));
#111639=CARTESIAN_POINT('Ctrl Pts',(4.31456663493016,-31.5851202866657,
54.4748935993468));
#111640=CARTESIAN_POINT('Ctrl Pts',(4.29902897515919,-31.6385095041705,
54.6821459150766));
#111641=CARTESIAN_POINT('Ctrl Pts',(4.29181562246724,-31.6547580337849,
54.7819936210726));
#111642=CARTESIAN_POINT('Ctrl Pts',(4.28339373083651,-31.6633951059486,
54.9043743263053));
#111643=CARTESIAN_POINT('Ctrl Pts',(4.2819160403144,-31.6645002647794,54.9260642591598));
#111644=CARTESIAN_POINT('Ctrl Pts',(4.27962408977165,-31.6655657412128,
54.9600337944312));
#111645=CARTESIAN_POINT('Ctrl Pts',(4.2788009375129,-31.6658149139237,54.9723012203511));
#111646=CARTESIAN_POINT('Ctrl Pts',(4.27727034224551,-31.6660272999848,
54.9952327216606));
#111647=CARTESIAN_POINT('Ctrl Pts',(4.27656190223701,-31.6660236913173,
55.0058957819017));
#111648=CARTESIAN_POINT('Ctrl Pts',(4.27498107070525,-31.6657861469652,
55.0297949516669));
#111649=CARTESIAN_POINT('Ctrl Pts',(4.27411044877809,-31.665496824531,55.0430298835917));
#111650=CARTESIAN_POINT('Ctrl Pts',(4.27188990265222,-31.6643503819525,
55.0769593938813));
#111651=CARTESIAN_POINT('Ctrl Pts',(4.27054707101667,-31.6632650371319,
55.0976443502016));
#111652=CARTESIAN_POINT('Ctrl Pts',(4.2594866804815,-31.651052387174,55.2691925189657));
#111653=CARTESIAN_POINT('Ctrl Pts',(4.25046988720103,-31.6198129178493,
55.4179068699138));
#111654=CARTESIAN_POINT('Ctrl Pts',(4.23743998382687,-31.5487380940279,
55.616903896742));
#111655=CARTESIAN_POINT('Ctrl Pts',(4.23368794479393,-31.5255061695279,
55.6723016491408));
#111656=CARTESIAN_POINT('Ctrl Pts',(4.22880675416902,-31.4927428213331,
55.7399349819324));
#111657=CARTESIAN_POINT('Ctrl Pts',(4.22781494287351,-31.4859618934619,
55.7534600984559));
#111658=CARTESIAN_POINT('Ctrl Pts',(4.22631796239106,-31.4755633446396,
55.7735143760035));
#111659=CARTESIAN_POINT('Ctrl Pts',(4.22582091840187,-31.4720843017999,
55.7801150408666));
#111660=CARTESIAN_POINT('Ctrl Pts',(4.22491911749055,-31.4657276486024,
55.7919813548612));
#111661=CARTESIAN_POINT('Ctrl Pts',(4.2245153365082,-31.4628657704036,55.7972551292189));
#111662=CARTESIAN_POINT('Ctrl Pts',(4.22360115058551,-31.4563512872595,
55.8091066267131));
#111663=CARTESIAN_POINT('Ctrl Pts',(4.22308977112509,-31.4526826068413,
55.8156750845549));
#111664=CARTESIAN_POINT('Ctrl Pts',(4.22152029045961,-31.4413446078695,
55.83565568618));
#111665=CARTESIAN_POINT('Ctrl Pts',(4.22045392214018,-31.4335333431051,
55.848985757357));
#111666=CARTESIAN_POINT('Ctrl Pts',(4.21206353661835,-31.3711586920197,
55.9521137626122));
#111667=CARTESIAN_POINT('Ctrl Pts',(4.2043607910329,-31.3083999367107,56.0366691711607));
#111668=CARTESIAN_POINT('Ctrl Pts',(4.18875597665751,-31.1647656503903,
56.1961981873379));
#111669=CARTESIAN_POINT('Ctrl Pts',(4.18090317924967,-31.0835570647785,
56.2702288097924));
#111670=CARTESIAN_POINT('Ctrl Pts',(4.17196571236912,-30.9790234395173,
56.3481465552009));
#111671=CARTESIAN_POINT('Ctrl Pts',(4.17055605016112,-30.9621663993536,
56.3602286266402));
#111672=CARTESIAN_POINT('Ctrl Pts',(4.16834536007593,-30.9351525385659,
56.3788369258308));
#111673=CARTESIAN_POINT('Ctrl Pts',(4.16753644962788,-30.9251433248385,
56.3855725820712));
#111674=CARTESIAN_POINT('Ctrl Pts',(4.16601860007384,-30.9061300254342,
56.3980696023578));
#111675=CARTESIAN_POINT('Ctrl Pts',(4.16530881937272,-30.8971419947323,
56.4038541542522));
#111676=CARTESIAN_POINT('Ctrl Pts',(4.16370694898828,-30.8766410822502,
56.4167709075377));
#111677=CARTESIAN_POINT('Ctrl Pts',(4.16281684299518,-30.8650955627986,
56.4238500892831));
#111678=CARTESIAN_POINT('Ctrl Pts',(4.16050974938813,-30.8347804155901,
56.4419330692133));
#111679=CARTESIAN_POINT('Ctrl Pts',(4.15910085133093,-30.815878943252,56.4527115811984));
#111680=CARTESIAN_POINT('Ctrl Pts',(4.14831711560297,-30.6683914941956,
56.5330289548121));
#111681=CARTESIAN_POINT('Ctrl Pts',(4.1395835121069,-30.5313752272314,56.5857386897001));
#111682=CARTESIAN_POINT('Ctrl Pts',(4.1277278313492,-30.3441572616773,56.6307240559534));
#111683=CARTESIAN_POINT('Ctrl Pts',(4.12484548830372,-30.2986516729565,
56.6396681855563));
#111684=CARTESIAN_POINT('Ctrl Pts',(4.12015853858643,-30.2259539257416,
56.6508302438842));
#111685=CARTESIAN_POINT('Ctrl Pts',(4.11840145701979,-30.1989768295528,
56.6542985494061));
#111686=CARTESIAN_POINT('Ctrl Pts',(4.11599532056623,-30.1626246429899,
56.6580701810744));
#111687=CARTESIAN_POINT('Ctrl Pts',(4.11537559377679,-30.1533127533312,
56.6589571089811));
#111688=CARTESIAN_POINT('Ctrl Pts',(4.11433490021571,-30.1377711863339,
56.6603054288524));
#111689=CARTESIAN_POINT('Ctrl Pts',(4.1139163008067,-30.131545313265,56.6608102978583));
#111690=CARTESIAN_POINT('Ctrl Pts',(4.11305876459616,-30.1188465916916,
56.6617682117781));
#111691=CARTESIAN_POINT('Ctrl Pts',(4.11261969730611,-30.1123737091335,
56.6622184717697));
#111692=CARTESIAN_POINT('Ctrl Pts',(4.11146557317384,-30.0954304551078,
56.6632976440805));
#111693=CARTESIAN_POINT('Ctrl Pts',(4.11074730601297,-30.08495667814,56.6638654913282));
#111694=CARTESIAN_POINT('Ctrl Pts',(4.10764834969443,-30.0400404992496,
56.6658754799896));
#111695=CARTESIAN_POINT('Ctrl Pts',(4.10522278003539,-30.0055655661888,
56.6663472017879));
#111696=CARTESIAN_POINT('Ctrl Pts',(4.09512949626596,-29.8639607440026,
56.6638907429518));
#111697=CARTESIAN_POINT('Ctrl Pts',(4.08723575310939,-29.7572488287963,
56.6516994522656));
#111698=CARTESIAN_POINT('Ctrl Pts',(4.07545478092333,-29.5975221193336,
56.6176283697018));
#111699=CARTESIAN_POINT('Ctrl Pts',(4.0714518503984,-29.543220820414,56.6031418548263));
#111700=CARTESIAN_POINT('Ctrl Pts',(4.06492484580193,-29.4543116654028,
56.5745368063034));
#111701=CARTESIAN_POINT('Ctrl Pts',(4.06235864332962,-29.4192627504,56.5619495957426));
#111702=CARTESIAN_POINT('Ctrl Pts',(4.05880921038728,-29.3706808727808,
56.5426405296941));
#111703=CARTESIAN_POINT('Ctrl Pts',(4.05779406452489,-29.3567747521713,
56.5368941648966));
#111704=CARTESIAN_POINT('Ctrl Pts',(4.05605441962116,-29.3329310158615,
56.5266609943642));
#111705=CARTESIAN_POINT('Ctrl Pts',(4.05532694819434,-29.3229562883377,
56.5222636576955));
#111706=CARTESIAN_POINT('Ctrl Pts',(4.05393561719765,-29.3038755060226,
56.5136272847745));
#111707=CARTESIAN_POINT('Ctrl Pts',(4.05327128487744,-29.294763252735,56.5094031953438));
#111708=CARTESIAN_POINT('Ctrl Pts',(4.05152828726064,-29.2708566692665,
56.4980572668541));
#111709=CARTESIAN_POINT('Ctrl Pts',(4.05045438316149,-29.2561282163702,
56.4907985687313));
#111710=CARTESIAN_POINT('Ctrl Pts',(4.04654743223306,-29.2025869646305,
56.4634204772381));
#111711=CARTESIAN_POINT('Ctrl Pts',(4.04375994240473,-29.1644610870358,
56.4419924659824));
#111712=CARTESIAN_POINT('Ctrl Pts',(4.03383248155881,-29.0299387395775,
56.3592573039316));
#111713=CARTESIAN_POINT('Ctrl Pts',(4.02696968234985,-28.939069625645,56.2895838950884));
#111714=CARTESIAN_POINT('Ctrl Pts',(4.01698224638606,-28.8210110952625,
56.1780759261994));
#111715=CARTESIAN_POINT('Ctrl Pts',(4.01399126515501,-28.7874358938281,
56.1434882484943));
#111716=CARTESIAN_POINT('Ctrl Pts',(4.00914829142771,-28.7368695567408,
56.0866624481503));
#111717=CARTESIAN_POINT('Ctrl Pts',(4.00734777507053,-28.7188573426948,
56.0653671051593));
#111718=CARTESIAN_POINT('Ctrl Pts',(4.00489109669797,-28.6954762554006,
56.0362735644389));
#111719=CARTESIAN_POINT('Ctrl Pts',(4.00426585454349,-28.6896260048181,
56.0288659207905));
#111720=CARTESIAN_POINT('Ctrl Pts',(4.00321848191607,-28.6799990377026,
56.0164608660014));
#111721=CARTESIAN_POINT('Ctrl Pts',(4.00279878496326,-28.6761868804898,
56.0114910059185));
#111722=CARTESIAN_POINT('Ctrl Pts',(4.00194178692412,-28.6684971252078,
56.0013480365853));
#111723=CARTESIAN_POINT('Ctrl Pts',(4.00150437897295,-28.6646214671163,
55.996173662705));
#111724=CARTESIAN_POINT('Ctrl Pts',(4.00035939204268,-28.6546012462752,
55.9826321582129));
#111725=CARTESIAN_POINT('Ctrl Pts',(3.99964869153961,-28.6485047112594,
55.9742300732526));
#111726=CARTESIAN_POINT('Ctrl Pts',(3.99662843692014,-28.6230961752453,
55.9385152084614));
#111727=CARTESIAN_POINT('Ctrl Pts',(3.99427666864257,-28.6045318480446,
55.9106828325461));
#111728=CARTESIAN_POINT('Ctrl Pts',(3.98422447510363,-28.5297646077199,
55.7909298343998));
#111729=CARTESIAN_POINT('Ctrl Pts',(3.97628765621781,-28.4817092264681,
55.694229975399));
#111730=CARTESIAN_POINT('Ctrl Pts',(3.96805085260525,-28.4410366537565,
55.5875632574752));
#111731=CARTESIAN_POINT('Ctrl Pts',(3.96758778209095,-28.4387819867155,
55.5815458727116));
#111732=CARTESIAN_POINT('Ctrl Pts',(3.96712537028317,-28.4365623116664,
55.5755159378315));
#111733=CARTESIAN_POINT('Origin',(5.,-30.,55.));
#111734=CARTESIAN_POINT('',(3.26653910946692,-28.436562310676,55.575515935141));
#111735=CARTESIAN_POINT('',(3.46016010521239,-28.436562259669,55.5755157965761));
#111736=CARTESIAN_POINT('',(5.,-28.4365623102018,55.5755159338528));
#111737=CARTESIAN_POINT('',(4.12032058488633,-28.3340002417459,54.9991025049737));
#111738=CARTESIAN_POINT('Ctrl Pts',(3.46016010521239,-28.436562259669,55.5755157965761));
#111739=CARTESIAN_POINT('Ctrl Pts',(3.46533507067826,-28.4612024188361,
55.6424528902211));
#111740=CARTESIAN_POINT('Ctrl Pts',(3.47055209814345,-28.4901263132498,
55.7077667856819));
#111741=CARTESIAN_POINT('Ctrl Pts',(3.4816728450369,-28.561500676386,55.8444740038002));
#111742=CARTESIAN_POINT('Ctrl Pts',(3.48753193624495,-28.6052619862572,
55.9149460362316));
#111743=CARTESIAN_POINT('Ctrl Pts',(3.4945442331466,-28.6656515254426,55.9977248446239));
#111744=CARTESIAN_POINT('Ctrl Pts',(3.49587587405831,-28.6774907555878,
56.0133657151434));
#111745=CARTESIAN_POINT('Ctrl Pts',(3.49799327515109,-28.6969081840013,
56.0380980826434));
#111746=CARTESIAN_POINT('Ctrl Pts',(3.49878581952017,-28.7043115090283,
56.0473238548627));
#111747=CARTESIAN_POINT('Ctrl Pts',(3.50029048938778,-28.7186233711836,
56.0647747587509));
#111748=CARTESIAN_POINT('Ctrl Pts',(3.50100326721198,-28.7255143901523,
56.0730134161581));
#111749=CARTESIAN_POINT('Ctrl Pts',(3.50263620373059,-28.741555089818,56.0918185523204));
#111750=CARTESIAN_POINT('Ctrl Pts',(3.50355407445497,-28.7507591137388,
56.1023377753521));
#111751=CARTESIAN_POINT('Ctrl Pts',(3.50646359854809,-28.7805221397302,
56.1355021517643));
#111752=CARTESIAN_POINT('Ctrl Pts',(3.50843461858365,-28.8015734698569,
56.1576983321546));
#111753=CARTESIAN_POINT('Ctrl Pts',(3.51308990961696,-28.8532907294034,
56.2093047022373));
#111754=CARTESIAN_POINT('Ctrl Pts',(3.51575165480754,-28.8844940383775,
56.2381465353354));
#111755=CARTESIAN_POINT('Ctrl Pts',(3.52295598512166,-28.9727797848721,
56.3137007959192));
#111756=CARTESIAN_POINT('Ctrl Pts',(3.52743086962242,-29.0319135147452,
56.3578660005447));
#111757=CARTESIAN_POINT('Ctrl Pts',(3.53278088196181,-29.1052964903932,
56.4054358932715));
#111758=CARTESIAN_POINT('Ctrl Pts',(3.53362178043204,-29.1169064909165,
56.4127598057533));
#111759=CARTESIAN_POINT('Ctrl Pts',(3.53899018210172,-29.1914013093267,
56.458476102786));
#111760=CARTESIAN_POINT('Ctrl Pts',(3.54357009068761,-29.2566766513578,
56.4928000648305));
#111761=CARTESIAN_POINT('Ctrl Pts',(3.54918363924978,-29.3352220551691,
56.5276704678041));
#111762=CARTESIAN_POINT('Ctrl Pts',(3.5499920180097,-29.3464991429991,56.5325284278827));
#111763=CARTESIAN_POINT('Ctrl Pts',(3.55126921776027,-29.3642418616072,
56.5399402256163));
#111764=CARTESIAN_POINT('Ctrl Pts',(3.55173316131602,-29.3706717949457,
56.5425791114077));
#111765=CARTESIAN_POINT('Ctrl Pts',(3.55260580793278,-29.3827331852131,
56.5474412216904));
#111766=CARTESIAN_POINT('Ctrl Pts',(3.55301393648577,-29.3883604910852,
56.5496740824049));
#111767=CARTESIAN_POINT('Ctrl Pts',(3.55398031389767,-29.4016542852369,
56.5548652455937));
#111768=CARTESIAN_POINT('Ctrl Pts',(3.55454004827901,-29.4093306284353,
56.5577975519136));
#111769=CARTESIAN_POINT('Ctrl Pts',(3.55642513769437,-29.4351150229484,
56.5674290233935));
#111770=CARTESIAN_POINT('Ctrl Pts',(3.55776404703404,-29.4533170357476,
56.5738698922835));
#111771=CARTESIAN_POINT('Ctrl Pts',(3.56109729789562,-29.4984526808686,
56.5889639546728));
#111772=CARTESIAN_POINT('Ctrl Pts',(3.56310623189366,-29.5255021717906,
56.5972500721407));
#111773=CARTESIAN_POINT('Ctrl Pts',(3.57231570895063,-29.6493106982567,
56.6317541477482));
#111774=CARTESIAN_POINT('Ctrl Pts',(3.57968871738581,-29.7481045565724,
56.6498950674548));
#111775=CARTESIAN_POINT('Ctrl Pts',(3.59286273765847,-29.9300606427894,
56.666573260525));
#111776=CARTESIAN_POINT('Ctrl Pts',(3.59869576996069,-30.0126457335807,
56.6679933202466));
#111777=CARTESIAN_POINT('Ctrl Pts',(3.60568291042129,-30.1145793844572,
56.6621708288185));
#111778=CARTESIAN_POINT('Ctrl Pts',(3.60701381194024,-30.1341304728216,
56.660707491624));
#111779=CARTESIAN_POINT('Ctrl Pts',(3.6091303264183,-30.1654276195149,56.6578086618428));
#111780=CARTESIAN_POINT('Ctrl Pts',(3.60992271348219,-30.1771916203264,
56.6565925868325));
#111781=CARTESIAN_POINT('Ctrl Pts',(3.6114272615719,-30.1996134157015,56.6540332065644));
#111782=CARTESIAN_POINT('Ctrl Pts',(3.61214007307276,-30.2102730664417,
56.6527118959124));
#111783=CARTESIAN_POINT('Ctrl Pts',(3.61377333599463,-30.2347769944241,
56.6494336096584));
#111784=CARTESIAN_POINT('Ctrl Pts',(3.61469149623948,-30.2486110288411,
56.6474052463979));
#111785=CARTESIAN_POINT('Ctrl Pts',(3.61760298378825,-30.2926462580163,
56.6403814030073));
#111786=CARTESIAN_POINT('Ctrl Pts',(3.61957563716275,-30.3227370362852,
56.634727492153));
#111787=CARTESIAN_POINT('Ctrl Pts',(3.62423561685806,-30.3942162897078,
56.6192460450048));
#111788=CARTESIAN_POINT('Ctrl Pts',(3.62690035273671,-30.435418097124,56.6086564886076));
#111789=CARTESIAN_POINT('Ctrl Pts',(3.6341062637875,-30.5468017408791,56.5754352462528));
#111790=CARTESIAN_POINT('Ctrl Pts',(3.63857993307601,-30.6159574009169,
56.5497048762593));
#111791=CARTESIAN_POINT('Ctrl Pts',(3.64394271292471,-30.6959079561773,
56.5137578416862));
#111792=CARTESIAN_POINT('Ctrl Pts',(3.64479751632439,-30.7085613637542,
56.5078764785417));
#111793=CARTESIAN_POINT('Ctrl Pts',(3.6501623613977,-30.7872918596637,56.4700723375306));
#111794=CARTESIAN_POINT('Ctrl Pts',(3.65472492856013,-30.8512653739252,
56.4339754843858));
#111795=CARTESIAN_POINT('Ctrl Pts',(3.66031922293849,-30.9229147782607,
56.3870598614524));
#111796=CARTESIAN_POINT('Ctrl Pts',(3.66112753103553,-30.933111520811,56.3802208573828));
#111797=CARTESIAN_POINT('Ctrl Pts',(3.66240464314722,-30.9489603845603,
56.3693350554648));
#111798=CARTESIAN_POINT('Ctrl Pts',(3.66286857080968,-30.9546645855542,
56.3653643580756));
#111799=CARTESIAN_POINT('Ctrl Pts',(3.66374120540813,-30.9652909567697,
56.3578681911965));
#111800=CARTESIAN_POINT('Ctrl Pts',(3.66414933803981,-30.9702189693318,
56.3543514325137));
#111801=CARTESIAN_POINT('Ctrl Pts',(3.66511574942603,-30.9817907538313,
56.3459979380169));
#111802=CARTESIAN_POINT('Ctrl Pts',(3.6656755140195,-30.9884180268185,56.3411388185554));
#111803=CARTESIAN_POINT('Ctrl Pts',(3.66756081403966,-31.0104967772053,
56.3246981333178));
#111804=CARTESIAN_POINT('Ctrl Pts',(3.66889990773721,-31.0257821586928,
56.3128974691884));
#111805=CARTESIAN_POINT('Ctrl Pts',(3.67223372046557,-31.0629492180813,
56.2831583764351));
#111806=CARTESIAN_POINT('Ctrl Pts',(3.67424303785215,-31.0845852220542,
56.2649233868526));
#111807=CARTESIAN_POINT('Ctrl Pts',(3.68345592262898,-31.1807565686212,
56.1795875781764));
#111808=CARTESIAN_POINT('Ctrl Pts',(3.6908320486152,-31.2496045598371,56.1063913594428));
#111809=CARTESIAN_POINT('Ctrl Pts',(3.70400536495773,-31.3622862393517,
55.9625623488482));
#111810=CARTESIAN_POINT('Ctrl Pts',(3.70983489406662,-31.4082404947078,
55.8939868349359));
#111811=CARTESIAN_POINT('Ctrl Pts',(3.71681864975773,-31.4586091730715,
55.8052325889746));
#111812=CARTESIAN_POINT('Ctrl Pts',(3.7181494496141,-31.4679828039877,55.7880144581521));
#111813=CARTESIAN_POINT('Ctrl Pts',(3.72026584218626,-31.4825209316052,
55.7601496803738));
#111814=CARTESIAN_POINT('Ctrl Pts',(3.72105820762084,-31.4878794624363,
55.7496069416447));
#111815=CARTESIAN_POINT('Ctrl Pts',(3.72256273897859,-31.4978898526126,
55.7293814881765));
#111816=CARTESIAN_POINT('Ctrl Pts',(3.7232755551223,-31.5025611900257,55.7197091393741));
#111817=CARTESIAN_POINT('Ctrl Pts',(3.72490886298606,-31.5130972652106,
55.6973436407032));
#111818=CARTESIAN_POINT('Ctrl Pts',(3.72582706308861,-31.5188964588693,
55.6846203723183));
#111819=CARTESIAN_POINT('Ctrl Pts',(3.72873882102058,-31.5368801186652,
55.6438110745932));
#111820=CARTESIAN_POINT('Ctrl Pts',(3.73071169932679,-31.5484513546906,
55.6154606320993));
#111821=CARTESIAN_POINT('Ctrl Pts',(3.7353723248432,-31.5742155165618,55.5470012129056));
#111822=CARTESIAN_POINT('Ctrl Pts',(3.73803747269969,-31.5876666826755,
55.5066356725296));
#111823=CARTESIAN_POINT('Ctrl Pts',(3.74524358970001,-31.6201652502446,
55.3950348188002));
#111824=CARTESIAN_POINT('Ctrl Pts',(3.74971708030216,-31.6360535934458,
55.3229813453965));
#111825=CARTESIAN_POINT('Ctrl Pts',(3.75508132925589,-31.6492173559422,
55.2362912268376));
#111826=CARTESIAN_POINT('Ctrl Pts',(3.7559377695857,-31.651142025191,55.2224442348912));
#111827=CARTESIAN_POINT('Ctrl Pts',(3.76130212598135,-31.6620749542148,
55.1358040696191));
#111828=CARTESIAN_POINT('Ctrl Pts',(3.76586258171806,-31.6664408270576,
55.0625151886453));
#111829=CARTESIAN_POINT('Ctrl Pts',(3.77145453224788,-31.6658852283461,
54.9769099621336));
#111830=CARTESIAN_POINT('Ctrl Pts',(3.77226283165594,-31.6656698286316,
54.9646341393723));
#111831=CARTESIAN_POINT('Ctrl Pts',(3.77353993299118,-31.6651200478486,
54.9454149157525));
#111832=CARTESIAN_POINT('Ctrl Pts',(3.77400385869929,-31.6648778456966,
54.938469034597));
#111833=CARTESIAN_POINT('Ctrl Pts',(3.77487649182004,-31.6643433506988,
54.9254757291173));
#111834=CARTESIAN_POINT('Ctrl Pts',(3.77528462495342,-31.6640615444062,
54.9194281208315));
#111835=CARTESIAN_POINT('Ctrl Pts',(3.77625104051829,-31.6633195249161,
54.9051754653926));
#111836=CARTESIAN_POINT('Ctrl Pts',(3.77681080882754,-31.6628315570884,
54.8969721396775));
#111837=CARTESIAN_POINT('Ctrl Pts',(3.77869613475052,-31.6609937109529,
54.8695056104935));
#111838=CARTESIAN_POINT('Ctrl Pts',(3.78003525112307,-31.6593696638124,
54.8502631212124));
#111839=CARTESIAN_POINT('Ctrl Pts',(3.78336913296018,-31.6545424981376,
54.8029070838807));
#111840=CARTESIAN_POINT('Ctrl Pts',(3.7853784975037,-31.6509569595678,54.7748390961061));
#111841=CARTESIAN_POINT('Ctrl Pts',(3.79459180154555,-31.6314213865786,
54.6477526221542));
#111842=CARTESIAN_POINT('Ctrl Pts',(3.80196831110846,-31.6072648526433,
54.5502065840207));
#111843=CARTESIAN_POINT('Ctrl Pts',(3.81514154092422,-31.5475406464638,
54.377531484538));
#111844=CARTESIAN_POINT('Ctrl Pts',(3.82097063911164,-31.5148531962473,
54.301736026339));
#111845=CARTESIAN_POINT('Ctrl Pts',(3.82795397840051,-31.4676077985264,
54.2112873877401));
#111846=CARTESIAN_POINT('Ctrl Pts',(3.82928476571399,-31.4582260962093,
54.1940738592707));
#111847=CARTESIAN_POINT('Ctrl Pts',(3.83140114324562,-31.4427007411339,
54.1667470853075));
#111848=CARTESIAN_POINT('Ctrl Pts',(3.83219350601165,-31.4367496184512,
54.1565271820183));
#111849=CARTESIAN_POINT('Ctrl Pts',(3.8336980353053,-31.4251866204119,54.1371474847553));
#111850=CARTESIAN_POINT('Ctrl Pts',(3.83441085202203,-31.4195940172651,
54.1279769490283));
#111851=CARTESIAN_POINT('Ctrl Pts',(3.83604416543163,-31.4065181254434,
54.1069948196298));
#111852=CARTESIAN_POINT('Ctrl Pts',(3.83696237045255,-31.398973982648,54.0952219581659));
#111853=CARTESIAN_POINT('Ctrl Pts',(3.83987416175062,-31.3744417056323,
54.0579791808063));
#111854=CARTESIAN_POINT('Ctrl Pts',(3.84184706781425,-31.3568988139562,
54.0328810707788));
#111855=CARTESIAN_POINT('Ctrl Pts',(3.84650777302961,-31.3133557949168,
53.9741045631673));
#111856=CARTESIAN_POINT('Ctrl Pts',(3.84917297172773,-31.2867377822684,
53.9409102249999));
#111857=CARTESIAN_POINT('Ctrl Pts',(3.85637911395052,-31.2106025379552,
53.8530782982882));
#111858=CARTESIAN_POINT('Ctrl Pts',(3.86085258231618,-31.1586846644668,
53.8006509653216));
#111859=CARTESIAN_POINT('Ctrl Pts',(3.86621700799498,-31.0929898031349,
53.7425721447289));
#111860=CARTESIAN_POINT('Ctrl Pts',(3.86707364594395,-31.0823977313833,
53.7334429874551));
#111861=CARTESIAN_POINT('Ctrl Pts',(3.87243794205832,-31.015537602767,53.6772684931629));
#111862=CARTESIAN_POINT('Ctrl Pts',(3.87699814160988,-30.956335654659,53.6338540861278));
#111863=CARTESIAN_POINT('Ctrl Pts',(3.88258980776084,-30.8841173114052,
53.587894011364));
#111864=CARTESIAN_POINT('Ctrl Pts',(3.8833981061131,-30.8736870466041,53.581417021706));
#111865=CARTESIAN_POINT('Ctrl Pts',(3.88467520613897,-30.8572419752615,
53.5714551106219));
#111866=CARTESIAN_POINT('Ctrl Pts',(3.88513913160962,-30.8512750792828,
53.5678914007186));
#111867=CARTESIAN_POINT('Ctrl Pts',(3.88601176455082,-30.8400689488414,
53.5612933526364));
#111868=CARTESIAN_POINT('Ctrl Pts',(3.88641989774516,-30.8348352473261,
53.5582501045202));
#111869=CARTESIAN_POINT('Ctrl Pts',(3.88738631381759,-30.822458519497,53.5511433755737));
#111870=CARTESIAN_POINT('Ctrl Pts',(3.88794608257821,-30.8153018862798,
53.5471041463385));
#111871=CARTESIAN_POINT('Ctrl Pts',(3.88983141164857,-30.7912292369109,
53.5337513206564));
#111872=CARTESIAN_POINT('Ctrl Pts',(3.89117053077613,-30.7741819237347,
53.5246793011302));
#111873=CARTESIAN_POINT('Ctrl Pts',(3.89450442100987,-30.7317778661351,
53.5030505503537));
#111874=CARTESIAN_POINT('Ctrl Pts',(3.89651379128293,-30.7062519868691,
53.4908398194811));
#111875=CARTESIAN_POINT('Ctrl Pts',(3.90572714626701,-30.5888850592815,
53.4383251082537));
#111876=CARTESIAN_POINT('Ctrl Pts',(3.91310370243606,-30.4938301291272,
53.4057144697383));
#111877=CARTESIAN_POINT('Ctrl Pts',(3.92627692173973,-30.3163660216553,
53.3622388672596));
#111878=CARTESIAN_POINT('Ctrl Pts',(3.93210596757001,-30.2349591536741,
53.3485924605103));
#111879=CARTESIAN_POINT('Ctrl Pts',(3.93908925626508,-30.1333458377287,
53.3392293590827));
#111880=CARTESIAN_POINT('Ctrl Pts',(3.94042004205404,-30.1137957260913,
53.3377753389391));
#111881=CARTESIAN_POINT('Ctrl Pts',(3.9425364177577,-30.0824169444836,53.335997807855));
#111882=CARTESIAN_POINT('Ctrl Pts',(3.94332878019931,-30.0706030880016,
53.3354546973279));
#111883=CARTESIAN_POINT('Ctrl Pts',(3.94483330924203,-30.048050008775,53.3346584246025));
#111884=CARTESIAN_POINT('Ctrl Pts',(3.9455461260284,-30.0373122139648,53.3343832451624));
#111885=CARTESIAN_POINT('Ctrl Pts',(3.94717944011199,-30.0125923084443,
53.3339889185848));
#111886=CARTESIAN_POINT('Ctrl Pts',(3.94809764573079,-29.9986097332567,
53.3339419048151));
#111887=CARTESIAN_POINT('Ctrl Pts',(3.95100944108458,-29.9540149647219,
53.3343533970871));
#111888=CARTESIAN_POINT('Ctrl Pts',(3.95298235052212,-29.923414261244,53.3354796359063));
#111889=CARTESIAN_POINT('Ctrl Pts',(3.95764306542494,-29.8504172318816,
53.340183776567));
#111890=CARTESIAN_POINT('Ctrl Pts',(3.96030827030289,-29.808092467181,53.3445433320651));
#111891=CARTESIAN_POINT('Ctrl Pts',(3.96751441558857,-29.6930079632713,
53.3608710307328));
#111892=CARTESIAN_POINT('Ctrl Pts',(3.97198788124859,-29.6208031332967,
53.3760548073667));
#111893=CARTESIAN_POINT('Ctrl Pts',(3.98145087481888,-29.471874998016,53.4178503811606));
#111894=CARTESIAN_POINT('Ctrl Pts',(3.98643588803758,-29.3956171781785,
53.4453837472909));
#111895=CARTESIAN_POINT('Ctrl Pts',(3.99272796473029,-29.3069340813158,
53.4849171505347));
#111896=CARTESIAN_POINT('Ctrl Pts',(3.99378385082902,-29.2922919792224,
53.4917010512792));
#111897=CARTESIAN_POINT('Ctrl Pts',(3.99536579942446,-29.27075368414,53.5020627143139));
#111898=CARTESIAN_POINT('Ctrl Pts',(3.99588254882001,-29.2637797692355,
53.5054779804612));
#111899=CARTESIAN_POINT('Ctrl Pts',(3.99680463588934,-29.2514503874433,
53.5116231628943));
#111900=CARTESIAN_POINT('Ctrl Pts',(3.99720877349272,-29.2460854477374,
53.5143334905181));
#111901=CARTESIAN_POINT('Ctrl Pts',(3.99810471271478,-29.2342783552774,
53.5203787706192));
#111902=CARTESIAN_POINT('Ctrl Pts',(3.99859728165862,-29.2278433465843,
53.5237267470937));
#111903=CARTESIAN_POINT('Ctrl Pts',(4.00005306909992,-29.2089834454017,
53.533696132518));
#111904=CARTESIAN_POINT('Ctrl Pts',(4.00102296014675,-29.1966207411293,
53.5404329562588));
#111905=CARTESIAN_POINT('Ctrl Pts',(4.00784050609912,-29.1110213806209,
53.5884956873026));
#111906=CARTESIAN_POINT('Ctrl Pts',(4.01394266999757,-29.0409270220139,
53.6351543874145));
#111907=CARTESIAN_POINT('Ctrl Pts',(4.0293952595558,-28.8735844489236,53.7658241952184));
#111908=CARTESIAN_POINT('Ctrl Pts',(4.03868615453698,-28.7819389527459,
53.85617264269));
#111909=CARTESIAN_POINT('Ctrl Pts',(4.04895765924964,-28.6883939578906,
53.9725336430833));
#111910=CARTESIAN_POINT('Ctrl Pts',(4.05039121667119,-28.6755389650117,
53.9891584887335));
#111911=CARTESIAN_POINT('Ctrl Pts',(4.05271392806205,-28.6550495416177,
54.0167188082507));
#111912=CARTESIAN_POINT('Ctrl Pts',(4.05361034633035,-28.64722612561,54.0275101541731));
#111913=CARTESIAN_POINT('Ctrl Pts',(4.05521556900639,-28.6333727921665,
54.0471096729604));
#111914=CARTESIAN_POINT('Ctrl Pts',(4.05592612315437,-28.6272965001879,
54.0558840054014));
#111915=CARTESIAN_POINT('Ctrl Pts',(4.05744287378617,-28.6144492577345,
54.0748220359052));
#111916=CARTESIAN_POINT('Ctrl Pts',(4.05824804070232,-28.6077048660541,
54.0850030612331));
#111917=CARTESIAN_POINT('Ctrl Pts',(4.06045475455164,-28.5894362048065,
54.113250355165));
#111918=CARTESIAN_POINT('Ctrl Pts',(4.06184759497065,-28.5781473441289,
54.1314666120708));
#111919=CARTESIAN_POINT('Ctrl Pts',(4.06493627537763,-28.5536938984248,
54.1726810988376));
#111920=CARTESIAN_POINT('Ctrl Pts',(4.06662544909748,-28.5407200937467,
54.1957859911961));
#111921=CARTESIAN_POINT('Ctrl Pts',(4.07209536195944,-28.500141370793,54.2722703133314));
#111922=CARTESIAN_POINT('Ctrl Pts',(4.07580684446593,-28.4748711253273,
54.3268364918782));
#111923=CARTESIAN_POINT('Ctrl Pts',(4.0836312306726,-28.4275588387586,54.4454257478977));
#111924=CARTESIAN_POINT('Ctrl Pts',(4.0877288233016,-28.4063581487556,54.5096642743236));
#111925=CARTESIAN_POINT('Ctrl Pts',(4.09533197393208,-28.3749100600871,
54.6288655045144));
#111926=CARTESIAN_POINT('Ctrl Pts',(4.09881090675606,-28.3634129653081,
54.6833932601575));
#111927=CARTESIAN_POINT('Ctrl Pts',(4.10355711618487,-28.3518829483987,
54.7559080583615));
#111928=CARTESIAN_POINT('Ctrl Pts',(4.10471576887663,-28.3493774464063,
54.7734700553919));
#111929=CARTESIAN_POINT('Ctrl Pts',(4.10640909984927,-28.346166758398,54.7988695730129));
#111930=CARTESIAN_POINT('Ctrl Pts',(4.10693206266747,-28.3452358361631,
54.8066780002246));
#111931=CARTESIAN_POINT('Ctrl Pts',(4.1078614480346,-28.3436888460894,54.8204847663319));
#111932=CARTESIAN_POINT('Ctrl Pts',(4.10826660606492,-28.3430500097013,
54.826480301797));
#111933=CARTESIAN_POINT('Ctrl Pts',(4.10905777157065,-28.3418715261223,
54.8381409699613));
#111934=CARTESIAN_POINT('Ctrl Pts',(4.10944352491412,-28.341328355765,54.8438053916598));
#111935=CARTESIAN_POINT('Ctrl Pts',(4.1103115111552,-28.3401760698506,54.856506425341));
#111936=CARTESIAN_POINT('Ctrl Pts',(4.11079456179747,-28.3395826655597,
54.8635443068639));
#111937=CARTESIAN_POINT('Ctrl Pts',(4.11238834707366,-28.3377806470898,
54.8866722676899));
#111938=CARTESIAN_POINT('Ctrl Pts',(4.1135081812535,-28.3367610745716,54.9027756044905));
#111939=CARTESIAN_POINT('Ctrl Pts',(4.11650947216456,-28.3346732105405,
54.9456097457554));
#111940=CARTESIAN_POINT('Ctrl Pts',(4.11840674262356,-28.3340146510312,
54.9723548740222));
#111941=CARTESIAN_POINT('Ctrl Pts',(4.12032058488633,-28.3340002417459,
54.9991025049737));
#111942=CARTESIAN_POINT('Ctrl Pts',(4.1203204113275,-28.3340002430544,54.9991000793355));
#111943=CARTESIAN_POINT('Ctrl Pts',(4.12609722619094,-28.3339566319437,
55.0798361960743));
#111944=CARTESIAN_POINT('Ctrl Pts',(4.13201002271519,-28.3397818578504,
55.1604689461328));
#111945=CARTESIAN_POINT('Ctrl Pts',(4.14421232624134,-28.3640341023962,
55.3268078040519));
#111946=CARTESIAN_POINT('Ctrl Pts',(4.15047178471177,-28.3834192393927,
55.4121386308245));
#111947=CARTESIAN_POINT('Ctrl Pts',(4.15848277482955,-28.4177846659238,
55.5224394374832));
#111948=CARTESIAN_POINT('Ctrl Pts',(4.16041355774539,-28.4268376910685,
55.5490981838307));
#111949=CARTESIAN_POINT('Ctrl Pts',(4.16232238521864,-28.4365623101738,
55.5755159337767));
#111950=CARTESIAN_POINT('Ctrl Pts',(3.96712537028317,-28.4365623116664,
55.5755159378315));
#111951=CARTESIAN_POINT('Ctrl Pts',(3.9635169617427,-28.419241183033,55.5284616278987));
#111952=CARTESIAN_POINT('Ctrl Pts',(3.95994984272749,-28.4040508085702,
55.4806430184928));
#111953=CARTESIAN_POINT('Ctrl Pts',(3.95382913432262,-28.3813333530033,
55.3960732284496));
#111954=CARTESIAN_POINT('Ctrl Pts',(3.95124985306976,-28.3728467099228,
55.3596224024264));
#111955=CARTESIAN_POINT('Ctrl Pts',(3.94768579525725,-28.3626726004268,
55.3081268934566));
#111956=CARTESIAN_POINT('Ctrl Pts',(3.94666874832452,-28.3599517911125,
55.2933003483287));
#111957=CARTESIAN_POINT('Ctrl Pts',(3.94492688194108,-28.3556098970241,
55.267686597003));
#111958=CARTESIAN_POINT('Ctrl Pts',(3.94419906991847,-28.3538928762381,
55.256916857802));
#111959=CARTESIAN_POINT('Ctrl Pts',(3.94271781014448,-28.350598719155,55.2348641821718));
#111960=CARTESIAN_POINT('Ctrl Pts',(3.94196470550827,-28.3490313136447,
55.2235803589091));
#111961=CARTESIAN_POINT('Ctrl Pts',(3.94005978507564,-28.3453421666476,
55.194863619123));
#111962=CARTESIAN_POINT('Ctrl Pts',(3.93891301636762,-28.3433800574488,
55.1774113292266));
#111963=CARTESIAN_POINT('Ctrl Pts',(3.93428743136639,-28.3365316744345,
55.1064011240595));
#111964=CARTESIAN_POINT('Ctrl Pts',(3.93088053675959,-28.3339636933345,
55.0526495474743));
#111965=CARTESIAN_POINT('Ctrl Pts',(3.92156616836595,-28.3340655770633,
54.903309587721));
#111966=CARTESIAN_POINT('Ctrl Pts',(3.91579736750292,-28.3423511625915,
54.8079391988554));
#111967=CARTESIAN_POINT('Ctrl Pts',(3.90524395331732,-28.3718971366683,
54.6385037980415));
#111968=CARTESIAN_POINT('Ctrl Pts',(3.90050169416086,-28.3901927356272,
54.5642064794781));
#111969=CARTESIAN_POINT('Ctrl Pts',(3.89470760145473,-28.417270374608,54.4797366842595));
#111970=CARTESIAN_POINT('Ctrl Pts',(3.89389867128788,-28.4211504787493,
54.4680778701374));
#111971=CARTESIAN_POINT('Ctrl Pts',(3.89262087655178,-28.4274268422726,
54.4498927552401));
#111972=CARTESIAN_POINT('Ctrl Pts',(3.8921568987256,-28.4297356891334,54.4433364510008));
#111973=CARTESIAN_POINT('Ctrl Pts',(3.89128439993776,-28.4341312707437,
54.4310995290871));
#111974=CARTESIAN_POINT('Ctrl Pts',(3.89087645551415,-28.4362080159269,
54.4254155858815));
#111975=CARTESIAN_POINT('Ctrl Pts',(3.88991082123848,-28.4411748994157,
54.412047877239));
#111976=CARTESIAN_POINT('Ctrl Pts',(3.88935165077797,-28.4440909153328,
54.4043740216686));
#111977=CARTESIAN_POINT('Ctrl Pts',(3.88746986060579,-28.4540406526268,
54.3787617555055));
#111978=CARTESIAN_POINT('Ctrl Pts',(3.88613374530733,-28.4613285520364,
54.3609246082099));
#111979=CARTESIAN_POINT('Ctrl Pts',(3.88280884321164,-28.4800448998022,
54.3172933998151));
#111980=CARTESIAN_POINT('Ctrl Pts',(3.88080554814264,-28.4918221445719,
54.2916560260077));
#111981=CARTESIAN_POINT('Ctrl Pts',(3.87164500573624,-28.5481262188826,
54.1768668966667));
#111982=CARTESIAN_POINT('Ctrl Pts',(3.86431660325594,-28.5999461676628,
54.0915203632211));
#111983=CARTESIAN_POINT('Ctrl Pts',(3.85113159288279,-28.7084397443199,
53.9443744512792));
#111984=CARTESIAN_POINT('Ctrl Pts',(3.84524752264212,-28.7627459035744,
53.8812152726242));
#111985=CARTESIAN_POINT('Ctrl Pts',(3.83821140374396,-28.8354202650434,
53.8084904525874));
#111986=CARTESIAN_POINT('Ctrl Pts',(3.83687933048297,-28.8495337534513,
53.79485750498));
#111987=CARTESIAN_POINT('Ctrl Pts',(3.83476157476816,-28.8725358396175,
53.7734110506687));
#111988=CARTESIAN_POINT('Ctrl Pts',(3.83396910060841,-28.8812721895702,
53.7654377365938));
#111989=CARTESIAN_POINT('Ctrl Pts',(3.83246477495646,-28.8980994235554,
53.7504055132469));
#111990=CARTESIAN_POINT('Ctrl Pts',(3.83175226931959,-28.9061750462882,
53.7433304962984));
#111991=CARTESIAN_POINT('Ctrl Pts',(3.83012026231281,-28.9249122106184,
53.7272324229452));
#111992=CARTESIAN_POINT('Ctrl Pts',(3.82920304345483,-28.9356200482597,
53.7182643025602));
#111993=CARTESIAN_POINT('Ctrl Pts',(3.82629692619005,-28.9700984734691,
53.6901177101134));
#111994=CARTESIAN_POINT('Ctrl Pts',(3.82432859635999,-28.9942849835688,
53.6714570911085));
#111995=CARTESIAN_POINT('Ctrl Pts',(3.81968081595669,-29.0532376064061,
53.6285065378173));
#111996=CARTESIAN_POINT('Ctrl Pts',(3.817023792213,-29.0884450596126,53.6048579588468));
#111997=CARTESIAN_POINT('Ctrl Pts',(3.80982204312389,-29.1872660040813,
53.5438204829187));
#111998=CARTESIAN_POINT('Ctrl Pts',(3.80534532601377,-29.2525193868902,
53.5092725138221));
#111999=CARTESIAN_POINT('Ctrl Pts',(3.80002284717559,-29.331943104722,53.4737524598691));
#112000=CARTESIAN_POINT('Ctrl Pts',(3.79921119577326,-29.3441028520772,
53.46848751379));
#112001=CARTESIAN_POINT('Ctrl Pts',(3.79383685374464,-29.4248266442524,
53.4346733190953));
#112002=CARTESIAN_POINT('Ctrl Pts',(3.78922201898326,-29.4951630752107,
53.4105948032067));
#112003=CARTESIAN_POINT('Ctrl Pts',(3.78356981673008,-29.5787171797105,
53.3880981564084));
#112004=CARTESIAN_POINT('Ctrl Pts',(3.7827614546676,-29.5906082037673,53.3850371200989));
#112005=CARTESIAN_POINT('Ctrl Pts',(3.7814843644999,-29.6092799571756,53.3804500199643));
#112006=CARTESIAN_POINT('Ctrl Pts',(3.78102051442992,-29.6160385264455,
53.3788344093982));
#112007=CARTESIAN_POINT('Ctrl Pts',(3.78014811242765,-29.6287018309195,
53.3758909217718));
#112008=CARTESIAN_POINT('Ctrl Pts',(3.77974013539755,-29.6346039490077,
53.3745528770239));
#112009=CARTESIAN_POINT('Ctrl Pts',(3.77877422882975,-29.6485324508578,
53.3714748967726));
#112010=CARTESIAN_POINT('Ctrl Pts',(3.77821481614667,-29.6565645540976,
53.3697621224577));
#112011=CARTESIAN_POINT('Ctrl Pts',(3.77633133886228,-29.6835028210192,
53.3642256881099));
#112012=CARTESIAN_POINT('Ctrl Pts',(3.77499374696187,-29.7024618906122,
53.3606711562403));
#112013=CARTESIAN_POINT('Ctrl Pts',(3.77166434712926,-29.7493317837924,
53.3527235741344));
#112014=CARTESIAN_POINT('Ctrl Pts',(3.76965798395742,-29.7773003318921,
53.3487099420319));
#112015=CARTESIAN_POINT('Ctrl Pts',(3.76047031364741,-29.9046493373813,
53.3337287394431));
#112016=CARTESIAN_POINT('Ctrl Pts',(3.75311710831985,-30.004792066411,53.3310095464614));
#112017=CARTESIAN_POINT('Ctrl Pts',(3.73993780162785,-30.1872003055034,
53.3424819979876));
#112018=CARTESIAN_POINT('Ctrl Pts',(3.73408173161187,-30.2693328883665,
53.3538306889441));
#112019=CARTESIAN_POINT('Ctrl Pts',(3.72707260638483,-30.3694633944301,
53.3753654786031));
#112020=CARTESIAN_POINT('Ctrl Pts',(3.72574129900404,-30.3885608084496,
53.3798268354637));
#112021=CARTESIAN_POINT('Ctrl Pts',(3.72362446165702,-30.4190413072739,
53.3875173765517));
#112022=CARTESIAN_POINT('Ctrl Pts',(3.72283215043316,-30.4304760036318,
53.3905323082146));
#112023=CARTESIAN_POINT('Ctrl Pts',(3.72132795111338,-30.4522299477943,
53.3965164956323));
#112024=CARTESIAN_POINT('Ctrl Pts',(3.7206154107873,-30.462554435464,53.3994642528518));
#112025=CARTESIAN_POINT('Ctrl Pts',(3.71898306666611,-30.4862464468943,
53.4064769899088));
#112026=CARTESIAN_POINT('Ctrl Pts',(3.71806554869362,-30.4995928942776,
53.4106107618042));
#112027=CARTESIAN_POINT('Ctrl Pts',(3.71515740431842,-30.5419696072504,
53.4243225733271));
#112028=CARTESIAN_POINT('Ctrl Pts',(3.71318738833584,-30.5707899371035,
53.4345321965595));
#112029=CARTESIAN_POINT('Ctrl Pts',(3.70853477023838,-30.6389193463788,
53.4607989853292));
#112030=CARTESIAN_POINT('Ctrl Pts',(3.70587466147067,-30.6779279677004,
53.4775770153992));
#112031=CARTESIAN_POINT('Ctrl Pts',(3.69867103140397,-30.7828292599355,
53.5275288119121));
#112032=CARTESIAN_POINT('Ctrl Pts',(3.6941953284477,-30.847226636022,53.5636154952525));
#112033=CARTESIAN_POINT('Ctrl Pts',(3.68885253381612,-30.9204158627209,
53.6112683830241));
#112034=CARTESIAN_POINT('Ctrl Pts',(3.68801962789674,-30.9317187329648,
53.6188262015581));
#112035=CARTESIAN_POINT('Ctrl Pts',(3.68264894870969,-31.0038112018581,
53.6683195040345));
#112036=CARTESIAN_POINT('Ctrl Pts',(3.67805883917794,-31.0618406433122,
53.7141144866898));
#112037=CARTESIAN_POINT('Ctrl Pts',(3.67243410827982,-31.1257451785403,
53.7718287890793));
#112038=CARTESIAN_POINT('Ctrl Pts',(3.67162584508035,-31.1347649953463,
53.7801577503949));
#112039=CARTESIAN_POINT('Ctrl Pts',(3.67034887752532,-31.1487443118484,
53.793355565662));
#112040=CARTESIAN_POINT('Ctrl Pts',(3.6698850496902,-31.1537670046734,53.7981572567605));
#112041=CARTESIAN_POINT('Ctrl Pts',(3.66901266451562,-31.1631078723631,
53.807199636773));
#112042=CARTESIAN_POINT('Ctrl Pts',(3.66860468179352,-31.167433166583,53.8114326160646));
#112043=CARTESIAN_POINT('Ctrl Pts',(3.66763872775876,-31.1775738989273,
53.8214656676801));
#112044=CARTESIAN_POINT('Ctrl Pts',(3.66707927285857,-31.1833696140813,
53.8272852822221));
#112045=CARTESIAN_POINT('Ctrl Pts',(3.66519550140865,-31.2026342775704,
53.8469176098963));
#112046=CARTESIAN_POINT('Ctrl Pts',(3.6638576520264,-31.2159057288332,53.8609208178176));
#112047=CARTESIAN_POINT('Ctrl Pts',(3.66052746770596,-31.2480104546234,
53.8959961518953));
#112048=CARTESIAN_POINT('Ctrl Pts',(3.65852056932849,-31.2665560840594,
53.9173227178944));
#112049=CARTESIAN_POINT('Ctrl Pts',(3.64932815603016,-31.3482512745239,
54.0162410139549));
#112050=CARTESIAN_POINT('Ctrl Pts',(3.6419706130645,-31.4048763560687,54.0989527719164));
#112051=CARTESIAN_POINT('Ctrl Pts',(3.6287922962335,-31.4941451099922,54.2584278528237));
#112052=CARTESIAN_POINT('Ctrl Pts',(3.62294111344197,-31.5291230919963,
54.3335278367503));
#112053=CARTESIAN_POINT('Ctrl Pts',(3.61593670414302,-31.5653130633097,
54.4292676070656));
#112054=CARTESIAN_POINT('Ctrl Pts',(3.61460553384762,-31.5719218770181,
54.4477300297358));
#112055=CARTESIAN_POINT('Ctrl Pts',(3.61248886088143,-31.5819913839723,
54.4775068620174));
#112056=CARTESIAN_POINT('Ctrl Pts',(3.61169657882252,-31.5856600152315,
54.4887484505886));
#112057=CARTESIAN_POINT('Ctrl Pts',(3.61019240209761,-31.5924308501639,
54.5102702130772));
#112058=CARTESIAN_POINT('Ctrl Pts',(3.60947985554459,-31.5955539471479,
54.5205431325975));
#112059=CARTESIAN_POINT('Ctrl Pts',(3.60784745099199,-31.6025121410359,
54.5442522056277));
#112060=CARTESIAN_POINT('Ctrl Pts',(3.60692987940837,-31.6062779933274,
54.5577079674059));
#112061=CARTESIAN_POINT('Ctrl Pts',(3.60402137159618,-31.617742986394,54.6007527929264));
#112062=CARTESIAN_POINT('Ctrl Pts',(3.60205105329454,-31.6247974077053,
54.6305080864498));
#112063=CARTESIAN_POINT('Ctrl Pts',(3.59739756763203,-31.6396824175065,
54.7020066362002));
#112064=CARTESIAN_POINT('Ctrl Pts',(3.59473690555963,-31.6467439858054,
54.7438885023124));
#112065=CARTESIAN_POINT('Ctrl Pts',(3.58753295657385,-31.661669401561,54.859119212564));
#112066=CARTESIAN_POINT('Ctrl Pts',(3.58305745313266,-31.666276078668,54.9327914153874));
#112067=CARTESIAN_POINT('Ctrl Pts',(3.57771154800517,-31.6659337407174,
55.0201766843736));
#112068=CARTESIAN_POINT('Ctrl Pts',(3.57687534593039,-31.665712507855,55.03382547379));
#112069=CARTESIAN_POINT('Ctrl Pts',(3.57150532411575,-31.6632212291599,
55.1212237108034));
#112070=CARTESIAN_POINT('Ctrl Pts',(3.56691913931639,-31.6562218217219,
55.1947474301107));
#112071=CARTESIAN_POINT('Ctrl Pts',(3.56129876762668,-31.6424037056981,
55.279672651212));
#112072=CARTESIAN_POINT('Ctrl Pts',(3.56049052019865,-31.640298242381,55.2917676791794));
#112073=CARTESIAN_POINT('Ctrl Pts',(3.55921357220381,-31.6367921102805,
55.310670036992));
#112074=CARTESIAN_POINT('Ctrl Pts',(3.55874974791583,-31.6354821369628,
55.3174940305964));
#112075=CARTESIAN_POINT('Ctrl Pts',(3.55787736542533,-31.6329513959881,
55.3302459201189));
#112076=CARTESIAN_POINT('Ctrl Pts',(3.55746938179472,-31.631740965999,55.3361756157435));
#112077=CARTESIAN_POINT('Ctrl Pts',(3.55650342018544,-31.6288117052746,
55.3501369592597));
#112078=CARTESIAN_POINT('Ctrl Pts',(3.55594395854869,-31.6270657579701,
55.3581626357571));
#112079=CARTESIAN_POINT('Ctrl Pts',(3.55406014015536,-31.621020085398,55.3849962455256));
#112080=CARTESIAN_POINT('Ctrl Pts',(3.55272224968321,-31.6164531836484,
55.4037415660234));
#112081=CARTESIAN_POINT('Ctrl Pts',(3.54939194016605,-31.6043968064112,
55.4497394190887));
#112082=CARTESIAN_POINT('Ctrl Pts',(3.54738495637288,-31.5965375188805,
55.4768882762972));
#112083=CARTESIAN_POINT('Ctrl Pts',(3.53819178582436,-31.5577368996198,
55.5991834801321));
#112084=CARTESIAN_POINT('Ctrl Pts',(3.53083355029357,-31.5189538622006,
55.6916246799748));
#112085=CARTESIAN_POINT('Ctrl Pts',(3.51765539129601,-31.433385450734,55.8531138554362));
#112086=CARTESIAN_POINT('Ctrl Pts',(3.51180498855318,-31.3892664238125,
55.9232224102179));
#112087=CARTESIAN_POINT('Ctrl Pts',(3.5048013320846,-31.3284658300934,56.0055441195572));
#112088=CARTESIAN_POINT('Ctrl Pts',(3.50347018376456,-31.316539307935,56.021109565988));
#112089=CARTESIAN_POINT('Ctrl Pts',(3.50135353714934,-31.2969840591638,
56.0457189712757));
#112090=CARTESIAN_POINT('Ctrl Pts',(3.50056125976577,-31.2895292830279,
56.0548981265043));
#112091=CARTESIAN_POINT('Ctrl Pts',(3.49905708666253,-31.2751201958198,
56.0722591866397));
#112092=CARTESIAN_POINT('Ctrl Pts',(3.49834453911081,-31.2681833098963,
56.0804547092898));
#112093=CARTESIAN_POINT('Ctrl Pts',(3.49671212486831,-31.2520380524084,
56.099159648696));
#112094=CARTESIAN_POINT('Ctrl Pts',(3.49579454468861,-31.2427756490096,
56.1096215228316));
#112095=CARTESIAN_POINT('Ctrl Pts',(3.49288597859922,-31.2128293854217,
56.1426003813374));
#112096=CARTESIAN_POINT('Ctrl Pts',(3.49091561182028,-31.191656167289,56.1646658389564));
#112097=CARTESIAN_POINT('Ctrl Pts',(3.48626198703707,-31.139658511577,56.215951099881));
#112098=CARTESIAN_POINT('Ctrl Pts',(3.48360123623655,-31.1083004862128,
56.2445999403378));
#112099=CARTESIAN_POINT('Ctrl Pts',(3.47639723661924,-31.0195840607264,
56.3196366414693));
#112100=CARTESIAN_POINT('Ctrl Pts',(3.47192176566036,-30.9601875487601,
56.3634635166959));
#112101=CARTESIAN_POINT('Ctrl Pts',(3.46657537581815,-30.8865788856192,
56.4105745055347));
#112102=CARTESIAN_POINT('Ctrl Pts',(3.46573865877656,-30.8749847526216,
56.4177955540933));
#112103=CARTESIAN_POINT('Ctrl Pts',(3.46036874236968,-30.8002074105462,
56.4631017066652));
#112104=CARTESIAN_POINT('Ctrl Pts',(3.45578317346601,-30.7346496825615,
56.4970923778875));
#112105=CARTESIAN_POINT('Ctrl Pts',(3.45016348581876,-30.6558154538616,
56.5315393608582));
#112106=CARTESIAN_POINT('Ctrl Pts',(3.44935524086905,-30.6445120013537,
56.5363303621741));
#112107=CARTESIAN_POINT('Ctrl Pts',(3.44807829594802,-30.6267297502404,
56.5436366490223));
#112108=CARTESIAN_POINT('Ctrl Pts',(3.4476144722174,-30.6202861413578,56.5462371689067));
#112109=CARTESIAN_POINT('Ctrl Pts',(3.44674209014855,-30.6082001465491,
56.5510271471433));
#112110=CARTESIAN_POINT('Ctrl Pts',(3.4463341063751,-30.6025618553427,56.5532262665976));
#112111=CARTESIAN_POINT('Ctrl Pts',(3.44536814357594,-30.5892435805364,
56.5583374039422));
#112112=CARTESIAN_POINT('Ctrl Pts',(3.44480868088069,-30.5815539066334,
56.5612234011634));
#112113=CARTESIAN_POINT('Ctrl Pts',(3.44292485511082,-30.5557307660925,
56.5706977893494));
#112114=CARTESIAN_POINT('Ctrl Pts',(3.44158695818191,-30.5375049952772,
56.5770277520163));
#112115=CARTESIAN_POINT('Ctrl Pts',(3.4382566289914,-30.492320984845,56.5918463229098));
#112116=CARTESIAN_POINT('Ctrl Pts',(3.43624963177599,-30.4652492729126,
56.5999680002081));
#112117=CARTESIAN_POINT('Ctrl Pts',(3.42705634222611,-30.3414580852053,
56.6336987965965));
#112118=CARTESIAN_POINT('Ctrl Pts',(3.41969799785833,-30.2427582081686,
56.6512523358386));
#112119=CARTESIAN_POINT('Ctrl Pts',(3.40651986365603,-30.0606750507911,
56.6669479183889));
#112120=CARTESIAN_POINT('Ctrl Pts',(3.40066958348873,-29.9778469003161,
56.6679058063101));
#112121=CARTESIAN_POINT('Ctrl Pts',(3.39366604532178,-29.8757105066716,
56.6614730085073));
#112122=CARTESIAN_POINT('Ctrl Pts',(3.39233490045728,-29.8561648296538,
56.659895158409));
#112123=CARTESIAN_POINT('Ctrl Pts',(3.39021825798574,-29.8248833920187,
56.656813203101));
#112124=CARTESIAN_POINT('Ctrl Pts',(3.38942598133736,-29.8131283916478,
56.6555285653924));
#112125=CARTESIAN_POINT('Ctrl Pts',(3.38792180880369,-29.7907276453987,
56.6528388786504));
#112126=CARTESIAN_POINT('Ctrl Pts',(3.38720926109497,-29.7800799094665,
56.6514558547426));
#112127=CARTESIAN_POINT('Ctrl Pts',(3.38557684532886,-29.7556084439227,
56.6480364030898));
#112128=CARTESIAN_POINT('Ctrl Pts',(3.38465926379753,-29.741795352084,56.6459287949629));
#112129=CARTESIAN_POINT('Ctrl Pts',(3.38175068854431,-29.6978464588485,
56.638656155075));
#112130=CARTESIAN_POINT('Ctrl Pts',(3.37978031414253,-29.6678245957053,
56.6328350944521));
#112131=CARTESIAN_POINT('Ctrl Pts',(3.37512666748297,-29.5965356135099,
56.6169647828039));
#112132=CARTESIAN_POINT('Ctrl Pts',(3.37246590273011,-29.5554587893254,
56.6061575610529));
#112133=CARTESIAN_POINT('Ctrl Pts',(3.36526189516412,-29.4443004641779,
56.5723201126431));
#112134=CARTESIAN_POINT('Ctrl Pts',(3.36078642932549,-29.3752651540996,
56.5461886207057));
#112135=CARTESIAN_POINT('Ctrl Pts',(3.35132895099948,-29.2346291878216,
56.4819925197743));
#112136=CARTESIAN_POINT('Ctrl Pts',(3.34635159749342,-29.1636211361858,
56.4431083058159));
#112137=CARTESIAN_POINT('Ctrl Pts',(3.34004643120265,-29.0818813094028,
56.3902826238861));
#112138=CARTESIAN_POINT('Ctrl Pts',(3.33896798008594,-29.0681714683268,
56.3811311457641));
#112139=CARTESIAN_POINT('Ctrl Pts',(3.33736589551659,-29.0482443730791,
56.367397825104));
#112140=CARTESIAN_POINT('Ctrl Pts',(3.33685214541117,-29.0419191201869,
56.3629734433732));
#112141=CARTESIAN_POINT('Ctrl Pts',(3.3359333402193,-29.0307270834271,56.3550284468596));
#112142=CARTESIAN_POINT('Ctrl Pts',(3.33552945234985,-29.0258482634933,
56.3515252385991));
#112143=CARTESIAN_POINT('Ctrl Pts',(3.33463150824678,-29.0150926534159,
56.3437137392996));
#112144=CARTESIAN_POINT('Ctrl Pts',(3.33413665804466,-29.0092252062333,
56.3393932945706));
#112145=CARTESIAN_POINT('Ctrl Pts',(3.33266692581943,-28.9919691647904,
56.3265115272862));
#112146=CARTESIAN_POINT('Ctrl Pts',(3.33168518247879,-28.9806621729188,
56.3178426906261));
#112147=CARTESIAN_POINT('Ctrl Pts',(3.32938715348942,-28.9546698786251,
56.2973803029542));
#112148=CARTESIAN_POINT('Ctrl Pts',(3.32806509178823,-28.9400707968081,
56.2854807401345));
#112149=CARTESIAN_POINT('Ctrl Pts',(3.32335736482795,-28.8892261061332,
56.2425827361353));
#112150=CARTESIAN_POINT('Ctrl Pts',(3.31991666830189,-28.8541145153204,
56.2102794680983));
#112151=CARTESIAN_POINT('Ctrl Pts',(3.30829271145983,-28.7410322505317,
56.0969046396222));
#112152=CARTESIAN_POINT('Ctrl Pts',(3.300066135971,-28.66987902042,56.0094469981921));
#112153=CARTESIAN_POINT('Ctrl Pts',(3.28892499432238,-28.5830020896006,
55.8773569025731));
#112154=CARTESIAN_POINT('Ctrl Pts',(3.28575955836855,-28.5595023575564,
55.8382156284401));
#112155=CARTESIAN_POINT('Ctrl Pts',(3.28151599604221,-28.5296509133886,
55.7835224758517));
#112156=CARTESIAN_POINT('Ctrl Pts',(3.28038843228126,-28.521884153901,55.7687701134053));
#112157=CARTESIAN_POINT('Ctrl Pts',(3.27859100767267,-28.5097744564672,
55.7449064462911));
#112158=CARTESIAN_POINT('Ctrl Pts',(3.27791625165747,-28.5052907656171,
55.7358682604314));
#112159=CARTESIAN_POINT('Ctrl Pts',(3.27652062666157,-28.496148559462,55.7170111165739));
#112160=CARTESIAN_POINT('Ctrl Pts',(3.27580024899632,-28.4915034508356,
55.7071861616145));
#112161=CARTESIAN_POINT('Ctrl Pts',(3.27410331088587,-28.4807395036109,
55.683830418164));
#112162=CARTESIAN_POINT('Ctrl Pts',(3.27312966679654,-28.4747047114319,
55.6702617420705));
#112163=CARTESIAN_POINT('Ctrl Pts',(3.27026543266706,-28.4573823375009,
55.6298679555056));
#112164=CARTESIAN_POINT('Ctrl Pts',(3.26839229184022,-28.4466154441205,
55.6028261219895));
#112165=CARTESIAN_POINT('Ctrl Pts',(3.26653910946692,-28.436562310676,55.575515935141));
#112166=CARTESIAN_POINT('Origin',(5.,-30.,55.));
#112167=CARTESIAN_POINT('',(2.56903904312142,-28.4365623153847,55.5755159479327));
#112168=CARTESIAN_POINT('',(2.75980443758381,-28.4365622822719,55.5755158579788));
#112169=CARTESIAN_POINT('',(5.,-28.4365623102018,55.5755159338528));
#112170=CARTESIAN_POINT('Ctrl Pts',(2.75980443758381,-28.4365622822719,
55.5755158579788));
#112171=CARTESIAN_POINT('Ctrl Pts',(2.76084862674717,-28.4423847804517,
55.5913331689));
#112172=CARTESIAN_POINT('Ctrl Pts',(2.76189838302494,-28.4484491493631,
55.6070671061794));
#112173=CARTESIAN_POINT('Ctrl Pts',(2.76472966975531,-28.4653300576938,
55.6489567060463));
#112174=CARTESIAN_POINT('Ctrl Pts',(2.76652343433635,-28.4765725895492,
55.6749262053549));
#112175=CARTESIAN_POINT('Ctrl Pts',(2.76959232887108,-28.4965912984897,
55.7181164371627));
#112176=CARTESIAN_POINT('Ctrl Pts',(2.77085111394464,-28.5050159636729,
55.7354941156935));
#112177=CARTESIAN_POINT('Ctrl Pts',(2.77267007075862,-28.5174533808426,
55.7600520112067));
#112178=CARTESIAN_POINT('Ctrl Pts',(2.77321617963206,-28.5212205412668,
55.7673557474457));
#112179=CARTESIAN_POINT('Ctrl Pts',(2.77417042327773,-28.5278565440596,
55.7799912180931));
#112180=CARTESIAN_POINT('Ctrl Pts',(2.77457702756173,-28.5307006638238,
55.7853356699778));
#112181=CARTESIAN_POINT('Ctrl Pts',(2.7754544672218,-28.5368723641967,55.7967821690365));
#112182=CARTESIAN_POINT('Ctrl Pts',(2.77592582828356,-28.5402089645767,
55.8028788401981));
#112183=CARTESIAN_POINT('Ctrl Pts',(2.77723612513202,-28.5495449665656,
55.8196870909652));
#112184=CARTESIAN_POINT('Ctrl Pts',(2.77807980798882,-28.5556246380549,
55.8303532518169));
#112185=CARTESIAN_POINT('Ctrl Pts',(2.78399612441273,-28.5987665067569,
55.9041336780491));
#112186=CARTESIAN_POINT('Ctrl Pts',(2.78927092568923,-28.6398312245519,
55.9648064774068));
#112187=CARTESIAN_POINT('Ctrl Pts',(2.79561403829376,-28.6934222218326,
56.0337361065216));
#112188=CARTESIAN_POINT('Ctrl Pts',(2.79664245169486,-28.7022404609474,
56.0447851469678));
#112189=CARTESIAN_POINT('Ctrl Pts',(2.80303532269296,-28.7579000780151,
56.1127332544735));
#112190=CARTESIAN_POINT('Ctrl Pts',(2.80839967758463,-28.8083365515119,
56.1665877798951));
#112191=CARTESIAN_POINT('Ctrl Pts',(2.8166948171388,-28.8932415220021,56.2459736713992));
#112192=CARTESIAN_POINT('Ctrl Pts',(2.81969336519339,-28.9254095838873,
56.2738212822276));
#112193=CARTESIAN_POINT('Ctrl Pts',(2.82477033726503,-28.9825059802322,
56.3195450319847));
#112194=CARTESIAN_POINT('Ctrl Pts',(2.82687028547511,-29.0069255550884,
56.3380196307692));
#112195=CARTESIAN_POINT('Ctrl Pts',(2.82989136153209,-29.0432202700187,
56.3639369611078));
#112196=CARTESIAN_POINT('Ctrl Pts',(2.83083295848849,-29.0547008075624,
56.3719187086164));
#112197=CARTESIAN_POINT('Ctrl Pts',(2.83248817738217,-29.0751761748341,
56.3857749666196));
#112198=CARTESIAN_POINT('Ctrl Pts',(2.8332040067372,-29.0841297540399,56.3917086863124));
#112199=CARTESIAN_POINT('Ctrl Pts',(2.83470118034477,-29.1030605825925,
56.4039927105872));
#112200=CARTESIAN_POINT('Ctrl Pts',(2.83548179739137,-29.1130493569947,
56.4103242247415));
#112201=CARTESIAN_POINT('Ctrl Pts',(2.83754610966426,-29.1397721154538,
56.4268665791687));
#112202=CARTESIAN_POINT('Ctrl Pts',(2.83882292401875,-29.156620646126,56.4368895455709));
#112203=CARTESIAN_POINT('Ctrl Pts',(2.84541462351944,-29.2451874203696,
56.4874820591694));
#112204=CARTESIAN_POINT('Ctrl Pts',(2.85054703465835,-29.3196698669227,
56.522989919062));
#112205=CARTESIAN_POINT('Ctrl Pts',(2.86177072510637,-29.4899883195561,
56.5891847440522));
#112206=CARTESIAN_POINT('Ctrl Pts',(2.86780258761651,-29.5865793393545,
56.6170037339531));
#112207=CARTESIAN_POINT('Ctrl Pts',(2.87586481445836,-29.7128649715601,
56.6413135413438));
#112208=CARTESIAN_POINT('Ctrl Pts',(2.87765860862119,-29.7407810978298,
56.6459532331609));
#112209=CARTESIAN_POINT('Ctrl Pts',(2.88072754865766,-29.7879252352958,
56.6525596039357));
#112210=CARTESIAN_POINT('Ctrl Pts',(2.88198634902052,-29.8070944534942,
56.6549067413306));
#112211=CARTESIAN_POINT('Ctrl Pts',(2.88380532410374,-29.8344724979168,
56.65777688017));
#112212=CARTESIAN_POINT('Ctrl Pts',(2.88435143557233,-29.8426518971075,
56.658573213905));
#112213=CARTESIAN_POINT('Ctrl Pts',(2.8853056821432,-29.8568666806896,56.6598510499845));
#112214=CARTESIAN_POINT('Ctrl Pts',(2.88571228672807,-29.8628993408856,
56.6603602209035));
#112215=CARTESIAN_POINT('Ctrl Pts',(2.88658972512328,-29.8758633342632,
56.6613832765049));
#112216=CARTESIAN_POINT('Ctrl Pts',(2.88706108460031,-29.8827950427904,
56.6618866678659));
#112217=CARTESIAN_POINT('Ctrl Pts',(2.88837137285151,-29.9019797746057,
56.6631592719984));
#112218=CARTESIAN_POINT('Ctrl Pts',(2.88921504859943,-29.9142381750231,
56.6638364150015));
#112219=CARTESIAN_POINT('Ctrl Pts',(2.89512948429612,-29.9995957990739,
56.6676057352042));
#112220=CARTESIAN_POINT('Ctrl Pts',(2.90040226330886,-30.072814599904,56.666014619831));
#112221=CARTESIAN_POINT('Ctrl Pts',(2.90674476459987,-30.1597836940589,
56.6583803967387));
#112222=CARTESIAN_POINT('Ctrl Pts',(2.90777456706569,-30.1738682384566,
56.6569629449716));
#112223=CARTESIAN_POINT('Ctrl Pts',(2.91416864688873,-30.2611588673225,
56.6470528813881));
#112224=CARTESIAN_POINT('Ctrl Pts',(2.91953283646889,-30.3337571152297,
56.6338894229793));
#112225=CARTESIAN_POINT('Ctrl Pts',(2.92782827166228,-30.4465059785372,
56.6056144106314));
#112226=CARTESIAN_POINT('Ctrl Pts',(2.93082725500764,-30.4873546511607,
56.593691052775));
#112227=CARTESIAN_POINT('Ctrl Pts',(2.93590487360403,-30.5567449880516,
56.5705185069125));
#112228=CARTESIAN_POINT('Ctrl Pts',(2.93800504049296,-30.5855135870241,
56.5600216073858));
#112229=CARTESIAN_POINT('Ctrl Pts',(2.94102636787263,-30.6269762568795,
56.5435842296558));
#112230=CARTESIAN_POINT('Ctrl Pts',(2.94196800228605,-30.6399092148182,
56.5382677654497));
#112231=CARTESIAN_POINT('Ctrl Pts',(2.94362326341745,-30.6626561433115,
56.5285804535323));
#112232=CARTESIAN_POINT('Ctrl Pts',(2.94433909793452,-30.6724974899078,
56.5242763865341));
#112233=CARTESIAN_POINT('Ctrl Pts',(2.945836259308,-30.6930850663282,56.5150343013674));
#112234=CARTESIAN_POINT('Ctrl Pts',(2.94661685918045,-30.7038217632145,
56.5100764156993));
#112235=CARTESIAN_POINT('Ctrl Pts',(2.94868107213386,-30.7322118146042,
56.4965981614257));
#112236=CARTESIAN_POINT('Ctrl Pts',(2.94995780555345,-30.7497694714839,
56.4878796962328));
#112237=CARTESIAN_POINT('Ctrl Pts',(2.95654978905709,-30.8403138118442,
56.4409089163907));
#112238=CARTESIAN_POINT('Ctrl Pts',(2.96168253516177,-30.9105467642476,
56.3975882351707));
#112239=CARTESIAN_POINT('Ctrl Pts',(2.97290639597626,-31.0585363428373,
56.2903954326488));
#112240=CARTESIAN_POINT('Ctrl Pts',(2.97893811419045,-31.1342936735202,
56.2243345446972));
#112241=CARTESIAN_POINT('Ctrl Pts',(2.98700016752665,-31.2232081506081,
56.1314232046287));
#112242=CARTESIAN_POINT('Ctrl Pts',(2.98879394240773,-31.2422466352296,
56.110486273842));
#112243=CARTESIAN_POINT('Ctrl Pts',(2.99186285278546,-31.2733658988316,
56.0744618336756));
#112244=CARTESIAN_POINT('Ctrl Pts',(2.9931216431824,-31.2857344224755,56.059630058646));
#112245=CARTESIAN_POINT('Ctrl Pts',(2.99494060635712,-31.3029945020249,
56.0381853715191));
#112246=CARTESIAN_POINT('Ctrl Pts',(2.99548671613375,-31.30809973222,56.0317454247556));
#112247=CARTESIAN_POINT('Ctrl Pts',(2.99644096079728,-31.3168828671844,
56.0204960408095));
#112248=CARTESIAN_POINT('Ctrl Pts',(2.99684756518578,-31.3205825397465,
56.0157038985675));
#112249=CARTESIAN_POINT('Ctrl Pts',(2.99772500440536,-31.3284732640311,
56.0053671419888));
#112250=CARTESIAN_POINT('Ctrl Pts',(2.9981963649154,-31.3326557032567,55.9998165209716));
#112251=CARTESIAN_POINT('Ctrl Pts',(2.99950665876987,-31.3441300297743,
55.9843887409465));
#112252=CARTESIAN_POINT('Ctrl Pts',(3.00035033915101,-31.3513474805704,
55.9744571282957));
#112253=CARTESIAN_POINT('Ctrl Pts',(3.00626600008934,-31.4008193853317,
55.904774380765));
#112254=CARTESIAN_POINT('Ctrl Pts',(3.01154009654297,-31.4392021283956,
55.8423814402288));
#112255=CARTESIAN_POINT('Ctrl Pts',(3.01788299767828,-31.4799571554667,
55.7651685012765));
#112256=CARTESIAN_POINT('Ctrl Pts',(3.01891189680001,-31.4863993190228,
55.7525776225502));
#112257=CARTESIAN_POINT('Ctrl Pts',(3.02530519155831,-31.5254111935584,
55.6738754167684));
#112258=CARTESIAN_POINT('Ctrl Pts',(3.03066948964701,-31.553726557103,55.6057412675533));
#112259=CARTESIAN_POINT('Ctrl Pts',(3.03896473157217,-31.5911203218191,
55.4956823727837));
#112260=CARTESIAN_POINT('Ctrl Pts',(3.04196342995015,-31.6032563661161,
55.4549004515107));
#112261=CARTESIAN_POINT('Ctrl Pts',(3.04704062529491,-31.6214210699778,
55.3840402991145));
#112262=CARTESIAN_POINT('Ctrl Pts',(3.04914064902566,-31.6282046634651,
55.354179368634));
#112263=CARTESIAN_POINT('Ctrl Pts',(3.05216181187759,-31.6368822271656,
55.310432062136));
#112264=CARTESIAN_POINT('Ctrl Pts',(3.05310342177044,-31.6394299215402,
55.2966834067954));
#112265=CARTESIAN_POINT('Ctrl Pts',(3.05475865525201,-31.6436282107965,
55.2723190608297));
#112266=CARTESIAN_POINT('Ctrl Pts',(3.05547448639007,-31.6453497509308,
55.2617165883497));
#112267=CARTESIAN_POINT('Ctrl Pts',(3.05697165577289,-31.6487510314567,
55.2394073598353));
#112268=CARTESIAN_POINT('Ctrl Pts',(3.05775226688843,-31.6504089053787,
55.2276978367452));
#112269=CARTESIAN_POINT('Ctrl Pts',(3.0598165448598,-31.6544830698815,55.1965349901438));
#112270=CARTESIAN_POINT('Ctrl Pts',(3.06109333126192,-31.6566810024698,
55.1770546230399));
#112271=CARTESIAN_POINT('Ctrl Pts',(3.06768711141143,-31.666329154324,55.0754812808575));
#112272=CARTESIAN_POINT('Ctrl Pts',(3.07282146880245,-31.6680237074741,
54.9929526851745));
#112273=CARTESIAN_POINT('Ctrl Pts',(3.08404543505332,-31.6582209977923,
54.8104796978346));
#112274=CARTESIAN_POINT('Ctrl Pts',(3.090075794086,-31.6438088121805,54.7110275696209));
#112275=CARTESIAN_POINT('Ctrl Pts',(3.09813621308581,-31.6139789957503,
54.5859610155698));
#112276=CARTESIAN_POINT('Ctrl Pts',(3.09992980631561,-31.6067153458938,
54.5586134391347));
#112277=CARTESIAN_POINT('Ctrl Pts',(3.10299843727901,-31.5933286944746,
54.5129347490476));
#112278=CARTESIAN_POINT('Ctrl Pts',(3.10425713378501,-31.5875765118503,
54.4945006148859));
#112279=CARTESIAN_POINT('Ctrl Pts',(3.10607598476422,-31.578921655433,54.4683704862345));
#112280=CARTESIAN_POINT('Ctrl Pts',(3.10662207859731,-31.5762801411878,
54.460588799343));
#112281=CARTESIAN_POINT('Ctrl Pts',(3.10757630528491,-31.5715927824681,
54.4471087078719));
#112282=CARTESIAN_POINT('Ctrl Pts',(3.10798290782014,-31.5695732711773,
54.4414013964579));
#112283=CARTESIAN_POINT('Ctrl Pts',(3.10886035480113,-31.5651685128829,
54.4291656705731));
#112284=CARTESIAN_POINT('Ctrl Pts',(3.10933172504006,-31.5627735463399,
54.4226412347365));
#112285=CARTESIAN_POINT('Ctrl Pts',(3.11064207167359,-31.5560349762906,
54.4046329719528));
#112286=CARTESIAN_POINT('Ctrl Pts',(3.11148579569767,-31.5516052410342,
54.3931821530273));
#112287=CARTESIAN_POINT('Ctrl Pts',(3.11741308369604,-31.519831068272,54.3136694242717));
#112288=CARTESIAN_POINT('Ctrl Pts',(3.12269968353565,-31.4881469966343,
54.2474362038162));
#112289=CARTESIAN_POINT('Ctrl Pts',(3.12897795831892,-31.4457954860863,
54.1721095617963));
#112290=CARTESIAN_POINT('Ctrl Pts',(3.12992968542177,-31.4392495773928,
54.1607814253002));
#112291=CARTESIAN_POINT('Ctrl Pts',(3.13636420917426,-31.394116640355,54.0847572765692));
#112292=CARTESIAN_POINT('Ctrl Pts',(3.14184842700386,-31.3513108831972,
54.0226613941766));
#112293=CARTESIAN_POINT('Ctrl Pts',(3.15022708427755,-31.2782492633003,
53.9306971672022));
#112294=CARTESIAN_POINT('Ctrl Pts',(3.15319539232901,-31.2508087987226,
53.898724572899));
#112295=CARTESIAN_POINT('Ctrl Pts',(3.15822740938044,-31.2015272498147,
53.8455251350235));
#112296=CARTESIAN_POINT('Ctrl Pts',(3.16031212852798,-31.1802630076731,
53.8237944958652));
#112297=CARTESIAN_POINT('Ctrl Pts',(3.16331569393269,-31.148393479347,53.7929611251073));
#112298=CARTESIAN_POINT('Ctrl Pts',(3.16425467538618,-31.1382505965271,
53.7833915876739));
#112299=CARTESIAN_POINT('Ctrl Pts',(3.16590694772803,-31.1200875666372,
53.7666812634142));
#112300=CARTESIAN_POINT('Ctrl Pts',(3.16662241940188,-31.1121164071001,
53.7594886662014));
#112301=CARTESIAN_POINT('Ctrl Pts',(3.16812046145024,-31.0952057819338,
53.7445237572471));
#112302=CARTESIAN_POINT('Ctrl Pts',(3.16890228902653,-31.0862518020579,
53.7367686927485));
#112303=CARTESIAN_POINT('Ctrl Pts',(3.17097360174201,-31.0621939122129,
53.716377055268));
#112304=CARTESIAN_POINT('Ctrl Pts',(3.172256120478,-31.0469470934892,53.7039114196437));
#112305=CARTESIAN_POINT('Ctrl Pts',(3.17908433607625,-30.963964087262,53.6384855088989));
#112306=CARTESIAN_POINT('Ctrl Pts',(3.18442954900959,-30.8924222062561,
53.590555502987));
#112307=CARTESIAN_POINT('Ctrl Pts',(3.19567077599505,-30.7327633334874,
53.5006436441105));
#112308=CARTESIAN_POINT('Ctrl Pts',(3.20152533741797,-30.6440259628007,
53.4604416593067));
#112309=CARTESIAN_POINT('Ctrl Pts',(3.20937399290479,-30.5259733183579,
53.4189603130667));
#112310=CARTESIAN_POINT('Ctrl Pts',(3.21114360969615,-30.4994240480951,
53.4103742990245));
#112311=CARTESIAN_POINT('Ctrl Pts',(3.21417532913787,-30.4543438232803,
53.3970361604525));
#112312=CARTESIAN_POINT('Ctrl Pts',(3.21542159763641,-30.4359233300001,
53.3919290577827));
#112313=CARTESIAN_POINT('Ctrl Pts',(3.21722559179305,-30.4094958711268,
53.3850894360244));
#112314=CARTESIAN_POINT('Ctrl Pts',(3.2177695676107,-30.4015569161318,53.3830970856943));
#112315=CARTESIAN_POINT('Ctrl Pts',(3.21872141050845,-30.3877248162805,
53.3797339500482));
#112316=CARTESIAN_POINT('Ctrl Pts',(3.21912777105963,-30.3818383667019,
53.3783366360069));
#112317=CARTESIAN_POINT('Ctrl Pts',(3.22000626805444,-30.3691550877092,
53.3753987913549));
#112318=CARTESIAN_POINT('Ctrl Pts',(3.22047894557644,-30.3623562672298,
53.3738688561274));
#112319=CARTESIAN_POINT('Ctrl Pts',(3.22179639049477,-30.3434714283287,
53.3697435213393));
#112320=CARTESIAN_POINT('Ctrl Pts',(3.22264598555996,-30.3313661035989,
53.3672399774821));
#112321=CARTESIAN_POINT('Ctrl Pts',(3.22915571341237,-30.2390844380402,
53.3492233565304));
#112322=CARTESIAN_POINT('Ctrl Pts',(3.23506652234412,-30.1579008249054,
53.3394912537596));
#112323=CARTESIAN_POINT('Ctrl Pts',(3.24534818864056,-30.0167183015033,
53.3330150359672));
#112324=CARTESIAN_POINT('Ctrl Pts',(3.24969974366852,-29.9569894683763,
53.3334860006485));
#112325=CARTESIAN_POINT('Ctrl Pts',(3.25789042500893,-29.8434997288736,
53.3404875977497));
#112326=CARTESIAN_POINT('Ctrl Pts',(3.26173451339523,-29.7897757528789,
53.3464340184039));
#112327=CARTESIAN_POINT('Ctrl Pts',(3.26803762893499,-29.7006328938803,
53.3607166948735));
#112328=CARTESIAN_POINT('Ctrl Pts',(3.27053506647565,-29.6650291418784,
53.3676197457849));
#112329=CARTESIAN_POINT('Ctrl Pts',(3.27400762581134,-29.6151476306214,
53.3789920683604));
#112330=CARTESIAN_POINT('Ctrl Pts',(3.27501282437738,-29.6006634406929,
53.3824993359752));
#112331=CARTESIAN_POINT('Ctrl Pts',(3.2767410473374,-29.5756899766321,53.3889024391067));
#112332=CARTESIAN_POINT('Ctrl Pts',(3.27746693728155,-29.565178621745,53.3917075125066));
#112333=CARTESIAN_POINT('Ctrl Pts',(3.27895011610086,-29.5436604818607,
53.3976762562637));
#112334=CARTESIAN_POINT('Ctrl Pts',(3.27970700707528,-29.5326573117655,
53.4008508642494));
#112335=CARTESIAN_POINT('Ctrl Pts',(3.28163342629008,-29.5046036094821,
53.4092591366056));
#112336=CARTESIAN_POINT('Ctrl Pts',(3.28279767479856,-29.4876025180866,
53.4146536849117));
#112337=CARTESIAN_POINT('Ctrl Pts',(3.28760670020865,-29.4172441155678,
53.4382289406238));
#112338=CARTESIAN_POINT('Ctrl Pts',(3.29117179504496,-29.3647372953229,
53.4588395436778));
#112339=CARTESIAN_POINT('Ctrl Pts',(3.3024876846289,-29.1991307741788,53.5337510418467));
#112340=CARTESIAN_POINT('Ctrl Pts',(3.30995634925944,-29.091096712291,53.5981549779476));
#112341=CARTESIAN_POINT('Ctrl Pts',(3.32065902743955,-28.9547435124863,
53.7018835770136));
#112342=CARTESIAN_POINT('Ctrl Pts',(3.32357745043948,-28.9193431756693,
53.7312023903951));
#112343=CARTESIAN_POINT('Ctrl Pts',(3.32731439418433,-28.8769639798445,
53.7693623509025));
#112344=CARTESIAN_POINT('Ctrl Pts',(3.32804618964863,-28.868799275869,53.7768631183228));
#112345=CARTESIAN_POINT('Ctrl Pts',(3.32922442078874,-28.855879760206,53.788972044402));
#112346=CARTESIAN_POINT('Ctrl Pts',(3.32966704946267,-28.8510763403816,
53.7935281798187));
#112347=CARTESIAN_POINT('Ctrl Pts',(3.33052174706599,-28.8419001819753,
53.8023364360759));
#112348=CARTESIAN_POINT('Ctrl Pts',(3.33093348881995,-28.8375234473256,
53.806584120905));
#112349=CARTESIAN_POINT('Ctrl Pts',(3.33195017462254,-28.8268213461241,
53.8170853941172));
#112350=CARTESIAN_POINT('Ctrl Pts',(3.33255713651355,-28.8205226053615,
53.8233657384761));
#112351=CARTESIAN_POINT('Ctrl Pts',(3.33468472875068,-28.7987465153784,
53.845428777766));
#112352=CARTESIAN_POINT('Ctrl Pts',(3.33622318731427,-28.7835339507551,
53.8614681042838));
#112353=CARTESIAN_POINT('Ctrl Pts',(3.3451861371016,-28.6977040653504,53.9556468510971));
#112354=CARTESIAN_POINT('Ctrl Pts',(3.35292769577762,-28.6343074301702,
54.0400364727233));
#112355=CARTESIAN_POINT('Ctrl Pts',(3.36765412257765,-28.528273717525,54.2131561119856));
#112356=CARTESIAN_POINT('Ctrl Pts',(3.3746252771296,-28.4846644689147,54.3008107779306));
#112357=CARTESIAN_POINT('Ctrl Pts',(3.38281215200732,-28.4411161655249,
54.4118657443026));
#112358=CARTESIAN_POINT('Ctrl Pts',(3.38427884864516,-28.4336362920606,
54.4320866948534));
#112359=CARTESIAN_POINT('Ctrl Pts',(3.38655784839013,-28.4225282563106,
54.4640068240206));
#112360=CARTESIAN_POINT('Ctrl Pts',(3.38737887548464,-28.4186332403263,
54.4756099046659));
#112361=CARTESIAN_POINT('Ctrl Pts',(3.38890777118908,-28.4115825937538,
54.4974067430999));
#112362=CARTESIAN_POINT('Ctrl Pts',(3.3896166116414,-28.4083963724233,54.5075898659803));
#112363=CARTESIAN_POINT('Ctrl Pts',(3.39120122627427,-28.4014616623823,
54.5305239116674));
#112364=CARTESIAN_POINT('Ctrl Pts',(3.39207519595345,-28.39776745023,54.5432905870902));
#112365=CARTESIAN_POINT('Ctrl Pts',(3.39431003004672,-28.3886625402012,
54.5762269210969));
#112366=CARTESIAN_POINT('Ctrl Pts',(3.39566364477448,-28.3834774723459,
54.5964569274004));
#112367=CARTESIAN_POINT('Ctrl Pts',(3.40533441856615,-28.3488788598153,
54.7428365674983));
#112368=CARTESIAN_POINT('Ctrl Pts',(3.41316148703126,-28.3338854148425,
54.8719377623552));
#112369=CARTESIAN_POINT('Ctrl Pts',(3.42170258281582,-28.3340095764059,
55.0115057284734));
#112370=CARTESIAN_POINT('Ctrl Pts',(3.42231667494751,-28.3341089554762,
55.0215290255626));
#112371=CARTESIAN_POINT('Ctrl Pts',(3.42758545230639,-28.3357347633383,
55.1073624654341));
#112372=CARTESIAN_POINT('Ctrl Pts',(3.43229182281094,-28.3423445945348,
55.1829783514376));
#112373=CARTESIAN_POINT('Ctrl Pts',(3.43804603572568,-28.3559800045717,
55.2700096847301));
#112374=CARTESIAN_POINT('Ctrl Pts',(3.43885494151344,-28.3580160363671,
55.2821269511806));
#112375=CARTESIAN_POINT('Ctrl Pts',(3.44013279489624,-28.3614136273147,
55.3010631723082));
#112376=CARTESIAN_POINT('Ctrl Pts',(3.44059685697841,-28.3626842169741,
55.3078982896115));
#112377=CARTESIAN_POINT('Ctrl Pts',(3.44146959330465,-28.365141176209,55.3206700431645));
#112378=CARTESIAN_POINT('Ctrl Pts',(3.44187769152197,-28.3663171716823,
55.3266084231833));
#112379=CARTESIAN_POINT('Ctrl Pts',(3.44284381593315,-28.3691650760195,
55.3405890838047));
#112380=CARTESIAN_POINT('Ctrl Pts',(3.44340332529196,-28.3708641278656,
55.3486255531894));
#112381=CARTESIAN_POINT('Ctrl Pts',(3.44528684667179,-28.3767516048983,
55.3754899210434));
#112382=CARTESIAN_POINT('Ctrl Pts',(3.44662438349436,-28.3812073886652,
55.3942568138681));
#112383=CARTESIAN_POINT('Ctrl Pts',(3.44995345228143,-28.3929894026953,
55.4403077294224));
#112384=CARTESIAN_POINT('Ctrl Pts',(3.45195953299621,-28.4006856057976,
55.4674903687714));
#112385=CARTESIAN_POINT('Ctrl Pts',(3.45602870270282,-28.4175410426145,
55.521722666911));
#112386=CARTESIAN_POINT('Ctrl Pts',(3.45809074295246,-28.4267091667749,
55.5487490294756));
#112387=CARTESIAN_POINT('Ctrl Pts',(3.46016010521239,-28.436562259669,55.5755157965761));
#112388=CARTESIAN_POINT('',(3.22999374427404,-28.3340001086967,54.9993981883037));
#112389=CARTESIAN_POINT('Ctrl Pts',(3.26653910946692,-28.436562310676,55.575515935141));
#112390=CARTESIAN_POINT('Ctrl Pts',(3.26610426142956,-28.4342033494585,
55.5691076175777));
#112391=CARTESIAN_POINT('Ctrl Pts',(3.26567050549283,-28.4318836884431,
55.5626845247273));
#112392=CARTESIAN_POINT('Ctrl Pts',(3.26185948662694,-28.4118015327416,
55.5059885842083));
#112393=CARTESIAN_POINT('Ctrl Pts',(3.25854909571553,-28.3964216962971,
55.4549022657807));
#112394=CARTESIAN_POINT('Ctrl Pts',(3.25151246114565,-28.3687308606398,
55.3438758887792));
#112395=CARTESIAN_POINT('Ctrl Pts',(3.24780182374277,-28.3572170598544,
55.2838201505538));
#112396=CARTESIAN_POINT('Ctrl Pts',(3.23947059422819,-28.3389924365888,
55.14905659201));
#112397=CARTESIAN_POINT('Ctrl Pts',(3.23484347681183,-28.3339730649767,
55.0742635237064));
#112398=CARTESIAN_POINT('Ctrl Pts',(3.22999374427404,-28.3340001086967,
54.9993981883037));
#112399=CARTESIAN_POINT('Ctrl Pts',(3.22999363096242,-28.3340001093295,
54.9993964391124));
#112400=CARTESIAN_POINT('Ctrl Pts',(3.22944627893864,-28.3340031704154,
54.9909469702904));
#112401=CARTESIAN_POINT('Ctrl Pts',(3.22889614275794,-28.3340705112933,
54.9824978038024));
#112402=CARTESIAN_POINT('Ctrl Pts',(3.22781978152219,-28.3343265807982,
54.9660602437476));
#112403=CARTESIAN_POINT('Ctrl Pts',(3.22729389686768,-28.3345085160145,
54.9580719987756));
#112404=CARTESIAN_POINT('Ctrl Pts',(3.22635468175902,-28.3349336617773,
54.9438882301297));
#112405=CARTESIAN_POINT('Ctrl Pts',(3.22594253609832,-28.3351540116596,
54.9376921072977));
#112406=CARTESIAN_POINT('Ctrl Pts',(3.22514990380104,-28.335642051126,54.9258328918709));
#112407=CARTESIAN_POINT('Ctrl Pts',(3.22476972683143,-28.3359040749976,
54.920169598038));
#112408=CARTESIAN_POINT('Ctrl Pts',(3.22394836010653,-28.3365298882734,
54.9079903447517));
#112409=CARTESIAN_POINT('Ctrl Pts',(3.2235066653871,-28.3369030628881,54.9014750623392));
#112410=CARTESIAN_POINT('Ctrl Pts',(3.22233807798199,-28.3379866273858,
54.8843228713518));
#112411=CARTESIAN_POINT('Ctrl Pts',(3.22160783262883,-28.3387608407594,
54.8736904999473));
#112412=CARTESIAN_POINT('Ctrl Pts',(3.21836852194565,-28.3426221046375,
54.8268713771079));
#112413=CARTESIAN_POINT('Ctrl Pts',(3.21580953598852,-28.3467897288866,
54.790786312995));
#112414=CARTESIAN_POINT('Ctrl Pts',(3.20731403660343,-28.3643024104152,
54.6730589349306));
#112415=CARTESIAN_POINT('Ctrl Pts',(3.20125683106105,-28.3825472288322,
54.5922711479893));
#112416=CARTESIAN_POINT('Ctrl Pts',(3.1877162694469,-28.4370344941116,54.4139447672884));
#112417=CARTESIAN_POINT('Ctrl Pts',(3.18030069668878,-28.4765622657465,
54.3177491133614));
#112418=CARTESIAN_POINT('Ctrl Pts',(3.17176083280522,-28.5344476544525,
54.2074445994328));
#112419=CARTESIAN_POINT('Ctrl Pts',(3.17034830519417,-28.5444466599546,
54.1892273545916));
#112420=CARTESIAN_POINT('Ctrl Pts',(3.16813418766622,-28.5607901277092,
54.1607284754705));
#112421=CARTESIAN_POINT('Ctrl Pts',(3.16732467365762,-28.5669097891404,
54.1503211140598));
#112422=CARTESIAN_POINT('Ctrl Pts',(3.16580630126171,-28.5786588857188,
54.1308281849853));
#112423=CARTESIAN_POINT('Ctrl Pts',(3.16509659458045,-28.5842636368123,
54.1217285350187));
#112424=CARTESIAN_POINT('Ctrl Pts',(3.16349570110759,-28.5971608547623,
54.1012334308335));
#112425=CARTESIAN_POINT('Ctrl Pts',(3.16260648819195,-28.6045054017531,
54.0898715159586));
#112426=CARTESIAN_POINT('Ctrl Pts',(3.16030338536082,-28.6239933445402,
54.0605145535657));
#112427=CARTESIAN_POINT('Ctrl Pts',(3.15889753767737,-28.636351718973,54.0426648157582));
#112428=CARTESIAN_POINT('Ctrl Pts',(3.14810055666687,-28.7347428904244,
53.9063270784758));
#112429=CARTESIAN_POINT('Ctrl Pts',(3.13935341336748,-28.8357038579149,
53.799411666546));
#112430=CARTESIAN_POINT('Ctrl Pts',(3.1264851680095,-28.9978850741701,53.6676210004575));
#112431=CARTESIAN_POINT('Ctrl Pts',(3.12258401545807,-29.0486037724197,
53.6309449749112));
#112432=CARTESIAN_POINT('Ctrl Pts',(3.11752381426487,-29.1142390716444,
53.588893602026));
#112433=CARTESIAN_POINT('Ctrl Pts',(3.11651358879216,-29.1273347335693,
53.580757603548));
#112434=CARTESIAN_POINT('Ctrl Pts',(3.11499421644602,-29.1469806019274,
53.568926830563));
#112435=CARTESIAN_POINT('Ctrl Pts',(3.11449355491824,-29.1534463871775,
53.565092516941));
#112436=CARTESIAN_POINT('Ctrl Pts',(3.11358816554865,-29.1651195387486,
53.5582765101685));
#112437=CARTESIAN_POINT('Ctrl Pts',(3.11318445542479,-29.1703173683475,
53.5552790118577));
#112438=CARTESIAN_POINT('Ctrl Pts',(3.11227419952155,-29.1820204819202,
53.548614016058));
#112439=CARTESIAN_POINT('Ctrl Pts',(3.11176672144735,-29.1885342371351,
53.5449621734525));
#112440=CARTESIAN_POINT('Ctrl Pts',(3.11022112087113,-29.2083465956974,
53.5340290734638));
#112441=CARTESIAN_POINT('Ctrl Pts',(3.10917507923877,-29.2217198319965,
53.5268856766034));
#112442=CARTESIAN_POINT('Ctrl Pts',(3.10057284982028,-29.3315512107026,
53.470131519646));
#112443=CARTESIAN_POINT('Ctrl Pts',(3.09261133568641,-29.43253896802,53.4298707541041));
#112444=CARTESIAN_POINT('Ctrl Pts',(3.07698197601865,-29.6391638771441,
53.3700524321576));
#112445=CARTESIAN_POINT('Ctrl Pts',(3.06935006233231,-29.7442415509271,
53.3502949241533));
#112446=CARTESIAN_POINT('Ctrl Pts',(3.06061437130328,-29.8711612708734,
53.3388597899902));
#112447=CARTESIAN_POINT('Ctrl Pts',(3.05920439733073,-29.8918529525876,
53.3373844404174));
#112448=CARTESIAN_POINT('Ctrl Pts',(3.0569933343112,-29.9246158785417,53.3356626557412));
#112449=CARTESIAN_POINT('Ctrl Pts',(3.05618435818009,-29.936670918022,53.3351603675124));
#112450=CARTESIAN_POINT('Ctrl Pts',(3.05466645180861,-29.9594135456323,
53.3344601558104));
#112451=CARTESIAN_POINT('Ctrl Pts',(3.05395667924349,-29.9700995852406,
53.3342340479073));
#112452=CARTESIAN_POINT('Ctrl Pts',(3.05235491557288,-29.9943270642431,
53.3339546320657));
#112453=CARTESIAN_POINT('Ctrl Pts',(3.051464907086,-30.0078685717886,53.3339635496848));
#112454=CARTESIAN_POINT('Ctrl Pts',(3.04915824930715,-30.0431576168594,
53.3344170662982));
#112455=CARTESIAN_POINT('Ctrl Pts',(3.04774968439721,-30.0648996237534,
53.3351224676973));
#112456=CARTESIAN_POINT('Ctrl Pts',(3.03870910392438,-30.2055001305203,
53.3424427865775));
#112457=CARTESIAN_POINT('Ctrl Pts',(3.03147792461151,-30.3233742061746,
53.3613545167691));
#112458=CARTESIAN_POINT('Ctrl Pts',(3.01863056307776,-30.5262288172144,
53.4166625110284));
#112459=CARTESIAN_POINT('Ctrl Pts',(3.01304287671953,-30.6120920187647,
53.4478359225096));
#112460=CARTESIAN_POINT('Ctrl Pts',(3.0061689366359,-30.7081609296605,53.4919300270745));
#112461=CARTESIAN_POINT('Ctrl Pts',(3.00521596248045,-30.7212805608765,
53.4981607066755));
#112462=CARTESIAN_POINT('Ctrl Pts',(3.0037663020653,-30.7409068238937,53.5077979416642));
#112463=CARTESIAN_POINT('Ctrl Pts',(3.00327700526436,-30.7474755216954,
53.5110774889336));
#112464=CARTESIAN_POINT('Ctrl Pts',(3.00238268345898,-30.7593756964178,
53.5171174709025));
#112465=CARTESIAN_POINT('Ctrl Pts',(3.00197854401409,-30.7647142128652,
53.5198634479797));
#112466=CARTESIAN_POINT('Ctrl Pts',(3.00105503280201,-30.7768248621168,
53.5261758204016));
#112467=CARTESIAN_POINT('Ctrl Pts',(3.00053458915641,-30.78358730203,53.5297600491469));
#112468=CARTESIAN_POINT('Ctrl Pts',(2.9989087684212,-30.8045266660954,53.5410438278637));
#112469=CARTESIAN_POINT('Ctrl Pts',(2.99779427442511,-30.8186161365642,
53.5489025388923));
#112470=CARTESIAN_POINT('Ctrl Pts',(2.99015730724839,-30.9135268269829,
53.6036631766884));
#112471=CARTESIAN_POINT('Ctrl Pts',(2.98333816764977,-30.9903854703331,
53.6570847502175));
#112472=CARTESIAN_POINT('Ctrl Pts',(2.96786974510205,-31.1541054690272,
53.7926128824164));
#112473=CARTESIAN_POINT('Ctrl Pts',(2.95929418444401,-31.2374634431106,
53.8781990854792));
#112474=CARTESIAN_POINT('Ctrl Pts',(2.94965601886661,-31.3241494977233,
53.988743843993));
#112475=CARTESIAN_POINT('Ctrl Pts',(2.9482052314118,-31.3369876837706,54.0057792437966));
#112476=CARTESIAN_POINT('Ctrl Pts',(2.94594538787192,-31.3566430109031,
54.0329300449955));
#112477=CARTESIAN_POINT('Ctrl Pts',(2.94512784481786,-31.3636818870867,
54.0428812605454));
#112478=CARTESIAN_POINT('Ctrl Pts',(2.94360236659168,-31.3766774430358,
54.0616881694945));
#112479=CARTESIAN_POINT('Ctrl Pts',(2.94289349500745,-31.3826594275714,
54.0705255302949));
#112480=CARTESIAN_POINT('Ctrl Pts',(2.94130485505719,-31.3959338397611,
54.0905479793892));
#112481=CARTESIAN_POINT('Ctrl Pts',(2.9404269364868,-31.4031776041989,54.1017645680989));
#112482=CARTESIAN_POINT('Ctrl Pts',(2.93817410278817,-31.4215191215799,
54.1309288822595));
#112483=CARTESIAN_POINT('Ctrl Pts',(2.93680664500663,-31.4324123541753,
54.1490028599927));
#112484=CARTESIAN_POINT('Ctrl Pts',(2.92584690603423,-31.5176417988483,
54.2966906670115));
#112485=CARTESIAN_POINT('Ctrl Pts',(2.9169332446144,-31.5745735196394,54.4355529411328));
#112486=CARTESIAN_POINT('Ctrl Pts',(2.90396652503318,-31.6275957747198,
54.6391590427815));
#112487=CARTESIAN_POINT('Ctrl Pts',(2.90015847426865,-31.639709805863,54.6989611730654));
#112488=CARTESIAN_POINT('Ctrl Pts',(2.89521003509339,-31.6507200674583,
54.7743642884269));
#112489=CARTESIAN_POINT('Ctrl Pts',(2.89421124586475,-31.6527147589818,
54.7894718528435));
#112490=CARTESIAN_POINT('Ctrl Pts',(2.89270577674961,-31.6553794641724,
54.8120350550889));
#112491=CARTESIAN_POINT('Ctrl Pts',(2.89220735767949,-31.6562069748809,
54.8194717698079));
#112492=CARTESIAN_POINT('Ctrl Pts',(2.89130419949058,-31.6576077442492,
54.8328815655753));
#112493=CARTESIAN_POINT('Ctrl Pts',(2.89090045222045,-31.6581988690253,
54.8388525125584));
#112494=CARTESIAN_POINT('Ctrl Pts',(2.88998778994189,-31.659456482078,54.8522960232315));
#112495=CARTESIAN_POINT('Ctrl Pts',(2.88947791669023,-31.660104754796,54.8597699094282));
#112496=CARTESIAN_POINT('Ctrl Pts',(2.88791768108065,-31.6619247164145,
54.8825372410852));
#112497=CARTESIAN_POINT('Ctrl Pts',(2.88685918718747,-31.6629356605656,
54.8978422300975));
#112498=CARTESIAN_POINT('Ctrl Pts',(2.87834111157345,-31.669314901281,55.0200573273979));
#112499=CARTESIAN_POINT('Ctrl Pts',(2.87048803290338,-31.6645786189451,
55.1272364564882));
#112500=CARTESIAN_POINT('Ctrl Pts',(2.85496826171191,-31.6346843038774,
55.3386910226096));
#112501=CARTESIAN_POINT('Ctrl Pts',(2.84733960055973,-31.60968734588,55.4425137060117));
#112502=CARTESIAN_POINT('Ctrl Pts',(2.83855559392522,-31.5679459582342,
55.5635258536358));
#112503=CARTESIAN_POINT('Ctrl Pts',(2.83709665743696,-31.5605618518459,
55.5836631705559));
#112504=CARTESIAN_POINT('Ctrl Pts',(2.83482708438295,-31.5483654761976,
55.6150361844531));
#112505=CARTESIAN_POINT('Ctrl Pts',(2.83400783891793,-31.5438151425258,
55.6263704778624));
#112506=CARTESIAN_POINT('Ctrl Pts',(2.83248082019742,-31.5350572091674,
55.6475099833509));
#112507=CARTESIAN_POINT('Ctrl Pts',(2.83177209206372,-31.5308792864683,
55.6573267325063));
#112508=CARTESIAN_POINT('Ctrl Pts',(2.83018588366596,-31.5212752165224,
55.6793048166104));
#112509=CARTESIAN_POINT('Ctrl Pts',(2.82931022832937,-31.5157969373391,
55.6914426803144));
#112510=CARTESIAN_POINT('Ctrl Pts',(2.82706742469511,-31.5013145261524,
55.7225308452343));
#112511=CARTESIAN_POINT('Ctrl Pts',(2.82570761951889,-31.4920967516918,
55.7413794408279));
#112512=CARTESIAN_POINT('Ctrl Pts',(2.816093852784,-31.4238710771484,55.8744579580612));
#112513=CARTESIAN_POINT('Ctrl Pts',(2.80832125224955,-31.3521716760421,
55.9816929400111));
#112514=CARTESIAN_POINT('Ctrl Pts',(2.79533865777135,-31.2146708268911,
56.143293390646));
#112515=CARTESIAN_POINT('Ctrl Pts',(2.79018909716237,-31.1557861385896,
56.2027883453288));
#112516=CARTESIAN_POINT('Ctrl Pts',(2.78382474576343,-31.0819521131929,
56.266940479258));
#112517=CARTESIAN_POINT('Ctrl Pts',(2.7828904986132,-31.0710900428015,56.2761366072337));
#112518=CARTESIAN_POINT('Ctrl Pts',(2.7814637003255,-31.0544933075837,56.2898266988611));
#112519=CARTESIAN_POINT('Ctrl Pts',(2.7809781954083,-31.0488444705833,56.2944243200642));
#112520=CARTESIAN_POINT('Ctrl Pts',(2.78008742011743,-31.038482297435,56.302745792299));
#112521=CARTESIAN_POINT('Ctrl Pts',(2.77968299052434,-31.0337787315782,
56.3064813859954));
#112522=CARTESIAN_POINT('Ctrl Pts',(2.77875441001977,-31.0229814783373,
56.3149618015025));
#112523=CARTESIAN_POINT('Ctrl Pts',(2.77822913570513,-31.016874951954,56.3196897251195));
#112524=CARTESIAN_POINT('Ctrl Pts',(2.77657277686449,-30.9976161550111,
56.3343876463584));
#112525=CARTESIAN_POINT('Ctrl Pts',(2.77543209781001,-30.9843489264619,
56.3442044202042));
#112526=CARTESIAN_POINT('Ctrl Pts',(2.7684956901135,-30.903523275283,56.4021712369296));
#112527=CARTESIAN_POINT('Ctrl Pts',(2.7624677182888,-30.8325967535362,56.4454129443026));
#112528=CARTESIAN_POINT('Ctrl Pts',(2.74996617596909,-30.6796953435356,
56.5236325105155));
#112529=CARTESIAN_POINT('Ctrl Pts',(2.74351347344466,-30.5975230270371,
56.5576941062641));
#112530=CARTESIAN_POINT('Ctrl Pts',(2.73375019136946,-30.4660212316411,
56.6002564040124));
#112531=CARTESIAN_POINT('Ctrl Pts',(2.73031840039953,-30.4183648002468,
56.6133716575618));
#112532=CARTESIAN_POINT('Ctrl Pts',(2.7258217092867,-30.353983897029,56.6280441415306));
#112533=CARTESIAN_POINT('Ctrl Pts',(2.72469743180069,-30.3377215460728,
56.631495178735));
#112534=CARTESIAN_POINT('Ctrl Pts',(2.72282870837987,-30.310420992386,56.6368629228397));
#112535=CARTESIAN_POINT('Ctrl Pts',(2.72208008336844,-30.299410512033,56.638912681182));
#112536=CARTESIAN_POINT('Ctrl Pts',(2.7206091570574,-30.2776352411253,56.6427396896492));
#112537=CARTESIAN_POINT('Ctrl Pts',(2.71988671274985,-30.2668720189564,
56.6445225295421));
#112538=CARTESIAN_POINT('Ctrl Pts',(2.71829620642966,-30.2430302827037,
56.6482314809183));
#112539=CARTESIAN_POINT('Ctrl Pts',(2.71742974330725,-30.22994470645,56.6501079302735));
#112540=CARTESIAN_POINT('Ctrl Pts',(2.71488330973983,-30.1912158848906,
56.6551919175608));
#112541=CARTESIAN_POINT('Ctrl Pts',(2.71321697365155,-30.1655181001968,
56.6579588870477));
#112542=CARTESIAN_POINT('Ctrl Pts',(2.7023991179353,-29.9967065247133,56.6721710427702));
#112543=CARTESIAN_POINT('Ctrl Pts',(2.6938380018832,-29.8526983311679,56.6656739724049));
#112544=CARTESIAN_POINT('Ctrl Pts',(2.68230599518897,-29.6686435396513,
56.6332896460315));
#112545=CARTESIAN_POINT('Ctrl Pts',(2.67960534020977,-29.626295757772,56.6241233966154));
#112546=CARTESIAN_POINT('Ctrl Pts',(2.67518135412202,-29.5591748399306,
56.6068308471363));
#112547=CARTESIAN_POINT('Ctrl Pts',(2.67349926900117,-29.5341503899648,
56.599755029947));
#112548=CARTESIAN_POINT('Ctrl Pts',(2.67118061195524,-29.5005093711111,
56.5893866093527));
#112549=CARTESIAN_POINT('Ctrl Pts',(2.67057071900159,-29.4917381382286,
56.586603464184));
#112550=CARTESIAN_POINT('Ctrl Pts',(2.66954188643043,-29.4770812997456,
56.5818187869957));
#112551=CARTESIAN_POINT('Ctrl Pts',(2.66912519735029,-29.4711828578901,
56.579856661386));
#112552=CARTESIAN_POINT('Ctrl Pts',(2.66832066823801,-29.4598699187782,
56.5760229420342));
#112553=CARTESIAN_POINT('Ctrl Pts',(2.66793315373526,-29.4544538763469,
56.5741563591074));
#112554=CARTESIAN_POINT('Ctrl Pts',(2.66687217266515,-29.4397119780404,
56.5689905002283));
#112555=CARTESIAN_POINT('Ctrl Pts',(2.66619560923379,-29.430405889308,56.5656360989789));
#112556=CARTESIAN_POINT('Ctrl Pts',(2.66350352891703,-29.3937266106652,
56.5520446721225));
#112557=CARTESIAN_POINT('Ctrl Pts',(2.66145600574359,-29.3665965656147,
56.541171609305));
#112558=CARTESIAN_POINT('Ctrl Pts',(2.65156626645615,-29.2385575443992,
56.4859049675584));
#112559=CARTESIAN_POINT('Ctrl Pts',(2.64344145086671,-29.1419352694405,
56.4322823150409));
#112560=CARTESIAN_POINT('Ctrl Pts',(2.63127112856187,-29.0034187262987,
56.3363297165009));
#112561=CARTESIAN_POINT('Ctrl Pts',(2.62711164560393,-28.957289154711,56.3006562105568));
#112562=CARTESIAN_POINT('Ctrl Pts',(2.62036568228315,-28.8841961997182,
56.2377376027337));
#112563=CARTESIAN_POINT('Ctrl Pts',(2.61773324718341,-28.8561344807863,
56.2118517138311));
#112564=CARTESIAN_POINT('Ctrl Pts',(2.61410985880653,-28.8181846730051,
56.1743504890903));
#112565=CARTESIAN_POINT('Ctrl Pts',(2.61308517346219,-28.807530787673,56.1635307226346));
#112566=CARTESIAN_POINT('Ctrl Pts',(2.61133436822402,-28.7894681821005,
56.1446781488531));
#112567=CARTESIAN_POINT('Ctrl Pts',(2.61060517438068,-28.7819879934138,
56.1367154913242));
#112568=CARTESIAN_POINT('Ctrl Pts',(2.60921400741425,-28.7678024719221,
56.1213141955596));
#112569=CARTESIAN_POINT('Ctrl Pts',(2.60855152997597,-28.761084852487,56.1138875787272));
#112570=CARTESIAN_POINT('Ctrl Pts',(2.60682113852235,-28.743641190483,56.0942498255165));
#112571=CARTESIAN_POINT('Ctrl Pts',(2.60575785076168,-28.7330259884047,
56.0819413216085));
#112572=CARTESIAN_POINT('Ctrl Pts',(2.60193837916156,-28.6952985371508,
56.0368788814984));
#112573=CARTESIAN_POINT('Ctrl Pts',(2.59922503288759,-28.6692611985757,
56.003243954617));
#112574=CARTESIAN_POINT('Ctrl Pts',(2.58929251678008,-28.5774875695183,
55.8748218620233));
#112575=CARTESIAN_POINT('Ctrl Pts',(2.58236295841184,-28.5203615719412,
55.7742904733263));
#112576=CARTESIAN_POINT('Ctrl Pts',(2.57321250994743,-28.4606342676709,
55.637989541466));
#112577=CARTESIAN_POINT('Ctrl Pts',(2.57114030558061,-28.448124746154,55.6069262677602));
#112578=CARTESIAN_POINT('Ctrl Pts',(2.56903904312142,-28.4365623153847,
55.5755159479327));
#112579=CARTESIAN_POINT('Origin',(5.,-30.,55.));
#112580=CARTESIAN_POINT('',(1.86810673741824,-28.4365624617973,55.5755163456747));
#112581=CARTESIAN_POINT('',(2.06220428404732,-28.4365623101862,55.5755159338105));
#112582=CARTESIAN_POINT('',(5.,-28.4365623102018,55.5755159338528));
#112583=CARTESIAN_POINT('',(2.72303743726837,-28.3340004588354,54.9999657623987));
#112584=CARTESIAN_POINT('Ctrl Pts',(2.06220428404731,-28.4365623101862,
55.5755159338105));
#112585=CARTESIAN_POINT('Ctrl Pts',(2.06232537164583,-28.4372097346566,
55.5772747171192));
#112586=CARTESIAN_POINT('Ctrl Pts',(2.06244636879248,-28.4378601333206,
55.5790324253072));
#112587=CARTESIAN_POINT('Ctrl Pts',(2.06925635199033,-28.474660488052,55.6779724051352));
#112588=CARTESIAN_POINT('Ctrl Pts',(2.07563303131421,-28.5198024133307,
55.7715737442157));
#112589=CARTESIAN_POINT('Ctrl Pts',(2.08880064720991,-28.631104512992,55.956129471173));
#112590=CARTESIAN_POINT('Ctrl Pts',(2.09555584618043,-28.6983337519922,
56.0458089234561));
#112591=CARTESIAN_POINT('Ctrl Pts',(2.1037874159976,-28.7841067908732,56.1390265532599));
#112592=CARTESIAN_POINT('Ctrl Pts',(2.10476402048816,-28.794336702512,56.1498494512293));
#112593=CARTESIAN_POINT('Ctrl Pts',(2.1062425814088,-28.8098761402488,56.1658542797185));
#112594=CARTESIAN_POINT('Ctrl Pts',(2.10673670555073,-28.8150777485499,
56.1711405790335));
#112595=CARTESIAN_POINT('Ctrl Pts',(2.10763579219869,-28.8245533382064,
56.180642699559));
#112596=CARTESIAN_POINT('Ctrl Pts',(2.1080398139472,-28.8288150430316,56.1848703862104));
#112597=CARTESIAN_POINT('Ctrl Pts',(2.10895787655775,-28.8385070444761,
56.1943816458927));
#112598=CARTESIAN_POINT('Ctrl Pts',(2.10947293032625,-28.843950554172,56.1996512305486));
#112599=CARTESIAN_POINT('Ctrl Pts',(2.11106459631092,-28.8607968180041,
56.2157381079754));
#112600=CARTESIAN_POINT('Ctrl Pts',(2.1121498029255,-28.872316489137,56.2264309567949));
#112601=CARTESIAN_POINT('Ctrl Pts',(2.1177880363432,-28.9324223258129,56.2806599319491));
#112602=CARTESIAN_POINT('Ctrl Pts',(2.12248669566025,-28.9833800445922,
56.3214742366377));
#112603=CARTESIAN_POINT('Ctrl Pts',(2.13556722442658,-29.1303544521544,
56.4256509187734));
#112604=CARTESIAN_POINT('Ctrl Pts',(2.1439715499686,-29.2307540869289,56.4822384412262));
#112605=CARTESIAN_POINT('Ctrl Pts',(2.15507093025407,-29.3755552514984,
56.545143054548));
#112606=CARTESIAN_POINT('Ctrl Pts',(2.15804335451875,-29.4155719639695,
56.5607186637322));
#112607=CARTESIAN_POINT('Ctrl Pts',(2.16207531836975,-29.4715675354315,
56.580057346495));
#112608=CARTESIAN_POINT('Ctrl Pts',(2.16317807720657,-29.4870639426854,
56.5851557405528));
#112609=CARTESIAN_POINT('Ctrl Pts',(2.16494659793527,-29.5122025762183,
56.5930192107853));
#112610=CARTESIAN_POINT('Ctrl Pts',(2.16561696100031,-29.5217989332165,
56.5959261511413));
#112611=CARTESIAN_POINT('Ctrl Pts',(2.16701151724068,-29.5419003896495,
56.6018177159694));
#112612=CARTESIAN_POINT('Ctrl Pts',(2.16773515153564,-29.552409796694,56.604786050461));
#112613=CARTESIAN_POINT('Ctrl Pts',(2.16945432388753,-29.577560171593,56.6116233716226));
#112614=CARTESIAN_POINT('Ctrl Pts',(2.17044673116837,-29.5922263582524,
56.6153965403498));
#112615=CARTESIAN_POINT('Ctrl Pts',(2.1738991728499,-29.643739004778,56.6279029164711));
#112616=CARTESIAN_POINT('Ctrl Pts',(2.17632568794083,-29.6808314817495,
56.6355798976115));
#112617=CARTESIAN_POINT('Ctrl Pts',(2.18236256735586,-29.7749133965924,
56.651728902515));
#112618=CARTESIAN_POINT('Ctrl Pts',(2.18592628177591,-29.8321409245678,
56.6585223567415));
#112619=CARTESIAN_POINT('Ctrl Pts',(2.19615394835175,-29.9984806117492,
56.6695685422116));
#112620=CARTESIAN_POINT('Ctrl Pts',(2.20270296308616,-30.1077894711117,
56.6660848557805));
#112621=CARTESIAN_POINT('Ctrl Pts',(2.21158248489456,-30.2467011034689,
56.6479246333367));
#112622=CARTESIAN_POINT('Ctrl Pts',(2.21357624777269,-30.2773196429087,
56.6430491658818));
#112623=CARTESIAN_POINT('Ctrl Pts',(2.21627658998945,-30.3177159250042,
56.6354555208864));
#112624=CARTESIAN_POINT('Ctrl Pts',(2.21694510200407,-30.3276323380065,
56.6334978445986));
#112625=CARTESIAN_POINT('Ctrl Pts',(2.21800315353894,-30.3431823633909,
56.6302807065075));
#112626=CARTESIAN_POINT('Ctrl Pts',(2.21838935393333,-30.3488284870189,
56.629081950256));
#112627=CARTESIAN_POINT('Ctrl Pts',(2.21919292922282,-30.3605118456347,
56.626537877586));
#112628=CARTESIAN_POINT('Ctrl Pts',(2.21961056482069,-30.3665479364537,
56.6251882547481));
#112629=CARTESIAN_POINT('Ctrl Pts',(2.22064266066459,-30.3813796825504,
56.6217851643071));
#112630=CARTESIAN_POINT('Ctrl Pts',(2.22125920328352,-30.3901663460958,
56.6196937347975));
#112631=CARTESIAN_POINT('Ctrl Pts',(2.22357609493654,-30.422928819136,56.6116134523345));
#112632=CARTESIAN_POINT('Ctrl Pts',(2.22529937686746,-30.4467861772772,
56.6051631257141));
#112633=CARTESIAN_POINT('Ctrl Pts',(2.22987418722147,-30.5090089635778,
56.586845361317));
#112634=CARTESIAN_POINT('Ctrl Pts',(2.23275607171611,-30.5471034083806,
56.5741174618133));
#112635=CARTESIAN_POINT('Ctrl Pts',(2.24419054467396,-30.6951232592355,
56.5186395969525));
#112636=CARTESIAN_POINT('Ctrl Pts',(2.25285324302594,-30.8008562305663,
56.4656388529966));
#112637=CARTESIAN_POINT('Ctrl Pts',(2.26476217240214,-30.9425238823466,
56.3746801249062));
#112638=CARTESIAN_POINT('Ctrl Pts',(2.26826856786382,-30.983684970585,56.3455339113695));
#112639=CARTESIAN_POINT('Ctrl Pts',(2.27287768223769,-31.0370360334894,
56.3039969655379));
#112640=CARTESIAN_POINT('Ctrl Pts',(2.27404186700073,-31.0504433003046,
56.2932210685962));
#112641=CARTESIAN_POINT('Ctrl Pts',(2.27595844493011,-31.072393577105,56.2750122117591));
#112642=CARTESIAN_POINT('Ctrl Pts',(2.27671548372277,-31.0810317185521,
56.2676965562624));
#112643=CARTESIAN_POINT('Ctrl Pts',(2.27819812991193,-31.0978821783893,
56.2531283806536));
#112644=CARTESIAN_POINT('Ctrl Pts',(2.27892392746534,-31.1060988290708,
56.2458817785384));
#112645=CARTESIAN_POINT('Ctrl Pts',(2.28065803308938,-31.125647952973,56.2282947562899));
#112646=CARTESIAN_POINT('Ctrl Pts',(2.2816630632547,-31.1369103858714,56.2178777125427));
#112647=CARTESIAN_POINT('Ctrl Pts',(2.28521602191174,-31.1764587641485,
56.1802711568812));
#112648=CARTESIAN_POINT('Ctrl Pts',(2.28772766795328,-31.2039275785866,
56.1522386865298));
#112649=CARTESIAN_POINT('Ctrl Pts',(2.2940420544524,-31.2713335873471,56.0784043599753));
#112650=CARTESIAN_POINT('Ctrl Pts',(2.29779197162577,-31.3098029094427,
56.0313400000281));
#112651=CARTESIAN_POINT('Ctrl Pts',(2.30692224562847,-31.3976704159359,
55.910970646456));
#112652=CARTESIAN_POINT('Ctrl Pts',(2.31225296111814,-31.4439697563155,
55.8356433702257));
#112653=CARTESIAN_POINT('Ctrl Pts',(2.3205469139733,-31.5042476474273,55.7174711414809));
#112654=CARTESIAN_POINT('Ctrl Pts',(2.32336742338587,-31.5228247228412,
55.6771483885607));
#112655=CARTESIAN_POINT('Ctrl Pts',(2.32701661797487,-31.5441024545265,
55.625645625704));
#112656=CARTESIAN_POINT('Ctrl Pts',(2.32776542395504,-31.5483290824238,
55.6151112696775));
#112657=CARTESIAN_POINT('Ctrl Pts',(2.32896461272201,-31.5548708405906,
55.5983120136017));
#112658=CARTESIAN_POINT('Ctrl Pts',(2.32941094913306,-31.5572565922799,
55.5920747405724));
#112659=CARTESIAN_POINT('Ctrl Pts',(2.3302721886907,-31.5617646490663,55.5800731948575));
#112660=CARTESIAN_POINT('Ctrl Pts',(2.33068675504299,-31.5638926652388,
55.5743112892845));
#112661=CARTESIAN_POINT('Ctrl Pts',(2.33169946406485,-31.5689903492804,
55.5602701574488));
#112662=CARTESIAN_POINT('Ctrl Pts',(2.33229951492806,-31.5719263800903,
55.5519789963861));
#112663=CARTESIAN_POINT('Ctrl Pts',(2.33448305351163,-31.582311545585,55.5218970223855));
#112664=CARTESIAN_POINT('Ctrl Pts',(2.33608630911952,-31.5893739469681,
55.4999766557985));
#112665=CARTESIAN_POINT('Ctrl Pts',(2.34688195458569,-31.6333724849818,
55.353046209968));
#112666=CARTESIAN_POINT('Ctrl Pts',(2.35653951194391,-31.6559809784502,
55.2242203392077));
#112667=CARTESIAN_POINT('Ctrl Pts',(2.3713837843607,-31.6676404691382,55.0180706027472));
#112668=CARTESIAN_POINT('Ctrl Pts',(2.37675188179722,-31.6667252280184,
54.9418515613006));
#112669=CARTESIAN_POINT('Ctrl Pts',(2.38328298878817,-31.6590431426242,
54.846684956322));
#112670=CARTESIAN_POINT('Ctrl Pts',(2.38459490360139,-31.6571525643435,
54.8274454149686));
#112671=CARTESIAN_POINT('Ctrl Pts',(2.38668864642201,-31.6535729990847,
54.7965526561828));
#112672=CARTESIAN_POINT('Ctrl Pts',(2.38747699158815,-31.6520946505789,
54.7848773307288));
#112673=CARTESIAN_POINT('Ctrl Pts',(2.38897846674383,-31.6490284765637,
54.7625620394904));
#112674=CARTESIAN_POINT('Ctrl Pts',(2.38969219923063,-31.6474610718561,
54.7519199170015));
#112675=CARTESIAN_POINT('Ctrl Pts',(2.39133412842055,-31.643601005332,54.7273636665469));
#112676=CARTESIAN_POINT('Ctrl Pts',(2.39225994897923,-31.6412345179996,
54.7134618485977));
#112677=CARTESIAN_POINT('Ctrl Pts',(2.39522375499666,-31.6330471136552,
54.6688005721892));
#112678=CARTESIAN_POINT('Ctrl Pts',(2.39723996913978,-31.626535501754,54.638173523921));
#112679=CARTESIAN_POINT('Ctrl Pts',(2.40865774937288,-31.584311833556,54.4638804725321));
#112680=CARTESIAN_POINT('Ctrl Pts',(2.41744539140517,-31.5304448980797,
54.3253108118202));
#112681=CARTESIAN_POINT('Ctrl Pts',(2.43005911113584,-31.4322182909615,
54.1471343942842));
#112682=CARTESIAN_POINT('Ctrl Pts',(2.43355100001086,-31.4030518897346,
54.0999594254477));
#112683=CARTESIAN_POINT('Ctrl Pts',(2.43795956684985,-31.3647790702097,
54.0444487600586));
#112684=CARTESIAN_POINT('Ctrl Pts',(2.43875046842822,-31.3578592136122,
54.0346407828298));
#112685=CARTESIAN_POINT('Ctrl Pts',(2.44000150399177,-31.3468428827081,
54.0193794035324));
#112686=CARTESIAN_POINT('Ctrl Pts',(2.44045697382574,-31.3428177103678,
54.0138747049737));
#112687=CARTESIAN_POINT('Ctrl Pts',(2.44132361103844,-31.3351346272211,
54.003501828411));
#112688=CARTESIAN_POINT('Ctrl Pts',(2.44173431498744,-31.3314836717503,
53.9986287872728));
#112689=CARTESIAN_POINT('Ctrl Pts',(2.44272061236917,-31.3226911512107,
53.9870262388145));
#112690=CARTESIAN_POINT('Ctrl Pts',(2.44329787484986,-31.3175248797891,
53.9803157813484));
#112691=CARTESIAN_POINT('Ctrl Pts',(2.44530828720449,-31.299455578073,53.9572121864804));
#112692=CARTESIAN_POINT('Ctrl Pts',(2.44675745515867,-31.2862965224039,
53.941022955255));
#112693=CARTESIAN_POINT('Ctrl Pts',(2.45043219755399,-31.252516669011,53.901023222342));
#112694=CARTESIAN_POINT('Ctrl Pts',(2.45267615215947,-31.23151847852,53.8775428884371));
#112695=CARTESIAN_POINT('Ctrl Pts',(2.4644000109941,-31.1193868060104,53.7590923163931));
#112696=CARTESIAN_POINT('Ctrl Pts',(2.47411700419691,-31.0178819210741,
53.6745559900337));
#112697=CARTESIAN_POINT('Ctrl Pts',(2.48700607651239,-30.8650922961737,
53.5753152824368));
#112698=CARTESIAN_POINT('Ctrl Pts',(2.49052275850408,-30.8214658255248,
53.5497220805052));
#112699=CARTESIAN_POINT('Ctrl Pts',(2.4951428077502,-30.7615098031002,53.5181244475952));
#112700=CARTESIAN_POINT('Ctrl Pts',(2.4963080232623,-30.746156961148,53.510334882938));
#112701=CARTESIAN_POINT('Ctrl Pts',(2.49822583472365,-30.7205104297312,
53.4978186146416));
#112702=CARTESIAN_POINT('Ctrl Pts',(2.49898308859381,-30.7102846613519,
53.4929565684259));
#112703=CARTESIAN_POINT('Ctrl Pts',(2.50046582294605,-30.690070508046,53.4835967996442));
#112704=CARTESIAN_POINT('Ctrl Pts',(2.50119149677422,-30.6800857761678,
53.4790926001512));
#112705=CARTESIAN_POINT('Ctrl Pts',(2.50292475912295,-30.6560225347886,
53.4685218203231));
#112706=CARTESIAN_POINT('Ctrl Pts',(2.50392907806751,-30.6419031343307,
53.462550367359));
#112707=CARTESIAN_POINT('Ctrl Pts',(2.50747629739231,-30.5914336491069,
53.4420220368113));
#112708=CARTESIAN_POINT('Ctrl Pts',(2.5099830763626,-30.5546536001011,53.4285519879416));
#112709=CARTESIAN_POINT('Ctrl Pts',(2.51628140465738,-30.4598709784488,
53.3975826063392));
#112710=CARTESIAN_POINT('Ctrl Pts',(2.5200205008995,-30.401325838068,53.3819267040085));
#112711=CARTESIAN_POINT('Ctrl Pts',(2.52911069557165,-30.2561234165271,
53.3514654878174));
#112712=CARTESIAN_POINT('Ctrl Pts',(2.53441259504023,-30.1689058108366,
53.3402607070238));
#112713=CARTESIAN_POINT('Ctrl Pts',(2.54271454378882,-30.0362002277193,
53.333783670764));
#112714=CARTESIAN_POINT('Ctrl Pts',(2.54557713043139,-29.99111731265,53.3334143789789));
#112715=CARTESIAN_POINT('Ctrl Pts',(2.54927382481636,-29.9346904436815,
53.3352416067863));
#112716=CARTESIAN_POINT('Ctrl Pts',(2.55002548734156,-29.923305888315,53.3357272334477));
#112717=CARTESIAN_POINT('Ctrl Pts',(2.55122819544278,-29.9052492522322,
53.3366831266628));
#112718=CARTESIAN_POINT('Ctrl Pts',(2.55167515386943,-29.8985732399226,
53.3370768707666));
#112719=CARTESIAN_POINT('Ctrl Pts',(2.55253671827702,-29.8857745982139,
53.3379090771366));
#112720=CARTESIAN_POINT('Ctrl Pts',(2.55295097855857,-29.8796517665738,
53.338341197505));
#112721=CARTESIAN_POINT('Ctrl Pts',(2.55396169143693,-29.8647856678546,
53.3394729693465));
#112722=CARTESIAN_POINT('Ctrl Pts',(2.55456003425262,-29.8560453433546,
53.34020784932));
#112723=CARTESIAN_POINT('Ctrl Pts',(2.55673016520325,-29.824547395081,53.3431068301361));
#112724=CARTESIAN_POINT('Ctrl Pts',(2.55832141637395,-29.8018302012381,
53.3456701668783));
#112725=CARTESIAN_POINT('Ctrl Pts',(2.57014304077642,-29.6353238787771,
53.3679367817011));
#112726=CARTESIAN_POINT('Ctrl Pts',(2.58093805936272,-29.494603708959,53.4058866255745));
#112727=CARTESIAN_POINT('Ctrl Pts',(2.5958109354758,-29.3022010270493,53.4858570500897));
#112728=CARTESIAN_POINT('Ctrl Pts',(2.60024015860938,-29.2452490993818,
53.5134250434331));
#112729=CARTESIAN_POINT('Ctrl Pts',(2.60582443997335,-29.1738202688117,
53.5531670132731));
#112730=CARTESIAN_POINT('Ctrl Pts',(2.60707949169387,-29.157795432562,53.5624360347152));
#112731=CARTESIAN_POINT('Ctrl Pts',(2.60910500518627,-29.1319899343932,
53.5779420032617));
#112732=CARTESIAN_POINT('Ctrl Pts',(2.60988123722554,-29.1221144376701,
53.5840171712596));
#112733=CARTESIAN_POINT('Ctrl Pts',(2.6113742371713,-29.1031511415047,53.5959575906852));
#112734=CARTESIAN_POINT('Ctrl Pts',(2.61209145801452,-29.0940554880607,
53.6018092001378));
#112735=CARTESIAN_POINT('Ctrl Pts',(2.61376303092771,-29.072895216172,53.6157156612731));
#112736=CARTESIAN_POINT('Ctrl Pts',(2.61471471752167,-29.0608774158467,
53.6238404145796));
#112737=CARTESIAN_POINT('Ctrl Pts',(2.6178607294643,-29.0212697443292,53.6513780940761));
#112738=CARTESIAN_POINT('Ctrl Pts',(2.62002922316321,-28.9941624439332,
53.6714726132932));
#112739=CARTESIAN_POINT('Ctrl Pts',(2.62526424652121,-28.9294581597486,
53.7225541529866));
#112740=CARTESIAN_POINT('Ctrl Pts',(2.62829939636591,-28.892573652032,53.7543936711335));
#112741=CARTESIAN_POINT('Ctrl Pts',(2.63539054523375,-28.8089273258662,
53.8332559756977));
#112742=CARTESIAN_POINT('Ctrl Pts',(2.63941263783197,-28.7634737634398,
53.8815418020753));
#112743=CARTESIAN_POINT('Ctrl Pts',(2.64822466703058,-28.671238693962,53.9920400139026));
#112744=CARTESIAN_POINT('Ctrl Pts',(2.6530166086471,-28.6256986445518,54.0550751933649));
#112745=CARTESIAN_POINT('Ctrl Pts',(2.65910972067198,-28.5760893625325,
54.1349551968652));
#112746=CARTESIAN_POINT('Ctrl Pts',(2.66018099248169,-28.5676580842231,
54.1489884829723));
#112747=CARTESIAN_POINT('Ctrl Pts',(2.66177448828764,-28.555567660035,54.16980092671));
#112748=CARTESIAN_POINT('Ctrl Pts',(2.66228698183378,-28.5517462608473,
54.1764853448608));
#112749=CARTESIAN_POINT('Ctrl Pts',(2.66320459873939,-28.5450261128556,
54.1884317176277));
#112750=CARTESIAN_POINT('Ctrl Pts',(2.66360857029623,-28.5421092927669,
54.1936832057829));
#112751=CARTESIAN_POINT('Ctrl Pts',(2.66450803698854,-28.5357072809428,
54.2053577960637));
#112752=CARTESIAN_POINT('Ctrl Pts',(2.6650043408485,-28.5322359574577,54.2117880299653));
#112753=CARTESIAN_POINT('Ctrl Pts',(2.66648223450761,-28.5220760152506,
54.2309080266732));
#112754=CARTESIAN_POINT('Ctrl Pts',(2.66747079372325,-28.5155090597173,
54.2436611990011));
#112755=CARTESIAN_POINT('Ctrl Pts',(2.669787532922,-28.5006283879976,54.2735003215386));
#112756=CARTESIAN_POINT('Ctrl Pts',(2.67112161085381,-28.4924407775574,
54.2906466755577));
#112757=CARTESIAN_POINT('Ctrl Pts',(2.67589012380187,-28.4644569974568,
54.351923666433));
#112758=CARTESIAN_POINT('Ctrl Pts',(2.67938092240163,-28.4462919916914,
54.396770281843));
#112759=CARTESIAN_POINT('Ctrl Pts',(2.69259541230682,-28.3853722202072,
54.5682685761565));
#112760=CARTESIAN_POINT('Ctrl Pts',(2.70235946782802,-28.3559458481188,
54.6991469049287));
#112761=CARTESIAN_POINT('Ctrl Pts',(2.71369123867573,-28.3394891846822,
54.8616547109419));
#112762=CARTESIAN_POINT('Ctrl Pts',(2.71572545086426,-28.3372894008935,
54.8912376681486));
#112763=CARTESIAN_POINT('Ctrl Pts',(2.71867277504418,-28.3352233232247,
54.9346851049013));
#112764=CARTESIAN_POINT('Ctrl Pts',(2.71960486850662,-28.3347383030971,
54.9485129148139));
#112765=CARTESIAN_POINT('Ctrl Pts',(2.72102151940647,-28.334260260276,54.9696582383626));
#112766=CARTESIAN_POINT('Ctrl Pts',(2.72150992748456,-28.3341430975167,
54.976972052061));
#112767=CARTESIAN_POINT('Ctrl Pts',(2.72234473947519,-28.3340248097476,
54.9895127770705));
#112768=CARTESIAN_POINT('Ctrl Pts',(2.72269187194403,-28.3340001073699,
54.9947392960198));
#112769=CARTESIAN_POINT('Ctrl Pts',(2.72303824113791,-28.3340000003493,
54.9999658866651));
#112770=CARTESIAN_POINT('Ctrl Pts',(2.72303822942304,-28.3340000003529,
54.9999657098917));
#112771=CARTESIAN_POINT('Ctrl Pts',(2.72328729578586,-28.3339999229979,
55.003724034477));
#112772=CARTESIAN_POINT('Ctrl Pts',(2.72353596649594,-28.3340125632317,
55.0074823807488));
#112773=CARTESIAN_POINT('Ctrl Pts',(2.72421539065123,-28.3340819571948,
55.0177671377999));
#112774=CARTESIAN_POINT('Ctrl Pts',(2.72464534569333,-28.3341643443612,
55.0242933522203));
#112775=CARTESIAN_POINT('Ctrl Pts',(2.7262307742564,-28.3346107689681,55.048421854334));
#112776=CARTESIAN_POINT('Ctrl Pts',(2.72737878432969,-28.3352154790134,
55.0660189655808));
#112777=CARTESIAN_POINT('Ctrl Pts',(2.73222385219982,-28.3389708721576,
55.1407596639566));
#112778=CARTESIAN_POINT('Ctrl Pts',(2.73583856341932,-28.344785934576,55.197733325189));
#112779=CARTESIAN_POINT('Ctrl Pts',(2.74629491638921,-28.3704529590116,
55.3639159669714));
#112780=CARTESIAN_POINT('Ctrl Pts',(2.75293891978614,-28.3982795014471,
55.4715174317822));
#112781=CARTESIAN_POINT('Ctrl Pts',(2.75980443758381,-28.4365622822719,
55.5755158579788));
#112782=CARTESIAN_POINT('Ctrl Pts',(2.56903904312142,-28.4365623153847,
55.5755159479327));
#112783=CARTESIAN_POINT('Ctrl Pts',(2.56703835108036,-28.4255532845451,
55.5456089857579));
#112784=CARTESIAN_POINT('Ctrl Pts',(2.56501128067198,-28.415402857017,55.5153874046099));
#112785=CARTESIAN_POINT('Ctrl Pts',(2.56192254398484,-28.4015461573019,
55.4698390721243));
#112786=CARTESIAN_POINT('Ctrl Pts',(2.56089227150846,-28.3971814487163,
55.4547263888258));
#112787=CARTESIAN_POINT('Ctrl Pts',(2.55934855448598,-28.3910323585701,
55.4322459322886));
#112788=CARTESIAN_POINT('Ctrl Pts',(2.55884399565741,-28.3890830825208,
55.4249236361458));
#112789=CARTESIAN_POINT('Ctrl Pts',(2.55793467883482,-28.3856796228417,
55.411778745954));
#112790=CARTESIAN_POINT('Ctrl Pts',(2.55753098331845,-28.3842068552135,
55.4059612374387));
#112791=CARTESIAN_POINT('Ctrl Pts',(2.55662469014299,-28.3809857071768,
55.3929422785539));
#112792=CARTESIAN_POINT('Ctrl Pts',(2.55612120362156,-28.3792539435179,
55.3857371252025));
#112793=CARTESIAN_POINT('Ctrl Pts',(2.55459981462748,-28.3741919823816,
55.3640403647579));
#112794=CARTESIAN_POINT('Ctrl Pts',(2.55357433846662,-28.3710077738259,
55.3495159313299));
#112795=CARTESIAN_POINT('Ctrl Pts',(2.5447505544529,-28.3454989159792,55.2252293185456));
#112796=CARTESIAN_POINT('Ctrl Pts',(2.53651830970599,-28.3341036274991,
55.1135246394297));
#112797=CARTESIAN_POINT('Ctrl Pts',(2.52138069507772,-28.3339120416039,
54.9050563349742));
#112798=CARTESIAN_POINT('Ctrl Pts',(2.51447543413713,-28.3422033913261,
54.8087432211969));
#112799=CARTESIAN_POINT('Ctrl Pts',(2.50627879320001,-28.3626384096543,
54.6916093334645));
#112800=CARTESIAN_POINT('Ctrl Pts',(2.50474821514035,-28.3669330379638,
54.6696211831237));
#112801=CARTESIAN_POINT('Ctrl Pts',(2.50230220635249,-28.3745727123223,
54.6343080775627));
#112802=CARTESIAN_POINT('Ctrl Pts',(2.50137815646881,-28.3776412226831,
54.6209268317182));
#112803=CARTESIAN_POINT('Ctrl Pts',(2.49974279163186,-28.3833969408986,
54.5971784515154));
#112804=CARTESIAN_POINT('Ctrl Pts',(2.49902944573445,-28.3860193355058,
54.5867965701316));
#112805=CARTESIAN_POINT('Ctrl Pts',(2.49752649549474,-28.3917808996816,
54.5648790645174));
#112806=CARTESIAN_POINT('Ctrl Pts',(2.49673772442098,-28.3949445198246,
54.5533504492246));
#112807=CARTESIAN_POINT('Ctrl Pts',(2.49462546461138,-28.4037920440569,
54.5224175976414));
#112808=CARTESIAN_POINT('Ctrl Pts',(2.49330945477949,-28.4097056550107,
54.5030807475177));
#112809=CARTESIAN_POINT('Ctrl Pts',(2.48464430264063,-28.4512847352377,
54.3754759257311));
#112810=CARTESIAN_POINT('Ctrl Pts',(2.47767019940445,-28.4976297409374,
54.2710026203267));
#112811=CARTESIAN_POINT('Ctrl Pts',(2.4645277693078,-28.6045895067659,54.0842316977445));
#112812=CARTESIAN_POINT('Ctrl Pts',(2.45837431571896,-28.6627868525958,
54.0011719123958));
#112813=CARTESIAN_POINT('Ctrl Pts',(2.45078834182361,-28.7383130714074,
53.9119054837793));
#112814=CARTESIAN_POINT('Ctrl Pts',(2.44975778235109,-28.7486454778635,
53.9000384561234));
#112815=CARTESIAN_POINT('Ctrl Pts',(2.44821371706354,-28.7642007284754,
53.8826757003381));
#112816=CARTESIAN_POINT('Ctrl Pts',(2.44770910276128,-28.7692958458465,
53.8770660262105));
#112817=CARTESIAN_POINT('Ctrl Pts',(2.44679972961303,-28.7784940892631,
53.8670766460264));
#112818=CARTESIAN_POINT('Ctrl Pts',(2.44639603388026,-28.7825828549661,
53.8626840772073));
#112819=CARTESIAN_POINT('Ctrl Pts',(2.4454897952363,-28.7917730550158,53.8529173733814));
#112820=CARTESIAN_POINT('Ctrl Pts',(2.44498636406658,-28.7968866048078,
53.84755518314));
#112821=CARTESIAN_POINT('Ctrl Pts',(2.44346530923389,-28.8123661527817,
53.8315382665714));
#112822=CARTESIAN_POINT('Ctrl Pts',(2.44244011659792,-28.8228388400482,
53.820988319422));
#112823=CARTESIAN_POINT('Ctrl Pts',(2.44002156029704,-28.8476672351425,
53.7966373306589));
#112824=CARTESIAN_POINT('Ctrl Pts',(2.43862160262966,-28.862131830105,53.782950917727));
#112825=CARTESIAN_POINT('Ctrl Pts',(2.43350940658966,-28.9153944255774,
53.7343333684519));
#112826=CARTESIAN_POINT('Ctrl Pts',(2.42973301407763,-28.9555819868563,
53.7009728140392));
#112827=CARTESIAN_POINT('Ctrl Pts',(2.41656146691648,-29.1002856582031,
53.5919120668428));
#112828=CARTESIAN_POINT('Ctrl Pts',(2.40715987144216,-29.2119941384566,
53.5264820533905));
#112829=CARTESIAN_POINT('Ctrl Pts',(2.3961897696172,-29.3568803729204,53.4628579853087));
#112830=CARTESIAN_POINT('Ctrl Pts',(2.3941883938128,-29.3839181213363,53.4518230939087));
#112831=CARTESIAN_POINT('Ctrl Pts',(2.3912773375423,-29.4241239345395,53.4366341965357));
#112832=CARTESIAN_POINT('Ctrl Pts',(2.39034937294933,-29.437074635501,53.4319244495153));
#112833=CARTESIAN_POINT('Ctrl Pts',(2.38870750341623,-29.4602227096479,
53.4238299993902));
#112834=CARTESIAN_POINT('Ctrl Pts',(2.38799154866458,-29.4703970496479,
53.4203822873007));
#112835=CARTESIAN_POINT('Ctrl Pts',(2.3864956940411,-29.491819396112,53.4133532859725));
#112836=CARTESIAN_POINT('Ctrl Pts',(2.38571650565754,-29.5030735847893,
53.4097926326291));
#112837=CARTESIAN_POINT('Ctrl Pts',(2.38365967646332,-29.5330261765167,
53.4006651291111));
#112838=CARTESIAN_POINT('Ctrl Pts',(2.38238882909739,-29.5517864870996,
53.395306484153));
#112839=CARTESIAN_POINT('Ctrl Pts',(2.37528923996673,-29.6579175994826,
53.3669980200577));
#112840=CARTESIAN_POINT('Ctrl Pts',(2.36968483959418,-29.7469520122311,
53.3508530768575));
#112841=CARTESIAN_POINT('Ctrl Pts',(2.36069739872477,-29.8929118451649,
53.3364917698487));
#112842=CARTESIAN_POINT('Ctrl Pts',(2.35727588964617,-29.9492003328648,
53.3338226953154));
#112843=CARTESIAN_POINT('Ctrl Pts',(2.3492002131386,-30.0807564356624,53.3342582193225));
#112844=CARTESIAN_POINT('Ctrl Pts',(2.3445281650401,-30.1558849720682,53.3396041865704));
#112845=CARTESIAN_POINT('Ctrl Pts',(2.33881232788712,-30.2425488653579,
53.3517048489213));
#112846=CARTESIAN_POINT('Ctrl Pts',(2.33800373221752,-30.254693659358,53.3535377394982));
#112847=CARTESIAN_POINT('Ctrl Pts',(2.33672635232354,-30.2736768174056,
53.3566177253608));
#112848=CARTESIAN_POINT('Ctrl Pts',(2.33626244971412,-30.280529811979,53.3577736693134));
#112849=CARTESIAN_POINT('Ctrl Pts',(2.33539000788557,-30.2933364589578,
53.3600163573909));
#112850=CARTESIAN_POINT('Ctrl Pts',(2.33498204424106,-30.2992916804859,
53.3610927080827));
#112851=CARTESIAN_POINT('Ctrl Pts',(2.3340162496017,-30.31331317584,53.3637059309768));
#112852=CARTESIAN_POINT('Ctrl Pts',(2.33345693650485,-30.3213740963753,
53.3652700193635));
#112853=CARTESIAN_POINT('Ctrl Pts',(2.33157415325444,-30.3483226184663,
53.370705954563));
#112854=CARTESIAN_POINT('Ctrl Pts',(2.33023716885546,-30.3671537350826,
53.3748459184671));
#112855=CARTESIAN_POINT('Ctrl Pts',(2.32690961976266,-30.4133745851862,
53.3858517246691));
#112856=CARTESIAN_POINT('Ctrl Pts',(2.32490451916805,-30.4406692358917,
53.3930887867935));
#112857=CARTESIAN_POINT('Ctrl Pts',(2.31572802510407,-30.563590940929,53.4290481676522));
#112858=CARTESIAN_POINT('Ctrl Pts',(2.3083850395483,-30.6567020471508,53.4656378357968));
#112859=CARTESIAN_POINT('Ctrl Pts',(2.29520339350666,-30.8201431983275,
53.5474845819436));
#112860=CARTESIAN_POINT('Ctrl Pts',(2.28933579930071,-30.8914405336698,
53.5901158117819));
#112861=CARTESIAN_POINT('Ctrl Pts',(2.28231555892406,-30.9753107606886,
53.6491818670247));
#112862=CARTESIAN_POINT('Ctrl Pts',(2.28098393227696,-30.9911469095463,
53.6607582111378));
#112863=CARTESIAN_POINT('Ctrl Pts',(2.2788667120394,-31.016197820083,53.6797584153974));
#112864=CARTESIAN_POINT('Ctrl Pts',(2.2780743328379,-31.0255439463336,53.6870051493337));
#112865=CARTESIAN_POINT('Ctrl Pts',(2.27657008073348,-31.0432264373216,
53.7010196808139));
#112866=CARTESIAN_POINT('Ctrl Pts',(2.27585755480261,-31.051576047011,53.707769720322));
#112867=CARTESIAN_POINT('Ctrl Pts',(2.27422535106344,-31.0706378458176,
53.7234868823847));
#112868=CARTESIAN_POINT('Ctrl Pts',(2.2733079576977,-31.0813037655132,53.732509044325));
#112869=CARTESIAN_POINT('Ctrl Pts',(2.27040065826232,-31.1149349528493,
53.7616907595333));
#112870=CARTESIAN_POINT('Ctrl Pts',(2.26843134516235,-31.1374604122517,
53.7823490967137));
#112871=CARTESIAN_POINT('Ctrl Pts',(2.26378074398716,-31.1898721913184,
53.8331409470337));
#112872=CARTESIAN_POINT('Ctrl Pts',(2.26112192150893,-31.2192008410207,
53.8638197464072));
#112873=CARTESIAN_POINT('Ctrl Pts',(2.25391905425235,-31.2962132114888,
53.9507977488816));
#112874=CARTESIAN_POINT('Ctrl Pts',(2.24944290793472,-31.3413799036468,
54.0091950863668));
#112875=CARTESIAN_POINT('Ctrl Pts',(2.24410794920097,-31.3900407675514,
54.0815644312773));
#112876=CARTESIAN_POINT('Ctrl Pts',(2.2432832906862,-31.3974167380233,54.0928265412012));
#112877=CARTESIAN_POINT('Ctrl Pts',(2.23791108319823,-31.4444538425068,
54.1665809545085));
#112878=CARTESIAN_POINT('Ctrl Pts',(2.23331127110286,-31.4800446055248,
54.2315604178246));
#112879=CARTESIAN_POINT('Ctrl Pts',(2.22767576188936,-31.516362482387,54.3098177290135));
#112880=CARTESIAN_POINT('Ctrl Pts',(2.22686745979227,-31.5214075005587,
54.3210110894427));
#112881=CARTESIAN_POINT('Ctrl Pts',(2.2255904439769,-31.529113305343,54.3386250789237));
#112882=CARTESIAN_POINT('Ctrl Pts',(2.22512660737437,-31.5318585268876,
54.3450085985029));
#112883=CARTESIAN_POINT('Ctrl Pts',(2.2242542155818,-31.5369198486099,54.3569836643989));
#112884=CARTESIAN_POINT('Ctrl Pts',(2.22384623512155,-31.5392455178413,
54.3625708980347));
#112885=CARTESIAN_POINT('Ctrl Pts',(2.22288029982929,-31.544655492089,54.375770181163));
#112886=CARTESIAN_POINT('Ctrl Pts',(2.22232086158404,-31.5477140058777,
54.3833925033628));
#112887=CARTESIAN_POINT('Ctrl Pts',(2.22043720596458,-31.5577673375764,
54.4089931720024));
#112888=CARTESIAN_POINT('Ctrl Pts',(2.21909945793434,-31.5645059374945,
54.4270696019089));
#112889=CARTESIAN_POINT('Ctrl Pts',(2.21576958235504,-31.5803375905998,
54.4719019708231));
#112890=CARTESIAN_POINT('Ctrl Pts',(2.21376289459154,-31.5890665002595,
54.4987795831598));
#112891=CARTESIAN_POINT('Ctrl Pts',(2.20457234774951,-31.6255705800626,
54.621742186336));
#112892=CARTESIAN_POINT('Ctrl Pts',(2.19721651169948,-31.6453425273582,
54.7199873379671));
#112893=CARTESIAN_POINT('Ctrl Pts',(2.18403780551838,-31.665153196257,54.9016738693175));
#112894=CARTESIAN_POINT('Ctrl Pts',(2.1781846997846,-31.6679827934126,54.9844979088606));
#112895=CARTESIAN_POINT('Ctrl Pts',(2.17117843492911,-31.6638531943162,
55.0867930224263));
#112896=CARTESIAN_POINT('Ctrl Pts',(2.16984721069288,-31.6627164115778,
55.1063704500606));
#112897=CARTESIAN_POINT('Ctrl Pts',(2.16773047312117,-31.6603404632456,
55.137714807446));
#112898=CARTESIAN_POINT('Ctrl Pts',(2.16693817966036,-31.6593211783186,
55.1494960258417));
#112899=CARTESIAN_POINT('Ctrl Pts',(2.16543399423523,-31.6571372362708,
55.1719519001914));
#112900=CARTESIAN_POINT('Ctrl Pts',(2.16472145024848,-31.6559946498985,
55.1826280496733));
#112901=CARTESIAN_POINT('Ctrl Pts',(2.16308906981575,-31.6531279019413,
55.2071698451742));
#112902=CARTESIAN_POINT('Ctrl Pts',(2.1621715195509,-31.6513323492107,55.2210264623908));
#112903=CARTESIAN_POINT('Ctrl Pts',(2.15926315580417,-31.6450529981877,
55.2651249119903));
#112904=CARTESIAN_POINT('Ctrl Pts',(2.1572929572791,-31.6399109089102,55.2952676489055));
#112905=CARTESIAN_POINT('Ctrl Pts',(2.1526398152762,-31.6256540345434,55.3668884381332));
#112906=CARTESIAN_POINT('Ctrl Pts',(2.14997937236171,-31.6157774278917,
55.408193395815));
#112907=CARTESIAN_POINT('Ctrl Pts',(2.14277554881109,-31.5844576153759,
55.520083496558));
#112908=CARTESIAN_POINT('Ctrl Pts',(2.13829996551363,-31.5598897025359,
55.5896925150088));
#112909=CARTESIAN_POINT('Ctrl Pts',(2.13295527386606,-31.5254128186204,
55.6699682736316));
#112910=CARTESIAN_POINT('Ctrl Pts',(2.13212035963713,-31.5198809678143,
55.6824247892904));
#112911=CARTESIAN_POINT('Ctrl Pts',(2.12675007713731,-31.4834142531925,
55.7618963491714));
#112912=CARTESIAN_POINT('Ctrl Pts',(2.12216235501318,-31.4482111809464,
55.8268527713405));
#112913=CARTESIAN_POINT('Ctrl Pts',(2.11654027588311,-31.4022709623842,
55.8996348563199));
#112914=CARTESIAN_POINT('Ctrl Pts',(2.11573202235905,-31.395603561099,55.9099436274539));
#112915=CARTESIAN_POINT('Ctrl Pts',(2.11445506685338,-31.3849851264321,
55.9259700232764));
#112916=CARTESIAN_POINT('Ctrl Pts',(2.11399124124554,-31.3811110526101,
55.9317384506558));
#112917=CARTESIAN_POINT('Ctrl Pts',(2.11311885789158,-31.3737954245023,
55.9424854168378));
#112918=CARTESIAN_POINT('Ctrl Pts',(2.11271087473568,-31.3703626813043,
55.9474696545795));
#112919=CARTESIAN_POINT('Ctrl Pts',(2.11174491645276,-31.3622073660227,
55.9591738907788));
#112920=CARTESIAN_POINT('Ctrl Pts',(2.11118545769657,-31.3574621719033,
55.9658777901899));
#112921=CARTESIAN_POINT('Ctrl Pts',(2.10930165882308,-31.3414052657541,
55.988210569702));
#112922=CARTESIAN_POINT('Ctrl Pts',(2.10796378534965,-31.3298721402424,
56.0036773527398));
#112923=CARTESIAN_POINT('Ctrl Pts',(2.10463352754408,-31.3007896000602,
56.0412977703782));
#112924=CARTESIAN_POINT('Ctrl Pts',(2.1026265789964,-31.2829403714896,56.063211386878));
#112925=CARTESIAN_POINT('Ctrl Pts',(2.09343372188809,-31.1994108899654,
56.1605937453689));
#112926=CARTESIAN_POINT('Ctrl Pts',(2.08607577300004,-31.1275715857393,
56.2305068409151));
#112927=CARTESIAN_POINT('Ctrl Pts',(2.07289754164681,-30.9856695232517,
56.3456795436961));
#112928=CARTESIAN_POINT('Ctrl Pts',(2.06704680935116,-30.9176452464735,
56.3929568406548));
#112929=CARTESIAN_POINT('Ctrl Pts',(2.06004283481689,-30.8294914373563,
56.4449513482183));
#112930=CARTESIAN_POINT('Ctrl Pts',(2.05871167716821,-30.812427847237,56.4546138640165));
#112931=CARTESIAN_POINT('Ctrl Pts',(2.05659501942459,-30.7848064540562,
56.4696171770011));
#112932=CARTESIAN_POINT('Ctrl Pts',(2.05580274011233,-30.7743558871533,
56.4751504295406));
#112933=CARTESIAN_POINT('Ctrl Pts',(2.05429856561854,-30.7543053576852,
56.4854947675108));
#112934=CARTESIAN_POINT('Ctrl Pts',(2.0535860185813,-30.7447161082256,56.4903252008502));
#112935=CARTESIAN_POINT('Ctrl Pts',(2.05195360872115,-30.7225422267729,
56.5012274800501));
#112936=CARTESIAN_POINT('Ctrl Pts',(2.05103603236773,-30.7099264563181,
56.5072344418335));
#112937=CARTESIAN_POINT('Ctrl Pts',(2.04812749185214,-30.6694691962174,
56.5258773621193));
#112938=CARTESIAN_POINT('Ctrl Pts',(2.04615714629515,-30.6413538804128,
56.5379064070614));
#112939=CARTESIAN_POINT('Ctrl Pts',(2.04150358224,-30.5734432120206,56.5647752005727));
#112940=CARTESIAN_POINT('Ctrl Pts',(2.0388428701114,-30.5333800312772,56.5788808273197));
#112941=CARTESIAN_POINT('Ctrl Pts',(2.03163889322003,-30.4223862329931,
56.6132521263377));
#112942=CARTESIAN_POINT('Ctrl Pts',(2.0271634087151,-30.3505811790887,56.6303636887563));
#112943=CARTESIAN_POINT('Ctrl Pts',(2.02181723499935,-30.2644150546329,
56.6449398570226));
#112944=CARTESIAN_POINT('Ctrl Pts',(2.02098074667628,-30.2509241126987,
56.6470517716352));
#112945=CARTESIAN_POINT('Ctrl Pts',(2.0156107855745,-30.1643838527792,56.6595111123436));
#112946=CARTESIAN_POINT('Ctrl Pts',(2.0110249452427,-30.0907500079712,56.6651609107663));
#112947=CARTESIAN_POINT('Ctrl Pts',(2.00540495613297,-30.0047183005893,
56.666038553412));
#112948=CARTESIAN_POINT('Ctrl Pts',(2.00459671004535,-29.9924414094366,
56.666028081927));
#112949=CARTESIAN_POINT('Ctrl Pts',(2.00331976367859,-29.9732180186805,
56.6657992104633));
#112950=CARTESIAN_POINT('Ctrl Pts',(2.00285593965653,-29.9662705776211,
56.6656730188718));
#112951=CARTESIAN_POINT('Ctrl Pts',(2.00198355701048,-29.9532738610787,
56.6653556068995));
#112952=CARTESIAN_POINT('Ctrl Pts',(2.00157557295156,-29.9472245764896,
56.6651748795512));
#112953=CARTESIAN_POINT('Ctrl Pts',(2.00060960959139,-29.9329681142962,
56.6646711951904));
#112954=CARTESIAN_POINT('Ctrl Pts',(2.00005014662097,-29.924762192847,56.6643205001155));
#112955=CARTESIAN_POINT('Ctrl Pts',(1.99816632100341,-29.8972903773353,
56.6629428622291));
#112956=CARTESIAN_POINT('Ctrl Pts',(1.99682842453156,-29.878040582076,56.6616419742938));
#112957=CARTESIAN_POINT('Ctrl Pts',(1.99349809715418,-29.8306597380197,
56.6576123016473));
#112958=CARTESIAN_POINT('Ctrl Pts',(1.99149110134063,-29.8025677331954,
56.6545014314531));
#112959=CARTESIAN_POINT('Ctrl Pts',(1.9822978236645,-29.6754434739068,56.6371403166034));
#112960=CARTESIAN_POINT('Ctrl Pts',(1.97493949047844,-29.577738480749,56.6147015224257));
#112961=CARTESIAN_POINT('Ctrl Pts',(1.96175688810711,-29.4039568504639,
56.5579280046778));
#112962=CARTESIAN_POINT('Ctrl Pts',(1.95590231956057,-29.327293171844,56.5263932489599));
#112963=CARTESIAN_POINT('Ctrl Pts',(1.94889711022973,-29.2357832756456,
56.4805107078214));
#112964=CARTESIAN_POINT('Ctrl Pts',(1.947568230824,-29.2184405232332,56.4714292367417));
#112965=CARTESIAN_POINT('Ctrl Pts',(1.94545430454428,-29.1908904451282,
56.4563781723088));
#112966=CARTESIAN_POINT('Ctrl Pts',(1.9446625095041,-29.1805800547817,56.4506021571734));
#112967=CARTESIAN_POINT('Ctrl Pts',(1.9431587085359,-29.1610195756471,56.4393690156069));
#112968=CARTESIAN_POINT('Ctrl Pts',(1.94244605645959,-29.1517591318772,
56.4339312237316));
#112969=CARTESIAN_POINT('Ctrl Pts',(1.94081263598737,-29.1305603358802,
56.4212059240331));
#112970=CARTESIAN_POINT('Ctrl Pts',(1.93989416397002,-29.1186597745658,
56.4138567943191));
#112971=CARTESIAN_POINT('Ctrl Pts',(1.93697954947175,-29.0809763893301,
56.389924910659));
#112972=CARTESIAN_POINT('Ctrl Pts',(1.93500415124032,-29.055557208528,56.3727795369857));
#112973=CARTESIAN_POINT('Ctrl Pts',(1.93033607971217,-28.9959698514808,
56.3301485203659));
#112974=CARTESIAN_POINT('Ctrl Pts',(1.92766611300871,-28.962277761855,56.3040339581454));
#112975=CARTESIAN_POINT('Ctrl Pts',(1.92045757524315,-28.8731696716777,
56.229323608626));
#112976=CARTESIAN_POINT('Ctrl Pts',(1.91598616736384,-28.8199174860712,
56.1782990893257));
#112977=CARTESIAN_POINT('Ctrl Pts',(1.91060735737232,-28.7606049003929,
56.1133996617428));
#112978=CARTESIAN_POINT('Ctrl Pts',(1.90973439785307,-28.7511279748243,
56.1027591205603));
#112979=CARTESIAN_POINT('Ctrl Pts',(1.90437535863507,-28.6939532131089,
56.036881802974));
#112980=CARTESIAN_POINT('Ctrl Pts',(1.89983659378609,-28.6497967557562,
55.9786882018082));
#112981=CARTESIAN_POINT('Ctrl Pts',(1.8942688632865,-28.6028406309548,55.9075529447326));
#112982=CARTESIAN_POINT('Ctrl Pts',(1.89346081078101,-28.5961925808969,
55.897235397393));
#112983=CARTESIAN_POINT('Ctrl Pts',(1.8921841044149,-28.5859608110775,55.8809639305689));
#112984=CARTESIAN_POINT('Ctrl Pts',(1.89172032384338,-28.5822991612967,
55.8750591993351));
#112985=CARTESIAN_POINT('Ctrl Pts',(1.89084797465748,-28.5755171882501,
55.8639683733889));
#112986=CARTESIAN_POINT('Ctrl Pts',(1.89043998005691,-28.5723880528177,
55.8587879568165));
#112987=CARTESIAN_POINT('Ctrl Pts',(1.88947392559671,-28.5650783935967,
55.8465361566159));
#112988=CARTESIAN_POINT('Ctrl Pts',(1.88891438121063,-28.5609218685731,
55.8394507761383));
#112989=CARTESIAN_POINT('Ctrl Pts',(1.88702998383444,-28.5471755609521,
55.8156161179621));
#112990=CARTESIAN_POINT('Ctrl Pts',(1.88569158620767,-28.5378248627358,
55.7987316765901));
#112991=CARTESIAN_POINT('Ctrl Pts',(1.88235973073603,-28.5155034379875,
55.7567201798113));
#112992=CARTESIAN_POINT('Ctrl Pts',(1.88035169195056,-28.5028753255672,
55.7314184861613));
#112993=CARTESIAN_POINT('Ctrl Pts',(1.87494997068406,-28.4709372529807,
55.6631311780316));
#112994=CARTESIAN_POINT('Ctrl Pts',(1.87153014927533,-28.4528121848193,
55.619660056186));
#112995=CARTESIAN_POINT('Ctrl Pts',(1.86810673741825,-28.4365624617974,
55.5755163456748));
#112996=CARTESIAN_POINT('Origin',(5.,-30.,55.));
#112997=CARTESIAN_POINT('',(1.16624546596858,-28.4365623102019,55.575515933853));
#112998=CARTESIAN_POINT('',(1.36116732170967,-28.4365623080758,55.5755159280775));
#112999=CARTESIAN_POINT('',(5.,-28.4365623102018,55.5755159338528));
#113000=CARTESIAN_POINT('Ctrl Pts',(1.36116732170967,-28.4365623080758,
55.5755159280775));
#113001=CARTESIAN_POINT('Ctrl Pts',(1.36158377376753,-28.4385480585766,
55.5809103872544));
#113002=CARTESIAN_POINT('Ctrl Pts',(1.36199991354639,-28.4405618822783,
55.5862949867732));
#113003=CARTESIAN_POINT('Ctrl Pts',(1.36679795800594,-28.4641243692031,
55.6483163168118));
#113004=CARTESIAN_POINT('Ctrl Pts',(1.37113052084416,-28.4887212500842,
55.7037512298974));
#113005=CARTESIAN_POINT('Ctrl Pts',(1.37811663022607,-28.5341033774531,
55.7926144392078));
#113006=CARTESIAN_POINT('Ctrl Pts',(1.38082054814088,-28.5531462531665,
55.8268647007203));
#113007=CARTESIAN_POINT('Ctrl Pts',(1.38452366318565,-28.5812986814334,
55.8735431494178));
#113008=CARTESIAN_POINT('Ctrl Pts',(1.38555860306899,-28.5893979635029,
55.886562455289));
#113009=CARTESIAN_POINT('Ctrl Pts',(1.38732161837705,-28.6035899400703,
55.9086885762336));
#113010=CARTESIAN_POINT('Ctrl Pts',(1.3880528760382,-28.6095947284154,55.9178503007989));
#113011=CARTESIAN_POINT('Ctrl Pts',(1.38944448722421,-28.6212468563099,
55.9352515864444));
#113012=CARTESIAN_POINT('Ctrl Pts',(1.39010537741692,-28.6268787693484,
55.9435008502789));
#113013=CARTESIAN_POINT('Ctrl Pts',(1.39165339328923,-28.6402996604933,
55.9627841850654));
#113014=CARTESIAN_POINT('Ctrl Pts',(1.39253817562486,-28.6481493740455,
55.9737752836327));
#113015=CARTESIAN_POINT('Ctrl Pts',(1.3956428073009,-28.6763152921145,56.0122158522167));
#113016=CARTESIAN_POINT('Ctrl Pts',(1.39783537785293,-28.6973416669029,
56.0391360159408));
#113017=CARTESIAN_POINT('Ctrl Pts',(1.40782879589833,-28.7981005882645,
56.1602687109848));
#113018=CARTESIAN_POINT('Ctrl Pts',(1.41524524747757,-28.8873147448464,
56.2460813457704));
#113019=CARTESIAN_POINT('Ctrl Pts',(1.42593905146676,-29.025414153285,56.3521504015004));
#113020=CARTESIAN_POINT('Ctrl Pts',(1.42908047856126,-29.0670239356125,
56.3811890635867));
#113021=CARTESIAN_POINT('Ctrl Pts',(1.43413817753778,-29.134254715251,56.4236825118854));
#113022=CARTESIAN_POINT('Ctrl Pts',(1.43599727016874,-29.1590132576931,
56.4384463340088));
#113023=CARTESIAN_POINT('Ctrl Pts',(1.43852209839875,-29.1924695345722,
56.4572377318534));
#113024=CARTESIAN_POINT('Ctrl Pts',(1.43915470291399,-29.2008384826829,
56.4618440813738));
#113025=CARTESIAN_POINT('Ctrl Pts',(1.44021111351293,-29.2147812443813,
56.4693628039732));
#113026=CARTESIAN_POINT('Ctrl Pts',(1.44063239791733,-29.2203329214534,
56.472316130487));
#113027=CARTESIAN_POINT('Ctrl Pts',(1.44143674182715,-29.2309130587344,
56.4778678266063));
#113028=CARTESIAN_POINT('Ctrl Pts',(1.44181940019445,-29.2359382891956,
56.4804721327332));
#113029=CARTESIAN_POINT('Ctrl Pts',(1.44285024496362,-29.2494565464955,
56.4873907589411));
#113030=CARTESIAN_POINT('Ctrl Pts',(1.44350123900518,-29.2579733145221,
56.491657847043));
#113031=CARTESIAN_POINT('Ctrl Pts',(1.44597108186289,-29.2902267666097,
56.5074729660901));
#113032=CARTESIAN_POINT('Ctrl Pts',(1.44781584560412,-29.3141988886506,
56.5185287072503));
#113033=CARTESIAN_POINT('Ctrl Pts',(1.45686863883772,-29.4317108359299,
56.5693742619728));
#113034=CARTESIAN_POINT('Ctrl Pts',(1.46433887448437,-29.528493799993,56.6011148018832));
#113035=CARTESIAN_POINT('Ctrl Pts',(1.47864601908454,-29.7208336424597,
56.6452293062189));
#113036=CARTESIAN_POINT('Ctrl Pts',(1.48546807433489,-29.81578817088,56.658549001633));
#113037=CARTESIAN_POINT('Ctrl Pts',(1.49351610959751,-29.9328893440817,
56.6647871745137));
#113038=CARTESIAN_POINT('Ctrl Pts',(1.49498194168079,-29.9544246297646,
56.6655158773369));
#113039=CARTESIAN_POINT('Ctrl Pts',(1.49725990951138,-29.9882037641785,
56.6660031728523));
#113040=CARTESIAN_POINT('Ctrl Pts',(1.49808075620676,-30.0004404784882,
56.666044880234));
#113041=CARTESIAN_POINT('Ctrl Pts',(1.49960948678899,-30.023346292887,56.6658705815975));
#113042=CARTESIAN_POINT('Ctrl Pts',(1.5003183405736,-30.0340149354649,56.6656868965212));
#113043=CARTESIAN_POINT('Ctrl Pts',(1.50190320405074,-30.0579697901595,
56.6650442080287));
#113044=CARTESIAN_POINT('Ctrl Pts',(1.50277740667697,-30.0712538532933,
56.6645286470046));
#113045=CARTESIAN_POINT('Ctrl Pts',(1.50501327182793,-30.1053975453121,
56.6627940066699));
#113046=CARTESIAN_POINT('Ctrl Pts',(1.50636767301957,-30.1262433519794,
56.661341394616));
#113047=CARTESIAN_POINT('Ctrl Pts',(1.51738141038033,-30.296878431497,56.6462204887977));
#113048=CARTESIAN_POINT('Ctrl Pts',(1.52635033113338,-30.4442044229351,
56.6127190239061));
#113049=CARTESIAN_POINT('Ctrl Pts',(1.53935047374397,-30.6416530600251,
56.538666105376));
#113050=CARTESIAN_POINT('Ctrl Pts',(1.54312811204966,-30.69706373042,56.5143687270485));
#113051=CARTESIAN_POINT('Ctrl Pts',(1.5480401612387,-30.7645766858779,56.4802732766343));
#113052=CARTESIAN_POINT('Ctrl Pts',(1.54903529964396,-30.7780334669659,
56.4732448427409));
#113053=CARTESIAN_POINT('Ctrl Pts',(1.5505364217496,-30.7979677990191,56.4624839274267));
#113054=CARTESIAN_POINT('Ctrl Pts',(1.55103421669152,-30.8045197453253,
56.458889927402));
#113055=CARTESIAN_POINT('Ctrl Pts',(1.55193689319192,-30.8162902601501,
56.4523299350908));
#113056=CARTESIAN_POINT('Ctrl Pts',(1.55234079135825,-30.8215172802137,
56.4493796550496));
#113057=CARTESIAN_POINT('Ctrl Pts',(1.5532546393959,-30.8332545330335,56.4426709221335));
#113058=CARTESIAN_POINT('Ctrl Pts',(1.5537655575938,-30.8397552866358,56.4388966465526));
#113059=CARTESIAN_POINT('Ctrl Pts',(1.55533170968354,-30.8595029812325,
56.4272519227815));
#113060=CARTESIAN_POINT('Ctrl Pts',(1.5563951593331,-30.8726660450193,56.4192418248951));
#113061=CARTESIAN_POINT('Ctrl Pts',(1.56484260049718,-30.975447404128,56.3547260380023));
#113062=CARTESIAN_POINT('Ctrl Pts',(1.57261173086794,-31.0595945916183,
56.2899752531431));
#113063=CARTESIAN_POINT('Ctrl Pts',(1.58824998057803,-31.2168488490078,
56.143138002274));
#113064=CARTESIAN_POINT('Ctrl Pts',(1.59607195954014,-31.2891686879162,
56.0609136030713));
#113065=CARTESIAN_POINT('Ctrl Pts',(1.60496450033353,-31.3648933195608,
55.9555327181075));
#113066=CARTESIAN_POINT('Ctrl Pts',(1.60635818377756,-31.3765521821325,
55.9386589924853));
#113067=CARTESIAN_POINT('Ctrl Pts',(1.60854991746957,-31.3945448132776,
55.9115619512726));
#113068=CARTESIAN_POINT('Ctrl Pts',(1.60935561873642,-31.4010842605642,
55.9014784163549));
#113069=CARTESIAN_POINT('Ctrl Pts',(1.6108709861859,-31.4132387076742,55.8822850121191));
#113070=CARTESIAN_POINT('Ctrl Pts',(1.61158145570637,-31.4188761307601,
55.8731901408965));
#113071=CARTESIAN_POINT('Ctrl Pts',(1.61318963616946,-31.4314941809594,
55.852388505316));
#113072=CARTESIAN_POINT('Ctrl Pts',(1.61408530408609,-31.4384196131465,
55.8406490284063));
#113073=CARTESIAN_POINT('Ctrl Pts',(1.6164167855927,-31.4561698107631,55.8096984972154));
#113074=CARTESIAN_POINT('Ctrl Pts',(1.61784422097093,-31.4667588284361,
55.7903548481227));
#113075=CARTESIAN_POINT('Ctrl Pts',(1.62641717429374,-31.5285556132645,
55.6719444359103));
#113076=CARTESIAN_POINT('Ctrl Pts',(1.63321815399214,-31.5700957679772,
55.5681499806008));
#113077=CARTESIAN_POINT('Ctrl Pts',(1.64434109877295,-31.6204936921444,
55.3931185874683));
#113078=CARTESIAN_POINT('Ctrl Pts',(1.64865250916417,-31.6356965734774,
55.3240946915944));
#113079=CARTESIAN_POINT('Ctrl Pts',(1.65460713659497,-31.6500970577635,
55.2308656271097));
#113080=CARTESIAN_POINT('Ctrl Pts',(1.65612113009439,-31.6532181480619,
55.2073375929617));
#113081=CARTESIAN_POINT('Ctrl Pts',(1.65875532433683,-31.6577067397094,
55.1668898026132));
#113082=CARTESIAN_POINT('Ctrl Pts',(1.65986459893477,-31.6593202220615,
55.1500006248846));
#113083=CARTESIAN_POINT('Ctrl Pts',(1.66150401994203,-31.661299293818,55.1253061928711));
#113084=CARTESIAN_POINT('Ctrl Pts',(1.66202361951538,-31.6618683953676,
55.1175177264249));
#113085=CARTESIAN_POINT('Ctrl Pts',(1.66291046489379,-31.6627411269317,
55.1042955431842));
#113086=CARTESIAN_POINT('Ctrl Pts',(1.66327614922529,-31.6630729238847,
55.0988638669398));
#113087=CARTESIAN_POINT('Ctrl Pts',(1.66411376151794,-31.6637690586954,
55.0864703220316));
#113088=CARTESIAN_POINT('Ctrl Pts',(1.66458659609144,-31.6641163084086,
55.0795078921204));
#113089=CARTESIAN_POINT('Ctrl Pts',(1.66590489407934,-31.6649585498489,
55.0601837556508));
#113090=CARTESIAN_POINT('Ctrl Pts',(1.66675519481662,-31.6653595428168,
55.0478186962362));
#113091=CARTESIAN_POINT('Ctrl Pts',(1.67329071850763,-31.6673681631933,
54.9534454968093));
#113092=CARTESIAN_POINT('Ctrl Pts',(1.67922873497755,-31.6630547889557,
54.8714319950975));
#113093=CARTESIAN_POINT('Ctrl Pts',(1.68952751499371,-31.645217831155,54.7309999733622));
#113094=CARTESIAN_POINT('Ctrl Pts',(1.69386917297553,-31.634551075954,54.6723630773916));
#113095=CARTESIAN_POINT('Ctrl Pts',(1.70203870642488,-31.6083004137768,
54.5620191174013));
#113096=CARTESIAN_POINT('Ctrl Pts',(1.70587163033355,-31.5932988559749,
54.5102478536596));
#113097=CARTESIAN_POINT('Ctrl Pts',(1.71135976433464,-31.5677848162377,
54.4358911910482));
#113098=CARTESIAN_POINT('Ctrl Pts',(1.71307124944709,-31.5592353788256,
54.4126729003733));
#113099=CARTESIAN_POINT('Ctrl Pts',(1.7161581454993,-31.542727846442,54.3707467680355));
#113100=CARTESIAN_POINT('Ctrl Pts',(1.71753870266278,-31.5349385846823,
54.3519780537993));
#113101=CARTESIAN_POINT('Ctrl Pts',(1.71971472260656,-31.5220147298226,
54.3223786968741));
#113102=CARTESIAN_POINT('Ctrl Pts',(1.7205176495593,-31.5171034984931,54.3114533740682));
#113103=CARTESIAN_POINT('Ctrl Pts',(1.72203068432302,-31.5075796754232,
54.2908637887608));
#113104=CARTESIAN_POINT('Ctrl Pts',(1.72274156417849,-31.5029909297819,
54.2811892335459));
#113105=CARTESIAN_POINT('Ctrl Pts',(1.72435458142107,-31.4923199847364,
54.2592404646978));
#113106=CARTESIAN_POINT('Ctrl Pts',(1.7252546276115,-31.4861789862258,54.2469955740609));
#113107=CARTESIAN_POINT('Ctrl Pts',(1.72804513691277,-31.4665624730002,
54.2090561119216));
#113108=CARTESIAN_POINT('Ctrl Pts',(1.72991734886921,-31.452565930064,54.1836360480317));
#113109=CARTESIAN_POINT('Ctrl Pts',(1.74004413338332,-31.3724407003726,
54.0467070077865));
#113110=CARTESIAN_POINT('Ctrl Pts',(1.74783797284851,-31.2941362849517,
53.9428460046709));
#113111=CARTESIAN_POINT('Ctrl Pts',(1.75900569603257,-31.1684067593939,
53.8112514110225));
#113112=CARTESIAN_POINT('Ctrl Pts',(1.762244451456,-31.1304737551301,53.7751220930884));
#113113=CARTESIAN_POINT('Ctrl Pts',(1.7674401334203,-31.0686766339808,53.7215825064583));
#113114=CARTESIAN_POINT('Ctrl Pts',(1.76933604140751,-31.045942990068,53.702917100652));
#113115=CARTESIAN_POINT('Ctrl Pts',(1.7719035484822,-31.0151338353942,53.6789580366621));
#113116=CARTESIAN_POINT('Ctrl Pts',(1.77254058547048,-31.0074878766252,
53.673117661519));
#113117=CARTESIAN_POINT('Ctrl Pts',(1.77360239123595,-30.9947504309796,
53.6635617099247));
#113118=CARTESIAN_POINT('Ctrl Pts',(1.77402458427284,-30.9896875355378,
53.6598081098155));
#113119=CARTESIAN_POINT('Ctrl Pts',(1.7748810234561,-30.9794239757351,53.6522886422584));
#113120=CARTESIAN_POINT('Ctrl Pts',(1.77531532900213,-30.9742226225317,
53.6485239527666));
#113121=CARTESIAN_POINT('Ctrl Pts',(1.77644280925468,-30.9607249784893,
53.6388728957903));
#113122=CARTESIAN_POINT('Ctrl Pts',(1.7771389361446,-30.9523964487101,53.6330323816554));
#113123=CARTESIAN_POINT('Ctrl Pts',(1.78001289075266,-30.9180127465532,
53.6093870127789));
#113124=CARTESIAN_POINT('Ctrl Pts',(1.78222819415428,-30.8915093582224,
53.5922490831907));
#113125=CARTESIAN_POINT('Ctrl Pts',(1.79220598298561,-30.7715131215519,
53.5194034597294));
#113126=CARTESIAN_POINT('Ctrl Pts',(1.80022484751124,-30.6731817972066,
53.4721830317116));
#113127=CARTESIAN_POINT('Ctrl Pts',(1.81221881958467,-30.5170898176883,
53.4152410410755));
#113128=CARTESIAN_POINT('Ctrl Pts',(1.81630861242007,-30.4622483300041,
53.3983850611159));
#113129=CARTESIAN_POINT('Ctrl Pts',(1.82295747958886,-30.3700317537936,
53.3751745533046));
#113130=CARTESIAN_POINT('Ctrl Pts',(1.8255607791396,-30.333116416724,53.367206357309));
#113131=CARTESIAN_POINT('Ctrl Pts',(1.82915186403274,-30.2810740499241,
53.3578117721664));
#113132=CARTESIAN_POINT('Ctrl Pts',(1.83017257370876,-30.2661522825533,
53.3553274532956));
#113133=CARTESIAN_POINT('Ctrl Pts',(1.8319189010864,-30.2404059490489,53.3514005445967));
#113134=CARTESIAN_POINT('Ctrl Pts',(1.83264754870688,-30.2295974517406,
53.3498605499463));
#113135=CARTESIAN_POINT('Ctrl Pts',(1.8340392244325,-30.2088310859813,53.3471097491684));
#113136=CARTESIAN_POINT('Ctrl Pts',(1.83470274295007,-30.1988759289686,
53.3458824176942));
#113137=CARTESIAN_POINT('Ctrl Pts',(1.83643933543539,-30.1726833119128,
53.3428931198305));
#113138=CARTESIAN_POINT('Ctrl Pts',(1.83750771980573,-30.1564297106569,
53.3412798562905));
#113139=CARTESIAN_POINT('Ctrl Pts',(1.84136744435496,-30.0972416953909,
53.3362828696846));
#113140=CARTESIAN_POINT('Ctrl Pts',(1.84411471653995,-30.0542020692733,
53.3343249844645));
#113141=CARTESIAN_POINT('Ctrl Pts',(1.8540445815078,-29.8963276800815,53.3332700731374));
#113142=CARTESIAN_POINT('Ctrl Pts',(1.8609433174609,-29.7817540046521,53.3443714336091));
#113143=CARTESIAN_POINT('Ctrl Pts',(1.87097680323465,-29.6218425238484,
53.3767653787616));
#113144=CARTESIAN_POINT('Ctrl Pts',(1.87397762291709,-29.5748986522819,
53.3884225391352));
#113145=CARTESIAN_POINT('Ctrl Pts',(1.87883478097776,-29.501721712393,53.4100138071475));
#113146=CARTESIAN_POINT('Ctrl Pts',(1.88063928356007,-29.4751169833749,
53.418597158505));
#113147=CARTESIAN_POINT('Ctrl Pts',(1.88310071464198,-29.4398260357812,
53.4309715073326));
#113148=CARTESIAN_POINT('Ctrl Pts',(1.88372657702852,-29.4309364430022,
53.4341737201425));
#113149=CARTESIAN_POINT('Ctrl Pts',(1.88477479559862,-29.4161970469491,
53.4396252416666));
#113150=CARTESIAN_POINT('Ctrl Pts',(1.88519471164361,-29.4103316638861,
53.4418323178598));
#113151=CARTESIAN_POINT('Ctrl Pts',(1.88599904600432,-29.3991746295811,
53.4461025993532));
#113152=CARTESIAN_POINT('Ctrl Pts',(1.88638308493371,-29.3938808279137,
53.4481598651098));
#113153=CARTESIAN_POINT('Ctrl Pts',(1.88742247861135,-29.3796397709683,
53.4537781785265));
#113154=CARTESIAN_POINT('Ctrl Pts',(1.8880807219464,-29.3707128677528,53.4573897352087));
#113155=CARTESIAN_POINT('Ctrl Pts',(1.89061139769923,-29.3367229548156,
53.4714851566882));
#113156=CARTESIAN_POINT('Ctrl Pts',(1.8925113448145,-29.3118878457891,53.4825035335824));
#113157=CARTESIAN_POINT('Ctrl Pts',(1.90232689287817,-29.1865087707893,
53.5418399197771));
#113158=CARTESIAN_POINT('Ctrl Pts',(1.91054975613207,-29.0907330446859,
53.5995601913861));
#113159=CARTESIAN_POINT('Ctrl Pts',(1.92287923202993,-28.9541497866542,
53.7018303857256));
#113160=CARTESIAN_POINT('Ctrl Pts',(1.92709931101957,-28.9087678960131,
53.7397378488051));
#113161=CARTESIAN_POINT('Ctrl Pts',(1.93306883925825,-28.846292181743,53.7978345760744));
#113162=CARTESIAN_POINT('Ctrl Pts',(1.93488620282228,-28.8275151795685,
53.8161406703138));
#113163=CARTESIAN_POINT('Ctrl Pts',(1.93814323006128,-28.7943118953648,
53.8500765214844));
#113164=CARTESIAN_POINT('Ctrl Pts',(1.93958896378713,-28.7797381701592,
53.8655534603913));
#113165=CARTESIAN_POINT('Ctrl Pts',(1.94184293614615,-28.7572882929765,
53.8903280402484));
#113166=CARTESIAN_POINT('Ctrl Pts',(1.94265958481592,-28.7492115339136,
53.8994399281399));
#113167=CARTESIAN_POINT('Ctrl Pts',(1.94418451565449,-28.7342411759457,
53.9167066003439));
#113168=CARTESIAN_POINT('Ctrl Pts',(1.94489372217523,-28.7273247206171,
53.9248406477522));
#113169=CARTESIAN_POINT('Ctrl Pts',(1.94648457654274,-28.7119174661925,
53.9433172541798));
#113170=CARTESIAN_POINT('Ctrl Pts',(1.9473643560252,-28.7034720497542,53.9536968265269));
#113171=CARTESIAN_POINT('Ctrl Pts',(1.94962493590604,-28.6819764386631,
53.9807752986874));
#113172=CARTESIAN_POINT('Ctrl Pts',(1.95099819348587,-28.669117935779,53.9976237752586));
#113173=CARTESIAN_POINT('Ctrl Pts',(1.96048448451935,-28.581819184619,54.11665368373));
#113174=CARTESIAN_POINT('Ctrl Pts',(1.96813527651343,-28.5188990470452,
54.2267722058592));
#113175=CARTESIAN_POINT('Ctrl Pts',(1.9811030231244,-28.435283548501,54.4216031967692));
#113176=CARTESIAN_POINT('Ctrl Pts',(1.98636858792426,-28.4076456044622,
54.5027233223497));
#113177=CARTESIAN_POINT('Ctrl Pts',(1.99285439274383,-28.3828589393575,
54.5992391735961));
#113178=CARTESIAN_POINT('Ctrl Pts',(1.99377933897153,-28.3795281878337,
54.6129269787273));
#113179=CARTESIAN_POINT('Ctrl Pts',(1.99519486431358,-28.3747455891304,
54.6337258630041));
#113180=CARTESIAN_POINT('Ctrl Pts',(1.99567856583511,-28.3731658846417,
54.6408072945396));
#113181=CARTESIAN_POINT('Ctrl Pts',(1.99656783200992,-28.3703621506975,
54.6537737577348));
#113182=CARTESIAN_POINT('Ctrl Pts',(1.99697257868926,-28.3691236488181,
54.6596553891418));
#113183=CARTESIAN_POINT('Ctrl Pts',(1.99790425559076,-28.366358485514,54.6731488548685));
#113184=CARTESIAN_POINT('Ctrl Pts',(1.99843233794233,-28.3648531863368,
54.6807647252102));
#113185=CARTESIAN_POINT('Ctrl Pts',(2.00006589113265,-28.3603848585366,
54.7042327622797));
#113186=CARTESIAN_POINT('Ctrl Pts',(2.00118036224702,-28.3575988311037,
54.7201171251284));
#113187=CARTESIAN_POINT('Ctrl Pts',(2.00843431037383,-28.3411136633396,
54.8228495109306));
#113188=CARTESIAN_POINT('Ctrl Pts',(2.01483590118353,-28.3340785096767,
54.9106190072649));
#113189=CARTESIAN_POINT('Ctrl Pts',(2.02993613776549,-28.3338947857698,
55.1180568449114));
#113190=CARTESIAN_POINT('Ctrl Pts',(2.03856942696008,-28.3466535323101,
55.2372744075942));
#113191=CARTESIAN_POINT('Ctrl Pts',(2.04830033618961,-28.3766865549533,
55.3753416420334));
#113192=CARTESIAN_POINT('Ctrl Pts',(2.0497835389115,-28.3817187648502,55.3964767460031));
#113193=CARTESIAN_POINT('Ctrl Pts',(2.05216951937095,-28.3905550413753,
55.4306113334118));
#113194=CARTESIAN_POINT('Ctrl Pts',(2.0530802414723,-28.3941066103615,55.4436728921056));
#113195=CARTESIAN_POINT('Ctrl Pts',(2.05470106395927,-28.400747566364,55.4669710265837));
#113196=CARTESIAN_POINT('Ctrl Pts',(2.05541305864357,-28.4037770236732,
55.4772237474747));
#113197=CARTESIAN_POINT('Ctrl Pts',(2.05692245471112,-28.4104380414905,
55.498993577318));
#113198=CARTESIAN_POINT('Ctrl Pts',(2.05771893068484,-28.4140965693085,
55.5105018428584));
#113199=CARTESIAN_POINT('Ctrl Pts',(2.05975208248151,-28.4238030084701,
55.5399226223487));
#113200=CARTESIAN_POINT('Ctrl Pts',(2.06098279722393,-28.4300313320395,
55.557773979529));
#113201=CARTESIAN_POINT('Ctrl Pts',(2.06220428404731,-28.4365623101862,
55.5755159338105));
#113202=CARTESIAN_POINT('',(1.82701798699663,-28.334000473818,54.999675424517));
#113203=CARTESIAN_POINT('Ctrl Pts',(1.86810673741825,-28.4365624617974,
55.5755163456748));
#113204=CARTESIAN_POINT('Ctrl Pts',(1.86162183563071,-28.4057809308945,
55.4918957825778));
#113205=CARTESIAN_POINT('Ctrl Pts',(1.85513252908068,-28.3817289129791,
55.405861033452));
#113206=CARTESIAN_POINT('Ctrl Pts',(1.84519626206848,-28.3549112155355,
55.2680536719336));
#113207=CARTESIAN_POINT('Ctrl Pts',(1.84163835190104,-28.3474595851737,
55.2174419664774));
#113208=CARTESIAN_POINT('Ctrl Pts',(1.83699847475443,-28.3406553066266,
55.1497249555348));
#113209=CARTESIAN_POINT('Ctrl Pts',(1.83585277227586,-28.339220020485,55.1328618458178));
#113210=CARTESIAN_POINT('Ctrl Pts',(1.83394918425833,-28.3372487394932,
55.1046138034724));
#113211=CARTESIAN_POINT('Ctrl Pts',(1.83318696520669,-28.3365721954689,
55.0932402941342));
#113212=CARTESIAN_POINT('Ctrl Pts',(1.83175229460624,-28.3355134147814,
55.0717183369838));
#113213=CARTESIAN_POINT('Ctrl Pts',(1.83107912628968,-28.3351071949762,
55.0615716475465));
#113214=CARTESIAN_POINT('Ctrl Pts',(1.82982343023142,-28.3345200432967,
55.0425577109211));
#113215=CARTESIAN_POINT('Ctrl Pts',(1.82924024488316,-28.3343170982553,
55.0336915544102));
#113216=CARTESIAN_POINT('Ctrl Pts',(1.82810993935358,-28.3340600375524,
55.0164415288973));
#113217=CARTESIAN_POINT('Ctrl Pts',(1.82756260927594,-28.3339983934517,
55.0080580818904));
#113218=CARTESIAN_POINT('Ctrl Pts',(1.82701715464812,-28.3340000318124,
54.9996744250059));
#113219=CARTESIAN_POINT('Ctrl Pts',(1.82701722290713,-28.3340000316078,
54.9996754741491));
#113220=CARTESIAN_POINT('Ctrl Pts',(1.82545459593269,-28.3340047100833,
54.9756578493269));
#113221=CARTESIAN_POINT('Ctrl Pts',(1.82390764189692,-28.3345287558541,
54.9516419897929));
#113222=CARTESIAN_POINT('Ctrl Pts',(1.81315018159099,-28.3418484033513,
54.7832643812592));
#113223=CARTESIAN_POINT('Ctrl Pts',(1.80453968563037,-28.3668823381416,
54.6403221171576));
#113224=CARTESIAN_POINT('Ctrl Pts',(1.79300176085031,-28.4226849666057,
54.4620188620413));
#113225=CARTESIAN_POINT('Ctrl Pts',(1.79036101234513,-28.4368561165743,
54.4221357064352));
#113226=CARTESIAN_POINT('Ctrl Pts',(1.78602430489043,-28.4620122921717,
54.359059143433));
#113227=CARTESIAN_POINT('Ctrl Pts',(1.78436761316333,-28.4720419925298,
54.3355035531236));
#113228=CARTESIAN_POINT('Ctrl Pts',(1.78207864037288,-28.4863870643553,
54.303856628424));
#113229=CARTESIAN_POINT('Ctrl Pts',(1.78147216978569,-28.490232909638,54.2955548026208));
#113230=CARTESIAN_POINT('Ctrl Pts',(1.78044744986378,-28.4968017594048,
54.2816758642341));
#113231=CARTESIAN_POINT('Ctrl Pts',(1.78003141074779,-28.4994879777933,
54.2760813690753));
#113232=CARTESIAN_POINT('Ctrl Pts',(1.77922668688876,-28.5047191620114,
54.2653407773242));
#113233=CARTESIAN_POINT('Ctrl Pts',(1.77883831547864,-28.5072595651708,
54.2601926266778));
#113234=CARTESIAN_POINT('Ctrl Pts',(1.77777216609402,-28.5142776829682,
54.246153667092));
#113235=CARTESIAN_POINT('Ctrl Pts',(1.77709124111117,-28.5188084708371,
54.2372898724368));
#113236=CARTESIAN_POINT('Ctrl Pts',(1.77435944763071,-28.5371877492326,
54.2021150661963));
#113237=CARTESIAN_POINT('Ctrl Pts',(1.77227541512984,-28.5516592441943,
54.176137848277));
#113238=CARTESIAN_POINT('Ctrl Pts',(1.76236681954623,-28.6228628248663,
54.0560019743048));
#113239=CARTESIAN_POINT('Ctrl Pts',(1.75426551738015,-28.6881281584836,
53.9672217407039));
#113240=CARTESIAN_POINT('Ctrl Pts',(1.74213391251971,-28.8005049419681,
53.8423561157109));
#113241=CARTESIAN_POINT('Ctrl Pts',(1.73798949091869,-28.8415820610622,
53.8012520011758));
#113242=CARTESIAN_POINT('Ctrl Pts',(1.73211361606381,-28.9039918434947,
53.7450120573343));
#113243=CARTESIAN_POINT('Ctrl Pts',(1.73031659305481,-28.9236617508805,
53.7281019242605));
#113244=CARTESIAN_POINT('Ctrl Pts',(1.72749016375896,-28.9555309877658,
53.7019731222036));
#113245=CARTESIAN_POINT('Ctrl Pts',(1.72644902278615,-28.967475491935,53.692451736991));
#113246=CARTESIAN_POINT('Ctrl Pts',(1.72446900398966,-28.9905816965725,
53.6745470681092));
#113247=CARTESIAN_POINT('Ctrl Pts',(1.723529133526,-29.0017210593077,53.6661372022929));
#113248=CARTESIAN_POINT('Ctrl Pts',(1.72187605247386,-29.0216130206805,
53.6515081929718));
#113249=CARTESIAN_POINT('Ctrl Pts',(1.72116065031392,-29.0303223889424,
53.64523191106));
#113250=CARTESIAN_POINT('Ctrl Pts',(1.71966350028497,-29.0487577170484,
53.6322156166884));
#113251=CARTESIAN_POINT('Ctrl Pts',(1.71888248749652,-29.0584960754086,
53.6254941352461));
#113252=CARTESIAN_POINT('Ctrl Pts',(1.71681510708784,-29.0845901064971,
53.6078913120709));
#113253=CARTESIAN_POINT('Ctrl Pts',(1.71553566132635,-29.101068330534,53.5971943189823));
#113254=CARTESIAN_POINT('Ctrl Pts',(1.70892850342153,-29.1877984928466,
53.5430486125507));
#113255=CARTESIAN_POINT('Ctrl Pts',(1.70378418414734,-29.2610249375565,
53.5045746495378));
#113256=CARTESIAN_POINT('Ctrl Pts',(1.69256312457214,-29.4286294051293,
53.4318451480556));
#113257=CARTESIAN_POINT('Ctrl Pts',(1.68654448256831,-29.5238448176661,
53.4003600724119));
#113258=CARTESIAN_POINT('Ctrl Pts',(1.67849823295412,-29.6488286995577,
53.3711864298665));
#113259=CARTESIAN_POINT('Ctrl Pts',(1.67670630962728,-29.6765116430934,
53.3654633588148));
#113260=CARTESIAN_POINT('Ctrl Pts',(1.67364031922123,-29.7233143455223,
53.3570230171086));
#113261=CARTESIAN_POINT('Ctrl Pts',(1.6723825597674,-29.7423606414123,53.353928859136));
#113262=CARTESIAN_POINT('Ctrl Pts',(1.67056493028423,-29.7695846220246,
53.3499902358845));
#113263=CARTESIAN_POINT('Ctrl Pts',(1.67001909855973,-29.7777222584166,
53.3488743031841));
#113264=CARTESIAN_POINT('Ctrl Pts',(1.66906527695937,-29.7918696053892,
53.3470407240329));
#113265=CARTESIAN_POINT('Ctrl Pts',(1.66865881543818,-29.7978755138257,
53.3462955766185));
#113266=CARTESIAN_POINT('Ctrl Pts',(1.66778162367742,-29.8107857417327,
53.3447651989941));
#113267=CARTESIAN_POINT('Ctrl Pts',(1.66731036749063,-29.8176908487408,
53.3439904435792));
#113268=CARTESIAN_POINT('Ctrl Pts',(1.66600025365635,-29.8368083497858,
53.341966469347));
#113269=CARTESIAN_POINT('Ctrl Pts',(1.66515664924455,-29.8490297284857,
53.3408090349567));
#113270=CARTESIAN_POINT('Ctrl Pts',(1.6592169541169,-29.934537538994,53.3336634738373));
#113271=CARTESIAN_POINT('Ctrl Pts',(1.65391681879628,-30.0081299795949,
53.332398651033));
#113272=CARTESIAN_POINT('Ctrl Pts',(1.64756637559429,-30.0954316173639,
53.3366774825345));
#113273=CARTESIAN_POINT('Ctrl Pts',(1.6465556910797,-30.1092979591638,53.3375310699811));
#113274=CARTESIAN_POINT('Ctrl Pts',(1.64017849207702,-30.1966772738093,
53.344007932512));
#113275=CARTESIAN_POINT('Ctrl Pts',(1.63481225275999,-30.2697644061377,
53.3543329137724));
#113276=CARTESIAN_POINT('Ctrl Pts',(1.62652043124555,-30.3834887613324,
53.3781814539819));
#113277=CARTESIAN_POINT('Ctrl Pts',(1.62352679304667,-30.4247011320883,
53.3884825549899));
#113278=CARTESIAN_POINT('Ctrl Pts',(1.61845723681767,-30.4948365980091,
53.4088910587602));
#113279=CARTESIAN_POINT('Ctrl Pts',(1.61635987529078,-30.5239561804558,
53.4182411512532));
#113280=CARTESIAN_POINT('Ctrl Pts',(1.61334194993097,-30.5659846040451,
53.4330243583449));
#113281=CARTESIAN_POINT('Ctrl Pts',(1.6124009718399,-30.5791070675546,53.4378264313719));
#113282=CARTESIAN_POINT('Ctrl Pts',(1.61074663871965,-30.6022036257754,
53.446609491173));
#113283=CARTESIAN_POINT('Ctrl Pts',(1.61003108089109,-30.61220240098,53.4505228271049));
#113284=CARTESIAN_POINT('Ctrl Pts',(1.60853428473231,-30.6331316275402,
53.4589483607161));
#113285=CARTESIAN_POINT('Ctrl Pts',(1.60775377493972,-30.6440533139186,
53.463480831979));
#113286=CARTESIAN_POINT('Ctrl Pts',(1.6056893188338,-30.6729537060661,53.4758367181291));
#113287=CARTESIAN_POINT('Ctrl Pts',(1.60441225858804,-30.6908444744905,
53.483862023093));
#113288=CARTESIAN_POINT('Ctrl Pts',(1.59780144012474,-30.7834256033647,
53.5273705345931));
#113289=CARTESIAN_POINT('Ctrl Pts',(1.592651598315,-30.8555439458057,53.5680641524787));
#113290=CARTESIAN_POINT('Ctrl Pts',(1.58142600451561,-31.007609306604,53.669475746203));
#113291=CARTESIAN_POINT('Ctrl Pts',(1.57540813560007,-31.0856912252472,
53.732386680518));
#113292=CARTESIAN_POINT('Ctrl Pts',(1.56736281516442,-31.1779768935513,
53.8215581169088));
#113293=CARTESIAN_POINT('Ctrl Pts',(1.56557099432716,-31.197798120355,53.8417106076669));
#113294=CARTESIAN_POINT('Ctrl Pts',(1.56250516123563,-31.2302716121272,
53.8764520276478));
#113295=CARTESIAN_POINT('Ctrl Pts',(1.56124745438774,-31.2432006320562,
53.8907748666653));
#113296=CARTESIAN_POINT('Ctrl Pts',(1.55942988734562,-31.2612743516383,
53.9115100019598));
#113297=CARTESIAN_POINT('Ctrl Pts',(1.55888406410575,-31.2666253817316,
53.9177414351029));
#113298=CARTESIAN_POINT('Ctrl Pts',(1.55793025420933,-31.2758387673183,
53.9286326174512));
#113299=CARTESIAN_POINT('Ctrl Pts',(1.55752379583824,-31.2797221643495,
53.9332742576878));
#113300=CARTESIAN_POINT('Ctrl Pts',(1.55664661161026,-31.2880098899131,
53.9432905770505));
#113301=CARTESIAN_POINT('Ctrl Pts',(1.55617535981127,-31.2924058454848,
53.948671598777));
#113302=CARTESIAN_POINT('Ctrl Pts',(1.55486524594626,-31.3044749452165,
53.9636352851151));
#113303=CARTESIAN_POINT('Ctrl Pts',(1.55402163691192,-31.3120758486463,
53.9732752802004));
#113304=CARTESIAN_POINT('Ctrl Pts',(1.5480786297716,-31.3644848040678,54.0412763733764));
#113305=CARTESIAN_POINT('Ctrl Pts',(1.54277491849894,-31.40548547083,54.1024600486782));
#113306=CARTESIAN_POINT('Ctrl Pts',(1.53642362639942,-31.4492389004914,
54.1781395662555));
#113307=CARTESIAN_POINT('Ctrl Pts',(1.53541563133018,-31.4560236223852,
54.1902202948951));
#113308=CARTESIAN_POINT('Ctrl Pts',(1.52904087508932,-31.4979560207691,
54.2671153463555));
#113309=CARTESIAN_POINT('Ctrl Pts',(1.5236744067401,-31.5289213978872,54.3341225103229));
#113310=CARTESIAN_POINT('Ctrl Pts',(1.51538286771513,-31.5705614975592,
54.442599739866));
#113311=CARTESIAN_POINT('Ctrl Pts',(1.51238970901964,-31.5842563859728,
54.4828049963383));
#113312=CARTESIAN_POINT('Ctrl Pts',(1.50732087084965,-31.6051455920761,
54.552788265643));
#113313=CARTESIAN_POINT('Ctrl Pts',(1.50522375552059,-31.613082435228,54.5823207244749));
#113314=CARTESIAN_POINT('Ctrl Pts',(1.50220612315584,-31.6234559173839,
54.6256444245092));
#113315=CARTESIAN_POINT('Ctrl Pts',(1.50126519680947,-31.626538414856,54.6392729310961));
#113316=CARTESIAN_POINT('Ctrl Pts',(1.49961093247191,-31.6316858303462,
54.6634400120583));
#113317=CARTESIAN_POINT('Ctrl Pts',(1.49889539207807,-31.6338209569508,
54.6739626335194));
#113318=CARTESIAN_POINT('Ctrl Pts',(1.49739861112907,-31.6380934496863,
54.6961157064468));
#113319=CARTESIAN_POINT('Ctrl Pts',(1.49661809930098,-31.6402090236074,
54.7077497907877));
#113320=CARTESIAN_POINT('Ctrl Pts',(1.49455358906428,-31.6455028833275,
54.7387325252692));
#113321=CARTESIAN_POINT('Ctrl Pts',(1.49327647768644,-31.6484638307345,
54.7581167971921));
#113322=CARTESIAN_POINT('Ctrl Pts',(1.48666342347386,-31.6621272788716,
54.85953025339));
#113323=CARTESIAN_POINT('Ctrl Pts',(1.48151156671246,-31.6670523059732,
54.9422250182093));
#113324=CARTESIAN_POINT('Ctrl Pts',(1.47028582541274,-31.6643146832485,
55.1249884167226));
#113325=CARTESIAN_POINT('Ctrl Pts',(1.46426964397116,-31.6538084112718,
55.2246794791036));
#113326=CARTESIAN_POINT('Ctrl Pts',(1.45622635190676,-31.628948715306,55.3505434407319));
#113327=CARTESIAN_POINT('Ctrl Pts',(1.45443476177725,-31.6227685955833,
55.3781223692615));
#113328=CARTESIAN_POINT('Ctrl Pts',(1.45136928620479,-31.6111943438156,
55.4242416742124));
#113329=CARTESIAN_POINT('Ctrl Pts',(1.45011170165141,-31.6061737456621,
55.4428702209807));
#113330=CARTESIAN_POINT('Ctrl Pts',(1.44829428500646,-31.5985563452328,
55.4692984877839));
#113331=CARTESIAN_POINT('Ctrl Pts',(1.44774848710103,-31.5962233413036,
55.4771734456194));
#113332=CARTESIAN_POINT('Ctrl Pts',(1.44679470863462,-31.5920702998738,
55.4908205249506));
#113333=CARTESIAN_POINT('Ctrl Pts',(1.44638825612012,-31.590276884126,55.4966005013321));
#113334=CARTESIAN_POINT('Ctrl Pts',(1.44551106694425,-31.5863566544626,
55.5089959214516));
#113335=CARTESIAN_POINT('Ctrl Pts',(1.44503980417734,-31.5842199678471,
55.5156077698054));
#113336=CARTESIAN_POINT('Ctrl Pts',(1.44372963375321,-31.5781938671376,
55.533864063917));
#113337=CARTESIAN_POINT('Ctrl Pts',(1.4428859784995,-31.5742170946578,55.5454789068228));
#113338=CARTESIAN_POINT('Ctrl Pts',(1.43693167733926,-31.545456337168,55.6265448101438));
#113339=CARTESIAN_POINT('Ctrl Pts',(1.43161582018813,-31.5162159050044,
55.6943202488002));
#113340=CARTESIAN_POINT('Ctrl Pts',(1.42526178333954,-31.4763256382389,
55.7721444531892));
#113341=CARTESIAN_POINT('Ctrl Pts',(1.42426305371873,-31.4699132207546,
55.7842828359576));
#113342=CARTESIAN_POINT('Ctrl Pts',(1.41789691160616,-31.4281045777199,
55.8611101992064));
#113343=CARTESIAN_POINT('Ctrl Pts',(1.41252985279945,-31.3885940690259,
55.9234724087597));
#113344=CARTESIAN_POINT('Ctrl Pts',(1.40423951896968,-31.3200424791767,
56.0172729969052));
#113345=CARTESIAN_POINT('Ctrl Pts',(1.40124805728931,-31.2937042856933,
56.0505647139523));
#113346=CARTESIAN_POINT('Ctrl Pts',(1.39618173151308,-31.2462585178706,
56.1060423491436));
#113347=CARTESIAN_POINT('Ctrl Pts',(1.39408546079869,-31.2257590757972,
56.1287182430763));
#113348=CARTESIAN_POINT('Ctrl Pts',(1.39106879197606,-31.1949962423499,
56.1609199531276));
#113349=CARTESIAN_POINT('Ctrl Pts',(1.39012800336942,-31.185219404729,56.1708997139368));
#113350=CARTESIAN_POINT('Ctrl Pts',(1.38847388694842,-31.1677086170226,
56.1883298603443));
#113351=CARTESIAN_POINT('Ctrl Pts',(1.38775835822321,-31.1600261138563,
56.1958305463998));
#113352=CARTESIAN_POINT('Ctrl Pts',(1.38626150947457,-31.1437305898784,
56.2114355866072));
#113353=CARTESIAN_POINT('Ctrl Pts',(1.3854809190765,-31.1351026778822,56.2195235813728));
#113354=CARTESIAN_POINT('Ctrl Pts',(1.38341598425799,-31.1119387311018,
56.2407791504558));
#113355=CARTESIAN_POINT('Ctrl Pts',(1.38213853180769,-31.0972547860331,
56.253783326236));
#113356=CARTESIAN_POINT('Ctrl Pts',(1.37551361237887,-31.0193215770003,
56.3203832809695));
#113357=CARTESIAN_POINT('Ctrl Pts',(1.3703511082947,-30.9523631047568,56.3694654113419));
#113358=CARTESIAN_POINT('Ctrl Pts',(1.35912473791162,-30.7972790047845,
56.4662469516713));
#113359=CARTESIAN_POINT('Ctrl Pts',(1.35311761352187,-30.7079582197976,
56.511398940935));
#113360=CARTESIAN_POINT('Ctrl Pts',(1.34508522170745,-30.5888933548515,
56.5587039859287));
#113361=CARTESIAN_POINT('Ctrl Pts',(1.34329484229251,-30.562389398754,56.568461502123));
#113362=CARTESIAN_POINT('Ctrl Pts',(1.34023122512766,-30.5173927026961,
56.5837400752557));
#113363=CARTESIAN_POINT('Ctrl Pts',(1.33897426179721,-30.4990282418087,
56.589622147231));
#113364=CARTESIAN_POINT('Ctrl Pts',(1.33715758004984,-30.4727039996028,
56.5975526168379));
#113365=CARTESIAN_POINT('Ctrl Pts',(1.33661187967724,-30.4648239866077,
56.5998631470506));
#113366=CARTESIAN_POINT('Ctrl Pts',(1.33565819654879,-30.4511074010679,
56.6037751527371));
#113367=CARTESIAN_POINT('Ctrl Pts',(1.33525174054363,-30.4452786617929,
56.6054032327856));
#113368=CARTESIAN_POINT('Ctrl Pts',(1.33437444193052,-30.4327369789256,
56.6088328104112));
#113369=CARTESIAN_POINT('Ctrl Pts',(1.33390307222236,-30.4260216964146,
56.6106240450719));
#113370=CARTESIAN_POINT('Ctrl Pts',(1.33259240895874,-30.4074084651998,
56.6154643917785));
#113371=CARTESIAN_POINT('Ctrl Pts',(1.33174836305431,-30.395487982673,56.6184239531236));
#113372=CARTESIAN_POINT('Ctrl Pts',(1.32569201328955,-30.310347850174,56.6385653906965));
#113373=CARTESIAN_POINT('Ctrl Pts',(1.32026632864406,-30.2360787506473,
56.6509017665711));
#113374=CARTESIAN_POINT('Ctrl Pts',(1.31071174694016,-30.105230094,56.6636253733694));
#113375=CARTESIAN_POINT('Ctrl Pts',(1.30660505217434,-30.0489791341576,
56.6662304853437));
#113376=CARTESIAN_POINT('Ctrl Pts',(1.29818034983908,-29.9324625332999,
56.6657201918926));
#113377=CARTESIAN_POINT('Ctrl Pts',(1.293874257319,-29.8722753298122,56.6621891322544));
#113378=CARTESIAN_POINT('Ctrl Pts',(1.28692486917766,-29.7736355106187,
56.6510110881028));
#113379=CARTESIAN_POINT('Ctrl Pts',(1.28423188850251,-29.7350282983485,
56.645256493113));
#113380=CARTESIAN_POINT('Ctrl Pts',(1.28054109828775,-29.681604535636,56.6353637637584));
#113381=CARTESIAN_POINT('Ctrl Pts',(1.27950785663442,-29.6665918837104,
56.6323692494965));
#113382=CARTESIAN_POINT('Ctrl Pts',(1.2777469913615,-29.6409172469014,56.626879040463));
#113383=CARTESIAN_POINT('Ctrl Pts',(1.27701620246075,-29.6302349127606,
56.6244844185117));
#113384=CARTESIAN_POINT('Ctrl Pts',(1.27562499871827,-29.6098515305301,
56.6197036624504));
#113385=CARTESIAN_POINT('Ctrl Pts',(1.27496405197059,-29.6001468640776,
56.6173352340937));
#113386=CARTESIAN_POINT('Ctrl Pts',(1.27341518106666,-29.5773607253018,
56.6115566322762));
#113387=CARTESIAN_POINT('Ctrl Pts',(1.27252960892119,-29.5642981700632,
56.6080742111692));
#113388=CARTESIAN_POINT('Ctrl Pts',(1.26941814569736,-29.518301895172,56.5952101729372));
#113389=CARTESIAN_POINT('Ctrl Pts',(1.26721970094342,-29.4856152201851,
56.5849722758909));
#113390=CARTESIAN_POINT('Ctrl Pts',(1.25644329243025,-29.3251037661909,
56.529208605666));
#113391=CARTESIAN_POINT('Ctrl Pts',(1.248346180035,-29.2028665800843,56.4691978589594));
#113392=CARTESIAN_POINT('Ctrl Pts',(1.23734904010953,-29.0537438296414,
56.3718433069069));
#113393=CARTESIAN_POINT('Ctrl Pts',(1.23470237003611,-29.0191304515592,
56.3473118598639));
#113394=CARTESIAN_POINT('Ctrl Pts',(1.23035701783487,-28.9651548660094,
56.3058747946619));
#113395=CARTESIAN_POINT('Ctrl Pts',(1.22869779540035,-28.94518109911,56.2897946913068));
#113396=CARTESIAN_POINT('Ctrl Pts',(1.22640585725787,-28.9185909337418,
56.2673571883539));
#113397=CARTESIAN_POINT('Ctrl Pts',(1.22579903730385,-28.911643200382,56.2613957660774));
#113398=CARTESIAN_POINT('Ctrl Pts',(1.22477389829932,-28.9000679651241,
56.2512969456098));
#113399=CARTESIAN_POINT('Ctrl Pts',(1.22435779357978,-28.8954136839243,
56.2471902806685));
#113400=CARTESIAN_POINT('Ctrl Pts',(1.22349866152291,-28.8858970352757,
56.23869829113));
#113401=CARTESIAN_POINT('Ctrl Pts',(1.22305544590985,-28.8810374233475,
56.2343101801323));
#113402=CARTESIAN_POINT('Ctrl Pts',(1.22187836034643,-28.8682593442517,
56.2226344100305));
#113403=CARTESIAN_POINT('Ctrl Pts',(1.22114105218907,-28.860385560112,56.2152986158212));
#113404=CARTESIAN_POINT('Ctrl Pts',(1.21782200567632,-28.8254954723313,
56.1821552449488));
#113405=CARTESIAN_POINT('Ctrl Pts',(1.21518739896034,-28.7992827764792,
56.1555213468577));
#113406=CARTESIAN_POINT('Ctrl Pts',(1.20585345298221,-28.7108156574795,
56.0593701281318));
#113407=CARTESIAN_POINT('Ctrl Pts',(1.19900163014399,-28.6535225746133,
55.9855249726162));
#113408=CARTESIAN_POINT('Ctrl Pts',(1.18770474561607,-28.5685446476298,
55.8546509067454));
#113409=CARTESIAN_POINT('Ctrl Pts',(1.18321236827063,-28.5373735321406,
55.8001360995782));
#113410=CARTESIAN_POINT('Ctrl Pts',(1.17690866172103,-28.4972007095769,
55.7196460339274));
#113411=CARTESIAN_POINT('Ctrl Pts',(1.17502064751211,-28.4856491628171,
55.6950092144419));
#113412=CARTESIAN_POINT('Ctrl Pts',(1.17165090234293,-28.4659090902918,
55.6500764368256));
#113413=CARTESIAN_POINT('Ctrl Pts',(1.17016244036602,-28.4575073397739,
55.629881548414));
#113414=CARTESIAN_POINT('Ctrl Pts',(1.16786921729795,-28.4450673872868,
55.5982371668454));
#113415=CARTESIAN_POINT('Ctrl Pts',(1.16705527994685,-28.440752793604,55.5868997362884));
#113416=CARTESIAN_POINT('Ctrl Pts',(1.16624546596859,-28.4365623102019,
55.575515933853));
#113417=CARTESIAN_POINT('Origin',(5.,-30.,55.));
#113418=CARTESIAN_POINT('',(0.468131487137801,-28.4365623373493,55.5755160076012));
#113419=CARTESIAN_POINT('',(0.659214745210771,-28.4365623102018,55.5755159338528));
#113420=CARTESIAN_POINT('',(5.,-28.4365623102018,55.5755159338528));
#113421=CARTESIAN_POINT('',(0.428519636557289,-28.3340004401721,55.0012110545587));
#113422=CARTESIAN_POINT('Ctrl Pts',(0.468131487137799,-28.4365623373493,
55.5755160076012));
#113423=CARTESIAN_POINT('Ctrl Pts',(0.464559665450955,-28.4163576335939,
55.5206282296826));
#113424=CARTESIAN_POINT('Ctrl Pts',(0.460978297772835,-28.3990503155309,
55.4646953498218));
#113425=CARTESIAN_POINT('Ctrl Pts',(0.454816291795371,-28.3750168253862,
55.369534079064));
#113426=CARTESIAN_POINT('Ctrl Pts',(0.452288494775125,-28.3666894253552,
55.3307896060807));
#113427=CARTESIAN_POINT('Ctrl Pts',(0.448975349890733,-28.3578371707525,
55.2810279403499));
#113428=CARTESIAN_POINT('Ctrl Pts',(0.448253722146548,-28.3560288899956,
55.2702488384788));
#113429=CARTESIAN_POINT('Ctrl Pts',(0.447089391460057,-28.3533044885334,
55.2529683566067));
#113430=CARTESIAN_POINT('Ctrl Pts',(0.446650389253277,-28.3523204816432,
55.2464777839124));
#113431=CARTESIAN_POINT('Ctrl Pts',(0.44582750414188,-28.3505568582534,
55.2343620528578));
#113432=CARTESIAN_POINT('Ctrl Pts',(0.445444173184423,-28.3497675964323,
55.2287384104872));
#113433=CARTESIAN_POINT('Ctrl Pts',(0.44464178135063,-28.3481822399086,
55.2170069741934));
#113434=CARTESIAN_POINT('Ctrl Pts',(0.444222447831723,-28.3473912330323,
55.2108985532282));
#113435=CARTESIAN_POINT('Ctrl Pts',(0.443221768061731,-28.3455919301614,
55.1963716527654));
#113436=CARTESIAN_POINT('Ctrl Pts',(0.442638889947717,-28.3446140027119,
55.1879496748707));
#113437=CARTESIAN_POINT('Ctrl Pts',(0.440656114804364,-28.3415220427165,
55.1594225538021));
#113438=CARTESIAN_POINT('Ctrl Pts',(0.439242468058708,-28.3397097701379,
55.1392873099145));
#113439=CARTESIAN_POINT('Ctrl Pts',(0.435037745367989,-28.3354495891085,
55.0798599353537));
#113440=CARTESIAN_POINT('Ctrl Pts',(0.432212098543957,-28.3340275642907,
55.0405100936272));
#113441=CARTESIAN_POINT('Ctrl Pts',(0.429364773524748,-28.3340003968516,
55.0011499171688));
#113442=CARTESIAN_POINT('',(0.,-31.2690708798524,56.0793586530485));
#113443=CARTESIAN_POINT('Ctrl Pts',(0.428519636557289,-28.3340004401721,
55.0012110545587));
#113444=CARTESIAN_POINT('Ctrl Pts',(0.424501125412418,-28.3339569165041,
54.9413372767136));
#113445=CARTESIAN_POINT('Ctrl Pts',(0.420482614267547,-28.3371452968995,
54.8813422610129));
#113446=CARTESIAN_POINT('Ctrl Pts',(0.416464103122675,-28.3435783380043,
54.821609199589));
#113447=CARTESIAN_POINT('Ctrl Pts',(0.412450057461902,-28.3500042305304,
54.7619425152452));
#113448=CARTESIAN_POINT('Ctrl Pts',(0.408436011801128,-28.3596675898715,
54.7025377291128));
#113449=CARTESIAN_POINT('Ctrl Pts',(0.404421966140355,-28.3725291627882,
54.643777212934));
#113450=CARTESIAN_POINT('Ctrl Pts',(0.400410795178421,-28.3853815247612,
54.5850587786851));
#113451=CARTESIAN_POINT('Ctrl Pts',(0.396399624216488,-28.4014274513206,
54.5269842136769));
#113452=CARTESIAN_POINT('Ctrl Pts',(0.392388453254553,-28.4205762710958,
54.4699276609986));
#113453=CARTESIAN_POINT('Ctrl Pts',(0.388378570694002,-28.4397189402068,
54.4128894350737));
#113454=CARTESIAN_POINT('Ctrl Pts',(0.384368688133449,-28.4619623584441,
54.3568690721377));
#113455=CARTESIAN_POINT('Ctrl Pts',(0.380358805572897,-28.4871661075506,
54.3022252413161));
#113456=CARTESIAN_POINT('Ctrl Pts',(0.376345831298646,-28.51238928934,54.2475392788167));
#113457=CARTESIAN_POINT('Ctrl Pts',(0.372332857024395,-28.5405771449676,
54.1942324502499));
#113458=CARTESIAN_POINT('Ctrl Pts',(0.368319882750144,-28.5715418157655,
54.1426417225608));
#113459=CARTESIAN_POINT('Ctrl Pts',(0.364305505297722,-28.6025173136824,
54.0910329556375));
#113460=CARTESIAN_POINT('Ctrl Pts',(0.3602911278453,-28.6362712667164,54.0411419232217));
#113461=CARTESIAN_POINT('Ctrl Pts',(0.356276750392879,-28.6725724488726,
53.9932765541084));
#113462=CARTESIAN_POINT('Ctrl Pts',(0.352255019302422,-28.7089401284513,
53.9453235040028));
#113463=CARTESIAN_POINT('Ctrl Pts',(0.348233288211964,-28.7478640170129,
53.899403933109));
#113464=CARTESIAN_POINT('Ctrl Pts',(0.344211557121507,-28.7890732686805,
53.8557917797114));
#113465=CARTESIAN_POINT('Ctrl Pts',(0.340609642252897,-28.8259808124639,
53.8167321657687));
#113466=CARTESIAN_POINT('Ctrl Pts',(0.337007727384288,-28.86472077612,53.7795230582427));
#113467=CARTESIAN_POINT('Ctrl Pts',(0.333405812515678,-28.9050764107094,
53.7443335101966));
#113468=CARTESIAN_POINT('Ctrl Pts',(0.329325377332539,-28.9507933577289,
53.7044689728148));
#113469=CARTESIAN_POINT('Ctrl Pts',(0.325244942149401,-28.9987826271463,
53.6670238660387));
#113470=CARTESIAN_POINT('Ctrl Pts',(0.321164506966262,-29.0487579722144,
53.6322666178767));
#113471=CARTESIAN_POINT('Ctrl Pts',(0.317043925079215,-29.0992250161556,
53.5971673990945));
#113472=CARTESIAN_POINT('Ctrl Pts',(0.312923343192167,-29.1517170913018,
53.5648096294597));
#113473=CARTESIAN_POINT('Ctrl Pts',(0.308802761305119,-29.2059030293678,
53.5354297554461));
#113474=CARTESIAN_POINT('Ctrl Pts',(0.304733346342263,-29.2594161188262,
53.5064147031561));
#113475=CARTESIAN_POINT('Ctrl Pts',(0.300663931379406,-29.314580782465,
53.4803042617932));
#113476=CARTESIAN_POINT('Ctrl Pts',(0.29659451641655,-29.3710489165639,
53.45728274313));
#113477=CARTESIAN_POINT('Ctrl Pts',(0.29252752005979,-29.4274834895307,
53.4342749070196));
#113478=CARTESIAN_POINT('Ctrl Pts',(0.288460523703031,-29.4852195246385,
53.4143525458554));
#113479=CARTESIAN_POINT('Ctrl Pts',(0.28439352734627,-29.5438872246229,
53.3976526168968));
#113480=CARTESIAN_POINT('Ctrl Pts',(0.280327444740207,-29.6025417434664,
53.3809564399877));
#113481=CARTESIAN_POINT('Ctrl Pts',(0.276261362134141,-29.6621270203941,
53.3674813976669));
#113482=CARTESIAN_POINT('Ctrl Pts',(0.272195279528077,-29.7222583109853,
53.3573145297461));
#113483=CARTESIAN_POINT('Ctrl Pts',(0.268034884707164,-29.7837843384146,
53.3469118427521));
#113484=CARTESIAN_POINT('Ctrl Pts',(0.263874489886252,-29.8458814862898,
53.339972864249));
#113485=CARTESIAN_POINT('Ctrl Pts',(0.259714095065338,-29.9081292883171,
53.3365350101866));
#113486=CARTESIAN_POINT('Ctrl Pts',(0.255642712986453,-29.9690452822391,
53.3331707099165));
#113487=CARTESIAN_POINT('Ctrl Pts',(0.251571330907568,-30.0301050229311,
53.3331591191531));
#113488=CARTESIAN_POINT('Ctrl Pts',(0.247499948828683,-30.0909144776033,
53.336482474465));
#113489=CARTESIAN_POINT('Ctrl Pts',(0.243295047636755,-30.1537181505274,
53.3399148176942));
#113490=CARTESIAN_POINT('Ctrl Pts',(0.239090146444827,-30.2162542433769,
53.3469046314213));
#113491=CARTESIAN_POINT('Ctrl Pts',(0.2348852452529,-30.2780973747092,53.3573747079203));
#113492=CARTESIAN_POINT('Ctrl Pts',(0.230680344060973,-30.3399405060415,
53.3678447844194));
#113493=CARTESIAN_POINT('Ctrl Pts',(0.226475442869046,-30.4010901142077,
53.3817949221457));
#113494=CARTESIAN_POINT('Ctrl Pts',(0.222270541677118,-30.4611382343937,
53.3990916550969));
#113495=CARTESIAN_POINT('Ctrl Pts',(0.218232105035426,-30.5188091564334,
53.4157036411921));
#113496=CARTESIAN_POINT('Ctrl Pts',(0.214193668393735,-30.5757132364291,
53.4354740797279));
#113497=CARTESIAN_POINT('Ctrl Pts',(0.210155231752043,-30.6314753353094,
53.458314266494));
#113498=CARTESIAN_POINT('Ctrl Pts',(0.206029400047314,-30.688444171494,
53.4816487335323));
#113499=CARTESIAN_POINT('Ctrl Pts',(0.201903568342585,-30.7442204617963,
53.508187329055));
#113500=CARTESIAN_POINT('Ctrl Pts',(0.197777736637857,-30.7984179174006,
53.5377808546002));
#113501=CARTESIAN_POINT('Ctrl Pts',(0.193750411658712,-30.8513213759957,
53.5666678168368));
#113502=CARTESIAN_POINT('Ctrl Pts',(0.189723086679567,-30.9027200696696,
53.5984651822622));
#113503=CARTESIAN_POINT('Ctrl Pts',(0.185695761700423,-30.9522751223287,
53.6329857018327));
#113504=CARTESIAN_POINT('Ctrl Pts',(0.181670784440974,-31.0018012869855,
53.6674860977468));
#113505=CARTESIAN_POINT('Ctrl Pts',(0.177645807181524,-31.049485511849,
53.7047062047229));
#113506=CARTESIAN_POINT('Ctrl Pts',(0.173620829922075,-31.0950167085855,
53.744414714996));
#113507=CARTESIAN_POINT('Ctrl Pts',(0.169596634189296,-31.1405390645653,
53.7841155150989));
#113508=CARTESIAN_POINT('Ctrl Pts',(0.165572438456518,-31.1839088281068,
53.8263034164061));
#113509=CARTESIAN_POINT('Ctrl Pts',(0.16154824272374,-31.2248486564817,
53.8707074034091));
#113510=CARTESIAN_POINT('Ctrl Pts',(0.157347161733308,-31.2675880126558,
53.9170631867966));
#113511=CARTESIAN_POINT('Ctrl Pts',(0.153146080742876,-31.3076784050157,
53.965833974631));
#113512=CARTESIAN_POINT('Ctrl Pts',(0.148944999752445,-31.3448498765588,
54.0166715657931));
#113513=CARTESIAN_POINT('Ctrl Pts',(0.144914712435887,-31.380510153197,
54.0654423701008));
#113514=CARTESIAN_POINT('Ctrl Pts',(0.140884425119329,-31.4134840489688,
54.1161146630918));
#113515=CARTESIAN_POINT('Ctrl Pts',(0.136854137802771,-31.4435782915124,
54.1683524086043));
#113516=CARTESIAN_POINT('Ctrl Pts',(0.132820591304928,-31.4736968704331,
54.2206323973291));
#113517=CARTESIAN_POINT('Ctrl Pts',(0.128787044807085,-31.5009309364345,
54.2744798873931));
#113518=CARTESIAN_POINT('Ctrl Pts',(0.124753498309242,-31.5251345724958,
54.3295370735245));
#113519=CARTESIAN_POINT('Ctrl Pts',(0.120712473306291,-31.5493830839579,
54.3846963399091));
#113520=CARTESIAN_POINT('Ctrl Pts',(0.116671448303339,-31.5705897898519,
54.4410692839238));
#113521=CARTESIAN_POINT('Ctrl Pts',(0.112630423300388,-31.5886584275105,
54.4982825489384));
#113522=CARTESIAN_POINT('Ctrl Pts',(0.112132039146445,-31.5908868528941,
54.5053387251951));
#113523=CARTESIAN_POINT('Ctrl Pts',(0.111633654992502,-31.5930676105852,
54.5124076720023));
#113524=CARTESIAN_POINT('Ctrl Pts',(0.11113527083856,-31.5952005742277,
54.5194886806913));
#113525=CARTESIAN_POINT('Ctrl Pts',(0.10694773985886,-31.6131221940476,
54.5789848404677));
#113526=CARTESIAN_POINT('Ctrl Pts',(0.102760208879161,-31.6277416901261,
54.6395863054358));
#113527=CARTESIAN_POINT('Ctrl Pts',(0.0985726778994609,-31.6389317870598,
54.7009036988445));
#113528=CARTESIAN_POINT('Ctrl Pts',(0.0943940903940186,-31.6500979848644,
54.7620901342896));
#113529=CARTESIAN_POINT('Ctrl Pts',(0.090215502888577,-31.6578492651913,
54.8239889898453));
#113530=CARTESIAN_POINT('Ctrl Pts',(0.0860369153831346,-31.6621086094138,
54.8861976691256));
#113531=CARTESIAN_POINT('Ctrl Pts',(0.0818635996917905,-31.6663625799375,
54.9483278643268));
#113532=CARTESIAN_POINT('Ctrl Pts',(0.077690284000446,-31.6671333299212,
55.0107666325594));
#113533=CARTESIAN_POINT('Ctrl Pts',(0.0735169683091019,-31.6643953215423,
55.0731041286663));
#113534=CARTESIAN_POINT('Ctrl Pts',(0.0693476782178636,-31.6616599542593,
55.1353814937289));
#113535=CARTESIAN_POINT('Ctrl Pts',(0.0651783881266246,-31.6554225724169,
55.1975573043719));
#113536=CARTESIAN_POINT('Ctrl Pts',(0.0610090980353863,-31.6457096786985,
55.2592212441872));
#113537=CARTESIAN_POINT('Ctrl Pts',(0.0568425928731666,-31.636003272828,
55.3208439948092));
#113538=CARTESIAN_POINT('Ctrl Pts',(0.0526760877109474,-31.6228260427918,
55.3819550822746));
#113539=CARTESIAN_POINT('Ctrl Pts',(0.0485095825487276,-31.6062561827473,
55.4421505121406));
#113540=CARTESIAN_POINT('Ctrl Pts',(0.0443433163955318,-31.5896872732227,
55.5023424889324));
#113541=CARTESIAN_POINT('Ctrl Pts',(0.0401770502423353,-31.569726233976,
55.5616184474993));
#113542=CARTESIAN_POINT('Ctrl Pts',(0.0360107840891395,-31.5465018284697,
55.619587035484));
#113543=CARTESIAN_POINT('Ctrl Pts',(0.0318450104360858,-31.5232801683529,
55.6775487709208));
#113544=CARTESIAN_POINT('Ctrl Pts',(0.0276792367830336,-31.4967960926715,
55.734203000793));
#113545=CARTESIAN_POINT('Ctrl Pts',(0.02351346312998,-31.4672267106425,
55.7891779137668));
#113546=CARTESIAN_POINT('Ctrl Pts',(0.0193444149573671,-31.4376340855072,
55.8441960399448));
#113547=CARTESIAN_POINT('Ctrl Pts',(0.0151753667847533,-31.4049515381844,
55.8975317907779));
#113548=CARTESIAN_POINT('Ctrl Pts',(0.0110063186121403,-31.3694019533152,
55.9488383899572));
#113549=CARTESIAN_POINT('Ctrl Pts',(0.00733754574142688,-31.3381182292772,
55.993988326193));
#113550=CARTESIAN_POINT('Ctrl Pts',(0.00366877287071343,-31.3046150543095,
56.0375670978278));
#113551=CARTESIAN_POINT('Ctrl Pts',(0.,-31.2690708798524,56.0793586530485));
#113552=CARTESIAN_POINT('',(0.,-28.7475028281235,56.0985476022646));
#113553=CARTESIAN_POINT('Origin',(0.,-30.,55.));
#113554=CARTESIAN_POINT('Ctrl Pts',(1.62023172656234E-14,-28.7475028281236,
56.0985476022648));
#113555=CARTESIAN_POINT('Ctrl Pts',(3.75357402200702E-5,-28.7478625803039,
56.0989577698236));
#113556=CARTESIAN_POINT('Ctrl Pts',(7.48508279364976E-5,-28.7482202958009,
56.0993652087435));
#113557=CARTESIAN_POINT('Ctrl Pts',(0.000932278812672465,-28.7564416618929,
56.1087202727867));
#113558=CARTESIAN_POINT('Ctrl Pts',(0.00175868013715661,-28.7644030580975,
56.1175858633979));
#113559=CARTESIAN_POINT('Ctrl Pts',(0.0107130193140845,-28.8511361178773,
56.2121097718193));
#113560=CARTESIAN_POINT('Ctrl Pts',(0.0192885215002732,-28.9385755977656,
56.2893695022278));
#113561=CARTESIAN_POINT('Ctrl Pts',(0.0346719272342822,-29.1113734614591,
56.4124720618206));
#113562=CARTESIAN_POINT('Ctrl Pts',(0.0415003586744818,-29.1940618415998,
56.4612335904689));
#113563=CARTESIAN_POINT('Ctrl Pts',(0.0495712580011992,-29.3001267556719,
56.5120208776402));
#113564=CARTESIAN_POINT('Ctrl Pts',(0.0510520476430112,-29.3199399305453,
56.5210351973345));
#113565=CARTESIAN_POINT('Ctrl Pts',(0.0533548169406772,-29.3512950504097,
56.534565489637));
#113566=CARTESIAN_POINT('Ctrl Pts',(0.0541855673846926,-29.362719818038,
56.5393451001824));
#113567=CARTESIAN_POINT('Ctrl Pts',(0.0557339708160195,-29.3842215115695,
56.5480600280857));
#113568=CARTESIAN_POINT('Ctrl Pts',(0.0564525915581555,-29.3942854618892,
56.5520254202119));
#113569=CARTESIAN_POINT('Ctrl Pts',(0.0580613783573555,-29.4170021737305,
56.5607216226821));
#113570=CARTESIAN_POINT('Ctrl Pts',(0.0589496921570372,-29.4296753804327,
56.565397168395));
#113571=CARTESIAN_POINT('Ctrl Pts',(0.061227793507911,-29.4624979999319,
56.5770549412087));
#113572=CARTESIAN_POINT('Ctrl Pts',(0.0626101184269552,-29.482727475378,
56.5838055080911));
#113573=CARTESIAN_POINT('Ctrl Pts',(0.0731854464751945,-29.6397047570472,
56.6328600575719));
#113574=CARTESIAN_POINT('Ctrl Pts',(0.0817782006599408,-29.781254490794,
56.6577686126975));
#113575=CARTESIAN_POINT('Ctrl Pts',(0.0943890865181255,-29.9850953182022,
56.6670463540227));
#113576=CARTESIAN_POINT('Ctrl Pts',(0.0981994555451711,-30.0460397150593,
56.666476680097));
#113577=CARTESIAN_POINT('Ctrl Pts',(0.103152500170303,-30.1221192704565,
56.661589072911));
#113578=CARTESIAN_POINT('Ctrl Pts',(0.10415830102058,-30.1374143067386,
56.6603941194457));
#113579=CARTESIAN_POINT('Ctrl Pts',(0.105679039932593,-30.160266827608,
56.6582908184455));
#113580=CARTESIAN_POINT('Ctrl Pts',(0.106185867033484,-30.1678386050706,
56.6575415806849));
#113581=CARTESIAN_POINT('Ctrl Pts',(0.107104957588992,-30.181483254212,
56.6560969748654));
#113582=CARTESIAN_POINT('Ctrl Pts',(0.107516219708491,-30.1875578043628,
56.6554200160817));
#113583=CARTESIAN_POINT('Ctrl Pts',(0.108447945740051,-30.2012487235869,
56.653817950112));
#113584=CARTESIAN_POINT('Ctrl Pts',(0.108969405992014,-30.2088623772444,
56.6528736680248));
#113585=CARTESIAN_POINT('Ctrl Pts',(0.110585995213957,-30.2323241071582,
56.6497991420235));
#113586=CARTESIAN_POINT('Ctrl Pts',(0.111689953793306,-30.2481477225314,
56.6474933569477));
#113587=CARTESIAN_POINT('Ctrl Pts',(0.119511069272,-30.3590326351629,56.6297017996245));
#113588=CARTESIAN_POINT('Ctrl Pts',(0.126541406312297,-30.4526197329216,
56.6062268309948));
#113589=CARTESIAN_POINT('Ctrl Pts',(0.141905327855665,-30.6523773093463,
56.5372674590541));
#113590=CARTESIAN_POINT('Ctrl Pts',(0.150172738911815,-30.7569468805903,
56.4885656596627));
#113591=CARTESIAN_POINT('Ctrl Pts',(0.159565076372559,-30.8743405843089,
56.4182939421622));
#113592=CARTESIAN_POINT('Ctrl Pts',(0.161045410770459,-30.8927847011483,
56.4067568084943));
#113593=CARTESIAN_POINT('Ctrl Pts',(0.16334364918861,-30.9213143126495,
56.3881238235734));
#113594=CARTESIAN_POINT('Ctrl Pts',(0.164170395069581,-30.9315554393837,
56.3812719825102));
#113595=CARTESIAN_POINT('Ctrl Pts',(0.165709004674219,-30.9505690861189,
56.3682432133675));
#113596=CARTESIAN_POINT('Ctrl Pts',(0.166421855639546,-30.9593597174167,
56.3620939836012));
#113597=CARTESIAN_POINT('Ctrl Pts',(0.168014349531454,-30.9789515544843,
56.3481053198735));
#113598=CARTESIAN_POINT('Ctrl Pts',(0.168892189568057,-30.989719271434,
56.3402200865601));
#113599=CARTESIAN_POINT('Ctrl Pts',(0.171134944282373,-31.0171347972556,
56.3196329911025));
#113600=CARTESIAN_POINT('Ctrl Pts',(0.172492615266876,-31.0336402935467,
56.3067448997139));
#113601=CARTESIAN_POINT('Ctrl Pts',(0.183562612263131,-31.1672891739787,
56.1982697855029));
#113602=CARTESIAN_POINT('Ctrl Pts',(0.19257856866068,-31.2711586006143,
56.087461188863));
#113603=CARTESIAN_POINT('Ctrl Pts',(0.205633605993383,-31.3936879586553,
55.9147969208517));
#113604=CARTESIAN_POINT('Ctrl Pts',(0.209416025636807,-31.4259969972004,
55.8635684960944));
#113605=CARTESIAN_POINT('Ctrl Pts',(0.214334831993184,-31.4628461254091,
55.7974136858428));
#113606=CARTESIAN_POINT('Ctrl Pts',(0.215332049689358,-31.470065360942,
55.784024979009));
#113607=CARTESIAN_POINT('Ctrl Pts',(0.21683648963492,-31.4805643848506,
55.7638986909951));
#113608=CARTESIAN_POINT('Ctrl Pts',(0.217335518587385,-31.4839839024865,
55.7572343623819));
#113609=CARTESIAN_POINT('Ctrl Pts',(0.218239093383336,-31.4900597795696,
55.7451938083046));
#113610=CARTESIAN_POINT('Ctrl Pts',(0.218642638681212,-31.4927322136535,
55.7398259894008));
#113611=CARTESIAN_POINT('Ctrl Pts',(0.219553678015184,-31.4986730022683,
55.7277301540787));
#113612=CARTESIAN_POINT('Ctrl Pts',(0.220062113914561,-31.5019250134053,
55.7209945863529));
#113613=CARTESIAN_POINT('Ctrl Pts',(0.221620217123942,-31.5117017353367,
55.7003918433673));
#113614=CARTESIAN_POINT('Ctrl Pts',(0.222678048221896,-31.5180803414009,
55.6864567766573));
#113615=CARTESIAN_POINT('Ctrl Pts',(0.231187528639727,-31.5674149526258,
55.5746260460575));
#113616=CARTESIAN_POINT('Ctrl Pts',(0.239033421441629,-31.6010462240505,
55.472897739143));
#113617=CARTESIAN_POINT('Ctrl Pts',(0.25454182033073,-31.6482501071324,
55.2648675104554));
#113618=CARTESIAN_POINT('Ctrl Pts',(0.262166353587474,-31.661805049623,
55.15904262621));
#113619=CARTESIAN_POINT('Ctrl Pts',(0.27095201622974,-31.6658489648646,
55.0311009220826));
#113620=CARTESIAN_POINT('Ctrl Pts',(0.272417672274158,-31.6661118691617,
55.0095580556456));
#113621=CARTESIAN_POINT('Ctrl Pts',(0.274692181369376,-31.6658692077285,
54.9758265970315));
#113622=CARTESIAN_POINT('Ctrl Pts',(0.275509829500226,-31.6656477607705,
54.9636390116038));
#113623=CARTESIAN_POINT('Ctrl Pts',(0.277030712186308,-31.6649836824572,
54.9408585589592));
#113624=CARTESIAN_POINT('Ctrl Pts',(0.277734932829164,-31.6645736608853,
54.9302654366796));
#113625=CARTESIAN_POINT('Ctrl Pts',(0.279306851781938,-31.6634276760127,
54.9065239900043));
#113626=CARTESIAN_POINT('Ctrl Pts',(0.280172784135655,-31.6626368700546,
54.89337892894));
#113627=CARTESIAN_POINT('Ctrl Pts',(0.282705833005443,-31.6598526530429,
54.8547460586797));
#113628=CARTESIAN_POINT('Ctrl Pts',(0.28435944189621,-31.6574283051908,
54.8292924608546));
#113629=CARTESIAN_POINT('Ctrl Pts',(0.296517854340955,-31.635083120541,
54.6407714281719));
#113630=CARTESIAN_POINT('Ctrl Pts',(0.306191047854637,-31.5917304354458,
54.4814125429551));
#113631=CARTESIAN_POINT('Ctrl Pts',(0.318502913361422,-31.5122874053803,
54.3002362145878));
#113632=CARTESIAN_POINT('Ctrl Pts',(0.320615923008884,-31.4978838293999,
54.2699134934715));
#113633=CARTESIAN_POINT('Ctrl Pts',(0.324169684140878,-31.4726294239121,
54.2206451466195));
#113634=CARTESIAN_POINT('Ctrl Pts',(0.325586297798577,-31.4623041448519,
54.2014401178944));
#113635=CARTESIAN_POINT('Ctrl Pts',(0.327590724173834,-31.4473961563363,
54.1749703355599));
#113636=CARTESIAN_POINT('Ctrl Pts',(0.328160045905645,-31.4431291732388,
54.1675291224502));
#113637=CARTESIAN_POINT('Ctrl Pts',(0.329139310499817,-31.4357387001571,
54.1548684238715));
#113638=CARTESIAN_POINT('Ctrl Pts',(0.329547435343278,-31.4326437677014,
54.1496325325326));
#113639=CARTESIAN_POINT('Ctrl Pts',(0.330411739038064,-31.4260597131908,
54.13863184582));
#113640=CARTESIAN_POINT('Ctrl Pts',(0.330868283351245,-31.422564320962,
54.1328713179069));
#113641=CARTESIAN_POINT('Ctrl Pts',(0.33211830593615,-31.4129437626281,
54.1172310317389));
#113642=CARTESIAN_POINT('Ctrl Pts',(0.332915978117594,-31.4067501158323,
54.1073941405651));
#113643=CARTESIAN_POINT('Ctrl Pts',(0.337072936175573,-31.3741680925198,
54.056828086171));
#113644=CARTESIAN_POINT('Ctrl Pts',(0.340521544944614,-31.3461143916216,
54.0172048407093));
#113645=CARTESIAN_POINT('Ctrl Pts',(0.351235652704874,-31.2548821998936,
53.8995946118062));
#113646=CARTESIAN_POINT('Ctrl Pts',(0.358610955290783,-31.1863544693423,
53.826038462252));
#113647=CARTESIAN_POINT('Ctrl Pts',(0.369452580184512,-31.0739700808081,
53.7253629304253));
#113648=CARTESIAN_POINT('Ctrl Pts',(0.37304047129974,-31.0347993219239,
53.6933621194328));
#113649=CARTESIAN_POINT('Ctrl Pts',(0.378979569212961,-30.9664288754677,
53.6425127227984));
#113650=CARTESIAN_POINT('Ctrl Pts',(0.381363495022356,-30.9379872362941,
53.6227067374863));
#113651=CARTESIAN_POINT('Ctrl Pts',(0.384709398161686,-30.8966532279324,
53.5957976753192));
#113652=CARTESIAN_POINT('Ctrl Pts',(0.385698478023701,-30.8842543038273,
53.5879569660136));
#113653=CARTESIAN_POINT('Ctrl Pts',(0.387409121334323,-30.8625007400884,
53.5745995805627));
#113654=CARTESIAN_POINT('Ctrl Pts',(0.388133366006338,-30.8531928943661,
53.5690088131035));
#113655=CARTESIAN_POINT('Ctrl Pts',(0.389622336670036,-30.8338578731183,
53.5576509338085));
#113656=CARTESIAN_POINT('Ctrl Pts',(0.390386577941943,-30.8238239363243,
53.5518964420303));
#113657=CARTESIAN_POINT('Ctrl Pts',(0.392351109702528,-30.7977534769141,
53.5373036403333));
#113658=CARTESIAN_POINT('Ctrl Pts',(0.393545729129202,-30.7816294527555,
53.5286242178936));
#113659=CARTESIAN_POINT('Ctrl Pts',(0.398667264531292,-30.7113889561795,
53.4922949417827));
#113660=CARTESIAN_POINT('Ctrl Pts',(0.402500690228721,-30.6559223034154,
53.4673500339213));
#113661=CARTESIAN_POINT('Ctrl Pts',(0.413730943686305,-30.4871627820572,
53.4022989049097));
#113662=CARTESIAN_POINT('Ctrl Pts',(0.420900872275422,-30.3707808667734,
53.3713517363182));
#113663=CARTESIAN_POINT('Ctrl Pts',(0.431234977027151,-30.2074115523137,
53.3463436296408));
#113664=CARTESIAN_POINT('Ctrl Pts',(0.434107958570272,-30.1624774325154,
53.3413260598535));
#113665=CARTESIAN_POINT('Ctrl Pts',(0.437794345600006,-30.1063698172342,
53.3373624194594));
#113666=CARTESIAN_POINT('Ctrl Pts',(0.438524247324552,-30.0953329595042,
53.3366930911864));
#113667=CARTESIAN_POINT('Ctrl Pts',(0.439701051414267,-30.0776712032297,
53.3357983555512));
#113668=CARTESIAN_POINT('Ctrl Pts',(0.440144194818643,-30.0710499832864,
53.3355025307177));
#113669=CARTESIAN_POINT('Ctrl Pts',(0.441000630524023,-30.0583147198418,
53.3350096657094));
#113670=CARTESIAN_POINT('Ctrl Pts',(0.441413603588024,-30.0522010996308,
53.3348067799563));
#113671=CARTESIAN_POINT('Ctrl Pts',(0.442338965069219,-30.0385602267756,
53.3344292871092));
#113672=CARTESIAN_POINT('Ctrl Pts',(0.442852275525089,-30.0310326363063,
53.334272032771));
#113673=CARTESIAN_POINT('Ctrl Pts',(0.444639979192116,-30.0049427669413,
53.3339039125524));
#113674=CARTESIAN_POINT('Ctrl Pts',(0.445927102676751,-29.9863789654471,
53.3339522814767));
#113675=CARTESIAN_POINT('Ctrl Pts',(0.454821841236573,-29.8593408374988,
53.3364065098491));
#113676=CARTESIAN_POINT('Ctrl Pts',(0.462797073776145,-29.7513322394771,
53.3490941794592));
#113677=CARTESIAN_POINT('Ctrl Pts',(0.476889661467134,-29.5615685736355,
53.3904400938668));
#113678=CARTESIAN_POINT('Ctrl Pts',(0.48302888112474,-29.4793301556177,
53.41513036437));
#113679=CARTESIAN_POINT('Ctrl Pts',(0.491051378892342,-29.3714337221862,
53.4568356911214));
#113680=CARTESIAN_POINT('Ctrl Pts',(0.493103164567633,-29.3438134259284,
53.4683763420509));
#113681=CARTESIAN_POINT('Ctrl Pts',(0.496069104295478,-29.3038727409577,
53.4863438025928));
#113682=CARTESIAN_POINT('Ctrl Pts',(0.497002663246154,-29.2912992262281,
53.4921898401472));
#113683=CARTESIAN_POINT('Ctrl Pts',(0.498649156748737,-29.2691264770014,
53.502837668713));
#113684=CARTESIAN_POINT('Ctrl Pts',(0.499364212908342,-29.2594980512346,
53.5075764589182));
#113685=CARTESIAN_POINT('Ctrl Pts',(0.500865110186966,-29.2392944549664,
53.5177636588023));
#113686=CARTESIAN_POINT('Ctrl Pts',(0.501650172003646,-29.2287304620333,
53.5232329873811));
#113687=CARTESIAN_POINT('Ctrl Pts',(0.503738921525196,-29.2006427511085,
53.5381585417489));
#113688=CARTESIAN_POINT('Ctrl Pts',(0.505035436693089,-29.1832281218627,
53.5478167420967));
#113689=CARTESIAN_POINT('Ctrl Pts',(0.512573733888914,-29.082206352273,
53.6062360177406));
#113690=CARTESIAN_POINT('Ctrl Pts',(0.518554975603383,-29.0027990410851,
53.6618980286231));
#113691=CARTESIAN_POINT('Ctrl Pts',(0.529880515505819,-28.8610237036824,
53.7809468026903));
#113692=CARTESIAN_POINT('Ctrl Pts',(0.535220759653745,-28.7980097953967,
53.8430318666004));
#113693=CARTESIAN_POINT('Ctrl Pts',(0.543256131918304,-28.7143304190063,
53.9397288976512));
#113694=CARTESIAN_POINT('Ctrl Pts',(0.545782499591792,-28.6895186927909,
53.9705539015747));
#113695=CARTESIAN_POINT('Ctrl Pts',(0.549073921677668,-28.6594732815697,
54.0107291766534));
#113696=CARTESIAN_POINT('Ctrl Pts',(0.54977512792125,-28.6531984528712,
54.0192889197349));
#113697=CARTESIAN_POINT('Ctrl Pts',(0.550915700674219,-28.6432033011031,
54.0332005418519));
#113698=CARTESIAN_POINT('Ctrl Pts',(0.551351676551874,-28.6394317372136,
54.0385154847581));
#113699=CARTESIAN_POINT('Ctrl Pts',(0.552203489425921,-28.6321601877708,
54.0488911165766));
#113700=CARTESIAN_POINT('Ctrl Pts',(0.552619097602689,-28.628656897173,
54.0539492879644));
#113701=CARTESIAN_POINT('Ctrl Pts',(0.55366065604612,-28.6199861054858,
54.0666178312412));
#113702=CARTESIAN_POINT('Ctrl Pts',(0.554288852055143,-28.6148535176734,
54.0742517433201));
#113703=CARTESIAN_POINT('Ctrl Pts',(0.556572629816215,-28.5965334536372,
54.1019933836642));
#113704=CARTESIAN_POINT('Ctrl Pts',(0.558249525702292,-28.5837191447751,
54.1223425361972));
#113705=CARTESIAN_POINT('Ctrl Pts',(0.567251634879455,-28.5180457917415,
54.2318173097701));
#113706=CARTESIAN_POINT('Ctrl Pts',(0.574868118399485,-28.4731497831658,
54.3254486004659));
#113707=CARTESIAN_POINT('Ctrl Pts',(0.588424553480013,-28.4083725499691,
54.5007825568729));
#113708=CARTESIAN_POINT('Ctrl Pts',(0.594384960335272,-28.3854007867015,
54.5809907471399));
#113709=CARTESIAN_POINT('Ctrl Pts',(0.602235533419829,-28.3624744736332,
54.6918463944742));
#113710=CARTESIAN_POINT('Ctrl Pts',(0.604283616471256,-28.3572117588969,
54.7212608960795));
#113711=CARTESIAN_POINT('Ctrl Pts',(0.60724453931131,-28.3506716616341,
54.7644926035828));
#113712=CARTESIAN_POINT('Ctrl Pts',(0.608176741524404,-28.348771343716,
54.7782081014048));
#113713=CARTESIAN_POINT('Ctrl Pts',(0.609820926989279,-28.3457038117893,
54.8025791898692));
#113714=CARTESIAN_POINT('Ctrl Pts',(0.610535028087741,-28.3444680509492,
54.8132251903913));
#113715=CARTESIAN_POINT('Ctrl Pts',(0.612033979505358,-28.3420791336145,
54.8356967654067));
#113716=CARTESIAN_POINT('Ctrl Pts',(0.612818051047757,-28.3409495725663,
54.8475242850854));
#113717=CARTESIAN_POINT('Ctrl Pts',(0.614904240245468,-28.338267729879,
54.8791802963705));
#113718=CARTESIAN_POINT('Ctrl Pts',(0.616199193150838,-28.3369437888853,
54.8990265781233));
#113719=CARTESIAN_POINT('Ctrl Pts',(0.623783176792384,-28.3312278387557,
55.0162966637291));
#113720=CARTESIAN_POINT('Ctrl Pts',(0.629806890393584,-28.3350410166939,
55.1139348987395));
#113721=CARTESIAN_POINT('Ctrl Pts',(0.640245363638023,-28.356624779606,
55.2832355454365));
#113722=CARTESIAN_POINT('Ctrl Pts',(0.644678590323032,-28.3706400013324,
55.3550910777214));
#113723=CARTESIAN_POINT('Ctrl Pts',(0.652476636674378,-28.4027065631766,
55.4763917838337));
#113724=CARTESIAN_POINT('Ctrl Pts',(0.655783585865192,-28.4184591678063,
55.526329641042));
#113725=CARTESIAN_POINT('Ctrl Pts',(0.659211111289602,-28.4365431355012,
55.5754638423972));
#113726=CARTESIAN_POINT('Ctrl Pts',(0.659212928209264,-28.4365527225674,
55.5754898882335));
#113727=CARTESIAN_POINT('Ctrl Pts',(0.659214745210768,-28.4365623102018,
55.5755159338528));
#113728=CARTESIAN_POINT('Origin',(5.,-30.,125.));
#113729=CARTESIAN_POINT('',(9.56913309254615,-28.4365599842513,125.575509615172));
#113730=CARTESIAN_POINT('',(9.75970369730367,-28.4365599837282,125.575509613751));
#113731=CARTESIAN_POINT('',(5.,-28.4365599837785,125.575509613888));
#113732=CARTESIAN_POINT('',(10.,-31.3346917155535,125.997072727755));
#113733=CARTESIAN_POINT('Ctrl Pts',(9.75970369730367,-28.4365599837282,
125.575509613751));
#113734=CARTESIAN_POINT('Ctrl Pts',(9.75994451571396,-28.4379065492441,
125.579167718432));
#113735=CARTESIAN_POINT('Ctrl Pts',(9.76018561618856,-28.439266103374,125.582821504279));
#113736=CARTESIAN_POINT('Ctrl Pts',(9.76396616505077,-28.4607604410501,
125.639972574818));
#113737=CARTESIAN_POINT('Ctrl Pts',(9.76756188217567,-28.4836202388558,
125.6923974909));
#113738=CARTESIAN_POINT('Ctrl Pts',(9.77207491623637,-28.5144274149677,
125.754169230963));
#113739=CARTESIAN_POINT('Ctrl Pts',(9.77285759273999,-28.5198428497737,
125.764743045133));
#113740=CARTESIAN_POINT('Ctrl Pts',(9.77410232503199,-28.5285590500868,
125.781322261152));
#113741=CARTESIAN_POINT('Ctrl Pts',(9.77455987107205,-28.5317847034412,
125.78736699422));
#113742=CARTESIAN_POINT('Ctrl Pts',(9.7754118944931,-28.5378290951926,125.798527621339));
#113743=CARTESIAN_POINT('Ctrl Pts',(9.77580572358126,-28.5406376614943,
125.803648978627));
#113744=CARTESIAN_POINT('Ctrl Pts',(9.77672967135821,-28.5472593623224,
125.815574320486));
#113745=CARTESIAN_POINT('Ctrl Pts',(9.77726113849169,-28.5510933601628,
125.822366326629));
#113746=CARTESIAN_POINT('Ctrl Pts',(9.77905624837008,-28.5641318539652,
125.845090060905));
#113747=CARTESIAN_POINT('Ctrl Pts',(9.7803331085325,-28.5735521639723,125.860895487567));
#113748=CARTESIAN_POINT('Ctrl Pts',(9.78350149743746,-28.5973271953013,
125.89932348826));
#113749=CARTESIAN_POINT('Ctrl Pts',(9.78540724587401,-28.6119693144433,
125.921761561951));
#113750=CARTESIAN_POINT('Ctrl Pts',(9.79378251429947,-28.6780255606532,
126.017843607809));
#113751=CARTESIAN_POINT('Ctrl Pts',(9.80041826342814,-28.7348055181594,
126.08761403733));
#113752=CARTESIAN_POINT('Ctrl Pts',(9.81454454270551,-28.8686960009257,
126.227383426841));
#113753=CARTESIAN_POINT('Ctrl Pts',(9.8219702729316,-28.947313719987,126.295445072283));
#113754=CARTESIAN_POINT('Ctrl Pts',(9.83042357402043,-29.0477427120753,
126.367167655443));
#113755=CARTESIAN_POINT('Ctrl Pts',(9.8317569649978,-29.0639182836909,126.378293299996));
#113756=CARTESIAN_POINT('Ctrl Pts',(9.83385413702969,-29.0898827351996,
126.395483785136));
#113757=CARTESIAN_POINT('Ctrl Pts',(9.83462524832458,-29.0995438831628,
126.401737216424));
#113758=CARTESIAN_POINT('Ctrl Pts',(9.83607463095884,-29.1179157793364,
126.413360574966));
#113759=CARTESIAN_POINT('Ctrl Pts',(9.83675368055385,-29.1266126615979,
126.418751300482));
#113760=CARTESIAN_POINT('Ctrl Pts',(9.8382884089348,-29.1464682625006,126.430806937075));
#113761=CARTESIAN_POINT('Ctrl Pts',(9.83914217914352,-29.1576565085309,
126.43742212901));
#113762=CARTESIAN_POINT('Ctrl Pts',(9.84176038765198,-29.1923941659267,
126.457416318034));
#113763=CARTESIAN_POINT('Ctrl Pts',(9.84350852502053,-29.2161940004395,
126.470352950626));
#113764=CARTESIAN_POINT('Ctrl Pts',(9.85217889303779,-29.3370203882264,
126.532261338954));
#113765=CARTESIAN_POINT('Ctrl Pts',(9.85878029389206,-29.4383597227391,
126.572237248646));
#113766=CARTESIAN_POINT('Ctrl Pts',(9.87101604579307,-29.6313419490597,
126.627301443516));
#113767=CARTESIAN_POINT('Ctrl Pts',(9.8766300372631,-29.7217317355538,126.645168986635));
#113768=CARTESIAN_POINT('Ctrl Pts',(9.88352498252932,-29.8273483986049,
126.657091565063));
#113769=CARTESIAN_POINT('Ctrl Pts',(9.88446223307119,-29.8415964405245,
126.658514187078));
#113770=CARTESIAN_POINT('Ctrl Pts',(9.88588934250875,-29.8630909875837,
126.660380859115));
#113771=CARTESIAN_POINT('Ctrl Pts',(9.88637190756385,-29.870325381615,126.660961517718));
#113772=CARTESIAN_POINT('Ctrl Pts',(9.88726167851064,-29.8835968076819,
126.661939499302));
#113773=CARTESIAN_POINT('Ctrl Pts',(9.88766807118888,-29.889632499381,126.662351230676));
#113774=CARTESIAN_POINT('Ctrl Pts',(9.88852639150201,-29.9023254722685,
126.663147663766));
#113775=CARTESIAN_POINT('Ctrl Pts',(9.88897867336083,-29.9089828816488,
126.663525276355));
#113776=CARTESIAN_POINT('Ctrl Pts',(9.89019244811108,-29.9267710924219,
126.6644271378));
#113777=CARTESIAN_POINT('Ctrl Pts',(9.89095770818538,-29.9379049575182,
126.664879682921));
#113778=CARTESIAN_POINT('Ctrl Pts',(9.8948510116117,-29.9941790262757,126.66660174095));
#113779=CARTESIAN_POINT('Ctrl Pts',(9.89805839363356,-30.0393490765158,
126.666147076887));
#113780=CARTESIAN_POINT('Ctrl Pts',(9.90936116946916,-30.1960286472457,
126.658195662987));
#113781=CARTESIAN_POINT('Ctrl Pts',(9.91764203974498,-30.3067643456311,
126.641321646206));
#113782=CARTESIAN_POINT('Ctrl Pts',(9.93203831717597,-30.4993665145325,
126.591785582919));
#113783=CARTESIAN_POINT('Ctrl Pts',(9.93821217710515,-30.5819314146435,
126.563492354797));
#113784=CARTESIAN_POINT('Ctrl Pts',(9.94565819888396,-30.6815914325746,
126.520344977419));
#113785=CARTESIAN_POINT('Ctrl Pts',(9.94711621840112,-30.7011022622152,
126.511446796632));
#113786=CARTESIAN_POINT('Ctrl Pts',(9.94944303030874,-30.7322104700222,
126.496527425594));
#113787=CARTESIAN_POINT('Ctrl Pts',(9.9503192101316,-30.7439177602343,126.490742395386));
#113788=CARTESIAN_POINT('Ctrl Pts',(9.95199065133982,-30.766230001092,126.479388731336));
#113789=CARTESIAN_POINT('Ctrl Pts',(9.95278655215591,-30.7768452374353,
126.473842230897));
#113790=CARTESIAN_POINT('Ctrl Pts',(9.95462617365112,-30.8013502788028,
126.460699941063));
#113791=CARTESIAN_POINT('Ctrl Pts',(9.95566714467698,-30.815193594718,126.453019619794));
#113792=CARTESIAN_POINT('Ctrl Pts',(9.95908941541234,-30.8605932621434,
126.426978631489));
#113793=CARTESIAN_POINT('Ctrl Pts',(9.961444339829,-30.8916566270398,126.407777503271));
#113794=CARTESIAN_POINT('Ctrl Pts',(9.96910762261717,-30.9916281706381,
126.341344598547));
#113795=CARTESIAN_POINT('Ctrl Pts',(9.97429816414406,-31.0576177915449,
126.289952476888));
#113796=CARTESIAN_POINT('Ctrl Pts',(9.98457090092396,-31.1795816150135,
126.179292029512));
#113797=CARTESIAN_POINT('Ctrl Pts',(9.98964040694053,-31.2356155639976,
126.120443806729));
#113798=CARTESIAN_POINT('Ctrl Pts',(9.995854392969,-31.2962772040964,126.046627351688));
#113799=CARTESIAN_POINT('Ctrl Pts',(9.99679738131947,-31.3052758614811,
126.03538316696));
#113800=CARTESIAN_POINT('Ctrl Pts',(9.99815926204356,-31.3179580649797,
126.019108129792));
#113801=CARTESIAN_POINT('Ctrl Pts',(9.99857202460429,-31.3217611232338,
126.014170780477));
#113802=CARTESIAN_POINT('Ctrl Pts',(9.99932318648219,-31.3286066166782,
126.005179658991));
#113803=CARTESIAN_POINT('Ctrl Pts',(9.99966107564483,-31.3316584429384,
126.001133097393));
#113804=CARTESIAN_POINT('Ctrl Pts',(10.,-31.3346917155535,125.997072727755));
#113805=CARTESIAN_POINT('',(10.,-30.7923075365013,123.534460929349));
#113806=CARTESIAN_POINT('Origin',(10.,-30.,125.));
#113807=CARTESIAN_POINT('Ctrl Pts',(9.99999999999994,-30.7923075365013,
123.534460929349));
#113808=CARTESIAN_POINT('Ctrl Pts',(9.99926708496121,-30.8016756586983,
123.539525573458));
#113809=CARTESIAN_POINT('Ctrl Pts',(9.99852930854555,-30.8109947629585,
123.544679796411));
#113810=CARTESIAN_POINT('Ctrl Pts',(9.99204966954295,-30.8919287972562,
123.590461664261));
#113811=CARTESIAN_POINT('Ctrl Pts',(9.98606976217558,-30.9604834673963,
123.636253610317));
#113812=CARTESIAN_POINT('Ctrl Pts',(9.97464534962519,-31.0841521385255,
123.732824677345));
#113813=CARTESIAN_POINT('Ctrl Pts',(9.9692155793381,-31.1397932651847,123.782629121173));
#113814=CARTESIAN_POINT('Ctrl Pts',(9.96087158743111,-31.2215068019947,
123.866301916725));
#113815=CARTESIAN_POINT('Ctrl Pts',(9.95788607305659,-31.2499370011715,
123.89772589531));
#113816=CARTESIAN_POINT('Ctrl Pts',(9.95282145460603,-31.2968042730688,
123.95367671475));
#113817=CARTESIAN_POINT('Ctrl Pts',(9.95072128046115,-31.3158181625168,
123.977690596857));
#113818=CARTESIAN_POINT('Ctrl Pts',(9.94769358097189,-31.3425896985432,
124.013487460142));
#113819=CARTESIAN_POINT('Ctrl Pts',(9.94674581584978,-31.3508760673856,
124.024865157323));
#113820=CARTESIAN_POINT('Ctrl Pts',(9.94507701084002,-31.3652948307072,
124.045199600773));
#113821=CARTESIAN_POINT('Ctrl Pts',(9.94435378369102,-31.3714856496421,
124.054113696361));
#113822=CARTESIAN_POINT('Ctrl Pts',(9.94283810955629,-31.3843342124285,
124.073005583975));
#113823=CARTESIAN_POINT('Ctrl Pts',(9.94204642672205,-31.3909722185667,
124.082996096683));
#113824=CARTESIAN_POINT('Ctrl Pts',(9.93994450295174,-31.40839393213,124.109841108067));
#113825=CARTESIAN_POINT('Ctrl Pts',(9.93864137206597,-31.418983087874,124.126819965796));
#113826=CARTESIAN_POINT('Ctrl Pts',(9.93128242964598,-31.47749510852,124.2245159632));
#113827=CARTESIAN_POINT('Ctrl Pts',(9.92546528087725,-31.5188366449002,
124.30898220434));
#113828=CARTESIAN_POINT('Ctrl Pts',(9.91546646844782,-31.5778393588891,
124.460797771252));
#113829=CARTESIAN_POINT('Ctrl Pts',(9.91126613611847,-31.5988125887474,
124.52659341407));
#113830=CARTESIAN_POINT('Ctrl Pts',(9.90469624315624,-31.6245855734625,
124.629028198606));
#113831=CARTESIAN_POINT('Ctrl Pts',(9.90239307114696,-31.6323502358026,
124.664842213327));
#113832=CARTESIAN_POINT('Ctrl Pts',(9.89855311395586,-31.6431009015141,
124.723747014169));
#113833=CARTESIAN_POINT('Ctrl Pts',(9.89704430793271,-31.6467949659221,
124.746696826641));
#113834=CARTESIAN_POINT('Ctrl Pts',(9.8949225422075,-31.6512420537353,124.778560511889));
#113835=CARTESIAN_POINT('Ctrl Pts',(9.89433002993274,-31.6524054017544,
124.787415554464));
#113836=CARTESIAN_POINT('Ctrl Pts',(9.89331615589468,-31.6542620781662,
124.802485252524));
#113837=CARTESIAN_POINT('Ctrl Pts',(9.89289675076957,-31.6549917358788,
124.808695397122));
#113838=CARTESIAN_POINT('Ctrl Pts',(9.89201864101834,-31.6564393303941,
124.821644531724));
#113839=CARTESIAN_POINT('Ctrl Pts',(9.89155962314301,-31.657151132115,124.828384005428));
#113840=CARTESIAN_POINT('Ctrl Pts',(9.89030675651547,-31.6589731106979,
124.846704316409));
#113841=CARTESIAN_POINT('Ctrl Pts',(9.88950875995965,-31.6600031060348,
124.858292492427));
#113842=CARTESIAN_POINT('Ctrl Pts',(9.88541804075691,-31.6646282137652,
124.917334077948));
#113843=CARTESIAN_POINT('Ctrl Pts',(9.88204024862677,-31.6663098884451,
124.964911150791));
#113844=CARTESIAN_POINT('Ctrl Pts',(9.87138706030857,-31.6651989797993,
125.11308774233));
#113845=CARTESIAN_POINT('Ctrl Pts',(9.8639970731756,-31.6553348053409,125.213411225608));
#113846=CARTESIAN_POINT('Ctrl Pts',(9.85314568841142,-31.6270179378176,
125.361824975351));
#113847=CARTESIAN_POINT('Ctrl Pts',(9.84956356623129,-31.6153065176612,
125.410962673781));
#113848=CARTESIAN_POINT('Ctrl Pts',(9.84363234818514,-31.5918340521378,
125.492766015986));
#113849=CARTESIAN_POINT('Ctrl Pts',(9.84125091452813,-31.5812527360129,
125.525731951912));
#113850=CARTESIAN_POINT('Ctrl Pts',(9.8379055887241,-31.5647272725196,125.572189154445));
#113851=CARTESIAN_POINT('Ctrl Pts',(9.83691482977229,-31.5596202099386,
125.585966458468));
#113852=CARTESIAN_POINT('Ctrl Pts',(9.83520016874323,-31.5504112729223,
125.609835629471));
#113853=CARTESIAN_POINT('Ctrl Pts',(9.83447359869569,-31.5463915142819,
125.619957985975));
#113854=CARTESIAN_POINT('Ctrl Pts',(9.83297878814657,-31.5378790884301,
125.640795509862));
#113855=CARTESIAN_POINT('Ctrl Pts',(9.83221104427392,-31.5333730031845,
125.651504582234));
#113856=CARTESIAN_POINT('Ctrl Pts',(9.83023519456374,-31.5214312643373,
125.679074705769));
#113857=CARTESIAN_POINT('Ctrl Pts',(9.8290328316294,-31.5138271127673,125.695861383162));
#113858=CARTESIAN_POINT('Ctrl Pts',(9.82385531164028,-31.4796386149013,
125.768120541713));
#113859=CARTESIAN_POINT('Ctrl Pts',(9.81997596267147,-31.4502706515343,
125.822226168476));
#113860=CARTESIAN_POINT('Ctrl Pts',(9.80868217627455,-31.3547531666863,
125.977089155921));
#113861=CARTESIAN_POINT('Ctrl Pts',(9.80149390773205,-31.2806090285349,
126.072425797119));
#113862=CARTESIAN_POINT('Ctrl Pts',(9.7911298764295,-31.1652975344011,126.191509063384));
#113863=CARTESIAN_POINT('Ctrl Pts',(9.78824757627212,-31.1324397928708,
126.222780238562));
#113864=CARTESIAN_POINT('Ctrl Pts',(9.78455035449333,-31.0900275382096,
126.259967663639));
#113865=CARTESIAN_POINT('Ctrl Pts',(9.78381951595969,-31.0816316308882,
126.267182522886));
#113866=CARTESIAN_POINT('Ctrl Pts',(9.78264157686225,-31.0680935572103,
126.27858363382));
#113867=CARTESIAN_POINT('Ctrl Pts',(9.78219824618454,-31.062997047823,126.28282392717));
#113868=CARTESIAN_POINT('Ctrl Pts',(9.78134369140809,-31.0531741136247,
126.290897874293));
#113869=CARTESIAN_POINT('Ctrl Pts',(9.78093280515532,-31.048451813452,126.294736199133));
#113870=CARTESIAN_POINT('Ctrl Pts',(9.77991766498423,-31.0367848042294,
126.304113561151));
#113871=CARTESIAN_POINT('Ctrl Pts',(9.77931139296962,-31.0298166945629,
126.309623028735));
#113872=CARTESIAN_POINT('Ctrl Pts',(9.77717984611495,-31.0053059946969,
126.328686308018));
#113873=CARTESIAN_POINT('Ctrl Pts',(9.77563654795875,-30.9875380349221,
126.341944842871));
#113874=CARTESIAN_POINT('Ctrl Pts',(9.76558283681481,-30.8713418957222,
126.4250935548));
#113875=CARTESIAN_POINT('Ctrl Pts',(9.75666116340628,-30.7658316028005,
126.484462632965));
#113876=CARTESIAN_POINT('Ctrl Pts',(9.74379121782298,-30.6019536338763,
126.554514488182));
#113877=CARTESIAN_POINT('Ctrl Pts',(9.73968728152694,-30.5479327926763,
126.574367884202));
#113878=CARTESIAN_POINT('Ctrl Pts',(9.73302212813713,-30.4568910276268,
126.602571267814));
#113879=CARTESIAN_POINT('Ctrl Pts',(9.7304160144128,-30.4204211770606,126.612523026939));
#113880=CARTESIAN_POINT('Ctrl Pts',(9.72682554439009,-30.3689667297245,
126.624699038706));
#113881=CARTESIAN_POINT('Ctrl Pts',(9.72580795972714,-30.3542448790846,
126.627972360263));
#113882=CARTESIAN_POINT('Ctrl Pts',(9.72406854753942,-30.328846868538,126.633258614709));
#113883=CARTESIAN_POINT('Ctrl Pts',(9.72334367629279,-30.3181919573441,
126.635367803717));
#113884=CARTESIAN_POINT('Ctrl Pts',(9.72196035843565,-30.2977265666011,
126.63921143368));
#113885=CARTESIAN_POINT('Ctrl Pts',(9.72130141341689,-30.2879197031116,
126.640962365404));
#113886=CARTESIAN_POINT('Ctrl Pts',(9.71957957789169,-30.2621464061597,
126.645325801574));
#113887=CARTESIAN_POINT('Ctrl Pts',(9.71852130296157,-30.2461563396241,
126.647793924736));
#113888=CARTESIAN_POINT('Ctrl Pts',(9.71471939950037,-30.1882072611637,
126.655876183282));
#113889=CARTESIAN_POINT('Ctrl Pts',(9.71201851712529,-30.1460721221638,
126.660123883524));
#113890=CARTESIAN_POINT('Ctrl Pts',(9.70135702509057,-29.976919647339,126.67068526608));
#113891=CARTESIAN_POINT('Ctrl Pts',(9.69376943843848,-29.8495372173957,
126.664056046763));
#113892=CARTESIAN_POINT('Ctrl Pts',(9.68335700841577,-29.6832518572427,
126.636137609831));
#113893=CARTESIAN_POINT('Ctrl Pts',(9.68076828175081,-29.6426286992141,
126.627747203136));
#113894=CARTESIAN_POINT('Ctrl Pts',(9.67650822926257,-29.5778575876894,
126.61182772459));
#113895=CARTESIAN_POINT('Ctrl Pts',(9.67487490877224,-29.553493017766,126.605248946307));
#113896=CARTESIAN_POINT('Ctrl Pts',(9.67261535893484,-29.5205920247129,
126.595558269083));
#113897=CARTESIAN_POINT('Ctrl Pts',(9.67201438451142,-29.5119164787226,
126.592925818661));
#113898=CARTESIAN_POINT('Ctrl Pts',(9.67099780997606,-29.4973767537795,
126.588384053768));
#113899=CARTESIAN_POINT('Ctrl Pts',(9.67058438312519,-29.4915007504997,
126.586512698332));
#113900=CARTESIAN_POINT('Ctrl Pts',(9.66972743422822,-29.4794004140336,
126.582584923653));
#113901=CARTESIAN_POINT('Ctrl Pts',(9.66928370309871,-29.473177682019,126.580524346861));
#113902=CARTESIAN_POINT('Ctrl Pts',(9.66810411914285,-29.4567442585325,
126.574974803239));
#113903=CARTESIAN_POINT('Ctrl Pts',(9.66736480496803,-29.4465552234503,
126.57142333425));
#113904=CARTESIAN_POINT('Ctrl Pts',(9.66402282935719,-29.4009598221346,
126.555032259623));
#113905=CARTESIAN_POINT('Ctrl Pts',(9.66136644399632,-29.3659630504794,
126.541094132434));
#113906=CARTESIAN_POINT('Ctrl Pts',(9.65113870839662,-29.2348569551235,
126.483656995352));
#113907=CARTESIAN_POINT('Ctrl Pts',(9.64337156100733,-29.1424811795041,
126.432251327956));
#113908=CARTESIAN_POINT('Ctrl Pts',(9.63180784087054,-29.0103148238149,
126.341304978151));
#113909=CARTESIAN_POINT('Ctrl Pts',(9.62789452512773,-28.9666102920846,
126.307930612521));
#113910=CARTESIAN_POINT('Ctrl Pts',(9.62149233049919,-28.8966010984201,
126.248764895171));
#113911=CARTESIAN_POINT('Ctrl Pts',(9.61896349987556,-28.8693590389266,
126.224154516576));
#113912=CARTESIAN_POINT('Ctrl Pts',(9.61545480067594,-28.8321708862205,
126.188257389433));
#113913=CARTESIAN_POINT('Ctrl Pts',(9.61444407248696,-28.8215320587777,
126.177707009184));
#113914=CARTESIAN_POINT('Ctrl Pts',(9.61270859179761,-28.8033982516775,
126.1592321436));
#113915=CARTESIAN_POINT('Ctrl Pts',(9.61198092727424,-28.7958362496777,
126.151375081794));
#113916=CARTESIAN_POINT('Ctrl Pts',(9.61058688283756,-28.7814320304424,
126.136111681118));
#113917=CARTESIAN_POINT('Ctrl Pts',(9.60992005080986,-28.7745788611619,
126.128716389728));
#113918=CARTESIAN_POINT('Ctrl Pts',(9.60816507076817,-28.7566447788359,
126.109007744648));
#113919=CARTESIAN_POINT('Ctrl Pts',(9.60708178667373,-28.7456794655501,
126.096590357779));
#113920=CARTESIAN_POINT('Ctrl Pts',(9.60310258716954,-28.7058205602204,
126.050072876008));
#113921=CARTESIAN_POINT('Ctrl Pts',(9.60025437984429,-28.6781160208182,
126.014976229816));
#113922=CARTESIAN_POINT('Ctrl Pts',(9.59035504899481,-28.5855318754205,
125.887456594161));
#113923=CARTESIAN_POINT('Ctrl Pts',(9.58356758144573,-28.528666386121,125.78960572766));
#113924=CARTESIAN_POINT('Ctrl Pts',(9.57415340819301,-28.4656058209318,
125.650228987696));
#113925=CARTESIAN_POINT('Ctrl Pts',(9.57166688472001,-28.4504056391673,
125.613122976217));
#113926=CARTESIAN_POINT('Ctrl Pts',(9.56913309254614,-28.4365599842513,
125.575509615172));
#113927=CARTESIAN_POINT('Origin',(5.,-30.,125.));
#113928=CARTESIAN_POINT('',(8.86798217145003,-28.436560143385,125.575510047478));
#113929=CARTESIAN_POINT('',(9.06223779754793,-28.4365599835583,125.57550961329));
#113930=CARTESIAN_POINT('',(5.,-28.4365599837785,125.575509613888));
#113931=CARTESIAN_POINT('Ctrl Pts',(9.06223779754793,-28.4365599835583,
125.57550961329));
#113932=CARTESIAN_POINT('Ctrl Pts',(9.06389059933002,-28.4453428407573,
125.599369284938));
#113933=CARTESIAN_POINT('Ctrl Pts',(9.06552590189583,-28.4546713138373,
125.623026366844));
#113934=CARTESIAN_POINT('Ctrl Pts',(9.06986227677821,-28.4810815118922,
125.68575523031));
#113935=CARTESIAN_POINT('Ctrl Pts',(9.07253365247076,-28.499127595394,125.724400453568));
#113936=CARTESIAN_POINT('Ctrl Pts',(9.07974290865302,-28.5523418183504,
125.827808846025));
#113937=CARTESIAN_POINT('Ctrl Pts',(9.08421372303455,-28.5903535329045,
125.890998817763));
#113938=CARTESIAN_POINT('Ctrl Pts',(9.0895973824134,-28.6406101871138,125.963234591888));
#113939=CARTESIAN_POINT('Ctrl Pts',(9.09047576512338,-28.6489495266976,
125.974896996808));
#113940=CARTESIAN_POINT('Ctrl Pts',(9.09583344681536,-28.7005825621802,
126.045169713907));
#113941=CARTESIAN_POINT('Ctrl Pts',(9.10036545821814,-28.7475274932461,
126.100988353071));
#113942=CARTESIAN_POINT('Ctrl Pts',(9.10592591400627,-28.8064683343981,
126.162406510963));
#113943=CARTESIAN_POINT('Ctrl Pts',(9.10673418688796,-28.815066603373,126.171170165829));
#113944=CARTESIAN_POINT('Ctrl Pts',(9.10801130200919,-28.8286830919664,
126.184745126469));
#113945=CARTESIAN_POINT('Ctrl Pts',(9.10847526922015,-28.8336361085751,
126.18962161301));
#113946=CARTESIAN_POINT('Ctrl Pts',(9.1093477861865,-28.8429585073051,126.198685785176));
#113947=CARTESIAN_POINT('Ctrl Pts',(9.10975575974265,-28.8473203780158,
126.20288083858));
#113948=CARTESIAN_POINT('Ctrl Pts',(9.11072168512997,-28.8576554453067,
126.212712815134));
#113949=CARTESIAN_POINT('Ctrl Pts',(9.11128112062213,-28.8636475715681,
126.218329432031));
#113950=CARTESIAN_POINT('Ctrl Pts',(9.11316534606356,-28.8838586605985,
126.236995136783));
#113951=CARTESIAN_POINT('Ctrl Pts',(9.11450369092158,-28.8982622088678,
126.249840877123));
#113952=CARTESIAN_POINT('Ctrl Pts',(9.11783548206529,-28.9343097006044,
126.280882350314));
#113953=CARTESIAN_POINT('Ctrl Pts',(9.11984352247364,-28.9561995799827,
126.298782472974));
#113954=CARTESIAN_POINT('Ctrl Pts',(9.12904500388289,-29.0576419177724,
126.37751414196));
#113955=CARTESIAN_POINT('Ctrl Pts',(9.13641092388408,-29.1421247782131,
126.43165446924));
#113956=CARTESIAN_POINT('Ctrl Pts',(9.14959464477476,-29.3043084007384,
126.516049526275));
#113957=CARTESIAN_POINT('Ctrl Pts',(9.15544338239801,-29.3804062666587,
126.548709232751));
#113958=CARTESIAN_POINT('Ctrl Pts',(9.16244526156718,-29.4771676818996,
126.581956619876));
#113959=CARTESIAN_POINT('Ctrl Pts',(9.16377630918558,-29.4958209598727,
126.587999978756));
#113960=CARTESIAN_POINT('Ctrl Pts',(9.16589271451769,-29.5258867656511,
126.597157603824));
#113961=CARTESIAN_POINT('Ctrl Pts',(9.16668485541362,-29.5372328399044,
126.600481908193));
#113962=CARTESIAN_POINT('Ctrl Pts',(9.16818871277626,-29.5589462469017,
126.606593541876));
#113963=CARTESIAN_POINT('Ctrl Pts',(9.16890108177321,-29.5693069628799,
126.609401981762));
#113964=CARTESIAN_POINT('Ctrl Pts',(9.1705329997968,-29.5932099264239,126.61563390805));
#113965=CARTESIAN_POINT('Ctrl Pts',(9.17145026311751,-29.6067696512427,
126.618987647053));
#113966=CARTESIAN_POINT('Ctrl Pts',(9.17435741631522,-29.6501237576559,
126.629133624891));
#113967=CARTESIAN_POINT('Ctrl Pts',(9.17632669996584,-29.6800645233558,
126.635277111439));
#113968=CARTESIAN_POINT('Ctrl Pts',(9.18097738764118,-29.7519404547603,
126.647975316782));
#113969=CARTESIAN_POINT('Ctrl Pts',(9.18363630873181,-29.7939906266829,
126.653758355772));
#113970=CARTESIAN_POINT('Ctrl Pts',(9.19083902256052,-29.9096040396609,
126.665179456619));
#113971=CARTESIAN_POINT('Ctrl Pts',(9.19531490061675,-29.9833920116409,
126.667548678803));
#113972=CARTESIAN_POINT('Ctrl Pts',(9.20064313679382,-30.0704430943989,
126.664563657246));
#113973=CARTESIAN_POINT('Ctrl Pts',(9.20146128200233,-30.0837857593542,
126.663945413749));
#113974=CARTESIAN_POINT('Ctrl Pts',(9.2068326810085,-30.1711080730042,126.658846289221));
#113975=CARTESIAN_POINT('Ctrl Pts',(9.21143820699762,-30.2447169095172,
126.649593836059));
#113976=CARTESIAN_POINT('Ctrl Pts',(9.21708018019915,-30.3295075734238,
126.633135479342));
#113977=CARTESIAN_POINT('Ctrl Pts',(9.21788845555639,-30.3415333703881,
126.630662954129));
#113978=CARTESIAN_POINT('Ctrl Pts',(9.21916541540654,-30.3603203827648,
126.626583382721));
#113979=CARTESIAN_POINT('Ctrl Pts',(9.21962921976291,-30.3671010165151,
126.625066496633));
#113980=CARTESIAN_POINT('Ctrl Pts',(9.22050173671547,-30.3797718203926,
126.622148581547));
#113981=CARTESIAN_POINT('Ctrl Pts',(9.22090987601783,-30.3856640991398,
126.620757802419));
#113982=CARTESIAN_POINT('Ctrl Pts',(9.22187628250806,-30.3995360148918,
126.617403629936));
#113983=CARTESIAN_POINT('Ctrl Pts',(9.22243603601175,-30.4075088535818,
126.615413277307));
#113984=CARTESIAN_POINT('Ctrl Pts',(9.22432068300024,-30.4341571944914,
126.608550913612));
#113985=CARTESIAN_POINT('Ctrl Pts',(9.22565911926247,-30.4527619309364,
126.603413566659));
#113986=CARTESIAN_POINT('Ctrl Pts',(9.22899068390954,-30.4983872675725,
126.589957643326));
#113987=CARTESIAN_POINT('Ctrl Pts',(9.23099838462509,-30.5252929153879,
126.581272382818));
#113988=CARTESIAN_POINT('Ctrl Pts',(9.24019357069396,-30.6463715918789,
126.538756552732));
#113989=CARTESIAN_POINT('Ctrl Pts',(9.24755316658955,-30.7376010584079,
126.497168354391));
#113990=CARTESIAN_POINT('Ctrl Pts',(9.260738185935,-30.896480138873,126.406674143785));
#113991=CARTESIAN_POINT('Ctrl Pts',(9.26659387469504,-30.965266892046,126.360394184085));
#113992=CARTESIAN_POINT('Ctrl Pts',(9.27360364815253,-31.0457561850253,
126.297048589284));
#113993=CARTESIAN_POINT('Ctrl Pts',(9.27493587962849,-31.060960949827,126.284641180069));
#113994=CARTESIAN_POINT('Ctrl Pts',(9.27705432048739,-31.0849792795904,
126.264324335906));
#113995=CARTESIAN_POINT('Ctrl Pts',(9.27784731605055,-31.0939335112525,
126.256584875355));
#113996=CARTESIAN_POINT('Ctrl Pts',(9.27935291402748,-31.1108602494669,
126.241636423269));
#113997=CARTESIAN_POINT('Ctrl Pts',(9.28006616848645,-31.1188469138541,
126.234444447523));
#113998=CARTESIAN_POINT('Ctrl Pts',(9.28170031317826,-31.1370666739329,
126.217715494352));
#113999=CARTESIAN_POINT('Ctrl Pts',(9.28261891221082,-31.1472504658255,
126.20812583557));
#114000=CARTESIAN_POINT('Ctrl Pts',(9.28553136420732,-31.1793366056851,
126.177140005287));
#114001=CARTESIAN_POINT('Ctrl Pts',(9.28750454801023,-31.2007711915046,
126.155267136093));
#114002=CARTESIAN_POINT('Ctrl Pts',(9.29216586624923,-31.2505134483854,
126.101626647788));
#114003=CARTESIAN_POINT('Ctrl Pts',(9.29483141592322,-31.2782313613824,
126.069340975862));
#114004=CARTESIAN_POINT('Ctrl Pts',(9.30203587260516,-31.3504928408421,
125.97834107053));
#114005=CARTESIAN_POINT('Ctrl Pts',(9.30650750206485,-31.3924256232248,
125.917678271393));
#114006=CARTESIAN_POINT('Ctrl Pts',(9.31185900726484,-31.4372839428721,
125.842592026091));
#114007=CARTESIAN_POINT('Ctrl Pts',(9.31270455652755,-31.4442142736856,
125.830657318496));
#114008=CARTESIAN_POINT('Ctrl Pts',(9.3180653150418,-31.4870942822952,125.754654616862));
#114009=CARTESIAN_POINT('Ctrl Pts',(9.32263291722558,-31.5189170355347,
125.688361320747));
#114010=CARTESIAN_POINT('Ctrl Pts',(9.32823297603165,-31.5508320274583,
125.608791401724));
#114011=CARTESIAN_POINT('Ctrl Pts',(9.32904181279348,-31.5552792746956,
125.597338517201));
#114012=CARTESIAN_POINT('Ctrl Pts',(9.33031988017727,-31.5620455872949,
125.579325452338));
#114013=CARTESIAN_POINT('Ctrl Pts',(9.33078423533308,-31.5644510154057,
125.572797881044));
#114014=CARTESIAN_POINT('Ctrl Pts',(9.33165835073149,-31.5688786352828,
125.560546764479));
#114015=CARTESIAN_POINT('Ctrl Pts',(9.33206754265318,-31.5709105207891,
125.554826980509));
#114016=CARTESIAN_POINT('Ctrl Pts',(9.3330371624904,-31.575630104756,125.541307520354));
#114017=CARTESIAN_POINT('Ctrl Pts',(9.33359908930249,-31.5782911797907,
125.53349883155));
#114018=CARTESIAN_POINT('Ctrl Pts',(9.33549396820274,-31.5870212102404,
125.507244280964));
#114019=CARTESIAN_POINT('Ctrl Pts',(9.33684058618207,-31.5928253841288,
125.488712898948));
#114020=CARTESIAN_POINT('Ctrl Pts',(9.34019636727919,-31.6063450960727,
125.442745478243));
#114021=CARTESIAN_POINT('Ctrl Pts',(9.34222028491288,-31.6136829011744,
125.415205295821));
#114022=CARTESIAN_POINT('Ctrl Pts',(9.35156962251807,-31.6440319446479,
125.288299826575));
#114023=CARTESIAN_POINT('Ctrl Pts',(9.35907015794566,-31.6585950088456,
125.187139251635));
#114024=CARTESIAN_POINT('Ctrl Pts',(9.37216406600614,-31.6679040950355,
125.0055192896));
#114025=CARTESIAN_POINT('Ctrl Pts',(9.37780517404365,-31.6662521772768,
124.925558278909));
#114026=CARTESIAN_POINT('Ctrl Pts',(9.38460671077072,-31.657064149822,124.826577323893));
#114027=CARTESIAN_POINT('Ctrl Pts',(9.38593173746895,-31.6549184496565,
124.80717364725));
#114028=CARTESIAN_POINT('Ctrl Pts',(9.38804210089221,-31.6509265233338,
124.776086264705));
#114029=CARTESIAN_POINT('Ctrl Pts',(9.38883411121953,-31.6492961101253,
124.764377208505));
#114030=CARTESIAN_POINT('Ctrl Pts',(9.39033996624531,-31.6459428838921,
124.742038871597));
#114031=CARTESIAN_POINT('Ctrl Pts',(9.39105444144772,-31.6442413922971,
124.731407047884));
#114032=CARTESIAN_POINT('Ctrl Pts',(9.39269443897607,-31.6400807316658,
124.706932001561));
#114033=CARTESIAN_POINT('Ctrl Pts',(9.3936176271612,-31.6375491352972,124.693101796001));
#114034=CARTESIAN_POINT('Ctrl Pts',(9.39655772892414,-31.6288799828841,
124.648908098807));
#114035=CARTESIAN_POINT('Ctrl Pts',(9.39855342602875,-31.6220703891944,
124.618682063026));
#114036=CARTESIAN_POINT('Ctrl Pts',(9.40992510334145,-31.5779885409697,
124.445669446299));
#114037=CARTESIAN_POINT('Ctrl Pts',(9.41868980673958,-31.5227236440366,
124.308160350397));
#114038=CARTESIAN_POINT('Ctrl Pts',(9.43132944099916,-31.4222745625069,
124.130587281867));
#114039=CARTESIAN_POINT('Ctrl Pts',(9.43488291763592,-31.3920003381725,
124.082897461114));
#114040=CARTESIAN_POINT('Ctrl Pts',(9.43935225533778,-31.3524773652413,
124.027116120467));
#114041=CARTESIAN_POINT('Ctrl Pts',(9.4401374574757,-31.3454826528222,124.017465279244));
#114042=CARTESIAN_POINT('Ctrl Pts',(9.44138594402702,-31.3342939762659,
124.002371419115));
#114043=CARTESIAN_POINT('Ctrl Pts',(9.4418447011448,-31.3301686997754,123.9968776613));
#114044=CARTESIAN_POINT('Ctrl Pts',(9.44271162772101,-31.3223498553831,
123.986598102644));
#114045=CARTESIAN_POINT('Ctrl Pts',(9.44311927172541,-31.3186640759014,
123.981806700079));
#114046=CARTESIAN_POINT('Ctrl Pts',(9.44409127822239,-31.3098529446529,
123.970480580788));
#114047=CARTESIAN_POINT('Ctrl Pts',(9.44465720653217,-31.3047047343026,
123.963964035327));
#114048=CARTESIAN_POINT('Ctrl Pts',(9.44659894595935,-31.2869722515712,
123.941860240634));
#114049=CARTESIAN_POINT('Ctrl Pts',(9.4479895726608,-31.2741561937267,123.926462282038));
#114050=CARTESIAN_POINT('Ctrl Pts',(9.45148446122763,-31.2415898580862,
123.888739942417));
#114051=CARTESIAN_POINT('Ctrl Pts',(9.45360523614729,-31.2215125710045,
123.866707838631));
#114052=CARTESIAN_POINT('Ctrl Pts',(9.46388437932644,-31.1222786429749,
123.763513752125));
#114053=CARTESIAN_POINT('Ctrl Pts',(9.47224659940962,-31.0355649220604,
123.690032390207));
#114054=CARTESIAN_POINT('Ctrl Pts',(9.48533161008495,-30.8849547222947,
123.586775213546));
#114055=CARTESIAN_POINT('Ctrl Pts',(9.49019755252259,-30.825462663382,123.551220229114));
#114056=CARTESIAN_POINT('Ctrl Pts',(9.49621708007272,-30.747204530449,123.510840740678));
#114057=CARTESIAN_POINT('Ctrl Pts',(9.49749312562583,-30.7303408507461,
123.502498012576));
#114058=CARTESIAN_POINT('Ctrl Pts',(9.49954097883193,-30.7028409503989,
123.489468456255));
#114059=CARTESIAN_POINT('Ctrl Pts',(9.50031888945334,-30.6922910832407,
123.484604337422));
#114060=CARTESIAN_POINT('Ctrl Pts',(9.50180756042947,-30.6719063342073,
123.475463063823));
#114061=CARTESIAN_POINT('Ctrl Pts',(9.50251884739219,-30.6620793764762,
123.47116976084));
#114062=CARTESIAN_POINT('Ctrl Pts',(9.50416526665393,-30.6391347185475,
123.461408188155));
#114063=CARTESIAN_POINT('Ctrl Pts',(9.5050979041059,-30.6259870151238,123.456012231391));
#114064=CARTESIAN_POINT('Ctrl Pts',(9.50812737656557,-30.5828068281466,
123.438932878497));
#114065=CARTESIAN_POINT('Ctrl Pts',(9.5102008008245,-30.5525031341213,123.427952016501));
#114066=CARTESIAN_POINT('Ctrl Pts',(9.51515772415006,-30.4784710356829,
123.403531206414));
#114067=CARTESIAN_POINT('Ctrl Pts',(9.51801409559071,-30.434470366514,123.390999349362));
#114068=CARTESIAN_POINT('Ctrl Pts',(9.52512372644802,-30.3226277650559,
123.364068906182));
#114069=CARTESIAN_POINT('Ctrl Pts',(9.52932924226855,-30.2543003760714,
123.352064693413));
#114070=CARTESIAN_POINT('Ctrl Pts',(9.53431792129586,-30.1732516179027,
123.342987657701));
#114071=CARTESIAN_POINT('Ctrl Pts',(9.53506815284999,-30.1610646414383,
123.341758701882));
#114072=CARTESIAN_POINT('Ctrl Pts',(9.54035796771801,-30.0752469660574,
123.334059672392));
#114073=CARTESIAN_POINT('Ctrl Pts',(9.54495067255575,-30.0012797032774,
123.332362493317));
#114074=CARTESIAN_POINT('Ctrl Pts',(9.5505778095653,-29.9152174870883,123.336113598137));
#114075=CARTESIAN_POINT('Ctrl Pts',(9.5513842367218,-29.9029870138944,123.336781886941));
#114076=CARTESIAN_POINT('Ctrl Pts',(9.55265793484031,-29.8838537580744,
123.338039101398));
#114077=CARTESIAN_POINT('Ctrl Pts',(9.55312032287477,-29.876945104284,123.338536348191));
#114078=CARTESIAN_POINT('Ctrl Pts',(9.5539919168578,-29.8639969877972,123.339549482477));
#114079=CARTESIAN_POINT('Ctrl Pts',(9.5544005661202,-29.8579569586731,123.340055269005));
#114080=CARTESIAN_POINT('Ctrl Pts',(9.55536868591195,-29.8437177275803,
123.341325932042));
#114081=CARTESIAN_POINT('Ctrl Pts',(9.55592965549295,-29.8355212460014,
123.342118657815));
#114082=CARTESIAN_POINT('Ctrl Pts',(9.55781629932395,-29.8081248077636,
123.344973474094));
#114083=CARTESIAN_POINT('Ctrl Pts',(9.55915548848551,-29.7889556700667,
123.347308527785));
#114084=CARTESIAN_POINT('Ctrl Pts',(9.56248722154647,-29.7418430948287,
123.353880422655));
#114085=CARTESIAN_POINT('Ctrl Pts',(9.56449427818051,-29.7139590926442,
123.358496095079));
#114086=CARTESIAN_POINT('Ctrl Pts',(9.57366386920714,-29.5882807641671,
123.382599104441));
#114087=CARTESIAN_POINT('Ctrl Pts',(9.5809974097623,-29.4922384660791,123.410133026382));
#114088=CARTESIAN_POINT('Ctrl Pts',(9.59421679974319,-29.3213071919836,
123.47621776069));
#114089=CARTESIAN_POINT('Ctrl Pts',(9.60012881080644,-29.2457477538774,
123.512168155588));
#114090=CARTESIAN_POINT('Ctrl Pts',(9.60719866112001,-29.1560795089531,
123.563426691946));
#114091=CARTESIAN_POINT('Ctrl Pts',(9.60853738784968,-29.1391384805706,
123.573514049607));
#114092=CARTESIAN_POINT('Ctrl Pts',(9.6106663654073,-29.1122703566486,123.590165422435));
#114093=CARTESIAN_POINT('Ctrl Pts',(9.61146343371866,-29.1022280294976,
123.596538936272));
#114094=CARTESIAN_POINT('Ctrl Pts',(9.61297698854849,-29.0831953322957,
123.608906213186));
#114095=CARTESIAN_POINT('Ctrl Pts',(9.61369412811207,-29.0741933766686,
123.614880933651));
#114096=CARTESIAN_POINT('Ctrl Pts',(9.61533762704353,-29.0536050307787,
123.628836089473));
#114097=CARTESIAN_POINT('Ctrl Pts',(9.61626167655271,-29.0420602272945,
123.636876630982));
#114098=CARTESIAN_POINT('Ctrl Pts',(9.61919439613349,-29.0055370186924,
123.663006937264));
#114099=CARTESIAN_POINT('Ctrl Pts',(9.62118219217877,-28.9809576125359,
123.681645011811));
#114100=CARTESIAN_POINT('Ctrl Pts',(9.62588348790906,-28.9234366565551,
123.72783252063));
#114101=CARTESIAN_POINT('Ctrl Pts',(9.6285740587608,-28.891014572963,123.755994197638));
#114102=CARTESIAN_POINT('Ctrl Pts',(9.63575157497526,-28.8066361848038,
123.835208527477));
#114103=CARTESIAN_POINT('Ctrl Pts',(9.64017526535042,-28.7568799290371,
123.888465386057));
#114104=CARTESIAN_POINT('Ctrl Pts',(9.64536565406243,-28.7031969632477,
123.954055102617));
#114105=CARTESIAN_POINT('Ctrl Pts',(9.64609844104944,-28.695726875889,123.963385096283));
#114106=CARTESIAN_POINT('Ctrl Pts',(9.65143268905923,-28.6421988854006,
124.031735172149));
#114107=CARTESIAN_POINT('Ctrl Pts',(9.65608507259707,-28.6000708598512,
124.093712947131));
#114108=CARTESIAN_POINT('Ctrl Pts',(9.66178032184662,-28.5560187562625,
124.16896049655));
#114109=CARTESIAN_POINT('Ctrl Pts',(9.66259319329784,-28.5498988856904,
124.179685898596));
#114110=CARTESIAN_POINT('Ctrl Pts',(9.66387840151904,-28.5404954779628,
124.196599966775));
#114111=CARTESIAN_POINT('Ctrl Pts',(9.66434587004967,-28.5371306505963,
124.202743250026));
#114112=CARTESIAN_POINT('Ctrl Pts',(9.66523007251182,-28.5308725435921,
124.214341901285));
#114113=CARTESIAN_POINT('Ctrl Pts',(9.66564627335725,-28.5279707042067,
124.219792413206));
#114114=CARTESIAN_POINT('Ctrl Pts',(9.6666366200846,-28.5211680713316,124.23274281235));
#114115=CARTESIAN_POINT('Ctrl Pts',(9.66721234151501,-28.5172939582916,
124.240256456666));
#114116=CARTESIAN_POINT('Ctrl Pts',(9.66916988677307,-28.5043864337242,
124.265764704886));
#114117=CARTESIAN_POINT('Ctrl Pts',(9.67056608814642,-28.4956224834149,
124.28389273905));
#114118=CARTESIAN_POINT('Ctrl Pts',(9.68032290249009,-28.4372644051163,
124.410406683955));
#114119=CARTESIAN_POINT('Ctrl Pts',(9.68909376329002,-28.3991001928916,
124.523679457309));
#114120=CARTESIAN_POINT('Ctrl Pts',(9.70382032119808,-28.3549258039464,
124.723308590907));
#114121=CARTESIAN_POINT('Ctrl Pts',(9.7098524581643,-28.3429193192993,124.807867778118));
#114122=CARTESIAN_POINT('Ctrl Pts',(9.71703355873765,-28.3361764024113,
124.912625356863));
#114123=CARTESIAN_POINT('Ctrl Pts',(9.71836925881555,-28.335260331937,124.932285995));
#114124=CARTESIAN_POINT('Ctrl Pts',(9.72049724830729,-28.3343488790973,
124.963880856001));
#114125=CARTESIAN_POINT('Ctrl Pts',(9.72129623747585,-28.3341329801179,
124.975806326301));
#114126=CARTESIAN_POINT('Ctrl Pts',(9.72281611609816,-28.3339650959009,
124.998606983978));
#114127=CARTESIAN_POINT('Ctrl Pts',(9.72353763388513,-28.3339914898998,
125.009481345367));
#114128=CARTESIAN_POINT('Ctrl Pts',(9.72519522352925,-28.3342981007914,
125.03457485386));
#114129=CARTESIAN_POINT('Ctrl Pts',(9.72612891418908,-28.3346539206633,
125.048792357817));
#114130=CARTESIAN_POINT('Ctrl Pts',(9.72911022938338,-28.3363812386608,
125.0944347978));
#114131=CARTESIAN_POINT('Ctrl Pts',(9.73113605243017,-28.3384606393052,
125.125827142653));
#114132=CARTESIAN_POINT('Ctrl Pts',(9.74228319104025,-28.3549758076651,
125.300136629054));
#114133=CARTESIAN_POINT('Ctrl Pts',(9.75083237414512,-28.3869548981719,
125.440751524718));
#114134=CARTESIAN_POINT('Ctrl Pts',(9.75970369730367,-28.4365599837282,
125.575509613751));
#114135=CARTESIAN_POINT('Ctrl Pts',(9.56913309254614,-28.4365599842513,
125.575509615172));
#114136=CARTESIAN_POINT('Ctrl Pts',(9.56864907652894,-28.4339151269433,
125.568324547117));
#114137=CARTESIAN_POINT('Ctrl Pts',(9.56816332838147,-28.4313196967858,
125.561120966193));
#114138=CARTESIAN_POINT('Ctrl Pts',(9.56590951223272,-28.4195543508702,
125.527746639993));
#114139=CARTESIAN_POINT('Ctrl Pts',(9.56411880548602,-28.4109898327577,
125.501369566884));
#114140=CARTESIAN_POINT('Ctrl Pts',(9.5616726110363,-28.4003989635077,125.465748386525));
#114141=CARTESIAN_POINT('Ctrl Pts',(9.56104756284543,-28.3977868054281,
125.456681403509));
#114142=CARTESIAN_POINT('Ctrl Pts',(9.55999962570631,-28.3935660290641,
125.441548720156));
#114143=CARTESIAN_POINT('Ctrl Pts',(9.55957915432647,-28.3919143628956,
125.435495070804));
#114144=CARTESIAN_POINT('Ctrl Pts',(9.5587733120997,-28.3888293866305,125.423931209732));
#114145=CARTESIAN_POINT('Ctrl Pts',(9.55838831516424,-28.3873900524238,
125.418422717458));
#114146=CARTESIAN_POINT('Ctrl Pts',(9.55734420574154,-28.3835787110721,
125.403524486058));
#114147=CARTESIAN_POINT('Ctrl Pts',(9.55668216604186,-28.3812603439051,
125.394121438962));
#114148=CARTESIAN_POINT('Ctrl Pts',(9.55412129549575,-28.3726629844751,
125.357895423551));
#114149=CARTESIAN_POINT('Ctrl Pts',(9.55219417358964,-28.3669680326369,
125.330939994153));
#114150=CARTESIAN_POINT('Ctrl Pts',(9.54311627988201,-28.3435782332267,
125.20484877221));
#114151=CARTESIAN_POINT('Ctrl Pts',(9.53571699610879,-28.3342272104926,
125.104382936422));
#114152=CARTESIAN_POINT('Ctrl Pts',(9.52129044764897,-28.333786189495,124.905355962508));
#114153=CARTESIAN_POINT('Ctrl Pts',(9.51428778498704,-28.3422749160066,
124.807180107484));
#114154=CARTESIAN_POINT('Ctrl Pts',(9.50620104424878,-28.362816952133,124.690842168768));
#114155=CARTESIAN_POINT('Ctrl Pts',(9.50485849955833,-28.366601233408,124.671434291939));
#114156=CARTESIAN_POINT('Ctrl Pts',(9.50272785511388,-28.3732077457406,
124.640495178933));
#114157=CARTESIAN_POINT('Ctrl Pts',(9.50193282781672,-28.3758091674126,
124.628919271821));
#114158=CARTESIAN_POINT('Ctrl Pts',(9.500425924596,-28.3809997232743,124.606923216332));
#114159=CARTESIAN_POINT('Ctrl Pts',(9.49971337030503,-28.3835663497061,
124.596498429626));
#114160=CARTESIAN_POINT('Ctrl Pts',(9.49809968516449,-28.3896339863144,
124.572841209062));
#114161=CARTESIAN_POINT('Ctrl Pts',(9.49720061826433,-28.3931976836133,
124.559625539693));
#114162=CARTESIAN_POINT('Ctrl Pts',(9.49436252145478,-28.4050268150634,
124.517814924124));
#114163=CARTESIAN_POINT('Ctrl Pts',(9.49244296538531,-28.4138961174369,
124.48939589123));
#114164=CARTESIAN_POINT('Ctrl Pts',(9.4814725659988,-28.4695220239556,124.326631245233));
#114165=CARTESIAN_POINT('Ctrl Pts',(9.47298949485508,-28.5325657372751,
124.198485425495));
#114166=CARTESIAN_POINT('Ctrl Pts',(9.4615463728839,-28.6349691757038,124.043908408253));
#114167=CARTESIAN_POINT('Ctrl Pts',(9.4588538890971,-28.6602038694527,124.008856159938));
#114168=CARTESIAN_POINT('Ctrl Pts',(9.45444160141901,-28.7027388407429,
123.954369582316));
#114169=CARTESIAN_POINT('Ctrl Pts',(9.45276276222877,-28.7191829359519,
123.93429039739));
#114170=CARTESIAN_POINT('Ctrl Pts',(9.45044779106971,-28.7420800491302,
123.907627359893));
#114171=CARTESIAN_POINT('Ctrl Pts',(9.44983821927761,-28.7481294795623,
123.90069986897));
#114172=CARTESIAN_POINT('Ctrl Pts',(9.44880971677453,-28.7583630566993,
123.889174928192));
#114173=CARTESIAN_POINT('Ctrl Pts',(9.44839303204895,-28.7625162569413,
123.884550035595));
#114174=CARTESIAN_POINT('Ctrl Pts',(9.44753432992432,-28.7710873037546,
123.87511233255));
#114175=CARTESIAN_POINT('Ctrl Pts',(9.44709213744048,-28.7755077153033,
123.870302111011));
#114176=CARTESIAN_POINT('Ctrl Pts',(9.44592030073135,-28.7872426498607,
123.85768213506));
#114177=CARTESIAN_POINT('Ctrl Pts',(9.44518726799707,-28.7946041801413,
123.849916786776));
#114178=CARTESIAN_POINT('Ctrl Pts',(9.44191822389892,-28.8275469582656,
123.815830651404));
#114179=CARTESIAN_POINT('Ctrl Pts',(9.43933119501081,-28.8539173218618,
123.790290438666));
#114180=CARTESIAN_POINT('Ctrl Pts',(9.42914507243602,-28.9596135366402,
123.694481166278));
#114181=CARTESIAN_POINT('Ctrl Pts',(9.42134135126428,-29.0447287841113,
123.630970901488));
#114182=CARTESIAN_POINT('Ctrl Pts',(9.40777103491111,-29.2056163465733,
123.533276402163));
#114183=CARTESIAN_POINT('Ctrl Pts',(9.40195325074701,-29.2790071232635,
123.495840289644));
#114184=CARTESIAN_POINT('Ctrl Pts',(9.39498164264185,-29.3729336953591,
123.456391397641));
#114185=CARTESIAN_POINT('Ctrl Pts',(9.39365185614205,-29.3911259752948,
123.449125360777));
#114186=CARTESIAN_POINT('Ctrl Pts',(9.39153712379415,-29.4204917834884,
123.437993005859));
#114187=CARTESIAN_POINT('Ctrl Pts',(9.39074541017417,-29.4315851936955,
123.433922018805));
#114188=CARTESIAN_POINT('Ctrl Pts',(9.38924216635695,-29.4528344412019,
123.426379647442));
#114189=CARTESIAN_POINT('Ctrl Pts',(9.38852998602496,-29.4629822968068,
123.422887715356));
#114190=CARTESIAN_POINT('Ctrl Pts',(9.38689823119501,-29.4864144897609,
123.415076965411));
#114191=CARTESIAN_POINT('Ctrl Pts',(9.38598094467362,-29.4997209358332,
123.410826636408));
#114192=CARTESIAN_POINT('Ctrl Pts',(9.38307267387077,-29.5423190467943,
123.397808082202));
#114193=CARTESIAN_POINT('Ctrl Pts',(9.38110232824733,-29.5718002799732,
123.389678297914));
#114194=CARTESIAN_POINT('Ctrl Pts',(9.37644857239736,-29.642719189676,123.372207193458));
#114195=CARTESIAN_POINT('Ctrl Pts',(9.3737876965006,-29.6843233715002,123.363629735032));
#114196=CARTESIAN_POINT('Ctrl Pts',(9.36658171166315,-29.7989784721036,
123.344527787625));
#114197=CARTESIAN_POINT('Ctrl Pts',(9.36210454696657,-29.8724712589146,
123.337250863823));
#114198=CARTESIAN_POINT('Ctrl Pts',(9.35676857231092,-29.959659213745,123.334434078629));
#114199=CARTESIAN_POINT('Ctrl Pts',(9.35594402320497,-29.9731185752571,
123.334162492568));
#114200=CARTESIAN_POINT('Ctrl Pts',(9.35057190384155,-30.0605995332203,
123.333457772531));
#114201=CARTESIAN_POINT('Ctrl Pts',(9.34597195985089,-30.1345678489389,
123.33779543764));
#114202=CARTESIAN_POINT('Ctrl Pts',(9.34033630074149,-30.2201707949272,
123.348566839258));
#114203=CARTESIAN_POINT('Ctrl Pts',(9.33952823014974,-30.2323315150685,
123.350233741198));
#114204=CARTESIAN_POINT('Ctrl Pts',(9.33825167019404,-30.2513426124542,
123.353053998569));
#114205=CARTESIAN_POINT('Ctrl Pts',(9.33778806013631,-30.2582063648558,
123.354116131301));
#114206=CARTESIAN_POINT('Ctrl Pts',(9.33691594499232,-30.2710375217351,
123.35618392687));
#114207=CARTESIAN_POINT('Ctrl Pts',(9.3365080131288,-30.2770063484849,123.357179225034));
#114208=CARTESIAN_POINT('Ctrl Pts',(9.33554219669211,-30.2910623881309,
123.359601839103));
#114209=CARTESIAN_POINT('Ctrl Pts',(9.33498282827726,-30.2991446201065,
123.361056459406));
#114210=CARTESIAN_POINT('Ctrl Pts',(9.333100012791,-30.3261649799327,123.366126037049));
#114211=CARTESIAN_POINT('Ctrl Pts',(9.33176305338781,-30.3450502734016,
123.370009831118));
#114212=CARTESIAN_POINT('Ctrl Pts',(9.3284356778858,-30.3914140428957,123.380386424095));
#114213=CARTESIAN_POINT('Ctrl Pts',(9.32643073005886,-30.4188025074075,
123.38725161038));
#114214=CARTESIAN_POINT('Ctrl Pts',(9.31725632167081,-30.5421739020631,
123.421530302263));
#114215=CARTESIAN_POINT('Ctrl Pts',(9.30991534878841,-30.6357493821585,
123.456840167597));
#114216=CARTESIAN_POINT('Ctrl Pts',(9.29673260043725,-30.8003028269684,
123.536457087596));
#114217=CARTESIAN_POINT('Ctrl Pts',(9.29086212744621,-30.8722075629032,
123.578134961831));
#114218=CARTESIAN_POINT('Ctrl Pts',(9.28383875660147,-30.9569084544208,
123.636083893992));
#114219=CARTESIAN_POINT('Ctrl Pts',(9.28250673464296,-30.9729047650104,
123.64744785325));
#114220=CARTESIAN_POINT('Ctrl Pts',(9.2803888512693,-30.9982186861673,123.66611267322));
#114221=CARTESIAN_POINT('Ctrl Pts',(9.27959620221406,-31.0076653179181,
123.673234547663));
#114222=CARTESIAN_POINT('Ctrl Pts',(9.2780914076956,-31.025542395378,123.687013270293));
#114223=CARTESIAN_POINT('Ctrl Pts',(9.27737860923445,-31.0339858475429,
123.693652177482));
#114224=CARTESIAN_POINT('Ctrl Pts',(9.275745726344,-31.0532666418938,123.709116314394));
#114225=CARTESIAN_POINT('Ctrl Pts',(9.274827928131,-31.0640584155899,123.717997263415));
#114226=CARTESIAN_POINT('Ctrl Pts',(9.27191901945845,-31.0981000399246,
123.746737394697));
#114227=CARTESIAN_POINT('Ctrl Pts',(9.26994852185422,-31.1209163030937,
123.767101916279));
#114228=CARTESIAN_POINT('Ctrl Pts',(9.26529460691424,-31.1740465702702,
123.817217941104));
#114229=CARTESIAN_POINT('Ctrl Pts',(9.26263368789692,-31.2038092043832,
123.847523307756));
#114230=CARTESIAN_POINT('Ctrl Pts',(9.25543144447707,-31.2819757327842,
123.933451474673));
#114231=CARTESIAN_POINT('Ctrl Pts',(9.2509577468347,-31.3278973198496,123.991200411082));
#114232=CARTESIAN_POINT('Ctrl Pts',(9.2456057615673,-31.3776860342753,124.063129131166));
#114233=CARTESIAN_POINT('Ctrl Pts',(9.24476165889348,-31.3853868652131,
124.074554668351));
#114234=CARTESIAN_POINT('Ctrl Pts',(9.23939448547394,-31.4333197340001,
124.147610774164));
#114235=CARTESIAN_POINT('Ctrl Pts',(9.23481904682353,-31.4695673785132,
124.211747610035));
#114236=CARTESIAN_POINT('Ctrl Pts',(9.22921055783351,-31.5067734932096,
124.289127006863));
#114237=CARTESIAN_POINT('Ctrl Pts',(9.22840217872281,-31.5119717115942,
124.300251263814));
#114238=CARTESIAN_POINT('Ctrl Pts',(9.22712493159828,-31.5199192813636,
124.317761260788));
#114239=CARTESIAN_POINT('Ctrl Pts',(9.22666093853779,-31.5227525474073,
124.324108740897));
#114240=CARTESIAN_POINT('Ctrl Pts',(9.22578823132324,-31.5279791158545,
124.336017711999));
#114241=CARTESIAN_POINT('Ctrl Pts',(9.22538009188315,-31.5303819303747,
124.341574757637));
#114242=CARTESIAN_POINT('Ctrl Pts',(9.22441366196081,-31.5359747770561,
124.354705477475));
#114243=CARTESIAN_POINT('Ctrl Pts',(9.22385388600149,-31.5391391169627,
124.362289793001));
#114244=CARTESIAN_POINT('Ctrl Pts',(9.22196833959125,-31.5495517990776,
124.387775990224));
#114245=CARTESIAN_POINT('Ctrl Pts',(9.22062900664261,-31.5565446294652,
124.405779709907));
#114246=CARTESIAN_POINT('Ctrl Pts',(9.21729441983968,-31.5730086491381,
124.450454112424));
#114247=CARTESIAN_POINT('Ctrl Pts',(9.21528456002422,-31.5821160283495,
124.477251891612));
#114248=CARTESIAN_POINT('Ctrl Pts',(9.20606642334074,-31.6203960571586,
124.600071562395));
#114249=CARTESIAN_POINT('Ctrl Pts',(9.19868545122572,-31.6415390275105,
124.698377334602));
#114250=CARTESIAN_POINT('Ctrl Pts',(9.1855137419008,-31.6636920637042,124.879727323645));
#114251=CARTESIAN_POINT('Ctrl Pts',(9.17969015143798,-31.6676043530301,
124.962102909666));
#114252=CARTESIAN_POINT('Ctrl Pts',(9.17271225983601,-31.6648843659895,
125.064032142613));
#114253=CARTESIAN_POINT('Ctrl Pts',(9.17138176776003,-31.6640159353249,
125.083612745987));
#114254=CARTESIAN_POINT('Ctrl Pts',(9.16926582094754,-31.6620699455326,
125.114975194841));
#114255=CARTESIAN_POINT('Ctrl Pts',(9.16847359734726,-31.661212090601,125.126768299615));
#114256=CARTESIAN_POINT('Ctrl Pts',(9.16696931233731,-31.6593356193819,
125.149253588732));
#114257=CARTESIAN_POINT('Ctrl Pts',(9.16625660116129,-31.658339021785,125.159946958506));
#114258=CARTESIAN_POINT('Ctrl Pts',(9.16462350646613,-31.655807256875,125.184536630692));
#114259=CARTESIAN_POINT('Ctrl Pts',(9.16370541409725,-31.6542004209905,
125.198424864662));
#114260=CARTESIAN_POINT('Ctrl Pts',(9.16079391990177,-31.6485182629067,
125.242653209634));
#114261=CARTESIAN_POINT('Ctrl Pts',(9.15882119412287,-31.6437813747341,
125.27290295694));
#114262=CARTESIAN_POINT('Ctrl Pts',(9.15416095088509,-31.6304788127535,
125.344823618399));
#114263=CARTESIAN_POINT('Ctrl Pts',(9.15149602891097,-31.6211456337839,
125.386331077069));
#114264=CARTESIAN_POINT('Ctrl Pts',(9.14428942280601,-31.5913215126241,
125.498683700995));
#114265=CARTESIAN_POINT('Ctrl Pts',(9.13981526786953,-31.5677012878763,
125.568597068817));
#114266=CARTESIAN_POINT('Ctrl Pts',(9.13445109923829,-31.5341903013582,
125.649623905231));
#114267=CARTESIAN_POINT('Ctrl Pts',(9.13359539420121,-31.5286899816869,
125.662463608741));
#114268=CARTESIAN_POINT('Ctrl Pts',(9.12822988086904,-31.4932880070493,
125.742314961656));
#114269=CARTESIAN_POINT('Ctrl Pts',(9.12366753319143,-31.4591511726609,
125.80735104298));
#114270=CARTESIAN_POINT('Ctrl Pts',(9.11807355409343,-31.4144346422765,
125.88038705076));
#114271=CARTESIAN_POINT('Ctrl Pts',(9.11726532568212,-31.4079089687935,
125.890785625307));
#114272=CARTESIAN_POINT('Ctrl Pts',(9.11598836799763,-31.3975105639601,
125.906955629354));
#114273=CARTESIAN_POINT('Ctrl Pts',(9.11552451437639,-31.3937154673444,
125.912776797311));
#114274=CARTESIAN_POINT('Ctrl Pts',(9.11465206218794,-31.3865468481967,
125.923623556525));
#114275=CARTESIAN_POINT('Ctrl Pts',(9.11424403813389,-31.3831822127602,
125.92865472488));
#114276=CARTESIAN_POINT('Ctrl Pts',(9.1132779456481,-31.3751865206967,125.94047090122));
#114277=CARTESIAN_POINT('Ctrl Pts',(9.11271839285482,-31.3705326132634,
125.94724011299));
#114278=CARTESIAN_POINT('Ctrl Pts',(9.11083406479607,-31.3547780050052,
125.969796377645));
#114279=CARTESIAN_POINT('Ctrl Pts',(9.10949574629724,-31.3434535369851,
125.985424259676));
#114280=CARTESIAN_POINT('Ctrl Pts',(9.10616416475786,-31.3148762880254,
126.023452812909));
#114281=CARTESIAN_POINT('Ctrl Pts',(9.10415632369449,-31.2973201302102,
126.045617335541));
#114282=CARTESIAN_POINT('Ctrl Pts',(9.09495578448027,-31.2150584476086,
126.144209722006));
#114283=CARTESIAN_POINT('Ctrl Pts',(9.08759083604433,-31.1441066983528,
126.21515564163));
#114284=CARTESIAN_POINT('Ctrl Pts',(9.07441425822697,-31.0037799005452,
126.33221838848));
#114285=CARTESIAN_POINT('Ctrl Pts',(9.06857146151652,-30.9364915102122,
126.38035041791));
#114286=CARTESIAN_POINT('Ctrl Pts',(9.06157511407242,-30.8491509219734,
126.433486328067));
#114287=CARTESIAN_POINT('Ctrl Pts',(9.06024413815668,-30.8322231672953,
126.443379713669));
#114288=CARTESIAN_POINT('Ctrl Pts',(9.05812767127939,-30.8048117235281,
126.458757657672));
#114289=CARTESIAN_POINT('Ctrl Pts',(9.05733540338543,-30.7944378455855,
126.46443311084));
#114290=CARTESIAN_POINT('Ctrl Pts',(9.05583118930943,-30.7745299231472,
126.47505074231));
#114291=CARTESIAN_POINT('Ctrl Pts',(9.05511859180318,-30.7650068464543,
126.480012104115));
#114292=CARTESIAN_POINT('Ctrl Pts',(9.05348597866258,-30.7429811213187,
126.491217736126));
#114293=CARTESIAN_POINT('Ctrl Pts',(9.05256825105334,-30.730446430936,126.497397513828));
#114294=CARTESIAN_POINT('Ctrl Pts',(9.04965885607282,-30.6902354266995,
126.516596999777));
#114295=CARTESIAN_POINT('Ctrl Pts',(9.04768782563769,-30.6622767929369,
126.529013094004));
#114296=CARTESIAN_POINT('Ctrl Pts',(9.04303234529681,-30.5947098508056,
126.556817415281));
#114297=CARTESIAN_POINT('Ctrl Pts',(9.04037042920156,-30.5548233946614,
126.571474355906));
#114298=CARTESIAN_POINT('Ctrl Pts',(9.03316567933843,-30.4442925020958,
126.607356845071));
#114299=CARTESIAN_POINT('Ctrl Pts',(9.02869056061395,-30.3727314978194,
126.62544254042));
#114300=CARTESIAN_POINT('Ctrl Pts',(9.02333971540549,-30.2866961602502,
126.641203826451));
#114301=CARTESIAN_POINT('Ctrl Pts',(9.022498226784,-30.2731546356077,126.643511858074));
#114302=CARTESIAN_POINT('Ctrl Pts',(9.01712959590003,-30.1868139379441,
126.657131295132));
#114303=CARTESIAN_POINT('Ctrl Pts',(9.01255003170936,-30.1133691972112,
126.663769290262));
#114304=CARTESIAN_POINT('Ctrl Pts',(9.00693696281334,-30.027463160572,126.66581886804));
#114305=CARTESIAN_POINT('Ctrl Pts',(9.00612871172942,-30.0151871692735,
126.665976006561));
#114306=CARTESIAN_POINT('Ctrl Pts',(9.00485174531684,-29.9959621186229,
126.666009598637));
#114307=CARTESIAN_POINT('Ctrl Pts',(9.00438790659187,-29.9890133767509,
126.665978264256));
#114308=CARTESIAN_POINT('Ctrl Pts',(9.00351545960601,-29.9760125771056,
126.665838300057));
#114309=CARTESIAN_POINT('Ctrl Pts',(9.003107425652,-29.9699606533227,126.665740157217));
#114310=CARTESIAN_POINT('Ctrl Pts',(9.0021413106944,-29.9556964194323,126.665431079037));
#114311=CARTESIAN_POINT('Ctrl Pts',(9.00158174520495,-29.9474849864777,
126.665192377042));
#114312=CARTESIAN_POINT('Ctrl Pts',(8.99969748271359,-29.9199906239966,
126.664189567124));
#114313=CARTESIAN_POINT('Ctrl Pts',(8.99835924538192,-29.9007200598256,
126.663151174646));
#114314=CARTESIAN_POINT('Ctrl Pts',(8.99502795234815,-29.8532752075023,
126.659767150037));
#114315=CARTESIAN_POINT('Ctrl Pts',(8.99302032323471,-29.8251347733289,
126.657038662555));
#114316=CARTESIAN_POINT('Ctrl Pts',(8.98382188715087,-29.6977154067481,
126.641402399791));
#114317=CARTESIAN_POINT('Ctrl Pts',(8.97645890361031,-29.5996537396147,
126.6202781039));
#114318=CARTESIAN_POINT('Ctrl Pts',(8.96327727135493,-29.4251281942028,
126.565860126711));
#114319=CARTESIAN_POINT('Ctrl Pts',(8.95742785399945,-29.3481088389755,
126.535394789005));
#114320=CARTESIAN_POINT('Ctrl Pts',(8.95042765424983,-29.2560471219849,
126.490796152483));
#114321=CARTESIAN_POINT('Ctrl Pts',(8.94909896203622,-29.2385845019613,
126.481953288398));
#114322=CARTESIAN_POINT('Ctrl Pts',(8.94698517657294,-29.2108334308248,
126.467280407598));
#114323=CARTESIAN_POINT('Ctrl Pts',(8.94619333879618,-29.2004446155483,
126.461645260682));
#114324=CARTESIAN_POINT('Ctrl Pts',(8.94468935663384,-29.1807302927506,
126.450678636941));
#114325=CARTESIAN_POINT('Ctrl Pts',(8.94397656697666,-29.1713947079991,
126.445366610994));
#114326=CARTESIAN_POINT('Ctrl Pts',(8.94234268517443,-29.1500182190073,
126.432928023052));
#114327=CARTESIAN_POINT('Ctrl Pts',(8.94142389195574,-29.1380143048349,
126.425739256799));
#114328=CARTESIAN_POINT('Ctrl Pts',(8.93850761017328,-29.0999862349143,
126.402309580254));
#114329=CARTESIAN_POINT('Ctrl Pts',(8.93653089643965,-29.0743185702054,
126.385500276577));
#114330=CARTESIAN_POINT('Ctrl Pts',(8.93185913279897,-29.0141084881935,
126.343649076758));
#114331=CARTESIAN_POINT('Ctrl Pts',(8.92918683710026,-28.9800346423822,
126.31797039676));
#114332=CARTESIAN_POINT('Ctrl Pts',(8.92200100880832,-28.8902056538236,
126.244701031015));
#114333=CARTESIAN_POINT('Ctrl Pts',(8.91755341277782,-28.8365448712948,
126.194695220975));
#114334=CARTESIAN_POINT('Ctrl Pts',(8.9122688064988,-28.7773653248804,126.131765195463));
#114335=CARTESIAN_POINT('Ctrl Pts',(8.91146544165359,-28.7684937983376,
126.122105376911));
#114336=CARTESIAN_POINT('Ctrl Pts',(8.90609014291122,-28.7100458568767,
126.056935844696));
#114337=CARTESIAN_POINT('Ctrl Pts',(8.90146615293136,-28.6641290480692,
125.998269026665));
#114338=CARTESIAN_POINT('Ctrl Pts',(8.8958037174643,-28.6153879818003,125.926583169957));
#114339=CARTESIAN_POINT('Ctrl Pts',(8.89499523942802,-28.6085957710182,
125.916352040206));
#114340=CARTESIAN_POINT('Ctrl Pts',(8.89371795615981,-28.5981376803837,
125.9002146091));
#114341=CARTESIAN_POINT('Ctrl Pts',(8.89325402995178,-28.594394451634,125.894358621373));
#114342=CARTESIAN_POINT('Ctrl Pts',(8.89238148360055,-28.5874599118728,
125.883359009665));
#114343=CARTESIAN_POINT('Ctrl Pts',(8.89197343850685,-28.584259850916,125.878221194301));
#114344=CARTESIAN_POINT('Ctrl Pts',(8.89100735056332,-28.5767831340685,
125.866069991195));
#114345=CARTESIAN_POINT('Ctrl Pts',(8.89044782392765,-28.5725302735253,
125.859042286531));
#114346=CARTESIAN_POINT('Ctrl Pts',(8.88856383190261,-28.5584624455144,
125.835402756564));
#114347=CARTESIAN_POINT('Ctrl Pts',(8.88722583127268,-28.5488845276075,
125.818652608353));
#114348=CARTESIAN_POINT('Ctrl Pts',(8.88389525848572,-28.525999143992,125.776966057176));
#114349=CARTESIAN_POINT('Ctrl Pts',(8.88188812044822,-28.5130314891505,
125.751850546977));
#114350=CARTESIAN_POINT('Ctrl Pts',(8.87594100326836,-28.4768414696524,
125.677156251079));
#114351=CARTESIAN_POINT('Ctrl Pts',(8.87195997478123,-28.4554367586926,
125.626790564402));
#114352=CARTESIAN_POINT('Ctrl Pts',(8.86798217145003,-28.4365601433851,
125.575510047478));
#114353=CARTESIAN_POINT('Origin',(5.,-30.,125.));
#114354=CARTESIAN_POINT('',(8.16626341820841,-28.4365599837785,125.575509613888));
#114355=CARTESIAN_POINT('',(8.36102756272879,-28.4365599800807,125.575509603842));
#114356=CARTESIAN_POINT('',(5.,-28.4365599837785,125.575509613888));
#114357=CARTESIAN_POINT('Ctrl Pts',(8.36102756272879,-28.4365599800807,
125.575509603842));
#114358=CARTESIAN_POINT('Ctrl Pts',(8.36145770696862,-28.4386070099079,
125.581070602881));
#114359=CARTESIAN_POINT('Ctrl Pts',(8.36188760913549,-28.4406839228182,
125.586621259518));
#114360=CARTESIAN_POINT('Ctrl Pts',(8.36819138196828,-28.4715968984599,
125.667913252586));
#114361=CARTESIAN_POINT('Ctrl Pts',(8.3739849424497,-28.5058953475837,125.741470545045));
#114362=CARTESIAN_POINT('Ctrl Pts',(8.38168331840411,-28.5600129458592,
125.838385065995));
#114363=CARTESIAN_POINT('Ctrl Pts',(8.3837357830561,-28.5753112481217,125.864126376972));
#114364=CARTESIAN_POINT('Ctrl Pts',(8.38670227849407,-28.598697583844,125.901165772368));
#114365=CARTESIAN_POINT('Ctrl Pts',(8.38763574447603,-28.6062455229821,
125.912796082803));
#114366=CARTESIAN_POINT('Ctrl Pts',(8.38928189758351,-28.6198897564361,
125.933256016873));
#114367=CARTESIAN_POINT('Ctrl Pts',(8.38999670869459,-28.6259277256678,
125.942123384479));
#114368=CARTESIAN_POINT('Ctrl Pts',(8.39149691209831,-28.6388369564555,
125.960693764744));
#114369=CARTESIAN_POINT('Ctrl Pts',(8.39228152708727,-28.6457273066304,
125.970382823967));
#114370=CARTESIAN_POINT('Ctrl Pts',(8.39436865484977,-28.6644230631664,
125.996085339622));
#114371=CARTESIAN_POINT('Ctrl Pts',(8.39566400793597,-28.6764127919527,
126.011962803471));
#114372=CARTESIAN_POINT('Ctrl Pts',(8.40340709727707,-28.7503497877074,
126.10631141169));
#114373=CARTESIAN_POINT('Ctrl Pts',(8.40957459561342,-28.8189757604072,
126.179294686223));
#114374=CARTESIAN_POINT('Ctrl Pts',(8.42058850569829,-28.9536663980121,
126.29890927781));
#114375=CARTESIAN_POINT('Ctrl Pts',(8.42544476690868,-29.0173510923646,
126.347731077068));
#114376=CARTESIAN_POINT('Ctrl Pts',(8.43230669257294,-29.1089407382553,
126.407991321287));
#114377=CARTESIAN_POINT('Ctrl Pts',(8.43417384748565,-29.1340087992832,
126.423546700542));
#114378=CARTESIAN_POINT('Ctrl Pts',(8.43735537156928,-29.1766599513997,
126.448469303392));
#114379=CARTESIAN_POINT('Ctrl Pts',(8.43865179517252,-29.1940225292612,
126.458201765976));
#114380=CARTESIAN_POINT('Ctrl Pts',(8.44051571475404,-29.2188803277021,
126.471556053164));
#114381=CARTESIAN_POINT('Ctrl Pts',(8.44106818664587,-29.2262354935232,
126.475436762904));
#114382=CARTESIAN_POINT('Ctrl Pts',(8.44202968137124,-29.2390069042951,
126.482053415615));
#114383=CARTESIAN_POINT('Ctrl Pts',(8.44243710258017,-29.244409552681,126.484815104019));
#114384=CARTESIAN_POINT('Ctrl Pts',(8.44331174683502,-29.2559862385061,
126.490653246658));
#114385=CARTESIAN_POINT('Ctrl Pts',(8.44377945191003,-29.2621642379322,
126.493720845059));
#114386=CARTESIAN_POINT('Ctrl Pts',(8.44506982522805,-29.2791796717585,
126.502038303693));
#114387=CARTESIAN_POINT('Ctrl Pts',(8.44589701834114,-29.2900550103824,
126.507209043946));
#114388=CARTESIAN_POINT('Ctrl Pts',(8.45102183791747,-29.3572903797278,
126.538287357102));
#114389=CARTESIAN_POINT('Ctrl Pts',(8.45546527715576,-29.414999519399,126.561145869374));
#114390=CARTESIAN_POINT('Ctrl Pts',(8.46974303275754,-29.6020544615563,
126.623408517052));
#114391=CARTESIAN_POINT('Ctrl Pts',(8.47965820117329,-29.7350088150674,
126.650335252346));
#114392=CARTESIAN_POINT('Ctrl Pts',(8.49150670112938,-29.9043325929816,
126.663612346825));
#114393=CARTESIAN_POINT('Ctrl Pts',(8.49389458874195,-29.9389788086658,
126.665243230035));
#114394=CARTESIAN_POINT('Ctrl Pts',(8.49717168016257,-29.9872360426982,
126.666006490485));
#114395=CARTESIAN_POINT('Ctrl Pts',(8.4980889041296,-30.0008215326724,126.666055187869));
#114396=CARTESIAN_POINT('Ctrl Pts',(8.49967283470738,-30.0244139784297,
126.665851168518));
#114397=CARTESIAN_POINT('Ctrl Pts',(8.50034187447292,-30.0344207015195,
126.665674452242));
#114398=CARTESIAN_POINT('Ctrl Pts',(8.5017362461051,-30.0553596647767,126.665115896981));
#114399=CARTESIAN_POINT('Ctrl Pts',(8.50246099746376,-30.0662909907093,
126.664716539569));
#114400=CARTESIAN_POINT('Ctrl Pts',(8.50418756080041,-30.0924411594482,
126.663503195412));
#114401=CARTESIAN_POINT('Ctrl Pts',(8.50518617047491,-30.1076544924927,
126.662587978036));
#114402=CARTESIAN_POINT('Ctrl Pts',(8.5086871853002,-30.161273441952,126.658623234945));
#114403=CARTESIAN_POINT('Ctrl Pts',(8.51115475382142,-30.1995853021649,
126.65445042986));
#114404=CARTESIAN_POINT('Ctrl Pts',(8.517324472727,-30.2962062008685,126.640521123376));
#114405=CARTESIAN_POINT('Ctrl Pts',(8.52097708010476,-30.3542048991576,
126.628983525005));
#114406=CARTESIAN_POINT('Ctrl Pts',(8.53143349804796,-30.5194756534759,
126.586859746785));
#114407=CARTESIAN_POINT('Ctrl Pts',(8.53812306285762,-30.6244340137254,
126.54856582347));
#114408=CARTESIAN_POINT('Ctrl Pts',(8.54695407241359,-30.7492968912502,
126.488237894541));
#114409=CARTESIAN_POINT('Ctrl Pts',(8.54871242000477,-30.7735256449567,
126.475789869132));
#114410=CARTESIAN_POINT('Ctrl Pts',(8.55113800532702,-30.805900510132,126.45814035454));
#114411=CARTESIAN_POINT('Ctrl Pts',(8.55177622972547,-30.8143238361179,
126.453452993632));
#114412=CARTESIAN_POINT('Ctrl Pts',(8.55279783590509,-30.8276465154202,
126.445887108063));
#114413=CARTESIAN_POINT('Ctrl Pts',(8.55317826351522,-30.832572790982,126.443056072724));
#114414=CARTESIAN_POINT('Ctrl Pts',(8.55398171053166,-30.8429011889788,
126.437050051014));
#114415=CARTESIAN_POINT('Ctrl Pts',(8.55440508917953,-30.8483000099712,
126.433869712394));
#114416=CARTESIAN_POINT('Ctrl Pts',(8.5554711854043,-30.8617885321296,126.425821051457));
#114417=CARTESIAN_POINT('Ctrl Pts',(8.55611629030951,-30.8698549398162,
126.420914324672));
#114418=CARTESIAN_POINT('Ctrl Pts',(8.55868225842405,-30.9015808691078,
126.401244326766));
#114419=CARTESIAN_POINT('Ctrl Pts',(8.56063261557264,-30.9249084335177,
126.385957393763));
#114420=CARTESIAN_POINT('Ctrl Pts',(8.56601614850504,-30.9874577232244,
126.342685381898));
#114421=CARTESIAN_POINT('Ctrl Pts',(8.56949274009445,-31.0258659620074,
126.313573463172));
#114422=CARTESIAN_POINT('Ctrl Pts',(8.58127918681224,-31.1508695917134,
126.20999596664));
#114423=CARTESIAN_POINT('Ctrl Pts',(8.58962954009622,-31.2310737857826,
126.128297093791));
#114424=CARTESIAN_POINT('Ctrl Pts',(8.60074104305059,-31.3295720190128,
126.004841848937));
#114425=CARTESIAN_POINT('Ctrl Pts',(8.6037714646891,-31.3554942382202,125.969590053118));
#114426=CARTESIAN_POINT('Ctrl Pts',(8.60786746237645,-31.389203368946,125.919749860271));
#114427=CARTESIAN_POINT('Ctrl Pts',(8.60897807989324,-31.3982042510058,
125.906008119057));
#114428=CARTESIAN_POINT('Ctrl Pts',(8.61075585636904,-31.412381248504,125.883649345891));
#114429=CARTESIAN_POINT('Ctrl Pts',(8.61142770806204,-31.417685001841,125.875114964341));
#114430=CARTESIAN_POINT('Ctrl Pts',(8.61282284294003,-31.4285835791482,
125.857218692879));
#114431=CARTESIAN_POINT('Ctrl Pts',(8.61354558812298,-31.4341643546033,
125.847848774036));
#114432=CARTESIAN_POINT('Ctrl Pts',(8.61525806876907,-31.4472282967277,
125.825416771546));
#114433=CARTESIAN_POINT('Ctrl Pts',(8.61624474050465,-31.4546273099731,
125.812306594301));
#114434=CARTESIAN_POINT('Ctrl Pts',(8.61965193810057,-31.4797153038824,
125.766411286217));
#114435=CARTESIAN_POINT('Ctrl Pts',(8.62204015231128,-31.4964824288276,
125.733133212663));
#114436=CARTESIAN_POINT('Ctrl Pts',(8.62795432106819,-31.535713954565,125.648303806195));
#114437=CARTESIAN_POINT('Ctrl Pts',(8.63143620982289,-31.5567115990926,
125.596124878231));
#114438=CARTESIAN_POINT('Ctrl Pts',(8.64146547144384,-31.6099530610728,
125.441686777283));
#114439=CARTESIAN_POINT('Ctrl Pts',(8.64789702667453,-31.6350176433205,
125.337268236808));
#114440=CARTESIAN_POINT('Ctrl Pts',(8.65683367474016,-31.6546591846119,
125.197088219706));
#114441=CARTESIAN_POINT('Ctrl Pts',(8.6590402273004,-31.6583774982597,125.162863370849));
#114442=CARTESIAN_POINT('Ctrl Pts',(8.66198709830412,-31.6618421828736,
125.118095422794));
#114443=CARTESIAN_POINT('Ctrl Pts',(8.66268009871064,-31.6625525854659,
125.107632970125));
#114444=CARTESIAN_POINT('Ctrl Pts',(8.66381059374463,-31.6635426584482,
125.090685956784));
#114445=CARTESIAN_POINT('Ctrl Pts',(8.6642448059996,-31.6638832965665,125.084205053423));
#114446=CARTESIAN_POINT('Ctrl Pts',(8.66510147008029,-31.6644776698322,
125.071478389391));
#114447=CARTESIAN_POINT('Ctrl Pts',(8.66552377080596,-31.6647341337085,
125.065232913471));
#114448=CARTESIAN_POINT('Ctrl Pts',(8.66658353726255,-31.6652870367743,
125.049626599976));
#114449=CARTESIAN_POINT('Ctrl Pts',(8.66722333292179,-31.6655396939478,
125.040264523982));
#114450=CARTESIAN_POINT('Ctrl Pts',(8.66974085755674,-31.6662191445097,
125.003638962121));
#114451=CARTESIAN_POINT('Ctrl Pts',(8.67164673455173,-31.6660554953507,
124.976370359353));
#114452=CARTESIAN_POINT('Ctrl Pts',(8.67686677678667,-31.6638016864866,
124.902606669074));
#114453=CARTESIAN_POINT('Ctrl Pts',(8.68022154841539,-31.6604323670643,
124.856176053179));
#114454=CARTESIAN_POINT('Ctrl Pts',(8.68858056675474,-31.6472905409691,
124.741725024608));
#114455=CARTESIAN_POINT('Ctrl Pts',(8.69360024140499,-31.6352453148678,
124.674047129665));
#114456=CARTESIAN_POINT('Ctrl Pts',(8.70469005641908,-31.5990268085286,
124.52472031556));
#114457=CARTESIAN_POINT('Ctrl Pts',(8.71070706558514,-31.572704481169,124.443778701327));
#114458=CARTESIAN_POINT('Ctrl Pts',(8.71787117024162,-31.5328192040067,
124.347000557882));
#114459=CARTESIAN_POINT('Ctrl Pts',(8.7192068155053,-31.5250016211873,124.328946278973));
#114460=CARTESIAN_POINT('Ctrl Pts',(8.72132909676774,-31.5119686888015,
124.300252251159));
#114461=CARTESIAN_POINT('Ctrl Pts',(8.72212257058555,-31.5069566563289,
124.289522782629));
#114462=CARTESIAN_POINT('Ctrl Pts',(8.72362810178253,-31.4971820201652,
124.269166692261));
#114463=CARTESIAN_POINT('Ctrl Pts',(8.72434082110673,-31.4924399209179,
124.259530948068));
#114464=CARTESIAN_POINT('Ctrl Pts',(8.72597235829699,-31.4813217974705,
124.237480167335));
#114465=CARTESIAN_POINT('Ctrl Pts',(8.72688890380039,-31.4748822248631,
124.225097938261));
#114466=CARTESIAN_POINT('Ctrl Pts',(8.72978896865646,-31.4538960487608,
124.185954574458));
#114467=CARTESIAN_POINT('Ctrl Pts',(8.73175205306949,-31.4387703709172,
124.159509856633));
#114468=CARTESIAN_POINT('Ctrl Pts',(8.73638448146635,-31.4009625006906,
124.097423950052));
#114469=CARTESIAN_POINT('Ctrl Pts',(8.73903161606981,-31.377633150419,124.062201124308));
#114470=CARTESIAN_POINT('Ctrl Pts',(8.74634984147412,-31.3087737864522,
123.966361124478));
#114471=CARTESIAN_POINT('Ctrl Pts',(8.75094660920688,-31.2604112096926,
123.907909299828));
#114472=CARTESIAN_POINT('Ctrl Pts',(8.75616197691216,-31.2017358639728,
123.84610396226));
#114473=CARTESIAN_POINT('Ctrl Pts',(8.756740416765,-31.1951768934233,123.839311693734));
#114474=CARTESIAN_POINT('Ctrl Pts',(8.76200330791184,-31.1350764746444,
123.778123160089));
#114475=CARTESIAN_POINT('Ctrl Pts',(8.76673908697932,-31.077920185203,123.72741731741));
#114476=CARTESIAN_POINT('Ctrl Pts',(8.7725261499066,-31.007766949544,123.673307559569));
#114477=CARTESIAN_POINT('Ctrl Pts',(8.77333526805991,-30.9979525769807,
123.665909415232));
#114478=CARTESIAN_POINT('Ctrl Pts',(8.77461342140452,-30.9824589323018,
123.65449682322));
#114479=CARTESIAN_POINT('Ctrl Pts',(8.77507756830051,-30.9768346165369,
123.650408032056));
#114480=CARTESIAN_POINT('Ctrl Pts',(8.77595041269201,-30.966265809128,123.642825346319));
#114481=CARTESIAN_POINT('Ctrl Pts',(8.77635853348204,-30.9613276566661,
123.639323041152));
#114482=CARTESIAN_POINT('Ctrl Pts',(8.77732466610054,-30.9496448243202,
123.631132520136));
#114483=CARTESIAN_POINT('Ctrl Pts',(8.77788416071585,-30.9428844415474,
123.626467185465));
#114484=CARTESIAN_POINT('Ctrl Pts',(8.77976750109632,-30.9201364819341,
123.61101591297));
#114485=CARTESIAN_POINT('Ctrl Pts',(8.78110486883277,-30.9039968209665,
123.600458072118));
#114486=CARTESIAN_POINT('Ctrl Pts',(8.78443339708765,-30.8637785118332,
123.575134974258));
#114487=CARTESIAN_POINT('Ctrl Pts',(8.78643910137207,-30.8395011064841,
123.560697609492));
#114488=CARTESIAN_POINT('Ctrl Pts',(8.7956196274884,-30.7277457099274,123.498028019629));
#114489=CARTESIAN_POINT('Ctrl Pts',(8.80296613486707,-30.6364048238903,
123.457105650151));
#114490=CARTESIAN_POINT('Ctrl Pts',(8.8161466944176,-30.4635686265864,123.397648489073));
#114491=CARTESIAN_POINT('Ctrl Pts',(8.82201005164917,-30.3832775355713,
123.376568971746));
#114492=CARTESIAN_POINT('Ctrl Pts',(8.82902649887282,-30.2824471380455,
123.357999870828));
#114493=CARTESIAN_POINT('Ctrl Pts',(8.83035830359465,-30.2630930625698,
123.354787883739));
#114494=CARTESIAN_POINT('Ctrl Pts',(8.83247592321245,-30.2319840472416,
123.350188091914));
#114495=CARTESIAN_POINT('Ctrl Pts',(8.83326852473787,-30.2202637135715,
123.348582475806));
#114496=CARTESIAN_POINT('Ctrl Pts',(8.83477327834336,-30.1978708635722,
123.345757429507));
#114497=CARTESIAN_POINT('Ctrl Pts',(8.83548608309976,-30.1872017630164,
123.34451612215));
#114498=CARTESIAN_POINT('Ctrl Pts',(8.83711904754025,-30.1626233001798,
123.341897166478));
#114499=CARTESIAN_POINT('Ctrl Pts',(8.83803691933775,-30.1487069903583,
123.340591191106));
#114500=CARTESIAN_POINT('Ctrl Pts',(8.8409463129405,-30.1042935960718,123.336986435659));
#114501=CARTESIAN_POINT('Ctrl Pts',(8.84291720362924,-30.0737479136646,
123.335352078473));
#114502=CARTESIAN_POINT('Ctrl Pts',(8.84757209503965,-30.0007176856076,
123.333458928047));
#114503=CARTESIAN_POINT('Ctrl Pts',(8.8502335747362,-29.9582339355169,123.333982102552));
#114504=CARTESIAN_POINT('Ctrl Pts',(8.85743770377063,-29.8421837670007,
123.339853813939));
#114505=CARTESIAN_POINT('Ctrl Pts',(8.86191263519807,-29.7688801425367,
123.348462746118));
#114506=CARTESIAN_POINT('Ctrl Pts',(8.86726034163982,-29.6829284990999,
123.364393374043));
#114507=CARTESIAN_POINT('Ctrl Pts',(8.86809888772666,-29.6695007055871,
123.367053711127));
#114508=CARTESIAN_POINT('Ctrl Pts',(8.87346749486712,-29.5839739241192,
123.385096566236));
#114509=CARTESIAN_POINT('Ctrl Pts',(8.8780499484194,-29.5129388937597,123.405083224761));
#114510=CARTESIAN_POINT('Ctrl Pts',(8.88366636573933,-29.43189618427,123.433805617918));
#114511=CARTESIAN_POINT('Ctrl Pts',(8.8844747809977,-29.4203681357607,123.438035317908));
#114512=CARTESIAN_POINT('Ctrl Pts',(8.88575204124957,-29.4023897340531,
123.444858114584));
#114513=CARTESIAN_POINT('Ctrl Pts',(8.88621600803788,-29.3959067982081,
123.447364913152));
#114514=CARTESIAN_POINT('Ctrl Pts',(8.88708871705689,-29.3838062349024,
123.452131172887));
#114515=CARTESIAN_POINT('Ctrl Pts',(8.88749688485231,-29.3781849939084,
123.454380785702));
#114516=CARTESIAN_POINT('Ctrl Pts',(8.88846337037872,-29.3649628894959,
123.459756054751));
#114517=CARTESIAN_POINT('Ctrl Pts',(8.88902317416903,-29.357372754441,123.462907368186));
#114518=CARTESIAN_POINT('Ctrl Pts',(8.89090852735885,-29.3320274878815,
123.473650888658));
#114519=CARTESIAN_POINT('Ctrl Pts',(8.89224763517326,-29.314381828731,123.481495297868));
#114520=CARTESIAN_POINT('Ctrl Pts',(8.89558141882648,-29.2712289204826,
123.501584459649));
#114521=CARTESIAN_POINT('Ctrl Pts',(8.89759069203603,-29.2458900926084,
123.514175486556));
#114522=CARTESIAN_POINT('Ctrl Pts',(8.90680243132826,-29.1322573003871,
123.574295837154));
#114523=CARTESIAN_POINT('Ctrl Pts',(8.91417742840122,-29.0480436727267,
123.629091772331));
#114524=CARTESIAN_POINT('Ctrl Pts',(8.92735212823738,-28.9044852908043,
123.742143564441));
#114525=CARTESIAN_POINT('Ctrl Pts',(8.93318399979611,-28.8435723673284,
123.797904286862));
#114526=CARTESIAN_POINT('Ctrl Pts',(8.94017018094361,-28.7735927445204,
123.872229806077));
#114527=CARTESIAN_POINT('Ctrl Pts',(8.94150120287582,-28.7604058538469,
123.886740472133));
#114528=CARTESIAN_POINT('Ctrl Pts',(8.94361794419042,-28.739678799933,123.910373290353));
#114529=CARTESIAN_POINT('Ctrl Pts',(8.9444104382666,-28.7319746775606,123.919348489172));
#114530=CARTESIAN_POINT('Ctrl Pts',(8.94591521416387,-28.7174568379781,
123.936630618989));
#114531=CARTESIAN_POINT('Ctrl Pts',(8.94662814636664,-28.7106266467982,
123.944922861496));
#114532=CARTESIAN_POINT('Ctrl Pts',(8.94826172465711,-28.6950910938163,
123.964160099813));
#114533=CARTESIAN_POINT('Ctrl Pts',(8.94918007843716,-28.6864422986704,
123.975149895211));
#114534=CARTESIAN_POINT('Ctrl Pts',(8.9520923738276,-28.6593008148525,124.0105459818));
#114535=CARTESIAN_POINT('Ctrl Pts',(8.95406562903356,-28.6413415073779,
124.035354547882));
#114536=CARTESIAN_POINT('Ctrl Pts',(8.95872726382163,-28.6000894251401,
124.095778755504));
#114537=CARTESIAN_POINT('Ctrl Pts',(8.96139303398346,-28.577456933059,124.131819557973));
#114538=CARTESIAN_POINT('Ctrl Pts',(8.96859914867215,-28.5194565331449,
124.232551293325));
#114539=CARTESIAN_POINT('Ctrl Pts',(8.97307208223782,-28.4869622831259,
124.298784123701));
#114540=CARTESIAN_POINT('Ctrl Pts',(8.97843591740039,-28.4536471547153,
124.379883592678));
#114541=CARTESIAN_POINT('Ctrl Pts',(8.97929248196261,-28.4484975178083,
124.392882612287));
#114542=CARTESIAN_POINT('Ctrl Pts',(8.98465558066968,-28.4173666473452,
124.474448806567));
#114543=CARTESIAN_POINT('Ctrl Pts',(8.98921465188718,-28.3957753455328,
124.544595864343));
#114544=CARTESIAN_POINT('Ctrl Pts',(8.99480513081464,-28.3760449815618,
124.627875181981));
#114545=CARTESIAN_POINT('Ctrl Pts',(8.99561353105724,-28.3733464392908,
124.639854260382));
#114546=CARTESIAN_POINT('Ctrl Pts',(8.9968908195505,-28.3693280228528,124.658659662157));
#114547=CARTESIAN_POINT('Ctrl Pts',(8.99735483134072,-28.3679179873674,
124.665466559286));
#114548=CARTESIAN_POINT('Ctrl Pts',(8.99822773302511,-28.3653591270608,
124.678220719373));
#114549=CARTESIAN_POINT('Ctrl Pts',(8.99863604950941,-28.3642000834639,
124.684165680641));
#114550=CARTESIAN_POINT('Ctrl Pts',(8.99960301584995,-28.3615439219884,
124.698196580603));
#114551=CARTESIAN_POINT('Ctrl Pts',(9.00016315392076,-28.3600742262815,
124.706287431088));
#114552=CARTESIAN_POINT('Ctrl Pts',(9.0020501190838,-28.3553508627016,124.733431391799));
#114553=CARTESIAN_POINT('Ctrl Pts',(9.00339052502644,-28.3523690250318,
124.752529398956));
#114554=CARTESIAN_POINT('Ctrl Pts',(9.00672814727556,-28.3458379487924,
124.799734265238));
#114555=CARTESIAN_POINT('Ctrl Pts',(9.0087399910164,-28.3426721571202,124.827887547695));
#114556=CARTESIAN_POINT('Ctrl Pts',(9.01797556390105,-28.3315398552732,
124.956295463057));
#114557=CARTESIAN_POINT('Ctrl Pts',(9.02537231383394,-28.33194321021,125.05706476187));
#114558=CARTESIAN_POINT('Ctrl Pts',(9.03853419354012,-28.3491703078742,
125.238841313797));
#114559=CARTESIAN_POINT('Ctrl Pts',(9.04433408946599,-28.3629297385434,
125.319825626506));
#114560=CARTESIAN_POINT('Ctrl Pts',(9.05128940886092,-28.3873006207887,
125.41849797493));
#114561=CARTESIAN_POINT('Ctrl Pts',(9.05261949376751,-28.3923337298054,
125.437434638829));
#114562=CARTESIAN_POINT('Ctrl Pts',(9.05473521130915,-28.4009388470119,
125.46765295942));
#114563=CARTESIAN_POINT('Ctrl Pts',(9.05552760338496,-28.404298886696,125.47899251657));
#114564=CARTESIAN_POINT('Ctrl Pts',(9.0570324786278,-28.4109418706488,125.50056541187));
#114565=CARTESIAN_POINT('Ctrl Pts',(9.05774560923411,-28.414203624293,125.510804594771));
#114566=CARTESIAN_POINT('Ctrl Pts',(9.05938006241585,-28.4219407943758,
125.534304209144));
#114567=CARTESIAN_POINT('Ctrl Pts',(9.06029908669143,-28.4264847238471,
125.547541359049));
#114568=CARTESIAN_POINT('Ctrl Pts',(9.06155524212669,-28.4329600900784,
125.565658398423));
#114569=CARTESIAN_POINT('Ctrl Pts',(9.06189689051117,-28.4347484306822,
125.570588315377));
#114570=CARTESIAN_POINT('Ctrl Pts',(9.06223779754793,-28.4365599835583,
125.57550961329));
#114571=CARTESIAN_POINT('',(8.82706574074257,-28.3340000603266,124.999551660593));
#114572=CARTESIAN_POINT('Ctrl Pts',(8.86798217145003,-28.4365601433851,
125.575510047478));
#114573=CARTESIAN_POINT('Ctrl Pts',(8.86185962239668,-28.4075056644279,
125.496580182371));
#114574=CARTESIAN_POINT('Ctrl Pts',(8.85575036351493,-28.3844406215789,
125.415482508081));
#114575=CARTESIAN_POINT('Ctrl Pts',(8.84633165537642,-28.3578042058915,
125.284872792836));
#114576=CARTESIAN_POINT('Ctrl Pts',(8.84292409524228,-28.3501319539516,
125.236422943428));
#114577=CARTESIAN_POINT('Ctrl Pts',(8.83842238551622,-28.3426894408775,
125.170785037085));
#114578=CARTESIAN_POINT('Ctrl Pts',(8.83727034630692,-28.341030750582,125.153840453454));
#114579=CARTESIAN_POINT('Ctrl Pts',(8.83536839463526,-28.3387051589693,
125.125629325156));
#114580=CARTESIAN_POINT('Ctrl Pts',(8.83461397978074,-28.3378925069161,
125.114376432987));
#114581=CARTESIAN_POINT('Ctrl Pts',(8.83319044802623,-28.3365686097304,
125.093027798251));
#114582=CARTESIAN_POINT('Ctrl Pts',(8.83252065816331,-28.3360348207541,
125.082934017713));
#114583=CARTESIAN_POINT('Ctrl Pts',(8.83106752375674,-28.3350720243024,
125.060932680886));
#114584=CARTESIAN_POINT('Ctrl Pts',(8.83028532486699,-28.3346788267911,
125.049024056637));
#114585=CARTESIAN_POINT('Ctrl Pts',(8.82868900352269,-28.3341344862232,
125.024594036931));
#114586=CARTESIAN_POINT('Ctrl Pts',(8.82787533746247,-28.3339966906545,
125.012073141787));
#114587=CARTESIAN_POINT('Ctrl Pts',(8.82706574074257,-28.3340000603266,
124.999551660593));
#114588=CARTESIAN_POINT('Ctrl Pts',(8.82706582501452,-28.3340000599764,
124.99955296397));
#114589=CARTESIAN_POINT('Ctrl Pts',(8.82552293670077,-28.3340064630552,
124.975690169399));
#114590=CARTESIAN_POINT('Ctrl Pts',(8.82399512451827,-28.3345255587479,
124.951829175653));
#114591=CARTESIAN_POINT('Ctrl Pts',(8.8139693057654,-28.3413530734983,124.794025566948));
#114592=CARTESIAN_POINT('Ctrl Pts',(8.80595594332984,-28.3632988322378,
124.661259729756));
#114593=CARTESIAN_POINT('Ctrl Pts',(8.79398870050104,-28.4177504440931,
124.474985621226));
#114594=CARTESIAN_POINT('Ctrl Pts',(8.79023980714995,-28.4376750408818,
124.41837042761));
#114595=CARTESIAN_POINT('Ctrl Pts',(8.78536234457686,-28.4663889185449,
124.348984026802));
#114596=CARTESIAN_POINT('Ctrl Pts',(8.78437087525542,-28.4723619244685,
124.335089015429));
#114597=CARTESIAN_POINT('Ctrl Pts',(8.78287427379261,-28.4815625950485,
124.314464068068));
#114598=CARTESIAN_POINT('Ctrl Pts',(8.78237725978755,-28.4846478491526,
124.307670945061));
#114599=CARTESIAN_POINT('Ctrl Pts',(8.78147543525583,-28.4902968726483,
124.295451575151));
#114600=CARTESIAN_POINT('Ctrl Pts',(8.78107159982884,-28.49284447342,124.290018147171));
#114601=CARTESIAN_POINT('Ctrl Pts',(8.78015718461895,-28.4986532435748,
124.277801578143));
#114602=CARTESIAN_POINT('Ctrl Pts',(8.7796456288921,-28.5019310283025,124.271026753521));
#114603=CARTESIAN_POINT('Ctrl Pts',(8.77807525536332,-28.5120820218852,
124.25040336544));
#114604=CARTESIAN_POINT('Ctrl Pts',(8.77700815827029,-28.5191019771699,
124.236628512749));
#114605=CARTESIAN_POINT('Ctrl Pts',(8.76863194953328,-28.5752199948783,
124.130199253173));
#114606=CARTESIAN_POINT('Ctrl Pts',(8.76094569801021,-28.6327712984183,
124.04227682885));
#114607=CARTESIAN_POINT('Ctrl Pts',(8.74537603323542,-28.7664233159057,
123.874923256554));
#114608=CARTESIAN_POINT('Ctrl Pts',(8.73754138196926,-28.8429040124052,
123.79640292199));
#114609=CARTESIAN_POINT('Ctrl Pts',(8.72899729874516,-28.9381855270799,
123.716123894898));
#114610=CARTESIAN_POINT('Ctrl Pts',(8.72795953209783,-28.9499637290812,
123.706473160498));
#114611=CARTESIAN_POINT('Ctrl Pts',(8.72598517823142,-28.9727626091331,
123.688309030333));
#114612=CARTESIAN_POINT('Ctrl Pts',(8.72504761257469,-28.9837609029819,
123.679769726437));
#114613=CARTESIAN_POINT('Ctrl Pts',(8.7233970517507,-29.0034237573007,123.664894400473));
#114614=CARTESIAN_POINT('Ctrl Pts',(8.72268188913507,-29.0120447906744,
123.658502447624));
#114615=CARTESIAN_POINT('Ctrl Pts',(8.72118373294742,-29.0303151053736,
123.645227818769));
#114616=CARTESIAN_POINT('Ctrl Pts',(8.72040148920367,-29.0399773118707,
123.638363885468));
#114617=CARTESIAN_POINT('Ctrl Pts',(8.71832728964169,-29.0659178584358,
123.620349380235));
#114618=CARTESIAN_POINT('Ctrl Pts',(8.71704233780558,-29.0823227321151,
123.609383674257));
#114619=CARTESIAN_POINT('Ctrl Pts',(8.7104526164313,-29.1681057082518,123.554222010733));
#114620=CARTESIAN_POINT('Ctrl Pts',(8.70532934453711,-29.2404965211612,
123.514914469575));
#114621=CARTESIAN_POINT('Ctrl Pts',(8.69411968592561,-29.4068882977375,
123.439928897928));
#114622=CARTESIAN_POINT('Ctrl Pts',(8.6880926206815,-29.50179762959,123.407079603888));
#114623=CARTESIAN_POINT('Ctrl Pts',(8.68003620877506,-29.6265301752924,
123.376153855184));
#114624=CARTESIAN_POINT('Ctrl Pts',(8.67824311719694,-29.6541508031264,
123.370047802957));
#114625=CARTESIAN_POINT('Ctrl Pts',(8.67517530208143,-29.700862167431,123.36096209351));
#114626=CARTESIAN_POINT('Ctrl Pts',(8.67391691030504,-29.7198741584461,
123.35760597397));
#114627=CARTESIAN_POINT('Ctrl Pts',(8.67209848650151,-29.747053801267,123.353293673558));
#114628=CARTESIAN_POINT('Ctrl Pts',(8.67155250820096,-29.7551776472432,
123.352066289686));
#114629=CARTESIAN_POINT('Ctrl Pts',(8.67059847890346,-29.769301739739,123.350039105652));
#114630=CARTESIAN_POINT('Ctrl Pts',(8.67019195752396,-29.7752978053332,
123.349211835961));
#114631=CARTESIAN_POINT('Ctrl Pts',(8.66931468778569,-29.7881870900808,
123.347505044789));
#114632=CARTESIAN_POINT('Ctrl Pts',(8.66884341385409,-29.7950812388545,
123.346635979969));
#114633=CARTESIAN_POINT('Ctrl Pts',(8.66753335845075,-29.8141684803774,
123.344351087112));
#114634=CARTESIAN_POINT('Ctrl Pts',(8.66668983160653,-29.8263718078877,
123.343026884577));
#114635=CARTESIAN_POINT('Ctrl Pts',(8.66078865563074,-29.9112203821212,
123.334767402788));
#114636=CARTESIAN_POINT('Ctrl Pts',(8.65553002066224,-29.9842309334713,
123.332477766137));
#114637=CARTESIAN_POINT('Ctrl Pts',(8.64288099834985,-30.1582473398906,
123.338450412223));
#114638=CARTESIAN_POINT('Ctrl Pts',(8.63548791381896,-30.2588318271421,
123.35112189794));
#114639=CARTESIAN_POINT('Ctrl Pts',(8.62457909681576,-30.4092647338153,
123.384187167215));
#114640=CARTESIAN_POINT('Ctrl Pts',(8.62090051317587,-30.4603142394905,
123.397982339724));
#114641=CARTESIAN_POINT('Ctrl Pts',(8.616140548432,-30.5268040293666,123.419391775582));
#114642=CARTESIAN_POINT('Ctrl Pts',(8.61499049166957,-30.5429013245915,
123.42484825068));
#114643=CARTESIAN_POINT('Ctrl Pts',(8.61309090891086,-30.5695351975844,
123.434333112344));
#114644=CARTESIAN_POINT('Ctrl Pts',(8.61233690392399,-30.5801190980823,
123.438223771718));
#114645=CARTESIAN_POINT('Ctrl Pts',(8.61086399930962,-30.6008134435513,
123.446070448043));
#114646=CARTESIAN_POINT('Ctrl Pts',(8.61014487534427,-30.610926313427,123.450018420937));
#114647=CARTESIAN_POINT('Ctrl Pts',(8.60841344476983,-30.6352912295891,
123.459805776321));
#114648=CARTESIAN_POINT('Ctrl Pts',(8.60740452813876,-30.6495024668347,
123.465744556872));
#114649=CARTESIAN_POINT('Ctrl Pts',(8.60398822907375,-30.6976404115853,
123.486649828974));
#114650=CARTESIAN_POINT('Ctrl Pts',(8.6016124394286,-30.7311503151428,123.502552030318));
#114651=CARTESIAN_POINT('Ctrl Pts',(8.59088850788345,-30.8818178038314,
123.580316482313));
#114652=CARTESIAN_POINT('Ctrl Pts',(8.58297964008849,-30.9918606323425,
123.654891688397));
#114653=CARTESIAN_POINT('Ctrl Pts',(8.57220093315785,-31.1236541146117,
123.769258812822));
#114654=CARTESIAN_POINT('Ctrl Pts',(8.56957720492188,-31.154341771547,123.797994574212));
#114655=CARTESIAN_POINT('Ctrl Pts',(8.56526531006402,-31.2018386734637,
123.845968240012));
#114656=CARTESIAN_POINT('Ctrl Pts',(8.56361585415679,-31.2193502032082,
123.864486718003));
#114657=CARTESIAN_POINT('Ctrl Pts',(8.56133529690855,-31.2425515427887,
123.89017789152));
#114658=CARTESIAN_POINT('Ctrl Pts',(8.56072975989833,-31.2486180747974,
123.897007550888));
#114659=CARTESIAN_POINT('Ctrl Pts',(8.55970611857505,-31.2587096693473,
123.90855854209));
#114660=CARTESIAN_POINT('Ctrl Pts',(8.5592902130915,-31.2627651945177,123.913253226494));
#114661=CARTESIAN_POINT('Ctrl Pts',(8.55843070622539,-31.2710523731426,
123.922955504012));
#114662=CARTESIAN_POINT('Ctrl Pts',(8.5579869098732,-31.2752808161903,123.927965570644));
#114663=CARTESIAN_POINT('Ctrl Pts',(8.55680691887714,-31.2863933945528,
123.941291082138));
#114664=CARTESIAN_POINT('Ctrl Pts',(8.55606725849165,-31.2932263310104,
123.949648544672));
#114665=CARTESIAN_POINT('Ctrl Pts',(8.55272065672722,-31.3235702235797,
123.987507547628));
#114666=CARTESIAN_POINT('Ctrl Pts',(8.55005981193214,-31.3461545558332,
124.017733983163));
#114667=CARTESIAN_POINT('Ctrl Pts',(8.53983105719722,-31.4278908573883,
124.135246671807));
#114668=CARTESIAN_POINT('Ctrl Pts',(8.53206803216505,-31.4797384613907,
124.227313033232));
#114669=CARTESIAN_POINT('Ctrl Pts',(8.52051604782475,-31.5448063504319,
124.373790739904));
#114670=CARTESIAN_POINT('Ctrl Pts',(8.51661011256681,-31.5645866171088,
124.424991831235));
#114671=CARTESIAN_POINT('Ctrl Pts',(8.51103072563614,-31.5896603680191,
124.500838622117));
#114672=CARTESIAN_POINT('Ctrl Pts',(8.50929887529829,-31.5969786858944,
124.524772309841));
#114673=CARTESIAN_POINT('Ctrl Pts',(8.50617920746973,-31.6093064321642,
124.568596437648));
#114674=CARTESIAN_POINT('Ctrl Pts',(8.50478607108701,-31.6144929945769,
124.588431461658));
#114675=CARTESIAN_POINT('Ctrl Pts',(8.50259508822357,-31.6221367611784,
124.620035947924));
#114676=CARTESIAN_POINT('Ctrl Pts',(8.5017895976725,-31.6248348184241,124.631744411082));
#114677=CARTESIAN_POINT('Ctrl Pts',(8.50027456753053,-31.6296953744908,
124.653931461807));
#114678=CARTESIAN_POINT('Ctrl Pts',(8.49956422553636,-31.6318840430296,
124.664403626383));
#114679=CARTESIAN_POINT('Ctrl Pts',(8.49795625940507,-31.6366310732582,
124.688262212454));
#114680=CARTESIAN_POINT('Ctrl Pts',(8.49706067837911,-31.6391263787626,
124.701660510648));
#114681=CARTESIAN_POINT('Ctrl Pts',(8.49472928081337,-31.6452278498938,
124.73681281002));
#114682=CARTESIAN_POINT('Ctrl Pts',(8.49330184338597,-31.6485671119436,
124.758610843183));
#114683=CARTESIAN_POINT('Ctrl Pts',(8.48473219217271,-31.6661604373065,
124.890961061172));
#114684=CARTESIAN_POINT('Ctrl Pts',(8.4779341523219,-31.6697235097824,125.002650670489));
#114685=CARTESIAN_POINT('Ctrl Pts',(8.46681184918821,-31.6572749674427,
125.184357105146));
#114686=CARTESIAN_POINT('Ctrl Pts',(8.4624980195575,-31.6479671603043,125.254461620818));
#114687=CARTESIAN_POINT('Ctrl Pts',(8.45654042125751,-31.6296255397651,
125.347044887742));
#114688=CARTESIAN_POINT('Ctrl Pts',(8.45502601485619,-31.6245152515883,
125.370229166802));
#114689=CARTESIAN_POINT('Ctrl Pts',(8.45239121013011,-31.6149057962378,
125.40978434658));
#114690=CARTESIAN_POINT('Ctrl Pts',(8.45128174588971,-31.6106484358086,
125.426210632598));
#114691=CARTESIAN_POINT('Ctrl Pts',(8.44964215357477,-31.6040666987849,
125.450096663259));
#114692=CARTESIAN_POINT('Ctrl Pts',(8.4491225770084,-31.6019394062509,125.457610219579));
#114693=CARTESIAN_POINT('Ctrl Pts',(8.44823581653339,-31.5982403949592,
125.470333121899));
#114694=CARTESIAN_POINT('Ctrl Pts',(8.4478701943089,-31.5966958480847,125.475550179448));
#114695=CARTESIAN_POINT('Ctrl Pts',(8.44703279875574,-31.5931147039456,
125.487432155117));
#114696=CARTESIAN_POINT('Ctrl Pts',(8.44656011987035,-31.5910618745412,
125.494091765476));
#114697=CARTESIAN_POINT('Ctrl Pts',(8.44524243188948,-31.5852508900668,
125.5125314725));
#114698=CARTESIAN_POINT('Ctrl Pts',(8.44439259132426,-31.5814033638846,
125.524282626921));
#114699=CARTESIAN_POINT('Ctrl Pts',(8.43787001537452,-31.5510942786992,
125.613482754506));
#114700=CARTESIAN_POINT('Ctrl Pts',(8.43194553276739,-31.5190911362583,
125.688922152097));
#114701=CARTESIAN_POINT('Ctrl Pts',(8.42576263423915,-31.4802346283364,
125.764507317313));
#114702=CARTESIAN_POINT('Ctrl Pts',(8.42553261645292,-31.478781331009,125.767314647441));
#114703=CARTESIAN_POINT('Ctrl Pts',(8.42036077280776,-31.4459293078638,
125.830334812944));
#114704=CARTESIAN_POINT('Ctrl Pts',(8.41541389751153,-31.4108845771325,
125.888579233453));
#114705=CARTESIAN_POINT('Ctrl Pts',(8.40717200905783,-31.34567703784,125.983324932337));
#114706=CARTESIAN_POINT('Ctrl Pts',(8.4038380267175,-31.3173376050465,126.020978406953));
#114707=CARTESIAN_POINT('Ctrl Pts',(8.39826772126613,-31.2665284780896,
126.082842090486));
#114708=CARTESIAN_POINT('Ctrl Pts',(8.39600375305034,-31.2448670212946,
126.107676732343));
#114709=CARTESIAN_POINT('Ctrl Pts',(8.39279521128459,-31.2127156672078,
126.142402448857));
#114710=CARTESIAN_POINT('Ctrl Pts',(8.39182641095768,-31.2028130528618,
126.152824109311));
#114711=CARTESIAN_POINT('Ctrl Pts',(8.39014036328775,-31.1852409873848,
126.170844269367));
#114712=CARTESIAN_POINT('Ctrl Pts',(8.38942062880467,-31.1776303920657,
126.178498693424));
#114713=CARTESIAN_POINT('Ctrl Pts',(8.38793130047828,-31.1616566632953,
126.194255148347));
#114714=CARTESIAN_POINT('Ctrl Pts',(8.3871622811226,-31.1532818811087,126.202344575004));
#114715=CARTESIAN_POINT('Ctrl Pts',(8.38516464951079,-31.13120143802,126.223229677761));
#114716=CARTESIAN_POINT('Ctrl Pts',(8.38394212636076,-31.1173631253853,
126.235883178226));
#114717=CARTESIAN_POINT('Ctrl Pts',(8.37839671643114,-31.0531544979173,
126.292634128942));
#114718=CARTESIAN_POINT('Ctrl Pts',(8.37418970793322,-31.0003655186899,
126.333906948898));
#114719=CARTESIAN_POINT('Ctrl Pts',(8.36295581817705,-30.8508071343742,
126.436952156236));
#114720=CARTESIAN_POINT('Ctrl Pts',(8.35610045906975,-30.7499261126979,
126.492083246674));
#114721=CARTESIAN_POINT('Ctrl Pts',(8.34705591980557,-30.6165818596045,
126.547991926128));
#114722=CARTESIAN_POINT('Ctrl Pts',(8.34516208627364,-30.5886684558691,
126.558820526579));
#114723=CARTESIAN_POINT('Ctrl Pts',(8.34193984248377,-30.541537474199,126.575657890066));
#114724=CARTESIAN_POINT('Ctrl Pts',(8.34062998071377,-30.5224747480987,
126.582081120766));
#114725=CARTESIAN_POINT('Ctrl Pts',(8.33875014869806,-30.4953425455757,
126.590679561886));
#114726=CARTESIAN_POINT('Ctrl Pts',(8.33819555479961,-30.4873649934236,
126.593141883801));
#114727=CARTESIAN_POINT('Ctrl Pts',(8.33723174466375,-30.4735554231775,
126.597290867606));
#114728=CARTESIAN_POINT('Ctrl Pts',(8.33682415486096,-30.4677321314326,
126.599005786909));
#114729=CARTESIAN_POINT('Ctrl Pts',(8.33595078186691,-30.4552921359627,
126.602595508025));
#114730=CARTESIAN_POINT('Ctrl Pts',(8.33548453244945,-30.4486732571209,
126.604461154245));
#114731=CARTESIAN_POINT('Ctrl Pts',(8.3342016428989,-30.4305167608695,126.609457746696));
#114732=CARTESIAN_POINT('Ctrl Pts',(8.33338055829408,-30.4189569526958,
126.612505494897));
#114733=CARTESIAN_POINT('Ctrl Pts',(8.32844967808664,-30.3498399263896,
126.629934871194));
#114734=CARTESIAN_POINT('Ctrl Pts',(8.32420638531486,-30.2915861159059,
126.64135666306));
#114735=CARTESIAN_POINT('Ctrl Pts',(8.3124039159444,-30.1300562869054,126.664157245159));
#114736=CARTESIAN_POINT('Ctrl Pts',(8.30478438900738,-30.0261175441198,
126.669028062859));
#114737=CARTESIAN_POINT('Ctrl Pts',(8.29440852544147,-29.8807623930906,
126.662250227872));
#114738=CARTESIAN_POINT('Ctrl Pts',(8.29147189746632,-29.8392101024742,
126.658746669104));
#114739=CARTESIAN_POINT('Ctrl Pts',(8.28648713322641,-29.7678857257353,
126.650026977369));
#114740=CARTESIAN_POINT('Ctrl Pts',(8.28441851695031,-29.7380448280005,
126.64555332789));
#114741=CARTESIAN_POINT('Ctrl Pts',(8.28143359034581,-29.6946528216197,
126.637837710602));
#114742=CARTESIAN_POINT('Ctrl Pts',(8.28049749407267,-29.6809961659564,
126.635232656175));
#114743=CARTESIAN_POINT('Ctrl Pts',(8.27884857909498,-29.6568602126853,
126.63031475525));
#114744=CARTESIAN_POINT('Ctrl Pts',(8.27813360795498,-29.6463678081762,
126.62807106632));
#114745=CARTESIAN_POINT('Ctrl Pts',(8.27663492649095,-29.6243217382988,
126.623133563683));
#114746=CARTESIAN_POINT('Ctrl Pts',(8.27585197495847,-29.6127736569231,
126.620417382449));
#114747=CARTESIAN_POINT('Ctrl Pts',(8.27377370492735,-29.5820480380202,
126.612843295144));
#114748=CARTESIAN_POINT('Ctrl Pts',(8.27248544026783,-29.5629259874137,
126.607766680447));
#114749=CARTESIAN_POINT('Ctrl Pts',(8.26533875559389,-29.4565354583767,
126.57748309987));
#114750=CARTESIAN_POINT('Ctrl Pts',(8.25970675943806,-29.3713474206997,
126.545511438966));
#114751=CARTESIAN_POINT('Ctrl Pts',(8.24843378544306,-29.2049260288125,
126.467001142149));
#114752=CARTESIAN_POINT('Ctrl Pts',(8.24281433605841,-29.1241582531405,
126.420258450694));
#114753=CARTESIAN_POINT('Ctrl Pts',(8.23441941445586,-29.0144255121978,
126.343817671257));
#114754=CARTESIAN_POINT('Ctrl Pts',(8.23183010945709,-28.9819870817916,
126.319413547021));
#114755=CARTESIAN_POINT('Ctrl Pts',(8.22846711326601,-28.942169566976,126.287115045455));
#114756=CARTESIAN_POINT('Ctrl Pts',(8.22776070308026,-28.9339295688024,
126.280298475448));
#114757=CARTESIAN_POINT('Ctrl Pts',(8.22661379182093,-28.9207618367548,
126.269190166702));
#114758=CARTESIAN_POINT('Ctrl Pts',(8.22617675178774,-28.9157925776939,
126.264947806824));
#114759=CARTESIAN_POINT('Ctrl Pts',(8.22532448641645,-28.9061989371415,
126.256659456414));
#114760=CARTESIAN_POINT('Ctrl Pts',(8.22490950596848,-28.9015717771517,
126.252616936301));
#114761=CARTESIAN_POINT('Ctrl Pts',(8.2239724693165,-28.8912200668231,126.243471700029));
#114762=CARTESIAN_POINT('Ctrl Pts',(8.22344940399404,-28.8855081814775,
126.238354872295));
#114763=CARTESIAN_POINT('Ctrl Pts',(8.22159070833133,-28.865438307072,126.220124535378));
#114764=CARTESIAN_POINT('Ctrl Pts',(8.22024101243933,-28.8512754051141,
126.206799834927));
#114765=CARTESIAN_POINT('Ctrl Pts',(8.21132992198955,-28.7602258823685,
126.118083778963));
#114766=CARTESIAN_POINT('Ctrl Pts',(8.20341412264587,-28.6905741590765,
126.035641207627));
#114767=CARTESIAN_POINT('Ctrl Pts',(8.18941166089258,-28.5808753524287,
125.876879753582));
#114768=CARTESIAN_POINT('Ctrl Pts',(8.18330323894413,-28.5378390236045,
125.803070198172));
#114769=CARTESIAN_POINT('Ctrl Pts',(8.17530625105535,-28.4875743270153,
125.699301885762));
#114770=CARTESIAN_POINT('Ctrl Pts',(8.17325108324174,-28.4752364448803,
125.6719753311));
#114771=CARTESIAN_POINT('Ctrl Pts',(8.17028164887843,-28.4582784058146,
125.63154006513));
#114772=CARTESIAN_POINT('Ctrl Pts',(8.16934788677825,-28.4530745996968,
125.618684211802));
#114773=CARTESIAN_POINT('Ctrl Pts',(8.16770159193498,-28.4441321197757,
125.595773585964));
#114774=CARTESIAN_POINT('Ctrl Pts',(8.16698693047251,-28.440328942492,125.585745019665));
#114775=CARTESIAN_POINT('Ctrl Pts',(8.16627145758177,-28.4366018553033,
125.575623353271));
#114776=CARTESIAN_POINT('Ctrl Pts',(8.16626743784335,-28.436580917989,125.57556648415));
#114777=CARTESIAN_POINT('Ctrl Pts',(8.16626341820841,-28.4365599837785,
125.575509613888));
#114778=CARTESIAN_POINT('Origin',(5.,-30.,125.));
#114779=CARTESIAN_POINT('',(7.46828914249572,-28.4365600390074,125.575509763924));
#114780=CARTESIAN_POINT('',(7.65924494691568,-28.4365599837121,125.575509613707));
#114781=CARTESIAN_POINT('',(5.,-28.4365599837785,125.575509613888));
#114782=CARTESIAN_POINT('Ctrl Pts',(7.65924494691568,-28.4365599837121,
125.575509613707));
#114783=CARTESIAN_POINT('Ctrl Pts',(7.66000437687175,-28.4406054932687,
125.586499719479));
#114784=CARTESIAN_POINT('Ctrl Pts',(7.66076922565613,-28.4447668020627,
125.597446945435));
#114785=CARTESIAN_POINT('Ctrl Pts',(7.66215647700585,-28.4524612023065,
125.617063437286));
#114786=CARTESIAN_POINT('Ctrl Pts',(7.66277660823055,-28.4559524641237,
125.625748202422));
#114787=CARTESIAN_POINT('Ctrl Pts',(7.66381792132597,-28.4618964043691,
125.640181525617));
#114788=CARTESIAN_POINT('Ctrl Pts',(7.66423673220792,-28.4643086518056,
125.645946698855));
#114789=CARTESIAN_POINT('Ctrl Pts',(7.66504125856129,-28.4689822593511,
125.656942271152));
#114790=CARTESIAN_POINT('Ctrl Pts',(7.66542661388327,-28.4712381138844,
125.662174873351));
#114791=CARTESIAN_POINT('Ctrl Pts',(7.66647392120915,-28.4774167327331,
125.676306719916));
#114792=CARTESIAN_POINT('Ctrl Pts',(7.66713883665129,-28.4813905789815,
125.685183187278));
#114793=CARTESIAN_POINT('Ctrl Pts',(7.66972642803558,-28.4970601637743,
125.719378684095));
#114794=CARTESIAN_POINT('Ctrl Pts',(7.67167815781493,-28.5093125957213,
125.744435818369));
#114795=CARTESIAN_POINT('Ctrl Pts',(7.68151928548853,-28.5734708238799,
125.867703271747));
#114796=CARTESIAN_POINT('Ctrl Pts',(7.68970708961808,-28.6344781316498,
125.960855783906));
#114797=CARTESIAN_POINT('Ctrl Pts',(7.70197988037505,-28.7412590674603,
126.092970378632));
#114798=CARTESIAN_POINT('Ctrl Pts',(7.7061785023585,-28.7806157559364,126.136712898359));
#114799=CARTESIAN_POINT('Ctrl Pts',(7.71212159124836,-28.8406942322164,
126.196766241463));
#114800=CARTESIAN_POINT('Ctrl Pts',(7.71393329980538,-28.8596150626884,
126.214809295234));
#114801=CARTESIAN_POINT('Ctrl Pts',(7.71718130508527,-28.8946409844701,
126.246670434491));
#114802=CARTESIAN_POINT('Ctrl Pts',(7.7186236199752,-28.9105999999297,126.260640090308));
#114803=CARTESIAN_POINT('Ctrl Pts',(7.72087357102241,-28.9361278205838,
126.282138838925));
#114804=CARTESIAN_POINT('Ctrl Pts',(7.7216895657369,-28.9455193633209,126.289873876349));
#114805=CARTESIAN_POINT('Ctrl Pts',(7.72321400907695,-28.9633122119621,
126.30420415486));
#114806=CARTESIAN_POINT('Ctrl Pts',(7.72392337402123,-28.9716937855505,
126.310822789633));
#114807=CARTESIAN_POINT('Ctrl Pts',(7.72551554159998,-28.9907331496529,
126.325562500279));
#114808=CARTESIAN_POINT('Ctrl Pts',(7.72639646404369,-29.0014265145047,
126.333636580506));
#114809=CARTESIAN_POINT('Ctrl Pts',(7.72866192503662,-29.0293285735346,
126.354180399429));
#114810=CARTESIAN_POINT('Ctrl Pts',(7.73003886593481,-29.0466808411547,
126.366451689241));
#114811=CARTESIAN_POINT('Ctrl Pts',(7.7409594064645,-29.187286200686,126.461903418399));
#114812=CARTESIAN_POINT('Ctrl Pts',(7.74983288404353,-29.3209286143421,
126.528570914357));
#114813=CARTESIAN_POINT('Ctrl Pts',(7.76277512159135,-29.5197027483694,
126.596444099852));
#114814=CARTESIAN_POINT('Ctrl Pts',(7.76660500095504,-29.5788013268332,
126.613043486413));
#114815=CARTESIAN_POINT('Ctrl Pts',(7.77157981327122,-29.6535932176645,
126.629660065105));
#114816=CARTESIAN_POINT('Ctrl Pts',(7.77258148058685,-29.6685572380419,
126.632769194257));
#114817=CARTESIAN_POINT('Ctrl Pts',(7.77409057973926,-29.6909182437501,
126.63709517713));
#114818=CARTESIAN_POINT('Ctrl Pts',(7.77458969599311,-29.6982845737826,
126.638468781275));
#114819=CARTESIAN_POINT('Ctrl Pts',(7.77549373189191,-29.7115684346454,
126.640853213922));
#114820=CARTESIAN_POINT('Ctrl Pts',(7.77589765335625,-29.7174825042249,
126.641881816439));
#114821=CARTESIAN_POINT('Ctrl Pts',(7.77681024290389,-29.7307965028565,
126.644123384841));
#114822=CARTESIAN_POINT('Ctrl Pts',(7.77731986480762,-29.7381990743511,
126.645318357439));
#114823=CARTESIAN_POINT('Ctrl Pts',(7.77887788073116,-29.7607395687476,
126.648801030067));
#114824=CARTESIAN_POINT('Ctrl Pts',(7.77993437047395,-29.7759007061343,
126.650929997241));
#114825=CARTESIAN_POINT('Ctrl Pts',(7.78847933956808,-29.8977055023577,
126.666325494422));
#114826=CARTESIAN_POINT('Ctrl Pts',(7.79636454579978,-30.0053676162317,
126.669452772226));
#114827=CARTESIAN_POINT('Ctrl Pts',(7.81188321619623,-30.2184360115704,
126.655022786106));
#114828=CARTESIAN_POINT('Ctrl Pts',(7.81948051818708,-30.3233897372144,
126.637754883678));
#114829=CARTESIAN_POINT('Ctrl Pts',(7.82823765499373,-30.4467600627743,
126.605123817649));
#114830=CARTESIAN_POINT('Ctrl Pts',(7.8296983865248,-30.4674104259716,126.599232500944));
#114831=CARTESIAN_POINT('Ctrl Pts',(7.83197032956753,-30.4996277824114,
126.589363850631));
#114832=CARTESIAN_POINT('Ctrl Pts',(7.83279017451538,-30.5112740880835,
126.585655760655));
#114833=CARTESIAN_POINT('Ctrl Pts',(7.83431808891986,-30.5330123233518,
126.578470073101));
#114834=CARTESIAN_POINT('Ctrl Pts',(7.83502711655958,-30.543113611665,126.575023022818));
#114835=CARTESIAN_POINT('Ctrl Pts',(7.83661372121867,-30.5657432301982,
126.567057099743));
#114836=CARTESIAN_POINT('Ctrl Pts',(7.8374894748619,-30.5782519976698,126.562484560147));
#114837=CARTESIAN_POINT('Ctrl Pts',(7.83973201163526,-30.6103158649109,
126.550325912969));
#114838=CARTESIAN_POINT('Ctrl Pts',(7.84109145927099,-30.6297853127081,
126.54251950204));
#114839=CARTESIAN_POINT('Ctrl Pts',(7.85071025735473,-30.7675865123462,
126.484222948799));
#114840=CARTESIAN_POINT('Ctrl Pts',(7.85848751998315,-30.8798661069955,
126.420544315833));
#114841=CARTESIAN_POINT('Ctrl Pts',(7.87148636541487,-31.0513226072828,
126.295104554463));
#114842=CARTESIAN_POINT('Ctrl Pts',(7.87664729544417,-31.1151021462972,
126.240612190912));
#114843=CARTESIAN_POINT('Ctrl Pts',(7.88301531431186,-31.1844898286138,
126.171639041958));
#114844=CARTESIAN_POINT('Ctrl Pts',(7.8839396881213,-31.1943478660608,126.161588283968));
#114845=CARTESIAN_POINT('Ctrl Pts',(7.88535454869376,-31.2090905776309,
126.146171278649));
#114846=CARTESIAN_POINT('Ctrl Pts',(7.88583816855855,-31.214069792629,126.140895770265));
#114847=CARTESIAN_POINT('Ctrl Pts',(7.88672741656866,-31.2231120765137,
126.131189192866));
#114848=CARTESIAN_POINT('Ctrl Pts',(7.88713222824153,-31.2271858215076,
126.126768431189));
#114849=CARTESIAN_POINT('Ctrl Pts',(7.88806423387845,-31.2364680019656,
126.11658551333));
#114850=CARTESIAN_POINT('Ctrl Pts',(7.88859258235956,-31.2416601150417,
126.11080893098));
#114851=CARTESIAN_POINT('Ctrl Pts',(7.89022755541026,-31.2575188109682,
126.092914931793));
#114852=CARTESIAN_POINT('Ctrl Pts',(7.89134320069149,-31.2680494545389,
126.080679018488));
#114853=CARTESIAN_POINT('Ctrl Pts',(7.89779499688969,-31.3273880940981,
126.009669891017));
#114854=CARTESIAN_POINT('Ctrl Pts',(7.90332903467554,-31.3722811430271,
125.947752432297));
#114855=CARTESIAN_POINT('Ctrl Pts',(7.91550006698255,-31.4609421525688,
125.805895369061));
#114856=CARTESIAN_POINT('Ctrl Pts',(7.92212219944983,-31.5027352138685,
125.724988980278));
#114857=CARTESIAN_POINT('Ctrl Pts',(7.93233305350001,-31.5581957147618,
125.591957370601));
#114858=CARTESIAN_POINT('Ctrl Pts',(7.93603780869256,-31.5763081381189,
125.5418866475));
#114859=CARTESIAN_POINT('Ctrl Pts',(7.94082573787058,-31.5970154400235,
125.474750368841));
#114860=CARTESIAN_POINT('Ctrl Pts',(7.94197860831124,-31.6017867418814,
125.458394480075));
#114861=CARTESIAN_POINT('Ctrl Pts',(7.94388171486389,-31.60930065671,125.431085586249));
#114862=CARTESIAN_POINT('Ctrl Pts',(7.94463646168098,-31.6121842311618,
125.420173061941));
#114863=CARTESIAN_POINT('Ctrl Pts',(7.94611002326954,-31.6176229532318,
125.398710164754));
#114864=CARTESIAN_POINT('Ctrl Pts',(7.94682907005252,-31.6201863206409,
125.3881624791));
#114865=CARTESIAN_POINT('Ctrl Pts',(7.94855898392565,-31.6261319955883,
125.362611692892));
#114866=CARTESIAN_POINT('Ctrl Pts',(7.94956647928676,-31.6294100417488,
125.347585167669));
#114867=CARTESIAN_POINT('Ctrl Pts',(7.95297067585508,-31.6398471340722,
125.2963443465));
#114868=CARTESIAN_POINT('Ctrl Pts',(7.95533610573655,-31.6460108411502,
125.259936959417));
#114869=CARTESIAN_POINT('Ctrl Pts',(7.96531081243936,-31.6671504769284,
125.103678655359));
#114870=CARTESIAN_POINT('Ctrl Pts',(7.97256764901129,-31.670280963747,124.982601434739));
#114871=CARTESIAN_POINT('Ctrl Pts',(7.98305894509792,-31.6561609203659,
124.812418379638));
#114872=CARTESIAN_POINT('Ctrl Pts',(7.9861577038636,-31.6497860554771,124.762805698741));
#114873=CARTESIAN_POINT('Ctrl Pts',(7.99115473589603,-31.6362799452474,
124.685421298988));
#114874=CARTESIAN_POINT('Ctrl Pts',(7.99299747899562,-31.6306466453361,
124.657417008517));
#114875=CARTESIAN_POINT('Ctrl Pts',(7.9955033767907,-31.6221794629302,124.620288960294));
#114876=CARTESIAN_POINT('Ctrl Pts',(7.99613402677024,-31.619982614706,124.611023135585));
#114877=CARTESIAN_POINT('Ctrl Pts',(7.99718809379577,-31.6162047844782,
124.595676409116));
#114878=CARTESIAN_POINT('Ctrl Pts',(7.99760901319832,-31.6146685763034,
124.589584530164));
#114879=CARTESIAN_POINT('Ctrl Pts',(7.99846598969639,-31.6114862086979,
124.577259223798));
#114880=CARTESIAN_POINT('Ctrl Pts',(7.99890213248015,-31.6098382609255,
124.571026417159));
#114881=CARTESIAN_POINT('Ctrl Pts',(8.00003959029246,-31.6054661577713,
124.554870460968));
#114882=CARTESIAN_POINT('Ctrl Pts',(8.00074395204116,-31.6026862138655,
124.544962884227));
#114883=CARTESIAN_POINT('Ctrl Pts',(8.00369842596939,-31.5907183554662,
124.50378066051));
#114884=CARTESIAN_POINT('Ctrl Pts',(8.00598857808518,-31.5807059464587,
124.47275537061));
#114885=CARTESIAN_POINT('Ctrl Pts',(8.0151938016667,-31.537375166918,124.350845152625));
#114886=CARTESIAN_POINT('Ctrl Pts',(8.0223044474517,-31.4970744495799,124.262645456113));
#114887=CARTESIAN_POINT('Ctrl Pts',(8.03396386060595,-31.4177073146066,
124.122629857593));
#114888=CARTESIAN_POINT('Ctrl Pts',(8.03856192451762,-31.3828681528981,
124.068683991876));
#114889=CARTESIAN_POINT('Ctrl Pts',(8.04591207161824,-31.3210041081768,
123.984048353026));
#114890=CARTESIAN_POINT('Ctrl Pts',(8.04872170209543,-31.2958120642838,
123.952106308627));
#114891=CARTESIAN_POINT('Ctrl Pts',(8.05254195012938,-31.2594097257565,
123.909273324487));
#114892=CARTESIAN_POINT('Ctrl Pts',(8.05359138800184,-31.2491797150288,
123.89757194974));
#114893=CARTESIAN_POINT('Ctrl Pts',(8.05537152884012,-31.2314366506489,
123.87784108989));
#114894=CARTESIAN_POINT('Ctrl Pts',(8.05610557031029,-31.2240052778759,
123.869739882231));
#114895=CARTESIAN_POINT('Ctrl Pts',(8.05749757399433,-31.2096955902363,
123.854447038344));
#114896=CARTESIAN_POINT('Ctrl Pts',(8.05815611827572,-31.2028319954567,
123.847242346812));
#114897=CARTESIAN_POINT('Ctrl Pts',(8.05969135825602,-31.1866139799571,
123.830520920362));
#114898=CARTESIAN_POINT('Ctrl Pts',(8.0605658108241,-31.1772088669591,123.821054133674));
#114899=CARTESIAN_POINT('Ctrl Pts',(8.06359536363938,-31.144052615423,123.788472894193));
#114900=CARTESIAN_POINT('Ctrl Pts',(8.06572493619712,-31.1197254532927,
123.765954028922));
#114901=CARTESIAN_POINT('Ctrl Pts',(8.07749848007033,-30.9799485525973,
123.644106237465));
#114902=CARTESIAN_POINT('Ctrl Pts',(8.08650217796176,-30.8519889151635,
123.560257356629));
#114903=CARTESIAN_POINT('Ctrl Pts',(8.09804410529499,-30.6846874278325,
123.480841452316));
#114904=CARTESIAN_POINT('Ctrl Pts',(8.1001190462817,-30.6545400475449,123.467610809832));
#114905=CARTESIAN_POINT('Ctrl Pts',(8.10361637507494,-30.60406152731,123.447218902795));
#114906=CARTESIAN_POINT('Ctrl Pts',(8.10501588074681,-30.5839472294856,
123.439543338569));
#114907=CARTESIAN_POINT('Ctrl Pts',(8.10700231137587,-30.5556238076518,
123.429359468825));
#114908=CARTESIAN_POINT('Ctrl Pts',(8.10757141894178,-30.5475345268512,
123.426521233759));
#114909=CARTESIAN_POINT('Ctrl Pts',(8.1085520634946,-30.5336470861384,123.421768690094));
#114910=CARTESIAN_POINT('Ctrl Pts',(8.10896182186858,-30.5278595287723,
123.419823555145));
#114911=CARTESIAN_POINT('Ctrl Pts',(8.10983015602446,-30.5156298130903,
123.415787967065));
#114912=CARTESIAN_POINT('Ctrl Pts',(8.11028911923891,-30.5091854915316,
123.413704945302));
#114913=CARTESIAN_POINT('Ctrl Pts',(8.11155262025018,-30.491493708333,123.408105277584));
#114914=CARTESIAN_POINT('Ctrl Pts',(8.11236149926928,-30.4802216033861,
123.404668666235));
#114915=CARTESIAN_POINT('Ctrl Pts',(8.1167573412069,-30.4192038931694,123.386770990382));
#114916=CARTESIAN_POINT('Ctrl Pts',(8.12044612402867,-30.3688451313495,
123.374517941011));
#114917=CARTESIAN_POINT('Ctrl Pts',(8.13130096307024,-30.2210730302732,
123.34578314236));
#114918=CARTESIAN_POINT('Ctrl Pts',(8.1385553547343,-30.122657798709,123.335589232585));
#114919=CARTESIAN_POINT('Ctrl Pts',(8.1491802482279,-29.974661944702,123.333464566189));
#114920=CARTESIAN_POINT('Ctrl Pts',(8.15267294200117,-29.9253982768887,
123.334942134734));
#114921=CARTESIAN_POINT('Ctrl Pts',(8.15847357563449,-29.8423562670606,
123.34112662357));
#114922=CARTESIAN_POINT('Ctrl Pts',(8.16081231774195,-29.8085272436336,
123.344690089323));
#114923=CARTESIAN_POINT('Ctrl Pts',(8.16410594938206,-29.7604117114463,
123.351253454494));
#114924=CARTESIAN_POINT('Ctrl Pts',(8.16508687295615,-29.7460206465406,
123.353408906049));
#114925=CARTESIAN_POINT('Ctrl Pts',(8.16678703625533,-29.7209776680386,
123.357495913684));
#114926=CARTESIAN_POINT('Ctrl Pts',(8.16750888694876,-29.7103131046261,
123.359343226796));
#114927=CARTESIAN_POINT('Ctrl Pts',(8.16899619163889,-29.6882781544591,
123.363381670807));
#114928=CARTESIAN_POINT('Ctrl Pts',(8.16976113115143,-29.6769110635224,
123.365587685135));
#114929=CARTESIAN_POINT('Ctrl Pts',(8.17173429317091,-29.6475091856344,
123.371612445821));
#114930=CARTESIAN_POINT('Ctrl Pts',(8.17293671189603,-29.6295128260624,
123.375612392682));
#114931=CARTESIAN_POINT('Ctrl Pts',(8.17821635309224,-29.550214806565,123.394623972619));
#114932=CARTESIAN_POINT('Ctrl Pts',(8.18219163219968,-29.4897251942165,
123.412813855749));
#114933=CARTESIAN_POINT('Ctrl Pts',(8.19511354842859,-29.2938358495133,
123.484081471318));
#114934=CARTESIAN_POINT('Ctrl Pts',(8.20369107127314,-29.1643719335063,
123.55141715803));
#114935=CARTESIAN_POINT('Ctrl Pts',(8.2144747122442,-29.0265129832222,123.647814896298));
#114936=CARTESIAN_POINT('Ctrl Pts',(8.21596258752668,-29.0080002473793,
123.661337274887));
#114937=CARTESIAN_POINT('Ctrl Pts',(8.21805347439158,-28.9827908967551,
123.680561198768));
#114938=CARTESIAN_POINT('Ctrl Pts',(8.21863608796822,-28.9758506744648,
123.685940921998));
#114939=CARTESIAN_POINT('Ctrl Pts',(8.21963255000446,-28.9641302862768,
123.695175245265));
#114940=CARTESIAN_POINT('Ctrl Pts',(8.22004446622471,-28.9593281941136,
123.699001961707));
#114941=CARTESIAN_POINT('Ctrl Pts',(8.22090890415184,-28.9493423766639,
123.707050175428));
#114942=CARTESIAN_POINT('Ctrl Pts',(8.22136173714491,-28.9441627934153,
123.711276414596));
#114943=CARTESIAN_POINT('Ctrl Pts',(8.22259120594472,-28.9302345479803,
123.722781382444));
#114944=CARTESIAN_POINT('Ctrl Pts',(8.2233718160776,-28.9215349904661,123.730118617861));
#114945=CARTESIAN_POINT('Ctrl Pts',(8.22725424727641,-28.8789392164369,
123.766797422974));
#114946=CARTESIAN_POINT('Ctrl Pts',(8.2304323118313,-28.8461645595898,123.797407427969));
#114947=CARTESIAN_POINT('Ctrl Pts',(8.23996918740608,-28.7528544772965,
123.891883681567));
#114948=CARTESIAN_POINT('Ctrl Pts',(8.24642377711056,-28.6960961697525,
123.959265375396));
#114949=CARTESIAN_POINT('Ctrl Pts',(8.25716882936448,-28.6096611677064,
124.08011520575));
#114950=CARTESIAN_POINT('Ctrl Pts',(8.26150268712672,-28.5771132068232,
124.131308724844));
#114951=CARTESIAN_POINT('Ctrl Pts',(8.26761239925455,-28.5343810256616,
124.207392527624));
#114952=CARTESIAN_POINT('Ctrl Pts',(8.26945976700469,-28.5218948344833,
124.230928586426));
#114953=CARTESIAN_POINT('Ctrl Pts',(8.2727648135219,-28.5003519183986,124.274000902871));
#114954=CARTESIAN_POINT('Ctrl Pts',(8.27422883713139,-28.4910994270867,
124.293432102383));
#114955=CARTESIAN_POINT('Ctrl Pts',(8.27650470944068,-28.4771819893589,
124.324181296994));
#114956=CARTESIAN_POINT('Ctrl Pts',(8.2773252411017,-28.4722611314191,124.3353801266));
#114957=CARTESIAN_POINT('Ctrl Pts',(8.27885378060327,-28.4632787287989,
124.356449209166));
#114958=CARTESIAN_POINT('Ctrl Pts',(8.27956275405594,-28.4591878580258,
124.366306195432));
#114959=CARTESIAN_POINT('Ctrl Pts',(8.28114839612405,-28.4502107048298,
124.388537717765));
#114960=CARTESIAN_POINT('Ctrl Pts',(8.28202325124273,-28.4453773282874,
124.400932935555));
#114961=CARTESIAN_POINT('Ctrl Pts',(8.28426181045815,-28.4333247079794,
124.432970537949));
#114962=CARTESIAN_POINT('Ctrl Pts',(8.2856182241134,-28.426326000243,124.452693790982));
#114963=CARTESIAN_POINT('Ctrl Pts',(8.2966237809029,-28.3721289735597,124.615072452251));
#114964=CARTESIAN_POINT('Ctrl Pts',(8.30558432046893,-28.3440583939598,
124.763373237726));
#114965=CARTESIAN_POINT('Ctrl Pts',(8.31760122228488,-28.333929230156,124.958047270103));
#114966=CARTESIAN_POINT('Ctrl Pts',(8.32038311470479,-28.3334035203741,
125.002734166932));
#114967=CARTESIAN_POINT('Ctrl Pts',(8.3249251277759,-28.335429007757,125.073919232414));
#114968=CARTESIAN_POINT('Ctrl Pts',(8.32664125314046,-28.336818028131,125.100429981403));
#114969=CARTESIAN_POINT('Ctrl Pts',(8.32899981068632,-28.339546028376,125.13614192483));
#114970=CARTESIAN_POINT('Ctrl Pts',(8.32961437993956,-28.340329624558,125.145383116617));
#114971=CARTESIAN_POINT('Ctrl Pts',(8.33064897671064,-28.3417687262063,
125.160822528058));
#114972=CARTESIAN_POINT('Ctrl Pts',(8.33106669954043,-28.3423819486823,
125.167024660113));
#114973=CARTESIAN_POINT('Ctrl Pts',(8.33187140242276,-28.3436243188825,
125.178908581248));
#114974=CARTESIAN_POINT('Ctrl Pts',(8.33225804133579,-28.3442479330186,
125.184590811351));
#114975=CARTESIAN_POINT('Ctrl Pts',(8.33331315286667,-28.3460222784039,
125.200025318645));
#114976=CARTESIAN_POINT('Ctrl Pts',(8.33398466373152,-28.3472299904756,
125.209770625929));
#114977=CARTESIAN_POINT('Ctrl Pts',(8.33663011011154,-28.3522954838519,
125.247881673198));
#114978=CARTESIAN_POINT('Ctrl Pts',(8.33863471079156,-28.3567977482924,
125.276155070562));
#114979=CARTESIAN_POINT('Ctrl Pts',(8.34732083498592,-28.3791834713274,
125.396653522729));
#114980=CARTESIAN_POINT('Ctrl Pts',(8.35421071389529,-28.4041190181944,
125.487379887572));
#114981=CARTESIAN_POINT('Ctrl Pts',(8.36102756272879,-28.4365599800807,
125.575509603842));
#114982=CARTESIAN_POINT('Ctrl Pts',(8.16626341820841,-28.4365599837785,
125.575509613888));
#114983=CARTESIAN_POINT('Ctrl Pts',(8.16547942547945,-28.4324769590612,
125.564417593744));
#114984=CARTESIAN_POINT('Ctrl Pts',(8.16469937320103,-28.4285120041026,
125.553282201909));
#114985=CARTESIAN_POINT('Ctrl Pts',(8.1626186044127,-28.4182017872195,125.523321164882));
#114986=CARTESIAN_POINT('Ctrl Pts',(8.16132506106394,-28.4120740470098,
125.504422293387));
#114987=CARTESIAN_POINT('Ctrl Pts',(8.15401452785318,-28.3791009035015,
125.39616547033));
#114988=CARTESIAN_POINT('Ctrl Pts',(8.14823771962926,-28.3594598761445,
125.304782308935));
#114989=CARTESIAN_POINT('Ctrl Pts',(8.13815381465029,-28.338478564275,125.141417546437));
#114990=CARTESIAN_POINT('Ctrl Pts',(8.13382720892913,-28.333945478382,125.070101000919));
#114991=CARTESIAN_POINT('Ctrl Pts',(8.1258696786412,-28.3340445101056,124.941605154235));
#114992=CARTESIAN_POINT('Ctrl Pts',(8.12227689942226,-28.3370251665466,
124.884540405244));
#114993=CARTESIAN_POINT('Ctrl Pts',(8.11776286945087,-28.3441647769812,
124.815857010106));
#114994=CARTESIAN_POINT('Ctrl Pts',(8.11697534779172,-28.3455287698328,
124.803979963053));
#114995=CARTESIAN_POINT('Ctrl Pts',(8.11572407869919,-28.3478785085063,
124.785295855632));
#114996=CARTESIAN_POINT('Ctrl Pts',(8.11526489406306,-28.3487788220798,
124.778478196097));
#114997=CARTESIAN_POINT('Ctrl Pts',(8.11439583277433,-28.3505533421466,
124.765652867563));
#114998=CARTESIAN_POINT('Ctrl Pts',(8.1139864698656,-28.3514182109223,124.759644148285));
#114999=CARTESIAN_POINT('Ctrl Pts',(8.11300979062025,-28.3535504749372,
124.745383296907));
#115000=CARTESIAN_POINT('Ctrl Pts',(8.11244089225243,-28.3548470860646,
124.737135802287));
#115001=CARTESIAN_POINT('Ctrl Pts',(8.11049068977032,-28.3594787420168,
124.709052248364));
#115002=CARTESIAN_POINT('Ctrl Pts',(8.10909457544795,-28.3631108672285,
124.689267848386));
#115003=CARTESIAN_POINT('Ctrl Pts',(8.10558542532627,-28.373037526978,124.640215053393));
#115004=CARTESIAN_POINT('Ctrl Pts',(8.10345589762585,-28.3797643675872,
124.611041924188));
#115005=CARTESIAN_POINT('Ctrl Pts',(8.09307956532922,-28.4160314348977,
124.471093734306));
#115006=CARTESIAN_POINT('Ctrl Pts',(8.08462915601719,-28.4561674029286,
124.363382620243));
#115007=CARTESIAN_POINT('Ctrl Pts',(8.07163710921463,-28.5367638877434,
124.200638129734));
#115008=CARTESIAN_POINT('Ctrl Pts',(8.06693700100534,-28.5700724169644,
124.142475376262));
#115009=CARTESIAN_POINT('Ctrl Pts',(8.06107839197189,-28.6170776229805,
124.070788901293));
#115010=CARTESIAN_POINT('Ctrl Pts',(8.05980672125489,-28.6276233442741,
124.055283147441));
#115011=CARTESIAN_POINT('Ctrl Pts',(8.05776136156508,-28.6451384948061,
124.030442436719));
#115012=CARTESIAN_POINT('Ctrl Pts',(8.05698168664499,-28.6519477334164,
124.020997106625));
#115013=CARTESIAN_POINT('Ctrl Pts',(8.05548658681987,-28.6652589860843,
124.002934843657));
#115014=CARTESIAN_POINT('Ctrl Pts',(8.05477066377694,-28.6717467994374,
123.994308225768));
#115015=CARTESIAN_POINT('Ctrl Pts',(8.05310884323275,-28.6870694278685,
123.974341213398));
#115016=CARTESIAN_POINT('Ctrl Pts',(8.05216551819546,-28.6959681772884,
123.963050791733));
#115017=CARTESIAN_POINT('Ctrl Pts',(8.04907873652986,-28.7257373928665,
123.926270033047));
#115018=CARTESIAN_POINT('Ctrl Pts',(8.04695975395307,-28.7472185535769,
123.901282514337));
#115019=CARTESIAN_POINT('Ctrl Pts',(8.04187247679382,-28.8011767256037,
123.842158475678));
#115020=CARTESIAN_POINT('Ctrl Pts',(8.03893313996667,-28.8343880669925,
123.808730281568));
#115021=CARTESIAN_POINT('Ctrl Pts',(8.03182964268563,-28.9188421181164,
123.730643236722));
#115022=CARTESIAN_POINT('Ctrl Pts',(8.02770660979172,-28.9714839982173,
123.687626584171));
#115023=CARTESIAN_POINT('Ctrl Pts',(8.02333105031825,-29.0295008712684,
123.645858141884));
#115024=CARTESIAN_POINT('Ctrl Pts',(8.02311257283382,-29.0324032148564,
123.64378276369));
#115025=CARTESIAN_POINT('Ctrl Pts',(8.01790381433809,-29.1017223679453,
123.594550513803));
#115026=CARTESIAN_POINT('Ctrl Pts',(8.01286811306646,-29.1714937959449,
123.552324310014));
#115027=CARTESIAN_POINT('Ctrl Pts',(8.00674276202954,-29.2550727596199,
123.509767776961));
#115028=CARTESIAN_POINT('Ctrl Pts',(8.0059294233641,-29.2661452647006,123.504284158882));
#115029=CARTESIAN_POINT('Ctrl Pts',(8.00464612531833,-29.2835545550346,
123.495902110174));
#115030=CARTESIAN_POINT('Ctrl Pts',(8.00418112007286,-29.2898505320337,
123.492919289974));
#115031=CARTESIAN_POINT('Ctrl Pts',(8.0033077663485,-29.3016478447872,123.487420461107));
#115032=CARTESIAN_POINT('Ctrl Pts',(8.00290000687352,-29.3071444133693,
123.484894813681));
#115033=CARTESIAN_POINT('Ctrl Pts',(8.00193626362902,-29.3201100772512,
123.479022458936));
#115034=CARTESIAN_POINT('Ctrl Pts',(8.0013788177423,-29.3275902106154,123.475700798524));
#115035=CARTESIAN_POINT('Ctrl Pts',(7.99950926179686,-29.3526223541858,
123.464805020734));
#115036=CARTESIAN_POINT('Ctrl Pts',(7.99818388648282,-29.3702795010093,
123.457478215209));
#115037=CARTESIAN_POINT('Ctrl Pts',(7.99489170691469,-29.41401192889,123.440207496968));
#115038=CARTESIAN_POINT('Ctrl Pts',(7.99291073520473,-29.44021803352,123.430612015065));
#115039=CARTESIAN_POINT('Ctrl Pts',(7.98394489144086,-29.5588073172379,
123.39053811178));
#115040=CARTESIAN_POINT('Ctrl Pts',(7.9767942255221,-29.6535127139069,123.367527859017));
#115041=CARTESIAN_POINT('Ctrl Pts',(7.96356668136652,-29.8346409159076,
123.340001031527));
#115042=CARTESIAN_POINT('Ctrl Pts',(7.95747970818973,-29.9204789632291,
123.33368048114));
#115043=CARTESIAN_POINT('Ctrl Pts',(7.95024903481309,-30.0261227812028,
123.334088458429));
#115044=CARTESIAN_POINT('Ctrl Pts',(7.94891218700895,-30.0458096207103,
123.334513524405));
#115045=CARTESIAN_POINT('Ctrl Pts',(7.94678863913994,-30.0773187574682,
123.335753004221));
#115046=CARTESIAN_POINT('Ctrl Pts',(7.94599508283325,-30.0891474164829,
123.336344685974));
#115047=CARTESIAN_POINT('Ctrl Pts',(7.94448979560155,-30.1116832310394,
123.337712999148));
#115048=CARTESIAN_POINT('Ctrl Pts',(7.94377739893271,-30.1223911023939,
123.338467079907));
#115049=CARTESIAN_POINT('Ctrl Pts',(7.94214717200413,-30.1469871171889,
123.340438273105));
#115050=CARTESIAN_POINT('Ctrl Pts',(7.94123160522727,-30.1608688902596,
123.341726332081));
#115051=CARTESIAN_POINT('Ctrl Pts',(7.93833707832414,-30.2049525104772,
123.346375547093));
#115052=CARTESIAN_POINT('Ctrl Pts',(7.93637844587613,-30.2350803351481,
123.350388899318));
#115053=CARTESIAN_POINT('Ctrl Pts',(7.93175853781775,-30.3066464127872,
123.361922969449));
#115054=CARTESIAN_POINT('Ctrl Pts',(7.92911930605668,-30.3479427795192,
123.370194927597));
#115055=CARTESIAN_POINT('Ctrl Pts',(7.9218396038667,-30.462077105722,123.397593453428));
#115056=CARTESIAN_POINT('Ctrl Pts',(7.91727239400856,-30.5339959481434,
123.420104213306));
#115057=CARTESIAN_POINT('Ctrl Pts',(7.91183715133302,-30.6167785394866,
123.452316590263));
#115058=CARTESIAN_POINT('Ctrl Pts',(7.91100664316762,-30.6293491455522,
123.457385546901));
#115059=CARTESIAN_POINT('Ctrl Pts',(7.90569050749756,-30.7091992493756,
123.49072270242));
#115060=CARTESIAN_POINT('Ctrl Pts',(7.9011519654138,-30.7746138627548,123.523229125894));
#115061=CARTESIAN_POINT('Ctrl Pts',(7.89558442436585,-30.848288926322,123.566084879981));
#115062=CARTESIAN_POINT('Ctrl Pts',(7.89477630857707,-30.8588304348841,
123.572373670629));
#115063=CARTESIAN_POINT('Ctrl Pts',(7.89349948739961,-30.8752289248917,
123.582403931149));
#115064=CARTESIAN_POINT('Ctrl Pts',(7.89303565586442,-30.8811338647551,
123.586066694147));
#115065=CARTESIAN_POINT('Ctrl Pts',(7.89216319647963,-30.8921395265004,
123.592989087817));
#115066=CARTESIAN_POINT('Ctrl Pts',(7.89175514263403,-30.8972456191498,
123.596239715626));
#115067=CARTESIAN_POINT('Ctrl Pts',(7.89078892106941,-30.9092405956053,
123.603968107052));
#115068=CARTESIAN_POINT('Ctrl Pts',(7.89022926811205,-30.916114193393,123.608469086074));
#115069=CARTESIAN_POINT('Ctrl Pts',(7.888344374703,-30.9390265986613,123.623715957769));
#115070=CARTESIAN_POINT('Ctrl Pts',(7.88700558181857,-30.9549111982721,
123.634689324039));
#115071=CARTESIAN_POINT('Ctrl Pts',(7.8836725896048,-30.9935898775746,123.662414410329));
#115072=CARTESIAN_POINT('Ctrl Pts',(7.88166379887218,-31.0161544425717,
123.679475095754));
#115073=CARTESIAN_POINT('Ctrl Pts',(7.87245499813857,-31.1166619364988,
123.759568910331));
#115074=CARTESIAN_POINT('Ctrl Pts',(7.86508252586005,-31.1892534186918,
123.828983374719));
#115075=CARTESIAN_POINT('Ctrl Pts',(7.85190793376787,-31.3094070397529,
123.966649377347));
#115076=CARTESIAN_POINT('Ctrl Pts',(7.84607386977252,-31.3589642359754,
124.032746053603));
#115077=CARTESIAN_POINT('Ctrl Pts',(7.83908588263193,-31.4139889545182,
124.118764804695));
#115078=CARTESIAN_POINT('Ctrl Pts',(7.83775509849655,-31.4242598199741,
124.135462982231));
#115079=CARTESIAN_POINT('Ctrl Pts',(7.83563882127667,-31.4402501886613,
124.162518532701));
#115080=CARTESIAN_POINT('Ctrl Pts',(7.83484655480527,-31.4461579802632,
124.172761870677));
#115081=CARTESIAN_POINT('Ctrl Pts',(7.83334227108706,-31.4572220766442,
124.192426389377));
#115082=CARTESIAN_POINT('Ctrl Pts',(7.83262960322967,-31.4623972947206,
124.201836182956));
#115083=CARTESIAN_POINT('Ctrl Pts',(7.83099672465691,-31.4740983186649,
124.223607371765));
#115084=CARTESIAN_POINT('Ctrl Pts',(7.83007880347991,-31.4805603226038,
124.236002279373));
#115085=CARTESIAN_POINT('Ctrl Pts',(7.82716834081315,-31.5006682525393,
124.27578523552));
#115086=CARTESIAN_POINT('Ctrl Pts',(7.82519645511471,-31.5137164783339,
124.303469425794));
#115087=CARTESIAN_POINT('Ctrl Pts',(7.82053855599107,-31.543049812716,124.370428966258));
#115088=CARTESIAN_POINT('Ctrl Pts',(7.81787510659863,-31.558608981378,124.409999293157));
#115089=CARTESIAN_POINT('Ctrl Pts',(7.81066971969658,-31.596968769538,124.519707737668));
#115090=CARTESIAN_POINT('Ctrl Pts',(7.80619538013148,-31.6166543896218,
124.590831504046));
#115091=CARTESIAN_POINT('Ctrl Pts',(7.80083666926066,-31.6343716467981,
124.676614972478));
#115092=CARTESIAN_POINT('Ctrl Pts',(7.79998656953,-31.6370084600261,124.690239040858));
#115093=CARTESIAN_POINT('Ctrl Pts',(7.79461998770719,-31.6525367813739,
124.776216091977));
#115094=CARTESIAN_POINT('Ctrl Pts',(7.79005102148958,-31.6607974236268,
124.849314116242));
#115095=CARTESIAN_POINT('Ctrl Pts',(7.78444971239173,-31.6647756820226,
124.934971923929));
#115096=CARTESIAN_POINT('Ctrl Pts',(7.78364147022368,-31.6652096554362,
124.947241078298));
#115097=CARTESIAN_POINT('Ctrl Pts',(7.78236449233671,-31.6656768597908,
124.966460616492));
#115098=CARTESIAN_POINT('Ctrl Pts',(7.78190063240834,-31.6658022645961,
124.973408603235));
#115099=CARTESIAN_POINT('Ctrl Pts',(7.78102815158764,-31.6659555652293,
124.986409737236));
#115100=CARTESIAN_POINT('Ctrl Pts',(7.78062010506356,-31.6659939442218,
124.992462513743));
#115101=CARTESIAN_POINT('Ctrl Pts',(7.77965394435065,-31.666006659998,125.006730743812));
#115102=CARTESIAN_POINT('Ctrl Pts',(7.77909434548976,-31.6659532123358,
125.01494594611));
#115103=CARTESIAN_POINT('Ctrl Pts',(7.77720982911279,-31.6655706896432,
125.04245957913));
#115104=CARTESIAN_POINT('Ctrl Pts',(7.77587136626035,-31.6649670177052,
125.061751831152));
#115105=CARTESIAN_POINT('Ctrl Pts',(7.7725393798046,-31.6626531408596,125.109270567233));
#115106=CARTESIAN_POINT('Ctrl Pts',(7.77053127531928,-31.6605591952488,
125.137471823562));
#115107=CARTESIAN_POINT('Ctrl Pts',(7.76132856963111,-31.6477925620909,
125.265269538704));
#115108=CARTESIAN_POINT('Ctrl Pts',(7.75396167292581,-31.6288690136447,
125.363832992559));
#115109=CARTESIAN_POINT('Ctrl Pts',(7.74078581811461,-31.5784023305153,
125.539463151853));
#115110=CARTESIAN_POINT('Ctrl Pts',(7.73494548422716,-31.5497265639478,
125.617029726385));
#115111=CARTESIAN_POINT('Ctrl Pts',(7.7279514412154,-31.5072661236998,125.70999237117));
#115112=CARTESIAN_POINT('Ctrl Pts',(7.72662047674095,-31.4988068007017,
125.727680263514));
#115113=CARTESIAN_POINT('Ctrl Pts',(7.72450398327123,-31.4847475651856,
125.755791303693));
#115114=CARTESIAN_POINT('Ctrl Pts',(7.72371167843047,-31.479345651537,125.766310826506));
#115115=CARTESIAN_POINT('Ctrl Pts',(7.72220736501307,-31.4688252736245,
125.78627198206));
#115116=CARTESIAN_POINT('Ctrl Pts',(7.72149470537442,-31.4637266469606,
125.795723335335));
#115117=CARTESIAN_POINT('Ctrl Pts',(7.71986190644102,-31.4517826150671,
125.817360736742));
#115118=CARTESIAN_POINT('Ctrl Pts',(7.71894405590255,-31.4448744725493,
125.82951137043));
#115119=CARTESIAN_POINT('Ctrl Pts',(7.71603407230868,-31.4223608703319,
125.867975457935));
#115120=CARTESIAN_POINT('Ctrl Pts',(7.71406258513979,-31.4061827120815,
125.89394754291));
#115121=CARTESIAN_POINT('Ctrl Pts',(7.70940583001876,-31.3658476543687,
125.95489348398));
#115122=CARTESIAN_POINT('Ctrl Pts',(7.70674311032931,-31.3410496734596,
125.989417775061));
#115123=CARTESIAN_POINT('Ctrl Pts',(7.69953811031672,-31.2696919709715,
126.081144248231));
#115124=CARTESIAN_POINT('Ctrl Pts',(7.69506347539834,-31.2206134033656,
126.136263117505));
#115125=CARTESIAN_POINT('Ctrl Pts',(7.68970794153499,-31.1581908575605,
126.197639735466));
#115126=CARTESIAN_POINT('Ctrl Pts',(7.68886129530606,-31.148216161876,126.207206129174));
#115127=CARTESIAN_POINT('Ctrl Pts',(7.68349384736662,-31.0844009071469,
126.266902687337));
#115128=CARTESIAN_POINT('Ctrl Pts',(7.67892059112954,-31.0274149761528,
126.313538531284));
#115129=CARTESIAN_POINT('Ctrl Pts',(7.67331451884676,-30.9575484231261,
126.363380998167));
#115130=CARTESIAN_POINT('Ctrl Pts',(7.67250625920492,-30.9474757254317,
126.370400108274));
#115131=CARTESIAN_POINT('Ctrl Pts',(7.67122925964101,-30.9315816785885,
126.381216807186));
#115132=CARTESIAN_POINT('Ctrl Pts',(7.67076539577713,-30.9258123381129,
126.38509053948));
#115133=CARTESIAN_POINT('Ctrl Pts',(7.66989291196878,-30.9149726262504,
126.392270711324));
#115134=CARTESIAN_POINT('Ctrl Pts',(7.66948486644286,-30.9099082525484,
126.395585757904));
#115135=CARTESIAN_POINT('Ctrl Pts',(7.6685187140959,-30.8979278907113,126.403334954812));
#115136=CARTESIAN_POINT('Ctrl Pts',(7.66795912268106,-30.8909970451717,
126.407745627142));
#115137=CARTESIAN_POINT('Ctrl Pts',(7.66607465823961,-30.8676748186116,
126.422346273744));
#115138=CARTESIAN_POINT('Ctrl Pts',(7.66473624085459,-30.8511397077952,
126.432302213832));
#115139=CARTESIAN_POINT('Ctrl Pts',(7.66140439296249,-30.8099638976418,
126.456129779611));
#115140=CARTESIAN_POINT('Ctrl Pts',(7.65939638302319,-30.7851362865985,
126.469665363804));
#115141=CARTESIAN_POINT('Ctrl Pts',(7.65019451669854,-30.6708541981889,
126.528247639604));
#115142=CARTESIAN_POINT('Ctrl Pts',(7.64282838778472,-30.5777933509493,
126.565803787186));
#115143=CARTESIAN_POINT('Ctrl Pts',(7.62965235893061,-30.4028672185788,
126.618664374487));
#115144=CARTESIAN_POINT('Ctrl Pts',(7.62381116140066,-30.3221361288222,
126.636645461328));
#115145=CARTESIAN_POINT('Ctrl Pts',(7.61681628438287,-30.2209931574098,
126.6513940696));
#115146=CARTESIAN_POINT('Ctrl Pts',(7.61548529519009,-30.2015444046224,
126.653880364072));
#115147=CARTESIAN_POINT('Ctrl Pts',(7.61336877207036,-30.1703014436118,
126.657315071783));
#115148=CARTESIAN_POINT('Ctrl Pts',(7.61257646196115,-30.1585336554849,
126.658482113685));
#115149=CARTESIAN_POINT('Ctrl Pts',(7.61107214444826,-30.1360574884488,
126.660469714761));
#115150=CARTESIAN_POINT('Ctrl Pts',(7.61035948592068,-30.1253517022893,
126.661312214409));
#115151=CARTESIAN_POINT('Ctrl Pts',(7.60872669785634,-30.100695335414,126.663012862423));
#115152=CARTESIAN_POINT('Ctrl Pts',(7.60780885696898,-30.0867404816529,
126.663799098365));
#115153=CARTESIAN_POINT('Ctrl Pts',(7.60489893888342,-30.042215576272,126.665745968945));
#115154=CARTESIAN_POINT('Ctrl Pts',(7.60292750621691,-30.0116217133338,
126.666240352381));
#115155=CARTESIAN_POINT('Ctrl Pts',(7.59827090755342,-29.938544610728,126.665408200689));
#115156=CARTESIAN_POINT('Ctrl Pts',(7.59560828766221,-29.8960913656353,
126.663299316137));
#115157=CARTESIAN_POINT('Ctrl Pts',(7.58840334126734,-29.7803270874141,
126.653098451153));
#115158=CARTESIAN_POINT('Ctrl Pts',(7.58392866662734,-29.7074002054776,
126.641760154257));
#115159=CARTESIAN_POINT('Ctrl Pts',(7.57446014648976,-29.5563768260499,
126.60789420372));
#115160=CARTESIAN_POINT('Ctrl Pts',(7.56947081470208,-29.4786984847162,
126.584413729969));
#115161=CARTESIAN_POINT('Ctrl Pts',(7.56317443575743,-29.3879893331913,
126.549599652459));
#115162=CARTESIAN_POINT('Ctrl Pts',(7.56211908234472,-29.3730168390307,
126.543602347795));
#115163=CARTESIAN_POINT('Ctrl Pts',(7.56053784015299,-29.3509708518339,
126.534398066715));
#115164=CARTESIAN_POINT('Ctrl Pts',(7.56002125403971,-29.3438284157962,
126.531357276545));
#115165=CARTESIAN_POINT('Ctrl Pts',(7.55909941258379,-29.3311947700974,
126.525874071297));
#115166=CARTESIAN_POINT('Ctrl Pts',(7.55869535611452,-29.3256951451234,
126.523451698449));
#115167=CARTESIAN_POINT('Ctrl Pts',(7.55779954987719,-29.3135867348158,
126.518039998779));
#115168=CARTESIAN_POINT('Ctrl Pts',(7.55730703257641,-29.3069843959243,
126.515037285367));
#115169=CARTESIAN_POINT('Ctrl Pts',(7.55585127908362,-29.2876241795882,
126.506079320415));
#115170=CARTESIAN_POINT('Ctrl Pts',(7.55488136958126,-29.2749223076002,
126.500005512053));
#115171=CARTESIAN_POINT('Ctrl Pts',(7.5480422291824,-29.1866225044816,126.456398573499));
#115172=CARTESIAN_POINT('Ctrl Pts',(7.54191663462614,-29.1139025864465,
126.413332312008));
#115173=CARTESIAN_POINT('Ctrl Pts',(7.52646891785952,-28.9400105864096,
126.291637216763));
#115174=CARTESIAN_POINT('Ctrl Pts',(7.51720686455405,-28.8440226685185,
126.206495914544));
#115175=CARTESIAN_POINT('Ctrl Pts',(7.50695850663711,-28.744671498522,126.095513320632));
#115176=CARTESIAN_POINT('Ctrl Pts',(7.50552236270976,-28.7309297559286,
126.079564666007));
#115177=CARTESIAN_POINT('Ctrl Pts',(7.50319643927016,-28.7089803982537,
126.053091771589));
#115178=CARTESIAN_POINT('Ctrl Pts',(7.5022993597384,-28.7005907968368,126.042722221962));
#115179=CARTESIAN_POINT('Ctrl Pts',(7.50069354247894,-28.6857144652872,
126.023876657793));
#115180=CARTESIAN_POINT('Ctrl Pts',(7.49998304725718,-28.6791830212844,
126.015437046281));
#115181=CARTESIAN_POINT('Ctrl Pts',(7.49846705315504,-28.665358742141,125.997214908737));
#115182=CARTESIAN_POINT('Ctrl Pts',(7.4976625770582,-28.6580913391826,125.987413804187));
#115183=CARTESIAN_POINT('Ctrl Pts',(7.49545942954509,-28.6383853515719,
125.960218097117));
#115184=CARTESIAN_POINT('Ctrl Pts',(7.49406941880257,-28.6261726995768,
125.942662113951));
#115185=CARTESIAN_POINT('Ctrl Pts',(7.48820579676779,-28.5756697713551,
125.866995841285));
#115186=CARTESIAN_POINT('Ctrl Pts',(7.48385361238211,-28.5407003449968,
125.80674934718));
#115187=CARTESIAN_POINT('Ctrl Pts',(7.47577564638596,-28.4821412597061,
125.689518808267));
#115188=CARTESIAN_POINT('Ctrl Pts',(7.47204379419599,-28.457761504673,125.633106038967));
#115189=CARTESIAN_POINT('Ctrl Pts',(7.46828914249572,-28.4365600390074,
125.575509763924));
#115190=CARTESIAN_POINT('Origin',(5.,-30.,125.));
#115191=CARTESIAN_POINT('',(6.7689357756443,-28.4365600093868,125.575509683456));
#115192=CARTESIAN_POINT('',(6.96167308954663,-28.4365599688247,125.575509573264));
#115193=CARTESIAN_POINT('',(5.,-28.4365599837785,125.575509613888));
#115194=CARTESIAN_POINT('Ctrl Pts',(6.96167308954662,-28.4365599688247,
125.575509573264));
#115195=CARTESIAN_POINT('Ctrl Pts',(6.96619326604114,-28.461605418403,125.643548508303));
#115196=CARTESIAN_POINT('Ctrl Pts',(6.97060995840626,-28.49107241895,125.709898686597));
#115197=CARTESIAN_POINT('Ctrl Pts',(6.98041879830601,-28.5656959162624,
125.852103833634));
#115198=CARTESIAN_POINT('Ctrl Pts',(6.98580004343452,-28.6127230432211,
125.926697481698));
#115199=CARTESIAN_POINT('Ctrl Pts',(6.99272049307737,-28.6769792923376,
126.012692150223));
#115200=CARTESIAN_POINT('Ctrl Pts',(6.99397967804428,-28.6888101283685,
126.027964117312));
#115201=CARTESIAN_POINT('Ctrl Pts',(6.99579915129659,-28.7060493096574,
126.049435646233));
#115202=CARTESIAN_POINT('Ctrl Pts',(6.99634536729574,-28.7112426605574,
126.05580683728));
#115203=CARTESIAN_POINT('Ctrl Pts',(6.9972997737851,-28.7203432178703,126.066804192495));
#115204=CARTESIAN_POINT('Ctrl Pts',(6.9977064329797,-28.7242288438188,126.071447908622));
#115205=CARTESIAN_POINT('Ctrl Pts',(6.99858396809871,-28.7326292603818,
126.081376770711));
#115206=CARTESIAN_POINT('Ctrl Pts',(6.99905536960203,-28.737151767051,126.086654797074));
#115207=CARTESIAN_POINT('Ctrl Pts',(7.00036573562785,-28.7497539111416,
126.101177305723));
#115208=CARTESIAN_POINT('Ctrl Pts',(7.00120944724854,-28.7579027283144,
126.110360791321));
#115209=CARTESIAN_POINT('Ctrl Pts',(7.00711659039268,-28.8152430606139,
126.173560633232));
#115210=CARTESIAN_POINT('Ctrl Pts',(7.01238145257386,-28.8678349230907,
126.224374713504));
#115211=CARTESIAN_POINT('Ctrl Pts',(7.01866721911848,-28.933874431748,126.280278891081));
#115212=CARTESIAN_POINT('Ctrl Pts',(7.01964797433931,-28.9442698815991,
126.288864492452));
#115213=CARTESIAN_POINT('Ctrl Pts',(7.02603794076691,-29.0126394783319,
126.343948747429));
#115214=CARTESIAN_POINT('Ctrl Pts',(7.03144851220877,-29.0735692764677,
126.386652977837));
#115215=CARTESIAN_POINT('Ctrl Pts',(7.0397952601921,-29.1736113126269,126.447223022306));
#115216=CARTESIAN_POINT('Ctrl Pts',(7.0428007017934,-29.210908576136,126.467892356308));
#115217=CARTESIAN_POINT('Ctrl Pts',(7.04788795810297,-29.2763309864504,
126.500932839584));
#115218=CARTESIAN_POINT('Ctrl Pts',(7.04999141354889,-29.304079488496,126.513998377334));
#115219=CARTESIAN_POINT('Ctrl Pts',(7.05301658893146,-29.3449925089903,
126.531899782452));
#115220=CARTESIAN_POINT('Ctrl Pts',(7.05395885418,-29.3578809947853,126.537346727527));
#115221=CARTESIAN_POINT('Ctrl Pts',(7.05561489945898,-29.3807845566007,
126.546687961624));
#115222=CARTESIAN_POINT('Ctrl Pts',(7.05633089303632,-29.3907714001008,
126.550648876547));
#115223=CARTESIAN_POINT('Ctrl Pts',(7.05782807308561,-29.4118281901591,
126.558765445241));
#115224=CARTESIAN_POINT('Ctrl Pts',(7.05860853541367,-29.4229055041951,
126.562900427479));
#115225=CARTESIAN_POINT('Ctrl Pts',(7.06067165743154,-29.4524474931904,
126.573571057137));
#115226=CARTESIAN_POINT('Ctrl Pts',(7.06194745217296,-29.4709853442732,
126.579899732921));
#115227=CARTESIAN_POINT('Ctrl Pts',(7.06853355814901,-29.5679949117098,
126.611119011648));
#115228=CARTESIAN_POINT('Ctrl Pts',(7.07366172258311,-29.6481250676711,
126.630496663849));
#115229=CARTESIAN_POINT('Ctrl Pts',(7.08488649056641,-29.8284384768893,
126.660181791797));
#115230=CARTESIAN_POINT('Ctrl Pts',(7.09092319526859,-29.9287736694686,
126.667501543961));
#115231=CARTESIAN_POINT('Ctrl Pts',(7.09899127111867,-30.0574534116637,
126.665249653017));
#115232=CARTESIAN_POINT('Ctrl Pts',(7.10078575072611,-30.0857375596243,
126.664033110103));
#115233=CARTESIAN_POINT('Ctrl Pts',(7.10385577202603,-30.1332479948339,
126.660775166727));
#115234=CARTESIAN_POINT('Ctrl Pts',(7.10511495455522,-30.1524952218776,
126.659118534576));
#115235=CARTESIAN_POINT('Ctrl Pts',(7.10693442489503,-30.1798842568459,
126.656280537426));
#115236=CARTESIAN_POINT('Ctrl Pts',(7.10748064048046,-30.1880536526125,
126.655372882842));
#115237=CARTESIAN_POINT('Ctrl Pts',(7.10843504650317,-30.2022288180361,
126.653691679341));
#115238=CARTESIAN_POINT('Ctrl Pts',(7.10884170564949,-30.2082376293783,
126.652945780579));
#115239=CARTESIAN_POINT('Ctrl Pts',(7.10971924096942,-30.221135385906,126.651273282356));
#115240=CARTESIAN_POINT('Ctrl Pts',(7.11019064272452,-30.2280225345039,
126.650336338834));
#115241=CARTESIAN_POINT('Ctrl Pts',(7.11150101011798,-30.2470584964309,
126.647625212566));
#115242=CARTESIAN_POINT('Ctrl Pts',(7.1123447228701,-30.2591935843518,126.645759826177));
#115243=CARTESIAN_POINT('Ctrl Pts',(7.11825216250102,-30.3433940836757,
126.631862338454));
#115244=CARTESIAN_POINT('Ctrl Pts',(7.12351734343573,-30.4146132440537,
126.615236106916));
#115245=CARTESIAN_POINT('Ctrl Pts',(7.12985706691742,-30.498108591718,126.589857242714));
#115246=CARTESIAN_POINT('Ctrl Pts',(7.13089161018272,-30.5116608441542,
126.58554766501));
#115247=CARTESIAN_POINT('Ctrl Pts',(7.13728951150637,-30.5950835079316,
126.557838541981));
#115248=CARTESIAN_POINT('Ctrl Pts',(7.14265284876418,-30.6633973025621,
126.529996938432));
#115249=CARTESIAN_POINT('Ctrl Pts',(7.15094946853164,-30.7679086970577,
126.479082041508));
#115250=CARTESIAN_POINT('Ctrl Pts',(7.15395036909879,-30.8054449652055,
126.458981276297));
#115251=CARTESIAN_POINT('Ctrl Pts',(7.15903088243546,-30.8686017285939,
126.421979352316));
#115252=CARTESIAN_POINT('Ctrl Pts',(7.16113205814459,-30.8945999687192,
126.405768598104));
#115253=CARTESIAN_POINT('Ctrl Pts',(7.16415461381213,-30.9317970226308,
126.381124870327));
#115254=CARTESIAN_POINT('Ctrl Pts',(7.16509648884991,-30.9433586433093,
126.373253832919));
#115255=CARTESIAN_POINT('Ctrl Pts',(7.16675209401653,-30.9636232207307,
126.359081192915));
#115256=CARTESIAN_POINT('Ctrl Pts',(7.1674680337163,-30.9723667688724,126.35283933878));
#115257=CARTESIAN_POINT('Ctrl Pts',(7.16896534069072,-30.9906077675845,
126.339549218365));
#115258=CARTESIAN_POINT('Ctrl Pts',(7.16974598151359,-31.0000918031732,
126.332483491451));
#115259=CARTESIAN_POINT('Ctrl Pts',(7.17181013579085,-31.0250915219491,
126.313441094717));
#115260=CARTESIAN_POINT('Ctrl Pts',(7.17308677172273,-31.0404727551062,
126.301290373489));
#115261=CARTESIAN_POINT('Ctrl Pts',(7.17967257876229,-31.119311036206,126.236718671754));
#115262=CARTESIAN_POINT('Ctrl Pts',(7.18479971111164,-31.179037516089,126.179916639213));
#115263=CARTESIAN_POINT('Ctrl Pts',(7.19602299766147,-31.301754702461,126.044542998536));
#115264=CARTESIAN_POINT('Ctrl Pts',(7.20205925630102,-31.3623170540397,
125.964222628287));
#115265=CARTESIAN_POINT('Ctrl Pts',(7.21012679584731,-31.4302114809766,
125.854899038405));
#115266=CARTESIAN_POINT('Ctrl Pts',(7.21192121591318,-31.4445291713042,
125.830477295724));
#115267=CARTESIAN_POINT('Ctrl Pts',(7.21499114563072,-31.4675592278534,
125.788795966392));
#115268=CARTESIAN_POINT('Ctrl Pts',(7.21625029738875,-31.4766061834217,
125.771727455041));
#115269=CARTESIAN_POINT('Ctrl Pts',(7.21806973095802,-31.4890764227335,
125.747178004529));
#115270=CARTESIAN_POINT('Ctrl Pts',(7.21861594131848,-31.4927446113176,
125.739822331082));
#115271=CARTESIAN_POINT('Ctrl Pts',(7.219570341449,-31.4990202169218,125.727001412862));
#115272=CARTESIAN_POINT('Ctrl Pts',(7.2199769999868,-31.5016525127705,125.721548608612));
#115273=CARTESIAN_POINT('Ctrl Pts',(7.22085453784462,-31.5072426669158,
125.709805505463));
#115274=CARTESIAN_POINT('Ctrl Pts',(7.22132594278407,-31.5101908596986,
125.703511105409));
#115275=CARTESIAN_POINT('Ctrl Pts',(7.22263632745684,-31.5182376458712,
125.686047518329));
#115276=CARTESIAN_POINT('Ctrl Pts',(7.2234800544977,-31.5232521673389,125.674840395447));
#115277=CARTESIAN_POINT('Ctrl Pts',(7.22939124540841,-31.5572651286404,
125.596512693993));
#115278=CARTESIAN_POINT('Ctrl Pts',(7.23466045948267,-31.581938280695,125.527608739796));
#115279=CARTESIAN_POINT('Ctrl Pts',(7.24100152105412,-31.6058978594324,
125.443676965507));
#115280=CARTESIAN_POINT('Ctrl Pts',(7.24203341270642,-31.6096169901336,
125.429988750864));
#115281=CARTESIAN_POINT('Ctrl Pts',(7.24842908470747,-31.6315724094788,
125.344902346293));
#115282=CARTESIAN_POINT('Ctrl Pts',(7.25379281108063,-31.6452307940476,
125.272402458721));
#115283=CARTESIAN_POINT('Ctrl Pts',(7.26208879086746,-31.6591324128804,
125.156990316707));
#115284=CARTESIAN_POINT('Ctrl Pts',(7.26508872035481,-31.662600834382,125.114565667326));
#115285=CARTESIAN_POINT('Ctrl Pts',(7.27016779150484,-31.6657656411109,
125.04145654363));
#115286=CARTESIAN_POINT('Ctrl Pts',(7.27226847948869,-31.6662463085384,
125.01082909845));
#115287=CARTESIAN_POINT('Ctrl Pts',(7.27529047464868,-31.6657162157421,
124.966220514559));
#115288=CARTESIAN_POINT('Ctrl Pts',(7.27623226616479,-31.6653739834145,
124.952239335256));
#115289=CARTESIAN_POINT('Ctrl Pts',(7.27788777714381,-31.664457666796,124.927528815414));
#115290=CARTESIAN_POINT('Ctrl Pts',(7.27860370532655,-31.6639557676617,
124.916797778223));
#115291=CARTESIAN_POINT('Ctrl Pts',(7.28010103954658,-31.6626833165531,
124.894264193733));
#115292=CARTESIAN_POINT('Ctrl Pts',(7.28088171863763,-31.6618908035528,
124.882463447901));
#115293=CARTESIAN_POINT('Ctrl Pts',(7.28294609422568,-31.6594509950476,
124.851128767655));
#115294=CARTESIAN_POINT('Ctrl Pts',(7.28422291050307,-31.6575844636793,
124.831613399686));
#115295=CARTESIAN_POINT('Ctrl Pts',(7.29081479276253,-31.6460823826263,
124.730262817037));
#115296=CARTESIAN_POINT('Ctrl Pts',(7.29594737289473,-31.6307294451463,
124.649187639915));
#115297=CARTESIAN_POINT('Ctrl Pts',(7.30717101264205,-31.5835197207545,
124.47266269227));
#115298=CARTESIAN_POINT('Ctrl Pts',(7.31320267380424,-31.5489039131112,
124.378297769228));
#115299=CARTESIAN_POINT('Ctrl Pts',(7.32126468549303,-31.4939147787945,
124.262046538924));
#115300=CARTESIAN_POINT('Ctrl Pts',(7.32305849152792,-31.4811663901989,
124.236781406804));
#115301=CARTESIAN_POINT('Ctrl Pts',(7.32612747677053,-31.4586453461783,
124.194839938157));
#115302=CARTESIAN_POINT('Ctrl Pts',(7.32738631117671,-31.4492143872971,
124.177986281896));
#115303=CARTESIAN_POINT('Ctrl Pts',(7.32920536552759,-31.4353555740465,
124.154199831174));
#115304=CARTESIAN_POINT('Ctrl Pts',(7.32975152200273,-31.4311656482883,
124.147129300723));
#115305=CARTESIAN_POINT('Ctrl Pts',(7.33070586137993,-31.4237983543817,
124.134904103676));
#115306=CARTESIAN_POINT('Ctrl Pts',(7.33111251365515,-31.4206449218808,
124.129735288336));
#115307=CARTESIAN_POINT('Ctrl Pts',(7.33199007775181,-31.4138107125555,
124.118669421745));
#115308=CARTESIAN_POINT('Ctrl Pts',(7.33246151557791,-31.4101212419726,
124.11277827031));
#115309=CARTESIAN_POINT('Ctrl Pts',(7.33377207864045,-31.3998121816725,
124.096544049527));
#115310=CARTESIAN_POINT('Ctrl Pts',(7.33461595318881,-31.3931150888306,
124.086251059891));
#115311=CARTESIAN_POINT('Ctrl Pts',(7.34056679290618,-31.3454380539383,
124.014717178169));
#115312=CARTESIAN_POINT('Ctrl Pts',(7.34587865060716,-31.3005523478014,
123.956186328974));
#115313=CARTESIAN_POINT('Ctrl Pts',(7.35215028781879,-31.2436017988192,
123.891320361461));
#115314=CARTESIAN_POINT('Ctrl Pts',(7.35307038129763,-31.2351490313212,
123.881911075728));
#115315=CARTESIAN_POINT('Ctrl Pts',(7.35947775295334,-31.1755717840124,
123.817092209638));
#115316=CARTESIAN_POINT('Ctrl Pts',(7.36496666235236,-31.1208413238072,
123.765108914887));
#115317=CARTESIAN_POINT('Ctrl Pts',(7.37335111413028,-31.0303287238141,
123.690132118193));
#115318=CARTESIAN_POINT('Ctrl Pts',(7.37632065589549,-30.9968724566929,
123.6644937505));
#115319=CARTESIAN_POINT('Ctrl Pts',(7.38135455556256,-30.9376591394278,
123.622583627847));
#115320=CARTESIAN_POINT('Ctrl Pts',(7.38343994298495,-30.9123631164856,
123.605699359097));
#115321=CARTESIAN_POINT('Ctrl Pts',(7.38644434586241,-30.8748101400577,
123.582093895129));
#115322=CARTESIAN_POINT('Ctrl Pts',(7.38738351006768,-30.8629096404324,
123.574820195075));
#115323=CARTESIAN_POINT('Ctrl Pts',(7.38903606105674,-30.8416875795425,
123.56221235493));
#115324=CARTESIAN_POINT('Ctrl Pts',(7.3897516298043,-30.8324032894817,123.556817382723));
#115325=CARTESIAN_POINT('Ctrl Pts',(7.39124983564941,-30.8127680189271,
123.545660124952));
#115326=CARTESIAN_POINT('Ctrl Pts',(7.39203173014164,-30.8024063961036,
123.53991770354));
#115327=CARTESIAN_POINT('Ctrl Pts',(7.39410313441399,-30.7746592887629,
123.52492482474));
#115328=CARTESIAN_POINT('Ctrl Pts',(7.39538567809875,-30.7571692211627,
123.515871093816));
#115329=CARTESIAN_POINT('Ctrl Pts',(7.40221086126839,-30.6625199597613,
123.468984768642));
#115330=CARTESIAN_POINT('Ctrl Pts',(7.40755326618122,-30.5826772649763,
123.436852453945));
#115331=CARTESIAN_POINT('Ctrl Pts',(7.41879401586944,-30.407923474442,123.381785807161));
#115332=CARTESIAN_POINT('Ctrl Pts',(7.42465069980157,-30.3127680694217,
123.360734124953));
#115333=CARTESIAN_POINT('Ctrl Pts',(7.4325019441944,-30.1886570919505,123.344480978544));
#115334=CARTESIAN_POINT('Ctrl Pts',(7.43427189498057,-30.160902477878,123.341553453677));
#115335=CARTESIAN_POINT('Ctrl Pts',(7.43730415572979,-30.1140320690139,
123.337797187808));
#115336=CARTESIAN_POINT('Ctrl Pts',(7.43855062547048,-30.0949511785318,
123.336598154541));
#115337=CARTESIAN_POINT('Ctrl Pts',(7.44035489873692,-30.0676770247961,
123.335355041839));
#115338=CARTESIAN_POINT('Ctrl Pts',(7.44089894804567,-30.0594967343944,
123.335042598718));
#115339=CARTESIAN_POINT('Ctrl Pts',(7.44185091585677,-30.0452665246496,
123.334604084087));
#115340=CARTESIAN_POINT('Ctrl Pts',(7.44225732740366,-30.0392176863733,
123.33445066519));
#115341=CARTESIAN_POINT('Ctrl Pts',(7.44313593620846,-30.0261995315224,
123.334191438699));
#115342=CARTESIAN_POINT('Ctrl Pts',(7.44360867468025,-30.0192304516878,
123.334096412261));
#115343=CARTESIAN_POINT('Ctrl Pts',(7.44492630011381,-29.9998981815117,
123.333954130075));
#115344=CARTESIAN_POINT('Ctrl Pts',(7.44577601603251,-29.9875350422296,
123.334000764306));
#115345=CARTESIAN_POINT('Ctrl Pts',(7.45228787447881,-29.8934910367533,
123.335402320559));
#115346=CARTESIAN_POINT('Ctrl Pts',(7.4582008533018,-29.8120168919971,123.342625867577));
#115347=CARTESIAN_POINT('Ctrl Pts',(7.46848348868089,-29.6725219105499,
123.365413023157));
#115348=CARTESIAN_POINT('Ctrl Pts',(7.47283385869959,-29.614190015485,123.378190028458));
#115349=CARTESIAN_POINT('Ctrl Pts',(7.48102255727653,-29.5046100153875,
123.408440596109));
#115350=CARTESIAN_POINT('Ctrl Pts',(7.48486584250961,-29.4532776781101,
123.425335522503));
#115351=CARTESIAN_POINT('Ctrl Pts',(7.49036700591859,-29.3797193267496,
123.453577703023));
#115352=CARTESIAN_POINT('Ctrl Pts',(7.49208145596446,-29.3567861375947,
123.46297492795));
#115353=CARTESIAN_POINT('Ctrl Pts',(7.49517316506172,-29.3154207105719,
123.48101312359));
#115354=CARTESIAN_POINT('Ctrl Pts',(7.49655559460631,-29.2969212194321,
123.4894867673));
#115355=CARTESIAN_POINT('Ctrl Pts',(7.49873391844987,-29.2677782856679,
123.503487057141));
#115356=CARTESIAN_POINT('Ctrl Pts',(7.49953730276435,-29.2570317907059,
123.508793146455));
#115357=CARTESIAN_POINT('Ctrl Pts',(7.50105082283565,-29.2367939691114,
123.519058675857));
#115358=CARTESIAN_POINT('Ctrl Pts',(7.50176173486675,-29.2272914329899,
123.523994535665));
#115359=CARTESIAN_POINT('Ctrl Pts',(7.50337431742757,-29.2057491287152,
123.535449222082));
#115360=CARTESIAN_POINT('Ctrl Pts',(7.50427390254093,-29.1937407040056,
123.542025585331));
#115361=CARTESIAN_POINT('Ctrl Pts',(7.50662277965274,-29.162424195563,123.559681196279));
#115362=CARTESIAN_POINT('Ctrl Pts',(7.50806348355918,-29.1432543395918,
123.571000898366));
#115363=CARTESIAN_POINT('Ctrl Pts',(7.51904980360839,-28.997596454177,123.660996236589));
#115364=CARTESIAN_POINT('Ctrl Pts',(7.52792892745521,-28.8819547580372,
123.755926061958));
#115365=CARTESIAN_POINT('Ctrl Pts',(7.54078984904522,-28.7398984062878,
123.908557759468));
#115366=CARTESIAN_POINT('Ctrl Pts',(7.54451308157894,-28.7016979975512,
123.954288467086));
#115367=CARTESIAN_POINT('Ctrl Pts',(7.54935985009843,-28.6569998292364,
124.014031528025));
#115368=CARTESIAN_POINT('Ctrl Pts',(7.55034822099687,-28.6481329918666,
124.026224440762));
#115369=CARTESIAN_POINT('Ctrl Pts',(7.55184114426868,-28.6351320442016,
124.044622059117));
#115370=CARTESIAN_POINT('Ctrl Pts',(7.55233763938041,-28.6308718612701,
124.05073729605));
#115371=CARTESIAN_POINT('Ctrl Pts',(7.55323909002869,-28.6232544544476,
124.061829576595));
#115372=CARTESIAN_POINT('Ctrl Pts',(7.55364307773244,-28.6198829069617,
124.066796460053));
#115373=CARTESIAN_POINT('Ctrl Pts',(7.55455858030701,-28.6123374276834,
124.078042607479));
#115374=CARTESIAN_POINT('Ctrl Pts',(7.55507108010478,-28.6081792649811,
124.084332001072));
#115375=CARTESIAN_POINT('Ctrl Pts',(7.55664676956547,-28.5955908428902,
124.103656371831));
#115376=CARTESIAN_POINT('Ctrl Pts',(7.55771831451886,-28.5873002316814,
124.116780717));
#115377=CARTESIAN_POINT('Ctrl Pts',(7.56600866908977,-28.5251211143859,
124.218328180392));
#115378=CARTESIAN_POINT('Ctrl Pts',(7.57359506488849,-28.4794031811977,
124.311479489786));
#115379=CARTESIAN_POINT('Ctrl Pts',(7.58919660152276,-28.4031904057528,
124.512060742581));
#115380=CARTESIAN_POINT('Ctrl Pts',(7.59715701738913,-28.3742206318665,
124.61955899875));
#115381=CARTESIAN_POINT('Ctrl Pts',(7.60619182603659,-28.352793720861,124.749606347116));
#115382=CARTESIAN_POINT('Ctrl Pts',(7.60760061138425,-28.3498062521622,
124.77011705312));
#115383=CARTESIAN_POINT('Ctrl Pts',(7.60981047905332,-28.3456863192798,
124.802648026804));
#115384=CARTESIAN_POINT('Ctrl Pts',(7.61061942888788,-28.3443005084163,
124.814633437821));
#115385=CARTESIAN_POINT('Ctrl Pts',(7.61213767996794,-28.3419321814745,
124.837268737546));
#115386=CARTESIAN_POINT('Ctrl Pts',(7.61284781990361,-28.3409217848343,
124.847915024808));
#115387=CARTESIAN_POINT('Ctrl Pts',(7.61445094883416,-28.3388631484173,
124.872077651338));
#115388=CARTESIAN_POINT('Ctrl Pts',(7.61534194689051,-28.3378772261518,
124.885598646541));
#115389=CARTESIAN_POINT('Ctrl Pts',(7.61765231313363,-28.3357369428939,
124.920883550426));
#115390=CARTESIAN_POINT('Ctrl Pts',(7.61906355764825,-28.3348443731604,
124.942661143777));
#115391=CARTESIAN_POINT('Ctrl Pts',(7.62983741626248,-28.3312639782071,
125.110416882985));
#115392=CARTESIAN_POINT('Ctrl Pts',(7.6385608707445,-28.3473477973736,125.256153014513));
#115393=CARTESIAN_POINT('Ctrl Pts',(7.65040919414744,-28.3933123002938,
125.443019724587));
#115394=CARTESIAN_POINT('Ctrl Pts',(7.65329581305405,-28.4062818674135,
125.487620514038));
#115395=CARTESIAN_POINT('Ctrl Pts',(7.65724268492099,-28.4260463842847,
125.546321056607));
#115396=CARTESIAN_POINT('Ctrl Pts',(7.65823906327717,-28.4312016068929,
125.56095294855));
#115397=CARTESIAN_POINT('Ctrl Pts',(7.65924494691568,-28.4365599837121,
125.575509613707));
#115398=CARTESIAN_POINT('',(7.42925547773031,-28.3340002666303,125.00126447839));
#115399=CARTESIAN_POINT('Ctrl Pts',(7.46828914249572,-28.4365600390074,
125.575509763924));
#115400=CARTESIAN_POINT('Ctrl Pts',(7.46566403364243,-28.4217367851707,
125.535240651473));
#115401=CARTESIAN_POINT('Ctrl Pts',(7.46302721323805,-28.4084671937405,
125.4943930358));
#115402=CARTESIAN_POINT('Ctrl Pts',(7.45746219409187,-28.3842248370625,
125.408607547837));
#115403=CARTESIAN_POINT('Ctrl Pts',(7.45453113574382,-28.3735189901549,
125.363659456007));
#115404=CARTESIAN_POINT('Ctrl Pts',(7.45075731402903,-28.3625047376426,
125.307077621908));
#115405=CARTESIAN_POINT('Ctrl Pts',(7.45000126478169,-28.3604307183729,
125.295803909537));
#115406=CARTESIAN_POINT('Ctrl Pts',(7.44879320517343,-28.3573287892267,
125.277906829833));
#115407=CARTESIAN_POINT('Ctrl Pts',(7.44834534534316,-28.3562241901259,
125.271296877405));
#115408=CARTESIAN_POINT('Ctrl Pts',(7.44748341995341,-28.3541855607317,
125.258627946203));
#115409=CARTESIAN_POINT('Ctrl Pts',(7.44706971401807,-28.3532450518384,
125.252570225264));
#115410=CARTESIAN_POINT('Ctrl Pts',(7.44623518833265,-28.3514234566647,
125.240394645433));
#115411=CARTESIAN_POINT('Ctrl Pts',(7.44581434796839,-28.3505429368899,
125.234276756687));
#115412=CARTESIAN_POINT('Ctrl Pts',(7.4448067979077,-28.3485247804576,125.219678865607));
#115413=CARTESIAN_POINT('Ctrl Pts',(7.44421850973425,-28.3474183988451,
125.211194812517));
#115414=CARTESIAN_POINT('Ctrl Pts',(7.44213373575981,-28.343748285315,125.181254517956));
#115415=CARTESIAN_POINT('Ctrl Pts',(7.44062121653562,-28.341536808702,125.159758208545));
#115416=CARTESIAN_POINT('Ctrl Pts',(7.4358635283949,-28.3359510074493,125.092666290553));
#115417=CARTESIAN_POINT('Ctrl Pts',(7.43257070150379,-28.3340351188065,
125.046972984103));
#115418=CARTESIAN_POINT('Ctrl Pts',(7.42925570628143,-28.3340004783878,
125.001262532282));
#115419=CARTESIAN_POINT('Ctrl Pts',(7.42925584547015,-28.3340004798433,
125.001264451555));
#115420=CARTESIAN_POINT('Ctrl Pts',(7.41937356250201,-28.3338970568045,
124.864997678517));
#115421=CARTESIAN_POINT('Ctrl Pts',(7.40939540494581,-28.3505132779832,
124.729197461488));
#115422=CARTESIAN_POINT('Ctrl Pts',(7.39773132741014,-28.3911308944978,
124.566304272887));
#115423=CARTESIAN_POINT('Ctrl Pts',(7.39556511349714,-28.3996344491601,
124.535907207785));
#115424=CARTESIAN_POINT('Ctrl Pts',(7.39246814011792,-28.4131923344622,
124.492262430278));
#115425=CARTESIAN_POINT('Ctrl Pts',(7.3915154280401,-28.4175596931546,124.478810299596));
#115426=CARTESIAN_POINT('Ctrl Pts',(7.38984774049602,-28.4255507270181,
124.455223648547));
#115427=CARTESIAN_POINT('Ctrl Pts',(7.38913044314721,-28.4291022414426,
124.445065744617));
#115428=CARTESIAN_POINT('Ctrl Pts',(7.3876370005742,-28.4367355615591,124.42389389732));
#115429=CARTESIAN_POINT('Ctrl Pts',(7.38686151707715,-28.4408359388719,
124.412887243857));
#115430=CARTESIAN_POINT('Ctrl Pts',(7.38482643944949,-28.4519554683061,
124.383977367569));
#115431=CARTESIAN_POINT('Ctrl Pts',(7.38357337554834,-28.4591689007725,
124.366150389133));
#115432=CARTESIAN_POINT('Ctrl Pts',(7.37751434511364,-28.4958143138997,
124.279911516966));
#115433=CARTESIAN_POINT('Ctrl Pts',(7.37285459654274,-28.5295037414308,
124.213396714037));
#115434=CARTESIAN_POINT('Ctrl Pts',(7.36165100731372,-28.6223364616383,
124.057069095073));
#115435=CARTESIAN_POINT('Ctrl Pts',(7.35521642813294,-28.6859235125185,
123.9703029597));
#115436=CARTESIAN_POINT('Ctrl Pts',(7.34666551916549,-28.7768993101918,
123.868436096094));
#115437=CARTESIAN_POINT('Ctrl Pts',(7.34481288550097,-28.7969603816424,
123.847130689847));
#115438=CARTESIAN_POINT('Ctrl Pts',(7.34167301274474,-28.8312979142142,
123.812535837829));
#115439=CARTESIAN_POINT('Ctrl Pts',(7.34040383027099,-28.8452658892386,
123.798948479201));
#115440=CARTESIAN_POINT('Ctrl Pts',(7.33859563195503,-28.8652266594629,
123.780201707463));
#115441=CARTESIAN_POINT('Ctrl Pts',(7.33807115532862,-28.8710233718836,
123.77483463326));
#115442=CARTESIAN_POINT('Ctrl Pts',(7.33753990228832,-28.8768990011261,
123.769471597473));
#115443=CARTESIAN_POINT('Ctrl Pts',(7.3375361850848,-28.8769401133886,123.769434075646));
#115444=CARTESIAN_POINT('Ctrl Pts',(7.33752867773757,-28.8770231450277,
123.769358302991));
#115445=CARTESIAN_POINT('Ctrl Pts',(7.33752488757879,-28.8770650645789,
123.769320052154));
#115446=CARTESIAN_POINT('Ctrl Pts',(7.3375172304766,-28.8771497533367,123.769242783113));
#115447=CARTESIAN_POINT('Ctrl Pts',(7.33751336352829,-28.8771925226056,
123.769203765013));
#115448=CARTESIAN_POINT('Ctrl Pts',(7.3375055487759,-28.8772789558496,123.769124920833));
#115449=CARTESIAN_POINT('Ctrl Pts',(7.33750160096349,-28.8773226199255,
123.769085094833));
#115450=CARTESIAN_POINT('Ctrl Pts',(7.33749362014911,-28.8774108907405,
123.769004591635));
#115451=CARTESIAN_POINT('Ctrl Pts',(7.33748958715301,-28.877455497424,123.768963914672));
#115452=CARTESIAN_POINT('Ctrl Pts',(7.33748143137279,-28.8775457043416,
123.768881663703));
#115453=CARTESIAN_POINT('Ctrl Pts',(7.3374773085818,-28.8775913046616,123.768840089819));
#115454=CARTESIAN_POINT('Ctrl Pts',(7.33746896833499,-28.8776835528198,
123.768755996411));
#115455=CARTESIAN_POINT('Ctrl Pts',(7.33746475083882,-28.8777302011151,
123.768713476686));
#115456=CARTESIAN_POINT('Ctrl Pts',(7.33745621592777,-28.8778246033652,
123.768627439252));
#115457=CARTESIAN_POINT('Ctrl Pts',(7.33745189852428,-28.8778723572058,
123.76858392188));
#115458=CARTESIAN_POINT('Ctrl Pts',(7.3374431582116,-28.8779690323747,123.768495833515));
#115459=CARTESIAN_POINT('Ctrl Pts',(7.33743873528734,-28.8780179538823,
123.768451262609));
#115460=CARTESIAN_POINT('Ctrl Pts',(7.33742977795473,-28.8781170305464,
123.76836100766));
#115461=CARTESIAN_POINT('Ctrl Pts',(7.33742524354762,-28.8781671857026,
123.768315323888));
#115462=CARTESIAN_POINT('Ctrl Pts',(7.33741605686236,-28.8782688003468,
123.768222779652));
#115463=CARTESIAN_POINT('Ctrl Pts',(7.33741140455526,-28.8783202601695,
123.768175919176));
#115464=CARTESIAN_POINT('Ctrl Pts',(7.33740197519525,-28.8784245602297,
123.768080953143));
#115465=CARTESIAN_POINT('Ctrl Pts',(7.33739719814064,-28.8784774005015,
123.768032847873));
#115466=CARTESIAN_POINT('Ctrl Pts',(7.33738751191134,-28.8785845430714,
123.767935318925));
#115467=CARTESIAN_POINT('Ctrl Pts',(7.33738260271761,-28.8786388455971,
123.767885895386));
#115468=CARTESIAN_POINT('Ctrl Pts',(7.33737264427328,-28.878749000513,123.767785651012));
#115469=CARTESIAN_POINT('Ctrl Pts',(7.33736759501287,-28.8788048530301,
123.767734830439));
#115470=CARTESIAN_POINT('Ctrl Pts',(7.33735734788781,-28.8789182025261,
123.767631707072));
#115471=CARTESIAN_POINT('Ctrl Pts',(7.33735215000152,-28.8789756997641,
123.767579404456));
#115472=CARTESIAN_POINT('Ctrl Pts',(7.33734159640269,-28.879092440767,123.767473225416));
#115473=CARTESIAN_POINT('Ctrl Pts',(7.3373362406618,-28.8791516848669,123.767419349139));
#115474=CARTESIAN_POINT('Ctrl Pts',(7.33732536135549,-28.8792720302513,
123.767309923524));
#115475=CARTESIAN_POINT('Ctrl Pts',(7.3373198377936,-28.8793331315201,123.767254374694));
#115476=CARTESIAN_POINT('Ctrl Pts',(7.33730861205778,-28.8794573106368,
123.767141496935));
#115477=CARTESIAN_POINT('Ctrl Pts',(7.33730290984146,-28.8795203889788,
123.767084168099));
#115478=CARTESIAN_POINT('Ctrl Pts',(7.33729131506578,-28.8796486520813,
123.76696761398));
#115479=CARTESIAN_POINT('Ctrl Pts',(7.33728542249567,-28.8797138369881,
123.766908389161));
#115480=CARTESIAN_POINT('Ctrl Pts',(7.33727343427613,-28.8798464541867,
123.76678791682));
#115481=CARTESIAN_POINT('Ctrl Pts',(7.33726733858723,-28.8799138869453,
123.766726669533));
#115482=CARTESIAN_POINT('Ctrl Pts',(7.33725493025597,-28.8800511534114,
123.766602014789));
#115483=CARTESIAN_POINT('Ctrl Pts',(7.33724861758046,-28.8801209875185,
123.766538607698));
#115484=CARTESIAN_POINT('Ctrl Pts',(7.33723576012546,-28.8802632243746,
123.766409483308));
#115485=CARTESIAN_POINT('Ctrl Pts',(7.33722921531702,-28.8803356274802,
123.766343766493));
#115486=CARTESIAN_POINT('Ctrl Pts',(7.33721587703332,-28.8804831856614,
123.766209858723));
#115487=CARTESIAN_POINT('Ctrl Pts',(7.33720908352888,-28.8805583410998,
123.766141668336));
#115488=CARTESIAN_POINT('Ctrl Pts',(7.33719522971353,-28.8807116047312,
123.766002633983));
#115489=CARTESIAN_POINT('Ctrl Pts',(7.33718816935918,-28.8807897134486,
123.765931790541));
#115490=CARTESIAN_POINT('Ctrl Pts',(7.33717376191652,-28.8809491042154,
123.765787253071));
#115491=CARTESIAN_POINT('Ctrl Pts',(7.3371664147823,-28.8810303868209,123.765713559655));
#115492=CARTESIAN_POINT('Ctrl Pts',(7.33715141183802,-28.8811963682422,
123.765563105448));
#115493=CARTESIAN_POINT('Ctrl Pts',(7.33714375597763,-28.8812810676682,
123.765486345354));
#115494=CARTESIAN_POINT('Ctrl Pts',(7.33712811137022,-28.8814541507277,
123.765329518739));
#115495=CARTESIAN_POINT('Ctrl Pts',(7.3371201225614,-28.8815425351041,123.76524945295));
#115496=CARTESIAN_POINT('Ctrl Pts',(7.33710378526031,-28.8817232846925,
123.765085750537));
#115497=CARTESIAN_POINT('Ctrl Pts',(7.33709543670959,-28.8818156506169,
123.765002114852));
#115498=CARTESIAN_POINT('Ctrl Pts',(7.33707835020737,-28.8820046922629,
123.764830979631));
#115499=CARTESIAN_POINT('Ctrl Pts',(7.33706961217501,-28.8821013689524,
123.764743481011));
#115500=CARTESIAN_POINT('Ctrl Pts',(7.33705171364309,-28.88229939817,123.764564294126));
#115501=CARTESIAN_POINT('Ctrl Pts',(7.33704255305717,-28.8824007517355,
123.764472606958));
#115502=CARTESIAN_POINT('Ctrl Pts',(7.33663053392987,-28.8869594097029,
123.76034974194));
#115503=CARTESIAN_POINT('Ctrl Pts',(7.33622585682368,-28.8914382500251,
123.756342908708));
#115504=CARTESIAN_POINT('Ctrl Pts',(7.33529423576552,-28.9017526234754,
123.747215512634));
#115505=CARTESIAN_POINT('Ctrl Pts',(7.33476613887717,-28.9076023211805,
123.742111460775));
#115506=CARTESIAN_POINT('Ctrl Pts',(7.33313221068919,-28.9257165314535,
123.726527868962));
#115507=CARTESIAN_POINT('Ctrl Pts',(7.33201737203806,-28.9380973441982,
123.716185784042));
#115508=CARTESIAN_POINT('Ctrl Pts',(7.32524300079625,-29.0135665541961,
123.654982531475));
#115509=CARTESIAN_POINT('Ctrl Pts',(7.31936060053549,-29.0801418395196,
123.608604505391));
#115510=CARTESIAN_POINT('Ctrl Pts',(7.30809840553617,-29.2132134421988,
123.529640580684));
#115511=CARTESIAN_POINT('Ctrl Pts',(7.30273296111614,-29.2790383951908,
123.496269443176));
#115512=CARTESIAN_POINT('Ctrl Pts',(7.29443954209551,-29.3859518810057,
123.450707724317));
#115513=CARTESIAN_POINT('Ctrl Pts',(7.29144364339463,-29.4256686705819,
123.435549401915));
#115514=CARTESIAN_POINT('Ctrl Pts',(7.28637067906987,-29.4949032954147,
123.412117991926));
#115515=CARTESIAN_POINT('Ctrl Pts',(7.28427213274951,-29.5241482047487,
123.403110136906));
#115516=CARTESIAN_POINT('Ctrl Pts',(7.2812527744722,-29.5670919198683,123.391167523035));
#115517=CARTESIAN_POINT('Ctrl Pts',(7.28031152315644,-29.5806044218695,
123.38759226171));
#115518=CARTESIAN_POINT('Ctrl Pts',(7.27865680691216,-29.6045756792918,
123.38157146536));
#115519=CARTESIAN_POINT('Ctrl Pts',(7.27794113709066,-29.6150159289277,
123.379056265799));
#115520=CARTESIAN_POINT('Ctrl Pts',(7.27644419888003,-29.6370020031624,
123.373983924632));
#115521=CARTESIAN_POINT('Ctrl Pts',(7.27566365833539,-29.6485522407399,
123.371448401889));
#115522=CARTESIAN_POINT('Ctrl Pts',(7.27359932949598,-29.6793201674347,
123.365036774304));
#115523=CARTESIAN_POINT('Ctrl Pts',(7.27232242428435,-29.6985812996632,
123.361376454428));
#115524=CARTESIAN_POINT('Ctrl Pts',(7.26572003761559,-29.7992701004747,
123.344077448166));
#115525=CARTESIAN_POINT('Ctrl Pts',(7.26057783867157,-29.8815687264981,
123.336164517924));
#115526=CARTESIAN_POINT('Ctrl Pts',(7.24935299960241,-30.0642848271456,
123.332228919761));
#115527=CARTESIAN_POINT('Ctrl Pts',(7.24332891776974,-30.1644297034915,
123.339110646512));
#115528=CARTESIAN_POINT('Ctrl Pts',(7.2352760958641,-30.291265492037,123.359414721593));
#115529=CARTESIAN_POINT('Ctrl Pts',(7.23348340206691,-30.3190680616087,
123.364594535179));
#115530=CARTESIAN_POINT('Ctrl Pts',(7.23041619746381,-30.3656033433355,
123.374496147947));
#115531=CARTESIAN_POINT('Ctrl Pts',(7.22915800970899,-30.3844107486517,
123.378840885009));
#115532=CARTESIAN_POINT('Ctrl Pts',(7.22733982705669,-30.411108918281,123.385499162527));
#115533=CARTESIAN_POINT('Ctrl Pts',(7.22679388058043,-30.419065389015,123.387546065891));
#115534=CARTESIAN_POINT('Ctrl Pts',(7.22583988544353,-30.43285706367,123.391203119674));
#115535=CARTESIAN_POINT('Ctrl Pts',(7.22543336601706,-30.4386991592339,
123.392786359547));
#115536=CARTESIAN_POINT('Ctrl Pts',(7.22455607664872,-30.4512298385684,
123.396255655373));
#115537=CARTESIAN_POINT('Ctrl Pts',(7.22408478089844,-30.4579151878881,
123.398151703052));
#115538=CARTESIAN_POINT('Ctrl Pts',(7.22277460481303,-30.4763777855145,
123.403512944941));
#115539=CARTESIAN_POINT('Ctrl Pts',(7.22193097773102,-30.4881286172494,
123.407066497805));
#115540=CARTESIAN_POINT('Ctrl Pts',(7.21600304099805,-30.5698194900865,
123.432759272902));
#115541=CARTESIAN_POINT('Ctrl Pts',(7.21071563021698,-30.6382626970609,
123.459365035987));
#115542=CARTESIAN_POINT('Ctrl Pts',(7.2043685736538,-30.7174246406035,123.49631971207));
#115543=CARTESIAN_POINT('Ctrl Pts',(7.20334869084487,-30.7300519515729,
123.502409713044));
#115544=CARTESIAN_POINT('Ctrl Pts',(7.19696317027417,-30.8085877946221,
123.541515964453));
#115545=CARTESIAN_POINT('Ctrl Pts',(7.19159772852778,-30.8723254076313,
123.578719028349));
#115546=CARTESIAN_POINT('Ctrl Pts',(7.18330430391382,-30.9685899044678,
123.643830669137));
#115547=CARTESIAN_POINT('Ctrl Pts',(7.18030839739543,-31.0028661240677,
123.668977199263));
#115548=CARTESIAN_POINT('Ctrl Pts',(7.17523542145845,-31.0601023804654,
123.714435960794));
#115549=CARTESIAN_POINT('Ctrl Pts',(7.1731368712097,-31.0835317051256,123.734120379615));
#115550=CARTESIAN_POINT('Ctrl Pts',(7.17011750841782,-31.1168563945396,
123.763722062387));
#115551=CARTESIAN_POINT('Ctrl Pts',(7.16917625642977,-31.1271888306669,
123.773135416704));
#115552=CARTESIAN_POINT('Ctrl Pts',(7.16752153942846,-31.1452483215704,
123.790009257428));
#115553=CARTESIAN_POINT('Ctrl Pts',(7.16680586951508,-31.1530238678371,
123.797416412614));
#115554=CARTESIAN_POINT('Ctrl Pts',(7.16530893152689,-31.1692098174702,
123.813136812569));
#115555=CARTESIAN_POINT('Ctrl Pts',(7.16452839129268,-31.1776044514178,
123.821465490075));
#115556=CARTESIAN_POINT('Ctrl Pts',(7.16246406424493,-31.1996785387533,
123.843837508329));
#115557=CARTESIAN_POINT('Ctrl Pts',(7.16118716049282,-31.2132002642859,
123.858034381055));
#115558=CARTESIAN_POINT('Ctrl Pts',(7.15458482406676,-31.2823433796613,
123.93324448832));
#115559=CARTESIAN_POINT('Ctrl Pts',(7.14944267019436,-31.3336267731865,
123.998094823561));
#115560=CARTESIAN_POINT('Ctrl Pts',(7.13821783412521,-31.4360320549009,
124.149467822659));
#115561=CARTESIAN_POINT('Ctrl Pts',(7.13219371430047,-31.484565796549,124.237336837175));
#115562=CARTESIAN_POINT('Ctrl Pts',(7.12414084670429,-31.5362989646492,
124.354909976433));
#115563=CARTESIAN_POINT('Ctrl Pts',(7.1223481478214,-31.5470263291784,124.38107754618));
#115564=CARTESIAN_POINT('Ctrl Pts',(7.11928093539525,-31.5639466675181,
124.425544257186));
#115565=CARTESIAN_POINT('Ctrl Pts',(7.11802274501155,-31.5704969411154,
124.443701645393));
#115566=CARTESIAN_POINT('Ctrl Pts',(7.11620455921831,-31.5793831768821,
124.469743196566));
#115567=CARTESIAN_POINT('Ctrl Pts',(7.11565861229608,-31.5819787905467,
124.477537947534));
#115568=CARTESIAN_POINT('Ctrl Pts',(7.1147046166567,-31.5863864520248,124.491108396063));
#115569=CARTESIAN_POINT('Ctrl Pts',(7.11429809717877,-31.5882248464276,
124.496875288251));
#115570=CARTESIAN_POINT('Ctrl Pts',(7.11342080802908,-31.5921063296269,
124.509284476255));
#115571=CARTESIAN_POINT('Ctrl Pts',(7.11294951255185,-31.5941392697469,
124.515929473807));
#115572=CARTESIAN_POINT('Ctrl Pts',(7.1116393379471,-31.59964850111,124.534348430723));
#115573=CARTESIAN_POINT('Ctrl Pts',(7.11079571208955,-31.6030362313227,
124.546148118841));
#115574=CARTESIAN_POINT('Ctrl Pts',(7.10486810396721,-31.6257555532954,
124.62871044262));
#115575=CARTESIAN_POINT('Ctrl Pts',(7.09958104660358,-31.6405233864013,
124.700637864255));
#115576=CARTESIAN_POINT('Ctrl Pts',(7.09323408216949,-31.6524113279818,
124.787186876037));
#115577=CARTESIAN_POINT('Ctrl Pts',(7.09221394195506,-31.6541439652191,
124.801102133685));
#115578=CARTESIAN_POINT('Ctrl Pts',(7.08582818790081,-31.6638846674983,
124.888296515404));
#115579=CARTESIAN_POINT('Ctrl Pts',(7.0804627678863,-31.6671979128064,124.962022529068));
#115580=CARTESIAN_POINT('Ctrl Pts',(7.07216929790442,-31.6647055032124,
125.078213287153));
#115581=CARTESIAN_POINT('Ctrl Pts',(7.06917332793634,-31.6621690309992,
125.120649678821));
#115582=CARTESIAN_POINT('Ctrl Pts',(7.06410025774465,-31.6550199938247,
125.193392874174));
#115583=CARTESIAN_POINT('Ctrl Pts',(7.06200167560689,-31.6511894478119,
125.223753445864));
#115584=CARTESIAN_POINT('Ctrl Pts',(7.05898227616285,-31.6443938353568,
125.267806388092));
#115585=CARTESIAN_POINT('Ctrl Pts',(7.05804101871024,-31.6420892000036,
125.281592661778));
#115586=CARTESIAN_POINT('Ctrl Pts',(7.05638629554762,-31.6377075609206,
125.305917080741));
#115587=CARTESIAN_POINT('Ctrl Pts',(7.05567062488179,-31.6357016648871,
125.316467041181));
#115588=CARTESIAN_POINT('Ctrl Pts',(7.05417368868203,-31.6312729607665,
125.33859171503));
#115589=CARTESIAN_POINT('Ctrl Pts',(7.05339315095625,-31.6288286352117,
125.350161550237));
#115590=CARTESIAN_POINT('Ctrl Pts',(7.05132883841502,-31.6220051785355,
125.380840513879));
#115591=CARTESIAN_POINT('Ctrl Pts',(7.0500519464842,-31.6174115181461,125.399900399846));
#115592=CARTESIAN_POINT('Ctrl Pts',(7.04345001705135,-31.5917266271684,
125.498775696548));
#115593=CARTESIAN_POINT('Ctrl Pts',(7.03830822828367,-31.5650597775483,
125.577027929199));
#115594=CARTESIAN_POINT('Ctrl Pts',(7.02708341661256,-31.4934279498487,
125.745162450392));
#115595=CARTESIAN_POINT('Ctrl Pts',(7.02105898912504,-31.445926384267,125.833599824145));
#115596=CARTESIAN_POINT('Ctrl Pts',(7.01300575153124,-31.3752031879176,
125.940835733467));
#115597=CARTESIAN_POINT('Ctrl Pts',(7.01121301146626,-31.3590364583208,
125.964041186931));
#115598=CARTESIAN_POINT('Ctrl Pts',(7.00814573569051,-31.3308544565283,
126.002374684314));
#115599=CARTESIAN_POINT('Ctrl Pts',(7.00688752401667,-31.3191520825185,
126.017726042458));
#115600=CARTESIAN_POINT('Ctrl Pts',(7.0050693127822,-31.302092779623,126.039316068949));
#115601=CARTESIAN_POINT('Ctrl Pts',(7.00452336224373,-31.2969518038483,
126.045724394579));
#115602=CARTESIAN_POINT('Ctrl Pts',(7.00356936252713,-31.2879411982705,
126.056787636949));
#115603=CARTESIAN_POINT('Ctrl Pts',(7.00316284262883,-31.2840932562691,
126.061459913361));
#115604=CARTESIAN_POINT('Ctrl Pts',(7.00228555524054,-31.2757729511287,
126.071451196654));
#115605=CARTESIAN_POINT('Ctrl Pts',(7.00181426197055,-31.2712928142239,
126.076763142823));
#115606=CARTESIAN_POINT('Ctrl Pts',(7.00050409934027,-31.2588063705757,
126.091381339864));
#115607=CARTESIAN_POINT('Ctrl Pts',(6.99966048338448,-31.250730417711,126.10062714291));
#115608=CARTESIAN_POINT('Ctrl Pts',(6.99373552866349,-31.1937139035421,
126.164464929997));
#115609=CARTESIAN_POINT('Ctrl Pts',(6.98845132493557,-31.1413232049315,
126.215857893132));
#115610=CARTESIAN_POINT('Ctrl Pts',(6.98210511512545,-31.0750684962294,
126.272784801032));
#115611=CARTESIAN_POINT('Ctrl Pts',(6.98108290718335,-31.0642959778432,
126.2818063384));
#115612=CARTESIAN_POINT('Ctrl Pts',(6.97469528415801,-30.9963042459605,
126.337298509323));
#115613=CARTESIAN_POINT('Ctrl Pts',(6.96933004491224,-30.9361638930803,
126.380068089586));
#115614=CARTESIAN_POINT('Ctrl Pts',(6.96103620405767,-30.8371928219746,
126.440996362045));
#115615=CARTESIAN_POINT('Ctrl Pts',(6.95803971253382,-30.8001585946025,
126.461885447702));
#115616=CARTESIAN_POINT('Ctrl Pts',(6.95296586758419,-30.7351571617461,
126.495338142216));
#115617=CARTESIAN_POINT('Ctrl Pts',(6.95086702333251,-30.7075690942456,
126.508588214968));
#115618=CARTESIAN_POINT('Ctrl Pts',(6.94784732262703,-30.666868660664,126.526773576812));
#115619=CARTESIAN_POINT('Ctrl Pts',(6.94690602026148,-30.6540356781177,
126.532314823348));
#115620=CARTESIAN_POINT('Ctrl Pts',(6.9452512464592,-30.631222573742,126.541826637324));
#115621=CARTESIAN_POINT('Ctrl Pts',(6.94453556960922,-30.6212710976615,
126.545863367073));
#115622=CARTESIAN_POINT('Ctrl Pts',(6.94303864810687,-30.6002814658965,
126.554142199428));
#115623=CARTESIAN_POINT('Ctrl Pts',(6.94225813099632,-30.5892357413782,
126.558363586445));
#115624=CARTESIAN_POINT('Ctrl Pts',(6.94019393767106,-30.5597619733041,
126.569269501898));
#115625=CARTESIAN_POINT('Ctrl Pts',(6.93891714288803,-30.5412589630261,
126.575747131965));
#115626=CARTESIAN_POINT('Ctrl Pts',(6.93231854793044,-30.4443083444405,
126.607778791493));
#115627=CARTESIAN_POINT('Ctrl Pts',(6.92717975028263,-30.3641521168646,
126.627807810239));
#115628=CARTESIAN_POINT('Ctrl Pts',(6.91595513760539,-30.18405382767,126.658833050549));
#115629=CARTESIAN_POINT('Ctrl Pts',(6.90992818902548,-30.0839471097344,
126.666899348882));
#115630=CARTESIAN_POINT('Ctrl Pts',(6.90187191962886,-29.9554464691717,
126.66564431401));
#115631=CARTESIAN_POINT('Ctrl Pts',(6.9000788422117,-29.9271767683142,126.664647889031));
#115632=CARTESIAN_POINT('Ctrl Pts',(6.89701104750156,-29.8796779515927,
126.661761505974));
#115633=CARTESIAN_POINT('Ctrl Pts',(6.89575266143302,-29.8604309189347,
126.660255730827));
#115634=CARTESIAN_POINT('Ctrl Pts',(6.89393424180196,-29.8330366551162,
126.657632874581));
#115635=CARTESIAN_POINT('Ctrl Pts',(6.89338826164524,-29.8248640052282,
126.656789329324));
#115636=CARTESIAN_POINT('Ctrl Pts',(6.892434228536,-29.8106817515041,126.655219393704));
#115637=CARTESIAN_POINT('Ctrl Pts',(6.89202770519594,-29.8046693250667,
126.654520645563));
#115638=CARTESIAN_POINT('Ctrl Pts',(6.89115043223224,-29.7917627761054,
126.652949347267));
#115639=CARTESIAN_POINT('Ctrl Pts',(6.89067915704018,-29.7848703689007,
126.652066440391));
#115640=CARTESIAN_POINT('Ctrl Pts',(6.88936909248049,-29.7658181847186,
126.649504639765));
#115641=CARTESIAN_POINT('Ctrl Pts',(6.88852555761921,-29.7536714157406,
126.647734470626));
#115642=CARTESIAN_POINT('Ctrl Pts',(6.88262203406951,-29.6694203980064,
126.634504047185));
#115643=CARTESIAN_POINT('Ctrl Pts',(6.87736087397863,-29.598125213307,126.618450075721));
#115644=CARTESIAN_POINT('Ctrl Pts',(6.87107459106674,-29.5151362300872,
126.593940539202));
#115645=CARTESIAN_POINT('Ctrl Pts',(6.87008966013403,-29.50219848629,126.589947473144));
#115646=CARTESIAN_POINT('Ctrl Pts',(6.86362724625123,-29.417678652807,126.562728761375));
#115647=CARTESIAN_POINT('Ctrl Pts',(6.85814858885033,-29.347687078278,126.534831778095));
#115648=CARTESIAN_POINT('Ctrl Pts',(6.84977682634256,-29.2418592223927,
126.48409924935));
#115649=CARTESIAN_POINT('Ctrl Pts',(6.84681000740223,-29.2046011283282,
126.464468895143));
#115650=CARTESIAN_POINT('Ctrl Pts',(6.8417802780461,-29.1417982028294,126.428274802709));
#115651=CARTESIAN_POINT('Ctrl Pts',(6.83969638087453,-29.1158909670876,
126.412384743522));
#115652=CARTESIAN_POINT('Ctrl Pts',(6.83669386733622,-29.0787521044276,
126.388183216752));
#115653=CARTESIAN_POINT('Ctrl Pts',(6.8357551326363,-29.0671685556515,126.38042596517));
#115654=CARTESIAN_POINT('Ctrl Pts',(6.83410325132563,-29.0468403746469,
126.366439879747));
#115655=CARTESIAN_POINT('Ctrl Pts',(6.83338792544044,-29.0380561584206,
126.360270293465));
#115656=CARTESIAN_POINT('Ctrl Pts',(6.83189015047112,-29.0197067624715,
126.347115965969));
#115657=CARTESIAN_POINT('Ctrl Pts',(6.83110844423959,-29.0101551691849,
126.340113234175));
#115658=CARTESIAN_POINT('Ctrl Pts',(6.82903737442185,-28.9849243587417,
126.321198372519));
#115659=CARTESIAN_POINT('Ctrl Pts',(6.82775497627883,-28.9693799756157,
126.309108901373));
#115660=CARTESIAN_POINT('Ctrl Pts',(6.82092612384948,-28.8871211774187,
126.242759497642));
#115661=CARTESIAN_POINT('Ctrl Pts',(6.81558021507435,-28.8244652367482,
126.18366852511));
#115662=CARTESIAN_POINT('Ctrl Pts',(6.80433857306496,-28.7012775650826,
126.048012769568));
#115663=CARTESIAN_POINT('Ctrl Pts',(6.79848425521836,-28.6423411790938,
125.970448862313));
#115664=CARTESIAN_POINT('Ctrl Pts',(6.79063594300864,-28.5756346710899,
125.864591084913));
#115665=CARTESIAN_POINT('Ctrl Pts',(6.78886641990585,-28.5613571208815,
125.840619311241));
#115666=CARTESIAN_POINT('Ctrl Pts',(6.78583488723391,-28.5383237954122,
125.79963991741));
#115667=CARTESIAN_POINT('Ctrl Pts',(6.78458871081901,-28.529246546389,125.782818962133));
#115668=CARTESIAN_POINT('Ctrl Pts',(6.78278488693997,-28.5166990017146,
125.758578359584));
#115669=CARTESIAN_POINT('Ctrl Pts',(6.78224098759198,-28.5129905523876,
125.751282819538));
#115670=CARTESIAN_POINT('Ctrl Pts',(6.78128929646074,-28.5066348190222,
125.738547918945));
#115671=CARTESIAN_POINT('Ctrl Pts',(6.78088301092258,-28.5039631655978,
125.733120986649));
#115672=CARTESIAN_POINT('Ctrl Pts',(6.78000470670348,-28.4982778978357,
125.721411997249));
#115673=CARTESIAN_POINT('Ctrl Pts',(6.77953214744316,-28.4952741615286,
125.715125645257));
#115674=CARTESIAN_POINT('Ctrl Pts',(6.77821511087333,-28.4870524111867,
125.697637655391));
#115675=CARTESIAN_POINT('Ctrl Pts',(6.77736580947579,-28.4819195884693,
125.686396784898));
#115676=CARTESIAN_POINT('Ctrl Pts',(6.77402887620946,-28.4623887797075,
125.642333507151));
#115677=CARTESIAN_POINT('Ctrl Pts',(6.77149707433844,-28.4489317881972,
125.609119081009));
#115678=CARTESIAN_POINT('Ctrl Pts',(6.7689357756443,-28.4365600093868,125.575509683456));
#115679=CARTESIAN_POINT('Origin',(5.,-30.,125.));
#115680=CARTESIAN_POINT('',(6.06644913825629,-28.4365599905855,125.57550963238));
#115681=CARTESIAN_POINT('',(6.2618827045692,-28.4365599067946,125.575509404752));
#115682=CARTESIAN_POINT('',(5.,-28.4365599837785,125.575509613888));
#115683=CARTESIAN_POINT('',(6.92206959391605,-28.3340008189938,124.998531925366));
#115684=CARTESIAN_POINT('Ctrl Pts',(6.2618827045692,-28.4365599067946,125.575509404752));
#115685=CARTESIAN_POINT('Ctrl Pts',(6.26453319938667,-28.4494969610584,
125.610654459128));
#115686=CARTESIAN_POINT('Ctrl Pts',(6.26715307047973,-28.4636223241704,
125.645372127239));
#115687=CARTESIAN_POINT('Ctrl Pts',(6.27126995743702,-28.4879893075809,
125.699910307995));
#115688=CARTESIAN_POINT('Ctrl Pts',(6.27278955539158,-28.4974691391647,
125.720036018624));
#115689=CARTESIAN_POINT('Ctrl Pts',(6.27522184522568,-28.5134282592118,
125.752228530355));
#115690=CARTESIAN_POINT('Ctrl Pts',(6.27614299564413,-28.5196579464052,
125.764415283831));
#115691=CARTESIAN_POINT('Ctrl Pts',(6.27777541001437,-28.5310278216,125.785997060839));
#115692=CARTESIAN_POINT('Ctrl Pts',(6.27848867307505,-28.5361096813697,
125.795421765339));
#115693=CARTESIAN_POINT('Ctrl Pts',(6.27999366462139,-28.5470727723749,
125.81529268462));
#115694=CARTESIAN_POINT('Ctrl Pts',(6.28078453734769,-28.5529766250115,
125.825725774838));
#115695=CARTESIAN_POINT('Ctrl Pts',(6.28290789256535,-28.5692094452626,
125.853703011054));
#115696=CARTESIAN_POINT('Ctrl Pts',(6.28423276079966,-28.579748426927,125.871123395666));
#115697=CARTESIAN_POINT('Ctrl Pts',(6.29281959222204,-28.6506788814484,
125.983657215931));
#115698=CARTESIAN_POINT('Ctrl Pts',(6.29971676160355,-28.7202679858104,
126.072631895048));
#115699=CARTESIAN_POINT('Ctrl Pts',(6.31285660422745,-28.869308642933,126.227843451257));
#115700=CARTESIAN_POINT('Ctrl Pts',(6.31908333450307,-28.9469656087316,
126.295058065134));
#115701=CARTESIAN_POINT('Ctrl Pts',(6.32674536027513,-29.0429755123075,
126.363782769096));
#115702=CARTESIAN_POINT('Ctrl Pts',(6.32776719432771,-29.0557856711485,
126.37268298221));
#115703=CARTESIAN_POINT('Ctrl Pts',(6.32930079888376,-29.0749820401044,
126.38562435));
#115704=CARTESIAN_POINT('Ctrl Pts',(6.32980385475558,-29.0812742455049,
126.389804320019));
#115705=CARTESIAN_POINT('Ctrl Pts',(6.33071183219028,-29.0926176796934,
126.397229175008));
#115706=CARTESIAN_POINT('Ctrl Pts',(6.33111571019184,-29.0976583218239,
126.400489748536));
#115707=CARTESIAN_POINT('Ctrl Pts',(6.33202416789549,-29.1089846153035,
126.407729706354));
#115708=CARTESIAN_POINT('Ctrl Pts',(6.33252965653828,-29.115279296855,126.411694235309));
#115709=CARTESIAN_POINT('Ctrl Pts',(6.33406249443389,-29.1343507452311,
126.423528202029));
#115710=CARTESIAN_POINT('Ctrl Pts',(6.33509757646537,-29.1472070915657,
126.431267057696));
#115711=CARTESIAN_POINT('Ctrl Pts',(6.33754361639287,-29.1775755955892,
126.448992916798));
#115712=CARTESIAN_POINT('Ctrl Pts',(6.33896136022004,-29.1951677578577,
126.45883767407));
#115713=CARTESIAN_POINT('Ctrl Pts',(6.3441679257121,-29.2598762787358,126.49352256554));
#115714=CARTESIAN_POINT('Ctrl Pts',(6.34802308250029,-29.3079961382248,
126.51641773694));
#115715=CARTESIAN_POINT('Ctrl Pts',(6.36157881677038,-29.479994884436,126.588360321446));
#115716=CARTESIAN_POINT('Ctrl Pts',(6.3712730371265,-29.608607765328,126.62484414707));
#115717=CARTESIAN_POINT('Ctrl Pts',(6.38223429718041,-29.7654675838344,
126.649607367618));
#115718=CARTESIAN_POINT('Ctrl Pts',(6.38398169376901,-29.7908162471649,
126.653013068482));
#115719=CARTESIAN_POINT('Ctrl Pts',(6.38660460147052,-29.8293711843941,
126.657291918874));
#115720=CARTESIAN_POINT('Ctrl Pts',(6.3874933582728,-29.8425250357522,126.658593485513));
#115721=CARTESIAN_POINT('Ctrl Pts',(6.38909041106804,-29.8663188666728,
126.660662250527));
#115722=CARTESIAN_POINT('Ctrl Pts',(6.38980037860481,-29.8769532460782,
126.661484053838));
#115723=CARTESIAN_POINT('Ctrl Pts',(6.39132185615373,-29.8998610367381,
126.663033172167));
#115724=CARTESIAN_POINT('Ctrl Pts',(6.39213227568952,-29.9121361457776,
126.663726870733));
#115725=CARTESIAN_POINT('Ctrl Pts',(6.3943693927692,-29.9462132249856,126.665274448983));
#115726=CARTESIAN_POINT('Ctrl Pts',(6.39578697157501,-29.9680264713172,
126.665836058176));
#115727=CARTESIAN_POINT('Ctrl Pts',(6.39893926136341,-30.0169624392807,
126.666134340882));
#115728=CARTESIAN_POINT('Ctrl Pts',(6.40066686821204,-30.044080590703,126.665637532037));
#115729=CARTESIAN_POINT('Ctrl Pts',(6.40631730562073,-30.1335205402861,
126.6618129418));
#115730=CARTESIAN_POINT('Ctrl Pts',(6.41016538120923,-30.1956695284297,
126.655646177167));
#115731=CARTESIAN_POINT('Ctrl Pts',(6.4196488368188,-30.348702894728,126.631721641554));
#115732=CARTESIAN_POINT('Ctrl Pts',(6.42523114005937,-30.4387221513904,
126.609853990699));
#115733=CARTESIAN_POINT('Ctrl Pts',(6.4334649209599,-30.5629835375019,126.568466721425));
#115734=CARTESIAN_POINT('Ctrl Pts',(6.43592404130443,-30.5990758195875,
126.555038896514));
#115735=CARTESIAN_POINT('Ctrl Pts',(6.4391603060366,-30.6447134498778,126.536235211082));
#115736=CARTESIAN_POINT('Ctrl Pts',(6.43987777696164,-30.6547184479179,
126.531997974782));
#115737=CARTESIAN_POINT('Ctrl Pts',(6.44103839619328,-30.6707078416453,
126.525041045625));
#115738=CARTESIAN_POINT('Ctrl Pts',(6.44147793490054,-30.6767190256917,
126.522383183106));
#115739=CARTESIAN_POINT('Ctrl Pts',(6.44233620694843,-30.6883673546834,
126.517150221002));
#115740=CARTESIAN_POINT('Ctrl Pts',(6.44275470492931,-30.6940060996796,
126.51457912859));
#115741=CARTESIAN_POINT('Ctrl Pts',(6.4437918939359,-30.7078830558456,126.508157906864));
#115742=CARTESIAN_POINT('Ctrl Pts',(6.44441271237697,-30.716104267001,126.504271704889));
#115743=CARTESIAN_POINT('Ctrl Pts',(6.44676505233764,-30.7469521745781,
126.48937958442));
#115744=CARTESIAN_POINT('Ctrl Pts',(6.44852038672317,-30.7693591700143,
126.477929429874));
#115745=CARTESIAN_POINT('Ctrl Pts',(6.45320553925439,-30.8277805917852,
126.446387076662));
#115746=CARTESIAN_POINT('Ctrl Pts',(6.45616736969528,-30.8633224172604,
126.425457913083));
#115747=CARTESIAN_POINT('Ctrl Pts',(6.46827432337109,-31.0042098561678,
126.335292007246));
#115748=CARTESIAN_POINT('Ctrl Pts',(6.47752956685181,-31.1023346033881,
126.255511168682));
#115749=CARTESIAN_POINT('Ctrl Pts',(6.4893893111207,-31.2203660844488,126.134937154781));
#115750=CARTESIAN_POINT('Ctrl Pts',(6.49234296369616,-31.2490271784583,
126.103316544031));
#115751=CARTESIAN_POINT('Ctrl Pts',(6.49635425942368,-31.2869047943292,
126.058157346815));
#115752=CARTESIAN_POINT('Ctrl Pts',(6.49745453764131,-31.2971815376834,
126.045533840314));
#115753=CARTESIAN_POINT('Ctrl Pts',(6.49922021503165,-31.3134840836536,
126.024898036044));
#115754=CARTESIAN_POINT('Ctrl Pts',(6.49989018589651,-31.3196252470397,
126.016978680825));
#115755=CARTESIAN_POINT('Ctrl Pts',(6.50128479102593,-31.3323125993615,
126.000309221005));
#115756=CARTESIAN_POINT('Ctrl Pts',(6.50200885903743,-31.3388449260318,
125.99154912826));
#115757=CARTESIAN_POINT('Ctrl Pts',(6.50373065270819,-31.3542429075739,
125.970470233193));
#115758=CARTESIAN_POINT('Ctrl Pts',(6.50472522313699,-31.3630274473054,
125.958093173536));
#115759=CARTESIAN_POINT('Ctrl Pts',(6.50819419780949,-31.3932607329634,
125.914238105718));
#115760=CARTESIAN_POINT('Ctrl Pts',(6.51063463981055,-31.4137989571279,
125.882144909165));
#115761=CARTESIAN_POINT('Ctrl Pts',(6.51671632950467,-31.4628378040119,
125.799397515676));
#115762=CARTESIAN_POINT('Ctrl Pts',(6.52030996584898,-31.4898226486207,
125.747903768538));
#115763=CARTESIAN_POINT('Ctrl Pts',(6.5306130663636,-31.5599071729842,125.595246586069));
#115764=CARTESIAN_POINT('Ctrl Pts',(6.53720786217767,-31.5957554721044,
125.491109977333));
#115765=CARTESIAN_POINT('Ctrl Pts',(6.54606922763657,-31.6279484766227,
125.355280140688));
#115766=CARTESIAN_POINT('Ctrl Pts',(6.54798403109222,-31.6340298106704,
125.326169501329));
#115767=CARTESIAN_POINT('Ctrl Pts',(6.5505925204446,-31.6411032107873,125.28711566778));
#115768=CARTESIAN_POINT('Ctrl Pts',(6.55125131463722,-31.6427899269998,
125.277301999324));
#115769=CARTESIAN_POINT('Ctrl Pts',(6.55229767160672,-31.6453105760916,
125.261805446907));
#115770=CARTESIAN_POINT('Ctrl Pts',(6.5526820208343,-31.6462032962194,125.256132170632));
#115771=CARTESIAN_POINT('Ctrl Pts',(6.55348542643119,-31.6480001160509,
125.244315724879));
#115772=CARTESIAN_POINT('Ctrl Pts',(6.55390477425739,-31.648899225091,125.238171989441));
#115773=CARTESIAN_POINT('Ctrl Pts',(6.55494710838994,-31.6510390707485,
125.222956981187));
#115774=CARTESIAN_POINT('Ctrl Pts',(6.55557226829297,-31.6522393985809,
125.213880314075));
#115775=CARTESIAN_POINT('Ctrl Pts',(6.5579614695847,-31.6565153810407,125.179359075986));
#115776=CARTESIAN_POINT('Ctrl Pts',(6.55975025928964,-31.6590783718404,
125.153855997126));
#115777=CARTESIAN_POINT('Ctrl Pts',(6.56455193761555,-31.664315894548,125.086050778279));
#115778=CARTESIAN_POINT('Ctrl Pts',(6.56759863363915,-31.665966066748,125.043689216899));
#115779=CARTESIAN_POINT('Ctrl Pts',(6.58047350559178,-31.6661062488206,
124.865917736589));
#115780=CARTESIAN_POINT('Ctrl Pts',(6.59040798074068,-31.6497063668685,
124.730986984933));
#115781=CARTESIAN_POINT('Ctrl Pts',(6.60225665207569,-31.6088689371866,
124.56608364022));
#115782=CARTESIAN_POINT('Ctrl Pts',(6.60462858419402,-31.5995526368281,
124.532908651128));
#115783=CARTESIAN_POINT('Ctrl Pts',(6.60788787289367,-31.5851467686922,
124.487116597681));
#115784=CARTESIAN_POINT('Ctrl Pts',(6.60880284621934,-31.5809221451636,
124.474238787605));
#115785=CARTESIAN_POINT('Ctrl Pts',(6.61038399442401,-31.5733079049395,
124.451950515089));
#115786=CARTESIAN_POINT('Ctrl Pts',(6.61105248224384,-31.5699898703658,
124.44251653286));
#115787=CARTESIAN_POINT('Ctrl Pts',(6.61244674602053,-31.5628627273512,
124.422820744788));
#115788=CARTESIAN_POINT('Ctrl Pts',(6.61317193274186,-31.5590370175724,
124.41256542088));
#115789=CARTESIAN_POINT('Ctrl Pts',(6.61490146548797,-31.5496293665892,
124.388086385591));
#115790=CARTESIAN_POINT('Ctrl Pts',(6.61590258005776,-31.5439522131185,
124.373900140193));
#115791=CARTESIAN_POINT('Ctrl Pts',(6.61942355040095,-31.5231720155337,
124.32397621279));
#115792=CARTESIAN_POINT('Ctrl Pts',(6.62190801953996,-31.5070161152784,
124.288688574357));
#115793=CARTESIAN_POINT('Ctrl Pts',(6.62813293145819,-31.4629013726425,
124.200599140311));
#115794=CARTESIAN_POINT('Ctrl Pts',(6.63182259687753,-31.4333080699181,
124.148676960642));
#115795=CARTESIAN_POINT('Ctrl Pts',(6.64237913559423,-31.3401040996549,
124.003839500944));
#115796=CARTESIAN_POINT('Ctrl Pts',(6.64913194514274,-31.2697983494857,
123.915646887389));
#115797=CARTESIAN_POINT('Ctrl Pts',(6.65794791548176,-31.1732156821294,
123.816877362549));
#115798=CARTESIAN_POINT('Ctrl Pts',(6.65960692389917,-31.1548584334054,
123.798952107329));
#115799=CARTESIAN_POINT('Ctrl Pts',(6.66191575738511,-31.1292029041182,
123.775032402144));
#115800=CARTESIAN_POINT('Ctrl Pts',(6.66254001999159,-31.1222557180147,
123.768664583661));
#115801=CARTESIAN_POINT('Ctrl Pts',(6.66354492540437,-31.1110640106714,
123.758579606982));
#115802=CARTESIAN_POINT('Ctrl Pts',(6.66392278602291,-31.1068538585194,
123.754824365202));
#115803=CARTESIAN_POINT('Ctrl Pts',(6.66472686477968,-31.0978930675363,
123.746913150258));
#115804=CARTESIAN_POINT('Ctrl Pts',(6.66515349106686,-31.0931377583651,
123.742762680333));
#115805=CARTESIAN_POINT('Ctrl Pts',(6.66623812964722,-31.0810429026558,
123.732326690308));
#115806=CARTESIAN_POINT('Ctrl Pts',(6.66689869691037,-31.0736721395653,
123.726077905448));
#115807=CARTESIAN_POINT('Ctrl Pts',(6.66961085642554,-31.0433737036929,
123.700841221238));
#115808=CARTESIAN_POINT('Ctrl Pts',(6.67169619280759,-31.0199948213183,
123.68240654186));
#115809=CARTESIAN_POINT('Ctrl Pts',(6.67759242938557,-30.9533535359595,
123.632695379766));
#115810=CARTESIAN_POINT('Ctrl Pts',(6.68145604984246,-30.9090640498384,
123.60285764462));
#115811=CARTESIAN_POINT('Ctrl Pts',(6.69505368842306,-30.7491287746903,
123.505937712207));
#115812=CARTESIAN_POINT('Ctrl Pts',(6.70477986328375,-30.6268932145498,
123.450666696313));
#115813=CARTESIAN_POINT('Ctrl Pts',(6.71558872697801,-30.4774265375474,
123.403708044208));
#115814=CARTESIAN_POINT('Ctrl Pts',(6.71715990626993,-30.4553614562229,
123.397274152549));
#115815=CARTESIAN_POINT('Ctrl Pts',(6.71964746889766,-30.4198950015234,
123.387724225972));
#115816=CARTESIAN_POINT('Ctrl Pts',(6.72057318091282,-30.4065766013591,
123.384314241345));
#115817=CARTESIAN_POINT('Ctrl Pts',(6.72221275884133,-30.3827788450401,
123.378534076148));
#115818=CARTESIAN_POINT('Ctrl Pts',(6.72292864974069,-30.372316045031,123.37609970801));
#115819=CARTESIAN_POINT('Ctrl Pts',(6.72442607246351,-30.3502838645565,
123.371197638648));
#115820=CARTESIAN_POINT('Ctrl Pts',(6.72520687573671,-30.3387102359802,
123.368751611096));
#115821=CARTESIAN_POINT('Ctrl Pts',(6.72727196947351,-30.3078815593857,
123.362578382068));
#115822=CARTESIAN_POINT('Ctrl Pts',(6.72854937096296,-30.2885847211309,
123.359067484357));
#115823=CARTESIAN_POINT('Ctrl Pts',(6.73583250017285,-30.177367094609,123.340855056472));
#115824=CARTESIAN_POINT('Ctrl Pts',(6.74159860185873,-30.0843999756339,
123.333536416551));
#115825=CARTESIAN_POINT('Ctrl Pts',(6.75291404096309,-29.899610665351,123.334501647568));
#115826=CARTESIAN_POINT('Ctrl Pts',(6.75844863262275,-29.8081255883498,
123.342548676133));
#115827=CARTESIAN_POINT('Ctrl Pts',(6.76669327797358,-29.6787340016579,
123.3647895315));
#115828=CARTESIAN_POINT('Ctrl Pts',(6.76922090942779,-29.6399495437974,
123.372889606036));
#115829=CARTESIAN_POINT('Ctrl Pts',(6.77253559312887,-29.5908493472666,
123.384985470093));
#115830=CARTESIAN_POINT('Ctrl Pts',(6.77325937274455,-29.5802310440417,
123.387712743889));
#115831=CARTESIAN_POINT('Ctrl Pts',(6.77442776287269,-29.5632705911494,
123.39224787228));
#115832=CARTESIAN_POINT('Ctrl Pts',(6.7748686775115,-29.5569107077642,123.393988992545));
#115833=CARTESIAN_POINT('Ctrl Pts',(6.77572748713438,-29.54460539846,123.397436423727));
#115834=CARTESIAN_POINT('Ctrl Pts',(6.77614512583801,-29.5386588863692,
123.399138159927));
#115835=CARTESIAN_POINT('Ctrl Pts',(6.77717705264136,-29.5240548550127,
123.403405575777));
#115836=CARTESIAN_POINT('Ctrl Pts',(6.77779342092862,-29.5154085291638,
123.406008584202));
#115837=CARTESIAN_POINT('Ctrl Pts',(6.78010853803244,-29.4832013957348,
123.415990918984));
#115838=CARTESIAN_POINT('Ctrl Pts',(6.78183017395441,-29.4597856269238,
123.423823030178));
#115839=CARTESIAN_POINT('Ctrl Pts',(6.78639924812052,-29.3988196238663,
123.445732987378));
#115840=CARTESIAN_POINT('Ctrl Pts',(6.78927695477294,-29.3615892951226,
123.460651059185));
#115841=CARTESIAN_POINT('Ctrl Pts',(6.80068390173899,-29.2174159488322,
123.524551022688));
#115842=CARTESIAN_POINT('Ctrl Pts',(6.80932329822938,-29.1152304523408,
123.583463511025));
#115843=CARTESIAN_POINT('Ctrl Pts',(6.82123600089791,-28.9790678616202,
123.682491876728));
#115844=CARTESIAN_POINT('Ctrl Pts',(6.82476601493298,-28.9394176715411,
123.714194360977));
#115845=CARTESIAN_POINT('Ctrl Pts',(6.8294003253749,-28.888317161365,123.759026870483));
#115846=CARTESIAN_POINT('Ctrl Pts',(6.83056696496207,-28.8755383640317,
123.770594001194));
#115847=CARTESIAN_POINT('Ctrl Pts',(6.83248654397586,-28.8546619422436,
123.790088827657));
#115848=CARTESIAN_POINT('Ctrl Pts',(6.83324415767988,-28.8464618409549,
123.797904314091));
#115849=CARTESIAN_POINT('Ctrl Pts',(6.83472718553359,-28.8304914096011,
123.8134395907));
#115850=CARTESIAN_POINT('Ctrl Pts',(6.83545279700059,-28.8227162478945,
123.821153561868));
#115851=CARTESIAN_POINT('Ctrl Pts',(6.83619066777848,-28.8148515459285,
123.829111791164));
#115852=CARTESIAN_POINT('Ctrl Pts',(6.83620624170887,-28.8146855680861,
123.829279814269));
#115853=CARTESIAN_POINT('Ctrl Pts',(6.83623583013961,-28.8143702683017,
123.829599135125));
#115854=CARTESIAN_POINT('Ctrl Pts',(6.83624984493426,-28.8142209395846,
123.829750426162));
#115855=CARTESIAN_POINT('Ctrl Pts',(6.83627655291757,-28.8139363935831,
123.830038821749));
#115856=CARTESIAN_POINT('Ctrl Pts',(6.83628924632489,-28.8138011711808,
123.830175921094));
#115857=CARTESIAN_POINT('Ctrl Pts',(6.83631350256281,-28.8135427947668,
123.83043797474));
#115858=CARTESIAN_POINT('Ctrl Pts',(6.83632506558081,-28.8134196365894,
123.830562925186));
#115859=CARTESIAN_POINT('Ctrl Pts',(6.83634721640795,-28.8131837275465,
123.830802342948));
#115860=CARTESIAN_POINT('Ctrl Pts',(6.83635780434501,-28.8130709736074,
123.830916807014));
#115861=CARTESIAN_POINT('Ctrl Pts',(6.83637813275086,-28.8128545077565,
123.831136619574));
#115862=CARTESIAN_POINT('Ctrl Pts',(6.83638787332317,-28.812750793376,123.831241965493));
#115863=CARTESIAN_POINT('Ctrl Pts',(6.83643223615479,-28.8122784670355,
123.831721849778));
#115864=CARTESIAN_POINT('Ctrl Pts',(6.83646685136234,-28.8119100179505,
123.832096549064));
#115865=CARTESIAN_POINT('Ctrl Pts',(6.83653604626115,-28.8111736889653,
123.832846077836));
#115866=CARTESIAN_POINT('Ctrl Pts',(6.83657062595841,-28.8108058088897,
123.833220907085));
#115867=CARTESIAN_POINT('Ctrl Pts',(6.83767795873292,-28.7990283896695,
123.845232155369));
#115868=CARTESIAN_POINT('Ctrl Pts',(6.83874329689679,-28.7877897099164,
123.857035509234));
#115869=CARTESIAN_POINT('Ctrl Pts',(6.84301520154557,-28.7431301836051,
123.905338743654));
#115870=CARTESIAN_POINT('Ctrl Pts',(6.84616095838745,-28.7111682803419,
123.943156345533));
#115871=CARTESIAN_POINT('Ctrl Pts',(6.85485758441965,-28.6263125093629,
124.053144652801));
#115872=CARTESIAN_POINT('Ctrl Pts',(6.86028018796973,-28.5774782027905,
124.128228780105));
#115873=CARTESIAN_POINT('Ctrl Pts',(6.87077987473199,-28.4957493985147,
124.279201320023));
#115874=CARTESIAN_POINT('Ctrl Pts',(6.87583847403425,-28.4620086311546,
124.354322141641));
#115875=CARTESIAN_POINT('Ctrl Pts',(6.88222971323214,-28.4283560689041,
124.447043659558));
#115876=CARTESIAN_POINT('Ctrl Pts',(6.88330360939275,-28.4229853013396,
124.462552373413));
#115877=CARTESIAN_POINT('Ctrl Pts',(6.88490031704324,-28.4154303061508,
124.485457195498));
#115878=CARTESIAN_POINT('Ctrl Pts',(6.88541334322756,-28.4130667369984,
124.492793705419));
#115879=CARTESIAN_POINT('Ctrl Pts',(6.88633156415561,-28.408951467608,124.505877879494));
#115880=CARTESIAN_POINT('Ctrl Pts',(6.88673560149617,-28.4071798291052,
124.511618997854));
#115881=CARTESIAN_POINT('Ctrl Pts',(6.88763478572709,-28.4033237748579,
124.524359003226));
#115882=CARTESIAN_POINT('Ctrl Pts',(6.88813073693747,-28.4012543254014,
124.531361985501));
#115883=CARTESIAN_POINT('Ctrl Pts',(6.88960635955107,-28.3952640490912,
124.552134505304));
#115884=CARTESIAN_POINT('Ctrl Pts',(6.89059296867327,-28.3914747200839,
124.565940829975));
#115885=CARTESIAN_POINT('Ctrl Pts',(6.89290428349614,-28.3830838604319,
124.598132652908));
#115886=CARTESIAN_POINT('Ctrl Pts',(6.89423485063796,-28.3786172580569,
124.616551038582));
#115887=CARTESIAN_POINT('Ctrl Pts',(6.90423166997339,-28.3476777675406,
124.754355990659));
#115888=CARTESIAN_POINT('Ctrl Pts',(6.91327216383534,-28.3341084014325,
124.876251723394));
#115889=CARTESIAN_POINT('Ctrl Pts',(6.92206989104865,-28.3340006468508,
124.99853190384));
#115890=CARTESIAN_POINT('Ctrl Pts',(6.92206979048547,-28.3340006480831,
124.998530506106));
#115891=CARTESIAN_POINT('Ctrl Pts',(6.92753177905078,-28.3339336859568,
125.074447023654));
#115892=CARTESIAN_POINT('Ctrl Pts',(6.93289216561482,-28.3390557540501,
125.150289817465));
#115893=CARTESIAN_POINT('Ctrl Pts',(6.93911162664111,-28.3513445759967,
125.240232116867));
#115894=CARTESIAN_POINT('Ctrl Pts',(6.94012218279109,-28.353549658344,125.254906795077));
#115895=CARTESIAN_POINT('Ctrl Pts',(6.94186359326972,-28.3577121892431,
125.280295014377));
#115896=CARTESIAN_POINT('Ctrl Pts',(6.94259723577587,-28.3595791353605,
125.291022241554));
#115897=CARTESIAN_POINT('Ctrl Pts',(6.94406284090429,-28.3635365850972,
125.312511870141));
#115898=CARTESIAN_POINT('Ctrl Pts',(6.94479472140027,-28.3656284244834,
125.323273476083));
#115899=CARTESIAN_POINT('Ctrl Pts',(6.94618651850421,-28.3698274805669,
125.343792349891));
#115900=CARTESIAN_POINT('Ctrl Pts',(6.94684698110349,-28.3719164533771,
125.353552818573));
#115901=CARTESIAN_POINT('Ctrl Pts',(6.9485622490246,-28.377592885062,125.378957441186));
#115902=CARTESIAN_POINT('Ctrl Pts',(6.94961259269553,-28.381318968508,125.394569812067));
#115903=CARTESIAN_POINT('Ctrl Pts',(6.95332698054743,-28.3953833556236,
125.449943441757));
#115904=CARTESIAN_POINT('Ctrl Pts',(6.95595133756798,-28.4069663656086,
125.4893750524));
#115905=CARTESIAN_POINT('Ctrl Pts',(6.95959035233196,-28.4252824963323,
125.544149468564));
#115906=CARTESIAN_POINT('Ctrl Pts',(6.96063434584027,-28.4308044849064,
125.5598741184));
#115907=CARTESIAN_POINT('Ctrl Pts',(6.96167308954662,-28.4365599688247,
125.575509573264));
#115908=CARTESIAN_POINT('Ctrl Pts',(6.7689357756443,-28.4365600093868,125.575509683456));
#115909=CARTESIAN_POINT('Ctrl Pts',(6.76566848506476,-28.420778095137,125.532636250435));
#115910=CARTESIAN_POINT('Ctrl Pts',(6.76235350240954,-28.4067621010019,
125.489120073969));
#115911=CARTESIAN_POINT('Ctrl Pts',(6.75469878842849,-28.378651974293,125.38772188101));
#115912=CARTESIAN_POINT('Ctrl Pts',(6.75035980893607,-28.3658371653365,
125.329560227213));
#115913=CARTESIAN_POINT('Ctrl Pts',(6.74216812851736,-28.3473522964619,
125.217366497062));
#115914=CARTESIAN_POINT('Ctrl Pts',(6.73831113630137,-28.341156118264,125.163494805165));
#115915=CARTESIAN_POINT('Ctrl Pts',(6.73198983938758,-28.3352104610111,
125.073156967422));
#115916=CARTESIAN_POINT('Ctrl Pts',(6.729486824718,-28.3340108073496,125.036830930799));
#115917=CARTESIAN_POINT('Ctrl Pts',(6.72610900406875,-28.3339961064373,
124.9870664239));
#115918=CARTESIAN_POINT('Ctrl Pts',(6.72520278314316,-28.3341544305092,
124.973640804401));
#115919=CARTESIAN_POINT('Ctrl Pts',(6.72363259450369,-28.3347130475935,
124.950253447738));
#115920=CARTESIAN_POINT('Ctrl Pts',(6.72296639062987,-28.3350404882023,
124.940290831137));
#115921=CARTESIAN_POINT('Ctrl Pts',(6.72157292296929,-28.3359160260347,
124.919372174836));
#115922=CARTESIAN_POINT('Ctrl Pts',(6.7208462812632,-28.3364829577567,124.908417367689));
#115923=CARTESIAN_POINT('Ctrl Pts',(6.71910585380683,-28.3381073583385,
124.882072999952));
#115924=CARTESIAN_POINT('Ctrl Pts',(6.71809541042726,-28.3392704585849,
124.866690786944));
#115925=CARTESIAN_POINT('Ctrl Pts',(6.71449765318875,-28.3442028793999,
124.811639768621));
#115926=CARTESIAN_POINT('Ctrl Pts',(6.71194789671585,-28.34918152188,124.77209118515));
#115927=CARTESIAN_POINT('Ctrl Pts',(6.70550674341121,-28.3655498553303,
124.671372101888));
#115928=CARTESIAN_POINT('Ctrl Pts',(6.70167115359441,-28.3789555107175,
124.610591255652));
#115929=CARTESIAN_POINT('Ctrl Pts',(6.69223211632216,-28.4205291939749,
124.46214848252));
#115930=CARTESIAN_POINT('Ctrl Pts',(6.68668135806102,-28.4526164707771,
124.375809040903));
#115931=CARTESIAN_POINT('Ctrl Pts',(6.67844004874595,-28.5083229885934,
124.257035943605));
#115932=CARTESIAN_POINT('Ctrl Pts',(6.67593524040467,-28.526234795142,124.222110883728));
#115933=CARTESIAN_POINT('Ctrl Pts',(6.67264687822897,-28.5506879960217,
124.17831263442));
#115934=CARTESIAN_POINT('Ctrl Pts',(6.67192539151807,-28.5561085634468,
124.168824377533));
#115935=CARTESIAN_POINT('Ctrl Pts',(6.67075991272595,-28.5649444428561,
124.153705187675));
#115936=CARTESIAN_POINT('Ctrl Pts',(6.6703195858635,-28.5683005963175,124.148039804224));
#115937=CARTESIAN_POINT('Ctrl Pts',(6.66946123327384,-28.5748751627257,
124.137090109082));
#115938=CARTESIAN_POINT('Ctrl Pts',(6.66904345692316,-28.5780895614228,
124.131803604381));
#115939=CARTESIAN_POINT('Ctrl Pts',(6.66801020449228,-28.586076454115,124.118831427133));
#115940=CARTESIAN_POINT('Ctrl Pts',(6.6673926346831,-28.5908822091461,124.111166556878));
#115941=CARTESIAN_POINT('Ctrl Pts',(6.66506668193613,-28.6091098437405,
124.082614032058));
#115942=CARTESIAN_POINT('Ctrl Pts',(6.66333513962677,-28.6229349829396,
124.061989221668));
#115943=CARTESIAN_POINT('Ctrl Pts',(6.65873182740592,-28.6604729417816,
124.008607990808));
#115944=CARTESIAN_POINT('Ctrl Pts',(6.65582927364801,-28.6849259992527,
123.976393230019));
#115945=CARTESIAN_POINT('Ctrl Pts',(6.64422750792679,-28.7864659750026,
123.85227386869));
#115946=CARTESIAN_POINT('Ctrl Pts',(6.63541794614295,-28.8722199805286,
123.767904940636));
#115947=CARTESIAN_POINT('Ctrl Pts',(6.62352598431755,-29.0042637056442,
123.663433766239));
#115948=CARTESIAN_POINT('Ctrl Pts',(6.62016185090898,-29.0435269750317,
123.635060356369));
#115949=CARTESIAN_POINT('Ctrl Pts',(6.61570424466294,-29.0981664409287,
123.599092818538));
#115950=CARTESIAN_POINT('Ctrl Pts',(6.61455448351329,-29.1125012202855,
123.589967854092));
#115951=CARTESIAN_POINT('Ctrl Pts',(6.61273094015243,-29.1356170530476,
123.575745418554));
#115952=CARTESIAN_POINT('Ctrl Pts',(6.61205199631276,-29.1443091173042,
123.570506343875));
#115953=CARTESIAN_POINT('Ctrl Pts',(6.61065440296462,-29.1623761000877,
123.559840451813));
#115954=CARTESIAN_POINT('Ctrl Pts',(6.60993618910334,-29.1717571804574,
123.554424971422));
#115955=CARTESIAN_POINT('Ctrl Pts',(6.60825606070921,-29.1939251968672,
123.54191453245));
#115956=CARTESIAN_POINT('Ctrl Pts',(6.60729689706585,-29.2067541799568,
123.534895597441));
#115957=CARTESIAN_POINT('Ctrl Pts',(6.60409583263791,-29.2501321935008,
123.51189964288));
#115958=CARTESIAN_POINT('Ctrl Pts',(6.60188106785313,-29.2810854776876,
123.496701435788));
#115959=CARTESIAN_POINT('Ctrl Pts',(6.59650605610566,-29.3582430179661,
123.461745473911));
#115960=CARTESIAN_POINT('Ctrl Pts',(6.59337959913883,-29.4049122626889,
123.443095972488));
#115961=CARTESIAN_POINT('Ctrl Pts',(6.58628634375605,-29.5136340053649,
123.405254234714));
#115962=CARTESIAN_POINT('Ctrl Pts',(6.58234749730337,-29.5761059118787,
123.387523694431));
#115963=CARTESIAN_POINT('Ctrl Pts',(6.57368799047526,-29.7141547719017,
123.35692268656));
#115964=CARTESIAN_POINT('Ctrl Pts',(6.56896412098794,-29.7899001867891,
123.345531539426));
#115965=CARTESIAN_POINT('Ctrl Pts',(6.56296075072051,-29.8822425262484,
123.33808850214));
#115966=CARTESIAN_POINT('Ctrl Pts',(6.56190438691834,-29.8983522551874,
123.337025454719));
#115967=CARTESIAN_POINT('Ctrl Pts',(6.56032191091518,-29.9222299153552,
123.335798051685));
#115968=CARTESIAN_POINT('Ctrl Pts',(6.55980512214208,-29.9299881816379,
123.335453620304));
#115969=CARTESIAN_POINT('Ctrl Pts',(6.55888306643245,-29.9437541129448,
123.334938884169));
#115970=CARTESIAN_POINT('Ctrl Pts',(6.55847900066332,-29.9497607046222,
123.334746826969));
#115971=CARTESIAN_POINT('Ctrl Pts',(6.55758335627051,-29.9630164713693,
123.334394767318));
#115972=CARTESIAN_POINT('Ctrl Pts',(6.55709101203843,-29.9702656164729,
123.334249588323));
#115973=CARTESIAN_POINT('Ctrl Pts',(6.5556362788004,-29.9915811577864,123.333961882986));
#115974=CARTESIAN_POINT('Ctrl Pts',(6.55466723003914,-30.0056482792319,
123.333950196247));
#115975=CARTESIAN_POINT('Ctrl Pts',(6.54798406726279,-30.101878269984,123.335088936061));
#115976=CARTESIAN_POINT('Ctrl Pts',(6.54202674199773,-30.183850511154,123.342138653558));
#115977=CARTESIAN_POINT('Ctrl Pts',(6.52653932635934,-30.3939658285482,
123.375985950159));
#115978=CARTESIAN_POINT('Ctrl Pts',(6.51706480653485,-30.5201058514035,
123.411877491657));
#115979=CARTESIAN_POINT('Ctrl Pts',(6.50664773052694,-30.6599278677778,
123.470136603068));
#115980=CARTESIAN_POINT('Ctrl Pts',(6.50523209566115,-30.6789369387628,
123.478477241566));
#115981=CARTESIAN_POINT('Ctrl Pts',(6.50293236403428,-30.7098190625436,
123.492721492463));
#115982=CARTESIAN_POINT('Ctrl Pts',(6.50204124124716,-30.7217858200303,
123.498415221026));
#115983=CARTESIAN_POINT('Ctrl Pts',(6.50044185124528,-30.7432587058715,
123.508947943201));
#115984=CARTESIAN_POINT('Ctrl Pts',(6.4997318867413,-30.752788602039,123.513736540968));
#115985=CARTESIAN_POINT('Ctrl Pts',(6.49821248466088,-30.7731752236963,
123.524226836731));
#115986=CARTESIAN_POINT('Ctrl Pts',(6.49740411579749,-30.7840163596878,
123.5299575798));
#115987=CARTESIAN_POINT('Ctrl Pts',(6.49517823416996,-30.813843142863,123.546148166046));
#115988=CARTESIAN_POINT('Ctrl Pts',(6.49376968994446,-30.8326898564463,
123.556859851032));
#115989=CARTESIAN_POINT('Ctrl Pts',(6.49064055108185,-30.8744377913088,
123.581677868949));
#115990=CARTESIAN_POINT('Ctrl Pts',(6.48892690102477,-30.8972174735286,
123.59597719349));
#115991=CARTESIAN_POINT('Ctrl Pts',(6.4833420696504,-30.9709730480013,123.644803720927));
#115992=CARTESIAN_POINT('Ctrl Pts',(6.47954362482003,-31.0203838273396,
123.68160579439));
#115993=CARTESIAN_POINT('Ctrl Pts',(6.47023692267696,-31.1370369912806,
123.778986745744));
#115994=CARTESIAN_POINT('Ctrl Pts',(6.46478012548521,-31.2015936094042,
123.84246063489));
#115995=CARTESIAN_POINT('Ctrl Pts',(6.45651942298891,-31.2877405891338,
123.942175069479));
#115996=CARTESIAN_POINT('Ctrl Pts',(6.45388232485946,-31.3136223248683,
123.974492723018));
#115997=CARTESIAN_POINT('Ctrl Pts',(6.45044103592729,-31.344904517884,124.016683233437));
#115998=CARTESIAN_POINT('Ctrl Pts',(6.44970604635026,-31.3514473891593,
124.025695138365));
#115999=CARTESIAN_POINT('Ctrl Pts',(6.44852393290883,-31.3617407716749,
124.040176039178));
#116000=CARTESIAN_POINT('Ctrl Pts',(6.44808066098892,-31.3655499588191,
124.045603189895));
#116001=CARTESIAN_POINT('Ctrl Pts',(6.44722104596509,-31.3728370379993,
124.056118412725));
#116002=CARTESIAN_POINT('Ctrl Pts',(6.44680499624314,-31.376319241199,124.061203256842));
#116003=CARTESIAN_POINT('Ctrl Pts',(6.44578248167053,-31.384770143057,124.073691653643));
#116004=CARTESIAN_POINT('Ctrl Pts',(6.44517401946421,-31.3897077297389,
124.081115938429));
#116005=CARTESIAN_POINT('Ctrl Pts',(6.44292288200507,-31.4076503349595,
124.108570322492));
#116006=CARTESIAN_POINT('Ctrl Pts',(6.44125886223176,-31.4202831634038,
124.128838747474));
#116007=CARTESIAN_POINT('Ctrl Pts',(6.43688510372683,-31.4519771114395,
124.182211909521));
#116008=CARTESIAN_POINT('Ctrl Pts',(6.43414792421252,-31.4703426829046,
124.21571247241));
#116009=CARTESIAN_POINT('Ctrl Pts',(6.42636814161454,-31.5188303104101,
124.31185809634));
#116010=CARTESIAN_POINT('Ctrl Pts',(6.4212844975024,-31.5462082224433,124.37580054661));
#116011=CARTESIAN_POINT('Ctrl Pts',(6.40925870486,-31.6018701258222,124.532157712738));
#116012=CARTESIAN_POINT('Ctrl Pts',(6.40239231032963,-31.6262750023347,
124.625701162495));
#116013=CARTESIAN_POINT('Ctrl Pts',(6.39442228899993,-31.6457805472773,
124.740464988821));
#116014=CARTESIAN_POINT('Ctrl Pts',(6.39307076223008,-31.6487633962984,
124.760143054257));
#116015=CARTESIAN_POINT('Ctrl Pts',(6.39092961805284,-31.6529637974901,
124.791654127011));
#116016=CARTESIAN_POINT('Ctrl Pts',(6.39013294220872,-31.6544083989397,
124.803454379842));
#116017=CARTESIAN_POINT('Ctrl Pts',(6.38862518575324,-31.656915636688,124.825926559411));
#116018=CARTESIAN_POINT('Ctrl Pts',(6.38791340311213,-31.6580017705635,
124.836595202634));
#116019=CARTESIAN_POINT('Ctrl Pts',(6.38628937938659,-31.6602548754232,
124.861069503379));
#116020=CARTESIAN_POINT('Ctrl Pts',(6.38537934069859,-31.6613528069016,
124.874880838876));
#116021=CARTESIAN_POINT('Ctrl Pts',(6.38252197418721,-31.6642754973892,
124.91853336968));
#116022=CARTESIAN_POINT('Ctrl Pts',(6.3805942197333,-31.6654694771846,124.948411823421));
#116023=CARTESIAN_POINT('Ctrl Pts',(6.37342763472322,-31.6669328141901,
125.060789075925));
#116024=CARTESIAN_POINT('Ctrl Pts',(6.3683461659369,-31.6618798136474,125.143240126127));
#116025=CARTESIAN_POINT('Ctrl Pts',(6.35705023005063,-31.6369343992204,
125.326267763607));
#116026=CARTESIAN_POINT('Ctrl Pts',(6.35088117107393,-31.6138393747341,
125.42605534833));
#116027=CARTESIAN_POINT('Ctrl Pts',(6.34271788078855,-31.5736725685779,
125.547514990068));
#116028=CARTESIAN_POINT('Ctrl Pts',(6.34105421172018,-31.5650297130898,
125.57175155696));
#116029=CARTESIAN_POINT('Ctrl Pts',(6.33873999859542,-31.5524564706115,
125.604585713514));
#116030=CARTESIAN_POINT('Ctrl Pts',(6.33811517573018,-31.5490085523667,
125.61336569229));
#116031=CARTESIAN_POINT('Ctrl Pts',(6.33710968377548,-31.5433795310543,
125.627349548043));
#116032=CARTESIAN_POINT('Ctrl Pts',(6.33673180434864,-31.5412461635949,
125.632572599087));
#116033=CARTESIAN_POINT('Ctrl Pts',(6.33592803487865,-31.5366718060309,
125.643611327701));
#116034=CARTESIAN_POINT('Ctrl Pts',(6.33550173973639,-31.5342242572817,
125.64942413331));
#116035=CARTESIAN_POINT('Ctrl Pts',(6.3344185612339,-31.5279498091341,125.664092194107));
#116036=CARTESIAN_POINT('Ctrl Pts',(6.33375913461186,-31.5240789420989,
125.672928249213));
#116037=CARTESIAN_POINT('Ctrl Pts',(6.33105697484544,-31.5080021169505,
125.708776596779));
#116038=CARTESIAN_POINT('Ctrl Pts',(6.32898079148647,-31.4951537457605,
125.735492805451));
#116039=CARTESIAN_POINT('Ctrl Pts',(6.32311980225455,-31.4573567763721,
125.808998103495));
#116040=CARTESIAN_POINT('Ctrl Pts',(6.319282930209,-31.4308775663393,125.854959309563));
#116041=CARTESIAN_POINT('Ctrl Pts',(6.305817962956,-31.3308762716336,126.010840622041));
#116042=CARTESIAN_POINT('Ctrl Pts',(6.29619306128808,-31.2464947843344,
126.113235510768));
#116043=CARTESIAN_POINT('Ctrl Pts',(6.28520854980733,-31.1315499810503,
126.223055818523));
#116044=CARTESIAN_POINT('Ctrl Pts',(6.28338036365473,-31.1117749281198,
126.241059042647));
#116045=CARTESIAN_POINT('Ctrl Pts',(6.28067435487289,-31.0815458536922,
126.26727691448));
#116046=CARTESIAN_POINT('Ctrl Pts',(6.2797816399537,-31.071413820254,126.275854480371));
#116047=CARTESIAN_POINT('Ctrl Pts',(6.27818053670851,-31.0529573126989,
126.291104439105));
#116048=CARTESIAN_POINT('Ctrl Pts',(6.27747043499808,-31.0446693175428,
126.297819633503));
#116049=CARTESIAN_POINT('Ctrl Pts',(6.27595196692837,-31.0267292877109,
126.312071994415));
#116050=CARTESIAN_POINT('Ctrl Pts',(6.27514465683307,-31.0170574464703,
126.319583310284));
#116051=CARTESIAN_POINT('Ctrl Pts',(6.27292496469938,-30.9901022018194,
126.340044777561));
#116052=CARTESIAN_POINT('Ctrl Pts',(6.2715214669039,-30.9726480943924,126.352766842425));
#116053=CARTESIAN_POINT('Ctrl Pts',(6.26342092083833,-30.8696349798483,
126.424826851887));
#116054=CARTESIAN_POINT('Ctrl Pts',(6.25702543657572,-30.778908785925,126.476381153419));
#116055=CARTESIAN_POINT('Ctrl Pts',(6.24397338457015,-30.5840757522166,
126.564100105994));
#116056=CARTESIAN_POINT('Ctrl Pts',(6.23734732374487,-30.4800207197973,
126.59910194209));
#116057=CARTESIAN_POINT('Ctrl Pts',(6.22925225068398,-30.3585575131978,
126.627028396531));
#116058=CARTESIAN_POINT('Ctrl Pts',(6.22826047036556,-30.3437681206091,
126.630217265675));
#116059=CARTESIAN_POINT('Ctrl Pts',(6.22676348905146,-30.3216229043059,
126.634677457065));
#116060=CARTESIAN_POINT('Ctrl Pts',(6.22626641215246,-30.314298171416,126.636101566321));
#116061=CARTESIAN_POINT('Ctrl Pts',(6.22536452278877,-30.3010657002205,
126.638582149385));
#116062=CARTESIAN_POINT('Ctrl Pts',(6.22496068611918,-30.2951614856038,
126.639655973216));
#116063=CARTESIAN_POINT('Ctrl Pts',(6.22404633030813,-30.2818405099807,
126.642004432791));
#116064=CARTESIAN_POINT('Ctrl Pts',(6.22353483591524,-30.2744208960654,
126.643260720841));
#116065=CARTESIAN_POINT('Ctrl Pts',(6.2219648526068,-30.2517373153726,126.646943593896));
#116066=CARTESIAN_POINT('Ctrl Pts',(6.22089809026885,-30.2364483615836,
126.649207993917));
#116067=CARTESIAN_POINT('Ctrl Pts',(6.21544461656102,-30.158805719062,126.659605622754));
#116068=CARTESIAN_POINT('Ctrl Pts',(6.21092192441388,-30.0960638788738,
126.664415893714));
#116069=CARTESIAN_POINT('Ctrl Pts',(6.20137953052586,-29.9645776445958,
126.667037234323));
#116070=CARTESIAN_POINT('Ctrl Pts',(6.19636205424312,-29.8959270886012,
126.664162592765));
#116071=CARTESIAN_POINT('Ctrl Pts',(6.18526919213416,-29.7430576156658,
126.648262647192));
#116072=CARTESIAN_POINT('Ctrl Pts',(6.17924716673526,-29.6592535197048,
126.632998773393));
#116073=CARTESIAN_POINT('Ctrl Pts',(6.1720785295216,-29.5579450683226,126.606402919354));
#116074=CARTESIAN_POINT('Ctrl Pts',(6.17074302629156,-29.5390091900488,
126.601071651302));
#116075=CARTESIAN_POINT('Ctrl Pts',(6.1686210905763,-29.5088343485104,126.591996375173));
#116076=CARTESIAN_POINT('Ctrl Pts',(6.16782782025468,-29.4975336760191,
126.588465851555));
#116077=CARTESIAN_POINT('Ctrl Pts',(6.1663227564773,-29.4760595092905,126.581504853401));
#116078=CARTESIAN_POINT('Ctrl Pts',(6.16561030062586,-29.4658797137806,
126.578095931237));
#116079=CARTESIAN_POINT('Ctrl Pts',(6.16397949045133,-29.442550089541,126.570031898233));
#116080=CARTESIAN_POINT('Ctrl Pts',(6.16306340534582,-29.4294242362088,
126.565309516204));
#116081=CARTESIAN_POINT('Ctrl Pts',(6.16016537561502,-29.3878542613355,
126.549761200043));
#116082=CARTESIAN_POINT('Ctrl Pts',(6.15820383055342,-29.3596458006872,
126.53832014464));
#116083=CARTESIAN_POINT('Ctrl Pts',(6.1535755828014,-29.2931196045941,126.509190486473));
#116084=CARTESIAN_POINT('Ctrl Pts',(6.15093103753098,-29.255129008656,126.490806291018));
#116085=CARTESIAN_POINT('Ctrl Pts',(6.14362504959845,-29.1511081797027,
126.435498780649));
#116086=CARTESIAN_POINT('Ctrl Pts',(6.13903760215144,-29.086835209857,126.395494359554));
#116087=CARTESIAN_POINT('Ctrl Pts',(6.13372869077102,-29.0164700688166,
126.344748618992));
#116088=CARTESIAN_POINT('Ctrl Pts',(6.1330465013984,-29.007504775263,126.338145432928));
#116089=CARTESIAN_POINT('Ctrl Pts',(6.12776556764452,-28.9387599463996,
126.286442041436));
#116090=CARTESIAN_POINT('Ctrl Pts',(6.12311457543217,-28.8820236671828,
126.237452880374));
#116091=CARTESIAN_POINT('Ctrl Pts',(6.11742211172923,-28.8200469106952,
126.176187721045));
#116092=CARTESIAN_POINT('Ctrl Pts',(6.11661353930724,-28.8114082721725,
126.167457292948));
#116093=CARTESIAN_POINT('Ctrl Pts',(6.1153361518231,-28.7980335833544,126.153638175816));
#116094=CARTESIAN_POINT('Ctrl Pts',(6.11487221761166,-28.7932313154153,
126.148613792785));
#116095=CARTESIAN_POINT('Ctrl Pts',(6.11399968056643,-28.7843059688965,
126.139157873265));
#116096=CARTESIAN_POINT('Ctrl Pts',(6.11359165305245,-28.7801754214001,
126.134733726586));
#116097=CARTESIAN_POINT('Ctrl Pts',(6.11262565089614,-28.7704967715143,
126.124253206343));
#116098=CARTESIAN_POINT('Ctrl Pts',(6.11206619305883,-28.7649692482964,
126.118178204093));
#116099=CARTESIAN_POINT('Ctrl Pts',(6.11027255066844,-28.7474875722705,
126.0986772845));
#116100=CARTESIAN_POINT('Ctrl Pts',(6.10902700859033,-28.7357061518161,
126.085099146581));
#116101=CARTESIAN_POINT('Ctrl Pts',(6.1025554996016,-28.6762057392147,126.014240032712));
#116102=CARTESIAN_POINT('Ctrl Pts',(6.09715138893323,-28.632154729726,125.953997603251));
#116103=CARTESIAN_POINT('Ctrl Pts',(6.08526294993754,-28.5447743063688,
125.815945593676));
#116104=CARTESIAN_POINT('Ctrl Pts',(6.07879307504246,-28.5033359053839,
125.737189425107));
#116105=CARTESIAN_POINT('Ctrl Pts',(6.07046004283884,-28.4570812673408,
125.629111752382));
#116106=CARTESIAN_POINT('Ctrl Pts',(6.06844399518573,-28.4464731093221,
125.602439792326));
#116107=CARTESIAN_POINT('Ctrl Pts',(6.06644913825629,-28.4365599905855,
125.57550963238));
#116108=CARTESIAN_POINT('Origin',(5.,-30.,125.));
#116109=CARTESIAN_POINT('',(5.3678724416903,-28.4365599837785,125.575509613888));
#116110=CARTESIAN_POINT('',(5.55934601859666,-28.436559980232,125.575509604253));
#116111=CARTESIAN_POINT('',(5.,-28.4365599837785,125.575509613888));
#116112=CARTESIAN_POINT('Ctrl Pts',(5.55934601859666,-28.436559980232,125.575509604253));
#116113=CARTESIAN_POINT('Ctrl Pts',(5.56387671087001,-28.4589277274792,
125.636274239526));
#116114=CARTESIAN_POINT('Ctrl Pts',(5.56855161395396,-28.4848198285364,
125.695685446484));
#116115=CARTESIAN_POINT('Ctrl Pts',(5.5740981650682,-28.5193379989006,125.763760391978));
#116116=CARTESIAN_POINT('Ctrl Pts',(5.5749399462272,-28.5246784771278,125.774026033106));
#116117=CARTESIAN_POINT('Ctrl Pts',(5.58242649944295,-28.5731019919598,
125.864785151984));
#116118=CARTESIAN_POINT('Ctrl Pts',(5.58906862584462,-28.6226313221648,
125.941673974154));
#116119=CARTESIAN_POINT('Ctrl Pts',(5.59905977370649,-28.7086796213221,
126.053827427168));
#116120=CARTESIAN_POINT('Ctrl Pts',(5.6025380965924,-28.7409192708118,126.092143388595));
#116121=CARTESIAN_POINT('Ctrl Pts',(5.60706181648059,-28.7859235576508,
126.14098290456));
#116122=CARTESIAN_POINT('Ctrl Pts',(5.60816858031253,-28.79718560053,126.152849144488));
#116123=CARTESIAN_POINT('Ctrl Pts',(5.60930315698163,-28.8089881810292,
126.164923655471));
#116124=CARTESIAN_POINT('Ctrl Pts',(5.60933845108678,-28.8093555914467,
126.165299175485));
#116125=CARTESIAN_POINT('Ctrl Pts',(5.60940902617381,-28.8100907933492,
126.166049894289));
#116126=CARTESIAN_POINT('Ctrl Pts',(5.60944430715177,-28.810458584829,126.166425093025));
#116127=CARTESIAN_POINT('Ctrl Pts',(5.60948912068581,-28.8109260786037,
126.166901550967));
#116128=CARTESIAN_POINT('Ctrl Pts',(5.60949866045186,-28.811025616166,126.167002971196));
#116129=CARTESIAN_POINT('Ctrl Pts',(5.60951854566114,-28.811233137171,126.167214363172));
#116130=CARTESIAN_POINT('Ctrl Pts',(5.60952889101054,-28.8113411229734,
126.167324332746));
#116131=CARTESIAN_POINT('Ctrl Pts',(5.60955050534072,-28.8115667820757,
126.167554073577));
#116132=CARTESIAN_POINT('Ctrl Pts',(5.60956177419511,-28.8116844582179,
126.167673842026));
#116133=CARTESIAN_POINT('Ctrl Pts',(5.60958537820657,-28.8119310008479,
126.167924692368));
#116134=CARTESIAN_POINT('Ctrl Pts',(5.60959771320737,-28.8120598709518,
126.168055770752));
#116135=CARTESIAN_POINT('Ctrl Pts',(5.60962362388296,-28.8123306396708,
126.168331088123));
#116136=CARTESIAN_POINT('Ctrl Pts',(5.60963719934727,-28.8124725427914,
126.16847532251));
#116137=CARTESIAN_POINT('Ctrl Pts',(5.6096658065174,-28.8127716518829,126.168779234774));
#116138=CARTESIAN_POINT('Ctrl Pts',(5.60968083796983,-28.8129288638965,
126.16893890689));
#116139=CARTESIAN_POINT('Ctrl Pts',(5.60971262712999,-28.8132614421574,
126.169276553155));
#116140=CARTESIAN_POINT('Ctrl Pts',(5.6097293844874,-28.8134368161937,126.169454519536));
#116141=CARTESIAN_POINT('Ctrl Pts',(5.60976496866988,-28.8138093465418,
126.169832386489));
#116142=CARTESIAN_POINT('Ctrl Pts',(5.60978379502933,-28.8140065133557,
126.170032276678));
#116143=CARTESIAN_POINT('Ctrl Pts',(5.6098239608815,-28.8144273244565,126.17045868459));
#116144=CARTESIAN_POINT('Ctrl Pts',(5.60984529974307,-28.8146509832175,
126.170685188144));
#116145=CARTESIAN_POINT('Ctrl Pts',(5.60989107542949,-28.8151309751109,
126.171171006646));
#116146=CARTESIAN_POINT('Ctrl Pts',(5.60991551135984,-28.8153873285028,
126.171430301588));
#116147=CARTESIAN_POINT('Ctrl Pts',(5.60996826986791,-28.8159410784756,
126.171990037956));
#116148=CARTESIAN_POINT('Ctrl Pts',(5.60999659115661,-28.8162385044083,
126.172290450471));
#116149=CARTESIAN_POINT('Ctrl Pts',(5.61005821318731,-28.8168860140822,
126.172943964375));
#116150=CARTESIAN_POINT('Ctrl Pts',(5.61009151199381,-28.8172361416954,
126.173297022381));
#116151=CARTESIAN_POINT('Ctrl Pts',(5.61084441121101,-28.8251579027286,
126.181277935234));
#116152=CARTESIAN_POINT('Ctrl Pts',(5.61156074400305,-28.8328031636369,
126.188832649401));
#116153=CARTESIAN_POINT('Ctrl Pts',(5.61305714493872,-28.8489987124434,
126.204529541568));
#116154=CARTESIAN_POINT('Ctrl Pts',(5.61383650325648,-28.8575635475978,
126.212655905345));
#116155=CARTESIAN_POINT('Ctrl Pts',(5.61589324046518,-28.8805052743641,
126.233964335834));
#116156=CARTESIAN_POINT('Ctrl Pts',(5.61716383197746,-28.8950287745099,
126.246986393483));
#116157=CARTESIAN_POINT('Ctrl Pts',(5.62375586413986,-28.9721473883346,
126.313726892015));
#116158=CARTESIAN_POINT('Ctrl Pts',(5.62889417640534,-29.0384428790275,
126.363000267641));
#116159=CARTESIAN_POINT('Ctrl Pts',(5.64012856737408,-29.1929248389875,
126.460912683838));
#116160=CARTESIAN_POINT('Ctrl Pts',(5.64616505641996,-29.2824057093656,
126.506881637926));
#116161=CARTESIAN_POINT('Ctrl Pts',(5.65423287298559,-29.4017163655147,
126.555125064875));
#116162=CARTESIAN_POINT('Ctrl Pts',(5.65602732380753,-29.4282237334719,
126.565065172765));
#116163=CARTESIAN_POINT('Ctrl Pts',(5.65909730083182,-29.4732245688206,
126.580644431431));
#116164=CARTESIAN_POINT('Ctrl Pts',(5.66035646848474,-29.4915868580442,
126.586645887563));
#116165=CARTESIAN_POINT('Ctrl Pts',(5.66217592104807,-29.5179045951558,
126.594743736312));
#116166=CARTESIAN_POINT('Ctrl Pts',(5.66272213410759,-29.5257784073134,
126.597102826339));
#116167=CARTESIAN_POINT('Ctrl Pts',(5.66367653728221,-29.5394822716513,
126.601098400157));
#116168=CARTESIAN_POINT('Ctrl Pts',(5.66408319613472,-29.5453043114087,
126.602761521419));
#116169=CARTESIAN_POINT('Ctrl Pts',(5.66496073268302,-29.5578291318377,
126.606265618003));
#116170=CARTESIAN_POINT('Ctrl Pts',(5.6654321359787,-29.5645343039123,126.608096370046));
#116171=CARTESIAN_POINT('Ctrl Pts',(5.66674251172949,-29.583114826629,126.61304479057));
#116172=CARTESIAN_POINT('Ctrl Pts',(5.66758623139195,-29.595013208627,126.616073148363));
#116173=CARTESIAN_POINT('Ctrl Pts',(5.6734954828419,-29.67796922657,126.636213365583));
#116174=CARTESIAN_POINT('Ctrl Pts',(5.67876261169556,-29.7500451611886,
126.648762629497));
#116175=CARTESIAN_POINT('Ctrl Pts',(5.68510299049547,-29.836825261145,126.658050580784));
#116176=CARTESIAN_POINT('Ctrl Pts',(5.68613626212294,-29.8509662411422,
126.659381408442));
#116177=CARTESIAN_POINT('Ctrl Pts',(5.69253310073032,-29.9385672252456,
126.666496846603));
#116178=CARTESIAN_POINT('Ctrl Pts',(5.69789663062693,-30.0123315240616,
126.667583571493));
#116179=CARTESIAN_POINT('Ctrl Pts',(5.70619293750442,-30.1284269870043,
126.661587616317));
#116180=CARTESIAN_POINT('Ctrl Pts',(5.70919336109643,-30.170827989108,126.657765121979));
#116181=CARTESIAN_POINT('Ctrl Pts',(5.71427316607011,-30.2434150200868,
126.648406248613));
#116182=CARTESIAN_POINT('Ctrl Pts',(5.71637410222801,-30.2736787240765,
126.643652701305));
#116183=CARTESIAN_POINT('Ctrl Pts',(5.71939638259966,-30.3175465571194,
126.635516972178));
#116184=CARTESIAN_POINT('Ctrl Pts',(5.72033821661738,-30.3312648437227,
126.632793681469));
#116185=CARTESIAN_POINT('Ctrl Pts',(5.72199377552585,-30.3554571823847,
126.627673674398));
#116186=CARTESIAN_POINT('Ctrl Pts',(5.72270970956948,-30.3659452277947,
126.625347808435));
#116187=CARTESIAN_POINT('Ctrl Pts',(5.72420702992422,-30.3879308874943,
126.620248589306));
#116188=CARTESIAN_POINT('Ctrl Pts',(5.72498768954085,-30.3994229807926,
126.617453912535));
#116189=CARTESIAN_POINT('Ctrl Pts',(5.72705195250144,-30.429879945526,126.609702899502));
#116190=CARTESIAN_POINT('Ctrl Pts',(5.72832867699853,-30.4487891203636,
126.604533754795));
#116191=CARTESIAN_POINT('Ctrl Pts',(5.73491745995534,-30.5466439093596,
126.575918174931));
#116192=CARTESIAN_POINT('Ctrl Pts',(5.74004726074812,-30.6238670634926,
126.546974472556));
#116193=CARTESIAN_POINT('Ctrl Pts',(5.75127071968234,-30.7897471518108,
126.47034926399));
#116194=CARTESIAN_POINT('Ctrl Pts',(5.75730472599273,-30.8768584874213,
126.420121250978));
#116195=CARTESIAN_POINT('Ctrl Pts',(5.765369557475,-30.9820587448928,126.346074882379));
#116196=CARTESIAN_POINT('Ctrl Pts',(5.76716367680494,-31.0047819481238,
126.329199015752));
#116197=CARTESIAN_POINT('Ctrl Pts',(5.77023314394908,-31.0422710021246,
126.299846232284));
#116198=CARTESIAN_POINT('Ctrl Pts',(5.77149214028249,-31.057269986804,126.287675877856));
#116199=CARTESIAN_POINT('Ctrl Pts',(5.77331138812889,-31.0783446967249,
126.26995916137));
#116200=CARTESIAN_POINT('Ctrl Pts',(5.77385757210018,-31.0845967939543,
126.264623795458));
#116201=CARTESIAN_POINT('Ctrl Pts',(5.7748119424772,-31.095385740118,126.255277955183));
#116202=CARTESIAN_POINT('Ctrl Pts',(5.77521859794716,-31.0999406187617,
126.251288655058));
#116203=CARTESIAN_POINT('Ctrl Pts',(5.77609614865013,-31.1096777138217,
126.242666361985));
#116204=CARTESIAN_POINT('Ctrl Pts',(5.77656756969137,-31.1148526357052,
126.238025812338));
#116205=CARTESIAN_POINT('Ctrl Pts',(5.77787804170919,-31.1290884354201,
126.22509839484));
#116206=CARTESIAN_POINT('Ctrl Pts',(5.77872184097471,-31.1380867558584,
126.216743722423));
#116207=CARTESIAN_POINT('Ctrl Pts',(5.78465224986635,-31.2002211056147,
126.157761577216));
#116208=CARTESIAN_POINT('Ctrl Pts',(5.78994213002371,-31.2500478152111,
126.103775631436));
#116209=CARTESIAN_POINT('Ctrl Pts',(5.79628915138742,-31.3049340404179,
126.035808245437));
#116210=CARTESIAN_POINT('Ctrl Pts',(5.79730656214647,-31.3135827305999,
126.024818021595));
#116211=CARTESIAN_POINT('Ctrl Pts',(5.80368943377926,-31.3669443041776,
125.955223962102));
#116212=CARTESIAN_POINT('Ctrl Pts',(5.80905469631131,-31.4078677272737,
125.89381168292));
#116213=CARTESIAN_POINT('Ctrl Pts',(5.81734777316818,-31.465756668967,125.793044031523));
#116214=CARTESIAN_POINT('Ctrl Pts',(5.82034350862756,-31.485506661922,125.755401818718));
#116215=CARTESIAN_POINT('Ctrl Pts',(5.825416350126,-31.5169645549511,125.689427674944));
#116216=CARTESIAN_POINT('Ctrl Pts',(5.82751493078528,-31.5293695850263,
125.661453600573));
#116217=CARTESIAN_POINT('Ctrl Pts',(5.83053450396068,-31.5463105872289,
125.620221723893));
#116218=CARTESIAN_POINT('Ctrl Pts',(5.83147593444493,-31.5514604800356,
125.607224685383));
#116219=CARTESIAN_POINT('Ctrl Pts',(5.83313103835407,-31.5602772227666,
125.584128728075));
#116220=CARTESIAN_POINT('Ctrl Pts',(5.83384691682046,-31.5640110636554,
125.574056430066));
#116221=CARTESIAN_POINT('Ctrl Pts',(5.83534436914983,-31.5716515929452,
125.55281751416));
#116222=CARTESIAN_POINT('Ctrl Pts',(5.8361252139267,-31.5755372999715,125.541643944042));
#116223=CARTESIAN_POINT('Ctrl Pts',(5.8381905476821,-31.5855487314031,125.51183586277));
#116224=CARTESIAN_POINT('Ctrl Pts',(5.83946814475944,-31.5914650557284,
125.493132597964));
#116225=CARTESIAN_POINT('Ctrl Pts',(5.84608704699126,-31.620625500087,125.39495026224));
#116226=CARTESIAN_POINT('Ctrl Pts',(5.85124386845245,-31.6382520012093,
125.313919743571));
#116227=CARTESIAN_POINT('Ctrl Pts',(5.86246913978206,-31.6636950448597,
125.132917490952));
#116228=CARTESIAN_POINT('Ctrl Pts',(5.86848038039449,-31.6686714861518,
125.032884592881));
#116229=CARTESIAN_POINT('Ctrl Pts',(5.87651783294262,-31.6635169570918,
124.904787197624));
#116230=CARTESIAN_POINT('Ctrl Pts',(5.87830890381491,-31.6616632716858,
124.8765936146));
#116231=CARTESIAN_POINT('Ctrl Pts',(5.88137368146036,-31.6573392221696,
124.829252187381));
#116232=CARTESIAN_POINT('Ctrl Pts',(5.88263110168593,-31.6552511806857,
124.810074846506));
#116233=CARTESIAN_POINT('Ctrl Pts',(5.88444846607165,-31.6517998740989,
124.782788894));
#116234=CARTESIAN_POINT('Ctrl Pts',(5.88499438230133,-31.6507087391817,
124.774646632965));
#116235=CARTESIAN_POINT('Ctrl Pts',(5.88594845086659,-31.6487089190083,
124.760518145733));
#116236=CARTESIAN_POINT('Ctrl Pts',(5.88635507527444,-31.6478277469296,
124.754528263866));
#116237=CARTESIAN_POINT('Ctrl Pts',(5.88723275659524,-31.6458644240482,
124.741669502414));
#116238=CARTESIAN_POINT('Ctrl Pts',(5.88770434123275,-31.6447719336788,
124.734802658193));
#116239=CARTESIAN_POINT('Ctrl Pts',(5.88901570084698,-31.6416296636297,
124.715818584914));
#116240=CARTESIAN_POINT('Ctrl Pts',(5.88986023408982,-31.6394887905003,
124.703717174243));
#116241=CARTESIAN_POINT('Ctrl Pts',(5.89598295086757,-31.6231181001006,
124.616797935887));
#116242=CARTESIAN_POINT('Ctrl Pts',(5.90147988936187,-31.6039079215513,
124.543017509895));
#116243=CARTESIAN_POINT('Ctrl Pts',(5.90771780544969,-31.5766499887535,
124.46164660416));
#116244=CARTESIAN_POINT('Ctrl Pts',(5.90842150588969,-31.5734977018988,
124.45250155542));
#116245=CARTESIAN_POINT('Ctrl Pts',(5.91463667402113,-31.5449648643984,
124.372007670209));
#116246=CARTESIAN_POINT('Ctrl Pts',(5.92015091202742,-31.5148248629015,
124.3024343415));
#116247=CARTESIAN_POINT('Ctrl Pts',(5.92856624835229,-31.4606718669075,
124.197643409191));
#116248=CARTESIAN_POINT('Ctrl Pts',(5.9315420805563,-31.4398697219119,124.160884943123));
#116249=CARTESIAN_POINT('Ctrl Pts',(5.93658533760329,-31.4016978052337,
124.099041323859));
#116250=CARTESIAN_POINT('Ctrl Pts',(5.93867389843221,-31.3849954304947,
124.073570757555));
#116251=CARTESIAN_POINT('Ctrl Pts',(5.94168195137679,-31.3596340961814,
124.037115869749));
#116252=CARTESIAN_POINT('Ctrl Pts',(5.94262166163607,-31.3515211574746,
124.025761166212));
#116253=CARTESIAN_POINT('Ctrl Pts',(5.94427482736665,-31.3369141438955,
124.005851174607));
#116254=CARTESIAN_POINT('Ctrl Pts',(5.94499047036058,-31.3304783062755,
123.99725436875));
#116255=CARTESIAN_POINT('Ctrl Pts',(5.94648849271052,-31.3167715243964,
123.97930955603));
#116256=CARTESIAN_POINT('Ctrl Pts',(5.94727013273233,-31.3094831004363,
123.969975606245));
#116257=CARTESIAN_POINT('Ctrl Pts',(5.9493400654138,-31.2898229747473,123.94534378201));
#116258=CARTESIAN_POINT('Ctrl Pts',(5.95062140999309,-31.2772785396692,
123.930185703219));
#116259=CARTESIAN_POINT('Ctrl Pts',(5.95738993451073,-31.2090775466254,
123.850685167063));
#116260=CARTESIAN_POINT('Ctrl Pts',(5.96268129293519,-31.1488195097103,
123.790450709512));
#116261=CARTESIAN_POINT('Ctrl Pts',(5.97211489582155,-31.0321022020777,
123.690407567738));
#116262=CARTESIAN_POINT('Ctrl Pts',(5.97627484188539,-30.9772778145826,
123.649002173353));
#116263=CARTESIAN_POINT('Ctrl Pts',(5.98437098580799,-30.8676481578466,
123.576379748542));
#116264=CARTESIAN_POINT('Ctrl Pts',(5.98829093449839,-30.8133219704435,
123.544660308136));
#116265=CARTESIAN_POINT('Ctrl Pts',(5.9933738649866,-30.7435740464345,123.509063209239));
#116266=CARTESIAN_POINT('Ctrl Pts',(5.9943865547912,-30.7297111673908,123.502229507906));
#116267=CARTESIAN_POINT('Ctrl Pts',(5.99590905208018,-30.7089591788538,
123.492356297438));
#116268=CARTESIAN_POINT('Ctrl Pts',(5.99641032695816,-30.7021408462258,
123.489168812293));
#116269=CARTESIAN_POINT('Ctrl Pts',(5.99731651449941,-30.6898458835086,
123.48352227317));
#116270=CARTESIAN_POINT('Ctrl Pts',(5.99772040408426,-30.6843772391891,
123.481046468587));
#116271=CARTESIAN_POINT('Ctrl Pts',(5.99863069424564,-30.672077620677,123.475558001356));
#116272=CARTESIAN_POINT('Ctrl Pts',(5.99913802378278,-30.6652397721613,
123.472561694998));
#116273=CARTESIAN_POINT('Ctrl Pts',(6.00068204607961,-30.6444738457948,
123.463628070545));
#116274=CARTESIAN_POINT('Ctrl Pts',(6.00172663185114,-30.6304851862709,
123.457834758111));
#116275=CARTESIAN_POINT('Ctrl Pts',(6.01039377130432,-30.5147596914464,
123.411745435089));
#116276=CARTESIAN_POINT('Ctrl Pts',(6.01842867603435,-30.409365919462,123.381375223097));
#116277=CARTESIAN_POINT('Ctrl Pts',(6.03394527829849,-30.199303985209,123.342686399179));
#116278=CARTESIAN_POINT('Ctrl Pts',(6.04139989670306,-30.095283035604,123.333465123683));
#116279=CARTESIAN_POINT('Ctrl Pts',(6.05003539576169,-29.969467437326,123.33413977014));
#116280=CARTESIAN_POINT('Ctrl Pts',(6.05150504361922,-29.9478716090723,
123.334675632282));
#116281=CARTESIAN_POINT('Ctrl Pts',(6.05378762748829,-29.9140548488339,
123.33617324886));
#116282=CARTESIAN_POINT('Ctrl Pts',(6.05460933133339,-29.9018243733904,
123.33685010085));
#116283=CARTESIAN_POINT('Ctrl Pts',(6.05613894212797,-29.8789556658657,
123.338368838315));
#116284=CARTESIAN_POINT('Ctrl Pts',(6.05684782734328,-29.8683159780741,
123.339178162555));
#116285=CARTESIAN_POINT('Ctrl Pts',(6.05843184712057,-29.8444534132373,
123.34122406272));
#116286=CARTESIAN_POINT('Ctrl Pts',(6.05930518487314,-29.8312359708868,
123.342516645566));
#116287=CARTESIAN_POINT('Ctrl Pts',(6.06153703149892,-29.7973150966523,
123.346243872056));
#116288=CARTESIAN_POINT('Ctrl Pts',(6.06288832566957,-29.7766389808975,
123.348909324813));
#116289=CARTESIAN_POINT('Ctrl Pts',(6.07257998852718,-29.6275345315832,
123.370983372838));
#116290=CARTESIAN_POINT('Ctrl Pts',(6.08042704077471,-29.5017165019639,
123.404963027084));
#116291=CARTESIAN_POINT('Ctrl Pts',(6.09344431203597,-29.3042387870999,
123.483976163813));
#116292=CARTESIAN_POINT('Ctrl Pts',(6.09854832142122,-29.229772869255,123.520419457875));
#116293=CARTESIAN_POINT('Ctrl Pts',(6.10485235763993,-29.1461892512382,
123.569349360332));
#116294=CARTESIAN_POINT('Ctrl Pts',(6.10577638650614,-29.1341353518918,
123.576612341434));
#116295=CARTESIAN_POINT('Ctrl Pts',(6.10719082544782,-29.1160107174131,
123.587848606771));
#116296=CARTESIAN_POINT('Ctrl Pts',(6.10767437480609,-29.1098712051099,
123.591710494001));
#116297=CARTESIAN_POINT('Ctrl Pts',(6.1085635586109,-29.0986894110263,123.598846416347));
#116298=CARTESIAN_POINT('Ctrl Pts',(6.10896837742722,-29.0936393785891,
123.602107814244));
#116299=CARTESIAN_POINT('Ctrl Pts',(6.10990048498639,-29.0821041072831,
123.609646275242));
#116300=CARTESIAN_POINT('Ctrl Pts',(6.11042892926396,-29.0756310736528,
123.613941403914));
#116301=CARTESIAN_POINT('Ctrl Pts',(6.11206447971331,-29.0557940126292,
123.627304882392));
#116302=CARTESIAN_POINT('Ctrl Pts',(6.11318061534033,-29.0425320701174,
123.636522113214));
#116303=CARTESIAN_POINT('Ctrl Pts',(6.12028371876759,-28.9597281500227,
123.695875715826));
#116304=CARTESIAN_POINT('Ctrl Pts',(6.12651987594059,-28.8940149442416,
123.751120491557));
#116305=CARTESIAN_POINT('Ctrl Pts',(6.13647447605889,-28.7964324388262,
123.846923358677));
#116306=CARTESIAN_POINT('Ctrl Pts',(6.14018735931351,-28.7616753258736,
123.884332955355));
#116307=CARTESIAN_POINT('Ctrl Pts',(6.14767734478265,-28.6944288972366,
123.963732527376));
#116308=CARTESIAN_POINT('Ctrl Pts',(6.15144707800656,-28.6621160872555,
124.005799963437));
#116309=CARTESIAN_POINT('Ctrl Pts',(6.15764471505079,-28.6114389279093,
124.078731794292));
#116310=CARTESIAN_POINT('Ctrl Pts',(6.16010934781647,-28.591967208349,124.108775587284));
#116311=CARTESIAN_POINT('Ctrl Pts',(6.16354511030201,-28.5658158918386,
124.152125057064));
#116312=CARTESIAN_POINT('Ctrl Pts',(6.16454545768899,-28.5583243549196,
124.164926749288));
#116313=CARTESIAN_POINT('Ctrl Pts',(6.16626810636348,-28.5456411601574,
124.187279580959));
#116314=CARTESIAN_POINT('Ctrl Pts',(6.16699322149103,-28.5403702800372,
124.196784459317));
#116315=CARTESIAN_POINT('Ctrl Pts',(6.16838576952037,-28.5303815074185,
124.215220105879));
#116316=CARTESIAN_POINT('Ctrl Pts',(6.16905362342998,-28.525651092268,124.224143504363));
#116317=CARTESIAN_POINT('Ctrl Pts',(6.1708190435125,-28.5133096692025,124.247944738807));
#116318=CARTESIAN_POINT('Ctrl Pts',(6.17191160988917,-28.5058407407028,
124.262895260788));
#116319=CARTESIAN_POINT('Ctrl Pts',(6.17597884358671,-28.4786947299313,
124.319342077429));
#116320=CARTESIAN_POINT('Ctrl Pts',(6.17890271693425,-28.4605101785177,
124.361535749782));
#116321=CARTESIAN_POINT('Ctrl Pts',(6.18882374878948,-28.4039846192959,
124.509207109504));
#116322=CARTESIAN_POINT('Ctrl Pts',(6.19556586069116,-28.374564794865,124.617764990719));
#116323=CARTESIAN_POINT('Ctrl Pts',(6.20539762039084,-28.3485178108549,
124.77543452399));
#116324=CARTESIAN_POINT('Ctrl Pts',(6.20835465869034,-28.3427751774363,
124.822719603926));
#116325=CARTESIAN_POINT('Ctrl Pts',(6.21314911311099,-28.3369089056542,
124.897774693167));
#116326=CARTESIAN_POINT('Ctrl Pts',(6.21493631096052,-28.3354403449275,
124.925414848332));
#116327=CARTESIAN_POINT('Ctrl Pts',(6.21737766336993,-28.3343957306038,
124.962488970179));
#116328=CARTESIAN_POINT('Ctrl Pts',(6.21800139367624,-28.3342103356652,
124.971902962946));
#116329=CARTESIAN_POINT('Ctrl Pts',(6.21904706341704,-28.3340345460499,
124.98757811068));
#116330=CARTESIAN_POINT('Ctrl Pts',(6.21946658871795,-28.3339996297195,
124.993838730686));
#116331=CARTESIAN_POINT('Ctrl Pts',(6.22032415080722,-28.3340003890238,
125.00657498276));
#116332=CARTESIAN_POINT('Ctrl Pts',(6.220762302291,-28.3340385309373,125.013050446491));
#116333=CARTESIAN_POINT('Ctrl Pts',(6.22191082718516,-28.3342365605299,
125.029946127955));
#116334=CARTESIAN_POINT('Ctrl Pts',(6.2226243540981,-28.3344564712401,125.040365167481));
#116335=CARTESIAN_POINT('Ctrl Pts',(6.22591359864517,-28.3359113208777,
125.088072924458));
#116336=CARTESIAN_POINT('Ctrl Pts',(6.22854275201821,-28.3383008200076,
125.125312927896));
#116337=CARTESIAN_POINT('Ctrl Pts',(6.23683045955873,-28.3496178692986,
125.240830095917));
#116338=CARTESIAN_POINT('Ctrl Pts',(6.24259339284647,-28.3628473382319,
125.318576038942));
#116339=CARTESIAN_POINT('Ctrl Pts',(6.25289099295345,-28.3964544071425,
125.456245786719));
#116340=CARTESIAN_POINT('Ctrl Pts',(6.2574309774459,-28.4148310450808,125.516480354484));
#116341=CARTESIAN_POINT('Ctrl Pts',(6.2618827045692,-28.4365599067946,125.575509404752));
#116342=CARTESIAN_POINT('',(6.02851963656825,-28.3340006962934,124.998476829274));
#116343=CARTESIAN_POINT('Ctrl Pts',(6.06644913825629,-28.4365599905855,
125.57550963238));
#116344=CARTESIAN_POINT('Ctrl Pts',(6.0647519761627,-28.4281262181678,125.552598291741));
#116345=CARTESIAN_POINT('Ctrl Pts',(6.06307012626867,-28.4201955224898,
125.529500065226));
#116346=CARTESIAN_POINT('Ctrl Pts',(6.06021111114331,-28.4074578948752,
125.489562813823));
#116347=CARTESIAN_POINT('Ctrl Pts',(6.05902639191263,-28.4024043292916,
125.472810975716));
#116348=CARTESIAN_POINT('Ctrl Pts',(6.0570853241414,-28.3945009537609,125.445037411799));
#116349=CARTESIAN_POINT('Ctrl Pts',(6.056324082195,-28.3914986397866,125.434060906635));
#116350=CARTESIAN_POINT('Ctrl Pts',(6.05483979642889,-28.3858373294429,
125.412497278553));
#116351=CARTESIAN_POINT('Ctrl Pts',(6.05411649930734,-28.3831694592067,
125.401913104826));
#116352=CARTESIAN_POINT('Ctrl Pts',(6.0526836420675,-28.3780674746594,125.380798727961));
#116353=CARTESIAN_POINT('Ctrl Pts',(6.05197405189187,-28.3756314279088,
125.370269549237));
#116354=CARTESIAN_POINT('Ctrl Pts',(6.05031190153342,-28.3701410357475,
125.345441067135));
#116355=CARTESIAN_POINT('Ctrl Pts',(6.04936204384721,-28.3671721072557,
125.331123645304));
#116356=CARTESIAN_POINT('Ctrl Pts',(6.04151867578899,-28.3440813688305,
125.211896568066));
#116357=CARTESIAN_POINT('Ctrl Pts',(6.03495492927364,-28.3339033738713,
125.105313603942));
#116358=CARTESIAN_POINT('Ctrl Pts',(6.02842899135889,-28.3340006912401,
124.99848236646));
#116359=CARTESIAN_POINT('Ctrl Pts',(6.02851963656825,-28.3340006962934,
124.998476829274));
#116360=CARTESIAN_POINT('Ctrl Pts',(6.02319560875472,-28.3340734949187,
124.918851835839));
#116361=CARTESIAN_POINT('Ctrl Pts',(6.01787158094119,-28.3398584615601,
124.839481023852));
#116362=CARTESIAN_POINT('Ctrl Pts',(6.01254755312766,-28.3512247099835,
124.761052216937));
#116363=CARTESIAN_POINT('Ctrl Pts',(6.00879991051251,-28.359225539141,124.705845304173));
#116364=CARTESIAN_POINT('Ctrl Pts',(6.00505226789736,-28.3699908306089,
124.651104499726));
#116365=CARTESIAN_POINT('Ctrl Pts',(6.00130462528221,-28.3834612365898,
124.597062751297));
#116366=CARTESIAN_POINT('Ctrl Pts',(5.99722727558203,-28.3981167311039,
124.538266561431));
#116367=CARTESIAN_POINT('Ctrl Pts',(5.99314992588185,-28.4160144422315,
124.480149579522));
#116368=CARTESIAN_POINT('Ctrl Pts',(5.98907257618167,-28.4370742327457,
124.423095288585));
#116369=CARTESIAN_POINT('Ctrl Pts',(5.98495160860925,-28.4583593125581,
124.365430653441));
#116370=CARTESIAN_POINT('Ctrl Pts',(5.98083064103684,-28.4828744868681,
124.308852114328));
#116371=CARTESIAN_POINT('Ctrl Pts',(5.97670967346442,-28.5104841015508,
124.253743751606));
#116372=CARTESIAN_POINT('Ctrl Pts',(5.97264355643894,-28.5377262291229,
124.199368887458));
#116373=CARTESIAN_POINT('Ctrl Pts',(5.96857743941347,-28.5679806888366,
124.146425773315));
#116374=CARTESIAN_POINT('Ctrl Pts',(5.96451132238799,-28.6010683663941,
124.095264522362));
#116375=CARTESIAN_POINT('Ctrl Pts',(5.96044769316854,-28.634135799644,124.04413457382));
#116376=CARTESIAN_POINT('Ctrl Pts',(5.9563840639491,-28.6700327363219,123.994784755901));
#116377=CARTESIAN_POINT('Ctrl Pts',(5.95232043472965,-28.7085351232899,
123.947538850017));
#116378=CARTESIAN_POINT('Ctrl Pts',(5.9482577821129,-28.7470282570674,123.900304298633));
#116379=CARTESIAN_POINT('Ctrl Pts',(5.94419512949615,-28.7881252748384,
123.855173052227));
#116380=CARTESIAN_POINT('Ctrl Pts',(5.94013247687939,-28.8315612467258,
123.8124365786));
#116381=CARTESIAN_POINT('Ctrl Pts',(5.93596888334308,-28.876076431472,123.768638271891));
#116382=CARTESIAN_POINT('Ctrl Pts',(5.93180528980677,-28.9230479927252,
123.727355765403));
#116383=CARTESIAN_POINT('Ctrl Pts',(5.92764169627046,-28.9721516994952,
123.68886161251));
#116384=CARTESIAN_POINT('Ctrl Pts',(5.92357385644441,-29.0201261264568,
123.65125274247));
#116385=CARTESIAN_POINT('Ctrl Pts',(5.91950601661836,-29.0701351964431,
123.616305575435));
#116386=CARTESIAN_POINT('Ctrl Pts',(5.91543817679231,-29.121846243511,123.584230958113));
#116387=CARTESIAN_POINT('Ctrl Pts',(5.91122670640087,-29.1753831458841,
123.551023824366));
#116388=CARTESIAN_POINT('Ctrl Pts',(5.90701523600943,-29.2307439592215,
123.520896213987));
#116389=CARTESIAN_POINT('Ctrl Pts',(5.90280376561798,-29.2875334118873,
123.494029428965));
#116390=CARTESIAN_POINT('Ctrl Pts',(5.89859229522654,-29.3443228645532,
123.467162643943));
#116391=CARTESIAN_POINT('Ctrl Pts',(5.8943808248351,-29.4025403724686,123.443556842906));
#116392=CARTESIAN_POINT('Ctrl Pts',(5.89016935444365,-29.4617725659751,
123.423336678532));
#116393=CARTESIAN_POINT('Ctrl Pts',(5.88609200474355,-29.5191184200315,
123.4037604561));
#116394=CARTESIAN_POINT('Ctrl Pts',(5.88201465504344,-29.5776521037458,
123.387276539074));
#116395=CARTESIAN_POINT('Ctrl Pts',(5.87793730534333,-29.6370079727795,
123.374025588094));
#116396=CARTESIAN_POINT('Ctrl Pts',(5.8738163377709,-29.696998807393,123.360632883687));
#116397=CARTESIAN_POINT('Ctrl Pts',(5.86969537019848,-29.7578290526703,
123.350542981847));
#116398=CARTESIAN_POINT('Ctrl Pts',(5.86557440262605,-29.8191024520453,
123.343850225027));
#116399=CARTESIAN_POINT('Ctrl Pts',(5.86150828560065,-29.8795602955066,
123.337246549561));
#116400=CARTESIAN_POINT('Ctrl Pts',(5.85744216857525,-29.9404490441904,
123.333950195322));
#116401=CARTESIAN_POINT('Ctrl Pts',(5.85337605154985,-30.0013774075983,
123.334000569403));
#116402=CARTESIAN_POINT('Ctrl Pts',(5.84931242233048,-30.0622684927014,
123.334050912664));
#116403=CARTESIAN_POINT('Ctrl Pts',(5.84524879311111,-30.1231986335682,
123.33744392392));
#116404=CARTESIAN_POINT('Ctrl Pts',(5.84118516389174,-30.1837742889544,
123.34416697378));
#116405=CARTESIAN_POINT('Ctrl Pts',(5.83712251127506,-30.2443353863322,
123.350888407906));
#116406=CARTESIAN_POINT('Ctrl Pts',(5.83305985865839,-30.3045416587418,
123.360938235477));
#116407=CARTESIAN_POINT('Ctrl Pts',(5.82899720604172,-30.3640045429381,
123.374251959029));
#116408=CARTESIAN_POINT('Ctrl Pts',(5.82483361250533,-30.4249448456552,
123.387896476186));
#116409=CARTESIAN_POINT('Ctrl Pts',(5.82067001896895,-30.4851037654203,
123.404969181928));
#116410=CARTESIAN_POINT('Ctrl Pts',(5.81650642543256,-30.544076467027,123.425345498839));
#116411=CARTESIAN_POINT('Ctrl Pts',(5.81243858560659,-30.601692923135,123.445253204217));
#116412=CARTESIAN_POINT('Ctrl Pts',(5.80837074578062,-30.6581766839114,
123.468313913943));
#116413=CARTESIAN_POINT('Ctrl Pts',(5.80430290595464,-30.7131701817936,
123.494362496548));
#116414=CARTESIAN_POINT('Ctrl Pts',(5.80009143556305,-30.7701054344017,
123.521330823493));
#116415=CARTESIAN_POINT('Ctrl Pts',(5.79587996517146,-30.82544266909,123.551501720361));
#116416=CARTESIAN_POINT('Ctrl Pts',(5.79166849477987,-30.8788151850225,
123.584641433921));
#116417=CARTESIAN_POINT('Ctrl Pts',(5.78745702438828,-30.932187700955,123.617781147481));
#116418=CARTESIAN_POINT('Ctrl Pts',(5.78324555399669,-30.9835950480775,
123.653889273056));
#116419=CARTESIAN_POINT('Ctrl Pts',(5.7790340836051,-31.0327083033886,123.692686127928));
#116420=CARTESIAN_POINT('Ctrl Pts',(5.77495673390501,-31.0802574722521,
123.730247437842));
#116421=CARTESIAN_POINT('Ctrl Pts',(5.77087938420491,-31.1258528967944,
123.770483850586));
#116422=CARTESIAN_POINT('Ctrl Pts',(5.76680203450482,-31.1691780895278,
123.813164461702));
#116423=CARTESIAN_POINT('Ctrl Pts',(5.76268106693239,-31.212966758015,123.856301653092));
#116424=CARTESIAN_POINT('Ctrl Pts',(5.75856009935996,-31.2544358643982,
123.901935391438));
#116425=CARTESIAN_POINT('Ctrl Pts',(5.75443913178754,-31.2932912321427,
123.949783932296));
#116426=CARTESIAN_POINT('Ctrl Pts',(5.75037301476215,-31.3316294305236,
123.996995603634));
#116427=CARTESIAN_POINT('Ctrl Pts',(5.74630689773677,-31.3674227117968,
124.046363069472));
#116428=CARTESIAN_POINT('Ctrl Pts',(5.74224078071139,-31.4004257464336,
124.097578962609));
#116429=CARTESIAN_POINT('Ctrl Pts',(5.73817715149204,-31.4334085885506,
124.148763519902));
#116430=CARTESIAN_POINT('Ctrl Pts',(5.73411352227268,-31.4636042921268,
124.201793832714));
#116431=CARTESIAN_POINT('Ctrl Pts',(5.73004989305333,-31.4908100250261,
124.256332420176));
#116432=CARTESIAN_POINT('Ctrl Pts',(5.72598724043667,-31.518009219634,124.310857900503));
#116433=CARTESIAN_POINT('Ctrl Pts',(5.72192458782002,-31.5422196416099,
124.366890477986));
#116434=CARTESIAN_POINT('Ctrl Pts',(5.71786193520336,-31.5632847353325,
124.42406872261));
#116435=CARTESIAN_POINT('Ctrl Pts',(5.71369834166696,-31.5848732136847,
124.482667621457));
#116436=CARTESIAN_POINT('Ctrl Pts',(5.70953474813056,-31.6031577274293,
124.542469372818));
#116437=CARTESIAN_POINT('Ctrl Pts',(5.70537115459415,-31.6180233714039,
124.603066290685));
#116438=CARTESIAN_POINT('Ctrl Pts',(5.7013033147682,-31.6325471374895,124.662269609566));
#116439=CARTESIAN_POINT('Ctrl Pts',(5.69723547494225,-31.643807594015,124.72223137808));
#116440=CARTESIAN_POINT('Ctrl Pts',(5.6931676351163,-31.651749543316,124.782561626764));
#116441=CARTESIAN_POINT('Ctrl Pts',(5.68895616472467,-31.659971913361,124.845022064472));
#116442=CARTESIAN_POINT('Ctrl Pts',(5.68474469433304,-31.6646369573864,
124.907876896626));
#116443=CARTESIAN_POINT('Ctrl Pts',(5.68053322394141,-31.6657421763008,
124.970691262523));
#116444=CARTESIAN_POINT('Ctrl Pts',(5.67632175354978,-31.6668473952153,
125.03350562842));
#116445=CARTESIAN_POINT('Ctrl Pts',(5.67211028315816,-31.6643928849113,
125.096278930468));
#116446=CARTESIAN_POINT('Ctrl Pts',(5.66789881276653,-31.6584352230018,
125.158583136263));
#116447=CARTESIAN_POINT('Ctrl Pts',(5.66382146306639,-31.6526672919133,
125.218903169694));
#116448=CARTESIAN_POINT('Ctrl Pts',(5.65974411336626,-31.6435922496629,
125.279032657119));
#116449=CARTESIAN_POINT('Ctrl Pts',(5.65566676366613,-31.6312324376956,
125.338580469327));
#116450=CARTESIAN_POINT('Ctrl Pts',(5.6515457960937,-31.6187404053549,125.398765300447));
#116451=CARTESIAN_POINT('Ctrl Pts',(5.64742482852128,-31.6028928679922,
125.458355403813));
#116452=CARTESIAN_POINT('Ctrl Pts',(5.64330386094886,-31.5837669805991,
125.516950820837));
#116453=CARTESIAN_POINT('Ctrl Pts',(5.63923774392343,-31.564895660942,125.574766326198));
#116454=CARTESIAN_POINT('Ctrl Pts',(5.63517162689801,-31.542832892783,125.631612961355));
#116455=CARTESIAN_POINT('Ctrl Pts',(5.63110550987258,-31.5177038507697,
125.687117909357));
#116456=CARTESIAN_POINT('Ctrl Pts',(5.62704188065318,-31.4925901836661,
125.742588897307));
#116457=CARTESIAN_POINT('Ctrl Pts',(5.62297825143379,-31.4644141731075,
125.796719360269));
#116458=CARTESIAN_POINT('Ctrl Pts',(5.61891462221439,-31.4333493426061,
125.849155852627));
#116459=CARTESIAN_POINT('Ctrl Pts',(5.61485196959769,-31.4022919778441,
125.901579743043));
#116460=CARTESIAN_POINT('Ctrl Pts',(5.61078931698099,-31.3683474321801,
125.952310030756));
#116461=CARTESIAN_POINT('Ctrl Pts',(5.60672666436429,-31.3317344485663,
126.001019159907));
#116462=CARTESIAN_POINT('Ctrl Pts',(5.60256307082793,-31.2942117764839,
126.050938519112));
#116463=CARTESIAN_POINT('Ctrl Pts',(5.59839947729157,-31.2538865838682,
126.098734457738));
#116464=CARTESIAN_POINT('Ctrl Pts',(5.59423588375521,-31.2110390650589,
126.144089324704));
#116465=CARTESIAN_POINT('Ctrl Pts',(5.59016804392921,-31.1691769471707,
126.188401127125));
#116466=CARTESIAN_POINT('Ctrl Pts',(5.58610020410322,-31.1249077208041,
126.230382636882));
#116467=CARTESIAN_POINT('Ctrl Pts',(5.58203236427722,-31.0785290790597,
126.269775974581));
#116468=CARTESIAN_POINT('Ctrl Pts',(5.57782089388568,-31.030512862871,126.310560243982));
#116469=CARTESIAN_POINT('Ctrl Pts',(5.57360942349414,-30.9802359328558,
126.348569754225));
#116470=CARTESIAN_POINT('Ctrl Pts',(5.5693979531026,-30.9280622790153,126.383566552888));
#116471=CARTESIAN_POINT('Ctrl Pts',(5.56518648271105,-30.8758886251748,
126.41856335155));
#116472=CARTESIAN_POINT('Ctrl Pts',(5.56097501231951,-30.8218188015804,
126.450547195083));
#116473=CARTESIAN_POINT('Ctrl Pts',(5.55676354192797,-30.7662431025642,
126.479333467401));
#116474=CARTESIAN_POINT('Ctrl Pts',(5.55268619222786,-30.7124372963612,
126.507202997017));
#116475=CARTESIAN_POINT('Ctrl Pts',(5.54860884252774,-30.6569979178379,
126.532190733182));
#116476=CARTESIAN_POINT('Ctrl Pts',(5.54453149282763,-30.6002656888768,
126.554103311481));
#116477=CARTESIAN_POINT('Ctrl Pts',(5.5404105252552,-30.5429265609983,126.576250301866));
#116478=CARTESIAN_POINT('Ctrl Pts',(5.53628955768278,-30.484267184399,126.595255627346));
#116479=CARTESIAN_POINT('Ctrl Pts',(5.53216859011035,-30.4246654278064,
126.610967186018));
#116480=CARTESIAN_POINT('Ctrl Pts',(5.52810247308495,-30.3658569773718,
126.626469622057));
#116481=CARTESIAN_POINT('Ctrl Pts',(5.52403635605954,-30.3061315899492,
126.638765302794));
#116482=CARTESIAN_POINT('Ctrl Pts',(5.51997023903413,-30.2458703755337,
126.647757190376));
#116483=CARTESIAN_POINT('Ctrl Pts',(5.51590660981476,-30.1856460312358,
126.656743576377));
#116484=CARTESIAN_POINT('Ctrl Pts',(5.51184298059538,-30.124887015264,126.662430101641));
#116485=CARTESIAN_POINT('Ctrl Pts',(5.507779351376,-30.0639843855967,126.664770854622));
#116486=CARTESIAN_POINT('Ctrl Pts',(5.50371669875932,-30.0030963925188,
126.667111045055));
#116487=CARTESIAN_POINT('Ctrl Pts',(5.49965404614264,-29.942065365614,126.66610703977));
#116488=CARTESIAN_POINT('Ctrl Pts',(5.49559139352596,-29.8812851371463,
126.661764959715));
#116489=CARTESIAN_POINT('Ctrl Pts',(5.49142779998959,-29.8189947593402,
126.65731499607));
#116490=CARTESIAN_POINT('Ctrl Pts',(5.48726420645321,-29.7569683731697,
126.64935884579));
#116491=CARTESIAN_POINT('Ctrl Pts',(5.48310061291683,-29.6956248184908,
126.637959629808));
#116492=CARTESIAN_POINT('Ctrl Pts',(5.47903277309085,-29.6356920338398,
126.626822571315));
#116493=CARTESIAN_POINT('Ctrl Pts',(5.47496493326487,-29.5764115003722,
126.612399329089));
#116494=CARTESIAN_POINT('Ctrl Pts',(5.47089709343889,-29.5181613318449,
126.594800143551));
#116495=CARTESIAN_POINT('Ctrl Pts',(5.46668562304731,-29.4578544194412,
126.576579551792));
#116496=CARTESIAN_POINT('Ctrl Pts',(5.46247415265573,-29.3986525730831,
126.554954706161));
#116497=CARTESIAN_POINT('Ctrl Pts',(5.45826268226415,-29.3409531220702,
126.530102353665));
#116498=CARTESIAN_POINT('Ctrl Pts',(5.45405121187257,-29.2832536710573,
126.505250001169));
#116499=CARTESIAN_POINT('Ctrl Pts',(5.44983974148099,-29.2270571205141,
126.477170475215));
#116500=CARTESIAN_POINT('Ctrl Pts',(5.44562827108941,-29.1727302560843,
126.446091549938));
#116501=CARTESIAN_POINT('Ctrl Pts',(5.44155183031644,-29.1201452383499,
126.4160090879));
#116502=CARTESIAN_POINT('Ctrl Pts',(5.43747538954347,-29.0690946646957,
126.382992519672));
#116503=CARTESIAN_POINT('Ctrl Pts',(5.43339894877049,-29.0199255545782,
126.347223100096));
#116504=CARTESIAN_POINT('Ctrl Pts',(5.42932840898429,-28.9708276208335,
126.311505459726));
#116505=CARTESIAN_POINT('Ctrl Pts',(5.42525786919808,-28.9236061619891,
126.273043165973));
#116506=CARTESIAN_POINT('Ctrl Pts',(5.42118732941187,-28.8785820263563,
126.232062388188));
#116507=CARTESIAN_POINT('Ctrl Pts',(5.41712116917619,-28.8336063328189,
126.191125702195));
#116508=CARTESIAN_POINT('Ctrl Pts',(5.41305500894051,-28.7908236503885,
126.147676249286));
#116509=CARTESIAN_POINT('Ctrl Pts',(5.40898884870483,-28.7505226465905,
126.101981099346));
#116510=CARTESIAN_POINT('Ctrl Pts',(5.40492500380744,-28.7102445908447,
126.056311968974));
#116511=CARTESIAN_POINT('Ctrl Pts',(5.40086115891004,-28.6724457521372,
126.008400058139));
#116512=CARTESIAN_POINT('Ctrl Pts',(5.39679731401265,-28.6373773381303,
125.958548632756));
#116513=CARTESIAN_POINT('Ctrl Pts',(5.392734798567,-28.602320396452,125.908713515837));
#116514=CARTESIAN_POINT('Ctrl Pts',(5.38867228312134,-28.5699923969535,
125.856940565118));
#116515=CARTESIAN_POINT('Ctrl Pts',(5.38460976767569,-28.54060233297,125.803563593916));
#116516=CARTESIAN_POINT('Ctrl Pts',(5.38054576390131,-28.5112015017471,
125.750167067717));
#116517=CARTESIAN_POINT('Ctrl Pts',(5.37648176012692,-28.4847409988668,
125.695165798197));
#116518=CARTESIAN_POINT('Ctrl Pts',(5.37241775635254,-28.4613839509542,
125.638918346597));
#116519=CARTESIAN_POINT('Ctrl Pts',(5.37090265146513,-28.4526761890001,
125.617948683783));
#116520=CARTESIAN_POINT('Ctrl Pts',(5.36938754657771,-28.4443992926494,
125.596806024743));
#116521=CARTESIAN_POINT('Ctrl Pts',(5.3678724416903,-28.4365599837785,125.575509613888));
#116522=CARTESIAN_POINT('Origin',(5.,-30.,125.));
#116523=CARTESIAN_POINT('',(4.66781556895434,-28.4339562630661,125.576468403481));
#116524=CARTESIAN_POINT('',(4.86075486118656,-28.4365599784656,125.575509599455));
#116525=CARTESIAN_POINT('',(5.,-28.4365599837785,125.575509613888));
#116526=CARTESIAN_POINT('',(5.52205821453768,-28.3340005850234,125.001396172494));
#116527=CARTESIAN_POINT('Ctrl Pts',(4.86075486118656,-28.4365599784656,
125.575509599455));
#116528=CARTESIAN_POINT('Ctrl Pts',(4.86238043919705,-28.4457530879321,
125.600483770652));
#116529=CARTESIAN_POINT('Ctrl Pts',(4.86400410782707,-28.4555447508684,
125.625238079615));
#116530=CARTESIAN_POINT('Ctrl Pts',(4.86651230638005,-28.471533401758,125.662987554203));
#116531=CARTESIAN_POINT('Ctrl Pts',(4.86739308927612,-28.4773107607449,
125.676150954234));
#116532=CARTESIAN_POINT('Ctrl Pts',(4.87273750404912,-28.5132941123096,
125.755336207118));
#116533=CARTESIAN_POINT('Ctrl Pts',(4.87725398811927,-28.547615579312,125.819392473812));
#116534=CARTESIAN_POINT('Ctrl Pts',(4.88279718916779,-28.592490550416,125.891416759702));
#116535=CARTESIAN_POINT('Ctrl Pts',(4.88360534816387,-28.5990967308248,
125.901763105706));
#116536=CARTESIAN_POINT('Ctrl Pts',(4.88488230900459,-28.6096212186161,
125.917851376678));
#116537=CARTESIAN_POINT('Ctrl Pts',(4.88534623716257,-28.6134623137335,
125.923643624771));
#116538=CARTESIAN_POINT('Ctrl Pts',(4.88621893813826,-28.6207175626951,
125.934437063524));
#116539=CARTESIAN_POINT('Ctrl Pts',(4.88662713725671,-28.6241228851158,
125.939443892735));
#116540=CARTESIAN_POINT('Ctrl Pts',(4.88759380217016,-28.6322155109139,
125.951204063062));
#116541=CARTESIAN_POINT('Ctrl Pts',(4.88815375538808,-28.6369255886961,
125.957941397128));
#116542=CARTESIAN_POINT('Ctrl Pts',(4.89004013162794,-28.6528735222028,
125.98039768879));
#116543=CARTESIAN_POINT('Ctrl Pts',(4.89138013178083,-28.6643344913381,
125.995955292534));
#116544=CARTESIAN_POINT('Ctrl Pts',(4.89471664534451,-28.6932522011111,
126.033812390676));
#116545=CARTESIAN_POINT('Ctrl Pts',(4.89672778407849,-28.7110116039955,
126.055872436836));
#116546=CARTESIAN_POINT('Ctrl Pts',(4.90595650221888,-28.7943058631281,
126.154102798447));
#116547=CARTESIAN_POINT('Ctrl Pts',(4.91334705981141,-28.8660872086386,
126.22470155148));
#116548=CARTESIAN_POINT('Ctrl Pts',(4.92651682306763,-29.0073635626406,
126.340517048636));
#116549=CARTESIAN_POINT('Ctrl Pts',(4.93232985908405,-29.0747113701787,
126.387860820313));
#116550=CARTESIAN_POINT('Ctrl Pts',(4.93929776894664,-29.1621105600168,
126.440097673046));
#116551=CARTESIAN_POINT('Ctrl Pts',(4.94062817726602,-29.1791082423171,
126.449854061832));
#116552=CARTESIAN_POINT('Ctrl Pts',(4.94274416254166,-29.206633147188,126.465013610755));
#116553=CARTESIAN_POINT('Ctrl Pts',(4.94353650619432,-29.2170522097914,
126.470608245974));
#116554=CARTESIAN_POINT('Ctrl Pts',(4.94504113085666,-29.2370482583143,
126.481072599086));
#116555=CARTESIAN_POINT('Ctrl Pts',(4.94575406081811,-29.2466144604934,
126.485961521032));
#116556=CARTESIAN_POINT('Ctrl Pts',(4.94738782273622,-29.2687431492796,
126.497002021461));
#116557=CARTESIAN_POINT('Ctrl Pts',(4.94830636003383,-29.2813372668548,
126.503088663298));
#116558=CARTESIAN_POINT('Ctrl Pts',(4.9512200213547,-29.3217579626969,126.521999484024));
#116559=CARTESIAN_POINT('Ctrl Pts',(4.95319442882247,-29.3498632007468,
126.534215441782));
#116560=CARTESIAN_POINT('Ctrl Pts',(4.95785936667107,-29.4177907695341,
126.561538051706));
#116561=CARTESIAN_POINT('Ctrl Pts',(4.96052724007215,-29.4578870085852,
126.575906901092));
#116562=CARTESIAN_POINT('Ctrl Pts',(4.96773457412782,-29.568755230396,126.610904347099));
#116563=CARTESIAN_POINT('Ctrl Pts',(4.9722067458145,-29.6404140538691,126.628398960873));
#116564=CARTESIAN_POINT('Ctrl Pts',(4.97757843672751,-29.7269056389501,
126.643525136016));
#116565=CARTESIAN_POINT('Ctrl Pts',(4.97844356417774,-29.7408457863712,
126.645780814707));
#116566=CARTESIAN_POINT('Ctrl Pts',(4.98380457014615,-29.8271614618932,
126.658623842087));
#116567=CARTESIAN_POINT('Ctrl Pts',(4.98835306559782,-29.9001317687946,
126.664611019222));
#116568=CARTESIAN_POINT('Ctrl Pts',(4.99393179432279,-29.985525347942,126.665982362427));
#116569=CARTESIAN_POINT('Ctrl Pts',(4.99474010364641,-29.9978030533051,
126.66604378668));
#116570=CARTESIAN_POINT('Ctrl Pts',(4.99601725093119,-30.0170304720378,
126.665927452106));
#116571=CARTESIAN_POINT('Ctrl Pts',(4.99648121290226,-30.0239805867628,
126.665841901184));
#116572=CARTESIAN_POINT('Ctrl Pts',(4.99735393942934,-30.0369840179344,
126.665600446852));
#116573=CARTESIAN_POINT('Ctrl Pts',(4.99776212985249,-30.043037281797,126.665455029062));
#116574=CARTESIAN_POINT('Ctrl Pts',(4.99872872240624,-30.0573056249283,
126.665034422571));
#116575=CARTESIAN_POINT('Ctrl Pts',(4.9992886112851,-30.065519608345,126.664731430842));
#116576=CARTESIAN_POINT('Ctrl Pts',(5.00117453888885,-30.0930292488551,
126.663512765216));
#116577=CARTESIAN_POINT('Ctrl Pts',(5.0025141462926,-30.1123103650977,126.662322310361));
#116578=CARTESIAN_POINT('Ctrl Pts',(5.00584946262772,-30.1597830797899,
126.658561606865));
#116579=CARTESIAN_POINT('Ctrl Pts',(5.00785978434464,-30.1879377026819,
126.655607584944));
#116580=CARTESIAN_POINT('Ctrl Pts',(5.01708122616136,-30.3155424992718,
126.638922420814));
#116581=CARTESIAN_POINT('Ctrl Pts',(5.02446512550131,-30.4137024591961,
126.616936771744));
#116582=CARTESIAN_POINT('Ctrl Pts',(5.03763638152116,-30.5876504326763,
126.561088328707));
#116583=CARTESIAN_POINT('Ctrl Pts',(5.04345688619681,-30.6640509648988,
126.530153515268));
#116584=CARTESIAN_POINT('Ctrl Pts',(5.05043201840522,-30.7554342714904,
126.485011517827));
#116585=CARTESIAN_POINT('Ctrl Pts',(5.05176264828876,-30.7728528799514,
126.476021215801));
#116586=CARTESIAN_POINT('Ctrl Pts',(5.05387889924891,-30.8005210812038,
126.46111664744));
#116587=CARTESIAN_POINT('Ctrl Pts',(5.05467129004169,-30.8108729231281,
126.455397187677));
#116588=CARTESIAN_POINT('Ctrl Pts',(5.05617595113781,-30.8305101034968,
126.444272954867));
#116589=CARTESIAN_POINT('Ctrl Pts',(5.05688887094814,-30.8398057360168,
126.438887672872));
#116590=CARTESIAN_POINT('Ctrl Pts',(5.05852253475496,-30.8610818807263,
126.426285241668));
#116591=CARTESIAN_POINT('Ctrl Pts',(5.0594409850558,-30.8730250084303,126.419006324978));
#116592=CARTESIAN_POINT('Ctrl Pts',(5.06235405598912,-30.9108279266776,
126.395308818645));
#116593=CARTESIAN_POINT('Ctrl Pts',(5.0643279722908,-30.936328077378,126.378326569357));
#116594=CARTESIAN_POINT('Ctrl Pts',(5.06899149950454,-30.9961067443332,
126.336090848631));
#116595=CARTESIAN_POINT('Ctrl Pts',(5.07165847292855,-31.029914401008,126.310207658955));
#116596=CARTESIAN_POINT('Ctrl Pts',(5.0788653922523,-31.1194453933778,126.236053341707));
#116597=CARTESIAN_POINT('Ctrl Pts',(5.08333798792775,-31.1730155419773,
126.185335713181));
#116598=CARTESIAN_POINT('Ctrl Pts',(5.08870730168159,-31.2326097943606,
126.120904645166));
#116599=CARTESIAN_POINT('Ctrl Pts',(5.08956965213516,-31.2420360638132,
126.110450601654));
#116600=CARTESIAN_POINT('Ctrl Pts',(5.09493172130901,-31.2996610953757,
126.044890763764));
#116601=CARTESIAN_POINT('Ctrl Pts',(5.09948403184024,-31.3443105863923,
125.986783670037));
#116602=CARTESIAN_POINT('Ctrl Pts',(5.10506699466941,-31.3918132310617,
125.91573068278));
#116603=CARTESIAN_POINT('Ctrl Pts',(5.10587531991308,-31.398523963689,125.905448758776));
#116604=CARTESIAN_POINT('Ctrl Pts',(5.10715248694237,-31.4088546555001,
125.889231619491));
#116605=CARTESIAN_POINT('Ctrl Pts',(5.10761645249436,-31.4125523042486,
125.883346079864));
#116606=CARTESIAN_POINT('Ctrl Pts',(5.10848918172814,-31.4194020673945,
125.872290339888));
#116607=CARTESIAN_POINT('Ctrl Pts',(5.10889737123119,-31.4225629633968,
125.867125871183));
#116608=CARTESIAN_POINT('Ctrl Pts',(5.10986395612519,-31.4299481768046,
125.854910388895));
#116609=CARTESIAN_POINT('Ctrl Pts',(5.11042383819312,-31.4341485424474,
125.847845217301));
#116610=CARTESIAN_POINT('Ctrl Pts',(5.11230971830816,-31.448044594566,125.824072806649));
#116611=CARTESIAN_POINT('Ctrl Pts',(5.11364928413995,-31.4575015556837,
125.807228761969));
#116612=CARTESIAN_POINT('Ctrl Pts',(5.11698447375815,-31.4800887441408,
125.765306787422));
#116613=CARTESIAN_POINT('Ctrl Pts',(5.11899470900334,-31.4928765283363,
125.740051795234));
#116614=CARTESIAN_POINT('Ctrl Pts',(5.12821538114816,-31.5480627377876,
125.623805773471));
#116615=CARTESIAN_POINT('Ctrl Pts',(5.13559857624145,-31.5828279437222,
125.529422384309));
#116616=CARTESIAN_POINT('Ctrl Pts',(5.1487699904762,-31.6302543442041,125.352990577226));
#116617=CARTESIAN_POINT('Ctrl Pts',(5.15459128551917,-31.6457044703404,
125.272014770313));
#116618=CARTESIAN_POINT('Ctrl Pts',(5.16156718184215,-31.6573431207567,
125.170745248412));
#116619=CARTESIAN_POINT('Ctrl Pts',(5.16289783502591,-31.6592372530369,
125.151234767285));
#116620=CARTESIAN_POINT('Ctrl Pts',(5.16501411392607,-31.6617215638531,
125.119905399332));
#116621=CARTESIAN_POINT('Ctrl Pts',(5.16580650967613,-31.6625308744097,
125.10810626569));
#116622=CARTESIAN_POINT('Ctrl Pts',(5.16731117460445,-31.6638354357006,
125.085574778323));
#116623=CARTESIAN_POINT('Ctrl Pts',(5.1680240933481,-31.6643526467217,125.074844347471));
#116624=CARTESIAN_POINT('Ctrl Pts',(5.16965774684138,-31.6653042169947,
125.050134387123));
#116625=CARTESIAN_POINT('Ctrl Pts',(5.17057618799685,-31.6656664099426,
125.036152765577));
#116626=CARTESIAN_POINT('Ctrl Pts',(5.1734891968717,-31.6662600665422,124.991541176395));
#116627=CARTESIAN_POINT('Ctrl Pts',(5.17546306154493,-31.6658229611774,
124.960907648763));
#116628=CARTESIAN_POINT('Ctrl Pts',(5.18012644049014,-31.6627609546134,
124.887780233753));
#116629=CARTESIAN_POINT('Ctrl Pts',(5.18279331932223,-31.6593516971863,
124.845340392403));
#116630=CARTESIAN_POINT('Ctrl Pts',(5.1900001943174,-31.645610503253,124.729903673284));
#116631=CARTESIAN_POINT('Ctrl Pts',(5.19447283384993,-31.6320551303181,
124.65738889661));
#116632=CARTESIAN_POINT('Ctrl Pts',(5.19984188142381,-31.6102469581482,
124.572380166922));
#116633=CARTESIAN_POINT('Ctrl Pts',(5.20070392437248,-31.6065779481966,
124.558795650451));
#116634=CARTESIAN_POINT('Ctrl Pts',(5.20606610542568,-31.5827525323426,
124.474822766881));
#116635=CARTESIAN_POINT('Ctrl Pts',(5.21061883258998,-31.5581485787204,
124.405788754817));
#116636=CARTESIAN_POINT('Ctrl Pts',(5.21620225783166,-31.5242147919116,
124.32733662035));
#116637=CARTESIAN_POINT('Ctrl Pts',(5.217010584809,-31.5192161497886,124.316122070349));
#116638=CARTESIAN_POINT('Ctrl Pts',(5.21828775398837,-31.5111944078119,
124.298647182006));
#116639=CARTESIAN_POINT('Ctrl Pts',(5.21875171993036,-31.5082551791437,
124.292348515355));
#116640=CARTESIAN_POINT('Ctrl Pts',(5.219624449459,-31.5026818342507,124.280597490286));
#116641=CARTESIAN_POINT('Ctrl Pts',(5.2200326388619,-31.5000572963385,124.275140862658));
#116642=CARTESIAN_POINT('Ctrl Pts',(5.22099922292171,-31.4938000177251,
124.262310994892));
#116643=CARTESIAN_POINT('Ctrl Pts',(5.22155910424794,-31.4901423918131,
124.254950198812));
#116644=CARTESIAN_POINT('Ctrl Pts',(5.22344497919173,-31.4777069085841,
124.23038228427));
#116645=CARTESIAN_POINT('Ctrl Pts',(5.22478454049656,-31.4686846406716,
124.213301529963));
#116646=CARTESIAN_POINT('Ctrl Pts',(5.22811971631613,-31.4457147433573,
124.171588240694));
#116647=CARTESIAN_POINT('Ctrl Pts',(5.23012994214515,-31.4314326310571,
124.14714737267));
#116648=CARTESIAN_POINT('Ctrl Pts',(5.23935053048307,-31.3637009524461,
124.037736319938));
#116649=CARTESIAN_POINT('Ctrl Pts',(5.24673364889391,-31.3032614797006,
123.957339139325));
#116650=CARTESIAN_POINT('Ctrl Pts',(5.25990508035964,-31.1807560127768,
123.821803494397));
#116651=CARTESIAN_POINT('Ctrl Pts',(5.26572646146689,-31.1211035184108,
123.764903917407));
#116652=CARTESIAN_POINT('Ctrl Pts',(5.27270244099332,-31.0423340409034,
123.700200050631));
#116653=CARTESIAN_POINT('Ctrl Pts',(5.27403309671259,-31.0269697176762,
123.688026899243));
#116654=CARTESIAN_POINT('Ctrl Pts',(5.27614937865315,-31.0019959179074,
123.668947769153));
#116655=CARTESIAN_POINT('Ctrl Pts',(5.27694177494266,-30.9925218869149,
123.661868400633));
#116656=CARTESIAN_POINT('Ctrl Pts',(5.27844644028799,-30.9742997460758,
123.648552108096));
#116657=CARTESIAN_POINT('Ctrl Pts',(5.2791593589156,-30.9655651623088,123.642297777018));
#116658=CARTESIAN_POINT('Ctrl Pts',(5.28079301128667,-30.9453213609007,
123.628096535429));
#116659=CARTESIAN_POINT('Ctrl Pts',(5.28171145144698,-30.9337712454245,
123.620209120028));
#116660=CARTESIAN_POINT('Ctrl Pts',(5.28462445356896,-30.8966131735221,
123.595514694759));
#116661=CARTESIAN_POINT('Ctrl Pts',(5.28659831262428,-30.8706396207975,
123.579267444194));
#116662=CARTESIAN_POINT('Ctrl Pts',(5.29126167543586,-30.8075416051257,
123.542178402699));
#116663=CARTESIAN_POINT('Ctrl Pts',(5.29392854397502,-30.770037145724,123.522024888971));
#116664=CARTESIAN_POINT('Ctrl Pts',(5.30113541413808,-30.6656011137827,
123.470960719107));
#116665=CARTESIAN_POINT('Ctrl Pts',(5.30560805843472,-30.597326287486,123.44301970664));
#116666=CARTESIAN_POINT('Ctrl Pts',(5.3109770768539,-30.5140792409551,123.41523613542));
#116667=CARTESIAN_POINT('Ctrl Pts',(5.31183908615908,-30.5006768831049,
123.410951031273));
#116668=CARTESIAN_POINT('Ctrl Pts',(5.31720127938764,-30.4172053775509,
123.385423742675));
#116669=CARTESIAN_POINT('Ctrl Pts',(5.32175405207011,-30.3458618548013,
123.368652799818));
#116670=CARTESIAN_POINT('Ctrl Pts',(5.32733752783174,-30.261545568793,123.35461230413));
#116671=CARTESIAN_POINT('Ctrl Pts',(5.32814585499848,-30.2494126499903,
123.352729511422));
#116672=CARTESIAN_POINT('Ctrl Pts',(5.32942302441272,-30.2303805268127,
123.349991173847));
#116673=CARTESIAN_POINT('Ctrl Pts',(5.32988699039733,-30.2234946098815,
123.349044377187));
#116674=CARTESIAN_POINT('Ctrl Pts',(5.33075971995818,-30.2105992792555,
123.347353452929));
#116675=CARTESIAN_POINT('Ctrl Pts',(5.33116790935014,-30.2045914737466,
123.346598962697));
#116676=CARTESIAN_POINT('Ctrl Pts',(5.33213449331878,-30.1904188211004,
123.344897515631));
#116677=CARTESIAN_POINT('Ctrl Pts',(5.33269437456398,-30.1822509319145,
123.343978215141));
#116678=CARTESIAN_POINT('Ctrl Pts',(5.33458024894301,-30.1548658053897,
123.341101052477));
#116679=CARTESIAN_POINT('Ctrl Pts',(5.33591980975339,-30.1356221725721,
123.339417065443));
#116680=CARTESIAN_POINT('Ctrl Pts',(5.33925498406594,-30.0881189949893,
123.336091287347));
#116681=CARTESIAN_POINT('Ctrl Pts',(5.34126520886653,-30.059839066475,123.334834462726));
#116682=CARTESIAN_POINT('Ctrl Pts',(5.35048578805117,-29.9311829713013,
123.33239816749));
#116683=CARTESIAN_POINT('Ctrl Pts',(5.35786889808692,-29.8308577096969,
123.339571435432));
#116684=CARTESIAN_POINT('Ctrl Pts',(5.37104209114812,-29.650521632075,123.368987836374));
#116685=CARTESIAN_POINT('Ctrl Pts',(5.37686516662464,-29.5703409067214,
123.388251713395));
#116686=CARTESIAN_POINT('Ctrl Pts',(5.3838418129469,-29.4732488167275,123.419344170878));
#116687=CARTESIAN_POINT('Ctrl Pts',(5.38517157920922,-29.4547009015659,
123.425646605975));
#116688=CARTESIAN_POINT('Ctrl Pts',(5.38728679456708,-29.4251416407104,
123.436275707448));
#116689=CARTESIAN_POINT('Ctrl Pts',(5.38807900161115,-29.4140582086348,
123.440394913458));
#116690=CARTESIAN_POINT('Ctrl Pts',(5.38958352077166,-29.3929895943905,
123.448481459267));
#116691=CARTESIAN_POINT('Ctrl Pts',(5.3902964802308,-29.3829971488306,123.452428061243));
#116692=CARTESIAN_POINT('Ctrl Pts',(5.39193052687161,-29.3600810017637,
123.461736231927));
#116693=CARTESIAN_POINT('Ctrl Pts',(5.39284931659802,-29.3471851515069,
123.467164543131));
#116694=CARTESIAN_POINT('Ctrl Pts',(5.39576469149395,-29.3062517407561,
123.485005137055));
#116695=CARTESIAN_POINT('Ctrl Pts',(5.39774052460512,-29.2784868415909,
123.498029616269));
#116696=CARTESIAN_POINT('Ctrl Pts',(5.40240955778406,-29.2130255967973,
123.530971864591));
#116697=CARTESIAN_POINT('Ctrl Pts',(5.40508004422706,-29.1757028321056,
123.551584681367));
#116698=CARTESIAN_POINT('Ctrl Pts',(5.41233686025362,-29.0754755121674,
123.612069231686));
#116699=CARTESIAN_POINT('Ctrl Pts',(5.41685382822784,-29.0143905616757,
123.654759599325));
#116700=CARTESIAN_POINT('Ctrl Pts',(5.42221445115768,-28.9461024652947,
123.709639854212));
#116701=CARTESIAN_POINT('Ctrl Pts',(5.4230211358357,-28.9359387851882,123.718008172611));
#116702=CARTESIAN_POINT('Ctrl Pts',(5.42833055829348,-28.8698708299322,
123.773732547345));
#116703=CARTESIAN_POINT('Ctrl Pts',(5.43288614633392,-28.8170499867948,
123.824606295463));
#116704=CARTESIAN_POINT('Ctrl Pts',(5.43847274690479,-28.759491573965,123.887864395107));
#116705=CARTESIAN_POINT('Ctrl Pts',(5.4392810857625,-28.7513291738461,123.897036761771));
#116706=CARTESIAN_POINT('Ctrl Pts',(5.44055826967646,-28.738706087534,123.911541465898));
#116707=CARTESIAN_POINT('Ctrl Pts',(5.44102223829059,-28.7341759407456,
123.916813145981));
#116708=CARTESIAN_POINT('Ctrl Pts',(5.44189496983914,-28.7257613351789,
123.926730000916));
#116709=CARTESIAN_POINT('Ctrl Pts',(5.44230315855554,-28.7218690420643,
123.931368203944));
#116710=CARTESIAN_POINT('Ctrl Pts',(5.44326973689955,-28.7127528939033,
123.94235239902));
#116711=CARTESIAN_POINT('Ctrl Pts',(5.44382961314334,-28.7075506235169,
123.948715946017));
#116712=CARTESIAN_POINT('Ctrl Pts',(5.44571545265216,-28.6902809929302,
123.970162516875));
#116713=CARTESIAN_POINT('Ctrl Pts',(5.4470549829368,-28.6784294002208,123.985416248211));
#116714=CARTESIAN_POINT('Ctrl Pts',(5.45450747594605,-28.6146156901012,
124.070563956309));
#116715=CARTESIAN_POINT('Ctrl Pts',(5.46085766180495,-28.567934519736,124.144238879998));
#116716=CARTESIAN_POINT('Ctrl Pts',(5.47370801870482,-28.4854054804999,
124.300311162647));
#116717=CARTESIAN_POINT('Ctrl Pts',(5.4801850158172,-28.4500167530918,124.382653781712));
#116718=CARTESIAN_POINT('Ctrl Pts',(5.48939016492012,-28.4081136754622,
124.50686285228));
#116719=CARTESIAN_POINT('Ctrl Pts',(5.49226834727872,-28.3962967092375,
124.546764304565));
#116720=CARTESIAN_POINT('Ctrl Pts',(5.49619599336575,-28.3819883320362,
124.602691235687));
#116721=CARTESIAN_POINT('Ctrl Pts',(5.49728578887273,-28.3782185524634,
124.618370624752));
#116722=CARTESIAN_POINT('Ctrl Pts',(5.49903921563436,-28.372481873467,124.643853071922));
#116723=CARTESIAN_POINT('Ctrl Pts',(5.49970729688571,-28.3703745997395,
124.65362311146));
#116724=CARTESIAN_POINT('Ctrl Pts',(5.50110147936075,-28.3661429895898,
124.674136255641));
#116725=CARTESIAN_POINT('Ctrl Pts',(5.5018269849342,-28.36403639343,124.684882564649));
#116726=CARTESIAN_POINT('Ctrl Pts',(5.50326582985179,-28.3600506634912,
124.706333075816));
#116727=CARTESIAN_POINT('Ctrl Pts',(5.50397918423974,-28.3581700086626,
124.717036437893));
#116728=CARTESIAN_POINT('Ctrl Pts',(5.50565525387928,-28.3539788256483,
124.742339822065));
#116729=CARTESIAN_POINT('Ctrl Pts',(5.50661517444864,-28.3517575830418,
124.756953850244));
#116730=CARTESIAN_POINT('Ctrl Pts',(5.51253201801181,-28.3391927720227,
124.847737316833));
#116731=CARTESIAN_POINT('Ctrl Pts',(5.51732909613142,-28.3339361594531,
124.924519595377));
#116732=CARTESIAN_POINT('Ctrl Pts',(5.52205821453768,-28.3340005850234,
125.001396172494));
#116733=CARTESIAN_POINT('Ctrl Pts',(5.52205812845195,-28.3340005838512,
125.001394773084));
#116734=CARTESIAN_POINT('Ctrl Pts',(5.53023876175647,-28.3341119182617,
125.134379173918));
#116735=CARTESIAN_POINT('Ctrl Pts',(5.538148581464,-28.3501451314225,125.266857640374));
#116736=CARTESIAN_POINT('Ctrl Pts',(5.54796471122472,-28.3863380832262,
125.414757645535));
#116737=CARTESIAN_POINT('Ctrl Pts',(5.5492230763142,-28.3912522236007,125.43342727207));
#116738=CARTESIAN_POINT('Ctrl Pts',(5.55104156984201,-28.3987189244339,
125.459915694842));
#116739=CARTESIAN_POINT('Ctrl Pts',(5.55158764660967,-28.401006898531,125.467808276731));
#116740=CARTESIAN_POINT('Ctrl Pts',(5.55254189612542,-28.4050819304441,
125.481486254538));
#116741=CARTESIAN_POINT('Ctrl Pts',(5.55294853914217,-28.4068422903595,
125.48727935804));
#116742=CARTESIAN_POINT('Ctrl Pts',(5.55382614207314,-28.4106916992212,
125.499703365874));
#116743=CARTESIAN_POINT('Ctrl Pts',(5.55429762856221,-28.412790651181,125.506330729269));
#116744=CARTESIAN_POINT('Ctrl Pts',(5.55560845564577,-28.4187128176287,
125.524631033915));
#116745=CARTESIAN_POINT('Ctrl Pts',(5.55645254851924,-28.4226236546171,
125.536274852816));
#116746=CARTESIAN_POINT('Ctrl Pts',(5.55798021472545,-28.4298810537396,
125.557116027919));
#116747=CARTESIAN_POINT('Ctrl Pts',(5.55866144585198,-28.433180286975,125.566328267133));
#116748=CARTESIAN_POINT('Ctrl Pts',(5.55934601859666,-28.436559980232,125.575509604253));
#116749=CARTESIAN_POINT('',(5.32851907197511,-28.3320235394521,125.000530942666));
#116750=CARTESIAN_POINT('Ctrl Pts',(5.3678724416903,-28.4365599837785,125.575509613888));
#116751=CARTESIAN_POINT('Ctrl Pts',(5.36380377119692,-28.41550826323,125.518320122137));
#116752=CARTESIAN_POINT('Ctrl Pts',(5.35973510070354,-28.3976158268008,
125.460021074581));
#116753=CARTESIAN_POINT('Ctrl Pts',(5.35566643021015,-28.3829781651687,
125.400994246441));
#116754=CARTESIAN_POINT('Ctrl Pts',(5.35159020293631,-28.3683133168683,
125.341857787211));
#116755=CARTESIAN_POINT('Ctrl Pts',(5.34751397566247,-28.3569154130502,
125.28199135154));
#116756=CARTESIAN_POINT('Ctrl Pts',(5.34343774838862,-28.348828605094,125.221785988385));
#116757=CARTESIAN_POINT('Ctrl Pts',(5.34045616567603,-28.3429134572912,
125.177748387455));
#116758=CARTESIAN_POINT('Ctrl Pts',(5.33747458296344,-28.3387687514707,
125.133529630053));
#116759=CARTESIAN_POINT('Ctrl Pts',(5.33449300025085,-28.3363941013021,
125.089282774473));
#116760=CARTESIAN_POINT('Ctrl Pts',(5.33250187903717,-28.3348082937691,
125.059734423387));
#116761=CARTESIAN_POINT('Ctrl Pts',(5.33051075782348,-28.3340096599776,
125.030143448947));
#116762=CARTESIAN_POINT('Ctrl Pts',(5.32851963660979,-28.3340000870979,
125.000538711647));
#116763=CARTESIAN_POINT('Ctrl Pts',(5.32851890483142,-28.3314384399868,
125.000528642885));
#116764=CARTESIAN_POINT('Ctrl Pts',(5.29346517969172,-28.3336501290359,
124.47853450853));
#116765=CARTESIAN_POINT('Ctrl Pts',(5.22136636427249,-28.8783523852238,
123.400922781091));
#116766=CARTESIAN_POINT('Ctrl Pts',(5.11222245857373,-30.7133320434846,
123.164583819203));
#116767=CARTESIAN_POINT('Ctrl Pts',(5.00108718773517,-31.9288987627743,
124.603837503091));
#116768=CARTESIAN_POINT('Ctrl Pts',(4.88995191689662,-31.3789987832528,
126.405687560155));
#116769=CARTESIAN_POINT('Ctrl Pts',(4.77886137730299,-29.5676694072103,
126.920744002413));
#116770=CARTESIAN_POINT('Ctrl Pts',(4.70481592798891,-28.6242856685622,
126.09333226611));
#116771=CARTESIAN_POINT('Ctrl Pts',(4.66781556895434,-28.4339562630661,
125.576468403481));
#116772=CARTESIAN_POINT('Origin',(5.,-30.,125.));
#116773=CARTESIAN_POINT('',(3.96713564162385,-28.4365599852621,125.575509617918));
#116774=CARTESIAN_POINT('',(4.16231116930939,-28.436559983762,125.575509613843));
#116775=CARTESIAN_POINT('',(5.,-28.4365599837785,125.575509613888));
#116776=CARTESIAN_POINT('Ctrl Pts',(4.16231116930939,-28.436559983762,125.575509613843));
#116777=CARTESIAN_POINT('Ctrl Pts',(4.16317922697514,-28.4409822920616,
125.587523338016));
#116778=CARTESIAN_POINT('Ctrl Pts',(4.16404268008447,-28.4455430622354,
125.599486059615));
#116779=CARTESIAN_POINT('Ctrl Pts',(4.16563891938588,-28.4542751614591,
125.621620092053));
#116780=CARTESIAN_POINT('Ctrl Pts',(4.16637286785923,-28.4584100737857,
125.631804815354));
#116781=CARTESIAN_POINT('Ctrl Pts',(4.16776485836637,-28.4664801403983,
125.651131226606));
#116782=CARTESIAN_POINT('Ctrl Pts',(4.16842348095199,-28.4703969876596,
125.660279990594));
#116783=CARTESIAN_POINT('Ctrl Pts',(4.17012589727787,-28.4807758879012,
125.683934389042));
#116784=CARTESIAN_POINT('Ctrl Pts',(4.17116536468675,-28.4873638687723,
125.698383930497));
#116785=CARTESIAN_POINT('Ctrl Pts',(4.17479569757736,-28.5112448409967,
125.748838663549));
#116786=CARTESIAN_POINT('Ctrl Pts',(4.17734928696242,-28.5296256928894,
125.784315662723));
#116787=CARTESIAN_POINT('Ctrl Pts',(4.18801181564254,-28.6127404528174,
125.931522928704));
#116788=CARTESIAN_POINT('Ctrl Pts',(4.195723419553,-28.6890648901925,126.036181896769));
#116789=CARTESIAN_POINT('Ctrl Pts',(4.20627235726083,-28.8049600963661,
126.161536737027));
#116790=CARTESIAN_POINT('Ctrl Pts',(4.20887139195282,-28.8343453468672,
126.19102339734));
#116791=CARTESIAN_POINT('Ctrl Pts',(4.21263383407759,-28.8774501499696,
126.231152502855));
#116792=CARTESIAN_POINT('Ctrl Pts',(4.21374791304859,-28.8902807566091,
126.242729979486));
#116793=CARTESIAN_POINT('Ctrl Pts',(4.21550022286791,-28.9105152726094,
126.260425004797));
#116794=CARTESIAN_POINT('Ctrl Pts',(4.21612984725988,-28.9177962573231,
126.266681970031));
#116795=CARTESIAN_POINT('Ctrl Pts',(4.21728735702848,-28.9311906267264,
126.277992735665));
#116796=CARTESIAN_POINT('Ctrl Pts',(4.21781389315024,-28.9372868591462,
126.283066515352));
#116797=CARTESIAN_POINT('Ctrl Pts',(4.21834735396957,-28.9434634153534,
126.288132931266));
#116798=CARTESIAN_POINT('Ctrl Pts',(4.21835119581947,-28.9435078973568,
126.288169414465));
#116799=CARTESIAN_POINT('Ctrl Pts',(4.21835894487734,-28.9435976181108,
126.288242993756));
#116800=CARTESIAN_POINT('Ctrl Pts',(4.21836285207824,-28.9436428567798,
126.288280089651));
#116801=CARTESIAN_POINT('Ctrl Pts',(4.21837073555032,-28.9437341338438,
126.288354929178));
#116802=CARTESIAN_POINT('Ctrl Pts',(4.21837471184787,-28.9437801725446,
126.28839267292));
#116803=CARTESIAN_POINT('Ctrl Pts',(4.21877605287532,-28.9484270132244,
126.292201859092));
#116804=CARTESIAN_POINT('Ctrl Pts',(4.21917515494819,-28.9530479165009,
126.295948581132));
#116805=CARTESIAN_POINT('Ctrl Pts',(4.22002521016993,-28.9628876238562,
126.303839840958));
#116806=CARTESIAN_POINT('Ctrl Pts',(4.22047658143271,-28.968111321352,126.307977890708));
#116807=CARTESIAN_POINT('Ctrl Pts',(4.22169796302618,-28.982247085991,126.31903841948));
#116808=CARTESIAN_POINT('Ctrl Pts',(4.2224718624188,-28.9912047083257,126.325901726405));
#116809=CARTESIAN_POINT('Ctrl Pts',(4.22624720919268,-29.0349388505564,
126.35871099675));
#116810=CARTESIAN_POINT('Ctrl Pts',(4.22932004107227,-29.0706475086381,
126.38338058524));
#116811=CARTESIAN_POINT('Ctrl Pts',(4.23881210239701,-29.1823387683896,
126.45426624988));
#116812=CARTESIAN_POINT('Ctrl Pts',(4.24533677897331,-29.2610949036596,
126.495820653806));
#116813=CARTESIAN_POINT('Ctrl Pts',(4.256183647702,-29.3988872592886,126.554974692873));
#116814=CARTESIAN_POINT('Ctrl Pts',(4.26054976332195,-29.4562698463316,
126.575957365829));
#116815=CARTESIAN_POINT('Ctrl Pts',(4.26758220213828,-29.5523386448093,
126.605211824967));
#116816=CARTESIAN_POINT('Ctrl Pts',(4.27029977497475,-29.590394516047,126.615341910125));
#116817=CARTESIAN_POINT('Ctrl Pts',(4.27401811929543,-29.6437505532854,
126.627537486277));
#116818=CARTESIAN_POINT('Ctrl Pts',(4.27505502323509,-29.6587716727772,
126.630752952986));
#116819=CARTESIAN_POINT('Ctrl Pts',(4.27682040968263,-29.6845832739236,
126.635905989399));
#116820=CARTESIAN_POINT('Ctrl Pts',(4.27755209498397,-29.6953521120446,
126.637945600897));
#116821=CARTESIAN_POINT('Ctrl Pts',(4.27894388251059,-29.7159680330845,
126.641639888374));
#116822=CARTESIAN_POINT('Ctrl Pts',(4.27960452739117,-29.7258113555464,
126.643312592277));
#116823=CARTESIAN_POINT('Ctrl Pts',(4.28132105893931,-29.7515320906149,
126.647445848561));
#116824=CARTESIAN_POINT('Ctrl Pts',(4.28237247059705,-29.7674313551585,
126.649765432095));
#116825=CARTESIAN_POINT('Ctrl Pts',(4.28609523790505,-29.8242076784766,
126.657211547177));
#116826=CARTESIAN_POINT('Ctrl Pts',(4.2887266612414,-29.8652401110334,126.661051851689));
#116827=CARTESIAN_POINT('Ctrl Pts',(4.29936671143038,-30.0338614361575,
126.670542892513));
#116828=CARTESIAN_POINT('Ctrl Pts',(4.30699527934091,-30.1617439648984,
126.663039006415));
#116829=CARTESIAN_POINT('Ctrl Pts',(4.31744725702816,-30.3283331185741,
126.633851479204));
#116830=CARTESIAN_POINT('Ctrl Pts',(4.32003570993169,-30.3688679108526,
126.625179775387));
#116831=CARTESIAN_POINT('Ctrl Pts',(4.32429611365685,-30.4335076314715,
126.608808407346));
#116832=CARTESIAN_POINT('Ctrl Pts',(4.32593049324473,-30.4578352375551,
126.602054958244));
#116833=CARTESIAN_POINT('Ctrl Pts',(4.32819351345414,-30.4907138987437,
126.592117699225));
#116834=CARTESIAN_POINT('Ctrl Pts',(4.32879709762664,-30.4994074009803,
126.589412198611));
#116835=CARTESIAN_POINT('Ctrl Pts',(4.32981849029757,-30.5139821578055,
126.584745018771));
#116836=CARTESIAN_POINT('Ctrl Pts',(4.33023412369842,-30.5198755954111,
126.582821467148));
#116837=CARTESIAN_POINT('Ctrl Pts',(4.33109424879399,-30.5319913820317,
126.578792044713));
#116838=CARTESIAN_POINT('Ctrl Pts',(4.33153894578492,-30.5382121919578,
126.576682207571));
#116839=CARTESIAN_POINT('Ctrl Pts',(4.33272350719992,-30.5546730627074,
126.570990605243));
#116840=CARTESIAN_POINT('Ctrl Pts',(4.33346688174507,-30.5648906928265,
126.567345583404));
#116841=CARTESIAN_POINT('Ctrl Pts',(4.33685771742829,-30.6110233497129,
126.550378607468));
#116842=CARTESIAN_POINT('Ctrl Pts',(4.33956077585401,-30.6465053273742,
126.535921129286));
#116843=CARTESIAN_POINT('Ctrl Pts',(4.34892012649131,-30.765969748107,126.482371208142));
#116844=CARTESIAN_POINT('Ctrl Pts',(4.35572099626238,-30.8471770134883,
126.437506458466));
#116845=CARTESIAN_POINT('Ctrl Pts',(4.36694606887245,-30.9761988225833,
126.35147796924));
#116846=CARTESIAN_POINT('Ctrl Pts',(4.37141715323246,-31.0261779801031,
126.313931864512));
#116847=CARTESIAN_POINT('Ctrl Pts',(4.37859384109451,-31.1044841786287,
126.247905241694));
#116848=CARTESIAN_POINT('Ctrl Pts',(4.3813534991082,-31.1340990713949,126.22105387124));
#116849=CARTESIAN_POINT('Ctrl Pts',(4.38511849018135,-31.1737824707877,
126.182382858021));
#116850=CARTESIAN_POINT('Ctrl Pts',(4.3861611731732,-31.1846929800073,126.17145084519));
#116851=CARTESIAN_POINT('Ctrl Pts',(4.3879333567846,-31.2030942913225,126.152493200084));
#116852=CARTESIAN_POINT('Ctrl Pts',(4.38866612261558,-31.210660505082,126.14454252932));
#116853=CARTESIAN_POINT('Ctrl Pts',(4.39014604037217,-31.2258517883746,
126.128260133651));
#116854=CARTESIAN_POINT('Ctrl Pts',(4.39089295493148,-31.2334718142169,
126.119924475314));
#116855=CARTESIAN_POINT('Ctrl Pts',(4.39275988297913,-31.2523942840735,
126.098797474278));
#116856=CARTESIAN_POINT('Ctrl Pts',(4.39387526280677,-31.263586180322,126.085908528559));
#116857=CARTESIAN_POINT('Ctrl Pts',(4.39817085703018,-31.3062127915342,
126.035266794887));
#116858=CARTESIAN_POINT('Ctrl Pts',(4.4012921114574,-31.3361714257897,125.996301061924));
#116859=CARTESIAN_POINT('Ctrl Pts',(4.41182898467989,-31.4327874951286,
125.858423723178));
#116860=CARTESIAN_POINT('Ctrl Pts',(4.41896233633882,-31.4905269490875,
125.753724112213));
#116861=CARTESIAN_POINT('Ctrl Pts',(4.42883229370567,-31.5521821057682,
125.60655874918));
#116862=CARTESIAN_POINT('Ctrl Pts',(4.43135439936957,-31.5664103778371,
125.568806563515));
#116863=CARTESIAN_POINT('Ctrl Pts',(4.4355175105843,-31.587148284961,125.507080634077));
#116864=CARTESIAN_POINT('Ctrl Pts',(4.43712303788963,-31.5945167435998,
125.483411466825));
#116865=CARTESIAN_POINT('Ctrl Pts',(4.43935225454763,-31.6038486740857,
125.450896007729));
#116866=CARTESIAN_POINT('Ctrl Pts',(4.43995184251413,-31.6062724715152,
125.442183804796));
#116867=CARTESIAN_POINT('Ctrl Pts',(4.440968454533,-31.6102350609335,125.427477878964));
#116868=CARTESIAN_POINT('Ctrl Pts',(4.44138335021321,-31.6118116473372,
125.421494365992));
#116869=CARTESIAN_POINT('Ctrl Pts',(4.44218897272962,-31.614793987893,125.409914227204));
#116870=CARTESIAN_POINT('Ctrl Pts',(4.44257941218681,-31.616204051675,125.404318881318));
#116871=CARTESIAN_POINT('Ctrl Pts',(4.44365744131983,-31.6200014388658,
125.388912953585));
#116872=CARTESIAN_POINT('Ctrl Pts',(4.44434829230354,-31.6223286389151,
125.37908801357));
#116873=CARTESIAN_POINT('Ctrl Pts',(4.44717123920904,-31.6314148973058,
125.339110990885));
#116874=CARTESIAN_POINT('Ctrl Pts',(4.44933922696244,-31.6374233377766,
125.308796627838));
#116875=CARTESIAN_POINT('Ctrl Pts',(4.45929174660197,-31.6608311006076,
125.170656546464));
#116876=CARTESIAN_POINT('Ctrl Pts',(4.46733985017474,-31.6684446471276,
125.061447481425));
#116877=CARTESIAN_POINT('Ctrl Pts',(4.47938274580057,-31.6636667543472,
124.894710334348));
#116878=CARTESIAN_POINT('Ctrl Pts',(4.48349201426374,-31.6590328438972,
124.837260600529));
#116879=CARTESIAN_POINT('Ctrl Pts',(4.49016815258423,-31.6464347523035,
124.742623473705));
#116880=CARTESIAN_POINT('Ctrl Pts',(4.49277972340893,-31.6401589568326,
124.705264414348));
#116881=CARTESIAN_POINT('Ctrl Pts',(4.49638011527232,-31.6295981471039,
124.653308163883));
#116882=CARTESIAN_POINT('Ctrl Pts',(4.49740208683874,-31.6263792444703,
124.63850874182));
#116883=CARTESIAN_POINT('Ctrl Pts',(4.4991499583045,-31.6204924376931,124.613115603815));
#116884=CARTESIAN_POINT('Ctrl Pts',(4.49987890092369,-31.6179213734383,
124.602500671963));
#116885=CARTESIAN_POINT('Ctrl Pts',(4.50127073123814,-31.6127897165635,
124.582189171061));
#116886=CARTESIAN_POINT('Ctrl Pts',(4.50193411319018,-31.6102455989487,
124.572488974244));
#116887=CARTESIAN_POINT('Ctrl Pts',(4.50366943743377,-31.6033327614527,
124.54706929583));
#116888=CARTESIAN_POINT('Ctrl Pts',(4.50473670485607,-31.5988203827969,
124.531389734225));
#116889=CARTESIAN_POINT('Ctrl Pts',(4.50858671764909,-31.5816002536884,
124.474700316751));
#116890=CARTESIAN_POINT('Ctrl Pts',(4.51132569969776,-31.5675383663796,
124.434117441358));
#116891=CARTESIAN_POINT('Ctrl Pts',(4.5212560676488,-31.5101261917827,124.287059710301));
#116892=CARTESIAN_POINT('Ctrl Pts',(4.52816221625505,-31.4573642478251,
124.184613529117));
#116893=CARTESIAN_POINT('Ctrl Pts',(4.53820516738287,-31.3680019493107,
124.04791406236));
#116894=CARTESIAN_POINT('Ctrl Pts',(4.54120798632575,-31.3397779754479,
124.008591256163));
#116895=CARTESIAN_POINT('Ctrl Pts',(4.54549759964524,-31.2981416882681,
123.955612451002));
#116896=CARTESIAN_POINT('Ctrl Pts',(4.54671908262832,-31.2861438318098,
123.940872446406));
#116897=CARTESIAN_POINT('Ctrl Pts',(4.54888866438222,-31.2646505962483,
123.915370696626));
#116898=CARTESIAN_POINT('Ctrl Pts',(4.54983032932422,-31.2552632263514,
123.904520171332));
#116899=CARTESIAN_POINT('Ctrl Pts',(4.55126631461466,-31.2408844249614,
123.888327719142));
#116900=CARTESIAN_POINT('Ctrl Pts',(4.55175345507476,-31.2359957700664,
123.882894871786));
#116901=CARTESIAN_POINT('Ctrl Pts',(4.55264595044027,-31.2270234779623,
123.873054800333));
#116902=CARTESIAN_POINT('Ctrl Pts',(4.55305044705163,-31.2229515390824,
123.868637269474));
#116903=CARTESIAN_POINT('Ctrl Pts',(4.55397754462481,-31.2136061141802,
123.858608087518));
#116904=CARTESIAN_POINT('Ctrl Pts',(4.55450125068896,-31.2083175786257,
123.853010932244));
#116905=CARTESIAN_POINT('Ctrl Pts',(4.55614692958504,-31.1916639969083,
123.835628506113));
#116906=CARTESIAN_POINT('Ctrl Pts',(4.55727832479877,-31.1801642913592,
123.823974382642));
#116907=CARTESIAN_POINT('Ctrl Pts',(4.56383934253566,-31.1130903657118,
123.75797434218));
#116908=CARTESIAN_POINT('Ctrl Pts',(4.56947347362756,-31.0539431093971,
123.707405895845));
#116909=CARTESIAN_POINT('Ctrl Pts',(4.57996511771871,-30.9380733036565,
123.621597831199));
#116910=CARTESIAN_POINT('Ctrl Pts',(4.5848085495672,-30.8823353489816,123.585270636609));
#116911=CARTESIAN_POINT('Ctrl Pts',(4.59481078997831,-30.7611922637512,
123.516267214959));
#116912=CARTESIAN_POINT('Ctrl Pts',(4.59994275309543,-30.6955010452258,
123.484362325228));
#116913=CARTESIAN_POINT('Ctrl Pts',(4.60620255939373,-30.6106485002079,
123.449834800201));
#116914=CARTESIAN_POINT('Ctrl Pts',(4.60746712552473,-30.5932586344661,
123.443096669935));
#116915=CARTESIAN_POINT('Ctrl Pts',(4.60950411867562,-30.5648509195995,
123.432634517634));
#116916=CARTESIAN_POINT('Ctrl Pts',(4.61028243792012,-30.5539011922207,
123.428731532237));
#116917=CARTESIAN_POINT('Ctrl Pts',(4.61177693114594,-30.5326957796855,
123.421422171251));
#116918=CARTESIAN_POINT('Ctrl Pts',(4.61249358342784,-30.5224460773789,
123.418000360077));
#116919=CARTESIAN_POINT('Ctrl Pts',(4.61414356097127,-30.4986649796156,
123.410317494367));
#116920=CARTESIAN_POINT('Ctrl Pts',(4.61507447354788,-30.485110879281,123.406129024676));
#116921=CARTESIAN_POINT('Ctrl Pts',(4.61804825830917,-30.441391910178,123.393228420271));
#116922=CARTESIAN_POINT('Ctrl Pts',(4.62006929800454,-30.4110326720846,
123.385195345504));
#116923=CARTESIAN_POINT('Ctrl Pts',(4.63094836414409,-30.2445843243034,
123.346151952231));
#116924=CARTESIAN_POINT('Ctrl Pts',(4.63927417250506,-30.1052460073446,
123.331480130998));
#116925=CARTESIAN_POINT('Ctrl Pts',(4.65053548342524,-29.9228527188195,
123.335235272053));
#116926=CARTESIAN_POINT('Ctrl Pts',(4.65320915825484,-29.8800508211849,
123.337771073136));
#116927=CARTESIAN_POINT('Ctrl Pts',(4.65759399957326,-29.8116959010801,
123.344474558685));
#116928=CARTESIAN_POINT('Ctrl Pts',(4.6592648233259,-29.7860581394499,123.347592173183));
#116929=CARTESIAN_POINT('Ctrl Pts',(4.66157047847722,-29.7514188744154,
123.352623988826));
#116930=CARTESIAN_POINT('Ctrl Pts',(4.66217902060251,-29.7423441578602,
123.35401890788));
#116931=CARTESIAN_POINT('Ctrl Pts',(4.66320636170562,-29.72714768124,123.356483578421));
#116932=CARTESIAN_POINT('Ctrl Pts',(4.66362292730653,-29.7210193634386,
123.357512734094));
#116933=CARTESIAN_POINT('Ctrl Pts',(4.66448229276276,-29.7084490508006,
123.359696103062));
#116934=CARTESIAN_POINT('Ctrl Pts',(4.66492527469808,-29.702007901545,123.360854022418));
#116935=CARTESIAN_POINT('Ctrl Pts',(4.66610039206937,-29.685018117183,123.364011709505));
#116936=CARTESIAN_POINT('Ctrl Pts',(4.6668359428259,-29.6744819062216,123.366075513184));
#116937=CARTESIAN_POINT('Ctrl Pts',(4.67013111700079,-29.6276841847637,
123.375712714981));
#116938=CARTESIAN_POINT('Ctrl Pts',(4.67274268786714,-29.5916638930089,
123.384391937964));
#116939=CARTESIAN_POINT('Ctrl Pts',(4.68206712786217,-29.4658281804642,
123.419189261915));
#116940=CARTESIAN_POINT('Ctrl Pts',(4.68893509065443,-29.3779514092269,
123.45165984287));
#116941=CARTESIAN_POINT('Ctrl Pts',(4.70025433355752,-29.2363703406212,
123.517983458252));
#116942=CARTESIAN_POINT('Ctrl Pts',(4.70475305418314,-29.1810247568318,
123.547834649225));
#116943=CARTESIAN_POINT('Ctrl Pts',(4.71196759048416,-29.0933198112044,
123.601752450571));
#116944=CARTESIAN_POINT('Ctrl Pts',(4.71473821155468,-29.0599141254374,
123.623989754725));
#116945=CARTESIAN_POINT('Ctrl Pts',(4.7185153371643,-29.0147853061878,123.656442340097));
#116946=CARTESIAN_POINT('Ctrl Pts',(4.71955951191594,-29.0023552929254,
123.665646132072));
#116947=CARTESIAN_POINT('Ctrl Pts',(4.72133345166069,-28.981323282175,123.681677474529));
#116948=CARTESIAN_POINT('Ctrl Pts',(4.72206649802086,-28.9726575237358,
123.688419280786));
#116949=CARTESIAN_POINT('Ctrl Pts',(4.72354633329308,-28.9552188643451,
123.702265132343));
#116950=CARTESIAN_POINT('Ctrl Pts',(4.72429289088067,-28.9464502473169,
123.709373664694));
#116951=CARTESIAN_POINT('Ctrl Pts',(4.72615767511359,-28.9246267143451,
123.727436176202));
#116952=CARTESIAN_POINT('Ctrl Pts',(4.7272712908582,-28.9116661605151,123.73850252555));
#116953=CARTESIAN_POINT('Ctrl Pts',(4.73154804558759,-28.8622119478054,
123.782058502115));
#116954=CARTESIAN_POINT('Ctrl Pts',(4.73465292780016,-28.826982656787,123.815950111589));
#116955=CARTESIAN_POINT('Ctrl Pts',(4.74606647368828,-28.7012718377728,
123.948014299602));
#116956=CARTESIAN_POINT('Ctrl Pts',(4.75399658311775,-28.6212084871078,
124.055383808113));
#116957=CARTESIAN_POINT('Ctrl Pts',(4.76430153766584,-28.5390722115101,
124.198596740525));
#116958=CARTESIAN_POINT('Ctrl Pts',(4.76629905873587,-28.5241163033265,
124.226485770754));
#116959=CARTESIAN_POINT('Ctrl Pts',(4.76967922578871,-28.5006015582395,
124.273502622169));
#116960=CARTESIAN_POINT('Ctrl Pts',(4.77104089798658,-28.4915928572346,
124.292397059673));
#116961=CARTESIAN_POINT('Ctrl Pts',(4.7729824502807,-28.4794381113972,124.319177365008));
#116962=CARTESIAN_POINT('Ctrl Pts',(4.77354556525418,-28.4759923298395,
124.326926058278));
#116963=CARTESIAN_POINT('Ctrl Pts',(4.77451926779054,-28.470173387285,124.340285182138));
#116964=CARTESIAN_POINT('Ctrl Pts',(4.77492813381232,-28.4677715825235,
124.345882899312));
#116965=CARTESIAN_POINT('Ctrl Pts',(4.77579853489,-28.4627475079176,124.357771672162));
#116966=CARTESIAN_POINT('Ctrl Pts',(4.77626048300065,-28.4601331616044,
124.364065596676));
#116967=CARTESIAN_POINT('Ctrl Pts',(4.77754063810094,-28.4530291819928,
124.38146878718));
#116968=CARTESIAN_POINT('Ctrl Pts',(4.77836337070612,-28.4486207721539,
124.392610467891));
#116969=CARTESIAN_POINT('Ctrl Pts',(4.78298345315674,-28.4247140732948,
124.454990131926));
#116970=CARTESIAN_POINT('Ctrl Pts',(4.78689457477958,-28.4076357984436,
124.507114096948));
#116971=CARTESIAN_POINT('Ctrl Pts',(4.80156354832864,-28.3539853336534,
124.703031438508));
#116972=CARTESIAN_POINT('Ctrl Pts',(4.81248202844361,-28.3340822986218,
124.850709193547));
#116973=CARTESIAN_POINT('Ctrl Pts',(4.82498050555705,-28.3339828214303,
125.030605074958));
#116974=CARTESIAN_POINT('Ctrl Pts',(4.82714463543918,-28.3348602620568,
125.062127258076));
#116975=CARTESIAN_POINT('Ctrl Pts',(4.83022909206343,-28.3374177715957,
125.10757319661));
#116976=CARTESIAN_POINT('Ctrl Pts',(4.83117144314779,-28.3383795779757,
125.121528814164));
#116977=CARTESIAN_POINT('Ctrl Pts',(4.83282998096261,-28.3403932604248,
125.14621073381));
#116978=CARTESIAN_POINT('Ctrl Pts',(4.83354835881832,-28.3413736517119,
125.156941883741));
#116979=CARTESIAN_POINT('Ctrl Pts',(4.83504069871296,-28.3436366818982,
125.179314545688));
#116980=CARTESIAN_POINT('Ctrl Pts',(4.83581403054194,-28.3449381027186,
125.190953595979));
#116981=CARTESIAN_POINT('Ctrl Pts',(4.83783589563745,-28.348679511804,125.221494568576));
#116982=CARTESIAN_POINT('Ctrl Pts',(4.83907805904064,-28.3513213373572,
125.240370369404));
#116983=CARTESIAN_POINT('Ctrl Pts',(4.84549040007951,-28.3667454337356,
125.338302097014));
#116984=CARTESIAN_POINT('Ctrl Pts',(4.85048818984653,-28.3848922241868,
125.416410867518));
#116985=CARTESIAN_POINT('Ctrl Pts',(4.8572016034264,-28.4171923328068,125.520693063046));
#116986=CARTESIAN_POINT('Ctrl Pts',(4.85897938281318,-28.4265191394924,
125.548232470602));
#116987=CARTESIAN_POINT('Ctrl Pts',(4.86075486118656,-28.4365599784656,
125.575509599455));
#116988=CARTESIAN_POINT('',(4.62852042919292,-28.3357497203589,125.001193953836));
#116989=CARTESIAN_POINT('Ctrl Pts',(4.66781556895434,-28.4339562630661,
125.576468403481));
#116990=CARTESIAN_POINT('Ctrl Pts',(4.66777083770939,-28.4337261660757,
125.575843545651));
#116991=CARTESIAN_POINT('Ctrl Pts',(4.65467245778892,-28.3664685496906,
125.392825950738));
#116992=CARTESIAN_POINT('Ctrl Pts',(4.64157407786846,-28.334468402925,125.196877811068));
#116993=CARTESIAN_POINT('Ctrl Pts',(4.62852042919292,-28.3357497203589,
125.001193953836));
#116994=CARTESIAN_POINT('Ctrl Pts',(4.6275136190416,-28.3340004723798,125.00125457927));
#116995=CARTESIAN_POINT('Ctrl Pts',(4.6239375618158,-28.3339624568575,124.950772442624));
#116996=CARTESIAN_POINT('Ctrl Pts',(4.62041976511974,-28.3362189480784,
124.900309774701));
#116997=CARTESIAN_POINT('Ctrl Pts',(4.61604554105104,-28.3419851644348,
124.836517043977));
#116998=CARTESIAN_POINT('Ctrl Pts',(4.61512462459214,-28.3433707318118,
124.823027237963));
#116999=CARTESIAN_POINT('Ctrl Pts',(4.61350377315945,-28.3461143487295,
124.799183530003));
#117000=CARTESIAN_POINT('Ctrl Pts',(4.61280178313282,-28.3474053112998,
124.788822809959));
#117001=CARTESIAN_POINT('Ctrl Pts',(4.61141212000764,-28.3501656184413,
124.768248018594));
#117002=CARTESIAN_POINT('Ctrl Pts',(4.61072440635864,-28.3516326308489,
124.758034109817));
#117003=CARTESIAN_POINT('Ctrl Pts',(4.60926076993725,-28.3549710616375,
124.736231993051));
#117004=CARTESIAN_POINT('Ctrl Pts',(4.60848576349747,-28.3568702538317,
124.724648554252));
#117005=CARTESIAN_POINT('Ctrl Pts',(4.60645344662114,-28.36219723033,124.694178998796));
#117006=CARTESIAN_POINT('Ctrl Pts',(4.60520263348851,-28.3658293058874,
124.675330030457));
#117007=CARTESIAN_POINT('Ctrl Pts',(4.59880832819561,-28.3862140855227,
124.578572740266));
#117008=CARTESIAN_POINT('Ctrl Pts',(4.59383504404583,-28.408215857731,124.501872029714));
#117009=CARTESIAN_POINT('Ctrl Pts',(4.58390751218169,-28.4637340275011,
124.350290617888));
#117010=CARTESIAN_POINT('Ctrl Pts',(4.57896992556178,-28.4974497369693,
124.275722699557));
#117011=CARTESIAN_POINT('Ctrl Pts',(4.57132676090821,-28.5565738161393,
124.16702842421));
#117012=CARTESIAN_POINT('Ctrl Pts',(4.56870420584042,-28.5780346285061,
124.130900001632));
#117013=CARTESIAN_POINT('Ctrl Pts',(4.5643940250378,-28.6146663041366,124.074227001829));
#117014=CARTESIAN_POINT('Ctrl Pts',(4.56274507237488,-28.6289845852772,
124.053151724226));
#117015=CARTESIAN_POINT('Ctrl Pts',(4.56046510581799,-28.64908431832,124.024978846363));
#117016=CARTESIAN_POINT('Ctrl Pts',(4.55985963947971,-28.6544500766305,
124.017587243912));
#117017=CARTESIAN_POINT('Ctrl Pts',(4.5588360844876,-28.6635617174338,124.005250181324));
#117018=CARTESIAN_POINT('Ctrl Pts',(4.55842019385935,-28.6672750409911,
124.000280705919));
#117019=CARTESIAN_POINT('Ctrl Pts',(4.55756067966869,-28.6749697654381,
123.990102053023));
#117020=CARTESIAN_POINT('Ctrl Pts',(4.55711686081514,-28.6789542769691,
123.984895483346));
#117021=CARTESIAN_POINT('Ctrl Pts',(4.55593674459495,-28.6895814628421,
123.971177455592));
#117022=CARTESIAN_POINT('Ctrl Pts',(4.55519698022075,-28.6962761955396,
123.962706986091));
#117023=CARTESIAN_POINT('Ctrl Pts',(4.55184909975054,-28.7267413816829,
123.924921924913));
#117024=CARTESIAN_POINT('Ctrl Pts',(4.54918703129522,-28.7514197832095,
123.896357244628));
#117025=CARTESIAN_POINT('Ctrl Pts',(4.53895755579082,-28.8486307895759,
123.791274337358));
#117026=CARTESIAN_POINT('Ctrl Pts',(4.53119518671602,-28.9273993093324,
123.720860840384));
#117027=CARTESIAN_POINT('Ctrl Pts',(4.51964436242677,-29.0564608674606,
123.625846490869));
#117028=CARTESIAN_POINT('Ctrl Pts',(4.51573892437174,-29.1022096527089,
123.595529483357));
#117029=CARTESIAN_POINT('Ctrl Pts',(4.51016015832971,-29.1708887879186,
123.554746849849));
#117030=CARTESIAN_POINT('Ctrl Pts',(4.50842844620163,-29.1926889401731,
123.542457192206));
#117031=CARTESIAN_POINT('Ctrl Pts',(4.50530900082085,-29.2328371772173,
123.521001224076));
#117032=CARTESIAN_POINT('Ctrl Pts',(4.50391594985222,-29.2510930955652,
123.511673863228));
#117033=CARTESIAN_POINT('Ctrl Pts',(4.50172506914042,-29.2803151867611,
123.497417517666));
#117034=CARTESIAN_POINT('Ctrl Pts',(4.5009195965488,-29.2911700440651,123.492266451494));
#117035=CARTESIAN_POINT('Ctrl Pts',(4.49940458149445,-29.3117939833515,
123.482751527787));
#117036=CARTESIAN_POINT('Ctrl Pts',(4.4986942368313,-29.3215511712721,123.478363498172));
#117037=CARTESIAN_POINT('Ctrl Pts',(4.49708623948698,-29.3438326293942,
123.468599950394));
#117038=CARTESIAN_POINT('Ctrl Pts',(4.49619063022583,-29.3563820535877,
123.463283471956));
#117039=CARTESIAN_POINT('Ctrl Pts',(4.49385910617347,-29.3894036755574,
123.449769574818));
#117040=CARTESIAN_POINT('Ctrl Pts',(4.4924315720158,-29.4099762526942,123.441823407701));
#117041=CARTESIAN_POINT('Ctrl Pts',(4.48374083056788,-29.5372268509231,
123.395554627666));
#117042=CARTESIAN_POINT('Ctrl Pts',(4.47683512781077,-29.6474296374407,
123.367792400218));
#117043=CARTESIAN_POINT('Ctrl Pts',(4.46400861349008,-29.85525008001,123.337488221073));
#117044=CARTESIAN_POINT('Ctrl Pts',(4.45810741105641,-29.951911980061,123.331893169279));
#117045=CARTESIAN_POINT('Ctrl Pts',(4.45088911827662,-30.0628214707039,
123.335123191926));
#117046=CARTESIAN_POINT('Ctrl Pts',(4.44994864637216,-30.0771379380591,
123.335725074394));
#117047=CARTESIAN_POINT('Ctrl Pts',(4.44851420767756,-30.0987368028933,
123.3369123939));
#117048=CARTESIAN_POINT('Ctrl Pts',(4.44802739989435,-30.1060264536135,
123.337361215442));
#117049=CARTESIAN_POINT('Ctrl Pts',(4.44713535547297,-30.1193052726517,
123.338266468655));
#117050=CARTESIAN_POINT('Ctrl Pts',(4.44673097448782,-30.1252952329037,
123.338707377272));
#117051=CARTESIAN_POINT('Ctrl Pts',(4.44580395327426,-30.1389598320813,
123.339787522105));
#117052=CARTESIAN_POINT('Ctrl Pts',(4.44528020639347,-30.1466324788901,
123.34044758536));
#117053=CARTESIAN_POINT('Ctrl Pts',(4.44363375921617,-30.1706126452903,
123.342678146121));
#117054=CARTESIAN_POINT('Ctrl Pts',(4.44250162191485,-30.1869011910927,
123.34443595813));
#117055=CARTESIAN_POINT('Ctrl Pts',(4.43589087854303,-30.28100575181,123.355997827549));
#117056=CARTESIAN_POINT('Ctrl Pts',(4.43020408697857,-30.3580713563141,
123.371046365756));
#117057=CARTESIAN_POINT('Ctrl Pts',(4.41966015512029,-30.4979667454167,
123.408772692479));
#117058=CARTESIAN_POINT('Ctrl Pts',(4.41481697701063,-30.5610605802085,
123.429908587048));
#117059=CARTESIAN_POINT('Ctrl Pts',(4.40659821662898,-30.6673515701857,
123.472743352658));
#117060=CARTESIAN_POINT('Ctrl Pts',(4.40318977590103,-30.7111813621061,
123.492653737976));
#117061=CARTESIAN_POINT('Ctrl Pts',(4.39751122011841,-30.783914391932,123.529573928426));
#117062=CARTESIAN_POINT('Ctrl Pts',(4.39521199812144,-30.8132767202812,
123.545608079141));
#117063=CARTESIAN_POINT('Ctrl Pts',(4.39196337816406,-30.8546124657938,
123.569824296462));
#117064=CARTESIAN_POINT('Ctrl Pts',(4.39098890782616,-30.8669912957543,
123.577294434659));
#117065=CARTESIAN_POINT('Ctrl Pts',(4.38929635097504,-30.888450015477,123.590628034534));
#117066=CARTESIAN_POINT('Ctrl Pts',(4.38857571876595,-30.8975728427396,
123.596420373301));
#117067=CARTESIAN_POINT('Ctrl Pts',(4.38708763826762,-30.9163789119354,
123.608619219607));
#117068=CARTESIAN_POINT('Ctrl Pts',(4.38632073511994,-30.9260528612506,
123.615039027277));
#117069=CARTESIAN_POINT('Ctrl Pts',(4.38433539213345,-30.9510419395565,
123.632001137973));
#117070=CARTESIAN_POINT('Ctrl Pts',(4.38312289914863,-30.9662493708966,
123.642699791613));
#117071=CARTESIAN_POINT('Ctrl Pts',(4.37775649630183,-31.0332488655607,
123.691531809118));
#117072=CARTESIAN_POINT('Ctrl Pts',(4.37370870515379,-31.0829891046085,
123.732392722253));
#117073=CARTESIAN_POINT('Ctrl Pts',(4.36078349152526,-31.2362894563955,
123.873954533147));
#117074=CARTESIAN_POINT('Ctrl Pts',(4.35225951593735,-31.329141929386,123.985228350538));
#117075=CARTESIAN_POINT('Ctrl Pts',(4.34155843054311,-31.4185612684161,
124.126073541137));
#117076=CARTESIAN_POINT('Ctrl Pts',(4.34009559672282,-31.430248340487,124.145334514263));
#117077=CARTESIAN_POINT('Ctrl Pts',(4.33803436412337,-31.4459127944192,
124.172371908705));
#117078=CARTESIAN_POINT('Ctrl Pts',(4.33745561601757,-31.4502255397583,
124.179952475699));
#117079=CARTESIAN_POINT('Ctrl Pts',(4.33646380079489,-31.4574671518285,
124.192916941977));
#117080=CARTESIAN_POINT('Ctrl Pts',(4.33605262262066,-31.4604262612337,
124.198283905885));
#117081=CARTESIAN_POINT('Ctrl Pts',(4.33518750371661,-31.4665608975553,
124.209557023808));
#117082=CARTESIAN_POINT('Ctrl Pts',(4.33473323193015,-31.4697304457395,
124.215466139844));
#117083=CARTESIAN_POINT('Ctrl Pts',(4.33349540021967,-31.4782297501892,
124.231544005287));
#117084=CARTESIAN_POINT('Ctrl Pts',(4.33270777533694,-31.4834900892777,
124.241748757439));
#117085=CARTESIAN_POINT('Ctrl Pts',(4.32870343820016,-31.5095142975284,
124.293541722267));
#117086=CARTESIAN_POINT('Ctrl Pts',(4.32540472585382,-31.5286348485165,
124.33592818055));
#117087=CARTESIAN_POINT('Ctrl Pts',(4.32117889486761,-31.5505428244502,
124.390472023849));
#117088=CARTESIAN_POINT('Ctrl Pts',(4.32029137841869,-31.5550022663463,
124.401940348357));
#117089=CARTESIAN_POINT('Ctrl Pts',(4.31119280338278,-31.5993052171702,
124.519720439028));
#117090=CARTESIAN_POINT('Ctrl Pts',(4.30285176938574,-31.628313544663,124.629804183977));
#117091=CARTESIAN_POINT('Ctrl Pts',(4.29083621630954,-31.6545315070307,
124.797051188914));
#117092=CARTESIAN_POINT('Ctrl Pts',(4.28695000220397,-31.660395617532,124.852520020277));
#117093=CARTESIAN_POINT('Ctrl Pts',(4.28197072407766,-31.6644205951122,
124.92544241941));
#117094=CARTESIAN_POINT('Ctrl Pts',(4.28080065422388,-31.6651045619957,
124.942714862513));
#117095=CARTESIAN_POINT('Ctrl Pts',(4.27887713041502,-31.6657918151533,
124.971327414729));
#117096=CARTESIAN_POINT('Ctrl Pts',(4.27811895961906,-31.6659483480288,
124.982662144019));
#117097=CARTESIAN_POINT('Ctrl Pts',(4.27664430148294,-31.6660281607841,
125.004815346992));
#117098=CARTESIAN_POINT('Ctrl Pts',(4.27592752877229,-31.6659617740972,
125.015633192928));
#117099=CARTESIAN_POINT('Ctrl Pts',(4.274212422453,-31.6655489446354,125.041632860686));
#117100=CARTESIAN_POINT('Ctrl Pts',(4.27321731690479,-31.665100289338,125.056812266337));
#117101=CARTESIAN_POINT('Ctrl Pts',(4.26992389061443,-31.6629151975043,
125.107336985913));
#117102=CARTESIAN_POINT('Ctrl Pts',(4.26765394037276,-31.660260202349,125.142634234797));
#117103=CARTESIAN_POINT('Ctrl Pts',(4.25594730946091,-31.6405356194274,
125.326376338418));
#117104=CARTESIAN_POINT('Ctrl Pts',(4.24710776268307,-31.6046805705133,
125.472097272328));
#117105=CARTESIAN_POINT('Ctrl Pts',(4.23575366586114,-31.5378713234268,
125.641545058589));
#117106=CARTESIAN_POINT('Ctrl Pts',(4.23368914925321,-31.5249655788896,
125.671645734975));
#117107=CARTESIAN_POINT('Ctrl Pts',(4.23020763861349,-31.5021534629487,
125.72079883118));
#117108=CARTESIAN_POINT('Ctrl Pts',(4.22881326754233,-31.4927504221238,
125.740075708319));
#117109=CARTESIAN_POINT('Ctrl Pts',(4.22683302510541,-31.4790783596106,
125.766783189641));
#117110=CARTESIAN_POINT('Ctrl Pts',(4.22626482784102,-31.4751197107079,
125.774371412831));
#117111=CARTESIAN_POINT('Ctrl Pts',(4.22528533890743,-31.4682388932838,
125.787316828047));
#117112=CARTESIAN_POINT('Ctrl Pts',(4.22487582712739,-31.4653454544112,
125.792689052272));
#117113=CARTESIAN_POINT('Ctrl Pts',(4.22400753710567,-31.4591769182905,
125.803992927678));
#117114=CARTESIAN_POINT('Ctrl Pts',(4.22354837816044,-31.45589517375,125.809920456328));
#117115=CARTESIAN_POINT('Ctrl Pts',(4.22228338892511,-31.4467975385827,
125.826118754195));
#117116=CARTESIAN_POINT('Ctrl Pts',(4.22147319932365,-31.4409086411515,
125.83634776362));
#117117=CARTESIAN_POINT('Ctrl Pts',(4.21704433047729,-31.4083572570148,
125.891525139464));
#117118=CARTESIAN_POINT('Ctrl Pts',(4.21332202333584,-31.3797020102034,
125.93525851543));
#117119=CARTESIAN_POINT('Ctrl Pts',(4.20252035818099,-31.291821509232,126.056533442922));
#117120=CARTESIAN_POINT('Ctrl Pts',(4.19535735206574,-31.2277738738686,
126.130326679629));
#117121=CARTESIAN_POINT('Ctrl Pts',(4.1829910097119,-31.1039288223965,126.249990126512));
#117122=CARTESIAN_POINT('Ctrl Pts',(4.17773177839953,-31.046783184364,126.298222604811));
#117123=CARTESIAN_POINT('Ctrl Pts',(4.17134452873138,-30.9714748825422,
126.353567208739));
#117124=CARTESIAN_POINT('Ctrl Pts',(4.17007273007814,-30.9561776380079,
126.364416362567));
#117125=CARTESIAN_POINT('Ctrl Pts',(4.16802721681029,-30.9310899839611,
126.381579899126));
#117126=CARTESIAN_POINT('Ctrl Pts',(4.16724751458468,-30.9214111797332,
126.388053682562));
#117127=CARTESIAN_POINT('Ctrl Pts',(4.16575239607922,-30.9026311239892,
126.400331943234));
#117128=CARTESIAN_POINT('Ctrl Pts',(4.1650364813213,-30.8935398041171,126.406150463156));
#117129=CARTESIAN_POINT('Ctrl Pts',(4.16339109487335,-30.8724210997654,
126.419379078216));
#117130=CARTESIAN_POINT('Ctrl Pts',(4.16246399573286,-30.8603546234547,
126.426725441425));
#117131=CARTESIAN_POINT('Ctrl Pts',(4.15943007726731,-30.8203337315293,
126.450398736041));
#117132=CARTESIAN_POINT('Ctrl Pts',(4.15734689018052,-30.7919958340841,
126.46606505455));
#117133=CARTESIAN_POINT('Ctrl Pts',(4.14727366930413,-30.651196338731,126.538629670035));
#117134=CARTESIAN_POINT('Ctrl Pts',(4.13969898072987,-30.5329881880253,
126.583465614267));
#117135=CARTESIAN_POINT('Ctrl Pts',(4.12880549058354,-30.3610194039377,
126.627226121469));
#117136=CARTESIAN_POINT('Ctrl Pts',(4.1256225041865,-30.3106319928343,126.637591795652));
#117137=CARTESIAN_POINT('Ctrl Pts',(4.12050586464599,-30.2311307506781,
126.65014542667));
#117138=CARTESIAN_POINT('Ctrl Pts',(4.11863101967559,-30.2022998654994,
126.653927409427));
#117139=CARTESIAN_POINT('Ctrl Pts',(4.11608799650355,-30.1638576399227,
126.657950082375));
#117140=CARTESIAN_POINT('Ctrl Pts',(4.11545355900496,-30.1543202001754,
126.658864993546));
#117141=CARTESIAN_POINT('Ctrl Pts',(4.11439497470346,-30.1385060590429,
126.660244463591));
#117142=CARTESIAN_POINT('Ctrl Pts',(4.1139733723927,-30.1322334888595,126.66075582468));
#117143=CARTESIAN_POINT('Ctrl Pts',(4.1131169529277,-30.1195475435465,126.661717701202));
#117144=CARTESIAN_POINT('Ctrl Pts',(4.11268206649378,-30.1131341958608,
126.66216665345));
#117145=CARTESIAN_POINT('Ctrl Pts',(4.11155114247452,-30.0965256544854,
126.663232732119));
#117146=CARTESIAN_POINT('Ctrl Pts',(4.11085211903813,-30.0863272766544,
126.663793229741));
#117147=CARTESIAN_POINT('Ctrl Pts',(4.10794928637258,-30.0442270075574,
126.665718933189));
#117148=CARTESIAN_POINT('Ctrl Pts',(4.10570708694556,-30.0122963143604,
126.666260507857));
#117149=CARTESIAN_POINT('Ctrl Pts',(4.09571478728842,-29.8717746359347,
126.664604866642));
#117150=CARTESIAN_POINT('Ctrl Pts',(4.08771233275723,-29.7635647252818,
126.652709689751));
#117151=CARTESIAN_POINT('Ctrl Pts',(4.07574585805454,-29.6013226152742,
126.618605039537));
#117152=CARTESIAN_POINT('Ctrl Pts',(4.07166703450062,-29.5460008205429,
126.603967506771));
#117153=CARTESIAN_POINT('Ctrl Pts',(4.06503359477111,-29.4556492874781,
126.575010635209));
#117154=CARTESIAN_POINT('Ctrl Pts',(4.06243501874747,-29.4201601198509,
126.56229392441));
#117155=CARTESIAN_POINT('Ctrl Pts',(4.05884932327329,-29.3710827959981,
126.542805107416));
#117156=CARTESIAN_POINT('Ctrl Pts',(4.05782940784878,-29.3571115029106,
126.537035736547));
#117157=CARTESIAN_POINT('Ctrl Pts',(4.05608411417787,-29.3331905109617,
126.526774446916));
#117158=CARTESIAN_POINT('Ctrl Pts',(4.05535571354866,-29.3232030915294,
126.522373495853));
#117159=CARTESIAN_POINT('Ctrl Pts',(4.05396429482689,-29.3041211614648,
126.513740150738));
#117160=CARTESIAN_POINT('Ctrl Pts',(4.05330078846113,-29.2950202509714,
126.50952315742));
#117161=CARTESIAN_POINT('Ctrl Pts',(4.0515637535685,-29.2711954313356,126.498221235096));
#117162=CARTESIAN_POINT('Ctrl Pts',(4.05049492103353,-29.256536464309,126.491001331569));
#117163=CARTESIAN_POINT('Ctrl Pts',(4.04663067059832,-29.2035794786347,
126.463943461823));
#117164=CARTESIAN_POINT('Ctrl Pts',(4.04387946595003,-29.1659475932882,
126.442835117309));
#117165=CARTESIAN_POINT('Ctrl Pts',(4.03394974542766,-29.0313492304479,
126.360308465389));
#117166=CARTESIAN_POINT('Ctrl Pts',(4.02705443893515,-28.9399840379235,
126.290383762643));
#117167=CARTESIAN_POINT('Ctrl Pts',(4.01702527179702,-28.8213762301946,
126.178447413574));
#117168=CARTESIAN_POINT('Ctrl Pts',(4.01402531442402,-28.7876864617562,
126.143760262708));
#117169=CARTESIAN_POINT('Ctrl Pts',(4.00916944944701,-28.7369742924151,
126.086785648973));
#117170=CARTESIAN_POINT('Ctrl Pts',(4.00736534809849,-28.71892344232,126.065448084705));
#117171=CARTESIAN_POINT('Ctrl Pts',(4.00490445364709,-28.6955009042766,
126.036304663281));
#117172=CARTESIAN_POINT('Ctrl Pts',(4.00427871249933,-28.6896457259004,
126.028891107864));
#117173=CARTESIAN_POINT('Ctrl Pts',(4.00323069623234,-28.6800125485721,
126.016478424503));
#117174=CARTESIAN_POINT('Ctrl Pts',(4.00281086026394,-28.6761990253808,
126.011506913893));
#117175=CARTESIAN_POINT('Ctrl Pts',(4.00195378036007,-28.6685083570726,
126.001362966315));
#117176=CARTESIAN_POINT('Ctrl Pts',(4.00151643124816,-28.6646331247064,
125.996189284355));
#117177=CARTESIAN_POINT('Ctrl Pts',(4.00037193420677,-28.6546169296553,
125.982653565336));
#117178=CARTESIAN_POINT('Ctrl Pts',(3.99966167019552,-28.6485239077102,
125.974256636452));
#117179=CARTESIAN_POINT('Ctrl Pts',(3.99664638996665,-28.6231559708506,
125.93860060631));
#117180=CARTESIAN_POINT('Ctrl Pts',(3.99429932888321,-28.6046255831409,
125.910824057031));
#117181=CARTESIAN_POINT('Ctrl Pts',(3.98424977189428,-28.5298567213915,
125.791106001401));
#117182=CARTESIAN_POINT('Ctrl Pts',(3.97631022084783,-28.4817745581952,
125.694378489058));
#117183=CARTESIAN_POINT('Ctrl Pts',(3.96806748132605,-28.4410652415147,
125.587639587124));
#117184=CARTESIAN_POINT('Ctrl Pts',(3.96760122759222,-28.4387948763755,
125.581580964228));
#117185=CARTESIAN_POINT('Ctrl Pts',(3.96713564162385,-28.4365599852621,
125.575509617918));
#117186=CARTESIAN_POINT('Origin',(5.,-30.,125.));
#117187=CARTESIAN_POINT('',(3.26654944485247,-28.4365599843055,125.57550961532));
#117188=CARTESIAN_POINT('',(3.46014888220092,-28.4365599331867,125.575509476449));
#117189=CARTESIAN_POINT('',(5.,-28.4365599837785,125.575509613888));
#117190=CARTESIAN_POINT('',(4.12030991028152,-28.3340002413346,124.999103268726));
#117191=CARTESIAN_POINT('Ctrl Pts',(3.46014888220092,-28.4365599331867,
125.575509476449));
#117192=CARTESIAN_POINT('Ctrl Pts',(3.46532991775447,-28.4612287593674,
125.642525282149));
#117193=CARTESIAN_POINT('Ctrl Pts',(3.47055310032042,-28.4901913607366,
125.707913999253));
#117194=CARTESIAN_POINT('Ctrl Pts',(3.48167381485054,-28.5615879239327,
125.844614835882));
#117195=CARTESIAN_POINT('Ctrl Pts',(3.48752709335552,-28.6053125474045,
125.915015928909));
#117196=CARTESIAN_POINT('Ctrl Pts',(3.49453388119038,-28.6656551191771,
125.997729631814));
#117197=CARTESIAN_POINT('Ctrl Pts',(3.49586545408808,-28.6774938168255,
126.013369691517));
#117198=CARTESIAN_POINT('Ctrl Pts',(3.49798283583202,-28.6969111525982,
126.038101817227));
#117199=CARTESIAN_POINT('Ctrl Pts',(3.49877542725244,-28.7043149569333,
126.047328128534));
#117200=CARTESIAN_POINT('Ctrl Pts',(3.5002802435704,-28.7186283026569,126.064780708679));
#117201=CARTESIAN_POINT('Ctrl Pts',(3.50099312033602,-28.7255203366588,
126.073020494341));
#117202=CARTESIAN_POINT('Ctrl Pts',(3.50262636737665,-28.7415642556874,
126.091829158633));
#117203=CARTESIAN_POINT('Ctrl Pts',(3.50354444804996,-28.7507705234206,
126.102350746716));
#117204=CARTESIAN_POINT('Ctrl Pts',(3.50645501158062,-28.7805447547872,
126.135526786545));
#117205=CARTESIAN_POINT('Ctrl Pts',(3.50842684198261,-28.8016055044676,
126.157731833981));
#117206=CARTESIAN_POINT('Ctrl Pts',(3.51308438016914,-28.8533503061446,
126.209362014637));
#117207=CARTESIAN_POINT('Ctrl Pts',(3.51574753310864,-28.88457245638,126.238217984662));
#117208=CARTESIAN_POINT('Ctrl Pts',(3.5229525464642,-28.9728743250068,126.313774157698));
#117209=CARTESIAN_POINT('Ctrl Pts',(3.52742680294526,-29.0320031187659,
126.357929340266));
#117210=CARTESIAN_POINT('Ctrl Pts',(3.53278268559425,-29.1054688779818,
126.405546651875));
#117211=CARTESIAN_POINT('Ctrl Pts',(3.53363004522545,-29.1171689882141,
126.412924880407));
#117212=CARTESIAN_POINT('Ctrl Pts',(3.53899665000148,-29.1916463202109,
126.458604895782));
#117213=CARTESIAN_POINT('Ctrl Pts',(3.5435683560016,-29.256802455335,126.492855848905));
#117214=CARTESIAN_POINT('Ctrl Pts',(3.54917284952906,-29.3352211517049,
126.527670077878));
#117215=CARTESIAN_POINT('Ctrl Pts',(3.54998125458917,-29.3464986056246,
126.532528201948));
#117216=CARTESIAN_POINT('Ctrl Pts',(3.55125852061003,-29.364242243006,126.539940385763));
#117217=CARTESIAN_POINT('Ctrl Pts',(3.55172250411449,-29.3706727284248,
126.542579494923));
#117218=CARTESIAN_POINT('Ctrl Pts',(3.55259524691991,-29.3827354427691,
126.547442125453));
#117219=CARTESIAN_POINT('Ctrl Pts',(3.55300343181197,-29.388363521192,126.549675281582));
#117220=CARTESIAN_POINT('Ctrl Pts',(3.55396997831247,-29.4016596287601,
126.55486731057));
#117221=CARTESIAN_POINT('Ctrl Pts',(3.55452982624035,-29.4093375182824,
126.557800172983));
#117222=CARTESIAN_POINT('Ctrl Pts',(3.55641546833364,-29.4351294277933,
126.567434292581));
#117223=CARTESIAN_POINT('Ctrl Pts',(3.5577548258011,-29.4533374744489,126.573877069074));
#117224=CARTESIAN_POINT('Ctrl Pts',(3.56108938031962,-29.4984906209931,
126.588976141008));
#117225=CARTESIAN_POINT('Ctrl Pts',(3.56309918218078,-29.5255516882073,
126.597264991331));
#117226=CARTESIAN_POINT('Ctrl Pts',(3.57231599811235,-29.6494586680582,
126.631791410014));
#117227=CARTESIAN_POINT('Ctrl Pts',(3.57969566492214,-29.7483427282499,
126.649936823387));
#117228=CARTESIAN_POINT('Ctrl Pts',(3.59286787274552,-29.9302851552353,
126.666577422531));
#117229=CARTESIAN_POINT('Ctrl Pts',(3.59869312869536,-30.0127638957753,
126.667987175944));
#117230=CARTESIAN_POINT('Ctrl Pts',(3.60567285382405,-30.1145896885818,
126.66217009621));
#117231=CARTESIAN_POINT('Ctrl Pts',(3.60700362335552,-30.1341388844873,
126.660706789916));
#117232=CARTESIAN_POINT('Ctrl Pts',(3.60912004177136,-30.1654346609528,
126.657807962926));
#117233=CARTESIAN_POINT('Ctrl Pts',(3.60991246227526,-30.1771991782469,
126.656591782154));
#117234=CARTESIAN_POINT('Ctrl Pts',(3.61141714634194,-30.1996230396647,
126.654032055268));
#117235=CARTESIAN_POINT('Ctrl Pts',(3.61213005976159,-30.2102842377848,
126.652710484742));
#117236=CARTESIAN_POINT('Ctrl Pts',(3.61376366176776,-30.2347933147538,
126.64943131754));
#117237=CARTESIAN_POINT('Ctrl Pts',(3.61468205726588,-30.2486309416167,
126.647402272233));
#117238=CARTESIAN_POINT('Ctrl Pts',(3.61759475633636,-30.2926846761326,
126.640374832179));
#117239=CARTESIAN_POINT('Ctrl Pts',(3.61956836327565,-30.3227902324913,
126.634717273503));
#117240=CARTESIAN_POINT('Ctrl Pts',(3.62423100207547,-30.3943108343342,
126.61922375425));
#117241=CARTESIAN_POINT('Ctrl Pts',(3.62689740871858,-30.4355388687808,
126.608624528928));
#117242=CARTESIAN_POINT('Ctrl Pts',(3.63410406030919,-30.5469337260266,
126.575388827143));
#117243=CARTESIAN_POINT('Ctrl Pts',(3.63857691673909,-30.6160751916339,
126.549657439062));
#117244=CARTESIAN_POINT('Ctrl Pts',(3.6439445879609,-30.6960954875547,126.513672466843));
#117245=CARTESIAN_POINT('Ctrl Pts',(3.64480505028118,-30.708831504118,126.50775036306));
#117246=CARTESIAN_POINT('Ctrl Pts',(3.65016779017718,-30.7875183002385,
126.469944525175));
#117247=CARTESIAN_POINT('Ctrl Pts',(3.65472264274787,-30.8513734072728,
126.433904665862));
#117248=CARTESIAN_POINT('Ctrl Pts',(3.66030842699278,-30.9229138819223,
126.387060461597));
#117249=CARTESIAN_POINT('Ctrl Pts',(3.66111676280043,-30.9331109793367,
126.380221227214));
#117250=CARTESIAN_POINT('Ctrl Pts',(3.66239394293167,-30.9489606881828,
126.3693348481));
#117251=CARTESIAN_POINT('Ctrl Pts',(3.66285791085971,-30.9546653803884,
126.365363805382));
#117252=CARTESIAN_POINT('Ctrl Pts',(3.66373064188961,-30.9652929101285,
126.35786680626));
#117253=CARTESIAN_POINT('Ctrl Pts',(3.66413883078226,-30.9702215891158,
126.354349559463));
#117254=CARTESIAN_POINT('Ctrl Pts',(3.66510541059366,-30.9817953481934,
126.34599459679));
#117255=CARTESIAN_POINT('Ctrl Pts',(3.66566528814227,-30.9884239203541,
126.34113448502));
#117256=CARTESIAN_POINT('Ctrl Pts',(3.66755113674812,-31.0105089247112,
126.324688958416));
#117257=CARTESIAN_POINT('Ctrl Pts',(3.66889067499644,-31.0257991423795,
126.312884291714));
#117258=CARTESIAN_POINT('Ctrl Pts',(3.67222578053739,-31.0629797880686,
126.283133311526));
#117259=CARTESIAN_POINT('Ctrl Pts',(3.67423595840849,-31.0846242931938,
126.264890148074));
#117260=CARTESIAN_POINT('Ctrl Pts',(3.68345611992189,-31.1808671940163,
126.179484337047));
#117261=CARTESIAN_POINT('Ctrl Pts',(3.69083884779448,-31.2497674287165,
126.106215386806));
#117262=CARTESIAN_POINT('Ctrl Pts',(3.70401036702836,-31.3624104493522,
125.962377534351));
#117263=CARTESIAN_POINT('Ctrl Pts',(3.70983218646979,-31.408298938585,125.893885068763));
#117264=CARTESIAN_POINT('Ctrl Pts',(3.71680858975323,-31.4586141220279,
125.805223578588));
#117265=CARTESIAN_POINT('Ctrl Pts',(3.71813925838095,-31.4679867582043,
125.78800704512));
#117266=CARTESIAN_POINT('Ctrl Pts',(3.72025555580035,-31.4825241516162,
125.760143408546));
#117267=CARTESIAN_POINT('Ctrl Pts',(3.72104795483627,-31.4878828749239,
125.749600176543));
#117268=CARTESIAN_POINT('Ctrl Pts',(3.72255262230491,-31.4978940955259,
125.729372797756));
#117269=CARTESIAN_POINT('Ctrl Pts',(3.72326554034158,-31.5025660537777,
125.719699008456));
#117270=CARTESIAN_POINT('Ctrl Pts',(3.72489918699927,-31.5131041798168,
125.697328710352));
#117271=CARTESIAN_POINT('Ctrl Pts',(3.72581762209329,-31.5189047473797,
125.684602057698));
#117272=CARTESIAN_POINT('Ctrl Pts',(3.72873058983711,-31.5368954121266,
125.643775286773));
#117273=CARTESIAN_POINT('Ctrl Pts',(3.73070442029226,-31.5484715910502,
125.615410471343));
#117274=CARTESIAN_POINT('Ctrl Pts',(3.73536770096955,-31.5742480175744,
125.546909826777));
#117275=CARTESIAN_POINT('Ctrl Pts',(3.73803451710919,-31.5877052751456,
125.506517047856));
#117276=CARTESIAN_POINT('Ctrl Pts',(3.74524136264681,-31.6201977354068,
125.394899125859));
#117277=CARTESIAN_POINT('Ctrl Pts',(3.74971403117173,-31.6360775111014,
125.3228571845));
#117278=CARTESIAN_POINT('Ctrl Pts',(3.75508290058745,-31.6492465947405,
125.236092277556));
#117279=CARTESIAN_POINT('Ctrl Pts',(3.75594473806314,-31.6511813048847,
125.22215802037));
#117280=CARTESIAN_POINT('Ctrl Pts',(3.76130699327965,-31.6620898394809,
125.1355535307));
#117281=CARTESIAN_POINT('Ctrl Pts',(3.76585999824478,-31.6664399486111,
125.062390575192));
#117282=CARTESIAN_POINT('Ctrl Pts',(3.77144373181391,-31.6658852474748,
124.976911108947));
#117283=CARTESIAN_POINT('Ctrl Pts',(3.77225205994675,-31.6656698468975,
124.964634847378));
#117284=CARTESIAN_POINT('Ctrl Pts',(3.77352923055926,-31.6651200394101,
124.945414581429));
#117285=CARTESIAN_POINT('Ctrl Pts',(3.77399319676115,-31.6648778135567,
124.938468096763));
#117286=CARTESIAN_POINT('Ctrl Pts',(3.77486592648628,-31.6643432477886,
124.925473363823));
#117287=CARTESIAN_POINT('Ctrl Pts',(3.77527411582245,-31.6640613929902,
124.919424931681));
#117288=CARTESIAN_POINT('Ctrl Pts',(3.77624069932617,-31.6633192115683,
124.90516982799));
#117289=CARTESIAN_POINT('Ctrl Pts',(3.77680058015803,-31.6628311152389,
124.896964878775));
#117290=CARTESIAN_POINT('Ctrl Pts',(3.77868645165528,-31.660992597261,124.869490512831));
#117291=CARTESIAN_POINT('Ctrl Pts',(3.78002600994291,-31.6593678146676,
124.850241826587));
#117292=CARTESIAN_POINT('Ctrl Pts',(3.7833611765657,-31.6545380464134,124.80286803854));
#117293=CARTESIAN_POINT('Ctrl Pts',(3.78537139611885,-31.650950265369,124.774788549093));
#117294=CARTESIAN_POINT('Ctrl Pts',(3.79459192860026,-31.6313948185806,
124.647604644421));
#117295=CARTESIAN_POINT('Ctrl Pts',(3.80197499590304,-31.6072057302879,
124.549975824683));
#117296=CARTESIAN_POINT('Ctrl Pts',(3.81514643885347,-31.5474533217331,
124.377328245949));
#117297=CARTESIAN_POINT('Ctrl Pts',(3.82096787732227,-31.514799756558,124.301632433047));
#117298=CARTESIAN_POINT('Ctrl Pts',(3.82794391230333,-31.4676029552573,
124.211278421824));
#117299=CARTESIAN_POINT('Ctrl Pts',(3.82927456971232,-31.4582220471357,
124.194066578225));
#117300=CARTESIAN_POINT('Ctrl Pts',(3.83139085367901,-31.4426972420499,
124.16674101946));
#117301=CARTESIAN_POINT('Ctrl Pts',(3.83218325032808,-31.4367458075771,
124.156520683263));
#117302=CARTESIAN_POINT('Ctrl Pts',(3.83368791595135,-31.4251816412912,
124.137139241225));
#117303=CARTESIAN_POINT('Ctrl Pts',(3.83440083450162,-31.4195881653953,
124.127967403364));
#117304=CARTESIAN_POINT('Ctrl Pts',(3.83603448612494,-31.4065093590034,
124.106980955285));
#117305=CARTESIAN_POINT('Ctrl Pts',(3.83695292562201,-31.3989631228259,
124.095205110582));
#117306=CARTESIAN_POINT('Ctrl Pts',(3.83986592324375,-31.3744199963634,
124.057947015548));
#117307=CARTESIAN_POINT('Ctrl Pts',(3.84183977855529,-31.3568677387098,
124.03283699387));
#117308=CARTESIAN_POINT('Ctrl Pts',(3.84650313061535,-31.3132968234182,
123.974027925592));
#117309=CARTESIAN_POINT('Ctrl Pts',(3.84916999229536,-31.2866592920587,
123.940813759968));
#117310=CARTESIAN_POINT('Ctrl Pts',(3.85637685923743,-31.2105064667283,
123.852977739293));
#117311=CARTESIAN_POINT('Ctrl Pts',(3.86084950670794,-31.1585936370154,
123.800563832764));
#117312=CARTESIAN_POINT('Ctrl Pts',(3.86621850567641,-31.0928394189226,
123.742440471932));
#117313=CARTESIAN_POINT('Ctrl Pts',(3.86708049254056,-31.0821800812025,
123.733256052763));
#117314=CARTESIAN_POINT('Ctrl Pts',(3.87244269388305,-31.0153366855485,
123.677121204314));
#117315=CARTESIAN_POINT('Ctrl Pts',(3.87699549691995,-30.9562312757209,
123.633787742421));
#117316=CARTESIAN_POINT('Ctrl Pts',(3.88257900637132,-30.8841182976005,
123.587894624976));
#117317=CARTESIAN_POINT('Ctrl Pts',(3.8833873336643,-30.8736876608711,123.5814173962));
#117318=CARTESIAN_POINT('Ctrl Pts',(3.88466450323518,-30.8572416958763,
123.571454940026));
#117319=CARTESIAN_POINT('Ctrl Pts',(3.88512846924817,-30.8512742793772,
123.567890922304));
#117320=CARTESIAN_POINT('Ctrl Pts',(3.88600119883046,-30.8400669108008,
123.561292159143));
#117321=CARTESIAN_POINT('Ctrl Pts',(3.88640938821511,-30.834832490976,123.558248505014));
#117322=CARTESIAN_POINT('Ctrl Pts',(3.88737597212307,-30.8224536197502,
123.551140584963));
#117323=CARTESIAN_POINT('Ctrl Pts',(3.88793585331422,-30.8152955540348,
123.547100583774));
#117324=CARTESIAN_POINT('Ctrl Pts',(3.88982172731652,-30.7912159644553,
123.533744076505));
#117325=CARTESIAN_POINT('Ctrl Pts',(3.89116128779708,-30.7741630531813,
123.524669317359));
#117326=CARTESIAN_POINT('Ctrl Pts',(3.89449646110404,-30.7317426926238,
123.503033135777));
#117327=CARTESIAN_POINT('Ctrl Pts',(3.89650668521849,-30.7062059489065,
123.490818056826));
#117328=CARTESIAN_POINT('Ctrl Pts',(3.90572725829652,-30.5887465190894,
123.438267251891));
#117329=CARTESIAN_POINT('Ctrl Pts',(3.91311036274472,-30.4936045096298,
123.405639091831));
#117330=CARTESIAN_POINT('Ctrl Pts',(3.92628179734783,-30.3161482211605,
123.36220205613));
#117331=CARTESIAN_POINT('Ctrl Pts',(3.93210319412599,-30.2348433056025,
123.348581189028));
#117332=CARTESIAN_POINT('Ctrl Pts',(3.9390791888024,-30.1333356982793,123.339228566891));
#117333=CARTESIAN_POINT('Ctrl Pts',(3.94040984498329,-30.1137874286749,
123.337774792795));
#117334=CARTESIAN_POINT('Ctrl Pts',(3.9425261274773,-30.0824099611487,123.33599745821));
#117335=CARTESIAN_POINT('Ctrl Pts',(3.94331852386509,-30.0705955709546,
123.335454374724));
#117336=CARTESIAN_POINT('Ctrl Pts',(3.94482318928658,-30.0480403915748,
123.334658137047));
#117337=CARTESIAN_POINT('Ctrl Pts',(3.94553610789297,-30.0373010296701,
123.334382984557));
#117338=CARTESIAN_POINT('Ctrl Pts',(3.94716976005973,-30.0125759171249,
123.333988764232));
#117339=CARTESIAN_POINT('Ctrl Pts',(3.9480882000388,-29.9985897020255,123.333941891105));
#117340=CARTESIAN_POINT('Ctrl Pts',(3.9510012009313,-29.9539761922974,123.334354190202));
#117341=CARTESIAN_POINT('Ctrl Pts',(3.95297505896388,-29.9233604119264,
123.335481836395));
#117342=CARTESIAN_POINT('Ctrl Pts',(3.95763841883828,-29.8503209270508,
123.34019175022));
#117343=CARTESIAN_POINT('Ctrl Pts',(3.96030528550364,-29.8079689377568,
123.344556946585));
#117344=CARTESIAN_POINT('Ctrl Pts',(3.96751215478685,-29.6928714715943,
123.360897186192));
#117345=CARTESIAN_POINT('Ctrl Pts',(3.97198479995059,-29.6206806504457,
123.37608400442));
#117346=CARTESIAN_POINT('Ctrl Pts',(3.98144490244575,-29.4718021718128,
123.417876513893));
#117347=CARTESIAN_POINT('Ctrl Pts',(3.98642785149998,-29.3955789386686,
123.445400466576));
#117348=CARTESIAN_POINT('Ctrl Pts',(3.99271754940338,-29.3069297739578,
123.484919135945));
#117349=CARTESIAN_POINT('Ctrl Pts',(3.99377334547296,-29.2922889685515,
123.491702479008));
#117350=CARTESIAN_POINT('Ctrl Pts',(3.99535521992618,-29.2707517182,123.50206367003));
#117351=CARTESIAN_POINT('Ctrl Pts',(3.99587198756371,-29.2637775704583,
123.505479062234));
#117352=CARTESIAN_POINT('Ctrl Pts',(3.9967941408829,-29.2514473301767,123.511624697639));
#117353=CARTESIAN_POINT('Ctrl Pts',(3.99719832673008,-29.246081766641,123.514335355673));
#117354=CARTESIAN_POINT('Ctrl Pts',(3.99809442097233,-29.2342726764778,
123.520381701839));
#117355=CARTESIAN_POINT('Ctrl Pts',(3.99858709737131,-29.22783629977,123.523730425256));
#117356=CARTESIAN_POINT('Ctrl Pts',(4.00004334439385,-29.2089705797939,
123.533703024247));
#117357=CARTESIAN_POINT('Ctrl Pts',(4.0010135927777,-29.1966034770277,123.540442409874));
#117358=CARTESIAN_POINT('Ctrl Pts',(4.00788448135043,-29.1103358552988,
123.588882046302));
#117359=CARTESIAN_POINT('Ctrl Pts',(4.01404416544292,-29.0396373519479,
123.636014360602));
#117360=CARTESIAN_POINT('Ctrl Pts',(4.02948371415978,-28.8726242102543,
123.766799735977));
#117361=CARTESIAN_POINT('Ctrl Pts',(4.0387027844885,-28.7817102821561,123.856522496258));
#117362=CARTESIAN_POINT('Ctrl Pts',(4.04891683104113,-28.6886644222319,
123.972186528897));
#117363=CARTESIAN_POINT('Ctrl Pts',(4.05035702854925,-28.6757473174831,
123.988883571246));
#117364=CARTESIAN_POINT('Ctrl Pts',(4.05268827165657,-28.655179906664,124.016540128322));
#117365=CARTESIAN_POINT('Ctrl Pts',(4.05358667030016,-28.6473383166857,
124.027353717342));
#117366=CARTESIAN_POINT('Ctrl Pts',(4.05519411568284,-28.6334645112329,
124.046978105102));
#117367=CARTESIAN_POINT('Ctrl Pts',(4.05590493145794,-28.6273854188557,
124.055754695563));
#117368=CARTESIAN_POINT('Ctrl Pts',(4.05742083903453,-28.6145441314777,
124.074680194685));
#117369=CARTESIAN_POINT('Ctrl Pts',(4.05822491512972,-28.6078081264228,
124.084846184434));
#117370=CARTESIAN_POINT('Ctrl Pts',(4.06042496870552,-28.5895921877436,
124.113004360132));
#117371=CARTESIAN_POINT('Ctrl Pts',(4.06181233070301,-28.5783451597669,
124.131144980734));
#117372=CARTESIAN_POINT('Ctrl Pts',(4.06803814907085,-28.5290376122545,
124.214196528902));
#117373=CARTESIAN_POINT('Ctrl Pts',(4.07273134890063,-28.4950504888545,
124.281427564177));
#117374=CARTESIAN_POINT('Ctrl Pts',(4.08222523325239,-28.4348971950192,
124.42357532095));
#117375=CARTESIAN_POINT('Ctrl Pts',(4.08700717862264,-28.4092993999039,
124.498518771395));
#117376=CARTESIAN_POINT('Ctrl Pts',(4.09532078163864,-28.3749114021091,
124.628858268459));
#117377=CARTESIAN_POINT('Ctrl Pts',(4.09880027393672,-28.3634123427282,
124.683394885247));
#117378=CARTESIAN_POINT('Ctrl Pts',(4.10354692297196,-28.3518817806926,
124.75591613204));
#117379=CARTESIAN_POINT('Ctrl Pts',(4.10470540968413,-28.3493767186088,
124.773475562353));
#117380=CARTESIAN_POINT('Ctrl Pts',(4.10639857849468,-28.3461663881126,
124.798872613458));
#117381=CARTESIAN_POINT('Ctrl Pts',(4.10692154951149,-28.3452354674114,
124.806681152133));
#117382=CARTESIAN_POINT('Ctrl Pts',(4.10785098795096,-28.3436884188277,
124.820488686389));
#117383=CARTESIAN_POINT('Ctrl Pts',(4.10825619117933,-28.3430495279652,
124.826484879077));
#117384=CARTESIAN_POINT('Ctrl Pts',(4.10904746182334,-28.3418709276439,
124.838147070533));
#117385=CARTESIAN_POINT('Ctrl Pts',(4.10943327520248,-28.3413276967457,
124.84381235849));
#117386=CARTESIAN_POINT('Ctrl Pts',(4.11030142907303,-28.3401752523307,
124.856515805792));
#117387=CARTESIAN_POINT('Ctrl Pts',(4.1107845878385,-28.3395817608714,124.863555235486));
#117388=CARTESIAN_POINT('Ctrl Pts',(4.11237843502179,-28.3377798553157,
124.886683990698));
#117389=CARTESIAN_POINT('Ctrl Pts',(4.11349822041555,-28.3367604410981,
124.902786569273));
#117390=CARTESIAN_POINT('Ctrl Pts',(4.11649924622742,-28.3346730304706,
124.945616809692));
#117391=CARTESIAN_POINT('Ctrl Pts',(4.11839629444807,-28.334014636662,124.972358788451));
#117392=CARTESIAN_POINT('Ctrl Pts',(4.12030991028152,-28.3340002413346,
124.999103268726));
#117393=CARTESIAN_POINT('Ctrl Pts',(4.12030973512622,-28.3340002426541,
124.999100820774));
#117394=CARTESIAN_POINT('Ctrl Pts',(4.12666726406915,-28.333952287056,125.08795297888));
#117395=CARTESIAN_POINT('Ctrl Pts',(4.13318681829467,-28.3410123763757,
125.176667750711));
#117396=CARTESIAN_POINT('Ctrl Pts',(4.14426204756692,-28.3652763865857,
125.327620293619));
#117397=CARTESIAN_POINT('Ctrl Pts',(4.14885076896109,-28.3790760497282,
125.390209339223));
#117398=CARTESIAN_POINT('Ctrl Pts',(4.15618819211529,-28.4074615666325,
125.490944771156));
#117399=CARTESIAN_POINT('Ctrl Pts',(4.15899418050003,-28.4199031649118,
125.52962242359));
#117400=CARTESIAN_POINT('Ctrl Pts',(4.16194038544885,-28.4346784063753,
125.570378624622));
#117401=CARTESIAN_POINT('Ctrl Pts',(4.16212588216124,-28.435616040836,125.572945281105));
#117402=CARTESIAN_POINT('Ctrl Pts',(4.16231116930939,-28.436559983762,125.575509613843));
#117403=CARTESIAN_POINT('Ctrl Pts',(3.96713564162385,-28.4365599852621,
125.575509617918));
#117404=CARTESIAN_POINT('Ctrl Pts',(3.96352864762869,-28.4192458061984,
125.528473600573));
#117405=CARTESIAN_POINT('Ctrl Pts',(3.95996290866004,-28.4040607105344,
125.480673858322));
#117406=CARTESIAN_POINT('Ctrl Pts',(3.9538426667242,-28.3813426200198,125.396112216372));
#117407=CARTESIAN_POINT('Ctrl Pts',(3.95126254740571,-28.3728525443762,
125.359650031383));
#117408=CARTESIAN_POINT('Ctrl Pts',(3.94769747204483,-28.3626750665644,
125.308140141014));
#117409=CARTESIAN_POINT('Ctrl Pts',(3.94668022427208,-28.3599536216725,
125.293310734621));
#117410=CARTESIAN_POINT('Ctrl Pts',(3.94493805013225,-28.3556108522336,
125.267692530268));
#117411=CARTESIAN_POINT('Ctrl Pts',(3.94421012975797,-28.3538935446072,
125.256921208376));
#117412=CARTESIAN_POINT('Ctrl Pts',(3.94272867798882,-28.3505989262102,
125.234865697589));
#117413=CARTESIAN_POINT('Ctrl Pts',(3.9419754895445,-28.3490313406727,125.22358062291));
#117414=CARTESIAN_POINT('Ctrl Pts',(3.94007040858907,-28.3453418994321,
125.194861456443));
#117415=CARTESIAN_POINT('Ctrl Pts',(3.93892356348225,-28.3433796873595,
125.177407990238));
#117416=CARTESIAN_POINT('Ctrl Pts',(3.93429800904611,-28.3365315365952,
125.106398168395));
#117417=CARTESIAN_POINT('Ctrl Pts',(3.93089121430676,-28.3339637011001,
125.052648173956));
#117418=CARTESIAN_POINT('Ctrl Pts',(3.92157743179926,-28.3340655593804,
124.903317728497));
#117419=CARTESIAN_POINT('Ctrl Pts',(3.91580908409069,-28.3423497631894,
124.807955221799));
#117420=CARTESIAN_POINT('Ctrl Pts',(3.90525577943598,-28.37189304426,124.638520869716));
#117421=CARTESIAN_POINT('Ctrl Pts',(3.90051314394173,-28.3901895479928,
124.564217127033));
#117422=CARTESIAN_POINT('Ctrl Pts',(3.89471857364882,-28.4172692269698,
124.479740151251));
#117423=CARTESIAN_POINT('Ctrl Pts',(3.89390957665405,-28.421149634481,124.468080352304));
#117424=CARTESIAN_POINT('Ctrl Pts',(3.89263166261146,-28.4274265704979,
124.449893522324));
#117425=CARTESIAN_POINT('Ctrl Pts',(3.89216763292323,-28.4297356740866,
124.443336483732));
#117426=CARTESIAN_POINT('Ctrl Pts',(3.89129502354381,-28.4341318165259,
124.431098017651));
#117427=CARTESIAN_POINT('Ctrl Pts',(3.8908870203951,-28.4362088654996,124.425413264577));
#117428=CARTESIAN_POINT('Ctrl Pts',(3.88992122171976,-28.4411766137068,
124.412043310677));
#117429=CARTESIAN_POINT('Ctrl Pts',(3.88936194489439,-28.4440932030299,
124.404368024486));
#117430=CARTESIAN_POINT('Ctrl Pts',(3.88747967205802,-28.4540455820203,
124.378749320774));
#117431=CARTESIAN_POINT('Ctrl Pts',(3.88614317290184,-28.4613357025898,
124.360907229159));
#117432=CARTESIAN_POINT('Ctrl Pts',(3.88281716880542,-28.4800587435126,
124.317262168115));
#117433=CARTESIAN_POINT('Ctrl Pts',(3.88081314549017,-28.4918407476356,
124.29161602209));
#117434=CARTESIAN_POINT('Ctrl Pts',(3.87164657880397,-28.5481849909733,
124.176754425839));
#117435=CARTESIAN_POINT('Ctrl Pts',(3.86431272939907,-28.6000513117406,
124.091350356092));
#117436=CARTESIAN_POINT('Ctrl Pts',(3.85112931401377,-28.7085597220535,
123.944234629508));
#117437=CARTESIAN_POINT('Ctrl Pts',(3.84525172148636,-28.7628133358153,
123.881147271579));
#117438=CARTESIAN_POINT('Ctrl Pts',(3.83822173658365,-28.8354248298719,
123.80848600785));
#117439=CARTESIAN_POINT('Ctrl Pts',(3.83688973546746,-28.8495376276999,
123.794853823229));
#117440=CARTESIAN_POINT('Ctrl Pts',(3.83477199894841,-28.8725395918999,
123.773407594073));
#117441=CARTESIAN_POINT('Ctrl Pts',(3.83397947356079,-28.8812765472154,
123.765433780314));
#117442=CARTESIAN_POINT('Ctrl Pts',(3.83247498925245,-28.8981056482833,
123.750400010187));
#117443=CARTESIAN_POINT('Ctrl Pts',(3.83176237667684,-28.9061825426724,
123.743323957362));
#117444=CARTESIAN_POINT('Ctrl Pts',(3.83013003461322,-28.9249237256984,
123.727222657881));
#117445=CARTESIAN_POINT('Ctrl Pts',(3.82921258939444,-28.9356343465705,
123.718252390808));
#117446=CARTESIAN_POINT('Ctrl Pts',(3.82630535355008,-28.9701266212994,
123.690095255444));
#117447=CARTESIAN_POINT('Ctrl Pts',(3.82433615205136,-28.9943246121907,
123.671426773606));
#117448=CARTESIAN_POINT('Ctrl Pts',(3.81968595623702,-29.0533104293303,
123.628455492344));
#117449=CARTESIAN_POINT('Ctrl Pts',(3.81702741989229,-29.0885402237399,
123.604795020764));
#117450=CARTESIAN_POINT('Ctrl Pts',(3.8098248175971,-29.1873802507635,123.543757166018));
#117451=CARTESIAN_POINT('Ctrl Pts',(3.80534866127199,-29.2526285159713,
123.509218230986));
#117452=CARTESIAN_POINT('Ctrl Pts',(3.80001615027389,-29.3322036468676,
123.473636941602));
#117453=CARTESIAN_POINT('Ctrl Pts',(3.79919394292238,-29.3445223859449,
123.468306411996));
#117454=CARTESIAN_POINT('Ctrl Pts',(3.79382151976482,-29.4252238015701,
123.434537392432));
#117455=CARTESIAN_POINT('Ctrl Pts',(3.78921906393103,-29.4953654259717,
123.410540339049));
#117456=CARTESIAN_POINT('Ctrl Pts',(3.78358055975889,-29.5787170185263,
123.38809819681));
#117457=CARTESIAN_POINT('Ctrl Pts',(3.78277218261997,-29.5906082617706,
123.385037103674));
#117458=CARTESIAN_POINT('Ctrl Pts',(3.78149503733048,-29.6092808166135,
123.380449810057));
#117459=CARTESIAN_POINT('Ctrl Pts',(3.78103114703818,-29.616039968685,123.378834065251));
#117460=CARTESIAN_POINT('Ctrl Pts',(3.78015864323567,-29.6287047408907,
123.375890253134));
#117461=CARTESIAN_POINT('Ctrl Pts',(3.77975060448261,-29.6346077444194,
123.374552020461));
#117462=CARTESIAN_POINT('Ctrl Pts',(3.77878450858412,-29.6485389539525,
123.371473483915));
#117463=CARTESIAN_POINT('Ctrl Pts',(3.77822496737115,-29.6565728831131,
123.369760358476));
#117464=CARTESIAN_POINT('Ctrl Pts',(3.7763408527856,-29.6835201823927,123.364222242629));
#117465=CARTESIAN_POINT('Ctrl Pts',(3.7750027416377,-29.702486500201,123.360666603587));
#117466=CARTESIAN_POINT('Ctrl Pts',(3.77167182689829,-29.7493773842434,
123.352716398822));
#117467=CARTESIAN_POINT('Ctrl Pts',(3.76966445363248,-29.7773597339886,
123.348701695674));
#117468=CARTESIAN_POINT('Ctrl Pts',(3.76046823664936,-29.9048260302872,
123.333712416959));
#117469=CARTESIAN_POINT('Ctrl Pts',(3.7531072750159,-30.0050733627839,123.331004163876));
#117470=CARTESIAN_POINT('Ctrl Pts',(3.73993007223488,-30.187459174884,123.342517418871));
#117471=CARTESIAN_POINT('Ctrl Pts',(3.7340830592895,-30.2694675356135,123.353858935357));
#117472=CARTESIAN_POINT('Ctrl Pts',(3.72708256762523,-30.3694749307159,
123.37536812854));
#117473=CARTESIAN_POINT('Ctrl Pts',(3.72575141293428,-30.3885701861821,
123.379829110991));
#117474=CARTESIAN_POINT('Ctrl Pts',(3.72363469136726,-30.4190490512539,
123.387519385085));
#117475=CARTESIAN_POINT('Ctrl Pts',(3.7228423460522,-30.4304842523267,123.390534510524));
#117476=CARTESIAN_POINT('Ctrl Pts',(3.72133800128878,-30.4522403237117,
123.396519410584));
#117477=CARTESIAN_POINT('Ctrl Pts',(3.72062535030276,-30.4625664281834,
123.39946770737));
#117478=CARTESIAN_POINT('Ctrl Pts',(3.71899263530128,-30.486263856021,123.406482267074));
#117479=CARTESIAN_POINT('Ctrl Pts',(3.71807485921755,-30.4996140826859,
123.410617386871));
#117480=CARTESIAN_POINT('Ctrl Pts',(3.71516538054259,-30.5420103226763,
123.424336253497));
#117481=CARTESIAN_POINT('Ctrl Pts',(3.71319431340135,-30.5708461291343,
123.434552358949));
#117482=CARTESIAN_POINT('Ctrl Pts',(3.70853876390975,-30.6390185278826,
123.46083931436));
#117483=CARTESIAN_POINT('Ctrl Pts',(3.70587681320953,-30.6780540780491,
123.477632323725));
#117484=CARTESIAN_POINT('Ctrl Pts',(3.6986722306304,-30.7829671285244,123.527602718632));
#117485=CARTESIAN_POINT('Ctrl Pts',(3.6941972937502,-30.847350731505,123.563689315279));
#117486=CARTESIAN_POINT('Ctrl Pts',(3.68884536145513,-30.9206605933198,
123.611429034442));
#117487=CARTESIAN_POINT('Ctrl Pts',(3.68800259901805,-30.9320951823863,
123.619078633755));
#117488=CARTESIAN_POINT('Ctrl Pts',(3.68263423726541,-31.0041327414484,
123.668573293278));
#117489=CARTESIAN_POINT('Ctrl Pts',(3.67805621681543,-31.0619923647512,
123.714251538116));
#117490=CARTESIAN_POINT('Ctrl Pts',(3.67244485434571,-31.1257450231763,
123.771828644301));
#117491=CARTESIAN_POINT('Ctrl Pts',(3.67163657537568,-31.1347650147263,
123.780157766036));
#117492=CARTESIAN_POINT('Ctrl Pts',(3.67035955183838,-31.1487449382285,
123.793356158528));
#117493=CARTESIAN_POINT('Ctrl Pts',(3.66989568362529,-31.1537680617216,
123.798158268055));
#117494=CARTESIAN_POINT('Ctrl Pts',(3.66902319652695,-31.1631099995716,
123.807201706442));
#117495=CARTESIAN_POINT('Ctrl Pts',(3.66861515211598,-31.1674359316296,
123.811435327346));
#117496=CARTESIAN_POINT('Ctrl Pts',(3.66764900905809,-31.1775785968597,
123.821470348873));
#117497=CARTESIAN_POINT('Ctrl Pts',(3.66708942590384,-31.1833755946098,
123.827291304127));
#117498=CARTESIAN_POINT('Ctrl Pts',(3.66520501902391,-31.2026465510491,
123.846930288713));
#117499=CARTESIAN_POINT('Ctrl Pts',(3.66386665202302,-31.2159228483038,
123.860938968508));
#117500=CARTESIAN_POINT('Ctrl Pts',(3.6605349576626,-31.2480411180231,123.896030463615));
#117501=CARTESIAN_POINT('Ctrl Pts',(3.65852705247634,-31.2665951050291,
123.917368008497));
#117502=CARTESIAN_POINT('Ctrl Pts',(3.64932611594672,-31.3483604993028,
124.016380208844));
#117503=CARTESIAN_POINT('Ctrl Pts',(3.64196083751902,-31.4050329845057,
124.099185538469));
#117504=CARTESIAN_POINT('Ctrl Pts',(3.62878461566318,-31.4942554506541,
124.25866393905));
#117505=CARTESIAN_POINT('Ctrl Pts',(3.62294246124247,-31.5291722871855,
124.333656002243));
#117506=CARTESIAN_POINT('Ctrl Pts',(3.61594666024645,-31.5653171195069,
124.429278807524));
#117507=CARTESIAN_POINT('Ctrl Pts',(3.61461564372652,-31.571925071051,124.447739199168));
#117508=CARTESIAN_POINT('Ctrl Pts',(3.61249908784277,-31.5819939093794,
124.477514496356));
#117509=CARTESIAN_POINT('Ctrl Pts',(3.61170677192388,-31.5856626502827,
124.488756610987));
#117510=CARTESIAN_POINT('Ctrl Pts',(3.61020244992106,-31.5924340390956,
124.510280545138));
#117511=CARTESIAN_POINT('Ctrl Pts',(3.60948979264503,-31.595557559744,124.52055511673));
#117512=CARTESIAN_POINT('Ctrl Pts',(3.60785701666444,-31.6025171618662,
124.544269737237));
#117513=CARTESIAN_POINT('Ctrl Pts',(3.6069391864906,-31.6062839330776,124.557729412545));
#117514=CARTESIAN_POINT('Ctrl Pts',(3.60402934103103,-31.6177536012827,
124.600794520789));
#117515=CARTESIAN_POINT('Ctrl Pts',(3.60205796877612,-31.6248109782942,
124.630566376625));
#117516=CARTESIAN_POINT('Ctrl Pts',(3.59740154351628,-31.6397023786624,
124.702112113262));
#117517=CARTESIAN_POINT('Ctrl Pts',(3.59473903422782,-31.6467659725939,
124.744024816263));
#117518=CARTESIAN_POINT('Ctrl Pts',(3.58753414740038,-31.6616820781218,
124.85927527001));
#117519=CARTESIAN_POINT('Ctrl Pts',(3.58305942888017,-31.6662813395355,
124.932935537576));
#117520=CARTESIAN_POINT('Ctrl Pts',(3.57770485414219,-31.6659315276349,
125.020461602146));
#117521=CARTESIAN_POINT('Ctrl Pts',(3.57685924522518,-31.6657048173855,
125.034263500966));
#117522=CARTESIAN_POINT('Ctrl Pts',(3.57149154731326,-31.6631838030986,
125.121616499952));
#117523=CARTESIAN_POINT('Ctrl Pts',(3.56691701269625,-31.6561901805754,
125.194941733526));
#117524=CARTESIAN_POINT('Ctrl Pts',(3.56130952094965,-31.6424037617841,
125.279672333373));
#117525=CARTESIAN_POINT('Ctrl Pts',(3.56050125611048,-31.6402982548054,
125.291767620381));
#117526=CARTESIAN_POINT('Ctrl Pts',(3.55922425009882,-31.6367919619569,
125.310670832005));
#117527=CARTESIAN_POINT('Ctrl Pts',(3.55876038506388,-31.6354818698118,
125.317495420012));
#117528=CARTESIAN_POINT('Ctrl Pts',(3.55788790036956,-31.6329508195242,
125.330248787076));
#117529=CARTESIAN_POINT('Ctrl Pts',(3.55747985514373,-31.6317401968368,
125.336179365369));
#117530=CARTESIAN_POINT('Ctrl Pts',(3.55651370529558,-31.62881033213,125.350143390252));
#117531=CARTESIAN_POINT('Ctrl Pts',(3.55595411610255,-31.6270639564911,
125.358170861749));
#117532=CARTESIAN_POINT('Ctrl Pts',(3.55406966713526,-31.6210161208298,
125.385013300963));
#117533=CARTESIAN_POINT('Ctrl Pts',(3.5527312632936,-31.6164472662686,125.403765602707));
#117534=CARTESIAN_POINT('Ctrl Pts',(3.54939945666924,-31.6043847099869,
125.449783426928));
#117535=CARTESIAN_POINT('Ctrl Pts',(3.54739147488572,-31.5965207720785,
125.476945146376));
#117536=CARTESIAN_POINT('Ctrl Pts',(3.53818985847344,-31.5576797020486,
125.599349262024));
#117537=CARTESIAN_POINT('Ctrl Pts',(3.53082395815422,-31.5188442387067,
125.69188020891));
#117538=CARTESIAN_POINT('Ctrl Pts',(3.5176478774254,-31.4332481974446,125.853332606013));
#117539=CARTESIAN_POINT('Ctrl Pts',(3.51180642270418,-31.3891861688273,
125.923332236672));
#117540=CARTESIAN_POINT('Ctrl Pts',(3.50481129734239,-31.3284587015546,
126.005553494918));
#117541=CARTESIAN_POINT('Ctrl Pts',(3.50348030080581,-31.3165334018153,
126.021117139094));
#117542=CARTESIAN_POINT('Ctrl Pts',(3.50136376888445,-31.2969790596035,
126.045725178207));
#117543=CARTESIAN_POINT('Ctrl Pts',(3.50057145721713,-31.2895238974997,
126.054904715906));
#117544=CARTESIAN_POINT('Ctrl Pts',(3.49906713850575,-31.2751132838785,
126.072267423245));
#117545=CARTESIAN_POINT('Ctrl Pts',(3.49835448031952,-31.2681752410406,
126.080464196953));
#117546=CARTESIAN_POINT('Ctrl Pts',(3.49672169551722,-31.2520260962374,
126.099173318561));
#117547=CARTESIAN_POINT('Ctrl Pts',(3.49580385751861,-31.2427609118106,
126.109638078695));
#117548=CARTESIAN_POINT('Ctrl Pts',(3.49289395899629,-31.2128001999143,
126.142631807354));
#117549=CARTESIAN_POINT('Ctrl Pts',(3.49092254260018,-31.1916147206059,
126.164708683709));
#117550=CARTESIAN_POINT('Ctrl Pts',(3.48626599063703,-31.1395810391596,
126.216024774802));
#117551=CARTESIAN_POINT('Ctrl Pts',(3.4836034005325,-31.1081983106632,126.244691962512));
#117552=CARTESIAN_POINT('Ctrl Pts',(3.47639847013452,-31.0194603774264,
126.31973150444));
#117553=CARTESIAN_POINT('Ctrl Pts',(3.47192378363465,-30.9600698863122,
126.363545703123));
#117554=CARTESIAN_POINT('Ctrl Pts',(3.46656883816062,-30.8863404659918,
126.41072580271));
#117555=CARTESIAN_POINT('Ctrl Pts',(3.46572282856574,-30.8746163232636,
126.418024327502));
#117556=CARTESIAN_POINT('Ctrl Pts',(3.46035522666701,-30.7998608440643,
126.463281358925));
#117557=CARTESIAN_POINT('Ctrl Pts',(3.45578118530074,-30.734471221513,126.497170327168));
#117558=CARTESIAN_POINT('Ctrl Pts',(3.45017424124447,-30.6558157807406,
126.531539223051));
#117559=CARTESIAN_POINT('Ctrl Pts',(3.44936597840817,-30.6445120802031,
126.536330331253));
#117560=CARTESIAN_POINT('Ctrl Pts',(3.44808897488056,-30.6267290162988,
126.543636949745));
#117561=CARTESIAN_POINT('Ctrl Pts',(3.44762511029616,-30.6202848420764,
126.546237692855));
#117562=CARTESIAN_POINT('Ctrl Pts',(3.44675262594267,-30.6081974370016,
126.551028213152));
#117563=CARTESIAN_POINT('Ctrl Pts',(3.44634458060134,-30.602558300073,126.55322764935));
#117564=CARTESIAN_POINT('Ctrl Pts',(3.44537842979062,-30.5892374480436,
126.558339732477));
#117565=CARTESIAN_POINT('Ctrl Pts',(3.44481883974155,-30.5815460365203,
126.56122634244));
#117566=CARTESIAN_POINT('Ctrl Pts',(3.44293438480842,-30.5557143240098,
126.570703695432));
#117567=CARTESIAN_POINT('Ctrl Pts',(3.44159597574447,-30.5374816454557,
126.577035798642));
#117568=CARTESIAN_POINT('Ctrl Pts',(3.4382641532061,-30.4922775556296,126.59185999554));
#117569=CARTESIAN_POINT('Ctrl Pts',(3.43625616056449,-30.4651925495935,
126.599984733842));
#117570=CARTESIAN_POINT('Ctrl Pts',(3.42705444776999,-30.3412882249394,
126.633740547108));
#117571=CARTESIAN_POINT('Ctrl Pts',(3.41968845928897,-30.2424847931028,
126.651298702795));
#117572=CARTESIAN_POINT('Ctrl Pts',(3.40651239856147,-30.0604175165886,
126.666951238755));
#117573=CARTESIAN_POINT('Ctrl Pts',(3.40067104302616,-29.9777114721474,
126.667897967212));
#117574=CARTESIAN_POINT('Ctrl Pts',(3.39367601344119,-29.875698805718,126.661472107613));
#117575=CARTESIAN_POINT('Ctrl Pts',(3.39234501973915,-29.8561552968963,
126.659894306766));
#117576=CARTESIAN_POINT('Ctrl Pts',(3.39022849121663,-29.8248754878884,
126.656812371525));
#117577=CARTESIAN_POINT('Ctrl Pts',(3.38943618015248,-29.8131199549463,
126.655527616931));
#117578=CARTESIAN_POINT('Ctrl Pts',(3.38793186190808,-29.7907169954979,
126.652837541245));
#117579=CARTESIAN_POINT('Ctrl Pts',(3.3872192035928,-29.7800675814883,126.651454224076));
#117580=CARTESIAN_POINT('Ctrl Pts',(3.38558641753944,-29.7555904981363,
126.648033775679));
#117581=CARTESIAN_POINT('Ctrl Pts',(3.3846685784309,-29.7417734770215,126.645925397134));
#117582=CARTESIAN_POINT('Ctrl Pts',(3.38175867238197,-29.6978042794605,
126.638648688608));
#117583=CARTESIAN_POINT('Ctrl Pts',(3.37978724972477,-29.6677661939915,
126.632823525222));
#117584=CARTESIAN_POINT('Ctrl Pts',(3.3751306797895,-29.5964318315708,126.616939685752));
#117585=CARTESIAN_POINT('Ctrl Pts',(3.37246807822157,-29.5553262339756,
126.606121675122));
#117586=CARTESIAN_POINT('Ctrl Pts',(3.36526314165245,-29.4441538842884,
126.572267722166));
#117587=CARTESIAN_POINT('Ctrl Pts',(3.36078845970326,-29.3751324787787,
126.54613441899));
#117588=CARTESIAN_POINT('Ctrl Pts',(3.35133283275612,-29.2345305104796,
126.481940490019));
#117589=CARTESIAN_POINT('Ctrl Pts',(3.34635652891028,-29.1635420043293,
126.443061348241));
#117590=CARTESIAN_POINT('Ctrl Pts',(3.34005347758473,-29.0818343203882,
126.390251401994));
#117591=CARTESIAN_POINT('Ctrl Pts',(3.33897605130137,-29.0681380819878,
126.381108428689));
#117592=CARTESIAN_POINT('Ctrl Pts',(3.33737516673439,-29.0482263438027,
126.367385262525));
#117593=CARTESIAN_POINT('Ctrl Pts',(3.33686156950279,-29.0419030929203,
126.362962163664));
#117594=CARTESIAN_POINT('Ctrl Pts',(3.33594287299062,-29.0307125584315,
126.355018059597));
#117595=CARTESIAN_POINT('Ctrl Pts',(3.33553893870879,-29.0258332618245,
126.351514428391));
#117596=CARTESIAN_POINT('Ctrl Pts',(3.33464067964683,-29.0150740699191,
126.343700139059));
#117597=CARTESIAN_POINT('Ctrl Pts',(3.33414555844965,-29.0092035435339,
126.339377291231));
#117598=CARTESIAN_POINT('Ctrl Pts',(3.3326744102038,-28.9919313533606,126.326482970932));
#117599=CARTESIAN_POINT('Ctrl Pts',(3.33169150373857,-28.9806115199769,
126.317803688489));
#117600=CARTESIAN_POINT('Ctrl Pts',(3.3293903085834,-28.9545851807178,126.297312462731));
#117601=CARTESIAN_POINT('Ctrl Pts',(3.32806622371377,-28.9399652336104,
126.285394102995));
#117602=CARTESIAN_POINT('Ctrl Pts',(3.32334839010026,-28.8890179718232,
126.24240094211));
#117603=CARTESIAN_POINT('Ctrl Pts',(3.31989939184916,-28.8538305107332,
126.210014918448));
#117604=CARTESIAN_POINT('Ctrl Pts',(3.30823783897726,-28.7404211193762,
126.096243905696));
#117605=CARTESIAN_POINT('Ctrl Pts',(3.29998260206738,-28.6690713312461,
126.008426556909));
#117606=CARTESIAN_POINT('Ctrl Pts',(3.28884869862378,-28.5823529747546,
125.876284658765));
#117607=CARTESIAN_POINT('Ctrl Pts',(3.2857149161221,-28.5591060801767,125.837510160612));
#117608=CARTESIAN_POINT('Ctrl Pts',(3.28150576136979,-28.529505610907,125.783248574592));
#117609=CARTESIAN_POINT('Ctrl Pts',(3.28038200205312,-28.5217669450595,
125.768543523804));
#117610=CARTESIAN_POINT('Ctrl Pts',(3.27858897635145,-28.5096890640931,
125.744735467308));
#117611=CARTESIAN_POINT('Ctrl Pts',(3.27791486065339,-28.505210403529,125.735704881014));
#117612=CARTESIAN_POINT('Ctrl Pts',(3.27651932666431,-28.496070304631,125.716847094642));
#117613=CARTESIAN_POINT('Ctrl Pts',(3.27579841013671,-28.4914225744092,
125.707013752518));
#117614=CARTESIAN_POINT('Ctrl Pts',(3.2740979973745,-28.4806387795556,125.683607583983));
#117615=CARTESIAN_POINT('Ctrl Pts',(3.27312145001788,-28.4745877174355,
125.669996447003));
#117616=CARTESIAN_POINT('Ctrl Pts',(3.27026165608738,-28.4572987162818,
125.629658068445));
#117617=CARTESIAN_POINT('Ctrl Pts',(3.26839564415477,-28.4465751377881,
125.602716965642));
#117618=CARTESIAN_POINT('Ctrl Pts',(3.26654944485247,-28.4365599843055,
125.575509615319));
#117619=CARTESIAN_POINT('Origin',(5.,-30.,125.));
#117620=CARTESIAN_POINT('',(2.56904935605388,-28.4365599852179,125.575509617798));
#117621=CARTESIAN_POINT('',(2.75979328931693,-28.4365599629713,125.575509557363));
#117622=CARTESIAN_POINT('',(5.,-28.4365599837785,125.575509613888));
#117623=CARTESIAN_POINT('Ctrl Pts',(2.75979328931693,-28.4365599629713,
125.575509557363));
#117624=CARTESIAN_POINT('Ctrl Pts',(2.76303723577968,-28.4546483265453,
125.624648744461));
#117625=CARTESIAN_POINT('Ctrl Pts',(2.76633054043747,-28.4750492326942,
125.672923875654));
#117626=CARTESIAN_POINT('Ctrl Pts',(2.7706819059645,-28.5039739496871,125.733261737967));
#117627=CARTESIAN_POINT('Ctrl Pts',(2.7716343813265,-28.5104195017411,125.746268466288));
#117628=CARTESIAN_POINT('Ctrl Pts',(2.77308356141338,-28.5203797917236,
125.765724460543));
#117629=CARTESIAN_POINT('Ctrl Pts',(2.77357288732662,-28.5237687615016,
125.77223781026));
#117630=CARTESIAN_POINT('Ctrl Pts',(2.77446743413919,-28.5300081696669,
125.784038326005));
#117631=CARTESIAN_POINT('Ctrl Pts',(2.77487177096086,-28.5328442928684,
125.789332759664));
#117632=CARTESIAN_POINT('Ctrl Pts',(2.77579597963266,-28.5393629527035,
125.801345185537));
#117633=CARTESIAN_POINT('Ctrl Pts',(2.77631692712918,-28.5430632194322,
125.808053155397));
#117634=CARTESIAN_POINT('Ctrl Pts',(2.77794519969519,-28.5547128226005,
125.828831799026));
#117635=CARTESIAN_POINT('Ctrl Pts',(2.77906167589533,-28.562820457572,125.842812013932));
#117636=CARTESIAN_POINT('Ctrl Pts',(2.78665470255186,-28.6188382658271,
125.936245944434));
#117637=CARTESIAN_POINT('Ctrl Pts',(2.79342359513652,-28.6731064091108,
126.011688978999));
#117638=CARTESIAN_POINT('Ctrl Pts',(2.80888647816696,-28.8111140384918,
126.173214271089));
#117639=CARTESIAN_POINT('Ctrl Pts',(2.81750623029459,-28.8984566979736,
126.255585129596));
#117640=CARTESIAN_POINT('Ctrl Pts',(2.82718609808875,-29.0109076803959,
126.340786439122));
#117641=CARTESIAN_POINT('Ctrl Pts',(2.82863849244357,-29.0281730411125,
126.353352994413));
#117642=CARTESIAN_POINT('Ctrl Pts',(2.83090048200251,-29.0556732312801,
126.372571204452));
#117643=CARTESIAN_POINT('Ctrl Pts',(2.8317185857514,-29.0657471791156,126.379447874255));
#117644=CARTESIAN_POINT('Ctrl Pts',(2.8332449232388,-29.0847787417583,126.39213505717));
#117645=CARTESIAN_POINT('Ctrl Pts',(2.83395409627308,-29.0937183949588,
126.397971255201));
#117646=CARTESIAN_POINT('Ctrl Pts',(2.83554318125725,-29.1139651043763,
126.410913351021));
#117647=CARTESIAN_POINT('Ctrl Pts',(2.83642124444281,-29.1253028258325,
126.417970095287));
#117648=CARTESIAN_POINT('Ctrl Pts',(2.83867401517774,-29.1547682521237,
126.435821847576));
#117649=CARTESIAN_POINT('Ctrl Pts',(2.8400412707289,-29.1730186891746,126.446410405486));
#117650=CARTESIAN_POINT('Ctrl Pts',(2.85100218251702,-29.322122896621,126.529172794167));
#117651=CARTESIAN_POINT('Ctrl Pts',(2.85991699057071,-29.4619359898843,
126.583785188738));
#117652=CARTESIAN_POINT('Ctrl Pts',(2.87288408100499,-29.6664043028776,
126.63339711441));
#117653=CARTESIAN_POINT('Ctrl Pts',(2.8766911564648,-29.7263844408796,126.644507576731));
#117654=CARTESIAN_POINT('Ctrl Pts',(2.88163859224958,-29.8019455984172,
126.654255934489));
#117655=CARTESIAN_POINT('Ctrl Pts',(2.88263743899645,-29.8170852406489,
126.655998307196));
#117656=CARTESIAN_POINT('Ctrl Pts',(2.88414310800062,-29.8396927948922,
126.658286351301));
#117657=CARTESIAN_POINT('Ctrl Pts',(2.88464166978938,-29.8471444153487,
126.658989809426));
#117658=CARTESIAN_POINT('Ctrl Pts',(2.88554515627021,-29.8605805798354,
126.660166938295));
#117659=CARTESIAN_POINT('Ctrl Pts',(2.88594908919052,-29.8665632881203,
126.66065850754));
#117660=CARTESIAN_POINT('Ctrl Pts',(2.88686228370704,-29.8800336942816,
126.661692041892));
#117661=CARTESIAN_POINT('Ctrl Pts',(2.88737250561811,-29.8875224131172,
126.662215733161));
#117662=CARTESIAN_POINT('Ctrl Pts',(2.88893419636274,-29.910337954678,126.663656355837));
#117663=CARTESIAN_POINT('Ctrl Pts',(2.88999381456226,-29.9256736535506,
126.664411999825));
#117664=CARTESIAN_POINT('Ctrl Pts',(2.89849926954696,-30.0477938556502,
126.668738257653));
#117665=CARTESIAN_POINT('Ctrl Pts',(2.90633703524342,-30.1546782396629,
126.662240304402));
#117666=CARTESIAN_POINT('Ctrl Pts',(2.92182256375358,-30.3651432359935,
126.628961598417));
#117667=CARTESIAN_POINT('Ctrl Pts',(2.92943272492981,-30.4682792175521,
126.602363042429));
#117668=CARTESIAN_POINT('Ctrl Pts',(2.93821829738369,-30.5885916222314,
126.558713180971));
#117669=CARTESIAN_POINT('Ctrl Pts',(2.93969491328196,-30.6088445811729,
126.550914321091));
#117670=CARTESIAN_POINT('Ctrl Pts',(2.94198580975405,-30.6403018166897,
126.538089764389));
#117671=CARTESIAN_POINT('Ctrl Pts',(2.9428089637918,-30.6516121229509,126.533332382412));
#117672=CARTESIAN_POINT('Ctrl Pts',(2.94433990679496,-30.6726562443397,
126.524205819835));
#117673=CARTESIAN_POINT('Ctrl Pts',(2.94504868964055,-30.682402574858,126.519867276819));
#117674=CARTESIAN_POINT('Ctrl Pts',(2.94663073617421,-30.7041599715204,
126.509930566909));
#117675=CARTESIAN_POINT('Ctrl Pts',(2.94750222340795,-30.7161473621253,
126.504282072947));
#117676=CARTESIAN_POINT('Ctrl Pts',(2.94972589219146,-30.7467265634955,
126.489424667644));
#117677=CARTESIAN_POINT('Ctrl Pts',(2.95107095081675,-30.7652163918327,
126.480010248559));
#117678=CARTESIAN_POINT('Ctrl Pts',(2.96212269049807,-30.9168808117756,
126.399185326102));
#117679=CARTESIAN_POINT('Ctrl Pts',(2.97113055886323,-31.0399406938127,
126.310310959368));
#117680=CARTESIAN_POINT('Ctrl Pts',(2.98415461116663,-31.192850805905,126.164592670322));
#117681=CARTESIAN_POINT('Ctrl Pts',(2.98791110691808,-31.2340849480302,
126.120804152586));
#117682=CARTESIAN_POINT('Ctrl Pts',(2.9927978158539,-31.2826277639255,126.063320871063));
#117683=CARTESIAN_POINT('Ctrl Pts',(2.9937903628562,-31.2922381549223,126.051620543336));
#117684=CARTESIAN_POINT('Ctrl Pts',(2.99528836821473,-31.3063468530237,
126.03395823717));
#117685=CARTESIAN_POINT('Ctrl Pts',(2.99578568858537,-31.310967002989,126.02809398809));
#117686=CARTESIAN_POINT('Ctrl Pts',(2.99668794986928,-31.3192308556153,
126.017458593071));
#117687=CARTESIAN_POINT('Ctrl Pts',(2.99709191338061,-31.3228883961609,
126.012698537217));
#117688=CARTESIAN_POINT('Ctrl Pts',(2.99800648412334,-31.3310737207185,
126.001925845536));
#117689=CARTESIAN_POINT('Ctrl Pts',(2.99851806637632,-31.3355864978393,
125.995902279951));
#117690=CARTESIAN_POINT('Ctrl Pts',(3.00008810806472,-31.3492408612435,
125.977416984754));
#117691=CARTESIAN_POINT('Ctrl Pts',(3.00115483941066,-31.3582496934169,
125.964858845395));
#117692=CARTESIAN_POINT('Ctrl Pts',(3.00954132285919,-31.4271006533988,
125.866006594887));
#117693=CARTESIAN_POINT('Ctrl Pts',(3.01723931917393,-31.4788324081438,
125.774361024761));
#117694=CARTESIAN_POINT('Ctrl Pts',(3.03286601043087,-31.566374232507,125.578031377637));
#117695=CARTESIAN_POINT('Ctrl Pts',(3.04074435836625,-31.6011104510511,
125.473394065915));
#117696=CARTESIAN_POINT('Ctrl Pts',(3.04969298501259,-31.6298020047711,
125.346012365552));
#117697=CARTESIAN_POINT('Ctrl Pts',(3.05109103788851,-31.6339501264954,
125.325862212821));
#117698=CARTESIAN_POINT('Ctrl Pts',(3.05328806407711,-31.6399315242076,
125.293811785721));
#117699=CARTESIAN_POINT('Ctrl Pts',(3.05409475028053,-31.6420107357334,
125.281960150391));
#117700=CARTESIAN_POINT('Ctrl Pts',(3.05561105901622,-31.6456959110216,
125.259529261526));
#117701=CARTESIAN_POINT('Ctrl Pts',(3.05632149497792,-31.6473286971399,
125.248955100047));
#117702=CARTESIAN_POINT('Ctrl Pts',(3.05792837934829,-31.6508067561278,
125.224896143383));
#117703=CARTESIAN_POINT('Ctrl Pts',(3.05882279918665,-31.6525888963804,
125.211402883611));
#117704=CARTESIAN_POINT('Ctrl Pts',(3.06114848406786,-31.6568161582198,
125.176066097184));
#117705=CARTESIAN_POINT('Ctrl Pts',(3.06257144218391,-31.6589947738764,
125.154192946908));
#117706=CARTESIAN_POINT('Ctrl Pts',(3.07129303488564,-31.669782835021,125.018754025983));
#117707=CARTESIAN_POINT('Ctrl Pts',(3.07823001012504,-31.6671616317556,
124.904595001293));
#117708=CARTESIAN_POINT('Ctrl Pts',(3.09106482445217,-31.6408724091839,
124.696097335447));
#117709=CARTESIAN_POINT('Ctrl Pts',(3.09694266222433,-31.6205819418205,
124.601843979847));
#117710=CARTESIAN_POINT('Ctrl Pts',(3.10413444886149,-31.5880596548816,
124.496186641115));
#117711=CARTESIAN_POINT('Ctrl Pts',(3.10507502122013,-31.5836673728014,
124.482545667123));
#117712=CARTESIAN_POINT('Ctrl Pts',(3.10650967241133,-31.5767713247972,
124.462039448031));
#117713=CARTESIAN_POINT('Ctrl Pts',(3.10699659132192,-31.5743973297258,
124.455130832859));
#117714=CARTESIAN_POINT('Ctrl Pts',(3.10788888020944,-31.5699881132764,
124.442568905563));
#117715=CARTESIAN_POINT('Ctrl Pts',(3.10829339451344,-31.5679676445182,
124.43691069709));
#117716=CARTESIAN_POINT('Ctrl Pts',(3.10922079153111,-31.5632864158377,
124.424021751059));
#117717=CARTESIAN_POINT('Ctrl Pts',(3.10974478238464,-31.5606060849227,
124.416798488511));
#117718=CARTESIAN_POINT('Ctrl Pts',(3.11139226506257,-31.5520658880556,
124.394263873374));
#117719=CARTESIAN_POINT('Ctrl Pts',(3.11252520759992,-31.546030253153,124.37902078772));
#117720=CARTESIAN_POINT('Ctrl Pts',(3.11968339923107,-31.5068308287761,
124.284137456742));
#117721=CARTESIAN_POINT('Ctrl Pts',(3.1259604110031,-31.4677503881054,124.207091174072));
#117722=CARTESIAN_POINT('Ctrl Pts',(3.13853769810426,-31.3778793126392,
124.059526098402));
#117723=CARTESIAN_POINT('Ctrl Pts',(3.14481785445178,-31.3271802787721,
123.989238982583));
#117724=CARTESIAN_POINT('Ctrl Pts',(3.15436579044093,-31.2397668605522,
123.886040319072));
#117725=CARTESIAN_POINT('Ctrl Pts',(3.15774782496874,-31.2066710245822,
123.850272246344));
#117726=CARTESIAN_POINT('Ctrl Pts',(3.16219141597261,-31.1602912437535,
123.804360383796));
#117727=CARTESIAN_POINT('Ctrl Pts',(3.16331054781866,-31.1483571435837,
123.79289363879));
#117728=CARTESIAN_POINT('Ctrl Pts',(3.16517336737757,-31.1280718939009,
123.773975951726));
#117729=CARTESIAN_POINT('Ctrl Pts',(3.16592117269069,-31.1198131836275,
123.766428109485));
#117730=CARTESIAN_POINT('Ctrl Pts',(3.16739244875795,-31.1033386864626,
123.751673457782));
#117731=CARTESIAN_POINT('Ctrl Pts',(3.16811604407364,-31.0951267901952,
123.744463168161));
#117732=CARTESIAN_POINT('Ctrl Pts',(3.16987650177474,-31.074883982123,123.727039096408));
#117733=CARTESIAN_POINT('Ctrl Pts',(3.17090968656239,-31.0627775933392,
123.716914323882));
#117734=CARTESIAN_POINT('Ctrl Pts',(3.17449247680874,-31.0200285212339,
123.682182815405));
#117735=CARTESIAN_POINT('Ctrl Pts',(3.17700613153684,-30.9886593561573,
123.65848840083));
#117736=CARTESIAN_POINT('Ctrl Pts',(3.18695772998778,-30.859551855189,123.567959220499));
#117737=CARTESIAN_POINT('Ctrl Pts',(3.19407110799303,-30.7556585173268,
123.510519760892));
#117738=CARTESIAN_POINT('Ctrl Pts',(3.20543037199233,-30.5853175200925,
123.438790895298));
#117739=CARTESIAN_POINT('Ctrl Pts',(3.20956163794169,-30.5226023275228,
123.416694806712));
#117740=CARTESIAN_POINT('Ctrl Pts',(3.21489817815105,-30.4435076682524,
123.394039813981));
#117741=CARTESIAN_POINT('Ctrl Pts',(3.21593601011778,-30.4282111414821,
123.389893685387));
#117742=CARTESIAN_POINT('Ctrl Pts',(3.21748902981047,-30.4054937158935,
123.384082726381));
#117743=CARTESIAN_POINT('Ctrl Pts',(3.21799518012268,-30.3981163137638,
123.382249344336));
#117744=CARTESIAN_POINT('Ctrl Pts',(3.21890629753049,-30.3848897441146,
123.379058317125));
#117745=CARTESIAN_POINT('Ctrl Pts',(3.21931018559243,-30.3790454227592,
123.377681714563));
#117746=CARTESIAN_POINT('Ctrl Pts',(3.22021559204696,-30.3659867841699,
123.374680229223));
#117747=CARTESIAN_POINT('Ctrl Pts',(3.22071798560091,-30.358769098873,123.373071786491));
#117748=CARTESIAN_POINT('Ctrl Pts',(3.22223212381146,-30.3370935583827,
123.368392696824));
#117749=CARTESIAN_POINT('Ctrl Pts',(3.22325133687287,-30.3226057435778,
123.365466440969));
#117750=CARTESIAN_POINT('Ctrl Pts',(3.23212354858208,-30.1972125092384,
123.341871417778));
#117751=CARTESIAN_POINT('Ctrl Pts',(3.24041737436664,-30.0845200328496,
123.332326168378));
#117752=CARTESIAN_POINT('Ctrl Pts',(3.25503508915634,-29.8832117013865,
123.335741756485));
#117753=CARTESIAN_POINT('Ctrl Pts',(3.26138040624311,-29.7949363292103,
123.344298365489));
#117754=CARTESIAN_POINT('Ctrl Pts',(3.26956477278181,-29.6787015467723,
123.365009530248));
#117755=CARTESIAN_POINT('Ctrl Pts',(3.27158688540903,-29.6497954147557,
123.370956270561));
#117756=CARTESIAN_POINT('Ctrl Pts',(3.27451836075723,-29.6076350878411,
123.380803946309));
#117757=CARTESIAN_POINT('Ctrl Pts',(3.27544651154424,-29.5942484564904,
123.384106504325));
#117758=CARTESIAN_POINT('Ctrl Pts',(3.27708671680372,-29.5705303573283,
123.390271231361));
#117759=CARTESIAN_POINT('Ctrl Pts',(3.27780084133571,-29.5601827666061,
123.393067614056));
#117760=CARTESIAN_POINT('Ctrl Pts',(3.2793030203289,-29.5383763515598,123.399187102454));
#117761=CARTESIAN_POINT('Ctrl Pts',(3.2800902642641,-29.526924742605,123.402533837904));
#117762=CARTESIAN_POINT('Ctrl Pts',(3.28219261162426,-29.4962893596308,
123.411845364699));
#117763=CARTESIAN_POINT('Ctrl Pts',(3.28350036576453,-29.4771755042877,
123.418034716562));
#117764=CARTESIAN_POINT('Ctrl Pts',(3.29110903947386,-29.3657587148261,
123.456353179857));
#117765=CARTESIAN_POINT('Ctrl Pts',(3.29714414454831,-29.2763107966007,
123.496209819013));
#117766=CARTESIAN_POINT('Ctrl Pts',(3.30753287686947,-29.1278328355663,
123.578704881674));
#117767=CARTESIAN_POINT('Ctrl Pts',(3.31190565576419,-29.0671441417323,
123.617779124584));
#117768=CARTESIAN_POINT('Ctrl Pts',(3.31965788762433,-28.9668560906495,
123.691970440996));
#117769=CARTESIAN_POINT('Ctrl Pts',(3.32298359356863,-28.9260444377097,
123.725266327141));
#117770=CARTESIAN_POINT('Ctrl Pts',(3.32718149695955,-28.8783324892821,
123.768111196788));
#117771=CARTESIAN_POINT('Ctrl Pts',(3.32793931228265,-28.8698631883654,
123.775876314673));
#117772=CARTESIAN_POINT('Ctrl Pts',(3.32914963445409,-28.8565772762266,
123.788312959258));
#117773=CARTESIAN_POINT('Ctrl Pts',(3.32959796612986,-28.8517072234968,
123.792927216193));
#117774=CARTESIAN_POINT('Ctrl Pts',(3.33046034977326,-28.8424407088608,
123.801813842122));
#117775=CARTESIAN_POINT('Ctrl Pts',(3.33087403725293,-28.838039774063,123.806081238236));
#117776=CARTESIAN_POINT('Ctrl Pts',(3.33188076421478,-28.8274346961004,
123.816478695595));
#117777=CARTESIAN_POINT('Ctrl Pts',(3.33247565728877,-28.8212550014351,
123.822633323954));
#117778=CARTESIAN_POINT('Ctrl Pts',(3.33450925422983,-28.8004148341158,
123.843717486912));
#117779=CARTESIAN_POINT('Ctrl Pts',(3.33596378607817,-28.7859880532031,
123.858873926947));
#117780=CARTESIAN_POINT('Ctrl Pts',(3.34490328341289,-28.6999851259749,
123.9527036415));
#117781=CARTESIAN_POINT('Ctrl Pts',(3.35272158264864,-28.6357965609123,
124.037807141351));
#117782=CARTESIAN_POINT('Ctrl Pts',(3.36756449678118,-28.5287667472807,
124.212167569368));
#117783=CARTESIAN_POINT('Ctrl Pts',(3.37457575800662,-28.4848717773251,
124.300286083396));
#117784=CARTESIAN_POINT('Ctrl Pts',(3.38280003822794,-28.4411231274983,
124.411847118787));
#117785=CARTESIAN_POINT('Ctrl Pts',(3.38426706216923,-28.4336414058478,
124.432072411769));
#117786=CARTESIAN_POINT('Ctrl Pts',(3.38654651510395,-28.4225309915491,
124.463998730343));
#117787=CARTESIAN_POINT('Ctrl Pts',(3.38736767229037,-28.4186353134346,
124.475603608291));
#117788=CARTESIAN_POINT('Ctrl Pts',(3.3888967829006,-28.4115836232334,124.49740346241));
#117789=CARTESIAN_POINT('Ctrl Pts',(3.38960570869245,-28.408397003706,124.507587797854));
#117790=CARTESIAN_POINT('Ctrl Pts',(3.39119048212472,-28.4014615886841,
124.530524130972));
#117791=CARTESIAN_POINT('Ctrl Pts',(3.39206452519877,-28.3977670719286,
124.54329188173));
#117792=CARTESIAN_POINT('Ctrl Pts',(3.39429949116731,-28.3886616688604,
124.576230189131));
#117793=CARTESIAN_POINT('Ctrl Pts',(3.39565316420881,-28.38347642017,124.596461094854));
#117794=CARTESIAN_POINT('Ctrl Pts',(3.40532389064964,-28.3488784010632,
124.742840270653));
#117795=CARTESIAN_POINT('Ctrl Pts',(3.41315087624358,-28.3338853611642,
124.871939983007));
#117796=CARTESIAN_POINT('Ctrl Pts',(3.42169050166202,-28.3340095611656,
125.011483767236));
#117797=CARTESIAN_POINT('Ctrl Pts',(3.42230320369506,-28.3341085155098,
125.021484389441));
#117798=CARTESIAN_POINT('Ctrl Pts',(3.42757183754949,-28.3357308221565,
125.107316137673));
#117799=CARTESIAN_POINT('Ctrl Pts',(3.43227943676868,-28.3423408481876,
125.182953074876));
#117800=CARTESIAN_POINT('Ctrl Pts',(3.43803507207486,-28.355979408971,125.270006104254));
#117801=CARTESIAN_POINT('Ctrl Pts',(3.4388440434325,-28.3580155855769,125.282124371585));
#117802=CARTESIAN_POINT('Ctrl Pts',(3.44012201179036,-28.3614134660585,
125.301062311549));
#117803=CARTESIAN_POINT('Ctrl Pts',(3.44058612265394,-28.3626841874184,
125.307898148971));
#117804=CARTESIAN_POINT('Ctrl Pts',(3.44145896183371,-28.3651414399192,
125.320671402663));
#117805=CARTESIAN_POINT('Ctrl Pts',(3.44186711410878,-28.3663175964764,
125.326610562742));
#117806=CARTESIAN_POINT('Ctrl Pts',(3.44283338866173,-28.3691659644831,
125.340593371787));
#117807=CARTESIAN_POINT('Ctrl Pts',(3.44339299472492,-28.3708653306969,
125.348631207018));
#117808=CARTESIAN_POINT('Ctrl Pts',(3.4452769512217,-28.3767542662811,125.375501676292));
#117809=CARTESIAN_POINT('Ctrl Pts',(3.44661483323226,-28.3812113386784,
125.394273270264));
#117810=CARTESIAN_POINT('Ctrl Pts',(3.44994489161394,-28.3929973763394,
125.44033740325));
#117811=CARTESIAN_POINT('Ctrl Pts',(3.45195162577028,-28.4006965880919,
125.467528477889));
#117812=CARTESIAN_POINT('Ctrl Pts',(3.45602015148294,-28.4175507825368,
125.521751199743));
#117813=CARTESIAN_POINT('Ctrl Pts',(3.45808086076826,-28.4267133184061,
125.548759974138));
#117814=CARTESIAN_POINT('Ctrl Pts',(3.46014888220092,-28.4365599331867,
125.575509476449));
#117815=CARTESIAN_POINT('',(3.23000357748363,-28.3339996803007,124.999395781857));
#117816=CARTESIAN_POINT('Ctrl Pts',(3.26654944485247,-28.4365599843055,
125.575509615319));
#117817=CARTESIAN_POINT('Ctrl Pts',(3.26608922769779,-28.4340634253296,
125.568727417246));
#117818=CARTESIAN_POINT('Ctrl Pts',(3.26563023416981,-28.4316108879902,
125.561928675024));
#117819=CARTESIAN_POINT('Ctrl Pts',(3.26175558114333,-28.4112291570977,
125.504254788388));
#117820=CARTESIAN_POINT('Ctrl Pts',(3.2584081392242,-28.3957355881006,125.452550575385));
#117821=CARTESIAN_POINT('Ctrl Pts',(3.25136299090292,-28.3682060469397,
125.341297853109));
#117822=CARTESIAN_POINT('Ctrl Pts',(3.24767920080253,-28.356861969498,125.281661433611));
#117823=CARTESIAN_POINT('Ctrl Pts',(3.23940931230418,-28.3389145332975,
125.14789329267));
#117824=CARTESIAN_POINT('Ctrl Pts',(3.23481638056788,-28.3339731665333,
125.073679451112));
#117825=CARTESIAN_POINT('Ctrl Pts',(3.23000431809184,-28.334000109585,124.999395734044));
#117826=CARTESIAN_POINT('Ctrl Pts',(3.23000443222266,-28.3340001089469,
124.99939749588));
#117827=CARTESIAN_POINT('Ctrl Pts',(3.22944765207874,-28.3340032173081,
124.99080248525));
#117828=CARTESIAN_POINT('Ctrl Pts',(3.22888799167503,-28.3340728389642,
124.982207796535));
#117829=CARTESIAN_POINT('Ctrl Pts',(3.22781269690895,-28.334332897955,124.965789723787));
#117830=CARTESIAN_POINT('Ctrl Pts',(3.22729762093207,-28.3345119609543,
124.957966394242));
#117831=CARTESIAN_POINT('Ctrl Pts',(3.22636905139114,-28.3349318006083,
124.943942991113));
#117832=CARTESIAN_POINT('Ctrl Pts',(3.22595661885278,-28.3351521138087,
124.937742392473));
#117833=CARTESIAN_POINT('Ctrl Pts',(3.22516382038836,-28.3356399400738,
124.925880411748));
#117834=CARTESIAN_POINT('Ctrl Pts',(3.22478376786043,-28.3359017200144,
124.920218825853));
#117835=CARTESIAN_POINT('Ctrl Pts',(3.22396282176298,-28.3365268562504,
124.908045476843));
#117836=CARTESIAN_POINT('Ctrl Pts',(3.22352142450034,-28.3368995659726,
124.90153438694));
#117837=CARTESIAN_POINT('Ctrl Pts',(3.22235463998572,-28.337980836864,124.884408105469));
#117838=CARTESIAN_POINT('Ctrl Pts',(3.22162591865072,-28.3387528541982,
124.873797422681));
#117839=CARTESIAN_POINT('Ctrl Pts',(3.21840447577815,-28.3425894175858,
124.827233785174));
#117840=CARTESIAN_POINT('Ctrl Pts',(3.21586248797687,-28.3467197210186,
124.791380994332));
#117841=CARTESIAN_POINT('Ctrl Pts',(3.20675625161801,-28.3654318790196,
124.665156461374));
#117842=CARTESIAN_POINT('Ctrl Pts',(3.20003860255776,-28.3862911370221,
124.575881812017));
#117843=CARTESIAN_POINT('Ctrl Pts',(3.18870595356972,-28.4342797884443,
124.427039702591));
#117844=CARTESIAN_POINT('Ctrl Pts',(3.18405531527007,-28.4577736244841,
124.366515535751));
#117845=CARTESIAN_POINT('Ctrl Pts',(3.17755872570092,-28.4962789591194,
124.282260673336));
#117846=CARTESIAN_POINT('Ctrl Pts',(3.175630798603,-28.5084482323227,124.25730208862));
#117847=CARTESIAN_POINT('Ctrl Pts',(3.17219748904402,-28.5314683041218,
124.212939537316));
#117848=CARTESIAN_POINT('Ctrl Pts',(3.17068499063485,-28.5420941575238,
124.193426909159));
#117849=CARTESIAN_POINT('Ctrl Pts',(3.1683514925556,-28.5592417593999,124.163384905577));
#117850=CARTESIAN_POINT('Ctrl Pts',(3.16752106545981,-28.5654956362802,
124.152706444695));
#117851=CARTESIAN_POINT('Ctrl Pts',(3.16598356732774,-28.5773551536463,
124.132964139113));
#117852=CARTESIAN_POINT('Ctrl Pts',(3.1652754226223,-28.582929862062,124.123882555756));
#117853=CARTESIAN_POINT('Ctrl Pts',(3.16370355342378,-28.5955531094982,
124.103754150159));
#117854=CARTESIAN_POINT('Ctrl Pts',(3.16284150333715,-28.6026456673121,
124.092735663181));
#117855=CARTESIAN_POINT('Ctrl Pts',(3.16065891811887,-28.6210299769782,
124.064902215425));
#117856=CARTESIAN_POINT('Ctrl Pts',(3.159345056047,-28.632499902251,124.04820709676));
#117857=CARTESIAN_POINT('Ctrl Pts',(3.14935022289263,-28.7227633509899,
123.921824962499));
#117858=CARTESIAN_POINT('Ctrl Pts',(3.14121161098739,-28.8143249215306,
123.821877307221));
#117859=CARTESIAN_POINT('Ctrl Pts',(3.12950949166578,-28.9594687004654,
123.697701675156));
#117860=CARTESIAN_POINT('Ctrl Pts',(3.12605852812399,-29.0037845957564,
123.663496988023));
#117861=CARTESIAN_POINT('Ctrl Pts',(3.12056433444249,-29.0749099493234,
123.614105370924));
#117862=CARTESIAN_POINT('Ctrl Pts',(3.11859088267162,-29.1005623311369,
123.597321446204));
#117863=CARTESIAN_POINT('Ctrl Pts',(3.11593372863336,-29.1349728163845,
123.576139319918));
#117864=CARTESIAN_POINT('Ctrl Pts',(3.1152877027733,-29.1433291697959,123.571096104715));
#117865=CARTESIAN_POINT('Ctrl Pts',(3.11421497743865,-29.1571781164444,
123.562903150098));
#117866=CARTESIAN_POINT('Ctrl Pts',(3.11379096471093,-29.1626453600842,
123.559710693161));
#117867=CARTESIAN_POINT('Ctrl Pts',(3.11298645255106,-29.1730026787887,
123.553741706294));
#117868=CARTESIAN_POINT('Ctrl Pts',(3.11260639591673,-29.1778888863421,
123.55095861487));
#117869=CARTESIAN_POINT('Ctrl Pts',(3.11159165561475,-29.1909197475348,
123.543623606031));
#117870=CARTESIAN_POINT('Ctrl Pts',(3.11095431455985,-29.1990885674555,
123.539115362905));
#117871=CARTESIAN_POINT('Ctrl Pts',(3.10859503984988,-29.2292855036084,
123.522779537778));
#117872=CARTESIAN_POINT('Ctrl Pts',(3.10684997113187,-29.2515400644324,
123.511380272746));
#117873=CARTESIAN_POINT('Ctrl Pts',(3.09710823055981,-29.3757527453012,
123.451245228638));
#117874=CARTESIAN_POINT('Ctrl Pts',(3.08877653802414,-29.4822062905465,
123.412481624518));
#117875=CARTESIAN_POINT('Ctrl Pts',(3.0762739792328,-29.6498767610489,123.370103398674));
#117876=CARTESIAN_POINT('Ctrl Pts',(3.07199006260309,-29.708747569502,123.358560858257));
#117877=CARTESIAN_POINT('Ctrl Pts',(3.06507128106493,-29.8066310188968,
123.344803026003));
#117878=CARTESIAN_POINT('Ctrl Pts',(3.06238730485174,-29.8453246685053,
123.340739755491));
#117879=CARTESIAN_POINT('Ctrl Pts',(3.05870646566697,-29.8993808422484,
123.33697096679));
#117880=CARTESIAN_POINT('Ctrl Pts',(3.05767442569999,-29.914648029691,123.336117537671));
#117881=CARTESIAN_POINT('Ctrl Pts',(3.05591492279765,-29.9408601509746,
123.335014035461));
#117882=CARTESIAN_POINT('Ctrl Pts',(3.05518430783682,-29.9517995353801,
123.334661443155));
#117883=CARTESIAN_POINT('Ctrl Pts',(3.05370418021214,-29.9740691671504,
123.334163283902));
#117884=CARTESIAN_POINT('Ctrl Pts',(3.05295494718087,-29.9853990248037,
123.334025451862));
#117885=CARTESIAN_POINT('Ctrl Pts',(3.05107334301465,-30.0139893152647,
123.333969329119));
#117886=CARTESIAN_POINT('Ctrl Pts',(3.04994576544092,-30.0312489693785,
123.334203663239));
#117887=CARTESIAN_POINT('Ctrl Pts',(3.04551733134659,-30.0994837089373,
123.33619102974));
#117888=CARTESIAN_POINT('Ctrl Pts',(3.04228052562196,-30.150373106521,123.340016267766));
#117889=CARTESIAN_POINT('Ctrl Pts',(3.03175858757404,-30.3175008056871,
123.360329421028));
#117890=CARTESIAN_POINT('Ctrl Pts',(3.0247352411413,-30.4321639410099,123.386754836161));
#117891=CARTESIAN_POINT('Ctrl Pts',(3.0149957152648,-30.5809785240957,123.438069938713));
#117892=CARTESIAN_POINT('Ctrl Pts',(3.01248945811593,-30.618373150999,123.4524936875));
#117893=CARTESIAN_POINT('Ctrl Pts',(3.00834972853951,-30.6778966753075,
123.477954989147));
#117894=CARTESIAN_POINT('Ctrl Pts',(3.00675124647266,-30.7003646194376,
123.488161991748));
#117895=CARTESIAN_POINT('Ctrl Pts',(3.00453040013058,-30.7307292238523,
123.502778481542));
#117896=CARTESIAN_POINT('Ctrl Pts',(3.00393190845015,-30.7388301149392,
123.506759387757));
#117897=CARTESIAN_POINT('Ctrl Pts',(3.002916700434,-30.7524250303608,123.513577850802));
#117898=CARTESIAN_POINT('Ctrl Pts',(3.00250210054275,-30.7579364831412,
123.516380602017));
#117899=CARTESIAN_POINT('Ctrl Pts',(3.00164141584703,-30.7692912746533,
123.522234663947));
#117900=CARTESIAN_POINT('Ctrl Pts',(3.00119510237882,-30.7751322643815,
123.525290054752));
#117901=CARTESIAN_POINT('Ctrl Pts',(3.00000124373214,-30.7906357325751,
123.533517388024));
#117902=CARTESIAN_POINT('Ctrl Pts',(2.99925009251312,-30.8002653759703,
123.53875004711));
#117903=CARTESIAN_POINT('Ctrl Pts',(2.99576166307805,-30.8444458914135,
123.563325012214));
#117904=CARTESIAN_POINT('Ctrl Pts',(2.99296494096236,-30.8783492785341,
123.583798786644));
#117905=CARTESIAN_POINT('Ctrl Pts',(2.98356991448956,-30.9882449259592,
123.655627833474));
#117906=CARTESIAN_POINT('Ctrl Pts',(2.97683741232306,-31.0607272402754,
123.712047354065));
#117907=CARTESIAN_POINT('Ctrl Pts',(2.96570787016637,-31.1738806301788,
123.816186362098));
#117908=CARTESIAN_POINT('Ctrl Pts',(2.96126455456212,-31.2171805883191,
123.860753227679));
#117909=CARTESIAN_POINT('Ctrl Pts',(2.95502073909017,-31.2756190494248,
123.928047229529));
#117910=CARTESIAN_POINT('Ctrl Pts',(2.95314517855461,-31.2928444983341,
123.948886330292));
#117911=CARTESIAN_POINT('Ctrl Pts',(2.94979521966981,-31.3230090925628,
123.987243088179));
#117912=CARTESIAN_POINT('Ctrl Pts',(2.94831421059811,-31.3361261673319,
124.004612354817));
#117913=CARTESIAN_POINT('Ctrl Pts',(2.94601823454732,-31.356106917401,124.032177271664));
#117914=CARTESIAN_POINT('Ctrl Pts',(2.94519432558859,-31.3632041392255,
124.042199763156));
#117915=CARTESIAN_POINT('Ctrl Pts',(2.94366292850998,-31.376255777431,124.061069897053));
#117916=CARTESIAN_POINT('Ctrl Pts',(2.94295443620894,-31.3822372742697,
124.069897946572));
#117917=CARTESIAN_POINT('Ctrl Pts',(2.94137425400026,-31.3954472966771,
124.089803438395));
#117918=CARTESIAN_POINT('Ctrl Pts',(2.9405043252574,-31.4026295443798,124.100910840577));
#117919=CARTESIAN_POINT('Ctrl Pts',(2.93828704686988,-31.4206954743156,
124.129593398409));
#117920=CARTESIAN_POINT('Ctrl Pts',(2.93694675193302,-31.4313859126302,
124.147288025016));
#117921=CARTESIAN_POINT('Ctrl Pts',(2.92587605213686,-31.5176403004289,
124.296250024484));
#117922=CARTESIAN_POINT('Ctrl Pts',(2.91684869953472,-31.5753053454347,
124.437051863492));
#117923=CARTESIAN_POINT('Ctrl Pts',(2.90381231805844,-31.6281289826934,
124.641747977118));
#117924=CARTESIAN_POINT('Ctrl Pts',(2.90006603072716,-31.6399613368566,
124.700544168891));
#117925=CARTESIAN_POINT('Ctrl Pts',(2.89519169770525,-31.6507790765647,
124.774804455902));
#117926=CARTESIAN_POINT('Ctrl Pts',(2.89420055436652,-31.6527546880626,
124.789794161532));
#117927=CARTESIAN_POINT('Ctrl Pts',(2.89270434814951,-31.6553999760959,
124.812216690311));
#117928=CARTESIAN_POINT('Ctrl Pts',(2.89220739704106,-31.6562242173595,
124.819630965089));
#117929=CARTESIAN_POINT('Ctrl Pts',(2.89130563139368,-31.6576216264516,
124.833019282977));
#117930=CARTESIAN_POINT('Ctrl Pts',(2.89090179119244,-31.6582123470696,
124.838991225973));
#117931=CARTESIAN_POINT('Ctrl Pts',(2.88998729403304,-31.6594712673837,
124.852460943545));
#117932=CARTESIAN_POINT('Ctrl Pts',(2.88947566031924,-31.6601209215356,
124.859960074218));
#117933=CARTESIAN_POINT('Ctrl Pts',(2.88790482011062,-31.6619501026632,
124.882880171667));
#117934=CARTESIAN_POINT('Ctrl Pts',(2.88683732756775,-31.662965690117,124.898312887684));
#117935=CARTESIAN_POINT('Ctrl Pts',(2.87846947113451,-31.6691878791066,
125.018348647222));
#117936=CARTESIAN_POINT('Ctrl Pts',(2.87079289439822,-31.6647344414331,
125.123209914435));
#117937=CARTESIAN_POINT('Ctrl Pts',(2.85515229486171,-31.6354264593641,
125.336349294407));
#117938=CARTESIAN_POINT('Ctrl Pts',(2.84724021019601,-31.609541227926,125.443999776096));
#117939=CARTESIAN_POINT('Ctrl Pts',(2.83826869110657,-31.5664504405343,
125.567633418755));
#117940=CARTESIAN_POINT('Ctrl Pts',(2.83687817705804,-31.5593604804076,
125.58683016078));
#117941=CARTESIAN_POINT('Ctrl Pts',(2.83469033306039,-31.5475517718996,
125.617076716792));
#117942=CARTESIAN_POINT('Ctrl Pts',(2.83388539649639,-31.5430642847155,
125.628213966274));
#117943=CARTESIAN_POINT('Ctrl Pts',(2.83237083530556,-31.5343509574631,
125.649182267367));
#117944=CARTESIAN_POINT('Ctrl Pts',(2.83166041450026,-31.530150066814,125.659022957931));
#117945=CARTESIAN_POINT('Ctrl Pts',(2.83005149781574,-31.5203782097541,
125.681316508919));
#117946=CARTESIAN_POINT('Ctrl Pts',(2.82915505453099,-31.5147484645711,
125.693742887154));
#117947=CARTESIAN_POINT('Ctrl Pts',(2.82681978764157,-31.4996015547241,
125.726112540495));
#117948=CARTESIAN_POINT('Ctrl Pts',(2.82538938994307,-31.4898389617098,
125.745938459639));
#117949=CARTESIAN_POINT('Ctrl Pts',(2.81693112508418,-31.4292794145189,
125.862987976907));
#117950=CARTESIAN_POINT('Ctrl Pts',(2.81023497601403,-31.3693750838475,
125.95519801829));
#117951=CARTESIAN_POINT('Ctrl Pts',(2.79744385927754,-31.2385046022361,
126.118756259709));
#117952=CARTESIAN_POINT('Ctrl Pts',(2.79136696910473,-31.1693115083733,
126.190888054312));
#117953=CARTESIAN_POINT('Ctrl Pts',(2.78393195888616,-31.0830734200047,
126.26598640281));
#117954=CARTESIAN_POINT('Ctrl Pts',(2.78297312960808,-31.0719261967078,
126.275438668985));
#117955=CARTESIAN_POINT('Ctrl Pts',(2.78151628894705,-31.0549802816593,
126.289428860244));
#117956=CARTESIAN_POINT('Ctrl Pts',(2.78102577539371,-31.0492731662119,
126.294077276615));
#117957=CARTESIAN_POINT('Ctrl Pts',(2.78013024060899,-31.0388555439189,
126.302448157598));
#117958=CARTESIAN_POINT('Ctrl Pts',(2.77972611867871,-31.0341554706231,
126.306183181476));
#117959=CARTESIAN_POINT('Ctrl Pts',(2.77880394364658,-31.0234326070543,
126.314610202835));
#117960=CARTESIAN_POINT('Ctrl Pts',(2.77828483342275,-31.0173977200388,
126.319286231299));
#117961=CARTESIAN_POINT('Ctrl Pts',(2.77666758969991,-30.9985938969649,
126.333650303977));
#117962=CARTESIAN_POINT('Ctrl Pts',(2.77556047243615,-30.9857175611156,
126.343195349507));
#117963=CARTESIAN_POINT('Ctrl Pts',(2.76778914102209,-30.8951772161083,
126.408308634197));
#117964=CARTESIAN_POINT('Ctrl Pts',(2.76081459039106,-30.8130047831794,
126.457290485201));
#117965=CARTESIAN_POINT('Ctrl Pts',(2.75117948116407,-30.6938751103934,
126.515076509239));
#117966=CARTESIAN_POINT('Ctrl Pts',(2.7484973952017,-30.6601244382253,126.530083447696));
#117967=CARTESIAN_POINT('Ctrl Pts',(2.74179567226525,-30.5740148055645,
126.564991295717));
#117968=CARTESIAN_POINT('Ctrl Pts',(2.73780545641421,-30.5210961787657,
126.583398419821));
#117969=CARTESIAN_POINT('Ctrl Pts',(2.73212095964041,-30.4430147266682,
126.606218091231));
#117970=CARTESIAN_POINT('Ctrl Pts',(2.73036578829342,-30.4185227321709,
126.612773215769));
#117971=CARTESIAN_POINT('Ctrl Pts',(2.72720859277426,-30.3737698827831,
126.623662785618));
#117972=CARTESIAN_POINT('Ctrl Pts',(2.72580104947853,-30.3535599892662,
126.6281830879));
#117973=CARTESIAN_POINT('Ctrl Pts',(2.72359282670168,-30.3214554943502,
126.634737829919));
#117974=CARTESIAN_POINT('Ctrl Pts',(2.72278429605972,-30.3096146280348,
126.637021747798));
#117975=CARTESIAN_POINT('Ctrl Pts',(2.72126666514748,-30.2872311877455,
126.641087607402));
#117976=CARTESIAN_POINT('Ctrl Pts',(2.72055672850573,-30.2766942917686,
126.642897004801));
#117977=CARTESIAN_POINT('Ctrl Pts',(2.71895384483305,-30.2527591156964,
126.646770348281));
#117978=CARTESIAN_POINT('Ctrl Pts',(2.71806289004406,-30.2393514887902,
126.648772462592));
#117979=CARTESIAN_POINT('Ctrl Pts',(2.71575221448119,-30.2043234528106,
126.653566781445));
#117980=CARTESIAN_POINT('Ctrl Pts',(2.71434062435975,-30.1826696365118,
126.656098743493));
#117981=CARTESIAN_POINT('Ctrl Pts',(2.70356851059332,-30.0156865390077,
126.67230875617));
#117982=CARTESIAN_POINT('Ctrl Pts',(2.69484679753411,-29.869184328285,126.667258761376));
#117983=CARTESIAN_POINT('Ctrl Pts',(2.68299947068425,-29.6793974205192,
126.635520530801));
#117984=CARTESIAN_POINT('Ctrl Pts',(2.68011183035185,-29.6339290017304,
126.625947371667));
#117985=CARTESIAN_POINT('Ctrl Pts',(2.67541721334043,-29.5625335777578,
126.607768855673));
#117986=CARTESIAN_POINT('Ctrl Pts',(2.67365794842134,-29.5363143869195,
126.600404015855));
#117987=CARTESIAN_POINT('Ctrl Pts',(2.67124922143442,-29.5013435437212,
126.589649437266));
#117988=CARTESIAN_POINT('Ctrl Pts',(2.67062916534392,-29.4924213995331,
126.586823099472));
#117989=CARTESIAN_POINT('Ctrl Pts',(2.66958803473497,-29.4775836727864,
126.581984898113));
#117990=CARTESIAN_POINT('Ctrl Pts',(2.66916933113692,-29.4716545704037,
126.580014601789));
#117991=CARTESIAN_POINT('Ctrl Pts',(2.66836506858315,-29.4603416462313,
126.576184413364));
#117992=CARTESIAN_POINT('Ctrl Pts',(2.66797987001052,-29.4549560404357,
126.574330182458));
#117993=CARTESIAN_POINT('Ctrl Pts',(2.66693311404226,-29.4404061907541,
126.569237153005));
#117994=CARTESIAN_POINT('Ctrl Pts',(2.66626859713171,-29.4312607821679,
126.565945773137));
#117995=CARTESIAN_POINT('Ctrl Pts',(2.66368354362812,-29.396015323223,126.552911666027));
#117996=CARTESIAN_POINT('Ctrl Pts',(2.66173401726768,-29.3701339332928,
126.542595427654));
#117997=CARTESIAN_POINT('Ctrl Pts',(2.65189391475221,-29.2423859207266,
126.487924735122));
#117998=CARTESIAN_POINT('Ctrl Pts',(2.64370454372534,-29.144878354173,126.434107886226));
#117999=CARTESIAN_POINT('Ctrl Pts',(2.63142898803704,-29.0050566248126,
126.337573385563));
#118000=CARTESIAN_POINT('Ctrl Pts',(2.62722918029416,-28.9584583119658,
126.301617055311));
#118001=CARTESIAN_POINT('Ctrl Pts',(2.62128476376028,-28.8940325753155,
126.246224494745));
#118002=CARTESIAN_POINT('Ctrl Pts',(2.61947287141277,-28.8746126106295,
126.228715910518));
#118003=CARTESIAN_POINT('Ctrl Pts',(2.61622465596887,-28.8401996363471,
126.196189307542));
#118004=CARTESIAN_POINT('Ctrl Pts',(2.61478231155967,-28.8250664269051,
126.181328452982));
#118005=CARTESIAN_POINT('Ctrl Pts',(2.61253248466898,-28.8017058533694,
126.157495183164));
#118006=CARTESIAN_POINT('Ctrl Pts',(2.61171664156733,-28.7932864457656,
126.148715096323));
#118007=CARTESIAN_POINT('Ctrl Pts',(2.61019258419445,-28.7776596370705,
126.132057422774));
#118008=CARTESIAN_POINT('Ctrl Pts',(2.60948345299235,-28.7704303825584,
126.12420128813));
#118009=CARTESIAN_POINT('Ctrl Pts',(2.60789195184058,-28.7543040693199,
126.106334934564));
#118010=CARTESIAN_POINT('Ctrl Pts',(2.60701145917471,-28.745451121731,126.096285760466));
#118011=CARTESIAN_POINT('Ctrl Pts',(2.60434700526554,-28.7188837744712,
126.065385246686));
#118012=CARTESIAN_POINT('Ctrl Pts',(2.60257894104523,-28.7015604300619,
126.044202723347));
#118013=CARTESIAN_POINT('Ctrl Pts',(2.59241916691543,-28.604052602405,125.918791653858));
#118014=CARTESIAN_POINT('Ctrl Pts',(2.58451199478791,-28.5359139983762,
125.805792754862));
#118015=CARTESIAN_POINT('Ctrl Pts',(2.57400318728507,-28.4653822822955,
125.649683244292));
#118016=CARTESIAN_POINT('Ctrl Pts',(2.57154703270053,-28.4503035415831,
125.612845615846));
#118017=CARTESIAN_POINT('Ctrl Pts',(2.56904935605388,-28.4365599852179,
125.575509617798));
#118018=CARTESIAN_POINT('Origin',(5.,-30.,125.));
#118019=CARTESIAN_POINT('',(1.86811697181266,-28.4365600386127,125.575509762851));
#118020=CARTESIAN_POINT('',(2.06219309044095,-28.4365599837628,125.575509613845));
#118021=CARTESIAN_POINT('',(5.,-28.4365599837785,125.575509613888));
#118022=CARTESIAN_POINT('',(2.72302673015923,-28.3340004556389,124.999966473191));
#118023=CARTESIAN_POINT('Ctrl Pts',(2.06219309044095,-28.4365599837628,
125.575509613845));
#118024=CARTESIAN_POINT('Ctrl Pts',(2.06231481742157,-28.4372108183064,
125.577277682953));
#118025=CARTESIAN_POINT('Ctrl Pts',(2.06243645299245,-28.4378646585235,
125.579044665562));
#118026=CARTESIAN_POINT('Ctrl Pts',(2.06925163019703,-28.4746946580413,
125.678060174038));
#118027=CARTESIAN_POINT('Ctrl Pts',(2.07563241278995,-28.5198750093322,
125.771722573598));
#118028=CARTESIAN_POINT('Ctrl Pts',(2.08879836885796,-28.6311900822544,
125.95624065934));
#118029=CARTESIAN_POINT('Ctrl Pts',(2.09554809795371,-28.6983657674872,
126.04583843714));
#118030=CARTESIAN_POINT('Ctrl Pts',(2.10377393077897,-28.7840779043172,
126.138995862746));
#118031=CARTESIAN_POINT('Ctrl Pts',(2.10475125216527,-28.7943152577931,
126.14982710997));
#118032=CARTESIAN_POINT('Ctrl Pts',(2.10623072174372,-28.8098641976026,
126.165842105749));
#118033=CARTESIAN_POINT('Ctrl Pts',(2.1067250244591,-28.8150676754099,126.171130404598));
#118034=CARTESIAN_POINT('Ctrl Pts',(2.10762433699979,-28.8245456339976,
126.180635032828));
#118035=CARTESIAN_POINT('Ctrl Pts',(2.10802840448228,-28.8288078176796,
126.184863247879));
#118036=CARTESIAN_POINT('Ctrl Pts',(2.10894645072438,-28.8384996378183,
126.194374437489));
#118037=CARTESIAN_POINT('Ctrl Pts',(2.10946144124541,-28.8439424732035,
126.199643437607));
#118038=CARTESIAN_POINT('Ctrl Pts',(2.11105252360253,-28.860782537141,126.215724628787));
#118039=CARTESIAN_POINT('Ctrl Pts',(2.11213720004111,-28.8722965462877,
126.226412523041));
#118040=CARTESIAN_POINT('Ctrl Pts',(2.11776954070583,-28.9323392160363,
126.280586774353));
#118041=CARTESIAN_POINT('Ctrl Pts',(2.12246251647973,-28.9832338004666,
126.321357966518));
#118042=CARTESIAN_POINT('Ctrl Pts',(2.13552178348418,-29.1299560432527,
126.425390658499));
#118043=CARTESIAN_POINT('Ctrl Pts',(2.14391087005518,-29.2301488679622,
126.481907669679));
#118044=CARTESIAN_POINT('Ctrl Pts',(2.15501351459777,-29.374929441546,126.544896341994));
#118045=CARTESIAN_POINT('Ctrl Pts',(2.1580021549344,-29.4151534589742,126.560568171068));
#118046=CARTESIAN_POINT('Ctrl Pts',(2.16205210126152,-29.4713929261248,
126.579999278967));
#118047=CARTESIAN_POINT('Ctrl Pts',(2.16315713109171,-29.4869200155011,
126.585109498637));
#118048=CARTESIAN_POINT('Ctrl Pts',(2.16492836668002,-29.5120958456072,
126.592986567285));
#118049=CARTESIAN_POINT('Ctrl Pts',(2.16559919963509,-29.5216984476141,
126.595896080581));
#118050=CARTESIAN_POINT('Ctrl Pts',(2.16699403399123,-29.5418030077233,
126.601789841456));
#118051=CARTESIAN_POINT('Ctrl Pts',(2.16771748221308,-29.5523092224007,
126.604757974655));
#118052=CARTESIAN_POINT('Ctrl Pts',(2.16943493757064,-29.5774332733477,
126.611589881155));
#118053=CARTESIAN_POINT('Ctrl Pts',(2.17042583212048,-29.5920761837414,
126.615358402468));
#118054=CARTESIAN_POINT('Ctrl Pts',(2.17386592794236,-29.643400741383,126.627824941497));
#118055=CARTESIAN_POINT('Ctrl Pts',(2.17628194413063,-29.6803260982737,
126.635477302222));
#118056=CARTESIAN_POINT('Ctrl Pts',(2.18228497170247,-29.773858712866,126.651571554493));
#118057=CARTESIAN_POINT('Ctrl Pts',(2.18582605746478,-29.8307008979953,
126.658362751919));
#118058=CARTESIAN_POINT('Ctrl Pts',(2.19599789533564,-29.9960892642132,
126.669528209492));
#118059=CARTESIAN_POINT('Ctrl Pts',(2.202513487661,-30.1048410644254,126.666236523335));
#118060=CARTESIAN_POINT('Ctrl Pts',(2.21140765119618,-30.2441754539222,
126.648318826746));
#118061=CARTESIAN_POINT('Ctrl Pts',(2.21346040468707,-30.2757353487152,
126.643333902262));
#118062=CARTESIAN_POINT('Ctrl Pts',(2.21622928866247,-30.3171723554896,
126.635561706165));
#118063=CARTESIAN_POINT('Ctrl Pts',(2.2169048903658,-30.327196900393,126.633585802203));
#118064=CARTESIAN_POINT('Ctrl Pts',(2.21801398624008,-30.3435004358817,
126.630216185413));
#118065=CARTESIAN_POINT('Ctrl Pts',(2.21844442342664,-30.3497908238771,
126.628878060701));
#118066=CARTESIAN_POINT('Ctrl Pts',(2.21930041417302,-30.3622232327263,
126.626158037645));
#118067=CARTESIAN_POINT('Ctrl Pts',(2.21972587955541,-30.3683654526088,
126.624777684136));
#118068=CARTESIAN_POINT('Ctrl Pts',(2.22080393617889,-30.3838389275887,
126.621208050756));
#118069=CARTESIAN_POINT('Ctrl Pts',(2.22145902274012,-30.3931592707069,
126.618973021103));
#118070=CARTESIAN_POINT('Ctrl Pts',(2.2241183758424,-30.4306863069507,126.609630837722));
#118071=CARTESIAN_POINT('Ctrl Pts',(2.22615481698908,-30.4587222214789,
126.601866351039));
#118072=CARTESIAN_POINT('Ctrl Pts',(2.2318623315178,-30.5357459961899,126.578347041504));
#118073=CARTESIAN_POINT('Ctrl Pts',(2.2355826130043,-30.5842282488699,126.561050885177));
#118074=CARTESIAN_POINT('Ctrl Pts',(2.24848865580523,-30.7485437608804,
126.493703091887));
#118075=CARTESIAN_POINT('Ctrl Pts',(2.25768881958384,-30.8594685118196,
126.432756202053));
#118076=CARTESIAN_POINT('Ctrl Pts',(2.26870369820073,-30.9887774723958,
126.341236268437));
#118077=CARTESIAN_POINT('Ctrl Pts',(2.27091825153586,-31.0145508856175,
126.321848087803));
#118078=CARTESIAN_POINT('Ctrl Pts',(2.27406023594464,-31.0507696648818,
126.292918454136));
#118079=CARTESIAN_POINT('Ctrl Pts',(2.27501085241741,-31.0616804081071,
126.283974201449));
#118080=CARTESIAN_POINT('Ctrl Pts',(2.27667888391339,-31.0807359635062,
126.267944112093));
#118081=CARTESIAN_POINT('Ctrl Pts',(2.27739857301846,-31.0889278513462,
126.260915793462));
#118082=CARTESIAN_POINT('Ctrl Pts',(2.27888877958168,-31.1058242453155,
126.24613186868));
#118083=CARTESIAN_POINT('Ctrl Pts',(2.27965871294223,-31.114516833776,126.238363490476));
#118084=CARTESIAN_POINT('Ctrl Pts',(2.28166088330865,-31.1370170336625,
126.21782671612));
#118085=CARTESIAN_POINT('Ctrl Pts',(2.28288698172451,-31.1506914958848,
126.204914425715));
#118086=CARTESIAN_POINT('Ctrl Pts',(2.28899093174138,-31.2181727752003,
126.138997519325));
#118087=CARTESIAN_POINT('Ctrl Pts',(2.29371702165791,-31.2685531066315,
126.082605807923));
#118088=CARTESIAN_POINT('Ctrl Pts',(2.30236830557441,-31.3547684106108,
125.971785129724));
#118089=CARTESIAN_POINT('Ctrl Pts',(2.30630613785602,-31.3915751445283,
125.918304142636));
#118090=CARTESIAN_POINT('Ctrl Pts',(2.31496273358526,-31.4647802129463,
125.797386090421));
#118091=CARTESIAN_POINT('Ctrl Pts',(2.31968471471535,-31.4998334536118,
125.729316481363));
#118092=CARTESIAN_POINT('Ctrl Pts',(2.32568607543219,-31.5364714998573,
125.644260832969));
#118093=CARTESIAN_POINT('Ctrl Pts',(2.32674252078714,-31.5426428276835,
125.629340726388));
#118094=CARTESIAN_POINT('Ctrl Pts',(2.32832518810266,-31.5514603679344,
125.607113715113));
#118095=CARTESIAN_POINT('Ctrl Pts',(2.32884208597202,-31.554274069415,125.59987369297));
#118096=CARTESIAN_POINT('Ctrl Pts',(2.32976437696333,-31.5591754297697,
125.586995843966));
#118097=CARTESIAN_POINT('Ctrl Pts',(2.3301685687761,-31.5612833518188,125.581366007593));
#118098=CARTESIAN_POINT('Ctrl Pts',(2.33106455896732,-31.5658675558016,
125.568917759249));
#118099=CARTESIAN_POINT('Ctrl Pts',(2.33155712411249,-31.5683297662948,
125.562094616843));
#118100=CARTESIAN_POINT('Ctrl Pts',(2.3330127152157,-31.5754387364072,125.541984253349));
#118101=CARTESIAN_POINT('Ctrl Pts',(2.33398241021494,-31.5799616115333,
125.528654344981));
#118102=CARTESIAN_POINT('Ctrl Pts',(2.34075274720278,-31.6101139538162,
125.435943980549));
#118103=CARTESIAN_POINT('Ctrl Pts',(2.34680388408158,-31.6299164062079,
125.354801012144));
#118104=CARTESIAN_POINT('Ctrl Pts',(2.36226796283999,-31.6646747087329,
125.145179694918));
#118105=CARTESIAN_POINT('Ctrl Pts',(2.37162264222884,-31.6709224711773,
125.015785402748));
#118106=CARTESIAN_POINT('Ctrl Pts',(2.3819450237651,-31.6607400010836,124.866072492029));
#118107=CARTESIAN_POINT('Ctrl Pts',(2.38337259339451,-31.6589266742306,
124.845221813287));
#118108=CARTESIAN_POINT('Ctrl Pts',(2.38568771757015,-31.6553187325703,
124.811180285239));
#118109=CARTESIAN_POINT('Ctrl Pts',(2.38658245541412,-31.6537581113795,
124.797967532445));
#118110=CARTESIAN_POINT('Ctrl Pts',(2.38818594032121,-31.650660696371,124.774192223803));
#118111=CARTESIAN_POINT('Ctrl Pts',(2.38889641941629,-31.6491803707634,
124.763623181936));
#118112=CARTESIAN_POINT('Ctrl Pts',(2.39041436900415,-31.6457856493461,
124.740972581627));
#118113=CARTESIAN_POINT('Ctrl Pts',(2.39122079594665,-31.6438395401406,
124.728896354288));
#118114=CARTESIAN_POINT('Ctrl Pts',(2.39343456569231,-31.6381033701174,
124.695637783608));
#118115=CARTESIAN_POINT('Ctrl Pts',(2.39483310826594,-31.634035578599,124.674505289315));
#118116=CARTESIAN_POINT('Ctrl Pts',(2.40253184634665,-31.6091855082056,
124.557652165559));
#118117=CARTESIAN_POINT('Ctrl Pts',(2.40856905912572,-31.5804019658594,
124.463825998978));
#118118=CARTESIAN_POINT('Ctrl Pts',(2.42101562493036,-31.5037849811704,
124.275192745723));
#118119=CARTESIAN_POINT('Ctrl Pts',(2.42739148430075,-31.4548193755125,
124.181336248532));
#118120=CARTESIAN_POINT('Ctrl Pts',(2.43556571651037,-31.3854594827054,
124.074510198276));
#118121=CARTESIAN_POINT('Ctrl Pts',(2.43697872959875,-31.3732559770193,
124.056497342415));
#118122=CARTESIAN_POINT('Ctrl Pts',(2.43899612297903,-31.3556033068122,
124.031509513785));
#118123=CARTESIAN_POINT('Ctrl Pts',(2.43958255187393,-31.3504453863978,
124.024330282792));
#118124=CARTESIAN_POINT('Ctrl Pts',(2.44057946784205,-31.3416380872528,
124.012275174306));
#118125=CARTESIAN_POINT('Ctrl Pts',(2.44098794219871,-31.3380185674872,
124.007377513695));
#118126=CARTESIAN_POINT('Ctrl Pts',(2.44184592498239,-31.3303953762181,
123.997179846196));
#118127=CARTESIAN_POINT('Ctrl Pts',(2.44229575068526,-31.3263867752225,
123.991883817919));
#118128=CARTESIAN_POINT('Ctrl Pts',(2.44350859264121,-31.3155440201311,
123.977735355829));
#118129=CARTESIAN_POINT('Ctrl Pts',(2.4442754087304,-31.3086523586475,123.968927714065));
#118130=CARTESIAN_POINT('Ctrl Pts',(2.44832063953449,-31.272081365715,123.923146767727));
#118131=CARTESIAN_POINT('Ctrl Pts',(2.45168540501488,-31.2409248864403,
123.887386667002));
#118132=CARTESIAN_POINT('Ctrl Pts',(2.46498909721191,-31.1135505170592,
123.753205232102));
#118133=CARTESIAN_POINT('Ctrl Pts',(2.47515119374629,-31.0067929304287,
123.665508072469));
#118134=CARTESIAN_POINT('Ctrl Pts',(2.4880242878335,-30.8523328001831,123.567826747251));
#118135=CARTESIAN_POINT('Ctrl Pts',(2.49115297688998,-30.813235621971,123.545269813954));
#118136=CARTESIAN_POINT('Ctrl Pts',(2.49535677662772,-30.7585555726385,
123.516616935911));
#118137=CARTESIAN_POINT('Ctrl Pts',(2.49648010337844,-30.7437287618295,
123.509127961513));
#118138=CARTESIAN_POINT('Ctrl Pts',(2.49827276881014,-30.719726819475,123.497451854677));
#118139=CARTESIAN_POINT('Ctrl Pts',(2.49894695043675,-30.7106216759104,
123.493124270177));
#118140=CARTESIAN_POINT('Ctrl Pts',(2.50034287098579,-30.6916083227468,
123.48429807652));
#118141=CARTESIAN_POINT('Ctrl Pts',(2.50106410571186,-30.681694168892,123.479813346136));
#118142=CARTESIAN_POINT('Ctrl Pts',(2.50276572553247,-30.658093888883,123.46941491926));
#118143=CARTESIAN_POINT('Ctrl Pts',(2.5037431532549,-30.6443707709508,123.463587103249));
#118144=CARTESIAN_POINT('Ctrl Pts',(2.50707938351856,-30.5969797601342,
123.444208173712));
#118145=CARTESIAN_POINT('Ctrl Pts',(2.50940771438994,-30.5629470321415,
123.43157276741));
#118146=CARTESIAN_POINT('Ctrl Pts',(2.51513281198041,-30.4772270836863,
123.402897482673));
#118147=CARTESIAN_POINT('Ctrl Pts',(2.51848929427493,-30.4251198576961,
123.388244468241));
#118148=CARTESIAN_POINT('Ctrl Pts',(2.5254767648598,-30.3143158819693,123.362834353216));
#118149=CARTESIAN_POINT('Ctrl Pts',(2.5290957655144,-30.2555704712064,123.352641632794));
#118150=CARTESIAN_POINT('Ctrl Pts',(2.53774699646188,-30.1153322516718,
123.335992804739));
#118151=CARTESIAN_POINT('Ctrl Pts',(2.54279356215285,-30.0336717308764,
123.332341719573));
#118152=CARTESIAN_POINT('Ctrl Pts',(2.54893151189941,-29.9397265177367,
123.335044756533));
#118153=CARTESIAN_POINT('Ctrl Pts',(2.5497453288015,-29.9273729500061,123.335537881227));
#118154=CARTESIAN_POINT('Ctrl Pts',(2.5510293060358,-29.9080656820036,123.336523922599));
#118155=CARTESIAN_POINT('Ctrl Pts',(2.55149450568713,-29.9011073539954,
123.336923086846));
#118156=CARTESIAN_POINT('Ctrl Pts',(2.55236817543867,-29.8881130059662,
123.337750344702));
#118157=CARTESIAN_POINT('Ctrl Pts',(2.55277605558448,-29.8820765503423,
123.338167676521));
#118158=CARTESIAN_POINT('Ctrl Pts',(2.5537400353919,-29.8678789954351,123.33922697052));
#118159=CARTESIAN_POINT('Ctrl Pts',(2.55429759741748,-29.8597202113756,
123.339896211318));
#118160=CARTESIAN_POINT('Ctrl Pts',(2.55616735457015,-29.8325252425241,
123.34232883484));
#118161=CARTESIAN_POINT('Ctrl Pts',(2.55749281551937,-29.8135152947768,
123.344359681681));
#118162=CARTESIAN_POINT('Ctrl Pts',(2.56078509930181,-29.7668536721785,
123.350158349507));
#118163=CARTESIAN_POINT('Ctrl Pts',(2.56276608779761,-29.739254141181,123.354294648412));
#118164=CARTESIAN_POINT('Ctrl Pts',(2.57173114335664,-29.6159755305234,
123.375949032978));
#118165=CARTESIAN_POINT('Ctrl Pts',(2.5788809553325,-29.5218366518924,123.401132799071));
#118166=CARTESIAN_POINT('Ctrl Pts',(2.59208211650717,-29.350011927202,123.463642330184));
#118167=CARTESIAN_POINT('Ctrl Pts',(2.59814461275216,-29.2719553757112,
123.499055468843));
#118168=CARTESIAN_POINT('Ctrl Pts',(2.60536629389388,-29.1795357897617,
123.549900082901));
#118169=CARTESIAN_POINT('Ctrl Pts',(2.60671652400811,-29.1622883831308,
123.559794946468));
#118170=CARTESIAN_POINT('Ctrl Pts',(2.60885627281193,-29.1350191398783,
123.576095019926));
#118171=CARTESIAN_POINT('Ctrl Pts',(2.60965283040887,-29.1248820492152,
123.582302618487));
#118172=CARTESIAN_POINT('Ctrl Pts',(2.61116076684659,-29.1057236703578,
123.594318338043));
#118173=CARTESIAN_POINT('Ctrl Pts',(2.6118728438471,-29.0966904034283,123.600106121719));
#118174=CARTESIAN_POINT('Ctrl Pts',(2.61349810833563,-29.0761089593788,
123.6135752151));
#118175=CARTESIAN_POINT('Ctrl Pts',(2.61440908479322,-29.0645994305063,
123.621314345836));
#118176=CARTESIAN_POINT('Ctrl Pts',(2.61727176942696,-29.0285331656084,
123.646225273701));
#118177=CARTESIAN_POINT('Ctrl Pts',(2.61920380248792,-29.0043415153599,
123.663916851643));
#118178=CARTESIAN_POINT('Ctrl Pts',(2.62656294866053,-28.913051869991,123.734535152209));
#118179=CARTESIAN_POINT('Ctrl Pts',(2.63181896097461,-28.8495841056786,
123.79194253248));
#118180=CARTESIAN_POINT('Ctrl Pts',(2.64363902708161,-28.7165561467008,
123.93230367782));
#118181=CARTESIAN_POINT('Ctrl Pts',(2.65015358676409,-28.6501125172907,
124.017655035499));
#118182=CARTESIAN_POINT('Ctrl Pts',(2.65834846640939,-28.5820754160901,
124.125118240397));
#118183=CARTESIAN_POINT('Ctrl Pts',(2.6596052238993,-28.5720396152025,124.141596085127));
#118184=CARTESIAN_POINT('Ctrl Pts',(2.6613804055424,-28.558456066797,124.164796581569));
#118185=CARTESIAN_POINT('Ctrl Pts',(2.66188442110346,-28.5546643347953,
124.171375554957));
#118186=CARTESIAN_POINT('Ctrl Pts',(2.66280018617779,-28.5478949656625,
124.183308808472));
#118187=CARTESIAN_POINT('Ctrl Pts',(2.66321095049384,-28.5449015863085,
124.188654119309));
#118188=CARTESIAN_POINT('Ctrl Pts',(2.66406626433856,-28.5387591018982,
124.199766153918));
#118189=CARTESIAN_POINT('Ctrl Pts',(2.66451106641684,-28.5356145417786,
124.205535150756));
#118190=CARTESIAN_POINT('Ctrl Pts',(2.66569620664442,-28.5273654130038,
124.220884340886));
#118191=CARTESIAN_POINT('Ctrl Pts',(2.66644006075658,-28.5223203143431,
124.230495894707));
#118192=CARTESIAN_POINT('Ctrl Pts',(2.67013111884252,-28.4979172579362,
124.27811185158));
#118193=CARTESIAN_POINT('Ctrl Pts',(2.67314824164962,-28.4799313031453,
124.316797581612));
#118194=CARTESIAN_POINT('Ctrl Pts',(2.6819460233931,-28.4325012417849,124.429985415987));
#118195=CARTESIAN_POINT('Ctrl Pts',(2.68781168610613,-28.4069179176067,
124.505977696194));
#118196=CARTESIAN_POINT('Ctrl Pts',(2.70097322623689,-28.361566048642,124.681630796932));
#118197=CARTESIAN_POINT('Ctrl Pts',(2.70819996968239,-28.345234088113,124.781869147136));
#118198=CARTESIAN_POINT('Ctrl Pts',(2.71647448556716,-28.3367452754212,
124.902431012962));
#118199=CARTESIAN_POINT('Ctrl Pts',(2.71779853598483,-28.3357174743766,
124.92189931528));
#118200=CARTESIAN_POINT('Ctrl Pts',(2.71988325154906,-28.3346287717819,
124.952822457251));
#118201=CARTESIAN_POINT('Ctrl Pts',(2.72065081836281,-28.3343439074036,
124.964267090192));
#118202=CARTESIAN_POINT('Ctrl Pts',(2.72195415943265,-28.3340591730269,
124.983797565021));
#118203=CARTESIAN_POINT('Ctrl Pts',(2.72249175600273,-28.334000162432,124.991881975512));
#118204=CARTESIAN_POINT('Ctrl Pts',(2.72302752844612,-28.3340000003349,
124.999966596608));
#118205=CARTESIAN_POINT('Ctrl Pts',(2.72302751681176,-28.3340000003384,
124.999966421049));
#118206=CARTESIAN_POINT('Ctrl Pts',(2.72341003707426,-28.3339998839993,
125.005738519388));
#118207=CARTESIAN_POINT('Ctrl Pts',(2.72379162305297,-28.3340297650592,
125.011510654778));
#118208=CARTESIAN_POINT('Ctrl Pts',(2.72478818356262,-28.3341865271217,
125.026621321881));
#118209=CARTESIAN_POINT('Ctrl Pts',(2.72540164493891,-28.3343619356514,
125.035959222548));
#118210=CARTESIAN_POINT('Ctrl Pts',(2.7274071184179,-28.3351952588838,125.066598225843));
#118211=CARTESIAN_POINT('Ctrl Pts',(2.72878894568904,-28.3361833704955,
125.087888788886));
#118212=CARTESIAN_POINT('Ctrl Pts',(2.7379957085408,-28.3455645420212,125.230762699901));
#118213=CARTESIAN_POINT('Ctrl Pts',(2.74539422571528,-28.3668678458642,
125.351128679346));
#118214=CARTESIAN_POINT('Ctrl Pts',(2.75514841777084,-28.4117154118108,
125.504312956938));
#118215=CARTESIAN_POINT('Ctrl Pts',(2.75745803106252,-28.4235384779283,
125.540135147333));
#118216=CARTESIAN_POINT('Ctrl Pts',(2.75979328931693,-28.4365599629713,
125.575509557363));
#118217=CARTESIAN_POINT('Ctrl Pts',(2.56904935605388,-28.4365599852179,
125.575509617798));
#118218=CARTESIAN_POINT('Ctrl Pts',(2.56823105408791,-28.4320572489617,
125.563277401652));
#118219=CARTESIAN_POINT('Ctrl Pts',(2.56740827376691,-28.4276978294066,
125.550991692691));
#118220=CARTESIAN_POINT('Ctrl Pts',(2.56530560429473,-28.4169970304824,
125.519672955597));
#118221=CARTESIAN_POINT('Ctrl Pts',(2.56401862826457,-28.4108550117471,
125.500576182282));
#118222=CARTESIAN_POINT('Ctrl Pts',(2.56174409682684,-28.4007402472956,
125.467062855529));
#118223=CARTESIAN_POINT('Ctrl Pts',(2.5607638775511,-28.3966139292905,125.452694751303));
#118224=CARTESIAN_POINT('Ctrl Pts',(2.55928096941336,-28.3907279549038,
125.431108617603));
#118225=CARTESIAN_POINT('Ctrl Pts',(2.55878618226911,-28.3888222061937,
125.423930733468));
#118226=CARTESIAN_POINT('Ctrl Pts',(2.5578865334742,-28.3854632353537,125.410929504263));
#118227=CARTESIAN_POINT('Ctrl Pts',(2.55748262103918,-28.3839934039219,
125.405110725782));
#118228=CARTESIAN_POINT('Ctrl Pts',(2.55656564180777,-28.380742613805,125.39194222151));
#118229=CARTESIAN_POINT('Ctrl Pts',(2.55605157199553,-28.3789802491961,
125.384588285914));
#118230=CARTESIAN_POINT('Ctrl Pts',(2.55446570287488,-28.3737249873275,
125.361981270724));
#118231=CARTESIAN_POINT('Ctrl Pts',(2.55338539455546,-28.3703969872883,
125.346691266283));
#118232=CARTESIAN_POINT('Ctrl Pts',(2.54519340993738,-28.347000244132,125.231407231135));
#118233=CARTESIAN_POINT('Ctrl Pts',(2.53772584557607,-28.3359379662311,
125.129814135697));
#118234=CARTESIAN_POINT('Ctrl Pts',(2.52221525519045,-28.3323717256583,
124.916563484871));
#118235=CARTESIAN_POINT('Ctrl Pts',(2.51422881501946,-28.341668410633,124.805345556746));
#118236=CARTESIAN_POINT('Ctrl Pts',(2.50512604426723,-28.3658885666801,
124.67489880836));
#118237=CARTESIAN_POINT('Ctrl Pts',(2.50367516624649,-28.3701848784543,
124.654003317728));
#118238=CARTESIAN_POINT('Ctrl Pts',(2.50141514689657,-28.3775652745733,
124.621304674162));
#118239=CARTESIAN_POINT('Ctrl Pts',(2.50059751802699,-28.3803795646112,
124.60944366983));
#118240=CARTESIAN_POINT('Ctrl Pts',(2.4990718571732,-28.3859015830823,124.587257701146));
#118241=CARTESIAN_POINT('Ctrl Pts',(2.49836288880667,-28.3885788282974,
124.576925867953));
#118242=CARTESIAN_POINT('Ctrl Pts',(2.49677399946516,-28.3948289891224,
124.55372614781));
#118243=CARTESIAN_POINT('Ctrl Pts',(2.49589592915852,-28.3984577363053,
124.54087396046));
#118244=CARTESIAN_POINT('Ctrl Pts',(2.49364263217726,-28.4082192282444,
124.507825843319));
#118245=CARTESIAN_POINT('Ctrl Pts',(2.49227486670575,-28.4145820243575,
124.487699958644));
#118246=CARTESIAN_POINT('Ctrl Pts',(2.4813162999072,-28.4690578344515,124.326137863247));
#118247=CARTESIAN_POINT('Ctrl Pts',(2.47240385014623,-28.535609663832,124.191645719875));
#118248=CARTESIAN_POINT('Ctrl Pts',(2.45943795445118,-28.6533260477269,
124.017276925459));
#118249=CARTESIAN_POINT('Ctrl Pts',(2.45562933404548,-28.690196198818,123.968647588215));
#118250=CARTESIAN_POINT('Ctrl Pts',(2.450680162438,-28.7395042671362,123.910532799219));
#118251=CARTESIAN_POINT('Ctrl Pts',(2.44968124960086,-28.7495229629386,
123.899047951195));
#118252=CARTESIAN_POINT('Ctrl Pts',(2.44817559155413,-28.7646937986434,
123.882131226772));
#118253=CARTESIAN_POINT('Ctrl Pts',(2.44767710906758,-28.7697275983366,
123.876593654285));
#118254=CARTESIAN_POINT('Ctrl Pts',(2.44677383246375,-28.7788649428169,
123.866676927444));
#118255=CARTESIAN_POINT('Ctrl Pts',(2.44637003040627,-28.7829550730582,
123.862285775118));
#118256=CARTESIAN_POINT('Ctrl Pts',(2.44545723270482,-28.7922125268839,
123.8524540453));
#118257=CARTESIAN_POINT('Ctrl Pts',(2.44494727845425,-28.7973928890774,
123.847026266711));
#118258=CARTESIAN_POINT('Ctrl Pts',(2.44338674920808,-28.8132764150256,
123.830607640808));
#118259=CARTESIAN_POINT('Ctrl Pts',(2.44232803947089,-28.8240945471019,
123.819729827089));
#118260=CARTESIAN_POINT('Ctrl Pts',(2.4338121221954,-28.9115604862978,123.734177525658));
#118261=CARTESIAN_POINT('Ctrl Pts',(2.42596169614753,-28.9950850129513,
123.666902276812));
#118262=CARTESIAN_POINT('Ctrl Pts',(2.41037437473203,-29.1742816987032,
123.549034862569));
#118263=CARTESIAN_POINT('Ctrl Pts',(2.40267823468151,-29.2696082320333,
123.498785161512));
#118264=CARTESIAN_POINT('Ctrl Pts',(2.39387012274102,-29.3884976536493,
123.450142306569));
#118265=CARTESIAN_POINT('Ctrl Pts',(2.39244717805493,-29.4080156595347,
123.442582715088));
#118266=CARTESIAN_POINT('Ctrl Pts',(2.3902205359124,-29.4390402266528,123.431234029817));
#118267=CARTESIAN_POINT('Ctrl Pts',(2.38940876344116,-29.4504539689033,
123.42719940564));
#118268=CARTESIAN_POINT('Ctrl Pts',(2.38788831217923,-29.4720219512251,
123.41983883121));
#118269=CARTESIAN_POINT('Ctrl Pts',(2.38717876111291,-29.4821661172456,
123.416485485291));
#118270=CARTESIAN_POINT('Ctrl Pts',(2.38558106504151,-29.5051820639366,
123.409121955857));
#118271=CARTESIAN_POINT('Ctrl Pts',(2.38469486008043,-29.5180717746173,
123.405169932399));
#118272=CARTESIAN_POINT('Ctrl Pts',(2.38240539291069,-29.5516791550761,
123.395310473407));
#118273=CARTESIAN_POINT('Ctrl Pts',(2.38101001075511,-29.5724663383989,
123.389647525277));
#118274=CARTESIAN_POINT('Ctrl Pts',(2.37016783612676,-29.7361573683702,
123.348447258276));
#118275=CARTESIAN_POINT('Ctrl Pts',(2.36137449331452,-29.8830845085621,
123.331595990745));
#118276=CARTESIAN_POINT('Ctrl Pts',(2.34847944699122,-30.0924128707277,
123.335406118444));
#118277=CARTESIAN_POINT('Ctrl Pts',(2.3446045348747,-30.1543886036571,123.3400073984));
#118278=CARTESIAN_POINT('Ctrl Pts',(2.33957578283868,-30.2311939476657,
123.35004802096));
#118279=CARTESIAN_POINT('Ctrl Pts',(2.33856870707222,-30.2464033072549,
123.352250764334));
#118280=CARTESIAN_POINT('Ctrl Pts',(2.33705312407168,-30.2689946005218,
123.355842379625));
#118281=CARTESIAN_POINT('Ctrl Pts',(2.33655303955399,-30.2764016192379,
123.357071360284));
#118282=CARTESIAN_POINT('Ctrl Pts',(2.33564817119637,-30.2897134214183,
123.359372635758));
#118283=CARTESIAN_POINT('Ctrl Pts',(2.33524439790885,-30.2956210648319,
123.360426824452));
#118284=CARTESIAN_POINT('Ctrl Pts',(2.33433332917205,-30.3088780243002,
123.362866439439));
#118285=CARTESIAN_POINT('Ctrl Pts',(2.33382509373115,-30.3162237164752,
123.364269433943));
#118286=CARTESIAN_POINT('Ctrl Pts',(2.33227507557799,-30.3384841785334,
123.368676630185));
#118287=CARTESIAN_POINT('Ctrl Pts',(2.33122531097994,-30.3533670004421,
123.371835635345));
#118288=CARTESIAN_POINT('Ctrl Pts',(2.32260864438357,-30.4741294941207,
123.399202173474));
#118289=CARTESIAN_POINT('Ctrl Pts',(2.31463595337783,-30.5774453402395,
123.433505227745));
#118290=CARTESIAN_POINT('Ctrl Pts',(2.29903129538714,-30.7737095874203,
123.520741962037));
#118291=CARTESIAN_POINT('Ctrl Pts',(2.29143363259745,-30.866409045802,123.573054461167));
#118292=CARTESIAN_POINT('Ctrl Pts',(2.28271944799927,-30.9706295582843,
123.645795390551));
#118293=CARTESIAN_POINT('Ctrl Pts',(2.28130003910408,-30.9875239259045,
123.658065415845));
#118294=CARTESIAN_POINT('Ctrl Pts',(2.27907762457224,-31.0138344413362,
123.677940242375));
#118295=CARTESIAN_POINT('Ctrl Pts',(2.27826659553927,-31.0234055454233,
123.685335259418));
#118296=CARTESIAN_POINT('Ctrl Pts',(2.27674679514816,-31.0412792126381,
123.699458661196));
#118297=CARTESIAN_POINT('Ctrl Pts',(2.27603715972085,-31.0495991672993,
123.706163932447));
#118298=CARTESIAN_POINT('Ctrl Pts',(2.27443829424766,-31.0682818947892,
123.721519656968));
#118299=CARTESIAN_POINT('Ctrl Pts',(2.27355101603783,-31.078605285717,123.730217006848));
#118300=CARTESIAN_POINT('Ctrl Pts',(2.27125676268263,-31.1051705655109,
123.753155753816));
#118301=CARTESIAN_POINT('Ctrl Pts',(2.26985772381813,-31.1212435205954,
123.767589520874));
#118302=CARTESIAN_POINT('Ctrl Pts',(2.25903124056536,-31.2444474272381,
123.882634675188));
#118303=CARTESIAN_POINT('Ctrl Pts',(2.2502539445275,-31.338115328509,123.99670351579));
#118304=CARTESIAN_POINT('Ctrl Pts',(2.23736827676881,-31.4484327637146,
124.174485340228));
#118305=CARTESIAN_POINT('Ctrl Pts',(2.23348431139957,-31.4782638916926,
124.229178275905));
#118306=CARTESIAN_POINT('Ctrl Pts',(2.22844469208572,-31.5115611045266,
124.299303394237));
#118307=CARTESIAN_POINT('Ctrl Pts',(2.22743650942295,-31.5179671535999,
124.313291630023));
#118308=CARTESIAN_POINT('Ctrl Pts',(2.22591958102072,-31.5272110812655,
124.33423822638));
#118309=CARTESIAN_POINT('Ctrl Pts',(2.22541927980277,-31.5301972913025,
124.341130763955));
#118310=CARTESIAN_POINT('Ctrl Pts',(2.22451419531994,-31.5354851901925,
124.35356574525));
#118311=CARTESIAN_POINT('Ctrl Pts',(2.22411042510577,-31.5378036833083,
124.359100753839));
#118312=CARTESIAN_POINT('Ctrl Pts',(2.22319958662066,-31.5429430484147,
124.371558571465));
#118313=CARTESIAN_POINT('Ctrl Pts',(2.22269158084853,-31.5457472361146,
124.378487846955));
#118314=CARTESIAN_POINT('Ctrl Pts',(2.22114296374925,-31.5541107451346,
124.399561199408));
#118315=CARTESIAN_POINT('Ctrl Pts',(2.22009439080216,-31.5595230737227,
124.413762246723));
#118316=CARTESIAN_POINT('Ctrl Pts',(2.21146593757035,-31.6020934679014,
124.530223166829));
#118317=CARTESIAN_POINT('Ctrl Pts',(2.2034787453441,-31.6293436541267,124.635816611436));
#118318=CARTESIAN_POINT('Ctrl Pts',(2.18798034707729,-31.6622123776669,
124.846591911234));
#118319=CARTESIAN_POINT('Ctrl Pts',(2.18049848314152,-31.6685646192756,
124.951183019841));
#118320=CARTESIAN_POINT('Ctrl Pts',(2.17183048515137,-31.6643432746323,
125.077385054417));
#118321=CARTESIAN_POINT('Ctrl Pts',(2.17035370169061,-31.6631939893173,
125.099059646083));
#118322=CARTESIAN_POINT('Ctrl Pts',(2.16806276524559,-31.6607326560642,
125.132941862874));
#118323=CARTESIAN_POINT('Ctrl Pts',(2.16723973460431,-31.6597086983541,
125.145167297901));
#118324=CARTESIAN_POINT('Ctrl Pts',(2.16570914858946,-31.6575423523039,
125.167997258063));
#118325=CARTESIAN_POINT('Ctrl Pts',(2.16500059846276,-31.6564329973489,
125.17860420693));
#118326=CARTESIAN_POINT('Ctrl Pts',(2.16341924168835,-31.6537178187908,
125.202358029223));
#118327=CARTESIAN_POINT('Ctrl Pts',(2.16254820835617,-31.6520569106524,
125.215497974481));
#118328=CARTESIAN_POINT('Ctrl Pts',(2.16032605332972,-31.6473948331044,
125.249150515399));
#118329=CARTESIAN_POINT('Ctrl Pts',(2.1589820407665,-31.6441671294819,125.269629795479));
#118330=CARTESIAN_POINT('Ctrl Pts',(2.14922885388604,-31.6177636497037,
125.418974035585));
#118331=CARTESIAN_POINT('Ctrl Pts',(2.14132266935337,-31.5798515228248,
125.544767212036));
#118332=CARTESIAN_POINT('Ctrl Pts',(2.12828874690645,-31.4948802408172,
125.74000725143));
#118333=CARTESIAN_POINT('Ctrl Pts',(2.12323215411156,-31.4566625351929,
125.812655207168));
#118334=CARTESIAN_POINT('Ctrl Pts',(2.11698149246651,-31.4058119570296,
125.894117775523));
#118335=CARTESIAN_POINT('Ctrl Pts',(2.11605790290485,-31.3982131173285,
125.905954690659));
#118336=CARTESIAN_POINT('Ctrl Pts',(2.11464409045213,-31.3864717978894,
125.923744836594));
#118337=CARTESIAN_POINT('Ctrl Pts',(2.11416072132097,-31.3824386013927,
125.929769905908));
#118338=CARTESIAN_POINT('Ctrl Pts',(2.11327184604019,-31.3749905762786,
125.940740684307));
#118339=CARTESIAN_POINT('Ctrl Pts',(2.11286715469574,-31.3715881469888,
125.945694491507));
#118340=CARTESIAN_POINT('Ctrl Pts',(2.11193532804392,-31.3637275080613,
125.957007627283));
#118341=CARTESIAN_POINT('Ctrl Pts',(2.11140703774528,-31.3592515954944,
125.963354248985));
#118342=CARTESIAN_POINT('Ctrl Pts',(2.10977194315397,-31.3453340755478,
125.982798513255));
#118343=CARTESIAN_POINT('Ctrl Pts',(2.10865611384413,-31.3357466221887,
125.995789940629));
#118344=CARTESIAN_POINT('Ctrl Pts',(2.10219031879693,-31.2796001024131,
126.069600991527));
#118345=CARTESIAN_POINT('Ctrl Pts',(2.09664144320763,-31.2290832996542,
126.127286433246));
#118346=CARTESIAN_POINT('Ctrl Pts',(2.08425634874461,-31.1083853806444,
126.247319922864));
#118347=CARTESIAN_POINT('Ctrl Pts',(2.07743596914106,-31.0365309125931,
126.3076436892));
#118348=CARTESIAN_POINT('Ctrl Pts',(2.06721888907106,-30.9184473538711,
126.390896527044));
#118349=CARTESIAN_POINT('Ctrl Pts',(2.06368547969969,-30.8755907895555,
126.418266687986));
#118350=CARTESIAN_POINT('Ctrl Pts',(2.05907999370103,-30.8170045138383,
126.452012817673));
#118351=CARTESIAN_POINT('Ctrl Pts',(2.05794479117482,-30.8023372274195,
126.460168691488));
#118352=CARTESIAN_POINT('Ctrl Pts',(2.05606295950073,-30.7776508851159,
126.473411436188));
#118353=CARTESIAN_POINT('Ctrl Pts',(2.05531202532798,-30.7676993864426,
126.47862091901));
#118354=CARTESIAN_POINT('Ctrl Pts',(2.05384022634437,-30.7480001088232,
126.488680744058));
#118355=CARTESIAN_POINT('Ctrl Pts',(2.05311918385441,-30.7382559790634,
126.493536956175));
#118356=CARTESIAN_POINT('Ctrl Pts',(2.05137473239474,-30.7144595178811,
126.50510667727));
#118357=CARTESIAN_POINT('Ctrl Pts',(2.05035484342123,-30.7003591295661,
126.511719428098));
#118358=CARTESIAN_POINT('Ctrl Pts',(2.04686699878162,-30.6515177542459,
126.533794805252));
#118359=CARTESIAN_POINT('Ctrl Pts',(2.04443245035103,-30.6163399647606,
126.548265894764));
#118360=CARTESIAN_POINT('Ctrl Pts',(2.03446983786867,-30.46856192392,126.603221305574));
#118361=CARTESIAN_POINT('Ctrl Pts',(2.02728095451647,-30.3522652084886,
126.632721399917));
#118362=CARTESIAN_POINT('Ctrl Pts',(2.01687602083308,-30.1846084127871,
126.656485738769));
#118363=CARTESIAN_POINT('Ctrl Pts',(2.01379546927359,-30.1351243690185,
126.661254342302));
#118364=CARTESIAN_POINT('Ctrl Pts',(2.00882447676607,-30.0570939783004,
126.665264422025));
#118365=CARTESIAN_POINT('Ctrl Pts',(2.00698887534482,-30.0286522006169,
126.665996440925));
#118366=CARTESIAN_POINT('Ctrl Pts',(2.0044913845513,-29.9907002587713,126.66600117233));
#118367=CARTESIAN_POINT('Ctrl Pts',(2.003861730469,-29.981193262172,126.665920972743));
#118368=CARTESIAN_POINT('Ctrl Pts',(2.00280896408529,-29.9654105323057,
126.665652719988));
#118369=CARTESIAN_POINT('Ctrl Pts',(2.00238833818513,-29.9591340614226,
126.665510548644));
#118370=CARTESIAN_POINT('Ctrl Pts',(2.0015315809664,-29.9464131118345,126.665150450689));
#118371=CARTESIAN_POINT('Ctrl Pts',(2.00109536080901,-29.9399688436851,
126.664930579547));
#118372=CARTESIAN_POINT('Ctrl Pts',(1.99995708470832,-29.9232333377424,
126.664262296203));
#118373=CARTESIAN_POINT('Ctrl Pts',(1.99925197261299,-29.9129448782246,
126.663755842457));
#118374=CARTESIAN_POINT('Ctrl Pts',(1.99628883654584,-29.8700078801283,
126.661242908119));
#118375=CARTESIAN_POINT('Ctrl Pts',(1.99399048395441,-29.8374194820291,
126.658370643786));
#118376=CARTESIAN_POINT('Ctrl Pts',(1.9847821400071,-29.7088971794409,126.643218630175));
#118377=CARTESIAN_POINT('Ctrl Pts',(1.97767766267397,-29.6140263671326,
126.623555325442));
#118378=CARTESIAN_POINT('Ctrl Pts',(1.96602669877626,-29.4599741942231,
126.577352386796));
#118379=CARTESIAN_POINT('Ctrl Pts',(1.96143096148941,-29.3996591133522,
126.555397273978));
#118380=CARTESIAN_POINT('Ctrl Pts',(1.95408413825634,-29.3034231438573,
126.513931664385));
#118381=CARTESIAN_POINT('Ctrl Pts',(1.95127556320853,-29.2666900433779,
126.496484346559));
#118382=CARTESIAN_POINT('Ctrl Pts',(1.94745667723266,-29.2168485114291,
126.470534301521));
#118383=CARTESIAN_POINT('Ctrl Pts',(1.9464075744234,-29.2031685027838,126.463166764062));
#118384=CARTESIAN_POINT('Ctrl Pts',(1.9446279972284,-29.1799914855315,126.450263012224));
#118385=CARTESIAN_POINT('Ctrl Pts',(1.94389418643111,-29.1704427602291,
126.444822329682));
#118386=CARTESIAN_POINT('Ctrl Pts',(1.94250262176393,-29.1523548397572,
126.434277737483));
#118387=CARTESIAN_POINT('Ctrl Pts',(1.94184428615079,-29.1438061974481,
126.429191073884));
#118388=CARTESIAN_POINT('Ctrl Pts',(1.94014297667687,-29.1217413344862,
126.415792875408));
#118389=CARTESIAN_POINT('Ctrl Pts',(1.93910432035509,-29.1082971724193,
126.407364148115));
#118390=CARTESIAN_POINT('Ctrl Pts',(1.93547895302539,-29.0614959649165,
126.377082519161));
#118391=CARTESIAN_POINT('Ctrl Pts',(1.93292938595661,-29.0288035226204,
126.354224458256));
#118392=CARTESIAN_POINT('Ctrl Pts',(1.92226532871704,-28.8938147118927,
126.252436993267));
#118393=CARTESIAN_POINT('Ctrl Pts',(1.91454912530594,-28.8000690141589,
126.162931517357));
#118394=CARTESIAN_POINT('Ctrl Pts',(1.9039947584171,-28.6910323785338,126.031451693134));
#118395=CARTESIAN_POINT('Ctrl Pts',(1.90139509278425,-28.6656715165416,
125.998426696306));
#118396=CARTESIAN_POINT('Ctrl Pts',(1.8971183709763,-28.6269165740481,125.943842713647));
#118397=CARTESIAN_POINT('Ctrl Pts',(1.89547924924855,-28.6127310450253,
125.922866102869));
#118398=CARTESIAN_POINT('Ctrl Pts',(1.89321078763743,-28.594098223647,125.893912325633));
#118399=CARTESIAN_POINT('Ctrl Pts',(1.89260666460085,-28.5892296013874,
125.886208735957));
#118400=CARTESIAN_POINT('Ctrl Pts',(1.89158472016883,-28.58115555032,125.873198066411));
#118401=CARTESIAN_POINT('Ctrl Pts',(1.89116908103375,-28.5779160102204,
125.867912184542));
#118402=CARTESIAN_POINT('Ctrl Pts',(1.89030935615627,-28.5713079126132,
125.856993578101));
#118403=CARTESIAN_POINT('Ctrl Pts',(1.88986506879942,-28.5679430360797,
125.851358867813));
#118404=CARTESIAN_POINT('Ctrl Pts',(1.88868237142817,-28.5591153662076,
125.836375934526));
#118405=CARTESIAN_POINT('Ctrl Pts',(1.88794046844187,-28.5537103693259,
125.82699426869));
#118406=CARTESIAN_POINT('Ctrl Pts',(1.88456627219145,-28.5297061820507,
125.784374151944));
#118407=CARTESIAN_POINT('Ctrl Pts',(1.88187901589238,-28.5121601141909,
125.750558922616));
#118408=CARTESIAN_POINT('Ctrl Pts',(1.87551696457238,-28.4738981862066,
125.670195938835));
#118409=CARTESIAN_POINT('Ctrl Pts',(1.87181988333564,-28.4541362594963,
125.623257634171));
#118410=CARTESIAN_POINT('Ctrl Pts',(1.86811697181266,-28.4365600386127,
125.575509762851));
#118411=CARTESIAN_POINT('Origin',(5.,-30.,125.));
#118412=CARTESIAN_POINT('',(1.16625578224439,-28.4365599837819,125.575509613897));
#118413=CARTESIAN_POINT('',(1.36115610141821,-28.4365599811973,125.575509606876));
#118414=CARTESIAN_POINT('',(5.,-28.4365599837785,125.575509613888));
#118415=CARTESIAN_POINT('Ctrl Pts',(1.36115610141822,-28.4365599811973,
125.575509606876));
#118416=CARTESIAN_POINT('Ctrl Pts',(1.36788846393626,-28.4686612718869,
125.662716565578));
#118417=CARTESIAN_POINT('Ctrl Pts',(1.37450638750137,-28.5080098087128,
125.747104294689));
#118418=CARTESIAN_POINT('Ctrl Pts',(1.38236658826502,-28.5649155593372,
125.846494758489));
#118419=CARTESIAN_POINT('Ctrl Pts',(1.38383330985978,-28.5759893934428,
125.864993986104));
#118420=CARTESIAN_POINT('Ctrl Pts',(1.38611240424284,-28.5939088699272,
125.893651803653));
#118421=CARTESIAN_POINT('Ctrl Pts',(1.3869335006038,-28.6005124280402,125.903958163869));
#118422=CARTESIAN_POINT('Ctrl Pts',(1.38846255903877,-28.6130846243825,
125.923111916019));
#118423=CARTESIAN_POINT('Ctrl Pts',(1.38917149278923,-28.6190258112384,
125.931976484495));
#118424=CARTESIAN_POINT('Ctrl Pts',(1.39075636246848,-28.6325578833415,
125.95175350691));
#118425=CARTESIAN_POINT('Ctrl Pts',(1.39163049290498,-28.6401950784762,
125.962633509062));
#118426=CARTESIAN_POINT('Ctrl Pts',(1.39386583866521,-28.6601657541862,
125.99037187657));
#118427=CARTESIAN_POINT('Ctrl Pts',(1.39521979993452,-28.6726877511813,
126.007092109214));
#118428=CARTESIAN_POINT('Ctrl Pts',(1.40488791976394,-28.7650752513151,
126.125736692284));
#118429=CARTESIAN_POINT('Ctrl Pts',(1.41271241556014,-28.8562674498513,
126.218278205338));
#118430=CARTESIAN_POINT('Ctrl Pts',(1.42572359794038,-29.022087177955,126.351351409861));
#118431=CARTESIAN_POINT('Ctrl Pts',(1.43084590381139,-29.0907035378142,
126.398442171754));
#118432=CARTESIAN_POINT('Ctrl Pts',(1.43717049648412,-29.1747029688786,
126.4472867398));
#118433=CARTESIAN_POINT('Ctrl Pts',(1.43809463791653,-29.1869588290539,
126.454207041323));
#118434=CARTESIAN_POINT('Ctrl Pts',(1.43950921612305,-29.2056613105414,
126.464457121626));
#118435=CARTESIAN_POINT('Ctrl Pts',(1.43999279022645,-29.2120447812719,
126.467901625791));
#118436=CARTESIAN_POINT('Ctrl Pts',(1.44088199819808,-29.2237596985939,
126.474124532455));
#118437=CARTESIAN_POINT('Ctrl Pts',(1.4412868161592,-29.2290839555731,126.476915905331));
#118438=CARTESIAN_POINT('Ctrl Pts',(1.44221889466395,-29.2413225440079,
126.483248078116));
#118439=CARTESIAN_POINT('Ctrl Pts',(1.44274731042079,-29.2482465935679,
126.486769367908));
#118440=CARTESIAN_POINT('Ctrl Pts',(1.44438268730008,-29.269639468863,126.497461271443));
#118441=CARTESIAN_POINT('Ctrl Pts',(1.44549867523161,-29.2841876430793,
126.504469802498));
#118442=CARTESIAN_POINT('Ctrl Pts',(1.45226602641753,-29.3722362966567,
126.545320773489));
#118443=CARTESIAN_POINT('Ctrl Pts',(1.45813949948361,-29.4480146701336,
126.573980078569));
#118444=CARTESIAN_POINT('Ctrl Pts',(1.46939065190613,-29.5961995291802,
126.61800200194));
#118445=CARTESIAN_POINT('Ctrl Pts',(1.47475398573363,-29.6681511236861,
126.634277494848));
#118446=CARTESIAN_POINT('Ctrl Pts',(1.48305059776605,-29.7829908697459,
126.652354225002));
#118447=CARTESIAN_POINT('Ctrl Pts',(1.48605149397676,-29.8252751271432,
126.657359095166));
#118448=CARTESIAN_POINT('Ctrl Pts',(1.49113200054262,-29.898241701715,126.663171514866));
#118449=CARTESIAN_POINT('Ctrl Pts',(1.4932331737568,-29.9288385499524,126.664761394697));
#118450=CARTESIAN_POINT('Ctrl Pts',(1.49625572646403,-29.9734451812655,
126.66584706387));
#118451=CARTESIAN_POINT('Ctrl Pts',(1.49719760097907,-29.987430784996,126.666011294724));
#118452=CARTESIAN_POINT('Ctrl Pts',(1.49885320545711,-30.0121596317582,
126.665990259205));
#118453=CARTESIAN_POINT('Ctrl Pts',(1.49956914498663,-30.0229019565679,
126.665877219391));
#118454=CARTESIAN_POINT('Ctrl Pts',(1.50106645181812,-30.0454663869723,
126.665421467763));
#118455=CARTESIAN_POINT('Ctrl Pts',(1.50184709266683,-30.0572874877419,
126.665056759849));
#118456=CARTESIAN_POINT('Ctrl Pts',(1.50391124746068,-30.0886865343674,
126.663753237886));
#118457=CARTESIAN_POINT('Ctrl Pts',(1.50518788387196,-30.108253868072,126.66259474635));
#118458=CARTESIAN_POINT('Ctrl Pts',(1.51177369321979,-30.2098603590109,
126.654777599387));
#118459=CARTESIAN_POINT('Ctrl Pts',(1.51690082711429,-30.2913484268968,
126.642391195443));
#118460=CARTESIAN_POINT('Ctrl Pts',(1.52812413300367,-30.4694627902114,
126.601636704204));
#118461=CARTESIAN_POINT('Ctrl Pts',(1.53416040838146,-30.5650989567957,
126.570444607145));
#118462=CARTESIAN_POINT('Ctrl Pts',(1.54222796926133,-30.6833492661583,
126.519668065507));
#118463=CARTESIAN_POINT('Ctrl Pts',(1.54402239215024,-30.7090687950657,
126.507839020593));
#118464=CARTESIAN_POINT('Ctrl Pts',(1.54709232618714,-30.7518119106759,
126.486844987105));
#118465=CARTESIAN_POINT('Ctrl Pts',(1.54835147935201,-30.769000471379,126.478028200564));
#118466=CARTESIAN_POINT('Ctrl Pts',(1.5501709142979,-30.7932782447822,126.465036924288));
#118467=CARTESIAN_POINT('Ctrl Pts',(1.55071712457215,-30.8004965645595,
126.461105337165));
#118468=CARTESIAN_POINT('Ctrl Pts',(1.55167152424277,-30.8129812863723,
126.45418502708));
#118469=CARTESIAN_POINT('Ctrl Pts',(1.55207818240303,-30.8182609667826,
126.451220746086));
#118470=CARTESIAN_POINT('Ctrl Pts',(1.55295571898963,-30.8295666701918,
126.444791836937));
#118471=CARTESIAN_POINT('Ctrl Pts',(1.55342712302998,-30.8355871155184,
126.441318313332));
#118472=CARTESIAN_POINT('Ctrl Pts',(1.5547375040737,-30.8521816641599,126.431605098145));
#118473=CARTESIAN_POINT('Ctrl Pts',(1.55558122835395,-30.8627085477605,
126.425286176622));
#118474=CARTESIAN_POINT('Ctrl Pts',(1.5614918217239,-30.9354270189733,126.380535081448));
#118475=CARTESIAN_POINT('Ctrl Pts',(1.56676039407081,-30.9950935147074,
126.338165665287));
#118476=CARTESIAN_POINT('Ctrl Pts',(1.57310125013654,-31.062782657917,126.283062887893));
#118477=CARTESIAN_POINT('Ctrl Pts',(1.57413357105327,-31.0736722706845,
126.273964365105));
#118478=CARTESIAN_POINT('Ctrl Pts',(1.58052960975855,-31.1403843568098,
126.216761910754));
#118479=CARTESIAN_POINT('Ctrl Pts',(1.5858932786639,-31.1930839691579,126.165134318634));
#118480=CARTESIAN_POINT('Ctrl Pts',(1.59418936030154,-31.2705486823036,
126.078458410821));
#118481=CARTESIAN_POINT('Ctrl Pts',(1.59718944031677,-31.2976789687186,
126.045655916539));
#118482=CARTESIAN_POINT('Ctrl Pts',(1.60226873464178,-31.34212541195,125.987518739219));
#118483=CARTESIAN_POINT('Ctrl Pts',(1.60436949788008,-31.3600520776271,
125.962679823125));
#118484=CARTESIAN_POINT('Ctrl Pts',(1.60739157896747,-31.3851531554695,
125.925798199347));
#118485=CARTESIAN_POINT('Ctrl Pts',(1.60833338284062,-31.3928758001722,
125.914138171189));
#118486=CARTESIAN_POINT('Ctrl Pts',(1.60998890717904,-31.4062694541386,
125.893351901445));
#118487=CARTESIAN_POINT('Ctrl Pts',(1.61070483649738,-31.4120006269298,
125.884265591495));
#118488=CARTESIAN_POINT('Ctrl Pts',(1.61220216491526,-31.4238559820603,
125.865060698267));
#118489=CARTESIAN_POINT('Ctrl Pts',(1.61298283714817,-31.4299611282615,
125.854931022444));
#118490=CARTESIAN_POINT('Ctrl Pts',(1.61504717540823,-31.4458970170011,
125.827841800432));
#118491=CARTESIAN_POINT('Ctrl Pts',(1.61632396165289,-31.4555373799171,
125.810771989272));
#118492=CARTESIAN_POINT('Ctrl Pts',(1.62291485042368,-31.5041143827149,
125.721098339484));
#118493=CARTESIAN_POINT('Ctrl Pts',(1.62804654001342,-31.5379299118089,
125.645845921156));
#118494=CARTESIAN_POINT('Ctrl Pts',(1.63927012383836,-31.6002711740445,
125.474082420563));
#118495=CARTESIAN_POINT('Ctrl Pts',(1.64530253830474,-31.6259093333768,
125.376879907786));
#118496=CARTESIAN_POINT('Ctrl Pts',(1.65336545592648,-31.647368550382,125.250067249801));
#118497=CARTESIAN_POINT('Ctrl Pts',(1.65515936240895,-31.6513780868515,
125.222051804522));
#118498=CARTESIAN_POINT('Ctrl Pts',(1.65822850200758,-31.6569204286489,
125.17476754759));
#118499=CARTESIAN_POINT('Ctrl Pts',(1.65948738815723,-31.6588349678136,
125.155548944385));
#118500=CARTESIAN_POINT('Ctrl Pts',(1.66130650407048,-31.6610873317372,
125.12811099888));
#118501=CARTESIAN_POINT('Ctrl Pts',(1.66185266904523,-31.6616991175698,
125.119914917138));
#118502=CARTESIAN_POINT('Ctrl Pts',(1.66280701784266,-31.6626562465918,
125.105673410175));
#118503=CARTESIAN_POINT('Ctrl Pts',(1.66321367094054,-31.6630293168683,
125.099630085021));
#118504=CARTESIAN_POINT('Ctrl Pts',(1.66409123053968,-31.6637599111632,
125.086644538431));
#118505=CARTESIAN_POINT('Ctrl Pts',(1.66456266298428,-31.6641069305862,
125.079702178145));
#118506=CARTESIAN_POINT('Ctrl Pts',(1.66587319650753,-31.6649467681416,
125.060490074267));
#118507=CARTESIAN_POINT('Ctrl Pts',(1.66671704656343,-31.6653473769055,
125.048217029552));
#118508=CARTESIAN_POINT('Ctrl Pts',(1.67266115851203,-31.6671998582417,
124.962367891315));
#118509=CARTESIAN_POINT('Ctrl Pts',(1.67796577810366,-31.6639107048638,
124.888778109899));
#118510=CARTESIAN_POINT('Ctrl Pts',(1.68431641348504,-31.6542389518277,
124.801906925831));
#118511=CARTESIAN_POINT('Ctrl Pts',(1.68532286335365,-31.6525370415844,
124.78817767238));
#118512=CARTESIAN_POINT('Ctrl Pts',(1.69169564117011,-31.6406841614922,
124.701425412049));
#118513=CARTESIAN_POINT('Ctrl Pts',(1.69706168589184,-31.6258656535747,
124.629117950333));
#118514=CARTESIAN_POINT('Ctrl Pts',(1.70535296391837,-31.5950414206202,
124.517090609858));
#118515=CARTESIAN_POINT('Ctrl Pts',(1.70834625675692,-31.5822165137071,
124.476597652801));
#118516=CARTESIAN_POINT('Ctrl Pts',(1.71341546965152,-31.557517975688,124.407860939935));
#118517=CARTESIAN_POINT('Ctrl Pts',(1.71551282260845,-31.5463877333739,
124.379374426795));
#118518=CARTESIAN_POINT('Ctrl Pts',(1.71853098494236,-31.5290362697914,
124.338335870974));
#118519=CARTESIAN_POINT('Ctrl Pts',(1.71947220528007,-31.523431603388,124.325531687589));
#118520=CARTESIAN_POINT('Ctrl Pts',(1.72112707262475,-31.5132357084331,
124.303014300458));
#118521=CARTESIAN_POINT('Ctrl Pts',(1.72184292252847,-31.5087104824101,
124.293272284258));
#118522=CARTESIAN_POINT('Ctrl Pts',(1.72334044487439,-31.499003658873,124.272893404998));
#118523=CARTESIAN_POINT('Ctrl Pts',(1.7241213869792,-31.4938023175698,124.262266567121));
#118524=CARTESIAN_POINT('Ctrl Pts',(1.72618728224493,-31.4796747643113,
124.234164767091));
#118525=CARTESIAN_POINT('Ctrl Pts',(1.72746533666611,-31.4705521158834,
124.216790232864));
#118526=CARTESIAN_POINT('Ctrl Pts',(1.73410063103621,-31.4212220551095,
124.126740784834));
#118527=CARTESIAN_POINT('Ctrl Pts',(1.73927216798448,-31.3759265373484,
124.056982253318));
#118528=CARTESIAN_POINT('Ctrl Pts',(1.7504984708822,-31.2651939515627,123.911519598761));
#118529=CARTESIAN_POINT('Ctrl Pts',(1.75649733878881,-31.197775103907,123.837744525143));
#118530=CARTESIAN_POINT('Ctrl Pts',(1.76451990582776,-31.1033380194236,
123.75140165755));
#118531=CARTESIAN_POINT('Ctrl Pts',(1.76630931321811,-31.082028329863,123.732890249487));
#118532=CARTESIAN_POINT('Ctrl Pts',(1.76937153156413,-31.0453909336996,
123.702662192452));
#118533=CARTESIAN_POINT('Ctrl Pts',(1.77062809137023,-31.0303108124198,
123.690653925292));
#118534=CARTESIAN_POINT('Ctrl Pts',(1.77244442768709,-31.0085139627873,
123.673906851498));
#118535=CARTESIAN_POINT('Ctrl Pts',(1.77299019788344,-31.0019646339259,
123.668951421994));
#118536=CARTESIAN_POINT('Ctrl Pts',(1.77394410206363,-30.9905241849914,
123.660427495915));
#118537=CARTESIAN_POINT('Ctrl Pts',(1.77435070976286,-30.9856498185388,
123.656836909152));
#118538=CARTESIAN_POINT('Ctrl Pts',(1.77522846308756,-30.9751340403509,
123.649178779574));
#118539=CARTESIAN_POINT('Ctrl Pts',(1.77570013748638,-30.9694867843727,
123.645120028667));
#118540=CARTESIAN_POINT('Ctrl Pts',(1.77701198407323,-30.9537856616645,
123.633983864675));
#118541=CARTESIAN_POINT('Ctrl Pts',(1.77785692000406,-30.9436788409369,
123.626982376905));
#118542=CARTESIAN_POINT('Ctrl Pts',(1.78405502730907,-30.8695188432329,
123.576813719439));
#118543=CARTESIAN_POINT('Ctrl Pts',(1.78963313685824,-30.8026162129568,
123.538040089812));
#118544=CARTESIAN_POINT('Ctrl Pts',(1.79585997646524,-30.7257112831898,
123.500343346361));
#118545=CARTESIAN_POINT('Ctrl Pts',(1.7964727563374,-30.7181201262464,123.496693501344));
#118546=CARTESIAN_POINT('Ctrl Pts',(1.80260485524155,-30.641906087462,123.460758635482));
#118547=CARTESIAN_POINT('Ctrl Pts',(1.80812732608967,-30.5711776929982,
123.43313533958));
#118548=CARTESIAN_POINT('Ctrl Pts',(1.81655269258082,-30.4585014349004,
123.397777422521));
#118549=CARTESIAN_POINT('Ctrl Pts',(1.81953056155232,-30.4177240239027,
123.386665599608));
#118550=CARTESIAN_POINT('Ctrl Pts',(1.82457684760902,-30.3468879632765,
123.37022918647));
#118551=CARTESIAN_POINT('Ctrl Pts',(1.82666643521057,-30.317025763236,123.364158002776));
#118552=CARTESIAN_POINT('Ctrl Pts',(1.82967566896759,-30.2732638543434,
123.356504438408));
#118553=CARTESIAN_POINT('Ctrl Pts',(1.83061555574374,-30.2594856061424,
123.354272794217));
#118554=CARTESIAN_POINT('Ctrl Pts',(1.83226892021003,-30.2350591650315,
123.350630874847));
#118555=CARTESIAN_POINT('Ctrl Pts',(1.83298458722008,-30.224422490641,123.349149953191));
#118556=CARTESIAN_POINT('Ctrl Pts',(1.83448255040342,-30.2020293257339,
123.346252633924));
#118557=CARTESIAN_POINT('Ctrl Pts',(1.83526410829843,-30.1902705182994,
123.344858513205));
#118558=CARTESIAN_POINT('Ctrl Pts',(1.83733356618749,-30.1589434349058,
123.341482653211));
#118559=CARTESIAN_POINT('Ctrl Pts',(1.83861452390815,-30.1393528672581,
123.339721819512));
#118560=CARTESIAN_POINT('Ctrl Pts',(1.84536578976562,-30.035145169582,123.332213019835));
#118561=CARTESIAN_POINT('Ctrl Pts',(1.85064160769523,-29.9502080533539,
123.332585236987));
#118562=CARTESIAN_POINT('Ctrl Pts',(1.86006752721349,-29.7971209348398,
123.344969977609));
#118563=CARTESIAN_POINT('Ctrl Pts',(1.86423485193548,-29.728992509241,123.354752603964));
#118564=CARTESIAN_POINT('Ctrl Pts',(1.87133723664868,-29.6160284193556,
123.378181863404));
#118565=CARTESIAN_POINT('Ctrl Pts',(1.87423435735936,-29.5708126132314,
123.389557254645));
#118566=CARTESIAN_POINT('Ctrl Pts',(1.87894271517298,-29.4999695551892,
123.410575409003));
#118567=CARTESIAN_POINT('Ctrl Pts',(1.88070590574773,-29.4739991571203,
123.418980112047));
#118568=CARTESIAN_POINT('Ctrl Pts',(1.88311931772348,-29.4394087048879,
123.431121045746));
#118569=CARTESIAN_POINT('Ctrl Pts',(1.88373999266335,-29.4305952629905,
123.434298237665));
#118570=CARTESIAN_POINT('Ctrl Pts',(1.88478196336245,-29.4159466653346,
123.439719006075));
#118571=CARTESIAN_POINT('Ctrl Pts',(1.88520088162678,-29.4100963275817,
123.441921461211));
#118572=CARTESIAN_POINT('Ctrl Pts',(1.88600539554548,-29.3989387397343,
123.446193766397));
#118573=CARTESIAN_POINT('Ctrl Pts',(1.88639062922018,-29.3936294732509,
123.448258000827));
#118574=CARTESIAN_POINT('Ctrl Pts',(1.88743719341928,-29.3792930887035,
123.453916774434));
#118575=CARTESIAN_POINT('Ctrl Pts',(1.88810148028092,-29.3702868302251,
123.457563057199));
#118576=CARTESIAN_POINT('Ctrl Pts',(1.8906836233059,-29.3356183124169,123.471953222355));
#118577=CARTESIAN_POINT('Ctrl Pts',(1.89263038386391,-29.3101962941188,
123.483259873022));
#118578=CARTESIAN_POINT('Ctrl Pts',(1.90246903495523,-29.1846998615746,
123.542882969278));
#118579=CARTESIAN_POINT('Ctrl Pts',(1.91066017172317,-29.0893545877398,
123.600489859609));
#118580=CARTESIAN_POINT('Ctrl Pts',(1.92293836202486,-28.9533952033453,
123.702450529702));
#118581=CARTESIAN_POINT('Ctrl Pts',(1.92713903414929,-28.9082333200005,
123.740213148905));
#118582=CARTESIAN_POINT('Ctrl Pts',(1.93308465529382,-28.8460169087158,
123.798100368657));
#118583=CARTESIAN_POINT('Ctrl Pts',(1.93489690987478,-28.8272948395158,
123.816360513253));
#118584=CARTESIAN_POINT('Ctrl Pts',(1.93814578960179,-28.7941773683414,
123.850218407817));
#118585=CARTESIAN_POINT('Ctrl Pts',(1.93958843785458,-28.7796356634218,
123.865664561606));
#118586=CARTESIAN_POINT('Ctrl Pts',(1.94183878705443,-28.7572227873252,
123.890401495792));
#118587=CARTESIAN_POINT('Ctrl Pts',(1.94265485150414,-28.7491521068725,
123.89950756352));
#118588=CARTESIAN_POINT('Ctrl Pts',(1.9441793570525,-28.734186424162,123.916770552509));
#118589=CARTESIAN_POINT('Ctrl Pts',(1.94488871523273,-28.7272687395855,
123.924906891229));
#118590=CARTESIAN_POINT('Ctrl Pts',(1.94648077899595,-28.7118503751862,
123.943398835323));
#118591=CARTESIAN_POINT('Ctrl Pts',(1.94736160544205,-28.7033953461322,
123.953791671745));
#118592=CARTESIAN_POINT('Ctrl Pts',(1.9496266402695,-28.681858800459,123.980926336417));
#118593=CARTESIAN_POINT('Ctrl Pts',(1.95100325590952,-28.6689702771839,
123.997818730983));
#118594=CARTESIAN_POINT('Ctrl Pts',(1.96045592283178,-28.581995373103,124.116451518948));
#118595=CARTESIAN_POINT('Ctrl Pts',(1.96807467217359,-28.5193221244078,
124.226054404614));
#118596=CARTESIAN_POINT('Ctrl Pts',(1.98103479774366,-28.4355857479652,
124.420718322886));
#118597=CARTESIAN_POINT('Ctrl Pts',(1.98632695518618,-28.4077646928326,
124.502263051839));
#118598=CARTESIAN_POINT('Ctrl Pts',(1.99284280428935,-28.3828620791189,
124.599226384169));
#118599=CARTESIAN_POINT('Ctrl Pts',(1.993767970265,-28.3795304253225,124.612917487288));
#118600=CARTESIAN_POINT('Ctrl Pts',(1.99518379916742,-28.3747467083531,
124.633720872586));
#118601=CARTESIAN_POINT('Ctrl Pts',(1.99566758099685,-28.3731667190938,
124.640803490568));
#118602=CARTESIAN_POINT('Ctrl Pts',(1.99655697683751,-28.3703625519003,
124.653771856634));
#118603=CARTESIAN_POINT('Ctrl Pts',(1.99696177244465,-28.3691238937258,
124.659654202665));
#118604=CARTESIAN_POINT('Ctrl Pts',(1.99789354529921,-28.366358440957,124.673149061158));
#118605=CARTESIAN_POINT('Ctrl Pts',(1.99842167473617,-28.3648530103468,
124.680765609844));
#118606=CARTESIAN_POINT('Ctrl Pts',(2.00005532707843,-28.3603844361573,
124.704235063094));
#118607=CARTESIAN_POINT('Ctrl Pts',(2.00116985069899,-28.3575983056336,
124.720120165698));
#118608=CARTESIAN_POINT('Ctrl Pts',(2.00842378542596,-28.3411134208396,
124.822852298433));
#118609=CARTESIAN_POINT('Ctrl Pts',(2.01482529538982,-28.3340784703978,
124.910620762262));
#118610=CARTESIAN_POINT('Ctrl Pts',(2.02992528091123,-28.3338948384011,
125.118055337291));
#118611=CARTESIAN_POINT('Ctrl Pts',(2.03855840379883,-28.3466531596518,
125.237270689548));
#118612=CARTESIAN_POINT('Ctrl Pts',(2.04828924071552,-28.3766854319895,
125.375336843758));
#118613=CARTESIAN_POINT('Ctrl Pts',(2.04977251375399,-28.3817178198129,
125.396472944023));
#118614=CARTESIAN_POINT('Ctrl Pts',(2.05215864167958,-28.3905545774915,
125.430609635674));
#118615=CARTESIAN_POINT('Ctrl Pts',(2.05306944116974,-28.3941064383024,
125.443672304342));
#118616=CARTESIAN_POINT('Ctrl Pts',(2.05469042476507,-28.4007480633653,
125.466972757659));
#118617=CARTESIAN_POINT('Ctrl Pts',(2.05540250324634,-28.4037778943884,
125.477226688204));
#118618=CARTESIAN_POINT('Ctrl Pts',(2.05691210379892,-28.4104398791914,
125.498999476005));
#118619=CARTESIAN_POINT('Ctrl Pts',(2.05770869996323,-28.4140990152609,
125.510509484949));
#118620=CARTESIAN_POINT('Ctrl Pts',(2.05974160437747,-28.4238044731072,
125.539926704309));
#118621=CARTESIAN_POINT('Ctrl Pts',(2.06097195868479,-28.4300309897374,
125.55777282843));
#118622=CARTESIAN_POINT('Ctrl Pts',(2.06219309044095,-28.4365599837628,
125.575509613845));
#118623=CARTESIAN_POINT('Ctrl Pts',(1.86811697181266,-28.4365600386127,
125.575509762851));
#118624=CARTESIAN_POINT('Ctrl Pts',(1.86507380622595,-28.4221153644137,
125.536269106429));
#118625=CARTESIAN_POINT('Ctrl Pts',(1.86202653433009,-28.4091469471883,
125.49648167022));
#118626=CARTESIAN_POINT('Ctrl Pts',(1.85221160981063,-28.3720165764368,
125.366077255002));
#118627=CARTESIAN_POINT('Ctrl Pts',(1.84555050434239,-28.3539977609925,
125.273905982475));
#118628=CARTESIAN_POINT('Ctrl Pts',(1.83779011161915,-28.3416990096445,
125.161180470645));
#118629=CARTESIAN_POINT('Ctrl Pts',(1.83645740575205,-28.3399149612747,
125.14162994074));
#118630=CARTESIAN_POINT('Ctrl Pts',(1.83433882467471,-28.3376101060971,
125.110253315698));
#118631=CARTESIAN_POINT('Ctrl Pts',(1.8335461498498,-28.3368690990637,125.098445781118));
#118632=CARTESIAN_POINT('Ctrl Pts',(1.83204155045042,-28.3356955867723,
125.075908530718));
#118633=CARTESIAN_POINT('Ctrl Pts',(1.8313289704571,-28.3352409240709,125.06518062015));
#118634=CARTESIAN_POINT('Ctrl Pts',(1.82971233006984,-28.3344411814591,
125.04072354665));
#118635=CARTESIAN_POINT('Ctrl Pts',(1.82881036880894,-28.3341620764283,
125.026992894911));
#118636=CARTESIAN_POINT('Ctrl Pts',(1.82595102331795,-28.3338135964352,
124.9832109419));
#118637=CARTESIAN_POINT('Ctrl Pts',(1.82401355860867,-28.3343874538904,
124.953159536054));
#118638=CARTESIAN_POINT('Ctrl Pts',(1.81305815017193,-28.3423150355948,
124.781509306069));
#118639=CARTESIAN_POINT('Ctrl Pts',(1.80460210868433,-28.3669068000732,
124.641301231028));
#118640=CARTESIAN_POINT('Ctrl Pts',(1.79319080210218,-28.4217437194828,
124.464722451907));
#118641=CARTESIAN_POINT('Ctrl Pts',(1.79050206848774,-28.4361236548606,
124.424061444828));
#118642=CARTESIAN_POINT('Ctrl Pts',(1.78609539047946,-28.4616485909794,
124.3599195207));
#118643=CARTESIAN_POINT('Ctrl Pts',(1.78441829244063,-28.4717943011066,
124.336060813831));
#118644=CARTESIAN_POINT('Ctrl Pts',(1.78210541589467,-28.4862855740065,
124.304076769783));
#118645=CARTESIAN_POINT('Ctrl Pts',(1.78149614364694,-28.4901484884623,
124.295735199441));
#118646=CARTESIAN_POINT('Ctrl Pts',(1.78046801842268,-28.4967383658165,
124.281808462095));
#118647=CARTESIAN_POINT('Ctrl Pts',(1.78005140828074,-28.4994279859631,
124.276205654222));
#118648=CARTESIAN_POINT('Ctrl Pts',(1.77924673172392,-28.5046583715688,
124.26546458883));
#118649=CARTESIAN_POINT('Ctrl Pts',(1.77885898841059,-28.5071944037697,
124.26032418903));
#118650=CARTESIAN_POINT('Ctrl Pts',(1.77779679374661,-28.5141856959868,
124.246335622485));
#118651=CARTESIAN_POINT('Ctrl Pts',(1.77711923438104,-28.5186933455285,
124.237514115988));
#118652=CARTESIAN_POINT('Ctrl Pts',(1.77441855530079,-28.5368592990006,
124.202732307009));
#118653=CARTESIAN_POINT('Ctrl Pts',(1.7723631833118,-28.5511227456628,124.177096033721));
#118654=CARTESIAN_POINT('Ctrl Pts',(1.76323958719341,-28.6166122338677,
124.066374415666));
#118655=CARTESIAN_POINT('Ctrl Pts',(1.75594226835794,-28.6747096118142,
123.985592427633));
#118656=CARTESIAN_POINT('Ctrl Pts',(1.74289414544669,-28.7924506631414,
123.849392142191));
#118657=CARTESIAN_POINT('Ctrl Pts',(1.73712358656608,-28.8496239719627,
123.792228526141));
#118658=CARTESIAN_POINT('Ctrl Pts',(1.72944788712227,-28.9333659717816,
123.719865926375));
#118659=CARTESIAN_POINT('Ctrl Pts',(1.72739640814584,-28.9565313351256,
123.700913882034));
#118660=CARTESIAN_POINT('Ctrl Pts',(1.7244312253868,-28.9911550936886,123.674111609039));
#118661=CARTESIAN_POINT('Ctrl Pts',(1.72349810535745,-29.0022198876238,
123.665765036519));
#118662=CARTESIAN_POINT('Ctrl Pts',(1.72185253039298,-29.0220290460688,
123.651206533345));
#118663=CARTESIAN_POINT('Ctrl Pts',(1.72113795325958,-29.0307315363274,
123.644939242323));
#118664=CARTESIAN_POINT('Ctrl Pts',(1.71963821619544,-29.0492051457759,
123.631904096242));
#118665=CARTESIAN_POINT('Ctrl Pts',(1.71885383327985,-29.0589894300226,
123.625155872033));
#118666=CARTESIAN_POINT('Ctrl Pts',(1.71676728307705,-29.0853371754616,
123.607396875484));
#118667=CARTESIAN_POINT('Ctrl Pts',(1.71547227186718,-29.1020273093401,
123.59657681126));
#118668=CARTESIAN_POINT('Ctrl Pts',(1.70786663011725,-29.2019532968336,
123.53430834638));
#118669=CARTESIAN_POINT('Ctrl Pts',(1.70182310428485,-29.2894007701753,
123.489972588029));
#118670=CARTESIAN_POINT('Ctrl Pts',(1.69132001184899,-29.4487947514026,
123.426093190352));
#118671=CARTESIAN_POINT('Ctrl Pts',(1.68684291800265,-29.5190929260357,
123.403210285008));
#118672=CARTESIAN_POINT('Ctrl Pts',(1.68009638892401,-29.6242251188271,
123.376563138935));
#118673=CARTESIAN_POINT('Ctrl Pts',(1.67791885507917,-29.6580311902958,
123.369107287598));
#118674=CARTESIAN_POINT('Ctrl Pts',(1.67426724128406,-29.7139608452303,
123.358587497524));
#118675=CARTESIAN_POINT('Ctrl Pts',(1.67281870032706,-29.7359583037017,
123.354905696476));
#118676=CARTESIAN_POINT('Ctrl Pts',(1.67077435051358,-29.7666177373059,
123.350404836485));
#118677=CARTESIAN_POINT('Ctrl Pts',(1.67019777112628,-29.7752232667888,
123.349210220518));
#118678=CARTESIAN_POINT('Ctrl Pts',(1.669208500349,-29.7899088440469,123.347288531397));
#118679=CARTESIAN_POINT('Ctrl Pts',(1.66879767318598,-29.7959844151418,
123.346527553219));
#118680=CARTESIAN_POINT('Ctrl Pts',(1.6679319489996,-29.8087358772128,123.345001756501));
#118681=CARTESIAN_POINT('Ctrl Pts',(1.667476708849,-29.8154123293023,123.34424381672));
#118682=CARTESIAN_POINT('Ctrl Pts',(1.66623351460583,-29.83357147366,123.342293506081));
#118683=CARTESIAN_POINT('Ctrl Pts',(1.66544143815951,-29.8450620205992,
123.34118009468));
#118684=CARTESIAN_POINT('Ctrl Pts',(1.66137119312437,-29.9037525662682,
123.336108195918));
#118685=CARTESIAN_POINT('Ctrl Pts',(1.65800790581231,-29.9510904001124,
123.334044873267));
#118686=CARTESIAN_POINT('Ctrl Pts',(1.64734994428443,-30.0992582882437,
123.333906739861));
#118687=CARTESIAN_POINT('Ctrl Pts',(1.63993754762206,-30.1998709535915,
123.342962959158));
#118688=CARTESIAN_POINT('Ctrl Pts',(1.62718882987642,-30.3743591862255,
123.374801130531));
#118689=CARTESIAN_POINT('Ctrl Pts',(1.621793337005,-30.4486393844416,123.393717996614));
#118690=CARTESIAN_POINT('Ctrl Pts',(1.6152699581377,-30.5392789919135,123.423583198221));
#118691=CARTESIAN_POINT('Ctrl Pts',(1.61399054570287,-30.5570923822157,
123.42978985722));
#118692=CARTESIAN_POINT('Ctrl Pts',(1.61193589368605,-30.5857478222201,
123.440323235905));
#118693=CARTESIAN_POINT('Ctrl Pts',(1.61115456716329,-30.5966561094524,
123.444463559178));
#118694=CARTESIAN_POINT('Ctrl Pts',(1.60965832785233,-30.6175628961522,
123.452651173079));
#118695=CARTESIAN_POINT('Ctrl Pts',(1.60894289641922,-30.6275673117454,
123.45668162668));
#118696=CARTESIAN_POINT('Ctrl Pts',(1.60728520335356,-30.6507607309003,
123.466288328642));
#118697=CARTESIAN_POINT('Ctrl Pts',(1.60634547388183,-30.6639185159585,
123.471938075514));
#118698=CARTESIAN_POINT('Ctrl Pts',(1.60328416879503,-30.7067917353428,
123.491005504918));
#118699=CARTESIAN_POINT('Ctrl Pts',(1.60118649386411,-30.7361874085937,
123.505126337104));
#118700=CARTESIAN_POINT('Ctrl Pts',(1.59616232716592,-30.8063831766521,
123.541419630566));
#118701=CARTESIAN_POINT('Ctrl Pts',(1.59326379285336,-30.8467079619909,
123.564452503418));
#118702=CARTESIAN_POINT('Ctrl Pts',(1.58617264115953,-30.9438936146995,
123.625485157041));
#118703=CARTESIAN_POINT('Ctrl Pts',(1.58202372174999,-30.9994758592016,
123.66535606554));
#118704=CARTESIAN_POINT('Ctrl Pts',(1.57720953188181,-31.060458843643,123.715052646713));
#118705=CARTESIAN_POINT('Ctrl Pts',(1.57657680197812,-31.0684038611822,
123.721651124768));
#118706=CARTESIAN_POINT('Ctrl Pts',(1.57130492344091,-31.1339656892536,
123.777139540133));
#118707=CARTESIAN_POINT('Ctrl Pts',(1.56661391594483,-31.1882492572264,
123.829817680767));
#118708=CARTESIAN_POINT('Ctrl Pts',(1.56087690935004,-31.2469782870881,
123.895123506874));
#118709=CARTESIAN_POINT('Ctrl Pts',(1.56006816542347,-31.2550911584685,
123.9043481047));
#118710=CARTESIAN_POINT('Ctrl Pts',(1.55879056472725,-31.2676334544057,
123.918931204264));
#118711=CARTESIAN_POINT('Ctrl Pts',(1.55832659142073,-31.2721327971966,
123.924229365635));
#118712=CARTESIAN_POINT('Ctrl Pts',(1.55745402692494,-31.2804877712706,
123.934193402581));
#118713=CARTESIAN_POINT('Ctrl Pts',(1.55704601157548,-31.2843512996369,
123.938852333591));
#118714=CARTESIAN_POINT('Ctrl Pts',(1.55608009878621,-31.2933970186093,
123.949882104392));
#118715=CARTESIAN_POINT('Ctrl Pts',(1.5555207189523,-31.2985575829968,123.956270322833));
#118716=CARTESIAN_POINT('Ctrl Pts',(1.55363771165736,-31.3156765433867,
123.977785221583));
#118717=CARTESIAN_POINT('Ctrl Pts',(1.55230056703928,-31.3274190199453,
123.993080695204));
#118718=CARTESIAN_POINT('Ctrl Pts',(1.54897259289164,-31.3556972302696,
124.031269682337));
#118719=CARTESIAN_POINT('Ctrl Pts',(1.54696722421238,-31.3719210836055,
124.054386035962));
#118720=CARTESIAN_POINT('Ctrl Pts',(1.53778875379205,-31.4428221876711,
124.161076157434));
#118721=CARTESIAN_POINT('Ctrl Pts',(1.53044401739243,-31.4905049128045,
124.249050862079));
#118722=CARTESIAN_POINT('Ctrl Pts',(1.51726303442301,-31.5628314648221,
124.416914521819));
#118723=CARTESIAN_POINT('Ctrl Pts',(1.51139766484842,-31.5899143449385,
124.495414052926));
#118724=CARTESIAN_POINT('Ctrl Pts',(1.50437947005127,-31.6160376457289,
124.594582861553));
#118725=CARTESIAN_POINT('Ctrl Pts',(1.50304780839145,-31.620698918698,124.613637734058));
#118726=CARTESIAN_POINT('Ctrl Pts',(1.50093048344589,-31.6276297275352,
124.644307230836));
#118727=CARTESIAN_POINT('Ctrl Pts',(1.5001380347067,-31.6301138226258,124.655870934442));
#118728=CARTESIAN_POINT('Ctrl Pts',(1.4986336177817,-31.6346179270985,124.677982092531));
#118729=CARTESIAN_POINT('Ctrl Pts',(1.49792099676429,-31.6366594993558,
124.688524491013));
#118730=CARTESIAN_POINT('Ctrl Pts',(1.49628852560322,-31.641122634375,124.712828083852));
#118731=CARTESIAN_POINT('Ctrl Pts',(1.49537096111671,-31.6434733171178,
124.726601598204));
#118732=CARTESIAN_POINT('Ctrl Pts',(1.49246288915985,-31.6504133584525,
124.770596330839));
#118733=CARTESIAN_POINT('Ctrl Pts',(1.4904929884044,-31.6543445967275,124.80091599706));
#118734=CARTESIAN_POINT('Ctrl Pts',(1.48584078088412,-31.6617364871279,
124.873551828445));
#118735=CARTESIAN_POINT('Ctrl Pts',(1.48318096006398,-31.6644185921562,
124.915926095558));
#118736=CARTESIAN_POINT('Ctrl Pts',(1.47597758258143,-31.6673225367432,
125.032072502706));
#118737=CARTESIAN_POINT('Ctrl Pts',(1.47150185678151,-31.6642697272068,
125.105828779475));
#118738=CARTESIAN_POINT('Ctrl Pts',(1.46616138228397,-31.65488286836,125.192620150486));
#118739=CARTESIAN_POINT('Ctrl Pts',(1.46533081335207,-31.6532604815924,
125.206081549259));
#118740=CARTESIAN_POINT('Ctrl Pts',(1.45995991371941,-31.641737361191,125.292770689231));
#118741=CARTESIAN_POINT('Ctrl Pts',(1.4553672672533,-31.6271393720648,125.3652819901));
#118742=CARTESIAN_POINT('Ctrl Pts',(1.44973966190952,-31.6045629908535,
125.448424314081));
#118743=CARTESIAN_POINT('Ctrl Pts',(1.44893132812255,-31.6012146814024,
125.460237199035));
#118744=CARTESIAN_POINT('Ctrl Pts',(1.44765423888298,-31.5957673048699,
125.478676304118));
#118745=CARTESIAN_POINT('Ctrl Pts',(1.44719036069773,-31.5937567357226,
125.485328505634));
#118746=CARTESIAN_POINT('Ctrl Pts',(1.44631786977977,-31.5899172011883,
125.497750873927));
#118747=CARTESIAN_POINT('Ctrl Pts',(1.44590983168935,-31.58809833254,125.503523902745));
#118748=CARTESIAN_POINT('Ctrl Pts',(1.44494372540347,-31.5837368542093,
125.517108363582));
#118749=CARTESIAN_POINT('Ctrl Pts',(1.44438417298862,-31.5811678829483,
125.524911041919));
#118750=CARTESIAN_POINT('Ctrl Pts',(1.44249997093948,-31.572371154149,125.550978531556));
#118751=CARTESIAN_POINT('Ctrl Pts',(1.44116178172606,-31.5658840312772,
125.56915332724));
#118752=CARTESIAN_POINT('Ctrl Pts',(1.43783062883177,-31.5491195024646,
125.61366428117));
#118753=CARTESIAN_POINT('Ctrl Pts',(1.43582309281918,-31.5384848063226,
125.639858893239));
#118754=CARTESIAN_POINT('Ctrl Pts',(1.42662547824706,-31.4871879703489,
125.757527368973));
#118755=CARTESIAN_POINT('Ctrl Pts',(1.41926324016873,-31.4389985613409,
125.845493561222));
#118756=CARTESIAN_POINT('Ctrl Pts',(1.40608610372879,-31.3371370522766,
125.997221735599));
#118757=CARTESIAN_POINT('Ctrl Pts',(1.40024031433766,-31.286022652747,126.062325811389));
#118758=CARTESIAN_POINT('Ctrl Pts',(1.39324099829267,-31.2170577152728,
126.137853656378));
#118759=CARTESIAN_POINT('Ctrl Pts',(1.39190987258097,-31.203581940568,126.152098517906));
#118760=CARTESIAN_POINT('Ctrl Pts',(1.38979318485049,-31.1815802686629,
126.174548384569));
#118761=CARTESIAN_POINT('Ctrl Pts',(1.38900084479733,-31.1732133457474,
126.182905869809));
#118762=CARTESIAN_POINT('Ctrl Pts',(1.38749650259467,-31.1570801498742,
126.198681291522));
#118763=CARTESIAN_POINT('Ctrl Pts',(1.38678384898385,-31.1493297886649,
126.206114570833));
#118764=CARTESIAN_POINT('Ctrl Pts',(1.38515111750396,-31.1313286923256,
126.223048117867));
#118765=CARTESIAN_POINT('Ctrl Pts',(1.3842333277029,-31.1210291115083,126.23249546026));
#118766=CARTESIAN_POINT('Ctrl Pts',(1.38132376112342,-31.0878132640032,
126.262201966602));
#118767=CARTESIAN_POINT('Ctrl Pts',(1.37935262149001,-31.0644567011252,
126.281960850171));
#118768=CARTESIAN_POINT('Ctrl Pts',(1.37469686096672,-31.007393866691,126.32759861474));
#118769=CARTESIAN_POINT('Ctrl Pts',(1.37203477449641,-30.9732154852828,
126.352853459575));
#118770=CARTESIAN_POINT('Ctrl Pts',(1.36483014601865,-30.8771827560328,
126.41828822623));
#118771=CARTESIAN_POINT('Ctrl Pts',(1.36035528791055,-30.8135686718883,
126.455712012325));
#118772=CARTESIAN_POINT('Ctrl Pts',(1.35500291977246,-30.7353836908596,
126.494977026586));
#118773=CARTESIAN_POINT('Ctrl Pts',(1.35415964654401,-30.7230065298141,
126.501002010302));
#118774=CARTESIAN_POINT('Ctrl Pts',(1.34879149638914,-30.6439561367631,
126.538277715496));
#118775=CARTESIAN_POINT('Ctrl Pts',(1.34421419432254,-30.5753553621518,
126.56522883206));
#118776=CARTESIAN_POINT('Ctrl Pts',(1.33860362850015,-30.4935078477781,
126.591275193368));
#118777=CARTESIAN_POINT('Ctrl Pts',(1.33779534773215,-30.4817680948006,
126.594868714949));
#118778=CARTESIAN_POINT('Ctrl Pts',(1.33651831903953,-30.4633230019829,
126.600292501335));
#118779=CARTESIAN_POINT('Ctrl Pts',(1.33605444740146,-30.4566438269569,
126.602211192361));
#118780=CARTESIAN_POINT('Ctrl Pts',(1.33518194067076,-30.4441245916519,
126.605722887128));
#118781=CARTESIAN_POINT('Ctrl Pts',(1.33477387992873,-30.4382876014881,
126.607325921168));
#118782=CARTESIAN_POINT('Ctrl Pts',(1.33380768559873,-30.4245079269523,
126.611029645546));
#118783=CARTESIAN_POINT('Ctrl Pts',(1.33324806727611,-30.4165582965145,
126.613103430473));
#118784=CARTESIAN_POINT('Ctrl Pts',(1.33136350594978,-30.3898817256404,
126.619852089884));
#118785=CARTESIAN_POINT('Ctrl Pts',(1.3300250179637,-30.3710897109862,126.62426010852));
#118786=CARTESIAN_POINT('Ctrl Pts',(1.32669297214444,-30.3245891781903,
126.634318640945));
#118787=CARTESIAN_POINT('Ctrl Pts',(1.32468483402052,-30.2968057496918,
126.63959193741));
#118788=CARTESIAN_POINT('Ctrl Pts',(1.31548177323326,-30.170050631906,126.660322863488));
#118789=CARTESIAN_POINT('Ctrl Pts',(1.30811456342572,-30.0699421225484,
126.667542438152));
#118790=CARTESIAN_POINT('Ctrl Pts',(1.29493956998774,-29.8872451506476,
126.664229037536));
#118791=CARTESIAN_POINT('Ctrl Pts',(1.28910034246893,-29.8049155354336,
126.656598228925));
#118792=CARTESIAN_POINT('Ctrl Pts',(1.28210734922354,-29.7041476141675,
126.639637670252));
#118793=CARTESIAN_POINT('Ctrl Pts',(1.28077640473921,-29.6848736145989,
126.636042707907));
#118794=CARTESIAN_POINT('Ctrl Pts',(1.27865991865501,-29.6540823485395,
126.62973519622));
#118795=CARTESIAN_POINT('Ctrl Pts',(1.27786760187127,-29.6425232182577,
126.627238825245));
#118796=CARTESIAN_POINT('Ctrl Pts',(1.27636324985426,-29.6205192690064,
126.622240949328));
#118797=CARTESIAN_POINT('Ctrl Pts',(1.27565056370567,-29.6100701938365,
126.61976111768));
#118798=CARTESIAN_POINT('Ctrl Pts',(1.27401768056143,-29.5860780685762,
126.613821549831));
#118799=CARTESIAN_POINT('Ctrl Pts',(1.27309977271339,-29.5725529990944,
126.610292035984));
#118800=CARTESIAN_POINT('Ctrl Pts',(1.27018950330272,-29.5295695274094,
126.598495301101));
#118801=CARTESIAN_POINT('Ctrl Pts',(1.26821779246539,-29.5002927490674,
126.589586395517));
#118802=CARTESIAN_POINT('Ctrl Pts',(1.26356042384791,-29.4309771687159,
126.566389138686));
#118803=CARTESIAN_POINT('Ctrl Pts',(1.26089732183558,-29.3912068677028,
126.551364953231));
#118804=CARTESIAN_POINT('Ctrl Pts',(1.25369207673303,-29.2841383915049,
126.506164823711));
#118805=CARTESIAN_POINT('Ctrl Pts',(1.24921755584633,-29.2182006897815,
126.473017489033));
#118806=CARTESIAN_POINT('Ctrl Pts',(1.24385974689897,-29.1427325433927,
126.428579917327));
#118807=CARTESIAN_POINT('Ctrl Pts',(1.24301071820361,-29.1308783650678,
126.421399187487));
#118808=CARTESIAN_POINT('Ctrl Pts',(1.23764363505311,-29.0567142633553,
126.37519924064));
#118809=CARTESIAN_POINT('Ctrl Pts',(1.23307310874791,-28.9969623534156,
126.332243850096));
#118810=CARTESIAN_POINT('Ctrl Pts',(1.22747006464366,-28.9307767818416,
126.27768088221));
#118811=CARTESIAN_POINT('Ctrl Pts',(1.22666180965119,-28.921390696961,126.269767174192));
#118812=CARTESIAN_POINT('Ctrl Pts',(1.225384812915,-28.9068301951148,126.257212818276));
#118813=CARTESIAN_POINT('Ctrl Pts',(1.22492094706501,-28.9015956841964,
126.25264210667));
#118814=CARTESIAN_POINT('Ctrl Pts',(1.2240484838881,-28.891855752849,126.244029325954));
#118815=CARTESIAN_POINT('Ctrl Pts',(1.22364046120809,-28.8873435676677,
126.239995280331));
#118816=CARTESIAN_POINT('Ctrl Pts',(1.2226743783183,-28.8767594002408,126.230428395339));
#118817=CARTESIAN_POINT('Ctrl Pts',(1.22211483383591,-28.8707062487426,
126.224875135393));
#118818=CARTESIAN_POINT('Ctrl Pts',(1.22023053591187,-28.8505705235727,
126.206126164516));
#118819=CARTESIAN_POINT('Ctrl Pts',(1.21889223925896,-28.8366767947949,
126.192731104189));
#118820=CARTESIAN_POINT('Ctrl Pts',(1.21556072260696,-28.8030106663786,
126.159125452884));
#118821=CARTESIAN_POINT('Ctrl Pts',(1.21355292466535,-28.7835144406899,
126.138647436167));
#118822=CARTESIAN_POINT('Ctrl Pts',(1.20435287453867,-28.6973758016848,
126.043432737066));
#118823=CARTESIAN_POINT('Ctrl Pts',(1.19698837360285,-28.6370327986885,
125.963276978598));
#118824=CARTESIAN_POINT('Ctrl Pts',(1.1838111571639,-28.5407003015419,125.807976853129));
#118825=CARTESIAN_POINT('Ctrl Pts',(1.17796734596364,-28.5024267616088,
125.734615752706));
#118826=CARTESIAN_POINT('Ctrl Pts',(1.17097000890308,-28.4619995623678,
125.640698850335));
#118827=CARTESIAN_POINT('Ctrl Pts',(1.16963899419521,-28.4545662236487,
125.622555108296));
#118828=CARTESIAN_POINT('Ctrl Pts',(1.1676281026626,-28.4437346288164,125.594726220909));
#118829=CARTESIAN_POINT('Ctrl Pts',(1.16694046674226,-28.4401029340819,
125.585134457932));
#118830=CARTESIAN_POINT('Ctrl Pts',(1.16625578224439,-28.4365599837819,
125.575509613897));
#118831=CARTESIAN_POINT('Origin',(5.,-30.,125.));
#118832=CARTESIAN_POINT('',(0.468139978699824,-28.4365599867671,125.575509622007));
#118833=CARTESIAN_POINT('',(0.659203971007262,-28.4365599837785,125.575509613888));
#118834=CARTESIAN_POINT('',(5.,-28.4365599837785,125.575509613888));
#118835=CARTESIAN_POINT('',(0.,-31.2690708798524,126.079358653049));
#118836=CARTESIAN_POINT('Ctrl Pts',(0.468139978699828,-28.4365599867671,
125.575509622007));
#118837=CARTESIAN_POINT('Ctrl Pts',(0.467368748069218,-28.4321976756175,
125.563658887387));
#118838=CARTESIAN_POINT('Ctrl Pts',(0.46659689192531,-28.4279697232914,
125.551757515043));
#118839=CARTESIAN_POINT('Ctrl Pts',(0.461140943886784,-28.3990928442639,
125.467443220244));
#118840=CARTESIAN_POINT('Ctrl Pts',(0.456419851168978,-28.3793245969748,
125.393465849614));
#118841=CARTESIAN_POINT('Ctrl Pts',(0.450407026927721,-28.3615908870582,
125.302386837636));
#118842=CARTESIAN_POINT('Ctrl Pts',(0.449339284521711,-28.3587081421932,
125.286327102347));
#118843=CARTESIAN_POINT('Ctrl Pts',(0.447751303682339,-28.3548178634009,
125.26266053574));
#118844=CARTESIAN_POINT('Ctrl Pts',(0.447240785306152,-28.3536261759322,
125.255084388493));
#118845=CARTESIAN_POINT('Ctrl Pts',(0.446325473091858,-28.3515952030916,
125.241565002395));
#118846=CARTESIAN_POINT('Ctrl Pts',(0.445921813156161,-28.3507356650182,
125.235625073383));
#118847=CARTESIAN_POINT('Ctrl Pts',(0.445021439516117,-28.3488983811264,
125.222425493121));
#118848=CARTESIAN_POINT('Ctrl Pts',(0.444523896583313,-28.3479364122372,
125.215164013547));
#118849=CARTESIAN_POINT('Ctrl Pts',(0.443043358912694,-28.3452299649791,
125.193645158876));
#118850=CARTESIAN_POINT('Ctrl Pts',(0.442053398234113,-28.3436220033341,
125.179371720183));
#118851=CARTESIAN_POINT('Ctrl Pts',(0.434511562346096,-28.3328672750034,
125.071368248408));
#118852=CARTESIAN_POINT('Ctrl Pts',(0.427644809121563,-28.3314993061057,
124.97704308329));
#118853=CARTESIAN_POINT('Ctrl Pts',(0.412301175541919,-28.3462867398635,
124.766787187021));
#118854=CARTESIAN_POINT('Ctrl Pts',(0.403887832506857,-28.3666615733685,
124.651617514269));
#118855=CARTESIAN_POINT('Ctrl Pts',(0.394336778889793,-28.4049792138424,
124.518390809573));
#118856=CARTESIAN_POINT('Ctrl Pts',(0.392836116317528,-28.4114694578954,
124.497397257524));
#118857=CARTESIAN_POINT('Ctrl Pts',(0.390425163645169,-28.4226607832197,
124.463583005454));
#118858=CARTESIAN_POINT('Ctrl Pts',(0.389506752829867,-28.4271073096314,
124.450681512634));
#118859=CARTESIAN_POINT('Ctrl Pts',(0.387873944840566,-28.4353402863902,
124.427713706725));
#118860=CARTESIAN_POINT('Ctrl Pts',(0.387157617190256,-28.4390665929141,
124.417626813142));
#118861=CARTESIAN_POINT('Ctrl Pts',(0.38564067839487,-28.4472004636079,
124.396247971283));
#118862=CARTESIAN_POINT('Ctrl Pts',(0.384840982115183,-28.451634147513,
124.384966576334));
#118863=CARTESIAN_POINT('Ctrl Pts',(0.382679879299442,-28.4640094803565,
124.354460107499));
#118864=CARTESIAN_POINT('Ctrl Pts',(0.381326458947623,-28.472188837654,
124.335333359092));
#118865=CARTESIAN_POINT('Ctrl Pts',(0.372837115258115,-28.5261676930721,
124.215373670924));
#118866=CARTESIAN_POINT('Ctrl Pts',(0.366048427726499,-28.5815683830622,
124.119161806243));
#118867=CARTESIAN_POINT('Ctrl Pts',(0.352975786852313,-28.7061986620622,
123.945360216557));
#118868=CARTESIAN_POINT('Ctrl Pts',(0.346709127500906,-28.773924212927,
123.867339647326));
#118869=CARTESIAN_POINT('Ctrl Pts',(0.3390079119112,-28.8596678157877,123.785322642221));
#118870=CARTESIAN_POINT('Ctrl Pts',(0.337987558499198,-28.8710726403485,
123.774715727569));
#118871=CARTESIAN_POINT('Ctrl Pts',(0.336453321402609,-28.8882529839161,
123.75918084932));
#118872=CARTESIAN_POINT('Ctrl Pts',(0.335947999885583,-28.8939165599583,
123.754129617259));
#118873=CARTESIAN_POINT('Ctrl Pts',(0.335031387501064,-28.9041940363187,
123.745088650751));
#118874=CARTESIAN_POINT('Ctrl Pts',(0.334621091419679,-28.9087956159959,
123.741085311536));
#118875=CARTESIAN_POINT('Ctrl Pts',(0.333691633453243,-28.9192227552468,
123.732113899224));
#118876=CARTESIAN_POINT('Ctrl Pts',(0.333171471614641,-28.9250606613696,
123.727160642531));
#118877=CARTESIAN_POINT('Ctrl Pts',(0.331579571740426,-28.94294051283,123.712200955946));
#118878=CARTESIAN_POINT('Ctrl Pts',(0.330499591107477,-28.9550891848959,
123.702324199624));
#118879=CARTESIAN_POINT('Ctrl Pts',(0.324968622064915,-29.0174852076867,
123.653041099372));
#118880=CARTESIAN_POINT('Ctrl Pts',(0.320382356874171,-29.0698254037879,
123.616378914318));
#118881=CARTESIAN_POINT('Ctrl Pts',(0.307594145872618,-29.2201247827609,
123.523489179777));
#118882=CARTESIAN_POINT('Ctrl Pts',(0.299371107691596,-29.32190694204,123.474062568239));
#118883=CARTESIAN_POINT('Ctrl Pts',(0.288538190039219,-29.4669380836437,
123.421035900165));
#118884=CARTESIAN_POINT('Ctrl Pts',(0.28566477727477,-29.506486954433,123.408231166247));
#118885=CARTESIAN_POINT('Ctrl Pts',(0.281736140891163,-29.5620666088561,
123.392507277488));
#118886=CARTESIAN_POINT('Ctrl Pts',(0.280641395479728,-29.5777207845674,
123.388324224919));
#118887=CARTESIAN_POINT('Ctrl Pts',(0.278876966986034,-29.6032151612703,
123.381908679414));
#118888=CARTESIAN_POINT('Ctrl Pts',(0.278202872197144,-29.6130186742796,
123.37953611852));
#118889=CARTESIAN_POINT('Ctrl Pts',(0.276793528398858,-29.6336454703021,
123.374742067139));
#118890=CARTESIAN_POINT('Ctrl Pts',(0.276058904642824,-29.6444726371476,
123.372339318523));
#118891=CARTESIAN_POINT('Ctrl Pts',(0.274300036745198,-29.6705712816732,
123.366820395673));
#118892=CARTESIAN_POINT('Ctrl Pts',(0.273279172806765,-29.6858642494674,
123.363810017885));
#118893=CARTESIAN_POINT('Ctrl Pts',(0.269644912271854,-29.7407968926573,
123.35379528363));
#118894=CARTESIAN_POINT('Ctrl Pts',(0.26706962256692,-29.7806469542651,
123.348013055479));
#118895=CARTESIAN_POINT('Ctrl Pts',(0.260566485341825,-29.8830994927785,
123.336920507761));
#118896=CARTESIAN_POINT('Ctrl Pts',(0.256695438207355,-29.945864358662,
123.333695911863));
#118897=CARTESIAN_POINT('Ctrl Pts',(0.24718554235897,-30.1012499221996,
123.334504061874));
#118898=CARTESIAN_POINT('Ctrl Pts',(0.241599868013843,-30.1936275022724,
123.342702671986));
#118899=CARTESIAN_POINT('Ctrl Pts',(0.233335296901047,-30.3232338269278,
123.365192840516));
#118900=CARTESIAN_POINT('Ctrl Pts',(0.230847500990398,-30.3613798305607,
123.373199876346));
#118901=CARTESIAN_POINT('Ctrl Pts',(0.227579176300134,-30.409780455689,
123.385145642556));
#118902=CARTESIAN_POINT('Ctrl Pts',(0.226860039358787,-30.4203281403454,
123.387858921663));
#118903=CARTESIAN_POINT('Ctrl Pts',(0.225698073261801,-30.437191994417,
123.392373709684));
#118904=CARTESIAN_POINT('Ctrl Pts',(0.22525889397465,-30.4435256372307,
123.394109550851));
#118905=CARTESIAN_POINT('Ctrl Pts',(0.224417262638342,-30.4555826264015,
123.397490738284));
#118906=CARTESIAN_POINT('Ctrl Pts',(0.224015204558463,-30.4613075824727,
123.399129369328));
#118907=CARTESIAN_POINT('Ctrl Pts',(0.223037323746592,-30.4751457723425,
123.403170614169));
#118908=CARTESIAN_POINT('Ctrl Pts',(0.22245970028393,-30.4832493309913,
123.405604293667));
#118909=CARTESIAN_POINT('Ctrl Pts',(0.220318835722793,-30.5130386605514,
123.41479865206));
#118910=CARTESIAN_POINT('Ctrl Pts',(0.218734838832397,-30.5346028945158,
123.421940561418));
#118911=CARTESIAN_POINT('Ctrl Pts',(0.208556855507809,-30.6705895275747,
123.470085303734));
#118912=CARTESIAN_POINT('Ctrl Pts',(0.19951277548354,-30.7803774165809,
123.523064373845));
#118913=CARTESIAN_POINT('Ctrl Pts',(0.183896431781186,-30.9624118037013,
123.636915427585));
#118914=CARTESIAN_POINT('Ctrl Pts',(0.177260327323807,-31.0371295421189,
123.692864231471));
#118915=CARTESIAN_POINT('Ctrl Pts',(0.169541363277904,-31.1213726954637,
123.767741887473));
#118916=CARTESIAN_POINT('Ctrl Pts',(0.168216069356784,-31.1357293849087,
123.780961197852));
#118917=CARTESIAN_POINT('Ctrl Pts',(0.166128770897804,-31.1581587203012,
123.802353900289));
#118918=CARTESIAN_POINT('Ctrl Pts',(0.165359549936311,-31.1663844159419,
123.810363413593));
#118919=CARTESIAN_POINT('Ctrl Pts',(0.163912054030019,-31.1817835519453,
123.825671114083));
#118920=CARTESIAN_POINT('Ctrl Pts',(0.163233019402845,-31.1889737836234,
123.832951566518));
#118921=CARTESIAN_POINT('Ctrl Pts',(0.161696094026265,-31.2051676171977,
123.849653606238));
#118922=CARTESIAN_POINT('Ctrl Pts',(0.160840137624069,-31.2141287390983,
123.85911559188));
#118923=CARTESIAN_POINT('Ctrl Pts',(0.158206827834837,-31.2415056523198,
123.888710600534));
#118924=CARTESIAN_POINT('Ctrl Pts',(0.156446062762316,-31.2595391593644,
123.909192198364));
#118925=CARTESIAN_POINT('Ctrl Pts',(0.149694644171677,-31.327445614566,
123.990247873303));
#118926=CARTESIAN_POINT('Ctrl Pts',(0.144853617646977,-31.3735205912213,
124.053874076849));
#118927=CARTESIAN_POINT('Ctrl Pts',(0.134500700346386,-31.462944085684,
124.197741698956));
#118928=CARTESIAN_POINT('Ctrl Pts',(0.12902276847542,-31.504538618876,124.278761376881));
#118929=CARTESIAN_POINT('Ctrl Pts',(0.120838387311833,-31.5544245244596,
124.399266115525));
#118930=CARTESIAN_POINT('Ctrl Pts',(0.118317679904426,-31.5682311914639,
124.436291599819));
#118931=CARTESIAN_POINT('Ctrl Pts',(0.115021240922941,-31.5841009440153,
124.483961629491));
#118932=CARTESIAN_POINT('Ctrl Pts',(0.114311247484056,-31.5873953367889,
124.494186368444));
#118933=CARTESIAN_POINT('Ctrl Pts',(0.113166954893524,-31.592503463104,
124.510581897636));
#118934=CARTESIAN_POINT('Ctrl Pts',(0.112736358545873,-31.5943808162653,
124.516732816865));
#118935=CARTESIAN_POINT('Ctrl Pts',(0.111886622773607,-31.5979968891285,
124.528830888064));
#118936=CARTESIAN_POINT('Ctrl Pts',(0.111467684181202,-31.5997381022603,
124.534777052739));
#118937=CARTESIAN_POINT('Ctrl Pts',(0.110439249006086,-31.6039122804174,
124.549332238158));
#118938=CARTESIAN_POINT('Ctrl Pts',(0.10982773797051,-31.6063091129287,
124.557951292892));
#118939=CARTESIAN_POINT('Ctrl Pts',(0.107583414180774,-31.6148008910839,
124.589469142002));
#118940=CARTESIAN_POINT('Ctrl Pts',(0.105929425526354,-31.6204762004279,
124.612476783305));
#118941=CARTESIAN_POINT('Ctrl Pts',(0.0954109898203623,-31.6530612283824,
124.75784331079));
#118942=CARTESIAN_POINT('Ctrl Pts',(0.0861013588996853,-31.66658639838,
124.88278541144));
#118943=CARTESIAN_POINT('Ctrl Pts',(0.069786220291986,-31.6655014734882,
125.107103876206));
#118944=CARTESIAN_POINT('Ctrl Pts',(0.0627319670394635,-31.6561907621357,
125.205923910599));
#118945=CARTESIAN_POINT('Ctrl Pts',(0.0544430292549055,-31.6341886360106,
125.324741380724));
#118946=CARTESIAN_POINT('Ctrl Pts',(0.0529628846407981,-31.6298077898648,
125.34605794817));
#118947=CARTESIAN_POINT('Ctrl Pts',(0.0506097543590494,-31.622117493711,
125.380082929194));
#118948=CARTESIAN_POINT('Ctrl Pts',(0.0497290710686916,-31.61907337331,
125.392848092743));
#118949=CARTESIAN_POINT('Ctrl Pts',(0.0480545747151445,-31.6129687432941,
125.417169885291));
#118950=CARTESIAN_POINT('Ctrl Pts',(0.0472600647941401,-31.6099340626304,
125.42873209057));
#118951=CARTESIAN_POINT('Ctrl Pts',(0.0454316673840891,-31.602631992534,
125.455381710269));
#118952=CARTESIAN_POINT('Ctrl Pts',(0.0444004241194634,-31.5982755012176,
125.470443675996));
#118953=CARTESIAN_POINT('Ctrl Pts',(0.0410488349128261,-31.583344462313,
125.519462274029));
#118954=CARTESIAN_POINT('Ctrl Pts',(0.0387533432384561,-31.571894892015,
125.553143229767));
#118955=CARTESIAN_POINT('Ctrl Pts',(0.0310873261977083,-31.5296613810816,
125.66544563161));
#118956=CARTESIAN_POINT('Ctrl Pts',(0.0258405408557333,-31.493984571933,
125.742086931177));
#118957=CARTESIAN_POINT('Ctrl Pts',(0.0154858401155532,-31.4127069888122,
125.886831798866));
#118958=CARTESIAN_POINT('Ctrl Pts',(0.0103909023578657,-31.3675954258118,
125.954930399638));
#118959=CARTESIAN_POINT('Ctrl Pts',(0.00414849682931046,-31.3088624321337,
126.030845732748));
#118960=CARTESIAN_POINT('Ctrl Pts',(0.00320463889004048,-31.2998944321788,
126.042131579948));
#118961=CARTESIAN_POINT('Ctrl Pts',(0.00184163870806128,-31.2868388690884,
126.058130715643));
#118962=CARTESIAN_POINT('Ctrl Pts',(0.00142863808420865,-31.2828692994149,
126.062939906396));
#118963=CARTESIAN_POINT('Ctrl Pts',(0.000677096287041342,-31.2756232242257,
126.071618915495));
#118964=CARTESIAN_POINT('Ctrl Pts',(0.000339066147284323,-31.2723558546131,
126.075496298494));
#118965=CARTESIAN_POINT('Ctrl Pts',(2.16137329388244E-13,-31.2690708798521,
126.079358653049));
#118966=CARTESIAN_POINT('',(0.,-28.7475103790669,126.098556211331));
#118967=CARTESIAN_POINT('Origin',(0.,-30.,125.));
#118968=CARTESIAN_POINT('Ctrl Pts',(-9.99200722162641E-15,-28.7475103790668,
126.098556211331));
#118969=CARTESIAN_POINT('Ctrl Pts',(0.000120204341514316,-28.7486620881253,
126.099869301756));
#118970=CARTESIAN_POINT('Ctrl Pts',(0.000240539935814629,-28.7498158573408,
126.101180575583));
#118971=CARTESIAN_POINT('Ctrl Pts',(0.0019350791672964,-28.7660745390613,
126.119600292189));
#118972=CARTESIAN_POINT('Ctrl Pts',(0.00353091054824124,-28.7815265364712,
126.136397446123));
#118973=CARTESIAN_POINT('Ctrl Pts',(0.013267754718737,-28.8769048167952,
126.235896674939));
#118974=CARTESIAN_POINT('Ctrl Pts',(0.0217551835120301,-28.9648722034378,
126.31045526773));
#118975=CARTESIAN_POINT('Ctrl Pts',(0.0343325086991831,-29.1085621231512,
126.408680644857));
#118976=CARTESIAN_POINT('Ctrl Pts',(0.0385493452439517,-29.1590496255426,
126.439390945862));
#118977=CARTESIAN_POINT('Ctrl Pts',(0.0445220131853722,-29.2342377070862,
126.479816293358));
#118978=CARTESIAN_POINT('Ctrl Pts',(0.0463454003814986,-29.2577024860493,
126.491724734376));
#118979=CARTESIAN_POINT('Ctrl Pts',(0.0496163886690653,-29.3007239761896,
126.512291596447));
#118980=CARTESIAN_POINT('Ctrl Pts',(0.0510700092075192,-29.3201836705438,
126.521138606934));
#118981=CARTESIAN_POINT('Ctrl Pts',(0.0533392675662641,-29.3510894382467,
126.534477772672));
#118982=CARTESIAN_POINT('Ctrl Pts',(0.0541632985448379,-29.362423610862,
126.539221658455));
#118983=CARTESIAN_POINT('Ctrl Pts',(0.0557040059123447,-29.3838205497343,
126.547900382581));
#118984=CARTESIAN_POINT('Ctrl Pts',(0.0564215939495652,-29.3938710611742,
126.551863533987));
#118985=CARTESIAN_POINT('Ctrl Pts',(0.0580342969124515,-29.416645468968,
126.56058900559));
#118986=CARTESIAN_POINT('Ctrl Pts',(0.0589274892305356,-29.4293905930541,
126.565294054114));
#118987=CARTESIAN_POINT('Ctrl Pts',(0.0612305467946988,-29.4625811686856,
126.577087568334));
#118988=CARTESIAN_POINT('Ctrl Pts',(0.0626326217166769,-29.4831100767161,
126.583934680824));
#118989=CARTESIAN_POINT('Ctrl Pts',(0.0713886819164829,-29.6131755552651,
126.624517896457));
#118990=CARTESIAN_POINT('Ctrl Pts',(0.0783816309159184,-29.7258164134769,
126.647276009909));
#118991=CARTESIAN_POINT('Ctrl Pts',(0.0909557853171158,-29.9299645456178,
126.666984180384));
#118992=CARTESIAN_POINT('Ctrl Pts',(0.0965126677234015,-30.0205655419375,
126.668326739641));
#118993=CARTESIAN_POINT('Ctrl Pts',(0.103345882081162,-30.1253657355237,
126.661340457183));
#118994=CARTESIAN_POINT('Ctrl Pts',(0.104302997915769,-30.1399031154778,
126.66017943787));
#118995=CARTESIAN_POINT('Ctrl Pts',(0.105763601487577,-30.161836951895,
126.658137583951));
#118996=CARTESIAN_POINT('Ctrl Pts',(0.106259850560081,-30.1692462386301,
126.65739770478));
#118997=CARTESIAN_POINT('Ctrl Pts',(0.107167828049092,-30.1827191650552,
126.655961037762));
#118998=CARTESIAN_POINT('Ctrl Pts',(0.107578668309061,-30.1887842664221,
126.655280565308));
#118999=CARTESIAN_POINT('Ctrl Pts',(0.108520533122658,-30.2026171334899,
126.653651575062));
#119000=CARTESIAN_POINT('Ctrl Pts',(0.109052678358275,-30.2103819408131,
126.65268165941));
#119001=CARTESIAN_POINT('Ctrl Pts',(0.110697145176755,-30.2342309139984,
126.649531852205));
#119002=CARTESIAN_POINT('Ctrl Pts',(0.111818497343242,-30.2502897539471,
126.647171649622));
#119003=CARTESIAN_POINT('Ctrl Pts',(0.118574562361602,-30.3459805350638,
126.631676186124));
#119004=CARTESIAN_POINT('Ctrl Pts',(0.124428019876327,-30.424600201384,
126.613004011741));
#119005=CARTESIAN_POINT('Ctrl Pts',(0.135602500289087,-30.5711266866351,
126.566746248814));
#119006=CARTESIAN_POINT('Ctrl Pts',(0.140909348804023,-30.6391903173131,
126.54023260657));
#119007=CARTESIAN_POINT('Ctrl Pts',(0.149160123011709,-30.7439571606213,
126.49127612494));
#119008=CARTESIAN_POINT('Ctrl Pts',(0.152168354429658,-30.7819090177159,
126.471732152215));
#119009=CARTESIAN_POINT('Ctrl Pts',(0.15726155955831,-30.8458096511564,
126.435654857519));
#119010=CARTESIAN_POINT('Ctrl Pts',(0.159368004072816,-30.8721270293933,
126.419821641805));
#119011=CARTESIAN_POINT('Ctrl Pts',(0.162399996212021,-30.9098230967158,
126.39569881646));
#119012=CARTESIAN_POINT('Ctrl Pts',(0.163345975461693,-30.9215570243161,
126.387979079584));
#119013=CARTESIAN_POINT('Ctrl Pts',(0.165009689961135,-30.942139661815,
126.374061685756));
#119014=CARTESIAN_POINT('Ctrl Pts',(0.165729631335259,-30.9510282078058,
126.36792471137));
#119015=CARTESIAN_POINT('Ctrl Pts',(0.167236288040144,-30.9695872863125,
126.354842510094));
#119016=CARTESIAN_POINT('Ctrl Pts',(0.168022262852501,-30.9792443504468,
126.347879166459));
#119017=CARTESIAN_POINT('Ctrl Pts',(0.170103074216175,-31.0047367826617,
126.329078939674));
#119018=CARTESIAN_POINT('Ctrl Pts',(0.171390933410031,-31.0204378084636,
126.317062475006));
#119019=CARTESIAN_POINT('Ctrl Pts',(0.17821391475362,-31.1031151901479,
126.251420738147));
#119020=CARTESIAN_POINT('Ctrl Pts',(0.183550467761074,-31.1660915861063,
126.192958548426));
#119021=CARTESIAN_POINT('Ctrl Pts',(0.19481921028437,-31.2906143135585,
126.058033159491));
#119022=CARTESIAN_POINT('Ctrl Pts',(0.200707971409592,-31.3504777518552,
125.980472867717));
#119023=CARTESIAN_POINT('Ctrl Pts',(0.208599612696059,-31.4182912815847,
125.874523028184));
#119024=CARTESIAN_POINT('Ctrl Pts',(0.210376585110017,-31.4327939970555,
125.850553862308));
#119025=CARTESIAN_POINT('Ctrl Pts',(0.213420572835703,-31.4562002149904,
125.809570915041));
#119026=CARTESIAN_POINT('Ctrl Pts',(0.214671685018553,-31.4654266404986,
125.792747638014));
#119027=CARTESIAN_POINT('Ctrl Pts',(0.216482560034626,-31.4781849013655,
125.768500403063));
#119028=CARTESIAN_POINT('Ctrl Pts',(0.217028522218047,-31.4819558884386,
125.761203133127));
#119029=CARTESIAN_POINT('Ctrl Pts',(0.217982960258905,-31.4884141875288,
125.748475725674));
#119030=CARTESIAN_POINT('Ctrl Pts',(0.218389913920641,-31.4911261009793,
125.743058312257));
#119031=CARTESIAN_POINT('Ctrl Pts',(0.219267007427853,-31.4968804830601,
125.731404786));
#119032=CARTESIAN_POINT('Ctrl Pts',(0.21973766624871,-31.4999135191273,
125.725164513949));
#119033=CARTESIAN_POINT('Ctrl Pts',(0.221049079958931,-31.5082157304375,
125.70780833454));
#119034=CARTESIAN_POINT('Ctrl Pts',(0.221894633332486,-31.51340077538,125.696652997369));
#119035=CARTESIAN_POINT('Ctrl Pts',(0.22829599029076,-31.5514373335683,
125.612390462723));
#119036=CARTESIAN_POINT('Ctrl Pts',(0.234094616544042,-31.579094916581,
125.53706264139));
#119037=CARTESIAN_POINT('Ctrl Pts',(0.240287625540146,-31.6025987786272,
125.455255975213));
#119038=CARTESIAN_POINT('Ctrl Pts',(0.240650432153012,-31.6039537630155,
125.450458848506));
#119039=CARTESIAN_POINT('Ctrl Pts',(0.245965032970622,-31.6234827844638,
125.38011376667));
#119040=CARTESIAN_POINT('Ctrl Pts',(0.25092170439923,-31.6376482144507,
125.313515622568));
#119041=CARTESIAN_POINT('Ctrl Pts',(0.259167209986624,-31.6546523477645,
125.199731189429));
#119042=CARTESIAN_POINT('Ctrl Pts',(0.262495760858726,-31.6596306104476,
125.152950442901));
#119043=CARTESIAN_POINT('Ctrl Pts',(0.268055402483936,-31.6647150429517,
125.073214095539));
#119044=CARTESIAN_POINT('Ctrl Pts',(0.270314240050564,-31.6658356270203,
125.040353522546));
#119045=CARTESIAN_POINT('Ctrl Pts',(0.273513716974237,-31.6660474913257,
124.993160975686));
#119046=CARTESIAN_POINT('Ctrl Pts',(0.274478631268238,-31.6659271842176,
124.978842144537));
#119047=CARTESIAN_POINT('Ctrl Pts',(0.276157107376378,-31.6653936232467,
124.953789509818));
#119048=CARTESIAN_POINT('Ctrl Pts',(0.276873158753556,-31.6650611427352,
124.943055026095));
#119049=CARTESIAN_POINT('Ctrl Pts',(0.278353993333672,-31.6641548314609,
124.920762416001));
#119050=CARTESIAN_POINT('Ctrl Pts',(0.279118213419217,-31.6635643273077,
124.909205516887));
#119051=CARTESIAN_POINT('Ctrl Pts',(0.281101127305262,-31.6617108473527,
124.879090911699));
#119052=CARTESIAN_POINT('Ctrl Pts',(0.282313805138082,-31.6602574010555,
124.860546224265));
#119053=CARTESIAN_POINT('Ctrl Pts',(0.287734266903797,-31.6523143985141,
124.777154774385));
#119054=CARTESIAN_POINT('Ctrl Pts',(0.291832029579267,-31.6423336616721,
124.712694490506));
#119055=CARTESIAN_POINT('Ctrl Pts',(0.304768062870247,-31.5982816110112,
124.508310382987));
#119056=CARTESIAN_POINT('Ctrl Pts',(0.313258034757407,-31.5498706940095,
124.372183610993));
#119057=CARTESIAN_POINT('Ctrl Pts',(0.323943474852953,-31.47421009323,124.223608656929));
#119058=CARTESIAN_POINT('Ctrl Pts',(0.325427401204644,-31.4634152842268,
124.20344837163));
#119059=CARTESIAN_POINT('Ctrl Pts',(0.327511557238231,-31.4479269098858,
124.175900473021));
#119060=CARTESIAN_POINT('Ctrl Pts',(0.328091318448439,-31.4435843987947,
124.168317102551));
#119061=CARTESIAN_POINT('Ctrl Pts',(0.329082906064293,-31.4361044052984,
124.155489800982));
#119062=CARTESIAN_POINT('Ctrl Pts',(0.329492796542649,-31.4329973814433,
124.150228358442));
#119063=CARTESIAN_POINT('Ctrl Pts',(0.330354501210045,-31.4264357188536,
124.139255151278));
#119064=CARTESIAN_POINT('Ctrl Pts',(0.330806622722977,-31.4229757247761,
124.133547094536));
#119065=CARTESIAN_POINT('Ctrl Pts',(0.332032104127468,-31.4135487213855,
124.118203847396));
#119066=CARTESIAN_POINT('Ctrl Pts',(0.332809395876531,-31.4075176660362,
124.108608702864));
#119067=CARTESIAN_POINT('Ctrl Pts',(0.336637513100385,-31.3775421894471,
124.061981769726));
#119068=CARTESIAN_POINT('Ctrl Pts',(0.33976209209934,-31.35223369061,124.025852166006));
#119069=CARTESIAN_POINT('Ctrl Pts',(0.349282392928046,-31.2718963871914,
123.920336734674));
#119070=CARTESIAN_POINT('Ctrl Pts',(0.355779027187453,-31.2127399536266,
123.854288437971));
#119071=CARTESIAN_POINT('Ctrl Pts',(0.366584571824769,-31.1045260057245,
123.751287315702));
#119072=CARTESIAN_POINT('Ctrl Pts',(0.370937290428969,-31.058165900498,
123.711765836677));
#119073=CARTESIAN_POINT('Ctrl Pts',(0.377952695974848,-30.9784753914571,
123.651042190002));
#119074=CARTESIAN_POINT('Ctrl Pts',(0.380666211539674,-30.9463729349424,
123.628329493749));
#119075=CARTESIAN_POINT('Ctrl Pts',(0.384381121927475,-30.9006433589569,
123.598346087419));
#119076=CARTESIAN_POINT('Ctrl Pts',(0.385418476396555,-30.8876758896001,
123.590097984554));
#119077=CARTESIAN_POINT('Ctrl Pts',(0.387185294083296,-30.8652551525701,
123.576269000164));
#119078=CARTESIAN_POINT('Ctrl Pts',(0.387917951829374,-30.8558576529953,
123.570600081619));
#119079=CARTESIAN_POINT('Ctrl Pts',(0.389312059920929,-30.8377874922977,
123.559941596044));
#119080=CARTESIAN_POINT('Ctrl Pts',(0.389974049303338,-30.8291245953965,
123.55493650598));
#119081=CARTESIAN_POINT('Ctrl Pts',(0.391695180620037,-30.8063906234806,
123.542073429595));
#119082=CARTESIAN_POINT('Ctrl Pts',(0.392749823247401,-30.7922494692561,
123.534340922807));
#119083=CARTESIAN_POINT('Ctrl Pts',(0.396492028696302,-30.7413490218364,
123.507460095458));
#119084=CARTESIAN_POINT('Ctrl Pts',(0.399139228099406,-30.7039886155014,
123.48947883064));
#119085=CARTESIAN_POINT('Ctrl Pts',(0.409052066066855,-30.559753083363,
123.426574947428));
#119086=CARTESIAN_POINT('Ctrl Pts',(0.416020550711431,-30.4489695066851,
123.391454981954));
#119087=CARTESIAN_POINT('Ctrl Pts',(0.426138482222719,-30.2878392845479,
123.358334498815));
#119088=CARTESIAN_POINT('Ctrl Pts',(0.42915439222678,-30.2398414308243,
123.350638756414));
#119089=CARTESIAN_POINT('Ctrl Pts',(0.433461001687293,-30.1726439262062,
123.342859862002));
#119090=CARTESIAN_POINT('Ctrl Pts',(0.434686160684013,-30.1536729257287,
123.340993089404));
#119091=CARTESIAN_POINT('Ctrl Pts',(0.436861951107176,-30.1203358867991,
123.33828936478));
#119092=CARTESIAN_POINT('Ctrl Pts',(0.437806129845592,-30.105982960015,
123.337312254507));
#119093=CARTESIAN_POINT('Ctrl Pts',(0.439245955362327,-30.0843024506078,
123.336118152477));
#119094=CARTESIAN_POINT('Ctrl Pts',(0.439734406324747,-30.0769827165876,
123.335763429683));
#119095=CARTESIAN_POINT('Ctrl Pts',(0.440628984963814,-30.0636465873523,
123.335205313235));
#119096=CARTESIAN_POINT('Ctrl Pts',(0.441034248602557,-30.057631117649,
123.334986219872));
#119097=CARTESIAN_POINT('Ctrl Pts',(0.441962986400886,-30.0439048031624,
123.334560758922));
#119098=CARTESIAN_POINT('Ctrl Pts',(0.442487565447425,-30.0361936693959,
123.334375339444));
#119099=CARTESIAN_POINT('Ctrl Pts',(0.444137173083129,-30.0120669123418,
123.333962811249));
#119100=CARTESIAN_POINT('Ctrl Pts',(0.445271670251234,-29.995649607398,
123.333924807098));
#119101=CARTESIAN_POINT('Ctrl Pts',(0.452144291417191,-29.8970892486183,
123.33515334501));
#119102=CARTESIAN_POINT('Ctrl Pts',(0.458110486290468,-29.8151390762679,
123.342251851057));
#119103=CARTESIAN_POINT('Ctrl Pts',(0.470596567811082,-29.6457821167786,
123.369637585095));
#119104=CARTESIAN_POINT('Ctrl Pts',(0.477095767494718,-29.558792907082,
123.390996844334));
#119105=CARTESIAN_POINT('Ctrl Pts',(0.485765742644005,-29.4423471582797,
123.429749246961));
#119106=CARTESIAN_POINT('Ctrl Pts',(0.488091863309416,-29.4110823230837,
123.441205483309));
#119107=CARTESIAN_POINT('Ctrl Pts',(0.492149731540387,-29.3564885356729,
123.463087365615));
#119108=CARTESIAN_POINT('Ctrl Pts',(0.493893030193381,-29.3330174631778,
123.473126766624));
#119109=CARTESIAN_POINT('Ctrl Pts',(0.496500009373458,-29.2979105507213,
123.489107340217));
#119110=CARTESIAN_POINT('Ctrl Pts',(0.49737699208755,-29.2860995412653,
123.494652074773));
#119111=CARTESIAN_POINT('Ctrl Pts',(0.498961880112305,-29.264757979387,
123.504978652865));
#119112=CARTESIAN_POINT('Ctrl Pts',(0.499671333702006,-29.255205977259,
123.509714279069));
#119113=CARTESIAN_POINT('Ctrl Pts',(0.501201638294757,-29.2346093398998,
123.520173032558));
#119114=CARTESIAN_POINT('Ctrl Pts',(0.502021295994636,-29.2235819566312,
123.525928851067));
#119115=CARTESIAN_POINT('Ctrl Pts',(0.504271013462008,-29.1933385476306,
123.542148158332));
#119116=CARTESIAN_POINT('Ctrl Pts',(0.505691989787461,-29.17426216427,123.552867735928));
#119117=CARTESIAN_POINT('Ctrl Pts',(0.515967654530167,-29.0367014191603,
123.633773281269));
#119118=CARTESIAN_POINT('Ctrl Pts',(0.524255789374191,-28.927115819782,
123.718031720228));
#119119=CARTESIAN_POINT('Ctrl Pts',(0.536044031092211,-28.7903072247371,
123.853187260546));
#119120=CARTESIAN_POINT('Ctrl Pts',(0.5394147654645,-28.7533841412355,123.893435887647));
#119121=CARTESIAN_POINT('Ctrl Pts',(0.544796753517581,-28.6992120515421,
123.958645898043));
#119122=CARTESIAN_POINT('Ctrl Pts',(0.546741615648602,-28.6805545984744,
123.982389457186));
#119123=CARTESIAN_POINT('Ctrl Pts',(0.549365902173527,-28.6567628881214,
124.01442180021));
#119124=CARTESIAN_POINT('Ctrl Pts',(0.550008823850018,-28.6510403258825,
124.022268895351));
#119125=CARTESIAN_POINT('Ctrl Pts',(0.551077882752288,-28.6417061783036,
124.03530633295));
#119126=CARTESIAN_POINT('Ctrl Pts',(0.551501372973584,-28.6380548515351,
124.040468141798));
#119127=CARTESIAN_POINT('Ctrl Pts',(0.552305889581432,-28.6312075727591,
124.050265828746));
#119128=CARTESIAN_POINT('Ctrl Pts',(0.552686482466124,-28.6280055616643,
124.054897379275));
#119129=CARTESIAN_POINT('Ctrl Pts',(0.553704843285209,-28.6195350499821,
124.06728331745));
#119130=CARTESIAN_POINT('Ctrl Pts',(0.554345304258772,-28.6143085140447,
124.075065957171));
#119131=CARTESIAN_POINT('Ctrl Pts',(0.556730305460815,-28.5952058099277,
124.104036410153));
#119132=CARTESIAN_POINT('Ctrl Pts',(0.558498628462718,-28.5817483947251,
124.125494604019));
#119133=CARTESIAN_POINT('Ctrl Pts',(0.56752911242005,-28.516294748761,124.235348758641));
#119134=CARTESIAN_POINT('Ctrl Pts',(0.575066613691092,-28.4720523084894,
124.328101890912));
#119135=CARTESIAN_POINT('Ctrl Pts',(0.588498201089292,-28.4080490681001,
124.501919031425));
#119136=CARTESIAN_POINT('Ctrl Pts',(0.594412569370975,-28.3852913269368,
124.581536584095));
#119137=CARTESIAN_POINT('Ctrl Pts',(0.602220893425202,-28.3624842367964,
124.691793209031));
#119138=CARTESIAN_POINT('Ctrl Pts',(0.604269924089063,-28.3572183076328,
124.721220855761));
#119139=CARTESIAN_POINT('Ctrl Pts',(0.607232070429548,-28.3506748515629,
124.764470014339));
#119140=CARTESIAN_POINT('Ctrl Pts',(0.608164564956312,-28.3487737789373,
124.778189706246));
#119141=CARTESIAN_POINT('Ctrl Pts',(0.60980921757349,-28.3457051817319,
124.802567569709));
#119142=CARTESIAN_POINT('Ctrl Pts',(0.61052349496063,-28.3444690548966,
124.813216142772));
#119143=CARTESIAN_POINT('Ctrl Pts',(0.612022773382726,-28.3420795381667,
124.835692521125));
#119144=CARTESIAN_POINT('Ctrl Pts',(0.612806995771749,-28.3409497416052,
124.847522271075));
#119145=CARTESIAN_POINT('Ctrl Pts',(0.614893497658181,-28.3382675101724,
124.879182921056));
#119146=CARTESIAN_POINT('Ctrl Pts',(0.616188612046181,-28.3369434543,124.899031613677));
#119147=CARTESIAN_POINT('Ctrl Pts',(0.623772420962331,-28.3312281813285,
125.016298603042));
#119148=CARTESIAN_POINT('Ctrl Pts',(0.62979586893043,-28.3350410932901,
125.113931273434));
#119149=CARTESIAN_POINT('Ctrl Pts',(0.640240300793025,-28.3566359154911,
125.283326066998));
#119150=CARTESIAN_POINT('Ctrl Pts',(0.644679613834121,-28.3706765037622,
125.355279190346));
#119151=CARTESIAN_POINT('Ctrl Pts',(0.652478488434351,-28.4027650855182,
125.476577295957));
#119152=CARTESIAN_POINT('Ctrl Pts',(0.655779574329153,-28.4184927710903,
125.52642095483));
#119153=CARTESIAN_POINT('Ctrl Pts',(0.659200637484241,-28.4365423944709,
125.575461829013));
#119154=CARTESIAN_POINT('Ctrl Pts',(0.659202304206952,-28.4365511888928,
125.575485721539));
#119155=CARTESIAN_POINT('Ctrl Pts',(0.659203971007256,-28.4365599837785,
125.575509613888));
#119156=CARTESIAN_POINT('Origin',(5.,30.,125.));
#119157=CARTESIAN_POINT('',(9.56913306840647,31.5634400114683,125.575509626801));
#119158=CARTESIAN_POINT('',(9.75970370682547,31.5634400119926,125.575509625376));
#119159=CARTESIAN_POINT('',(5.,31.5634400119422,125.575509625513));
#119160=CARTESIAN_POINT('',(10.,28.6653082844465,125.997072727755));
#119161=CARTESIAN_POINT('Ctrl Pts',(9.75970370682547,31.5634400119926,125.575509625376));
#119162=CARTESIAN_POINT('Ctrl Pts',(9.75994459139466,31.5620930770963,125.579168733439));
#119163=CARTESIAN_POINT('Ctrl Pts',(9.76018575818481,31.5607331464613,125.582823520293));
#119164=CARTESIAN_POINT('Ctrl Pts',(9.76396628152904,31.5392388666679,125.639974101608));
#119165=CARTESIAN_POINT('Ctrl Pts',(9.76756190554505,31.5163796603936,125.692397583835));
#119166=CARTESIAN_POINT('Ctrl Pts',(9.77207483843158,31.4855732267757,125.754167966873));
#119167=CARTESIAN_POINT('Ctrl Pts',(9.77285751500153,31.4801578002206,125.764741787096));
#119168=CARTESIAN_POINT('Ctrl Pts',(9.77410224807535,31.4714416077863,125.7813210223));
#119169=CARTESIAN_POINT('Ctrl Pts',(9.77455979485348,31.4682159539979,125.787365768384));
#119170=CARTESIAN_POINT('Ctrl Pts',(9.77541181945527,31.46217156249,125.798526417119));
#119171=CARTESIAN_POINT('Ctrl Pts',(9.77580564898278,31.4593629969158,125.803647783058));
#119172=CARTESIAN_POINT('Ctrl Pts',(9.77672959500891,31.4527413176242,125.815573109029));
#119173=CARTESIAN_POINT('Ctrl Pts',(9.77726105993558,31.4489073410184,125.822365090935));
#119174=CARTESIAN_POINT('Ctrl Pts',(9.77905616486145,31.4358689016285,125.845088776269));
#119175=CARTESIAN_POINT('Ctrl Pts',(9.78033302229518,31.4264486253917,125.860894178829));
#119176=CARTESIAN_POINT('Ctrl Pts',(9.78350140602102,31.4026736679402,125.899322140857));
#119177=CARTESIAN_POINT('Ctrl Pts',(9.78540715205928,31.3880315890365,125.921760200467));
#119178=CARTESIAN_POINT('Ctrl Pts',(9.79378242249019,31.3219754251849,126.017842332533));
#119179=CARTESIAN_POINT('Ctrl Pts',(9.80041817703831,31.2651954969747,126.087612861256));
#119180=CARTESIAN_POINT('Ctrl Pts',(9.81454442273501,31.1313054550444,126.227382041363));
#119181=CARTESIAN_POINT('Ctrl Pts',(9.82197011540505,31.0526882199104,126.295443454695));
#119182=CARTESIAN_POINT('Ctrl Pts',(9.83042336813809,30.9522599057718,126.36716582979));
#119183=CARTESIAN_POINT('Ctrl Pts',(9.83175674799993,30.936084486356,126.378291416433));
#119184=CARTESIAN_POINT('Ctrl Pts',(9.83385390086391,30.910120300584,126.395481804265));
#119185=CARTESIAN_POINT('Ctrl Pts',(9.83462500408079,30.900459264765,126.401735193274));
#119186=CARTESIAN_POINT('Ctrl Pts',(9.83607437031181,30.8820875978143,126.413358466382));
#119187=CARTESIAN_POINT('Ctrl Pts',(9.8367534115864,30.8733908325676,126.418749148576));
#119188=CARTESIAN_POINT('Ctrl Pts',(9.83828811921684,30.8535355246368,126.430804676216));
#119189=CARTESIAN_POINT('Ctrl Pts',(9.83914187704127,30.8423474554919,126.437419804376));
#119190=CARTESIAN_POINT('Ctrl Pts',(9.84176003815002,30.8076104740441,126.457413737022));
#119191=CARTESIAN_POINT('Ctrl Pts',(9.84350814097426,30.7838111478326,126.470350196461));
#119192=CARTESIAN_POINT('Ctrl Pts',(9.85258879217069,30.6572674520097,126.535188599539));
#119193=CARTESIAN_POINT('Ctrl Pts',(9.85955502127682,30.5496647418267,126.576919847836));
#119194=CARTESIAN_POINT('Ctrl Pts',(9.87177897248656,30.3564027375561,126.629660856546));
#119195=CARTESIAN_POINT('Ctrl Pts',(9.8770017977947,30.2726050549933,126.645752159744));
#119196=CARTESIAN_POINT('Ctrl Pts',(9.88356980597318,30.1719574979488,126.657180104862));
#119197=CARTESIAN_POINT('Ctrl Pts',(9.88462442759328,30.1559333474297,126.658764607608));
#119198=CARTESIAN_POINT('Ctrl Pts',(9.88618948312394,30.1324045698738,126.660747257134));
#119199=CARTESIAN_POINT('Ctrl Pts',(9.8866900713217,30.1249156322456,126.661327331197));
#119200=CARTESIAN_POINT('Ctrl Pts',(9.8875932127674,30.111476506953,126.662276910837));
#119201=CARTESIAN_POINT('Ctrl Pts',(9.8879946960257,30.105527839588,126.662665152759));
#119202=CARTESIAN_POINT('Ctrl Pts',(9.88889106872669,30.0923012641878,126.663457125401));
#119203=CARTESIAN_POINT('Ctrl Pts',(9.88938682424562,30.0850225581548,126.663845032129));
#119204=CARTESIAN_POINT('Ctrl Pts',(9.89084623625951,30.0636955621998,126.664841313866));
#119205=CARTESIAN_POINT('Ctrl Pts',(9.89181657197186,30.0496422441511,126.665319590807));
#119206=CARTESIAN_POINT('Ctrl Pts',(9.89407522113535,30.0171861406494,126.666012999601));
#119207=CARTESIAN_POINT('Ctrl Pts',(9.89536902846809,29.9987827042178,126.666101177692));
#119208=CARTESIAN_POINT('Ctrl Pts',(9.89988294160567,29.9351132153575,126.665351402391));
#119209=CARTESIAN_POINT('Ctrl Pts',(9.90315495945869,29.8898874761054,126.662973319785));
#119210=CARTESIAN_POINT('Ctrl Pts',(9.91521616358714,29.7250558894377,126.647552805197));
#119211=CARTESIAN_POINT('Ctrl Pts',(9.92409883915684,29.6068440151953,126.623409493784));
#119212=CARTESIAN_POINT('Ctrl Pts',(9.93686594271568,29.4360947377721,126.568771596439));
#119213=CARTESIAN_POINT('Ctrl Pts',(9.94098731420158,29.3809188867373,126.54782862083));
#119214=CARTESIAN_POINT('Ctrl Pts',(9.9463461503922,29.3092019759589,126.516156693602));
#119215=CARTESIAN_POINT('Ctrl Pts',(9.94766344887194,29.2915776404115,126.508002268485));
#119216=CARTESIAN_POINT('Ctrl Pts',(9.94982184362611,29.2627265518777,126.494035980163));
#119217=CARTESIAN_POINT('Ctrl Pts',(9.95066847590616,29.2514165912527,126.488401337476));
#119218=CARTESIAN_POINT('Ctrl Pts',(9.95232208590052,29.2293477426935,126.477091406567));
#119219=CARTESIAN_POINT('Ctrl Pts',(9.9531293103512,29.2185847635262,126.471425895264));
#119220=CARTESIAN_POINT('Ctrl Pts',(9.95505641867882,29.1929242938889,126.457557541801));
#119221=CARTESIAN_POINT('Ctrl Pts',(9.95617270637998,29.1780883064762,126.449243382604));
#119222=CARTESIAN_POINT('Ctrl Pts',(9.96020750324361,29.1246142158177,126.418190912052));
#119223=CARTESIAN_POINT('Ctrl Pts',(9.96308428783827,29.0867691561011,126.394121807055));
#119224=CARTESIAN_POINT('Ctrl Pts',(9.9707685764379,28.9872908689865,126.32506318033));
#119225=CARTESIAN_POINT('Ctrl Pts',(9.97550377578497,28.9277020871985,126.277321416801));
#119226=CARTESIAN_POINT('Ctrl Pts',(9.98509064503516,28.8146820719787,126.173269511672));
#119227=CARTESIAN_POINT('Ctrl Pts',(9.98993265788907,28.7614950083516,126.11697951251));
#119228=CARTESIAN_POINT('Ctrl Pts',(9.99589057874712,28.7033764422887,126.04619608118));
#119229=CARTESIAN_POINT('Ctrl Pts',(9.99682341121584,28.6944793874846,126.035072362502));
#119230=CARTESIAN_POINT('Ctrl Pts',(9.99817185487695,28.6819257142596,126.018957518433));
#119231=CARTESIAN_POINT('Ctrl Pts',(9.99858147442229,28.6781523448154,126.014057701144));
#119232=CARTESIAN_POINT('Ctrl Pts',(9.9993273882682,28.6713554335786,126.005129338138));
#119233=CARTESIAN_POINT('Ctrl Pts',(9.99966318296832,28.6683226971404,126.00110785131));
#119234=CARTESIAN_POINT('Ctrl Pts',(10.,28.6653082844465,125.997072727755));
#119235=CARTESIAN_POINT('',(10.,29.2076925604819,123.534460876918));
#119236=CARTESIAN_POINT('Origin',(10.,30.,125.));
#119237=CARTESIAN_POINT('Ctrl Pts',(9.99999999999989,29.2076925604819,123.534460876918));
#119238=CARTESIAN_POINT('Ctrl Pts',(9.99926836029946,29.1983407334261,123.53951671066));
#119239=CARTESIAN_POINT('Ctrl Pts',(9.99853187606714,29.1890377534795,123.544661812123));
#119240=CARTESIAN_POINT('Ctrl Pts',(9.99208084888614,29.1084579028524,123.590239774574));
#119241=CARTESIAN_POINT('Ctrl Pts',(9.98613037893974,29.0402114633257,123.635787921533));
#119242=CARTESIAN_POINT('Ctrl Pts',(9.97478930496467,28.917371786035,123.731566384957));
#119243=CARTESIAN_POINT('Ctrl Pts',(9.9694133315424,28.8622228045054,123.780790397032));
#119244=CARTESIAN_POINT('Ctrl Pts',(9.96107116435099,28.7804042760972,123.86422177828));
#119245=CARTESIAN_POINT('Ctrl Pts',(9.95803791514138,28.7514881025938,123.896086751998));
#119246=CARTESIAN_POINT('Ctrl Pts',(9.95290232109893,28.7039302985686,123.952756878366));
#119247=CARTESIAN_POINT('Ctrl Pts',(9.9507780919654,28.6846890676815,123.977027762911));
#119248=CARTESIAN_POINT('Ctrl Pts',(9.94772273497591,28.6576659677329,124.013138752683));
#119249=CARTESIAN_POINT('Ctrl Pts',(9.94677083906848,28.6493416519085,124.024562752636));
#119250=CARTESIAN_POINT('Ctrl Pts',(9.9450973829791,28.6348801425166,124.044949365195));
#119251=CARTESIAN_POINT('Ctrl Pts',(9.9443735934591,28.6286834205053,124.053868514092));
#119252=CARTESIAN_POINT('Ctrl Pts',(9.942859306635,28.6158443772112,124.07273933266));
#119253=CARTESIAN_POINT('Ctrl Pts',(9.94206954878145,28.6092211293346,124.082703276691));
#119254=CARTESIAN_POINT('Ctrl Pts',(9.93997879188096,28.5918876987556,124.109398875837));
#119255=CARTESIAN_POINT('Ctrl Pts',(9.93868476651747,28.581368262413,124.126252518104));
#119256=CARTESIAN_POINT('Ctrl Pts',(9.93125846200095,28.5222853356233,124.224792961299));
#119257=CARTESIAN_POINT('Ctrl Pts',(9.92537191052699,28.4804782994499,124.310330856594));
#119258=CARTESIAN_POINT('Ctrl Pts',(9.91507039455771,28.4199297270125,124.466865446259));
#119259=CARTESIAN_POINT('Ctrl Pts',(9.91064078618597,28.3981483822722,124.536399846889));
#119260=CARTESIAN_POINT('Ctrl Pts',(9.90298349575962,28.3692031925257,124.655683602719));
#119261=CARTESIAN_POINT('Ctrl Pts',(9.89981746831812,28.3596129071907,124.704735377485));
#119262=CARTESIAN_POINT('Ctrl Pts',(9.89579478947652,28.3505492412692,124.76547988562));
#119263=CARTESIAN_POINT('Ctrl Pts',(9.89503826657815,28.3489741982092,124.776838010076));
#119264=CARTESIAN_POINT('Ctrl Pts',(9.89382393908063,28.3466534158236,124.794945920801));
#119265=CARTESIAN_POINT('Ctrl Pts',(9.89337014896009,28.3458314540211,124.801685804175));
#119266=CARTESIAN_POINT('Ctrl Pts',(9.8924999356591,28.3443418279684,124.814554522555));
#119267=CARTESIAN_POINT('Ctrl Pts',(9.89208390114965,28.3436669549775,124.820682274528));
#119268=CARTESIAN_POINT('Ctrl Pts',(9.89115568319814,28.3422434822918,124.834301449103));
#119269=CARTESIAN_POINT('Ctrl Pts',(9.89064262202549,28.3415116295774,124.841794432531));
#119270=CARTESIAN_POINT('Ctrl Pts',(9.88911188262665,28.3394896764623,124.864054441157));
#119271=CARTESIAN_POINT('Ctrl Pts',(9.88808703414315,28.3383458870185,124.878833577842));
#119272=CARTESIAN_POINT('Ctrl Pts',(9.88134986456065,28.3321736065462,124.975304301392));
#119273=CARTESIAN_POINT('Ctrl Pts',(9.87541090078437,28.3329742887738,125.057249823764));
#119274=CARTESIAN_POINT('Ctrl Pts',(9.86410502872961,28.3459251905703,125.212161974066));
#119275=CARTESIAN_POINT('Ctrl Pts',(9.85875226363202,28.3569155002326,125.285045313465));
#119276=CARTESIAN_POINT('Ctrl Pts',(9.85053346758975,28.3816209954979,125.39767069975));
#119277=CARTESIAN_POINT('Ctrl Pts',(9.8475981786668,28.392074584836,125.438028444428));
#119278=CARTESIAN_POINT('Ctrl Pts',(9.84261362292443,28.4126897425999,125.506865836783));
#119279=CARTESIAN_POINT('Ctrl Pts',(9.84054410428431,28.4221324407004,125.535538045768));
#119280=CARTESIAN_POINT('Ctrl Pts',(9.83755478201414,28.4370715275392,125.577066020499));
#119281=CARTESIAN_POINT('Ctrl Pts',(9.83661534623579,28.4419583863854,125.590132995784));
#119282=CARTESIAN_POINT('Ctrl Pts',(9.83495917503574,28.4509138585718,125.613192034038));
#119283=CARTESIAN_POINT('Ctrl Pts',(9.83424029828365,28.4549164216817,125.623208704637));
#119284=CARTESIAN_POINT('Ctrl Pts',(9.83273196700223,28.4635569859417,125.644237234464));
#119285=CARTESIAN_POINT('Ctrl Pts',(9.83194329023348,28.4682167527892,125.655239533094));
#119286=CARTESIAN_POINT('Ctrl Pts',(9.82984608415284,28.4809846486782,125.684505383807));
#119287=CARTESIAN_POINT('Ctrl Pts',(9.82854473747946,28.4893038181359,125.70267514506));
#119288=CARTESIAN_POINT('Ctrl Pts',(9.82097238886605,28.540002793598,125.808341009415));
#119289=CARTESIAN_POINT('Ctrl Pts',(9.81496336481829,28.589650613333,125.892146335419));
#119290=CARTESIAN_POINT('Ctrl Pts',(9.80467100192769,28.68769523141,126.028808808049));
#119291=CARTESIAN_POINT('Ctrl Pts',(9.80036643622977,28.7326996666267,126.083762224968));
#119292=CARTESIAN_POINT('Ctrl Pts',(9.79365745014556,28.8063903186663,126.162855005261));
#119293=CARTESIAN_POINT('Ctrl Pts',(9.7913262553079,28.8326123663793,126.189176856684));
#119294=CARTESIAN_POINT('Ctrl Pts',(9.78744409000612,28.8767853829111,126.230648101506));
#119295=CARTESIAN_POINT('Ctrl Pts',(9.78592274972215,28.8942163341931,126.246333894596));
#119296=CARTESIAN_POINT('Ctrl Pts',(9.78379141831008,28.9186907759503,126.267440369686));
#119297=CARTESIAN_POINT('Ctrl Pts',(9.78320274610423,28.9254561537052,126.273181150679));
#119298=CARTESIAN_POINT('Ctrl Pts',(9.78219858965437,28.9369985243572,126.28281793624));
#119299=CARTESIAN_POINT('Ctrl Pts',(9.78178509695071,28.941751997332,126.286742071262));
#119300=CARTESIAN_POINT('Ctrl Pts',(9.78092290866195,28.9516618765897,126.294830919954));
#119301=CARTESIAN_POINT('Ctrl Pts',(9.78047394156271,28.9568215101036,126.298991365103));
#119302=CARTESIAN_POINT('Ctrl Pts',(9.77926024722766,28.970771235138,126.310102947866));
#119303=CARTESIAN_POINT('Ctrl Pts',(9.77849167455775,28.9796066820226,126.316996220147));
#119304=CARTESIAN_POINT('Ctrl Pts',(9.77476830526531,29.0224495855222,126.349731642557));
#119305=CARTESIAN_POINT('Ctrl Pts',(9.77174403425812,29.0573701830882,126.374346635588));
#119306=CARTESIAN_POINT('Ctrl Pts',(9.76226003425398,29.1682670325332,126.446300396185));
#119307=CARTESIAN_POINT('Ctrl Pts',(9.75568929087881,29.2471412809544,126.488881541108));
#119308=CARTESIAN_POINT('Ctrl Pts',(9.74478446278907,29.3850799915816,126.549572856507));
#119309=CARTESIAN_POINT('Ctrl Pts',(9.74040536224569,29.4424269877839,126.571119436276));
#119310=CARTESIAN_POINT('Ctrl Pts',(9.73335874784092,29.5384160479382,126.60126446523));
#119311=CARTESIAN_POINT('Ctrl Pts',(9.73063926940642,29.5764063858856,126.611730912066));
#119312=CARTESIAN_POINT('Ctrl Pts',(9.72692272228067,29.6296304519756,126.624381977367));
#119313=CARTESIAN_POINT('Ctrl Pts',(9.72588921945157,29.6445744322476,126.627717144845));
#119314=CARTESIAN_POINT('Ctrl Pts',(9.72413112226573,29.6702350317118,126.633073766658));
#119315=CARTESIAN_POINT('Ctrl Pts',(9.72340331328317,29.6809291764201,126.635196832492));
#119316=CARTESIAN_POINT('Ctrl Pts',(9.72193226891773,29.7026850433936,126.639294376947));
#119317=CARTESIAN_POINT('Ctrl Pts',(9.72118927962108,29.7137474486734,126.641262235324));
#119318=CARTESIAN_POINT('Ctrl Pts',(9.719330252277,29.741606072966,126.645927682956));
#119319=CARTESIAN_POINT('Ctrl Pts',(9.71821885658562,29.7584255282048,126.64848026034));
#119320=CARTESIAN_POINT('Ctrl Pts',(9.71392938616291,29.8239344429659,126.657397924007));
#119321=CARTESIAN_POINT('Ctrl Pts',(9.71081065952237,29.8728592425205,126.661867288073));
#119322=CARTESIAN_POINT('Ctrl Pts',(9.70023348150523,30.0417630132157,126.669792588948));
#119323=CARTESIAN_POINT('Ctrl Pts',(9.69306460946781,30.1618636872509,126.662453276365));
#119324=CARTESIAN_POINT('Ctrl Pts',(9.68314484900705,30.3200833785907,126.635464783275));
#119325=CARTESIAN_POINT('Ctrl Pts',(9.68061253924705,30.3597686874985,126.62719528075));
#119326=CARTESIAN_POINT('Ctrl Pts',(9.67643521808628,30.4232330692483,126.611535637181));
#119327=CARTESIAN_POINT('Ctrl Pts',(9.67482640763888,30.4472182085229,126.605044876782));
#119328=CARTESIAN_POINT('Ctrl Pts',(9.67259556538434,30.4796939535801,126.595472019438));
#119329=CARTESIAN_POINT('Ctrl Pts',(9.67199796926011,30.4883191676482,126.592853299981));
#119330=CARTESIAN_POINT('Ctrl Pts',(9.67098541774517,30.5027994397358,126.588328251699));
#119331=CARTESIAN_POINT('Ctrl Pts',(9.67057259587047,30.508666102462,126.586459172744));
#119332=CARTESIAN_POINT('Ctrl Pts',(9.66971506999163,30.5207731853111,126.582527877569));
#119333=CARTESIAN_POINT('Ctrl Pts',(9.6692701406393,30.5270119031628,126.580461212425));
#119334=CARTESIAN_POINT('Ctrl Pts',(9.66808395754688,30.5435348657518,126.57487903491));
#119335=CARTESIAN_POINT('Ctrl Pts',(9.66733917599276,30.5537970130761,126.571299773282));
#119336=CARTESIAN_POINT('Ctrl Pts',(9.66392967791013,30.600300566692,126.554567996119));
#119337=CARTESIAN_POINT('Ctrl Pts',(9.66120863146903,30.6361110292305,126.540261233719));
#119338=CARTESIAN_POINT('Ctrl Pts',(9.65094279156276,30.7675062283601,126.482403396383));
#119339=CARTESIAN_POINT('Ctrl Pts',(9.64321022821429,30.8594045934907,126.431086964612));
#119340=CARTESIAN_POINT('Ctrl Pts',(9.63170809265067,30.9908026570209,126.340465030825));
#119341=CARTESIAN_POINT('Ctrl Pts',(9.62782140772832,31.0341966287455,126.307277592613));
#119342=CARTESIAN_POINT('Ctrl Pts',(9.62145682970451,31.1037817760943,126.248421669904));
#119343=CARTESIAN_POINT('Ctrl Pts',(9.61893960249259,31.1308955366265,126.22391442491));
#119344=CARTESIAN_POINT('Ctrl Pts',(9.61544391609849,31.167943667768,126.188144480954));
#119345=CARTESIAN_POINT('Ctrl Pts',(9.61443490562762,31.1785639124622,126.177610652233));
#119346=CARTESIAN_POINT('Ctrl Pts',(9.61270142660526,31.1966761367847,126.159155312624));
#119347=CARTESIAN_POINT('Ctrl Pts',(9.61197406417985,31.204234727627,126.151300805881));
#119348=CARTESIAN_POINT('Ctrl Pts',(9.61057995439297,31.2186391182505,126.136035415064));
#119349=CARTESIAN_POINT('Ctrl Pts',(9.60991276077203,31.2254957346616,126.128635448981));
#119350=CARTESIAN_POINT('Ctrl Pts',(9.60815535416587,31.2434538238869,126.108897664633));
#119351=CARTESIAN_POINT('Ctrl Pts',(9.607070031325,31.2544390590741,126.09645525319));
#119352=CARTESIAN_POINT('Ctrl Pts',(9.60307316080922,31.294471345934,126.049723411253));
#119353=CARTESIAN_POINT('Ctrl Pts',(9.60020989792636,31.3223148262538,126.014425624678));
#119354=CARTESIAN_POINT('Ctrl Pts',(9.59031124964165,31.414839344165,125.886836374096));
#119355=CARTESIAN_POINT('Ctrl Pts',(9.5835370976321,31.471556489273,125.789158496023));
#119356=CARTESIAN_POINT('Ctrl Pts',(9.57414193141392,31.5344641741873,125.650058102091));
#119357=CARTESIAN_POINT('Ctrl Pts',(9.57166102470114,31.5496262471594,125.613036352373));
#119358=CARTESIAN_POINT('Ctrl Pts',(9.56913306840647,31.5634400114683,125.575509626801));
#119359=CARTESIAN_POINT('Origin',(5.,30.,125.));
#119360=CARTESIAN_POINT('',(8.86798214956472,31.5634398523358,125.575510059103));
#119361=CARTESIAN_POINT('',(9.06223782796602,31.5634400121624,125.575509624915));
#119362=CARTESIAN_POINT('',(5.,31.5634400119422,125.575509625513));
#119363=CARTESIAN_POINT('Ctrl Pts',(9.06223782796602,31.5634400121624,125.575509624915));
#119364=CARTESIAN_POINT('Ctrl Pts',(9.06389062877664,31.5546571597327,125.59936928306));
#119365=CARTESIAN_POINT('Ctrl Pts',(9.06552593039392,31.5453286920362,125.623026351691));
#119366=CARTESIAN_POINT('Ctrl Pts',(9.06986230611145,31.5189184897683,125.685755228381));
#119367=CARTESIAN_POINT('Ctrl Pts',(9.07253368351343,31.5008723940766,125.72440047704));
#119368=CARTESIAN_POINT('Ctrl Pts',(9.07974294086227,31.4476581580646,125.827808886655));
#119369=CARTESIAN_POINT('Ctrl Pts',(9.08421375479368,31.4096464454391,125.890998851454));
#119370=CARTESIAN_POINT('Ctrl Pts',(9.08959742043858,31.3593897315873,125.963234708243));
#119371=CARTESIAN_POINT('Ctrl Pts',(9.09047580983357,31.351050327314,125.974897200724));
#119372=CARTESIAN_POINT('Ctrl Pts',(9.09583349033581,31.2994172908424,126.04516988738));
#119373=CARTESIAN_POINT('Ctrl Pts',(9.100365493913,31.2524724401225,126.100988420088));
#119374=CARTESIAN_POINT('Ctrl Pts',(9.10592594088404,31.193531694105,126.162406481669));
#119375=CARTESIAN_POINT('Ctrl Pts',(9.10673421359536,31.1849334271892,126.17117013488));
#119376=CARTESIAN_POINT('Ctrl Pts',(9.10801132842461,31.1713169420958,126.184745092782));
#119377=CARTESIAN_POINT('Ctrl Pts',(9.10847529551549,31.1663639269091,126.18962157821));
#119378=CARTESIAN_POINT('Ctrl Pts',(9.10934781214595,31.1570415320287,126.198685747192));
#119379=CARTESIAN_POINT('Ctrl Pts',(9.10975578548555,31.1526796637549,126.202880798536));
#119380=CARTESIAN_POINT('Ctrl Pts',(9.11072171024584,31.1423446034807,126.212712769137));
#119381=CARTESIAN_POINT('Ctrl Pts',(9.11128114532463,31.1363524818378,126.218329382178));
#119382=CARTESIAN_POINT('Ctrl Pts',(9.11316536903013,31.1161414121232,126.236995070868));
#119383=CARTESIAN_POINT('Ctrl Pts',(9.11450371254273,31.1017378789253,126.249840799439));
#119384=CARTESIAN_POINT('Ctrl Pts',(9.11783549987676,31.0656904302382,126.280882240694));
#119385=CARTESIAN_POINT('Ctrl Pts',(9.11984353779017,31.0438005795086,126.298782344046));
#119386=CARTESIAN_POINT('Ctrl Pts',(9.12904499849737,30.9423584789533,126.37751385227));
#119387=CARTESIAN_POINT('Ctrl Pts',(9.13641089983079,30.8578758516824,126.431654074186));
#119388=CARTESIAN_POINT('Ctrl Pts',(9.14959462764769,30.6956922180221,126.516049259841));
#119389=CARTESIAN_POINT('Ctrl Pts',(9.15544338884661,30.6195940658896,126.548709116859));
#119390=CARTESIAN_POINT('Ctrl Pts',(9.16244529028004,30.5228323443837,126.581956611231));
#119391=CARTESIAN_POINT('Ctrl Pts',(9.16377633813259,30.5041790633144,126.587999971436));
#119392=CARTESIAN_POINT('Ctrl Pts',(9.16589274344447,30.4741132579814,126.597157596781));
#119393=CARTESIAN_POINT('Ctrl Pts',(9.16668488409393,30.4627671873311,126.600481900291));
#119394=CARTESIAN_POINT('Ctrl Pts',(9.16818874073528,30.4410537909091,126.606593531448));
#119395=CARTESIAN_POINT('Ctrl Pts',(9.16890110925921,30.4306930819234,126.609401969724));
#119396=CARTESIAN_POINT('Ctrl Pts',(9.17053302582577,30.4067901400571,126.615633891181));
#119397=CARTESIAN_POINT('Ctrl Pts',(9.17145028816966,30.3932304299766,126.618987627196));
#119398=CARTESIAN_POINT('Ctrl Pts',(9.17435743659877,30.3498763959247,126.629133590807));
#119399=CARTESIAN_POINT('Ctrl Pts',(9.17632671654041,30.3199356884272,126.635277068908));
#119400=CARTESIAN_POINT('Ctrl Pts',(9.18097739394434,30.2480599214561,126.647975257419));
#119401=CARTESIAN_POINT('Ctrl Pts',(9.18363630859977,30.2060098563406,126.653758292877));
#119402=CARTESIAN_POINT('Ctrl Pts',(9.19083901894009,30.0903965122107,126.665179428479));
#119403=CARTESIAN_POINT('Ctrl Pts',(9.19531489950267,30.0166084997682,126.667548675528));
#119404=CARTESIAN_POINT('Ctrl Pts',(9.200643094285,29.9295580872039,126.664563701532));
#119405=CARTESIAN_POINT('Ctrl Pts',(9.20146119573136,29.9162161335331,126.663945503343));
#119406=CARTESIAN_POINT('Ctrl Pts',(9.20683260273836,29.8288936515202,126.658846506115));
#119407=CARTESIAN_POINT('Ctrl Pts',(9.21143818011781,29.7552839386996,126.649594001097));
#119408=CARTESIAN_POINT('Ctrl Pts',(9.2170802102421,29.6704924191865,126.633135477842));
#119409=CARTESIAN_POINT('Ctrl Pts',(9.21788848552087,29.6584666233909,126.630662952818));
#119410=CARTESIAN_POINT('Ctrl Pts',(9.21916544511396,29.6396796148329,126.626583382178));
#119411=CARTESIAN_POINT('Ctrl Pts',(9.21962924929007,29.6328989837258,126.625066496676));
#119412=CARTESIAN_POINT('Ctrl Pts',(9.22050176579212,29.6202281863918,126.62214858312));
#119413=CARTESIAN_POINT('Ctrl Pts',(9.22090990482348,29.6143359115425,126.620757804946));
#119414=CARTESIAN_POINT('Ctrl Pts',(9.22187631047224,29.6004640078077,126.617403635501));
#119415=CARTESIAN_POINT('Ctrl Pts',(9.22243606340184,29.5924911772155,126.615413285033));
#119416=CARTESIAN_POINT('Ctrl Pts',(9.224320707475,29.5658428771384,126.608550932538));
#119417=CARTESIAN_POINT('Ctrl Pts',(9.2256591413514,29.5472381731496,126.603413595641));
#119418=CARTESIAN_POINT('Ctrl Pts',(9.22899069894387,29.5016129306525,126.589957704299));
#119419=CARTESIAN_POINT('Ctrl Pts',(9.23099839492724,29.4747073438418,126.581272467764));
#119420=CARTESIAN_POINT('Ctrl Pts',(9.2401935388186,29.3536292096072,126.53875685569));
#119421=CARTESIAN_POINT('Ctrl Pts',(9.2475530962725,29.2624001899776,126.497168934755));
#119422=CARTESIAN_POINT('Ctrl Pts',(9.26073813260729,29.1035208529412,126.406674816822));
#119423=CARTESIAN_POINT('Ctrl Pts',(9.26659387250964,29.034733496332,126.360394502034));
#119424=CARTESIAN_POINT('Ctrl Pts',(9.27360369517304,28.9542436488877,126.297048455659));
#119425=CARTESIAN_POINT('Ctrl Pts',(9.27493592796731,28.9390388711654,126.284641032517));
#119426=CARTESIAN_POINT('Ctrl Pts',(9.27705437023721,28.915020529009,126.264324171669));
#119427=CARTESIAN_POINT('Ctrl Pts',(9.27784736591292,28.9060662974466,126.256584708829));
#119428=CARTESIAN_POINT('Ctrl Pts',(9.27935296367374,28.8891395643087,126.241636256614));
#119429=CARTESIAN_POINT('Ctrl Pts',(9.28006621780825,28.8811529048086,126.234444283122));
#119430=CARTESIAN_POINT('Ctrl Pts',(9.28170036114069,28.8629331627562,126.217715341672));
#119431=CARTESIAN_POINT('Ctrl Pts',(9.2826189591478,28.8527493838038,126.20812569259));
#119432=CARTESIAN_POINT('Ctrl Pts',(9.28553140525843,28.8206633136011,126.17713992245));
#119433=CARTESIAN_POINT('Ctrl Pts',(9.28750458431834,28.7992287819021,126.155267106442));
#119434=CARTESIAN_POINT('Ctrl Pts',(9.29216588929718,28.7494866701461,126.101626776961));
#119435=CARTESIAN_POINT('Ctrl Pts',(9.29483143063456,28.7217688432505,126.069341214927));
#119436=CARTESIAN_POINT('Ctrl Pts',(9.30203588235172,28.6495073996171,125.978341405609));
#119437=CARTESIAN_POINT('Ctrl Pts',(9.30650751469573,28.6075745791044,125.917678581757));
#119438=CARTESIAN_POINT('Ctrl Pts',(9.31185899291285,28.5627164708772,125.842592723949));
#119439=CARTESIAN_POINT('Ctrl Pts',(9.31270451253243,28.5557863750801,125.830658438441));
#119440=CARTESIAN_POINT('Ctrl Pts',(9.31806527959504,28.5129062079765,125.754655645326));
#119441=CARTESIAN_POINT('Ctrl Pts',(9.32263291966874,28.481083144172,125.688361785598));
#119442=CARTESIAN_POINT('Ctrl Pts',(9.32823302040352,28.4491679200935,125.608791268149));
#119443=CARTESIAN_POINT('Ctrl Pts',(9.32904185726714,28.4447206732827,125.597338381785));
#119444=CARTESIAN_POINT('Ctrl Pts',(9.3303199247623,28.437954361659,125.579325314704));
#119445=CARTESIAN_POINT('Ctrl Pts',(9.33078427992747,28.4355489340645,125.572797743037));
#119446=CARTESIAN_POINT('Ctrl Pts',(9.33165839559378,28.4311213138859,125.560546622252));
#119447=CARTESIAN_POINT('Ctrl Pts',(9.33206758777648,28.4290894275987,125.554826834419));
#119448=CARTESIAN_POINT('Ctrl Pts',(9.33303720840305,28.4243698410351,125.541307362684));
#119449=CARTESIAN_POINT('Ctrl Pts',(9.33359913574653,28.4217087642537,125.533498666134));
#119450=CARTESIAN_POINT('Ctrl Pts',(9.33549401670571,28.4129787270715,125.507244085695));
#119451=CARTESIAN_POINT('Ctrl Pts',(9.3368406362249,28.407174548846,125.488712681394));
#119452=CARTESIAN_POINT('Ctrl Pts',(9.34019642174467,28.3936548256269,125.442745196853));
#119453=CARTESIAN_POINT('Ctrl Pts',(9.34222034228052,28.3863170149145,125.415204972576));
#119454=CARTESIAN_POINT('Ctrl Pts',(9.35156970863305,28.3559679050901,125.288299099347));
#119455=CARTESIAN_POINT('Ctrl Pts',(9.35907027026344,28.3414048444474,125.187138151239));
#119456=CARTESIAN_POINT('Ctrl Pts',(9.372164154986,28.3320959320033,125.005518437495));
#119457=CARTESIAN_POINT('Ctrl Pts',(9.37780521709078,28.3337478627129,124.925558053323));
#119458=CARTESIAN_POINT('Ctrl Pts',(9.38460670912955,28.3429358067847,124.826577741219));
#119459=CARTESIAN_POINT('Ctrl Pts',(9.38593173415139,28.3450814992874,124.807174087865));
#119460=CARTESIAN_POINT('Ctrl Pts',(9.38804209578857,28.3490734135898,124.776086729871));
#119461=CARTESIAN_POINT('Ctrl Pts',(9.38883410597609,28.3507038232307,124.76437767509));
#119462=CARTESIAN_POINT('Ctrl Pts',(9.39033996129603,28.3540570438136,124.742039332603));
#119463=CARTESIAN_POINT('Ctrl Pts',(9.39105443692671,28.3557585334912,124.731407501921));
#119464=CARTESIAN_POINT('Ctrl Pts',(9.39269443624668,28.3599191920535,124.706932427447));
#119465=CARTESIAN_POINT('Ctrl Pts',(9.39361762578411,28.362450788668,124.693102200754));
#119466=CARTESIAN_POINT('Ctrl Pts',(9.39655773535488,28.3711199539213,124.648908383196));
#119467=CARTESIAN_POINT('Ctrl Pts',(9.39855343876987,28.3779295651696,124.618682249049));
#119468=CARTESIAN_POINT('Ctrl Pts',(9.40992512657868,28.422011448229,124.445669455774));
#119469=CARTESIAN_POINT('Ctrl Pts',(9.41868983410944,28.4772763776186,124.308160285715));
#119470=CARTESIAN_POINT('Ctrl Pts',(9.43132946666871,28.5777254521937,124.13058726598));
#119471=CARTESIAN_POINT('Ctrl Pts',(9.43488293577421,28.607999607853,124.082897550771));
#119472=CARTESIAN_POINT('Ctrl Pts',(9.43935226483786,28.6475224960859,124.027116313338));
#119473=CARTESIAN_POINT('Ctrl Pts',(9.44013746648668,28.6545172026832,124.017465477207));
#119474=CARTESIAN_POINT('Ctrl Pts',(9.44138595240005,28.6657058712102,124.002371623125));
#119475=CARTESIAN_POINT('Ctrl Pts',(9.44184470937689,28.6698311455922,123.996877866362));
#119476=CARTESIAN_POINT('Ctrl Pts',(9.44271163534225,28.6776499829049,123.986598313697));
#119477=CARTESIAN_POINT('Ctrl Pts',(9.44311927887378,28.6813357573731,123.981806916047));
#119478=CARTESIAN_POINT('Ctrl Pts',(9.44409128401035,28.6901468744469,123.970480811052));
#119479=CARTESIAN_POINT('Ctrl Pts',(9.44465721142636,28.6952950755365,123.963964274905));
#119480=CARTESIAN_POINT('Ctrl Pts',(9.4465989478592,28.7130275268391,123.94186051072));
#119481=CARTESIAN_POINT('Ctrl Pts',(9.44798957243805,28.7258435618516,123.926462572703));
#119482=CARTESIAN_POINT('Ctrl Pts',(9.45148445529768,28.7584098351155,123.88874028656));
#119483=CARTESIAN_POINT('Ctrl Pts',(9.45360522660707,28.778487081513,123.866708214499));
#119484=CARTESIAN_POINT('Ctrl Pts',(9.46388433594104,28.8777206459923,123.763514436302));
#119485=CARTESIAN_POINT('Ctrl Pts',(9.47224652539027,28.964433988561,123.690033288061));
#119486=CARTESIAN_POINT('Ctrl Pts',(9.48533154932152,29.1150441728456,123.586775878831));
#119487=CARTESIAN_POINT('Ctrl Pts',(9.49019753131637,29.1745366771242,123.55122057893));
#119488=CARTESIAN_POINT('Ctrl Pts',(9.49621709775722,29.2527953075334,123.510840821687));
#119489=CARTESIAN_POINT('Ctrl Pts',(9.49749314487559,29.2696590066946,123.502498081818));
#119490=CARTESIAN_POINT('Ctrl Pts',(9.49954099911461,29.2971589197535,123.489468516729));
#119491=CARTESIAN_POINT('Ctrl Pts',(9.50031890924003,29.3077087797483,123.484604400071));
#119492=CARTESIAN_POINT('Ctrl Pts',(9.50180757828612,29.3280935015322,123.475463136368));
#119493=CARTESIAN_POINT('Ctrl Pts',(9.5025188638239,29.3379204390714,123.47116984087));
#119494=CARTESIAN_POINT('Ctrl Pts',(9.50416527830476,29.360865028963,123.461408293511));
#119495=CARTESIAN_POINT('Ctrl Pts',(9.505097912426,29.3740126842085,123.456012353762));
#119496=CARTESIAN_POINT('Ctrl Pts',(9.50812736701992,29.4171926113231,123.438933092395));
#119497=CARTESIAN_POINT('Ctrl Pts',(9.51020077707883,29.4474960896393,123.427952293913));
#119498=CARTESIAN_POINT('Ctrl Pts',(9.51515765977125,29.5215275542217,123.403531641257));
#119499=CARTESIAN_POINT('Ctrl Pts',(9.51801400534572,29.5655277995352,123.390999856712));
#119500=CARTESIAN_POINT('Ctrl Pts',(9.52512364974521,29.6773705502116,123.364069212202));
#119501=CARTESIAN_POINT('Ctrl Pts',(9.52932920236756,29.7456985407943,123.352064834511));
#119502=CARTESIAN_POINT('Ctrl Pts',(9.53431798473983,29.8267489886206,123.342987586275));
#119503=CARTESIAN_POINT('Ctrl Pts',(9.53506828261862,29.8389370440741,123.341758530166));
#119504=CARTESIAN_POINT('Ctrl Pts',(9.54035810917796,29.9247549024237,123.334059628491));
#119505=CARTESIAN_POINT('Ctrl Pts',(9.54495075986615,29.9987212513298,123.332362533013));
#119506=CARTESIAN_POINT('Ctrl Pts',(9.55057783631371,30.0847825397663,123.336113599624));
#119507=CARTESIAN_POINT('Ctrl Pts',(9.55138426242192,30.0970129967992,123.336781887684));
#119508=CARTESIAN_POINT('Ctrl Pts',(9.55265795879871,30.1161462260015,123.338039100329));
#119509=CARTESIAN_POINT('Ctrl Pts',(9.55312034614369,30.1230548693247,123.33853634628));
#119510=CARTESIAN_POINT('Ctrl Pts',(9.55399193859455,30.1360029627462,123.339549478472));
#119511=CARTESIAN_POINT('Ctrl Pts',(9.55440058701291,30.1420429792716,123.340055263741));
#119512=CARTESIAN_POINT('Ctrl Pts',(9.55536870442133,30.1562821750216,123.341325922979));
#119513=CARTESIAN_POINT('Ctrl Pts',(9.55592967245522,30.1644786338746,123.342118646011));
#119514=CARTESIAN_POINT('Ctrl Pts',(9.55781630920489,30.1918749689669,123.344973449155));
#119515=CARTESIAN_POINT('Ctrl Pts',(9.55915549274808,30.2110440265521,123.347308489991));
#119516=CARTESIAN_POINT('Ctrl Pts',(9.56248720925415,30.2581563689506,123.353880341232));
#119517=CARTESIAN_POINT('Ctrl Pts',(9.56449425482874,30.286040219293,123.358495977858));
#119518=CARTESIAN_POINT('Ctrl Pts',(9.57366374245559,30.4117171385766,123.382598650216));
#119519=CARTESIAN_POINT('Ctrl Pts',(9.58099718867245,30.5077582331624,123.410132053281));
#119520=CARTESIAN_POINT('Ctrl Pts',(9.59421664708468,30.6786904021136,123.476216576636));
#119521=CARTESIAN_POINT('Ctrl Pts',(9.60012880930738,30.7542517363511,123.512167781886));
#119522=CARTESIAN_POINT('Ctrl Pts',(9.60719880541295,30.8439217731816,123.563427444288));
#119523=CARTESIAN_POINT('Ctrl Pts',(9.60853753652738,30.8608628458774,123.573514849237));
#119524=CARTESIAN_POINT('Ctrl Pts',(9.61066651903751,30.8877310138302,123.590166285313));
#119525=CARTESIAN_POINT('Ctrl Pts',(9.61146358798281,30.8977733419323,123.596539813483));
#119526=CARTESIAN_POINT('Ctrl Pts',(9.61297714274904,30.9168060247153,123.608907107617));
#119527=CARTESIAN_POINT('Ctrl Pts',(9.61369428162765,30.9258079652071,123.614881830643));
#119528=CARTESIAN_POINT('Ctrl Pts',(9.61533777717813,30.9463962535605,123.628836976373));
#119529=CARTESIAN_POINT('Ctrl Pts',(9.61626182401774,30.9579410150674,123.636877504492));
#119530=CARTESIAN_POINT('Ctrl Pts',(9.61919452745109,30.9944639949957,123.663007696109));
#119531=CARTESIAN_POINT('Ctrl Pts',(9.62118231034945,31.0190432202443,123.68164566045));
#119532=CARTESIAN_POINT('Ctrl Pts',(9.62588356945235,31.0765636881982,123.727832825373));
#119533=CARTESIAN_POINT('Ctrl Pts',(9.62857411733407,31.1089854761103,123.755994254681));
#119534=CARTESIAN_POINT('Ctrl Pts',(9.63575162178631,31.1933637022315,123.835208402818));
#119535=CARTESIAN_POINT('Ctrl Pts',(9.64017532207441,31.2431200588934,123.888465363202));
#119536=CARTESIAN_POINT('Ctrl Pts',(9.64536570077535,31.2968029093329,123.954054948268));
#119537=CARTESIAN_POINT('Ctrl Pts',(9.6460984683413,31.3042728001394,123.963384692323));
#119538=CARTESIAN_POINT('Ctrl Pts',(9.65143273124897,31.3578009760821,124.031734934387));
#119539=CARTESIAN_POINT('Ctrl Pts',(9.65608514848103,31.3999293187771,124.093713176586));
#119540=CARTESIAN_POINT('Ctrl Pts',(9.66178043508395,31.4439816721087,124.168961240757));
#119541=CARTESIAN_POINT('Ctrl Pts',(9.66259330704902,31.4501015409512,124.179686652672));
#119542=CARTESIAN_POINT('Ctrl Pts',(9.66387851619824,31.4595049466089,124.196600738023));
#119543=CARTESIAN_POINT('Ctrl Pts',(9.6643459851462,31.4628697737392,124.202744028575));
#119544=CARTESIAN_POINT('Ctrl Pts',(9.66523019048358,31.4691278949307,124.214342721006));
#119545=CARTESIAN_POINT('Ctrl Pts',(9.665646393804,31.4720297484639,124.219793266977));
#119546=CARTESIAN_POINT('Ctrl Pts',(9.66663674769495,31.4788324228329,124.232743764053));
#119547=CARTESIAN_POINT('Ctrl Pts',(9.66721247383979,31.4827065626442,124.240257472547));
#119548=CARTESIAN_POINT('Ctrl Pts',(9.66917003941979,31.495614202851,124.265765995321));
#119549=CARTESIAN_POINT('Ctrl Pts',(9.67056625661295,31.5043782354683,124.283894242856));
#119550=CARTESIAN_POINT('Ctrl Pts',(9.68032333574324,31.5627377542587,124.410411688846));
#119551=CARTESIAN_POINT('Ctrl Pts',(9.68909446134691,31.600902621213,124.523688025507));
#119552=CARTESIAN_POINT('Ctrl Pts',(9.70382089364437,31.6450752332532,124.723316246679));
#119553=CARTESIAN_POINT('Ctrl Pts',(9.70985267453206,31.6570807667373,124.807870666166));
#119554=CARTESIAN_POINT('Ctrl Pts',(9.71703343871411,31.6638234915555,124.912623351592));
#119555=CARTESIAN_POINT('Ctrl Pts',(9.71836913443617,31.6647395832279,124.932283927229));
#119556=CARTESIAN_POINT('Ctrl Pts',(9.72049712123613,31.6656510753911,124.963878749423));
#119557=CARTESIAN_POINT('Ctrl Pts',(9.72129611195126,31.6658669897983,124.975804243232));
#119558=CARTESIAN_POINT('Ctrl Pts',(9.72281599628191,31.6660349028388,124.998604987353));
#119559=CARTESIAN_POINT('Ctrl Pts',(9.72353751820475,31.6660085215143,125.009479411651));
#119560=CARTESIAN_POINT('Ctrl Pts',(9.72519512144482,31.6657019362699,125.034573127701));
#119561=CARTESIAN_POINT('Ctrl Pts',(9.72612882149797,31.6653461269038,125.048790776343));
#119562=CARTESIAN_POINT('Ctrl Pts',(9.72911018517412,31.6636188199951,125.094433965659));
#119563=CARTESIAN_POINT('Ctrl Pts',(9.73113604645711,31.6615393894272,125.125826914274));
#119564=CARTESIAN_POINT('Ctrl Pts',(9.74228321099633,31.6450241359012,125.300136882798));
#119565=CARTESIAN_POINT('Ctrl Pts',(9.75083238762177,31.6130450549854,125.440751655063));
#119566=CARTESIAN_POINT('Ctrl Pts',(9.75970370682547,31.5634400119926,125.575509625376));
#119567=CARTESIAN_POINT('Ctrl Pts',(9.56913306840647,31.5634400114683,125.575509626801));
#119568=CARTESIAN_POINT('Ctrl Pts',(9.56864716996237,31.5660951549131,125.568296615402));
#119569=CARTESIAN_POINT('Ctrl Pts',(9.5681595259895,31.5687004854742,125.561064948305));
#119570=CARTESIAN_POINT('Ctrl Pts',(9.5659052451564,31.5804661087518,125.527684127776));
#119571=CARTESIAN_POINT('Ctrl Pts',(9.56411601704802,31.5890224936162,125.501329196451));
#119572=CARTESIAN_POINT('Ctrl Pts',(9.56167154232831,31.5996054289806,125.465733241958));
#119573=CARTESIAN_POINT('Ctrl Pts',(9.56104668084311,31.6022167108484,125.456669007324));
#119574=CARTESIAN_POINT('Ctrl Pts',(9.55999897001426,31.6064364641037,125.441539641122));
#119575=CARTESIAN_POINT('Ctrl Pts',(9.55957853599634,31.6080879427172,125.435486548686));
#119576=CARTESIAN_POINT('Ctrl Pts',(9.55877269141859,31.6111728577567,125.423922687406));
#119577=CARTESIAN_POINT('Ctrl Pts',(9.5583876541566,31.6126123061516,125.418413635119));
#119578=CARTESIAN_POINT('Ctrl Pts',(9.55734329597031,31.6164244484165,125.403511902199));
#119579=CARTESIAN_POINT('Ctrl Pts',(9.5566810454587,31.6187434567815,125.39410590263));
#119580=CARTESIAN_POINT('Ctrl Pts',(9.55411836420225,31.6273464125161,125.357854465012));
#119581=CARTESIAN_POINT('Ctrl Pts',(9.55218959334705,31.6330452551839,125.330876333946));
#119582=CARTESIAN_POINT('Ctrl Pts',(9.54311115963848,31.656429207402,125.204779484353));
#119583=CARTESIAN_POINT('Ctrl Pts',(9.53571324710989,31.665774868943,125.104331873209));
#119584=CARTESIAN_POINT('Ctrl Pts',(9.52128883831654,31.6662119385057,124.905333820171));
#119585=CARTESIAN_POINT('Ctrl Pts',(9.51428695032684,31.6577231140409,124.807168482993));
#119586=CARTESIAN_POINT('Ctrl Pts',(9.50620094519701,31.6371828415255,124.690841094219));
#119587=CARTESIAN_POINT('Ctrl Pts',(9.50485842021703,31.6333986035078,124.671433498286));
#119588=CARTESIAN_POINT('Ctrl Pts',(9.5027277995363,31.6267921537136,124.640494726012));
#119589=CARTESIAN_POINT('Ctrl Pts',(9.50193277656213,31.6241907427051,124.628918880407));
#119590=CARTESIAN_POINT('Ctrl Pts',(9.50042587698607,31.6190001941022,124.606922875716));
#119591=CARTESIAN_POINT('Ctrl Pts',(9.49971332206483,31.6164335627545,124.596498078643));
#119592=CARTESIAN_POINT('Ctrl Pts',(9.4980996294026,31.6103658915538,124.572840745214));
#119593=CARTESIAN_POINT('Ctrl Pts',(9.49720055568629,31.6068021622483,124.559624973969));
#119594=CARTESIAN_POINT('Ctrl Pts',(9.49436241208394,31.5949728153653,124.517813663338));
#119595=CARTESIAN_POINT('Ctrl Pts',(9.49244281698285,31.5861033002369,124.489394046141));
#119596=CARTESIAN_POINT('Ctrl Pts',(9.48147243276875,31.5304771818831,124.326629596053));
#119597=CARTESIAN_POINT('Ctrl Pts',(9.47298940546583,31.4674336864022,124.198484501313));
#119598=CARTESIAN_POINT('Ctrl Pts',(9.46154633329198,31.3650306648649,124.043908184054));
#119599=CARTESIAN_POINT('Ctrl Pts',(9.45885385407333,31.3397960104764,124.008856000932));
#119600=CARTESIAN_POINT('Ctrl Pts',(9.45444157308856,31.2972611012484,123.954369511132));
#119601=CARTESIAN_POINT('Ctrl Pts',(9.45276273588887,31.2808170251525,123.934290351413));
#119602=CARTESIAN_POINT('Ctrl Pts',(9.45044776720107,31.2579199363108,123.907627343182));
#119603=CARTESIAN_POINT('Ctrl Pts',(9.44983819582955,31.2518705100522,123.900699857198));
#119604=CARTESIAN_POINT('Ctrl Pts',(9.44880969396276,31.241636939281,123.889174923717));
#119605=CARTESIAN_POINT('Ctrl Pts',(9.4483930094494,31.2374837411765,123.884550033525));
#119606=CARTESIAN_POINT('Ctrl Pts',(9.44753430771095,31.2289126982773,123.875112334785));
#119607=CARTESIAN_POINT('Ctrl Pts',(9.44709211540075,31.2244922885013,123.87030211515));
#119608=CARTESIAN_POINT('Ctrl Pts',(9.44592027908621,31.2127573580111,123.857682143448));
#119609=CARTESIAN_POINT('Ctrl Pts',(9.44518724657377,31.2053958300472,123.849916797485));
#119610=CARTESIAN_POINT('Ctrl Pts',(9.44191820299046,31.1724530575859,123.815830667233));
#119611=CARTESIAN_POINT('Ctrl Pts',(9.43933117439354,31.146082697487,123.790290457129));
#119612=CARTESIAN_POINT('Ctrl Pts',(9.42914505173448,31.040386484491,123.694481182765));
#119613=CARTESIAN_POINT('Ctrl Pts',(9.42134133008691,30.9552712344495,123.630970914103));
#119614=CARTESIAN_POINT('Ctrl Pts',(9.40777101218967,30.7943836572881,123.533276403464));
#119615=CARTESIAN_POINT('Ctrl Pts',(9.40195322697442,30.7209928679223,123.495840284648));
#119616=CARTESIAN_POINT('Ctrl Pts',(9.39498161824195,30.6270662864124,123.456391390294));
#119617=CARTESIAN_POINT('Ctrl Pts',(9.39365183205418,30.6088740105948,123.449125355294));
#119618=CARTESIAN_POINT('Ctrl Pts',(9.39153710031163,30.5795082106172,123.437993003705));
#119619=CARTESIAN_POINT('Ctrl Pts',(9.39074538698554,30.568414804482,123.433922018177));
#119620=CARTESIAN_POINT('Ctrl Pts',(9.38924214380341,30.5471655659103,123.42637964995));
#119621=CARTESIAN_POINT('Ctrl Pts',(9.38852996381217,30.537017715169,123.422887719469));
#119622=CARTESIAN_POINT('Ctrl Pts',(9.38689820988419,30.5135855352467,123.41507697359));
#119623=CARTESIAN_POINT('Ctrl Pts',(9.38598092392063,30.5002790973745,123.410826646936));
#119624=CARTESIAN_POINT('Ctrl Pts',(9.38307265547898,30.4576810215181,123.397808102247));
#119625=CARTESIAN_POINT('Ctrl Pts',(9.38110231162277,30.4281998155988,123.389678323856));
#119626=CARTESIAN_POINT('Ctrl Pts',(9.37644856057148,30.3572809816464,123.372207232335));
#119627=CARTESIAN_POINT('Ctrl Pts',(9.37378768765131,30.3156768487121,123.36362977878));
#119628=CARTESIAN_POINT('Ctrl Pts',(9.36658170407566,30.2010217742872,123.34452781641));
#119629=CARTESIAN_POINT('Ctrl Pts',(9.36210453789624,30.1275289630816,123.33725087972));
#119630=CARTESIAN_POINT('Ctrl Pts',(9.35676858294957,30.0403413269084,123.334434094504));
#119631=CARTESIAN_POINT('Ctrl Pts',(9.35594405497878,30.0268823094354,123.334162509623));
#119632=CARTESIAN_POINT('Ctrl Pts',(9.35057193163556,29.9394012713396,123.333457724416));
#119633=CARTESIAN_POINT('Ctrl Pts',(9.34597196269281,29.8654325288746,123.337795388156));
#119634=CARTESIAN_POINT('Ctrl Pts',(9.34033627599718,29.7798291636796,123.348566844789));
#119635=CARTESIAN_POINT('Ctrl Pts',(9.33952820551658,29.7676684451976,123.350233746805));
#119636=CARTESIAN_POINT('Ctrl Pts',(9.33825164582206,29.7486573516972,123.353054004049));
#119637=CARTESIAN_POINT('Ctrl Pts',(9.33778803591536,29.7417936015258,123.354116136584));
#119638=CARTESIAN_POINT('Ctrl Pts',(9.33691592106518,29.7289624489481,123.356183931711));
#119639=CARTESIAN_POINT('Ctrl Pts',(9.33650798934424,29.7229936242695,123.357179229636));
#119640=CARTESIAN_POINT('Ctrl Pts',(9.33554217333016,29.7089375907119,123.359601842878));
#119641=CARTESIAN_POINT('Ctrl Pts',(9.3349828051974,29.7008553627503,123.361056462556));
#119642=CARTESIAN_POINT('Ctrl Pts',(9.33309999122663,29.6738350243931,123.366126036395));
#119643=CARTESIAN_POINT('Ctrl Pts',(9.33176303308278,29.6549497482706,123.37000982674));
#119644=CARTESIAN_POINT('Ctrl Pts',(9.32843566130366,29.60858602914,123.380386407281));
#119645=CARTESIAN_POINT('Ctrl Pts',(9.32643071597727,29.5811975973753,123.387251583767));
#119646=CARTESIAN_POINT('Ctrl Pts',(9.31725632910224,29.4578264844409,123.42153018603));
#119647=CARTESIAN_POINT('Ctrl Pts',(9.30991537579628,29.3642512390301,123.456839928591));
#119648=CARTESIAN_POINT('Ctrl Pts',(9.29673262182983,29.1996977010349,123.536456780961));
#119649=CARTESIAN_POINT('Ctrl Pts',(9.29086212567876,29.1277926793247,123.578134794794));
#119650=CARTESIAN_POINT('Ctrl Pts',(9.28383873261389,29.0430915215764,123.636083910724));
#119651=CARTESIAN_POINT('Ctrl Pts',(9.28250671013498,29.0270952051103,123.647447874634));
#119652=CARTESIAN_POINT('Ctrl Pts',(9.2803888262205,29.0017812781593,123.666112699913));
#119653=CARTESIAN_POINT('Ctrl Pts',(9.27959617713721,28.9923346463331,123.673234574811));
#119654=CARTESIAN_POINT('Ctrl Pts',(9.27809138274418,28.9744575708709,123.687013296674));
#119655=CARTESIAN_POINT('Ctrl Pts',(9.27737858443528,28.9660141207505,123.693652202597));
#119656=CARTESIAN_POINT('Ctrl Pts',(9.27574570214914,28.9467333340873,123.709116334068));
#119657=CARTESIAN_POINT('Ctrl Pts',(9.274827904384,28.9359415659544,123.717997278809));
#119658=CARTESIAN_POINT('Ctrl Pts',(9.27191899822293,28.9018999718918,123.74673738513));
#119659=CARTESIAN_POINT('Ctrl Pts',(9.26994850263097,28.8790837323931,123.767101884815));
#119660=CARTESIAN_POINT('Ctrl Pts',(9.26529459330476,28.8259535292162,123.817217844472));
#119661=CARTESIAN_POINT('Ctrl Pts',(9.26263367781123,28.7961909334648,123.847523165944));
#119662=CARTESIAN_POINT('Ctrl Pts',(9.25543143681679,28.7180244234719,123.933451286025));
#119663=CARTESIAN_POINT('Ctrl Pts',(9.25095773826373,28.6721028206199,123.9912002253));
#119664=CARTESIAN_POINT('Ctrl Pts',(9.24560576632945,28.6223142210004,124.063128759169));
#119665=CARTESIAN_POINT('Ctrl Pts',(9.244761677796,28.6146135150153,124.074554102582));
#119666=CARTESIAN_POINT('Ctrl Pts',(9.23939450072776,28.5666805691533,124.147610238665));
#119667=CARTESIAN_POINT('Ctrl Pts',(9.23481904443503,28.5304327596079,124.211747324718));
#119668=CARTESIAN_POINT('Ctrl Pts',(9.22921053597087,28.4932265149786,124.28912698951));
#119669=CARTESIAN_POINT('Ctrl Pts',(9.22840215686886,28.488028296534,124.300251246254));
#119670=CARTESIAN_POINT('Ctrl Pts',(9.22712490978736,28.4800807268359,124.317761242526));
#119671=CARTESIAN_POINT('Ctrl Pts',(9.22666091676075,28.4772474609219,124.324108722137));
#119672=CARTESIAN_POINT('Ctrl Pts',(9.2257882096669,28.4720208930417,124.336017691538));
#119673=CARTESIAN_POINT('Ctrl Pts',(9.225380070314,28.4696180789519,124.341574735971));
#119674=CARTESIAN_POINT('Ctrl Pts',(9.22441364065567,28.4640252335839,124.354705452181));
#119675=CARTESIAN_POINT('Ctrl Pts',(9.22385386487468,28.4608608945387,124.362289765275));
#119676=CARTESIAN_POINT('Ctrl Pts',(9.22196831925048,28.4504482161981,124.387775951836));
#119677=CARTESIAN_POINT('Ctrl Pts',(9.22062898692214,28.4434553884755,124.405779663196));
#119678=CARTESIAN_POINT('Ctrl Pts',(9.21729440188898,28.4269913757312,124.450454042056));
#119679=CARTESIAN_POINT('Ctrl Pts',(9.21528454323937,28.417884000301,124.477251805759));
#119680=CARTESIAN_POINT('Ctrl Pts',(9.20606641611484,28.3796040026176,124.600071349076));
#119681=CARTESIAN_POINT('Ctrl Pts',(9.19868545263399,28.358461040177,124.698377004531));
#119682=CARTESIAN_POINT('Ctrl Pts',(9.18551374117176,28.3363079525061,124.879727007108));
#119683=CARTESIAN_POINT('Ctrl Pts',(9.17969014083037,28.3323956444406,124.962102727797));
#119684=CARTESIAN_POINT('Ctrl Pts',(9.17271223990494,28.3351156322315,125.064032096668));
#119685=CARTESIAN_POINT('Ctrl Pts',(9.17138174775636,28.3359840624065,125.083612701075));
#119686=CARTESIAN_POINT('Ctrl Pts',(9.16926580099379,28.3379300513207,125.114975149166));
#119687=CARTESIAN_POINT('Ctrl Pts',(9.16847357751368,28.338787905789,125.126768252138));
#119688=CARTESIAN_POINT('Ctrl Pts',(9.16696929283938,28.3406643759151,125.14925353621));
#119689=CARTESIAN_POINT('Ctrl Pts',(9.16625658187803,28.3416609728578,125.159946902741));
#119690=CARTESIAN_POINT('Ctrl Pts',(9.16462348783413,28.3441927358669,125.184536565057));
#119691=CARTESIAN_POINT('Ctrl Pts',(9.16370539589856,28.3457995704,125.198424792414));
#119692=CARTESIAN_POINT('Ctrl Pts',(9.16079390380021,28.3514817222167,125.242653105299));
#119693=CARTESIAN_POINT('Ctrl Pts',(9.15882117964728,28.3562186042313,125.272902827336));
#119694=CARTESIAN_POINT('Ctrl Pts',(9.15416094092926,28.3695211461486,125.344823418261));
#119695=CARTESIAN_POINT('Ctrl Pts',(9.15149602179119,28.378854309098,125.3863308322));
#119696=CARTESIAN_POINT('Ctrl Pts',(9.14428941665975,28.4086784048964,125.498683441747));
#119697=CARTESIAN_POINT('Ctrl Pts',(9.13981526008009,28.4322986273763,125.568596838621));
#119698=CARTESIAN_POINT('Ctrl Pts',(9.13445110096442,28.4658095445839,125.649623537523));
#119699=CARTESIAN_POINT('Ctrl Pts',(9.13359540701092,28.4713097894908,125.662463076913));
#119700=CARTESIAN_POINT('Ctrl Pts',(9.12822988966241,28.5067117578528,125.742314513883));
#119701=CARTESIAN_POINT('Ctrl Pts',(9.12366752697258,28.5408486961765,125.807350829049));
#119702=CARTESIAN_POINT('Ctrl Pts',(9.11807353132014,28.585565359013,125.880387052816));
#119703=CARTESIAN_POINT('Ctrl Pts',(9.11726530298087,28.5920910319217,125.890785626423));
#119704=CARTESIAN_POINT('Ctrl Pts',(9.11598834546718,28.6024894353629,125.9069556283));
#119705=CARTESIAN_POINT('Ctrl Pts',(9.11552449194505,28.6062845311625,125.91277679502));
#119706=CARTESIAN_POINT('Ctrl Pts',(9.11465203999268,28.6134531483526,125.923623551332));
#119707=CARTESIAN_POINT('Ctrl Pts',(9.11424401607584,28.6168177826448,125.928654718023));
#119708=CARTESIAN_POINT('Ctrl Pts',(9.11327792400074,28.6248134712663,125.940470889433));
#119709=CARTESIAN_POINT('Ctrl Pts',(9.11271837148313,28.629467376369,125.947240097954));
#119710=CARTESIAN_POINT('Ctrl Pts',(9.11083404476517,28.6452219732414,125.96979634695));
#119711=CARTESIAN_POINT('Ctrl Pts',(9.10949572735296,28.656546431822,125.985424216849));
#119712=CARTESIAN_POINT('Ctrl Pts',(9.10616414897365,28.685123652693,126.023452735951));
#119713=CARTESIAN_POINT('Ctrl Pts',(9.10415631001334,28.7026797911337,126.045617237172));
#119714=CARTESIAN_POINT('Ctrl Pts',(9.09495578857043,28.7849413079796,126.144209443588));
#119715=CARTESIAN_POINT('Ctrl Pts',(9.08759085625378,28.8558928834684,126.215155230123));
#119716=CARTESIAN_POINT('Ctrl Pts',(9.07441427394306,28.9962196575627,126.332218071535));
#119717=CARTESIAN_POINT('Ctrl Pts',(9.06857145829816,29.0635082467873,126.380350268506));
#119718=CARTESIAN_POINT('Ctrl Pts',(9.0615750928155,29.1508490586062,126.433486316624));
#119719=CARTESIAN_POINT('Ctrl Pts',(9.06024411658716,29.1677768170299,126.443379704692));
#119720=CARTESIAN_POINT('Ctrl Pts',(9.05812764948606,29.1951882634531,126.458757650479));
#119721=CARTESIAN_POINT('Ctrl Pts',(9.0573353816748,29.2055621402121,126.464433103125));
#119722=CARTESIAN_POINT('Ctrl Pts',(9.05583116792962,29.2254700580637,126.475050732417));
#119723=CARTESIAN_POINT('Ctrl Pts',(9.0551185706702,29.2349931313293,126.480012092604));
#119724=CARTESIAN_POINT('Ctrl Pts',(9.05348595834825,29.2570188450594,126.491217719292));
#119725=CARTESIAN_POINT('Ctrl Pts',(9.05256823130631,29.2695535273992,126.497397493422));
#119726=CARTESIAN_POINT('Ctrl Pts',(9.04965883924049,29.3097644901472,126.516596961196));
#119727=CARTESIAN_POINT('Ctrl Pts',(9.04768781109885,29.3377230897316,126.529013042453));
#119728=CARTESIAN_POINT('Ctrl Pts',(9.04303233715148,29.4052899337179,126.556817331149));
#119729=CARTESIAN_POINT('Ctrl Pts',(9.04037042507345,29.445176324879,126.571474255084));
#119730=CARTESIAN_POINT('Ctrl Pts',(9.03316567721225,29.5557071724755,126.607356756388));
#119731=CARTESIAN_POINT('Ctrl Pts',(9.02869055674728,29.6272682001601,126.625442472419));
#119732=CARTESIAN_POINT('Ctrl Pts',(9.02333973042141,29.7133032336722,126.641203717781));
#119733=CARTESIAN_POINT('Ctrl Pts',(9.02249826232157,29.7268444278566,126.643511699627));
#119734=CARTESIAN_POINT('Ctrl Pts',(9.01712962638129,29.8131852107088,126.657131218315));
#119735=CARTESIAN_POINT('Ctrl Pts',(9.01255003678489,29.8866303794313,126.663769280485));
#119736=CARTESIAN_POINT('Ctrl Pts',(9.00693693979593,29.9725368461396,126.665818868146));
#119737=CARTESIAN_POINT('Ctrl Pts',(9.00612868875217,29.9848128368429,126.665976006613));
#119738=CARTESIAN_POINT('Ctrl Pts',(9.00485172247082,30.0040378855395,126.666009598622));
#119739=CARTESIAN_POINT('Ctrl Pts',(9.00438788383683,30.0109866260611,126.665978264232));
#119740=CARTESIAN_POINT('Ctrl Pts',(9.00351543706875,30.0239874224951,126.665838300056));
#119741=CARTESIAN_POINT('Ctrl Pts',(9.00310740324179,30.0300393444174,126.665740157251));
#119742=CARTESIAN_POINT('Ctrl Pts',(9.00214128867261,30.0443035726448,126.665431079229));
#119743=CARTESIAN_POINT('Ctrl Pts',(9.00158172344623,30.0525150018009,126.665192377392));
#119744=CARTESIAN_POINT('Ctrl Pts',(8.99969746228032,30.0800093452069,126.664189568427));
#119745=CARTESIAN_POINT('Ctrl Pts',(8.9983592260331,30.0992798941254,126.663151177217));
#119746=CARTESIAN_POINT('Ctrl Pts',(8.99502793617251,30.1467247024318,126.659767157506));
#119747=CARTESIAN_POINT('Ctrl Pts',(8.99302030917817,30.1748651079416,126.657038674591));
#119748=CARTESIAN_POINT('Ctrl Pts',(8.98382189110826,30.3022842302785,126.64140245331));
#119749=CARTESIAN_POINT('Ctrl Pts',(8.97645892392758,30.4003456884862,126.620278231699));
#119750=CARTESIAN_POINT('Ctrl Pts',(8.96327728746326,30.5748712970012,126.565860327092));
#119751=CARTESIAN_POINT('Ctrl Pts',(8.95742785122725,30.6518909001427,126.535394913637));
#119752=CARTESIAN_POINT('Ctrl Pts',(8.95042763332085,30.7439528556987,126.490796163709));
#119753=CARTESIAN_POINT('Ctrl Pts',(8.94909894063734,30.7614154818554,126.481953296802));
#119754=CARTESIAN_POINT('Ctrl Pts',(8.94698515473778,30.7891665586458,126.467280413257));
#119755=CARTESIAN_POINT('Ctrl Pts',(8.94619331698695,30.7995553735554,126.461645266639));
#119756=CARTESIAN_POINT('Ctrl Pts',(8.94468933507047,30.8192696930831,126.450678644916));
#119757=CARTESIAN_POINT('Ctrl Pts',(8.94397654563138,30.8286052749591,126.445366620738));
#119758=CARTESIAN_POINT('Ctrl Pts',(8.94234266461335,30.8499817536594,126.432928039181));
#119759=CARTESIAN_POINT('Ctrl Pts',(8.94142387195601,30.8619856604941,126.425739277675));
#119760=CARTESIAN_POINT('Ctrl Pts',(8.93850759319652,30.9000136910563,126.402309626929));
#119761=CARTESIAN_POINT('Ctrl Pts',(8.9365308818662,30.9256813247731,126.385500345896));
#119762=CARTESIAN_POINT('Ctrl Pts',(8.93185912496166,30.9858913214588,126.343649214182));
#119763=CARTESIAN_POINT('Ctrl Pts',(8.92918683350596,31.0199651149679,126.317970582259));
#119764=CARTESIAN_POINT('Ctrl Pts',(8.92200100675805,31.1097940948035,126.244701257382));
#119765=CARTESIAN_POINT('Ctrl Pts',(8.91755340833453,31.1634549148331,126.194695431589));
#119766=CARTESIAN_POINT('Ctrl Pts',(8.91226882714098,31.2226341911993,126.131765713061));
#119767=CARTESIAN_POINT('Ctrl Pts',(8.91146548971117,31.2315054209678,126.122106228499));
#119768=CARTESIAN_POINT('Ctrl Pts',(8.90609018670832,31.2899534827182,126.056936688228));
#119769=CARTESIAN_POINT('Ctrl Pts',(8.90146616531748,31.3358706493544,125.99826947128));
#119770=CARTESIAN_POINT('Ctrl Pts',(8.89580369504892,31.3846120154415,125.926583174079));
#119771=CARTESIAN_POINT('Ctrl Pts',(8.89499521700938,31.3914042262869,125.916352044299));
#119772=CARTESIAN_POINT('Ctrl Pts',(8.89371793380427,31.4018623164603,125.900214614007));
#119773=CARTESIAN_POINT('Ctrl Pts',(8.89325400766306,31.4056055446989,125.894358627129));
#119774=CARTESIAN_POINT('Ctrl Pts',(8.89238146149913,31.4125400830397,125.883359017788));
#119775=CARTESIAN_POINT('Ctrl Pts',(8.89197341652628,31.4157401430931,125.878221203947));
#119776=CARTESIAN_POINT('Ctrl Pts',(8.89100732896184,31.4232168571379,125.86607000561));
#119777=CARTESIAN_POINT('Ctrl Pts',(8.89044780258653,31.4274697158115,125.859042304214));
#119778=CARTESIAN_POINT('Ctrl Pts',(8.88856381186247,31.4415375345811,125.835402790564));
#119779=CARTESIAN_POINT('Ctrl Pts',(8.88722581229469,31.4511154455202,125.818652655633));
#119780=CARTESIAN_POINT('Ctrl Pts',(8.88389524261034,31.474000810046,125.776966143342));
#119781=CARTESIAN_POINT('Ctrl Pts',(8.88188810664293,31.4869684535879,125.751850659163));
#119782=CARTESIAN_POINT('Ctrl Pts',(8.87594098827087,31.5231584883341,125.677156349413));
#119783=CARTESIAN_POINT('Ctrl Pts',(8.87195995633795,31.5445632203393,125.626790620188));
#119784=CARTESIAN_POINT('Ctrl Pts',(8.86798214956472,31.5634398523358,125.575510059103));
#119785=CARTESIAN_POINT('Origin',(5.,30.,125.));
#119786=CARTESIAN_POINT('',(8.1662633962835,31.5634400119422,125.575509625513));
#119787=CARTESIAN_POINT('',(8.36102759409884,31.5634400156515,125.575509615436));
#119788=CARTESIAN_POINT('',(5.,31.5634400119422,125.575509625513));
#119789=CARTESIAN_POINT('Ctrl Pts',(8.36102759409884,31.5634400156515,125.575509615436));
#119790=CARTESIAN_POINT('Ctrl Pts',(8.36145852083983,31.5613892619103,125.581080730801));
#119791=CARTESIAN_POINT('Ctrl Pts',(8.36188920460623,31.5593085163546,125.586641465852));
#119792=CARTESIAN_POINT('Ctrl Pts',(8.36819296046608,31.5283939536364,125.667932879917));
#119793=CARTESIAN_POINT('Ctrl Pts',(8.37398572743088,31.4940993543677,125.741480043892));
#119794=CARTESIAN_POINT('Ctrl Pts',(8.38168335485436,31.4399870101799,125.838385140646));
#119795=CARTESIAN_POINT('Ctrl Pts',(8.38373581782508,31.4246887189983,125.864126430352));
#119796=CARTESIAN_POINT('Ctrl Pts',(8.38670231113614,31.4013023989325,125.901165799042));
#119797=CARTESIAN_POINT('Ctrl Pts',(8.38763577663898,31.3937544634111,125.912796103473));
#119798=CARTESIAN_POINT('Ctrl Pts',(8.38928192900608,31.380110235804,125.933256028303));
#119799=CARTESIAN_POINT('Ctrl Pts',(8.38999673985287,31.3740722687193,125.942123392621));
#119800=CARTESIAN_POINT('Ctrl Pts',(8.39149694279808,31.3611630417819,125.960693767205));
#119801=CARTESIAN_POINT('Ctrl Pts',(8.39228155759251,31.3542726932988,125.97038282403));
#119802=CARTESIAN_POINT('Ctrl Pts',(8.3943686850467,31.335576939568,125.996085335921));
#119803=CARTESIAN_POINT('Ctrl Pts',(8.39566403801901,31.3235872118942,126.011962798405));
#119804=CARTESIAN_POINT('Ctrl Pts',(8.40340712935528,31.2496501976135,126.106311431212));
#119805=CARTESIAN_POINT('Ctrl Pts',(8.40957462958438,31.1810242007115,126.179294727921));
#119806=CARTESIAN_POINT('Ctrl Pts',(8.42058854287345,31.0463335164611,126.298909348018));
#119807=CARTESIAN_POINT('Ctrl Pts',(8.42544480537767,30.9826488016226,126.347731155626));
#119808=CARTESIAN_POINT('Ctrl Pts',(8.43230673082812,30.8910591565401,126.407991387263));
#119809=CARTESIAN_POINT('Ctrl Pts',(8.43417388398498,30.8659911190021,126.423546749655));
#119810=CARTESIAN_POINT('Ctrl Pts',(8.43735540530436,30.8233400039988,126.448469328534));
#119811=CARTESIAN_POINT('Ctrl Pts',(8.43865182793557,30.8059774392345,126.45820178318));
#119812=CARTESIAN_POINT('Ctrl Pts',(8.4405157462498,30.7811196577645,126.471556060855));
#119813=CARTESIAN_POINT('Ctrl Pts',(8.44106821786963,30.7737644955833,126.475436768593));
#119814=CARTESIAN_POINT('Ctrl Pts',(8.44202971216977,30.7609930904826,126.482053418287));
#119815=CARTESIAN_POINT('Ctrl Pts',(8.44243713322745,30.7555904441105,126.484815105642));
#119816=CARTESIAN_POINT('Ctrl Pts',(8.44331177719675,30.744013762075,126.490653246359));
#119817=CARTESIAN_POINT('Ctrl Pts',(8.44377948213751,30.7378357644251,126.493720843886));
#119818=CARTESIAN_POINT('Ctrl Pts',(8.4450698551519,30.7208203346055,126.502038300619));
#119819=CARTESIAN_POINT('Ctrl Pts',(8.44589704809475,30.709944998219,126.507209039875));
#119820=CARTESIAN_POINT('Ctrl Pts',(8.45102186771389,30.6427096283131,126.538287353876));
#119821=CARTESIAN_POINT('Ctrl Pts',(8.45546530719541,30.5850004856562,126.56114586761));
#119822=CARTESIAN_POINT('Ctrl Pts',(8.46974306413475,30.3979455265239,126.623408521195));
#119823=CARTESIAN_POINT('Ctrl Pts',(8.47965823365812,30.2649911581475,126.65033525785));
#119824=CARTESIAN_POINT('Ctrl Pts',(8.49150673398063,30.0956673731849,126.663612348605));
#119825=CARTESIAN_POINT('Ctrl Pts',(8.49389462102906,30.0610211654159,126.66524323082));
#119826=CARTESIAN_POINT('Ctrl Pts',(8.49717171162583,30.0127639432865,126.666006490561));
#119827=CARTESIAN_POINT('Ctrl Pts',(8.49808893532242,29.9991784572749,126.666055187832));
#119828=CARTESIAN_POINT('Ctrl Pts',(8.49967286541058,29.9755860187698,126.665851168457));
#119829=CARTESIAN_POINT('Ctrl Pts',(8.50034190495544,29.9655792989757,126.665674452232));
#119830=CARTESIAN_POINT('Ctrl Pts',(8.50173627610054,29.9446403430466,126.665115897215));
#119831=CARTESIAN_POINT('Ctrl Pts',(8.50246102719351,29.9337090211443,126.664716540014));
#119832=CARTESIAN_POINT('Ctrl Pts',(8.50418758983578,29.9075588630099,126.663503196599));
#119833=CARTESIAN_POINT('Ctrl Pts',(8.5051861990846,29.8923455365339,126.662587979855));
#119834=CARTESIAN_POINT('Ctrl Pts',(8.5086872119435,29.8387266175708,126.658623240173));
#119835=CARTESIAN_POINT('Ctrl Pts',(8.51115477896851,29.8004147811303,126.654450439348));
#119836=CARTESIAN_POINT('Ctrl Pts',(8.51732449331676,29.7037939551105,126.640521149728));
#119837=CARTESIAN_POINT('Ctrl Pts',(8.52097709772414,29.6457953049644,126.628983567565));
#119838=CARTESIAN_POINT('Ctrl Pts',(8.53143350738073,29.4805246785236,126.586859849257));
#119839=CARTESIAN_POINT('Ctrl Pts',(8.53812306685359,29.3755663929442,126.548565981097));
#119840=CARTESIAN_POINT('Ctrl Pts',(8.54695407795666,29.2507034520346,126.488238069897));
#119841=CARTESIAN_POINT('Ctrl Pts',(8.54871243418737,29.2264745734536,126.47578998615));
#119842=CARTESIAN_POINT('Ctrl Pts',(8.55113802951733,29.1940995719078,126.458140399991));
#119843=CARTESIAN_POINT('Ctrl Pts',(8.55177625497132,29.185676231403,126.453453031571));
#119844=CARTESIAN_POINT('Ctrl Pts',(8.55279786232767,29.1723535360796,126.445887137549));
#119845=CARTESIAN_POINT('Ctrl Pts',(8.55317829004431,29.1674272588959,126.443056101508));
#119846=CARTESIAN_POINT('Ctrl Pts',(8.55398173673604,29.1570988645817,126.437050082402));
#119847=CARTESIAN_POINT('Ctrl Pts',(8.55440511494797,29.1517000488509,126.433869747167));
#119848=CARTESIAN_POINT('Ctrl Pts',(8.55547120913263,29.1382115516744,126.425821101955));
#119849=CARTESIAN_POINT('Ctrl Pts',(8.55611631241708,29.1301451635377,126.420914387789));
#119850=CARTESIAN_POINT('Ctrl Pts',(8.55868226675073,29.0984194010315,126.401244497095));
#119851=CARTESIAN_POINT('Ctrl Pts',(8.56063261135995,29.075091979303,126.385957665736));
#119852=CARTESIAN_POINT('Ctrl Pts',(8.56601609817774,29.0125431963903,126.342686041623));
#119853=CARTESIAN_POINT('Ctrl Pts',(8.56949265539986,28.9741353028369,126.313574434025));
#119854=CARTESIAN_POINT('Ctrl Pts',(8.58127894628778,28.8491331781839,126.209998444722));
#119855=CARTESIAN_POINT('Ctrl Pts',(8.58962918093296,28.7689299331193,126.128300983447));
#119856=CARTESIAN_POINT('Ctrl Pts',(8.60074071123726,28.6704310918054,126.004846043431));
#119857=CARTESIAN_POINT('Ctrl Pts',(8.60377126111752,28.6445077130205,125.969592862229));
#119858=CARTESIAN_POINT('Ctrl Pts',(8.60786739974862,28.6107973889234,125.919751009295));
#119859=CARTESIAN_POINT('Ctrl Pts',(8.60897803404597,28.6017963636637,125.906009072045));
#119860=CARTESIAN_POINT('Ctrl Pts',(8.61075583000625,28.5876192024087,125.883650067073));
#119861=CARTESIAN_POINT('Ctrl Pts',(8.61142768460174,28.582315423162,125.875115653316));
#119862=CARTESIAN_POINT('Ctrl Pts',(8.61282281995839,28.5714168362554,125.857219384673));
#119863=CARTESIAN_POINT('Ctrl Pts',(8.6135455627643,28.5658360758292,125.847849501632));
#119864=CARTESIAN_POINT('Ctrl Pts',(8.6152580276974,28.5527722449584,125.825417717538));
#119865=CARTESIAN_POINT('Ctrl Pts',(8.61624468624745,28.5453733237219,125.812307725258));
#119866=CARTESIAN_POINT('Ctrl Pts',(8.61965178295648,28.5202860417297,125.766413817886));
#119867=CARTESIAN_POINT('Ctrl Pts',(8.62203991211518,28.5035194603453,125.733136999518));
#119868=CARTESIAN_POINT('Ctrl Pts',(8.62795381039532,28.4642894959505,125.648311716775));
#119869=CARTESIAN_POINT('Ctrl Pts',(8.63143551930446,28.4432926685673,125.596135736531));
#119870=CARTESIAN_POINT('Ctrl Pts',(8.64146435503369,28.3900521903403,125.441704908605));
#119871=CARTESIAN_POINT('Ctrl Pts',(8.64789566207008,28.364987274512,125.337290756297));
#119872=CARTESIAN_POINT('Ctrl Pts',(8.65683244781597,28.3453429844221,125.197107740404));
#119873=CARTESIAN_POINT('Ctrl Pts',(8.65903946635646,28.3416235330142,125.162875457893));
#119874=CARTESIAN_POINT('Ctrl Pts',(8.66198687524166,28.3381580846026,125.118099256063));
#119875=CARTESIAN_POINT('Ctrl Pts',(8.66267992615894,28.3374476073891,125.107636025148));
#119876=CARTESIAN_POINT('Ctrl Pts',(8.6638104832514,28.3364574557726,125.090688064136));
#119877=CARTESIAN_POINT('Ctrl Pts',(8.66424470639012,28.3361168008911,125.084206992194));
#119878=CARTESIAN_POINT('Ctrl Pts',(8.66510137274591,28.3355224119753,125.071480283535));
#119879=CARTESIAN_POINT('Ctrl Pts',(8.66552366468333,28.3352659458463,125.065234931787));
#119880=CARTESIAN_POINT('Ctrl Pts',(8.66658338028155,28.3347130486683,125.049629352022));
#119881=CARTESIAN_POINT('Ctrl Pts',(8.66722313341433,28.3344603907533,125.040267885759));
#119882=CARTESIAN_POINT('Ctrl Pts',(8.66974027598701,28.3337809548505,125.003647822239));
#119883=CARTESIAN_POINT('Ctrl Pts',(8.67164580298702,28.3339443896708,124.976384108168));
#119884=CARTESIAN_POINT('Ctrl Pts',(8.67686456943339,28.3361968348608,124.902638029354));
#119885=CARTESIAN_POINT('Ctrl Pts',(8.68021839370413,28.3395641776208,124.856220077551));
#119886=CARTESIAN_POINT('Ctrl Pts',(8.68857530716182,28.3526988531599,124.741796847259));
#119887=CARTESIAN_POINT('Ctrl Pts',(8.6935938417762,28.3647380596105,124.67413385293));
#119888=CARTESIAN_POINT('Ctrl Pts',(8.70468506646875,28.4009513860754,124.524787742649));
#119889=CARTESIAN_POINT('Ctrl Pts',(8.71070451656663,28.4272814014683,124.443813539551));
#119890=CARTESIAN_POINT('Ctrl Pts',(8.71787095621603,28.4671793787881,124.347003861594));
#119891=CARTESIAN_POINT('Ctrl Pts',(8.71920665444058,28.4749972299187,124.328948867533));
#119892=CARTESIAN_POINT('Ctrl Pts',(8.72132899904051,28.4880305081195,124.3002539837));
#119893=CARTESIAN_POINT('Ctrl Pts',(8.72212248396117,28.493042596378,124.289524365015));
#119894=CARTESIAN_POINT('Ctrl Pts',(8.72362802353031,28.5028172631068,124.269168161197));
#119895=CARTESIAN_POINT('Ctrl Pts',(8.72434074025671,28.5075593332783,124.259532451903));
#119896=CARTESIAN_POINT('Ctrl Pts',(8.72597225366272,28.5186772664773,124.237481991774));
#119897=CARTESIAN_POINT('Ctrl Pts',(8.72688877820963,28.5251166713647,124.225100044994));
#119898=CARTESIAN_POINT('Ctrl Pts',(8.72978870234118,28.5461017498443,124.185958575804));
#119899=CARTESIAN_POINT('Ctrl Pts',(8.73175166987347,28.5612264160809,124.159515424189));
#119900=CARTESIAN_POINT('Ctrl Pts',(8.7363837636112,28.5990311677978,124.097433943471));
#119901=CARTESIAN_POINT('Ctrl Pts',(8.73903068500187,28.622358272983,124.062213883016));
#119902=CARTESIAN_POINT('Ctrl Pts',(8.74634785136885,28.6912063606978,123.966387282686));
#119903=CARTESIAN_POINT('Ctrl Pts',(8.7509438030195,28.7395586389947,123.907945064896));
#119904=CARTESIAN_POINT('Ctrl Pts',(8.75616757583938,28.7983265636739,123.846037699088));
#119905=CARTESIAN_POINT('Ctrl Pts',(8.75675531252979,28.8049915747812,123.839137001509));
#119906=CARTESIAN_POINT('Ctrl Pts',(8.76201973715487,28.8651212870059,123.777947621603));
#119907=CARTESIAN_POINT('Ctrl Pts',(8.76674784870889,28.922185654505,123.727335490899));
#119908=CARTESIAN_POINT('Ctrl Pts',(8.7725263572259,28.992235197421,123.673305934496));
#119909=CARTESIAN_POINT('Ctrl Pts',(8.77333543522115,29.0020490825062,123.665908179616));
#119910=CARTESIAN_POINT('Ctrl Pts',(8.77461353866993,29.0175421215255,123.654496054466));
#119911=CARTESIAN_POINT('Ctrl Pts',(8.77507767644332,29.0231663263354,123.650407350332));
#119912=CARTESIAN_POINT('Ctrl Pts',(8.77595051372792,29.03373504688,123.642824736743));
#119913=CARTESIAN_POINT('Ctrl Pts',(8.77635863664875,29.0386732246568,123.639322418366));
#119914=CARTESIAN_POINT('Ctrl Pts',(8.7773247879708,29.0503562823087,123.631131750977));
#119915=CARTESIAN_POINT('Ctrl Pts',(8.77788429933565,29.0571168669394,123.626466285797));
#119916=CARTESIAN_POINT('Ctrl Pts',(8.77976775712462,29.0798662433206,123.611014087461));
#119917=CARTESIAN_POINT('Ctrl Pts',(8.7811052277329,29.0960071449061,123.600455490474));
#119918=CARTESIAN_POINT('Ctrl Pts',(8.78443406955368,29.1362292528909,123.575130209165));
#119919=CARTESIAN_POINT('Ctrl Pts',(8.78643998781241,29.1605092661512,123.56069150209));
#119920=CARTESIAN_POINT('Ctrl Pts',(8.7956224088175,29.2722879488188,123.498010173361));
#119921=CARTESIAN_POINT('Ctrl Pts',(8.8029706490421,29.3636512883739,123.45708100833));
#119922=CARTESIAN_POINT('Ctrl Pts',(8.81615081259195,29.5364872015663,123.397633715322));
#119923=CARTESIAN_POINT('Ctrl Pts',(8.82201221639358,29.616752996857,123.376563123351));
#119924=CARTESIAN_POINT('Ctrl Pts',(8.82902677928226,29.717556485459,123.357999256891));
#119925=CARTESIAN_POINT('Ctrl Pts',(8.83035852964539,29.7369097947053,123.354787436159));
#119926=CARTESIAN_POINT('Ctrl Pts',(8.83247608388773,29.7680178738376,123.350187823001));
#119927=CARTESIAN_POINT('Ctrl Pts',(8.83326867365714,29.7797380415854,123.348582242919));
#119928=CARTESIAN_POINT('Ctrl Pts',(8.83477341781172,29.8021307638273,123.345757234603));
#119929=CARTESIAN_POINT('Ctrl Pts',(8.83548622473827,29.8127999031348,123.344515933498));
#119930=CARTESIAN_POINT('Ctrl Pts',(8.83711921226534,29.837378728107,123.341896964821));
#119931=CARTESIAN_POINT('Ctrl Pts',(8.838037104748,29.8512953619975,123.340590977576));
#119932=CARTESIAN_POINT('Ctrl Pts',(8.84094663978793,29.8957109544765,123.336986115787));
#119933=CARTESIAN_POINT('Ctrl Pts',(8.84291764829771,29.9262585166631,123.335351759133));
#119934=CARTESIAN_POINT('Ctrl Pts',(8.84757287809975,29.9992942154751,123.333458831552));
#119935=CARTESIAN_POINT('Ctrl Pts',(8.85023457369954,30.0417815520664,123.333982399425));
#119936=CARTESIAN_POINT('Ctrl Pts',(8.85743882329956,30.157833975101,123.339855556705));
#119937=CARTESIAN_POINT('Ctrl Pts',(8.86191367315608,30.2311362519815,123.348465096912));
#119938=CARTESIAN_POINT('Ctrl Pts',(8.86726246431578,30.317105092997,123.364399728107));
#119939=CARTESIAN_POINT('Ctrl Pts',(8.86810217116482,30.3305513612015,123.367064091462));
#119940=CARTESIAN_POINT('Ctrl Pts',(8.87347052154384,30.4160725063227,123.385109617529));
#119941=CARTESIAN_POINT('Ctrl Pts',(8.87805156770615,30.4870840567518,123.405091335915));
#119942=CARTESIAN_POINT('Ctrl Pts',(8.88366642188338,30.5681041855749,123.433805752786));
#119943=CARTESIAN_POINT('Ctrl Pts',(8.88447483126632,30.5796321475535,123.438035423761));
#119944=CARTESIAN_POINT('Ctrl Pts',(8.88575208412609,30.5976104425406,123.444858182544));
#119945=CARTESIAN_POINT('Ctrl Pts',(8.88621604948673,30.6040933575983,123.447364973871));
#119946=CARTESIAN_POINT('Ctrl Pts',(8.88708875721947,30.6161939017649,123.452131227286));
#119947=CARTESIAN_POINT('Ctrl Pts',(8.88749692517266,30.6218151443017,123.454380841298));
#119948=CARTESIAN_POINT('Ctrl Pts',(8.88846341295131,30.6350372780574,123.459756123671));
#119949=CARTESIAN_POINT('Ctrl Pts',(8.88902321885964,30.6426274407528,123.46290744963));
#119950=CARTESIAN_POINT('Ctrl Pts',(8.890908587557,30.6679729114838,123.473651060988));
#119951=CARTESIAN_POINT('Ctrl Pts',(8.89224770905777,30.6856187446232,123.481495554287));
#119952=CARTESIAN_POINT('Ctrl Pts',(8.89558153460426,30.7287721731277,123.501584984143));
#119953=CARTESIAN_POINT('Ctrl Pts',(8.89759083646413,30.754111341289,123.514176206856));
#119954=CARTESIAN_POINT('Ctrl Pts',(8.90680283125409,30.8677471659709,123.574298336104));
#119955=CARTESIAN_POINT('Ctrl Pts',(8.91417806222237,30.9519632063012,123.629096320781));
#119956=CARTESIAN_POINT('Ctrl Pts',(8.9273527113519,31.0955204788528,123.742148822495));
#119957=CARTESIAN_POINT('Ctrl Pts',(8.93318432209167,31.1564305675864,123.797907354295));
#119958=CARTESIAN_POINT('Ctrl Pts',(8.94017025098004,31.2264076446241,123.872230231214));
#119959=CARTESIAN_POINT('Ctrl Pts',(8.94150126510173,31.2395944550552,123.886740818072));
#119960=CARTESIAN_POINT('Ctrl Pts',(8.94361799687578,31.2603214122776,123.910373536095));
#119961=CARTESIAN_POINT('Ctrl Pts',(8.94441048911714,31.2680255156898,123.91934871622));
#119962=CARTESIAN_POINT('Ctrl Pts',(8.94591526328482,31.2825433366579,123.936630829599));
#119963=CARTESIAN_POINT('Ctrl Pts',(8.9466281955744,31.2893735277293,123.944923074759));
#119964=CARTESIAN_POINT('Ctrl Pts',(8.94826177652706,31.3049091038059,123.964160348231));
#119965=CARTESIAN_POINT('Ctrl Pts',(8.94918013285224,31.3135579213929,123.975150176724));
#119966=CARTESIAN_POINT('Ctrl Pts',(8.95209244659461,31.3406995704015,124.010546496219));
#119967=CARTESIAN_POINT('Ctrl Pts',(8.95406571722126,31.3586590105093,124.035355269509));
#119968=CARTESIAN_POINT('Ctrl Pts',(8.95872739653469,31.3999114568146,124.095780098686));
#119969=CARTESIAN_POINT('Ctrl Pts',(8.96139319518157,31.4225441609179,124.131821327306));
#119970=CARTESIAN_POINT('Ctrl Pts',(8.96859932375573,31.480544542999,124.232553388569));
#119971=CARTESIAN_POINT('Ctrl Pts',(8.97307224462647,31.5130386151843,124.298786083015));
#119972=CARTESIAN_POINT('Ctrl Pts',(8.97843617056716,31.5463542077416,124.379886952487));
#119973=CARTESIAN_POINT('Ctrl Pts',(8.97929283784044,31.5515044255601,124.392887540137));
#119974=CARTESIAN_POINT('Ctrl Pts',(8.98465590276752,31.5826347314577,124.474453279298));
#119975=CARTESIAN_POINT('Ctrl Pts',(8.98921483840908,31.6042252067548,124.544598179623));
#119976=CARTESIAN_POINT('Ctrl Pts',(8.99480516670045,31.6239550344586,124.627875252257));
#119977=CARTESIAN_POINT('Ctrl Pts',(8.9956135662341,31.6266535738346,124.63985432004));
#119978=CARTESIAN_POINT('Ctrl Pts',(8.99689085376639,31.6306719866406,124.658659707585));
#119979=CARTESIAN_POINT('Ctrl Pts',(8.99735486531452,31.6320820211966,124.665466601144));
#119980=CARTESIAN_POINT('Ctrl Pts',(8.99822776670442,31.6346408803267,124.678220756916));
#119981=CARTESIAN_POINT('Ctrl Pts',(8.99863608313842,31.63579992364,124.684165717449));
#119982=CARTESIAN_POINT('Ctrl Pts',(8.99960304953536,31.6384560849532,124.698196618246));
#119983=CARTESIAN_POINT('Ctrl Pts',(9.00016318771426,31.63992578075,124.706287470304));
#119984=CARTESIAN_POINT('Ctrl Pts',(9.00205015390863,31.6446491462258,124.733431445904));
#119985=CARTESIAN_POINT('Ctrl Pts',(9.00339056079286,31.6476309852622,124.752529466443));
#119986=CARTESIAN_POINT('Ctrl Pts',(9.00672818600977,31.6541620649319,124.799734374569));
#119987=CARTESIAN_POINT('Ctrl Pts',(9.00874003180645,31.6573278576865,124.827887685586));
#119988=CARTESIAN_POINT('Ctrl Pts',(9.01797562427636,31.6684601701077,124.956295872632));
#119989=CARTESIAN_POINT('Ctrl Pts',(9.02537239223562,31.6680567820779,125.057065415937));
#119990=CARTESIAN_POINT('Ctrl Pts',(9.03853426560753,31.6508295925412,125.2388418975));
#119991=CARTESIAN_POINT('Ctrl Pts',(9.04433413913181,31.6370701917772,125.31982590499));
#119992=CARTESIAN_POINT('Ctrl Pts',(9.05128943664876,31.6126993867303,125.418497945355));
#119993=CARTESIAN_POINT('Ctrl Pts',(9.05261952066453,31.6076662814296,125.437434596963));
#119994=CARTESIAN_POINT('Ctrl Pts',(9.05473523703392,31.5990611699335,125.467652901369));
#119995=CARTESIAN_POINT('Ctrl Pts',(9.05552762881655,31.5957011318969,125.478992454524));
#119996=CARTESIAN_POINT('Ctrl Pts',(9.05703250364877,31.5890581506228,125.500565344305));
#119997=CARTESIAN_POINT('Ctrl Pts',(9.05774563413572,31.5857963979551,125.510804525664));
#119998=CARTESIAN_POINT('Ctrl Pts',(9.05938008724483,31.57805922925,125.534304139384));
#119999=CARTESIAN_POINT('Ctrl Pts',(9.06029911156577,31.5735153001287,125.547541290166));
#120000=CARTESIAN_POINT('Ctrl Pts',(9.06155526888709,31.5670399249498,125.565658357052));
#120001=CARTESIAN_POINT('Ctrl Pts',(9.06189691910435,31.565251574817,125.570588300551));
#120002=CARTESIAN_POINT('Ctrl Pts',(9.06223782796602,31.5634400121624,125.575509624915));
#120003=CARTESIAN_POINT('',(8.82706654161307,31.6659995121743,124.999552917719));
#120004=CARTESIAN_POINT('Ctrl Pts',(8.86798214956472,31.5634398523358,125.575510059103));
#120005=CARTESIAN_POINT('Ctrl Pts',(8.86185959862923,31.5924943407706,125.496580170059));
#120006=CARTESIAN_POINT('Ctrl Pts',(8.85575033786931,31.6155593894588,125.41548247043));
#120007=CARTESIAN_POINT('Ctrl Pts',(8.84633162917246,31.6421958019909,125.284872744603));
#120008=CARTESIAN_POINT('Ctrl Pts',(8.84292407020463,31.6498680502033,125.236422911066));
#120009=CARTESIAN_POINT('Ctrl Pts',(8.83842236191684,31.6573105602946,125.170785025261));
#120010=CARTESIAN_POINT('Ctrl Pts',(8.83727032301696,31.6589692500531,125.153840446107));
#120011=CARTESIAN_POINT('Ctrl Pts',(8.83536837185457,31.6612948409996,125.125629325297));
#120012=CARTESIAN_POINT('Ctrl Pts',(8.83461395720211,31.6621074928471,125.114376436131));
#120013=CARTESIAN_POINT('Ctrl Pts',(8.83319042582845,31.6634313897574,125.093027807114));
#120014=CARTESIAN_POINT('Ctrl Pts',(8.83252063614475,31.6639651786523,125.082934029292));
#120015=CARTESIAN_POINT('Ctrl Pts',(8.83106750172905,31.6649279752969,125.060932692383));
#120016=CARTESIAN_POINT('Ctrl Pts',(8.83028530265433,31.6653211729731,125.04902406533));
#120017=CARTESIAN_POINT('Ctrl Pts',(8.82868898103002,31.6658655137231,125.02459404133));
#120018=CARTESIAN_POINT('Ctrl Pts',(8.827875314874,31.6660033093356,125.012073144697));
#120019=CARTESIAN_POINT('Ctrl Pts',(8.82706571805936,31.6659999396738,124.999551662012));
#120020=CARTESIAN_POINT('Ctrl Pts',(8.82706580233264,31.665999940024,124.99955296541));
#120021=CARTESIAN_POINT('Ctrl Pts',(8.82311191219987,31.6659835311962,124.938400860403));
#120022=CARTESIAN_POINT('Ctrl Pts',(8.81926106119894,31.6626002355637,124.877290397594));
#120023=CARTESIAN_POINT('Ctrl Pts',(8.80644804764151,31.6398369726596,124.671882810155));
#120024=CARTESIAN_POINT('Ctrl Pts',(8.79786135123866,31.604938388399,124.530012045354));
#120025=CARTESIAN_POINT('Ctrl Pts',(8.78706288842619,31.5437082326314,124.373062880477));
#120026=CARTESIAN_POINT('Ctrl Pts',(8.78556987258757,31.5349043321249,124.351807263532));
#120027=CARTESIAN_POINT('Ctrl Pts',(8.78347303192169,31.5221320866681,124.322691208441));
#120028=CARTESIAN_POINT('Ctrl Pts',(8.78288976210561,31.5185368793,124.314668674204));
#120029=CARTESIAN_POINT('Ctrl Pts',(8.78189262552663,31.5123229318677,124.301091524065));
#120030=CARTESIAN_POINT('Ctrl Pts',(8.78148069941551,31.5097366028299,124.295522110435));
#120031=CARTESIAN_POINT('Ctrl Pts',(8.78061676449524,31.5042736057273,124.283926323756));
#120032=CARTESIAN_POINT('Ctrl Pts',(8.78016444924453,31.5013914359647,124.277902816256));
#120033=CARTESIAN_POINT('Ctrl Pts',(8.77893744183874,31.4935117291653,124.261685978332));
#120034=CARTESIAN_POINT('Ctrl Pts',(8.77815879962782,31.4884461898224,124.251526351833));
#120035=CARTESIAN_POINT('Ctrl Pts',(8.77430621951915,31.463046613068,124.201861714845));
#120036=CARTESIAN_POINT('Ctrl Pts',(8.77115739764556,31.4412432644848,124.163132492397));
#120037=CARTESIAN_POINT('Ctrl Pts',(8.76163131245482,31.3715888915748,124.050217019742));
#120038=CARTESIAN_POINT('Ctrl Pts',(8.75515555536039,31.3193632980177,123.978910242169));
#120039=CARTESIAN_POINT('Ctrl Pts',(8.74273248152964,31.2071932368506,123.848819424931));
#120040=CARTESIAN_POINT('Ctrl Pts',(8.73679255303544,31.1479647878587,123.789746834459));
#120041=CARTESIAN_POINT('Ctrl Pts',(8.72987429344803,31.0716779565566,123.724323810785));
#120042=CARTESIAN_POINT('Ctrl Pts',(8.72871509926703,31.0586415470875,123.713484748001));
#120043=CARTESIAN_POINT('Ctrl Pts',(8.72653656167878,31.033662639708,123.693352989191));
#120044=CARTESIAN_POINT('Ctrl Pts',(8.72551569827136,31.0217546541001,123.684020396574));
#120045=CARTESIAN_POINT('Ctrl Pts',(8.72376930046346,31.0010382537288,123.668235166541));
#120046=CARTESIAN_POINT('Ctrl Pts',(8.72304073351015,30.9922906720167,123.661704670461));
#120047=CARTESIAN_POINT('Ctrl Pts',(8.72164934351712,30.975385905112,123.649341317512));
#120048=CARTESIAN_POINT('Ctrl Pts',(8.72098602904161,30.9672390377362,123.643495229719));
#120049=CARTESIAN_POINT('Ctrl Pts',(8.71925027353451,30.9456930492278,123.628326906264));
#120050=CARTESIAN_POINT('Ctrl Pts',(8.71818251493026,30.9322086308161,123.61912726183));
#120051=CARTESIAN_POINT('Ctrl Pts',(8.7143270631873,30.882710583457,123.586413157544));
#120052=CARTESIAN_POINT('Ctrl Pts',(8.71158331086487,30.8459235203386,123.564096237216));
#120053=CARTESIAN_POINT('Ctrl Pts',(8.70165305561416,30.707874526144,123.487497799325));
#120054=CARTESIAN_POINT('Ctrl Pts',(8.69475101905403,30.6019460250435,123.442305901425));
#120055=CARTESIAN_POINT('Ctrl Pts',(8.68471319411838,30.4460009885597,123.394080178988));
#120056=CARTESIAN_POINT('Ctrl Pts',(8.68171136033691,30.3991959169987,123.381810478194));
#120057=CARTESIAN_POINT('Ctrl Pts',(8.67742310757907,30.3333560991082,123.367581334883));
#120058=CARTESIAN_POINT('Ctrl Pts',(8.67620196428344,30.3147187069327,123.363885988645));
#120059=CARTESIAN_POINT('Ctrl Pts',(8.67403298271044,30.2819076000493,123.357961679316));
#120060=CARTESIAN_POINT('Ctrl Pts',(8.6730915748514,30.2677604039843,123.355595526105));
#120061=CARTESIAN_POINT('Ctrl Pts',(8.67165599586849,30.2463637083167,123.352300298216));
#120062=CARTESIAN_POINT('Ctrl Pts',(8.6711690009513,30.2391353382487,123.351235714542));
#120063=CARTESIAN_POINT('Ctrl Pts',(8.67027678372557,30.2259525935307,123.349382691082));
#120064=CARTESIAN_POINT('Ctrl Pts',(8.66987241930273,30.2200006508454,123.348578858952));
#120065=CARTESIAN_POINT('Ctrl Pts',(8.66894565782454,30.2064107093069,123.346818258179));
#120066=CARTESIAN_POINT('Ctrl Pts',(8.66842215671462,30.1987703711942,123.345882233315));
#120067=CARTESIAN_POINT('Ctrl Pts',(8.66677726855011,30.1748680301569,123.34312192567));
#120068=CARTESIAN_POINT('Ctrl Pts',(8.66564646899085,30.1585860166767,123.341484336362));
#120069=CARTESIAN_POINT('Ctrl Pts',(8.6591084614552,30.0651567378163,123.333475828782));
#120070=CARTESIAN_POINT('Ctrl Pts',(8.65349839423687,29.9876703296727,123.332248847061));
#120071=CARTESIAN_POINT('Ctrl Pts',(8.6475393364023,29.9058929549144,123.336653936853));
#120072=CARTESIAN_POINT('Ctrl Pts',(8.64721173805971,29.9013991726717,123.336914272052));
#120073=CARTESIAN_POINT('Ctrl Pts',(8.64035413409775,29.8073644820645,123.342744391764));
#120074=CARTESIAN_POINT('Ctrl Pts',(8.63383225169681,29.7184085455744,123.355520200013));
#120075=CARTESIAN_POINT('Ctrl Pts',(8.62398292990317,29.5824669872475,123.386404693268));
#120076=CARTESIAN_POINT('Ctrl Pts',(8.62053144395442,29.534538749924,123.399571827955));
#120077=CARTESIAN_POINT('Ctrl Pts',(8.61601355290141,29.4714194077108,123.419988622866));
#120078=CARTESIAN_POINT('Ctrl Pts',(8.61488705457271,29.4556499168614,123.425351970631));
#120079=CARTESIAN_POINT('Ctrl Pts',(8.6130156103648,29.4294084817164,123.434718265363));
#120080=CARTESIAN_POINT('Ctrl Pts',(8.61226646048581,29.4188920324227,123.438591939901));
#120081=CARTESIAN_POINT('Ctrl Pts',(8.61079521016866,29.3982198087819,123.446444224937));
#120082=CARTESIAN_POINT('Ctrl Pts',(8.61007296001439,29.3880624469165,123.45041702852));
#120083=CARTESIAN_POINT('Ctrl Pts',(8.60832045953376,29.3633998946243,123.460343503968));
#120084=CARTESIAN_POINT('Ctrl Pts',(8.60729380984965,29.3489381422298,123.466402821849));
#120085=CARTESIAN_POINT('Ctrl Pts',(8.6037616198176,29.2991657970233,123.488087873988));
#120086=CARTESIAN_POINT('Ctrl Pts',(8.6012906372966,29.2643128725904,123.504736923961));
#120087=CARTESIAN_POINT('Ctrl Pts',(8.59133451022103,29.1245037321512,123.57759622948));
#120088=CARTESIAN_POINT('Ctrl Pts',(8.58418159188789,29.0251415541858,123.643763196199));
#120089=CARTESIAN_POINT('Ctrl Pts',(8.5738225311856,28.8956234625868,123.75165653871));
#120090=CARTESIAN_POINT('Ctrl Pts',(8.57075175376744,28.8590051762603,123.785035363904));
#120091=CARTESIAN_POINT('Ctrl Pts',(8.56579469825905,28.8038237119711,123.840032686575));
#120092=CARTESIAN_POINT('Ctrl Pts',(8.56396288707236,28.7842337097326,123.860581735628));
#120093=CARTESIAN_POINT('Ctrl Pts',(8.56146979561538,28.7588021093787,123.888661144796));
#120094=CARTESIAN_POINT('Ctrl Pts',(8.56084060681494,28.7524851554267,123.89575683983));
#120095=CARTESIAN_POINT('Ctrl Pts',(8.55978840419957,28.7420961062591,123.907629554276));
#120096=CARTESIAN_POINT('Ctrl Pts',(8.55936787112815,28.737989585219,123.912376394481));
#120097=CARTESIAN_POINT('Ctrl Pts',(8.55851107498217,28.7297177188876,123.922047993255));
#120098=CARTESIAN_POINT('Ctrl Pts',(8.55807472113558,28.7255539862377,123.926973925302));
#120099=CARTESIAN_POINT('Ctrl Pts',(8.5569357083593,28.7148094489037,123.939836079498));
#120100=CARTESIAN_POINT('Ctrl Pts',(8.55622998620274,28.708273641222,123.947809289384));
#120101=CARTESIAN_POINT('Ctrl Pts',(8.55326073039812,28.6812619414789,123.981392583222));
#120102=CARTESIAN_POINT('Ctrl Pts',(8.55095666864024,28.6614717498443,124.007541978785));
#120103=CARTESIAN_POINT('Ctrl Pts',(8.54174628197452,28.5864429952765,124.113008823578));
#120104=CARTESIAN_POINT('Ctrl Pts',(8.53464624056418,28.5373793468705,124.196484719431));
#120105=CARTESIAN_POINT('Ctrl Pts',(8.52068717676047,28.4545344817127,124.370461919366));
#120106=CARTESIAN_POINT('Ctrl Pts',(8.51385425221636,28.4208105372209,124.460603908105));
#120107=CARTESIAN_POINT('Ctrl Pts',(8.50592953605485,28.3897566002235,124.572144459933));
#120108=CARTESIAN_POINT('Ctrl Pts',(8.50459179682329,28.3848092618782,124.591217530965));
#120109=CARTESIAN_POINT('Ctrl Pts',(8.50246718043537,28.3774309196519,124.621891685846));
#120110=CARTESIAN_POINT('Ctrl Pts',(8.5016734348206,28.3747834602172,124.633438232905));
#120111=CARTESIAN_POINT('Ctrl Pts',(8.50016799988828,28.3699722979114,124.655499066481));
#120112=CARTESIAN_POINT('Ctrl Pts',(8.49945564260801,28.3677866298647,124.666007894823));
#120113=CARTESIAN_POINT('Ctrl Pts',(8.4978411199076,28.3630420606848,124.689979862989));
#120114=CARTESIAN_POINT('Ctrl Pts',(8.4969410333358,28.3605473831199,124.703455035379));
#120115=CARTESIAN_POINT('Ctrl Pts',(8.49409439533492,28.3531425097773,124.746407162936));
#120116=CARTESIAN_POINT('Ctrl Pts',(8.49216750629334,28.3488587813619,124.77598711571));
#120117=CARTESIAN_POINT('Ctrl Pts',(8.48120701128608,28.3288096242296,124.946694203732));
#120118=CARTESIAN_POINT('Ctrl Pts',(8.47273828431608,28.3303433339884,125.08925242879));
#120119=CARTESIAN_POINT('Ctrl Pts',(8.4613123919638,28.3558905109907,125.272618818602));
#120120=CARTESIAN_POINT('Ctrl Pts',(8.4586222083635,28.3635003107159,125.315095700026));
#120121=CARTESIAN_POINT('Ctrl Pts',(8.45421341975417,28.3783099999797,125.382557350146));
#120122=CARTESIAN_POINT('Ctrl Pts',(8.4525357093555,28.3844612129153,125.407753397292));
#120123=CARTESIAN_POINT('Ctrl Pts',(8.45022211731647,28.3935859313128,125.441672241644));
#120124=CARTESIAN_POINT('Ctrl Pts',(8.44961276298937,28.3960477285878,125.450530388016));
#120125=CARTESIAN_POINT('Ctrl Pts',(8.44858453916677,28.4002963728728,125.465341739297));
#120126=CARTESIAN_POINT('Ctrl Pts',(8.44816791347502,28.4020434962221,125.47130631162));
#120127=CARTESIAN_POINT('Ctrl Pts',(8.44736324161128,28.4054659130842,125.482752419264));
#120128=CARTESIAN_POINT('Ctrl Pts',(8.44697551883245,28.4071361834842,125.488235304096));
#120129=CARTESIAN_POINT('Ctrl Pts',(8.4459134477172,28.4117699900738,125.503169500219));
#120130=CARTESIAN_POINT('Ctrl Pts',(8.44523599256275,28.4147895183836,125.512602991908));
#120131=CARTESIAN_POINT('Ctrl Pts',(8.44253625675836,28.4270803566041,125.549854138065));
#120132=CARTESIAN_POINT('Ctrl Pts',(8.44048175119273,28.4370007090071,125.577450209979));
#120133=CARTESIAN_POINT('Ctrl Pts',(8.43058845761243,28.4876378018054,125.707428689183));
#120134=CARTESIAN_POINT('Ctrl Pts',(8.42246820876931,28.5377160101224,125.805865894639));
#120135=CARTESIAN_POINT('Ctrl Pts',(8.41030548490949,28.6285524042213,125.947669838855));
#120136=CARTESIAN_POINT('Ctrl Pts',(8.40614900568784,28.6625124924165,125.995025092727));
#120137=CARTESIAN_POINT('Ctrl Pts',(8.4002581521145,28.7151123243326,126.060799068439));
#120138=CARTESIAN_POINT('Ctrl Pts',(8.39845783866359,28.7318119003453,126.080708135181));
#120139=CARTESIAN_POINT('Ctrl Pts',(8.39522817505633,28.7629090461731,126.116067833763));
#120140=CARTESIAN_POINT('Ctrl Pts',(8.39379290784193,28.7771473837845,126.13165055896));
#120141=CARTESIAN_POINT('Ctrl Pts',(8.39155153739882,28.8000380962516,126.155765923685));
#120142=CARTESIAN_POINT('Ctrl Pts',(8.39073717819677,28.8084938418462,126.164481227588));
#120143=CARTESIAN_POINT('Ctrl Pts',(8.38921444443899,28.8245634863263,126.180685831148));
#120144=CARTESIAN_POINT('Ctrl Pts',(8.38850516916867,28.8321555301534,126.188195831027));
#120145=CARTESIAN_POINT('Ctrl Pts',(8.38691145295182,28.8494532312489,126.204980635389));
#120146=CARTESIAN_POINT('Ctrl Pts',(8.38602891180433,28.8591999109625,126.214212243859));
#120147=CARTESIAN_POINT('Ctrl Pts',(8.38375575684629,28.8847306489732,126.237814961218));
#120148=CARTESIAN_POINT('Ctrl Pts',(8.38237283288687,28.9006815022897,126.25200259995));
#120149=CARTESIAN_POINT('Ctrl Pts',(8.37298877237357,29.0116577515645,126.34695489566));
#120150=CARTESIAN_POINT('Ctrl Pts',(8.36543506173788,29.1152179281998,126.417135241382));
#120151=CARTESIAN_POINT('Ctrl Pts',(8.35251044376639,29.30236585554,126.515377811488));
#120152=CARTESIAN_POINT('Ctrl Pts',(8.34718468790678,29.3820978145835,126.54959874999));
#120153=CARTESIAN_POINT('Ctrl Pts',(8.34061835408789,29.4776645857624,126.582063983745));
#120154=CARTESIAN_POINT('Ctrl Pts',(8.33967920348933,29.4912708609437,126.586491526321));
#120155=CARTESIAN_POINT('Ctrl Pts',(8.33824637861165,29.5119015835442,126.592912181252));
#120156=CARTESIAN_POINT('Ctrl Pts',(8.33775983924086,29.518885275295,126.595035390825));
#120157=CARTESIAN_POINT('Ctrl Pts',(8.33686804492697,29.5316408330934,126.598821994754));
#120158=CARTESIAN_POINT('Ctrl Pts',(8.33646364246367,29.537408038012,126.600500157221));
#120159=CARTESIAN_POINT('Ctrl Pts',(8.33553625818704,29.5505948952862,126.604260089533));
#120160=CARTESIAN_POINT('Ctrl Pts',(8.33501216603918,29.5580199711224,126.606321583988));
#120161=CARTESIAN_POINT('Ctrl Pts',(8.33336353085078,29.581300465874,126.612611538694));
#120162=CARTESIAN_POINT('Ctrl Pts',(8.33222951640808,29.597203680645,126.616657152698));
#120163=CARTESIAN_POINT('Ctrl Pts',(8.32533956440547,29.6933153841576,126.639600868683));
#120164=CARTESIAN_POINT('Ctrl Pts',(8.31935390558644,29.77476926883,126.652759826452));
#120165=CARTESIAN_POINT('Ctrl Pts',(8.3079945711629,29.9302519368262,126.666168843073));
#120166=CARTESIAN_POINT('Ctrl Pts',(8.30263490766846,30.0039942237203,126.667623701327));
#120167=CARTESIAN_POINT('Ctrl Pts',(8.29440884702313,30.1192327446014,126.662250604774));
#120168=CARTESIAN_POINT('Ctrl Pts',(8.29147213707223,30.1607861631104,126.658747059286));
#120169=CARTESIAN_POINT('Ctrl Pts',(8.2864872507338,30.2321122535858,126.650027272425));
#120170=CARTESIAN_POINT('Ctrl Pts',(8.28441859296429,30.2619537407256,126.645553566569));
#120171=CARTESIAN_POINT('Ctrl Pts',(8.28143361873136,30.3053464331246,126.637837850405));
#120172=CARTESIAN_POINT('Ctrl Pts',(8.28049751542141,30.319003189854,126.63523278271));
#120173=CARTESIAN_POINT('Ctrl Pts',(8.27884859269855,30.343139254354,126.630314867491));
#120174=CARTESIAN_POINT('Ctrl Pts',(8.27813362077775,30.353631669446,126.628071179851));
#120175=CARTESIAN_POINT('Ctrl Pts',(8.27663494226303,30.3756776942224,126.623133694604));
#120176=CARTESIAN_POINT('Ctrl Pts',(8.27585199441556,30.3872257202403,126.620417530863));
#120177=CARTESIAN_POINT('Ctrl Pts',(8.27377374505151,30.4179510307577,126.612843533235));
#120178=CARTESIAN_POINT('Ctrl Pts',(8.27248549712261,30.4370728304289,126.607766998581));
#120179=CARTESIAN_POINT('Ctrl Pts',(8.26533958107234,30.5434519017089,126.577486782053));
#120180=CARTESIAN_POINT('Ctrl Pts',(8.25970827242814,30.628629315451,126.545520215033));
#120181=CARTESIAN_POINT('Ctrl Pts',(8.24843537639549,30.7950507561807,126.467014348336));
#120182=CARTESIAN_POINT('Ctrl Pts',(8.24281535967413,30.8758276975229,126.420267759495));
#120183=CARTESIAN_POINT('Ctrl Pts',(8.23441970976056,30.9855704936985,126.34382066184));
#120184=CARTESIAN_POINT('Ctrl Pts',(8.2318302798772,31.0180106046631,126.319415394432));
#120185=CARTESIAN_POINT('Ctrl Pts',(8.22846714159822,31.0578298363242,126.287115537185));
#120186=CARTESIAN_POINT('Ctrl Pts',(8.22776072110762,31.0660699602434,126.280298868931));
#120187=CARTESIAN_POINT('Ctrl Pts',(8.22661379723479,31.0792378430255,126.26919043917));
#120188=CARTESIAN_POINT('Ctrl Pts',(8.22617675503122,31.0842071287889,126.264948058576));
#120189=CARTESIAN_POINT('Ctrl Pts',(8.22532448910126,31.0938007790999,126.256659703285));
#120190=CARTESIAN_POINT('Ctrl Pts',(8.22490951030006,31.0984279225647,126.252617199508));
#120191=CARTESIAN_POINT('Ctrl Pts',(8.22397248119027,31.1087795539742,126.243472037631));
#120192=CARTESIAN_POINT('Ctrl Pts',(8.22344942181113,31.1144913775475,126.238355268635));
#120193=CARTESIAN_POINT('Ctrl Pts',(8.22159076799756,31.1345608133872,126.220125344995));
#120194=CARTESIAN_POINT('Ctrl Pts',(8.22024110880068,31.1487233501495,126.206801011429));
#120195=CARTESIAN_POINT('Ctrl Pts',(8.21133002619227,31.2397729788634,126.118085089767));
#120196=CARTESIAN_POINT('Ctrl Pts',(8.20341418999369,31.3094250999261,126.035642196394));
#120197=CARTESIAN_POINT('Ctrl Pts',(8.18941167158819,31.4191244138898,125.876880158043));
#120198=CARTESIAN_POINT('Ctrl Pts',(8.18330322973614,31.4621608940694,125.803070376775));
#120199=CARTESIAN_POINT('Ctrl Pts',(8.17530622432523,31.5124256970906,125.69930183296));
#120200=CARTESIAN_POINT('Ctrl Pts',(8.17325105760495,31.5247635719941,125.671975292116));
#120201=CARTESIAN_POINT('Ctrl Pts',(8.17028162465115,31.5417216024768,125.63154004478));
#120202=CARTESIAN_POINT('Ctrl Pts',(8.16934786288843,31.5469254065904,125.618684195971));
#120203=CARTESIAN_POINT('Ctrl Pts',(8.16770156858408,31.5558678834473,125.595773577493));
#120204=CARTESIAN_POINT('Ctrl Pts',(8.16698690732518,31.5596710596102,125.585745014012));
#120205=CARTESIAN_POINT('Ctrl Pts',(8.1662714349765,31.5633981439605,125.57562335527));
#120206=CARTESIAN_POINT('Ctrl Pts',(8.16626741557826,31.563419079503,125.575566490962));
#120207=CARTESIAN_POINT('Ctrl Pts',(8.1662633962835,31.5634400119422,125.575509625513));
#120208=CARTESIAN_POINT('Origin',(5.,30.,125.));
#120209=CARTESIAN_POINT('',(7.46828911258472,31.5634400017109,125.575509653308));
#120210=CARTESIAN_POINT('',(7.65924497815242,31.5634400119497,125.575509625493));
#120211=CARTESIAN_POINT('',(5.,31.5634400119422,125.575509625513));
#120212=CARTESIAN_POINT('Ctrl Pts',(7.65924497815242,31.5634400119496,125.575509625493));
#120213=CARTESIAN_POINT('Ctrl Pts',(7.66017729015006,31.5584735537155,125.58900159709));
#120214=CARTESIAN_POINT('Ctrl Pts',(7.66111773020847,31.5533327778235,125.602428385792));
#120215=CARTESIAN_POINT('Ctrl Pts',(7.66261080835764,31.5449808147374,125.623424291053));
#120216=CARTESIAN_POINT('Ctrl Pts',(7.66315702419078,31.5418862215632,125.631039172576));
#120217=CARTESIAN_POINT('Ctrl Pts',(7.66411143038786,31.5364143463579,125.644223269884));
#120218=CARTESIAN_POINT('Ctrl Pts',(7.66451808945713,31.5340628459776,125.649802930435));
#120219=CARTESIAN_POINT('Ctrl Pts',(7.66539562430481,31.5289466590125,125.661760096817));
#120220=CARTESIAN_POINT('Ctrl Pts',(7.66586702566179,31.5261725065432,125.66813306138));
#120221=CARTESIAN_POINT('Ctrl Pts',(7.66717739120733,31.5183879447439,125.685714802585));
#120222=CARTESIAN_POINT('Ctrl Pts',(7.66802110248971,31.5132934994877,125.696885574195));
#120223=CARTESIAN_POINT('Ctrl Pts',(7.6739281957247,31.4770288850266,125.774131212128));
#120224=CARTESIAN_POINT('Ctrl Pts',(7.67919300440629,31.4416683139265,125.838142928507));
#120225=CARTESIAN_POINT('Ctrl Pts',(7.68553260137612,31.3945459696026,125.911591934296));
#120226=CARTESIAN_POINT('Ctrl Pts',(7.68656738638667,31.3867123306757,125.923464793082));
#120227=CARTESIAN_POINT('Ctrl Pts',(7.69296548856018,31.337364382259,125.996213697452));
#120228=CARTESIAN_POINT('Ctrl Pts',(7.69832878806617,31.2919986891319,126.054384141325));
#120229=CARTESIAN_POINT('Ctrl Pts',(7.70662546771097,31.2145866562511,126.141116477023));
#120230=CARTESIAN_POINT('Ctrl Pts',(7.70962646036876,31.1850367874528,126.171774669521));
#120231=CARTESIAN_POINT('Ctrl Pts',(7.71470711035421,31.1322561156653,126.222493505136));
#120232=CARTESIAN_POINT('Ctrl Pts',(7.7168083321998,31.1095870509708,126.243105414682));
#120233=CARTESIAN_POINT('Ctrl Pts',(7.71983094073532,31.0757577996573,126.27220154002));
#120234=CARTESIAN_POINT('Ctrl Pts',(7.72077282352162,31.0650397620834,126.281187702036));
#120235=CARTESIAN_POINT('Ctrl Pts',(7.72242843726573,31.0458912994405,126.296835683684));
#120236=CARTESIAN_POINT('Ctrl Pts',(7.72314437787457,31.0375073376343,126.303552812267));
#120237=CARTESIAN_POINT('Ctrl Pts',(7.72464168182622,31.0197584625874,126.317493276704));
#120238=CARTESIAN_POINT('Ctrl Pts',(7.72542231876526,31.0103803947095,126.32469895686));
#120239=CARTESIAN_POINT('Ctrl Pts',(7.72748645123638,30.9852585790615,126.343579420491));
#120240=CARTESIAN_POINT('Ctrl Pts',(7.72876306950882,30.9693838961959,126.355077503749));
#120241=CARTESIAN_POINT('Ctrl Pts',(7.73534829110199,30.8858172584015,126.413384802853));
#120242=CARTESIAN_POINT('Ctrl Pts',(7.74047489869333,30.8149242760387,126.455413931142));
#120243=CARTESIAN_POINT('Ctrl Pts',(7.75169815211647,30.6512876792323,126.536704684808));
#120244=CARTESIAN_POINT('Ctrl Pts',(7.75773485436627,30.5575201688452,126.573151563584));
#120245=CARTESIAN_POINT('Ctrl Pts',(7.76580292719123,30.4338471508407,126.608767836171));
#120246=CARTESIAN_POINT('Ctrl Pts',(7.76759740637812,30.4064517008403,126.615906598519));
#120247=CARTESIAN_POINT('Ctrl Pts',(7.77066742696375,30.3600776052865,126.626737010258));
#120248=CARTESIAN_POINT('Ctrl Pts',(7.77192660920649,30.3411918761311,126.630802626916));
#120249=CARTESIAN_POINT('Ctrl Pts',(7.77374607910833,30.3141761986648,126.636128625957));
#120250=CARTESIAN_POINT('Ctrl Pts',(7.77429229454883,30.3061002147552,126.637658760548));
#120251=CARTESIAN_POINT('Ctrl Pts',(7.77524670028917,30.2920559386583,126.640212179517));
#120252=CARTESIAN_POINT('Ctrl Pts',(7.77565335929858,30.2860928543941,126.641262788972));
#120253=CARTESIAN_POINT('Ctrl Pts',(7.77653089424722,30.2732722807136,126.643449595354));
#120254=CARTESIAN_POINT('Ctrl Pts',(7.77700229576726,30.2664134726515,126.644575376521));
#120255=CARTESIAN_POINT('Ctrl Pts',(7.77831266241106,30.2474202036857,126.647570934548));
#120256=CARTESIAN_POINT('Ctrl Pts',(7.77915637464264,30.2352720943578,126.649349496335));
#120257=CARTESIAN_POINT('Ctrl Pts',(7.78506373574391,30.1507022124981,126.66077778977));
#120258=CARTESIAN_POINT('Ctrl Pts',(7.79032883252951,30.077741003739,126.665787499988));
#120259=CARTESIAN_POINT('Ctrl Pts',(7.79666852811906,29.9904745394112,126.666033465635));
#120260=CARTESIAN_POINT('Ctrl Pts',(7.79770312672476,29.9762535160704,126.665891456134));
#120261=CARTESIAN_POINT('Ctrl Pts',(7.80410107461282,29.8883715695728,126.663888331602));
#120262=CARTESIAN_POINT('Ctrl Pts',(7.80946440379635,29.8148949028771,126.65732395683));
#120263=CARTESIAN_POINT('Ctrl Pts',(7.81776103740661,29.7000423700989,126.639326964603));
#120264=CARTESIAN_POINT('Ctrl Pts',(7.8207619586742,29.6582592767303,126.631128829586));
#120265=CARTESIAN_POINT('Ctrl Pts',(7.82584250257533,29.5870233032342,126.614293807885));
#120266=CARTESIAN_POINT('Ctrl Pts',(7.82794368850995,29.5574119551091,126.606427803198));
#120267=CARTESIAN_POINT('Ctrl Pts',(7.83096625567725,29.5146198444375,126.593787220432));
#120268=CARTESIAN_POINT('Ctrl Pts',(7.83190813222009,29.5012571874778,126.58965632358));
#120269=CARTESIAN_POINT('Ctrl Pts',(7.83356373882031,29.4777252986039,126.58205579444));
#120270=CARTESIAN_POINT('Ctrl Pts',(7.83427967846663,29.4675347998188,126.578655193615));
#120271=CARTESIAN_POINT('Ctrl Pts',(7.83577698413783,29.4461964307767,126.571304382951));
#120272=CARTESIAN_POINT('Ctrl Pts',(7.83655762372302,29.4350562596176,126.567333544434));
#120273=CARTESIAN_POINT('Ctrl Pts',(7.83862177191416,29.4055685634763,126.556467603902));
#120274=CARTESIAN_POINT('Ctrl Pts',(7.83989840306588,29.3872984798224,126.549366655922));
#120275=CARTESIAN_POINT('Ctrl Pts',(7.84648406016985,29.2929821945624,126.510779838452));
#120276=CARTESIAN_POINT('Ctrl Pts',(7.85161105833248,29.2192162249487,126.474011216018));
#120277=CARTESIAN_POINT('Ctrl Pts',(7.86283433713142,29.0621701508971,126.380619771661));
#120278=CARTESIAN_POINT('Ctrl Pts',(7.8688707098774,28.9806985101051,126.32161185825));
#120279=CARTESIAN_POINT('Ctrl Pts',(7.87693838655805,28.8837049712049,126.237029776872));
#120280=CARTESIAN_POINT('Ctrl Pts',(7.87873282171588,28.862849639222,126.217885929157));
#120281=CARTESIAN_POINT('Ctrl Pts',(7.88180277455025,28.8285997012969,126.184799775797));
#120282=CARTESIAN_POINT('Ctrl Pts',(7.88306193400523,28.8149413199946,126.171138341701));
#120283=CARTESIAN_POINT('Ctrl Pts',(7.88488137662834,28.7958146793757,126.151330220693));
#120284=CARTESIAN_POINT('Ctrl Pts',(7.88542758814761,28.7901490660582,126.14537516741));
#120285=CARTESIAN_POINT('Ctrl Pts',(7.88638198941899,28.7803867654472,126.134960890579));
#120286=CARTESIAN_POINT('Ctrl Pts',(7.88678864792402,28.7762699463427,126.130520862025));
#120287=CARTESIAN_POINT('Ctrl Pts',(7.88766618462007,28.7674792814555,126.120935765638));
#120288=CARTESIAN_POINT('Ctrl Pts',(7.8881375884195,28.7628134715875,126.115783940482));
#120289=CARTESIAN_POINT('Ctrl Pts',(7.88944796753677,28.74999538904,126.10145141416));
#120290=CARTESIAN_POINT('Ctrl Pts',(7.89029169010397,28.7419123498506,126.092209772709));
#120291=CARTESIAN_POINT('Ctrl Pts',(7.8962017589591,28.6864178995672,126.027327494601));
#120292=CARTESIAN_POINT('Ctrl Pts',(7.90146976693902,28.6426161805956,125.968713845724));
#120293=CARTESIAN_POINT('Ctrl Pts',(7.90781043800223,28.595077571397,125.895516871823));
#120294=CARTESIAN_POINT('Ctrl Pts',(7.90884313218526,28.5874984690762,125.883513961057));
#120295=CARTESIAN_POINT('Ctrl Pts',(7.91523948632845,28.5415306055414,125.808611735073));
#120296=CARTESIAN_POINT('Ctrl Pts',(7.92060310201217,28.5071943045998,125.743315799317));
#120297=CARTESIAN_POINT('Ctrl Pts',(7.92889927250416,28.4600279591175,125.637065747959));
#120298=CARTESIAN_POINT('Ctrl Pts',(7.93189948654414,28.4442583857804,125.59752421494));
#120299=CARTESIAN_POINT('Ctrl Pts',(7.93697898019848,28.4197722488643,125.528558601444));
#120300=CARTESIAN_POINT('Ctrl Pts',(7.93907981101,28.4103225133051,125.499419305726));
#120301=CARTESIAN_POINT('Ctrl Pts',(7.9421019700887,28.3977353790991,125.456617629355));
#120302=CARTESIAN_POINT('Ctrl Pts',(7.94304378584589,28.3939587872263,125.443151462155));
#120303=CARTESIAN_POINT('Ctrl Pts',(7.94469932392174,28.3875817959398,125.419259982886));
#120304=CARTESIAN_POINT('Ctrl Pts',(7.9454152552096,28.3849118850133,125.408854238275));
#120305=CARTESIAN_POINT('Ctrl Pts',(7.94691258078027,28.3795144366944,125.386939797216));
#120306=CARTESIAN_POINT('Ctrl Pts',(7.94769324826333,28.3768084172636,125.375426378172));
#120307=CARTESIAN_POINT('Ctrl Pts',(7.94975755769356,28.3699438593298,125.344756717018));
#120308=CARTESIAN_POINT('Ctrl Pts',(7.95103432022259,28.3660003246257,125.32555388056));
#120309=CARTESIAN_POINT('Ctrl Pts',(7.95762439611037,28.3472531151046,125.225318895443));
#120310=CARTESIAN_POINT('Ctrl Pts',(7.96275535660239,28.3381341228507,125.143335800659));
#120311=CARTESIAN_POINT('Ctrl Pts',(7.97397889053894,28.3314430746386,124.960733044532));
#120312=CARTESIAN_POINT('Ctrl Pts',(7.9800119179566,28.3368352743163,124.860340216216));
#120313=CARTESIAN_POINT('Ctrl Pts',(7.98807557233017,28.3552840326611,124.733042638468));
#120314=CARTESIAN_POINT('Ctrl Pts',(7.9898695608054,28.3600556409009,124.70514551971));
#120315=CARTESIAN_POINT('Ctrl Pts',(7.99293882661262,28.3692751412895,124.658436735692));
#120316=CARTESIAN_POINT('Ctrl Pts',(7.99419775525374,28.3733442420051,124.639555836097));
#120317=CARTESIAN_POINT('Ctrl Pts',(7.99601692213102,28.3796114167166,124.61274763689));
#120318=CARTESIAN_POINT('Ctrl Pts',(7.99656309452805,28.3815415677023,124.604758492202));
#120319=CARTESIAN_POINT('Ctrl Pts',(7.9975174518509,28.384996194286,124.590909091179));
#120320=CARTESIAN_POINT('Ctrl Pts',(7.99792410597136,28.3864936324497,124.585042333868));
#120321=CARTESIAN_POINT('Ctrl Pts',(7.99880166242837,28.3897788385109,124.57245803915));
#120322=CARTESIAN_POINT('Ctrl Pts',(7.99927309065674,28.3915766469335,124.565743589457));
#120323=CARTESIAN_POINT('Ctrl Pts',(8.00058360118448,28.3966665024585,124.547199294584));
#120324=CARTESIAN_POINT('Ctrl Pts',(8.00142743219962,28.4000473265462,124.535394571977));
#120325=CARTESIAN_POINT('Ctrl Pts',(8.007366396333,28.4245792473758,124.453181837674));
#120326=CARTESIAN_POINT('Ctrl Pts',(8.01266547828767,28.4502379979847,124.384211081478));
#120327=CARTESIAN_POINT('Ctrl Pts',(8.01901480169053,28.4860564108427,124.304497467385));
#120328=CARTESIAN_POINT('Ctrl Pts',(8.02002541510096,28.4919081042523,124.291898457524));
#120329=CARTESIAN_POINT('Ctrl Pts',(8.02640205195574,28.529804264357,124.212907130112));
#120330=CARTESIAN_POINT('Ctrl Pts',(8.0317678226661,28.5660704902492,124.148625720939));
#120331=CARTESIAN_POINT('Ctrl Pts',(8.04005974970625,28.6297525680149,124.051431814825));
#120332=CARTESIAN_POINT('Ctrl Pts',(8.04305391622489,28.6543788849495,124.016809305059));
#120333=CARTESIAN_POINT('Ctrl Pts',(8.04812442687762,28.6989693020672,123.958937842279));
#120334=CARTESIAN_POINT('Ctrl Pts',(8.05022221882604,28.7182997490558,123.935229614866));
#120335=CARTESIAN_POINT('Ctrl Pts',(8.05324088556407,28.7474005751394,123.901480066102));
#120336=CARTESIAN_POINT('Ctrl Pts',(8.05418218096618,28.7566611294397,123.891009541086));
#120337=CARTESIAN_POINT('Ctrl Pts',(8.05583713272232,28.7732694808934,123.872700744684));
#120338=CARTESIAN_POINT('Ctrl Pts',(8.05655299273948,28.7805632667765,123.864814799031));
#120339=CARTESIAN_POINT('Ctrl Pts',(8.05805048979114,28.7960494514399,123.848392847619));
#120340=CARTESIAN_POINT('Ctrl Pts',(8.05883139693659,28.8042575599505,123.839872426838));
#120341=CARTESIAN_POINT('Ctrl Pts',(8.06089709085245,28.8263171085823,123.817456393452));
#120342=CARTESIAN_POINT('Ctrl Pts',(8.06217498133404,28.8403246869818,123.803716533545));
#120343=CARTESIAN_POINT('Ctrl Pts',(8.06880434749208,28.9148163948325,123.733186887875));
#120344=CARTESIAN_POINT('Ctrl Pts',(8.07397056175925,28.9792408411131,123.680722860206));
#120345=CARTESIAN_POINT('Ctrl Pts',(8.08519649246316,29.1292056399887,123.576188905894));
#120346=CARTESIAN_POINT('Ctrl Pts',(8.09119983785487,29.216057022665,123.526584944874));
#120347=CARTESIAN_POINT('Ctrl Pts',(8.09922779230884,29.3324935823875,123.473308038464));
#120348=CARTESIAN_POINT('Ctrl Pts',(8.10101780225709,29.358460750046,123.462215758249));
#120349=CARTESIAN_POINT('Ctrl Pts',(8.10408094761068,29.402614024032,123.444667953206));
#120350=CARTESIAN_POINT('Ctrl Pts',(8.10533781904149,29.4206537265812,123.437858649841));
#120351=CARTESIAN_POINT('Ctrl Pts',(8.10715452754884,29.4465402580152,123.428597512091));
#120352=CARTESIAN_POINT('Ctrl Pts',(8.10770035047911,29.4542940961943,123.425888020323));
#120353=CARTESIAN_POINT('Ctrl Pts',(8.10865431373779,29.4677975712148,123.421281142596));
#120354=CARTESIAN_POINT('Ctrl Pts',(8.10906092718512,29.4735380290792,123.419357583844));
#120355=CARTESIAN_POINT('Ctrl Pts',(8.10993865335319,29.4858947250929,123.415291785253));
#120356=CARTESIAN_POINT('Ctrl Pts',(8.11041029446289,29.4925138288406,123.413159698885));
#120357=CARTESIAN_POINT('Ctrl Pts',(8.1117219620347,29.5108702874787,123.407373476646));
#120358=CARTESIAN_POINT('Ctrl Pts',(8.11256675023826,29.5226347608772,123.403807804541));
#120359=CARTESIAN_POINT('Ctrl Pts',(8.11874017630656,29.6082612112354,123.378886690644));
#120360=CARTESIAN_POINT('Ctrl Pts',(8.12429172306605,29.6834762305766,123.362539245164));
#120361=CARTESIAN_POINT('Ctrl Pts',(8.13680093034895,29.8537423756648,123.33770420625));
#120362=CARTESIAN_POINT('Ctrl Pts',(8.143749501351,29.9489566396222,123.332062285043));
#120363=CARTESIAN_POINT('Ctrl Pts',(8.15436594312315,30.0986156273441,123.336028553768));
#120364=CARTESIAN_POINT('Ctrl Pts',(8.15816306033289,30.1529953555493,123.340144709919));
#120365=CARTESIAN_POINT('Ctrl Pts',(8.16304867591075,30.2241139134745,123.349053717936));
#120366=CARTESIAN_POINT('Ctrl Pts',(8.1642105450047,30.2411133496201,123.35145061845));
#120367=CARTESIAN_POINT('Ctrl Pts',(8.16612441458717,30.2692499629297,123.355862400187));
#120368=CARTESIAN_POINT('Ctrl Pts',(8.16688103248263,30.280408744844,123.357728726312));
#120369=CARTESIAN_POINT('Ctrl Pts',(8.16835536296679,30.3022174807017,123.361605044283));
#120370=CARTESIAN_POINT('Ctrl Pts',(8.16907333515373,30.3128685197425,123.36360556853));
#120371=CARTESIAN_POINT('Ctrl Pts',(8.17079581853744,30.3384891189188,123.368677037219));
#120372=CARTESIAN_POINT('Ctrl Pts',(8.17179703180715,30.3534376019871,123.371850320277));
#120373=CARTESIAN_POINT('Ctrl Pts',(8.17514719167736,30.4036171077776,123.383226172473));
#120374=CARTESIAN_POINT('Ctrl Pts',(8.1774662877337,30.4386254930111,123.392370578873));
#120375=CARTESIAN_POINT('Ctrl Pts',(8.18744535598168,30.5897709479583,123.437156411244));
#120376=CARTESIAN_POINT('Ctrl Pts',(8.19474448068092,30.7021062656688,123.484296219092));
#120377=CARTESIAN_POINT('Ctrl Pts',(8.20528952279636,30.8522083280496,123.5675838564));
#120378=CARTESIAN_POINT('Ctrl Pts',(8.20839964569837,30.894969264776,123.593904569692));
#120379=CARTESIAN_POINT('Ctrl Pts',(8.21341285794739,30.9601546792472,123.638207501934));
#120380=CARTESIAN_POINT('Ctrl Pts',(8.21525998050454,30.9834150026727,123.654908733025));
#120381=CARTESIAN_POINT('Ctrl Pts',(8.21777096111479,31.0138280500334,123.67795630691));
#120382=CARTESIAN_POINT('Ctrl Pts',(8.21840214741607,31.021374548354,123.68377780645));
#120383=CARTESIAN_POINT('Ctrl Pts',(8.21945686594944,31.03381319667,123.6935445789));
#120384=CARTESIAN_POINT('Ctrl Pts',(8.21987789402631,31.038733857771,123.697453469815));
#120385=CARTESIAN_POINT('Ctrl Pts',(8.22068232362156,31.0480479374128,123.704938760973));
#120386=CARTESIAN_POINT('Ctrl Pts',(8.22106532869029,31.0524454473363,123.708509903293));
#120387=CARTESIAN_POINT('Ctrl Pts',(8.22209816859498,31.064207119915,123.718161317854));
#120388=CARTESIAN_POINT('Ctrl Pts',(8.22275082937282,31.0715372221164,123.724282487425));
#120389=CARTESIAN_POINT('Ctrl Pts',(8.22523420258614,31.0990590368401,123.747669749681));
#120390=CARTESIAN_POINT('Ctrl Pts',(8.22709117926231,31.1188882605249,123.765354021507));
#120391=CARTESIAN_POINT('Ctrl Pts',(8.23614896413271,31.2124158385421,123.852868474948));
#120392=CARTESIAN_POINT('Ctrl Pts',(8.24361003557906,31.2800479139355,123.928860971623));
#120393=CARTESIAN_POINT('Ctrl Pts',(8.25790072237452,31.3971163123766,124.087442794647));
#120394=CARTESIAN_POINT('Ctrl Pts',(8.26471553660821,31.4471754551548,124.169106930208));
#120395=CARTESIAN_POINT('Ctrl Pts',(8.27275692385634,31.4995977406789,124.273896132744));
#120396=CARTESIAN_POINT('Ctrl Pts',(8.27422280918255,31.5088629398133,124.293350925686));
#120397=CARTESIAN_POINT('Ctrl Pts',(8.27650090312042,31.5227948779878,124.324129073434));
#120398=CARTESIAN_POINT('Ctrl Pts',(8.27732182275284,31.5277183528788,124.335332866823));
#120399=CARTESIAN_POINT('Ctrl Pts',(8.27885071595576,31.5367032983413,124.35640630369));
#120400=CARTESIAN_POINT('Ctrl Pts',(8.27955965933285,31.5407942182755,124.366262626123));
#120401=CARTESIAN_POINT('Ctrl Pts',(8.28114476056929,31.5497688249438,124.388486009195));
#120402=CARTESIAN_POINT('Ctrl Pts',(8.28201911048519,31.5545997715853,124.400873686974));
#120403=CARTESIAN_POINT('Ctrl Pts',(8.28425543471283,31.5666414909333,124.432878149566));
#120404=CARTESIAN_POINT('Ctrl Pts',(8.28561014383738,31.573632506011,124.452575527924));
#120405=CARTESIAN_POINT('Ctrl Pts',(8.29662267006727,31.6278765267608,124.615045539408));
#120406=CARTESIAN_POINT('Ctrl Pts',(8.30559035061524,31.6559677911309,124.763474909878));
#120407=CARTESIAN_POINT('Ctrl Pts',(8.3176124521911,31.666073919873,124.958227368355));
#120408=CARTESIAN_POINT('Ctrl Pts',(8.32039128140837,31.6665948890141,125.002862943127));
#120409=CARTESIAN_POINT('Ctrl Pts',(8.3249288582424,31.6645681280028,125.073976470512));
#120410=CARTESIAN_POINT('Ctrl Pts',(8.32664371599238,31.6631794123358,125.100467035911));
#120411=CARTESIAN_POINT('Ctrl Pts',(8.3290007945212,31.6604527800136,125.136156282169));
#120412=CARTESIAN_POINT('Ctrl Pts',(8.3296151970263,31.6596693286104,125.145394902405));
#120413=CARTESIAN_POINT('Ctrl Pts',(8.33064959263819,31.658230427495,125.160831234165));
#120414=CARTESIAN_POINT('Ctrl Pts',(8.33106728303625,31.6576172236508,125.16703285496));
#120415=CARTESIAN_POINT('Ctrl Pts',(8.33187199221239,31.6563747934697,125.1789168169));
#120416=CARTESIAN_POINT('Ctrl Pts',(8.33225867042812,31.6557510893514,125.184599597587));
#120417=CARTESIAN_POINT('Ctrl Pts',(8.33331402068823,31.6539762632975,125.200037518568));
#120418=CARTESIAN_POINT('Ctrl Pts',(8.33398573327863,31.6527681155502,125.209785683135));
#120419=CARTESIAN_POINT('Ctrl Pts',(8.33663297112653,31.6476988166234,125.247922195983));
#120420=CARTESIAN_POINT('Ctrl Pts',(8.33863921217874,31.6431920673948,125.276218032144));
#120421=CARTESIAN_POINT('Ctrl Pts',(8.34732511271102,31.6208011871795,125.39670936142));
#120422=CARTESIAN_POINT('Ctrl Pts',(8.35421284492904,31.5958709859904,125.487407044403));
#120423=CARTESIAN_POINT('Ctrl Pts',(8.36102759409884,31.5634400156515,125.575509615436));
#120424=CARTESIAN_POINT('Ctrl Pts',(8.1662633962835,31.5634400119422,125.575509625513));
#120425=CARTESIAN_POINT('Ctrl Pts',(8.16547940338663,31.5675230376026,125.564417603061));
#120426=CARTESIAN_POINT('Ctrl Pts',(8.16469935094199,31.5714879934552,125.553282208899));
#120427=CARTESIAN_POINT('Ctrl Pts',(8.16261858217722,31.5817982102992,125.523321172272));
#120428=CARTESIAN_POINT('Ctrl Pts',(8.16132503901361,31.5879259497238,125.504422303556));
#120429=CARTESIAN_POINT('Ctrl Pts',(8.15401450562091,31.6208990948384,125.396165478388));
#120430=CARTESIAN_POINT('Ctrl Pts',(8.14823769707328,31.6405401236333,125.304782311777));
#120431=CARTESIAN_POINT('Ctrl Pts',(8.13815379187163,31.6615214357682,125.14141754525));
#120432=CARTESIAN_POINT('Ctrl Pts',(8.1338271862413,31.6660545215536,125.070101001078));
#120433=CARTESIAN_POINT('Ctrl Pts',(8.12586965586689,31.6659554899448,124.941605152703));
#120434=CARTESIAN_POINT('Ctrl Pts',(8.12227687646165,31.6629748332408,124.884540400681));
#120435=CARTESIAN_POINT('Ctrl Pts',(8.11775371755643,31.6558207837429,124.815718104112));
#120436=CARTESIAN_POINT('Ctrl Pts',(8.11695692623532,31.6544393470652,124.803702493656));
#120437=CARTESIAN_POINT('Ctrl Pts',(8.1156986941528,31.6520722827159,124.784918770768));
#120438=CARTESIAN_POINT('Ctrl Pts',(8.11524200733928,31.651175557281,124.778139599428));
#120439=CARTESIAN_POINT('Ctrl Pts',(8.11437467022709,31.6494024998621,124.765341988591));
#120440=CARTESIAN_POINT('Ctrl Pts',(8.11396450064347,31.6485349133915,124.759322574243));
#120441=CARTESIAN_POINT('Ctrl Pts',(8.11298173515628,31.6463868167796,124.744975613812));
#120442=CARTESIAN_POINT('Ctrl Pts',(8.11240750137777,31.6450760665032,124.736652860589));
#120443=CARTESIAN_POINT('Ctrl Pts',(8.11041880368796,31.6403444299506,124.708023618481));
#120444=CARTESIAN_POINT('Ctrl Pts',(8.10898876159608,31.6366103579801,124.687771722417));
#120445=CARTESIAN_POINT('Ctrl Pts',(8.10537394454592,31.6263309118788,124.637287408729));
#120446=CARTESIAN_POINT('Ctrl Pts',(8.10317148301915,31.6193172228626,124.607158853233));
#120447=CARTESIAN_POINT('Ctrl Pts',(8.09197161397868,31.5797573301492,124.456363388652));
#120448=CARTESIAN_POINT('Ctrl Pts',(8.0827492786961,31.5345391916822,124.339418226514));
#120449=CARTESIAN_POINT('Ctrl Pts',(8.06983431307662,31.4504007392126,124.178347955077));
#120450=CARTESIAN_POINT('Ctrl Pts',(8.06587361593285,31.4215804840318,124.129434323745));
#120451=CARTESIAN_POINT('Ctrl Pts',(8.06078102752913,31.3804668005706,124.067161834185));
#120452=CARTESIAN_POINT('Ctrl Pts',(8.05956981262259,31.3703765665007,124.052401065682));
#120453=CARTESIAN_POINT('Ctrl Pts',(8.05759698623261,31.3534321454635,124.028450341525));
#120454=CARTESIAN_POINT('Ctrl Pts',(8.05683015656659,31.3467174801256,124.019163952884));
#120455=CARTESIAN_POINT('Ctrl Pts',(8.05534300263878,31.3334467009033,124.001203680129));
#120456=CARTESIAN_POINT('Ctrl Pts',(8.05462234735522,31.3269004557831,123.992523259468));
#120457=CARTESIAN_POINT('Ctrl Pts',(8.05292384508931,31.3112009674688,123.97212398091));
#120458=CARTESIAN_POINT('Ctrl Pts',(8.05194892831283,31.3019747844053,123.960462231522));
#120459=CARTESIAN_POINT('Ctrl Pts',(8.04863056139839,31.2698482352999,123.920953559997));
#120460=CARTESIAN_POINT('Ctrl Pts',(8.04631713578434,31.2461998773373,123.893726107727));
#120461=CARTESIAN_POINT('Ctrl Pts',(8.04063836038355,31.1852560975805,123.827995392861));
#120462=CARTESIAN_POINT('Ctrl Pts',(8.03731240113142,31.1469511931257,123.790483397542));
#120463=CARTESIAN_POINT('Ctrl Pts',(8.03042966977431,31.0632888621334,123.716108161257));
#120464=CARTESIAN_POINT('Ctrl Pts',(8.02688373322862,31.0176680829258,123.679654143026));
#120465=CARTESIAN_POINT('Ctrl Pts',(8.01856846521728,30.9072627973995,123.600560960724));
#120466=CARTESIAN_POINT('Ctrl Pts',(8.01378953276452,30.8412350824564,123.559904125507));
#120467=CARTESIAN_POINT('Ctrl Pts',(8.00771114135584,30.7581293055201,123.51640174419));
#120468=CARTESIAN_POINT('Ctrl Pts',(8.00664023293826,30.7435197795543,123.509026453329));
#120469=CARTESIAN_POINT('Ctrl Pts',(8.00504723388949,30.721882482574,123.49850043697));
#120470=CARTESIAN_POINT('Ctrl Pts',(8.00453486656568,30.7149372173345,123.49518106542));
#120471=CARTESIAN_POINT('Ctrl Pts',(8.00361745592655,30.7025324198043,123.489357661751));
#120472=CARTESIAN_POINT('Ctrl Pts',(8.00321356364716,30.697081992667,123.486834851005));
#120473=CARTESIAN_POINT('Ctrl Pts',(8.00231425875376,30.6849709846306,123.481308414496));
#120474=CARTESIAN_POINT('Ctrl Pts',(8.00181803756103,30.6783043106643,123.478319140316));
#120475=CARTESIAN_POINT('Ctrl Pts',(8.00034036016486,30.6584927477178,123.469591879847));
#120476=CARTESIAN_POINT('Ctrl Pts',(7.99935193623896,30.6452935674306,123.463979853512));
#120477=CARTESIAN_POINT('Ctrl Pts',(7.99703551064283,30.6144464083375,123.451332013878));
#120478=CARTESIAN_POINT('Ctrl Pts',(7.99570161230325,30.5967474608037,123.444426368702));
#120479=CARTESIAN_POINT('Ctrl Pts',(7.99093377029377,30.5335897778804,123.421020408171));
#120480=CARTESIAN_POINT('Ctrl Pts',(7.98744347377121,30.4875369236231,123.406198954746));
#120481=CARTESIAN_POINT('Ctrl Pts',(7.97559565026444,30.3301799489671,123.363014573685));
#120482=CARTESIAN_POINT('Ctrl Pts',(7.96719875114672,30.2165916068098,123.344151491891));
#120483=CARTESIAN_POINT('Ctrl Pts',(7.95609761582235,30.0590035474612,123.334489079746));
#120484=CARTESIAN_POINT('Ctrl Pts',(7.95311713213314,30.0159598904829,123.333520505956));
#120485=CARTESIAN_POINT('Ctrl Pts',(7.94907638977623,29.956599414166,123.334485384452));
#120486=CARTESIAN_POINT('Ctrl Pts',(7.94797265909548,29.9402796496154,123.334990673249));
#120487=CARTESIAN_POINT('Ctrl Pts',(7.94620309146414,29.9139521404799,123.336193424277));
#120488=CARTESIAN_POINT('Ctrl Pts',(7.94553264128268,29.9039390013121,123.33674149704));
#120489=CARTESIAN_POINT('Ctrl Pts',(7.94413829492636,29.8830379102962,123.338074906346));
#120490=CARTESIAN_POINT('Ctrl Pts',(7.94341495412745,29.8721514707935,123.338876912879));
#120491=CARTESIAN_POINT('Ctrl Pts',(7.94169720050561,29.8462007216866,123.341045342342));
#120492=CARTESIAN_POINT('Ctrl Pts',(7.94070590647955,29.8311454264068,123.342510050721));
#120493=CARTESIAN_POINT('Ctrl Pts',(7.93726143839548,29.7785836839113,123.348347330616));
#120494=CARTESIAN_POINT('Ctrl Pts',(7.93484157359096,29.7412061589878,123.353789863707));
#120495=CARTESIAN_POINT('Ctrl Pts',(7.92882591070616,29.6476065425237,123.37068610308));
#120496=CARTESIAN_POINT('Ctrl Pts',(7.92527631368619,29.5917303668433,123.383781711775));
#120497=CARTESIAN_POINT('Ctrl Pts',(7.91508382551709,29.4321716469966,123.429982439392));
#120498=CARTESIAN_POINT('Ctrl Pts',(7.90855600761051,29.3309279800054,123.47038475019));
#120499=CARTESIAN_POINT('Ctrl Pts',(7.89966723044288,29.2062870285207,123.534880792568));
#120500=CARTESIAN_POINT('Ctrl Pts',(7.8976360741054,29.178642565453,123.550197862887));
#120501=CARTESIAN_POINT('Ctrl Pts',(7.89489237100837,29.1426951649625,123.571473495394));
#120502=CARTESIAN_POINT('Ctrl Pts',(7.89421944458202,29.1339857973103,123.576736516854));
#120503=CARTESIAN_POINT('Ctrl Pts',(7.89311372364442,29.1198606530076,123.585449909621));
#120504=CARTESIAN_POINT('Ctrl Pts',(7.89268395275239,29.1144154962051,123.588852484168));
#120505=CARTESIAN_POINT('Ctrl Pts',(7.89182829161612,29.103666686415,123.595655923485));
#120506=CARTESIAN_POINT('Ctrl Pts',(7.89140248040706,29.0983624082315,123.599055553105));
#120507=CARTESIAN_POINT('Ctrl Pts',(7.89032204265401,29.0850128985059,123.607718765476));
#120508=CARTESIAN_POINT('Ctrl Pts',(7.88966489768543,29.0769938146294,123.613021989139));
#120509=CARTESIAN_POINT('Ctrl Pts',(7.88698477430282,29.0446751223538,123.634799555874));
#120510=CARTESIAN_POINT('Ctrl Pts',(7.88492900238214,29.0207685383274,123.651844457387));
#120511=CARTESIAN_POINT('Ctrl Pts',(7.87914695340166,28.9556304836782,123.700933313278));
#120512=CARTESIAN_POINT('Ctrl Pts',(7.87537008386222,28.9154370496436,123.734296839081));
#120513=CARTESIAN_POINT('Ctrl Pts',(7.86219594576666,28.7815763555194,123.856475254525));
#120514=CARTESIAN_POINT('Ctrl Pts',(7.85279232132601,28.6966841254842,123.954254516698));
#120515=CARTESIAN_POINT('Ctrl Pts',(7.84182238365393,28.6074816347841,124.084959302965));
#120516=CARTESIAN_POINT('Ctrl Pts',(7.83982287605718,28.59167324514,124.109481717511));
#120517=CARTESIAN_POINT('Ctrl Pts',(7.83691392227666,28.5693587284,124.146178401709));
#120518=CARTESIAN_POINT('Ctrl Pts',(7.83598623183796,28.5623474722054,124.15803741245));
#120519=CARTESIAN_POINT('Ctrl Pts',(7.83434459552105,28.5501317531604,124.179296963083));
#120520=CARTESIAN_POINT('Ctrl Pts',(7.83362860328781,28.5448696935481,124.188663319862));
#120521=CARTESIAN_POINT('Ctrl Pts',(7.83213241674886,28.5340147828956,124.208430185137));
#120522=CARTESIAN_POINT('Ctrl Pts',(7.83135293656554,28.528441150779,124.218840609135));
#120523=CARTESIAN_POINT('Ctrl Pts',(7.82929473910204,28.513946225919,124.246620008103));
#120524=CARTESIAN_POINT('Ctrl Pts',(7.82802283033789,28.5052186200826,124.26408838172));
#120525=CARTESIAN_POINT('Ctrl Pts',(7.82089597060359,28.4576774834777,124.363579566852));
#120526=CARTESIAN_POINT('Ctrl Pts',(7.81526758462706,28.425306763893,124.44851656933));
#120527=CARTESIAN_POINT('Ctrl Pts',(7.80433881143629,28.3755953875649,124.619814571025));
#120528=CARTESIAN_POINT('Ctrl Pts',(7.79904847125346,28.3578543909645,124.705742324073));
#120529=CARTESIAN_POINT('Ctrl Pts',(7.79074311066009,28.3413084843429,124.837657812602));
#120530=CARTESIAN_POINT('Ctrl Pts',(7.78786345525984,28.3375047801776,124.882861691838));
#120531=CARTESIAN_POINT('Ctrl Pts',(7.78414759032397,28.3350575775181,124.939560393859));
#120532=CARTESIAN_POINT('Ctrl Pts',(7.78339488069868,28.3346826716383,124.950965376616));
#120533=CARTESIAN_POINT('Ctrl Pts',(7.78219093552553,28.3342738578325,124.96906165323));
#120534=CARTESIAN_POINT('Ctrl Pts',(7.78174380255814,28.3341630486648,124.975751090097));
#120535=CARTESIAN_POINT('Ctrl Pts',(7.78088226895111,28.3340278724356,124.988575816032));
#120536=CARTESIAN_POINT('Ctrl Pts',(7.78046821761287,28.3339971004304,124.994710827184));
#120537=CARTESIAN_POINT('Ctrl Pts',(7.77945854909367,28.3340046610185,125.009604853838));
#120538=CARTESIAN_POINT('Ctrl Pts',(7.77886105007367,28.3340781852903,125.018363592065));
#120539=CARTESIAN_POINT('Ctrl Pts',(7.77669705871863,28.3345916740203,125.049902096294));
#120540=CARTESIAN_POINT('Ctrl Pts',(7.77511123981863,28.3354298441543,125.072671740563));
#120541=CARTESIAN_POINT('Ctrl Pts',(7.76331096249049,28.345034490146,125.240097979747));
#120542=CARTESIAN_POINT('Ctrl Pts',(7.75253210682085,28.3721755996099,125.383078773499));
#120543=CARTESIAN_POINT('Ctrl Pts',(7.73764260775917,28.4373656924348,125.581186869983));
#120544=CARTESIAN_POINT('Ctrl Pts',(7.73318430821949,28.4607010085987,125.64044090245));
#120545=CARTESIAN_POINT('Ctrl Pts',(7.72757582582287,28.4951096077819,125.714983742574));
#120546=CARTESIAN_POINT('Ctrl Pts',(7.72632414020747,28.5031253860173,125.731616895899));
#120547=CARTESIAN_POINT('Ctrl Pts',(7.72430276290603,28.5166172616756,125.758462787412));
#120548=CARTESIAN_POINT('Ctrl Pts',(7.72352734323422,28.5219261306994,125.768757306863));
#120549=CARTESIAN_POINT('Ctrl Pts',(7.72203505804241,28.5323997074546,125.788557150542));
#120550=CARTESIAN_POINT('Ctrl Pts',(7.72131774822327,28.5375504662946,125.798069150583));
#120551=CARTESIAN_POINT('Ctrl Pts',(7.71964469751258,28.5498350382943,125.820236928453));
#120552=CARTESIAN_POINT('Ctrl Pts',(7.71869163853259,28.5570425427458,125.832851027241));
#120553=CARTESIAN_POINT('Ctrl Pts',(7.71553504002844,28.5816042387835,125.874561091506));
#120554=CARTESIAN_POINT('Ctrl Pts',(7.71335758306803,28.5996813934821,125.903222945534));
#120555=CARTESIAN_POINT('Ctrl Pts',(7.70809545278324,28.6460105336811,125.971940920347));
#120556=CARTESIAN_POINT('Ctrl Pts',(7.70504261989538,28.6751801135217,126.011340408464));
#120557=CARTESIAN_POINT('Ctrl Pts',(7.69595441545285,28.768005958698,126.125798667521));
#120558=CARTESIAN_POINT('Ctrl Pts',(7.6900402606431,28.836607764046,126.196557224185));
#120559=CARTESIAN_POINT('Ctrl Pts',(7.68066372424506,28.9508398064102,126.29521557618));
#120560=CARTESIAN_POINT('Ctrl Pts',(7.67734412115297,28.9922324149247,126.327676101586));
#120561=CARTESIAN_POINT('Ctrl Pts',(7.67313254270442,29.0447190292049,126.364966637521));
#120562=CARTESIAN_POINT('Ctrl Pts',(7.67235362444439,29.0544249119742,126.371708200758));
#120563=CARTESIAN_POINT('Ctrl Pts',(7.67111739632021,29.0698095114343,126.382153249063));
#120564=CARTESIAN_POINT('Ctrl Pts',(7.67066457148278,29.0754407375763,126.385926446496));
#120565=CARTESIAN_POINT('Ctrl Pts',(7.66979974185772,29.0861838383295,126.393030238777));
#120566=CARTESIAN_POINT('Ctrl Pts',(7.66938816571084,29.0912911931432,126.396367259283));
#120567=CARTESIAN_POINT('Ctrl Pts',(7.66839526749728,29.1036014817378,126.404314363718));
#120568=CARTESIAN_POINT('Ctrl Pts',(7.66781221520989,29.1108217379869,126.408897138234));
#120569=CARTESIAN_POINT('Ctrl Pts',(7.66575853836856,29.1362343295871,126.424753636516));
#120570=CARTESIAN_POINT('Ctrl Pts',(7.66427099435488,29.1546075098037,126.435731691455));
#120571=CARTESIAN_POINT('Ctrl Pts',(7.66047464353693,29.2015303646166,126.462555363645));
#120572=CARTESIAN_POINT('Ctrl Pts',(7.65814600305316,29.2303433361172,126.47792094369));
#120573=CARTESIAN_POINT('Ctrl Pts',(7.64516265713269,29.3919913425261,126.558116536754));
#120574=CARTESIAN_POINT('Ctrl Pts',(7.63424581479998,29.5325789428854,126.605905413153));
#120575=CARTESIAN_POINT('Ctrl Pts',(7.62134585339485,29.713652597349,126.641617849186));
#120576=CARTESIAN_POINT('Ctrl Pts',(7.61881405646138,29.7499010111748,126.647529926132));
#120577=CARTESIAN_POINT('Ctrl Pts',(7.61527680714111,29.8015385445396,126.654208148241));
#120578=CARTESIAN_POINT('Ctrl Pts',(7.61424077930881,29.8167862213805,126.655966269499));
#120579=CARTESIAN_POINT('Ctrl Pts',(7.61248389057747,29.8428473532705,126.658606850407));
#120580=CARTESIAN_POINT('Ctrl Pts',(7.61175976728051,29.8536488696803,126.659594828515));
#120581=CARTESIAN_POINT('Ctrl Pts',(7.61028862612303,29.8757120741823,126.661395791455));
#120582=CARTESIAN_POINT('Ctrl Pts',(7.6095419220133,29.8869739334423,126.662199922772));
#120583=CARTESIAN_POINT('Ctrl Pts',(7.60767544364632,29.9152762451372,126.663931817031));
#120584=CARTESIAN_POINT('Ctrl Pts',(7.60656030149541,29.9323246544792,126.664712374313));
#120585=CARTESIAN_POINT('Ctrl Pts',(7.60197943443788,30.0028814755744,126.666857064561));
#120586=CARTESIAN_POINT('Ctrl Pts',(7.59858554710241,30.05643108293,126.665904314293));
#120587=CARTESIAN_POINT('Ctrl Pts',(7.58950602481521,30.2015769896193,126.656313364939));
#120588=CARTESIAN_POINT('Ctrl Pts',(7.58394572145114,30.2926485133906,126.642670006646));
#120589=CARTESIAN_POINT('Ctrl Pts',(7.5737204231737,30.4550977610937,126.604388273474));
#120590=CARTESIAN_POINT('Ctrl Pts',(7.56908774313582,30.5268119690066,126.582290193669));
#120591=CARTESIAN_POINT('Ctrl Pts',(7.56317059711611,30.6120673691395,126.549579762324));
#120592=CARTESIAN_POINT('Ctrl Pts',(7.56209954095448,30.627261036796,126.543491965252));
#120593=CARTESIAN_POINT('Ctrl Pts',(7.56050636309539,30.6494648494323,126.534213372519));
#120594=CARTESIAN_POINT('Ctrl Pts',(7.55999396781632,30.6565470229436,126.531196023996));
#120595=CARTESIAN_POINT('Ctrl Pts',(7.55907652799532,30.6691170721733,126.525737336162));
#120596=CARTESIAN_POINT('Ctrl Pts',(7.55867263480671,30.674613021977,126.523315247564));
#120597=CARTESIAN_POINT('Ctrl Pts',(7.55777335390008,30.6867653101072,126.517881018139));
#120598=CARTESIAN_POINT('Ctrl Pts',(7.55727715788175,30.6934149093771,126.514854823003));
#120599=CARTESIAN_POINT('Ctrl Pts',(7.55579963001501,30.713057652568,126.505759092814));
#120600=CARTESIAN_POINT('Ctrl Pts',(7.55481133247162,30.7259921883703,126.499565593588));
#120601=CARTESIAN_POINT('Ctrl Pts',(7.55249525598461,30.7558692866738,126.484782281322));
#120602=CARTESIAN_POINT('Ctrl Pts',(7.55116158268466,30.7727478972863,126.476068231195));
#120603=CARTESIAN_POINT('Ctrl Pts',(7.54639489054645,30.8320464692208,126.444157899682));
#120604=CARTESIAN_POINT('Ctrl Pts',(7.54290554430773,30.873599932571,126.419406899207));
#120605=CARTESIAN_POINT('Ctrl Pts',(7.53106201613659,31.0099762168683,126.329916404571));
#120606=CARTESIAN_POINT('Ctrl Pts',(7.5226683822198,31.0991858730792,126.257189773572));
#120607=CARTESIAN_POINT('Ctrl Pts',(7.51156652673191,31.2106227338073,126.145340503689));
#120608=CARTESIAN_POINT('Ctrl Pts',(7.50858254789901,31.2398384763245,126.113648690396));
#120609=CARTESIAN_POINT('Ctrl Pts',(7.50453794722115,31.2783913784705,126.068427934785));
#120610=CARTESIAN_POINT('Ctrl Pts',(7.50343374417013,31.288804792686,126.055843268544));
#120611=CARTESIAN_POINT('Ctrl Pts',(7.50166362390539,31.3053110616948,126.035287212402));
#120612=CARTESIAN_POINT('Ctrl Pts',(7.50099308793677,31.3115197145778,126.02741064128));
#120613=CARTESIAN_POINT('Ctrl Pts',(7.49959871809119,31.3243358946151,126.010845964487));
#120614=CARTESIAN_POINT('Ctrl Pts',(7.49887543829594,31.3309299465244,126.002147999434));
#120615=CARTESIAN_POINT('Ctrl Pts',(7.49715811276073,31.3464535458631,125.981247905099));
#120616=CARTESIAN_POINT('Ctrl Pts',(7.49616718161414,31.3553034952546,125.968987648509));
#120617=CARTESIAN_POINT('Ctrl Pts',(7.49272555565311,31.3856443051889,125.92572602529));
#120618=CARTESIAN_POINT('Ctrl Pts',(7.49030809399141,31.406249144935,125.894115482181));
#120619=CARTESIAN_POINT('Ctrl Pts',(7.48276440726234,31.4679467320688,125.792046451093));
#120620=CARTESIAN_POINT('Ctrl Pts',(7.47776961305755,31.5049504781821,125.719257086047));
#120621=CARTESIAN_POINT('Ctrl Pts',(7.4712888155576,31.5459710599474,125.621395714317));
#120622=CARTESIAN_POINT('Ctrl Pts',(7.46979075119214,31.5549606711069,125.598544757198));
#120623=CARTESIAN_POINT('Ctrl Pts',(7.46828911258472,31.5634400017109,125.575509653308));
#120624=CARTESIAN_POINT('Origin',(5.,30.,125.));
#120625=CARTESIAN_POINT('',(6.76893575384937,31.5634399863339,125.575509695081));
#120626=CARTESIAN_POINT('',(6.96167312081938,31.563440026896,125.575509584889));
#120627=CARTESIAN_POINT('',(5.,31.5634400119422,125.575509625513));
#120628=CARTESIAN_POINT('Ctrl Pts',(6.96167312081939,31.563440026896,125.575509584889));
#120629=CARTESIAN_POINT('Ctrl Pts',(6.966193296855,31.5383945792393,125.643548513147));
#120630=CARTESIAN_POINT('Ctrl Pts',(6.97060998878207,31.508927581491,125.709898684935));
#120631=CARTESIAN_POINT('Ctrl Pts',(6.98041882974021,31.434304076632,125.852103848172));
#120632=CARTESIAN_POINT('Ctrl Pts',(6.98580007636323,31.3872769350315,125.926697516622));
#120633=CARTESIAN_POINT('Ctrl Pts',(6.99272052682677,31.3230206764459,126.012692190723));
#120634=CARTESIAN_POINT('Ctrl Pts',(6.99397971085297,31.3111898490752,126.027964145805));
#120635=CARTESIAN_POINT('Ctrl Pts',(6.99579918287312,31.2939506793452,126.049435659761));
#120636=CARTESIAN_POINT('Ctrl Pts',(6.99634539860296,31.2887573309838,126.055806847573));
#120637=CARTESIAN_POINT('Ctrl Pts',(6.9972998046712,31.2796567776652,126.066804197838));
#120638=CARTESIAN_POINT('Ctrl Pts',(6.99770646371591,31.2757711531439,126.071447912225));
#120639=CARTESIAN_POINT('Ctrl Pts',(6.99858399855288,31.2673707392771,126.081376771098));
#120640=CARTESIAN_POINT('Ctrl Pts',(6.99905539992462,31.2628482338718,126.086654795989));
#120641=CARTESIAN_POINT('Ctrl Pts',(7.00036576565738,31.2502460926146,126.101177301433));
#120642=CARTESIAN_POINT('Ctrl Pts',(7.00120947711509,31.2420972770347,126.110360785311));
#120643=CARTESIAN_POINT('Ctrl Pts',(7.00711662413704,31.1847569073055,126.173560669269));
#120644=CARTESIAN_POINT('Ctrl Pts',(7.01238149070013,31.132165000168,126.224374787963));
#120645=CARTESIAN_POINT('Ctrl Pts',(7.0186672546681,31.0661255139492,126.280278935297));
#120646=CARTESIAN_POINT('Ctrl Pts',(7.01964800295812,31.0557301374573,126.288864475846));
#120647=CARTESIAN_POINT('Ctrl Pts',(7.02603795929059,30.9873606527184,126.343948648749));
#120648=CARTESIAN_POINT('Ctrl Pts',(7.03144852766284,30.9264308950238,126.386652860934));
#120649=CARTESIAN_POINT('Ctrl Pts',(7.03979527649104,30.8263888625795,126.447222923726));
#120650=CARTESIAN_POINT('Ctrl Pts',(7.04280072172926,30.7890915576832,126.467892285816));
#120651=CARTESIAN_POINT('Ctrl Pts',(7.04788798330599,30.7236690833864,126.500932806407));
#120652=CARTESIAN_POINT('Ctrl Pts',(7.04999144044879,30.695920559973,126.513998355545));
#120653=CARTESIAN_POINT('Ctrl Pts',(7.05301661758845,30.655007516378,126.531899771618));
#120654=CARTESIAN_POINT('Ctrl Pts',(7.05395888293745,30.6421190293987,126.537346717438));
#120655=CARTESIAN_POINT('Ctrl Pts',(7.0556149281266,30.6192154691299,126.546687951303));
#120656=CARTESIAN_POINT('Ctrl Pts',(7.05633092151664,30.6092286283953,126.550648865331));
#120657=CARTESIAN_POINT('Ctrl Pts',(7.05782810090738,30.5881718479604,126.558765430803));
#120658=CARTESIAN_POINT('Ctrl Pts',(7.05860856276711,30.5770945408188,126.562900410803));
#120659=CARTESIAN_POINT('Ctrl Pts',(7.06067168290318,30.5475525795693,126.573571031546));
#120660=CARTESIAN_POINT('Ctrl Pts',(7.06194747625012,30.5290147495355,126.579899701239));
#120661=CARTESIAN_POINT('Ctrl Pts',(7.06853353903769,30.432005823576,126.611118781296));
#120662=CARTESIAN_POINT('Ctrl Pts',(7.07366166483805,30.3518763143641,126.630496332782));
#120663=CARTESIAN_POINT('Ctrl Pts',(7.08488643070133,30.1715630175352,126.660181672029));
#120664=CARTESIAN_POINT('Ctrl Pts',(7.09092316836261,30.0712272551629,126.667501538973));
#120665=CARTESIAN_POINT('Ctrl Pts',(7.09899128376423,29.9425468691838,126.665249663901));
#120666=CARTESIAN_POINT('Ctrl Pts',(7.1007857676625,29.9142626508337,126.664033122141));
#120667=CARTESIAN_POINT('Ctrl Pts',(7.10385579548681,29.8667521117274,126.660775175668));
#120668=CARTESIAN_POINT('Ctrl Pts',(7.10511498015536,29.8475048510824,126.659118541673));
#120669=CARTESIAN_POINT('Ctrl Pts',(7.10693445294361,29.8201157786704,126.656280541303));
#120670=CARTESIAN_POINT('Ctrl Pts',(7.1074806687826,29.8119463789569,126.655372886448));
#120671=CARTESIAN_POINT('Ctrl Pts',(7.10843507497376,29.7977712108058,126.653691682864));
#120672=CARTESIAN_POINT('Ctrl Pts',(7.10884173403102,29.7917624006745,126.652945784361));
#120673=CARTESIAN_POINT('Ctrl Pts',(7.10971926881462,29.7788646517967,126.651273287378));
#120674=CARTESIAN_POINT('Ctrl Pts',(7.11019067011921,29.7719775096223,126.650336344903));
#120675=CARTESIAN_POINT('Ctrl Pts',(7.11150103548905,29.7529415765722,126.647625223343));
#120676=CARTESIAN_POINT('Ctrl Pts',(7.11234474664724,29.7408065110413,126.645759841031));
#120677=CARTESIAN_POINT('Ctrl Pts',(7.11825181547121,29.6566112920883,126.631863231038));
#120678=CARTESIAN_POINT('Ctrl Pts',(7.12351659796537,29.5853972575236,126.615238561539));
#120679=CARTESIAN_POINT('Ctrl Pts',(7.12985618616815,29.5019033539565,126.589861017168));
#120680=CARTESIAN_POINT('Ctrl Pts',(7.13089098830388,29.4883476775932,126.585550446938));
#120681=CARTESIAN_POINT('Ctrl Pts',(7.1372891050192,29.404922107127,126.557840658739));
#120682=CARTESIAN_POINT('Ctrl Pts',(7.14265240217251,29.3366087604331,126.529999538607));
#120683=CARTESIAN_POINT('Ctrl Pts',(7.15094908680955,29.2320964648863,126.479084760424));
#120684=CARTESIAN_POINT('Ctrl Pts',(7.15395008642306,29.1945589397529,126.458983471565));
#120685=CARTESIAN_POINT('Ctrl Pts',(7.1590307467202,29.1314003294049,126.421980624633));
#120686=CARTESIAN_POINT('Ctrl Pts',(7.16113197204303,29.105401469555,126.405769528781));
#120687=CARTESIAN_POINT('Ctrl Pts',(7.16415458453434,29.0682037118246,126.381125367054));
#120688=CARTESIAN_POINT('Ctrl Pts',(7.1650964678777,29.0566419879583,126.373254267792));
#120689=CARTESIAN_POINT('Ctrl Pts',(7.16675208220771,29.0363772965739,126.359081559794));
#120690=CARTESIAN_POINT('Ctrl Pts',(7.16746802285157,29.027633736103,126.352839701833));
#120691=CARTESIAN_POINT('Ctrl Pts',(7.16896532649102,29.0093927762997,126.339549619986));
#120692=CARTESIAN_POINT('Ctrl Pts',(7.16974596308683,28.9999087909649,126.33248393679));
#120693=CARTESIAN_POINT('Ctrl Pts',(7.17181009374439,28.9749093546767,126.313441774409));
#120694=CARTESIAN_POINT('Ctrl Pts',(7.17308671056739,28.9595283480561,126.301291251019));
#120695=CARTESIAN_POINT('Ctrl Pts',(7.17967188543802,28.8806976045962,126.23672585809));
#120696=CARTESIAN_POINT('Ctrl Pts',(7.18479845117593,28.8209775130676,126.179930992096));
#120697=CARTESIAN_POINT('Ctrl Pts',(7.19602170186277,28.6982586781219,126.044560473895));
#120698=CARTESIAN_POINT('Ctrl Pts',(7.20205843940251,28.6376904265412,125.964234063907));
#120699=CARTESIAN_POINT('Ctrl Pts',(7.21012655465839,28.5697907063525,125.85490273231));
#120700=CARTESIAN_POINT('Ctrl Pts',(7.21192103853971,28.5554724320103,125.830480120127));
#120701=CARTESIAN_POINT('Ctrl Pts',(7.21499106633762,28.5324415648769,125.788797453938));
#120702=CARTESIAN_POINT('Ctrl Pts',(7.21625025099701,28.5233943524098,125.771728493233));
#120703=CARTESIAN_POINT('Ctrl Pts',(7.21806972377346,28.5109238310133,125.74717851116));
#120704=CARTESIAN_POINT('Ctrl Pts',(7.21861593961022,28.5072556024047,125.739822763249));
#120705=CARTESIAN_POINT('Ctrl Pts',(7.21957034579791,28.5009799526793,125.72700176264));
#120706=CARTESIAN_POINT('Ctrl Pts',(7.21997700485396,28.4983476516984,125.721548950972));
#120707=CARTESIAN_POINT('Ctrl Pts',(7.22085453963506,28.4927575135064,125.709805888072));
#120708=CARTESIAN_POINT('Ctrl Pts',(7.22132594093839,28.4898093411323,125.703511536007));
#120709=CARTESIAN_POINT('Ctrl Pts',(7.22263630630562,28.4817626660433,125.686048204548));
#120710=CARTESIAN_POINT('Ctrl Pts',(7.22348001746242,28.4767482312665,125.674841291059));
#120711=CARTESIAN_POINT('Ctrl Pts',(7.22938708606425,28.442758916984,125.596568200993));
#120712=CARTESIAN_POINT('Ctrl Pts',(7.23465186832113,28.418102092124,125.52772156801));
#120713=CARTESIAN_POINT('Ctrl Pts',(7.24099145646593,28.3941387776321,125.443810835012));
#120714=CARTESIAN_POINT('Ctrl Pts',(7.24202625877757,28.390408162747,125.430084220041));
#120715=CARTESIAN_POINT('Ctrl Pts',(7.24842437566815,28.3684413288612,125.344965968219));
#120716=CARTESIAN_POINT('Ctrl Pts',(7.25378767282275,28.3547811606937,125.272472926459));
#120717=CARTESIAN_POINT('Ctrl Pts',(7.26208435754627,28.3408731677075,125.157053246447));
#120718=CARTESIAN_POINT('Ctrl Pts',(7.26508535724185,28.3374021304523,125.114614118249));
#120719=CARTESIAN_POINT('Ctrl Pts',(7.27016601766141,28.3342348719602,125.041482801664));
#120720=CARTESIAN_POINT('Ctrl Pts',(7.27226724302612,28.3337536718893,125.010847710264));
#120721=CARTESIAN_POINT('Ctrl Pts',(7.27528985556495,28.3342835778378,124.966230144794));
#120722=CARTESIAN_POINT('Ctrl Pts',(7.27623173891497,28.3346257674137,124.952247635315));
#120723=CARTESIAN_POINT('Ctrl Pts',(7.27788735325175,28.3355420359784,124.927535617478));
#120724=CARTESIAN_POINT('Ctrl Pts',(7.27860329389593,28.3360438995755,124.916804411885));
#120725=CARTESIAN_POINT('Ctrl Pts',(7.28010059753142,28.3373162347825,124.894271323985));
#120726=CARTESIAN_POINT('Ctrl Pts',(7.28088123412269,28.338108649987,124.882471242065));
#120727=CARTESIAN_POINT('Ctrl Pts',(7.28294536475721,28.34054800367,124.851140342079));
#120728=CARTESIAN_POINT('Ctrl Pts',(7.28422198156203,28.342414082035,124.831628081226));
#120729=CARTESIAN_POINT('Ctrl Pts',(7.29080715586865,28.353903316031,124.730380998343));
#120730=CARTESIAN_POINT('Ctrl Pts',(7.29593372110214,28.3692291218998,124.649404060856));
#120731=CARTESIAN_POINT('Ctrl Pts',(7.30715697173942,28.4164014992063,124.472882515546));
#120732=CARTESIAN_POINT('Ctrl Pts',(7.31319370968902,28.4510371724665,124.378430322264));
#120733=CARTESIAN_POINT('Ctrl Pts',(7.32126182543699,28.5060648200421,124.262087414743));
#120734=CARTESIAN_POINT('Ctrl Pts',(7.32305630937317,28.5188176029647,124.236812060255));
#120735=CARTESIAN_POINT('Ctrl Pts',(7.32612633725581,28.5413459119135,124.194855643275));
#120736=CARTESIAN_POINT('Ctrl Pts',(7.32738552194384,28.5507794064118,124.177997094348));
#120737=CARTESIAN_POINT('Ctrl Pts',(7.32920499475501,28.5646413530681,124.154205037103));
#120738=CARTESIAN_POINT('Ctrl Pts',(7.32975121059729,28.5688317218884,124.147133704909));
#120739=CARTESIAN_POINT('Ctrl Pts',(7.33070561679346,28.5761995160184,124.134907607844));
#120740=CARTESIAN_POINT('Ctrl Pts',(7.33111227585242,28.5793529951318,124.129738687883));
#120741=CARTESIAN_POINT('Ctrl Pts',(7.33198981064104,28.5861869636679,124.118673153631));
#120742=CARTESIAN_POINT('Ctrl Pts',(7.33246121194913,28.5898761402413,124.112782435044));
#120743=CARTESIAN_POINT('Ctrl Pts',(7.33377157732532,28.6001836181937,124.096550588903));
#120744=CARTESIAN_POINT('Ctrl Pts',(7.33461528848609,28.6068793850868,124.086259516398));
#120745=CARTESIAN_POINT('Ctrl Pts',(7.34052235688253,28.6542054326214,124.015251102541));
#120746=CARTESIAN_POINT('Ctrl Pts',(7.34578713890975,28.6986735096762,123.957195891152));
#120747=CARTESIAN_POINT('Ctrl Pts',(7.35212672693545,28.7561737291237,123.891553099738));
#120748=CARTESIAN_POINT('Ctrl Pts',(7.35316152935754,28.7656827057463,123.880974023523));
#120749=CARTESIAN_POINT('Ctrl Pts',(7.35955964627689,28.8252802352485,123.816353646246));
#120750=CARTESIAN_POINT('Ctrl Pts',(7.36492294335048,28.8787760118712,123.765559522229));
#120751=CARTESIAN_POINT('Ctrl Pts',(7.37321962798843,28.9682019155929,123.691275322744));
#120752=CARTESIAN_POINT('Ctrl Pts',(7.37622062767511,29.0019743096699,123.665341694156));
#120753=CARTESIAN_POINT('Ctrl Pts',(7.38130128808386,29.0616973067255,123.623016942581));
#120754=CARTESIAN_POINT('Ctrl Pts',(7.38340251344613,29.0871741957121,123.605997292045));
#120755=CARTESIAN_POINT('Ctrl Pts',(7.38642512598808,29.1249467578543,123.582243523875));
#120756=CARTESIAN_POINT('Ctrl Pts',(7.38736700934347,29.1368796645049,123.574947401198));
#120757=CARTESIAN_POINT('Ctrl Pts',(7.38902262369281,29.1581382583909,123.562314287215));
#120758=CARTESIAN_POINT('Ctrl Pts',(7.38973856434393,29.1674262045092,123.556915704096));
#120759=CARTESIAN_POINT('Ctrl Pts',(7.39123586799713,29.1870473022802,123.545763510524));
#120760=CARTESIAN_POINT('Ctrl Pts',(7.39201650459929,29.1973908427705,123.540029312306));
#120761=CARTESIAN_POINT('Ctrl Pts',(7.39408063527072,29.2250363148598,123.525085964332));
#120762=CARTESIAN_POINT('Ctrl Pts',(7.39535725210117,29.2424415093435,123.516070988316));
#120763=CARTESIAN_POINT('Ctrl Pts',(7.40194242698856,29.3337349497125,123.470810808562));
#120764=CARTESIAN_POINT('Ctrl Pts',(7.40706899273668,29.4100793770008,123.439767700186));
#120765=CARTESIAN_POINT('Ctrl Pts',(7.41829224342091,29.5839674214316,123.383660324616));
#120766=CARTESIAN_POINT('Ctrl Pts',(7.42432898094934,29.6821059613598,123.361531787285));
#120767=CARTESIAN_POINT('Ctrl Pts',(7.43239709619095,29.809695717242,123.344662697421));
#120768=CARTESIAN_POINT('Ctrl Pts',(7.43419158007314,29.8378472940619,123.341668421405));
#120769=CARTESIAN_POINT('Ctrl Pts',(7.43726160787373,29.8853152518913,123.337839781371));
#120770=CARTESIAN_POINT('Ctrl Pts',(7.43852079253511,29.9045952413721,123.336621799531));
#120771=CARTESIAN_POINT('Ctrl Pts',(7.44034026531624,29.9321022065677,123.335363867318));
#120772=CARTESIAN_POINT('Ctrl Pts',(7.44088648115566,29.9403158462684,123.335049142056));
#120773=CARTESIAN_POINT('Ctrl Pts',(7.44184088734762,29.9545835498231,123.334608150853));
#120774=CARTESIAN_POINT('Ctrl Pts',(7.44224754640526,29.9606365184279,123.334454089457));
#120775=CARTESIAN_POINT('Ctrl Pts',(7.44312508118727,29.973639654747,123.33419405571));
#120776=CARTESIAN_POINT('Ctrl Pts',(7.44359648249007,29.9805895808218,123.334098579431));
#120777=CARTESIAN_POINT('Ctrl Pts',(7.44490684785871,29.999817067539,123.333954770206));
#120778=CARTESIAN_POINT('Ctrl Pts',(7.44575055901746,30.0120945892691,123.333998667474));
#120779=CARTESIAN_POINT('Ctrl Pts',(7.45165762904086,30.0974198227322,123.335246928159));
#120780=CARTESIAN_POINT('Ctrl Pts',(7.45692241283013,30.1703124459516,123.341119438285));
#120781=CARTESIAN_POINT('Ctrl Pts',(7.4632620014523,30.2566478753397,123.353825589296));
#120782=CARTESIAN_POINT('Ctrl Pts',(7.46429680272615,30.2706931298021,123.356076781613));
#120783=CARTESIAN_POINT('Ctrl Pts',(7.47069491871232,30.3573070701426,123.371099489073));
#120784=CARTESIAN_POINT('Ctrl Pts',(7.47605821598763,30.4289956167446,123.388494714266));
#120785=CARTESIAN_POINT('Ctrl Pts',(7.48435490041269,30.5399064039931,123.423336230416));
#120786=CARTESIAN_POINT('Ctrl Pts',(7.48735589971121,30.5800113034398,123.437644419683));
#120787=CARTESIAN_POINT('Ctrl Pts',(7.49243655953587,30.6479617717169,123.464864883197));
#120788=CARTESIAN_POINT('Ctrl Pts',(7.49453778469617,30.6760784683834,123.477038279151));
#120789=CARTESIAN_POINT('Ctrl Pts',(7.4975603969953,30.7165215215942,123.495889461756));
#120790=CARTESIAN_POINT('Ctrl Pts',(7.49850228030555,30.7291232914694,123.50195766124));
#120791=CARTESIAN_POINT('Ctrl Pts',(7.50015789459243,30.7512668178171,123.512966184254));
#120792=CARTESIAN_POINT('Ctrl Pts',(7.50087383522634,30.7608398508293,123.517841394651));
#120793=CARTESIAN_POINT('Ctrl Pts',(7.5023711388598,30.7808510729231,123.528277384162));
#120794=CARTESIAN_POINT('Ctrl Pts',(7.50315177545901,30.7912785874679,123.533857419891));
#120795=CARTESIAN_POINT('Ctrl Pts',(7.50521590615963,30.8188270566152,123.548978850164));
#120796=CARTESIAN_POINT('Ctrl Pts',(7.50649252302161,30.8358408834732,123.558712313236));
#120797=CARTESIAN_POINT('Ctrl Pts',(7.51307769939527,30.9233802351038,123.610864425048));
#120798=CARTESIAN_POINT('Ctrl Pts',(7.51820426648427,30.9908673957531,123.658168051287));
#120799=CARTESIAN_POINT('Ctrl Pts',(7.52942751729442,31.1323162742686,123.773828354633));
#120800=CARTESIAN_POINT('Ctrl Pts',(7.53546425372712,31.2041342265591,123.844277081419));
#120801=CARTESIAN_POINT('Ctrl Pts',(7.54353236765408,31.2875067704446,123.942321588919));
#120802=CARTESIAN_POINT('Ctrl Pts',(7.54532685138454,31.3052907946921,123.964348965258));
#120803=CARTESIAN_POINT('Ctrl Pts',(7.54839687894824,31.3342523150708,124.002152344534));
#120804=CARTESIAN_POINT('Ctrl Pts',(7.54965606352714,31.3457323677236,124.017689712884));
#120805=CARTESIAN_POINT('Ctrl Pts',(7.55147553620363,31.3617080004292,124.04011725396));
#120806=CARTESIAN_POINT('Ctrl Pts',(7.55202175202278,31.3664271978291,124.046847194516));
#120807=CARTESIAN_POINT('Ctrl Pts',(7.55297615818503,31.3745359834704,124.058594935591));
#120808=CARTESIAN_POINT('Ctrl Pts',(7.55338281723334,31.3779483298579,124.063596740689));
#120809=CARTESIAN_POINT('Ctrl Pts',(7.55426035200048,31.3852192295387,124.074380208753));
#120810=CARTESIAN_POINT('Ctrl Pts',(7.55473175329769,31.3890688335681,124.0801673614));
#120811=CARTESIAN_POINT('Ctrl Pts',(7.55604211865959,31.3996179521425,124.096243213456));
#120812=CARTESIAN_POINT('Ctrl Pts',(7.55688582981733,31.4062399589624,124.106581902531));
#120813=CARTESIAN_POINT('Ctrl Pts',(7.56279289993928,31.4514685836792,124.178944360683));
#120814=CARTESIAN_POINT('Ctrl Pts',(7.5680576838424,31.4860691735957,124.243369668355));
#120815=CARTESIAN_POINT('Ctrl Pts',(7.57439727268539,31.5222194197738,124.322795185727));
#120816=CARTESIAN_POINT('Ctrl Pts',(7.57543207406137,31.5279457371311,124.335816182902));
#120817=CARTESIAN_POINT('Ctrl Pts',(7.58183019034967,31.5623007978282,124.416732107576));
#120818=CARTESIAN_POINT('Ctrl Pts',(7.58719348782527,31.5865676047445,124.486395326085));
#120819=CARTESIAN_POINT('Ctrl Pts',(7.59549017257246,31.6174497571123,124.598473100837));
#120820=CARTESIAN_POINT('Ctrl Pts',(7.59849117199816,31.6271802811094,124.639927223499));
#120821=CARTESIAN_POINT('Ctrl Pts',(7.60357183201865,31.6411650772316,124.71177877631));
#120822=CARTESIAN_POINT('Ctrl Pts',(7.60567305724997,31.6461871632694,124.742003251707));
#120823=CARTESIAN_POINT('Ctrl Pts',(7.60869566962982,31.6522843227317,124.786205427981));
#120824=CARTESIAN_POINT('Ctrl Pts',(7.60963755295165,31.6540209112374,124.800083897414));
#120825=CARTESIAN_POINT('Ctrl Pts',(7.61129316725043,31.6567820246177,124.824658266149));
#120826=CARTESIAN_POINT('Ctrl Pts',(7.61200910788456,31.6578782171453,124.835345127209));
#120827=CARTESIAN_POINT('Ctrl Pts',(7.61350641150992,31.659963855613,124.857817532346));
#120828=CARTESIAN_POINT('Ctrl Pts',(7.61428704810103,31.660931333749,124.869604552378));
#120829=CARTESIAN_POINT('Ctrl Pts',(7.6163511787599,31.6631684612917,124.900950541348));
#120830=CARTESIAN_POINT('Ctrl Pts',(7.61762779558879,31.6642186433368,124.920523678669));
#120831=CARTESIAN_POINT('Ctrl Pts',(7.62421297105267,31.6678815810625,125.022354719317));
#120832=CARTESIAN_POINT('Ctrl Pts',(7.629339537333,31.6647423567958,125.104709396858));
#120833=CARTESIAN_POINT('Ctrl Pts',(7.64056278794753,31.6442878921592,125.286276751473));
#120834=CARTESIAN_POINT('Ctrl Pts',(7.6465995249291,31.6240523245838,125.384823009938));
#120835=CARTESIAN_POINT('Ctrl Pts',(7.6546676395099,31.5868991330003,125.508043745124));
#120836=CARTESIAN_POINT('Ctrl Pts',(7.65646212331654,31.5780383901506,125.534931737467));
#120837=CARTESIAN_POINT('Ctrl Pts',(7.65860526371597,31.5668323255569,125.566230402364));
#120838=CARTESIAN_POINT('Ctrl Pts',(7.65892464110724,31.5651464584609,125.570873861579));
#120839=CARTESIAN_POINT('Ctrl Pts',(7.65924497815242,31.5634400119496,125.575509625493));
#120840=CARTESIAN_POINT('',(7.4292556837088,31.665999521611,125.001262533919));
#120841=CARTESIAN_POINT('Ctrl Pts',(7.46828911258472,31.5634400017109,125.575509653308));
#120842=CARTESIAN_POINT('Ctrl Pts',(7.46528247231107,31.5804176531656,125.529387856276));
#120843=CARTESIAN_POINT('Ctrl Pts',(7.46226192838087,31.5953496106608,125.482527794622));
#120844=CARTESIAN_POINT('Ctrl Pts',(7.45662573031151,31.6188128575682,125.395797693496));
#120845=CARTESIAN_POINT('Ctrl Pts',(7.45403248721639,31.6279934835074,125.356156576094));
#120846=CARTESIAN_POINT('Ctrl Pts',(7.45064112335473,31.6378167593212,125.305344127953));
#120847=CARTESIAN_POINT('Ctrl Pts',(7.44990977216345,31.6398112597121,125.294444884129));
#120848=CARTESIAN_POINT('Ctrl Pts',(7.44873214131851,31.6428231626362,125.277005159377));
#120849=CARTESIAN_POINT('Ctrl Pts',(7.44828966293518,31.643910597604,125.270476884929));
#120850=CARTESIAN_POINT('Ctrl Pts',(7.44743040643905,31.6459364819821,125.257851038113));
#120851=CARTESIAN_POINT('Ctrl Pts',(7.44701390997584,31.6468800014469,125.251754476398));
#120852=CARTESIAN_POINT('Ctrl Pts',(7.44617153378019,31.6487115998284,125.239468491965));
#120853=CARTESIAN_POINT('Ctrl Pts',(7.44574561059107,31.649598743314,125.233278976747));
#120854=CARTESIAN_POINT('Ctrl Pts',(7.44471964986124,31.6516431637521,125.218420136887));
#120855=CARTESIAN_POINT('Ctrl Pts',(7.44411793239531,31.6527670413154,125.209746503644));
#120856=CARTESIAN_POINT('Ctrl Pts',(7.44202256058211,31.6564236033363,125.17967008459));
#120857=CARTESIAN_POINT('Ctrl Pts',(7.4405132147872,31.6586091277853,125.158228174088));
#120858=CARTESIAN_POINT('Ctrl Pts',(7.43579240609516,31.664090141318,125.091679863765));
#120859=CARTESIAN_POINT('Ctrl Pts',(7.43253489000666,31.6659652551283,125.046479492374));
#120860=CARTESIAN_POINT('Ctrl Pts',(7.4292556837088,31.665999521611,125.001262533919));
#120861=CARTESIAN_POINT('Ctrl Pts',(7.42925582289325,31.6659995201555,125.001264453133));
#120862=CARTESIAN_POINT('Ctrl Pts',(7.41937353690219,31.6661029433549,124.864997638634));
#120863=CARTESIAN_POINT('Ctrl Pts',(7.40939537630788,31.6494867121614,124.729197380578));
#120864=CARTESIAN_POINT('Ctrl Pts',(7.39773129809934,31.6088690801473,124.566304180783));
#120865=CARTESIAN_POINT('Ctrl Pts',(7.39556508607674,31.6003655312297,124.535907141989));
#120866=CARTESIAN_POINT('Ctrl Pts',(7.39246811501382,31.5868076548228,124.492262396981));
#120867=CARTESIAN_POINT('Ctrl Pts',(7.3915154034024,31.5824402979764,124.478810272853));
#120868=CARTESIAN_POINT('Ctrl Pts',(7.38984771654489,31.5744492670533,124.455223631478));
#120869=CARTESIAN_POINT('Ctrl Pts',(7.38913041941947,31.5708977536186,124.445065730701));
#120870=CARTESIAN_POINT('Ctrl Pts',(7.38763697719301,31.5632644351025,124.423893888299));
#120871=CARTESIAN_POINT('Ctrl Pts',(7.38686149381992,31.559164058377,124.412887236588));
#120872=CARTESIAN_POINT('Ctrl Pts',(7.3848264162618,31.5480445291983,124.383977361271));
#120873=CARTESIAN_POINT('Ctrl Pts',(7.38357335230851,31.5408310963366,124.36615038208));
#120874=CARTESIAN_POINT('Ctrl Pts',(7.37751431785362,31.5041856583478,124.279911452624));
#120875=CARTESIAN_POINT('Ctrl Pts',(7.37285456558696,31.4704961988646,124.213396596589));
#120876=CARTESIAN_POINT('Ctrl Pts',(7.36165097278908,31.3776634283298,124.057068934145));
#120877=CARTESIAN_POINT('Ctrl Pts',(7.35521639351726,31.3140763664132,123.970302805046));
#120878=CARTESIAN_POINT('Ctrl Pts',(7.3466654863898,31.2231005808139,123.868435979257));
#120879=CARTESIAN_POINT('Ctrl Pts',(7.34481285502146,31.2030395334059,123.847130602155));
#120880=CARTESIAN_POINT('Ctrl Pts',(7.34167298585398,31.1687020394077,123.812535792505));
#120881=CARTESIAN_POINT('Ctrl Pts',(7.34040380462425,31.1547340779628,123.798948447985));
#120882=CARTESIAN_POINT('Ctrl Pts',(7.33859560784482,31.1347733246387,123.780201692698));
#120883=CARTESIAN_POINT('Ctrl Pts',(7.33807113148018,31.1289766151009,123.774834621293));
#120884=CARTESIAN_POINT('Ctrl Pts',(7.33753987871096,31.1231009888508,123.769471588325));
#120885=CARTESIAN_POINT('Ctrl Pts',(7.33753616151487,31.1230598766707,123.769434066573));
#120886=CARTESIAN_POINT('Ctrl Pts',(7.33752865416081,31.1229768449558,123.769358293851));
#120887=CARTESIAN_POINT('Ctrl Pts',(7.33752486401972,31.1229349256002,123.769320043193));
#120888=CARTESIAN_POINT('Ctrl Pts',(7.33751720695663,31.1228502372749,123.769242774548));
#120889=CARTESIAN_POINT('Ctrl Pts',(7.33751334000804,31.1228074680027,123.769203756445));
#120890=CARTESIAN_POINT('Ctrl Pts',(7.33750552526399,31.1227210348509,123.769124912351));
#120891=CARTESIAN_POINT('Ctrl Pts',(7.33750157745753,31.1226773708409,123.769085086412));
#120892=CARTESIAN_POINT('Ctrl Pts',(7.33749359666524,31.1225891002702,123.769004583437));
#120893=CARTESIAN_POINT('Ctrl Pts',(7.3374895636713,31.1225444936103,123.768963906496));
#120894=CARTESIAN_POINT('Ctrl Pts',(7.33748140788969,31.1224542866775,123.768881655515));
#120895=CARTESIAN_POINT('Ctrl Pts',(7.33747728511051,31.1224086864881,123.768840081751));
#120896=CARTESIAN_POINT('Ctrl Pts',(7.33746894485562,31.1223164382404,123.768755988263));
#120897=CARTESIAN_POINT('Ctrl Pts',(7.33746472737942,31.1222697901659,123.768713468739));
#120898=CARTESIAN_POINT('Ctrl Pts',(7.33745619252152,31.1221753885036,123.768627431842));
#120899=CARTESIAN_POINT('Ctrl Pts',(7.33745187511125,31.1221276345881,123.768583914403));
#120900=CARTESIAN_POINT('Ctrl Pts',(7.33744313479236,31.1220309593503,123.768495825976));
#120901=CARTESIAN_POINT('Ctrl Pts',(7.33743871187758,31.1219820379475,123.768451255166));
#120902=CARTESIAN_POINT('Ctrl Pts',(7.33742975457208,31.1218829615832,123.768361000491));
#120903=CARTESIAN_POINT('Ctrl Pts',(7.33742522016576,31.1218328064357,123.768315316728));
#120904=CARTESIAN_POINT('Ctrl Pts',(7.33741603348765,31.1217311918706,123.768222772565));
#120905=CARTESIAN_POINT('Ctrl Pts',(7.33741138118688,31.1216797321178,123.768175912153));
#120906=CARTESIAN_POINT('Ctrl Pts',(7.33740195183875,31.1215754321889,123.76808094624));
#120907=CARTESIAN_POINT('Ctrl Pts',(7.33739717479071,31.1215225919898,123.768032841037));
#120908=CARTESIAN_POINT('Ctrl Pts',(7.3373874885513,31.121415449308,123.767935311988));
#120909=CARTESIAN_POINT('Ctrl Pts',(7.3373825793752,31.1213611469773,123.767885888628));
#120910=CARTESIAN_POINT('Ctrl Pts',(7.33737262096932,31.1212509924865,123.767785644642));
#120911=CARTESIAN_POINT('Ctrl Pts',(7.33736757170755,31.1211951399545,123.767734824056));
#120912=CARTESIAN_POINT('Ctrl Pts',(7.33735732457755,31.1210817904038,123.76763170064));
#120913=CARTESIAN_POINT('Ctrl Pts',(7.33735212670209,31.1210242932854,123.767579398133));
#120914=CARTESIAN_POINT('Ctrl Pts',(7.33734157312457,31.1209075525183,123.767473219309));
#120915=CARTESIAN_POINT('Ctrl Pts',(7.33733621738728,31.1208483084581,123.76741934307));
#120916=CARTESIAN_POINT('Ctrl Pts',(7.33732533810009,31.1207279632852,123.767309917648));
#120917=CARTESIAN_POINT('Ctrl Pts',(7.33731981453915,31.1206668620269,123.767254368828));
#120918=CARTESIAN_POINT('Ctrl Pts',(7.33730858880094,31.1205426828837,123.767141491046));
#120919=CARTESIAN_POINT('Ctrl Pts',(7.33730288659491,31.1204796046552,123.767084162314));
#120920=CARTESIAN_POINT('Ctrl Pts',(7.33729129183352,31.1203513417109,123.76696760834));
#120921=CARTESIAN_POINT('Ctrl Pts',(7.33728539926978,31.1202861568746,123.766908383585));
#120922=CARTESIAN_POINT('Ctrl Pts',(7.33727341106456,31.1201535398343,123.76678791139));
#120923=CARTESIAN_POINT('Ctrl Pts',(7.33726731537992,31.1200861071227,123.766726664146));
#120924=CARTESIAN_POINT('Ctrl Pts',(7.33725490705958,31.1199488407774,123.766602009512));
#120925=CARTESIAN_POINT('Ctrl Pts',(7.33724859438879,31.1198790067224,123.766538602469));
#120926=CARTESIAN_POINT('Ctrl Pts',(7.33723573693869,31.1197367699204,123.766409478129));
#120927=CARTESIAN_POINT('Ctrl Pts',(7.33722919213803,31.1196643669009,123.766343761393));
#120928=CARTESIAN_POINT('Ctrl Pts',(7.33721585387418,31.1195168089391,123.766209853824));
#120929=CARTESIAN_POINT('Ctrl Pts',(7.33720906037137,31.1194416535188,123.766141663453));
#120930=CARTESIAN_POINT('Ctrl Pts',(7.33719520656172,31.1192883899504,123.766002629159));
#120931=CARTESIAN_POINT('Ctrl Pts',(7.33718814621274,31.1192102812924,123.765931785771));
#120932=CARTESIAN_POINT('Ctrl Pts',(7.3371737387784,31.1190508906176,123.765787248386));
#120933=CARTESIAN_POINT('Ctrl Pts',(7.3371663916499,31.1189696080753,123.765713555028));
#120934=CARTESIAN_POINT('Ctrl Pts',(7.33715138871921,31.1188036268043,123.765563100958));
#120935=CARTESIAN_POINT('Ctrl Pts',(7.33714373286178,31.118718927411,123.765486340894));
#120936=CARTESIAN_POINT('Ctrl Pts',(7.3371280882549,31.1185458443574,123.765329514286));
#120937=CARTESIAN_POINT('Ctrl Pts',(7.33712009945392,31.1184574600676,123.765249448576));
#120938=CARTESIAN_POINT('Ctrl Pts',(7.33710376216209,31.1182767105816,123.765085746257));
#120939=CARTESIAN_POINT('Ctrl Pts',(7.33709541361698,31.1181843447192,123.765002110629));
#120940=CARTESIAN_POINT('Ctrl Pts',(7.33707832712759,31.1179953032151,123.764830975538));
#120941=CARTESIAN_POINT('Ctrl Pts',(7.33706958909751,31.1178986265508,123.764743476942));
#120942=CARTESIAN_POINT('Ctrl Pts',(7.3370516905616,31.117700597289,123.764564290018));
#120943=CARTESIAN_POINT('Ctrl Pts',(7.33704252998437,31.1175992438194,123.764472602937));
#120944=CARTESIAN_POINT('Ctrl Pts',(7.33663051097191,31.1130405871212,123.760349739096));
#120945=CARTESIAN_POINT('Ctrl Pts',(7.33622583397279,31.1085617479838,123.756342906941));
#120946=CARTESIAN_POINT('Ctrl Pts',(7.33529421312361,31.098247376848,123.747215512927));
#120947=CARTESIAN_POINT('Ctrl Pts',(7.33476611633774,31.0923976802799,123.742111462052));
#120948=CARTESIAN_POINT('Ctrl Pts',(7.3331321883631,31.0742834723832,123.726527872219));
#120949=CARTESIAN_POINT('Ctrl Pts',(7.33201734982392,31.0619026608961,123.716185788276));
#120950=CARTESIAN_POINT('Ctrl Pts',(7.325242972604,30.986433384442,123.654982481198));
#120951=CARTESIAN_POINT('Ctrl Pts',(7.31936056575535,30.9198580235857,123.608604409793));
#120952=CARTESIAN_POINT('Ctrl Pts',(7.30809836245104,30.7867863116177,123.529640447671));
#120953=CARTESIAN_POINT('Ctrl Pts',(7.30273291631078,30.7209613298933,123.496269310114));
#120954=CARTESIAN_POINT('Ctrl Pts',(7.29443950023808,30.6140478668175,123.450707626018));
#120955=CARTESIAN_POINT('Ctrl Pts',(7.29144360593981,30.5743311312966,123.435549330816));
#120956=CARTESIAN_POINT('Ctrl Pts',(7.28637064825851,30.505096592487,123.412117956902));
#120957=CARTESIAN_POINT('Ctrl Pts',(7.28427210425098,30.4758517140761,123.403110113347));
#120958=CARTESIAN_POINT('Ctrl Pts',(7.28125274878252,30.4329080379419,123.391167511752));
#120959=CARTESIAN_POINT('Ctrl Pts',(7.28031149801141,30.4193955435292,123.387592252779));
#120960=CARTESIAN_POINT('Ctrl Pts',(7.2786567825405,30.3954242970259,123.381571459597));
#120961=CARTESIAN_POINT('Ctrl Pts',(7.27794111295128,30.3849840506785,123.379056260978));
#120962=CARTESIAN_POINT('Ctrl Pts',(7.27644417505223,30.3629979808563,123.373983921072));
#120963=CARTESIAN_POINT('Ctrl Pts',(7.27566363458848,30.3514477443983,123.37144839869));
#120964=CARTESIAN_POINT('Ctrl Pts',(7.27359930557026,30.320679814854,123.365036770782));
#120965=CARTESIAN_POINT('Ctrl Pts',(7.2723224001043,30.3014186786258,123.361376450386));
#120966=CARTESIAN_POINT('Ctrl Pts',(7.26571999820734,30.2007296445294,123.344077405669));
#120967=CARTESIAN_POINT('Ctrl Pts',(7.26057778543781,30.1184307844295,123.336164471575));
#120968=CARTESIAN_POINT('Ctrl Pts',(7.24935294498439,29.9357146444029,123.332228951831));
#120969=CARTESIAN_POINT('Ctrl Pts',(7.24332887437045,29.8355699653185,123.339110691048));
#120970=CARTESIAN_POINT('Ctrl Pts',(7.23527606601592,29.7087343964665,123.359414741836));
#120971=CARTESIAN_POINT('Ctrl Pts',(7.23348337380518,29.6809318527754,123.364594552332));
#120972=CARTESIAN_POINT('Ctrl Pts',(7.23041617170141,29.6343966103914,123.374496158519));
#120973=CARTESIAN_POINT('Ctrl Pts',(7.22915798482784,29.6155892186855,123.378840892919));
#120974=CARTESIAN_POINT('Ctrl Pts',(7.22733980331298,29.5888910660702,123.38549916653));
#120975=CARTESIAN_POINT('Ctrl Pts',(7.22679385707214,29.5809345988379,123.387546069066));
#120976=CARTESIAN_POINT('Ctrl Pts',(7.22583986229258,29.5671429294275,123.391203121538));
#120977=CARTESIAN_POINT('Ctrl Pts',(7.22543334298627,29.5613008356146,123.39278636096));
#120978=CARTESIAN_POINT('Ctrl Pts',(7.22455605382618,29.5487701592848,123.396255655983));
#120979=CARTESIAN_POINT('Ctrl Pts',(7.22408475816362,29.5420848112174,123.398151703314));
#120980=CARTESIAN_POINT('Ctrl Pts',(7.22277458222512,29.5236222156625,123.403512944597));
#120981=CARTESIAN_POINT('Ctrl Pts',(7.22193095520257,29.5118713847495,123.407066497199));
#120982=CARTESIAN_POINT('Ctrl Pts',(7.21600299706765,29.4301802168941,123.432759364924));
#120983=CARTESIAN_POINT('Ctrl Pts',(7.21071556310233,29.3617367273716,123.459365259678));
#120984=CARTESIAN_POINT('Ctrl Pts',(7.20436849991623,29.2825747268916,123.496320015939));
#120985=CARTESIAN_POINT('Ctrl Pts',(7.20334863341958,29.2699476203082,123.502409923847));
#120986=CARTESIAN_POINT('Ctrl Pts',(7.19696312729404,29.1914119613713,123.541516098445));
#120987=CARTESIAN_POINT('Ctrl Pts',(7.19159768383466,29.1276743327996,123.578719186341));
#120988=CARTESIAN_POINT('Ctrl Pts',(7.18330426215173,29.0314098772701,123.643830826896));
#120989=CARTESIAN_POINT('Ctrl Pts',(7.18030836001311,28.9971337095694,123.668977326521));
#120990=CARTESIAN_POINT('Ctrl Pts',(7.17523539068563,28.9398975297436,123.714436035617));
#120991=CARTESIAN_POINT('Ctrl Pts',(7.17313684273824,28.9164682313566,123.734120434774));
#120992=CARTESIAN_POINT('Ctrl Pts',(7.17011748274211,28.8831435732529,123.763722091573));
#120993=CARTESIAN_POINT('Ctrl Pts',(7.16917623129671,28.8728111431952,123.773135440809));
#120994=CARTESIAN_POINT('Ctrl Pts',(7.16752151506618,28.8547516608461,123.790009274101));
#120995=CARTESIAN_POINT('Ctrl Pts',(7.16680584538502,28.8469761171536,123.797416427036));
#120996=CARTESIAN_POINT('Ctrl Pts',(7.16530890770955,28.8307901709854,123.813136823953));
#120997=CARTESIAN_POINT('Ctrl Pts',(7.16452836755698,28.8223955379555,123.821465500705));
#120998=CARTESIAN_POINT('Ctrl Pts',(7.16246404033559,28.8003214488568,123.843837521118));
#120999=CARTESIAN_POINT('Ctrl Pts',(7.16118713633342,28.7867997207624,123.858034396872));
#121000=CARTESIAN_POINT('Ctrl Pts',(7.1545847848286,28.7176564481081,123.933244677546));
#121001=CARTESIAN_POINT('Ctrl Pts',(7.14944261726476,28.6663729256509,123.998095205464));
#121002=CARTESIAN_POINT('Ctrl Pts',(7.13821777982035,28.5639676879752,124.149468279496));
#121003=CARTESIAN_POINT('Ctrl Pts',(7.13219367110133,28.5154340626107,124.237337136652));
#121004=CARTESIAN_POINT('Ctrl Pts',(7.12414081692024,28.4637009922747,124.354910080149));
#121005=CARTESIAN_POINT('Ctrl Pts',(7.12234811960874,28.4529736390788,124.381077626699));
#121006=CARTESIAN_POINT('Ctrl Pts',(7.11928090965876,28.4360533164031,124.425544301422));
#121007=CARTESIAN_POINT('Ctrl Pts',(7.11802272014844,28.4295030479053,124.443701676865));
#121008=CARTESIAN_POINT('Ctrl Pts',(7.11620453548328,28.4206168180352,124.469743211761));
#121009=CARTESIAN_POINT('Ctrl Pts',(7.11565858879512,28.4180212055672,124.477537959357));
#121010=CARTESIAN_POINT('Ctrl Pts',(7.1147045935116,28.4136135458241,124.49110840279));
#121011=CARTESIAN_POINT('Ctrl Pts',(7.11429807415367,28.411775151991,124.496875293265));
#121012=CARTESIAN_POINT('Ctrl Pts',(7.11342078521269,28.4078936697478,124.509284478302));
#121013=CARTESIAN_POINT('Ctrl Pts',(7.11294948982388,28.4058607300169,124.515929474603));
#121014=CARTESIAN_POINT('Ctrl Pts',(7.1116393153706,28.4003514992859,124.534348429388));
#121015=CARTESIAN_POINT('Ctrl Pts',(7.11079568957607,28.396963769312,124.546148116624));
#121016=CARTESIAN_POINT('Ctrl Pts',(7.10486806103463,28.3742443689039,124.628710724814));
#121017=CARTESIAN_POINT('Ctrl Pts',(7.09958098154403,28.3594764950987,124.700638441158));
#121018=CARTESIAN_POINT('Ctrl Pts',(7.09323401074213,28.3475885882259,124.787187540729));
#121019=CARTESIAN_POINT('Ctrl Pts',(7.09221388604955,28.3458559820897,124.801102586954));
#121020=CARTESIAN_POINT('Ctrl Pts',(7.08582814571166,28.3361153134979,124.888296782242));
#121021=CARTESIAN_POINT('Ctrl Pts',(7.08046272403968,28.3328020794517,124.962022821129));
#121022=CARTESIAN_POINT('Ctrl Pts',(7.07216925686224,28.3352945104118,125.078213545914));
#121023=CARTESIAN_POINT('Ctrl Pts',(7.06917329110161,28.3378309850588,125.120649879804));
#121024=CARTESIAN_POINT('Ctrl Pts',(7.06410022726345,28.3449800198226,125.193392985981));
#121025=CARTESIAN_POINT('Ctrl Pts',(7.0620016473404,28.3488105636538,125.223753526165));
#121026=CARTESIAN_POINT('Ctrl Pts',(7.05898225059248,28.3556061714426,125.26780642944));
#121027=CARTESIAN_POINT('Ctrl Pts',(7.05804099366769,28.3579108058421,125.281592695485));
#121028=CARTESIAN_POINT('Ctrl Pts',(7.05638627125911,28.3622924433477,125.305917103472));
#121029=CARTESIAN_POINT('Ctrl Pts',(7.05567060082343,28.3642983388838,125.316467060556));
#121030=CARTESIAN_POINT('Ctrl Pts',(7.05417366494116,28.368727042303,125.338591729773));
#121031=CARTESIAN_POINT('Ctrl Pts',(7.05339312730385,28.3711713676912,125.350161563697));
#121032=CARTESIAN_POINT('Ctrl Pts',(7.05132881462839,28.3779948250668,125.380840529399));
#121033=CARTESIAN_POINT('Ctrl Pts',(7.05005192247959,28.3825884864676,125.399900418676));
#121034=CARTESIAN_POINT('Ctrl Pts',(7.04344997908207,28.4082734333065,125.498775924849));
#121035=CARTESIAN_POINT('Ctrl Pts',(7.03830817762255,28.4349403681072,125.57702835479));
#121036=CARTESIAN_POINT('Ctrl Pts',(7.02708336464363,28.5065722764158,125.745162879906));
#121037=CARTESIAN_POINT('Ctrl Pts',(7.02105894741988,28.5540737781649,125.83360008448));
#121038=CARTESIAN_POINT('Ctrl Pts',(7.01300572222854,28.6247968715355,125.940835819651));
#121039=CARTESIAN_POINT('Ctrl Pts',(7.0112129836221,28.6409635887543,125.964041252593));
#121040=CARTESIAN_POINT('Ctrl Pts',(7.00814571014895,28.6691455701068,126.002374719431));
#121041=CARTESIAN_POINT('Ctrl Pts',(7.00688749929019,28.6808479366916,126.017726067114));
#121042=CARTESIAN_POINT('Ctrl Pts',(7.00506928911407,28.6979072297578,126.039316080675));
#121043=CARTESIAN_POINT('Ctrl Pts',(7.0045233387998,28.7030482034408,126.045724403592));
#121044=CARTESIAN_POINT('Ctrl Pts',(7.00356933942795,28.7120588057818,126.056787641877));
#121045=CARTESIAN_POINT('Ctrl Pts',(7.00316281964853,28.7159067466625,126.061459916897));
#121046=CARTESIAN_POINT('Ctrl Pts',(7.00228553247384,28.7242270497817,126.071451197729));
#121047=CARTESIAN_POINT('Ctrl Pts',(7.00181423929839,28.7287071857878,126.076763142828));
#121048=CARTESIAN_POINT('Ctrl Pts',(7.00050407685232,28.7411936276725,126.091381337829));
#121049=CARTESIAN_POINT('Ctrl Pts',(6.9996604609868,28.7492695796623,126.100627139911));
#121050=CARTESIAN_POINT('Ctrl Pts',(6.99373549318338,28.8062862196025,126.164465068223));
#121051=CARTESIAN_POINT('Ctrl Pts',(6.98845127521954,28.8586770632103,126.215858156313));
#121052=CARTESIAN_POINT('Ctrl Pts',(6.98210506099176,28.924931834679,126.272785079067));
#121053=CARTESIAN_POINT('Ctrl Pts',(6.98108286271784,28.9357042530065,126.281806528618));
#121054=CARTESIAN_POINT('Ctrl Pts',(6.97469524803576,29.0036959012725,126.337298620006));
#121055=CARTESIAN_POINT('Ctrl Pts',(6.96933000756723,29.0638362738374,126.380068203777));
#121056=CARTESIAN_POINT('Ctrl Pts',(6.96103616855051,29.1628073348391,126.44099645199));
#121057=CARTESIAN_POINT('Ctrl Pts',(6.9580396799083,29.1998415299242,126.461885514717));
#121058=CARTESIAN_POINT('Ctrl Pts',(6.95296583934262,29.2648429102593,126.495338177166));
#121059=CARTESIAN_POINT('Ctrl Pts',(6.95086699663923,29.2924309584427,126.508588239233));
#121060=CARTESIAN_POINT('Ctrl Pts',(6.94784729786394,29.3331313667887,126.526773588747));
#121061=CARTESIAN_POINT('Ctrl Pts',(6.94690599591197,29.3459643438783,126.532314832681));
#121062=CARTESIAN_POINT('Ctrl Pts',(6.94525122273482,29.368777439849,126.541826642866));
#121063=CARTESIAN_POINT('Ctrl Pts',(6.94453554609937,29.3787289130146,126.545863371341));
#121064=CARTESIAN_POINT('Ctrl Pts',(6.94303862495206,29.3997185398932,126.554142201648));
#121065=CARTESIAN_POINT('Ctrl Pts',(6.94225810798242,29.4107642624478,126.558363587875));
#121066=CARTESIAN_POINT('Ctrl Pts',(6.94019391482633,29.4402380281446,126.569269502409));
#121067=CARTESIAN_POINT('Ctrl Pts',(6.93891712007254,29.4587410380198,126.575747132319));
#121068=CARTESIAN_POINT('Ctrl Pts',(6.93231851969021,29.555691736407,126.60777881817));
#121069=CARTESIAN_POINT('Ctrl Pts',(6.92717971701196,29.635848047797,126.627807851358));
#121070=CARTESIAN_POINT('Ctrl Pts',(6.91595510354097,29.8159463599422,126.658833067378));
#121071=CARTESIAN_POINT('Ctrl Pts',(6.90992815877011,29.9160530124556,126.666899351068));
#121072=CARTESIAN_POINT('Ctrl Pts',(6.90187189401322,30.0445535772375,126.665644312603));
#121073=CARTESIAN_POINT('Ctrl Pts',(6.90007881719033,30.0728232683213,126.664647887263));
#121074=CARTESIAN_POINT('Ctrl Pts',(6.89701102345314,30.1203220694846,126.66176150438));
#121075=CARTESIAN_POINT('Ctrl Pts',(6.89575263775295,30.1395690963481,126.660255729475));
#121076=CARTESIAN_POINT('Ctrl Pts',(6.89393421864653,30.1669633521387,126.657632873839));
#121077=CARTESIAN_POINT('Ctrl Pts',(6.89338823863804,30.1751359997823,126.656789328783));
#121078=CARTESIAN_POINT('Ctrl Pts',(6.89243420578799,30.1893182496334,126.655219393568));
#121079=CARTESIAN_POINT('Ctrl Pts',(6.89202768255808,30.1953306744409,126.654520645615));
#121080=CARTESIAN_POINT('Ctrl Pts',(6.89115040984466,30.2082372197349,126.652949347782));
#121081=CARTESIAN_POINT('Ctrl Pts',(6.89067913479338,30.2151296248998,126.652066441189));
#121082=CARTESIAN_POINT('Ctrl Pts',(6.88936907066973,30.2341818028201,126.649504641502));
#121083=CARTESIAN_POINT('Ctrl Pts',(6.88852553610683,30.2463285675887,126.647734473086));
#121084=CARTESIAN_POINT('Ctrl Pts',(6.88262205409705,30.3305789933017,126.634504143708));
#121085=CARTESIAN_POINT('Ctrl Pts',(6.87736093849703,30.4018736043471,126.618450342471));
#121086=CARTESIAN_POINT('Ctrl Pts',(6.87107463938203,30.4848628382286,126.593940829652));
#121087=CARTESIAN_POINT('Ctrl Pts',(6.87008964816212,30.4978013753195,126.58994752353));
#121088=CARTESIAN_POINT('Ctrl Pts',(6.86362718487559,30.582321842406,126.562728569554));
#121089=CARTESIAN_POINT('Ctrl Pts',(6.85814853884835,30.6523132682235,126.534831623407));
#121090=CARTESIAN_POINT('Ctrl Pts',(6.84977679037718,30.7581409439591,126.484099163215));
#121091=CARTESIAN_POINT('Ctrl Pts',(6.84680997441759,30.7953989999941,126.464468824276));
#121092=CARTESIAN_POINT('Ctrl Pts',(6.84178024959967,30.8582018681293,126.428274759587));
#121093=CARTESIAN_POINT('Ctrl Pts',(6.8396963540326,30.8841090837144,126.41238471123));
#121094=CARTESIAN_POINT('Ctrl Pts',(6.83669384249032,30.92124792151,126.388183199477));
#121095=CARTESIAN_POINT('Ctrl Pts',(6.83575510821472,30.9328314650066,126.380425951147));
#121096=CARTESIAN_POINT('Ctrl Pts',(6.83410322754093,30.9531596381203,126.366439870816));
#121097=CARTESIAN_POINT('Ctrl Pts',(6.83338790187141,30.9619438516806,126.360270286297));
#121098=CARTESIAN_POINT('Ctrl Pts',(6.83189012725186,30.9802932433207,126.347115961736));
#121099=CARTESIAN_POINT('Ctrl Pts',(6.83110842115497,30.9898448349546,126.3401132311));
#121100=CARTESIAN_POINT('Ctrl Pts',(6.82903735147019,31.015075643772,126.321198370588));
#121101=CARTESIAN_POINT('Ctrl Pts',(6.82775495332686,31.0306200269001,126.309108899393));
#121102=CARTESIAN_POINT('Ctrl Pts',(6.82092609152769,31.1128789379639,126.242759404361));
#121103=CARTESIAN_POINT('Ctrl Pts',(6.81558017414355,31.1755349768754,126.183668323503));
#121104=CARTESIAN_POINT('Ctrl Pts',(6.80433853084959,31.29872263266,126.048012513782));
#121105=CARTESIAN_POINT('Ctrl Pts',(6.79848421968039,31.3576589359036,125.970448689836));
#121106=CARTESIAN_POINT('Ctrl Pts',(6.79063591558927,31.4243653675363,125.864591020742));
#121107=CARTESIAN_POINT('Ctrl Pts',(6.7888663935003,31.438642908284,125.840619260776));
#121108=CARTESIAN_POINT('Ctrl Pts',(6.78583486244883,31.4616762200661,125.799639888896));
#121109=CARTESIAN_POINT('Ctrl Pts',(6.78458868662136,31.4707534644218,125.782818941596));
#121110=CARTESIAN_POINT('Ctrl Pts',(6.78278486352893,31.4833010033453,125.75857834966));
#121111=CARTESIAN_POINT('Ctrl Pts',(6.78224096436679,31.487009451346,125.751282812117));
#121112=CARTESIAN_POINT('Ctrl Pts',(6.7812892735369,31.4933651826408,125.738547915569));
#121113=CARTESIAN_POINT('Ctrl Pts',(6.78088298811303,31.4960368353003,125.733120984802));
#121114=CARTESIAN_POINT('Ctrl Pts',(6.78000468412576,31.501722101558,125.721411998494));
#121115=CARTESIAN_POINT('Ctrl Pts',(6.77953212498298,31.5047258371292,125.715125648064));
#121116=CARTESIAN_POINT('Ctrl Pts',(6.77821508872227,31.5129475856079,125.697637662293));
#121117=CARTESIAN_POINT('Ctrl Pts',(6.77736578751824,31.518080407234,125.686396794351));
#121118=CARTESIAN_POINT('Ctrl Pts',(6.77402885444147,31.5376112153215,125.642333519064));
#121119=CARTESIAN_POINT('Ctrl Pts',(6.77149705255902,31.5510682071831,125.609119092788));
#121120=CARTESIAN_POINT('Ctrl Pts',(6.76893575384937,31.5634399863339,125.575509695081));
#121121=CARTESIAN_POINT('Origin',(5.,30.,125.));
#121122=CARTESIAN_POINT('',(6.06644911688889,31.5634400025946,125.575509650907));
#121123=CARTESIAN_POINT('',(6.2618827359479,31.5634400889265,125.575509416376));
#121124=CARTESIAN_POINT('',(5.,31.5634400119422,125.575509625513));
#121125=CARTESIAN_POINT('',(6.92206962423701,31.6659991809955,124.998531923256));
#121126=CARTESIAN_POINT('Ctrl Pts',(6.26188273594789,31.5634400889265,125.575509416376));
#121127=CARTESIAN_POINT('Ctrl Pts',(6.26453323098372,31.5505030333263,125.610654473577));
#121128=CARTESIAN_POINT('Ctrl Pts',(6.2671531022909,31.5363776686696,125.64537214447));
#121129=CARTESIAN_POINT('Ctrl Pts',(6.27126998919214,31.5120106847638,125.699910324414));
#121130=CARTESIAN_POINT('Ctrl Pts',(6.27278958688585,31.5025308545777,125.720036031566));
#121131=CARTESIAN_POINT('Ctrl Pts',(6.27522187622556,31.4865717375308,125.752228536729));
#121132=CARTESIAN_POINT('Ctrl Pts',(6.27614302640899,31.4803420518802,125.764415287089));
#121133=CARTESIAN_POINT('Ctrl Pts',(6.27777544030934,31.4689721799572,125.78599705788));
#121134=CARTESIAN_POINT('Ctrl Pts',(6.27848870313448,31.4638903219023,125.795421759269));
#121135=CARTESIAN_POINT('Ctrl Pts',(6.2799936941221,31.4529272351232,125.815292671185));
#121136=CARTESIAN_POINT('Ctrl Pts',(6.28078456652666,31.447023385029,125.825725757171));
#121137=CARTESIAN_POINT('Ctrl Pts',(6.28290792070682,31.4307905732418,125.853702979776));
#121138=CARTESIAN_POINT('Ctrl Pts',(6.28423278823446,31.4202515977551,125.871123355166));
#121139=CARTESIAN_POINT('Ctrl Pts',(6.28714785562688,31.3961720472937,125.909326465987));
#121140=CARTESIAN_POINT('Ctrl Pts',(6.28873250811245,31.3824812442445,125.930008984485));
#121141=CARTESIAN_POINT('Ctrl Pts',(6.29372835811387,31.3374866682258,125.994791115195));
#121142=CARTESIAN_POINT('Ctrl Pts',(6.29708363774178,31.3044947913601,126.037677183274));
#121143=CARTESIAN_POINT('Ctrl Pts',(6.30407114563171,31.2308770651783,126.124299695415));
#121144=CARTESIAN_POINT('Ctrl Pts',(6.30769132644786,31.1898716407773,126.167610234891));
#121145=CARTESIAN_POINT('Ctrl Pts',(6.31634451591232,31.0873952216886,126.264830117245));
#121146=CARTESIAN_POINT('Ctrl Pts',(6.32139183620691,31.0241127901276,126.316591446482));
#121147=CARTESIAN_POINT('Ctrl Pts',(6.32753065126077,30.9471827882536,126.370603381623));
#121148=CARTESIAN_POINT('Ctrl Pts',(6.32834449073214,30.9369855006192,126.377594647753));
#121149=CARTESIAN_POINT('Ctrl Pts',(6.32962849585779,30.9209195993999,126.388348541046));
#121150=CARTESIAN_POINT('Ctrl Pts',(6.33009370048239,30.9151033358208,126.392189089291));
#121151=CARTESIAN_POINT('Ctrl Pts',(6.33096737387406,30.9041928781788,126.399295485162));
#121152=CARTESIAN_POINT('Ctrl Pts',(6.33137525262167,30.8991047701905,126.402570220464));
#121153=CARTESIAN_POINT('Ctrl Pts',(6.33233922137343,30.8870913130234,126.410209918899));
#121154=CARTESIAN_POINT('Ctrl Pts',(6.33289677364094,30.8801515104572,126.414551633784));
#121155=CARTESIAN_POINT('Ctrl Pts',(6.33476646386004,30.8568993759404,126.428861404817));
#121156=CARTESIAN_POINT('Ctrl Pts',(6.33609186639121,30.8404481684083,126.43859940693));
#121157=CARTESIAN_POINT('Ctrl Pts',(6.33938397300423,30.7995810649746,126.46184975642));
#121158=CARTESIAN_POINT('Ctrl Pts',(6.34136484092547,30.7749866741457,126.475035616516));
#121159=CARTESIAN_POINT('Ctrl Pts',(6.35032886249905,30.6632367264032,126.531382034958));
#121160=CARTESIAN_POINT('Ctrl Pts',(6.35747773264583,30.5727331987659,126.567479107099));
#121161=CARTESIAN_POINT('Ctrl Pts',(6.37070495662873,30.3972865369762,126.620218098892));
#121162=CARTESIAN_POINT('Ctrl Pts',(6.37679326992271,30.3131741211006,126.638557104524));
#121163=CARTESIAN_POINT('Ctrl Pts',(6.38402546998996,30.2085020180894,126.653018670417));
#121164=CARTESIAN_POINT('Ctrl Pts',(6.38536258494941,30.1889473276658,126.655367868903));
#121165=CARTESIAN_POINT('Ctrl Pts',(6.38748661161821,30.1575701563187,126.658574078676));
#121166=CARTESIAN_POINT('Ctrl Pts',(6.388280381661,30.1457727188137,126.659652570755));
#121167=CARTESIAN_POINT('Ctrl Pts',(6.38978611472357,30.1232618295957,126.661468571554));
#121168=CARTESIAN_POINT('Ctrl Pts',(6.39049874344686,30.1125508419617,126.66222850718));
#121169=CARTESIAN_POINT('Ctrl Pts',(6.39212956673031,30.0879130012123,126.663737298468));
#121170=CARTESIAN_POINT('Ctrl Pts',(6.39304549550791,30.0739824717173,126.664414944528));
#121171=CARTESIAN_POINT('Ctrl Pts',(6.39594149479883,30.0296602633358,126.666013410678));
#121172=CARTESIAN_POINT('Ctrl Pts',(6.39790121280371,29.9992501158025,126.666277299375));
#121173=CARTESIAN_POINT('Ctrl Pts',(6.40252402836766,29.9267261118602,126.664920967144));
#121174=CARTESIAN_POINT('Ctrl Pts',(6.40516504666239,29.8846471549676,126.662535708677));
#121175=CARTESIAN_POINT('Ctrl Pts',(6.41245305829984,29.7676578177247,126.65144037819));
#121176=CARTESIAN_POINT('Ctrl Pts',(6.41702657266004,29.6931832877958,126.639238265844));
#121177=CARTESIAN_POINT('Ctrl Pts',(6.42242697299816,29.6072559608185,126.619096614067));
#121178=CARTESIAN_POINT('Ctrl Pts',(6.42321578123079,29.5947567912209,126.616013509519));
#121179=CARTESIAN_POINT('Ctrl Pts',(6.42852037429965,29.5111563866242,126.594361328546));
#121180=CARTESIAN_POINT('Ctrl Pts',(6.43308895516093,29.4413236799063,126.571252417981));
#121181=CARTESIAN_POINT('Ctrl Pts',(6.43868997878531,29.3618765073843,126.53899486264));
#121182=CARTESIAN_POINT('Ctrl Pts',(6.43949837093124,29.3505511643521,126.534249968932));
#121183=CARTESIAN_POINT('Ctrl Pts',(6.44077562084146,29.3328987137899,126.52662378816));
#121184=CARTESIAN_POINT('Ctrl Pts',(6.44123960134599,29.3265351710516,126.523827233131));
#121185=CARTESIAN_POINT('Ctrl Pts',(6.44211234169883,29.3146613139832,126.518520184515));
#121186=CARTESIAN_POINT('Ctrl Pts',(6.44252052717498,29.3091469461265,126.51601936617));
#121187=CARTESIAN_POINT('Ctrl Pts',(6.44348707937824,29.2961796725674,126.510053145173));
#121188=CARTESIAN_POINT('Ctrl Pts',(6.44404693248017,29.2887386444359,126.506562587998));
#121189=CARTESIAN_POINT('Ctrl Pts',(6.4459326113132,29.2638991334082,126.494685437374));
#121190=CARTESIAN_POINT('Ctrl Pts',(6.44727200104214,29.2466214371786,126.486051716484));
#121191=CARTESIAN_POINT('Ctrl Pts',(6.45060665406564,29.2044072083047,126.464031760517));
#121192=CARTESIAN_POINT('Ctrl Pts',(6.45261652320512,29.1796546718011,126.450306949463));
#121193=CARTESIAN_POINT('Ctrl Pts',(6.46183393868985,29.0687809783488,126.385083042454));
#121194=CARTESIAN_POINT('Ctrl Pts',(6.4692141542084,28.9870703369412,126.326498349653));
#121195=CARTESIAN_POINT('Ctrl Pts',(6.48238623938157,28.8487927532436,126.207087800662));
#121196=CARTESIAN_POINT('Ctrl Pts',(6.48821088004376,28.7905285921975,126.148704342915));
#121197=CARTESIAN_POINT('Ctrl Pts',(6.49519001018681,28.7240349991667,126.071379266078));
#121198=CARTESIAN_POINT('Ctrl Pts',(6.49652076142678,28.7115176079655,126.056292287906));
#121199=CARTESIAN_POINT('Ctrl Pts',(6.49863715773475,28.6918791743119,126.031753736607));
#121200=CARTESIAN_POINT('Ctrl Pts',(6.49942957417504,28.6845878073523,126.02244151105));
#121201=CARTESIAN_POINT('Ctrl Pts',(6.50093425479178,28.6708639055627,126.004524086572));
#121202=CARTESIAN_POINT('Ctrl Pts',(6.50164716877997,28.6644142669889,125.99593280749));
#121203=CARTESIAN_POINT('Ctrl Pts',(6.50328077809434,28.6497605818281,125.976014901765));
#121204=CARTESIAN_POINT('Ctrl Pts',(6.50419918025611,28.6416150822143,125.964646054125));
#121205=CARTESIAN_POINT('Ctrl Pts',(6.5071119256167,28.6160913479543,125.928057536032));
#121206=CARTESIAN_POINT('Ctrl Pts',(6.50908557121767,28.5992643440476,125.90245983752));
#121207=CARTESIAN_POINT('Ctrl Pts',(6.51374832126198,28.5607667677671,125.840222830019));
#121208=CARTESIAN_POINT('Ctrl Pts',(6.51641479894631,28.5397754581317,125.803188252582));
#121209=CARTESIAN_POINT('Ctrl Pts',(6.52362148459172,28.4863692014257,125.699934417149));
#121210=CARTESIAN_POINT('Ctrl Pts',(6.52809430880673,28.4568936053249,125.632304831701));
#121211=CARTESIAN_POINT('Ctrl Pts',(6.5334621940821,28.4272451267642,125.549723098583));
#121212=CARTESIAN_POINT('Ctrl Pts',(6.53432290077695,28.4226653916835,125.536440960096));
#121213=CARTESIAN_POINT('Ctrl Pts',(6.53968555690888,28.3952555125483,125.453559589253));
#121214=CARTESIAN_POINT('Ctrl Pts',(6.54424008350693,28.376870929878,125.382583954629));
#121215=CARTESIAN_POINT('Ctrl Pts',(6.54982550579754,28.3609274233676,125.298576364644));
#121216=CARTESIAN_POINT('Ctrl Pts',(6.55063384008586,28.3587715387297,125.286488870896));
#121217=CARTESIAN_POINT('Ctrl Pts',(6.55191101823856,28.3556047751723,125.267523192279));
#121218=CARTESIAN_POINT('Ctrl Pts',(6.55237498572978,28.3545029651142,125.260660349208));
#121219=CARTESIAN_POINT('Ctrl Pts',(6.55324771624495,28.3525217295595,125.247806404879));
#121220=CARTESIAN_POINT('Ctrl Pts',(6.55365590506358,28.351631979949,125.241817145095));
#121221=CARTESIAN_POINT('Ctrl Pts',(6.55462248509758,28.3496114358677,125.227686512057));
#121222=CARTESIAN_POINT('Ctrl Pts',(6.55518236294708,28.3485082214955,125.219541474079));
#121223=CARTESIAN_POINT('Ctrl Pts',(6.55706821431895,28.3450144030586,125.192228506631));
#121224=CARTESIAN_POINT('Ctrl Pts',(6.55840775508845,28.3428970003459,125.173028014631));
#121225=CARTESIAN_POINT('Ctrl Pts',(6.56174286848806,28.3385011081693,125.125612744714));
#121226=CARTESIAN_POINT('Ctrl Pts',(6.56375305178258,28.3366070086541,125.09736890993));
#121227=CARTESIAN_POINT('Ctrl Pts',(6.5729732626186,28.3312706460676,124.968805515804));
#121228=CARTESIAN_POINT('Ctrl Pts',(6.5803560357767,28.3361793615962,124.868348519008));
#121229=CARTESIAN_POINT('Ctrl Pts',(6.59352754570157,28.3615173680557,124.687418324636));
#121230=CARTESIAN_POINT('Ctrl Pts',(6.59934931514316,28.3789623229815,124.606842074978));
#121231=CARTESIAN_POINT('Ctrl Pts',(6.60632566981298,28.4078517187159,124.50907839942));
#121232=CARTESIAN_POINT('Ctrl Pts',(6.60765633670465,28.4137376553053,124.490380535847));
#121233=CARTESIAN_POINT('Ctrl Pts',(6.60977263186832,28.4237019717756,124.460574020175));
#121234=CARTESIAN_POINT('Ctrl Pts',(6.61056503036285,28.4275709375132,124.449397859226));
#121235=CARTESIAN_POINT('Ctrl Pts',(6.61206969710485,28.4351807621224,124.428150236314));
#121236=CARTESIAN_POINT('Ctrl Pts',(6.61278261495284,28.4389006562751,124.418071956595));
#121237=CARTESIAN_POINT('Ctrl Pts',(6.61441626159378,28.4476871690297,124.394957469147));
#121238=CARTESIAN_POINT('Ctrl Pts',(6.61533469685582,28.4528210240405,124.381947554457));
#121239=CARTESIAN_POINT('Ctrl Pts',(6.61824766681568,28.4697189036466,124.340656466048));
#121240=CARTESIAN_POINT('Ctrl Pts',(6.62022149926635,28.4820996323642,124.312633436655));
#121241=CARTESIAN_POINT('Ctrl Pts',(6.62488478589524,28.5135121920068,124.24652725224));
#121242=CARTESIAN_POINT('Ctrl Pts',(6.62755160590334,28.5332447520683,124.208800525387));
#121243=CARTESIAN_POINT('Ctrl Pts',(6.63475845347621,28.5910305894367,124.107928692374));
#121244=CARTESIAN_POINT('Ctrl Pts',(6.6392311204136,28.6318622486393,124.046487822005));
#121245=CARTESIAN_POINT('Ctrl Pts',(6.64460000274253,28.6851732601604,123.976777372913));
#121246=CARTESIAN_POINT('Ctrl Pts',(6.64546185461863,28.6938601246875,123.965711587453));
#121247=CARTESIAN_POINT('Ctrl Pts',(6.65082410561159,28.7486247698257,123.897739875715));
#121248=CARTESIAN_POINT('Ctrl Pts',(6.65537709208036,28.7982669053413,123.843819992595));
#121249=CARTESIAN_POINT('Ctrl Pts',(6.66096080497191,28.8601792063967,123.784880535494));
#121250=CARTESIAN_POINT('Ctrl Pts',(6.66176913286139,28.8691650911879,123.776513530192));
#121251=CARTESIAN_POINT('Ctrl Pts',(6.66304630307807,28.8833813569835,123.763566775114));
#121252=CARTESIAN_POINT('Ctrl Pts',(6.66351026912993,28.8885495321933,123.758918952376));
#121253=CARTESIAN_POINT('Ctrl Pts',(6.6643829985571,28.8982741276389,123.750282924777));
#121254=CARTESIAN_POINT('Ctrl Pts',(6.66479118774555,28.9028234015672,123.746287045173));
#121255=CARTESIAN_POINT('Ctrl Pts',(6.66575777085838,28.9135993257459,123.736925522379));
#121256=CARTESIAN_POINT('Ctrl Pts',(6.66631765144547,28.9198440136909,123.731581063215));
#121257=CARTESIAN_POINT('Ctrl Pts',(6.66820352190422,28.9408961192109,123.713832007997));
#121258=CARTESIAN_POINT('Ctrl Pts',(6.66954307938242,28.9558790734049,123.701639285459));
#121259=CARTESIAN_POINT('Ctrl Pts',(6.67287824371164,28.9933311099518,123.672229348907));
#121260=CARTESIAN_POINT('Ctrl Pts',(6.67488846176037,29.0160330930262,123.655319331158));
#121261=CARTESIAN_POINT('Ctrl Pts',(6.68410898190789,29.1211541314611,123.58110555354));
#121262=CARTESIAN_POINT('Ctrl Pts',(6.69149203808143,29.208218275861,123.5307438313));
#121263=CARTESIAN_POINT('Ctrl Pts',(6.70466348439964,29.373968172544,123.453902953511));
#121264=CARTESIAN_POINT('Ctrl Pts',(6.71048493618625,29.4511213636809,123.424859424188));
#121265=CARTESIAN_POINT('Ctrl Pts',(6.71746098376527,29.5489211848458,123.396108462286));
#121266=CARTESIAN_POINT('Ctrl Pts',(6.71879164130262,29.5678222669254,123.390912486472));
#121267=CARTESIAN_POINT('Ctrl Pts',(6.72090792524934,29.5982681498962,123.383118006338));
#121268=CARTESIAN_POINT('Ctrl Pts',(6.72170032175374,29.6097560903192,123.380306953692));
#121269=CARTESIAN_POINT('Ctrl Pts',(6.72320498695728,29.6317344195238,123.375176359769));
#121270=CARTESIAN_POINT('Ctrl Pts',(6.72391790523362,29.6422191658679,123.372835508142));
#121271=CARTESIAN_POINT('Ctrl Pts',(6.72555155601529,29.6664042068442,123.367680963252));
#121272=CARTESIAN_POINT('Ctrl Pts',(6.72646999494893,29.6801188784146,123.364938019905));
#121273=CARTESIAN_POINT('Ctrl Pts',(6.72938298982267,29.7239745065552,123.356739802464));
#121274=CARTESIAN_POINT('Ctrl Pts',(6.73135684299987,29.7542330657226,123.351942673112));
#121275=CARTESIAN_POINT('Ctrl Pts',(6.7360201891513,29.8268097561523,123.342480051985));
#121276=CARTESIAN_POINT('Ctrl Pts',(6.73868704713319,29.8692084892348,123.338596617197));
#121277=CARTESIAN_POINT('Ctrl Pts',(6.74589391255398,29.9852966392249,123.332435971777));
#121278=CARTESIAN_POINT('Ctrl Pts',(6.75036656193504,30.059061136963,123.333417232298));
#121279=CARTESIAN_POINT('Ctrl Pts',(6.75573555229408,30.1465436339659,123.340397963137));
#121280=CARTESIAN_POINT('Ctrl Pts',(6.75659752874064,30.1605539400058,123.341694725452));
#121281=CARTESIAN_POINT('Ctrl Pts',(6.76195973481106,30.2473614434156,123.350839835931));
#121282=CARTESIAN_POINT('Ctrl Pts',(6.76651255289934,30.3195831444888,123.363301849301));
#121283=CARTESIAN_POINT('Ctrl Pts',(6.77209607890747,30.4026769742861,123.383349756854));
#121284=CARTESIAN_POINT('Ctrl Pts',(6.77290440609658,30.4145800704601,123.38636122453));
#121285=CARTESIAN_POINT('Ctrl Pts',(6.77418157544481,30.4331675823993,123.391283070563));
#121286=CARTESIAN_POINT('Ctrl Pts',(6.77464554133918,30.4398754509814,123.393104266996));
#121287=CARTESIAN_POINT('Ctrl Pts',(6.77551827064704,30.4524052233899,123.396590451635));
#121288=CARTESIAN_POINT('Ctrl Pts',(6.77592645987569,30.4582296991918,123.398245273447));
#121289=CARTESIAN_POINT('Ctrl Pts',(6.7768930433258,30.4719392011326,123.402221244495));
#121290=CARTESIAN_POINT('Ctrl Pts',(6.77745292421245,30.479816212621,123.404569037491));
#121291=CARTESIAN_POINT('Ctrl Pts',(6.7793387967593,30.5061459016077,123.41262938756));
#121292=CARTESIAN_POINT('Ctrl Pts',(6.78067835606566,30.5245157794411,123.418604333972));
#121293=CARTESIAN_POINT('Ctrl Pts',(6.78401352596746,30.569537060273,123.434118556207));
#121294=CARTESIAN_POINT('Ctrl Pts',(6.78602374781892,30.596056690669,123.44402011593));
#121295=CARTESIAN_POINT('Ctrl Pts',(6.79524430181211,30.7154212177369,123.49208618448));
#121296=CARTESIAN_POINT('Ctrl Pts',(6.80262738895412,30.8049531052218,123.537918412208));
#121297=CARTESIAN_POINT('Ctrl Pts',(6.81581202222102,30.9595618433797,123.635594239608));
#121298=CARTESIAN_POINT('Ctrl Pts',(6.82164607199979,31.0259469056759,123.684781900821));
#121299=CARTESIAN_POINT('Ctrl Pts',(6.8286270269019,31.1031886744835,123.751436361586));
#121300=CARTESIAN_POINT('Ctrl Pts',(6.82995102338177,31.11773059282,123.764437460648));
#121301=CARTESIAN_POINT('Ctrl Pts',(6.83205931931205,31.1407031295016,123.785713481385));
#121302=CARTESIAN_POINT('Ctrl Pts',(6.83285029829913,31.1492795270704,123.793827557926));
#121303=CARTESIAN_POINT('Ctrl Pts',(6.83435387418819,31.1654975062067,123.809501332601));
#121304=CARTESIAN_POINT('Ctrl Pts',(6.83506710392819,31.1731535618737,123.81704512193));
#121305=CARTESIAN_POINT('Ctrl Pts',(6.8358099347739,31.1810865677337,123.825014567701));
#121306=CARTESIAN_POINT('Ctrl Pts',(6.8358427323928,31.1814367437494,123.825366666948));
#121307=CARTESIAN_POINT('Ctrl Pts',(6.83590340358551,31.1820843671655,123.826018429797));
#121308=CARTESIAN_POINT('Ctrl Pts',(6.8359312790547,31.182381858045,123.826318049879));
#121309=CARTESIAN_POINT('Ctrl Pts',(6.83598319034381,31.1829357493136,123.826876329775));
#121310=CARTESIAN_POINT('Ctrl Pts',(6.83600722742855,31.1831921787587,123.827134960547));
#121311=CARTESIAN_POINT('Ctrl Pts',(6.83605224364996,31.1836723303381,123.827619551723));
#121312=CARTESIAN_POINT('Ctrl Pts',(6.83607322366717,31.1838960726408,123.82784549214));
#121313=CARTESIAN_POINT('Ctrl Pts',(6.83611270482746,31.184317056052,123.828270854925));
#121314=CARTESIAN_POINT('Ctrl Pts',(6.83613120659242,31.1845143114719,123.828470263036));
#121315=CARTESIAN_POINT('Ctrl Pts',(6.83616617017156,31.1848870225307,123.828847231933));
#121316=CARTESIAN_POINT('Ctrl Pts',(6.83618263243793,31.1850624885993,123.829024782317));
#121317=CARTESIAN_POINT('Ctrl Pts',(6.83621385628806,31.1853952531242,123.829361651066));
#121318=CARTESIAN_POINT('Ctrl Pts',(6.83622861821685,31.1855525594419,123.829520961774));
#121319=CARTESIAN_POINT('Ctrl Pts',(6.83625670813026,31.1858518588694,123.8298241971));
#121320=CARTESIAN_POINT('Ctrl Pts',(6.83627003636292,31.1859938578017,123.829968115762));
#121321=CARTESIAN_POINT('Ctrl Pts',(6.83629547171104,31.1862648190436,123.830242840227));
#121322=CARTESIAN_POINT('Ctrl Pts',(6.83630757902373,31.1863937859098,123.830373641501));
#121323=CARTESIAN_POINT('Ctrl Pts',(6.83633074456984,31.1866405226297,123.830623970568));
#121324=CARTESIAN_POINT('Ctrl Pts',(6.83634180296788,31.1867582961606,123.830743494929));
#121325=CARTESIAN_POINT('Ctrl Pts',(6.83636301139702,31.1869841503641,123.830972775975));
#121326=CARTESIAN_POINT('Ctrl Pts',(6.83637316154242,31.1870922337808,123.831082529763));
#121327=CARTESIAN_POINT('Ctrl Pts',(6.83639266973831,31.187299950285,123.831293514937));
#121328=CARTESIAN_POINT('Ctrl Pts',(6.83640202788553,31.1873995856289,123.831394744055));
#121329=CARTESIAN_POINT('Ctrl Pts',(6.83644599565934,31.1878676737873,123.831870441451));
#121330=CARTESIAN_POINT('Ctrl Pts',(6.83648059819211,31.1882359627286,123.832245071574));
#121331=CARTESIAN_POINT('Ctrl Pts',(6.83654978594269,31.1889721651694,123.832994658793));
#121332=CARTESIAN_POINT('Ctrl Pts',(6.83658437116217,31.1893400786978,123.833369615878));
#121333=CARTESIAN_POINT('Ctrl Pts',(6.83769552992994,31.2011573758218,123.84542455043));
#121334=CARTESIAN_POINT('Ctrl Pts',(6.83876463532282,31.2124346360422,123.857272650799));
#121335=CARTESIAN_POINT('Ctrl Pts',(6.84307431199839,31.257482519891,123.906018547587));
#121336=CARTESIAN_POINT('Ctrl Pts',(6.8462526482211,31.2897598023664,123.944264195551));
#121337=CARTESIAN_POINT('Ctrl Pts',(6.85509057777599,31.3758971638434,124.05618760401));
#121338=CARTESIAN_POINT('Ctrl Pts',(6.86061604731787,31.4254956588701,124.132914148576));
#121339=CARTESIAN_POINT('Ctrl Pts',(6.86695878713564,31.4744411549266,124.224284794228));
#121340=CARTESIAN_POINT('Ctrl Pts',(6.86772113622544,31.4801930975265,124.235317589096));
#121341=CARTESIAN_POINT('Ctrl Pts',(6.87301921800923,31.5192130050196,124.312251833965));
#121342=CARTESIAN_POINT('Ctrl Pts',(6.87760764457699,31.5481880979843,124.380228636115));
#121343=CARTESIAN_POINT('Ctrl Pts',(6.88323070623185,31.5766126688508,124.461484167233));
#121344=CARTESIAN_POINT('Ctrl Pts',(6.88403917876402,31.58053919779,124.473119907191));
#121345=CARTESIAN_POINT('Ctrl Pts',(6.88531652837233,31.5864862515534,124.49140812614));
#121346=CARTESIAN_POINT('Ctrl Pts',(6.88578052695712,31.5885944632874,124.498031925956));
#121347=CARTESIAN_POINT('Ctrl Pts',(6.88665328098075,31.5924614110914,124.510449881254));
#121348=CARTESIAN_POINT('Ctrl Pts',(6.88706146181564,31.5942300905237,124.516240681366));
#121349=CARTESIAN_POINT('Ctrl Pts',(6.88802797536398,31.598324991112,124.529914083135));
#121350=CARTESIAN_POINT('Ctrl Pts',(6.88858779409208,31.6006244922968,124.537804398521));
#121351=CARTESIAN_POINT('Ctrl Pts',(6.89047323329542,31.6081313233629,124.564290721975));
#121352=CARTESIAN_POINT('Ctrl Pts',(6.89181241325579,31.61307346818,124.582959432531));
#121353=CARTESIAN_POINT('Ctrl Pts',(6.90253161359105,31.6496630424049,124.731570746258));
#121354=CARTESIAN_POINT('Ctrl Pts',(6.91244836012507,31.6658815080754,124.86480119885));
#121355=CARTESIAN_POINT('Ctrl Pts',(6.92206992138496,31.6659993531474,124.998531901728));
#121356=CARTESIAN_POINT('Ctrl Pts',(6.92206982081665,31.665999351915,124.998530503923));
#121357=CARTESIAN_POINT('Ctrl Pts',(6.92753181140456,31.6660663141654,125.074447049386));
#121358=CARTESIAN_POINT('Ctrl Pts',(6.93289219990884,31.6609442423801,125.150289871046));
#121359=CARTESIAN_POINT('Ctrl Pts',(6.93911166202533,31.6486554136217,125.240232187486));
#121360=CARTESIAN_POINT('Ctrl Pts',(6.94012221746603,31.6464503321999,125.254906855563));
#121361=CARTESIAN_POINT('Ctrl Pts',(6.94186362685613,31.6422878030681,125.280295059211));
#121362=CARTESIAN_POINT('Ctrl Pts',(6.94259726897818,31.6404208576317,125.291022280846));
#121363=CARTESIAN_POINT('Ctrl Pts',(6.94406287339542,31.6364634093353,125.312511899126));
#121364=CARTESIAN_POINT('Ctrl Pts',(6.94479475356403,31.634371570694,125.323273500301));
#121365=CARTESIAN_POINT('Ctrl Pts',(6.94618655018325,31.6301725158045,125.343792367028));
#121366=CARTESIAN_POINT('Ctrl Pts',(6.94684701262364,31.6280835433912,125.353552833388));
#121367=CARTESIAN_POINT('Ctrl Pts',(6.9485622804204,31.6224071119003,125.378957454216));
#121368=CARTESIAN_POINT('Ctrl Pts',(6.94961262412396,31.6186810281943,125.394569825618));
#121369=CARTESIAN_POINT('Ctrl Pts',(6.95332701362548,31.6046166342835,125.44994348004));
#121370=CARTESIAN_POINT('Ctrl Pts',(6.95595137220481,31.5930336159903,125.489375114406));
#121371=CARTESIAN_POINT('Ctrl Pts',(6.95959038684336,31.5747174825424,125.544149528908));
#121372=CARTESIAN_POINT('Ctrl Pts',(6.96063437872422,31.5691955020297,125.559874154248));
#121373=CARTESIAN_POINT('Ctrl Pts',(6.96167312081939,31.563440026896,125.575509584889));
#121374=CARTESIAN_POINT('Ctrl Pts',(6.76893575384937,31.5634399863339,125.575509695081));
#121375=CARTESIAN_POINT('Ctrl Pts',(6.76566846517258,31.5792218917318,125.532636287091));
#121376=CARTESIAN_POINT('Ctrl Pts',(6.7623534844689,31.5932378790754,125.48912013638));
#121377=CARTESIAN_POINT('Ctrl Pts',(6.7546987721579,31.6213480053,125.38772196693));
#121378=CARTESIAN_POINT('Ctrl Pts',(6.75035979235393,31.6341628180893,125.329560310083));
#121379=CARTESIAN_POINT('Ctrl Pts',(6.74216811017329,31.6526476961366,125.217366558126));
#121380=CARTESIAN_POINT('Ctrl Pts',(6.7383111165396,31.6588438782114,125.163494847297));
#121381=CARTESIAN_POINT('Ctrl Pts',(6.73198981774126,31.6647895384476,125.073156983302));
#121382=CARTESIAN_POINT('Ctrl Pts',(6.72948680256719,31.6659891926143,125.036830939512));
#121383=CARTESIAN_POINT('Ctrl Pts',(6.72610898150434,31.6660038935743,124.987066426564));
#121384=CARTESIAN_POINT('Ctrl Pts',(6.72520276065366,31.6658455695417,124.973640808191));
#121385=CARTESIAN_POINT('Ctrl Pts',(6.72363257222695,31.665286952603,124.950253454733));
#121386=CARTESIAN_POINT('Ctrl Pts',(6.7229663684906,31.6649595121106,124.94029084021));
#121387=CARTESIAN_POINT('Ctrl Pts',(6.72157290120123,31.6640839746543,124.919372189542));
#121388=CARTESIAN_POINT('Ctrl Pts',(6.72084625972782,31.663517043225,124.908417385948));
#121389=CARTESIAN_POINT('Ctrl Pts',(6.71910583299487,31.6618926436736,124.882073029297));
#121390=CARTESIAN_POINT('Ctrl Pts',(6.71809539010171,31.6607295443041,124.86669082381));
#121391=CARTESIAN_POINT('Ctrl Pts',(6.71449763569955,31.6557971289075,124.811639849404));
#121392=CARTESIAN_POINT('Ctrl Pts',(6.71194788150291,31.6508184933732,124.772091302045));
#121393=CARTESIAN_POINT('Ctrl Pts',(6.70550673554532,31.6344501884969,124.671372335618));
#121394=CARTESIAN_POINT('Ctrl Pts',(6.70167115063231,31.6210445612681,124.610591568612));
#121395=CARTESIAN_POINT('Ctrl Pts',(6.69223213099618,31.5794709929212,124.46214906716));
#121396=CARTESIAN_POINT('Ctrl Pts',(6.68668138531257,31.5473838265913,124.375809808904));
#121397=CARTESIAN_POINT('Ctrl Pts',(6.67844007291379,31.4916773452116,124.25703659814));
#121398=CARTESIAN_POINT('Ctrl Pts',(6.6759352462958,31.4737654155543,124.222111267959));
#121399=CARTESIAN_POINT('Ctrl Pts',(6.67264686331178,31.4493120621227,124.178312736655));
#121400=CARTESIAN_POINT('Ctrl Pts',(6.67192537503852,31.4438914832879,124.1688244584));
#121401=CARTESIAN_POINT('Ctrl Pts',(6.6707598943962,31.4350555901827,124.153705243666));
#121402=CARTESIAN_POINT('Ctrl Pts',(6.67031956726799,31.4316994348043,124.148039856491));
#121403=CARTESIAN_POINT('Ctrl Pts',(6.66946121476285,31.4251248692273,124.137090161889));
#121404=CARTESIAN_POINT('Ctrl Pts',(6.6690434387682,31.4219104733702,124.1318036614));
#121405=CARTESIAN_POINT('Ctrl Pts',(6.66801018811353,31.4139235946949,124.118831505665));
#121406=CARTESIAN_POINT('Ctrl Pts',(6.66739261973903,31.4091178510767,124.111166652563));
#121407=CARTESIAN_POINT('Ctrl Pts',(6.66506667823885,31.3908903058785,124.082614262726));
#121408=CARTESIAN_POINT('Ctrl Pts',(6.66333514601541,31.3770652496449,124.061989566856));
#121409=CARTESIAN_POINT('Ctrl Pts',(6.65873186824812,31.3395275833869,124.008608714111));
#121410=CARTESIAN_POINT('Ctrl Pts',(6.65582933936729,31.3150747499944,123.976394205894));
#121411=CARTESIAN_POINT('Ctrl Pts',(6.64422777868077,31.2135366659428,123.852276918859));
#121412=CARTESIAN_POINT('Ctrl Pts',(6.63541839725036,31.1277847013632,123.767909466563));
#121413=CARTESIAN_POINT('Ctrl Pts',(6.62352641523548,30.995741565389,123.663437604996));
#121414=CARTESIAN_POINT('Ctrl Pts',(6.62016210801722,30.9564764107155,123.635062642549));
#121415=CARTESIAN_POINT('Ctrl Pts',(6.61570431649433,30.9018347339696,123.599093571785));
#121416=CARTESIAN_POINT('Ctrl Pts',(6.61455453767669,30.887499746302,123.589968459404));
#121417=CARTESIAN_POINT('Ctrl Pts',(6.61273097368413,30.8643836653132,123.575745854207));
#121418=CARTESIAN_POINT('Ctrl Pts',(6.61205202666465,30.8556915649227,123.570506751934));
#121419=CARTESIAN_POINT('Ctrl Pts',(6.6106544320865,30.8376245748689,123.559840844616));
#121420=CARTESIAN_POINT('Ctrl Pts',(6.60993622013046,30.8282435240922,123.554425375328));
#121421=CARTESIAN_POINT('Ctrl Pts',(6.60825610543794,30.8060757000681,123.541915030134));
#121422=CARTESIAN_POINT('Ctrl Pts',(6.60729695346035,30.793246881779,123.534896174114));
#121423=CARTESIAN_POINT('Ctrl Pts',(6.60409597356454,30.7498700496152,123.511900799454));
#121424=CARTESIAN_POINT('Ctrl Pts',(6.60188127962806,30.7189178113786,123.496703034692));
#121425=CARTESIAN_POINT('Ctrl Pts',(6.59650648304181,30.6417635497319,123.461748290888));
#121426=CARTESIAN_POINT('Ctrl Pts',(6.59338016661069,30.5950965893341,123.443099432007));
#121427=CARTESIAN_POINT('Ctrl Pts',(6.58628694986402,30.486375883835,123.405257187973));
#121428=CARTESIAN_POINT('Ctrl Pts',(6.58234800923876,30.423902590394,123.38752586745));
#121429=CARTESIAN_POINT('Ctrl Pts',(6.57368827061504,30.2858500804228,123.356923422177));
#121430=CARTESIAN_POINT('Ctrl Pts',(6.56896426463972,30.2101023782979,123.345531757429));
#121431=CARTESIAN_POINT('Ctrl Pts',(6.56296074054861,30.117757664634,123.338088515151));
#121432=CARTESIAN_POINT('Ctrl Pts',(6.5619043733652,30.1016478830074,123.337025462653));
#121433=CARTESIAN_POINT('Ctrl Pts',(6.5603218933115,30.0777701608207,123.335798055202));
#121434=CARTESIAN_POINT('Ctrl Pts',(6.55980510393975,30.0700118852934,123.335453623076));
#121435=CARTESIAN_POINT('Ctrl Pts',(6.55888304769967,30.0562459456892,123.334938886153));
#121436=CARTESIAN_POINT('Ctrl Pts',(6.55847898200649,30.0502393549644,123.33474682877));
#121437=CARTESIAN_POINT('Ctrl Pts',(6.55758333846138,30.036983600381,123.33439476896));
#121438=CARTESIAN_POINT('Ctrl Pts',(6.55709099500868,30.0297344664941,123.334249589853));
#121439=CARTESIAN_POINT('Ctrl Pts',(6.55563626598367,30.0084189860264,123.333961884132));
#121440=CARTESIAN_POINT('Ctrl Pts',(6.55466722071023,29.994351914211,123.33395019601));
#121441=CARTESIAN_POINT('Ctrl Pts',(6.54798466243464,29.8981306186771,123.335088818889));
#121442=CARTESIAN_POINT('Ctrl Pts',(6.54202798855866,29.8161669707849,123.342137143349));
#121443=CARTESIAN_POINT('Ctrl Pts',(6.52654041030243,29.6060487682507,123.375981521745));
#121444=CARTESIAN_POINT('Ctrl Pts',(6.51706505609792,29.4798978137246,123.411875382835));
#121445=CARTESIAN_POINT('Ctrl Pts',(6.5066473226768,29.3400669615481,123.47013884988));
#121446=CARTESIAN_POINT('Ctrl Pts',(6.50523177199624,29.3210590203445,123.47847906116));
#121447=CARTESIAN_POINT('Ctrl Pts',(6.50293214807661,29.2901783428614,123.492722717465));
#121448=CARTESIAN_POINT('Ctrl Pts',(6.50204104992566,29.2782119164071,123.498416312229));
#121449=CARTESIAN_POINT('Ctrl Pts',(6.50044168657876,29.2567393890003,123.508948893068));
#121450=CARTESIAN_POINT('Ctrl Pts',(6.49973172434151,29.2472095236347,123.51373749051));
#121451=CARTESIAN_POINT('Ctrl Pts',(6.49821230823,29.2268227148164,123.52422791467));
#121452=CARTESIAN_POINT('Ctrl Pts',(6.49740392325962,29.2159813637002,123.529958791876));
#121453=CARTESIAN_POINT('Ctrl Pts',(6.49517794678016,29.1861533133621,123.546150131607));
#121454=CARTESIAN_POINT('Ctrl Pts',(6.49376932510773,29.1673055684959,123.556862472511));
#121455=CARTESIAN_POINT('Ctrl Pts',(6.49063998672077,29.1255549961917,123.581682278525));
#121456=CARTESIAN_POINT('Ctrl Pts',(6.48892621597124,29.1027737337512,123.595982774814));
#121457=CARTESIAN_POINT('Ctrl Pts',(6.48334081515579,29.0290107900213,123.644814968658));
#121458=CARTESIAN_POINT('Ctrl Pts',(6.47954193904515,28.9795946482407,123.681622112195));
#121459=CARTESIAN_POINT('Ctrl Pts',(6.47023368799811,28.862923746602,123.779021946069));
#121460=CARTESIAN_POINT('Ctrl Pts',(6.46477578823116,28.7983563015707,123.842511196219));
#121461=CARTESIAN_POINT('Ctrl Pts',(6.45651536395954,28.7122196526121,123.942224488467));
#121462=CARTESIAN_POINT('Ctrl Pts',(6.45387986474419,28.6863551673293,123.974522604075));
#121463=CARTESIAN_POINT('Ctrl Pts',(6.45044039445048,28.6550899515346,124.016690820631));
#121464=CARTESIAN_POINT('Ctrl Pts',(6.44970553512465,28.6485483109278,124.025701125809));
#121465=CARTESIAN_POINT('Ctrl Pts',(6.44852358223024,28.6382563994411,124.040180055691));
#121466=CARTESIAN_POINT('Ctrl Pts',(6.44808033878806,28.6344474811615,124.045606855845));
#121467=CARTESIAN_POINT('Ctrl Pts',(6.44722073702929,28.6271605547018,124.056121912629));
#121468=CARTESIAN_POINT('Ctrl Pts',(6.44680467167672,28.6236782416112,124.061206945738));
#121469=CARTESIAN_POINT('Ctrl Pts',(6.4457820581066,28.6152265756055,124.073696547416));
#121470=CARTESIAN_POINT('Ctrl Pts',(6.44517351164284,28.6102883488275,124.081121857456));
#121471=CARTESIAN_POINT('Ctrl Pts',(6.44292169165269,28.5923405043771,124.10858455724));
#121472=CARTESIAN_POINT('Ctrl Pts',(6.44125705738956,28.5797033742168,124.12886045977));
#121473=CARTESIAN_POINT('Ctrl Pts',(6.43688123202123,28.5479958749019,124.182258936347));
#121474=CARTESIAN_POINT('Ctrl Pts',(6.43414257082114,28.5296219412697,124.215777819422));
#121475=CARTESIAN_POINT('Ctrl Pts',(6.42636297470662,28.481141548104,124.311922639527));
#121476=CARTESIAN_POINT('Ctrl Pts',(6.42128110692228,28.4537753625509,124.375843885437));
#121477=CARTESIAN_POINT('Ctrl Pts',(6.40925762727111,28.3981261400603,124.532172052491));
#121478=CARTESIAN_POINT('Ctrl Pts',(6.40239179061435,28.3737237958675,124.625708328326));
#121479=CARTESIAN_POINT('Ctrl Pts',(6.394422281649,28.3542194874083,124.740464765179));
#121480=CARTESIAN_POINT('Ctrl Pts',(6.39307075153351,28.351236628781,124.760142877868));
#121481=CARTESIAN_POINT('Ctrl Pts',(6.39092960348249,28.3470362176849,124.791654006149));
#121482=CARTESIAN_POINT('Ctrl Pts',(6.39013292706237,28.3455916144051,124.803454267017));
#121483=CARTESIAN_POINT('Ctrl Pts',(6.3886251703804,28.3430843749332,124.825926449132));
#121484=CARTESIAN_POINT('Ctrl Pts',(6.38791338807996,28.3419982408849,124.836595086831));
#121485=CARTESIAN_POINT('Ctrl Pts',(6.38628936633682,28.3397451370627,124.861069356698));
#121486=CARTESIAN_POINT('Ctrl Pts',(6.38537932927415,28.3386472062693,124.8748806668));
#121487=CARTESIAN_POINT('Ctrl Pts',(6.38252197281539,28.3357245210372,124.918533041298));
#121488=CARTESIAN_POINT('Ctrl Pts',(6.38059422659175,28.334530539402,124.948411363841));
#121489=CARTESIAN_POINT('Ctrl Pts',(6.37342718024813,28.3330670685648,125.060795833283));
#121490=CARTESIAN_POINT('Ctrl Pts',(6.36834527609445,28.3381210360748,125.143254217431));
#121491=CARTESIAN_POINT('Ctrl Pts',(6.35704814479076,28.3630714757776,125.326301131831));
#121492=CARTESIAN_POINT('Ctrl Pts',(6.35087833401576,28.3861717177644,125.426100341294));
#121493=CARTESIAN_POINT('Ctrl Pts',(6.3427150414444,28.4263419848175,125.547556112928));
#121494=CARTESIAN_POINT('Ctrl Pts',(6.34105231593054,28.4349803240993,125.571778355805));
#121495=CARTESIAN_POINT('Ctrl Pts',(6.33873921413658,28.4475477194582,125.60459643992));
#121496=CARTESIAN_POINT('Ctrl Pts',(6.33811452722373,28.4509949253843,125.613374442734));
#121497=CARTESIAN_POINT('Ctrl Pts',(6.33710919758382,28.4566230793419,125.627355966506));
#121498=CARTESIAN_POINT('Ctrl Pts',(6.33673134286049,28.4587563212774,125.632578649919));
#121499=CARTESIAN_POINT('Ctrl Pts',(6.33592756514873,28.463330752225,125.643617440336));
#121500=CARTESIAN_POINT('Ctrl Pts',(6.33550123657487,28.4657785085624,125.649430672004));
#121501=CARTESIAN_POINT('Ctrl Pts',(6.33441786867087,28.4720540980336,125.664101216503));
#121502=CARTESIAN_POINT('Ctrl Pts',(6.33375828435987,28.4759259296848,125.672939315327));
#121503=CARTESIAN_POINT('Ctrl Pts',(6.33105459344575,28.4920120766179,125.708807621319));
#121504=CARTESIAN_POINT('Ctrl Pts',(6.328976990741,28.5048697243589,125.735541311528));
#121505=CARTESIAN_POINT('Ctrl Pts',(6.32311048891109,28.5427047417038,125.809112607265));
#121506=CARTESIAN_POINT('Ctrl Pts',(6.31926942004885,28.569216484543,125.855120189009));
#121507=CARTESIAN_POINT('Ctrl Pts',(6.30578385549763,28.6693921821795,126.011223354872));
#121508=CARTESIAN_POINT('Ctrl Pts',(6.29614326225557,28.7539536768138,126.113764170959));
#121509=CARTESIAN_POINT('Ctrl Pts',(6.28518173627638,28.8687449970032,126.223317399741));
#121510=CARTESIAN_POINT('Ctrl Pts',(6.28338919329618,28.8881365293536,126.240968613648));
#121511=CARTESIAN_POINT('Ctrl Pts',(6.28071304786774,28.9180165719773,126.266904093456));
#121512=CARTESIAN_POINT('Ctrl Pts',(6.27981537483889,28.9282005529466,126.275531294723));
#121513=CARTESIAN_POINT('Ctrl Pts',(6.27820891482175,28.9467125941445,126.290835207247));
#121514=CARTESIAN_POINT('Ctrl Pts',(6.27749836434077,28.9550031269339,126.297555947149));
#121515=CARTESIAN_POINT('Ctrl Pts',(6.27598269763902,28.9729044143073,126.311784804919));
#121516=CARTESIAN_POINT('Ctrl Pts',(6.27517859971786,28.9825342277472,126.31926802892));
#121517=CARTESIAN_POINT('Ctrl Pts',(6.27297765691045,29.00925064968,126.339562525642));
#121518=CARTESIAN_POINT('Ctrl Pts',(6.27158944310107,29.026503126198,126.352152335843));
#121519=CARTESIAN_POINT('Ctrl Pts',(6.26328593824872,29.1320038354848,126.426074065688));
#121520=CARTESIAN_POINT('Ctrl Pts',(6.25669533492763,29.2257775596631,126.479083512348));
#121521=CARTESIAN_POINT('Ctrl Pts',(6.24364533706041,29.4210792246415,126.56578579227));
#121522=CARTESIAN_POINT('Ctrl Pts',(6.23720834210651,29.522028794827,126.59949108886));
#121523=CARTESIAN_POINT('Ctrl Pts',(6.22931655961956,29.6404821282031,126.626818944679));
#121524=CARTESIAN_POINT('Ctrl Pts',(6.22830780916112,29.6555288243556,126.630071331798));
#121525=CARTESIAN_POINT('Ctrl Pts',(6.22679019075446,29.6779828867365,126.634600082726));
#121526=CARTESIAN_POINT('Ctrl Pts',(6.22628977852532,29.6853577986835,126.636035675464));
#121527=CARTESIAN_POINT('Ctrl Pts',(6.22538458333702,29.6986403021103,126.638528103996));
#121528=CARTESIAN_POINT('Ctrl Pts',(6.22498081470885,29.7045442391213,126.639602971935));
#121529=CARTESIAN_POINT('Ctrl Pts',(6.22407009415916,29.7178137820148,126.6419448203));
#121530=CARTESIAN_POINT('Ctrl Pts',(6.22356220601175,29.7251821135943,126.643194138997));
#121531=CARTESIAN_POINT('Ctrl Pts',(6.22201430603384,29.7475501934873,126.646832047732));
#121532=CARTESIAN_POINT('Ctrl Pts',(6.22096634294683,29.7625739607222,126.64906504833));
#121533=CARTESIAN_POINT('Ctrl Pts',(6.214239988704,29.8583733281886,126.661967621428));
#121534=CARTESIAN_POINT('Ctrl Pts',(6.20832952025617,29.9398024230305,126.666903753681));
#121535=CARTESIAN_POINT('Ctrl Pts',(6.19299247442665,30.1505254695771,126.664214898999));
#121536=CARTESIAN_POINT('Ctrl Pts',(6.18362314896035,30.2791884326212,126.647523921862));
#121537=CARTESIAN_POINT('Ctrl Pts',(6.17328928026487,30.4249206014095,126.61103553132));
#121538=CARTESIAN_POINT('Ctrl Pts',(6.17186325968043,30.4451025863081,126.605576767734));
#121539=CARTESIAN_POINT('Ctrl Pts',(6.1695502604646,30.4779436504929,126.596027138637));
#121540=CARTESIAN_POINT('Ctrl Pts',(6.1686561176047,30.4906654123736,126.592162124659));
#121541=CARTESIAN_POINT('Ctrl Pts',(6.16705347505006,30.5135093931105,126.584922051913));
#121542=CARTESIAN_POINT('Ctrl Pts',(6.16634324753615,30.5236479197711,126.581601300156));
#121543=CARTESIAN_POINT('Ctrl Pts',(6.16482560319896,30.5453399946238,126.574264869246));
#121544=CARTESIAN_POINT('Ctrl Pts',(6.16401923158058,30.5568826830236,126.57021886341));
#121545=CARTESIAN_POINT('Ctrl Pts',(6.16180502113609,30.5886139269804,126.558702340121));
#121546=CARTESIAN_POINT('Ctrl Pts',(6.16040599219921,30.6087043053468,126.550966949264));
#121547=CARTESIAN_POINT('Ctrl Pts',(6.15303681439696,30.7146044578148,126.507817377358));
#121548=CARTESIAN_POINT('Ctrl Pts',(6.14729965965831,30.7974960563683,126.465665662885));
#121549=CARTESIAN_POINT('Ctrl Pts',(6.13569639994598,30.9587634419109,126.365904948752));
#121550=CARTESIAN_POINT('Ctrl Pts',(6.12985525162857,31.0364735784667,126.307915587103));
#121551=CARTESIAN_POINT('Ctrl Pts',(6.12167168058232,31.1330236320952,126.221832648336));
#121552=CARTESIAN_POINT('Ctrl Pts',(6.11957939928412,31.1566997671829,126.199442742693));
#121553=CARTESIAN_POINT('Ctrl Pts',(6.11676481224766,31.1869660424645,126.169090857237));
#121554=CARTESIAN_POINT('Ctrl Pts',(6.11608473173688,31.1941617878221,126.161739828757));
#121555=CARTESIAN_POINT('Ctrl Pts',(6.1149702181184,31.205754326921,126.149675624323));
#121556=CARTESIAN_POINT('Ctrl Pts',(6.11453890025574,31.2101927808608,126.145002605959));
#121557=CARTESIAN_POINT('Ctrl Pts',(6.11368305905451,31.2189027413773,126.135725122369));
#121558=CARTESIAN_POINT('Ctrl Pts',(6.11325864120831,31.2231755214743,126.131122047296));
#121559=CARTESIAN_POINT('Ctrl Pts',(6.11218614603746,31.2338586912055,126.119481731413));
#121560=CARTESIAN_POINT('Ctrl Pts',(6.11153562212534,31.2402349066889,126.112413584198));
#121561=CARTESIAN_POINT('Ctrl Pts',(6.108999354549,31.2647084935015,126.084812220464));
#121562=CARTESIAN_POINT('Ctrl Pts',(6.10708545722772,31.2823583280782,126.063890049858));
#121563=CARTESIAN_POINT('Ctrl Pts',(6.10179136357219,31.3291770104192,126.005532707082));
#121564=CARTESIAN_POINT('Ctrl Pts',(6.09836858901783,31.3572738784761,125.967271735084));
#121565=CARTESIAN_POINT('Ctrl Pts',(6.08793005323057,31.437368953623,125.847828505974));
#121566=CARTESIAN_POINT('Ctrl Pts',(6.08087903640557,31.4839989688586,125.763277419907));
#121567=CARTESIAN_POINT('Ctrl Pts',(6.07146606012556,31.5375894141665,125.642386490861));
#121568=CARTESIAN_POINT('Ctrl Pts',(6.06894107617486,31.5510566138041,125.609150590502));
#121569=CARTESIAN_POINT('Ctrl Pts',(6.06644911688889,31.5634400025946,125.575509650907));
#121570=CARTESIAN_POINT('Origin',(5.,30.,125.));
#121571=CARTESIAN_POINT('',(5.36787244251734,31.5634400119422,125.575509625513));
#121572=CARTESIAN_POINT('',(5.55934605048515,31.5634400125327,125.575509623909));
#121573=CARTESIAN_POINT('',(5.,31.5634400119422,125.575509625513));
#121574=CARTESIAN_POINT('Ctrl Pts',(5.55934605048515,31.5634400125327,125.575509623909));
#121575=CARTESIAN_POINT('Ctrl Pts',(5.56457325969903,31.5376336036079,125.645615788283));
#121576=CARTESIAN_POINT('Ctrl Pts',(5.56999012258899,31.507141899839,125.713904230111));
#121577=CARTESIAN_POINT('Ctrl Pts',(5.5821568579232,31.4288705775657,125.861650140254));
#121578=CARTESIAN_POINT('Ctrl Pts',(5.58889024925279,31.3788321131222,125.939647398461));
#121579=CARTESIAN_POINT('Ctrl Pts',(5.59899374878281,31.2919283036445,126.053098701067));
#121580=CARTESIAN_POINT('Ctrl Pts',(5.60249704164566,31.2594815404164,126.09169720192));
#121581=CARTESIAN_POINT('Ctrl Pts',(5.60704747128831,31.2142220122951,126.140828541928));
#121582=CARTESIAN_POINT('Ctrl Pts',(5.60815689890244,31.2029348422995,126.152724015447));
#121583=CARTESIAN_POINT('Ctrl Pts',(5.60929411181592,31.191106268656,126.16482708282));
#121584=CARTESIAN_POINT('Ctrl Pts',(5.60932941348466,31.1907388238759,126.165202698855));
#121585=CARTESIAN_POINT('Ctrl Pts',(5.60939999170995,31.1900036779194,126.165953482131));
#121586=CARTESIAN_POINT('Ctrl Pts',(5.60943526826434,31.1896359769058,126.166328649398));
#121587=CARTESIAN_POINT('Ctrl Pts',(5.60947983086635,31.1891711569369,126.166802459147));
#121588=CARTESIAN_POINT('Ctrl Pts',(5.60948912415662,31.1890742032685,126.166901263297));
#121589=CARTESIAN_POINT('Ctrl Pts',(5.60950848156975,31.1888722166713,126.167107053747));
#121590=CARTESIAN_POINT('Ctrl Pts',(5.60951854560201,31.1887671815783,126.16721403799));
#121591=CARTESIAN_POINT('Ctrl Pts',(5.6095395554274,31.1885478647307,126.167437364418));
#121592=CARTESIAN_POINT('Ctrl Pts',(5.6095505010958,31.1884335804163,126.167553703919));
#121593=CARTESIAN_POINT('Ctrl Pts',(5.60957340793005,31.1881943567315,126.167797158071));
#121594=CARTESIAN_POINT('Ctrl Pts',(5.60958536894441,31.1880694140929,126.167924269405));
#121595=CARTESIAN_POINT('Ctrl Pts',(5.609610469325,31.1878071574507,126.168190992542));
#121596=CARTESIAN_POINT('Ctrl Pts',(5.6096236085078,31.1876698391951,126.168330600221));
#121597=CARTESIAN_POINT('Ctrl Pts',(5.60965126576703,31.1873807161161,126.168624440027));
#121598=CARTESIAN_POINT('Ctrl Pts',(5.60966578360975,31.1872289057797,126.168778666863));
#121599=CARTESIAN_POINT('Ctrl Pts',(5.60969644824963,31.1869081586972,126.169104392588));
#121600=CARTESIAN_POINT('Ctrl Pts',(5.60971259472704,31.1867392148708,126.1692758844));
#121601=CARTESIAN_POINT('Ctrl Pts',(5.60974683284431,31.1863808593938,126.169639486871));
#121602=CARTESIAN_POINT('Ctrl Pts',(5.60976492407513,31.1861914381201,126.16983158827));
#121603=CARTESIAN_POINT('Ctrl Pts',(5.60980345807131,31.1857878288947,126.17024070935));
#121604=CARTESIAN_POINT('Ctrl Pts',(5.60982390026522,31.1855736280023,126.170457716263));
#121605=CARTESIAN_POINT('Ctrl Pts',(5.60986766819247,31.185114824843,126.170922274555));
#121606=CARTESIAN_POINT('Ctrl Pts',(5.60989099313652,31.184870204477,126.171169808207));
#121607=CARTESIAN_POINT('Ctrl Pts',(5.60994123826933,31.1843430141136,126.171702942872));
#121608=CARTESIAN_POINT('Ctrl Pts',(5.609968157316,31.1840604183304,126.171988518356));
#121609=CARTESIAN_POINT('Ctrl Pts',(5.61002656736855,31.1834469022115,126.172608055014));
#121610=CARTESIAN_POINT('Ctrl Pts',(5.61005805669007,31.1831159436978,126.172941978449));
#121611=CARTESIAN_POINT('Ctrl Pts',(5.61012698942341,31.1823909947736,126.173672802887));
#121612=CARTESIAN_POINT('Ctrl Pts',(5.61016443024702,31.1819969456538,126.174069645815));
#121613=CARTESIAN_POINT('Ctrl Pts',(5.61024729666775,31.1811241626173,126.17494773214));
#121614=CARTESIAN_POINT('Ctrl Pts',(5.61029271808654,31.1806453340635,126.175428881701));
#121615=CARTESIAN_POINT('Ctrl Pts',(5.61056165950892,31.1778076227556,126.178276864748));
#121616=CARTESIAN_POINT('Ctrl Pts',(5.61078487736116,31.1754419033654,126.180636903674));
#121617=CARTESIAN_POINT('Ctrl Pts',(5.61172144478894,31.1654721204463,126.190523078419));
#121618=CARTESIAN_POINT('Ctrl Pts',(5.61243186680322,31.1578026198435,126.197983124417));
#121619=CARTESIAN_POINT('Ctrl Pts',(5.61403858074731,31.1402166881517,126.214762141136));
#121620=CARTESIAN_POINT('Ctrl Pts',(5.61493284580725,31.1302567997614,126.224034615652));
#121621=CARTESIAN_POINT('Ctrl Pts',(5.61725783755841,31.1039217845292,126.247956480633));
#121622=CARTESIAN_POINT('Ctrl Pts',(5.61868026565278,31.0873682083727,126.262406089641));
#121623=CARTESIAN_POINT('Ctrl Pts',(5.62747313631323,30.9824138034119,126.350424100891));
#121624=CARTESIAN_POINT('Ctrl Pts',(5.63447378993395,30.8868779082634,126.415002938947));
#121625=CARTESIAN_POINT('Ctrl Pts',(5.64731086811544,30.7015324742168,126.514087601024));
#121626=CARTESIAN_POINT('Ctrl Pts',(5.65312596698492,30.6139450501004,126.551668663773));
#121627=CARTESIAN_POINT('Ctrl Pts',(5.66024628090668,30.5100417646885,126.586070206986));
#121628=CARTESIAN_POINT('Ctrl Pts',(5.66118670807923,30.4963825505974,126.590397947976));
#121629=CARTESIAN_POINT('Ctrl Pts',(5.66262118188542,30.475678312678,126.596665119041));
#121630=CARTESIAN_POINT('Ctrl Pts',(5.66310807124715,30.4686731600006,126.598735382602));
#121631=CARTESIAN_POINT('Ctrl Pts',(5.6640003324627,30.4558816505424,126.602424420016));
#121632=CARTESIAN_POINT('Ctrl Pts',(5.66440484899187,30.4500998541532,126.604058047231));
#121633=CARTESIAN_POINT('Ctrl Pts',(5.66533228546413,30.4368832366709,126.607715275486));
#121634=CARTESIAN_POINT('Ctrl Pts',(5.66585631394989,30.4294431594788,126.609718589194));
#121635=CARTESIAN_POINT('Ctrl Pts',(5.66750403563471,30.4061270759994,126.615823526705));
#121636=CARTESIAN_POINT('Ctrl Pts',(5.66863718330682,30.3902047867189,126.619742277491));
#121637=CARTESIAN_POINT('Ctrl Pts',(5.67562178609053,30.2925929659798,126.642243516335));
#121638=CARTESIAN_POINT('Ctrl Pts',(5.68171073253202,30.2096622307838,126.654875692006));
#121639=CARTESIAN_POINT('Ctrl Pts',(5.69423683596305,30.0380747589092,126.667904948228));
#121640=CARTESIAN_POINT('Ctrl Pts',(5.70065309217485,29.9496065178747,126.667579077431));
#121641=CARTESIAN_POINT('Ctrl Pts',(5.71037123417081,29.8124878954803,126.656146572711));
#121642=CARTESIAN_POINT('Ctrl Pts',(5.71379282929853,29.7636029262947,126.64987864419));
#121643=CARTESIAN_POINT('Ctrl Pts',(5.71827889062258,29.6986963837706,126.638611628788));
#121644=CARTESIAN_POINT('Ctrl Pts',(5.71940235811241,29.682372639126,126.635525858399));
#121645=CARTESIAN_POINT('Ctrl Pts',(5.72127034752949,29.6551242288974,126.629951578646));
#121646=CARTESIAN_POINT('Ctrl Pts',(5.72201903697238,29.644173899557,126.627596154777));
#121647=CARTESIAN_POINT('Ctrl Pts',(5.72349054832347,29.622598328577,126.622727077587));
#121648=CARTESIAN_POINT('Ctrl Pts',(5.72421350898735,29.6119724082001,126.620219055424));
#121649=CARTESIAN_POINT('Ctrl Pts',(5.72596978311197,29.5861024843057,126.613843906288));
#121650=CARTESIAN_POINT('Ctrl Pts',(5.72699946111895,29.5708869104211,126.609864991698));
#121651=CARTESIAN_POINT('Ctrl Pts',(5.73055307472606,29.5182397148198,126.595298126329));
#121652=CARTESIAN_POINT('Ctrl Pts',(5.73304187817072,29.4811226802842,126.583614782041));
#121653=CARTESIAN_POINT('Ctrl Pts',(5.74372333143259,29.3216196833483,126.527196780995));
#121654=CARTESIAN_POINT('Ctrl Pts',(5.75150405627262,29.2043184327592,126.469496694858));
#121655=CARTESIAN_POINT('Ctrl Pts',(5.76213358570567,29.059874621473,126.376032109371));
#121656=CARTESIAN_POINT('Ctrl Pts',(5.76474133504684,29.0256800414665,126.352035594465));
#121657=CARTESIAN_POINT('Ctrl Pts',(5.76902996662426,28.9722147815773,126.311433408143));
#121658=CARTESIAN_POINT('Ctrl Pts',(5.77067265823775,28.9523587442249,126.295626362772));
#121659=CARTESIAN_POINT('Ctrl Pts',(5.7729454084626,28.9258673488297,126.273529845309));
#121660=CARTESIAN_POINT('Ctrl Pts',(5.77355013204621,28.9189102414311,126.267629340032));
#121661=CARTESIAN_POINT('Ctrl Pts',(5.77457289000334,28.9073047204626,126.257621366232));
#121662=CARTESIAN_POINT('Ctrl Pts',(5.77498873591552,28.9026300221485,126.253544416811));
#121663=CARTESIAN_POINT('Ctrl Pts',(5.77584867806959,28.8930560434106,126.245100057384));
#121664=CARTESIAN_POINT('Ctrl Pts',(5.77629297421402,28.888159659177,126.240729675914));
#121665=CARTESIAN_POINT('Ctrl Pts',(5.77747532839682,28.8752581774155,126.229076463896));
#121666=CARTESIAN_POINT('Ctrl Pts',(5.77821687431527,28.8672981585801,126.221744508696));
#121667=CARTESIAN_POINT('Ctrl Pts',(5.78158509077229,28.8317070770929,126.188314860766));
#121668=CARTESIAN_POINT('Ctrl Pts',(5.78426648446888,28.8049046033917,126.161355698573));
#121669=CARTESIAN_POINT('Ctrl Pts',(5.7936175718252,28.7158896607248,126.065473724263));
#121670=CARTESIAN_POINT('Ctrl Pts',(5.80043429861472,28.658527688714,125.992282870422));
#121671=CARTESIAN_POINT('Ctrl Pts',(5.81168160693744,28.5732219271696,125.862422226442));
#121672=CARTESIAN_POINT('Ctrl Pts',(5.81615920509418,28.5418510314233,125.808251634476));
#121673=CARTESIAN_POINT('Ctrl Pts',(5.82334481840903,28.4955342557765,125.716755562493));
#121674=CARTESIAN_POINT('Ctrl Pts',(5.82610706460244,28.478759785408,125.68042956269));
#121675=CARTESIAN_POINT('Ctrl Pts',(5.82987492082888,28.4573404512171,125.629282278208));
#121676=CARTESIAN_POINT('Ctrl Pts',(5.83091795629424,28.4515712688815,125.6149497229));
#121677=CARTESIAN_POINT('Ctrl Pts',(5.83269055460315,28.442045658395,125.590300550476));
#121678=CARTESIAN_POINT('Ctrl Pts',(5.83342338647556,28.4381903965146,125.580023484712));
#121679=CARTESIAN_POINT('Ctrl Pts',(5.83490328386405,28.4305755164743,125.559097751976));
#121680=CARTESIAN_POINT('Ctrl Pts',(5.83565011344544,28.4268220354759,125.548447452646));
#121681=CARTESIAN_POINT('Ctrl Pts',(5.8375165322432,28.417669726288,125.52161097868));
#121682=CARTESIAN_POINT('Ctrl Pts',(5.83863149320454,28.4124106436824,125.50537825348));
#121683=CARTESIAN_POINT('Ctrl Pts',(5.84292260665953,28.3929994513573,125.442167638477));
#121684=CARTESIAN_POINT('Ctrl Pts',(5.84603996684777,28.3806750011564,125.394652025608));
#121685=CARTESIAN_POINT('Ctrl Pts',(5.85596082405347,28.3476928012931,125.239612611489));
#121686=CARTESIAN_POINT('Ctrl Pts',(5.8625386665665,28.3355238834389,125.130586327015));
#121687=CARTESIAN_POINT('Ctrl Pts',(5.87317034740403,28.3333308227973,124.95787782252));
#121688=CARTESIAN_POINT('Ctrl Pts',(5.87711492428867,28.3361332355556,124.894614577595));
#121689=CARTESIAN_POINT('Ctrl Pts',(5.88222741517975,28.3440918674147,124.816248607254));
#121690=CARTESIAN_POINT('Ctrl Pts',(5.88324308642268,28.3458732912283,124.800849034407));
#121691=CARTESIAN_POINT('Ctrl Pts',(5.88476920586318,28.3488395895283,124.778004312739));
#121692=CARTESIAN_POINT('Ctrl Pts',(5.88527106230205,28.3498605886854,124.77053822974));
#121693=CARTESIAN_POINT('Ctrl Pts',(5.88617783273807,28.3517859057663,124.757137200296));
#121694=CARTESIAN_POINT('Ctrl Pts',(5.88658171696137,28.3526716999606,124.751199861386));
#121695=CARTESIAN_POINT('Ctrl Pts',(5.88749140192732,28.3547297454272,124.737898120819));
#121696=CARTESIAN_POINT('Ctrl Pts',(5.88799812504275,28.3559193502293,124.730536797822));
#121697=CARTESIAN_POINT('Ctrl Pts',(5.88953845833747,28.3596666390805,124.708297476768));
#121698=CARTESIAN_POINT('Ctrl Pts',(5.89057990850622,28.362377088442,124.693446486329));
#121699=CARTESIAN_POINT('Ctrl Pts',(5.89927507152819,28.3864848932785,124.570815513254));
#121700=CARTESIAN_POINT('Ctrl Pts',(5.90734487442019,28.4182941018893,124.465366209693));
#121701=CARTESIAN_POINT('Ctrl Pts',(5.92284609007664,28.4997823262785,124.268138138674));
#121702=CARTESIAN_POINT('Ctrl Pts',(5.930253221389,28.5481559517931,124.176331084483));
#121703=CARTESIAN_POINT('Ctrl Pts',(5.93885599461161,28.6166351377654,124.071382371052));
#121704=CARTESIAN_POINT('Ctrl Pts',(5.94033607771004,28.6288764127222,124.053401231306));
#121705=CARTESIAN_POINT('Ctrl Pts',(5.94263110922004,28.648574791763,124.02565062655));
#121706=CARTESIAN_POINT('Ctrl Pts',(5.94345498385429,28.6557934362825,124.015715730568));
#121707=CARTESIAN_POINT('Ctrl Pts',(5.94498659138499,28.6694866247886,123.997301669683));
#121708=CARTESIAN_POINT('Ctrl Pts',(5.94569532590523,28.6759339946595,123.988803181479));
#121709=CARTESIAN_POINT('Ctrl Pts',(5.94727640487547,28.6905637486762,123.969899078162));
#121710=CARTESIAN_POINT('Ctrl Pts',(5.94814698287283,28.6987894773204,123.959527800489));
#121711=CARTESIAN_POINT('Ctrl Pts',(5.95036663735369,28.7201921856478,123.93319338448));
#121712=CARTESIAN_POINT('Ctrl Pts',(5.9517086357629,28.7335448560628,123.9173754919));
#121713=CARTESIAN_POINT('Ctrl Pts',(5.96277271526625,28.8469472964873,123.78800645423));
#121714=CARTESIAN_POINT('Ctrl Pts',(5.97179323522894,28.9617397211405,123.688330864023));
#121715=CARTESIAN_POINT('Ctrl Pts',(5.98482514095229,29.1386333198886,123.572693847425));
#121716=CARTESIAN_POINT('Ctrl Pts',(5.98857484555124,29.1905820295968,123.542606284667));
#121717=CARTESIAN_POINT('Ctrl Pts',(5.99345340023804,29.2575146114485,123.508524119668));
#121718=CARTESIAN_POINT('Ctrl Pts',(5.99444509664196,29.2710877446885,123.501843887122));
#121719=CARTESIAN_POINT('Ctrl Pts',(5.99594206689023,29.291489682272,123.492145621225));
#121720=CARTESIAN_POINT('Ctrl Pts',(5.99643921922003,29.2982512873055,123.488986950152));
#121721=CARTESIAN_POINT('Ctrl Pts',(5.99734131504561,29.3104897315577,123.48336964656));
#121722=CARTESIAN_POINT('Ctrl Pts',(5.9977452830855,29.3159589462932,123.48089504212));
#121723=CARTESIAN_POINT('Ctrl Pts',(5.9986600419308,29.3283179270791,123.475383365257));
#121724=CARTESIAN_POINT('Ctrl Pts',(5.99917180976277,29.3352149243644,123.472363430751));
#121725=CARTESIAN_POINT('Ctrl Pts',(6.00074299328435,29.3563438963562,123.463282032669));
#121726=CARTESIAN_POINT('Ctrl Pts',(6.00181069771191,29.3706395712153,123.457372145034));
#121727=CARTESIAN_POINT('Ctrl Pts',(6.01017667108098,29.4823217640223,123.413013023175));
#121728=CARTESIAN_POINT('Ctrl Pts',(6.01785091234201,29.5830472697835,123.383625836273));
#121729=CARTESIAN_POINT('Ctrl Pts',(6.03333780873458,29.7922555946841,123.343456370911));
#121730=CARTESIAN_POINT('Ctrl Pts',(6.04110419612859,29.9004123296194,123.333451318377));
#121731=CARTESIAN_POINT('Ctrl Pts',(6.05002753583856,30.0304167987172,123.334137305565));
#121732=CARTESIAN_POINT('Ctrl Pts',(6.05149904397454,30.0520393938018,123.334672501828));
#121733=CARTESIAN_POINT('Ctrl Pts',(6.05378384717539,30.0858885010986,123.336170282431));
#121734=CARTESIAN_POINT('Ctrl Pts',(6.05460593822486,30.0981245764871,123.336847046999));
#121735=CARTESIAN_POINT('Ctrl Pts',(6.05613590370432,30.1209983339723,123.338365491635));
#121736=CARTESIAN_POINT('Ctrl Pts',(6.05684476057622,30.1316374790162,123.339174476537));
#121737=CARTESIAN_POINT('Ctrl Pts',(6.05842824886481,30.1554917767242,123.341218986328));
#121738=CARTESIAN_POINT('Ctrl Pts',(6.05930108894348,30.1687015118014,123.342510343673));
#121739=CARTESIAN_POINT('Ctrl Pts',(6.06153073589555,30.2025884449256,123.346232386923));
#121740=CARTESIAN_POINT('Ctrl Pts',(6.06288035280219,30.2232384314512,123.348893080274));
#121741=CARTESIAN_POINT('Ctrl Pts',(6.07258663013868,30.3725637997045,123.370986079972));
#121742=CARTESIAN_POINT('Ctrl Pts',(6.08044769594742,30.4986189752606,123.405047667186));
#121743=CARTESIAN_POINT('Ctrl Pts',(6.0934687629512,30.6961172590375,123.484150280772));
#121744=CARTESIAN_POINT('Ctrl Pts',(6.09856140046476,30.7704004292598,123.520520603427));
#121745=CARTESIAN_POINT('Ctrl Pts',(6.10485266390874,30.8538143567022,123.56935152415));
#121746=CARTESIAN_POINT('Ctrl Pts',(6.10577662360586,30.8658673172546,123.576613975761));
#121747=CARTESIAN_POINT('Ctrl Pts',(6.10719097789564,30.8839908355671,123.587849580047));
#121748=CARTESIAN_POINT('Ctrl Pts',(6.10767451300823,30.8901301578181,123.591711356592));
#121749=CARTESIAN_POINT('Ctrl Pts',(6.10856368367182,30.9013117728976,123.59884717786));
#121750=CARTESIAN_POINT('Ctrl Pts',(6.10896850376115,30.9063618147695,123.602108587929));
#121751=CARTESIAN_POINT('Ctrl Pts',(6.10990063128414,30.9178973185441,123.609647215044));
#121752=CARTESIAN_POINT('Ctrl Pts',(6.11042909445382,30.9243705732351,123.613942500713));
#121753=CARTESIAN_POINT('Ctrl Pts',(6.11206475935497,30.9442089845233,123.62730692776));
#121754=CARTESIAN_POINT('Ctrl Pts',(6.11318099227888,30.9574720354773,123.636524979944));
#121755=CARTESIAN_POINT('Ctrl Pts',(6.12028434315648,31.0402784231018,123.69588083174));
#121756=CARTESIAN_POINT('Ctrl Pts',(6.12652065243238,31.1059928106279,123.751127226154));
#121757=CARTESIAN_POINT('Ctrl Pts',(6.13647511919247,31.2035733040398,123.846929520133));
#121758=CARTESIAN_POINT('Ctrl Pts',(6.14018772461461,31.2383276964915,123.884336482728));
#121759=CARTESIAN_POINT('Ctrl Pts',(6.1476774249638,31.3055715319364,123.963733076918));
#121760=CARTESIAN_POINT('Ctrl Pts',(6.15144714540973,31.3378842210959,124.005800387596));
#121761=CARTESIAN_POINT('Ctrl Pts',(6.15764476412742,31.3885612194047,124.078732019532));
#121762=CARTESIAN_POINT('Ctrl Pts',(6.16010939106544,31.4080328899557,124.108775745907));
#121763=CARTESIAN_POINT('Ctrl Pts',(6.1635451467901,31.4341841530298,124.152125133234));
#121764=CARTESIAN_POINT('Ctrl Pts',(6.1645454930962,31.4416756813994,124.164926812268));
#121765=CARTESIAN_POINT('Ctrl Pts',(6.16626814032352,31.4543588649423,124.187279625948));
#121766=CARTESIAN_POINT('Ctrl Pts',(6.16699325507513,31.4596297421235,124.196784499662));
#121767=CARTESIAN_POINT('Ctrl Pts',(6.16838580266179,31.4696185112332,124.215220140819));
#121768=CARTESIAN_POINT('Ctrl Pts',(6.16905365650199,31.4743489257356,124.224143538587));
#121769=CARTESIAN_POINT('Ctrl Pts',(6.17081907703487,31.4866903515453,124.247944779643));
#121770=CARTESIAN_POINT('Ctrl Pts',(6.17191164392309,31.4941592832044,124.262895309067));
#121771=CARTESIAN_POINT('Ctrl Pts',(6.17597888409622,31.5213053355789,124.319342217589));
#121772=CARTESIAN_POINT('Ctrl Pts',(6.17890276317572,31.5394899186674,124.361535977443));
#121773=CARTESIAN_POINT('Ctrl Pts',(6.18882379509985,31.5960154523824,124.509207360837));
#121774=CARTESIAN_POINT('Ctrl Pts',(6.19556590220482,31.6254352413948,124.617765168342));
#121775=CARTESIAN_POINT('Ctrl Pts',(6.20539765587632,31.6514821995445,124.775434604708));
#121776=CARTESIAN_POINT('Ctrl Pts',(6.20835469298737,31.657224828524,124.822719665012));
#121777=CARTESIAN_POINT('Ctrl Pts',(6.21314914560204,31.66309109616,124.897774725197));
#121778=CARTESIAN_POINT('Ctrl Pts',(6.21493634287029,31.6645596559382,124.925414871101));
#121779=CARTESIAN_POINT('Ctrl Pts',(6.21737769447918,31.6656042696135,124.962488980599));
#121780=CARTESIAN_POINT('Ctrl Pts',(6.21800142458465,31.6657896644415,124.9719029703));
#121781=CARTESIAN_POINT('Ctrl Pts',(6.21904709398241,31.6659654539585,124.987578112864));
#121782=CARTESIAN_POINT('Ctrl Pts',(6.21946661914249,31.6660003702729,124.993838730766));
#121783=CARTESIAN_POINT('Ctrl Pts',(6.22032418092333,31.6659996109844,125.006574978272));
#121784=CARTESIAN_POINT('Ctrl Pts',(6.22076233223928,31.6659614691076,125.013050439539));
#121785=CARTESIAN_POINT('Ctrl Pts',(6.2219108566375,31.6657634396951,125.029946113778));
#121786=CARTESIAN_POINT('Ctrl Pts',(6.22262438321931,31.665543529189,125.040365148543));
#121787=CARTESIAN_POINT('Ctrl Pts',(6.22591362540958,31.6640886812597,125.088072871787));
#121788=CARTESIAN_POINT('Ctrl Pts',(6.2285427766786,31.6616991854907,125.125312846353));
#121789=CARTESIAN_POINT('Ctrl Pts',(6.2368304743083,31.650382157143,125.240829879691));
#121790=CARTESIAN_POINT('Ctrl Pts',(6.24259339957814,31.6371527188931,125.318575718898));
#121791=CARTESIAN_POINT('Ctrl Pts',(6.25289100296512,31.6035456758948,125.456245515323));
#121792=CARTESIAN_POINT('Ctrl Pts',(6.25743099835426,31.5851690022004,125.516480227392));
#121793=CARTESIAN_POINT('Ctrl Pts',(6.26188273594789,31.5634400889265,125.575509416376));
#121794=CARTESIAN_POINT('',(6.02851963656823,31.6659993037066,124.998476829273));
#121795=CARTESIAN_POINT('Ctrl Pts',(6.06644911688889,31.5634400025946,125.575509650907));
#121796=CARTESIAN_POINT('Ctrl Pts',(6.06485626759794,31.571355409626,125.554006511958));
#121797=CARTESIAN_POINT('Ctrl Pts',(6.06327683483192,31.578827998692,125.532337889805));
#121798=CARTESIAN_POINT('Ctrl Pts',(6.06046683788409,31.5914378618506,125.493167072324));
#121799=CARTESIAN_POINT('Ctrl Pts',(6.05923143504398,31.5967383372352,125.475725716762));
#121800=CARTESIAN_POINT('Ctrl Pts',(6.057229595139,31.6049235121702,125.447112425146));
#121801=CARTESIAN_POINT('Ctrl Pts',(6.05645763721405,31.6079801734448,125.435991713235));
#121802=CARTESIAN_POINT('Ctrl Pts',(6.0549675145839,31.6136847571051,125.41436089562));
#121803=CARTESIAN_POINT('Ctrl Pts',(6.05424895043071,31.6163460733296,125.40385495888));
#121804=CARTESIAN_POINT('Ctrl Pts',(6.05282974809935,31.6214225497731,125.382960377269));
#121805=CARTESIAN_POINT('Ctrl Pts',(6.05212904065077,31.6238408409157,125.37257303663));
#121806=CARTESIAN_POINT('Ctrl Pts',(6.05050106010127,31.629251148826,125.348280045128));
#121807=CARTESIAN_POINT('Ctrl Pts',(6.04957626062148,31.6321651911645,125.334357749262));
#121808=CARTESIAN_POINT('Ctrl Pts',(6.04651039208248,31.6412854194013,125.287820012642));
#121809=CARTESIAN_POINT('Ctrl Pts',(6.04439352764609,31.6466952091796,125.255055479839));
#121810=CARTESIAN_POINT('Ctrl Pts',(6.03758378161774,31.6610970214292,125.148014208556));
#121811=CARTESIAN_POINT('Ctrl Pts',(6.03299866726444,31.6660674538522,125.073289477035));
#121812=CARTESIAN_POINT('Ctrl Pts',(6.02842896873232,31.6659993087612,124.998482367842));
#121813=CARTESIAN_POINT('Ctrl Pts',(6.02851963656823,31.6659993037066,124.998476829273));
#121814=CARTESIAN_POINT('Ctrl Pts',(6.02319560875282,31.6659265050813,124.91885183581));
#121815=CARTESIAN_POINT('Ctrl Pts',(6.0178715809374,31.6601415384358,124.839481023796));
#121816=CARTESIAN_POINT('Ctrl Pts',(6.01254755312199,31.6487752900045,124.761052216854));
#121817=CARTESIAN_POINT('Ctrl Pts',(6.00879991050873,31.6407744608483,124.705845304119));
#121818=CARTESIAN_POINT('Ctrl Pts',(6.00505226789547,31.6300091693845,124.651104499699));
#121819=CARTESIAN_POINT('Ctrl Pts',(6.00130462528221,31.6165387634105,124.597062751298));
#121820=CARTESIAN_POINT('Ctrl Pts',(5.99722727558211,31.6018832688967,124.538266561433));
#121821=CARTESIAN_POINT('Ctrl Pts',(5.99314992588201,31.5839855577696,124.480149579525));
#121822=CARTESIAN_POINT('Ctrl Pts',(5.9890725761819,31.5629257672559,124.42309528859));
#121823=CARTESIAN_POINT('Ctrl Pts',(5.98495160860948,31.5416406874437,124.365430653445));
#121824=CARTESIAN_POINT('Ctrl Pts',(5.98083064103705,31.5171255131338,124.308852114332));
#121825=CARTESIAN_POINT('Ctrl Pts',(5.97670967346462,31.4895158984512,124.25374375161));
#121826=CARTESIAN_POINT('Ctrl Pts',(5.97264355643923,31.4622737708798,124.199368887463));
#121827=CARTESIAN_POINT('Ctrl Pts',(5.96857743941384,31.4320193111668,124.146425773321));
#121828=CARTESIAN_POINT('Ctrl Pts',(5.96451132238844,31.3989316336102,124.095264522369));
#121829=CARTESIAN_POINT('Ctrl Pts',(5.96044769316908,31.3658642003612,124.044134573828));
#121830=CARTESIAN_POINT('Ctrl Pts',(5.95638406394971,31.3299672636843,123.994784755909));
#121831=CARTESIAN_POINT('Ctrl Pts',(5.95232043473035,31.2914648767174,123.947538850026));
#121832=CARTESIAN_POINT('Ctrl Pts',(5.94825778211368,31.2529717429409,123.900304298643));
#121833=CARTESIAN_POINT('Ctrl Pts',(5.94419512949701,31.2118747251711,123.855173052237));
#121834=CARTESIAN_POINT('Ctrl Pts',(5.94013247688035,31.1684387532848,123.812436578611));
#121835=CARTESIAN_POINT('Ctrl Pts',(5.93596888334396,31.1239235685381,123.7686382719));
#121836=CARTESIAN_POINT('Ctrl Pts',(5.93180528980757,31.0769520072842,123.727355765411));
#121837=CARTESIAN_POINT('Ctrl Pts',(5.92764169627117,31.0278483005135,123.688861612517));
#121838=CARTESIAN_POINT('Ctrl Pts',(5.92357385644521,30.979873873553,123.651252742477));
#121839=CARTESIAN_POINT('Ctrl Pts',(5.91950601661925,30.9298648035679,123.616305575443));
#121840=CARTESIAN_POINT('Ctrl Pts',(5.91543817679328,30.8781537565013,123.584230958121));
#121841=CARTESIAN_POINT('Ctrl Pts',(5.91122670640168,30.8246168541263,123.551023824372));
#121842=CARTESIAN_POINT('Ctrl Pts',(5.90701523601007,30.769256040787,123.520896213992));
#121843=CARTESIAN_POINT('Ctrl Pts',(5.90280376561847,30.712466588119,123.494029428968));
#121844=CARTESIAN_POINT('Ctrl Pts',(5.89859229522686,30.655677135451,123.467162643945));
#121845=CARTESIAN_POINT('Ctrl Pts',(5.89438082483526,30.5974596275333,123.443556842907));
#121846=CARTESIAN_POINT('Ctrl Pts',(5.89016935444365,30.5382274340245,123.423336678532));
#121847=CARTESIAN_POINT('Ctrl Pts',(5.88609200474354,30.4808815799681,123.4037604561));
#121848=CARTESIAN_POINT('Ctrl Pts',(5.88201465504342,30.4223478962537,123.387276539074));
#121849=CARTESIAN_POINT('Ctrl Pts',(5.87793730534331,30.3629920272199,123.374025588093));
#121850=CARTESIAN_POINT('Ctrl Pts',(5.87381633777088,30.3030011926064,123.360632883687));
#121851=CARTESIAN_POINT('Ctrl Pts',(5.86969537019845,30.2421709473292,123.350542981847));
#121852=CARTESIAN_POINT('Ctrl Pts',(5.86557440262603,30.1808975479542,123.343850225027));
#121853=CARTESIAN_POINT('Ctrl Pts',(5.86150828560062,30.1204397044928,123.337246549561));
#121854=CARTESIAN_POINT('Ctrl Pts',(5.85744216857521,30.0595509558089,123.333950195322));
#121855=CARTESIAN_POINT('Ctrl Pts',(5.85337605154981,29.9986225924009,123.334000569403));
#121856=CARTESIAN_POINT('Ctrl Pts',(5.84931242233043,29.9377315072977,123.334050912664));
#121857=CARTESIAN_POINT('Ctrl Pts',(5.84524879311105,29.8768013664308,123.33744392392));
#121858=CARTESIAN_POINT('Ctrl Pts',(5.84118516389167,29.8162257110445,123.344166973781));
#121859=CARTESIAN_POINT('Ctrl Pts',(5.83712251127499,29.7556646136666,123.350888407906));
#121860=CARTESIAN_POINT('Ctrl Pts',(5.83305985865831,29.6954583412569,123.360938235477));
#121861=CARTESIAN_POINT('Ctrl Pts',(5.82899720604163,29.6359954570605,123.37425195903));
#121862=CARTESIAN_POINT('Ctrl Pts',(5.82483361250525,29.5750551543435,123.387896476186));
#121863=CARTESIAN_POINT('Ctrl Pts',(5.82067001896887,29.5148962345785,123.404969181928));
#121864=CARTESIAN_POINT('Ctrl Pts',(5.81650642543249,29.4559235329719,123.425345498839));
#121865=CARTESIAN_POINT('Ctrl Pts',(5.81243858560652,29.3983070768638,123.445253204218));
#121866=CARTESIAN_POINT('Ctrl Pts',(5.80837074578054,29.3418233160874,123.468313913944));
#121867=CARTESIAN_POINT('Ctrl Pts',(5.80430290595456,29.2868298182051,123.494362496549));
#121868=CARTESIAN_POINT('Ctrl Pts',(5.80009143556298,29.2298945655971,123.521330823493));
#121869=CARTESIAN_POINT('Ctrl Pts',(5.7958799651714,29.174557330909,123.551501720362));
#121870=CARTESIAN_POINT('Ctrl Pts',(5.79166849477982,29.1211848149767,123.584641433921));
#121871=CARTESIAN_POINT('Ctrl Pts',(5.78745702438825,29.0678122990443,123.617781147481));
#121872=CARTESIAN_POINT('Ctrl Pts',(5.78324555399667,29.016404951922,123.653889273057));
#121873=CARTESIAN_POINT('Ctrl Pts',(5.77903408360509,28.967291696611,123.692686127928));
#121874=CARTESIAN_POINT('Ctrl Pts',(5.77495673390497,28.9197425277472,123.730247437843));
#121875=CARTESIAN_POINT('Ctrl Pts',(5.77087938420486,28.8741471032045,123.770483850587));
#121876=CARTESIAN_POINT('Ctrl Pts',(5.76680203450474,28.8308219104709,123.813164461703));
#121877=CARTESIAN_POINT('Ctrl Pts',(5.76268106693231,28.7870332419838,123.856301653093));
#121878=CARTESIAN_POINT('Ctrl Pts',(5.75856009935989,28.7455641356007,123.901935391439));
#121879=CARTESIAN_POINT('Ctrl Pts',(5.75443913178746,28.7067087678563,123.949783932298));
#121880=CARTESIAN_POINT('Ctrl Pts',(5.75037301476205,28.6683705694751,123.996995603636));
#121881=CARTESIAN_POINT('Ctrl Pts',(5.74630689773664,28.6325772882018,124.046363069474));
#121882=CARTESIAN_POINT('Ctrl Pts',(5.74224078071123,28.5995742535649,124.097578962611));
#121883=CARTESIAN_POINT('Ctrl Pts',(5.73817715149185,28.5665914114478,124.148763519905));
#121884=CARTESIAN_POINT('Ctrl Pts',(5.73411352227247,28.5363957078714,124.201793832718));
#121885=CARTESIAN_POINT('Ctrl Pts',(5.73004989305309,28.5091899749721,124.256332420179));
#121886=CARTESIAN_POINT('Ctrl Pts',(5.72598724043641,28.4819907803642,124.310857900507));
#121887=CARTESIAN_POINT('Ctrl Pts',(5.72192458781972,28.4577803583883,124.366890477991));
#121888=CARTESIAN_POINT('Ctrl Pts',(5.71786193520304,28.4367152646657,124.424068722615));
#121889=CARTESIAN_POINT('Ctrl Pts',(5.71369834166666,28.4151267863139,124.482667621462));
#121890=CARTESIAN_POINT('Ctrl Pts',(5.70953474813029,28.3968422725696,124.542469372822));
#121891=CARTESIAN_POINT('Ctrl Pts',(5.70537115459391,28.3819766285952,124.603066290688));
#121892=CARTESIAN_POINT('Ctrl Pts',(5.70130331476793,28.3674528625097,124.66226960957));
#121893=CARTESIAN_POINT('Ctrl Pts',(5.69723547494195,28.3561924059842,124.722231378084));
#121894=CARTESIAN_POINT('Ctrl Pts',(5.69316763511597,28.3482504566834,124.782561626769));
#121895=CARTESIAN_POINT('Ctrl Pts',(5.68895616472439,28.3400280866387,124.845022064476));
#121896=CARTESIAN_POINT('Ctrl Pts',(5.68474469433282,28.3353630426135,124.907876896629));
#121897=CARTESIAN_POINT('Ctrl Pts',(5.68053322394125,28.3342578236991,124.970691262525));
#121898=CARTESIAN_POINT('Ctrl Pts',(5.67632175354967,28.3331526047847,125.033505628421));
#121899=CARTESIAN_POINT('Ctrl Pts',(5.6721102831581,28.3356071150888,125.096278930468));
#121900=CARTESIAN_POINT('Ctrl Pts',(5.66789881276653,28.3415647769982,125.158583136263));
#121901=CARTESIAN_POINT('Ctrl Pts',(5.66382146306642,28.3473327080867,125.218903169694));
#121902=CARTESIAN_POINT('Ctrl Pts',(5.6597441133663,28.3564077503369,125.279032657118));
#121903=CARTESIAN_POINT('Ctrl Pts',(5.65566676366619,28.3687675623041,125.338580469326));
#121904=CARTESIAN_POINT('Ctrl Pts',(5.65154579609376,28.3812595946448,125.398765300446));
#121905=CARTESIAN_POINT('Ctrl Pts',(5.64742482852134,28.3971071320074,125.458355403812));
#121906=CARTESIAN_POINT('Ctrl Pts',(5.64330386094891,28.4162330194005,125.516950820836));
#121907=CARTESIAN_POINT('Ctrl Pts',(5.63923774392351,28.4351043390575,125.574766326196));
#121908=CARTESIAN_POINT('Ctrl Pts',(5.6351716268981,28.4571671072163,125.631612961354));
#121909=CARTESIAN_POINT('Ctrl Pts',(5.63110550987269,28.4822961492294,125.687117909355));
#121910=CARTESIAN_POINT('Ctrl Pts',(5.62704188065332,28.5074098163328,125.742588897304));
#121911=CARTESIAN_POINT('Ctrl Pts',(5.62297825143394,28.5355858268912,125.796719360266));
#121912=CARTESIAN_POINT('Ctrl Pts',(5.61891462221457,28.5666506573924,125.849155852624));
#121913=CARTESIAN_POINT('Ctrl Pts',(5.61485196959789,28.5977080221541,125.901579743041));
#121914=CARTESIAN_POINT('Ctrl Pts',(5.61078931698121,28.6316525678179,125.952310030753));
#121915=CARTESIAN_POINT('Ctrl Pts',(5.60672666436453,28.6682655514314,126.001019159904));
#121916=CARTESIAN_POINT('Ctrl Pts',(5.60256307082815,28.7057882235139,126.05093851911));
#121917=CARTESIAN_POINT('Ctrl Pts',(5.59839947729177,28.7461134161297,126.098734457736));
#121918=CARTESIAN_POINT('Ctrl Pts',(5.59423588375539,28.7889609349392,126.144089324702));
#121919=CARTESIAN_POINT('Ctrl Pts',(5.59016804392941,28.8308230528271,126.188401127123));
#121920=CARTESIAN_POINT('Ctrl Pts',(5.58610020410344,28.8750922791935,126.23038263688));
#121921=CARTESIAN_POINT('Ctrl Pts',(5.58203236427746,28.9214709209375,126.269775974578));
#121922=CARTESIAN_POINT('Ctrl Pts',(5.57782089388588,28.9694871371266,126.31056024398));
#121923=CARTESIAN_POINT('Ctrl Pts',(5.5736094234943,29.0197640671423,126.348569754223));
#121924=CARTESIAN_POINT('Ctrl Pts',(5.56939795310271,29.0719377209833,126.383566552887));
#121925=CARTESIAN_POINT('Ctrl Pts',(5.56518648271113,29.1241113748242,126.41856335155));
#121926=CARTESIAN_POINT('Ctrl Pts',(5.56097501231955,29.1781811984191,126.450547195083));
#121927=CARTESIAN_POINT('Ctrl Pts',(5.55676354192797,29.2337568974358,126.479333467401));
#121928=CARTESIAN_POINT('Ctrl Pts',(5.55268619222785,29.2875627036389,126.507202997017));
#121929=CARTESIAN_POINT('Ctrl Pts',(5.54860884252774,29.3430020821622,126.532190733182));
#121930=CARTESIAN_POINT('Ctrl Pts',(5.54453149282762,29.3997343111234,126.554103311481));
#121931=CARTESIAN_POINT('Ctrl Pts',(5.54041052525519,29.4570734390019,126.576250301866));
#121932=CARTESIAN_POINT('Ctrl Pts',(5.53628955768277,29.5157328156011,126.595255627346));
#121933=CARTESIAN_POINT('Ctrl Pts',(5.53216859011034,29.5753345721938,126.610967186018));
#121934=CARTESIAN_POINT('Ctrl Pts',(5.52810247308494,29.6341430226284,126.626469622057));
#121935=CARTESIAN_POINT('Ctrl Pts',(5.52403635605953,29.693868410051,126.638765302794));
#121936=CARTESIAN_POINT('Ctrl Pts',(5.51997023903412,29.7541296244665,126.647757190376));
#121937=CARTESIAN_POINT('Ctrl Pts',(5.51590660981474,29.8143539687645,126.656743576377));
#121938=CARTESIAN_POINT('Ctrl Pts',(5.51184298059536,29.8751129847364,126.662430101641));
#121939=CARTESIAN_POINT('Ctrl Pts',(5.50777935137598,29.9360156144037,126.664770854622));
#121940=CARTESIAN_POINT('Ctrl Pts',(5.5037166987593,29.9969036074816,126.667111045055));
#121941=CARTESIAN_POINT('Ctrl Pts',(5.49965404614262,30.0579346343865,126.66610703977));
#121942=CARTESIAN_POINT('Ctrl Pts',(5.49559139352594,30.1187148628542,126.661764959715));
#121943=CARTESIAN_POINT('Ctrl Pts',(5.49142779998956,30.1810052406603,126.65731499607));
#121944=CARTESIAN_POINT('Ctrl Pts',(5.48726420645318,30.2430316268307,126.64935884579));
#121945=CARTESIAN_POINT('Ctrl Pts',(5.4831006129168,30.3043751815096,126.637959629808));
#121946=CARTESIAN_POINT('Ctrl Pts',(5.47903277309083,30.3643079661606,126.626822571315));
#121947=CARTESIAN_POINT('Ctrl Pts',(5.47496493326485,30.4235884996283,126.612399329089));
#121948=CARTESIAN_POINT('Ctrl Pts',(5.47089709343887,30.4818386681556,126.594800143551));
#121949=CARTESIAN_POINT('Ctrl Pts',(5.46668562304729,30.5421455805592,126.576579551792));
#121950=CARTESIAN_POINT('Ctrl Pts',(5.46247415265571,30.6013474269172,126.554954706161));
#121951=CARTESIAN_POINT('Ctrl Pts',(5.45826268226414,30.6590468779301,126.530102353665));
#121952=CARTESIAN_POINT('Ctrl Pts',(5.45405121187256,30.7167463289429,126.505250001169));
#121953=CARTESIAN_POINT('Ctrl Pts',(5.44983974148098,30.7729428794861,126.477170475215));
#121954=CARTESIAN_POINT('Ctrl Pts',(5.44562827108941,30.8272697439158,126.446091549938));
#121955=CARTESIAN_POINT('Ctrl Pts',(5.44155183031641,30.8798547616506,126.416009087899));
#121956=CARTESIAN_POINT('Ctrl Pts',(5.43747538954341,30.9309053353052,126.382992519671));
#121957=CARTESIAN_POINT('Ctrl Pts',(5.43339894877041,30.9800744454229,126.347223100095));
#121958=CARTESIAN_POINT('Ctrl Pts',(5.42932840898418,31.0291723791678,126.311505459725));
#121959=CARTESIAN_POINT('Ctrl Pts',(5.42525786919795,31.0763938380124,126.273043165971));
#121960=CARTESIAN_POINT('Ctrl Pts',(5.42118732941172,31.1214179736454,126.232062388187));
#121961=CARTESIAN_POINT('Ctrl Pts',(5.41712116917604,31.1663936671829,126.191125702193));
#121962=CARTESIAN_POINT('Ctrl Pts',(5.41305500894035,31.2091763496132,126.147676249284));
#121963=CARTESIAN_POINT('Ctrl Pts',(5.40898884870466,31.2494773534112,126.101981099345));
#121964=CARTESIAN_POINT('Ctrl Pts',(5.40492500380731,31.2897554091565,126.056311968973));
#121965=CARTESIAN_POINT('Ctrl Pts',(5.40086115890996,31.3275542478635,126.008400058138));
#121966=CARTESIAN_POINT('Ctrl Pts',(5.39679731401261,31.36262266187,125.958548632756));
#121967=CARTESIAN_POINT('Ctrl Pts',(5.392734798567,31.3976796035479,125.908713515837));
#121968=CARTESIAN_POINT('Ctrl Pts',(5.3886722831214,31.430007603046,125.856940565119));
#121969=CARTESIAN_POINT('Ctrl Pts',(5.38460976767579,31.4593976670292,125.803563593918));
#121970=CARTESIAN_POINT('Ctrl Pts',(5.38054576390159,31.4887984982509,125.75016706772));
#121971=CARTESIAN_POINT('Ctrl Pts',(5.37648176012739,31.5152590011302,125.695165798204));
#121972=CARTESIAN_POINT('Ctrl Pts',(5.37241775635318,31.538616049042,125.638918346606));
#121973=CARTESIAN_POINT('Ctrl Pts',(5.37090265174123,31.5473238094131,125.617948687605));
#121974=CARTESIAN_POINT('Ctrl Pts',(5.36938754712929,31.5556007043374,125.59680603244));
#121975=CARTESIAN_POINT('Ctrl Pts',(5.36787244251734,31.5634400119422,125.575509625513));
#121976=CARTESIAN_POINT('Origin',(5.,30.,125.));
#121977=CARTESIAN_POINT('',(4.66781556978768,31.5660436956742,125.576468401513));
#121978=CARTESIAN_POINT('',(4.86075489241547,31.5634400172546,125.575509611081));
#121979=CARTESIAN_POINT('',(5.,31.5634400119422,125.575509625513));
#121980=CARTESIAN_POINT('',(5.52205786626619,31.6659992468011,125.001394788999));
#121981=CARTESIAN_POINT('Ctrl Pts',(4.86075489241547,31.5634400172546,125.575509611081));
#121982=CARTESIAN_POINT('Ctrl Pts',(4.86238037643612,31.554247439111,125.600482338304));
#121983=CARTESIAN_POINT('Ctrl Pts',(4.86400395132135,31.5444563766197,125.625235228954));
#121984=CARTESIAN_POINT('Ctrl Pts',(4.86651208868844,31.5284682148076,125.662983839313));
#121985=CARTESIAN_POINT('Ctrl Pts',(4.86739290510976,31.5226906633799,125.676147758858));
#121986=CARTESIAN_POINT('Ctrl Pts',(4.87273741189656,31.4867068185035,125.755334469012));
#121987=CARTESIAN_POINT('Ctrl Pts',(4.87725395371479,31.4523849452009,125.819391630691));
#121988=CARTESIAN_POINT('Ctrl Pts',(4.88279721873322,31.4075094565573,125.891416748726));
#121989=CARTESIAN_POINT('Ctrl Pts',(4.88360537788959,31.4009032748706,125.901763096892));
#121990=CARTESIAN_POINT('Ctrl Pts',(4.88488233883513,31.3903787862481,125.917851369303));
#121991=CARTESIAN_POINT('Ctrl Pts',(4.88534626693394,31.3865376916344,125.923643616706));
#121992=CARTESIAN_POINT('Ctrl Pts',(4.88621896768022,31.3792824446093,125.934437052726));
#121993=CARTESIAN_POINT('Ctrl Pts',(4.88662716662745,31.3758771236352,125.939443879902));
#121994=CARTESIAN_POINT('Ctrl Pts',(4.88759383095554,31.3677845027958,125.951204043296));
#121995=CARTESIAN_POINT('Ctrl Pts',(4.88815378375568,31.3630744285798,125.957941372494));
#121996=CARTESIAN_POINT('Ctrl Pts',(4.89004015775076,31.3471265142947,125.980397638121));
#121997=CARTESIAN_POINT('Ctrl Pts',(4.8913801560382,31.3356655614814,125.995955221188));
#121998=CARTESIAN_POINT('Ctrl Pts',(4.89471666408884,31.3067479010221,126.033812260193));
#121999=CARTESIAN_POINT('Ctrl Pts',(4.89672779912124,31.288988532416,126.05587226895));
#122000=CARTESIAN_POINT('Ctrl Pts',(4.90595648533575,31.2056945727883,126.15410230925));
#122001=CARTESIAN_POINT('Ctrl Pts',(4.91334701386877,31.1339135416843,126.224700824916));
#122002=CARTESIAN_POINT('Ctrl Pts',(4.92651678449591,30.9926372350616,126.340516485883));
#122003=CARTESIAN_POINT('Ctrl Pts',(4.93232985392164,30.9252890744389,126.387860550889));
#122004=CARTESIAN_POINT('Ctrl Pts',(4.93929779582167,30.8378894863385,126.440097646218));
#122005=CARTESIAN_POINT('Ctrl Pts',(4.94062820487365,30.8208917951965,126.449854040734));
#122006=CARTESIAN_POINT('Ctrl Pts',(4.94274419085391,30.7933668817169,126.465013595099));
#122007=CARTESIAN_POINT('Ctrl Pts',(4.94353653449039,30.7829478195366,126.470608230357));
#122008=CARTESIAN_POINT('Ctrl Pts',(4.94504115883189,30.76295177568,126.481072581541));
#122009=CARTESIAN_POINT('Ctrl Pts',(4.9457540884917,30.7533855777773,126.485961501595));
#122010=CARTESIAN_POINT('Ctrl Pts',(4.94738784930017,30.7312569046288,126.497001995012));
#122011=CARTESIAN_POINT('Ctrl Pts',(4.94830638579662,30.7186627985128,126.503088631929));
#122012=CARTESIAN_POINT('Ctrl Pts',(4.95122004275614,30.6782421650691,126.521999425974));
#122013=CARTESIAN_POINT('Ctrl Pts',(4.95319444674746,30.6501369790614,126.534215364481));
#122014=CARTESIAN_POINT('Ctrl Pts',(4.95785937483207,30.5822095607378,126.561537925775));
#122015=CARTESIAN_POINT('Ctrl Pts',(4.96052724207514,30.5421134216512,126.575906750325));
#122016=CARTESIAN_POINT('Ctrl Pts',(4.96773457354951,30.4312452615663,126.610904217683));
#122017=CARTESIAN_POINT('Ctrl Pts',(4.97220674837597,30.3595863944731,126.62839886413));
#122018=CARTESIAN_POINT('Ctrl Pts',(4.97757842588871,30.2730950261339,126.643525023215));
#122019=CARTESIAN_POINT('Ctrl Pts',(4.97844353696784,30.2591551426606,126.645780666132));
#122020=CARTESIAN_POINT('Ctrl Pts',(4.98380455056035,30.1728393402246,126.658623776316));
#122021=CARTESIAN_POINT('Ctrl Pts',(4.9883530698556,30.0998686316507,126.664611012936));
#122022=CARTESIAN_POINT('Ctrl Pts',(4.99393182489342,30.0144746497704,126.66598236244));
#122023=CARTESIAN_POINT('Ctrl Pts',(4.99474013415032,30.0021969454228,126.666043786675));
#122024=CARTESIAN_POINT('Ctrl Pts',(4.99601728125774,29.9829695293546,126.665927452113));
#122025=CARTESIAN_POINT('Ctrl Pts',(4.99648124311894,29.9760194162668,126.66584190122));
#122026=CARTESIAN_POINT('Ctrl Pts',(4.99735396937867,29.9630159890462,126.665600446998));
#122027=CARTESIAN_POINT('Ctrl Pts',(4.99776215964407,29.9569627274974,126.665455029293));
#122028=CARTESIAN_POINT('Ctrl Pts',(4.99872875172116,29.942694391322,126.665034423107));
#122029=CARTESIAN_POINT('Ctrl Pts',(4.9992886402795,29.934480412536,126.664731431641));
#122030=CARTESIAN_POINT('Ctrl Pts',(5.00117456631664,29.906970794567,126.663512767436));
#122031=CARTESIAN_POINT('Ctrl Pts',(5.00251417244876,29.8876896962,126.662322314294));
#122032=CARTESIAN_POINT('Ctrl Pts',(5.00584948508166,29.8402170328163,126.658561617138));
#122033=CARTESIAN_POINT('Ctrl Pts',(5.00785980433287,29.8120624432313,126.655607600932));
#122034=CARTESIAN_POINT('Ctrl Pts',(5.01708122525734,29.6844579294815,126.638922487842));
#122035=CARTESIAN_POINT('Ctrl Pts',(5.02446510563703,29.5862982109609,126.616936927469));
#122036=CARTESIAN_POINT('Ctrl Pts',(5.03763636678413,29.4123501603004,126.56108856782));
#122037=CARTESIAN_POINT('Ctrl Pts',(5.04345689356615,29.3359493383585,126.530153663104));
#122038=CARTESIAN_POINT('Ctrl Pts',(5.05043204686999,29.2445657553768,126.485011531568));
#122039=CARTESIAN_POINT('Ctrl Pts',(5.05176267714154,29.2271471418306,126.47602122728));
#122040=CARTESIAN_POINT('Ctrl Pts',(5.05387892839298,29.1994789367576,126.461116657269));
#122041=CARTESIAN_POINT('Ctrl Pts',(5.05467131909631,29.1891270959937,126.455397198319));
#122042=CARTESIAN_POINT('Ctrl Pts',(5.05617597981531,29.169489920522,126.444272968646));
#122043=CARTESIAN_POINT('Ctrl Pts',(5.0568888993397,29.1601942917123,126.438887689023));
#122044=CARTESIAN_POINT('Ctrl Pts',(5.05852256218956,29.1389181594045,126.426285265794));
#122045=CARTESIAN_POINT('Ctrl Pts',(5.05944101182486,29.1269750402998,126.419006354857));
#122046=CARTESIAN_POINT('Ctrl Pts',(5.06235407931748,29.0891721664285,126.395308878475));
#122047=CARTESIAN_POINT('Ctrl Pts',(5.06432799290853,29.063672050337,126.378326655157));
#122048=CARTESIAN_POINT('Ctrl Pts',(5.06899151255869,29.003893478202,126.336091012022));
#122049=CARTESIAN_POINT('Ctrl Pts',(5.07165848122883,28.9700858794517,126.310207876848));
#122050=CARTESIAN_POINT('Ctrl Pts',(5.07886539854358,28.8805548991423,126.236053608914));
#122051=CARTESIAN_POINT('Ctrl Pts',(5.08333799662581,28.826984711163,126.185335966073));
#122052=CARTESIAN_POINT('Ctrl Pts',(5.08870729896525,28.7673905716162,126.120905044818));
#122053=CARTESIAN_POINT('Ctrl Pts',(5.08956963572815,28.7579644472012,126.110451170399));
#122054=CARTESIAN_POINT('Ctrl Pts',(5.09493171087788,28.7003393052001,126.044891285209));
#122055=CARTESIAN_POINT('Ctrl Pts',(5.09948404095198,28.6556895946933,125.986783941282));
#122056=CARTESIAN_POINT('Ctrl Pts',(5.10506702532268,28.6081867669985,125.915730679814));
#122057=CARTESIAN_POINT('Ctrl Pts',(5.10587535048109,28.6014760351014,125.90544875689));
#122058=CARTESIAN_POINT('Ctrl Pts',(5.1071525173104,28.5911453449174,125.889231620139));
#122059=CARTESIAN_POINT('Ctrl Pts',(5.10761648274811,28.5874476970702,125.88334608196));
#122060=CARTESIAN_POINT('Ctrl Pts',(5.10848921171111,28.5805979360069,125.872290345407));
#122061=CARTESIAN_POINT('Ctrl Pts',(5.10889740105742,28.5774370411825,125.867125878679));
#122062=CARTESIAN_POINT('Ctrl Pts',(5.1098639854839,28.5700518312273,125.854910402286));
#122063=CARTESIAN_POINT('Ctrl Pts',(5.11042386723923,28.5658514678204,125.847845234625));
#122064=CARTESIAN_POINT('Ctrl Pts',(5.11230974584357,28.5519554263393,125.824072842979));
#122065=CARTESIAN_POINT('Ctrl Pts',(5.11364931045251,28.5424984731596,125.807228813635));
#122066=CARTESIAN_POINT('Ctrl Pts',(5.11698449651718,28.5199113062932,125.765306883766));
#122067=CARTESIAN_POINT('Ctrl Pts',(5.11899472939815,28.5071235348106,125.740051921382));
#122068=CARTESIAN_POINT('Ctrl Pts',(5.12821538155622,28.451937431038,125.623806153446));
#122069=CARTESIAN_POINT('Ctrl Pts',(5.13559855851799,28.4171722790135,125.529423004262));
#122070=CARTESIAN_POINT('Ctrl Pts',(5.14876997769516,28.3697457712846,125.352991177952));
#122071=CARTESIAN_POINT('Ctrl Pts',(5.15459129391607,28.3542955681113,125.272015090418));
#122072=CARTESIAN_POINT('Ctrl Pts',(5.16156721043594,28.342656882081,125.170745276547));
#122073=CARTESIAN_POINT('Ctrl Pts',(5.16289786397962,28.340762749002,125.151234790322));
#122074=CARTESIAN_POINT('Ctrl Pts',(5.16501414313744,28.3382784375587,125.119905418752));
#122075=CARTESIAN_POINT('Ctrl Pts',(5.16580653879206,28.3374691269613,125.10810628661));
#122076=CARTESIAN_POINT('Ctrl Pts',(5.1673112033387,28.3361645657059,125.085574805121));
#122077=CARTESIAN_POINT('Ctrl Pts',(5.16802412179771,28.3356473547087,125.07484437865));
#122078=CARTESIAN_POINT('Ctrl Pts',(5.16965777434659,28.3346957844673,125.05013443285));
#122079=CARTESIAN_POINT('Ctrl Pts',(5.17057621484759,28.334333591356,125.036152821475));
#122080=CARTESIAN_POINT('Ctrl Pts',(5.17348922035691,28.3337399336835,124.99154128465));
#122081=CARTESIAN_POINT('Ctrl Pts',(5.17546308238214,28.3341770360683,124.960907799184));
#122082=CARTESIAN_POINT('Ctrl Pts',(5.18012645394362,28.3372390291876,124.887780503026));
#122083=CARTESIAN_POINT('Ctrl Pts',(5.18279332813655,28.3406482725798,124.845340738013));
#122084=CARTESIAN_POINT('Ctrl Pts',(5.19000020116968,28.3543894324385,124.729904054905));
#122085=CARTESIAN_POINT('Ctrl Pts',(5.19447284304928,28.367944796246,124.657389238388));
#122086=CARTESIAN_POINT('Ctrl Pts',(5.19984187937073,28.3897529073344,124.572380680672));
#122087=CARTESIAN_POINT('Ctrl Pts',(5.2007039088472,28.3934218549189,124.558796374364));
#122088=CARTESIAN_POINT('Ctrl Pts',(5.20606609574129,28.4172472508609,124.47482337492));
#122089=CARTESIAN_POINT('Ctrl Pts',(5.21061884209723,28.4418512940101,124.405789048505));
#122090=CARTESIAN_POINT('Ctrl Pts',(5.21620228849069,28.475785209564,124.327336617031));
#122091=CARTESIAN_POINT('Ctrl Pts',(5.21701061538136,28.4807838511674,124.316122068249));
#122092=CARTESIAN_POINT('Ctrl Pts',(5.21828778435916,28.4888055918879,124.29864718267));
#122093=CARTESIAN_POINT('Ctrl Pts',(5.21875175018648,28.4917448198266,124.292348517567));
#122094=CARTESIAN_POINT('Ctrl Pts',(5.21962447944393,28.4973181629705,124.280597496109));
#122095=CARTESIAN_POINT('Ctrl Pts',(5.22003266869008,28.49994269986,124.275140870545));
#122096=CARTESIAN_POINT('Ctrl Pts',(5.2209992522832,28.5061999753993,124.262311008866));
#122097=CARTESIAN_POINT('Ctrl Pts',(5.22155913329749,28.5098575992237,124.254950216788));
#122098=CARTESIAN_POINT('Ctrl Pts',(5.22344500673452,28.5222930722812,124.230382321442));
#122099=CARTESIAN_POINT('Ctrl Pts',(5.22478456682007,28.5313153316397,124.213301582077));
#122100=CARTESIAN_POINT('Ctrl Pts',(5.22811973909698,28.5542852032068,124.171588335049));
#122101=CARTESIAN_POINT('Ctrl Pts',(5.23012996256916,28.5685672974179,124.147147493787));
#122102=CARTESIAN_POINT('Ctrl Pts',(5.23935053098661,28.636298820608,124.037736666752));
#122103=CARTESIAN_POINT('Ctrl Pts',(5.24673363132664,28.6967381215495,123.957339660999));
#122104=CARTESIAN_POINT('Ctrl Pts',(5.25990506772165,28.8192435466228,123.82180391584));
#122105=CARTESIAN_POINT('Ctrl Pts',(5.2657264699393,28.8788962343529,123.764904122622));
#122106=CARTESIAN_POINT('Ctrl Pts',(5.27270246959723,28.9576659371131,123.700200068183));
#122107=CARTESIAN_POINT('Ctrl Pts',(5.2740331256744,28.9730302641684,123.688026913378));
#122108=CARTESIAN_POINT('Ctrl Pts',(5.27614940787022,28.99800406661,123.668947780821));
#122109=CARTESIAN_POINT('Ctrl Pts',(5.27694180406383,29.0074780963142,123.661868413085));
#122110=CARTESIAN_POINT('Ctrl Pts',(5.27844646902708,29.0257002322304,123.64855212377));
#122111=CARTESIAN_POINT('Ctrl Pts',(5.27915938737013,29.0344348123309,123.642297795088));
#122112=CARTESIAN_POINT('Ctrl Pts',(5.28079303879772,29.0546786015462,123.628096561409));
#122113=CARTESIAN_POINT('Ctrl Pts',(5.28171147830432,29.0662287083991,123.620209151381));
#122114=CARTESIAN_POINT('Ctrl Pts',(5.28462447706611,29.1033867358027,123.595514753564));
#122115=CARTESIAN_POINT('Ctrl Pts',(5.28659833347796,29.1293602515496,123.579267523329));
#122116=CARTESIAN_POINT('Ctrl Pts',(5.29126168891873,29.1924581602637,123.542178534906));
#122117=CARTESIAN_POINT('Ctrl Pts',(5.29392855282703,29.2299625480471,123.522025050736));
#122118=CARTESIAN_POINT('Ctrl Pts',(5.30113542103113,29.3343985313334,123.470960871794));
#122119=CARTESIAN_POINT('Ctrl Pts',(5.30560806767021,29.402673386095,123.443019830104));
#122120=CARTESIAN_POINT('Ctrl Pts',(5.31097707484294,29.4859202551149,123.415236300833));
#122121=CARTESIAN_POINT('Ctrl Pts',(5.31183907068656,29.4993224027386,123.410951258228));
#122122=CARTESIAN_POINT('Ctrl Pts',(5.31720126974645,29.5827939947003,123.385423890155));
#122123=CARTESIAN_POINT('Ctrl Pts',(5.32175406160045,29.6541378297784,123.368652852121));
#122124=CARTESIAN_POINT('Ctrl Pts',(5.32733755849163,29.7384544348061,123.354612303568));
#122125=CARTESIAN_POINT('Ctrl Pts',(5.32814588557151,29.7505873522995,123.352729511085));
#122126=CARTESIAN_POINT('Ctrl Pts',(5.32942305478397,29.7696194724705,123.349991173954));
#122127=CARTESIAN_POINT('Ctrl Pts',(5.32988702065385,29.7765053877053,123.349044377521));
#122128=CARTESIAN_POINT('Ctrl Pts',(5.33075974994338,29.789400714346,123.347353453753));
#122129=CARTESIAN_POINT('Ctrl Pts',(5.33116793917849,29.7954085175658,123.34659896378));
#122130=CARTESIAN_POINT('Ctrl Pts',(5.33213452268102,29.8095811634394,123.344897517432));
#122131=CARTESIAN_POINT('Ctrl Pts',(5.33269440361449,29.8177490481325,123.34397821736));
#122132=CARTESIAN_POINT('Ctrl Pts',(5.33458027648687,29.8451341530161,123.34110105656));
#122133=CARTESIAN_POINT('Ctrl Pts',(5.33591983607837,29.8643777686456,123.339417070444));
#122134=CARTESIAN_POINT('Ctrl Pts',(5.33925500684945,29.9118808967923,123.336091293626));
#122135=CARTESIAN_POINT('Ctrl Pts',(5.34126522929403,29.9401607930236,123.334834468322));
#122136=CARTESIAN_POINT('Ctrl Pts',(5.35048578856561,30.0688166143859,123.332398164924));
#122137=CARTESIAN_POINT('Ctrl Pts',(5.35786888053724,30.1691416359921,123.339571383381));
#122138=CARTESIAN_POINT('Ctrl Pts',(5.37104207867903,30.3494777771977,123.368987695162));
#122139=CARTESIAN_POINT('Ctrl Pts',(5.37686517540465,30.4296587910167,123.388251617995));
#122140=CARTESIAN_POINT('Ctrl Pts',(5.38384184190729,30.5267511615722,123.419344163597));
#122141=CARTESIAN_POINT('Ctrl Pts',(5.38517160844966,30.5452990806009,123.425646599748));
#122142=CARTESIAN_POINT('Ctrl Pts',(5.38728682396925,30.5748583436767,123.436275701722));
#122143=CARTESIAN_POINT('Ctrl Pts',(5.38807903090096,30.5859417741661,123.440394907009));
#122144=CARTESIAN_POINT('Ctrl Pts',(5.3895835496665,30.6070103828556,123.448481450394));
#122145=CARTESIAN_POINT('Ctrl Pts',(5.39029650884441,30.6170028244621,123.452428050625));
#122146=CARTESIAN_POINT('Ctrl Pts',(5.39193055457517,30.6399189587419,123.461736215586));
#122147=CARTESIAN_POINT('Ctrl Pts',(5.39284934367759,30.6528148002263,123.467164522663));
#122148=CARTESIAN_POINT('Ctrl Pts',(5.39576471541366,30.6937481665943,123.485005095427));
#122149=CARTESIAN_POINT('Ctrl Pts',(5.39774054604783,30.7215130309643,123.498029555853));
#122150=CARTESIAN_POINT('Ctrl Pts',(5.40240957233133,30.7869741797879,123.530971746993));
#122151=CARTESIAN_POINT('Ctrl Pts',(5.40508005444592,30.8242968849747,123.551584522475));
#122152=CARTESIAN_POINT('Ctrl Pts',(5.4123368675085,30.9245241718314,123.612069020306));
#122153=CARTESIAN_POINT('Ctrl Pts',(5.41685383658555,30.9856091454516,123.654759383831));
#122154=CARTESIAN_POINT('Ctrl Pts',(5.42221449123898,31.0538976593136,123.709639950839));
#122155=CARTESIAN_POINT('Ctrl Pts',(5.42302120683429,31.0640617267757,123.718008592365));
#122156=CARTESIAN_POINT('Ctrl Pts',(5.42833063752569,31.1301297359296,123.773733091716));
#122157=CARTESIAN_POINT('Ctrl Pts',(5.4328862029799,31.1829502843929,123.824606592241));
#122158=CARTESIAN_POINT('Ctrl Pts',(5.43847277833247,31.2405084362413,123.887864406536));
#122159=CARTESIAN_POINT('Ctrl Pts',(5.43928111693002,31.2486708336146,123.897036770262));
#122160=CARTESIAN_POINT('Ctrl Pts',(5.44055830042732,31.2612939157065,123.911541469668));
#122161=CARTESIAN_POINT('Ctrl Pts',(5.44102226888773,31.2658240609743,123.916813148005));
#122162=CARTESIAN_POINT('Ctrl Pts',(5.44189500013556,31.2742386636389,123.926729999525));
#122163=CARTESIAN_POINT('Ctrl Pts',(5.44230318870524,31.2781309553681,123.931368200886));
#122164=CARTESIAN_POINT('Ctrl Pts',(5.44326976666608,31.2872470999813,123.942352391604));
#122165=CARTESIAN_POINT('Ctrl Pts',(5.44382964267218,31.2924493682281,123.948715935895));
#122166=CARTESIAN_POINT('Ctrl Pts',(5.44571548119146,31.3097189900807,123.970162495472));
#122167=CARTESIAN_POINT('Ctrl Pts',(5.44705501070969,31.3215705764539,123.985416218034));
#122168=CARTESIAN_POINT('Ctrl Pts',(5.4545075053824,31.3853843042896,124.070563944558));
#122169=CARTESIAN_POINT('Ctrl Pts',(5.46085769394969,31.4320654938738,124.144238899093));
#122170=CARTESIAN_POINT('Ctrl Pts',(5.47370805071857,31.514594526569,124.300311182841));
#122171=CARTESIAN_POINT('Ctrl Pts',(5.4801850450461,31.5499832386887,124.382653766623));
#122172=CARTESIAN_POINT('Ctrl Pts',(5.48939019275632,31.5918863134997,124.506862815249));
#122173=CARTESIAN_POINT('Ctrl Pts',(5.49226837628911,31.6037032851654,124.546764283238));
#122174=CARTESIAN_POINT('Ctrl Pts',(5.49619602346351,31.6180116664799,124.602691229674));
#122175=CARTESIAN_POINT('Ctrl Pts',(5.49728581892356,31.6217814459432,124.618370618012));
#122176=CARTESIAN_POINT('Ctrl Pts',(5.49903924546741,31.6275181243303,124.643853061928));
#122177=CARTESIAN_POINT('Ctrl Pts',(5.49970732654887,31.6296253975822,124.653623098934));
#122178=CARTESIAN_POINT('Ctrl Pts',(5.5011015085536,31.6338570064753,124.674136236065));
#122179=CARTESIAN_POINT('Ctrl Pts',(5.50182701382798,31.6359636018971,124.684882540548));
#122180=CARTESIAN_POINT('Ctrl Pts',(5.50326585811388,31.6399493304295,124.706333042058));
#122181=CARTESIAN_POINT('Ctrl Pts',(5.50397921216962,31.6418299846005,124.717036399002));
#122182=CARTESIAN_POINT('Ctrl Pts',(5.50565528089859,31.6460211659661,124.742339769015));
#122183=CARTESIAN_POINT('Ctrl Pts',(5.50661520089376,31.6482424077205,124.756953788149));
#122184=CARTESIAN_POINT('Ctrl Pts',(5.5125320454875,31.6608072246128,124.847737268346));
#122185=CARTESIAN_POINT('Ctrl Pts',(5.51732912507926,31.6660638404818,124.924519570155));
#122186=CARTESIAN_POINT('Ctrl Pts',(5.52205824491057,31.6659994149782,125.001396170626));
#122187=CARTESIAN_POINT('Ctrl Pts',(5.52205815882027,31.6659994161504,125.001394771142));
#122188=CARTESIAN_POINT('Ctrl Pts',(5.52952817550204,31.6658977530252,125.12282738621));
#122189=CARTESIAN_POINT('Ctrl Pts',(5.53677883282065,31.6525201216262,125.243875523706));
#122190=CARTESIAN_POINT('Ctrl Pts',(5.54571783249626,31.6219777811608,125.380926412135));
#122191=CARTESIAN_POINT('Ctrl Pts',(5.54693875696725,31.617529138693,125.399394886252));
#122192=CARTESIAN_POINT('Ctrl Pts',(5.549107440675,31.6091692314404,125.43166664503));
#122193=CARTESIAN_POINT('Ctrl Pts',(5.55004877350797,31.6053935658685,125.445503280201));
#122194=CARTESIAN_POINT('Ctrl Pts',(5.55148435318858,31.5994253101844,125.466313283183));
#122195=CARTESIAN_POINT('Ctrl Pts',(5.55197142621871,31.5973645787756,125.473324200069));
#122196=CARTESIAN_POINT('Ctrl Pts',(5.55286385855791,31.5935256100598,125.486074304289));
#122197=CARTESIAN_POINT('Ctrl Pts',(5.55326836036909,31.5917623625524,125.491817727222));
#122198=CARTESIAN_POINT('Ctrl Pts',(5.55419554837357,31.5876679445464,125.504901787628));
#122199=CARTESIAN_POINT('Ctrl Pts',(5.55471934058999,31.5853169223576,125.512235851038));
#122200=CARTESIAN_POINT('Ctrl Pts',(5.5563655655747,31.5778072627781,125.535115423373));
#122201=CARTESIAN_POINT('Ctrl Pts',(5.55749742930064,31.5724703467732,125.550600792995));
#122202=CARTESIAN_POINT('Ctrl Pts',(5.55887450521995,31.565760403058,125.569176366074));
#122203=CARTESIAN_POINT('Ctrl Pts',(5.55911008052214,31.5646049816606,125.572344847383));
#122204=CARTESIAN_POINT('Ctrl Pts',(5.55934605048515,31.5634400125327,125.575509623909));
#122205=CARTESIAN_POINT('',(5.32851907198357,31.6679764309607,125.000530942783));
#122206=CARTESIAN_POINT('Ctrl Pts',(5.36787244251734,31.5634400119422,125.575509625513));
#122207=CARTESIAN_POINT('Ctrl Pts',(5.36380377202413,31.5844917329173,125.518320133915));
#122208=CARTESIAN_POINT('Ctrl Pts',(5.35973510153093,31.6023841697817,125.460021086487));
#122209=CARTESIAN_POINT('Ctrl Pts',(5.35566643103772,31.6170218318539,125.400994258448));
#122210=CARTESIAN_POINT('Ctrl Pts',(5.35159020376397,31.6316866805955,125.341857799317));
#122211=CARTESIAN_POINT('Ctrl Pts',(5.34751397649022,31.6430845848598,125.281991363721));
#122212=CARTESIAN_POINT('Ctrl Pts',(5.34343774921647,31.6511713932636,125.221786000613));
#122213=CARTESIAN_POINT('Ctrl Pts',(5.34045616622793,31.6570865419413,125.17774839564));
#122214=CARTESIAN_POINT('Ctrl Pts',(5.33747458323939,31.6612312483094,125.133529634148));
#122215=CARTESIAN_POINT('Ctrl Pts',(5.33449300025085,31.6636058986978,125.089282774474));
#122216=CARTESIAN_POINT('Ctrl Pts',(5.33250187903717,31.6651917062308,125.059734423388));
#122217=CARTESIAN_POINT('Ctrl Pts',(5.33051075782348,31.6659903400224,125.030143448948));
#122218=CARTESIAN_POINT('Ctrl Pts',(5.3285196366098,31.6659999129021,125.000538711647));
#122219=CARTESIAN_POINT('Ctrl Pts',(5.32851890484269,31.6685615206205,125.00052864304));
#122220=CARTESIAN_POINT('Ctrl Pts',(5.29346517969922,31.6663498316797,124.478534520954));
#122221=CARTESIAN_POINT('Ctrl Pts',(5.22136636427624,31.1216475883581,123.40092281885));
#122222=CARTESIAN_POINT('Ctrl Pts',(5.11222245857374,29.2866679733565,123.164583862537));
#122223=CARTESIAN_POINT('Ctrl Pts',(5.00108718773517,28.0711012827654,124.603837512444));
#122224=CARTESIAN_POINT('Ctrl Pts',(4.88995191689663,28.6210012493043,126.405687526968));
#122225=CARTESIAN_POINT('Ctrl Pts',(4.77886137758078,30.4323305780535,126.920743955777));
#122226=CARTESIAN_POINT('Ctrl Pts',(4.70481592854447,31.3757142918801,126.093332246506));
#122227=CARTESIAN_POINT('Ctrl Pts',(4.66781556978768,31.5660436956742,125.576468401513));
#122228=CARTESIAN_POINT('Origin',(5.,30.,125.));
#122229=CARTESIAN_POINT('',(3.96713561979274,31.5634400104587,125.575509629543));
#122230=CARTESIAN_POINT('',(4.16231120066723,31.5634400119557,125.575509625476));
#122231=CARTESIAN_POINT('',(5.,31.5634400119422,125.575509625513));
#122232=CARTESIAN_POINT('Ctrl Pts',(4.16231120066723,31.5634400119558,125.575509625476));
#122233=CARTESIAN_POINT('Ctrl Pts',(4.16319058703546,31.5589599896281,125.587680136362));
#122234=CARTESIAN_POINT('Ctrl Pts',(4.16406524665906,31.554337873318,125.59979828981));
#122235=CARTESIAN_POINT('Ctrl Pts',(4.16567097839286,31.5455459090605,125.62206444262));
#122236=CARTESIAN_POINT('Ctrl Pts',(4.16640334762147,31.5414164942572,125.632227434503));
#122237=CARTESIAN_POINT('Ctrl Pts',(4.16779517503746,31.5333413397352,125.651551851126));
#122238=CARTESIAN_POINT('Ctrl Pts',(4.16845518751511,31.5294131298379,125.660720034854));
#122239=CARTESIAN_POINT('Ctrl Pts',(4.17016732897336,31.5189663013785,125.684509778734));
#122240=CARTESIAN_POINT('Ctrl Pts',(4.17121502931073,31.5123187561079,125.699073866687));
#122241=CARTESIAN_POINT('Ctrl Pts',(4.17490877765944,31.4879873140498,125.750409529617));
#122242=CARTESIAN_POINT('Ctrl Pts',(4.17751573861791,31.4691630315169,125.786626413127));
#122243=CARTESIAN_POINT('Ctrl Pts',(4.18745721451471,31.3913217619973,125.923825785018));
#122244=CARTESIAN_POINT('Ctrl Pts',(4.19448379154936,31.3230706609143,126.019173786773));
#122245=CARTESIAN_POINT('Ctrl Pts',(4.20468121314224,31.21288702587,126.143178243967));
#122246=CARTESIAN_POINT('Ctrl Pts',(4.20771729517768,31.1787836554665,126.178312296051));
#122247=CARTESIAN_POINT('Ctrl Pts',(4.21205002789272,31.1292622752695,126.22502616147));
#122248=CARTESIAN_POINT('Ctrl Pts',(4.21327996640977,31.1151138180846,126.237919015802));
#122249=CARTESIAN_POINT('Ctrl Pts',(4.21519394755994,31.093025012955,126.257361582333));
#122250=CARTESIAN_POINT('Ctrl Pts',(4.21586732731321,31.0852404281857,126.264086638059));
#122251=CARTESIAN_POINT('Ctrl Pts',(4.21709875135551,31.0709930528768,126.276166255583));
#122252=CARTESIAN_POINT('Ctrl Pts',(4.21765518008878,31.0645510649365,126.281544948101));
#122253=CARTESIAN_POINT('Ctrl Pts',(4.2186246014314,31.0533269192791,126.290773445787));
#122254=CARTESIAN_POINT('Ctrl Pts',(4.21903599390885,31.0485635082625,126.294645995778));
#122255=CARTESIAN_POINT('Ctrl Pts',(4.21983196103034,31.0393495033326,126.302052574293));
#122256=CARTESIAN_POINT('Ctrl Pts',(4.22021623946143,31.0349020409072,126.305590310768));
#122257=CARTESIAN_POINT('Ctrl Pts',(4.22125694631312,31.0228574639984,126.315070965117));
#122258=CARTESIAN_POINT('Ctrl Pts',(4.22191627524253,31.0152268362459,126.32097066385));
#122259=CARTESIAN_POINT('Ctrl Pts',(4.22445583620608,30.9858202384963,126.343301391327));
#122260=CARTESIAN_POINT('Ctrl Pts',(4.22636381832533,30.9636943533992,126.359261990562));
#122261=CARTESIAN_POINT('Ctrl Pts',(4.23828066895123,30.8247539430314,126.454389530815));
#122262=CARTESIAN_POINT('Ctrl Pts',(4.24875982908233,30.6986629412363,126.518993915378));
#122263=CARTESIAN_POINT('Ctrl Pts',(4.26177503365491,30.5269491191074,126.581011789793));
#122264=CARTESIAN_POINT('Ctrl Pts',(4.26469428421219,30.487454794372,126.593631684596));
#122265=CARTESIAN_POINT('Ctrl Pts',(4.26965324794239,30.4185891917061,126.612836531113));
#122266=CARTESIAN_POINT('Ctrl Pts',(4.27171314914196,30.3894358271902,126.620122997255));
#122267=CARTESIAN_POINT('Ctrl Pts',(4.27468821168877,30.3465451244102,126.629618116513));
#122268=CARTESIAN_POINT('Ctrl Pts',(4.27562296846786,30.3329532924104,126.632449342017));
#122269=CARTESIAN_POINT('Ctrl Pts',(4.27727056627474,30.3087966052571,126.637166998658));
#122270=CARTESIAN_POINT('Ctrl Pts',(4.27798554443899,30.2982460896326,126.639121839336));
#122271=CARTESIAN_POINT('Ctrl Pts',(4.27948527629863,30.2759768807872,126.643025826409));
#122272=CARTESIAN_POINT('Ctrl Pts',(4.28026926066304,30.2642547028447,126.644951844067));
#122273=CARTESIAN_POINT('Ctrl Pts',(4.28235275218274,30.232894844977,126.649760558191));
#122274=CARTESIAN_POINT('Ctrl Pts',(4.28364514455263,30.2132241916118,126.652418048444));
#122275=CARTESIAN_POINT('Ctrl Pts',(4.29092516026438,30.1012955810992,126.665507431881));
#122276=CARTESIAN_POINT('Ctrl Pts',(4.29667517862958,30.008335689306,126.668565096381));
#122277=CARTESIAN_POINT('Ctrl Pts',(4.30674853932338,29.8440315204372,126.660230209088));
#122278=CARTESIAN_POINT('Ctrl Pts',(4.31109083183077,29.7727790608835,126.651986857076));
#122279=CARTESIAN_POINT('Ctrl Pts',(4.31795495956892,29.6637088657278,126.632176816563));
#122280=CARTESIAN_POINT('Ctrl Pts',(4.32040918598953,29.6253984908349,126.62381224196));
#122281=CARTESIAN_POINT('Ctrl Pts',(4.32447237417068,29.5638658489251,126.608083990391));
#122282=CARTESIAN_POINT('Ctrl Pts',(4.32604793989103,29.5404463517141,126.601548442702));
#122283=CARTESIAN_POINT('Ctrl Pts',(4.32824200481638,29.5085869564058,126.591901324369));
#122284=CARTESIAN_POINT('Ctrl Pts',(4.32883737485338,29.5000155841861,126.589230059145));
#122285=CARTESIAN_POINT('Ctrl Pts',(4.32984895519503,29.4855855493209,126.58460465465));
#122286=CARTESIAN_POINT('Ctrl Pts',(4.3302630862102,29.4797152426027,126.582686926873));
#122287=CARTESIAN_POINT('Ctrl Pts',(4.3311246768605,29.4675822858722,126.57864850247));
#122288=CARTESIAN_POINT('Ctrl Pts',(4.33157238172558,29.4613214357542,126.576523110283));
#122289=CARTESIAN_POINT('Ctrl Pts',(4.33277352031084,29.4446362270969,126.570747932771));
#122290=CARTESIAN_POINT('Ctrl Pts',(4.33353063290721,29.4342354436852,126.567031728767));
#122291=CARTESIAN_POINT('Ctrl Pts',(4.33706867090928,29.3861340105069,126.549303782684));
#122292=CARTESIAN_POINT('Ctrl Pts',(4.33991086584414,29.3489145563841,126.534034169986));
#122293=CARTESIAN_POINT('Ctrl Pts',(4.3493206248095,29.2292066346742,126.479781658319));
#122294=CARTESIAN_POINT('Ctrl Pts',(4.35601718698825,29.1493599045371,126.43537011905));
#122295=CARTESIAN_POINT('Ctrl Pts',(4.36709643973142,29.0221146494648,126.350231925024));
#122296=CARTESIAN_POINT('Ctrl Pts',(4.37152507249643,28.9726325240827,126.312975018402));
#122297=CARTESIAN_POINT('Ctrl Pts',(4.37864351690706,28.894982183219,126.247425100924));
#122298=CARTESIAN_POINT('Ctrl Pts',(4.3813862397343,28.8655540471636,126.220723800427));
#122299=CARTESIAN_POINT('Ctrl Pts',(4.38513247215379,28.826071308131,126.182237245629));
#122300=CARTESIAN_POINT('Ctrl Pts',(4.3861728394732,28.8151856987691,126.171327698753));
#122301=CARTESIAN_POINT('Ctrl Pts',(4.38794229809535,28.7968135455444,126.152396924661));
#122302=CARTESIAN_POINT('Ctrl Pts',(4.38867462956843,28.7892521599083,126.144450083571));
#122303=CARTESIAN_POINT('Ctrl Pts',(4.39015468248037,28.7740601524281,126.128164539176));
#122304=CARTESIAN_POINT('Ctrl Pts',(4.39090215712362,28.7664347948603,126.119821696806));
#122305=CARTESIAN_POINT('Ctrl Pts',(4.39277244530255,28.7474793569807,126.098654109383));
#122306=CARTESIAN_POINT('Ctrl Pts',(4.39389058943712,28.7362606958482,126.085731007152));
#122307=CARTESIAN_POINT('Ctrl Pts',(4.39821587929387,28.6933446490841,126.034728158176));
#122308=CARTESIAN_POINT('Ctrl Pts',(4.40136294724094,28.6631514106822,125.99541304205));
#122309=CARTESIAN_POINT('Ctrl Pts',(4.41189628154717,28.5666641679311,125.857449200472));
#122310=CARTESIAN_POINT('Ctrl Pts',(4.41900492270334,28.5091870388347,125.753091473105));
#122311=CARTESIAN_POINT('Ctrl Pts',(4.42884562177325,28.4477416979857,125.606359832775));
#122312=CARTESIAN_POINT('Ctrl Pts',(4.43136421206043,28.4335382621367,125.568660954391));
#122313=CARTESIAN_POINT('Ctrl Pts',(4.4355221579014,28.4128303397632,125.507012530812));
#122314=CARTESIAN_POINT('Ctrl Pts',(4.43712614451108,28.4054699875807,125.483366445528));
#122315=CARTESIAN_POINT('Ctrl Pts',(4.43935355468554,28.3961461537136,125.45087754303));
#122316=CARTESIAN_POINT('Ctrl Pts',(4.4399529273415,28.3937233385711,125.442168516331));
#122317=CARTESIAN_POINT('Ctrl Pts',(4.44096928204918,28.3897618869612,125.427466372996));
#122318=CARTESIAN_POINT('Ctrl Pts',(4.44138413823894,28.3881855015162,125.421483453766));
#122319=CARTESIAN_POINT('Ctrl Pts',(4.44218977871404,28.3852031845383,125.409903099919));
#122320=CARTESIAN_POINT('Ctrl Pts',(4.44258027642,28.3837929585358,125.404306941705));
#122321=CARTESIAN_POINT('Ctrl Pts',(4.44365865606108,28.3799944816574,125.388896070233));
#122322=CARTESIAN_POINT('Ctrl Pts',(4.44434980275872,28.3776664207772,125.379066983391));
#122323=CARTESIAN_POINT('Ctrl Pts',(4.44717556007952,28.368571834471,125.339050448907));
#122324=CARTESIAN_POINT('Ctrl Pts',(4.44934614872122,28.3625578221788,125.308700328386));
#122325=CARTESIAN_POINT('Ctrl Pts',(4.4593000480868,28.33915876353,125.170544040238));
#122326=CARTESIAN_POINT('Ctrl Pts',(4.46734653090748,28.3315534069206,125.061356211219));
#122327=CARTESIAN_POINT('Ctrl Pts',(4.47938671832493,28.3363372292898,124.894655331219));
#122328=CARTESIAN_POINT('Ctrl Pts',(4.48349491064335,28.3409716220761,124.837220208576));
#122329=CARTESIAN_POINT('Ctrl Pts',(4.49016954584143,28.3535684389535,124.742604002876));
#122330=CARTESIAN_POINT('Ctrl Pts',(4.49278066319695,28.3598435421195,124.705251332033));
#122331=CARTESIAN_POINT('Ctrl Pts',(4.49638054881835,28.3704031023441,124.653302332234));
#122332=CARTESIAN_POINT('Ctrl Pts',(4.49740245511979,28.3736218531016,124.638503843338));
#122333=CARTESIAN_POINT('Ctrl Pts',(4.49915025000755,28.3795084708342,124.613111803149));
#122334=CARTESIAN_POINT('Ctrl Pts',(4.49987918061958,28.3820795198762,124.602497040587));
#122335=CARTESIAN_POINT('Ctrl Pts',(4.50127101140126,28.3872112272003,124.582185523349));
#122336=CARTESIAN_POINT('Ctrl Pts',(4.50193440561334,28.3897554171307,124.572485142534));
#122337=CARTESIAN_POINT('Ctrl Pts',(4.50366981427321,28.396668662493,124.547064215024));
#122338=CARTESIAN_POINT('Ctrl Pts',(4.50473715294574,28.4011814047808,124.531383596488));
#122339=CARTESIAN_POINT('Ctrl Pts',(4.50858775156105,28.4184044451597,124.47468551383));
#122340=CARTESIAN_POINT('Ctrl Pts',(4.51132723006017,28.4324694376922,124.434095215161));
#122341=CARTESIAN_POINT('Ctrl Pts',(4.52125756321136,28.4898846005365,124.287038054555));
#122342=CARTESIAN_POINT('Ctrl Pts',(4.52816326411835,28.5426443521346,124.18459921125));
#122343=CARTESIAN_POINT('Ctrl Pts',(4.5382056402252,28.632002177851,124.047908238331));
#122344=CARTESIAN_POINT('Ctrl Pts',(4.54120833510575,28.6602250770414,124.008587232885));
#122345=CARTESIAN_POINT('Ctrl Pts',(4.54549778742929,28.7018598538428,123.955610543496));
#122346=CARTESIAN_POINT('Ctrl Pts',(4.54671923867236,28.7138574075062,123.94087095061));
#122347=CARTESIAN_POINT('Ctrl Pts',(4.54888876933783,28.7353501460472,123.915369835031));
#122348=CARTESIAN_POINT('Ctrl Pts',(4.54983041535226,28.7447373294063,123.904519538375));
#122349=CARTESIAN_POINT('Ctrl Pts',(4.55126637743371,28.759115900008,123.8883273568));
#122350=CARTESIAN_POINT('Ctrl Pts',(4.55175351395751,28.764004515797,123.882894555896));
#122351=CARTESIAN_POINT('Ctrl Pts',(4.55264600549826,28.7729767699733,123.873054530373));
#122352=CARTESIAN_POINT('Ctrl Pts',(4.55305050226626,28.777048710634,123.868636999535));
#122353=CARTESIAN_POINT('Ctrl Pts',(4.55397760457306,28.7863941837865,123.858607770252));
#122354=CARTESIAN_POINT('Ctrl Pts',(4.55450131526568,28.791682766488,123.853010568232));
#122355=CARTESIAN_POINT('Ctrl Pts',(4.55614702402541,28.8083366521187,123.83562783675));
#122356=CARTESIAN_POINT('Ctrl Pts',(4.5572784449458,28.8198366214168,123.823973461583));
#122357=CARTESIAN_POINT('Ctrl Pts',(4.56384081447224,28.886924392363,123.757959929136));
#122358=CARTESIAN_POINT('Ctrl Pts',(4.56947637030779,28.9460870302979,123.707380181069));
#122359=CARTESIAN_POINT('Ctrl Pts',(4.57997711671616,29.062060175513,123.621501892103));
#122360=CARTESIAN_POINT('Ctrl Pts',(4.58482823244832,29.117891823969,123.585123999372));
#122361=CARTESIAN_POINT('Ctrl Pts',(4.59482948120842,29.2390456792669,123.516150641602));
#122362=CARTESIAN_POINT('Ctrl Pts',(4.5999533195312,29.3046403192063,123.48430282542));
#122363=CARTESIAN_POINT('Ctrl Pts',(4.60620495545551,29.3893839370133,123.449822107671));
#122364=CARTESIAN_POINT('Ctrl Pts',(4.60746903192942,29.406767345019,123.443086855244));
#122365=CARTESIAN_POINT('Ctrl Pts',(4.60950543731256,29.4351671576774,123.432628014138));
#122366=CARTESIAN_POINT('Ctrl Pts',(4.61028365211428,29.4461155158327,123.428725653531));
#122367=CARTESIAN_POINT('Ctrl Pts',(4.6117780754605,29.4673201051505,123.421416807166));
#122368=CARTESIAN_POINT('Ctrl Pts',(4.61249476099101,29.4775703675198,123.41799492556));
#122369=CARTESIAN_POINT('Ctrl Pts',(4.61414500163495,29.5013554597621,123.410311051165));
#122370=CARTESIAN_POINT('Ctrl Pts',(4.61507614156788,29.5149130180437,123.406121719806));
#122371=CARTESIAN_POINT('Ctrl Pts',(4.61805143589898,29.5586547473912,123.393215214038));
#122372=CARTESIAN_POINT('Ctrl Pts',(4.62007372595736,29.5890335590473,123.385178100508));
#122373=CARTESIAN_POINT('Ctrl Pts',(4.63095222128706,29.7554788903902,123.346144728701));
#122374=CARTESIAN_POINT('Ctrl Pts',(4.63927654918687,29.8947923300856,123.331479819019));
#122375=CARTESIAN_POINT('Ctrl Pts',(4.65053615341447,30.077157536108,123.33523582151));
#122376=CARTESIAN_POINT('Ctrl Pts',(4.65320965586474,30.1199565405167,123.337771678674));
#122377=CARTESIAN_POINT('Ctrl Pts',(4.65759424598209,30.1883074183726,123.344474954379));
#122378=CARTESIAN_POINT('Ctrl Pts',(4.65926499660684,30.2139440209308,123.347592471049));
#122379=CARTESIAN_POINT('Ctrl Pts',(4.66157056615668,30.2485819808267,123.352624118736));
#122380=CARTESIAN_POINT('Ctrl Pts',(4.66217909830849,30.257656544573,123.354019018695));
#122381=CARTESIAN_POINT('Ctrl Pts',(4.66320642732542,30.2728528374561,123.356483664653));
#122382=CARTESIAN_POINT('Ctrl Pts',(4.6636229909301,30.278981123993,123.357512817004));
#122383=CARTESIAN_POINT('Ctrl Pts',(4.6644823574858,30.2915514491688,123.359696191749));
#122384=CARTESIAN_POINT('Ctrl Pts',(4.66492534256169,30.2979926420563,123.360854121065));
#122385=CARTESIAN_POINT('Ctrl Pts',(4.66610047765069,30.314982676704,123.36401186097));
#122386=CARTESIAN_POINT('Ctrl Pts',(4.66683604316334,30.3255190936232,123.366075710992));
#122387=CARTESIAN_POINT('Ctrl Pts',(4.67013139659234,30.37231933019,123.375713466757));
#122388=CARTESIAN_POINT('Ctrl Pts',(4.67274313869128,30.4083418970573,123.384393347198));
#122389=CARTESIAN_POINT('Ctrl Pts',(4.68206764426872,30.5341780830882,123.419191478542));
#122390=CARTESIAN_POINT('Ctrl Pts',(4.68893548139201,30.6220531464908,123.451661775286));
#122391=CARTESIAN_POINT('Ctrl Pts',(4.70025454787673,30.7636319255206,123.517984655344));
#122392=CARTESIAN_POINT('Ctrl Pts',(4.70475321673696,30.8189768571155,123.547835589487));
#122393=CARTESIAN_POINT('Ctrl Pts',(4.71196768202377,30.9066809251967,123.601752936437));
#122394=CARTESIAN_POINT('Ctrl Pts',(4.71473828244273,30.9400863584744,123.623990093825));
#122395=CARTESIAN_POINT('Ctrl Pts',(4.71851538498551,30.9852148999651,123.656442491769));
#122396=CARTESIAN_POINT('Ctrl Pts',(4.71955955672165,30.9976448768381,123.665646259504));
#122397=CARTESIAN_POINT('Ctrl Pts',(4.72133349273079,31.018676842668,123.681677571086));
#122398=CARTESIAN_POINT('Ctrl Pts',(4.72206653833957,31.0273425919794,123.688419371514));
#122399=CARTESIAN_POINT('Ctrl Pts',(4.72354637324233,31.0447812465562,123.702265221575));
#122400=CARTESIAN_POINT('Ctrl Pts',(4.72429293120188,31.0535498676956,123.709373758527));
#122401=CARTESIAN_POINT('Ctrl Pts',(4.72615771856068,31.0753734365306,123.727436303128));
#122402=CARTESIAN_POINT('Ctrl Pts',(4.72727133702211,31.0883340213392,123.738502681865));
#122403=CARTESIAN_POINT('Ctrl Pts',(4.73154812285012,31.1377885901312,123.782058986931));
#122404=CARTESIAN_POINT('Ctrl Pts',(4.73465303227406,31.1730181807384,123.815950923078));
#122405=CARTESIAN_POINT('Ctrl Pts',(4.74606657253298,31.2987288526957,123.94801521169));
#122406=CARTESIAN_POINT('Ctrl Pts',(4.75399665507499,31.3787918609511,124.055384382602));
#122407=CARTESIAN_POINT('Ctrl Pts',(4.76430157832991,31.4609278659618,124.198596883284));
#122408=CARTESIAN_POINT('Ctrl Pts',(4.76629909704706,31.4758837534199,124.226485880613));
#122409=CARTESIAN_POINT('Ctrl Pts',(4.76967926044928,31.4993984699941,124.273502681005));
#122410=CARTESIAN_POINT('Ctrl Pts',(4.77104093140285,31.5084071619223,124.292397101091));
#122411=CARTESIAN_POINT('Ctrl Pts',(4.77298248210799,31.5205618972558,124.319177384393));
#122412=CARTESIAN_POINT('Ctrl Pts',(4.7735455967691,31.5240076767844,124.326926073336));
#122413=CARTESIAN_POINT('Ctrl Pts',(4.77451929883274,31.5298266163881,124.340285190678));
#122414=CARTESIAN_POINT('Ctrl Pts',(4.77492816469663,31.5322284201851,124.345882905679));
#122415=CARTESIAN_POINT('Ctrl Pts',(4.77579856550045,31.537252493166,124.357771674774));
#122416=CARTESIAN_POINT('Ctrl Pts',(4.77626051349565,31.5398668388154,124.364065597711));
#122417=CARTESIAN_POINT('Ctrl Pts',(4.7775406683905,31.5469708172924,124.381468785417));
#122418=CARTESIAN_POINT('Ctrl Pts',(4.77836340090532,31.5513792266664,124.392610464904));
#122419=CARTESIAN_POINT('Ctrl Pts',(4.7829834856537,31.5752859376067,124.454990159955));
#122420=CARTESIAN_POINT('Ctrl Pts',(4.78689460982024,31.5923642217666,124.507114158395));
#122421=CARTESIAN_POINT('Ctrl Pts',(4.80156358365905,31.6460146750772,124.703031503824));
#122422=CARTESIAN_POINT('Ctrl Pts',(4.81248206114835,31.6659177012127,124.850709225393));
#122423=CARTESIAN_POINT('Ctrl Pts',(4.82498053605921,31.6660171786085,125.030605074771));
#122424=CARTESIAN_POINT('Ctrl Pts',(4.82714466607129,31.6651397379159,125.062127259757));
#122425=CARTESIAN_POINT('Ctrl Pts',(4.83022912265091,31.6625822283161,125.107573197646));
#122426=CARTESIAN_POINT('Ctrl Pts',(4.83117147356669,31.6616204221105,125.121528812696));
#122427=CARTESIAN_POINT('Ctrl Pts',(4.83283001099022,31.6596067401981,125.146210726491));
#122428=CARTESIAN_POINT('Ctrl Pts',(4.83354838862347,31.6586263492754,125.156941873076));
#122429=CARTESIAN_POINT('Ctrl Pts',(4.83504072795697,31.6563633201379,125.179314526542));
#122430=CARTESIAN_POINT('Ctrl Pts',(4.83581405944858,31.6550619000457,125.190953571702));
#122431=CARTESIAN_POINT('Ctrl Pts',(4.83783592342047,31.651320493612,125.22149452715));
#122432=CARTESIAN_POINT('Ctrl Pts',(4.83907808604678,31.6486786702876,125.240370316004));
#122433=CARTESIAN_POINT('Ctrl Pts',(4.84549041615057,31.6332546043597,125.33830187556));
#122434=CARTESIAN_POINT('Ctrl Pts',(4.85048819649043,31.6151078641715,125.4164104943));
#122435=CARTESIAN_POINT('Ctrl Pts',(4.85720161207947,31.5828077818136,125.520692724916));
#122436=CARTESIAN_POINT('Ctrl Pts',(4.85897940275955,31.5734809202704,125.548232308875));
#122437=CARTESIAN_POINT('Ctrl Pts',(4.86075489241547,31.5634400172546,125.575509611081));
#122438=CARTESIAN_POINT('',(4.62852042921073,31.6642502403512,125.001193954075));
#122439=CARTESIAN_POINT('Ctrl Pts',(4.66781556978768,31.5660436956742,125.576468401513));
#122440=CARTESIAN_POINT('Ctrl Pts',(4.66777083826495,31.5662737940932,125.575843539819));
#122441=CARTESIAN_POINT('Ctrl Pts',(4.65467245807264,31.633531411034,125.392825945703));
#122442=CARTESIAN_POINT('Ctrl Pts',(4.64157407788033,31.6655315577241,125.196877806597));
#122443=CARTESIAN_POINT('Ctrl Pts',(4.62852042921073,31.6642502403512,125.001193954075));
#122444=CARTESIAN_POINT('Ctrl Pts',(4.62751359642243,31.665999527619,125.001254580872));
#122445=CARTESIAN_POINT('Ctrl Pts',(4.6239375376834,31.6660375432059,124.950772422952));
#122446=CARTESIAN_POINT('Ctrl Pts',(4.620419739526,31.6637810501156,124.900309733779));
#122447=CARTESIAN_POINT('Ctrl Pts',(4.61604551457903,31.6580148301263,124.836516989429));
#122448=CARTESIAN_POINT('Ctrl Pts',(4.61512459863438,31.6566292630902,124.823027190808));
#122449=CARTESIAN_POINT('Ctrl Pts',(4.61350374798853,31.6538856469017,124.799183494231));
#122450=CARTESIAN_POINT('Ctrl Pts',(4.61280175823768,31.6525946846149,124.788822778187));
#122451=CARTESIAN_POINT('Ctrl Pts',(4.61141209549366,31.649834377863,124.768247992353));
#122452=CARTESIAN_POINT('Ctrl Pts',(4.61072438195141,31.6483673655148,124.75803408511));
#122453=CARTESIAN_POINT('Ctrl Pts',(4.60926074568572,31.6450289347522,124.736231970565));
#122454=CARTESIAN_POINT('Ctrl Pts',(4.60848573929539,31.6431297425108,124.724648532455));
#122455=CARTESIAN_POINT('Ctrl Pts',(4.6064534220572,31.6378027646385,124.69417897145));
#122456=CARTESIAN_POINT('Ctrl Pts',(4.60520260852067,31.634170687524,124.675329996917));
#122457=CARTESIAN_POINT('Ctrl Pts',(4.59880830461285,31.6137859097119,124.578572727055));
#122458=CARTESIAN_POINT('Ctrl Pts',(4.59383502211434,31.5917841448493,124.501872042224));
#122459=CARTESIAN_POINT('Ctrl Pts',(4.58254820986431,31.5286644162865,124.329536060907));
#122460=CARTESIAN_POINT('Ctrl Pts',(4.57631401501912,31.4839215685967,124.235597580406));
#122461=CARTESIAN_POINT('Ctrl Pts',(4.56803212861921,31.4162381294626,124.122147074781));
#122462=CARTESIAN_POINT('Ctrl Pts',(4.56623883557412,31.4011295787923,124.098228454284));
#122463=CARTESIAN_POINT('Ctrl Pts',(4.56317070923784,31.3746972486314,124.058651902695));
#122464=CARTESIAN_POINT('Ctrl Pts',(4.56191221176865,31.3636963750407,124.042784828558));
#122465=CARTESIAN_POINT('Ctrl Pts',(4.56009365910278,31.3476247189508,124.020443402823));
#122466=CARTESIAN_POINT('Ctrl Pts',(4.55954766011369,31.3427774369491,124.013809218244));
#122467=CARTESIAN_POINT('Ctrl Pts',(4.55859360586352,31.3342742505681,124.002350329422));
#122468=CARTESIAN_POINT('Ctrl Pts',(4.55818708042727,31.3306408025923,123.997509254872));
#122469=CARTESIAN_POINT('Ctrl Pts',(4.55730981695369,31.322779588904,123.987153297438));
#122470=CARTESIAN_POINT('Ctrl Pts',(4.55683855348448,31.3185437440771,123.981645113792));
#122471=CARTESIAN_POINT('Ctrl Pts',(4.55552855219161,31.3067304602129,123.966480689454));
#122472=CARTESIAN_POINT('Ctrl Pts',(4.55468506958303,31.2990807494605,123.956881672482));
#122473=CARTESIAN_POINT('Ctrl Pts',(4.54879413520227,31.2453107467731,123.890918802521));
#122474=CARTESIAN_POINT('Ctrl Pts',(4.54354650317086,31.1956484151725,123.83755323724));
#122475=CARTESIAN_POINT('Ctrl Pts',(4.53721259282661,31.1321971526107,123.777751100028));
#122476=CARTESIAN_POINT('Ctrl Pts',(4.53616650612087,31.1216057700827,123.768024651911));
#122477=CARTESIAN_POINT('Ctrl Pts',(4.52975899118879,31.0559976953666,123.709321774576));
#122478=CARTESIAN_POINT('Ctrl Pts',(4.52439743288553,30.9979052861488,123.663898298047));
#122479=CARTESIAN_POINT('Ctrl Pts',(4.51609773864597,30.901750659307,123.598494185376));
#122480=CARTESIAN_POINT('Ctrl Pts',(4.51309225307635,30.8655977837028,123.575881401399));
#122481=CARTESIAN_POINT('Ctrl Pts',(4.50800505152788,30.8020142829812,123.539428454368));
#122482=CARTESIAN_POINT('Ctrl Pts',(4.50590169074892,30.774996552601,123.524914677643));
#122483=CARTESIAN_POINT('Ctrl Pts',(4.50287679986803,30.7350909498831,123.504876936965));
#122484=CARTESIAN_POINT('Ctrl Pts',(4.5019347243888,30.7225110323898,123.498757345723));
#122485=CARTESIAN_POINT('Ctrl Pts',(4.50027907880937,30.7001388763902,123.488220617423));
#122486=CARTESIAN_POINT('Ctrl Pts',(4.49956329541892,30.6903783494703,123.483738448787));
#122487=CARTESIAN_POINT('Ctrl Pts',(4.49806662613094,30.6697873561553,123.474522835288));
#122488=CARTESIAN_POINT('Ctrl Pts',(4.4972864632009,30.6589484537709,123.469809609913));
#122489=CARTESIAN_POINT('Ctrl Pts',(4.49522431741981,30.6300261086534,123.457597227897));
#122490=CARTESIAN_POINT('Ctrl Pts',(4.49394919106735,30.6118587484649,123.450300631313));
#122491=CARTESIAN_POINT('Ctrl Pts',(4.48734481868632,30.5163742815439,123.413892008877));
#122492=CARTESIAN_POINT('Ctrl Pts',(4.48219918854202,30.4370949166804,123.39023868696));
#122493=CARTESIAN_POINT('Ctrl Pts',(4.47097106952106,30.258514571176,123.351132824828));
#122494=CARTESIAN_POINT('Ctrl Pts',(4.4649470365792,30.1589230178527,123.33857474555));
#122495=CARTESIAN_POINT('Ctrl Pts',(4.45689427352911,30.0305533785609,123.334040178307));
#122496=CARTESIAN_POINT('Ctrl Pts',(4.4551015863614,30.0022738875131,123.333761636019));
#122497=CARTESIAN_POINT('Ctrl Pts',(4.45203439201522,29.9547028075906,123.334504055862));
#122498=CARTESIAN_POINT('Ctrl Pts',(4.45077620774895,29.9354106359493,123.335140633047));
#122499=CARTESIAN_POINT('Ctrl Pts',(4.44895802935054,29.9079296833214,123.336525758087));
#122500=CARTESIAN_POINT('Ctrl Pts',(4.44841208355267,29.8997278445778,123.337000004639));
#122501=CARTESIAN_POINT('Ctrl Pts',(4.44745808927257,29.8854898336433,123.337928984224));
#122502=CARTESIAN_POINT('Ctrl Pts',(4.44705157001777,29.8794520882996,123.338355982972));
#122503=CARTESIAN_POINT('Ctrl Pts',(4.44617428064305,29.8664875990031,123.339343886004));
#122504=CARTESIAN_POINT('Ctrl Pts',(4.44570298471046,29.8595621020924,123.339915218249));
#122505=CARTESIAN_POINT('Ctrl Pts',(4.44439280730621,29.8404121811999,123.341615714017));
#122506=CARTESIAN_POINT('Ctrl Pts',(4.44354917907181,29.8281966399155,123.342836672123));
#122507=CARTESIAN_POINT('Ctrl Pts',(4.43762089560038,29.7430796205433,123.352295415229));
#122508=CARTESIAN_POINT('Ctrl Pts',(4.4323331117368,29.6707856942883,123.365205200804));
#122509=CARTESIAN_POINT('Ctrl Pts',(4.42598595763153,29.5859824652277,123.386202646103));
#122510=CARTESIAN_POINT('Ctrl Pts',(4.42496634626789,29.5724214434115,123.389742569395));
#122511=CARTESIAN_POINT('Ctrl Pts',(4.41858107174438,29.4878220241583,123.412970171694));
#122512=CARTESIAN_POINT('Ctrl Pts',(4.41321560691376,29.4181065104412,123.437184836468));
#122513=CARTESIAN_POINT('Ctrl Pts',(4.40492223001949,29.3110938963762,123.482511957329));
#122514=CARTESIAN_POINT('Ctrl Pts',(4.40192639044384,29.2726128410122,123.500576776877));
#122515=CARTESIAN_POINT('Ctrl Pts',(4.39685351405384,29.2076862771862,123.534144996522));
#122516=CARTESIAN_POINT('Ctrl Pts',(4.39475499754981,29.1809013668893,123.548941913927));
#122517=CARTESIAN_POINT('Ctrl Pts',(4.39173567369348,29.142494529767,123.571561793016));
#122518=CARTESIAN_POINT('Ctrl Pts',(4.39079442763599,29.1305409147393,123.578806043363));
#122519=CARTESIAN_POINT('Ctrl Pts',(4.38913971748014,29.1095666750761,123.591880754784));
#122520=CARTESIAN_POINT('Ctrl Pts',(4.38842404854045,29.1005087538223,123.597649536594));
#122521=CARTESIAN_POINT('Ctrl Pts',(4.38692710910026,29.0815952054365,123.609953793155));
#122522=CARTESIAN_POINT('Ctrl Pts',(4.38614656647374,29.0717520764694,123.616507452699));
#122523=CARTESIAN_POINT('Ctrl Pts',(4.38408222494615,29.0457781071075,123.63420320327));
#122524=CARTESIAN_POINT('Ctrl Pts',(4.38280530928595,29.0297724322667,123.64552636413));
#122525=CARTESIAN_POINT('Ctrl Pts',(4.37620255613942,28.9474190767965,123.705996018596));
#122526=CARTESIAN_POINT('Ctrl Pts',(4.37106002826708,28.8845886462763,123.75974482309));
#122527=CARTESIAN_POINT('Ctrl Pts',(4.35983516673441,28.7549170786552,123.888532289982));
#122528=CARTESIAN_POINT('Ctrl Pts',(4.35381136163362,28.6903545612229,123.965389719219));
#122529=CARTESIAN_POINT('Ctrl Pts',(4.34575887258919,28.6169245027203,124.070775712212));
#122530=CARTESIAN_POINT('Ctrl Pts',(4.34396621592166,28.6013530076224,124.094383072906));
#122531=CARTESIAN_POINT('Ctrl Pts',(4.34089906849349,28.5761763226775,124.134751653046));
#122532=CARTESIAN_POINT('Ctrl Pts',(4.33964089999516,28.5662478922055,124.151304894849));
#122533=CARTESIAN_POINT('Ctrl Pts',(4.33782274043886,28.5525070632302,124.17514383433));
#122534=CARTESIAN_POINT('Ctrl Pts',(4.33727679731929,28.5484571370885,124.18229173529));
#122535=CARTESIAN_POINT('Ctrl Pts',(4.33632280605877,28.5415154515645,124.194757513792));
#122536=CARTESIAN_POINT('Ctrl Pts',(4.33591628711518,28.5385995386652,124.200061671198));
#122537=CARTESIAN_POINT('Ctrl Pts',(4.33503899643536,28.5323980381598,124.211489523151));
#122538=CARTESIAN_POINT('Ctrl Pts',(4.33456769886762,28.5291218881997,124.217617825919));
#122539=CARTESIAN_POINT('Ctrl Pts',(4.33325751259384,28.5201642622918,124.234628911002));
#122540=CARTESIAN_POINT('Ctrl Pts',(4.33241387702492,28.5145647264256,124.245554017583));
#122541=CARTESIAN_POINT('Ctrl Pts',(4.32648362199371,28.4763343381828,124.322220099976));
#122542=CARTESIAN_POINT('Ctrl Pts',(4.32119371768404,28.4479615462381,124.389986153815));
#122543=CARTESIAN_POINT('Ctrl Pts',(4.31484601842944,28.4196101608446,124.47262937442));
#122544=CARTESIAN_POINT('Ctrl Pts',(4.31382795901488,28.4152362960595,124.485922360479));
#122545=CARTESIAN_POINT('Ctrl Pts',(4.30744409686147,28.3888740511055,124.569577633223));
#122546=CARTESIAN_POINT('Ctrl Pts',(4.30207850537624,28.3714072476193,124.641283959141));
#122547=CARTESIAN_POINT('Ctrl Pts',(4.29378539742429,28.3514511564899,124.755770895924));
#122548=CARTESIAN_POINT('Ctrl Pts',(4.29078993197952,28.3457586356449,124.797893209285));
#122549=CARTESIAN_POINT('Ctrl Pts',(4.28571761137024,28.3387481885042,124.870639335085));
#122550=CARTESIAN_POINT('Ctrl Pts',(4.28361928290735,28.3366528773597,124.901165159404));
#122551=CARTESIAN_POINT('Ctrl Pts',(4.28060017518036,28.3348265654864,124.945697489825));
#122552=CARTESIAN_POINT('Ctrl Pts',(4.27965896134667,28.3344296038693,124.95966879837));
#122553=CARTESIAN_POINT('Ctrl Pts',(4.27800428752195,28.3340386086976,124.984380899615));
#122554=CARTESIAN_POINT('Ctrl Pts',(4.27728862301793,28.3339725379405,124.995119574565));
#122555=CARTESIAN_POINT('Ctrl Pts',(4.27579167302631,28.3340518817492,125.017683230656));
#122556=CARTESIAN_POINT('Ctrl Pts',(4.27501111560342,28.334219358815,125.029507574273));
#122557=CARTESIAN_POINT('Ctrl Pts',(4.27294668851087,28.3349990703969,125.060928303955));
#122558=CARTESIAN_POINT('Ctrl Pts',(4.27166970312514,28.3358313485668,125.080517737309));
#122559=CARTESIAN_POINT('Ctrl Pts',(4.26506454224581,28.34197166826,125.182540285609));
#122560=CARTESIAN_POINT('Ctrl Pts',(4.25991985433236,28.3530592852464,125.264514039844));
#122561=CARTESIAN_POINT('Ctrl Pts',(4.24869484790847,28.3909433744583,125.443308460205));
#122562=CARTESIAN_POINT('Ctrl Pts',(4.24267286268373,28.4204927891004,125.539203341651));
#122563=CARTESIAN_POINT('Ctrl Pts',(4.23462256229896,28.4691942727592,125.658019154722));
#122564=CARTESIAN_POINT('Ctrl Pts',(4.23283014930831,28.4805810417531,125.683901478033));
#122565=CARTESIAN_POINT('Ctrl Pts',(4.22976337672776,28.5008391903916,125.726942471238));
#122566=CARTESIAN_POINT('Ctrl Pts',(4.22850533420944,28.5093606480927,125.744259856653));
#122567=CARTESIAN_POINT('Ctrl Pts',(4.22668732519725,28.5219352283501,125.768731436477));
#122568=CARTESIAN_POINT('Ctrl Pts',(4.22614140347588,28.5257438126068,125.776010423612));
#122569=CARTESIAN_POINT('Ctrl Pts',(4.22518743633911,28.5324517720066,125.788603092583));
#122570=CARTESIAN_POINT('Ctrl Pts',(4.22478091988075,28.5353265241769,125.793929623452));
#122571=CARTESIAN_POINT('Ctrl Pts',(4.22390361877397,28.541564168575,125.805337953106));
#122572=CARTESIAN_POINT('Ctrl Pts',(4.22343230814111,28.544936053455,125.811414320898));
#122573=CARTESIAN_POINT('Ctrl Pts',(4.22212205098766,28.5543700339596,125.828167094421));
#122574=CARTESIAN_POINT('Ctrl Pts',(4.22127835680807,28.5605121433436,125.838797605755));
#122575=CARTESIAN_POINT('Ctrl Pts',(4.21533221368887,28.6043050045739,125.912694757357));
#122576=CARTESIAN_POINT('Ctrl Pts',(4.21002521897172,28.6459921360164,125.973466251084));
#122577=CARTESIAN_POINT('Ctrl Pts',(4.19736356040869,28.7538672361296,126.110334323629));
#122578=CARTESIAN_POINT('Ctrl Pts',(4.19000833253669,28.8232231628061,126.183591601516));
#122579=CARTESIAN_POINT('Ctrl Pts',(4.17914469474326,28.9383328515318,126.284989557615));
#122580=CARTESIAN_POINT('Ctrl Pts',(4.17547523752923,28.979527497469,126.317942415896));
#122581=CARTESIAN_POINT('Ctrl Pts',(4.17072495952773,29.035969628908,126.358856077292));
#122582=CARTESIAN_POINT('Ctrl Pts',(4.1695758183336,29.0498714072905,126.368612468738));
#122583=CARTESIAN_POINT('Ctrl Pts',(4.16767733256486,29.0732457618727,126.384488954336));
#122584=CARTESIAN_POINT('Ctrl Pts',(4.16692351974461,29.0826353721918,126.390728310275));
#122585=CARTESIAN_POINT('Ctrl Pts',(4.16545069464834,29.1011913482187,126.402788969361));
#122586=CARTESIAN_POINT('Ctrl Pts',(4.16473146085928,29.1103527058597,126.408616905545));
#122587=CARTESIAN_POINT('Ctrl Pts',(4.16315787876189,29.1306118786374,126.421228146816));
#122588=CARTESIAN_POINT('Ctrl Pts',(4.16230500461638,29.1417335416142,126.427971937081));
#122589=CARTESIAN_POINT('Ctrl Pts',(4.15936955957198,29.1804875647951,126.450854682549));
#122590=CARTESIAN_POINT('Ctrl Pts',(4.1573107349061,29.2085061529089,126.466327945709));
#122591=CARTESIAN_POINT('Ctrl Pts',(4.14726467295489,29.3489411795435,126.538684028992));
#122592=CARTESIAN_POINT('Ctrl Pts',(4.13969282258815,29.4671084462327,126.58349440859));
#122593=CARTESIAN_POINT('Ctrl Pts',(4.12880290138125,29.6390212026807,126.627234737882));
#122594=CARTESIAN_POINT('Ctrl Pts',(4.12562065060112,29.6893966584587,126.637596840689));
#122595=CARTESIAN_POINT('Ctrl Pts',(4.1205050544084,29.7688813713826,126.650147046079));
#122596=CARTESIAN_POINT('Ctrl Pts',(4.11863048822673,29.7977078628706,126.653928276468));
#122597=CARTESIAN_POINT('Ctrl Pts',(4.1160877883894,29.836145151061,126.657950355198));
#122598=CARTESIAN_POINT('Ctrl Pts',(4.11545338462258,29.8456820735412,126.658865202054));
#122599=CARTESIAN_POINT('Ctrl Pts',(4.11439484146624,29.8614955879011,126.660244600571));
#122600=CARTESIAN_POINT('Ctrl Pts',(4.11397324615907,29.8677680493433,126.660755946739));
#122601=CARTESIAN_POINT('Ctrl Pts',(4.1131168247805,29.8804540146102,126.661717813797));
#122602=CARTESIAN_POINT('Ctrl Pts',(4.11268192929386,29.886867491127,126.66216676877));
#122603=CARTESIAN_POINT('Ctrl Pts',(4.11155095500766,29.9034767576726,126.663232875771));
#122604=CARTESIAN_POINT('Ctrl Pts',(4.11085188987724,29.9136757323124,126.663793389524));
#122605=CARTESIAN_POINT('Ctrl Pts',(4.10794864798838,29.9557818777473,126.665719270336));
#122606=CARTESIAN_POINT('Ctrl Pts',(4.10570606803766,29.9877178581445,126.666260713563));
#122607=CARTESIAN_POINT('Ctrl Pts',(4.09571356291661,30.1282417104813,126.664603405995));
#122608=CARTESIAN_POINT('Ctrl Pts',(4.08771134013885,30.2364484263436,126.652707605576));
#122609=CARTESIAN_POINT('Ctrl Pts',(4.07574525631691,30.3986852341966,126.618603031214));
#122610=CARTESIAN_POINT('Ctrl Pts',(4.07166659013704,30.4540049130392,126.603965808263));
#122611=CARTESIAN_POINT('Ctrl Pts',(4.06503337067012,30.54435346129,126.575009662619));
#122612=CARTESIAN_POINT('Ctrl Pts',(4.06243486137301,30.579841721536,126.562293218225));
#122613=CARTESIAN_POINT('Ctrl Pts',(4.05884924057299,30.6289180251403,126.542804771297));
#122614=CARTESIAN_POINT('Ctrl Pts',(4.05782933492302,30.6428891846669,126.537035447567));
#122615=CARTESIAN_POINT('Ctrl Pts',(4.05608405283442,30.6668100182096,126.526774215611));
#122616=CARTESIAN_POINT('Ctrl Pts',(4.05535565411528,30.6767974115517,126.522373272007));
#122617=CARTESIAN_POINT('Ctrl Pts',(4.05396423560397,30.6958793388433,126.51373992092));
#122618=CARTESIAN_POINT('Ctrl Pts',(4.05330072757054,30.7049802722395,126.509522913247));
#122619=CARTESIAN_POINT('Ctrl Pts',(4.05156368060672,30.7288052574025,126.498220901817));
#122620=CARTESIAN_POINT('Ctrl Pts',(4.05049483779986,30.7434643651665,126.491000919728));
#122621=CARTESIAN_POINT('Ctrl Pts',(4.04663050152185,30.796422525431,126.463942406264));
#122622=CARTESIAN_POINT('Ctrl Pts',(4.0438792239805,30.8340554032095,126.442833420357));
#122623=CARTESIAN_POINT('Ctrl Pts',(4.03394950825957,30.9686536103306,126.360306350369));
#122624=CARTESIAN_POINT('Ctrl Pts',(4.02705426726375,31.0600178031161,126.290382153097));
#122625=CARTESIAN_POINT('Ctrl Pts',(4.01702518417021,31.1786245043795,126.178446666427));
#122626=CARTESIAN_POINT('Ctrl Pts',(4.01402524486027,31.212314042209,126.143759715701));
#122627=CARTESIAN_POINT('Ctrl Pts',(4.0091694058192,31.2630259181156,126.086785401346));
#122628=CARTESIAN_POINT('Ctrl Pts',(4.00736531167835,31.2810766905238,126.065447921962));
#122629=CARTESIAN_POINT('Ctrl Pts',(4.00490442570335,31.3044991452293,126.036304600822));
#122630=CARTESIAN_POINT('Ctrl Pts',(4.00427868555851,31.3103543137012,126.028891057287));
#122631=CARTESIAN_POINT('Ctrl Pts',(4.00323067058586,31.3199874785417,126.016478389267));
#122632=CARTESIAN_POINT('Ctrl Pts',(4.00281083489726,31.3238009989842,126.011506881978));
#122633=CARTESIAN_POINT('Ctrl Pts',(4.00195375515965,31.3314916654427,126.001362936387));
#122634=CARTESIAN_POINT('Ctrl Pts',(4.00151640593082,31.3353668986533,125.996189253052));
#122635=CARTESIAN_POINT('Ctrl Pts',(4.00037190791011,31.3453831017511,125.982653522468));
#122636=CARTESIAN_POINT('Ctrl Pts',(3.99966164302565,31.3514761307239,125.974256583269));
#122637=CARTESIAN_POINT('Ctrl Pts',(3.99664635284777,31.3768441487848,125.938600435456));
#122638=CARTESIAN_POINT('Ctrl Pts',(3.99429928234992,31.3953746043831,125.910823774527));
#122639=CARTESIAN_POINT('Ctrl Pts',(3.98424972008916,31.4701434628719,125.791105649042));
#122640=CARTESIAN_POINT('Ctrl Pts',(3.97631017450905,31.5182255724779,125.694378192039));
#122641=CARTESIAN_POINT('Ctrl Pts',(3.96806744683423,31.5589348157813,125.587639434157));
#122642=CARTESIAN_POINT('Ctrl Pts',(3.9676011994398,31.5612051496513,125.581580893384));
#122643=CARTESIAN_POINT('Ctrl Pts',(3.96713561979274,31.5634400104587,125.575509629543));
#122644=CARTESIAN_POINT('Origin',(5.,30.,125.));
#122645=CARTESIAN_POINT('',(3.26654942290125,31.5634400114153,125.575509626944));
#122646=CARTESIAN_POINT('',(3.46014891354655,31.5634400625338,125.575509488075));
#122647=CARTESIAN_POINT('',(5.,31.5634400119422,125.575509625513));
#122648=CARTESIAN_POINT('',(4.12030994055874,31.6659997586642,124.99910326656));
#122649=CARTESIAN_POINT('Ctrl Pts',(3.46014891354656,31.5634400625339,125.575509488075));
#122650=CARTESIAN_POINT('Ctrl Pts',(3.46532993227505,31.5387713160517,125.642525075727));
#122651=CARTESIAN_POINT('Ctrl Pts',(3.47055309778454,31.509808822216,125.707913585587));
#122652=CARTESIAN_POINT('Ctrl Pts',(3.4816738125574,31.4384123201443,125.844614441927));
#122653=CARTESIAN_POINT('Ctrl Pts',(3.48752710731656,31.3946875940775,125.915015733321));
#122654=CARTESIAN_POINT('Ctrl Pts',(3.49453391055907,31.3343448909579,125.997729618313));
#122655=CARTESIAN_POINT('Ctrl Pts',(3.495865483649,31.3225061918041,126.013369680307));
#122656=CARTESIAN_POINT('Ctrl Pts',(3.49798286544945,31.3030888557521,126.038101806722));
#122657=CARTESIAN_POINT('Ctrl Pts',(3.49877545673878,31.2956850527535,126.047328116527));
#122658=CARTESIAN_POINT('Ctrl Pts',(3.5002802726476,31.2813717111757,126.06478069199));
#122659=CARTESIAN_POINT('Ctrl Pts',(3.50099314913645,31.2744796800137,126.073020474495));
#122660=CARTESIAN_POINT('Ctrl Pts',(3.50262639530776,31.2584357699984,126.091829128911));
#122661=CARTESIAN_POINT('Ctrl Pts',(3.50354447539312,31.2492295085491,126.10235071037));
#122662=CARTESIAN_POINT('Ctrl Pts',(3.50645503601106,31.2194553085823,126.135526717517));
#122663=CARTESIAN_POINT('Ctrl Pts',(3.50842686414188,31.1983945853018,126.157731740102));
#122664=CARTESIAN_POINT('Ctrl Pts',(3.51308439602941,31.1466498608286,126.209361854017));
#122665=CARTESIAN_POINT('Ctrl Pts',(3.51574754502253,31.1154277634125,126.238217784413));
#122666=CARTESIAN_POINT('Ctrl Pts',(3.52295255650722,31.0271259394368,126.313773952552));
#122667=CARTESIAN_POINT('Ctrl Pts',(3.52742681479081,30.9679971312345,126.357929163602));
#122668=CARTESIAN_POINT('Ctrl Pts',(3.53278268226031,30.8945315865238,126.405546353547));
#122669=CARTESIAN_POINT('Ctrl Pts',(3.53363002501478,30.8828317117301,126.412924440375));
#122670=CARTESIAN_POINT('Ctrl Pts',(3.53899663482922,30.808354329522,126.458604554307));
#122671=CARTESIAN_POINT('Ctrl Pts',(3.54356836259951,30.7431978780145,126.492855701118));
#122672=CARTESIAN_POINT('Ctrl Pts',(3.54917288014986,30.6647788454937,126.527670079088));
#122673=CARTESIAN_POINT('Ctrl Pts',(3.54998128513186,30.6535013926619,126.532528202669));
#122674=CARTESIAN_POINT('Ctrl Pts',(3.55125855096193,30.6357577579263,126.539940385371));
#122675=CARTESIAN_POINT('Ctrl Pts',(3.55172253435364,30.6293272740659,126.5425794939));
#122676=CARTESIAN_POINT('Ctrl Pts',(3.55259527688928,30.6172645634356,126.547442122969));
#122677=CARTESIAN_POINT('Ctrl Pts',(3.55300346162404,30.6116364871698,126.549675278273));
#122678=CARTESIAN_POINT('Ctrl Pts',(3.55397000765372,30.5983403860437,126.554867304849));
#122679=CARTESIAN_POINT('Ctrl Pts',(3.55452985526582,30.5906625008217,126.557800165715));
#122680=CARTESIAN_POINT('Ctrl Pts',(3.55641549582653,30.5648706121503,126.567434277971));
#122681=CARTESIAN_POINT('Ctrl Pts',(3.55775485205199,30.546662582218,126.573877049177));
#122682=CARTESIAN_POINT('Ctrl Pts',(3.5610894029587,30.5015094841628,126.588976107234));
#122683=CARTESIAN_POINT('Ctrl Pts',(3.56309920241594,30.4744484490152,126.597264949989));
#122684=CARTESIAN_POINT('Ctrl Pts',(3.57231599801876,30.3505417418867,126.631791306795));
#122685=CARTESIAN_POINT('Ctrl Pts',(3.57969564638525,30.251657931563,126.649936707753));
#122686=CARTESIAN_POINT('Ctrl Pts',(3.59286785922977,30.0697154667537,126.66657741103));
#122687=CARTESIAN_POINT('Ctrl Pts',(3.59869313671815,29.9872364316415,126.667987192966));
#122688=CARTESIAN_POINT('Ctrl Pts',(3.60567288238736,29.8854103400715,126.662170098247));
#122689=CARTESIAN_POINT('Ctrl Pts',(3.60700365228553,29.8658611389089,126.660706791867));
#122690=CARTESIAN_POINT('Ctrl Pts',(3.60912007096686,29.8345653586577,126.657807964873));
#122691=CARTESIAN_POINT('Ctrl Pts',(3.60991249137689,29.8228008428132,126.656591784396));
#122692=CARTESIAN_POINT('Ctrl Pts',(3.61141717506324,29.8003769871737,126.654032058479));
#122693=CARTESIAN_POINT('Ctrl Pts',(3.61213008819787,29.7897157933807,126.652710488679));
#122694=CARTESIAN_POINT('Ctrl Pts',(3.61376368925664,29.7652067307976,126.649431323938));
#122695=CARTESIAN_POINT('Ctrl Pts',(3.61468208409774,29.7513691139675,126.647402280536));
#122696=CARTESIAN_POINT('Ctrl Pts',(3.61759477978564,29.7073154311185,126.640374850524));
#122697=CARTESIAN_POINT('Ctrl Pts',(3.61956838406271,29.677209916018,126.634717302033));
#122698=CARTESIAN_POINT('Ctrl Pts',(3.62423101543838,29.6056894296176,126.619223816489));
#122699=CARTESIAN_POINT('Ctrl Pts',(3.62689741741674,29.5644614683956,126.608624618168));
#122700=CARTESIAN_POINT('Ctrl Pts',(3.63410406699923,29.4530666415299,126.575388956479));
#122701=CARTESIAN_POINT('Ctrl Pts',(3.63857692575548,29.3839251354062,126.549657570839));
#122702=CARTESIAN_POINT('Ctrl Pts',(3.64394458484375,29.3039050115591,126.513672694208));
#122703=CARTESIAN_POINT('Ctrl Pts',(3.64480503283153,29.29116920407,126.507750693825));
#122704=CARTESIAN_POINT('Ctrl Pts',(3.65016777860263,29.2124822883973,126.46994485749));
#122705=CARTESIAN_POINT('Ctrl Pts',(3.65472265125325,29.1486268732331,126.433904849781));
#122706=CARTESIAN_POINT('Ctrl Pts',(3.66030845763685,29.077086115248,126.387060459703));
#122707=CARTESIAN_POINT('Ctrl Pts',(3.66111679336123,29.0668890189016,126.380221226011));
#122708=CARTESIAN_POINT('Ctrl Pts',(3.66239397329506,29.0510393125109,126.369334848572));
#122709=CARTESIAN_POINT('Ctrl Pts',(3.66285794110926,29.0453346216952,126.365363806831));
#122710=CARTESIAN_POINT('Ctrl Pts',(3.66373067186867,29.0347070952065,126.357866810042));
#122711=CARTESIAN_POINT('Ctrl Pts',(3.66413886060442,29.0297784180783,126.354349564606));
#122712=CARTESIAN_POINT('Ctrl Pts',(3.66510543994742,29.0182046644932,126.345994606016));
#122713=CARTESIAN_POINT('Ctrl Pts',(3.66566531718262,29.0115760959378,126.341134497));
#122714=CARTESIAN_POINT('Ctrl Pts',(3.66755116427151,28.9894911088743,126.324688983783));
#122715=CARTESIAN_POINT('Ctrl Pts',(3.66889070129161,28.9742009045673,126.31288432814));
#122716=CARTESIAN_POINT('Ctrl Pts',(3.67222580326294,28.9370202963898,126.283133380777));
#122717=CARTESIAN_POINT('Ctrl Pts',(3.67423597875879,28.9153758147292,126.26489023989));
#122718=CARTESIAN_POINT('Ctrl Pts',(3.68345612018844,28.8191331113837,126.179484622085));
#122719=CARTESIAN_POINT('Ctrl Pts',(3.69083882984096,28.7502330208457,126.106215872603));
#122720=CARTESIAN_POINT('Ctrl Pts',(3.70401035403832,28.6375898934945,125.962378044533));
#122721=CARTESIAN_POINT('Ctrl Pts',(3.7098321947585,28.5917012227628,125.89388534971));
#122722=CARTESIAN_POINT('Ctrl Pts',(3.7168086183357,28.5413858916655,125.805223603519));
#122723=CARTESIAN_POINT('Ctrl Pts',(3.71813928732583,28.5320132527416,125.78800706564));
#122724=CARTESIAN_POINT('Ctrl Pts',(3.72025558500587,28.5174758573163,125.760143425944));
#122725=CARTESIAN_POINT('Ctrl Pts',(3.72104798394689,28.5121171345539,125.749600195332));
#122726=CARTESIAN_POINT('Ctrl Pts',(3.72255265103414,28.5021059162805,125.729372821938));
#122727=CARTESIAN_POINT('Ctrl Pts',(3.7232655687861,28.4974339597639,125.719699036662));
#122728=CARTESIAN_POINT('Ctrl Pts',(3.72489921449837,28.4868958394483,125.69732875195));
#122729=CARTESIAN_POINT('Ctrl Pts',(3.72581764893689,28.4810952757181,125.684602108737));
#122730=CARTESIAN_POINT('Ctrl Pts',(3.72873061330856,28.4631046304957,125.643775386516));
#122731=CARTESIAN_POINT('Ctrl Pts',(3.73070444111024,28.4515284653459,125.61541061114));
#122732=CARTESIAN_POINT('Ctrl Pts',(3.73536771438811,28.4257520729958,125.546910081464));
#122733=CARTESIAN_POINT('Ctrl Pts',(3.73803452587861,28.4122948323951,125.506517378453));
#122734=CARTESIAN_POINT('Ctrl Pts',(3.74524136944499,28.3798023548413,125.3948995031));
#122735=CARTESIAN_POINT('Ctrl Pts',(3.74971404031728,28.3639225551281,125.322857528649));
#122736=CARTESIAN_POINT('Ctrl Pts',(3.75508289834654,28.3507534828001,125.236092806036));
#122737=CARTESIAN_POINT('Ctrl Pts',(3.75594472221589,28.3488187977033,125.222158768837));
#122738=CARTESIAN_POINT('Ctrl Pts',(3.76130698328557,28.3379101990462,125.135554180075));
#122739=CARTESIAN_POINT('Ctrl Pts',(3.76586000758779,28.3335600490799,125.062390897778));
#122740=CARTESIAN_POINT('Ctrl Pts',(3.77144376247034,28.3341147525847,124.976911105354));
#122741=CARTESIAN_POINT('Ctrl Pts',(3.7722520905171,28.3343301531606,124.964634845102));
#122742=CARTESIAN_POINT('Ctrl Pts',(3.77352926092877,28.3348799605726,124.945414582176));
#122743=CARTESIAN_POINT('Ctrl Pts',(3.77399322701611,28.3351221863597,124.938468099218));
#122744=CARTESIAN_POINT('Ctrl Pts',(3.77486595647011,28.3356567519304,124.925473370286));
#122745=CARTESIAN_POINT('Ctrl Pts',(3.77527414564945,28.3359386065939,124.919424940444));
#122746=CARTESIAN_POINT('Ctrl Pts',(3.77624072868633,28.3366807875664,124.905169843559));
#122747=CARTESIAN_POINT('Ctrl Pts',(3.77680060920601,28.3371688835396,124.896964898848));
#122748=CARTESIAN_POINT('Ctrl Pts',(3.77868647919485,28.3390073996597,124.869490554571));
#122749=CARTESIAN_POINT('Ctrl Pts',(3.78002603626177,28.3406321802209,124.850241885446));
#122750=CARTESIAN_POINT('Ctrl Pts',(3.78336119933753,28.3454619412868,124.802868146404));
#122751=CARTESIAN_POINT('Ctrl Pts',(3.7853714165309,28.3490497161394,124.774788688702));
#122752=CARTESIAN_POINT('Ctrl Pts',(3.79459192906553,28.3686051080659,124.647605052887));
#122753=CARTESIAN_POINT('Ctrl Pts',(3.80197497827345,28.392794106492,124.549976461569));
#122754=CARTESIAN_POINT('Ctrl Pts',(3.81514642615884,28.45254643723,124.377328806859));
#122755=CARTESIAN_POINT('Ctrl Pts',(3.82096788576526,28.4852000959407,124.30163271898));
#122756=CARTESIAN_POINT('Ctrl Pts',(3.82794394090392,28.5323970313496,124.211278446618));
#122757=CARTESIAN_POINT('Ctrl Pts',(3.82927459867152,28.5417779416629,124.194066598367));
#122758=CARTESIAN_POINT('Ctrl Pts',(3.83139088289436,28.55730274825,124.166741036276));
#122759=CARTESIAN_POINT('Ctrl Pts',(3.83218327944765,28.5632541818446,124.156520701303));
#122760=CARTESIAN_POINT('Ctrl Pts',(3.83368794468906,28.5748183448608,124.137139264152));
#122761=CARTESIAN_POINT('Ctrl Pts',(3.83440086295466,28.5804118183179,124.127967429931));
#122762=CARTESIAN_POINT('Ctrl Pts',(3.83603451363388,28.5934906165754,124.106980993908));
#122763=CARTESIAN_POINT('Ctrl Pts',(3.83695295247706,28.6010368469153,124.095205157524));
#122764=CARTESIAN_POINT('Ctrl Pts',(3.83986594673684,28.6255799431405,124.057947105179));
#122765=CARTESIAN_POINT('Ctrl Pts',(3.84183979940321,28.6431321746941,124.032837116693));
#122766=CARTESIAN_POINT('Ctrl Pts',(3.84650314408774,28.6867030122478,123.974028139143));
#122767=CARTESIAN_POINT('Ctrl Pts',(3.84917000113386,28.7133404892142,123.940814028766));
#122768=CARTESIAN_POINT('Ctrl Pts',(3.85637686611507,28.7894932661763,123.852978018775));
#122769=CARTESIAN_POINT('Ctrl Pts',(3.86084951592899,28.8414061106628,123.800564074202));
#122770=CARTESIAN_POINT('Ctrl Pts',(3.86621850363203,28.9071601815433,123.742440821587));
#122771=CARTESIAN_POINT('Ctrl Pts',(3.86708047701465,28.9178193495902,123.733256541473));
#122772=CARTESIAN_POINT('Ctrl Pts',(3.87244268419204,28.9846627937088,123.677121585994));
#122773=CARTESIAN_POINT('Ctrl Pts',(3.87699550642383,29.0437684540843,123.633787914116));
#122774=CARTESIAN_POINT('Ctrl Pts',(3.88257903703063,29.1158817054854,123.587894623055));
#122775=CARTESIAN_POINT('Ctrl Pts',(3.88338736423698,29.1263123411007,123.581417394997));
#122776=CARTESIAN_POINT('Ctrl Pts',(3.88466453360653,29.1427583035081,123.571454940404));
#122777=CARTESIAN_POINT('Ctrl Pts',(3.88512849950472,29.1487257185332,123.567890923554));
#122778=CARTESIAN_POINT('Ctrl Pts',(3.88600122881559,29.159933083632,123.561292162403));
#122779=CARTESIAN_POINT('Ctrl Pts',(3.88640941804338,29.1651675014516,123.558248509409));
#122780=CARTESIAN_POINT('Ctrl Pts',(3.88737600148491,29.1775463667203,123.551140592669));
#122781=CARTESIAN_POINT('Ctrl Pts',(3.88793588236415,29.1847044284616,123.547100593622));
#122782=CARTESIAN_POINT('Ctrl Pts',(3.88982175485984,29.2087839988527,123.533744096531));
#122783=CARTESIAN_POINT('Ctrl Pts',(3.89116131412128,29.225836894663,123.524669344952));
#122784=CARTESIAN_POINT('Ctrl Pts',(3.89449648388623,29.2682572102138,123.503033183881));
#122785=CARTESIAN_POINT('Ctrl Pts',(3.89650670564428,29.2937939239464,123.490818116928));
#122786=CARTESIAN_POINT('Ctrl Pts',(3.90572725880528,29.4112530985108,123.438267411568));
#122787=CARTESIAN_POINT('Ctrl Pts',(3.91311034518584,29.5063948676848,123.40563929982));
#122788=CARTESIAN_POINT('Ctrl Pts',(3.92628178471754,29.6838511777597,123.36220215769));
#122789=CARTESIAN_POINT('Ctrl Pts',(3.93210320260243,29.7651563746571,123.348581220137));
#122790=CARTESIAN_POINT('Ctrl Pts',(3.93907921740668,29.8666642736799,123.339228569082));
#122791=CARTESIAN_POINT('Ctrl Pts',(3.94040987394538,29.8862125483689,123.337774794306));
#122792=CARTESIAN_POINT('Ctrl Pts',(3.94252615669465,29.9175900194915,123.335997459179));
#122793=CARTESIAN_POINT('Ctrl Pts',(3.94331855298645,29.9294044081779,123.33545437562));
#122794=CARTESIAN_POINT('Ctrl Pts',(3.94482321802553,29.9519595816701,123.334658137847));
#122795=CARTESIAN_POINT('Ctrl Pts',(3.94553613634749,29.9626989391974,123.334382985283));
#122796=CARTESIAN_POINT('Ctrl Pts',(3.94716978757093,29.9874240372146,123.333988764662));
#122797=CARTESIAN_POINT('Ctrl Pts',(3.94808822689634,30.0014102421621,123.333941891143));
#122798=CARTESIAN_POINT('Ctrl Pts',(3.951001224429,30.0460236996587,123.334354187991));
#122799=CARTESIAN_POINT('Ctrl Pts',(3.95297507981826,30.0766394380173,123.33548183026));
#122800=CARTESIAN_POINT('Ctrl Pts',(3.95763843232247,30.1496788045913,123.340191727994));
#122801=CARTESIAN_POINT('Ctrl Pts',(3.96030529435738,30.1920307180263,123.344556908635));
#122802=CARTESIAN_POINT('Ctrl Pts',(3.96751216168179,30.3071281490144,123.360897113427));
#122803=CARTESIAN_POINT('Ctrl Pts',(3.97198480918777,30.3793190101193,123.376083923441));
#122804=CARTESIAN_POINT('Ctrl Pts',(3.98144491979491,30.5281976279092,123.417876441958));
#122805=CARTESIAN_POINT('Ctrl Pts',(3.98642787460068,30.6044209573295,123.445400420983));
#122806=CARTESIAN_POINT('Ctrl Pts',(3.99271757909824,30.6930702159501,123.484919131293));
#122807=CARTESIAN_POINT('Ctrl Pts',(3.9937733753815,30.7077110244348,123.491702475682));
#122808=CARTESIAN_POINT('Ctrl Pts',(3.99535524999535,30.7292482770566,123.502063667725));
#122809=CARTESIAN_POINT('Ctrl Pts',(3.99587201757454,30.7362224240439,123.50547905953));
#122810=CARTESIAN_POINT('Ctrl Pts',(3.99679417070097,30.7485526618185,123.511624693621));
#122811=CARTESIAN_POINT('Ctrl Pts',(3.99719835641313,30.753918223606,123.514335350732));
#122812=CARTESIAN_POINT('Ctrl Pts',(3.99809445022717,30.7657273082469,123.520381693954));
#122813=CARTESIAN_POINT('Ctrl Pts',(3.9985871263319,30.7721636812068,123.523730415327));
#122814=CARTESIAN_POINT('Ctrl Pts',(4.00004337210746,30.7910293853934,123.533703005599));
#122815=CARTESIAN_POINT('Ctrl Pts',(4.0010136195239,30.8033964762513,123.54044238429));
#122816=CARTESIAN_POINT('Ctrl Pts',(4.00788436451526,30.889662299283,123.588881006176));
#122817=CARTESIAN_POINT('Ctrl Pts',(4.01404389374448,30.9603591773377,123.636012044499));
#122818=CARTESIAN_POINT('Ctrl Pts',(4.0294834768799,31.1273731969797,123.766797102822));
#122819=CARTESIAN_POINT('Ctrl Pts',(4.03870273966068,31.21828908597,123.856521539238));
#122820=CARTESIAN_POINT('Ctrl Pts',(4.04891694059792,31.3113362887856,123.97218744119));
#122821=CARTESIAN_POINT('Ctrl Pts',(4.05035712062509,31.3242532299976,123.988884293505));
#122822=CARTESIAN_POINT('Ctrl Pts',(4.0526883412668,31.3448204354563,124.016540597177));
#122823=CARTESIAN_POINT('Ctrl Pts',(4.0535867346915,31.3526619775464,124.027354127569));
#122824=CARTESIAN_POINT('Ctrl Pts',(4.0551941741983,31.3665357289057,124.046978449541));
#122825=CARTESIAN_POINT('Ctrl Pts',(4.0559049892657,31.3726148137569,124.055755033809));
#122826=CARTESIAN_POINT('Ctrl Pts',(4.05742089899463,31.3854561162687,124.074680565043));
#122827=CARTESIAN_POINT('Ctrl Pts',(4.05822497791378,31.3921921430221,124.084846593739));
#122828=CARTESIAN_POINT('Ctrl Pts',(4.06042504878695,31.4104082186223,124.113005000897));
#122829=CARTESIAN_POINT('Ctrl Pts',(4.06181242502166,31.4216553553276,124.131145818043));
#122830=CARTESIAN_POINT('Ctrl Pts',(4.06801589487877,31.4707858618911,124.213899302527));
#122831=CARTESIAN_POINT('Ctrl Pts',(4.07268825199925,31.5046367602592,124.280809140658));
#122832=CARTESIAN_POINT('Ctrl Pts',(4.08218333822555,31.5648784907217,124.422919019021));
#122833=CARTESIAN_POINT('Ctrl Pts',(4.08698583571402,31.5906121945652,124.498183682773));
#122834=CARTESIAN_POINT('Ctrl Pts',(4.09532081336199,31.6250886016307,124.628858288635));
#122835=CARTESIAN_POINT('Ctrl Pts',(4.09880030409581,31.636587655521,124.683394880651));
#122836=CARTESIAN_POINT('Ctrl Pts',(4.10354695190264,31.648118216037,124.755916109427));
#122837=CARTESIAN_POINT('Ctrl Pts',(4.10470543907957,31.6506232793526,124.773475546927));
#122838=CARTESIAN_POINT('Ctrl Pts',(4.10639860834429,31.6538336108501,124.798872604941));
#122839=CARTESIAN_POINT('Ctrl Pts',(4.10692157933837,31.6547645315561,124.806681143307));
#122840=CARTESIAN_POINT('Ctrl Pts',(4.10785101762972,31.6563115799768,124.820488675419));
#122841=CARTESIAN_POINT('Ctrl Pts',(4.10825622073179,31.6569504706871,124.826484866271));
#122842=CARTESIAN_POINT('Ctrl Pts',(4.10904749108155,31.6581290706816,124.838147053464));
#122843=CARTESIAN_POINT('Ctrl Pts',(4.10943330429272,31.6586723014105,124.843812338997));
#122844=CARTESIAN_POINT('Ctrl Pts',(4.11030145769451,31.6598247453823,124.85651577955));
#122845=CARTESIAN_POINT('Ctrl Pts',(4.11078461615754,31.6604182365978,124.863555204913));
#122846=CARTESIAN_POINT('Ctrl Pts',(4.11237846316793,31.6622201424697,124.886683957907));
#122847=CARTESIAN_POINT('Ctrl Pts',(4.11349824869852,31.6632395571304,124.902786538608));
#122848=CARTESIAN_POINT('Ctrl Pts',(4.11649927525144,31.6653269690255,124.945616789931));
#122849=CARTESIAN_POINT('Ctrl Pts',(4.11839632409284,31.6659853632973,124.972358777486));
#122850=CARTESIAN_POINT('Ctrl Pts',(4.12030994055874,31.6659997586642,124.99910326656));
#122851=CARTESIAN_POINT('Ctrl Pts',(4.12030976540797,31.6659997573448,124.999100818672));
#122852=CARTESIAN_POINT('Ctrl Pts',(4.12690058450125,31.6660494727944,125.091213415329));
#122853=CARTESIAN_POINT('Ctrl Pts',(4.13366432505074,31.6584599294103,125.183173080206));
#122854=CARTESIAN_POINT('Ctrl Pts',(4.144812852646,31.6331199009412,125.335129094415));
#122855=CARTESIAN_POINT('Ctrl Pts',(4.14924516230143,31.6195324395953,125.39561107137));
#122856=CARTESIAN_POINT('Ctrl Pts',(4.15636865642105,31.5917480049583,125.493430538165));
#122857=CARTESIAN_POINT('Ctrl Pts',(4.15911285061266,31.5795242165704,125.531261815179));
#122858=CARTESIAN_POINT('Ctrl Pts',(4.1619795480403,31.565123709874,125.570920088539));
#122859=CARTESIAN_POINT('Ctrl Pts',(4.16214545821458,31.5642843847085,125.573215786958));
#122860=CARTESIAN_POINT('Ctrl Pts',(4.16231120066723,31.5634400119558,125.575509625476));
#122861=CARTESIAN_POINT('Ctrl Pts',(3.96713561979274,31.5634400104587,125.575509629543));
#122862=CARTESIAN_POINT('Ctrl Pts',(3.96352862299315,31.5807542032736,125.52847357592));
#122863=CARTESIAN_POINT('Ctrl Pts',(3.95996288128871,31.5959393093763,125.480673796253));
#122864=CARTESIAN_POINT('Ctrl Pts',(3.95384263844318,31.6186573985309,125.396112138332));
#122865=CARTESIAN_POINT('Ctrl Pts',(3.95126252080062,31.6271474673079,125.359649976059));
#122866=CARTESIAN_POINT('Ctrl Pts',(3.94769744747633,31.6373249383762,125.308140114473));
#122867=CARTESIAN_POINT('Ctrl Pts',(3.94668020010676,31.6400463819926,125.293310713825));
#122868=CARTESIAN_POINT('Ctrl Pts',(3.94493802658564,31.6443891496727,125.267692518425));
#122869=CARTESIAN_POINT('Ctrl Pts',(3.94421010642985,31.6461064567215,125.256921199726));
#122870=CARTESIAN_POINT('Ctrl Pts',(3.94272865504895,31.6494010741873,125.234865694673));
#122871=CARTESIAN_POINT('Ctrl Pts',(3.94197546677462,31.6509686593607,125.223580622533));
#122872=CARTESIAN_POINT('Ctrl Pts',(3.94007038614763,31.6546581000016,125.194861461032));
#122873=CARTESIAN_POINT('Ctrl Pts',(3.93892354119861,31.6566203118629,125.177407997258));
#122874=CARTESIAN_POINT('Ctrl Pts',(3.93429798673835,31.6634684630543,125.106398175224));
#122875=CARTESIAN_POINT('Ctrl Pts',(3.93089119182993,31.6660362988545,125.052648178121));
#122876=CARTESIAN_POINT('Ctrl Pts',(3.92157740828373,31.6659344406967,124.90331771581));
#122877=CARTESIAN_POINT('Ctrl Pts',(3.91580905976596,31.6576502345239,124.807955195007));
#122878=CARTESIAN_POINT('Ctrl Pts',(3.9052557548619,31.6281069486617,124.638520840064));
#122879=CARTESIAN_POINT('Ctrl Pts',(3.90051311998408,31.6098104463343,124.564217107924));
#122880=CARTESIAN_POINT('Ctrl Pts',(3.89471855049518,31.5827307707288,124.479740144298));
#122881=CARTESIAN_POINT('Ctrl Pts',(3.89390955363458,31.5788503638266,124.468080347329));
#122882=CARTESIAN_POINT('Ctrl Pts',(3.89263163983194,31.5725734289611,124.449893520797));
#122883=CARTESIAN_POINT('Ctrl Pts',(3.89216761024834,31.5702643258904,124.443336483687));
#122884=CARTESIAN_POINT('Ctrl Pts',(3.89129500109225,31.5658681845837,124.431098020723));
#122885=CARTESIAN_POINT('Ctrl Pts',(3.89088699806223,31.5637911362241,124.425413269286));
#122886=CARTESIAN_POINT('Ctrl Pts',(3.88992119971945,31.5588233897662,124.412043319928));
#122887=CARTESIAN_POINT('Ctrl Pts',(3.88936192310935,31.5559068016037,124.404368036632));
#122888=CARTESIAN_POINT('Ctrl Pts',(3.88747965125037,31.5459544279629,124.378749345957));
#122889=CARTESIAN_POINT('Ctrl Pts',(3.88614315287176,31.5386643118929,124.360907264358));
#122890=CARTESIAN_POINT('Ctrl Pts',(3.88281715100822,31.5199412845325,124.317262231384));
#122891=CARTESIAN_POINT('Ctrl Pts',(3.88081312916866,31.5081592900544,124.291616103136));
#122892=CARTESIAN_POINT('Ctrl Pts',(3.8716465746977,31.4518151281689,124.176754653832));
#122893=CARTESIAN_POINT('Ctrl Pts',(3.86431273633819,31.3999489014488,124.091350700761));
#122894=CARTESIAN_POINT('Ctrl Pts',(3.85112931772382,31.2914405212585,123.944234913046));
#122895=CARTESIAN_POINT('Ctrl Pts',(3.84525171206695,31.2371868009904,123.88114740955));
#122896=CARTESIAN_POINT('Ctrl Pts',(3.83822171472868,31.1645751794945,123.80848601697));
#122897=CARTESIAN_POINT('Ctrl Pts',(3.83688971346384,31.1504623802431,123.794853830778));
#122898=CARTESIAN_POINT('Ctrl Pts',(3.83477197690267,31.127460415763,123.773407601132));
#122899=CARTESIAN_POINT('Ctrl Pts',(3.83397945161786,31.1187234616638,123.765433788375));
#122900=CARTESIAN_POINT('Ctrl Pts',(3.83247496762936,31.1018943643616,123.750400021365));
#122901=CARTESIAN_POINT('Ctrl Pts',(3.83176235527004,31.0938174725448,123.743323970636));
#122902=CARTESIAN_POINT('Ctrl Pts',(3.83013001388486,31.0750762976567,123.727222677686));
#122903=CARTESIAN_POINT('Ctrl Pts',(3.82921256912457,31.0643656824223,123.718252414961));
#122904=CARTESIAN_POINT('Ctrl Pts',(3.82630533554839,31.0298734357762,123.690095300974));
#122905=CARTESIAN_POINT('Ctrl Pts',(3.82433613581767,31.0056754681708,123.671426835084));
#122906=CARTESIAN_POINT('Ctrl Pts',(3.81968594490355,30.9466897183713,123.628455595871));
#122907=CARTESIAN_POINT('Ctrl Pts',(3.81702741162792,30.9114599692911,123.60479514842));
#122908=CARTESIAN_POINT('Ctrl Pts',(3.80982481102461,30.8126199804357,123.543757294105));
#122909=CARTESIAN_POINT('Ctrl Pts',(3.80534865352413,30.7473717042517,123.509218340482));
#122910=CARTESIAN_POINT('Ctrl Pts',(3.8000161615178,30.6677968601917,123.473637166322));
#122911=CARTESIAN_POINT('Ctrl Pts',(3.79919397425709,30.6554784237595,123.468306761371));
#122912=CARTESIAN_POINT('Ctrl Pts',(3.79382154719974,30.5747769618755,123.43453765363));
#122913=CARTESIAN_POINT('Ctrl Pts',(3.78921906755502,30.5046349627858,123.410540443666));
#122914=CARTESIAN_POINT('Ctrl Pts',(3.78358053704357,30.4212829808363,123.388098196648));
#122915=CARTESIAN_POINT('Ctrl Pts',(3.78277215993997,30.4093917381067,123.385037103647));
#122916=CARTESIAN_POINT('Ctrl Pts',(3.78149501476816,30.3907191849761,123.380449810446));
#122917=CARTESIAN_POINT('Ctrl Pts',(3.78103112455801,30.3839600340956,123.378834065915));
#122918=CARTESIAN_POINT('Ctrl Pts',(3.78015862096159,30.371295264862,123.375890254456));
#122919=CARTESIAN_POINT('Ctrl Pts',(3.77975058233277,30.3653922631154,123.374552022162));
#122920=CARTESIAN_POINT('Ctrl Pts',(3.77878448681502,30.3514610590279,123.371473486735));
#122921=CARTESIAN_POINT('Ctrl Pts',(3.77822494585976,30.3434271335287,123.369760362));
#122922=CARTESIAN_POINT('Ctrl Pts',(3.7763408325478,30.3164798522999,123.364222249514));
#122923=CARTESIAN_POINT('Ctrl Pts',(3.77500272243682,30.2975135489668,123.360666612683));
#122924=CARTESIAN_POINT('Ctrl Pts',(3.77167181072081,30.250622706819,123.35271641315));
#122925=CARTESIAN_POINT('Ctrl Pts',(3.76966443947044,30.2226403846133,123.348701712137));
#122926=CARTESIAN_POINT('Ctrl Pts',(3.76046823954153,30.0951743223672,123.333712449522));
#122927=CARTESIAN_POINT('Ctrl Pts',(3.7531072933845,29.9949271986037,123.331004174576));
#122928=CARTESIAN_POINT('Ctrl Pts',(3.73993008640346,29.8125413417562,123.34251734815));
#122929=CARTESIAN_POINT('Ctrl Pts',(3.73408305538641,29.730532733163,123.353858878976));
#122930=CARTESIAN_POINT('Ctrl Pts',(3.72708254649382,29.6305250923967,123.37536812323));
#122931=CARTESIAN_POINT('Ctrl Pts',(3.72575139149734,29.6114298326118,123.379829106431));
#122932=CARTESIAN_POINT('Ctrl Pts',(3.72363466969997,29.5809509642906,123.387519381053));
#122933=CARTESIAN_POINT('Ctrl Pts',(3.72284232445438,29.5695157642461,123.3905345061));
#122934=CARTESIAN_POINT('Ctrl Pts',(3.72133797998545,29.547759697168,123.396519404718));
#122935=CARTESIAN_POINT('Ctrl Pts',(3.7206253292228,29.5374335959599,123.399467700415));
#122936=CARTESIAN_POINT('Ctrl Pts',(3.7189926149693,29.5137361790457,123.406482256444));
#122937=CARTESIAN_POINT('Ctrl Pts',(3.71807483940607,29.5003859600017,123.410617373523));
#122938=CARTESIAN_POINT('Ctrl Pts',(3.71516536342022,29.4579897593647,123.424336225931));
#122939=CARTESIAN_POINT('Ctrl Pts',(3.71319429839723,29.4291539840933,123.43455231832));
#122940=CARTESIAN_POINT('Ctrl Pts',(3.70853875481299,29.3609816719742,123.460839233088));
#122941=CARTESIAN_POINT('Ctrl Pts',(3.70587680782465,29.3219461760718,123.477632212263));
#122942=CARTESIAN_POINT('Ctrl Pts',(3.69867222710805,29.2170331484494,123.527602570088));
#122943=CARTESIAN_POINT('Ctrl Pts',(3.69419728862964,29.152649516931,123.563689167423));
#122944=CARTESIAN_POINT('Ctrl Pts',(3.68884537306649,29.0793398752456,123.611428726712));
#122945=CARTESIAN_POINT('Ctrl Pts',(3.68800262886321,29.067905529692,123.619078156074));
#122946=CARTESIAN_POINT('Ctrl Pts',(3.682634262437,28.9958678630912,123.668572816012));
#122947=CARTESIAN_POINT('Ctrl Pts',(3.67805621923547,28.9380079202976,123.714251280594));
#122948=CARTESIAN_POINT('Ctrl Pts',(3.6724448316176,28.8742549761992,123.771828644879));
#122949=CARTESIAN_POINT('Ctrl Pts',(3.67163655268575,28.865234985076,123.780157766226));
#122950=CARTESIAN_POINT('Ctrl Pts',(3.6703595292693,28.8512550628881,123.793356157472));
#122951=CARTESIAN_POINT('Ctrl Pts',(3.66989566113923,28.8462319402818,123.798158266138));
#122952=CARTESIAN_POINT('Ctrl Pts',(3.66902317424784,28.8368900046065,123.807201702377));
#122953=CARTESIAN_POINT('Ctrl Pts',(3.66861512996107,28.8325640738332,123.81143532199));
#122954=CARTESIAN_POINT('Ctrl Pts',(3.66764898728223,28.8224214124804,123.821470339566));
#122955=CARTESIAN_POINT('Ctrl Pts',(3.6670894043844,28.8166244172952,123.827291292139));
#122956=CARTESIAN_POINT('Ctrl Pts',(3.66520499876969,28.7973534733861,123.846930263471));
#122957=CARTESIAN_POINT('Ctrl Pts',(3.66386663279833,28.7840771857697,123.860938932381));
#122958=CARTESIAN_POINT('Ctrl Pts',(3.66053494143929,28.751958942969,123.896030395364));
#122959=CARTESIAN_POINT('Ctrl Pts',(3.65852703825346,28.7334049725675,123.917367918429));
#122960=CARTESIAN_POINT('Ctrl Pts',(3.64932611865575,28.6516397177456,124.016379932212));
#122961=CARTESIAN_POINT('Ctrl Pts',(3.64196085559383,28.5949673266824,124.099185075933));
#122962=CARTESIAN_POINT('Ctrl Pts',(3.62878462957162,28.5057447685608,124.258663469944));
#122963=CARTESIAN_POINT('Ctrl Pts',(3.62294245721442,28.4708278105737,124.333655747558));
#122964=CARTESIAN_POINT('Ctrl Pts',(3.61594663911569,28.4346828885717,124.429278785217));
#122965=CARTESIAN_POINT('Ctrl Pts',(3.61461562229018,28.4280749353141,124.447739180896));
#122966=CARTESIAN_POINT('Ctrl Pts',(3.61249906617595,28.4180060956667,124.477514481102));
#122967=CARTESIAN_POINT('Ctrl Pts',(3.61170675032658,28.4143373549911,124.488756594655));
#122968=CARTESIAN_POINT('Ctrl Pts',(3.61020242861816,28.4075659673028,124.510280524408));
#122969=CARTESIAN_POINT('Ctrl Pts',(3.60948977156561,28.4044424475102,124.520555092666));
#122970=CARTESIAN_POINT('Ctrl Pts',(3.60785699633333,28.397482848226,124.544269701998));
#122971=CARTESIAN_POINT('Ctrl Pts',(3.60693916668006,28.3937160788647,124.557729369427));
#122972=CARTESIAN_POINT('Ctrl Pts',(3.6040293239106,28.3822464200609,124.600794436882));
#122973=CARTESIAN_POINT('Ctrl Pts',(3.60205795377475,28.3751890489907,124.630566259418));
#122974=CARTESIAN_POINT('Ctrl Pts',(3.59740153442503,28.3602976614656,124.702111901186));
#122975=CARTESIAN_POINT('Ctrl Pts',(3.59473902885037,28.3532340716015,124.744024542191));
#122976=CARTESIAN_POINT('Ctrl Pts',(3.58753414385141,28.3383179472313,124.859274957168));
#122977=CARTESIAN_POINT('Ctrl Pts',(3.58305942369869,28.3337186709136,124.932935249666));
#122978=CARTESIAN_POINT('Ctrl Pts',(3.57770486474803,28.3340684680187,125.020461058019));
#122979=CARTESIAN_POINT('Ctrl Pts',(3.57685927315372,28.33429516796,125.034262674931));
#122980=CARTESIAN_POINT('Ctrl Pts',(3.57149157056634,28.336816126696,125.121615763974));
#122981=CARTESIAN_POINT('Ctrl Pts',(3.56691701409882,28.3438097601599,125.194941369759));
#122982=CARTESIAN_POINT('Ctrl Pts',(3.56130949820639,28.3575962384021,125.279672334438));
#122983=CARTESIAN_POINT('Ctrl Pts',(3.56050123340875,28.3597017452784,125.291767620826));
#122984=CARTESIAN_POINT('Ctrl Pts',(3.55922422752216,28.3632080377829,125.310670830606));
#122985=CARTESIAN_POINT('Ctrl Pts',(3.55876036257101,28.3645181296845,125.317495417391));
#122986=CARTESIAN_POINT('Ctrl Pts',(3.55788787808429,28.367049179345,125.330248781452));
#122987=CARTESIAN_POINT('Ctrl Pts',(3.55747983298255,28.3682598016447,125.336179357965));
#122988=CARTESIAN_POINT('Ctrl Pts',(3.55651368351164,28.3711896651417,125.350143377474));
#122989=CARTESIAN_POINT('Ctrl Pts',(3.55595409457362,28.3729360399246,125.358170845382));
#122990=CARTESIAN_POINT('Ctrl Pts',(3.55406964686146,28.37898387128,125.385013267021));
#122991=CARTESIAN_POINT('Ctrl Pts',(3.55273124404052,28.3835527219579,125.403765554884));
#122992=CARTESIAN_POINT('Ctrl Pts',(3.54939944039085,28.395615265959,125.449783339423));
#122993=CARTESIAN_POINT('Ctrl Pts',(3.54739146058956,28.4034791946279,125.476945033324));
#122994=CARTESIAN_POINT('Ctrl Pts',(3.5381898609488,28.4423201843109,125.599348932699));
#122995=CARTESIAN_POINT('Ctrl Pts',(3.53082397584887,28.481155543515,125.691879701384));
#122996=CARTESIAN_POINT('Ctrl Pts',(3.5176478909884,28.5667515299219,125.853332171553));
#122997=CARTESIAN_POINT('Ctrl Pts',(3.5118064184972,28.6108136717573,125.923332018516));
#122998=CARTESIAN_POINT('Ctrl Pts',(3.50481127619276,28.6715412842545,126.005553476254));
#122999=CARTESIAN_POINT('Ctrl Pts',(3.5034802793548,28.6834665864198,126.021117124008));
#123000=CARTESIAN_POINT('Ctrl Pts',(3.50136374720814,28.7030209304076,126.045725165805));
#123001=CARTESIAN_POINT('Ctrl Pts',(3.50057143561116,28.7104760917228,126.054904702719));
#123002=CARTESIAN_POINT('Ctrl Pts',(3.4990671171947,28.7248867022551,126.072267406721));
#123003=CARTESIAN_POINT('Ctrl Pts',(3.49835445923184,28.7318247427581,126.080464177902));
#123004=CARTESIAN_POINT('Ctrl Pts',(3.4967216751761,28.7479738797309,126.099173291085));
#123005=CARTESIAN_POINT('Ctrl Pts',(3.49580383769647,28.7572390585602,126.109638045409));
#123006=CARTESIAN_POINT('Ctrl Pts',(3.4928939418534,28.7871997414039,126.142631744169));
#123007=CARTESIAN_POINT('Ctrl Pts',(3.49092252756731,28.8083851960636,126.164708597571));
#123008=CARTESIAN_POINT('Ctrl Pts',(3.48626598148828,28.8604188050897,126.216024626695));
#123009=CARTESIAN_POINT('Ctrl Pts',(3.48360339508098,28.8918014839276,126.24469177753));
#123010=CARTESIAN_POINT('Ctrl Pts',(3.47639846649747,28.9805393746336,126.319731314348));
#123011=CARTESIAN_POINT('Ctrl Pts',(3.47192377836683,29.0399298786321,126.363545539011));
#123012=CARTESIAN_POINT('Ctrl Pts',(3.46656884846885,29.1136590786099,126.410725513862));
#123013=CARTESIAN_POINT('Ctrl Pts',(3.46572285598404,29.1253829818725,126.418023896207));
#123014=CARTESIAN_POINT('Ctrl Pts',(3.46035524942957,29.2001385065439,126.463281022382));
#123015=CARTESIAN_POINT('Ctrl Pts',(3.45578118644328,29.2655284443782,126.497170181264));
#123016=CARTESIAN_POINT('Ctrl Pts',(3.45017421849734,29.3441842203121,126.531539223497));
#123017=CARTESIAN_POINT('Ctrl Pts',(3.44936595570352,29.3554879202592,126.536330331442));
#123018=CARTESIAN_POINT('Ctrl Pts',(3.44808895230225,29.3732709824101,126.543636949215));
#123019=CARTESIAN_POINT('Ctrl Pts',(3.44762508780179,29.3797151554707,126.546237691865));
#123020=CARTESIAN_POINT('Ctrl Pts',(3.44675260365591,29.3918025576823,126.55102821106));
#123021=CARTESIAN_POINT('Ctrl Pts',(3.44634455843855,29.397441692908,126.55322764662));
#123022=CARTESIAN_POINT('Ctrl Pts',(3.44537840800485,29.4107625397687,126.558339727849));
#123023=CARTESIAN_POINT('Ctrl Pts',(3.44481881821046,29.418453947817,126.561226336586));
#123024=CARTESIAN_POINT('Ctrl Pts',(3.44293436452967,29.4442856432646,126.570703683677));
#123025=CARTESIAN_POINT('Ctrl Pts',(3.44159595648408,29.4625183080825,126.577035782631));
#123026=CARTESIAN_POINT('Ctrl Pts',(3.43826413691347,29.5077223580024,126.59185996835));
#123027=CARTESIAN_POINT('Ctrl Pts',(3.43625614624933,29.5348073376272,126.599984700574));
#123028=CARTESIAN_POINT('Ctrl Pts',(3.42705445018405,29.658711437572,126.633740464172));
#123029=CARTESIAN_POINT('Ctrl Pts',(3.41968847688366,29.7575146637356,126.651298610726));
#123030=CARTESIAN_POINT('Ctrl Pts',(3.40651241203323,29.9395819718255,126.666951232189));
#123031=CARTESIAN_POINT('Ctrl Pts',(3.40067103877146,30.0222882588045,126.667897982785));
#123032=CARTESIAN_POINT('Ctrl Pts',(3.39367599228565,30.1243011709922,126.661472109407));
#123033=CARTESIAN_POINT('Ctrl Pts',(3.39234499828336,30.14384468412,126.659894308462));
#123034=CARTESIAN_POINT('Ctrl Pts',(3.39022846953704,30.1751244963244,126.656812373186));
#123035=CARTESIAN_POINT('Ctrl Pts',(3.38943615854334,30.1868800281768,126.655527618828));
#123036=CARTESIAN_POINT('Ctrl Pts',(3.38793184059409,30.2092829831432,126.652837543927));
#123037=CARTESIAN_POINT('Ctrl Pts',(3.38721918250205,30.2199323937662,126.65145422735));
#123038=CARTESIAN_POINT('Ctrl Pts',(3.38558639719452,30.2444094658033,126.648033780959));
#123039=CARTESIAN_POINT('Ctrl Pts',(3.38466855860457,30.2582264790076,126.645925403964));
#123040=CARTESIAN_POINT('Ctrl Pts',(3.38175865523192,30.3021956357366,126.63864870362));
#123041=CARTESIAN_POINT('Ctrl Pts',(3.37978723468221,30.3322336885918,126.632823548484));
#123042=CARTESIAN_POINT('Ctrl Pts',(3.3751306706239,30.403567959783,126.616939736214));
#123043=CARTESIAN_POINT('Ctrl Pts',(3.3724680727487,30.4446734995351,126.606121747278));
#123044=CARTESIAN_POINT('Ctrl Pts',(3.36526313799108,30.5558458219071,126.572267827239));
#123045=CARTESIAN_POINT('Ctrl Pts',(3.36078845441238,30.6248672562079,126.54613452732));
#123046=CARTESIAN_POINT('Ctrl Pts',(3.35133282169985,30.7654693231246,126.481940579878));
#123047=CARTESIAN_POINT('Ctrl Pts',(3.34635651373472,30.8364578959568,126.443061410053));
#123048=CARTESIAN_POINT('Ctrl Pts',(3.34005345722458,30.9181656501343,126.390251421584));
#123049=CARTESIAN_POINT('Ctrl Pts',(3.3389760302868,30.9318618972197,126.381108442841));
#123050=CARTESIAN_POINT('Ctrl Pts',(3.33737514500823,30.951773644525,126.367385270653));
#123051=CARTESIAN_POINT('Ctrl Pts',(3.33686154773424,30.9580968960103,126.362962171449));
#123052=CARTESIAN_POINT('Ctrl Pts',(3.33594285128177,30.9692874299057,126.355018067934));
#123053=CARTESIAN_POINT('Ctrl Pts',(3.3355389171035,30.9741667253314,126.351514437642));
#123054=CARTESIAN_POINT('Ctrl Pts',(3.33464065845415,30.9849259124668,126.343700151946));
#123055=CARTESIAN_POINT('Ctrl Pts',(3.33414553756842,30.9907964352877,126.339377306873));
#123056=CARTESIAN_POINT('Ctrl Pts',(3.33267439078484,31.0080686087668,126.326482999535));
#123057=CARTESIAN_POINT('Ctrl Pts',(3.33169148548803,31.0193884292462,126.317803727587));
#123058=CARTESIAN_POINT('Ctrl Pts',(3.3293902934715,31.0454147347688,126.297312530433));
#123059=CARTESIAN_POINT('Ctrl Pts',(3.32806621059145,31.0600346613704,126.285394189197));
#123060=CARTESIAN_POINT('Ctrl Pts',(3.32334838674721,31.1109818241644,126.242401120407));
#123061=CARTESIAN_POINT('Ctrl Pts',(3.31989939648284,31.1461692123785,126.210015176482));
#123062=CARTESIAN_POINT('Ctrl Pts',(3.30823788005546,31.2595782867348,126.096244548077));
#123063=CARTESIAN_POINT('Ctrl Pts',(3.2999826709812,31.3309278840731,126.008427549007));
#123064=CARTESIAN_POINT('Ctrl Pts',(3.2888487604919,31.4176463946644,125.87628570116));
#123065=CARTESIAN_POINT('Ctrl Pts',(3.28571494723918,31.4408935347018,125.837510846481));
#123066=CARTESIAN_POINT('Ctrl Pts',(3.28150575909692,31.4704942474655,125.783248841607));
#123067=CARTESIAN_POINT('Ctrl Pts',(3.28038199612462,31.4782329403291,125.768543745391));
#123068=CARTESIAN_POINT('Ctrl Pts',(3.27858896626285,31.490310851459,125.744735636403));
#123069=CARTESIAN_POINT('Ctrl Pts',(3.27791485001578,31.4947895164398,125.735705043725));
#123070=CARTESIAN_POINT('Ctrl Pts',(3.2765193161326,31.5039296161606,125.716847260663));
#123071=CARTESIAN_POINT('Ctrl Pts',(3.27579840024908,31.5085773430972,125.707013928379));
#123072=CARTESIAN_POINT('Ctrl Pts',(3.27409799123439,31.5193611164379,125.683607814098));
#123073=CARTESIAN_POINT('Ctrl Pts',(3.27312144694752,31.5254121613228,125.669996721972));
#123074=CARTESIAN_POINT('Ctrl Pts',(3.27026164857302,31.5427011961233,125.629658288214));
#123075=CARTESIAN_POINT('Ctrl Pts',(3.26839562934732,31.5534248189975,125.602717082415));
#123076=CARTESIAN_POINT('Ctrl Pts',(3.26654942290125,31.5634400114153,125.575509626944));
#123077=CARTESIAN_POINT('Origin',(5.,30.,125.));
#123078=CARTESIAN_POINT('',(2.56904933390813,31.5634400118358,125.575509625802));
#123079=CARTESIAN_POINT('',(2.75979332369797,31.5634400150579,125.575509617049));
#123080=CARTESIAN_POINT('',(5.,31.5634400119422,125.575509625513));
#123081=CARTESIAN_POINT('Ctrl Pts',(2.75979332369797,31.5634400150579,125.575509617049));
#123082=CARTESIAN_POINT('Ctrl Pts',(2.76041358651822,31.559981406667,125.584905336242));
#123083=CARTESIAN_POINT('Ctrl Pts',(2.76103576549018,31.5564377314933,125.594270881401));
#123084=CARTESIAN_POINT('Ctrl Pts',(2.76368036814329,31.5410732388471,125.633796936527));
#123085=CARTESIAN_POINT('Ctrl Pts',(2.76572347926925,31.528459758398,125.663638303974));
#123086=CARTESIAN_POINT('Ctrl Pts',(2.76917271010146,31.5061307195007,125.712445975781));
#123087=CARTESIAN_POINT('Ctrl Pts',(2.77055674212779,31.4969064936737,125.731628224946));
#123088=CARTESIAN_POINT('Ctrl Pts',(2.77252482942317,31.4834722581688,125.758247261965));
#123089=CARTESIAN_POINT('Ctrl Pts',(2.7730915014663,31.4795682324861,125.765837246845));
#123090=CARTESIAN_POINT('Ctrl Pts',(2.77406932080167,31.4727744530551,125.778799472925));
#123091=CARTESIAN_POINT('Ctrl Pts',(2.77447870635722,31.4699132169148,125.784186420574));
#123092=CARTESIAN_POINT('Ctrl Pts',(2.77534785585793,31.4638045537374,125.795536503927));
#123093=CARTESIAN_POINT('Ctrl Pts',(2.77580801108254,31.4605502817986,125.801495459022));
#123094=CARTESIAN_POINT('Ctrl Pts',(2.77707815531717,31.4515101517744,125.817811113318));
#123095=CARTESIAN_POINT('Ctrl Pts',(2.77789255871442,31.4456500826764,125.828125930106));
#123096=CARTESIAN_POINT('Ctrl Pts',(2.78241420296411,31.4127404635743,125.884639102952));
#123097=CARTESIAN_POINT('Ctrl Pts',(2.78623016575027,31.3835887736318,125.929571346781));
#123098=CARTESIAN_POINT('Ctrl Pts',(2.79713444714875,31.2953414870224,126.052220020763));
#123099=CARTESIAN_POINT('Ctrl Pts',(2.80430021625587,31.231502617139,126.12626787655));
#123100=CARTESIAN_POINT('Ctrl Pts',(2.81480762648961,31.1265367979438,126.228355150878));
#123101=CARTESIAN_POINT('Ctrl Pts',(2.81826965337511,31.0900406162061,126.260854359214));
#123102=CARTESIAN_POINT('Ctrl Pts',(2.82402596645811,31.0259569398931,126.313054091823));
#123103=CARTESIAN_POINT('Ctrl Pts',(2.82635043076461,30.9991026078242,126.333601498122));
#123104=CARTESIAN_POINT('Ctrl Pts',(2.8296278782315,30.9598467161995,126.361785978704));
#123105=CARTESIAN_POINT('Ctrl Pts',(2.83060654518557,30.9479430783254,126.370098797103));
#123106=CARTESIAN_POINT('Ctrl Pts',(2.83230410870678,30.9269825194263,126.384332487089));
#123107=CARTESIAN_POINT('Ctrl Pts',(2.83302559281953,30.9179739184319,126.390322595914));
#123108=CARTESIAN_POINT('Ctrl Pts',(2.83451334342174,30.8991931297128,126.40254842091));
#123109=CARTESIAN_POINT('Ctrl Pts',(2.83527908410116,30.8894129016869,126.408770761795));
#123110=CARTESIAN_POINT('Ctrl Pts',(2.83725690595954,30.8638623342852,126.424654299822));
#123111=CARTESIAN_POINT('Ctrl Pts',(2.83846313004437,30.847994383697,126.434156050182));
#123112=CARTESIAN_POINT('Ctrl Pts',(2.84373836423414,30.7773972657187,126.474848222531));
#123113=CARTESIAN_POINT('Ctrl Pts',(2.8477059680593,30.7210798780603,126.503186253981));
#123114=CARTESIAN_POINT('Ctrl Pts',(2.86062048426853,30.5299717219439,126.586129537178));
#123115=CARTESIAN_POINT('Ctrl Pts',(2.8691980346961,30.3896780366754,126.626289545261));
#123116=CARTESIAN_POINT('Ctrl Pts',(2.87998171472577,30.2233020437298,126.651126200779));
#123117=CARTESIAN_POINT('Ctrl Pts',(2.88146959984958,30.2005626630594,126.654042328997));
#123118=CARTESIAN_POINT('Ctrl Pts',(2.8835604985241,30.169040636722,126.657425224111));
#123119=CARTESIAN_POINT('Ctrl Pts',(2.88414311380086,30.1603024875565,126.658293162989));
#123120=CARTESIAN_POINT('Ctrl Pts',(2.88513957805721,30.1454431902161,126.659650560478));
#123121=CARTESIAN_POINT('Ctrl Pts',(2.88555149478189,30.1393253024884,126.660175341159));
#123122=CARTESIAN_POINT('Ctrl Pts',(2.8864159330681,30.1265409799594,126.661200791808));
#123123=CARTESIAN_POINT('Ctrl Pts',(2.88686876590961,30.119874290692,126.66169517084));
#123124=CARTESIAN_POINT('Ctrl Pts',(2.88809823298623,30.1018506238574,126.662922718974));
#123125=CARTESIAN_POINT('Ctrl Pts',(2.88887884151984,30.0904890540283,126.663579644047));
#123126=CARTESIAN_POINT('Ctrl Pts',(2.89276124346385,30.0343413814461,126.666249234226));
#123127=CARTESIAN_POINT('Ctrl Pts',(2.89593927887881,29.9894970689316,126.666569761793));
#123128=CARTESIAN_POINT('Ctrl Pts',(2.90547612845563,29.8567830012224,126.662162036695));
#123129=CARTESIAN_POINT('Ctrl Pts',(2.91193072300331,29.7692373708531,126.652283989316));
#123130=CARTESIAN_POINT('Ctrl Pts',(2.92267577694516,29.623374918835,126.624002354429));
#123131=CARTESIAN_POINT('Ctrl Pts',(2.92700963160559,29.5645381565499,126.609224762518));
#123132=CARTESIAN_POINT('Ctrl Pts',(2.933119339431,29.4811896525542,126.583382899251));
#123133=CARTESIAN_POINT('Ctrl Pts',(2.93496670580938,29.4559382285905,126.574884918794));
#123134=CARTESIAN_POINT('Ctrl Pts',(2.93827174992921,29.4106758654013,126.558433868167));
#123135=CARTESIAN_POINT('Ctrl Pts',(2.93973577249966,29.3905950687023,126.550691704362));
#123136=CARTESIAN_POINT('Ctrl Pts',(2.94201164346743,29.3593437024263,126.537941845825));
#123137=CARTESIAN_POINT('Ctrl Pts',(2.94283217480837,29.3480693167826,126.533196664119));
#123138=CARTESIAN_POINT('Ctrl Pts',(2.94436071387478,29.3270580963708,126.524079748587));
#123139=CARTESIAN_POINT('Ctrl Pts',(2.94506968721008,29.3173090972797,126.519737814926));
#123140=CARTESIAN_POINT('Ctrl Pts',(2.94665532922495,29.2955021949079,126.509773434883));
#123141=CARTESIAN_POINT('Ctrl Pts',(2.94753018440601,29.2834684735075,126.504099588021));
#123142=CARTESIAN_POINT('Ctrl Pts',(2.94976874416363,29.252684687574,126.48913186307));
#123143=CARTESIAN_POINT('Ctrl Pts',(2.95112515828914,29.2340390986472,126.479627602431));
#123144=CARTESIAN_POINT('Ctrl Pts',(2.9607714366619,29.1016695867877,126.40898157404));
#123145=CARTESIAN_POINT('Ctrl Pts',(2.96857500373158,28.9952149178294,126.335154390318));
#123146=CARTESIAN_POINT('Ctrl Pts',(2.98158070008948,28.8357769450745,126.194611997377));
#123147=CARTESIAN_POINT('Ctrl Pts',(2.98672011951199,28.7774446259738,126.134842683276));
#123148=CARTESIAN_POINT('Ctrl Pts',(2.99306394893745,28.7147909360834,126.060184796897));
#123149=CARTESIAN_POINT('Ctrl Pts',(2.99398819234034,28.7058795610027,126.04928852029));
#123150=CARTESIAN_POINT('Ctrl Pts',(2.99540289343865,28.6925869292023,126.032608193478));
#123151=CARTESIAN_POINT('Ctrl Pts',(2.99588648657258,28.6881033788603,126.026905969133));
#123152=CARTESIAN_POINT('Ctrl Pts',(2.9967757101234,28.6799723613746,126.016424702276));
#123153=CARTESIAN_POINT('Ctrl Pts',(2.99718052438614,28.6763133376372,126.011654960091));
#123154=CARTESIAN_POINT('Ctrl Pts',(2.99811256822277,28.6679857390021,126.000676943365));
#123155=CARTESIAN_POINT('Ctrl Pts',(2.99864095269692,28.6633347249646,125.994455767225));
#123156=CARTESIAN_POINT('Ctrl Pts',(3.00027614303048,28.6491503753529,125.975203560358));
#123157=CARTESIAN_POINT('Ctrl Pts',(3.00139197289242,28.6397631554656,125.962066718775));
#123158=CARTESIAN_POINT('Ctrl Pts',(3.00785170084655,28.5869974212952,125.88590805824));
#123159=CARTESIAN_POINT('Ctrl Pts',(3.01339405136169,28.5478138613454,125.820099113123));
#123160=CARTESIAN_POINT('Ctrl Pts',(3.02367981821342,28.4840154051156,125.693942296414));
#123161=CARTESIAN_POINT('Ctrl Pts',(3.0284089031753,28.4581425546146,125.634382764511));
#123162=CARTESIAN_POINT('Ctrl Pts',(3.03667846597153,28.4185187260463,125.526304092791));
#123163=CARTESIAN_POINT('Ctrl Pts',(3.04024277763164,28.403369279339,125.478382839419));
#123164=CARTESIAN_POINT('Ctrl Pts',(3.04614662244591,28.3815124549162,125.396538289062));
#123165=CARTESIAN_POINT('Ctrl Pts',(3.04851844013303,28.3736529454115,125.362960203776));
#123166=CARTESIAN_POINT('Ctrl Pts',(3.05184951356238,28.3639509549359,125.314822855414));
#123167=CARTESIAN_POINT('Ctrl Pts',(3.05283562313009,28.3612501464017,125.300447747825));
#123168=CARTESIAN_POINT('Ctrl Pts',(3.05454177222463,28.3568786869573,125.275364741452));
#123169=CARTESIAN_POINT('Ctrl Pts',(3.05526447664666,28.3551225933755,125.264672848878));
#123170=CARTESIAN_POINT('Ctrl Pts',(3.05665798183441,28.3519233047215,125.243930876256));
#123171=CARTESIAN_POINT('Ctrl Pts',(3.05732915303646,28.3504674328856,125.233883269289));
#123172=CARTESIAN_POINT('Ctrl Pts',(3.05911652231163,28.3468196776442,125.206977758677));
#123173=CARTESIAN_POINT('Ctrl Pts',(3.0602274796093,28.3447937737002,125.190098274724));
#123174=CARTESIAN_POINT('Ctrl Pts',(3.06447609585473,28.3379886392869,125.124991090773));
#123175=CARTESIAN_POINT('Ctrl Pts',(3.06755653922172,28.3350559042702,125.076592173165));
#123176=CARTESIAN_POINT('Ctrl Pts',(3.07809925085577,28.3322130159441,124.908249071328));
#123177=CARTESIAN_POINT('Ctrl Pts',(3.0852718322245,28.3431352879358,124.788504523533));
#123178=CARTESIAN_POINT('Ctrl Pts',(3.09518818485887,28.3747983060623,124.631340674317));
#123179=CARTESIAN_POINT('Ctrl Pts',(3.09771581674007,28.3842215499221,124.592017383705));
#123180=CARTESIAN_POINT('Ctrl Pts',(3.10188704564452,28.4017247032338,124.529161993919));
#123181=CARTESIAN_POINT('Ctrl Pts',(3.10349499226149,28.4089179978693,124.505398889994));
#123182=CARTESIAN_POINT('Ctrl Pts',(3.10572704502167,28.4194534531143,124.473207359104));
#123183=CARTESIAN_POINT('Ctrl Pts',(3.10632697040285,28.4223378002467,124.464631110683));
#123184=CARTESIAN_POINT('Ctrl Pts',(3.10734398546722,28.4273123026022,124.450229405107));
#123185=CARTESIAN_POINT('Ctrl Pts',(3.10775894284056,28.4293653758128,124.444391165977));
#123186=CARTESIAN_POINT('Ctrl Pts',(3.10856453673155,28.4333950685419,124.43313293382));
#123187=CARTESIAN_POINT('Ctrl Pts',(3.1089548846171,28.4353673799386,124.427711573005));
#123188=CARTESIAN_POINT('Ctrl Pts',(3.1100323637874,28.4408666520327,124.412836465196));
#123189=CARTESIAN_POINT('Ctrl Pts',(3.11072275096625,28.444451334304,124.403404534625));
#123190=CARTESIAN_POINT('Ctrl Pts',(3.11354129899314,28.459340532903,124.365275062926));
#123191=CARTESIAN_POINT('Ctrl Pts',(3.11570521700883,28.4713546087149,124.336863270827));
#123192=CARTESIAN_POINT('Ctrl Pts',(3.12486595233927,28.524862083711,124.219516980018));
#123193=CARTESIAN_POINT('Ctrl Pts',(3.13207592402463,28.5733823403823,124.134005360044));
#123194=CARTESIAN_POINT('Ctrl Pts',(3.14387363295889,28.6659059948645,124.000032957676));
#123195=CARTESIAN_POINT('Ctrl Pts',(3.14851138548278,28.7057399331862,123.948984659089));
#123196=CARTESIAN_POINT('Ctrl Pts',(3.15591551809863,28.775429196581,123.869666570163));
#123197=CARTESIAN_POINT('Ctrl Pts',(3.15874055968381,28.8035357619547,123.839956405336));
#123198=CARTESIAN_POINT('Ctrl Pts',(3.16257781918233,28.8438193544095,123.800398074729));
#123199=CARTESIAN_POINT('Ctrl Pts',(3.16362931632742,28.8550821858649,123.789643981373));
#123200=CARTESIAN_POINT('Ctrl Pts',(3.16541188485943,28.8745548122119,123.771565999191));
#123201=CARTESIAN_POINT('Ctrl Pts',(3.16614631717641,28.8826892142886,123.764162800692));
#123202=CARTESIAN_POINT('Ctrl Pts',(3.16753837535789,28.8983174211389,123.750219859778));
#123203=CARTESIAN_POINT('Ctrl Pts',(3.16819658966974,28.9057976044839,123.743665638305));
#123204=CARTESIAN_POINT('Ctrl Pts',(3.1698961300391,28.9253436652138,123.726846159011));
#123205=CARTESIAN_POINT('Ctrl Pts',(3.17093315991077,28.9374982456451,123.716685155119));
#123206=CARTESIAN_POINT('Ctrl Pts',(3.1745449639437,28.9806072719259,123.681679187845));
#123207=CARTESIAN_POINT('Ctrl Pts',(3.17708298180775,29.0123042012483,123.657767272609));
#123208=CARTESIAN_POINT('Ctrl Pts',(3.18703174815099,29.1415090216432,123.567354274854));
#123209=CARTESIAN_POINT('Ctrl Pts',(3.19412232044589,29.2451029463337,123.510163791845));
#123210=CARTESIAN_POINT('Ctrl Pts',(3.20545085458583,29.4149925939744,123.438680266656));
#123211=CARTESIAN_POINT('Ctrl Pts',(3.20957435327357,29.4775866670924,123.416637958818));
#123212=CARTESIAN_POINT('Ctrl Pts',(3.21490157245063,29.5565419525,123.394026251145));
#123213=CARTESIAN_POINT('Ctrl Pts',(3.21593849753998,29.5718249111311,123.389884236938));
#123214=CARTESIAN_POINT('Ctrl Pts',(3.21749041712337,29.5945260788391,123.384077771955));
#123215=CARTESIAN_POINT('Ctrl Pts',(3.21799639264703,29.6019008857442,123.382245124426));
#123216=CARTESIAN_POINT('Ctrl Pts',(3.21890733157072,29.6151247944122,123.379054865311));
#123217=CARTESIAN_POINT('Ctrl Pts',(3.21931121793574,29.6209690585979,123.377678331411));
#123218=CARTESIAN_POINT('Ctrl Pts',(3.2202167918883,29.6340300445327,123.374676428692));
#123219=CARTESIAN_POINT('Ctrl Pts',(3.22071935650986,29.6412501421166,123.37306753245));
#123220=CARTESIAN_POINT('Ctrl Pts',(3.22223452539326,29.6629402830115,123.368385592928));
#123221=CARTESIAN_POINT('Ctrl Pts',(3.22325461251871,29.6774403443719,123.365457232998));
#123222=CARTESIAN_POINT('Ctrl Pts',(3.23212030405779,29.8027395069395,123.341884537806));
#123223=CARTESIAN_POINT('Ctrl Pts',(3.24040579483127,29.9153219494606,123.332341553944));
#123224=CARTESIAN_POINT('Ctrl Pts',(3.25502125559649,30.1165959031958,123.335724323828));
#123225=CARTESIAN_POINT('Ctrl Pts',(3.26137212387327,30.2049461765468,123.344279852133));
#123226=CARTESIAN_POINT('Ctrl Pts',(3.26956240925985,30.3212642648536,123.365002632665));
#123227=CARTESIAN_POINT('Ctrl Pts',(3.27158521968818,30.3501802488817,123.370950858853));
#123228=CARTESIAN_POINT('Ctrl Pts',(3.27451750064764,30.3923520757415,123.380800820732));
#123229=CARTESIAN_POINT('Ctrl Pts',(3.27544577401502,30.4057404534445,123.384103704513));
#123230=CARTESIAN_POINT('Ctrl Pts',(3.27708611589577,30.4294604993485,123.390268790646));
#123231=CARTESIAN_POINT('Ctrl Pts',(3.27780025571393,30.4398082998792,123.39306516764));
#123232=CARTESIAN_POINT('Ctrl Pts',(3.27930238687223,30.4616139979326,123.399184326891));
#123233=CARTESIAN_POINT('Ctrl Pts',(3.28008956846626,30.473064686975,123.402530714929));
#123234=CARTESIAN_POINT('Ctrl Pts',(3.28219155590904,30.5036947891746,123.411840395599));
#123235=CARTESIAN_POINT('Ctrl Pts',(3.28349901697462,30.5228043285662,123.418028110187));
#123236=CARTESIAN_POINT('Ctrl Pts',(3.29110887254802,30.6342382453536,123.456350531951));
#123237=CARTESIAN_POINT('Ctrl Pts',(3.29714530477315,30.7237062879604,123.496216604328));
#123238=CARTESIAN_POINT('Ctrl Pts',(3.30753549303479,30.872203427531,123.578727027031));
#123239=CARTESIAN_POINT('Ctrl Pts',(3.31190841014993,30.9328928924409,123.617804008825));
#123240=CARTESIAN_POINT('Ctrl Pts',(3.31965997291716,31.0331691807712,123.69199097212));
#123241=CARTESIAN_POINT('Ctrl Pts',(3.32298482121273,31.0739693307999,123.725278511882));
#123242=CARTESIAN_POINT('Ctrl Pts',(3.32718175520478,31.1216700648778,123.768113529545));
#123243=CARTESIAN_POINT('Ctrl Pts',(3.32793952126156,31.1301387885983,123.775878147016));
#123244=CARTESIAN_POINT('Ctrl Pts',(3.32914978264526,31.1434240067198,123.788314170853));
#123245=CARTESIAN_POINT('Ctrl Pts',(3.32959810350882,31.1482939332931,123.792928317583));
#123246=CARTESIAN_POINT('Ctrl Pts',(3.33046048098246,31.1575603673239,123.801814881478));
#123247=CARTESIAN_POINT('Ctrl Pts',(3.33087417325538,31.1619613457941,123.806082327778));
#123248=CARTESIAN_POINT('Ctrl Pts',(3.33188093263697,31.1725667468185,123.816480122207));
#123249=CARTESIAN_POINT('Ctrl Pts',(3.3324758536315,31.1787467169499,123.822635041387));
#123250=CARTESIAN_POINT('Ctrl Pts',(3.33450972238414,31.199589608525,123.843722032137));
#123251=CARTESIAN_POINT('Ctrl Pts',(3.33596450408592,31.2140187469185,123.858881096811));
#123252=CARTESIAN_POINT('Ctrl Pts',(3.34490408043666,31.3000213075562,123.95271192715));
#123253=CARTESIAN_POINT('Ctrl Pts',(3.35272216199712,31.3642076253796,124.037813402579));
#123254=CARTESIAN_POINT('Ctrl Pts',(3.36756474752012,31.4712346299523,124.212170329023));
#123255=CARTESIAN_POINT('Ctrl Pts',(3.37457589674533,31.5151288015248,124.300287548376));
#123256=CARTESIAN_POINT('Ctrl Pts',(3.38280007253362,31.5588768919739,124.41184717088));
#123257=CARTESIAN_POINT('Ctrl Pts',(3.38426709555954,31.5663586084554,124.432072451718));
#123258=CARTESIAN_POINT('Ctrl Pts',(3.38654654722683,31.5774690161018,124.463998752982));
#123259=CARTESIAN_POINT('Ctrl Pts',(3.38736770404948,31.5813646923647,124.475603625904));
#123260=CARTESIAN_POINT('Ctrl Pts',(3.3888968140588,31.5884163796476,124.497403471591));
#123261=CARTESIAN_POINT('Ctrl Pts',(3.38960573961199,31.5916029980613,124.507587803644));
#123262=CARTESIAN_POINT('Ctrl Pts',(3.39119051260019,31.5985384111118,124.530524130365));
#123263=CARTESIAN_POINT('Ctrl Pts',(3.39206455546905,31.6022329270157,124.543291878118));
#123264=CARTESIAN_POINT('Ctrl Pts',(3.39429952106896,31.6113383287057,124.576230180002));
#123265=CARTESIAN_POINT('Ctrl Pts',(3.39565319394755,31.616523576891,124.596461083212));
#123266=CARTESIAN_POINT('Ctrl Pts',(3.40532392051984,31.651121597653,124.742840260298));
#123267=CARTESIAN_POINT('Ctrl Pts',(3.41315090634434,31.6661146386835,124.871939976784));
#123268=CARTESIAN_POINT('Ctrl Pts',(3.42169053587817,31.6659904387919,125.011483828701));
#123269=CARTESIAN_POINT('Ctrl Pts',(3.42230324180335,31.6658914832599,125.021484514393));
#123270=CARTESIAN_POINT('Ctrl Pts',(3.42757187605949,31.6642691668115,125.107316267364));
#123271=CARTESIAN_POINT('Ctrl Pts',(3.43227947183841,31.6576591413254,125.182953145629));
#123272=CARTESIAN_POINT('Ctrl Pts',(3.43803510316227,31.6440205893638,125.270006114265));
#123273=CARTESIAN_POINT('Ctrl Pts',(3.43884407433654,31.6419844131629,125.282124378797));
#123274=CARTESIAN_POINT('Ctrl Pts',(3.44012204237294,31.6385865334908,125.301062313955));
#123275=CARTESIAN_POINT('Ctrl Pts',(3.44058615310007,31.6373158124992,125.307898149363));
#123276=CARTESIAN_POINT('Ctrl Pts',(3.44145899199215,31.6348585608187,125.320671398859));
#123277=CARTESIAN_POINT('Ctrl Pts',(3.44186714411603,31.6336824047121,125.326610556756));
#123278=CARTESIAN_POINT('Ctrl Pts',(3.44283341824922,31.6308340380017,125.340593359794));
#123279=CARTESIAN_POINT('Ctrl Pts',(3.44339302404201,31.629134672667,125.348631191206));
#123280=CARTESIAN_POINT('Ctrl Pts',(3.44527697932228,31.6232457411608,125.375501643422));
#123281=CARTESIAN_POINT('Ctrl Pts',(3.44661486036773,31.6187886723666,125.39427322425));
#123282=CARTESIAN_POINT('Ctrl Pts',(3.44994491598246,31.6070026459566,125.440337320279));
#123283=CARTESIAN_POINT('Ctrl Pts',(3.45195164831175,31.599303442617,125.467528371332));
#123284=CARTESIAN_POINT('Ctrl Pts',(3.45602017567125,31.5824492453355,125.52175111791));
#123285=CARTESIAN_POINT('Ctrl Pts',(3.45808088852165,31.5732866945828,125.548759939466));
#123286=CARTESIAN_POINT('Ctrl Pts',(3.46014891354656,31.5634400625339,125.575509488075));
#123287=CARTESIAN_POINT('',(3.23000355491767,31.6660003196933,124.999395783345));
#123288=CARTESIAN_POINT('Ctrl Pts',(3.26654942290125,31.5634400114153,125.575509626944));
#123289=CARTESIAN_POINT('Ctrl Pts',(3.26608923191792,31.5659364284638,125.568727814589));
#123290=CARTESIAN_POINT('Ctrl Pts',(3.26563026442176,31.5683888288847,125.561929459962));
#123291=CARTESIAN_POINT('Ctrl Pts',(3.26175567718783,31.5887702507647,125.504256584977));
#123292=CARTESIAN_POINT('Ctrl Pts',(3.25840827363323,31.6042637027712,125.452553012212));
#123293=CARTESIAN_POINT('Ctrl Pts',(3.25136312741718,31.6317934377905,125.341300417692));
#123294=CARTESIAN_POINT('Ctrl Pts',(3.24767930295061,31.6431377050807,125.28166345445));
#123295=CARTESIAN_POINT('Ctrl Pts',(3.23940935061001,31.6610854010454,125.147894277671));
#123296=CARTESIAN_POINT('Ctrl Pts',(3.23481638988841,31.6660268335795,125.073679945117));
#123297=CARTESIAN_POINT('Ctrl Pts',(3.23000429551471,31.6659998904155,124.999395735533));
#123298=CARTESIAN_POINT('Ctrl Pts',(3.23000440964381,31.6659998910536,124.999397497343));
#123299=CARTESIAN_POINT('Ctrl Pts',(3.22944762951936,31.6659967827001,124.990802487001));
#123300=CARTESIAN_POINT('Ctrl Pts',(3.22888796913527,31.6659271610561,124.982207798573));
#123301=CARTESIAN_POINT('Ctrl Pts',(3.22781267407205,31.665667102016,124.965789721261));
#123302=CARTESIAN_POINT('Ctrl Pts',(3.22729759777495,31.6654880388823,124.957966386865));
#123303=CARTESIAN_POINT('Ctrl Pts',(3.22636902803633,31.6650681990382,124.943942980828));
#123304=CARTESIAN_POINT('Ctrl Pts',(3.2259565956253,31.664847885872,124.937742384129));
#123305=CARTESIAN_POINT('Ctrl Pts',(3.22516379738237,31.664360059699,124.925880406756));
#123306=CARTESIAN_POINT('Ctrl Pts',(3.2247837449481,31.664098279809,124.920218822269));
#123307=CARTESIAN_POINT('Ctrl Pts',(3.22396279904964,31.6634731437093,124.908045476223));
#123308=CARTESIAN_POINT('Ctrl Pts',(3.22352140189257,31.6631004340768,124.901534387878));
#123309=CARTESIAN_POINT('Ctrl Pts',(3.2223546176247,31.6620191634388,124.884408110011));
#123310=CARTESIAN_POINT('Ctrl Pts',(3.22162589643186,31.6612471462891,124.873797429269));
#123311=CARTESIAN_POINT('Ctrl Pts',(3.21840445398554,31.6574105836397,124.827233797765));
#123312=CARTESIAN_POINT('Ctrl Pts',(3.21586246647544,31.6532802809791,124.791381010853));
#123313=CARTESIAN_POINT('Ctrl Pts',(3.20562451751908,31.6322425991551,124.649469437146));
#123314=CARTESIAN_POINT('Ctrl Pts',(3.19771370889377,31.6062624843367,124.545017802866));
#123315=CARTESIAN_POINT('Ctrl Pts',(3.18602107104068,31.5521000669193,124.392094302889));
#123316=CARTESIAN_POINT('Ctrl Pts',(3.18211563770412,31.5312466637038,124.341328163862));
#123317=CARTESIAN_POINT('Ctrl Pts',(3.17653687767181,31.4972867537276,124.269031843283));
#123318=CARTESIAN_POINT('Ctrl Pts',(3.17480516696833,31.4861392970172,124.246626140132));
#123319=CARTESIAN_POINT('Ctrl Pts',(3.17168572395223,31.464948942663,124.206337117742));
#123320=CARTESIAN_POINT('Ctrl Pts',(3.17029267393445,31.4550727073158,124.188372217841));
#123321=CARTESIAN_POINT('Ctrl Pts',(3.16810179449721,31.4388857413205,124.160173726339));
#123322=CARTESIAN_POINT('Ctrl Pts',(3.16729632224105,31.432791771423,124.149818784408));
#123323=CARTESIAN_POINT('Ctrl Pts',(3.16578130769558,31.421060772584,124.130369774933));
#123324=CARTESIAN_POINT('Ctrl Pts',(3.16507096320784,31.4154471529324,124.121262374711));
#123325=CARTESIAN_POINT('Ctrl Pts',(3.16346296610323,31.4024837405915,124.100677428543));
#123326=CARTESIAN_POINT('Ctrl Pts',(3.16256735690727,31.3950799966663,124.089234634286));
#123327=CARTESIAN_POINT('Ctrl Pts',(3.160235832714,31.3753315034283,124.059518475247));
#123328=CARTESIAN_POINT('Ctrl Pts',(3.15880829835496,31.3627626754443,124.04139674227));
#123329=CARTESIAN_POINT('Ctrl Pts',(3.15024218807943,31.2845397643885,123.933264271455));
#123330=CARTESIAN_POINT('Ctrl Pts',(3.14344738531115,31.2103514671904,123.849773771238));
#123331=CARTESIAN_POINT('Ctrl Pts',(3.13062264146857,31.0558443368599,123.707534003338));
#123332=CARTESIAN_POINT('Ctrl Pts',(3.12461113188037,30.977537802283,123.647339615485));
#123333=CARTESIAN_POINT('Ctrl Pts',(3.11726684994839,30.8822912276902,123.586732995289));
#123334=CARTESIAN_POINT('Ctrl Pts',(3.1163261232019,30.8701003858477,123.579195044409));
#123335=CARTESIAN_POINT('Ctrl Pts',(3.11489137340451,30.8515526415955,123.568054661646));
#123336=CARTESIAN_POINT('Ctrl Pts',(3.11440451401603,30.8452664480177,123.564335004163));
#123337=CARTESIAN_POINT('Ctrl Pts',(3.11351242163061,30.8337669183006,123.55763222351));
#123338=CARTESIAN_POINT('Ctrl Pts',(3.11310804489819,30.8285616433028,123.554635798009));
#123339=CARTESIAN_POINT('Ctrl Pts',(3.11218109392786,30.8166461798106,123.547862159107));
#123340=CARTESIAN_POINT('Ctrl Pts',(3.11165741374762,30.8099259591167,123.544103291158));
#123341=CARTESIAN_POINT('Ctrl Pts',(3.11001138861411,30.7888311998346,123.532495460942));
#123342=CARTESIAN_POINT('Ctrl Pts',(3.10887961328207,30.7743673156416,123.524812064725));
#123343=CARTESIAN_POINT('Ctrl Pts',(3.10209237642772,30.6877357982926,123.480417399505));
#123344=CARTESIAN_POINT('Ctrl Pts',(3.09621494572295,30.6130889694828,123.448796836085));
#123345=CARTESIAN_POINT('Ctrl Pts',(3.08495771413926,30.4666583254375,123.39899407243));
#123346=CARTESIAN_POINT('Ctrl Pts',(3.07959224124605,30.3953660309375,123.3799145121));
#123347=CARTESIAN_POINT('Ctrl Pts',(3.07129888128102,30.2813555298315,123.357379953355));
#123348=CARTESIAN_POINT('Ctrl Pts',(3.06830306533877,30.2393676024499,123.350737981842));
#123349=CARTESIAN_POINT('Ctrl Pts',(3.06323022405642,30.1667908351939,123.342087839018));
#123350=CARTESIAN_POINT('Ctrl Pts',(3.06113171943038,30.1363175246406,123.339304464373));
#123351=CARTESIAN_POINT('Ctrl Pts',(3.05811240922627,30.0918347572182,123.336474310629));
#123352=CARTESIAN_POINT('Ctrl Pts',(3.05717116520443,30.0778755149462,123.335762406784));
#123353=CARTESIAN_POINT('Ctrl Pts',(3.0555164573438,30.0531780198984,123.334814300745));
#123354=CARTESIAN_POINT('Ctrl Pts',(3.05480078868459,30.0424435090379,123.334506117506));
#123355=CARTESIAN_POINT('Ctrl Pts',(3.05330384857882,30.0198839626366,123.334076696778));
#123356=CARTESIAN_POINT('Ctrl Pts',(3.052523305018,30.0080590671158,123.333977524833));
#123357=CARTESIAN_POINT('Ctrl Pts',(3.05045895808728,29.9766299898239,123.334048573286));
#123358=CARTESIAN_POINT('Ctrl Pts',(3.04918203802404,29.9570277972582,123.334438906566));
#123359=CARTESIAN_POINT('Ctrl Pts',(3.04257913310749,29.8549277744348,123.338275795651));
#123360=CARTESIAN_POINT('Ctrl Pts',(3.03743646908265,29.7727585324845,123.34750579861));
#123361=CARTESIAN_POINT('Ctrl Pts',(3.02621159844141,29.5931575752951,123.381336726373));
#123362=CARTESIAN_POINT('Ctrl Pts',(3.02018790806716,29.4965911241707,123.408721044981));
#123363=CARTESIAN_POINT('Ctrl Pts',(3.01213555699536,29.3766758060392,123.454741916964));
#123364=CARTESIAN_POINT('Ctrl Pts',(3.01034291568652,29.3505397920609,123.465543466888));
#123365=CARTESIAN_POINT('Ctrl Pts',(3.00727579188438,29.3070477952539,123.484828127528));
#123366=CARTESIAN_POINT('Ctrl Pts',(3.00601763132619,29.2895409791455,123.492957710288));
#123367=CARTESIAN_POINT('Ctrl Pts',(3.00419948125809,29.2647901500576,123.504978270309));
#123368=CARTESIAN_POINT('Ctrl Pts',(3.00365353948722,29.2574268638396,123.508621903689));
#123369=CARTESIAN_POINT('Ctrl Pts',(3.00269954974722,29.2446858423245,123.515044390292));
#123370=CARTESIAN_POINT('Ctrl Pts',(3.00229303096033,29.2392958145425,123.5177983334));
#123371=CARTESIAN_POINT('Ctrl Pts',(3.00141573962227,29.2277498676595,123.523777109051));
#123372=CARTESIAN_POINT('Ctrl Pts',(3.00094444123053,29.2215991742195,123.527011052084));
#123373=CARTESIAN_POINT('Ctrl Pts',(2.9996342504882,29.2046387967321,123.536064457668));
#123374=CARTESIAN_POINT('Ctrl Pts',(2.99879061122449,29.1938731841119,123.541964935139));
#123375=CARTESIAN_POINT('Ctrl Pts',(2.99285936166074,29.1191947573507,123.583974976772));
#123376=CARTESIAN_POINT('Ctrl Pts',(2.9875683876885,29.0576709083589,123.624151811937));
#123377=CARTESIAN_POINT('Ctrl Pts',(2.98122041712203,28.9878262569549,123.676649769886));
#123378=CARTESIAN_POINT('Ctrl Pts',(2.98020314425414,28.9767551095666,123.685191493708));
#123379=CARTESIAN_POINT('Ctrl Pts',(2.97382000014652,28.9079984609273,123.739633777752));
#123380=CARTESIAN_POINT('Ctrl Pts',(2.96845434657568,28.8533015165863,123.789184457528));
#123381=CARTESIAN_POINT('Ctrl Pts',(2.96016137272527,28.7725391977684,123.872746298215));
#123382=CARTESIAN_POINT('Ctrl Pts',(2.95716609284884,28.7441916692102,123.904414828906));
#123383=CARTESIAN_POINT('Ctrl Pts',(2.95209404791017,28.6975689721157,123.9606900851));
#123384=CARTESIAN_POINT('Ctrl Pts',(2.94999581271927,28.6787054374135,123.984779544265));
#123385=CARTESIAN_POINT('Ctrl Pts',(2.94697681219696,28.6522046429645,124.020612947446));
#123386=CARTESIAN_POINT('Ctrl Pts',(2.94603561434711,28.64403597099,124.031954083807));
#123387=CARTESIAN_POINT('Ctrl Pts',(2.94438095854266,28.6298448664701,124.052188719715));
#123388=CARTESIAN_POINT('Ctrl Pts',(2.9436652962379,28.6237640012545,124.06104004451));
#123389=CARTESIAN_POINT('Ctrl Pts',(2.9421683410089,28.6111676360915,124.079760630573));
#123390=CARTESIAN_POINT('Ctrl Pts',(2.94138777624414,28.6046707575993,124.089641746607));
#123391=CARTESIAN_POINT('Ctrl Pts',(2.93932330669706,28.5876834839577,124.11608686307));
#123392=CARTESIAN_POINT('Ctrl Pts',(2.9380462867162,28.5773791352406,124.132768598983));
#123393=CARTESIAN_POINT('Ctrl Pts',(2.93143992771044,28.525200352599,124.22067471995));
#123394=CARTESIAN_POINT('Ctrl Pts',(2.92629416486954,28.4883698025541,124.294763493629));
#123395=CARTESIAN_POINT('Ctrl Pts',(2.91506908605419,28.4193977524785,124.464015859961));
#123396=CARTESIAN_POINT('Ctrl Pts',(2.90904800629896,28.390049289096,124.559955877235));
#123397=CARTESIAN_POINT('Ctrl Pts',(2.90099879489973,28.3636883673267,124.685612482727));
#123398=CARTESIAN_POINT('Ctrl Pts',(2.89920650318679,28.3585893630659,124.713423289447));
#123399=CARTESIAN_POINT('Ctrl Pts',(2.89613991716965,28.3512044210566,124.760413709986));
#123400=CARTESIAN_POINT('Ctrl Pts',(2.89488193735399,28.3485398518485,124.77952834035));
#123401=CARTESIAN_POINT('Ctrl Pts',(2.89306400327071,28.3452153465866,124.806838827014));
#123402=CARTESIAN_POINT('Ctrl Pts',(2.89251809219995,28.3442830075713,124.815000751605));
#123403=CARTESIAN_POINT('Ctrl Pts',(2.89156413706995,28.3427686209241,124.829187836868));
#123404=CARTESIAN_POINT('Ctrl Pts',(2.89115762184814,28.3421589845353,124.835209815321));
#123405=CARTESIAN_POINT('Ctrl Pts',(2.89028031554994,28.340919903072,124.84815295074));
#123406=CARTESIAN_POINT('Ctrl Pts',(2.88980899841296,28.3403009503174,124.855074658979));
#123407=CARTESIAN_POINT('Ctrl Pts',(2.88849870597299,28.3387083217207,124.874235518156));
#123408=CARTESIAN_POINT('Ctrl Pts',(2.88765498261459,28.3378266359041,124.886481583925));
#123409=CARTESIAN_POINT('Ctrl Pts',(2.88170085173004,28.3325984551041,124.972336661931));
#123410=CARTESIAN_POINT('Ctrl Pts',(2.87638526315512,28.3330083071948,125.046146050823));
#123411=CARTESIAN_POINT('Ctrl Pts',(2.87011512066167,28.3392074572243,125.132220663024));
#123412=CARTESIAN_POINT('Ctrl Pts',(2.86920022172322,28.3402529134883,125.144754205294));
#123413=CARTESIAN_POINT('Ctrl Pts',(2.86279641950432,28.3485594398537,125.232351735376));
#123414=CARTESIAN_POINT('Ctrl Pts',(2.85730583372106,28.3607686736817,125.30686367938));
#123415=CARTESIAN_POINT('Ctrl Pts',(2.84891951398021,28.3876037615196,125.42131913763));
#123416=CARTESIAN_POINT('Ctrl Pts',(2.84594972126466,28.3987755656737,125.46196563411));
#123417=CARTESIAN_POINT('Ctrl Pts',(2.84091556729559,28.4206422099122,125.531139818426));
#123418=CARTESIAN_POINT('Ctrl Pts',(2.83883016903536,28.4305993735213,125.559877146311));
#123419=CARTESIAN_POINT('Ctrl Pts',(2.8358259288854,28.4462622815148,125.601373041239));
#123420=CARTESIAN_POINT('Ctrl Pts',(2.8348869358725,28.451350113537,125.614356559547));
#123421=CARTESIAN_POINT('Ctrl Pts',(2.83323476396836,28.4606421420797,125.637219437581));
#123422=CARTESIAN_POINT('Ctrl Pts',(2.83251940317294,28.4647798894719,125.647124754489));
#123423=CARTESIAN_POINT('Ctrl Pts',(2.83102171578353,28.473682733824,125.667871106731));
#123424=CARTESIAN_POINT('Ctrl Pts',(2.83024013049114,28.4784682753279,125.678702759118));
#123425=CARTESIAN_POINT('Ctrl Pts',(2.82816975939818,28.4915141137239,125.70739923356));
#123426=CARTESIAN_POINT('Ctrl Pts',(2.82688793048867,28.4999763349493,125.725170602168));
#123427=CARTESIAN_POINT('Ctrl Pts',(2.82008673483577,28.5469034763966,125.819383178545));
#123428=CARTESIAN_POINT('Ctrl Pts',(2.81476574922657,28.5909018149036,125.892929611599));
#123429=CARTESIAN_POINT('Ctrl Pts',(2.80352647892542,28.6967605444655,126.042423763495));
#123430=CARTESIAN_POINT('Ctrl Pts',(2.79765157040846,28.7600447450523,126.116955270718));
#123431=CARTESIAN_POINT('Ctrl Pts',(2.78977841579008,28.849368766442,126.20514924836));
#123432=CARTESIAN_POINT('Ctrl Pts',(2.78800603449176,28.8697443248551,126.224278922585));
#123433=CARTESIAN_POINT('Ctrl Pts',(2.78497009847331,28.9048667440436,126.255629471254));
#123434=CARTESIAN_POINT('Ctrl Pts',(2.7837224369373,28.9193611498396,126.268125315913));
#123435=CARTESIAN_POINT('Ctrl Pts',(2.78191683718211,28.9403595034149,126.285606884402));
#123436=CARTESIAN_POINT('Ctrl Pts',(2.78137268404044,28.9466905802202,126.290799094551));
#123437=CARTESIAN_POINT('Ctrl Pts',(2.78042070779235,28.9577653864412,126.299745978419));
#123438=CARTESIAN_POINT('Ctrl Pts',(2.78001439378176,28.9624917079205,126.303521822067));
#123439=CARTESIAN_POINT('Ctrl Pts',(2.77913621763289,28.972703854175,126.311589546725));
#123440=CARTESIAN_POINT('Ctrl Pts',(2.77866381676206,28.9781959755135,126.315872729946));
#123441=CARTESIAN_POINT('Ctrl Pts',(2.77734764052124,28.9934984812606,126.327653247953));
#123442=CARTESIAN_POINT('Ctrl Pts',(2.77649905079012,29.0033653714899,126.335075971174));
#123443=CARTESIAN_POINT('Ctrl Pts',(2.77002521186004,29.0787102163956,126.390456188607));
#123444=CARTESIAN_POINT('Ctrl Pts',(2.76415222016676,29.1475251621098,126.433676055205));
#123445=CARTESIAN_POINT('Ctrl Pts',(2.75366050534591,29.2749321145779,126.501270138842));
#123446=CARTESIAN_POINT('Ctrl Pts',(2.7490606523328,29.332294547713,126.527647032274));
#123447=CARTESIAN_POINT('Ctrl Pts',(2.73887014809178,29.4641319206823,126.579421344778));
#123448=CARTESIAN_POINT('Ctrl Pts',(2.73332826459998,29.5391952837345,126.602931260864));
#123449=CARTESIAN_POINT('Ctrl Pts',(2.72665930936424,29.6341094845195,126.625435361452));
#123450=CARTESIAN_POINT('Ctrl Pts',(2.72537215889611,29.6526449550512,126.629497010733));
#123451=CARTESIAN_POINT('Ctrl Pts',(2.72330822395127,29.6827072610619,126.635548223058));
#123452=CARTESIAN_POINT('Ctrl Pts',(2.72252525086594,29.6941922814834,126.637734509461));
#123453=CARTESIAN_POINT('Ctrl Pts',(2.7210278618457,29.7163074629667,126.641703595438));
#123454=CARTESIAN_POINT('Ctrl Pts',(2.72031290691692,29.7269337344024,126.643504479683));
#123455=CARTESIAN_POINT('Ctrl Pts',(2.71867534903226,29.7514215874654,126.647410490299));
#123456=CARTESIAN_POINT('Ctrl Pts',(2.71775504441344,29.7652938856565,126.649444030723));
#123457=CARTESIAN_POINT('Ctrl Pts',(2.71476910960261,29.8106422456316,126.655507939296));
#123458=CARTESIAN_POINT('Ctrl Pts',(2.71272605736257,29.842209151933,126.658814381774));
#123459=CARTESIAN_POINT('Ctrl Pts',(2.70264383453606,30.0001853716208,126.670810543705));
#123460=CARTESIAN_POINT('Ctrl Pts',(2.69502837993978,30.1271975408264,126.665962365335));
#123461=CARTESIAN_POINT('Ctrl Pts',(2.6840836703434,30.3034387242932,126.63894573199));
#123462=CARTESIAN_POINT('Ctrl Pts',(2.68089014888625,30.3540450708383,126.628763186564));
#123463=CARTESIAN_POINT('Ctrl Pts',(2.67575857260075,30.4323620649775,126.609182433477));
#123464=CARTESIAN_POINT('Ctrl Pts',(2.67387974124537,30.4604382687125,126.601374852077));
#123465=CARTESIAN_POINT('Ctrl Pts',(2.67133209660001,30.4974608902823,126.590025347803));
#123466=CARTESIAN_POINT('Ctrl Pts',(2.67069717887378,30.5066038302762,126.587135940091));
#123467=CARTESIAN_POINT('Ctrl Pts',(2.6696380099088,30.5217068213611,126.582219207083));
#123468=CARTESIAN_POINT('Ctrl Pts',(2.66921630901507,30.5276814041959,126.580236678435));
#123469=CARTESIAN_POINT('Ctrl Pts',(2.66835992027973,30.5397331294258,126.576161621997));
#123470=CARTESIAN_POINT('Ctrl Pts',(2.66792516509816,30.5458096487933,126.574067702927));
#123471=CARTESIAN_POINT('Ctrl Pts',(2.66679496470894,30.5615028776378,126.568558148879));
#123472=CARTESIAN_POINT('Ctrl Pts',(2.66609654053953,30.5711004209757,126.565089276706));
#123473=CARTESIAN_POINT('Ctrl Pts',(2.66319956791773,30.610523130223,126.550429707478));
#123474=CARTESIAN_POINT('Ctrl Pts',(2.66096281499383,30.6400542742139,126.538473589378));
#123475=CARTESIAN_POINT('Ctrl Pts',(2.65097345311355,30.7687205971854,126.482035546318));
#123476=CARTESIAN_POINT('Ctrl Pts',(2.64296767709374,30.8637088123153,126.428764377939));
#123477=CARTESIAN_POINT('Ctrl Pts',(2.63099559960946,30.999766338879,126.333902798652));
#123478=CARTESIAN_POINT('Ctrl Pts',(2.62691451983526,31.0449857240352,126.29878225012));
#123479=CARTESIAN_POINT('Ctrl Pts',(2.62027792440761,31.1168554941155,126.23677444253));
#123480=CARTESIAN_POINT('Ctrl Pts',(2.61767839377811,31.1445567531923,126.211184316766));
#123481=CARTESIAN_POINT('Ctrl Pts',(2.614091632524,31.1821170212712,126.174045934805));
#123482=CARTESIAN_POINT('Ctrl Pts',(2.61307157974278,31.1927213509525,126.16327138457));
#123483=CARTESIAN_POINT('Ctrl Pts',(2.61132612552146,31.210726921053,126.144471684482));
#123484=CARTESIAN_POINT('Ctrl Pts',(2.61059770023467,31.2181984833588,126.136515542723));
#123485=CARTESIAN_POINT('Ctrl Pts',(2.60911653368624,31.2333002529586,126.12011428141));
#123486=CARTESIAN_POINT('Ctrl Pts',(2.60836412313826,31.2409231959974,126.111663235817));
#123487=CARTESIAN_POINT('Ctrl Pts',(2.60646364308394,31.2600484018051,126.090018517044));
#123488=CARTESIAN_POINT('Ctrl Pts',(2.60532057092064,31.2714306282132,126.076720269119));
#123489=CARTESIAN_POINT('Ctrl Pts',(2.60073648248559,31.3165468031565,126.022296225832));
#123490=CARTESIAN_POINT('Ctrl Pts',(2.59736567137769,31.3485137854623,125.97974306972));
#123491=CARTESIAN_POINT('Ctrl Pts',(2.58601116936331,31.4507215337578,125.829184216894));
#123492=CARTESIAN_POINT('Ctrl Pts',(2.57834874049672,31.51044843214,125.714620214557));
#123493=CARTESIAN_POINT('Ctrl Pts',(2.56988925421428,31.5587739581986,125.588068557324));
#123494=CARTESIAN_POINT('Ctrl Pts',(2.56946987217007,31.5611259847506,125.581795954251));
#123495=CARTESIAN_POINT('Ctrl Pts',(2.56904933390813,31.5634400118358,125.575509625802));
#123496=CARTESIAN_POINT('Origin',(5.,30.,125.));
#123497=CARTESIAN_POINT('',(1.86811695019056,31.5634399562749,125.57550977674));
#123498=CARTESIAN_POINT('',(2.06219312175648,31.563440011958,125.57550962547));
#123499=CARTESIAN_POINT('',(5.,31.5634400119422,125.575509625513));
#123500=CARTESIAN_POINT('',(2.72302676052858,31.665999544352,124.999966471175));
#123501=CARTESIAN_POINT('Ctrl Pts',(2.06219312175648,31.563440011958,125.57550962547));
#123502=CARTESIAN_POINT('Ctrl Pts',(2.06231484708762,31.5627891862177,125.577277670622));
#123503=CARTESIAN_POINT('Ctrl Pts',(2.06243648101149,31.5621353548853,125.579044629305));
#123504=CARTESIAN_POINT('Ctrl Pts',(2.06925164381925,31.5253054375802,125.67805992843));
#123505=CARTESIAN_POINT('Ctrl Pts',(2.0756324149288,31.4801251938429,125.771722157109));
#123506=CARTESIAN_POINT('Ctrl Pts',(2.0887983756326,31.3688101572776,125.956240348087));
#123507=CARTESIAN_POINT('Ctrl Pts',(2.09554812002998,31.3016343222387,126.045838354362));
#123508=CARTESIAN_POINT('Ctrl Pts',(2.10377396890585,31.215922015026,126.138995948441));
#123509=CARTESIAN_POINT('Ctrl Pts',(2.1047512882903,31.2056846823302,126.149827172351));
#123510=CARTESIAN_POINT('Ctrl Pts',(2.10623075533151,31.1901357690531,126.165842139739));
#123511=CARTESIAN_POINT('Ctrl Pts',(2.10672505754805,31.184932296468,126.171130433003));
#123512=CARTESIAN_POINT('Ctrl Pts',(2.10762436945739,31.1754543445013,126.180635054225));
#123513=CARTESIAN_POINT('Ctrl Pts',(2.10802843681176,31.1711921621607,126.184863267796));
#123514=CARTESIAN_POINT('Ctrl Pts',(2.10894648309864,31.1615003415256,126.194374457592));
#123515=CARTESIAN_POINT('Ctrl Pts',(2.10946147379547,31.156057504266,126.199643459335));
#123516=CARTESIAN_POINT('Ctrl Pts',(2.11105255777801,31.1392174230616,126.21572466635));
#123517=CARTESIAN_POINT('Ctrl Pts',(2.11213723569339,31.1277033981437,126.226412574405));
#123518=CARTESIAN_POINT('Ctrl Pts',(2.11776959276997,31.0676605524709,126.280586978131));
#123519=CARTESIAN_POINT('Ctrl Pts',(2.12246258437263,31.0167657922176,126.321358290381));
#123520=CARTESIAN_POINT('Ctrl Pts',(2.1355219105744,30.8700428474146,126.425391383337));
#123521=CARTESIAN_POINT('Ctrl Pts',(2.14391103957429,30.7698494470602,126.481908590973));
#123522=CARTESIAN_POINT('Ctrl Pts',(2.15501367498537,30.6250688167146,126.544897028975));
#123523=CARTESIAN_POINT('Ctrl Pts',(2.15800227012495,30.5848453769678,126.560568589754));
#123524=CARTESIAN_POINT('Ctrl Pts',(2.1620521663546,30.5286065892752,126.579999440152));
#123525=CARTESIAN_POINT('Ctrl Pts',(2.16315718987412,30.5130795851568,126.585109626958));
#123526=CARTESIAN_POINT('Ctrl Pts',(2.16492841791662,30.487903858439,126.592986657812));
#123527=CARTESIAN_POINT('Ctrl Pts',(2.16559924956397,30.4783012738165,126.595896163953));
#123528=CARTESIAN_POINT('Ctrl Pts',(2.16699408313781,30.4581967224745,126.601789918692));
#123529=CARTESIAN_POINT('Ctrl Pts',(2.16771753186965,30.4476904990334,126.604758052427));
#123530=CARTESIAN_POINT('Ctrl Pts',(2.16943499196601,30.4225663754263,126.611589973862));
#123531=CARTESIAN_POINT('Ctrl Pts',(2.17042589069407,30.407923400741,126.615358508011));
#123532=CARTESIAN_POINT('Ctrl Pts',(2.173866020572,30.356598324263,126.627825156942));
#123533=CARTESIAN_POINT('Ctrl Pts',(2.17628206571861,30.3196725064753,126.635477585654));
#123534=CARTESIAN_POINT('Ctrl Pts',(2.18228518652278,30.2261383791953,126.651571989087));
#123535=CARTESIAN_POINT('Ctrl Pts',(2.18582633457376,30.1692951335907,126.658363193327));
#123536=CARTESIAN_POINT('Ctrl Pts',(2.19599832498569,30.003904166691,126.669528323762));
#123537=CARTESIAN_POINT('Ctrl Pts',(2.20251400819836,29.8951508506819,126.666236113557));
#123538=CARTESIAN_POINT('Ctrl Pts',(2.21140813023452,29.7558176380258,126.648317752978));
#123539=CARTESIAN_POINT('Ctrl Pts',(2.21346072168204,29.7242603312846,126.643333126849));
#123540=CARTESIAN_POINT('Ctrl Pts',(2.21622941755561,29.6828261808594,126.635561420476));
#123541=CARTESIAN_POINT('Ctrl Pts',(2.2169050000686,29.6728019286809,126.633585565818));
#123542=CARTESIAN_POINT('Ctrl Pts',(2.2180140722637,29.6564987501744,126.630216013647));
#123543=CARTESIAN_POINT('Ctrl Pts',(2.21844450520571,29.6502084273531,126.628877899647));
#123544=CARTESIAN_POINT('Ctrl Pts',(2.21930049520768,29.6377760348753,126.6261578747));
#123545=CARTESIAN_POINT('Ctrl Pts',(2.2197259641605,29.6316337664497,126.624777507278));
#123546=CARTESIAN_POINT('Ctrl Pts',(2.22080404156066,29.6161600013267,126.621207798638));
#123547=CARTESIAN_POINT('Ctrl Pts',(2.22145914551838,29.6068394175093,126.618972704018));
#123548=CARTESIAN_POINT('Ctrl Pts',(2.2241186656368,29.5693100586655,126.60962990419));
#123549=CARTESIAN_POINT('Ctrl Pts',(2.22615526131399,29.5412720904004,126.601864761229));
#123550=CARTESIAN_POINT('Ctrl Pts',(2.23186336714723,29.4642406198312,126.57834269446));
#123551=CARTESIAN_POINT('Ctrl Pts',(2.23558409626776,29.4157528725329,126.561044017813));
#123552=CARTESIAN_POINT('Ctrl Pts',(2.24849224655666,29.2514118472204,126.493682762023));
#123553=CARTESIAN_POINT('Ctrl Pts',(2.25769400967526,29.1404691927851,126.432720832713));
#123554=CARTESIAN_POINT('Ctrl Pts',(2.26870870646079,29.0111645325439,126.341192991018));
#123555=CARTESIAN_POINT('Ctrl Pts',(2.27092173493167,28.9854091633001,126.321816894845));
#123556=CARTESIAN_POINT('Ctrl Pts',(2.27406198197868,28.9492106248379,126.292902395978));
#123557=CARTESIAN_POINT('Ctrl Pts',(2.27501235043641,28.9383027832521,126.283960263277));
#123558=CARTESIAN_POINT('Ctrl Pts',(2.27668009619661,28.9192505697169,126.267932628841));
#123559=CARTESIAN_POINT('Ctrl Pts',(2.27739974508893,28.9110591727596,126.260904582646));
#123560=CARTESIAN_POINT('Ctrl Pts',(2.27889001156984,28.8941621673948,126.246119825689));
#123561=CARTESIAN_POINT('Ctrl Pts',(2.27966004370379,28.885468505363,126.238350310336));
#123562=CARTESIAN_POINT('Ctrl Pts',(2.28166278776605,28.8629619861222,126.217807241287));
#123563=CARTESIAN_POINT('Ctrl Pts',(2.28288935440913,28.8492824267927,126.204889636175));
#123564=CARTESIAN_POINT('Ctrl Pts',(2.2890017913848,28.7817082453176,126.138878546755));
#123565=CARTESIAN_POINT('Ctrl Pts',(2.29373535362855,28.7312522112861,126.082386373105));
#123566=CARTESIAN_POINT('Ctrl Pts',(2.30239056060592,28.6450207047523,125.971487511175));
#123567=CARTESIAN_POINT('Ctrl Pts',(2.3063251398579,28.6082550963964,125.918043077578));
#123568=CARTESIAN_POINT('Ctrl Pts',(2.31497358055427,28.5351393486953,125.797230345943));
#123569=CARTESIAN_POINT('Ctrl Pts',(2.31969069810125,28.5001297080804,125.729232017946));
#123570=CARTESIAN_POINT('Ctrl Pts',(2.32568657328166,28.4635257513297,125.644254228056));
#123571=CARTESIAN_POINT('Ctrl Pts',(2.32674289278498,28.4573552313602,125.629335918189));
#123572=CARTESIAN_POINT('Ctrl Pts',(2.32832540632171,28.448538604023,125.607111082976));
#123573=CARTESIAN_POINT('Ctrl Pts',(2.32884227884974,28.4457250555176,125.599871420605));
#123574=CARTESIAN_POINT('Ctrl Pts',(2.32976454291645,28.4408238590203,125.586993954589));
#123575=CARTESIAN_POINT('Ctrl Pts',(2.33016873343164,28.4387159526978,125.581364139575));
#123576=CARTESIAN_POINT('Ctrl Pts',(2.33106474337751,28.4341316668017,125.568915623458));
#123577=CARTESIAN_POINT('Ctrl Pts',(2.33155732981303,28.4316693626588,125.562092190422));
#123578=CARTESIAN_POINT('Ctrl Pts',(2.33301304691124,28.4245598212857,125.541980100141));
#123579=CARTESIAN_POINT('Ctrl Pts',(2.33398284829192,28.4200365011293,125.528648744649));
#123580=CARTESIAN_POINT('Ctrl Pts',(2.3407725054562,28.3897986134358,125.435673942654));
#123581=CARTESIAN_POINT('Ctrl Pts',(2.34684448950259,28.3699509518981,125.354256299569));
#123582=CARTESIAN_POINT('Ctrl Pts',(2.36230371302771,28.3353092941659,125.144687285004));
#123583=CARTESIAN_POINT('Ctrl Pts',(2.37163215567612,28.3291029829872,125.015642098542));
#123584=CARTESIAN_POINT('Ctrl Pts',(2.38193366428839,28.3392461574188,124.866238622592));
#123585=CARTESIAN_POINT('Ctrl Pts',(2.38336373979404,28.3410607293745,124.845352020939));
#123586=CARTESIAN_POINT('Ctrl Pts',(2.38568206348581,28.3446716199138,124.811264139324));
#123587=CARTESIAN_POINT('Ctrl Pts',(2.38657752852385,28.3462328467409,124.798040866294));
#123588=CARTESIAN_POINT('Ctrl Pts',(2.38818179854772,28.3493308181814,124.774254223855));
#123589=CARTESIAN_POINT('Ctrl Pts',(2.38889234291897,28.3508108592451,124.763684341683));
#123590=CARTESIAN_POINT('Ctrl Pts',(2.39040987926162,28.3542037689673,124.741040174056));
#123591=CARTESIAN_POINT('Ctrl Pts',(2.39121583326844,28.3561481745557,124.72897119179));
#123592=CARTESIAN_POINT('Ctrl Pts',(2.39342684271795,28.3618753986251,124.695754578958));
#123593=CARTESIAN_POINT('Ctrl Pts',(2.39482313524652,28.3659347605844,124.674656569582));
#123594=CARTESIAN_POINT('Ctrl Pts',(2.40352072320405,28.3939924887682,124.542646159419));
#123595=CARTESIAN_POINT('Ctrl Pts',(2.41045532144491,28.4288623700194,124.43434704776));
#123596=CARTESIAN_POINT('Ctrl Pts',(2.42343326398717,28.5142820621516,124.23973181976));
#123597=CARTESIAN_POINT('Ctrl Pts',(2.42946142027302,28.5620910209305,124.152782142219));
#123598=CARTESIAN_POINT('Ctrl Pts',(2.4369187935266,28.626246403007,124.05733749447));
#123599=CARTESIAN_POINT('Ctrl Pts',(2.43796541666402,28.6353543180777,124.044199988772));
#123600=CARTESIAN_POINT('Ctrl Pts',(2.43952909600102,28.6490852029212,124.024990565933));
#123601=CARTESIAN_POINT('Ctrl Pts',(2.44003693506263,28.6535634232798,124.018815652042));
#123602=CARTESIAN_POINT('Ctrl Pts',(2.44094978134239,28.6616427152804,124.007834770874));
#123603=CARTESIAN_POINT('Ctrl Pts',(2.44135369022403,28.6652275899375,124.003017214677));
#123604=CARTESIAN_POINT('Ctrl Pts',(2.44225749895012,28.6732709598002,123.992329224982));
#123605=CARTESIAN_POINT('Ctrl Pts',(2.44275825603309,28.6777423609436,123.98646901));
#123606=CARTESIAN_POINT('Ctrl Pts',(2.4442625596831,28.6912234478525,123.969041752596));
#123607=CARTESIAN_POINT('Ctrl Pts',(2.44527343738382,28.7003468249733,123.957564122197));
#123608=CARTESIAN_POINT('Ctrl Pts',(2.44765198017155,28.7219879545002,123.931064298304));
#123609=CARTESIAN_POINT('Ctrl Pts',(2.44902595940349,28.7346209170494,123.916139294703));
#123610=CARTESIAN_POINT('Ctrl Pts',(2.45400059784178,28.7809200023238,123.86335288));
#123611=CARTESIAN_POINT('Ctrl Pts',(2.4576622429291,28.8160450206779,123.826810886431));
#123612=CARTESIAN_POINT('Ctrl Pts',(2.47029424685196,28.9421087011361,123.707096917967));
#123613=CARTESIAN_POINT('Ctrl Pts',(2.47928650658561,29.0405886223175,123.632421515674));
#123614=CARTESIAN_POINT('Ctrl Pts',(2.49027513645961,29.1759058271934,123.551689187209));
#123615=CARTESIAN_POINT('Ctrl Pts',(2.49263963166935,29.2059370662376,123.535008610103));
#123616=CARTESIAN_POINT('Ctrl Pts',(2.49589057643095,29.248495607888,123.513063423203));
#123617=CARTESIAN_POINT('Ctrl Pts',(2.49680445631832,29.2606021770034,123.507006325224));
#123618=CARTESIAN_POINT('Ctrl Pts',(2.49838425131612,29.2817751986499,123.496733869181));
#123619=CARTESIAN_POINT('Ctrl Pts',(2.49905246958652,29.2908081090442,123.492451395588));
#123620=CARTESIAN_POINT('Ctrl Pts',(2.50044667841361,29.3098140892484,123.483649354386));
#123621=CARTESIAN_POINT('Ctrl Pts',(2.50117207549156,29.3197942986351,123.479146264294));
#123622=CARTESIAN_POINT('Ctrl Pts',(2.50290305226282,29.3438240237021,123.46858786835));
#123623=CARTESIAN_POINT('Ctrl Pts',(2.50390538625201,29.3579141327025,123.462626982969));
#123624=CARTESIAN_POINT('Ctrl Pts',(2.50743613085758,29.4081432165906,123.442188380183));
#123625=CARTESIAN_POINT('Ctrl Pts',(2.50992888344628,29.4447068368197,123.428783475297));
#123626=CARTESIAN_POINT('Ctrl Pts',(2.51618095379018,29.5387567160002,123.397996939118));
#123627=CARTESIAN_POINT('Ctrl Pts',(2.51988887958108,29.5967749617278,123.382418617265));
#123628=CARTESIAN_POINT('Ctrl Pts',(2.52702891407718,29.7107654582403,123.358327421136));
#123629=CARTESIAN_POINT('Ctrl Pts',(2.53046000823088,29.7665778892013,123.349466901731));
#123630=CARTESIAN_POINT('Ctrl Pts',(2.5385518614802,29.897655105699,123.335440214263));
#123631=CARTESIAN_POINT('Ctrl Pts',(2.54323033156511,29.973026660294,123.332515881254));
#123632=CARTESIAN_POINT('Ctrl Pts',(2.54895351809678,30.060607536818,123.335057455553));
#123633=CARTESIAN_POINT('Ctrl Pts',(2.5497623578414,30.0728837701607,123.335549675095));
#123634=CARTESIAN_POINT('Ctrl Pts',(2.55104016287578,30.0920964744503,123.33653296466));
#123635=CARTESIAN_POINT('Ctrl Pts',(2.55150424404567,30.0990375098509,123.336931779652));
#123636=CARTESIAN_POINT('Ctrl Pts',(2.55237706055531,30.1120182708224,123.337759172637));
#123637=CARTESIAN_POINT('Ctrl Pts',(2.55278522023267,30.1180584180493,123.338177245793));
#123638=CARTESIAN_POINT('Ctrl Pts',(2.55375155740589,30.1322896458728,123.339240246437));
#123639=CARTESIAN_POINT('Ctrl Pts',(2.55431121927308,30.1404783815892,123.339912855694));
#123640=CARTESIAN_POINT('Ctrl Pts',(2.55619556524564,30.1678824483649,123.342367987097));
#123641=CARTESIAN_POINT('Ctrl Pts',(2.557533788259,30.18707093269,123.344423727673));
#123642=CARTESIAN_POINT('Ctrl Pts',(2.56086488577724,30.2342676960707,123.350311042706));
#123643=CARTESIAN_POINT('Ctrl Pts',(2.56287232893253,30.2622219442267,123.354523023291));
#123644=CARTESIAN_POINT('Ctrl Pts',(2.57206819547035,30.3886012888545,123.376867161957));
#123645=CARTESIAN_POINT('Ctrl Pts',(2.57942869852923,30.485377674129,123.403134278938));
#123646=CARTESIAN_POINT('Ctrl Pts',(2.59260681628881,30.6567380705163,123.466674320744));
#123647=CARTESIAN_POINT('Ctrl Pts',(2.59845512517556,30.7320252577369,123.501155356578));
#123648=CARTESIAN_POINT('Ctrl Pts',(2.60545625046126,30.8216132380106,123.550554652936));
#123649=CARTESIAN_POINT('Ctrl Pts',(2.60678684558914,30.8386084050745,123.560320825025));
#123650=CARTESIAN_POINT('Ctrl Pts',(2.60890305469828,30.8655760375088,123.576457243498));
#123651=CARTESIAN_POINT('Ctrl Pts',(2.60969543792399,30.8756594224334,123.582637504135));
#123652=CARTESIAN_POINT('Ctrl Pts',(2.61120009286179,30.8947750738458,123.594635645858));
#123653=CARTESIAN_POINT('Ctrl Pts',(2.61191301399459,30.9038185011594,123.600434522128));
#123654=CARTESIAN_POINT('Ctrl Pts',(2.61354669239935,30.9245050753181,123.613983417353));
#123655=CARTESIAN_POINT('Ctrl Pts',(2.6144651558284,30.9361080885384,123.621793459603));
#123656=CARTESIAN_POINT('Ctrl Pts',(2.61737831692675,30.9728054088336,123.64717188037));
#123657=CARTESIAN_POINT('Ctrl Pts',(2.61935230839179,30.9975149960066,123.665287182066));
#123658=CARTESIAN_POINT('Ctrl Pts',(2.62401605168759,31.0553314988408,123.710177134437));
#123659=CARTESIAN_POINT('Ctrl Pts',(2.62668316303981,31.0879395739724,123.737559719633));
#123660=CARTESIAN_POINT('Ctrl Pts',(2.63389014695948,31.1740370188715,123.815676234277));
#123661=CARTESIAN_POINT('Ctrl Pts',(2.6383626786391,31.225265292257,123.868756865402));
#123662=CARTESIAN_POINT('Ctrl Pts',(2.6437323767735,31.2818980296044,123.935814032153));
#123663=CARTESIAN_POINT('Ctrl Pts',(2.64459517191213,31.2908479117433,123.94668808275));
#123664=CARTESIAN_POINT('Ctrl Pts',(2.64995707834337,31.3454557633846,124.014777709002));
#123665=CARTESIAN_POINT('Ctrl Pts',(2.65450878543387,31.3874339340077,124.074830530808));
#123666=CARTESIAN_POINT('Ctrl Pts',(2.66009107837441,31.4316798645555,124.14794394671));
#123667=CARTESIAN_POINT('Ctrl Pts',(2.66089940093836,31.437920239317,124.158517905049));
#123668=CARTESIAN_POINT('Ctrl Pts',(2.66217656454987,31.4475093262418,124.175184224375));
#123669=CARTESIAN_POINT('Ctrl Pts',(2.66264052940382,31.4509378877096,124.181230462884));
#123670=CARTESIAN_POINT('Ctrl Pts',(2.66351325792558,31.4572822840432,124.192583743911));
#123671=CARTESIAN_POINT('Ctrl Pts',(2.66392144742188,31.4602071498572,124.197885456556));
#123672=CARTESIAN_POINT('Ctrl Pts',(2.66488803309729,31.467034181087,124.210421458564));
#123673=CARTESIAN_POINT('Ctrl Pts',(2.66544791596296,31.4709117806914,124.217668811874));
#123674=CARTESIAN_POINT('Ctrl Pts',(2.66733380230659,31.4837220759187,124.242043574492));
#123675=CARTESIAN_POINT('Ctrl Pts',(2.66867337369049,31.4924101193453,124.259296889656));
#123676=CARTESIAN_POINT('Ctrl Pts',(2.67200858040578,31.5130845801798,124.302194703582));
#123677=CARTESIAN_POINT('Ctrl Pts',(2.67401882737852,31.5247209155569,124.328000649385));
#123678=CARTESIAN_POINT('Ctrl Pts',(2.68179150686038,31.5667759875388,124.427989187578));
#123679=CARTESIAN_POINT('Ctrl Pts',(2.68766344128463,31.5924827800888,124.504034784201));
#123680=CARTESIAN_POINT('Ctrl Pts',(2.70088063835712,31.6382248331295,124.680349949422));
#123681=CARTESIAN_POINT('Ctrl Pts',(2.70815570515403,31.6547206185765,124.78122367749));
#123682=CARTESIAN_POINT('Ctrl Pts',(2.71647465747929,31.6632548411833,124.902433088291));
#123683=CARTESIAN_POINT('Ctrl Pts',(2.71779867745289,31.6642825973897,124.921900954));
#123684=CARTESIAN_POINT('Ctrl Pts',(2.71988334606309,31.6653712535199,124.95282341065));
#123685=CARTESIAN_POINT('Ctrl Pts',(2.72065089605411,31.6656561060218,124.964267795548));
#123686=CARTESIAN_POINT('Ctrl Pts',(2.7219542101763,31.6659408291883,124.983797869167));
#123687=CARTESIAN_POINT('Ctrl Pts',(2.7224917965327,31.6659998375613,124.991882126584));
#123688=CARTESIAN_POINT('Ctrl Pts',(2.72302755883131,31.6659999996651,124.999966594594));
#123689=CARTESIAN_POINT('Ctrl Pts',(2.72302754719672,31.6659999996616,124.999966419032));
#123690=CARTESIAN_POINT('Ctrl Pts',(2.72339558096022,31.6660001116015,125.005519921113));
#123691=CARTESIAN_POINT('Ctrl Pts',(2.72376274997295,31.6659724551936,125.011073458905));
#123692=CARTESIAN_POINT('Ctrl Pts',(2.72472346752639,31.6658270924562,125.025638010347));
#123693=CARTESIAN_POINT('Ctrl Pts',(2.72531560230014,31.6656640414659,125.034648460313));
#123694=CARTESIAN_POINT('Ctrl Pts',(2.7272324465681,31.6648967006198,125.063920793919));
#123695=CARTESIAN_POINT('Ctrl Pts',(2.72854800141681,31.6639957203849,125.084173578587));
#123696=CARTESIAN_POINT('Ctrl Pts',(2.73600252008977,31.6567396460939,125.199731153278));
#123697=CARTESIAN_POINT('Ctrl Pts',(2.74189284273147,31.6425675085602,125.294370330194));
#123698=CARTESIAN_POINT('Ctrl Pts',(2.75174615151661,31.605106952336,125.451102252216));
#123699=CARTESIAN_POINT('Ctrl Pts',(2.75572966382173,31.5860991325912,125.51395344143));
#123700=CARTESIAN_POINT('Ctrl Pts',(2.75979332369797,31.5634400150579,125.575509617049));
#123701=CARTESIAN_POINT('Ctrl Pts',(2.56904933390813,31.5634400118358,125.575509625802));
#123702=CARTESIAN_POINT('Ctrl Pts',(2.56750768440673,31.5719229943011,125.552464599948));
#123703=CARTESIAN_POINT('Ctrl Pts',(2.56595051571147,31.5798953096122,125.529235120265));
#123704=CARTESIAN_POINT('Ctrl Pts',(2.56303659776313,31.5936510056218,125.486068913008));
#123705=CARTESIAN_POINT('Ctrl Pts',(2.56168650874348,31.5995806545989,125.466184673763));
#123706=CARTESIAN_POINT('Ctrl Pts',(2.55975881801057,31.6074002625116,125.438054564161));
#123707=CARTESIAN_POINT('Ctrl Pts',(2.55919766684648,31.6096013883969,125.429896229335));
#123708=CARTESIAN_POINT('Ctrl Pts',(2.55822633255545,31.6132807220529,125.4158345151));
#123709=CARTESIAN_POINT('Ctrl Pts',(2.55781784972441,31.6147888095325,125.409939180308));
#123710=CARTESIAN_POINT('Ctrl Pts',(2.55694707943159,31.6179200985488,125.397413075285));
#123711=CARTESIAN_POINT('Ctrl Pts',(2.5564843681348,31.619534834569,125.390780645791));
#123712=CARTESIAN_POINT('Ctrl Pts',(2.55519954180064,31.6238845656322,125.372424285793));
#123713=CARTESIAN_POINT('Ctrl Pts',(2.55437284706231,31.62653324698,125.360680615845));
#123714=CARTESIAN_POINT('Ctrl Pts',(2.54965622493531,31.6408145640836,125.294001354521));
#123715=CARTESIAN_POINT('Ctrl Pts',(2.54564696591654,31.6497900057805,125.238538991999));
#123716=CARTESIAN_POINT('Ctrl Pts',(2.53092411806609,31.6721389246965,125.036013588231));
#123717=CARTESIAN_POINT('Ctrl Pts',(2.52006485417299,31.6687604919269,124.887755290083));
#123718=CARTESIAN_POINT('Ctrl Pts',(2.50765667614603,31.6410743164775,124.711219905917));
#123719=CARTESIAN_POINT('Ctrl Pts',(2.50552745157347,31.6354108782717,124.680703372049));
#123720=CARTESIAN_POINT('Ctrl Pts',(2.50247286587228,31.625948858238,124.636621718354));
#123721=CARTESIAN_POINT('Ctrl Pts',(2.50152638550819,31.6228259662935,124.622919943099));
#123722=CARTESIAN_POINT('Ctrl Pts',(2.49986576324301,31.6170091144835,124.598810456889));
#123723=CARTESIAN_POINT('Ctrl Pts',(2.49914936313765,31.6143871225168,124.588386402332));
#123724=CARTESIAN_POINT('Ctrl Pts',(2.49765408285465,31.6086784916746,124.566585121346));
#123725=CARTESIAN_POINT('Ctrl Pts',(2.49687589991155,31.6055716032335,124.555213775471));
#123726=CARTESIAN_POINT('Ctrl Pts',(2.49482520500147,31.5970248560212,124.525189408577));
#123727=CARTESIAN_POINT('Ctrl Pts',(2.49355941074421,31.5913788398077,124.506596586992));
#123728=CARTESIAN_POINT('Ctrl Pts',(2.48725774246659,31.5614258265708,124.413827811878));
#123729=CARTESIAN_POINT('Ctrl Pts',(2.48238388449402,31.5322511863651,124.341321819731));
#123730=CARTESIAN_POINT('Ctrl Pts',(2.47117051387643,31.4525132725897,124.177432953324));
#123731=CARTESIAN_POINT('Ctrl Pts',(2.46491618176057,31.398245417011,124.08823322209));
#123732=CARTESIAN_POINT('Ctrl Pts',(2.45571450168454,31.3104986927239,123.970450451187));
#123733=CARTESIAN_POINT('Ctrl Pts',(2.4529952182635,31.2836854524679,123.937206475624));
#123734=CARTESIAN_POINT('Ctrl Pts',(2.44948437292046,31.2484924018074,123.896849697564));
#123735=CARTESIAN_POINT('Ctrl Pts',(2.4487674654407,31.2412773500014,123.888737478313));
#123736=CARTESIAN_POINT('Ctrl Pts',(2.44760762717081,31.2295700819844,123.875830719551));
#123737=CARTESIAN_POINT('Ctrl Pts',(2.44716829910654,31.2251277480399,123.870991074058));
#123738=CARTESIAN_POINT('Ctrl Pts',(2.44631517630151,31.2164892592834,123.861690997691));
#123739=CARTESIAN_POINT('Ctrl Pts',(2.4459016611756,31.2122969525896,123.857227233143));
#123740=CARTESIAN_POINT('Ctrl Pts',(2.44497164910762,31.2028548791652,123.847284196805));
#123741=CARTESIAN_POINT('Ctrl Pts',(2.44445418919199,31.1975920966534,123.841817480805));
#123742=CARTESIAN_POINT('Ctrl Pts',(2.44261357240089,31.1788336112256,123.822596658982));
#123743=CARTESIAN_POINT('Ctrl Pts',(2.44127656029826,31.165137397526,123.809041530215));
#123744=CARTESIAN_POINT('Ctrl Pts',(2.43236282805903,31.0731820713852,123.721137917035));
#123745=CARTESIAN_POINT('Ctrl Pts',(2.42442760407517,30.9880948382047,123.654312788474));
#123746=CARTESIAN_POINT('Ctrl Pts',(2.41039467056622,30.8251416040873,123.550172440081));
#123747=CARTESIAN_POINT('Ctrl Pts',(2.40427516634134,30.7496928316227,123.509757438197));
#123748=CARTESIAN_POINT('Ctrl Pts',(2.39626880572495,30.644045787585,123.46323107403));
#123749=CARTESIAN_POINT('Ctrl Pts',(2.39421461651924,30.6163031175517,123.451896522758));
#123750=CARTESIAN_POINT('Ctrl Pts',(2.39124631007734,30.5752955991356,123.436419738837));
#123751=CARTESIAN_POINT('Ctrl Pts',(2.39031271834411,30.5622620535688,123.43168572576));
#123752=CARTESIAN_POINT('Ctrl Pts',(2.38866661466185,30.539045255487,123.423579614265));
#123753=CARTESIAN_POINT('Ctrl Pts',(2.38795197572336,30.5288858375409,123.420142158257));
#123754=CARTESIAN_POINT('Ctrl Pts',(2.38645240894849,30.5074027180524,123.413103767499));
#123755=CARTESIAN_POINT('Ctrl Pts',(2.38566825521845,30.4960722215795,123.40952537452));
#123756=CARTESIAN_POINT('Ctrl Pts',(2.38358303030669,30.4656924247426,123.400287077126));
#123757=CARTESIAN_POINT('Ctrl Pts',(2.38228909880272,30.4465781508587,123.394846150684));
#123758=CARTESIAN_POINT('Ctrl Pts',(2.37459420560437,30.3314461354506,123.364289425666));
#123759=CARTESIAN_POINT('Ctrl Pts',(2.36846900019063,30.2334337937581,123.347451100979));
#123760=CARTESIAN_POINT('Ctrl Pts',(2.35712166498238,30.0484735090973,123.332470549024));
#123761=CARTESIAN_POINT('Ctrl Pts',(2.35189847504009,29.9620469648778,123.332198513648));
#123762=CARTESIAN_POINT('Ctrl Pts',(2.34401577394342,29.8370031962186,123.341531774075));
#123763=CARTESIAN_POINT('Ctrl Pts',(2.34151788091398,29.7981295065047,123.345813620046));
#123764=CARTESIAN_POINT('Ctrl Pts',(2.33825905284894,29.748983465588,123.352984974295));
#123765=CARTESIAN_POINT('Ctrl Pts',(2.3375604506864,29.7385360336302,123.354611178036));
#123766=CARTESIAN_POINT('Ctrl Pts',(2.33642315192652,29.7216848517864,123.357398701416));
#123767=CARTESIAN_POINT('Ctrl Pts',(2.33598781240839,29.7152709951856,123.358498328358));
#123768=CARTESIAN_POINT('Ctrl Pts',(2.33513609963773,29.7027977306627,123.360712115441));
#123769=CARTESIAN_POINT('Ctrl Pts',(2.33471994490285,29.6967377882096,123.361822358923));
#123770=CARTESIAN_POINT('Ctrl Pts',(2.33367560794991,29.6816132159569,123.364680129679));
#123771=CARTESIAN_POINT('Ctrl Pts',(2.3330451577626,29.6725567810803,123.366469421453));
#123772=CARTESIAN_POINT('Ctrl Pts',(2.33074381425698,29.6397485077054,123.373235180857));
#123773=CARTESIAN_POINT('Ctrl Pts',(2.32905120321328,29.6160924583892,123.378654951812));
#123774=CARTESIAN_POINT('Ctrl Pts',(2.32004493578621,29.4922764882314,123.409883530933));
#123775=CARTESIAN_POINT('Ctrl Pts',(2.31244298822751,29.3945667624941,123.444460727571));
#123776=CARTESIAN_POINT('Ctrl Pts',(2.29890959143051,29.2251886175557,123.522791682623));
#123777=CARTESIAN_POINT('Ctrl Pts',(2.29295775707005,29.1523924535725,123.563322617609));
#123778=CARTESIAN_POINT('Ctrl Pts',(2.28511457005254,29.0579737618701,123.62557811282));
#123779=CARTESIAN_POINT('Ctrl Pts',(2.28306595474137,29.033472041509,123.642696473962));
#123780=CARTESIAN_POINT('Ctrl Pts',(2.28010407320749,28.9983052906521,123.668701543796));
#123781=CARTESIAN_POINT('Ctrl Pts',(2.27917145221545,28.9872707862423,123.677076181351));
#123782=CARTESIAN_POINT('Ctrl Pts',(2.27752643649752,28.9678816254554,123.692176370919));
#123783=CARTESIAN_POINT('Ctrl Pts',(2.2768119246418,28.9594851772492,123.698846705138));
#123784=CARTESIAN_POINT('Ctrl Pts',(2.27531200665376,28.9419163829581,123.71308259512));
#123785=CARTESIAN_POINT('Ctrl Pts',(2.27452738061961,28.932759411369,123.720666233565));
#123786=CARTESIAN_POINT('Ctrl Pts',(2.27243942412201,28.9084897629472,123.741207854997));
#123787=CARTESIAN_POINT('Ctrl Pts',(2.27114326715865,28.8935265417639,123.754340013031));
#123788=CARTESIAN_POINT('Ctrl Pts',(2.2637871406152,28.8092949159083,123.830979824061));
#123789=CARTESIAN_POINT('Ctrl Pts',(2.25797112631215,28.7452592899401,123.899992839493));
#123790=CARTESIAN_POINT('Ctrl Pts',(2.24787115203191,28.6436509421557,124.029992093533));
#123791=CARTESIAN_POINT('Ctrl Pts',(2.24356696978252,28.6035459355214,124.088674833431));
#123792=CARTESIAN_POINT('Ctrl Pts',(2.23676400379598,28.5474935141545,124.183122848311));
#123793=CARTESIAN_POINT('Ctrl Pts',(2.23433250431504,28.5288531415018,124.217191017946));
#123794=CARTESIAN_POINT('Ctrl Pts',(2.23030294485382,28.5005759158235,124.273455658855));
#123795=CARTESIAN_POINT('Ctrl Pts',(2.22873760062581,28.4902020608207,124.295266503208));
#123796=CARTESIAN_POINT('Ctrl Pts',(2.22655564749562,28.4766373461281,124.325461344167));
#123797=CARTESIAN_POINT('Ctrl Pts',(2.225961842205,28.4730341304597,124.333658197502));
#123798=CARTESIAN_POINT('Ctrl Pts',(2.22495222010856,28.4670600209088,124.34755146802));
#123799=CARTESIAN_POINT('Ctrl Pts',(2.22453846530128,28.4646543164811,124.353232887994));
#123800=CARTESIAN_POINT('Ctrl Pts',(2.22367688566946,28.4597339908895,124.365035113364));
#123801=CARTESIAN_POINT('Ctrl Pts',(2.22322880898844,28.4572242117579,124.371157691105));
#123802=CARTESIAN_POINT('Ctrl Pts',(2.22202522766242,28.4506115663153,124.387567037897));
#123803=CARTESIAN_POINT('Ctrl Pts',(2.22126601736054,28.4465747724071,124.397879831561));
#123804=CARTESIAN_POINT('Ctrl Pts',(2.21769862511443,28.4282157522584,124.446195335171));
#123805=CARTESIAN_POINT('Ctrl Pts',(2.2148279607198,28.4151844929541,124.484670447427));
#123806=CARTESIAN_POINT('Ctrl Pts',(2.20540719597188,28.3775671166334,124.61072168151));
#123807=CARTESIAN_POINT('Ctrl Pts',(2.19873109221899,28.3587404135626,124.699845296651));
#123808=CARTESIAN_POINT('Ctrl Pts',(2.18768018724387,28.339495724135,124.851345490244));
#123809=CARTESIAN_POINT('Ctrl Pts',(2.18325963961434,28.3351249939939,124.913022177084));
#123810=CARTESIAN_POINT('Ctrl Pts',(2.17615245495413,28.3335905372008,125.014473291492));
#123811=CARTESIAN_POINT('Ctrl Pts',(2.17341311675692,28.3344076633956,125.054153481255));
#123812=CARTESIAN_POINT('Ctrl Pts',(2.16967082987506,28.3375077988401,125.109146075771));
#123813=CARTESIAN_POINT('Ctrl Pts',(2.16863111864284,28.338587818163,125.124510138092));
#123814=CARTESIAN_POINT('Ctrl Pts',(2.16686260137528,28.3408012169422,125.150783355902));
#123815=CARTESIAN_POINT('Ctrl Pts',(2.16613056069923,28.3418295296182,125.161700102593));
#123816=CARTESIAN_POINT('Ctrl Pts',(2.16473917933094,28.3439987313666,125.182524635184));
#123817=CARTESIAN_POINT('Ctrl Pts',(2.16407928631761,28.345120950561,125.19243384115));
#123818=CARTESIAN_POINT('Ctrl Pts',(2.1625361847491,28.3479649431131,125.215677847066));
#123819=CARTESIAN_POINT('Ctrl Pts',(2.16165528268827,28.3497593147327,125.22900318993));
#123820=CARTESIAN_POINT('Ctrl Pts',(2.15857813177452,28.3566280414943,125.275727725687));
#123821=CARTESIAN_POINT('Ctrl Pts',(2.15640851826147,28.3625568781979,125.308994244319));
#123822=CARTESIAN_POINT('Ctrl Pts',(2.14465579092078,28.4005873918265,125.490275631819));
#123823=CARTESIAN_POINT('Ctrl Pts',(2.1357002042975,28.4517410493955,125.633547186988));
#123824=CARTESIAN_POINT('Ctrl Pts',(2.12421330619666,28.5366927651692,125.797099847025));
#123825=CARTESIAN_POINT('Ctrl Pts',(2.12214143477398,28.5527014418604,125.825810420963));
#123826=CARTESIAN_POINT('Ctrl Pts',(2.11864881717407,28.5805707774142,125.872490161107));
#123827=CARTESIAN_POINT('Ctrl Pts',(2.11725087847344,28.5919497196416,125.890737167683));
#123828=CARTESIAN_POINT('Ctrl Pts',(2.11526640810246,28.6083512703442,125.915938434034));
#123829=CARTESIAN_POINT('Ctrl Pts',(2.11469765099059,28.6130797928288,125.923082733429));
#123830=CARTESIAN_POINT('Ctrl Pts',(2.11371751494314,28.62127083578,125.935253518153));
#123831=CARTESIAN_POINT('Ctrl Pts',(2.11330791156008,28.6247063311271,125.940298130768));
#123832=CARTESIAN_POINT('Ctrl Pts',(2.11243980955811,28.6320117988284,125.950899645255));
#123833=CARTESIAN_POINT('Ctrl Pts',(2.11198092285726,28.6358879942933,125.956451925442));
#123834=CARTESIAN_POINT('Ctrl Pts',(2.11071744974352,28.6466027983288,125.971602235303));
#123835=CARTESIAN_POINT('Ctrl Pts',(2.10990852067194,28.6535094207371,125.981151359045));
#123836=CARTESIAN_POINT('Ctrl Pts',(2.10550818269214,28.6913585325467,126.032329358542));
#123837=CARTESIAN_POINT('Ctrl Pts',(2.10181469510058,28.7241283320169,126.072565518666));
#123838=CARTESIAN_POINT('Ctrl Pts',(2.09095331498943,28.8245942356333,126.18479209712));
#123839=CARTESIAN_POINT('Ctrl Pts',(2.08369699422513,28.8968890502394,126.252381214588));
#123840=CARTESIAN_POINT('Ctrl Pts',(2.073074585622,29.0135313207396,126.343449647559));
#123841=CARTESIAN_POINT('Ctrl Pts',(2.0695856132006,29.0536429993486,126.372000939735));
#123842=CARTESIAN_POINT('Ctrl Pts',(2.06379048581444,29.1234919579681,126.417195925477));
#123843=CARTESIAN_POINT('Ctrl Pts',(2.06145360046727,29.1525805068665,126.434779123136));
#123844=CARTESIAN_POINT('Ctrl Pts',(2.05816225498934,29.1948592769611,126.458600676972));
#123845=CARTESIAN_POINT('Ctrl Pts',(2.05718180413031,29.2076233811371,126.465573893032));
#123846=CARTESIAN_POINT('Ctrl Pts',(2.05548236302441,29.2300392874922,126.477441557332));
#123847=CARTESIAN_POINT('Ctrl Pts',(2.05476076510907,29.2396503269645,126.482410684783));
#123848=CARTESIAN_POINT('Ctrl Pts',(2.05327389914097,29.2596433464019,126.492501934617));
#123849=CARTESIAN_POINT('Ctrl Pts',(2.05250914598858,29.2700316987983,126.497610192945));
#123850=CARTESIAN_POINT('Ctrl Pts',(2.05053630372098,29.2970966500618,126.51057029147));
#123851=CARTESIAN_POINT('Ctrl Pts',(2.04933401803458,29.3138520959994,126.518254531589));
#123852=CARTESIAN_POINT('Ctrl Pts',(2.04405306145618,29.3885465246893,126.551021070744));
#123853=CARTESIAN_POINT('Ctrl Pts',(2.04007641786547,29.4477595579309,126.573077726668));
#123854=CARTESIAN_POINT('Ctrl Pts',(2.02715479675985,29.6469140094264,126.634625291418));
#123855=CARTESIAN_POINT('Ctrl Pts',(2.01857863180699,29.7907363503682,126.659176908244));
#123856=CARTESIAN_POINT('Ctrl Pts',(2.00779634488768,29.9588105245502,126.66564857244));
#123857=CARTESIAN_POINT('Ctrl Pts',(2.00630817305725,29.9817369738419,126.666057644819));
#123858=CARTESIAN_POINT('Ctrl Pts',(2.00421704216577,30.013443408266,126.665968897727));
#123859=CARTESIAN_POINT('Ctrl Pts',(2.00363449149764,30.0222230877966,126.665874911073));
#123860=CARTESIAN_POINT('Ctrl Pts',(2.00263820106578,30.0371390944546,126.665597301974));
#123861=CARTESIAN_POINT('Ctrl Pts',(2.00222639368994,30.0432760482853,126.665449148775));
#123862=CARTESIAN_POINT('Ctrl Pts',(2.0013622704175,30.0560911705319,126.665068896678));
#123863=CARTESIAN_POINT('Ctrl Pts',(2.00090964418383,30.0627689041207,126.664830535167));
#123864=CARTESIAN_POINT('Ctrl Pts',(1.99968092741465,30.0808077533322,126.664077956934));
#123865=CARTESIAN_POINT('Ctrl Pts',(1.99890086883427,30.0921650928268,126.663487576623));
#123866=CARTESIAN_POINT('Ctrl Pts',(1.99502521720697,30.1481709589136,126.660000976265));
#123867=CARTESIAN_POINT('Ctrl Pts',(1.99185368136524,30.1926926728845,126.655423406051));
#123868=CARTESIAN_POINT('Ctrl Pts',(1.98231906174619,30.3241066326442,126.636539083468));
#123869=CARTESIAN_POINT('Ctrl Pts',(1.97585958504778,30.410111074259,126.61713147611));
#123870=CARTESIAN_POINT('Ctrl Pts',(1.96510770015513,30.5520915004783,126.573031583146));
#123871=CARTESIAN_POINT('Ctrl Pts',(1.9607718416773,30.6089829306542,126.551893821281));
#123872=CARTESIAN_POINT('Ctrl Pts',(1.95378127910273,30.7005374787702,126.512064543252));
#123873=CARTESIAN_POINT('Ctrl Pts',(1.95107611390662,30.7359146575836,126.495166211577));
#123874=CARTESIAN_POINT('Ctrl Pts',(1.94737173507689,30.7842589981586,126.469941805635));
#123875=CARTESIAN_POINT('Ctrl Pts',(1.94633674152783,30.7977543074398,126.462661676674));
#123876=CARTESIAN_POINT('Ctrl Pts',(1.94457376980897,30.8207140226308,126.449863595264));
#123877=CARTESIAN_POINT('Ctrl Pts',(1.94384260786403,30.8302278284621,126.444436815694));
#123878=CARTESIAN_POINT('Ctrl Pts',(1.94245127042418,30.8483118999807,126.433883756422));
#123879=CARTESIAN_POINT('Ctrl Pts',(1.94179055761511,30.8568909075131,126.428773490291));
#123880=CARTESIAN_POINT('Ctrl Pts',(1.94024309949947,30.8769590042724,126.416573734841));
#123881=CARTESIAN_POINT('Ctrl Pts',(1.93935869460053,30.8884090038081,126.409421051704));
#123882=CARTESIAN_POINT('Ctrl Pts',(1.93625622460555,30.9284877438922,126.383701827216));
#123883=CARTESIAN_POINT('Ctrl Pts',(1.93406539022289,30.9566329224646,126.364395083296));
#123884=CARTESIAN_POINT('Ctrl Pts',(1.92328624366364,31.0937548245079,126.264002893837));
#123885=CARTESIAN_POINT('Ctrl Pts',(1.91518068298333,31.1931157191803,126.170674153587));
#123886=CARTESIAN_POINT('Ctrl Pts',(1.90417378267724,31.3072035363218,126.033719077966));
#123887=CARTESIAN_POINT('Ctrl Pts',(1.90152611468047,31.3331030636473,126.00009597486));
#123888=CARTESIAN_POINT('Ctrl Pts',(1.89717927392726,31.3725533538331,125.94462219776));
#123889=CARTESIAN_POINT('Ctrl Pts',(1.89551959231258,31.3869317882335,125.923381746079));
#123890=CARTESIAN_POINT('Ctrl Pts',(1.89322707557086,31.4057697631156,125.894120357556));
#123891=CARTESIAN_POINT('Ctrl Pts',(1.89262015135067,31.4106625312169,125.886380874228));
#123892=CARTESIAN_POINT('Ctrl Pts',(1.89159484689329,31.418765014924,125.873327184444));
#123893=CARTESIAN_POINT('Ctrl Pts',(1.89117868182008,31.4220093648947,125.868034505788));
#123894=CARTESIAN_POINT('Ctrl Pts',(1.89031938970207,31.4286154701201,125.857121187626));
#123895=CARTESIAN_POINT('Ctrl Pts',(1.88987607418007,31.4319737667784,125.851498690118));
#123896=CARTESIAN_POINT('Ctrl Pts',(1.88869872797906,31.4407638003234,125.836583250243));
#123897=CARTESIAN_POINT('Ctrl Pts',(1.88796125805969,31.4461386692578,125.827257394608));
#123898=CARTESIAN_POINT('Ctrl Pts',(1.88464135417116,31.4697693782988,125.785321991227));
#123899=CARTESIAN_POINT('Ctrl Pts',(1.88200603188418,31.4870139095433,125.752158103781));
#123900=CARTESIAN_POINT('Ctrl Pts',(1.87563875356216,31.5254502461663,125.671741835603));
#123901=CARTESIAN_POINT('Ctrl Pts',(1.87188086914729,31.5455741574153,125.624044319361));
#123902=CARTESIAN_POINT('Ctrl Pts',(1.86811695019056,31.5634399562749,125.57550977674));
#123903=CARTESIAN_POINT('Origin',(5.,30.,125.));
#123904=CARTESIAN_POINT('',(1.16625576032278,31.5634400119388,125.575509625522));
#123905=CARTESIAN_POINT('',(1.36115613275098,31.5634400145948,125.575509618307));
#123906=CARTESIAN_POINT('',(5.,31.5634400119422,125.575509625513));
#123907=CARTESIAN_POINT('Ctrl Pts',(1.36115613275098,31.5634400145948,125.575509618307));
#123908=CARTESIAN_POINT('Ctrl Pts',(1.36788843714252,31.5313390004694,125.662715823723));
#123909=CARTESIAN_POINT('Ctrl Pts',(1.37450631330542,31.4919908242762,125.747102957969));
#123910=CARTESIAN_POINT('Ctrl Pts',(1.38236650476969,31.4350852948616,125.846493320159));
#123911=CARTESIAN_POINT('Ctrl Pts',(1.3838332531891,31.4240112791323,125.864992888475));
#123912=CARTESIAN_POINT('Ctrl Pts',(1.38611237940914,31.4060915723659,125.893651108808));
#123913=CARTESIAN_POINT('Ctrl Pts',(1.38693348118945,31.3994879769824,125.903957537879));
#123914=CARTESIAN_POINT('Ctrl Pts',(1.38846254431071,31.3869157521616,125.923111350145));
#123915=CARTESIAN_POINT('Ctrl Pts',(1.38917147738888,31.3809745757465,125.931975910933));
#123916=CARTESIAN_POINT('Ctrl Pts',(1.39075633862594,31.3674425867808,125.951752829778));
#123917=CARTESIAN_POINT('Ctrl Pts',(1.391630461375,31.3598054665056,125.962632737567));
#123918=CARTESIAN_POINT('Ctrl Pts',(1.39386577366159,31.3398351135063,125.99037069423));
#123919=CARTESIAN_POINT('Ctrl Pts',(1.39521970951885,31.3273133741414,126.007090617742));
#123920=CARTESIAN_POINT('Ctrl Pts',(1.40488805332882,31.2349239505862,126.125738004368));
#123921=CARTESIAN_POINT('Ctrl Pts',(1.41271276384103,31.1437288724805,126.21828206136));
#123922=CARTESIAN_POINT('Ctrl Pts',(1.42572400376261,30.9779077990288,126.351354860294));
#123923=CARTESIAN_POINT('Ctrl Pts',(1.43084613520645,30.909293792728,126.398443729326));
#123924=CARTESIAN_POINT('Ctrl Pts',(1.43717053171415,30.8252969675018,126.447286775893));
#123925=CARTESIAN_POINT('Ctrl Pts',(1.43809467192393,30.8130411236341,126.454207067591));
#123926=CARTESIAN_POINT('Ctrl Pts',(1.43950924853964,30.7943386632721,126.464457135803));
#123927=CARTESIAN_POINT('Ctrl Pts',(1.43999282229543,30.7879551971601,126.467901637342));
#123928=CARTESIAN_POINT('Ctrl Pts',(1.44088202979343,30.7762402861211,126.474124540496));
#123929=CARTESIAN_POINT('Ctrl Pts',(1.44128684763122,30.7709160307832,126.476915912445));
#123930=CARTESIAN_POINT('Ctrl Pts',(1.44221892605108,30.7586774434982,126.483248084509));
#123931=CARTESIAN_POINT('Ctrl Pts',(1.44274734184737,30.7517533934417,126.486769374479));
#123932=CARTESIAN_POINT('Ctrl Pts',(1.44438271947967,30.7303605083595,126.497461282664));
#123933=CARTESIAN_POINT('Ctrl Pts',(1.44549870813941,30.715812324722,126.504469817929));
#123934=CARTESIAN_POINT('Ctrl Pts',(1.45226606876418,30.6277635487778,126.545320842738));
#123935=CARTESIAN_POINT('Ctrl Pts',(1.45813955116446,30.5519850555145,126.573980181122));
#123936=CARTESIAN_POINT('Ctrl Pts',(1.46939071625332,30.4038000201976,126.618002116637));
#123937=CARTESIAN_POINT('Ctrl Pts',(1.47475405342166,30.3318483728441,126.634277599297));
#123938=CARTESIAN_POINT('Ctrl Pts',(1.4830506607513,30.2170086743266,126.652354282216));
#123939=CARTESIAN_POINT('Ctrl Pts',(1.48605154938794,30.1747245185688,126.657359129859));
#123940=CARTESIAN_POINT('Ctrl Pts',(1.49113204457282,30.1017581020467,126.663171525842));
#123941=CARTESIAN_POINT('Ctrl Pts',(1.49323321385457,30.0711613095641,126.664761399673));
#123942=CARTESIAN_POINT('Ctrl Pts',(1.49625576184964,30.0265547467054,126.665847064912));
#123943=CARTESIAN_POINT('Ctrl Pts',(1.49719763550133,30.0125691555328,126.666011295067));
#123944=CARTESIAN_POINT('Ctrl Pts',(1.49885323880198,29.9878403260271,126.665990258866));
#123945=CARTESIAN_POINT('Ctrl Pts',(1.49956917801096,29.9770980059061,126.665877218845));
#123946=CARTESIAN_POINT('Ctrl Pts',(1.50106648449706,29.9545335804967,126.665421466873));
#123947=CARTESIAN_POINT('Ctrl Pts',(1.50184712531767,29.9427124800443,126.665056758738));
#123948=CARTESIAN_POINT('Ctrl Pts',(1.50391128077752,29.911313423008,126.66375323574));
#123949=CARTESIAN_POINT('Ctrl Pts',(1.5051879178707,29.8917460785984,126.662594743005));
#123950=CARTESIAN_POINT('Ctrl Pts',(1.51177375811627,29.7901391093795,126.654777555307));
#123951=CARTESIAN_POINT('Ctrl Pts',(1.51690091992469,29.7086505813626,126.64239104304));
#123952=CARTESIAN_POINT('Ctrl Pts',(1.52812422821807,29.5305361858221,126.601636379029));
#123953=CARTESIAN_POINT('Ctrl Pts',(1.53416048059969,29.434900417567,126.57044435649));
#123954=CARTESIAN_POINT('Ctrl Pts',(1.54222801375701,29.316650531387,126.519667973499));
#123955=CARTESIAN_POINT('Ctrl Pts',(1.54402243346827,29.2909310511884,126.507838947316));
#123956=CARTESIAN_POINT('Ctrl Pts',(1.54709236254215,29.2481880080668,126.486844945667));
#123957=CARTESIAN_POINT('Ctrl Pts',(1.54835151398663,29.2309994718478,126.478028170672));
#123958=CARTESIAN_POINT('Ctrl Pts',(1.5501709467685,29.2067217280122,126.465036909522));
#123959=CARTESIAN_POINT('Ctrl Pts',(1.55071715664052,29.1995034137108,126.461105325225));
#123960=CARTESIAN_POINT('Ctrl Pts',(1.55167155573971,29.1870186995625,126.454185019206));
#123961=CARTESIAN_POINT('Ctrl Pts',(1.55207821373416,29.1817390213714,126.451220739397));
#123962=CARTESIAN_POINT('Ctrl Pts',(1.55295575010206,29.1704333208859,126.44479183181));
#123963=CARTESIAN_POINT('Ctrl Pts',(1.55342715409083,29.1644128762686,126.441318308567));
#123964=CARTESIAN_POINT('Ctrl Pts',(1.55473753527695,29.1478183259475,126.43160509228));
#123965=CARTESIAN_POINT('Ctrl Pts',(1.55558125975455,29.137291439999,126.425286169237));
#123966=CARTESIAN_POINT('Ctrl Pts',(1.56149195184508,29.0645717552314,126.38053432621));
#123967=CARTESIAN_POINT('Ctrl Pts',(1.5667606305462,29.0049041505482,126.338164006801));
#123968=CARTESIAN_POINT('Ctrl Pts',(1.57310152214887,28.9372147896413,126.283060763051));
#123969=CARTESIAN_POINT('Ctrl Pts',(1.57413377338813,28.9263259284823,126.273962836714));
#123970=CARTESIAN_POINT('Ctrl Pts',(1.5805297536356,28.8596145021991,126.216760850669));
#123971=CARTESIAN_POINT('Ctrl Pts',(1.5858934328867,28.8069148305002,126.165133099205));
#123972=CARTESIAN_POINT('Ctrl Pts',(1.59418949790209,28.7294503436004,126.078457249508));
#123973=CARTESIAN_POINT('Ctrl Pts',(1.59718955248034,28.7023203053945,126.045655001549));
#123974=CARTESIAN_POINT('Ctrl Pts',(1.60226880889453,28.6578742134838,125.987518224455));
#123975=CARTESIAN_POINT('Ctrl Pts',(1.60436955922799,28.6399476634801,125.962679451522));
#123976=CARTESIAN_POINT('Ctrl Pts',(1.60739162529151,28.614846714531,125.92579800432));
#123977=CARTESIAN_POINT('Ctrl Pts',(1.60833342676447,28.6071240905643,125.914138004172));
#123978=CARTESIAN_POINT('Ctrl Pts',(1.60998894819264,28.59373046158,125.893351768683));
#123979=CARTESIAN_POINT('Ctrl Pts',(1.61070487697827,28.5879992936424,125.884265464572));
#123980=CARTESIAN_POINT('Ctrl Pts',(1.61220220555134,28.5761439384451,125.865060567569));
#123981=CARTESIAN_POINT('Ctrl Pts',(1.61298287846048,28.5700387876429,125.854930881935));
#123982=CARTESIAN_POINT('Ctrl Pts',(1.61504722145929,28.5541028643732,125.827841594732));
#123983=CARTESIAN_POINT('Ctrl Pts',(1.61632401170468,28.5444624732624,125.810771727214));
#123984=CARTESIAN_POINT('Ctrl Pts',(1.62291504384544,28.495884428535,125.721096107323));
#123985=CARTESIAN_POINT('Ctrl Pts',(1.62804686221697,28.4620681710365,125.645841632242));
#123986=CARTESIAN_POINT('Ctrl Pts',(1.63927045501971,28.3997275171634,125.474077605111));
#123987=CARTESIAN_POINT('Ctrl Pts',(1.64530276138104,28.3740900755344,125.376876857683));
#123988=CARTESIAN_POINT('Ctrl Pts',(1.6533655489414,28.3526313051633,125.250066271206));
#123989=CARTESIAN_POINT('Ctrl Pts',(1.65515944087159,28.3486218171002,125.222051059855));
#123990=CARTESIAN_POINT('Ctrl Pts',(1.65822855801079,28.343079531499,125.17476715656));
#123991=CARTESIAN_POINT('Ctrl Pts',(1.65948743656081,28.3411650080246,125.155548671883));
#123992=CARTESIAN_POINT('Ctrl Pts',(1.66130654328476,28.3389126581761,125.128110866713));
#123993=CARTESIAN_POINT('Ctrl Pts',(1.66185270685914,28.338300874547,125.11991480642));
#123994=CARTESIAN_POINT('Ctrl Pts',(1.66280705396003,28.337343748033,125.105673325348));
#123995=CARTESIAN_POINT('Ctrl Pts',(1.66321370677633,28.3369706783309,125.099630004616));
#123996=CARTESIAN_POINT('Ctrl Pts',(1.66409126664441,28.3362400844329,125.086644454505));
#123997=CARTESIAN_POINT('Ctrl Pts',(1.66456269964768,28.3358930649802,125.079702086268));
#123998=CARTESIAN_POINT('Ctrl Pts',(1.66587323662131,28.3350532264047,125.060489932643));
#123999=CARTESIAN_POINT('Ctrl Pts',(1.66671708960978,28.3346526174751,125.04821684611));
#124000=CARTESIAN_POINT('Ctrl Pts',(1.67266204871686,28.3327998838993,124.962355479993));
#124001=CARTESIAN_POINT('Ctrl Pts',(1.67796757987229,28.3360904001255,124.888753519978));
#124002=CARTESIAN_POINT('Ctrl Pts',(1.68431842629328,28.3457643669062,124.801879876537));
#124003=CARTESIAN_POINT('Ctrl Pts',(1.68532418592172,28.3474652940615,124.788160071502));
#124004=CARTESIAN_POINT('Ctrl Pts',(1.69169632094496,28.3593174067707,124.701416633705));
#124005=CARTESIAN_POINT('Ctrl Pts',(1.69706240822283,28.374136446682,124.629108613771));
#124006=CARTESIAN_POINT('Ctrl Pts',(1.70535358077061,28.4049610309634,124.517082680831));
#124007=CARTESIAN_POINT('Ctrl Pts',(1.70834673343382,28.417785537069,124.476591608923));
#124008=CARTESIAN_POINT('Ctrl Pts',(1.71341573792905,28.4424832714218,124.407857711538));
#124009=CARTESIAN_POINT('Ctrl Pts',(1.7155130202741,28.4536131983008,124.379372154915));
#124010=CARTESIAN_POINT('Ctrl Pts',(1.71853110124874,28.4709642368116,124.338334704028));
#124011=CARTESIAN_POINT('Ctrl Pts',(1.71947230929001,28.4765688409329,124.325530687684));
#124012=CARTESIAN_POINT('Ctrl Pts',(1.72112716257105,28.4867646642519,124.303013491713));
#124013=CARTESIAN_POINT('Ctrl Pts',(1.72184301058404,28.4912898845768,124.293271501212));
#124014=CARTESIAN_POINT('Ctrl Pts',(1.72334053634561,28.500996742821,124.272892575523));
#124015=CARTESIAN_POINT('Ctrl Pts',(1.72412148368649,28.506198126562,124.262265666496));
#124016=CARTESIAN_POINT('Ctrl Pts',(1.72618741005727,28.5203259151761,124.234163443987));
#124017=CARTESIAN_POINT('Ctrl Pts',(1.72746548996388,28.529448767495,124.216788564199));
#124018=CARTESIAN_POINT('Ctrl Pts',(1.73410172018248,28.5787859400112,124.126726427666));
#124019=CARTESIAN_POINT('Ctrl Pts',(1.73927409767307,28.624090176007,124.056956621597));
#124020=CARTESIAN_POINT('Ctrl Pts',(1.75050046146239,28.7348278079584,123.911495430027));
#124021=CARTESIAN_POINT('Ctrl Pts',(1.756498624146,28.8022395048367,123.837730521627));
#124022=CARTESIAN_POINT('Ctrl Pts',(1.76452034257048,28.8966668096847,123.751397425456));
#124023=CARTESIAN_POINT('Ctrl Pts',(1.76630965489659,28.9179753863162,123.732887110786));
#124024=CARTESIAN_POINT('Ctrl Pts',(1.76937172689543,28.9546110445973,123.702660609856));
#124025=CARTESIAN_POINT('Ctrl Pts',(1.7706282374366,28.9696905753923,123.690652844637));
#124026=CARTESIAN_POINT('Ctrl Pts',(1.7724445147675,28.9914867171358,123.673906335216));
#124027=CARTESIAN_POINT('Ctrl Pts',(1.77299027647761,28.9980359440086,123.668950987754));
#124028=CARTESIAN_POINT('Ctrl Pts',(1.77394417097862,29.0094762765465,123.66042715472));
#124029=CARTESIAN_POINT('Ctrl Pts',(1.77435077757914,29.0143506296302,123.656836580355));
#124030=CARTESIAN_POINT('Ctrl Pts',(1.77522853465085,29.0248664523636,123.649178423531));
#124031=CARTESIAN_POINT('Ctrl Pts',(1.77570021395467,29.0305137668903,123.64511963385));
#124032=CARTESIAN_POINT('Ctrl Pts',(1.77701208757998,29.046215212826,123.633983251205));
#124033=CARTESIAN_POINT('Ctrl Pts',(1.77785704595068,29.0563223017492,123.62698158867));
#124034=CARTESIAN_POINT('Ctrl Pts',(1.78405869542625,29.1305246831192,123.576784369876));
#124035=CARTESIAN_POINT('Ctrl Pts',(1.78964061639427,29.197473222275,123.537988310393));
#124036=CARTESIAN_POINT('Ctrl Pts',(1.79586696042007,29.27437487689,123.500301981295));
#124037=CARTESIAN_POINT('Ctrl Pts',(1.7964754996018,29.2819136316209,123.496677701413));
#124038=CARTESIAN_POINT('Ctrl Pts',(1.80260370465787,29.3580788605175,123.460764674209));
#124039=CARTESIAN_POINT('Ctrl Pts',(1.80812653922023,29.4288115508352,123.43313902632));
#124040=CARTESIAN_POINT('Ctrl Pts',(1.8165523485444,29.5414934588872,123.39777885141));
#124041=CARTESIAN_POINT('Ctrl Pts',(1.81953030723498,29.582272023511,123.386666590883));
#124042=CARTESIAN_POINT('Ctrl Pts',(1.82457672658104,29.6531098765742,123.370229634247));
#124043=CARTESIAN_POINT('Ctrl Pts',(1.82666635927882,29.6829726992655,123.364158288784));
#124044=CARTESIAN_POINT('Ctrl Pts',(1.82967564470528,29.7267353441532,123.356504570745));
#124045=CARTESIAN_POINT('Ctrl Pts',(1.83061553904464,29.7405136992961,123.354272902803));
#124046=CARTESIAN_POINT('Ctrl Pts',(1.83226891182424,29.7649402578377,123.350630957027));
#124047=CARTESIAN_POINT('Ctrl Pts',(1.83298457966375,29.7755769423046,123.349150030209));
#124048=CARTESIAN_POINT('Ctrl Pts',(1.83448253969067,29.7979700554958,123.346252709959));
#124049=CARTESIAN_POINT('Ctrl Pts',(1.83526409364735,29.8097288009486,123.344858591905));
#124050=CARTESIAN_POINT('Ctrl Pts',(1.83733352958761,29.8410555440159,123.341482754373));
#124051=CARTESIAN_POINT('Ctrl Pts',(1.83861446956224,29.8606458325574,123.339721931946));
#124052=CARTESIAN_POINT('Ctrl Pts',(1.84536496575442,29.9648415987415,123.332213892433));
#124053=CARTESIAN_POINT('Ctrl Pts',(1.85064009096393,30.0497669918163,123.332585086059));
#124054=CARTESIAN_POINT('Ctrl Pts',(1.86006566838607,30.202848239972,123.344965970038));
#124055=CARTESIAN_POINT('Ctrl Pts',(1.86423332221204,30.2709823084041,123.354748225466));
#124056=CARTESIAN_POINT('Ctrl Pts',(1.87133630242154,30.3839564865597,123.378178160646));
#124057=CARTESIAN_POINT('Ctrl Pts',(1.87423369101479,30.429176750271,123.389554289904));
#124058=CARTESIAN_POINT('Ctrl Pts',(1.8789424342582,30.5000258497311,123.410573933885));
#124059=CARTESIAN_POINT('Ctrl Pts',(1.88070573276224,30.525997903815,123.418979104566));
#124060=CARTESIAN_POINT('Ctrl Pts',(1.88311927028536,30.5605901873607,123.431120648662));
#124061=CARTESIAN_POINT('Ctrl Pts',(1.88373995892311,30.5694038303257,123.434297906662));
#124062=CARTESIAN_POINT('Ctrl Pts',(1.88478194609291,30.5840526673782,123.439718756127));
#124063=CARTESIAN_POINT('Ctrl Pts',(1.88520086696497,30.589903044506,123.441921223312));
#124064=CARTESIAN_POINT('Ctrl Pts',(1.88600538029486,30.601060629361,123.446193522512));
#124065=CARTESIAN_POINT('Ctrl Pts',(1.88639061072643,30.6063698538341,123.448257738043));
#124066=CARTESIAN_POINT('Ctrl Pts',(1.8874371555427,30.6207059806807,123.453916402289));
#124067=CARTESIAN_POINT('Ctrl Pts',(1.88810142608172,30.6297120248546,123.457562591248));
#124068=CARTESIAN_POINT('Ctrl Pts',(1.89068342876682,30.6643786924457,123.471951952564));
#124069=CARTESIAN_POINT('Ctrl Pts',(1.89263006146988,30.6897991089644,123.483257815077));
#124070=CARTESIAN_POINT('Ctrl Pts',(1.90246864897745,30.8152952126032,123.542880125558));
#124071=CARTESIAN_POINT('Ctrl Pts',(1.91065987168029,30.910641652665,123.600487322182));
#124072=CARTESIAN_POINT('Ctrl Pts',(1.92293820138425,31.0466027330274,123.702448832827));
#124073=CARTESIAN_POINT('Ctrl Pts',(1.9271389265445,31.0917652175097,123.740211848135));
#124074=CARTESIAN_POINT('Ctrl Pts',(1.93308461304396,31.1539823375902,123.798099640762));
#124075=CARTESIAN_POINT('Ctrl Pts',(1.93489688160465,31.1727045570917,123.816359911119));
#124076=CARTESIAN_POINT('Ctrl Pts',(1.93814578362795,31.2058222630889,123.850218019044));
#124077=CARTESIAN_POINT('Ctrl Pts',(1.93958844032543,31.2203640556432,123.865664257095));
#124078=CARTESIAN_POINT('Ctrl Pts',(1.94183879943864,31.2427770329806,123.890401294279));
#124079=CARTESIAN_POINT('Ctrl Pts',(1.94265486548425,31.250847730041,123.899507377898));
#124080=CARTESIAN_POINT('Ctrl Pts',(1.94417937218529,31.2658134254406,123.916770376831));
#124081=CARTESIAN_POINT('Ctrl Pts',(1.94488872994252,31.2727311065784,123.924906709183));
#124082=CARTESIAN_POINT('Ctrl Pts',(1.94648079036711,31.2881494403024,123.943398610948));
#124083=CARTESIAN_POINT('Ctrl Pts',(1.94736161392708,31.2966044428568,123.953791410809));
#124084=CARTESIAN_POINT('Ctrl Pts',(1.94962663647813,31.3181408757305,123.980925920629));
#124085=CARTESIAN_POINT('Ctrl Pts',(1.95100324286549,31.331029316296,123.997818194174));
#124086=CARTESIAN_POINT('Ctrl Pts',(1.96045600370541,31.4180051242381,124.116452092594));
#124087=CARTESIAN_POINT('Ctrl Pts',(1.96807484248614,31.4806790616155,124.226056417331));
#124088=CARTESIAN_POINT('Ctrl Pts',(1.98103498906011,31.5644150982949,124.420720799116));
#124089=CARTESIAN_POINT('Ctrl Pts',(1.98632707210239,31.5922356404503,124.502264339919));
#124090=CARTESIAN_POINT('Ctrl Pts',(1.99284283712311,31.6171379296576,124.599226419919));
#124091=CARTESIAN_POINT('Ctrl Pts',(1.99376800248439,31.6204695809314,124.612917513817));
#124092=CARTESIAN_POINT('Ctrl Pts',(1.99518383053812,31.6252532947745,124.633720886531));
#124093=CARTESIAN_POINT('Ctrl Pts',(1.995667612143,31.6268332832375,124.640803501195));
#124094=CARTESIAN_POINT('Ctrl Pts',(1.99655700762109,31.6296374492197,124.653771861941));
#124095=CARTESIAN_POINT('Ctrl Pts',(1.9969618030914,31.6308761069571,124.659654205974));
#124096=CARTESIAN_POINT('Ctrl Pts',(1.99789357567764,31.6336415589165,124.673149060572));
#124097=CARTESIAN_POINT('Ctrl Pts',(1.99842170498291,31.6351469891592,124.68076560736));
#124098=CARTESIAN_POINT('Ctrl Pts',(2.00005535704772,31.6396155626593,124.704235056647));
#124099=CARTESIAN_POINT('Ctrl Pts',(2.00116988052132,31.6424016928945,124.720120157181));
#124100=CARTESIAN_POINT('Ctrl Pts',(2.00842381528541,31.6588865784798,124.822852290617));
#124101=CARTESIAN_POINT('Ctrl Pts',(2.01482532547526,31.6659215294908,124.910620757329));
#124102=CARTESIAN_POINT('Ctrl Pts',(2.02992531169939,31.6661051617482,125.118055341483));
#124103=CARTESIAN_POINT('Ctrl Pts',(2.03855843505277,31.6533468393091,125.237270699926));
#124104=CARTESIAN_POINT('Ctrl Pts',(2.04828927217212,31.6233145648734,125.375336857162));
#124105=CARTESIAN_POINT('Ctrl Pts',(2.04977254501389,31.618282177548,125.396472954639));
#124106=CARTESIAN_POINT('Ctrl Pts',(2.05215867252703,31.6094454212157,125.430609640405));
#124107=CARTESIAN_POINT('Ctrl Pts',(2.05306947180075,31.6058935612211,125.443672305969));
#124108=CARTESIAN_POINT('Ctrl Pts',(2.05469045494552,31.5992519380296,125.466972752801));
#124109=CARTESIAN_POINT('Ctrl Pts',(2.05540253319247,31.5962221080516,125.477226679963));
#124110=CARTESIAN_POINT('Ctrl Pts',(2.05691213317322,31.589560125953,125.498999459493));
#124111=CARTESIAN_POINT('Ctrl Pts',(2.05770872900135,31.5859009915848,125.510509463561));
#124112=CARTESIAN_POINT('Ctrl Pts',(2.05974163396675,31.576195531666,125.539926690842));
#124113=CARTESIAN_POINT('Ctrl Pts',(2.0609719891437,31.5699690107231,125.557772827586));
#124114=CARTESIAN_POINT('Ctrl Pts',(2.06219312175648,31.563440011958,125.57550962547));
#124115=CARTESIAN_POINT('Ctrl Pts',(1.86811695019056,31.5634399562749,125.57550977674));
#124116=CARTESIAN_POINT('Ctrl Pts',(1.8650975957568,31.5777716089006,125.536576157781));
#124117=CARTESIAN_POINT('Ctrl Pts',(1.86207416272325,31.5906501488235,125.497103921108));
#124118=CARTESIAN_POINT('Ctrl Pts',(1.85225960628685,31.6278521720039,125.366739431899));
#124119=CARTESIAN_POINT('Ctrl Pts',(1.84557562255184,31.645959334402,125.274269386285));
#124120=CARTESIAN_POINT('Ctrl Pts',(1.83779330177858,31.6582965364205,125.161227512936));
#124121=CARTESIAN_POINT('Ctrl Pts',(1.83645989763197,31.6600819946652,125.141667010593));
#124122=CARTESIAN_POINT('Ctrl Pts',(1.83434047940836,31.6623882543454,125.110278263081));
#124123=CARTESIAN_POINT('Ctrl Pts',(1.83354765617931,31.6631295647758,125.098468608018));
#124124=CARTESIAN_POINT('Ctrl Pts',(1.83204294171875,31.6643034403869,125.075929780786));
#124125=CARTESIAN_POINT('Ctrl Pts',(1.83133039332371,31.664758218864,125.065202417317));
#124126=CARTESIAN_POINT('Ctrl Pts',(1.82971404962073,31.6655581377755,125.040749997231));
#124127=CARTESIAN_POINT('Ctrl Pts',(1.82881235060955,31.6658373942977,125.027023453554));
#124128=CARTESIAN_POINT('Ctrl Pts',(1.82595478419034,31.6661865645428,124.983269170221));
#124129=CARTESIAN_POINT('Ctrl Pts',(1.82401880020484,31.6656144187612,124.953241310217));
#124130=CARTESIAN_POINT('Ctrl Pts',(1.81306268485349,31.6576973888719,124.781584047833));
#124131=CARTESIAN_POINT('Ctrl Pts',(1.80460487138785,31.6331054437484,124.641345075194));
#124132=CARTESIAN_POINT('Ctrl Pts',(1.79319152746903,31.578260222233,124.46473380145));
#124133=CARTESIAN_POINT('Ctrl Pts',(1.79050259143215,31.5638794088472,124.424069510597));
#124134=CARTESIAN_POINT('Ctrl Pts',(1.78609561888315,31.5383529214723,124.359923100736));
#124135=CARTESIAN_POINT('Ctrl Pts',(1.78441843546376,31.5282067261145,124.336063125251));
#124136=CARTESIAN_POINT('Ctrl Pts',(1.78210545923976,31.5137148434697,124.304077675527));
#124137=CARTESIAN_POINT('Ctrl Pts',(1.78149617563148,31.5098518598556,124.2957359439));
#124138=CARTESIAN_POINT('Ctrl Pts',(1.78046803682817,31.5032618987868,124.281809015657));
#124139=CARTESIAN_POINT('Ctrl Pts',(1.78005142460269,31.5005722663843,124.276206177107));
#124140=CARTESIAN_POINT('Ctrl Pts',(1.77924674889782,31.4953418884016,124.265465118399));
#124141=CARTESIAN_POINT('Ctrl Pts',(1.77885900856078,31.4928058767948,124.26032475559));
#124142=CARTESIAN_POINT('Ctrl Pts',(1.77779683150709,31.4858147039284,124.246336413686));
#124143=CARTESIAN_POINT('Ctrl Pts',(1.77711928694477,31.4813071561139,124.2375150933));
#124144=CARTESIAN_POINT('Ctrl Pts',(1.77441874119394,31.4631421169201,124.202734968191));
#124145=CARTESIAN_POINT('Ctrl Pts',(1.77236349159094,31.4488795584703,124.177100151305));
#124146=CARTESIAN_POINT('Ctrl Pts',(1.76323993688256,31.3833906809416,124.066378591908));
#124147=CARTESIAN_POINT('Ctrl Pts',(1.75594251866082,31.3252927288633,123.985595354362));
#124148=CARTESIAN_POINT('Ctrl Pts',(1.74289423580892,31.2075504571697,123.849393260035));
#124149=CARTESIAN_POINT('Ctrl Pts',(1.73712361616642,31.1503766023283,123.792229017934));
#124150=CARTESIAN_POINT('Ctrl Pts',(1.72944786058439,31.0666339856568,123.719865891249));
#124151=CARTESIAN_POINT('Ctrl Pts',(1.72739638262212,31.0434686329461,123.700913856721));
#124152=CARTESIAN_POINT('Ctrl Pts',(1.7244312011817,31.0088448891291,123.674111596015));
#124153=CARTESIAN_POINT('Ctrl Pts',(1.72349808147628,30.9977800988859,123.66576502648));
#124154=CARTESIAN_POINT('Ctrl Pts',(1.72185250703582,30.9779709465843,123.651206528042));
#124155=CARTESIAN_POINT('Ctrl Pts',(1.72113793010426,30.9692684587398,123.644939238819));
#124156=CARTESIAN_POINT('Ctrl Pts',(1.71963819342284,30.9507948539696,123.631904096089));
#124157=CARTESIAN_POINT('Ctrl Pts',(1.71885381068788,30.9410105719847,123.62515587343));
#124158=CARTESIAN_POINT('Ctrl Pts',(1.71676726088378,30.9146628316728,123.607396880218));
#124159=CARTESIAN_POINT('Ctrl Pts',(1.71547224989026,30.8979727006939,123.596576817728));
#124160=CARTESIAN_POINT('Ctrl Pts',(1.70786660590026,30.7980466847075,123.534308333818));
#124161=CARTESIAN_POINT('Ctrl Pts',(1.70182307785615,30.7105991765247,123.489972560508));
#124162=CARTESIAN_POINT('Ctrl Pts',(1.69131998367277,30.5512051637506,123.426093160997));
#124163=CARTESIAN_POINT('Ctrl Pts',(1.68684289026914,30.4809069952529,123.403210261657));
#124164=CARTESIAN_POINT('Ctrl Pts',(1.68009636241854,30.375774821969,123.376563125523));
#124165=CARTESIAN_POINT('Ctrl Pts',(1.6779188293992,30.3419687636271,123.369107278227));
#124166=CARTESIAN_POINT('Ctrl Pts',(1.67426721690907,30.2860391290879,123.358587493148));
#124167=CARTESIAN_POINT('Ctrl Pts',(1.67281867641262,30.2640416777576,123.354905693599));
#124168=CARTESIAN_POINT('Ctrl Pts',(1.67077432723228,30.2333822537574,123.350404835233));
#124169=CARTESIAN_POINT('Ctrl Pts',(1.67019774800596,30.224776726699,123.349210219644));
#124170=CARTESIAN_POINT('Ctrl Pts',(1.6692084775017,30.2100911535124,123.347288531093));
#124171=CARTESIAN_POINT('Ctrl Pts',(1.66879765044966,30.2040155840612,123.346527553127));
#124172=CARTESIAN_POINT('Ctrl Pts',(1.66793192650467,30.191264125538,123.345001756826));
#124173=CARTESIAN_POINT('Ctrl Pts',(1.6674766864847,30.184587675353,123.344243817247));
#124174=CARTESIAN_POINT('Ctrl Pts',(1.6662334926318,30.1664285366477,123.342293507142));
#124175=CARTESIAN_POINT('Ctrl Pts',(1.66544141644789,30.154937993463,123.34118009602));
#124176=CARTESIAN_POINT('Ctrl Pts',(1.66137117460098,30.0962474934186,123.336108200566));
#124177=CARTESIAN_POINT('Ctrl Pts',(1.65800789036152,30.0489097016657,123.334044877448));
#124178=CARTESIAN_POINT('Ctrl Pts',(1.64734993075662,29.9007418367087,123.333906731279));
#124179=CARTESIAN_POINT('Ctrl Pts',(1.6399375326435,29.8001291518946,123.342962945291));
#124180=CARTESIAN_POINT('Ctrl Pts',(1.62718881121054,29.6256408696133,123.374801116256));
#124181=CARTESIAN_POINT('Ctrl Pts',(1.62179331615814,29.5513606417542,123.393717987868));
#124182=CARTESIAN_POINT('Ctrl Pts',(1.61526993533219,29.4607210070736,123.423583198583));
#124183=CARTESIAN_POINT('Ctrl Pts',(1.61399052298572,29.4429076180026,123.429789857158));
#124184=CARTESIAN_POINT('Ctrl Pts',(1.61193587120959,29.4142521813549,123.44032323458));
#124185=CARTESIAN_POINT('Ctrl Pts',(1.61115454483907,29.4033438962492,123.444463557008));
#124186=CARTESIAN_POINT('Ctrl Pts',(1.60965830588906,29.382437114595,123.452651168812));
#124187=CARTESIAN_POINT('Ctrl Pts',(1.60894287466394,29.3724327019125,123.456681621149));
#124188=CARTESIAN_POINT('Ctrl Pts',(1.60728518219,29.3492392910392,123.466288319388));
#124189=CARTESIAN_POINT('Ctrl Pts',(1.60634545309903,29.3360815113137,123.47193806372));
#124190=CARTESIAN_POINT('Ctrl Pts',(1.60328414981054,29.2932083170981,123.491005480833));
#124191=CARTESIAN_POINT('Ctrl Pts',(1.60118647626245,29.2638126631903,123.505126302234));
#124192=CARTESIAN_POINT('Ctrl Pts',(1.59616231346269,29.1936169490497,123.54141956238));
#124193=CARTESIAN_POINT('Ctrl Pts',(1.59326378160945,29.1532921971898,123.56445241086));
#124194=CARTESIAN_POINT('Ctrl Pts',(1.58617262825909,29.0561065167093,123.625485063611));
#124195=CARTESIAN_POINT('Ctrl Pts',(1.58202370498385,29.0005242168353,123.665356005313));
#124196=CARTESIAN_POINT('Ctrl Pts',(1.57720950396108,28.9395410898399,123.715052700657));
#124197=CARTESIAN_POINT('Ctrl Pts',(1.5765767667947,28.9315959817358,123.721651255095));
#124198=CARTESIAN_POINT('Ctrl Pts',(1.57130488719242,28.866034153506,123.777139692381));
#124199=CARTESIAN_POINT('Ctrl Pts',(1.56661388582035,28.8117506658058,123.829817765646));
#124200=CARTESIAN_POINT('Ctrl Pts',(1.56087688616262,28.7530217076119,123.895123512882));
#124201=CARTESIAN_POINT('Ctrl Pts',(1.56006814239335,28.7449088378722,123.904348108919));
#124202=CARTESIAN_POINT('Ctrl Pts',(1.55879054196527,28.7323665446149,123.918931205423));
#124203=CARTESIAN_POINT('Ctrl Pts',(1.5583265687682,28.7278672028904,123.924229365542));
#124204=CARTESIAN_POINT('Ctrl Pts',(1.55745400450032,28.7195122309835,123.934193399882));
#124205=CARTESIAN_POINT('Ctrl Pts',(1.55704598926925,28.7156487037191,123.938852329539));
#124206=CARTESIAN_POINT('Ctrl Pts',(1.55608007680387,28.7066029877078,123.949882096635));
#124207=CARTESIAN_POINT('Ctrl Pts',(1.55552069717715,28.7014424251636,123.956270312704));
#124208=CARTESIAN_POINT('Ctrl Pts',(1.55363769079733,28.6843234727806,123.977785200966));
#124209=CARTESIAN_POINT('Ctrl Pts',(1.55230054690105,28.6725810021383,123.993080666286));
#124210=CARTESIAN_POINT('Ctrl Pts',(1.54897257481461,28.6443028078553,124.031269629524));
#124211=CARTESIAN_POINT('Ctrl Pts',(1.54696720749342,28.628078964157,124.054385967221));
#124212=CARTESIAN_POINT('Ctrl Pts',(1.53778874825973,28.5571779386006,124.16107595635));
#124213=CARTESIAN_POINT('Ctrl Pts',(1.5304440219652,28.5094952621727,124.249050532757));
#124214=CARTESIAN_POINT('Ctrl Pts',(1.51726303597941,28.4371686474596,124.416914197472));
#124215=CARTESIAN_POINT('Ctrl Pts',(1.51139765433763,28.410085701166,124.495413880593));
#124216=CARTESIAN_POINT('Ctrl Pts',(1.50437944812438,28.3839623571727,124.594582849902));
#124217=CARTESIAN_POINT('Ctrl Pts',(1.50304778634159,28.3793010836614,124.613637724073));
#124218=CARTESIAN_POINT('Ctrl Pts',(1.50093046138679,28.3723702746541,124.644307220874));
#124219=CARTESIAN_POINT('Ctrl Pts',(1.50013801275799,28.3698861798404,124.655870922818));
#124220=CARTESIAN_POINT('Ctrl Pts',(1.49863359616269,28.365382076191,124.677982075944));
#124221=CARTESIAN_POINT('Ctrl Pts',(1.49792097536365,28.3633405044518,124.68852447112));
#124222=CARTESIAN_POINT('Ctrl Pts',(1.49628850487941,28.3588773709665,124.71282805367));
#124223=CARTESIAN_POINT('Ctrl Pts',(1.49537094084789,28.3565266891281,124.726601561018));
#124224=CARTESIAN_POINT('Ctrl Pts',(1.49246287112248,28.3495866520175,124.770596259197));
#124225=CARTESIAN_POINT('Ctrl Pts',(1.49049297210273,28.3456554157299,124.800915897787));
#124226=CARTESIAN_POINT('Ctrl Pts',(1.48584076938843,28.3382635276247,124.873551651356));
#124227=CARTESIAN_POINT('Ctrl Pts',(1.48318095157678,28.3355814206046,124.915925868181));
#124228=CARTESIAN_POINT('Ctrl Pts',(1.47597757567576,28.332677457431,125.032072244088));
#124229=CARTESIAN_POINT('Ctrl Pts',(1.47150184865063,28.3357302567508,125.105828540613));
#124230=CARTESIAN_POINT('Ctrl Pts',(1.46616139066561,28.3451170752842,125.192619646064));
#124231=CARTESIAN_POINT('Ctrl Pts',(1.46533083939547,28.3467394223706,125.206080759893));
#124232=CARTESIAN_POINT('Ctrl Pts',(1.45995993592433,28.3582624962417,125.292769981152));
#124233=CARTESIAN_POINT('Ctrl Pts',(1.45536726811178,28.3728605335367,125.365281642797));
#124234=CARTESIAN_POINT('Ctrl Pts',(1.44973963917309,28.395437009501,125.44842431533));
#124235=CARTESIAN_POINT('Ctrl Pts',(1.44893130543299,28.3987853187646,125.460237199597));
#124236=CARTESIAN_POINT('Ctrl Pts',(1.4476542163264,28.4042326947301,125.478676302766));
#124237=CARTESIAN_POINT('Ctrl Pts',(1.44719033822738,28.4062432634974,125.485328503054));
#124238=CARTESIAN_POINT('Ctrl Pts',(1.4463178475217,28.4100827970753,125.497750868358));
#124239=CARTESIAN_POINT('Ctrl Pts',(1.44590980955758,28.4119016651429,125.503523895415));
#124240=CARTESIAN_POINT('Ctrl Pts',(1.44494370365468,28.4162631416855,125.517108350949));
#124241=CARTESIAN_POINT('Ctrl Pts',(1.44438415149831,28.4188321117056,125.524911025757));
#124242=CARTESIAN_POINT('Ctrl Pts',(1.44249995071792,28.4276288343304,125.550978498169));
#124243=CARTESIAN_POINT('Ctrl Pts',(1.44116176253548,28.4341159518442,125.56915328031));
#124244=CARTESIAN_POINT('Ctrl Pts',(1.43783061264571,28.4508804641549,125.613664195643));
#124245=CARTESIAN_POINT('Ctrl Pts',(1.43582307863503,28.4615151483336,125.639858783005));
#124246=CARTESIAN_POINT('Ctrl Pts',(1.42662548102339,28.5128118807922,125.757527049544));
#124247=CARTESIAN_POINT('Ctrl Pts',(1.41926325833615,28.5610011663348,125.845493073363));
#124248=CARTESIAN_POINT('Ctrl Pts',(1.40608611756473,28.6628626288872,125.997221328557));
#124249=CARTESIAN_POINT('Ctrl Pts',(1.40024031005497,28.7139771662845,126.062325611546));
#124250=CARTESIAN_POINT('Ctrl Pts',(1.39324097673362,28.7829422723837,126.137853643252));
#124251=CARTESIAN_POINT('Ctrl Pts',(1.39190985071197,28.7964180500025,126.152098508131));
#124252=CARTESIAN_POINT('Ctrl Pts',(1.38979316274644,28.8184197241252,126.174548377303));
#124253=CARTESIAN_POINT('Ctrl Pts',(1.38900082276235,28.8267866462151,126.182905861826));
#124254=CARTESIAN_POINT('Ctrl Pts',(1.38749648085482,28.8429198387189,126.19868128048));
#124255=CARTESIAN_POINT('Ctrl Pts',(1.38678382746859,28.8506701973549,126.20611455748));
#124256=CARTESIAN_POINT('Ctrl Pts',(1.38515109674147,28.8686712850179,126.223048096816));
#124257=CARTESIAN_POINT('Ctrl Pts',(1.38423330746454,28.8789708596368,126.232495433923));
#124258=CARTESIAN_POINT('Ctrl Pts',(1.38132374359486,28.9121866748853,126.26220191311));
#124259=CARTESIAN_POINT('Ctrl Pts',(1.37935260609621,28.9355432106215,126.281960776079));
#124260=CARTESIAN_POINT('Ctrl Pts',(1.37469685152446,28.992605965859,126.327598485688));
#124261=CARTESIAN_POINT('Ctrl Pts',(1.37203476879308,29.0267842935368,126.352853298509));
#124262=CARTESIAN_POINT('Ctrl Pts',(1.36483014220288,29.1228169789706,126.41828806364));
#124263=CARTESIAN_POINT('Ctrl Pts',(1.36035528249527,29.18643107814,126.455711873894));
#124264=CARTESIAN_POINT('Ctrl Pts',(1.35500293105549,29.2646158106712,126.494976778658));
#124265=CARTESIAN_POINT('Ctrl Pts',(1.35415967602753,29.2769927027013,126.501001637901));
#124266=CARTESIAN_POINT('Ctrl Pts',(1.3487915211988,29.356043150369,126.538277435509));
#124267=CARTESIAN_POINT('Ctrl Pts',(1.3442141964137,29.424644275302,126.5652287169));
#124268=CARTESIAN_POINT('Ctrl Pts',(1.33860360548016,29.5064921560772,126.591275194559));
#124269=CARTESIAN_POINT('Ctrl Pts',(1.33779532474864,29.5182319085358,126.594868715952));
#124270=CARTESIAN_POINT('Ctrl Pts',(1.33651829617363,29.5366769996734,126.60029250181));
#124271=CARTESIAN_POINT('Ctrl Pts',(1.33605442461696,29.543356173537,126.602211192496));
#124272=CARTESIAN_POINT('Ctrl Pts',(1.33518191808346,29.5558754060376,126.605722886482));
#124273=CARTESIAN_POINT('Ctrl Pts',(1.33477385745745,29.5617123945586,126.607325920083));
#124274=CARTESIAN_POINT('Ctrl Pts',(1.33380766348178,29.5754920640902,126.611029643168));
#124275=CARTESIAN_POINT('Ctrl Pts',(1.3332480453986,29.5834416911668,126.613103427274));
#124276=CARTESIAN_POINT('Ctrl Pts',(1.33136348526455,29.6101182453291,126.619852082733));
#124277=CARTESIAN_POINT('Ctrl Pts',(1.33002499825152,29.6289102465318,126.624260098651));
#124278=CARTESIAN_POINT('Ctrl Pts',(1.32669295527103,29.6754107403253,126.634318624314));
#124279=CARTESIAN_POINT('Ctrl Pts',(1.32468481904022,29.7031941431251,126.639591917562));
#124280=CARTESIAN_POINT('Ctrl Pts',(1.31548177421981,29.8299490429691,126.660322818526));
#124281=CARTESIAN_POINT('Ctrl Pts',(1.30811457890264,29.9300573564844,126.667542404684));
#124282=CARTESIAN_POINT('Ctrl Pts',(1.29493958186778,30.1127543627972,126.664229081732));
#124283=CARTESIAN_POINT('Ctrl Pts',(1.28910033775239,30.1950842061433,126.656598270649));
#124284=CARTESIAN_POINT('Ctrl Pts',(1.28210732868493,30.2958523550384,126.639637675855));
#124285=CARTESIAN_POINT('Ctrl Pts',(1.28077638392426,30.3151263585623,126.636042713124));
#124286=CARTESIAN_POINT('Ctrl Pts',(1.27865989763603,30.3459176275524,126.629735201287));
#124287=CARTESIAN_POINT('Ctrl Pts',(1.27786758091951,30.3574767568382,126.627238830709));
#124288=CARTESIAN_POINT('Ctrl Pts',(1.27636322918002,30.3794807020006,126.622240956089));
#124289=CARTESIAN_POINT('Ctrl Pts',(1.27565054324009,30.3899297740913,126.61976112538));
#124290=CARTESIAN_POINT('Ctrl Pts',(1.27401766079166,30.4139218890745,126.613821560628));
#124291=CARTESIAN_POINT('Ctrl Pts',(1.27309975342713,30.4274469513864,126.610292049063));
#124292=CARTESIAN_POINT('Ctrl Pts',(1.27018948650855,30.4704303860945,126.598495325958));
#124293=CARTESIAN_POINT('Ctrl Pts',(1.26821777763292,30.4997071350736,126.589586431336));
#124294=CARTESIAN_POINT('Ctrl Pts',(1.26356041448887,30.5690226336343,126.566389208934));
#124295=CARTESIAN_POINT('Ctrl Pts',(1.26089731591647,30.6087928832071,126.551365049412));
#124296=CARTESIAN_POINT('Ctrl Pts',(1.25369207243897,30.7158613383938,126.506164953304));
#124297=CARTESIAN_POINT('Ctrl Pts',(1.2492175499748,30.7817990681317,126.473017618766));
#124298=CARTESIAN_POINT('Ctrl Pts',(1.24385975445351,30.8572670334666,126.428580168892));
#124299=CARTESIAN_POINT('Ctrl Pts',(1.2430107406695,30.8691210068066,126.421399569191));
#124300=CARTESIAN_POINT('Ctrl Pts',(1.23764365312306,30.9432852055279,126.375199622325));
#124301=CARTESIAN_POINT('Ctrl Pts',(1.23307310763841,31.0030373928751,126.332244059039));
#124302=CARTESIAN_POINT('Ctrl Pts',(1.22747004235412,31.0692232147379,126.277680885065));
#124303=CARTESIAN_POINT('Ctrl Pts',(1.22666178740936,31.078609299087,126.269767177542));
#124304=CARTESIAN_POINT('Ctrl Pts',(1.22538479080401,31.0931697994912,126.25721282296));
#124305=CARTESIAN_POINT('Ctrl Pts',(1.22492092503705,31.0984043095,126.25264211219));
#124306=CARTESIAN_POINT('Ctrl Pts',(1.22404846207362,31.1081442385341,126.24402933362));
#124307=CARTESIAN_POINT('Ctrl Pts',(1.22364043952439,31.1126564223152,126.23999528931));
#124308=CARTESIAN_POINT('Ctrl Pts',(1.22267435703036,31.1232405855415,126.230428408292));
#124309=CARTESIAN_POINT('Ctrl Pts',(1.22211481281497,31.1292937342623,126.224875151036));
#124310=CARTESIAN_POINT('Ctrl Pts',(1.22023051617607,31.1494294461739,126.206126193112));
#124311=CARTESIAN_POINT('Ctrl Pts',(1.21889222056169,31.1633231647867,126.192731143373));
#124312=CARTESIAN_POINT('Ctrl Pts',(1.21556070692504,31.1969892648387,126.159125523245));
#124313=CARTESIAN_POINT('Ctrl Pts',(1.21355291098837,31.216485472978,126.138647527719));
#124314=CARTESIAN_POINT('Ctrl Pts',(1.20435287778152,31.3026239646651,126.043433009063));
#124315=CARTESIAN_POINT('Ctrl Pts',(1.19698839218701,31.3629668656202,125.963277432235));
#124316=CARTESIAN_POINT('Ctrl Pts',(1.18381117140529,31.4592994560645,125.807977316129));
#124317=CARTESIAN_POINT('Ctrl Pts',(1.17796734212128,31.4975731280804,125.734616005332));
#124318=CARTESIAN_POINT('Ctrl Pts',(1.17096998784353,31.5380004281088,125.640698873322));
#124319=CARTESIAN_POINT('Ctrl Pts',(1.16963897284778,31.5454337686396,125.622555127569));
#124320=CARTESIAN_POINT('Ctrl Pts',(1.16762808093418,31.556265365759,125.594726235129));
#124321=CARTESIAN_POINT('Ctrl Pts',(1.16694044491676,31.5598970610783,125.585134470859));
#124322=CARTESIAN_POINT('Ctrl Pts',(1.16625576032278,31.5634400119388,125.575509625522));
#124323=CARTESIAN_POINT('Origin',(5.,30.,125.));
#124324=CARTESIAN_POINT('',(0.46813995976768,31.5634400089539,125.575509633631));
#124325=CARTESIAN_POINT('',(0.659204001356836,31.5634400119422,125.575509625513));
#124326=CARTESIAN_POINT('',(5.,31.5634400119422,125.575509625513));
#124327=CARTESIAN_POINT('',(0.,28.7309291201476,126.079358653049));
#124328=CARTESIAN_POINT('Ctrl Pts',(0.468139959767684,31.5634400089539,
125.575509633631));
#124329=CARTESIAN_POINT('Ctrl Pts',(0.467368770690193,31.567802085591,125.563659536364));
#124330=CARTESIAN_POINT('Ctrl Pts',(0.466596956162903,31.5720298178673,
125.551758806788));
#124331=CARTESIAN_POINT('Ctrl Pts',(0.461141010456295,31.6009067962447,
125.46744456039));
#124332=CARTESIAN_POINT('Ctrl Pts',(0.456419879107899,31.6206752627371,
125.393466556818));
#124333=CARTESIAN_POINT('Ctrl Pts',(0.450407011445989,31.638409104359,125.302386884556));
#124334=CARTESIAN_POINT('Ctrl Pts',(0.449339268556211,31.6412918510075,
125.286327141761));
#124335=CARTESIAN_POINT('Ctrl Pts',(0.447751287487431,31.6451821308189,
125.262660571821));
#124336=CARTESIAN_POINT('Ctrl Pts',(0.447240769391864,31.6463738178038,
125.255084428795));
#124337=CARTESIAN_POINT('Ctrl Pts',(0.446325458016176,31.648404789134,125.241565055238));
#124338=CARTESIAN_POINT('Ctrl Pts',(0.445921798641823,31.6492643262127,
125.235625134549));
#124339=CARTESIAN_POINT('Ctrl Pts',(0.445021426772412,31.651101607034,125.222425580418));
#124340=CARTESIAN_POINT('Ctrl Pts',(0.44452388505581,31.6520635739916,125.215164118675));
#124341=CARTESIAN_POINT('Ctrl Pts',(0.443043352510583,31.6547700134784,
125.193645338723));
#124342=CARTESIAN_POINT('Ctrl Pts',(0.442053395789655,31.656377970519,125.179371957054));
#124343=CARTESIAN_POINT('Ctrl Pts',(0.434513415275642,31.6671300724779,
125.071395054618));
#124344=CARTESIAN_POINT('Ctrl Pts',(0.42764868542884,31.6684999275946,124.977096703258));
#124345=CARTESIAN_POINT('Ctrl Pts',(0.412304827135571,31.653722402769,124.766837295084));
#124346=CARTESIAN_POINT('Ctrl Pts',(0.403889262908525,31.6333448864033,
124.651637932408));
#124347=CARTESIAN_POINT('Ctrl Pts',(0.394336279461322,31.595018794061,124.518384267772));
#124348=CARTESIAN_POINT('Ctrl Pts',(0.392835702202461,31.588528832241,124.497391906723));
#124349=CARTESIAN_POINT('Ctrl Pts',(0.390424858204483,31.5773379130571,
124.463579180904));
#124350=CARTESIAN_POINT('Ctrl Pts',(0.389506471943513,31.5728914726194,
124.450678034635));
#124351=CARTESIAN_POINT('Ctrl Pts',(0.387873691290787,31.5646585834181,
124.427710617482));
#124352=CARTESIAN_POINT('Ctrl Pts',(0.387157366668118,31.5609322709169,
124.417623768616));
#124353=CARTESIAN_POINT('Ctrl Pts',(0.385640417512856,31.5527982994039,
124.396244785696));
#124354=CARTESIAN_POINT('Ctrl Pts',(0.384840708010599,31.5483645157232,
124.384963206909));
#124355=CARTESIAN_POINT('Ctrl Pts',(0.382679527278756,31.5359886582273,
124.354455646217));
#124356=CARTESIAN_POINT('Ctrl Pts',(0.381326043245242,31.5278088458072,
124.335328002947));
#124357=CARTESIAN_POINT('Ctrl Pts',(0.372816736258931,31.4737024844142,
124.215086270981));
#124358=CARTESIAN_POINT('Ctrl Pts',(0.366010330351707,31.4181195833027,
124.118620703354));
#124359=CARTESIAN_POINT('Ctrl Pts',(0.352940332421378,31.2934163691235,
123.944922250076));
#124360=CARTESIAN_POINT('Ctrl Pts',(0.346693658205991,31.2259025825912,
123.867183949264));
#124361=CARTESIAN_POINT('Ctrl Pts',(0.339013873587773,31.1403992568927,
123.785385291027));
#124362=CARTESIAN_POINT('Ctrl Pts',(0.33799191278734,31.1289765556816,123.77476073737));
#124363=CARTESIAN_POINT('Ctrl Pts',(0.336455722723449,31.1117743934971,
123.759205349809));
#124364=CARTESIAN_POINT('Ctrl Pts',(0.335950087347881,31.1061073081551,
123.754150778275));
#124365=CARTESIAN_POINT('Ctrl Pts',(0.335033168053102,31.0958263971097,
123.745106494143));
#124366=CARTESIAN_POINT('Ctrl Pts',(0.334622882564975,31.0912249366391,
123.74110312682));
#124367=CARTESIAN_POINT('Ctrl Pts',(0.333693765673588,31.0808016304986,
123.73213471557));
#124368=CARTESIAN_POINT('Ctrl Pts',(0.333173937905942,31.0749674812954,
123.727184438947));
#124369=CARTESIAN_POINT('Ctrl Pts',(0.331584096848049,31.0571107958942,
123.712243376026));
#124370=CARTESIAN_POINT('Ctrl Pts',(0.330505870857499,31.0449819336647,
123.702381769159));
#124371=CARTESIAN_POINT('Ctrl Pts',(0.32499257597472,30.9827861411625,123.653249761813));
#124372=CARTESIAN_POINT('Ctrl Pts',(0.320423120177883,30.9306413534343,
123.616703221994));
#124373=CARTESIAN_POINT('Ctrl Pts',(0.307698517681965,30.7811244703153,
123.52419866703));
#124374=CARTESIAN_POINT('Ctrl Pts',(0.299521308008059,30.67997659713,123.474948408541));
#124375=CARTESIAN_POINT('Ctrl Pts',(0.288679174945068,30.534995564185,123.421671925826));
#124376=CARTESIAN_POINT('Ctrl Pts',(0.28575732732078,30.494810505844,123.408616054369));
#124377=CARTESIAN_POINT('Ctrl Pts',(0.28177491245182,30.4384865965643,123.392657098812));
#124378=CARTESIAN_POINT('Ctrl Pts',(0.280673378841057,30.4227389239297,
123.388443754657));
#124379=CARTESIAN_POINT('Ctrl Pts',(0.278901027352942,30.3971341915459,
123.381994279869));
#124380=CARTESIAN_POINT('Ctrl Pts',(0.278225719759276,30.387314498595,123.379615612478));
#124381=CARTESIAN_POINT('Ctrl Pts',(0.276816168551184,30.3666874725309,
123.374817261534));
#124382=CARTESIAN_POINT('Ctrl Pts',(0.276082530698485,30.355876395902,123.372415705186));
#124383=CARTESIAN_POINT('Ctrl Pts',(0.274330374375297,30.3298812737826,
123.366912588925));
#124384=CARTESIAN_POINT('Ctrl Pts',(0.273315169406157,30.3146761516838,
123.363914704848));
#124385=CARTESIAN_POINT('Ctrl Pts',(0.269726970706268,30.2604530153548,
123.354007829728));
#124386=CARTESIAN_POINT('Ctrl Pts',(0.26719076948498,30.221231264432,123.348278742434));
#124387=CARTESIAN_POINT('Ctrl Pts',(0.260817490673064,30.1208997243022,
123.337261974428));
#124388=CARTESIAN_POINT('Ctrl Pts',(0.257034128238834,30.0596335023462,
123.333939030875));
#124389=CARTESIAN_POINT('Ctrl Pts',(0.247839320171625,29.9094801953683,
123.334090415222));
#124390=CARTESIAN_POINT('Ctrl Pts',(0.242477938268877,29.8207947027282,
123.341285927766));
#124391=CARTESIAN_POINT('Ctrl Pts',(0.234159662091679,29.6894615256933,
123.362600436931));
#124392=CARTESIAN_POINT('Ctrl Pts',(0.231349311652282,29.6461152983617,
123.371418915673));
#124393=CARTESIAN_POINT('Ctrl Pts',(0.227712284229607,29.5921767632879,
123.38464726608));
#124394=CARTESIAN_POINT('Ctrl Pts',(0.226965162534283,29.581206228346,123.387456665141));
#124395=CARTESIAN_POINT('Ctrl Pts',(0.225768717193004,29.563829096667,123.392095984191));
#124396=CARTESIAN_POINT('Ctrl Pts',(0.225323434430909,29.5574031382573,
123.393852934802));
#124397=CARTESIAN_POINT('Ctrl Pts',(0.224477673033089,29.545279881108,123.397245886415));
#124398=CARTESIAN_POINT('Ctrl Pts',(0.224077670321568,29.5395805739931,
123.398873806956));
#124399=CARTESIAN_POINT('Ctrl Pts',(0.223118448933726,29.5259975931469,
123.402832101328));
#124400=CARTESIAN_POINT('Ctrl Pts',(0.222557613118673,29.5181226345996,
123.405190363881));
#124401=CARTESIAN_POINT('Ctrl Pts',(0.220548127685299,29.490131162165,123.413799031918));
#124402=CARTESIAN_POINT('Ctrl Pts',(0.219081790091245,29.4701171161197,
123.42037227058));
#124403=CARTESIAN_POINT('Ctrl Pts',(0.215326067188745,29.4197529847743,
123.437978216238));
#124404=CARTESIAN_POINT('Ctrl Pts',(0.213015409762782,29.3895897780316,
123.44951693326));
#124405=CARTESIAN_POINT('Ctrl Pts',(0.200529610501357,29.2300646652659,
123.515918521441));
#124406=CARTESIAN_POINT('Ctrl Pts',(0.190064542815158,29.1076728703631,
123.58611876236));
#124407=CARTESIAN_POINT('Ctrl Pts',(0.176589423172343,28.9559563764781,
123.700772690116));
#124408=CARTESIAN_POINT('Ctrl Pts',(0.173134986376414,28.9177180680903,
123.732449039431));
#124409=CARTESIAN_POINT('Ctrl Pts',(0.168612282644377,28.8685655253681,
123.777015381181));
#124410=CARTESIAN_POINT('Ctrl Pts',(0.167481173164388,28.8563528711332,
123.788428033549));
#124411=CARTESIAN_POINT('Ctrl Pts',(0.165626985887512,28.8364739180026,
123.807573262244));
#124412=CARTESIAN_POINT('Ctrl Pts',(0.164899249616014,28.8287082396161,
123.815200400668));
#124413=CARTESIAN_POINT('Ctrl Pts',(0.163480579706886,28.8136446596442,
123.830288110655));
#124414=CARTESIAN_POINT('Ctrl Pts',(0.162789399244573,28.8063410261192,
123.83774221427));
#124415=CARTESIAN_POINT('Ctrl Pts',(0.161149985660963,28.7891064289632,
123.855665709101));
#124416=CARTESIAN_POINT('Ctrl Pts',(0.160204680457111,28.779240386751,123.866196578458));
#124417=CARTESIAN_POINT('Ctrl Pts',(0.156942374811789,28.7454615307051,
123.903203783401));
#124418=CARTESIAN_POINT('Ctrl Pts',(0.154655988771575,28.7222622101635,
123.930320071177));
#124419=CARTESIAN_POINT('Ctrl Pts',(0.14901271229703,28.6664752093685,123.999933478309));
#124420=CARTESIAN_POINT('Ctrl Pts',(0.145696720407851,28.6350312584555,
124.043296079065));
#124421=CARTESIAN_POINT('Ctrl Pts',(0.136010305398242,28.5486172949571,
124.175420816695));
#124422=CARTESIAN_POINT('Ctrl Pts',(0.129760520647114,28.4998402846621,
124.267906791714));
#124423=CARTESIAN_POINT('Ctrl Pts',(0.120761037950463,28.445148887449,124.400403266088));
#124424=CARTESIAN_POINT('Ctrl Pts',(0.118270580114547,28.4315352623153,
124.436975987133));
#124425=CARTESIAN_POINT('Ctrl Pts',(0.115008671259818,28.4158399621266,
124.484143906482));
#124426=CARTESIAN_POINT('Ctrl Pts',(0.114301287857148,28.4125589999163,
124.494330551949));
#124427=CARTESIAN_POINT('Ctrl Pts',(0.113160173153524,28.4074664239155,
124.510680000478));
#124428=CARTESIAN_POINT('Ctrl Pts',(0.112730107672887,28.4055918425637,
124.516823138953));
#124429=CARTESIAN_POINT('Ctrl Pts',(0.111880549185385,28.4019773047899,
124.528918352972));
#124430=CARTESIAN_POINT('Ctrl Pts',(0.111461248669659,28.4002350013568,
124.534869482342));
#124431=CARTESIAN_POINT('Ctrl Pts',(0.110430701722022,28.3960533375199,
124.549454117648));
#124432=CARTESIAN_POINT('Ctrl Pts',(0.109817422587184,28.3936504488922,
124.558097749877));
#124433=CARTESIAN_POINT('Ctrl Pts',(0.10755902290542,28.3851094317105,124.589811783972));
#124434=CARTESIAN_POINT('Ctrl Pts',(0.105892391064636,28.3793978953718,
124.612992775244));
#124435=CARTESIAN_POINT('Ctrl Pts',(0.0953374774786414,28.346769127222,
124.758844787492));
#124436=CARTESIAN_POINT('Ctrl Pts',(0.0860039510206011,28.3332983044055,
124.884103984439));
#124437=CARTESIAN_POINT('Ctrl Pts',(0.0697063715490643,28.3346008157314,
125.108220445731));
#124438=CARTESIAN_POINT('Ctrl Pts',(0.0626898594723843,28.343914664283,
125.206527192335));
#124439=CARTESIAN_POINT('Ctrl Pts',(0.054437159096772,28.3658285735266,
125.324826806449));
#124440=CARTESIAN_POINT('Ctrl Pts',(0.0529582260633922,28.3702069174437,
125.346126113057));
#124441=CARTESIAN_POINT('Ctrl Pts',(0.0506065414160396,28.3778936493717,
125.380130358099));
#124442=CARTESIAN_POINT('Ctrl Pts',(0.0497261093003398,28.3809372930433,
125.392891929786));
#124443=CARTESIAN_POINT('Ctrl Pts',(0.0480517958143798,28.3870419178504,
125.417211135297));
#124444=CARTESIAN_POINT('Ctrl Pts',(0.0472572206844655,28.3900771757282,
125.428774320061));
#124445=CARTESIAN_POINT('Ctrl Pts',(0.0454282488283537,28.397382327402,
125.455432374105));
#124446=CARTESIAN_POINT('Ctrl Pts',(0.044396501792675,28.4017415133624,
125.470501738964));
#124447=CARTESIAN_POINT('Ctrl Pts',(0.0410412543902908,28.4166910837999,
125.519573952442));
#124448=CARTESIAN_POINT('Ctrl Pts',(0.0387426856803513,28.4281592505517,
125.553300207085));
#124449=CARTESIAN_POINT('Ctrl Pts',(0.0310769026755918,28.4704076382907,
125.66559821414));
#124450=CARTESIAN_POINT('Ctrl Pts',(0.0258331118161244,28.5060708126985,
125.742192994397));
#124451=CARTESIAN_POINT('Ctrl Pts',(0.0154827819627932,28.5873200683497,
125.8868727954));
#124452=CARTESIAN_POINT('Ctrl Pts',(0.010389205693264,28.6324204876046,
125.954951236689));
#124453=CARTESIAN_POINT('Ctrl Pts',(0.00414832869307692,28.6911391688753,
126.030847754724));
#124454=CARTESIAN_POINT('Ctrl Pts',(0.00320452041853181,28.700106702341,
126.042132984382));
#124455=CARTESIAN_POINT('Ctrl Pts',(0.00184158482903431,28.7131616496016,
126.05813134517));
#124456=CARTESIAN_POINT('Ctrl Pts',(0.00142859836214397,28.7171310837055,
126.062940367519));
#124457=CARTESIAN_POINT('Ctrl Pts',(0.000677079262193936,28.724376940454,
126.07161911092));
#124458=CARTESIAN_POINT('Ctrl Pts',(0.000339057602576914,28.7276442281703,
126.075496395827));
#124459=CARTESIAN_POINT('Ctrl Pts',(1.87192926090485E-13,28.7309291201478,
126.079358653049));
#124460=CARTESIAN_POINT('',(0.,31.2524897196664,126.098556098763));
#124461=CARTESIAN_POINT('Origin',(0.,30.,125.));
#124462=CARTESIAN_POINT('Ctrl Pts',(1.19418364086243E-13,31.2524897196665,
126.098556098763));
#124463=CARTESIAN_POINT('Ctrl Pts',(0.000120419872249425,31.2513359446956,
126.099871544821));
#124464=CARTESIAN_POINT('Ctrl Pts',(0.000240971468816246,31.2501801021712,
126.101185167756));
#124465=CARTESIAN_POINT('Ctrl Pts',(0.00193646291216417,31.233912230833,
126.119615089179));
#124466=CARTESIAN_POINT('Ctrl Pts',(0.0035330494313661,31.2184528025057,
126.136419811813));
#124467=CARTESIAN_POINT('Ctrl Pts',(0.0132700945587604,31.1230711888905,
126.235917611428));
#124468=CARTESIAN_POINT('Ctrl Pts',(0.021756819076212,31.0351097558255,
126.310468700313));
#124469=CARTESIAN_POINT('Ctrl Pts',(0.0343332838466417,30.8914286708614,
126.408686373077));
#124470=CARTESIAN_POINT('Ctrl Pts',(0.0385499468194289,30.8409429808811,
126.439395170051));
#124471=CARTESIAN_POINT('Ctrl Pts',(0.0445224030564696,30.7657573349109,
126.479818848122));
#124472=CARTESIAN_POINT('Ctrl Pts',(0.0463457463768341,30.7422930627286,
126.491726938576));
#124473=CARTESIAN_POINT('Ctrl Pts',(0.0496166659792298,30.6992723961174,
126.512293268752));
#124474=CARTESIAN_POINT('Ctrl Pts',(0.0510702612592213,30.6798130112003,
126.521140084812));
#124475=CARTESIAN_POINT('Ctrl Pts',(0.0533394920189012,30.6489075855109,
126.534479030971));
#124476=CARTESIAN_POINT('Ctrl Pts',(0.0541635202143546,30.6375734396752,
126.539222879867));
#124477=CARTESIAN_POINT('Ctrl Pts',(0.0557042291348595,30.6161764593036,
126.547901573664));
#124478=CARTESIAN_POINT('Ctrl Pts',(0.0564218214363469,30.6061258787205,
126.551864729663));
#124479=CARTESIAN_POINT('Ctrl Pts',(0.0580345429839894,30.5833511871357,
126.560590257455));
#124480=CARTESIAN_POINT('Ctrl Pts',(0.0589277495074523,30.570605847082,
126.565295353718));
#124481=CARTESIAN_POINT('Ctrl Pts',(0.061230862686238,30.5374144326067,
126.577089076055));
#124482=CARTESIAN_POINT('Ctrl Pts',(0.0626329784772223,30.516884895882,
126.58393633018));
#124483=CARTESIAN_POINT('Ctrl Pts',(0.0713881304400068,30.3868326848086,
126.624514897965));
#124484=CARTESIAN_POINT('Ctrl Pts',(0.0783802403871928,30.2742065579199,
126.647271164091));
#124485=CARTESIAN_POINT('Ctrl Pts',(0.0909542344985003,30.0700614129422,
126.666983748548));
#124486=CARTESIAN_POINT('Ctrl Pts',(0.0965118220669303,29.9794482348121,
126.668327567464));
#124487=CARTESIAN_POINT('Ctrl Pts',(0.103345836149256,29.87463576077,126.661340571532));
#124488=CARTESIAN_POINT('Ctrl Pts',(0.104302962662541,29.8600982165223,
126.660179551556));
#124489=CARTESIAN_POINT('Ctrl Pts',(0.105763581129966,29.8381641540326,
126.658137692169));
#124490=CARTESIAN_POINT('Ctrl Pts',(0.106259834300462,29.8307548053142,
126.65739781166));
#124491=CARTESIAN_POINT('Ctrl Pts',(0.107167817586604,29.8172817915208,
126.655961143403));
#124492=CARTESIAN_POINT('Ctrl Pts',(0.107578659519283,29.8112166647196,
126.655280671597));
#124493=CARTESIAN_POINT('Ctrl Pts',(0.108520526137026,29.797383769729,126.653651685739));
#124494=CARTESIAN_POINT('Ctrl Pts',(0.109052671483722,29.7896189599143,
126.65268177408));
#124495=CARTESIAN_POINT('Ctrl Pts',(0.110697137358969,29.7657699975256,
126.649531981497));
#124496=CARTESIAN_POINT('Ctrl Pts',(0.111818488437504,29.749711170695,126.647171789978));
#124497=CARTESIAN_POINT('Ctrl Pts',(0.118574861806228,29.6540160048456,
126.631675672434));
#124498=CARTESIAN_POINT('Ctrl Pts',(0.124428652658414,29.5753920586676,
126.613002196761));
#124499=CARTESIAN_POINT('Ctrl Pts',(0.135603602004164,29.4288597830144,
126.566741408986));
#124500=CARTESIAN_POINT('Ctrl Pts',(0.140910586278219,29.3607945398787,
126.540226416423));
#124501=CARTESIAN_POINT('Ctrl Pts',(0.149161203294748,29.2560298529204,
126.491269538329));
#124502=CARTESIAN_POINT('Ctrl Pts',(0.152169158710906,29.2180815027312,
126.47172700641));
#124503=CARTESIAN_POINT('Ctrl Pts',(0.157261953427681,29.1541860318168,
126.435652271797));
#124504=CARTESIAN_POINT('Ctrl Pts',(0.15936825883863,29.1278703901019,126.419820013881));
#124505=CARTESIAN_POINT('Ctrl Pts',(0.162400090719225,29.0901763019751,
126.395698420953));
#124506=CARTESIAN_POINT('Ctrl Pts',(0.16334604576855,29.0784426697601,126.387978872917));
#124507=CARTESIAN_POINT('Ctrl Pts',(0.165009732633383,29.0578603643131,
126.374061703277));
#124508=CARTESIAN_POINT('Ctrl Pts',(0.165729670330972,29.048971859355,126.367924757666));
#124509=CARTESIAN_POINT('Ctrl Pts',(0.167236333917631,29.0304126867199,
126.354842492236));
#124510=CARTESIAN_POINT('Ctrl Pts',(0.168022319148125,29.0207554900144,
126.347879052001));
#124511=CARTESIAN_POINT('Ctrl Pts',(0.170103192254091,28.9952622904181,
126.329078250773));
#124512=CARTESIAN_POINT('Ctrl Pts',(0.171391102004005,28.9795606446763,
126.317061288452));
#124513=CARTESIAN_POINT('Ctrl Pts',(0.178216470464427,28.8968543440787,
126.25139636933));
#124514=CARTESIAN_POINT('Ctrl Pts',(0.183555173863248,28.8338532511722,
126.192907235631));
#124515=CARTESIAN_POINT('Ctrl Pts',(0.194824144986091,28.7093355564115,
126.057969197731));
#124516=CARTESIAN_POINT('Ctrl Pts',(0.200711153308162,28.6494938617959,
125.980430737206));
#124517=CARTESIAN_POINT('Ctrl Pts',(0.208600682002403,28.5817001482742,
125.874509002213));
#124518=CARTESIAN_POINT('Ctrl Pts',(0.210377412201224,28.5671996919254,
125.850543100639));
#124519=CARTESIAN_POINT('Ctrl Pts',(0.21342102665041,28.5437966293544,125.809565191917));
#124520=CARTESIAN_POINT('Ctrl Pts',(0.214672012808006,28.5345712120699,
125.79274362048));
#124521=CARTESIAN_POINT('Ctrl Pts',(0.216482736540219,28.5218140695251,
125.768498419952));
#124522=CARTESIAN_POINT('Ctrl Pts',(0.217028676566177,28.5180432482695,
125.761201448732));
#124523=CARTESIAN_POINT('Ctrl Pts',(0.217983088824172,28.5115851404496,
125.748474388849));
#124524=CARTESIAN_POINT('Ctrl Pts',(0.218390039097989,28.5088732564213,
125.743057022276));
#124525=CARTESIAN_POINT('Ctrl Pts',(0.219267141160128,28.5031188319966,
125.731403385843));
#124526=CARTESIAN_POINT('Ctrl Pts',(0.219737812071764,28.5000857266515,
125.725162955584));
#124527=CARTESIAN_POINT('Ctrl Pts',(0.221049293472486,28.4917831141627,
125.707805886538));
#124528=CARTESIAN_POINT('Ctrl Pts',(0.22189490322558,28.4865977515219,125.696649811398));
#124529=CARTESIAN_POINT('Ctrl Pts',(0.228299151452013,28.4485442980768,
125.612349266656));
#124530=CARTESIAN_POINT('Ctrl Pts',(0.234100851802819,28.4208755617529,
125.536981920421));
#124531=CARTESIAN_POINT('Ctrl Pts',(0.240293458575491,28.3973795694616,
125.45517923896));
#124532=CARTESIAN_POINT('Ctrl Pts',(0.2406528604165,28.396037463859,125.450427093416));
#124533=CARTESIAN_POINT('Ctrl Pts',(0.245962791381931,28.3765250131813,
125.380143966479));
#124534=CARTESIAN_POINT('Ctrl Pts',(0.250918207616037,28.3623616103307,
125.313563174657));
#124535=CARTESIAN_POINT('Ctrl Pts',(0.25916348053512,28.3453536468021,125.199783868053));
#124536=CARTESIAN_POINT('Ctrl Pts',(0.262492976182862,28.3403727147697,
125.15299046966));
#124537=CARTESIAN_POINT('Ctrl Pts',(0.268053993240698,28.335285751493,125.073235019719));
#124538=CARTESIAN_POINT('Ctrl Pts',(0.27031327992051,28.3341645998031,125.040368080396));
#124539=CARTESIAN_POINT('Ctrl Pts',(0.273513266818834,28.333952470457,124.993168119654));
#124540=CARTESIAN_POINT('Ctrl Pts',(0.274478252745838,28.3340727293236,
124.978848251524));
#124541=CARTESIAN_POINT('Ctrl Pts',(0.276156810082106,28.3346062390976,
124.953794438435));
#124542=CARTESIAN_POINT('Ctrl Pts',(0.27687287180603,28.3349386926446,124.943059813253));
#124543=CARTESIAN_POINT('Ctrl Pts',(0.27835368746437,28.3358449289516,124.920767514385));
#124544=CARTESIAN_POINT('Ctrl Pts',(0.279117878664363,28.3364353729257,
124.909211067412));
#124545=CARTESIAN_POINT('Ctrl Pts',(0.281100629030457,28.3382885882748,
124.879098988909));
#124546=CARTESIAN_POINT('Ctrl Pts',(0.28231317409968,28.3397417700217,124.860556371253));
#124547=CARTESIAN_POINT('Ctrl Pts',(0.287731413302196,28.3476808759991,
124.777199329844));
#124548=CARTESIAN_POINT('Ctrl Pts',(0.291827206387565,28.3576542608388,
124.712770921812));
#124549=CARTESIAN_POINT('Ctrl Pts',(0.304762928305831,28.4016909800989,
124.508392544346));
#124550=CARTESIAN_POINT('Ctrl Pts',(0.313254178368665,28.4501038627908,
124.372240989306));
#124551=CARTESIAN_POINT('Ctrl Pts',(0.323941609087643,28.5257761912828,
124.223634412228));
#124552=CARTESIAN_POINT('Ctrl Pts',(0.325426153653166,28.53657532494,124.203465343797));
#124553=CARTESIAN_POINT('Ctrl Pts',(0.327511038110602,28.552069024776,124.17590760082));
#124554=CARTESIAN_POINT('Ctrl Pts',(0.328090890717785,28.5564122027791,
124.168322986537));
#124555=CARTESIAN_POINT('Ctrl Pts',(0.329082585095573,28.5638929812083,
124.155494243625));
#124556=CARTESIAN_POINT('Ctrl Pts',(0.329492489877153,28.5670001060839,
124.150232593667));
#124557=CARTESIAN_POINT('Ctrl Pts',(0.330354170156425,28.573561568467,124.139259651117));
#124558=CARTESIAN_POINT('Ctrl Pts',(0.330806252477442,28.5770212534269,
124.133552061565));
#124559=CARTESIAN_POINT('Ctrl Pts',(0.332031517224733,28.5864465606485,
124.118211443503));
#124560=CARTESIAN_POINT('Ctrl Pts',(0.332808629225396,28.5924761903665,
124.108618436396));
#124561=CARTESIAN_POINT('Ctrl Pts',(0.336633882415379,28.6224290199547,
124.062025865209));
#124562=CARTESIAN_POINT('Ctrl Pts',(0.339755647276421,28.6477138004997,
124.02592680392));
#124563=CARTESIAN_POINT('Ctrl Pts',(0.349274887476877,28.7280359353408,
123.920414244656));
#124564=CARTESIAN_POINT('Ctrl Pts',(0.355773539922679,28.7872069940285,
123.854342503203));
#124565=CARTESIAN_POINT('Ctrl Pts',(0.366581855952751,28.8954451058935,
123.751312360873));
#124566=CARTESIAN_POINT('Ctrl Pts',(0.370935350416607,28.9418123787886,
123.711783185823));
#124567=CARTESIAN_POINT('Ctrl Pts',(0.377951826521861,29.0215140838698,
123.651049694617));
#124568=CARTESIAN_POINT('Ctrl Pts',(0.380665657124409,29.0536200283644,
123.628334221189));
#124569=CARTESIAN_POINT('Ctrl Pts',(0.38438091751618,29.0993537831104,123.59834791684));
#124570=CARTESIAN_POINT('Ctrl Pts',(0.385418315944144,29.1123217737337,
123.590099448794));
#124571=CARTESIAN_POINT('Ctrl Pts',(0.387185185521635,29.1347431347277,
123.57627004013));
#124572=CARTESIAN_POINT('Ctrl Pts',(0.387917851668388,29.1441407287606,
123.570601049642));
#124573=CARTESIAN_POINT('Ctrl Pts',(0.389311960667801,29.1622108778907,
123.559942545048));
#124574=CARTESIAN_POINT('Ctrl Pts',(0.38997394269656,29.1708736664756,123.554937504075));
#124575=CARTESIAN_POINT('Ctrl Pts',(0.391695021873892,29.1936069158011,
123.542074798301));
#124576=CARTESIAN_POINT('Ctrl Pts',(0.392749620275369,29.2077474471295,
123.534342597254));
#124577=CARTESIAN_POINT('Ctrl Pts',(0.396491474681653,29.2586429840492,
123.507464199005));
#124578=CARTESIAN_POINT('Ctrl Pts',(0.399138377662074,29.2959989525964,
123.489484755959));
#124579=CARTESIAN_POINT('Ctrl Pts',(0.409051233442797,29.4402334131195,
123.426579428819));
#124580=CARTESIAN_POINT('Ctrl Pts',(0.416019982644108,29.5510209455288,
123.391457331225));
#124581=CARTESIAN_POINT('Ctrl Pts',(0.426138251613408,29.7121565240423,
123.358335198261));
#124582=CARTESIAN_POINT('Ctrl Pts',(0.429154233192449,29.7601555452664,
123.350639160858));
#124583=CARTESIAN_POINT('Ctrl Pts',(0.433460935383947,29.8273545219931,
123.342860020302));
#124584=CARTESIAN_POINT('Ctrl Pts',(0.434686112669329,29.8463258125067,
123.340993202916));
#124585=CARTESIAN_POINT('Ctrl Pts',(0.436861932572467,29.8796633116692,
123.338289421349));
#124586=CARTESIAN_POINT('Ctrl Pts',(0.437806122271101,29.8940164080375,
123.337312293315));
#124587=CARTESIAN_POINT('Ctrl Pts',(0.439245961409634,29.9156971251417,
123.336118173804));
#124588=CARTESIAN_POINT('Ctrl Pts',(0.439734414844805,29.9230168970012,
123.33576344739));
#124589=CARTESIAN_POINT('Ctrl Pts',(0.440628995988438,29.9363530647816,
123.335205326532));
#124590=CARTESIAN_POINT('Ctrl Pts',(0.441034259632286,29.9423685351658,
123.334986231886));
#124591=CARTESIAN_POINT('Ctrl Pts',(0.441962994899013,29.9560948135542,
123.334560769196));
#124592=CARTESIAN_POINT('Ctrl Pts',(0.442487571378068,29.9638059105064,
123.334375348743));
#124593=CARTESIAN_POINT('Ctrl Pts',(0.444137162823976,29.9879324341714,
123.333962817919));
#124594=CARTESIAN_POINT('Ctrl Pts',(0.445271646113914,30.0043495425571,
123.333924806814));
#124595=CARTESIAN_POINT('Ctrl Pts',(0.452149199731338,30.1029806714545,
123.335154164901));
#124596=CARTESIAN_POINT('Ctrl Pts',(0.458120736128249,30.1850013857375,
123.342264002874));
#124597=CARTESIAN_POINT('Ctrl Pts',(0.470608274499982,30.3543741164985,
123.369674358478));
#124598=CARTESIAN_POINT('Ctrl Pts',(0.477103570605014,30.4413113746485,
123.391028303444));
#124599=CARTESIAN_POINT('Ctrl Pts',(0.485769101215786,30.5576975206259,
123.429765325448));
#124600=CARTESIAN_POINT('Ctrl Pts',(0.488094502943807,30.5889527240976,
123.441218936991));
#124601=CARTESIAN_POINT('Ctrl Pts',(0.492151258319918,30.6435315700449,
123.463095879849));
#124602=CARTESIAN_POINT('Ctrl Pts',(0.493894154064312,30.6669972250208,
123.473133279331));
#124603=CARTESIAN_POINT('Ctrl Pts',(0.496500659639892,30.7020977641217,
123.489111213766));
#124604=CARTESIAN_POINT('Ctrl Pts',(0.497377564370255,30.7139077240488,
123.494655530092));
#124605=CARTESIAN_POINT('Ctrl Pts',(0.498962370100576,30.7352481782841,
123.504981681577));
#124606=CARTESIAN_POINT('Ctrl Pts',(0.499671818589518,30.7448001115646,
123.509717322466));
#124607=CARTESIAN_POINT('Ctrl Pts',(0.501202177328026,30.7653974762926,
123.520176550304));
#124608=CARTESIAN_POINT('Ctrl Pts',(0.502021893598458,30.7764256458123,
123.525932847675));
#124609=CARTESIAN_POINT('Ctrl Pts',(0.504271941509844,30.8066734874212,
123.542154754372));
#124610=CARTESIAN_POINT('Ctrl Pts',(0.505693185222492,30.8257534459316,
123.552876579499));
#124611=CARTESIAN_POINT('Ctrl Pts',(0.51596710352404,30.9632905553324,123.633770685432));
#124612=CARTESIAN_POINT('Ctrl Pts',(0.524253532652145,31.0728529698589,
123.718008864406));
#124613=CARTESIAN_POINT('Ctrl Pts',(0.536040815112307,31.209656949812,123.853148707026));
#124614=CARTESIAN_POINT('Ctrl Pts',(0.539412498956275,31.2465919908856,
123.893408206995));
#124615=CARTESIAN_POINT('Ctrl Pts',(0.544795821256298,31.3007786776399,
123.958634157515));
#124616=CARTESIAN_POINT('Ctrl Pts',(0.546741028654071,31.3194397187668,
123.982381925061));
#124617=CARTESIAN_POINT('Ctrl Pts',(0.549365714333144,31.3432351649281,
124.014419140651));
#124618=CARTESIAN_POINT('Ctrl Pts',(0.55000867594225,31.3489581047971,124.022266724061));
#124619=CARTESIAN_POINT('Ctrl Pts',(0.551077783483638,31.3582927024894,
124.03530475626));
#124620=CARTESIAN_POINT('Ctrl Pts',(0.551501281917573,31.3619441092458,
124.040466665902));
#124621=CARTESIAN_POINT('Ctrl Pts',(0.552305799385169,31.368791410968,124.050264364683));
#124622=CARTESIAN_POINT('Ctrl Pts',(0.552686384795243,31.3719933671395,
124.054895824862));
#124623=CARTESIAN_POINT('Ctrl Pts',(0.553704699010479,31.3804635139322,
124.067281197679));
#124624=CARTESIAN_POINT('Ctrl Pts',(0.554345120421671,31.3856897469891,
124.075063357688));
#124625=CARTESIAN_POINT('Ctrl Pts',(0.556729805589084,31.4047900136592,
124.104029974355));
#124626=CARTESIAN_POINT('Ctrl Pts',(0.558497844305222,31.418245439427,124.125484719619));
#124627=CARTESIAN_POINT('Ctrl Pts',(0.567528240818528,31.4836997811928,
124.235337699133));
#124628=CARTESIAN_POINT('Ctrl Pts',(0.575065987911613,31.5279442536527,
124.328093566176));
#124629=CARTESIAN_POINT('Ctrl Pts',(0.588497965147215,31.591949911208,124.501915443828));
#124630=CARTESIAN_POINT('Ctrl Pts',(0.594412477961797,31.6147083244348,
124.581534851399));
#124631=CARTESIAN_POINT('Ctrl Pts',(0.602220934874307,31.6375157908092,
124.691793359584));
#124632=CARTESIAN_POINT('Ctrl Pts',(0.604269962726265,31.642781710564,124.721220967286));
#124633=CARTESIAN_POINT('Ctrl Pts',(0.607232105492085,31.6493251569751,
124.764470074825));
#124634=CARTESIAN_POINT('Ctrl Pts',(0.608164599205063,31.6512262275195,
124.778189755053));
#124635=CARTESIAN_POINT('Ctrl Pts',(0.609809250555115,31.6542948218558,
124.802567600137));
#124636=CARTESIAN_POINT('Ctrl Pts',(0.610523527484548,31.6555309477397,
124.813216166525));
#124637=CARTESIAN_POINT('Ctrl Pts',(0.612022805099943,31.6579204629778,
124.835692533048));
#124638=CARTESIAN_POINT('Ctrl Pts',(0.612807027139203,31.6590502589798,
124.847522277845));
#124639=CARTESIAN_POINT('Ctrl Pts',(0.614893528427083,31.6617324896373,
124.879182919037));
#124640=CARTESIAN_POINT('Ctrl Pts',(0.616188642564974,31.6630565453131,
124.899031608022));
#124641=CARTESIAN_POINT('Ctrl Pts',(0.623772434758818,31.6687718064019,
125.016298340099));
#124642=CARTESIAN_POINT('Ctrl Pts',(0.629795867719878,31.6649589272272,
125.113930756203));
#124643=CARTESIAN_POINT('Ctrl Pts',(0.640240285887603,31.6433642118955,
125.283325335272));
#124644=CARTESIAN_POINT('Ctrl Pts',(0.64467960019994,31.6293236497559,125.355278492019));
#124645=CARTESIAN_POINT('Ctrl Pts',(0.652478489251387,31.5972350524001,
125.476576858804));
#124646=CARTESIAN_POINT('Ctrl Pts',(0.655779588951016,31.5815073081684,
125.526420739406));
#124647=CARTESIAN_POINT('Ctrl Pts',(0.659200667255647,31.5634576043012,
125.57546183235));
#124648=CARTESIAN_POINT('Ctrl Pts',(0.659202334267445,31.5634488083536,
125.57548572902));
#124649=CARTESIAN_POINT('Ctrl Pts',(0.659204001356838,31.5634400119422,
125.575509625513));
#124650=CARTESIAN_POINT('Origin',(5.,30.,125.));
#124651=CARTESIAN_POINT('',(1.3202051089041,31.6659997343953,125.000940741602));
#124652=CARTESIAN_POINT('Ctrl Pts',(0.659204001356838,31.5634400119422,
125.575509625513));
#124653=CARTESIAN_POINT('Ctrl Pts',(0.659952818579036,31.5594888714704,
125.58624336624));
#124654=CARTESIAN_POINT('Ctrl Pts',(0.660707209088037,31.5554274335712,
125.59693576341));
#124655=CARTESIAN_POINT('Ctrl Pts',(0.661913462714968,31.5488129268718,
125.613823595541));
#124656=CARTESIAN_POINT('Ctrl Pts',(0.662361198565082,31.5463319310609,
125.620047130398));
#124657=CARTESIAN_POINT('Ctrl Pts',(0.663223043581735,31.5415087804316,
125.631936920441));
#124658=CARTESIAN_POINT('Ctrl Pts',(0.663636794203542,31.5391727896203,
125.637605450252));
#124659=CARTESIAN_POINT('Ctrl Pts',(0.664644208306056,31.5334345380658,
125.651314628873));
#124660=CARTESIAN_POINT('Ctrl Pts',(0.665239732984002,31.5300002824465,
125.659341607683));
#124661=CARTESIAN_POINT('Ctrl Pts',(0.667387495713215,31.5174590041267,
125.688029042452));
#124662=CARTESIAN_POINT('Ctrl Pts',(0.668958690484256,31.5079957187007,
125.708529873833));
#124663=CARTESIAN_POINT('Ctrl Pts',(0.68070975642583,31.4349176589108,125.858742594515));
#124664=CARTESIAN_POINT('Ctrl Pts',(0.69145408655341,31.3550877098455,125.979881810146));
#124665=CARTESIAN_POINT('Ctrl Pts',(0.706353123477042,31.2187010461449,
126.137732923072));
#124666=CARTESIAN_POINT('Ctrl Pts',(0.710848360648883,31.1740040118202,
126.183801013888));
#124667=CARTESIAN_POINT('Ctrl Pts',(0.716500696364889,31.1130668513934,
126.239751416371));
#124668=CARTESIAN_POINT('Ctrl Pts',(0.717760885644108,31.0991674888283,
126.252091158872));
#124669=CARTESIAN_POINT('Ctrl Pts',(0.7197927482922,31.0762523264584,126.271759323671));
#124670=CARTESIAN_POINT('Ctrl Pts',(0.720570254941475,31.0673615787215,
126.279230284049));
#124671=CARTESIAN_POINT('Ctrl Pts',(0.722064445742197,31.050042414074,126.293477427806));
#124672=CARTESIAN_POINT('Ctrl Pts',(0.722781595637464,31.0416247365479,
126.300265682542));
#124673=CARTESIAN_POINT('Ctrl Pts',(0.724451127881559,31.0217858453109,
126.315948027207));
#124674=CARTESIAN_POINT('Ctrl Pts',(0.725400869349282,31.0103135106441,
126.324776266404));
#124675=CARTESIAN_POINT('Ctrl Pts',(0.728531657477741,30.9718925022953,
126.353552741498));
#124676=CARTESIAN_POINT('Ctrl Pts',(0.730687241748473,30.9444558325748,
126.372837748582));
#124677=CARTESIAN_POINT('Ctrl Pts',(0.735883479201286,30.8761378346528,
126.417839617048));
#124678=CARTESIAN_POINT('Ctrl Pts',(0.738893417719294,30.8346842554547,
126.442632797124));
#124679=CARTESIAN_POINT('Ctrl Pts',(0.745995230933175,30.7334358222402,
126.497361544146));
#124680=CARTESIAN_POINT('Ctrl Pts',(0.750051128482708,30.6728038918927,
126.525567033434));
#124681=CARTESIAN_POINT('Ctrl Pts',(0.758902128955931,30.5382987635135,
126.578555078483));
#124682=CARTESIAN_POINT('Ctrl Pts',(0.763698665792319,30.4640577037242,
126.601951716197));
#124683=CARTESIAN_POINT('Ctrl Pts',(0.769796878259095,30.3725425064711,
126.623895369703));
#124684=CARTESIAN_POINT('Ctrl Pts',(0.770868306932346,30.35656566161,126.627478101455));
#124685=CARTESIAN_POINT('Ctrl Pts',(0.772462133810009,30.3329995914776,
126.632399031748));
#124686=CARTESIAN_POINT('Ctrl Pts',(0.772974803978947,30.325449187111,126.633921095877));
#124687=CARTESIAN_POINT('Ctrl Pts',(0.773892751723442,30.3119893872091,
126.636537423632));
#124688=CARTESIAN_POINT('Ctrl Pts',(0.774296877163166,30.3060842358617,
126.6376521471));
#124689=CARTESIAN_POINT('Ctrl Pts',(0.775196718014226,30.2929819943888,
126.640052132557));
#124690=CARTESIAN_POINT('Ctrl Pts',(0.775693242797695,30.2857825020341,
126.641321968107));
#124691=CARTESIAN_POINT('Ctrl Pts',(0.777172121290137,30.264421454863,126.644944795683));
#124692=CARTESIAN_POINT('Ctrl Pts',(0.778161455541685,30.2502380004913,
126.647162103504));
#124693=CARTESIAN_POINT('Ctrl Pts',(0.780480263962006,30.217201524402,126.651890191334));
#124694=CARTESIAN_POINT('Ctrl Pts',(0.781815648233726,30.1983308546577,
126.654261923864));
#124695=CARTESIAN_POINT('Ctrl Pts',(0.786590563466671,30.1312698577639,
126.661526501931));
#124696=CARTESIAN_POINT('Ctrl Pts',(0.790086589152524,30.082913377996,126.664640166428));
#124697=CARTESIAN_POINT('Ctrl Pts',(0.801961065874912,29.919409229959,126.668026122323));
#124698=CARTESIAN_POINT('Ctrl Pts',(0.810378374963458,29.8043718472874,
126.658475759223));
#124699=CARTESIAN_POINT('Ctrl Pts',(0.821474117974972,29.6492547775654,
126.629220199659));
#124700=CARTESIAN_POINT('Ctrl Pts',(0.824431891531851,29.607595737263,126.619691368837));
#124701=CARTESIAN_POINT('Ctrl Pts',(0.828447769148284,29.5506222132914,
126.604331885885));
#124702=CARTESIAN_POINT('Ctrl Pts',(0.829548632789009,29.5349612879075,
126.599862564166));
#124703=CARTESIAN_POINT('Ctrl Pts',(0.831315013146628,29.509771220983,126.592272653086));
#124704=CARTESIAN_POINT('Ctrl Pts',(0.831985108009481,29.5002006393613,
126.589294517775));
#124705=CARTESIAN_POINT('Ctrl Pts',(0.833379791687525,29.480254229731,126.582889673207));
#124706=CARTESIAN_POINT('Ctrl Pts',(0.834103815727575,29.4698840356168,
126.579446883321));
#124707=CARTESIAN_POINT('Ctrl Pts',(0.835825175608085,29.4451982358715,
126.570980949779));
#124708=CARTESIAN_POINT('Ctrl Pts',(0.836819360979899,29.4309157381964,
126.565863745683));
#124709=CARTESIAN_POINT('Ctrl Pts',(0.840285127572467,29.3810676016894,
126.547231760538));
#124710=CARTESIAN_POINT('Ctrl Pts',(0.842722834844815,29.3458952993867,
126.532693975326));
#124711=CARTESIAN_POINT('Ctrl Pts',(0.848795560938966,29.2584458742504,
126.492989105741));
#124712=CARTESIAN_POINT('Ctrl Pts',(0.852383163650852,29.2069274277764,
126.466272698576));
#124713=CARTESIAN_POINT('Ctrl Pts',(0.862670243545594,29.0622800374831,
126.381402728523));
#124714=CARTESIAN_POINT('Ctrl Pts',(0.869255011291786,28.9733801675694,
126.316677504005));
#124715=CARTESIAN_POINT('Ctrl Pts',(0.878120473650786,28.869088274024,126.223722013611));
#124716=CARTESIAN_POINT('Ctrl Pts',(0.880052719187994,28.8472270646883,
126.203150529413));
#124717=CARTESIAN_POINT('Ctrl Pts',(0.882681529434413,28.8188461883467,
126.174960213398));
#124718=CARTESIAN_POINT('Ctrl Pts',(0.883342512649087,28.811821082035,126.167855588923));
#124719=CARTESIAN_POINT('Ctrl Pts',(0.884391506669561,28.8008547513549,
126.15656376032));
#124720=CARTESIAN_POINT('Ctrl Pts',(0.884776275815562,28.7968704397023,
126.152418464643));
#124721=CARTESIAN_POINT('Ctrl Pts',(0.885579694648213,28.7886321161988,
126.143757987326));
#124722=CARTESIAN_POINT('Ctrl Pts',(0.885998628644832,28.7843817779742,
126.139239578341));
#124723=CARTESIAN_POINT('Ctrl Pts',(0.887038553534329,28.7739406751601,
126.128014996122));
#124724=CARTESIAN_POINT('Ctrl Pts',(0.887661696806021,28.767779651318,126.121281544598));
#124725=CARTESIAN_POINT('Ctrl Pts',(0.890033896506755,28.7446733891965,
126.095608035311));
#124726=CARTESIAN_POINT('Ctrl Pts',(0.891807269866931,28.728107887861,126.076332732886));
#124727=CARTESIAN_POINT('Ctrl Pts',(0.896555147256173,28.6854461416704,
126.02433181204));
#124728=CARTESIAN_POINT('Ctrl Pts',(0.899562627305037,28.6601316737754,
125.990989372923));
#124729=CARTESIAN_POINT('Ctrl Pts',(0.912076439066468,28.5608792446586,
125.849496931349));
#124730=CARTESIAN_POINT('Ctrl Pts',(0.921691452239241,28.4985538138432,
125.733745386815));
#124731=CARTESIAN_POINT('Ctrl Pts',(0.933543598717862,28.4363725259767,
125.576273050132));
#124732=CARTESIAN_POINT('Ctrl Pts',(0.936186469382574,28.4235430828048,
125.540190249118));
#124733=CARTESIAN_POINT('Ctrl Pts',(0.939850840103563,28.4072440800358,
125.488803278875));
#124734=CARTESIAN_POINT('Ctrl Pts',(0.940905888925251,28.4027303364164,
125.473845667598));
#124735=CARTESIAN_POINT('Ctrl Pts',(0.942685251681564,28.3954262235344,
125.448350037626));
#124736=CARTESIAN_POINT('Ctrl Pts',(0.943413034264247,28.3925277302467,
125.437844346847));
#124737=CARTESIAN_POINT('Ctrl Pts',(0.944883589146057,28.3868537524629,
125.416462665857));
#124738=CARTESIAN_POINT('Ctrl Pts',(0.945626121342268,28.3840846737134,
125.405585547953));
#124739=CARTESIAN_POINT('Ctrl Pts',(0.947466774148661,28.3774623333828,
125.378427542424));
#124740=CARTESIAN_POINT('Ctrl Pts',(0.948560536708781,28.3737439347172,
125.362114799254));
#124741=CARTESIAN_POINT('Ctrl Pts',(0.952914978220962,28.3598267199175,
125.296514254568));
#124742=CARTESIAN_POINT('Ctrl Pts',(0.956112837826936,28.351617389738,125.24682910196));
#124743=CARTESIAN_POINT('Ctrl Pts',(0.965014141073731,28.3348077580783,
125.10555676311));
#124744=CARTESIAN_POINT('Ctrl Pts',(0.97058122621504,28.3315200463238,125.01352615613));
#124745=CARTESIAN_POINT('Ctrl Pts',(0.97651601084138,28.3360778930133,124.916666153156));
#124746=CARTESIAN_POINT('Ctrl Pts',(0.976824089541183,28.3363371165403,
124.911642102236));
#124747=CARTESIAN_POINT('Ctrl Pts',(0.982046211373305,28.3411132169989,
124.826565896748));
#124748=CARTESIAN_POINT('Ctrl Pts',(0.987007554900982,28.3513800315247,
124.746951485922));
#124749=CARTESIAN_POINT('Ctrl Pts',(0.993048223344464,28.3697888909617,
124.656314457611));
#124750=CARTESIAN_POINT('Ctrl Pts',(0.993859839462372,28.3723768980549,
124.644259886892));
#124751=CARTESIAN_POINT('Ctrl Pts',(0.995141065074082,28.3766351740338,
124.625445451774));
#124752=CARTESIAN_POINT('Ctrl Pts',(0.995605747122006,28.3782144998812,
124.618665166829));
#124753=CARTESIAN_POINT('Ctrl Pts',(0.996479002658836,28.3812462210789,
124.60600909048));
#124754=CARTESIAN_POINT('Ctrl Pts',(0.996886992587754,28.3826881998646,
124.60013105892));
#124755=CARTESIAN_POINT('Ctrl Pts',(0.997851965809552,28.3861589690541,
124.586308868633));
#124756=CARTESIAN_POINT('Ctrl Pts',(0.998410420994445,28.3882144110028,
124.57837168809));
#124757=CARTESIAN_POINT('Ctrl Pts',(1.00028635216151,28.3952771152164,124.551905291348));
#124758=CARTESIAN_POINT('Ctrl Pts',(1.00161720896866,28.4005457857632,124.533448241567));
#124759=CARTESIAN_POINT('Ctrl Pts',(1.00492587989113,28.4142983909995,124.488244555675));
#124760=CARTESIAN_POINT('Ctrl Pts',(1.00691802891608,28.4231412964133,124.461613819438));
#124761=CARTESIAN_POINT('Ctrl Pts',(1.01597949388326,28.4660223570574,124.342612389942));
#124762=CARTESIAN_POINT('Ctrl Pts',(1.02321720301547,28.5075344275784,124.253144807469));
#124763=CARTESIAN_POINT('Ctrl Pts',(1.03642265546007,28.5989391316009,124.094607835047));
#124764=CARTESIAN_POINT('Ctrl Pts',(1.04240890848009,28.6466968307238,124.024663641592));
#124765=CARTESIAN_POINT('Ctrl Pts',(1.04954358140924,28.711857745256,123.943291839808));
#124766=CARTESIAN_POINT('Ctrl Pts',(1.05087855734872,28.7244191307929,123.928162275411));
#124767=CARTESIAN_POINT('Ctrl Pts',(1.05300003611701,28.7449690258938,123.904284054407));
#124768=CARTESIAN_POINT('Ctrl Pts',(1.05379336763362,28.7527877697174,123.895392447721));
#124769=CARTESIAN_POINT('Ctrl Pts',(1.05529878780915,28.7678781759838,123.878595903846));
#124770=CARTESIAN_POINT('Ctrl Pts',(1.05601153674331,28.7751327553615,123.87067649528));
#124771=CARTESIAN_POINT('Ctrl Pts',(1.05764336520534,28.7919921784295,123.852625615239));
#124772=CARTESIAN_POINT('Ctrl Pts',(1.05856016952897,28.8016488856344,123.842543520416));
#124773=CARTESIAN_POINT('Ctrl Pts',(1.06146198922086,28.8327903696453,123.810837786707));
#124774=CARTESIAN_POINT('Ctrl Pts',(1.06342653393592,28.8547430612517,123.789681107625));
#124775=CARTESIAN_POINT('Ctrl Pts',(1.06806317226052,28.9084988238109,123.740647623599));
#124776=CARTESIAN_POINT('Ctrl Pts',(1.07071299943881,28.9408070988456,123.713355527454));
#124777=CARTESIAN_POINT('Ctrl Pts',(1.0779091005603,29.0322434778389,123.641896566375));
#124778=CARTESIAN_POINT('Ctrl Pts',(1.08238699243441,29.0933205750657,123.600382045042));
#124779=CARTESIAN_POINT('Ctrl Pts',(1.08763840827616,29.1673634778397,123.55694135908));
#124780=CARTESIAN_POINT('Ctrl Pts',(1.08837798832119,29.1778448805665,123.550944178062));
#124781=CARTESIAN_POINT('Ctrl Pts',(1.09376010146922,29.2544242382338,123.508225852885));
#124782=CARTESIAN_POINT('Ctrl Pts',(1.09845400542489,29.322881007457,123.475932988059));
#124783=CARTESIAN_POINT('Ctrl Pts',(1.10419437901174,29.4047272492038,123.443928879114));
#124784=CARTESIAN_POINT('Ctrl Pts',(1.10500330146222,29.4162196539468,123.439580996383));
#124785=CARTESIAN_POINT('Ctrl Pts',(1.10628122189851,29.4342887051178,123.432972535078));
#124786=CARTESIAN_POINT('Ctrl Pts',(1.10674533487703,29.4408334698775,123.430625241637));
#124787=CARTESIAN_POINT('Ctrl Pts',(1.10761819081847,29.4531047513464,123.426310624824));
#124788=CARTESIAN_POINT('Ctrl Pts',(1.10802635787912,29.4588275466715,123.424333463698));
#124789=CARTESIAN_POINT('Ctrl Pts',(1.10899269581838,29.4723413166809,123.419746912091));
#124790=CARTESIAN_POINT('Ctrl Pts',(1.10955235086725,29.480140956618,123.417163913771));
#124791=CARTESIAN_POINT('Ctrl Pts',(1.11143662837365,29.5063221126128,123.408707909851));
#124792=CARTESIAN_POINT('Ctrl Pts',(1.11277478822223,29.5247857488185,123.403096837993));
#124793=CARTESIAN_POINT('Ctrl Pts',(1.11610568808141,29.5705240079117,123.390060474166));
#124794=CARTESIAN_POINT('Ctrl Pts',(1.11811299445784,29.5978976384193,123.383006365152));
#124795=CARTESIAN_POINT('Ctrl Pts',(1.12730763320554,29.7229349798826,123.354155791651));
#124796=CARTESIAN_POINT('Ctrl Pts',(1.13466700934437,29.8222618537179,123.340488692602));
#124797=CARTESIAN_POINT('Ctrl Pts',(1.14784369775615,30.004803028561,123.331956693205));
#124798=CARTESIAN_POINT('Ctrl Pts',(1.15369166135275,30.0875729025551,123.334249046508));
#124799=CARTESIAN_POINT('Ctrl Pts',(1.16069331953902,30.1893506945456,123.344679212863));
#124800=CARTESIAN_POINT('Ctrl Pts',(1.16202474155987,30.2088234492544,123.347022862252));
#124801=CARTESIAN_POINT('Ctrl Pts',(1.16414194306474,30.2399681137035,123.351330469495));
#124802=CARTESIAN_POINT('Ctrl Pts',(1.16493450303635,30.2516678618541,123.353075831675));
#124803=CARTESIAN_POINT('Ctrl Pts',(1.16643929615208,30.2739550846055,123.3566436787));
#124804=CARTESIAN_POINT('Ctrl Pts',(1.1671521807826,30.2845454096222,123.358444242123));
#124805=CARTESIAN_POINT('Ctrl Pts',(1.1687854972134,30.3088774222517,123.362823711763));
#124806=CARTESIAN_POINT('Ctrl Pts',(1.16970363874614,30.322605665053,123.365473443055));
#124807=CARTESIAN_POINT('Ctrl Pts',(1.17261460969725,30.3662717155549,123.374473150756));
#124808=CARTESIAN_POINT('Ctrl Pts',(1.17458677823152,30.3960696321055,123.381475504621));
#124809=CARTESIAN_POINT('Ctrl Pts',(1.17924528002188,30.466755745292,123.40015565067));
#124810=CARTESIAN_POINT('Ctrl Pts',(1.18190904512399,30.5074233584667,123.412585503692));
#124811=CARTESIAN_POINT('Ctrl Pts',(1.18911444875213,30.6171889142565,123.450784996727));
#124812=CARTESIAN_POINT('Ctrl Pts',(1.19358851883807,30.6851215217037,123.479605923504));
#124813=CARTESIAN_POINT('Ctrl Pts',(1.20304788111868,30.823147536297,123.549299960639));
#124814=CARTESIAN_POINT('Ctrl Pts',(1.20802859471426,30.8926117881279,123.590977809746));
#124815=CARTESIAN_POINT('Ctrl Pts',(1.21433279756274,30.9721804331959,123.64696995769));
#124816=CARTESIAN_POINT('Ctrl Pts',(1.21540616685556,30.9854549760152,123.656607454636));
#124817=CARTESIAN_POINT('Ctrl Pts',(1.21700223551545,31.0047530616942,123.671058062475));
#124818=CARTESIAN_POINT('Ctrl Pts',(1.2175151606351,31.0108894104195,123.675719824828));
#124819=CARTESIAN_POINT('Ctrl Pts',(1.2184173343787,31.0215635000866,123.683946311164));
#124820=CARTESIAN_POINT('Ctrl Pts',(1.21880528522261,31.0261153966085,123.687492290473));
#124821=CARTESIAN_POINT('Ctrl Pts',(1.21920080715234,31.0307171248432,123.69111565977));
#124822=CARTESIAN_POINT('Ctrl Pts',(1.21920667341311,31.0307853676731,123.691169402353));
#124823=CARTESIAN_POINT('Ctrl Pts',(1.21922183236524,31.0309616911448,123.691308282932));
#124824=CARTESIAN_POINT('Ctrl Pts',(1.21923112559518,31.0310697650798,123.691393428693));
#124825=CARTESIAN_POINT('Ctrl Pts',(1.21924929405809,31.0312810097945,123.691559899692));
#124826=CARTESIAN_POINT('Ctrl Pts',(1.21925816922612,31.0313841817224,123.691641223918));
#124827=CARTESIAN_POINT('Ctrl Pts',(1.21927553586896,31.0315860268068,123.691800364971));
#124828=CARTESIAN_POINT('Ctrl Pts',(1.2192840272588,31.0316847006437,123.691878180654));
#124829=CARTESIAN_POINT('Ctrl Pts',(1.21930065697599,31.0318779104089,123.69203058426));
#124830=CARTESIAN_POINT('Ctrl Pts',(1.21930879523635,31.031972447027,123.692105171248));
#124831=CARTESIAN_POINT('Ctrl Pts',(1.21932474616484,31.0321577057908,123.692251368292));
#124832=CARTESIAN_POINT('Ctrl Pts',(1.21933255878525,31.0322484286796,123.692322977625));
#124833=CARTESIAN_POINT('Ctrl Pts',(1.21934788320445,31.0324263514604,123.692463445576));
#124834=CARTESIAN_POINT('Ctrl Pts',(1.21935539494409,31.032513551816,123.692532303396));
#124835=CARTESIAN_POINT('Ctrl Pts',(1.21937013993988,31.0326846922427,123.69266747235));
#124836=CARTESIAN_POINT('Ctrl Pts',(1.21937737314511,31.0327686327463,123.69273378279));
#124837=CARTESIAN_POINT('Ctrl Pts',(1.21939158129738,31.0329334912076,123.692864041739));
#124838=CARTESIAN_POINT('Ctrl Pts',(1.21939855620023,31.0330144095663,123.69292798964));
#124839=CARTESIAN_POINT('Ctrl Pts',(1.21941226611225,31.0331734394942,123.693053691295));
#124840=CARTESIAN_POINT('Ctrl Pts',(1.21941900108266,31.0332515514322,123.69311544451));
#124841=CARTESIAN_POINT('Ctrl Pts',(1.21943224784002,31.0334051647447,123.69323690948));
#124842=CARTESIAN_POINT('Ctrl Pts',(1.21943875959904,31.0334806665304,123.693296620815));
#124843=CARTESIAN_POINT('Ctrl Pts',(1.21945157515994,31.0336292382594,123.693414141169));
#124844=CARTESIAN_POINT('Ctrl Pts',(1.21945787895093,31.0337023087384,123.693471949941));
#124845=CARTESIAN_POINT('Ctrl Pts',(1.21947029255831,31.0338461818934,123.693585792967));
#124846=CARTESIAN_POINT('Ctrl Pts',(1.21947640234328,31.0339169848029,123.693641826799));
#124847=CARTESIAN_POINT('Ctrl Pts',(1.21948844072825,31.0340564728022,123.693752236852));
#124848=CARTESIAN_POINT('Ctrl Pts',(1.21949436929992,31.0341251581047,123.693806612691));
#124849=CARTESIAN_POINT('Ctrl Pts',(1.21950605700752,31.0342605486142,123.693913814168));
#124850=CARTESIAN_POINT('Ctrl Pts',(1.21951181611796,31.0343272540166,123.693966639462));
#124851=CARTESIAN_POINT('Ctrl Pts',(1.21952317574618,31.0344588117726,123.694070838984));
#124852=CARTESIAN_POINT('Ctrl Pts',(1.21952877623557,31.0345236642437,123.694122212853));
#124853=CARTESIAN_POINT('Ctrl Pts',(1.21953982852408,31.0346516321283,123.694223600068));
#124854=CARTESIAN_POINT('Ctrl Pts',(1.21954528034411,31.0347147481906,123.694273613515));
#124855=CARTESIAN_POINT('Ctrl Pts',(1.21955604459482,31.0348393521421,123.694372364947));
#124856=CARTESIAN_POINT('Ctrl Pts',(1.21956135699385,31.0349008400361,123.694421102557));
#124857=CARTESIAN_POINT('Ctrl Pts',(1.21957185096577,31.035022287867,123.694517380631));
#124858=CARTESIAN_POINT('Ctrl Pts',(1.21957703250395,31.0350822477416,123.694564920701));
#124859=CARTESIAN_POINT('Ctrl Pts',(1.21958727266399,31.0352007320731,123.694658876042));
#124860=CARTESIAN_POINT('Ctrl Pts',(1.21959233127398,31.0352592567035,123.694705291136));
#124861=CARTESIAN_POINT('Ctrl Pts',(1.21960233292773,31.0353749565056,123.694797063761));
#124862=CARTESIAN_POINT('Ctrl Pts',(1.21960727597216,31.0354321319706,123.694842421234));
#124863=CARTESIAN_POINT('Ctrl Pts',(1.21961705343487,31.0355452145648,123.694932142115));
#124864=CARTESIAN_POINT('Ctrl Pts',(1.21962188781855,31.035601121556,123.694976505144));
#124865=CARTESIAN_POINT('Ctrl Pts',(1.21963145426949,31.0357117409508,123.695064294865));
#124866=CARTESIAN_POINT('Ctrl Pts',(1.21963618636369,31.0357664539071,123.695107721749));
#124867=CARTESIAN_POINT('Ctrl Pts',(1.21964555432574,31.0358747563637,123.695193694907));
#124868=CARTESIAN_POINT('Ctrl Pts',(1.21965019015896,31.035928345686,123.695236240814));
#124869=CARTESIAN_POINT('Ctrl Pts',(1.21965937114814,31.0360344656818,123.695320502798));
#124870=CARTESIAN_POINT('Ctrl Pts',(1.21966391631347,31.0360869966688,123.695362218915));
#124871=CARTESIAN_POINT('Ctrl Pts',(1.21967292122972,31.0361910614302,123.695444869489));
#124872=CARTESIAN_POINT('Ctrl Pts',(1.21967738098021,31.036242595389,123.695485803898));
#124873=CARTESIAN_POINT('Ctrl Pts',(1.21968622007376,31.036344724515,123.695566936886));
#124874=CARTESIAN_POINT('Ctrl Pts',(1.21969059938012,31.0363953194332,123.695607135088));
#124875=CARTESIAN_POINT('Ctrl Pts',(1.21969928215642,31.0364956238086,123.695686837505));
#124876=CARTESIAN_POINT('Ctrl Pts',(1.21970358563773,31.0365453335592,123.695726341787));
#124877=CARTESIAN_POINT('Ctrl Pts',(1.21971212122168,31.0366439195734,123.695804697175));
#124878=CARTESIAN_POINT('Ctrl Pts',(1.21971635329085,31.0366927956005,123.695843547941));
#124879=CARTESIAN_POINT('Ctrl Pts',(1.21972475011958,31.0367897616077,123.69592063355));
#124880=CARTESIAN_POINT('Ctrl Pts',(1.21972891489335,31.0368378518908,123.695958868493));
#124881=CARTESIAN_POINT('Ctrl Pts',(1.21973718105,31.036933292073,123.696034758343));
#124882=CARTESIAN_POINT('Ctrl Pts',(1.21974128243751,31.0369806421544,123.696072413262));
#124883=CARTESIAN_POINT('Ctrl Pts',(1.22028397769698,31.0432454572721,123.701055033715));
#124884=CARTESIAN_POINT('Ctrl Pts',(1.22082562537764,31.0494273201492,123.706044280924));
#124885=CARTESIAN_POINT('Ctrl Pts',(1.22202868314172,31.063007270087,123.717165685881));
#124886=CARTESIAN_POINT('Ctrl Pts',(1.2226913751114,31.0703884151777,123.723317986299));
#124887=CARTESIAN_POINT('Ctrl Pts',(1.22455787967135,31.0909123956658,123.740728141102));
#124888=CARTESIAN_POINT('Ctrl Pts',(1.22576982250827,31.1039332970036,123.752127132211));
#124889=CARTESIAN_POINT('Ctrl Pts',(1.22993490269307,31.1477219639052,123.791683125796));
#124890=CARTESIAN_POINT('Ctrl Pts',(1.23293161995211,31.1776076635566,123.820790463895));
#124891=CARTESIAN_POINT('Ctrl Pts',(1.24534838092547,31.2958928554335,123.944979981985));
#124892=CARTESIAN_POINT('Ctrl Pts',(1.25487755850006,31.3741410617327,124.049131547035));
#124893=CARTESIAN_POINT('Ctrl Pts',(1.26673032546307,31.4592919610593,124.195283835595));
#124894=CARTESIAN_POINT('Ctrl Pts',(1.26944596021835,31.4778731338379,124.229939887222));
#124895=CARTESIAN_POINT('Ctrl Pts',(1.2731921198376,31.502172933079,124.279388061748));
#124896=CARTESIAN_POINT('Ctrl Pts',(1.27425822595668,31.5089322424796,124.293651216599));
#124897=CARTESIAN_POINT('Ctrl Pts',(1.27605066006876,31.5200270579677,124.317949297389));
#124898=CARTESIAN_POINT('Ctrl Pts',(1.27678057790763,31.5244682347428,124.327934505453));
#124899=CARTESIAN_POINT('Ctrl Pts',(1.27825095082319,31.5332565239658,124.348228885664));
#124900=CARTESIAN_POINT('Ctrl Pts',(1.27899120722439,31.537598684842,124.358539597106));
#124901=CARTESIAN_POINT('Ctrl Pts',(1.28081775627551,31.5481048919435,124.384206985614));
#124902=CARTESIAN_POINT('Ctrl Pts',(1.28189983863684,31.5541447227466,124.399613452858));
#124903=CARTESIAN_POINT('Ctrl Pts',(1.28613710096058,31.5770468556965,124.460695271514));
#124904=CARTESIAN_POINT('Ctrl Pts',(1.289233864174,31.5921340232231,124.50701287269));
#124905=CARTESIAN_POINT('Ctrl Pts',(1.30175015240752,31.6456276915849,124.699507841544));
#124906=CARTESIAN_POINT('Ctrl Pts',(1.31064630109017,31.6660850299523,124.849887173953));
#124907=CARTESIAN_POINT('Ctrl Pts',(1.3202051089041,31.6659997343953,125.000940741602));
#124908=CARTESIAN_POINT('Ctrl Pts',(1.32020526047221,31.6659997330411,125.000943136764));
#124909=CARTESIAN_POINT('Ctrl Pts',(1.32219893801785,31.6659818976929,125.032448308161));
#124910=CARTESIAN_POINT('Ctrl Pts',(1.32422173835897,31.6650703897071,125.063944775686));
#124911=CARTESIAN_POINT('Ctrl Pts',(1.32680936405944,31.6628115005492,125.103330023435));
#124912=CARTESIAN_POINT('Ctrl Pts',(1.32733346424632,31.6622995925459,125.111262027454));
#124913=CARTESIAN_POINT('Ctrl Pts',(1.3282558745491,31.6613044281163,125.125136490565));
#124914=CARTESIAN_POINT('Ctrl Pts',(1.32865288126487,31.6608459899292,125.131080659028));
#124915=CARTESIAN_POINT('Ctrl Pts',(1.32944779578682,31.6598685577877,125.142924622143));
#124916=CARTESIAN_POINT('Ctrl Pts',(1.32984567753739,31.6593500037223,125.148824193138));
#124917=CARTESIAN_POINT('Ctrl Pts',(1.3307184216827,31.6581490151828,125.16170026855));
#124918=CARTESIAN_POINT('Ctrl Pts',(1.33119393266027,31.6574540172209,125.168675160255));
#124919=CARTESIAN_POINT('Ctrl Pts',(1.33252665365269,31.6553928067528,125.188116833037));
#124920=CARTESIAN_POINT('Ctrl Pts',(1.33338886477738,31.6539298363843,125.200572581251));
#124921=CARTESIAN_POINT('Ctrl Pts',(1.33795703000348,31.6454968392836,125.265987604827));
#124922=CARTESIAN_POINT('Ctrl Pts',(1.34176854934652,31.6361239516461,125.318600890097));
#124923=CARTESIAN_POINT('Ctrl Pts',(1.3504369306267,31.6094152752173,125.435636654983));
#124924=CARTESIAN_POINT('Ctrl Pts',(1.35530991971809,31.5907040896157,125.499657140944));
#124925=CARTESIAN_POINT('Ctrl Pts',(1.36048146718461,31.5666375771793,125.566766595078));
#124926=CARTESIAN_POINT('Ctrl Pts',(1.36081892588276,31.5650478864037,125.571141644177));
#124927=CARTESIAN_POINT('Ctrl Pts',(1.36115613275098,31.5634400145948,125.575509618307));
#124928=CARTESIAN_POINT('Ctrl Pts',(1.16625576032278,31.5634400119388,125.575509625522));
#124929=CARTESIAN_POINT('Ctrl Pts',(1.16615104541434,31.5639818669451,125.574037612267));
#124930=CARTESIAN_POINT('Ctrl Pts',(1.16604639949232,31.5645216461886,125.572564825237));
#124931=CARTESIAN_POINT('Ctrl Pts',(1.1652259625993,31.5687400693189,125.561004356859));
#124932=CARTESIAN_POINT('Ctrl Pts',(1.16451336704287,31.5723232598739,125.55088190129));
#124933=CARTESIAN_POINT('Ctrl Pts',(1.16288077169874,31.5803439224431,125.527507690019));
#124934=CARTESIAN_POINT('Ctrl Pts',(1.16196305973342,31.5847130653475,125.514233212133));
#124935=CARTESIAN_POINT('Ctrl Pts',(1.15905376820061,31.5981099678571,125.471737056413));
#124936=CARTESIAN_POINT('Ctrl Pts',(1.15708282306876,31.606500675845,125.442320117487));
#124937=CARTESIAN_POINT('Ctrl Pts',(1.15242757306978,31.624598565457,125.371536763432));
#124938=CARTESIAN_POINT('Ctrl Pts',(1.14976579838331,31.6335428965921,125.329997045072));
#124939=CARTESIAN_POINT('Ctrl Pts',(1.14256128485893,31.6536422265335,125.215543399428));
#124940=CARTESIAN_POINT('Ctrl Pts',(1.13808625857221,31.6615602323168,125.14216023227));
#124941=CARTESIAN_POINT('Ctrl Pts',(1.13273557453383,31.6651561164103,125.054770113502));
#124942=CARTESIAN_POINT('Ctrl Pts',(1.13189415096574,31.6655510682859,125.04104010977));
#124943=CARTESIAN_POINT('Ctrl Pts',(1.12652557143184,31.6669837310359,124.953644787307));
#124944=CARTESIAN_POINT('Ctrl Pts',(1.121945997636,31.6633036550011,124.87999264205));
#124945=CARTESIAN_POINT('Ctrl Pts',(1.11633292104252,31.6533404778681,124.79464180066));
#124946=CARTESIAN_POINT('Ctrl Pts',(1.11552466937479,31.651782321632,124.782464104157));
#124947=CARTESIAN_POINT('Ctrl Pts',(1.11424769822748,31.6491317170624,124.763422596876));
#124948=CARTESIAN_POINT('Ctrl Pts',(1.11378385527769,31.6481306211017,124.756546227583));
#124949=CARTESIAN_POINT('Ctrl Pts',(1.11291140865508,31.646177088406,124.743692311869));
#124950=CARTESIAN_POINT('Ctrl Pts',(1.11250337937553,31.6452350561548,124.737713433993));
#124951=CARTESIAN_POINT('Ctrl Pts',(1.11153727988101,31.6429377259955,124.723632288774));
#124952=CARTESIAN_POINT('Ctrl Pts',(1.11097772525339,31.6415550575652,124.71553476624));
#124953=CARTESIAN_POINT('Ctrl Pts',(1.1090934975894,31.6367239002156,124.688450205421));
#124954=CARTESIAN_POINT('Ctrl Pts',(1.10775528409002,31.6330055499766,124.669513700042));
#124955=CARTESIAN_POINT('Ctrl Pts',(1.10442406724899,31.6230315611231,124.623007081869));
#124956=CARTESIAN_POINT('Ctrl Pts',(1.10241649043974,31.6164015710208,124.595523932047));
#124957=CARTESIAN_POINT('Ctrl Pts',(1.0932188414337,31.5831337189889,124.471546332358));
#124958=CARTESIAN_POINT('Ctrl Pts',(1.08585659497729,31.5485315442009,124.377403698515));
#124959=CARTESIAN_POINT('Ctrl Pts',(1.07267823814797,31.4703067631554,124.212226378259));
#124960=CARTESIAN_POINT('Ctrl Pts',(1.06683129443048,31.4294105282845,124.140245089017));
#124961=CARTESIAN_POINT('Ctrl Pts',(1.05983080640134,31.3724051956386,124.055307217959));
#124962=CARTESIAN_POINT('Ctrl Pts',(1.05849959388575,31.3611912868546,124.039219686378));
#124963=CARTESIAN_POINT('Ctrl Pts',(1.05638278288682,31.3427628122987,124.013752626706));
#124964=CARTESIAN_POINT('Ctrl Pts',(1.05559040554109,31.3357281098834,124.004245873536));
#124965=CARTESIAN_POINT('Ctrl Pts',(1.05408600133388,31.3221134044702,123.986250787895));
#124966=CARTESIAN_POINT('Ctrl Pts',(1.05337332289603,31.3155514170519,123.977749640437));
#124967=CARTESIAN_POINT('Ctrl Pts',(1.05174054621389,31.3002614353206,123.958332338911));
#124968=CARTESIAN_POINT('Ctrl Pts',(1.05082273596291,31.2914772837104,123.947461277807));
#124969=CARTESIAN_POINT('Ctrl Pts',(1.04791314522152,31.2630361558175,123.913155407181));
#124970=CARTESIAN_POINT('Ctrl Pts',(1.04594200063166,31.2428695406762,123.890150013382));
#124971=CARTESIAN_POINT('Ctrl Pts',(1.04128622263145,31.1932091019712,123.836551452902));
#124972=CARTESIAN_POINT('Ctrl Pts',(1.03862412209428,31.1631558104998,123.806505373867));
#124973=CARTESIAN_POINT('Ctrl Pts',(1.03141968496264,31.0778966978345,123.727549917461));
#124974=CARTESIAN_POINT('Ctrl Pts',(1.0269450135002,31.020542054095,123.68110470999));
#124975=CARTESIAN_POINT('Ctrl Pts',(1.02159392370077,30.9490659496804,123.630686737188));
#124976=CARTESIAN_POINT('Ctrl Pts',(1.02075174300647,30.9377346247631,123.622902052726));
#124977=CARTESIAN_POINT('Ctrl Pts',(1.01538394693864,30.8650963458796,123.574311433637));
#124978=CARTESIAN_POINT('Ctrl Pts',(1.01080592116414,30.8012440445017,123.537473142206));
#124979=CARTESIAN_POINT('Ctrl Pts',(1.00519454109444,30.7241560373828,123.499565133853));
#124980=CARTESIAN_POINT('Ctrl Pts',(1.0043862151566,30.7130788047338,123.494269163991));
#124981=CARTESIAN_POINT('Ctrl Pts',(1.00310910495451,30.6956415117699,123.486168044705));
#124982=CARTESIAN_POINT('Ctrl Pts',(1.00264519684143,30.6893204507745,123.483279322505));
#124983=CARTESIAN_POINT('Ctrl Pts',(1.00177254203339,30.6774588086583,123.477948021258));
#124984=CARTESIAN_POINT('Ctrl Pts',(1.00136436896197,30.6719227467918,123.475495988502));
#124985=CARTESIAN_POINT('Ctrl Pts',(1.0003978307594,30.6588404471331,123.469786674817));
#124986=CARTESIAN_POINT('Ctrl Pts',(0.999837979457446,30.6512833337974,
123.466555000208));
#124987=CARTESIAN_POINT('Ctrl Pts',(0.997952403917785,30.6258895824725,
123.455917351632));
#124988=CARTESIAN_POINT('Ctrl Pts',(0.996613123784626,30.6079488668393,
123.448765946));
#124989=CARTESIAN_POINT('Ctrl Pts',(0.993278775046426,30.5634241947271,
123.43190882006));
#124990=CARTESIAN_POINT('Ctrl Pts',(0.991269110342212,30.5367099625444,
123.422565688461));
#124991=CARTESIAN_POINT('Ctrl Pts',(0.982051976004868,30.414243428537,123.383204761397));
#124992=CARTESIAN_POINT('Ctrl Pts',(0.974671960578939,30.3161367357605,
123.361194794368));
#124993=CARTESIAN_POINT('Ctrl Pts',(0.961505591149596,30.1350541980818,
123.337445376626));
#124994=CARTESIAN_POINT('Ctrl Pts',(0.955686222244953,30.0527732855876,
123.332802905411));
#124995=CARTESIAN_POINT('Ctrl Pts',(0.948712314266306,29.950881064108,123.334608945481));
#124996=CARTESIAN_POINT('Ctrl Pts',(0.947381888523307,29.9312943118038,
123.335301943406));
#124997=CARTESIAN_POINT('Ctrl Pts',(0.945265920871936,29.899915231188,123.336966966903));
#124998=CARTESIAN_POINT('Ctrl Pts',(0.944473613316821,29.8881136146423,
123.337719253745));
#124999=CARTESIAN_POINT('Ctrl Pts',(0.942969084660503,29.8656086898683,
123.33939458038));
#125000=CARTESIAN_POINT('Ctrl Pts',(0.942256214547882,29.8549043950995,
123.340295611091));
#125001=CARTESIAN_POINT('Ctrl Pts',(0.94062262953714,29.8302855494874,123.342607895621));
#125002=CARTESIAN_POINT('Ctrl Pts',(0.939704207962742,29.8163784335405,
123.344090967942));
#125003=CARTESIAN_POINT('Ctrl Pts',(0.936791097864563,29.772076179508,123.349380420096));
#125004=CARTESIAN_POINT('Ctrl Pts',(0.934817112327998,29.7417656123787,
123.353850111493));
#125005=CARTESIAN_POINT('Ctrl Pts',(0.930153404728529,29.6696745211926,
123.366521318667));
#125006=CARTESIAN_POINT('Ctrl Pts',(0.927486320210308,29.6280509444095,
123.375493365516));
#125007=CARTESIAN_POINT('Ctrl Pts',(0.920278729470461,29.5154207041526,
123.404327720658));
#125008=CARTESIAN_POINT('Ctrl Pts',(0.915805598831463,29.445316897942,123.427322621771));
#125009=CARTESIAN_POINT('Ctrl Pts',(0.910429136892259,29.3638109894641,
123.460188086302));
#125010=CARTESIAN_POINT('Ctrl Pts',(0.90956014794745,29.3507245215536,123.465660228814));
#125011=CARTESIAN_POINT('Ctrl Pts',(0.904197065286935,29.2706206185653,
123.500364225849));
#125012=CARTESIAN_POINT('Ctrl Pts',(0.899650350216493,29.2055258592992,
123.533811103953));
#125013=CARTESIAN_POINT('Ctrl Pts',(0.894073721140564,29.1323200037801,
123.577734861494));
#125014=CARTESIAN_POINT('Ctrl Pts',(0.893265536754654,29.1218639504466,
123.584166762371));
#125015=CARTESIAN_POINT('Ctrl Pts',(0.891988617515621,29.1056018994423,
123.594419575672));
#125016=CARTESIAN_POINT('Ctrl Pts',(0.891524757164687,29.0997468694983,
123.598162424464));
#125017=CARTESIAN_POINT('Ctrl Pts',(0.890652489745682,29.0888386116333,
123.605232088714));
#125018=CARTESIAN_POINT('Ctrl Pts',(0.890244659052364,29.0837798704517,
123.608549939243));
#125019=CARTESIAN_POINT('Ctrl Pts',(0.889279155980788,29.0718997256016,
123.616434581438));
#125020=CARTESIAN_POINT('Ctrl Pts',(0.888720001926843,29.0650938859424,
123.6210243158));
#125021=CARTESIAN_POINT('Ctrl Pts',(0.886837125733698,29.0424146041814,
123.636563872111));
#125022=CARTESIAN_POINT('Ctrl Pts',(0.885499870838667,29.0266980624203,
123.647738514862));
#125023=CARTESIAN_POINT('Ctrl Pts',(0.882171241948214,28.9884478451966,
123.675947121282));
#125024=CARTESIAN_POINT('Ctrl Pts',(0.880165303956652,28.9661470653072,
123.693285908564));
#125025=CARTESIAN_POINT('Ctrl Pts',(0.870981480686386,28.8669962839387,
123.774502633823));
#125026=CARTESIAN_POINT('Ctrl Pts',(0.863631571630988,28.7955475808231,
123.844648966041));
#125027=CARTESIAN_POINT('Ctrl Pts',(0.850443421795366,28.6770853776692,
123.983962454178));
#125028=CARTESIAN_POINT('Ctrl Pts',(0.84457590690708,28.628143072863,124.051080766918));
#125029=CARTESIAN_POINT('Ctrl Pts',(0.837556162480866,28.5740591741384,
124.138238258094));
#125030=CARTESIAN_POINT('Ctrl Pts',(0.836224832608533,28.5640143082487,
124.15508243668));
#125031=CARTESIAN_POINT('Ctrl Pts',(0.834108248050821,28.5483945145437,
124.182358728252));
#125032=CARTESIAN_POINT('Ctrl Pts',(0.833316204751512,28.5426294515965,
124.19267922621));
#125033=CARTESIAN_POINT('Ctrl Pts',(0.83181270470213,28.5318417559076,124.212483329035));
#125034=CARTESIAN_POINT('Ctrl Pts',(0.831100593998624,28.5267999751587,
124.221955764274));
#125035=CARTESIAN_POINT('Ctrl Pts',(0.829469518582781,28.5154109610429,
124.243860976518));
#125036=CARTESIAN_POINT('Ctrl Pts',(0.828552834871153,28.5091277034344,
124.256326245983));
#125037=CARTESIAN_POINT('Ctrl Pts',(0.82564862643093,28.4896076228686,124.296293831737));
#125038=CARTESIAN_POINT('Ctrl Pts',(0.823681652593458,28.4769690788082,
124.324082472258));
#125039=CARTESIAN_POINT('Ctrl Pts',(0.819037388497101,28.4486289372169,
124.391232127994));
#125040=CARTESIAN_POINT('Ctrl Pts',(0.816382497106407,28.4336511640838,
124.4308759382));
#125041=CARTESIAN_POINT('Ctrl Pts',(0.80918211559994,28.3967798458641,124.540998420847));
#125042=CARTESIAN_POINT('Ctrl Pts',(0.804704797706259,28.3780306001838,
124.612426844358));
#125043=CARTESIAN_POINT('Ctrl Pts',(0.799406715139897,28.361647415525,124.697474363291));
#125044=CARTESIAN_POINT('Ctrl Pts',(0.798620069040916,28.3593639243095,
124.710113445385));
#125045=CARTESIAN_POINT('Ctrl Pts',(0.793243648806473,28.3447918609733,
124.796465027007));
#125046=CARTESIAN_POINT('Ctrl Pts',(0.78860190390421,28.3373304790088,124.870896631371));
#125047=CARTESIAN_POINT('Ctrl Pts',(0.782919806619903,28.3344883440115,
124.957837733997));
#125048=CARTESIAN_POINT('Ctrl Pts',(0.782111537013232,28.3342228761568,
124.970112129245));
#125049=CARTESIAN_POINT('Ctrl Pts',(0.780834670687406,28.3340196555056,
124.989334509761));
#125050=CARTESIAN_POINT('Ctrl Pts',(0.78037095485496,28.3339896674098,124.996281363847));
#125051=CARTESIAN_POINT('Ctrl Pts',(0.779498674049345,28.3340148542163,
125.009280299266));
#125052=CARTESIAN_POINT('Ctrl Pts',(0.779090682784958,28.3340595598204,
125.015332155614));
#125053=CARTESIAN_POINT('Ctrl Pts',(0.778124739261436,28.3342426536421,
125.029595895695));
#125054=CARTESIAN_POINT('Ctrl Pts',(0.777565303041478,28.3344087937849,
125.037807151429));
#125055=CARTESIAN_POINT('Ctrl Pts',(0.775682254334744,28.3351682259923,
125.065291377494));
#125056=CARTESIAN_POINT('Ctrl Pts',(0.774345125880129,28.3360353760421,
125.084554424996));
#125057=CARTESIAN_POINT('Ctrl Pts',(0.771017386764214,28.3389957014857,
125.131976986764));
#125058=CARTESIAN_POINT('Ctrl Pts',(0.769012240783627,28.3414708173332,
125.160106136882));
#125059=CARTESIAN_POINT('Ctrl Pts',(0.759838698169651,28.3559303565895,
125.287316109779));
#125060=CARTESIAN_POINT('Ctrl Pts',(0.752498754756179,28.3760880869748,
125.385261015734));
#125061=CARTESIAN_POINT('Ctrl Pts',(0.739308435077516,28.4288719284735,
125.560372404515));
#125062=CARTESIAN_POINT('Ctrl Pts',(0.733429820491881,28.4587745338714,
125.638034853079));
#125063=CARTESIAN_POINT('Ctrl Pts',(0.726398187296024,28.5027557609034,
125.730890518723));
#125064=CARTESIAN_POINT('Ctrl Pts',(0.725065564549435,28.5114709305134,
125.748480145571));
#125065=CARTESIAN_POINT('Ctrl Pts',(0.722946813425933,28.5259355536561,
125.776421305557));
#125066=CARTESIAN_POINT('Ctrl Pts',(0.722153891958588,28.5314877927967,
125.786872254876));
#125067=CARTESIAN_POINT('Ctrl Pts',(0.720648632632085,28.5422921512439,
125.806696499387));
#125068=CARTESIAN_POINT('Ctrl Pts',(0.719935641032287,28.547524484198,125.816079836574));
#125069=CARTESIAN_POINT('Ctrl Pts',(0.718302386126289,28.5597725077789,
125.837553667904));
#125070=CARTESIAN_POINT('Ctrl Pts',(0.717384408841334,28.5668503880867,
125.849607901068));
#125071=CARTESIAN_POINT('Ctrl Pts',(0.714475190960476,28.5898920516393,
125.88774236557));
#125072=CARTESIAN_POINT('Ctrl Pts',(0.712504558122011,28.606422982935,125.913473710069));
#125073=CARTESIAN_POINT('Ctrl Pts',(0.70785036019596,28.647578339997,125.973814396864));
#125074=CARTESIAN_POINT('Ctrl Pts',(0.705189286004692,28.6728363165386,
126.007966151164));
#125075=CARTESIAN_POINT('Ctrl Pts',(0.697986956610556,28.7454262638781,
126.09864991108));
#125076=CARTESIAN_POINT('Ctrl Pts',(0.693513284049057,28.7952471826995,
126.153064569791));
#125077=CARTESIAN_POINT('Ctrl Pts',(0.688176206903143,28.858288579375,126.213356590394));
#125078=CARTESIAN_POINT('Ctrl Pts',(0.6873470021138,28.8681834119047,126.222591668937));
#125079=CARTESIAN_POINT('Ctrl Pts',(0.681980499194111,28.9327778016449,
126.28142284487));
#125080=CARTESIAN_POINT('Ctrl Pts',(0.677390966578049,28.99060419533,126.327450592712));
#125081=CARTESIAN_POINT('Ctrl Pts',(0.671766700678755,29.0613820205161,
126.376482187741));
#125082=CARTESIAN_POINT('Ctrl Pts',(0.670957926524988,29.0715573650559,
126.38336588668));
#125083=CARTESIAN_POINT('Ctrl Pts',(0.669680022733904,29.0876111068642,
126.393969469991));
#125084=CARTESIAN_POINT('Ctrl Pts',(0.66921576842484,29.0934384966343,126.397766293706));
#125085=CARTESIAN_POINT('Ctrl Pts',(0.668341896917066,29.104394164388,126.404807107438));
#125086=CARTESIAN_POINT('Ctrl Pts',(0.66793284828064,29.1095166161575,126.408059714717));
#125087=CARTESIAN_POINT('Ctrl Pts',(0.666963659612877,29.1216415317055,
126.415666059009));
#125088=CARTESIAN_POINT('Ctrl Pts',(0.666402022771516,29.1286586857989,
126.419995879042));
#125089=CARTESIAN_POINT('Ctrl Pts',(0.664508563905053,29.1522946861015,
126.434338925018));
#125090=CARTESIAN_POINT('Ctrl Pts',(0.663163099641827,29.1690555728924,
126.444113475416));
#125091=CARTESIAN_POINT('Ctrl Pts',(0.659810683398703,29.2108201689025,
126.467501814608));
#125092=CARTESIAN_POINT('Ctrl Pts',(0.657789009349254,29.2360090062294,
126.480771407286));
#125093=CARTESIAN_POINT('Ctrl Pts',(0.6484590393188,29.3527353388503,126.538492228506));
#125094=CARTESIAN_POINT('Ctrl Pts',(0.640976122976484,29.4478866494741,
126.575144875196));
#125095=CARTESIAN_POINT('Ctrl Pts',(0.627877905708863,29.6228926231761,
126.624736398472));
#125096=CARTESIAN_POINT('Ctrl Pts',(0.622216764615846,29.7014811773404,
126.640996111611));
#125097=CARTESIAN_POINT('Ctrl Pts',(0.615395910433173,29.8003033203065,
126.654103545578));
#125098=CARTESIAN_POINT('Ctrl Pts',(0.614070380700639,29.819705101918,126.656330615932));
#125099=CARTESIAN_POINT('Ctrl Pts',(0.611959571554278,29.8509076833447,
126.659357468475));
#125100=CARTESIAN_POINT('Ctrl Pts',(0.611167610191796,29.8626851432515,
126.660373563277));
#125101=CARTESIAN_POINT('Ctrl Pts',(0.609662074371933,29.8852046054757,
126.662075163477));
#125102=CARTESIAN_POINT('Ctrl Pts',(0.608947867417984,29.8959443377139,
126.662782084356));
#125103=CARTESIAN_POINT('Ctrl Pts',(0.607308815025502,29.9207169894568,
126.66417173663));
#125104=CARTESIAN_POINT('Ctrl Pts',(0.606386297959672,29.9347533275941,
126.664781143722));
#125105=CARTESIAN_POINT('Ctrl Pts',(0.603449792534127,29.9797120701522,
126.666163588421));
#125106=CARTESIAN_POINT('Ctrl Pts',(0.601456950722025,30.0106499918481,
126.666253124582));
#125107=CARTESIAN_POINT('Ctrl Pts',(0.596740447039811,30.0846742076842,
126.664405315339));
#125108=CARTESIAN_POINT('Ctrl Pts',(0.594040121294101,30.1277182675217,
126.661656767285));
#125109=CARTESIAN_POINT('Ctrl Pts',(0.586842660233912,30.2432627289797,
126.649761697095));
#125110=CARTESIAN_POINT('Ctrl Pts',(0.58240957196995,30.3153468908837,126.637512470602));
#125111=CARTESIAN_POINT('Ctrl Pts',(0.577016471332671,30.4010959915034,
126.617067228247));
#125112=CARTESIAN_POINT('Ctrl Pts',(0.576090424704046,30.4157487919857,
126.613362125855));
#125113=CARTESIAN_POINT('Ctrl Pts',(0.570735612060012,30.4999191911044,
126.59085601265));
#125114=CARTESIAN_POINT('Ctrl Pts',(0.566253895149197,30.5682016592702,
126.567764755207));
#125115=CARTESIAN_POINT('Ctrl Pts',(0.560749370323946,30.6461126659113,
126.535657840446));
#125116=CARTESIAN_POINT('Ctrl Pts',(0.559941500548798,30.6574057464283,
126.530857355476));
#125117=CARTESIAN_POINT('Ctrl Pts',(0.558664973549813,30.6750082834363,
126.523144147176));
#125118=CARTESIAN_POINT('Ctrl Pts',(0.558201186201658,30.6813545573832,
126.52031583513));
#125119=CARTESIAN_POINT('Ctrl Pts',(0.557371232117855,30.6926199447267,
126.515210544299));
#125120=CARTESIAN_POINT('Ctrl Pts',(0.557006011680592,30.6975458987382,
126.512949139164));
#125121=CARTESIAN_POINT('Ctrl Pts',(0.556112857223938,30.7095166972507,
126.507382701346));
#125122=CARTESIAN_POINT('Ctrl Pts',(0.555583406191478,30.7165494215158,
126.504052350291));
#125123=CARTESIAN_POINT('Ctrl Pts',(0.553889413758413,30.7388581186891,
126.49329607934));
#125124=CARTESIAN_POINT('Ctrl Pts',(0.552714545376632,30.7540434219739,
126.485686024027));
#125125=CARTESIAN_POINT('Ctrl Pts',(0.549867236056007,30.7902234496698,
126.466857003386));
#125126=CARTESIAN_POINT('Ctrl Pts',(0.548184731357374,30.8110989331917,
126.455417799357));
#125127=CARTESIAN_POINT('Ctrl Pts',(0.541418138772753,30.893316645787,126.40804648008));
#125128=CARTESIAN_POINT('Ctrl Pts',(0.536227271511378,30.9525747682982,
126.36865260101));
#125129=CARTESIAN_POINT('Ctrl Pts',(0.522908170011819,31.0981049568245,
126.257865285868));
#125130=CARTESIAN_POINT('Ctrl Pts',(0.514852835877638,31.1800462963872,
126.181337565979));
#125131=CARTESIAN_POINT('Ctrl Pts',(0.505625127887404,31.2682350069771,
126.080565781917));
#125132=CARTESIAN_POINT('Ctrl Pts',(0.504118606412817,31.2824294126384,
126.063681025808));
#125133=CARTESIAN_POINT('Ctrl Pts',(0.501705780468279,31.3048223410172,
126.035943712146));
#125134=CARTESIAN_POINT('Ctrl Pts',(0.500791124888508,31.3132302114156,
126.025264427983));
#125135=CARTESIAN_POINT('Ctrl Pts',(0.499169604700596,31.3279868665607,
126.006041814014));
#125136=CARTESIAN_POINT('Ctrl Pts',(0.498460762918687,31.3343861512601,
125.997538399112));
#125137=CARTESIAN_POINT('Ctrl Pts',(0.496964616802881,31.3477804158328,
125.979380451607));
#125138=CARTESIAN_POINT('Ctrl Pts',(0.496178166579844,31.3547541564008,
125.969710939655));
#125139=CARTESIAN_POINT('Ctrl Pts',(0.494065885852746,31.3732967140546,
125.943410056116));
#125140=CARTESIAN_POINT('Ctrl Pts',(0.49274763566798,31.384667188492,125.926640833353));
#125141=CARTESIAN_POINT('Ctrl Pts',(0.489846976954011,31.4092054278564,
125.888991108142));
#125142=CARTESIAN_POINT('Ctrl Pts',(0.488270089023461,31.4222208209061,
125.868016796208));
#125143=CARTESIAN_POINT('Ctrl Pts',(0.483300369326884,31.462104782962,125.800436684676));
#125144=CARTESIAN_POINT('Ctrl Pts',(0.479963116353044,31.4871856101745,
125.752813978256));
#125145=CARTESIAN_POINT('Ctrl Pts',(0.473803296962714,31.5295458105348,
125.661968556735));
#125146=CARTESIAN_POINT('Ctrl Pts',(0.470975552750166,31.5474010448887,
125.619081377102));
#125147=CARTESIAN_POINT('Ctrl Pts',(0.468139959767684,31.5634400089539,
125.575509633631));
#125148=CARTESIAN_POINT('Origin',(5.,-30.,125.));
#125149=CARTESIAN_POINT('',(1.32020507860662,-28.3340002656058,125.000940743489));
#125150=CARTESIAN_POINT('Ctrl Pts',(0.659203971007256,-28.4365599837785,
125.575509613888));
#125151=CARTESIAN_POINT('Ctrl Pts',(0.659952788000284,-28.4405111228567,
125.586243351075));
#125152=CARTESIAN_POINT('Ctrl Pts',(0.660707178275404,-28.4445725592891,
125.596935744733));
#125153=CARTESIAN_POINT('Ctrl Pts',(0.661913431714573,-28.4511870645999,
125.613823574029));
#125154=CARTESIAN_POINT('Ctrl Pts',(0.662361167616503,-28.4536680605702,
125.620047109534));
#125155=CARTESIAN_POINT('Ctrl Pts',(0.663223012937918,-28.4584912126697,
125.631936903649));
#125156=CARTESIAN_POINT('Ctrl Pts',(0.663636763814656,-28.4608272048218,
125.63760543687));
#125157=CARTESIAN_POINT('Ctrl Pts',(0.664644178966683,-28.4665654621471,
125.651314629528));
#125158=CARTESIAN_POINT('Ctrl Pts',(0.665239704446657,-28.4699997223272,
125.659341618913));
#125159=CARTESIAN_POINT('Ctrl Pts',(0.66738747270351,-28.4825410329116,
125.688029126372));
#125160=CARTESIAN_POINT('Ctrl Pts',(0.668958672319821,-28.4920043483959,
125.708530018805));
#125161=CARTESIAN_POINT('Ctrl Pts',(0.680709757870277,-28.5650825441696,
125.858742966811));
#125162=CARTESIAN_POINT('Ctrl Pts',(0.691454103024878,-28.6449126402584,
125.979882323236));
#125163=CARTESIAN_POINT('Ctrl Pts',(0.70635313264515,-28.7812993357348,
126.137733317166));
#125164=CARTESIAN_POINT('Ctrl Pts',(0.710848350620454,-28.8259961962093,
126.183801205807));
#125165=CARTESIAN_POINT('Ctrl Pts',(0.716500666851209,-28.8869331488791,
126.239751416357));
#125166=CARTESIAN_POINT('Ctrl Pts',(0.717760854930286,-28.9008324984542,
126.252091147451));
#125167=CARTESIAN_POINT('Ctrl Pts',(0.71979271624179,-28.9237476457165,
126.271759300105));
#125168=CARTESIAN_POINT('Ctrl Pts',(0.720570222738542,-28.9326383916829,
126.279230259336));
#125169=CARTESIAN_POINT('Ctrl Pts',(0.722064413641303,-28.9499575574367,
126.293477404711));
#125170=CARTESIAN_POINT('Ctrl Pts',(0.72278156378737,-28.9583752379163,
126.300265662119));
#125171=CARTESIAN_POINT('Ctrl Pts',(0.724451097211425,-28.9782141433035,
126.315948018525));
#125172=CARTESIAN_POINT('Ctrl Pts',(0.725400839598706,-28.9896864893521,
126.324776266559));
#125173=CARTESIAN_POINT('Ctrl Pts',(0.728531633613869,-29.0281075714805,
126.35355279639));
#125174=CARTESIAN_POINT('Ctrl Pts',(0.730687222715632,-29.0555443061314,
126.372837845898));
#125175=CARTESIAN_POINT('Ctrl Pts',(0.735883474388284,-29.1238625039574,
126.417839831529));
#125176=CARTESIAN_POINT('Ctrl Pts',(0.738893422057637,-29.1653162225518,
126.442633078843));
#125177=CARTESIAN_POINT('Ctrl Pts',(0.745995229778165,-29.2665646144079,
126.497361747878));
#125178=CARTESIAN_POINT('Ctrl Pts',(0.750051113498307,-29.3271963442272,
126.525567127607));
#125179=CARTESIAN_POINT('Ctrl Pts',(0.758902099603246,-29.4617012585901,
126.578555085847));
#125180=CARTESIAN_POINT('Ctrl Pts',(0.7636986361377,-29.5359423153221,126.601951721544));
#125181=CARTESIAN_POINT('Ctrl Pts',(0.769796848439415,-29.6274575112708,
126.623895373793));
#125182=CARTESIAN_POINT('Ctrl Pts',(0.770868277232152,-29.6434343580739,
126.627478105787));
#125183=CARTESIAN_POINT('Ctrl Pts',(0.772462104297826,-29.6670004311443,
126.632399036367));
#125184=CARTESIAN_POINT('Ctrl Pts',(0.772974774531412,-29.6745508365018,
126.633921100585));
#125185=CARTESIAN_POINT('Ctrl Pts',(0.773892722424834,-29.6880106386339,
126.636537428563));
#125186=CARTESIAN_POINT('Ctrl Pts',(0.774296847948697,-29.6939157912203,
126.637652152166));
#125187=CARTESIAN_POINT('Ctrl Pts',(0.775196689044128,-29.7070180362633,
126.640052138043));
#125188=CARTESIAN_POINT('Ctrl Pts',(0.775693213989008,-29.7142175309546,
126.641321973861));
#125189=CARTESIAN_POINT('Ctrl Pts',(0.777172093011416,-29.7355785857425,
126.644944802257));
#125190=CARTESIAN_POINT('Ctrl Pts',(0.778161427636895,-29.7497620454105,
126.647162110524));
#125191=CARTESIAN_POINT('Ctrl Pts',(0.780480236995961,-29.7827985346632,
126.65189019919));
#125192=CARTESIAN_POINT('Ctrl Pts',(0.781815621837031,-29.8016692122806,
126.65426193198));
#125193=CARTESIAN_POINT('Ctrl Pts',(0.786590539582907,-29.8687302437716,
126.661526510729));
#125194=CARTESIAN_POINT('Ctrl Pts',(0.790086567261338,-29.9170867503672,
126.664640173597));
#125195=CARTESIAN_POINT('Ctrl Pts',(0.801961053567282,-30.0805910286992,
126.66802611696));
#125196=CARTESIAN_POINT('Ctrl Pts',(0.810378370068741,-30.1956285135019,
126.658475723849));
#125197=CARTESIAN_POINT('Ctrl Pts',(0.821474111727933,-30.3507455707969,
126.629220121835));
#125198=CARTESIAN_POINT('Ctrl Pts',(0.824431877616766,-30.392404504127,
126.61969130751));
#125199=CARTESIAN_POINT('Ctrl Pts',(0.828447746977999,-30.4493779111564,
126.604331850906));
#125200=CARTESIAN_POINT('Ctrl Pts',(0.829548609789823,-30.4650388247494,
126.599862531299));
#125201=CARTESIAN_POINT('Ctrl Pts',(0.831314989341577,-30.4902288801112,
126.592272621963));
#125202=CARTESIAN_POINT('Ctrl Pts',(0.831985084216166,-30.4997994618681,
126.589294485942));
#125203=CARTESIAN_POINT('Ctrl Pts',(0.8333797683235,-30.5197458775554,126.582889638024));
#125204=CARTESIAN_POINT('Ctrl Pts',(0.834103792777535,-30.5301160775566,
126.579446845381));
#125205=CARTESIAN_POINT('Ctrl Pts',(0.835825154396519,-30.5548019021225,
126.570980901244));
#125206=CARTESIAN_POINT('Ctrl Pts',(0.836819341079492,-30.5690844185817,
126.565863688903));
#125207=CARTESIAN_POINT('Ctrl Pts',(0.840285116630252,-30.6189326836981,
126.547231649304));
#125208=CARTESIAN_POINT('Ctrl Pts',(0.842722831317173,-30.6541050929578,
126.532693810843));
#125209=CARTESIAN_POINT('Ctrl Pts',(0.84879558111837,-30.7415548564192,
126.492988753184));
#125210=CARTESIAN_POINT('Ctrl Pts',(0.852383199621562,-30.7930735250193,
126.466272193781));
#125211=CARTESIAN_POINT('Ctrl Pts',(0.862670320436195,-30.9377214396954,
126.381401759193));
#125212=CARTESIAN_POINT('Ctrl Pts',(0.869255113445024,-31.0266215752484,
126.316676180117));
#125213=CARTESIAN_POINT('Ctrl Pts',(0.878120565810813,-31.1309131168693,
126.223720711109));
#125214=CARTESIAN_POINT('Ctrl Pts',(0.880052767804596,-31.1527737991446,
126.203149684368));
#125215=CARTESIAN_POINT('Ctrl Pts',(0.882681527470541,-31.1811541142419,
126.174959908517));
#125216=CARTESIAN_POINT('Ctrl Pts',(0.883342505382893,-31.1881791612443,
126.167855340709));
#125217=CARTESIAN_POINT('Ctrl Pts',(0.884391493103859,-31.1991454228612,
126.156563579617));
#125218=CARTESIAN_POINT('Ctrl Pts',(0.884776261322163,-31.2031297238217,
126.152418293851));
#125219=CARTESIAN_POINT('Ctrl Pts',(0.885579680345145,-31.2113680472079,
126.143757814347));
#125220=CARTESIAN_POINT('Ctrl Pts',(0.885998615477635,-31.2156183957721,
126.139239393033));
#125221=CARTESIAN_POINT('Ctrl Pts',(0.887038546669201,-31.2260595587147,
126.128014742525));
#125222=CARTESIAN_POINT('Ctrl Pts',(0.887661695162183,-31.2322206315728,
126.121281234328));
#125223=CARTESIAN_POINT('Ctrl Pts',(0.890033938164367,-31.2553273030339,
126.095607254887));
#125224=CARTESIAN_POINT('Ctrl Pts',(0.891807350696535,-31.2718931466652,
126.076331523339));
#125225=CARTESIAN_POINT('Ctrl Pts',(0.896555364268742,-31.314556022892,
126.024329088885));
#125226=CARTESIAN_POINT('Ctrl Pts',(0.899562943419358,-31.3398712180821,
125.990985519493));
#125227=CARTESIAN_POINT('Ctrl Pts',(0.912077654603941,-31.4391301885819,
125.849482640872));
#125228=CARTESIAN_POINT('Ctrl Pts',(0.921693463471601,-31.5014593082718,
125.733720494547));
#125229=CARTESIAN_POINT('Ctrl Pts',(0.933545634833785,-31.5636376122723,
125.576244937981));
#125230=CARTESIAN_POINT('Ctrl Pts',(0.936187861162518,-31.5764634633483,
125.5401705015));
#125231=CARTESIAN_POINT('Ctrl Pts',(0.939851490197423,-31.5927588579299,
125.488793652399));
#125232=CARTESIAN_POINT('Ctrl Pts',(0.94090642416339,-31.5972720388305,
125.473837606134));
#125233=CARTESIAN_POINT('Ctrl Pts',(0.942685651888065,-31.6045755080865,
125.448343833051));
#125234=CARTESIAN_POINT('Ctrl Pts',(0.943413413033034,-31.6074738814749,
125.43783842213));
#125235=CARTESIAN_POINT('Ctrl Pts',(0.94488397245525,-31.6131478112168,
125.416456619934));
#125236=CARTESIAN_POINT('Ctrl Pts',(0.945626530187649,-31.6159169481621,
125.405579097346));
#125237=CARTESIAN_POINT('Ctrl Pts',(0.947467337420167,-31.6225397421857,
125.378418731322));
#125238=CARTESIAN_POINT('Ctrl Pts',(0.948561227260991,-31.6262584857579,
125.362104020899));
#125239=CARTESIAN_POINT('Ctrl Pts',(0.952916961696848,-31.6401793689172,
125.29648365487));
#125240=CARTESIAN_POINT('Ctrl Pts',(0.956115937444605,-31.6483904627062,
125.246780360908));
#125241=CARTESIAN_POINT('Ctrl Pts',(0.965022166420443,-31.6652039047736,
125.105427193662));
#125242=CARTESIAN_POINT('Ctrl Pts',(0.970592851241548,-31.6684849518826,
125.013333446826));
#125243=CARTESIAN_POINT('Ctrl Pts',(0.976476273650288,-31.6639519553479,
124.917314311575));
#125244=CARTESIAN_POINT('Ctrl Pts',(0.976728993283109,-31.6637420180873,
124.913192570066));
#125245=CARTESIAN_POINT('Ctrl Pts',(0.981942939262595,-31.6590975300757,
124.828222541442));
#125246=CARTESIAN_POINT('Ctrl Pts',(0.986950336421848,-31.648790639554,
124.747813445692));
#125247=CARTESIAN_POINT('Ctrl Pts',(0.993043460817581,-31.6302260786282,
124.656384872667));
#125248=CARTESIAN_POINT('Ctrl Pts',(0.993856149516315,-31.627635035567,
124.644313913594));
#125249=CARTESIAN_POINT('Ctrl Pts',(0.995138705276603,-31.6233726973217,
124.62547949956));
#125250=CARTESIAN_POINT('Ctrl Pts',(0.99560362837449,-31.6217926611739,
124.618695555468));
#125251=CARTESIAN_POINT('Ctrl Pts',(0.996477068376249,-31.6187604666437,
124.606036580946));
#125252=CARTESIAN_POINT('Ctrl Pts',(0.996884998644199,-31.6173187788029,
124.600159297963));
#125253=CARTESIAN_POINT('Ctrl Pts',(0.997849466516603,-31.613850024864,
124.586344084224));
#125254=CARTESIAN_POINT('Ctrl Pts',(0.998407471292178,-31.6117963913303,
124.578413110631));
#125255=CARTESIAN_POINT('Ctrl Pts',(1.00028027613092,-31.604746086708,124.55199004273));
#125256=CARTESIAN_POINT('Ctrl Pts',(1.00160839860681,-31.599489197655,124.533569776379));
#125257=CARTESIAN_POINT('Ctrl Pts',(1.00490875905489,-31.585774838564,124.488475759881));
#125258=CARTESIAN_POINT('Ctrl Pts',(1.0068952458719,-31.576960836835,124.461917078837));
#125259=CARTESIAN_POINT('Ctrl Pts',(1.01590761029936,-31.53433686381,124.34354058279));
#125260=CARTESIAN_POINT('Ctrl Pts',(1.02310053201971,-31.4931467962678,
124.254586388757));
#125261=CARTESIAN_POINT('Ctrl Pts',(1.03631690639912,-31.4018999306265,
124.095841930695));
#125262=CARTESIAN_POINT('Ctrl Pts',(1.04235452313837,-31.35379455986,124.025284881628));
#125263=CARTESIAN_POINT('Ctrl Pts',(1.04953835166265,-31.2881908987373,
123.943350836977));
#125264=CARTESIAN_POINT('Ctrl Pts',(1.05087445908436,-31.2756197223439,
123.928208216638));
#125265=CARTESIAN_POINT('Ctrl Pts',(1.05299729466008,-31.2550575658085,
123.904314475793));
#125266=CARTESIAN_POINT('Ctrl Pts',(1.05379086698088,-31.2472367401788,
123.895420085311));
#125267=CARTESIAN_POINT('Ctrl Pts',(1.05529647517862,-31.2321449294111,
123.878621299215));
#125268=CARTESIAN_POINT('Ctrl Pts',(1.05600917415139,-31.2248910952324,
123.87070237241));
#125269=CARTESIAN_POINT('Ctrl Pts',(1.05764051056466,-31.208037317787,123.852656754201));
#125270=CARTESIAN_POINT('Ctrl Pts',(1.05855687764223,-31.1983856230341,
123.842579331887));
#125271=CARTESIAN_POINT('Ctrl Pts',(1.06145573908754,-31.1672774503254,
123.810905361708));
#125272=CARTESIAN_POINT('Ctrl Pts',(1.06341782363415,-31.1453544374955,
123.789774358659));
#125273=CARTESIAN_POINT('Ctrl Pts',(1.06804741290466,-31.0916878542415,
123.740811947588));
#125274=CARTESIAN_POINT('Ctrl Pts',(1.07069274749435,-31.059441319136,123.713562521073));
#125275=CARTESIAN_POINT('Ctrl Pts',(1.07800220401919,-30.9665882968917,
123.640960710175));
#125276=CARTESIAN_POINT('Ctrl Pts',(1.08259225305527,-30.9038778200993,
123.598470128191));
#125277=CARTESIAN_POINT('Ctrl Pts',(1.08786899299986,-30.829368119352,123.555072289489));
#125278=CARTESIAN_POINT('Ctrl Pts',(1.08851612439677,-30.8201906482293,
123.549843158828));
#125279=CARTESIAN_POINT('Ctrl Pts',(1.09379079653486,-30.7451279522311,
123.508014515775));
#125280=CARTESIAN_POINT('Ctrl Pts',(1.09847029713675,-30.6768861982096,
123.475841703367));
#125281=CARTESIAN_POINT('Ctrl Pts',(1.10419462993725,-30.5952687498334,
123.443927356345));
#125282=CARTESIAN_POINT('Ctrl Pts',(1.10500348888736,-30.583777257668,123.439579848731));
#125283=CARTESIAN_POINT('Ctrl Pts',(1.10628133065542,-30.5657093295162,
123.432971826538));
#125284=CARTESIAN_POINT('Ctrl Pts',(1.10674542943947,-30.5591647685032,
123.430624614947));
#125285=CARTESIAN_POINT('Ctrl Pts',(1.10761827480739,-30.5468936415534,
123.426310066122));
#125286=CARTESIAN_POINT('Ctrl Pts',(1.10802644567243,-30.5411707958751,
123.42433289424));
#125287=CARTESIAN_POINT('Ctrl Pts',(1.10899281456034,-30.5276565998648,
123.419746214365));
#125288=CARTESIAN_POINT('Ctrl Pts',(1.10955249703968,-30.5198565825867,
123.417163103519));
#125289=CARTESIAN_POINT('Ctrl Pts',(1.11143696502406,-30.493672798988,123.408706302729));
#125290=CARTESIAN_POINT('Ctrl Pts',(1.11277529150004,-30.4752068903733,
123.403094619134));
#125291=CARTESIAN_POINT('Ctrl Pts',(1.11610669889285,-30.4294617379501,
123.39005658859));
#125292=CARTESIAN_POINT('Ctrl Pts',(1.11811435147819,-30.4020834479405,
123.383001579213));
#125293=CARTESIAN_POINT('Ctrl Pts',(1.12731205982333,-30.2770045639129,
123.354143337078));
#125294=CARTESIAN_POINT('Ctrl Pts',(1.13467424331126,-30.177639681118,123.340475888893));
#125295=CARTESIAN_POINT('Ctrl Pts',(1.14785029236992,-29.9951033935346,
123.331959099954));
#125296=CARTESIAN_POINT('Ctrl Pts',(1.15369509473113,-29.912376869125,123.334253827135));
#125297=CARTESIAN_POINT('Ctrl Pts',(1.16069370150931,-29.8106432788171,
123.344679917503));
#125298=CARTESIAN_POINT('Ctrl Pts',(1.16202503416068,-29.7911718099492,
123.347023476445));
#125299=CARTESIAN_POINT('Ctrl Pts',(1.16414212867657,-29.760028697994,123.351330935507));
#125300=CARTESIAN_POINT('Ctrl Pts',(1.16493466980795,-29.748329221065,123.353076279386));
#125301=CARTESIAN_POINT('Ctrl Pts',(1.16643944864941,-29.7260421986319,
123.356644131116));
#125302=CARTESIAN_POINT('Ctrl Pts',(1.16715233762151,-29.71545180378,123.358444724667));
#125303=CARTESIAN_POINT('Ctrl Pts',(1.16878569430159,-29.6911191792949,
123.36282434819));
#125304=CARTESIAN_POINT('Ctrl Pts',(1.1697038713505,-29.6773903968712,123.365474215564));
#125305=CARTESIAN_POINT('Ctrl Pts',(1.17261508210444,-29.6337207185938,
123.374474795799));
#125306=CARTESIAN_POINT('Ctrl Pts',(1.1745874499727,-29.6039197497773,123.381478042994));
#125307=CARTESIAN_POINT('Ctrl Pts',(1.17924652379521,-29.5332248658153,
123.400161146468));
#125308=CARTESIAN_POINT('Ctrl Pts',(1.18191065371257,-29.4925516225319,
123.412593338978));
#125309=CARTESIAN_POINT('Ctrl Pts',(1.18911624590242,-29.3827833289793,
123.450796168208));
#125310=CARTESIAN_POINT('Ctrl Pts',(1.19359016368393,-29.3148534168532,
123.479617332439));
#125311=CARTESIAN_POINT('Ctrl Pts',(1.20304885159216,-29.1768385354342,
123.549308360876));
#125312=CARTESIAN_POINT('Ctrl Pts',(1.20802904347214,-29.1073822496287,
123.590982098273));
#125313=CARTESIAN_POINT('Ctrl Pts',(1.21433268730004,-29.0278205573635,
123.646969241793));
#125314=CARTESIAN_POINT('Ctrl Pts',(1.2154060785304,-29.0145457307697,123.65660693198));
#125315=CARTESIAN_POINT('Ctrl Pts',(1.21700217383662,-28.995247313429,123.671057778482));
#125316=CARTESIAN_POINT('Ctrl Pts',(1.21751510320364,-28.9891109113589,
123.675719578817));
#125317=CARTESIAN_POINT('Ctrl Pts',(1.21841728125938,-28.9784367671974,
123.683946103684));
#125318=CARTESIAN_POINT('Ctrl Pts',(1.2188052321189,-28.9738848689808,123.687492082831));
#125319=CARTESIAN_POINT('Ctrl Pts',(1.21920075568198,-28.9692831202466,
123.691115466765));
#125320=CARTESIAN_POINT('Ctrl Pts',(1.21920662355708,-28.9692148586174,
123.691169224134));
#125321=CARTESIAN_POINT('Ctrl Pts',(1.21922178435846,-28.9690385135907,
123.691308121645));
#125322=CARTESIAN_POINT('Ctrl Pts',(1.2192310778624,-28.9689304364423,123.69139326991));
#125323=CARTESIAN_POINT('Ctrl Pts',(1.21924924690886,-28.9687191848912,
123.691559746245));
#125324=CARTESIAN_POINT('Ctrl Pts',(1.21925812235001,-28.9686160097637,
123.691641072968));
#125325=CARTESIAN_POINT('Ctrl Pts',(1.21927548947839,-28.9684141589893,
123.691800218461));
#125326=CARTESIAN_POINT('Ctrl Pts',(1.21928398111029,-28.9683154823172,
123.691878036357));
#125327=CARTESIAN_POINT('Ctrl Pts',(1.21930061129616,-28.9681222670639,
123.692030444249));
#125328=CARTESIAN_POINT('Ctrl Pts',(1.2193087497812,-28.9680277278153,123.692105033291));
#125329=CARTESIAN_POINT('Ctrl Pts',(1.21932470114206,-28.9678424639905,
123.692251234289));
#125330=CARTESIAN_POINT('Ctrl Pts',(1.21933251397122,-28.9677517386588,
123.692322845532));
#125331=CARTESIAN_POINT('Ctrl Pts',(1.21934783878755,-28.9675738112311,
123.692463317115));
#125332=CARTESIAN_POINT('Ctrl Pts',(1.2193553507183,-28.9674866086396,123.692532176684));
#125333=CARTESIAN_POINT('Ctrl Pts',(1.21937009609573,-28.9673154637501,
123.692667349129));
#125334=CARTESIAN_POINT('Ctrl Pts',(1.21937732948593,-28.9672315210839,
123.692733661261));
#125335=CARTESIAN_POINT('Ctrl Pts',(1.21939153797072,-28.9670666587335,
123.692863923251));
#125336=CARTESIAN_POINT('Ctrl Pts',(1.21939851303747,-28.9669857384585,
123.692927872652));
#125337=CARTESIAN_POINT('Ctrl Pts',(1.21941222328814,-28.9668267045739,
123.693053577405));
#125338=CARTESIAN_POINT('Ctrl Pts',(1.21941895842297,-28.9667485907153,
123.693115332125));
#125339=CARTESIAN_POINT('Ctrl Pts',(1.21943220545572,-28.9665949741827,
123.693236799614));
#125340=CARTESIAN_POINT('Ctrl Pts',(1.21943871735016,-28.966519470814,123.693296512188));
#125341=CARTESIAN_POINT('Ctrl Pts',(1.21945153321689,-28.9663708955148,
123.693414035341));
#125342=CARTESIAN_POINT('Ctrl Pts',(1.2194578371461,-28.9662978234217,123.693471845378));
#125343=CARTESIAN_POINT('Ctrl Pts',(1.21947025101568,-28.9661539472047,
123.693585690804));
#125344=CARTESIAN_POINT('Ctrl Pts',(1.21947636092835,-28.9660831428042,
123.693641725804));
#125345=CARTESIAN_POINT('Ctrl Pts',(1.21948839957223,-28.9659436517833,
123.693752138227));
#125346=CARTESIAN_POINT('Ctrl Pts',(1.2194943282726,-28.9658749649792,123.693806515244));
#125347=CARTESIAN_POINT('Ctrl Pts',(1.2195060161932,-28.9657395719821,123.693913718671));
#125348=CARTESIAN_POINT('Ctrl Pts',(1.21951177541156,-28.9656728653199,
123.693966544952));
#125349=CARTESIAN_POINT('Ctrl Pts',(1.21952313526533,-28.9655413049327,
123.694070746539));
#125350=CARTESIAN_POINT('Ctrl Pts',(1.21952873585499,-28.9654764512913,
123.694122121325));
#125351=CARTESIAN_POINT('Ctrl Pts',(1.21953978836484,-28.965348480826,123.694223510567));
#125352=CARTESIAN_POINT('Ctrl Pts',(1.21954524028525,-28.9652853635928,
123.694273524933));
#125353=CARTESIAN_POINT('Ctrl Pts',(1.21955600474592,-28.965160757194,123.694372278287));
#125354=CARTESIAN_POINT('Ctrl Pts',(1.21956131725224,-28.9650992680499,
123.69442101688));
#125355=CARTESIAN_POINT('Ctrl Pts',(1.21957181139231,-28.9649778182569,
123.694517296493));
#125356=CARTESIAN_POINT('Ctrl Pts',(1.21957699302637,-28.9649178572651,
123.694564837441));
#125357=CARTESIAN_POINT('Ctrl Pts',(1.21958723333976,-28.9647993711441,
123.694658794186));
#125358=CARTESIAN_POINT('Ctrl Pts',(1.21959229202362,-28.9647408456518,
123.694705209955));
#125359=CARTESIAN_POINT('Ctrl Pts',(1.21960229387362,-28.964625143565,123.694796984378));
#125360=CARTESIAN_POINT('Ctrl Pts',(1.21960723700523,-28.9645679670848,
123.69484234265));
#125361=CARTESIAN_POINT('Ctrl Pts',(1.21961701460404,-28.9644548829029,
123.694932064776));
#125362=CARTESIAN_POINT('Ctrl Pts',(1.2196218490546,-28.9643989751315,123.694976428418));
#125363=CARTESIAN_POINT('Ctrl Pts',(1.21963141568774,-28.9642883536169,
123.695064219808));
#125364=CARTESIAN_POINT('Ctrl Pts',(1.21963614786677,-28.9642336396734,
123.695107647468));
#125365=CARTESIAN_POINT('Ctrl Pts',(1.21964551593236,-28.9641253360074,
123.695193621574));
#125366=CARTESIAN_POINT('Ctrl Pts',(1.21965015181907,-28.9640717460609,
123.69523616797));
#125367=CARTESIAN_POINT('Ctrl Pts',(1.21965933297478,-28.9639656241284,
123.69532043148));
#125368=CARTESIAN_POINT('Ctrl Pts',(1.21966387820487,-28.9639130923872,
123.695362148191));
#125369=CARTESIAN_POINT('Ctrl Pts',(1.21967288326782,-28.9638090259192,
123.695444800108));
#125370=CARTESIAN_POINT('Ctrl Pts',(1.21967734309576,-28.9637574910599,
123.695485735227));
#125371=CARTESIAN_POINT('Ctrl Pts',(1.21968618227514,-28.9636553609314,
123.695566869));
#125372=CARTESIAN_POINT('Ctrl Pts',(1.21969056163286,-28.9636047654146,
123.695607067673));
#125373=CARTESIAN_POINT('Ctrl Pts',(1.21969924454946,-28.963504459408,123.695686771376));
#125374=CARTESIAN_POINT('Ctrl Pts',(1.2197035480933,-28.9634547489301,123.69572627623));
#125375=CARTESIAN_POINT('Ctrl Pts',(1.21971208379459,-28.9633561615505,
123.695804632694));
#125376=CARTESIAN_POINT('Ctrl Pts',(1.21971631593383,-28.9633072847094,
123.695843484101));
#125377=CARTESIAN_POINT('Ctrl Pts',(1.21972471282815,-28.9632103179353,
123.695920570311));
#125378=CARTESIAN_POINT('Ctrl Pts',(1.21972887764312,-28.9631622271718,
123.695958805631));
#125379=CARTESIAN_POINT('Ctrl Pts',(1.21973714391899,-28.9630667856039,
123.696034696573));
#125380=CARTESIAN_POINT('Ctrl Pts',(1.21974124535099,-28.9630194350046,
123.696072351899));
#125381=CARTESIAN_POINT('Ctrl Pts',(1.22028393924562,-28.9567546350548,
123.701054959689));
#125382=CARTESIAN_POINT('Ctrl Pts',(1.22082558548529,-28.9505727878688,
123.706044193446));
#125383=CARTESIAN_POINT('Ctrl Pts',(1.22202863962478,-28.9369928768266,
123.717165564375));
#125384=CARTESIAN_POINT('Ctrl Pts',(1.22269132940012,-28.9296117547805,
123.723317844037));
#125385=CARTESIAN_POINT('Ctrl Pts',(1.22455782570845,-28.9090878603758,
123.740727920465));
#125386=CARTESIAN_POINT('Ctrl Pts',(1.22576976240379,-28.8960670206688,
123.752126852365));
#125387=CARTESIAN_POINT('Ctrl Pts',(1.22993481286726,-28.8522786474751,
123.791682556353));
#125388=CARTESIAN_POINT('Ctrl Pts',(1.2329315059388,-28.8223931646664,123.82078964835));
#125389=CARTESIAN_POINT('Ctrl Pts',(1.24534804968517,-28.7041099104753,
123.944976909866));
#125390=CARTESIAN_POINT('Ctrl Pts',(1.25487703514157,-28.6258629693803,
124.049126082904));
#125391=CARTESIAN_POINT('Ctrl Pts',(1.26672980387923,-28.5407114183588,
124.195277594783));
#125392=CARTESIAN_POINT('Ctrl Pts',(1.26944560205847,-28.5221290323072,
124.229935612407));
#125393=CARTESIAN_POINT('Ctrl Pts',(1.27319194526195,-28.4978279849176,
124.279386140264));
#125394=CARTESIAN_POINT('Ctrl Pts',(1.27425807616971,-28.491068505303,124.293649611147));
#125395=CARTESIAN_POINT('Ctrl Pts',(1.27605053971841,-28.4799734914073,
124.31794807193));
#125396=CARTESIAN_POINT('Ctrl Pts',(1.27678046247768,-28.4755322784921,
124.327933340134));
#125397=CARTESIAN_POINT('Ctrl Pts',(1.27825083547488,-28.4667439771098,
124.348227708216));
#125398=CARTESIAN_POINT('Ctrl Pts',(1.27899108712776,-28.4624018375552,
124.358538346231));
#125399=CARTESIAN_POINT('Ctrl Pts',(1.28081760606239,-28.4518957858664,
124.384205292149));
#125400=CARTESIAN_POINT('Ctrl Pts',(1.28189966337131,-28.4458560796823,
124.399611386536));
#125401=CARTESIAN_POINT('Ctrl Pts',(1.28613667752862,-28.4229552088,124.460689548178));
#125402=CARTESIAN_POINT('Ctrl Pts',(1.28923322675697,-28.4078689017657,
124.507003769619));
#125403=CARTESIAN_POINT('Ctrl Pts',(1.30174960511128,-28.3543734897741,
124.699499177115));
#125404=CARTESIAN_POINT('Ctrl Pts',(1.31064599465137,-28.3339149674139,
124.849882812604));
#125405=CARTESIAN_POINT('Ctrl Pts',(1.32020507860662,-28.3340002656058,
125.000940743489));
#125406=CARTESIAN_POINT('Ctrl Pts',(1.32020523017832,-28.33400026696,125.000943138708));
#125407=CARTESIAN_POINT('Ctrl Pts',(1.32219890698379,-28.3340181023383,
125.032448298303));
#125408=CARTESIAN_POINT('Ctrl Pts',(1.32422170656257,-28.3349296096847,
125.063944754036));
#125409=CARTESIAN_POINT('Ctrl Pts',(1.32680933174148,-28.3371884976266,
125.103329994415));
#125410=CARTESIAN_POINT('Ctrl Pts',(1.32733343221065,-28.3377004057832,
125.111262002803));
#125411=CARTESIAN_POINT('Ctrl Pts',(1.32825584296946,-28.3386955705439,
125.125136472903));
#125412=CARTESIAN_POINT('Ctrl Pts',(1.32865284985722,-28.3391540088743,
125.131080643988));
#125413=CARTESIAN_POINT('Ctrl Pts',(1.329447764642,-28.3401314412556,125.142924611089));
#125414=CARTESIAN_POINT('Ctrl Pts',(1.32984564648262,-28.3406499954039,
125.148824183451));
#125415=CARTESIAN_POINT('Ctrl Pts',(1.33071839080185,-28.3418509841225,
125.161700261481));
#125416=CARTESIAN_POINT('Ctrl Pts',(1.33119390186315,-28.3425459821816,
125.168675154436));
#125417=CARTESIAN_POINT('Ctrl Pts',(1.33252662288963,-28.3446071926527,
125.188116827758));
#125418=CARTESIAN_POINT('Ctrl Pts',(1.33338883396304,-28.3460701628955,
125.200572575268));
#125419=CARTESIAN_POINT('Ctrl Pts',(1.3379570008922,-28.3545031629007,125.26598762346));
#125420=CARTESIAN_POINT('Ctrl Pts',(1.34176852209445,-28.3638760560123,
125.318600933699));
#125421=CARTESIAN_POINT('Ctrl Pts',(1.35044146688248,-28.3905987980285,
125.43569831053));
#125422=CARTESIAN_POINT('Ctrl Pts',(1.35531912301383,-28.4093313976143,
125.499778532008));
#125423=CARTESIAN_POINT('Ctrl Pts',(1.36049059062027,-28.4334055482443,
125.566885271663));
#125424=CARTESIAN_POINT('Ctrl Pts',(1.36082346855069,-28.4349739191953,
125.571200881571));
#125425=CARTESIAN_POINT('Ctrl Pts',(1.36115610141822,-28.4365599811973,
125.575509606876));
#125426=CARTESIAN_POINT('Ctrl Pts',(1.16625578224439,-28.4365599837819,
125.575509613897));
#125427=CARTESIAN_POINT('Ctrl Pts',(1.16615106715064,-28.4360181278264,
125.574037598029));
#125428=CARTESIAN_POINT('Ctrl Pts',(1.16604642104355,-28.4354783476409,
125.572564808384));
#125429=CARTESIAN_POINT('Ctrl Pts',(1.16522598371781,-28.4312599224099,
125.561004333803));
#125430=CARTESIAN_POINT('Ctrl Pts',(1.16451338791583,-28.4276767307586,
125.550881874627));
#125431=CARTESIAN_POINT('Ctrl Pts',(1.16288079176412,-28.419656064612,125.527507651467));
#125432=CARTESIAN_POINT('Ctrl Pts',(1.16196307924118,-28.4152869193639,
125.514233165253));
#125433=CARTESIAN_POINT('Ctrl Pts',(1.15905378485932,-28.4018900050275,
125.471736966863));
#125434=CARTESIAN_POINT('Ctrl Pts',(1.15708283748867,-28.393499289232,125.44231999311));
#125435=CARTESIAN_POINT('Ctrl Pts',(1.15242758125335,-28.3754013816926,
125.371536539769));
#125436=CARTESIAN_POINT('Ctrl Pts',(1.14976580265002,-28.3664570433951,
125.329996756368));
#125437=CARTESIAN_POINT('Ctrl Pts',(1.14256128716452,-28.346357731558,125.215543068738));
#125438=CARTESIAN_POINT('Ctrl Pts',(1.13808626256621,-28.3384397427388,
125.142159926808));
#125439=CARTESIAN_POINT('Ctrl Pts',(1.13273556033149,-28.3348438611616,
125.054769512405));
#125440=CARTESIAN_POINT('Ctrl Pts',(1.13189411697792,-28.334448906308,125.041039186489));
#125441=CARTESIAN_POINT('Ctrl Pts',(1.1265255423805,-28.3330163104506,124.953643957334));
#125442=CARTESIAN_POINT('Ctrl Pts',(1.12194599314035,-28.3366963931124,
124.879992230711));
#125443=CARTESIAN_POINT('Ctrl Pts',(1.11633294369522,-28.346659521943,124.79464180214));
#125444=CARTESIAN_POINT('Ctrl Pts',(1.11552469198212,-28.3482176782578,
124.782464104954));
#125445=CARTESIAN_POINT('Ctrl Pts',(1.11424772069684,-28.3508682831121,
124.763422595618));
#125446=CARTESIAN_POINT('Ctrl Pts',(1.113783877654,-28.3518693792809,124.756546224953));
#125447=CARTESIAN_POINT('Ctrl Pts',(1.11291143080005,-28.3538229125227,
124.743692305856));
#125448=CARTESIAN_POINT('Ctrl Pts',(1.11250340138189,-28.3547649451166,
124.737713425971));
#125449=CARTESIAN_POINT('Ctrl Pts',(1.1115373014639,-28.3570622763596,124.72363227465));
#125450=CARTESIAN_POINT('Ctrl Pts',(1.11097774654946,-28.3584449455696,
124.71553474803));
#125451=CARTESIAN_POINT('Ctrl Pts',(1.10909351746417,-28.3632761068919,
124.688450167068));
#125452=CARTESIAN_POINT('Ctrl Pts',(1.10775530280762,-28.3669944608212,
124.669513645733));
#125453=CARTESIAN_POINT('Ctrl Pts',(1.10442408258247,-28.3769684616018,
124.623006981712));
#125454=CARTESIAN_POINT('Ctrl Pts',(1.10241650351457,-28.3835984609188,
124.595523802243));
#125455=CARTESIAN_POINT('Ctrl Pts',(1.09321883513799,-28.4168663943231,
124.471545948245));
#125456=CARTESIAN_POINT('Ctrl Pts',(1.08585657108412,-28.4514686801848,
124.377403102497));
#125457=CARTESIAN_POINT('Ctrl Pts',(1.07267821986524,-28.5296935240147,
124.212225872802));
#125458=CARTESIAN_POINT('Ctrl Pts',(1.06683129749109,-28.5705896333804,
124.140244848222));
#125459=CARTESIAN_POINT('Ctrl Pts',(1.05983082986308,-28.6275948005129,
124.055307223673));
#125460=CARTESIAN_POINT('Ctrl Pts',(1.05849961776267,-28.6388087058061,
124.039219696898));
#125461=CARTESIAN_POINT('Ctrl Pts',(1.0563828071248,-28.6572371770517,124.013752641196));
#125462=CARTESIAN_POINT('Ctrl Pts',(1.05559042973218,-28.6642718798303,
124.004245887325));
#125463=CARTESIAN_POINT('Ctrl Pts',(1.05408602524642,-28.6778865876812,
123.986250798093));
#125464=CARTESIAN_POINT('Ctrl Pts',(1.05337334657858,-28.6844485772155,
123.977749647777));
#125465=CARTESIAN_POINT('Ctrl Pts',(1.05174056909496,-28.6997385665339,
123.958332336478));
#125466=CARTESIAN_POINT('Ctrl Pts',(1.05082275827726,-28.7085227237348,
123.947461268555));
#125467=CARTESIAN_POINT('Ctrl Pts',(1.04791316454007,-28.736963881813,123.913155362386));
#125468=CARTESIAN_POINT('Ctrl Pts',(1.04594201757812,-28.7571305229629,
123.890149941074));
#125469=CARTESIAN_POINT('Ctrl Pts',(1.04128623296005,-28.806791038723,123.836551306082));
#125470=CARTESIAN_POINT('Ctrl Pts',(1.03862412826436,-28.8368443834861,
123.806505182348));
#125471=CARTESIAN_POINT('Ctrl Pts',(1.03141968890869,-28.9221035442637,
123.727549713869));
#125472=CARTESIAN_POINT('Ctrl Pts',(1.0269450191103,-28.9794581763953,123.681104533079));
#125473=CARTESIAN_POINT('Ctrl Pts',(1.02159391043209,-29.0509345397209,
123.630686394644));
#125474=CARTESIAN_POINT('Ctrl Pts',(1.02075170930233,-29.0622661425251,
123.62290152692));
#125475=CARTESIAN_POINT('Ctrl Pts',(1.01538391823107,-29.1349043791237,
123.574311015818));
#125476=CARTESIAN_POINT('Ctrl Pts',(1.01080591771019,-29.1987563224001,
123.537472962735));
#125477=CARTESIAN_POINT('Ctrl Pts',(1.00519456556864,-29.2758439453853,
123.499565142168));
#125478=CARTESIAN_POINT('Ctrl Pts',(1.004386239616,-29.2869211781704,123.494269172085));
#125479=CARTESIAN_POINT('Ctrl Pts',(1.00310912933111,-29.3043584721581,
123.486168052086));
#125480=CARTESIAN_POINT('Ctrl Pts',(1.00264522114973,-29.3106795340434,
123.4832793294));
#125481=CARTESIAN_POINT('Ctrl Pts',(1.00177256620039,-29.3225411779991,
123.477948027192));
#125482=CARTESIAN_POINT('Ctrl Pts',(1.00136439305603,-29.3280772408143,
123.475495993961));
#125483=CARTESIAN_POINT('Ctrl Pts',(1.00039785463017,-29.3411595433869,
123.469786678887));
#125484=CARTESIAN_POINT('Ctrl Pts',(0.99983800317666,-29.3487166586959,
123.466555003385));
#125485=CARTESIAN_POINT('Ctrl Pts',(0.997952426810626,-29.3741104208787,
123.455917350153));
#125486=CARTESIAN_POINT('Ctrl Pts',(0.996613145986367,-29.3920511455114,
123.448765941039));
#125487=CARTESIAN_POINT('Ctrl Pts',(0.993278795220195,-29.4365758439961,
123.431908805816));
#125488=CARTESIAN_POINT('Ctrl Pts',(0.991269129156873,-29.4632900937476,
123.42256566898));
#125489=CARTESIAN_POINT('Ctrl Pts',(0.982051983685102,-29.5857567736997,
123.383204701323));
#125490=CARTESIAN_POINT('Ctrl Pts',(0.974671958152577,-29.6838636007809,
123.361194721295));
#125491=CARTESIAN_POINT('Ctrl Pts',(0.961505589281053,-29.8649461454338,
123.337445355301));
#125492=CARTESIAN_POINT('Ctrl Pts',(0.955686230085221,-29.9472269253968,
123.332802905299));
#125493=CARTESIAN_POINT('Ctrl Pts',(0.948712331337758,-30.0491190120977,
123.334608947749));
#125494=CARTESIAN_POINT('Ctrl Pts',(0.947381905713893,-30.0687057626552,
123.3353019465));
#125495=CARTESIAN_POINT('Ctrl Pts',(0.945265938121997,-30.1000848423782,
123.336966971324));
#125496=CARTESIAN_POINT('Ctrl Pts',(0.944473630508666,-30.1118864597902,
123.337719258749));
#125497=CARTESIAN_POINT('Ctrl Pts',(0.942969101659076,-30.1343913874589,
123.339394586624));
#125498=CARTESIAN_POINT('Ctrl Pts',(0.942256231412057,-30.1450956842545,
123.340295618014));
#125499=CARTESIAN_POINT('Ctrl Pts',(0.940622645972129,-30.1697145363664,
123.342607904374));
#125500=CARTESIAN_POINT('Ctrl Pts',(0.93970422410551,-30.1836216567743,
123.344090977918));
#125501=CARTESIAN_POINT('Ctrl Pts',(0.936791112539374,-30.2279239332839,
123.349380435329));
#125502=CARTESIAN_POINT('Ctrl Pts',(0.934817125855642,-30.2582345182754,
123.353850131647));
#125503=CARTESIAN_POINT('Ctrl Pts',(0.93015341504093,-30.3303256597539,
123.366521354377));
#125504=CARTESIAN_POINT('Ctrl Pts',(0.927486328497796,-30.371949268577,
123.375493413394));
#125505=CARTESIAN_POINT('Ctrl Pts',(0.920278737169879,-30.4845795175345,
123.404327788921));
#125506=CARTESIAN_POINT('Ctrl Pts',(0.915805607809372,-30.5546833012663,
123.427322692987));
#125507=CARTESIAN_POINT('Ctrl Pts',(0.910429142862871,-30.6361892506851,
123.46018818489));
#125508=CARTESIAN_POINT('Ctrl Pts',(0.90956014969723,-30.649275780915,123.465660356173));
#125509=CARTESIAN_POINT('Ctrl Pts',(0.904197070038578,-30.7293796271543,
123.50036435128));
#125510=CARTESIAN_POINT('Ctrl Pts',(0.899650362145599,-30.7944742737766,
123.533811182113));
#125511=CARTESIAN_POINT('Ctrl Pts',(0.894073740930451,-30.8676800253446,
123.577734879252));
#125512=CARTESIAN_POINT('Ctrl Pts',(0.893265556468678,-30.8781360795331,
123.584166780955));
#125513=CARTESIAN_POINT('Ctrl Pts',(0.891988637072149,-30.8943981323138,
123.594419595873));
#125514=CARTESIAN_POINT('Ctrl Pts',(0.891524776639683,-30.9002531631936,
123.598162445453));
#125515=CARTESIAN_POINT('Ctrl Pts',(0.890652508969474,-30.9111614240045,
123.605232111984));
#125516=CARTESIAN_POINT('Ctrl Pts',(0.890244678105772,-30.9162201671904,
123.608549964018));
#125517=CARTESIAN_POINT('Ctrl Pts',(0.889279174523455,-30.9281003180437,
123.616434610686));
#125518=CARTESIAN_POINT('Ctrl Pts',(0.888720020126513,-30.9349061616793,
123.621024348056));
#125519=CARTESIAN_POINT('Ctrl Pts',(0.886837142423207,-30.9575854608541,
123.63656391755));
#125520=CARTESIAN_POINT('Ctrl Pts',(0.885499886339679,-30.973302015754,
123.647738570888));
#125521=CARTESIAN_POINT('Ctrl Pts',(0.882171254050822,-31.0115522694112,
123.675947208183));
#125522=CARTESIAN_POINT('Ctrl Pts',(0.880165313821002,-31.0338530719746,
123.693286016514));
#125523=CARTESIAN_POINT('Ctrl Pts',(0.870981471847521,-31.1330040430234,
123.774502917571));
#125524=CARTESIAN_POINT('Ctrl Pts',(0.863631545894803,-31.2044528863925,
123.844649433441));
#125525=CARTESIAN_POINT('Ctrl Pts',(0.850443401970882,-31.3229149775003,
123.983962939969));
#125526=CARTESIAN_POINT('Ctrl Pts',(0.844575908090151,-31.3718570945992,
124.051081034038));
#125527=CARTESIAN_POINT('Ctrl Pts',(0.83755618354263,-31.4259408390617,
124.138238280016));
#125528=CARTESIAN_POINT('Ctrl Pts',(0.836224853915574,-31.4359857029084,
124.155082455724));
#125529=CARTESIAN_POINT('Ctrl Pts',(0.834108269421008,-31.4516054958727,
124.182358746707));
#125530=CARTESIAN_POINT('Ctrl Pts',(0.833316225946469,-31.4573705599678,
124.192679247047));
#125531=CARTESIAN_POINT('Ctrl Pts',(0.831812725354296,-31.4681582592602,
124.212483357237));
#125532=CARTESIAN_POINT('Ctrl Pts',(0.831100614285069,-31.4732000424193,
124.221955797481));
#125533=CARTESIAN_POINT('Ctrl Pts',(0.829469537723204,-31.4845890640284,
124.243861025522));
#125534=CARTESIAN_POINT('Ctrl Pts',(0.828552853236997,-31.4908723265472,
124.256326305864));
#125535=CARTESIAN_POINT('Ctrl Pts',(0.825648640970225,-31.5103924311854,
124.296293945706));
#125536=CARTESIAN_POINT('Ctrl Pts',(0.823681664147706,-31.5230309923198,
124.324082630396));
#125537=CARTESIAN_POINT('Ctrl Pts',(0.819037391774664,-31.5513711766943,
124.391232412323));
#125538=CARTESIAN_POINT('Ctrl Pts',(0.816382495195395,-31.566348971826,
124.430876305876));
#125539=CARTESIAN_POINT('Ctrl Pts',(0.809182110492082,-31.6032202771721,
124.540998854901));
#125540=CARTESIAN_POINT('Ctrl Pts',(0.804704794253211,-31.6219694972719,
124.612427257312));
#125541=CARTESIAN_POINT('Ctrl Pts',(0.799406664717733,-31.6383528061114,
124.697475530023));
#125542=CARTESIAN_POINT('Ctrl Pts',(0.798619970096382,-31.6406364258722,
124.710115392251));
#125543=CARTESIAN_POINT('Ctrl Pts',(0.79324355618884,-31.655208323417,124.796466865955));
#125544=CARTESIAN_POINT('Ctrl Pts',(0.788601865667353,-31.6626695510857,
124.870897553711));
#125545=CARTESIAN_POINT('Ctrl Pts',(0.782919828727749,-31.6655116559534,
124.957837732638));
#125546=CARTESIAN_POINT('Ctrl Pts',(0.782111559124968,-31.6657771238166,
124.970112127799));
#125547=CARTESIAN_POINT('Ctrl Pts',(0.780834692681443,-31.6659803445043,
124.989334510083));
#125548=CARTESIAN_POINT('Ctrl Pts',(0.780370976724859,-31.6660103326028,
124.996281366027));
#125549=CARTESIAN_POINT('Ctrl Pts',(0.779498695584072,-31.6659851457551,
125.009280306434));
#125550=CARTESIAN_POINT('Ctrl Pts',(0.779090704107883,-31.6659404400962,
125.015332165912));
#125551=CARTESIAN_POINT('Ctrl Pts',(0.77812475990824,-31.6657573460318,
125.029595915936));
#125552=CARTESIAN_POINT('Ctrl Pts',(0.777565323220713,-31.6655912056346,
125.037807178484));
#125553=CARTESIAN_POINT('Ctrl Pts',(0.775682272090778,-31.6648317718971,
125.065291439682));
#125554=CARTESIAN_POINT('Ctrl Pts',(0.774345141642842,-31.6639646196891,
125.084554515466));
#125555=CARTESIAN_POINT('Ctrl Pts',(0.771017396621862,-31.661004285685,
125.131977159938));
#125556=CARTESIAN_POINT('Ctrl Pts',(0.769012246675701,-31.6585291616439,
125.160106364307));
#125557=CARTESIAN_POINT('Ctrl Pts',(0.7598386688879,-31.6440695458233,125.287316818176));
#125558=CARTESIAN_POINT('Ctrl Pts',(0.752498693421345,-31.6239116732194,
125.385262138454));
#125559=CARTESIAN_POINT('Ctrl Pts',(0.739308387318392,-31.5711277066871,
125.560373342479));
#125560=CARTESIAN_POINT('Ctrl Pts',(0.733429814837493,-31.5412252745476,
125.638035241197));
#125561=CARTESIAN_POINT('Ctrl Pts',(0.726398222103071,-31.4972443070696,
125.730890379078));
#125562=CARTESIAN_POINT('Ctrl Pts',(0.725065600402682,-31.4885291458107,
125.748479993391));
#125563=CARTESIAN_POINT('Ctrl Pts',(0.722946850400739,-31.4740645331745,
125.776421140688));
#125564=CARTESIAN_POINT('Ctrl Pts',(0.72215392902457,-31.4685122957506,
125.786872089606));
#125565=CARTESIAN_POINT('Ctrl Pts',(0.720648669531772,-31.4577079381769,
125.806696337857));
#125566=CARTESIAN_POINT('Ctrl Pts',(0.719935677677714,-31.4524756042906,
125.816079679133));
#125567=CARTESIAN_POINT('Ctrl Pts',(0.718302421703189,-31.4402275747301,
125.837553526235));
#125568=CARTESIAN_POINT('Ctrl Pts',(0.717384443611637,-31.4331496891641,
125.849607770966));
#125569=CARTESIAN_POINT('Ctrl Pts',(0.714475221098579,-31.4101079913955,
125.887742299267));
#125570=CARTESIAN_POINT('Ctrl Pts',(0.712504584526768,-31.3935770285898,
125.913473694485));
#125571=CARTESIAN_POINT('Ctrl Pts',(0.707850376161537,-31.3524215746607,
125.973814520167));
#125572=CARTESIAN_POINT('Ctrl Pts',(0.705189295406144,-31.3271635286492,
126.007966359622));
#125573=CARTESIAN_POINT('Ctrl Pts',(0.697986961690473,-31.2545735091527,
126.098650168494));
#125574=CARTESIAN_POINT('Ctrl Pts',(0.69351329100442,-31.2047525974259,
126.153064797835));
#125575=CARTESIAN_POINT('Ctrl Pts',(0.688176181758693,-31.1417108112333,
126.213357169947));
#125576=CARTESIAN_POINT('Ctrl Pts',(0.687346943166105,-31.1318155697849,
126.222592617736));
#125577=CARTESIAN_POINT('Ctrl Pts',(0.681980447100824,-31.0672212088951,
126.2814236296));
#125578=CARTESIAN_POINT('Ctrl Pts',(0.67739095481364,-31.0093953255646,
126.32745091908));
#125579=CARTESIAN_POINT('Ctrl Pts',(0.671766733598932,-30.9386180658002,
126.376482128867));
#125580=CARTESIAN_POINT('Ctrl Pts',(0.670957959561977,-30.9284427231868,
126.38336582744));
#125581=CARTESIAN_POINT('Ctrl Pts',(0.669680055901379,-30.9123889837533,
126.393969410678));
#125582=CARTESIAN_POINT('Ctrl Pts',(0.669215801605281,-30.9065615944165,
126.397766234651));
#125583=CARTESIAN_POINT('Ctrl Pts',(0.668341930295656,-30.8956059296626,
126.404807047466));
#125584=CARTESIAN_POINT('Ctrl Pts',(0.667932881846171,-30.8904834804768,
126.408059653592));
#125585=CARTESIAN_POINT('Ctrl Pts',(0.666963693731415,-30.878358572475,
126.415665994338));
#125586=CARTESIAN_POINT('Ctrl Pts',(0.666402057257771,-30.8713414233687,
126.419995812023));
#125587=CARTESIAN_POINT('Ctrl Pts',(0.664508599745873,-30.8477054414036,
126.434338849463));
#125588=CARTESIAN_POINT('Ctrl Pts',(0.663163136475742,-30.8309445681685,
126.444113394053));
#125589=CARTESIAN_POINT('Ctrl Pts',(0.659810723061453,-30.7891800108563,
126.467501717418));
#125590=CARTESIAN_POINT('Ctrl Pts',(0.657789050857232,-30.7639911990428,
126.480771300861));
#125591=CARTESIAN_POINT('Ctrl Pts',(0.648459099339785,-30.6472651122729,
126.538492023009));
#125592=CARTESIAN_POINT('Ctrl Pts',(0.640976199854946,-30.5521140381387,
126.575144618829));
#125593=CARTESIAN_POINT('Ctrl Pts',(0.627877965661515,-30.377107912237,
126.624736295201));
#125594=CARTESIAN_POINT('Ctrl Pts',(0.622216793183016,-30.298518942658,
126.64099611059));
#125595=CARTESIAN_POINT('Ctrl Pts',(0.615395908507051,-30.1996963591046,
126.654103584471));
#125596=CARTESIAN_POINT('Ctrl Pts',(0.614070377653021,-30.1802945611189,
126.656330652801));
#125597=CARTESIAN_POINT('Ctrl Pts',(0.611959567323206,-30.1490919619853,
126.65935750035));
#125598=CARTESIAN_POINT('Ctrl Pts',(0.611167605878462,-30.1373145007617,
126.660373592725));
#125599=CARTESIAN_POINT('Ctrl Pts',(0.609662070284355,-30.1147950417186,
126.662075187814));
#125600=CARTESIAN_POINT('Ctrl Pts',(0.608947863634468,-30.1040553139814,
126.662782106122));
#125601=CARTESIAN_POINT('Ctrl Pts',(0.607308812492061,-30.0792826810204,
126.664171752207));
#125602=CARTESIAN_POINT('Ctrl Pts',(0.606386296364463,-30.0652463571903,
126.664781155955));
#125603=CARTESIAN_POINT('Ctrl Pts',(0.603449796313902,-30.0202876973036,
126.66616358998));
#125604=CARTESIAN_POINT('Ctrl Pts',(0.601456958839757,-29.9893498441647,
126.666253122262));
#125605=CARTESIAN_POINT('Ctrl Pts',(0.596740467267545,-29.91532582262,126.664405313624));
#125606=CARTESIAN_POINT('Ctrl Pts',(0.594040149136078,-29.8722818882341,
126.661656775995));
#125607=CARTESIAN_POINT('Ctrl Pts',(0.586842690992665,-29.7567374825711,
126.649761731282));
#125608=CARTESIAN_POINT('Ctrl Pts',(0.582409598552956,-29.6846532524469,
126.637512501222));
#125609=CARTESIAN_POINT('Ctrl Pts',(0.577016503721894,-29.5989042411632,
126.617067284458));
#125610=CARTESIAN_POINT('Ctrl Pts',(0.57609046697172,-29.5842515955794,
126.613362224224));
#125611=CARTESIAN_POINT('Ctrl Pts',(0.57073564931471,-29.5000811012224,
126.590856115885));
#125612=CARTESIAN_POINT('Ctrl Pts',(0.566253917592269,-29.4317983918142,
126.567764785254));
#125613=CARTESIAN_POINT('Ctrl Pts',(0.560749376253956,-29.3538871549404,
126.535657765087));
#125614=CARTESIAN_POINT('Ctrl Pts',(0.559941506354228,-29.3425940732412,
126.53085727805));
#125615=CARTESIAN_POINT('Ctrl Pts',(0.558664979174158,-29.3249915347029,
126.523144066585));
#125616=CARTESIAN_POINT('Ctrl Pts',(0.558201191772277,-29.3186452603866,
126.520315753464));
#125617=CARTESIAN_POINT('Ctrl Pts',(0.557371237326707,-29.3073798688148,
126.515210459083));
#125618=CARTESIAN_POINT('Ctrl Pts',(0.557006016579308,-29.3024539109558,
126.512949051439));
#125619=CARTESIAN_POINT('Ctrl Pts',(0.556112861077067,-29.2904830992487,
126.507382605615));
#125620=CARTESIAN_POINT('Ctrl Pts',(0.555583409303405,-29.2834503656735,
126.504052248961));
#125621=CARTESIAN_POINT('Ctrl Pts',(0.553889414205153,-29.2611416352582,
126.493295957914));
#125622=CARTESIAN_POINT('Ctrl Pts',(0.552714543876437,-29.2459563083808,
126.48568588749));
#125623=CARTESIAN_POINT('Ctrl Pts',(0.549867229395235,-29.2097762194701,
126.466856825882));
#125624=CARTESIAN_POINT('Ctrl Pts',(0.548184721456098,-29.1889006988942,
126.455417595061));
#125625=CARTESIAN_POINT('Ctrl Pts',(0.541418110010879,-29.1066827715153,
126.408046121392));
#125626=CARTESIAN_POINT('Ctrl Pts',(0.536227226792752,-29.0474244857738,
126.368652093163));
#125627=CARTESIAN_POINT('Ctrl Pts',(0.522908139521502,-28.9018945116724,
126.25786478686));
#125628=CARTESIAN_POINT('Ctrl Pts',(0.514852835373573,-28.8199534865787,
126.181337311866));
#125629=CARTESIAN_POINT('Ctrl Pts',(0.50562515322859,-28.7317650209868,
126.080565815076));
#125630=CARTESIAN_POINT('Ctrl Pts',(0.50411863058937,-28.7175706042957,
126.063681046568));
#125631=CARTESIAN_POINT('Ctrl Pts',(0.501705802567479,-28.6951776569899,
126.03594370981));
#125632=CARTESIAN_POINT('Ctrl Pts',(0.500791146072882,-28.6867697784389,
126.025264415164));
#125633=CARTESIAN_POINT('Ctrl Pts',(0.499169624106025,-28.6720131077862,
126.006041780287));
#125634=CARTESIAN_POINT('Ctrl Pts',(0.498460781459573,-28.6656138156697,
125.99753835501));
#125635=CARTESIAN_POINT('Ctrl Pts',(0.496964633333417,-28.6522195341151,
125.979380382936));
#125636=CARTESIAN_POINT('Ctrl Pts',(0.496178181967775,-28.6452457840825,
125.969710856716));
#125637=CARTESIAN_POINT('Ctrl Pts',(0.494065897637493,-28.626703196969,
125.943409927396));
#125638=CARTESIAN_POINT('Ctrl Pts',(0.492747645016592,-28.6153327033637,
125.92664067257));
#125639=CARTESIAN_POINT('Ctrl Pts',(0.489846980583185,-28.5907944208838,
125.888990869792));
#125640=CARTESIAN_POINT('Ctrl Pts',(0.488270089392217,-28.5777790046832,
125.868016511898));
#125641=CARTESIAN_POINT('Ctrl Pts',(0.483300356898985,-28.5378949550602,
125.800436216336));
#125642=CARTESIAN_POINT('Ctrl Pts',(0.479963094649077,-28.5128140745072,
125.752813366189));
#125643=CARTESIAN_POINT('Ctrl Pts',(0.473803282860917,-28.4704539722927,
125.661968035598));
#125644=CARTESIAN_POINT('Ctrl Pts',(0.470975555099976,-28.4525988551096,
125.619081106435));
#125645=CARTESIAN_POINT('Ctrl Pts',(0.468139978699828,-28.4365599867671,
125.575509622007));
#125646=CARTESIAN_POINT('Origin',(5.,-30.,55.));
#125647=CARTESIAN_POINT('',(1.32021575923829,-28.3340002652327,55.0009400825958));
#125648=CARTESIAN_POINT('Ctrl Pts',(0.659214745210768,-28.4365623102018,
55.5755159338528));
#125649=CARTESIAN_POINT('Ctrl Pts',(0.659963641292018,-28.4405139534956,
55.5862509069418));
#125650=CARTESIAN_POINT('Ctrl Pts',(0.660718112395066,-28.4445759197288,
55.5969445264719));
#125651=CARTESIAN_POINT('Ctrl Pts',(0.661924434192335,-28.4511909595541,
55.6138333999505));
#125652=CARTESIAN_POINT('Ctrl Pts',(0.662372155669629,-28.4536719329351,
55.6200567649136));
#125653=CARTESIAN_POINT('Ctrl Pts',(0.663233890173186,-28.4584945714238,
55.6319450832073));
#125654=CARTESIAN_POINT('Ctrl Pts',(0.663647543837139,-28.4608300603191,
55.6376123165684));
#125655=CARTESIAN_POINT('Ctrl Pts',(0.664654545452568,-28.4665660606024,
55.6513159771192));
#125656=CARTESIAN_POINT('Ctrl Pts',(0.665249751707099,-28.4699985149372,
55.6593387565258));
#125657=CARTESIAN_POINT('Ctrl Pts',(0.667395281146444,-28.4825267915646,
55.687996809844));
#125658=CARTESIAN_POINT('Ctrl Pts',(0.668964512435956,-28.4919779215533,
55.7084728909968));
#125659=CARTESIAN_POINT('Ctrl Pts',(0.680707788462809,-28.5650020372384,
55.8585954186811));
#125660=CARTESIAN_POINT('Ctrl Pts',(0.691446198038116,-28.6447740481354,
55.9796792143553));
#125661=CARTESIAN_POINT('Ctrl Pts',(0.706348215234274,-28.7811489998703,
56.1375782492685));
#125662=CARTESIAN_POINT('Ctrl Pts',(0.710851108539443,-28.825915457073,
56.1837268875902));
#125663=CARTESIAN_POINT('Ctrl Pts',(0.716511229173992,-28.8869357299301,
56.2397538400991));
#125664=CARTESIAN_POINT('Ctrl Pts',(0.717771910094331,-28.9008404423981,
56.2520982265341));
#125665=CARTESIAN_POINT('Ctrl Pts',(0.719804332451236,-28.9237619754479,
56.2717714362838));
#125666=CARTESIAN_POINT('Ctrl Pts',(0.720581913525034,-28.9326536036333,
56.2792429611344));
#125667=CARTESIAN_POINT('Ctrl Pts',(0.722076094015,-28.9499727184326,56.2934897010616));
#125668=CARTESIAN_POINT('Ctrl Pts',(0.72279316063993,-28.9583894354873,
56.3002770243558));
#125669=CARTESIAN_POINT('Ctrl Pts',(0.724462268379914,-28.9782232838014,
56.3159550573192));
#125670=CARTESIAN_POINT('Ctrl Pts',(0.72541167226813,-28.9896914662681,
56.3247800040469));
#125671=CARTESIAN_POINT('Ctrl Pts',(0.728540249029682,-29.0280848532284,
56.3535357580327));
#125672=CARTESIAN_POINT('Ctrl Pts',(0.730694011293115,-29.0554970934145,
56.3728046485986));
#125673=CARTESIAN_POINT('Ctrl Pts',(0.735884881361671,-29.1237397587507,
56.4177619905098));
#125674=CARTESIAN_POINT('Ctrl Pts',(0.738891364809314,-29.1651407596486,
56.442529593517));
#125675=CARTESIAN_POINT('Ctrl Pts',(0.745995233323475,-29.266404573629,
56.4972871703079));
#125676=CARTESIAN_POINT('Ctrl Pts',(0.750056334966432,-29.3271119036571,
56.5255336385376));
#125677=CARTESIAN_POINT('Ctrl Pts',(0.758912614853314,-29.4616954151474,
56.5785530440077));
#125678=CARTESIAN_POINT('Ctrl Pts',(0.763709136771604,-29.5359354234534,
56.6019496767449));
#125679=CARTESIAN_POINT('Ctrl Pts',(0.76980726565648,-29.6274488471113,
56.6238933788813));
#125680=CARTESIAN_POINT('Ctrl Pts',(0.770878651015154,-29.6434249755122,
56.6274760429261));
#125681=CARTESIAN_POINT('Ctrl Pts',(0.772472415436527,-29.6669900525349,
56.6323969178816));
#125682=CARTESIAN_POINT('Ctrl Pts',(0.772985068171922,-29.6745401826819,
56.6339189772137));
#125683=CARTESIAN_POINT('Ctrl Pts',(0.773902973631897,-29.6879993405186,
56.6365352733002));
#125684=CARTESIAN_POINT('Ctrl Pts',(0.774307074264652,-29.6939041239484,
56.637649970112));
#125685=CARTESIAN_POINT('Ctrl Pts',(0.775206840638491,-29.707005271969,
56.6400498545001));
#125686=CARTESIAN_POINT('Ctrl Pts',(0.775703315393402,-29.7142040375561,
56.6413196211194));
#125687=CARTESIAN_POINT('Ctrl Pts',(0.777182043165073,-29.7355629128225,
56.6449422701476));
#125688=CARTESIAN_POINT('Ctrl Pts',(0.778171275327273,-29.7497449188664,
56.6471594959333));
#125689=CARTESIAN_POINT('Ctrl Pts',(0.780489834331059,-29.7827778964682,
56.6518874618695));
#125690=CARTESIAN_POINT('Ctrl Pts',(0.781825070041427,-29.8016465136671,
56.6542591869629));
#125691=CARTESIAN_POINT('Ctrl Pts',(0.786599363794931,-29.8686989762837,
56.6615238516719));
#125692=CARTESIAN_POINT('Ctrl Pts',(0.790094904868642,-29.9170489575495,
56.6646381026969));
#125693=CARTESIAN_POINT('Ctrl Pts',(0.801966995933811,-30.0805207792727,
56.6680277218472));
#125694=CARTESIAN_POINT('Ctrl Pts',(0.810382446848105,-30.1955326990349,
56.6584852228168));
#125695=CARTESIAN_POINT('Ctrl Pts',(0.821478443120727,-30.3506519603713,
56.6292409537629));
#125696=CARTESIAN_POINT('Ctrl Pts',(0.824438057573833,-30.3923367446291,
56.619708408388));
#125697=CARTESIAN_POINT('Ctrl Pts',(0.828455890430732,-30.4493380675934,
56.6043430359028));
#125698=CARTESIAN_POINT('Ctrl Pts',(0.829556926894114,-30.4650014798904,
56.5998734113248));
#125699=CARTESIAN_POINT('Ctrl Pts',(0.831323450748539,-30.4901936579209,
56.5922834629587));
#125700=CARTESIAN_POINT('Ctrl Pts',(0.831993518833882,-30.4997638833363,
56.5893056714085));
#125701=CARTESIAN_POINT('Ctrl Pts',(0.833388042719641,-30.5197080667199,
56.5829020386295));
#125702=CARTESIAN_POINT('Ctrl Pts',(0.83411193475826,-30.530076401145,56.5794601473679));
#125703=CARTESIAN_POINT('Ctrl Pts',(0.835832785829586,-30.5547549817536,
56.5709974143047));
#125704=CARTESIAN_POINT('Ctrl Pts',(0.836826598044922,-30.5690321616613,
56.5658826231637));
#125705=CARTESIAN_POINT('Ctrl Pts',(0.840289916299863,-30.6188452550762,
56.5472658228053));
#125706=CARTESIAN_POINT('Ctrl Pts',(0.842725610946042,-30.6539886139836,
56.5327427099798));
#125707=CARTESIAN_POINT('Ctrl Pts',(0.848791916699208,-30.7413466796475,
56.4930893241426));
#125708=CARTESIAN_POINT('Ctrl Pts',(0.852375246155066,-30.792805214712,
56.466414422777));
#125709=CARTESIAN_POINT('Ctrl Pts',(0.862651125810953,-30.9373096076258,
56.3816720105806));
#125710=CARTESIAN_POINT('Ctrl Pts',(0.869228930686582,-31.0261365411004,
56.3170445643393));
#125711=CARTESIAN_POINT('Ctrl Pts',(0.878097227136037,-31.1305267278775,
56.2240824572584));
#125712=CARTESIAN_POINT('Ctrl Pts',(0.88004155115911,-31.1525341799814,
56.2033840792647));
#125713=CARTESIAN_POINT('Ctrl Pts',(0.88268437638759,-31.18107055971,56.1750440895643));
#125714=CARTESIAN_POINT('Ctrl Pts',(0.883346812629502,-31.1881119242406,
56.1679239370166));
#125715=CARTESIAN_POINT('Ctrl Pts',(0.884397523809826,-31.199097091447,
56.1566137076135));
#125716=CARTESIAN_POINT('Ctrl Pts',(0.884782538026635,-31.2030842410492,
56.1524657954881));
#125717=CARTESIAN_POINT('Ctrl Pts',(0.885585877276413,-31.211322322205,
56.143806214921));
#125718=CARTESIAN_POINT('Ctrl Pts',(0.886004481639483,-31.2155696457618,
56.1392913836904));
#125719=CARTESIAN_POINT('Ctrl Pts',(0.887042618707048,-31.2259936761341,
56.1280861758301));
#125720=CARTESIAN_POINT('Ctrl Pts',(0.887664288533123,-31.2321408607672,
56.121368718919));
#125721=CARTESIAN_POINT('Ctrl Pts',(0.890024387995303,-31.2551327325838,
56.0958265989553));
#125722=CARTESIAN_POINT('Ctrl Pts',(0.891786831028371,-31.2716026938486,
56.0766710422131));
#125723=CARTESIAN_POINT('Ctrl Pts',(0.896496804446941,-31.3139498103398,
56.0250914029554));
#125724=CARTESIAN_POINT('Ctrl Pts',(0.899476732144382,-31.3390618911845,
55.9920631579025));
#125725=CARTESIAN_POINT('Ctrl Pts',(0.911742955187062,-31.436512417141,
55.8534431135917));
#125726=CARTESIAN_POINT('Ctrl Pts',(0.921138969129262,-31.4978151011057,
55.7406019954244));
#125727=CARTESIAN_POINT('Ctrl Pts',(0.932994445367097,-31.5608703064797,
55.5838791540793));
#125728=CARTESIAN_POINT('Ctrl Pts',(0.935824974923883,-31.574743222478,
55.545357921975));
#125729=CARTESIAN_POINT('Ctrl Pts',(0.939699465085544,-31.5920548005865,
55.4910950090183));
#125730=CARTESIAN_POINT('Ctrl Pts',(0.940782341143438,-31.5967049905873,
55.4757583421885));
#125731=CARTESIAN_POINT('Ctrl Pts',(0.942527586162851,-31.6038897272558,
55.4507696182194));
#125732=CARTESIAN_POINT('Ctrl Pts',(0.943194326698031,-31.6065600285174,
55.4411580081438));
#125733=CARTESIAN_POINT('Ctrl Pts',(0.944587994716938,-31.6119836600457,
55.4209333448612));
#125734=CARTESIAN_POINT('Ctrl Pts',(0.945314307638591,-31.61471888452,55.4103158963638));
#125735=CARTESIAN_POINT('Ctrl Pts',(0.947052218707638,-31.6210414861569,
55.3847302801767));
#125736=CARTESIAN_POINT('Ctrl Pts',(0.948060499974413,-31.6245266806757,
55.3697377154156));
#125737=CARTESIAN_POINT('Ctrl Pts',(0.951640215251125,-31.6362344790149,
55.3160075949944));
#125738=CARTESIAN_POINT('Ctrl Pts',(0.954174604394025,-31.6432835844108,
55.2770262066794));
#125739=CARTESIAN_POINT('Ctrl Pts',(0.960564404724356,-31.6577309517901,
55.1768580372996));
#125740=CARTESIAN_POINT('Ctrl Pts',(0.964365223745703,-31.6631368409799,
55.1154441197577));
#125741=CARTESIAN_POINT('Ctrl Pts',(0.973680422779509,-31.6680548877707,
54.9634230593059));
#125742=CARTESIAN_POINT('Ctrl Pts',(0.979143253785267,-31.6636067451724,
54.8728950791873));
#125743=CARTESIAN_POINT('Ctrl Pts',(0.987402570717024,-31.6464623037035,
54.7422797707631));
#125744=CARTESIAN_POINT('Ctrl Pts',(0.990031037836238,-31.6395765784195,
54.7015944670879));
#125745=CARTESIAN_POINT('Ctrl Pts',(0.993462558443658,-31.6289264133717,
54.6503165183594));
#125746=CARTESIAN_POINT('Ctrl Pts',(0.994196884827876,-31.6265547956662,
54.6394458741157));
#125747=CARTESIAN_POINT('Ctrl Pts',(0.995378206655547,-31.6225968145929,
54.6221382295046));
#125748=CARTESIAN_POINT('Ctrl Pts',(0.995821359168282,-31.6210805523774,
54.6156853122823));
#125749=CARTESIAN_POINT('Ctrl Pts',(0.996681022140957,-31.6180797379266,
54.6032482193401));
#125750=CARTESIAN_POINT('Ctrl Pts',(0.997097241816606,-31.6166004158405,
54.5972629838045));
#125751=CARTESIAN_POINT('Ctrl Pts',(0.998120537342818,-31.6128983525958,
54.582633777008));
#125752=CARTESIAN_POINT('Ctrl Pts',(0.998729616657382,-31.61063932153,54.5739992642144));
#125753=CARTESIAN_POINT('Ctrl Pts',(1.00098522511608,-31.6020664926277,
54.5422752550403));
#125754=CARTESIAN_POINT('Ctrl Pts',(1.0026532021352,-31.5953249728398,54.5193056316508));
#125755=CARTESIAN_POINT('Ctrl Pts',(1.00704012273649,-31.5765093364595,
54.4599602500243));
#125756=CARTESIAN_POINT('Ctrl Pts',(1.00978669059544,-31.5636709241073,
54.4238424729003));
#125757=CARTESIAN_POINT('Ctrl Pts',(1.0175652224386,-31.5241375833952,54.3237100179675));
#125758=CARTESIAN_POINT('Ctrl Pts',(1.0226375406149,-31.4946744638198,54.2608709199988));
#125759=CARTESIAN_POINT('Ctrl Pts',(1.03464843330274,-31.4150800113469,
54.1154644229076));
#125760=CARTESIAN_POINT('Ctrl Pts',(1.04151112617786,-31.361515594002,54.0350463214709));
#125761=CARTESIAN_POINT('Ctrl Pts',(1.04947794848679,-31.2888556764999,
53.9441575882492));
#125762=CARTESIAN_POINT('Ctrl Pts',(1.05082968622706,-31.2761492812382,
53.9288346416686));
#125763=CARTESIAN_POINT('Ctrl Pts',(1.05297120198867,-31.2554182870267,
53.9047272940103));
#125764=CARTESIAN_POINT('Ctrl Pts',(1.05376803998593,-31.2475692633859,
53.8957951631918));
#125765=CARTESIAN_POINT('Ctrl Pts',(1.0552761313253,-31.2324591194727,53.878966742388));
#125766=CARTESIAN_POINT('Ctrl Pts',(1.05598808668145,-31.2252160867848,
53.8710550962479));
#125767=CARTESIAN_POINT('Ctrl Pts',(1.05761255005021,-31.2084409905437,
53.8530830806558));
#125768=CARTESIAN_POINT('Ctrl Pts',(1.05852285411219,-31.1988587122944,
53.843070505736));
#125769=CARTESIAN_POINT('Ctrl Pts',(1.06138128369846,-31.1682056598785,
53.8118308114439));
#125770=CARTESIAN_POINT('Ctrl Pts',(1.06330981930706,-31.1466869563556,
53.7910501726467));
#125771=CARTESIAN_POINT('Ctrl Pts',(1.07043446628666,-31.0642544911494,
53.715627459757));
#125772=CARTESIAN_POINT('Ctrl Pts',(1.07547632256952,-30.9999001979576,
53.6649150074561));
#125773=CARTESIAN_POINT('Ctrl Pts',(1.08666462366743,-30.8482724542223,
53.5625674788946));
#125774=CARTESIAN_POINT('Ctrl Pts',(1.09276640156089,-30.75950366134,53.5137534967374));
#125775=CARTESIAN_POINT('Ctrl Pts',(1.10093007852872,-30.6420524393445,
53.4624506456449));
#125776=CARTESIAN_POINT('Ctrl Pts',(1.10267860066395,-30.6169771469631,
53.4522182471399));
#125777=CARTESIAN_POINT('Ctrl Pts',(1.1050926392708,-30.5826737458718,53.439186165975));
#125778=CARTESIAN_POINT('Ctrl Pts',(1.10572949521159,-30.5736529521352,
53.4358482176635));
#125779=CARTESIAN_POINT('Ctrl Pts',(1.10674944642822,-30.5592623409872,
53.4306645132565));
#125780=CARTESIAN_POINT('Ctrl Pts',(1.10712960461376,-30.5539109522798,
53.4287677159289));
#125781=CARTESIAN_POINT('Ctrl Pts',(1.10793302524484,-30.542630143941,53.4248340297426));
#125782=CARTESIAN_POINT('Ctrl Pts',(1.10835665129977,-30.5366987801322,
53.4228032076037));
#125783=CARTESIAN_POINT('Ctrl Pts',(1.10942431157411,-30.5217884717841,
53.4177919554728));
#125784=CARTESIAN_POINT('Ctrl Pts',(1.11007074770082,-30.5127954371229,
53.414854475276));
#125785=CARTESIAN_POINT('Ctrl Pts',(1.11264930593903,-30.4770414154817,
53.4035118904902));
#125786=CARTESIAN_POINT('Ctrl Pts',(1.11461127806468,-30.4500965777982,
53.3957071202711));
#125787=CARTESIAN_POINT('Ctrl Pts',(1.12003804526655,-30.3759520788193,
53.3762454035932));
#125788=CARTESIAN_POINT('Ctrl Pts',(1.12354701370819,-30.3284197424937,
53.3659685303982));
#125789=CARTESIAN_POINT('Ctrl Pts',(1.13547970136026,-30.1664360243814,
53.3382998293558));
#125790=CARTESIAN_POINT('Ctrl Pts',(1.14394117757766,-30.0506264895923,
53.3307511443493));
#125791=CARTESIAN_POINT('Ctrl Pts',(1.15502814538573,-29.8929283312015,
53.3369121636872));
#125792=CARTESIAN_POINT('Ctrl Pts',(1.15793962131046,-29.850969421449,53.3401458132592));
#125793=CARTESIAN_POINT('Ctrl Pts',(1.16190413889962,-29.7930899355848,
53.346819314464));
#125794=CARTESIAN_POINT('Ctrl Pts',(1.16299852222704,-29.777032751387,53.3489083029754));
#125795=CARTESIAN_POINT('Ctrl Pts',(1.16475725076074,-29.7511064147828,
53.3526663707886));
#125796=CARTESIAN_POINT('Ctrl Pts',(1.16542609961355,-29.741217711071,53.3541908260158));
#125797=CARTESIAN_POINT('Ctrl Pts',(1.16682028678175,-29.7205480095359,
53.357568195804));
#125798=CARTESIAN_POINT('Ctrl Pts',(1.16754504294498,-29.7097702888344,
53.3594383977234));
#125799=CARTESIAN_POINT('Ctrl Pts',(1.16927200883321,-29.6840165445165,
53.3641690513153));
#125800=CARTESIAN_POINT('Ctrl Pts',(1.17027101109583,-29.6690596652992,
53.3671292283001));
#125801=CARTESIAN_POINT('Ctrl Pts',(1.17377560962581,-29.6164110960138,
53.3783022677858));
#125802=CARTESIAN_POINT('Ctrl Pts',(1.1762462678384,-29.5789645509273,53.3876186887177));
#125803=CARTESIAN_POINT('Ctrl Pts',(1.18242614099913,-29.4849493492021,
53.4145082238645));
#125804=CARTESIAN_POINT('Ctrl Pts',(1.18608558387259,-29.4289313316328,
53.4338126901721));
#125805=CARTESIAN_POINT('Ctrl Pts',(1.19655994573354,-29.2705929944841,
53.4980060801958));
#125806=CARTESIAN_POINT('Ctrl Pts',(1.20326065921172,-29.1716182010739,
53.5502417494761));
#125807=CARTESIAN_POINT('Ctrl Pts',(1.21208881541147,-29.0561632499323,
53.6268813743853));
#125808=CARTESIAN_POINT('Ctrl Pts',(1.21382945801558,-29.0340723299868,
53.6423306323007));
#125809=CARTESIAN_POINT('Ctrl Pts',(1.21623422885395,-29.0046349399247,
53.6639997806444));
#125810=CARTESIAN_POINT('Ctrl Pts',(1.21686997369886,-28.9969520651439,
53.6697582857092));
#125811=CARTESIAN_POINT('Ctrl Pts',(1.21788857533824,-28.9848088374216,
53.6790249436114));
#125812=CARTESIAN_POINT('Ctrl Pts',(1.21826850845923,-28.9803157540354,
53.6824901395899));
#125813=CARTESIAN_POINT('Ctrl Pts',(1.21905930458946,-28.9710411111115,
53.6897188727172));
#125814=CARTESIAN_POINT('Ctrl Pts',(1.21947041646921,-28.9662623424226,
53.6934857525445));
#125815=CARTESIAN_POINT('Ctrl Pts',(1.22045299713856,-28.9549398472241,
53.7025117508851));
#125816=CARTESIAN_POINT('Ctrl Pts',(1.2210260689708,-28.9484150728044,53.7077942838033));
#125817=CARTESIAN_POINT('Ctrl Pts',(1.2223077814754,-28.9339903933139,53.7196542701509));
#125818=CARTESIAN_POINT('Ctrl Pts',(1.22301794647307,-28.9261109354356,
53.7262559385422));
#125819=CARTESIAN_POINT('Ctrl Pts',(1.22506093262138,-28.9037508370259,
53.7453449124877));
#125820=CARTESIAN_POINT('Ctrl Pts',(1.22640372360606,-28.8894238278728,
53.7580088103662));
#125821=CARTESIAN_POINT('Ctrl Pts',(1.23121688973683,-28.8392705232512,
53.8039019162475));
#125822=CARTESIAN_POINT('Ctrl Pts',(1.23474462079593,-28.804693204456,53.8384559331168));
#125823=CARTESIAN_POINT('Ctrl Pts',(1.24676234642063,-28.6928931196582,
53.9604663629038));
#125824=CARTESIAN_POINT('Ctrl Pts',(1.25528841883712,-28.6233358799653,
54.0545048294473));
#125825=CARTESIAN_POINT('Ctrl Pts',(1.26636223392244,-28.5433199730105,
54.1904758995821));
#125826=CARTESIAN_POINT('Ctrl Pts',(1.26920574386274,-28.523787467326,54.226667578192));
#125827=CARTESIAN_POINT('Ctrl Pts',(1.27309474604692,-28.4985164994813,
54.2779466913659));
#125828=CARTESIAN_POINT('Ctrl Pts',(1.27417953476662,-28.4916287921005,
54.292447872342));
#125829=CARTESIAN_POINT('Ctrl Pts',(1.27592705245948,-28.4808001858974,
54.3161231551476));
#125830=CARTESIAN_POINT('Ctrl Pts',(1.27659417429594,-28.4767304062588,
54.3252368071961));
#125831=CARTESIAN_POINT('Ctrl Pts',(1.27798801302688,-28.4683637848074,
54.3444341142369));
#125832=CARTESIAN_POINT('Ctrl Pts',(1.27871412054514,-28.464084044836,54.3545247373503));
#125833=CARTESIAN_POINT('Ctrl Pts',(1.28045036987591,-28.4540431656761,
54.3788642176465));
#125834=CARTESIAN_POINT('Ctrl Pts',(1.28145721243702,-28.448378938272,54.3931521603375));
#125835=CARTESIAN_POINT('Ctrl Pts',(1.2850248863174,-28.4288891562718,54.444372662124));
#125836=CARTESIAN_POINT('Ctrl Pts',(1.28754901973547,-28.4161774351021,
54.4817167879635));
#125837=CARTESIAN_POINT('Ctrl Pts',(1.2939047253306,-28.3871475977008,54.5780879430202));
#125838=CARTESIAN_POINT('Ctrl Pts',(1.29768251325451,-28.3727354337739,
54.6376279524458));
#125839=CARTESIAN_POINT('Ctrl Pts',(1.30766056230485,-28.3431899516063,
54.7978233223371));
#125840=CARTESIAN_POINT('Ctrl Pts',(1.31378284441053,-28.3339429029157,
54.8992834777778));
#125841=CARTESIAN_POINT('Ctrl Pts',(1.32021575923829,-28.3340002652327,
55.0009400825958));
#125842=CARTESIAN_POINT('Ctrl Pts',(1.32021590954351,-28.3340002665747,
55.000942457804));
#125843=CARTESIAN_POINT('Ctrl Pts',(1.32220985562038,-28.3340180915062,
55.0324519122196));
#125844=CARTESIAN_POINT('Ctrl Pts',(1.32423293252513,-28.3349298320778,
55.0639526592521));
#125845=CARTESIAN_POINT('Ctrl Pts',(1.32682074830839,-28.3371891639739,
55.1033405957195));
#125846=CARTESIAN_POINT('Ctrl Pts',(1.32734474700025,-28.3377010174839,
55.1112710289715));
#125847=CARTESIAN_POINT('Ctrl Pts',(1.32826699345549,-28.3386960641558,
55.1251429808795));
#125848=CARTESIAN_POINT('Ctrl Pts',(1.32866393842213,-28.3391544514235,
55.1310862081801));
#125849=CARTESIAN_POINT('Ctrl Pts',(1.32945875925557,-28.3401317993643,
55.1429287499632));
#125850=CARTESIAN_POINT('Ctrl Pts',(1.3298566093499,-28.340650325113,55.1488278403667));
#125851=CARTESIAN_POINT('Ctrl Pts',(1.33072929281893,-28.3418512531499,
55.1617030012841));
#125852=CARTESIAN_POINT('Ctrl Pts',(1.331204774772,-28.3425462185789,55.1686774592109));
#125853=CARTESIAN_POINT('Ctrl Pts',(1.3325374877822,-28.3446074371047,55.1881189991655));
#125854=CARTESIAN_POINT('Ctrl Pts',(1.33339972061422,-28.3460704603213,
55.2005750468619));
#125855=CARTESIAN_POINT('Ctrl Pts',(1.33796728344874,-28.3545024450872,
55.2659813549176));
#125856=CARTESIAN_POINT('Ctrl Pts',(1.34177814116433,-28.363873396488,55.3185857505541));
#125857=CARTESIAN_POINT('Ctrl Pts',(1.35078342266844,-28.391618412814,55.4401709101938));
#125858=CARTESIAN_POINT('Ctrl Pts',(1.35600155264901,-28.4119305928387,
55.5086017904495));
#125859=CARTESIAN_POINT('Ctrl Pts',(1.36116732170967,-28.4365623080758,
55.5755159280775));
#125860=CARTESIAN_POINT('Ctrl Pts',(1.16624546596859,-28.4365623102019,
55.575515933853));
#125861=CARTESIAN_POINT('Ctrl Pts',(1.16623406145781,-28.4365032961389,
55.5753556171617));
#125862=CARTESIAN_POINT('Ctrl Pts',(1.16622265776398,-28.4364443066904,
55.5751952912736));
#125863=CARTESIAN_POINT('Ctrl Pts',(1.16549980768447,-28.4327064137748,
55.5650313454292));
#125864=CARTESIAN_POINT('Ctrl Pts',(1.16479157876853,-28.4291235001549,
55.5549924666191));
#125865=CARTESIAN_POINT('Ctrl Pts',(1.16321390103826,-28.4213222899542,
55.5324534831877));
#125866=CARTESIAN_POINT('Ctrl Pts',(1.16234619052926,-28.4171555947951,
55.5199361783316));
#125867=CARTESIAN_POINT('Ctrl Pts',(1.16013833760378,-28.406876906967,55.4877883429162));
#125868=CARTESIAN_POINT('Ctrl Pts',(1.15880514823918,-28.4009786949724,
55.4680914253662));
#125869=CARTESIAN_POINT('Ctrl Pts',(1.14770621329044,-28.3545505755323,
55.3019122474401));
#125870=CARTESIAN_POINT('Ctrl Pts',(1.13864993213321,-28.3338772243859,
55.1506356236224));
#125871=CARTESIAN_POINT('Ctrl Pts',(1.12530416485984,-28.334052803967,54.9342472504104));
#125872=CARTESIAN_POINT('Ctrl Pts',(1.12127417411137,-28.3378392579978,
54.869910826422));
#125873=CARTESIAN_POINT('Ctrl Pts',(1.11627530334294,-28.3467489465006,
54.7939328377005));
#125874=CARTESIAN_POINT('Ctrl Pts',(1.11547762566429,-28.3482908250023,
54.7819185896074));
#125875=CARTESIAN_POINT('Ctrl Pts',(1.11421381289345,-28.3509180014544,
54.7630773733838));
#125876=CARTESIAN_POINT('Ctrl Pts',(1.11375239404336,-28.351915058325,54.756238252291));
#125877=CARTESIAN_POINT('Ctrl Pts',(1.11288183398201,-28.3538662063784,
54.7434142206414));
#125878=CARTESIAN_POINT('Ctrl Pts',(1.11247323670157,-28.3548104370481,
54.737428055846));
#125879=CARTESIAN_POINT('Ctrl Pts',(1.1115021446493,-28.3571218253109,54.72327659247));
#125880=CARTESIAN_POINT('Ctrl Pts',(1.11093811813268,-28.3585172123379,
54.7151161785498));
#125881=CARTESIAN_POINT('Ctrl Pts',(1.10902222587865,-28.3634365821474,
54.6875838185676));
#125882=CARTESIAN_POINT('Ctrl Pts',(1.10765621507157,-28.3672430045154,
54.668264863394));
#125883=CARTESIAN_POINT('Ctrl Pts',(1.104239881799,-28.3775137553063,54.6206069001332));
#125884=CARTESIAN_POINT('Ctrl Pts',(1.10217408030968,-28.3843789473843,
54.5923614838859));
#125885=CARTESIAN_POINT('Ctrl Pts',(1.09432056936455,-28.4130189305222,
54.4866581517853));
#125886=CARTESIAN_POINT('Ctrl Pts',(1.0884267795435,-28.4396557592631,54.4106323466519));
#125887=CARTESIAN_POINT('Ctrl Pts',(1.07530638859385,-28.5116588000358,
54.2446965534111));
#125888=CARTESIAN_POINT('Ctrl Pts',(1.06814665844362,-28.5598923465102,
54.156353663732));
#125889=CARTESIAN_POINT('Ctrl Pts',(1.05990691753729,-28.6268670473983,
54.0563595152035));
#125890=CARTESIAN_POINT('Ctrl Pts',(1.05855636733932,-28.6382290561309,
54.0400357163173));
#125891=CARTESIAN_POINT('Ctrl Pts',(1.05641644138395,-28.6568437020813,
54.0142878770965));
#125892=CARTESIAN_POINT('Ctrl Pts',(1.05562002030217,-28.6639093480471,
54.0047316882814));
#125893=CARTESIAN_POINT('Ctrl Pts',(1.05411255135894,-28.6775436475373,
53.9866983789375));
#125894=CARTESIAN_POINT('Ctrl Pts',(1.0534008036682,-28.6840930426992,53.9782075218927));
#125895=CARTESIAN_POINT('Ctrl Pts',(1.05177659261749,-28.6992932435353,
53.9588900335077));
#125896=CARTESIAN_POINT('Ctrl Pts',(1.05086633451863,-28.7079981432164,
53.948106825792));
#125897=CARTESIAN_POINT('Ctrl Pts',(1.04800720552964,-28.7359192230794,
53.9143891314306));
#125898=CARTESIAN_POINT('Ctrl Pts',(1.04607794402249,-28.7556198149369,
53.8918622376811));
#125899=CARTESIAN_POINT('Ctrl Pts',(1.03901442524823,-28.8307620313791,
53.8104726236096));
#125900=CARTESIAN_POINT('Ctrl Pts',(1.03403000485387,-28.8898606397321,
53.7551364483433));
#125901=CARTESIAN_POINT('Ctrl Pts',(1.02299686358755,-29.0301372817023,
53.641757151509));
#125902=CARTESIAN_POINT('Ctrl Pts',(1.01699173984669,-29.1129663323208,
53.586272645239));
#125903=CARTESIAN_POINT('Ctrl Pts',(1.00882317195071,-29.2257573147217,
53.5245508088232));
#125904=CARTESIAN_POINT('Ctrl Pts',(1.00694893069188,-29.2516331498732,
53.5112593010003));
#125905=CARTESIAN_POINT('Ctrl Pts',(1.00438787609396,-29.2867415356805,
53.4943719263102));
#125906=CARTESIAN_POINT('Ctrl Pts',(1.00373437504665,-29.2956790001159,
53.4901703902266));
#125907=CARTESIAN_POINT('Ctrl Pts',(1.00269448035717,-29.3098564742229,
53.4836587780271));
#125908=CARTESIAN_POINT('Ctrl Pts',(1.00231123296883,-29.3150721180615,
53.4812957556926));
#125909=CARTESIAN_POINT('Ctrl Pts',(1.00150802720176,-29.3259806095401,
53.4764211284065));
#125910=CARTESIAN_POINT('Ctrl Pts',(1.00108776034537,-29.3316754693969,
53.4739144736553));
#125911=CARTESIAN_POINT('Ctrl Pts',(1.00003988045341,-29.3458461348936,
53.467771628282));
#125912=CARTESIAN_POINT('Ctrl Pts',(0.999410044857784,-29.35433826898,53.4641738439509));
#125913=CARTESIAN_POINT('Ctrl Pts',(0.996980507169826,-29.3870159065608,
53.45064852419));
#125914=CARTESIAN_POINT('Ctrl Pts',(0.995155025085117,-29.4114026488488,
53.4412208402037));
#125915=CARTESIAN_POINT('Ctrl Pts',(0.99022383204168,-29.4770840403755,
53.4175900217503));
#125916=CARTESIAN_POINT('Ctrl Pts',(0.987082286576581,-29.5187314527544,
53.4044303373608));
#125917=CARTESIAN_POINT('Ctrl Pts',(0.973279874152865,-29.7024637997197,
53.3542230395125));
#125918=CARTESIAN_POINT('Ctrl Pts',(0.962524276868997,-29.8486113982833,
53.334404853455));
#125919=CARTESIAN_POINT('Ctrl Pts',(0.950598892162561,-30.0213236605926,
53.3339359706849));
#125920=CARTESIAN_POINT('Ctrl Pts',(0.948832291167848,-30.0471694992282,
53.3344672875928));
#125921=CARTESIAN_POINT('Ctrl Pts',(0.946186726389482,-30.0862532601435,
53.336181342138));
#125922=CARTESIAN_POINT('Ctrl Pts',(0.945294172911729,-30.0995056080924,
53.336921287858));
#125923=CARTESIAN_POINT('Ctrl Pts',(0.9436931362223,-30.1233915632246,53.3385415057917));
#125924=CARTESIAN_POINT('Ctrl Pts',(0.942982942691258,-30.1340281142516,
53.3393656996426));
#125925=CARTESIAN_POINT('Ctrl Pts',(0.941464033961621,-30.1568606527204,
53.3413557298148));
#125926=CARTESIAN_POINT('Ctrl Pts',(0.940656377603993,-30.1690532350134,
53.3425540441495));
#125927=CARTESIAN_POINT('Ctrl Pts',(0.938435069860581,-30.2027187878852,
53.3462381326349));
#125928=CARTESIAN_POINT('Ctrl Pts',(0.93703032077653,-30.2241587654593,
53.3490075292339));
#125929=CARTESIAN_POINT('Ctrl Pts',(0.928761603677918,-30.3510850959352,
53.367920818445));
#125930=CARTESIAN_POINT('Ctrl Pts',(0.922216310365715,-30.4548798673067,
53.3937524230652));
#125931=CARTESIAN_POINT('Ctrl Pts',(0.909190829915431,-30.6559510039607,
53.464865905101));
#125932=CARTESIAN_POINT('Ctrl Pts',(0.902734071567557,-30.7527479627162,
53.5099420591852));
#125933=CARTESIAN_POINT('Ctrl Pts',(0.89482074879949,-30.8578161669773,
53.5717340019465));
#125934=CARTESIAN_POINT('Ctrl Pts',(0.893813333509112,-30.870958545872,
53.5797100620832));
#125935=CARTESIAN_POINT('Ctrl Pts',(0.892297356381249,-30.8903529844528,
53.591850877824));
#125936=CARTESIAN_POINT('Ctrl Pts',(0.891797223519456,-30.8966907125267,
53.5958781577637));
#125937=CARTESIAN_POINT('Ctrl Pts',(0.890892525057947,-30.9080413722192,
53.6031990684467));
#125938=CARTESIAN_POINT('Ctrl Pts',(0.89048897293095,-30.9130640394406,
53.6064771142445));
#125939=CARTESIAN_POINT('Ctrl Pts',(0.88957877330433,-30.9243015955239,
53.6138981470499));
#125940=CARTESIAN_POINT('Ctrl Pts',(0.88907119092711,-30.9305063269588,
53.6180558056394));
#125941=CARTESIAN_POINT('Ctrl Pts',(0.887523648197904,-30.9492427515387,
53.630794073457));
#125942=CARTESIAN_POINT('Ctrl Pts',(0.886475727312991,-30.9616848630911,
53.6395041880975));
#125943=CARTESIAN_POINT('Ctrl Pts',(0.879750634011209,-31.0400912972663,
53.696005618615));
#125944=CARTESIAN_POINT('Ctrl Pts',(0.873841249761727,-31.1025889396038,
53.748406510031));
#125945=CARTESIAN_POINT('Ctrl Pts',(0.858494524399951,-31.2538123075522,
53.8953467709984));
#125946=CARTESIAN_POINT('Ctrl Pts',(0.849114437939133,-31.3358207167937,
53.9960581539459));
#125947=CARTESIAN_POINT('Ctrl Pts',(0.838771987341453,-31.4165702836705,
54.1228904173036));
#125948=CARTESIAN_POINT('Ctrl Pts',(0.837346648791826,-31.4274597475475,
54.1407262796545));
#125949=CARTESIAN_POINT('Ctrl Pts',(0.835034953584482,-31.4447199387857,
54.1702308652387));
#125950=CARTESIAN_POINT('Ctrl Pts',(0.834141431539081,-31.4512913830487,
54.1817788454352));
#125951=CARTESIAN_POINT('Ctrl Pts',(0.832540049376055,-31.462884502025,
54.2027305733635));
#125952=CARTESIAN_POINT('Ctrl Pts',(0.831830461129028,-31.4679553376095,
54.212106136104));
#125953=CARTESIAN_POINT('Ctrl Pts',(0.83031436203537,-31.4786445855784,
54.2323311618035));
#125954=CARTESIAN_POINT('Ctrl Pts',(0.82950889333664,-31.4842343603653,
54.2431951159927));
#125955=CARTESIAN_POINT('Ctrl Pts',(0.827297705722188,-31.4993268412837,
54.2733384737363));
#125956=CARTESIAN_POINT('Ctrl Pts',(0.825900773112623,-31.508576957018,
54.2927422081236));
#125957=CARTESIAN_POINT('Ctrl Pts',(0.82280112519334,-31.5284310914414,
54.3365527809227));
#125958=CARTESIAN_POINT('Ctrl Pts',(0.821105162298961,-31.5388311954838,
54.3610457919199));
#125959=CARTESIAN_POINT('Ctrl Pts',(0.815601995257463,-31.5709531990043,
54.4420351969047));
#125960=CARTESIAN_POINT('Ctrl Pts',(0.811865118567678,-31.5901849074589,
54.4994688481055));
#125961=CARTESIAN_POINT('Ctrl Pts',(0.802783956080069,-31.6295249209977,
54.6423756857888));
#125962=CARTESIAN_POINT('Ctrl Pts',(0.797488790093301,-31.6460869352314,
54.7286277771464));
#125963=CARTESIAN_POINT('Ctrl Pts',(0.789184423591483,-31.6607855854843,
54.8607385156302));
#125964=CARTESIAN_POINT('Ctrl Pts',(0.786311587025967,-31.6639541013579,
54.905880479385));
#125965=CARTESIAN_POINT('Ctrl Pts',(0.782603682227426,-31.6656165636806,
54.9624847188622));
#125966=CARTESIAN_POINT('Ctrl Pts',(0.781851773580448,-31.6658342456913,
54.9738813914868));
#125967=CARTESIAN_POINT('Ctrl Pts',(0.780649029015884,-31.6659940248568,
54.9919631699322));
#125968=CARTESIAN_POINT('Ctrl Pts',(0.780202289534688,-31.6660128595703,
54.9986474787928));
#125969=CARTESIAN_POINT('Ctrl Pts',(0.77934123350569,-31.6659718388379,
55.011465496239));
#125970=CARTESIAN_POINT('Ctrl Pts',(0.778927263617136,-31.6659183338037,
55.0175990182009));
#125971=CARTESIAN_POINT('Ctrl Pts',(0.777917704064818,-31.6657061974064,
55.0324896424649));
#125972=CARTESIAN_POINT('Ctrl Pts',(0.777320231466912,-31.665512375544,
55.0412459860966));
#125973=CARTESIAN_POINT('Ctrl Pts',(0.775156322922067,-31.6645657689097,
55.0727726170826));
#125974=CARTESIAN_POINT('Ctrl Pts',(0.773570558434099,-31.6634149990333,
55.0955273151611));
#125975=CARTESIAN_POINT('Ctrl Pts',(0.761777916473459,-31.6515198482567,
55.2626932155156));
#125976=CARTESIAN_POINT('Ctrl Pts',(0.751007005008851,-31.6224544700863,
55.4051798530242));
#125977=CARTESIAN_POINT('Ctrl Pts',(0.736115130301,-31.5545905070751,55.6023838077631));
#125978=CARTESIAN_POINT('Ctrl Pts',(0.731648427581999,-31.5304086840699,
55.6614143490946));
#125979=CARTESIAN_POINT('Ctrl Pts',(0.726025326849968,-31.4948935124071,
55.7356586554303));
#125980=CARTESIAN_POINT('Ctrl Pts',(0.724767201104126,-31.4866074373264,
55.7522623520767));
#125981=CARTESIAN_POINT('Ctrl Pts',(0.722737892684079,-31.4726908064105,
55.7790201900131));
#125982=CARTESIAN_POINT('Ctrl Pts',(0.721960903523555,-31.4672286612023,
55.7892596120809));
#125983=CARTESIAN_POINT('Ctrl Pts',(0.720467211776136,-31.4564709513518,
55.8089284877257));
#125984=CARTESIAN_POINT('Ctrl Pts',(0.719750048647606,-31.4511897066254,
55.8183650622773));
#125985=CARTESIAN_POINT('Ctrl Pts',(0.718079753404172,-31.4386194148121,
55.8403213841295));
#125986=CARTESIAN_POINT('Ctrl Pts',(0.717129270570933,-31.4312581356779,
55.85279893306));
#125987=CARTESIAN_POINT('Ctrl Pts',(0.71399260796866,-31.4062828836215,
55.8938980905331));
#125988=CARTESIAN_POINT('Ctrl Pts',(0.711832020490769,-31.387965105435,
55.9220837577085));
#125989=CARTESIAN_POINT('Ctrl Pts',(0.706620482125906,-31.3411915824033,
55.9894987808133));
#125990=CARTESIAN_POINT('Ctrl Pts',(0.703600490750051,-31.3118528933047,
56.0280784000104));
#125991=CARTESIAN_POINT('Ctrl Pts',(0.696505448911896,-31.2383217635587,
56.1164869739304));
#125992=CARTESIAN_POINT('Ctrl Pts',(0.692465420791772,-31.1927438745192,
56.1650519945106));
#125993=CARTESIAN_POINT('Ctrl Pts',(0.683632256201668,-31.087899989496,
56.2641479728702));
#125994=CARTESIAN_POINT('Ctrl Pts',(0.678837433618865,-31.027756542017,
56.313510616572));
#125995=CARTESIAN_POINT('Ctrl Pts',(0.672754215512254,-30.9512069767532,
56.3678533993608));
#125996=CARTESIAN_POINT('Ctrl Pts',(0.671695895796978,-30.937882381046,
56.3770236841965));
#125997=CARTESIAN_POINT('Ctrl Pts',(0.670110755775963,-30.917957443895,
56.3903131322876));
#125998=CARTESIAN_POINT('Ctrl Pts',(0.669593282966531,-30.9114579191173,
56.3945827083055));
#125999=CARTESIAN_POINT('Ctrl Pts',(0.668669726593056,-30.8998724836048,
56.4020776658342));
#126000=CARTESIAN_POINT('Ctrl Pts',(0.66826484204571,-30.8947986298631,
56.405321200796));
#126001=CARTESIAN_POINT('Ctrl Pts',(0.667366701809323,-30.8835558053559,
56.4124227681519));
#126002=CARTESIAN_POINT('Ctrl Pts',(0.666872671499463,-30.8773791657986,
56.4162678883598));
#126003=CARTESIAN_POINT('Ctrl Pts',(0.665412459139005,-30.8591392915425,
56.4274575799269));
#126004=CARTESIAN_POINT('Ctrl Pts',(0.664439590437624,-30.8470079618816,
56.434689145578));
#126005=CARTESIAN_POINT('Ctrl Pts',(0.662166838642417,-30.8186839734351,
56.4510888245021));
#126006=CARTESIAN_POINT('Ctrl Pts',(0.660861378299215,-30.8024269061112,
56.460141508049));
#126007=CARTESIAN_POINT('Ctrl Pts',(0.656239668831929,-30.7448092058579,
56.4909728770553));
#126008=CARTESIAN_POINT('Ctrl Pts',(0.652870583563433,-30.7026886030704,
56.5112806029566));
#126009=CARTESIAN_POINT('Ctrl Pts',(0.64154904114023,-30.5593663034603,
56.5730931427838));
#126010=CARTESIAN_POINT('Ctrl Pts',(0.633549622447796,-30.4549280125623,
56.6064115039828));
#126011=CARTESIAN_POINT('Ctrl Pts',(0.622393051233916,-30.3004469393127,
56.6394051642707));
#126012=CARTESIAN_POINT('Ctrl Pts',(0.619016261141123,-30.2524968739035,
56.6474719432033));
#126013=CARTESIAN_POINT('Ctrl Pts',(0.614543968262986,-30.187361226336,
56.6555185405715));
#126014=CARTESIAN_POINT('Ctrl Pts',(0.613391881250385,-30.1704326578384,
56.6573468598146));
#126015=CARTESIAN_POINT('Ctrl Pts',(0.611564736807413,-30.1433540543122,
56.6598521007722));
#126016=CARTESIAN_POINT('Ctrl Pts',(0.610884507356309,-30.1332210798639,
56.6606960989632));
#126017=CARTESIAN_POINT('Ctrl Pts',(0.609484289612966,-30.1122588079788,
56.6622489941722));
#126018=CARTESIAN_POINT('Ctrl Pts',(0.608764737727573,-30.101429013331,
56.6629449549879));
#126019=CARTESIAN_POINT('Ctrl Pts',(0.60708144742816,-30.0759643992842,
56.6643317096555));
#126020=CARTESIAN_POINT('Ctrl Pts',(0.606120466413455,-30.0613255871529,
56.6649353815292));
#126021=CARTESIAN_POINT('Ctrl Pts',(0.602912778805024,-30.0121466847089,
56.6663138861494));
#126022=CARTESIAN_POINT('Ctrl Pts',(0.600693295279663,-29.9775895644834,
56.6662075340011));
#126023=CARTESIAN_POINT('Ctrl Pts',(0.59530640700282,-29.8927428511392,
56.6633059102952));
#126024=CARTESIAN_POINT('Ctrl Pts',(0.592172932785695,-29.8425285284031,
56.6593052584522));
#126025=CARTESIAN_POINT('Ctrl Pts',(0.582906926889831,-29.6933085474579,
56.6405804570941));
#126026=CARTESIAN_POINT('Ctrl Pts',(0.57689533921652,-29.5953764194341,
56.6192103106182));
#126027=CARTESIAN_POINT('Ctrl Pts',(0.567606146855471,-29.4530995130802,
56.5744424032324));
#126028=CARTESIAN_POINT('Ctrl Pts',(0.564496395484269,-29.4069214705016,
56.5576347153741));
#126029=CARTESIAN_POINT('Ctrl Pts',(0.560520020241607,-29.3507948586255,
56.5343482252573));
#126030=CARTESIAN_POINT('Ctrl Pts',(0.559751716019859,-29.3400790147403,
56.5297699390206));
#126031=CARTESIAN_POINT('Ctrl Pts',(0.558528558300658,-29.3232398187259,
56.5223656344813));
#126032=CARTESIAN_POINT('Ctrl Pts',(0.558078032595549,-29.3170838560514,
56.519614097171));
#126033=CARTESIAN_POINT('Ctrl Pts',(0.557217019932719,-29.3054111737008,
56.514311495));
#126034=CARTESIAN_POINT('Ctrl Pts',(0.556806951378812,-29.2998915039549,
56.5117675186392));
#126035=CARTESIAN_POINT('Ctrl Pts',(0.555815032476529,-29.2866331659693,
56.5055686650774));
#126036=CARTESIAN_POINT('Ctrl Pts',(0.555231426341487,-29.2789086081284,
56.5018842970498));
#126037=CARTESIAN_POINT('Ctrl Pts',(0.55315739431752,-29.2517125119825,
56.4886544570432));
#126038=CARTESIAN_POINT('Ctrl Pts',(0.551649395663401,-29.2324002279826,
56.4787889425007));
#126039=CARTESIAN_POINT('Ctrl Pts',(0.547784117502843,-29.1839256256531,
56.4528207469828));
#126040=CARTESIAN_POINT('Ctrl Pts',(0.54540590785726,-29.1550441329977,
56.4362154506226));
#126041=CARTESIAN_POINT('Ctrl Pts',(0.531573373523371,-28.9915056759951,
56.33554904769));
#126042=CARTESIAN_POINT('Ctrl Pts',(0.519839473796115,-28.8688787605094,
56.2334242836303));
#126043=CARTESIAN_POINT('Ctrl Pts',(0.50676852445426,-28.7426736331756,
56.093420531934));
#126044=CARTESIAN_POINT('Ctrl Pts',(0.5047326476553,-28.7233806477863,56.0708320497424));
#126045=CARTESIAN_POINT('Ctrl Pts',(0.501799048754285,-28.6961343404467,
56.0371479573592));
#126046=CARTESIAN_POINT('Ctrl Pts',(0.500881968650037,-28.6876978821238,
56.0264524900288));
#126047=CARTESIAN_POINT('Ctrl Pts',(0.499256145630107,-28.6728908968879,
56.007199679074));
#126048=CARTESIAN_POINT('Ctrl Pts',(0.498545415866182,-28.6664696865922,
55.9986824707877));
#126049=CARTESIAN_POINT('Ctrl Pts',(0.497057403954751,-28.6531380219633,
55.9806412452735));
#126050=CARTESIAN_POINT('Ctrl Pts',(0.496280857520036,-28.6462457545938,
55.9711044716594));
#126051=CARTESIAN_POINT('Ctrl Pts',(0.494224169513516,-28.628171475085,
55.9455288163754));
#126052=CARTESIAN_POINT('Ctrl Pts',(0.492950927267009,-28.6171695690114,
55.9293644580919));
#126053=CARTESIAN_POINT('Ctrl Pts',(0.485637773665962,-28.5551409659613,
55.8346889052855));
#126054=CARTESIAN_POINT('Ctrl Pts',(0.47984189674057,-28.5105183090986,
55.7521773320803));
#126055=CARTESIAN_POINT('Ctrl Pts',(0.472112722188003,-28.4600025376136,
55.6364195169717));
#126056=CARTESIAN_POINT('Ctrl Pts',(0.470123713197726,-28.447831751358,
55.6061303190444));
#126057=CARTESIAN_POINT('Ctrl Pts',(0.468131487137799,-28.4365623373493,
55.5755160076012));
#126058=CARTESIAN_POINT('Origin',(5.,30.,55.));
#126059=CARTESIAN_POINT('',(1.3202157917438,31.6659997347684,55.0009400806026));
#126060=CARTESIAN_POINT('Ctrl Pts',(0.659214778542432,31.5634376782623,
55.5755159651912));
#126061=CARTESIAN_POINT('Ctrl Pts',(0.659963674773577,31.5594860338117,
55.5862509407588));
#126062=CARTESIAN_POINT('Ctrl Pts',(0.660718146030943,31.5554240663698,
55.5969445627462));
#126063=CARTESIAN_POINT('Ctrl Pts',(0.661924467957585,31.5488090252237,
55.613833438356));
#126064=CARTESIAN_POINT('Ctrl Pts',(0.662372189405329,31.5463280517853,
55.6200568030159));
#126065=CARTESIAN_POINT('Ctrl Pts',(0.66323392355848,31.5415054148437,55.6319451166599));
#126066=CARTESIAN_POINT('Ctrl Pts',(0.663647576898634,31.5391699275969,
55.6376123456943));
#126067=CARTESIAN_POINT('Ctrl Pts',(0.664654577091319,31.5334339350216,
55.6513159872087));
#126068=CARTESIAN_POINT('Ctrl Pts',(0.665249782236512,31.5300014869306,
55.6593387519811));
#126069=CARTESIAN_POINT('Ctrl Pts',(0.667395303766544,31.5174732562376,
55.6879967012015));
#126070=CARTESIAN_POINT('Ctrl Pts',(0.668964528083185,31.5080221693331,
55.7084726944259));
#126071=CARTESIAN_POINT('Ctrl Pts',(0.680707776955766,31.434998241425,55.8585949080955));
#126072=CARTESIAN_POINT('Ctrl Pts',(0.691446166056638,31.3552264309243,
55.9796785122895));
#126073=CARTESIAN_POINT('Ctrl Pts',(0.706348193913444,31.2188515169005,
56.1375777165001));
#126074=CARTESIAN_POINT('Ctrl Pts',(0.710851114015021,31.1740848164214,
56.183726636443));
#126075=CARTESIAN_POINT('Ctrl Pts',(0.716511261941901,31.1130642518199,
56.2397538568652));
#126076=CARTESIAN_POINT('Ctrl Pts',(0.71777194462588,31.0991595200653,56.2520982598632));
#126077=CARTESIAN_POINT('Ctrl Pts',(0.719804369030032,31.0762379635695,
56.2717714879298));
#126078=CARTESIAN_POINT('Ctrl Pts',(0.720581950409677,31.0673463317197,
56.2792430151123));
#126079=CARTESIAN_POINT('Ctrl Pts',(0.722076130964953,31.0500272157867,
56.2934897544291));
#126080=CARTESIAN_POINT('Ctrl Pts',(0.72279319735446,31.0416105013657,56.3002770749091));
#126081=CARTESIAN_POINT('Ctrl Pts',(0.724462303762982,31.0217766686898,
56.3159550940202));
#126082=CARTESIAN_POINT('Ctrl Pts',(0.72541170656721,31.0103084994599,56.3247800299974));
#126083=CARTESIAN_POINT('Ctrl Pts',(0.72854027604579,30.9719152031312,56.3535357151689));
#126084=CARTESIAN_POINT('Ctrl Pts',(0.730694032283207,30.9445030435336,
56.3728045520156));
#126085=CARTESIAN_POINT('Ctrl Pts',(0.735884884584433,30.8762606271322,
56.4177617454544));
#126086=CARTESIAN_POINT('Ctrl Pts',(0.738891356592106,30.8348598001479,
56.4425292630904));
#126087=CARTESIAN_POINT('Ctrl Pts',(0.745995231813121,30.7335959365295,
56.4972869328982));
#126088=CARTESIAN_POINT('Ctrl Pts',(0.750056350595555,30.6728883584316,
56.5255335352461));
#126089=CARTESIAN_POINT('Ctrl Pts',(0.758912647442102,30.5383045961151,
56.5785530396186));
#126090=CARTESIAN_POINT('Ctrl Pts',(0.763709168879551,30.4640645987096,
56.6019496697849));
#126091=CARTESIAN_POINT('Ctrl Pts',(0.769794313488902,30.3727460295175,
56.6238466503994));
#126092=CARTESIAN_POINT('Ctrl Pts',(0.770852462074844,30.3569660635819,
56.6273883152812));
#126093=CARTESIAN_POINT('Ctrl Pts',(0.772437302118265,30.3335281211712,
56.6322914670152));
#126094=CARTESIAN_POINT('Ctrl Pts',(0.772954640244863,30.3259076144078,
56.6338300590287));
#126095=CARTESIAN_POINT('Ctrl Pts',(0.773877471459437,30.3123742586365,
56.6364640180472));
#126096=CARTESIAN_POINT('Ctrl Pts',(0.774281759344064,30.306465840248,56.637580790813));
#126097=CARTESIAN_POINT('Ctrl Pts',(0.775177653612938,30.293419209587,56.6399737029599));
#126098=CARTESIAN_POINT('Ctrl Pts',(0.77567002350507,30.2862787488537,56.6412352213943));
#126099=CARTESIAN_POINT('Ctrl Pts',(0.77712445941937,30.265266708266,56.6448061673337));
#126100=CARTESIAN_POINT('Ctrl Pts',(0.778093178502888,30.2513742527611,
56.6469865534037));
#126101=CARTESIAN_POINT('Ctrl Pts',(0.784689935432296,30.1573501703635,
56.6605261228646));
#126102=CARTESIAN_POINT('Ctrl Pts',(0.790553974769039,30.0765178487816,
56.6662077882946));
#126103=CARTESIAN_POINT('Ctrl Pts',(0.806063510907355,29.8633650116075,
56.6656451293248));
#126104=CARTESIAN_POINT('Ctrl Pts',(0.815656604586156,29.7316125475259,
56.6495526434039));
#126105=CARTESIAN_POINT('Ctrl Pts',(0.826166746061048,29.5831461540704,
56.6131374478684));
#126106=CARTESIAN_POINT('Ctrl Pts',(0.827570139913132,29.5632499976581,
56.6078647504266));
#126107=CARTESIAN_POINT('Ctrl Pts',(0.829854328291138,29.5307598483869,
56.5986068797755));
#126108=CARTESIAN_POINT('Ctrl Pts',(0.830741985896256,29.5181069842943,
56.5948383663475));
#126109=CARTESIAN_POINT('Ctrl Pts',(0.832337806176316,29.4953167834712,
56.5877545672487));
#126110=CARTESIAN_POINT('Ctrl Pts',(0.833047629721722,29.485164066098,56.5844916172385));
#126111=CARTESIAN_POINT('Ctrl Pts',(0.834569600723171,29.4633660279139,
56.5772543759887));
#126112=CARTESIAN_POINT('Ctrl Pts',(0.835380649743124,29.4517319373144,
56.5732480833068));
#126113=CARTESIAN_POINT('Ctrl Pts',(0.837621661865729,29.4195466305778,
56.5617644194604));
#126114=CARTESIAN_POINT('Ctrl Pts',(0.839042451604891,29.3990961879455,
56.5540105845071));
#126115=CARTESIAN_POINT('Ctrl Pts',(0.847871545164079,29.2719069539899,
56.5029000673142));
#126116=CARTESIAN_POINT('Ctrl Pts',(0.854901810203552,29.1697508616464,
56.4489715324176));
#126117=CARTESIAN_POINT('Ctrl Pts',(0.867843281551346,28.9935758290465,
56.3311719757932));
#126118=CARTESIAN_POINT('Ctrl Pts',(0.873738399752646,28.9180269742054,
56.2705266337626));
#126119=CARTESIAN_POINT('Ctrl Pts',(0.881042755825898,28.8366476961067,
56.192653310532));
#126120=CARTESIAN_POINT('Ctrl Pts',(0.882087291892754,28.8252811193462,
56.1814592705049));
#126121=CARTESIAN_POINT('Ctrl Pts',(0.883648396481805,28.8087249421397,
56.1646792765745));
#126122=CARTESIAN_POINT('Ctrl Pts',(0.884155789803154,28.8034097488822,
56.1592177733404));
#126123=CARTESIAN_POINT('Ctrl Pts',(0.885068105851131,28.7939745280309,
56.1493887979365));
#126124=CARTESIAN_POINT('Ctrl Pts',(0.885471934599636,28.7898403750829,
56.1450352516483));
#126125=CARTESIAN_POINT('Ctrl Pts',(0.886375889732285,28.7806806084086,
56.1352843723342));
#126126=CARTESIAN_POINT('Ctrl Pts',(0.88687687662457,28.7756673070899,56.1298760271112));
#126127=CARTESIAN_POINT('Ctrl Pts',(0.888382867171218,28.76078025105,56.1136004676827));
#126128=CARTESIAN_POINT('Ctrl Pts',(0.889395227501982,28.7510143813196,
56.1026361482085));
#126129=CARTESIAN_POINT('Ctrl Pts',(0.891777961222555,28.7285593866664,
56.0767444311353));
#126130=CARTESIAN_POINT('Ctrl Pts',(0.893154679035589,28.7159862886877,
56.0617196057646));
#126131=CARTESIAN_POINT('Ctrl Pts',(0.898143930548396,28.6717555545062,
56.0069290121172));
#126132=CARTESIAN_POINT('Ctrl Pts',(0.901817792886701,28.6416578810171,
55.9659427518692));
#126133=CARTESIAN_POINT('Ctrl Pts',(0.914506057533618,28.5448501336338,
55.8206215257514));
#126134=CARTESIAN_POINT('Ctrl Pts',(0.923540887224526,28.4879032779091,
55.7102487288947));
#126135=CARTESIAN_POINT('Ctrl Pts',(0.934524493244932,28.4316602796097,
55.5630333153845));
#126136=CARTESIAN_POINT('Ctrl Pts',(0.936848123405035,28.4205713274763,
55.5311321359396));
#126137=CARTESIAN_POINT('Ctrl Pts',(0.940052720156528,28.4064332387933,
55.4860881432053));
#126138=CARTESIAN_POINT('Ctrl Pts',(0.940960112133307,28.4025628689944,
55.4732138377933));
#126139=CARTESIAN_POINT('Ctrl Pts',(0.942531789310143,28.396093430618,55.4507096223187));
#126140=CARTESIAN_POINT('Ctrl Pts',(0.943198320871191,28.3934242713645,
55.4411007623922));
#126141=CARTESIAN_POINT('Ctrl Pts',(0.944591957268216,28.3880013610972,
55.4208760517827));
#126142=CARTESIAN_POINT('Ctrl Pts',(0.945318444150124,28.3852658209177,
55.4102557780982));
#126143=CARTESIAN_POINT('Ctrl Pts',(0.947057532354182,28.3789398176874,
55.3846521176276));
#126144=CARTESIAN_POINT('Ctrl Pts',(0.948066805141481,28.3754519024687,
55.3696442495976));
#126145=CARTESIAN_POINT('Ctrl Pts',(0.951654600013756,28.3637209195867,
55.3157904183378));
#126146=CARTESIAN_POINT('Ctrl Pts',(0.954195847185852,28.3566586619238,
55.2766992129396));
#126147=CARTESIAN_POINT('Ctrl Pts',(0.960608477038097,28.3421848769875,
55.1761590171424));
#126148=CARTESIAN_POINT('Ctrl Pts',(0.964424727524717,28.3367868788208,
55.1144811052257));
#126149=CARTESIAN_POINT('Ctrl Pts',(0.973795099258164,28.3319518174995,
54.961540822956));
#126150=CARTESIAN_POINT('Ctrl Pts',(0.97929714832269,28.3365530150519,54.8703621973523));
#126151=CARTESIAN_POINT('Ctrl Pts',(0.987546786681617,28.3539117228408,
54.7400462640853));
#126152=CARTESIAN_POINT('Ctrl Pts',(0.99011849501523,28.360686374524,54.7002787648945));
#126153=CARTESIAN_POINT('Ctrl Pts',(0.993485357352461,28.3711465983728,
54.6499789235106));
#126154=CARTESIAN_POINT('Ctrl Pts',(0.994214910994948,28.3735044579729,
54.6391809407212));
#126155=CARTESIAN_POINT('Ctrl Pts',(0.995390352702229,28.3774444053126,
54.6219615512177));
#126156=CARTESIAN_POINT('Ctrl Pts',(0.995832464198432,28.3789576453801,
54.6155245036074));
#126157=CARTESIAN_POINT('Ctrl Pts',(0.996691663417114,28.3819577276792,
54.6030953252751));
#126158=CARTESIAN_POINT('Ctrl Pts',(0.997108475790868,28.3834396171674,
54.5971021972253));
#126159=CARTESIAN_POINT('Ctrl Pts',(0.998135483652145,28.3871563348902,
54.5824215272881));
#126160=CARTESIAN_POINT('Ctrl Pts',(0.998747715927455,28.389428068324,54.5737436067658));
#126161=CARTESIAN_POINT('Ctrl Pts',(1.00102901243452,28.3981033413843,54.5416641718702));
#126162=CARTESIAN_POINT('Ctrl Pts',(1.00272014057986,28.4049474384177,54.5183862415263));
#126163=CARTESIAN_POINT('Ctrl Pts',(1.00718530026382,28.424137671168,54.4580208052705));
#126164=CARTESIAN_POINT('Ctrl Pts',(1.00998807895293,28.43728477872,54.4212044542003));
#126165=CARTESIAN_POINT('Ctrl Pts',(1.01797729513375,28.4780893895311,54.3184961284334));
#126166=CARTESIAN_POINT('Ctrl Pts',(1.02320480885816,28.5087083946863,54.2538707123977));
#126167=CARTESIAN_POINT('Ctrl Pts',(1.03512347050194,28.5886228123156,54.109910463198));
#126168=CARTESIAN_POINT('Ctrl Pts',(1.04174799528417,28.6406304124562,54.0323407351921));
#126169=CARTESIAN_POINT('Ctrl Pts',(1.04949123279008,28.7112681920914,53.9440071906692));
#126170=CARTESIAN_POINT('Ctrl Pts',(1.0508400584708,28.7239494120389,53.9287178512361));
#126171=CARTESIAN_POINT('Ctrl Pts',(1.05297808378099,28.7446488621043,53.9046504280458));
#126172=CARTESIAN_POINT('Ctrl Pts',(1.05377430308946,28.75249252959,53.8957254471249));
#126173=CARTESIAN_POINT('Ctrl Pts',(1.05528189985961,28.7675989285154,53.8789029086026));
#126174=CARTESIAN_POINT('Ctrl Pts',(1.05599397217408,28.7748437448607,53.8709901466265));
#126175=CARTESIAN_POINT('Ctrl Pts',(1.05761964209106,28.7916327038708,53.8530052342212));
#126176=CARTESIAN_POINT('Ctrl Pts',(1.05853102383887,28.8012273367748,53.8429811426392));
#126177=CARTESIAN_POINT('Ctrl Pts',(1.06139667209143,28.8319616524653,53.8116639289647));
#126178=CARTESIAN_POINT('Ctrl Pts',(1.06333120326394,28.8535525653389,53.7908206680888));
#126179=CARTESIAN_POINT('Ctrl Pts',(1.06788218003509,28.9062255612992,53.7426515877071));
#126180=CARTESIAN_POINT('Ctrl Pts',(1.07047751114992,28.9377860812315,53.7158779265474));
#126181=CARTESIAN_POINT('Ctrl Pts',(1.08276478671506,29.0934265415283,53.5935127062661));
#126182=CARTESIAN_POINT('Ctrl Pts',(1.09195761566225,29.2295508095331,53.5145791717377));
#126183=CARTESIAN_POINT('Ctrl Pts',(1.10317170578295,29.3900128559393,53.449598139637));
#126184=CARTESIAN_POINT('Ctrl Pts',(1.10425507158038,29.4054534543692,53.4436116812001));
#126185=CARTESIAN_POINT('Ctrl Pts',(1.1058632136874,29.4282329461096,53.4351682938226));
#126186=CARTESIAN_POINT('Ctrl Pts',(1.10637800404369,29.4355043527415,53.432530545467));
#126187=CARTESIAN_POINT('Ctrl Pts',(1.10729804200894,29.4484570688819,53.427933681803));
#126188=CARTESIAN_POINT('Ctrl Pts',(1.10770211194395,29.4541309910689,53.4259545316262));
#126189=CARTESIAN_POINT('Ctrl Pts',(1.1085996984854,29.466701181022,53.4216459995717));
#126190=CARTESIAN_POINT('Ctrl Pts',(1.10909400146366,29.4736019768989,53.4193311234645));
#126191=CARTESIAN_POINT('Ctrl Pts',(1.11056001178771,29.4940113049587,53.4126332711549));
#126192=CARTESIAN_POINT('Ctrl Pts',(1.11153852804422,29.5075605748194,53.4083778493662));
#126193=CARTESIAN_POINT('Ctrl Pts',(1.11910413224452,29.6118816777519,53.3770732230114));
#126194=CARTESIAN_POINT('Ctrl Pts',(1.12601146325622,29.7047489583111,53.3576387176011));
#126195=CARTESIAN_POINT('Ctrl Pts',(1.14132830868975,29.9136428125962,53.3322190242885));
#126196=CARTESIAN_POINT('Ctrl Pts',(1.14967533091106,30.0296951607165,53.3302461267074));
#126197=CARTESIAN_POINT('Ctrl Pts',(1.15915999706084,30.1668561083711,53.3422319109193));
#126198=CARTESIAN_POINT('Ctrl Pts',(1.16065619284714,30.1886428967115,53.3445695621347));
#126199=CARTESIAN_POINT('Ctrl Pts',(1.1630586979109,30.2238580689484,53.3490523275096));
#126200=CARTESIAN_POINT('Ctrl Pts',(1.16397313375916,30.2373168109122,53.3509331721888));
#126201=CARTESIAN_POINT('Ctrl Pts',(1.1655980449246,30.2613253048975,53.3545883541528));
#126202=CARTESIAN_POINT('Ctrl Pts',(1.16631045208938,30.2718836795725,53.3563000051061));
#126203=CARTESIAN_POINT('Ctrl Pts',(1.16781813103271,30.2942928872174,53.3601546690648));
#126204=CARTESIAN_POINT('Ctrl Pts',(1.16861250303092,30.3061384919742,53.3623247423918));
#126205=CARTESIAN_POINT('Ctrl Pts',(1.17075643389708,30.338203111707,53.3685589382604));
#126206=CARTESIAN_POINT('Ctrl Pts',(1.17209811365845,30.3583722912001,53.3728704278661));
#126207=CARTESIAN_POINT('Ctrl Pts',(1.17505597317585,30.4030134065257,53.3832835671536));
#126208=CARTESIAN_POINT('Ctrl Pts',(1.1766663398387,30.4274375227992,53.3895686624122));
#126209=CARTESIAN_POINT('Ctrl Pts',(1.18177668028163,30.5051478955028,53.4114586140517));
#126210=CARTESIAN_POINT('Ctrl Pts',(1.18521766952564,30.5578021788056,53.4291736117712));
#126211=CARTESIAN_POINT('Ctrl Pts',(1.19515096346947,30.7083264333205,53.4883417151074));
#126212=CARTESIAN_POINT('Ctrl Pts',(1.20152694237223,30.8032261729406,53.5365583087831));
#126213=CARTESIAN_POINT('Ctrl Pts',(1.21049707279574,30.9233995796738,53.6128461814064));
#126214=CARTESIAN_POINT('Ctrl Pts',(1.21281057002896,30.9532745631696,53.633204596608));
#126215=CARTESIAN_POINT('Ctrl Pts',(1.21588022871239,30.9910653381725,53.6607991207853));
#126216=CARTESIAN_POINT('Ctrl Pts',(1.21658401888085,30.9996085963038,53.6671638739113));
#126217=CARTESIAN_POINT('Ctrl Pts',(1.21772775460492,31.0132854923741,53.6775586602082));
#126218=CARTESIAN_POINT('Ctrl Pts',(1.21816427452302,31.0184576772661,53.6815378116196));
#126219=CARTESIAN_POINT('Ctrl Pts',(1.21900877905731,31.0283689957166,53.6892560705806));
#126220=CARTESIAN_POINT('Ctrl Pts',(1.2194164563968,31.0331114052629,53.6929907193143));
#126221=CARTESIAN_POINT('Ctrl Pts',(1.22038104170437,31.0442355238733,53.7018493335292));
#126222=CARTESIAN_POINT('Ctrl Pts',(1.22093941704082,31.0505999455364,53.706994690768));
#126223=CARTESIAN_POINT('Ctrl Pts',(1.22218434736042,31.0646298189081,53.7185091992837));
#126224=CARTESIAN_POINT('Ctrl Pts',(1.22287231140984,31.0722764984545,53.7249006222609));
#126225=CARTESIAN_POINT('Ctrl Pts',(1.22483234739306,31.0937748572291,53.743200005788));
#126226=CARTESIAN_POINT('Ctrl Pts',(1.22611350427427,31.107488292973,53.7552673839139));
#126227=CARTESIAN_POINT('Ctrl Pts',(1.23061560482753,31.1545949602295,53.7981144612208));
#126228=CARTESIAN_POINT('Ctrl Pts',(1.23388712409717,31.1869244959774,53.8300307286654));
#126229=CARTESIAN_POINT('Ctrl Pts',(1.24794376716423,31.3191713370836,53.9717162195025));
#126230=CARTESIAN_POINT('Ctrl Pts',(1.25880023520702,31.4055088503652,54.0932791123764));
#126231=CARTESIAN_POINT('Ctrl Pts',(1.27048477212937,31.4845138953527,54.2435422931743));
#126232=CARTESIAN_POINT('Ctrl Pts',(1.2719385409479,31.4940650473768,54.2625859544202));
#126233=CARTESIAN_POINT('Ctrl Pts',(1.27428702924811,31.5090307050563,54.2939106096332));
#126234=CARTESIAN_POINT('Ctrl Pts',(1.27518928693818,31.5146664612768,54.3060825514971));
#126235=CARTESIAN_POINT('Ctrl Pts',(1.27680084095772,31.5245243762305,54.3280658723908));
#126236=CARTESIAN_POINT('Ctrl Pts',(1.27751194612753,31.5288002881486,54.3378521814277));
#126237=CARTESIAN_POINT('Ctrl Pts',(1.27902552219088,31.537740727347,54.3588625951354));
#126238=CARTESIAN_POINT('Ctrl Pts',(1.27982700722774,31.5423771441183,54.3700980434219));
#126239=CARTESIAN_POINT('Ctrl Pts',(1.28201229344357,31.5547447610464,54.4010240629602));
#126240=CARTESIAN_POINT('Ctrl Pts',(1.28338767433082,31.5622247230256,54.4208131342422));
#126241=CARTESIAN_POINT('Ctrl Pts',(1.28643158955148,31.5780725691943,54.4652833983786));
#126242=CARTESIAN_POINT('Ctrl Pts',(1.28809375679505,31.5862424285784,54.490029467944));
#126243=CARTESIAN_POINT('Ctrl Pts',(1.29343886300011,31.6108588879297,54.5709181818392));
#126244=CARTESIAN_POINT('Ctrl Pts',(1.29705621264224,31.6249308483184,54.6277392667515));
#126245=CARTESIAN_POINT('Ctrl Pts',(1.30714294227936,31.6560116465503,54.7892559436727));
#126246=CARTESIAN_POINT('Ctrl Pts',(1.31351093898179,31.6660595218301,54.894986156346));
#126247=CARTESIAN_POINT('Ctrl Pts',(1.3202157917438,31.6659997347684,55.0009400806026));
#126248=CARTESIAN_POINT('Ctrl Pts',(1.32021594204516,31.6659997334265,55.00094245575));
#126249=CARTESIAN_POINT('Ctrl Pts',(1.32220988897509,31.6659819085261,55.032451923777));
#126250=CARTESIAN_POINT('Ctrl Pts',(1.32423296675841,31.6650701672133,55.06395268441));
#126251=CARTESIAN_POINT('Ctrl Pts',(1.32682078314898,31.6628108339044,55.1033406294786));
#126252=CARTESIAN_POINT('Ctrl Pts',(1.32734478152174,31.6622989805633,55.1112710577923));
#126253=CARTESIAN_POINT('Ctrl Pts',(1.32826702746228,31.6613039342568,55.1251430018115));
#126254=CARTESIAN_POINT('Ctrl Pts',(1.32866397223534,31.6608455471467,55.1310862261613));
#126255=CARTESIAN_POINT('Ctrl Pts',(1.32945879277765,31.6598681994625,55.1429287635264));
#126256=CARTESIAN_POINT('Ctrl Pts',(1.32985664277534,31.659349673797,55.1488278524614));
#126257=CARTESIAN_POINT('Ctrl Pts',(1.33072932606067,31.6581487459355,55.1617030106065));
#126258=CARTESIAN_POINT('Ctrl Pts',(1.33120480792667,31.6574537805996,55.1686774672297));
#126259=CARTESIAN_POINT('Ctrl Pts',(1.33253752092831,31.655392562013,55.1881190070045));
#126260=CARTESIAN_POINT('Ctrl Pts',(1.33339975384111,31.653929538601,55.2005750558197));
#126261=CARTESIAN_POINT('Ctrl Pts',(1.33796731482122,31.6454975568926,55.2659813370139));
#126262=CARTESIAN_POINT('Ctrl Pts',(1.34177817048429,31.6361266114523,55.3185857050561));
#126263=CARTESIAN_POINT('Ctrl Pts',(1.35078326094407,31.6083821889067,55.4401682876052));
#126264=CARTESIAN_POINT('Ctrl Pts',(1.35600139652401,31.5880703088527,55.5085993456218));
#126265=CARTESIAN_POINT('Ctrl Pts',(1.36116735710803,31.5634376788384,55.575515963626));
#126266=CARTESIAN_POINT('Ctrl Pts',(1.16624544379888,31.5634376782622,55.5755159651914));
#126267=CARTESIAN_POINT('Ctrl Pts',(1.16623403829253,31.5634966974797,55.5753556345072));
#126268=CARTESIAN_POINT('Ctrl Pts',(1.16622263360327,31.5635556920785,55.5751952946246));
#126269=CARTESIAN_POINT('Ctrl Pts',(1.16549978278659,31.5672935887586,55.5650313383302));
#126270=CARTESIAN_POINT('Ctrl Pts',(1.16479155412673,31.5708765010653,55.5549924630923));
#126271=CARTESIAN_POINT('Ctrl Pts',(1.16321387684814,31.5786777090593,55.5324534860398));
#126272=CARTESIAN_POINT('Ctrl Pts',(1.16234616653486,31.5828444033223,55.5199361839881));
#126273=CARTESIAN_POINT('Ctrl Pts',(1.1601383138976,31.5931230899973,55.4877883527716));
#126274=CARTESIAN_POINT('Ctrl Pts',(1.15880512462655,31.5990213017183,55.4680914366092));
#126275=CARTESIAN_POINT('Ctrl Pts',(1.14770618951907,31.6454494232188,55.3019122563605));
#126276=CARTESIAN_POINT('Ctrl Pts',(1.13864990821346,31.6661227755638,55.1506356284136));
#126277=CARTESIAN_POINT('Ctrl Pts',(1.12530414052524,31.6659471960532,54.9342472468964));
#126278=CARTESIAN_POINT('Ctrl Pts',(1.12127414953928,31.6621607415656,54.8699108188114));
#126279=CARTESIAN_POINT('Ctrl Pts',(1.1162752786559,31.6532510523558,54.793932828679));
#126280=CARTESIAN_POINT('Ctrl Pts',(1.11547760114754,31.6517091741316,54.7819185831932));
#126281=CARTESIAN_POINT('Ctrl Pts',(1.11421378868947,31.6490819982911,54.7630773716748));
#126282=CARTESIAN_POINT('Ctrl Pts',(1.1137523699807,31.6480849417241,54.7562382526835));
#126283=CARTESIAN_POINT('Ctrl Pts',(1.11288181022897,31.6461337943836,54.7434142255889));
#126284=CARTESIAN_POINT('Ctrl Pts',(1.11247321311694,31.6451895641239,54.7374280632467));
#126285=CARTESIAN_POINT('Ctrl Pts',(1.11150212154691,31.6428781770869,54.723276606843));
#126286=CARTESIAN_POINT('Ctrl Pts',(1.1109380953463,31.6414827909169,54.7151161974368));
#126287=CARTESIAN_POINT('Ctrl Pts',(1.1090222045819,31.6365634252889,54.6875838585901));
#126288=CARTESIAN_POINT('Ctrl Pts',(1.10765619497171,31.632757006768,54.668264919935));
#126289=CARTESIAN_POINT('Ctrl Pts',(1.10423986519777,31.6224862684322,54.6206070041068));
#126290=CARTESIAN_POINT('Ctrl Pts',(1.10217406604258,31.6156210860061,54.5923616185086));
#126291=CARTESIAN_POINT('Ctrl Pts',(1.09432055537429,31.5869811140024,54.4866582845914));
#126292=CARTESIAN_POINT('Ctrl Pts',(1.08842676319786,31.5603442806905,54.4106324482154));
#126293=CARTESIAN_POINT('Ctrl Pts',(1.07530636567537,31.4883412133279,54.2446965723646));
#126294=CARTESIAN_POINT('Ctrl Pts',(1.0681466313918,31.4401076398284,54.1563536337982));
#126295=CARTESIAN_POINT('Ctrl Pts',(1.0599068869644,31.3731329048861,54.0563594458513));
#126296=CARTESIAN_POINT('Ctrl Pts',(1.05855633702873,31.3617708975396,54.0400356506754));
#126297=CARTESIAN_POINT('Ctrl Pts',(1.05641641155044,31.3431562545548,54.0142878180469));
#126298=CARTESIAN_POINT('Ctrl Pts',(1.05561999068524,31.336090610107,54.0047316321445));
#126299=CARTESIAN_POINT('Ctrl Pts',(1.05411252219701,31.3224563140401,53.9866983288307));
#126300=CARTESIAN_POINT('Ctrl Pts',(1.05340077474465,31.3159069207834,53.9782074749021));
#126301=CARTESIAN_POINT('Ctrl Pts',(1.05177656430949,31.3007067251372,53.9588899944462));
#126302=CARTESIAN_POINT('Ctrl Pts',(1.05086630658539,31.2920018288,53.9481067914974));
#126303=CARTESIAN_POINT('Ctrl Pts',(1.04800717911774,31.2640807632862,53.9143891160484));
#126304=CARTESIAN_POINT('Ctrl Pts',(1.04607791873211,31.2443801830687,53.8918622359251));
#126305=CARTESIAN_POINT('Ctrl Pts',(1.03901434101723,31.169237342049,53.8104719438515));
#126306=CARTESIAN_POINT('Ctrl Pts',(1.03402986482835,31.1101379987447,53.7551351731194));
#126307=CARTESIAN_POINT('Ctrl Pts',(1.02299657396941,30.9698592406278,53.6417545557324));
#126308=CARTESIAN_POINT('Ctrl Pts',(1.0169913574635,30.887028736885,53.586269443464));
#126309=CARTESIAN_POINT('Ctrl Pts',(1.00882279596341,30.7742378446537,53.5245483071496));
#126310=CARTESIAN_POINT('Ctrl Pts',(1.00694867667202,30.7483637088535,53.5112577600136));
#126311=CARTESIAN_POINT('Ctrl Pts',(1.00438776453645,30.7132572841634,53.4943713688402));
#126312=CARTESIAN_POINT('Ctrl Pts',(1.00373427929968,30.7043200378587,53.4901699430492));
#126313=CARTESIAN_POINT('Ctrl Pts',(1.0026944037241,30.6901428265271,53.4836584599552));
#126314=CARTESIAN_POINT('Ctrl Pts',(1.00231115943869,30.6849272256988,53.4812954599143));
#126315=CARTESIAN_POINT('Ctrl Pts',(1.00150795393641,30.6740187393585,53.4764208401987));
#126316=CARTESIAN_POINT('Ctrl Pts',(1.00108768419088,30.6683238412235,53.4739141715872));
#126317=CARTESIAN_POINT('Ctrl Pts',(1.00003978700348,30.6541529439843,53.4677712337712));
#126318=CARTESIAN_POINT('Ctrl Pts',(0.999409936846762,30.6456606152799,
53.4641733736404));
#126319=CARTESIAN_POINT('Ctrl Pts',(0.996980272384737,30.6129812800444,
53.450647383833));
#126320=CARTESIAN_POINT('Ctrl Pts',(0.99515467477545,30.5885930081612,53.441219173195));
#126321=CARTESIAN_POINT('Ctrl Pts',(0.990223071858972,30.5229061866649,
53.4175866802113));
#126322=CARTESIAN_POINT('Ctrl Pts',(0.987081225495934,30.4812548006023,
53.4044260799589));
#126323=CARTESIAN_POINT('Ctrl Pts',(0.973275756936014,30.2974815630265,
53.3542097944964));
#126324=CARTESIAN_POINT('Ctrl Pts',(0.96251745536523,30.1512951460901,53.3343930279766));
#126325=CARTESIAN_POINT('Ctrl Pts',(0.950591734803027,29.9785721445165,
53.333937727724));
#126326=CARTESIAN_POINT('Ctrl Pts',(0.948827029643659,29.9527534430484,
53.3344698921893));
#126327=CARTESIAN_POINT('Ctrl Pts',(0.946183708033942,29.9137023296954,
53.3361836890162));
#126328=CARTESIAN_POINT('Ctrl Pts',(0.945291536352232,29.9004555142163,
53.336923658514));
#126329=CARTESIAN_POINT('Ctrl Pts',(0.94369091073918,29.8765754986089,53.3385439548971));
#126330=CARTESIAN_POINT('Ctrl Pts',(0.94298075034712,29.8659393610362,53.3393683275592));
#126331=CARTESIAN_POINT('Ctrl Pts',(0.941461618673189,29.8431033009809,
53.3413591098246));
#126332=CARTESIAN_POINT('Ctrl Pts',(0.940653709210325,29.8309067927053,
53.3425580922916));
#126333=CARTESIAN_POINT('Ctrl Pts',(0.93843092168224,29.7972184928342,53.3462455734345));
#126334=CARTESIAN_POINT('Ctrl Pts',(0.937024966057036,29.7757597774687,
53.3490183418476));
#126335=CARTESIAN_POINT('Ctrl Pts',(0.933902588934588,29.7278298552886,
53.356163353642));
#126336=CARTESIAN_POINT('Ctrl Pts',(0.932193062671097,29.7013977718548,
53.3607586102609));
#126337=CARTESIAN_POINT('Ctrl Pts',(0.926628040775296,29.6149603799195,
53.3779461628909));
#126338=CARTESIAN_POINT('Ctrl Pts',(0.922844664320479,29.5555363798742,
53.3932121901108));
#126339=CARTESIAN_POINT('Ctrl Pts',(0.913593322738773,29.4115448535048,
53.4388057515699));
#126340=CARTESIAN_POINT('Ctrl Pts',(0.908176262808959,29.328336818378,53.4727561737609));
#126341=CARTESIAN_POINT('Ctrl Pts',(0.899904699423246,29.2104833508854,
53.5323445526535));
#126342=CARTESIAN_POINT('Ctrl Pts',(0.897209163146009,29.1734401492577,
53.5528831405394));
#126343=CARTESIAN_POINT('Ctrl Pts',(0.893701527215476,29.1276350308805,
53.580612463476));
#126344=CARTESIAN_POINT('Ctrl Pts',(0.892961937286515,29.1181062444252,
53.5865131747315));
#126345=CARTESIAN_POINT('Ctrl Pts',(0.891774173536246,29.1030233592756,
53.5960651460512));
#126346=CARTESIAN_POINT('Ctrl Pts',(0.891329915986969,29.0974301284945,
53.5996544028974));
#126347=CARTESIAN_POINT('Ctrl Pts',(0.890470221332444,29.0867027366668,
53.6066292918335));
#126348=CARTESIAN_POINT('Ctrl Pts',(0.890055095152861,29.0815656347868,
53.610010024027));
#126349=CARTESIAN_POINT('Ctrl Pts',(0.88903715500841,29.0690707331154,53.6183324356169));
#126350=CARTESIAN_POINT('Ctrl Pts',(0.888432379421689,29.0617334892426,
53.6233044982939));
#126351=CARTESIAN_POINT('Ctrl Pts',(0.886208436377775,29.0350530367429,
53.6416967862867));
#126352=CARTESIAN_POINT('Ctrl Pts',(0.884568532850984,29.0159561887648,
53.6554674039132));
#126353=CARTESIAN_POINT('Ctrl Pts',(0.880274988250084,28.9672784494778,
53.69216118529));
#126354=CARTESIAN_POINT('Ctrl Pts',(0.877594993253211,28.9381672569238,
53.7156842112387));
#126355=CARTESIAN_POINT('Ctrl Pts',(0.869806054999817,28.8566070072196,
53.7862577004912));
#126356=CARTESIAN_POINT('Ctrl Pts',(0.864651643722582,28.8063166503866,
53.8356813250772));
#126357=CARTESIAN_POINT('Ctrl Pts',(0.852526539317233,28.6946564412618,
53.9602798842364));
#126358=CARTESIAN_POINT('Ctrl Pts',(0.845631044149412,28.6364131696759,
54.0379311614804));
#126359=CARTESIAN_POINT('Ctrl Pts',(0.837635025485726,28.5747386586289,
54.1371084991372));
#126360=CARTESIAN_POINT('Ctrl Pts',(0.836284189287029,28.5645378103655,
54.1541867847296));
#126361=CARTESIAN_POINT('Ctrl Pts',(0.834144343814903,28.5487371450569,
54.1817498965096));
#126362=CARTESIAN_POINT('Ctrl Pts',(0.833348275666138,28.5429396920421,
54.1921185868982));
#126363=CARTESIAN_POINT('Ctrl Pts',(0.831841815384134,28.5321255584706,
54.21195470068));
#126364=CARTESIAN_POINT('Ctrl Pts',(0.831130720372282,28.5270883629943,
54.221410192333));
#126365=CARTESIAN_POINT('Ctrl Pts',(0.829508494149889,28.5157548244046,
54.2431884452231));
#126366=CARTESIAN_POINT('Ctrl Pts',(0.828599559893766,28.5095200439121,
54.2555424858402));
#126367=CARTESIAN_POINT('Ctrl Pts',(0.825746749503835,28.4903271304715,
54.2947805943529));
#126368=CARTESIAN_POINT('Ctrl Pts',(0.823822384930057,28.4779365815331,
54.3219367958556));
#126369=CARTESIAN_POINT('Ctrl Pts',(0.816519047277932,28.4332119272116,
54.4273723233963));
#126370=CARTESIAN_POINT('Ctrl Pts',(0.811307955225365,28.4061327360044,
54.507743464591));
#126371=CARTESIAN_POINT('Ctrl Pts',(0.799647107030315,28.3591662828282,
54.6926375990911));
#126372=CARTESIAN_POINT('Ctrl Pts',(0.793245369348885,28.3429325806394,
54.7976900760107));
#126373=CARTESIAN_POINT('Ctrl Pts',(0.785068161700053,28.335562014142,54.9248006017527));
#126374=CARTESIAN_POINT('Ctrl Pts',(0.783685474318799,28.334737404848,54.9460635019496));
#126375=CARTESIAN_POINT('Ctrl Pts',(0.781704316928369,28.3341484662617,
54.9760952577574));
#126376=CARTESIAN_POINT('Ctrl Pts',(0.781122965769341,28.334045789722,54.984856353958));
#126377=CARTESIAN_POINT('Ctrl Pts',(0.780132315556956,28.3339889628622,
54.9996898057422));
#126378=CARTESIAN_POINT('Ctrl Pts',(0.779724974732296,28.3339988984451,
55.0057619937108));
#126379=CARTESIAN_POINT('Ctrl Pts',(0.778866540186639,28.3340893727542,
55.0184987328981));
#126380=CARTESIAN_POINT('Ctrl Pts',(0.778415105289353,28.3341767077085,
55.025162989298));
#126381=CARTESIAN_POINT('Ctrl Pts',(0.777192885164705,28.3345198133665,
55.0431200885004));
#126382=CARTESIAN_POINT('Ctrl Pts',(0.77641819953582,28.3348504484209,55.0544109132017));
#126383=CARTESIAN_POINT('Ctrl Pts',(0.772236304599404,28.3372384702508,
55.1149211838566));
#126384=CARTESIAN_POINT('Ctrl Pts',(0.768735890934266,28.341363235936,55.1640301718498));
#126385=CARTESIAN_POINT('Ctrl Pts',(0.75384952111547,28.3677864031852,55.3691239121344));
#126386=CARTESIAN_POINT('Ctrl Pts',(0.742214657580388,28.4099837168053,
55.5217660675314));
#126387=CARTESIAN_POINT('Ctrl Pts',(0.729199729424099,28.4850158501175,
55.6937445200622));
#126388=CARTESIAN_POINT('Ctrl Pts',(0.72713997536398,28.4977717882302,55.7209500921857));
#126389=CARTESIAN_POINT('Ctrl Pts',(0.72417509256806,28.5174218994855,55.7600702611463));
#126390=CARTESIAN_POINT('Ctrl Pts',(0.723250262152292,28.5237382485796,
55.7722667200562));
#126391=CARTESIAN_POINT('Ctrl Pts',(0.721611635753326,28.535261719143,55.7938596400568));
#126392=CARTESIAN_POINT('Ctrl Pts',(0.72089582484082,28.5404101869745,55.803286341546));
#126393=CARTESIAN_POINT('Ctrl Pts',(0.719397961123313,28.5514232858508,
55.8229955067832));
#126394=CARTESIAN_POINT('Ctrl Pts',(0.718616642452789,28.5573070822822,
55.8332666189716));
#126395=CARTESIAN_POINT('Ctrl Pts',(0.716548754468793,28.5732465218691,
55.8604164575752));
#126396=CARTESIAN_POINT('Ctrl Pts',(0.715269103039929,28.5834922957881,
55.8771818196099));
#126397=CARTESIAN_POINT('Ctrl Pts',(0.707913424028041,28.6445549642229,
55.9732387813358));
#126398=CARTESIAN_POINT('Ctrl Pts',(0.702083065101889,28.7017278787835,
56.0482927723663));
#126399=CARTESIAN_POINT('Ctrl Pts',(0.690587632322136,28.8277413581298,
56.1874849758101));
#126400=CARTESIAN_POINT('Ctrl Pts',(0.684939420233994,28.8962656891405,
56.2514308033437));
#126401=CARTESIAN_POINT('Ctrl Pts',(0.67672268997073,28.9988126347639,56.3321200353707));
#126402=CARTESIAN_POINT('Ctrl Pts',(0.674360470722042,29.0285854034851,
56.3539841775009));
#126403=CARTESIAN_POINT('Ctrl Pts',(0.671234809158863,29.0679126331245,
56.3808998108574));
#126404=CARTESIAN_POINT('Ctrl Pts',(0.670526040649685,29.0768259980924,
56.3868745056533));
#126405=CARTESIAN_POINT('Ctrl Pts',(0.669375955721784,29.0912686810264,
56.3963546260907));
#126406=CARTESIAN_POINT('Ctrl Pts',(0.668938124725499,29.0967622029471,
56.3999144010123));
#126407=CARTESIAN_POINT('Ctrl Pts',(0.668079047827891,29.1075282332294,
56.4068009852452));
#126408=CARTESIAN_POINT('Ctrl Pts',(0.667657999454671,29.1127986741173,
56.4101307277259));
#126409=CARTESIAN_POINT('Ctrl Pts',(0.666609254673614,29.1259138992273,
56.4183139944637));
#126410=CARTESIAN_POINT('Ctrl Pts',(0.665979347765396,29.133780469857,56.4231320438587));
#126411=CARTESIAN_POINT('Ctrl Pts',(0.663556970511623,29.1640060283959,
56.4413008871406));
#126412=CARTESIAN_POINT('Ctrl Pts',(0.661739036458412,29.1866356999515,
56.4541913568609));
#126413=CARTESIAN_POINT('Ctrl Pts',(0.656835581106417,29.2477549135031,
56.4871335917686));
#126414=CARTESIAN_POINT('Ctrl Pts',(0.65371484967794,29.2867407747695,56.506220368829));
#126415=CARTESIAN_POINT('Ctrl Pts',(0.640076189821123,29.4589623937029,
56.582350519456));
#126416=CARTESIAN_POINT('Ctrl Pts',(0.629462598419139,29.5986092714402,
56.6234086133886));
#126417=CARTESIAN_POINT('Ctrl Pts',(0.617561620180513,29.7686874948643,
56.6500879181067));
#126418=CARTESIAN_POINT('Ctrl Pts',(0.615701457171254,29.7956552060657,
56.653644147925));
#126419=CARTESIAN_POINT('Ctrl Pts',(0.612957121000256,29.835998568582,56.657962130611));
#126420=CARTESIAN_POINT('Ctrl Pts',(0.612057486776425,29.8493147962743,
56.6592253865871));
#126421=CARTESIAN_POINT('Ctrl Pts',(0.610447721933842,29.8733009036232,
56.661209698211));
#126422=CARTESIAN_POINT('Ctrl Pts',(0.609735821961458,29.8839651165113,
56.6619886393708));
#126423=CARTESIAN_POINT('Ctrl Pts',(0.608217440895881,29.9068273772939,
56.6634374293711));
#126424=CARTESIAN_POINT('Ctrl Pts',(0.607411978681493,29.919026839703,56.6640758936066));
#126425=CARTESIAN_POINT('Ctrl Pts',(0.60520759669882,29.9526008428531,56.665462910222));
#126426=CARTESIAN_POINT('Ctrl Pts',(0.603817320110536,29.9739849476055,
56.6659341733854));
#126427=CARTESIAN_POINT('Ctrl Pts',(0.595896665760208,30.0968653934603,
56.6662754507159));
#126428=CARTESIAN_POINT('Ctrl Pts',(0.589651416925288,30.1981760767792,
56.6572828877345));
#126429=CARTESIAN_POINT('Ctrl Pts',(0.576644099756275,30.4076116534788,
56.6192003237016));
#126430=CARTESIAN_POINT('Ctrl Pts',(0.569920155937744,30.5148861087348,
56.5883458173367));
#126431=CARTESIAN_POINT('Ctrl Pts',(0.561662264105647,30.633149300932,56.5410823750858));
#126432=CARTESIAN_POINT('Ctrl Pts',(0.560612884267485,30.6479462416258,
56.5349197196464));
#126433=CARTESIAN_POINT('Ctrl Pts',(0.559045953680191,30.6696561357093,
56.5255080955093));
#126434=CARTESIAN_POINT('Ctrl Pts',(0.558537676427858,30.6766398528819,
56.5224233292216));
#126435=CARTESIAN_POINT('Ctrl Pts',(0.557625806109177,30.6890592359119,
56.5168352517106));
#126436=CARTESIAN_POINT('Ctrl Pts',(0.55722333295034,30.6945029726856,56.5143504978949));
#126437=CARTESIAN_POINT('Ctrl Pts',(0.556325795834287,30.7065577552782,
56.5087695076465));
#126438=CARTESIAN_POINT('Ctrl Pts',(0.555829912306552,30.7131617844598,
56.5056591755241));
#126439=CARTESIAN_POINT('Ctrl Pts',(0.554343599794483,30.7327956957268,
56.4962539464864));
#126440=CARTESIAN_POINT('Ctrl Pts',(0.553345980772109,30.7457638374317,
56.4898327648505));
#126441=CARTESIAN_POINT('Ctrl Pts',(0.546088146329676,30.8387189767206,
56.4422882825654));
#126442=CARTESIAN_POINT('Ctrl Pts',(0.539537884083121,30.915336030933,56.3949199888804));
#126443=CARTESIAN_POINT('Ctrl Pts',(0.524133826461675,31.0856074310675,
56.2695589093804));
#126444=CARTESIAN_POINT('Ctrl Pts',(0.51534630348892,31.1753074655953,56.1870071311232));
#126445=CARTESIAN_POINT('Ctrl Pts',(0.505485110241221,31.2694579066818,
56.0791202099465));
#126446=CARTESIAN_POINT('Ctrl Pts',(0.504008422704584,31.2833609669245,
56.0625481210254));
#126447=CARTESIAN_POINT('Ctrl Pts',(0.501633853707625,31.3053884812245,
56.0352285593731));
#126448=CARTESIAN_POINT('Ctrl Pts',(0.500728035043655,31.3137118554183,
56.0246455175189));
#126449=CARTESIAN_POINT('Ctrl Pts',(0.499116706646434,31.3283712533504,
56.0055340115715));
#126450=CARTESIAN_POINT('Ctrl Pts',(0.498409304206956,31.3347556301056,
55.9970437563527));
#126451=CARTESIAN_POINT('Ctrl Pts',(0.496910589125443,31.3481689769721,
55.9788462723328));
#126452=CARTESIAN_POINT('Ctrl Pts',(0.496120185035914,31.355175316799,55.9691230513945));
#126453=CARTESIAN_POINT('Ctrl Pts',(0.493983313289197,31.3739259121142,
55.9425004312645));
#126454=CARTESIAN_POINT('Ctrl Pts',(0.492644753405512,31.3854631966573,
55.9254573282705));
#126455=CARTESIAN_POINT('Ctrl Pts',(0.484129435350948,31.4574196212838,
55.8147991138387));
#126456=CARTESIAN_POINT('Ctrl Pts',(0.477309236783129,31.5086369027444,
55.7155336274773));
#126457=CARTESIAN_POINT('Ctrl Pts',(0.469715587863468,31.554331224466,55.5998157085011));
#126458=CARTESIAN_POINT('Ctrl Pts',(0.468923766207712,31.5589558739021,
55.5876911645927));
#126459=CARTESIAN_POINT('Ctrl Pts',(0.468131466136093,31.5634376737814,
55.5755159773639));
#126460=CARTESIAN_POINT('Origin',(-1.54592528053767,-30.,125.));
#126461=CARTESIAN_POINT('',(0.904074719503818,-27.9452506257245,124.99839643692));
#126462=CARTESIAN_POINT('Ctrl Pts',(0.452117106605179,-31.2520409112987,
126.629230222815));
#126463=CARTESIAN_POINT('Ctrl Pts',(0.455981894727876,-31.3083783410325,
126.585935686613));
#126464=CARTESIAN_POINT('Ctrl Pts',(0.459846682850573,-31.3625576973326,
126.539646253954));
#126465=CARTESIAN_POINT('Ctrl Pts',(0.463711470973271,-31.4142452973653,
126.490606521313));
#126466=CARTESIAN_POINT('Ctrl Pts',(0.467571428034043,-31.4658682868712,
126.441628089312));
#126467=CARTESIAN_POINT('Ctrl Pts',(0.471431385094814,-31.5150053569671,
126.389906519012));
#126468=CARTESIAN_POINT('Ctrl Pts',(0.475291342155586,-31.5613556938613,
126.335726753399));
#126469=CARTESIAN_POINT('Ctrl Pts',(0.479148671756006,-31.6076744802303,
126.281583867779));
#126470=CARTESIAN_POINT('Ctrl Pts',(0.483006001356426,-31.6512099818744,
126.224986474436));
#126471=CARTESIAN_POINT('Ctrl Pts',(0.486863330956846,-31.6916990980054,
126.166255428415));
#126472=CARTESIAN_POINT('Ctrl Pts',(0.490719324021933,-31.7321741849659,
126.107544732255));
#126473=CARTESIAN_POINT('Ctrl Pts',(0.49457531708702,-31.7696047062383,
126.0467022504));
#126474=CARTESIAN_POINT('Ctrl Pts',(0.498431310152108,-31.8037696906984,
125.984079501574));
#126475=CARTESIAN_POINT('Ctrl Pts',(0.502287255796065,-31.8379342549964,
125.921457522884));
#126476=CARTESIAN_POINT('Ctrl Pts',(0.506143201440022,-31.8688331313069,
125.857055747879));
#126477=CARTESIAN_POINT('Ctrl Pts',(0.509999147083979,-31.896291146279,
125.791250561481));
#126478=CARTESIAN_POINT('Ctrl Pts',(0.513859005452489,-31.9237770235862,
125.725378600913));
#126479=CARTESIAN_POINT('Ctrl Pts',(0.517718863821,-31.9478148798075,125.658100834341));
#126480=CARTESIAN_POINT('Ctrl Pts',(0.521578722189511,-31.9682779451068,
125.589813100318));
#126481=CARTESIAN_POINT('Ctrl Pts',(0.525440585853742,-31.9887516414949,
125.52148988906));
#126482=CARTESIAN_POINT('Ctrl Pts',(0.529302449517972,-32.0056467333534,
125.452156137726));
#126483=CARTESIAN_POINT('Ctrl Pts',(0.533164313182203,-32.0188872512256,
125.382219608784));
#126484=CARTESIAN_POINT('Ctrl Pts',(0.537033128459735,-32.032151602917,
125.312157189405));
#126485=CARTESIAN_POINT('Ctrl Pts',(0.540901943737267,-32.0417481756389,
125.241490307152));
#126486=CARTESIAN_POINT('Ctrl Pts',(0.544770759014798,-32.0476527861995,
125.170633026315));
#126487=CARTESIAN_POINT('Ctrl Pts',(0.547681165584014,-32.0520946672745,
125.11732898339));
#126488=CARTESIAN_POINT('Ctrl Pts',(0.550591572153229,-32.0544482948932,
125.063917320894));
#126489=CARTESIAN_POINT('Ctrl Pts',(0.553501978722444,-32.054722795758,
125.010573319835));
#126490=CARTESIAN_POINT('Ctrl Pts',(0.557370585381146,-32.0550876711967,
124.939666746204));
#126491=CARTESIAN_POINT('Ctrl Pts',(0.561239192039847,-32.0517785733045,
124.86860204487));
#126492=CARTESIAN_POINT('Ctrl Pts',(0.565107798698548,-32.0447760923756,
124.797791457774));
#126493=CARTESIAN_POINT('Ctrl Pts',(0.568970633233783,-32.037784059442,
124.727086523045));
#126494=CARTESIAN_POINT('Ctrl Pts',(0.572833467769018,-32.0271096293515,
124.656635429572));
#126495=CARTESIAN_POINT('Ctrl Pts',(0.576696302304252,-32.0127854036125,
124.586850533699));
#126496=CARTESIAN_POINT('Ctrl Pts',(0.580554596587112,-31.9984780141111,
124.517147660766));
#126497=CARTESIAN_POINT('Ctrl Pts',(0.584412890869972,-31.9805294472387,
124.448109903765));
#126498=CARTESIAN_POINT('Ctrl Pts',(0.588271185152831,-31.9590239119133,
124.380142859159));
#126499=CARTESIAN_POINT('Ctrl Pts',(0.592127043638286,-31.9375319533458,
124.312218723139));
#126500=CARTESIAN_POINT('Ctrl Pts',(0.595982902123741,-31.9124876276894,
124.245364420624));
#126501=CARTESIAN_POINT('Ctrl Pts',(0.599838760609196,-31.8840255135458,
124.179972301194));
#126502=CARTESIAN_POINT('Ctrl Pts',(0.60369347558556,-31.8555718402427,
124.114599574718));
#126503=CARTESIAN_POINT('Ctrl Pts',(0.607548190561925,-31.8237025845142,
124.050688615762));
#126504=CARTESIAN_POINT('Ctrl Pts',(0.611402905538289,-31.7886005409679,
123.988612009489));
#126505=CARTESIAN_POINT('Ctrl Pts',(0.615257767676156,-31.7534971573306,
123.926533033317));
#126506=CARTESIAN_POINT('Ctrl Pts',(0.619112629814023,-31.7151609819453,
123.866288970761));
#126507=CARTESIAN_POINT('Ctrl Pts',(0.62296749195189,-31.6738200106235,
123.808226475149));
#126508=CARTESIAN_POINT('Ctrl Pts',(0.626826387848944,-31.6324357797721,
123.750103222468));
#126509=CARTESIAN_POINT('Ctrl Pts',(0.630685283745995,-31.5880407587821,
123.694166490385));
#126510=CARTESIAN_POINT('Ctrl Pts',(0.634544179643048,-31.5409048822941,
123.640731922606));
#126511=CARTESIAN_POINT('Ctrl Pts',(0.638405258875845,-31.4937423366638,
123.58726712193));
#126512=CARTESIAN_POINT('Ctrl Pts',(0.642266338108641,-31.443836188636,
123.536307651104));
#126513=CARTESIAN_POINT('Ctrl Pts',(0.646127417341438,-31.3914931636325,
123.488132169115));
#126514=CARTESIAN_POINT('Ctrl Pts',(0.649995255646101,-31.3390585087384,
123.439872352793));
#126515=CARTESIAN_POINT('Ctrl Pts',(0.653863093950765,-31.2841788341738,
123.394406565587));
#126516=CARTESIAN_POINT('Ctrl Pts',(0.657730932255428,-31.2271932805672,
123.351972629284));
#126517=CARTESIAN_POINT('Ctrl Pts',(0.660033038023954,-31.1932759444877,
123.326716296973));
#126518=CARTESIAN_POINT('Ctrl Pts',(0.66233514379248,-31.158613154127,123.302533177827));
#126519=CARTESIAN_POINT('Ctrl Pts',(0.664637249561006,-31.1232806678074,
123.279465750463));
#126520=CARTESIAN_POINT('Ctrl Pts',(0.668506416678538,-31.0638970825189,
123.240696145407));
#126521=CARTESIAN_POINT('Ctrl Pts',(0.672375583796069,-31.0023876857733,
123.204928638054));
#126522=CARTESIAN_POINT('Ctrl Pts',(0.6762447509136,-30.9390884475194,123.17240309416));
#126523=CARTESIAN_POINT('Ctrl Pts',(0.680108153533234,-30.8758835159508,
123.13992600861));
#126524=CARTESIAN_POINT('Ctrl Pts',(0.683971556152868,-30.8108944645568,
123.110681519179));
#126525=CARTESIAN_POINT('Ctrl Pts',(0.687834958772501,-30.7444855552332,
123.084865847898));
#126526=CARTESIAN_POINT('Ctrl Pts',(0.691693829694629,-30.6781545422923,
123.059080457906));
#126527=CARTESIAN_POINT('Ctrl Pts',(0.695552700616756,-30.6104074301625,
123.036716072269));
#126528=CARTESIAN_POINT('Ctrl Pts',(0.699411571538884,-30.5416307797413,
123.017921883241));
#126529=CARTESIAN_POINT('Ctrl Pts',(0.703268011629716,-30.4728974540225,
122.999139533298));
#126530=CARTESIAN_POINT('Ctrl Pts',(0.707124451720549,-30.4031363441796,
122.983923045746));
#126531=CARTESIAN_POINT('Ctrl Pts',(0.710980891811382,-30.3327501894497,
122.972372106643));
#126532=CARTESIAN_POINT('Ctrl Pts',(0.714836192489223,-30.2623848308161,
122.960824580347));
#126533=CARTESIAN_POINT('Ctrl Pts',(0.718691493167064,-30.1913952730109,
122.952940531037));
#126534=CARTESIAN_POINT('Ctrl Pts',(0.722546793844905,-30.1201937916367,
122.948768415085));
#126535=CARTESIAN_POINT('Ctrl Pts',(0.726402244915015,-30.0489895327484,
122.944596136382));
#126536=CARTESIAN_POINT('Ctrl Pts',(0.730257695985126,-29.9775738189337,
122.944136104734));
#126537=CARTESIAN_POINT('Ctrl Pts',(0.734113147055236,-29.9063616475896,
122.947384736133));
#126538=CARTESIAN_POINT('Ctrl Pts',(0.737972632756789,-29.8350749545201,
122.950636767143));
#126539=CARTESIAN_POINT('Ctrl Pts',(0.741832118458341,-29.7639927153693,
122.95760518641));
#126540=CARTESIAN_POINT('Ctrl Pts',(0.745691604159893,-29.6935266156856,
122.968234357214));
#126541=CARTESIAN_POINT('Ctrl Pts',(0.749553274580396,-29.6230206276243,
122.978869544816));
#126542=CARTESIAN_POINT('Ctrl Pts',(0.753414945000898,-29.5531319494602,
122.993169511702));
#126543=CARTESIAN_POINT('Ctrl Pts',(0.757276615421401,-29.4842611454871,
123.011027653172));
#126544=CARTESIAN_POINT('Ctrl Pts',(0.761145040678233,-29.4152698726602,
123.028917032115));
#126545=CARTESIAN_POINT('Ctrl Pts',(0.765013465935067,-29.3473004921461,
123.050376865672));
#126546=CARTESIAN_POINT('Ctrl Pts',(0.768881891191899,-29.2807368380768,
123.07525116797));
#126547=CARTESIAN_POINT('Ctrl Pts',(0.771178767594455,-29.2412146872921,
123.090020277927));
#126548=CARTESIAN_POINT('Ctrl Pts',(0.773475643997011,-29.2021877165685,
123.105992201612));
#126549=CARTESIAN_POINT('Ctrl Pts',(0.775772520399567,-29.1637321695312,
123.123126621686));
#126550=CARTESIAN_POINT('Ctrl Pts',(0.779641657361591,-29.0989529858227,
123.151989915313));
#126551=CARTESIAN_POINT('Ctrl Pts',(0.783510794323616,-29.0355430214481,
123.184267382036));
#126552=CARTESIAN_POINT('Ctrl Pts',(0.78737993128564,-28.9738860106988,
123.219806852204));
#126553=CARTESIAN_POINT('Ctrl Pts',(0.79124330480375,-28.912320843874,123.255293382983));
#126554=CARTESIAN_POINT('Ctrl Pts',(0.795106678321859,-28.8525038649618,
123.294032031484));
#126555=CARTESIAN_POINT('Ctrl Pts',(0.798970051839968,-28.7947974852949,
123.335823188165));
#126556=CARTESIAN_POINT('Ctrl Pts',(0.802828895384963,-28.7371587688626,
123.377565342902));
#126557=CARTESIAN_POINT('Ctrl Pts',(0.806687738929957,-28.6816261274668,
123.422352612775));
#126558=CARTESIAN_POINT('Ctrl Pts',(0.810546582474951,-28.628534554461,
123.469941146821));
#126559=CARTESIAN_POINT('Ctrl Pts',(0.81440299627091,-28.5754764109521,
123.517499716398));
#126560=CARTESIAN_POINT('Ctrl Pts',(0.818259410066869,-28.5248566472431,
123.567855727257));
#126561=CARTESIAN_POINT('Ctrl Pts',(0.822115823862828,-28.4769774383036,
123.620724886376));
#126562=CARTESIAN_POINT('Ctrl Pts',(0.82597109937082,-28.4291123617499,
123.673578440238));
#126563=CARTESIAN_POINT('Ctrl Pts',(0.829826374878813,-28.3839865599273,
123.728943309816));
#126564=CARTESIAN_POINT('Ctrl Pts',(0.833681650386806,-28.3418643390767,
123.786499405655));
#126565=CARTESIAN_POINT('Ctrl Pts',(0.837537077455988,-28.299740462289,
123.844057764179));
#126566=CARTESIAN_POINT('Ctrl Pts',(0.841392504525171,-28.2606206860118,
123.903807126687));
#126567=CARTESIAN_POINT('Ctrl Pts',(0.845247931594353,-28.2247270707112,
123.96539689299));
#126568=CARTESIAN_POINT('Ctrl Pts',(0.849107395262291,-28.1887958751061,
124.027051143246));
#126569=CARTESIAN_POINT('Ctrl Pts',(0.852966858930228,-28.1560978283416,
124.090549223239));
#126570=CARTESIAN_POINT('Ctrl Pts',(0.856826322598166,-28.1268094624695,
124.155515084441));
#126571=CARTESIAN_POINT('Ctrl Pts',(0.860687972062339,-28.097504509215,
124.220517738873));
#126572=CARTESIAN_POINT('Ctrl Pts',(0.864549621526512,-28.0716132573966,
124.286989376467));
#126573=CARTESIAN_POINT('Ctrl Pts',(0.868411270990685,-28.0492633864212,
124.354535650138));
#126574=CARTESIAN_POINT('Ctrl Pts',(0.872279677238259,-28.0268744095564,
124.422200110491));
#126575=CARTESIAN_POINT('Ctrl Pts',(0.876148083485833,-28.0080393132444,
124.490942492359));
#126576=CARTESIAN_POINT('Ctrl Pts',(0.880016489733406,-27.9928352155008,
124.560355722923));
#126577=CARTESIAN_POINT('Ctrl Pts',(0.88231359023498,-27.9838068616213,
124.60157403262));
#126578=CARTESIAN_POINT('Ctrl Pts',(0.884610690736553,-27.9760578526443,
124.643028722785));
#126579=CARTESIAN_POINT('Ctrl Pts',(0.886907791238126,-27.969595668015,
124.684633845893));
#126580=CARTESIAN_POINT('Ctrl Pts',(0.892630100646193,-27.9534977132778,
124.788276410603));
#126581=CARTESIAN_POINT('Ctrl Pts',(0.898352410054259,-27.9453327368298,
124.893182202474));
#126582=CARTESIAN_POINT('Ctrl Pts',(0.904074719462325,-27.9452506257251,
124.998396436157));
#126583=CARTESIAN_POINT('Ctrl Pts',(0.904074719503818,-27.9452506257245,
124.99839643692));
#126584=CARTESIAN_POINT('Ctrl Pts',(0.907990067111021,-27.9451944432742,
125.070386654283));
#126585=CARTESIAN_POINT('Ctrl Pts',(0.911905414718225,-27.9489263631045,
125.142516745463));
#126586=CARTESIAN_POINT('Ctrl Pts',(0.915820762325428,-27.9564608111608,
125.214348189119));
#126587=CARTESIAN_POINT('Ctrl Pts',(0.919623075698889,-27.9637777432651,
125.284105892968));
#126588=CARTESIAN_POINT('Ctrl Pts',(0.923425389072348,-27.9746805797795,
125.353581419206));
#126589=CARTESIAN_POINT('Ctrl Pts',(0.927227702445809,-27.9891298100322,
125.422372633582));
#126590=CARTESIAN_POINT('Ctrl Pts',(0.931027545776556,-28.0035696538372,
125.4911191601));
#126591=CARTESIAN_POINT('Ctrl Pts',(0.934827389107304,-28.0215512222172,
125.55918176638));
#126592=CARTESIAN_POINT('Ctrl Pts',(0.93862723243805,-28.0429835185496,
125.626166155131));
#126593=CARTESIAN_POINT('Ctrl Pts',(0.942425966459145,-28.0644095580311,
125.693130988752));
#126594=CARTESIAN_POINT('Ctrl Pts',(0.946224700480239,-28.0892841740311,
125.75901775194));
#126595=CARTESIAN_POINT('Ctrl Pts',(0.950023434501334,-28.1174663973963,
125.823446900272));
#126596=CARTESIAN_POINT('Ctrl Pts',(0.953822418190325,-28.1456504730093,
125.887880283144));
#126597=CARTESIAN_POINT('Ctrl Pts',(0.957621401879316,-28.1771423830415,
125.95085540307));
#126598=CARTESIAN_POINT('Ctrl Pts',(0.961420385568307,-28.2117536492897,
126.012014106459));
#126599=CARTESIAN_POINT('Ctrl Pts',(0.965223301434588,-28.2464007402864,
126.073236112794));
#126600=CARTESIAN_POINT('Ctrl Pts',(0.969026217300869,-28.2841733783799,
126.132637516528));
#126601=CARTESIAN_POINT('Ctrl Pts',(0.972829133167149,-28.3248385009404,
126.189887185648));
#126602=CARTESIAN_POINT('Ctrl Pts',(0.976634453101162,-28.3655293305405,
126.247173045965));
#126603=CARTESIAN_POINT('Ctrl Pts',(0.980439773035174,-28.4091159674221,
126.302304075996));
#126604=CARTESIAN_POINT('Ctrl Pts',(0.984245092969186,-28.4553254313972,
126.354982671333));
#126605=CARTESIAN_POINT('Ctrl Pts',(0.988056543848615,-28.5016093458013,
126.407746139846));
#126606=CARTESIAN_POINT('Ctrl Pts',(0.991867994728043,-28.5505241611592,
126.458048940715));
#126607=CARTESIAN_POINT('Ctrl Pts',(0.995679445607472,-28.6017613924464,
126.505631548171));
#126608=CARTESIAN_POINT('Ctrl Pts',(0.996467317763876,-28.6123527365773,
126.515467438158));
#126609=CARTESIAN_POINT('Ctrl Pts',(0.99725518992028,-28.623043212392,126.525187238548));
#126610=CARTESIAN_POINT('Ctrl Pts',(0.998043062076684,-28.6338299377042,
126.534788885608));
#126611=CARTESIAN_POINT('Ctrl Pts',(1.00191215041398,-28.6868014671125,
126.581940724086));
#126612=CARTESIAN_POINT('Ctrl Pts',(1.00578123875128,-28.7423207029647,
126.626439315564));
#126613=CARTESIAN_POINT('Ctrl Pts',(1.00965032708858,-28.8000910094635,
126.667997595001));
#126614=CARTESIAN_POINT('Ctrl Pts',(1.01351365059778,-28.8577752399007,
126.709493953822));
#126615=CARTESIAN_POINT('Ctrl Pts',(1.01737697410698,-28.9177034921955,
126.748058415354));
#126616=CARTESIAN_POINT('Ctrl Pts',(1.02124029761618,-28.9795446740498,
126.783442875519));
#126617=CARTESIAN_POINT('Ctrl Pts',(1.02509908933243,-29.0413133143655,
126.818785828664));
#126618=CARTESIAN_POINT('Ctrl Pts',(1.02895788104868,-29.1049900074564,
126.850955949871));
#126619=CARTESIAN_POINT('Ctrl Pts',(1.03281667276493,-29.1702146287174,
126.879748334247));
#126620=CARTESIAN_POINT('Ctrl Pts',(1.03667303363584,-29.2353981617367,
126.908522580864));
#126621=CARTESIAN_POINT('Ctrl Pts',(1.04052939450675,-29.3021272449515,
126.933923116469));
#126622=CARTESIAN_POINT('Ctrl Pts',(1.04438575537766,-29.3700184070463,
126.955791592946));
#126623=CARTESIAN_POINT('Ctrl Pts',(1.04824097694197,-29.4378895116695,
126.977653608695));
#126624=CARTESIAN_POINT('Ctrl Pts',(1.05209619850629,-29.506921551454,126.995985488087));
#126625=CARTESIAN_POINT('Ctrl Pts',(1.0559514200706,-29.5767140212836,127.010678130065));
#126626=CARTESIAN_POINT('Ctrl Pts',(1.05980679225408,-29.6465092178263,
127.025371346068));
#126627=CARTESIAN_POINT('Ctrl Pts',(1.06366216443755,-29.7170644275819,
127.03642494446));
#126628=CARTESIAN_POINT('Ctrl Pts',(1.06751753662103,-29.7879687307261,
127.043780884378));
#126629=CARTESIAN_POINT('Ctrl Pts',(1.07137694433534,-29.8589472514783,
127.051144523975));
#126630=CARTESIAN_POINT('Ctrl Pts',(1.07523635204964,-29.9302751108738,
127.054802728585));
#126631=CARTESIAN_POINT('Ctrl Pts',(1.07909575976395,-30.0015369395232,
127.05474942519));
#126632=CARTESIAN_POINT('Ctrl Pts',(1.08295735258731,-30.0728391150027,
127.054696091615));
#126633=CARTESIAN_POINT('Ctrl Pts',(1.08681894541067,-30.1440746999807,
127.050927092529));
#126634=CARTESIAN_POINT('Ctrl Pts',(1.09068053823403,-30.2148317599149,
127.04348840893));
#126635=CARTESIAN_POINT('Ctrl Pts',(1.09454888736175,-30.2857126175292,
127.036036710492));
#126636=CARTESIAN_POINT('Ctrl Pts',(1.09841723648948,-30.3561127985652,
127.024902584658));
#126637=CARTESIAN_POINT('Ctrl Pts',(1.1022855856172,-30.4256295856275,127.010183329535));
#126638=CARTESIAN_POINT('Ctrl Pts',(1.10458316804988,-30.4669186584224,
127.001440917494));
#126639=CARTESIAN_POINT('Ctrl Pts',(1.10688075048256,-30.5078963491774,
126.991434748811));
#126640=CARTESIAN_POINT('Ctrl Pts',(1.10917833291525,-30.5484811992541,
126.980193408878));
#126641=CARTESIAN_POINT('Ctrl Pts',(1.11304631609095,-30.6168058500052,
126.961268597688));
#126642=CARTESIAN_POINT('Ctrl Pts',(1.11691429926665,-30.6842836647767,
126.938766367269));
#126643=CARTESIAN_POINT('Ctrl Pts',(1.12078228244236,-30.7505129247959,
126.912780152609));
#126644=CARTESIAN_POINT('Ctrl Pts',(1.12464523167393,-30.8166559914737,
126.886827757421));
#126645=CARTESIAN_POINT('Ctrl Pts',(1.12850818090551,-30.8815532773588,
126.857400544484));
#126646=CARTESIAN_POINT('Ctrl Pts',(1.13237113013709,-30.9448168729143,
126.824642057817));
#126647=CARTESIAN_POINT('Ctrl Pts',(1.13622985099915,-31.0080112203791,
126.791919428466));
#126648=CARTESIAN_POINT('Ctrl Pts',(1.1400885718612,-31.069574998631,126.755872986999));
#126649=CARTESIAN_POINT('Ctrl Pts',(1.14394729272326,-31.1291407496662,
126.716694128243));
#126650=CARTESIAN_POINT('Ctrl Pts',(1.146668096559,-31.1711408656863,126.689068914345));
#126651=CARTESIAN_POINT('Ctrl Pts',(1.14938890039474,-31.212148009238,126.659887366754));
#126652=CARTESIAN_POINT('Ctrl Pts',(1.15210970423049,-31.2520409112987,
126.629230222815));
#126653=CARTESIAN_POINT('',(0.845925280586436,-27.945250330481,125.00116538046));
#126654=CARTESIAN_POINT('Ctrl Pts',(0.845925280586436,-27.945250330481,
125.00116538046));
#126655=CARTESIAN_POINT('Ctrl Pts',(0.85022219368581,-27.9452954735043,
125.080759654999));
#126656=CARTESIAN_POINT('Ctrl Pts',(0.854519106785184,-27.9499695693127,
125.160186918996));
#126657=CARTESIAN_POINT('Ctrl Pts',(0.858816019884558,-27.9591900445396,
125.23893992591));
#126658=CARTESIAN_POINT('Ctrl Pts',(0.86313050384008,-27.9684482239602,
125.318014968137));
#126659=CARTESIAN_POINT('Ctrl Pts',(0.867444987795601,-27.9822899038121,
125.396409967232));
#126660=CARTESIAN_POINT('Ctrl Pts',(0.871759471751123,-28.0005817423557,
125.473628750709));
#126661=CARTESIAN_POINT('Ctrl Pts',(0.876096088705256,-28.0189674167418,
125.551243661104));
#126662=CARTESIAN_POINT('Ctrl Pts',(0.88043270565939,-28.0418488879396,
125.62767000483));
#126663=CARTESIAN_POINT('Ctrl Pts',(0.884769322613523,-28.0690426460444,
125.702425269836));
#126664=CARTESIAN_POINT('Ctrl Pts',(0.88620693731184,-28.0780575410115,
125.727207091447));
#126665=CARTESIAN_POINT('Ctrl Pts',(0.887644552010157,-28.0875459587084,
125.751805457319));
#126666=CARTESIAN_POINT('Ctrl Pts',(0.889082166708475,-28.0975000961443,
125.776203374335));
#126667=CARTESIAN_POINT('Ctrl Pts',(0.892951333584334,-28.1242904586036,
125.841867430545));
#126668=CARTESIAN_POINT('Ctrl Pts',(0.896820500460194,-28.15453682424,125.906271445725));
#126669=CARTESIAN_POINT('Ctrl Pts',(0.900689667336053,-28.1880992959586,
125.969027038423));
#126670=CARTESIAN_POINT('Ctrl Pts',(0.904553069711517,-28.2216117644367,
126.031689134342));
#126671=CARTESIAN_POINT('Ctrl Pts',(0.90841647208698,-28.2584303049682,
126.092707257843));
#126672=CARTESIAN_POINT('Ctrl Pts',(0.912279874462444,-28.2983669267469,
126.151712831617));
#126673=CARTESIAN_POINT('Ctrl Pts',(0.916138745137886,-28.3382567036019,
126.210649192937));
#126674=CARTESIAN_POINT('Ctrl Pts',(0.919997615813329,-28.3812570258022,
126.267577293327));
#126675=CARTESIAN_POINT('Ctrl Pts',(0.923856486488771,-28.4271348119871,
126.32215455331));
#126676=CARTESIAN_POINT('Ctrl Pts',(0.927712926331499,-28.4729836982081,
126.376697433237));
#126677=CARTESIAN_POINT('Ctrl Pts',(0.931569366174226,-28.521706140386,
126.428892039833));
#126678=CARTESIAN_POINT('Ctrl Pts',(0.935425806016954,-28.5730275921944,
126.478427309631));
#126679=CARTESIAN_POINT('Ctrl Pts',(0.939281106445644,-28.6243338806954,
126.527947943862));
#126680=CARTESIAN_POINT('Ctrl Pts',(0.943136406874334,-28.6782373050151,
126.574810464008));
#126681=CARTESIAN_POINT('Ctrl Pts',(0.946991707303024,-28.7344263364808,
126.618740518028));
#126682=CARTESIAN_POINT('Ctrl Pts',(0.950847158123302,-28.7906175598271,
126.662672285718));
#126683=CARTESIAN_POINT('Ctrl Pts',(0.954702608943581,-28.8490941832946,
126.703671062714));
#126684=CARTESIAN_POINT('Ctrl Pts',(0.958558059763859,-28.9095128396272,
126.741503751234));
#126685=CARTESIAN_POINT('Ctrl Pts',(0.962417545216279,-28.9699947225614,
126.77937603071));
#126686=CARTESIAN_POINT('Ctrl Pts',(0.966277030668698,-29.0324222827182,
126.814075349425));
#126687=CARTESIAN_POINT('Ctrl Pts',(0.970136516121118,-29.0964252698175,
126.845413305868));
#126688=CARTESIAN_POINT('Ctrl Pts',(0.973998186292504,-29.1604644867567,
126.876769001626));
#126689=CARTESIAN_POINT('Ctrl Pts',(0.977859856463891,-29.2260804589129,
126.904759356628));
#126690=CARTESIAN_POINT('Ctrl Pts',(0.981721526635277,-29.292883093083,
126.929244215348));
#126691=CARTESIAN_POINT('Ctrl Pts',(0.985589951645727,-29.3598025785177,
126.953771903018));
#126692=CARTESIAN_POINT('Ctrl Pts',(0.989458376656176,-29.4279124058617,
126.974781708812));
#126693=CARTESIAN_POINT('Ctrl Pts',(0.993326801666625,-29.4968081547775,
126.992183608356));
#126694=CARTESIAN_POINT('Ctrl Pts',(0.99562368029343,-29.5377150284366,
127.002515991954));
#126695=CARTESIAN_POINT('Ctrl Pts',(0.997920558920233,-29.5788987710876,
127.0115774254));
#126696=CARTESIAN_POINT('Ctrl Pts',(1.00021743754704,-29.6202737412824,
127.019357702573));
#126697=CARTESIAN_POINT('Ctrl Pts',(1.00411924001165,-29.6905591097799,
127.032574380325));
#126698=CARTESIAN_POINT('Ctrl Pts',(1.00802104247626,-29.7616741112237,
127.042143266183));
#126699=CARTESIAN_POINT('Ctrl Pts',(1.01192284494087,-29.8332062447118,
127.047969092955));
#126700=CARTESIAN_POINT('Ctrl Pts',(1.01578547045942,-29.9040201433429,
127.053736424171));
#126701=CARTESIAN_POINT('Ctrl Pts',(1.01964809597797,-29.9752423456309,
127.055835443642));
#126702=CARTESIAN_POINT('Ctrl Pts',(1.02351072149651,-30.0464614134387,
127.05422464681));
#126703=CARTESIAN_POINT('Ctrl Pts',(1.02736946478645,-30.117608900737,127.052615468949));
#126704=CARTESIAN_POINT('Ctrl Pts',(1.03122820807639,-30.1887527767806,
127.047303883675));
#126705=CARTESIAN_POINT('Ctrl Pts',(1.03508695136633,-30.2594788442955,
127.03830034388));
#126706=CARTESIAN_POINT('Ctrl Pts',(1.03894310717835,-30.3301574864897,
127.029302841403));
#126707=CARTESIAN_POINT('Ctrl Pts',(1.04279926299038,-30.4004183956563,
127.016618359994));
#126708=CARTESIAN_POINT('Ctrl Pts',(1.0466554188024,-30.4698514739257,127.000309264826));
#126709=CARTESIAN_POINT('Ctrl Pts',(1.05058919196034,-30.5406821127495,
126.983671897477));
#126710=CARTESIAN_POINT('Ctrl Pts',(1.05452296511828,-30.6106507113064,
126.963262454806));
#126711=CARTESIAN_POINT('Ctrl Pts',(1.05845673827622,-30.6793332005368,
126.939201888703));
#126712=CARTESIAN_POINT('Ctrl Pts',(1.06231299626292,-30.7466622983283,
126.915615437102));
#126713=CARTESIAN_POINT('Ctrl Pts',(1.06616925424962,-30.8127550614049,
126.888520672006));
#126714=CARTESIAN_POINT('Ctrl Pts',(1.07002551223631,-30.8772297845218,
126.858081125152));
#126715=CARTESIAN_POINT('Ctrl Pts',(1.07399804297988,-30.9436485305311,
126.826723774033));
#126716=CARTESIAN_POINT('Ctrl Pts',(1.07797057372345,-31.0083495876843,
126.791816908259));
#126717=CARTESIAN_POINT('Ctrl Pts',(1.08194310446701,-31.0709426864352,
126.753590409666));
#126718=CARTESIAN_POINT('Ctrl Pts',(1.08591563521058,-31.1335357851862,
126.715363911072));
#126719=CARTESIAN_POINT('Ctrl Pts',(1.08988816595415,-31.1940204803808,
126.67381812217));
#126720=CARTESIAN_POINT('Ctrl Pts',(1.09386069669771,-31.2520409112987,
126.629230222815));
#126721=CARTESIAN_POINT('Ctrl Pts',(0.393902764517251,-31.2520409112987,
126.629230222815));
#126722=CARTESIAN_POINT('Ctrl Pts',(0.397765020730025,-31.3086816915374,
126.585702565942));
#126723=CARTESIAN_POINT('Ctrl Pts',(0.401627276942799,-31.3630392040398,
126.539226023053));
#126724=CARTESIAN_POINT('Ctrl Pts',(0.405489533155574,-31.4148028017945,
126.490077378707));
#126725=CARTESIAN_POINT('Ctrl Pts',(0.409356059028123,-31.4666236233425,
126.440874401355));
#126726=CARTESIAN_POINT('Ctrl Pts',(0.413222584900672,-31.5158444569778,
126.388993762238));
#126727=CARTESIAN_POINT('Ctrl Pts',(0.417089110773222,-31.5621914994499,
126.33474914555));
#126728=CARTESIAN_POINT('Ctrl Pts',(0.42095811694271,-31.6085682725979,
126.280469732055));
#126729=CARTESIAN_POINT('Ctrl Pts',(0.424827123112198,-31.6520672913701,
126.223823706893));
#126730=CARTESIAN_POINT('Ctrl Pts',(0.428696129281686,-31.6924567108541,
126.165155716797));
#126731=CARTESIAN_POINT('Ctrl Pts',(0.432571643378787,-31.7329140680478,
126.106389043211));
#126732=CARTESIAN_POINT('Ctrl Pts',(0.436447157475887,-31.7702511359751,
126.045594029938));
#126733=CARTESIAN_POINT('Ctrl Pts',(0.440322671572987,-31.8042812499767,
125.983141258153));
#126734=CARTESIAN_POINT('Ctrl Pts',(0.441728808833403,-31.8166282599669,
125.960481769057));
#126735=CARTESIAN_POINT('Ctrl Pts',(0.443134946093818,-31.828540390247,
125.937604245957));
#126736=CARTESIAN_POINT('Ctrl Pts',(0.444541083354234,-31.8400103070147,
125.914526999372));
#126737=CARTESIAN_POINT('Ctrl Pts',(0.44840642658579,-31.8715400633143,
125.851089750817));
#126738=CARTESIAN_POINT('Ctrl Pts',(0.452271769817345,-31.8998482225227,
125.785893454723));
#126739=CARTESIAN_POINT('Ctrl Pts',(0.456137113048901,-31.9247355213386,
125.719298780339));
#126740=CARTESIAN_POINT('Ctrl Pts',(0.459996637425455,-31.9495853550253,
125.652804357015));
#126741=CARTESIAN_POINT('Ctrl Pts',(0.463856161802009,-31.9710243806548,
125.584916185923));
#126742=CARTESIAN_POINT('Ctrl Pts',(0.467715686178562,-31.988899935638,
125.516018031196));
#126743=CARTESIAN_POINT('Ctrl Pts',(0.471570616814023,-32.0067542145096,
125.447201881465));
#126744=CARTESIAN_POINT('Ctrl Pts',(0.475425547449484,-32.0210533254499,
125.377378604707));
#126745=CARTESIAN_POINT('Ctrl Pts',(0.479280478084945,-32.0316938889068,
125.306948699751));
#126746=CARTESIAN_POINT('Ctrl Pts',(0.483132941660506,-32.0423276426672,
125.236563868186));
#126747=CARTESIAN_POINT('Ctrl Pts',(0.486985405236067,-32.0493074212925,
125.165573658832));
#126748=CARTESIAN_POINT('Ctrl Pts',(0.490837868811627,-32.0525808856403,
125.094388931576));
#126749=CARTESIAN_POINT('Ctrl Pts',(0.494689162603668,-32.0558533560152,
125.023225819248));
#126750=CARTESIAN_POINT('Ctrl Pts',(0.498540456395708,-32.0554217238142,
124.951868792349));
#126751=CARTESIAN_POINT('Ctrl Pts',(0.502391750187749,-32.0512856380332,
124.880732260444));
#126752=CARTESIAN_POINT('Ctrl Pts',(0.506243169824716,-32.0471494171013,
124.80959340408));
#126753=CARTESIAN_POINT('Ctrl Pts',(0.510094589461684,-32.0393085327444,
124.73867554294));
#126754=CARTESIAN_POINT('Ctrl Pts',(0.513946009098651,-32.0278146390282,
124.668389758537));
#126755=CARTESIAN_POINT('Ctrl Pts',(0.517801453495946,-32.0163087341131,
124.598030525001));
#126756=CARTESIAN_POINT('Ctrl Pts',(0.52165689789324,-32.0011422781157,
124.528305168249));
#126757=CARTESIAN_POINT('Ctrl Pts',(0.525512342290535,-31.9824182414273,
124.459615434569));
#126758=CARTESIAN_POINT('Ctrl Pts',(0.529369959655217,-31.9636836516829,
124.390886986662));
#126759=CARTESIAN_POINT('Ctrl Pts',(0.5332275770199,-31.9413876423888,124.323195786347));
#126760=CARTESIAN_POINT('Ctrl Pts',(0.537085194384582,-31.9156825106371,
124.256926597879));
#126761=CARTESIAN_POINT('Ctrl Pts',(0.540949591980453,-31.8899321989934,
124.190540933262));
#126762=CARTESIAN_POINT('Ctrl Pts',(0.544813989576324,-31.8607610014774,
124.125582714751));
#126763=CARTESIAN_POINT('Ctrl Pts',(0.548678387172195,-31.8283683107149,
124.062414333048));
#126764=CARTESIAN_POINT('Ctrl Pts',(0.551011042845729,-31.8088152000389,
124.024284176844));
#126765=CARTESIAN_POINT('Ctrl Pts',(0.553343698519263,-31.7880891683627,
123.986805673443));
#126766=CARTESIAN_POINT('Ctrl Pts',(0.555676354192797,-31.7662416108555,
123.950053270598));
#126767=CARTESIAN_POINT('Ctrl Pts',(0.559545932806801,-31.7299992960307,
123.889085716031));
#126768=CARTESIAN_POINT('Ctrl Pts',(0.563415511420805,-31.6905256384392,
123.829877628157));
#126769=CARTESIAN_POINT('Ctrl Pts',(0.56728509003481,-31.6480166895168,
123.772792375523));
#126770=CARTESIAN_POINT('Ctrl Pts',(0.571148902574401,-31.6055710833475,
123.71579218585));
#126771=CARTESIAN_POINT('Ctrl Pts',(0.575012715113993,-31.5600994514413,
123.660908938752));
#126772=CARTESIAN_POINT('Ctrl Pts',(0.578876527653584,-31.5118424650373,
123.608479276687));
#126773=CARTESIAN_POINT('Ctrl Pts',(0.582735804066608,-31.4636421324683,
123.556111167189));
#126774=CARTESIAN_POINT('Ctrl Pts',(0.586595080479631,-31.4126632681155,
123.506191276576));
#126775=CARTESIAN_POINT('Ctrl Pts',(0.590454356892654,-31.3591872739167,
123.459023842844));
#126776=CARTESIAN_POINT('Ctrl Pts',(0.594311199502693,-31.3057450036651,
123.411886154647));
#126777=CARTESIAN_POINT('Ctrl Pts',(0.598168042112731,-31.2498090912909,
123.367497799978));
#126778=CARTESIAN_POINT('Ctrl Pts',(0.602024884722769,-31.1916972663116,
123.326125695291));
#126779=CARTESIAN_POINT('Ctrl Pts',(0.605880584327041,-31.1336026632306,
123.284765851553));
#126780=CARTESIAN_POINT('Ctrl Pts',(0.609736283931313,-31.0733338231633,
123.246420764666));
#126781=CARTESIAN_POINT('Ctrl Pts',(0.613591983535585,-31.0112396003772,
123.211315557979));
#126782=CARTESIAN_POINT('Ctrl Pts',(0.617447829314859,-30.9491430235117,
123.176209020403));
#126783=CARTESIAN_POINT('Ctrl Pts',(0.621303675094133,-30.8852213503721,
123.144342843979));
#126784=CARTESIAN_POINT('Ctrl Pts',(0.625159520873407,-30.8198488004311,
123.115896630508));
#126785=CARTESIAN_POINT('Ctrl Pts',(0.629019392036878,-30.7544080035621,
123.087420720066));
#126786=CARTESIAN_POINT('Ctrl Pts',(0.63287926320035,-30.6875137524757,
123.062372093968));
#126787=CARTESIAN_POINT('Ctrl Pts',(0.636739134363821,-30.6195602206645,
123.040882163965));
#126788=CARTESIAN_POINT('Ctrl Pts',(0.640601185605821,-30.5515683082884,
123.01938009632));
#126789=CARTESIAN_POINT('Ctrl Pts',(0.644463236847821,-30.4825163944218,
123.001440848258));
#126790=CARTESIAN_POINT('Ctrl Pts',(0.648325288089821,-30.4128111208673,
122.987145176376));
#126791=CARTESIAN_POINT('Ctrl Pts',(0.652194082616269,-30.3429841393247,
122.97282454372));
#126792=CARTESIAN_POINT('Ctrl Pts',(0.656062877142717,-30.2725020007958,
122.962160261539));
#126793=CARTESIAN_POINT('Ctrl Pts',(0.659931671669165,-30.2017780807413,
122.955181384907));
#126794=CARTESIAN_POINT('Ctrl Pts',(0.662224989456562,-30.1598548349481,
122.951044493736));
#126795=CARTESIAN_POINT('Ctrl Pts',(0.664518307243959,-30.1178466836125,
122.948201584349));
#126796=CARTESIAN_POINT('Ctrl Pts',(0.666811625031356,-30.0758394270535,
122.946650067864));
#126797=CARTESIAN_POINT('Ctrl Pts',(0.670681339064105,-30.0049569392113,
122.944032059515));
#126798=CARTESIAN_POINT('Ctrl Pts',(0.674551053096854,-29.9338004265351,
122.945083589534));
#126799=CARTESIAN_POINT('Ctrl Pts',(0.678420767129603,-29.8627815495254,
122.949836918841));
#126800=CARTESIAN_POINT('Ctrl Pts',(0.682284730142912,-29.791868218026,
122.954583183933));
#126801=CARTESIAN_POINT('Ctrl Pts',(0.686148693156222,-29.7210925967539,
122.963020295739));
#126802=CARTESIAN_POINT('Ctrl Pts',(0.690012656169532,-29.6508680762893,
122.975128531895));
#126803=CARTESIAN_POINT('Ctrl Pts',(0.693872104829046,-29.5807256006914,
122.98722262173));
#126804=CARTESIAN_POINT('Ctrl Pts',(0.697731553488561,-29.5111334231914,
123.002979234233));
#126805=CARTESIAN_POINT('Ctrl Pts',(0.701591002148075,-29.4424997873939,
123.022326853233));
#126806=CARTESIAN_POINT('Ctrl Pts',(0.705448030375005,-29.3739091948138,
123.041662338476));
#126807=CARTESIAN_POINT('Ctrl Pts',(0.709305058601936,-29.3062764175459,
123.06458423062));
#126808=CARTESIAN_POINT('Ctrl Pts',(0.713162086828866,-29.2399980313748,
123.090970254243));
#126809=CARTESIAN_POINT('Ctrl Pts',(0.717017985171078,-29.1737390609121,
123.117348548296));
#126810=CARTESIAN_POINT('Ctrl Pts',(0.720873883513291,-29.1088341447766,
123.147188779646));
#126811=CARTESIAN_POINT('Ctrl Pts',(0.724729781855503,-29.0456616135279,
123.180319861458));
#126812=CARTESIAN_POINT('Ctrl Pts',(0.728585839258048,-28.982486476338,
123.213452309965));
#126813=CARTESIAN_POINT('Ctrl Pts',(0.732441896660594,-28.9210442949365,
123.249875650967));
#126814=CARTESIAN_POINT('Ctrl Pts',(0.736297954063139,-28.8616888998584,
123.289372804555));
#126815=CARTESIAN_POINT('Ctrl Pts',(0.740158055211578,-28.8022712603399,
123.328911377769));
#126816=CARTESIAN_POINT('Ctrl Pts',(0.744018156360015,-28.7449451806828,
123.371529928666));
#126817=CARTESIAN_POINT('Ctrl Pts',(0.747878257508454,-28.6900348175087,
123.416968483207));
#126818=CARTESIAN_POINT('Ctrl Pts',(0.751740549446914,-28.6350932901056,
123.462432826277));
#126819=CARTESIAN_POINT('Ctrl Pts',(0.755602841385376,-28.5825705661525,
123.510720030277));
#126820=CARTESIAN_POINT('Ctrl Pts',(0.759465133323836,-28.5327549971333,
123.561532181777));
#126821=CARTESIAN_POINT('Ctrl Pts',(0.763334183008087,-28.4828522671855,
123.612433237899));
#126822=CARTESIAN_POINT('Ctrl Pts',(0.767203232692338,-28.4356664705326,
123.665867697753));
#126823=CARTESIAN_POINT('Ctrl Pts',(0.771072282376589,-28.3914461665989,
123.721503958727));
#126824=CARTESIAN_POINT('Ctrl Pts',(0.773363820207697,-28.3652556268962,
123.75445587385));
#126825=CARTESIAN_POINT('Ctrl Pts',(0.775655358038806,-28.3401045395053,
123.788179572696));
#126826=CARTESIAN_POINT('Ctrl Pts',(0.777946895869915,-28.3160371429284,
123.822601741761));
#126827=CARTESIAN_POINT('Ctrl Pts',(0.781859926298845,-28.2749396520329,
123.881381044094));
#126828=CARTESIAN_POINT('Ctrl Pts',(0.785772956727774,-28.236845311038,
123.942426078789));
#126829=CARTESIAN_POINT('Ctrl Pts',(0.789685987156704,-28.2020089815868,
124.005401658856));
#126830=CARTESIAN_POINT('Ctrl Pts',(0.793592843665999,-28.1672276163641,
124.068277877016));
#126831=CARTESIAN_POINT('Ctrl Pts',(0.797499700175295,-28.135694282503,
124.133078184039));
#126832=CARTESIAN_POINT('Ctrl Pts',(0.80140655668459,-28.1076211970859,
124.199437679639));
#126833=CARTESIAN_POINT('Ctrl Pts',(0.805307700426477,-28.0795891612971,
124.265700141636));
#126834=CARTESIAN_POINT('Ctrl Pts',(0.809208844168363,-28.0550074979398,
124.333516828244));
#126835=CARTESIAN_POINT('Ctrl Pts',(0.813109987910249,-28.0340421790454,
124.402499030354));
#126836=CARTESIAN_POINT('Ctrl Pts',(0.81700774558199,-28.0130950573889,
124.471421358081));
#126837=CARTESIAN_POINT('Ctrl Pts',(0.820905503253732,-27.9957581837704,
124.541506743162));
#126838=CARTESIAN_POINT('Ctrl Pts',(0.824803260925473,-27.9821487118791,
124.612348427671));
#126839=CARTESIAN_POINT('Ctrl Pts',(0.82869925686719,-27.9685453912721,
124.683158092765));
#126840=CARTESIAN_POINT('Ctrl Pts',(0.832595252808908,-27.9586662201479,
124.75472291711));
#126841=CARTESIAN_POINT('Ctrl Pts',(0.836491248750625,-27.9525776100896,
124.826624339097));
#126842=CARTESIAN_POINT('Ctrl Pts',(0.839635926012976,-27.9476631507585,
124.884660017326));
#126843=CARTESIAN_POINT('Ctrl Pts',(0.842780603275327,-27.9452172927798,
124.942914654077));
#126844=CARTESIAN_POINT('Ctrl Pts',(0.845925280537678,-27.9452503304805,
125.001165379557));
#126845=CARTESIAN_POINT('Origin',(-1.54592528053767,30.,125.));
#126846=CARTESIAN_POINT('',(0.904074719503814,32.0547493742749,124.998396436228));
#126847=CARTESIAN_POINT('Ctrl Pts',(0.452117107018789,28.7479590808042,
126.629230216746));
#126848=CARTESIAN_POINT('Ctrl Pts',(0.455981895232545,28.6916216498318,
126.585935679157));
#126849=CARTESIAN_POINT('Ctrl Pts',(0.4598466834463,28.6374422924799,126.539646245016));
#126850=CARTESIAN_POINT('Ctrl Pts',(0.463711471660055,28.5857546915823,
126.490606510827));
#126851=CARTESIAN_POINT('Ctrl Pts',(0.46757142881513,28.5341317011676,126.441628077236));
#126852=CARTESIAN_POINT('Ctrl Pts',(0.471431385970206,28.4849946303537,
126.389906505276));
#126853=CARTESIAN_POINT('Ctrl Pts',(0.475291343125281,28.4386442929298,
126.335726737959));
#126854=CARTESIAN_POINT('Ctrl Pts',(0.479148672821944,28.3923255060073,
126.281583850608));
#126855=CARTESIAN_POINT('Ctrl Pts',(0.483006002518608,28.3487900040007,
126.224986455488));
#126856=CARTESIAN_POINT('Ctrl Pts',(0.486863332215272,28.3083008876935,
126.166255407671));
#126857=CARTESIAN_POINT('Ctrl Pts',(0.490719325378409,28.2678258005376,
126.107544709687));
#126858=CARTESIAN_POINT('Ctrl Pts',(0.494575318541546,28.2303952792588,
126.046702225986));
#126859=CARTESIAN_POINT('Ctrl Pts',(0.498431311704683,28.1962302949751,
125.984079475314));
#126860=CARTESIAN_POINT('Ctrl Pts',(0.502287257448356,28.1620657308387,
125.921457494752));
#126861=CARTESIAN_POINT('Ctrl Pts',(0.506143203192031,28.1311668548754,
125.857055717875));
#126862=CARTESIAN_POINT('Ctrl Pts',(0.509999148935705,28.1037088404285,
125.791250529625));
#126863=CARTESIAN_POINT('Ctrl Pts',(0.513859007405818,28.0762229636345,
125.725378567172));
#126864=CARTESIAN_POINT('Ctrl Pts',(0.51771886587593,28.0521851081078,125.658100798736));
#126865=CARTESIAN_POINT('Ctrl Pts',(0.521578724346043,28.0317220436767,
125.589813062887));
#126866=CARTESIAN_POINT('Ctrl Pts',(0.525440588113093,28.011248348151,125.521489849782));
#126867=CARTESIAN_POINT('Ctrl Pts',(0.529302451880144,27.9943532573307,
125.452156096639));
#126868=CARTESIAN_POINT('Ctrl Pts',(0.533164315647195,27.9811127406638,
125.382219565944));
#126869=CARTESIAN_POINT('Ctrl Pts',(0.537033131028333,27.9678483901779,
125.312157144797));
#126870=CARTESIAN_POINT('Ctrl Pts',(0.540901946409472,27.9582518188302,
125.241490260834));
#126871=CARTESIAN_POINT('Ctrl Pts',(0.544770761790611,27.9523472098042,
125.170632978358));
#126872=CARTESIAN_POINT('Ctrl Pts',(0.547681167434558,27.9479053314146,
125.117328952573));
#126873=CARTESIAN_POINT('Ctrl Pts',(0.550591573078505,27.9455517051314,
125.063917307332));
#126874=CARTESIAN_POINT('Ctrl Pts',(0.553501978722452,27.9452772042607,
125.010573323468));
#126875=CARTESIAN_POINT('Ctrl Pts',(0.557370585230107,27.9449123287125,
124.93966675292));
#126876=CARTESIAN_POINT('Ctrl Pts',(0.561239191737762,27.9482214261752,
124.868602054561));
#126877=CARTESIAN_POINT('Ctrl Pts',(0.565107798245418,27.9552239063853,
124.797791470304));
#126878=CARTESIAN_POINT('Ctrl Pts',(0.568970632627215,27.9622159385964,
124.727086538457));
#126879=CARTESIAN_POINT('Ctrl Pts',(0.572833467009012,27.9728903676711,
124.656635447727));
#126880=CARTESIAN_POINT('Ctrl Pts',(0.57669630139081,27.9872145921315,124.586850554434));
#126881=CARTESIAN_POINT('Ctrl Pts',(0.580554595517413,28.0015219803447,
124.51714768413));
#126882=CARTESIAN_POINT('Ctrl Pts',(0.584412889644017,28.0194705456612,
124.448109929595));
#126883=CARTESIAN_POINT('Ctrl Pts',(0.588271183770621,28.0409760791931,
124.380142887266));
#126884=CARTESIAN_POINT('Ctrl Pts',(0.592127042098162,28.0624680359586,
124.312218753553));
#126885=CARTESIAN_POINT('Ctrl Pts',(0.595982900425703,28.0875123595725,
124.245364453157));
#126886=CARTESIAN_POINT('Ctrl Pts',(0.599838758753245,28.1159744714627,
124.179972335637));
#126887=CARTESIAN_POINT('Ctrl Pts',(0.603693473570268,28.1444281425023,
124.114599611096));
#126888=CARTESIAN_POINT('Ctrl Pts',(0.607548188387292,28.1762973957539,
124.050688653865));
#126889=CARTESIAN_POINT('Ctrl Pts',(0.611402903204315,28.2113994366381,
123.988612049092));
#126890=CARTESIAN_POINT('Ctrl Pts',(0.615257765181646,28.2465028176025,
123.926533074439));
#126891=CARTESIAN_POINT('Ctrl Pts',(0.619112627158977,28.2848389901278,
123.866289013174));
#126892=CARTESIAN_POINT('Ctrl Pts',(0.622967489136308,28.3261799584297,
123.808226518613));
#126893=CARTESIAN_POINT('Ctrl Pts',(0.626826384872089,28.3675641862521,
123.750103266992));
#126894=CARTESIAN_POINT('Ctrl Pts',(0.63068528060787,28.411959204052,123.694166535726));
#126895=CARTESIAN_POINT('Ctrl Pts',(0.634544176343651,28.459095077215,123.640731968508));
#126896=CARTESIAN_POINT('Ctrl Pts',(0.638405255414516,28.5062576195114,
123.587267168401));
#126897=CARTESIAN_POINT('Ctrl Pts',(0.64226633448538,28.5561637640696,123.536307697886));
#126898=CARTESIAN_POINT('Ctrl Pts',(0.646127413556245,28.6085067854929,
123.488132215939));
#126899=CARTESIAN_POINT('Ctrl Pts',(0.649995251699682,28.660941436814,123.439872399646));
#126900=CARTESIAN_POINT('Ctrl Pts',(0.653863089843119,28.7158211076959,
123.394406612201));
#126901=CARTESIAN_POINT('Ctrl Pts',(0.657730927986555,28.7728066575346,
123.351972675376));
#126902=CARTESIAN_POINT('Ctrl Pts',(0.660033035178038,28.8067240137499,
123.326716326091));
#126903=CARTESIAN_POINT('Ctrl Pts',(0.662335142369521,28.8413868252004,
123.302533191287));
#126904=CARTESIAN_POINT('Ctrl Pts',(0.664637249561004,28.8767193334179,
123.279465749663));
#126905=CARTESIAN_POINT('Ctrl Pts',(0.668506416735362,28.9361029196769,
123.240696144034));
#126906=CARTESIAN_POINT('Ctrl Pts',(0.672375583909721,28.9976123174276,
123.204928636224));
#126907=CARTESIAN_POINT('Ctrl Pts',(0.676244751084079,29.0609115567066,
123.172403091989));
#126908=CARTESIAN_POINT('Ctrl Pts',(0.680108153761125,29.1241164893097,
123.139926006092));
#126909=CARTESIAN_POINT('Ctrl Pts',(0.683971556438171,29.1891055417586,
123.110681516429));
#126910=CARTESIAN_POINT('Ctrl Pts',(0.687834959115217,29.255514452144,123.08486584503));
#126911=CARTESIAN_POINT('Ctrl Pts',(0.691693830095352,29.3218454661568,
123.059080454915));
#126912=CARTESIAN_POINT('Ctrl Pts',(0.695552701075488,29.3895925793658,
123.03671606927));
#126913=CARTESIAN_POINT('Ctrl Pts',(0.699411572055622,29.4583692308609,
123.017921880343));
#126914=CARTESIAN_POINT('Ctrl Pts',(0.703268012204796,29.5271025576596,
122.9991395305));
#126915=CARTESIAN_POINT('Ctrl Pts',(0.707124452353968,29.5968636685773,
122.98392304316));
#126916=CARTESIAN_POINT('Ctrl Pts',(0.710980892503141,29.6672498243653,
122.972372104375));
#126917=CARTESIAN_POINT('Ctrl Pts',(0.714836193239567,29.7376151840615,
122.960824578398));
#126918=CARTESIAN_POINT('Ctrl Pts',(0.718691493975995,29.8086047429128,
122.952940529514));
#126919=CARTESIAN_POINT('Ctrl Pts',(0.722546794712421,29.8798062253056,
122.948768414092));
#126920=CARTESIAN_POINT('Ctrl Pts',(0.726402245841275,29.9510104852156,
122.94459613592));
#126921=CARTESIAN_POINT('Ctrl Pts',(0.730257696970128,30.0224262000244,
122.944136104907));
#126922=CARTESIAN_POINT('Ctrl Pts',(0.734113148098982,30.0936383723252,
122.947384737042));
#126923=CARTESIAN_POINT('Ctrl Pts',(0.737972633859116,30.1649250663482,
122.950636768788));
#126924=CARTESIAN_POINT('Ctrl Pts',(0.74183211961925,30.2360073064148,122.957605188893));
#126925=CARTESIAN_POINT('Ctrl Pts',(0.745691605379384,30.3064734069668,
122.968234360631));
#126926=CARTESIAN_POINT('Ctrl Pts',(0.749553275858465,30.3769793958963,
122.978869549168));
#126927=CARTESIAN_POINT('Ctrl Pts',(0.753414946337548,30.4468680748809,
122.993169517086));
#126928=CARTESIAN_POINT('Ctrl Pts',(0.757276616816629,30.5157388796174,
123.011027659682));
#126929=CARTESIAN_POINT('Ctrl Pts',(0.761145042131397,30.5847301531956,
123.028917039749));
#126930=CARTESIAN_POINT('Ctrl Pts',(0.765013467446165,30.652699534404,123.050376874523));
#126931=CARTESIAN_POINT('Ctrl Pts',(0.768881892760934,30.7192631891007,
123.075251178126));
#126932=CARTESIAN_POINT('Ctrl Pts',(0.771178768640478,30.7587853306666,
123.090020285274));
#126933=CARTESIAN_POINT('Ctrl Pts',(0.773475644520022,30.7978122923884,
123.105992205597));
#126934=CARTESIAN_POINT('Ctrl Pts',(0.775772520399567,30.8362678306938,
123.123126621786));
#126935=CARTESIAN_POINT('Ctrl Pts',(0.779641657374848,30.9010470146657,
123.15198991554));
#126936=CARTESIAN_POINT('Ctrl Pts',(0.783510794350128,30.9644569792795,
123.184267382412));
#126937=CARTESIAN_POINT('Ctrl Pts',(0.787379931325409,31.0261139902426,
123.219806852747));
#126938=CARTESIAN_POINT('Ctrl Pts',(0.791243304857167,31.0876791572874,
123.255293383696));
#126939=CARTESIAN_POINT('Ctrl Pts',(0.795106678388925,31.147496136394,123.294032032385));
#126940=CARTESIAN_POINT('Ctrl Pts',(0.798970051920683,31.2052025162291,
123.335823189269));
#126941=CARTESIAN_POINT('Ctrl Pts',(0.802828895479853,31.2628412328375,
123.377565344213));
#126942=CARTESIAN_POINT('Ctrl Pts',(0.806687739039024,31.3183738743825,
123.422352614309));
#126943=CARTESIAN_POINT('Ctrl Pts',(0.810546582598194,31.3714654475106,
123.469941148588));
#126944=CARTESIAN_POINT('Ctrl Pts',(0.81440299640865,31.4245235911463,123.517499718403));
#126945=CARTESIAN_POINT('Ctrl Pts',(0.818259410219106,31.4751433549548,
123.567855729509));
#126946=CARTESIAN_POINT('Ctrl Pts',(0.822115824029562,31.5230225639667,
123.620724888882));
#126947=CARTESIAN_POINT('Ctrl Pts',(0.825971099552345,31.5708876405964,
123.673578443003));
#126948=CARTESIAN_POINT('Ctrl Pts',(0.829826375075127,31.6160134424675,
123.728943312848));
#126949=CARTESIAN_POINT('Ctrl Pts',(0.83368165059791,31.6581356633396,123.786499408957));
#126950=CARTESIAN_POINT('Ctrl Pts',(0.837537077682162,31.7002595401519,
123.844057767755));
#126951=CARTESIAN_POINT('Ctrl Pts',(0.841392504766413,31.7393793164261,
123.90380713054));
#126952=CARTESIAN_POINT('Ctrl Pts',(0.845247931850665,31.7752729316972,
123.965396897123));
#126953=CARTESIAN_POINT('Ctrl Pts',(0.849107395533993,31.8112041272755,
124.027051147662));
#126954=CARTESIAN_POINT('Ctrl Pts',(0.852966859217321,31.8439021739859,
124.090549227941));
#126955=CARTESIAN_POINT('Ctrl Pts',(0.856826322900649,31.8731905397776,
124.155515089426));
#126956=CARTESIAN_POINT('Ctrl Pts',(0.86068797238042,31.9024954929531,124.220517744144));
#126957=CARTESIAN_POINT('Ctrl Pts',(0.864549621860191,31.9283867446657,
124.286989382022));
#126958=CARTESIAN_POINT('Ctrl Pts',(0.868411271339961,31.9507366155094,
124.354535655973));
#126959=CARTESIAN_POINT('Ctrl Pts',(0.87227967760329,31.9731255922432,124.422200116608));
#126960=CARTESIAN_POINT('Ctrl Pts',(0.876148083866617,31.991960688398,124.490942498754));
#126961=CARTESIAN_POINT('Ctrl Pts',(0.880016490129945,32.0071647859594,
124.56035572959));
#126962=CARTESIAN_POINT('Ctrl Pts',(0.882313590499338,32.0161931391744,
124.601574036908));
#126963=CARTESIAN_POINT('Ctrl Pts',(0.884610690868732,32.0239421476356,
124.643028724662));
#126964=CARTESIAN_POINT('Ctrl Pts',(0.886907791238125,32.0304043318996,
124.684633845342));
#126965=CARTESIAN_POINT('Ctrl Pts',(0.892630100646191,32.0465022866529,
124.788276409971));
#126966=CARTESIAN_POINT('Ctrl Pts',(0.898352410054257,32.0546672631343,
124.893182201794));
#126967=CARTESIAN_POINT('Ctrl Pts',(0.904074719462323,32.0547493742743,
124.998396435465));
#126968=CARTESIAN_POINT('Ctrl Pts',(0.904074719503815,32.0547493742749,
124.998396436228));
#126969=CARTESIAN_POINT('Ctrl Pts',(0.907990067111018,32.0548055567495,
125.070386653581));
#126970=CARTESIAN_POINT('Ctrl Pts',(0.91190541471822,32.0510736369444,125.142516744769));
#126971=CARTESIAN_POINT('Ctrl Pts',(0.915820762325423,32.0435391889099,
125.214348188444));
#126972=CARTESIAN_POINT('Ctrl Pts',(0.919623075674049,32.0362222568748,
125.284105891857));
#126973=CARTESIAN_POINT('Ctrl Pts',(0.923425389022675,32.0253194204732,
125.353581417674));
#126974=CARTESIAN_POINT('Ctrl Pts',(0.9272277023713,32.0108701903739,125.422372631649));
#126975=CARTESIAN_POINT('Ctrl Pts',(0.931027545677041,31.9964303467229,
125.491119157763));
#126976=CARTESIAN_POINT('Ctrl Pts',(0.934827388982782,31.9784487785375,
125.559181763658));
#126977=CARTESIAN_POINT('Ctrl Pts',(0.938627232288522,31.9570164824372,
125.626166152047));
#126978=CARTESIAN_POINT('Ctrl Pts',(0.942425966284456,31.9355904431887,
125.693130985303));
#126979=CARTESIAN_POINT('Ctrl Pts',(0.946224700280389,31.9107158274593,
125.75901774815));
#126980=CARTESIAN_POINT('Ctrl Pts',(0.950023434276323,31.8825336043991,
125.823446896168));
#126981=CARTESIAN_POINT('Ctrl Pts',(0.953822417940025,31.8543495290922,
125.887880278722));
#126982=CARTESIAN_POINT('Ctrl Pts',(0.957621401603728,31.8228576194006,
125.950855398358));
#126983=CARTESIAN_POINT('Ctrl Pts',(0.96142038526743,31.7882463535246,126.012014101486));
#126984=CARTESIAN_POINT('Ctrl Pts',(0.965223301108344,31.753599262901,126.07323610756));
#126985=CARTESIAN_POINT('Ctrl Pts',(0.969026216949257,31.7158266252122,
126.132637511061));
#126986=CARTESIAN_POINT('Ctrl Pts',(0.97282913279017,31.675161503085,126.189887179981));
#126987=CARTESIAN_POINT('Ctrl Pts',(0.976634452698739,31.634470673919,126.247173040098));
#126988=CARTESIAN_POINT('Ctrl Pts',(0.980439772607308,31.5908840375004,
126.30230406996));
#126989=CARTESIAN_POINT('Ctrl Pts',(0.984245092515878,31.5446745740139,
126.354982665164));
#126990=CARTESIAN_POINT('Ctrl Pts',(0.988056543369924,31.4983906600981,
126.407746133546));
#126991=CARTESIAN_POINT('Ctrl Pts',(0.99186799422397,31.449475845254,126.458048934318));
#126992=CARTESIAN_POINT('Ctrl Pts',(0.995679445078016,31.3982386145035,
126.505631541716));
#126993=CARTESIAN_POINT('Ctrl Pts',(0.996467317410906,31.3876472680404,
126.515467433961));
#126994=CARTESIAN_POINT('Ctrl Pts',(0.997255189743795,31.3769567898488,
126.525187236556));
#126995=CARTESIAN_POINT('Ctrl Pts',(0.998043062076684,31.366170062117,126.534788885767));
#126996=CARTESIAN_POINT('Ctrl Pts',(1.0019121504236,31.3131985325603,126.581940724366));
#126997=CARTESIAN_POINT('Ctrl Pts',(1.00578123877052,31.2576792965509,126.626439315946));
#126998=CARTESIAN_POINT('Ctrl Pts',(1.00965032711744,31.1999089898887,126.667997595467));
#126999=CARTESIAN_POINT('Ctrl Pts',(1.01351365063637,31.1422247592866,126.709493954372));
#127000=CARTESIAN_POINT('Ctrl Pts',(1.01737697415529,31.0822965068207,126.74805841597));
#127001=CARTESIAN_POINT('Ctrl Pts',(1.02124029767421,31.0204553247912,126.783442876182));
#127002=CARTESIAN_POINT('Ctrl Pts',(1.0250990894003,30.9586866842988,126.818785829375));
#127003=CARTESIAN_POINT('Ctrl Pts',(1.02895788112638,30.8950099910271,126.850955950611));
#127004=CARTESIAN_POINT('Ctrl Pts',(1.03281667285247,30.8297853695835,126.879748334997));
#127005=CARTESIAN_POINT('Ctrl Pts',(1.03667303373327,30.7646018363806,126.908522581625));
#127006=CARTESIAN_POINT('Ctrl Pts',(1.04052939461407,30.6978727529803,126.933923117222));
#127007=CARTESIAN_POINT('Ctrl Pts',(1.04438575549487,30.6299815907003,126.955791593672));
#127008=CARTESIAN_POINT('Ctrl Pts',(1.04824097706913,30.562110485891,126.977653609394));
#127009=CARTESIAN_POINT('Ctrl Pts',(1.05209619864339,30.4930784459205,126.995985488741));
#127010=CARTESIAN_POINT('Ctrl Pts',(1.05595142021765,30.423285975907,127.010678130657));
#127011=CARTESIAN_POINT('Ctrl Pts',(1.0598067924111,30.3534907791797,127.025371346597));
#127012=CARTESIAN_POINT('Ctrl Pts',(1.06366216460456,30.2829355692416,127.036424944907));
#127013=CARTESIAN_POINT('Ctrl Pts',(1.06751753679801,30.2120312659187,127.043780884726));
#127014=CARTESIAN_POINT('Ctrl Pts',(1.07137694452228,30.1410527449883,127.051144524223));
#127015=CARTESIAN_POINT('Ctrl Pts',(1.07523635224654,30.0697248854185,127.054802728717));
#127016=CARTESIAN_POINT('Ctrl Pts',(1.07909575997081,29.9984630566003,127.054749425187));
#127017=CARTESIAN_POINT('Ctrl Pts',(1.08295735280413,29.9271608809521,127.054696091478));
#127018=CARTESIAN_POINT('Ctrl Pts',(1.08681894563745,29.855925295811,127.050927092239));
#127019=CARTESIAN_POINT('Ctrl Pts',(1.09068053847077,29.7851682357209,127.043488408471));
#127020=CARTESIAN_POINT('Ctrl Pts',(1.09454888760835,29.7142873779527,127.036036709864));
#127021=CARTESIAN_POINT('Ctrl Pts',(1.09841723674594,29.6438871967701,127.024902583843));
#127022=CARTESIAN_POINT('Ctrl Pts',(1.10228558588353,29.5743704095703,127.010183328518));
#127023=CARTESIAN_POINT('Ctrl Pts',(1.10458316822743,29.5330813383943,127.001440916717));
#127024=CARTESIAN_POINT('Ctrl Pts',(1.10688075057134,29.4921036492357,126.991434748372));
#127025=CARTESIAN_POINT('Ctrl Pts',(1.10917833291525,29.4515188007233,126.980193408872));
#127026=CARTESIAN_POINT('Ctrl Pts',(1.11304631609241,29.3831941499399,126.961268597672));
#127027=CARTESIAN_POINT('Ctrl Pts',(1.11691429926958,29.3157163351387,126.938766367241));
#127028=CARTESIAN_POINT('Ctrl Pts',(1.12078228244674,29.2494870750926,126.912780152565));
#127029=CARTESIAN_POINT('Ctrl Pts',(1.12464523167984,29.1833440083867,126.886827757362));
#127030=CARTESIAN_POINT('Ctrl Pts',(1.12850818091294,29.1184467224764,126.857400544407));
#127031=CARTESIAN_POINT('Ctrl Pts',(1.13237113014605,29.0551831268984,126.82464205772));
#127032=CARTESIAN_POINT('Ctrl Pts',(1.13622985100971,28.9919887794099,126.791919428348));
#127033=CARTESIAN_POINT('Ctrl Pts',(1.14008857187337,28.9304250011371,126.755872986859));
#127034=CARTESIAN_POINT('Ctrl Pts',(1.14394729273703,28.8708592500841,126.716694128079));
#127035=CARTESIAN_POINT('Ctrl Pts',(1.14666809674701,28.8288591313792,126.689068912407));
#127036=CARTESIAN_POINT('Ctrl Pts',(1.14938890075699,28.7878519852708,126.659887362842));
#127037=CARTESIAN_POINT('Ctrl Pts',(1.15210970476697,28.7479590808042,126.629230216746));
#127038=CARTESIAN_POINT('',(0.845925280586436,32.05474966952,125.001165378589));
#127039=CARTESIAN_POINT('Ctrl Pts',(0.845925280586436,32.05474966952,125.001165378589));
#127040=CARTESIAN_POINT('Ctrl Pts',(0.850222193392141,32.054704526572,125.080759648224));
#127041=CARTESIAN_POINT('Ctrl Pts',(0.854519106197847,32.0500304314087,
125.160186907327));
#127042=CARTESIAN_POINT('Ctrl Pts',(0.858816019003553,32.0408099573904,
125.238939909425));
#127043=CARTESIAN_POINT('Ctrl Pts',(0.863130502657197,32.0315517791984,
125.318014946689));
#127044=CARTESIAN_POINT('Ctrl Pts',(0.867444986310841,32.0177101011583,
125.3964099409));
#127045=CARTESIAN_POINT('Ctrl Pts',(0.871759469964486,31.9994182650028,
125.473628719646));
#127046=CARTESIAN_POINT('Ctrl Pts',(0.876096086614631,31.9810325930193,
125.551243625274));
#127047=CARTESIAN_POINT('Ctrl Pts',(0.880432703264777,31.9581511248076,
125.627669964385));
#127048=CARTESIAN_POINT('Ctrl Pts',(0.884769319914922,31.9309573702644,
125.702425225004));
#127049=CARTESIAN_POINT('Ctrl Pts',(0.886206935512773,31.9219424702053,
125.727207062403));
#127050=CARTESIAN_POINT('Ctrl Pts',(0.887644551110624,31.9124540468206,
125.751805443833));
#127051=CARTESIAN_POINT('Ctrl Pts',(0.889082166708474,31.9024999031172,
125.776203376145));
#127052=CARTESIAN_POINT('Ctrl Pts',(0.892951333660256,31.8757095400272,
125.841867433723));
#127053=CARTESIAN_POINT('Ctrl Pts',(0.896820500612038,31.8454631736331,
125.906271450168));
#127054=CARTESIAN_POINT('Ctrl Pts',(0.90068966756382,31.8119007010479,125.96902704402));
#127055=CARTESIAN_POINT('Ctrl Pts',(0.904553070015992,31.7783882316965,
126.031689141106));
#127056=CARTESIAN_POINT('Ctrl Pts',(0.908416472468163,31.7415696901814,
126.092707265663));
#127057=CARTESIAN_POINT('Ctrl Pts',(0.912279874920336,31.7016330673258,
126.151712840375));
#127058=CARTESIAN_POINT('Ctrl Pts',(0.916138745673275,31.6617432893861,
126.210649202644));
#127059=CARTESIAN_POINT('Ctrl Pts',(0.919997616426214,31.6187429660066,
126.267577303863));
#127060=CARTESIAN_POINT('Ctrl Pts',(0.923856487179154,31.5728651785641,
126.32215456455));
#127061=CARTESIAN_POINT('Ctrl Pts',(0.927712927099826,31.5270162910805,
126.376697445188));
#127062=CARTESIAN_POINT('Ctrl Pts',(0.931569367020499,31.4782938475611,
126.428892052369));
#127063=CARTESIAN_POINT('Ctrl Pts',(0.935425806941171,31.4269723943476,
126.47842732262));
#127064=CARTESIAN_POINT('Ctrl Pts',(0.939281107448132,31.3756661044372,
126.52794795731));
#127065=CARTESIAN_POINT('Ctrl Pts',(0.943136407955094,31.3217626786443,
126.574810477783));
#127066=CARTESIAN_POINT('Ctrl Pts',(0.946991708462056,31.2655736456561,
126.618740531994));
#127067=CARTESIAN_POINT('Ctrl Pts',(0.950847159360819,31.2093824207842,
126.662672299878));
#127068=CARTESIAN_POINT('Ctrl Pts',(0.954702610259581,31.1509057957416,
126.703671076931));
#127069=CARTESIAN_POINT('Ctrl Pts',(0.958558061158344,31.0904871377984,
126.74150376537));
#127070=CARTESIAN_POINT('Ctrl Pts',(0.962417546689029,31.0300052532568,
126.77937604476));
#127071=CARTESIAN_POINT('Ctrl Pts',(0.966277032219715,30.9675776914572,
126.814075363251));
#127072=CARTESIAN_POINT('Ctrl Pts',(0.9701365177504,30.9035747026936,126.845413319328));
#127073=CARTESIAN_POINT('Ctrl Pts',(0.973998188000047,30.8395354840899,
126.876769014718));
#127074=CARTESIAN_POINT('Ctrl Pts',(0.977859858249693,30.7739195102478,
126.904759369209));
#127075=CARTESIAN_POINT('Ctrl Pts',(0.98172152849934,30.7071168743834,126.929244227272));
#127076=CARTESIAN_POINT('Ctrl Pts',(0.98558995358719,30.6401973872688,126.953771914278));
#127077=CARTESIAN_POINT('Ctrl Pts',(0.989458378675041,30.5720875582374,
126.974781719263));
#127078=CARTESIAN_POINT('Ctrl Pts',(0.993326803762892,30.50319180764,126.992183617849));
#127079=CARTESIAN_POINT('Ctrl Pts',(0.995623681690939,30.4622849462456,
127.002515997528));
#127080=CARTESIAN_POINT('Ctrl Pts',(0.997920559618986,30.4211012160408,
127.011577427828));
#127081=CARTESIAN_POINT('Ctrl Pts',(1.00021743754703,30.3797262583935,127.019357702634));
#127082=CARTESIAN_POINT('Ctrl Pts',(1.00411924003509,30.3094408894063,127.032574380467));
#127083=CARTESIAN_POINT('Ctrl Pts',(1.00802104252315,30.2383258874802,127.042143266351));
#127084=CARTESIAN_POINT('Ctrl Pts',(1.01192284501121,30.166793753524,127.047969093098));
#127085=CARTESIAN_POINT('Ctrl Pts',(1.01578547054818,30.0959798545174,127.053736424283));
#127086=CARTESIAN_POINT('Ctrl Pts',(1.01964809608515,30.0247576518687,127.055835443684));
#127087=CARTESIAN_POINT('Ctrl Pts',(1.02351072162212,29.9535385837193,127.054224646746));
#127088=CARTESIAN_POINT('Ctrl Pts',(1.02736946493094,29.8823910960708,127.052615468779));
#127089=CARTESIAN_POINT('Ctrl Pts',(1.03122820823977,29.811247219696,127.047303883362));
#127090=CARTESIAN_POINT('Ctrl Pts',(1.0350869515486,29.7405211518721,127.038300343393));
#127091=CARTESIAN_POINT('Ctrl Pts',(1.03894310737994,29.669842509361,127.02930284074));
#127092=CARTESIAN_POINT('Ctrl Pts',(1.04279926321129,29.5995815998998,127.016618359122));
#127093=CARTESIAN_POINT('Ctrl Pts',(1.04665541904263,29.530148521361,127.000309263719));
#127094=CARTESIAN_POINT('Ctrl Pts',(1.05058919222745,29.4593178821334,126.983671896099));
#127095=CARTESIAN_POINT('Ctrl Pts',(1.05452296541227,29.3893492832019,126.963262453114));
#127096=CARTESIAN_POINT('Ctrl Pts',(1.05845673859709,29.3206667936306,126.93920188666));
#127097=CARTESIAN_POINT('Ctrl Pts',(1.06231299660405,29.2533376956111,126.915615434752));
#127098=CARTESIAN_POINT('Ctrl Pts',(1.06616925461102,29.187244932335,126.888520669323));
#127099=CARTESIAN_POINT('Ctrl Pts',(1.07002551261798,29.1227702090487,126.858081122117));
#127100=CARTESIAN_POINT('Ctrl Pts',(1.07399804339173,29.0563514627095,126.826723770561));
#127101=CARTESIAN_POINT('Ctrl Pts',(1.07797057416548,28.9916504052664,126.791816904311));
#127102=CARTESIAN_POINT('Ctrl Pts',(1.08194310493923,28.9290573062697,126.75359040521));
#127103=CARTESIAN_POINT('Ctrl Pts',(1.08591563571297,28.8664642072729,126.715363906109));
#127104=CARTESIAN_POINT('Ctrl Pts',(1.08988816648672,28.8059795118765,126.673818116667));
#127105=CARTESIAN_POINT('Ctrl Pts',(1.09386069726047,28.7479590808042,126.629230216746));
#127106=CARTESIAN_POINT('Ctrl Pts',(0.393902765004298,28.7479590808042,
126.629230216746));
#127107=CARTESIAN_POINT('Ctrl Pts',(0.397765021747291,28.6913182945486,
126.585702554812));
#127108=CARTESIAN_POINT('Ctrl Pts',(0.401627278490284,28.63696077667,126.539226006323));
#127109=CARTESIAN_POINT('Ctrl Pts',(0.405489535233277,28.5851971742094,
126.490077355923));
#127110=CARTESIAN_POINT('Ctrl Pts',(0.409356061646295,28.5333763478207,
126.440874372388));
#127111=CARTESIAN_POINT('Ctrl Pts',(0.413222588059313,28.4841555100294,
126.388993726621));
#127112=CARTESIAN_POINT('Ctrl Pts',(0.417089114472331,28.4378084641117,
126.334749102902));
#127113=CARTESIAN_POINT('Ctrl Pts',(0.420958121188522,28.3914316874453,
126.280469682289));
#127114=CARTESIAN_POINT('Ctrl Pts',(0.424827127904714,28.3479326658746,
126.223823649619));
#127115=CARTESIAN_POINT('Ctrl Pts',(0.428696134620905,28.307543244335,126.165155651707));
#127116=CARTESIAN_POINT('Ctrl Pts',(0.432571649270529,28.267085885031,126.106388970216));
#127117=CARTESIAN_POINT('Ctrl Pts',(0.436447163920152,28.2297488157466,
126.045593948724));
#127118=CARTESIAN_POINT('Ctrl Pts',(0.440322678569775,28.1957187011626,
125.983141168483));
#127119=CARTESIAN_POINT('Ctrl Pts',(0.441728813497928,28.1833717132005,
125.960481717133));
#127120=CARTESIAN_POINT('Ctrl Pts',(0.443134948426081,28.1714596034836,
125.937604232533));
#127121=CARTESIAN_POINT('Ctrl Pts',(0.444541083354233,28.1599897057763,
125.914527025107));
#127122=CARTESIAN_POINT('Ctrl Pts',(0.448406425456853,28.1284599587848,
125.851089797506));
#127123=CARTESIAN_POINT('Ctrl Pts',(0.452271767559472,28.1001518064021,
125.7858935227));
#127124=CARTESIAN_POINT('Ctrl Pts',(0.456137109662091,28.0752645120309,
125.719298869631));
#127125=CARTESIAN_POINT('Ctrl Pts',(0.459996632892445,28.0504146829042,
125.652804467916));
#127126=CARTESIAN_POINT('Ctrl Pts',(0.463856156122799,28.0289756594278,
125.584916318474));
#127127=CARTESIAN_POINT('Ctrl Pts',(0.467715679353152,28.0111001043075,
125.516018185158));
#127128=CARTESIAN_POINT('Ctrl Pts',(0.471570608822083,27.9932458253994,
125.447202057202));
#127129=CARTESIAN_POINT('Ctrl Pts',(0.475425538291014,27.9789467120985,
125.377378801993));
#127130=CARTESIAN_POINT('Ctrl Pts',(0.479280467759945,27.968306144083,125.30694891811));
#127131=CARTESIAN_POINT('Ctrl Pts',(0.483132930157,27.957672385802,125.236564107837));
#127132=CARTESIAN_POINT('Ctrl Pts',(0.486985392554054,27.9506926004373,
125.165573919304));
#127133=CARTESIAN_POINT('Ctrl Pts',(0.490837854951109,27.947419127263,125.094389212171));
#127134=CARTESIAN_POINT('Ctrl Pts',(0.494689147554331,27.9441466480735,
125.023226120157));
#127135=CARTESIAN_POINT('Ctrl Pts',(0.498540440157554,27.9445782693539,
124.951869112878));
#127136=CARTESIAN_POINT('Ctrl Pts',(0.502391732760776,27.948714342242,124.880732599692));
#127137=CARTESIAN_POINT('Ctrl Pts',(0.506243151200269,27.9528505502711,
124.809593762207));
#127138=CARTESIAN_POINT('Ctrl Pts',(0.510094569639761,27.9606914197365,
124.738675919046));
#127139=CARTESIAN_POINT('Ctrl Pts',(0.513945988079253,27.9721852967047,
124.668390151534));
#127140=CARTESIAN_POINT('Ctrl Pts',(0.517801431273902,27.9836911848427,
124.598030934977));
#127141=CARTESIAN_POINT('Ctrl Pts',(0.521656874468552,27.9988576221953,
124.528305594113));
#127142=CARTESIAN_POINT('Ctrl Pts',(0.525512317663202,28.0175816385012,
124.459615875055));
#127143=CARTESIAN_POINT('Ctrl Pts',(0.52936993382045,28.0363162078317,124.390887441852));
#127144=CARTESIAN_POINT('Ctrl Pts',(0.533227549977698,28.0586121949647,
124.32319625497));
#127145=CARTESIAN_POINT('Ctrl Pts',(0.537085166134947,28.0843173029351,
124.2569270785));
#127146=CARTESIAN_POINT('Ctrl Pts',(0.540949562528794,28.1100675908058,
124.190541425772));
#127147=CARTESIAN_POINT('Ctrl Pts',(0.544813958922641,28.1392387629363,
124.125583217714));
#127148=CARTESIAN_POINT('Ctrl Pts',(0.548678355316488,28.1716314268244,
124.062414844868));
#127149=CARTESIAN_POINT('Ctrl Pts',(0.551011021608591,28.1911846163687,
124.024284508575));
#127150=CARTESIAN_POINT('Ctrl Pts',(0.553343687900694,28.2119107377833,
123.986805830846));
#127151=CARTESIAN_POINT('Ctrl Pts',(0.555676354192796,28.233758395163,123.950053260473));
#127152=CARTESIAN_POINT('Ctrl Pts',(0.55954593324945,28.2700007148295,123.889085698557));
#127153=CARTESIAN_POINT('Ctrl Pts',(0.563415512306104,28.3094743779065,
123.829877604035));
#127154=CARTESIAN_POINT('Ctrl Pts',(0.567285091362758,28.3519833328474,
123.77279234549));
#127155=CARTESIAN_POINT('Ctrl Pts',(0.571148904349671,28.3944289450848,
123.715792149837));
#127156=CARTESIAN_POINT('Ctrl Pts',(0.575012717336582,28.4399005835988,
123.6609088975));
#127157=CARTESIAN_POINT('Ctrl Pts',(0.578876530323495,28.4881575770453,
123.608479230965));
#127158=CARTESIAN_POINT('Ctrl Pts',(0.582735807188568,28.5363579167142,
123.556111116932));
#127159=CARTESIAN_POINT('Ctrl Pts',(0.586595084053642,28.587336788608,123.506191222558));
#127160=CARTESIAN_POINT('Ctrl Pts',(0.590454360918715,28.6408127906897,
123.459023785859));
#127161=CARTESIAN_POINT('Ctrl Pts',(0.594311203983475,28.69425506886,123.411886094661));
#127162=CARTESIAN_POINT('Ctrl Pts',(0.598168047048235,28.7501909894982,
123.36749773779));
#127163=CARTESIAN_POINT('Ctrl Pts',(0.602024890112995,28.8083028229929,
123.326125631711));
#127164=CARTESIAN_POINT('Ctrl Pts',(0.60588059017397,28.8663974346187,123.284765786561));
#127165=CARTESIAN_POINT('Ctrl Pts',(0.609736290234945,28.9266662834845,
123.246420699076));
#127166=CARTESIAN_POINT('Ctrl Pts',(0.61359199029592,28.988760515234,123.211315492618));
#127167=CARTESIAN_POINT('Ctrl Pts',(0.61744783653321,29.0508571010842,123.176208955259));
#127168=CARTESIAN_POINT('Ctrl Pts',(0.6213036827705,29.1147787833747,123.14434277988));
#127169=CARTESIAN_POINT('Ctrl Pts',(0.62515952900779,29.1801513425479,123.115896568292));
#127170=CARTESIAN_POINT('Ctrl Pts',(0.629019400628104,29.2455921486309,
123.087420659747));
#127171=CARTESIAN_POINT('Ctrl Pts',(0.632879272248418,29.3124864090116,
123.062372036382));
#127172=CARTESIAN_POINT('Ctrl Pts',(0.636739143868732,29.3804399501159,
123.040882109957));
#127173=CARTESIAN_POINT('Ctrl Pts',(0.640601195567596,29.4484318717861,
123.019380045892));
#127174=CARTESIAN_POINT('Ctrl Pts',(0.644463247266461,29.5174837949454,
123.001440802256));
#127175=CARTESIAN_POINT('Ctrl Pts',(0.648325298965326,29.5871890777104,
122.98714513565));
#127176=CARTESIAN_POINT('Ctrl Pts',(0.652194093943705,29.6570160683762,
122.972824508302));
#127177=CARTESIAN_POINT('Ctrl Pts',(0.656062888922084,29.727498215944,122.962160232273));
#127178=CARTESIAN_POINT('Ctrl Pts',(0.659931683900464,29.7982221448728,
122.955181362644));
#127179=CARTESIAN_POINT('Ctrl Pts',(0.662224997610761,29.8401453164972,
122.951044483462));
#127180=CARTESIAN_POINT('Ctrl Pts',(0.664518311321058,29.8821533932848,
122.948201581459));
#127181=CARTESIAN_POINT('Ctrl Pts',(0.666811625031356,29.9241605753862,
122.946650067774));
#127182=CARTESIAN_POINT('Ctrl Pts',(0.670681339183318,29.9950430657896,
122.944032059414));
#127183=CARTESIAN_POINT('Ctrl Pts',(0.674551053335281,30.0661995809263,
122.945083589692));
#127184=CARTESIAN_POINT('Ctrl Pts',(0.678420767487243,30.1372184602691,
122.949836919496));
#127185=CARTESIAN_POINT('Ctrl Pts',(0.682284730622962,30.20813179416,122.954583185089));
#127186=CARTESIAN_POINT('Ctrl Pts',(0.68614869375868,30.2789074176964,122.963020297639));
#127187=CARTESIAN_POINT('Ctrl Pts',(0.6900126568944,30.349131940276,122.975128534751));
#127188=CARTESIAN_POINT('Ctrl Pts',(0.693872105680565,30.4192744180661,
122.987222625555));
#127189=CARTESIAN_POINT('Ctrl Pts',(0.697731554466732,30.4888665976082,
123.002979239247));
#127190=CARTESIAN_POINT('Ctrl Pts',(0.701591003252898,30.5575002352797,
123.022326859624));
#127191=CARTESIAN_POINT('Ctrl Pts',(0.705448031609014,30.626090829779,123.041662346258));
#127192=CARTESIAN_POINT('Ctrl Pts',(0.70930505996513,30.693723608797,123.064584239985));
#127193=CARTESIAN_POINT('Ctrl Pts',(0.713162088321247,30.7600019965348,
123.090970265354));
#127194=CARTESIAN_POINT('Ctrl Pts',(0.717017986794997,30.8262609686048,
123.11734856117));
#127195=CARTESIAN_POINT('Ctrl Pts',(0.720873885268748,30.8911658861629,
123.147188794448));
#127196=CARTESIAN_POINT('Ctrl Pts',(0.724729783742498,30.9543384186385,
123.180319878327));
#127197=CARTESIAN_POINT('Ctrl Pts',(0.72858584127878,31.0175135570912,123.213452328921));
#127198=CARTESIAN_POINT('Ctrl Pts',(0.732441898815062,31.078955739558,123.249875672151));
#127199=CARTESIAN_POINT('Ctrl Pts',(0.736297956351344,31.1383111354956,
123.289372828081));
#127200=CARTESIAN_POINT('Ctrl Pts',(0.740158057635936,31.1977287759096,
123.328911403662));
#127201=CARTESIAN_POINT('Ctrl Pts',(0.744018158920527,31.2550548562536,
123.371529957045));
#127202=CARTESIAN_POINT('Ctrl Pts',(0.747878260205119,31.3099652199,123.416968514163));
#127203=CARTESIAN_POINT('Ctrl Pts',(0.751740552281313,31.3649067477969,
123.462432859829));
#127204=CARTESIAN_POINT('Ctrl Pts',(0.755602844357507,31.4174294720272,
123.510720066518));
#127205=CARTESIAN_POINT('Ctrl Pts',(0.759465136433701,31.4672450411022,
123.561532220778));
#127206=CARTESIAN_POINT('Ctrl Pts',(0.763334186256716,31.5171477711161,
123.612433279674));
#127207=CARTESIAN_POINT('Ctrl Pts',(0.76720323607973,31.5643335676119,123.665867742371));
#127208=CARTESIAN_POINT('Ctrl Pts',(0.771072285902744,31.608553871162,123.721504006236));
#127209=CARTESIAN_POINT('Ctrl Pts',(0.773363822558468,31.6347443962645,
123.754455904988));
#127210=CARTESIAN_POINT('Ctrl Pts',(0.775655359214192,31.659895470117,123.788179586632));
#127211=CARTESIAN_POINT('Ctrl Pts',(0.777946895869915,31.6839628542883,
123.822601737781));
#127212=CARTESIAN_POINT('Ctrl Pts',(0.781859926094245,31.7250603429308,
123.881381036595));
#127213=CARTESIAN_POINT('Ctrl Pts',(0.785772956318574,31.7631546821155,
123.942426067642));
#127214=CARTESIAN_POINT('Ctrl Pts',(0.789685986542903,31.7979910101894,
124.00540164399));
#127215=CARTESIAN_POINT('Ctrl Pts',(0.793592842844341,31.8327723740052,
124.068277858378));
#127216=CARTESIAN_POINT('Ctrl Pts',(0.797499699145779,31.8643057068968,
124.133078161557));
#127217=CARTESIAN_POINT('Ctrl Pts',(0.801406555447216,31.8923787917684,
124.199437653293));
#127218=CARTESIAN_POINT('Ctrl Pts',(0.805307698977523,31.9204108269836,
124.265700111363));
#127219=CARTESIAN_POINT('Ctrl Pts',(0.80920884250783,31.9449924901972,124.333516794022));
#127220=CARTESIAN_POINT('Ctrl Pts',(0.813109986038136,31.9659578093617,
124.40249899221));
#127221=CARTESIAN_POINT('Ctrl Pts',(0.817007743496307,31.9869049312765,
124.471421315981));
#127222=CARTESIAN_POINT('Ctrl Pts',(0.820905500954478,32.0042418055704,
124.541506697131));
#127223=CARTESIAN_POINT('Ctrl Pts',(0.824803258412648,32.0178512785365,
124.612348377782));
#127224=CARTESIAN_POINT('Ctrl Pts',(0.828699254139108,32.0314546002117,
124.683158038986));
#127225=CARTESIAN_POINT('Ctrl Pts',(0.832595249865569,32.0413337728066,
124.754722859513));
#127226=CARTESIAN_POINT('Ctrl Pts',(0.83649124559203,32.0474223847194,124.826624277795));
#127227=CARTESIAN_POINT('Ctrl Pts',(0.839635923907246,32.0523368474643,
124.88465997567));
#127228=CARTESIAN_POINT('Ctrl Pts',(0.842780602222461,32.0547827071795,
124.942914632312));
#127229=CARTESIAN_POINT('Ctrl Pts',(0.845925280537677,32.0547496695206,
125.001165377686));
#127230=CARTESIAN_POINT('Origin',(-1.54592528053767,30.,55.));
#127231=CARTESIAN_POINT('',(0.904074719503237,32.0547493739418,54.9983960094259));
#127232=CARTESIAN_POINT('Ctrl Pts',(0.452117494115148,28.7479524050421,
56.6292250864936));
#127233=CARTESIAN_POINT('Ctrl Pts',(0.455982334291425,28.6916143219704,
56.5859296805983));
#127234=CARTESIAN_POINT('Ctrl Pts',(0.459847174467703,28.6374344239205,
56.5396393262805));
#127235=CARTESIAN_POINT('Ctrl Pts',(0.46371201464398,28.5857463933444,56.4905986376492));
#127236=CARTESIAN_POINT('Ctrl Pts',(0.467572025665764,28.5341229474532,
56.4416192258239));
#127237=CARTESIAN_POINT('Ctrl Pts',(0.471432036687546,28.4849855344149,
56.3898966386622));
#127238=CARTESIAN_POINT('Ctrl Pts',(0.475292047709329,28.4386349661428,
56.3357158356282));
#127239=CARTESIAN_POINT('Ctrl Pts',(0.479149432414872,28.3923159343738,
56.2815718967177));
#127240=CARTESIAN_POINT('Ctrl Pts',(0.483006817120415,28.3487803004197,
56.2249734280577));
#127241=CARTESIAN_POINT('Ctrl Pts',(0.486864201825958,28.3082911618458,
56.1662412998222));
#127242=CARTESIAN_POINT('Ctrl Pts',(0.490720251061402,28.2678160410684,
56.107529505312));
#127243=CARTESIAN_POINT('Ctrl Pts',(0.494576300296846,28.2303855974567,
56.0466859170156));
#127244=CARTESIAN_POINT('Ctrl Pts',(0.498432349532289,28.1962207978899,
55.9840620674201));
#127245=CARTESIAN_POINT('Ctrl Pts',(0.502288352334105,28.1620564097275,
55.921438971926));
#127246=CARTESIAN_POINT('Ctrl Pts',(0.506144355135921,28.1311578184329,
55.8570360848732));
#127247=CARTESIAN_POINT('Ctrl Pts',(0.510000357937737,28.1037001923878,
55.7912298036284));
#127248=CARTESIAN_POINT('Ctrl Pts',(0.513860274577921,28.0762146968841,
55.7253567290845));
#127249=CARTESIAN_POINT('Ctrl Pts',(0.517720191218106,28.0521773284542,
55.6580778649955));
#127250=CARTESIAN_POINT('Ctrl Pts',(0.52158010785829,28.0317148515083,55.5897890612133));
#127251=CARTESIAN_POINT('Ctrl Pts',(0.525442030519987,28.011241740092,55.5214647673358));
#127252=CARTESIAN_POINT('Ctrl Pts',(0.529303953181685,27.9943473351431,
55.4521299607925));
#127253=CARTESIAN_POINT('Ctrl Pts',(0.533165875843382,27.9811076004398,
55.3821924142338));
#127254=CARTESIAN_POINT('Ctrl Pts',(0.537034750574321,27.967844032128,55.3121289690725));
#127255=CARTESIAN_POINT('Ctrl Pts',(0.540903625305261,27.9582483400407,
55.2414610986422));
#127256=CARTESIAN_POINT('Ctrl Pts',(0.5447725000362,27.9523447016016,55.1706028764146));
#127257=CARTESIAN_POINT('Ctrl Pts',(0.547682326264951,27.9479045056351,
55.1173095733486));
#127258=CARTESIAN_POINT('Ctrl Pts',(0.550592152493701,27.9455517174084,
55.063908723299));
#127259=CARTESIAN_POINT('Ctrl Pts',(0.553501978722452,27.9452772154524,
55.010575498138));
#127260=CARTESIAN_POINT('Ctrl Pts',(0.557370495096533,27.9449122743088,
54.9396707641098));
#127261=CARTESIAN_POINT('Ctrl Pts',(0.561239011470614,27.9482211155754,
54.8686078387497));
#127262=CARTESIAN_POINT('Ctrl Pts',(0.565107527844695,27.9552231671876,
54.7977989453697));
#127263=CARTESIAN_POINT('Ctrl Pts',(0.568970270673785,27.9622147686281,
54.727095730315));
#127264=CARTESIAN_POINT('Ctrl Pts',(0.572833013502874,27.9728885921152,
54.6566462743214));
#127265=CARTESIAN_POINT('Ctrl Pts',(0.576695756331965,27.9872120544266,
54.5868629178416));
#127266=CARTESIAN_POINT('Ctrl Pts',(0.580553957234481,28.00151867479,54.5171616146837));
#127267=CARTESIAN_POINT('Ctrl Pts',(0.584412158136999,28.0194663127297,
54.4481253290154));
#127268=CARTESIAN_POINT('Ctrl Pts',(0.588270359039516,28.0409707773654,
54.380159643647));
#127269=CARTESIAN_POINT('Ctrl Pts',(0.59212612316034,28.0624616601046,54.3122368843837));
#127270=CARTESIAN_POINT('Ctrl Pts',(0.595981887281165,28.0875047664499,
54.2453838461247));
#127271=CARTESIAN_POINT('Ctrl Pts',(0.599837651401989,28.1159655353422,
54.1799928668105));
#127272=CARTESIAN_POINT('Ctrl Pts',(0.603692271167429,28.1444178573397,
54.1146212949386));
#127273=CARTESIAN_POINT('Ctrl Pts',(0.607546890932868,28.176285634357,54.0507113658897));
#127274=CARTESIAN_POINT('Ctrl Pts',(0.611401510698308,28.2113860886913,
53.9886356547846));
#127275=CARTESIAN_POINT('Ctrl Pts',(0.615256276916005,28.2464878766308,
53.9265575851776));
#127276=CARTESIAN_POINT('Ctrl Pts',(0.619111043133703,28.2848223446265,
53.8663142937954));
#127277=CARTESIAN_POINT('Ctrl Pts',(0.622965809351401,28.3261615130957,
53.8082524251093));
#127278=CARTESIAN_POINT('Ctrl Pts',(0.626824608897236,28.3675439356617,
53.750129804991));
#127279=CARTESIAN_POINT('Ctrl Pts',(0.630683408443071,28.4119370521812,
53.694193560574));
#127280=CARTESIAN_POINT('Ctrl Pts',(0.634542207988907,28.4590709436111,
53.6407593275374));
#127281=CARTESIAN_POINT('Ctrl Pts',(0.638403190481053,28.5062314989694,
53.5872948664311));
#127282=CARTESIAN_POINT('Ctrl Pts',(0.6422641729732,28.5561355755575,53.5363355816682));
#127283=CARTESIAN_POINT('Ctrl Pts',(0.646125155465346,28.608476463058,53.4881601246705));
#127284=CARTESIAN_POINT('Ctrl Pts',(0.649992897456676,28.6609089847958,
53.4399003259378));
#127285=CARTESIAN_POINT('Ctrl Pts',(0.653860639448007,28.7157864606461,
53.3944343955679));
#127286=CARTESIAN_POINT('Ctrl Pts',(0.657728381439337,28.77276976465,53.3520001480756));
#127287=CARTESIAN_POINT('Ctrl Pts',(0.660031337479892,28.8066991333775,
53.3267336730088));
#127288=CARTESIAN_POINT('Ctrl Pts',(0.662334293520448,28.841374526437,53.3025411983353));
#127289=CARTESIAN_POINT('Ctrl Pts',(0.664637249561003,28.8767200983988,
53.2794652502321));
#127290=CARTESIAN_POINT('Ctrl Pts',(0.668506451727346,28.9361042816819,
53.2406952924827));
#127291=CARTESIAN_POINT('Ctrl Pts',(0.67237565389369,28.9976142977631,53.2049275043511));
#127292=CARTESIAN_POINT('Ctrl Pts',(0.676244856060033,29.0609141675609,
53.1724017504352));
#127293=CARTESIAN_POINT('Ctrl Pts',(0.680108294091384,29.1241197365239,
53.1399244516861));
#127294=CARTESIAN_POINT('Ctrl Pts',(0.683971732122735,29.1891094378702,
53.1106798202829));
#127295=CARTESIAN_POINT('Ctrl Pts',(0.687835170154086,29.2555190013059,
53.0848640766036));
#127296=CARTESIAN_POINT('Ctrl Pts',(0.691694076853992,29.321850674598,53.0590786115751));
#127297=CARTESIAN_POINT('Ctrl Pts',(0.695552983553898,29.3895984515335,
53.0367142210235));
#127298=CARTESIAN_POINT('Ctrl Pts',(0.699411890253804,29.4583757634714,
53.017920095227));
#127299=CARTESIAN_POINT('Ctrl Pts',(0.703268366328725,29.527109754369,52.9991378073617));
#127300=CARTESIAN_POINT('Ctrl Pts',(0.707124842403646,29.5968715262351,
52.9839214503626));
#127301=CARTESIAN_POINT('Ctrl Pts',(0.710981318478567,29.6672583326809,
52.9723707081101));
#127302=CARTESIAN_POINT('Ctrl Pts',(0.714836655293049,29.7376243458164,
52.9608233781189));
#127303=CARTESIAN_POINT('Ctrl Pts',(0.718691992107531,29.8086145478841,
52.9529395916762));
#127304=CARTESIAN_POINT('Ctrl Pts',(0.722547328922012,29.8798166566084,
52.9487678028874));
#127305=CARTESIAN_POINT('Ctrl Pts',(0.726402816227741,29.9510215446733,
52.9445958512549));
#127306=CARTESIAN_POINT('Ctrl Pts',(0.73025830353347,30.0224378707715,52.9441362111621));
#127307=CARTESIAN_POINT('Ctrl Pts',(0.734113790839199,30.0936506311823,
52.9473852963161));
#127308=CARTESIAN_POINT('Ctrl Pts',(0.737973312677396,30.1649379114063,
52.9506377814398));
#127309=CARTESIAN_POINT('Ctrl Pts',(0.741832834515594,30.236020714471,52.9576067168871));
#127310=CARTESIAN_POINT('Ctrl Pts',(0.74569235635379,30.3064873487565,52.968236463672));
#127311=CARTESIAN_POINT('Ctrl Pts',(0.749554062909574,30.376993871324,52.9788722275221));
#127312=CARTESIAN_POINT('Ctrl Pts',(0.753415769465359,30.446883054666,52.9931728304852));
#127313=CARTESIAN_POINT('Ctrl Pts',(0.757277476021143,30.5157543284872,
53.0110316656249));
#127314=CARTESIAN_POINT('Ctrl Pts',(0.761145937018379,30.5847460638143,
53.0289217373319));
#127315=CARTESIAN_POINT('Ctrl Pts',(0.765014398015613,30.6527158716266,
53.050382320605));
#127316=CARTESIAN_POINT('Ctrl Pts',(0.768882859012849,30.7192799118218,
53.0752574273556));
#127317=CARTESIAN_POINT('Ctrl Pts',(0.771179412808421,30.7587963756735,
53.0900248040629));
#127318=CARTESIAN_POINT('Ctrl Pts',(0.773475966603994,30.7978177932748,
53.1059946535758));
#127319=CARTESIAN_POINT('Ctrl Pts',(0.775772520399566,30.8362679536972,
53.1231266765924));
#127320=CARTESIAN_POINT('Ctrl Pts',(0.779641665029999,30.9010472904688,
53.1519900435167));
#127321=CARTESIAN_POINT('Ctrl Pts',(0.783510809660432,30.9644573937457,
53.1842675964721));
#127322=CARTESIAN_POINT('Ctrl Pts',(0.787379954290865,31.0261145286024,
53.2198071630604));
#127323=CARTESIAN_POINT('Ctrl Pts',(0.791243335712682,31.0876798232813,
53.2552937923833));
#127324=CARTESIAN_POINT('Ctrl Pts',(0.7951067171345,31.1474969150771,53.2940325499976));
#127325=CARTESIAN_POINT('Ctrl Pts',(0.798970098556317,31.2052033923354,
53.3358238237484));
#127326=CARTESIAN_POINT('Ctrl Pts',(0.802828950318409,31.2628422110641,
53.3775660989074));
#127327=CARTESIAN_POINT('Ctrl Pts',(0.8066878020805,31.3183749391514,53.4223534976467));
#127328=CARTESIAN_POINT('Ctrl Pts',(0.810546653842592,31.3714665831634,
53.469942166529));
#127329=CARTESIAN_POINT('Ctrl Pts',(0.814403076044992,31.4245248003102,
53.517500873257));
#127330=CARTESIAN_POINT('Ctrl Pts',(0.818259498247393,31.4751446217494,
53.5678570275087));
#127331=CARTESIAN_POINT('Ctrl Pts',(0.822115920449793,31.5230238726558,
53.6207263339639));
#127332=CARTESIAN_POINT('Ctrl Pts',(0.825971204541594,31.5708889933969,
53.6735800375845));
#127333=CARTESIAN_POINT('Ctrl Pts',(0.829826488633396,31.6160148234011,
53.7289450610951));
#127334=CARTESIAN_POINT('Ctrl Pts',(0.833681772725197,31.6581370567484,
53.786501312923));
#127335=CARTESIAN_POINT('Ctrl Pts',(0.837537208543773,31.7002609478389,
53.8440598299081));
#127336=CARTESIAN_POINT('Ctrl Pts',(0.84139264436235,31.7393807224787,53.9038093531206));
#127337=CARTESIAN_POINT('Ctrl Pts',(0.845248080180926,31.7752743206541,
53.9653992804343));
#127338=CARTESIAN_POINT('Ctrl Pts',(0.84910755279315,31.8112055008452,54.0270536948355));
#127339=CARTESIAN_POINT('Ctrl Pts',(0.852967025405373,31.8439035163674,
54.0905519394591));
#127340=CARTESIAN_POINT('Ctrl Pts',(0.856826498017596,31.8731918357075,
54.1555179639928));
#127341=CARTESIAN_POINT('Ctrl Pts',(0.860688156549584,31.9024967433027,
54.2205207838432));
#127342=CARTESIAN_POINT('Ctrl Pts',(0.864549815081573,31.9283879339482,
54.2869925856471));
#127343=CARTESIAN_POINT('Ctrl Pts',(0.868411473613561,31.9507377288338,
54.3545390206958));
#127344=CARTESIAN_POINT('Ctrl Pts',(0.872279889027977,31.9731266299571,
54.4222036441644));
#127345=CARTESIAN_POINT('Ctrl Pts',(0.876148304442392,31.9919616354081,
54.4909461863541));
#127346=CARTESIAN_POINT('Ctrl Pts',(0.880016719856808,32.007165627798,54.5603595729619));
#127347=CARTESIAN_POINT('Ctrl Pts',(0.88231374365058,32.0161935962395,54.6015765012294));
#127348=CARTESIAN_POINT('Ctrl Pts',(0.884610767444353,32.0239423062121,
54.6430297915521));
#127349=CARTESIAN_POINT('Ctrl Pts',(0.886907791238125,32.0304042790898,
54.6846335053405));
#127350=CARTESIAN_POINT('Ctrl Pts',(0.892630100646191,32.0465022438967,
54.7882760202622));
#127351=CARTESIAN_POINT('Ctrl Pts',(0.898352410054257,32.0546672409534,
54.8931817831011));
#127352=CARTESIAN_POINT('Ctrl Pts',(0.904074719462322,32.0547493739412,
54.9983960086736));
#127353=CARTESIAN_POINT('Ctrl Pts',(0.904074719503237,32.0547493739418,
54.9983960094259));
#127354=CARTESIAN_POINT('Ctrl Pts',(0.907990067110464,32.0548055713655,
55.070386221239));
#127355=CARTESIAN_POINT('Ctrl Pts',(0.911905414717691,32.0510736670533,
55.1425163169785));
#127356=CARTESIAN_POINT('Ctrl Pts',(0.915820762324918,32.0435392324816,
55.2143477730435));
#127357=CARTESIAN_POINT('Ctrl Pts',(0.919623060278423,32.0362223431458,
55.2841052060461));
#127358=CARTESIAN_POINT('Ctrl Pts',(0.923425358231927,32.0253195766014,
55.3535804711167));
#127359=CARTESIAN_POINT('Ctrl Pts',(0.927227656185431,32.0108704414169,
55.4223714364582));
#127360=CARTESIAN_POINT('Ctrl Pts',(0.931027483988993,31.996430693064,55.4911177119828));
#127361=CARTESIAN_POINT('Ctrl Pts',(0.934827311792556,31.9784492454175,
55.5591800794248));
#127362=CARTESIAN_POINT('Ctrl Pts',(0.938627139596119,31.9570170930322,
55.6261642436932));
#127363=CARTESIAN_POINT('Ctrl Pts',(0.942425857996128,31.9355911980109,
55.6931288511622));
#127364=CARTESIAN_POINT('Ctrl Pts',(0.946224576396138,31.9107167498486,
55.7590154025972));
#127365=CARTESIAN_POINT('Ctrl Pts',(0.950023294796147,31.8825347156863,
55.8234443555797));
#127366=CARTESIAN_POINT('Ctrl Pts',(0.953822262783287,31.8543508298802,
55.8878775417366));
#127367=CARTESIAN_POINT('Ctrl Pts',(0.957621230770428,31.8228591311617,
55.9508524814108));
#127368=CARTESIAN_POINT('Ctrl Pts',(0.961420198757568,31.7882480957827,
56.0120110228795));
#127369=CARTESIAN_POINT('Ctrl Pts',(0.96522309887351,31.7536012361879,56.0732328666089));
#127370=CARTESIAN_POINT('Ctrl Pts',(0.969025998989452,31.7158288491463,
56.1326341261334));
#127371=CARTESIAN_POINT('Ctrl Pts',(0.972828899105393,31.6751639953886,
56.1898836712275));
#127372=CARTESIAN_POINT('Ctrl Pts',(0.976634203238837,31.6344734351918,
56.2471694068352));
#127373=CARTESIAN_POINT('Ctrl Pts',(0.98043950737228,31.5908870855503,56.3023003324072));
#127374=CARTESIAN_POINT('Ctrl Pts',(0.984244811505724,31.5446779247817,
56.3549788452932));
#127375=CARTESIAN_POINT('Ctrl Pts',(0.988056246624191,31.4983943132825,
56.4077422321242));
#127376=CARTESIAN_POINT('Ctrl Pts',(0.991867681742658,31.4494798167601,
56.4580449733025));
#127377=CARTESIAN_POINT('Ctrl Pts',(0.995679116861126,31.398242918379,56.5056275448141));
#127378=CARTESIAN_POINT('Ctrl Pts',(0.996467098599645,31.3876501261609,
56.5154648360856));
#127379=CARTESIAN_POINT('Ctrl Pts',(0.997255080338164,31.3769581744616,
56.5251860055168));
#127380=CARTESIAN_POINT('Ctrl Pts',(0.998043062076684,31.3661699466928,
56.5347889885106));
#127381=CARTESIAN_POINT('Ctrl Pts',(1.00191215656167,31.3131983224499,56.5819409042527));
#127382=CARTESIAN_POINT('Ctrl Pts',(1.00578125104665,31.2576789862063,56.626439560984));
#127383=CARTESIAN_POINT('Ctrl Pts',(1.00965034553163,31.1999085753941,56.6679978936425));
#127384=CARTESIAN_POINT('Ctrl Pts',(1.0135136752563,31.1422242396501,56.7094943064311));
#127385=CARTESIAN_POINT('Ctrl Pts',(1.01737700498097,31.0822958780486,56.7480588098205));
#127386=CARTESIAN_POINT('Ctrl Pts',(1.02124033470564,31.020454584405,56.7834432998183));
#127387=CARTESIAN_POINT('Ctrl Pts',(1.02509913270775,30.9586858311878,56.8187862834724));
#127388=CARTESIAN_POINT('Ctrl Pts',(1.02895793070986,30.8950090226413,56.8509564230656));
#127389=CARTESIAN_POINT('Ctrl Pts',(1.03281672871197,30.8297842847801,56.8797488138664));
#127390=CARTESIAN_POINT('Ctrl Pts',(1.03667309590875,30.7646006344909,56.9085230672323));
#127391=CARTESIAN_POINT('Ctrl Pts',(1.04052946310553,30.6978714328268,56.9339235975645));
#127392=CARTESIAN_POINT('Ctrl Pts',(1.04438583030231,30.6299801524122,56.9557920569597));
#127393=CARTESIAN_POINT('Ctrl Pts',(1.04824105822307,30.5621089289329,56.9776540558157));
#127394=CARTESIAN_POINT('Ctrl Pts',(1.05209628614383,30.4930767704008,56.9959859064551));
#127395=CARTESIAN_POINT('Ctrl Pts',(1.05595151406459,30.4232841831565,57.0106785080638));
#127396=CARTESIAN_POINT('Ctrl Pts',(1.05980689262569,30.3534888688156,57.0253716837756));
#127397=CARTESIAN_POINT('Ctrl Pts',(1.06366227118679,30.2829335425852,57.0364252302183));
#127398=CARTESIAN_POINT('Ctrl Pts',(1.06751764974788,30.21202912545,57.0437811067873));
#127399=CARTESIAN_POINT('Ctrl Pts',(1.07137706382818,30.1410504909242,57.0511446829326));
#127400=CARTESIAN_POINT('Ctrl Pts',(1.07523647790847,30.0697225202458,57.0548028127025));
#127401=CARTESIAN_POINT('Ctrl Pts',(1.07909589198877,29.9984605839173,57.0547494233356));
#127402=CARTESIAN_POINT('Ctrl Pts',(1.08295749118116,29.9271583007081,57.0546960037409));
#127403=CARTESIAN_POINT('Ctrl Pts',(1.08681909037356,29.8559226116065,57.050926907492));
#127404=CARTESIAN_POINT('Ctrl Pts',(1.09068068956595,29.7851654522512,57.0434881158435));
#127405=CARTESIAN_POINT('Ctrl Pts',(1.09454904499834,29.7142844964256,57.0360363093119));
#127406=CARTESIAN_POINT('Ctrl Pts',(1.09841740043072,29.6438842218769,57.0249020646029));
#127407=CARTESIAN_POINT('Ctrl Pts',(1.10228575586311,29.5743673470875,57.0101826800753));
#127408=CARTESIAN_POINT('Ctrl Pts',(1.10458328154716,29.5330793092908,57.0014404213566));
#127409=CARTESIAN_POINT('Ctrl Pts',(1.1068808072312,29.4921026391673,56.991434468854));
#127410=CARTESIAN_POINT('Ctrl Pts',(1.10917833291525,29.4515187891883,56.980193405677));
#127411=CARTESIAN_POINT('Ctrl Pts',(1.11304631691874,29.3831941199109,56.9612685889262));
#127412=CARTESIAN_POINT('Ctrl Pts',(1.11691430092223,29.3157162880953,56.9387663512784));
#127413=CARTESIAN_POINT('Ctrl Pts',(1.12078228492572,29.2494870126202,56.912780128053));
#127414=CARTESIAN_POINT('Ctrl Pts',(1.1246452350137,29.1833439299984,56.8868277241122));
#127415=CARTESIAN_POINT('Ctrl Pts',(1.12850818510168,29.1184466297722,56.8574005010361));
#127416=CARTESIAN_POINT('Ctrl Pts',(1.13237113518965,29.0551830215408,56.8246420031653));
#127417=CARTESIAN_POINT('Ctrl Pts',(1.1362298569753,28.9919886602983,56.7919193620438));
#127418=CARTESIAN_POINT('Ctrl Pts',(1.14008857876095,28.9304248699874,56.7558729076272));
#127419=CARTESIAN_POINT('Ctrl Pts',(1.1439473005466,28.8708591086472,56.7166940350497));
#127420=CARTESIAN_POINT('Ctrl Pts',(1.1466682533244,28.8288566962466,56.6890673057614));
#127421=CARTESIAN_POINT('Ctrl Pts',(1.14938920610221,28.7878473654915,56.6598840725942));
#127422=CARTESIAN_POINT('Ctrl Pts',(1.15211015888001,28.7479524050421,56.6292250864936));
#127423=CARTESIAN_POINT('',(0.845925280586868,32.0547496699795,55.0011645681513));
#127424=CARTESIAN_POINT('Ctrl Pts',(0.845925280586868,32.0547496699795,
55.0011645681513));
#127425=CARTESIAN_POINT('Ctrl Pts',(0.850222060205272,32.0547045596875,
55.0807566105182));
#127426=CARTESIAN_POINT('Ctrl Pts',(0.854518839823676,32.0500307559347,
55.1601816477493));
#127427=CARTESIAN_POINT('Ctrl Pts',(0.85881561944208,32.0408108291358,55.2389324636425));
#127428=CARTESIAN_POINT('Ctrl Pts',(0.863129966126428,32.0315532073474,
55.3180052464269));
#127429=CARTESIAN_POINT('Ctrl Pts',(0.867444312810776,32.0177123505107,
55.3963980230681));
#127430=CARTESIAN_POINT('Ctrl Pts',(0.871758659495125,31.9994215971072,
55.4736146529843));
#127431=CARTESIAN_POINT('Ctrl Pts',(0.87609513814191,31.9810370148352,55.5512273928281));
#127432=CARTESIAN_POINT('Ctrl Pts',(0.880431616788695,31.9581569012951,
55.6276516357164));
#127433=CARTESIAN_POINT('Ctrl Pts',(0.88476809543548,31.9309647626119,55.7024049032084));
#127434=CARTESIAN_POINT('Ctrl Pts',(0.886206119193146,31.9219475519594,
55.7271939044633));
#127435=CARTESIAN_POINT('Ctrl Pts',(0.88764414295081,31.9124565475937,55.7517993452135));
#127436=CARTESIAN_POINT('Ctrl Pts',(0.889082166708476,31.9024995598415,
55.7762042175245));
#127437=CARTESIAN_POINT('Ctrl Pts',(0.892951368473773,31.875708907474,55.8418689011044));
#127438=CARTESIAN_POINT('Ctrl Pts',(0.89682057023907,31.8454621937363,55.9062734968565));
#127439=CARTESIAN_POINT('Ctrl Pts',(0.900689772004367,31.811899323857,55.969029619107));
#127440=CARTESIAN_POINT('Ctrl Pts',(0.904553209630516,31.7783864542268,
56.0316922504921));
#127441=CARTESIAN_POINT('Ctrl Pts',(0.908416647256666,31.7415674619314,
56.0927108582529));
#127442=CARTESIAN_POINT('Ctrl Pts',(0.912280084882815,31.7016303455885,
56.1517168616776));
#127443=CARTESIAN_POINT('Ctrl Pts',(0.916138991173326,31.6617400705553,
56.2106536583409));
#127444=CARTESIAN_POINT('Ctrl Pts',(0.919997897463837,31.618739206825,56.2675821391834));
#127445=CARTESIAN_POINT('Ctrl Pts',(0.923856803754348,31.5728608432167,
56.3221597219609));
#127446=CARTESIAN_POINT('Ctrl Pts',(0.927713279417508,31.5270113772277,
56.3767029277012));
#127447=CARTESIAN_POINT('Ctrl Pts',(0.931569755080669,31.4782883190936,
56.4288978022599));
#127448=CARTESIAN_POINT('Ctrl Pts',(0.935426230743829,31.4269662222281,
56.4784332799015));
#127449=CARTESIAN_POINT('Ctrl Pts',(0.9392815671448,31.3756592866988,56.5279541240015));
#127450=CARTESIAN_POINT('Ctrl Pts',(0.94313690354577,31.3217551860451,56.5748167937198));
#127451=CARTESIAN_POINT('Ctrl Pts',(0.946992239946741,31.2655654556863,
56.6187469350931));
#127452=CARTESIAN_POINT('Ctrl Pts',(0.950847726837816,31.2093735320045,
56.662678791246));
#127453=CARTESIAN_POINT('Ctrl Pts',(0.954703213728891,31.1508961855199,
56.7036775943421));
#127454=CARTESIAN_POINT('Ctrl Pts',(0.958558700619966,31.0904767899601,
56.7415102448904));
#127455=CARTESIAN_POINT('Ctrl Pts',(0.962418222044635,31.029994169161,56.779382485017));
#127456=CARTESIAN_POINT('Ctrl Pts',(0.966277743469305,30.9675658550251,
56.8140817004074));
#127457=CARTESIAN_POINT('Ctrl Pts',(0.970137264893974,30.9035621040846,
56.8454194879653));
#127458=CARTESIAN_POINT('Ctrl Pts',(0.973998971036238,30.8395221232323,
56.8767750145661));
#127459=CARTESIAN_POINT('Ctrl Pts',(0.977860677178502,30.7739053772985,
56.9047651348175));
#127460=CARTESIAN_POINT('Ctrl Pts',(0.981722383320766,30.7071019656674,
56.9292496916287));
#127461=CARTESIAN_POINT('Ctrl Pts',(0.985590843908987,30.6401817093007,
56.9537770739707));
#127462=CARTESIAN_POINT('Ctrl Pts',(0.98945930449721,30.5720711075993,56.9747865078759));
#127463=CARTESIAN_POINT('Ctrl Pts',(0.993327765085431,30.5031745870426,
56.9921879674003));
#127464=CARTESIAN_POINT('Ctrl Pts',(0.995624322572632,30.4622733508743,
57.0025185501341));
#127465=CARTESIAN_POINT('Ctrl Pts',(0.997920880059832,30.421095329188,57.0115785376082));
#127466=CARTESIAN_POINT('Ctrl Pts',(1.00021743754703,30.3797261264494,57.019357727445));
#127467=CARTESIAN_POINT('Ctrl Pts',(1.00411925951087,30.3094403771173,57.0325744720444));
#127468=CARTESIAN_POINT('Ctrl Pts',(1.00802108147471,30.2383249941629,57.0421433837288));
#127469=CARTESIAN_POINT('Ctrl Pts',(1.01192290343855,30.1667924843784,57.0479691964614));
#127470=CARTESIAN_POINT('Ctrl Pts',(1.01578553689087,30.0959784216706,57.0537364968038));
#127471=CARTESIAN_POINT('Ctrl Pts',(1.01964817034319,30.0247560628285,57.0558354679589));
#127472=CARTESIAN_POINT('Ctrl Pts',(1.02351080379551,29.9535368477729,57.0542246074821));
#127473=CARTESIAN_POINT('Ctrl Pts',(1.02736955523059,29.8823892093306,57.0526153659496));
#127474=CARTESIAN_POINT('Ctrl Pts',(1.03122830666567,29.8112451914293,57.0473037012904));
#127475=CARTESIAN_POINT('Ctrl Pts',(1.03508705810074,29.7405189927952,57.0383000685375));
#127476=CARTESIAN_POINT('Ctrl Pts',(1.03894322225702,29.66984021582,57.0293024726876));
#127477=CARTESIAN_POINT('Ctrl Pts',(1.04279938641329,29.5995791826385,57.016617883963));
#127478=CARTESIAN_POINT('Ctrl Pts',(1.04665555056957,29.5301459922717,57.0003086696612));
#127479=CARTESIAN_POINT('Ctrl Pts',(1.05058935174537,29.4593148878801,56.9836710982828));
#127480=CARTESIAN_POINT('Ctrl Pts',(1.05452315292117,29.3893458447176,56.9632614018325));
#127481=CARTESIAN_POINT('Ctrl Pts',(1.05845695409698,29.3206629389884,56.9392005363129));
#127482=CARTESIAN_POINT('Ctrl Pts',(1.06231322087807,29.2533337589013,56.9156139053976));
#127483=CARTESIAN_POINT('Ctrl Pts',(1.06616948765916,29.187240928555,56.8885189511515));
#127484=CARTESIAN_POINT('Ctrl Pts',(1.07002575444025,29.1227661537687,56.8580792075491));
#127485=CARTESIAN_POINT('Ctrl Pts',(1.07399832281341,29.056346876856,56.8267214282287));
#127486=CARTESIAN_POINT('Ctrl Pts',(1.07797089118657,28.9916453300971,56.7918140750785));
#127487=CARTESIAN_POINT('Ctrl Pts',(1.08194345955972,28.92905179168,56.7535870373598));
#127488=CARTESIAN_POINT('Ctrl Pts',(1.08591602793288,28.8664582532629,56.715359999641));
#127489=CARTESIAN_POINT('Ctrl Pts',(1.08988859630604,28.8059731683529,56.6738136198787));
#127490=CARTESIAN_POINT('Ctrl Pts',(1.0938611646792,28.7479524050421,56.6292250864936));
#127491=CARTESIAN_POINT('Ctrl Pts',(0.393903217269906,28.7479524050421,
56.6292250864936));
#127492=CARTESIAN_POINT('Ctrl Pts',(0.397765692980319,28.6913092315187,
56.5856952208116));
#127493=CARTESIAN_POINT('Ctrl Pts',(0.401628168690733,28.6369495977553,
56.5392162516049));
#127494=CARTESIAN_POINT('Ctrl Pts',(0.405490644401147,28.5851841620823,
56.4900650010242));
#127495=CARTESIAN_POINT('Ctrl Pts',(0.409357394093613,28.5333614459085,
56.4408593626418));
#127496=CARTESIAN_POINT('Ctrl Pts',(0.413224143786079,28.4841390070372,
56.3889758765177));
#127497=CARTESIAN_POINT('Ctrl Pts',(0.417090893478545,28.4377906583134,
56.3347282626989));
#127498=CARTESIAN_POINT('Ctrl Pts',(0.42096012610705,28.3914125481636,56.2804458151396));
#127499=CARTESIAN_POINT('Ctrl Pts',(0.424829358735555,28.3479124954103,
56.2237966025194));
#127500=CARTESIAN_POINT('Ctrl Pts',(0.42869859136406,28.3075223532751,56.1651253056374));
#127501=CARTESIAN_POINT('Ctrl Pts',(0.432574334358801,28.2670642507347,
56.1063552885007));
#127502=CARTESIAN_POINT('Ctrl Pts',(0.436450077353541,28.2297267531038,
56.0455568097575));
#127503=CARTESIAN_POINT('Ctrl Pts',(0.440325820348281,28.1956965327029,
55.9831004833686));
#127504=CARTESIAN_POINT('Ctrl Pts',(0.441730908016932,28.1833594290529,
55.9604579567208));
#127505=CARTESIAN_POINT('Ctrl Pts',(0.443135995685583,28.171456547217,55.9375977354635));
#127506=CARTESIAN_POINT('Ctrl Pts',(0.444541083354234,28.1599952039845,
55.9145380873096));
#127507=CARTESIAN_POINT('Ctrl Pts',(0.448405941216207,28.1284694397995,
55.8511098298063));
#127508=CARTESIAN_POINT('Ctrl Pts',(0.45227079907818,28.1001642080859,55.7859226688689));
#127509=CARTESIAN_POINT('Ctrl Pts',(0.456135656940153,28.0752788153013,
55.7193371418688));
#127510=CARTESIAN_POINT('Ctrl Pts',(0.459994688596713,28.0504309368096,
55.6528519913822));
#127511=CARTESIAN_POINT('Ctrl Pts',(0.463853720253272,28.0289928339176,
55.5849731111926));
#127512=CARTESIAN_POINT('Ctrl Pts',(0.467712751909832,28.0111172190746,
55.5160841464706));
#127513=CARTESIAN_POINT('Ctrl Pts',(0.471567181193553,27.9932629231145,
55.4472773403647));
#127514=CARTESIAN_POINT('Ctrl Pts',(0.475421610477274,27.9789627980082,
55.377463311472));
#127515=CARTESIAN_POINT('Ctrl Pts',(0.479276039760995,27.9683202772573,
55.3070424509678));
#127516=CARTESIAN_POINT('Ctrl Pts',(0.483127996899415,27.9576845823828,
55.2366667568388));
#127517=CARTESIAN_POINT('Ctrl Pts',(0.486979954037834,27.9507019106231,
55.1656854835747));
#127518=CARTESIAN_POINT('Ctrl Pts',(0.490831911176254,27.9474246574332,
55.0945093941715));
#127519=CARTESIAN_POINT('Ctrl Pts',(0.494682694160181,27.9441484032163,
55.0233550006808));
#127520=CARTESIAN_POINT('Ctrl Pts',(0.498533477144108,27.9445753478264,
54.9520063951509));
#127521=CARTESIAN_POINT('Ctrl Pts',(0.502384260128034,27.9487058992826,
54.8808778993558));
#127522=CARTESIAN_POINT('Ctrl Pts',(0.506235165295295,27.952836581799,54.8097471466906));
#127523=CARTESIAN_POINT('Ctrl Pts',(0.510086070462555,27.9606710740166,
54.7388370036943));
#127524=CARTESIAN_POINT('Ctrl Pts',(0.513936975629815,27.9721577784347,
54.6685584713146));
#127525=CARTESIAN_POINT('Ctrl Pts',(0.517791903410963,27.9836564817401,
54.5982065267401));
#127526=CARTESIAN_POINT('Ctrl Pts',(0.52164683119211,27.9988149342846,54.5284879914766));
#127527=CARTESIAN_POINT('Ctrl Pts',(0.525501758973257,28.0175302211821,
54.4598045366966));
#127528=CARTESIAN_POINT('Ctrl Pts',(0.529358857706701,28.0362560478348,
54.3910824019431));
#127529=CARTESIAN_POINT('Ctrl Pts',(0.533215956440145,28.0585425436682,
54.323396970801));
#127530=CARTESIAN_POINT('Ctrl Pts',(0.537073055173589,28.084237465828,54.2571329357396));
#127531=CARTESIAN_POINT('Ctrl Pts',(0.540936936527285,28.109977571923,54.1907523768821));
#127532=CARTESIAN_POINT('Ctrl Pts',(0.544800817880983,28.1391378711156,
54.1257986487736));
#127533=CARTESIAN_POINT('Ctrl Pts',(0.54866469923468,28.1715190236334,54.0626340727521));
#127534=CARTESIAN_POINT('Ctrl Pts',(0.551001917554052,28.1911060181446,
54.0244265320181));
#127535=CARTESIAN_POINT('Ctrl Pts',(0.553339135873424,28.2118706089704,
53.9868731216588));
#127536=CARTESIAN_POINT('Ctrl Pts',(0.555676354192796,28.2337610839925,
53.9500487372831));
#127537=CARTESIAN_POINT('Ctrl Pts',(0.559546127776258,28.2700055294806,
53.8890779547493));
#127538=CARTESIAN_POINT('Ctrl Pts',(0.56341590135972,28.3094816006687,53.8298669467456));
#127539=CARTESIAN_POINT('Ctrl Pts',(0.567285674943182,28.3519931974908,
53.7727790983758));
#127540=CARTESIAN_POINT('Ctrl Pts',(0.571149684492805,28.3944414732225,
53.7157762824459));
#127541=CARTESIAN_POINT('Ctrl Pts',(0.575013694042429,28.439916011926,53.6608907349997));
#127542=CARTESIAN_POINT('Ctrl Pts',(0.578877703592051,28.4881760962043,
53.6084591107654));
#127543=CARTESIAN_POINT('Ctrl Pts',(0.582737179080315,28.536379551693,53.5560890102407));
#127544=CARTESIAN_POINT('Ctrl Pts',(0.586596654568578,28.5873617328976,
53.5061674688283));
#127545=CARTESIAN_POINT('Ctrl Pts',(0.590456130056842,28.6408411942136,
53.4589987335653));
#127546=CARTESIAN_POINT('Ctrl Pts',(0.594313172906131,28.6942869472648,
53.4118597288976));
#127547=CARTESIAN_POINT('Ctrl Pts',(0.598170215755419,28.7502264941943,
53.3674704083578));
#127548=CARTESIAN_POINT('Ctrl Pts',(0.602027258604707,28.8083420642981,
53.3260976949718));
#127549=CARTESIAN_POINT('Ctrl Pts',(0.605883159311579,28.8664404252962,
53.284737232819));
#127550=CARTESIAN_POINT('Ctrl Pts',(0.609739060018451,28.926713134852,53.2463918858627));
#127551=CARTESIAN_POINT('Ctrl Pts',(0.613594960725322,28.9888112996955,
53.2112867823833));
#127552=CARTESIAN_POINT('Ctrl Pts',(0.617451008170922,29.0509118277238,
53.1761803429571));
#127553=CARTESIAN_POINT('Ctrl Pts',(0.621307055616521,29.1148375251662,
53.1443146288754));
#127554=CARTESIAN_POINT('Ctrl Pts',(0.62516310306212,29.180214135265,53.1158692459172));
#127555=CARTESIAN_POINT('Ctrl Pts',(0.629023175358348,29.2456589839147,
53.0873941723447));
#127556=CARTESIAN_POINT('Ctrl Pts',(0.632883247654576,29.3125573221994,
53.0623467506991));
#127557=CARTESIAN_POINT('Ctrl Pts',(0.636743319950804,29.3805149406725,
53.0408583961923));
#127558=CARTESIAN_POINT('Ctrl Pts',(0.640605572326229,29.4485109400305,
53.0193579055619));
#127559=CARTESIAN_POINT('Ctrl Pts',(0.644467824701654,29.5175669403351,
53.0014206057529));
#127560=CARTESIAN_POINT('Ctrl Pts',(0.648330077077079,29.5872762642552,
52.9871272567664));
#127561=CARTESIAN_POINT('Ctrl Pts',(0.652199070552378,29.657107257468,52.9728089604476));
#127562=CARTESIAN_POINT('Ctrl Pts',(0.656068064027678,29.7275933706668,
52.9621473857586));
#127563=CARTESIAN_POINT('Ctrl Pts',(0.659937057502978,29.7983211930969,
52.9551715912219));
#127564=CARTESIAN_POINT('Ctrl Pts',(0.662228580012437,29.8402117773479,
52.9510399765514));
#127565=CARTESIAN_POINT('Ctrl Pts',(0.664520102521896,29.8821871002605,
52.948200316185));
#127566=CARTESIAN_POINT('Ctrl Pts',(0.666811625031355,29.9241615682704,
52.9466500311022));
#127567=CARTESIAN_POINT('Ctrl Pts',(0.670681389893222,29.9950451492649,
52.9440320167844));
#127568=CARTESIAN_POINT('Ctrl Pts',(0.674551154755091,30.0662027119619,
52.9450836557535));
#127569=CARTESIAN_POINT('Ctrl Pts',(0.678420919616958,30.1372225844074,
52.9498371955309));
#127570=CARTESIAN_POINT('Ctrl Pts',(0.682284934848094,30.208136936736,52.9545836725799));
#127571=CARTESIAN_POINT('Ctrl Pts',(0.68614895007923,30.2789135243227,52.9630211003315));
#127572=CARTESIAN_POINT('Ctrl Pts',(0.690012965310366,30.3491389472087,
52.9751297429114));
#127573=CARTESIAN_POINT('Ctrl Pts',(0.693872468011491,30.4192823584284,
52.9872242446016));
#127574=CARTESIAN_POINT('Ctrl Pts',(0.697731970712618,30.4888754072847,
53.0029813627833));
#127575=CARTESIAN_POINT('Ctrl Pts',(0.701591473413743,30.5575098425005,
53.0223295678968));
#127576=CARTESIAN_POINT('Ctrl Pts',(0.705448556780905,30.6261012541369,
53.0416656445644));
#127577=CARTESIAN_POINT('Ctrl Pts',(0.709305640148067,30.6937347780694,
53.0645882105555));
#127578=CARTESIAN_POINT('Ctrl Pts',(0.713162723515229,30.7600138325188,
53.0909749774086));
#127579=CARTESIAN_POINT('Ctrl Pts',(0.717018678017908,30.826273488873,53.1173540215653));
#127580=CARTESIAN_POINT('Ctrl Pts',(0.720874632520587,30.8911790118523,
53.1471950742087));
#127581=CARTESIAN_POINT('Ctrl Pts',(0.724730587023266,30.9543520663278,
53.1803270359771));
#127582=CARTESIAN_POINT('Ctrl Pts',(0.728586701529236,31.0175277421768,
53.2134603725602));
#127583=CARTESIAN_POINT('Ctrl Pts',(0.732442816035207,31.0789703777892,
53.2498846619025));
#127584=CARTESIAN_POINT('Ctrl Pts',(0.736298930541177,31.1383261392231,
53.2893828121811));
#127585=CARTESIAN_POINT('Ctrl Pts',(0.74015908985444,31.1977441608976,53.3289223933887));
#127586=CARTESIAN_POINT('Ctrl Pts',(0.744019249167702,31.2550705336062,
53.3715420023265));
#127587=CARTESIAN_POINT('Ctrl Pts',(0.747879408480964,31.3099810981801,
53.4169816536404));
#127588=CARTESIAN_POINT('Ctrl Pts',(0.751741759271153,31.3649228363987,
53.4624471018035));
#127589=CARTESIAN_POINT('Ctrl Pts',(0.755604110061343,31.417445678612,53.5107354506283));
#127590=CARTESIAN_POINT('Ctrl Pts',(0.759466460851533,31.4672612714758,
53.5615487760347));
#127591=CARTESIAN_POINT('Ctrl Pts',(0.763335569848735,31.5171640299305,
53.6124510128298));
#127592=CARTESIAN_POINT('Ctrl Pts',(0.767204678845938,31.5643497598586,
53.6658866830124));
#127593=CARTESIAN_POINT('Ctrl Pts',(0.77107378784314,31.6085699004703,53.7215241739474));
#127594=CARTESIAN_POINT('Ctrl Pts',(0.773364823852066,31.6347542066076,
53.7544690962203));
#127595=CARTESIAN_POINT('Ctrl Pts',(0.77565585986099,31.6598995138589,53.7881854473603));
#127596=CARTESIAN_POINT('Ctrl Pts',(0.777946895869916,31.683961613921,53.8225999637589));
#127597=CARTESIAN_POINT('Ctrl Pts',(0.781859836390422,31.7250581161037,
53.8813777198417));
#127598=CARTESIAN_POINT('Ctrl Pts',(0.785772776910929,31.7631516630838,
53.9424211513269));
#127599=CARTESIAN_POINT('Ctrl Pts',(0.789685717431435,31.7979873888736,
54.0053950975631));
#127600=CARTESIAN_POINT('Ctrl Pts',(0.79359248258054,31.8327681371999,54.0682696588216));
#127601=CARTESIAN_POINT('Ctrl Pts',(0.797499247729644,31.8643010465251,
54.1330682768469));
#127602=CARTESIAN_POINT('Ctrl Pts',(0.801406012878749,31.892373893761,54.1994260754236));
#127603=CARTESIAN_POINT('Ctrl Pts',(0.805307063592873,31.9204056787743,
54.2656868122852));
#127604=CARTESIAN_POINT('Ctrl Pts',(0.809208114306997,31.9449872803149,
54.3335017643087));
#127605=CARTESIAN_POINT('Ctrl Pts',(0.813109165021121,31.9659527192365,
54.4024822444255));
#127606=CARTESIAN_POINT('Ctrl Pts',(0.817006828775115,31.986899955599,54.4714028344888));
#127607=CARTESIAN_POINT('Ctrl Pts',(0.820904492529109,32.0042371272175,
54.541486493878));
#127608=CARTESIAN_POINT('Ctrl Pts',(0.824802156283103,32.0178470725133,
54.6123264847203));
#127609=CARTESIAN_POINT('Ctrl Pts',(0.828698057535242,32.0314508634676,
54.6831344421129));
#127610=CARTESIAN_POINT('Ctrl Pts',(0.832593958787382,32.0413306817161,
54.7546975904148));
#127611=CARTESIAN_POINT('Ctrl Pts',(0.836489860039521,32.0474201073761,
54.8265973863746));
#127612=CARTESIAN_POINT('Ctrl Pts',(0.839635000205574,32.0523360680208,
54.8846417056654));
#127613=CARTESIAN_POINT('Ctrl Pts',(0.842780140371627,32.0547826896117,
54.9429050911716));
#127614=CARTESIAN_POINT('Ctrl Pts',(0.84592528053768,32.0547496699801,55.0011645672402));
#127615=CARTESIAN_POINT('Origin',(-1.54592528053767,-30.,55.));
#127616=CARTESIAN_POINT('',(0.904074719503239,-27.9452506260572,54.9983960106767));
#127617=CARTESIAN_POINT('Ctrl Pts',(0.452117492759457,-31.2520475724682,
56.6292251037768));
#127618=CARTESIAN_POINT('Ctrl Pts',(0.455982332793877,-31.3083856538667,
56.5859297004043));
#127619=CARTESIAN_POINT('Ctrl Pts',(0.459847172828296,-31.3625655505572,
56.5396393487449));
#127620=CARTESIAN_POINT('Ctrl Pts',(0.463712012862715,-31.4142535800857,
56.4905986628582));
#127621=CARTESIAN_POINT('Ctrl Pts',(0.46757202373732,-31.4658770248571,
56.4416192538439));
#127622=CARTESIAN_POINT('Ctrl Pts',(0.471432034611924,-31.5150144370937,
56.3898966695869));
#127623=CARTESIAN_POINT('Ctrl Pts',(0.475292045486528,-31.5613650048761,
56.3357158695053));
#127624=CARTESIAN_POINT('Ctrl Pts',(0.479149430041697,-31.607684036116,
56.2815719335914));
#127625=CARTESIAN_POINT('Ctrl Pts',(0.483006814596865,-31.6512196698572,
56.2249734679798));
#127626=CARTESIAN_POINT('Ctrl Pts',(0.486864199152033,-31.6917088085244,
56.1662413428021));
#127627=CARTESIAN_POINT('Ctrl Pts',(0.490720248234121,-31.7321839293632,
56.1075295513949));
#127628=CARTESIAN_POINT('Ctrl Pts',(0.494576297316209,-31.7696143733469,
56.0466859662144));
#127629=CARTESIAN_POINT('Ctrl Pts',(0.498432346398297,-31.8037791735835,
55.9840621197092));
#127630=CARTESIAN_POINT('Ctrl Pts',(0.502288349043991,-31.8379435623911,
55.9214390273503));
#127631=CARTESIAN_POINT('Ctrl Pts',(0.506144351689685,-31.8688421546333,
55.8570361434098));
#127632=CARTESIAN_POINT('Ctrl Pts',(0.510000354335379,-31.8962997819133,
55.7912298652196));
#127633=CARTESIAN_POINT('Ctrl Pts',(0.513860270816316,-31.9237852786321,
55.725356793784));
#127634=CARTESIAN_POINT('Ctrl Pts',(0.517720187297254,-31.9478226485702,
55.658077932748));
#127635=CARTESIAN_POINT('Ctrl Pts',(0.521580103778191,-31.9682851273012,
55.5897891319318));
#127636=CARTESIAN_POINT('Ctrl Pts',(0.525442026278597,-31.9887582404931,
55.5214648410566));
#127637=CARTESIAN_POINT('Ctrl Pts',(0.529303948779003,-32.0056526474982,
55.4521300374299));
#127638=CARTESIAN_POINT('Ctrl Pts',(0.533165871279409,-32.0188923845216,
55.3821924936739));
#127639=CARTESIAN_POINT('Ctrl Pts',(0.537034745847787,-32.0321559551542,
55.3121290513381));
#127640=CARTESIAN_POINT('Ctrl Pts',(0.540903620416166,-32.0417516498287,
55.2414611836194));
#127641=CARTESIAN_POINT('Ctrl Pts',(0.544772494984544,-32.0476552911041,
55.1706029639645));
#127642=CARTESIAN_POINT('Ctrl Pts',(0.54768232289718,-32.0520954919598,
55.1173096297538));
#127643=CARTESIAN_POINT('Ctrl Pts',(0.550592150809814,-32.0544482826237,
55.0639087483478));
#127644=CARTESIAN_POINT('Ctrl Pts',(0.55350197872245,-32.0547227845796,
55.0105754919346));
#127645=CARTESIAN_POINT('Ctrl Pts',(0.557370495353025,-32.0550877255359,
54.9396707526882));
#127646=CARTESIAN_POINT('Ctrl Pts',(0.561239011983601,-32.0517788835405,
54.8686078222902));
#127647=CARTESIAN_POINT('Ctrl Pts',(0.565107528614176,-32.0447768307097,
54.7977989241054));
#127648=CARTESIAN_POINT('Ctrl Pts',(0.568970271703778,-32.0377852280443,
54.7270957041724));
#127649=CARTESIAN_POINT('Ctrl Pts',(0.57283301479338,-32.0271114028356,
54.6566462435337));
#127650=CARTESIAN_POINT('Ctrl Pts',(0.576695757882982,-32.0127879383576,
54.5868628826867));
#127651=CARTESIAN_POINT('Ctrl Pts',(0.580553959050737,-31.9984813158116,
54.5171615750759));
#127652=CARTESIAN_POINT('Ctrl Pts',(0.584412160218493,-31.9805336752359,
54.4481252852337));
#127653=CARTESIAN_POINT('Ctrl Pts',(0.588270361386249,-31.9590292075618,
54.3801595960091));
#127654=CARTESIAN_POINT('Ctrl Pts',(0.59212612577509,-31.9375383217699,
54.3122368328403));
#127655=CARTESIAN_POINT('Ctrl Pts',(0.595981890163931,-31.9124952119648,
54.2453837909946));
#127656=CARTESIAN_POINT('Ctrl Pts',(0.599837654552772,-31.8840344392551,
54.1799928084458));
#127657=CARTESIAN_POINT('Ctrl Pts',(0.603692274588616,-31.8555821134233,
54.1146212332983));
#127658=CARTESIAN_POINT('Ctrl Pts',(0.60754689462446,-31.82371433221,54.0507113013275));
#127659=CARTESIAN_POINT('Ctrl Pts',(0.611401514660303,-31.7886138733661,
53.9886355876825));
#127660=CARTESIAN_POINT('Ctrl Pts',(0.615256281150403,-31.7535120808988,
53.9265575155035));
#127661=CARTESIAN_POINT('Ctrl Pts',(0.619111047640502,-31.7151776080581,
53.8663142219333));
#127662=CARTESIAN_POINT('Ctrl Pts',(0.622965814130601,-31.673838434473,
53.8082523514682));
#127663=CARTESIAN_POINT('Ctrl Pts',(0.62682461395004,-31.6324560067758,
53.7501297295552));
#127664=CARTESIAN_POINT('Ctrl Pts',(0.630683413769478,-31.5880628848521,
53.6941934837545));
#127665=CARTESIAN_POINT('Ctrl Pts',(0.634542213588916,-31.5409289877891,
53.640759249768));
#127666=CARTESIAN_POINT('Ctrl Pts',(0.638403196355759,-31.493768426783,
53.5872947876981));
#127667=CARTESIAN_POINT('Ctrl Pts',(0.642264179122601,-31.4438643443167,
53.5363355024071));
#127668=CARTESIAN_POINT('Ctrl Pts',(0.646125161889444,-31.3915234507503,
53.4881600453382));
#127669=CARTESIAN_POINT('Ctrl Pts',(0.649992904154239,-31.3390909229591,
53.4399002465555));
#127670=CARTESIAN_POINT('Ctrl Pts',(0.653860646419034,-31.2842134408693,
53.3944343165916));
#127671=CARTESIAN_POINT('Ctrl Pts',(0.657728388683829,-31.2272301304811,
53.352000069982));
#127672=CARTESIAN_POINT('Ctrl Pts',(0.660031342309557,-31.1933007959288,
53.3267336237211));
#127673=CARTESIAN_POINT('Ctrl Pts',(0.662334295935285,-31.1586254386636,
53.302541175617));
#127674=CARTESIAN_POINT('Ctrl Pts',(0.664637249561013,-31.1232799038679,
53.279465251712));
#127675=CARTESIAN_POINT('Ctrl Pts',(0.668506451624919,-31.063895722331,
53.240695294991));
#127676=CARTESIAN_POINT('Ctrl Pts',(0.672375653688824,-31.0023857080583,
53.2049275076779));
#127677=CARTESIAN_POINT('Ctrl Pts',(0.676244855752729,-30.9390858401043,
53.1724017543739));
#127678=CARTESIAN_POINT('Ctrl Pts',(0.68010829368058,-30.8758802730024,
53.139924456246));
#127679=CARTESIAN_POINT('Ctrl Pts',(0.683971731608431,-30.8108905735538,
53.110679825256));
#127680=CARTESIAN_POINT('Ctrl Pts',(0.687835169536282,-30.7444810120277,
53.0848640817868));
#127681=CARTESIAN_POINT('Ctrl Pts',(0.691694076131616,-30.6781493406635,
53.0590786169762));
#127682=CARTESIAN_POINT('Ctrl Pts',(0.695552982726951,-30.6104015656689,
53.0367142264377));
#127683=CARTESIAN_POINT('Ctrl Pts',(0.699411889322285,-30.5416242556622,
53.0179201004555));
#127684=CARTESIAN_POINT('Ctrl Pts',(0.70326836529203,-30.4728902667065,
52.9991378124078));
#127685=CARTESIAN_POINT('Ctrl Pts',(0.707124841261774,-30.4031284967729,
52.9839214550263));
#127686=CARTESIAN_POINT('Ctrl Pts',(0.710981317231519,-30.3327416922295,
52.972370712198));
#127687=CARTESIAN_POINT('Ctrl Pts',(0.714836653940378,-30.2623756810045,
52.9608233816326));
#127688=CARTESIAN_POINT('Ctrl Pts',(0.718691990649237,-30.1913854808174,
52.9529395944213));
#127689=CARTESIAN_POINT('Ctrl Pts',(0.722547327358096,-30.1201833739241,
52.9487678046764));
#127690=CARTESIAN_POINT('Ctrl Pts',(0.72640281455791,-30.0489784876957,
52.9445958520879));
#127691=CARTESIAN_POINT('Ctrl Pts',(0.730258301757724,-29.9775621633845,
52.944136210851));
#127692=CARTESIAN_POINT('Ctrl Pts',(0.734113788957539,-29.9063494046929,
52.9473852946793));
#127693=CARTESIAN_POINT('Ctrl Pts',(0.737973310690108,-29.8350621261825,
52.9506377784762));
#127694=CARTESIAN_POINT('Ctrl Pts',(0.741832832422678,-29.7639793247635,
52.9576067124157));
#127695=CARTESIAN_POINT('Ctrl Pts',(0.745692354155247,-29.693512692038,
52.9682364575182));
#127696=CARTESIAN_POINT('Ctrl Pts',(0.749554060605406,-29.6230061710303,
52.9788722196852));
#127697=CARTESIAN_POINT('Ctrl Pts',(0.753415767055565,-29.5531169891623,
52.9931728207905));
#127698=CARTESIAN_POINT('Ctrl Pts',(0.757277473505724,-29.4842457167119,
53.0110316539045));
#127699=CARTESIAN_POINT('Ctrl Pts',(0.761145934398485,-29.4152539827343,
53.0289217235882));
#127700=CARTESIAN_POINT('Ctrl Pts',(0.765014395291245,-29.3472841761686,
53.050382304672));
#127701=CARTESIAN_POINT('Ctrl Pts',(0.768882856184006,-29.2807201370997,
53.0752574090736));
#127702=CARTESIAN_POINT('Ctrl Pts',(0.771179410922525,-29.2412036566243,
53.0900247908485));
#127703=CARTESIAN_POINT('Ctrl Pts',(0.773475965661045,-29.2021822227904,
53.1059946464256));
#127704=CARTESIAN_POINT('Ctrl Pts',(0.775772520399564,-29.1637320466221,
53.1231266764501));
#127705=CARTESIAN_POINT('Ctrl Pts',(0.779641665008882,-29.0989527102737,
53.1519900431726));
#127706=CARTESIAN_POINT('Ctrl Pts',(0.783510809618202,-29.0355426073808,
53.1842675958906));
#127707=CARTESIAN_POINT('Ctrl Pts',(0.787379954227521,-28.973885472867,
53.2198071622134));
#127708=CARTESIAN_POINT('Ctrl Pts',(0.791243335627565,-28.9123201785415,
53.2552937912649));
#127709=CARTESIAN_POINT('Ctrl Pts',(0.79510671702761,-28.8525030870576,
53.2940325485787));
#127710=CARTESIAN_POINT('Ctrl Pts',(0.798970098427655,-28.7947966100688,
53.3358238220073));
#127711=CARTESIAN_POINT('Ctrl Pts',(0.80282895016708,-28.737157791623,53.3775660968344));
#127712=CARTESIAN_POINT('Ctrl Pts',(0.806687801906505,-28.6816250637753,
53.4223534952188));
#127713=CARTESIAN_POINT('Ctrl Pts',(0.81054665364593,-28.6285334199595,
53.4699421637298));
#127714=CARTESIAN_POINT('Ctrl Pts',(0.814403075825124,-28.5754752030164,
53.5175008700799));
#127715=CARTESIAN_POINT('Ctrl Pts',(0.818259498004319,-28.5248553817368,
53.5678570239367));
#127716=CARTESIAN_POINT('Ctrl Pts',(0.822115920183513,-28.4769761309464,
53.6207263299863));
#127717=CARTESIAN_POINT('Ctrl Pts',(0.825971204251606,-28.4291110103275,
53.6735800331944));
#127718=CARTESIAN_POINT('Ctrl Pts',(0.829826488319699,-28.3839851804013,
53.7289450562814));
#127719=CARTESIAN_POINT('Ctrl Pts',(0.833681772387792,-28.3418629470885,
53.7865013076801));
#127720=CARTESIAN_POINT('Ctrl Pts',(0.837537208182194,-28.2997390560378,
53.8440598242291));
#127721=CARTESIAN_POINT('Ctrl Pts',(0.841392643976596,-28.2606192813935,
53.9038093469996));
#127722=CARTESIAN_POINT('Ctrl Pts',(0.845248079770998,-28.224725683171,
53.9653992738707));
#127723=CARTESIAN_POINT('Ctrl Pts',(0.849107552358481,-28.1887945029378,
54.0270536878203));
#127724=CARTESIAN_POINT('Ctrl Pts',(0.852967024945965,-28.1560964873298,
54.0905519319911));
#127725=CARTESIAN_POINT('Ctrl Pts',(0.856826497533448,-28.1268081678616,
54.155517956076));
#127726=CARTESIAN_POINT('Ctrl Pts',(0.860688156040342,-28.0975032601409,
54.2205207754715));
#127727=CARTESIAN_POINT('Ctrl Pts',(0.864549814547237,-28.0716120693271,
54.2869925768243));
#127728=CARTESIAN_POINT('Ctrl Pts',(0.868411473054131,-28.0492622742321,
54.3545390114299));
#127729=CARTESIAN_POINT('Ctrl Pts',(0.87227988844316,-28.0268733729005,
54.4222036344503));
#127730=CARTESIAN_POINT('Ctrl Pts',(0.876148303832189,-28.0080383671996,
54.4909461761997));
#127731=CARTESIAN_POINT('Ctrl Pts',(0.880016719221218,-27.9928343745199,
54.5603595623795));
#127732=CARTESIAN_POINT('Ctrl Pts',(0.882313743226854,-27.9838064050144,
54.6015764944648));
#127733=CARTESIAN_POINT('Ctrl Pts',(0.884610767232489,-27.9760576942167,
54.6430297886563));
#127734=CARTESIAN_POINT('Ctrl Pts',(0.886907791238125,-27.969595720755,
54.6846335063398));
#127735=CARTESIAN_POINT('Ctrl Pts',(0.892630100646191,-27.9534977559779,
54.7882760214057));
#127736=CARTESIAN_POINT('Ctrl Pts',(0.898352410054257,-27.9453327589816,
54.8931817843288));
#127737=CARTESIAN_POINT('Ctrl Pts',(0.904074719462322,-27.9452506260578,
54.9983960099243));
#127738=CARTESIAN_POINT('Ctrl Pts',(0.904074719503241,-27.9452506260572,
54.9983960106767));
#127739=CARTESIAN_POINT('Ctrl Pts',(0.907990067110467,-27.9451944286773,
55.0703862225056));
#127740=CARTESIAN_POINT('Ctrl Pts',(0.911905414717693,-27.9489263330349,
55.1425163182313));
#127741=CARTESIAN_POINT('Ctrl Pts',(0.91582076232492,-27.956460767646,55.2143477742593));
#127742=CARTESIAN_POINT('Ctrl Pts',(0.919623060323791,-27.9637776571072,
55.2841052080584));
#127743=CARTESIAN_POINT('Ctrl Pts',(0.923425358322662,-27.9746804238571,
55.353580473897));
#127744=CARTESIAN_POINT('Ctrl Pts',(0.927227656321533,-27.9891295593209,
55.4223714399708));
#127745=CARTESIAN_POINT('Ctrl Pts',(0.931027484170776,-28.0035693079543,
55.4911177162335));
#127746=CARTESIAN_POINT('Ctrl Pts',(0.934827312020019,-28.0215507559555,
55.5591800843778));
#127747=CARTESIAN_POINT('Ctrl Pts',(0.938627139869262,-28.0429829087638,
55.6261642493064));
#127748=CARTESIAN_POINT('Ctrl Pts',(0.942425858315227,-28.0644088042096,
55.6931288574405));
#127749=CARTESIAN_POINT('Ctrl Pts',(0.946224576761191,-28.0892832528651,
55.7590154094981));
#127750=CARTESIAN_POINT('Ctrl Pts',(0.950023295207156,-28.1174652875836,
55.8234443630551));
#127751=CARTESIAN_POINT('Ctrl Pts',(0.953822263240489,-28.1456491739475,
55.8878775497905));
#127752=CARTESIAN_POINT('Ctrl Pts',(0.957621231273823,-28.1771408732871,
55.9508524899949));
#127753=CARTESIAN_POINT('Ctrl Pts',(0.961420199307156,-28.2117519093447,
56.0120110319398));
#127754=CARTESIAN_POINT('Ctrl Pts',(0.965223099469433,-28.2463987696197,
56.0732328761475));
#127755=CARTESIAN_POINT('Ctrl Pts',(0.96902599963171,-28.2841711573993,
56.1326341360962));
#127756=CARTESIAN_POINT('Ctrl Pts',(0.972828899793987,-28.3248360119472,
56.1898836815551));
#127757=CARTESIAN_POINT('Ctrl Pts',(0.976634203973915,-28.3655265729359,
56.2471694175296));
#127758=CARTESIAN_POINT('Ctrl Pts',(0.980439508153843,-28.4091129234218,
56.302300343409));
#127759=CARTESIAN_POINT('Ctrl Pts',(0.984244812333771,-28.4553220850818,
56.3549788565376));
#127760=CARTESIAN_POINT('Ctrl Pts',(0.988056247498605,-28.5016056974715,
56.407742243609));
#127761=CARTESIAN_POINT('Ctrl Pts',(0.991867682663438,-28.5505201949312,
56.4580449849629));
#127762=CARTESIAN_POINT('Ctrl Pts',(0.995679117828272,-28.601757094291,
56.5056275565804));
#127763=CARTESIAN_POINT('Ctrl Pts',(0.996467099244409,-28.6123498822488,
56.5154648437295));
#127764=CARTESIAN_POINT('Ctrl Pts',(0.997255080660547,-28.623041829606,
56.5251860091331));
#127765=CARTESIAN_POINT('Ctrl Pts',(0.998043062076684,-28.6338300529546,
56.5347889881968));
#127766=CARTESIAN_POINT('Ctrl Pts',(1.00191215654311,-28.6868016769114,
56.5819409037059));
#127767=CARTESIAN_POINT('Ctrl Pts',(1.00578125100953,-28.742321012852,56.6264395602405));
#127768=CARTESIAN_POINT('Ctrl Pts',(1.00965034547595,-28.8000914233495,
56.6679978927386));
#127769=CARTESIAN_POINT('Ctrl Pts',(1.01351367518186,-28.8577757587759,
56.7094943053647));
#127770=CARTESIAN_POINT('Ctrl Pts',(1.01737700488776,-28.9177041200476,
56.748058808628));
#127771=CARTESIAN_POINT('Ctrl Pts',(1.02124033459367,-28.979545413354,56.783443298536));
#127772=CARTESIAN_POINT('Ctrl Pts',(1.02509913257681,-29.0413141662306,
56.8187862820983));
#127773=CARTESIAN_POINT('Ctrl Pts',(1.02895793055994,-29.1049909744289,
56.8509564216362));
#127774=CARTESIAN_POINT('Ctrl Pts',(1.03281672854308,-29.1702157119384,
56.8797488124178));
#127775=CARTESIAN_POINT('Ctrl Pts',(1.03667309572076,-29.235399361874,56.9085230657636));
#127776=CARTESIAN_POINT('Ctrl Pts',(1.04052946289844,-29.3021285631809,
56.9339235961119));
#127777=CARTESIAN_POINT('Ctrl Pts',(1.04438583007612,-29.3700198432387,
56.9557920555588));
#127778=CARTESIAN_POINT('Ctrl Pts',(1.04824105797769,-29.4378910663595,
56.977654054466));
#127779=CARTESIAN_POINT('Ctrl Pts',(1.05209628587926,-29.5069232245335,
56.9959859051922));
#127780=CARTESIAN_POINT('Ctrl Pts',(1.05595151378083,-29.5767158114237,
57.0106785069228));
#127781=CARTESIAN_POINT('Ctrl Pts',(1.05980689232267,-29.6465111254094,
57.0253716827563));
#127782=CARTESIAN_POINT('Ctrl Pts',(1.06366227086452,-29.7170664512887,
57.0364252293559));
#127783=CARTESIAN_POINT('Ctrl Pts',(1.06751764940637,-29.7879708680803,
57.0437811061162));
#127784=CARTESIAN_POINT('Ctrl Pts',(1.07137706346744,-29.858949502263,57.051144682453));
#127785=CARTESIAN_POINT('Ctrl Pts',(1.07523647752851,-29.9302774726059,
57.0548028124487));
#127786=CARTESIAN_POINT('Ctrl Pts',(1.07909589158959,-30.0015394086098,
57.0547494233412));
#127787=CARTESIAN_POINT('Ctrl Pts',(1.08295749076274,-30.072841691494,57.054696004006));
#127788=CARTESIAN_POINT('Ctrl Pts',(1.0868190899359,-30.1440773802816,57.0509269080504));
#127789=CARTESIAN_POINT('Ctrl Pts',(1.09068068910905,-30.214834539337,57.0434881167278));
#127790=CARTESIAN_POINT('Ctrl Pts',(1.0945490445224,-30.2857154948666,57.0360363105224));
#127791=CARTESIAN_POINT('Ctrl Pts',(1.09841739993575,-30.3561157691335,
57.024902066172));
#127792=CARTESIAN_POINT('Ctrl Pts',(1.1022857553491,-30.4256326436585,57.0101826820347));
#127793=CARTESIAN_POINT('Ctrl Pts',(1.10458328120448,-30.4669206845804,
57.0014404228529));
#127794=CARTESIAN_POINT('Ctrl Pts',(1.10688080705986,-30.5078973577857,
56.9914344696973));
#127795=CARTESIAN_POINT('Ctrl Pts',(1.10917833291525,-30.5484812107845,
56.9801934056845));
#127796=CARTESIAN_POINT('Ctrl Pts',(1.1130463169165,-30.6168058800112,56.9612685889488));
#127797=CARTESIAN_POINT('Ctrl Pts',(1.11691430091776,-30.6842837117802,
56.9387663513206));
#127798=CARTESIAN_POINT('Ctrl Pts',(1.12078228491901,-30.750512987213,56.9127801281184));
#127799=CARTESIAN_POINT('Ctrl Pts',(1.12464523500466,-30.8166560697911,
56.8868277242015));
#127800=CARTESIAN_POINT('Ctrl Pts',(1.12850818509031,-30.881553369978,56.857400501153));
#127801=CARTESIAN_POINT('Ctrl Pts',(1.13237113517596,-30.9448169781747,
56.8246420033126));
#127802=CARTESIAN_POINT('Ctrl Pts',(1.13622985695909,-31.0080113393794,
56.7919193622232));
#127803=CARTESIAN_POINT('Ctrl Pts',(1.14008857874222,-31.0695751296572,
56.7558729078419));
#127804=CARTESIAN_POINT('Ctrl Pts',(1.14394730052535,-31.1291408909691,
56.716694035302));
#127805=CARTESIAN_POINT('Ctrl Pts',(1.1466682528,-31.1711432956104,56.6890673111309));
#127806=CARTESIAN_POINT('Ctrl Pts',(1.14938920507465,-31.2121526189746,
56.659884083656));
#127807=CARTESIAN_POINT('Ctrl Pts',(1.15211015734929,-31.2520475724682,
56.6292251037768));
#127808=CARTESIAN_POINT('',(0.845925280586865,-27.9452503300222,55.0011645711683));
#127809=CARTESIAN_POINT('Ctrl Pts',(0.845925280586864,-27.9452503300222,
55.0011645711683));
#127810=CARTESIAN_POINT('Ctrl Pts',(0.850222060722874,-27.945295440436,
55.0807566222002));
#127811=CARTESIAN_POINT('Ctrl Pts',(0.854518840858883,-27.9499692453172,
55.1601816680743));
#127812=CARTESIAN_POINT('Ctrl Pts',(0.858815620994894,-27.9591891742394,
55.2389324924709));
#127813=CARTESIAN_POINT('Ctrl Pts',(0.863129968211751,-27.9684467981871,
55.3180052840278));
#127814=CARTESIAN_POINT('Ctrl Pts',(0.867444315428608,-27.9822876582133,
55.3963980692969));
#127815=CARTESIAN_POINT('Ctrl Pts',(0.871758662645465,-28.0005784158235,
55.4736147075728));
#127816=CARTESIAN_POINT('Ctrl Pts',(0.87609514182901,-28.0189630023301,
55.5512274558463));
#127817=CARTESIAN_POINT('Ctrl Pts',(0.880431621012555,-28.0418431211359,
55.6276517068927));
#127818=CARTESIAN_POINT('Ctrl Pts',(0.8847681001961,-28.0690352661005,55.702404982141));
#127819=CARTESIAN_POINT('Ctrl Pts',(0.886206122366891,-28.0780524677693,
55.7271939555446));
#127820=CARTESIAN_POINT('Ctrl Pts',(0.887644144537682,-28.0875434620998,
55.7517993688499));
#127821=CARTESIAN_POINT('Ctrl Pts',(0.889082166708474,-28.0975004387939,
55.77620421418));
#127822=CARTESIAN_POINT('Ctrl Pts',(0.892951368337054,-28.1242910900254,
55.8418688953053));
#127823=CARTESIAN_POINT('Ctrl Pts',(0.896820569965634,-28.1545378023993,
55.9062734887861));
#127824=CARTESIAN_POINT('Ctrl Pts',(0.900689771594214,-28.1881006707189,
55.969029608965));
#127825=CARTESIAN_POINT('Ctrl Pts',(0.90455320908223,-28.2216135387777,
56.0316922382554));
#127826=CARTESIAN_POINT('Ctrl Pts',(0.908416646570245,-28.2584325293038,
56.0927108441219));
#127827=CARTESIAN_POINT('Ctrl Pts',(0.912280084058261,-28.2983696437099,
56.1517168458662));
#127828=CARTESIAN_POINT('Ctrl Pts',(0.916138990209208,-28.3382599167921,
56.2106536408268));
#127829=CARTESIAN_POINT('Ctrl Pts',(0.919997896360154,-28.3812607784018,
56.2675821201815));
#127830=CARTESIAN_POINT('Ctrl Pts',(0.923856802511101,-28.4271391397493,
56.3221597016969));
#127831=CARTESIAN_POINT('Ctrl Pts',(0.927713278033892,-28.4729886034681,
56.3767029061633));
#127832=CARTESIAN_POINT('Ctrl Pts',(0.931569753556685,-28.5217116591905,
56.4288977796746));
#127833=CARTESIAN_POINT('Ctrl Pts',(0.935426229079476,-28.5730337535307,
56.4784332565041));
#127834=CARTESIAN_POINT('Ctrl Pts',(0.939281565339479,-28.6243406865268,
56.5279540997841));
#127835=CARTESIAN_POINT('Ctrl Pts',(0.943136901599481,-28.6782447845327,
56.5748167689184));
#127836=CARTESIAN_POINT('Ctrl Pts',(0.946992237859484,-28.7344345121555,
56.6187469099513));
#127837=CARTESIAN_POINT('Ctrl Pts',(0.950847724609213,-28.7906264330959,
56.6626787657594));
#127838=CARTESIAN_POINT('Ctrl Pts',(0.954703211358941,-28.8491037767504,
56.703677568755));
#127839=CARTESIAN_POINT('Ctrl Pts',(0.958558698108669,-28.9095231694168,
56.7415102194536));
#127840=CARTESIAN_POINT('Ctrl Pts',(0.962418219392364,-28.9700057873276,
56.7793824597356));
#127841=CARTESIAN_POINT('Ctrl Pts',(0.96627774067606,-29.0324340985123,
56.8140816755319));
#127842=CARTESIAN_POINT('Ctrl Pts',(0.970137261959756,-29.0964378464631,
56.8454194637523));
#127843=CARTESIAN_POINT('Ctrl Pts',(0.97399896796105,-29.1604778243254,
56.8767749910166));
#127844=CARTESIAN_POINT('Ctrl Pts',(0.977860673962344,-29.2260945672309,
56.9047651121883));
#127845=CARTESIAN_POINT('Ctrl Pts',(0.981722379963638,-29.2928979758192,
56.9292496701825));
#127846=CARTESIAN_POINT('Ctrl Pts',(0.985590840412425,-29.3598182291688,
56.9537770537211));
#127847=CARTESIAN_POINT('Ctrl Pts',(0.989459300861211,-29.4279288278397,
56.9747864890832));
#127848=CARTESIAN_POINT('Ctrl Pts',(0.993327761309998,-29.4968253453767,
56.9921879503312));
#127849=CARTESIAN_POINT('Ctrl Pts',(0.995624320055678,-29.5377266036399,
57.0025185401216));
#127850=CARTESIAN_POINT('Ctrl Pts',(0.997920878801357,-29.5789046477481,
57.0115785332614));
#127851=CARTESIAN_POINT('Ctrl Pts',(1.00021743754704,-29.620273873091,57.0193577273585));
#127852=CARTESIAN_POINT('Ctrl Pts',(1.00411925944499,-29.6905596211249,
57.0325744717304));
#127853=CARTESIAN_POINT('Ctrl Pts',(1.00802108134294,-29.7616750027816,
57.0421433833276));
#127854=CARTESIAN_POINT('Ctrl Pts',(1.01192290324089,-29.8332075112887,
57.0479691961085));
#127855=CARTESIAN_POINT('Ctrl Pts',(1.01578553666388,-29.90402157339,57.0537364965524));
#127856=CARTESIAN_POINT('Ctrl Pts',(1.01964817008687,-29.9752439316532,
57.0558354678734));
#127857=CARTESIAN_POINT('Ctrl Pts',(1.02351080350986,-30.0464631461639,
57.0542246076193));
#127858=CARTESIAN_POINT('Ctrl Pts',(1.02736955491481,-30.1176107840465,
57.0526153663095));
#127859=CARTESIAN_POINT('Ctrl Pts',(1.03122830631976,-30.1887548014223,
57.0473037019312));
#127860=CARTESIAN_POINT('Ctrl Pts',(1.03508705772471,-30.2594809995703,
57.0383000695094));
#127861=CARTESIAN_POINT('Ctrl Pts',(1.03894322185011,-30.3301597760455,
57.0293024739922));
#127862=CARTESIAN_POINT('Ctrl Pts',(1.0427993859755,-30.4004208087665,57.0166178856518));
#127863=CARTESIAN_POINT('Ctrl Pts',(1.04665555010089,-30.4698539987165,
57.000308671778));
#127864=CARTESIAN_POINT('Ctrl Pts',(1.05058935118398,-30.5406851015808,
56.9836711010951));
#127865=CARTESIAN_POINT('Ctrl Pts',(1.05452315226706,-30.6106541432883,
56.9632614055032));
#127866=CARTESIAN_POINT('Ctrl Pts',(1.05845695335014,-30.6793370476578,
56.9392005409909));
#127867=CARTESIAN_POINT('Ctrl Pts',(1.06231322009866,-30.7466662274301,
56.9156139107065));
#127868=CARTESIAN_POINT('Ctrl Pts',(1.06616948684717,-30.8127590575158,
56.8885189571279));
#127869=CARTESIAN_POINT('Ctrl Pts',(1.07002575359569,-30.8772338320979,
56.8580792142217));
#127870=CARTESIAN_POINT('Ctrl Pts',(1.07399832184605,-30.9436531073082,
56.8267214363229));
#127871=CARTESIAN_POINT('Ctrl Pts',(1.07797089009642,-31.0083546525018,
56.7918140847842));
#127872=CARTESIAN_POINT('Ctrl Pts',(1.08194345834679,-31.0709481895177,
56.7535870488427));
#127873=CARTESIAN_POINT('Ctrl Pts',(1.08591602659716,-31.1335417265337,
56.7153600129011));
#127874=CARTESIAN_POINT('Ctrl Pts',(1.08988859484753,-31.1940268102068,
56.6738136350815));
#127875=CARTESIAN_POINT('Ctrl Pts',(1.09386116309789,-31.2520475724682,
56.6292251037768));
#127876=CARTESIAN_POINT('Ctrl Pts',(0.393903215690563,-31.2520475724682,
56.6292251037768));
#127877=CARTESIAN_POINT('Ctrl Pts',(0.39776569061235,-31.3086907373524,
56.5856952459777));
#127878=CARTESIAN_POINT('Ctrl Pts',(0.401628165534137,-31.3630503634527,
56.5392162854362));
#127879=CARTESIAN_POINT('Ctrl Pts',(0.405490640455925,-31.4148157924792,
56.490065044168));
#127880=CARTESIAN_POINT('Ctrl Pts',(0.409357389344096,-31.4666385018009,
56.4408594152967));
#127881=CARTESIAN_POINT('Ctrl Pts',(0.413224138232267,-31.5158609348587,
56.3889759393529));
#127882=CARTESIAN_POINT('Ctrl Pts',(0.417090887120438,-31.5622092788417,
56.3347283362546));
#127883=CARTESIAN_POINT('Ctrl Pts',(0.420960118935074,-31.6085873841392,
56.2804458995498));
#127884=CARTESIAN_POINT('Ctrl Pts',(0.424829350749709,-31.6520874331276,
56.2237966983362));
#127885=CARTESIAN_POINT('Ctrl Pts',(0.428698582564345,-31.6924775726151,
56.1651254132904));
#127886=CARTESIAN_POINT('Ctrl Pts',(0.432574324736315,-31.7329356724247,
56.106355408124));
#127887=CARTESIAN_POINT('Ctrl Pts',(0.436450066908286,-31.7702731684576,
56.0455569417902));
#127888=CARTESIAN_POINT('Ctrl Pts',(0.440325809080256,-31.8043033884208,
55.9831006281319));
#127889=CARTESIAN_POINT('Ctrl Pts',(0.441730900504915,-31.81664052751,55.9604580407659));
#127890=CARTESIAN_POINT('Ctrl Pts',(0.443135991929574,-31.8285434424312,
55.9375977575761));
#127891=CARTESIAN_POINT('Ctrl Pts',(0.444541083354233,-31.8400048163345,
55.9145380464287));
#127892=CARTESIAN_POINT('Ctrl Pts',(0.44840594300457,-31.8715305951977,
55.851109755858));
#127893=CARTESIAN_POINT('Ctrl Pts',(0.452270802654908,-31.8998358376757,
55.7859225613206));
#127894=CARTESIAN_POINT('Ctrl Pts',(0.456135662305245,-31.9247212374688,
55.7193370006726));
#127895=CARTESIAN_POINT('Ctrl Pts',(0.459994695776998,-31.9495691231484,
55.6528518160803));
#127896=CARTESIAN_POINT('Ctrl Pts',(0.463853729248751,-31.9710072294324,
55.5849729017156));
#127897=CARTESIAN_POINT('Ctrl Pts',(0.467712762720505,-31.9888828440538,
55.5160839031867));
#127898=CARTESIAN_POINT('Ctrl Pts',(0.471567193850847,-32.0067371399481,
55.4472770627144));
#127899=CARTESIAN_POINT('Ctrl Pts',(0.47542162498119,-32.0210372613224,
55.3774629998046));
#127900=CARTESIAN_POINT('Ctrl Pts',(0.479276056111532,-32.0316797748725,
55.3070421060282));
#127901=CARTESIAN_POINT('Ctrl Pts',(0.483128015115094,-32.0423154626052,
55.2366663782884));
#127902=CARTESIAN_POINT('Ctrl Pts',(0.486979974118655,-32.0492981237219,
55.1656850721509));
#127903=CARTESIAN_POINT('Ctrl Pts',(0.490831933122217,-32.0525753629738,
55.0945089509679));
#127904=CARTESIAN_POINT('Ctrl Pts',(0.494682717987179,-32.0558516032708,
55.0233545254029));
#127905=CARTESIAN_POINT('Ctrl Pts',(0.498533502852141,-32.0554246414167,
54.9520058888896));
#127906=CARTESIAN_POINT('Ctrl Pts',(0.502384287717103,-32.0512940696008,
54.8808773635249));
#127907=CARTESIAN_POINT('Ctrl Pts',(0.506235194778705,-32.0471633667097,
54.8097465810445));
#127908=CARTESIAN_POINT('Ctrl Pts',(0.510086101840306,-32.0393288509765,
54.7388364096479));
#127909=CARTESIAN_POINT('Ctrl Pts',(0.513937008901907,-32.0278421201088,
54.6685578505792));
#127910=CARTESIAN_POINT('Ctrl Pts',(0.517791938585007,-32.0163433903094,
54.5982058791851));
#127911=CARTESIAN_POINT('Ctrl Pts',(0.521646868268107,-32.0011849083202,
54.5284873188182));
#127912=CARTESIAN_POINT('Ctrl Pts',(0.525501797951207,-31.9824695892304,
54.4598038409277));
#127913=CARTESIAN_POINT('Ctrl Pts',(0.529358898593875,-31.9637437303373,
54.3910816829403));
#127914=CARTESIAN_POINT('Ctrl Pts',(0.533215999236543,-31.9414571995012,
54.3233962305621));
#127915=CARTESIAN_POINT('Ctrl Pts',(0.537073099879211,-31.9157622397753,
54.2571321765271));
#127916=CARTESIAN_POINT('Ctrl Pts',(0.540936983133111,-31.8900220961305,
54.1907515988753));
#127917=CARTESIAN_POINT('Ctrl Pts',(0.544800866387012,-31.8608617568373,
54.1257978542333));
#127918=CARTESIAN_POINT('Ctrl Pts',(0.548664749640912,-31.8284805618616,
54.0626332641948));
#127919=CARTESIAN_POINT('Ctrl Pts',(0.551001951158207,-31.8088936921102,
54.0244260084429));
#127920=CARTESIAN_POINT('Ctrl Pts',(0.553339152675502,-31.7881292432781,
53.9868728739325));
#127921=CARTESIAN_POINT('Ctrl Pts',(0.555676354192796,-31.7662389263135,
53.95004875462));
#127922=CARTESIAN_POINT('Ctrl Pts',(0.559546127041688,-31.7299944888457,
53.8890779842155));
#127923=CARTESIAN_POINT('Ctrl Pts',(0.56341589989058,-31.6905184267416,
53.8298669871839));
#127924=CARTESIAN_POINT('Ctrl Pts',(0.567285672739472,-31.6480068398848,
53.7727791485666));
#127925=CARTESIAN_POINT('Ctrl Pts',(0.571149681546897,-31.6055585741993,
53.7157763425034));
#127926=CARTESIAN_POINT('Ctrl Pts',(0.575013690354322,-31.5600840464339,
53.6608908036987));
#127927=CARTESIAN_POINT('Ctrl Pts',(0.578877699161747,-31.5118239738126,
53.6084591868344));
#127928=CARTESIAN_POINT('Ctrl Pts',(0.582737173900105,-31.4636205300742,
53.5560890937875));
#127929=CARTESIAN_POINT('Ctrl Pts',(0.586596648638463,-31.4126383613493,
53.5061675585738));
#127930=CARTESIAN_POINT('Ctrl Pts',(0.590456123376821,-31.3591589130782,
53.4589988281964));
#127931=CARTESIAN_POINT('Ctrl Pts',(0.594313165471867,-31.3057131731303,
53.4118598284699));
#127932=CARTESIAN_POINT('Ctrl Pts',(0.598170207566914,-31.249773639875,
53.3674705115531));
#127933=CARTESIAN_POINT('Ctrl Pts',(0.60202724966196,-31.1916580838614,
53.3260978004472));
#127934=CARTESIAN_POINT('Ctrl Pts',(0.605883149611384,-31.1335597370009,
53.2847373406104));
#127935=CARTESIAN_POINT('Ctrl Pts',(0.609739049560808,-31.0732870420026,
53.2463919946229));
#127936=CARTESIAN_POINT('Ctrl Pts',(0.613594949510231,-31.0111888919898,
53.2112868907462));
#127937=CARTESIAN_POINT('Ctrl Pts',(0.617450996196304,-30.9490883788258,
53.1761804509413));
#127938=CARTESIAN_POINT('Ctrl Pts',(0.621307042882376,-30.885162696523,
53.1443147351114));
#127939=CARTESIAN_POINT('Ctrl Pts',(0.625163089568449,-30.819786101699,
53.1158693490203));
#127940=CARTESIAN_POINT('Ctrl Pts',(0.62902316110723,-30.7543412682912,
53.0873942722905));
#127941=CARTESIAN_POINT('Ctrl Pts',(0.632883232646012,-30.687442945382,
53.0623468461053));
#127942=CARTESIAN_POINT('Ctrl Pts',(0.636743304184793,-30.6194853422827,
53.0408584856635));
#127943=CARTESIAN_POINT('Ctrl Pts',(0.640605555802807,-30.551489358299,
53.019357989092));
#127944=CARTESIAN_POINT('Ctrl Pts',(0.644467807420821,-30.4824333733671,
53.0014206819458));
#127945=CARTESIAN_POINT('Ctrl Pts',(0.648330059038836,-30.4127240646842,
52.9871273242128));
#127946=CARTESIAN_POINT('Ctrl Pts',(0.652199051765006,-30.342893086562,
52.9728090190969));
#127947=CARTESIAN_POINT('Ctrl Pts',(0.656068044491176,-30.2724069883148,
52.9621474342147));
#127948=CARTESIAN_POINT('Ctrl Pts',(0.659937037217347,-30.2016791805648,
52.9551716280757));
#127949=CARTESIAN_POINT('Ctrl Pts',(0.662228566488683,-30.1597884732859,
52.9510399935418));
#127950=CARTESIAN_POINT('Ctrl Pts',(0.664520095760019,-30.1178130267174,
52.9482003209458));
#127951=CARTESIAN_POINT('Ctrl Pts',(0.666811625031356,-30.0758384352019,
52.9466500312304));
#127952=CARTESIAN_POINT('Ctrl Pts',(0.670681389707337,-30.0049548582094,
52.9440320169404));
#127953=CARTESIAN_POINT('Ctrl Pts',(0.674551154383317,-29.933797299356,
52.9450836555165));
#127954=CARTESIAN_POINT('Ctrl Pts',(0.678420919059298,-29.8627774305534,
52.9498371945296));
#127955=CARTESIAN_POINT('Ctrl Pts',(0.682284934099417,-29.7918630819617,
52.9545836708086));
#127956=CARTESIAN_POINT('Ctrl Pts',(0.686148949139536,-29.7210864979116,
52.9630210974097));
#127957=CARTESIAN_POINT('Ctrl Pts',(0.690012964179655,-29.6508610783276,
52.9751297385083));
#127958=CARTESIAN_POINT('Ctrl Pts',(0.693872466683003,-29.5807176705331,
52.9872242386971));
#127959=CARTESIAN_POINT('Ctrl Pts',(0.697731969186351,-29.5111246248659,
53.002981355034));
#127960=CARTESIAN_POINT('Ctrl Pts',(0.701591471689699,-29.4424901925755,
53.0223295580088));
#127961=CARTESIAN_POINT('Ctrl Pts',(0.705448554854998,-29.3738987839373,
53.041665632518));
#127962=CARTESIAN_POINT('Ctrl Pts',(0.709305638020299,-29.3062652627375,
53.0645881960493));
#127963=CARTESIAN_POINT('Ctrl Pts',(0.713162721185598,-29.2399862107333,
53.0909749601892));
#127964=CARTESIAN_POINT('Ctrl Pts',(0.717018675482635,-29.1737265568896,
53.1173540016073));
#127965=CARTESIAN_POINT('Ctrl Pts',(0.720874629779671,-29.1088210361309,
53.1471950512521));
#127966=CARTESIAN_POINT('Ctrl Pts',(0.724730584076708,-29.0456479835695,
53.1803270098078));
#127967=CARTESIAN_POINT('Ctrl Pts',(0.728586698373548,-28.9824723096917,
53.2134603431483));
#127968=CARTESIAN_POINT('Ctrl Pts',(0.732442812670388,-28.9210296757409,
53.249884629028));
#127969=CARTESIAN_POINT('Ctrl Pts',(0.736298926967228,-28.8616739156467,
53.2893827756681));
#127970=CARTESIAN_POINT('Ctrl Pts',(0.74015908606738,-28.8022558953714,
53.3289223531948));
#127971=CARTESIAN_POINT('Ctrl Pts',(0.744019245167533,-28.7449295237354,
53.3715419582693));
#127972=CARTESIAN_POINT('Ctrl Pts',(0.747879404267685,-28.6900189598985,
53.4169816055792));
#127973=CARTESIAN_POINT('Ctrl Pts',(0.751741754842204,-28.635077222452,
53.4624470497072));
#127974=CARTESIAN_POINT('Ctrl Pts',(0.755604105416722,-28.5825543806718,
53.5107353943525));
#127975=CARTESIAN_POINT('Ctrl Pts',(0.759466455991241,-28.5327387878957,
53.5615487154741));
#127976=CARTESIAN_POINT('Ctrl Pts',(0.763335564771012,-28.4828360295466,
53.6124509479586));
#127977=CARTESIAN_POINT('Ctrl Pts',(0.767204673550783,-28.4356502993757,
53.6658866137231));
#127978=CARTESIAN_POINT('Ctrl Pts',(0.771073782330553,-28.3914301581678,
53.7215241001693));
#127979=CARTESIAN_POINT('Ctrl Pts',(0.773364820177007,-28.3652458292049,
53.7544690480591));
#127980=CARTESIAN_POINT('Ctrl Pts',(0.775655858023461,-28.3401005007883,
53.7881854261158));
#127981=CARTESIAN_POINT('Ctrl Pts',(0.777946895869916,-28.316038381332,
53.8225999705482));
#127982=CARTESIAN_POINT('Ctrl Pts',(0.781859836728712,-28.2749418754339,
53.8813777324496));
#127983=CARTESIAN_POINT('Ctrl Pts',(0.785772777587509,-28.2368483254715,
53.9424211699665));
#127984=CARTESIAN_POINT('Ctrl Pts',(0.789685718446306,-28.2020125974159,
54.0053951223482));
#127985=CARTESIAN_POINT('Ctrl Pts',(0.793592483939231,-28.1672318467734,
54.0682696898399));
#127986=CARTESIAN_POINT('Ctrl Pts',(0.797499249432156,-28.1356989358561,
54.1330683142181));
#127987=CARTESIAN_POINT('Ctrl Pts',(0.801406014925082,-28.1076260877293,
54.1994261191761));
#127988=CARTESIAN_POINT('Ctrl Pts',(0.805307065989411,-28.079594301777,
54.2656868625268));
#127989=CARTESIAN_POINT('Ctrl Pts',(0.80920811705374,-28.0550127000085,
54.3335018210736));
#127990=CARTESIAN_POINT('Ctrl Pts',(0.813109168118069,-28.0340472615431,
54.4024823076646));
#127991=CARTESIAN_POINT('Ctrl Pts',(0.817006832225679,-28.0131000256163,
54.4714029042622));
#127992=CARTESIAN_POINT('Ctrl Pts',(0.82090449633329,-27.9957628551231,
54.5414865701392));
#127993=CARTESIAN_POINT('Ctrl Pts',(0.8248021604409,-27.9821529116122,54.6123265673472));
#127994=CARTESIAN_POINT('Ctrl Pts',(0.828698062049659,-27.9685491224309,
54.6831345311603));
#127995=CARTESIAN_POINT('Ctrl Pts',(0.832593963658419,-27.9586693066202,
54.7546976857619));
#127996=CARTESIAN_POINT('Ctrl Pts',(0.836489865267178,-27.9525798840312,
54.8265974878318));
#127997=CARTESIAN_POINT('Ctrl Pts',(0.839635003690678,-27.9476639290393,
54.8846417745827));
#127998=CARTESIAN_POINT('Ctrl Pts',(0.842780142114177,-27.9452173103231,
54.9429051271427));
#127999=CARTESIAN_POINT('Ctrl Pts',(0.845925280537677,-27.9452503300217,
55.0011645702572));
#128000=CARTESIAN_POINT('Origin',(80.,-9.,134.));
#128001=CARTESIAN_POINT('',(78.3340002645784,-8.99906107773531,138.679802703723));
#128002=CARTESIAN_POINT('Ctrl Pts',(78.4365593749993,-8.42449203993574,
139.340802385574));
#128003=CARTESIAN_POINT('Ctrl Pts',(78.4404068256367,-8.41403995056995,
139.340073131));
#128004=CARTESIAN_POINT('Ctrl Pts',(78.4443588637281,-8.40362705661283,
139.339338587103));
#128005=CARTESIAN_POINT('Ctrl Pts',(78.450721004147,-8.38735761703001,139.338177103129));
#128006=CARTESIAN_POINT('Ctrl Pts',(78.4530606904758,-8.38147363376576,
139.337754185242));
#128007=CARTESIAN_POINT('Ctrl Pts',(78.4572880769896,-8.37101637513597,
139.336997211539));
#128008=CARTESIAN_POINT('Ctrl Pts',(78.4591626864472,-8.3664379679219,139.336663938979));
#128009=CARTESIAN_POINT('Ctrl Pts',(78.4637554384923,-8.35536191966457,
139.335853231315));
#128010=CARTESIAN_POINT('Ctrl Pts',(78.4664944016446,-8.34887314395052,
139.335374571223));
#128011=CARTESIAN_POINT('Ctrl Pts',(78.4751941165289,-8.32862235513383,
139.333869501142));
#128012=CARTESIAN_POINT('Ctrl Pts',(78.4812994162062,-8.3149237838157,139.332835100129));
#128013=CARTESIAN_POINT('Ctrl Pts',(78.5143713886673,-8.24333489887553,
139.327350021681));
#128014=CARTESIAN_POINT('Ctrl Pts',(78.5444630974817,-8.1869531698572,139.322756877021));
#128015=CARTESIAN_POINT('Ctrl Pts',(78.6346517897326,-8.03909622286664,
139.310189682049));
#128016=CARTESIAN_POINT('Ctrl Pts',(78.7006497236031,-7.95157005770015,
139.302185330614));
#128017=CARTESIAN_POINT('Ctrl Pts',(78.8088854917817,-7.83409277274342,
139.290895045155));
#128018=CARTESIAN_POINT('Ctrl Pts',(78.8446829265701,-7.79861046733643,
139.287394266339));
#128019=CARTESIAN_POINT('Ctrl Pts',(78.8941308511983,-7.75385574502929,
139.282852431406));
#128020=CARTESIAN_POINT('Ctrl Pts',(78.9063852206201,-7.74308758234494,
139.281749041542));
#128021=CARTESIAN_POINT('Ctrl Pts',(78.9267516322524,-7.72571459899383,
139.279950590039));
#128022=CARTESIAN_POINT('Ctrl Pts',(78.9347709786541,-7.71900332444436,
139.279251179898));
#128023=CARTESIAN_POINT('Ctrl Pts',(78.9505043452793,-7.7060862197635,139.277895611099));
#128024=CARTESIAN_POINT('Ctrl Pts',(78.9582115228496,-7.69987278467009,
139.277239162322));
#128025=CARTESIAN_POINT('Ctrl Pts',(78.9765383417246,-7.68536553366061,
139.275695685906));
#128026=CARTESIAN_POINT('Ctrl Pts',(78.9872042244231,-7.6771310417617,139.274811034834));
#128027=CARTESIAN_POINT('Ctrl Pts',(79.0235620733276,-7.64975882722003,
139.271839678635));
#128028=CARTESIAN_POINT('Ctrl Pts',(79.0497066872027,-7.63123227537913,
139.269776519917));
#128029=CARTESIAN_POINT('Ctrl Pts',(79.1149223844842,-7.58778919564296,
139.264789027379));
#128030=CARTESIAN_POINT('Ctrl Pts',(79.1545301201519,-7.56372603772657,
139.261893507738));
#128031=CARTESIAN_POINT('Ctrl Pts',(79.2558412699803,-7.50782103574636,
139.254738139325));
#128032=CARTESIAN_POINT('Ctrl Pts',(79.3186268530432,-7.47812577495616,
139.25052548465));
#128033=CARTESIAN_POINT('Ctrl Pts',(79.4047570279563,-7.44379104376631,
139.244851496986));
#128034=CARTESIAN_POINT('Ctrl Pts',(79.42661178888,-7.43560668773582,139.243420092094));
#128035=CARTESIAN_POINT('Ctrl Pts',(79.5093040189332,-7.40660504285213,
139.238012131354));
#128036=CARTESIAN_POINT('Ctrl Pts',(79.5711511706588,-7.38885856077627,
139.233984518759));
#128037=CARTESIAN_POINT('Ctrl Pts',(79.645020838286,-7.3722172548364,139.229029798449));
#128038=CARTESIAN_POINT('Ctrl Pts',(79.6562062440389,-7.36981819839152,
139.228275698206));
#128039=CARTESIAN_POINT('Ctrl Pts',(79.6736845488838,-7.3662573140173,139.227090081093));
#128040=CARTESIAN_POINT('Ctrl Pts',(79.6799611875879,-7.36501617966122,
139.226662860076));
#128041=CARTESIAN_POINT('Ctrl Pts',(79.6910965948281,-7.36288085561345,
139.225902100367));
#128042=CARTESIAN_POINT('Ctrl Pts',(79.6959524107364,-7.36197207964264,
139.225569389795));
#128043=CARTESIAN_POINT('Ctrl Pts',(79.7076584209494,-7.35983511981965,
139.224765019745));
#128044=CARTESIAN_POINT('Ctrl Pts',(79.7145122729696,-7.35862826076438,
139.224292190922));
#128045=CARTESIAN_POINT('Ctrl Pts',(79.7357207741475,-7.35503061934712,
139.222823712972));
#128046=CARTESIAN_POINT('Ctrl Pts',(79.7500988928056,-7.35278502519239,
139.221820598745));
#128047=CARTESIAN_POINT('Ctrl Pts',(79.8237555849773,-7.3422677417297,139.216649342557));
#128048=CARTESIAN_POINT('Ctrl Pts',(79.8834144880129,-7.33700729622843,
139.212355050607));
#128049=CARTESIAN_POINT('Ctrl Pts',(80.049545421667,-7.33134203810467,139.20030964474));
#128050=CARTESIAN_POINT('Ctrl Pts',(80.1559845018728,-7.33790895035622,
139.192510301768));
#128051=CARTESIAN_POINT('Ctrl Pts',(80.3168552909091,-7.36343389448626,
139.18094372524));
#128052=CARTESIAN_POINT('Ctrl Pts',(80.3721553983385,-7.37511615084551,
139.177004371144));
#128053=CARTESIAN_POINT('Ctrl Pts',(80.4432516755323,-7.39395672751375,
139.171989438108));
#128054=CARTESIAN_POINT('Ctrl Pts',(80.4596747997823,-7.39857995610281,
139.170834357321));
#128055=CARTESIAN_POINT('Ctrl Pts',(80.4861969677707,-7.4064877830627,139.168973820899));
#128056=CARTESIAN_POINT('Ctrl Pts',(80.4963403561506,-7.40961799027086,
139.168263415141));
#128057=CARTESIAN_POINT('Ctrl Pts',(80.5158196689459,-7.41583374298972,
139.166901131199));
#128058=CARTESIAN_POINT('Ctrl Pts',(80.5251595237089,-7.41890539737718,
139.166248831528));
#128059=CARTESIAN_POINT('Ctrl Pts',(80.5468327157855,-7.42624642897226,
139.164736927369));
#128060=CARTESIAN_POINT('Ctrl Pts',(80.559144276443,-7.43057844554725,139.163879422684));
#128061=CARTESIAN_POINT('Ctrl Pts',(80.5990935705138,-7.44516501676963,
139.161100159304));
#128062=CARTESIAN_POINT('Ctrl Pts',(80.6265112179921,-7.45600880997235,
139.159197893095));
#128063=CARTESIAN_POINT('Ctrl Pts',(80.6916105920269,-7.48377576698143,
139.154680964787));
#128064=CARTESIAN_POINT('Ctrl Pts',(80.7289794051964,-7.50138379780424,
139.152088145992));
#128065=CARTESIAN_POINT('Ctrl Pts',(80.8623561745392,-7.57040135230035,
139.142761079237));
#128066=CARTESIAN_POINT('Ctrl Pts',(80.9539129070601,-7.62979577890478,
139.136233145291));
#128067=CARTESIAN_POINT('Ctrl Pts',(81.0837382271023,-7.73337446686093,
139.125942516964));
#128068=CARTESIAN_POINT('Ctrl Pts',(81.1265853934548,-7.77132890007261,
139.122340462722));
#128069=CARTESIAN_POINT('Ctrl Pts',(81.1754549745402,-7.81932673492763,
139.117856955963));
#128070=CARTESIAN_POINT('Ctrl Pts',(81.1834378663579,-7.8273284537776,139.117111704332));
#128071=CARTESIAN_POINT('Ctrl Pts',(81.1957887035048,-7.83996297203915,
139.115937137606));
#128072=CARTESIAN_POINT('Ctrl Pts',(81.2002127297484,-7.84454081437404,
139.115511994429));
#128073=CARTESIAN_POINT('Ctrl Pts',(81.2080252573827,-7.85271824908043,
139.114753077978));
#128074=CARTESIAN_POINT('Ctrl Pts',(81.2114241279721,-7.8563077256886,139.114420111112));
#128075=CARTESIAN_POINT('Ctrl Pts',(81.219597008072,-7.86501624100604,139.113612707633));
#128076=CARTESIAN_POINT('Ctrl Pts',(81.224354739907,-7.87015024817455,139.113137074994));
#128077=CARTESIAN_POINT('Ctrl Pts',(81.2390495351768,-7.88620902058621,
139.111650882181));
#128078=CARTESIAN_POINT('Ctrl Pts',(81.2488734714249,-7.89723569545139,
139.110632602807));
#128079=CARTESIAN_POINT('Ctrl Pts',(81.2990284598913,-7.95506090269255,
139.105310447461));
#128080=CARTESIAN_POINT('Ctrl Pts',(81.3368766919029,-8.00394184402509,
139.100872666353));
#128081=CARTESIAN_POINT('Ctrl Pts',(81.4570882857847,-8.17842517040699,
139.085508070088));
#128082=CARTESIAN_POINT('Ctrl Pts',(81.5251785484698,-8.31302113873978,
139.074524324563));
#128083=CARTESIAN_POINT('Ctrl Pts',(81.5811030584779,-8.47454789597075,
139.062769785278));
#128084=CARTESIAN_POINT('Ctrl Pts',(81.587526807376,-8.49428713845587,139.061354270288));
#128085=CARTESIAN_POINT('Ctrl Pts',(81.5972254986323,-8.52609817184272,
139.059105574938));
#128086=CARTESIAN_POINT('Ctrl Pts',(81.6007361444671,-8.53809519726469,
139.058264818814));
#128087=CARTESIAN_POINT('Ctrl Pts',(81.6067534547674,-8.55955129749134,
139.056773805271));
#128088=CARTESIAN_POINT('Ctrl Pts',(81.6093123974102,-8.56899496695653,
139.056121879899));
#128089=CARTESIAN_POINT('Ctrl Pts',(81.614512959671,-8.58887972317174,139.054758002613));
#128090=CARTESIAN_POINT('Ctrl Pts',(81.6171368357983,-8.59932501643513,
139.054046649405));
#128091=CARTESIAN_POINT('Ctrl Pts',(81.6238244612891,-8.62708396658456,
139.052169138659));
#128092=CARTESIAN_POINT('Ctrl Pts',(81.6277126660476,-8.64443880207056,
139.051008621214));
#128093=CARTESIAN_POINT('Ctrl Pts',(81.646684389425,-8.73596411027016,139.044952676544));
#128094=CARTESIAN_POINT('Ctrl Pts',(81.6569794717248,-8.81104083498744,
139.040211539027));
#128095=CARTESIAN_POINT('Ctrl Pts',(81.6692157845001,-8.99033709402061,
139.029131904));
#128096=CARTESIAN_POINT('Ctrl Pts',(81.6665639372429,-9.09453784548305,
139.022889697919));
#128097=CARTESIAN_POINT('Ctrl Pts',(81.6485596052606,-9.24510491714907,
139.013428296461));
#128098=CARTESIAN_POINT('Ctrl Pts',(81.6408782397394,-9.29213504358959,
139.010406203584));
#128099=CARTESIAN_POINT('Ctrl Pts',(81.6289718448549,-9.34946549794788,
139.006569086307));
#128100=CARTESIAN_POINT('Ctrl Pts',(81.6266447414103,-9.36014202085136,
139.005847883685));
#128101=CARTESIAN_POINT('Ctrl Pts',(81.622828921443,-9.37685667925658,139.004707275751));
#128102=CARTESIAN_POINT('Ctrl Pts',(81.6214110816232,-9.38291091157659,
139.004291750468));
#128103=CARTESIAN_POINT('Ctrl Pts',(81.6186685003208,-9.39433343660984,
139.003503021156));
#128104=CARTESIAN_POINT('Ctrl Pts',(81.6173508844832,-9.39970324732988,
139.003130217162));
#128105=CARTESIAN_POINT('Ctrl Pts',(81.6141616867702,-9.41242650897211,
139.002242202601));
#128106=CARTESIAN_POINT('Ctrl Pts',(81.6122665676593,-9.4197738504856,139.001725684514));
#128107=CARTESIAN_POINT('Ctrl Pts',(81.6056823884638,-9.44459813193324,
138.99996853776));
#128108=CARTESIAN_POINT('Ctrl Pts',(81.6007589903592,-9.46201084391851,
138.998715814736));
#128109=CARTESIAN_POINT('Ctrl Pts',(81.5879289415297,-9.50471762477543,
138.995599043641));
#128110=CARTESIAN_POINT('Ctrl Pts',(81.5797006411595,-9.52990936294555,
138.993721808239));
#128111=CARTESIAN_POINT('Ctrl Pts',(81.5407094005852,-9.64029176324238,
138.985353711912));
#128112=CARTESIAN_POINT('Ctrl Pts',(81.5036303681489,-9.72308662970838,
138.978706454975));
#128113=CARTESIAN_POINT('Ctrl Pts',(81.4133986209474,-9.887256275759,138.965137209152));
#128114=CARTESIAN_POINT('Ctrl Pts',(81.3594846578721,-9.96784638168643,
138.958256394555));
#128115=CARTESIAN_POINT('Ctrl Pts',(81.2871068676301,-10.0579530477069,
138.950352436821));
#128116=CARTESIAN_POINT('Ctrl Pts',(81.2750981212901,-10.0723961819373,
138.949077814952));
#128117=CARTESIAN_POINT('Ctrl Pts',(81.255614451474,-10.0950394144237,138.947066337866));
#128118=CARTESIAN_POINT('Ctrl Pts',(81.2482977415181,-10.1033728874261,
138.946323108888));
#128119=CARTESIAN_POINT('Ctrl Pts',(81.234469922968,-10.1188086629687,138.944940642752));
#128120=CARTESIAN_POINT('Ctrl Pts',(81.2279793960653,-10.1259286942567,
138.944300586777));
#128121=CARTESIAN_POINT('Ctrl Pts',(81.213184158602,-10.1418787674245,138.94286109795));
#128122=CARTESIAN_POINT('Ctrl Pts',(81.2048440499005,-10.1506753454214,
138.942063215308));
#128123=CARTESIAN_POINT('Ctrl Pts',(81.1794611121129,-10.1768689610236,
138.939674376835));
#128124=CARTESIAN_POINT('Ctrl Pts',(81.1621316509018,-10.1939845856308,
138.938095900388));
#128125=CARTESIAN_POINT('Ctrl Pts',(81.1211872542965,-10.23268741861,138.934478500816));
#128126=CARTESIAN_POINT('Ctrl Pts',(81.097313156499,-10.2539869040337,138.93245113995));
#128127=CARTESIAN_POINT('Ctrl Pts',(81.0072187051488,-10.329820797807,138.925062898522));
#128128=CARTESIAN_POINT('Ctrl Pts',(80.9374294033046,-10.3799058304871,
138.919846998417));
#128129=CARTESIAN_POINT('Ctrl Pts',(80.7867978735428,-10.4712843910356,
138.909083028692));
#128130=CARTESIAN_POINT('Ctrl Pts',(80.7058266837974,-10.5117979899266,
138.903548120027));
#128131=CARTESIAN_POINT('Ctrl Pts',(80.6073565927027,-10.5514259613815,
138.896661246888));
#128132=CARTESIAN_POINT('Ctrl Pts',(80.5926490493154,-10.5571035946484,
138.89562856959));
#128133=CARTESIAN_POINT('Ctrl Pts',(80.5711965936094,-10.5650370547405,
138.894113377604));
#128134=CARTESIAN_POINT('Ctrl Pts',(80.5645138102336,-10.5674599467685,
138.893640126414));
#128135=CARTESIAN_POINT('Ctrl Pts',(80.5526467059649,-10.5716767200934,
138.892797194074));
#128136=CARTESIAN_POINT('Ctrl Pts',(80.5474687308649,-10.5734878714346,
138.892428530702));
#128137=CARTESIAN_POINT('Ctrl Pts',(80.5362057212862,-10.5773651187782,
138.891624647997));
#128138=CARTESIAN_POINT('Ctrl Pts',(80.5301177430218,-10.5794215613716,
138.891188912372));
#128139=CARTESIAN_POINT('Ctrl Pts',(80.5127235205137,-10.5851852152572,
138.889940802131));
#128140=CARTESIAN_POINT('Ctrl Pts',(80.5013895207989,-10.5888065028011,
138.889123758127));
#128141=CARTESIAN_POINT('Ctrl Pts',(80.4754563525984,-10.5967872066983,
138.887247212396));
#128142=CARTESIAN_POINT('Ctrl Pts',(80.4608343613467,-10.6010683250892,
138.886184082174));
#128143=CARTESIAN_POINT('Ctrl Pts',(80.3060670505471,-10.6440864178984,
138.874892248395));
#128144=CARTESIAN_POINT('Ctrl Pts',(80.1614840342172,-10.664519051482,138.864075581864));
#128145=CARTESIAN_POINT('Ctrl Pts',(79.9507120684992,-10.666553286255,138.849022903426));
#128146=CARTESIAN_POINT('Ctrl Pts',(79.8853587767227,-10.6633365494475,
138.844443159493));
#128147=CARTESIAN_POINT('Ctrl Pts',(79.8028201934209,-10.6543842482472,
138.838777170037));
#128148=CARTESIAN_POINT('Ctrl Pts',(79.7853152806429,-10.6522038705261,
138.837582081662));
#128149=CARTESIAN_POINT('Ctrl Pts',(79.7572137075095,-10.6482494159339,
138.835673439323));
#128150=CARTESIAN_POINT('Ctrl Pts',(79.746594227845,-10.6466501889977,138.834954450985));
#128151=CARTESIAN_POINT('Ctrl Pts',(79.7263216489237,-10.6433965010427,
138.833586008472));
#128152=CARTESIAN_POINT('Ctrl Pts',(79.7166662623906,-10.6417593915083,
138.832936037184));
#128153=CARTESIAN_POINT('Ctrl Pts',(79.6944492618709,-10.6377905728283,
138.831444293622));
#128154=CARTESIAN_POINT('Ctrl Pts',(79.6818988072796,-10.6353992969059,
138.830604443108));
#128155=CARTESIAN_POINT('Ctrl Pts',(79.6420374199767,-10.6273281405852,
138.827945004566));
#128156=CARTESIAN_POINT('Ctrl Pts',(79.614840198836,-10.6211064611918,138.82614258319));
#128157=CARTESIAN_POINT('Ctrl Pts',(79.5156892451251,-10.5957881311155,
138.819599937934));
#128158=CARTESIAN_POINT('Ctrl Pts',(79.4448791678645,-10.5725581631489,
138.814987170475));
#128159=CARTESIAN_POINT('Ctrl Pts',(79.2563727472063,-10.496389367791,138.802521098322));
#128160=CARTESIAN_POINT('Ctrl Pts',(79.1429144477376,-10.4344187789382,
138.794823601157));
#128161=CARTESIAN_POINT('Ctrl Pts',(79.0263614493235,-10.3519535891143,
138.785554713314));
#128162=CARTESIAN_POINT('Ctrl Pts',(79.0150776629315,-10.3437553698324,
138.784641540473));
#128163=CARTESIAN_POINT('Ctrl Pts',(78.9983272179701,-10.3312610367618,
138.783259831104));
#128164=CARTESIAN_POINT('Ctrl Pts',(78.9927820373413,-10.3270705639592,
138.782798048324));
#128165=CARTESIAN_POINT('Ctrl Pts',(78.9828227851343,-10.3194460161396,
138.781960421194));
#128166=CARTESIAN_POINT('Ctrl Pts',(78.9783994072971,-10.3160241273241,
138.781585413341));
#128167=CARTESIAN_POINT('Ctrl Pts',(78.9694186609889,-10.3090041325214,
138.780817760678));
#128168=CARTESIAN_POINT('Ctrl Pts',(78.9648627588378,-10.3054043835621,
138.780425014286));
#128169=CARTESIAN_POINT('Ctrl Pts',(78.9535305410094,-10.2963538487905,
138.779439982242));
#128170=CARTESIAN_POINT('Ctrl Pts',(78.9467780071182,-10.2908737565632,
138.778845701987));
#128171=CARTESIAN_POINT('Ctrl Pts',(78.9317431800531,-10.2784755846167,
138.777506569767));
#128172=CARTESIAN_POINT('Ctrl Pts',(78.9234846425289,-10.2715294431498,
138.776759968635));
#128173=CARTESIAN_POINT('Ctrl Pts',(78.8991134467303,-10.2506235570128,
138.774525111573));
#128174=CARTESIAN_POINT('Ctrl Pts',(78.8832011607647,-10.2364346921585,
138.773024144763));
#128175=CARTESIAN_POINT('Ctrl Pts',(78.8231402598813,-10.1807734479365,
138.767209270554));
#128176=CARTESIAN_POINT('Ctrl Pts',(78.7809950559529,-10.1372118943443,
138.762810883504));
#128177=CARTESIAN_POINT('Ctrl Pts',(78.6562619125777,-9.99336781705434,
138.748954119857));
#128178=CARTESIAN_POINT('Ctrl Pts',(78.5829465834908,-9.88565436811021,
138.739549489168));
#128179=CARTESIAN_POINT('Ctrl Pts',(78.5134952003582,-9.7525099803891,138.729229690625));
#128180=CARTESIAN_POINT('Ctrl Pts',(78.5044393173238,-9.73434739552867,
138.72784644108));
#128181=CARTESIAN_POINT('Ctrl Pts',(78.4903442080147,-9.70473518234833,
138.725629613013));
#128182=CARTESIAN_POINT('Ctrl Pts',(78.4850983435307,-9.69338681378128,
138.724788985808));
#128183=CARTESIAN_POINT('Ctrl Pts',(78.4759856550359,-9.67307616041793,
138.723299962849));
#128184=CARTESIAN_POINT('Ctrl Pts',(78.4720689647162,-9.66413703387003,
138.722649884185));
#128185=CARTESIAN_POINT('Ctrl Pts',(78.46395169687,-9.64515891166399,138.721280601481));
#128186=CARTESIAN_POINT('Ctrl Pts',(78.4597704593522,-9.63511210225471,
138.720562078149));
#128187=CARTESIAN_POINT('Ctrl Pts',(78.448820388865,-9.60805665503589,138.718643617584));
#128188=CARTESIAN_POINT('Ctrl Pts',(78.4422328186799,-9.59097591628757,
138.717449777295));
#128189=CARTESIAN_POINT('Ctrl Pts',(78.4060847467122,-9.49244119123581,
138.710655162977));
#128190=CARTESIAN_POINT('Ctrl Pts',(78.3826313546794,-9.40888344053641,
138.705261407724));
#128191=CARTESIAN_POINT('Ctrl Pts',(78.3445816311609,-9.21688870063967,
138.693247528272));
#128192=CARTESIAN_POINT('Ctrl Pts',(78.3339388140977,-9.10809724434987,
138.686703611574));
#128193=CARTESIAN_POINT('Ctrl Pts',(78.3340002645784,-8.99906107773531,
138.679802703723));
#128194=CARTESIAN_POINT('Ctrl Pts',(78.3340002659352,-8.9990586732761,138.679802551545));
#128195=CARTESIAN_POINT('Ctrl Pts',(78.3340122908892,-8.97777640250722,
138.678455593874));
#128196=CARTESIAN_POINT('Ctrl Pts',(78.3344321193602,-8.95649709999227,
138.677095246544));
#128197=CARTESIAN_POINT('Ctrl Pts',(78.3358009540242,-8.92131348367504,
138.67481502874));
#128198=CARTESIAN_POINT('Ctrl Pts',(78.3365170051759,-8.90740232859391,
138.673905425437));
#128199=CARTESIAN_POINT('Ctrl Pts',(78.3378248684508,-8.88698456957304,
138.672556420238));
#128200=CARTESIAN_POINT('Ctrl Pts',(78.3382806792744,-8.88046945513672,
138.672123874439));
#128201=CARTESIAN_POINT('Ctrl Pts',(78.3391689393945,-8.86876230860699,
138.671342591399));
#128202=CARTESIAN_POINT('Ctrl Pts',(78.3395874622305,-8.86356926269507,
138.67099460244));
#128203=CARTESIAN_POINT('Ctrl Pts',(78.3404626590702,-8.85331094236375,
138.6703042116));
#128204=CARTESIAN_POINT('Ctrl Pts',(78.3409181710623,-8.84824576329396,
138.669961869966));
#128205=CARTESIAN_POINT('Ctrl Pts',(78.3420395514555,-8.83638530291543,
138.669156852411));
#128206=CARTESIAN_POINT('Ctrl Pts',(78.3427239995179,-8.82959204207361,
138.668693172819));
#128207=CARTESIAN_POINT('Ctrl Pts',(78.3449257623353,-8.80900852954848,
138.667280747579));
#128208=CARTESIAN_POINT('Ctrl Pts',(78.3465735514021,-8.79523325050894,
138.666325306197));
#128209=CARTESIAN_POINT('Ctrl Pts',(78.3545977592447,-8.73458488322595,
138.66207839854));
#128210=CARTESIAN_POINT('Ctrl Pts',(78.3627964138434,-8.68797865093281,
138.658708642598));
#128211=CARTESIAN_POINT('Ctrl Pts',(78.3892162346329,-8.56797690308466,
138.649852340649));
#128212=CARTESIAN_POINT('Ctrl Pts',(78.4104657701459,-8.49537864982559,
138.644319845945));
#128213=CARTESIAN_POINT('Ctrl Pts',(78.436559345854,-8.42449211911253,138.638847691527));
#128214=CARTESIAN_POINT('Ctrl Pts',(78.4365593750041,-8.42449203992252,
138.833737849951));
#128215=CARTESIAN_POINT('Ctrl Pts',(78.4357654627803,-8.42664880352886,
138.833891290677));
#128216=CARTESIAN_POINT('Ctrl Pts',(78.4349760076973,-8.42880722551953,
138.834044583115));
#128217=CARTESIAN_POINT('Ctrl Pts',(78.4308396898992,-8.44018914343849,
138.834851539479));
#128218=CARTESIAN_POINT('Ctrl Pts',(78.4275698389047,-8.44944058502104,
138.835502628057));
#128219=CARTESIAN_POINT('Ctrl Pts',(78.4201791056846,-8.47095437667124,
138.83700585588));
#128220=CARTESIAN_POINT('Ctrl Pts',(78.4161188918261,-8.48323701707355,
138.837855968269));
#128221=CARTESIAN_POINT('Ctrl Pts',(78.4034747020729,-8.52303690839969,
138.840585659804));
#128222=CARTESIAN_POINT('Ctrl Pts',(78.3954613590095,-8.55073089736053,
138.842446720717));
#128223=CARTESIAN_POINT('Ctrl Pts',(78.3649421910079,-8.66747049985526,
138.850153225424));
#128224=CARTESIAN_POINT('Ctrl Pts',(78.3490992446991,-8.75809293572287,
138.855791524017));
#128225=CARTESIAN_POINT('Ctrl Pts',(78.3307435608108,-8.96054648702028,
138.868210307207));
#128226=CARTESIAN_POINT('Ctrl Pts',(78.3318429385482,-9.07223950797057,
138.874946240725));
#128227=CARTESIAN_POINT('Ctrl Pts',(78.345676015335,-9.19743340964611,138.883137059902));
#128228=CARTESIAN_POINT('Ctrl Pts',(78.3474637306941,-9.21187647540124,
138.884091970012));
#128229=CARTESIAN_POINT('Ctrl Pts',(78.3503854186024,-9.23318692748227,
138.885518151753));
#128230=CARTESIAN_POINT('Ctrl Pts',(78.3513736460147,-9.24007405299294,
138.885981735949));
#128231=CARTESIAN_POINT('Ctrl Pts',(78.3532149466878,-9.25235856789412,
138.886813725034));
#128232=CARTESIAN_POINT('Ctrl Pts',(78.3540514732453,-9.25775822795488,
138.887181205429));
#128233=CARTESIAN_POINT('Ctrl Pts',(78.3559612207556,-9.2696968667602,138.887997699576));
#128234=CARTESIAN_POINT('Ctrl Pts',(78.3570468824366,-9.27623351948151,
138.888447373386));
#128235=CARTESIAN_POINT('Ctrl Pts',(78.3603559833217,-9.29544738024032,
138.889776537574));
#128236=CARTESIAN_POINT('Ctrl Pts',(78.362687311603,-9.30810516225522,138.890661655817));
#128237=CARTESIAN_POINT('Ctrl Pts',(78.3684118462298,-9.33728406070953,
138.89272206758));
#128238=CARTESIAN_POINT('Ctrl Pts',(78.3719097151171,-9.35378300890375,
138.893902022913));
#128239=CARTESIAN_POINT('Ctrl Pts',(78.3848745738333,-9.4106655989781,138.898015580042));
#128240=CARTESIAN_POINT('Ctrl Pts',(78.3955983074982,-9.45074510014426,
138.900993480983));
#128241=CARTESIAN_POINT('Ctrl Pts',(78.4451145988264,-9.61151751358259,
138.913166572));
#128242=CARTESIAN_POINT('Ctrl Pts',(78.4961331980123,-9.72802109726034,
138.922476660456));
#128243=CARTESIAN_POINT('Ctrl Pts',(78.5817385502336,-9.875203573505,138.93444442158));
#128244=CARTESIAN_POINT('Ctrl Pts',(78.6050656555788,-9.91192412359391,
138.93745427323));
#128245=CARTESIAN_POINT('Ctrl Pts',(78.6386422790772,-9.96046994167867,
138.941468598723));
#128246=CARTESIAN_POINT('Ctrl Pts',(78.6476581072446,-9.97312321248951,
138.942518391084));
#128247=CARTESIAN_POINT('Ctrl Pts',(78.6623297722622,-9.9931163850955,138.944183255617));
#128248=CARTESIAN_POINT('Ctrl Pts',(78.6678719369064,-10.0005381662012,
138.944802656392));
#128249=CARTESIAN_POINT('Ctrl Pts',(78.6794382270635,-10.0157606670721,
138.946076128631));
#128250=CARTESIAN_POINT('Ctrl Pts',(78.6854702666044,-10.0235549404123,
138.94672985669));
#128251=CARTESIAN_POINT('Ctrl Pts',(78.699755812662,-10.0416793497508,138.948254268952));
#128252=CARTESIAN_POINT('Ctrl Pts',(78.7080639106748,-10.0519657657019,
138.949122740492));
#128253=CARTESIAN_POINT('Ctrl Pts',(78.7359439856612,-10.085656079992,138.951979430824));
#128254=CARTESIAN_POINT('Ctrl Pts',(78.7560370060276,-10.1086221124858,
138.953946565433));
#128255=CARTESIAN_POINT('Ctrl Pts',(78.8777093875024,-10.2402157882939,
138.965372180505));
#128256=CARTESIAN_POINT('Ctrl Pts',(78.9928255613813,-10.3353914340398,
138.974203251278));
#128257=CARTESIAN_POINT('Ctrl Pts',(79.1676650222503,-10.4443185494194,
138.986966430809));
#128258=CARTESIAN_POINT('Ctrl Pts',(79.2178108548987,-10.472078889972,138.990573127886));
#128259=CARTESIAN_POINT('Ctrl Pts',(79.2794407214493,-10.5021578317847,
138.995061827805));
#128260=CARTESIAN_POINT('Ctrl Pts',(79.2896510534084,-10.5070130000715,
138.995807276204));
#128261=CARTESIAN_POINT('Ctrl Pts',(79.3056866175785,-10.5144389909557,
138.996982042738));
#128262=CARTESIAN_POINT('Ctrl Pts',(79.311478740144,-10.5170810794716,138.997407186286));
#128263=CARTESIAN_POINT('Ctrl Pts',(79.3217950848453,-10.5217156538283,
138.998166097348));
#128264=CARTESIAN_POINT('Ctrl Pts',(79.3263132329559,-10.523721291979,138.998499058561));
#128265=CARTESIAN_POINT('Ctrl Pts',(79.3372499262112,-10.5285180166273,
138.999306413092));
#128266=CARTESIAN_POINT('Ctrl Pts',(79.343677146171,-10.5312887691616,138.999782001796));
#128267=CARTESIAN_POINT('Ctrl Pts',(79.363714522277,-10.5397774914202,139.001267754765));
#128268=CARTESIAN_POINT('Ctrl Pts',(79.3773829243795,-10.5453549339939,
139.002285627907));
#128269=CARTESIAN_POINT('Ctrl Pts',(79.4485795306223,-10.5733091368075,
139.007603595204));
#128270=CARTESIAN_POINT('Ctrl Pts',(79.5072399477876,-10.5926557040071,
139.012037311236));
#128271=CARTESIAN_POINT('Ctrl Pts',(79.7118081413373,-10.6477389056236,
139.027398716744));
#128272=CARTESIAN_POINT('Ctrl Pts',(79.8614335449113,-10.6670079403707,
139.038383640353));
#128273=CARTESIAN_POINT('Ctrl Pts',(80.0323665402619,-10.6658146426545,
139.050137982387));
#128274=CARTESIAN_POINT('Ctrl Pts',(80.0530991329156,-10.6652827284884,
139.051552181808));
#128275=CARTESIAN_POINT('Ctrl Pts',(80.0862990603242,-10.6638102580642,
139.053799212641));
#128276=CARTESIAN_POINT('Ctrl Pts',(80.0987745577488,-10.6631162629689,
139.054639599674));
#128277=CARTESIAN_POINT('Ctrl Pts',(80.1210027308491,-10.6616287341169,
139.056130199461));
#128278=CARTESIAN_POINT('Ctrl Pts',(80.1307583240794,-10.660889514271,139.056782076316));
#128279=CARTESIAN_POINT('Ctrl Pts',(80.1512408935126,-10.6591558798163,
139.058146094951));
#128280=CARTESIAN_POINT('Ctrl Pts',(80.1619659080164,-10.658143267402,139.058857636047));
#128281=CARTESIAN_POINT('Ctrl Pts',(80.190381465752,-10.6551820510527,139.06073620679));
#128282=CARTESIAN_POINT('Ctrl Pts',(80.2080522030789,-10.653053854273,139.06189758614));
#128283=CARTESIAN_POINT('Ctrl Pts',(80.3009130684846,-10.640357347065,139.067969907922));
#128284=CARTESIAN_POINT('Ctrl Pts',(80.3753541586966,-10.6249406998734,
139.072725524982));
#128285=CARTESIAN_POINT('Ctrl Pts',(80.5500972025953,-10.5760962469182,
139.083910609427));
#128286=CARTESIAN_POINT('Ctrl Pts',(80.648769083236,-10.5381101484378,139.090239133787));
#128287=CARTESIAN_POINT('Ctrl Pts',(80.7844210682072,-10.4704974628363,
139.099708393852));
#128288=CARTESIAN_POINT('Ctrl Pts',(80.8247861040395,-10.4482424687139,
139.102635401686));
#128289=CARTESIAN_POINT('Ctrl Pts',(80.8734287501862,-10.4187302157357,
139.106364745582));
#128290=CARTESIAN_POINT('Ctrl Pts',(80.8826293490558,-10.4130246366018,
139.10707941089));
#128291=CARTESIAN_POINT('Ctrl Pts',(80.8970066692135,-10.4039136087939,
139.108211930331));
#128292=CARTESIAN_POINT('Ctrl Pts',(80.9022213035857,-10.4005681353655,
139.108625994407));
#128293=CARTESIAN_POINT('Ctrl Pts',(80.9120557258954,-10.3941811023156,
139.109413403265));
#128294=CARTESIAN_POINT('Ctrl Pts',(80.9166791767232,-10.3911455266973,
139.109786363018));
#128295=CARTESIAN_POINT('Ctrl Pts',(80.9276385213664,-10.3838716993669,
139.110676941632));
#128296=CARTESIAN_POINT('Ctrl Pts',(80.9339605435542,-10.3796129181916,
139.111195893278));
#128297=CARTESIAN_POINT('Ctrl Pts',(80.955388482954,-10.3649633710228,139.112972057691));
#128298=CARTESIAN_POINT('Ctrl Pts',(80.9703513945365,-10.3543671067065,
139.114241727563));
#128299=CARTESIAN_POINT('Ctrl Pts',(81.0068974031942,-10.32756989012,139.117410391055));
#128300=CARTESIAN_POINT('Ctrl Pts',(81.0282671182901,-10.3110876264722,
139.119323123501));
#128301=CARTESIAN_POINT('Ctrl Pts',(81.1223055716679,-10.2348431425141,
139.127982044712));
#128302=CARTESIAN_POINT('Ctrl Pts',(81.1902335271836,-10.1695090043202,
139.134893419425));
#128303=CARTESIAN_POINT('Ctrl Pts',(81.3135590047839,-10.0289559907336,
139.148420685002));
#128304=CARTESIAN_POINT('Ctrl Pts',(81.3688940057096,-9.9541080016211,139.155014791111));
#128305=CARTESIAN_POINT('Ctrl Pts',(81.4275744848557,-9.8590344266445,139.162653017737));
#128306=CARTESIAN_POINT('Ctrl Pts',(81.4371724637305,-9.84287864824879,
139.163927794711));
#128307=CARTESIAN_POINT('Ctrl Pts',(81.451942601725,-9.81703073625185,139.165931753165));
#128308=CARTESIAN_POINT('Ctrl Pts',(81.4572955243766,-9.80744430601168,
139.166667391658));
#128309=CARTESIAN_POINT('Ctrl Pts',(81.4667474109426,-9.79011691281913,
139.167983746783));
#128310=CARTESIAN_POINT('Ctrl Pts',(81.4708807948246,-9.7823952938621,139.168565672047));
#128311=CARTESIAN_POINT('Ctrl Pts',(81.480454589229,-9.76416634305832,139.169928705837));
#128312=CARTESIAN_POINT('Ctrl Pts',(81.4858443843175,-9.75363284715538,
139.170708010123));
#128313=CARTESIAN_POINT('Ctrl Pts',(81.5013392258646,-9.72253813808178,
139.172984966399));
#128314=CARTESIAN_POINT('Ctrl Pts',(81.511133180982,-9.701824354067,139.174471836469));
#128315=CARTESIAN_POINT('Ctrl Pts',(81.5545678892191,-9.60483365950251,
139.181307329184));
#128316=CARTESIAN_POINT('Ctrl Pts',(81.5828824965542,-9.52629880540434,
139.186476374112));
#128317=CARTESIAN_POINT('Ctrl Pts',(81.6283618491473,-9.36260144581922,
139.196889616307));
#128318=CARTESIAN_POINT('Ctrl Pts',(81.6449922152124,-9.27756328726469,
139.202114256777));
#128319=CARTESIAN_POINT('Ctrl Pts',(81.6605055395375,-9.14358313068467,
139.210524640583));
#128320=CARTESIAN_POINT('Ctrl Pts',(81.6639730348982,-9.09532865618125,
139.21359091935));
#128321=CARTESIAN_POINT('Ctrl Pts',(81.6656425916159,-9.0361679198286,139.217469048152));
#128322=CARTESIAN_POINT('Ctrl Pts',(81.6658425518073,-9.02533651086294,
139.218183950568));
#128323=CARTESIAN_POINT('Ctrl Pts',(81.6659913384069,-9.00824713174338,
139.21932067823));
#128324=CARTESIAN_POINT('Ctrl Pts',(81.6660105618148,-9.00198985817584,
139.219738748212));
#128325=CARTESIAN_POINT('Ctrl Pts',(81.6659804065235,-8.99021679746421,
139.220529091812));
#128326=CARTESIAN_POINT('Ctrl Pts',(81.665938884974,-8.98470118065836,139.220900933308));
#128327=CARTESIAN_POINT('Ctrl Pts',(81.665776247815,-8.97168436904526,139.221782089728));
#128328=CARTESIAN_POINT('Ctrl Pts',(81.6656318524333,-8.96418367016243,
139.222292656523));
#128329=CARTESIAN_POINT('Ctrl Pts',(81.6649796485914,-8.93910716416467,
139.224008449677));
#128330=CARTESIAN_POINT('Ctrl Pts',(81.6642442727935,-8.92153913792775,
139.225225038674));
#128331=CARTESIAN_POINT('Ctrl Pts',(81.6617623174051,-8.87854430881846,
139.228232910677));
#128332=CARTESIAN_POINT('Ctrl Pts',(81.6597100664976,-8.85314007145961,
139.230036297735));
#128333=CARTESIAN_POINT('Ctrl Pts',(81.6484208755317,-8.74450804695441,
139.237834262732));
#128334=CARTESIAN_POINT('Ctrl Pts',(81.6334992484543,-8.66199558686887,
139.243968580014));
#128335=CARTESIAN_POINT('Ctrl Pts',(81.5880354831232,-8.48705516877,139.257090678194));
#128336=CARTESIAN_POINT('Ctrl Pts',(81.5554728734917,-8.39545161228709,
139.264029326413));
#128337=CARTESIAN_POINT('Ctrl Pts',(81.5052710113702,-8.28566429093416,
139.272340679899));
#128338=CARTESIAN_POINT('Ctrl Pts',(81.4949692404908,-8.26434832108724,
139.273955102075));
#128339=CARTESIAN_POINT('Ctrl Pts',(81.478699577489,-8.23243823474725,139.276374176812));
#128340=CARTESIAN_POINT('Ctrl Pts',(81.4730646652475,-8.2216787234766,139.277190258056));
#128341=CARTESIAN_POINT('Ctrl Pts',(81.4627059432925,-8.20241493857962,
139.278652437866));
#128342=CARTESIAN_POINT('Ctrl Pts',(81.4580244058265,-8.19388868905047,
139.279299990825));
#128343=CARTESIAN_POINT('Ctrl Pts',(81.4478369629443,-8.17571393194336,
139.280681405892));
#128344=CARTESIAN_POINT('Ctrl Pts',(81.442308662733,-8.16607846609383,139.281414429577));
#128345=CARTESIAN_POINT('Ctrl Pts',(81.4268821689816,-8.13980345713761,
139.283415691732));
#128346=CARTESIAN_POINT('Ctrl Pts',(81.4167894605229,-8.12327969583428,
139.284676868815));
#128347=CARTESIAN_POINT('Ctrl Pts',(81.3465725830168,-8.0127012163698,139.293143772132));
#128348=CARTESIAN_POINT('Ctrl Pts',(81.2774132635477,-7.92471572678365,
139.299989343676));
#128349=CARTESIAN_POINT('Ctrl Pts',(81.1262955392844,-7.76780996550157,
139.313294437602));
#128350=CARTESIAN_POINT('Ctrl Pts',(81.0454917251394,-7.69854900069521,
139.319734685963));
#128351=CARTESIAN_POINT('Ctrl Pts',(80.9465992895673,-7.62896997803671,
139.327592255134));
#128352=CARTESIAN_POINT('Ctrl Pts',(80.9344250221196,-7.62064385393388,
139.328559383554));
#128353=CARTESIAN_POINT('Ctrl Pts',(80.9162291843967,-7.60855093843947,
139.330007170816));
#128354=CARTESIAN_POINT('Ctrl Pts',(80.9102911040183,-7.60465899844532,
139.330480003006));
#128355=CARTESIAN_POINT('Ctrl Pts',(80.8997246339761,-7.59782967077172,
139.331322355417));
#128356=CARTESIAN_POINT('Ctrl Pts',(80.8951063650861,-7.59487700086125,
139.331690863198));
#128357=CARTESIAN_POINT('Ctrl Pts',(80.8849473958799,-7.58845231815264,
139.332502299767));
#128358=CARTESIAN_POINT('Ctrl Pts',(80.8794008690894,-7.58499015572465,
139.332945819337));
#128359=CARTESIAN_POINT('Ctrl Pts',(80.8632818028448,-7.57505995086257,
139.334235864697));
#128360=CARTESIAN_POINT('Ctrl Pts',(80.8526575485988,-7.56867729113766,
139.335087517461));
#128361=CARTESIAN_POINT('Ctrl Pts',(80.8281114789083,-7.55430118142076,
139.337056565091));
#128362=CARTESIAN_POINT('Ctrl Pts',(80.814143503225,-7.54638931972059,139.338178072111));
#128363=CARTESIAN_POINT('Ctrl Pts',(80.766367502663,-7.52023222950363,139.342012187541));
#128364=CARTESIAN_POINT('Ctrl Pts',(80.7320450405205,-7.50295574849416,
139.344763249164));
#128365=CARTESIAN_POINT('Ctrl Pts',(80.6328625112713,-7.45725809061481,
139.35264864543));
#128366=CARTESIAN_POINT('Ctrl Pts',(80.5667439989889,-7.431762503023,139.357826474518));
#128367=CARTESIAN_POINT('Ctrl Pts',(80.4070366551528,-7.3816026603498,139.369947844441));
#128368=CARTESIAN_POINT('Ctrl Pts',(80.3125131974446,-7.36072270970312,
139.376816046572));
#128369=CARTESIAN_POINT('Ctrl Pts',(80.1980779205702,-7.34571048063891,
139.384708637636));
#128370=CARTESIAN_POINT('Ctrl Pts',(80.1794171779391,-7.34358272082952,
139.385983097254));
#128371=CARTESIAN_POINT('Ctrl Pts',(80.1496787973133,-7.34070032995489,
139.387994920842));
#128372=CARTESIAN_POINT('Ctrl Pts',(80.1386231842156,-7.33974015272477,
139.388738641321));
#128373=CARTESIAN_POINT('Ctrl Pts',(80.1179405065252,-7.33815190540202,
139.390122410837));
#128374=CARTESIAN_POINT('Ctrl Pts',(80.1083160440931,-7.33749685898879,
139.390763275428));
#128375=CARTESIAN_POINT('Ctrl Pts',(80.0865629160185,-7.33620603602546,
139.39220511338));
#128376=CARTESIAN_POINT('Ctrl Pts',(80.0744318096969,-7.33561921072226,
139.393004528911));
#128377=CARTESIAN_POINT('Ctrl Pts',(80.0378816720721,-7.33425157098279,
139.395399930388));
#128378=CARTESIAN_POINT('Ctrl Pts',(80.0134501600528,-7.33387514206634,
139.39698335957));
#128379=CARTESIAN_POINT('Ctrl Pts',(79.9569122344079,-7.33424783383181,
139.400613212122));
#128380=CARTESIAN_POINT('Ctrl Pts',(79.9248178057395,-7.33538753403498,
139.402647977563));
#128381=CARTESIAN_POINT('Ctrl Pts',(79.8066594070181,-7.3430081095544,139.41007559726));
#128382=CARTESIAN_POINT('Ctrl Pts',(79.7211041821049,-7.35524441251809,
139.415321710573));
#128383=CARTESIAN_POINT('Ctrl Pts',(79.549169724019,-7.39364246086482,139.426085428576));
#128384=CARTESIAN_POINT('Ctrl Pts',(79.4632007283571,-7.42029278227903,
139.431589757663));
#128385=CARTESIAN_POINT('Ctrl Pts',(79.3652150567596,-7.45959374814087,
139.438440030539));
#128386=CARTESIAN_POINT('Ctrl Pts',(79.3507024823065,-7.46565452569573,
139.439470267458));
#128387=CARTESIAN_POINT('Ctrl Pts',(79.3297659706607,-7.47474829581623,
139.440982438017));
#128388=CARTESIAN_POINT('Ctrl Pts',(79.3232717054569,-7.47761856751154,
139.441455156496));
#128389=CARTESIAN_POINT('Ctrl Pts',(79.31180577059,-7.48277403096381,139.442296607062));
#128390=CARTESIAN_POINT('Ctrl Pts',(79.3068267075362,-7.48504233585205,
139.44266431683));
#128391=CARTESIAN_POINT('Ctrl Pts',(79.2960636870118,-7.49000980008923,
139.443464321018));
#128392=CARTESIAN_POINT('Ctrl Pts',(79.2902841397156,-7.49271763402121,
139.443897114828));
#128393=CARTESIAN_POINT('Ctrl Pts',(79.2738498905341,-7.50053288548231,
139.445136638163));
#128394=CARTESIAN_POINT('Ctrl Pts',(79.2632340257019,-7.5057204116621,139.445948006113));
#128395=CARTESIAN_POINT('Ctrl Pts',(79.1670791002145,-7.55398098386478,
139.453388948551));
#128396=CARTESIAN_POINT('Ctrl Pts',(79.0853565530412,-7.60423795889812,
139.46036873848));
#128397=CARTESIAN_POINT('Ctrl Pts',(78.9109705802748,-7.73340036811098,
139.47617715688));
#128398=CARTESIAN_POINT('Ctrl Pts',(78.8216819984057,-7.81600815811391,
139.484937470301));
#128399=CARTESIAN_POINT('Ctrl Pts',(78.7283665603689,-7.92345651350948,
139.494728244193));
#128400=CARTESIAN_POINT('Ctrl Pts',(78.7148900055743,-7.93958033989662,
139.496161656021));
#128401=CARTESIAN_POINT('Ctrl Pts',(78.6938650444635,-7.96572506198106,
139.498430543781));
#128402=CARTESIAN_POINT('Ctrl Pts',(78.6861189059643,-7.97558326096429,
139.499273907597));
#128403=CARTESIAN_POINT('Ctrl Pts',(78.6725513831199,-7.99325717798711,
139.500764844494));
#128404=CARTESIAN_POINT('Ctrl Pts',(78.6666859840328,-8.00103819796508,
139.501414142837));
#128405=CARTESIAN_POINT('Ctrl Pts',(78.6545511924222,-8.01743346206989,
139.502767757607));
#128406=CARTESIAN_POINT('Ctrl Pts',(78.6482954684241,-8.02605730993669,
139.503471521148));
#128407=CARTESIAN_POINT('Ctrl Pts',(78.6320287865222,-8.04894044397087,
139.50531786036));
#128408=CARTESIAN_POINT('Ctrl Pts',(78.6221578606527,-8.06329802149247,
139.506455058233));
#128409=CARTESIAN_POINT('Ctrl Pts',(78.5734443906988,-8.13659001803001,
139.512158771233));
#128410=CARTESIAN_POINT('Ctrl Pts',(78.5381473041907,-8.19779915812948,
139.516592024258));
#128411=CARTESIAN_POINT('Ctrl Pts',(78.4805144020893,-8.31425847162602,
139.524620536356));
#128412=CARTESIAN_POINT('Ctrl Pts',(78.457055835973,-8.36881079569985,139.528231549375));
#128413=CARTESIAN_POINT('Ctrl Pts',(78.4365593777415,-8.42449203248626,
139.531855306428));
#128414=CARTESIAN_POINT('Origin',(80.,-9.,141.545925280538));
#128415=CARTESIAN_POINT('',(77.9452506264311,-9.00160446819347,139.095925280496));
#128416=CARTESIAN_POINT('Ctrl Pts',(81.2520391107129,-7.37076839346111,
139.547882946156));
#128417=CARTESIAN_POINT('Ctrl Pts',(81.308376492207,-7.41406279355911,139.544018177529));
#128418=CARTESIAN_POINT('Ctrl Pts',(81.3625557941979,-7.46035206945108,
139.540153408901));
#128419=CARTESIAN_POINT('Ctrl Pts',(81.4142433388808,-7.50939162053498,
139.536288640274));
#128420=CARTESIAN_POINT('Ctrl Pts',(81.4658662946457,-7.55836989164198,
139.532428701074));
#128421=CARTESIAN_POINT('Ctrl Pts',(81.515003327894,-7.61009127859361,139.528568761873));
#128422=CARTESIAN_POINT('Ctrl Pts',(81.5613536305889,-7.66427083480709,
139.524708822673));
#128423=CARTESIAN_POINT('Ctrl Pts',(81.6076723958972,-7.71841352650165,
139.520851509828));
#128424=CARTESIAN_POINT('Ctrl Pts',(81.6512078775579,-7.7750107012777,139.516994196984));
#128425=CARTESIAN_POINT('Ctrl Pts',(81.6916969813358,-7.83374150127879,
139.51313688414));
#128426=CARTESIAN_POINT('Ctrl Pts',(81.7321720676574,-7.89245196849052,
139.509280906709));
#128427=CARTESIAN_POINT('Ctrl Pts',(81.7696025941656,-7.95329419518399,
139.505424929279));
#128428=CARTESIAN_POINT('Ctrl Pts',(81.8037675969863,-8.01591666076381,
139.501568951848));
#128429=CARTESIAN_POINT('Ctrl Pts',(81.8379321897393,-8.07853837471322,
139.497713020699));
#128430=CARTESIAN_POINT('Ctrl Pts',(81.8688311057131,-8.14293985793319,
139.493857089551));
#128431=CARTESIAN_POINT('Ctrl Pts',(81.896289179377,-8.20874472470788,139.490001158402));
#128432=CARTESIAN_POINT('Ctrl Pts',(81.9237751180498,-8.27461637159319,
139.486141314176));
#128433=CARTESIAN_POINT('Ctrl Pts',(81.9478130540654,-8.34189379684482,
139.48228146995));
#128434=CARTESIAN_POINT('Ctrl Pts',(81.9682762259155,-8.41018116256268,
139.478421625724));
#128435=CARTESIAN_POINT('Ctrl Pts',(81.9887500346486,-8.47850402447474,
139.474559775128));
#128436=CARTESIAN_POINT('Ctrl Pts',(82.0056452636483,-8.54783740001086,
139.470697924531));
#128437=CARTESIAN_POINT('Ctrl Pts',(82.0188859519888,-8.61777352870029,
139.466836073934));
#128438=CARTESIAN_POINT('Ctrl Pts',(82.0321504672958,-8.68783550929022,
139.462967273836));
#128439=CARTESIAN_POINT('Ctrl Pts',(82.0417472410663,-8.7585019275549,139.459098473738));
#128440=CARTESIAN_POINT('Ctrl Pts',(82.0476520986989,-8.82935872365122,
139.45522967364));
#128441=CARTESIAN_POINT('Ctrl Pts',(82.052086736227,-8.88257325084868,139.452324146162));
#128442=CARTESIAN_POINT('Ctrl Pts',(82.0544401302615,-8.93589502683532,
139.449418618684));
#128443=CARTESIAN_POINT('Ctrl Pts',(82.0547213515201,-8.98914964943005,
139.446513091206));
#128444=CARTESIAN_POINT('Ctrl Pts',(82.0550957922083,-9.06005715348447,
139.442644437343));
#128445=CARTESIAN_POINT('Ctrl Pts',(82.0517961792383,-9.1311232476299,139.438775783481));
#128446=CARTESIAN_POINT('Ctrl Pts',(82.0448030571631,-9.20193568262351,
139.434907129618));
#128447=CARTESIAN_POINT('Ctrl Pts',(82.0378203675282,-9.27264247860433,
139.431044247069));
#128448=CARTESIAN_POINT('Ctrl Pts',(82.0271551533183,-9.34309588696136,
139.427181364519));
#128449=CARTESIAN_POINT('Ctrl Pts',(82.0128399703195,-9.41288353852396,
139.42331848197));
#128450=CARTESIAN_POINT('Ctrl Pts',(81.998541609247,-9.48258918186285,139.419460138736));
#128451=CARTESIAN_POINT('Ctrl Pts',(81.9806018961423,-9.55163014870729,
139.415601795502));
#128452=CARTESIAN_POINT('Ctrl Pts',(81.9591049949775,-9.61960082404249,
139.411743452268));
#128453=CARTESIAN_POINT('Ctrl Pts',(81.9376216617892,-9.68752859903064,
139.407887544264));
#128454=CARTESIAN_POINT('Ctrl Pts',(81.9125857410267,-9.75438696053742,
139.404031636261));
#128455=CARTESIAN_POINT('Ctrl Pts',(81.8841317678587,-9.81978353474901,
139.400175728257));
#128456=CARTESIAN_POINT('Ctrl Pts',(81.8556862293651,-9.8851607233089,139.396320963269));
#128457=CARTESIAN_POINT('Ctrl Pts',(81.8238248437278,-9.9490765395105,139.392466198281));
#128458=CARTESIAN_POINT('Ctrl Pts',(81.7887303644301,-10.0111583683408,
139.388611433293));
#128459=CARTESIAN_POINT('Ctrl Pts',(81.7536345415136,-10.0732425740212,
139.384756520722));
#128460=CARTESIAN_POINT('Ctrl Pts',(81.7153056202243,-10.133492231011,139.380901608151));
#128461=CARTESIAN_POINT('Ctrl Pts',(81.6739715583618,-10.1915606506997,
139.37704669558));
#128462=CARTESIAN_POINT('Ctrl Pts',(81.6325942438482,-10.2496898341503,
139.373187749165));
#128463=CARTESIAN_POINT('Ctrl Pts',(81.5882057937322,-10.3056328272753,
139.369328802749));
#128464=CARTESIAN_POINT('Ctrl Pts',(81.5410761084176,-10.3590739459516,
139.365469856334));
#128465=CARTESIAN_POINT('Ctrl Pts',(81.4939197547027,-10.4125453043619,
139.361608726328));
#128466=CARTESIAN_POINT('Ctrl Pts',(81.444019418087,-10.4635116227775,139.357747596322));
#128467=CARTESIAN_POINT('Ctrl Pts',(81.3916817944375,-10.5116941970952,
139.353886466316));
#128468=CARTESIAN_POINT('Ctrl Pts',(81.339252561045,-10.559961108319,139.350018577938));
#128469=CARTESIAN_POINT('Ctrl Pts',(81.2843778974373,-10.6054342371213,
139.34615068956));
#128470=CARTESIAN_POINT('Ctrl Pts',(81.2273969197782,-10.6478757124914,
139.342282801182));
#128471=CARTESIAN_POINT('Ctrl Pts',(81.1934998810702,-10.6731234423926,
139.339981858526));
#128472=CARTESIAN_POINT('Ctrl Pts',(81.1588580068394,-10.6972991413891,
139.337680915871));
#128473=CARTESIAN_POINT('Ctrl Pts',(81.1235469328426,-10.7203603843962,
139.335379973215));
#128474=CARTESIAN_POINT('Ctrl Pts',(81.064169403796,-10.7591391433384,139.331510810544));
#128475=CARTESIAN_POINT('Ctrl Pts',(81.0026656025668,-10.7949161392637,
139.327641647873));
#128476=CARTESIAN_POINT('Ctrl Pts',(80.9393714614606,-10.8274514548664,
139.323772485202));
#128477=CARTESIAN_POINT('Ctrl Pts',(80.8761716184376,-10.8599382980854,
139.319909086961));
#128478=CARTESIAN_POINT('Ctrl Pts',(80.8111871586046,-10.8891928273149,
139.31604568872));
#128479=CARTESIAN_POINT('Ctrl Pts',(80.7447823129528,-10.9150187646111,
139.312182290478));
#128480=CARTESIAN_POINT('Ctrl Pts',(80.6784553574967,-10.9408144091283,
139.308323423847));
#128481=CARTESIAN_POINT('Ctrl Pts',(80.610711776106,-10.9631892747637,139.304464557215));
#128482=CARTESIAN_POINT('Ctrl Pts',(80.5419381060237,-10.9819941099154,
139.300605690584));
#128483=CARTESIAN_POINT('Ctrl Pts',(80.4732077575516,-11.0007870996075,
139.296749254713));
#128484=CARTESIAN_POINT('Ctrl Pts',(80.4034490751883,-11.016014392627,139.292892818841));
#128485=CARTESIAN_POINT('Ctrl Pts',(80.3330647821262,-11.0275762410837,
139.28903638297));
#128486=CARTESIAN_POINT('Ctrl Pts',(80.2627012832298,-11.0391346737358,
139.285181086435));
#128487=CARTESIAN_POINT('Ctrl Pts',(80.1917130196465,-11.0470297330092,
139.2813257899));
#128488=CARTESIAN_POINT('Ctrl Pts',(80.1205122587922,-11.0512128992332,
139.277470493365));
#128489=CARTESIAN_POINT('Ctrl Pts',(80.0493087189167,-11.0553962287295,
139.273615046355));
#128490=CARTESIAN_POINT('Ctrl Pts',(79.9778931503567,-11.0558673512484,
139.269759599345));
#128491=CARTESIAN_POINT('Ctrl Pts',(79.9066805502896,-11.0526297870794,
139.265904152335));
#128492=CARTESIAN_POINT('Ctrl Pts',(79.8353934290479,-11.0493888349274,
139.262044670751));
#128493=CARTESIAN_POINT('Ctrl Pts',(79.764310186547,-11.0424314708572,139.258185189168));
#128494=CARTESIAN_POINT('Ctrl Pts',(79.6938425160225,-11.0318132683651,
139.254325707585));
#128495=CARTESIAN_POINT('Ctrl Pts',(79.6233349545345,-11.0211890550269,
139.250464041192));
#128496=CARTESIAN_POINT('Ctrl Pts',(79.5534441348589,-11.0068999751735,
139.246602374799));
#128497=CARTESIAN_POINT('Ctrl Pts',(79.4845706367511,-10.989052571955,139.242740708406));
#128498=CARTESIAN_POINT('Ctrl Pts',(79.4155766714858,-10.9711739517083,
139.238872287543));
#128499=CARTESIAN_POINT('Ctrl Pts',(79.3476040438129,-10.949724728142,139.23500386668));
#128500=CARTESIAN_POINT('Ctrl Pts',(79.2810366107104,-10.92486082805,139.231135445818));
#128501=CARTESIAN_POINT('Ctrl Pts',(79.2415238646542,-10.9101022452939,
139.228839248953));
#128502=CARTESIAN_POINT('Ctrl Pts',(79.2025058194015,-10.8941414848041,
139.226543052088));
#128503=CARTESIAN_POINT('Ctrl Pts',(79.1640586576305,-10.8770188157335,
139.224246855223));
#128504=CARTESIAN_POINT('Ctrl Pts',(79.0992743299609,-10.8481667353053,
139.220377712139));
#128505=CARTESIAN_POINT('Ctrl Pts',(79.035858637873,-10.8159002327603,139.216508569054));
#128506=CARTESIAN_POINT('Ctrl Pts',(78.9741953427939,-10.7803714128671,
139.21263942597));
#128507=CARTESIAN_POINT('Ctrl Pts',(78.912623899062,-10.7448955153804,139.208776046217));
#128508=CARTESIAN_POINT('Ctrl Pts',(78.8528000884208,-10.7061671869215,
139.204912666463));
#128509=CARTESIAN_POINT('Ctrl Pts',(78.7950863573877,-10.664385975772,139.20104928671));
#128510=CARTESIAN_POINT('Ctrl Pts',(78.7374402965986,-10.6226537537402,
139.19719043683));
#128511=CARTESIAN_POINT('Ctrl Pts',(78.6818997925833,-10.5778760426978,
139.193331586949));
#128512=CARTESIAN_POINT('Ctrl Pts',(78.6287998814073,-10.5302966370189,
139.189472737069));
#128513=CARTESIAN_POINT('Ctrl Pts',(78.5757334039231,-10.4827471891149,
139.185616316865));
#128514=CARTESIAN_POINT('Ctrl Pts',(78.5251048314328,-10.4323998698312,
139.181759896661));
#128515=CARTESIAN_POINT('Ctrl Pts',(78.4772163885171,-10.3795389211976,
139.177903476456));
#128516=CARTESIAN_POINT('Ctrl Pts',(78.4293420799125,-10.3266935745141,
139.174048194478));
#128517=CARTESIAN_POINT('Ctrl Pts',(78.3842066212449,-10.2713364311666,
139.170192912499));
#128518=CARTESIAN_POINT('Ctrl Pts',(78.342074374492,-10.2137875360968,139.16633763052));
#128519=CARTESIAN_POINT('Ctrl Pts',(78.2999404708373,-10.1562363778468,
139.162482196928));
#128520=CARTESIAN_POINT('Ctrl Pts',(78.2608102987546,-10.0964936900018,
139.158626763336));
#128521=CARTESIAN_POINT('Ctrl Pts',(78.2249059796854,-10.0349100354831,
139.154771329743));
#128522=CARTESIAN_POINT('Ctrl Pts',(78.1889640708374,-9.97326190638249,
139.150911859731));
#128523=CARTESIAN_POINT('Ctrl Pts',(78.1562550019824,-9.90976938362367,
139.147052389719));
#128524=CARTESIAN_POINT('Ctrl Pts',(78.1269553705043,-9.84480848623664,
139.143192919707));
#128525=CARTESIAN_POINT('Ctrl Pts',(78.0976391450011,-9.77981079784868,
139.139331263861));
#128526=CARTESIAN_POINT('Ctrl Pts',(78.0717363772824,-9.71334353215134,
139.135469608015));
#128527=CARTESIAN_POINT('Ctrl Pts',(78.0493748152645,-9.64580101515523,
139.131607952168));
#128528=CARTESIAN_POINT('Ctrl Pts',(78.026974130229,-9.57814032810112,139.127739540102));
#128529=CARTESIAN_POINT('Ctrl Pts',(78.0081271490154,-9.50940110245736,
139.123871128036));
#128530=CARTESIAN_POINT('Ctrl Pts',(77.9929110603408,-9.4399903985291,139.12000271597));
#128531=CARTESIAN_POINT('Ctrl Pts',(77.9838786451825,-9.39878754359592,
139.117706389724));
#128532=CARTESIAN_POINT('Ctrl Pts',(77.9761246711039,-9.35734824655245,
139.115410063478));
#128533=CARTESIAN_POINT('Ctrl Pts',(77.9696566259696,-9.31575836652541,
139.113113737232));
#128534=CARTESIAN_POINT('Ctrl Pts',(77.9535184264028,-9.21198887050296,
139.107384251667));
#128535=CARTESIAN_POINT('Ctrl Pts',(77.9453328874797,-9.10695137253559,
139.101654766102));
#128536=CARTESIAN_POINT('Ctrl Pts',(77.9452506264317,-9.00160446896122,
139.095925280538));
#128537=CARTESIAN_POINT('Ctrl Pts',(77.9452506264311,-9.00160446819347,
139.095925280496));
#128538=CARTESIAN_POINT('Ctrl Pts',(77.9451944260495,-8.9296318985583,139.092010919611));
#128539=CARTESIAN_POINT('Ctrl Pts',(77.9489244684886,-8.85751959834465,
139.088096558725));
#128540=CARTESIAN_POINT('Ctrl Pts',(77.9564551529281,-8.78570576184602,
139.084182197839));
#128541=CARTESIAN_POINT('Ctrl Pts',(77.9637702774153,-8.71594754025189,
139.080379882473));
#128542=CARTESIAN_POINT('Ctrl Pts',(77.9746713407522,-8.64647146490485,
139.076577567106));
#128543=CARTESIAN_POINT('Ctrl Pts',(77.989118824301,-8.57767967167147,139.072775251739));
#128544=CARTESIAN_POINT('Ctrl Pts',(78.0035569312041,-8.50893252540201,
139.068975404136));
#128545=CARTESIAN_POINT('Ctrl Pts',(78.0215367933465,-8.44086927047645,
139.065175556532));
#128546=CARTESIAN_POINT('Ctrl Pts',(78.04296740632,-8.37388420418094,139.061375708928));
#128547=CARTESIAN_POINT('Ctrl Pts',(78.0643917757445,-8.3069186531715,139.057576968364));
#128548=CARTESIAN_POINT('Ctrl Pts',(78.0892647486508,-8.24103114499242,
139.053778227799));
#128549=CARTESIAN_POINT('Ctrl Pts',(78.1174453485376,-8.17660122251894,
139.049979487235));
#128550=CARTESIAN_POINT('Ctrl Pts',(78.1456278173538,-8.11216702707126,
139.046180494739));
#128551=CARTESIAN_POINT('Ctrl Pts',(78.1771181441239,-8.04919106713867,
139.042381502244));
#128552=CARTESIAN_POINT('Ctrl Pts',(78.2117278439726,-7.98803149333731,
139.038582509748));
#128553=CARTESIAN_POINT('Ctrl Pts',(78.2463733781589,-7.92680859587732,
139.034779583835));
#128554=CARTESIAN_POINT('Ctrl Pts',(78.284144478339,-7.86740627170997,139.030976657923));
#128555=CARTESIAN_POINT('Ctrl Pts',(78.3248080762865,-7.81015564831994,
139.02717373201));
#128556=CARTESIAN_POINT('Ctrl Pts',(78.3654974020029,-7.75286880258645,
139.023368399995));
#128557=CARTESIAN_POINT('Ctrl Pts',(78.4090825513877,-7.69773675553732,
139.019563067979));
#128558=CARTESIAN_POINT('Ctrl Pts',(78.4552905398303,-7.64505710594054,
139.015757735964));
#128559=CARTESIAN_POINT('Ctrl Pts',(78.5015729500498,-7.59229261142271,
139.011946275147));
#128560=CARTESIAN_POINT('Ctrl Pts',(78.5504862702189,-7.5419887443633,139.00813481433));
#128561=CARTESIAN_POINT('Ctrl Pts',(78.6017220132516,-7.49440502316367,
139.004323353514));
#128562=CARTESIAN_POINT('Ctrl Pts',(78.6122194521588,-7.48465582901318,
139.003542442089));
#128563=CARTESIAN_POINT('Ctrl Pts',(78.622814278579,-7.47502067954326,139.002761530665));
#128564=CARTESIAN_POINT('Ctrl Pts',(78.6335036862727,-7.46550158453334,
139.001980619241));
#128565=CARTESIAN_POINT('Ctrl Pts',(78.6864653129501,-7.41833837674232,
138.99811152373));
#128566=CARTESIAN_POINT('Ctrl Pts',(78.741975216377,-7.37382789140775,138.994242428218));
#128567=CARTESIAN_POINT('Ctrl Pts',(78.7997368192305,-7.33225725623249,
138.990373332707));
#128568=CARTESIAN_POINT('Ctrl Pts',(78.8574123619349,-7.29074855796495,
138.986510001838));
#128569=CARTESIAN_POINT('Ctrl Pts',(78.9173325537051,-7.25217129684877,
138.982646670968));
#128570=CARTESIAN_POINT('Ctrl Pts',(78.9791663526586,-7.21677364674147,
138.978783340098));
#128571=CARTESIAN_POINT('Ctrl Pts',(79.0409276221684,-7.18141751716047,
138.974924540816));
#128572=CARTESIAN_POINT('Ctrl Pts',(79.1045976207614,-7.14923383050781,
138.971065741533));
#128573=CARTESIAN_POINT('Ctrl Pts',(79.1698162652816,-7.12042756747473,
138.967206942251));
#128574=CARTESIAN_POINT('Ctrl Pts',(79.234993827726,-7.09163944988286,138.963350573676));
#128575=CARTESIAN_POINT('Ctrl Pts',(79.3017176573821,-7.06622473082228,
138.959494205102));
#128576=CARTESIAN_POINT('Ctrl Pts',(79.3696043147107,-7.04434183905555,
138.955637836527));
#128577=CARTESIAN_POINT('Ctrl Pts',(79.437470918147,-7.02246541155104,138.951782607134));
#128578=CARTESIAN_POINT('Ctrl Pts',(79.5064992052078,-7.00411888903381,
138.94792737774));
#128579=CARTESIAN_POINT('Ctrl Pts',(79.5762886922953,-6.98941145675622,
138.944072148347));
#128580=CARTESIAN_POINT('Ctrl Pts',(79.6460809080327,-6.9747034494431,138.940216768221));
#128581=CARTESIAN_POINT('Ctrl Pts',(79.7166339070914,-6.9636349128697,138.936361388094));
#128582=CARTESIAN_POINT('Ctrl Pts',(79.7875367805005,-6.95626397427165,
138.932506007968));
#128583=CARTESIAN_POINT('Ctrl Pts',(79.8585138681322,-6.94888532049294,
138.928646592405));
#128584=CARTESIAN_POINT('Ctrl Pts',(79.929841076995,-6.94521204097988,138.924787176843));
#128585=CARTESIAN_POINT('Ctrl Pts',(80.0011030377304,-6.94525029606821,
138.92092776128));
#128586=CARTESIAN_POINT('Ctrl Pts',(80.0724053469192,-6.94528857281654,
138.91706616052));
#128587=CARTESIAN_POINT('Ctrl Pts',(80.1436418491016,-6.94904254196509,
138.91320455976));
#128588=CARTESIAN_POINT('Ctrl Pts',(80.2144005988324,-6.95646630913011,
138.909342959));
#128589=CARTESIAN_POINT('Ctrl Pts',(80.2852831397793,-6.96390306404816,
138.905474602435));
#128590=CARTESIAN_POINT('Ctrl Pts',(80.3556857795533,-6.97502235938342,
138.901606245871));
#128591=CARTESIAN_POINT('Ctrl Pts',(80.425205779222,-6.98972698177183,138.897737889307));
#128592=CARTESIAN_POINT('Ctrl Pts',(80.4664825477539,-6.99845769663903,
138.895441093288));
#128593=CARTESIAN_POINT('Ctrl Pts',(80.5074484142674,-7.00845136765168,
138.893144297268));
#128594=CARTESIAN_POINT('Ctrl Pts',(80.5480219975304,-7.01967945707702,
138.890847501249));
#128595=CARTESIAN_POINT('Ctrl Pts',(80.6163512059742,-7.03858847129437,
138.886979510272));
#128596=CARTESIAN_POINT('Ctrl Pts',(80.6838343956939,-7.06107511666485,
138.883111519295));
#128597=CARTESIAN_POINT('Ctrl Pts',(80.7500698253181,-7.08704604873845,
138.879243528319));
#128598=CARTESIAN_POINT('Ctrl Pts',(80.8162190584746,-7.11298318315084,
138.87538057101));
#128599=CARTESIAN_POINT('Ctrl Pts',(80.8811233032238,-7.1423954376098,138.871517613701));
#128600=CARTESIAN_POINT('Ctrl Pts',(80.9443946161016,-7.17513935557307,
138.867654656392));
#128601=CARTESIAN_POINT('Ctrl Pts',(81.0075967034356,-7.20784744820844,
138.86379592557));
#128602=CARTESIAN_POINT('Ctrl Pts',(81.0691689767197,-7.24387974524783,
138.859937194747));
#128603=CARTESIAN_POINT('Ctrl Pts',(81.1287439327008,-7.28304493451599,
138.856078463924));
#128604=CARTESIAN_POINT('Ctrl Pts',(81.1708819766027,-7.31074691830482,
138.853349139728));
#128605=CARTESIAN_POINT('Ctrl Pts',(81.21202117558,-7.34001523367997,138.850619815533));
#128606=CARTESIAN_POINT('Ctrl Pts',(81.2520391107129,-7.37076839346111,
138.847890491337));
#128607=CARTESIAN_POINT('',(77.9452503313529,-8.99883308321583,139.154074719413));
#128608=CARTESIAN_POINT('Ctrl Pts',(77.9452503313529,-8.99883308321583,
139.154074719413));
#128609=CARTESIAN_POINT('Ctrl Pts',(77.9452955388054,-8.91923015076267,
139.149777319356));
#128610=CARTESIAN_POINT('Ctrl Pts',(77.9499707048544,-8.83979433416053,
139.145479919299));
#128611=CARTESIAN_POINT('Ctrl Pts',(77.9591932155917,-8.761032991371,139.141182519242));
#128612=CARTESIAN_POINT('Ctrl Pts',(77.9684534931109,-8.68194911575514,
139.136867521052));
#128613=CARTESIAN_POINT('Ctrl Pts',(77.9822982979791,-8.60354550943924,
139.132552522862));
#128614=CARTESIAN_POINT('Ctrl Pts',(78.0005942479508,-8.52631846017337,
139.128237524672));
#128615=CARTESIAN_POINT('Ctrl Pts',(78.0189841118794,-8.44869500089355,
139.123900377397));
#128616=CARTESIAN_POINT('Ctrl Pts',(78.0418707971446,-8.37226046029615,
139.119563230122));
#128617=CARTESIAN_POINT('Ctrl Pts',(78.069070752716,-8.29749747012325,139.115226082847));
#128618=CARTESIAN_POINT('Ctrl Pts',(78.0780409913188,-8.2728414790961,139.113795740587));
#128619=CARTESIAN_POINT('Ctrl Pts',(78.0874799658388,-8.2483670990492,139.112365398327));
#128620=CARTESIAN_POINT('Ctrl Pts',(78.0973799938381,-8.22409106549,139.110935056068));
#128621=CARTESIAN_POINT('Ctrl Pts',(78.1241601719728,-8.15842291756506,
139.107065893222));
#128622=CARTESIAN_POINT('Ctrl Pts',(78.1543965425552,-8.09401427390062,
139.103196730376));
#128623=CARTESIAN_POINT('Ctrl Pts',(78.1879492686742,-8.03125353698621,
139.09932756753));
#128624=CARTESIAN_POINT('Ctrl Pts',(78.2214520066495,-7.96858630343507,
139.095464169112));
#128625=CARTESIAN_POINT('Ctrl Pts',(78.2582610655738,-7.90756252818727,
139.091600770694));
#128626=CARTESIAN_POINT('Ctrl Pts',(78.2981885117691,-7.84855081700258,
139.087737372276));
#128627=CARTESIAN_POINT('Ctrl Pts',(78.3380691247073,-7.78960832413534,
139.083878505466));
#128628=CARTESIAN_POINT('Ctrl Pts',(78.3810605885034,-7.73267360779941,
139.080019638656));
#128629=CARTESIAN_POINT('Ctrl Pts',(78.4269298749198,-7.67808928286357,
139.076160771846));
#128630=CARTESIAN_POINT('Ctrl Pts',(78.4727702675689,-7.62353934143152,
139.072304335796));
#128631=CARTESIAN_POINT('Ctrl Pts',(78.5214845745239,-7.57133722501943,
139.068447899745));
#128632=CARTESIAN_POINT('Ctrl Pts',(78.5727982977411,-7.52179403885339,
139.064591463694));
#128633=CARTESIAN_POINT('Ctrl Pts',(78.6240968609664,-7.47226548959643,
139.060736166979));
#128634=CARTESIAN_POINT('Ctrl Pts',(78.6779929665586,-7.42539464827194,
139.056880870264));
#128635=CARTESIAN_POINT('Ctrl Pts',(78.7341751285011,-7.3814559143493,139.053025573549));
#128636=CARTESIAN_POINT('Ctrl Pts',(78.7903594832843,-7.33751546545815,
139.049170126358));
#128637=CARTESIAN_POINT('Ctrl Pts',(78.8488296875721,-7.29650764869656,
139.045314679167));
#128638=CARTESIAN_POINT('Ctrl Pts',(78.9092424104538,-7.25866561414891,
139.041459231976));
#128639=CARTESIAN_POINT('Ctrl Pts',(78.969718352854,-7.22078397941294,139.037599750212));
#128640=CARTESIAN_POINT('Ctrl Pts',(79.0321404592024,-7.18607499850772,
139.033740268449));
#128641=CARTESIAN_POINT('Ctrl Pts',(79.0961385087842,-7.15472712933909,
139.029880786685));
#128642=CARTESIAN_POINT('Ctrl Pts',(79.1601727869471,-7.12336151449182,
139.026019120112));
#128643=CARTESIAN_POINT('Ctrl Pts',(79.2257843373035,-7.09536098981289,
139.022157453539));
#128644=CARTESIAN_POINT('Ctrl Pts',(79.2925830888667,-7.0708657702631,139.018295786966));
#128645=CARTESIAN_POINT('Ctrl Pts',(79.3594986785926,-7.04632770595379,
139.014427365925));
#128646=CARTESIAN_POINT('Ctrl Pts',(79.4276051510998,-7.02530733110495,
139.010558944884));
#128647=CARTESIAN_POINT('Ctrl Pts',(79.4964981007915,-7.0078947316988,139.006690523843));
#128648=CARTESIAN_POINT('Ctrl Pts',(79.5373911841844,-6.99755906044666,
139.004394328587));
#128649=CARTESIAN_POINT('Ctrl Pts',(79.5785611680086,-6.98849353941898,
139.002098133332));
#128650=CARTESIAN_POINT('Ctrl Pts',(79.6199224887927,-6.98070837966023,
138.999801938076));
#128651=CARTESIAN_POINT('Ctrl Pts',(79.6902200529322,-6.96747674785778,
138.995899332206));
#128652=CARTESIAN_POINT('Ctrl Pts',(79.7613482220587,-6.95789427115864,
138.991996726337));
#128653=CARTESIAN_POINT('Ctrl Pts',(79.8328942558139,-6.95205634043317,
138.988094120467));
#128654=CARTESIAN_POINT('Ctrl Pts',(79.9037074294676,-6.94627820878081,
138.984231489758));
#128655=CARTESIAN_POINT('Ctrl Pts',(79.9749294567065,-6.94416834348739,
138.980368859048));
#128656=CARTESIAN_POINT('Ctrl Pts',(80.0461489039904,-6.94576830879268,
138.976506228338));
#128657=CARTESIAN_POINT('Ctrl Pts',(80.1172967808345,-6.94736666624752,
138.972647479296));
#128658=CARTESIAN_POINT('Ctrl Pts',(80.1884415998422,-6.95266744653637,
138.968788730253));
#128659=CARTESIAN_POINT('Ctrl Pts',(80.2591691608483,-6.9616602568352,138.964929981211));
#128660=CARTESIAN_POINT('Ctrl Pts',(80.3298493056808,-6.97064703830099,
138.961073819096));
#128661=CARTESIAN_POINT('Ctrl Pts',(80.4001122671532,-6.98332087521417,
138.957217656981));
#128662=CARTESIAN_POINT('Ctrl Pts',(80.4695479369975,-6.99961946186196,
138.953361494867));
#128663=CARTESIAN_POINT('Ctrl Pts',(80.5404063424309,-7.01625200624832,
138.949426320062));
#128664=CARTESIAN_POINT('Ctrl Pts',(80.6104026566569,-7.0366594470523,138.945491145257));
#128665=CARTESIAN_POINT('Ctrl Pts',(80.6791123432621,-7.06072075560815,
138.941555970452));
#128666=CARTESIAN_POINT('Ctrl Pts',(80.7464442673682,-7.08429958825344,
138.937699703536));
#128667=CARTESIAN_POINT('Ctrl Pts',(80.8125402343916,-7.11138688392842,
138.933843436619));
#128668=CARTESIAN_POINT('Ctrl Pts',(80.877018521144,-7.1418191487182,138.929987169702));
#128669=CARTESIAN_POINT('Ctrl Pts',(80.9434758638943,-7.17318548231151,
138.926012540953));
#128670=CARTESIAN_POINT('Ctrl Pts',(81.0082140902805,-7.20810526770631,
138.922037912204));
#128671=CARTESIAN_POINT('Ctrl Pts',(81.0708422988144,-7.24634828612698,
138.918063283455));
#128672=CARTESIAN_POINT('Ctrl Pts',(81.1334705073483,-7.28459130454764,
138.914088654706));
#128673=CARTESIAN_POINT('Ctrl Pts',(81.1939882517061,-7.32615721258586,
138.910114025957));
#128674=CARTESIAN_POINT('Ctrl Pts',(81.2520391107129,-7.37076839346111,
138.906139397208));
#128675=CARTESIAN_POINT('Ctrl Pts',(81.2520391107129,-7.37076839346111,
139.606097362913));
#128676=CARTESIAN_POINT('Ctrl Pts',(81.3086788835608,-7.4142951766041,139.60223519659));
#128677=CARTESIAN_POINT('Ctrl Pts',(81.3630354864183,-7.46077074580535,
139.598373030266));
#128678=CARTESIAN_POINT('Ctrl Pts',(81.4147982803809,-7.50991832830168,
139.594510863943));
#128679=CARTESIAN_POINT('Ctrl Pts',(81.466618276899,-7.55912022330893,139.590644429577));
#128680=CARTESIAN_POINT('Ctrl Pts',(81.5158383936151,-7.61099968960752,
139.586777995211));
#128681=CARTESIAN_POINT('Ctrl Pts',(81.5621848353351,-7.66524305480394,
139.582911560846));
#128682=CARTESIAN_POINT('Ctrl Pts',(81.6085610024906,-7.71952121032284,
139.579042646647));
#128683=CARTESIAN_POINT('Ctrl Pts',(81.652059532174,-7.7761658982234,139.575173732448));
#128684=CARTESIAN_POINT('Ctrl Pts',(81.6924485874334,-7.83483248354808,
139.571304818249));
#128685=CARTESIAN_POINT('Ctrl Pts',(81.7329055584333,-7.89359771897892,
139.567429398323));
#128686=CARTESIAN_POINT('Ctrl Pts',(81.7702423687397,-7.95439122419767,
139.563553978397));
#128687=CARTESIAN_POINT('Ctrl Pts',(81.8042723619686,-8.0168424305656,139.559678558471));
#128688=CARTESIAN_POINT('Ctrl Pts',(81.8165980230159,-8.03946225292367,
139.558274881659));
#128689=CARTESIAN_POINT('Ctrl Pts',(81.8284903220569,-8.06229934988405,
139.556871204846));
#128690=CARTESIAN_POINT('Ctrl Pts',(81.8399419628445,-8.0853355063938,139.555467528034));
#128691=CARTESIAN_POINT('Ctrl Pts',(81.8714784322706,-8.14877436715937,
139.551601967482));
#128692=CARTESIAN_POINT('Ctrl Pts',(81.8997929599867,-8.21397258847203,
139.547736406931));
#128693=CARTESIAN_POINT('Ctrl Pts',(81.9246862746981,-8.28056945680009,
139.543870846379));
#128694=CARTESIAN_POINT('Ctrl Pts',(81.949542139255,-8.34706613505579,139.540011101278));
#128695=CARTESIAN_POINT('Ctrl Pts',(81.9709868376719,-8.41495683172817,
139.536151356177));
#128696=CARTESIAN_POINT('Ctrl Pts',(81.9888677006433,-8.48385774069773,
139.532291611075));
#128697=CARTESIAN_POINT('Ctrl Pts',(82.0067273008979,-8.55267671735107,
139.528436455723));
#128698=CARTESIAN_POINT('Ctrl Pts',(82.0210313614891,-8.62250305142058,
139.524581300371));
#128699=CARTESIAN_POINT('Ctrl Pts',(82.0316764967262,-8.69293620345219,
139.520726145018));
#128700=CARTESIAN_POINT('Ctrl Pts',(82.0423148262782,-8.76332432591449,
139.516873454357));
#128701=CARTESIAN_POINT('Ctrl Pts',(82.0492987985764,-8.8343180165325,139.513020763696));
#128702=CARTESIAN_POINT('Ctrl Pts',(82.0525760686228,-8.90550637578659,
139.509168073035));
#128703=CARTESIAN_POINT('Ctrl Pts',(82.0558523453396,-8.97667315808627,
139.505316550112));
#128704=CARTESIAN_POINT('Ctrl Pts',(82.0554241276904,-9.04803400587314,
139.501465027188));
#128705=CARTESIAN_POINT('Ctrl Pts',(82.0512910588627,-9.11917447012652,
139.497613504265));
#128706=CARTESIAN_POINT('Ctrl Pts',(82.0471578531392,-9.19031729069972,
139.493761853771));
#128707=CARTESIAN_POINT('Ctrl Pts',(82.0393195830591,-9.2612392273806,139.489910203277));
#128708=CARTESIAN_POINT('Ctrl Pts',(82.0278278969249,-9.33152915852604,
139.486058552784));
#128709=CARTESIAN_POINT('Ctrl Pts',(82.0163242000214,-9.4018925546219,139.482202876659));
#128710=CARTESIAN_POINT('Ctrl Pts',(82.0011595432771,-9.47162214513738,
139.478347200534));
#128711=CARTESIAN_POINT('Ctrl Pts',(81.9824368915262,-9.54031614228697,
139.47449152441));
#128712=CARTESIAN_POINT('Ctrl Pts',(81.9637036833706,-9.60904887121698,
139.470633674337));
#128713=CARTESIAN_POINT('Ctrl Pts',(81.9414086392753,-9.67674438189115,
139.466775824264));
#128714=CARTESIAN_POINT('Ctrl Pts',(81.9157040514693,-9.74301786632893,
139.462917974191));
#128715=CARTESIAN_POINT('Ctrl Pts',(81.8899542975128,-9.80940780150311,
139.459053345397));
#128716=CARTESIAN_POINT('Ctrl Pts',(81.8607832382982,-9.87437027759518,
139.455188716602));
#128717=CARTESIAN_POINT('Ctrl Pts',(81.8283902625532,-9.93754285784748,
139.451324087808));
#128718=CARTESIAN_POINT('Ctrl Pts',(81.808861309546,-9.97562810079643,139.448994195219));
#128719=CARTESIAN_POINT('Ctrl Pts',(81.7881621998911,-10.0130632909878,
139.446664302631));
#128720=CARTESIAN_POINT('Ctrl Pts',(81.7663441333031,-10.0497742448953,
139.444334410042));
#128721=CARTESIAN_POINT('Ctrl Pts',(81.7301084811426,-10.1107441457301,
139.440464902308));
#128722=CARTESIAN_POINT('Ctrl Pts',(81.6906414186229,-10.169955001328,139.436595394573));
#128723=CARTESIAN_POINT('Ctrl Pts',(81.6481389450854,-10.2270434304428,
139.432725886839));
#128724=CARTESIAN_POINT('Ctrl Pts',(81.605699812798,-10.2840467809218,139.428862145815));
#128725=CARTESIAN_POINT('Ctrl Pts',(81.5602345365568,-10.3389335971282,
139.424998404791));
#128726=CARTESIAN_POINT('Ctrl Pts',(81.5119837389329,-10.3913672181356,
139.421134663766));
#128727=CARTESIAN_POINT('Ctrl Pts',(81.4637895967741,-10.4437392722606,
139.417275459497));
#128728=CARTESIAN_POINT('Ctrl Pts',(81.4128167573264,-10.4936634972701,
139.413416255228));
#128729=CARTESIAN_POINT('Ctrl Pts',(81.3593465778319,-10.5408356316742,
139.409557050959));
#128730=CARTESIAN_POINT('Ctrl Pts',(81.3059101238675,-10.5879780129475,
139.405700280826));
#128731=CARTESIAN_POINT('Ctrl Pts',(81.249979818307,-10.6323714269904,139.401843510694));
#128732=CARTESIAN_POINT('Ctrl Pts',(81.1918733503977,-10.6737489295327,
139.397986740561));
#128733=CARTESIAN_POINT('Ctrl Pts',(81.1337841065074,-10.7151141668846,
139.394131113659));
#128734=CARTESIAN_POINT('Ctrl Pts',(81.0735203762951,-10.7534649859936,
139.390275486756));
#128735=CARTESIAN_POINT('Ctrl Pts',(81.0114309784969,-10.7885762321569,
139.386419859854));
#128736=CARTESIAN_POINT('Ctrl Pts',(80.949339228629,-10.8236888084041,139.382564086893));
#128737=CARTESIAN_POINT('Ctrl Pts',(80.885422097698,-10.8555613309118,139.378708313932));
#128738=CARTESIAN_POINT('Ctrl Pts',(80.8200537745665,-10.8840141637788,
139.374852540971));
#128739=CARTESIAN_POINT('Ctrl Pts',(80.7546172056999,-10.9124967019282,
139.370992742511));
#128740=CARTESIAN_POINT('Ctrl Pts',(80.6877268664157,-10.9375522292262,
139.367132944052));
#128741=CARTESIAN_POINT('Ctrl Pts',(80.6197769045767,-10.9590492977598,
139.363273145593));
#128742=CARTESIAN_POINT('Ctrl Pts',(80.5517885619752,-10.9805585086679,
139.35941116697));
#128743=CARTESIAN_POINT('Ctrl Pts',(80.4827398756082,-10.9985051373091,
139.355549188348));
#128744=CARTESIAN_POINT('Ctrl Pts',(80.4130374665832,-11.0128083897129,
139.351687209725));
#128745=CARTESIAN_POINT('Ctrl Pts',(80.3432133455862,-11.0271366179687,
139.347818487448));
#128746=CARTESIAN_POINT('Ctrl Pts',(80.2727337032124,-11.0378086954034,
139.34394976517));
#128747=CARTESIAN_POINT('Ctrl Pts',(80.2020118990309,-11.0447955289344,
139.340081042892));
#128748=CARTESIAN_POINT('Ctrl Pts',(80.1600903586339,-11.0489370921694,
139.337787792611));
#128749=CARTESIAN_POINT('Ctrl Pts',(80.1180837809894,-11.0517847582771,
139.335494542331));
#128750=CARTESIAN_POINT('Ctrl Pts',(80.0760779610836,-11.0533411081302,
139.333201292051));
#128751=CARTESIAN_POINT('Ctrl Pts',(80.0051960423676,-11.055967340972,139.329331590654));
#128752=CARTESIAN_POINT('Ctrl Pts',(79.9340396619645,-11.054924095133,139.325461889257));
#128753=CARTESIAN_POINT('Ctrl Pts',(79.8630204738569,-11.0501790585014,
139.32159218786));
#128754=CARTESIAN_POINT('Ctrl Pts',(79.7921068390491,-11.0454410742493,
139.317728237864));
#128755=CARTESIAN_POINT('Ctrl Pts',(79.7213304723844,-11.0370122524541,
139.313864287867));
#128756=CARTESIAN_POINT('Ctrl Pts',(79.6511047644822,-11.0249122640581,
139.31000033787));
#128757=CARTESIAN_POINT('Ctrl Pts',(79.5809611129923,-11.0128264140976,
139.30614090277));
#128758=CARTESIAN_POINT('Ctrl Pts',(79.5113673184356,-10.997078000316,139.302281467671));
#128759=CARTESIAN_POINT('Ctrl Pts',(79.4427316308838,-10.9777384880925,
139.298422032572));
#128760=CARTESIAN_POINT('Ctrl Pts',(79.374138993588,-10.9584111061614,139.29456501822));
#128761=CARTESIAN_POINT('Ctrl Pts',(79.3065037373071,-10.9354972260411,
139.290708003868));
#128762=CARTESIAN_POINT('Ctrl Pts',(79.2402224506115,-10.9091190737995,
139.286850989516));
#128763=CARTESIAN_POINT('Ctrl Pts',(79.1739605856351,-10.8827486508749,
139.282995105345));
#128764=CARTESIAN_POINT('Ctrl Pts',(79.1090523535346,-10.8529161505769,
139.279139221174));
#128765=CARTESIAN_POINT('Ctrl Pts',(79.0458761036871,-10.8197926126305,
139.275283337003));
#128766=CARTESIAN_POINT('Ctrl Pts',(78.9826972522886,-10.7866677106816,
139.27142729405));
#128767=CARTESIAN_POINT('Ctrl Pts',(78.9212509537941,-10.7502517294585,
139.267571251097));
#128768=CARTESIAN_POINT('Ctrl Pts',(78.8618910631971,-10.7107617047588,
139.263715208144));
#128769=CARTESIAN_POINT('Ctrl Pts',(78.802468931596,-10.6712302733322,139.259855121989));
#128770=CARTESIAN_POINT('Ctrl Pts',(78.7451379801005,-10.6286186336461,
139.255995035834));
#128771=CARTESIAN_POINT('Ctrl Pts',(78.6902223949398,-10.5831867191783,
139.25213494968));
#128772=CARTESIAN_POINT('Ctrl Pts',(78.6352756453157,-10.5377290222076,
139.248272672935));
#128773=CARTESIAN_POINT('Ctrl Pts',(78.5827473484004,-10.4894481931033,
139.244410396191));
#128774=CARTESIAN_POINT('Ctrl Pts',(78.5329258898893,-10.4386421090539,
139.240548119447));
#128775=CARTESIAN_POINT('Ctrl Pts',(78.4830172689758,-10.3877471400044,
139.236679085668));
#128776=CARTESIAN_POINT('Ctrl Pts',(78.4358252628058,-10.334318459567,139.232810051889));
#128777=CARTESIAN_POINT('Ctrl Pts',(78.3915984689724,-10.2786876387484,
139.22894101811));
#128778=CARTESIAN_POINT('Ctrl Pts',(78.3654107199297,-10.2457472908652,
139.226650070093));
#128779=CARTESIAN_POINT('Ctrl Pts',(78.3402617982504,-10.2120354314329,
139.224359122076));
#128780=CARTESIAN_POINT('Ctrl Pts',(78.3161959180139,-10.1776253122225,
139.222068174059));
#128781=CARTESIAN_POINT('Ctrl Pts',(78.2750915169463,-10.1188530035883,
139.218155246495));
#128782=CARTESIAN_POINT('Ctrl Pts',(78.2369898127519,-10.0578146704116,
139.214242318932));
#128783=CARTESIAN_POINT('Ctrl Pts',(78.2021456985161,-9.99484545188481,
139.210329391368));
#128784=CARTESIAN_POINT('Ctrl Pts',(78.1673565385612,-9.93197554505502,
139.206422635065));
#128785=CARTESIAN_POINT('Ctrl Pts',(78.1358149939178,-9.86718120799267,
139.202515878762));
#128786=CARTESIAN_POINT('Ctrl Pts',(78.1077333167647,-9.80082729849671,
139.198609122459));
#128787=CARTESIAN_POINT('Ctrl Pts',(78.0796926665112,-9.73457033104502,
139.194708073868));
#128788=CARTESIAN_POINT('Ctrl Pts',(78.0551020175886,-9.66675875233996,
139.190807025276));
#128789=CARTESIAN_POINT('Ctrl Pts',(78.0341273801337,-9.59778123503494,
139.186905976684));
#128790=CARTESIAN_POINT('Ctrl Pts',(78.0131709343877,-9.52886354326538,
139.183008311547));
#128791=CARTESIAN_POINT('Ctrl Pts',(77.9958244089983,-9.45878237028468,
139.17911064641));
#128792=CARTESIAN_POINT('Ctrl Pts',(77.9822049975602,-9.38794444270915,
139.175212981273));
#128793=CARTESIAN_POINT('Ctrl Pts',(77.9685917193691,-9.31713841566859,
139.171317071377));
#128794=CARTESIAN_POINT('Ctrl Pts',(77.9587023155159,-9.24557677214363,
139.167421161481));
#128795=CARTESIAN_POINT('Ctrl Pts',(77.9526032387532,-9.17367804851513,
139.163525251585));
#128796=CARTESIAN_POINT('Ctrl Pts',(77.9476716119619,-9.11554176240162,
139.16037507421));
#128797=CARTESIAN_POINT('Ctrl Pts',(77.9452171923888,-9.05718542585664,
139.157224896836));
#128798=CARTESIAN_POINT('Ctrl Pts',(77.9452503313524,-8.99883308411473,
139.154074719462));
#128799=CARTESIAN_POINT('Origin',(80.,9.,134.));
#128800=CARTESIAN_POINT('',(78.3340002645793,9.00093892397456,138.679802731044));
#128801=CARTESIAN_POINT('Ctrl Pts',(78.4365593737638,9.57550795670799,139.340802412607));
#128802=CARTESIAN_POINT('Ctrl Pts',(78.4404068226713,9.58596004144325,139.340073158341));
#128803=CARTESIAN_POINT('Ctrl Pts',(78.4443588589399,9.59637293080484,139.339338614757));
#128804=CARTESIAN_POINT('Ctrl Pts',(78.4507209975141,9.61264236620036,139.338177131073));
#128805=CARTESIAN_POINT('Ctrl Pts',(78.4530606839165,9.61852634983335,139.337754213156));
#128806=CARTESIAN_POINT('Ctrl Pts',(78.4572880712981,9.62898361092206,139.336997239269));
#128807=CARTESIAN_POINT('Ctrl Pts',(78.4591626815642,9.63356202021996,139.336663966555));
#128808=CARTESIAN_POINT('Ctrl Pts',(78.4637554368413,9.64463807647073,139.335853258296));
#128809=CARTESIAN_POINT('Ctrl Pts',(78.466494402472,9.65112685806699,139.335374597762));
#128810=CARTESIAN_POINT('Ctrl Pts',(78.4751941310678,9.67137767851389,139.333869525295));
#128811=CARTESIAN_POINT('Ctrl Pts',(78.4812994425996,9.68507627530903,139.332835122305));
#128812=CARTESIAN_POINT('Ctrl Pts',(78.5143715333345,9.75666540579144,139.327350024636));
#128813=CARTESIAN_POINT('Ctrl Pts',(78.5444633730473,9.81304734265798,139.322756861721));
#128814=CARTESIAN_POINT('Ctrl Pts',(78.6346526201113,9.96090503443917,139.310189598706));
#128815=CARTESIAN_POINT('Ctrl Pts',(78.7006510636092,10.0484316740427,139.302185198289));
#128816=CARTESIAN_POINT('Ctrl Pts',(78.8088869487155,10.165908680851,139.290894928653));
#128817=CARTESIAN_POINT('Ctrl Pts',(78.8446838450898,10.2013903821324,139.287394207462));
#128818=CARTESIAN_POINT('Ctrl Pts',(78.8941311229802,10.2461444950879,139.282852433657));
#128819=CARTESIAN_POINT('Ctrl Pts',(78.9063854330165,10.2569126013951,139.281749049446));
#128820=CARTESIAN_POINT('Ctrl Pts',(78.9267517724024,10.2742855189152,139.27995060464));
#128821=CARTESIAN_POINT('Ctrl Pts',(78.934771107336,10.2809967824331,139.279251195608));
#128822=CARTESIAN_POINT('Ctrl Pts',(78.9505044712475,10.2939138824925,139.277895627228));
#128823=CARTESIAN_POINT('Ctrl Pts',(78.9582116578861,10.3001273236168,139.277239177777));
#128824=CARTESIAN_POINT('Ctrl Pts',(78.9765385304608,10.3146346138431,139.275695697084));
#128825=CARTESIAN_POINT('Ctrl Pts',(78.9872044584987,10.3228691380142,139.274811042446));
#128826=CARTESIAN_POINT('Ctrl Pts',(79.0235626270761,10.3502415812307,139.271839660943));
#128827=CARTESIAN_POINT('Ctrl Pts',(79.0497075258949,10.3687683147958,139.269776481048));
#128828=CARTESIAN_POINT('Ctrl Pts',(79.114924104198,10.4122119044117,139.264788925647));
#128829=CARTESIAN_POINT('Ctrl Pts',(79.1545324549174,10.4362753585315,139.261893365329));
#128830=CARTESIAN_POINT('Ctrl Pts',(79.2558435354716,10.4921800527771,139.254738013854));
#128831=CARTESIAN_POINT('Ctrl Pts',(79.3186283502537,10.5218748548831,139.250525413001));
#128832=CARTESIAN_POINT('Ctrl Pts',(79.4047577048759,10.5562092149828,139.244851480178));
#128833=CARTESIAN_POINT('Ctrl Pts',(79.4266124587449,10.5643935576172,139.243420075882));
#128834=CARTESIAN_POINT('Ctrl Pts',(79.5093044828733,10.593395091149,139.238012128862));
#128835=CARTESIAN_POINT('Ctrl Pts',(79.5711514267309,10.6111414986151,139.23398452943));
#128836=CARTESIAN_POINT('Ctrl Pts',(79.6450208759008,10.6277827533342,139.229029823763));
#128837=CARTESIAN_POINT('Ctrl Pts',(79.6562062772238,10.6301818085748,139.228275723817));
#128838=CARTESIAN_POINT('Ctrl Pts',(79.6736845772325,10.6337426916433,139.227090107031));
#128839=CARTESIAN_POINT('Ctrl Pts',(79.6799612155504,10.6349838258107,139.226662886039));
#128840=CARTESIAN_POINT('Ctrl Pts',(79.6910966237643,10.6371191498506,139.225902126262));
#128841=CARTESIAN_POINT('Ctrl Pts',(79.695952441036,10.6380279259856,139.225569415596));
#128842=CARTESIAN_POINT('Ctrl Pts',(79.7076584566262,10.6401648865566,139.224765045173));
#128843=CARTESIAN_POINT('Ctrl Pts',(79.7145123126687,10.6413717461578,139.22429221607));
#128844=CARTESIAN_POINT('Ctrl Pts',(79.7357208331176,10.6449693902631,139.222823736774));
#128845=CARTESIAN_POINT('Ctrl Pts',(79.750098967077,10.6472149862114,139.221820621464));
#128846=CARTESIAN_POINT('Ctrl Pts',(79.8237557947681,10.6577322849405,139.21664935566));
#128847=CARTESIAN_POINT('Ctrl Pts',(79.883414819369,10.6629927313519,139.212355054702));
#128848=CARTESIAN_POINT('Ctrl Pts',(80.0495460003891,10.6686579526859,139.20030963045));
#128849=CARTESIAN_POINT('Ctrl Pts',(80.1559852038318,10.662090991782,139.1925102786));
#128850=CARTESIAN_POINT('Ctrl Pts',(80.3168558794727,10.6365659837214,139.180943711137));
#128851=CARTESIAN_POINT('Ctrl Pts',(80.3721557607356,10.6248837582514,139.177004373364));
#128852=CARTESIAN_POINT('Ctrl Pts',(80.4432517991695,10.6060432381723,139.171989457209));
#128853=CARTESIAN_POINT('Ctrl Pts',(80.4596749057441,10.6014200132898,139.17083437767));
#128854=CARTESIAN_POINT('Ctrl Pts',(80.4861970543714,10.593512190503,139.168973842607));
#128855=CARTESIAN_POINT('Ctrl Pts',(80.4963404409305,10.5903819832587,139.168263436977));
#128856=CARTESIAN_POINT('Ctrl Pts',(80.5158197563398,10.5841662285839,139.166901152849));
#128857=CARTESIAN_POINT('Ctrl Pts',(80.5251596155036,10.5810945721632,139.16624885287));
#128858=CARTESIAN_POINT('Ctrl Pts',(80.5468328269296,10.5737535325418,139.164736947359));
#128859=CARTESIAN_POINT('Ctrl Pts',(80.5591444024363,10.5694215096984,139.163879441639));
#128860=CARTESIAN_POINT('Ctrl Pts',(80.5990937860606,10.5548349017069,139.161100172025));
#128861=CARTESIAN_POINT('Ctrl Pts',(80.6265115068149,10.543991074371,139.159197900738));
#128862=CARTESIAN_POINT('Ctrl Pts',(80.6916110878453,10.5162240109812,139.154680958014));
#128863=CARTESIAN_POINT('Ctrl Pts',(80.7289800316512,10.4986159016409,139.152088130076));
#128864=CARTESIAN_POINT('Ctrl Pts',(80.8623365761505,10.4296087269023,139.142762476515));
#128865=CARTESIAN_POINT('Ctrl Pts',(80.9538751682516,10.3702286761206,139.136235854507));
#128866=CARTESIAN_POINT('Ctrl Pts',(81.0837028540863,10.2666567248658,139.12594551084));
#128867=CARTESIAN_POINT('Ctrl Pts',(81.1265662505306,10.2286896072184,139.122342222886));
#128868=CARTESIAN_POINT('Ctrl Pts',(81.1754514646162,10.180676770483,139.117857309997));
#128869=CARTESIAN_POINT('Ctrl Pts',(81.1834351897454,10.1726742584859,139.117111984074));
#128870=CARTESIAN_POINT('Ctrl Pts',(81.1957870321312,10.1600387522657,139.115937325167));
#128871=CARTESIAN_POINT('Ctrl Pts',(81.2002112447982,10.155460729518,139.115512165151));
#128872=CARTESIAN_POINT('Ctrl Pts',(81.208023934129,10.1472831440658,139.114753234609));
#128873=CARTESIAN_POINT('Ctrl Pts',(81.2114227823699,10.1436936994349,139.114420270673));
#128874=CARTESIAN_POINT('Ctrl Pts',(81.2195953961233,10.1349854888543,139.113612895331));
#128875=CARTESIAN_POINT('Ctrl Pts',(81.2243528870579,10.1298517573838,139.113137288134));
#128876=CARTESIAN_POINT('Ctrl Pts',(81.2390461532584,10.1137947158913,139.111651255061));
#128877=CARTESIAN_POINT('Ctrl Pts',(81.2488688365197,10.1027695275106,139.110633112279));
#128878=CARTESIAN_POINT('Ctrl Pts',(81.2990113950014,10.0449592768906,139.105312326445));
#128879=CARTESIAN_POINT('Ctrl Pts',(81.3368499205332,9.99609300183868,139.100875849382));
#128880=CARTESIAN_POINT('Ctrl Pts',(81.4570768493695,9.82160117787799,139.08551020595));
#128881=CARTESIAN_POINT('Ctrl Pts',(81.5251832678669,9.68697564742368,139.074523934561));
#128882=CARTESIAN_POINT('Ctrl Pts',(81.5811126946868,9.52542283135678,139.062767708023));
#128883=CARTESIAN_POINT('Ctrl Pts',(81.5875339559354,9.50569013338958,139.061352680344));
#128884=CARTESIAN_POINT('Ctrl Pts',(81.5972297090175,9.47388758510644,139.059104602231));
#128885=CARTESIAN_POINT('Ctrl Pts',(81.6007396985286,9.46189243229859,139.058263982643));
#128886=CARTESIAN_POINT('Ctrl Pts',(81.6067562634227,9.44043845065898,139.056773123634));
#128887=CARTESIAN_POINT('Ctrl Pts',(81.6093150786288,9.43099501572934,139.056121217502));
#128888=CARTESIAN_POINT('Ctrl Pts',(81.6145157169252,9.41110947581618,139.054757292526));
#128889=CARTESIAN_POINT('Ctrl Pts',(81.6171397726104,9.40066315819406,139.054045873163));
#128890=CARTESIAN_POINT('Ctrl Pts',(81.6238285502723,9.37289845794113,139.052167984069));
#128891=CARTESIAN_POINT('Ctrl Pts',(81.6277175965278,9.35553886739058,139.051007158595));
#128892=CARTESIAN_POINT('Ctrl Pts',(81.6467065083611,9.26392297529577,139.044945286787));
#128893=CARTESIAN_POINT('Ctrl Pts',(81.657006347636,9.18875841022886,139.040198916405));
#128894=CARTESIAN_POINT('Ctrl Pts',(81.6692599293877,9.00874863605022,139.029075772722));
#128895=CARTESIAN_POINT('Ctrl Pts',(81.6665149103011,8.90392049647273,139.022797288656));
#128896=CARTESIAN_POINT('Ctrl Pts',(81.6483191537308,8.75340945376733,139.013332909244));
#128897=CARTESIAN_POINT('Ctrl Pts',(81.6407112838855,8.70703492592829,139.010351004561));
#128898=CARTESIAN_POINT('Ctrl Pts',(81.62893935155,8.65038416620291,139.006558974952));
#128899=CARTESIAN_POINT('Ctrl Pts',(81.6266188276171,8.63974201409532,139.005840034976));
#128900=CARTESIAN_POINT('Ctrl Pts',(81.6228116393935,8.62306903299932,139.004702212132));
#128901=CARTESIAN_POINT('Ctrl Pts',(81.621395263543,8.61702223687432,139.004287178101));
#128902=CARTESIAN_POINT('Ctrl Pts',(81.618653519927,8.60560504589117,139.003498785897));
#128903=CARTESIAN_POINT('Ctrl Pts',(81.6173351739051,8.60023315677666,139.003125821843));
#128904=CARTESIAN_POINT('Ctrl Pts',(81.6141412395193,8.58749319333404,139.002236603353));
#128905=CARTESIAN_POINT('Ctrl Pts',(81.6122419339988,8.58013127374146,139.001719031333));
#128906=CARTESIAN_POINT('Ctrl Pts',(81.60562856751,8.55520378179635,138.999954458945));
#128907=CARTESIAN_POINT('Ctrl Pts',(81.6006774725734,8.53770319712688,138.998695230358));
#128908=CARTESIAN_POINT('Ctrl Pts',(81.5877579298106,8.49473497060424,138.995558735837));
#128909=CARTESIAN_POINT('Ctrl Pts',(81.5794623250883,8.46937150563186,138.993668081348));
#128910=CARTESIAN_POINT('Ctrl Pts',(81.5399122156118,8.35760812529544,138.985191840629));
#128911=CARTESIAN_POINT('Ctrl Pts',(81.5021515070241,8.2736822746639,138.978446679774));
#128912=CARTESIAN_POINT('Ctrl Pts',(81.411496417037,8.1098735246819,138.964892067466));
#128913=CARTESIAN_POINT('Ctrl Pts',(81.358244601958,8.03055456833383,138.958116998613));
#128914=CARTESIAN_POINT('Ctrl Pts',(81.2866515207404,7.94149122292979,138.950303546905));
#128915=CARTESIAN_POINT('Ctrl Pts',(81.2745642685879,7.92696740813512,138.949021584936));
#128916=CARTESIAN_POINT('Ctrl Pts',(81.2550477401424,7.90431193354309,138.947008570631));
#128917=CARTESIAN_POINT('Ctrl Pts',(81.2477807341328,7.89604328952335,138.946270974457));
#128918=CARTESIAN_POINT('Ctrl Pts',(81.2345818487011,7.8813220025922,138.944952264514));
#128919=CARTESIAN_POINT('Ctrl Pts',(81.2286800528808,7.87484306174711,138.944369928145));
#128920=CARTESIAN_POINT('Ctrl Pts',(81.2147005736506,7.85973767516507,138.943007385054));
#128921=CARTESIAN_POINT('Ctrl Pts',(81.2065816141077,7.85114993423826,138.94222896933));
#128922=CARTESIAN_POINT('Ctrl Pts',(81.1825296049206,7.8262454305747,138.939959626976));
#128923=CARTESIAN_POINT('Ctrl Pts',(81.1663517042526,7.81016814669137,138.938479352931));
#128924=CARTESIAN_POINT('Ctrl Pts',(81.0901643650076,7.73750236615975,138.931706266261));
#128925=CARTESIAN_POINT('Ctrl Pts',(81.0263323756214,7.68508449802901,138.926588875406));
#128926=CARTESIAN_POINT('Ctrl Pts',(80.9119012339443,7.60454613930618,138.918009272305));
#128927=CARTESIAN_POINT('Ctrl Pts',(80.8632511251667,7.5739380242485,138.914520117631));
#128928=CARTESIAN_POINT('Ctrl Pts',(80.7458212019398,7.50827224107048,138.906263423895));
#128929=CARTESIAN_POINT('Ctrl Pts',(80.67600185028,7.47536255512107,138.901477853062));
#128930=CARTESIAN_POINT('Ctrl Pts',(80.5933465041269,7.44319856504702,138.895676617026));
#128931=CARTESIAN_POINT('Ctrl Pts',(80.5824838966771,7.43910177352648,138.894911563568));
#128932=CARTESIAN_POINT('Ctrl Pts',(80.5655353298124,7.43291123424384,138.893712449777));
#128933=CARTESIAN_POINT('Ctrl Pts',(80.5594783073788,7.43073857209131,138.893282845821));
#128934=CARTESIAN_POINT('Ctrl Pts',(80.5482850922439,7.42679659036717,138.892486715536));
#128935=CARTESIAN_POINT('Ctrl Pts',(80.5431526463564,7.42501723497488,138.892120780624));
#128936=CARTESIAN_POINT('Ctrl Pts',(80.5312107586048,7.42094244348017,138.891267338891));
#128937=CARTESIAN_POINT('Ctrl Pts',(80.524395107462,7.41866594188989,138.890778764549));
#128938=CARTESIAN_POINT('Ctrl Pts',(80.5025736348129,7.41153391817042,138.889210249206));
#128939=CARTESIAN_POINT('Ctrl Pts',(80.4875140137342,7.40684752994001,138.888121364217));
#128940=CARTESIAN_POINT('Ctrl Pts',(80.4039927024236,7.38215167014042,138.882055582529));
#128941=CARTESIAN_POINT('Ctrl Pts',(80.3343728683518,7.36634272133175,138.876903749626));
#128942=CARTESIAN_POINT('Ctrl Pts',(80.1347254798889,7.3343057734282,138.862204453047));
#128943=CARTESIAN_POINT('Ctrl Pts',(80.0034697195409,7.32886632828541,138.852669560682));
#128944=CARTESIAN_POINT('Ctrl Pts',(79.8447127407914,7.34101175452654,138.841651452545));
#128945=CARTESIAN_POINT('Ctrl Pts',(79.8165667005079,7.34388752631555,138.839715470578));
#128946=CARTESIAN_POINT('Ctrl Pts',(79.7759022594195,7.34909186850973,138.836942130089));
#128947=CARTESIAN_POINT('Ctrl Pts',(79.7633171035397,7.3508491039305,138.836087104017));
#128948=CARTESIAN_POINT('Ctrl Pts',(79.7410500895531,7.35421834822134,138.83457978855));
#128949=CARTESIAN_POINT('Ctrl Pts',(79.7313601919956,7.35577222925397,138.833925701665));
#128950=CARTESIAN_POINT('Ctrl Pts',(79.7111656646915,7.35919393370254,138.832566155215));
#128951=CARTESIAN_POINT('Ctrl Pts',(79.7006640824533,7.36107723249207,138.83186121731));
#128952=CARTESIAN_POINT('Ctrl Pts',(79.6731713115377,7.36628071382591,138.830020649792));
#128953=CARTESIAN_POINT('Ctrl Pts',(79.6562122350053,7.36976513750182,138.82889025843));
#128954=CARTESIAN_POINT('Ctrl Pts',(79.5729583094963,7.38822754385139,138.823361087912));
#128955=CARTESIAN_POINT('Ctrl Pts',(79.5075645725196,7.40698900395815,138.819084530675));
#128956=CARTESIAN_POINT('Ctrl Pts',(79.3768020250966,7.45333046446893,138.81049777654));
#128957=CARTESIAN_POINT('Ctrl Pts',(79.3116826741024,7.48119062532437,138.806202147965));
#128958=CARTESIAN_POINT('Ctrl Pts',(79.175671963896,7.54992972835588,138.796878436688));
#128959=CARTESIAN_POINT('Ctrl Pts',(79.1056257332216,7.5920540089126,138.791851628775));
#128960=CARTESIAN_POINT('Ctrl Pts',(79.0260641671065,7.64824035246158,138.785532306932));
#128961=CARTESIAN_POINT('Ctrl Pts',(79.0133012696898,7.65752812970628,138.784498397428));
#128962=CARTESIAN_POINT('Ctrl Pts',(78.9949825298433,7.6712613265876,138.782981736006));
#128963=CARTESIAN_POINT('Ctrl Pts',(78.9893197284526,7.67556353053581,138.782508273499));
#128964=CARTESIAN_POINT('Ctrl Pts',(78.9795158616251,7.68311131662061,138.78168015851));
#128965=CARTESIAN_POINT('Ctrl Pts',(78.975362355064,7.68634046394217,138.781326647072));
#128966=CARTESIAN_POINT('Ctrl Pts',(78.9664098434199,7.69336889268544,138.780558786581));
#128967=CARTESIAN_POINT('Ctrl Pts',(78.9616165386678,7.69717489792751,138.780143986943));
#128968=CARTESIAN_POINT('Ctrl Pts',(78.9487827224328,7.70748108793751,138.779023702781));
#128969=CARTESIAN_POINT('Ctrl Pts',(78.9407817255431,7.71402972962652,138.778314965539));
#128970=CARTESIAN_POINT('Ctrl Pts',(78.9226228123415,7.72917683922673,138.77668365365));
#128971=CARTESIAN_POINT('Ctrl Pts',(78.9125060396484,7.73782332005442,138.775758184024));
#128972=CARTESIAN_POINT('Ctrl Pts',(78.8806777361102,7.76569268247144,138.772796060345));
#128973=CARTESIAN_POINT('Ctrl Pts',(78.8593648579604,7.78536089185063,138.770736390998));
#128974=CARTESIAN_POINT('Ctrl Pts',(78.7593527734994,7.88260952872156,138.760738120544));
#128975=CARTESIAN_POINT('Ctrl Pts',(78.687988437749,7.96733632513103,138.752595624068));
#128976=CARTESIAN_POINT('Ctrl Pts',(78.5836293190767,8.11968798760006,138.739342731608));
#128977=CARTESIAN_POINT('Ctrl Pts',(78.5458489314751,8.18360391158375,138.734124780613));
#128978=CARTESIAN_POINT('Ctrl Pts',(78.5042636115694,8.26606597521267,138.727816668625));
#128979=CARTESIAN_POINT('Ctrl Pts',(78.4963436930611,8.28243170883749,138.726584144183));
#128980=CARTESIAN_POINT('Ctrl Pts',(78.484125129964,8.30877123608531,138.724630503009));
#128981=CARTESIAN_POINT('Ctrl Pts',(78.4796535544265,8.31866269678607,138.723903483568));
#128982=CARTESIAN_POINT('Ctrl Pts',(78.4713436667529,8.3375340274822,138.722528747547));
#128983=CARTESIAN_POINT('Ctrl Pts',(78.4674870295011,8.34650527767667,138.721880428125));
#128984=CARTESIAN_POINT('Ctrl Pts',(78.4588544455196,8.36708303553032,138.720404943349));
#128985=CARTESIAN_POINT('Ctrl Pts',(78.4541302886478,8.37871073252396,138.719579554884));
#128986=CARTESIAN_POINT('Ctrl Pts',(78.4397898314646,8.41518384045414,138.717015504033));
#128987=CARTESIAN_POINT('Ctrl Pts',(78.4306374736656,8.44020798626491,138.715292267821));
#128988=CARTESIAN_POINT('Ctrl Pts',(78.3843189260331,8.57693133839935,138.70604944903));
#128989=CARTESIAN_POINT('Ctrl Pts',(78.358470220905,8.69211092607303,138.698908399452));
#128990=CARTESIAN_POINT('Ctrl Pts',(78.3376286856976,8.87276265300322,138.687793230822));
#128991=CARTESIAN_POINT('Ctrl Pts',(78.3339641330686,8.93682820906066,138.683860303415));
#128992=CARTESIAN_POINT('Ctrl Pts',(78.3340002645793,9.00093892397456,138.679802731044));
#128993=CARTESIAN_POINT('Ctrl Pts',(78.3340002659362,9.00094132848483,138.679802578862));
#128994=CARTESIAN_POINT('Ctrl Pts',(78.3340122909079,9.02222359066603,138.678455621731));
#128995=CARTESIAN_POINT('Ctrl Pts',(78.3344321190674,9.04350288459769,138.677095274952));
#128996=CARTESIAN_POINT('Ctrl Pts',(78.335800952913,9.07868649292419,138.674815057685));
#128997=CARTESIAN_POINT('Ctrl Pts',(78.3365170039007,9.09259764858293,138.673905454353));
#128998=CARTESIAN_POINT('Ctrl Pts',(78.3378248671248,9.11301541109249,138.672556448937));
#128999=CARTESIAN_POINT('Ctrl Pts',(78.3382806780811,9.11953052843225,138.672123902949));
#129000=CARTESIAN_POINT('Ctrl Pts',(78.3391689384659,9.13123767971605,138.671342619596));
#129001=CARTESIAN_POINT('Ctrl Pts',(78.3395874614174,9.13643072747922,138.670994630515));
#129002=CARTESIAN_POINT('Ctrl Pts',(78.3404626584501,9.14668905065455,138.670304239487));
#129003=CARTESIAN_POINT('Ctrl Pts',(78.3409181705115,9.15175423071767,138.669961897786));
#129004=CARTESIAN_POINT('Ctrl Pts',(78.3420395510613,9.16361469313387,138.669156880096));
#129005=CARTESIAN_POINT('Ctrl Pts',(78.3427239992148,9.17040795502056,138.668693200433));
#129006=CARTESIAN_POINT('Ctrl Pts',(78.3449257620241,9.19099146768943,138.667280775185));
#129007=CARTESIAN_POINT('Ctrl Pts',(78.346573550956,9.20476674582777,138.666325333866));
#129008=CARTESIAN_POINT('Ctrl Pts',(78.3545977611215,9.26541513195532,138.662078424901));
#129009=CARTESIAN_POINT('Ctrl Pts',(78.3627964198778,9.31202138374526,138.658708667515));
#129010=CARTESIAN_POINT('Ctrl Pts',(78.3852576384601,9.41404270652216,138.651179346744));
#129011=CARTESIAN_POINT('Ctrl Pts',(78.4004150068948,9.4692034413495,138.647007138059));
#129012=CARTESIAN_POINT('Ctrl Pts',(78.4241525990979,9.54092402435479,138.641512903841));
#129013=CARTESIAN_POINT('Ctrl Pts',(78.4302142694855,9.55827066911257,138.640178362243));
#129014=CARTESIAN_POINT('Ctrl Pts',(78.4365593294404,9.57550783629781,138.638847722432));
#129015=CARTESIAN_POINT('Ctrl Pts',(78.4365593737687,9.57550795672114,138.833737829798));
#129016=CARTESIAN_POINT('Ctrl Pts',(78.4357692491731,9.57336148267508,138.833890538484));
#129017=CARTESIAN_POINT('Ctrl Pts',(78.434983539282,9.57121336600505,138.834043100294));
#129018=CARTESIAN_POINT('Ctrl Pts',(78.4308510841927,9.55984277640087,138.834849266783));
#129019=CARTESIAN_POINT('Ctrl Pts',(78.4275813760033,9.55059234665785,138.835500295248));
#129020=CARTESIAN_POINT('Ctrl Pts',(78.4201928105344,9.52908637313912,138.837003003153));
#129021=CARTESIAN_POINT('Ctrl Pts',(78.4161344814598,9.51681058518315,138.837852660339));
#129022=CARTESIAN_POINT('Ctrl Pts',(78.4035034946116,9.47705698110891,138.840579250395));
#129023=CARTESIAN_POINT('Ctrl Pts',(78.3954995880927,9.44940298378392,138.842437725573));
#129024=CARTESIAN_POINT('Ctrl Pts',(78.3648350198884,9.332159038107,138.850178097835));
#129025=CARTESIAN_POINT('Ctrl Pts',(78.3489306474362,9.24097008691327,138.855849713538));
#129026=CARTESIAN_POINT('Ctrl Pts',(78.3307615371578,9.03852853225636,138.868266132359));
#129027=CARTESIAN_POINT('Ctrl Pts',(78.3318966575602,8.92743470978668,138.874968455501));
#129028=CARTESIAN_POINT('Ctrl Pts',(78.3456509678574,8.80277234630258,138.883123457903));
#129029=CARTESIAN_POINT('Ctrl Pts',(78.3474441632568,8.78827225429018,138.884082046146));
#129030=CARTESIAN_POINT('Ctrl Pts',(78.3503739193868,8.7668941091527,138.885512684605));
#129031=CARTESIAN_POINT('Ctrl Pts',(78.3513633794776,8.7599961431404,138.88597697809));
#129032=CARTESIAN_POINT('Ctrl Pts',(78.3532059284696,8.74770027724662,138.886809706563));
#129033=CARTESIAN_POINT('Ctrl Pts',(78.3540423403343,8.74230008741915,138.887177209765));
#129034=CARTESIAN_POINT('Ctrl Pts',(78.3559503006038,8.73036993477362,138.88799309534));
#129035=CARTESIAN_POINT('Ctrl Pts',(78.3570341766908,8.72384228091856,138.888442131348));
#129036=CARTESIAN_POINT('Ctrl Pts',(78.36033309306,8.70468164012298,138.889767550045));
#129037=CARTESIAN_POINT('Ctrl Pts',(78.362655106246,8.6920679081068,138.890649514557));
#129038=CARTESIAN_POINT('Ctrl Pts',(78.3683523979806,8.66300746293163,138.892701332986));
#129039=CARTESIAN_POINT('Ctrl Pts',(78.3718310932534,8.64658263923721,138.893875797502));
#129040=CARTESIAN_POINT('Ctrl Pts',(78.3846990049891,8.59005486258268,138.897962887116));
#129041=CARTESIAN_POINT('Ctrl Pts',(78.395326260614,8.55025109615191,138.9009192615));
#129042=CARTESIAN_POINT('Ctrl Pts',(78.4439959631655,8.39178014556828,138.912913224673));
#129043=CARTESIAN_POINT('Ctrl Pts',(78.4938274719577,8.27713667223757,138.922065989366));
#129044=CARTESIAN_POINT('Ctrl Pts',(78.5786993296101,8.12963487475271,138.93404814134));
#129045=CARTESIAN_POINT('Ctrl Pts',(78.6030292165121,8.09109716641648,138.937205119208));
#129046=CARTESIAN_POINT('Ctrl Pts',(78.6378754586152,8.0406138443944,138.941378731347));
#129047=CARTESIAN_POINT('Ctrl Pts',(78.6470248568391,8.02775345021318,138.942445514144));
#129048=CARTESIAN_POINT('Ctrl Pts',(78.6624702455775,8.0066837810718,138.944199786827));
#129049=CARTESIAN_POINT('Ctrl Pts',(78.6686622455977,7.99839990675778,138.944891219221));
#129050=CARTESIAN_POINT('Ctrl Pts',(78.6809650325927,7.98225649055595,138.946242297613));
#129051=CARTESIAN_POINT('Ctrl Pts',(78.6870699120153,7.97439301501973,138.946902135934));
#129052=CARTESIAN_POINT('Ctrl Pts',(78.7018142601135,7.95574876994713,138.948471082713));
#129053=CARTESIAN_POINT('Ctrl Pts',(78.7105181515312,7.94501970247346,138.949377584196));
#129054=CARTESIAN_POINT('Ctrl Pts',(78.7412614358887,7.9080722199774,138.95251355375));
#129055=CARTESIAN_POINT('Ctrl Pts',(78.7639759108039,7.88242505387744,138.954715645285));
#129056=CARTESIAN_POINT('Ctrl Pts',(78.822383092881,7.82043786565147,138.960124168288));
#129057=CARTESIAN_POINT('Ctrl Pts',(78.8589819740554,7.78499923645947,138.963294508447));
#129058=CARTESIAN_POINT('Ctrl Pts',(78.9772810613102,7.68051834483437,138.97302113719));
#129059=CARTESIAN_POINT('Ctrl Pts',(79.0640340870432,7.61762839794364,138.979431576538));
#129060=CARTESIAN_POINT('Ctrl Pts',(79.1942384289264,7.54114785047247,138.988881566925));
#129061=CARTESIAN_POINT('Ctrl Pts',(79.2331371563621,7.52033046286871,138.99168777954));
#129062=CARTESIAN_POINT('Ctrl Pts',(79.2824431925521,7.49641002125102,138.995280964287));
#129063=CARTESIAN_POINT('Ctrl Pts',(79.2921190555448,7.49183053013492,138.995987785118));
#129064=CARTESIAN_POINT('Ctrl Pts',(79.3074397010656,7.4847593276703,138.997110660218));
#129065=CARTESIAN_POINT('Ctrl Pts',(79.3130555430832,7.48220509528942,138.997523031445));
#129066=CARTESIAN_POINT('Ctrl Pts',(79.3237446737536,7.47741487222536,138.998309647952));
#129067=CARTESIAN_POINT('Ctrl Pts',(79.3288151011754,7.47517293917561,138.998683531523));
#129068=CARTESIAN_POINT('Ctrl Pts',(79.3409428793794,7.46988274621522,138.999579483106));
#129069=CARTESIAN_POINT('Ctrl Pts',(79.3480102592148,7.46685797439554,139.000102924389));
#129070=CARTESIAN_POINT('Ctrl Pts',(79.3723453572463,7.45664147219591,139.001909224417));
#129071=CARTESIAN_POINT('Ctrl Pts',(79.3897124140637,7.44969200302547,139.003205072442));
#129072=CARTESIAN_POINT('Ctrl Pts',(79.4331066815716,7.43316979192352,139.006453323264));
#129073=CARTESIAN_POINT('Ctrl Pts',(79.4592623958316,7.42395190272819,139.008420277806));
#129074=CARTESIAN_POINT('Ctrl Pts',(79.5681683902661,7.38860089929623,139.016615754553));
#129075=CARTESIAN_POINT('Ctrl Pts',(79.6526673643786,7.3682998958565,139.022979473595));
#129076=CARTESIAN_POINT('Ctrl Pts',(79.8357847192328,7.33918073794056,139.036415851139));
#129077=CARTESIAN_POINT('Ctrl Pts',(79.9344052656145,7.33236972653376,139.043434880908));
#129078=CARTESIAN_POINT('Ctrl Pts',(80.0519278264193,7.33470258459134,139.051471897582));
#129079=CARTESIAN_POINT('Ctrl Pts',(80.0707844850185,7.33539746834601,139.052752046667));
#129080=CARTESIAN_POINT('Ctrl Pts',(80.1006114830504,7.33700440126782,139.054762843428));
#129081=CARTESIAN_POINT('Ctrl Pts',(80.1115910922268,7.33770505923055,139.055500010075));
#129082=CARTESIAN_POINT('Ctrl Pts',(80.1313030568346,7.33915915625824,139.056818279471));
#129083=CARTESIAN_POINT('Ctrl Pts',(80.1400378425088,7.3398728335882,139.057400600822));
#129084=CARTESIAN_POINT('Ctrl Pts',(80.1605431207748,7.34171121201776,139.058763525863));
#129085=CARTESIAN_POINT('Ctrl Pts',(80.1723081792958,7.34289236880078,139.059542334698));
#129086=CARTESIAN_POINT('Ctrl Pts',(80.2067588999614,7.34672193281049,139.061814275838));
#129087=CARTESIAN_POINT('Ctrl Pts',(80.2294044232828,7.34971175169727,139.063296717616));
#129088=CARTESIAN_POINT('Ctrl Pts',(80.3337770024127,7.36568181396698,139.070089013551));
#129089=CARTESIAN_POINT('Ctrl Pts',(80.4145305097773,7.38427422003881,139.075222228073));
#129090=CARTESIAN_POINT('Ctrl Pts',(80.5482693859694,7.42575862916321,139.083806765298));
#129091=CARTESIAN_POINT('Ctrl Pts',(80.6020514041023,7.44553248866636,139.08728534675));
#129092=CARTESIAN_POINT('Ctrl Pts',(80.7254998019522,7.49829003881839,139.095524342095));
#129093=CARTESIAN_POINT('Ctrl Pts',(80.7941004190273,7.53341070020239,139.100302985286));
#129094=CARTESIAN_POINT('Ctrl Pts',(80.8699589936861,7.57913333599058,139.106096369263));
#129095=CARTESIAN_POINT('Ctrl Pts',(80.8798368561949,7.58522870556923,139.106861271032));
#129096=CARTESIAN_POINT('Ctrl Pts',(80.8950892173173,7.59486204170529,139.108060126745));
#129097=CARTESIAN_POINT('Ctrl Pts',(80.9005084941648,7.59832891259672,139.108489625891));
#129098=CARTESIAN_POINT('Ctrl Pts',(80.9105067571738,7.60480701003788,139.109288869155));
#129099=CARTESIAN_POINT('Ctrl Pts',(80.9150911278067,7.60780954652006,139.109658049459));
#129100=CARTESIAN_POINT('Ctrl Pts',(80.9256711350002,7.61481376335306,139.110516319469));
#129101=CARTESIAN_POINT('Ctrl Pts',(80.9316556693983,7.61883177374747,139.111006466169));
#129102=CARTESIAN_POINT('Ctrl Pts',(80.9507727503427,7.63184774057316,139.112586764383));
#129103=CARTESIAN_POINT('Ctrl Pts',(80.9638020164294,7.64099482908725,139.113686056936));
#129104=CARTESIAN_POINT('Ctrl Pts',(81.0357393633405,7.69305264070969,139.119871973738));
#129105=CARTESIAN_POINT('Ctrl Pts',(81.0919083323157,7.73960262617889,139.125140816355));
#129106=CARTESIAN_POINT('Ctrl Pts',(81.2435074045345,7.88299978946355,139.140315999192));
#129107=CARTESIAN_POINT('Ctrl Pts',(81.330409862682,7.98805958431232,139.150195079913));
#129108=CARTESIAN_POINT('Ctrl Pts',(81.4163593328022,8.12247881739747,139.161179912788));
#129109=CARTESIAN_POINT('Ctrl Pts',(81.4286942594245,8.14270775185891,139.162795588655));
#129110=CARTESIAN_POINT('Ctrl Pts',(81.4466923350692,8.17369213335468,139.165215588268));
#129111=CARTESIAN_POINT('Ctrl Pts',(81.4526757449046,8.1842570278951,139.166031378889));
#129112=CARTESIAN_POINT('Ctrl Pts',(81.4632388376915,8.20339312542098,139.167492574988));
#129113=CARTESIAN_POINT('Ctrl Pts',(81.4678599824138,8.2119406826567,139.168139439171));
#129114=CARTESIAN_POINT('Ctrl Pts',(81.4775943503616,8.23032870636824,139.169518874926));
#129115=CARTESIAN_POINT('Ctrl Pts',(81.4826846575776,8.24018082371478,139.170250613835));
#129116=CARTESIAN_POINT('Ctrl Pts',(81.496366277121,8.2673222644671,139.172246988692));
#129117=CARTESIAN_POINT('Ctrl Pts',(81.504756206573,8.28471159065525,139.173504602973));
#129118=CARTESIAN_POINT('Ctrl Pts',(81.560933364796,8.40651220572631,139.182174775952));
#129119=CARTESIAN_POINT('Ctrl Pts',(81.5981184416421,8.51547690452788,139.189202974856));
#129120=CARTESIAN_POINT('Ctrl Pts',(81.6467966474662,8.72762500633572,139.202493444823));
#129121=CARTESIAN_POINT('Ctrl Pts',(81.6604614833694,8.82973781925677,139.208740482576));
#129122=CARTESIAN_POINT('Ctrl Pts',(81.6651844740251,8.94611256066371,139.216305709975));
#129123=CARTESIAN_POINT('Ctrl Pts',(81.6655708385299,8.95978878752331,139.217201853024));
#129124=CARTESIAN_POINT('Ctrl Pts',(81.6658983279396,8.98034968508746,139.218561852008));
#129125=CARTESIAN_POINT('Ctrl Pts',(81.6659652912678,8.98723214651758,139.219019235916));
#129126=CARTESIAN_POINT('Ctrl Pts',(81.6660092905257,8.99968724595585,139.219851157759));
#129127=CARTESIAN_POINT('Ctrl Pts',(81.6660010165673,9.00525981466055,139.220224893772));
#129128=CARTESIAN_POINT('Ctrl Pts',(81.6659260856385,9.01678399480822,139.221001118786));
#129129=CARTESIAN_POINT('Ctrl Pts',(81.6658554929286,9.02273541648955,139.221403804207));
#129130=CARTESIAN_POINT('Ctrl Pts',(81.6655858267819,9.03839440896083,139.222467890329));
#129131=CARTESIAN_POINT('Ctrl Pts',(81.6653337777657,9.04810066860475,139.223132085162));
#129132=CARTESIAN_POINT('Ctrl Pts',(81.6637555761683,9.09355957250443,139.226262758297));
#129133=CARTESIAN_POINT('Ctrl Pts',(81.6613628834445,9.12926309794042,139.228779261488));
#129134=CARTESIAN_POINT('Ctrl Pts',(81.6503915938091,9.23959063454353,139.236681672161));
#129135=CARTESIAN_POINT('Ctrl Pts',(81.6379157083485,9.31373126292154,139.242168142917));
#129136=CARTESIAN_POINT('Ctrl Pts',(81.5953222533608,9.49218671842658,139.255513048377));
#129137=CARTESIAN_POINT('Ctrl Pts',(81.5599330956303,9.5949092957262,139.263299512595));
#129138=CARTESIAN_POINT('Ctrl Pts',(81.5050176944035,9.71486425501044,139.272380687931));
#129139=CARTESIAN_POINT('Ctrl Pts',(81.4947754805915,9.73604043644773,139.2739845395));
#129140=CARTESIAN_POINT('Ctrl Pts',(81.4785835593894,9.76778473759124,139.276391065084));
#129141=CARTESIAN_POINT('Ctrl Pts',(81.4729616380445,9.77851574914366,139.277204991305));
#129142=CARTESIAN_POINT('Ctrl Pts',(81.4626167011207,9.79774867279879,139.278664839818));
#129143=CARTESIAN_POINT('Ctrl Pts',(81.4579353892392,9.80627226606789,139.27931219662));
#129144=CARTESIAN_POINT('Ctrl Pts',(81.4477364844404,9.82446282526617,139.280694826209));
#129145=CARTESIAN_POINT('Ctrl Pts',(81.4421960800286,9.83411651193372,139.281429245587));
#129146=CARTESIAN_POINT('Ctrl Pts',(81.4267025032489,9.86049682182268,139.283438563704));
#129147=CARTESIAN_POINT('Ctrl Pts',(81.4165521173167,9.87710601612858,139.284706303334));
#129148=CARTESIAN_POINT('Ctrl Pts',(81.3469557760927,9.98662650915673,139.293092718759));
#129149=CARTESIAN_POINT('Ctrl Pts',(81.2786983865789,10.0736183654656,139.299861126766));
#129150=CARTESIAN_POINT('Ctrl Pts',(81.1279686121786,10.2307657788421,139.313161309424));
#129151=CARTESIAN_POINT('Ctrl Pts',(81.0462876306508,10.3009124991158,139.319671439941));
#129152=CARTESIAN_POINT('Ctrl Pts',(80.9474605814812,10.3704213160674,139.327523795779));
#129153=CARTESIAN_POINT('Ctrl Pts',(80.9363900032069,10.3780093873317,139.32840326883));
#129154=CARTESIAN_POINT('Ctrl Pts',(80.919554744259,10.3892521854819,139.329742461064));
#129155=CARTESIAN_POINT('Ctrl Pts',(80.9138569989904,10.3930067996752,139.330195998075));
#129156=CARTESIAN_POINT('Ctrl Pts',(80.9034714638576,10.3997593636885,139.331023534536));
#129157=CARTESIAN_POINT('Ctrl Pts',(80.8987913456885,10.4027690751538,139.331396768845));
#129158=CARTESIAN_POINT('Ctrl Pts',(80.8890336025733,10.4089752489483,139.332175763998));
#129159=CARTESIAN_POINT('Ctrl Pts',(80.8839536958779,10.4121677872447,139.332581750743));
#129160=CARTESIAN_POINT('Ctrl Pts',(80.8704576236274,10.4205482294225,139.333661289074));
#129161=CARTESIAN_POINT('Ctrl Pts',(80.862012483487,10.4256886802755,139.334337758768));
#129162=CARTESIAN_POINT('Ctrl Pts',(80.8211143979894,10.4500866147024,139.337616475561));
#129163=CARTESIAN_POINT('Ctrl Pts',(80.7880616347628,10.4683114143862,139.340274218421));
#129164=CARTESIAN_POINT('Ctrl Pts',(80.6803365676113,10.5230241602307,139.348897684124));
#129165=CARTESIAN_POINT('Ctrl Pts',(80.6035426474527,10.5550549722217,139.354981446099));
#129166=CARTESIAN_POINT('Ctrl Pts',(80.4244444872526,10.6144834426629,139.368676281499));
#129167=CARTESIAN_POINT('Ctrl Pts',(80.3212556839463,10.6381428675606,139.376213547164));
#129168=CARTESIAN_POINT('Ctrl Pts',(80.1976987827919,10.6543370055795,139.384734680179));
#129169=CARTESIAN_POINT('Ctrl Pts',(80.1788515345371,10.6564805814864,139.3860216645));
#129170=CARTESIAN_POINT('Ctrl Pts',(80.1489907367143,10.6593611573852,139.388041254577));
#129171=CARTESIAN_POINT('Ctrl Pts',(80.1379999067815,10.6603113340909,139.388780455287));
#129172=CARTESIAN_POINT('Ctrl Pts',(80.1182528024387,10.6618210611349,139.390101387859));
#129173=CARTESIAN_POINT('Ctrl Pts',(80.1095001019975,10.6624207341126,139.390684350556));
#129174=CARTESIAN_POINT('Ctrl Pts',(80.0889468035803,10.6636658695073,139.39204755524));
#129175=CARTESIAN_POINT('Ctrl Pts',(80.077143163462,10.664254969525,139.392826012649));
#129176=CARTESIAN_POINT('Ctrl Pts',(80.042587680798,10.6656111434507,139.39509277293));
#129177=CARTESIAN_POINT('Ctrl Pts',(80.0198246263635,10.6660375916688,139.396570485389));
#129178=CARTESIAN_POINT('Ctrl Pts',(79.9150083711597,10.6658525623273,139.403314013684));
#129179=CARTESIAN_POINT('Ctrl Pts',(79.8330756485913,10.6596466130065,139.408406458951));
#129180=CARTESIAN_POINT('Ctrl Pts',(79.623794575424,10.6281324774774,139.421384618289));
#129181=CARTESIAN_POINT('Ctrl Pts',(79.4983715315212,10.5939588600333,139.429121433734));
#129182=CARTESIAN_POINT('Ctrl Pts',(79.3639637242141,10.5398860845557,139.438528689698));
#129183=CARTESIAN_POINT('Ctrl Pts',(79.3498131381566,10.5339648957099,139.439534061743));
#129184=CARTESIAN_POINT('Ctrl Pts',(79.3292996749242,10.5250463921841,139.441016304928));
#129185=CARTESIAN_POINT('Ctrl Pts',(79.3228703531876,10.5222026347784,139.441484463366));
#129186=CARTESIAN_POINT('Ctrl Pts',(79.3114761846957,10.5170764035241,139.442320883757));
#129187=CARTESIAN_POINT('Ctrl Pts',(79.3065042822255,10.514810069531,139.442688168378));
#129188=CARTESIAN_POINT('Ctrl Pts',(79.2957037759191,10.5098225733702,139.443491175486));
#129189=CARTESIAN_POINT('Ctrl Pts',(79.289879855386,10.5070921508022,139.443927432893));
#129190=CARTESIAN_POINT('Ctrl Pts',(79.2731889810486,10.4991487614854,139.445186779839));
#129191=CARTESIAN_POINT('Ctrl Pts',(79.2623628622817,10.4938516319351,139.446014734336));
#129192=CARTESIAN_POINT('Ctrl Pts',(79.2377359605263,10.4814689287182,139.447922095803));
#129193=CARTESIAN_POINT('Ctrl Pts',(79.2239749092783,10.4743071839206,139.44900534099));
#129194=CARTESIAN_POINT('Ctrl Pts',(79.1781252738224,10.4496256410324,139.452668738487));
#129195=CARTESIAN_POINT('Ctrl Pts',(79.1465151992474,10.4312427889872,139.45528456391));
#129196=CARTESIAN_POINT('Ctrl Pts',(79.0542519521836,10.3734433281636,139.463142569012));
#129197=CARTESIAN_POINT('Ctrl Pts',(78.9955318730438,10.3311009278282,139.4684391669));
#129198=CARTESIAN_POINT('Ctrl Pts',(78.8627301698412,10.2215330967392,139.480926723629));
#129199=CARTESIAN_POINT('Ctrl Pts',(78.7915685120538,10.1511843896484,139.488036808255));
#129200=CARTESIAN_POINT('Ctrl Pts',(78.7151245231262,10.0606588081365,139.49613812222));
#129201=CARTESIAN_POINT('Ctrl Pts',(78.7033602644596,10.0462444951057,139.49740047211));
#129202=CARTESIAN_POINT('Ctrl Pts',(78.685021072553,10.0229895724865,139.499394449581));
#129203=CARTESIAN_POINT('Ctrl Pts',(78.6782884051204,10.0142759561069,139.500132349261));
#129204=CARTESIAN_POINT('Ctrl Pts',(78.6658601359839,9.99785701058727,139.501505879796));
#129205=CARTESIAN_POINT('Ctrl Pts',(78.6601436945794,9.9901681058014,139.502142314505));
#129206=CARTESIAN_POINT('Ctrl Pts',(78.6473754008669,9.9726810427655,139.503574805987));
#129207=CARTESIAN_POINT('Ctrl Pts',(78.6403630241468,9.96285462240757,139.504369310828));
#129208=CARTESIAN_POINT('Ctrl Pts',(78.6195548004498,9.93301545462512,139.506751514334));
#129209=CARTESIAN_POINT('Ctrl Pts',(78.606089124474,9.91277563334462,139.508326707875));
#129210=CARTESIAN_POINT('Ctrl Pts',(78.5759582657796,9.86526416330425,139.511938231557));
#129211=CARTESIAN_POINT('Ctrl Pts',(78.5596250305868,9.8377929747174,139.513962951576));
#129212=CARTESIAN_POINT('Ctrl Pts',(78.5023852446224,9.73489233014485,139.521348469257));
#129213=CARTESIAN_POINT('Ctrl Pts',(78.4665321901734,9.65680612437858,139.526563553791));
#129214=CARTESIAN_POINT('Ctrl Pts',(78.4367543527153,9.57603743440659,139.531820828887));
#129215=CARTESIAN_POINT('Ctrl Pts',(78.4366568293464,9.57577270720414,139.531838058773));
#129216=CARTESIAN_POINT('Ctrl Pts',(78.4365593737676,9.57550795671827,139.531855288841));
#129217=CARTESIAN_POINT('Origin',(80.,9.,141.545925280538));
#129218=CARTESIAN_POINT('',(77.9452506264307,8.99839553228233,139.095925280496));
#129219=CARTESIAN_POINT('Ctrl Pts',(81.252039109102,10.6292316077768,139.54788294617));
#129220=CARTESIAN_POINT('Ctrl Pts',(81.308376489574,10.585937208553,139.54401817761));
#129221=CARTESIAN_POINT('Ctrl Pts',(81.3625557906715,10.539647933612,139.54015340905));
#129222=CARTESIAN_POINT('Ctrl Pts',(81.4142433345909,10.4906083835351,139.53628864049));
#129223=CARTESIAN_POINT('Ctrl Pts',(81.4658662895611,10.4416301134644,139.532428701359));
#129224=CARTESIAN_POINT('Ctrl Pts',(81.5150033221473,10.3899087276083,139.528568762228));
#129225=CARTESIAN_POINT('Ctrl Pts',(81.5613536243118,10.3357291725303,139.524708823097));
#129226=CARTESIAN_POINT('Ctrl Pts',(81.6076723890728,10.2815864819905,139.520851510324));
#129227=CARTESIAN_POINT('Ctrl Pts',(81.6512078703199,10.2249893084108,139.51699419755));
#129228=CARTESIAN_POINT('Ctrl Pts',(81.6916969738153,10.1662585096298,139.513136884777));
#129229=CARTESIAN_POINT('Ctrl Pts',(81.7321720598409,10.1075480436577,139.509280907419));
#129230=CARTESIAN_POINT('Ctrl Pts',(81.7696025861863,10.0467058182288,139.505424930061));
#129231=CARTESIAN_POINT('Ctrl Pts',(81.803767588974,9.98408335392235,139.501568952702));
#129232=CARTESIAN_POINT('Ctrl Pts',(81.8379321816834,9.92146164126539,139.497713021627));
#129233=CARTESIAN_POINT('Ctrl Pts',(81.8688310977455,9.85706015934763,139.493857090552));
#129234=CARTESIAN_POINT('Ctrl Pts',(81.8962891716252,9.79125529386987,139.490001159476));
#129235=CARTESIAN_POINT('Ctrl Pts',(81.9237751105049,9.72538364830441,139.486141315325));
#129236=CARTESIAN_POINT('Ctrl Pts',(81.9478130468575,9.65810622436826,139.482281471174));
#129237=CARTESIAN_POINT('Ctrl Pts',(81.96827621917,9.58981885994765,139.478421627023));
#129238=CARTESIAN_POINT('Ctrl Pts',(81.9887500283614,9.52149599934791,139.474559776502));
#129239=CARTESIAN_POINT('Ctrl Pts',(82.0056452579464,9.45216262510631,139.470697925981));
#129240=CARTESIAN_POINT('Ctrl Pts',(82.0188859469942,9.38222649768085,139.46683607546));
#129241=CARTESIAN_POINT('Ctrl Pts',(82.0321504630082,9.31216451836531,139.462967275438));
#129242=CARTESIAN_POINT('Ctrl Pts',(82.0417472376092,9.2414981013445,139.459098475416));
#129243=CARTESIAN_POINT('Ctrl Pts',(82.0476520961904,9.17064130644974,139.455229675394));
#129244=CARTESIAN_POINT('Ctrl Pts',(82.0520867354107,9.11742676839861,139.452324147332));
#129245=CARTESIAN_POINT('Ctrl Pts',(82.0544401302839,9.06410498148714,139.449418619269));
#129246=CARTESIAN_POINT('Ctrl Pts',(82.0547213515336,9.0108503480071,139.446513091207));
#129247=CARTESIAN_POINT('Ctrl Pts',(82.055095792145,8.93994284176746,139.442644437237));
#129248=CARTESIAN_POINT('Ctrl Pts',(82.0517961788713,8.86887674551251,139.438775783267));
#129249=CARTESIAN_POINT('Ctrl Pts',(82.0448030562872,8.7980643085072,139.434907129298));
#129250=CARTESIAN_POINT('Ctrl Pts',(82.0378203661409,8.72735751048363,139.43104424664));
#129251=CARTESIAN_POINT('Ctrl Pts',(82.0271551512116,8.65690410018162,139.427181363982));
#129252=CARTESIAN_POINT('Ctrl Pts',(82.0128399673072,8.58711644679066,139.423318481324));
#129253=CARTESIAN_POINT('Ctrl Pts',(81.9985416053222,8.517410801587,139.41946013798));
#129254=CARTESIAN_POINT('Ctrl Pts',(81.9806018911152,8.44836983299485,139.415601794635));
#129255=CARTESIAN_POINT('Ctrl Pts',(81.9591049886799,8.3803991560452,139.41174345129));
#129256=CARTESIAN_POINT('Ctrl Pts',(81.9376216542149,8.31247137942159,139.407887543175));
#129257=CARTESIAN_POINT('Ctrl Pts',(81.9125857320053,8.24561301641311,139.404031635059));
#129258=CARTESIAN_POINT('Ctrl Pts',(81.8841317572407,8.18021644084738,139.400175726944));
#129259=CARTESIAN_POINT('Ctrl Pts',(81.8556862171433,8.11483925091596,139.396320961843));
#129260=CARTESIAN_POINT('Ctrl Pts',(81.8238248297509,8.05092343349106,139.392466196742));
#129261=CARTESIAN_POINT('Ctrl Pts',(81.7887303485671,7.98884160359757,139.388611431641));
#129262=CARTESIAN_POINT('Ctrl Pts',(81.7536345237565,7.9267573968403,139.384756518956));
#129263=CARTESIAN_POINT('Ctrl Pts',(81.7153056004407,7.86650773893452,139.380901606272));
#129264=CARTESIAN_POINT('Ctrl Pts',(81.6739715364385,7.80843931850121,139.377046693587));
#129265=CARTESIAN_POINT('Ctrl Pts',(81.6325942197785,7.750310134299,139.373187747058));
#129266=CARTESIAN_POINT('Ctrl Pts',(81.588205767402,7.69436714059467,139.369328800528));
#129267=CARTESIAN_POINT('Ctrl Pts',(81.5410760797314,7.64092602152064,139.365469853998));
#129268=CARTESIAN_POINT('Ctrl Pts',(81.4939197236542,7.58745466270674,139.361608723878));
#129269=CARTESIAN_POINT('Ctrl Pts',(81.4440193845799,7.53648834406992,139.357747593757));
#129270=CARTESIAN_POINT('Ctrl Pts',(81.3916817583935,7.48830576972232,139.353886463636));
#129271=CARTESIAN_POINT('Ctrl Pts',(81.3392525224691,7.44003885847724,139.350018575144));
#129272=CARTESIAN_POINT('Ctrl Pts',(81.2843778562518,7.39456572984455,139.346150686652));
#129273=CARTESIAN_POINT('Ctrl Pts',(81.2273968759229,7.35212425484364,139.34228279816));
#129274=CARTESIAN_POINT('Ctrl Pts',(81.1934998514691,7.32687653696197,139.339981856512));
#129275=CARTESIAN_POINT('Ctrl Pts',(81.1588579921675,7.3027008490532,139.337680914863));
#129276=CARTESIAN_POINT('Ctrl Pts',(81.1235469336721,7.27963961614549,139.335379973215));
#129277=CARTESIAN_POINT('Ctrl Pts',(81.0641694052924,7.24086085759806,139.331510810583));
#129278=CARTESIAN_POINT('Ctrl Pts',(81.0026656047539,7.20508386198724,139.327641647951));
#129279=CARTESIAN_POINT('Ctrl Pts',(80.9393714643523,7.17254854662003,139.323772485319));
#129280=CARTESIAN_POINT('Ctrl Pts',(80.8761716220403,7.14006170364008,139.319909087117));
#129281=CARTESIAN_POINT('Ctrl Pts',(80.8111871629325,7.11080717457016,139.316045688916));
#129282=CARTESIAN_POINT('Ctrl Pts',(80.7447823180106,7.08498123735595,139.312182290714));
#129283=CARTESIAN_POINT('Ctrl Pts',(80.6784553632913,7.05918559292363,139.308323424122));
#129284=CARTESIAN_POINT('Ctrl Pts',(80.6107117826425,7.03681072729491,139.30446455753));
#129285=CARTESIAN_POINT('Ctrl Pts',(80.5419381132986,7.01800589207375,139.300605690939));
#129286=CARTESIAN_POINT('Ctrl Pts',(80.4732077655688,6.99921290231356,139.296749255107));
#129287=CARTESIAN_POINT('Ctrl Pts',(80.4034490839446,6.98398560914946,139.292892819276));
#129288=CARTESIAN_POINT('Ctrl Pts',(80.3330647916101,6.97242376047416,139.289036383445));
#129289=CARTESIAN_POINT('Ctrl Pts',(80.2627012934443,6.96086532760408,139.285181086951));
#129290=CARTESIAN_POINT('Ctrl Pts',(80.1917130305803,6.95297026803838,139.281325790456));
#129291=CARTESIAN_POINT('Ctrl Pts',(80.1205122704267,6.94878710145032,139.277470493961));
#129292=CARTESIAN_POINT('Ctrl Pts',(80.0493087312538,6.94460377159011,139.273615046991));
#129293=CARTESIAN_POINT('Ctrl Pts',(79.9778931633775,6.94413264863522,139.269759600021));
#129294=CARTESIAN_POINT('Ctrl Pts',(79.9066805639685,6.94737021229868,139.265904153051));
#129295=CARTESIAN_POINT('Ctrl Pts',(79.8353934433826,6.95061116394483,139.262044671508));
#129296=CARTESIAN_POINT('Ctrl Pts',(79.7643102015117,6.95756852743989,139.258185189965));
#129297=CARTESIAN_POINT('Ctrl Pts',(79.6938425315846,6.96818672928996,139.254325708422));
#129298=CARTESIAN_POINT('Ctrl Pts',(79.6233349706938,6.9788109419859,139.250464042069));
#129299=CARTESIAN_POINT('Ctrl Pts',(79.5534441515828,6.99310002113018,139.246602375717));
#129300=CARTESIAN_POINT('Ctrl Pts',(79.4845706540003,7.01094742357516,139.242740709364));
#129301=CARTESIAN_POINT('Ctrl Pts',(79.415576689252,7.02882604304938,139.238872288541));
#129302=CARTESIAN_POINT('Ctrl Pts',(79.347604062057,7.05027526577957,139.235003867718));
#129303=CARTESIAN_POINT('Ctrl Pts',(79.2810366293864,7.07513916497426,139.231135446895));
#129304=CARTESIAN_POINT('Ctrl Pts',(79.2415238770009,7.08989774965758,139.228839249671));
#129305=CARTESIAN_POINT('Ctrl Pts',(79.2025058255676,7.105858512454,139.226543052447));
#129306=CARTESIAN_POINT('Ctrl Pts',(79.1640586578012,7.1229811841905,139.224246855223));
#129307=CARTESIAN_POINT('Ctrl Pts',(79.099274330323,7.15183326452633,139.220377712148));
#129308=CARTESIAN_POINT('Ctrl Pts',(79.035858638409,7.18409976696277,139.216508569073));
#129309=CARTESIAN_POINT('Ctrl Pts',(78.9741953434853,7.21962858673456,139.212639425999));
#129310=CARTESIAN_POINT('Ctrl Pts',(78.9126238999133,7.25510448409725,139.208776046255));
#129311=CARTESIAN_POINT('Ctrl Pts',(78.8528000894136,7.29383281241874,139.204912666512));
#129312=CARTESIAN_POINT('Ctrl Pts',(78.7950863585028,7.33561402342066,139.201049286769));
#129313=CARTESIAN_POINT('Ctrl Pts',(78.7374402978417,7.37734624530099,139.197190436899));
#129314=CARTESIAN_POINT('Ctrl Pts',(78.6818997939348,7.42212395618128,139.193331587029));
#129315=CARTESIAN_POINT('Ctrl Pts',(78.6287998828478,7.46970336169033,139.189472737159));
#129316=CARTESIAN_POINT('Ctrl Pts',(78.5757334054558,7.51725280942168,139.185616316965));
#129317=CARTESIAN_POINT('Ctrl Pts',(78.5251048330378,7.56760012852479,139.181759896771));
#129318=CARTESIAN_POINT('Ctrl Pts',(78.4772163901747,7.62046107697261,139.177903476578));
#129319=CARTESIAN_POINT('Ctrl Pts',(78.4293420816255,7.67330642346745,139.17404819461));
#129320=CARTESIAN_POINT('Ctrl Pts',(78.3842066229932,7.72866356662089,139.170192912642));
#129321=CARTESIAN_POINT('Ctrl Pts',(78.342074376256,7.78621246149379,139.166337630674));
#129322=CARTESIAN_POINT('Ctrl Pts',(78.2999404726191,7.84376361954402,139.162482197093));
#129323=CARTESIAN_POINT('Ctrl Pts',(78.2608103005342,7.90350630718624,139.158626763511));
#129324=CARTESIAN_POINT('Ctrl Pts',(78.2249059814435,7.96508996150155,139.15477132993));
#129325=CARTESIAN_POINT('Ctrl Pts',(78.1889640725758,8.02673809039502,139.150911859929));
#129326=CARTESIAN_POINT('Ctrl Pts',(78.1562550036814,8.0902306129459,139.147052389928));
#129327=CARTESIAN_POINT('Ctrl Pts',(78.1269553721447,8.15519151012636,139.143192919928));
#129328=CARTESIAN_POINT('Ctrl Pts',(78.0976391465839,8.22018919830535,139.139331264092));
#129329=CARTESIAN_POINT('Ctrl Pts',(78.0717363787881,8.28665646379498,139.135469608257));
#129330=CARTESIAN_POINT('Ctrl Pts',(78.0493748166742,8.35419898058668,139.131607952422));
#129331=CARTESIAN_POINT('Ctrl Pts',(78.0269741315431,8.42185966743443,139.127739540368));
#129332=CARTESIAN_POINT('Ctrl Pts',(78.0081271502149,8.49059889287508,139.123871128313));
#129333=CARTESIAN_POINT('Ctrl Pts',(77.9929110614074,8.56000959660532,139.120002716258));
#129334=CARTESIAN_POINT('Ctrl Pts',(77.9838786457656,8.60121245326676,139.117706389916));
#129335=CARTESIAN_POINT('Ctrl Pts',(77.9761246713115,8.64265175206147,139.115410063574));
#129336=CARTESIAN_POINT('Ctrl Pts',(77.969656625911,8.68424163385155,139.113113737232));
#129337=CARTESIAN_POINT('Ctrl Pts',(77.9535184263551,8.78801112993064,139.107384251667));
#129338=CARTESIAN_POINT('Ctrl Pts',(77.945332887455,8.89304862793086,139.101654766102));
#129339=CARTESIAN_POINT('Ctrl Pts',(77.9452506264313,8.99839553151457,139.095925280538));
#129340=CARTESIAN_POINT('Ctrl Pts',(77.9452506264307,8.99839553228234,139.095925280496));
#129341=CARTESIAN_POINT('Ctrl Pts',(77.9451944260658,9.07036810192396,139.092010919611));
#129342=CARTESIAN_POINT('Ctrl Pts',(77.9489244685222,9.14248040213294,139.088096558725));
#129343=CARTESIAN_POINT('Ctrl Pts',(77.9564551529768,9.21429423861822,139.084182197839));
#129344=CARTESIAN_POINT('Ctrl Pts',(77.9637702775113,9.28405246051092,139.080379882456));
#129345=CARTESIAN_POINT('Ctrl Pts',(77.9746713409255,9.35352853614584,139.076577567072));
#129346=CARTESIAN_POINT('Ctrl Pts',(77.9891188245793,9.42232032965372,139.072775251688));
#129347=CARTESIAN_POINT('Ctrl Pts',(78.0035569315878,9.49106747619983,139.068975404067));
#129348=CARTESIAN_POINT('Ctrl Pts',(78.0215367938635,9.55913073138864,139.065175556447));
#129349=CARTESIAN_POINT('Ctrl Pts',(78.0429674069959,9.62611579793157,139.061375708826));
#129350=CARTESIAN_POINT('Ctrl Pts',(78.0643917765798,9.69308134919031,139.057576968244));
#129351=CARTESIAN_POINT('Ctrl Pts',(78.0892647496713,9.7589688576028,139.053778227663));
#129352=CARTESIAN_POINT('Ctrl Pts',(78.1174453497669,9.82339878029161,139.049979487081));
#129353=CARTESIAN_POINT('Ctrl Pts',(78.1456278187924,9.88783297595597,139.046180494568));
#129354=CARTESIAN_POINT('Ctrl Pts',(78.1771181457956,9.95080893608708,139.042381502055));
#129355=CARTESIAN_POINT('Ctrl Pts',(78.2117278458989,10.0119685100668,139.038582509542));
#129356=CARTESIAN_POINT('Ctrl Pts',(78.2463733803406,10.0731914077059,139.034779583612));
#129357=CARTESIAN_POINT('Ctrl Pts',(78.2841444807975,10.1325937320322,139.030976657682));
#129358=CARTESIAN_POINT('Ctrl Pts',(78.3248080790415,10.1898443555589,139.027173731752));
#129359=CARTESIAN_POINT('Ctrl Pts',(78.3654974050552,10.2471312014299,139.023368399719));
#129360=CARTESIAN_POINT('Ctrl Pts',(78.4090825547568,10.3022632485942,139.019563067687));
#129361=CARTESIAN_POINT('Ctrl Pts',(78.4552905435339,10.3549428982818,139.015757735654));
#129362=CARTESIAN_POINT('Ctrl Pts',(78.5015729540876,10.4077073928896,139.01194627482));
#129363=CARTESIAN_POINT('Ctrl Pts',(78.5504862746083,10.4580112600147,139.008134813986));
#129364=CARTESIAN_POINT('Ctrl Pts',(78.6017220180081,10.5055949812539,139.004323353152));
#129365=CARTESIAN_POINT('Ctrl Pts',(78.6122194553207,10.5153441738616,139.003542441848));
#129366=CARTESIAN_POINT('Ctrl Pts',(78.6228142801158,10.5249793218239,139.002761530544));
#129367=CARTESIAN_POINT('Ctrl Pts',(78.6335036861555,10.5344984153623,139.001980619241));
#129368=CARTESIAN_POINT('Ctrl Pts',(78.6864653127342,10.5816616230727,138.998111523736));
#129369=CARTESIAN_POINT('Ctrl Pts',(78.7419752160566,10.6261721083391,138.994242428231));
#129370=CARTESIAN_POINT('Ctrl Pts',(78.7997368188016,10.6677427434588,138.990373332726));
#129371=CARTESIAN_POINT('Ctrl Pts',(78.8574123613961,10.7092514416698,138.986510001863));
#129372=CARTESIAN_POINT('Ctrl Pts',(78.9173325530523,10.7478287027422,138.982646671));
#129373=CARTESIAN_POINT('Ctrl Pts',(78.9791663518893,10.7832263528181,138.978783340137));
#129374=CARTESIAN_POINT('Ctrl Pts',(79.0409276212815,10.8185824823672,138.974924540861));
#129375=CARTESIAN_POINT('Ctrl Pts',(79.1045976197542,10.8507661690005,138.971065741585));
#129376=CARTESIAN_POINT('Ctrl Pts',(79.1698162641529,10.8795724320267,138.967206942309));
#129377=CARTESIAN_POINT('Ctrl Pts',(79.2349938264751,10.9083605496114,138.963350573741));
#129378=CARTESIAN_POINT('Ctrl Pts',(79.3017176560076,10.9337752686773,138.959494205173));
#129379=CARTESIAN_POINT('Ctrl Pts',(79.3696043132128,10.9556581604616,138.955637836605));
#129380=CARTESIAN_POINT('Ctrl Pts',(79.4374709165253,10.9775345879836,138.951782607218));
#129381=CARTESIAN_POINT('Ctrl Pts',(79.5064992034623,10.9958811105306,138.947927377831));
#129382=CARTESIAN_POINT('Ctrl Pts',(79.5762886904272,11.0105885428501,138.944072148445));
#129383=CARTESIAN_POINT('Ctrl Pts',(79.6460809060418,11.0252965502051,138.940216768325));
#129384=CARTESIAN_POINT('Ctrl Pts',(79.7166339049791,11.0363650868325,138.936361388205));
#129385=CARTESIAN_POINT('Ctrl Pts',(79.7875367782694,11.0437360254964,138.932506008086));
#129386=CARTESIAN_POINT('Ctrl Pts',(79.8585138657824,11.0511146793411,138.92864659253));
#129387=CARTESIAN_POINT('Ctrl Pts',(79.9298410745291,11.054787958932,138.924787176974));
#129388=CARTESIAN_POINT('Ctrl Pts',(80.0011030351522,11.0547497039332,138.920927761417));
#129389=CARTESIAN_POINT('Ctrl Pts',(80.0724053442286,11.0547114272744,138.917066160664));
#129390=CARTESIAN_POINT('Ctrl Pts',(80.1436418463023,11.050957458227,138.91320455991));
#129391=CARTESIAN_POINT('Ctrl Pts',(80.2144005959293,11.0435336911745,138.909342959157));
#129392=CARTESIAN_POINT('Ctrl Pts',(80.2852831367737,11.036096936369,138.905474602599));
#129393=CARTESIAN_POINT('Ctrl Pts',(80.35568577645,11.0249776411575,138.901606246042));
#129394=CARTESIAN_POINT('Ctrl Pts',(80.4252057760271,11.010273018904,138.897737889484));
#129395=CARTESIAN_POINT('Ctrl Pts',(80.4664825456352,11.0015423038777,138.895441093406));
#129396=CARTESIAN_POINT('Ctrl Pts',(80.5074484132099,10.9915486326406,138.893144297327));
#129397=CARTESIAN_POINT('Ctrl Pts',(80.5480219975128,10.9803205429278,138.890847501249));
#129398=CARTESIAN_POINT('Ctrl Pts',(80.6163512059331,10.9614115287177,138.886979510273));
#129399=CARTESIAN_POINT('Ctrl Pts',(80.683834395631,10.9389248833565,138.883111519298));
#129400=CARTESIAN_POINT('Ctrl Pts',(80.7500698252355,10.912953951294,138.879243528322));
#129401=CARTESIAN_POINT('Ctrl Pts',(80.8162190583714,10.8870168168929,138.875380571014));
#129402=CARTESIAN_POINT('Ctrl Pts',(80.8811233031021,10.8576045624471,138.871517613707));
#129403=CARTESIAN_POINT('Ctrl Pts',(80.9443946159635,10.8248606444984,138.867654656399));
#129404=CARTESIAN_POINT('Ctrl Pts',(81.0075967032803,10.792152551878,138.863795925577));
#129405=CARTESIAN_POINT('Ctrl Pts',(81.0691689765495,10.756120254855,138.859937194756));
#129406=CARTESIAN_POINT('Ctrl Pts',(81.1287439325178,10.7169550656043,138.856078463934));
#129407=CARTESIAN_POINT('Ctrl Pts',(81.1708819759179,10.6892530821518,138.853349139771));
#129408=CARTESIAN_POINT('Ctrl Pts',(81.2120211744178,10.6599847671502,138.850619815608));
#129409=CARTESIAN_POINT('Ctrl Pts',(81.252039109102,10.6292316077768,138.847890491445));
#129410=CARTESIAN_POINT('',(77.9452503313537,9.00116691815225,139.154074719413));
#129411=CARTESIAN_POINT('Ctrl Pts',(77.9452503313537,9.00116691815225,139.154074719413));
#129412=CARTESIAN_POINT('Ctrl Pts',(77.9452955388611,9.08076985405426,139.14977731915));
#129413=CARTESIAN_POINT('Ctrl Pts',(77.9499707053658,9.16020567409785,139.145479918886));
#129414=CARTESIAN_POINT('Ctrl Pts',(77.9591932169553,9.23896702027448,139.141182518622));
#129415=CARTESIAN_POINT('Ctrl Pts',(77.9684534953407,9.31805089938046,139.13686752022));
#129416=CARTESIAN_POINT('Ctrl Pts',(77.9822983014852,9.39645450913027,139.132552521817));
#129417=CARTESIAN_POINT('Ctrl Pts',(78.0005942531386,9.47368156172441,139.128237523415));
#129418=CARTESIAN_POINT('Ctrl Pts',(78.0189841187588,9.55130502435452,139.123900375926));
#129419=CARTESIAN_POINT('Ctrl Pts',(78.0418708061259,9.62773956819543,139.119563228437));
#129420=CARTESIAN_POINT('Ctrl Pts',(78.0690707642039,9.70250256145301,139.115226080948));
#129421=CARTESIAN_POINT('Ctrl Pts',(78.0780409992218,9.72715854137151,139.113795739321));
#129422=CARTESIAN_POINT('Ctrl Pts',(78.0874799697398,9.75163291047114,139.112365397694));
#129423=CARTESIAN_POINT('Ctrl Pts',(78.0973799933312,9.7759089332671,139.110935056068));
#129424=CARTESIAN_POINT('Ctrl Pts',(78.124160171027,9.84157708023847,139.107065893275));
#129425=CARTESIAN_POINT('Ctrl Pts',(78.1543965410821,9.90598572302029,139.103196730482));
#129426=CARTESIAN_POINT('Ctrl Pts',(78.1879492665976,9.96874645912945,139.099327567689));
#129427=CARTESIAN_POINT('Ctrl Pts',(78.2214520039649,10.0314136918665,139.095464169324));
#129428=CARTESIAN_POINT('Ctrl Pts',(78.2582610622044,10.0924374663779,139.09160077096));
#129429=CARTESIAN_POINT('Ctrl Pts',(78.2981885076497,10.151449176909,139.087737372595));
#129430=CARTESIAN_POINT('Ctrl Pts',(78.3380691198323,10.2103916691139,139.083878505839));
#129431=CARTESIAN_POINT('Ctrl Pts',(78.381060582807,10.2673263848709,139.080019639083));
#129432=CARTESIAN_POINT('Ctrl Pts',(78.4269298683473,10.3219107093152,139.076160772327));
#129433=CARTESIAN_POINT('Ctrl Pts',(78.4727702601167,10.3764606502512,139.072304336331));
#129434=CARTESIAN_POINT('Ctrl Pts',(78.5214845661371,10.428662766255,139.068447900334));
#129435=CARTESIAN_POINT('Ctrl Pts',(78.5727982883753,10.4782059521039,139.064591464338));
#129436=CARTESIAN_POINT('Ctrl Pts',(78.6240968506186,10.5277345010408,139.060736167677));
#129437=CARTESIAN_POINT('Ctrl Pts',(78.6779929551842,10.5746053421367,139.056880871016));
#129438=CARTESIAN_POINT('Ctrl Pts',(78.7341751160657,10.6185440759253,139.053025574356));
#129439=CARTESIAN_POINT('Ctrl Pts',(78.7903594697857,10.6624845246806,139.049170127219));
#129440=CARTESIAN_POINT('Ctrl Pts',(78.8488296729757,10.703492341401,139.045314680083));
#129441=CARTESIAN_POINT('Ctrl Pts',(78.9092423947348,10.7413343760048,139.041459232947));
#129442=CARTESIAN_POINT('Ctrl Pts',(78.9697183360146,10.7792160107991,139.037599751238));
#129443=CARTESIAN_POINT('Ctrl Pts',(79.0321404412179,10.8139249918597,139.033740269529));
#129444=CARTESIAN_POINT('Ctrl Pts',(79.0961384896395,10.8452728612833,139.029880787819));
#129445=CARTESIAN_POINT('Ctrl Pts',(79.1601727666421,10.876638476386,139.026019121301));
#129446=CARTESIAN_POINT('Ctrl Pts',(79.225784315823,10.90463900142,139.022157454782));
#129447=CARTESIAN_POINT('Ctrl Pts',(79.292583066205,10.9291342214268,139.018295788264));
#129448=CARTESIAN_POINT('Ctrl Pts',(79.3594986547597,10.9536722861984,139.014427367277));
#129449=CARTESIAN_POINT('Ctrl Pts',(79.4276051260904,10.9746926616106,139.010558946289));
#129450=CARTESIAN_POINT('Ctrl Pts',(79.4964980746094,10.9921052616837,139.006690525302));
#129451=CARTESIAN_POINT('Ctrl Pts',(79.537391166539,11.0024409356653,139.00439432956));
#129452=CARTESIAN_POINT('Ctrl Pts',(79.5785611590264,11.0115064588851,139.002098133818));
#129453=CARTESIAN_POINT('Ctrl Pts',(79.6199224885441,11.019291620293,138.999801938076));
#129454=CARTESIAN_POINT('Ctrl Pts',(79.6902200525406,11.0325232520775,138.995899332212));
#129455=CARTESIAN_POINT('Ctrl Pts',(79.7613482215346,11.0421057287759,138.991996726347));
#129456=CARTESIAN_POINT('Ctrl Pts',(79.8328942551689,11.0479436595142,138.988094120483));
#129457=CARTESIAN_POINT('Ctrl Pts',(79.9037074285486,11.0537217911667,138.984231489787));
#129458=CARTESIAN_POINT('Ctrl Pts',(79.9749294555231,11.0558316564894,138.980368859091));
#129459=CARTESIAN_POINT('Ctrl Pts',(80.0461489025551,11.0542316912396,138.976506228395));
#129460=CARTESIAN_POINT('Ctrl Pts',(80.1172967791412,11.0526333338403,138.972647479366));
#129461=CARTESIAN_POINT('Ctrl Pts',(80.1884415979034,11.0473325536336,138.968788730337));
#129462=CARTESIAN_POINT('Ctrl Pts',(80.2591691586792,11.0383397434406,138.964929981309));
#129463=CARTESIAN_POINT('Ctrl Pts',(80.3298493032757,11.0293529620813,138.961073819208));
#129464=CARTESIAN_POINT('Ctrl Pts',(80.4001122645271,11.0166791252986,138.957217657108));
#129465=CARTESIAN_POINT('Ctrl Pts',(80.4695479341675,11.0003805388023,138.953361495008));
#129466=CARTESIAN_POINT('Ctrl Pts',(80.5404063396775,10.9837479945037,138.949426320201));
#129467=CARTESIAN_POINT('Ctrl Pts',(80.610402653991,10.963340553779,138.945491145395));
#129468=CARTESIAN_POINT('Ctrl Pts',(80.6791123406911,10.9392792452922,138.941555970589));
#129469=CARTESIAN_POINT('Ctrl Pts',(80.7464442646084,10.9157004128132,138.937699703687));
#129470=CARTESIAN_POINT('Ctrl Pts',(80.8125402314606,10.8886131173241,138.933843436786));
#129471=CARTESIAN_POINT('Ctrl Pts',(80.8770185180608,10.858180852737,138.929987169884));
#129472=CARTESIAN_POINT('Ctrl Pts',(80.9434758610669,10.8268145191578,138.926012541126));
#129473=CARTESIAN_POINT('Ctrl Pts',(81.0082140877077,10.7918947337507,138.922037912367));
#129474=CARTESIAN_POINT('Ctrl Pts',(81.0708422964889,10.7536517152931,138.918063283609));
#129475=CARTESIAN_POINT('Ctrl Pts',(81.1334705052701,10.7154086968354,138.91408865485));
#129476=CARTESIAN_POINT('Ctrl Pts',(81.1939882498678,10.6738427887355,138.910114026092));
#129477=CARTESIAN_POINT('Ctrl Pts',(81.252039109102,10.6292316077768,138.906139397334));
#129478=CARTESIAN_POINT('Ctrl Pts',(81.252039109102,10.6292316077768,139.606097362941));
#129479=CARTESIAN_POINT('Ctrl Pts',(81.3086788770668,10.5857048284755,139.602235197034));
#129480=CARTESIAN_POINT('Ctrl Pts',(81.3630354755369,10.5392292635521,139.598373031127));
#129481=CARTESIAN_POINT('Ctrl Pts',(81.4147982656329,10.4900816857012,139.59451086522));
#129482=CARTESIAN_POINT('Ctrl Pts',(81.4666182581804,10.4408797954392,139.590644431278));
#129483=CARTESIAN_POINT('Ctrl Pts',(81.5158383714577,10.3890003342646,139.586777997337));
#129484=CARTESIAN_POINT('Ctrl Pts',(81.5621848102927,10.3347569745054,139.582911563396));
#129485=CARTESIAN_POINT('Ctrl Pts',(81.6085609745073,10.2804788244905,139.579042649626));
#129486=CARTESIAN_POINT('Ctrl Pts',(81.6520595018109,10.2238341424132,139.575173735856));
#129487=CARTESIAN_POINT('Ctrl Pts',(81.6924485552715,10.1651675631683,139.571304822086));
#129488=CARTESIAN_POINT('Ctrl Pts',(81.7329055244302,10.1064023338847,139.567429402594));
#129489=CARTESIAN_POINT('Ctrl Pts',(81.7702423334845,10.0456088350746,139.563553983102));
#129490=CARTESIAN_POINT('Ctrl Pts',(81.8042723260695,9.98315763531587,139.559678563609));
#129491=CARTESIAN_POINT('Ctrl Pts',(81.8165980033016,9.96053778522156,139.558274885084));
#129492=CARTESIAN_POINT('Ctrl Pts',(81.8284903174524,9.93770065997237,139.556871206559));
#129493=CARTESIAN_POINT('Ctrl Pts',(81.8399419722473,9.91466447469142,139.555467528034));
#129494=CARTESIAN_POINT('Ctrl Pts',(81.8714784485882,9.85122559838008,139.551601966646));
#129495=CARTESIAN_POINT('Ctrl Pts',(81.8997929813764,9.78602736127449,139.547736405259));
#129496=CARTESIAN_POINT('Ctrl Pts',(81.9246862993926,9.71943047713488,139.543870843871));
#129497=CARTESIAN_POINT('Ctrl Pts',(81.9495421673408,9.65293378284705,139.540011097921));
#129498=CARTESIAN_POINT('Ctrl Pts',(81.9709868673624,9.58504307011365,139.536151351971));
#129499=CARTESIAN_POINT('Ctrl Pts',(81.988867730239,9.51614214526027,139.532291606022));
#129500=CARTESIAN_POINT('Ctrl Pts',(82.0067273304742,9.44732315245196,139.528436449805));
#129501=CARTESIAN_POINT('Ctrl Pts',(82.021031389321,9.37749680239563,139.524581293589));
#129502=CARTESIAN_POINT('Ctrl Pts',(82.0316765211828,9.30706363473175,139.520726137372));
#129503=CARTESIAN_POINT('Ctrl Pts',(82.0423148473879,9.23667549647311,139.516873445838));
#129504=CARTESIAN_POINT('Ctrl Pts',(82.0492988146928,9.16568179040966,139.513020754304));
#129505=CARTESIAN_POINT('Ctrl Pts',(82.0525760781977,9.0944934162287,139.50916806277));
#129506=CARTESIAN_POINT('Ctrl Pts',(82.0558523483818,9.02332661885882,139.505316538966));
#129507=CARTESIAN_POINT('Ctrl Pts',(82.0554241226374,8.95196575651897,139.501465015162));
#129508=CARTESIAN_POINT('Ctrl Pts',(82.0512910442517,8.88082527838157,139.497613491358));
#129509=CARTESIAN_POINT('Ctrl Pts',(82.0471578289629,8.80968244380407,139.493761839977));
#129510=CARTESIAN_POINT('Ctrl Pts',(82.0393195478422,8.73876049378837,139.489910188596));
#129511=CARTESIAN_POINT('Ctrl Pts',(82.027827849291,8.66847055011675,139.486058537215));
#129512=CARTESIAN_POINT('Ctrl Pts',(82.0163241399483,8.59810714142592,139.482202860199));
#129513=CARTESIAN_POINT('Ctrl Pts',(82.0011594693797,8.5283775391265,139.478347183183));
#129514=CARTESIAN_POINT('Ctrl Pts',(81.9824368025165,8.45968353113359,139.474491506167));
#129515=CARTESIAN_POINT('Ctrl Pts',(81.9637035792248,8.3909507912984,139.470633655199));
#129516=CARTESIAN_POINT('Ctrl Pts',(81.9414085186979,8.32325527066213,139.466775804232));
#129517=CARTESIAN_POINT('Ctrl Pts',(81.9157039132598,8.25698177732901,139.462917953264));
#129518=CARTESIAN_POINT('Ctrl Pts',(81.8899541416765,8.19059183333773,139.459053323579));
#129519=CARTESIAN_POINT('Ctrl Pts',(81.8607830636398,8.12562934949478,139.455188693893));
#129520=CARTESIAN_POINT('Ctrl Pts',(81.8283900679697,8.06245676267714,139.451324064208));
#129521=CARTESIAN_POINT('Ctrl Pts',(81.8088611733903,8.02437165314194,139.448994179486));
#129522=CARTESIAN_POINT('Ctrl Pts',(81.7881621302068,7.98693659210319,139.446664294764));
#129523=CARTESIAN_POINT('Ctrl Pts',(81.7663441375903,7.95022576231819,139.444334410042));
#129524=CARTESIAN_POINT('Ctrl Pts',(81.7301084889346,7.88925586681367,139.440464902628));
#129525=CARTESIAN_POINT('Ctrl Pts',(81.6906414303863,7.83004501603826,139.436595395214));
#129526=CARTESIAN_POINT('Ctrl Pts',(81.6481389612067,7.77295659121104,139.432725887799));
#129527=CARTESIAN_POINT('Ctrl Pts',(81.6056998333134,7.71595324507047,139.428862147099));
#129528=CARTESIAN_POINT('Ctrl Pts',(81.5602345618575,7.66106643266508,139.424998406399));
#129529=CARTESIAN_POINT('Ctrl Pts',(81.5119837693341,7.60863281490103,139.421134665698));
#129530=CARTESIAN_POINT('Ctrl Pts',(81.4637896323175,7.55626076406748,139.417275461756));
#129531=CARTESIAN_POINT('Ctrl Pts',(81.4128167983318,7.50633654178831,139.413416257814));
#129532=CARTESIAN_POINT('Ctrl Pts',(81.3593466245471,7.45916440953868,139.409557053872));
#129533=CARTESIAN_POINT('Ctrl Pts',(81.3059101763189,7.41202203044485,139.405700284068));
#129534=CARTESIAN_POINT('Ctrl Pts',(81.2499798767448,7.36762861800326,139.401843514265));
#129535=CARTESIAN_POINT('Ctrl Pts',(81.1918734150042,7.32625111647348,139.397986744461));
#129536=CARTESIAN_POINT('Ctrl Pts',(81.133784177304,7.2848858801503,139.394131117889));
#129537=CARTESIAN_POINT('Ctrl Pts',(81.0735204534658,7.24653506147924,139.390275491317));
#129538=CARTESIAN_POINT('Ctrl Pts',(81.0114310621613,7.21142381515487,139.386419864745));
#129539=CARTESIAN_POINT('Ctrl Pts',(80.9493393188025,7.17631123875524,139.382564092116));
#129540=CARTESIAN_POINT('Ctrl Pts',(80.8854221945011,7.14443871549472,139.378708319486));
#129541=CARTESIAN_POINT('Ctrl Pts',(80.8200538780584,7.11598588126802,139.374852546856));
#129542=CARTESIAN_POINT('Ctrl Pts',(80.7546173158675,7.08750334174889,139.370992748728));
#129543=CARTESIAN_POINT('Ctrl Pts',(80.6877269833174,7.06244781247504,139.367132950599));
#129544=CARTESIAN_POINT('Ctrl Pts',(80.6197770282117,7.04095074135409,139.363273152471));
#129545=CARTESIAN_POINT('Ctrl Pts',(80.5517886923445,7.01944152785635,139.359411174179));
#129546=CARTESIAN_POINT('Ctrl Pts',(80.482740012711,7.00149489601355,139.355549195887));
#129547=CARTESIAN_POINT('Ctrl Pts',(80.41303761036,6.98719163979078,139.351687217595));
#129548=CARTESIAN_POINT('Ctrl Pts',(80.3432134959739,6.97286340769394,139.347818495644));
#129549=CARTESIAN_POINT('Ctrl Pts',(80.2727338601499,6.96219132580645,139.343949773694));
#129550=CARTESIAN_POINT('Ctrl Pts',(80.2020120623991,6.95520448720532,139.340081051743));
#129551=CARTESIAN_POINT('Ctrl Pts',(80.1600904683361,6.9510629152864,139.337787798512));
#129552=CARTESIAN_POINT('Ctrl Pts',(80.1180838367506,6.94821524382756,139.335494545281));
#129553=CARTESIAN_POINT('Ctrl Pts',(80.0760779629691,6.94665889193966,139.333201292051));
#129554=CARTESIAN_POINT('Ctrl Pts',(80.0051960461625,6.94403265910342,139.329331590743));
#129555=CARTESIAN_POINT('Ctrl Pts',(79.934039667594,6.94507590474726,139.325461889435));
#129556=CARTESIAN_POINT('Ctrl Pts',(79.8630204812265,6.94982094100623,139.321592188127));
#129557=CARTESIAN_POINT('Ctrl Pts',(79.7921068482023,6.95455892488306,139.317728238222));
#129558=CARTESIAN_POINT('Ctrl Pts',(79.7213304832265,6.96298774612134,139.313864288316));
#129559=CARTESIAN_POINT('Ctrl Pts',(79.6511047769023,6.97508773380188,139.310000338411));
#129560=CARTESIAN_POINT('Ctrl Pts',(79.5809611270469,6.98717358303777,139.306140903406));
#129561=CARTESIAN_POINT('Ctrl Pts',(79.5113673340132,7.00292199593063,139.302281468401));
#129562=CARTESIAN_POINT('Ctrl Pts',(79.4427316478592,7.02226150712429,139.298422033396));
#129563=CARTESIAN_POINT('Ctrl Pts',(79.3741390119948,7.04158888801658,139.29456501914));
#129564=CARTESIAN_POINT('Ctrl Pts',(79.3065037570193,7.06450276695379,139.290708004885));
#129565=CARTESIAN_POINT('Ctrl Pts',(79.2402224714927,7.09088091789029,139.286850990629));
#129566=CARTESIAN_POINT('Ctrl Pts',(79.1739606077154,7.11725133949825,139.282995106556));
#129567=CARTESIAN_POINT('Ctrl Pts',(79.1090523766764,7.14708383835458,139.279139222483));
#129568=CARTESIAN_POINT('Ctrl Pts',(79.0458761277446,7.18020737475601,139.275283338411));
#129569=CARTESIAN_POINT('Ctrl Pts',(78.9826972772882,7.21333227514625,139.271427295557));
#129570=CARTESIAN_POINT('Ctrl Pts',(78.9212509795886,7.24974825470462,139.267571252703));
#129571=CARTESIAN_POINT('Ctrl Pts',(78.8618910896333,7.28923827765412,139.26371520985));
#129572=CARTESIAN_POINT('Ctrl Pts',(78.8024689587002,7.32876970731177,139.259855123796));
#129573=CARTESIAN_POINT('Ctrl Pts',(78.7451380077172,7.37138134514055,139.255995037743));
#129574=CARTESIAN_POINT('Ctrl Pts',(78.6902224229091,7.41681325768247,139.25213495169));
#129575=CARTESIAN_POINT('Ctrl Pts',(78.6352756736537,7.46227095271314,139.248272675048));
#129576=CARTESIAN_POINT('Ctrl Pts',(78.5827473769454,7.51055177980714,139.244410398407));
#129577=CARTESIAN_POINT('Ctrl Pts',(78.5329259184762,7.5613578617943,139.240548121765));
#129578=CARTESIAN_POINT('Ctrl Pts',(78.4830172976119,7.61225282877056,139.23667908809));
#129579=CARTESIAN_POINT('Ctrl Pts',(78.4358252913247,7.665681507082,139.232810054414));
#129580=CARTESIAN_POINT('Ctrl Pts',(78.391598497205,7.72131232573913,139.228941020738));
#129581=CARTESIAN_POINT('Ctrl Pts',(78.3654107372799,7.75425268581786,139.226650071845));
#129582=CARTESIAN_POINT('Ctrl Pts',(78.3402618055092,7.78796455806452,139.224359122952));
#129583=CARTESIAN_POINT('Ctrl Pts',(78.3161959160251,7.82237469062124,139.222068174059));
#129584=CARTESIAN_POINT('Ctrl Pts',(78.2750915133202,7.88114700180774,139.218155246347));
#129585=CARTESIAN_POINT('Ctrl Pts',(78.2369898078095,7.94218533763197,139.214242318635));
#129586=CARTESIAN_POINT('Ctrl Pts',(78.2021456925714,8.0051545588583,139.210329390922));
#129587=CARTESIAN_POINT('Ctrl Pts',(78.1673565315928,8.06802446842476,139.206422634469));
#129588=CARTESIAN_POINT('Ctrl Pts',(78.1358149862431,8.1328188082781,139.202515878015));
#129589=CARTESIAN_POINT('Ctrl Pts',(78.1077333086913,8.19917272057976,139.198609121561));
#129590=CARTESIAN_POINT('Ctrl Pts',(78.0796926580191,8.26542969088187,139.194708072816));
#129591=CARTESIAN_POINT('Ctrl Pts',(78.0551020089896,8.33324127245433,139.190807024071));
#129592=CARTESIAN_POINT('Ctrl Pts',(78.0341273717282,8.40221879260742,139.186905975326));
#129593=CARTESIAN_POINT('Ctrl Pts',(78.0131709261672,8.47113648725012,139.183008310034));
#129594=CARTESIAN_POINT('Ctrl Pts',(77.9958244012656,8.54121766308561,139.179110644742));
#129595=CARTESIAN_POINT('Ctrl Pts',(77.9822049906054,8.61205559346455,139.17521297945));
#129596=CARTESIAN_POINT('Ctrl Pts',(77.9685917131875,8.6828616233298,139.171317069398));
#129597=CARTESIAN_POINT('Ctrl Pts',(77.9587023103997,8.75442326962861,139.167421159346));
#129598=CARTESIAN_POINT('Ctrl Pts',(77.9526032349813,8.82632199594982,139.163525249293));
#129599=CARTESIAN_POINT('Ctrl Pts',(77.9476716106702,8.88445826781668,139.160375072683));
#129600=CARTESIAN_POINT('Ctrl Pts',(77.9452171923589,8.94281458993765,139.157224896072));
#129601=CARTESIAN_POINT('Ctrl Pts',(77.9452503313532,9.00116691725337,139.154074719462));
#129602=CARTESIAN_POINT('Origin',(80.,9.,129.));
#129603=CARTESIAN_POINT('Ctrl Pts',(79.2300979593294,7.52256748114465,129.));
#129604=CARTESIAN_POINT('Ctrl Pts',(79.281830748178,7.48750058327585,129.));
#129605=CARTESIAN_POINT('Ctrl Pts',(79.3355405243692,7.45568942276443,129.));
#129606=CARTESIAN_POINT('Ctrl Pts',(79.3908959010939,7.42706960794827,129.));
#129607=CARTESIAN_POINT('Ctrl Pts',(79.4259930678064,7.40892368480008,129.));
#129608=CARTESIAN_POINT('Ctrl Pts',(79.4617526563836,7.39206132563758,129.));
#129609=CARTESIAN_POINT('Ctrl Pts',(79.4980977986663,7.37647332647928,129.));
#129610=CARTESIAN_POINT('Ctrl Pts',(79.5226963251973,7.36592331107759,129.));
#129611=CARTESIAN_POINT('Ctrl Pts',(79.5475631896663,7.35595715019795,129.));
#129612=CARTESIAN_POINT('Ctrl Pts',(79.5726757725026,7.34657353461922,129.));
#129613=CARTESIAN_POINT('Ctrl Pts',(79.5862857126981,7.34148801841897,129.));
#129614=CARTESIAN_POINT('Ctrl Pts',(79.599968045098,7.33657368647343,129.));
#129615=CARTESIAN_POINT('Ctrl Pts',(79.6137049524654,7.33183503949085,129.));
#129616=CARTESIAN_POINT('Ctrl Pts',(79.6760826347754,7.31031740031977,129.));
#129617=CARTESIAN_POINT('Ctrl Pts',(79.7396533189192,7.29239195390877,129.));
#129618=CARTESIAN_POINT('Ctrl Pts',(79.8040665846156,7.2780116608573,129.));
#129619=CARTESIAN_POINT('Ctrl Pts',(79.850512417162,7.26764260603894,129.));
#129620=CARTESIAN_POINT('Ctrl Pts',(79.8973972321369,7.25911760209265,129.));
#129621=CARTESIAN_POINT('Ctrl Pts',(79.9445987750863,7.25243304107414,129.));
#129622=CARTESIAN_POINT('Ctrl Pts',(79.9573802290497,7.25062296446254,129.));
#129623=CARTESIAN_POINT('Ctrl Pts',(79.9701849395111,7.24894790625536,129.));
#129624=CARTESIAN_POINT('Ctrl Pts',(79.9830105439016,7.24740795082224,129.));
#129625=CARTESIAN_POINT('Ctrl Pts',(79.9965305707581,7.2457846168896,129.));
#129626=CARTESIAN_POINT('Ctrl Pts',(80.010066274218,7.24431236541112,129.));
#129627=CARTESIAN_POINT('Ctrl Pts',(80.0236082610051,7.24299136914067,129.));
#129628=CARTESIAN_POINT('Ctrl Pts',(80.0912918487103,7.23638895781539,129.));
#129629=CARTESIAN_POINT('Ctrl Pts',(80.1591802213322,7.23355533205344,129.));
#129630=CARTESIAN_POINT('Ctrl Pts',(80.2269161369356,7.23444184514064,129.));
#129631=CARTESIAN_POINT('Ctrl Pts',(80.2955027350948,7.23533949177806,129.));
#129632=CARTESIAN_POINT('Ctrl Pts',(80.3639340445116,7.24005098621149,129.));
#129633=CARTESIAN_POINT('Ctrl Pts',(80.4318607174046,7.24857423381045,129.));
#129634=CARTESIAN_POINT('Ctrl Pts',(80.4737684724859,7.25383270088474,129.));
#129635=CARTESIAN_POINT('Ctrl Pts',(80.515484509682,7.26054302178907,129.));
#129636=CARTESIAN_POINT('Ctrl Pts',(80.5569281451476,7.26871452189268,129.));
#129637=CARTESIAN_POINT('Ctrl Pts',(80.59098326124,7.27542921720238,129.));
#129638=CARTESIAN_POINT('Ctrl Pts',(80.6248544845506,7.28313067078347,129.));
#129639=CARTESIAN_POINT('Ctrl Pts',(80.6584967044525,7.29182802522507,129.));
#129640=CARTESIAN_POINT('Ctrl Pts',(80.6723040435688,7.29539756738195,129.));
#129641=CARTESIAN_POINT('Ctrl Pts',(80.6860753217099,7.29913575892529,129.));
#129642=CARTESIAN_POINT('Ctrl Pts',(80.6997840581602,7.30303636166769,129.));
#129643=CARTESIAN_POINT('Ctrl Pts',(80.7675838280963,7.32232770697194,129.));
#129644=CARTESIAN_POINT('Ctrl Pts',(80.8339731467169,7.34561685223654,129.));
#129645=CARTESIAN_POINT('Ctrl Pts',(80.898588998481,7.37288464964485,129.));
#129646=CARTESIAN_POINT('Ctrl Pts',(80.9057659256999,7.37591330270869,129.));
#129647=CARTESIAN_POINT('Ctrl Pts',(80.9129209821764,7.37899109153126,129.));
#129648=CARTESIAN_POINT('Ctrl Pts',(80.9200536746534,7.3821180294085,129.));
#129649=CARTESIAN_POINT('Ctrl Pts',(80.984149627247,7.41021738495922,129.));
#129650=CARTESIAN_POINT('Ctrl Pts',(81.0464406059207,7.44228062654433,129.));
#129651=CARTESIAN_POINT('Ctrl Pts',(81.1067678836995,7.477962347096,129.));
#129652=CARTESIAN_POINT('Ctrl Pts',(81.1670951614783,7.51364406764767,129.));
#129653=CARTESIAN_POINT('Ctrl Pts',(81.2254594571749,7.55294494292302,129.));
#129654=CARTESIAN_POINT('Ctrl Pts',(81.2816840111194,7.59557425376097,129.));
#129655=CARTESIAN_POINT('Ctrl Pts',(81.2922356478337,7.60357447732499,129.));
#129656=CARTESIAN_POINT('Ctrl Pts',(81.3027118541411,7.61169206594889,129.));
#129657=CARTESIAN_POINT('Ctrl Pts',(81.313111358469,7.61992528231288,129.));
#129658=CARTESIAN_POINT('Ctrl Pts',(81.3222610024349,7.62716899278696,129.));
#129659=CARTESIAN_POINT('Ctrl Pts',(81.3313442109961,7.63449663645984,129.));
#129660=CARTESIAN_POINT('Ctrl Pts',(81.340358501486,7.64190506046335,129.));
#129661=CARTESIAN_POINT('Ctrl Pts',(81.3958400493656,7.68750275132147,129.));
#129662=CARTESIAN_POINT('Ctrl Pts',(81.4487348274871,7.73617414202039,129.));
#129663=CARTESIAN_POINT('Ctrl Pts',(81.4988881430576,7.78755864017411,129.));
#129664=CARTESIAN_POINT('Ctrl Pts',(81.5490414586282,7.83894313832784,129.));
#129665=CARTESIAN_POINT('Ctrl Pts',(81.596453992352,7.89304144632724,129.));
#129666=CARTESIAN_POINT('Ctrl Pts',(81.6409514014518,7.94954263372726,129.));
#129667=CARTESIAN_POINT('Ctrl Pts',(81.6861833091593,8.00697646067449,129.));
#129668=CARTESIAN_POINT('Ctrl Pts',(81.7284038904358,8.06689379464521,129.));
#129669=CARTESIAN_POINT('Ctrl Pts',(81.7673981934856,8.12900933410927,129.));
#129670=CARTESIAN_POINT('Ctrl Pts',(81.7770296357955,8.14435163255051,129.));
#129671=CARTESIAN_POINT('Ctrl Pts',(81.786464068092,8.15982820433461,129.));
#129672=CARTESIAN_POINT('Ctrl Pts',(81.7956978659394,8.17543505634213,129.));
#129673=CARTESIAN_POINT('Ctrl Pts',(81.8029371409721,8.18767079032106,129.));
#129674=CARTESIAN_POINT('Ctrl Pts',(81.8100538149155,8.19998811837099,129.));
#129675=CARTESIAN_POINT('Ctrl Pts',(81.8170357172675,8.21236610903634,129.));
#129676=CARTESIAN_POINT('Ctrl Pts',(81.854021820935,8.27793758552841,129.));
#129677=CARTESIAN_POINT('Ctrl Pts',(81.8872984696483,8.34532395025826,129.));
#129678=CARTESIAN_POINT('Ctrl Pts',(81.9166855007576,8.41417988544907,129.));
#129679=CARTESIAN_POINT('Ctrl Pts',(81.9459284893018,8.48269831851237,129.));
#129680=CARTESIAN_POINT('Ctrl Pts',(81.9713206084984,8.55267279654377,129.));
#129681=CARTESIAN_POINT('Ctrl Pts',(81.9926494449667,8.62379991350796,129.));
#129682=CARTESIAN_POINT('Ctrl Pts',(82.0137867709559,8.69428838390283,129.));
#129683=CARTESIAN_POINT('Ctrl Pts',(82.0309341246297,8.76590972191823,129.));
#129684=CARTESIAN_POINT('Ctrl Pts',(82.0438402050009,8.83839240103824,129.));
#129685=CARTESIAN_POINT('Ctrl Pts',(82.0465861966793,8.85381434387207,129.));
#129686=CARTESIAN_POINT('Ctrl Pts',(82.0491400035047,8.8692753399892,129.));
#129687=CARTESIAN_POINT('Ctrl Pts',(82.0514988962123,8.88477285886849,129.));
#129688=CARTESIAN_POINT('Ctrl Pts',(82.053488432599,8.89784377032416,129.));
#129689=CARTESIAN_POINT('Ctrl Pts',(82.0553393131761,8.9109406630385,129.));
#129690=CARTESIAN_POINT('Ctrl Pts',(82.0570523367261,8.92406189548185,129.));
#129691=CARTESIAN_POINT('Ctrl Pts',(81.8174278887596,9.95862058795901,129.));
#129692=CARTESIAN_POINT('Ctrl Pts',(81.7762160018567,10.0216592895785,129.));
#129693=CARTESIAN_POINT('Ctrl Pts',(81.7313405655059,10.0821005916704,129.));
#129694=CARTESIAN_POINT('Ctrl Pts',(81.6831396740662,10.1397906903828,129.));
#129695=CARTESIAN_POINT('Ctrl Pts',(81.6370503035558,10.1949535775186,129.));
#129696=CARTESIAN_POINT('Ctrl Pts',(81.5879193937338,10.2476011126225,129.));
#129697=CARTESIAN_POINT('Ctrl Pts',(81.5360172152856,10.2975621775029,129.));
#129698=CARTESIAN_POINT('Ctrl Pts',(81.5243247634357,10.3088173379403,129.));
#129699=CARTESIAN_POINT('Ctrl Pts',(81.5124900085598,10.3199374555242,129.));
#129700=CARTESIAN_POINT('Ctrl Pts',(81.5005210105629,10.3309156511376,129.));
#129701=CARTESIAN_POINT('Ctrl Pts',(81.4455937863517,10.381295959669,129.));
#129702=CARTESIAN_POINT('Ctrl Pts',(81.3879517403589,10.4285914676262,129.));
#129703=CARTESIAN_POINT('Ctrl Pts',(81.32791149294,10.4726299004967,129.));
#129704=CARTESIAN_POINT('Ctrl Pts',(81.2857591326134,10.5035478925167,129.));
#129705=CARTESIAN_POINT('Ctrl Pts',(81.2424240158456,10.5328595775406,129.));
#129706=CARTESIAN_POINT('Ctrl Pts',(81.198010382721,10.5604909361764,129.));
#129707=CARTESIAN_POINT('Ctrl Pts',(81.1811383966962,10.5709876207291,129.));
#129708=CARTESIAN_POINT('Ctrl Pts',(81.1641107403089,10.5812416863955,129.));
#129709=CARTESIAN_POINT('Ctrl Pts',(81.1469330529734,10.5912485887382,129.));
#129710=CARTESIAN_POINT('Ctrl Pts',(81.1305340848948,10.6008018463378,129.));
#129711=CARTESIAN_POINT('Ctrl Pts',(81.1139930505993,10.6101325847749,129.));
#129712=CARTESIAN_POINT('Ctrl Pts',(81.0973444947477,10.6192209212688,129.));
#129713=CARTESIAN_POINT('Ctrl Pts',(81.0336769966004,10.6539765872885,129.));
#129714=CARTESIAN_POINT('Ctrl Pts',(80.968373580833,10.6852316531886,129.));
#129715=CARTESIAN_POINT('Ctrl Pts',(80.9017255995023,10.7128251457784,129.));
#129716=CARTESIAN_POINT('Ctrl Pts',(80.8366062693887,10.7397857485914,129.));
#129717=CARTESIAN_POINT('Ctrl Pts',(80.7702024261762,10.7632509566609,129.));
#129718=CARTESIAN_POINT('Ctrl Pts',(80.7027772959504,10.783022803573,129.));
#129719=CARTESIAN_POINT('Ctrl Pts',(80.6364369119638,10.8024765578613,129.));
#129720=CARTESIAN_POINT('Ctrl Pts',(80.5691070645839,10.8183549948411,129.));
#129721=CARTESIAN_POINT('Ctrl Pts',(80.501042459281,10.8304204386017,129.));
#129722=CARTESIAN_POINT('Ctrl Pts',(80.4789907160657,10.8343294316298,129.));
#129723=CARTESIAN_POINT('Ctrl Pts',(80.4568619287533,10.8378377953482,129.));
#129724=CARTESIAN_POINT('Ctrl Pts',(80.4346650539684,10.8409362728209,129.));
#129725=CARTESIAN_POINT('Ctrl Pts',(80.4221749866782,10.8426797701603,129.));
#129726=CARTESIAN_POINT('Ctrl Pts',(80.4096620712929,10.8442935310645,129.));
#129727=CARTESIAN_POINT('Ctrl Pts',(80.3971456250734,10.8457740253543,129.));
#129728=CARTESIAN_POINT('Ctrl Pts',(80.3293080731436,10.8537981167383,129.));
#129729=CARTESIAN_POINT('Ctrl Pts',(80.2612484637432,10.8579293246703,129.));
#129730=CARTESIAN_POINT('Ctrl Pts',(80.1932129649845,10.8579897571609,129.));
#129731=CARTESIAN_POINT('Ctrl Pts',(80.183419062696,10.8579984565887,129.));
#129732=CARTESIAN_POINT('Ctrl Pts',(80.173625666279,10.8579227116332,129.));
#129733=CARTESIAN_POINT('Ctrl Pts',(80.1638335195185,10.8577619017594,129.));
#129734=CARTESIAN_POINT('Ctrl Pts',(80.094125774739,10.8566171381119,129.));
#129735=CARTESIAN_POINT('Ctrl Pts',(80.0244798679339,10.8511657002129,129.));
#129736=CARTESIAN_POINT('Ctrl Pts',(79.9552253060309,10.8415831053598,129.));
#129737=CARTESIAN_POINT('Ctrl Pts',(79.8912776929718,10.8327348208435,129.));
#129738=CARTESIAN_POINT('Ctrl Pts',(79.8276632746924,10.8203632855842,129.));
#129739=CARTESIAN_POINT('Ctrl Pts',(79.7646616788188,10.8045727994338,129.));
#129740=CARTESIAN_POINT('Ctrl Pts',(79.7507943070261,10.8010971328383,129.));
#129741=CARTESIAN_POINT('Ctrl Pts',(79.7369567233517,10.7974557117189,129.));
#129742=CARTESIAN_POINT('Ctrl Pts',(79.7231520870758,10.7936494709069,129.));
#129743=CARTESIAN_POINT('Ctrl Pts',(79.7120934934718,10.7906003742514,129.));
#129744=CARTESIAN_POINT('Ctrl Pts',(79.7010565962289,10.7874455711953,129.));
#129745=CARTESIAN_POINT('Ctrl Pts',(79.6900560633263,10.7841896646439,129.));
#129746=CARTESIAN_POINT('Ctrl Pts',(79.6245012361557,10.7647869326896,129.));
#129747=CARTESIAN_POINT('Ctrl Pts',(79.5601138344761,10.7417646897258,129.));
#129748=CARTESIAN_POINT('Ctrl Pts',(79.4971959262021,10.715304780306,129.));
#129749=CARTESIAN_POINT('Ctrl Pts',(79.4345683059016,10.6889669504927,129.));
#129750=CARTESIAN_POINT('Ctrl Pts',(79.3733957590305,10.6592224003991,129.));
#129751=CARTESIAN_POINT('Ctrl Pts',(79.3140059902934,10.6262089191606,129.));
#129752=CARTESIAN_POINT('Ctrl Pts',(79.2558864207415,10.5939015140336,129.));
#129753=CARTESIAN_POINT('Ctrl Pts',(79.1994735144971,10.558462809005,129.));
#129754=CARTESIAN_POINT('Ctrl Pts',(79.1451143324441,10.5199925315035,129.));
#129755=CARTESIAN_POINT('Ctrl Pts',(79.1336097299013,10.5118506641014,129.));
#129756=CARTESIAN_POINT('Ctrl Pts',(79.1221972825761,10.5035729216371,129.));
#129757=CARTESIAN_POINT('Ctrl Pts',(79.1108805595173,10.4951601203912,129.));
#129758=CARTESIAN_POINT('Ctrl Pts',(79.1002618280376,10.4872662029598,129.));
#129759=CARTESIAN_POINT('Ctrl Pts',(79.0897261684286,10.479252279507,129.));
#129760=CARTESIAN_POINT('Ctrl Pts',(79.0792930565818,10.4711322469418,129.));
#129761=CARTESIAN_POINT('Ctrl Pts',(79.0277338571515,10.4310040105575,129.));
#129762=CARTESIAN_POINT('Ctrl Pts',(78.978581104871,10.3882180036356,129.));
#129763=CARTESIAN_POINT('Ctrl Pts',(78.9321255592781,10.3429060921625,129.));
#129764=CARTESIAN_POINT('Ctrl Pts',(78.8871753821825,10.2990624903005,129.));
#129765=CARTESIAN_POINT('Ctrl Pts',(78.8447499809854,10.2528533437791,129.));
#129766=CARTESIAN_POINT('Ctrl Pts',(78.8051532326766,10.2043735161521,129.));
#129767=CARTESIAN_POINT('Ctrl Pts',(78.7657598821795,10.1561427163183,129.));
#129768=CARTESIAN_POINT('Ctrl Pts',(78.7291656220547,10.1056639886396,129.));
#129769=CARTESIAN_POINT('Ctrl Pts',(78.6957182918309,10.0530146622108,129.));
#129770=CARTESIAN_POINT('Ctrl Pts',(78.6902769744426,10.0444495033935,129.));
#129771=CARTESIAN_POINT('Ctrl Pts',(78.6849190588097,10.0358268728766,129.));
#129772=CARTESIAN_POINT('Ctrl Pts',(78.6796461810995,10.0271470773945,129.));
#129773=CARTESIAN_POINT('Ctrl Pts',(78.6739912646832,10.017838399921,129.));
#129774=CARTESIAN_POINT('Ctrl Pts',(78.6684341558143,10.0084639727813,129.));
#129775=CARTESIAN_POINT('Ctrl Pts',(78.6629752590626,9.99902545690085,129.));
#129776=CARTESIAN_POINT('Ctrl Pts',(81.2663555529872,10.0778216258784,139.998270369527));
#129777=CARTESIAN_POINT('Ctrl Pts',(81.624882726317,9.65660459345759,139.961212857736));
#129778=CARTESIAN_POINT('Ctrl Pts',(81.8817055576156,8.43521511269861,139.887110973282));
#129779=CARTESIAN_POINT('Ctrl Pts',(80.5443606420769,7.1101993889356,139.775964716164));
#129780=CARTESIAN_POINT('Ctrl Pts',(78.7083082983556,7.51894549756411,139.664831598172));
#129781=CARTESIAN_POINT('Ctrl Pts',(78.0547700623159,9.28127667726292,139.553698480181));
#129782=CARTESIAN_POINT('Ctrl Pts',(79.181430819152,10.7871147142069,139.442565362189));
#129783=CARTESIAN_POINT('Ctrl Pts',(81.0573526210883,10.6568543838274,139.331432244198));
#129784=CARTESIAN_POINT('Ctrl Pts',(81.9655073494158,9.01040090821446,139.220299126206));
#129785=CARTESIAN_POINT('Ctrl Pts',(81.0747701558528,7.35431801012218,139.109166008215));
#129786=CARTESIAN_POINT('Ctrl Pts',(79.2003523271827,7.20448187233449,138.998032890223));
#129787=CARTESIAN_POINT('Ctrl Pts',(78.0578077691287,8.69794827804849,138.886899772231));
#129788=CARTESIAN_POINT('Ctrl Pts',(78.6928319084955,10.4678771753584,138.77576665424));
#129789=CARTESIAN_POINT('Ctrl Pts',(80.5242287499213,10.8943408158948,138.664633536248));
#129790=CARTESIAN_POINT('Ctrl Pts',(81.8758303096953,9.58703225682554,138.553500418257));
#129791=CARTESIAN_POINT('Ctrl Pts',(81.5105983807109,7.74244716724272,138.442367300265));
#129792=CARTESIAN_POINT('Ctrl Pts',(79.7628072385,7.04882466216988,138.331234182274));
#129793=CARTESIAN_POINT('Ctrl Pts',(78.2321043054277,8.14099426435935,138.220101064282));
#129794=CARTESIAN_POINT('Ctrl Pts',(78.3194490673689,10.0193599016733,138.108967946291));
#129795=CARTESIAN_POINT('Ctrl Pts',(79.9449002025574,10.9647671494451,137.997834828299));
#129796=CARTESIAN_POINT('Ctrl Pts',(81.6207808342945,10.1119422115685,137.886701710307));
#129797=CARTESIAN_POINT('Ctrl Pts',(81.8132590564869,8.24142397550868,137.775568592316));
#129798=CARTESIAN_POINT('Ctrl Pts',(80.3461712193815,7.06518438436528,137.664435474324));
#129799=CARTESIAN_POINT('Ctrl Pts',(78.5622538579237,7.65976419334241,137.553302356333));
#129800=CARTESIAN_POINT('Ctrl Pts',(78.0942183544438,9.48098056613988,137.442169238341));
#129801=CARTESIAN_POINT('Ctrl Pts',(79.3704292240006,10.8619845924221,137.33103612035));
#129802=CARTESIAN_POINT('Ctrl Pts',(81.222848047324,10.5388270332939,137.219903002358));
#129803=CARTESIAN_POINT('Ctrl Pts',(81.9560682069516,8.80727440537282,137.108769884366));
#129804=CARTESIAN_POINT('Ctrl Pts',(80.8990177534605,7.25211182739711,136.997636766375));
#129805=CARTESIAN_POINT('Ctrl Pts',(79.0191508670193,7.2966853011286,136.886503648383));
#129806=CARTESIAN_POINT('Ctrl Pts',(78.0369957129224,8.90019942911323,136.775370530392));
#129807=CARTESIAN_POINT('Ctrl Pts',(78.8514593454574,10.5950549676696,136.6642374124));
#129808=CARTESIAN_POINT('Ctrl Pts',(80.7171125911482,10.8300534190709,136.553104294409));
#129809=CARTESIAN_POINT('Ctrl Pts',(81.9264361681442,9.39011495113394,136.441971176417));
#129810=CARTESIAN_POINT('Ctrl Pts',(81.3726095402657,7.59312792514629,136.330838058426));
#129811=CARTESIAN_POINT('Ctrl Pts',(79.562516635751,7.08376559600911,136.219704940434));
#129812=CARTESIAN_POINT('Ctrl Pts',(78.1528257253745,8.32821641565602,136.108571822443));
#129813=CARTESIAN_POINT('Ctrl Pts',(78.4337414152061,10.1875100128385,135.997438704451));
#129814=CARTESIAN_POINT('Ctrl Pts',(80.1481586091783,10.9599477063327,135.886305586459));
#129815=CARTESIAN_POINT('Ctrl Pts',(81.7269752125645,9.93856411620112,135.775172468468));
#129816=CARTESIAN_POINT('Ctrl Pts',(81.7251961283297,8.05816970539868,135.664039350476));
#129817=CARTESIAN_POINT('Ctrl Pts',(80.1444496443897,7.0397754502945,135.552906232485));
#129818=CARTESIAN_POINT('Ctrl Pts',(78.4314971604217,7.81545585676727,135.441773114493));
#129819=CARTESIAN_POINT('Ctrl Pts',(78.1541002109059,9.67527768632976,135.330639996501));
#129820=CARTESIAN_POINT('Ctrl Pts',(79.5661434022768,10.9170587986925,135.21950687851));
#129821=CARTESIAN_POINT('Ctrl Pts',(81.3752692283133,10.4042722437928,135.108373760518));
#129822=CARTESIAN_POINT('Ctrl Pts',(81.9256945265281,8.60624045975704,134.997240642527));
#129823=CARTESIAN_POINT('Ctrl Pts',(80.7136483994663,7.16859290517607,134.886107524535));
#129824=CARTESIAN_POINT('Ctrl Pts',(78.8484431682858,7.40712120725877,134.774974406544));
#129825=CARTESIAN_POINT('Ctrl Pts',(78.0371880743253,9.10351487555662,134.663841288552));
#129826=CARTESIAN_POINT('Ctrl Pts',(79.0223757102669,10.7051676554393,134.552708170561));
#129827=CARTESIAN_POINT('Ctrl Pts',(80.9023235750891,10.7461838823189,134.441575052569));
#129828=CARTESIAN_POINT('Ctrl Pts',(81.9564293888803,9.18902389097254,134.330441934578));
#129829=CARTESIAN_POINT('Ctrl Pts',(81.2199340216575,7.45886179470017,134.219308816586));
#129830=CARTESIAN_POINT('Ctrl Pts',(79.3669070216788,7.13921004252689,134.108175698594));
#129831=CARTESIAN_POINT('Ctrl Pts',(78.0933116337564,8.52262649941205,133.997042580603));
#129832=CARTESIAN_POINT('Ctrl Pts',(78.5647924851429,10.3429539732731,133.885909462611));
#129833=CARTESIAN_POINT('Ctrl Pts',(80.3498317433441,10.9341571126414,133.77477634462));
#129834=CARTESIAN_POINT('Ctrl Pts',(81.8146912207933,9.75514353483809,133.663643226628));
#129835=CARTESIAN_POINT('Ctrl Pts',(81.6186738674224,7.88499287179108,133.552510108637));
#129836=CARTESIAN_POINT('Ctrl Pts',(79.9411824802037,7.03534061873377,133.441376990645));
#129837=CARTESIAN_POINT('Ctrl Pts',(78.3175232021377,7.98382195965104,133.330243872653));
#129838=CARTESIAN_POINT('Ctrl Pts',(78.2337329111168,9.86234943947361,133.219110754662));
#129839=CARTESIAN_POINT('Ctrl Pts',(79.766499779437,10.9516207705468,133.10797763667));
#129840=CARTESIAN_POINT('Ctrl Pts',(81.5129752400956,10.2546919573705,132.996844518679));
#129841=CARTESIAN_POINT('Ctrl Pts',(81.8747162108936,8.40941968061457,132.885711400687));
#129842=CARTESIAN_POINT('Ctrl Pts',(80.5206431173708,7.10466975717507,132.774578282696));
#129843=CARTESIAN_POINT('Ctrl Pts',(78.6900569505169,7.53460067144032,132.663445164704));
#129844=CARTESIAN_POINT('Ctrl Pts',(78.0583822214058,9.30572272875902,132.552312046712));
#129845=CARTESIAN_POINT('Ctrl Pts',(79.2037525045956,10.7970353115879,132.441178928721));
#129846=CARTESIAN_POINT('Ctrl Pts',(81.0778798355747,10.6436304466314,132.330045810729));
#129847=CARTESIAN_POINT('Ctrl Pts',(81.9654891161006,8.98591030425289,132.218912692738));
#129848=CARTESIAN_POINT('Ctrl Pts',(81.0542053966701,7.34108560598915,132.107779574746));
#129849=CARTESIAN_POINT('Ctrl Pts',(79.1780714050938,7.21456465535435,131.996646456755));
#129850=CARTESIAN_POINT('Ctrl Pts',(78.0541988143562,8.72214440619798,131.885513338763));
#129851=CARTESIAN_POINT('Ctrl Pts',(78.7112000547364,10.4840285327618,131.774380220772));
#129852=CARTESIAN_POINT('Ctrl Pts',(80.5477617316354,10.887671335383,131.66324710278));
#129853=CARTESIAN_POINT('Ctrl Pts',(81.8829903121689,9.56364303377056,131.552113984788));
#129854=CARTESIAN_POINT('Ctrl Pts',(81.4948320449856,7.72374644302386,131.440980866797));
#129855=CARTESIAN_POINT('Ctrl Pts',(79.7385446547136,7.05192734017315,131.329847748805));
#129856=CARTESIAN_POINT('Ctrl Pts',(78.2215514862109,8.16306101160042,131.218714630814));
#129857=CARTESIAN_POINT('Ctrl Pts',(78.3322643986637,10.0401941855574,131.107581512822));
#129858=CARTESIAN_POINT('Ctrl Pts',(79.9693545706299,10.9653007018072,130.996448394831));
#129859=CARTESIAN_POINT('Ctrl Pts',(81.634492654468,10.0916866570469,130.885315276839));
#129860=CARTESIAN_POINT('Ctrl Pts',(81.8036787100972,8.2189180260953,130.774182158847));
#129861=CARTESIAN_POINT('Ctrl Pts',(80.3220670546241,7.06102633885022,130.663049040856));
#129862=CARTESIAN_POINT('Ctrl Pts',(78.5456868797065,7.67775970833857,130.551915922864));
#129863=CARTESIAN_POINT('Ctrl Pts',(78.1003514663068,9.50465934401503,130.440782804873));
#129864=CARTESIAN_POINT('Ctrl Pts',(79.3936488482192,10.8696750722296,130.329649686881));
#129865=CARTESIAN_POINT('Ctrl Pts',(81.2419033084764,10.5234902013865,130.21851656889));
#129866=CARTESIAN_POINT('Ctrl Pts',(81.9535176740369,8.78294791815207,130.107383450898));
#129867=CARTESIAN_POINT('Ctrl Pts',(80.8771984457467,7.24105863992984,129.996250332907));
#129868=CARTESIAN_POINT('Ctrl Pts',(78.9980272102543,7.30902500521152,129.885117214915));
#129869=CARTESIAN_POINT('Ctrl Pts',(78.0359120840056,8.92463153403525,129.773984096924));
#129870=CARTESIAN_POINT('Ctrl Pts',(78.8713846676021,10.6092319693557,129.662850978932));
#129871=CARTESIAN_POINT('Ctrl Pts',(80.7398571755473,10.8209719051349,129.551717860941));
#129872=CARTESIAN_POINT('Ctrl Pts',(81.9310876541967,9.36614407866247,129.440584742949));
#129873=CARTESIAN_POINT('Ctrl Pts',(81.3551062875205,7.57608937952851,129.329451624957));
#129874=CARTESIAN_POINT('Ctrl Pts',(79.5384782449276,7.08949384998904,129.218318506966));
#129875=CARTESIAN_POINT('Ctrl Pts',(78.1450715048774,8.35097752792031,129.107185388974));
#129876=CARTESIAN_POINT('Ctrl Pts',(78.4476865286044,10.2074757739787,128.996052270983));
#129877=CARTESIAN_POINT('Ctrl Pts',(80.1745002968193,10.9567650420694,128.884919152991));
#129878=CARTESIAN_POINT('Ctrl Pts',(81.2128991468495,10.264901734376,128.810830407663));
#129879=CARTESIAN_POINT('Ctrl Pts',(81.4708680456716,9.7758241190599,128.773786035));
#129880=CARTESIAN_POINT('Ctrl Pts',(81.3664711693111,10.1630321152291,140.074173738579));
#129881=CARTESIAN_POINT('Ctrl Pts',(81.7533428062807,9.70851448037676,140.037116226789));
#129882=CARTESIAN_POINT('Ctrl Pts',(82.0304695530007,8.39056431383793,139.963014342335));
#129883=CARTESIAN_POINT('Ctrl Pts',(80.5873967396842,6.96079541430976,139.851868085216));
#129884=CARTESIAN_POINT('Ctrl Pts',(78.6061896552104,7.40185619829842,139.740734967225));
#129885=CARTESIAN_POINT('Ctrl Pts',(77.9009839525276,9.30351386636456,139.629601849233));
#129886=CARTESIAN_POINT('Ctrl Pts',(79.116716325777,10.9284005407918,139.518468731242));
#129887=CARTESIAN_POINT('Ctrl Pts',(81.140944870581,10.7878420810855,139.40733561325));
#129888=CARTESIAN_POINT('Ctrl Pts',(82.1208965520861,9.01122318386506,139.296202495259));
#129889=CARTESIAN_POINT('Ctrl Pts',(81.1597394018957,7.22421358068219,139.185069377267));
#129890=CARTESIAN_POINT('Ctrl Pts',(79.1371337315701,7.06253168816407,139.073936259276));
#129891=CARTESIAN_POINT('Ctrl Pts',(77.9042618145551,8.67406865416758,138.962803141284));
#129892=CARTESIAN_POINT('Ctrl Pts',(78.5894897319551,10.5839247006777,138.851670023292));
#129893=CARTESIAN_POINT('Ctrl Pts',(80.5656732591424,11.0441037303175,138.740536905301));
#129894=CARTESIAN_POINT('Ctrl Pts',(82.0241298193638,9.63344188961423,138.629403787309));
#129895=CARTESIAN_POINT('Ctrl Pts',(81.6300233617486,7.64302747692412,138.518270669318));
#129896=CARTESIAN_POINT('Ctrl Pts',(79.7440552383615,6.89456852056587,138.407137551326));
#129897=CARTESIAN_POINT('Ctrl Pts',(78.0923378972964,8.0730829353124,138.296004433335));
#129898=CARTESIAN_POINT('Ctrl Pts',(78.186587966877,10.0999485203839,138.184871315343));
#129899=CARTESIAN_POINT('Ctrl Pts',(79.9405441193332,11.1200978333399,138.073738197351));
#129900=CARTESIAN_POINT('Ctrl Pts',(81.7489166266227,10.1998502083116,137.96260507936));
#129901=CARTESIAN_POINT('Ctrl Pts',(81.9566118041151,8.18145242483221,137.851471961368));
#129902=CARTESIAN_POINT('Ctrl Pts',(80.3735388452432,6.91222161069935,137.740338843377));
#129903=CARTESIAN_POINT('Ctrl Pts',(78.4485884337135,7.5538077473141,137.629205725385));
#129904=CARTESIAN_POINT('Ctrl Pts',(77.9435509501959,9.5190059577491,137.518072607394));
#129905=CARTESIAN_POINT('Ctrl Pts',(79.3206565783088,11.0091894865106,137.406939489402));
#129906=CARTESIAN_POINT('Ctrl Pts',(81.3195240445505,10.660483716909,137.295806371411));
#129907=CARTESIAN_POINT('Ctrl Pts',(82.1107111693078,8.79203789328744,137.184673253419));
#129908=CARTESIAN_POINT('Ctrl Pts',(80.9700923551089,7.11392717518595,137.073540135427));
#129909=CARTESIAN_POINT('Ctrl Pts',(78.9416068350628,7.16202454138493,136.962407017436));
#129910=CARTESIAN_POINT('Ctrl Pts',(77.8818043975107,8.89230938935288,136.851273899444));
#129911=CARTESIAN_POINT('Ctrl Pts',(78.760657946726,10.7211569228289,136.740140781453));
#129912=CARTESIAN_POINT('Ctrl Pts',(80.7738061231242,10.974733896464,136.629007663461));
#129913=CARTESIAN_POINT('Ctrl Pts',(82.0787364789275,9.42095668328237,136.51787454547));
#129914=CARTESIAN_POINT('Ctrl Pts',(81.4811253909457,7.48190334486909,136.406741427478));
#129915=CARTESIAN_POINT('Ctrl Pts',(79.5279300486431,6.93227181693272,136.295608309486));
#129916=CARTESIAN_POINT('Ctrl Pts',(78.0067917063145,8.27510650712824,136.184475191495));
#129917=CARTESIAN_POINT('Ctrl Pts',(78.3099160462811,10.2813922535296,136.073342073503));
#129918=CARTESIAN_POINT('Ctrl Pts',(80.1598717417471,11.1148973743932,135.962208955512));
#129919=CARTESIAN_POINT('Ctrl Pts',(81.863506526676,10.0127651766626,135.85107583752));
#129920=CARTESIAN_POINT('Ctrl Pts',(81.8615867914887,7.98371042720149,135.739942719529));
#129921=CARTESIAN_POINT('Ctrl Pts',(80.155869553389,6.8848038955334,135.628809601537));
#129922=CARTESIAN_POINT('Ctrl Pts',(78.3074943650616,7.72180809198056,135.517676483546));
#129923=CARTESIAN_POINT('Ctrl Pts',(78.0081669502028,9.72866383179037,135.406543365554));
#129924=CARTESIAN_POINT('Ctrl Pts',(79.531843540303,11.0686177528167,135.295410247562));
#129925=CARTESIAN_POINT('Ctrl Pts',(81.4839953487769,10.5152912864638,135.184277129571));
#129926=CARTESIAN_POINT('Ctrl Pts',(82.0779362045621,8.57511059345543,135.073144011579));
#129927=CARTESIAN_POINT('Ctrl Pts',(80.7700680591604,7.0238054088007,134.962010893588));
#129928=CARTESIAN_POINT('Ctrl Pts',(78.7574033164313,7.28119129627272,134.850877775596));
#129929=CARTESIAN_POINT('Ctrl Pts',(77.8820119666334,9.11169856104729,134.739744657605));
#129930=CARTESIAN_POINT('Ctrl Pts',(78.9450866281691,10.8399749063389,134.628611539613));
#129931=CARTESIAN_POINT('Ctrl Pts',(80.9736595285902,10.8842337966425,134.517478421622));
#129932=CARTESIAN_POINT('Ctrl Pts',(82.1111009055799,9.2039677535394,134.40634530363));
#129933=CARTESIAN_POINT('Ctrl Pts',(81.316379641661,7.33702239430447,134.295212185638));
#129934=CARTESIAN_POINT('Ctrl Pts',(79.3168559174961,6.99209959396283,134.184079067647));
#129935=CARTESIAN_POINT('Ctrl Pts',(77.9425725459279,8.4848862754163,134.072945949655));
#129936=CARTESIAN_POINT('Ctrl Pts',(78.4513277598819,10.4491253122873,133.961812831664));
#129937=CARTESIAN_POINT('Ctrl Pts',(80.3774887631374,11.0870678263366,133.850679713672));
#129938=CARTESIAN_POINT('Ctrl Pts',(81.9581571925566,9.81484371953338,133.739546595681));
#129939=CARTESIAN_POINT('Ctrl Pts',(81.746643087032,7.79684256867697,133.628413477689));
#129940=CARTESIAN_POINT('Ctrl Pts',(79.9365324810536,6.88001845478242,133.517280359698));
#129941=CARTESIAN_POINT('Ctrl Pts',(78.1845098464722,7.90348489273153,133.406147241706));
#129942=CARTESIAN_POINT('Ctrl Pts',(78.0940952573956,9.93052511526679,133.295014123714));
#129943=CARTESIAN_POINT('Ctrl Pts',(79.7480397044302,11.1059121271983,133.183881005723));
#129944=CARTESIAN_POINT('Ctrl Pts',(81.6325881310308,10.3538854724243,133.072747887731));
#129945=CARTESIAN_POINT('Ctrl Pts',(82.0229276420695,8.36272954487466,132.96161476974));
#129946=CARTESIAN_POINT('Ctrl Pts',(80.5618041534298,6.95482862057646,132.850481651748));
#129947=CARTESIAN_POINT('Ctrl Pts',(78.5864953911754,7.41874903988775,132.739348533757));
#129948=CARTESIAN_POINT('Ctrl Pts',(77.9048816819162,9.32989257532517,132.628215415765));
#129949=CARTESIAN_POINT('Ctrl Pts',(79.1408027204212,10.9391054413796,132.517082297773));
#129950=CARTESIAN_POINT('Ctrl Pts',(81.163094926871,10.7735726850374,132.405949179782));
#129951=CARTESIAN_POINT('Ctrl Pts',(82.1208768772803,8.98479640020736,132.29481606179));
#129952=CARTESIAN_POINT('Ctrl Pts',(81.1375488326983,7.20993504831756,132.183682943799));
#129953=CARTESIAN_POINT('Ctrl Pts',(79.1130913229525,7.07341159647303,132.072549825807));
#129954=CARTESIAN_POINT('Ctrl Pts',(77.9003675428109,8.70017768132606,131.961416707816));
#129955=CARTESIAN_POINT('Ctrl Pts',(78.6093100282476,10.6013529531025,131.850283589824));
#129956=CARTESIAN_POINT('Ctrl Pts',(80.5910667127933,11.0369069735992,131.739150471833));
#129957=CARTESIAN_POINT('Ctrl Pts',(82.0318558777597,9.60820355990355,131.628017353841));
#129958=CARTESIAN_POINT('Ctrl Pts',(81.6130105700699,7.62284830968311,131.51688423585));
#129959=CARTESIAN_POINT('Ctrl Pts',(79.7178745017121,6.8979164902803,131.405751117858));
#129960=CARTESIAN_POINT('Ctrl Pts',(78.0809507926393,8.09689423683374,131.294617999866));
#129961=CARTESIAN_POINT('Ctrl Pts',(78.200416453433,10.1224299223834,131.183484881875));
#129962=CARTESIAN_POINT('Ctrl Pts',(79.9669318023625,11.1206735673178,131.072351763883));
#129963=CARTESIAN_POINT('Ctrl Pts',(81.763712476731,10.1779932888968,130.961218645892));
#129964=CARTESIAN_POINT('Ctrl Pts',(81.9462740541028,8.15716719866583,130.8500855279));
#129965=CARTESIAN_POINT('Ctrl Pts',(80.3475290519243,6.90773483816252,130.738952409908));
#129966=CARTESIAN_POINT('Ctrl Pts',(78.4307117022989,7.57322595285769,130.627819291917));
#129967=CARTESIAN_POINT('Ctrl Pts',(77.9501689339994,9.54455673392297,130.516686173925));
#129968=CARTESIAN_POINT('Ctrl Pts',(79.3457119010278,11.0174879607505,130.405553055934));
#129969=CARTESIAN_POINT('Ctrl Pts',(81.3400857777279,10.6439343847877,130.294419937942));
#129970=CARTESIAN_POINT('Ctrl Pts',(82.107958996203,8.76578820112213,130.183286819951));
#129971=CARTESIAN_POINT('Ctrl Pts',(80.9465480552043,7.1020001441342,130.072153701959));
#129972=CARTESIAN_POINT('Ctrl Pts',(78.9188131829234,7.17533979856319,129.961020583968));
#129973=CARTESIAN_POINT('Ctrl Pts',(77.8806350989911,8.91867304915029,129.849887465976));
#129974=CARTESIAN_POINT('Ctrl Pts',(78.7821585262321,10.7364547307989,129.738754347984));
#129975=CARTESIAN_POINT('Ctrl Pts',(80.7983488502959,10.9649344156327,129.627621229993));
#129976=CARTESIAN_POINT('Ctrl Pts',(82.0837557024546,9.39509072007935,129.516488112001));
#129977=CARTESIAN_POINT('Ctrl Pts',(81.4622383649526,7.46351776484872,129.40535499401));
#129978=CARTESIAN_POINT('Ctrl Pts',(79.501991229218,6.93845293557322,129.294221876018));
#129979=CARTESIAN_POINT('Ctrl Pts',(77.9984244521695,8.29966706882612,129.183088758027));
#129980=CARTESIAN_POINT('Ctrl Pts',(78.3249636333244,10.3029364690596,129.071955640035));
#129981=CARTESIAN_POINT('Ctrl Pts',(80.1882959521733,11.11146309486,128.960822522044));
#129982=CARTESIAN_POINT('Ctrl Pts',(81.3087886032814,10.3649024146173,128.886733776716));
#129983=CARTESIAN_POINT('Ctrl Pts',(81.5871520234028,9.83715927067298,128.849689404052));
#129984=CARTESIAN_POINT('Ctrl Pts',(81.4665867856348,10.2482426045797,140.150077107631));
#129985=CARTESIAN_POINT('Ctrl Pts',(81.8818028862442,9.76042436729594,140.113019595841));
#129986=CARTESIAN_POINT('Ctrl Pts',(82.1792335483859,8.34591351497726,140.038917711386));
#129987=CARTESIAN_POINT('Ctrl Pts',(80.6304328372915,6.81139143968391,139.927771454269));
#129988=CARTESIAN_POINT('Ctrl Pts',(78.5040710120652,7.28476689903274,139.816638336277));
#129989=CARTESIAN_POINT('Ctrl Pts',(77.7471978427393,9.32575105546619,139.705505218286));
#129990=CARTESIAN_POINT('Ctrl Pts',(79.052001832402,11.0696863673767,139.594372100294));
#129991=CARTESIAN_POINT('Ctrl Pts',(81.2245371200737,10.9188297783435,139.483238982303));
#129992=CARTESIAN_POINT('Ctrl Pts',(82.2762857547564,9.01204545951565,139.372105864311));
#129993=CARTESIAN_POINT('Ctrl Pts',(81.2447086479385,7.09410915124218,139.260972746319));
#129994=CARTESIAN_POINT('Ctrl Pts',(79.0739151359574,6.92058150399365,139.149839628328));
#129995=CARTESIAN_POINT('Ctrl Pts',(77.7507158599816,8.65018903028666,139.038706510336));
#129996=CARTESIAN_POINT('Ctrl Pts',(78.4861475554145,10.6999722259972,138.927573392345));
#129997=CARTESIAN_POINT('Ctrl Pts',(80.6071177683635,11.1938666447401,138.816440274353));
#129998=CARTESIAN_POINT('Ctrl Pts',(82.1724293290323,9.67985152240289,138.705307156362));
#129999=CARTESIAN_POINT('Ctrl Pts',(81.7494483427865,7.54360778660553,138.59417403837));
#130000=CARTESIAN_POINT('Ctrl Pts',(79.7253032382228,6.74031237896183,138.483040920378));
#130001=CARTESIAN_POINT('Ctrl Pts',(77.952571489165,8.00517160626547,138.371907802387));
#130002=CARTESIAN_POINT('Ctrl Pts',(78.0537268663851,10.1805371390946,138.260774684395));
#130003=CARTESIAN_POINT('Ctrl Pts',(79.936188036109,11.2754285172347,138.149641566404));
#130004=CARTESIAN_POINT('Ctrl Pts',(81.8770524189507,10.2877582050546,138.038508448412));
#130005=CARTESIAN_POINT('Ctrl Pts',(82.0999645517432,8.12148087415575,137.927375330421));
#130006=CARTESIAN_POINT('Ctrl Pts',(80.4009064711046,6.75925883703344,137.816242212429));
#130007=CARTESIAN_POINT('Ctrl Pts',(78.3349230095036,7.44785130128577,137.705109094438));
#130008=CARTESIAN_POINT('Ctrl Pts',(77.792883545948,9.55703134935834,137.593975976446));
#130009=CARTESIAN_POINT('Ctrl Pts',(79.2708839326172,11.1563943805989,137.482842858454));
#130010=CARTESIAN_POINT('Ctrl Pts',(81.4162000417767,10.782140400524,137.371709740463));
#130011=CARTESIAN_POINT('Ctrl Pts',(82.265354131664,8.77680138120206,137.260576622471));
#130012=CARTESIAN_POINT('Ctrl Pts',(81.0411669567573,6.9757425229748,137.14944350448));
#130013=CARTESIAN_POINT('Ctrl Pts',(78.8640628031065,7.02736378164124,137.038310386488));
#130014=CARTESIAN_POINT('Ctrl Pts',(77.7266130820991,8.88441934959255,136.927177268497));
#130015=CARTESIAN_POINT('Ctrl Pts',(78.6698565479946,10.8472588779883,136.816044150505));
#130016=CARTESIAN_POINT('Ctrl Pts',(80.8304996551003,11.1194143738573,136.704911032514));
#130017=CARTESIAN_POINT('Ctrl Pts',(82.2310367897109,9.45179841543078,136.593777914522));
#130018=CARTESIAN_POINT('Ctrl Pts',(81.5896412416254,7.37067876459188,136.482644796531));
#130019=CARTESIAN_POINT('Ctrl Pts',(79.493343461535,6.78077803785633,136.371511678539));
#130020=CARTESIAN_POINT('Ctrl Pts',(77.8607576872547,8.22199659860045,136.260378560547));
#130021=CARTESIAN_POINT('Ctrl Pts',(78.1860906773558,10.3752744942207,136.149245442556));
#130022=CARTESIAN_POINT('Ctrl Pts',(80.1715848743162,11.2698470424537,136.038112324564));
#130023=CARTESIAN_POINT('Ctrl Pts',(82.0000378407876,10.086966237124,135.926979206573));
#130024=CARTESIAN_POINT('Ctrl Pts',(81.9979774546478,7.90925114900429,135.815846088581));
#130025=CARTESIAN_POINT('Ctrl Pts',(80.1672894623882,6.7298323407723,135.70471297059));
#130026=CARTESIAN_POINT('Ctrl Pts',(78.1834915697017,7.62816032719385,135.593579852598));
#130027=CARTESIAN_POINT('Ctrl Pts',(77.8622336894994,9.78204997725095,135.482446734607));
#130028=CARTESIAN_POINT('Ctrl Pts',(79.4975436783292,11.2201767069408,135.371313616615));
#130029=CARTESIAN_POINT('Ctrl Pts',(81.5927214692403,10.6263103291348,135.260180498623));
#130030=CARTESIAN_POINT('Ctrl Pts',(82.2301778825965,8.54398072715382,135.149047380632));
#130031=CARTESIAN_POINT('Ctrl Pts',(80.8264877188542,6.87901791242533,135.03791426264));
#130032=CARTESIAN_POINT('Ctrl Pts',(78.666363464577,7.15526138528666,134.926781144649));
#130033=CARTESIAN_POINT('Ctrl Pts',(77.7268358589415,9.11988224653797,134.815648026657));
#130034=CARTESIAN_POINT('Ctrl Pts',(78.8677975460713,10.9747821572384,134.704514908666));
#130035=CARTESIAN_POINT('Ctrl Pts',(81.0449954820912,11.022283710966,134.593381790674));
#130036=CARTESIAN_POINT('Ctrl Pts',(82.2657724222796,9.21891161610627,134.482248672683));
#130037=CARTESIAN_POINT('Ctrl Pts',(81.4128252616645,7.21518299390877,134.371115554691));
#130038=CARTESIAN_POINT('Ctrl Pts',(79.2668048133133,6.84498914539877,134.259982436699));
#130039=CARTESIAN_POINT('Ctrl Pts',(77.7918334580994,8.44714605142053,134.148849318708));
#130040=CARTESIAN_POINT('Ctrl Pts',(78.3378630346208,10.5552966513015,134.037716200716));
#130041=CARTESIAN_POINT('Ctrl Pts',(80.405145782931,11.2399785400318,133.926583082725));
#130042=CARTESIAN_POINT('Ctrl Pts',(82.1016231643198,9.87454390422866,133.815449964733));
#130043=CARTESIAN_POINT('Ctrl Pts',(81.8746123066417,7.70869226556286,133.704316846742));
#130044=CARTESIAN_POINT('Ctrl Pts',(79.9318824819036,6.72469629083107,133.59318372875));
#130045=CARTESIAN_POINT('Ctrl Pts',(78.0514964908067,7.82314782581201,133.482050610758));
#130046=CARTESIAN_POINT('Ctrl Pts',(77.9544576036744,9.99870079106,133.370917492767));
#130047=CARTESIAN_POINT('Ctrl Pts',(79.7295796294233,11.2602034838498,133.259784374775));
#130048=CARTESIAN_POINT('Ctrl Pts',(81.7522010219662,10.453078987478,133.148651256784));
#130049=CARTESIAN_POINT('Ctrl Pts',(82.1711390732453,8.31603940913473,133.037518138792));
#130050=CARTESIAN_POINT('Ctrl Pts',(80.6029651894892,6.80498748397788,132.926385020801));
#130051=CARTESIAN_POINT('Ctrl Pts',(78.482933831834,7.30289740833519,132.815251902809));
#130052=CARTESIAN_POINT('Ctrl Pts',(77.7513811424265,9.35406242189131,132.704118784817));
#130053=CARTESIAN_POINT('Ctrl Pts',(79.0778529362468,11.0811755711711,132.592985666826));
#130054=CARTESIAN_POINT('Ctrl Pts',(81.2483100181675,10.9035149234434,132.481852548834));
#130055=CARTESIAN_POINT('Ctrl Pts',(82.2762646384599,8.98368249616185,132.370719430843));
#130056=CARTESIAN_POINT('Ctrl Pts',(81.2208922687267,7.07878449064595,132.259586312851));
#130057=CARTESIAN_POINT('Ctrl Pts',(79.0481112408112,6.93225853759174,132.14845319486));
#130058=CARTESIAN_POINT('Ctrl Pts',(77.7465362712657,8.67821095645413,132.037320076868));
#130059=CARTESIAN_POINT('Ctrl Pts',(78.5074200017588,10.7186773734432,131.926186958876));
#130060=CARTESIAN_POINT('Ctrl Pts',(80.634371693951,11.1861426118154,131.815053840885));
#130061=CARTESIAN_POINT('Ctrl Pts',(82.1807214433505,9.65276408603656,131.703920722893));
#130062=CARTESIAN_POINT('Ctrl Pts',(81.7311890951541,7.52195017634236,131.592787604902));
#130063=CARTESIAN_POINT('Ctrl Pts',(79.6972043487107,6.74390564038746,131.48165448691));
#130064=CARTESIAN_POINT('Ctrl Pts',(77.9403500990677,8.03072746206706,131.370521368919));
#130065=CARTESIAN_POINT('Ctrl Pts',(78.0685685082022,10.2046656592093,131.259388250927));
#130066=CARTESIAN_POINT('Ctrl Pts',(79.9645090340951,11.2760464328285,131.148255132935));
#130067=CARTESIAN_POINT('Ctrl Pts',(81.892932298994,10.2642999207466,131.037122014944));
#130068=CARTESIAN_POINT('Ctrl Pts',(82.0888693981082,8.09541637123634,130.925988896952));
#130069=CARTESIAN_POINT('Ctrl Pts',(80.3729910492246,6.75444333747484,130.814855778961));
#130070=CARTESIAN_POINT('Ctrl Pts',(78.3157365248911,7.46869219737679,130.703722660969));
#130071=CARTESIAN_POINT('Ctrl Pts',(77.7999864016918,9.58445412383093,130.592589542978));
#130072=CARTESIAN_POINT('Ctrl Pts',(79.2977749538362,11.1653008492713,130.481456424986));
#130073=CARTESIAN_POINT('Ctrl Pts',(81.4382682469794,10.7643785681889,130.370323306995));
#130074=CARTESIAN_POINT('Ctrl Pts',(82.2624003183689,8.74862848409216,130.259190189003));
#130075=CARTESIAN_POINT('Ctrl Pts',(81.0158976646619,6.96294164833859,130.148057071012));
#130076=CARTESIAN_POINT('Ctrl Pts',(78.8395991555924,7.04165459191484,130.03692395302));
#130077=CARTESIAN_POINT('Ctrl Pts',(77.725358113977,8.91271456426536,129.925790835029));
#130078=CARTESIAN_POINT('Ctrl Pts',(78.6929323848621,10.8636774922421,129.814657717037));
#130079=CARTESIAN_POINT('Ctrl Pts',(80.8568405250446,11.1088969261305,129.703524599046));
#130080=CARTESIAN_POINT('Ctrl Pts',(82.2364237507125,9.42403736149622,129.592391481054));
#130081=CARTESIAN_POINT('Ctrl Pts',(81.5693704423849,7.35094615016893,129.481258363063));
#130082=CARTESIAN_POINT('Ctrl Pts',(79.4655042135082,6.7874120211574,129.370125245071));
#130083=CARTESIAN_POINT('Ctrl Pts',(77.8517773994617,8.24835660973194,129.258992127079));
#130084=CARTESIAN_POINT('Ctrl Pts',(78.2022407380443,10.3983971641407,129.147859009088));
#130085=CARTESIAN_POINT('Ctrl Pts',(80.2020916075274,11.2661611476506,129.036725891096));
#130086=CARTESIAN_POINT('Ctrl Pts',(81.4046780597132,10.4649030948587,128.962637145768));
#130087=CARTESIAN_POINT('Ctrl Pts',(81.7034360011341,9.89849442228607,128.925592773105));
#130088=CARTESIAN_POINT('Ctrl Pts',(81.5667024019587,10.3334530939303,140.225980476683));
#130089=CARTESIAN_POINT('Ctrl Pts',(82.0102629662079,9.81233425421511,140.188922964893));
#130090=CARTESIAN_POINT('Ctrl Pts',(82.327997543771,8.30126271611657,140.114821080439));
#130091=CARTESIAN_POINT('Ctrl Pts',(80.6734689348986,6.66198746505808,140.00367482332));
#130092=CARTESIAN_POINT('Ctrl Pts',(78.4019523689201,7.16767759976703,139.892541705329));
#130093=CARTESIAN_POINT('Ctrl Pts',(77.5934117329509,9.34798824456784,139.781408587337));
#130094=CARTESIAN_POINT('Ctrl Pts',(78.9872873390269,11.2109721939615,139.670275469346));
#130095=CARTESIAN_POINT('Ctrl Pts',(81.3081293695664,11.0498174756014,139.559142351354));
#130096=CARTESIAN_POINT('Ctrl Pts',(82.4316749574265,9.01286773516624,139.448009233363));
#130097=CARTESIAN_POINT('Ctrl Pts',(81.3296778939815,6.96400472180219,139.336876115371));
#130098=CARTESIAN_POINT('Ctrl Pts',(79.010696540345,6.77863131982322,139.225742997379));
#130099=CARTESIAN_POINT('Ctrl Pts',(77.5971699054081,8.62630940640575,139.114609879388));
#130100=CARTESIAN_POINT('Ctrl Pts',(78.3828053788741,10.8160197513165,139.003476761396));
#130101=CARTESIAN_POINT('Ctrl Pts',(80.6485622775848,11.3436295591627,138.892343643405));
#130102=CARTESIAN_POINT('Ctrl Pts',(82.3207288387009,9.72626115519157,138.781210525413));
#130103=CARTESIAN_POINT('Ctrl Pts',(81.8688733238243,7.44418809628693,138.670077407422));
#130104=CARTESIAN_POINT('Ctrl Pts',(79.7065512380843,6.58605623735781,138.55894428943));
#130105=CARTESIAN_POINT('Ctrl Pts',(77.8128050810336,7.93726027721854,138.447811171439));
#130106=CARTESIAN_POINT('Ctrl Pts',(77.9208657658932,10.2611257578052,138.336678053447));
#130107=CARTESIAN_POINT('Ctrl Pts',(79.9318319528847,11.4307592011295,138.225544935455));
#130108=CARTESIAN_POINT('Ctrl Pts',(82.0051882112789,10.3756662017978,138.114411817464));
#130109=CARTESIAN_POINT('Ctrl Pts',(82.2433172993713,8.06150932347929,138.003278699472));
#130110=CARTESIAN_POINT('Ctrl Pts',(80.4282740969664,6.60629606336752,137.892145581481));
#130111=CARTESIAN_POINT('Ctrl Pts',(78.2212575852933,7.34189485525748,137.781012463489));
#130112=CARTESIAN_POINT('Ctrl Pts',(77.6422161417002,9.59505674096755,137.669879345498));
#130113=CARTESIAN_POINT('Ctrl Pts',(79.2211112869253,11.3035992746874,137.558746227506));
#130114=CARTESIAN_POINT('Ctrl Pts',(81.5128760390032,10.9037970841391,137.447613109514));
#130115=CARTESIAN_POINT('Ctrl Pts',(82.4199970940205,8.7615648691167,137.336479991523));
#130116=CARTESIAN_POINT('Ctrl Pts',(81.1122415584055,6.83755787076364,137.225346873531));
#130117=CARTESIAN_POINT('Ctrl Pts',(78.78651877115,6.89270302189758,137.11421375554));
#130118=CARTESIAN_POINT('Ctrl Pts',(77.5714217666873,8.87652930983221,137.003080637548));
#130119=CARTESIAN_POINT('Ctrl Pts',(78.5790551492632,10.9733608331476,136.891947519557));
#130120=CARTESIAN_POINT('Ctrl Pts',(80.8871931870763,11.2640948512505,136.780814401565));
#130121=CARTESIAN_POINT('Ctrl Pts',(82.3833371004942,9.48264014757921,136.669681283574));
#130122=CARTESIAN_POINT('Ctrl Pts',(81.6981570923054,7.25945418431468,136.558548165582));
#130123=CARTESIAN_POINT('Ctrl Pts',(79.4587568744269,6.62928425877995,136.44741504759));
#130124=CARTESIAN_POINT('Ctrl Pts',(77.7147236681948,8.16888669007266,136.336281929599));
#130125=CARTESIAN_POINT('Ctrl Pts',(78.0622653084306,10.4691567349117,136.225148811607));
#130126=CARTESIAN_POINT('Ctrl Pts',(80.1832980068851,11.4247967105141,136.114015693616));
#130127=CARTESIAN_POINT('Ctrl Pts',(82.136569154899,10.1611672975854,136.002882575624));
#130128=CARTESIAN_POINT('Ctrl Pts',(82.134368117807,7.83479187080711,135.891749457633));
#130129=CARTESIAN_POINT('Ctrl Pts',(80.1787093713873,6.57486078601119,135.780616339641));
#130130=CARTESIAN_POINT('Ctrl Pts',(78.0594887743418,7.53451256240715,135.66948322165));
#130131=CARTESIAN_POINT('Ctrl Pts',(77.7163004287961,9.83543612271155,135.558350103658));
#130132=CARTESIAN_POINT('Ctrl Pts',(79.4632438163555,11.371735661065,135.447216985666));
#130133=CARTESIAN_POINT('Ctrl Pts',(81.7014475897037,10.7373293718058,135.336083867675));
#130134=CARTESIAN_POINT('Ctrl Pts',(82.3824195606306,8.51285086085221,135.224950749683));
#130135=CARTESIAN_POINT('Ctrl Pts',(80.8829073785483,6.73423041604996,135.113817631692));
#130136=CARTESIAN_POINT('Ctrl Pts',(78.5753236127225,7.0293314743006,135.0026845137));
#130137=CARTESIAN_POINT('Ctrl Pts',(77.5716597512496,9.12806593202865,134.891551395709));
#130138=CARTESIAN_POINT('Ctrl Pts',(78.7905084639736,11.1095894081381,134.780418277717));
#130139=CARTESIAN_POINT('Ctrl Pts',(81.1163314355921,11.1603336252896,134.669285159726));
#130140=CARTESIAN_POINT('Ctrl Pts',(82.4204439389795,9.23385547867315,134.558152041734));
#130141=CARTESIAN_POINT('Ctrl Pts',(81.5092708816678,7.09334359351305,134.447018923742));
#130142=CARTESIAN_POINT('Ctrl Pts',(79.2167537091307,6.69787869683471,134.335885805751));
#130143=CARTESIAN_POINT('Ctrl Pts',(77.6410943702708,8.40940582742477,134.224752687759));
#130144=CARTESIAN_POINT('Ctrl Pts',(78.2243983093599,10.6614679903157,134.113619569768));
#130145=CARTESIAN_POINT('Ctrl Pts',(80.4328028027243,11.3928892537269,134.002486451776));
#130146=CARTESIAN_POINT('Ctrl Pts',(82.2450891360831,9.93424408892397,133.891353333785));
#130147=CARTESIAN_POINT('Ctrl Pts',(82.0025815262513,7.62054196244875,133.780220215793));
#130148=CARTESIAN_POINT('Ctrl Pts',(79.9272324827536,6.56937412687972,133.669087097802));
#130149=CARTESIAN_POINT('Ctrl Pts',(77.9184831351412,7.74281075889249,133.55795397981));
#130150=CARTESIAN_POINT('Ctrl Pts',(77.8148199499532,10.0668764668532,133.446820861818));
#130151=CARTESIAN_POINT('Ctrl Pts',(79.7111195544165,11.4144948405014,133.335687743827));
#130152=CARTESIAN_POINT('Ctrl Pts',(81.8718139129015,10.5522725025318,133.224554625835));
#130153=CARTESIAN_POINT('Ctrl Pts',(82.3193505044213,8.26934927339481,133.113421507844));
#130154=CARTESIAN_POINT('Ctrl Pts',(80.6441262255484,6.65514634737931,133.002288389852));
#130155=CARTESIAN_POINT('Ctrl Pts',(78.3793722724926,7.18704577678262,132.891155271861));
#130156=CARTESIAN_POINT('Ctrl Pts',(77.597880602937,9.37823226845748,132.780022153869));
#130157=CARTESIAN_POINT('Ctrl Pts',(79.0149031520722,11.2232457009628,132.668889035877));
#130158=CARTESIAN_POINT('Ctrl Pts',(81.333525109464,11.0334571618495,132.557755917886));
#130159=CARTESIAN_POINT('Ctrl Pts',(82.4316523996396,8.98256859211635,132.446622799894));
#130160=CARTESIAN_POINT('Ctrl Pts',(81.3042357047549,6.94763393297434,132.335489681903));
#130161=CARTESIAN_POINT('Ctrl Pts',(78.98313115867,6.79110547871043,132.224356563911));
#130162=CARTESIAN_POINT('Ctrl Pts',(77.5927049997205,8.65624423158219,132.11322344592));
#130163=CARTESIAN_POINT('Ctrl Pts',(78.40552997527,10.836001793784,132.002090327928));
#130164=CARTESIAN_POINT('Ctrl Pts',(80.6776766751088,11.3353782500316,131.890957209937));
#130165=CARTESIAN_POINT('Ctrl Pts',(82.3295870089414,9.69732461216955,131.779824091945));
#130166=CARTESIAN_POINT('Ctrl Pts',(81.8493676202382,7.42105204300162,131.668690973954));
#130167=CARTESIAN_POINT('Ctrl Pts',(79.6765341957092,6.58989479049461,131.557557855962));
#130168=CARTESIAN_POINT('Ctrl Pts',(77.7997494054962,7.96456068730038,131.44642473797));
#130169=CARTESIAN_POINT('Ctrl Pts',(77.9367205629714,10.2869013960352,131.335291619979));
#130170=CARTESIAN_POINT('Ctrl Pts',(79.9620862658279,11.4314192983393,131.224158501987));
#130171=CARTESIAN_POINT('Ctrl Pts',(82.022152121257,10.3506065525964,131.113025383996));
#130172=CARTESIAN_POINT('Ctrl Pts',(82.2314647421138,8.03366554380687,131.001892266004));
#130173=CARTESIAN_POINT('Ctrl Pts',(80.3984530465246,6.60115183678714,130.890759148013));
#130174=CARTESIAN_POINT('Ctrl Pts',(78.2007613474834,7.36415844189591,130.779626030021));
#130175=CARTESIAN_POINT('Ctrl Pts',(77.6498038693843,9.62435151373887,130.668492912029));
#130176=CARTESIAN_POINT('Ctrl Pts',(79.2498380066448,11.3131137377922,130.557359794038));
#130177=CARTESIAN_POINT('Ctrl Pts',(81.5364507162309,10.8848227515901,130.446226676046));
#130178=CARTESIAN_POINT('Ctrl Pts',(82.416841640535,8.73146876706222,130.335093558055));
#130179=CARTESIAN_POINT('Ctrl Pts',(81.0852472741196,6.82388315254297,130.223960440063));
#130180=CARTESIAN_POINT('Ctrl Pts',(78.7603851282614,6.90796938526652,130.112827322072));
#130181=CARTESIAN_POINT('Ctrl Pts',(77.5700811289627,8.90675607938041,130.00169420408));
#130182=CARTESIAN_POINT('Ctrl Pts',(78.6037062434921,10.9909002536853,129.890561086088));
#130183=CARTESIAN_POINT('Ctrl Pts',(80.9153321997933,11.2528594366284,129.779427968097));
#130184=CARTESIAN_POINT('Ctrl Pts',(82.3890917989704,9.45298400291311,129.668294850105));
#130185=CARTESIAN_POINT('Ctrl Pts',(81.6765025198171,7.23837453548914,129.557161732114));
#130186=CARTESIAN_POINT('Ctrl Pts',(79.4290171977985,6.63637110674158,129.446028614122));
#130187=CARTESIAN_POINT('Ctrl Pts',(77.7051303467539,8.19704615063774,129.334895496131));
#130188=CARTESIAN_POINT('Ctrl Pts',(78.0795178427644,10.4938578592218,129.223762378139));
#130189=CARTESIAN_POINT('Ctrl Pts',(80.2158872628815,11.4208592004411,129.112629260147));
#130190=CARTESIAN_POINT('Ctrl Pts',(81.5005675161451,10.5649037751,129.03854051482));
#130191=CARTESIAN_POINT('Ctrl Pts',(81.8197199788653,9.95982957389915,129.001496142156));
#130192=CARTESIAN_POINT('Ctrl Pts',(81.2690708798525,10.0793586530483,140.));
#130193=CARTESIAN_POINT('Ctrl Pts',(81.3143922493461,10.037078625412,140.));
#130194=CARTESIAN_POINT('Ctrl Pts',(81.3569831621752,9.99222888973338,140.));
#130195=CARTESIAN_POINT('Ctrl Pts',(81.3968454123345,9.94515461985499,140.));
#130196=CARTESIAN_POINT('Ctrl Pts',(81.4393469149689,9.89496359458048,140.));
#130197=CARTESIAN_POINT('Ctrl Pts',(81.4787471926403,9.84224348169698,140.));
#130198=CARTESIAN_POINT('Ctrl Pts',(81.5150195594611,9.78735790922335,140.));
#130199=CARTESIAN_POINT('Ctrl Pts',(81.5467578804294,9.73933303330892,140.));
#130200=CARTESIAN_POINT('Ctrl Pts',(81.5761011504664,9.68964900085175,140.));
#130201=CARTESIAN_POINT('Ctrl Pts',(81.6030085858433,9.63852184375101,140.));
#130202=CARTESIAN_POINT('Ctrl Pts',(81.6165037566978,9.61287949951723,140.));
#130203=CARTESIAN_POINT('Ctrl Pts',(81.6293858497916,9.58687379163623,140.));
#130204=CARTESIAN_POINT('Ctrl Pts',(81.6416473796641,9.56053013392403,140.));
#130205=CARTESIAN_POINT('Ctrl Pts',(81.6472597696334,9.54847202357099,140.));
#130206=CARTESIAN_POINT('Ctrl Pts',(81.6527427313326,9.53634140530439,140.));
#130207=CARTESIAN_POINT('Ctrl Pts',(81.6580870166726,9.5241607216166,140.));
#130208=CARTESIAN_POINT('Ctrl Pts',(81.6852360971005,9.46228259571773,140.));
#130209=CARTESIAN_POINT('Ctrl Pts',(81.7088626185403,9.39900435672435,140.));
#130210=CARTESIAN_POINT('Ctrl Pts',(81.7289426467891,9.33469347024794,140.));
#130211=CARTESIAN_POINT('Ctrl Pts',(81.7490226750378,9.27038258377154,140.));
#130212=CARTESIAN_POINT('Ctrl Pts',(81.7655566446948,9.20503811827903,140.));
#130213=CARTESIAN_POINT('Ctrl Pts',(81.7784823019253,9.13899201824649,140.));
#130214=CARTESIAN_POINT('Ctrl Pts',(81.7914980138043,9.07248576688647,140.));
#130215=CARTESIAN_POINT('Ctrl Pts',(81.800855473018,9.00526711378445,140.));
#130216=CARTESIAN_POINT('Ctrl Pts',(81.8064450545183,8.93765313125535,140.));
#130217=CARTESIAN_POINT('Ctrl Pts',(81.8076966254415,8.92251359092883,140.));
#130218=CARTESIAN_POINT('Ctrl Pts',(81.8087590894417,8.90735417722168,140.));
#130219=CARTESIAN_POINT('Ctrl Pts',(81.8096308609416,8.8921783781706,140.));
#130220=CARTESIAN_POINT('Ctrl Pts',(81.8102881062911,8.8807370505378,140.));
#130221=CARTESIAN_POINT('Ctrl Pts',(81.8108368598249,8.86928658800379,140.));
#130222=CARTESIAN_POINT('Ctrl Pts',(81.8112761266604,8.85784267362559,140.));
#130223=CARTESIAN_POINT('Ctrl Pts',(81.8139681483841,8.78770929767787,140.));
#130224=CARTESIAN_POINT('Ctrl Pts',(81.8125602359496,8.71769045278861,140.));
#130225=CARTESIAN_POINT('Ctrl Pts',(81.8069981196216,8.64814732532177,140.));
#130226=CARTESIAN_POINT('Ctrl Pts',(81.8020258450083,8.58597898743637,140.));
#130227=CARTESIAN_POINT('Ctrl Pts',(81.793733374456,8.52418985638038,140.));
#130228=CARTESIAN_POINT('Ctrl Pts',(81.7820488148449,8.46302583141971,140.));
#130229=CARTESIAN_POINT('Ctrl Pts',(81.769316661712,8.39637807078986,140.));
#130230=CARTESIAN_POINT('Ctrl Pts',(81.7525579964158,8.33047169570494,140.));
#130231=CARTESIAN_POINT('Ctrl Pts',(81.7320178331077,8.26552006538765,140.));
#130232=CARTESIAN_POINT('Ctrl Pts',(81.7240897912002,8.2404501942579,140.));
#130233=CARTESIAN_POINT('Ctrl Pts',(81.7155978327267,8.2155226071289,140.));
#130234=CARTESIAN_POINT('Ctrl Pts',(81.7065540378326,8.19074989375515,140.));
#130235=CARTESIAN_POINT('Ctrl Pts',(81.7025873788784,8.17988444330244,140.));
#130236=CARTESIAN_POINT('Ctrl Pts',(81.6985146637445,8.16904935856075,140.));
#130237=CARTESIAN_POINT('Ctrl Pts',(81.6943419939996,8.15825823120868,140.));
#130238=CARTESIAN_POINT('Ctrl Pts',(81.6688285338256,8.09227673380644,140.));
#130239=CARTESIAN_POINT('Ctrl Pts',(81.6395390164229,8.0278166187107,140.));
#130240=CARTESIAN_POINT('Ctrl Pts',(81.6067965122877,7.96510411531983,140.));
#130241=CARTESIAN_POINT('Ctrl Pts',(81.5740540081525,7.90239161192896,140.));
#130242=CARTESIAN_POINT('Ctrl Pts',(81.5378580152312,7.84142593331998,140.));
#130243=CARTESIAN_POINT('Ctrl Pts',(81.4984773919093,7.78243697400106,140.));
#130244=CARTESIAN_POINT('Ctrl Pts',(81.4582451906682,7.72217242046859,140.));
#130245=CARTESIAN_POINT('Ctrl Pts',(81.4146887664041,7.66397006974518,140.));
#130246=CARTESIAN_POINT('Ctrl Pts',(81.3680445980429,7.60809196964191,140.));
#130247=CARTESIAN_POINT('Ctrl Pts',(81.3573469119398,7.59527651176268,140.));
#130248=CARTESIAN_POINT('Ctrl Pts',(81.3464866201888,7.58258341222455,140.));
#130249=CARTESIAN_POINT('Ctrl Pts',(81.3354662478833,7.57001603639548,140.));
#130250=CARTESIAN_POINT('Ctrl Pts',(81.3227850921236,7.55555474180744,140.));
#130251=CARTESIAN_POINT('Ctrl Pts',(81.3098875424283,7.54125535227706,140.));
#130252=CARTESIAN_POINT('Ctrl Pts',(81.2968012384801,7.52714834847591,140.));
#130253=CARTESIAN_POINT('Ctrl Pts',(81.2459376695597,7.47231754499339,140.));
#130254=CARTESIAN_POINT('Ctrl Pts',(81.1921776208598,7.42033184651139,140.));
#130255=CARTESIAN_POINT('Ctrl Pts',(81.1358057253517,7.37145486543547,140.));
#130256=CARTESIAN_POINT('Ctrl Pts',(81.0936523414515,7.33490597651479,140.));
#130257=CARTESIAN_POINT('Ctrl Pts',(81.050037349269,7.30009557097858,140.));
#130258=CARTESIAN_POINT('Ctrl Pts',(81.005063375939,7.26714361886256,140.));
#130259=CARTESIAN_POINT('Ctrl Pts',(80.9910000906874,7.25683959927322,140.));
#130260=CARTESIAN_POINT('Ctrl Pts',(80.9768038313551,7.24671737660939,140.));
#130261=CARTESIAN_POINT('Ctrl Pts',(80.9624774943437,7.23678084594061,140.));
#130262=CARTESIAN_POINT('Ctrl Pts',(80.9486909780282,7.22721872674186,140.));
#130263=CARTESIAN_POINT('Ctrl Pts',(80.9347910474626,7.21783351877335,140.));
#130264=CARTESIAN_POINT('Ctrl Pts',(80.9207856469263,7.20863142672219,140.));
#130265=CARTESIAN_POINT('Ctrl Pts',(80.8578389195166,7.16727298228203,140.));
#130266=CARTESIAN_POINT('Ctrl Pts',(80.7927341061665,7.12958962170196,140.));
#130267=CARTESIAN_POINT('Ctrl Pts',(80.7257321762408,7.09586020443097,140.));
#130268=CARTESIAN_POINT('Ctrl Pts',(80.6745101548169,7.07007454518227,140.));
#130269=CARTESIAN_POINT('Ctrl Pts',(80.6221784116493,7.04660013039904,140.));
#130270=CARTESIAN_POINT('Ctrl Pts',(80.5688396787843,7.02557680443979,140.));
#130271=CARTESIAN_POINT('Ctrl Pts',(80.5565366069901,7.02072757996939,140.));
#130272=CARTESIAN_POINT('Ctrl Pts',(80.5441799163443,7.0160088282093,140.));
#130273=CARTESIAN_POINT('Ctrl Pts',(80.5317714801634,7.01141998135025,140.));
#130274=CARTESIAN_POINT('Ctrl Pts',(79.4691328668544,7.01221613569387,139.998440578768));
#130275=CARTESIAN_POINT('Ctrl Pts',(78.8081758252084,7.18873450679631,139.961396206104));
#130276=CARTESIAN_POINT('Ctrl Pts',(77.687752744404,8.25079161293192,139.887307460776));
#130277=CARTESIAN_POINT('Ctrl Pts',(78.116148705963,10.5399996648632,139.776174342785));
#130278=CARTESIAN_POINT('Ctrl Pts',(80.2721800561424,11.416134581678,139.665041224793));
#130279=CARTESIAN_POINT('Ctrl Pts',(82.177427932532,10.0826818014991,139.553908106802));
#130280=CARTESIAN_POINT('Ctrl Pts',(82.090625956823,7.75746322787376,139.44277498881));
#130281=CARTESIAN_POINT('Ctrl Pts',(80.0900009572206,6.56988012499553,139.331641870819));
#130282=CARTESIAN_POINT('Ctrl Pts',(78.00719905694,7.60623453967738,139.220508752827));
#130283=CARTESIAN_POINT('Ctrl Pts',(77.7481914138751,9.91831763289069,139.109375634835));
#130284=CARTESIAN_POINT('Ctrl Pts',(79.5501743653611,11.3898715478751,138.998242516844));
#130285=CARTESIAN_POINT('Ctrl Pts',(81.7638325852258,10.6741447881572,138.887109398852));
#130286=CARTESIAN_POINT('Ctrl Pts',(82.3631729758628,8.426163172343,138.775976280861));
#130287=CARTESIAN_POINT('Ctrl Pts',(80.7996389804333,6.70338530479118,138.664843162869));
#130288=CARTESIAN_POINT('Ctrl Pts',(78.5042465888265,7.08255681422626,138.553710044878));
#130289=CARTESIAN_POINT('Ctrl Pts',(77.5778252847861,9.21664915934671,138.442576926886));
#130290=CARTESIAN_POINT('Ctrl Pts',(78.8682742548729,11.1524550005147,138.331443808895));
#130291=CARTESIAN_POINT('Ctrl Pts',(81.1945228587917,11.1182496311054,138.220310690903));
#130292=CARTESIAN_POINT('Ctrl Pts',(82.4274972791361,9.14533866655995,138.109177572911));
#130293=CARTESIAN_POINT('Ctrl Pts',(81.4387305695618,7.03940811177544,137.99804445492));
#130294=CARTESIAN_POINT('Ctrl Pts',(79.1331810513629,6.72788838316243,137.886911336928));
#130295=CARTESIAN_POINT('Ctrl Pts',(77.62097833476,8.49589465433908,137.775778218937));
#130296=CARTESIAN_POINT('Ctrl Pts',(78.2861498922971,10.7252779701539,137.664645100945));
#130297=CARTESIAN_POINT('Ctrl Pts',(80.519904520617,11.3756189858562,137.553511982953));
#130298=CARTESIAN_POINT('Ctrl Pts',(82.2778220705136,9.85170000007408,137.442378864962));
#130299=CARTESIAN_POINT('Ctrl Pts',(81.9509872062522,7.54827165270313,137.331245746971));
#130300=CARTESIAN_POINT('Ctrl Pts',(79.8385320612198,6.5735222277288,137.220112628979));
#130301=CARTESIAN_POINT('Ctrl Pts',(77.8738587288312,7.81958076542601,137.108979510988));
#130302=CARTESIAN_POINT('Ctrl Pts',(77.8551135720406,10.1460054473293,136.997846392996));
#130303=CARTESIAN_POINT('Ctrl Pts',(79.7994528959673,11.4235608375628,136.886713275004));
#130304=CARTESIAN_POINT('Ctrl Pts',(81.9273408229903,10.4829779588041,136.775580157013));
#130305=CARTESIAN_POINT('Ctrl Pts',(82.2912505694032,8.18511528271877,136.664447039021));
#130306=CARTESIAN_POINT('Ctrl Pts',(80.5581176119615,6.63306717343212,136.55331392103));
#130307=CARTESIAN_POINT('Ctrl Pts',(78.3141734487542,7.24732914859208,136.442180803038));
#130308=CARTESIAN_POINT('Ctrl Pts',(77.6131640987352,9.46570447141138,136.331047685047));
#130309=CARTESIAN_POINT('Ctrl Pts',(79.0966809104985,11.2578487320464,136.219914567055));
#130310=CARTESIAN_POINT('Ctrl Pts',(81.406950907267,10.9835209650521,136.108781449063));
#130311=CARTESIAN_POINT('Ctrl Pts',(82.4295240566564,8.89379674021785,135.997648331072));
#130312=CARTESIAN_POINT('Ctrl Pts',(81.228501164259,6.90127391885572,135.88651521308));
#130313=CARTESIAN_POINT('Ctrl Pts',(78.903105652997,6.82958781201049,135.775382095089));
#130314=CARTESIAN_POINT('Ctrl Pts',(77.5816310214531,8.74434836620449,135.664248977097));
#130315=CARTESIAN_POINT('Ctrl Pts',(78.4735428651507,10.8930913579985,135.553115859106));
#130316=CARTESIAN_POINT('Ctrl Pts',(80.7625283594298,11.3092026276025,135.441982741114));
#130317=CARTESIAN_POINT('Ctrl Pts',(82.3536178863351,9.61184076309495,135.330849623122));
#130318=CARTESIAN_POINT('Ctrl Pts',(81.7905836861691,7.35449815038521,135.219716505131));
#130319=CARTESIAN_POINT('Ctrl Pts',(79.5887368197341,6.60318359676461,135.108583387139));
#130320=CARTESIAN_POINT('Ctrl Pts',(77.7632942030395,8.04552975315939,134.997450269148));
#130321=CARTESIAN_POINT('Ctrl Pts',(77.9849727676055,10.3614446470455,134.886317151156));
#130322=CARTESIAN_POINT('Ctrl Pts',(80.050883565958,11.4313118140165,134.775184033165));
#130323=CARTESIAN_POINT('Ctrl Pts',(82.070223721988,10.2759467132991,134.664050915173));
#130324=CARTESIAN_POINT('Ctrl Pts',(82.1948136444431,7.95278495979708,134.552917797182));
#130325=CARTESIAN_POINT('Ctrl Pts',(80.3106237324807,6.58807562907116,134.44178467919));
#130326=CARTESIAN_POINT('Ctrl Pts',(78.1421387545208,7.43085441503748,134.330651561199));
#130327=CARTESIAN_POINT('Ctrl Pts',(77.6740415131297,9.70977700132987,134.219518443207));
#130328=CARTESIAN_POINT('Ctrl Pts',(79.3347530277562,11.3390837394547,134.108385325215));
#130329=CARTESIAN_POINT('Ctrl Pts',(81.6043247552459,10.8275689737917,133.997252207224));
#130330=CARTESIAN_POINT('Ctrl Pts',(82.4055553211276,8.64339115090071,133.886119089232));
#130331=CARTESIAN_POINT('Ctrl Pts',(81.0051269753784,6.78559578269294,133.774985971241));
#130332=CARTESIAN_POINT('Ctrl Pts',(78.6847668603508,6.95451031226528,133.663852853249));
#130333=CARTESIAN_POINT('Ctrl Pts',(77.5681598818021,8.995537513742,133.552719735258));
#130334=CARTESIAN_POINT('Ctrl Pts',(78.6772686957224,11.0406489582838,133.441586617266));
#130335=CARTESIAN_POINT('Ctrl Pts',(80.9969932615145,11.218078157044,133.330453499275));
#130336=CARTESIAN_POINT('Ctrl Pts',(82.4042303530961,9.36543492377197,133.219320381283));
#130337=CARTESIAN_POINT('Ctrl Pts',(81.6110211959397,7.17833126488543,133.108187263291));
#130338=CARTESIAN_POINT('Ctrl Pts',(79.3433420310828,6.65849053255848,132.9970541453));
#130339=CARTESIAN_POINT('Ctrl Pts',(77.6766620851849,8.2816914257486,132.885921027308));
#130340=CARTESIAN_POINT('Ctrl Pts',(78.1363924446149,10.5623165984436,132.774787909317));
#130341=CARTESIAN_POINT('Ctrl Pts',(80.3017697896119,11.4130481280609,132.663654791325));
#130342=CARTESIAN_POINT('Ctrl Pts',(82.1909555456132,10.0552630342281,132.552521673334));
#130343=CARTESIAN_POINT('Ctrl Pts',(82.0748925510988,7.73165967672142,132.441388555342));
#130344=CARTESIAN_POINT('Ctrl Pts',(80.0598062268449,6.56889130446804,132.33025543735));
#130345=CARTESIAN_POINT('Ctrl Pts',(77.9899828898302,7.63116929787119,132.219122319359));
#130346=CARTESIAN_POINT('Ctrl Pts',(77.7598063255501,9.94625502651435,132.107989201367));
#130347=CARTESIAN_POINT('Ctrl Pts',(79.5799431852807,11.3952909106561,131.996856083376));
#130348=CARTESIAN_POINT('Ctrl Pts',(81.7845325751376,10.6520622756351,131.885722965384));
#130349=CARTESIAN_POINT('Ctrl Pts',(82.3558475136698,8.39680122141269,131.774589847393));
#130350=CARTESIAN_POINT('Ctrl Pts',(80.7709980825209,6.69361143103145,131.663456729401));
#130351=CARTESIAN_POINT('Ctrl Pts',(78.4805008598881,7.10131923752851,131.55232361141));
#130352=CARTESIAN_POINT('Ctrl Pts',(77.580709057541,9.24677440920892,131.441190493418));
#130353=CARTESIAN_POINT('Ctrl Pts',(78.8951475473763,11.1663719285885,131.330057375426));
#130354=CARTESIAN_POINT('Ctrl Pts',(81.2207904898933,11.1032205914513,131.218924257435));
#130355=CARTESIAN_POINT('Ctrl Pts',(82.429117923205,9.11511898686653,131.107791139443));
#130356=CARTESIAN_POINT('Ctrl Pts',(81.4142210302046,7.02165595486222,130.996658021452));
#130357=CARTESIAN_POINT('Ctrl Pts',(79.104973374576,6.73885125901313,130.88552490346));
#130358=CARTESIAN_POINT('Ctrl Pts',(77.6148893401839,8.52553889053475,130.774391785469));
#130359=CARTESIAN_POINT('Ctrl Pts',(78.307752406047,10.7464720006261,130.663258667477));
#130360=CARTESIAN_POINT('Ctrl Pts',(80.5494271837866,11.3689652022709,130.552125549485));
#130361=CARTESIAN_POINT('Ctrl Pts',(82.288244357474,9.82328819493091,130.440992431494));
#130362=CARTESIAN_POINT('Ctrl Pts',(81.9327706811323,7.52410545653742,130.329859313502));
#130363=CARTESIAN_POINT('Ctrl Pts',(79.8083482832819,6.57571943513415,130.218726195511));
#130364=CARTESIAN_POINT('Ctrl Pts',(77.8593349635166,7.84613052780885,130.107593077519));
#130365=CARTESIAN_POINT('Ctrl Pts',(77.8695386886888,10.1726081270525,129.996459959528));
#130366=CARTESIAN_POINT('Ctrl Pts',(79.8296323383495,11.4258691267836,129.885326841536));
#130367=CARTESIAN_POINT('Ctrl Pts',(81.9456370655975,10.4588781737672,129.774193723544));
#130368=CARTESIAN_POINT('Ctrl Pts',(82.280951121822,8.15666663573472,129.663060605553));
#130369=CARTESIAN_POINT('Ctrl Pts',(80.5285815452698,6.62630260836619,129.551927487561));
#130370=CARTESIAN_POINT('Ctrl Pts',(78.2925711520252,7.2684488144164,129.44079436957));
#130371=CARTESIAN_POINT('Ctrl Pts',(77.6189849879312,9.49536050885278,129.329661251578));
#130372=CARTESIAN_POINT('Ctrl Pts',(79.1251739340349,11.2689362351057,129.218528133587));
#130373=CARTESIAN_POINT('Ctrl Pts',(81.4308590042111,10.9658155584414,129.107395015595));
#130374=CARTESIAN_POINT('Ctrl Pts',(82.429384248427,8.86366644097112,128.996261897604));
#130375=CARTESIAN_POINT('Ctrl Pts',(81.1993093722144,6.88573951185316,128.885115641378));
#130376=CARTESIAN_POINT('Ctrl Pts',(79.6553399314687,6.85926310844778,128.811013757815));
#130377=CARTESIAN_POINT('Ctrl Pts',(79.0485528000777,7.17575966835091,128.773956246917));
#130378=CARTESIAN_POINT('Ctrl Pts',(79.5030640075578,7.13926821666982,140.074365000815));
#130379=CARTESIAN_POINT('Ctrl Pts',(78.8843529912895,7.30450416075302,140.037320628152));
#130380=CARTESIAN_POINT('Ctrl Pts',(77.835543372364,8.29867835070604,139.963231882824));
#130381=CARTESIAN_POINT('Ctrl Pts',(78.2365577863739,10.4415683587053,139.852098764832));
#130382=CARTESIAN_POINT('Ctrl Pts',(80.2547832741512,11.2617038450006,139.740965646841));
#130383=CARTESIAN_POINT('Ctrl Pts',(82.0382544766191,10.0134806280791,139.629832528849));
#130384=CARTESIAN_POINT('Ctrl Pts',(81.9570005747449,7.83688176296831,139.518699410858));
#130385=CARTESIAN_POINT('Ctrl Pts',(80.0842484158553,6.7252047519253,139.407566292866));
#130386=CARTESIAN_POINT('Ctrl Pts',(78.1345718117616,7.69531907512722,139.296433174875));
#130387=CARTESIAN_POINT('Ctrl Pts',(77.8921190168525,9.85962203305674,139.185300056883));
#130388=CARTESIAN_POINT('Ctrl Pts',(79.5789256214626,11.2371194509922,139.074166938891));
#130389=CARTESIAN_POINT('Ctrl Pts',(81.6510946741933,10.5671394024057,138.9630338209));
#130390=CARTESIAN_POINT('Ctrl Pts',(82.212127356829,8.46284078322597,138.851900702908));
#130391=CARTESIAN_POINT('Ctrl Pts',(80.7485288983373,6.85017675504178,138.740767584917));
#130392=CARTESIAN_POINT('Ctrl Pts',(78.5998498316785,7.20511296898747,138.629634466925));
#130393=CARTESIAN_POINT('Ctrl Pts',(77.7326420853354,9.20280171494848,138.518501348934));
#130394=CARTESIAN_POINT('Ctrl Pts',(78.9406101428909,11.0148777256745,138.407368230942));
#130395=CARTESIAN_POINT('Ctrl Pts',(81.118173202419,10.9828586419285,138.296235112951));
#130396=CARTESIAN_POINT('Ctrl Pts',(82.2723402792148,9.13604913545734,138.185101994959));
#130397=CARTESIAN_POINT('Ctrl Pts',(81.3467720241138,7.16472217826751,138.073968876967));
#130398=CARTESIAN_POINT('Ctrl Pts',(79.188585038301,6.87311368371572,137.962835758976));
#130399=CARTESIAN_POINT('Ctrl Pts',(77.7730369457001,8.52811527668511,137.851702640984));
#130400=CARTESIAN_POINT('Ctrl Pts',(78.3956931009801,10.6150043331122,137.740569522993));
#130401=CARTESIAN_POINT('Ctrl Pts',(80.4866740711505,11.2237778620907,137.629436405001));
#130402=CARTESIAN_POINT('Ctrl Pts',(82.1322317780535,9.79726236260266,137.51830328701));
#130403=CARTESIAN_POINT('Ctrl Pts',(81.8262870369014,7.64106096991607,137.407170169018));
#130404=CARTESIAN_POINT('Ctrl Pts',(79.848852518087,6.72861406439414,137.296037051027));
#130405=CARTESIAN_POINT('Ctrl Pts',(78.0097541235979,7.89502896825616,137.184903933035));
#130406=CARTESIAN_POINT('Ctrl Pts',(77.9922070906181,10.0727568514897,137.073770815043));
#130407=CARTESIAN_POINT('Ctrl Pts',(79.8122711542087,11.2686554409985,136.962637697052));
#130408=CARTESIAN_POINT('Ctrl Pts',(81.8041520464296,10.3881912774696,136.85150457906));
#130409=CARTESIAN_POINT('Ctrl Pts',(82.1448019750125,8.23719981813793,136.740371461069));
#130410=CARTESIAN_POINT('Ctrl Pts',(80.5224447174872,6.78435310876227,136.629238343077));
#130411=CARTESIAN_POINT('Ctrl Pts',(78.4219254912908,7.35935364126247,136.518105225086));
#130412=CARTESIAN_POINT('Ctrl Pts',(77.7657221678739,9.43593829648909,136.406972107094));
#130413=CARTESIAN_POINT('Ctrl Pts',(79.1544178567368,11.1135350644055,136.295838989103));
#130414=CARTESIAN_POINT('Ctrl Pts',(81.3170236049032,10.8567413534482,136.184705871111));
#130415=CARTESIAN_POINT('Ctrl Pts',(82.2742375123182,8.90058487518767,136.073572753119));
#130416=CARTESIAN_POINT('Ctrl Pts',(81.1499797353433,7.03541703209655,135.962439635128));
#130417=CARTESIAN_POINT('Ctrl Pts',(78.9732152418211,6.9683128464628,135.851306517136));
#130418=CARTESIAN_POINT('Ctrl Pts',(77.7362045728382,8.76068871017342,135.740173399145));
#130419=CARTESIAN_POINT('Ctrl Pts',(78.5711085809138,10.7720916855339,135.629040281153));
#130420=CARTESIAN_POINT('Ctrl Pts',(80.7137902563551,11.1616066014447,135.517907163162));
#130421=CARTESIAN_POINT('Ctrl Pts',(82.2031829946697,9.57273407570653,135.40677404517));
#130422=CARTESIAN_POINT('Ctrl Pts',(81.6761359398247,7.45967278128821,135.295640927178));
#130423=CARTESIAN_POINT('Ctrl Pts',(79.6150233007846,6.75637958412346,135.184507809187));
#130424=CARTESIAN_POINT('Ctrl Pts',(77.9062564894017,8.10653609960796,135.073374691195));
#130425=CARTESIAN_POINT('Ctrl Pts',(78.1137661478597,10.2744259431277,134.962241573204));
#130426=CARTESIAN_POINT('Ctrl Pts',(80.0476312692378,11.2759110025806,134.851108455212));
#130427=CARTESIAN_POINT('Ctrl Pts',(81.9379023782607,10.1943927334876,134.739975337221));
#130428=CARTESIAN_POINT('Ctrl Pts',(82.0545289556053,8.01971922386687,134.628842219229));
#130429=CARTESIAN_POINT('Ctrl Pts',(80.2907697673081,6.7422372640385,134.517709101238));
#130430=CARTESIAN_POINT('Ctrl Pts',(78.2608866433841,7.53114862483747,134.406575983246));
#130431=CARTESIAN_POINT('Ctrl Pts',(77.8227085142696,9.66441057761191,134.295442865254));
#130432=CARTESIAN_POINT('Ctrl Pts',(79.3772732502533,11.1895778188105,134.184309747263));
#130433=CARTESIAN_POINT('Ctrl Pts',(81.5017820178913,10.7107572592905,134.073176629271));
#130434=CARTESIAN_POINT('Ctrl Pts',(82.2518007731909,8.66618432131833,133.96204351128));
#130435=CARTESIAN_POINT('Ctrl Pts',(80.9408828308515,6.92713263133267,133.850910393288));
#130436=CARTESIAN_POINT('Ctrl Pts',(78.7688318889294,7.08525074441597,133.739777275297));
#130437=CARTESIAN_POINT('Ctrl Pts',(77.7235944605638,8.99582274000608,133.628644157305));
#130438=CARTESIAN_POINT('Ctrl Pts',(78.7618129803392,10.910217928358,133.517511039313));
#130439=CARTESIAN_POINT('Ctrl Pts',(80.9332689950743,11.0763064832317,133.406377921322));
#130440=CARTESIAN_POINT('Ctrl Pts',(82.2505604924078,9.34207762202491,133.29524480333));
#130441=CARTESIAN_POINT('Ctrl Pts',(81.5080504458918,7.29476585709696,133.184111685339));
#130442=CARTESIAN_POINT('Ctrl Pts',(79.3853132750087,6.80815149711572,133.072978567347));
#130443=CARTESIAN_POINT('Ctrl Pts',(77.8251615886712,8.32760315729057,132.961845449356));
#130444=CARTESIAN_POINT('Ctrl Pts',(78.2555076171877,10.462458873195,132.850712331364));
#130445=CARTESIAN_POINT('Ctrl Pts',(80.2824817370051,11.2588146665309,132.739579213373));
#130446=CARTESIAN_POINT('Ctrl Pts',(82.0509174527428,9.98781437097895,132.628446095381));
#130447=CARTESIAN_POINT('Ctrl Pts',(81.9422727924055,7.81272748311218,132.51731297739));
#130448=CARTESIAN_POINT('Ctrl Pts',(80.0559836253476,6.72427913329213,132.406179859398));
#130449=CARTESIAN_POINT('Ctrl Pts',(78.1184560408754,7.71866009218345,132.295046741406));
#130450=CARTESIAN_POINT('Ctrl Pts',(77.902991544647,9.88577376775608,132.183913623415));
#130451=CARTESIAN_POINT('Ctrl Pts',(79.6067917241972,11.242192427362,132.072780505423));
#130452=CARTESIAN_POINT('Ctrl Pts',(81.6704715943076,10.5464683256135,131.961647387432));
#130453=CARTESIAN_POINT('Ctrl Pts',(82.2052701121483,8.43535554386083,131.85051426944));
#130454=CARTESIAN_POINT('Ctrl Pts',(80.7217186248435,6.84102759256112,131.739381151449));
#130455=CARTESIAN_POINT('Ctrl Pts',(78.577621845353,7.22267616486489,131.628248033457));
#130456=CARTESIAN_POINT('Ctrl Pts',(77.7353415375832,9.2310014658902,131.517114915466));
#130457=CARTESIAN_POINT('Ctrl Pts',(78.9657657900324,11.0279051331599,131.405981797474));
#130458=CARTESIAN_POINT('Ctrl Pts',(81.1427618998832,10.968790205083,131.294848679482));
#130459=CARTESIAN_POINT('Ctrl Pts',(82.2738573374737,9.10776099030368,131.183715561491));
#130460=CARTESIAN_POINT('Ctrl Pts',(81.3238290474173,7.14810467614153,131.072582443499));
#130461=CARTESIAN_POINT('Ctrl Pts',(79.1621802959776,6.88337585149887,130.961449325508));
#130462=CARTESIAN_POINT('Ctrl Pts',(77.76733713802,8.55586475864455,130.850316207516));
#130463=CARTESIAN_POINT('Ctrl Pts',(78.4159148588162,10.63484371647,130.739183089525));
#130464=CARTESIAN_POINT('Ctrl Pts',(80.5143097505996,11.217549364708,130.628049971533));
#130465=CARTESIAN_POINT('Ctrl Pts',(82.1419879094673,9.7706665390823,130.516916853541));
#130466=CARTESIAN_POINT('Ctrl Pts',(81.8092348473344,7.6184393911342,130.40578373555));
#130467=CARTESIAN_POINT('Ctrl Pts',(79.8205979799762,6.73067083410996,130.294650617558));
#130468=CARTESIAN_POINT('Ctrl Pts',(77.9961586657518,7.91988176417262,130.183517499567));
#130469=CARTESIAN_POINT('Ctrl Pts',(78.00571020507,10.0976591824581,130.072384381575));
#130470=CARTESIAN_POINT('Ctrl Pts',(79.8405216338773,11.270816192575,129.961251263584));
#130471=CARTESIAN_POINT('Ctrl Pts',(81.8212788582255,10.3656318650533,129.850118145592));
#130472=CARTESIAN_POINT('Ctrl Pts',(82.1351608315215,8.21056950757627,129.738985027601));
#130473=CARTESIAN_POINT('Ctrl Pts',(80.4947964912215,6.77802091065733,129.627851909609));
#130474=CARTESIAN_POINT('Ctrl Pts',(78.4017039366046,7.37912341309647,129.516718791617));
#130475=CARTESIAN_POINT('Ctrl Pts',(77.7711710065171,9.46369882540057,129.405585673626));
#130476=CARTESIAN_POINT('Ctrl Pts',(79.1810897074592,11.1239138936689,129.294452555634));
#130477=CARTESIAN_POINT('Ctrl Pts',(81.3394035812484,10.8401676135116,129.183319437643));
#130478=CARTESIAN_POINT('Ctrl Pts',(82.2741066401341,8.87238039760016,129.072186319651));
#130479=CARTESIAN_POINT('Ctrl Pts',(81.1226537789126,7.02087552918776,128.961040063426));
#130480=CARTESIAN_POINT('Ctrl Pts',(79.6773693782926,6.99609140340361,128.886938179863));
#130481=CARTESIAN_POINT('Ctrl Pts',(79.1093659241097,7.2923586278747,128.849880668964));
#130482=CARTESIAN_POINT('Ctrl Pts',(79.5369951482613,7.26632029764578,140.150289422863));
#130483=CARTESIAN_POINT('Ctrl Pts',(78.9605301573707,7.42027381470975,140.113245050199));
#130484=CARTESIAN_POINT('Ctrl Pts',(77.9833340003239,8.34656508848017,140.039156304871));
#130485=CARTESIAN_POINT('Ctrl Pts',(78.3569668667848,10.3431370525474,139.92802318688));
#130486=CARTESIAN_POINT('Ctrl Pts',(80.2373864921598,11.1072731083233,139.816890068888));
#130487=CARTESIAN_POINT('Ctrl Pts',(81.8990810207062,9.94427945465913,139.705756950897));
#130488=CARTESIAN_POINT('Ctrl Pts',(81.8233751926667,7.91630029806288,139.594623832905));
#130489=CARTESIAN_POINT('Ctrl Pts',(80.07849587449,6.88052937885506,139.483490714914));
#130490=CARTESIAN_POINT('Ctrl Pts',(78.2619445665833,7.78440361057707,139.372357596922));
#130491=CARTESIAN_POINT('Ctrl Pts',(78.0360466198298,9.80092643322281,139.26122447893));
#130492=CARTESIAN_POINT('Ctrl Pts',(79.6076768775642,11.0843673541092,139.150091360939));
#130493=CARTESIAN_POINT('Ctrl Pts',(81.5383567631607,10.4601340166544,139.038958242947));
#130494=CARTESIAN_POINT('Ctrl Pts',(82.0610817377952,8.49951839410893,138.927825124956));
#130495=CARTESIAN_POINT('Ctrl Pts',(80.6974188162415,6.99696820529239,138.816692006964));
#130496=CARTESIAN_POINT('Ctrl Pts',(78.6954530745305,7.32766912374867,138.705558888973));
#130497=CARTESIAN_POINT('Ctrl Pts',(77.8874588858846,9.18895427055025,138.594425770981));
#130498=CARTESIAN_POINT('Ctrl Pts',(79.012946030909,10.8773004508344,138.48329265299));
#130499=CARTESIAN_POINT('Ctrl Pts',(81.0418235460464,10.8474676527515,138.372159534998));
#130500=CARTESIAN_POINT('Ctrl Pts',(82.1171832792935,9.12675960435475,138.261026417006));
#130501=CARTESIAN_POINT('Ctrl Pts',(81.254813478666,7.29003624475958,138.149893299015));
#130502=CARTESIAN_POINT('Ctrl Pts',(79.243989025239,7.01833898426903,138.038760181023));
#130503=CARTESIAN_POINT('Ctrl Pts',(77.9250955566404,8.56033589903112,137.927627063032));
#130504=CARTESIAN_POINT('Ctrl Pts',(78.5052363096632,10.5047306960704,137.81649394504));
#130505=CARTESIAN_POINT('Ctrl Pts',(80.4534436216841,11.0719367383254,137.705360827049));
#130506=CARTESIAN_POINT('Ctrl Pts',(81.9866414855934,9.74282472513125,137.594227709057));
#130507=CARTESIAN_POINT('Ctrl Pts',(81.7015868675506,7.73385028712899,137.483094591066));
#130508=CARTESIAN_POINT('Ctrl Pts',(79.8591729749542,6.88370590105949,137.371961473074));
#130509=CARTESIAN_POINT('Ctrl Pts',(78.1456495183648,7.97047717108632,137.260828355082));
#130510=CARTESIAN_POINT('Ctrl Pts',(78.1293006091955,9.99950825565009,137.149695237091));
#130511=CARTESIAN_POINT('Ctrl Pts',(79.8250894124504,11.1137500444344,137.038562119099));
#130512=CARTESIAN_POINT('Ctrl Pts',(81.680963269869,10.2934045961353,136.927429001108));
#130513=CARTESIAN_POINT('Ctrl Pts',(81.9983533806219,8.28928435355709,136.816295883116));
#130514=CARTESIAN_POINT('Ctrl Pts',(80.486771823013,6.93563904409244,136.705162765125));
#130515=CARTESIAN_POINT('Ctrl Pts',(78.5296775338274,7.47137813393286,136.594029647133));
#130516=CARTESIAN_POINT('Ctrl Pts',(77.9182802370128,9.40617212156682,136.482896529142));
#130517=CARTESIAN_POINT('Ctrl Pts',(79.2121548029749,10.9692213967646,136.37176341115));
#130518=CARTESIAN_POINT('Ctrl Pts',(81.2270963025394,10.7299617418442,136.260630293158));
#130519=CARTESIAN_POINT('Ctrl Pts',(82.11895096798,8.9073730101575,136.149497175167));
#130520=CARTESIAN_POINT('Ctrl Pts',(81.0714583064278,7.16956014533737,136.038364057175));
#130521=CARTESIAN_POINT('Ctrl Pts',(79.0433248306451,7.10703788091514,135.927230939184));
#130522=CARTESIAN_POINT('Ctrl Pts',(77.8907781242235,8.77702905414233,135.816097821192));
#130523=CARTESIAN_POINT('Ctrl Pts',(78.6686742966767,10.6510920130694,135.704964703201));
#130524=CARTESIAN_POINT('Ctrl Pts',(80.6650521532805,11.0140105752869,135.593831585209));
#130525=CARTESIAN_POINT('Ctrl Pts',(82.0527481030041,9.53362738831814,135.482698467217));
#130526=CARTESIAN_POINT('Ctrl Pts',(81.5616881934805,7.56484741219121,135.371565349226));
#130527=CARTESIAN_POINT('Ctrl Pts',(79.6413097818351,6.90957557148231,135.260432231234));
#130528=CARTESIAN_POINT('Ctrl Pts',(78.0492187757636,8.16754244605654,135.149299113243));
#130529=CARTESIAN_POINT('Ctrl Pts',(78.2425595281141,10.1874072392099,135.038165995251));
#130530=CARTESIAN_POINT('Ctrl Pts',(80.0443789725174,11.1205101911448,134.92703287726));
#130531=CARTESIAN_POINT('Ctrl Pts',(81.8055810345334,10.1128387536762,134.815899759268));
#130532=CARTESIAN_POINT('Ctrl Pts',(81.9142442667676,8.08665348793663,134.704766641277));
#130533=CARTESIAN_POINT('Ctrl Pts',(80.2709158021357,6.89639889900585,134.593633523285));
#130534=CARTESIAN_POINT('Ctrl Pts',(78.3796345322474,7.63144283463743,134.482500405293));
#130535=CARTESIAN_POINT('Ctrl Pts',(77.9713755154094,9.61904415389396,134.371367287302));
#130536=CARTESIAN_POINT('Ctrl Pts',(79.4197934727505,11.0400718981662,134.26023416931));
#130537=CARTESIAN_POINT('Ctrl Pts',(81.3992392805367,10.5939455447894,134.149101051319));
#130538=CARTESIAN_POINT('Ctrl Pts',(82.0980462252544,8.68897749173593,134.037967933327));
#130539=CARTESIAN_POINT('Ctrl Pts',(80.8766386863244,7.06866947997241,133.926834815336));
#130540=CARTESIAN_POINT('Ctrl Pts',(78.852896917508,7.21599117656667,133.815701697344));
#130541=CARTESIAN_POINT('Ctrl Pts',(77.8790290393256,8.99610796627015,133.704568579353));
#130542=CARTESIAN_POINT('Ctrl Pts',(78.8463572649559,10.7797868984321,133.593435461361));
#130543=CARTESIAN_POINT('Ctrl Pts',(80.8695447286342,10.9345348094194,133.482302343369));
#130544=CARTESIAN_POINT('Ctrl Pts',(82.0968906317194,9.31872032027786,133.371169225378));
#130545=CARTESIAN_POINT('Ctrl Pts',(81.4050796958441,7.41120044930849,133.260036107386));
#130546=CARTESIAN_POINT('Ctrl Pts',(79.4272845189342,6.95781246167295,133.148902989395));
#130547=CARTESIAN_POINT('Ctrl Pts',(77.9736610921575,8.37351488883257,133.037769871403));
#130548=CARTESIAN_POINT('Ctrl Pts',(78.3746227897605,10.3626011479463,132.926636753412));
#130549=CARTESIAN_POINT('Ctrl Pts',(80.2631936843982,11.104581205001,132.81550363542));
#130550=CARTESIAN_POINT('Ctrl Pts',(81.9108793598724,9.92036570772979,132.704370517429));
#130551=CARTESIAN_POINT('Ctrl Pts',(81.8096530337122,7.89379528950295,132.593237399437));
#130552=CARTESIAN_POINT('Ctrl Pts',(80.0521610238504,6.87966696211622,132.482104281445));
#130553=CARTESIAN_POINT('Ctrl Pts',(78.2469291919207,7.80615088649572,132.370971163454));
#130554=CARTESIAN_POINT('Ctrl Pts',(78.0461767637439,9.8252925089978,132.259838045462));
#130555=CARTESIAN_POINT('Ctrl Pts',(79.6336402631136,11.089093944068,132.148704927471));
#130556=CARTESIAN_POINT('Ctrl Pts',(81.5564106134778,10.4408743755918,132.037571809479));
#130557=CARTESIAN_POINT('Ctrl Pts',(82.0546927106265,8.47390986630898,131.926438691488));
#130558=CARTESIAN_POINT('Ctrl Pts',(80.6724391671662,6.98844375409079,131.815305573496));
#130559=CARTESIAN_POINT('Ctrl Pts',(78.6747428308176,7.34403309220127,131.704172455504));
#130560=CARTESIAN_POINT('Ctrl Pts',(77.8899740176255,9.21522852257146,131.593039337513));
#130561=CARTESIAN_POINT('Ctrl Pts',(79.0363840326883,10.8894383377314,131.481906219521));
#130562=CARTESIAN_POINT('Ctrl Pts',(81.0647333098732,10.8343598187147,131.37077310153));
#130563=CARTESIAN_POINT('Ctrl Pts',(82.1185967517424,9.10040299374085,131.259639983538));
#130564=CARTESIAN_POINT('Ctrl Pts',(81.2334370646298,7.27455339742084,131.148506865547));
#130565=CARTESIAN_POINT('Ctrl Pts',(79.2193872173793,7.0279004439846,131.037373747555));
#130566=CARTESIAN_POINT('Ctrl Pts',(77.9197849358561,8.58619062675434,130.926240629564));
#130567=CARTESIAN_POINT('Ctrl Pts',(78.5240773115852,10.5232154323138,130.815107511572));
#130568=CARTESIAN_POINT('Ctrl Pts',(80.4791923174128,11.0661335271449,130.70397439358));
#130569=CARTESIAN_POINT('Ctrl Pts',(81.9957314614605,9.71804488323371,130.592841275589));
#130570=CARTESIAN_POINT('Ctrl Pts',(81.6856990135364,7.71277332573098,130.481708157597));
#130571=CARTESIAN_POINT('Ctrl Pts',(79.8328476766705,6.88562223308578,130.370575039606));
#130572=CARTESIAN_POINT('Ctrl Pts',(78.132982367987,7.99363300053637,130.259441921614));
#130573=CARTESIAN_POINT('Ctrl Pts',(78.1418817214514,10.0227102378639,130.148308803623));
#130574=CARTESIAN_POINT('Ctrl Pts',(79.8514109294049,11.1157632583664,130.037175685631));
#130575=CARTESIAN_POINT('Ctrl Pts',(81.6969206508535,10.2723855563395,129.926042567639));
#130576=CARTESIAN_POINT('Ctrl Pts',(81.9893705412209,8.26447237941779,129.814909449648));
#130577=CARTESIAN_POINT('Ctrl Pts',(80.4610114371731,6.9297392129485,129.703776331656));
#130578=CARTESIAN_POINT('Ctrl Pts',(78.5108367211839,7.48979801177652,129.592643213665));
#130579=CARTESIAN_POINT('Ctrl Pts',(77.9233570251033,9.43203714194838,129.481510095673));
#130580=CARTESIAN_POINT('Ctrl Pts',(79.2370054808835,10.9788915522322,129.370376977682));
#130581=CARTESIAN_POINT('Ctrl Pts',(81.247948158286,10.7145196685817,129.25924385969));
#130582=CARTESIAN_POINT('Ctrl Pts',(82.1188290318412,8.88109435422919,129.148110741698));
#130583=CARTESIAN_POINT('Ctrl Pts',(81.045998185611,7.15601154652237,129.036964485473));
#130584=CARTESIAN_POINT('Ctrl Pts',(79.6993988251165,7.13291969835944,128.96286260191));
#130585=CARTESIAN_POINT('Ctrl Pts',(79.1701790481417,7.4089575873985,128.925805091013));
#130586=CARTESIAN_POINT('Ctrl Pts',(79.5709262889649,7.39337237862174,140.22621384491));
#130587=CARTESIAN_POINT('Ctrl Pts',(79.0367073234519,7.53604346866648,140.189169472247));
#130588=CARTESIAN_POINT('Ctrl Pts',(78.1311246282838,8.39445182625427,140.115080726919));
#130589=CARTESIAN_POINT('Ctrl Pts',(78.4773759471957,10.2447057463896,140.003947608927));
#130590=CARTESIAN_POINT('Ctrl Pts',(80.2199897101685,10.9528423716459,139.892814490936));
#130591=CARTESIAN_POINT('Ctrl Pts',(81.7599075647934,9.87507828123918,139.781681372944));
#130592=CARTESIAN_POINT('Ctrl Pts',(81.6897498105885,7.99571883315742,139.670548254953));
#130593=CARTESIAN_POINT('Ctrl Pts',(80.0727433331246,7.03585400578483,139.559415136961));
#130594=CARTESIAN_POINT('Ctrl Pts',(78.3893173214049,7.87348814602691,139.44828201897));
#130595=CARTESIAN_POINT('Ctrl Pts',(78.1799742228073,9.74223083338886,139.337148900978));
#130596=CARTESIAN_POINT('Ctrl Pts',(79.6364281336657,10.9316152572264,139.226015782987));
#130597=CARTESIAN_POINT('Ctrl Pts',(81.4256188521281,10.353128630903,139.114882664995));
#130598=CARTESIAN_POINT('Ctrl Pts',(81.9100361187613,8.53619600499189,139.003749547003));
#130599=CARTESIAN_POINT('Ctrl Pts',(80.6463087341457,7.143759655543,138.892616429012));
#130600=CARTESIAN_POINT('Ctrl Pts',(78.7910563173825,7.45022527850987,138.78148331102));
#130601=CARTESIAN_POINT('Ctrl Pts',(78.0422756864338,9.17510682615201,138.670350193029));
#130602=CARTESIAN_POINT('Ctrl Pts',(79.085281918927,10.7397231759942,138.559217075037));
#130603=CARTESIAN_POINT('Ctrl Pts',(80.9654738896738,10.7120766635745,138.448083957046));
#130604=CARTESIAN_POINT('Ctrl Pts',(81.9620262793723,9.11747007325214,138.336950839054));
#130605=CARTESIAN_POINT('Ctrl Pts',(81.1628549332179,7.41535031125165,138.225817721063));
#130606=CARTESIAN_POINT('Ctrl Pts',(79.2993930121772,7.16356428482233,138.114684603071));
#130607=CARTESIAN_POINT('Ctrl Pts',(78.0771541675805,8.59255652137716,138.003551485079));
#130608=CARTESIAN_POINT('Ctrl Pts',(78.6147795183462,10.3944570590286,137.892418367088));
#130609=CARTESIAN_POINT('Ctrl Pts',(80.4202131722175,10.92009561456,137.781285249096));
#130610=CARTESIAN_POINT('Ctrl Pts',(81.8410511931334,9.68838708765981,137.670152131105));
#130611=CARTESIAN_POINT('Ctrl Pts',(81.5768866981997,7.82663960434193,137.559019013113));
#130612=CARTESIAN_POINT('Ctrl Pts',(79.8694934318215,7.03879773772482,137.447885895122));
#130613=CARTESIAN_POINT('Ctrl Pts',(78.2815449131314,8.04592537391647,137.33675277713));
#130614=CARTESIAN_POINT('Ctrl Pts',(78.2663941277731,9.92625965981055,137.225619659138));
#130615=CARTESIAN_POINT('Ctrl Pts',(79.837907670692,10.9588446478703,137.114486541147));
#130616=CARTESIAN_POINT('Ctrl Pts',(81.5577744933084,10.198617914801,137.003353423155));
#130617=CARTESIAN_POINT('Ctrl Pts',(81.8519047862312,8.34136888897625,136.892220305164));
#130618=CARTESIAN_POINT('Ctrl Pts',(80.4510989285387,7.0869249794226,136.781087187172));
#130619=CARTESIAN_POINT('Ctrl Pts',(78.6374295763639,7.58340262660325,136.66995406918));
#130620=CARTESIAN_POINT('Ctrl Pts',(78.0708383061516,9.37640594664453,136.558820951189));
#130621=CARTESIAN_POINT('Ctrl Pts',(79.269891749213,10.8249077291237,136.447687833197));
#130622=CARTESIAN_POINT('Ctrl Pts',(81.1371690001757,10.6031821302402,136.336554715206));
#130623=CARTESIAN_POINT('Ctrl Pts',(81.9636644236418,8.91416114512732,136.225421597214));
#130624=CARTESIAN_POINT('Ctrl Pts',(80.9929368775125,7.30370325857819,136.114288479223));
#130625=CARTESIAN_POINT('Ctrl Pts',(79.113434419469,7.24576291536748,136.003155361231));
#130626=CARTESIAN_POINT('Ctrl Pts',(78.0453516756087,8.79336939811123,135.89202224324));
#130627=CARTESIAN_POINT('Ctrl Pts',(78.7662400124398,10.5300923406048,135.780889125248));
#130628=CARTESIAN_POINT('Ctrl Pts',(80.6163140502057,10.8664145491293,135.669756007257));
#130629=CARTESIAN_POINT('Ctrl Pts',(81.9023132113388,9.49452070092974,135.558622889265));
#130630=CARTESIAN_POINT('Ctrl Pts',(81.4472404471363,7.67002204309423,135.447489771273));
#130631=CARTESIAN_POINT('Ctrl Pts',(79.6675962628857,7.06277155884116,135.336356653282));
#130632=CARTESIAN_POINT('Ctrl Pts',(78.1921810621257,8.2285487925051,135.22522353529));
#130633=CARTESIAN_POINT('Ctrl Pts',(78.3713529083684,10.100388535292,135.114090417299));
#130634=CARTESIAN_POINT('Ctrl Pts',(80.0411266757971,10.965109379709,135.002957299307));
#130635=CARTESIAN_POINT('Ctrl Pts',(81.6732596908063,10.0312847738648,134.891824181316));
#130636=CARTESIAN_POINT('Ctrl Pts',(81.7739595779298,8.15358775200641,134.780691063324));
#130637=CARTESIAN_POINT('Ctrl Pts',(80.2510618369633,7.05056053397319,134.669557945332));
#130638=CARTESIAN_POINT('Ctrl Pts',(78.4983824211106,7.73173704443741,134.558424827341));
#130639=CARTESIAN_POINT('Ctrl Pts',(78.1200425165492,9.573677730176,134.447291709349));
#130640=CARTESIAN_POINT('Ctrl Pts',(79.4623136952477,10.890565977522,134.336158591358));
#130641=CARTESIAN_POINT('Ctrl Pts',(81.2966965431822,10.4771338302882,134.225025473366));
#130642=CARTESIAN_POINT('Ctrl Pts',(81.9442916773176,8.71177066215355,134.113892355375));
#130643=CARTESIAN_POINT('Ctrl Pts',(80.8123945417976,7.21020632861215,134.002759237383));
#130644=CARTESIAN_POINT('Ctrl Pts',(78.9369619460865,7.34673160871737,133.891626119392));
#130645=CARTESIAN_POINT('Ctrl Pts',(78.0344636180874,8.99639319253423,133.7804930014));
#130646=CARTESIAN_POINT('Ctrl Pts',(78.9309015495727,10.6493558685063,133.669359883408));
#130647=CARTESIAN_POINT('Ctrl Pts',(80.8058204621942,10.7927631356071,133.558226765417));
#130648=CARTESIAN_POINT('Ctrl Pts',(81.9432207710311,9.29536301853081,133.447093647425));
#130649=CARTESIAN_POINT('Ctrl Pts',(81.3021089457963,7.52763504152003,133.335960529434));
#130650=CARTESIAN_POINT('Ctrl Pts',(79.4692557628599,7.10747342623018,133.224827411442));
#130651=CARTESIAN_POINT('Ctrl Pts',(78.1221605956438,8.41942662037456,133.113694293451));
#130652=CARTESIAN_POINT('Ctrl Pts',(78.4937379623332,10.2627434226976,133.002561175459));
#130653=CARTESIAN_POINT('Ctrl Pts',(80.2439056317912,10.9503477434711,132.891428057468));
#130654=CARTESIAN_POINT('Ctrl Pts',(81.770841267002,9.85291704448063,132.780294939476));
#130655=CARTESIAN_POINT('Ctrl Pts',(81.6770332750191,7.97486309589373,132.669161821485));
#130656=CARTESIAN_POINT('Ctrl Pts',(80.048338422353,7.0350547909403,132.558028703493));
#130657=CARTESIAN_POINT('Ctrl Pts',(78.375402342966,7.89364168080799,132.446895585501));
#130658=CARTESIAN_POINT('Ctrl Pts',(78.1893619828409,9.76481125023954,132.33576246751));
#130659=CARTESIAN_POINT('Ctrl Pts',(79.66048880203,10.935995460774,132.224629349518));
#130660=CARTESIAN_POINT('Ctrl Pts',(81.4423496326477,10.3352804255702,132.113496231527));
#130661=CARTESIAN_POINT('Ctrl Pts',(81.904115309105,8.51246418875713,132.002363113535));
#130662=CARTESIAN_POINT('Ctrl Pts',(80.6231597094889,7.13585991562045,131.891229995544));
#130663=CARTESIAN_POINT('Ctrl Pts',(78.7718638162824,7.46539001953766,131.780096877552));
#130664=CARTESIAN_POINT('Ctrl Pts',(78.0446064976679,9.1994555792527,131.668963759561));
#130665=CARTESIAN_POINT('Ctrl Pts',(79.1070022753443,10.7509715423028,131.557830641569));
#130666=CARTESIAN_POINT('Ctrl Pts',(80.9867047198631,10.6999294323463,131.446697523577));
#130667=CARTESIAN_POINT('Ctrl Pts',(81.9633361660112,9.093044997178,131.335564405586));
#130668=CARTESIAN_POINT('Ctrl Pts',(81.1430450818425,7.40100211870016,131.224431287594));
#130669=CARTESIAN_POINT('Ctrl Pts',(79.2765941387811,7.17242503647032,131.113298169603));
#130670=CARTESIAN_POINT('Ctrl Pts',(78.0722327336921,8.61651649486414,131.002165051611));
#130671=CARTESIAN_POINT('Ctrl Pts',(78.6322397643545,10.4115871481576,130.89103193362));
#130672=CARTESIAN_POINT('Ctrl Pts',(80.4440748842258,10.9147176895819,130.779898815628));
#130673=CARTESIAN_POINT('Ctrl Pts',(81.8494750134538,9.66542322738512,130.668765697637));
#130674=CARTESIAN_POINT('Ctrl Pts',(81.5621631797384,7.80710726032776,130.557632579645));
#130675=CARTESIAN_POINT('Ctrl Pts',(79.8450973733649,7.04057363206159,130.446499461653));
#130676=CARTESIAN_POINT('Ctrl Pts',(78.269806070222,8.06738423690015,130.335366343662));
#130677=CARTESIAN_POINT('Ctrl Pts',(78.2780532378328,9.94776129326954,130.22423322567));
#130678=CARTESIAN_POINT('Ctrl Pts',(79.8623002249327,10.9607103241578,130.113100107679));
#130679=CARTESIAN_POINT('Ctrl Pts',(81.5725624434815,10.1791392476256,130.001966989687));
#130680=CARTESIAN_POINT('Ctrl Pts',(81.8435802509203,8.31837525125933,129.890833871696));
#130681=CARTESIAN_POINT('Ctrl Pts',(80.4272263831248,7.08145751523965,129.779700753704));
#130682=CARTESIAN_POINT('Ctrl Pts',(78.6199695057632,7.60047261045659,129.668567635712));
#130683=CARTESIAN_POINT('Ctrl Pts',(78.0755430436893,9.40037545849617,129.557434517721));
#130684=CARTESIAN_POINT('Ctrl Pts',(79.2929212543077,10.8338692107953,129.446301399729));
#130685=CARTESIAN_POINT('Ctrl Pts',(81.1564927353234,10.5888717236517,129.335168281738));
#130686=CARTESIAN_POINT('Ctrl Pts',(81.9635514235481,8.88980831085824,129.224035163746));
#130687=CARTESIAN_POINT('Ctrl Pts',(80.9693425923095,7.29114756385696,129.112888907521));
#130688=CARTESIAN_POINT('Ctrl Pts',(79.7214282719405,7.26974799331527,129.038787023958));
#130689=CARTESIAN_POINT('Ctrl Pts',(79.2309921721737,7.5255565469223,129.00172951306));
#130690=CARTESIAN_POINT('',(78.7297156500765,10.0802549060841,140.000878868843));
#130691=CARTESIAN_POINT('Ctrl Pts',(78.7308621553943,10.0792799133634,140.000878868843));
#130692=CARTESIAN_POINT('Ctrl Pts',(78.736370574171,10.0857573272824,140.000585912562));
#130693=CARTESIAN_POINT('Ctrl Pts',(78.7419285829586,10.092192569647,140.000292956281));
#130694=CARTESIAN_POINT('Ctrl Pts',(78.7475355302757,10.0985848861505,140.));
#130695=CARTESIAN_POINT('Ctrl Pts',(79.4698297828112,7.01482567432834,140.));
#130696=CARTESIAN_POINT('Ctrl Pts',(79.4008201088926,7.04037739808265,140.));
#130697=CARTESIAN_POINT('Ctrl Pts',(79.333531264625,7.06986024816562,140.));
#130698=CARTESIAN_POINT('Ctrl Pts',(79.2681550277024,7.10297535276265,140.));
#130699=CARTESIAN_POINT('Ctrl Pts',(79.2013067432528,7.13683609537928,140.));
#130700=CARTESIAN_POINT('Ctrl Pts',(79.1364574168441,7.17449523887906,140.));
#130701=CARTESIAN_POINT('Ctrl Pts',(79.0738433838076,7.21567796853842,140.));
#130702=CARTESIAN_POINT('Ctrl Pts',(79.0212317769186,7.25028186607351,140.));
#130703=CARTESIAN_POINT('Ctrl Pts',(78.9701986946478,7.28737455147851,140.));
#130704=CARTESIAN_POINT('Ctrl Pts',(78.9209066494717,7.32681062951119,140.));
#130705=CARTESIAN_POINT('Ctrl Pts',(78.8988725699372,7.34443898469096,140.));
#130706=CARTESIAN_POINT('Ctrl Pts',(78.8771866812342,7.36253576994061,140.));
#130707=CARTESIAN_POINT('Ctrl Pts',(78.8558650479428,7.38108871910383,140.));
#130708=CARTESIAN_POINT('Ctrl Pts',(78.8441549123335,7.39127825513441,140.));
#130709=CARTESIAN_POINT('Ctrl Pts',(78.8325546668865,7.40160539314329,140.));
#130710=CARTESIAN_POINT('Ctrl Pts',(78.8210671070671,7.41206814268509,140.));
#130711=CARTESIAN_POINT('Ctrl Pts',(78.8104708100333,7.42171913938738,140.));
#130712=CARTESIAN_POINT('Ctrl Pts',(78.7999689523207,7.43148704191031,140.));
#130713=CARTESIAN_POINT('Ctrl Pts',(78.7895796274579,7.44135481790265,140.));
#130714=CARTESIAN_POINT('Ctrl Pts',(78.7364949706948,7.4917746005629,140.));
#130715=CARTESIAN_POINT('Ctrl Pts',(78.6862504774249,7.54488334682044,140.));
#130716=CARTESIAN_POINT('Ctrl Pts',(78.6390647471674,7.60042107429915,140.));
#130717=CARTESIAN_POINT('Ctrl Pts',(78.592610468946,7.65509788082504,140.));
#130718=CARTESIAN_POINT('Ctrl Pts',(78.5491204205517,7.71212983833611,140.));
#130719=CARTESIAN_POINT('Ctrl Pts',(78.5088467574884,7.77129247852492,140.));
#130720=CARTESIAN_POINT('Ctrl Pts',(78.474800950115,7.82130630141469,140.));
#130721=CARTESIAN_POINT('Ctrl Pts',(78.4430542558921,7.87284343154723,140.));
#130722=CARTESIAN_POINT('Ctrl Pts',(78.4137873790238,7.92577492972471,140.));
#130723=CARTESIAN_POINT('Ctrl Pts',(78.4016823401401,7.94766786508959,140.));
#130724=CARTESIAN_POINT('Ctrl Pts',(78.3900018581821,7.96979937807893,140.));
#130725=CARTESIAN_POINT('Ctrl Pts',(78.3787601693597,7.992160428703,140.));
#130726=CARTESIAN_POINT('Ctrl Pts',(78.3735606798431,8.00250282922102,140.));
#130727=CARTESIAN_POINT('Ctrl Pts',(78.3684550708377,8.01289433315706,140.));
#130728=CARTESIAN_POINT('Ctrl Pts',(78.3634448160861,8.02333404404232,140.));
#130729=CARTESIAN_POINT('Ctrl Pts',(78.3582119146326,8.03423767688612,140.));
#130730=CARTESIAN_POINT('Ctrl Pts',(78.3530866368273,8.04518644941609,140.));
#130731=CARTESIAN_POINT('Ctrl Pts',(78.3480720486465,8.05617503558337,140.));
#130732=CARTESIAN_POINT('Ctrl Pts',(78.3195311610532,8.11871736035694,140.));
#130733=CARTESIAN_POINT('Ctrl Pts',(78.2945512775789,8.18259159922865,140.));
#130734=CARTESIAN_POINT('Ctrl Pts',(78.2733558100535,8.24759283259564,140.));
#130735=CARTESIAN_POINT('Ctrl Pts',(78.2541541352166,8.30647959909913,140.));
#130736=CARTESIAN_POINT('Ctrl Pts',(78.2380587088044,8.36629190489806,140.));
#130737=CARTESIAN_POINT('Ctrl Pts',(78.2252723327201,8.42688219532759,140.));
#130738=CARTESIAN_POINT('Ctrl Pts',(78.2101393236097,8.49859238209378,140.));
#130739=CARTESIAN_POINT('Ctrl Pts',(78.1996408096421,8.5713938352022,140.));
#130740=CARTESIAN_POINT('Ctrl Pts',(78.1937017441597,8.64486393524295,140.));
#130741=CARTESIAN_POINT('Ctrl Pts',(78.1923945903257,8.66103427773769,140.));
#130742=CARTESIAN_POINT('Ctrl Pts',(78.1913085266392,8.67723692864844,140.));
#130743=CARTESIAN_POINT('Ctrl Pts',(78.1904431222916,8.69346721770384,140.));
#130744=CARTESIAN_POINT('Ctrl Pts',(78.1895475165414,8.71026392117007,140.));
#130745=CARTESIAN_POINT('Ctrl Pts',(78.1888882301811,8.72709641868181,140.));
#130746=CARTESIAN_POINT('Ctrl Pts',(78.1884653473802,8.74392526443646,140.));
#130747=CARTESIAN_POINT('Ctrl Pts',(78.1867426630314,8.81248040340845,140.));
#130748=CARTESIAN_POINT('Ctrl Pts',(78.1889312907711,8.88106164831567,140.));
#130749=CARTESIAN_POINT('Ctrl Pts',(78.1949107281129,8.94933109926134,140.));
#130750=CARTESIAN_POINT('Ctrl Pts',(78.2008889807299,9.01758702376556,140.));
#130751=CARTESIAN_POINT('Ctrl Pts',(78.2106569943201,9.08553234841923,140.));
#130752=CARTESIAN_POINT('Ctrl Pts',(78.2241439421755,9.15281433200293,140.));
#130753=CARTESIAN_POINT('Ctrl Pts',(78.2339020360718,9.20149427948872,140.));
#130754=CARTESIAN_POINT('Ctrl Pts',(78.2456079790146,9.24982671336545,140.));
#130755=CARTESIAN_POINT('Ctrl Pts',(78.2592491471692,9.29766838566998,140.));
#130756=CARTESIAN_POINT('Ctrl Pts',(78.2670120870047,9.32489420823299,140.));
#130757=CARTESIAN_POINT('Ctrl Pts',(78.2754019651411,9.3519609244368,140.));
#130758=CARTESIAN_POINT('Ctrl Pts',(78.284417996475,9.37884052478954,140.));
#130759=CARTESIAN_POINT('Ctrl Pts',(78.2903710440095,9.39658841548341,140.));
#130760=CARTESIAN_POINT('Ctrl Pts',(78.2965990797181,9.41425955524979,140.));
#130761=CARTESIAN_POINT('Ctrl Pts',(78.3030899812727,9.4318142879203,140.));
#130762=CARTESIAN_POINT('Ctrl Pts',(78.3040429931651,9.43439172171164,140.));
#130763=CARTESIAN_POINT('Ctrl Pts',(78.3050017082472,9.43696676507744,140.));
#130764=CARTESIAN_POINT('Ctrl Pts',(78.3059661198725,9.43953939093159,140.));
#130765=CARTESIAN_POINT('Ctrl Pts',(78.329146503839,9.50137445547726,140.));
#130766=CARTESIAN_POINT('Ctrl Pts',(78.3556159827812,9.56181902474221,140.));
#130767=CARTESIAN_POINT('Ctrl Pts',(78.38532430616,9.62053681691923,140.));
#130768=CARTESIAN_POINT('Ctrl Pts',(78.4060956394296,9.66159086142438,140.));
#130769=CARTESIAN_POINT('Ctrl Pts',(78.4284511313581,9.70180023814684,140.));
#130770=CARTESIAN_POINT('Ctrl Pts',(78.4523839013391,9.74103877789827,140.));
#130771=CARTESIAN_POINT('Ctrl Pts',(78.4600963609368,9.75368360140783,140.));
#130772=CARTESIAN_POINT('Ctrl Pts',(78.4679737809338,9.76622922088728,140.));
#130773=CARTESIAN_POINT('Ctrl Pts',(78.4760125858817,9.77866574969129,140.));
#130774=CARTESIAN_POINT('Ctrl Pts',(78.5102589136736,9.8316469384092,140.));
#130775=CARTESIAN_POINT('Ctrl Pts',(78.5473615905134,9.88254471555941,140.));
#130776=CARTESIAN_POINT('Ctrl Pts',(78.5872864455964,9.93104413524139,140.));
#130777=CARTESIAN_POINT('Ctrl Pts',(78.6240638497462,9.97572013356295,140.));
#130778=CARTESIAN_POINT('Ctrl Pts',(78.6632365895196,10.018361106523,140.));
#130779=CARTESIAN_POINT('Ctrl Pts',(78.7047993791355,10.0586880242349,140.));
#130780=CARTESIAN_POINT('Ctrl Pts',(78.7126175960375,10.0662737660143,140.));
#130781=CARTESIAN_POINT('Ctrl Pts',(78.7205204353165,10.0737775242579,140.));
#130782=CARTESIAN_POINT('Ctrl Pts',(78.7285063046483,10.0811986317636,140.));
#130783=CARTESIAN_POINT('Origin',(80.,-9.,129.));
#130784=CARTESIAN_POINT('Ctrl Pts',(79.2300979593296,-10.4774325188555,
129.));
#130785=CARTESIAN_POINT('Ctrl Pts',(79.2818307626562,-10.5124994265382,
129.));
#130786=CARTESIAN_POINT('Ctrl Pts',(79.3355405524417,-10.5443105979769,
129.));
#130787=CARTESIAN_POINT('Ctrl Pts',(79.3908959420258,-10.5729304242413,
129.));
#130788=CARTESIAN_POINT('Ctrl Pts',(79.4259931310383,-10.5910763619622,
129.));
#130789=CARTESIAN_POINT('Ctrl Pts',(79.4617527421542,-10.607938734873,129.));
#130790=CARTESIAN_POINT('Ctrl Pts',(79.4980979071617,-10.6235267468153,
129.));
#130791=CARTESIAN_POINT('Ctrl Pts',(79.5226967495725,-10.63407689975,129.));
#130792=CARTESIAN_POINT('Ctrl Pts',(79.5475639365611,-10.6440431834583,
129.));
#130793=CARTESIAN_POINT('Ctrl Pts',(79.572676847719,-10.6534269071554,129.));
#130794=CARTESIAN_POINT('Ctrl Pts',(79.5862865628442,-10.6585123313631,
129.));
#130795=CARTESIAN_POINT('Ctrl Pts',(79.5999686671651,-10.6634265769751,
129.));
#130796=CARTESIAN_POINT('Ctrl Pts',(79.6137053445211,-10.6681651435862,
129.));
#130797=CARTESIAN_POINT('Ctrl Pts',(79.6760830398119,-10.6896827825697,
129.));
#130798=CARTESIAN_POINT('Ctrl Pts',(79.7396537355289,-10.7076082288804,
129.));
#130799=CARTESIAN_POINT('Ctrl Pts',(79.8040670116738,-10.7219885211612,
129.));
#130800=CARTESIAN_POINT('Ctrl Pts',(79.850512820343,-10.7323575684114,129.));
#130801=CARTESIAN_POINT('Ctrl Pts',(79.8973976102623,-10.7408825669339,
129.));
#130802=CARTESIAN_POINT('Ctrl Pts',(79.9445991273204,-10.7475671243797,
129.));
#130803=CARTESIAN_POINT('Ctrl Pts',(79.9573807540249,-10.7493772254798,
129.));
#130804=CARTESIAN_POINT('Ctrl Pts',(79.97018563782,-10.7510523045138,129.));
#130805=CARTESIAN_POINT('Ctrl Pts',(79.9830114160439,-10.7525922771026,
129.));
#130806=CARTESIAN_POINT('Ctrl Pts',(79.996531159052,-10.7542155730365,129.));
#130807=CARTESIAN_POINT('Ctrl Pts',(80.0100665770587,-10.7556877927573,
129.));
#130808=CARTESIAN_POINT('Ctrl Pts',(80.0236082784729,-10.7570087636515,
129.));
#130809=CARTESIAN_POINT('Ctrl Pts',(80.091484178783,-10.7636299470602,129.));
#130810=CARTESIAN_POINT('Ctrl Pts',(80.1595660163247,-10.7664609181679,
129.));
#130811=CARTESIAN_POINT('Ctrl Pts',(80.2274935340178,-10.7655506742358,
129.));
#130812=CARTESIAN_POINT('Ctrl Pts',(80.296076466387,-10.7646316476003,129.));
#130813=CARTESIAN_POINT('Ctrl Pts',(80.3645031228694,-10.7598991585355,
129.));
#130814=CARTESIAN_POINT('Ctrl Pts',(80.4324242364423,-10.7513551603384,
129.));
#130815=CARTESIAN_POINT('Ctrl Pts',(80.4996588750007,-10.7428975158681,
129.));
#130816=CARTESIAN_POINT('Ctrl Pts',(80.5663992262361,-10.730705158574,129.));
#130817=CARTESIAN_POINT('Ctrl Pts',(80.6323115272082,-10.7147296965981,
129.));
#130818=CARTESIAN_POINT('Ctrl Pts',(80.6410547490952,-10.7126105624344,
129.));
#130819=CARTESIAN_POINT('Ctrl Pts',(80.6497833941471,-10.7104247863846,
129.));
#130820=CARTESIAN_POINT('Ctrl Pts',(80.6584966740677,-10.7081721860126,
129.));
#130821=CARTESIAN_POINT('Ctrl Pts',(80.6723039786817,-10.7046026530936,
129.));
#130822=CARTESIAN_POINT('Ctrl Pts',(80.6860752224786,-10.7008644715111,
129.));
#130823=CARTESIAN_POINT('Ctrl Pts',(80.6997839249182,-10.6969638794083,
129.));
#130824=CARTESIAN_POINT('Ctrl Pts',(80.767583687095,-10.6776725410715,129.));
#130825=CARTESIAN_POINT('Ctrl Pts',(80.8339729993893,-10.654383400419,129.));
#130826=CARTESIAN_POINT('Ctrl Pts',(80.8985888467434,-10.6271156045297,
129.));
#130827=CARTESIAN_POINT('Ctrl Pts',(80.9057657592136,-10.6240869576517,
129.));
#130828=CARTESIAN_POINT('Ctrl Pts',(80.9129208010519,-10.6210091751721,
129.));
#130829=CARTESIAN_POINT('Ctrl Pts',(80.9200534790049,-10.617882243794,129.));
#130830=CARTESIAN_POINT('Ctrl Pts',(80.9841494242166,-10.5897828926648,
129.));
#130831=CARTESIAN_POINT('Ctrl Pts',(81.0464403977837,-10.5577196528645,
129.));
#130832=CARTESIAN_POINT('Ctrl Pts',(81.1067676723926,-10.5220379319953,
129.));
#130833=CARTESIAN_POINT('Ctrl Pts',(81.1670949470016,-10.4863562111261,
129.));
#130834=CARTESIAN_POINT('Ctrl Pts',(81.2254592414653,-10.4470553334301,
129.));
#130835=CARTESIAN_POINT('Ctrl Pts',(81.2816837958061,-10.4044260185767,
129.));
#130836=CARTESIAN_POINT('Ctrl Pts',(81.2922353885737,-10.3964258276358,
129.));
#130837=CARTESIAN_POINT('Ctrl Pts',(81.3027115516211,-10.3883082725581,
129.));
#130838=CARTESIAN_POINT('Ctrl Pts',(81.31311101339,-10.380075090645,129.));
#130839=CARTESIAN_POINT('Ctrl Pts',(81.3222607011055,-10.3728313462008,
129.));
#130840=CARTESIAN_POINT('Ctrl Pts',(81.3313439530095,-10.3655036675837,
129.));
#130841=CARTESIAN_POINT('Ctrl Pts',(81.3403582861554,-10.3580952079013,
129.));
#130842=CARTESIAN_POINT('Ctrl Pts',(81.3951033706617,-10.3131027780881,
129.));
#130843=CARTESIAN_POINT('Ctrl Pts',(81.4473298717614,-10.2651175909719,
129.));
#130844=CARTESIAN_POINT('Ctrl Pts',(81.496889274164,-10.2144864134273,129.));
#130845=CARTESIAN_POINT('Ctrl Pts',(81.5478632629694,-10.1624100575344,
129.));
#130846=CARTESIAN_POINT('Ctrl Pts',(81.5960165224352,-10.1075340205125,
129.));
#130847=CARTESIAN_POINT('Ctrl Pts',(81.641166947533,-10.0501836096891,129.));
#130848=CARTESIAN_POINT('Ctrl Pts',(81.6863173726308,-9.99283319886575,
129.));
#130849=CARTESIAN_POINT('Ctrl Pts',(81.7284657192251,-9.93300764353711,
129.));
#130850=CARTESIAN_POINT('Ctrl Pts',(81.7673980299202,-9.87099085777822,
129.));
#130851=CARTESIAN_POINT('Ctrl Pts',(81.7770294648137,-9.85564857206042,
129.));
#130852=CARTESIAN_POINT('Ctrl Pts',(81.7864638901199,-9.84017201327144,
129.));
#130853=CARTESIAN_POINT('Ctrl Pts',(81.7956976814099,-9.82456517452716,
129.));
#130854=CARTESIAN_POINT('Ctrl Pts',(81.8029369736993,-9.81232941309025,
129.));
#130855=CARTESIAN_POINT('Ctrl Pts',(81.8100536644344,-9.80001205719501,
129.));
#130856=CARTESIAN_POINT('Ctrl Pts',(81.8170355830307,-9.78763403843294,
129.));
#130857=CARTESIAN_POINT('Ctrl Pts',(81.8540216960544,-9.72206254907344,
129.));
#130858=CARTESIAN_POINT('Ctrl Pts',(81.8872983542923,-9.6546761717898,129.));
#130859=CARTESIAN_POINT('Ctrl Pts',(81.9166853947369,-9.58582022495588,
129.));
#130860=CARTESIAN_POINT('Ctrl Pts',(81.9459283936586,-9.51730177775739,
129.));
#130861=CARTESIAN_POINT('Ctrl Pts',(81.9713205227596,-9.4473272863831,129.));
#130862=CARTESIAN_POINT('Ctrl Pts',(81.9926493682963,-9.37620015748104,
129.));
#130863=CARTESIAN_POINT('Ctrl Pts',(82.0137867027778,-9.30571167690551,
129.));
#130864=CARTESIAN_POINT('Ctrl Pts',(82.0309340643105,-9.23409033014075,
129.));
#130865=CARTESIAN_POINT('Ctrl Pts',(82.0438401515687,-9.1616076442864,129.));
#130866=CARTESIAN_POINT('Ctrl Pts',(82.0465861480475,-9.14618568128984,
129.));
#130867=CARTESIAN_POINT('Ctrl Pts',(82.0491399591624,-9.13072466500652,
129.));
#130868=CARTESIAN_POINT('Ctrl Pts',(82.0514988556353,-9.11522712597233,
129.));
#130869=CARTESIAN_POINT('Ctrl Pts',(82.0534883930455,-9.10215621165814,
129.));
#130870=CARTESIAN_POINT('Ctrl Pts',(82.0553392745732,-9.08905931614965,
129.));
#130871=CARTESIAN_POINT('Ctrl Pts',(82.0570522990024,-9.07593808097501,
129.));
#130872=CARTESIAN_POINT('Ctrl Pts',(81.8174278887595,-8.04137941204075,
129.));
#130873=CARTESIAN_POINT('Ctrl Pts',(81.7762159990727,-7.97834070616292,
129.));
#130874=CARTESIAN_POINT('Ctrl Pts',(81.7313405623381,-7.91789939904031,
129.));
#130875=CARTESIAN_POINT('Ctrl Pts',(81.6831396723547,-7.86020929481065,
129.));
#130876=CARTESIAN_POINT('Ctrl Pts',(81.6370503049079,-7.80504640439929,
129.));
#130877=CARTESIAN_POINT('Ctrl Pts',(81.5879194000536,-7.75239886539245,
129.));
#130878=CARTESIAN_POINT('Ctrl Pts',(81.5360172279659,-7.70243779621757,
129.));
#130879=CARTESIAN_POINT('Ctrl Pts',(81.5243247771145,-7.69118263439461,
129.));
#130880=CARTESIAN_POINT('Ctrl Pts',(81.5124900232915,-7.68006251540966,
129.));
#130881=CARTESIAN_POINT('Ctrl Pts',(81.5005210264171,-7.66908431840279,
129.));
#130882=CARTESIAN_POINT('Ctrl Pts',(81.4455928567033,-7.61870313151859,
129.));
#130883=CARTESIAN_POINT('Ctrl Pts',(81.3879497724495,-7.57140685173894,
129.));
#130884=CARTESIAN_POINT('Ctrl Pts',(81.3279084097019,-7.52736776321866,
129.));
#130885=CARTESIAN_POINT('Ctrl Pts',(81.2857570428461,-7.49645061391918,
129.));
#130886=CARTESIAN_POINT('Ctrl Pts',(81.2424229811911,-7.46713969363308,
129.));
#130887=CARTESIAN_POINT('Ctrl Pts',(81.1980104568253,-7.43950901649432,
129.));
#130888=CARTESIAN_POINT('Ctrl Pts',(81.1811384663816,-7.42901232603832,
129.));
#130889=CARTESIAN_POINT('Ctrl Pts',(81.1641108054664,-7.41875825468291,
129.));
#130890=CARTESIAN_POINT('Ctrl Pts',(81.14693311349,-7.40875134687659,129.));
#130891=CARTESIAN_POINT('Ctrl Pts',(81.1305341636591,-7.39919809727218,
129.));
#130892=CARTESIAN_POINT('Ctrl Pts',(81.1139931479043,-7.38986736642136,
129.));
#130893=CARTESIAN_POINT('Ctrl Pts',(81.0973446108032,-7.38077903707112,
129.));
#130894=CARTESIAN_POINT('Ctrl Pts',(81.0336771270485,-7.34602336708333,
129.));
#130895=CARTESIAN_POINT('Ctrl Pts',(80.9683737258037,-7.31476829705795,
129.));
#130896=CARTESIAN_POINT('Ctrl Pts',(80.9017257585264,-7.28717480040604,
129.));
#130897=CARTESIAN_POINT('Ctrl Pts',(80.8366064434856,-7.2602141941796,129.));
#130898=CARTESIAN_POINT('Ctrl Pts',(80.770202614952,-7.2367489826126,129.));
#130899=CARTESIAN_POINT('Ctrl Pts',(80.7027774984244,-7.2169771323118,129.));
#130900=CARTESIAN_POINT('Ctrl Pts',(80.6364371264415,-7.19752337425697,
129.));
#130901=CARTESIAN_POINT('Ctrl Pts',(80.5691072900731,-7.18164493377435,
129.));
#130902=CARTESIAN_POINT('Ctrl Pts',(80.5010426942184,-7.16957948697683,
129.));
#130903=CARTESIAN_POINT('Ctrl Pts',(80.4789909407811,-7.16567049061024,
129.));
#130904=CARTESIAN_POINT('Ctrl Pts',(80.4568621429895,-7.1621621240849,129.));
#130905=CARTESIAN_POINT('Ctrl Pts',(80.434665257464,-7.15906364436086,129.));
#130906=CARTESIAN_POINT('Ctrl Pts',(80.4221751971582,-7.15732014757321,
129.));
#130907=CARTESIAN_POINT('Ctrl Pts',(80.4096622887256,-7.15570638712659,
129.));
#130908=CARTESIAN_POINT('Ctrl Pts',(80.3971458493996,-7.15422589319744,
129.));
#130909=CARTESIAN_POINT('Ctrl Pts',(80.3293083065445,-7.14620180042234,
129.));
#130910=CARTESIAN_POINT('Ctrl Pts',(80.2612487043902,-7.14207059151351,
129.));
#130911=CARTESIAN_POINT('Ctrl Pts',(80.1932132104911,-7.14201015864512,
129.));
#130912=CARTESIAN_POINT('Ctrl Pts',(80.1834193046227,-7.14200145915915,
129.));
#130913=CARTESIAN_POINT('Ctrl Pts',(80.1736259045768,-7.14207720414265,
129.));
#130914=CARTESIAN_POINT('Ctrl Pts',(80.1638337541376,-7.14223801413209,
129.));
#130915=CARTESIAN_POINT('Ctrl Pts',(80.0941260097053,-7.14338277816691,
129.));
#130916=CARTESIAN_POINT('Ctrl Pts',(80.0244801006768,-7.14883421760917,
129.));
#130917=CARTESIAN_POINT('Ctrl Pts',(79.9552255344744,-7.15841681494381,
129.));
#130918=CARTESIAN_POINT('Ctrl Pts',(79.8912779185903,-7.16726510159306,
129.));
#130919=CARTESIAN_POINT('Ctrl Pts',(79.8276634957026,-7.17963663965979,
129.));
#130920=CARTESIAN_POINT('Ctrl Pts',(79.7646618938049,-7.19542712913009,
129.));
#130921=CARTESIAN_POINT('Ctrl Pts',(79.7507945251221,-7.19890279534443,
129.));
#130922=CARTESIAN_POINT('Ctrl Pts',(79.73695694447,-7.20254421600149,129.));
#130923=CARTESIAN_POINT('Ctrl Pts',(79.7231523111297,-7.20635045626908,
129.));
#130924=CARTESIAN_POINT('Ctrl Pts',(79.7120937153582,-7.20939955373447,
129.));
#130925=CARTESIAN_POINT('Ctrl Pts',(79.7010568159009,-7.21255435763673,
129.));
#130926=CARTESIAN_POINT('Ctrl Pts',(79.6900562807526,-7.21581026506554,
129.));
#130927=CARTESIAN_POINT('Ctrl Pts',(79.6245241542564,-7.2352062794056,129.));
#130928=CARTESIAN_POINT('Ctrl Pts',(79.5601586446492,-7.25821930074134,
129.));
#130929=CARTESIAN_POINT('Ctrl Pts',(79.497261502229,-7.28466766521021,129.));
#130930=CARTESIAN_POINT('Ctrl Pts',(79.4350282189579,-7.31083687568166,
129.));
#130931=CARTESIAN_POINT('Ctrl Pts',(79.3742316278236,-7.34037002111481,
129.));
#130932=CARTESIAN_POINT('Ctrl Pts',(79.3151931372451,-7.37313178272857,
129.));
#130933=CARTESIAN_POINT('Ctrl Pts',(79.2566545492536,-7.40561613736218,
129.));
#130934=CARTESIAN_POINT('Ctrl Pts',(79.1998436436882,-7.44127530985043,
129.));
#130935=CARTESIAN_POINT('Ctrl Pts',(79.1451144630058,-7.48000743341435,
129.));
#130936=CARTESIAN_POINT('Ctrl Pts',(79.1336098695569,-7.48814929356024,
129.));
#130937=CARTESIAN_POINT('Ctrl Pts',(79.1221974311397,-7.49642702849065,
129.));
#130938=CARTESIAN_POINT('Ctrl Pts',(79.1108807167964,-7.50483982192541,
129.));
#130939=CARTESIAN_POINT('Ctrl Pts',(79.1002619712711,-7.51273374854853,
129.));
#130940=CARTESIAN_POINT('Ctrl Pts',(79.0897262977731,-7.52074768146701,
129.));
#130941=CARTESIAN_POINT('Ctrl Pts',(79.0792931722657,-7.52886772372503,
129.));
#130942=CARTESIAN_POINT('Ctrl Pts',(79.0276936912682,-7.56902730638227,
129.));
#130943=CARTESIAN_POINT('Ctrl Pts',(78.9785044128779,-7.61184880861672,
129.));
#130944=CARTESIAN_POINT('Ctrl Pts',(78.9320167948803,-7.65720006725642,
129.));
#130945=CARTESIAN_POINT('Ctrl Pts',(78.8870712692266,-7.70104692898903,
129.));
#130946=CARTESIAN_POINT('Ctrl Pts',(78.8446506824178,-7.74725918924175,
129.));
#130947=CARTESIAN_POINT('Ctrl Pts',(78.8050589359191,-7.7957420041302,129.));
#130948=CARTESIAN_POINT('Ctrl Pts',(78.7657015104581,-7.84393787680228,
129.));
#130949=CARTESIAN_POINT('Ctrl Pts',(78.7291389707237,-7.8943780226341,129.));
#130950=CARTESIAN_POINT('Ctrl Pts',(78.6957183447143,-7.94698530266433,
129.));
#130951=CARTESIAN_POINT('Ctrl Pts',(78.6902770143314,-7.95555048008235,
129.));
#130952=CARTESIAN_POINT('Ctrl Pts',(78.6849190860989,-7.9641731294301,129.));
#130953=CARTESIAN_POINT('Ctrl Pts',(78.6796461961968,-7.97285294397019,
129.));
#130954=CARTESIAN_POINT('Ctrl Pts',(78.6739912788964,-7.98216162181429,
129.));
#130955=CARTESIAN_POINT('Ctrl Pts',(78.6684341691904,-7.99153604930243,
129.));
#130956=CARTESIAN_POINT('Ctrl Pts',(78.6629752716474,-8.00097456550985,
129.));
#130957=CARTESIAN_POINT('Ctrl Pts',(81.2663555976867,-7.92217834879833,
139.998270398006));
#130958=CARTESIAN_POINT('Ctrl Pts',(81.6248827770132,-8.34339539386142,
139.961212886432));
#130959=CARTESIAN_POINT('Ctrl Pts',(81.8817058969813,-9.56478460164107,
139.887111002195));
#130960=CARTESIAN_POINT('Ctrl Pts',(80.5443605470635,-10.8898007373938,
139.775964745293));
#130961=CARTESIAN_POINT('Ctrl Pts',(78.7083083354406,-10.4810544455385,
139.664831627301));
#130962=CARTESIAN_POINT('Ctrl Pts',(78.0547700220628,-8.71872336189441,
139.55369850931));
#130963=CARTESIAN_POINT('Ctrl Pts',(79.1814308219956,-7.21288524523363,
139.442565391318));
#130964=CARTESIAN_POINT('Ctrl Pts',(81.0573526260259,-7.34314561460427,
139.331432273327));
#130965=CARTESIAN_POINT('Ctrl Pts',(81.9655073696431,-8.98959908412584,
139.220299155335));
#130966=CARTESIAN_POINT('Ctrl Pts',(81.0747701647197,-10.6456820091187,
139.109166037344));
#130967=CARTESIAN_POINT('Ctrl Pts',(79.2003523202965,-10.7955181419101,
138.998032919352));
#130968=CARTESIAN_POINT('Ctrl Pts',(78.0578077510972,-9.30205172592216,
138.886899801361));
#130969=CARTESIAN_POINT('Ctrl Pts',(78.6928318965889,-7.53212281053173,
138.775766683369));
#130970=CARTESIAN_POINT('Ctrl Pts',(80.524228754692,-7.10565916705379,138.664633565377));
#130971=CARTESIAN_POINT('Ctrl Pts',(81.8758303269309,-8.41296773760928,
138.553500447386));
#130972=CARTESIAN_POINT('Ctrl Pts',(81.5105983945688,-10.2575528443921,
138.442367329394));
#130973=CARTESIAN_POINT('Ctrl Pts',(79.7628072363265,-10.9511753556914,
138.331234211403));
#130974=CARTESIAN_POINT('Ctrl Pts',(78.2321042891996,-9.85900574355044,
138.220101093411));
#130975=CARTESIAN_POINT('Ctrl Pts',(78.3194490519439,-7.98064008895766,
138.10896797542));
#130976=CARTESIAN_POINT('Ctrl Pts',(79.9449002020512,-7.0352328325274,137.997834857428));
#130977=CARTESIAN_POINT('Ctrl Pts',(81.6207808491711,-7.88805777822167,
137.886701739436));
#130978=CARTESIAN_POINT('Ctrl Pts',(81.8132590731305,-9.75857603145555,
137.775568621445));
#130979=CARTESIAN_POINT('Ctrl Pts',(80.3461712225592,-10.9348156333929,
137.664435503453));
#130980=CARTESIAN_POINT('Ctrl Pts',(78.5622538447273,-10.3402358189599,
137.553302385462));
#130981=CARTESIAN_POINT('Ctrl Pts',(78.094218336951,-8.51901942944539,137.44216926747));
#130982=CARTESIAN_POINT('Ctrl Pts',(79.3704292182216,-7.13801539048741,
137.331036149478));
#130983=CARTESIAN_POINT('Ctrl Pts',(81.222848058548,-7.46117295258134,137.219903031487));
#130984=CARTESIAN_POINT('Ctrl Pts',(81.9560682249059,-9.1927255963959,137.108769913495));
#130985=CARTESIAN_POINT('Ctrl Pts',(80.8990177617125,-10.7478881886462,
136.997636795504));
#130986=CARTESIAN_POINT('Ctrl Pts',(79.0191508580167,-10.7033147145058,
136.886503677512));
#130987=CARTESIAN_POINT('Ctrl Pts',(78.0369956949045,-9.0998005718031,136.775370559521));
#130988=CARTESIAN_POINT('Ctrl Pts',(78.8514593349149,-7.40494501768999,
136.664237441529));
#130989=CARTESIAN_POINT('Ctrl Pts',(80.7171125977301,-7.16994656413151,
136.553104323538));
#130990=CARTESIAN_POINT('Ctrl Pts',(81.9264361858263,-8.60988504528501,
136.441971205546));
#130991=CARTESIAN_POINT('Ctrl Pts',(81.3726095528648,-10.4068720877668,
136.330838087554));
#130992=CARTESIAN_POINT('Ctrl Pts',(79.5625166317358,-10.9162344215796,
136.219704969563));
#130993=CARTESIAN_POINT('Ctrl Pts',(78.15282570842,-9.67178359051037,136.108571851571));
#130994=CARTESIAN_POINT('Ctrl Pts',(78.4337414008296,-7.81248997626183,
135.99743873358));
#130995=CARTESIAN_POINT('Ctrl Pts',(80.148158610538,-7.04005227567747,135.886305615588));
#130996=CARTESIAN_POINT('Ctrl Pts',(81.7269752284157,-8.06143587518381,
135.775172497597));
#130997=CARTESIAN_POINT('Ctrl Pts',(81.7251961441649,-9.9418303032459,135.664039379605));
#130998=CARTESIAN_POINT('Ctrl Pts',(80.1444496457157,-10.9602245676979,
135.552906261614));
#130999=CARTESIAN_POINT('Ctrl Pts',(78.4314971460249,-10.1845441541056,
135.441773143622));
#131000=CARTESIAN_POINT('Ctrl Pts',(78.1541001939629,-8.32472230747231,
135.330640025631));
#131001=CARTESIAN_POINT('Ctrl Pts',(79.5661433982943,-7.08294118371136,
135.219506907639));
#131002=CARTESIAN_POINT('Ctrl Pts',(81.3752692409363,-7.59572774331752,
135.108373789647));
#131003=CARTESIAN_POINT('Ctrl Pts',(81.9256945442036,-9.39375954385691,
134.997240671656));
#131004=CARTESIAN_POINT('Ctrl Pts',(80.713648406017,-10.8314071116339,134.886107553664));
#131005=CARTESIAN_POINT('Ctrl Pts',(78.8484431577161,-10.592878807362,134.774974435673));
#131006=CARTESIAN_POINT('Ctrl Pts',(78.0371880563092,-8.89648512349353,
134.663841317681));
#131007=CARTESIAN_POINT('Ctrl Pts',(79.0223757012933,-7.29483232890963,
134.55270819969));
#131008=CARTESIAN_POINT('Ctrl Pts',(80.9023235833712,-7.25381610165316,
134.441575081698));
#131009=CARTESIAN_POINT('Ctrl Pts',(81.9564294068378,-8.81097610729224,
134.330441963706));
#131010=CARTESIAN_POINT('Ctrl Pts',(81.2199340328551,-10.5411382194453,
134.219308845715));
#131011=CARTESIAN_POINT('Ctrl Pts',(79.3669070158681,-10.8607899745529,
134.108175727723));
#131012=CARTESIAN_POINT('Ctrl Pts',(78.0933116162554,-9.4773735049699,133.997042609732));
#131013=CARTESIAN_POINT('Ctrl Pts',(78.5647924719695,-7.6570460144004,133.88590949174));
#131014=CARTESIAN_POINT('Ctrl Pts',(80.3498317465547,-7.06584286960547,
133.774776373749));
#131015=CARTESIAN_POINT('Ctrl Pts',(81.8146912374499,-8.24485645823041,
133.663643255757));
#131016=CARTESIAN_POINT('Ctrl Pts',(81.6186738822797,-10.1150071384431,
133.552510137766));
#131017=CARTESIAN_POINT('Ctrl Pts',(79.9411824796641,-10.9646593992994,
133.441377019774));
#131018=CARTESIAN_POINT('Ctrl Pts',(78.3175231866948,-10.0161780496764,
133.330243901783));
#131019=CARTESIAN_POINT('Ctrl Pts',(78.2337328949045,-8.13765055261137,
133.219110783791));
#131020=CARTESIAN_POINT('Ctrl Pts',(79.7664997772935,-7.04837921153991,
133.107977665799));
#131021=CARTESIAN_POINT('Ctrl Pts',(81.5129752539825,-7.74530803111284,
132.996844547808));
#131022=CARTESIAN_POINT('Ctrl Pts',(81.8747162281011,-9.59058032480595,
132.885711429816));
#131023=CARTESIAN_POINT('Ctrl Pts',(80.5206431221497,-10.8953302602216,
132.774578311825));
#131024=CARTESIAN_POINT('Ctrl Pts',(78.6900569384936,-10.4653993420104,
132.663445193833));
#131025=CARTESIAN_POINT('Ctrl Pts',(78.0583822035841,-8.69427726843509,
132.552312075842));
#131026=CARTESIAN_POINT('Ctrl Pts',(79.2037524972869,-7.20296467191772,
132.44117895785));
#131027=CARTESIAN_POINT('Ctrl Pts',(81.077879845468,-7.35636953828203,132.330045839859));
#131028=CARTESIAN_POINT('Ctrl Pts',(81.9654891341413,-9.01408969587618,
132.218912721867));
#131029=CARTESIAN_POINT('Ctrl Pts',(81.0542054063466,-10.6589144092374,
132.107779603875));
#131030=CARTESIAN_POINT('Ctrl Pts',(79.1780713975498,-10.7854353610338,
131.996646485884));
#131031=CARTESIAN_POINT('Ctrl Pts',(78.0541987964962,-9.27785559635263,
131.885513367892));
#131032=CARTESIAN_POINT('Ctrl Pts',(78.7112000429067,-7.51597145361696,
131.774380249901));
#131033=CARTESIAN_POINT('Ctrl Pts',(80.5477617366628,-7.11232864729046,
131.663247131909));
#131034=CARTESIAN_POINT('Ctrl Pts',(81.8829903294524,-8.43635696105569,
131.552114013917));
#131035=CARTESIAN_POINT('Ctrl Pts',(81.4948320587062,-10.2762535686903,
131.440980895926));
#131036=CARTESIAN_POINT('Ctrl Pts',(79.7385446523142,-10.9480726777078,
131.329847777934));
#131037=CARTESIAN_POINT('Ctrl Pts',(78.2215514698866,-9.83693899608168,
131.218714659943));
#131038=CARTESIAN_POINT('Ctrl Pts',(78.3322643833567,-7.95980580489549,
131.107581541951));
#131039=CARTESIAN_POINT('Ctrl Pts',(79.9693545703466,-7.03469928015326,
130.99644842396));
#131040=CARTESIAN_POINT('Ctrl Pts',(81.6344926694737,-7.90831333293382,
130.885315305968));
#131041=CARTESIAN_POINT('Ctrl Pts',(81.8036787266466,-9.78108198107158,
130.774182187977));
#131042=CARTESIAN_POINT('Ctrl Pts',(80.3220670575926,-10.9389736789513,
130.663049069985));
#131043=CARTESIAN_POINT('Ctrl Pts',(78.5456868663343,-10.3222403037902,
130.551915951993));
#131044=CARTESIAN_POINT('Ctrl Pts',(78.1003514489162,-8.49534065136783,
130.440782834002));
#131045=CARTESIAN_POINT('Ctrl Pts',(79.3936488425649,-7.13032491058225,
130.32964971601));
#131046=CARTESIAN_POINT('Ctrl Pts',(81.2419033200459,-7.47650978467848,
130.218516598019));
#131047=CARTESIAN_POINT('Ctrl Pts',(81.9535176916404,-9.21705208375298,
130.107383480027));
#131048=CARTESIAN_POINT('Ctrl Pts',(80.8771984544237,-10.7589413763661,
129.996250362036));
#131049=CARTESIAN_POINT('Ctrl Pts',(78.9980271998695,-10.6909750100548,
129.885117244044));
#131050=CARTESIAN_POINT('Ctrl Pts',(78.035912068222,-9.0753684670664,129.773984126053));
#131051=CARTESIAN_POINT('Ctrl Pts',(78.8713846530321,-7.39076801526417,
129.662851008061));
#131052=CARTESIAN_POINT('Ctrl Pts',(80.7398571901727,-7.17902807893094,
129.551717890069));
#131053=CARTESIAN_POINT('Ctrl Pts',(81.9310876574871,-8.63385591733535,
129.440584772078));
#131054=CARTESIAN_POINT('Ctrl Pts',(81.3551063262338,-10.4239106328993,
129.329451654086));
#131055=CARTESIAN_POINT('Ctrl Pts',(79.538478193619,-10.910506172836,129.218318536095));
#131056=CARTESIAN_POINT('Ctrl Pts',(78.1450715714801,-9.64902245878714,
129.107185418103));
#131057=CARTESIAN_POINT('Ctrl Pts',(78.4476863760178,-7.79252426730275,
128.996052300112));
#131058=CARTESIAN_POINT('Ctrl Pts',(80.1745006914082,-7.04323474754915,
128.88491918212));
#131059=CARTESIAN_POINT('Ctrl Pts',(81.2128991836478,-7.73509822724767,
128.810830436792));
#131060=CARTESIAN_POINT('Ctrl Pts',(81.4708680902966,-8.22417585740202,
128.773786064129));
#131061=CARTESIAN_POINT('Ctrl Pts',(81.3664711939768,-7.83696787750457,
140.074173751493));
#131062=CARTESIAN_POINT('Ctrl Pts',(81.7533428307448,-8.29148551815949,
140.03711623992));
#131063=CARTESIAN_POINT('Ctrl Pts',(82.0304698841766,-9.60943536740704,
139.963014355682));
#131064=CARTESIAN_POINT('Ctrl Pts',(80.5873966270283,-11.0392046868368,
139.85186809878));
#131065=CARTESIAN_POINT('Ctrl Pts',(78.6061897192665,-10.5981437127428,
139.740734980789));
#131066=CARTESIAN_POINT('Ctrl Pts',(77.900983945294,-8.69648618112318,139.629601862797));
#131067=CARTESIAN_POINT('Ctrl Pts',(79.1167163440794,-7.07159944870142,
139.518468744806));
#131068=CARTESIAN_POINT('Ctrl Pts',(81.1409448562311,-7.21215794805729,
139.407335626814));
#131069=CARTESIAN_POINT('Ctrl Pts',(82.1208965373333,-8.98877680806325,
139.296202508823));
#131070=CARTESIAN_POINT('Ctrl Pts',(81.1597393914615,-10.7757864094529,
139.185069390831));
#131071=CARTESIAN_POINT('Ctrl Pts',(79.1371337390217,-10.9374682937912,
139.073936272839));
#131072=CARTESIAN_POINT('Ctrl Pts',(77.9042618312433,-9.32593134449562,
138.962803154848));
#131073=CARTESIAN_POINT('Ctrl Pts',(78.5894897434344,-7.41607531141488,
138.851670036856));
#131074=CARTESIAN_POINT('Ctrl Pts',(80.565673254534,-6.95589628653788,138.740536918865));
#131075=CARTESIAN_POINT('Ctrl Pts',(82.0241298030518,-8.36655811530563,
138.629403800873));
#131076=CARTESIAN_POINT('Ctrl Pts',(81.630023348589,-10.3569725122268,138.518270682882));
#131077=CARTESIAN_POINT('Ctrl Pts',(79.7440552404305,-11.105431462395,138.40713756489));
#131078=CARTESIAN_POINT('Ctrl Pts',(78.0923379126866,-9.92691705723613,
138.296004446898));
#131079=CARTESIAN_POINT('Ctrl Pts',(78.1865879815086,-7.90005148847718,
138.184871328907));
#131080=CARTESIAN_POINT('Ctrl Pts',(79.9405441198124,-6.87990218377285,
138.073738210915));
#131081=CARTESIAN_POINT('Ctrl Pts',(81.7489166125117,-7.80014980136526,
137.962605092924));
#131082=CARTESIAN_POINT('Ctrl Pts',(81.9566117883287,-9.81854756856506,
137.851471974932));
#131083=CARTESIAN_POINT('Ctrl Pts',(80.3735388422295,-11.0877783724548,
137.740338856941));
#131084=CARTESIAN_POINT('Ctrl Pts',(78.4485884462312,-10.4461922410183,
137.629205738949));
#131085=CARTESIAN_POINT('Ctrl Pts',(77.9435509667878,-8.48099404643846,
137.518072620958));
#131086=CARTESIAN_POINT('Ctrl Pts',(79.3206565837898,-6.99081052970044,
137.406939502966));
#131087=CARTESIAN_POINT('Ctrl Pts',(81.3195240339037,-7.33951629648805,
137.295806384974));
#131088=CARTESIAN_POINT('Ctrl Pts',(82.1107111522781,-9.20796210503437,
137.184673266983));
#131089=CARTESIAN_POINT('Ctrl Pts',(80.970092347282,-10.8860728095965,137.073540148991));
#131090=CARTESIAN_POINT('Ctrl Pts',(78.9416068436026,-10.8379754437858,
136.962407031));
#131091=CARTESIAN_POINT('Ctrl Pts',(77.8818044146011,-9.10769060977854,
136.851273913008));
#131092=CARTESIAN_POINT('Ctrl Pts',(78.7606579567252,-7.2788430910581,136.740140795017));
#131093=CARTESIAN_POINT('Ctrl Pts',(80.7738061168806,-7.02526611946862,
136.629007677025));
#131094=CARTESIAN_POINT('Ctrl Pts',(82.0787364621556,-8.57904332011374,
136.517874559034));
#131095=CARTESIAN_POINT('Ctrl Pts',(81.4811253789957,-10.5180966428822,
136.406741441042));
#131096=CARTESIAN_POINT('Ctrl Pts',(79.5279300524522,-11.0677281663842,
136.29560832305));
#131097=CARTESIAN_POINT('Ctrl Pts',(78.0067917223965,-9.72489348702338,
136.184475205059));
#131098=CARTESIAN_POINT('Ctrl Pts',(78.309916059917,-7.71860775680932,136.073342087067));
#131099=CARTESIAN_POINT('Ctrl Pts',(80.159871740457,-6.88510264267047,135.962208969076));
#131100=CARTESIAN_POINT('Ctrl Pts',(81.8635065116406,-7.98723483150851,
135.851075851084));
#131101=CARTESIAN_POINT('Ctrl Pts',(81.861586776469,-10.0162895645985,135.739942733093));
#131102=CARTESIAN_POINT('Ctrl Pts',(80.1558695521316,-11.1151960874005,
135.628809615101));
#131103=CARTESIAN_POINT('Ctrl Pts',(78.3074943787175,-10.2781918977068,
135.51767649711));
#131104=CARTESIAN_POINT('Ctrl Pts',(78.0081669662734,-8.27133617408902,
135.406543379118));
#131105=CARTESIAN_POINT('Ctrl Pts',(79.5318435440799,-6.93138226387365,
135.295410261126));
#131106=CARTESIAN_POINT('Ctrl Pts',(81.4839953368033,-7.48470872576181,
135.184277143135));
#131107=CARTESIAN_POINT('Ctrl Pts',(82.0779361877968,-9.42488940311613,
135.073144025143));
#131108=CARTESIAN_POINT('Ctrl Pts',(80.7700680529474,-10.9761945752546,
134.962010907152));
#131109=CARTESIAN_POINT('Ctrl Pts',(78.7574033264573,-10.7188086898595,
134.85087778916));
#131110=CARTESIAN_POINT('Ctrl Pts',(77.8820119837219,-8.88830143985422,
134.739744671169));
#131111=CARTESIAN_POINT('Ctrl Pts',(78.9450866366803,-7.1600251085068,134.628611553177));
#131112=CARTESIAN_POINT('Ctrl Pts',(80.9736595207341,-7.11576621855994,
134.517478435185));
#131113=CARTESIAN_POINT('Ctrl Pts',(82.1111008885469,-8.79603224810603,
134.406345317194));
#131114=CARTESIAN_POINT('Ctrl Pts',(81.3163796310402,-10.6629775922779,
134.295212199202));
#131115=CARTESIAN_POINT('Ctrl Pts',(79.3168559230081,-11.0079003898369,
134.184079081211));
#131116=CARTESIAN_POINT('Ctrl Pts',(77.942572562528,-9.5151137204279,134.072945963219));
#131117=CARTESIAN_POINT('Ctrl Pts',(78.4513277723769,-7.55087469940482,
133.961812845228));
#131118=CARTESIAN_POINT('Ctrl Pts',(80.3774887600915,-6.9129321905025,133.850679727236));
#131119=CARTESIAN_POINT('Ctrl Pts',(81.9581571767575,-8.18515628704078,
133.739546609245));
#131120=CARTESIAN_POINT('Ctrl Pts',(81.7466430729396,-10.2031574216154,
133.628413491253));
#131121=CARTESIAN_POINT('Ctrl Pts',(79.9365324815659,-11.1199815281129,
133.517280373261));
#131122=CARTESIAN_POINT('Ctrl Pts',(78.1845098611203,-10.0965150984217,
133.40614725527));
#131123=CARTESIAN_POINT('Ctrl Pts',(78.0940952727729,-8.06947489224123,
133.295014137278));
#131124=CARTESIAN_POINT('Ctrl Pts',(79.7480397064628,-6.89408788979295,
133.183881019287));
#131125=CARTESIAN_POINT('Ctrl Pts',(81.6325881178585,-7.6461145384991,133.072747901295));
#131126=CARTESIAN_POINT('Ctrl Pts',(82.0229276257478,-9.63727044998339,
132.961614783304));
#131127=CARTESIAN_POINT('Ctrl Pts',(80.5618041488974,-11.0451713629224,
132.850481665312));
#131128=CARTESIAN_POINT('Ctrl Pts',(78.5864954025802,-10.5812509473544,
132.739348547321));
#131129=CARTESIAN_POINT('Ctrl Pts',(77.9048816988202,-8.67010742733677,
132.628215429329));
#131130=CARTESIAN_POINT('Ctrl Pts',(79.1408027273532,-7.06089457426592,
132.517082311337));
#131131=CARTESIAN_POINT('Ctrl Pts',(81.1630949174867,-7.22642732927219,
132.405949193346));
#131132=CARTESIAN_POINT('Ctrl Pts',(82.1208768601684,-9.01520359966968,
132.294816075354));
#131133=CARTESIAN_POINT('Ctrl Pts',(81.1375488235206,-10.7900649372395,
132.183682957363));
#131134=CARTESIAN_POINT('Ctrl Pts',(79.1130913301086,-10.9265883879828,
132.072549839371));
#131135=CARTESIAN_POINT('Ctrl Pts',(77.9003675597515,-9.29982231625516,
131.96141672138));
#131136=CARTESIAN_POINT('Ctrl Pts',(78.609310039468,-7.39864705981793,131.850283603388));
#131137=CARTESIAN_POINT('Ctrl Pts',(80.591066708024,-6.96309304283512,131.739150485397));
#131138=CARTESIAN_POINT('Ctrl Pts',(82.0318558613661,-8.39179644500338,
131.628017367405));
#131139=CARTESIAN_POINT('Ctrl Pts',(81.6130105570556,-10.3771516792053,
131.516884249414));
#131140=CARTESIAN_POINT('Ctrl Pts',(79.7178745039888,-11.1020834927595,
131.405751131422));
#131141=CARTESIAN_POINT('Ctrl Pts',(78.0809508081225,-9.90310575587979,
131.29461801343));
#131142=CARTESIAN_POINT('Ctrl Pts',(78.2004164679532,-7.87757008667339,
131.183484895439));
#131143=CARTESIAN_POINT('Ctrl Pts',(79.9669318026273,-6.87932644979174,
131.072351777447));
#131144=CARTESIAN_POINT('Ctrl Pts',(81.7637124625041,-7.82200672060876,
130.961218659456));
#131145=CARTESIAN_POINT('Ctrl Pts',(81.946274038393,-9.84283279453126,130.850085541464));
#131146=CARTESIAN_POINT('Ctrl Pts',(80.3475290491337,-11.092265144961,130.738952423472));
#131147=CARTESIAN_POINT('Ctrl Pts',(78.430711714935,-10.4267740356223,130.627819305481));
#131148=CARTESIAN_POINT('Ctrl Pts',(77.9501689505874,-8.45544327048684,
130.516686187489));
#131149=CARTESIAN_POINT('Ctrl Pts',(79.3457119062108,-6.98251205549822,
130.405553069498));
#131150=CARTESIAN_POINT('Ctrl Pts',(81.3400857670997,-7.35606562852865,
130.294419951506));
#131151=CARTESIAN_POINT('Ctrl Pts',(82.1079589788419,-9.23421179689408,
130.183286833515));
#131152=CARTESIAN_POINT('Ctrl Pts',(80.9465480482423,-10.8979998407152,
130.072153715523));
#131153=CARTESIAN_POINT('Ctrl Pts',(78.9188131903647,-10.8246601864401,
129.961020597532));
#131154=CARTESIAN_POINT('Ctrl Pts',(77.8806351185129,-9.08132695063578,
129.84988747954));
#131155=CARTESIAN_POINT('Ctrl Pts',(78.7821585315143,-7.26354528255374,
129.738754361548));
#131156=CARTESIAN_POINT('Ctrl Pts',(80.7983488523086,-7.03506560106271,
129.627621243557));
#131157=CARTESIAN_POINT('Ctrl Pts',(82.0837556700664,-8.6049092824162,129.516488125565));
#131158=CARTESIAN_POINT('Ctrl Pts',(81.4622383815074,-10.5364822220618,
129.405355007574));
#131159=CARTESIAN_POINT('Ctrl Pts',(79.5019911824421,-11.0615470535008,
129.294221889582));
#131160=CARTESIAN_POINT('Ctrl Pts',(77.9984245585591,-9.70033290475177,
129.183088771591));
#131161=CARTESIAN_POINT('Ctrl Pts',(78.3249634975641,-7.69706359795712,
129.071955653599));
#131162=CARTESIAN_POINT('Ctrl Pts',(80.1882963747102,-6.88853671454275,
128.960822535608));
#131163=CARTESIAN_POINT('Ctrl Pts',(81.3087886204161,-7.63509756751294,
128.88673379028));
#131164=CARTESIAN_POINT('Ctrl Pts',(81.5871520441821,-8.16284071836659,
128.849689417616));
#131165=CARTESIAN_POINT('Ctrl Pts',(81.4665867902668,-7.7517574062108,140.150077104981));
#131166=CARTESIAN_POINT('Ctrl Pts',(81.8818028844763,-8.23957564245756,
140.113019593406));
#131167=CARTESIAN_POINT('Ctrl Pts',(82.1792338713718,-9.65408613317302,
140.038917709168));
#131168=CARTESIAN_POINT('Ctrl Pts',(80.6304327069932,-11.1886086362797,
139.927771452267));
#131169=CARTESIAN_POINT('Ctrl Pts',(78.5040711030923,-10.715232979947,139.816638334275));
#131170=CARTESIAN_POINT('Ctrl Pts',(77.7471978685252,-8.67424900035197,
139.705505216284));
#131171=CARTESIAN_POINT('Ctrl Pts',(79.0520018661632,-6.93031365216921,
139.594372098292));
#131172=CARTESIAN_POINT('Ctrl Pts',(81.2245370864363,-7.0811702815103,139.483238980301));
#131173=CARTESIAN_POINT('Ctrl Pts',(82.2762857050234,-8.98795453200066,
139.372105862309));
#131174=CARTESIAN_POINT('Ctrl Pts',(81.2447086182033,-10.9058908097869,
139.260972744318));
#131175=CARTESIAN_POINT('Ctrl Pts',(79.0739151577466,-11.0794184456721,
139.149839626326));
#131176=CARTESIAN_POINT('Ctrl Pts',(77.7507159113895,-9.3498109630691,139.038706508334));
#131177=CARTESIAN_POINT('Ctrl Pts',(78.4861475902798,-7.30002781229801,
138.927573390343));
#131178=CARTESIAN_POINT('Ctrl Pts',(80.607117754376,-6.80613340602198,138.816440272351));
#131179=CARTESIAN_POINT('Ctrl Pts',(82.1724292791728,-8.32014849300197,
138.70530715436));
#131180=CARTESIAN_POINT('Ctrl Pts',(81.7494483026092,-10.4563921800615,
138.594174036368));
#131181=CARTESIAN_POINT('Ctrl Pts',(79.7253032445344,-11.2596875690987,
138.483040918377));
#131182=CARTESIAN_POINT('Ctrl Pts',(77.9525715361738,-9.99482837092183,
138.371907800385));
#131183=CARTESIAN_POINT('Ctrl Pts',(78.0537269110733,-7.81946288799671,
138.260774682393));
#131184=CARTESIAN_POINT('Ctrl Pts',(79.9361880375736,-6.72457153501829,
138.149641564402));
#131185=CARTESIAN_POINT('Ctrl Pts',(81.8770523758524,-7.71224182450884,
138.03850844641));
#131186=CARTESIAN_POINT('Ctrl Pts',(82.0999645035268,-9.8785191056746,137.927375328419));
#131187=CARTESIAN_POINT('Ctrl Pts',(80.4009064619,-11.2407411115166,137.816242210427));
#131188=CARTESIAN_POINT('Ctrl Pts',(78.3349230477351,-10.5521486630767,
137.705109092436));
#131189=CARTESIAN_POINT('Ctrl Pts',(77.7928835966247,-8.44296866343152,
137.593975974444));
#131190=CARTESIAN_POINT('Ctrl Pts',(79.2708839493578,-6.8436056689135,137.482842856453));
#131191=CARTESIAN_POINT('Ctrl Pts',(81.4162000092596,-7.21785964039476,
137.371709738461));
#131192=CARTESIAN_POINT('Ctrl Pts',(82.2653540796503,-9.22319861367285,
137.260576620469));
#131193=CARTESIAN_POINT('Ctrl Pts',(81.0411669328516,-11.0242574305468,
137.149443502478));
#131194=CARTESIAN_POINT('Ctrl Pts',(78.8640628291885,-10.9726361730659,
137.038310384486));
#131195=CARTESIAN_POINT('Ctrl Pts',(77.7266131342975,-9.11558064775398,
136.927177266495));
#131196=CARTESIAN_POINT('Ctrl Pts',(78.6698565785353,-7.15274116442619,
136.816044148503));
#131197=CARTESIAN_POINT('Ctrl Pts',(80.8304996360312,-6.88058567480575,
136.704911030512));
#131198=CARTESIAN_POINT('Ctrl Pts',(82.2310367384848,-8.54820159494246,
136.59377791252));
#131199=CARTESIAN_POINT('Ctrl Pts',(81.5896412051266,-10.6293211979976,
136.482644794529));
#131200=CARTESIAN_POINT('Ctrl Pts',(79.4933434731685,-11.219221911189,136.371511676537));
#131201=CARTESIAN_POINT('Ctrl Pts',(77.8607577363731,-9.77800338353641,
136.260378558545));
#131202=CARTESIAN_POINT('Ctrl Pts',(78.1860907190042,-7.62472553735678,
136.149245440554));
#131203=CARTESIAN_POINT('Ctrl Pts',(80.1715848703761,-6.73015300966351,
136.038112322562));
#131204=CARTESIAN_POINT('Ctrl Pts',(82.0000377948652,-7.91303378783318,
135.926979204571));
#131205=CARTESIAN_POINT('Ctrl Pts',(81.9979774087732,-10.0907488259511,
135.815846086579));
#131206=CARTESIAN_POINT('Ctrl Pts',(80.1672894585474,-11.2701676071032,
135.704712968588));
#131207=CARTESIAN_POINT('Ctrl Pts',(78.1834916114102,-10.3718396413081,
135.593579850596));
#131208=CARTESIAN_POINT('Ctrl Pts',(77.8622337385839,-8.21795004070572,
135.482446732605));
#131209=CARTESIAN_POINT('Ctrl Pts',(79.4975436898657,-6.77982334403592,
135.371313614613));
#131210=CARTESIAN_POINT('Ctrl Pts',(81.5927214326702,-7.37368970820611,
135.260180496621));
#131211=CARTESIAN_POINT('Ctrl Pts',(82.2301778313902,-9.45601926237537,
135.14904737863));
#131212=CARTESIAN_POINT('Ctrl Pts',(80.8264876998778,-11.1209820388755,
135.037914260638));
#131213=CARTESIAN_POINT('Ctrl Pts',(78.6663634951985,-10.8447385723571,
134.926781142647));
#131214=CARTESIAN_POINT('Ctrl Pts',(77.7268359111347,-8.88011775621491,
134.815648024655));
#131215=CARTESIAN_POINT('Ctrl Pts',(78.8677975720673,-7.02521788810393,
134.704514906664));
#131216=CARTESIAN_POINT('Ctrl Pts',(81.044995458097,-6.97771633546675,134.593381788672));
#131217=CARTESIAN_POINT('Ctrl Pts',(82.2657723702561,-8.7810883889198,134.482248670681));
#131218=CARTESIAN_POINT('Ctrl Pts',(81.4128252292252,-10.7848169651105,
134.371115552689));
#131219=CARTESIAN_POINT('Ctrl Pts',(79.2668048301483,-11.1550108051209,
134.259982434697));
#131220=CARTESIAN_POINT('Ctrl Pts',(77.7918335088003,-9.5528539358859,134.148849316706));
#131221=CARTESIAN_POINT('Ctrl Pts',(78.3378630727844,-7.44470338440925,
134.037716198714));
#131222=CARTESIAN_POINT('Ctrl Pts',(80.4051457736282,-6.76002151139955,
133.926583080723));
#131223=CARTESIAN_POINT('Ctrl Pts',(82.1016231160651,-8.12545611585114,
133.815449962731));
#131224=CARTESIAN_POINT('Ctrl Pts',(81.8746122635996,-10.2913077047877,
133.70431684474));
#131225=CARTESIAN_POINT('Ctrl Pts',(79.9318824834679,-11.2753036569265,
133.593183726748));
#131226=CARTESIAN_POINT('Ctrl Pts',(78.0514965355458,-10.176852147167,133.482050608757));
#131227=CARTESIAN_POINT('Ctrl Pts',(77.9544576506411,-8.00129923187109,
133.370917490765));
#131228=CARTESIAN_POINT('Ctrl Pts',(79.7295796356322,-6.73979656804598,
133.259784372773));
#131229=CARTESIAN_POINT('Ctrl Pts',(81.7522009817343,-7.54692104588537,
133.148651254782));
#131230=CARTESIAN_POINT('Ctrl Pts',(82.1711390233947,-9.6839605751608,133.03751813679));
#131231=CARTESIAN_POINT('Ctrl Pts',(80.6029651756449,-11.1950124656231,
132.926385018798));
#131232=CARTESIAN_POINT('Ctrl Pts',(78.482933866667,-10.6971025526985,132.815251900807));
#131233=CARTESIAN_POINT('Ctrl Pts',(77.7513811940564,-8.64593758623847,
132.704118782815));
#131234=CARTESIAN_POINT('Ctrl Pts',(79.0778529574195,-6.91882447661411,
132.592985664824));
#131235=CARTESIAN_POINT('Ctrl Pts',(81.2483099895054,-7.09648512026235,
132.481852546832));
#131236=CARTESIAN_POINT('Ctrl Pts',(82.2762645861953,-9.01631750346318,
132.370719428841));
#131237=CARTESIAN_POINT('Ctrl Pts',(81.2208922406947,-10.9212154652415,
132.259586310849));
#131238=CARTESIAN_POINT('Ctrl Pts',(79.0481112626675,-11.0677414149317,
132.148453192858));
#131239=CARTESIAN_POINT('Ctrl Pts',(77.7465363230069,-9.32178903615767,
132.037320074866));
#131240=CARTESIAN_POINT('Ctrl Pts',(78.5074200360291,-7.2813226660189,131.926186956875));
#131241=CARTESIAN_POINT('Ctrl Pts',(80.6343716793853,-6.81385743837979,
131.815053838883));
#131242=CARTESIAN_POINT('Ctrl Pts',(82.1807213932797,-8.34723592895108,
131.703920720891));
#131243=CARTESIAN_POINT('Ctrl Pts',(81.7311890554049,-10.4780497897204,
131.5927876029));
#131244=CARTESIAN_POINT('Ctrl Pts',(79.6972043556635,-11.2560943078113,
131.481654484908));
#131245=CARTESIAN_POINT('Ctrl Pts',(77.9403501463584,-9.96927251567788,
131.370521366917));
#131246=CARTESIAN_POINT('Ctrl Pts',(78.0685685525499,-7.79533436845129,
131.259388248925));
#131247=CARTESIAN_POINT('Ctrl Pts',(79.9645090349079,-6.72395361943023,
131.148255130934));
#131248=CARTESIAN_POINT('Ctrl Pts',(81.8929322555346,-7.73570010828368,
131.037122012942));
#131249=CARTESIAN_POINT('Ctrl Pts',(82.0888693501395,-9.90458360799097,
130.92598889495));
#131250=CARTESIAN_POINT('Ctrl Pts',(80.3729910406748,-11.2455566109706,
130.814855776959));
#131251=CARTESIAN_POINT('Ctrl Pts',(78.3157365635357,-10.5313077674544,
130.703722658967));
#131252=CARTESIAN_POINT('Ctrl Pts',(77.7999864522586,-8.41554588960587,
130.592589540976));
#131253=CARTESIAN_POINT('Ctrl Pts',(79.2977749698569,-6.8346992004142,130.481456422984));
#131254=CARTESIAN_POINT('Ctrl Pts',(81.4382682141534,-7.23562147237883,
130.370323304993));
#131255=CARTESIAN_POINT('Ctrl Pts',(82.2624002660436,-9.25137151003518,
130.259190187001));
#131256=CARTESIAN_POINT('Ctrl Pts',(81.0158976420608,-11.0370583050643,
130.14805706901));
#131257=CARTESIAN_POINT('Ctrl Pts',(78.8395991808601,-10.9583453628253,
130.036923951018));
#131258=CARTESIAN_POINT('Ctrl Pts',(77.7253581688036,-9.08728543420517,
129.925790833026));
#131259=CARTESIAN_POINT('Ctrl Pts',(78.6929324099967,-7.13632254984329,
129.814657715035));
#131260=CARTESIAN_POINT('Ctrl Pts',(80.8568405144443,-6.89110312319448,
129.703524597043));
#131261=CARTESIAN_POINT('Ctrl Pts',(82.2364236826459,-8.57596264749706,
129.592391479052));
#131262=CARTESIAN_POINT('Ctrl Pts',(81.5693704367807,-10.6490538112244,
129.48125836106));
#131263=CARTESIAN_POINT('Ctrl Pts',(79.4655041712653,-11.2125879341655,
129.370125243069));
#131264=CARTESIAN_POINT('Ctrl Pts',(77.8517775456378,-9.75164335071642,
129.258992125077));
#131265=CARTESIAN_POINT('Ctrl Pts',(78.2022406191104,-7.60160292861149,
129.147859007086));
#131266=CARTESIAN_POINT('Ctrl Pts',(80.2020920580122,-6.73383868153635,
129.036725889094));
#131267=CARTESIAN_POINT('Ctrl Pts',(81.4046780571844,-7.5350969077782,128.962637143766));
#131268=CARTESIAN_POINT('Ctrl Pts',(81.7034359980675,-8.10150557933116,
128.925592771103));
#131269=CARTESIAN_POINT('Ctrl Pts',(81.566702386557,-7.66654693491703,140.225980458467));
#131270=CARTESIAN_POINT('Ctrl Pts',(82.010262938208,-8.18766576675564,140.188922946894));
#131271=CARTESIAN_POINT('Ctrl Pts',(82.327997858567,-9.69873689893897,140.114821062656));
#131272=CARTESIAN_POINT('Ctrl Pts',(80.6734687869581,-11.3380125857227,
140.003674805754));
#131273=CARTESIAN_POINT('Ctrl Pts',(78.401952486918,-10.8323222471513,139.892541687763));
#131274=CARTESIAN_POINT('Ctrl Pts',(77.5934117917565,-8.65201181958074,
139.781408569771));
#131275=CARTESIAN_POINT('Ctrl Pts',(78.9872873882469,-6.78902785563699,
139.67027545178));
#131276=CARTESIAN_POINT('Ctrl Pts',(81.3081293166415,-6.95018261496333,
139.559142333788));
#131277=CARTESIAN_POINT('Ctrl Pts',(82.4316748727135,-8.98713225593806,
139.448009215796));
#131278=CARTESIAN_POINT('Ctrl Pts',(81.3296778449453,-11.035995210121,139.336876097805));
#131279=CARTESIAN_POINT('Ctrl Pts',(79.0106965764716,-11.2213685975531,
139.225742979813));
#131280=CARTESIAN_POINT('Ctrl Pts',(77.5971699915357,-9.37369058164258,
139.114609861822));
#131281=CARTESIAN_POINT('Ctrl Pts',(78.3828054371252,-7.18398031318115,
139.00347674383));
#131282=CARTESIAN_POINT('Ctrl Pts',(80.6485622542183,-6.65637052550606,
138.892343625839));
#131283=CARTESIAN_POINT('Ctrl Pts',(82.3207287552936,-8.27373887069834,
138.781210507847));
#131284=CARTESIAN_POINT('Ctrl Pts',(81.8688732566295,-10.5558118478961,
138.670077389856));
#131285=CARTESIAN_POINT('Ctrl Pts',(79.7065512486383,-11.4139436758023,
138.558944271864));
#131286=CARTESIAN_POINT('Ctrl Pts',(77.8128051596609,-10.0627396846075,
138.447811153873));
#131287=CARTESIAN_POINT('Ctrl Pts',(77.9208658406379,-7.73887428751625,
138.336678035881));
#131288=CARTESIAN_POINT('Ctrl Pts',(79.9318319553347,-6.56924088626373,
138.225544917889));
#131289=CARTESIAN_POINT('Ctrl Pts',(82.0051881391931,-7.62433384765245,
138.114411799898));
#131290=CARTESIAN_POINT('Ctrl Pts',(82.243317218725,-9.93849064278411,138.003278681906));
#131291=CARTESIAN_POINT('Ctrl Pts',(80.4282740815705,-11.3937038505785,
137.892145563915));
#131292=CARTESIAN_POINT('Ctrl Pts',(78.221257649239,-10.658105085135,137.781012445923));
#131293=CARTESIAN_POINT('Ctrl Pts',(77.6422162264616,-8.40494328042461,
137.669879327932));
#131294=CARTESIAN_POINT('Ctrl Pts',(79.2211113149259,-6.69640080812653,
137.55874620994));
#131295=CARTESIAN_POINT('Ctrl Pts',(81.5128759846153,-7.09620298430149,
137.447613091949));
#131296=CARTESIAN_POINT('Ctrl Pts',(82.4199970070225,-9.23843512231133,
137.336479973957));
#131297=CARTESIAN_POINT('Ctrl Pts',(81.1122415184211,-11.162442051497,137.225346855965));
#131298=CARTESIAN_POINT('Ctrl Pts',(78.7865188147747,-11.107296902346,137.114213737974));
#131299=CARTESIAN_POINT('Ctrl Pts',(77.5714218539939,-9.12347068572941,
137.003080619982));
#131300=CARTESIAN_POINT('Ctrl Pts',(78.5790552003455,-7.02663923779428,
136.891947501991));
#131301=CARTESIAN_POINT('Ctrl Pts',(80.8871931551817,-6.73590523014286,
136.780814383999));
#131302=CARTESIAN_POINT('Ctrl Pts',(82.3833370148139,-8.51735986977119,
136.669681266007));
#131303=CARTESIAN_POINT('Ctrl Pts',(81.6981570312575,-10.740545753113,136.558548148016));
#131304=CARTESIAN_POINT('Ctrl Pts',(79.4587568938848,-11.3707156559936,
136.447415030024));
#131305=CARTESIAN_POINT('Ctrl Pts',(77.7147237503498,-9.83111328004943,
136.336281912033));
#131306=CARTESIAN_POINT('Ctrl Pts',(78.0622653780914,-7.53084331790425,
136.225148794041));
#131307=CARTESIAN_POINT('Ctrl Pts',(80.1832980002954,-6.57520337665653,
136.11401567605));
#131308=CARTESIAN_POINT('Ctrl Pts',(82.13656907809,-7.83883274415787,136.002882558058));
#131309=CARTESIAN_POINT('Ctrl Pts',(82.1343680410774,-10.1652080873037,
135.891749440067));
#131310=CARTESIAN_POINT('Ctrl Pts',(80.1787093649632,-11.4251391268058,
135.780616322075));
#131311=CARTESIAN_POINT('Ctrl Pts',(78.0594888441027,-10.4654873849093,
135.669483204083));
#131312=CARTESIAN_POINT('Ctrl Pts',(77.7163005108943,-8.16456390732242,
135.558350086092));
#131313=CARTESIAN_POINT('Ctrl Pts',(79.4632438356514,-6.62826442419822,
135.4472169681));
#131314=CARTESIAN_POINT('Ctrl Pts',(81.7014475285372,-7.2626706906504,135.336083850109));
#131315=CARTESIAN_POINT('Ctrl Pts',(82.3824194749835,-9.48714912163461,
135.224950732117));
#131316=CARTESIAN_POINT('Ctrl Pts',(80.8829073468083,-11.2657695024962,
135.113817614126));
#131317=CARTESIAN_POINT('Ctrl Pts',(78.5753236639396,-10.9706684548548,
135.002684496134));
#131318=CARTESIAN_POINT('Ctrl Pts',(77.5716598385475,-8.8719340725756,134.891551378143));
#131319=CARTESIAN_POINT('Ctrl Pts',(78.7905085074542,-6.89041066770108,
134.780418260151));
#131320=CARTESIAN_POINT('Ctrl Pts',(81.11633139546,-6.83966645237353,134.66928514216));
#131321=CARTESIAN_POINT('Ctrl Pts',(82.4204438519653,-8.76614452973359,
134.558152024168));
#131322=CARTESIAN_POINT('Ctrl Pts',(81.5092708274104,-10.906656337943,134.447018906177));
#131323=CARTESIAN_POINT('Ctrl Pts',(79.2167537372884,-11.3021212204049,
134.335885788185));
#131324=CARTESIAN_POINT('Ctrl Pts',(77.6410944550728,-9.59059415134389,
134.224752670193));
#131325=CARTESIAN_POINT('Ctrl Pts',(78.224398373192,-7.33853206941367,134.113619552202));
#131326=CARTESIAN_POINT('Ctrl Pts',(80.432802787165,-6.60711083229659,134.00248643421));
#131327=CARTESIAN_POINT('Ctrl Pts',(82.2450890553728,-8.06575594466151,
133.891353316218));
#131328=CARTESIAN_POINT('Ctrl Pts',(82.0025814542595,-10.37945798796,133.780220198227));
#131329=CARTESIAN_POINT('Ctrl Pts',(79.9272324853697,-11.4306257857401,
133.669087080235));
#131330=CARTESIAN_POINT('Ctrl Pts',(77.9184832099714,-10.2571891959123,
133.557953962244));
#131331=CARTESIAN_POINT('Ctrl Pts',(77.8148200285094,-7.93312357150095,
133.446820844252));
#131332=CARTESIAN_POINT('Ctrl Pts',(79.7111195648015,-6.58550524629902,
133.335687726261));
#131333=CARTESIAN_POINT('Ctrl Pts',(81.8718138456102,-7.44772755327165,
133.224554608269));
#131334=CARTESIAN_POINT('Ctrl Pts',(82.3193504210416,-9.73065070033822,
133.113421490278));
#131335=CARTESIAN_POINT('Ctrl Pts',(80.6441262023926,-11.3448535683239,
133.002288372286));
#131336=CARTESIAN_POINT('Ctrl Pts',(78.3793723307539,-10.8129541580425,
132.891155254295));
#131337=CARTESIAN_POINT('Ctrl Pts',(77.5978806892923,-8.62176774514015,
132.780022136303));
#131338=CARTESIAN_POINT('Ctrl Pts',(79.014903187486,-6.77675437896232,132.668889018312));
#131339=CARTESIAN_POINT('Ctrl Pts',(81.3335250615239,-6.9665429112525,132.55775590032));
#131340=CARTESIAN_POINT('Ctrl Pts',(82.4316523122226,-9.01743140725671,
132.446622782328));
#131341=CARTESIAN_POINT('Ctrl Pts',(81.3042356578685,-11.0523659932435,
132.335489664337));
#131342=CARTESIAN_POINT('Ctrl Pts',(78.9831311952265,-11.2088944418807,
132.224356546345));
#131343=CARTESIAN_POINT('Ctrl Pts',(77.5927050862621,-9.34375575606019,
132.113223428354));
#131344=CARTESIAN_POINT('Ctrl Pts',(78.4055300325905,-7.16399827221987,
132.002090310362));
#131345=CARTESIAN_POINT('Ctrl Pts',(80.6776766507465,-6.66462183392446,
131.890957192371));
#131346=CARTESIAN_POINT('Ctrl Pts',(82.3295869251935,-8.30267541289877,
131.779824074379));
#131347=CARTESIAN_POINT('Ctrl Pts',(81.8493675537542,-10.5789479002354,
131.668690956388));
#131348=CARTESIAN_POINT('Ctrl Pts',(79.6765342073382,-11.4101051228631,
131.557557838396));
#131349=CARTESIAN_POINT('Ctrl Pts',(77.7997494845942,-10.035439275476,131.446424720404));
#131350=CARTESIAN_POINT('Ctrl Pts',(77.9367206371466,-7.71309865022921,
131.335291602413));
#131351=CARTESIAN_POINT('Ctrl Pts',(79.9620862671886,-6.56858078906871,
131.224158484421));
#131352=CARTESIAN_POINT('Ctrl Pts',(82.0221520485652,-7.6493934959586,131.11302536643));
#131353=CARTESIAN_POINT('Ctrl Pts',(82.2314646618857,-9.96633442145068,
131.001892248438));
#131354=CARTESIAN_POINT('Ctrl Pts',(80.3984530322158,-11.3988480769803,
130.890759130447));
#131355=CARTESIAN_POINT('Ctrl Pts',(78.2007614121363,-10.6358414992865,
130.779626012455));
#131356=CARTESIAN_POINT('Ctrl Pts',(77.6498039539297,-8.3756485087249,130.668492894463));
#131357=CARTESIAN_POINT('Ctrl Pts',(79.249838033503,-6.68688634533016,130.557359776472));
#131358=CARTESIAN_POINT('Ctrl Pts',(81.536450661207,-7.11517731622901,130.44622665848));
#131359=CARTESIAN_POINT('Ctrl Pts',(82.4168415532452,-9.26853122317627,
130.335093540489));
#131360=CARTESIAN_POINT('Ctrl Pts',(81.0852472358793,-11.1761167694134,
130.223960422497));
#131361=CARTESIAN_POINT('Ctrl Pts',(78.7603851713554,-11.0920305392106,
130.112827304506));
#131362=CARTESIAN_POINT('Ctrl Pts',(77.5700812190944,-9.09324391777456,
130.001694186514));
#131363=CARTESIAN_POINT('Ctrl Pts',(78.6037062884789,-7.00909981713288,
129.890561068523));
#131364=CARTESIAN_POINT('Ctrl Pts',(80.9153321765801,-6.74714064532625,
129.779427950531));
#131365=CARTESIAN_POINT('Ctrl Pts',(82.3890916952254,-8.54701601257792,
129.668294832539));
#131366=CARTESIAN_POINT('Ctrl Pts',(81.6765024920544,-10.7616254003869,
129.557161714548));
#131367=CARTESIAN_POINT('Ctrl Pts',(79.4290171600884,-11.3636288148302,
129.446028596556));
#131368=CARTESIAN_POINT('Ctrl Pts',(77.7051305327169,-9.80295379668104,
129.334895478565));
#131369=CARTESIAN_POINT('Ctrl Pts',(78.0795177406565,-7.50614225926586,
129.223762360573));
#131370=CARTESIAN_POINT('Ctrl Pts',(80.2158877413142,-6.57914064852994,
129.112629242582));
#131371=CARTESIAN_POINT('Ctrl Pts',(81.5005674939528,-7.43509624804347,
129.038540497254));
#131372=CARTESIAN_POINT('Ctrl Pts',(81.8197199519531,-8.04017044029572,
129.00149612459));
#131373=CARTESIAN_POINT('Ctrl Pts',(81.2690708798523,-7.92064134695145,
140.));
#131374=CARTESIAN_POINT('Ctrl Pts',(81.3143922592526,-7.96292138382976,
140.));
#131375=CARTESIAN_POINT('Ctrl Pts',(81.3569831825551,-8.00777112798572,
140.));
#131376=CARTESIAN_POINT('Ctrl Pts',(81.3968454433617,-8.05484540576437,
140.));
#131377=CARTESIAN_POINT('Ctrl Pts',(81.4393469469686,-8.10503642720478,
140.));
#131378=CARTESIAN_POINT('Ctrl Pts',(81.4787472273247,-8.15775653436478,
140.));
#131379=CARTESIAN_POINT('Ctrl Pts',(81.5150195980997,-8.21264209971973,
140.));
#131380=CARTESIAN_POINT('Ctrl Pts',(81.5467579225278,-8.26066696940532,
140.));
#131381=CARTESIAN_POINT('Ctrl Pts',(81.5761011969975,-8.31035099456426,
140.));
#131382=CARTESIAN_POINT('Ctrl Pts',(81.6030086375,-8.36147814360778,140.));
#131383=CARTESIAN_POINT('Ctrl Pts',(81.6165038148102,-8.38712049118233,
140.));
#131384=CARTESIAN_POINT('Ctrl Pts',(81.6293859141812,-8.41312620242211,
140.));
#131385=CARTESIAN_POINT('Ctrl Pts',(81.6416474501114,-8.4394698635273,140.));
#131386=CARTESIAN_POINT('Ctrl Pts',(81.6472598357352,-8.45152796013997,
140.));
#131387=CARTESIAN_POINT('Ctrl Pts',(81.6527427933622,-8.46365856446902,
140.));
#131388=CARTESIAN_POINT('Ctrl Pts',(81.6580870749244,-8.47583923409168,
140.));
#131389=CARTESIAN_POINT('Ctrl Pts',(81.6849965902534,-8.53717131626459,
140.));
#131390=CARTESIAN_POINT('Ctrl Pts',(81.7084453900242,-8.59987896898128,
140.));
#131391=CARTESIAN_POINT('Ctrl Pts',(81.7284103210218,-8.66360419268533,
140.));
#131392=CARTESIAN_POINT('Ctrl Pts',(81.7487859790682,-8.72864039878482,
140.));
#131393=CARTESIAN_POINT('Ctrl Pts',(81.7655335305298,-8.79473730760459,
140.));
#131394=CARTESIAN_POINT('Ctrl Pts',(81.7785886627868,-8.86155122472489,
140.));
#131395=CARTESIAN_POINT('Ctrl Pts',(81.7894440925633,-8.91710744362078,
140.));
#131396=CARTESIAN_POINT('Ctrl Pts',(81.7977459929751,-8.97316035289416,
140.));
#131397=CARTESIAN_POINT('Ctrl Pts',(81.8034327980193,-9.02952452320688,
140.));
#131398=CARTESIAN_POINT('Ctrl Pts',(81.806059918276,-9.05556294942861,140.));
#131399=CARTESIAN_POINT('Ctrl Pts',(81.8081286078971,-9.08166791525863,
140.));
#131400=CARTESIAN_POINT('Ctrl Pts',(81.8096310008458,-9.10782153849097,
140.));
#131401=CARTESIAN_POINT('Ctrl Pts',(81.8102882463636,-9.11926285393143,
140.));
#131402=CARTESIAN_POINT('Ctrl Pts',(81.8108370002414,-9.13071330424245,
140.));
#131403=CARTESIAN_POINT('Ctrl Pts',(81.8112762675986,-9.14215720643866,
140.));
#131404=CARTESIAN_POINT('Ctrl Pts',(81.813968295031,-9.21229057315298,140.));
#131405=CARTESIAN_POINT('Ctrl Pts',(81.8125603873038,-9.28230940983736,
140.));
#131406=CARTESIAN_POINT('Ctrl Pts',(81.8069982742316,-9.35185253060966,
140.));
#131407=CARTESIAN_POINT('Ctrl Pts',(81.8020260032913,-9.41402085297565,
140.));
#131408=CARTESIAN_POINT('Ctrl Pts',(81.7937335362703,-9.47580996983483,
140.));
#131409=CARTESIAN_POINT('Ctrl Pts',(81.7820489797618,-9.53697398237741,
140.));
#131410=CARTESIAN_POINT('Ctrl Pts',(81.7693168290942,-9.6036217342678,140.));
#131411=CARTESIAN_POINT('Ctrl Pts',(81.7525581651765,-9.6695281026167,140.));
#131412=CARTESIAN_POINT('Ctrl Pts',(81.7320180024232,-9.73447972793787,
140.));
#131413=CARTESIAN_POINT('Ctrl Pts',(81.7240899589877,-9.75954960264804,
140.));
#131414=CARTESIAN_POINT('Ctrl Pts',(81.7155979986156,-9.78447719355442,
140.));
#131415=CARTESIAN_POINT('Ctrl Pts',(81.7065542014754,-9.80924991088,140.));
#131416=CARTESIAN_POINT('Ctrl Pts',(81.702587541701,-9.82011536261413,140.));
#131417=CARTESIAN_POINT('Ctrl Pts',(81.6985148256868,-9.83095044867854,
140.));
#131418=CARTESIAN_POINT('Ctrl Pts',(81.6943421550071,-9.84174157738441,
140.));
#131419=CARTESIAN_POINT('Ctrl Pts',(81.6692401550965,-9.90665897264566,
140.));
#131420=CARTESIAN_POINT('Ctrl Pts',(81.6404827620673,-9.97010366580973,
140.));
#131421=CARTESIAN_POINT('Ctrl Pts',(81.6083781064462,-10.0318601884806,
140.));
#131422=CARTESIAN_POINT('Ctrl Pts',(81.575580286364,-10.0949500824628,140.));
#131423=CARTESIAN_POINT('Ctrl Pts',(81.5392887976022,-10.1562789155961,
140.));
#131424=CARTESIAN_POINT('Ctrl Pts',(81.499777343564,-10.21561337491,140.));
#131425=CARTESIAN_POINT('Ctrl Pts',(81.4596177776799,-10.2759211055673,
140.));
#131426=CARTESIAN_POINT('Ctrl Pts',(81.416131326886,-10.3341694205845,140.));
#131427=CARTESIAN_POINT('Ctrl Pts',(81.3695549575856,-10.3900965447165,
140.));
#131428=CARTESIAN_POINT('Ctrl Pts',(81.3583695251126,-10.4035275845288,
140.));
#131429=CARTESIAN_POINT('Ctrl Pts',(81.3470056786722,-10.4168246423396,
140.));
#131430=CARTESIAN_POINT('Ctrl Pts',(81.3354663202672,-10.4299838569706,
140.));
#131431=CARTESIAN_POINT('Ctrl Pts',(81.3227851686387,-10.444445145908,140.));
#131432=CARTESIAN_POINT('Ctrl Pts',(81.3098876232902,-10.4587445299804,
140.));
#131433=CARTESIAN_POINT('Ctrl Pts',(81.2968013238845,-10.4728515285403,
140.));
#131434=CARTESIAN_POINT('Ctrl Pts',(81.2459377457121,-10.527682340658,140.));
#131435=CARTESIAN_POINT('Ctrl Pts',(81.1921776876492,-10.5796680480248,
140.));
#131436=CARTESIAN_POINT('Ctrl Pts',(81.1358057830487,-10.6285450378629,
140.));
#131437=CARTESIAN_POINT('Ctrl Pts',(81.0936523916007,-10.6650939339847,
140.));
#131438=CARTESIAN_POINT('Ctrl Pts',(81.0500373919693,-10.6999043465923,
140.));
#131439=CARTESIAN_POINT('Ctrl Pts',(81.0050634114518,-10.7328563054907,
140.));
#131440=CARTESIAN_POINT('Ctrl Pts',(80.9910001257159,-10.7431603259091,
140.));
#131441=CARTESIAN_POINT('Ctrl Pts',(80.9768038659581,-10.7532825494193,
140.));
#131442=CARTESIAN_POINT('Ctrl Pts',(80.9624775285841,-10.7632190809483,
140.));
#131443=CARTESIAN_POINT('Ctrl Pts',(80.948691008792,-10.7727812031442,140.));
#131444=CARTESIAN_POINT('Ctrl Pts',(80.9347910747477,-10.782166414048,140.));
#131445=CARTESIAN_POINT('Ctrl Pts',(80.9207856707492,-10.7913685089582,
140.));
#131446=CARTESIAN_POINT('Ctrl Pts',(80.8578389347226,-10.8327269616862,
140.));
#131447=CARTESIAN_POINT('Ctrl Pts',(80.7927341134844,-10.8704103298825,
140.));
#131448=CARTESIAN_POINT('Ctrl Pts',(80.7257321767826,-10.9041397537238,
140.));
#131449=CARTESIAN_POINT('Ctrl Pts',(80.6745101487068,-10.9299254187363,
140.));
#131450=CARTESIAN_POINT('Ctrl Pts',(80.6221783994731,-10.9533998385397,
140.));
#131451=CARTESIAN_POINT('Ctrl Pts',(80.56883966131,-10.9744231685942,140.));
#131452=CARTESIAN_POINT('Ctrl Pts',(80.5565365876157,-10.9792723942765,
140.));
#131453=CARTESIAN_POINT('Ctrl Pts',(80.5441798951046,-10.9839911471849,
140.));
#131454=CARTESIAN_POINT('Ctrl Pts',(80.5317714570928,-10.98857999513,140.));
#131455=CARTESIAN_POINT('Ctrl Pts',(79.4691328777287,-10.9877838235895,
139.9984406031));
#131456=CARTESIAN_POINT('Ctrl Pts',(78.8081758496214,-10.811265456103,139.961396230436));
#131457=CARTESIAN_POINT('Ctrl Pts',(77.6877526904063,-9.74920906242341,
139.887307485108));
#131458=CARTESIAN_POINT('Ctrl Pts',(78.1161488323421,-7.46000016524759,
139.776174367117));
#131459=CARTESIAN_POINT('Ctrl Pts',(80.2721800425073,-6.58386568048153,
139.665041249125));
#131460=CARTESIAN_POINT('Ctrl Pts',(82.1774278168464,-7.91731817278388,
139.553908131134));
#131461=CARTESIAN_POINT('Ctrl Pts',(82.0906258630199,-10.2425367543248,
139.442775013142));
#131462=CARTESIAN_POINT('Ctrl Pts',(80.0900009463851,-11.4301197324817,
139.331641895151));
#131463=CARTESIAN_POINT('Ctrl Pts',(78.0071991588717,-10.3937654044698,
139.220508777159));
#131464=CARTESIAN_POINT('Ctrl Pts',(77.7481915217547,-8.0816824054986,139.109375659168));
#131465=CARTESIAN_POINT('Ctrl Pts',(79.550174388928,-6.61012857285443,138.998242541176));
#131466=CARTESIAN_POINT('Ctrl Pts',(81.763832497857,-7.32585529210686,138.887109423184));
#131467=CARTESIAN_POINT('Ctrl Pts',(82.3631728604374,-9.57383680047761,
138.775976305193));
#131468=CARTESIAN_POINT('Ctrl Pts',(80.7996389409501,-11.2966145820648,
138.664843187201));
#131469=CARTESIAN_POINT('Ctrl Pts',(78.5042466623318,-10.9174430919909,
138.55371006921));
#131470=CARTESIAN_POINT('Ctrl Pts',(77.5778254035081,-8.78335085114467,
138.442576951218));
#131471=CARTESIAN_POINT('Ctrl Pts',(78.8682743104211,-6.84754510512543,
138.331443833227));
#131472=CARTESIAN_POINT('Ctrl Pts',(81.1945228001823,-6.88175047275135,
138.220310715235));
#131473=CARTESIAN_POINT('Ctrl Pts',(82.4274971600873,-8.85466134058638,
138.109177597244));
#131474=CARTESIAN_POINT('Ctrl Pts',(81.4387304989914,-10.9605917920548,
137.998044479252));
#131475=CARTESIAN_POINT('Ctrl Pts',(79.1331810938808,-11.2721115054034,
137.88691136126));
#131476=CARTESIAN_POINT('Ctrl Pts',(77.6209784514413,-9.50410532093426,
137.775778243269));
#131477=CARTESIAN_POINT('Ctrl Pts',(78.286149976356,-7.27472211446641,137.664645125277));
#131478=CARTESIAN_POINT('Ctrl Pts',(80.5199044951167,-6.62438113065896,
137.553512007286));
#131479=CARTESIAN_POINT('Ctrl Pts',(82.2778219587944,-8.1483000416988,137.442378889294));
#131480=CARTESIAN_POINT('Ctrl Pts',(81.9509871105632,-10.4517282760942,
137.331245771303));
#131481=CARTESIAN_POINT('Ctrl Pts',(79.8385320691397,-11.4264776532609,
137.220112653311));
#131482=CARTESIAN_POINT('Ctrl Pts',(77.8738588331112,-10.1804191766788,
137.10897953532));
#131483=CARTESIAN_POINT('Ctrl Pts',(77.8551136772396,-7.85399460887872,
136.997846417328));
#131484=CARTESIAN_POINT('Ctrl Pts',(79.799452905803,-6.57643928130455,136.886713299336));
#131485=CARTESIAN_POINT('Ctrl Pts',(81.9273407284608,-7.51702211393059,
136.775580181345));
#131486=CARTESIAN_POINT('Ctrl Pts',(82.2912504570253,-9.81488467731359,
136.664447063353));
#131487=CARTESIAN_POINT('Ctrl Pts',(80.5581175845882,-11.366932710478,136.553313945362));
#131488=CARTESIAN_POINT('Ctrl Pts',(78.3141735314383,-10.7526707654457,
136.44218082737));
#131489=CARTESIAN_POINT('Ctrl Pts',(77.6131642158011,-8.5342955514302,136.331047709378));
#131490=CARTESIAN_POINT('Ctrl Pts',(79.0966809548029,-6.74215137869336,
136.219914591387));
#131491=CARTESIAN_POINT('Ctrl Pts',(81.4069508382607,-7.01647913223252,
136.108781473395));
#131492=CARTESIAN_POINT('Ctrl Pts',(82.4295239374967,-9.10620325457287,
135.997648355404));
#131493=CARTESIAN_POINT('Ctrl Pts',(81.2285011040056,-11.0987259782088,
135.886515237412));
#131494=CARTESIAN_POINT('Ctrl Pts',(78.9031057067962,-11.1704120815385,
135.775382119421));
#131495=CARTESIAN_POINT('Ctrl Pts',(77.5816311400657,-9.25565162125707,
135.664249001429));
#131496=CARTESIAN_POINT('Ctrl Pts',(78.4735429400179,-7.10690873485139,
135.553115883438));
#131497=CARTESIAN_POINT('Ctrl Pts',(80.76252832203,-6.69079748565583,135.441982765446));
#131498=CARTESIAN_POINT('Ctrl Pts',(82.3536177708982,-8.38815926691335,
135.330849647455));
#131499=CARTESIAN_POINT('Ctrl Pts',(81.7905835983475,-10.6455017689083,
135.219716529463));
#131500=CARTESIAN_POINT('Ctrl Pts',(79.5887368399055,-11.3968162856799,
135.108583411471));
#131501=CARTESIAN_POINT('Ctrl Pts',(77.7632943127424,-9.95447020002752,
134.99745029348));
#131502=CARTESIAN_POINT('Ctrl Pts',(77.9849728664353,-7.63855541972894,
134.886317175488));
#131503=CARTESIAN_POINT('Ctrl Pts',(80.0508835634619,-6.56868830523093,
134.775184057497));
#131504=CARTESIAN_POINT('Ctrl Pts',(82.0702236204505,-7.72405334928139,
134.664050939505));
#131505=CARTESIAN_POINT('Ctrl Pts',(82.1948135367953,-10.0472149888403,
134.552917821514));
#131506=CARTESIAN_POINT('Ctrl Pts',(80.3106237172459,-11.4119242526323,
134.441784703522));
#131507=CARTESIAN_POINT('Ctrl Pts',(78.1421388456428,-10.5691455080017,
134.33065158553));
#131508=CARTESIAN_POINT('Ctrl Pts',(77.6740416272099,-8.2902230334826,134.219518467539));
#131509=CARTESIAN_POINT('Ctrl Pts',(79.3347530603838,-6.6609163752694,134.108385349547));
#131510=CARTESIAN_POINT('Ctrl Pts',(81.6043246765592,-7.17243111584399,
133.997252231556));
#131511=CARTESIAN_POINT('Ctrl Pts',(82.4055552031433,-9.35660883160848,
133.886119113564));
#131512=CARTESIAN_POINT('Ctrl Pts',(81.0051269260808,-11.2144041086981,
133.774985995573));
#131513=CARTESIAN_POINT('Ctrl Pts',(78.6847669248588,-11.0454895874108,
133.663852877581));
#131514=CARTESIAN_POINT('Ctrl Pts',(77.5681600010754,-9.00446248603955,
133.55271975959));
#131515=CARTESIAN_POINT('Ctrl Pts',(78.6772687605974,-6.95935114180318,
133.441586641598));
#131516=CARTESIAN_POINT('Ctrl Pts',(80.996993212615,-6.78192195174491,133.330453523606));
#131517=CARTESIAN_POINT('Ctrl Pts',(82.4042302351769,-8.63456509415099,
133.219320405615));
#131518=CARTESIAN_POINT('Ctrl Pts',(81.611021116925,-10.8216686457678,133.108187287623));
#131519=CARTESIAN_POINT('Ctrl Pts',(79.3433420632901,-11.3415093525987,
132.997054169632));
#131520=CARTESIAN_POINT('Ctrl Pts',(77.6766621991367,-9.71830853902125,
132.88592105164));
#131521=CARTESIAN_POINT('Ctrl Pts',(78.1363925360183,-7.43768347818297,
132.774787933649));
#131522=CARTESIAN_POINT('Ctrl Pts',(80.3017697748106,-6.58695199029069,
132.663654815657));
#131523=CARTESIAN_POINT('Ctrl Pts',(82.1909554381543,-7.94473701752852,
132.552521697666));
#131524=CARTESIAN_POINT('Ctrl Pts',(82.0748924493326,-10.2683402610705,
132.441388579674));
#131525=CARTESIAN_POINT('Ctrl Pts',(80.0598062239121,-11.4311085762945,
132.330255461682));
#131526=CARTESIAN_POINT('Ctrl Pts',(77.9899829884147,-10.3688306349928,
132.219122343691));
#131527=CARTESIAN_POINT('Ctrl Pts',(77.7598064354237,-8.05374501989655,
132.107989225699));
#131528=CARTESIAN_POINT('Ctrl Pts',(79.5799432058827,-6.60470920682474,
131.996856107708));
#131529=CARTESIAN_POINT('Ctrl Pts',(81.7845324876121,-7.34793780539253,
131.885722989716));
#131530=CARTESIAN_POINT('Ctrl Pts',(82.3558473981236,-9.6031987490021,131.774589871725));
#131531=CARTESIAN_POINT('Ctrl Pts',(80.7709980447065,-11.3063884558481,
131.663456753733));
#131532=CARTESIAN_POINT('Ctrl Pts',(78.4805009344145,-10.8986806693481,
131.552323635741));
#131533=CARTESIAN_POINT('Ctrl Pts',(77.580709176199,-8.75322560289489,131.44119051775));
#131534=CARTESIAN_POINT('Ctrl Pts',(78.8951476015647,-6.83362817766481,
131.330057399758));
#131535=CARTESIAN_POINT('Ctrl Pts',(81.2207904300182,-6.89677951170404,
131.218924281767));
#131536=CARTESIAN_POINT('Ctrl Pts',(82.4291178040635,-8.8848810187796,131.107791163775));
#131537=CARTESIAN_POINT('Ctrl Pts',(81.4142209608452,-10.9783439481059,
130.996658045784));
#131538=CARTESIAN_POINT('Ctrl Pts',(79.1049734184687,-11.2611486300869,
130.885524927792));
#131539=CARTESIAN_POINT('Ctrl Pts',(77.6148894571761,-9.47446108619213,
130.774391809801));
#131540=CARTESIAN_POINT('Ctrl Pts',(78.3077524890248,-7.25352808503831,
130.663258691809));
#131541=CARTESIAN_POINT('Ctrl Pts',(80.5494271568789,-6.63103491390683,
130.552125573817));
#131542=CARTESIAN_POINT('Ctrl Pts',(82.2882442451662,-8.17671184547162,
130.440992455826));
#131543=CARTESIAN_POINT('Ctrl Pts',(81.9327705864848,-10.4758944710274,
130.329859337834));
#131544=CARTESIAN_POINT('Ctrl Pts',(79.8083482924002,-11.4242804460588,
130.218726219843));
#131545=CARTESIAN_POINT('Ctrl Pts',(77.8593350690433,-10.1538694154057,
130.107593101851));
#131546=CARTESIAN_POINT('Ctrl Pts',(77.8695387921742,-7.82739193084829,
129.99645998386));
#131547=CARTESIAN_POINT('Ctrl Pts',(79.8296323485855,-6.57413099141478,
129.885326865868));
#131548=CARTESIAN_POINT('Ctrl Pts',(81.9456369666873,-7.54112189936117,
129.774193747877));
#131549=CARTESIAN_POINT('Ctrl Pts',(82.2809510163317,-9.84333331972787,
129.663060629885));
#131550=CARTESIAN_POINT('Ctrl Pts',(80.5285815078084,-11.3736972816056,
129.551927511894));
#131551=CARTESIAN_POINT('Ctrl Pts',(78.2925712562624,-10.731551087784,129.440794393902));
#131552=CARTESIAN_POINT('Ctrl Pts',(77.6189850691365,-8.50463954136352,
129.32966127591));
#131553=CARTESIAN_POINT('Ctrl Pts',(79.1251740367243,-6.73106382404891,
129.218528157919));
#131554=CARTESIAN_POINT('Ctrl Pts',(81.4308588372317,-7.03418464412087,
129.107395039927));
#131555=CARTESIAN_POINT('Ctrl Pts',(82.4293842699421,-9.13633334838347,
128.996261921936));
#131556=CARTESIAN_POINT('Ctrl Pts',(81.1993089591602,-11.1142610176031,
128.885115666002));
#131557=CARTESIAN_POINT('Ctrl Pts',(79.65533995085,-11.1407368472887,128.811013782731));
#131558=CARTESIAN_POINT('Ctrl Pts',(79.0485528339274,-10.8242403017729,
128.773956272126));
#131559=CARTESIAN_POINT('Ctrl Pts',(79.5030640089439,-10.8607317781412,
140.074365003916));
#131560=CARTESIAN_POINT('Ctrl Pts',(78.884352994401,-10.6954958345189,140.037320631253));
#131561=CARTESIAN_POINT('Ctrl Pts',(77.835543283518,-9.70132229389272,139.963231885925));
#131562=CARTESIAN_POINT('Ctrl Pts',(78.2365578734717,-7.55843145675596,
139.852098767933));
#131563=CARTESIAN_POINT('Ctrl Pts',(80.2547832658959,-6.73829636038229,
139.740965649942));
#131564=CARTESIAN_POINT('Ctrl Pts',(82.0382544043942,-7.9865193299143,139.62983253195));
#131565=CARTESIAN_POINT('Ctrl Pts',(81.9570005215658,-10.1631182409492,
139.518699413959));
#131566=CARTESIAN_POINT('Ctrl Pts',(80.0842484072031,-11.2747951549134,
139.407566295967));
#131567=CARTESIAN_POINT('Ctrl Pts',(78.1345718741699,-10.3046808956759,
139.296433177976));
#131568=CARTESIAN_POINT('Ctrl Pts',(77.8921190805384,-8.14037798766803,
139.185300059984));
#131569=CARTESIAN_POINT('Ctrl Pts',(79.5789256360724,-6.76288062243545,
139.074166941992));
#131570=CARTESIAN_POINT('Ctrl Pts',(81.6510946216244,-7.4328606449979,138.963033824001));
#131571=CARTESIAN_POINT('Ctrl Pts',(82.2121272879242,-9.53715920083675,
138.851900706009));
#131572=CARTESIAN_POINT('Ctrl Pts',(80.7485288746228,-11.1498231770866,
138.740767588018));
#131573=CARTESIAN_POINT('Ctrl Pts',(78.5998498757103,-10.794886974984,138.629634470026));
#131574=CARTESIAN_POINT('Ctrl Pts',(77.7326421563487,-8.79719829128381,
138.518501352035));
#131575=CARTESIAN_POINT('Ctrl Pts',(78.9406101761429,-6.98512233756069,
138.407368234043));
#131576=CARTESIAN_POINT('Ctrl Pts',(81.1181731673415,-7.01714142020401,
138.296235116052));
#131577=CARTESIAN_POINT('Ctrl Pts',(82.2723402079837,-8.86395086882484,
138.18510199806));
#131578=CARTESIAN_POINT('Ctrl Pts',(81.3467719818848,-10.8352777641842,
138.073968880068));
#131579=CARTESIAN_POINT('Ctrl Pts',(79.1885850637436,-11.1268862496072,
137.962835762077));
#131580=CARTESIAN_POINT('Ctrl Pts',(77.7730370155179,-9.47188470851856,
137.851702644085));
#131581=CARTESIAN_POINT('Ctrl Pts',(78.3956931512785,-7.38499571752248,
137.740569526094));
#131582=CARTESIAN_POINT('Ctrl Pts',(80.4866740558917,-6.77622220762796,
137.629436408102));
#131583=CARTESIAN_POINT('Ctrl Pts',(82.1322317112042,-8.20273766239288,
137.518303290111));
#131584=CARTESIAN_POINT('Ctrl Pts',(81.8262869796441,-10.3589389874783,
137.407170172119));
#131585=CARTESIAN_POINT('Ctrl Pts',(79.8488525228262,-11.271385864394,137.296037054127));
#131586=CARTESIAN_POINT('Ctrl Pts',(78.0097541859958,-10.1049709971013,
137.184903936136));
#131587=CARTESIAN_POINT('Ctrl Pts',(77.9922071535657,-7.9272431821435,137.073770818144));
#131588=CARTESIAN_POINT('Ctrl Pts',(79.812271160094,-6.73134463012783,136.962637700153));
#131589=CARTESIAN_POINT('Ctrl Pts',(81.8041519898661,-7.61180876605229,
136.851504582161));
#131590=CARTESIAN_POINT('Ctrl Pts',(82.1448019077693,-9.76280015794658,
136.74037146417));
#131591=CARTESIAN_POINT('Ctrl Pts',(80.522444701108,-11.2156468217732,136.629238346178));
#131592=CARTESIAN_POINT('Ctrl Pts',(78.4219255407664,-10.6406463073006,
136.518105228187));
#131593=CARTESIAN_POINT('Ctrl Pts',(77.7657222379225,-8.56406171717871,
136.406972110195));
#131594=CARTESIAN_POINT('Ctrl Pts',(79.1544178832468,-6.88646500185769,
136.295838992204));
#131595=CARTESIAN_POINT('Ctrl Pts',(81.317023563612,-7.14325870476379,136.184705874212));
#131596=CARTESIAN_POINT('Ctrl Pts',(82.2742374410167,-9.09941512169513,
136.07357275622));
#131597=CARTESIAN_POINT('Ctrl Pts',(81.1499796992898,-10.9645829063101,
135.962439638229));
#131598=CARTESIAN_POINT('Ctrl Pts',(78.9732152740129,-11.0316870898403,
135.851306520237));
#131599=CARTESIAN_POINT('Ctrl Pts',(77.7362046438123,-9.23931128232413,
135.740173402246));
#131600=CARTESIAN_POINT('Ctrl Pts',(78.5711086257117,-7.22790837002455,
135.629040284254));
#131601=CARTESIAN_POINT('Ctrl Pts',(80.7137902339762,-6.8383934663254,135.517907166263));
#131602=CARTESIAN_POINT('Ctrl Pts',(82.2031829255959,-8.42726594224934,
135.406774048271));
#131603=CARTESIAN_POINT('Ctrl Pts',(81.6761358872752,-10.5403271704196,
135.29564093028));
#131604=CARTESIAN_POINT('Ctrl Pts',(79.6150233128547,-11.2436203455352,
135.184507812288));
#131605=CARTESIAN_POINT('Ctrl Pts',(77.9062565550443,-9.89346387238071,
135.073374694296));
#131606=CARTESIAN_POINT('Ctrl Pts',(78.1137662069962,-7.72557409682812,
134.962241576305));
#131607=CARTESIAN_POINT('Ctrl Pts',(80.0476312677441,-6.72408906877321,
134.851108458313));
#131608=CARTESIAN_POINT('Ctrl Pts',(81.9379023175039,-7.80560730395839,
134.739975340322));
#131609=CARTESIAN_POINT('Ctrl Pts',(82.0545288911924,-9.98028074539927,
134.62884222233));
#131610=CARTESIAN_POINT('Ctrl Pts',(80.2907697581922,-11.2577626651766,
134.517709104338));
#131611=CARTESIAN_POINT('Ctrl Pts',(78.2608866979087,-10.4688513291117,
134.406575986347));
#131612=CARTESIAN_POINT('Ctrl Pts',(77.8227085825314,-8.33558944321889,
134.295442868355));
#131613=CARTESIAN_POINT('Ctrl Pts',(79.3772732697765,-6.81042224983678,
134.184309750364));
#131614=CARTESIAN_POINT('Ctrl Pts',(81.5017819708075,-7.28924279434453,
134.073176632372));
#131615=CARTESIAN_POINT('Ctrl Pts',(82.251800702593,-9.3338156682156,133.962043514381));
#131616=CARTESIAN_POINT('Ctrl Pts',(80.9408828013534,-11.0728673036791,
133.850910396389));
#131617=CARTESIAN_POINT('Ctrl Pts',(78.768831927529,-10.9147491955534,133.739777278398));
#131618=CARTESIAN_POINT('Ctrl Pts',(77.7235945319332,-9.00417725986336,
133.628644160406));
#131619=CARTESIAN_POINT('Ctrl Pts',(78.7618130191583,-7.08978213153095,
133.517511042414));
#131620=CARTESIAN_POINT('Ctrl Pts',(80.9332689658142,-6.92369358186409,
133.406377924423));
#131621=CARTESIAN_POINT('Ctrl Pts',(82.2505604218487,-8.65792238869949,
133.295244806431));
#131622=CARTESIAN_POINT('Ctrl Pts',(81.508050398612,-10.7052340894407,133.18411168844));
#131623=CARTESIAN_POINT('Ctrl Pts',(79.3853132942805,-11.1918484341661,
133.072978570448));
#131624=CARTESIAN_POINT('Ctrl Pts',(77.8251616568562,-9.67239682162895,
132.961845452457));
#131625=CARTESIAN_POINT('Ctrl Pts',(78.2555076718805,-7.53754117265604,
132.850712334465));
#131626=CARTESIAN_POINT('Ctrl Pts',(80.2824817281482,-6.74118540428684,
132.739579216473));
#131627=CARTESIAN_POINT('Ctrl Pts',(82.0509173884428,-8.01218565999045,
132.628446098482));
#131628=CARTESIAN_POINT('Ctrl Pts',(81.9422727315119,-10.1872724796644,
132.51731298049));
#131629=CARTESIAN_POINT('Ctrl Pts',(80.0559836235928,-11.27572079536,132.406179862499));
#131630=CARTESIAN_POINT('Ctrl Pts',(78.1184560998653,-10.2813398676446,
132.295046744507));
#131631=CARTESIAN_POINT('Ctrl Pts',(77.9029916103919,-8.11422626001485,
132.183913626516));
#131632=CARTESIAN_POINT('Ctrl Pts',(79.6067917365245,-6.75780764293479,
132.072780508524));
#131633=CARTESIAN_POINT('Ctrl Pts',(81.6704715419352,-7.45353172287077,
131.961647390533));
#131634=CARTESIAN_POINT('Ctrl Pts',(82.2052700430089,-9.56464443843619,
131.850514272541));
#131635=CARTESIAN_POINT('Ctrl Pts',(80.7217186022169,-11.1589723397512,
131.73938115455));
#131636=CARTESIAN_POINT('Ctrl Pts',(78.5776218899472,-10.7773237794131,
131.628248036558));
#131637=CARTESIAN_POINT('Ctrl Pts',(77.7353416085845,-8.76899854135246,
131.517114918566));
#131638=CARTESIAN_POINT('Ctrl Pts',(78.9657658224566,-6.97209493041876,
131.405981800575));
#131639=CARTESIAN_POINT('Ctrl Pts',(81.142761864056,-7.03120985664177,131.294848682583));
#131640=CARTESIAN_POINT('Ctrl Pts',(82.2738572661827,-8.89223901307474,
131.183715564592));
#131641=CARTESIAN_POINT('Ctrl Pts',(81.3238290059157,-10.8518952657974,
131.0725824466));
#131642=CARTESIAN_POINT('Ctrl Pts',(79.16218032224,-11.1166240821426,130.961449328609));
#131643=CARTESIAN_POINT('Ctrl Pts',(77.767337208028,-9.44413522742874,130.850316210617));
#131644=CARTESIAN_POINT('Ctrl Pts',(78.4159149084603,-7.36515633479095,
130.739183092626));
#131645=CARTESIAN_POINT('Ctrl Pts',(80.5143097345124,-6.78245070480519,
130.628049974634));
#131646=CARTESIAN_POINT('Ctrl Pts',(82.1419878422397,-8.22933348510106,
130.516916856643));
#131647=CARTESIAN_POINT('Ctrl Pts',(81.8092347907504,-10.3815605655068,
130.405783738651));
#131648=CARTESIAN_POINT('Ctrl Pts',(79.8205979853371,-11.269329094832,130.294650620659));
#131649=CARTESIAN_POINT('Ctrl Pts',(77.9961587290761,-10.0801182017839,
130.183517502668));
#131650=CARTESIAN_POINT('Ctrl Pts',(78.0057102666526,-7.90234085231897,
130.072384384676));
#131651=CARTESIAN_POINT('Ctrl Pts',(79.840521640637,-6.72918387788704,129.961251266685));
#131652=CARTESIAN_POINT('Ctrl Pts',(81.8212787978642,-7.63436817923641,
129.850118148693));
#131653=CARTESIAN_POINT('Ctrl Pts',(82.1351607705549,-9.78943046470178,
129.738985030701));
#131654=CARTESIAN_POINT('Ctrl Pts',(80.4947964649098,-11.2219790256644,
129.62785191271));
#131655=CARTESIAN_POINT('Ctrl Pts',(78.4017040058978,-10.6208765240359,
129.516718794718));
#131656=CARTESIAN_POINT('Ctrl Pts',(77.7711710430936,-8.53630121340103,
129.405585676727));
#131657=CARTESIAN_POINT('Ctrl Pts',(79.1810897890947,-6.87608612412261,
129.294452558735));
#131658=CARTESIAN_POINT('Ctrl Pts',(81.3394034486423,-7.15983254354241,
129.183319440744));
#131659=CARTESIAN_POINT('Ctrl Pts',(82.2741067005136,-9.12761940747632,
129.072186322752));
#131660=CARTESIAN_POINT('Ctrl Pts',(81.1226534121246,-10.9791250014477,
128.961040066819));
#131661=CARTESIAN_POINT('Ctrl Pts',(79.6773693907263,-11.0039085906207,
128.886938183549));
#131662=CARTESIAN_POINT('Ctrl Pts',(79.1093659400363,-10.7076413743751,
128.849880672942));
#131663=CARTESIAN_POINT('Ctrl Pts',(79.5369951401592,-10.7336797326929,
140.150289404733));
#131664=CARTESIAN_POINT('Ctrl Pts',(78.9605301391807,-10.5797262129349,
140.113245032069));
#131665=CARTESIAN_POINT('Ctrl Pts',(77.9833338766298,-9.653435525362,140.039156286741));
#131666=CARTESIAN_POINT('Ctrl Pts',(78.3569669146011,-7.65686274826432,
139.92802316875));
#131667=CARTESIAN_POINT('Ctrl Pts',(80.2373864892844,-6.89272704028306,
139.816890050758));
#131668=CARTESIAN_POINT('Ctrl Pts',(81.8990809919417,-8.05572048704471,
139.705756932767));
#131669=CARTESIAN_POINT('Ctrl Pts',(81.8233751801121,-10.0836997275735,
139.594623814775));
#131670=CARTESIAN_POINT('Ctrl Pts',(80.0784958680211,-11.1194705773451,
139.483490696784));
#131671=CARTESIAN_POINT('Ctrl Pts',(78.2619445894682,-10.2155963868819,
139.372357578792));
#131672=CARTESIAN_POINT('Ctrl Pts',(78.036046639322,-8.19907356983747,139.261224460801));
#131673=CARTESIAN_POINT('Ctrl Pts',(79.6076768832169,-6.91563267201647,
139.150091342809));
#131674=CARTESIAN_POINT('Ctrl Pts',(81.5383567453918,-7.53986599788894,
139.038958224817));
#131675=CARTESIAN_POINT('Ctrl Pts',(82.061081715411,-9.50048160119588,138.927825106826));
#131676=CARTESIAN_POINT('Ctrl Pts',(80.6974188082955,-11.0030317721083,
138.816691988834));
#131677=CARTESIAN_POINT('Ctrl Pts',(78.6954530890887,-10.6723308579772,
138.705558870843));
#131678=CARTESIAN_POINT('Ctrl Pts',(77.8874589091894,-8.81104573142295,
138.594425752851));
#131679=CARTESIAN_POINT('Ctrl Pts',(79.0129460418649,-7.12269956999594,
138.48329263486));
#131680=CARTESIAN_POINT('Ctrl Pts',(81.0418235345008,-7.15253236765667,
138.372159516868));
#131681=CARTESIAN_POINT('Ctrl Pts',(82.11718325588,-8.87324039706331,138.261026398876));
#131682=CARTESIAN_POINT('Ctrl Pts',(81.2548134647783,-10.7099637363138,
138.149893280885));
#131683=CARTESIAN_POINT('Ctrl Pts',(79.2439890336062,-10.9816609938111,
138.038760162893));
#131684=CARTESIAN_POINT('Ctrl Pts',(77.9250955795947,-9.43966409610286,
137.927627044902));
#131685=CARTESIAN_POINT('Ctrl Pts',(78.505236326201,-7.49526932057854,137.81649392691));
#131686=CARTESIAN_POINT('Ctrl Pts',(80.4534436166667,-6.92806328459693,
137.705360808919));
#131687=CARTESIAN_POINT('Ctrl Pts',(81.9866414636141,-8.25717528308697,
137.594227690927));
#131688=CARTESIAN_POINT('Ctrl Pts',(81.7015868487251,-10.2661496988625,
137.483094572936));
#131689=CARTESIAN_POINT('Ctrl Pts',(79.8591729765127,-11.116294075527,137.371961454944));
#131690=CARTESIAN_POINT('Ctrl Pts',(78.1456495388805,-10.0295228175239,
137.260828336952));
#131691=CARTESIAN_POINT('Ctrl Pts',(78.1293006298919,-8.00049175540828,
137.149695218961));
#131692=CARTESIAN_POINT('Ctrl Pts',(79.8250894143851,-6.88624997895113,
137.038562100969));
#131693=CARTESIAN_POINT('Ctrl Pts',(81.6809632512715,-7.70659541817398,
136.927428982978));
#131694=CARTESIAN_POINT('Ctrl Pts',(81.9983533585131,-9.71071563857958,
136.816295864986));
#131695=CARTESIAN_POINT('Ctrl Pts',(80.4867718176279,-11.0643609330684,
136.705162746995));
#131696=CARTESIAN_POINT('Ctrl Pts',(78.5296775500945,-10.5286218491554,
136.594029629003));
#131697=CARTESIAN_POINT('Ctrl Pts',(77.9182802600438,-8.59382788292722,
136.482896511012));
#131698=CARTESIAN_POINT('Ctrl Pts',(79.2121548116908,-7.03077862502201,
136.37176339302));
#131699=CARTESIAN_POINT('Ctrl Pts',(81.2270962889633,-7.27003827729506,
136.260630275028));
#131700=CARTESIAN_POINT('Ctrl Pts',(82.1189509445369,-9.09262698881739,
136.149497157037));
#131701=CARTESIAN_POINT('Ctrl Pts',(81.071458294574,-10.8304398344114,136.038364039045));
#131702=CARTESIAN_POINT('Ctrl Pts',(79.0433248412296,-10.8929620981422,
135.927230921054));
#131703=CARTESIAN_POINT('Ctrl Pts',(77.8907781475588,-9.22297094339117,
135.816097803062));
#131704=CARTESIAN_POINT('Ctrl Pts',(78.6686743114057,-7.34890800519772,
135.704964685071));
#131705=CARTESIAN_POINT('Ctrl Pts',(80.6650521459222,-6.98598944699497,
135.593831567079));
#131706=CARTESIAN_POINT('Ctrl Pts',(82.0527480802936,-8.46637261758534,
135.482698449088));
#131707=CARTESIAN_POINT('Ctrl Pts',(81.5616881762029,-10.4351525719307,
135.371565331096));
#131708=CARTESIAN_POINT('Ctrl Pts',(79.6413097858039,-11.0904244053903,
135.260432213105));
#131709=CARTESIAN_POINT('Ctrl Pts',(78.0492187973462,-9.83245754473388,
135.149299095113));
#131710=CARTESIAN_POINT('Ctrl Pts',(78.2425595475572,-7.81259277392733,
135.038165977121));
#131711=CARTESIAN_POINT('Ctrl Pts',(80.0443789720261,-6.87948983231548,
134.92703285913));
#131712=CARTESIAN_POINT('Ctrl Pts',(81.8055810145572,-7.8871612586354,134.815899741138));
#131713=CARTESIAN_POINT('Ctrl Pts',(81.9142442455895,-9.91334650195824,
134.704766623147));
#131714=CARTESIAN_POINT('Ctrl Pts',(80.2709157991388,-11.1036010777208,
134.593633505155));
#131715=CARTESIAN_POINT('Ctrl Pts',(78.3796345501745,-10.3685571502218,
134.482500387163));
#131716=CARTESIAN_POINT('Ctrl Pts',(77.971375537853,-8.38095585295519,134.371367269172));
#131717=CARTESIAN_POINT('Ctrl Pts',(79.4197934791693,-6.95992812440418,
134.26023415118));
#131718=CARTESIAN_POINT('Ctrl Pts',(81.3992392650559,-7.40605447284507,
134.149101033189));
#131719=CARTESIAN_POINT('Ctrl Pts',(82.0980462020426,-9.31102250482272,
134.037967915197));
#131720=CARTESIAN_POINT('Ctrl Pts',(80.876638676626,-10.9313304986601,133.926834797206));
#131721=CARTESIAN_POINT('Ctrl Pts',(78.8528969301993,-10.7840088036961,
133.815701679214));
#131722=CARTESIAN_POINT('Ctrl Pts',(77.879029062791,-9.00389203368715,133.704568561223));
#131723=CARTESIAN_POINT('Ctrl Pts',(78.846357277719,-7.22021312125874,133.593435443231));
#131724=CARTESIAN_POINT('Ctrl Pts',(80.8695447190136,-7.06546521198324,
133.482302325239));
#131725=CARTESIAN_POINT('Ctrl Pts',(82.0968906085204,-8.68127968324799,
133.371169207248));
#131726=CARTESIAN_POINT('Ctrl Pts',(81.4050796802991,-10.5887995331135,
133.260036089256));
#131727=CARTESIAN_POINT('Ctrl Pts',(79.4272845252708,-11.0421875157334,
133.148902971265));
#131728=CARTESIAN_POINT('Ctrl Pts',(77.973661114576,-9.62648510423664,133.037769853273));
#131729=CARTESIAN_POINT('Ctrl Pts',(78.3746228077427,-7.63739886712913,
132.926636735282));
#131730=CARTESIAN_POINT('Ctrl Pts',(80.2631936814858,-6.89541881828299,
132.81550361729));
#131731=CARTESIAN_POINT('Ctrl Pts',(81.9108793387313,-8.07963430245237,
132.704370499299));
#131732=CARTESIAN_POINT('Ctrl Pts',(81.8096530136912,-10.1062046982582,
132.593237381307));
#131733=CARTESIAN_POINT('Ctrl Pts',(80.0521610232735,-11.1203330144254,
132.482104263315));
#131734=CARTESIAN_POINT('Ctrl Pts',(78.246929211316,-10.1938491002965,132.370971145324));
#131735=CARTESIAN_POINT('Ctrl Pts',(78.04617678536,-8.17470750013315,132.259838027332));
#131736=CARTESIAN_POINT('Ctrl Pts',(79.6336402671663,-6.91090607904484,
132.148704909341));
#131737=CARTESIAN_POINT('Ctrl Pts',(81.5564105962581,-7.55912564034901,
132.037571791349));
#131738=CARTESIAN_POINT('Ctrl Pts',(82.0546926878945,-9.52609012787027,
131.926438673358));
#131739=CARTESIAN_POINT('Ctrl Pts',(80.6724391597271,-11.0115562236542,
131.815305555366));
#131740=CARTESIAN_POINT('Ctrl Pts',(78.6747428454798,-10.6559668894782,
131.704172437375));
#131741=CARTESIAN_POINT('Ctrl Pts',(77.8899740409698,-8.78477147981007,
131.593039319383));
#131742=CARTESIAN_POINT('Ctrl Pts',(79.0363840433487,-7.1105616831727,131.481906201391));
#131743=CARTESIAN_POINT('Ctrl Pts',(81.0647332980937,-7.16564020157951,
131.3707730834));
#131744=CARTESIAN_POINT('Ctrl Pts',(82.118596728302,-8.8995970073699,131.259639965408));
#131745=CARTESIAN_POINT('Ctrl Pts',(81.2334370509863,-10.7254465834888,
131.148506847417));
#131746=CARTESIAN_POINT('Ctrl Pts',(79.2193872260113,-10.9720995341984,
131.037373729425));
#131747=CARTESIAN_POINT('Ctrl Pts',(77.9197849588799,-9.41380936866533,
130.926240611434));
#131748=CARTESIAN_POINT('Ctrl Pts',(78.5240773278958,-7.47678458454359,
130.815107493442));
#131749=CARTESIAN_POINT('Ctrl Pts',(80.4791923121458,-6.93386649570354,
130.70397437545));
#131750=CARTESIAN_POINT('Ctrl Pts',(81.9957314393132,-8.28195512473053,
130.592841257459));
#131751=CARTESIAN_POINT('Ctrl Pts',(81.6856989950159,-10.2872266599862,
130.481708139467));
#131752=CARTESIAN_POINT('Ctrl Pts',(79.8328476782742,-11.1143777436051,
130.370575021476));
#131753=CARTESIAN_POINT('Ctrl Pts',(78.1329823891089,-10.0063669881622,
130.259441903484));
#131754=CARTESIAN_POINT('Ctrl Pts',(78.141881741131,-7.97728977378966,130.148308785492));
#131755=CARTESIAN_POINT('Ctrl Pts',(79.8514109326885,-6.88423676435929,
130.037175667501));
#131756=CARTESIAN_POINT('Ctrl Pts',(81.6969206290413,-7.72761445911164,
129.926042549509));
#131757=CARTESIAN_POINT('Ctrl Pts',(81.9893705247781,-9.7355276096757,129.814909431518));
#131758=CARTESIAN_POINT('Ctrl Pts',(80.4610114220111,-11.0702607697232,
129.703776313526));
#131759=CARTESIAN_POINT('Ctrl Pts',(78.5108367555332,-10.5102019602878,
129.592643195535));
#131760=CARTESIAN_POINT('Ctrl Pts',(77.9233570170507,-8.56796288543854,
129.481510077543));
#131761=CARTESIAN_POINT('Ctrl Pts',(79.2370055414648,-7.02110842419632,
129.370376959552));
#131762=CARTESIAN_POINT('Ctrl Pts',(81.247948060053,-7.28548044296393,129.25924384156));
#131763=CARTESIAN_POINT('Ctrl Pts',(82.1188291310851,-9.11890546656919,
129.148110723569));
#131764=CARTESIAN_POINT('Ctrl Pts',(81.045997865089,-10.8439889852923,129.036964467635));
#131765=CARTESIAN_POINT('Ctrl Pts',(79.6993988306026,-10.8670803339528,
128.962862584365));
#131766=CARTESIAN_POINT('Ctrl Pts',(79.1701790461452,-10.5910424469771,
128.92580507376));
#131767=CARTESIAN_POINT('Ctrl Pts',(79.5709262713745,-10.6066276872446,
140.22621380555));
#131768=CARTESIAN_POINT('Ctrl Pts',(79.0367072839604,-10.4639565913509,
140.189169432887));
#131769=CARTESIAN_POINT('Ctrl Pts',(78.1311244697415,-9.6055487568313,140.115080687559));
#131770=CARTESIAN_POINT('Ctrl Pts',(78.4773759557306,-7.75529403977268,
140.003947569567));
#131771=CARTESIAN_POINT('Ctrl Pts',(80.2199897126731,-7.04715772018383,
139.892814451576));
#131772=CARTESIAN_POINT('Ctrl Pts',(81.7599075794896,-8.12492164417513,
139.781681333584));
#131773=CARTESIAN_POINT('Ctrl Pts',(81.689749838658,-10.0042812141978,139.670548215593));
#131774=CARTESIAN_POINT('Ctrl Pts',(80.0727433288392,-10.9641459997769,
139.559415097601));
#131775=CARTESIAN_POINT('Ctrl Pts',(78.3893173047664,-10.126511878088,139.44828197961));
#131776=CARTESIAN_POINT('Ctrl Pts',(78.1799741981056,-8.25776915200689,
139.337148861618));
#131777=CARTESIAN_POINT('Ctrl Pts',(79.6364281303614,-7.0683847215975,139.226015743626));
#131778=CARTESIAN_POINT('Ctrl Pts',(81.4256188691593,-7.64687135077996,
139.114882625635));
#131779=CARTESIAN_POINT('Ctrl Pts',(81.9100361428979,-9.46380400155503,
139.003749507643));
#131780=CARTESIAN_POINT('Ctrl Pts',(80.6463087419684,-10.8562403671301,
138.892616389652));
#131781=CARTESIAN_POINT('Ctrl Pts',(78.7910563024672,-10.5497747409704,
138.78148327166));
#131782=CARTESIAN_POINT('Ctrl Pts',(78.04227566203,-8.82489317156209,138.670350153669));
#131783=CARTESIAN_POINT('Ctrl Pts',(79.0852819075869,-7.26027680243122,
138.559217035677));
#131784=CARTESIAN_POINT('Ctrl Pts',(80.9654739016601,-7.28792331510932,
138.448083917685));
#131785=CARTESIAN_POINT('Ctrl Pts',(81.9620263037764,-8.88252992530179,
138.336950799694));
#131786=CARTESIAN_POINT('Ctrl Pts',(81.1628549476717,-10.5846497084434,
138.225817681702));
#131787=CARTESIAN_POINT('Ctrl Pts',(79.2993930034689,-10.836435738015,138.114684563711));
#131788=CARTESIAN_POINT('Ctrl Pts',(78.0771541436715,-9.40744348368716,
138.003551445719));
#131789=CARTESIAN_POINT('Ctrl Pts',(78.6147795011235,-7.6055429236346,137.892418327728));
#131790=CARTESIAN_POINT('Ctrl Pts',(80.4202131774415,-7.07990436156593,
137.781285209736));
#131791=CARTESIAN_POINT('Ctrl Pts',(81.8410512160243,-8.31161290378106,
137.670152091745));
#131792=CARTESIAN_POINT('Ctrl Pts',(81.5768867178061,-10.1733604102468,
137.559018973753));
#131793=CARTESIAN_POINT('Ctrl Pts',(79.8694934301991,-10.9612022866599,
137.447885855761));
#131794=CARTESIAN_POINT('Ctrl Pts',(78.281544891765,-9.9540746379463,137.33675273777));
#131795=CARTESIAN_POINT('Ctrl Pts',(78.266394106218,-8.07374032867307,137.225619619778));
#131796=CARTESIAN_POINT('Ctrl Pts',(79.8379076686761,-7.04115532777441,
137.114486501787));
#131797=CARTESIAN_POINT('Ctrl Pts',(81.5577745126769,-7.80138207029568,
137.003353383795));
#131798=CARTESIAN_POINT('Ctrl Pts',(81.851904809257,-9.65863111921257,136.892220265804));
#131799=CARTESIAN_POINT('Ctrl Pts',(80.4510989341479,-10.9130750443636,
136.781087147812));
#131800=CARTESIAN_POINT('Ctrl Pts',(78.6374295594225,-10.4165973910102,
136.669954029821));
#131801=CARTESIAN_POINT('Ctrl Pts',(78.0708382821652,-8.62359404867573,
136.558820911829));
#131802=CARTESIAN_POINT('Ctrl Pts',(79.2698917401348,-7.17509224818634,
136.447687793838));
#131803=CARTESIAN_POINT('Ctrl Pts',(81.1371690143145,-7.39681784982634,
136.336554675846));
#131804=CARTESIAN_POINT('Ctrl Pts',(81.9636644480571,-9.08583885593964,
136.225421557854));
#131805=CARTESIAN_POINT('Ctrl Pts',(80.9929368898583,-10.6962967625126,
136.114288439863));
#131806=CARTESIAN_POINT('Ctrl Pts',(79.1134344084462,-10.7542371064441,
136.003155321871));
#131807=CARTESIAN_POINT('Ctrl Pts',(78.0453516513057,-9.20663060445822,
135.89202220388));
#131808=CARTESIAN_POINT('Ctrl Pts',(78.7662399970995,-7.46990764037088,
135.780889085888));
#131809=CARTESIAN_POINT('Ctrl Pts',(80.6163140578685,-7.13358542766454,
135.669755967897));
#131810=CARTESIAN_POINT('Ctrl Pts',(81.9023132349912,-8.50547929292133,
135.558622849905));
#131811=CARTESIAN_POINT('Ctrl Pts',(81.4472404651308,-10.3299779734419,
135.447489731913));
#131812=CARTESIAN_POINT('Ctrl Pts',(79.6675962587529,-10.9372284652455,
135.336356613922));
#131813=CARTESIAN_POINT('Ctrl Pts',(78.1921810396483,-9.77145121708706,
135.22522349593));
#131814=CARTESIAN_POINT('Ctrl Pts',(78.3713528881184,-7.89961145102653,
135.114090377939));
#131815=CARTESIAN_POINT('Ctrl Pts',(80.0411266763082,-7.03489059585776,
135.002957259947));
#131816=CARTESIAN_POINT('Ctrl Pts',(81.6732597116106,-7.96871521331242,
134.891824141956));
#131817=CARTESIAN_POINT('Ctrl Pts',(81.7739595999865,-9.8464122585172,134.780691023964));
#131818=CARTESIAN_POINT('Ctrl Pts',(80.2510618400852,-10.9494394902652,
134.669557905973));
#131819=CARTESIAN_POINT('Ctrl Pts',(78.4983824024403,-10.2682629713319,
134.558424787981));
#131820=CARTESIAN_POINT('Ctrl Pts',(78.1200424931747,-8.42632226269147,
134.44729166999));
#131821=CARTESIAN_POINT('Ctrl Pts',(79.462313688562,-7.10943399897156,134.336158551998));
#131822=CARTESIAN_POINT('Ctrl Pts',(81.2966965593045,-7.5228661513456,134.225025434006));
#131823=CARTESIAN_POINT('Ctrl Pts',(81.9442917014921,-9.28822934142986,
134.113892316015));
#131824=CARTESIAN_POINT('Ctrl Pts',(80.8123945518987,-10.7897936936412,
134.002759198023));
#131825=CARTESIAN_POINT('Ctrl Pts',(78.9369619328696,-10.6532684118388,
133.891626080032));
#131826=CARTESIAN_POINT('Ctrl Pts',(78.0344635936487,-9.00360680751095,
133.78049296204));
#131827=CARTESIAN_POINT('Ctrl Pts',(78.9309015362798,-7.35064411098652,
133.669359844049));
#131828=CARTESIAN_POINT('Ctrl Pts',(80.805820472213,-7.20723684210242,133.558226726057));
#131829=CARTESIAN_POINT('Ctrl Pts',(81.9432207951922,-8.70463697779649,
133.447093608065));
#131830=CARTESIAN_POINT('Ctrl Pts',(81.3021089619863,-10.4723649767864,
133.335960490074));
#131831=CARTESIAN_POINT('Ctrl Pts',(79.4692557562613,-10.8925265973008,
133.224827372082));
#131832=CARTESIAN_POINT('Ctrl Pts',(78.1221605722958,-9.58057338684435,
133.113694254091));
#131833=CARTESIAN_POINT('Ctrl Pts',(78.4937379436049,-7.73725656160221,
133.002561136099));
#131834=CARTESIAN_POINT('Ctrl Pts',(80.2439056348234,-7.04965223227914,
132.891428018108));
#131835=CARTESIAN_POINT('Ctrl Pts',(81.7708412890197,-8.14708294491428,
132.780294900116));
#131836=CARTESIAN_POINT('Ctrl Pts',(81.6770332958706,-10.0251369168521,
132.669161782124));
#131837=CARTESIAN_POINT('Ctrl Pts',(80.0483384229543,-10.9649452334909,
132.558028664133));
#131838=CARTESIAN_POINT('Ctrl Pts',(78.3754023227666,-10.1063583329482,
132.446895546141));
#131839=CARTESIAN_POINT('Ctrl Pts',(78.1893619603281,-8.23518874025145,
132.33576242815));
#131840=CARTESIAN_POINT('Ctrl Pts',(79.6604887978082,-7.0640045151549,132.224629310158));
#131841=CARTESIAN_POINT('Ctrl Pts',(81.4423496505812,-7.66471955782726,
132.113496192167));
#131842=CARTESIAN_POINT('Ctrl Pts',(81.9041153327798,-9.48753581730435,
132.002363074175));
#131843=CARTESIAN_POINT('Ctrl Pts',(80.6231597172374,-10.8641401075573,
131.891229956184));
#131844=CARTESIAN_POINT('Ctrl Pts',(78.7718638010126,-10.5346099995432,
131.780096838192));
#131845=CARTESIAN_POINT('Ctrl Pts',(78.0446064733555,-8.80054441826766,
131.668963720201));
#131846=CARTESIAN_POINT('Ctrl Pts',(79.1070022642405,-7.24902843592665,
131.557830602209));
#131847=CARTESIAN_POINT('Ctrl Pts',(80.9867047321316,-7.30007054651723,
131.446697484217));
#131848=CARTESIAN_POINT('Ctrl Pts',(81.9633361904213,-8.90695500166506,
131.335564366226));
#131849=CARTESIAN_POINT('Ctrl Pts',(81.1430450960569,-10.5989979011803,
131.224431248234));
#131850=CARTESIAN_POINT('Ctrl Pts',(79.2765941297824,-10.8275749862541,
131.113298130243));
#131851=CARTESIAN_POINT('Ctrl Pts',(78.0722327097319,-9.38348350990194,
131.002165012251));
#131852=CARTESIAN_POINT('Ctrl Pts',(78.6322397473312,-7.58841283429622,
130.89103189426));
#131853=CARTESIAN_POINT('Ctrl Pts',(80.4440748897793,-7.08528228660189,
130.779898776268));
#131854=CARTESIAN_POINT('Ctrl Pts',(81.8494750363867,-8.33457676435999,
130.668765658276));
#131855=CARTESIAN_POINT('Ctrl Pts',(81.5621631992815,-10.1928927544656,
130.557632540285));
#131856=CARTESIAN_POINT('Ctrl Pts',(79.8450973712113,-10.9594263923782,
130.446499422293));
#131857=CARTESIAN_POINT('Ctrl Pts',(78.2698060491417,-9.93261577454027,
130.335366304302));
#131858=CARTESIAN_POINT('Ctrl Pts',(78.2780532156094,-8.05223869526036,
130.22423318631));
#131859=CARTESIAN_POINT('Ctrl Pts',(79.8623002247402,-7.03928965083155,
130.113100068319));
#131860=CARTESIAN_POINT('Ctrl Pts',(81.5725624602183,-7.82086073898689,
130.001966950327));
#131861=CARTESIAN_POINT('Ctrl Pts',(81.8435802790012,-9.68162475464961,
129.890833832335));
#131862=CARTESIAN_POINT('Ctrl Pts',(80.4272263791125,-10.9185425137821,
129.779700714344));
#131863=CARTESIAN_POINT('Ctrl Pts',(78.6199695051686,-10.3995273965398,
129.668567596352));
#131864=CARTESIAN_POINT('Ctrl Pts',(78.0755429910078,-8.59962455747607,
129.557434478361));
#131865=CARTESIAN_POINT('Ctrl Pts',(79.2929212938352,-7.16613072427,129.446301360369));
#131866=CARTESIAN_POINT('Ctrl Pts',(81.1564926714636,-7.41112834238548,
129.335168242378));
#131867=CARTESIAN_POINT('Ctrl Pts',(81.9635515616568,-9.11019152566204,
129.224035124386));
#131868=CARTESIAN_POINT('Ctrl Pts',(80.9693423180533,-10.7088529691368,
129.112888868452));
#131869=CARTESIAN_POINT('Ctrl Pts',(79.7214282704788,-10.7302520772847,
129.038786985182));
#131870=CARTESIAN_POINT('Ctrl Pts',(79.230992152254,-10.4744435195791,129.001729474576));
#131871=CARTESIAN_POINT('',(78.7297156613008,-7.9197450866006,140.000878852949));
#131872=CARTESIAN_POINT('Ctrl Pts',(78.7308621637076,-7.92072007686099,
140.000878852949));
#131873=CARTESIAN_POINT('Ctrl Pts',(78.7363705291969,-7.91424272570425,
140.000585901966));
#131874=CARTESIAN_POINT('Ctrl Pts',(78.7419284837365,-7.9078075452857,140.000292950983));
#131875=CARTESIAN_POINT('Ctrl Pts',(78.7475353758638,-7.90141528989,140.));
#131876=CARTESIAN_POINT('Ctrl Pts',(79.4698297828115,-10.9851743256717,
140.));
#131877=CARTESIAN_POINT('Ctrl Pts',(79.4008200957994,-10.9596225970694,
140.));
#131878=CARTESIAN_POINT('Ctrl Pts',(79.333531238509,-10.9301397446099,140.));
#131879=CARTESIAN_POINT('Ctrl Pts',(79.2681549888845,-10.8970246394104,
140.));
#131880=CARTESIAN_POINT('Ctrl Pts',(79.2013067023064,-10.8631639016782,
140.));
#131881=CARTESIAN_POINT('Ctrl Pts',(79.1364573734554,-10.8255047661518,
140.));
#131882=CARTESIAN_POINT('Ctrl Pts',(79.0738433378323,-10.7843220466833,
140.));
#131883=CARTESIAN_POINT('Ctrl Pts',(79.0212317311646,-10.7497181592862,
140.));
#131884=CARTESIAN_POINT('Ctrl Pts',(78.9701986488695,-10.7126254858123,
140.));
#131885=CARTESIAN_POINT('Ctrl Pts',(78.9209066035052,-10.6731894209709,
140.));
#131886=CARTESIAN_POINT('Ctrl Pts',(78.8988725316228,-10.6555610778773,
140.));
#131887=CARTESIAN_POINT('Ctrl Pts',(78.8771866502947,-10.6374643052944,
140.));
#131888=CARTESIAN_POINT('Ctrl Pts',(78.8558650240912,-10.6189113693179,
140.));
#131889=CARTESIAN_POINT('Ctrl Pts',(78.8441548842812,-10.6087218334872,
140.));
#131890=CARTESIAN_POINT('Ctrl Pts',(78.8325546346987,-10.5983946956447,
140.));
#131891=CARTESIAN_POINT('Ctrl Pts',(78.8210670708132,-10.58793194623,140.));
#131892=CARTESIAN_POINT('Ctrl Pts',(78.8104707785347,-10.5782809573921,
140.));
#131893=CARTESIAN_POINT('Ctrl Pts',(78.7999689254918,-10.5685130628946,
140.));
#131894=CARTESIAN_POINT('Ctrl Pts',(78.7895796051904,-10.5586452950551,
140.));
#131895=CARTESIAN_POINT('Ctrl Pts',(78.7365483625556,-10.5082762646108,
140.));
#131896=CARTESIAN_POINT('Ctrl Pts',(78.6863515775254,-10.4552236751168,
140.));
#131897=CARTESIAN_POINT('Ctrl Pts',(78.6392071691807,-10.3997467391998,
140.));
#131898=CARTESIAN_POINT('Ctrl Pts',(78.5923344111128,-10.3445894663248,
140.));
#131899=CARTESIAN_POINT('Ctrl Pts',(78.5484784305652,-10.2870348269277,
140.));
#131900=CARTESIAN_POINT('Ctrl Pts',(78.5078983274109,-10.2273132639917,
140.));
#131901=CARTESIAN_POINT('Ctrl Pts',(78.4742112341867,-10.177736114065,140.));
#131902=CARTESIAN_POINT('Ctrl Pts',(78.4427822939888,-10.1266650192556,
140.));
#131903=CARTESIAN_POINT('Ctrl Pts',(78.4137873452838,-10.0742253403816,
140.));
#131904=CARTESIAN_POINT('Ctrl Pts',(78.4016823044879,-10.0523324079764,
140.));
#131905=CARTESIAN_POINT('Ctrl Pts',(78.3900018207447,-10.0302008977002,
140.));
#131906=CARTESIAN_POINT('Ctrl Pts',(78.3787601302745,-10.0078398495078,
140.));
#131907=CARTESIAN_POINT('Ctrl Pts',(78.3735606382605,-9.99749744666275,
140.));
#131908=CARTESIAN_POINT('Ctrl Pts',(78.3684550268498,-9.98710594030671,
140.));
#131909=CARTESIAN_POINT('Ctrl Pts',(78.3634447697875,-9.97666622690583,
140.));
#131910=CARTESIAN_POINT('Ctrl Pts',(78.3582118701569,-9.96576260026162,
140.));
#131911=CARTESIAN_POINT('Ctrl Pts',(78.3530865941153,-9.95481383392318,
140.));
#131912=CARTESIAN_POINT('Ctrl Pts',(78.3480720076244,-9.94382525390416,
140.));
#131913=CARTESIAN_POINT('Ctrl Pts',(78.3195311208759,-9.88128294489856,
140.));
#131914=CARTESIAN_POINT('Ctrl Pts',(78.2945512381878,-9.81740871987298,
140.));
#131915=CARTESIAN_POINT('Ctrl Pts',(78.2733557714692,-9.75240749763881,
140.));
#131916=CARTESIAN_POINT('Ctrl Pts',(78.2541540953671,-9.69352073509912,
140.));
#131917=CARTESIAN_POINT('Ctrl Pts',(78.2380586683517,-9.63370843084546,
140.));
#131918=CARTESIAN_POINT('Ctrl Pts',(78.2252722924462,-9.57311813897071,
140.));
#131919=CARTESIAN_POINT('Ctrl Pts',(78.2101392841633,-9.50140795341181,
140.));
#131920=CARTESIAN_POINT('Ctrl Pts',(78.1996407717424,-9.42860649740764,
140.));
#131921=CARTESIAN_POINT('Ctrl Pts',(78.1937017083734,-9.35513639115956,
140.));
#131922=CARTESIAN_POINT('Ctrl Pts',(78.1923945550754,-9.33896604817427,
140.));
#131923=CARTESIAN_POINT('Ctrl Pts',(78.1913084919283,-9.32276339661601,
140.));
#131924=CARTESIAN_POINT('Ctrl Pts',(78.1904430881221,-9.30653310676373,
140.));
#131925=CARTESIAN_POINT('Ctrl Pts',(78.1895474828392,-9.28973640072695,
140.));
#131926=CARTESIAN_POINT('Ctrl Pts',(78.1888881969976,-9.27290390047659,
140.));
#131927=CARTESIAN_POINT('Ctrl Pts',(78.1884653147637,-9.25607505183301,
140.));
#131928=CARTESIAN_POINT('Ctrl Pts',(78.1867405462831,-9.18743686990091,
140.));
#131929=CARTESIAN_POINT('Ctrl Pts',(78.1889365602746,-9.11877251451354,
140.));
#131930=CARTESIAN_POINT('Ctrl Pts',(78.194932447553,-9.05042112078302,140.));
#131931=CARTESIAN_POINT('Ctrl Pts',(78.2009126413601,-8.98224862812093,
140.));
#131932=CARTESIAN_POINT('Ctrl Pts',(78.2106733153825,-8.91438639908554,
140.));
#131933=CARTESIAN_POINT('Ctrl Pts',(78.2241439281836,-8.84718590809215,
140.));
#131934=CARTESIAN_POINT('Ctrl Pts',(78.233903850027,-8.79849684326436,140.));
#131935=CARTESIAN_POINT('Ctrl Pts',(78.2456123494515,-8.7501554211586,140.));
#131936=CARTESIAN_POINT('Ctrl Pts',(78.259256796517,-8.70230497136332,140.));
#131937=CARTESIAN_POINT('Ctrl Pts',(78.26949384472,-8.66640411303307,140.));
#131938=CARTESIAN_POINT('Ctrl Pts',(78.2808209031763,-8.63077978202661,
140.));
#131939=CARTESIAN_POINT('Ctrl Pts',(78.2932365554045,-8.59549668869302,
140.));
#131940=CARTESIAN_POINT('Ctrl Pts',(78.2973629100911,-8.58377031662187,
140.));
#131941=CARTESIAN_POINT('Ctrl Pts',(78.3016063044215,-8.57209085321481,
140.));
#131942=CARTESIAN_POINT('Ctrl Pts',(78.3059661153362,-8.56046079440967,
140.));
#131943=CARTESIAN_POINT('Ctrl Pts',(78.3291465008772,-8.49862571664103,
140.));
#131944=CARTESIAN_POINT('Ctrl Pts',(78.3556159809548,-8.43818113391062,
140.));
#131945=CARTESIAN_POINT('Ctrl Pts',(78.3853243049125,-8.37946332859205,
140.));
#131946=CARTESIAN_POINT('Ctrl Pts',(78.406095636309,-8.3384092794008,140.));
#131947=CARTESIAN_POINT('Ctrl Pts',(78.428451125745,-8.29819989796544,140.));
#131948=CARTESIAN_POINT('Ctrl Pts',(78.4523838925721,-8.25896135362974,
140.));
#131949=CARTESIAN_POINT('Ctrl Pts',(78.4600963530419,-8.24631652554664,
140.));
#131950=CARTESIAN_POINT('Ctrl Pts',(78.4679737739132,-8.23377090157036,
140.));
#131951=CARTESIAN_POINT('Ctrl Pts',(78.4760125797683,-8.22133436830632,
140.));
#131952=CARTESIAN_POINT('Ctrl Pts',(78.5102589047579,-8.16835317090255,
140.));
#131953=CARTESIAN_POINT('Ctrl Pts',(78.5473615778501,-8.11745538563355,
140.));
#131954=CARTESIAN_POINT('Ctrl Pts',(78.5872864281299,-8.06895595885705,
140.));
#131955=CARTESIAN_POINT('Ctrl Pts',(78.6240638473892,-8.02427993027098,
140.));
#131956=CARTESIAN_POINT('Ctrl Pts',(78.663236603919,-7.98163893007374,140.));
#131957=CARTESIAN_POINT('Ctrl Pts',(78.7047994118345,-7.9413119889715,140.));
#131958=CARTESIAN_POINT('Ctrl Pts',(78.7126176289588,-7.93372624591629,
140.));
#131959=CARTESIAN_POINT('Ctrl Pts',(78.7205204684454,-7.9262224864657,140.));
#131960=CARTESIAN_POINT('Ctrl Pts',(78.7285063379699,-7.91880137781994,
140.));
#131961=CARTESIAN_POINT('Origin',(80.,-9.,128.));
#131962=CARTESIAN_POINT('Origin',(80.,9.,128.));
#131963=CARTESIAN_POINT('Origin',(70.,4.,140.));
#131964=CARTESIAN_POINT('',(90.,4.,111.633307652784));
#131965=CARTESIAN_POINT('',(70.,4.,111.633307652784));
#131966=CARTESIAN_POINT('',(60.,4.,111.633307652784));
#131967=CARTESIAN_POINT('',(90.,4.,140.));
#131968=CARTESIAN_POINT('',(90.,4.,140.));
#131969=CARTESIAN_POINT('',(70.,4.,140.));
#131970=CARTESIAN_POINT('',(65.,4.,140.));
#131971=CARTESIAN_POINT('',(70.,4.,140.));
#131972=CARTESIAN_POINT('Origin',(70.,-4.,140.));
#131973=CARTESIAN_POINT('',(70.,-4.,111.633307652784));
#131974=CARTESIAN_POINT('Origin',(70.,0.,90.));
#131975=CARTESIAN_POINT('',(70.,-4.,140.));
#131976=CARTESIAN_POINT('',(70.,-2.,140.));
#131977=CARTESIAN_POINT('',(70.,-4.,140.));
#131978=CARTESIAN_POINT('Origin',(90.,-4.,140.));
#131979=CARTESIAN_POINT('',(90.,-4.,111.633307652784));
#131980=CARTESIAN_POINT('',(60.,-4.,111.633307652784));
#131981=CARTESIAN_POINT('',(90.,-4.,140.));
#131982=CARTESIAN_POINT('',(75.,-4.,140.));
#131983=CARTESIAN_POINT('',(90.,-4.,140.));
#131984=CARTESIAN_POINT('Origin',(90.,4.,140.));
#131985=CARTESIAN_POINT('Origin',(90.,0.,90.));
#131986=CARTESIAN_POINT('',(90.,2.,140.));
#131987=CARTESIAN_POINT('Origin',(130.,-35.,35.));
#131988=CARTESIAN_POINT('',(125.5,-35.,40.));
#131989=CARTESIAN_POINT('Origin',(130.,-35.,40.));
#131990=CARTESIAN_POINT('',(125.5,-35.,30.));
#131991=CARTESIAN_POINT('',(125.5,-35.,35.));
#131992=CARTESIAN_POINT('Origin',(130.,-35.,30.));
#131993=CARTESIAN_POINT('Origin',(-10.,-35.,35.));
#131994=CARTESIAN_POINT('',(-14.5,-35.,40.));
#131995=CARTESIAN_POINT('Origin',(-10.,-35.,40.));
#131996=CARTESIAN_POINT('',(-14.5,-35.,30.));
#131997=CARTESIAN_POINT('',(-14.5,-35.,35.));
#131998=CARTESIAN_POINT('Origin',(-10.,-35.,30.));
#131999=CARTESIAN_POINT('Origin',(-10.,35.,35.));
#132000=CARTESIAN_POINT('',(-14.5,35.,40.));
#132001=CARTESIAN_POINT('Origin',(-10.,35.,40.));
#132002=CARTESIAN_POINT('',(-14.5,35.,30.));
#132003=CARTESIAN_POINT('',(-14.5,35.,35.));
#132004=CARTESIAN_POINT('Origin',(-10.,35.,30.));
#132005=CARTESIAN_POINT('Origin',(130.,35.,35.));
#132006=CARTESIAN_POINT('',(125.5,35.,40.));
#132007=CARTESIAN_POINT('Origin',(130.,35.,40.));
#132008=CARTESIAN_POINT('',(125.5,35.,30.));
#132009=CARTESIAN_POINT('',(125.5,35.,35.));
#132010=CARTESIAN_POINT('Origin',(130.,35.,30.));
#132011=CARTESIAN_POINT('Ctrl Pts',(0.00170278829429053,-31.2663976828551,
56.0778454928015));
#132012=CARTESIAN_POINT('Ctrl Pts',(0.0387608137938565,-31.624937451848,
55.6566083896577));
#132013=CARTESIAN_POINT('Ctrl Pts',(0.112863929572942,-31.8820300337866,
54.4354445242093));
#132014=CARTESIAN_POINT('Ctrl Pts',(0.224012135631548,-30.544181885415,
53.1100227718196));
#132015=CARTESIAN_POINT('Ctrl Pts',(0.335147406470108,-28.7082554303748,
53.5190716991923));
#132016=CARTESIAN_POINT('Ctrl Pts',(0.446282677308667,-28.0547317584378,
55.2813852137159));
#132017=CARTESIAN_POINT('Ctrl Pts',(0.557417948147225,-29.1816019930474,
56.787252268337));
#132018=CARTESIAN_POINT('Ctrl Pts',(0.668553218985785,-31.0575569454888,
56.6567445709802));
#132019=CARTESIAN_POINT('Ctrl Pts',(0.779688489824345,-31.9655456415866,
55.0101441815013));
#132020=CARTESIAN_POINT('Ctrl Pts',(0.890823760662904,-31.074532934791,
53.3541184147092));
#132021=CARTESIAN_POINT('Ctrl Pts',(1.00195903150147,-29.2000268959159,
53.204592662045));
#132022=CARTESIAN_POINT('Ctrl Pts',(1.11309430234002,-28.0577155228313,
54.6983168732093));
#132023=CARTESIAN_POINT('Ctrl Pts',(1.22422957317858,-28.6931214980771,
56.4681812061873));
#132024=CARTESIAN_POINT('Ctrl Pts',(1.33536484401714,-30.5246770131522,
56.894251534457));
#132025=CARTESIAN_POINT('Ctrl Pts',(1.4465001148557,-31.8760102052004,55.5865713892929));
#132026=CARTESIAN_POINT('Ctrl Pts',(1.55763538569426,-31.5102842230428,
53.7420166588749));
#132027=CARTESIAN_POINT('Ctrl Pts',(1.66877065653282,-29.7622375781494,
53.0488598107174));
#132028=CARTESIAN_POINT('Ctrl Pts',(1.77990592737138,-28.2318082099653,
54.1415260230505));
#132029=CARTESIAN_POINT('Ctrl Pts',(1.89104119820994,-28.3197549605855,
56.019929579839));
#132030=CARTESIAN_POINT('Ctrl Pts',(2.0021764690485,-29.9455826694406,56.9648201745416));
#132031=CARTESIAN_POINT('Ctrl Pts',(2.11331173988706,-31.621217024128,56.1113662898202));
#132032=CARTESIAN_POINT('Ctrl Pts',(2.22444701072562,-31.8129971096645,
54.240710110029));
#132033=CARTESIAN_POINT('Ctrl Pts',(2.33558228156418,-30.3453920134525,
53.0650105959154));
#132034=CARTESIAN_POINT('Ctrl Pts',(2.44671755240274,-28.5616593378144,
53.6603523633191));
#132035=CARTESIAN_POINT('Ctrl Pts',(2.5578528232413,-28.0943993507182,55.4818358784335));
#132036=CARTESIAN_POINT('Ctrl Pts',(2.66898809407986,-29.3712819556072,
56.8623085852841));
#132037=CARTESIAN_POINT('Ctrl Pts',(2.78012336491841,-31.2236124749314,
56.5382627081225));
#132038=CARTESIAN_POINT('Ctrl Pts',(2.89125863575698,-31.9560049662107,
54.8062883077869));
#132039=CARTESIAN_POINT('Ctrl Pts',(3.00239390659553,-30.8981212142627,
53.2516127626239));
#132040=CARTESIAN_POINT('Ctrl Pts',(3.1135291774341,-29.0182124157641,53.297186802082));
#132041=CARTESIAN_POINT('Ctrl Pts',(3.22466444827265,-28.0369061353021,
54.901297791946));
#132042=CARTESIAN_POINT('Ctrl Pts',(3.33579971911122,-28.8523643671384,
56.5957481322741));
#132043=CARTESIAN_POINT('Ctrl Pts',(3.44693498994977,-30.7182211638377,
56.8296551607653));
#132044=CARTESIAN_POINT('Ctrl Pts',(3.55807026078833,-31.9267103621918,
55.3889303635752));
#132045=CARTESIAN_POINT('Ctrl Pts',(3.66920553162689,-31.3717358431385,
53.5922285611165));
#132046=CARTESIAN_POINT('Ctrl Pts',(3.78034080246546,-29.5612501498527,
53.0840202985193));
#132047=CARTESIAN_POINT('Ctrl Pts',(3.891476073304,-28.1523398344416,54.3294542818737));
#132048=CARTESIAN_POINT('Ctrl Pts',(4.00261134414257,-28.434540818372,56.1886198711722));
#132049=CARTESIAN_POINT('Ctrl Pts',(4.11374661498113,-30.1495624908996,
56.9598751768429));
#132050=CARTESIAN_POINT('Ctrl Pts',(4.22488188581969,-31.7276938288123,
55.9373119445377));
#132051=CARTESIAN_POINT('Ctrl Pts',(4.33601715665825,-31.724515675851,54.0568534942901));
#132052=CARTESIAN_POINT('Ctrl Pts',(4.44715242749681,-30.1429369058903,
53.0396304714612));
#132053=CARTESIAN_POINT('Ctrl Pts',(4.55828769833536,-28.430532012625,53.8166784527888));
#132054=CARTESIAN_POINT('Ctrl Pts',(4.66942296917392,-28.1546169549256,
55.6767873110815));
#132055=CARTESIAN_POINT('Ctrl Pts',(4.78055824001249,-29.5677290123371,
56.9174518092285));
#132056=CARTESIAN_POINT('Ctrl Pts',(4.89169351085105,-31.3764865273067,
56.4031266826741));
#132057=CARTESIAN_POINT('Ctrl Pts',(5.0028287816896,-31.9253847006554,54.6045592307673));
#132058=CARTESIAN_POINT('Ctrl Pts',(5.11396405252817,-30.7120324972562,
53.1679275750288));
#132059=CARTESIAN_POINT('Ctrl Pts',(5.22509932336672,-28.8469770076932,
53.4081401987923));
#132060=CARTESIAN_POINT('Ctrl Pts',(5.33623459420528,-28.037250981328,55.105337254526));
#132061=CARTESIAN_POINT('Ctrl Pts',(5.44736986504384,-29.023973839406,56.7061220886341));
#132062=CARTESIAN_POINT('Ctrl Pts',(5.5585051358824,-30.9040259467696,56.7453414379588));
#132063=CARTESIAN_POINT('Ctrl Pts',(5.66964040672096,-31.9566485722524,
55.1870989369065));
#132064=CARTESIAN_POINT('Ctrl Pts',(5.78077567755952,-31.2184058800449,
53.4576100496434));
#132065=CARTESIAN_POINT('Ctrl Pts',(5.89191094839808,-29.3649906093859,
53.1398272334751));
#132066=CARTESIAN_POINT('Ctrl Pts',(6.00304621923664,-28.0927815451889,
54.524608147822));
#132067=CARTESIAN_POINT('Ctrl Pts',(6.1141814900752,-28.5661958046776,56.3445018322654));
#132068=CARTESIAN_POINT('Ctrl Pts',(6.22531676091376,-30.3519306526335,
56.9338108654224));
#132069=CARTESIAN_POINT('Ctrl Pts',(6.33645203175232,-31.8155532884263,
55.7531572905929));
#132070=CARTESIAN_POINT('Ctrl Pts',(6.44758730259087,-31.6174511450385,
53.8831600647792));
#132071=CARTESIAN_POINT('Ctrl Pts',(6.55872257342944,-29.9389415336019,
53.0353749693217));
#132072=CARTESIAN_POINT('Ctrl Pts',(6.66985784426799,-28.3163170163911,
53.9857558192458));
#132073=CARTESIAN_POINT('Ctrl Pts',(6.78099311510656,-28.2347201032599,
55.8644457956774));
#132074=CARTESIAN_POINT('Ctrl Pts',(6.89212838594511,-29.7688341501512,
56.9519328875076));
#132075=CARTESIAN_POINT('Ctrl Pts',(7.00326365678368,-31.514527787253,56.2528707950653));
#132076=CARTESIAN_POINT('Ctrl Pts',(7.11439892762223,-31.8740168062734,
54.4070913583285));
#132077=CARTESIAN_POINT('Ctrl Pts',(7.22553419846079,-30.518271035144,53.1039844986238));
#132078=CARTESIAN_POINT('Ctrl Pts',(7.33666946929935,-28.6881663857952,
53.5362472147991));
#132079=CARTESIAN_POINT('Ctrl Pts',(7.44780474013791,-28.0587460878319,
55.3082416203242));
#132080=CARTESIAN_POINT('Ctrl Pts',(7.55894001097647,-29.2061008092653,
56.7981111537161));
#132081=CARTESIAN_POINT('Ctrl Pts',(7.67007528181502,-31.080089094353,56.6422202034286));
#132082=CARTESIAN_POINT('Ctrl Pts',(7.78121055265359,-31.9655022600037,
54.9832513618084));
#132083=CARTESIAN_POINT('Ctrl Pts',(7.89234582349214,-31.051946573859,53.3396120806803));
#132084=CARTESIAN_POINT('Ctrl Pts',(8.00348109433071,-29.1755738291021,
53.2156790800412));
#132085=CARTESIAN_POINT('Ctrl Pts',(8.11461636516927,-28.0537751214917,
54.7248847664219));
#132086=CARTESIAN_POINT('Ctrl Pts',(8.22575163600783,-28.7133012426661,
56.485895646412));
#132087=CARTESIAN_POINT('Ctrl Pts',(8.33688690684639,-30.5505064407611,
56.8869081585993));
#132088=CARTESIAN_POINT('Ctrl Pts',(8.44802217768495,-31.8838486975197,
55.5608866733121));
#132089=CARTESIAN_POINT('Ctrl Pts',(8.55915744852351,-31.4929571214681,
53.7215016460962));
#132090=CARTESIAN_POINT('Ctrl Pts',(8.67029271936206,-29.7356043259867,
53.0522896908207));
#132091=CARTESIAN_POINT('Ctrl Pts',(8.78142799020063,-28.2202446973277,
54.1657630148673));
#132092=CARTESIAN_POINT('Ctrl Pts',(8.89256326103917,-28.3338464376506,
56.0427881618974));
#132093=CARTESIAN_POINT('Ctrl Pts',(9.00369853187775,-29.9724286669489,
56.9653822260781));
#132094=CARTESIAN_POINT('Ctrl Pts',(9.11483380271629,-31.6362519689162,
56.0891102760781));
#132095=CARTESIAN_POINT('Ctrl Pts',(9.22596907355487,-31.8024484231335,
54.2160203074161));
#132096=CARTESIAN_POINT('Ctrl Pts',(9.33710434439342,-30.3189374419903,
53.0604572371698));
#132097=CARTESIAN_POINT('Ctrl Pts',(9.44823961523198,-28.5434667432019,
53.6801577952576));
#132098=CARTESIAN_POINT('Ctrl Pts',(9.55937488607055,-28.1012096376717,
55.5077641444152));
#132099=CARTESIAN_POINT('Ctrl Pts',(9.67051015690909,-29.3966839478976,
56.8708435823807));
#132100=CARTESIAN_POINT('Ctrl Pts',(9.78164542774768,-31.244709241904,56.5211656955268));
#132101=CARTESIAN_POINT('Ctrl Pts',(9.8927806985862,-31.9527868925014,54.7800545118344));
#132102=CARTESIAN_POINT('Ctrl Pts',(10.0039159694248,-30.874933117478,53.2385687957247));
#132103=CARTESIAN_POINT('Ctrl Pts',(10.1150512402633,-28.9933745151999,
53.3126786820222));
#132104=CARTESIAN_POINT('Ctrl Pts',(10.1891414208223,-28.358348784767,54.3865918892037));
#132105=CARTESIAN_POINT('Ctrl Pts',(10.2261865111019,-28.338128692637,54.9391906103726));
#132106=CARTESIAN_POINT('Ctrl Pts',(-0.074183729153435,-31.3664915399073,
56.1630365146595));
#132107=CARTESIAN_POINT('Ctrl Pts',(-0.0371257036538689,-31.7533696649088,
55.7085055679165));
#132108=CARTESIAN_POINT('Ctrl Pts',(0.0369774121252169,-32.0307823946921,
54.3908230471987));
#132109=CARTESIAN_POINT('Ctrl Pts',(0.148125618183823,-30.5871930694899,
52.9606422785743));
#132110=CARTESIAN_POINT('Ctrl Pts',(0.259260889022382,-28.6061581997412,
53.4020217174587));
#132111=CARTESIAN_POINT('Ctrl Pts',(0.370396159860942,-27.9009811602368,
55.3036254086718));
#132112=CARTESIAN_POINT('Ctrl Pts',(0.481531430699501,-29.1169172465188,
56.9285135604929));
#132113=CARTESIAN_POINT('Ctrl Pts',(0.592666701538061,-31.1411443960659,
56.7876907630847));
#132114=CARTESIAN_POINT('Ctrl Pts',(0.70380197237662,-32.1208989300063,
55.010945959858));
#132115=CARTESIAN_POINT('Ctrl Pts',(0.81493724321518,-31.1594621378598,
53.2240308139867));
#132116=CARTESIAN_POINT('Ctrl Pts',(0.926072514053739,-29.1367984214722,
53.0626868074554));
#132117=CARTESIAN_POINT('Ctrl Pts',(1.0372077848923,-27.9042007561473,54.674472366719));
#132118=CARTESIAN_POINT('Ctrl Pts',(1.14834305573085,-28.5898281079144,
56.5842236798656));
#132119=CARTESIAN_POINT('Ctrl Pts',(1.25947832656941,-30.5661465662507,
57.0439698613918));
#132120=CARTESIAN_POINT('Ctrl Pts',(1.37061359740797,-32.0242867693873,
55.6329329655858));
#132121=CARTESIAN_POINT('Ctrl Pts',(1.48174886824653,-31.6296544455062,
53.6425878566706));
#132122=CARTESIAN_POINT('Ctrl Pts',(1.59288413908509,-29.7434452523364,
52.8946451040428));
#132123=CARTESIAN_POINT('Ctrl Pts',(1.70401940992365,-28.0920534246646,
54.0736737419738));
#132124=CARTESIAN_POINT('Ctrl Pts',(1.81515468076221,-28.1869513325744,
56.1005430292712));
#132125=CARTESIAN_POINT('Ctrl Pts',(1.92628995160077,-29.9412816188465,
57.1201161233154));
#132126=CARTESIAN_POINT('Ctrl Pts',(2.03742522243933,-31.7493551810914,
56.1992067368236));
#132127=CARTESIAN_POINT('Ctrl Pts',(2.14856049327789,-31.9562932290335,
54.1806971656458));
#132128=CARTESIAN_POINT('Ctrl Pts',(2.25969576411645,-30.3726911938675,
52.912072419044));
#132129=CARTESIAN_POINT('Ctrl Pts',(2.37083103495501,-28.4479754085223,
53.5544689580811));
#132130=CARTESIAN_POINT('Ctrl Pts',(2.48196630579357,-27.9437840096051,
55.5199193432025));
#132131=CARTESIAN_POINT('Ctrl Pts',(2.59310157663213,-29.3215891814387,
57.0095021974063));
#132132=CARTESIAN_POINT('Ctrl Pts',(2.70423684747069,-31.3203246640101,
56.659844301093));
#132133=CARTESIAN_POINT('Ctrl Pts',(2.81537211830925,-32.1106041763419,
54.7909776745694));
#132134=CARTESIAN_POINT('Ctrl Pts',(2.92650738914781,-30.9691071436062,
53.1134232945136));
#132135=CARTESIAN_POINT('Ctrl Pts',(3.03764265998637,-28.9406136429279,
53.1625994263101));
#132136=CARTESIAN_POINT('Ctrl Pts',(3.14877793082492,-27.8817466310379,
54.8934965421195));
#132137=CARTESIAN_POINT('Ctrl Pts',(3.25991320166349,-28.7616572547211,
56.721873272588));
#132138=CARTESIAN_POINT('Ctrl Pts',(3.37104847250204,-30.7749881079645,
56.9742679033468));
#132139=CARTESIAN_POINT('Ctrl Pts',(3.4821837433406,-32.0789941780779,55.4196707390054));
#132140=CARTESIAN_POINT('Ctrl Pts',(3.59331901417916,-31.4801554440706,
53.4809607697478));
#132141=CARTESIAN_POINT('Ctrl Pts',(3.70445428501772,-29.5265721293723,
52.9325846152807));
#132142=CARTESIAN_POINT('Ctrl Pts',(3.81558955585628,-28.0063040077843,
54.2764555215586));
#132143=CARTESIAN_POINT('Ctrl Pts',(3.92672482669484,-28.310809663721,56.282566306076));
#132144=CARTESIAN_POINT('Ctrl Pts',(4.0378600975334,-30.1613836484926,57.1147802816508));
#132145=CARTESIAN_POINT('Ctrl Pts',(4.14899536837196,-31.8642477261168,
56.0113954406308));
#132146=CARTESIAN_POINT('Ctrl Pts',(4.26013063921052,-31.8608183775063,
53.9823088446907));
#132147=CARTESIAN_POINT('Ctrl Pts',(4.37126591004908,-30.1542343888369,
52.8846862939603));
#132148=CARTESIAN_POINT('Ctrl Pts',(4.48240118088764,-28.3064840089819,
53.7231507881405));
#132149=CARTESIAN_POINT('Ctrl Pts',(4.5935364517262,-28.0087611078872,55.730279395983));
#132150=CARTESIAN_POINT('Ctrl Pts',(4.70467172256476,-29.5335630698115,
57.0690038452879));
#132151=CARTESIAN_POINT('Ctrl Pts',(4.81580699340331,-31.4852816140033,
56.5140273606391));
#132152=CARTESIAN_POINT('Ctrl Pts',(4.92694226424188,-32.077563738573,54.5733042842651));
#132153=CARTESIAN_POINT('Ctrl Pts',(5.03807753508044,-30.7683103000047,
53.0231237761138));
#132154=CARTESIAN_POINT('Ctrl Pts',(5.149212805919,-28.7558440878116,53.2823223853626));
#132155=CARTESIAN_POINT('Ctrl Pts',(5.26034807675755,-27.8821187330902,
55.1136629268163));
#132156=CARTESIAN_POINT('Ctrl Pts',(5.37148334759611,-28.9468304394138,
56.8409709933388));
#132157=CARTESIAN_POINT('Ctrl Pts',(5.48261861843467,-30.9754785758391,
56.8832901714124));
#132158=CARTESIAN_POINT('Ctrl Pts',(5.59375388927323,-32.1112986518792,
55.2018869095149));
#132159=CARTESIAN_POINT('Ctrl Pts',(5.70488916011179,-31.3147065489737,
53.3357022466681));
#132160=CARTESIAN_POINT('Ctrl Pts',(5.81602443095035,-29.31480057822,52.9928024327307));
#132161=CARTESIAN_POINT('Ctrl Pts',(5.92715970178891,-27.9420383355576,
54.4870340076132));
#132162=CARTESIAN_POINT('Ctrl Pts',(6.03829497262747,-28.4528704297891,
56.4507689046292));
#132163=CARTESIAN_POINT('Ctrl Pts',(6.14943024346604,-30.3797466356488,
57.08665589266));
#132164=CARTESIAN_POINT('Ctrl Pts',(6.26056551430458,-31.9590514436921,
55.8126855250512));
#132165=CARTESIAN_POINT('Ctrl Pts',(6.37170078514316,-31.7452916535078,
53.7948869904205));
#132166=CARTESIAN_POINT('Ctrl Pts',(6.4828360559817,-29.9341155792511,52.8800944443774));
#132167=CARTESIAN_POINT('Ctrl Pts',(6.59397132682027,-28.1832416592862,
53.9055917338097));
#132168=CARTESIAN_POINT('Ctrl Pts',(6.70510659765882,-28.0951954689103,
55.9327700788575));
#132169=CARTESIAN_POINT('Ctrl Pts',(6.81624186849739,-29.7505632058472,
57.106210247663));
#132170=CARTESIAN_POINT('Ctrl Pts',(6.92737713933594,-31.6342334136067,
56.3518955105745));
#132171=CARTESIAN_POINT('Ctrl Pts',(7.03851241017451,-32.0221358156968,
54.3602288966959));
#132172=CARTESIAN_POINT('Ctrl Pts',(7.14964768101306,-30.5592342709492,
52.9541267508301));
#132173=CARTESIAN_POINT('Ctrl Pts',(7.26078295185163,-28.5844813522277,
53.4205547557672));
#132174=CARTESIAN_POINT('Ctrl Pts',(7.37191822269018,-27.9053127752024,
55.332604498668));
#132175=CARTESIAN_POINT('Ctrl Pts',(7.48305349352875,-29.1433524063054,
56.9402307131726));
#132176=CARTESIAN_POINT('Ctrl Pts',(7.59418876436729,-31.1654574465519,
56.7720184149349));
#132177=CARTESIAN_POINT('Ctrl Pts',(7.70532403520587,-32.1208521196191,
54.9819275787506));
#132178=CARTESIAN_POINT('Ctrl Pts',(7.81645930604441,-31.1350905904786,
53.2083779246979));
#132179=CARTESIAN_POINT('Ctrl Pts',(7.92759457688299,-29.1104126270428,
53.0746494765322));
#132180=CARTESIAN_POINT('Ctrl Pts',(8.03872984772154,-27.8999489123803,
54.7031401397257));
#132181=CARTESIAN_POINT('Ctrl Pts',(8.1498651185601,-28.6116028242076,56.6033382384509));
#132182=CARTESIAN_POINT('Ctrl Pts',(8.26100038939866,-30.5940175066244,
57.0360460779548));
#132183=CARTESIAN_POINT('Ctrl Pts',(8.37213566023721,-32.0327448024245,
55.6052181745942));
#132184=CARTESIAN_POINT('Ctrl Pts',(8.48327093107578,-31.6109578401403,
53.6204513731766));
#132185=CARTESIAN_POINT('Ctrl Pts',(8.59440620191433,-29.7147069545225,
52.8983460758682));
#132186=CARTESIAN_POINT('Ctrl Pts',(8.7055414727529,-28.0795759522207,54.0998263832167));
#132187=CARTESIAN_POINT('Ctrl Pts',(8.81667674359147,-28.2021565753311,
56.1252083136601));
#132188=CARTESIAN_POINT('Ctrl Pts',(8.92781201443001,-29.9702494770258,
57.120722598422));
#132189=CARTESIAN_POINT('Ctrl Pts',(9.03894728526858,-31.7655784616092,
56.1751916466963));
#132190=CARTESIAN_POINT('Ctrl Pts',(9.15008255610713,-31.944910792776,54.154055924234));
#132191=CARTESIAN_POINT('Ctrl Pts',(9.26121782694571,-30.3441456993643,
52.90715917079));
#132192=CARTESIAN_POINT('Ctrl Pts',(9.37235309778425,-28.428344903063,53.5758397767066));
#132193=CARTESIAN_POINT('Ctrl Pts',(9.48348836862282,-27.9511325697238,
55.547896933961));
#132194=CARTESIAN_POINT('Ctrl Pts',(9.59462363946135,-29.3489989027542,
57.0187117857399));
#132195=CARTESIAN_POINT('Ctrl Pts',(9.70575891029995,-31.3430888825314,
56.6413959705362));
#132196=CARTESIAN_POINT('Ctrl Pts',(9.81689418113849,-32.1071317517173,
54.7626704052856));
#132197=CARTESIAN_POINT('Ctrl Pts',(9.92802945197706,-30.9440863002237,
53.0993483552936));
#132198=CARTESIAN_POINT('Ctrl Pts',(10.0391647228156,-28.9138125981616,
53.1793157573348));
#132199=CARTESIAN_POINT('Ctrl Pts',(10.1132549033747,-28.2285955450921,
54.3381091853991));
#132200=CARTESIAN_POINT('Ctrl Pts',(10.1502999936542,-28.2067772922589,
54.9343843426139));
#132201=CARTESIAN_POINT('Ctrl Pts',(-0.15007024660116,-31.4665853969597,
56.2482275365175));
#132202=CARTESIAN_POINT('Ctrl Pts',(-0.113012221101594,-31.8818018779696,
55.7604027461753));
#132203=CARTESIAN_POINT('Ctrl Pts',(-0.0389091053225084,-32.1795347555977,
54.3462015701881));
#132204=CARTESIAN_POINT('Ctrl Pts',(0.072239100736097,-30.6302042535647,
52.8112617853291));
#132205=CARTESIAN_POINT('Ctrl Pts',(0.183374371574657,-28.5040609691078,
53.284971735725));
#132206=CARTESIAN_POINT('Ctrl Pts',(0.294509642413217,-27.7472305620358,
55.3258656036276));
#132207=CARTESIAN_POINT('Ctrl Pts',(0.405644913251776,-29.0522324999903,
57.0697748526486));
#132208=CARTESIAN_POINT('Ctrl Pts',(0.516780184090336,-31.2247318466428,
56.9186369551892));
#132209=CARTESIAN_POINT('Ctrl Pts',(0.627915454928895,-32.2762522184261,
55.0117477382148));
#132210=CARTESIAN_POINT('Ctrl Pts',(0.739050725767455,-31.2443913409285,
53.0939432132643));
#132211=CARTESIAN_POINT('Ctrl Pts',(0.850185996606014,-29.0735699470287,
52.9207809528658));
#132212=CARTESIAN_POINT('Ctrl Pts',(0.961321267444574,-27.7506859894634,
54.6506278602288));
#132213=CARTESIAN_POINT('Ctrl Pts',(1.07245653828313,-28.4865347177518,
56.7002661535439));
#132214=CARTESIAN_POINT('Ctrl Pts',(1.1835918091217,-30.6076161193494,57.1936881883264));
#132215=CARTESIAN_POINT('Ctrl Pts',(1.29472707996025,-32.1725633335742,
55.6792945418786));
#132216=CARTESIAN_POINT('Ctrl Pts',(1.40586235079882,-31.7490246679696,
53.5431590544662));
#132217=CARTESIAN_POINT('Ctrl Pts',(1.51699762163737,-29.7246529265234,
52.7404303973681));
#132218=CARTESIAN_POINT('Ctrl Pts',(1.62813289247593,-27.9522986393639,
54.0058214608971));
#132219=CARTESIAN_POINT('Ctrl Pts',(1.73926816331449,-28.0541477045633,
56.1811564787034));
#132220=CARTESIAN_POINT('Ctrl Pts',(1.85040343415305,-29.9369805682525,
57.2754120720893));
#132221=CARTESIAN_POINT('Ctrl Pts',(1.96153870499161,-31.8774933380549,
56.2870471838269));
#132222=CARTESIAN_POINT('Ctrl Pts',(2.07267397583017,-32.0995893484024,
54.1206842212628));
#132223=CARTESIAN_POINT('Ctrl Pts',(2.18380924666873,-30.3999903742827,
52.7591342421725));
#132224=CARTESIAN_POINT('Ctrl Pts',(2.29494451750729,-28.3342914792303,
53.448585552843));
#132225=CARTESIAN_POINT('Ctrl Pts',(2.40607978834585,-27.7931686684921,
55.5580028079716));
#132226=CARTESIAN_POINT('Ctrl Pts',(2.51721505918441,-29.2718964072702,
57.1566958095285));
#132227=CARTESIAN_POINT('Ctrl Pts',(2.62835033002297,-31.4170368530889,
56.7814258940635));
#132228=CARTESIAN_POINT('Ctrl Pts',(2.73948560086153,-32.2652033864732,
54.7756670413518));
#132229=CARTESIAN_POINT('Ctrl Pts',(2.85062087170008,-31.0400930729498,
52.9752338264031));
#132230=CARTESIAN_POINT('Ctrl Pts',(2.96175614253865,-28.8630148700916,
53.0280120505382));
#132231=CARTESIAN_POINT('Ctrl Pts',(3.0728914133772,-27.7265871267736,54.885695292293));
#132232=CARTESIAN_POINT('Ctrl Pts',(3.18402668421577,-28.6709501423038,
56.8479984129019));
#132233=CARTESIAN_POINT('Ctrl Pts',(3.29516195505432,-30.8317550520915,
57.1188806459284));
#132234=CARTESIAN_POINT('Ctrl Pts',(3.40629722589288,-32.2312779939638,
55.4504111144357));
#132235=CARTESIAN_POINT('Ctrl Pts',(3.51743249673144,-31.5885750450029,
53.3696929783789));
#132236=CARTESIAN_POINT('Ctrl Pts',(3.62856776757001,-29.4918941088918,
52.781148932042));
#132237=CARTESIAN_POINT('Ctrl Pts',(3.73970303840856,-27.860268181127,54.2234567612437));
#132238=CARTESIAN_POINT('Ctrl Pts',(3.85083830924712,-28.18707850907,56.3765127409798));
#132239=CARTESIAN_POINT('Ctrl Pts',(3.96197358008568,-30.1732048060856,
57.2696853864588));
#132240=CARTESIAN_POINT('Ctrl Pts',(4.07310885092424,-32.0008016234211,
56.0854789367237));
#132241=CARTESIAN_POINT('Ctrl Pts',(4.1842441217628,-31.9971210791615,53.9077641950914));
#132242=CARTESIAN_POINT('Ctrl Pts',(4.29537939260136,-30.1655318717835,
52.7297421164591));
#132243=CARTESIAN_POINT('Ctrl Pts',(4.40651466343992,-28.1824360053388,
53.6296231234923));
#132244=CARTESIAN_POINT('Ctrl Pts',(4.51764993427848,-27.8629052608487,
55.7837714808843));
#132245=CARTESIAN_POINT('Ctrl Pts',(4.62878520511703,-29.4993971272859,
57.2205558813473));
#132246=CARTESIAN_POINT('Ctrl Pts',(4.7399204759556,-31.5940767006999,56.624928038604));
#132247=CARTESIAN_POINT('Ctrl Pts',(4.85105574679415,-32.2297427764907,
54.5420493377628));
#132248=CARTESIAN_POINT('Ctrl Pts',(4.96219101763272,-30.8245881027533,
52.8783199771989));
#132249=CARTESIAN_POINT('Ctrl Pts',(5.07332628847127,-28.6647111679299,
53.1565045719328));
#132250=CARTESIAN_POINT('Ctrl Pts',(5.18446155930983,-27.7269864848525,
55.1219885991068));
#132251=CARTESIAN_POINT('Ctrl Pts',(5.2955968301484,-28.8696870394214,56.9758198980433));
#132252=CARTESIAN_POINT('Ctrl Pts',(5.40673210098694,-31.0469312049086,
57.0212389048661));
#132253=CARTESIAN_POINT('Ctrl Pts',(5.51786737182552,-32.2659487315058,
55.2166748821232));
#132254=CARTESIAN_POINT('Ctrl Pts',(5.62900264266406,-31.4110072179026,
53.2137944436928));
#132255=CARTESIAN_POINT('Ctrl Pts',(5.74013791350264,-29.264610547054,52.8457776319862));
#132256=CARTESIAN_POINT('Ctrl Pts',(5.85127318434119,-27.7912951259262,
54.4494598674044));
#132257=CARTESIAN_POINT('Ctrl Pts',(5.96240845517975,-28.3395450549005,
56.5570359769931));
#132258=CARTESIAN_POINT('Ctrl Pts',(6.07354372601831,-30.4075626186642,
57.2395009198977));
#132259=CARTESIAN_POINT('Ctrl Pts',(6.18467899685687,-32.1025495989578,
55.8722137595095));
#132260=CARTESIAN_POINT('Ctrl Pts',(6.29581426769543,-31.873132161977,53.7066139160619));
#132261=CARTESIAN_POINT('Ctrl Pts',(6.40694953853399,-29.9292896249002,
52.724813919433));
#132262=CARTESIAN_POINT('Ctrl Pts',(6.51808480937254,-28.0501663021814,
53.8254276483735));
#132263=CARTESIAN_POINT('Ctrl Pts',(6.62922008021111,-27.9556708345606,
56.0010943620377));
#132264=CARTESIAN_POINT('Ctrl Pts',(6.74035535104966,-29.7322922615432,
57.2604876078183));
#132265=CARTESIAN_POINT('Ctrl Pts',(6.85149062188823,-31.7539390399603,
56.4509202260838));
#132266=CARTESIAN_POINT('Ctrl Pts',(6.96262589272678,-32.1702548251203,
54.3133664350632));
#132267=CARTESIAN_POINT('Ctrl Pts',(7.07376116356534,-30.6001975067545,
52.8042690030366));
#132268=CARTESIAN_POINT('Ctrl Pts',(7.18489643440391,-28.4807963186602,
53.3048622967354));
#132269=CARTESIAN_POINT('Ctrl Pts',(7.29603170524246,-27.7518794625729,
55.3569673770119));
#132270=CARTESIAN_POINT('Ctrl Pts',(7.40716697608102,-29.0806040033454,
57.0823502726293));
#132271=CARTESIAN_POINT('Ctrl Pts',(7.51830224691958,-31.2508257987508,
56.9018166264413));
#132272=CARTESIAN_POINT('Ctrl Pts',(7.62943751775815,-32.2762019792346,
54.9806037956928));
#132273=CARTESIAN_POINT('Ctrl Pts',(7.7405727885967,-31.2182346070983,53.0771437687153));
#132274=CARTESIAN_POINT('Ctrl Pts',(7.85170805943526,-29.0452514249833,
52.9336198730232));
#132275=CARTESIAN_POINT('Ctrl Pts',(7.96284333027382,-27.746122703269,54.6813955130294));
#132276=CARTESIAN_POINT('Ctrl Pts',(8.07397860111238,-28.509904405749,56.7207808304898));
#132277=CARTESIAN_POINT('Ctrl Pts',(8.18511387195094,-30.6375285724877,
57.1851839973102));
#132278=CARTESIAN_POINT('Ctrl Pts',(8.29624914278949,-32.1816409073294,
55.6495496758762));
#132279=CARTESIAN_POINT('Ctrl Pts',(8.40738441362806,-31.7289585588121,
53.519401100257));
#132280=CARTESIAN_POINT('Ctrl Pts',(8.51851968446662,-29.6938095830584,
52.7444024609157));
#132281=CARTESIAN_POINT('Ctrl Pts',(8.62965495530518,-27.9389072071136,
54.0338897515661));
#132282=CARTESIAN_POINT('Ctrl Pts',(8.74079022614373,-28.0704667130116,
56.2076284654227));
#132283=CARTESIAN_POINT('Ctrl Pts',(8.85192549698231,-29.9680702871027,
57.2760629707658));
#132284=CARTESIAN_POINT('Ctrl Pts',(8.96306076782084,-31.8949049543022,
56.2612730173147));
#132285=CARTESIAN_POINT('Ctrl Pts',(9.07419603865942,-32.0873731624184,
54.0920915410519));
#132286=CARTESIAN_POINT('Ctrl Pts',(9.18533130949797,-30.3693539567383,
52.7538611044103));
#132287=CARTESIAN_POINT('Ctrl Pts',(9.29646658033654,-28.3132230629242,
53.4715217581555));
#132288=CARTESIAN_POINT('Ctrl Pts',(9.40760185117508,-27.8010555017756,
55.5880297235069));
#132289=CARTESIAN_POINT('Ctrl Pts',(9.51873712201365,-29.3013138576107,
57.1665799890989));
#132290=CARTESIAN_POINT('Ctrl Pts',(9.62987239285222,-31.441468523159,56.7616262455456));
#132291=CARTESIAN_POINT('Ctrl Pts',(9.74100766369077,-32.2614766109332,
54.7452862987369));
#132292=CARTESIAN_POINT('Ctrl Pts',(9.85214293452933,-31.0132394829693,
52.9601279148623));
#132293=CARTESIAN_POINT('Ctrl Pts',(9.96327820536789,-28.8342506811234,
53.0459528326475));
#132294=CARTESIAN_POINT('Ctrl Pts',(10.037368385927,-28.0988423054172,54.2896264815944));
#132295=CARTESIAN_POINT('Ctrl Pts',(10.0744134762065,-28.075425891881,54.9295780748552));
#132296=CARTESIAN_POINT('Ctrl Pts',(-0.225956764048886,-31.5666792540119,
56.3334185583754));
#132297=CARTESIAN_POINT('Ctrl Pts',(-0.188898738549319,-32.0102340910304,
55.8122999244342));
#132298=CARTESIAN_POINT('Ctrl Pts',(-0.114795622770234,-32.3282871165031,
54.3015800931774));
#132299=CARTESIAN_POINT('Ctrl Pts',(-0.00364741671162839,-30.6732154376395,
52.6618812920838));
#132300=CARTESIAN_POINT('Ctrl Pts',(0.107487854126931,-28.4019637384743,
53.1679217539914));
#132301=CARTESIAN_POINT('Ctrl Pts',(0.218623124965491,-27.5934799638349,
55.3481057985834));
#132302=CARTESIAN_POINT('Ctrl Pts',(0.32975839580405,-28.9875477534618,
57.2110361448045));
#132303=CARTESIAN_POINT('Ctrl Pts',(0.44089366664261,-31.3083192972198,
57.0495831472937));
#132304=CARTESIAN_POINT('Ctrl Pts',(0.552028937481168,-32.4316055068458,
55.0125495165716));
#132305=CARTESIAN_POINT('Ctrl Pts',(0.66316420831973,-31.3293205439973,
52.9638556125418));
#132306=CARTESIAN_POINT('Ctrl Pts',(0.774299479158287,-29.010341472585,
52.7788750982762));
#132307=CARTESIAN_POINT('Ctrl Pts',(0.885434749996847,-27.5971712227794,
54.6267833537386));
#132308=CARTESIAN_POINT('Ctrl Pts',(0.996570020835408,-28.3832413275893,
56.8163086272222));
#132309=CARTESIAN_POINT('Ctrl Pts',(1.10770529167397,-30.649085672448,57.3434065152611));
#132310=CARTESIAN_POINT('Ctrl Pts',(1.21884056251252,-32.320839897761,55.7256561181716));
#132311=CARTESIAN_POINT('Ctrl Pts',(1.32997583335109,-31.868394890433,53.4437302522617));
#132312=CARTESIAN_POINT('Ctrl Pts',(1.44111110418964,-29.7058606007103,
52.5862156906935));
#132313=CARTESIAN_POINT('Ctrl Pts',(1.5522463750282,-27.8125438540631,53.9379691798205));
#132314=CARTESIAN_POINT('Ctrl Pts',(1.66338164586676,-27.9213440765523,
56.2617699281355));
#132315=CARTESIAN_POINT('Ctrl Pts',(1.77451691670532,-29.9326795176583,
57.4307080208631));
#132316=CARTESIAN_POINT('Ctrl Pts',(1.88565218754388,-32.0056314950183,
56.3748876308303));
#132317=CARTESIAN_POINT('Ctrl Pts',(1.99678745838244,-32.2428854677713,
54.0606712768798));
#132318=CARTESIAN_POINT('Ctrl Pts',(2.107922729221,-30.4272895546977,52.606196065301));
#132319=CARTESIAN_POINT('Ctrl Pts',(2.21905800005956,-28.2206075499382,
53.3427021476049));
#132320=CARTESIAN_POINT('Ctrl Pts',(2.33019327089812,-27.6425533273791,
55.5960862727407));
#132321=CARTESIAN_POINT('Ctrl Pts',(2.44132854173668,-29.2222036331016,
57.3038894216507));
#132322=CARTESIAN_POINT('Ctrl Pts',(2.55246381257524,-31.5137490421676,
56.903007487034));
#132323=CARTESIAN_POINT('Ctrl Pts',(2.6635990834138,-32.4198025966044,54.7603564081343));
#132324=CARTESIAN_POINT('Ctrl Pts',(2.77473435425236,-31.1110790022934,
52.8370443582928));
#132325=CARTESIAN_POINT('Ctrl Pts',(2.88586962509092,-28.7854160972553,
52.8934246747662));
#132326=CARTESIAN_POINT('Ctrl Pts',(2.99700489592947,-27.5714276225093,
54.8778940424664));
#132327=CARTESIAN_POINT('Ctrl Pts',(3.10814016676804,-28.5802430298865,
56.9741235532158));
#132328=CARTESIAN_POINT('Ctrl Pts',(3.2192754376066,-30.8885219962184,57.2634933885099));
#132329=CARTESIAN_POINT('Ctrl Pts',(3.33041070844515,-32.3835618098499,
55.481151489866));
#132330=CARTESIAN_POINT('Ctrl Pts',(3.44154597928371,-31.6969946459351,
53.2584251870102));
#132331=CARTESIAN_POINT('Ctrl Pts',(3.55268125012228,-29.4572160884115,
52.6297132488032));
#132332=CARTESIAN_POINT('Ctrl Pts',(3.66381652096083,-27.7142323544697,
54.1704580009286));
#132333=CARTESIAN_POINT('Ctrl Pts',(3.7749517917994,-28.063347354419,56.4704591758836));
#132334=CARTESIAN_POINT('Ctrl Pts',(3.88608706263795,-30.1850259636787,
57.4245904912667));
#132335=CARTESIAN_POINT('Ctrl Pts',(3.99722233347652,-32.1373555207256,
56.1595624328168));
#132336=CARTESIAN_POINT('Ctrl Pts',(4.10835760431506,-32.1334237808167,
53.833219545492));
#132337=CARTESIAN_POINT('Ctrl Pts',(4.21949287515364,-30.1768293547301,
52.5747979389581));
#132338=CARTESIAN_POINT('Ctrl Pts',(4.33062814599218,-28.0583880016956,
53.536095458844));
#132339=CARTESIAN_POINT('Ctrl Pts',(4.44176341683075,-27.7170494138102,
55.8372635657857));
#132340=CARTESIAN_POINT('Ctrl Pts',(4.5528986876693,-29.4652311847602,57.3721079174066));
#132341=CARTESIAN_POINT('Ctrl Pts',(4.66403395850787,-31.7028717873966,
56.735828716569));
#132342=CARTESIAN_POINT('Ctrl Pts',(4.77516922934643,-32.3819218144083,
54.5107943912606));
#132343=CARTESIAN_POINT('Ctrl Pts',(4.88630450018498,-30.8808659055018,
52.7335161782839));
#132344=CARTESIAN_POINT('Ctrl Pts',(4.99743977102355,-28.5735782480482,
53.0306867585031));
#132345=CARTESIAN_POINT('Ctrl Pts',(5.1085750418621,-27.5718542366147,55.1303142713972));
#132346=CARTESIAN_POINT('Ctrl Pts',(5.21971031270067,-28.7925436394291,
57.110668802748));
#132347=CARTESIAN_POINT('Ctrl Pts',(5.33084558353922,-31.1183838339782,
57.1591876383197));
#132348=CARTESIAN_POINT('Ctrl Pts',(5.44198085437779,-32.4205988111325,
55.2314628547315));
#132349=CARTESIAN_POINT('Ctrl Pts',(5.55311612521634,-31.5073078868314,
53.0918866407176));
#132350=CARTESIAN_POINT('Ctrl Pts',(5.66425139605491,-29.214420515888,52.6987528312416));
#132351=CARTESIAN_POINT('Ctrl Pts',(5.77538666689346,-27.6405519162949,
54.4118857271955));
#132352=CARTESIAN_POINT('Ctrl Pts',(5.88652193773202,-28.2262196800119,
56.6633030493568));
#132353=CARTESIAN_POINT('Ctrl Pts',(5.99765720857058,-30.4353786016796,
57.3923459471355));
#132354=CARTESIAN_POINT('Ctrl Pts',(6.10879247940914,-32.2460477542236,
55.9317419939679));
#132355=CARTESIAN_POINT('Ctrl Pts',(6.2199277502477,-32.0009726704464,53.6183408417034));
#132356=CARTESIAN_POINT('Ctrl Pts',(6.33106302108626,-29.9244636705494,
52.5695333944887));
#132357=CARTESIAN_POINT('Ctrl Pts',(6.44219829192482,-27.9170909450764,
53.7452635629374));
#132358=CARTESIAN_POINT('Ctrl Pts',(6.55333356276338,-27.816146200211,56.0694186452177));
#132359=CARTESIAN_POINT('Ctrl Pts',(6.66446883360194,-29.7140213172392,
57.4147649679738));
#132360=CARTESIAN_POINT('Ctrl Pts',(6.77560410444049,-31.873644666314,56.549944941593));
#132361=CARTESIAN_POINT('Ctrl Pts',(6.88673937527906,-32.3183738345439,
54.2665039734305));
#132362=CARTESIAN_POINT('Ctrl Pts',(6.99787464611762,-30.6411607425598,
52.6544112552431));
#132363=CARTESIAN_POINT('Ctrl Pts',(7.10900991695617,-28.3771112850928,
53.1891698377035));
#132364=CARTESIAN_POINT('Ctrl Pts',(7.22014518779474,-27.5984461499434,
55.3813302553558));
#132365=CARTESIAN_POINT('Ctrl Pts',(7.33128045863329,-29.0178556003855,
57.2244698320859));
#132366=CARTESIAN_POINT('Ctrl Pts',(7.44241572947186,-31.3361941509497,
57.0316148379476));
#132367=CARTESIAN_POINT('Ctrl Pts',(7.55355100031041,-32.4315518388499,
54.979280012635));
#132368=CARTESIAN_POINT('Ctrl Pts',(7.66468627114897,-31.3013786237181,
52.9459096127328));
#132369=CARTESIAN_POINT('Ctrl Pts',(7.77582154198753,-28.980090222924,52.7925902695143));
#132370=CARTESIAN_POINT('Ctrl Pts',(7.88695681282609,-27.5922964941576,
54.6596508863331));
#132371=CARTESIAN_POINT('Ctrl Pts',(7.99809208366465,-28.4082059872904,
56.8382234225286));
#132372=CARTESIAN_POINT('Ctrl Pts',(8.1092273545032,-30.6810396383511,57.3343219166659));
#132373=CARTESIAN_POINT('Ctrl Pts',(8.22036262534177,-32.3305370122343,
55.6938811771581));
#132374=CARTESIAN_POINT('Ctrl Pts',(8.33149789618033,-31.8469592774841,
53.4183508273375));
#132375=CARTESIAN_POINT('Ctrl Pts',(8.44263316701889,-29.6729122115943,
52.5904588459632));
#132376=CARTESIAN_POINT('Ctrl Pts',(8.55376843785744,-27.7982384620065,
53.9679531199155));
#132377=CARTESIAN_POINT('Ctrl Pts',(8.66490370869601,-27.938776850692,56.2900486171853));
#132378=CARTESIAN_POINT('Ctrl Pts',(8.77603897953457,-29.9658910971795,
57.4314033431097));
#132379=CARTESIAN_POINT('Ctrl Pts',(8.88717425037312,-32.0242314469952,
56.3473543879329));
#132380=CARTESIAN_POINT('Ctrl Pts',(8.99830952121169,-32.2298355320608,
54.0301271578697));
#132381=CARTESIAN_POINT('Ctrl Pts',(9.10944479205024,-30.3945622141122,
52.6005630380306));
#132382=CARTESIAN_POINT('Ctrl Pts',(9.22058006288882,-28.1981012227853,
53.3672037396045));
#132383=CARTESIAN_POINT('Ctrl Pts',(9.33171533372735,-27.6509784338276,
55.6281625130527));
#132384=CARTESIAN_POINT('Ctrl Pts',(9.44285060456594,-29.2536288124672,
57.3144481924582));
#132385=CARTESIAN_POINT('Ctrl Pts',(9.55398587540448,-31.5398481637865,
56.8818565205549));
#132386=CARTESIAN_POINT('Ctrl Pts',(9.66512114624305,-32.415821470149,54.7279021921883));
#132387=CARTESIAN_POINT('Ctrl Pts',(9.7762564170816,-31.082392665715,52.8209074744312));
#132388=CARTESIAN_POINT('Ctrl Pts',(9.88739168792017,-28.7546887640851,
52.9125899079599));
#132389=CARTESIAN_POINT('Ctrl Pts',(9.9614818684792,-27.9690890657423,54.2411437777897));
#132390=CARTESIAN_POINT('Ctrl Pts',(9.99852695875872,-27.944074491503,54.9247718070965));
#132391=CARTESIAN_POINT('',(10.0008699698353,-30.7705894968619,53.5212323702993));
#132392=CARTESIAN_POINT('Ctrl Pts',(10.,-27.9466241674713,54.9248651020699));
#132393=CARTESIAN_POINT('Ctrl Pts',(9.99999999999999,-27.9564039519262,
54.8501832546246));
#132394=CARTESIAN_POINT('Ctrl Pts',(9.99999999999998,-27.9706090922962,
54.7762523429086));
#132395=CARTESIAN_POINT('Ctrl Pts',(9.99999999999999,-27.9890023094346,
54.7033576472274));
#132396=CARTESIAN_POINT('Ctrl Pts',(10.,-28.0065895417162,54.633657173656));
#132397=CARTESIAN_POINT('Ctrl Pts',(10.,-28.0280067648394,54.5649035539299));
#132398=CARTESIAN_POINT('Ctrl Pts',(9.99999999999999,-28.0530852461662,
54.4973682348888));
#132399=CARTESIAN_POINT('Ctrl Pts',(9.99999999999999,-28.0587349917983,
54.4821537022067));
#132400=CARTESIAN_POINT('Ctrl Pts',(9.99999999999999,-28.0645714906859,
54.4669991037866));
#132401=CARTESIAN_POINT('Ctrl Pts',(10.,-28.0705904602987,54.451914165365));
#132402=CARTESIAN_POINT('Ctrl Pts',(10.,-28.0982103307347,54.3826923431025));
#132403=CARTESIAN_POINT('Ctrl Pts',(10.,-28.1296130964609,54.3150720673866));
#132404=CARTESIAN_POINT('Ctrl Pts',(10.,-28.1645888762895,54.249345890764));
#132405=CARTESIAN_POINT('Ctrl Pts',(10.,-28.1891445313107,54.2032011206712));
#132406=CARTESIAN_POINT('Ctrl Pts',(10.,-28.2154623661137,54.1579904820105));
#132407=CARTESIAN_POINT('Ctrl Pts',(10.,-28.2434807977927,54.113825883058));
#132408=CARTESIAN_POINT('Ctrl Pts',(10.,-28.2541311786634,54.0970380126577));
#132409=CARTESIAN_POINT('Ctrl Pts',(10.,-28.2650273632795,54.0804013902968));
#132410=CARTESIAN_POINT('Ctrl Pts',(10.,-28.2761662488052,54.0639225691025));
#132411=CARTESIAN_POINT('Ctrl Pts',(10.,-28.2867799276645,54.0482207364789));
#132412=CARTESIAN_POINT('Ctrl Pts',(10.,-28.2976175556647,54.032657412247));
#132413=CARTESIAN_POINT('Ctrl Pts',(10.,-28.3086567111279,54.0172654083652));
#132414=CARTESIAN_POINT('Ctrl Pts',(9.99999999999999,-28.3509657809783,
53.9582734529077));
#132415=CARTESIAN_POINT('Ctrl Pts',(10.,-28.3962731815781,53.9017302005496));
#132416=CARTESIAN_POINT('Ctrl Pts',(10.,-28.444386329927,53.8479078339097));
#132417=CARTESIAN_POINT('Ctrl Pts',(10.,-28.4913495953192,53.7953717980173));
#132418=CARTESIAN_POINT('Ctrl Pts',(10.,-28.5409868702555,53.74542762759));
#132419=CARTESIAN_POINT('Ctrl Pts',(10.,-28.5931475035754,53.6983678482907));
#132420=CARTESIAN_POINT('Ctrl Pts',(10.,-28.644420195856,53.6521091771583));
#132421=CARTESIAN_POINT('Ctrl Pts',(10.,-28.6981316928852,53.6086370584655));
#132422=CARTESIAN_POINT('Ctrl Pts',(10.,-28.7541565899177,53.5682751474532));
#132423=CARTESIAN_POINT('Ctrl Pts',(10.,-28.7723276241148,53.5551842235227));
#132424=CARTESIAN_POINT('Ctrl Pts',(10.,-28.7907421194074,53.5424208732304));
#132425=CARTESIAN_POINT('Ctrl Pts',(9.99999999999999,-28.8093960417122,
53.5299973248125));
#132426=CARTESIAN_POINT('Ctrl Pts',(9.99999999999998,-28.8198979217188,
53.5230030523689));
#132427=CARTESIAN_POINT('Ctrl Pts',(9.99999999999998,-28.8304768374501,
53.5161158780251));
#132428=CARTESIAN_POINT('Ctrl Pts',(9.99999999999999,-28.8411168980571,
53.5093473810421));
#132429=CARTESIAN_POINT('Ctrl Pts',(10.,-28.8987469337441,53.4726869956283));
#132430=CARTESIAN_POINT('Ctrl Pts',(10.,-28.9582678505386,53.439437211614));
#132431=CARTESIAN_POINT('Ctrl Pts',(10.,-29.0195356012334,53.4098650402476));
#132432=CARTESIAN_POINT('Ctrl Pts',(10.,-29.0283680962592,53.4056018503388));
#132433=CARTESIAN_POINT('Ctrl Pts',(9.99999999999997,-29.037236928022,53.4014151736005));
#132434=CARTESIAN_POINT('Ctrl Pts',(9.99999999999997,-29.0461416956092,
53.3973058954662));
#132435=CARTESIAN_POINT('Ctrl Pts',(9.99999999999997,-29.1094439341424,
53.3680938467391));
#132436=CARTESIAN_POINT('Ctrl Pts',(9.99999999999997,-29.1745617485033,
53.3427887894062));
#132437=CARTESIAN_POINT('Ctrl Pts',(9.99999999999996,-29.2411215698538,
53.3213755702336));
#132438=CARTESIAN_POINT('Ctrl Pts',(9.99999999999996,-29.3025810355913,
53.3016032063154));
#132439=CARTESIAN_POINT('Ctrl Pts',(9.99999999999997,-29.3652708265432,
53.2851497565554));
#132440=CARTESIAN_POINT('Ctrl Pts',(9.99999999999996,-29.4288933318821,
53.2720425880717));
#132441=CARTESIAN_POINT('Ctrl Pts',(9.99999999999995,-29.4429446720262,
53.2691478060805));
#132442=CARTESIAN_POINT('Ctrl Pts',(9.99999999999999,-29.4570414665537,
53.266416387187));
#132443=CARTESIAN_POINT('Ctrl Pts',(9.99999999999999,-29.4711804257353,
53.2638488655497));
#132444=CARTESIAN_POINT('Ctrl Pts',(9.99999999999998,-29.4823151499984,
53.2618268888891));
#132445=CARTESIAN_POINT('Ctrl Pts',(9.99999999999999,-29.4934754862078,
53.2599067415914));
#132446=CARTESIAN_POINT('Ctrl Pts',(9.99999999999998,-29.5046466791603,
53.2580905770623));
#132447=CARTESIAN_POINT('Ctrl Pts',(9.99999999999998,-29.5721359464321,
53.2471184621026));
#132448=CARTESIAN_POINT('Ctrl Pts',(9.99999999999995,-29.6401457101856,
53.2399139604603));
#132449=CARTESIAN_POINT('Ctrl Pts',(9.99999999999996,-29.7083244050125,
53.2364442314095));
#132450=CARTESIAN_POINT('Ctrl Pts',(9.99999999999996,-29.7757601728194,
53.2330123111708));
#132451=CARTESIAN_POINT('Ctrl Pts',(9.99999999999997,-29.8433622859179,
53.23323450567));
#132452=CARTESIAN_POINT('Ctrl Pts',(9.99999999999997,-29.91078197846,53.2371283063634));
#132453=CARTESIAN_POINT('Ctrl Pts',(9.99999999999997,-29.977606070675,53.2409877083688));
#132454=CARTESIAN_POINT('Ctrl Pts',(9.99999999999998,-30.044251924723,53.2484543816368));
#132455=CARTESIAN_POINT('Ctrl Pts',(9.99999999999999,-30.1103563112186,
53.2595900434352));
#132456=CARTESIAN_POINT('Ctrl Pts',(9.99999999999999,-30.1294385130765,
53.2628045494237));
#132457=CARTESIAN_POINT('Ctrl Pts',(9.99999999999997,-30.1484753926267,
53.26632506233));
#132458=CARTESIAN_POINT('Ctrl Pts',(9.99999999999998,-30.1674576666939,
53.2701537231559));
#132459=CARTESIAN_POINT('Ctrl Pts',(9.99999999999998,-30.1780436988077,
53.2722888902235));
#132460=CARTESIAN_POINT('Ctrl Pts',(9.99999999999996,-30.1886032905924,
53.2745179938254));
#132461=CARTESIAN_POINT('Ctrl Pts',(9.99999999999996,-30.1991346915138,
53.2768408806036));
#132462=CARTESIAN_POINT('Ctrl Pts',(9.99999999999999,-30.2629071303035,
53.2909070201399));
#132463=CARTESIAN_POINT('Ctrl Pts',(9.99999999999999,-30.3256519182632,
53.3084091752865));
#132464=CARTESIAN_POINT('Ctrl Pts',(9.99999999999999,-30.3870487756711,
53.3293566078869));
#132465=CARTESIAN_POINT('Ctrl Pts',(9.99999999999999,-30.4475549976041,
53.3500001727101));
#132466=CARTESIAN_POINT('Ctrl Pts',(9.99999999999998,-30.5067529547149,
53.3739900996769));
#132467=CARTESIAN_POINT('Ctrl Pts',(9.99999999999999,-30.5643079758142,
53.4013774025353));
#132468=CARTESIAN_POINT('Ctrl Pts',(10.,-30.6218629969135,53.4287647053938));
#132469=CARTESIAN_POINT('Ctrl Pts',(9.99999999999999,-30.6777759450102,
53.4595495876129));
#132470=CARTESIAN_POINT('Ctrl Pts',(10.,-30.7316710181693,53.4938218163979));
#132471=CARTESIAN_POINT('Ctrl Pts',(10.,-30.7357940686267,53.4964436910942));
#132472=CARTESIAN_POINT('Ctrl Pts',(10.,-30.7399052858608,53.4990859932845));
#132473=CARTESIAN_POINT('Ctrl Pts',(10.,-30.7440044894661,53.5017487719653));
#132474=CARTESIAN_POINT('Ctrl Pts',(10.,-30.753120839882,53.5076706109057));
#132475=CARTESIAN_POINT('Ctrl Pts',(9.99999999999998,-30.762177774796,53.5136937234875));
#132476=CARTESIAN_POINT('Ctrl Pts',(9.99999999999999,-30.7711742170104,
53.5198167964781));
#132477=CARTESIAN_POINT('Ctrl Pts',(-2.78423117894278E-16,-31.2690708798524,
56.0793586530485));
#132478=CARTESIAN_POINT('Ctrl Pts',(-2.57282377653238E-14,-31.3146241118499,
56.0368623223042));
#132479=CARTESIAN_POINT('Ctrl Pts',(-2.2197106541116E-14,-31.3574205812789,
55.9917717560589));
#132480=CARTESIAN_POINT('Ctrl Pts',(-2.5278390491934E-14,-31.3974616756518,
55.9444369337232));
#132481=CARTESIAN_POINT('Ctrl Pts',(-2.84724648645398E-14,-31.4389684745802,
55.8953694198661));
#132482=CARTESIAN_POINT('Ctrl Pts',(-7.29811795260109E-15,-31.4775150387688,
55.8438898979911));
#132483=CARTESIAN_POINT('Ctrl Pts',(-8.77076189453874E-15,-31.5130762861459,
55.7903375833125));
#132484=CARTESIAN_POINT('Ctrl Pts',(-1.01167848752535E-14,-31.5455799041824,
55.7413898070204));
#132485=CARTESIAN_POINT('Ctrl Pts',(-3.36001753813602E-15,-31.5755894343036,
55.6907093117701));
#132486=CARTESIAN_POINT('Ctrl Pts',(-6.01602101468757E-15,-31.6030614619887,
55.6385258325769));
#132487=CARTESIAN_POINT('Ctrl Pts',(-7.67020104658086E-15,-31.6165640542223,
55.6128774804074));
#132488=CARTESIAN_POINT('Ctrl Pts',(-1.92883565851348E-14,-31.6294532670974,
55.5868656683753));
#132489=CARTESIAN_POINT('Ctrl Pts',(-6.94583279781114E-15,-31.6417215732041,
55.5605158025313));
#132490=CARTESIAN_POINT('Ctrl Pts',(-1.26737980692756E-15,-31.6473278423374,
55.5484746586063));
#132491=CARTESIAN_POINT('Ctrl Pts',(-1.47443749393244E-14,-31.6528050246646,
55.5363612489351));
#132492=CARTESIAN_POINT('Ctrl Pts',(-1.35724764760425E-14,-31.6581439011687,
55.524197929143));
#132493=CARTESIAN_POINT('Ctrl Pts',(-6.89730998572226E-15,-31.6850933570533,
55.4628002081252));
#132494=CARTESIAN_POINT('Ctrl Pts',(-6.57763955012823E-15,-31.7085741592776,
55.4000241140312));
#132495=CARTESIAN_POINT('Ctrl Pts',(-5.54417622922188E-15,-31.7285626394371,
55.3362284938232));
#132496=CARTESIAN_POINT('Ctrl Pts',(-4.49070260999537E-15,-31.7489381439281,
55.2711976392667));
#132497=CARTESIAN_POINT('Ctrl Pts',(-3.16205974643209E-14,-31.7656853518822,
55.2051065542478));
#132498=CARTESIAN_POINT('Ctrl Pts',(-2.57155408078802E-14,-31.7787394756354,
55.1382984849778));
#132499=CARTESIAN_POINT('Ctrl Pts',(-2.08116559556361E-14,-31.7895803402464,
55.0828173781973));
#132500=CARTESIAN_POINT('Ctrl Pts',(-1.68020975472041E-14,-31.7978736664125,
55.0268408524174));
#132501=CARTESIAN_POINT('Ctrl Pts',(-1.25038868148408E-14,-31.8035578588702,
54.9705533929035));
#132502=CARTESIAN_POINT('Ctrl Pts',(-1.02026785998301E-14,-31.8061882803694,
54.9445057626131));
#132503=CARTESIAN_POINT('Ctrl Pts',(-9.94370814337888E-15,-31.808259630761,
54.9183914347958));
#132504=CARTESIAN_POINT('Ctrl Pts',(-2.18020046460765E-14,-31.8097640080344,
54.8922282921563));
#132505=CARTESIAN_POINT('Ctrl Pts',(-2.8149256454812E-14,-31.8105739898639,
54.8781416195417));
#132506=CARTESIAN_POINT('Ctrl Pts',(-2.39741397133629E-14,-31.8112192935178,
54.8640433553622));
#132507=CARTESIAN_POINT('Ctrl Pts',(-1.78329573330416E-14,-31.811698521278,
54.8499553064024));
#132508=CARTESIAN_POINT('Ctrl Pts',(1.15714359936816E-14,-31.8139930959514,
54.7825007826369));
#132509=CARTESIAN_POINT('Ctrl Pts',(-9.17816564628055E-15,-31.812490761091,
54.7151643158931));
#132510=CARTESIAN_POINT('Ctrl Pts',(-6.80011602582908E-16,-31.8071420452598,
54.6482666402681));
#132511=CARTESIAN_POINT('Ctrl Pts',(7.39918467707698E-15,-31.8021719907044,
54.5861049723127));
#132512=CARTESIAN_POINT('Ctrl Pts',(1.51061130160261E-14,-31.7938807595678,
54.5243213359004));
#132513=CARTESIAN_POINT('Ctrl Pts',(1.60982338570648E-14,-31.7821961531115,
54.4631612860264));
#132514=CARTESIAN_POINT('Ctrl Pts',(1.69344470150937E-14,-31.7694646642199,
54.3965216008566));
#132515=CARTESIAN_POINT('Ctrl Pts',(1.19364270054881E-14,-31.7527055889607,
54.3306214152988));
#132516=CARTESIAN_POINT('Ctrl Pts',(4.9960036108132E-16,-31.7321642059902,
54.2656743472661));
#132517=CARTESIAN_POINT('Ctrl Pts',(-4.13176169865794E-15,-31.7242361536314,
54.240607692472));
#132518=CARTESIAN_POINT('Ctrl Pts',(-1.3612586526406E-14,-31.7157441295239,
54.2156830625258));
#132519=CARTESIAN_POINT('Ctrl Pts',(-1.49880108324396E-15,-31.7067002269016,
54.1909130590085));
#132520=CARTESIAN_POINT('Ctrl Pts',(3.98752837147791E-15,-31.702733264022,
54.1800480941163));
#132521=CARTESIAN_POINT('Ctrl Pts',(-1.32089167663491E-14,-31.6986602242431,
54.1692134541154));
#132522=CARTESIAN_POINT('Ctrl Pts',(-1.05193631583234E-14,-31.6944872093316,
54.1584227272008));
#132523=CARTESIAN_POINT('Ctrl Pts',(4.54181674810102E-15,-31.6694832150762,
54.0937665302998));
#132524=CARTESIAN_POINT('Ctrl Pts',(-2.05732350039661E-14,-31.640852147275,
54.0305697527002));
#132525=CARTESIAN_POINT('Ctrl Pts',(-4.52415882534751E-15,-31.6088988590651,
53.9690455844801));
#132526=CARTESIAN_POINT('Ctrl Pts',(1.20570199622642E-14,-31.5758861685673,
53.9054815997583));
#132527=CARTESIAN_POINT('Ctrl Pts',(-1.76645667684946E-14,-31.5393271021827,
53.8437021556787));
#132528=CARTESIAN_POINT('Ctrl Pts',(-8.93729534823251E-15,-31.4995017172175,
53.7839459944069));
#132529=CARTESIAN_POINT('Ctrl Pts',(-2.19864240011066E-15,-31.4687510467178,
53.7378060254599));
#132530=CARTESIAN_POINT('Ctrl Pts',(-1.86107330608832E-14,-31.4360517893389,
53.6928722834116));
#132531=CARTESIAN_POINT('Ctrl Pts',(-1.52100554373646E-14,-31.4015126326392,
53.6492609538454));
#132532=CARTESIAN_POINT('Ctrl Pts',(-1.30940809355439E-14,-31.3802217602078,
53.6223777481425));
#132533=CARTESIAN_POINT('Ctrl Pts',(-5.96119017066866E-15,-31.3582314248551,
53.595997163054));
#132534=CARTESIAN_POINT('Ctrl Pts',(-1.52655665885959E-14,-31.3355641610242,
53.570148108709));
#132535=CARTESIAN_POINT('Ctrl Pts',(-2.03883579394625E-14,-31.3228721183306,
53.555674491435));
#132536=CARTESIAN_POINT('Ctrl Pts',(1.45111025983856E-14,-31.3099633641148,
53.5413629717455));
#132537=CARTESIAN_POINT('Ctrl Pts',(1.47937218031302E-14,-31.2968655882308,
53.5272440845563));
#132538=CARTESIAN_POINT('Ctrl Pts',(1.63603910997093E-14,-31.2460184014874,
53.4724328173702));
#132539=CARTESIAN_POINT('Ctrl Pts',(-5.80558094253327E-15,-31.1922776399754,
53.4204635517656));
#132540=CARTESIAN_POINT('Ctrl Pts',(-2.99760216648792E-15,-31.1359279003417,
53.3715998536437));
#132541=CARTESIAN_POINT('Ctrl Pts',(-8.95100641520165E-16,-31.0937354826062,
53.335012682582));
#132542=CARTESIAN_POINT('Ctrl Pts',(-2.28577618870274E-15,-31.0500792097546,
53.3001668168172));
#132543=CARTESIAN_POINT('Ctrl Pts',(-1.52655665885959E-15,-31.0050621224658,
53.2671826644093));
#132544=CARTESIAN_POINT('Ctrl Pts',(-1.22529459397018E-15,-30.9910114153834,
53.2568876699582));
#132545=CARTESIAN_POINT('Ctrl Pts',(5.50416399254457E-15,-30.9768280471771,
53.2467741178013));
#132546=CARTESIAN_POINT('Ctrl Pts',(1.66533453693773E-15,-30.962514910112,
53.2368458953558));
#132547=CARTESIAN_POINT('Ctrl Pts',(-2.32875220709882E-15,-30.9487200109087,
53.2272771455227));
#132548=CARTESIAN_POINT('Ctrl Pts',(2.32032892379646E-14,-30.9348115999123,
53.2178854875332));
#132549=CARTESIAN_POINT('Ctrl Pts',(1.97897254139434E-14,-30.9207976678547,
53.2086771606816));
#132550=CARTESIAN_POINT('Ctrl Pts',(4.17236467677409E-15,-30.8578426129519,
53.1673104179198));
#132551=CARTESIAN_POINT('Ctrl Pts',(1.73679733454129E-14,-30.7927302716737,
53.129619436727));
#132552=CARTESIAN_POINT('Ctrl Pts',(1.97064586870965E-15,-30.7257220056234,
53.0958834398336));
#132553=CARTESIAN_POINT('Ctrl Pts',(-9.63241745287261E-15,-30.6744687584743,
53.070079468346));
#132554=CARTESIAN_POINT('Ctrl Pts',(-1.67306283423615E-14,-30.622105344157,
53.0465897299349));
#132555=CARTESIAN_POINT('Ctrl Pts',(-1.8623991238087E-14,-30.5687348286521,
53.0255544534855));
#132556=CARTESIAN_POINT('Ctrl Pts',(-1.893565290737E-14,-30.556454937019,
53.0207144980752));
#132557=CARTESIAN_POINT('Ctrl Pts',(-1.99912525927446E-14,-30.5441216860115,
53.0160045481786));
#132558=CARTESIAN_POINT('Ctrl Pts',(5.27355936696949E-16,-30.5317369366261,
53.0114240379353));
#132559=CARTESIAN_POINT('Ctrl Pts',(10.,-30.7922981853442,53.5344558739157));
#132560=CARTESIAN_POINT('Ctrl Pts',(10.0002899899451,-30.7848609529314,
53.530435179049));
#132561=CARTESIAN_POINT('Ctrl Pts',(10.0005799798902,-30.777393114057,53.5264710981355));
#132562=CARTESIAN_POINT('Ctrl Pts',(10.0008699698353,-30.7698955341219,
53.5225640905477));
#132563=CARTESIAN_POINT('Ctrl Pts',(0.00154683520447944,-29.4691384916359,
53.0122371971775));
#132564=CARTESIAN_POINT('Ctrl Pts',(0.0385919254839992,-28.8081756493506,
53.1887571174265));
#132565=CARTESIAN_POINT('Ctrl Pts',(0.112682106043039,-27.6876746937628,
54.2503605089641));
#132566=CARTESIAN_POINT('Ctrl Pts',(0.223817376881599,-28.1162794172484,
56.540242738843));
#132567=CARTESIAN_POINT('Ctrl Pts',(0.334952647720158,-30.2723120807304,
57.4159505201799));
#132568=CARTESIAN_POINT('Ctrl Pts',(0.446087918558717,-32.1774584443673,
56.082555317456));
#132569=CARTESIAN_POINT('Ctrl Pts',(0.557223189397277,-32.0904669771016,
53.7572516909355));
#132570=CARTESIAN_POINT('Ctrl Pts',(0.668358460235836,-30.0897123148979,
52.5699426008396));
#132571=CARTESIAN_POINT('Ctrl Pts',(0.779493731074396,-28.0070571020679,
53.6065233138136));
#132572=CARTESIAN_POINT('Ctrl Pts',(0.890629001912955,-27.7483801793046,
55.9186517854682));
#132573=CARTESIAN_POINT('Ctrl Pts',(1.00176427275152,-29.5506010031038,
57.3898946665584));
#132574=CARTESIAN_POINT('Ctrl Pts',(1.11289954359007,-31.7641170624246,
56.673769327145));
#132575=CARTESIAN_POINT('Ctrl Pts',(1.22403481442863,-32.363000089887,54.4256724031027));
#132576=CARTESIAN_POINT('Ctrl Pts',(1.33517008526719,-30.7990888352776,
52.7032502602688));
#132577=CARTESIAN_POINT('Ctrl Pts',(1.44630535610575,-28.503797543915,53.082973959131));
#132578=CARTESIAN_POINT('Ctrl Pts',(1.55744062694431,-27.5779364648995,
55.2172998549449));
#132579=CARTESIAN_POINT('Ctrl Pts',(1.66857589778287,-28.8689227885836,
57.1527361723464));
#132580=CARTESIAN_POINT('Ctrl Pts',(1.77971116862143,-31.195151776353,57.1178342918897));
#132581=CARTESIAN_POINT('Ctrl Pts',(1.89084643945999,-32.4274922356383,
55.1445380547168));
#132582=CARTESIAN_POINT('Ctrl Pts',(2.00198171029855,-31.4380173232809,
53.0389503543588));
#132583=CARTESIAN_POINT('Ctrl Pts',(2.11311698113711,-29.1323657220718,
52.7282560762878));
#132584=CARTESIAN_POINT('Ctrl Pts',(2.22425225197567,-27.6208353047203,
54.4968250518511));
#132585=CARTESIAN_POINT('Ctrl Pts',(2.33538752281423,-28.2868873243009,
56.725935863788));
#132586=CARTESIAN_POINT('Ctrl Pts',(2.44652279365279,-30.5209031087717,
57.3753462101905));
#132587=CARTESIAN_POINT('Ctrl Pts',(2.55765806449135,-32.2781509557601,
55.850669081196));
#132588=CARTESIAN_POINT('Ctrl Pts',(2.66879333532991,-31.9502714085785,
53.5473985086807));
#132589=CARTESIAN_POINT('Ctrl Pts',(2.77992860616847,-29.8373633829036,
52.573653158907));
#132590=CARTESIAN_POINT('Ctrl Pts',(2.89106387700702,-27.8733120707697,
53.8206747210973));
#132591=CARTESIAN_POINT('Ctrl Pts',(3.00219914784558,-27.8557583098495,
56.1470994881393));
#132592=CARTESIAN_POINT('Ctrl Pts',(3.11333441868415,-29.8007685626502,
57.4236164086336));
#132593=CARTESIAN_POINT('Ctrl Pts',(3.2244696895227,-31.9281297375949,56.4818655056094));
#132594=CARTESIAN_POINT('Ctrl Pts',(3.33560496036126,-32.2907280807803,
54.1838048507812));
#132595=CARTESIAN_POINT('Ctrl Pts',(3.44674023119983,-30.5566875434458,
52.6327846230853));
#132596=CARTESIAN_POINT('Ctrl Pts',(3.55787550203837,-28.3131265799599,
53.2484099433732));
#132597=CARTESIAN_POINT('Ctrl Pts',(3.66901077287695,-27.613513337149,55.4672162986708));
#132598=CARTESIAN_POINT('Ctrl Pts',(3.7801460437155,-29.0981841074383,57.2583927376871));
#132599=CARTESIAN_POINT('Ctrl Pts',(3.89128131455406,-31.4082615592521,
56.9825259247851));
#132600=CARTESIAN_POINT('Ctrl Pts',(4.00241658539262,-32.4293968778352,
54.8921089824078));
#132601=CARTESIAN_POINT('Ctrl Pts',(4.11355185623118,-31.2269736723593,
52.9004416490485));
#132602=CARTESIAN_POINT('Ctrl Pts',(4.22468712706974,-28.9015360294886,
52.83044092793));
#132603=CARTESIAN_POINT('Ctrl Pts',(4.3358223979083,-27.5814915141413,54.7461765071108));
#132604=CARTESIAN_POINT('Ctrl Pts',(4.44695766874686,-28.4750396844126,
56.8942295789044));
#132605=CARTESIAN_POINT('Ctrl Pts',(4.55809293958541,-30.7643410720823,
57.3085476792218));
#132606=CARTESIAN_POINT('Ctrl Pts',(4.66922821042398,-32.3540626086281,
55.609917122544));
#132607=CARTESIAN_POINT('Ctrl Pts',(4.78036348126253,-31.789176955488,53.3530466054973));
#132608=CARTESIAN_POINT('Ctrl Pts',(4.8914987521011,-29.586708037661,52.6035861343293));
#132609=CARTESIAN_POINT('Ctrl Pts',(5.00263402293966,-27.7625136101689,
54.0474957653462));
#132610=CARTESIAN_POINT('Ctrl Pts',(5.11376929377821,-27.9862274433511,
56.363205689469));
#132611=CARTESIAN_POINT('Ctrl Pts',(5.22490456461678,-30.0530905679093,
57.4312118487108));
#132612=CARTESIAN_POINT('Ctrl Pts',(5.33603983545533,-32.0713613912677,
56.2739982921804));
#132613=CARTESIAN_POINT('Ctrl Pts',(5.44717510629389,-32.193773485251,53.9507299884574));
#132614=CARTESIAN_POINT('Ctrl Pts',(5.55831037713245,-30.3082865086915,
52.5878289674504));
#132615=CARTESIAN_POINT('Ctrl Pts',(5.66944564797101,-28.1406335754259,
53.4327201395797));
#132616=CARTESIAN_POINT('Ctrl Pts',(5.78058091880957,-27.6748063506032,
55.7120984163146));
#132617=CARTESIAN_POINT('Ctrl Pts',(5.89171618964813,-29.3371633703456,
57.3397130730287));
#132618=CARTESIAN_POINT('Ctrl Pts',(6.00285146048669,-31.6061960845262,
56.8258542657522));
#132619=CARTESIAN_POINT('Ctrl Pts',(6.11398673132524,-32.405122770481,54.6408424849358));
#132620=CARTESIAN_POINT('Ctrl Pts',(6.22512200216382,-31.002708339015,52.7845574598779));
#132621=CARTESIAN_POINT('Ctrl Pts',(6.33625727300236,-28.6825432120152,
52.9560045808502));
#132622=CARTESIAN_POINT('Ctrl Pts',(6.44739254384094,-27.5682091691533,
54.9982631278413));
#132623=CARTESIAN_POINT('Ctrl Pts',(6.55852781467948,-28.6796247681038,
57.0421113849897));
#132624=CARTESIAN_POINT('Ctrl Pts',(6.66966308551805,-30.9995426206869,
57.216872619512));
#132625=CARTESIAN_POINT('Ctrl Pts',(6.78079835635661,-32.4046072705466,
55.3625927966234));
#132626=CARTESIAN_POINT('Ctrl Pts',(6.89193362719516,-31.6088026255414,
53.1764420015434));
#132627=CARTESIAN_POINT('Ctrl Pts',(7.00306889803373,-29.3405062587718,
52.6593424712286));
#132628=CARTESIAN_POINT('Ctrl Pts',(7.11420416887228,-27.675825934788,54.2845808386533));
#132629=CARTESIAN_POINT('Ctrl Pts',(7.22533943971084,-28.1383966587829,
56.5646222104514));
#132630=CARTESIAN_POINT('Ctrl Pts',(7.3364747105494,-30.3048404778189,57.4126089498457));
#132631=CARTESIAN_POINT('Ctrl Pts',(7.44760998138796,-32.1922723955041,
56.0524026826328));
#132632=CARTESIAN_POINT('Ctrl Pts',(7.55874525222652,-32.0731791470605,
53.728961887316));
#132633=CARTESIAN_POINT('Ctrl Pts',(7.66988052306508,-30.0565634300485,
52.5688664698714));
#132634=CARTESIAN_POINT('Ctrl Pts',(7.78101579390364,-27.988176796027,53.6339190862362));
#132635=CARTESIAN_POINT('Ctrl Pts',(7.8921510647422,-27.7611552715967,55.9493070776374));
#132636=CARTESIAN_POINT('Ctrl Pts',(8.00328633558076,-29.5832852453598,
57.395821046943));
#132637=CARTESIAN_POINT('Ctrl Pts',(8.11442160641932,-31.7868225176538,
56.6495074978805));
#132638=CARTESIAN_POINT('Ctrl Pts',(8.22555687725788,-32.3549314306192,
54.3934462168881));
#132639=CARTESIAN_POINT('Ctrl Pts',(8.33669214809644,-30.7676380353678,
52.6925465010098));
#132640=CARTESIAN_POINT('Ctrl Pts',(8.447827418935,-28.4777469933738,53.1035940201946));
#132641=CARTESIAN_POINT('Ctrl Pts',(8.55896268977356,-27.581131598138,55.2503684093247));
#132642=CARTESIAN_POINT('Ctrl Pts',(8.67009796061211,-28.8984376095163,
57.1679878447293));
#132643=CARTESIAN_POINT('Ctrl Pts',(8.78123323145067,-31.2239740330287,
57.1013086868512));
#132644=CARTESIAN_POINT('Ctrl Pts',(8.89236850228924,-32.4292387518736,
55.1113616631365));
#132645=CARTESIAN_POINT('Ctrl Pts',(9.00350377312779,-31.4110951335146,
53.0194869004384));
#132646=CARTESIAN_POINT('Ctrl Pts',(9.11463904396635,-29.1014050665648,
52.740323050515));
#132647=CARTESIAN_POINT('Ctrl Pts',(9.22577431480492,-27.6141950937383,
54.5293717763318));
#132648=CARTESIAN_POINT('Ctrl Pts',(9.33690958564347,-28.3106025739419,
56.749185312287));
#132649=CARTESIAN_POINT('Ctrl Pts',(9.44804485648204,-30.5533523395227,
57.367994902382));
#132650=CARTESIAN_POINT('Ctrl Pts',(9.55918012732059,-32.2894669018336,
55.8194928724932));
#132651=CARTESIAN_POINT('Ctrl Pts',(9.67031539815916,-31.9304288651689,
53.5208380958941));
#132652=CARTESIAN_POINT('Ctrl Pts',(9.78145066899771,-29.8038652797079,
52.5762049459999));
#132653=CARTESIAN_POINT('Ctrl Pts',(9.89258593983627,-27.8581251142671,
53.8496336413402));
#132654=CARTESIAN_POINT('Ctrl Pts',(10.0037212106749,-27.8701762214051,
56.1766909537225));
#132655=CARTESIAN_POINT('Ctrl Pts',(10.1148694181389,-29.837170584603,57.4254741206559));
#132656=CARTESIAN_POINT('Ctrl Pts',(10.1889725353234,-31.2393300826299,
56.7791900932959));
#132657=CARTESIAN_POINT('Ctrl Pts',(10.2260305622284,-31.6487083722557,
56.2307621881824));
#132658=CARTESIAN_POINT('Ctrl Pts',(-0.0743643433070923,-29.503063713713,
53.1392671163936));
#132659=CARTESIAN_POINT('Ctrl Pts',(-0.0373192530275725,-28.8843403460478,
53.3045063591003));
#132660=CARTESIAN_POINT('Ctrl Pts',(0.0367709275314672,-27.8354460960829,
54.298266951248));
#132661=CARTESIAN_POINT('Ctrl Pts',(0.147906198370027,-28.23666041699,56.441812025475));
#132662=CARTESIAN_POINT('Ctrl Pts',(0.259041469208586,-30.2549097118121,
57.2615568475682));
#132663=CARTESIAN_POINT('Ctrl Pts',(0.370176740047145,-32.0383058402982,
56.0133735648203));
#132664=CARTESIAN_POINT('Ctrl Pts',(0.481312010885705,-31.9568736475312,
53.8366707328262));
#132665=CARTESIAN_POINT('Ctrl Pts',(0.592447281724263,-30.0839791619795,
52.7252377873014));
#132666=CARTESIAN_POINT('Ctrl Pts',(0.703582552562825,-28.1344180603106,
53.6955747995465));
#132667=CARTESIAN_POINT('Ctrl Pts',(0.814717823401383,-27.8922721384068,
55.8599444477868));
#132668=CARTESIAN_POINT('Ctrl Pts',(0.925853094239943,-29.579320283991,
57.2371661186667));
#132669=CARTESIAN_POINT('Ctrl Pts',(1.0369883650785,-31.6513794422169,56.5668054670145));
#132670=CARTESIAN_POINT('Ctrl Pts',(1.14812363591707,-32.2119902661294,
54.4623753679303));
#132671=CARTESIAN_POINT('Ctrl Pts',(1.25925890675562,-30.7480222844559,
52.8500262908311));
#132672=CARTESIAN_POINT('Ctrl Pts',(1.37039417759418,-28.5994138200912,
53.2054833766335));
#132673=CARTESIAN_POINT('Ctrl Pts',(1.48152944843274,-27.7327207956875,
55.2034130959311));
#132674=CARTESIAN_POINT('Ctrl Pts',(1.5926647192713,-28.941205380143,57.0151634691656));
#132675=CARTESIAN_POINT('Ctrl Pts',(1.70379999010986,-31.1187744372733,
56.9824920273952));
#132676=CARTESIAN_POINT('Ctrl Pts',(1.81493526094842,-32.2723609784515,
55.1353012094613));
#132677=CARTESIAN_POINT('Ctrl Pts',(1.92607053178698,-31.3461194247246,
53.1642731432303));
#132678=CARTESIAN_POINT('Ctrl Pts',(2.03720580262554,-29.1878127362114,
52.8734340858064));
#132679=CARTESIAN_POINT('Ctrl Pts',(2.1483410734641,-27.7728781433397,54.528980937314));
#132680=CARTESIAN_POINT('Ctrl Pts',(2.25947634430266,-28.3963654594653,
56.6156382502912));
#132681=CARTESIAN_POINT('Ctrl Pts',(2.37061161514122,-30.4876142879261,
57.2235473955822));
#132682=CARTESIAN_POINT('Ctrl Pts',(2.48174688597978,-32.1325634986141,
55.796306244488));
#132683=CARTESIAN_POINT('Ctrl Pts',(2.59288215681834,-31.8256374134512,
53.6402284227095));
#132684=CARTESIAN_POINT('Ctrl Pts',(2.7040174276569,-29.8477568344271,52.7287112185391));
#132685=CARTESIAN_POINT('Ctrl Pts',(2.81515269849545,-28.0092201355873,
53.8960406524328));
#132686=CARTESIAN_POINT('Ctrl Pts',(2.92628796933401,-27.9927881648669,
56.0737929773703));
#132687=CARTESIAN_POINT('Ctrl Pts',(3.03742324017257,-29.8135006418279,
57.2687328399489));
#132688=CARTESIAN_POINT('Ctrl Pts',(3.14855851101114,-31.8049107275313,
56.3871654462264));
#132689=CARTESIAN_POINT('Ctrl Pts',(3.25969378184969,-32.144336870202,54.2359645972673));
#132690=CARTESIAN_POINT('Ctrl Pts',(3.37082905268826,-30.5211118834263,
52.7840638288688));
#132691=CARTESIAN_POINT('Ctrl Pts',(3.48196432352681,-28.4209278699183,
53.3603470130664));
#132692=CARTESIAN_POINT('Ctrl Pts',(3.59309959436537,-27.7660240932422,
55.4373583857486));
#132693=CARTESIAN_POINT('Ctrl Pts',(3.70423486520393,-29.1558155309749,
57.1140679487238));
#132694=CARTESIAN_POINT('Ctrl Pts',(3.81537013604249,-31.3182652317965,
56.8558306733639));
#132695=CARTESIAN_POINT('Ctrl Pts',(3.92650540688105,-32.2741439026325,
54.8990038630393));
#132696=CARTESIAN_POINT('Ctrl Pts',(4.03764067771961,-31.1485627240013,
53.0346159717254));
#132697=CARTESIAN_POINT('Ctrl Pts',(4.14877594855817,-28.9717344401026,
52.9690887149137));
#132698=CARTESIAN_POINT('Ctrl Pts',(4.25991121939673,-27.7360486560428,
54.7623973448038));
#132699=CARTESIAN_POINT('Ctrl Pts',(4.37104649023528,-28.5724937596281,
56.7731769915215));
#132700=CARTESIAN_POINT('Ctrl Pts',(4.48218176107385,-30.7154951109333,
57.161017689838));
#132701=CARTESIAN_POINT('Ctrl Pts',(4.5933170319124,-32.2036239433209,55.5709397743939));
#132702=CARTESIAN_POINT('Ctrl Pts',(4.70445230275097,-31.6748378583903,
53.4582967673173));
#132703=CARTESIAN_POINT('Ctrl Pts',(4.81558757358953,-29.6131198633146,
52.7567312979939));
#132704=CARTESIAN_POINT('Ctrl Pts',(4.92672284442808,-27.905502358597,54.1083664767859));
#132705=CARTESIAN_POINT('Ctrl Pts',(5.03785811526665,-28.1149195412349,
56.2760887012839));
#132706=CARTESIAN_POINT('Ctrl Pts',(5.14899338610521,-30.0496977634243,
57.2758428860254));
#132707=CARTESIAN_POINT('Ctrl Pts',(5.26012865694376,-31.9389890227805,
56.1925821896618));
#132708=CARTESIAN_POINT('Ctrl Pts',(5.37126392778233,-32.0535782525933,
54.0177846111785));
#132709=CARTESIAN_POINT('Ctrl Pts',(5.48239919862088,-30.2885851588932,
52.7419811082214));
#132710=CARTESIAN_POINT('Ctrl Pts',(5.59353446945944,-28.2594581989532,
53.5328786865529));
#132711=CARTESIAN_POINT('Ctrl Pts',(5.704669740298,-27.8234001169346,55.6665910729988));
#132712=CARTESIAN_POINT('Ctrl Pts',(5.81580501113656,-29.3795225911736,
57.1901914287792));
#132713=CARTESIAN_POINT('Ctrl Pts',(5.92694028197513,-31.5035505583231,
56.709171269396));
#132714=CARTESIAN_POINT('Ctrl Pts',(6.03807555281367,-32.2514210557666,
54.6637947959758));
#132715=CARTESIAN_POINT('Ctrl Pts',(6.14921082365225,-30.9386292853566,
52.9261374746062));
#132716=CARTESIAN_POINT('Ctrl Pts',(6.26034609449079,-28.7667365720634,
53.0866281002179));
#132717=CARTESIAN_POINT('Ctrl Pts',(6.37148136532936,-27.7236151322564,
54.9983741243495));
#132718=CARTESIAN_POINT('Ctrl Pts',(6.48261663616792,-28.7640046341545,
56.9116082666613));
#132719=CARTESIAN_POINT('Ctrl Pts',(6.59375190700648,-30.9356658753436,
57.0752012141665));
#132720=CARTESIAN_POINT('Ctrl Pts',(6.70488717784504,-32.2509384993579,
55.3394209505671));
#132721=CARTESIAN_POINT('Ctrl Pts',(6.8160224486836,-31.5059905257943,53.2929782527002));
#132722=CARTESIAN_POINT('Ctrl Pts',(6.92715771952215,-29.382651849057,52.8089244718427));
#132723=CARTESIAN_POINT('Ctrl Pts',(7.03829299036072,-27.8243545435983,
54.3303003974168));
#132724=CARTESIAN_POINT('Ctrl Pts',(7.14942826119927,-28.2573642346483,
56.4646335031895));
#132725=CARTESIAN_POINT('Ctrl Pts',(7.26056353203784,-30.2853593499821,
57.258428823543));
#132726=CARTESIAN_POINT('Ctrl Pts',(7.37169880287639,-32.0521730914497,
55.9851478635125));
#132727=CARTESIAN_POINT('Ctrl Pts',(7.48283407371496,-31.9406906131178,
53.8101888166788));
#132728=CARTESIAN_POINT('Ctrl Pts',(7.59396934455351,-30.0529486889238,
52.7242304275315));
#132729=CARTESIAN_POINT('Ctrl Pts',(7.70510461539206,-28.1167443186283,
53.721219818432));
#132730=CARTESIAN_POINT('Ctrl Pts',(7.81623988623064,-27.9042308259751,
55.8886406836328));
#132731=CARTESIAN_POINT('Ctrl Pts',(7.92737515706918,-29.6099158078912,
57.2427137679369));
#132732=CARTESIAN_POINT('Ctrl Pts',(8.03851042790776,-31.6726338832006,
56.5440941135952));
#132733=CARTESIAN_POINT('Ctrl Pts',(8.1496456987463,-32.204437242396,54.4322086275537));
#132734=CARTESIAN_POINT('Ctrl Pts',(8.26078096958488,-30.7185813785667,
52.8400065657396));
#132735=CARTESIAN_POINT('Ctrl Pts',(8.37191624042342,-28.5750280553716,
53.2247856925982));
#132736=CARTESIAN_POINT('Ctrl Pts',(8.483051511262,-27.7357117408224,55.2343683721141));
#132737=CARTESIAN_POINT('Ctrl Pts',(8.59418678210054,-28.9688340276785,
57.0294404685603));
#132738=CARTESIAN_POINT('Ctrl Pts',(8.70532205293911,-31.1457547795456,
56.9670225072527));
#132739=CARTESIAN_POINT('Ctrl Pts',(8.81645732377767,-32.2739958818645,
55.1042449875192));
#132740=CARTESIAN_POINT('Ctrl Pts',(8.92759259461623,-31.3209177237342,
53.146053520302));
#132741=CARTESIAN_POINT('Ctrl Pts',(9.03872786545478,-29.1588306515692,
52.884729908285));
#132742=CARTESIAN_POINT('Ctrl Pts',(9.14986313629334,-27.7666622815123,
54.5594477316463));
#132743=CARTESIAN_POINT('Ctrl Pts',(9.26099840713191,-28.4185651629648,
56.6374019201245));
#132744=CARTESIAN_POINT('Ctrl Pts',(9.37213367797046,-30.5179898189604,
57.2166658802639));
#132745=CARTESIAN_POINT('Ctrl Pts',(9.48326894880902,-32.143156288125,55.7671223817873));
#132746=CARTESIAN_POINT('Ctrl Pts',(9.59440421964759,-31.8070629271169,
53.6153653789881));
#132747=CARTESIAN_POINT('Ctrl Pts',(9.70553949048613,-29.816399460164,52.7310999311908));
#132748=CARTESIAN_POINT('Ctrl Pts',(9.81667476132471,-27.9950037163415,
53.9231489246537));
#132749=CARTESIAN_POINT('Ctrl Pts',(9.92781003216325,-28.0062846857326,
56.1014933715052));
#132750=CARTESIAN_POINT('Ctrl Pts',(10.0389582396273,-29.8475763570898,
57.2704718330739));
#132751=CARTESIAN_POINT('Ctrl Pts',(10.1130613568119,-31.1601294858308,
56.66548921636));
#132752=CARTESIAN_POINT('Ctrl Pts',(10.1501193837169,-31.5433460568722,
56.1521091310284));
#132753=CARTESIAN_POINT('Ctrl Pts',(-0.150275521818664,-29.5369889357901,
53.2662970356098));
#132754=CARTESIAN_POINT('Ctrl Pts',(-0.113230431539144,-28.960505042745,
53.4202556007742));
#132755=CARTESIAN_POINT('Ctrl Pts',(-0.0391402509801043,-27.9832174984029,
54.3461733935319));
#132756=CARTESIAN_POINT('Ctrl Pts',(0.0719950198584549,-28.3570414167314,
56.3433813121067));
#132757=CARTESIAN_POINT('Ctrl Pts',(0.183130290697014,-30.2375073428938,
57.1071631749565));
#132758=CARTESIAN_POINT('Ctrl Pts',(0.294265561535574,-31.8991532362291,
55.9441918121845));
#132759=CARTESIAN_POINT('Ctrl Pts',(0.405400832374133,-31.8232803179608,
53.9160897747171));
#132760=CARTESIAN_POINT('Ctrl Pts',(0.516536103212693,-30.078246009061,
52.8805329737631));
#132761=CARTESIAN_POINT('Ctrl Pts',(0.627671374051251,-28.2617790185534,
53.7846262852794));
#132762=CARTESIAN_POINT('Ctrl Pts',(0.738806644889812,-28.0361640975088,
55.8012371101055));
#132763=CARTESIAN_POINT('Ctrl Pts',(0.84994191572837,-29.6080395648783,
57.0844375707751));
#132764=CARTESIAN_POINT('Ctrl Pts',(0.96107718656693,-31.5386418220091,
56.4598416068841));
#132765=CARTESIAN_POINT('Ctrl Pts',(1.07221245740549,-32.0609804423719,
54.4990783327577));
#132766=CARTESIAN_POINT('Ctrl Pts',(1.18334772824404,-30.6969557336342,
52.9968023213935));
#132767=CARTESIAN_POINT('Ctrl Pts',(1.29448299908261,-28.6950300962674,
53.3279927941359));
#132768=CARTESIAN_POINT('Ctrl Pts',(1.40561826992116,-27.8875051264756,
55.1895263369173));
#132769=CARTESIAN_POINT('Ctrl Pts',(1.51675354075972,-29.0134879717024,
56.8775907659846));
#132770=CARTESIAN_POINT('Ctrl Pts',(1.62788881159828,-31.0423970981937,
56.8471497629006));
#132771=CARTESIAN_POINT('Ctrl Pts',(1.73902408243684,-32.1172297212648,
55.1260643642059));
#132772=CARTESIAN_POINT('Ctrl Pts',(1.8501593532754,-31.2542215261682,53.2895959321017));
#132773=CARTESIAN_POINT('Ctrl Pts',(1.96129462411396,-29.2432597503511,
53.0186120953251));
#132774=CARTESIAN_POINT('Ctrl Pts',(2.07242989495252,-27.9249209819592,
54.5611368227768));
#132775=CARTESIAN_POINT('Ctrl Pts',(2.18356516579108,-28.5058435946297,
56.5053406367943));
#132776=CARTESIAN_POINT('Ctrl Pts',(2.29470043662964,-30.4543254670805,
57.0717485809739));
#132777=CARTESIAN_POINT('Ctrl Pts',(2.4058357074682,-31.9869760414681,55.7419434077801));
#132778=CARTESIAN_POINT('Ctrl Pts',(2.51697097830676,-31.7010034183238,
53.7330583367382));
#132779=CARTESIAN_POINT('Ctrl Pts',(2.62810624914532,-29.8581502859505,
52.8837692781711));
#132780=CARTESIAN_POINT('Ctrl Pts',(2.73924151998388,-28.145128200405,53.9714065837682));
#132781=CARTESIAN_POINT('Ctrl Pts',(2.85037679082244,-28.1298180198844,
56.0004864666014));
#132782=CARTESIAN_POINT('Ctrl Pts',(2.961512061661,-29.8262327210055,57.1138492712643));
#132783=CARTESIAN_POINT('Ctrl Pts',(3.07264733249956,-31.6816917174677,
56.2924653868433));
#132784=CARTESIAN_POINT('Ctrl Pts',(3.18378260333811,-31.9979456596237,
54.2881243437535));
#132785=CARTESIAN_POINT('Ctrl Pts',(3.29491787417668,-30.4855362234068,
52.9353430346521));
#132786=CARTESIAN_POINT('Ctrl Pts',(3.40605314501523,-28.5287291598767,
53.4722840827597));
#132787=CARTESIAN_POINT('Ctrl Pts',(3.5171884158538,-27.9185348493353,55.4075004728264));
#132788=CARTESIAN_POINT('Ctrl Pts',(3.62832368669235,-29.2134469545116,
56.9697431597603));
#132789=CARTESIAN_POINT('Ctrl Pts',(3.73945895753091,-31.2282689043408,
56.7291354219427));
#132790=CARTESIAN_POINT('Ctrl Pts',(3.85059422836948,-32.1188909274298,
54.9058987436705));
#132791=CARTESIAN_POINT('Ctrl Pts',(3.96172949920803,-31.0701517756433,
53.1687902944022));
#132792=CARTESIAN_POINT('Ctrl Pts',(4.07286477004659,-29.0419328507167,
53.1077365018973));
#132793=CARTESIAN_POINT('Ctrl Pts',(4.18400004088515,-27.8906057979442,
54.7786181824969));
#132794=CARTESIAN_POINT('Ctrl Pts',(4.2951353117237,-28.6699478348436,56.6521244041387));
#132795=CARTESIAN_POINT('Ctrl Pts',(4.40627058256227,-30.6666491497843,
57.013487700454));
#132796=CARTESIAN_POINT('Ctrl Pts',(4.51740585340082,-32.0531852780137,
55.5319624262439));
#132797=CARTESIAN_POINT('Ctrl Pts',(4.62854112423939,-31.5604987612927,
53.563546929137));
#132798=CARTESIAN_POINT('Ctrl Pts',(4.73967639507795,-29.6395316889681,
52.9098764616585));
#132799=CARTESIAN_POINT('Ctrl Pts',(4.85081166591652,-28.048491107025,54.1692371882256));
#132800=CARTESIAN_POINT('Ctrl Pts',(4.96194693675506,-28.2436116391189,
56.1889717130987));
#132801=CARTESIAN_POINT('Ctrl Pts',(5.07308220759364,-30.0463049589392,
57.1204739233401));
#132802=CARTESIAN_POINT('Ctrl Pts',(5.18421747843218,-31.8066166542933,
56.1111660871432));
#132803=CARTESIAN_POINT('Ctrl Pts',(5.29535274927075,-31.9133830199357,
54.0848392338995));
#132804=CARTESIAN_POINT('Ctrl Pts',(5.4064880201093,-30.2688838090949,52.8961332489926));
#132805=CARTESIAN_POINT('Ctrl Pts',(5.51762329094786,-28.3782828224804,
53.6330372335263));
#132806=CARTESIAN_POINT('Ctrl Pts',(5.62875856178643,-27.9719938832659,
55.621083729683));
#132807=CARTESIAN_POINT('Ctrl Pts',(5.73989383262498,-29.4218818120017,
57.0406697845298));
#132808=CARTESIAN_POINT('Ctrl Pts',(5.85102910346354,-31.40090503212,56.5924882730395));
#132809=CARTESIAN_POINT('Ctrl Pts',(5.9621643743021,-32.0977193410523,54.6867471070161));
#132810=CARTESIAN_POINT('Ctrl Pts',(6.07329964514066,-30.874550231698,53.0677174893343));
#132811=CARTESIAN_POINT('Ctrl Pts',(6.18443491597923,-28.8509299321116,
53.2172516195854));
#132812=CARTESIAN_POINT('Ctrl Pts',(6.29557018681779,-27.8790210953594,
54.9984851208576));
#132813=CARTESIAN_POINT('Ctrl Pts',(6.40670545765634,-28.8483845002052,
56.7811051483327));
#132814=CARTESIAN_POINT('Ctrl Pts',(6.51784072849489,-30.8717891300001,
56.9335298088213));
#132815=CARTESIAN_POINT('Ctrl Pts',(6.62897599933347,-32.0972697281694,
55.3162491045108));
#132816=CARTESIAN_POINT('Ctrl Pts',(6.74011127017202,-31.4031784260473,
53.409514503857));
#132817=CARTESIAN_POINT('Ctrl Pts',(6.85124654101057,-29.4247974393421,
52.9585064724569));
#132818=CARTESIAN_POINT('Ctrl Pts',(6.96238181184914,-27.9728831524087,
54.3760199561802));
#132819=CARTESIAN_POINT('Ctrl Pts',(7.07351708268769,-28.3763318105138,
56.3646447959276));
#132820=CARTESIAN_POINT('Ctrl Pts',(7.18465235352626,-30.2658782221452,
57.1042486972401));
#132821=CARTESIAN_POINT('Ctrl Pts',(7.29578762436481,-31.9120737873953,
55.9178930443925));
#132822=CARTESIAN_POINT('Ctrl Pts',(7.40692289520338,-31.8082020791752,
53.8914157460416));
#132823=CARTESIAN_POINT('Ctrl Pts',(7.51805816604193,-30.049333947799,52.8795943851916));
#132824=CARTESIAN_POINT('Ctrl Pts',(7.6291934368805,-28.2453118412296,53.8085205506278));
#132825=CARTESIAN_POINT('Ctrl Pts',(7.74032870771905,-28.0473063803536,
55.8279742896283));
#132826=CARTESIAN_POINT('Ctrl Pts',(7.85146397855761,-29.6365463704225,
57.0896064889309));
#132827=CARTESIAN_POINT('Ctrl Pts',(7.96259924939617,-31.5584452487474,
56.4386807293097));
#132828=CARTESIAN_POINT('Ctrl Pts',(8.07373452023473,-32.0539430541726,
54.4709710382194));
#132829=CARTESIAN_POINT('Ctrl Pts',(8.18486979107328,-30.6695247217656,
52.9874666304696));
#132830=CARTESIAN_POINT('Ctrl Pts',(8.29600506191187,-28.6723091173694,
53.3459773650017));
#132831=CARTESIAN_POINT('Ctrl Pts',(8.4071403327504,-27.8902918835068,55.2183683349037));
#132832=CARTESIAN_POINT('Ctrl Pts',(8.51827560358897,-29.0392304458407,
56.8908930923912));
#132833=CARTESIAN_POINT('Ctrl Pts',(8.62941087442753,-31.0675355260624,
56.8327363276544));
#132834=CARTESIAN_POINT('Ctrl Pts',(8.74054614526609,-32.1187530118556,
55.0971283119017));
#132835=CARTESIAN_POINT('Ctrl Pts',(8.85168141610465,-31.2307403139536,
53.2726201401656));
#132836=CARTESIAN_POINT('Ctrl Pts',(8.96281668694321,-29.2162562365738,
53.0291367660549));
#132837=CARTESIAN_POINT('Ctrl Pts',(9.07395195778177,-27.9191294692861,
54.5895236869607));
#132838=CARTESIAN_POINT('Ctrl Pts',(9.18508722862032,-28.5265277519878,
56.525618527962));
#132839=CARTESIAN_POINT('Ctrl Pts',(9.2962224994589,-30.4826272983983,57.0653368581459));
#132840=CARTESIAN_POINT('Ctrl Pts',(9.40735777029745,-31.9968456744164,
55.7147518910812));
#132841=CARTESIAN_POINT('Ctrl Pts',(9.518493041136,-31.6836969890651,53.7098926620822));
#132842=CARTESIAN_POINT('Ctrl Pts',(9.62962831197457,-29.8289336406198,
52.8859949163817));
#132843=CARTESIAN_POINT('Ctrl Pts',(9.74076358281312,-28.1318823184159,
53.9966642079673));
#132844=CARTESIAN_POINT('Ctrl Pts',(9.85189885365168,-28.1423931500601,
56.0262957892879));
#132845=CARTESIAN_POINT('Ctrl Pts',(9.96304706111574,-29.8579821295766,
57.115469545492));
#132846=CARTESIAN_POINT('Ctrl Pts',(10.0371501783003,-31.0809288890316,
56.551788339424));
#132847=CARTESIAN_POINT('Ctrl Pts',(10.0742082052053,-31.4379837414887,
56.0734560738743));
#132848=CARTESIAN_POINT('Ctrl Pts',(-0.226186700330235,-29.5709141578673,
53.3933269548259));
#132849=CARTESIAN_POINT('Ctrl Pts',(-0.189141610050715,-29.0366697394421,
53.536004842448));
#132850=CARTESIAN_POINT('Ctrl Pts',(-0.115051429491676,-28.130988900723,
54.3940798358158));
#132851=CARTESIAN_POINT('Ctrl Pts',(-0.00391615865311672,-28.477422416473,
56.2449505987386));
#132852=CARTESIAN_POINT('Ctrl Pts',(0.107219112185443,-30.2201049739755,
56.9527695023448));
#132853=CARTESIAN_POINT('Ctrl Pts',(0.218354383024002,-31.7600006321599,
55.8750100595487));
#132854=CARTESIAN_POINT('Ctrl Pts',(0.329489653862562,-31.6896869883905,
53.995508816608));
#132855=CARTESIAN_POINT('Ctrl Pts',(0.44062492470112,-30.0725128561426,
53.0358281602248));
#132856=CARTESIAN_POINT('Ctrl Pts',(0.55176019553968,-28.3891399767961,
53.8736777710121));
#132857=CARTESIAN_POINT('Ctrl Pts',(0.662895466378239,-28.1800560566109,
55.7425297724241));
#132858=CARTESIAN_POINT('Ctrl Pts',(0.774030737216799,-29.6367588457657,
56.9317090228835));
#132859=CARTESIAN_POINT('Ctrl Pts',(0.885166008055357,-31.4259042018014,
56.3528777467535));
#132860=CARTESIAN_POINT('Ctrl Pts',(0.996301278893918,-31.9099706186142,
54.5357812975853));
#132861=CARTESIAN_POINT('Ctrl Pts',(1.10743654973247,-30.6458891828125,
53.1435783519559));
#132862=CARTESIAN_POINT('Ctrl Pts',(1.21857182057104,-28.7906463724437,
53.4505022116384));
#132863=CARTESIAN_POINT('Ctrl Pts',(1.32970709140959,-28.0422894572636,
55.1756395779036));
#132864=CARTESIAN_POINT('Ctrl Pts',(1.44084236224816,-29.0857705632619,
56.7400180628036));
#132865=CARTESIAN_POINT('Ctrl Pts',(1.55197763308671,-30.966019759114,56.7118074984061));
#132866=CARTESIAN_POINT('Ctrl Pts',(1.66311290392527,-31.962098464078,55.1168275189504));
#132867=CARTESIAN_POINT('Ctrl Pts',(1.77424817476383,-31.162323627612,53.4149187209731));
#132868=CARTESIAN_POINT('Ctrl Pts',(1.88538344560239,-29.2987067644908,
53.1637901048438));
#132869=CARTESIAN_POINT('Ctrl Pts',(1.99651871644095,-28.0769638205787,
54.5932927082397));
#132870=CARTESIAN_POINT('Ctrl Pts',(2.10765398727951,-28.6153217297941,
56.3950430232974));
#132871=CARTESIAN_POINT('Ctrl Pts',(2.21878925811807,-30.4210366462349,
56.9199497663655));
#132872=CARTESIAN_POINT('Ctrl Pts',(2.32992452895663,-31.841388584322,55.6875805710721));
#132873=CARTESIAN_POINT('Ctrl Pts',(2.44105979979519,-31.5763694231964,
53.8258882507669));
#132874=CARTESIAN_POINT('Ctrl Pts',(2.55219507063375,-29.8685437374741,
53.0388273378032));
#132875=CARTESIAN_POINT('Ctrl Pts',(2.66333034147231,-28.2810362652226,
54.0467725151036));
#132876=CARTESIAN_POINT('Ctrl Pts',(2.77446561231087,-28.2668478749018,
55.9271799558324));
#132877=CARTESIAN_POINT('Ctrl Pts',(2.88560088314943,-29.8389648001831,
56.9589657025797));
#132878=CARTESIAN_POINT('Ctrl Pts',(2.99673615398798,-31.5584727074041,
56.1977653274602));
#132879=CARTESIAN_POINT('Ctrl Pts',(3.10787142482655,-31.8515544490454,
54.3402840902397));
#132880=CARTESIAN_POINT('Ctrl Pts',(3.21900669566511,-30.4499605633874,
53.0866222404354));
#132881=CARTESIAN_POINT('Ctrl Pts',(3.33014196650366,-28.6365304498351,
53.5842211524528));
#132882=CARTESIAN_POINT('Ctrl Pts',(3.44127723734223,-28.0710456054286,
55.3776425599043));
#132883=CARTESIAN_POINT('Ctrl Pts',(3.55241250818078,-29.2710783780484,
56.8254183707968));
#132884=CARTESIAN_POINT('Ctrl Pts',(3.66354777901934,-31.1382725768852,
56.6024401705214));
#132885=CARTESIAN_POINT('Ctrl Pts',(3.7746830498579,-31.9636379522272,54.9127936243018));
#132886=CARTESIAN_POINT('Ctrl Pts',(3.88581832069646,-30.9917408272851,
53.3029646170791));
#132887=CARTESIAN_POINT('Ctrl Pts',(3.99695359153502,-29.1121312613309,
53.2463842888809));
#132888=CARTESIAN_POINT('Ctrl Pts',(4.10808886237358,-28.0451629398456,
54.7948390201899));
#132889=CARTESIAN_POINT('Ctrl Pts',(4.21922413321213,-28.7674019100592,
56.5310718167557));
#132890=CARTESIAN_POINT('Ctrl Pts',(4.3303594040507,-30.6178031886351,56.8659577110701));
#132891=CARTESIAN_POINT('Ctrl Pts',(4.44149467488925,-31.9027466127066,
55.4929850780938));
#132892=CARTESIAN_POINT('Ctrl Pts',(4.55262994572782,-31.4461596641949,
53.6687970909568));
#132893=CARTESIAN_POINT('Ctrl Pts',(4.66376521656638,-29.6659435146215,
53.0630216253231));
#132894=CARTESIAN_POINT('Ctrl Pts',(4.77490048740493,-28.1914798554531,
54.2301078996653));
#132895=CARTESIAN_POINT('Ctrl Pts',(4.8860357582435,-28.3723037370028,56.1018547249136));
#132896=CARTESIAN_POINT('Ctrl Pts',(4.99717102908206,-30.042912154454,56.9651049606548));
#132897=CARTESIAN_POINT('Ctrl Pts',(5.10830629992061,-31.6742442858063,
56.0297499846246));
#132898=CARTESIAN_POINT('Ctrl Pts',(5.21944157075917,-31.773187787278,54.1518938566205));
#132899=CARTESIAN_POINT('Ctrl Pts',(5.33057684159773,-30.2491824592966,
53.0502853897639));
#132900=CARTESIAN_POINT('Ctrl Pts',(5.4417121124363,-28.4971074460077,53.7331957804995));
#132901=CARTESIAN_POINT('Ctrl Pts',(5.55284738327485,-28.1205876495973,
55.5755763863672));
#132902=CARTESIAN_POINT('Ctrl Pts',(5.66398265411341,-29.4642410328297,
56.8911481402805));
#132903=CARTESIAN_POINT('Ctrl Pts',(5.77511792495198,-31.2982595059169,
56.4758052766832));
#132904=CARTESIAN_POINT('Ctrl Pts',(5.88625319579053,-31.944017626338,54.7096994180563));
#132905=CARTESIAN_POINT('Ctrl Pts',(5.99738846662909,-30.8104711780395,
53.2092975040626));
#132906=CARTESIAN_POINT('Ctrl Pts',(6.10852373746765,-28.9351232921599,
53.3478751389531));
#132907=CARTESIAN_POINT('Ctrl Pts',(6.21965900830621,-28.0344270584624,
54.9985961173656));
#132908=CARTESIAN_POINT('Ctrl Pts',(6.33079427914477,-28.932764366256,56.6506020300043));
#132909=CARTESIAN_POINT('Ctrl Pts',(6.44192954998333,-30.8079123846567,
56.7918584034759));
#132910=CARTESIAN_POINT('Ctrl Pts',(6.55306482082189,-31.9436009569808,
55.2930772584545));
#132911=CARTESIAN_POINT('Ctrl Pts',(6.66420009166045,-31.3003663263002,
53.5260507550139));
#132912=CARTESIAN_POINT('Ctrl Pts',(6.775335362499,-29.4669430296272,53.1080884730709));
#132913=CARTESIAN_POINT('Ctrl Pts',(6.88647063333757,-28.121411761219,54.4217395149438));
#132914=CARTESIAN_POINT('Ctrl Pts',(6.99760590417612,-28.4952993863792,
56.2646560886658));
#132915=CARTESIAN_POINT('Ctrl Pts',(7.10874117501469,-30.2463970943083,
56.9500685709374));
#132916=CARTESIAN_POINT('Ctrl Pts',(7.21987644585324,-31.7719744833409,
55.8506382252722));
#132917=CARTESIAN_POINT('Ctrl Pts',(7.3310117166918,-31.6757135452325,53.9726426754045));
#132918=CARTESIAN_POINT('Ctrl Pts',(7.44214698753037,-30.0457192066742,
53.0349583428515));
#132919=CARTESIAN_POINT('Ctrl Pts',(7.55328225836892,-28.3738793638309,
53.8958212828239));
#132920=CARTESIAN_POINT('Ctrl Pts',(7.66441752920749,-28.1903819347319,
55.7673078956236));
#132921=CARTESIAN_POINT('Ctrl Pts',(7.77555280004603,-29.663176932954,56.936499209925));
#132922=CARTESIAN_POINT('Ctrl Pts',(7.88668807088461,-31.4442566142942,
56.3332673450242));
#132923=CARTESIAN_POINT('Ctrl Pts',(7.99782334172316,-31.9034488659494,
54.5097334488851));
#132924=CARTESIAN_POINT('Ctrl Pts',(8.10895861256172,-30.6204680649645,
53.1349266951994));
#132925=CARTESIAN_POINT('Ctrl Pts',(8.22009388340028,-28.7695901793672,
53.4671690374053));
#132926=CARTESIAN_POINT('Ctrl Pts',(8.33122915423884,-28.0448720261911,
55.2023682976932));
#132927=CARTESIAN_POINT('Ctrl Pts',(8.44236442507739,-29.1096268640029,
56.7523457162221));
#132928=CARTESIAN_POINT('Ctrl Pts',(8.55349969591596,-30.9893162725793,
56.698450148056));
#132929=CARTESIAN_POINT('Ctrl Pts',(8.66463496675452,-31.9635101418466,
55.0900116362843));
#132930=CARTESIAN_POINT('Ctrl Pts',(8.77577023759308,-31.140562904173,53.3991867600292));
#132931=CARTESIAN_POINT('Ctrl Pts',(8.88690550843164,-29.2736818215783,
53.173543623825));
#132932=CARTESIAN_POINT('Ctrl Pts',(8.99804077927019,-28.07159665706,54.6195996422751));
#132933=CARTESIAN_POINT('Ctrl Pts',(9.10917605010876,-28.6344903410107,
56.4138351357996));
#132934=CARTESIAN_POINT('Ctrl Pts',(9.22031132094731,-30.447264777836,56.9140078360277));
#132935=CARTESIAN_POINT('Ctrl Pts',(9.33144659178588,-31.8505350607078,
55.6623814003752));
#132936=CARTESIAN_POINT('Ctrl Pts',(9.44258186262443,-31.5603310510131,
53.8044199451762));
#132937=CARTESIAN_POINT('Ctrl Pts',(9.553717133463,-29.8414678210757,53.0408899015726));
#132938=CARTESIAN_POINT('Ctrl Pts',(9.66485240430155,-28.2687609204902,
54.0701794912807));
#132939=CARTESIAN_POINT('Ctrl Pts',(9.77598767514011,-28.2785016143876,
55.9510982070706));
#132940=CARTESIAN_POINT('Ctrl Pts',(9.88713588260416,-29.8683879020635,
56.96046725791));
#132941=CARTESIAN_POINT('Ctrl Pts',(9.96123899978869,-31.0017282922326,
56.4380874624881));
#132942=CARTESIAN_POINT('Ctrl Pts',(9.99829702669369,-31.3326214261051,
55.9948030167202));
#132943=CARTESIAN_POINT('Ctrl Pts',(10.,-31.3346917155535,55.997072727755));
#132944=CARTESIAN_POINT('Ctrl Pts',(10.,-31.3032909346448,56.0511234363458));
#132945=CARTESIAN_POINT('Ctrl Pts',(9.99999999999997,-31.2686972100049,
56.1030990415617));
#132946=CARTESIAN_POINT('Ctrl Pts',(9.99999999999999,-31.2312367751759,
56.1529134472441));
#132947=CARTESIAN_POINT('Ctrl Pts',(10.,-31.2074766111454,56.1845094085695));
#132948=CARTESIAN_POINT('Ctrl Pts',(9.99999999999998,-31.1825620753087,
56.2152357171833));
#132949=CARTESIAN_POINT('Ctrl Pts',(9.99999999999999,-31.1565664281997,
56.2450672023032));
#132950=CARTESIAN_POINT('Ctrl Pts',(10.,-31.1387986277207,56.2654567649627));
#132951=CARTESIAN_POINT('Ctrl Pts',(10.,-31.1205256172073,56.2854282470845));
#132952=CARTESIAN_POINT('Ctrl Pts',(9.99999999999999,-31.1017689652775,
56.3049727142744));
#132953=CARTESIAN_POINT('Ctrl Pts',(9.99999999999998,-31.0918278768739,
56.3153313474069));
#132954=CARTESIAN_POINT('Ctrl Pts',(9.99999999999998,-31.0817509756526,
56.3255697751785));
#132955=CARTESIAN_POINT('Ctrl Pts',(9.99999999999998,-31.0715517224076,
56.3356767875606));
#132956=CARTESIAN_POINT('Ctrl Pts',(9.99999999999998,-31.0246754291279,
56.382129137083));
#132957=CARTESIAN_POINT('Ctrl Pts',(9.99999999999999,-30.9751667282857,
56.4258621586488));
#132958=CARTESIAN_POINT('Ctrl Pts',(9.99999999999998,-30.9233613204925,
56.4667657821209));
#132959=CARTESIAN_POINT('Ctrl Pts',(9.99999999999997,-30.8860273825892,
56.4962432711278));
#132960=CARTESIAN_POINT('Ctrl Pts',(9.99999999999999,-30.8474994872535,
56.5242509659966));
#132961=CARTESIAN_POINT('Ctrl Pts',(10.,-30.8078890088004,56.5507389966442));
#132962=CARTESIAN_POINT('Ctrl Pts',(10.,-30.797015398732,56.5580103179711));
#132963=CARTESIAN_POINT('Ctrl Pts',(10.,-30.7860601469677,56.5651670716741));
#132964=CARTESIAN_POINT('Ctrl Pts',(10.,-30.7750254260934,56.5722081087175));
#132965=CARTESIAN_POINT('Ctrl Pts',(10.,-30.7637763630091,56.5793859132839));
#132966=CARTESIAN_POINT('Ctrl Pts',(10.,-30.7524515667651,56.5864390456066));
#132967=CARTESIAN_POINT('Ctrl Pts',(10.,-30.7410580144043,56.5933641088242));
#132968=CARTESIAN_POINT('Ctrl Pts',(10.,-30.6829437846755,56.6286862543647));
#132969=CARTESIAN_POINT('Ctrl Pts',(10.,-30.6230097365582,56.6607008904149));
#132970=CARTESIAN_POINT('Ctrl Pts',(10.,-30.5615984318091,56.6892964836472));
#132971=CARTESIAN_POINT('Ctrl Pts',(10.,-30.4994238831573,56.7182474741841));
#132972=CARTESIAN_POINT('Ctrl Pts',(10.,-30.4357343478421,56.7436946380252));
#132973=CARTESIAN_POINT('Ctrl Pts',(10.,-30.3708449452616,56.7654879565643));
#132974=CARTESIAN_POINT('Ctrl Pts',(10.,-30.3308185453291,56.7789309541727));
#132975=CARTESIAN_POINT('Ctrl Pts',(10.,-30.2903348574852,56.7909829777777));
#132976=CARTESIAN_POINT('Ctrl Pts',(10.,-30.249462365503,56.8016005644171));
#132977=CARTESIAN_POINT('Ctrl Pts',(10.,-30.2158480327199,56.8103326742871));
#132978=CARTESIAN_POINT('Ctrl Pts',(10.,-30.1819706297403,56.8180944670961));
#132979=CARTESIAN_POINT('Ctrl Pts',(9.99999999999999,-30.1478668356042,
56.8248580322968));
#132980=CARTESIAN_POINT('Ctrl Pts',(9.99999999999998,-30.1339192196307,
56.8276241647));
#132981=CARTESIAN_POINT('Ctrl Pts',(10.,-30.1199311692375,56.8302235991369));
#132982=CARTESIAN_POINT('Ctrl Pts',(10.,-30.1059290408562,56.8326505130612));
#132983=CARTESIAN_POINT('Ctrl Pts',(9.99999999999999,-30.036479877866,56.8446877645493));
#132984=CARTESIAN_POINT('Ctrl Pts',(10.,-29.9665653006914,56.8525100973381));
#132985=CARTESIAN_POINT('Ctrl Pts',(10.,-29.8965201495899,56.855976934255));
#132986=CARTESIAN_POINT('Ctrl Pts',(10.,-29.8887467804205,56.8563616718533));
#132987=CARTESIAN_POINT('Ctrl Pts',(9.99999999999999,-29.8809717732861,
56.8566927244466));
#132988=CARTESIAN_POINT('Ctrl Pts',(9.99999999999999,-29.8731955649853,
56.8569698661726));
#132989=CARTESIAN_POINT('Ctrl Pts',(10.,-29.8058138556625,56.8593713300357));
#132990=CARTESIAN_POINT('Ctrl Pts',(9.99999999999998,-29.7383430939132,
56.857729193759));
#132991=CARTESIAN_POINT('Ctrl Pts',(9.99999999999998,-29.6710457952579,
56.8522613874595));
#132992=CARTESIAN_POINT('Ctrl Pts',(9.99999999999998,-29.5986466816943,
56.8463790662203));
#132993=CARTESIAN_POINT('Ctrl Pts',(9.99999999999999,-29.5264474184432,
56.836069467537));
#132994=CARTESIAN_POINT('Ctrl Pts',(9.99999999999999,-29.4547662757674,
56.8215402711312));
#132995=CARTESIAN_POINT('Ctrl Pts',(9.99999999999999,-29.441748496888,56.8189016710888));
#132996=CARTESIAN_POINT('Ctrl Pts',(10.,-29.4287478079428,56.816123737079));
#132997=CARTESIAN_POINT('Ctrl Pts',(10.,-29.4157661281353,56.8132074934358));
#132998=CARTESIAN_POINT('Ctrl Pts',(10.,-29.4044168231439,56.8106579513869));
#132999=CARTESIAN_POINT('Ctrl Pts',(9.99999999999998,-29.3930909204653,
56.8080046750453));
#133000=CARTESIAN_POINT('Ctrl Pts',(9.99999999999998,-29.3817917769416,
56.8052493638686));
#133001=CARTESIAN_POINT('Ctrl Pts',(10.,-29.3127468519509,56.788412667076));
#133002=CARTESIAN_POINT('Ctrl Pts',(9.99999999999998,-29.2446768142312,
56.7677647231327));
#133003=CARTESIAN_POINT('Ctrl Pts',(9.99999999999998,-29.1778687398964,
56.7435558218946));
#133004=CARTESIAN_POINT('Ctrl Pts',(9.99999999999998,-29.1093809169293,
56.7187382387098));
#133005=CARTESIAN_POINT('Ctrl Pts',(10.,-29.042218379655,56.6901782595077));
#133006=CARTESIAN_POINT('Ctrl Pts',(10.,-28.9766863196167,56.6580897906909));
#133007=CARTESIAN_POINT('Ctrl Pts',(10.,-28.9112758404337,56.6260608552304));
#133008=CARTESIAN_POINT('Ctrl Pts',(10.,-28.8474887900981,56.5905161312587));
#133009=CARTESIAN_POINT('Ctrl Pts',(10.,-28.7856393264207,56.5516176578855));
#133010=CARTESIAN_POINT('Ctrl Pts',(10.,-28.7688957142038,56.5410872358694));
#133011=CARTESIAN_POINT('Ctrl Pts',(10.,-28.7522942908099,56.5303108130768));
#133012=CARTESIAN_POINT('Ctrl Pts',(10.,-28.7358413036534,56.5192908377815));
#133013=CARTESIAN_POINT('Ctrl Pts',(10.,-28.7254089766122,56.5123034144539));
#133014=CARTESIAN_POINT('Ctrl Pts',(10.,-28.7150370135204,56.5052184142791));
#133015=CARTESIAN_POINT('Ctrl Pts',(10.,-28.704739183828,56.4980452468686));
#133016=CARTESIAN_POINT('Ctrl Pts',(10.,-28.6429556743447,56.4550086585805));
#133017=CARTESIAN_POINT('Ctrl Pts',(10.,-28.5837268958653,56.4087277658481));
#133018=CARTESIAN_POINT('Ctrl Pts',(10.,-28.5273654175275,56.3594358051663));
#133019=CARTESIAN_POINT('Ctrl Pts',(10.,-28.4712788591607,56.3103842807682));
#133020=CARTESIAN_POINT('Ctrl Pts',(10.,-28.4180306882043,56.2583505378195));
#133021=CARTESIAN_POINT('Ctrl Pts',(10.,-28.3679443534525,56.2035160661832));
#133022=CARTESIAN_POINT('Ctrl Pts',(10.,-28.3183087377282,56.1491750413094));
#133023=CARTESIAN_POINT('Ctrl Pts',(10.,-28.2717773418937,56.0920830054598));
#133024=CARTESIAN_POINT('Ctrl Pts',(10.,-28.2286947931129,56.0323758423507));
#133025=CARTESIAN_POINT('Ctrl Pts',(10.,-28.2195095858647,56.0196462642993));
#133026=CARTESIAN_POINT('Ctrl Pts',(10.,-28.2104812826155,56.0067976831957));
#133027=CARTESIAN_POINT('Ctrl Pts',(10.,-28.2016134661306,55.9938312042311));
#133028=CARTESIAN_POINT('Ctrl Pts',(10.,-28.1941455433265,55.982911643129));
#133029=CARTESIAN_POINT('Ctrl Pts',(10.0000000000001,-28.1867914389921,
55.9719084678104));
#133030=CARTESIAN_POINT('Ctrl Pts',(10.,-28.1795511441573,55.9608235055809));
#133031=CARTESIAN_POINT('',(-0.000879000304030074,-28.729739644302,56.080266780513));
#133032=CARTESIAN_POINT('Ctrl Pts',(-0.000879000304030431,-28.7308780712584,
56.079298628734));
#133033=CARTESIAN_POINT('Ctrl Pts',(-0.000586000202687196,-28.7363705706892,
56.0857571299178));
#133034=CARTESIAN_POINT('Ctrl Pts',(-0.000293000101343235,-28.7419123715811,
56.0921737036785));
#133035=CARTESIAN_POINT('Ctrl Pts',(0.,-28.7475028281235,56.0985476022646));
#133036=CARTESIAN_POINT('Ctrl Pts',(-2.77989437025283E-16,-29.4698297828114,
53.0148256743283));
#133037=CARTESIAN_POINT('Ctrl Pts',(-1.0665791516157E-14,-29.4008110336088,
53.0403807583238));
#133038=CARTESIAN_POINT('Ctrl Pts',(-1.4405926639662E-14,-29.3335131533633,
53.0698652662575));
#133039=CARTESIAN_POINT('Ctrl Pts',(-1.08229397666193E-14,-29.2681280944835,
53.1029808141168));
#133040=CARTESIAN_POINT('Ctrl Pts',(-7.159689807959E-15,-29.2012783340112,
53.1368381888785));
#133041=CARTESIAN_POINT('Ctrl Pts',(8.43478140072747E-15,-29.1364273041799,
53.1744918375422));
#133042=CARTESIAN_POINT('Ctrl Pts',(-7.1505301679764E-15,-29.0738114589791,
53.2156675542709));
#133043=CARTESIAN_POINT('Ctrl Pts',(-2.02460281250629E-14,-29.0211987364619,
53.2502652915009));
#133044=CARTESIAN_POINT('Ctrl Pts',(-1.09741656434686E-14,-28.970164437306,
53.2873507054925));
#133045=CARTESIAN_POINT('Ctrl Pts',(3.01841884819964E-15,-28.9208711427474,
53.3267787632336));
#133046=CARTESIAN_POINT('Ctrl Pts',(9.13037560475156E-15,-28.8988436927425,
53.3443977838014));
#133047=CARTESIAN_POINT('Ctrl Pts',(-1.22852585041228E-14,-28.8771642000329,
53.3624847793734));
#133048=CARTESIAN_POINT('Ctrl Pts',(-1.06165076729781E-14,-28.8558487196368,
53.3810275283898));
#133049=CARTESIAN_POINT('Ctrl Pts',(-9.88881029091767E-15,-28.8441362670507,
53.3912164176212));
#133050=CARTESIAN_POINT('Ctrl Pts',(7.41477610914109E-15,-28.8325337381655,
53.4015429188335));
#133051=CARTESIAN_POINT('Ctrl Pts',(-6.03683769639929E-16,-28.8210439308083,
53.4120050460791));
#133052=CARTESIAN_POINT('Ctrl Pts',(-7.96620544898847E-15,-28.8104503093549,
53.421651144764));
#133053=CARTESIAN_POINT('Ctrl Pts',(-3.05068135553069E-14,-28.7999510772543,
53.4314140526976));
#133054=CARTESIAN_POINT('Ctrl Pts',(-2.68118860446975E-14,-28.7895643152319,
53.4412767583167));
#133055=CARTESIAN_POINT('Ctrl Pts',(-7.62295780683882E-15,-28.7365326250796,
53.4916327737262));
#133056=CARTESIAN_POINT('Ctrl Pts',(1.51656315868618E-14,-28.6863352196068,
53.5446717148978));
#133057=CARTESIAN_POINT('Ctrl Pts',(3.91353616180368E-15,-28.6391900995011,
53.6001349753071));
#133058=CARTESIAN_POINT('Ctrl Pts',(-7.27372162178762E-15,-28.5923166424305,
53.655278641289));
#133059=CARTESIAN_POINT('Ctrl Pts',(2.48947925224922E-14,-28.548459871344,
53.7128196446158));
#133060=CARTESIAN_POINT('Ctrl Pts',(1.70835567914196E-14,-28.5078789636859,
53.7725281427631));
#133061=CARTESIAN_POINT('Ctrl Pts',(1.05450601504418E-14,-28.4741885332485,
53.8220983746639));
#133062=CARTESIAN_POINT('Ctrl Pts',(-2.04280178585247E-15,-28.442756603648,
53.8731631816402));
#133063=CARTESIAN_POINT('Ctrl Pts',(-1.48492329543615E-15,-28.4137591004027,
53.9255975295555));
#133064=CARTESIAN_POINT('Ctrl Pts',(-1.22938169818173E-15,-28.4016536375506,
53.9474870710616));
#133065=CARTESIAN_POINT('Ctrl Pts',(-9.11589881619325E-15,-28.3899727624535,
53.9696153320029));
#133066=CARTESIAN_POINT('Ctrl Pts',(2.48412401759879E-15,-28.3787307158643,
53.9919732986115));
#133067=CARTESIAN_POINT('Ctrl Pts',(7.89954593962274E-15,-28.3735286790514,
54.0023190096382));
#133068=CARTESIAN_POINT('Ctrl Pts',(-2.36829711337499E-14,-28.3684206163503,
54.0127139050674));
#133069=CARTESIAN_POINT('Ctrl Pts',(-1.07414077632484E-14,-28.3634080039989,
54.0231570898446));
#133070=CARTESIAN_POINT('Ctrl Pts',(2.9082809691703E-15,-28.358177440751,
54.0340543495284));
#133071=CARTESIAN_POINT('Ctrl Pts',(-1.10461030585208E-15,-28.353054421572,
54.0449967292496));
#133072=CARTESIAN_POINT('Ctrl Pts',(9.99200722162641E-16,-28.3480419952893,
54.0559789414607));
#133073=CARTESIAN_POINT('Ctrl Pts',(1.25291893836216E-14,-28.3195017414189,
54.1185105592614));
#133074=CARTESIAN_POINT('Ctrl Pts',(-1.82419144324192E-14,-28.2945224341956,
54.1823754520524));
#133075=CARTESIAN_POINT('Ctrl Pts',(-9.99200722162641E-16,-28.2733275400369,
54.2473692544875));
#133076=CARTESIAN_POINT('Ctrl Pts',(1.45523611235135E-14,-28.2541213280901,
54.3062647948684));
#133077=CARTESIAN_POINT('Ctrl Pts',(-1.08023430877253E-14,-28.2380229966997,
54.36608793415));
#133078=CARTESIAN_POINT('Ctrl Pts',(-2.27595720048157E-15,-28.225235550378,
54.4266914343325));
#133079=CARTESIAN_POINT('Ctrl Pts',(7.749618433971E-15,-28.2101043131511,
54.4984028546557));
#133080=CARTESIAN_POINT('Ctrl Pts',(-1.67522331911175E-14,-28.1996082812463,
54.5712084333142));
#133081=CARTESIAN_POINT('Ctrl Pts',(8.04911692853238E-15,-28.1936722887569,
54.6446849507566));
#133082=CARTESIAN_POINT('Ctrl Pts',(1.33492669303424E-14,-28.1923656613117,
54.6608585618995));
#133083=CARTESIAN_POINT('Ctrl Pts',(9.42994019188542E-16,-28.191280203414,
54.6770645999387));
#133084=CARTESIAN_POINT('Ctrl Pts',(1.08801856413265E-14,-28.190415482858,
54.6932983865838));
#133085=CARTESIAN_POINT('Ctrl Pts',(2.12756282169907E-14,-28.1895217390097,
54.7100770405054));
#133086=CARTESIAN_POINT('Ctrl Pts',(1.01404829358878E-14,-28.1888637889881,
54.7268915103632));
#133087=CARTESIAN_POINT('Ctrl Pts',(5.19029264012261E-15,-28.188441715024,
54.7437024356232));
#133088=CARTESIAN_POINT('Ctrl Pts',(-1.44902179624514E-14,-28.1867182332684,
54.8123475676241));
#133089=CARTESIAN_POINT('Ctrl Pts',(-2.06499258425703E-14,-28.1889159285315,
54.8810206540149));
#133090=CARTESIAN_POINT('Ctrl Pts',(-2.19546603119625E-14,-28.1949137770878,
54.9493820494338));
#133091=CARTESIAN_POINT('Ctrl Pts',(-2.32559660595922E-14,-28.2008958638517,
55.017563797415));
#133092=CARTESIAN_POINT('Ctrl Pts',(-1.15115769682287E-14,-28.2106586298725,
55.0854365535916));
#133093=CARTESIAN_POINT('Ctrl Pts',(-7.88258347483861E-15,-28.2241314254406,
55.15264835974));
#133094=CARTESIAN_POINT('Ctrl Pts',(-5.00043810275242E-15,-28.233892766503,
55.201344813265));
#133095=CARTESIAN_POINT('Ctrl Pts',(-2.02964811291747E-14,-28.2456026680783,
55.2496940495499));
#133096=CARTESIAN_POINT('Ctrl Pts',(-1.63757896132211E-14,-28.2592484588431,
55.2975525606475));
#133097=CARTESIAN_POINT('Ctrl Pts',(-1.37739671341366E-14,-28.2694856535417,
55.3334564451883));
#133098=CARTESIAN_POINT('Ctrl Pts',(-2.0853126275729E-14,-28.2808126421487,
55.3690839879711));
#133099=CARTESIAN_POINT('Ctrl Pts',(-2.19269047363468E-15,-28.2932279901634,
55.4043704183004));
#133100=CARTESIAN_POINT('Ctrl Pts',(4.080860316094E-15,-28.297356610343,
55.4161046256824));
#133101=CARTESIAN_POINT('Ctrl Pts',(-5.64529113086221E-15,-28.3016023883907,
55.4277919105227));
#133102=CARTESIAN_POINT('Ctrl Pts',(-4.55191440096314E-15,-28.3059646859586,
55.4394297312791));
#133103=CARTESIAN_POINT('Ctrl Pts',(1.18430705547116E-15,-28.3291463512111,
55.5012742205299));
#133104=CARTESIAN_POINT('Ctrl Pts',(-2.93539877151333E-14,-28.3556167596801,
55.5617283395611));
#133105=CARTESIAN_POINT('Ctrl Pts',(-1.02418074021671E-14,-28.3853255649081,
55.6204553959407));
#133106=CARTESIAN_POINT('Ctrl Pts',(3.12256336159443E-15,-28.4060997247117,
55.6615208391538));
#133107=CARTESIAN_POINT('Ctrl Pts',(-2.86399248371055E-16,-28.428458203708,
55.7017412727147));
#133108=CARTESIAN_POINT('Ctrl Pts',(6.85562717706034E-15,-28.4523940833834,
55.7409903379818));
#133109=CARTESIAN_POINT('Ctrl Pts',(9.35284774839498E-15,-28.4601069023448,
55.7536374994363));
#133110=CARTESIAN_POINT('Ctrl Pts',(-7.98569581965833E-15,-28.4679846656324,
55.7661854163635));
#133111=CARTESIAN_POINT('Ctrl Pts',(-9.13158437754191E-15,-28.4760238017732,
55.7786242039287));
#133112=CARTESIAN_POINT('Ctrl Pts',(-1.32593519350506E-14,-28.5102686331161,
55.831610516739));
#133113=CARTESIAN_POINT('Ctrl Pts',(2.63092452167841E-14,-28.5473690403558,
55.8825129450324));
#133114=CARTESIAN_POINT('Ctrl Pts',(1.35447209004269E-14,-28.5872907667857,
55.9310162114176));
#133115=CARTESIAN_POINT('Ctrl Pts',(1.94148639868689E-15,-28.6240879045149,
55.9757232302042));
#133116=CARTESIAN_POINT('Ctrl Pts',(1.25238026008096E-14,-28.663282593062,
56.0183920404323));
#133117=CARTESIAN_POINT('Ctrl Pts',(1.53765888910584E-14,-28.7048694629046,
56.0587428197802));
#133118=CARTESIAN_POINT('Ctrl Pts',(1.59003142960975E-14,-28.7126726657512,
56.0663140872852));
#133119=CARTESIAN_POINT('Ctrl Pts',(1.71809312476446E-14,-28.7205601438141,
56.0738036401068));
#133120=CARTESIAN_POINT('Ctrl Pts',(1.67643676718399E-14,-28.728530314404,
56.0812108165541));
#133121=CARTESIAN_POINT('Ctrl Pts',(0.00170274486062548,28.7336022489738,
56.0778455314206));
#133122=CARTESIAN_POINT('Ctrl Pts',(0.0387607700302481,28.375062470833,
55.6566084090024));
#133123=CARTESIAN_POINT('Ctrl Pts',(0.11286388547939,28.1179694426535,54.4354449555209));
#133124=CARTESIAN_POINT('Ctrl Pts',(0.224012091208053,29.4558183203175,
53.1100225039009));
#133125=CARTESIAN_POINT('Ctrl Pts',(0.335147362046612,31.2917444909721,
53.519071810237));
#133126=CARTESIAN_POINT('Ctrl Pts',(0.446282632885172,31.9452683344491,
55.2813851316961));
#133127=CARTESIAN_POINT('Ctrl Pts',(0.557417903723731,30.8183979982367,
56.7872523586237));
#133128=CARTESIAN_POINT('Ctrl Pts',(0.668553174562291,28.9424430451878,
56.6567445746501));
#133129=CARTESIAN_POINT('Ctrl Pts',(0.779688445400849,28.034454310918,55.0101441995473));
#133130=CARTESIAN_POINT('Ctrl Pts',(0.89082371623941,28.9254670458642,53.3541183701554));
#133131=CARTESIAN_POINT('Ctrl Pts',(1.00195898707797,30.79997311927,53.2045926301162));
#133132=CARTESIAN_POINT('Ctrl Pts',(1.11309425791653,31.9422845185978,54.6983168637613));
#133133=CARTESIAN_POINT('Ctrl Pts',(1.22422952875509,31.3068785288967,56.4681812386422));
#133134=CARTESIAN_POINT('Ctrl Pts',(1.33536479959365,29.4753229760543,56.8942515731679));
#133135=CARTESIAN_POINT('Ctrl Pts',(1.44650007043221,28.1239897554366,55.5865714020816));
#133136=CARTESIAN_POINT('Ctrl Pts',(1.55763534127076,28.4897157453897,53.7420166322667));
#133137=CARTESIAN_POINT('Ctrl Pts',(1.66877061210933,30.2377624268046,53.0488597700237));
#133138=CARTESIAN_POINT('Ctrl Pts',(1.77990588294789,31.7681918270586,54.141526005001));
#133139=CARTESIAN_POINT('Ctrl Pts',(1.89104115378645,31.6802450745805,56.0199296012311));
#133140=CARTESIAN_POINT('Ctrl Pts',(2.00217642462501,30.0544173317013,56.9648202156473));
#133141=CARTESIAN_POINT('Ctrl Pts',(2.11331169546357,28.3787829419347,56.1113663130958));
#133142=CARTESIAN_POINT('Ctrl Pts',(2.22444696630212,28.1870028523858,54.2407100941288));
#133143=CARTESIAN_POINT('Ctrl Pts',(2.33558223714069,29.6546079793174,53.0650105554149));
#133144=CARTESIAN_POINT('Ctrl Pts',(2.44671750797925,31.4383406922937,53.6603523352754));
#133145=CARTESIAN_POINT('Ctrl Pts',(2.55785277881781,31.9056006891706,55.4818358885204));
#133146=CARTESIAN_POINT('Ctrl Pts',(2.66898804965636,30.6287180575535,56.8623086242662));
#133147=CARTESIAN_POINT('Ctrl Pts',(2.78012332049493,28.7763874994555,56.5382627403222));
#133148=CARTESIAN_POINT('Ctrl Pts',(2.89125859133347,28.0439949928455,54.806288303732));
#133149=CARTESIAN_POINT('Ctrl Pts',(3.00239386217205,29.1018787669375,53.251612726026));
#133150=CARTESIAN_POINT('Ctrl Pts',(3.1135291330106,30.9817876047871,53.297186766438));
#133151=CARTESIAN_POINT('Ctrl Pts',(3.22466440384917,31.9630939057901,54.9012977898799));
#133152=CARTESIAN_POINT('Ctrl Pts',(3.33579967468772,31.1476356568844,56.595748165677));
#133153=CARTESIAN_POINT('Ctrl Pts',(3.44693494552628,29.2817788211282,56.8296551990643));
#133154=CARTESIAN_POINT('Ctrl Pts',(3.55807021636484,28.0732895974775,55.3889303717164));
#133155=CARTESIAN_POINT('Ctrl Pts',(3.6692054872034,28.6282641281478,53.5922285316486));
#133156=CARTESIAN_POINT('Ctrl Pts',(3.78034075804196,30.4387498593314,53.0840202584133));
#133157=CARTESIAN_POINT('Ctrl Pts',(3.89147602888052,31.8476602042343,54.3294542678376));
#133158=CARTESIAN_POINT('Ctrl Pts',(4.00261129971908,31.5654592143968,56.1886198960528));
#133159=CARTESIAN_POINT('Ctrl Pts',(4.11374657055764,29.8504375059698,56.9598752178678));
#133160=CARTESIAN_POINT('Ctrl Pts',(4.2248818413962,28.272306135023,55.937311964158));
#133161=CARTESIAN_POINT('Ctrl Pts',(4.33601711223476,28.2754842880507,54.0568534745479));
#133162=CARTESIAN_POINT('Ctrl Pts',(4.44715238307332,29.8570630911178,53.0396304304259));
#133163=CARTESIAN_POINT('Ctrl Pts',(4.55828765391188,31.5694680202276,53.8166784280192));
#133164=CARTESIAN_POINT('Ctrl Pts',(4.66942292475044,31.8453830837027,55.6767873252483));
#133165=CARTESIAN_POINT('Ctrl Pts',(4.780558195589,30.4322709967113,56.9174518493654));
#133166=CARTESIAN_POINT('Ctrl Pts',(4.89169346642755,28.6235134438802,56.403126712045));
#133167=CARTESIAN_POINT('Ctrl Pts',(5.00282873726612,28.0746152590417,54.6045592224899));
#133168=CARTESIAN_POINT('Ctrl Pts',(5.11396400810467,29.2879674878394,53.1679275366791));
#133169=CARTESIAN_POINT('Ctrl Pts',(5.22509927894324,31.1530230164423,53.4081401654709));
#133170=CARTESIAN_POINT('Ctrl Pts',(5.33623454978178,31.9627490597571,55.1053372567309));
#133171=CARTESIAN_POINT('Ctrl Pts',(5.44736982062036,30.9760261810247,56.7061221243472));
#133172=CARTESIAN_POINT('Ctrl Pts',(5.55850509145891,29.0959740343069,56.7453414744931));
#133173=CARTESIAN_POINT('Ctrl Pts',(5.66964036229747,28.0433513867903,55.1870989408228));
#133174=CARTESIAN_POINT('Ctrl Pts',(5.78077563313603,28.781594094451,53.4576100173576));
#133175=CARTESIAN_POINT('Ctrl Pts',(5.89191090397459,30.6350094039064,53.1398271945372));
#133176=CARTESIAN_POINT('Ctrl Pts',(6.00304617481315,31.9072184947336,54.5246081378709));
#133177=CARTESIAN_POINT('Ctrl Pts',(6.11418144565171,31.4338042253354,56.3445018604091));
#133178=CARTESIAN_POINT('Ctrl Pts',(6.22531671649026,29.6480693399998,56.9338109059017));
#133179=CARTESIAN_POINT('Ctrl Pts',(6.33645198732883,28.1844466735699,55.7531573063582));
#133180=CARTESIAN_POINT('Ctrl Pts',(6.44758725816739,28.3825488211043,53.8831600414011));
#133181=CARTESIAN_POINT('Ctrl Pts',(6.55872252900594,30.0610584676762,53.0353749281974));
#133182=CARTESIAN_POINT('Ctrl Pts',(6.66985779984451,31.6836830188524,53.9857557980152));
#133183=CARTESIAN_POINT('Ctrl Pts',(6.78099307068307,31.7652799336917,55.8644458137724));
#133184=CARTESIAN_POINT('Ctrl Pts',(6.89212834152162,30.2311658546877,56.9519329283661));
#133185=CARTESIAN_POINT('Ctrl Pts',(7.00326361236018,28.4854721810444,56.252870821291));
#133186=CARTESIAN_POINT('Ctrl Pts',(7.11439888319874,28.125983154499,54.4070913459176));
#133187=CARTESIAN_POINT('Ctrl Pts',(7.2255341540373,29.4817289540074,53.1039844589357));
#133188=CARTESIAN_POINT('Ctrl Pts',(7.33666942487587,31.3118336416646,53.5362471841592));
#133189=CARTESIAN_POINT('Ctrl Pts',(7.44780469571442,31.9412539528034,55.3082416267767));
#133190=CARTESIAN_POINT('Ctrl Pts',(7.55893996655298,30.7938992073525,56.7981111913546));
#133191=CARTESIAN_POINT('Ctrl Pts',(7.67007523739155,28.9199108830388,56.6422202378048));
#133192=CARTESIAN_POINT('Ctrl Pts',(7.7812105082301,28.0344976988523,54.9832513614566));
#133193=CARTESIAN_POINT('Ctrl Pts',(7.89234577906866,28.9480534041238,53.3396120459267));
#133194=CARTESIAN_POINT('Ctrl Pts',(8.00348104990723,30.8244261881505,53.2156790426869));
#133195=CARTESIAN_POINT('Ctrl Pts',(8.11461632074577,31.9462249192566,54.724884760671));
#133196=CARTESIAN_POINT('Ctrl Pts',(8.22575159158435,31.2866987842503,56.4858956775006));
#133197=CARTESIAN_POINT('Ctrl Pts',(8.3368868624229,29.4494935477483,56.8869081981243));
#133198=CARTESIAN_POINT('Ctrl Pts',(8.44802213326146,28.1161512629849,55.560886685002));
#133199=CARTESIAN_POINT('Ctrl Pts',(8.55915740410001,28.5070428473976,53.721501619428));
#133200=CARTESIAN_POINT('Ctrl Pts',(8.67029267493858,30.2643956793274,53.0522896498785));
#133201=CARTESIAN_POINT('Ctrl Pts',(8.78142794577713,31.7797553403405,54.1657629977179));
#133202=CARTESIAN_POINT('Ctrl Pts',(8.8925632166157,31.6661535964514,56.0427881831597));
#133203=CARTESIAN_POINT('Ctrl Pts',(9.00369848745425,30.0275713350733,56.9653822682303));
#133204=CARTESIAN_POINT('Ctrl Pts',(9.11483375829281,28.3637479941479,56.0891102970866));
#133205=CARTESIAN_POINT('Ctrl Pts',(9.22596902913138,28.1975515441048,54.2160202941221));
#133206=CARTESIAN_POINT('Ctrl Pts',(9.33710429996993,29.6810625421903,53.0604571912458));
#133207=CARTESIAN_POINT('Ctrl Pts',(9.4482395708085,31.4565333040147,53.6801577764939));
#133208=CARTESIAN_POINT('Ctrl Pts',(9.55937484164705,31.8987903716828,55.507764140826));
#133209=CARTESIAN_POINT('Ctrl Pts',(9.67051011248561,30.6033161195011,56.8708436430855));
#133210=CARTESIAN_POINT('Ctrl Pts',(9.78164538332418,28.7552906341999,56.5211656977594));
#133211=CARTESIAN_POINT('Ctrl Pts',(9.89278065416272,28.047213240497,54.7800545406207));
#133212=CARTESIAN_POINT('Ctrl Pts',(10.0039159250013,29.1250665498602,53.2385687370523));
#133213=CARTESIAN_POINT('Ctrl Pts',(10.1150511958398,31.0066261676809,53.3126786467944));
#133214=CARTESIAN_POINT('Ctrl Pts',(10.1891413763989,31.6416512911897,54.3865918608222));
#133215=CARTESIAN_POINT('Ctrl Pts',(10.2261864666784,31.6618713842553,54.9391906075592));
#133216=CARTESIAN_POINT('Ctrl Pts',(-0.0741837504160435,28.6335084204081,
56.1630365274997));
#133217=CARTESIAN_POINT('Ctrl Pts',(-0.037125725246421,28.2466302951262,
55.7085055712267));
#133218=CARTESIAN_POINT('Ctrl Pts',(0.0369773902027212,27.9692170907089,
54.3908235277015));
#133219=CARTESIAN_POINT('Ctrl Pts',(0.148125595931384,29.4128071670596,
52.9606420400344));
#133220=CARTESIAN_POINT('Ctrl Pts',(0.259260866769943,31.3938416808363,
53.4020218768933));
#133221=CARTESIAN_POINT('Ctrl Pts',(0.370396137608503,32.0990188879581,
55.3036253126424));
#133222=CARTESIAN_POINT('Ctrl Pts',(0.481531408447062,30.883082722185,56.9285136101086));
#133223=CARTESIAN_POINT('Ctrl Pts',(0.592666679285622,28.8588556221624,
56.7876907227286));
#133224=CARTESIAN_POINT('Ctrl Pts',(0.70380195012418,27.8791010713203,55.0109459790591));
#133225=CARTESIAN_POINT('Ctrl Pts',(0.814937220962741,28.8405378700091,
53.2240308099369));
#133226=CARTESIAN_POINT('Ctrl Pts',(0.9260724918013,30.8632015735155,53.062686821028));
#133227=CARTESIAN_POINT('Ctrl Pts',(1.03720776263986,32.0957992366023,54.6744723645939));
#133228=CARTESIAN_POINT('Ctrl Pts',(1.14834303347842,31.4101718862337,56.5842236756135));
#133229=CARTESIAN_POINT('Ctrl Pts',(1.25947830431697,29.4338534361371,57.0439698524931));
#133230=CARTESIAN_POINT('Ctrl Pts',(1.37061357515554,27.9757132383196,55.6329329636953));
#133231=CARTESIAN_POINT('Ctrl Pts',(1.48174884599409,28.3703455608296,53.6425878616088));
#133232=CARTESIAN_POINT('Ctrl Pts',(1.59288411683265,30.2565547466493,52.8946451123234));
#133233=CARTESIAN_POINT('Ctrl Pts',(1.70401938767121,31.9079465679885,54.073673745461));
#133234=CARTESIAN_POINT('Ctrl Pts',(1.81515465850977,31.8130486604264,56.1005430250722));
#133235=CARTESIAN_POINT('Ctrl Pts',(1.92628992934833,30.0587183809301,57.1201161151134));
#133236=CARTESIAN_POINT('Ctrl Pts',(2.03742520018689,28.2506448256545,56.1992067322111));
#133237=CARTESIAN_POINT('Ctrl Pts',(2.14856047102545,28.043706778513,54.1806971687991));
#133238=CARTESIAN_POINT('Ctrl Pts',(2.25969574186401,29.6273088075695,52.912072427101));
#133239=CARTESIAN_POINT('Ctrl Pts',(2.37083101270257,31.5520245854915,53.5544689636547));
#133240=CARTESIAN_POINT('Ctrl Pts',(2.48196628354113,32.0562159824636,55.5199193411982));
#133241=CARTESIAN_POINT('Ctrl Pts',(2.59310155437969,30.6784108159447,57.0095021896548));
#133242=CARTESIAN_POINT('Ctrl Pts',(2.70423682521824,28.6796753410825,56.6598442946911));
#133243=CARTESIAN_POINT('Ctrl Pts',(2.81537209605682,27.889395831799,54.7909776753754));
#133244=CARTESIAN_POINT('Ctrl Pts',(2.92650736689538,29.0308928601318,53.1134233017903));
#133245=CARTESIAN_POINT('Ctrl Pts',(3.03764263773393,31.059386352986,53.1625994333971));
#133246=CARTESIAN_POINT('Ctrl Pts',(3.14877790857249,32.1182533607917,54.8934965425302));
#133247=CARTESIAN_POINT('Ctrl Pts',(3.25991317941105,31.2383427405024,56.7218732659465));
#133248=CARTESIAN_POINT('Ctrl Pts',(3.37104845024961,29.2250118950247,56.9742678957318));
#133249=CARTESIAN_POINT('Ctrl Pts',(3.48218372108817,27.9210058299411,55.4196707373867));
#133250=CARTESIAN_POINT('Ctrl Pts',(3.59331899192673,28.5198445616384,53.4809607756069));
#133251=CARTESIAN_POINT('Ctrl Pts',(3.70445426276529,30.4734278688017,52.9325846232549));
#133252=CARTESIAN_POINT('Ctrl Pts',(3.81558953360385,31.9936959845257,54.2764555243495));
#133253=CARTESIAN_POINT('Ctrl Pts',(3.92672480444241,31.6891903297635,56.282566301129));
#133254=CARTESIAN_POINT('Ctrl Pts',(4.03786007528097,29.8386163521299,57.1147802734938));
#133255=CARTESIAN_POINT('Ctrl Pts',(4.14899534611951,28.135752281074,56.0113954367296));
#133256=CARTESIAN_POINT('Ctrl Pts',(4.26013061695809,28.1391816296711,53.9823088486162));
#133257=CARTESIAN_POINT('Ctrl Pts',(4.37126588779665,29.845765611758,52.8846863021191));
#133258=CARTESIAN_POINT('Ctrl Pts',(4.4824011586352,31.693515984486,53.7231507930656));
#133259=CARTESIAN_POINT('Ctrl Pts',(4.59353642947377,31.9912388844324,55.7302793931661));
#133260=CARTESIAN_POINT('Ctrl Pts',(4.70467170031233,30.4664369283895,57.0690038373076));
#133261=CARTESIAN_POINT('Ctrl Pts',(4.81580697115087,28.5147183917256,56.5140273547993));
#133262=CARTESIAN_POINT('Ctrl Pts',(4.92694224198944,27.9224362694404,54.5733042859109));
#133263=CARTESIAN_POINT('Ctrl Pts',(5.03807751282801,29.2316897029588,53.0231237837388));
#133264=CARTESIAN_POINT('Ctrl Pts',(5.14921278366655,31.2441559073895,53.2823223919879));
#133265=CARTESIAN_POINT('Ctrl Pts',(5.26034805450513,32.1178812587409,55.1136629263779));
#133266=CARTESIAN_POINT('Ctrl Pts',(5.37148332534367,31.0531695565241,56.8409709862378));
#133267=CARTESIAN_POINT('Ctrl Pts',(5.48261859618223,29.0245214279234,56.8832901641483));
#133268=CARTESIAN_POINT('Ctrl Pts',(5.59375386702079,27.8887013562645,55.2018869087362));
#133269=CARTESIAN_POINT('Ctrl Pts',(5.70488913785936,28.6852934560972,53.3357022530876));
#133270=CARTESIAN_POINT('Ctrl Pts',(5.81602440869791,30.6851994191372,52.9928024404727));
#133271=CARTESIAN_POINT('Ctrl Pts',(5.92715967953647,32.0579616565045,54.4870340095917));
#133272=CARTESIAN_POINT('Ctrl Pts',(6.03829495037504,31.5471295642435,56.4507688990334));
#133273=CARTESIAN_POINT('Ctrl Pts',(6.1494302212136,29.6202533658159,57.0866558846116));
#133274=CARTESIAN_POINT('Ctrl Pts',(6.26056549205216,28.0409485638643,55.8126855219167));
#133275=CARTESIAN_POINT('Ctrl Pts',(6.37170076289071,28.2547083532241,53.7948869950688));
#133276=CARTESIAN_POINT('Ctrl Pts',(6.48283603372927,30.0658844204948,52.8800944525541));
#133277=CARTESIAN_POINT('Ctrl Pts',(6.59397130456782,31.8167583337063,53.9055917380309));
#133278=CARTESIAN_POINT('Ctrl Pts',(6.70510657540639,31.9048045237427,55.9327700752596));
#133279=CARTESIAN_POINT('Ctrl Pts',(6.81624184624495,30.2494367931908,57.106210239539));
#133280=CARTESIAN_POINT('Ctrl Pts',(6.92737711708351,28.3657665926968,56.3518955053601));
#133281=CARTESIAN_POINT('Ctrl Pts',(7.03851238792207,27.9778641921028,54.3602288991636));
#133282=CARTESIAN_POINT('Ctrl Pts',(7.14964765876062,29.4407657312078,52.9541267587214));
#133283=CARTESIAN_POINT('Ctrl Pts',(7.26078292959918,31.4155186423124,53.4205547618593));
#133284=CARTESIAN_POINT('Ctrl Pts',(7.37191820043774,32.0946872167183,55.3326044973854));
#133285=CARTESIAN_POINT('Ctrl Pts',(7.4830534712763,30.8566475903901,56.9402307056887));
#133286=CARTESIAN_POINT('Ctrl Pts',(7.59418874211486,28.8345425579441,56.7720184081006));
#133287=CARTESIAN_POINT('Ctrl Pts',(7.70532401295343,27.8791478885599,54.981927578819));
#133288=CARTESIAN_POINT('Ctrl Pts',(7.81645928379199,28.8649094139022,53.2083779316108));
#133289=CARTESIAN_POINT('Ctrl Pts',(7.92759455463055,30.889587369521,53.0746494839541));
#133290=CARTESIAN_POINT('Ctrl Pts',(8.0387298254691,32.1000510795293,54.7031401408792));
#133291=CARTESIAN_POINT('Ctrl Pts',(8.14986509630766,31.3883971704186,56.6033382322506));
#133292=CARTESIAN_POINT('Ctrl Pts',(8.26100036714621,29.4059824957022,57.0360460701312));
#133293=CARTESIAN_POINT('Ctrl Pts',(8.37213563798479,27.9672552053491,55.6052181722048));
#133294=CARTESIAN_POINT('Ctrl Pts',(8.48327090882334,28.3890421661998,53.620451378599));
#133295=CARTESIAN_POINT('Ctrl Pts',(8.5944061796619,30.2852930441393,52.8983460837889));
#133296=CARTESIAN_POINT('Ctrl Pts',(8.70554145050047,31.9204240408184,54.0998263870268));
#133297=CARTESIAN_POINT('Ctrl Pts',(8.81667672133901,31.7978434168986,56.1252083087096));
#133298=CARTESIAN_POINT('Ctrl Pts',(8.92781199217758,30.0297505244187,57.1207225913341));
#133299=CARTESIAN_POINT('Ctrl Pts',(9.03894726301614,28.2344215423033,56.1751916402329));
#133300=CARTESIAN_POINT('Ctrl Pts',(9.15008253385469,28.0550892200863,54.1540559308596));
#133301=CARTESIAN_POINT('Ctrl Pts',(9.26121780469326,29.6558542920972,52.9071591731169));
#133302=CARTESIAN_POINT('Ctrl Pts',(9.37235307553181,31.5716551089249,53.5758397917641));
#133303=CARTESIAN_POINT('Ctrl Pts',(9.48348834637038,32.0488673895799,55.5478969165061));
#133304=CARTESIAN_POINT('Ctrl Pts',(9.59462361720893,30.6510011538336,57.0187118011999));
#133305=CARTESIAN_POINT('Ctrl Pts',(9.70575888804748,28.6569110170744,56.6413959322557));
#133306=CARTESIAN_POINT('Ctrl Pts',(9.81689415888607,27.892868444028,54.7626704422307));
#133307=CARTESIAN_POINT('Ctrl Pts',(9.9280294297246,29.0559133642249,53.0993483390999));
#133308=CARTESIAN_POINT('Ctrl Pts',(10.0391647005632,31.0861881117667,53.1793157644567));
#133309=CARTESIAN_POINT('Ctrl Pts',(10.1132548811223,31.7714044929558,54.3381091711824));
#133310=CARTESIAN_POINT('Ctrl Pts',(10.1502999714018,31.7932227462577,54.9343843412047));
#133311=CARTESIAN_POINT('Ctrl Pts',(-0.150070245692712,28.5334145918423,
56.248227523579));
#133312=CARTESIAN_POINT('Ctrl Pts',(-0.11301222052309,28.1181981194195,
55.7604027334509));
#133313=CARTESIAN_POINT('Ctrl Pts',(-0.0389091050739475,27.8204647387642,
54.3462020998821));
#133314=CARTESIAN_POINT('Ctrl Pts',(0.0722391006547147,29.3697960138018,
52.8112615761681));
#133315=CARTESIAN_POINT('Ctrl Pts',(0.183374371493274,31.4959388707004,
53.2849719435495));
#133316=CARTESIAN_POINT('Ctrl Pts',(0.294509642331834,32.2527694414669,
55.3258654935888));
#133317=CARTESIAN_POINT('Ctrl Pts',(0.405644913170393,30.9477674461335,
57.0697748615937));
#133318=CARTESIAN_POINT('Ctrl Pts',(0.516780184008953,28.775268199137,56.9186368708072));
#133319=CARTESIAN_POINT('Ctrl Pts',(0.627915454847512,27.7237478317228,
55.0117477585708));
#133320=CARTESIAN_POINT('Ctrl Pts',(0.739050725686071,28.7556086941538,
53.0939432497185));
#133321=CARTESIAN_POINT('Ctrl Pts',(0.850185996524631,30.9264300277611,
52.9207810119399));
#133322=CARTESIAN_POINT('Ctrl Pts',(0.961321267363189,32.2493139546068,
54.6506278654266));
#133323=CARTESIAN_POINT('Ctrl Pts',(1.07245653820176,31.5134652435707,56.7002661125848));
#133324=CARTESIAN_POINT('Ctrl Pts',(1.1835918090403,29.39238389622,57.1936881318183));
#133325=CARTESIAN_POINT('Ctrl Pts',(1.29472707987888,27.8274367212027,55.679294525309));
#133326=CARTESIAN_POINT('Ctrl Pts',(1.40586235071743,28.2509753762695,53.5431590909509));
#133327=CARTESIAN_POINT('Ctrl Pts',(1.51699762155598,30.2753470664941,52.7404304546232));
#133328=CARTESIAN_POINT('Ctrl Pts',(1.62813289239454,32.0477013089184,54.005821485921));
#133329=CARTESIAN_POINT('Ctrl Pts',(1.73926816323311,31.9458522462723,56.1811564489131));
#133330=CARTESIAN_POINT('Ctrl Pts',(1.85040343407167,30.0630194301587,57.2754120145795));
#133331=CARTESIAN_POINT('Ctrl Pts',(1.96153870491023,28.1225067093746,56.2870471513263));
#133332=CARTESIAN_POINT('Ctrl Pts',(2.07267397574878,27.9004107046402,54.1206842434695));
#133333=CARTESIAN_POINT('Ctrl Pts',(2.18380924658734,29.6000096358219,52.7591342987872));
#133334=CARTESIAN_POINT('Ctrl Pts',(2.2949445174259,31.6657084786893,53.4485855920342));
#133335=CARTESIAN_POINT('Ctrl Pts',(2.40607978826446,32.2068312757568,55.5580027938758));
#133336=CARTESIAN_POINT('Ctrl Pts',(2.51721505910302,30.7281035743359,57.1566957550435));
#133337=CARTESIAN_POINT('Ctrl Pts',(2.62835032994158,28.5829631827096,56.7814258490598));
#133338=CARTESIAN_POINT('Ctrl Pts',(2.73948560078014,27.7347966707524,54.7756670470189));
#133339=CARTESIAN_POINT('Ctrl Pts',(2.8506208716187,28.959906953326,52.9752338775547));
#133340=CARTESIAN_POINT('Ctrl Pts',(2.96175614245727,31.1369851011849,53.0280121003562));
#133341=CARTESIAN_POINT('Ctrl Pts',(3.07289141329581,32.2734128157934,54.8856952951807));
#133342=CARTESIAN_POINT('Ctrl Pts',(3.18402668413438,31.3290498241205,56.847998366216));
#133343=CARTESIAN_POINT('Ctrl Pts',(3.29516195497293,29.1682449689211,57.1188805923993));
#133344=CARTESIAN_POINT('Ctrl Pts',(3.40629722581149,27.7687220624047,55.4504111030571));
#133345=CARTESIAN_POINT('Ctrl Pts',(3.51743249665005,28.4114249951292,53.3696930195652));
#133346=CARTESIAN_POINT('Ctrl Pts',(3.62856776748862,30.5081058782719,52.7811489880965));
#133347=CARTESIAN_POINT('Ctrl Pts',(3.73970303832718,32.1397317648171,54.2234567808614));
#133348=CARTESIAN_POINT('Ctrl Pts',(3.85083830916574,31.8129214451303,56.3765127062051));
#133349=CARTESIAN_POINT('Ctrl Pts',(3.96197358000429,29.82679519829,57.26968532912));
#133350=CARTESIAN_POINT('Ctrl Pts',(4.07310885084286,27.9991984271249,56.0854789093014));
#133351=CARTESIAN_POINT('Ctrl Pts',(4.18424412168142,28.0028789712916,53.9077642226845));
#133352=CARTESIAN_POINT('Ctrl Pts',(4.29537939251997,29.8344681323984,52.7297421738124));
#133353=CARTESIAN_POINT('Ctrl Pts',(4.40651466335854,31.8175639487442,53.6296231581121));
#133354=CARTESIAN_POINT('Ctrl Pts',(4.5176499341971,32.1370946851621,55.783771461084));
#133355=CARTESIAN_POINT('Ctrl Pts',(4.62878520503565,30.5006028600674,57.2205558252495));
#133356=CARTESIAN_POINT('Ctrl Pts',(4.73992047587422,28.4059233395712,56.6249279975537));
#133357=CARTESIAN_POINT('Ctrl Pts',(4.85105574671277,27.7702572798392,54.542049349332));
#133358=CARTESIAN_POINT('Ctrl Pts',(4.96219101755134,29.1754119180782,52.8783200307987));
#133359=CARTESIAN_POINT('Ctrl Pts',(5.07332628838988,31.3352887983368,53.1565046185048));
#133360=CARTESIAN_POINT('Ctrl Pts',(5.18446155922844,32.2730134577246,55.121988596025));
#133361=CARTESIAN_POINT('Ctrl Pts',(5.295596830067,31.1303129320237,56.9758198481282));
#133362=CARTESIAN_POINT('Ctrl Pts',(5.40673210090556,28.9530688215398,57.0212388538038));
#133363=CARTESIAN_POINT('Ctrl Pts',(5.51786737174412,27.7340513257388,55.2166748766493));
#133364=CARTESIAN_POINT('Ctrl Pts',(5.6290026425827,28.5889928177436,53.2137944888177));
#133365=CARTESIAN_POINT('Ctrl Pts',(5.74013791342125,30.735389434368,52.8457776864079));
#133366=CARTESIAN_POINT('Ctrl Pts',(5.85127318425982,32.2087048182755,54.4494598813127));
#133367=CARTESIAN_POINT('Ctrl Pts',(5.96240845509836,31.6604549031516,56.5570359376577));
#133368=CARTESIAN_POINT('Ctrl Pts',(6.07354372593693,29.592437391632,57.2395008633215));
#133369=CARTESIAN_POINT('Ctrl Pts',(6.18467899677548,27.8974504541587,55.8722137374748));
#133370=CARTESIAN_POINT('Ctrl Pts',(6.29581426761406,28.1268678853437,53.7066139487367));
#133371=CARTESIAN_POINT('Ctrl Pts',(6.4069495384526,30.0707103733134,52.7248139769108));
#133372=CARTESIAN_POINT('Ctrl Pts',(6.51808480929118,31.9498336485602,53.8254276780467));
#133373=CARTESIAN_POINT('Ctrl Pts',(6.62922008012973,32.0443291137937,56.001094336747));
#133374=CARTESIAN_POINT('Ctrl Pts',(6.74035535096829,30.2677077316937,57.2604875507119));
#133375=CARTESIAN_POINT('Ctrl Pts',(6.85149062180684,28.2460610043493,56.4509201894293));
#133376=CARTESIAN_POINT('Ctrl Pts',(6.9626258926454,27.8297452297067,54.3133664524095));
#133377=CARTESIAN_POINT('Ctrl Pts',(7.07376116348396,29.3998025084083,52.8042690585072));
#133378=CARTESIAN_POINT('Ctrl Pts',(7.18489643432252,31.5192036429601,53.3048623395593));
#133379=CARTESIAN_POINT('Ctrl Pts',(7.29603170516107,32.2481204806333,55.3569673679941));
#133380=CARTESIAN_POINT('Ctrl Pts',(7.40716697599964,30.9193959734275,57.0823502200226));
#133381=CARTESIAN_POINT('Ctrl Pts',(7.51830224683819,28.7491742328494,56.9018165783966));
#133382=CARTESIAN_POINT('Ctrl Pts',(7.62943751767676,27.7237980782675,54.9806037961815));
#133383=CARTESIAN_POINT('Ctrl Pts',(7.7405727885153,28.7817654236807,53.0771438172949));
#133384=CARTESIAN_POINT('Ctrl Pts',(7.85170805935387,30.9547485508914,52.9336199252212));
#133385=CARTESIAN_POINT('Ctrl Pts',(7.96284333019243,32.2538772398021,54.6813955210875));
#133386=CARTESIAN_POINT('Ctrl Pts',(8.07397860103099,31.4900955565868,56.7207807870007));
#133387=CARTESIAN_POINT('Ctrl Pts',(8.18511387186956,29.362471443656,57.185183942138));
#133388=CARTESIAN_POINT('Ctrl Pts',(8.29624914270812,27.8183591477134,55.6495496594077));
#133389=CARTESIAN_POINT('Ctrl Pts',(8.40738441354667,28.2710414850018,53.5194011377699));
#133390=CARTESIAN_POINT('Ctrl Pts',(8.51851968438524,30.3061904089512,52.7444025176994));
#133391=CARTESIAN_POINT('Ctrl Pts',(8.62965495522378,32.0610927412963,54.0338897763355));
#133392=CARTESIAN_POINT('Ctrl Pts',(8.74079022606235,31.9295332373459,56.2076284342593));
#133393=CARTESIAN_POINT('Ctrl Pts',(8.85192549690091,30.0319297137642,57.2760629144379));
#133394=CARTESIAN_POINT('Ctrl Pts',(8.96306076773945,28.1050950904588,56.2612729833792));
#133395=CARTESIAN_POINT('Ctrl Pts',(9.07419603857805,27.9126268960678,54.0920915675973));
#133396=CARTESIAN_POINT('Ctrl Pts',(9.18533130941658,29.6306460420042,52.753861154988));
#133397=CARTESIAN_POINT('Ctrl Pts',(9.29646658025515,31.686776913835,53.4715218070343));
#133398=CARTESIAN_POINT('Ctrl Pts',(9.40760185109372,32.1989444074769,55.5880296921861));
#133399=CARTESIAN_POINT('Ctrl Pts',(9.51873712193226,30.698686188166,57.1665799593141));
#133400=CARTESIAN_POINT('Ctrl Pts',(9.62987239277085,28.5585313999489,56.7616261667521));
#133401=CARTESIAN_POINT('Ctrl Pts',(9.74100766360938,27.7385236475588,54.7452863438404));
#133402=CARTESIAN_POINT('Ctrl Pts',(9.85214293444796,28.9867601785899,52.9601279411475));
#133403=CARTESIAN_POINT('Ctrl Pts',(9.9632782052865,31.1657500558526,53.0459528821187));
#133404=CARTESIAN_POINT('Ctrl Pts',(10.0373683858456,31.9011576947219,54.2896264815424));
#133405=CARTESIAN_POINT('Ctrl Pts',(10.0744134761251,31.9245741082599,54.9295780748502));
#133406=CARTESIAN_POINT('Ctrl Pts',(-0.225956740969381,28.4333207632767,
56.3334185196581));
#133407=CARTESIAN_POINT('Ctrl Pts',(-0.188898715799759,27.9897659437127,
55.8122998956753));
#133408=CARTESIAN_POINT('Ctrl Pts',(-0.114795600350617,27.6717123868196,
54.3015806720628));
#133409=CARTESIAN_POINT('Ctrl Pts',(-0.00364739462195415,29.326784860544,
52.6618811123017));
#133410=CARTESIAN_POINT('Ctrl Pts',(0.107487876216605,31.5980360605646,
53.1679220102057));
#133411=CARTESIAN_POINT('Ctrl Pts',(0.218623147055165,32.4065199949758,
55.3481056745352));
#133412=CARTESIAN_POINT('Ctrl Pts',(0.329758417893724,31.0124521700819,
57.2110361130788));
#133413=CARTESIAN_POINT('Ctrl Pts',(0.440893688732284,28.6916807761116,
57.0495830188858));
#133414=CARTESIAN_POINT('Ctrl Pts',(0.552028959570843,27.5683945921251,
55.0125495380824));
#133415=CARTESIAN_POINT('Ctrl Pts',(0.663164230409402,28.6706795182987,
52.9638556895));
#133416=CARTESIAN_POINT('Ctrl Pts',(0.774299501247962,30.9896584820065,
52.7788752028517));
#133417=CARTESIAN_POINT('Ctrl Pts',(0.885434772086521,32.4028286726114,
54.6267833662593));
#133418=CARTESIAN_POINT('Ctrl Pts',(0.996570042925081,31.6167586009078,
56.8163085495561));
#133419=CARTESIAN_POINT('Ctrl Pts',(1.10770531376365,29.3509143563028,57.3434064111436));
#133420=CARTESIAN_POINT('Ctrl Pts',(1.21884058460219,27.6791602040858,55.7256560869226));
#133421=CARTESIAN_POINT('Ctrl Pts',(1.32997585544075,28.1316051917093,53.4437303202929));
#133422=CARTESIAN_POINT('Ctrl Pts',(1.44111112627932,30.2941393863388,52.5862157969229));
#133423=CARTESIAN_POINT('Ctrl Pts',(1.55224639711788,32.1874560498483,53.937969226381));
#133424=CARTESIAN_POINT('Ctrl Pts',(1.66338166795644,32.0786558321182,56.261769872754));
#133425=CARTESIAN_POINT('Ctrl Pts',(1.77451693879499,30.0673204793875,57.4307079140457));
#133426=CARTESIAN_POINT('Ctrl Pts',(1.88565220963356,27.9943685930944,56.3748875704415));
#133427=CARTESIAN_POINT('Ctrl Pts',(1.99678748047212,27.7571146307674,54.06067131814));
#133428=CARTESIAN_POINT('Ctrl Pts',(2.10792275131068,29.5727104640742,52.6061961704733));
#133429=CARTESIAN_POINT('Ctrl Pts',(2.21905802214923,31.779392371887,53.3427022204136));
#133430=CARTESIAN_POINT('Ctrl Pts',(2.33019329298779,32.3574465690499,55.5960862465536));
#133431=CARTESIAN_POINT('Ctrl Pts',(2.44132856382636,30.7777963327271,57.3038893204322));
#133432=CARTESIAN_POINT('Ctrl Pts',(2.55246383466492,28.4862510243367,56.9030074034286));
#133433=CARTESIAN_POINT('Ctrl Pts',(2.66359910550347,27.5801975097059,54.7603564186625));
#133434=CARTESIAN_POINT('Ctrl Pts',(2.77473437634204,28.8889210465201,52.837044453319));
#133435=CARTESIAN_POINT('Ctrl Pts',(2.88586964718059,31.2145838493837,52.8934247673154));
#133436=CARTESIAN_POINT('Ctrl Pts',(2.99700491801916,32.428572270795,54.8778940478309));
#133437=CARTESIAN_POINT('Ctrl Pts',(3.10814018885771,31.4197569077386,56.9741234664856));
#133438=CARTESIAN_POINT('Ctrl Pts',(3.21927545969628,29.1114780428174,57.2634932890667));
#133439=CARTESIAN_POINT('Ctrl Pts',(3.33041073053483,27.6164382948684,55.4811514687273));
#133440=CARTESIAN_POINT('Ctrl Pts',(3.44154600137339,28.3030054286198,53.2584252635236));
#133441=CARTESIAN_POINT('Ctrl Pts',(3.55268127221196,30.5427838877422,52.6297133529383));
#133442=CARTESIAN_POINT('Ctrl Pts',(3.6638165430505,32.2857675451084,54.1704580373733));
#133443=CARTESIAN_POINT('Ctrl Pts',(3.77495181388906,31.9366525604971,56.4704591112811));
#133444=CARTESIAN_POINT('Ctrl Pts',(3.88608708472762,29.8149740444501,57.424590384746));
#133445=CARTESIAN_POINT('Ctrl Pts',(3.99722235556618,27.8626445731759,56.1595623818731));
#133446=CARTESIAN_POINT('Ctrl Pts',(4.10835762640474,27.866576312912,53.8332195967528));
#133447=CARTESIAN_POINT('Ctrl Pts',(4.21949289724331,29.8231706530387,52.5747980455056));
#133448=CARTESIAN_POINT('Ctrl Pts',(4.33062816808186,31.9416119130024,53.5360955231585));
#133449=CARTESIAN_POINT('Ctrl Pts',(4.44176343892042,32.2829504858917,55.8372635290018));
#133450=CARTESIAN_POINT('Ctrl Pts',(4.55289870975898,30.5347687917455,57.3721078131917));
#133451=CARTESIAN_POINT('Ctrl Pts',(4.66403398059754,28.2971282874166,56.7358286403078));
#133452=CARTESIAN_POINT('Ctrl Pts',(4.77516925143611,27.6180782902379,54.5107944127531));
#133453=CARTESIAN_POINT('Ctrl Pts',(4.88630452227465,29.1191341331977,52.7335162778585));
#133454=CARTESIAN_POINT('Ctrl Pts',(4.99743979311322,31.426421689284,53.0306868450219));
#133455=CARTESIAN_POINT('Ctrl Pts',(5.10857506395178,32.4281456567085,55.130314265672));
#133456=CARTESIAN_POINT('Ctrl Pts',(5.21971033479033,31.2074563075231,57.1106687100188));
#133457=CARTESIAN_POINT('Ctrl Pts',(5.3308456056289,28.8816162151564,57.1591875434591));
#133458=CARTESIAN_POINT('Ctrl Pts',(5.44198087646746,27.5794012952129,55.2314628445626));
#133459=CARTESIAN_POINT('Ctrl Pts',(5.55311614730602,28.4926921793899,53.0918867245477));
#133460=CARTESIAN_POINT('Ctrl Pts',(5.66425141814458,30.7855794495987,52.6987529323434));
#133461=CARTESIAN_POINT('Ctrl Pts',(5.77538668898315,32.3594479800464,54.4118857530334));
#133462=CARTESIAN_POINT('Ctrl Pts',(5.88652195982169,31.7737802420597,56.6633029762821));
#133463=CARTESIAN_POINT('Ctrl Pts',(5.99765723066025,29.5646214174482,57.3923458420313));
#133464=CARTESIAN_POINT('Ctrl Pts',(6.10879250149881,27.7539523444532,55.9317419530332));
#133465=CARTESIAN_POINT('Ctrl Pts',(6.21992777233738,27.9990274174633,53.6183409024045));
#133466=CARTESIAN_POINT('Ctrl Pts',(6.33106304317593,30.0755363261321,52.5695335012675));
#133467=CARTESIAN_POINT('Ctrl Pts',(6.44219831401451,32.082908963414,53.7452636180623));
#133468=CARTESIAN_POINT('Ctrl Pts',(6.55333358485306,32.1838537038447,56.0694185982343));
#133469=CARTESIAN_POINT('Ctrl Pts',(6.66446885569162,30.2859786701968,57.4147648618848));
#133470=CARTESIAN_POINT('Ctrl Pts',(6.77560412653018,28.1263554160018,56.5499448734984));
#133471=CARTESIAN_POINT('Ctrl Pts',(6.88673939736874,27.6816262673105,54.2665040056556));
#133472=CARTESIAN_POINT('Ctrl Pts',(6.9978746682073,29.3588392856087,52.6544113582929));
#133473=CARTESIAN_POINT('Ctrl Pts',(7.10900993904585,31.622888643608,53.1891699172596));
#133474=CARTESIAN_POINT('Ctrl Pts',(7.22014520988442,32.4015537445481,55.3813302386028));
#133475=CARTESIAN_POINT('Ctrl Pts',(7.33128048072298,30.982144356465,57.2244697343568));
#133476=CARTESIAN_POINT('Ctrl Pts',(7.44241575156153,28.6638059077547,57.0316147486923));
#133477=CARTESIAN_POINT('Ctrl Pts',(7.5535510224001,27.5684482679751,54.9792800135439));
#133478=CARTESIAN_POINT('Ctrl Pts',(7.66468629323865,28.6986214334592,52.9459097029788));
#133479=CARTESIAN_POINT('Ctrl Pts',(7.77582156407722,31.019909732262,52.7925903664883));
#133480=CARTESIAN_POINT('Ctrl Pts',(7.88695683491577,32.4077034000748,54.6596509012957));
#133481=CARTESIAN_POINT('Ctrl Pts',(7.99809210575433,31.591793942755,56.8382233417508));
#133482=CARTESIAN_POINT('Ctrl Pts',(8.10922737659289,29.3189603916098,57.3343218141449));
#133483=CARTESIAN_POINT('Ctrl Pts',(8.22036264743145,27.6694630900778,55.6938811466105));
#133484=CARTESIAN_POINT('Ctrl Pts',(8.33149791827,28.1530408038039,53.4183508969409));
#133485=CARTESIAN_POINT('Ctrl Pts',(8.44263318910856,30.3270877737631,52.5904589516098));
#133486=CARTESIAN_POINT('Ctrl Pts',(8.55376845994713,32.2017614417742,53.9679531656445));
#133487=CARTESIAN_POINT('Ctrl Pts',(8.66490373078569,32.061223057793,56.2900485598091));
#133488=CARTESIAN_POINT('Ctrl Pts',(8.77603900162424,30.0341089031096,57.4314032375418));
#133489=CARTESIAN_POINT('Ctrl Pts',(8.8871742724628,27.9757686386143,56.3473543265254));
#133490=CARTESIAN_POINT('Ctrl Pts',(8.99830954330136,27.7701645720494,54.0301272043351));
#133491=CARTESIAN_POINT('Ctrl Pts',(9.10944481413992,29.6054377919111,52.6005631368589));
#133492=CARTESIAN_POINT('Ctrl Pts',(9.22058008497849,31.8018987187452,53.3672038223045));
#133493=CARTESIAN_POINT('Ctrl Pts',(9.33171535581705,32.3490214253738,55.6281624678661));
#133494=CARTESIAN_POINT('Ctrl Pts',(9.44285062665559,30.7463712224987,57.3144481174284));
#133495=CARTESIAN_POINT('Ctrl Pts',(9.55398589749417,28.4601517828233,56.8818564012485));
#133496=CARTESIAN_POINT('Ctrl Pts',(9.66512116833272,27.5841788510897,54.7279022454503));
#133497=CARTESIAN_POINT('Ctrl Pts',(9.77625643917129,28.9176069929546,52.8209075431952));
#133498=CARTESIAN_POINT('Ctrl Pts',(9.88739171000984,31.2453119999385,52.9125899997809));
#133499=CARTESIAN_POINT('Ctrl Pts',(9.96148189056888,32.030910896488,54.2411437919026));
#133500=CARTESIAN_POINT('Ctrl Pts',(9.9985269808484,32.0559254702622,54.9247718084957));
#133501=CARTESIAN_POINT('',(10.0008693306327,29.2294100445698,53.5212313410887));
#133502=CARTESIAN_POINT('Ctrl Pts',(10.,32.0533758325287,54.9248651020699));
#133503=CARTESIAN_POINT('Ctrl Pts',(9.99999999999998,32.0436832069832,54.8508488304773));
#133504=CARTESIAN_POINT('Ctrl Pts',(10.,32.0296436856721,54.777570200097));
#133505=CARTESIAN_POINT('Ctrl Pts',(10.,32.011488473763,54.7053068406861));
#133506=CARTESIAN_POINT('Ctrl Pts',(10.,31.9938094546564,54.6349388759312));
#133507=CARTESIAN_POINT('Ctrl Pts',(9.99999999999998,31.9722270068482,54.5655330028697));
#133508=CARTESIAN_POINT('Ctrl Pts',(9.99999999999999,31.9469147886137,54.4973682067378));
#133509=CARTESIAN_POINT('Ctrl Pts',(9.99999999999999,31.9412650452606,54.4821536727806));
#133510=CARTESIAN_POINT('Ctrl Pts',(10.,31.9354285487349,54.4669990730982));
#133511=CARTESIAN_POINT('Ctrl Pts',(10.,31.9294095815725,54.4519141334687));
#133512=CARTESIAN_POINT('Ctrl Pts',(10.,31.9017891954822,54.3826909851324));
#133513=CARTESIAN_POINT('Ctrl Pts',(10.,31.8703857715094,54.3150694449083));
#133514=CARTESIAN_POINT('Ctrl Pts',(10.,31.8354092014842,54.2493420824359));
#133515=CARTESIAN_POINT('Ctrl Pts',(10.,31.8108541343843,54.2031986271272));
#133516=CARTESIAN_POINT('Ctrl Pts',(10.,31.7845369863314,54.1579892552018));
#133517=CARTESIAN_POINT('Ctrl Pts',(10.,31.7565193347055,54.1138258658698));
#133518=CARTESIAN_POINT('Ctrl Pts',(10.,31.7458689517922,54.0970379846649));
#133519=CARTESIAN_POINT('Ctrl Pts',(10.,31.7349727648439,54.080401351714));
#133520=CARTESIAN_POINT('Ctrl Pts',(10.,31.7238338766828,54.063922520157));
#133521=CARTESIAN_POINT('Ctrl Pts',(10.,31.7132202172074,54.0482207100508));
#133522=CARTESIAN_POINT('Ctrl Pts',(10.,31.702382609243,54.0326574079742));
#133523=CARTESIAN_POINT('Ctrl Pts',(10.,31.6913434743771,54.0172654257873));
#133524=CARTESIAN_POINT('Ctrl Pts',(9.99999999999999,31.6490748357409,53.9583298170775));
#133525=CARTESIAN_POINT('Ctrl Pts',(10.,31.6038135855978,53.9018382421701));
#133526=CARTESIAN_POINT('Ctrl Pts',(10.,31.5557517714265,53.8480620861241));
#133527=CARTESIAN_POINT('Ctrl Pts',(10.,31.5087931407094,53.7955202772746));
#133528=CARTESIAN_POINT('Ctrl Pts',(10.,31.4591602697449,53.7455701374524));
#133529=CARTESIAN_POINT('Ctrl Pts',(10.,31.4070038374311,53.6985041612426));
#133530=CARTESIAN_POINT('Ctrl Pts',(10.,31.3556856160202,53.6521945867392));
#133531=CARTESIAN_POINT('Ctrl Pts',(9.99999999999999,31.3019236685778,53.6086767368471));
#133532=CARTESIAN_POINT('Ctrl Pts',(9.99999999999999,31.2458437756219,53.5682751968982));
#133533=CARTESIAN_POINT('Ctrl Pts',(9.99999999999999,31.2276727281975,53.5551842607403));
#133534=CARTESIAN_POINT('Ctrl Pts',(10.,31.2092582189262,53.5424208988166));
#133535=CARTESIAN_POINT('Ctrl Pts',(10.,31.1906042818692,53.5299973393956));
#133536=CARTESIAN_POINT('Ctrl Pts',(10.,31.1801024108385,53.5230030722668));
#133537=CARTESIAN_POINT('Ctrl Pts',(10.,31.1695235040959,53.5161159030876));
#133538=CARTESIAN_POINT('Ctrl Pts',(10.,31.1588834524544,53.5093474110969));
#133539=CARTESIAN_POINT('Ctrl Pts',(10.,31.101253429008,53.4726870296196));
#133540=CARTESIAN_POINT('Ctrl Pts',(9.99999999999998,31.0417325215066,53.4394372488709));
#133541=CARTESIAN_POINT('Ctrl Pts',(9.99999999999999,30.9804647762413,53.409865079986));
#133542=CARTESIAN_POINT('Ctrl Pts',(9.99999999999999,30.9716322758967,53.4056018874899));
#133543=CARTESIAN_POINT('Ctrl Pts',(9.99999999999998,30.9627634386846,53.4014152082538));
#133544=CARTESIAN_POINT('Ctrl Pts',(9.99999999999999,30.9538586655155,53.3973059277124));
#133545=CARTESIAN_POINT('Ctrl Pts',(9.99999999999999,30.8905564254343,53.3680938794712));
#133546=CARTESIAN_POINT('Ctrl Pts',(9.99999999999997,30.8254386050166,53.3427888225031));
#133547=CARTESIAN_POINT('Ctrl Pts',(9.99999999999996,30.7588787740053,53.3213756036074));
#133548=CARTESIAN_POINT('Ctrl Pts',(9.99999999999995,30.697419300789,53.3016032404087));
#133549=CARTESIAN_POINT('Ctrl Pts',(9.99999999999996,30.6347294993411,53.2851497911376));
#133550=CARTESIAN_POINT('Ctrl Pts',(9.99999999999998,30.5711069811699,53.2720426229371));
#133551=CARTESIAN_POINT('Ctrl Pts',(9.99999999999999,30.557055646849,53.269147842792));
#133552=CARTESIAN_POINT('Ctrl Pts',(9.99999999999998,30.5429588580867,53.2664164255331));
#133553=CARTESIAN_POINT('Ctrl Pts',(9.99999999999997,30.5288199046136,53.2638489053184));
#133554=CARTESIAN_POINT('Ctrl Pts',(9.99999999999997,30.5176851752098,53.2618269280282));
#133555=CARTESIAN_POINT('Ctrl Pts',(9.99999999999999,30.5065248337635,53.2599067801427));
#133556=CARTESIAN_POINT('Ctrl Pts',(9.99999999999999,30.4953536355096,53.2580906150721));
#133557=CARTESIAN_POINT('Ctrl Pts',(9.99999999999998,30.4278879692109,53.247122338992));
#133558=CARTESIAN_POINT('Ctrl Pts',(9.99999999999995,30.3599021685379,53.2399190427721));
#133559=CARTESIAN_POINT('Ctrl Pts',(9.99999999999996,30.2917474304394,53.2364479110107));
#133560=CARTESIAN_POINT('Ctrl Pts',(9.99999999999997,30.2243114893283,53.2330133876953));
#133561=CARTESIAN_POINT('Ctrl Pts',(9.99999999999996,30.1567090796788,53.233233010574));
#133562=CARTESIAN_POINT('Ctrl Pts',(9.99999999999997,30.0892889665376,53.2371242546236));
#133563=CARTESIAN_POINT('Ctrl Pts',(9.99999999999998,30.0224411516751,53.2409824676953));
#133564=CARTESIAN_POINT('Ctrl Pts',(9.99999999999999,29.9557715754486,53.2484504808556));
#133565=CARTESIAN_POINT('Ctrl Pts',(9.99999999999998,29.8896438474063,53.2595900690709));
#133566=CARTESIAN_POINT('Ctrl Pts',(9.99999999999998,29.8705616649699,53.2628045701717));
#133567=CARTESIAN_POINT('Ctrl Pts',(9.99999999999998,29.851524804742,53.2663250773652));
#133568=CARTESIAN_POINT('Ctrl Pts',(9.99999999999999,29.8325425498808,53.2701537316448));
#133569=CARTESIAN_POINT('Ctrl Pts',(10.,29.8219564844318,53.2722889039455));
#133570=CARTESIAN_POINT('Ctrl Pts',(9.99999999999997,29.8113968593313,53.2745180133388));
#133571=CARTESIAN_POINT('Ctrl Pts',(9.99999999999996,29.8008654253447,53.2768409064225));
#133572=CARTESIAN_POINT('Ctrl Pts',(9.99999999999995,29.7370929698571,53.2909070436615));
#133573=CARTESIAN_POINT('Ctrl Pts',(9.99999999999996,29.6743481658389,53.3084091960948));
#133574=CARTESIAN_POINT('Ctrl Pts',(9.99999999999998,29.6129512937306,53.3293566255847));
#133575=CARTESIAN_POINT('Ctrl Pts',(9.99999999999999,29.5524450572685,53.350000187357));
#133576=CARTESIAN_POINT('Ctrl Pts',(10.,29.4932470869475,53.3739901108916));
#133577=CARTESIAN_POINT('Ctrl Pts',(9.99999999999999,29.4356920546672,53.4013774099463));
#133578=CARTESIAN_POINT('Ctrl Pts',(9.99999999999998,29.3781370223868,53.428764709001));
#133579=CARTESIAN_POINT('Ctrl Pts',(10.,29.3222240651368,53.4595495870449));
#133580=CARTESIAN_POINT('Ctrl Pts',(10.,29.2683289856055,53.4938218112857));
#133581=CARTESIAN_POINT('Ctrl Pts',(10.,29.2642059165283,53.4964436971648));
#133582=CARTESIAN_POINT('Ctrl Pts',(9.99999999999998,29.2600946807948,53.4990860107153));
#133583=CARTESIAN_POINT('Ctrl Pts',(9.99999999999999,29.2559954588133,53.5017488009346));
#133584=CARTESIAN_POINT('Ctrl Pts',(10.,29.2468791070862,53.5076706398406));
#133585=CARTESIAN_POINT('Ctrl Pts',(9.99999999999998,29.2378221709542,53.5136937523903));
#133586=CARTESIAN_POINT('Ctrl Pts',(9.99999999999999,29.2288257276126,53.5198168253508));
#133587=CARTESIAN_POINT('Ctrl Pts',(-1.11065670549415E-15,28.7309291201476,
56.0793586530485));
#133588=CARTESIAN_POINT('Ctrl Pts',(1.40820494214792E-14,28.6853758729853,
56.036862308157));
#133589=CARTESIAN_POINT('Ctrl Pts',(7.46374256104984E-15,28.6425793874778,
55.9917717289187));
#133590=CARTESIAN_POINT('Ctrl Pts',(3.6949610038306E-15,28.6025382767428,
55.9444368944416));
#133591=CARTESIAN_POINT('Ctrl Pts',(-2.11776492034417E-16,28.5610314644456,
55.8953693722451));
#133592=CARTESIAN_POINT('Ctrl Pts',(-1.42116051368288E-14,28.5224848860696,
55.8438898433626));
#133593=CARTESIAN_POINT('Ctrl Pts',(4.5102810375397E-16,28.4869236243661,
55.7903375225762));
#133594=CARTESIAN_POINT('Ctrl Pts',(1.38529299224628E-14,28.4544200126287,
55.7413897699068));
#133595=CARTESIAN_POINT('Ctrl Pts',(3.2556342786873E-15,28.4244104857153,
55.6907093010964));
#133596=CARTESIAN_POINT('Ctrl Pts',(4.71844785465692E-16,28.3969384585817,
55.6385258504283));
#133597=CARTESIAN_POINT('Ctrl Pts',(-9.03483966360219E-16,28.383435856458,
55.612877492978));
#133598=CARTESIAN_POINT('Ctrl Pts',(-2.82856510769481E-14,28.3705466339733,
55.5868656756228));
#133599=CARTESIAN_POINT('Ctrl Pts',(-1.21569421196455E-14,28.3582783186024,
55.5605158043874));
#133600=CARTESIAN_POINT('Ctrl Pts',(-4.6121945743922E-15,28.3526720561333,
55.5484746814046));
#133601=CARTESIAN_POINT('Ctrl Pts',(1.38947693528612E-14,28.3471948800546,
55.5363612929739));
#133602=CARTESIAN_POINT('Ctrl Pts',(9.5964902691037E-15,28.3418560093508,
55.524197994614));
#133603=CARTESIAN_POINT('Ctrl Pts',(-1.11574869560312E-14,28.3149353070124,
55.4628658229304));
#133604=CARTESIAN_POINT('Ctrl Pts',(-7.98462157858785E-15,28.2914758629066,
55.400158212843));
#133605=CARTESIAN_POINT('Ctrl Pts',(-9.95731275210687E-15,28.2715012520033,
55.3364328839772));
#133606=CARTESIAN_POINT('Ctrl Pts',(-1.19923092204882E-14,28.2511181538008,
55.2714043513795));
#133607=CARTESIAN_POINT('Ctrl Pts',(-3.07508960440585E-14,28.2343632979817,
55.2053152157044));
#133608=CARTESIAN_POINT('Ctrl Pts',(-2.47163400857175E-14,28.2213014270528,
55.1385087524746));
#133609=CARTESIAN_POINT('Ctrl Pts',(-1.96985779232646E-14,28.2104404188577,
55.0829588585445));
#133610=CARTESIAN_POINT('Ctrl Pts',(-3.14336743467927E-14,28.2021333189636,
55.0269120563622));
#133611=CARTESIAN_POINT('Ctrl Pts',(-2.94902990916057E-14,28.1964419417431,
54.9705535356952));
#133612=CARTESIAN_POINT('Ctrl Pts',(-2.86701166028188E-14,28.1938115155022,
54.9445058980301));
#133613=CARTESIAN_POINT('Ctrl Pts',(-1.27533407423501E-14,28.191740161086,
54.9183915626081));
#133614=CARTESIAN_POINT('Ctrl Pts',(-2.15660822533437E-14,28.1902357805568,
54.8922284121185));
#133615=CARTESIAN_POINT('Ctrl Pts',(-2.53088403276183E-14,28.1895788075958,
54.8808027906674));
#133616=CARTESIAN_POINT('Ctrl Pts',(2.03905128226202E-15,28.1890300817403,
54.8693680844173));
#133617=CARTESIAN_POINT('Ctrl Pts',(1.98452365651747E-15,28.1885905940451,
54.8579398818212));
#133618=CARTESIAN_POINT('Ctrl Pts',(1.7123297641234E-15,28.1858938459936,
54.7878150901245));
#133619=CARTESIAN_POINT('Ctrl Pts',(-2.75809254679551E-14,28.1872979880003,
54.7178038384048));
#133620=CARTESIAN_POINT('Ctrl Pts',(-6.75848266240564E-15,28.1928577234074,
54.6482668481114));
#133621=CARTESIAN_POINT('Ctrl Pts',(1.18107030287633E-14,28.1978277731874,
54.5861052022779));
#133622=CARTESIAN_POINT('Ctrl Pts',(2.36466186055739E-15,28.2061189999238,
54.5243215858547));
#133623=CARTESIAN_POINT('Ctrl Pts',(5.45397060847108E-15,28.2178036028124,
54.4631615531338));
#133624=CARTESIAN_POINT('Ctrl Pts',(8.86164441660497E-15,28.2305350890377,
54.3965218802625));
#133625=CARTESIAN_POINT('Ctrl Pts',(-2.00354280069877E-14,28.2472941633897,
54.3306217037811));
#133626=CARTESIAN_POINT('Ctrl Pts',(-6.66133814775094E-16,28.2678355467659,
54.2656746420521));
#133627=CARTESIAN_POINT('Ctrl Pts',(6.62424595565122E-15,28.2757636019639,
54.2406079812093));
#133628=CARTESIAN_POINT('Ctrl Pts',(-1.52339698000625E-14,28.2842556294877,
54.2156833448971));
#133629=CARTESIAN_POINT('Ctrl Pts',(-6.80011602582908E-15,28.293299536066,
54.1909133347334));
#133630=CARTESIAN_POINT('Ctrl Pts',(-3.37245178901788E-15,28.2972665004933,
54.1800483674392));
#133631=CARTESIAN_POINT('Ctrl Pts',(-2.17185403739263E-14,28.3013395419173,
54.1692137249702));
#133632=CARTESIAN_POINT('Ctrl Pts',(-1.84574577843932E-14,28.3055125585617,
54.1584229955393));
#133633=CARTESIAN_POINT('Ctrl Pts',(1.52368349615535E-15,28.3310282228841,
54.0924437164197));
#133634=CARTESIAN_POINT('Ctrl Pts',(1.85341033795595E-14,28.3603207357524,
54.0279841981644));
#133635=CARTESIAN_POINT('Ctrl Pts',(8.10462807976364E-15,28.3930667172485,
53.9652709772947));
#133636=CARTESIAN_POINT('Ctrl Pts',(-2.32484722003222E-15,28.4258126987446,
53.902557756425));
#133637=CARTESIAN_POINT('Ctrl Pts',(3.91496741470812E-15,28.4620126514484,
53.8415900456593));
#133638=CARTESIAN_POINT('Ctrl Pts',(8.29891710907305E-15,28.5013974153454,
53.7825980208192));
#133639=CARTESIAN_POINT('Ctrl Pts',(1.17608196074637E-14,28.5318861331045,
53.7369308384517));
#133640=CARTESIAN_POINT('Ctrl Pts',(1.13837602802617E-15,28.5642845662645,
53.6924475817031));
#133641=CARTESIAN_POINT('Ctrl Pts',(5.41233724504764E-15,28.5984872509066,
53.6492611078387));
#133642=CARTESIAN_POINT('Ctrl Pts',(7.69524181669997E-15,28.6197781352125,
53.6223778900957));
#133643=CARTESIAN_POINT('Ctrl Pts',(-1.25356090036905E-15,28.6417684828538,
53.5959972930288));
#133644=CARTESIAN_POINT('Ctrl Pts',(-2.83106871279415E-15,28.6644357593109,
53.5701482268476));
#133645=CARTESIAN_POINT('Ctrl Pts',(-3.72072440462852E-15,28.6771277964087,
53.5556746173897));
#133646=CARTESIAN_POINT('Ctrl Pts',(4.76010837754156E-15,28.6900365447023,
53.5413631052373));
#133647=CARTESIAN_POINT('Ctrl Pts',(7.04991620636974E-15,28.7031343143651,
53.5272442252728));
#133648=CARTESIAN_POINT('Ctrl Pts',(1.66473880124441E-14,28.7540075643444,
53.4724048649576));
#133649=CARTESIAN_POINT('Ctrl Pts',(-2.32322889134241E-14,28.8077773503859,
53.4204104165983));
#133650=CARTESIAN_POINT('Ctrl Pts',(-2.78110867668602E-14,28.8641586498734,
53.3715248576467));
#133651=CARTESIAN_POINT('Ctrl Pts',(-3.11620636517304E-14,28.9063242170955,
53.3349650879907));
#133652=CARTESIAN_POINT('Ctrl Pts',(1.24250061455589E-14,28.9499515635121,
53.3001443221104));
#133653=CARTESIAN_POINT('Ctrl Pts',(7.99360577730113E-15,28.9949378639353,
53.2671827247916));
#133654=CARTESIAN_POINT('Ctrl Pts',(6.58027310319314E-15,29.0089885716387,
53.2568877290927));
#133655=CARTESIAN_POINT('Ctrl Pts',(-7.25313467225921E-15,29.0231719403568,
53.2467741756668));
#133656=CARTESIAN_POINT('Ctrl Pts',(-1.13520304267922E-14,29.0374850778181,
53.2368459519368));
#133657=CARTESIAN_POINT('Ctrl Pts',(-1.54901283588251E-14,29.0512799828038,
53.2272771971196));
#133658=CARTESIAN_POINT('Ctrl Pts',(1.57215114802889E-14,29.0651883995786,
53.2178855342609));
#133659=CARTESIAN_POINT('Ctrl Pts',(1.40443212615082E-14,29.0792023373798,
53.2086772026791));
#133660=CARTESIAN_POINT('Ctrl Pts',(5.95643201164454E-15,29.1421574061881,
53.167310446485));
#133661=CARTESIAN_POINT('Ctrl Pts',(5.87521379537194E-15,29.2072697599874,
53.1296194531803));
#133662=CARTESIAN_POINT('Ctrl Pts',(6.55031584528842E-15,29.2742780365298,
53.0958834461281));
#133663=CARTESIAN_POINT('Ctrl Pts',(7.02525033480137E-15,29.3255312944275,
53.070079465499));
#133664=CARTESIAN_POINT('Ctrl Pts',(-8.85054505632768E-15,29.3778947184249,
53.0465897193344));
#133665=CARTESIAN_POINT('Ctrl Pts',(-1.17683640610267E-14,29.4312652422325,
53.0255544368292));
#133666=CARTESIAN_POINT('Ctrl Pts',(-1.23454027065879E-14,29.4435451349662,
53.0207144803446));
#133667=CARTESIAN_POINT('Ctrl Pts',(-2.95665940748309E-14,29.4558783869943,
53.0160045294466));
#133668=CARTESIAN_POINT('Ctrl Pts',(-2.77555756156289E-16,29.4682631373226,
53.0114240182723));
#133669=CARTESIAN_POINT('Ctrl Pts',(10.,29.207701741744,53.534455913333));
#133670=CARTESIAN_POINT('Ctrl Pts',(10.0002897768776,29.215139018462,53.530435194036));
#133671=CARTESIAN_POINT('Ctrl Pts',(10.0005795537551,29.2226069020107,53.5264710893684));
#133672=CARTESIAN_POINT('Ctrl Pts',(10.0008693306327,29.2301045269737,53.5225640587107));
#133673=CARTESIAN_POINT('Ctrl Pts',(0.00154681533403014,30.5308614994839,
53.0122372304288));
#133674=CARTESIAN_POINT('Ctrl Pts',(0.03859190561355,31.1918243307126,53.1887571477249));
#133675=CARTESIAN_POINT('Ctrl Pts',(0.11268208617259,32.3123254329236,54.2503594776237));
#133676=CARTESIAN_POINT('Ctrl Pts',(0.223817357011149,31.8837204066822,
56.5402431757408));
#133677=CARTESIAN_POINT('Ctrl Pts',(0.334952627849709,29.7276879431726,
57.4159501049812));
#133678=CARTESIAN_POINT('Ctrl Pts',(0.446087898688268,27.822541677856,56.08255543116));
#133679=CARTESIAN_POINT('Ctrl Pts',(0.557223169526827,27.9095331143253,
53.757251657784));
#133680=CARTESIAN_POINT('Ctrl Pts',(0.668358440365387,29.9102877014042,
52.5699427782862));
#133681=CARTESIAN_POINT('Ctrl Pts',(0.779493711203945,31.9929427887065,
53.6065233542934));
#133682=CARTESIAN_POINT('Ctrl Pts',(0.890628982042508,32.2516197117106,
55.9186517555512));
#133683=CARTESIAN_POINT('Ctrl Pts',(1.00176425288106,30.4493989709057,57.3898945361969));
#133684=CARTESIAN_POINT('Ctrl Pts',(1.11289952371963,28.2358830289503,56.6737692472272));
#133685=CARTESIAN_POINT('Ctrl Pts',(1.22403479455818,27.6370000288693,54.425672429537));
#133686=CARTESIAN_POINT('Ctrl Pts',(1.33517006539674,29.20091120588,52.7032503782176));
#133687=CARTESIAN_POINT('Ctrl Pts',(1.4463053362353,31.4962023798426,53.0829740555855));
#133688=CARTESIAN_POINT('Ctrl Pts',(1.55744060707386,32.4220634124452,55.2172998443405));
#133689=CARTESIAN_POINT('Ctrl Pts',(1.66857587791242,31.1310771539381,57.1527360629333));
#133690=CARTESIAN_POINT('Ctrl Pts',(1.77971114875098,28.8048482843264,57.1178341845877));
#133691=CARTESIAN_POINT('Ctrl Pts',(1.89084641958954,27.5725078874562,55.1445380473229));
#133692=CARTESIAN_POINT('Ctrl Pts',(2.0019816904281,28.5619827496753,53.0389504538599));
#133693=CARTESIAN_POINT('Ctrl Pts',(2.11311696126666,30.8676342339108,52.7282561914974));
#133694=CARTESIAN_POINT('Ctrl Pts',(2.22425223210522,32.3791645746092,54.4968250773821));
#133695=CARTESIAN_POINT('Ctrl Pts',(2.33538750294378,31.7131125888044,56.7259357762407));
#133696=CARTESIAN_POINT('Ctrl Pts',(2.44652277378234,29.4790969176509,57.3753460897111));
#133697=CARTESIAN_POINT('Ctrl Pts',(2.5576580446209,27.7218491597909,55.8506690380474));
#133698=CARTESIAN_POINT('Ctrl Pts',(2.66879331545945,28.0497286903431,53.5473985823599));
#133699=CARTESIAN_POINT('Ctrl Pts',(2.77992858629801,30.162636608847,52.5736532819753));
#133700=CARTESIAN_POINT('Ctrl Pts',(2.89106385713658,32.1266878213609,53.820674780915));
#133701=CARTESIAN_POINT('Ctrl Pts',(3.00219912797513,32.1442415813906,56.1470994299562));
#133702=CARTESIAN_POINT('Ctrl Pts',(3.1133343988137,30.1992314272445,57.4236162857034));
#133703=CARTESIAN_POINT('Ctrl Pts',(3.22446966965225,28.0718703602033,56.4818654304466));
#133704=CARTESIAN_POINT('Ctrl Pts',(3.33560494049081,27.7092720354094,54.1838048921801));
#133705=CARTESIAN_POINT('Ctrl Pts',(3.44674021132937,29.4433124847903,52.6327847431547));
#133706=CARTESIAN_POINT('Ctrl Pts',(3.55787548216793,31.6868733344789,53.2484100322169));
#133707=CARTESIAN_POINT('Ctrl Pts',(3.66901075300649,32.3864865418042,55.4672162749728));
#133708=CARTESIAN_POINT('Ctrl Pts',(3.78014602384505,30.90181584682,57.2583926231375));
#133709=CARTESIAN_POINT('Ctrl Pts',(3.89128129468361,28.5917385121774,56.9825258242279));
#133710=CARTESIAN_POINT('Ctrl Pts',(4.00241656552217,27.5706032453881,54.8921089878803));
#133711=CARTESIAN_POINT('Ctrl Pts',(4.11355183636073,28.7730263898749,52.9004417555418));
#133712=CARTESIAN_POINT('Ctrl Pts',(4.22468710719928,31.0984639147953,52.8304410379739));
#133713=CARTESIAN_POINT('Ctrl Pts',(4.33582237803785,32.4185083631876,54.7461765199851));
#133714=CARTESIAN_POINT('Ctrl Pts',(4.4469576488764,31.5249602382387,56.8942294828257));
#133715=CARTESIAN_POINT('Ctrl Pts',(4.55809291971497,29.2356589666865,57.3085475621284));
#133716=CARTESIAN_POINT('Ctrl Pts',(4.66922819055352,27.6459375107741,55.6099170916078));
#133717=CARTESIAN_POINT('Ctrl Pts',(4.78036346139209,28.2108231352622,53.3530466890339));
#133718=CARTESIAN_POINT('Ctrl Pts',(4.89149873223064,30.413291941376,52.6035862558796));
#133719=CARTESIAN_POINT('Ctrl Pts',(5.0026340030692,32.2374862763419,54.0474958136589));
#133720=CARTESIAN_POINT('Ctrl Pts',(5.11376927390777,32.0137724545067,56.3632056203247));
#133721=CARTESIAN_POINT('Ctrl Pts',(5.22490454474632,29.9469094347836,57.4312117253954));
#133722=CARTESIAN_POINT('Ctrl Pts',(5.33603981558489,27.9286387137954,56.2739982275609));
#133723=CARTESIAN_POINT('Ctrl Pts',(5.44717508642344,27.806226626021,53.9507300416783));
#133724=CARTESIAN_POINT('Ctrl Pts',(5.558310357262,29.6917135069452,52.5878290898));
#133725=CARTESIAN_POINT('Ctrl Pts',(5.66944562810056,31.8593663302637,53.4327202190748));
#133726=CARTESIAN_POINT('Ctrl Pts',(5.78058089893912,32.3251935314588,55.7120983801957));
#133727=CARTESIAN_POINT('Ctrl Pts',(5.89171616977768,30.6628365960341,57.3397129543542));
#133728=CARTESIAN_POINT('Ctrl Pts',(6.00285144061624,28.3938039969429,56.8258541731416));
#133729=CARTESIAN_POINT('Ctrl Pts',(6.1139867114548,27.5948773515111,54.6408425031529));
#133730=CARTESIAN_POINT('Ctrl Pts',(6.22512198229336,28.997291711844,52.7845575722491));
#133731=CARTESIAN_POINT('Ctrl Pts',(6.33625725313191,31.317456721161,52.9560046845253));
#133732=CARTESIAN_POINT('Ctrl Pts',(6.44739252397048,32.431790707502,54.9982631279294));
#133733=CARTESIAN_POINT('Ctrl Pts',(6.55852779480903,31.3203751649245,57.0421112814102));
#133734=CARTESIAN_POINT('Ctrl Pts',(6.66966306564759,29.0004574300117,57.2168725070682));
#133735=CARTESIAN_POINT('Ctrl Pts',(6.78079833648615,27.5953928514194,55.3625927782321));
#133736=CARTESIAN_POINT('Ctrl Pts',(6.89193360732472,28.3911974560599,53.1764420940374));
#133737=CARTESIAN_POINT('Ctrl Pts',(7.00306887816327,30.6594937077774,52.6593425899509));
#133738=CARTESIAN_POINT('Ctrl Pts',(7.11420414900184,32.3241739473258,54.2845808749405));
#133739=CARTESIAN_POINT('Ctrl Pts',(7.2253394198404,31.8616032467933,56.5646221310909));
#133740=CARTESIAN_POINT('Ctrl Pts',(7.33647469067895,29.6951595376434,57.4126088274738));
#133741=CARTESIAN_POINT('Ctrl Pts',(7.44760996151752,27.8077277156913,56.0524026292531));
#133742=CARTESIAN_POINT('Ctrl Pts',(7.55874523235607,27.9268209580955,53.7289619517855));
#133743=CARTESIAN_POINT('Ctrl Pts',(7.66988050319463,29.9434365728189,52.5688665931827));
#133744=CARTESIAN_POINT('Ctrl Pts',(7.78101577403319,32.0118231019326,53.6339191555266));
#133745=CARTESIAN_POINT('Ctrl Pts',(7.89215104487175,32.2388446148396,55.9493070294859));
#133746=CARTESIAN_POINT('Ctrl Pts',(8.00328631571031,30.4167147335142,57.3958209254241));
#133747=CARTESIAN_POINT('Ctrl Pts',(8.11442158654887,28.2131775729573,56.6495074142123));
#133748=CARTESIAN_POINT('Ctrl Pts',(8.22555685738743,27.6450686888643,54.3934462476575));
#133749=CARTESIAN_POINT('Ctrl Pts',(8.33669212822598,29.2323620034979,52.6925466180413));
#133750=CARTESIAN_POINT('Ctrl Pts',(8.44782739906455,31.5222529295465,53.1035941163948));
#133751=CARTESIAN_POINT('Ctrl Pts',(8.5589626699031,32.418868278926,55.2503683966076));
#133752=CARTESIAN_POINT('Ctrl Pts',(8.67009794074167,31.1015623350708,57.1679877347923));
#133753=CARTESIAN_POINT('Ctrl Pts',(8.78123321158022,28.7760260281981,57.1013085802318));
#133754=CARTESIAN_POINT('Ctrl Pts',(8.89236848241879,27.5707613729241,55.1113616575299));
#133755=CARTESIAN_POINT('Ctrl Pts',(9.00350375325735,28.5889049351466,53.0194870008748));
#133756=CARTESIAN_POINT('Ctrl Pts',(9.1146390240959,30.8985948931835,52.7403231650404));
#133757=CARTESIAN_POINT('Ctrl Pts',(9.22577429493447,32.3858047755745,54.5293718006317));
#133758=CARTESIAN_POINT('Ctrl Pts',(9.33690956577302,31.6893973577937,56.7491852222167));
#133759=CARTESIAN_POINT('Ctrl Pts',(9.44804483661158,29.4466476574818,57.3679947859353));
#133760=CARTESIAN_POINT('Ctrl Pts',(9.55918010745014,27.7105332689696,55.8194928217058));
#133761=CARTESIAN_POINT('Ctrl Pts',(9.67031537828869,28.0695711380181,53.5208381930937));
#133762=CARTESIAN_POINT('Ctrl Pts',(9.78145064912726,30.1961348712651,52.5762050172338));
#133763=CARTESIAN_POINT('Ctrl Pts',(9.89258591996582,32.1418745091302,53.8496338177819));
#133764=CARTESIAN_POINT('Ctrl Pts',(10.0037211908043,32.1298241188128,56.1766906279436));
#133765=CARTESIAN_POINT('Ctrl Pts',(10.1148693978264,30.1628285126107,57.4254746165565));
#133766=CARTESIAN_POINT('Ctrl Pts',(10.188972514569,28.7606699551445,56.7791900710538));
#133767=CARTESIAN_POINT('Ctrl Pts',(10.2260305410321,28.3512916699711,56.2307621872168));
#133768=CARTESIAN_POINT('Ctrl Pts',(-0.0743643367184447,30.4969362892315,
53.1392671053682));
#133769=CARTESIAN_POINT('Ctrl Pts',(-0.0373192464389249,31.1156596605629,
53.3045063490539));
#133770=CARTESIAN_POINT('Ctrl Pts',(0.0367709341201149,32.1645540715419,
54.2982659699198));
#133771=CARTESIAN_POINT('Ctrl Pts',(0.147906204958674,31.763339458138,56.4418124671141));
#133772=CARTESIAN_POINT('Ctrl Pts',(0.259041475797234,29.7450903047889,
57.2615565101349));
#133773=CARTESIAN_POINT('Ctrl Pts',(0.370176746635793,27.9616942279399,
56.0133736942143));
#133774=CARTESIAN_POINT('Ctrl Pts',(0.481312017474353,28.0431263937234,
53.8366706754401));
#133775=CARTESIAN_POINT('Ctrl Pts',(0.592447288312911,29.9160208513783,
52.7252379018771));
#133776=CARTESIAN_POINT('Ctrl Pts',(0.703582559151472,31.8655818797056,
53.6955748078898));
#133777=CARTESIAN_POINT('Ctrl Pts',(0.81471782999003,32.1077278073204,55.8599444392623));
#133778=CARTESIAN_POINT('Ctrl Pts',(0.92585310082859,30.4206797012092,57.2371660473154));
#133779=CARTESIAN_POINT('Ctrl Pts',(1.03698837166715,28.3486206059095,56.5668054276972));
#133780=CARTESIAN_POINT('Ctrl Pts',(1.14812364250571,27.7880097949288,54.4623753804963));
#133781=CARTESIAN_POINT('Ctrl Pts',(1.25925891334427,29.2519777371264,52.8500263525383));
#133782=CARTESIAN_POINT('Ctrl Pts',(1.37039418418283,31.4005861402667,53.2054834262723));
#133783=CARTESIAN_POINT('Ctrl Pts',(1.48152945502139,32.2672791408569,55.2034130906123));
#133784=CARTESIAN_POINT('Ctrl Pts',(1.59266472585995,31.058794590037,57.0151634123946));
#133785=CARTESIAN_POINT('Ctrl Pts',(1.70379999669851,28.8812255941844,56.9824919718604));
#133786=CARTESIAN_POINT('Ctrl Pts',(1.81493526753707,27.7276390853,55.135301205605));
#133787=CARTESIAN_POINT('Ctrl Pts',(1.92607053837562,28.6538806130752,53.1642731947873));
#133788=CARTESIAN_POINT('Ctrl Pts',(2.03720580921418,30.8121872409829,52.8734341454796));
#133789=CARTESIAN_POINT('Ctrl Pts',(2.14834108005275,32.227121794153,54.5289809505433));
#133790=CARTESIAN_POINT('Ctrl Pts',(2.2594763508913,31.6036344955207,56.6156382049381));
#133791=CARTESIAN_POINT('Ctrl Pts',(2.37061162172987,29.5123857257618,57.2235473331729));
#133792=CARTESIAN_POINT('Ctrl Pts',(2.48174689256842,27.867436561243,55.7963062221357));
#133793=CARTESIAN_POINT('Ctrl Pts',(2.59288216340698,28.1743626377921,53.6402284608768));
#133794=CARTESIAN_POINT('Ctrl Pts',(2.70401743424554,30.1522431612995,52.7287112822902));
#133795=CARTESIAN_POINT('Ctrl Pts',(2.8151527050841,31.9907798085346,53.8960406834195));
#133796=CARTESIAN_POINT('Ctrl Pts',(2.92628797592267,32.0072117787937,56.0737929472303));
#133797=CARTESIAN_POINT('Ctrl Pts',(3.03742324676122,30.1864993529374,57.2687327762693));
#133798=CARTESIAN_POINT('Ctrl Pts',(3.14855851759978,28.1950893231298,56.3871654072907));
#133799=CARTESIAN_POINT('Ctrl Pts',(3.25969378843834,27.8556631899861,54.2359646187127));
#133800=CARTESIAN_POINT('Ctrl Pts',(3.37082905927689,29.4788881312005,52.7840638910666));
#133801=CARTESIAN_POINT('Ctrl Pts',(3.48196433011546,31.5790720857596,53.360347059089));
#133802=CARTESIAN_POINT('Ctrl Pts',(3.59309960095402,32.2339758440535,55.4373583734727));
#133803=CARTESIAN_POINT('Ctrl Pts',(3.70423487179258,30.8441844453301,57.1140678893851));
#133804=CARTESIAN_POINT('Ctrl Pts',(3.81537014263114,28.6817348052052,56.8558306212735));
#133805=CARTESIAN_POINT('Ctrl Pts',(3.92650541346969,27.7258561611993,54.8990038658741));
#133806=CARTESIAN_POINT('Ctrl Pts',(4.03764068430826,28.8514373082371,53.0346160268907));
#133807=CARTESIAN_POINT('Ctrl Pts',(4.1487759551468,31.0282655310355,52.9690887719183));
#133808=CARTESIAN_POINT('Ctrl Pts',(4.25991122598538,32.2639512804115,54.7623973514728));
#133809=CARTESIAN_POINT('Ctrl Pts',(4.37104649682393,31.4275062003041,56.7731769417513));
#133810=CARTESIAN_POINT('Ctrl Pts',(4.4821817676625,29.2845049091495,57.1610176291815));
#133811=CARTESIAN_POINT('Ctrl Pts',(4.59331703850104,27.7963761185315,55.5709397583685));
#133812=CARTESIAN_POINT('Ctrl Pts',(4.70445230933962,28.3251621886198,53.4582968105905));
#133813=CARTESIAN_POINT('Ctrl Pts',(4.81558758017816,30.3868801258263,52.7567313609589));
#133814=CARTESIAN_POINT('Ctrl Pts',(4.92672285101673,32.0944975826136,54.1083665018127));
#133815=CARTESIAN_POINT('Ctrl Pts',(5.03785812185529,31.8850804058537,56.2760886654659));
#133816=CARTESIAN_POINT('Ctrl Pts',(5.14899339269384,29.9503022379707,57.275842822146));
#133817=CARTESIAN_POINT('Ctrl Pts',(5.2601286635324,28.061011031644,56.1925821561879));
#133818=CARTESIAN_POINT('Ctrl Pts',(5.37126393437097,27.9464218050474,54.0177846387478));
#133819=CARTESIAN_POINT('Ctrl Pts',(5.48239920520953,29.7114148492069,52.7419811716006));
#133820=CARTESIAN_POINT('Ctrl Pts',(5.59353447604809,31.7405417521925,53.5328787277328));
#133821=CARTESIAN_POINT('Ctrl Pts',(5.70466974688665,32.1765998219716,55.6665910542886));
#133822=CARTESIAN_POINT('Ctrl Pts',(5.81580501772522,30.6204773914105,57.190191367304));
#133823=CARTESIAN_POINT('Ctrl Pts',(5.92694028856376,28.4964494838793,56.7091712214221));
#133824=CARTESIAN_POINT('Ctrl Pts',(6.03807555940233,27.7485790074273,54.6637948054127));
#133825=CARTESIAN_POINT('Ctrl Pts',(6.14921083024089,29.0613707409894,52.9261375328163));
#133826=CARTESIAN_POINT('Ctrl Pts',(6.26034610107943,31.2332633933208,53.0866281539233));
#133827=CARTESIAN_POINT('Ctrl Pts',(6.37148137191802,32.276384803849,54.9983741243951));
#133828=CARTESIAN_POINT('Ctrl Pts',(6.48261664275655,31.235995331153,56.9116082130054));
#133829=CARTESIAN_POINT('Ctrl Pts',(6.59375191359513,29.0643341509192,57.0752011559189));
#133830=CARTESIAN_POINT('Ctrl Pts',(6.70488718443368,27.7490615638223,55.3394209410401));
#133831=CARTESIAN_POINT('Ctrl Pts',(6.81602245527225,28.4940095164765,53.2929783006137));
#133832=CARTESIAN_POINT('Ctrl Pts',(6.9271577261108,30.6173481336149,52.8089245333429));
#133833=CARTESIAN_POINT('Ctrl Pts',(7.03829299694936,32.1756453953347,54.3303004162143));
#133834=CARTESIAN_POINT('Ctrl Pts',(7.14942826778791,31.7426357164384,56.4646334620794));
#133835=CARTESIAN_POINT('Ctrl Pts',(7.26056353862649,29.7146406580278,57.2584287601524));
#133836=CARTESIAN_POINT('Ctrl Pts',(7.37169880946503,27.9478269661512,55.985147835861));
#133837=CARTESIAN_POINT('Ctrl Pts',(7.48283408030359,28.0593094413551,53.8101888500751));
#133838=CARTESIAN_POINT('Ctrl Pts',(7.59396935114215,29.947051312561,52.7242304914087));
#133839=CARTESIAN_POINT('Ctrl Pts',(7.70510462198073,31.8832556285142,53.7212198543257));
#133840=CARTESIAN_POINT('Ctrl Pts',(7.81623989281927,32.0957691151947,55.8886406586893));
#133841=CARTESIAN_POINT('Ctrl Pts',(7.92737516365785,30.3900841811695,57.2427137049886));
#133842=CARTESIAN_POINT('Ctrl Pts',(8.03851043449638,28.3273661637292,56.5440940702528));
#133843=CARTESIAN_POINT('Ctrl Pts',(8.14964570533495,27.7955628195141,54.4322086434944));
#133844=CARTESIAN_POINT('Ctrl Pts',(8.26078097617351,29.2814186415371,52.8400066263611));
#133845=CARTESIAN_POINT('Ctrl Pts',(8.37191624701208,31.424971904755,53.2247857424361));
#133846=CARTESIAN_POINT('Ctrl Pts',(8.48305151785062,32.2642881953915,55.2343683655191));
#133847=CARTESIAN_POINT('Ctrl Pts',(8.59418678868919,31.0311659438091,57.0294404116223));
#133848=CARTESIAN_POINT('Ctrl Pts',(8.70532205952775,28.8542452518133,56.9670224520066));
#133849=CARTESIAN_POINT('Ctrl Pts',(8.8164573303663,27.7260041834442,55.1042449846322));
#133850=CARTESIAN_POINT('Ctrl Pts',(8.92759260120488,28.6790823106162,53.146053572322));
#133851=CARTESIAN_POINT('Ctrl Pts',(9.03872787204343,30.8411693298065,52.8847299675736));
#133852=CARTESIAN_POINT('Ctrl Pts',(9.149863142882,32.2333376467449,54.5594477444133));
#133853=CARTESIAN_POINT('Ctrl Pts',(9.26099841372054,31.5814348089579,56.6374018729028));
#133854=CARTESIAN_POINT('Ctrl Pts',(9.3721336845591,29.4820101665014,57.2166658214737));
#133855=CARTESIAN_POINT('Ctrl Pts',(9.48326895539768,27.8568438232133,55.7671223516233));
#133856=CARTESIAN_POINT('Ctrl Pts',(9.59440422623621,28.1929370349304,53.6153654386096));
#133857=CARTESIAN_POINT('Ctrl Pts',(9.7055394970748,30.1836006853202,52.7310999464744));
#133858=CARTESIAN_POINT('Ctrl Pts',(9.81667476791335,32.0049959765427,53.9231490654255));
#133859=CARTESIAN_POINT('Ctrl Pts',(9.92781003875191,31.9937156779076,56.1014930914981));
#133860=CARTESIAN_POINT('Ctrl Pts',(10.038958245774,30.1524228012702,57.2704723487172));
#133861=CARTESIAN_POINT('Ctrl Pts',(10.1130613625166,28.8398705232488,56.6654892332682));
#133862=CARTESIAN_POINT('Ctrl Pts',(10.1501193889796,28.4566539476942,56.1521091562236));
#133863=CARTESIAN_POINT('Ctrl Pts',(-0.15027548877092,30.4630110789791,
53.2662969803077));
#133864=CARTESIAN_POINT('Ctrl Pts',(-0.1132303984914,31.0394949904132,53.4202555503831));
#133865=CARTESIAN_POINT('Ctrl Pts',(-0.0391402179323597,32.0167827101601,
54.346172462216));
#133866=CARTESIAN_POINT('Ctrl Pts',(0.0719950529061993,31.6429585095939,
56.3433817584873));
#133867=CARTESIAN_POINT('Ctrl Pts',(0.183130323744759,29.7624926664051,
57.1071629152887));
#133868=CARTESIAN_POINT('Ctrl Pts',(0.294265594583318,28.1008467780239,
55.9441919572683));
#133869=CARTESIAN_POINT('Ctrl Pts',(0.405400865421878,28.1767196731213,
53.9160896930964));
#133870=CARTESIAN_POINT('Ctrl Pts',(0.516536136260436,29.9217540013526,
52.8805330254681));
#133871=CARTESIAN_POINT('Ctrl Pts',(0.627671407098997,31.7382209707045,
53.7846262614862));
#133872=CARTESIAN_POINT('Ctrl Pts',(0.738806677937555,31.9638359029301,
55.8012371229733));
#133873=CARTESIAN_POINT('Ctrl Pts',(0.849941948776116,30.3919604315126,
57.084437558434));
#133874=CARTESIAN_POINT('Ctrl Pts',(0.961077219614675,28.4613581828686,
56.4598416081671));
#133875=CARTESIAN_POINT('Ctrl Pts',(1.07221249045323,27.9390195609882,54.4990783314556));
#133876=CARTESIAN_POINT('Ctrl Pts',(1.1833477612918,29.3030442683727,52.996802326859));
#133877=CARTESIAN_POINT('Ctrl Pts',(1.29448303213035,31.3049699006907,53.3279927969591));
#133878=CARTESIAN_POINT('Ctrl Pts',(1.40561830296891,32.1124948692687,55.1895263368842));
#133879=CARTESIAN_POINT('Ctrl Pts',(1.51675357380747,30.986512026136,56.877590761856));
#133880=CARTESIAN_POINT('Ctrl Pts',(1.62788884464603,28.9576029040423,56.8471497591331));
#133881=CARTESIAN_POINT('Ctrl Pts',(1.73902411548459,27.8827702831439,55.126064363887));
#133882=CARTESIAN_POINT('Ctrl Pts',(1.85015938632315,28.7457784764752,53.2895959357148));
#133883=CARTESIAN_POINT('Ctrl Pts',(1.96129465716171,30.7567402480549,53.0186120994619));
#133884=CARTESIAN_POINT('Ctrl Pts',(2.07242992800027,32.0750790136968,54.5611368237044));
#133885=CARTESIAN_POINT('Ctrl Pts',(2.18356519883883,31.4941564022369,56.5053406336356));
#133886=CARTESIAN_POINT('Ctrl Pts',(2.29470046967739,29.5456745338728,57.0717485766346));
#133887=CARTESIAN_POINT('Ctrl Pts',(2.40583574051595,28.013023962695,55.7419434062243));
#133888=CARTESIAN_POINT('Ctrl Pts',(2.5169710113545,28.298996585241,53.7330583393936));
#133889=CARTESIAN_POINT('Ctrl Pts',(2.62810628219307,30.1418497137519,52.8837692826054));
#133890=CARTESIAN_POINT('Ctrl Pts',(2.73924155303162,31.8548717957082,53.9714065859237));
#133891=CARTESIAN_POINT('Ctrl Pts',(2.85037682387019,31.8701819761967,56.0004864645048));
#133892=CARTESIAN_POINT('Ctrl Pts',(2.96151209470874,30.1737672786304,57.1138492668348));
#133893=CARTESIAN_POINT('Ctrl Pts',(3.07264736554731,28.3183082860562,56.2924653841349));
#133894=CARTESIAN_POINT('Ctrl Pts',(3.18378263638586,28.0020543445629,54.2881243452452));
#133895=CARTESIAN_POINT('Ctrl Pts',(3.29491790722442,29.5144637776106,52.9353430389786));
#133896=CARTESIAN_POINT('Ctrl Pts',(3.40605317806298,31.4712708370402,53.472284085961));
#133897=CARTESIAN_POINT('Ctrl Pts',(3.51718844890155,32.0814651463029,55.4075004719725));
#133898=CARTESIAN_POINT('Ctrl Pts',(3.6283237197401,30.7865530438401,56.9697431556326));
#133899=CARTESIAN_POINT('Ctrl Pts',(3.73945899057866,28.771731098233,56.7291354183192));
#133900=CARTESIAN_POINT('Ctrl Pts',(3.85059426141722,27.8811090770103,54.9058987438678));
#133901=CARTESIAN_POINT('Ctrl Pts',(3.96172953225578,28.9298482265992,53.1687902982395));
#133902=CARTESIAN_POINT('Ctrl Pts',(4.07286480309434,30.9580671472756,53.1077365058626));
#133903=CARTESIAN_POINT('Ctrl Pts',(4.1840000739329,32.1093941976355,54.7786181829607));
#133904=CARTESIAN_POINT('Ctrl Pts',(4.29513534477146,31.3300521623692,56.6521244006766));
#133905=CARTESIAN_POINT('Ctrl Pts',(4.40627061561002,29.3333508516128,57.0134876962348));
#133906=CARTESIAN_POINT('Ctrl Pts',(4.51740588644858,27.9468147262887,55.5319624251291));
#133907=CARTESIAN_POINT('Ctrl Pts',(4.62854115728713,28.4395012419773,53.5635469321471));
#133908=CARTESIAN_POINT('Ctrl Pts',(4.7396764281257,30.3604683102766,52.9098764660384));
#133909=CARTESIAN_POINT('Ctrl Pts',(4.85081169896425,31.9515088888855,54.1692371899665));
#133910=CARTESIAN_POINT('Ctrl Pts',(4.96194696980282,31.7563883572006,56.1889717106072));
#133911=CARTESIAN_POINT('Ctrl Pts',(5.07308224064137,29.9536950411579,57.1204739188966));
#133912=CARTESIAN_POINT('Ctrl Pts',(5.18421751147994,28.1933833494923,56.1111660848148));
#133913=CARTESIAN_POINT('Ctrl Pts',(5.29535278231849,28.0866169840739,54.0848392358172));
#133914=CARTESIAN_POINT('Ctrl Pts',(5.40648805315706,29.7311161914685,52.8961332534013));
#133915=CARTESIAN_POINT('Ctrl Pts',(5.51762332399561,31.6217171741212,53.6330372363906));
#133916=CARTESIAN_POINT('Ctrl Pts',(5.62875859483417,32.0280061124844,55.6210837283815));
#133917=CARTESIAN_POINT('Ctrl Pts',(5.73989386567274,30.5781181867869,57.0406697802536));
#133918=CARTESIAN_POINT('Ctrl Pts',(5.85102913651129,28.5990949708156,56.5924882697025));
#133919=CARTESIAN_POINT('Ctrl Pts',(5.96216440734985,27.9022806633435,54.6867471076725));
#133920=CARTESIAN_POINT('Ctrl Pts',(6.07329967818841,29.1254497701346,53.0677174933834));
#133921=CARTESIAN_POINT('Ctrl Pts',(6.18443494902697,31.1490700654805,53.2172516233213));
#133922=CARTESIAN_POINT('Ctrl Pts',(6.29557021986553,32.120978900196,54.9984851208607));
#133923=CARTESIAN_POINT('Ctrl Pts',(6.40670549070409,31.1516154973816,56.7811051446004));
#133924=CARTESIAN_POINT('Ctrl Pts',(6.51784076154265,29.1282108718268,56.9335298047696));
#133925=CARTESIAN_POINT('Ctrl Pts',(6.6289760323812,27.9027302762255,55.316249103848));
#133926=CARTESIAN_POINT('Ctrl Pts',(6.74011130321977,28.5968215768931,53.4095145071899));
#133927=CARTESIAN_POINT('Ctrl Pts',(6.85124657405832,30.5752025594525,52.9585064767349));
#133928=CARTESIAN_POINT('Ctrl Pts',(6.96238184489689,32.0271168433436,54.3760199574878));
#133929=CARTESIAN_POINT('Ctrl Pts',(7.07351711573544,31.6236681860837,56.3646447930679));
#133930=CARTESIAN_POINT('Ctrl Pts',(7.18465238657401,29.7341217784122,57.1042486928307));
#133931=CARTESIAN_POINT('Ctrl Pts',(7.29578765741256,28.0879262166111,55.9178930424689));
#133932=CARTESIAN_POINT('Ctrl Pts',(7.40692292825113,28.1917979246146,53.8914157483648));
#133933=CARTESIAN_POINT('Ctrl Pts',(7.51805819908967,29.9506660523031,52.8795943896346));
#133934=CARTESIAN_POINT('Ctrl Pts',(7.62919346992825,31.7546881550959,53.808520553125));
#133935=CARTESIAN_POINT('Ctrl Pts',(7.74032874076679,31.9526936155498,55.8279742878926));
#133936=CARTESIAN_POINT('Ctrl Pts',(7.85146401160537,30.3634536288249,57.0896064845533));
#133937=CARTESIAN_POINT('Ctrl Pts',(7.96259928244391,28.4415547545012,56.4386807262929));
#133938=CARTESIAN_POINT('Ctrl Pts',(8.07373455328248,27.9460569501639,54.4709710393315));
#133939=CARTESIAN_POINT('Ctrl Pts',(8.18486982412104,29.3304752795761,52.9874666346809));
#133940=CARTESIAN_POINT('Ctrl Pts',(8.29600509495959,31.3276908799634,53.3459773684774));
#133941=CARTESIAN_POINT('Ctrl Pts',(8.40714036579816,32.1097081118571,55.2183683344306));
#133942=CARTESIAN_POINT('Ctrl Pts',(8.51827563663671,30.9607695525475,56.8908930884524));
#133943=CARTESIAN_POINT('Ctrl Pts',(8.62941090747528,28.9324644754286,56.8327363237813));
#133944=CARTESIAN_POINT('Ctrl Pts',(8.74054617831384,27.8812469939644,55.0971283117347));
#133945=CARTESIAN_POINT('Ctrl Pts',(8.8516814491524,28.7692596860857,53.272620143769));
#133946=CARTESIAN_POINT('Ctrl Pts',(8.96281671999095,30.7837437664296,53.0291367701069));
#133947=CARTESIAN_POINT('Ctrl Pts',(9.07395199082952,32.0808705179151,54.5895236881948));
#133948=CARTESIAN_POINT('Ctrl Pts',(9.18508726166807,31.4734722601222,56.525618523589));
#133949=CARTESIAN_POINT('Ctrl Pts',(9.29622253250664,29.5173726755208,57.0653368570119));
#133950=CARTESIAN_POINT('Ctrl Pts',(9.40735780334519,28.0031543774569,55.7147518815408));
#133951=CARTESIAN_POINT('Ctrl Pts',(9.51849307418375,28.3163029318427,53.7098926841253));
#133952=CARTESIAN_POINT('Ctrl Pts',(9.62962834502232,30.1710664993754,52.8859948757149));
#133953=CARTESIAN_POINT('Ctrl Pts',(9.74076361586087,31.8681174439553,53.996664313069));
#133954=CARTESIAN_POINT('Ctrl Pts',(9.85189888669943,31.8576072370023,56.0262955550524));
#133955=CARTESIAN_POINT('Ctrl Pts',(9.9630470937215,30.1420170899297,57.1154700808779));
#133956=CARTESIAN_POINT('Ctrl Pts',(10.0371502104641,28.9190710913532,56.5517883954824));
#133957=CARTESIAN_POINT('Ctrl Pts',(10.0742082369271,28.5620162254173,56.0734561252304));
#133958=CARTESIAN_POINT('Ctrl Pts',(-0.226186640823395,30.4290858687267,
53.393326855247));
#133959=CARTESIAN_POINT('Ctrl Pts',(-0.189141550543875,30.9633303202635,
53.536004751712));
#133960=CARTESIAN_POINT('Ctrl Pts',(-0.115051369984835,31.8690113487782,
54.3940789545122));
#133961=CARTESIAN_POINT('Ctrl Pts',(-0.00391609914627541,31.5225775610498,
56.2449510498606));
#133962=CARTESIAN_POINT('Ctrl Pts',(0.107219171692284,29.7798950280212,
56.9527693204424));
#133963=CARTESIAN_POINT('Ctrl Pts',(0.218354442530843,28.2399993281078,
55.8750102203225));
#133964=CARTESIAN_POINT('Ctrl Pts',(0.329489713369402,28.3103129525194,
53.9955087107525));
#133965=CARTESIAN_POINT('Ctrl Pts',(0.440624984207962,29.9274871513269,
53.035828149059));
#133966=CARTESIAN_POINT('Ctrl Pts',(0.551760255046521,31.6108600617036,
53.8736777150826));
#133967=CARTESIAN_POINT('Ctrl Pts',(0.662895525885082,31.8199439985398,
55.7425298066844));
#133968=CARTESIAN_POINT('Ctrl Pts',(0.774030796723639,30.363241161816,56.9317090695523));
#133969=CARTESIAN_POINT('Ctrl Pts',(0.885166067562201,28.5740957598277,
56.3528777886373));
#133970=CARTESIAN_POINT('Ctrl Pts',(0.996301338400759,28.0900293270476,
54.5357812824147));
#133971=CARTESIAN_POINT('Ctrl Pts',(1.10743660923932,29.3541107996191,53.1435783011798));
#133972=CARTESIAN_POINT('Ctrl Pts',(1.21857188007787,31.2093536611147,53.4505021676458));
#133973=CARTESIAN_POINT('Ctrl Pts',(1.32970715091643,31.9577105976804,55.1756395831562));
#133974=CARTESIAN_POINT('Ctrl Pts',(1.440842421755,30.9142294622349,56.7400181113173));
#133975=CARTESIAN_POINT('Ctrl Pts',(1.55197769259355,29.0339802139003,56.7118075464059));
#133976=CARTESIAN_POINT('Ctrl Pts',(1.66311296343211,28.0379014809877,55.1168275221689));
#133977=CARTESIAN_POINT('Ctrl Pts',(1.77424823427067,28.837676339875,53.4149186766423));
#133978=CARTESIAN_POINT('Ctrl Pts',(1.88538350510923,30.701293255127,53.1637900534441));
#133979=CARTESIAN_POINT('Ctrl Pts',(1.99651877594779,31.9230362332406,54.5932926968657));
#133980=CARTESIAN_POINT('Ctrl Pts',(2.10765404678635,31.3846783089532,56.3950430623329));
#133981=CARTESIAN_POINT('Ctrl Pts',(2.21878931762491,29.5789633419837,56.9199498200965));
#133982=CARTESIAN_POINT('Ctrl Pts',(2.32992458846347,28.158611364147,55.6875805903127));
#133983=CARTESIAN_POINT('Ctrl Pts',(2.44105985930203,28.42363053269,53.8258882179105));
#133984=CARTESIAN_POINT('Ctrl Pts',(2.55219513014059,30.1314562662045,53.0388272829205));
#133985=CARTESIAN_POINT('Ctrl Pts',(2.66333040097915,31.7189637828817,54.046772488428));
#133986=CARTESIAN_POINT('Ctrl Pts',(2.77446567181771,31.7331521735996,55.927179981779));
#133987=CARTESIAN_POINT('Ctrl Pts',(2.88560094265627,30.1610352043235,56.9589657574004));
#133988=CARTESIAN_POINT('Ctrl Pts',(2.99673621349482,28.4415272489827,56.1977653609792));
#133989=CARTESIAN_POINT('Ctrl Pts',(3.10787148433339,28.1484454991397,54.3402840717779));
#133990=CARTESIAN_POINT('Ctrl Pts',(3.21900675517194,29.5500394240206,53.0866221868906));
#133991=CARTESIAN_POINT('Ctrl Pts',(3.33014202601051,31.3634695883209,53.584221112833));
#133992=CARTESIAN_POINT('Ctrl Pts',(3.44127729684907,31.9289544485523,55.3776425704724));
#133993=CARTESIAN_POINT('Ctrl Pts',(3.55241256768762,30.7289216423502,56.8254184218802));
#133994=CARTESIAN_POINT('Ctrl Pts',(3.66354783852618,28.8617273912608,56.6024402153649));
#133995=CARTESIAN_POINT('Ctrl Pts',(3.77468310936474,28.0363619928214,54.9127936218614));
#133996=CARTESIAN_POINT('Ctrl Pts',(3.88581838020331,29.0082591449614,53.3029645695884));
#133997=CARTESIAN_POINT('Ctrl Pts',(3.99695365104185,30.8878687635158,53.2463842398069));
#133998=CARTESIAN_POINT('Ctrl Pts',(4.10808892188042,31.9548371148595,54.7948390144485));
#133999=CARTESIAN_POINT('Ctrl Pts',(4.21922419271897,31.2325981244345,56.5310718596021));
#134000=CARTESIAN_POINT('Ctrl Pts',(4.33035946355754,29.382196794076,56.865957763288));
#134001=CARTESIAN_POINT('Ctrl Pts',(4.4414947343961,28.0972533340459,55.4929850918898));
#134002=CARTESIAN_POINT('Ctrl Pts',(4.55263000523466,28.553840295335,53.6687970537037));
#134003=CARTESIAN_POINT('Ctrl Pts',(4.66376527607322,30.334056494727,53.0630215711176));
#134004=CARTESIAN_POINT('Ctrl Pts',(4.77490054691178,31.8085201951574,54.2301078781202));
#134005=CARTESIAN_POINT('Ctrl Pts',(4.88603581775034,31.6276963085475,56.1018547557485));
#134006=CARTESIAN_POINT('Ctrl Pts',(4.99717108858889,29.957087844345,56.9651050156472));
#134007=CARTESIAN_POINT('Ctrl Pts',(5.10830635942746,28.3257556673408,56.0297500134417));
#134008=CARTESIAN_POINT('Ctrl Pts',(5.21944163026601,28.2268121631002,54.1518938328867));
#134009=CARTESIAN_POINT('Ctrl Pts',(5.33057690110458,29.7508175337302,53.050285335202));
#134010=CARTESIAN_POINT('Ctrl Pts',(5.44171217194313,31.50289259605,53.7331957450487));
#134011=CARTESIAN_POINT('Ctrl Pts',(5.55284744278169,31.8794124029971,55.5755764024744));
#134012=CARTESIAN_POINT('Ctrl Pts',(5.66398271362025,30.5357589821632,56.8911481932033));
#134013=CARTESIAN_POINT('Ctrl Pts',(5.77511798445881,28.701740457752,56.475805317983));
#134014=CARTESIAN_POINT('Ctrl Pts',(5.88625325529737,28.0559823192596,54.7096994099324));
#134015=CARTESIAN_POINT('Ctrl Pts',(5.99738852613593,29.1895287992798,53.2092974539506));
#134016=CARTESIAN_POINT('Ctrl Pts',(6.10852379697449,31.0648767376402,53.3478750927192));
#134017=CARTESIAN_POINT('Ctrl Pts',(6.21965906781306,31.9655729965431,54.9985961173263));
#134018=CARTESIAN_POINT('Ctrl Pts',(6.3307943386516,31.0672356636102,56.6506020761956));
#134019=CARTESIAN_POINT('Ctrl Pts',(6.44192960949018,29.1920875927343,56.7918584536201));
#134020=CARTESIAN_POINT('Ctrl Pts',(6.55306488032872,28.0563989886284,55.2930772666561));
#134021=CARTESIAN_POINT('Ctrl Pts',(6.66420015116729,28.6996336373097,53.5260507137662));
#134022=CARTESIAN_POINT('Ctrl Pts',(6.77533542200584,30.53305698529,53.1080884201267));
#134023=CARTESIAN_POINT('Ctrl Pts',(6.88647069284441,31.8785882913524,54.4217394987615));
#134024=CARTESIAN_POINT('Ctrl Pts',(6.99760596368297,31.5047006557289,56.2646561240565));
#134025=CARTESIAN_POINT('Ctrl Pts',(7.10874123452152,29.7536028987965,56.9500686255091));
#134026=CARTESIAN_POINT('Ctrl Pts',(7.21987650536009,28.228025467071,55.8506382490768));
#134027=CARTESIAN_POINT('Ctrl Pts',(7.33101177619865,28.3242864078741,53.9726426466545));
#134028=CARTESIAN_POINT('Ctrl Pts',(7.4421470470372,29.9542807920451,53.0349582878607));
#134029=CARTESIAN_POINT('Ctrl Pts',(7.55328231787577,31.6261206816776,53.8958212519243));
#134030=CARTESIAN_POINT('Ctrl Pts',(7.66441758871431,31.8096181159048,55.7673079170957));
#134031=CARTESIAN_POINT('Ctrl Pts',(7.77555285955289,30.3368230764804,56.9364992641179));
#134032=CARTESIAN_POINT('Ctrl Pts',(7.88668813039144,28.555743345273,56.3332673823333));
#134033=CARTESIAN_POINT('Ctrl Pts',(7.99782340123,28.0965510808136,54.5097334351684));
#134034=CARTESIAN_POINT('Ctrl Pts',(8.10895867206856,29.3795319176152,53.1349266430008));
#134035=CARTESIAN_POINT('Ctrl Pts',(8.22009394290712,31.2304098551717,53.4671689945188));
#134036=CARTESIAN_POINT('Ctrl Pts',(8.33122921374569,31.9551280283227,55.2023683033418));
#134037=CARTESIAN_POINT('Ctrl Pts',(8.44236448458424,30.8903731612859,56.7523457652825));
#134038=CARTESIAN_POINT('Ctrl Pts',(8.5534997554228,29.0106836990437,56.698450195556));
#134039=CARTESIAN_POINT('Ctrl Pts',(8.66463502626136,28.0364898044845,55.0900116388371));
#134040=CARTESIAN_POINT('Ctrl Pts',(8.77577029709992,28.8594370615552,53.3991867152161));
#134041=CARTESIAN_POINT('Ctrl Pts',(8.88690556793847,30.7263182030527,53.1735435726402));
#134042=CARTESIAN_POINT('Ctrl Pts',(8.99804083877704,31.9284033890853,54.6195996319764));
#134043=CARTESIAN_POINT('Ctrl Pts',(9.10917610961559,31.3655097112866,56.4138351742751));
#134044=CARTESIAN_POINT('Ctrl Pts',(9.22031138045416,29.5527351845403,56.9140078925503));
#134045=CARTESIAN_POINT('Ctrl Pts',(9.33144665129271,28.1494649317004,55.6623814114582));
#134046=CARTESIAN_POINT('Ctrl Pts',(9.44258192213128,28.4396688287551,53.8044199296412));
#134047=CARTESIAN_POINT('Ctrl Pts',(9.55371719296983,30.1585323134304,53.0408898049554));
#134048=CARTESIAN_POINT('Ctrl Pts',(9.66485246380839,31.7312389113679,54.0701795607126));
#134049=CARTESIAN_POINT('Ctrl Pts',(9.77598773464695,31.7214987960971,55.9510980186068));
#134050=CARTESIAN_POINT('Ctrl Pts',(9.88713594166903,30.1316113785892,56.9604678130387));
#134051=CARTESIAN_POINT('Ctrl Pts',(9.96123905841159,28.9982716594575,56.4380875576967));
#134052=CARTESIAN_POINT('Ctrl Pts',(9.99829708487463,28.6673785031403,55.994803094237));
#134053=CARTESIAN_POINT('Ctrl Pts',(10.,28.6653082844465,55.9970727277551));
#134054=CARTESIAN_POINT('Ctrl Pts',(10.,28.6967090787531,56.0511234594078));
#134055=CARTESIAN_POINT('Ctrl Pts',(10.,28.7313028149014,56.1030990886654));
#134056=CARTESIAN_POINT('Ctrl Pts',(10.,28.7687632599603,56.1529135186339));
#134057=CARTESIAN_POINT('Ctrl Pts',(10.,28.7925234449976,56.1845095146696));
#134058=CARTESIAN_POINT('Ctrl Pts',(10.,28.8174380027366,56.2152358570303));
#134059=CARTESIAN_POINT('Ctrl Pts',(10.,28.8434336726689,56.2450673747019));
#134060=CARTESIAN_POINT('Ctrl Pts',(10.,28.8612018283552,56.2654573493296));
#134061=CARTESIAN_POINT('Ctrl Pts',(10.,28.879475213815,56.2854292268814));
#134062=CARTESIAN_POINT('Ctrl Pts',(10.,28.8982322592198,56.3049740723664));
#134063=CARTESIAN_POINT('Ctrl Pts',(10.,28.9081731573242,56.3153324904029));
#134064=CARTESIAN_POINT('Ctrl Pts',(10.,28.9182498619851,56.3255707073213));
#134065=CARTESIAN_POINT('Ctrl Pts',(10.,28.9284489135861,56.3356775141706));
#134066=CARTESIAN_POINT('Ctrl Pts',(10.,28.9753089563359,56.3821137338849));
#134067=CARTESIAN_POINT('Ctrl Pts',(10.,29.0247995791763,56.4258325114299));
#134068=CARTESIAN_POINT('Ctrl Pts',(10.,29.0765854237513,56.4667238945408));
#134069=CARTESIAN_POINT('Ctrl Pts',(10.,29.1139361671967,56.4962169649394));
#134070=CARTESIAN_POINT('Ctrl Pts',(9.99999999999999,29.1524820705888,56.5242388499532));
#134071=CARTESIAN_POINT('Ctrl Pts',(10.,29.1921115967059,56.5507396091909));
#134072=CARTESIAN_POINT('Ctrl Pts',(10.,29.2029855373481,56.5580111491551));
#134073=CARTESIAN_POINT('Ctrl Pts',(10.,29.2139411245786,56.5651681145049));
#134074=CARTESIAN_POINT('Ctrl Pts',(10.,29.2249761856231,56.5722093560925));
#134075=CARTESIAN_POINT('Ctrl Pts',(9.99999999999999,29.2362247392384,56.5793868228231));
#134076=CARTESIAN_POINT('Ctrl Pts',(9.99999999999999,29.2475490172341,56.5864396275743));
#134077=CARTESIAN_POINT('Ctrl Pts',(10.,29.2589420457756,56.5933643753857));
#134078=CARTESIAN_POINT('Ctrl Pts',(10.,29.3169247868431,56.6286066165372));
#134079=CARTESIAN_POINT('Ctrl Pts',(10.,29.3767191373825,56.6605562853147));
#134080=CARTESIAN_POINT('Ctrl Pts',(10.,29.4379848073917,56.6891026354925));
#134081=CARTESIAN_POINT('Ctrl Pts',(10.,29.5001359672636,56.718061574053));
#134082=CARTESIAN_POINT('Ctrl Pts',(10.,29.5638020498636,56.7435188436963));
#134083=CARTESIAN_POINT('Ctrl Pts',(10.,29.6286681086957,56.7653246387053));
#134084=CARTESIAN_POINT('Ctrl Pts',(10.,29.6688530659824,56.778833474556));
#134085=CARTESIAN_POINT('Ctrl Pts',(9.99999999999999,29.709499312355,56.7909402012805));
#134086=CARTESIAN_POINT('Ctrl Pts',(9.99999999999999,29.7505375207727,56.8016008389451));
#134087=CARTESIAN_POINT('Ctrl Pts',(9.99999999999999,29.784151885417,56.8103329589771));
#134088=CARTESIAN_POINT('Ctrl Pts',(10.,29.8180293214886,56.8180947591621));
#134089=CARTESIAN_POINT('Ctrl Pts',(10.,29.8521331499728,56.8248583287514));
#134090=CARTESIAN_POINT('Ctrl Pts',(10.,29.8660806800435,56.827624443127));
#134091=CARTESIAN_POINT('Ctrl Pts',(9.99999999999999,29.8800686440204,56.8302238613979));
#134092=CARTESIAN_POINT('Ctrl Pts',(9.99999999999999,29.8940706859101,56.8326507611155));
#134093=CARTESIAN_POINT('Ctrl Pts',(9.99999999999999,29.9635198353059,56.8446880141378));
#134094=CARTESIAN_POINT('Ctrl Pts',(10.,30.0334344025252,56.8525103460855));
#134095=CARTESIAN_POINT('Ctrl Pts',(10.,30.1034795484966,56.8559771790632));
#134096=CARTESIAN_POINT('Ctrl Pts',(10.,30.1112528776822,56.8563619142735));
#134097=CARTESIAN_POINT('Ctrl Pts',(9.99999999999999,30.1190278448756,56.8566929649851));
#134098=CARTESIAN_POINT('Ctrl Pts',(9.99999999999999,30.1268040132865,56.8569701053381));
#134099=CARTESIAN_POINT('Ctrl Pts',(9.99999999999999,30.1941857015925,56.8593715688738));
#134100=CARTESIAN_POINT('Ctrl Pts',(10.,30.2616564470238,56.8577294314614));
#134101=CARTESIAN_POINT('Ctrl Pts',(10.,30.3289537333749,56.8522616236189));
#134102=CARTESIAN_POINT('Ctrl Pts',(10.,30.401352855462,56.8463792989518));
#134103=CARTESIAN_POINT('Ctrl Pts',(9.99999999999998,30.473552131762,56.8360696937098));
#134104=CARTESIAN_POINT('Ctrl Pts',(9.99999999999997,30.5452332909405,56.8215404883134));
#134105=CARTESIAN_POINT('Ctrl Pts',(9.99999999999997,30.5582509814866,56.8189019051501));
#134106=CARTESIAN_POINT('Ctrl Pts',(9.99999999999999,30.5712515824525,56.8161239898941));
#134107=CARTESIAN_POINT('Ctrl Pts',(9.99999999999999,30.5842331746687,56.8132077668621));
#134108=CARTESIAN_POINT('Ctrl Pts',(9.99999999999998,30.59558256849,56.8106582056751));
#134109=CARTESIAN_POINT('Ctrl Pts',(9.99999999999997,30.6069085600895,56.8080049084806));
#134110=CARTESIAN_POINT('Ctrl Pts',(9.99999999999998,30.6182077920376,56.8052495748911));
#134111=CARTESIAN_POINT('Ctrl Pts',(9.99999999999999,30.6870524499179,56.7884617083184));
#134112=CARTESIAN_POINT('Ctrl Pts',(10.,30.7549278753879,56.767884646354));
#134113=CARTESIAN_POINT('Ctrl Pts',(9.99999999999999,30.8215494692935,56.7437665839902));
#134114=CARTESIAN_POINT('Ctrl Pts',(9.99999999999999,30.8900781708933,56.7189581187164));
#134115=CARTESIAN_POINT('Ctrl Pts',(9.99999999999999,30.9572811586239,56.6904029319238));
#134116=CARTESIAN_POINT('Ctrl Pts',(9.99999999999998,31.0228528016449,56.6583153826992));
#134117=CARTESIAN_POINT('Ctrl Pts',(9.99999999999997,31.0884244446658,56.6262278334746));
#134118=CARTESIAN_POINT('Ctrl Pts',(9.99999999999999,31.1523657592502,56.5906075547783));
#134119=CARTESIAN_POINT('Ctrl Pts',(9.99999999999999,31.2143603894943,56.5516177870526));
#134120=CARTESIAN_POINT('Ctrl Pts',(9.99999999999999,31.2296939735553,56.541974163426));
#134121=CARTESIAN_POINT('Ctrl Pts',(9.99999999999998,31.2449083747354,56.5321241791562));
#134122=CARTESIAN_POINT('Ctrl Pts',(9.99999999999999,31.2599985921039,56.5220698622709));
#134123=CARTESIAN_POINT('Ctrl Pts',(10.,31.27183436846,56.5141839158221));
#134124=CARTESIAN_POINT('Ctrl Pts',(9.99999999999997,31.2835950627688,56.506171208362));
#134125=CARTESIAN_POINT('Ctrl Pts',(9.99999999999997,31.2952606081233,56.498045330906));
#134126=CARTESIAN_POINT('Ctrl Pts',(9.99999999999999,31.3571930817231,56.4549049824932));
#134127=CARTESIAN_POINT('Ctrl Pts',(10.,31.4165584957401,56.4085046904197));
#134128=CARTESIAN_POINT('Ctrl Pts',(10.,31.4730420025436,56.3590793199022));
#134129=CARTESIAN_POINT('Ctrl Pts',(10.,31.5293868312765,56.3097752983484));
#134130=CARTESIAN_POINT('Ctrl Pts',(10.,31.5828649228564,56.2574605914182));
#134131=CARTESIAN_POINT('Ctrl Pts',(9.99999999999997,31.6331479801363,56.2023191232462));
#134132=CARTESIAN_POINT('Ctrl Pts',(9.99999999999995,31.6823740195989,56.1483368032542));
#134133=CARTESIAN_POINT('Ctrl Pts',(10.,31.7285388297368,56.0916447820002));
#134134=CARTESIAN_POINT('Ctrl Pts',(9.99999999999997,31.7713051866725,56.0323758367667));
#134135=CARTESIAN_POINT('Ctrl Pts',(9.99999999999996,31.7804904155719,56.0196462318247));
#134136=CARTESIAN_POINT('Ctrl Pts',(9.99999999999997,31.7895187396851,56.0067976234562));
#134137=CARTESIAN_POINT('Ctrl Pts',(9.99999999999997,31.7983865762153,55.9938311168654));
#134138=CARTESIAN_POINT('Ctrl Pts',(9.99999999999996,31.8058544816558,55.9829115825703));
#134139=CARTESIAN_POINT('Ctrl Pts',(9.99999999999997,31.8132085690898,55.9719084345694));
#134140=CARTESIAN_POINT('Ctrl Pts',(9.99999999999996,31.8204488474911,55.9608235001519));
#134141=CARTESIAN_POINT('',(-0.000875592065448203,31.2702649910176,56.0802705037372));
#134142=CARTESIAN_POINT('Ctrl Pts',(-0.000875592065447961,31.2691220366182,
56.0792985018844));
#134143=CARTESIAN_POINT('Ctrl Pts',(-0.00058372804363219,31.2636294785081,
56.0857570733759));
#134144=CARTESIAN_POINT('Ctrl Pts',(-0.000291864021815771,31.2580876178677,
56.0921737165434));
#134145=CARTESIAN_POINT('Ctrl Pts',(0.,31.2524971005285,56.0985476836113));
#134146=CARTESIAN_POINT('Ctrl Pts',(-8.33100949337862E-16,30.5301702171886,
53.0148256743283));
#134147=CARTESIAN_POINT('Ctrl Pts',(1.52400929049043E-14,30.5991889862419,
53.0403807656738));
#134148=CARTESIAN_POINT('Ctrl Pts',(-6.40578742936595E-15,30.6664868862982,
53.0698652772264));
#134149=CARTESIAN_POINT('Ctrl Pts',(-3.05311331771918E-16,30.731871964553,
53.1029808260606));
#134150=CARTESIAN_POINT('Ctrl Pts',(5.93182098850016E-15,30.7987217281326,
53.13683819336));
#134151=CARTESIAN_POINT('Ctrl Pts',(-1.66504703272918E-14,30.8635727616145,
53.1744918299003));
#134152=CARTESIAN_POINT('Ctrl Pts',(-9.52363188311267E-15,30.9261886107377,
53.2156675311995));
#134153=CARTESIAN_POINT('Ctrl Pts',(-3.5353337505241E-15,30.9788013330987,
53.250265253195));
#134154=CARTESIAN_POINT('Ctrl Pts',(-1.39536846550042E-14,31.0298356324975,
53.28735064929));
#134155=CARTESIAN_POINT('Ctrl Pts',(-1.00613961606655E-14,31.0791289275649,
53.3267786872998));
#134156=CARTESIAN_POINT('Ctrl Pts',(-8.36857957455973E-15,31.1011563662468,
53.3443976898116));
#134157=CARTESIAN_POINT('Ctrl Pts',(-2.11056085633504E-14,31.1228358480513,
53.3624846664704));
#134158=CARTESIAN_POINT('Ctrl Pts',(-1.45300438347817E-14,31.144151317974,
53.3810273958102));
#134159=CARTESIAN_POINT('Ctrl Pts',(-1.08684591444371E-14,31.1558637768627,
53.3912162847189));
#134160=CARTESIAN_POINT('Ctrl Pts',(-2.68961571318634E-14,31.1674663119545,
53.4015427856613));
#134161=CARTESIAN_POINT('Ctrl Pts',(-2.51187959321442E-14,31.1789561254162,
53.4120049126992));
#134162=CARTESIAN_POINT('Ctrl Pts',(-2.36718143111391E-14,31.1895497398249,
53.421650999653));
#134163=CARTESIAN_POINT('Ctrl Pts',(1.14391065484607E-15,31.2000489650095,
53.4314138956186));
#134164=CARTESIAN_POINT('Ctrl Pts',(1.1518563880486E-15,31.2104357202779,
53.4412765890835));
#134165=CARTESIAN_POINT('Ctrl Pts',(8.1966554988569E-16,31.2635217526087,
53.4916841755357));
#134166=CARTESIAN_POINT('Ctrl Pts',(-3.26175822196583E-15,31.3137676963847,
53.5447801824368));
#134167=CARTESIAN_POINT('Ctrl Pts',(-9.28424004342787E-15,31.3609548581112,
53.6003052242583));
#134168=CARTESIAN_POINT('Ctrl Pts',(-1.52131118947695E-14,31.4074085699195,
53.6549672169815));
#134169=CARTESIAN_POINT('Ctrl Pts',(5.15834010684451E-15,31.450898285427,
53.7119842112287));
#134170=CARTESIAN_POINT('Ctrl Pts',(8.42381719934338E-15,31.491171791901,
53.7711323423525));
#134171=CARTESIAN_POINT('Ctrl Pts',(1.11846352470455E-14,31.5252212800365,
53.8211395000414));
#134172=CARTESIAN_POINT('Ctrl Pts',(9.24895866556134E-15,31.556971266667,
53.8726706304121));
#134173=CARTESIAN_POINT('Ctrl Pts',(-6.82787160144471E-15,31.5862409537777,
53.9255971284423));
#134174=CARTESIAN_POINT('Ctrl Pts',(-1.34890089303024E-14,31.5983464196043,
53.9474866659287));
#134175=CARTESIAN_POINT('Ctrl Pts',(-4.85517114680581E-15,31.6100272974802,
53.9696149232492));
#134176=CARTESIAN_POINT('Ctrl Pts',(-1.90125692967058E-14,31.6212693466356,
53.9919728866902));
#134177=CARTESIAN_POINT('Ctrl Pts',(-2.5771791364664E-14,31.6264713864379,
54.0023185998349));
#134178=CARTESIAN_POINT('Ctrl Pts',(-2.75258379892674E-14,31.6315794520179,
54.0127134975132));
#134179=CARTESIAN_POINT('Ctrl Pts',(-2.43693953905222E-14,31.6365920671342,
54.0231566846752));
#134180=CARTESIAN_POINT('Ctrl Pts',(-2.07974541930872E-14,31.6418226285869,
54.0340539370965));
#134181=CARTESIAN_POINT('Ctrl Pts',(-2.23959949028931E-14,31.646945646026,
54.0449963095968));
#134182=CARTESIAN_POINT('Ctrl Pts',(-2.29816166097407E-14,31.6519580706395,
54.0559785146692));
#134183=CARTESIAN_POINT('Ctrl Pts',(-2.63568282812162E-14,31.6804983232411,
54.1185101098663));
#134184=CARTESIAN_POINT('Ctrl Pts',(-1.07629757736254E-14,31.7054776292798,
54.1823749831571));
#134185=CARTESIAN_POINT('Ctrl Pts',(-4.12170297892089E-15,31.7266725222073,
54.247368770426));
#134186=CARTESIAN_POINT('Ctrl Pts',(1.92857175470246E-15,31.745878736449,
54.3062643075221));
#134187=CARTESIAN_POINT('Ctrl Pts',(-2.25561961424682E-14,31.7619770689939,
54.366087447406));
#134188=CARTESIAN_POINT('Ctrl Pts',(-2.02060590481778E-14,31.7747645151277,
54.426690952962));
#134189=CARTESIAN_POINT('Ctrl Pts',(-1.72961694481268E-14,31.7898957509816,
54.4984023741906));
#134190=CARTESIAN_POINT('Ctrl Pts',(-1.01685731942279E-14,31.8003917803375,
54.5712079602738));
#134191=CARTESIAN_POINT('Ctrl Pts',(-5.35682609381638E-15,31.806327769353,
54.6446844903357));
#134192=CARTESIAN_POINT('Ctrl Pts',(-4.30837113251911E-15,31.8076343958791,
54.6608581023443));
#134193=CARTESIAN_POINT('Ctrl Pts',(5.81263003671622E-15,31.8087198528652,
54.6770641414933));
#134194=CARTESIAN_POINT('Ctrl Pts',(8.74300631892311E-15,31.8095845725196,
54.6932979294799));
#134195=CARTESIAN_POINT('Ctrl Pts',(1.17064828251018E-14,31.8104783156427,
54.7100765886703));
#134196=CARTESIAN_POINT('Ctrl Pts',(-1.48807671551939E-15,31.8111362648404,
54.7268910640621));
#134197=CARTESIAN_POINT('Ctrl Pts',(1.80411241501588E-15,31.8115583378869,
54.7437019950884));
#134198=CARTESIAN_POINT('Ctrl Pts',(1.47366039221688E-14,31.8132818157269,
54.8123471439272));
#134199=CARTESIAN_POINT('Ctrl Pts',(-1.9678893150324E-14,31.8110841157504,
54.8810202510296));
#134200=CARTESIAN_POINT('Ctrl Pts',(-1.16850973341798E-14,31.805086261906,
54.9493816698622));
#134201=CARTESIAN_POINT('Ctrl Pts',(-3.71230872538842E-15,31.7991041700553,
55.0175634390598));
#134202=CARTESIAN_POINT('Ctrl Pts',(-2.16825510572882E-14,31.7893413986122,
55.085436219163));
#134203=CARTESIAN_POINT('Ctrl Pts',(-6.46704911844154E-15,31.7758685974957,
55.1526480508404));
#134204=CARTESIAN_POINT('Ctrl Pts',(4.77989727775678E-15,31.7661072564571,
55.2013445026887));
#134205=CARTESIAN_POINT('Ctrl Pts',(1.70591577400874E-14,31.7543973564531,
55.2496937384255));
#134206=CARTESIAN_POINT('Ctrl Pts',(1.11299858218672E-14,31.7407515688752,
55.2975522498582));
#134207=CARTESIAN_POINT('Ctrl Pts',(6.6694150280109E-15,31.730514376406,
55.333456135217));
#134208=CARTESIAN_POINT('Ctrl Pts',(-2.94485010351568E-14,31.7191873909037,
55.3690836793064));
#134209=CARTESIAN_POINT('Ctrl Pts',(2.41473507855972E-15,31.7067720469057,
55.4043701113268));
#134210=CARTESIAN_POINT('Ctrl Pts',(1.31535546200685E-14,31.7026434175627,
55.4161043491114));
#134211=CARTESIAN_POINT('Ctrl Pts',(1.33952048454485E-14,31.6983976298144,
55.4277916642713));
#134212=CARTESIAN_POINT('Ctrl Pts',(1.0547118733939E-14,31.694035322072,
55.4394295150765));
#134213=CARTESIAN_POINT('Ctrl Pts',(-4.75894157798451E-15,31.6709110098913,
55.5011210121069));
#134214=CARTESIAN_POINT('Ctrl Pts',(-6.26081247270993E-15,31.6445141936346,
55.5614289964144));
#134215=CARTESIAN_POINT('Ctrl Pts',(-3.13638004456607E-15,31.6148948930439,
55.6200193099657));
#134216=CARTESIAN_POINT('Ctrl Pts',(-4.45298702533462E-16,31.5940584883539,
55.6612360659228));
#134217=CARTESIAN_POINT('Ctrl Pts',(-1.57022272665468E-14,31.5716265001234,
55.7016022596676));
#134218=CARTESIAN_POINT('Ctrl Pts',(6.66133814775094E-15,31.5476059348169,
55.7409902049166));
#134219=CARTESIAN_POINT('Ctrl Pts',(1.38011075348573E-14,31.5398931143376,
55.7536373739935));
#134220=CARTESIAN_POINT('Ctrl Pts',(-2.65642106040399E-15,31.5320153495236,
55.7661852983957));
#134221=CARTESIAN_POINT('Ctrl Pts',(-2.3037127760972E-15,31.523976211793,
55.7786240933602));
#134222=CARTESIAN_POINT('Ctrl Pts',(2.60456430514903E-16,31.489731385867,
55.8316104188294));
#134223=CARTESIAN_POINT('Ctrl Pts',(1.23913251833813E-14,31.4526309856926,
55.8825128586331));
#134224=CARTESIAN_POINT('Ctrl Pts',(1.1296519275561E-14,31.4127092681578,
55.9310161346265));
#134225=CARTESIAN_POINT('Ctrl Pts',(9.71221749203167E-15,31.3759121039422,
55.9757232044103));
#134226=CARTESIAN_POINT('Ctrl Pts',(1.80240216455387E-14,31.3367173859466,
56.0183920601835));
#134227=CARTESIAN_POINT('Ctrl Pts',(1.6153745008296E-14,31.2951304838667,
56.0587428782121));
#134228=CARTESIAN_POINT('Ctrl Pts',(1.60754418658392E-14,31.2873272806742,
56.0663141474415));
#134229=CARTESIAN_POINT('Ctrl Pts',(-3.83560330923859E-15,31.2794398022902,
56.0738037018648));
#134230=CARTESIAN_POINT('Ctrl Pts',(-1.11022302462516E-15,31.2714696314036,
56.0812108797947));
#134231=CARTESIAN_POINT('Ctrl Pts',(0.00172041412894349,28.7336299816271,
126.077829820709));
#134232=CARTESIAN_POINT('Ctrl Pts',(0.0387785735230462,28.3750939246243,
125.656600540125));
#134233=CARTESIAN_POINT('Ctrl Pts',(0.112881823196669,28.1181816877044,
124.435269010958));
#134234=CARTESIAN_POINT('Ctrl Pts',(0.224030163149812,29.4557424409344,
123.110121783689));
#134235=CARTESIAN_POINT('Ctrl Pts',(0.335165433988371,31.2917730403109,
123.519030371424));
#134236=CARTESIAN_POINT('Ctrl Pts',(0.44630070482693,31.9452349105524,125.281415227633));
#134237=CARTESIAN_POINT('Ctrl Pts',(0.55743597566549,30.818400731034,126.787219544026));
#134238=CARTESIAN_POINT('Ctrl Pts',(0.668571246504049,28.9424467746888,
126.656743001303));
#134239=CARTESIAN_POINT('Ctrl Pts',(0.779706517342608,28.0344714474466,
125.010137817827));
#134240=CARTESIAN_POINT('Ctrl Pts',(0.890841788181168,28.9254742404942,
123.354134483461));
#134241=CARTESIAN_POINT('Ctrl Pts',(1.00197705901972,30.7999674965501,123.204604403169));
#134242=CARTESIAN_POINT('Ctrl Pts',(1.11311232985828,31.9422694308905,124.698320240969));
#134243=CARTESIAN_POINT('Ctrl Pts',(1.22424760069684,31.3068686523209,126.468169431628));
#134244=CARTESIAN_POINT('Ctrl Pts',(1.3353828715354,29.4753269319837,126.894237405488));
#134245=CARTESIAN_POINT('Ctrl Pts',(1.44651814237396,28.1240041248564,125.586566748605));
#134246=CARTESIAN_POINT('Ctrl Pts',(1.55765341321252,28.4897272792089,123.742026340277));
#134247=CARTESIAN_POINT('Ctrl Pts',(1.66878868405108,30.2377606151872,123.04887463911));
#134248=CARTESIAN_POINT('Ctrl Pts',(1.77992395488964,31.7681783056687,124.141532593809));
#134249=CARTESIAN_POINT('Ctrl Pts',(1.8910592257282,31.6802322299405,126.019921790054));
#134250=CARTESIAN_POINT('Ctrl Pts',(2.00219449656676,30.0544169149864,126.964805201012));
#134251=CARTESIAN_POINT('Ctrl Pts',(2.11332976740532,28.3787953370211,126.111357812589));
#134252=CARTESIAN_POINT('Ctrl Pts',(2.22446503824388,28.1870167132214,124.240715901116));
#134253=CARTESIAN_POINT('Ctrl Pts',(2.33560030908244,29.6546106200314,123.065025348056));
#134254=CARTESIAN_POINT('Ctrl Pts',(2.44673557992099,31.438329695648,123.660362577878));
#134255=CARTESIAN_POINT('Ctrl Pts',(2.55787085075956,31.9055861202118,125.481832204441));
#134256=CARTESIAN_POINT('Ctrl Pts',(2.66900612159811,30.6287132507792,126.862294386418));
#134257=CARTESIAN_POINT('Ctrl Pts',(2.78014139243668,28.7763968543991,126.538250979697));
#134258=CARTESIAN_POINT('Ctrl Pts',(2.89127666327523,28.0440099471773,124.806289784764));
#134259=CARTESIAN_POINT('Ctrl Pts',(3.0024119341138,29.1018856333851,123.251626093031));
#134260=CARTESIAN_POINT('Ctrl Pts',(3.11354720495235,30.9817800986816,123.297199785044));
#134261=CARTESIAN_POINT('Ctrl Pts',(3.22468247579091,31.9630788972596,124.901298544487));
#134262=CARTESIAN_POINT('Ctrl Pts',(3.33581774662947,31.1476268828135,126.595735965634));
#134263=CARTESIAN_POINT('Ctrl Pts',(3.44695301746803,29.2817843121772,126.829641210717));
#134264=CARTESIAN_POINT('Ctrl Pts',(3.55808828830659,28.0733043278437,125.38892739821));
#134265=CARTESIAN_POINT('Ctrl Pts',(3.66922355914515,28.6282746155421,123.592239294547));
#134266=CARTESIAN_POINT('Ctrl Pts',(3.78035882998371,30.4387465049373,123.08403490674));
#134267=CARTESIAN_POINT('Ctrl Pts',(3.89149410082227,31.8476460782342,124.329459394392));
#134268=CARTESIAN_POINT('Ctrl Pts',(4.00262937166083,31.5654472459206,126.188610808644));
#134269=CARTESIAN_POINT('Ctrl Pts',(4.11376464249939,29.8504386494267,126.959860233945));
#134270=CARTESIAN_POINT('Ctrl Pts',(4.22489991333795,28.2723193438391,125.937304798085));
#134271=CARTESIAN_POINT('Ctrl Pts',(4.3360351841765,28.2754974725687,124.056860685229));
#134272=CARTESIAN_POINT('Ctrl Pts',(4.44717045501507,29.8570641839197,123.039645418128));
#134273=CARTESIAN_POINT('Ctrl Pts',(4.55830572585362,31.5694560211028,123.816687474921));
#134274=CARTESIAN_POINT('Ctrl Pts',(4.66944099669219,31.8453689751119,125.676782150975));
#134275=CARTESIAN_POINT('Ctrl Pts',(4.78057626753074,30.4322676918504,126.917437189784));
#134276=CARTESIAN_POINT('Ctrl Pts',(4.89171153836931,28.6235239675951,126.403115984657));
#134277=CARTESIAN_POINT('Ctrl Pts',(5.00284680920786,28.0746299792728,124.604562245771));
#134278=CARTESIAN_POINT('Ctrl Pts',(5.11398208004642,29.2879729315736,123.167941543506));
#134279=CARTESIAN_POINT('Ctrl Pts',(5.22511735088498,31.1530142011832,123.408152335789));
#134280=CARTESIAN_POINT('Ctrl Pts',(5.33625262172354,31.9627340538628,125.105336451391));
#134281=CARTESIAN_POINT('Ctrl Pts',(5.4473878925621,30.9760187189675,126.706109080455));
#134282=CARTESIAN_POINT('Ctrl Pts',(5.55852316340066,29.0959809458976,126.745328130754));
#134283=CARTESIAN_POINT('Ctrl Pts',(5.66965843423922,28.0433663460444,125.187097510387));
#134284=CARTESIAN_POINT('Ctrl Pts',(5.78079370507778,28.7816034095847,123.457621809462));
#134285=CARTESIAN_POINT('Ctrl Pts',(5.89192897591634,30.6350045490403,123.139841416201));
#134286=CARTESIAN_POINT('Ctrl Pts',(6.0030642467549,31.9072039133898,124.524611772405));
#134287=CARTESIAN_POINT('Ctrl Pts',(6.11419951759346,31.433793263407,126.344491581228));
#134288=CARTESIAN_POINT('Ctrl Pts',(6.22533478843202,29.6480720306313,126.93379612125));
#134289=CARTESIAN_POINT('Ctrl Pts',(6.33647005927058,28.1844605541017,125.753151548211));
#134290=CARTESIAN_POINT('Ctrl Pts',(6.44760533010913,28.3825611870771,123.883168580029));
#134291=CARTESIAN_POINT('Ctrl Pts',(6.5587406009477,30.0610580008629,123.035389948434));
#134292=CARTESIAN_POINT('Ctrl Pts',(6.66987587178625,31.683670146515,123.985763552263));
#134293=CARTESIAN_POINT('Ctrl Pts',(6.78101114262482,31.7652664375161,125.864439204784));
#134294=CARTESIAN_POINT('Ctrl Pts',(6.89214641346337,30.231164087347,126.951918005167));
#134295=CARTESIAN_POINT('Ctrl Pts',(7.00328168430194,28.4854837601286,126.252861242657));
#134296=CARTESIAN_POINT('Ctrl Pts',(7.11441695514049,28.1259974820121,124.407095878917));
#134297=CARTESIAN_POINT('Ctrl Pts',(7.22555222597905,29.4817329163543,123.103998954614));
#134298=CARTESIAN_POINT('Ctrl Pts',(7.33668749681761,31.3118236122709,123.536258375082));
#134299=CARTESIAN_POINT('Ctrl Pts',(7.44782276765618,31.9412391111934,125.30823927011));
#134300=CARTESIAN_POINT('Ctrl Pts',(7.55895803849473,30.7938931378223,126.798097444275));
#134301=CARTESIAN_POINT('Ctrl Pts',(7.67009330933329,28.9199191404933,126.64220768227));
#134302=CARTESIAN_POINT('Ctrl Pts',(7.78122858017185,28.0345127261816,124.983251489876));
#134303=CARTESIAN_POINT('Ctrl Pts',(7.89236385101041,28.9480614458749,123.339624739461));
#134304=CARTESIAN_POINT('Ctrl Pts',(8.00349912184897,30.82441988656,123.215692685774));
#134305=CARTESIAN_POINT('Ctrl Pts',(8.11463439268753,31.9462100369406,124.724886861491));
#134306=CARTESIAN_POINT('Ctrl Pts',(8.22576966352609,31.2866889522822,126.48588432209));
#134307=CARTESIAN_POINT('Ctrl Pts',(8.33690493436464,29.4494977464259,126.886893763084));
#134308=CARTESIAN_POINT('Ctrl Pts',(8.44804020520321,28.1161656850418,125.560882413626));
#134309=CARTESIAN_POINT('Ctrl Pts',(8.55917547604176,28.507054224578,123.721511362706));
#134310=CARTESIAN_POINT('Ctrl Pts',(8.67031074688032,30.2643937283649,123.052304598731));
#134311=CARTESIAN_POINT('Ctrl Pts',(8.78144601771889,31.7797415997414,124.165769269162));
#134312=CARTESIAN_POINT('Ctrl Pts',(8.89258128855744,31.6661411113959,126.042780405246));
#134313=CARTESIAN_POINT('Ctrl Pts',(9.00371655939601,30.0275706462923,126.965366890392));
#134314=CARTESIAN_POINT('Ctrl Pts',(9.11485183023456,28.3637614026585,126.089102599277));
#134315=CARTESIAN_POINT('Ctrl Pts',(9.22598710107312,28.1975636414152,124.216025180308));
#134316=CARTESIAN_POINT('Ctrl Pts',(9.33712237191168,29.6810681170523,123.060473934073));
#134317=CARTESIAN_POINT('Ctrl Pts',(9.44825764275024,31.4565163554669,123.680164641892));
#134318=CARTESIAN_POINT('Ctrl Pts',(9.5593929135888,31.8987865585251,125.507765498923));
#134319=CARTESIAN_POINT('Ctrl Pts',(9.67052818442736,30.6032919443857,126.870821286213));
#134320=CARTESIAN_POINT('Ctrl Pts',(9.78166345526592,28.7553356095551,126.521165323933));
#134321=CARTESIAN_POINT('Ctrl Pts',(9.89279872610447,28.0471642005665,124.780043256774));
#134322=CARTESIAN_POINT('Ctrl Pts',(10.0039339969431,29.125189557685,123.238590719592));
#134323=CARTESIAN_POINT('Ctrl Pts',(10.1150692677816,31.0063485869877,123.312692118962));
#134324=CARTESIAN_POINT('Ctrl Pts',(10.1891594483406,31.641620391195,124.386603406702));
#134325=CARTESIAN_POINT('Ctrl Pts',(10.2262045386202,31.6618401036677,124.939191752144));
#134326=CARTESIAN_POINT('Ctrl Pts',(-0.0741753660804533,28.6335242142575,
126.163031601966));
#134327=CARTESIAN_POINT('Ctrl Pts',(-0.0371172066863504,28.2466461035143,
125.708504407061));
#134328=CARTESIAN_POINT('Ctrl Pts',(0.0369860429872722,27.9694251130308,
124.390627375262));
#134329=CARTESIAN_POINT('Ctrl Pts',(0.148134382940415,29.412719217227,122.960728078584));
#134330=CARTESIAN_POINT('Ctrl Pts',(0.259269653778974,31.3938869008663,
123.401960637484));
#134331=CARTESIAN_POINT('Ctrl Pts',(0.370404924617533,32.0990045281285,
125.303660927471));
#134332=CARTESIAN_POINT('Ctrl Pts',(0.481540195456093,30.8830948030726,
126.928498144528));
#134333=CARTESIAN_POINT('Ctrl Pts',(0.592675466294653,28.8588478457675,
126.787707511733));
#134334=CARTESIAN_POINT('Ctrl Pts',(0.703810737133211,27.8790976300112,
125.010939206061));
#134335=CARTESIAN_POINT('Ctrl Pts',(0.814946007971772,28.8405336432333,
123.22402983148));
#134336=CARTESIAN_POINT('Ctrl Pts',(0.92608127881033,30.8632044327939,123.062679490744));
#134337=CARTESIAN_POINT('Ctrl Pts',(1.03721654964889,32.0958046291319,124.674472642447));
#134338=CARTESIAN_POINT('Ctrl Pts',(1.14835182048745,31.4101758116771,126.584227317909));
#134339=CARTESIAN_POINT('Ctrl Pts',(1.259487091326,29.4338518501909,127.043975701803));
#134340=CARTESIAN_POINT('Ctrl Pts',(1.37062236216457,27.9757078102415,125.632934487599));
#134341=CARTESIAN_POINT('Ctrl Pts',(1.48175763300312,28.3703411539385,123.64258429987));
#134342=CARTESIAN_POINT('Ctrl Pts',(1.59289290384169,30.256555444888,122.894639385076));
#134343=CARTESIAN_POINT('Ctrl Pts',(1.70402817468025,31.907951708045,124.073671275859));
#134344=CARTESIAN_POINT('Ctrl Pts',(1.8151634455188,31.8130535493788,126.100545977274));
#134345=CARTESIAN_POINT('Ctrl Pts',(1.92629871635736,30.0587185384879,127.120121837955));
#134346=CARTESIAN_POINT('Ctrl Pts',(2.03743398719592,28.2506401102737,126.199209960885));
#134347=CARTESIAN_POINT('Ctrl Pts',(2.14856925803448,28.0437015047767,124.180694962316));
#134348=CARTESIAN_POINT('Ctrl Pts',(2.25970452887304,29.6273078029863,122.912066797581));
#134349=CARTESIAN_POINT('Ctrl Pts',(2.3708397997116,31.5520287692397,123.554465067519));
#134350=CARTESIAN_POINT('Ctrl Pts',(2.48197507055016,32.0562215254133,125.519920742442));
#134351=CARTESIAN_POINT('Ctrl Pts',(2.59311034138872,30.6784126447253,127.009507606816));
#134352=CARTESIAN_POINT('Ctrl Pts',(2.70424561222729,28.6796717818933,126.659848769045));
#134353=CARTESIAN_POINT('Ctrl Pts',(2.81538088306583,27.8893901422511,124.790977111957));
#134354=CARTESIAN_POINT('Ctrl Pts',(2.92651615390439,29.0308902477149,123.113418216132));
#134355=CARTESIAN_POINT('Ctrl Pts',(3.03765142474296,31.0593892087685,123.162594480336));
#134356=CARTESIAN_POINT('Ctrl Pts',(3.14878669558152,32.1182590709579,124.893496255424));
#134357=CARTESIAN_POINT('Ctrl Pts',(3.25992196642008,31.2383460786973,126.721877907595));
#134358=CARTESIAN_POINT('Ctrl Pts',(3.37105723725863,29.2250098058928,126.974273217756));
#134359=CARTESIAN_POINT('Ctrl Pts',(3.4821925080972,27.9210002256061,125.419671868692));
#134360=CARTESIAN_POINT('Ctrl Pts',(3.59332777893576,28.5198405715902,123.48095668074));
#134361=CARTESIAN_POINT('Ctrl Pts',(3.70446304977431,30.473429145019,122.932579050133));
#134362=CARTESIAN_POINT('Ctrl Pts',(3.81559832061288,31.9937013589228,124.276453573894));
#134363=CARTESIAN_POINT('Ctrl Pts',(3.92673359145143,31.6891948833062,126.282569758537));
#134364=CARTESIAN_POINT('Ctrl Pts',(4.03786886229,29.8386159170887,127.114785974297));
#134365=CARTESIAN_POINT('Ctrl Pts',(4.14900413312855,28.13574725563,126.011398163144));
#134366=CARTESIAN_POINT('Ctrl Pts',(4.2601394039671,28.1391766134716,123.98230610523));
#134367=CARTESIAN_POINT('Ctrl Pts',(4.37127467480567,29.8457651959891,122.884680599877));
#134368=CARTESIAN_POINT('Ctrl Pts',(4.48240994564422,31.6935205496892,123.723147351069));
#134369=CARTESIAN_POINT('Ctrl Pts',(4.5935452164828,31.9912442522059,125.730281361776));
#134370=CARTESIAN_POINT('Ctrl Pts',(4.70468048732134,30.4664381857613,127.069009414712));
#134371=CARTESIAN_POINT('Ctrl Pts',(4.81581575815992,28.5147143878589,126.514031436155));
#134372=CARTESIAN_POINT('Ctrl Pts',(4.92695102899846,27.9224306689614,124.573303135669));
#134373=CARTESIAN_POINT('Ctrl Pts',(5.03808629983704,29.2316876318282,123.023118454682));
#134374=CARTESIAN_POINT('Ctrl Pts',(5.14922157067558,31.2441592612549,123.282317761652));
#134375=CARTESIAN_POINT('Ctrl Pts',(5.26035684151415,32.1178869679037,125.113663232778));
#134376=CARTESIAN_POINT('Ctrl Pts',(5.3714921123527,31.0531723955484,126.840975948935));
#134377=CARTESIAN_POINT('Ctrl Pts',(5.48262738319128,29.0245187983303,126.883295240925));
#134378=CARTESIAN_POINT('Ctrl Pts',(5.59376265402982,27.8886956648464,125.201887452962));
#134379=CARTESIAN_POINT('Ctrl Pts',(5.7048979248684,28.6852899120488,123.335697766648));
#134380=CARTESIAN_POINT('Ctrl Pts',(5.81603319570694,30.6852012662261,122.992797029679));
#134381=CARTESIAN_POINT('Ctrl Pts',(5.92716846654552,32.0579672041423,124.487032626791));
#134382=CARTESIAN_POINT('Ctrl Pts',(6.03830373738406,31.5471337348335,126.450772809865));
#134383=CARTESIAN_POINT('Ctrl Pts',(6.14943900822263,29.6202523421347,127.0866615096));
#134384=CARTESIAN_POINT('Ctrl Pts',(6.26057427906118,28.0409432828582,125.812687712669));
#134385=CARTESIAN_POINT('Ctrl Pts',(6.37170954989974,28.2547036484494,123.794883746451));
#134386=CARTESIAN_POINT('Ctrl Pts',(6.4828448207383,30.0658845980988,122.880088737935));
#134387=CARTESIAN_POINT('Ctrl Pts',(6.59398009157685,31.816763231134,123.90558878784));
#134388=CARTESIAN_POINT('Ctrl Pts',(6.70511536241541,31.9048096585145,125.932772589723));
#134389=CARTESIAN_POINT('Ctrl Pts',(6.81625063325399,30.2494374655985,127.106215917242));
#134390=CARTESIAN_POINT('Ctrl Pts',(6.92738590409254,28.3657621872972,126.351899149654));
#134391=CARTESIAN_POINT('Ctrl Pts',(7.0385211749311,27.9778587410484,124.360227174544));
#134392=CARTESIAN_POINT('Ctrl Pts',(7.14965644576966,29.4407642236672,122.954121243655));
#134393=CARTESIAN_POINT('Ctrl Pts',(7.26079171660821,31.4155224581491,123.420550504186));
#134394=CARTESIAN_POINT('Ctrl Pts',(7.37192698744678,32.0946928632995,125.332605393929));
#134395=CARTESIAN_POINT('Ctrl Pts',(7.48306225828533,30.8566498997625,126.94023593607));
#134396=CARTESIAN_POINT('Ctrl Pts',(7.5941975291239,28.8345394160104,126.772023184714));
#134397=CARTESIAN_POINT('Ctrl Pts',(7.70533279996246,27.8791421718047,124.981927530501));
#134398=CARTESIAN_POINT('Ctrl Pts',(7.81646807080102,28.8649063532411,123.208373101183));
#134399=CARTESIAN_POINT('Ctrl Pts',(7.92760334163957,30.8895897691232,123.074644295238));
#134400=CARTESIAN_POINT('Ctrl Pts',(8.03873861247814,32.100056737655,124.703139337904));
#134401=CARTESIAN_POINT('Ctrl Pts',(8.14987388331669,31.3884009188208,126.603342559515));
#134402=CARTESIAN_POINT('Ctrl Pts',(8.26100915415525,29.4059808834766,127.036051549007));
#134403=CARTESIAN_POINT('Ctrl Pts',(8.37214442499382,27.9672497466033,125.605219821814));
#134404=CARTESIAN_POINT('Ctrl Pts',(8.48327969583238,28.3890377836314,123.620447626));
#134405=CARTESIAN_POINT('Ctrl Pts',(8.59441496667093,30.2852938892039,122.898340480884));
#134406=CARTESIAN_POINT('Ctrl Pts',(8.70555023750948,31.9204290733683,124.099823845421));
#134407=CARTESIAN_POINT('Ctrl Pts',(8.81668550834805,31.7978485366211,126.12521155187));
#134408=CARTESIAN_POINT('Ctrl Pts',(8.92782077918661,30.0297500888439,127.120727928533));
#134409=CARTESIAN_POINT('Ctrl Pts',(9.03895605002517,28.2344177526903,126.175195486713));
#134410=CARTESIAN_POINT('Ctrl Pts',(9.15009132086374,28.0550821611265,124.154052455286));
#134411=CARTESIAN_POINT('Ctrl Pts',(9.26122659170229,29.6558567487967,122.907155597137));
#134412=CARTESIAN_POINT('Ctrl Pts',(9.37236186254086,31.5716530732786,123.575832472457));
#134413=CARTESIAN_POINT('Ctrl Pts',(9.48349713337941,32.0488844625773,125.547904047827));
#134414=CARTESIAN_POINT('Ctrl Pts',(9.59463240421796,30.6509817997711,127.018708552771));
#134415=CARTESIAN_POINT('Ctrl Pts',(9.70576767505652,28.6569456586597,126.641412502749));
#134416=CARTESIAN_POINT('Ctrl Pts',(9.81690294589508,27.8927937374215,124.762655812148));
#134417=CARTESIAN_POINT('Ctrl Pts',(9.92803821673365,29.0560363328294,123.099352404481));
#134418=CARTESIAN_POINT('Ctrl Pts',(10.0391734875722,31.0858998208927,123.179311473677));
#134419=CARTESIAN_POINT('Ctrl Pts',(10.1132636681313,31.7713894686415,124.338114785064));
#134420=CARTESIAN_POINT('Ctrl Pts',(10.1503087584108,31.79320753689,124.934384897729));
#134421=CARTESIAN_POINT('Ctrl Pts',(-0.15007114628985,28.5334184468878,
126.248233383223));
#134422=CARTESIAN_POINT('Ctrl Pts',(-0.113012986895747,28.1181982824042,
125.760408273996));
#134423=CARTESIAN_POINT('Ctrl Pts',(-0.0389097372221243,27.8206685383571,
124.345985739566));
#134424=CARTESIAN_POINT('Ctrl Pts',(0.0722386027310179,29.3696959935194,
122.811334373478));
#134425=CARTESIAN_POINT('Ctrl Pts',(0.183373873569577,31.4960007614218,
123.284890903545));
#134426=CARTESIAN_POINT('Ctrl Pts',(0.294509144408137,32.2527741457047,
125.325906627308));
#134427=CARTESIAN_POINT('Ctrl Pts',(0.405644415246696,30.9477888751111,
127.06977674503));
#134428=CARTESIAN_POINT('Ctrl Pts',(0.516779686085255,28.7752489168462,
126.918672022163));
#134429=CARTESIAN_POINT('Ctrl Pts',(0.627914956923815,27.7237238125758,
125.011740594295));
#134430=CARTESIAN_POINT('Ctrl Pts',(0.739050227762374,28.7555930459725,
123.093925179498));
#134431=CARTESIAN_POINT('Ctrl Pts',(0.850185498600933,30.9264413690376,
122.920754578321));
#134432=CARTESIAN_POINT('Ctrl Pts',(0.961320769439493,32.2493398273734,
124.650625043926));
#134433=CARTESIAN_POINT('Ctrl Pts',(1.07245604027805,31.5134829710332,126.700285204189));
#134434=CARTESIAN_POINT('Ctrl Pts',(1.18359131111662,29.3923767683981,127.193713998118));
#134435=CARTESIAN_POINT('Ctrl Pts',(1.29472658195517,27.8274114956265,125.679302226594));
#134436=CARTESIAN_POINT('Ctrl Pts',(1.40586185279373,28.250955028668,123.543142259463));
#134437=CARTESIAN_POINT('Ctrl Pts',(1.51699712363229,30.2753502745888,122.74040413104));
#134438=CARTESIAN_POINT('Ctrl Pts',(1.62813239447085,32.0477251104213,124.00580995791));
#134439=CARTESIAN_POINT('Ctrl Pts',(1.73926766530941,31.9458748688171,126.181170164493));
#134440=CARTESIAN_POINT('Ctrl Pts',(1.85040293614797,30.0630201619894,127.275438474898));
#134441=CARTESIAN_POINT('Ctrl Pts',(1.96153820698653,28.1224848835262,126.287062109182));
#134442=CARTESIAN_POINT('Ctrl Pts',(2.07267347782509,27.9003862963319,124.120674023516));
#134443=CARTESIAN_POINT('Ctrl Pts',(2.18380874866365,29.6000049859411,122.759108247108));
#134444=CARTESIAN_POINT('Ctrl Pts',(2.29494401950221,31.6657278428315,123.44856755716));
#134445=CARTESIAN_POINT('Ctrl Pts',(2.40607929034077,32.2068569306149,125.558009280444));
#134446=CARTESIAN_POINT('Ctrl Pts',(2.51721456117933,30.7281120386715,127.156720827214));
#134447=CARTESIAN_POINT('Ctrl Pts',(2.62834983201789,28.5829467093875,126.781446558392));
#134448=CARTESIAN_POINT('Ctrl Pts',(2.73948510285645,27.7347703373249,124.77566443915));
#134449=CARTESIAN_POINT('Ctrl Pts',(2.85062037369501,28.9598948620446,122.975210339235));
#134450=CARTESIAN_POINT('Ctrl Pts',(2.96175564453356,31.1369983188555,123.027989175629));
#134451=CARTESIAN_POINT('Ctrl Pts',(3.07289091537213,32.273439244656,124.88569396636));
#134452=CARTESIAN_POINT('Ctrl Pts',(3.18402618621068,31.329065274581,126.848019849556));
#134453=CARTESIAN_POINT('Ctrl Pts',(3.29516145704925,29.1682352996085,127.118905224794));
#134454=CARTESIAN_POINT('Ctrl Pts',(3.4062967278878,27.7686961233683,125.450416339173));
#134455=CARTESIAN_POINT('Ctrl Pts',(3.51743199872636,28.4114065276384,123.369674066932));
#134456=CARTESIAN_POINT('Ctrl Pts',(3.62856726956492,30.5081117851007,122.781123193526));
#134457=CARTESIAN_POINT('Ctrl Pts',(3.73970254040348,32.1397566396115,124.223447753396));
#134458=CARTESIAN_POINT('Ctrl Pts',(3.85083781124204,31.8129425206918,126.37652870843));
#134459=CARTESIAN_POINT('Ctrl Pts',(3.9619730820806,29.8267931847508,127.269711714649));
#134460=CARTESIAN_POINT('Ctrl Pts',(4.07310835291916,27.9991751674208,126.085491528203));
#134461=CARTESIAN_POINT('Ctrl Pts',(4.18424362375772,28.0028557543744,123.907751525233));
#134462=CARTESIAN_POINT('Ctrl Pts',(4.29537889459628,29.8344662080584,122.729715781627));
#134463=CARTESIAN_POINT('Ctrl Pts',(4.40651416543484,31.8175850782756,123.629607227217));
#134464=CARTESIAN_POINT('Ctrl Pts',(4.5176494362734,32.1371195293,125.783780572579));
#134465=CARTESIAN_POINT('Ctrl Pts',(4.62878470711196,30.5006086796722,127.22058163964));
#134466=CARTESIAN_POINT('Ctrl Pts',(4.73991997795051,28.4059048081225,126.624946887655));
#134467=CARTESIAN_POINT('Ctrl Pts',(4.85105524878908,27.77023135865,124.542044025567));
#134468=CARTESIAN_POINT('Ctrl Pts',(4.96219051962763,29.1754023320827,122.87829536586));
#134469=CARTESIAN_POINT('Ctrl Pts',(5.07332579046619,31.3353043213265,123.156483187516));
#134470=CARTESIAN_POINT('Ctrl Pts',(5.18446106130475,32.2730398819445,125.121990014166));
#134471=CARTESIAN_POINT('Ctrl Pts',(5.29559633214331,31.1303260721294,126.975842817415));
#134472=CARTESIAN_POINT('Ctrl Pts',(5.40673160298187,28.9530566507631,127.021262351096));
#134473=CARTESIAN_POINT('Ctrl Pts',(5.51786687382043,27.7340249836483,125.216677395537));
#134474=CARTESIAN_POINT('Ctrl Pts',(5.62900214465898,28.5889764145129,123.213773723834));
#134475=CARTESIAN_POINT('Ctrl Pts',(5.74013741549755,30.7353979834119,122.845752643158));
#134476=CARTESIAN_POINT('Ctrl Pts',(5.85127268633611,32.2087304948949,124.449453481178));
#134477=CARTESIAN_POINT('Ctrl Pts',(5.96240795717467,31.6604742062601,126.557054038501));
#134478=CARTESIAN_POINT('Ctrl Pts',(6.07354322801323,29.5924326536382,127.239526897951));
#134479=CARTESIAN_POINT('Ctrl Pts',(6.18467849885179,27.8974260116147,125.872223877128));
#134480=CARTESIAN_POINT('Ctrl Pts',(6.29581376969034,28.1268461098218,123.706598912874));
#134481=CARTESIAN_POINT('Ctrl Pts',(6.40694904052891,30.0707111953348,122.724787527434));
#134482=CARTESIAN_POINT('Ctrl Pts',(6.51808431136746,31.949856315753,123.825414023417));
#134483=CARTESIAN_POINT('Ctrl Pts',(6.62921958220603,32.0443528795128,126.001105974661));
#134484=CARTESIAN_POINT('Ctrl Pts',(6.74035485304458,30.2677108438501,127.260513829318));
#134485=CARTESIAN_POINT('Ctrl Pts',(6.85149012388314,28.2460406144659,126.450937056652));
#134486=CARTESIAN_POINT('Ctrl Pts',(6.96262539472171,27.8297200000849,124.313358470171));
#134487=CARTESIAN_POINT('Ctrl Pts',(7.07376066556025,29.3997955309802,122.804243532695));
#134488=CARTESIAN_POINT('Ctrl Pts',(7.18489593639883,31.5192213040273,123.304842633289));
#134489=CARTESIAN_POINT('Ctrl Pts',(7.29603120723738,32.2481466154056,125.356971517748));
#134490=CARTESIAN_POINT('Ctrl Pts',(7.40716647807594,30.9194066617026,127.082374427863));
#134491=CARTESIAN_POINT('Ctrl Pts',(7.5183017489145,28.7491596915275,126.901838687156));
#134492=CARTESIAN_POINT('Ctrl Pts',(7.62943701975306,27.7237716174278,124.980603571126));
#134493=CARTESIAN_POINT('Ctrl Pts',(7.74057229059162,28.7817512606074,123.077121462905));
#134494=CARTESIAN_POINT('Ctrl Pts',(7.85170756143018,30.9547596516863,122.933595904703));
#134495=CARTESIAN_POINT('Ctrl Pts',(7.96284283226874,32.2539034383696,124.681391814318));
#134496=CARTESIAN_POINT('Ctrl Pts',(8.07397810310729,31.4901128853594,126.72080079694));
#134497=CARTESIAN_POINT('Ctrl Pts',(8.18511337394586,29.3624640205271,127.185209334929));
#134498=CARTESIAN_POINT('Ctrl Pts',(8.29624864478441,27.818333808165,125.649557230001));
#134499=CARTESIAN_POINT('Ctrl Pts',(8.40738391562298,28.2710213426847,123.519383889294));
#134500=CARTESIAN_POINT('Ctrl Pts',(8.51851918646153,30.3061940500428,122.744376363038));
#134501=CARTESIAN_POINT('Ctrl Pts',(8.62965445730009,32.0611165469952,124.033878421681));
#134502=CARTESIAN_POINT('Ctrl Pts',(8.74078972813866,31.9295559618465,126.207642698494));
#134503=CARTESIAN_POINT('Ctrl Pts',(8.85192499897721,30.0319295313953,127.276088966675));
#134504=CARTESIAN_POINT('Ctrl Pts',(8.96306026981578,28.105074102722,126.26128837415));
#134505=CARTESIAN_POINT('Ctrl Pts',(9.07419554065433,27.9126006808377,124.092079730265));
#134506=CARTESIAN_POINT('Ctrl Pts',(9.1853308114929,29.630645380541,122.7538372602));
#134507=CARTESIAN_POINT('Ctrl Pts',(9.29646608233145,31.6867897910901,123.471500303021));
#134508=CARTESIAN_POINT('Ctrl Pts',(9.40760135317001,32.1989823666295,125.588042596731));
#134509=CARTESIAN_POINT('Ctrl Pts',(9.51873662400857,30.6986716551566,127.166595819328));
#134510=CARTESIAN_POINT('Ctrl Pts',(9.62987189484713,28.5585557077642,126.761659681567));
#134511=CARTESIAN_POINT('Ctrl Pts',(9.74100716568569,27.7384232742764,124.745268367524));
#134512=CARTESIAN_POINT('Ctrl Pts',(9.85214243652425,28.9868831079738,122.960114089368));
#134513=CARTESIAN_POINT('Ctrl Pts',(9.96327770736281,31.1654510547976,123.045930828392));
#134514=CARTESIAN_POINT('Ctrl Pts',(10.0373678879219,31.9011585460881,124.289626163427));
#134515=CARTESIAN_POINT('Ctrl Pts',(10.0744129782014,31.9245749701123,124.929578043314));
#134516=CARTESIAN_POINT('Ctrl Pts',(-0.225966926499246,28.4333126795182,
126.33343516448));
#134517=CARTESIAN_POINT('Ctrl Pts',(-0.188908767105143,27.9897504612942,
125.812312140931));
#134518=CARTESIAN_POINT('Ctrl Pts',(-0.114805517431522,27.6719119636834,
124.301344103871));
#134519=CARTESIAN_POINT('Ctrl Pts',(-0.0036571774783789,29.3266727698119,
122.661940668373));
#134520=CARTESIAN_POINT('Ctrl Pts',(0.10747809336018,31.5981146219772,123.167821169605));
#134521=CARTESIAN_POINT('Ctrl Pts',(0.21861336419874,32.4065437632808,125.348152327146));
#134522=CARTESIAN_POINT('Ctrl Pts',(0.329748635037299,31.0124829471497,
127.211055345531));
#134523=CARTESIAN_POINT('Ctrl Pts',(0.440883905875859,28.6916499879248,
127.049636532593));
#134524=CARTESIAN_POINT('Ctrl Pts',(0.552019176714417,27.5683499951404,
125.01254198253));
#134525=CARTESIAN_POINT('Ctrl Pts',(0.663154447552977,28.6706524487117,
122.963820527516));
#134526=CARTESIAN_POINT('Ctrl Pts',(0.774289718391537,30.9896783052814,
122.778829665898));
#134527=CARTESIAN_POINT('Ctrl Pts',(0.885424989230096,32.4028750256148,
124.626777445404));
#134528=CARTESIAN_POINT('Ctrl Pts',(0.996560260068655,31.6167901303894,
126.81634309047));
#134529=CARTESIAN_POINT('Ctrl Pts',(1.10769553090722,29.3509016866054,127.343452294435));
#134530=CARTESIAN_POINT('Ctrl Pts',(1.21883080174578,27.6791151810116,125.725669965589));
#134531=CARTESIAN_POINT('Ctrl Pts',(1.32996607258433,28.1315689033976,123.443700219056));
#134532=CARTESIAN_POINT('Ctrl Pts',(1.44110134342289,30.2941451042897,122.586168877006));
#134533=CARTESIAN_POINT('Ctrl Pts',(1.55223661426145,32.1874985127976,123.93794863996));
#134534=CARTESIAN_POINT('Ctrl Pts',(1.66337188510001,32.0786961882554,126.261794351712));
#134535=CARTESIAN_POINT('Ctrl Pts',(1.77450715593857,30.0673217854909,127.430755111841));
#134536=CARTESIAN_POINT('Ctrl Pts',(1.88564242677713,27.9943296567787,126.374914257477));
#134537=CARTESIAN_POINT('Ctrl Pts',(1.99677769761569,27.7570710878872,124.060653084717));
#134538=CARTESIAN_POINT('Ctrl Pts',(2.10791296845425,29.572702168896,122.606149696634));
#134539=CARTESIAN_POINT('Ctrl Pts',(2.21904823929281,31.7794269164233,123.342670046801));
#134540=CARTESIAN_POINT('Ctrl Pts',(2.33018351013137,32.3574923358165,125.596097818445));
#134541=CARTESIAN_POINT('Ctrl Pts',(2.44131878096993,30.7778114326176,127.303934047614));
#134542=CARTESIAN_POINT('Ctrl Pts',(2.55245405180849,28.4862216368817,126.903044347739));
#134543=CARTESIAN_POINT('Ctrl Pts',(2.66358932264705,27.5801505323987,124.760351766343));
#134544=CARTESIAN_POINT('Ctrl Pts',(2.77472459348561,28.8888994763742,122.837002462337));
#134545=CARTESIAN_POINT('Ctrl Pts',(2.88585986432417,31.2146074289425,122.893383870921));
#134546=CARTESIAN_POINT('Ctrl Pts',(2.99699513516273,32.4286194183543,124.877891677296));
#134547=CARTESIAN_POINT('Ctrl Pts',(3.10813040600128,31.4197844704647,126.974161791518));
#134548=CARTESIAN_POINT('Ctrl Pts',(3.21926567683985,29.1114607933241,127.263537231831));
#134549=CARTESIAN_POINT('Ctrl Pts',(3.3304009476784,27.6163920211307,125.481160809656));
#134550=CARTESIAN_POINT('Ctrl Pts',(3.44153621851696,28.3029724836865,123.258391453124));
#134551=CARTESIAN_POINT('Ctrl Pts',(3.55267148935552,30.5427944251824,122.629667336919));
#134552=CARTESIAN_POINT('Ctrl Pts',(3.66380676019408,32.2858119203001,124.1704419329));
#134553=CARTESIAN_POINT('Ctrl Pts',(3.77494203103264,31.9366901580772,126.470487658325));
#134554=CARTESIAN_POINT('Ctrl Pts',(3.8860773018712,29.8149704524129,127.424637455002));
#134555=CARTESIAN_POINT('Ctrl Pts',(3.99721257270976,27.8626030792116,126.159584893262));
#134556=CARTESIAN_POINT('Ctrl Pts',(4.10834784354832,27.8665348952773,123.833196945235));
#134557=CARTESIAN_POINT('Ctrl Pts',(4.21948311438688,29.8231672201278,122.574750963377));
#134558=CARTESIAN_POINT('Ctrl Pts',(4.33061838522544,31.941649606862,123.536067103365));
#134559=CARTESIAN_POINT('Ctrl Pts',(4.441753656064,32.282994806394,125.83727978338));
#134560=CARTESIAN_POINT('Ctrl Pts',(4.55288892690256,30.5347791735832,127.372153864567));
#134561=CARTESIAN_POINT('Ctrl Pts',(4.66402419774111,28.2970952283862,126.735862339154));
#134562=CARTESIAN_POINT('Ctrl Pts',(4.77515946857968,27.6180320483386,124.510784915466));
#134563=CARTESIAN_POINT('Ctrl Pts',(4.88629473941823,29.1191170323373,122.733472277036));
#134564=CARTESIAN_POINT('Ctrl Pts',(4.99743001025679,31.4264493813982,123.030648613378));
#134565=CARTESIAN_POINT('Ctrl Pts',(5.10856528109536,32.4281927959853,125.130316795553));
#134566=CARTESIAN_POINT('Ctrl Pts',(5.21970055193391,31.2074797487104,127.110709685895));
#134567=CARTESIAN_POINT('Ctrl Pts',(5.33083582277248,28.8815945031958,127.159229461265));
#134568=CARTESIAN_POINT('Ctrl Pts',(5.44197109361103,27.5793543024504,125.231467338112));
#134569=CARTESIAN_POINT('Ctrl Pts',(5.55310636444959,28.492662916977,123.09184968102));
#134570=CARTESIAN_POINT('Ctrl Pts',(5.66424163528815,30.7855947005978,122.698708256637));
#134571=CARTESIAN_POINT('Ctrl Pts',(5.77537690612671,32.3594937856475,124.411874335563));
#134572=CARTESIAN_POINT('Ctrl Pts',(5.88651217696527,31.7738146776866,126.663335267137));
#134573=CARTESIAN_POINT('Ctrl Pts',(5.99764744780384,29.5646129651416,127.392392286301));
#134574=CARTESIAN_POINT('Ctrl Pts',(6.10878271864238,27.7539087403712,125.931760041586));
#134575=CARTESIAN_POINT('Ctrl Pts',(6.21991798948095,27.998988571194,123.618314079298));
#134576=CARTESIAN_POINT('Ctrl Pts',(6.33105326031951,30.0755377925708,122.569486316934));
#134577=CARTESIAN_POINT('Ctrl Pts',(6.44218853115807,32.082949400372,123.745239258995));
#134578=CARTESIAN_POINT('Ctrl Pts',(6.55332380199662,32.1838961005111,126.069439359598));
#134579=CARTESIAN_POINT('Ctrl Pts',(6.66445907283519,30.2859842221016,127.414811741394));
#134580=CARTESIAN_POINT('Ctrl Pts',(6.77559434367375,28.1263190416345,126.549974963649));
#134581=CARTESIAN_POINT('Ctrl Pts',(6.8867296145123,27.6815812591212,124.266489765798));
#134582=CARTESIAN_POINT('Ctrl Pts',(6.99786488535086,29.3588268382931,122.654365821735));
#134583=CARTESIAN_POINT('Ctrl Pts',(7.10900015618942,31.6229201499055,123.189134762393));
#134584=CARTESIAN_POINT('Ctrl Pts',(7.22013542702799,32.4016003675117,125.381337641565));
#134585=CARTESIAN_POINT('Ctrl Pts',(7.33127069786654,30.9821634236429,127.224512919657));
#134586=CARTESIAN_POINT('Ctrl Pts',(7.4424059687051,28.6637799670445,127.031654189599));
#134587=CARTESIAN_POINT('Ctrl Pts',(7.55354123954367,27.5684010630509,124.97927961175));
#134588=CARTESIAN_POINT('Ctrl Pts',(7.66467651038222,28.6985961679736,122.945869824627));
#134589=CARTESIAN_POINT('Ctrl Pts',(7.77581178122078,31.0199295342495,122.792547514168));
#134590=CARTESIAN_POINT('Ctrl Pts',(7.88694705205934,32.4077501390841,124.65964429073));
#134591=CARTESIAN_POINT('Ctrl Pts',(7.99808232289791,31.5918248518981,126.838259034364));
#134592=CARTESIAN_POINT('Ctrl Pts',(8.10921759373646,29.3189471575778,127.334367120851));
#134593=CARTESIAN_POINT('Ctrl Pts',(8.22035286457502,27.6694178697268,125.693894638187));
#134594=CARTESIAN_POINT('Ctrl Pts',(8.33148813541358,28.1530049017381,123.418320152587));
#134595=CARTESIAN_POINT('Ctrl Pts',(8.44262340625213,30.3270942108819,122.590412245191));
#134596=CARTESIAN_POINT('Ctrl Pts',(8.5537586770907,32.2018040206222,123.967932997941));
#134597=CARTESIAN_POINT('Ctrl Pts',(8.66489394792926,32.0612633870717,126.290073845118));
#134598=CARTESIAN_POINT('Ctrl Pts',(8.77602921876781,30.0341089739469,127.431450004816));
#134599=CARTESIAN_POINT('Ctrl Pts',(8.88716448960638,27.9757304527538,126.347381261586));
#134600=CARTESIAN_POINT('Ctrl Pts',(8.99829976044494,27.7701192005489,124.030107005244));
#134601=CARTESIAN_POINT('Ctrl Pts',(9.10943503128349,29.6054340122852,122.600518923263));
#134602=CARTESIAN_POINT('Ctrl Pts',(9.22057030212206,31.8019265089017,123.367168133586));
#134603=CARTESIAN_POINT('Ctrl Pts',(9.3317055729606,32.3490802706817,125.628181145636));
#134604=CARTESIAN_POINT('Ctrl Pts',(9.44284084379918,30.7463615105419,127.314483085886));
#134605=CARTESIAN_POINT('Ctrl Pts',(9.55397611463773,28.4601657568688,126.881906860385));
#134606=CARTESIAN_POINT('Ctrl Pts',(9.66511138547629,27.5840528111314,124.727880922899));
#134607=CARTESIAN_POINT('Ctrl Pts',(9.77624665631484,28.9177298831183,122.820875774256));
#134608=CARTESIAN_POINT('Ctrl Pts',(9.88738192715342,31.2450022887026,122.912550183106));
#134609=CARTESIAN_POINT('Ctrl Pts',(9.96147210771245,32.0309276235346,124.241137541789));
#134610=CARTESIAN_POINT('Ctrl Pts',(9.99851719799197,32.0559424033345,124.924771188899));
#134611=CARTESIAN_POINT('',(10.0008700299984,29.229417545743,123.521225009551));
#134612=CARTESIAN_POINT('Ctrl Pts',(10.,32.0533758325287,124.92486510207));
#134613=CARTESIAN_POINT('Ctrl Pts',(10.,32.0436838801938,124.850853971349));
#134614=CARTESIAN_POINT('Ctrl Pts',(9.99999999999998,32.0296437464646,124.777580246055));
#134615=CARTESIAN_POINT('Ctrl Pts',(9.99999999999997,32.011487005396,124.705321521794));
#134616=CARTESIAN_POINT('Ctrl Pts',(9.99999999999996,31.9938051114884,124.634952555719));
#134617=CARTESIAN_POINT('Ctrl Pts',(9.99999999999999,31.9722183073752,124.565545575943));
#134618=CARTESIAN_POINT('Ctrl Pts',(9.99999999999997,31.9469006329171,124.497379595077));
#134619=CARTESIAN_POINT('Ctrl Pts',(9.99999999999996,31.9412499679373,124.482165594221));
#134620=CARTESIAN_POINT('Ctrl Pts',(9.99999999999996,31.9354125162585,124.467011522081));
#134621=CARTESIAN_POINT('Ctrl Pts',(9.99999999999998,31.9293925581285,124.451927087433));
#134622=CARTESIAN_POINT('Ctrl Pts',(10.0000000000001,31.9017664039417,124.382703197761));
#134623=CARTESIAN_POINT('Ctrl Pts',(9.99999999999996,31.870356225898,124.315080819697));
#134624=CARTESIAN_POINT('Ctrl Pts',(10.0000000000001,31.8353723366309,124.249352545652));
#134625=CARTESIAN_POINT('Ctrl Pts',(10.0000000000001,31.810811842914,124.20320790892));
#134626=CARTESIAN_POINT('Ctrl Pts',(10.,31.7844889480599,124.157997341092));
#134627=CARTESIAN_POINT('Ctrl Pts',(10.0000000000001,31.7564653772615,124.113832752978));
#134628=CARTESIAN_POINT('Ctrl Pts',(10.0000000000001,31.745815848242,124.097049307851));
#134629=CARTESIAN_POINT('Ctrl Pts',(10.,31.7349206335243,124.080417022449));
#134630=CARTESIAN_POINT('Ctrl Pts',(9.99999999999998,31.7237828414283,124.063942444803));
#134631=CARTESIAN_POINT('Ctrl Pts',(9.99999999999993,31.7131612362719,124.048231390282));
#134632=CARTESIAN_POINT('Ctrl Pts',(10.0000000000001,31.702315414293,124.032658992084));
#134633=CARTESIAN_POINT('Ctrl Pts',(10.0000000000001,31.6912678340984,124.017258102486));
#134634=CARTESIAN_POINT('Ctrl Pts',(10.0000000000001,31.648949962443,123.958264833559));
#134635=CARTESIAN_POINT('Ctrl Pts',(10.,31.6036337000859,123.901720305621));
#134636=CARTESIAN_POINT('Ctrl Pts',(10.,31.5555120295465,123.847896734174));
#134637=CARTESIAN_POINT('Ctrl Pts',(10.,31.5084230386781,123.795228203843));
#134638=CARTESIAN_POINT('Ctrl Pts',(10.0000000000001,31.4586469877109,123.745164560953));
#134639=CARTESIAN_POINT('Ctrl Pts',(10.0000000000001,31.4063360139386,123.698000619784));
#134640=CARTESIAN_POINT('Ctrl Pts',(10.0000000000001,31.3551727086319,123.65187142456));
#134641=CARTESIAN_POINT('Ctrl Pts',(9.99999999999992,31.3015838507054,123.608515661013));
#134642=CARTESIAN_POINT('Ctrl Pts',(9.99999999999988,31.2456942589875,123.568254646092));
#134643=CARTESIAN_POINT('Ctrl Pts',(9.99999999999987,31.2275284079873,123.555168567348));
#134644=CARTESIAN_POINT('Ctrl Pts',(10.0000000000001,31.2091193946461,123.542409825234));
#134645=CARTESIAN_POINT('Ctrl Pts',(10.0000000000001,31.1904712619119,123.529990635087));
#134646=CARTESIAN_POINT('Ctrl Pts',(10.0000000000001,31.179965598328,123.522994125811));
#134647=CARTESIAN_POINT('Ctrl Pts',(10.0000000000002,31.1693828915675,123.516104777863));
#134648=CARTESIAN_POINT('Ctrl Pts',(10.0000000000001,31.1587390473461,123.509334179643));
#134649=CARTESIAN_POINT('Ctrl Pts',(9.99999999999996,31.1011038925273,123.472672192814));
#134650=CARTESIAN_POINT('Ctrl Pts',(10.,31.041579032397,123.439421075485));
#134651=CARTESIAN_POINT('Ctrl Pts',(9.99999999999991,30.9803088822866,123.409847885084));
#134652=CARTESIAN_POINT('Ctrl Pts',(9.9999999999999,30.9714786041448,123.405585785247));
#134653=CARTESIAN_POINT('Ctrl Pts',(10.,30.9626120424464,123.401400160729));
#134654=CARTESIAN_POINT('Ctrl Pts',(10.,30.9537095988913,123.39729189634));
#134655=CARTESIAN_POINT('Ctrl Pts',(9.99999999999998,30.8907195264398,123.368223487207));
#134656=CARTESIAN_POINT('Ctrl Pts',(9.9999999999998,30.8259335006331,123.343023769821));
#134657=CARTESIAN_POINT('Ctrl Pts',(9.99999999999985,30.7597192517224,123.321677672926));
#134658=CARTESIAN_POINT('Ctrl Pts',(9.99999999999989,30.6979479251232,123.301763881792));
#134659=CARTESIAN_POINT('Ctrl Pts',(10.,30.6349327477613,123.285204520595));
#134660=CARTESIAN_POINT('Ctrl Pts',(10.,30.5709758239915,123.272027286914));
#134661=CARTESIAN_POINT('Ctrl Pts',(10.,30.5569222627032,123.269131790223));
#134662=CARTESIAN_POINT('Ctrl Pts',(9.99999999999973,30.5428232716055,123.26639973771));
#134663=CARTESIAN_POINT('Ctrl Pts',(9.99999999999988,30.5286821398607,123.263831663828));
#134664=CARTESIAN_POINT('Ctrl Pts',(9.99999999999999,30.5175493411139,123.261809912654));
#134665=CARTESIAN_POINT('Ctrl Pts',(10.0000000000001,30.506390968432,123.259889975947));
#134666=CARTESIAN_POINT('Ctrl Pts',(10.0000000000001,30.4952217650004,123.258074005347));
#134667=CARTESIAN_POINT('Ctrl Pts',(9.99999999999998,30.4277390447172,123.247102172233));
#134668=CARTESIAN_POINT('Ctrl Pts',(10.0000000000001,30.3597367395742,123.23989796486));
#134669=CARTESIAN_POINT('Ctrl Pts',(9.99999999999997,30.2915660703205,123.236428532288));
#134670=CARTESIAN_POINT('Ctrl Pts',(9.99999999999985,30.2237084738309,123.232975033033));
#134671=CARTESIAN_POINT('Ctrl Pts',(9.99999999999983,30.1556829478191,123.233222328895));
#134672=CARTESIAN_POINT('Ctrl Pts',(9.99999999999995,30.0878446921053,123.237188390519));
#134673=CARTESIAN_POINT('Ctrl Pts',(10.0000000000001,30.0214572536015,123.241069632296));
#134674=CARTESIAN_POINT('Ctrl Pts',(9.99999999999994,29.9552482504001,123.248512619597));
#134675=CARTESIAN_POINT('Ctrl Pts',(9.99999999999983,29.8895737838068,123.259578024576));
#134676=CARTESIAN_POINT('Ctrl Pts',(9.9999999999998,29.8704842081868,123.262794402205));
#134677=CARTESIAN_POINT('Ctrl Pts',(10.0000000000001,29.8514399947749,123.266317103788));
#134678=CARTESIAN_POINT('Ctrl Pts',(10.0000000000001,29.8324504331394,123.270148273509));
#134679=CARTESIAN_POINT('Ctrl Pts',(10.0000000000002,29.821877140126,123.272281449662));
#134680=CARTESIAN_POINT('Ctrl Pts',(9.99999999999979,29.8113302806734,123.274508350105));
#134681=CARTESIAN_POINT('Ctrl Pts',(9.9999999999998,29.8008115170796,123.276828838321));
#134682=CARTESIAN_POINT('Ctrl Pts',(9.99999999999982,29.7370705081107,123.29089040163));
#134683=CARTESIAN_POINT('Ctrl Pts',(9.9999999999999,29.6743561255583,123.308385480754));
#134684=CARTESIAN_POINT('Ctrl Pts',(9.9999999999999,29.6129879890306,123.329323310669));
#134685=CARTESIAN_POINT('Ctrl Pts',(9.99999999999991,29.5501643704022,123.350757727875));
#134686=CARTESIAN_POINT('Ctrl Pts',(10.0000000000001,29.4887504504911,123.375800193779));
#134687=CARTESIAN_POINT('Ctrl Pts',(10.0000000000002,29.4291213825965,123.404508661191));
#134688=CARTESIAN_POINT('Ctrl Pts',(10.0000000000002,29.3738779432933,123.431105663844));
#134689=CARTESIAN_POINT('Ctrl Pts',(10.0000000000001,29.3201661528932,123.460849885524));
#134690=CARTESIAN_POINT('Ctrl Pts',(10.0000000000002,29.2683211125717,123.493821880151));
#134691=CARTESIAN_POINT('Ctrl Pts',(10.0000000000002,29.2642052737676,123.496439438438));
#134692=CARTESIAN_POINT('Ctrl Pts',(10.0000000000001,29.260101221769,123.499077355755));
#134693=CARTESIAN_POINT('Ctrl Pts',(10.0000000000002,29.2560091359247,123.501735680849));
#134694=CARTESIAN_POINT('Ctrl Pts',(10.0000000000003,29.2468933389776,123.507657538966));
#134695=CARTESIAN_POINT('Ctrl Pts',(10.,29.2378369215811,123.513680670008));
#134696=CARTESIAN_POINT('Ctrl Pts',(10.,29.2288409619357,123.519803760817));
#134697=CARTESIAN_POINT('Ctrl Pts',(-2.78639958328775E-16,28.7309291201476,
126.079358653049));
#134698=CARTESIAN_POINT('Ctrl Pts',(2.43951905577452E-13,28.6856045121037,
126.037075604188));
#134699=CARTESIAN_POINT('Ctrl Pts',(2.32264696777501E-14,28.6430101816999,
125.992223094823));
#134700=CARTESIAN_POINT('Ctrl Pts',(-1.23824561715224E-14,28.6031444611115,
125.945146237493));
#134701=CARTESIAN_POINT('Ctrl Pts',(-5.0440039678236E-14,28.5606416816283,
125.894955315159));
#134702=CARTESIAN_POINT('Ctrl Pts',(-1.53712585429092E-14,28.5212397133509,
125.842235804835));
#134703=CARTESIAN_POINT('Ctrl Pts',(-5.82867087928207E-16,28.4849653865329,
125.787351197263));
#134704=CARTESIAN_POINT('Ctrl Pts',(1.27498972438004E-14,28.4532253505671,
125.739327165638));
#134705=CARTESIAN_POINT('Ctrl Pts',(7.95844567888735E-14,28.4238801589872,
125.689644255155));
#134706=CARTESIAN_POINT('Ctrl Pts',(-1.85268467234323E-14,28.396970688999,
125.638518410175));
#134707=CARTESIAN_POINT('Ctrl Pts',(-6.76177436159774E-14,28.383472104572,
125.612872177263));
#134708=CARTESIAN_POINT('Ctrl Pts',(5.0431355625446E-14,28.3705867868154,
125.586862499757));
#134709=CARTESIAN_POINT('Ctrl Pts',(5.70862801474448E-14,28.3583222370606,
125.560514794078));
#134710=CARTESIAN_POINT('Ctrl Pts',(6.02689641839324E-14,28.3527132731747,
125.548465160574));
#134711=CARTESIAN_POINT('Ctrl Pts',(3.48561988117052E-14,28.3472335647089,
125.536343140102));
#134712=CARTESIAN_POINT('Ctrl Pts',(3.5978164891759E-14,28.3418923437833,
125.524171131458));
#134713=CARTESIAN_POINT('Ctrl Pts',(4.15921821842815E-14,28.3149790658411,
125.46283896484));
#134714=CARTESIAN_POINT('Ctrl Pts',(5.59872842514893E-14,28.2915266892741,
125.400131282304));
#134715=CARTESIAN_POINT('Ctrl Pts',(-1.64451785522601E-15,28.2715585090975,
125.336405988326));
#134716=CARTESIAN_POINT('Ctrl Pts',(-6.05299641908085E-14,28.2511803715366,
125.27137238009));
#134717=CARTESIAN_POINT('Ctrl Pts',(-1.51360821367708E-14,28.2344303837891,
125.205278113985));
#134718=CARTESIAN_POINT('Ctrl Pts',(-2.14273043752655E-14,28.2213730031473,
125.138466741869));
#134719=CARTESIAN_POINT('Ctrl Pts',(-2.6658648028734E-14,28.2105153918976,
125.082911043112));
#134720=CARTESIAN_POINT('Ctrl Pts',(6.74653547581201E-15,28.202211586376,
125.026858558113));
#134721=CARTESIAN_POINT('Ctrl Pts',(7.89646126264643E-15,28.196523242066,
124.970494651124));
#134722=CARTESIAN_POINT('Ctrl Pts',(8.51570007836861E-15,28.1938947698915,
124.944449996811));
#134723=CARTESIAN_POINT('Ctrl Pts',(-8.72662611035027E-15,28.1918250788729,
124.918338736059));
#134724=CARTESIAN_POINT('Ctrl Pts',(3.3584246494911E-15,28.1903220501733,
124.892178757629));
#134725=CARTESIAN_POINT('Ctrl Pts',(8.48608315006128E-15,28.1896651687426,
124.880745839508));
#134726=CARTESIAN_POINT('Ctrl Pts',(-2.44137855573384E-14,28.1891166383197,
124.86930381891));
#134727=CARTESIAN_POINT('Ctrl Pts',(-2.27873275804313E-14,28.1886774510598,
124.857868328144));
#134728=CARTESIAN_POINT('Ctrl Pts',(-1.28244564203572E-14,28.1859840496925,
124.787737954891));
#134729=CARTESIAN_POINT('Ctrl Pts',(-2.61029113609051E-14,28.1873908986415,
124.717721796522));
#134730=CARTESIAN_POINT('Ctrl Pts',(1.55431223447522E-15,28.1929524150393,
124.648180880013));
#134731=CARTESIAN_POINT('Ctrl Pts',(2.62922359085441E-14,28.1979245136766,
124.586010013027));
#134732=CARTESIAN_POINT('Ctrl Pts',(-1.89380643560603E-14,28.2062176594135,
124.524218028094));
#134733=CARTESIAN_POINT('Ctrl Pts',(5.73152636462737E-15,28.2179038679988,
124.463050764826));
#134734=CARTESIAN_POINT('Ctrl Pts',(3.25218004191036E-14,28.2306365799094,
124.396405955617));
#134735=CARTESIAN_POINT('Ctrl Pts',(-4.75594221305812E-14,28.2473961773284,
124.330501931656));
#134736=CARTESIAN_POINT('Ctrl Pts',(3.12527781431982E-14,28.267937556801,
124.265552134843));
#134737=CARTESIAN_POINT('Ctrl Pts',(6.17662707231035E-14,28.2758645232437,
124.240487856152));
#134738=CARTESIAN_POINT('Ctrl Pts',(-4.83646106192593E-14,28.2843552288597,
124.215565728878));
#134739=CARTESIAN_POINT('Ctrl Pts',(-8.82627304576999E-15,28.2933975953373,
124.190798339915));
#134740=CARTESIAN_POINT('Ctrl Pts',(8.52941477985801E-15,28.2973639657865,
124.179934298967));
#134741=CARTESIAN_POINT('Ctrl Pts',(-9.62032087635259E-15,28.3014363742385,
124.169100609291));
#134742=CARTESIAN_POINT('Ctrl Pts',(-2.72004641033163E-15,28.3056087226356,
124.158310852064));
#134743=CARTESIAN_POINT('Ctrl Pts',(3.85734597192918E-14,28.3308312619704,
124.093084976808));
#134744=CARTESIAN_POINT('Ctrl Pts',(6.02936583413694E-14,28.3597443603586,
124.029345353138));
#134745=CARTESIAN_POINT('Ctrl Pts',(9.81992265280951E-14,28.3920354848392,
123.967310636409));
#134746=CARTESIAN_POINT('Ctrl Pts',(1.37087657368489E-13,28.4250737751078,
123.90384053399));
#134747=CARTESIAN_POINT('Ctrl Pts',(1.3210876930124E-13,28.461648526632,
123.84215432989));
#134748=CARTESIAN_POINT('Ctrl Pts',(1.9595436384634E-14,28.5014811380923,
123.782489939349));
#134749=CARTESIAN_POINT('Ctrl Pts',(-6.6418823366357E-14,28.5319599761612,
123.736836359754));
#134750=CARTESIAN_POINT('Ctrl Pts',(3.98228911114656E-15,28.5643474730915,
123.692366499728));
#134751=CARTESIAN_POINT('Ctrl Pts',(8.70137295549966E-14,28.5985383356841,
123.649193044353));
#134752=CARTESIAN_POINT('Ctrl Pts',(1.38648056659717E-13,28.619824456337,
123.622314653156));
#134753=CARTESIAN_POINT('Ctrl Pts',(1.22190750202126E-13,28.6418098672274,
123.595938858562));
#134754=CARTESIAN_POINT('Ctrl Pts',(1.34087185799103E-13,28.6644720642652,
123.570094538783));
#134755=CARTESIAN_POINT('Ctrl Pts',(1.40798623008578E-13,28.6771664952139,
123.555617613518));
#134756=CARTESIAN_POINT('Ctrl Pts',(3.97015826307881E-14,28.6900777714248,
123.541302901776));
#134757=CARTESIAN_POINT('Ctrl Pts',(1.19348975147204E-14,28.7031781914608,
123.527180952641));
#134758=CARTESIAN_POINT('Ctrl Pts',(-9.64246718465023E-14,28.7540452177212,
123.472347477413));
#134759=CARTESIAN_POINT('Ctrl Pts',(-6.96814581978678E-14,28.8078087436982,
123.420359024874));
#134760=CARTESIAN_POINT('Ctrl Pts',(-7.75213226944516E-14,28.864184000068,
123.371479324179));
#134761=CARTESIAN_POINT('Ctrl Pts',(-8.33770163543804E-14,28.9063445726748,
123.334924347707));
#134762=CARTESIAN_POINT('Ctrl Pts',(1.58152049026456E-13,28.9499670126063,
123.300108259198));
#134763=CARTESIAN_POINT('Ctrl Pts',(-9.90596493721796E-14,28.9949486028232,
123.267151117223));
#134764=CARTESIAN_POINT('Ctrl Pts',(-1.7947882528363E-13,29.0089990364185,
123.256856636024));
#134765=CARTESIAN_POINT('Ctrl Pts',(1.56627630403963E-13,29.0231821727827,
123.246743606353));
#134766=CARTESIAN_POINT('Ctrl Pts',(3.36675132217579E-14,29.0374951222103,
123.236815913378));
#134767=CARTESIAN_POINT('Ctrl Pts',(-8.47289291612157E-14,29.0512877290505,
123.227249138428));
#134768=CARTESIAN_POINT('Ctrl Pts',(5.31593884409529E-14,29.0651938482479,
123.217859411298));
#134769=CARTESIAN_POINT('Ctrl Pts',(1.44884104713583E-14,29.0792055012066,
123.208652961744));
#134770=CARTESIAN_POINT('Ctrl Pts',(-1.59719470102946E-13,29.1421550047024,
123.167291572758));
#134771=CARTESIAN_POINT('Ctrl Pts',(-3.90017336220626E-14,29.2072623202427,
123.129605449444));
#134772=CARTESIAN_POINT('Ctrl Pts',(-9.32032229172819E-14,29.2742663398359,
123.095873566138));
#134773=CARTESIAN_POINT('Ctrl Pts',(-1.34974257368109E-13,29.3255152870948,
123.070073270588));
#134774=CARTESIAN_POINT('Ctrl Pts',(-1.96225293566553E-13,29.3778748117198,
123.046586677912));
#134775=CARTESIAN_POINT('Ctrl Pts',(-2.60125254669674E-13,29.4312419689629,
123.025553895645));
#134776=CARTESIAN_POINT('Ctrl Pts',(-2.74819563164584E-13,29.4435211852116,
123.020714475764));
#134777=CARTESIAN_POINT('Ctrl Pts',(-1.97358671919277E-13,29.4558537898234,
123.016005028946));
#134778=CARTESIAN_POINT('Ctrl Pts',(-5.10702591327572E-15,29.468237921027,
123.011424990249));
#134779=CARTESIAN_POINT('Ctrl Pts',(10.,29.2076925604819,123.534460876918));
#134780=CARTESIAN_POINT('Ctrl Pts',(10.0002900099995,29.215135678433,123.530436939492));
#134781=CARTESIAN_POINT('Ctrl Pts',(10.0005800199989,29.2226094518746,123.526469705855));
#134782=CARTESIAN_POINT('Ctrl Pts',(10.0008700299984,29.230113013341,123.522559636475));
#134783=CARTESIAN_POINT('Ctrl Pts',(0.00155432571019262,30.5308648559221,
123.01222466255));
#134784=CARTESIAN_POINT('Ctrl Pts',(0.0385994159897124,31.1918318661709,
123.188745695915));
#134785=CARTESIAN_POINT('Ctrl Pts',(0.112689596548752,32.3122910244663,
124.250671109051));
#134786=CARTESIAN_POINT('Ctrl Pts',(0.223824867387312,31.8837750190762,
126.540127999121));
#134787=CARTESIAN_POINT('Ctrl Pts',(0.334960138225871,29.72768122948,127.416072798206));
#134788=CARTESIAN_POINT('Ctrl Pts',(0.44609540906443,27.8224997759096,126.082528680968));
#134789=CARTESIAN_POINT('Ctrl Pts',(0.55723067990299,27.9095008630876,123.757255622762));
#134790=CARTESIAN_POINT('Ctrl Pts',(0.66836595074155,29.9102827683814,122.569885979054));
#134791=CARTESIAN_POINT('Ctrl Pts',(0.779501221580109,31.9929799341018,
123.606506840134));
#134792=CARTESIAN_POINT('Ctrl Pts',(0.890636492418669,32.251657659651,125.918663536734));
#134793=CARTESIAN_POINT('Ctrl Pts',(1.00177176325722,30.4494077016117,127.389938666344));
#134794=CARTESIAN_POINT('Ctrl Pts',(1.11290703409579,28.2358516598168,126.673797276444));
#134795=CARTESIAN_POINT('Ctrl Pts',(1.22404230493434,27.6369589836974,124.425663052317));
#134796=CARTESIAN_POINT('Ctrl Pts',(1.3351775757729,29.2008970629833,122.703209843518));
#134797=CARTESIAN_POINT('Ctrl Pts',(1.44631284661146,31.4962286446548,123.082940710024));
#134798=CARTESIAN_POINT('Ctrl Pts',(1.55744811745002,32.422105732079,125.217303545347));
#134799=CARTESIAN_POINT('Ctrl Pts',(1.66858338828858,31.1310969676118,127.152773774276));
#134800=CARTESIAN_POINT('Ctrl Pts',(1.77971865912714,28.8048273623399,127.117871204668));
#134801=CARTESIAN_POINT('Ctrl Pts',(1.8908539299657,27.5724654306094,125.144540590365));
#134802=CARTESIAN_POINT('Ctrl Pts',(2.00198920080426,28.5619575897349,123.038916141001));
#134803=CARTESIAN_POINT('Ctrl Pts',(2.11312447164282,30.8676494139743,122.728216455201));
#134804=CARTESIAN_POINT('Ctrl Pts',(2.22425974248138,32.3792061928279,124.496816273114));
#134805=CARTESIAN_POINT('Ctrl Pts',(2.33539501331994,31.7131425574306,126.725965969629));
#134806=CARTESIAN_POINT('Ctrl Pts',(2.4465302841585,29.4790878050011,127.37538764178));
#134807=CARTESIAN_POINT('Ctrl Pts',(2.55766555499706,27.7218093076021,125.850683919345));
#134808=CARTESIAN_POINT('Ctrl Pts',(2.66880082583561,28.0496945735768,123.547373171422));
#134809=CARTESIAN_POINT('Ctrl Pts',(2.77993609667418,30.1626394539462,122.573610837253));
#134810=CARTESIAN_POINT('Ctrl Pts',(2.89107136751274,32.1267250241147,123.82065415059));
#134811=CARTESIAN_POINT('Ctrl Pts',(3.00220663835129,32.1442790912563,126.147119496527));
#134812=CARTESIAN_POINT('Ctrl Pts',(3.11334190918986,30.1992349124517,127.42365868273));
#134813=CARTESIAN_POINT('Ctrl Pts',(3.22447718002841,28.0718366308647,126.481891353163));
#134814=CARTESIAN_POINT('Ctrl Pts',(3.33561245086697,27.7092319630256,124.183790614235));
#134815=CARTESIAN_POINT('Ctrl Pts',(3.44674772170553,29.443302746492,122.632743332759));
#134816=CARTESIAN_POINT('Ctrl Pts',(3.55788299254409,31.6869028434527,123.248379391135));
#134817=CARTESIAN_POINT('Ctrl Pts',(3.66901826338265,32.3865282893196,125.467224448126));
#134818=CARTESIAN_POINT('Ctrl Pts',(3.78015353422121,30.9018316225513,127.258432129867));
#134819=CARTESIAN_POINT('Ctrl Pts',(3.89128880505977,28.5917138770426,126.982560505139));
#134820=CARTESIAN_POINT('Ctrl Pts',(4.00242407589833,27.5705607472319,124.89210710051));
#134821=CARTESIAN_POINT('Ctrl Pts',(4.11355934673689,28.7730049260626,122.900405027348));
#134822=CARTESIAN_POINT('Ctrl Pts',(4.22469461757545,31.0984831305496,122.830403085237));
#134823=CARTESIAN_POINT('Ctrl Pts',(4.33582988841401,32.41855067087,124.746172079776));
#134824=CARTESIAN_POINT('Ctrl Pts',(4.44696515925257,31.5249869148193,126.894262619143));
#134825=CARTESIAN_POINT('Ctrl Pts',(4.55810043009113,29.2356455958426,127.308587946233));
#134826=CARTESIAN_POINT('Ctrl Pts',(4.6692357009297,27.6458963304626,125.609927761068));
#134827=CARTESIAN_POINT('Ctrl Pts',(4.78037097176824,28.210791836662,123.353017878392));
#134828=CARTESIAN_POINT('Ctrl Pts',(4.89150624260681,30.4132991712142,122.603544334705));
#134829=CARTESIAN_POINT('Ctrl Pts',(5.00264151344537,32.2375254173512,124.047479151221));
#134830=CARTESIAN_POINT('Ctrl Pts',(5.11377678428393,32.0138076820242,126.363229467284));
#134831=CARTESIAN_POINT('Ctrl Pts',(5.22491205512248,29.9469085060545,127.431254255301));
#134832=CARTESIAN_POINT('Ctrl Pts',(5.33604732596105,27.9286024788597,126.274020513989));
#134833=CARTESIAN_POINT('Ctrl Pts',(5.44718259679961,27.8061882496944,123.950711686488));
#134834=CARTESIAN_POINT('Ctrl Pts',(5.55831786763816,29.6917081139984,122.587786892981));
#134835=CARTESIAN_POINT('Ctrl Pts',(5.66945313847672,31.8593988567091,123.432692802186));
#134836=CARTESIAN_POINT('Ctrl Pts',(5.78058840931528,32.3252342067572,125.712110837143));
#134837=CARTESIAN_POINT('Ctrl Pts',(5.89172368015384,30.6628481912308,127.339753883645));
#134838=CARTESIAN_POINT('Ctrl Pts',(6.00285895099241,28.3937758992811,126.825886113349));
#134839=CARTESIAN_POINT('Ctrl Pts',(6.11399422183096,27.5948352779891,124.640836220304));
#134840=CARTESIAN_POINT('Ctrl Pts',(6.22512949266952,28.9972741711713,122.784518816859));
#134841=CARTESIAN_POINT('Ctrl Pts',(6.33626476350808,31.3174797678214,122.95596892831));
#134842=CARTESIAN_POINT('Ctrl Pts',(6.44740003434664,32.431833247536,124.998263097546));
#134843=CARTESIAN_POINT('Ctrl Pts',(6.55853530518519,31.3203982626383,127.042147004667));
#134844=CARTESIAN_POINT('Ctrl Pts',(6.66967057602377,29.0004399447169,127.216911287475));
#134845=CARTESIAN_POINT('Ctrl Pts',(6.78080584686232,27.5953507869168,125.362599121175));
#134846=CARTESIAN_POINT('Ctrl Pts',(6.89194111770087,28.3911693127978,123.176410193999));
#134847=CARTESIAN_POINT('Ctrl Pts',(7.00307638853944,30.6595052445024,122.65930164414));
#134848=CARTESIAN_POINT('Ctrl Pts',(7.11421165937799,32.3242146047758,124.2845683599));
#134849=CARTESIAN_POINT('Ctrl Pts',(7.22534693021657,31.8616358123939,126.564649501493));
#134850=CARTESIAN_POINT('Ctrl Pts',(7.33648220105513,29.6951542049319,127.412651031946));
#134851=CARTESIAN_POINT('Ctrl Pts',(7.44761747189367,27.8076893657145,126.05242103926));
#134852=CARTESIAN_POINT('Ctrl Pts',(7.55875274273224,27.9267846911862,123.728939717111));
#134853=CARTESIAN_POINT('Ctrl Pts',(7.66988801357079,29.9434355836753,122.568824064703));
#134854=CARTESIAN_POINT('Ctrl Pts',(7.78102328440936,32.0118582947014,123.633895258166));
#134855=CARTESIAN_POINT('Ctrl Pts',(7.89215855524792,32.2388837808543,125.949323636188));
#134856=CARTESIAN_POINT('Ctrl Pts',(8.00329382608648,30.4167220208466,127.395862835877));
#134857=CARTESIAN_POINT('Ctrl Pts',(8.11442909692502,28.2131463200964,126.649536270169));
#134858=CARTESIAN_POINT('Ctrl Pts',(8.2255643677636,27.6450274846715,124.393435635898));
#134859=CARTESIAN_POINT('Ctrl Pts',(8.33669963860214,29.2323485914987,122.692506255073));
#134860=CARTESIAN_POINT('Ctrl Pts',(8.44783490944072,31.5222795274243,123.103560938559));
#134861=CARTESIAN_POINT('Ctrl Pts',(8.55897018027927,32.4189106521937,125.250372782172));
#134862=CARTESIAN_POINT('Ctrl Pts',(8.67010545111782,31.1015814932564,127.168025650657));
#134863=CARTESIAN_POINT('Ctrl Pts',(8.7812407219564,28.7760048267531,127.101345353396));
#134864=CARTESIAN_POINT('Ctrl Pts',(8.89237599279495,27.5707184851016,125.111363585784));
#134865=CARTESIAN_POINT('Ctrl Pts',(9.00351126363351,28.5888809804667,123.019452377014));
#134866=CARTESIAN_POINT('Ctrl Pts',(9.11464653447208,30.8986092624814,122.740283627933));
#134867=CARTESIAN_POINT('Ctrl Pts',(9.22578180531062,32.3858489908478,124.529363511801));
#134868=CARTESIAN_POINT('Ctrl Pts',(9.3369170761492,31.6894223937398,126.749216077424));
#134869=CARTESIAN_POINT('Ctrl Pts',(9.44805234698775,29.4466461250334,127.368035407967));
#134870=CARTESIAN_POINT('Ctrl Pts',(9.55918761782632,27.7104787022057,125.819509343078));
#134871=CARTESIAN_POINT('Ctrl Pts',(9.67032288866486,28.0695628376466,123.520806777059));
#134872=CARTESIAN_POINT('Ctrl Pts',(9.78145815950342,30.1960944686997,122.576176052107));
#134873=CARTESIAN_POINT('Ctrl Pts',(9.89259343034199,32.1419859270096,123.849582003139));
#134874=CARTESIAN_POINT('Ctrl Pts',(10.0037287011806,32.1297374742994,126.176784120702));
#134875=CARTESIAN_POINT('Ctrl Pts',(10.1148770421612,30.1631027296072,127.425328374009));
#134876=CARTESIAN_POINT('Ctrl Pts',(10.1889802928623,28.7606569526153,126.779199041105));
#134877=CARTESIAN_POINT('Ctrl Pts',(10.2260384532841,28.3512768063378,126.230764021361));
#134878=CARTESIAN_POINT('Ctrl Pts',(-0.0743653418493182,30.4969358400317,
123.139268787356));
#134879=CARTESIAN_POINT('Ctrl Pts',(-0.0373202515697984,31.1156586520752,
123.304507881675));
#134880=CARTESIAN_POINT('Ctrl Pts',(0.0367699289892414,32.164506220034,
124.298562755228));
#134881=CARTESIAN_POINT('Ctrl Pts',(0.147905199827801,31.7633778373016,
126.441694232461));
#134882=CARTESIAN_POINT('Ctrl Pts',(0.25904047066636,29.7450858622959,127.261655018524));
#134883=CARTESIAN_POINT('Ctrl Pts',(0.37017574150492,27.9616697339138,126.013341330537));
#134884=CARTESIAN_POINT('Ctrl Pts',(0.481311012343479,28.0431103451318,
123.836682793825));
#134885=CARTESIAN_POINT('Ctrl Pts',(0.59244628318204,29.9160168405154,122.725201171447));
#134886=CARTESIAN_POINT('Ctrl Pts',(0.703581554020597,31.8656031693769,
123.695568775648));
#134887=CARTESIAN_POINT('Ctrl Pts',(0.814716824859158,32.1077480983721,
125.859949253074));
#134888=CARTESIAN_POINT('Ctrl Pts',(0.925852095697717,30.4206848338627,
127.237191190064));
#134889=CARTESIAN_POINT('Ctrl Pts',(1.03698736653628,28.348603175385,126.566820342944));
#134890=CARTESIAN_POINT('Ctrl Pts',(1.14812263737483,27.7879873580519,124.462370487754));
#134891=CARTESIAN_POINT('Ctrl Pts',(1.25925790821339,29.2519699037367,122.850003945343));
#134892=CARTESIAN_POINT('Ctrl Pts',(1.37039317905195,31.4006006050627,123.205465180021));
#134893=CARTESIAN_POINT('Ctrl Pts',(1.48152844989051,32.2673023711948,125.203415085109));
#134894=CARTESIAN_POINT('Ctrl Pts',(1.59266372072907,31.0588054859671,127.015184150888));
#134895=CARTESIAN_POINT('Ctrl Pts',(1.70379899156763,28.881214094222,126.982512299373));
#134896=CARTESIAN_POINT('Ctrl Pts',(1.81493426240619,27.7276157632423,125.135302608358));
#134897=CARTESIAN_POINT('Ctrl Pts',(1.92606953324475,28.6538667889307,123.164254340868));
#134898=CARTESIAN_POINT('Ctrl Pts',(2.03720480408331,30.8121955815617,122.873412316505));
#134899=CARTESIAN_POINT('Ctrl Pts',(2.14834007492187,32.2271446581029,124.528976112807));
#134900=CARTESIAN_POINT('Ctrl Pts',(2.25947534576043,31.6036509600772,126.615654793147));
#134901=CARTESIAN_POINT('Ctrl Pts',(2.37061061659899,29.5123807192795,127.223570161032));
#134902=CARTESIAN_POINT('Ctrl Pts',(2.48174588743755,27.8674146671234,125.796314397807));
#134903=CARTESIAN_POINT('Ctrl Pts',(2.59288115827611,28.1743438945219,123.640214500434));
#134904=CARTESIAN_POINT('Ctrl Pts',(2.70401642911466,30.1522447243727,122.728687963833));
#134905=CARTESIAN_POINT('Ctrl Pts',(2.81515169995323,31.9908002471535,123.896029349415));
#134906=CARTESIAN_POINT('Ctrl Pts',(2.92628697079178,32.0072323861502,126.073803971508));
#134907=CARTESIAN_POINT('Ctrl Pts',(3.03742224163035,30.1865012676549,127.268756068548));
#134908=CARTESIAN_POINT('Ctrl Pts',(3.1485575124689,28.195070792744,126.38717964884));
#134909=CARTESIAN_POINT('Ctrl Pts',(3.25969278330746,27.8556411748254,124.235956774625));
#134910=CARTESIAN_POINT('Ctrl Pts',(3.37082805414602,29.4788827811274,122.784041140824));
#134911=CARTESIAN_POINT('Ctrl Pts',(3.48196332498458,31.5790882975421,123.360330225342));
#134912=CARTESIAN_POINT('Ctrl Pts',(3.59309859582314,32.2339987795056,125.437362863679));
#134913=CARTESIAN_POINT('Ctrl Pts',(3.7042338666617,30.8441931122775,127.114089593783));
#134914=CARTESIAN_POINT('Ctrl Pts',(3.81536913750026,28.6817212710357,126.85584967444));
#134915=CARTESIAN_POINT('Ctrl Pts',(3.92650440833882,27.7258328133566,124.899002828982));
#134916=CARTESIAN_POINT('Ctrl Pts',(4.03763967917738,28.8514255163441,123.034595848978));
#134917=CARTESIAN_POINT('Ctrl Pts',(4.14877495001594,31.0282760878795,122.96906792126));
#134918=CARTESIAN_POINT('Ctrl Pts',(4.2599102208545,32.2639745236107,124.76239491209));
#134919=CARTESIAN_POINT('Ctrl Pts',(4.37104549169305,31.4275208560128,126.773195146342));
#134920=CARTESIAN_POINT('Ctrl Pts',(4.48218076253162,29.2844975634107,127.161039815597));
#134921=CARTESIAN_POINT('Ctrl Pts',(4.59331603337017,27.7963534946927,125.570945620008));
#134922=CARTESIAN_POINT('Ctrl Pts',(4.70445130420873,28.3251449936434,123.45828098246));
#134923=CARTESIAN_POINT('Ctrl Pts',(4.8155865750473,30.3868840977898,122.756708330102));
#134924=CARTESIAN_POINT('Ctrl Pts',(4.92672184588585,32.0945190860907,124.108357347723));
#134925=CARTESIAN_POINT('Ctrl Pts',(5.03785711672442,31.8850997593176,126.276101766624));
#134926=CARTESIAN_POINT('Ctrl Pts',(5.14899238756297,29.950301727741,127.275866187431));
#134927=CARTESIAN_POINT('Ctrl Pts',(5.26012765840153,28.0609911247196,126.192594400014));
#134928=CARTESIAN_POINT('Ctrl Pts',(5.3712629292401,27.9464007216756,124.017774554685));
#134929=CARTESIAN_POINT('Ctrl Pts',(5.48239820007865,29.7114118864037,122.741957989307));
#134930=CARTESIAN_POINT('Ctrl Pts',(5.59353347091722,31.7405596217284,123.532863665309));
#134931=CARTESIAN_POINT('Ctrl Pts',(5.70466874175577,32.1766221683637,125.666597897947));
#134932=CARTESIAN_POINT('Ctrl Pts',(5.81580401259433,30.6204837616357,127.190213853235));
#134933=CARTESIAN_POINT('Ctrl Pts',(5.9269392834329,28.4964340474499,126.709188768887));
#134934=CARTESIAN_POINT('Ctrl Pts',(6.03807455427144,27.7485558928723,124.66379135371));
#134935=CARTESIAN_POINT('Ctrl Pts',(6.14920982511002,29.0613611044097,122.926116241192));
#134936=CARTESIAN_POINT('Ctrl Pts',(6.26034509594857,31.2332760548066,123.086608510001));
#134937=CARTESIAN_POINT('Ctrl Pts',(6.37148036678712,32.2764081746986,124.998374107703));
#134938=CARTESIAN_POINT('Ctrl Pts',(6.4826156376257,31.2360080206869,126.911627838821));
#134939=CARTESIAN_POINT('Ctrl Pts',(6.59375090846424,29.0643245447631,127.075222461286));
#134940=CARTESIAN_POINT('Ctrl Pts',(6.70488617930281,27.7490384542232,125.339424425757));
#134941=CARTESIAN_POINT('Ctrl Pts',(6.81602145014137,28.4939940549937,123.292960775216));
#134942=CARTESIAN_POINT('Ctrl Pts',(6.92715672097993,30.6173544717193,122.808902038335));
#134943=CARTESIAN_POINT('Ctrl Pts',(7.03829199181848,32.1756677319163,124.330293540639));
#134944=CARTESIAN_POINT('Ctrl Pts',(7.14942726265705,31.7426536074951,126.464648498966));
#134945=CARTESIAN_POINT('Ctrl Pts',(7.2605625334956,29.7146377282987,127.258451946646));
#134946=CARTESIAN_POINT('Ctrl Pts',(7.37169780433417,27.9478058972905,125.985157950046));
#134947=CARTESIAN_POINT('Ctrl Pts',(7.48283307517272,28.0592895167973,123.81017663467));
#134948=CARTESIAN_POINT('Ctrl Pts',(7.59396834601129,29.9470507692709,122.724207126928));
#134949=CARTESIAN_POINT('Ctrl Pts',(7.70510361684984,31.8832749626372,123.721206725438));
#134950=CARTESIAN_POINT('Ctrl Pts',(7.8162388876884,32.0957906328901,125.888649782234));
#134951=CARTESIAN_POINT('Ctrl Pts',(7.92737415852696,30.3900881837985,127.24273672982));
#134952=CARTESIAN_POINT('Ctrl Pts',(8.03850942936553,28.3273489956417,126.544109923524));
#134953=CARTESIAN_POINT('Ctrl Pts',(8.14964470020408,27.7955401791978,124.432202813116));
#134954=CARTESIAN_POINT('Ctrl Pts',(8.26077997104264,29.281411279576,122.839984452331));
#134955=CARTESIAN_POINT('Ctrl Pts',(8.37191524188121,31.4249865051052,123.224767513704));
#134956=CARTESIAN_POINT('Ctrl Pts',(8.48305051271975,32.2643114975497,125.234370777121));
#134957=CARTESIAN_POINT('Ctrl Pts',(8.59418578355832,31.031176425804,127.029461238393));
#134958=CARTESIAN_POINT('Ctrl Pts',(8.70532105439688,28.8542336852274,126.967042660175));
#134959=CARTESIAN_POINT('Ctrl Pts',(8.81645632523543,27.7259804697702,125.104246036319));
#134960=CARTESIAN_POINT('Ctrl Pts',(8.927591596074,28.6790694325801,123.146034558943));
#134961=CARTESIAN_POINT('Ctrl Pts',(9.03872686691255,30.8411767019984,122.884708243426));
#134962=CARTESIAN_POINT('Ctrl Pts',(9.14986213775112,32.2333628968455,124.559443169003));
#134963=CARTESIAN_POINT('Ctrl Pts',(9.26099740858968,31.581446816522,126.637418923356));
#134964=CARTESIAN_POINT('Ctrl Pts',(9.37213267942823,29.4820124752587,127.216687828466));
#134965=CARTESIAN_POINT('Ctrl Pts',(9.48326795026681,27.8568082315158,125.767132273447));
#134966=CARTESIAN_POINT('Ctrl Pts',(9.59440322110534,28.1929423238309,123.615346036546));
#134967=CARTESIAN_POINT('Ctrl Pts',(9.70553849194393,30.1835615381989,122.731089228834));
#134968=CARTESIAN_POINT('Ctrl Pts',(9.81667376278246,32.0050857842635,123.92310834428));
#134969=CARTESIAN_POINT('Ctrl Pts',(9.92780903362104,31.9936201634588,126.10157264892));
#134970=CARTESIAN_POINT('Ctrl Pts',(10.0389573746017,30.152678390827,127.270319045319));
#134971=CARTESIAN_POINT('Ctrl Pts',(10.1130606253029,28.839866735443,126.665485594332));
#134972=CARTESIAN_POINT('Ctrl Pts',(10.1501187857246,28.4566511870538,126.152102547405));
#134973=CARTESIAN_POINT('Ctrl Pts',(-0.150285009408829,30.4630068241413,
123.266312912162));
#134974=CARTESIAN_POINT('Ctrl Pts',(-0.113239919129309,31.0394854379795,
123.420270067436));
#134975=CARTESIAN_POINT('Ctrl Pts',(-0.0391497385702692,32.0167214156017,
124.346454401407));
#134976=CARTESIAN_POINT('Ctrl Pts',(0.07198553226829,31.6429806555269,126.343260465802));
#134977=CARTESIAN_POINT('Ctrl Pts',(0.183120803106849,29.7624904951118,
127.107237238841));
#134978=CARTESIAN_POINT('Ctrl Pts',(0.294256073945408,28.100839691918,125.944153980106));
#134979=CARTESIAN_POINT('Ctrl Pts',(0.405391344783969,28.1767198271761,
123.91610996489));
#134980=CARTESIAN_POINT('Ctrl Pts',(0.516526615622528,29.9217509126493,
122.88051636384));
#134981=CARTESIAN_POINT('Ctrl Pts',(0.627661886461087,31.7382264046522,
123.78463071116));
#134982=CARTESIAN_POINT('Ctrl Pts',(0.738797157299648,31.9638385370933,
125.801234969414));
#134983=CARTESIAN_POINT('Ctrl Pts',(0.849932428138205,30.3919619661137,
127.084443713786));
#134984=CARTESIAN_POINT('Ctrl Pts',(0.961067698976766,28.4613546909533,
126.459843409443));
#134985=CARTESIAN_POINT('Ctrl Pts',(1.07220296981532,27.9390157324064,124.49907792319));
#134986=CARTESIAN_POINT('Ctrl Pts',(1.18333824065389,29.3030427444903,122.99679804717));
#134987=CARTESIAN_POINT('Ctrl Pts',(1.29447351149244,31.3049725654706,123.32798965002));
#134988=CARTESIAN_POINT('Ctrl Pts',(1.405608782331,32.1124990103107,125.189526624871));
#134989=CARTESIAN_POINT('Ctrl Pts',(1.51674405316956,30.9865140043224,126.8775945275));
#134990=CARTESIAN_POINT('Ctrl Pts',(1.62787932400812,28.9576008261042,126.847153394078));
#134991=CARTESIAN_POINT('Ctrl Pts',(1.73901459484668,27.8827660958751,125.12606462635));
#134992=CARTESIAN_POINT('Ctrl Pts',(1.85014986568524,28.7457759881265,123.289592540736));
#134993=CARTESIAN_POINT('Ctrl Pts',(1.9612851365238,30.7567417491492,123.018608177807));
#134994=CARTESIAN_POINT('Ctrl Pts',(2.07242040736236,32.0750831233779,124.561135952501));
#134995=CARTESIAN_POINT('Ctrl Pts',(2.18355567820092,31.494159362724,126.505343616665));
#134996=CARTESIAN_POINT('Ctrl Pts',(2.29469094903948,29.545673633558,127.071752680283));
#134997=CARTESIAN_POINT('Ctrl Pts',(2.40582621987804,28.0130200266448,125.741944876271));
#134998=CARTESIAN_POINT('Ctrl Pts',(2.5169614907166,28.298993215467,123.733055829446));
#134999=CARTESIAN_POINT('Ctrl Pts',(2.62809676155516,30.1418499947993,122.883765090414));
#135000=CARTESIAN_POINT('Ctrl Pts',(2.73923203239372,31.8548754701923,123.971404548242));
#135001=CARTESIAN_POINT('Ctrl Pts',(2.85036730323227,31.8701856810441,126.00048844649));
#135002=CARTESIAN_POINT('Ctrl Pts',(2.96150257407084,30.1737676228579,127.113853454367));
#135003=CARTESIAN_POINT('Ctrl Pts',(3.07263784490939,28.3183049546232,126.292467944518));
#135004=CARTESIAN_POINT('Ctrl Pts',(3.18377311574795,28.0020503866253,124.288122935015));
#135005=CARTESIAN_POINT('Ctrl Pts',(3.29490838658652,29.5144628157628,122.935338948888));
#135006=CARTESIAN_POINT('Ctrl Pts',(3.40604365742507,31.4712737516316,123.472281059551));
#135007=CARTESIAN_POINT('Ctrl Pts',(3.51717892826364,32.0814692696916,125.407501279233));
#135008=CARTESIAN_POINT('Ctrl Pts',(3.62831419910219,30.7865546020038,126.969747057699));
#135009=CARTESIAN_POINT('Ctrl Pts',(3.73944946994076,28.7717286650289,126.729138843742));
#135010=CARTESIAN_POINT('Ctrl Pts',(3.8505847407793,27.8811048794813,124.905898557453));
#135011=CARTESIAN_POINT('Ctrl Pts',(3.96172001161788,28.9298461066255,123.168786670608));
#135012=CARTESIAN_POINT('Ctrl Pts',(4.07285528245642,30.9580690452094,123.107732757283));
#135013=CARTESIAN_POINT('Ctrl Pts',(4.183990553295,32.1093983763515,124.778617744403));
#135014=CARTESIAN_POINT('Ctrl Pts',(4.29512582413354,31.3300547972064,126.65212767354));
#135015=CARTESIAN_POINT('Ctrl Pts',(4.40626109497212,29.3333495309789,127.01349168496));
#135016=CARTESIAN_POINT('Ctrl Pts',(4.51739636581066,27.9468106589228,125.531963478948));
#135017=CARTESIAN_POINT('Ctrl Pts',(4.62853163664923,28.4394981506248,123.563544086529));
#135018=CARTESIAN_POINT('Ctrl Pts',(4.73966690748779,30.3604690243655,122.909872325498));
#135019=CARTESIAN_POINT('Ctrl Pts',(4.85080217832634,31.9515127548303,124.169235544223));
#135020=CARTESIAN_POINT('Ctrl Pts',(4.96193744916491,31.7563918366111,126.188974065964));
#135021=CARTESIAN_POINT('Ctrl Pts',(5.07307272000346,29.9536949494275,127.120478119561));
#135022=CARTESIAN_POINT('Ctrl Pts',(5.18420799084203,28.1933797705796,126.111168286038));
#135023=CARTESIAN_POINT('Ctrl Pts',(5.29534326168058,28.0866131936566,124.084837422881));
#135024=CARTESIAN_POINT('Ctrl Pts',(5.40647853251915,29.7311156588089,122.896129085635));
#135025=CARTESIAN_POINT('Ctrl Pts',(5.5176138033577,31.6217203867477,123.633034528433));
#135026=CARTESIAN_POINT('Ctrl Pts',(5.62874907419627,32.0280101299703,125.621084958751));
#135027=CARTESIAN_POINT('Ctrl Pts',(5.73988434503482,30.5781193320407,127.040673822826));
#135028=CARTESIAN_POINT('Ctrl Pts',(5.85101961587339,28.5990921956187,126.592491424426));
#135029=CARTESIAN_POINT('Ctrl Pts',(5.96215488671193,27.9022765077555,124.686746487118));
#135030=CARTESIAN_POINT('Ctrl Pts',(6.0732901575505,29.125448037648,123.067713665527));
#135031=CARTESIAN_POINT('Ctrl Pts',(6.18442542838907,31.1490723417917,123.217248091692));
#135032=CARTESIAN_POINT('Ctrl Pts',(6.29556069922761,32.1209831018612,124.998485117859));
#135033=CARTESIAN_POINT('Ctrl Pts',(6.40669597006619,31.1516177787356,126.781108672975));
#135034=CARTESIAN_POINT('Ctrl Pts',(6.51783124090473,29.1282091448092,126.933533635097));
#135035=CARTESIAN_POINT('Ctrl Pts',(6.62896651174331,27.9027261215296,125.316249730339));
#135036=CARTESIAN_POINT('Ctrl Pts',(6.74010178258185,28.5968187971898,123.409511356433));
#135037=CARTESIAN_POINT('Ctrl Pts',(6.85123705342043,30.5752036989361,122.958502432531));
#135038=CARTESIAN_POINT('Ctrl Pts',(6.96237232425897,32.0271208590569,124.37601872138));
#135039=CARTESIAN_POINT('Ctrl Pts',(7.07350759509754,31.6236714025963,126.364647496437));
#135040=CARTESIAN_POINT('Ctrl Pts',(7.1846428659361,29.7341212516656,127.104252861346));
#135041=CARTESIAN_POINT('Ctrl Pts',(7.29577813677465,28.0879224288666,125.917894860832));
#135042=CARTESIAN_POINT('Ctrl Pts',(7.40691340761322,28.1917943424084,123.89141355223));
#135043=CARTESIAN_POINT('Ctrl Pts',(7.51804867845177,29.9506659548665,122.879590189155));
#135044=CARTESIAN_POINT('Ctrl Pts',(7.62918394929034,31.754691630573,123.808518192709));
#135045=CARTESIAN_POINT('Ctrl Pts',(7.74031922012889,31.952697484926,125.827975928281));
#135046=CARTESIAN_POINT('Ctrl Pts',(7.85145449096745,30.3634543467503,127.089610623763));
#135047=CARTESIAN_POINT('Ctrl Pts',(7.96258976180602,28.4415516711872,126.438683576878));
#135048=CARTESIAN_POINT('Ctrl Pts',(8.07372503264457,27.946052873724,124.470969990334));
#135049=CARTESIAN_POINT('Ctrl Pts',(8.18486030348314,29.3304739676535,122.987462649588));
#135050=CARTESIAN_POINT('Ctrl Pts',(8.29599557432169,31.3276934827861,123.345974088848));
#135051=CARTESIAN_POINT('Ctrl Pts',(8.40713084516025,32.1097123429055,125.218368772072));
#135052=CARTESIAN_POINT('Ctrl Pts',(8.51826611599881,30.9607713583517,126.890896826131));
#135053=CARTESIAN_POINT('Ctrl Pts',(8.62940138683738,28.9324625437016,126.832739966954));
#135054=CARTESIAN_POINT('Ctrl Pts',(8.74053665767593,27.8812424544389,125.097128486853));
#135055=CARTESIAN_POINT('Ctrl Pts',(8.85167192851449,28.7692578846935,123.272616740873));
#135056=CARTESIAN_POINT('Ctrl Pts',(8.96280719935305,30.7837441415154,123.029132858921));
#135057=CARTESIAN_POINT('Ctrl Pts',(9.0739424701916,32.0808768028432,124.589522826205));
#135058=CARTESIAN_POINT('Ctrl Pts',(9.18507774103017,31.4734712393041,126.525621769289));
#135059=CARTESIAN_POINT('Ctrl Pts',(9.29621301186872,29.5173788254838,127.065340248965));
#135060=CARTESIAN_POINT('Ctrl Pts',(9.4073482827073,28.0031377608259,125.714755203815));
#135061=CARTESIAN_POINT('Ctrl Pts',(9.51848355354583,28.3163218100152,123.709885296032));
#135062=CARTESIAN_POINT('Ctrl Pts',(9.62961882438441,30.1710286076982,122.886002405562));
#135063=CARTESIAN_POINT('Ctrl Pts',(9.74075409522296,31.8681856415175,123.996634685421));
#135064=CARTESIAN_POINT('Ctrl Pts',(9.85188936606152,31.857502852618,126.026361177139));
#135065=CARTESIAN_POINT('Ctrl Pts',(9.96303770704222,30.1422540520468,127.11530971663));
#135066=CARTESIAN_POINT('Ctrl Pts',(10.0371409577434,28.9190765182705,126.551772147558));
#135067=CARTESIAN_POINT('Ctrl Pts',(10.074199118165,28.5620255677698,126.073441073449));
#135068=CARTESIAN_POINT('Ctrl Pts',(-0.22620467696834,30.4290778082509,
123.393357036968));
#135069=CARTESIAN_POINT('Ctrl Pts',(-0.189159586688819,30.9633122238839,
123.536032253196));
#135070=CARTESIAN_POINT('Ctrl Pts',(-0.115069406129781,31.8689366111695,
124.394346047585));
#135071=CARTESIAN_POINT('Ctrl Pts',(-0.00393413529122068,31.5225834737523,
126.244826699143));
#135072=CARTESIAN_POINT('Ctrl Pts',(0.107201135547339,29.7798951279279,
126.95281945916));
#135073=CARTESIAN_POINT('Ctrl Pts',(0.218336406385899,28.2400096499221,
125.874966629674));
#135074=CARTESIAN_POINT('Ctrl Pts',(0.329471677224458,28.3103293092203,
123.995537135953));
#135075=CARTESIAN_POINT('Ctrl Pts',(0.440606948063018,29.9274849847832,
123.035831556234));
#135076=CARTESIAN_POINT('Ctrl Pts',(0.551742218901577,31.6108496399274,
123.873692646674));
#135077=CARTESIAN_POINT('Ctrl Pts',(0.662877489740137,31.8199289758145,
125.742520685753));
#135078=CARTESIAN_POINT('Ctrl Pts',(0.774012760578696,30.3632390983645,
126.931696237506));
#135079=CARTESIAN_POINT('Ctrl Pts',(0.885148031417255,28.5741062065216,
126.352866475942));
#135080=CARTESIAN_POINT('Ctrl Pts',(0.996283302255815,28.090044106761,124.535785358627));
#135081=CARTESIAN_POINT('Ctrl Pts',(1.10741857309438,29.3541155852438,123.143592148996));
#135082=CARTESIAN_POINT('Ctrl Pts',(1.21855384393294,31.2093445258783,123.450514120018));
#135083=CARTESIAN_POINT('Ctrl Pts',(1.32968911477149,31.9576956494266,125.175638164633));
#135084=CARTESIAN_POINT('Ctrl Pts',(1.44082438561006,30.9142225226776,126.740004904113));
#135085=CARTESIAN_POINT('Ctrl Pts',(1.55195965644861,29.0339875579863,126.711794488784));
#135086=CARTESIAN_POINT('Ctrl Pts',(1.66309492728717,28.037916428508,125.116826644344));
#135087=CARTESIAN_POINT('Ctrl Pts',(1.77423019812573,28.8376851873223,123.414930740604));
#135088=CARTESIAN_POINT('Ctrl Pts',(1.88536546896429,30.7012879167365,123.163804039111));
#135089=CARTESIAN_POINT('Ctrl Pts',(1.99650073980285,31.923021588653,124.593295792194));
#135090=CARTESIAN_POINT('Ctrl Pts',(2.10763601064141,31.3846677653708,126.395032440182));
#135091=CARTESIAN_POINT('Ctrl Pts',(2.21877128147997,29.5789665478364,126.919935199536));
#135092=CARTESIAN_POINT('Ctrl Pts',(2.32990655231853,28.1586253861661,125.687575354735));
#135093=CARTESIAN_POINT('Ctrl Pts',(2.44104182315709,28.4236425364121,123.825897158459));
#135094=CARTESIAN_POINT('Ctrl Pts',(2.55217709399565,30.1314552652258,123.038842216995));
#135095=CARTESIAN_POINT('Ctrl Pts',(2.66331236483421,31.7189506932312,124.046779747068));
#135096=CARTESIAN_POINT('Ctrl Pts',(2.77444763567277,31.733138975938,125.927172921471));
#135097=CARTESIAN_POINT('Ctrl Pts',(2.88558290651133,30.1610339780609,126.958950840186));
#135098=CARTESIAN_POINT('Ctrl Pts',(2.99671817734989,28.4415391165025,126.197756240195));
#135099=CARTESIAN_POINT('Ctrl Pts',(3.10785344818845,28.1484595984251,124.340289095405));
#135100=CARTESIAN_POINT('Ctrl Pts',(3.21898871902701,29.5500428503983,123.086636756953));
#135101=CARTESIAN_POINT('Ctrl Pts',(3.33012398986556,31.3634592057211,123.584231893759));
#135102=CARTESIAN_POINT('Ctrl Pts',(3.44125926070413,31.9289397598776,125.377639694786));
#135103=CARTESIAN_POINT('Ctrl Pts',(3.55239453154268,30.72891609173,126.825404521615));
#135104=CARTESIAN_POINT('Ctrl Pts',(3.66352980238124,28.861736059022,126.602428013043));
#135105=CARTESIAN_POINT('Ctrl Pts',(3.7746650732198,28.0363769456059,124.912794285924));
#135106=CARTESIAN_POINT('Ctrl Pts',(3.88580034405837,29.0082666969071,123.302977492238));
#135107=CARTESIAN_POINT('Ctrl Pts',(3.99693561489692,30.8878620025393,123.246397593306));
#135108=CARTESIAN_POINT('Ctrl Pts',(4.10807088573548,31.9548222290924,124.794840576717));
#135109=CARTESIAN_POINT('Ctrl Pts',(4.21920615657404,31.2325887383998,126.531060200739));
#135110=CARTESIAN_POINT('Ctrl Pts',(4.3303414274126,29.382201498547,126.865943554323));
#135111=CARTESIAN_POINT('Ctrl Pts',(4.44147669825116,28.0972678231528,125.492981337888));
#135112=CARTESIAN_POINT('Ctrl Pts',(4.55261196908972,28.5538513076063,123.668807190598));
#135113=CARTESIAN_POINT('Ctrl Pts',(4.66374723992828,30.334053950941,123.063036320894));
#135114=CARTESIAN_POINT('Ctrl Pts',(4.77488251076683,31.8085064235698,124.230113740723));
#135115=CARTESIAN_POINT('Ctrl Pts',(4.8860177816054,31.6276839139044,126.101846365303));
#135116=CARTESIAN_POINT('Ctrl Pts',(4.99715305244395,29.9570881711141,126.965090051692));
#135117=CARTESIAN_POINT('Ctrl Pts',(5.10828832328252,28.3257684164394,126.029742172062));
#135118=CARTESIAN_POINT('Ctrl Pts',(5.21942359412107,28.2268256656377,124.151900291077));
#135119=CARTESIAN_POINT('Ctrl Pts',(5.33055886495964,29.7508194312142,123.050300181963));
#135120=CARTESIAN_POINT('Ctrl Pts',(5.44169413579819,31.502881151767,123.733205391558));
#135121=CARTESIAN_POINT('Ctrl Pts',(5.55282940663676,31.8793980915768,125.575572019554));
#135122=CARTESIAN_POINT('Ctrl Pts',(5.66396467747531,30.5357549024456,126.891133792417));
#135123=CARTESIAN_POINT('Ctrl Pts',(5.77509994831388,28.7017503437876,126.475794079966));
#135124=CARTESIAN_POINT('Ctrl Pts',(5.88623521915243,28.0559971226385,124.709701620524));
#135125=CARTESIAN_POINT('Ctrl Pts',(5.99737048999099,29.1895349708864,123.209311089859));
#135126=CARTESIAN_POINT('Ctrl Pts',(6.10850576082955,31.0648686287769,123.347887673383));
#135127=CARTESIAN_POINT('Ctrl Pts',(6.21964103166811,31.9655580290238,124.998596128017));
#135128=CARTESIAN_POINT('Ctrl Pts',(6.33077630250668,31.0672275367842,126.650589507129));
#135129=CARTESIAN_POINT('Ctrl Pts',(6.44191157334522,29.1920937448553,126.791844808909));
#135130=CARTESIAN_POINT('Ctrl Pts',(6.5530468441838,28.0564137888359,125.29307503492));
#135131=CARTESIAN_POINT('Ctrl Pts',(6.66418211502234,28.6996435393857,123.52606193765));
#135132=CARTESIAN_POINT('Ctrl Pts',(6.77531738586092,30.533052926153,123.108102826727));
#135133=CARTESIAN_POINT('Ctrl Pts',(6.88645265669946,31.8785739861974,124.421743902119));
#135134=CARTESIAN_POINT('Ctrl Pts',(6.99758792753804,31.5046891976975,126.264646493909));
#135135=CARTESIAN_POINT('Ctrl Pts',(7.10872319837658,29.7536047750324,126.950053776046));
#135136=CARTESIAN_POINT('Ctrl Pts',(7.21985846921515,28.2280389604426,125.850631771618));
#135137=CARTESIAN_POINT('Ctrl Pts',(7.33099374005371,28.3242991680195,123.97265046979));
#135138=CARTESIAN_POINT('Ctrl Pts',(7.44212901089227,29.954281140462,123.03497325138));
#135139=CARTESIAN_POINT('Ctrl Pts',(7.55326428173082,31.626108298509,123.895829659981));
#135140=CARTESIAN_POINT('Ctrl Pts',(7.66439955256939,31.8096043369618,125.767302074327));
#135141=CARTESIAN_POINT('Ctrl Pts',(7.77553482340794,30.3368205097023,126.936484517706));
#135142=CARTESIAN_POINT('Ctrl Pts',(7.8866700942465,28.5557543467325,126.333257230232));
#135143=CARTESIAN_POINT('Ctrl Pts',(7.99780536508506,28.0965655682502,124.509737167552));
#135144=CARTESIAN_POINT('Ctrl Pts',(8.10894063592362,29.3795366557309,123.134940846845));
#135145=CARTESIAN_POINT('Ctrl Pts',(8.22007590676218,31.230400460467,123.467180663992));
#135146=CARTESIAN_POINT('Ctrl Pts',(8.33121117760075,31.9551131882614,125.202366767024));
#135147=CARTESIAN_POINT('Ctrl Pts',(8.44234644843929,30.8903662908993,126.752332413868));
#135148=CARTESIAN_POINT('Ctrl Pts',(8.55348171927787,29.0106914021759,126.698437273733));
#135149=CARTESIAN_POINT('Ctrl Pts',(8.6646169901164,28.0365044391075,125.090010937387));
#135150=CARTESIAN_POINT('Ctrl Pts',(8.77575226095499,28.8594463368069,123.399198922802));
#135151=CARTESIAN_POINT('Ctrl Pts',(8.88688753179353,30.7263115810325,123.173557474415));
#135152=CARTESIAN_POINT('Ctrl Pts',(8.9980228026321,31.928390708841,124.619602483407));
#135153=CARTESIAN_POINT('Ctrl Pts',(9.10915807347066,31.3654956620864,126.413824615221));
#135154=CARTESIAN_POINT('Ctrl Pts',(9.22029334430921,29.552745175709,126.913992669463));
#135155=CARTESIAN_POINT('Ctrl Pts',(9.33142861514778,28.1494672901359,125.662378134184));
#135156=CARTESIAN_POINT('Ctrl Pts',(9.44256388598633,28.4397012961995,123.804424555518));
#135157=CARTESIAN_POINT('Ctrl Pts',(9.5536991568249,30.1584956771975,123.040915582288));
#135158=CARTESIAN_POINT('Ctrl Pts',(9.66483442766346,31.7312854987716,124.070161026561));
#135159=CARTESIAN_POINT('Ctrl Pts',(9.77596969850201,31.7213855417773,125.951149705358));
#135160=CARTESIAN_POINT('Ctrl Pts',(9.8871180394827,30.1318297132667,126.960300387941));
#135161=CARTESIAN_POINT('Ctrl Pts',(9.96122129018386,28.9982863010982,126.438058700785));
#135162=CARTESIAN_POINT('Ctrl Pts',(9.99827945060551,28.6673999484858,125.994779599494));
#135163=CARTESIAN_POINT('Ctrl Pts',(10.,28.6653082844465,125.997072727755));
#135164=CARTESIAN_POINT('Ctrl Pts',(10.0000000000001,28.6967050287084,126.051116487996));
#135165=CARTESIAN_POINT('Ctrl Pts',(10.,28.7312952913176,126.103084852867));
#135166=CARTESIAN_POINT('Ctrl Pts',(10.,28.7687526561708,126.152891945816));
#135167=CARTESIAN_POINT('Ctrl Pts',(10.0000000000001,28.7925064920188,126.184477443477));
#135168=CARTESIAN_POINT('Ctrl Pts',(9.99999999999996,28.8174144318639,126.215193579688));
#135169=CARTESIAN_POINT('Ctrl Pts',(10.,28.8434032080411,126.245015253039));
#135170=CARTESIAN_POINT('Ctrl Pts',(10.0000000000001,28.8610650760105,126.265281942542));
#135171=CARTESIAN_POINT('Ctrl Pts',(9.99999999999991,28.8792262859797,126.285135469238));
#135172=CARTESIAN_POINT('Ctrl Pts',(9.99999999999992,28.8978656284541,126.304567075492));
#135173=CARTESIAN_POINT('Ctrl Pts',(9.99999999999992,28.9078692983068,126.314995950541));
#135174=CARTESIAN_POINT('Ctrl Pts',(10.0000000000001,28.9180108113656,126.325303204012));
#135175=CARTESIAN_POINT('Ctrl Pts',(10.0000000000001,28.9282763435345,126.335477297132));
#135176=CARTESIAN_POINT('Ctrl Pts',(9.99999999999998,28.9751289989059,126.381912617854));
#135177=CARTESIAN_POINT('Ctrl Pts',(9.99999999999992,29.0246129144767,126.425630794521));
#135178=CARTESIAN_POINT('Ctrl Pts',(9.99999999999994,29.0763924472693,126.466522146034));
#135179=CARTESIAN_POINT('Ctrl Pts',(9.99999999999995,29.1137524290861,126.496026084493));
#135180=CARTESIAN_POINT('Ctrl Pts',(9.99999999999988,29.1523086592386,126.524058047823));
#135181=CARTESIAN_POINT('Ctrl Pts',(9.99999999999993,29.191949375433,126.55056814615));
#135182=CARTESIAN_POINT('Ctrl Pts',(9.99999999999994,29.2027336731786,126.557780245755));
#135183=CARTESIAN_POINT('Ctrl Pts',(10.0000000000001,29.2135982956353,126.564879660816));
#135184=CARTESIAN_POINT('Ctrl Pts',(10.0000000000001,29.224541120581,126.571865272476));
#135185=CARTESIAN_POINT('Ctrl Pts',(10.0000000000001,29.2359307117797,126.579136087962));
#135186=CARTESIAN_POINT('Ctrl Pts',(9.99999999999999,29.2473984635858,126.586279379619));
#135187=CARTESIAN_POINT('Ctrl Pts',(9.99999999999997,29.2589365233135,126.593291232705));
#135188=CARTESIAN_POINT('Ctrl Pts',(9.99999999999987,29.3169202191603,126.628528800049));
#135189=CARTESIAN_POINT('Ctrl Pts',(10.0000000000002,29.3767154320219,126.660474363582));
#135190=CARTESIAN_POINT('Ctrl Pts',(10.0000000000001,29.4379816057261,126.6890174197));
#135191=CARTESIAN_POINT('Ctrl Pts',(10.0000000000001,29.5001391867863,126.717975770077));
#135192=CARTESIAN_POINT('Ctrl Pts',(10.0000000000001,29.5638116094751,126.74343262034));
#135193=CARTESIAN_POINT('Ctrl Pts',(9.99999999999995,29.6286835625344,126.76523838423));
#135194=CARTESIAN_POINT('Ctrl Pts',(9.99999999999989,29.6688787895444,126.778749425417));
#135195=CARTESIAN_POINT('Ctrl Pts',(10.0000000000001,29.7095352866061,126.790858044881));
#135196=CARTESIAN_POINT('Ctrl Pts',(9.99999999999995,29.7505836069801,126.801520293352));
#135197=CARTESIAN_POINT('Ctrl Pts',(9.99999999999985,29.7841900744798,126.810249530102));
#135198=CARTESIAN_POINT('Ctrl Pts',(9.9999999999998,29.8180592674631,126.818009191325));
#135199=CARTESIAN_POINT('Ctrl Pts',(9.99999999999999,29.8521544944741,126.82477142239));
#135200=CARTESIAN_POINT('Ctrl Pts',(10.0000000000001,29.8661247094476,126.827542186217));
#135201=CARTESIAN_POINT('Ctrl Pts',(10.0000000000001,29.8801354878125,126.830145768473));
#135202=CARTESIAN_POINT('Ctrl Pts',(10.,29.8941603582459,126.832576321549));
#135203=CARTESIAN_POINT('Ctrl Pts',(9.9999999999998,29.9636137929348,126.844612814874));
#135204=CARTESIAN_POINT('Ctrl Pts',(10.0000000000002,30.0335315560267,126.852435094899));
#135205=CARTESIAN_POINT('Ctrl Pts',(9.99999999999991,30.1035784530787,126.85590279931));
#135206=CARTESIAN_POINT('Ctrl Pts',(9.99999999999988,30.1113621962958,126.85628813716));
#135207=CARTESIAN_POINT('Ctrl Pts',(10.0000000000001,30.119147563991,126.856619660668));
#135208=CARTESIAN_POINT('Ctrl Pts',(10.0000000000001,30.1269341171633,126.856897143374));
#135209=CARTESIAN_POINT('Ctrl Pts',(10.0000000000001,30.1968734287048,126.859389510539));
#135210=CARTESIAN_POINT('Ctrl Pts',(10.0000000000001,30.2669070801432,126.857526934753));
#135211=CARTESIAN_POINT('Ctrl Pts',(10.0000000000001,30.3367420640854,126.851551839746));
#135212=CARTESIAN_POINT('Ctrl Pts',(10.,30.4065770480275,126.845576744738));
#135213=CARTESIAN_POINT('Ctrl Pts',(9.99999999999998,30.4762143055634,126.835488833351));
#135214=CARTESIAN_POINT('Ctrl Pts',(9.9999999999999,30.5453683176971,126.821473427802));
#135215=CARTESIAN_POINT('Ctrl Pts',(9.99999999999988,30.558412278624,126.818829815426));
#135216=CARTESIAN_POINT('Ctrl Pts',(9.99999999999984,30.5714390442574,126.816046313978));
#135217=CARTESIAN_POINT('Ctrl Pts',(9.99999999999995,30.584446685237,126.813123952926));
#135218=CARTESIAN_POINT('Ctrl Pts',(10.,30.5957697829836,126.8105800497));
#135219=CARTESIAN_POINT('Ctrl Pts',(9.99999999999987,30.6070694510325,126.807932918437));
#135220=CARTESIAN_POINT('Ctrl Pts',(9.99999999999987,30.6183425063254,126.805184212759));
#135221=CARTESIAN_POINT('Ctrl Pts',(9.99999999999988,30.6873871245024,126.788349084293));
#135222=CARTESIAN_POINT('Ctrl Pts',(9.9999999999999,30.7554558673819,126.767702776233));
#135223=CARTESIAN_POINT('Ctrl Pts',(10.,30.8222618925395,126.743495436202));
#135224=CARTESIAN_POINT('Ctrl Pts',(10.0000000000002,30.8904746787203,126.71877835259));
#135225=CARTESIAN_POINT('Ctrl Pts',(9.99999999999986,30.9573719317382,126.690348530093));
#135226=CARTESIAN_POINT('Ctrl Pts',(9.99999999999997,31.0226523342096,126.658417278966));
#135227=CARTESIAN_POINT('Ctrl Pts',(10.0000000000001,31.0883272019745,126.626293079115));
#135228=CARTESIAN_POINT('Ctrl Pts',(9.99999999999989,31.1523666455233,126.590624692189));
#135229=CARTESIAN_POINT('Ctrl Pts',(9.99999999999989,31.2144530767094,126.551575995527));
#135230=CARTESIAN_POINT('Ctrl Pts',(9.99999999999989,31.2297926762732,126.541928293785));
#135231=CARTESIAN_POINT('Ctrl Pts',(9.99999999999993,31.2450129650166,126.532074017689));
#135232=CARTESIAN_POINT('Ctrl Pts',(10.,31.2601089384186,126.522015195508));
#135233=CARTESIAN_POINT('Ctrl Pts',(10.0000000000001,31.2719311826033,126.51413774045));
#135234=CARTESIAN_POINT('Ctrl Pts',(10.0000000000001,31.283678470288,126.506133794645));
#135235=CARTESIAN_POINT('Ctrl Pts',(10.0000000000001,31.2953308003886,126.49801690638));
#135236=CARTESIAN_POINT('Ctrl Pts',(10.,31.3572558121971,126.454880606831));
#135237=CARTESIAN_POINT('Ctrl Pts',(10.,31.4166138612528,126.408484217952));
#135238=CARTESIAN_POINT('Ctrl Pts',(10.,31.4730903954254,126.359062410629));
#135239=CARTESIAN_POINT('Ctrl Pts',(10.,31.5294280870934,126.309762102396));
#135240=CARTESIAN_POINT('Ctrl Pts',(10.,31.5828994498296,126.25745079026));
#135241=CARTESIAN_POINT('Ctrl Pts',(10.,31.6331764759971,126.202312206008));
#135242=CARTESIAN_POINT('Ctrl Pts',(10.,31.6823970284773,126.148332251608));
#135243=CARTESIAN_POINT('Ctrl Pts',(10.0000000000001,31.7285569678729,126.091642060811));
#135244=CARTESIAN_POINT('Ctrl Pts',(9.99999999999998,31.7713193360823,126.03237423032));
#135245=CARTESIAN_POINT('Ctrl Pts',(9.99999999999995,31.7804981155288,126.019652616267));
#135246=CARTESIAN_POINT('Ctrl Pts',(9.99999999999993,31.7895202218754,126.006812110665));
#135247=CARTESIAN_POINT('Ctrl Pts',(10.,31.7983820815757,125.993853814881));
#135248=CARTESIAN_POINT('Ctrl Pts',(10.0000000000001,31.8058537413279,125.982928345472));
#135249=CARTESIAN_POINT('Ctrl Pts',(10.0000000000001,31.8132114861588,125.97191914214));
#135250=CARTESIAN_POINT('Ctrl Pts',(10.,31.8204553240174,125.960828035951));
#135251=CARTESIAN_POINT('',(-0.00087680738617197,31.2702792793494,126.080257521478));
#135252=CARTESIAN_POINT('Ctrl Pts',(-0.000876807386172018,31.2691344289485,
126.079283929862));
#135253=CARTESIAN_POINT('Ctrl Pts',(-0.000584538257448223,31.2636353971113,
126.085750264102));
#135254=CARTESIAN_POINT('Ctrl Pts',(-0.000292269128723795,31.2580869446366,
126.092174570554));
#135255=CARTESIAN_POINT('Ctrl Pts',(0.,31.2524897196664,126.098556098763));
#135256=CARTESIAN_POINT('Ctrl Pts',(-2.77772596590786E-16,30.5301702171886,
123.014825674328));
#135257=CARTESIAN_POINT('Ctrl Pts',(-8.75743131328376E-15,30.598829973896,
123.040247836712));
#135258=CARTESIAN_POINT('Ctrl Pts',(-2.39681854255766E-13,30.6657864177248,
123.069560482627));
#135259=CARTESIAN_POINT('Ctrl Pts',(-2.5254277835618E-13,30.7308507067716,
123.102469346234));
#135260=CARTESIAN_POINT('Ctrl Pts',(-2.65638855218647E-13,30.7977302451018,
123.136296344688));
#135261=CARTESIAN_POINT('Ctrl Pts',(-6.11451911266343E-14,30.8626113478622,
123.173923712712));
#135262=CARTESIAN_POINT('Ctrl Pts',(-1.69683711526147E-13,30.9252577077206,
123.21507651753));
#135263=CARTESIAN_POINT('Ctrl Pts',(-2.61344823476963E-13,30.9781920191894,
123.24984941404));
#135264=CARTESIAN_POINT('Ctrl Pts',(-8.4631591032592E-14,31.0295304465062,
123.287140434778));
#135265=CARTESIAN_POINT('Ctrl Pts',(-1.73687453308702E-13,31.0791076863594,
123.326801732865));
#135266=CARTESIAN_POINT('Ctrl Pts',(-2.13342330293228E-13,31.1011385797417,
123.34442622814));
#135267=CARTESIAN_POINT('Ctrl Pts',(-1.10073476274008E-13,31.1228213894366,
123.362518959318));
#135268=CARTESIAN_POINT('Ctrl Pts',(3.95516952522712E-15,31.1441400562127,
123.381067676726));
#135269=CARTESIAN_POINT('Ctrl Pts',(6.66452089179545E-14,31.1558506001259,
123.391256661432));
#135270=CARTESIAN_POINT('Ctrl Pts',(-1.34022555091032E-13,31.1674512495831,
123.401583242396));
#135271=CARTESIAN_POINT('Ctrl Pts',(-8.07479083597684E-14,31.178939208613,
123.412045430858));
#135272=CARTESIAN_POINT('Ctrl Pts',(-3.16896073044118E-14,31.1895349701113,
123.421695086938));
#135273=CARTESIAN_POINT('Ctrl Pts',(-6.15876490622071E-14,31.200036303322,
123.43146162442));
#135274=CARTESIAN_POINT('Ctrl Pts',(-7.96654409107589E-14,31.2104251173888,
123.441328016445));
#135275=CARTESIAN_POINT('Ctrl Pts',(-1.71607632518157E-13,31.2635091616281,
123.491742624636));
#135276=CARTESIAN_POINT('Ctrl Pts',(5.49748712918573E-14,31.3137531838448,
123.544845896782));
#135277=CARTESIAN_POINT('Ctrl Pts',(4.07729405793589E-14,31.3609385689379,
123.600378065046));
#135278=CARTESIAN_POINT('Ctrl Pts',(2.6523705644377E-14,31.4077587712736,
123.655480452134));
#135279=CARTESIAN_POINT('Ctrl Pts',(-1.80781432573089E-13,31.4515680052721,
123.712975168858));
#135280=CARTESIAN_POINT('Ctrl Pts',(-9.5215502149415E-14,31.4921078981635,
123.77263267036));
#135281=CARTESIAN_POINT('Ctrl Pts',(-2.38087088306119E-14,31.5257972460783,
123.822209079681));
#135282=CARTESIAN_POINT('Ctrl Pts',(-4.4744082398028E-14,31.5572281772826,
123.873279737524));
#135283=CARTESIAN_POINT('Ctrl Pts',(-4.78783679369599E-14,31.5862248073375,
123.925719379271));
#135284=CARTESIAN_POINT('Ctrl Pts',(-4.95707857465004E-14,31.5983293795196,
123.947610179255));
#135285=CARTESIAN_POINT('Ctrl Pts',(-1.23896470668944E-13,31.6100094226953,
123.969739580722));
#135286=CARTESIAN_POINT('Ctrl Pts',(-6.71823707776298E-14,31.6212507011121,
123.992098553664));
#135287=CARTESIAN_POINT('Ctrl Pts',(-4.1055023269343E-14,31.626451748782,
124.002443469946));
#135288=CARTESIAN_POINT('Ctrl Pts',(4.20872296912592E-14,31.6315588588845,
124.012837529915));
#135289=CARTESIAN_POINT('Ctrl Pts',(-1.66672231571852E-14,31.6365705562371,
124.023279837204));
#135290=CARTESIAN_POINT('Ctrl Pts',(-7.76815753353117E-14,31.6418017627402,
124.034179510898));
#135291=CARTESIAN_POINT('Ctrl Pts',(-6.18625599143113E-14,31.6469254048826,
124.045124295143));
#135292=CARTESIAN_POINT('Ctrl Pts',(-5.67601521339611E-14,31.6519384284677,
124.05610888875));
#135293=CARTESIAN_POINT('Ctrl Pts',(-2.74607999713858E-14,31.6804790658224,
124.118647454013));
#135294=CARTESIAN_POINT('Ctrl Pts',(-4.39722585003227E-15,31.7054587309027,
124.182518376153));
#135295=CARTESIAN_POINT('Ctrl Pts',(1.14908083048704E-14,31.7266539957321,
124.247516921405));
#135296=CARTESIAN_POINT('Ctrl Pts',(2.48997376757104E-14,31.7458595519117,
124.306413718519));
#135297=CARTESIAN_POINT('Ctrl Pts',(1.79531194258059E-14,31.7619575585816,
124.366236962781));
#135298=CARTESIAN_POINT('Ctrl Pts',(2.72004641033163E-15,31.7747450702918,
124.426839150922));
#135299=CARTESIAN_POINT('Ctrl Pts',(-1.50013263895926E-14,31.7898767105001,
124.498550561833));
#135300=CARTESIAN_POINT('Ctrl Pts',(-1.25000641635101E-14,31.8003734925573,
124.571354192565));
#135301=CARTESIAN_POINT('Ctrl Pts',(-5.63438184997267E-15,31.8063105084585,
124.644827210979));
#135302=CARTESIAN_POINT('Ctrl Pts',(-4.15408756744793E-15,31.8076174032829,
124.661000573001));
#135303=CARTESIAN_POINT('Ctrl Pts',(-1.03439185283564E-14,31.808703127552,
124.677206288828));
#135304=CARTESIAN_POINT('Ctrl Pts',(3.02535774210355E-15,31.8095681127238,
124.693439683831));
#135305=CARTESIAN_POINT('Ctrl Pts',(1.65497979186504E-14,31.8104620745258,
124.710216890567));
#135306=CARTESIAN_POINT('Ctrl Pts',(-9.80120482820878E-15,31.811120270022,
124.727029834275));
#135307=CARTESIAN_POINT('Ctrl Pts',(-1.05193631583234E-14,31.8115426155158,
124.743839163738));
#135308=CARTESIAN_POINT('Ctrl Pts',(-1.34948166120589E-14,31.8132672489494,
124.812479487862));
#135309=CARTESIAN_POINT('Ctrl Pts',(-1.60405791084441E-14,31.8110709449073,
124.881146605068));
#135310=CARTESIAN_POINT('Ctrl Pts',(-1.80688797257744E-14,31.8050746611966,
124.949501213653));
#135311=CARTESIAN_POINT('Ctrl Pts',(-2.00918682248362E-14,31.7990940817499,
125.017676801554));
#135312=CARTESIAN_POINT('Ctrl Pts',(1.91766302506283E-15,31.7893329284663,
125.085542577925));
#135313=CARTESIAN_POINT('Ctrl Pts',(-1.30451205393456E-14,31.7758617893156,
125.152746909433));
#135314=CARTESIAN_POINT('Ctrl Pts',(-2.4101450158528E-14,31.7661004735783,
125.201443808146));
#135315=CARTESIAN_POINT('Ctrl Pts',(6.03490530108545E-14,31.7543901513868,
125.249793146236));
#135316=CARTESIAN_POINT('Ctrl Pts',(3.41393580072236E-15,31.7407434738878,
125.297651488221));
#135317=CARTESIAN_POINT('Ctrl Pts',(-3.93869884415215E-14,31.7305056909709,
125.333554975794));
#135318=CARTESIAN_POINT('Ctrl Pts',(-1.37967821082287E-15,31.7191778680749,
125.369181973231));
#135319=CARTESIAN_POINT('Ctrl Pts',(-1.89293025698589E-14,31.7067614289762,
125.404467741074));
#135320=CARTESIAN_POINT('Ctrl Pts',(-2.47700547482771E-14,31.7026354143409,
125.416193292448));
#135321=CARTESIAN_POINT('Ctrl Pts',(1.15236377331479E-14,31.6983923938271,
125.427871943742));
#135322=CARTESIAN_POINT('Ctrl Pts',(-2.44249065417534E-15,31.6940329877996,
125.439501206732));
#135323=CARTESIAN_POINT('Ctrl Pts',(-7.59147689133786E-14,31.6709092331424,
125.501186725936));
#135324=CARTESIAN_POINT('Ctrl Pts',(6.73746093792032E-14,31.6445127108641,
125.561488649643));
#135325=CARTESIAN_POINT('Ctrl Pts',(-3.60822483003176E-15,31.6148933850985,
125.620073088418));
#135326=CARTESIAN_POINT('Ctrl Pts',(-5.37075275596212E-14,31.594056103009,
125.661287412014));
#135327=CARTESIAN_POINT('Ctrl Pts',(1.77541335953307E-14,31.5716229476758,
125.701651195217));
#135328=CARTESIAN_POINT('Ctrl Pts',(4.9960036108132E-16,31.5476009047189,
125.741036831029));
#135329=CARTESIAN_POINT('Ctrl Pts',(-5.33872078257124E-15,31.5398884957193,
125.753681806006));
#135330=CARTESIAN_POINT('Ctrl Pts',(3.16358140217142E-14,31.5320111431503,
125.766227577131));
#135331=CARTESIAN_POINT('Ctrl Pts',(2.75057754350883E-14,31.5239724343926,
125.778664238771));
#135332=CARTESIAN_POINT('Ctrl Pts',(1.03649137560407E-14,31.4897260852599,
125.831646660379));
#135333=CARTESIAN_POINT('Ctrl Pts',(-5.08270772809619E-14,31.4526236846046,
125.882545515417));
#135334=CARTESIAN_POINT('Ctrl Pts',(1.04083408558608E-14,31.4126994357374,
125.931045747963));
#135335=CARTESIAN_POINT('Ctrl Pts',(6.66773404040496E-14,31.3759099756901,
125.975737819026));
#135336=CARTESIAN_POINT('Ctrl Pts',(-1.45729917785235E-13,31.3367238178986,
126.018393245589));
#135337=CARTESIAN_POINT('Ctrl Pts',(3.38895578266829E-14,31.2951462810091,
126.058732615753));
#135338=CARTESIAN_POINT('Ctrl Pts',(6.77098686975264E-14,31.287343182337,
126.06630334046));
#135339=CARTESIAN_POINT('Ctrl Pts',(-1.39523139557582E-13,31.2794558011521,
126.073792385657));
#135340=CARTESIAN_POINT('Ctrl Pts',(-2.51743070833754E-14,31.2714857203022,
126.08119908863));
#135341=CARTESIAN_POINT('Ctrl Pts',(0.00172044862969348,-31.2663699642227,
126.077829790033));
#135342=CARTESIAN_POINT('Ctrl Pts',(0.0387786082858811,-31.6249060139602,
125.656600524761));
#135343=CARTESIAN_POINT('Ctrl Pts',(0.112881858221588,-31.8818178994089,
124.435268666319));
#135344=CARTESIAN_POINT('Ctrl Pts',(0.224030198436815,-30.5442576915066,
123.110121958068));
#135345=CARTESIAN_POINT('Ctrl Pts',(0.335165469275375,-28.7082269099583,
123.519030297083));
#135346=CARTESIAN_POINT('Ctrl Pts',(0.446300740113934,-28.0547651464445,
125.281415280471));
#135347=CARTESIAN_POINT('Ctrl Pts',(0.557436010952494,-29.181599264857,
126.787219487406));
#135348=CARTESIAN_POINT('Ctrl Pts',(0.668571281791053,-31.0575532184307,
126.656742998468));
#135349=CARTESIAN_POINT('Ctrl Pts',(0.779706552629611,-31.9655285234099,
125.010137807065));
#135350=CARTESIAN_POINT('Ctrl Pts',(0.890841823468172,-31.074525746938,
123.354134510974));
#135351=CARTESIAN_POINT('Ctrl Pts',(1.00197709430673,-29.2000325132351,
123.204604423553));
#135352=CARTESIAN_POINT('Ctrl Pts',(1.11311236514529,-28.0577305949802,
124.698320246674));
#135353=CARTESIAN_POINT('Ctrl Pts',(1.22424763598385,-28.6931313646975,
126.468169411394));
#135354=CARTESIAN_POINT('Ctrl Pts',(1.33538290682241,-30.5246730611939,
126.894237381088));
#135355=CARTESIAN_POINT('Ctrl Pts',(1.44651817766097,-31.8759958504512,
125.58656674063));
#135356=CARTESIAN_POINT('Ctrl Pts',(1.55765344849953,-31.5102727009557,
123.742026356952));
#135357=CARTESIAN_POINT('Ctrl Pts',(1.66878871933809,-29.7622393879308,
123.048874664683));
#135358=CARTESIAN_POINT('Ctrl Pts',(1.77992399017665,-28.2318217175757,
124.141532605131));
#135359=CARTESIAN_POINT('Ctrl Pts',(1.89105926101521,-28.3197677921431,
126.019921776628));
#135360=CARTESIAN_POINT('Ctrl Pts',(2.00219453185377,-29.9455830857295,
126.964805175196));
#135361=CARTESIAN_POINT('Ctrl Pts',(2.11332980269233,-31.6212046416694,
126.111357797976));
#135362=CARTESIAN_POINT('Ctrl Pts',(2.22446507353089,-31.8129832629486,
124.240715911099));
#135363=CARTESIAN_POINT('Ctrl Pts',(2.33560034436945,-30.3453893754288,
123.065025373487));
#135364=CARTESIAN_POINT('Ctrl Pts',(2.44673561520801,-28.5616703232575,
123.660362595487));
#135365=CARTESIAN_POINT('Ctrl Pts',(2.55787088604656,-28.0944139048355,
125.481832198108));
#135366=CARTESIAN_POINT('Ctrl Pts',(2.66900615688513,-29.3712867574847,
126.86229436194));
#135367=CARTESIAN_POINT('Ctrl Pts',(2.78014142772368,-31.2236031295178,
126.538250959478));
#135368=CARTESIAN_POINT('Ctrl Pts',(2.89127669856224,-31.9559900271131,
124.80628978731));
#135369=CARTESIAN_POINT('Ctrl Pts',(3.00241196940081,-30.89811435481,123.251626116011));
#135370=CARTESIAN_POINT('Ctrl Pts',(3.11354724023936,-29.0182199142231,
123.297199807425));
#135371=CARTESIAN_POINT('Ctrl Pts',(3.22468251107792,-28.0369211285432,
124.901298545784));
#135372=CARTESIAN_POINT('Ctrl Pts',(3.33581778191648,-28.852373132271,126.595735944659));
#135373=CARTESIAN_POINT('Ctrl Pts',(3.44695305275504,-30.7182156783826,
126.829641186668));
#135374=CARTESIAN_POINT('Ctrl Pts',(3.5580883235936,-31.9266956468316,125.388927393098));
#135375=CARTESIAN_POINT('Ctrl Pts',(3.66922359443216,-31.3717253664279,
123.59223931305));
#135376=CARTESIAN_POINT('Ctrl Pts',(3.78035886527072,-29.5612535008297,
123.084034931924));
#135377=CARTESIAN_POINT('Ctrl Pts',(3.89149413610928,-28.1523539460514,
124.329459403205));
#135378=CARTESIAN_POINT('Ctrl Pts',(4.00262940694784,-28.4345527746557,
126.18861079302));
#135379=CARTESIAN_POINT('Ctrl Pts',(4.1137646777864,-30.1495613486075,126.959860208184));
#135380=CARTESIAN_POINT('Ctrl Pts',(4.22489994862496,-31.7276806334521,
125.937304785764));
#135381=CARTESIAN_POINT('Ctrl Pts',(4.33603521946352,-31.7245025047645,
124.056860697625));
#135382=CARTESIAN_POINT('Ctrl Pts',(4.44717049030208,-30.1429358142016,
123.039645443895));
#135383=CARTESIAN_POINT('Ctrl Pts',(4.55830576114063,-28.4305439995263,
123.816687490475));
#135384=CARTESIAN_POINT('Ctrl Pts',(4.6694410319792,-28.1546310491437,125.67678214208));
#135385=CARTESIAN_POINT('Ctrl Pts',(4.78057630281775,-29.5677323138313,
126.917437164581));
#135386=CARTESIAN_POINT('Ctrl Pts',(4.89171157365632,-31.3764760143124,
126.403115966214));
#135387=CARTESIAN_POINT('Ctrl Pts',(5.00284684449487,-31.92536999542,124.604562250968));
#135388=CARTESIAN_POINT('Ctrl Pts',(5.11398211533343,-30.7120270590674,
123.167941567586));
#135389=CARTESIAN_POINT('Ctrl Pts',(5.225117386172,-28.8469858139721,123.408152356713));
#135390=CARTESIAN_POINT('Ctrl Pts',(5.33625265701055,-28.0372659719354,
125.105336450006));
#135391=CARTESIAN_POINT('Ctrl Pts',(5.44738792784911,-29.0239812938614,
126.70610905803));
#135392=CARTESIAN_POINT('Ctrl Pts',(5.55852319868768,-30.9040190422199,
126.745328107815));
#135393=CARTESIAN_POINT('Ctrl Pts',(5.66965846952622,-31.9566336282375,
125.187097507927));
#135394=CARTESIAN_POINT('Ctrl Pts',(5.7807937403648,-31.2183965744007,123.457621829735));
#135395=CARTESIAN_POINT('Ctrl Pts',(5.89192901120334,-29.3649954593064,
123.139841440651));
#135396=CARTESIAN_POINT('Ctrl Pts',(6.00306428204191,-28.0927961116786,
124.524611778654));
#135397=CARTESIAN_POINT('Ctrl Pts',(6.11419955288046,-28.5662067554389,
126.344491563556));
#135398=CARTESIAN_POINT('Ctrl Pts',(6.22533482371902,-30.3519279647429,
126.933796095832));
#135399=CARTESIAN_POINT('Ctrl Pts',(6.33647009455759,-31.8155394220347,
125.753151538311));
#135400=CARTESIAN_POINT('Ctrl Pts',(6.44760536539615,-31.6174387916631,
123.883168594708));
#135401=CARTESIAN_POINT('Ctrl Pts',(6.5587406362347,-29.9389419999398,123.035389974257));
#135402=CARTESIAN_POINT('Ctrl Pts',(6.66987590707327,-28.3163298756153,
123.985763565594));
#135403=CARTESIAN_POINT('Ctrl Pts',(6.78101117791182,-28.2347335856866,
125.864439193422));
#135404=CARTESIAN_POINT('Ctrl Pts',(6.89214644875039,-29.7688359156915,
126.951917979511));
#135405=CARTESIAN_POINT('Ctrl Pts',(7.00328171958894,-31.5145162199645,
126.252861226189));
#135406=CARTESIAN_POINT('Ctrl Pts',(7.1144169904275,-31.8740024933559,124.40709588671));
#135407=CARTESIAN_POINT('Ctrl Pts',(7.22555226126606,-30.5182670768337,
123.103998979536));
#135408=CARTESIAN_POINT('Ctrl Pts',(7.33668753210462,-28.6881764049717,
123.536258394322));
#135409=CARTESIAN_POINT('Ctrl Pts',(7.44782280294318,-28.0587609143225,
125.308239266059));
#135410=CARTESIAN_POINT('Ctrl Pts',(7.55895807378174,-29.2061068726125,
126.798097420642));
#135411=CARTESIAN_POINT('Ctrl Pts',(7.6700933446203,-31.0800808453102,126.642207660685));
#135412=CARTESIAN_POINT('Ctrl Pts',(7.78122861545886,-31.9654872479834,
124.983251490096));
#135413=CARTESIAN_POINT('Ctrl Pts',(7.89236388629742,-31.0519385402995,
123.339624761284));
#135414=CARTESIAN_POINT('Ctrl Pts',(8.00349915713598,-29.1755801242742,
123.215692709229));
#135415=CARTESIAN_POINT('Ctrl Pts',(8.11463442797453,-28.0537899886445,
124.724886865103));
#135416=CARTESIAN_POINT('Ctrl Pts',(8.2257696988131,-28.7133110646225,126.485884302567));
#135417=CARTESIAN_POINT('Ctrl Pts',(8.33690496965165,-30.5505022463529,
126.886893738269));
#135418=CARTESIAN_POINT('Ctrl Pts',(8.44804024049022,-31.8838342901685,
125.560882406281));
#135419=CARTESIAN_POINT('Ctrl Pts',(8.55917551132877,-31.4929457558537,
123.721511379461));
#135420=CARTESIAN_POINT('Ctrl Pts',(8.67031078216733,-29.7356062750041,
123.052304624424));
#135421=CARTESIAN_POINT('Ctrl Pts',(8.78144605300589,-28.220258423856,124.165769279955));
#135422=CARTESIAN_POINT('Ctrl Pts',(8.89258132384446,-28.3338589101122,
126.042780391858));
#135423=CARTESIAN_POINT('Ctrl Pts',(9.00371659468301,-29.9724293548191,
126.965366863976));
#135424=CARTESIAN_POINT('Ctrl Pts',(9.11485186552158,-31.6362385744073,
126.089102586015));
#135425=CARTESIAN_POINT('Ctrl Pts',(9.22598713636013,-31.8024363376022,
124.216025188734));
#135426=CARTESIAN_POINT('Ctrl Pts',(9.3371224071987,-30.3189318736382,123.060473962851));
#135427=CARTESIAN_POINT('Ctrl Pts',(9.44825767803725,-28.5434836732957,
123.680164653635));
#135428=CARTESIAN_POINT('Ctrl Pts',(9.55939294887581,-28.1012134484641,
125.507765501478));
#135429=CARTESIAN_POINT('Ctrl Pts',(9.67052821971438,-29.3967080968805,
126.870821247227));
#135430=CARTESIAN_POINT('Ctrl Pts',(9.78166349055292,-31.2446643127262,
126.521165324413));
#135431=CARTESIAN_POINT('Ctrl Pts',(9.89279876139149,-31.9528358863139,
124.780043235528));
#135432=CARTESIAN_POINT('Ctrl Pts',(10.00393403223,-30.8748102268758,123.238590758769));
#135433=CARTESIAN_POINT('Ctrl Pts',(10.1150693030686,-28.9936519546155,
123.312692143422));
#135434=CARTESIAN_POINT('Ctrl Pts',(10.1891594836276,-28.3583796691399,
124.386603429246));
#135435=CARTESIAN_POINT('Ctrl Pts',(10.2262045739072,-28.3381599574103,
124.939191754379));
#135436=CARTESIAN_POINT('Ctrl Pts',(-0.0741753502519805,-31.3664757556195,
126.163031592958));
#135437=CARTESIAN_POINT('Ctrl Pts',(-0.0371171905957929,-31.7533538665377,
125.708504405161));
#135438=CARTESIAN_POINT('Ctrl Pts',(0.0369860593399143,-32.0305744835093,
124.390626990756));
#135439=CARTESIAN_POINT('Ctrl Pts',(0.148134399555141,-30.5872809378495,
122.960728224503));
#135440=CARTESIAN_POINT('Ctrl Pts',(0.259269670393701,-28.6061130165961,
123.401960524163));
#135441=CARTESIAN_POINT('Ctrl Pts',(0.37040494123226,-27.9009954898912,
125.303660990775));
#135442=CARTESIAN_POINT('Ctrl Pts',(0.481540212070819,-29.1169051741997,
126.928498123382));
#135443=CARTESIAN_POINT('Ctrl Pts',(0.59267548290938,-31.1411521704481,
126.787707545708));
#135444=CARTESIAN_POINT('Ctrl Pts',(0.703810753747938,-32.1209023824778,
125.010939194675));
#135445=CARTESIAN_POINT('Ctrl Pts',(0.814946024586498,-31.1594663672247,
123.224029824376));
#135446=CARTESIAN_POINT('Ctrl Pts',(0.926081295425056,-29.1367955598828,
123.062679472607));
#135447=CARTESIAN_POINT('Ctrl Pts',(1.03721656626361,-27.9041953553674,
124.67447264186));
#135448=CARTESIAN_POINT('Ctrl Pts',(1.14835183710217,-28.5898241774735,
126.584227328894));
#135449=CARTESIAN_POINT('Ctrl Pts',(1.25948710794074,-30.5661481541757,
127.043975717818));
#135450=CARTESIAN_POINT('Ctrl Pts',(1.37062237877929,-32.0242922050491,
125.632934492105));
#135451=CARTESIAN_POINT('Ctrl Pts',(1.48175764961785,-31.6296588584181,
123.642584289743));
#135452=CARTESIAN_POINT('Ctrl Pts',(1.59289292045641,-29.7434445531617,
122.894639369055));
#135453=CARTESIAN_POINT('Ctrl Pts',(1.70402819129497,-28.0920482775119,
124.073671268887));
#135454=CARTESIAN_POINT('Ctrl Pts',(1.81516346213353,-28.1869464368915,
126.100545985585));
#135455=CARTESIAN_POINT('Ctrl Pts',(1.92629873297209,-29.9412814610682,
127.120121854019));
#135456=CARTESIAN_POINT('Ctrl Pts',(2.03743400381065,-31.7493599029718,
126.19920996996));
#135457=CARTESIAN_POINT('Ctrl Pts',(2.14856927464921,-31.9562985100362,
124.180694956115));
#135458=CARTESIAN_POINT('Ctrl Pts',(2.25970454548777,-30.3726921998356,
122.91206678177));
#135459=CARTESIAN_POINT('Ctrl Pts',(2.37083981632633,-28.4479712190086,
123.554465056575));
#135460=CARTESIAN_POINT('Ctrl Pts',(2.48197508716489,-27.9437784590173,
125.519920746379));
#135461=CARTESIAN_POINT('Ctrl Pts',(2.59311035800345,-29.3215873501379,
127.009507622032));
#135462=CARTESIAN_POINT('Ctrl Pts',(2.70424562884201,-31.320328228104,126.659848781613));
#135463=CARTESIAN_POINT('Ctrl Pts',(2.81538089968056,-32.11060987373,124.790977110375));
#135464=CARTESIAN_POINT('Ctrl Pts',(2.92651617051912,-30.9691097596231,
123.113418201847));
#135465=CARTESIAN_POINT('Ctrl Pts',(3.03765144135768,-28.9406107832101,
123.162594466423));
#135466=CARTESIAN_POINT('Ctrl Pts',(3.14878671219624,-27.8817409130031,
124.893496254617));
#135467=CARTESIAN_POINT('Ctrl Pts',(3.2599219830348,-28.7616539119262,126.721877920633));
#135468=CARTESIAN_POINT('Ctrl Pts',(3.37105725387336,-30.7749901999753,
126.974273232704));
#135469=CARTESIAN_POINT('Ctrl Pts',(3.48219252471192,-32.0789997901358,
125.41967187187));
#135470=CARTESIAN_POINT('Ctrl Pts',(3.59332779555048,-31.4801594396173,
123.480956669238));
#135471=CARTESIAN_POINT('Ctrl Pts',(3.70446306638904,-29.5265708513964,
122.932579034479));
#135472=CARTESIAN_POINT('Ctrl Pts',(3.8155983372276,-28.0062986259812,124.276453568415));
#135473=CARTESIAN_POINT('Ctrl Pts',(3.92673360806616,-28.3108051039036,
126.282569768248));
#135474=CARTESIAN_POINT('Ctrl Pts',(4.03786887890472,-30.1613840841332,
127.11478599031));
#135475=CARTESIAN_POINT('Ctrl Pts',(4.14900414974328,-31.8642527584858,
126.011398170802));
#135476=CARTESIAN_POINT('Ctrl Pts',(4.26013942058184,-31.8608234006184,
123.982306097525));
#135477=CARTESIAN_POINT('Ctrl Pts',(4.37127469142039,-30.1542348051788,
122.884680583861));
#135478=CARTESIAN_POINT('Ctrl Pts',(4.48240996225896,-28.3064794374878,
123.723147341401));
#135479=CARTESIAN_POINT('Ctrl Pts',(4.59354523309752,-28.0087557327167,
125.730281367306));
#135480=CARTESIAN_POINT('Ctrl Pts',(4.70468050393607,-29.5335618107069,
127.069009430378));
#135481=CARTESIAN_POINT('Ctrl Pts',(4.81581577477464,-31.4852856233874,
126.51403144762));
#135482=CARTESIAN_POINT('Ctrl Pts',(4.92695104561319,-32.0775693467696,
124.573303132439));
#135483=CARTESIAN_POINT('Ctrl Pts',(5.03808631645175,-30.7683123739893,
123.023118439714));
#135484=CARTESIAN_POINT('Ctrl Pts',(5.14922158729032,-28.7558407293246,
123.282317748647));
#135485=CARTESIAN_POINT('Ctrl Pts',(5.26035685812887,-27.8821130160601,
125.11366323364));
#135486=CARTESIAN_POINT('Ctrl Pts',(5.37149212896743,-28.946827596477,126.840975962874));
#135487=CARTESIAN_POINT('Ctrl Pts',(5.48262739980599,-30.9754812090559,
126.883295255185));
#135488=CARTESIAN_POINT('Ctrl Pts',(5.59376267064455,-32.1113043511401,
125.20188745449));
#135489=CARTESIAN_POINT('Ctrl Pts',(5.70489794148311,-31.3147100979059,
123.335697754046));
#135490=CARTESIAN_POINT('Ctrl Pts',(5.81603321232167,-29.3147987285858,
122.992797014481));
#135491=CARTESIAN_POINT('Ctrl Pts',(5.92716848316023,-27.942032780275,124.487032622907));
#135492=CARTESIAN_POINT('Ctrl Pts',(6.03830375399879,-28.4528662534518,
126.45077282085));
#135493=CARTESIAN_POINT('Ctrl Pts',(6.14943902483735,-30.3797476607406,
127.0866615254));
#135494=CARTESIAN_POINT('Ctrl Pts',(6.26057429567591,-31.9590567319754,
125.812687718823));
#135495=CARTESIAN_POINT('Ctrl Pts',(6.37170956651447,-31.7452963647656,
123.794883737326));
#135496=CARTESIAN_POINT('Ctrl Pts',(6.48284483735302,-29.9341154014023,
122.880088721882));
#135497=CARTESIAN_POINT('Ctrl Pts',(6.59398010819159,-28.1832367551099,
123.905588779554));
#135498=CARTESIAN_POINT('Ctrl Pts',(6.70511537903014,-28.0951903270626,
125.932772596785));
#135499=CARTESIAN_POINT('Ctrl Pts',(6.81625064986871,-29.7505625325129,
127.10621593319));
#135500=CARTESIAN_POINT('Ctrl Pts',(6.92738592070726,-31.6342378250768,
126.35189915989));
#135501=CARTESIAN_POINT('Ctrl Pts',(7.03852119154583,-32.0221412742628,
124.360227169699));
#135502=CARTESIAN_POINT('Ctrl Pts',(7.14965646238439,-30.5592357805672,
122.954121228164));
#135503=CARTESIAN_POINT('Ctrl Pts',(7.26079173322294,-28.5844775311327,
123.420550492226));
#135504=CARTESIAN_POINT('Ctrl Pts',(7.37192700406151,-27.90530712084,125.332605396447));
#135505=CARTESIAN_POINT('Ctrl Pts',(7.48306227490006,-29.1433500937509,
126.94023595076));
#135506=CARTESIAN_POINT('Ctrl Pts',(7.59419754573863,-31.1654605928145,
126.772023198131));
#135507=CARTESIAN_POINT('Ctrl Pts',(7.70533281657718,-32.1208578442534,
124.981927530364));
#135508=CARTESIAN_POINT('Ctrl Pts',(7.81646808741574,-31.1350936553549,
123.208373087617));
#135509=CARTESIAN_POINT('Ctrl Pts',(7.9276033582543,-29.1104102241388,123.074644280663));
#135510=CARTESIAN_POINT('Ctrl Pts',(8.03873862909285,-27.8999432464479,
124.703139335652));
#135511=CARTESIAN_POINT('Ctrl Pts',(8.14987389993142,-28.6115990706583,
126.603342571663));
#135512=CARTESIAN_POINT('Ctrl Pts',(8.26100917076997,-30.594019121037,127.036051564408));
#135513=CARTESIAN_POINT('Ctrl Pts',(8.37214444160854,-32.0327502687575,
125.605219826424));
#135514=CARTESIAN_POINT('Ctrl Pts',(8.48327971244709,-31.6109622286261,
123.620447615501));
#135515=CARTESIAN_POINT('Ctrl Pts',(8.59441498328566,-29.7147061085213,
122.898340465071));
#135516=CARTESIAN_POINT('Ctrl Pts',(8.70555025412421,-28.079570912311,124.09982383842));
#135517=CARTESIAN_POINT('Ctrl Pts',(8.81668552496278,-28.2021514493431,
126.125211560733));
#135518=CARTESIAN_POINT('Ctrl Pts',(8.92782079580133,-29.9702499117393,
127.120727943962));
#135519=CARTESIAN_POINT('Ctrl Pts',(9.03895606663989,-31.7655822591382,
126.175195496748));
#135520=CARTESIAN_POINT('Ctrl Pts',(9.15009133747845,-31.9449178565231,
124.154052446854));
#135521=CARTESIAN_POINT('Ctrl Pts',(9.26122660831701,-30.3441432482872,
122.907155584834));
#135522=CARTESIAN_POINT('Ctrl Pts',(9.37236187915557,-28.4283469251996,
123.575832455625));
#135523=CARTESIAN_POINT('Ctrl Pts',(9.48349714999413,-27.9511155025199,
125.547904061935));
#135524=CARTESIAN_POINT('Ctrl Pts',(9.59463242083269,-29.3490182312716,
127.018708552522));
#135525=CARTESIAN_POINT('Ctrl Pts',(9.70576769167125,-31.3430542853006,
126.641412537272));
#135526=CARTESIAN_POINT('Ctrl Pts',(9.81690296250981,-32.1072063999793,
124.762655784306));
#135527=CARTESIAN_POINT('Ctrl Pts',(9.92803823334836,-30.9439634542561,
123.09935240738));
#135528=CARTESIAN_POINT('Ctrl Pts',(10.0391735041869,-28.9141007410287,
123.179311462354));
#135529=CARTESIAN_POINT('Ctrl Pts',(10.113263684746,-28.2286105597669,124.338114795679));
#135530=CARTESIAN_POINT('Ctrl Pts',(10.1503087750255,-28.2067924918683,
124.934384898781));
#135531=CARTESIAN_POINT('Ctrl Pts',(-0.150071149133654,-31.4665815470164,
126.248233395883));
#135532=CARTESIAN_POINT('Ctrl Pts',(-0.113012989477467,-31.8818017191152,
125.760408285559));
#135533=CARTESIAN_POINT('Ctrl Pts',(-0.0389097395417594,-32.1793310676097,
124.345985315194));
#135534=CARTESIAN_POINT('Ctrl Pts',(0.0722386006734674,-30.6303041841925,
122.811334490936));
#135535=CARTESIAN_POINT('Ctrl Pts',(0.183373871512027,-28.5039991232338,
123.284890751242));
#135536=CARTESIAN_POINT('Ctrl Pts',(0.294509142350586,-27.747225833338,
125.32590670108));
#135537=CARTESIAN_POINT('Ctrl Pts',(0.405644413189146,-29.0522110835422,
127.069776759358));
#135538=CARTESIAN_POINT('Ctrl Pts',(0.516779684027705,-31.2247511224655,
126.918672092948));
#135539=CARTESIAN_POINT('Ctrl Pts',(0.627914954866265,-32.2762762415459,
125.011740582285));
#135540=CARTESIAN_POINT('Ctrl Pts',(0.739050225704823,-31.2444069875114,
123.093925137778));
#135541=CARTESIAN_POINT('Ctrl Pts',(0.850185496543384,-29.0735586065304,
122.920754521663));
#135542=CARTESIAN_POINT('Ctrl Pts',(0.961320767381941,-27.7506601157544,
124.650625037046));
#135543=CARTESIAN_POINT('Ctrl Pts',(1.07245603822051,-28.4865169902498,
126.700285246394));
#135544=CARTESIAN_POINT('Ctrl Pts',(1.18359130905906,-30.6076232471574,
127.193714054548));
#135545=CARTESIAN_POINT('Ctrl Pts',(1.29472657989762,-32.1725885596471,
125.679302243581));
#135546=CARTESIAN_POINT('Ctrl Pts',(1.40586185073618,-31.7490450158803,
123.543142222534));
#135547=CARTESIAN_POINT('Ctrl Pts',(1.51699712157474,-29.7246497183924,
122.740404073427));
#135548=CARTESIAN_POINT('Ctrl Pts',(1.6281323924133,-27.9522748374482,124.005809932643));
#135549=CARTESIAN_POINT('Ctrl Pts',(1.73926766325186,-28.0541250816399,
126.181170194542));
#135550=CARTESIAN_POINT('Ctrl Pts',(1.85040293409042,-29.9369798364069,
127.275438532842));
#135551=CARTESIAN_POINT('Ctrl Pts',(1.96153820492898,-31.8775151642743,
126.287062141943));
#135552=CARTESIAN_POINT('Ctrl Pts',(2.07267347576754,-32.0996137571237,
124.120674001133));
#135553=CARTESIAN_POINT('Ctrl Pts',(2.1838087466061,-30.3999950242426,122.759108190054));
#135554=CARTESIAN_POINT('Ctrl Pts',(2.29494401744466,-28.3342721147596,
123.448567517662));
#135555=CARTESIAN_POINT('Ctrl Pts',(2.40607928828322,-27.7931430131993,
125.55800929465));
#135556=CARTESIAN_POINT('Ctrl Pts',(2.51721455912178,-29.2718879427911,
127.156720882125));
#135557=CARTESIAN_POINT('Ctrl Pts',(2.62834982996034,-31.4170533266902,
126.781446603746));
#135558=CARTESIAN_POINT('Ctrl Pts',(2.7394851007989,-32.265229720347,124.775664433439));
#135559=CARTESIAN_POINT('Ctrl Pts',(2.85062037163745,-31.0401051644362,
122.975210287685));
#135560=CARTESIAN_POINT('Ctrl Pts',(2.96175564247602,-28.863001652197,123.027989125423));
#135561=CARTESIAN_POINT('Ctrl Pts',(3.07289091331457,-27.726560697463,124.88569396345));
#135562=CARTESIAN_POINT('Ctrl Pts',(3.18402618415313,-28.6709346915815,
126.848019896607));
#135563=CARTESIAN_POINT('Ctrl Pts',(3.2951614549917,-30.831764721568,127.11890527874));
#135564=CARTESIAN_POINT('Ctrl Pts',(3.40629672583025,-32.2313039334398,
125.450416350642));
#135565=CARTESIAN_POINT('Ctrl Pts',(3.51743199666881,-31.5885935128067,
123.369674025424));
#135566=CARTESIAN_POINT('Ctrl Pts',(3.62856726750737,-29.491888201963,122.781123137034));
#135567=CARTESIAN_POINT('Ctrl Pts',(3.73970253834593,-27.8602433059111,
124.223447733626));
#135568=CARTESIAN_POINT('Ctrl Pts',(3.85083780918449,-28.1870574331513,
126.376528743476));
#135569=CARTESIAN_POINT('Ctrl Pts',(3.96197308002305,-30.173206819659,127.269711772436));
#135570=CARTESIAN_POINT('Ctrl Pts',(4.07310835086161,-32.0008248835195,
126.085491555839));
#135571=CARTESIAN_POINT('Ctrl Pts',(4.18424362170017,-31.9971442964722,
123.907751497425));
#135572=CARTESIAN_POINT('Ctrl Pts',(4.29537889253873,-30.165533796156,122.729715723827));
#135573=CARTESIAN_POINT('Ctrl Pts',(4.40651416337728,-28.1824148754493,
123.629607192327));
#135574=CARTESIAN_POINT('Ctrl Pts',(4.51764943421585,-27.8628804162897,
125.783780592533));
#135575=CARTESIAN_POINT('Ctrl Pts',(4.6287847050544,-29.4993913075824,127.220581696175));
#135576=CARTESIAN_POINT('Ctrl Pts',(4.73991997589297,-31.5940952324625,
126.624946929026));
#135577=CARTESIAN_POINT('Ctrl Pts',(4.85105524673152,-32.2297686981192,
124.542044013908));
#135578=CARTESIAN_POINT('Ctrl Pts',(4.96219051757009,-30.8245976889112,
122.878295311842));
#135579=CARTESIAN_POINT('Ctrl Pts',(5.07332578840864,-28.6646956446771,
123.156483140581));
#135580=CARTESIAN_POINT('Ctrl Pts',(5.1844610592472,-27.7269600601847,125.121990017272));
#135581=CARTESIAN_POINT('Ctrl Pts',(5.29559633008576,-28.8696738990929,
126.975842867719));
#135582=CARTESIAN_POINT('Ctrl Pts',(5.40673160092433,-31.0469433758917,
127.021262402556));
#135583=CARTESIAN_POINT('Ctrl Pts',(5.51786687176288,-32.2659750740426,
125.216677401053));
#135584=CARTESIAN_POINT('Ctrl Pts',(5.62900214260144,-31.4110236214113,
123.213773678358));
#135585=CARTESIAN_POINT('Ctrl Pts',(5.74013741344,-29.2646019978652,122.845752588311));
#135586=CARTESIAN_POINT('Ctrl Pts',(5.85127268427856,-27.7912694488716,
124.44945346716));
#135587=CARTESIAN_POINT('Ctrl Pts',(5.96240795511712,-28.3395257514648,
126.557054078143));
#135588=CARTESIAN_POINT('Ctrl Pts',(6.07354322595567,-30.4075673567382,
127.239526954969));
#135589=CARTESIAN_POINT('Ctrl Pts',(6.18467849679424,-32.1025740419161,
125.872223899334));
#135590=CARTESIAN_POINT('Ctrl Pts',(6.2958137676328,-31.8731539378682,123.706598879945));
#135591=CARTESIAN_POINT('Ctrl Pts',(6.40694903847135,-29.9292888028649,
122.724787469508));
#135592=CARTESIAN_POINT('Ctrl Pts',(6.51808430930992,-28.0501436346044,
123.825413993513));
#135593=CARTESIAN_POINT('Ctrl Pts',(6.62921958014847,-27.9556470684387,
126.001106000148));
#135594=CARTESIAN_POINT('Ctrl Pts',(6.74035485098703,-29.7322891493341,
127.260513886869));
#135595=CARTESIAN_POINT('Ctrl Pts',(6.85149012182559,-31.7539594301893,
126.450937093592));
#135596=CARTESIAN_POINT('Ctrl Pts',(6.96262539266416,-32.1702800551697,
124.313358452689));
#135597=CARTESIAN_POINT('Ctrl Pts',(7.07376066350271,-30.6002044843009,
122.804243476792));
#135598=CARTESIAN_POINT('Ctrl Pts',(7.18489593434127,-28.4807786572938,
123.304842590131));
#135599=CARTESIAN_POINT('Ctrl Pts',(7.29603120517984,-27.7518533273575,
125.356971526835));
#135600=CARTESIAN_POINT('Ctrl Pts',(7.40716647601839,-29.0805933148894,
127.08237448088));
#135601=CARTESIAN_POINT('Ctrl Pts',(7.51830174685695,-31.2508403403189,
126.901838735577));
#135602=CARTESIAN_POINT('Ctrl Pts',(7.62943701769551,-32.2762284405235,
124.980603570633));
#135603=CARTESIAN_POINT('Ctrl Pts',(7.74057228853406,-31.2182487704101,
123.077121413948));
#135604=CARTESIAN_POINT('Ctrl Pts',(7.85170755937263,-29.0452403240035,
122.933595852095));
#135605=CARTESIAN_POINT('Ctrl Pts',(7.96284283021118,-27.7460965042514,
124.681391806202));
#135606=CARTESIAN_POINT('Ctrl Pts',(8.07397810104976,-28.509887076694,126.720800840759));
#135607=CARTESIAN_POINT('Ctrl Pts',(8.1851133718883,-30.6375359957213,127.185209390547));
#135608=CARTESIAN_POINT('Ctrl Pts',(8.29624864272688,-32.1816662473463,
125.649557246568));
#135609=CARTESIAN_POINT('Ctrl Pts',(8.40738391356542,-31.7289787013983,
123.51938385154));
#135610=CARTESIAN_POINT('Ctrl Pts',(8.51851918440399,-29.6938059420385,
122.744376305717));
#135611=CARTESIAN_POINT('Ctrl Pts',(8.62965445524254,-27.9388834007661,
124.033878396884));
#135612=CARTESIAN_POINT('Ctrl Pts',(8.74078972608111,-28.070443988574,126.207642729609));
#135613=CARTESIAN_POINT('Ctrl Pts',(8.85192499691966,-29.9680704686594,
127.276089023948));
#135614=CARTESIAN_POINT('Ctrl Pts',(8.96306026775823,-31.8949259438691,
126.261288407482));
#135615=CARTESIAN_POINT('Ctrl Pts',(9.07419553859677,-32.0873993754438,
124.092079704975));
#135616=CARTESIAN_POINT('Ctrl Pts',(9.18533080943535,-30.3693546229362,
122.753837206818));
#135617=CARTESIAN_POINT('Ctrl Pts',(9.2964660802739,-28.3132101771035,123.471500257614));
#135618=CARTESIAN_POINT('Ctrl Pts',(9.40760135111246,-27.8010175565758,
125.588042622392));
#135619=CARTESIAN_POINT('Ctrl Pts',(9.51873662195103,-29.3013283656625,
127.166595857817));
#135620=CARTESIAN_POINT('Ctrl Pts',(9.62987189278957,-31.4414442578748,
126.76165975013));
#135621=CARTESIAN_POINT('Ctrl Pts',(9.74100716362815,-32.2615769136449,
124.745268333085));
#135622=CARTESIAN_POINT('Ctrl Pts',(9.85214243446669,-31.0131166816364,
122.960114055991));
#135623=CARTESIAN_POINT('Ctrl Pts',(9.96327770530527,-28.8345495274418,
123.045930781285));
#135624=CARTESIAN_POINT('Ctrl Pts',(10.0373678858643,-28.0988414503939,
124.289626162113));
#135625=CARTESIAN_POINT('Ctrl Pts',(10.0744129761438,-28.0754250263263,
124.929578043184));
#135626=CARTESIAN_POINT('Ctrl Pts',(-0.225966948015328,-31.5666873384132,
126.333435198808));
#135627=CARTESIAN_POINT('Ctrl Pts',(-0.188908788359141,-32.0102495716926,
125.812312165957));
#135628=CARTESIAN_POINT('Ctrl Pts',(-0.114805538423433,-32.3280876517101,
124.301343639632));
#135629=CARTESIAN_POINT('Ctrl Pts',(-0.00365719820820642,-30.6733274305354,
122.661940757371));
#135630=CARTESIAN_POINT('Ctrl Pts',(0.107478072630353,-28.4018852298716,
123.167820978322));
#135631=CARTESIAN_POINT('Ctrl Pts',(0.218613343468912,-27.5934561767846,
125.348152411385));
#135632=CARTESIAN_POINT('Ctrl Pts',(0.329748614307472,-28.9875169928847,
127.211055395334));
#135633=CARTESIAN_POINT('Ctrl Pts',(0.440883885146031,-31.3083500744829,
127.049636640188));
#135634=CARTESIAN_POINT('Ctrl Pts',(0.55201915598459,-32.4316501006138,
125.012541969895));
#135635=CARTESIAN_POINT('Ctrl Pts',(0.66315442682315,-31.329347607798,122.963820451181));
#135636=CARTESIAN_POINT('Ctrl Pts',(0.77428969766171,-29.0103216531781,
122.778829570717));
#135637=CARTESIAN_POINT('Ctrl Pts',(0.885424968500269,-27.5971248761416,
124.626777432233));
#135638=CARTESIAN_POINT('Ctrl Pts',(0.996560239338828,-28.3832098030258,
126.816343163895));
#135639=CARTESIAN_POINT('Ctrl Pts',(1.10769551017739,-30.6490983401391,
127.343452391279));
#135640=CARTESIAN_POINT('Ctrl Pts',(1.21883078101594,-32.3208849142452,
125.725669995058));
#135641=CARTESIAN_POINT('Ctrl Pts',(1.3299660518545,-31.8684311733427,123.443700155325));
#135642=CARTESIAN_POINT('Ctrl Pts',(1.44110132269306,-29.7058548836233,
122.586168777798));
#135643=CARTESIAN_POINT('Ctrl Pts',(1.55223659353162,-27.8125013973844,
123.937948596399));
#135644=CARTESIAN_POINT('Ctrl Pts',(1.66337186437018,-27.9213037263882,
126.261794403498));
#135645=CARTESIAN_POINT('Ctrl Pts',(1.77450713520874,-29.9326782117456,
127.430755211664));
#135646=CARTESIAN_POINT('Ctrl Pts',(1.8856424060473,-32.0056704255768,126.374914313927));
#135647=CARTESIAN_POINT('Ctrl Pts',(1.99677767688586,-32.2429290042112,
124.06065304615));
#135648=CARTESIAN_POINT('Ctrl Pts',(2.10791294772442,-30.4272978486494,
122.606149598337));
#135649=CARTESIAN_POINT('Ctrl Pts',(2.21904821856298,-28.2205730105108,
123.34266997875));
#135650=CARTESIAN_POINT('Ctrl Pts',(2.33018348940154,-27.6425075673812,
125.596097842922));
#135651=CARTESIAN_POINT('Ctrl Pts',(2.4413187602401,-29.2221885354442,127.303934142217));
#135652=CARTESIAN_POINT('Ctrl Pts',(2.55245403107866,-31.5137784252764,
126.903044425881));
#135653=CARTESIAN_POINT('Ctrl Pts',(2.66358930191722,-32.4198495669641,
124.760351756503));
#135654=CARTESIAN_POINT('Ctrl Pts',(2.77472457275578,-31.1111005692493,
122.837002373521));
#135655=CARTESIAN_POINT('Ctrl Pts',(2.88585984359434,-28.7853925211838,
122.893383784421));
#135656=CARTESIAN_POINT('Ctrl Pts',(2.99699511443289,-27.5713804819229,
124.877891672283));
#135657=CARTESIAN_POINT('Ctrl Pts',(3.10813038527145,-28.5802154712366,
126.97416187258));
#135658=CARTESIAN_POINT('Ctrl Pts',(3.21926565611002,-30.8885392431607,
127.263537324776));
#135659=CARTESIAN_POINT('Ctrl Pts',(3.33040092694857,-32.3836080767439,
125.481160829412));
#135660=CARTESIAN_POINT('Ctrl Pts',(3.44153619778713,-31.6970275859962,
123.258391381611));
#135661=CARTESIAN_POINT('Ctrl Pts',(3.55267146862569,-29.4572055525297,
122.629667239589));
#135662=CARTESIAN_POINT('Ctrl Pts',(3.66380673946425,-27.7141879858409,
124.170441898836));
#135663=CARTESIAN_POINT('Ctrl Pts',(3.77494201030281,-28.0633097623991,
126.470487718705));
#135664=CARTESIAN_POINT('Ctrl Pts',(3.88607728114137,-30.1850295551847,
127.424637554561));
#135665=CARTESIAN_POINT('Ctrl Pts',(3.99721255197993,-32.1373970085532,
126.159584940877));
#135666=CARTESIAN_POINT('Ctrl Pts',(4.10834782281849,-32.1334651923261,
123.833196897325));
#135667=CARTESIAN_POINT('Ctrl Pts',(4.21948309365705,-30.1768327871333,
122.574750863792));
#135668=CARTESIAN_POINT('Ctrl Pts',(4.33061836449561,-28.0583503134108,
123.536067043254));
#135669=CARTESIAN_POINT('Ctrl Pts',(4.44175363533417,-27.7170050998627,
125.83727981776));
#135670=CARTESIAN_POINT('Ctrl Pts',(4.55288890617273,-29.4652208044579,
127.372153961972));
#135671=CARTESIAN_POINT('Ctrl Pts',(4.66402417701129,-31.7029048415377,
126.735862410431));
#135672=CARTESIAN_POINT('Ctrl Pts',(4.77515944784984,-32.3819680494687,
124.510784895378));
#135673=CARTESIAN_POINT('Ctrl Pts',(4.88629471868841,-30.8808830038331,
122.733472183969));
#135674=CARTESIAN_POINT('Ctrl Pts',(4.99742998952697,-28.5735505600296,
123.030648532515));
#135675=CARTESIAN_POINT('Ctrl Pts',(5.10856526036552,-27.5718071043093,
125.130316800904));
#135676=CARTESIAN_POINT('Ctrl Pts',(5.21970053120408,-28.7925202017086,
127.110709772564));
#135677=CARTESIAN_POINT('Ctrl Pts',(5.33083580204264,-31.1184055427276,
127.159229549927));
#135678=CARTESIAN_POINT('Ctrl Pts',(5.4419710728812,-32.4206457969451,125.231467347616));
#135679=CARTESIAN_POINT('Ctrl Pts',(5.55310634371976,-31.5073371449166,
123.091849602668));
#135680=CARTESIAN_POINT('Ctrl Pts',(5.66424161455832,-29.2144052671446,
122.698708162142));
#135681=CARTESIAN_POINT('Ctrl Pts',(5.77537688539688,-27.6405061174681,
124.411874311414));
#135682=CARTESIAN_POINT('Ctrl Pts',(5.88651215623544,-28.2261852494778,
126.663335335437));
#135683=CARTESIAN_POINT('Ctrl Pts',(5.997647427074,-30.435387052736,127.392392384537));
#135684=CARTESIAN_POINT('Ctrl Pts',(6.10878269791256,-32.2460913518569,
125.931760079845));
#135685=CARTESIAN_POINT('Ctrl Pts',(6.21991796875111,-32.0010115109706,
123.618314022564));
#135686=CARTESIAN_POINT('Ctrl Pts',(6.33105323958968,-29.9244622043275,
122.569486217133));
#135687=CARTESIAN_POINT('Ctrl Pts',(6.44218851042824,-27.9170505140989,
123.745239207473));
#135688=CARTESIAN_POINT('Ctrl Pts',(6.55332378126679,-27.8161038098147,
126.069439403511));
#135689=CARTESIAN_POINT('Ctrl Pts',(6.66445905210537,-29.7140157661554,
127.414811840549));
#135690=CARTESIAN_POINT('Ctrl Pts',(6.77559432294391,-31.8736810353017,
126.549975027294));
#135691=CARTESIAN_POINT('Ctrl Pts',(6.88672959378247,-32.3184188360767,
124.266489735679));
#135692=CARTESIAN_POINT('Ctrl Pts',(6.99786486462104,-30.6411731880345,
122.65436572542));
#135693=CARTESIAN_POINT('Ctrl Pts',(7.10900013545958,-28.3770797834548,
123.189134688036));
#135694=CARTESIAN_POINT('Ctrl Pts',(7.22013540629817,-27.598399533875,125.381337657224));
#135695=CARTESIAN_POINT('Ctrl Pts',(7.3312706771367,-29.0178365360278,127.224513010999));
#135696=CARTESIAN_POINT('Ctrl Pts',(7.44240594797528,-31.3362200878231,
127.031654273023));
#135697=CARTESIAN_POINT('Ctrl Pts',(7.55354121881383,-32.4315990367936,
124.9792796109));
#135698=CARTESIAN_POINT('Ctrl Pts',(7.66467648965239,-31.3014038854654,
122.94586974028));
#135699=CARTESIAN_POINT('Ctrl Pts',(7.77581176049095,-28.980070423868,122.792547423528));
#135700=CARTESIAN_POINT('Ctrl Pts',(7.88694703132951,-27.5922497620548,
124.65964427675));
#135701=CARTESIAN_POINT('Ctrl Pts',(7.99808230216807,-28.4081750827298,
126.838259109854));
#135702=CARTESIAN_POINT('Ctrl Pts',(8.10921757300663,-30.6810528704055,
127.334367216686));
#135703=CARTESIAN_POINT('Ctrl Pts',(8.22035284384519,-32.3305822259353,
125.693894666712));
#135704=CARTESIAN_POINT('Ctrl Pts',(8.33148811468374,-31.8469951741706,
123.41832008758));
#135705=CARTESIAN_POINT('Ctrl Pts',(8.44262338552231,-29.6729057755557,
122.590412146364));
#135706=CARTESIAN_POINT('Ctrl Pts',(8.55375865636087,-27.798195889221,123.967932955349));
#135707=CARTESIAN_POINT('Ctrl Pts',(8.66489392719942,-27.9387365278048,
126.290073898485));
#135708=CARTESIAN_POINT('Ctrl Pts',(8.77602919803799,-29.9658910255794,
127.431450103935));
#135709=CARTESIAN_POINT('Ctrl Pts',(8.88716446887655,-32.0242696285999,
126.347381318216));
#135710=CARTESIAN_POINT('Ctrl Pts',(8.9982997397151,-32.2298808943646,124.030106963096));
#135711=CARTESIAN_POINT('Ctrl Pts',(9.10943501055366,-30.3945659975851,
122.600518828802));
#135712=CARTESIAN_POINT('Ctrl Pts',(9.22057028139223,-28.1980734290074,
123.367168059605));
#135713=CARTESIAN_POINT('Ctrl Pts',(9.33170555223079,-27.6509196106317,
125.628181182848));
#135714=CARTESIAN_POINT('Ctrl Pts',(9.44284082306934,-29.2536385000535,
127.314483163113));
#135715=CARTESIAN_POINT('Ctrl Pts',(9.5539760939079,-31.5398342304492,126.881906962989));
#135716=CARTESIAN_POINT('Ctrl Pts',(9.66511136474646,-32.4159474273104,
124.727880881864));
#135717=CARTESIAN_POINT('Ctrl Pts',(9.77624663558503,-31.0822699090167,
122.820875704601));
#135718=CARTESIAN_POINT('Ctrl Pts',(9.88738190642358,-28.7549983138549,
122.912550100216));
#135719=CARTESIAN_POINT('Ctrl Pts',(9.96147208698262,-27.9690723410208,
124.241137528545));
#135720=CARTESIAN_POINT('Ctrl Pts',(9.99851717726214,-27.9440575607844,
124.924771187586));
#135721=CARTESIAN_POINT('',(10.0008700344079,-30.7705824472418,123.521224995955));
#135722=CARTESIAN_POINT('Ctrl Pts',(10.,-27.9466241674713,124.92486510207));
#135723=CARTESIAN_POINT('Ctrl Pts',(10.,-27.9563161184906,124.850853981395));
#135724=CARTESIAN_POINT('Ctrl Pts',(10.,-27.9703562534103,124.777580265674));
#135725=CARTESIAN_POINT('Ctrl Pts',(10.,-27.9885129974625,124.705321550446));
#135726=CARTESIAN_POINT('Ctrl Pts',(10.,-28.0061948969839,124.63495258239));
#135727=CARTESIAN_POINT('Ctrl Pts',(9.99999999999999,-28.0277817096079,
124.565545600416));
#135728=CARTESIAN_POINT('Ctrl Pts',(10.0000000000001,-28.0530993947356,
124.497379617191));
#135729=CARTESIAN_POINT('Ctrl Pts',(10.0000000000001,-28.0587500616534,
124.482165617002));
#135730=CARTESIAN_POINT('Ctrl Pts',(10.,-28.0645875153452,124.46701154552));
#135731=CARTESIAN_POINT('Ctrl Pts',(10.,-28.0706074755671,124.45192711149));
#135732=CARTESIAN_POINT('Ctrl Pts',(10.,-28.0982336410484,124.382703220408));
#135733=CARTESIAN_POINT('Ctrl Pts',(9.99999999999995,-28.1296438323157,
124.315080840735));
#135734=CARTESIAN_POINT('Ctrl Pts',(9.99999999999993,-28.1646277359223,
124.249352564926));
#135735=CARTESIAN_POINT('Ctrl Pts',(9.99999999999992,-28.1891882402768,
124.203207925883));
#135736=CARTESIAN_POINT('Ctrl Pts',(10.0000000000001,-28.2155111464007,
124.157997355713));
#135737=CARTESIAN_POINT('Ctrl Pts',(10.0000000000001,-28.2435347288156,
124.113832765246));
#135738=CARTESIAN_POINT('Ctrl Pts',(10.0000000000001,-28.2541842563361,
124.097049328544));
#135739=CARTESIAN_POINT('Ctrl Pts',(10.,-28.2650794693322,124.080417051398));
#135740=CARTESIAN_POINT('Ctrl Pts',(9.99999999999997,-28.276217259473,124.063942481829));
#135741=CARTESIAN_POINT('Ctrl Pts',(9.99999999999989,-28.2868388799486,
124.048231409593));
#135742=CARTESIAN_POINT('Ctrl Pts',(9.99999999999993,-28.2976847177624,
124.032658993963));
#135743=CARTESIAN_POINT('Ctrl Pts',(9.99999999999997,-28.3087323142363,
124.017258087294));
#135744=CARTESIAN_POINT('Ctrl Pts',(10.0000000000001,-28.3509004273892,
123.958473610816));
#135745=CARTESIAN_POINT('Ctrl Pts',(10.0000000000001,-28.3960457650924,
123.902120594903));
#135746=CARTESIAN_POINT('Ctrl Pts',(10.,-28.4439773242738,123.848468307574));
#135747=CARTESIAN_POINT('Ctrl Pts',(9.99999999999994,-28.4912171255121,
123.795590340892));
#135748=CARTESIAN_POINT('Ctrl Pts',(9.9999999999999,-28.5411640434952,123.745335118217));
#135749=CARTESIAN_POINT('Ctrl Pts',(9.99999999999988,-28.5936642386043,
123.698000585234));
#135750=CARTESIAN_POINT('Ctrl Pts',(9.99999999999987,-28.6448275591752,
123.651871387427));
#135751=CARTESIAN_POINT('Ctrl Pts',(9.99999999999992,-28.698416431159,123.608515621588));
#135752=CARTESIAN_POINT('Ctrl Pts',(9.99999999999992,-28.7543060349939,
123.568254604751));
#135753=CARTESIAN_POINT('Ctrl Pts',(9.99999999999991,-28.7724718760314,
123.555168535398));
#135754=CARTESIAN_POINT('Ctrl Pts',(10.0000000000001,-28.7908808788323,
123.542409802214));
#135755=CARTESIAN_POINT('Ctrl Pts',(10.,-28.8095290004319,123.529990620511));
#135756=CARTESIAN_POINT('Ctrl Pts',(9.99999999999998,-28.8200346714515,
123.522994106862));
#135757=CARTESIAN_POINT('Ctrl Pts',(9.99999999999988,-28.8306173856636,
123.516104754664));
#135758=CARTESIAN_POINT('Ctrl Pts',(9.99999999999992,-28.8412612373231,
123.509334152335));
#135759=CARTESIAN_POINT('Ctrl Pts',(10.0000000000001,-28.8988964024382,
123.47267216233));
#135760=CARTESIAN_POINT('Ctrl Pts',(10.0000000000001,-28.9584212706046,
123.439421042338));
#135761=CARTESIAN_POINT('Ctrl Pts',(10.0000000000002,-29.019691425777,123.40984784988));
#135762=CARTESIAN_POINT('Ctrl Pts',(10.0000000000002,-29.0285216998097,
123.405585752082));
#135763=CARTESIAN_POINT('Ctrl Pts',(10.,-29.0373882572974,123.401400129531));
#135764=CARTESIAN_POINT('Ctrl Pts',(10.,-29.0462906965386,123.397291867037));
#135765=CARTESIAN_POINT('Ctrl Pts',(10.0000000000002,-29.109280769285,123.368223457094));
#135766=CARTESIAN_POINT('Ctrl Pts',(9.99999999999996,-29.1740667919833,
123.343023739063));
#135767=CARTESIAN_POINT('Ctrl Pts',(9.99999999999996,-29.2402810350378,
123.321677641666));
#135768=CARTESIAN_POINT('Ctrl Pts',(9.99999999999997,-29.3020523561828,
123.30176385006));
#135769=CARTESIAN_POINT('Ctrl Pts',(9.99999999999982,-29.3650675256982,
123.285204488516));
#135770=CARTESIAN_POINT('Ctrl Pts',(10.0000000000001,-29.4290244397517,
123.272027254596));
#135771=CARTESIAN_POINT('Ctrl Pts',(10.0000000000002,-29.4430780050743,
123.269131756582));
#135772=CARTESIAN_POINT('Ctrl Pts',(9.99999999999994,-29.4571770001559,
123.266399702894));
#135773=CARTESIAN_POINT('Ctrl Pts',(10.0000000000001,-29.4713181358355,
123.263831627986));
#135774=CARTESIAN_POINT('Ctrl Pts',(10.0000000000002,-29.4824509309542,
123.261809877226));
#135775=CARTESIAN_POINT('Ctrl Pts',(10.0000000000002,-29.493609299935,123.259889940904));
#135776=CARTESIAN_POINT('Ctrl Pts',(10.0000000000001,-29.5047784996148,
123.258073970657));
#135777=CARTESIAN_POINT('Ctrl Pts',(10.0000000000001,-29.5722612076497,
123.247102137987));
#135778=CARTESIAN_POINT('Ctrl Pts',(10.0000000000001,-29.640263498764,123.239897931082));
#135779=CARTESIAN_POINT('Ctrl Pts',(10.0000000000001,-29.7084341528629,
123.236428498985));
#135780=CARTESIAN_POINT('Ctrl Pts',(10.0000000000001,-29.776291735959,123.232975000116));
#135781=CARTESIAN_POINT('Ctrl Pts',(9.99999999999987,-29.8443172474683,
123.233222296554));
#135782=CARTESIAN_POINT('Ctrl Pts',(9.99999999999985,-29.9121554881824,
123.237188358926));
#135783=CARTESIAN_POINT('Ctrl Pts',(9.99999999999982,-29.9785429160644,
123.241069601673));
#135784=CARTESIAN_POINT('Ctrl Pts',(10.0000000000002,-30.0447519081449,
123.248512590545));
#135785=CARTESIAN_POINT('Ctrl Pts',(10.0000000000002,-30.1104263636383,
123.259577997692));
#135786=CARTESIAN_POINT('Ctrl Pts',(10.0000000000002,-30.129515952431,123.262794378714));
#135787=CARTESIAN_POINT('Ctrl Pts',(10.0000000000001,-30.1485601789394,
123.266317084266));
#135788=CARTESIAN_POINT('Ctrl Pts',(10.0000000000001,-30.1675497535845,
123.270148258539));
#135789=CARTESIAN_POINT('Ctrl Pts',(10.0000000000001,-30.178123023576,123.272281431121));
#135790=CARTESIAN_POINT('Ctrl Pts',(10.0000000000001,-30.1886698600177,
123.274508327613));
#135791=CARTESIAN_POINT('Ctrl Pts',(10.0000000000001,-30.1991886007708,
123.276828811527));
#135792=CARTESIAN_POINT('Ctrl Pts',(9.99999999999994,-30.2629295969814,
123.290890376484));
#135793=CARTESIAN_POINT('Ctrl Pts',(10.0000000000001,-30.3256439671593,
123.30838545758));
#135794=CARTESIAN_POINT('Ctrl Pts',(10.0000000000001,-30.3870120922313,
123.329323289776));
#135795=CARTESIAN_POINT('Ctrl Pts',(10.0000000000001,-30.4498356918113,
123.35075770682));
#135796=CARTESIAN_POINT('Ctrl Pts',(10.0000000000001,-30.5112495939634,
123.375800172046));
#135797=CARTESIAN_POINT('Ctrl Pts',(10.,-30.5708786461142,123.404508638235));
#135798=CARTESIAN_POINT('Ctrl Pts',(9.99999999999995,-30.6261220841815,
123.431105646182));
#135799=CARTESIAN_POINT('Ctrl Pts',(10.,-30.6798338743358,123.460849874209));
#135800=CARTESIAN_POINT('Ctrl Pts',(9.9999999999999,-30.7316789157771,123.493821876261));
#135801=CARTESIAN_POINT('Ctrl Pts',(9.99999999999989,-30.7357947411469,
123.496439426537));
#135802=CARTESIAN_POINT('Ctrl Pts',(10.0000000000002,-30.7398987797973,
123.499077335717));
#135803=CARTESIAN_POINT('Ctrl Pts',(10.0000000000002,-30.7439908523812,
123.501735652545));
#135804=CARTESIAN_POINT('Ctrl Pts',(10.,-30.753106648206,123.50765751071));
#135805=CARTESIAN_POINT('Ctrl Pts',(10.0000000000001,-30.7621630645469,
123.5136806418));
#135806=CARTESIAN_POINT('Ctrl Pts',(9.99999999999995,-30.7711590232015,
123.519803732655));
#135807=CARTESIAN_POINT('Ctrl Pts',(-5.55328352747075E-16,-31.2690708798524,
126.079358653049));
#135808=CARTESIAN_POINT('Ctrl Pts',(1.40620977341373E-13,-31.3143954758567,
126.03707561542));
#135809=CARTESIAN_POINT('Ctrl Pts',(-1.82722262030262E-14,-31.3569897935278,
125.992223116373));
#135810=CARTESIAN_POINT('Ctrl Pts',(5.40453098940574E-14,-31.3968555011726,
125.945146268677));
#135811=CARTESIAN_POINT('Ctrl Pts',(1.30912518458065E-13,-31.4393582794698,
125.894955341718));
#135812=CARTESIAN_POINT('Ctrl Pts',(6.08222559450276E-14,-31.478760244481,
125.842235824494));
#135813=CARTESIAN_POINT('Ctrl Pts',(2.52541043632704E-14,-31.5150345664964,
125.787351208348));
#135814=CARTESIAN_POINT('Ctrl Pts',(-5.65129697731147E-15,-31.5467745982599,
125.739327169221));
#135815=CARTESIAN_POINT('Ctrl Pts',(1.45041605914566E-15,-31.57611978446,
125.689644249953));
#135816=CARTESIAN_POINT('Ctrl Pts',(-5.9834082133392E-14,-31.6030292482344,
125.638518395284));
#135817=CARTESIAN_POINT('Ctrl Pts',(-9.02967013637418E-14,-31.6165278248273,
125.612872166473));
#135818=CARTESIAN_POINT('Ctrl Pts',(-3.10225958482436E-15,-31.6294131349682,
125.586862493095));
#135819=CARTESIAN_POINT('Ctrl Pts',(3.85247389544929E-14,-31.6416776773763,
125.560514791589));
#135820=CARTESIAN_POINT('Ctrl Pts',(5.75210116800135E-14,-31.6472866465359,
125.548465141447));
#135821=CARTESIAN_POINT('Ctrl Pts',(-3.60961809090547E-14,-31.6527663599446,
125.536343104099));
#135822=CARTESIAN_POINT('Ctrl Pts',(-2.28012053682392E-14,-31.6581075854569,
125.524171078425));
#135823=CARTESIAN_POINT('Ctrl Pts',(4.36540846169443E-14,-31.6850208488875,
125.462838911733));
#135824=CARTESIAN_POINT('Ctrl Pts',(4.94852571796735E-14,-31.7084732116299,
125.400131228953));
#135825=CARTESIAN_POINT('Ctrl Pts',(-8.56953397132543E-15,-31.7284413792091,
125.336405934918));
#135826=CARTESIAN_POINT('Ctrl Pts',(-6.74212432052424E-14,-31.7487645533631,
125.27154769274));
#135827=CARTESIAN_POINT('Ctrl Pts',(-3.05921264967593E-14,-31.7654790997968,
125.205634492719));
#135828=CARTESIAN_POINT('Ctrl Pts',(3.73312492030209E-15,-31.7785211409705,
125.139007153357));
#135829=CARTESIAN_POINT('Ctrl Pts',(3.2589687151767E-14,-31.7894305875867,
125.083274512103));
#135830=CARTESIAN_POINT('Ctrl Pts',(-2.04083765805674E-14,-31.7977698129652,
125.027041243318));
#135831=CARTESIAN_POINT('Ctrl Pts',(-5.9535709695524E-15,-31.8034765988388,
124.970494534412));
#135832=CARTESIAN_POINT('Ctrl Pts',(9.02866769369479E-16,-31.8061050671481,
124.944449885875));
#135833=CARTESIAN_POINT('Ctrl Pts',(1.54065700236016E-15,-31.8081747548663,
124.918338631073));
#135834=CARTESIAN_POINT('Ctrl Pts',(-5.13478148889135E-15,-31.809677780871,
124.892178658778));
#135835=CARTESIAN_POINT('Ctrl Pts',(-8.15445944510913E-15,-31.8103346621044,
124.880745726271));
#135836=CARTESIAN_POINT('Ctrl Pts',(5.75406636603668E-16,-31.8108831921244,
124.869303691251));
#135837=CARTESIAN_POINT('Ctrl Pts',(1.41553435639707E-15,-31.8113223787737,
124.857868186114));
#135838=CARTESIAN_POINT('Ctrl Pts',(6.29323886627523E-15,-31.8140157734359,
124.787737801816));
#135839=CARTESIAN_POINT('Ctrl Pts',(-6.06599144194739E-15,-31.8126089190124,
124.717721633684));
#135840=CARTESIAN_POINT('Ctrl Pts',(-1.77635683940025E-15,-31.8070473989234,
124.648180709286));
#135841=CARTESIAN_POINT('Ctrl Pts',(1.9596435517566E-15,-31.8020752960732,
124.586009823832));
#135842=CARTESIAN_POINT('Ctrl Pts',(2.43016174079474E-14,-31.7937821463294,
124.524217822068));
#135843=CARTESIAN_POINT('Ctrl Pts',(1.95399252334028E-14,-31.7820959342962,
124.463050544159));
#135844=CARTESIAN_POINT('Ctrl Pts',(1.43444283326989E-14,-31.7693632197095,
124.396405724654));
#135845=CARTESIAN_POINT('Ctrl Pts',(8.99293850601339E-15,-31.75260362096,
124.330501692871));
#135846=CARTESIAN_POINT('Ctrl Pts',(2.66175970153881E-14,-31.7320622411714,
124.265551890376));
#135847=CARTESIAN_POINT('Ctrl Pts',(3.37988617717994E-14,-31.7241352767211,
124.240487616178));
#135848=CARTESIAN_POINT('Ctrl Pts',(5.56272031405345E-14,-31.7156445735492,
124.215565493641));
#135849=CARTESIAN_POINT('Ctrl Pts',(4.77395900588817E-14,-31.706602209939,
124.19079810963));
#135850=CARTESIAN_POINT('Ctrl Pts',(4.43131798314357E-14,-31.7026358405724,
124.179934070373));
#135851=CARTESIAN_POINT('Ctrl Pts',(5.36000528057561E-14,-31.6985634332776,
124.16910038244));
#135852=CARTESIAN_POINT('Ctrl Pts',(6.00353100566053E-14,-31.6943910861053,
124.158310626993));
#135853=CARTESIAN_POINT('Ctrl Pts',(9.76408670109977E-14,-31.6691685481284,
124.093084746864));
#135854=CARTESIAN_POINT('Ctrl Pts',(-2.81031955616449E-14,-31.6402554518206,
124.029345120458));
#135855=CARTESIAN_POINT('Ctrl Pts',(-2.42861286636753E-14,-31.6079643298064,
123.96731040277));
#135856=CARTESIAN_POINT('Ctrl Pts',(-2.01425376075046E-14,-31.5748912639704,
123.903773486918));
#135857=CARTESIAN_POINT('Ctrl Pts',(5.74024171858222E-14,-31.5382742971337,
123.842024226929));
#135858=CARTESIAN_POINT('Ctrl Pts',(1.85407245112401E-14,-31.4983928835297,
123.782301295738));
#135859=CARTESIAN_POINT('Ctrl Pts',(-1.11230404567022E-14,-31.4679507489155,
123.736713806565));
#135860=CARTESIAN_POINT('Ctrl Pts',(4.72011644752096E-14,-31.4356053574396,
123.692306933135));
#135861=CARTESIAN_POINT('Ctrl Pts',(1.03889119529299E-13,-31.4014615571113,
123.649192900504));
#135862=CARTESIAN_POINT('Ctrl Pts',(1.39474512305205E-13,-31.3801754456228,
123.622314518588));
#135863=CARTESIAN_POINT('Ctrl Pts',(-5.99846713652865E-14,-31.3581900442438,
123.595938733229));
#135864=CARTESIAN_POINT('Ctrl Pts',(-3.4777736246383E-14,-31.3355278570067,
123.57009442258));
#135865=CARTESIAN_POINT('Ctrl Pts',(-2.07796655249921E-14,-31.3228334211773,
123.555617490602));
#135866=CARTESIAN_POINT('Ctrl Pts',(-7.74124701957694E-14,-31.3099221398224,
123.541302772379));
#135867=CARTESIAN_POINT('Ctrl Pts',(-4.70179450928754E-14,-31.2968217144024,
123.527180817023));
#135868=CARTESIAN_POINT('Ctrl Pts',(7.0510271335355E-14,-31.2459805955745,
123.472375267789));
#135869=CARTESIAN_POINT('Ctrl Pts',(-3.08159693383178E-14,-31.1922459214608,
123.420411847386));
#135870=CARTESIAN_POINT('Ctrl Pts',(-2.18713935851156E-14,-31.1359020383884,
123.371553876303));
#135871=CARTESIAN_POINT('Ctrl Pts',(-1.51741762347561E-14,-31.0937147685043,
123.334971654778));
#135872=CARTESIAN_POINT('Ctrl Pts',(-1.86234104118756E-14,-31.0500635672472,
123.300130609683));
#135873=CARTESIAN_POINT('Ctrl Pts',(7.78266340262235E-14,-31.0050513657681,
123.267151041331));
#135874=CARTESIAN_POINT('Ctrl Pts',(1.08037011731502E-13,-30.9910009326709,
123.256856561091));
#135875=CARTESIAN_POINT('Ctrl Pts',(5.25799844816238E-14,-30.976817796727,
123.246743532399));
#135876=CARTESIAN_POINT('Ctrl Pts',(4.6074255521944E-15,-30.9625048476372,
123.236815840421));
#135877=CARTESIAN_POINT('Ctrl Pts',(-4.16956105884885E-14,-30.9487122452095,
123.227249069267));
#135878=CARTESIAN_POINT('Ctrl Pts',(-1.04201132457139E-13,-30.9348061304262,
123.21785934585));
#135879=CARTESIAN_POINT('Ctrl Pts',(-6.62525589945062E-14,-30.92079448186,
123.20865289991));
#135880=CARTESIAN_POINT('Ctrl Pts',(1.04251430563816E-13,-30.8578449890432,
123.167291521208));
#135881=CARTESIAN_POINT('Ctrl Pts',(6.69980452307654E-14,-30.7927376832244,
123.129605407283));
#135882=CARTESIAN_POINT('Ctrl Pts',(-1.89015469942433E-14,-30.7257336719143,
123.095873532002));
#135883=CARTESIAN_POINT('Ctrl Pts',(-8.47522016279924E-14,-30.6744847329293,
123.070073243566));
#135884=CARTESIAN_POINT('Ctrl Pts',(-2.96517112328656E-13,-30.622125215821,
123.046586657031));
#135885=CARTESIAN_POINT('Ctrl Pts',(-1.39083189409916E-13,-30.5687580651082,
123.025553879704));
#135886=CARTESIAN_POINT('Ctrl Pts',(-1.03033770214677E-13,-30.5564788506438,
123.020714461071));
#135887=CARTESIAN_POINT('Ctrl Pts',(-1.42521024204696E-13,-30.5441462477664,
123.016005015431));
#135888=CARTESIAN_POINT('Ctrl Pts',(-1.66533453693773E-15,-30.5317621182487,
123.011424977843));
#135889=CARTESIAN_POINT('Ctrl Pts',(10.,-30.7923075365013,123.534460929349));
#135890=CARTESIAN_POINT('Ctrl Pts',(10.0002900114693,-30.7848643828255,
123.530436971974));
#135891=CARTESIAN_POINT('Ctrl Pts',(10.0005800229386,-30.7773905733591,
123.526469718933));
#135892=CARTESIAN_POINT('Ctrl Pts',(10.0008700344079,-30.7698869755801,
123.522559630702));
#135893=CARTESIAN_POINT('Ctrl Pts',(0.00155434972953121,-29.4691351333435,
123.012224622356));
#135894=CARTESIAN_POINT('Ctrl Pts',(0.038599440009051,-28.8081681097297,
123.188745659291));
#135895=CARTESIAN_POINT('Ctrl Pts',(0.112689620568091,-27.6877090541907,
124.250671923409));
#135896=CARTESIAN_POINT('Ctrl Pts',(0.223824891406651,-28.1162248339476,
126.540127744107));
#135897=CARTESIAN_POINT('Ctrl Pts',(0.33496016224521,-30.2723187871224,
127.416073114121));
#135898=CARTESIAN_POINT('Ctrl Pts',(0.44609543308377,-32.1775003475611,
126.082528630612));
#135899=CARTESIAN_POINT('Ctrl Pts',(0.557230703922329,-32.090499234442,
123.757255617341));
#135900=CARTESIAN_POINT('Ctrl Pts',(0.668365974760889,-30.0897172445553,
122.569885820561));
#135901=CARTESIAN_POINT('Ctrl Pts',(0.779501245599448,-28.0070199569619,
123.606506785386));
#135902=CARTESIAN_POINT('Ctrl Pts',(0.890636516438007,-27.7483422269096,
125.918663574952));
#135903=CARTESIAN_POINT('Ctrl Pts',(1.00177178727657,-29.5505922730324,
127.389938795433));
#135904=CARTESIAN_POINT('Ctrl Pts',(1.11290705811512,-31.7641484329131,
126.673797360623));
#135905=CARTESIAN_POINT('Ctrl Pts',(1.22404232895368,-32.3630411382761,
124.425663023932));
#135906=CARTESIAN_POINT('Ctrl Pts',(1.33517759979224,-30.799102978858,122.70320972357));
#135907=CARTESIAN_POINT('Ctrl Pts',(1.4463128706308,-28.503771277491,123.082940610925));
#135908=CARTESIAN_POINT('Ctrl Pts',(1.55744814146936,-27.5778941423288,
125.21730355642));
#135909=CARTESIAN_POINT('Ctrl Pts',(1.66858341230792,-28.868902973627,127.152773886107));
#135910=CARTESIAN_POINT('Ctrl Pts',(1.77971868314648,-31.1951726997191,
127.117871314526));
#135911=CARTESIAN_POINT('Ctrl Pts',(1.89085395398504,-32.427534695358,125.144540597895));
#135912=CARTESIAN_POINT('Ctrl Pts',(2.0019892248236,-31.4380424849057,123.038916039209));
#135913=CARTESIAN_POINT('Ctrl Pts',(2.11312449566216,-29.1323505409916,
122.728216337308));
#135914=CARTESIAN_POINT('Ctrl Pts',(2.22425976650072,-27.6207936836985,
124.496816246995));
#135915=CARTESIAN_POINT('Ctrl Pts',(2.33539503733928,-28.2868573536594,
126.725966059205));
#135916=CARTESIAN_POINT('Ctrl Pts',(2.44653030817784,-30.5209122220338,
127.375387765058));
#135917=CARTESIAN_POINT('Ctrl Pts',(2.5576655790164,-32.2781908106313,125.850683963494));
#135918=CARTESIAN_POINT('Ctrl Pts',(2.66880084985495,-31.9503055276404,
123.547373096034));
#135919=CARTESIAN_POINT('Ctrl Pts',(2.77993612069352,-29.8373605376131,
122.573610711328));
#135920=CARTESIAN_POINT('Ctrl Pts',(2.89107139153207,-27.8732748655125,
123.820654089384));
#135921=CARTESIAN_POINT('Ctrl Pts',(3.00220666237064,-27.8557207974597,
126.14711955606));
#135922=CARTESIAN_POINT('Ctrl Pts',(3.11334193320919,-29.8007650772084,
127.423658808513));
#135923=CARTESIAN_POINT('Ctrl Pts',(3.22447720404775,-31.9281634692032,
126.48189143007));
#135924=CARTESIAN_POINT('Ctrl Pts',(3.33561247488631,-32.2907681558608,
124.183790571875));
#135925=CARTESIAN_POINT('Ctrl Pts',(3.44674774572488,-30.5566972823996,
122.632743209903));
#135926=CARTESIAN_POINT('Ctrl Pts',(3.55788301656343,-28.3130970690004,
123.248379300229));
#135927=CARTESIAN_POINT('Ctrl Pts',(3.669018287402,-27.6134715868242,125.467224472374));
#135928=CARTESIAN_POINT('Ctrl Pts',(3.78015355824055,-29.0981683306454,
127.258432247076));
#135929=CARTESIAN_POINT('Ctrl Pts',(3.89128882907911,-31.4082861960447,
126.982560608029));
#135930=CARTESIAN_POINT('Ctrl Pts',(4.00242409991767,-32.4294393788512,
124.892107094911));
#135931=CARTESIAN_POINT('Ctrl Pts',(4.11355937075623,-31.2269951376161,
122.900404918383));
#135932=CARTESIAN_POINT('Ctrl Pts',(4.22469464159479,-28.9015168124413,
122.83040297264));
#135933=CARTESIAN_POINT('Ctrl Pts',(4.33582991243335,-27.581449203612,124.746172066603));
#135934=CARTESIAN_POINT('Ctrl Pts',(4.44696518327191,-28.4750130060368,
126.894262717451));
#135935=CARTESIAN_POINT('Ctrl Pts',(4.55810045411047,-30.7643544438259,
127.308588066045));
#135936=CARTESIAN_POINT('Ctrl Pts',(4.66923572494902,-32.3541037917107,
125.609927792723));
#135937=CARTESIAN_POINT('Ctrl Pts',(4.78037099578759,-31.7892082561945,
123.353017792917));
#135938=CARTESIAN_POINT('Ctrl Pts',(4.89150626662615,-29.5867008073364,
122.603544210334));
#135939=CARTESIAN_POINT('Ctrl Pts',(5.0026415374647,-27.7624744665255,124.047479101787));
#135940=CARTESIAN_POINT('Ctrl Pts',(5.11377680830327,-27.9861922134631,
126.363229538033));
#135941=CARTESIAN_POINT('Ctrl Pts',(5.22491207914182,-30.0530914967008,
127.431254381478));
#135942=CARTESIAN_POINT('Ctrl Pts',(5.33604734998039,-32.0713976286418,
126.274020580108));
#135943=CARTESIAN_POINT('Ctrl Pts',(5.44718262081894,-32.1938118641602,
123.950711632033));
#135944=CARTESIAN_POINT('Ctrl Pts',(5.5583178916575,-30.3082919020013,122.587786767791));
#135945=CARTESIAN_POINT('Ctrl Pts',(5.66945316249606,-28.1406010467917,
123.432692720846));
#135946=CARTESIAN_POINT('Ctrl Pts',(5.78058843333462,-27.6747656725676,
125.7121108741));
#135947=CARTESIAN_POINT('Ctrl Pts',(5.89172370417318,-29.3371517743687,
127.339754005074));
#135948=CARTESIAN_POINT('Ctrl Pts',(6.00285897501174,-31.6062241840789,
126.825886208109));
#135949=CARTESIAN_POINT('Ctrl Pts',(6.1139942458503,-32.4051648468343,124.640836201665));
#135950=CARTESIAN_POINT('Ctrl Pts',(6.22512951668886,-31.0027258808682,
122.78451870188));
#135951=CARTESIAN_POINT('Ctrl Pts',(6.33626478752742,-28.682520163804,122.955968822229));
#135952=CARTESIAN_POINT('Ctrl Pts',(6.44740005836598,-27.5681666262566,
124.998263097456));
#135953=CARTESIAN_POINT('Ctrl Pts',(6.55853532920454,-28.6796016688356,
127.042147110651));
#135954=CARTESIAN_POINT('Ctrl Pts',(6.6696706000431,-30.9995601071582,127.216911402528));
#135955=CARTESIAN_POINT('Ctrl Pts',(6.78080587088166,-32.4046493378798,
125.362599139994));
#135956=CARTESIAN_POINT('Ctrl Pts',(6.89194114172022,-31.6088307706975,
123.176410099358));
#135957=CARTESIAN_POINT('Ctrl Pts',(7.00307641255877,-29.3404947212706,
122.659301522662));
#135958=CARTESIAN_POINT('Ctrl Pts',(7.11421168339733,-27.6757852746021,
124.284568322771));
#135959=CARTESIAN_POINT('Ctrl Pts',(7.22534695423589,-28.1383640909908,
126.564649582695));
#135960=CARTESIAN_POINT('Ctrl Pts',(7.33648222507445,-30.3048458108891,
127.412651157157));
#135961=CARTESIAN_POINT('Ctrl Pts',(7.44761749591301,-32.1923107480619,
126.052421093879));
#135962=CARTESIAN_POINT('Ctrl Pts',(7.55875276675157,-32.0732154164101,
123.728939651145));
#135963=CARTESIAN_POINT('Ctrl Pts',(7.66988803759013,-30.0565644192597,
122.56882393853));
#135964=CARTESIAN_POINT('Ctrl Pts',(7.7810233084287,-27.9881416008883,123.633895187267));
#135965=CARTESIAN_POINT('Ctrl Pts',(7.89215857926725,-27.7611161029497,
125.949323685456));
#135966=CARTESIAN_POINT('Ctrl Pts',(8.00329385010582,-29.583277957531,127.395862960217));
#135967=CARTESIAN_POINT('Ctrl Pts',(8.11442912094438,-31.7868537726289,
126.649536355778));
#135968=CARTESIAN_POINT('Ctrl Pts',(8.22556439178294,-32.3549726375641,
124.393435604416));
#135969=CARTESIAN_POINT('Ctrl Pts',(8.33669966262149,-30.767651448308,122.692506135324));
#135970=CARTESIAN_POINT('Ctrl Pts',(8.44783493346005,-28.4777203936358,
123.103560840128));
#135971=CARTESIAN_POINT('Ctrl Pts',(8.55897020429861,-27.5810892221483,
125.250372795181));
#135972=CARTESIAN_POINT('Ctrl Pts',(8.67010547513716,-28.8984184498051,
127.168025763146));
#135973=CARTESIAN_POINT('Ctrl Pts',(8.78124074597574,-31.22399523633,127.101345462494));
#135974=CARTESIAN_POINT('Ctrl Pts',(8.89237601681429,-32.4292816418055,
125.1113635915));
#135975=CARTESIAN_POINT('Ctrl Pts',(9.00351128765285,-31.4111190912015,
123.019452274317));
#135976=CARTESIAN_POINT('Ctrl Pts',(9.11464655849142,-29.1013906938143,
122.740283510567));
#135977=CARTESIAN_POINT('Ctrl Pts',(9.22578182932996,-27.6141508798812,
124.529363487384));
#135978=CARTESIAN_POINT('Ctrl Pts',(9.33691710016854,-28.3105775286338,
126.749216168547));
#135979=CARTESIAN_POINT('Ctrl Pts',(9.4480523710071,-30.5533538853258,127.368035529446));
#135980=CARTESIAN_POINT('Ctrl Pts',(9.55918764184564,-32.289521449751,125.81950938995));
#135981=CARTESIAN_POINT('Ctrl Pts',(9.67032291268421,-31.93043720362,123.520806688524));
#135982=CARTESIAN_POINT('Ctrl Pts',(9.78145818352276,-29.8039056239228,
122.576175956181));
#135983=CARTESIAN_POINT('Ctrl Pts',(9.89259345436133,-27.858013785853,123.84958187036));
#135984=CARTESIAN_POINT('Ctrl Pts',(10.0037287251999,-27.8702627078603,
126.176784351898));
#135985=CARTESIAN_POINT('Ctrl Pts',(10.1148770665318,-29.8368965496469,
127.425328002316));
#135986=CARTESIAN_POINT('Ctrl Pts',(10.1889803175841,-31.2393430859939,
126.779199071106));
#135987=CARTESIAN_POINT('Ctrl Pts',(10.226038478357,-31.6487232386396,126.230764030654));
#135988=CARTESIAN_POINT('Ctrl Pts',(-0.0743653415986168,-29.5030641598563,
123.139268786936));
#135989=CARTESIAN_POINT('Ctrl Pts',(-0.037320251319097,-28.8843413476733,
123.304507881293));
#135990=CARTESIAN_POINT('Ctrl Pts',(0.0367699292399429,-27.8354938968754,
124.298563531564));
#135991=CARTESIAN_POINT('Ctrl Pts',(0.147905200078501,-28.2366220603748,
126.441693964919));
#135992=CARTESIAN_POINT('Ctrl Pts',(0.259040470917062,-30.2549141481483,
127.261655269027));
#135993=CARTESIAN_POINT('Ctrl Pts',(0.370175741755621,-32.0383303409089,
126.013341263137));
#135994=CARTESIAN_POINT('Ctrl Pts',(0.481311012594181,-31.9568897070361,
123.836682812011));
#135995=CARTESIAN_POINT('Ctrl Pts',(0.592446283432741,-30.0839831699153,
122.725201068568));
#135996=CARTESIAN_POINT('Ctrl Pts',(0.703581554271301,-28.1343967659521,
123.695568750481));
#135997=CARTESIAN_POINT('Ctrl Pts',(0.814716825109859,-27.8922518375834,
125.859949271654));
#135998=CARTESIAN_POINT('Ctrl Pts',(0.925852095948419,-29.5793151508136,
127.237191266171));
#135999=CARTESIAN_POINT('Ctrl Pts',(1.03698736678697,-31.6513968783983,
126.566820390414));
#136000=CARTESIAN_POINT('Ctrl Pts',(1.14812263762554,-32.2120127118963,
124.462370471932));
#136001=CARTESIAN_POINT('Ctrl Pts',(1.25925790846409,-30.7480301204735,
122.850003876052));
#136002=CARTESIAN_POINT('Ctrl Pts',(1.37039317930265,-28.5993993500641,
123.205465123138));
#136003=CARTESIAN_POINT('Ctrl Pts',(1.48152845014121,-27.7326975565748,
125.203415091407));
#136004=CARTESIAN_POINT('Ctrl Pts',(1.59266372097977,-28.9411944801982,
127.015184215278));
#136005=CARTESIAN_POINT('Ctrl Pts',(1.70379899181833,-31.1187859415003,
126.982512362569));
#136006=CARTESIAN_POINT('Ctrl Pts',(1.81493426265689,-32.2723843092376,
125.135302612701));
#136007=CARTESIAN_POINT('Ctrl Pts',(1.92606953349545,-31.3461332540233,
123.164254282289));
#136008=CARTESIAN_POINT('Ctrl Pts',(2.03720480433401,-29.1878043925225,
122.873412248667));
#136009=CARTESIAN_POINT('Ctrl Pts',(2.14834007517257,-27.7728552708471,
124.528976097777));
#136010=CARTESIAN_POINT('Ctrl Pts',(2.25947534601113,-28.3963489887604,
126.615654844693));
#136011=CARTESIAN_POINT('Ctrl Pts',(2.37061061684969,-30.4876192962776,
127.22357023197));
#136012=CARTESIAN_POINT('Ctrl Pts',(2.48174588768825,-32.1325854009119,
125.796314423213));
#136013=CARTESIAN_POINT('Ctrl Pts',(2.59288115852681,-31.825656163722,123.640214457053));
#136014=CARTESIAN_POINT('Ctrl Pts',(2.70401642936537,-29.8477552707702,
122.728687891372));
#136015=CARTESIAN_POINT('Ctrl Pts',(2.81515170020393,-28.0091996893342,
123.896029314195));
#136016=CARTESIAN_POINT('Ctrl Pts',(2.92628697104248,-27.9927675498132,
126.073804005766));
#136017=CARTESIAN_POINT('Ctrl Pts',(3.03742224188105,-29.8134987263952,
127.268756140928));
#136018=CARTESIAN_POINT('Ctrl Pts',(3.1485575127196,-31.8049292648385,126.387179693095));
#136019=CARTESIAN_POINT('Ctrl Pts',(3.25969278355817,-32.1443588935859,
124.23595675025));
#136020=CARTESIAN_POINT('Ctrl Pts',(3.37082805439672,-30.5211172354979,
122.784041070128));
#136021=CARTESIAN_POINT('Ctrl Pts',(3.48196332523528,-28.4209116520804,
123.360330173033));
#136022=CARTESIAN_POINT('Ctrl Pts',(3.59309859607384,-27.7660011492234,
125.437362877633));
#136023=CARTESIAN_POINT('Ctrl Pts',(3.7042338669124,-29.1558068607902,127.114089661229));
#136024=CARTESIAN_POINT('Ctrl Pts',(3.81536913775096,-31.3182787710212,
126.855849733647));
#136025=CARTESIAN_POINT('Ctrl Pts',(3.92650440858952,-32.274167259196,124.89900282576));
#136026=CARTESIAN_POINT('Ctrl Pts',(4.03763967942808,-31.1485745202988,
123.034595786276));
#136027=CARTESIAN_POINT('Ctrl Pts',(4.14877495026664,-28.9717238793155,
122.969067856468));
#136028=CARTESIAN_POINT('Ctrl Pts',(4.2599102211052,-27.7360254041619,124.762394904509));
#136029=CARTESIAN_POINT('Ctrl Pts',(4.37104549194376,-28.572479098445,126.773195202911));
#136030=CARTESIAN_POINT('Ctrl Pts',(4.48218076278232,-30.7155024594159,
127.16103988454));
#136031=CARTESIAN_POINT('Ctrl Pts',(4.59331603362088,-32.2036465756101,
125.570945638223));
#136032=CARTESIAN_POINT('Ctrl Pts',(4.70445130445944,-31.6748550597894,
123.458280933275));
#136033=CARTESIAN_POINT('Ctrl Pts',(4.815586575298,-29.6131158898675,122.756708258534));
#136034=CARTESIAN_POINT('Ctrl Pts',(4.92672184613655,-27.905480847088,124.108357319276));
#136035=CARTESIAN_POINT('Ctrl Pts',(5.03785711697512,-28.1149001805423,
126.276101807335));
#136036=CARTESIAN_POINT('Ctrl Pts',(5.14899238781368,-30.0496982738444,
127.275866260038));
#136037=CARTESIAN_POINT('Ctrl Pts',(5.26012765865223,-31.9390089371404,
126.192594438061));
#136038=CARTESIAN_POINT('Ctrl Pts',(5.3712629294908,-32.0535993438403,124.017774523349));
#136039=CARTESIAN_POINT('Ctrl Pts',(5.48239820032934,-30.2885881228032,
122.741957917269));
#136040=CARTESIAN_POINT('Ctrl Pts',(5.59353347116793,-28.2594403227427,
123.532863618504));
#136041=CARTESIAN_POINT('Ctrl Pts',(5.70466874200646,-27.8233777621957,
125.666597919213));
#136042=CARTESIAN_POINT('Ctrl Pts',(5.81580401284504,-29.379516218569,127.19021392311));
#136043=CARTESIAN_POINT('Ctrl Pts',(5.92693928368359,-31.5035660005183,
126.709188823416));
#136044=CARTESIAN_POINT('Ctrl Pts',(6.03807455452215,-32.2514441789554,
124.663791342985));
#136045=CARTESIAN_POINT('Ctrl Pts',(6.14920982536071,-30.9386389255357,
122.92611617503));
#136046=CARTESIAN_POINT('Ctrl Pts',(6.26034509619927,-28.7667239058484,
123.086608448958));
#136047=CARTESIAN_POINT('Ctrl Pts',(6.37148036703783,-27.7235917526774,
124.99837410765));
#136048=CARTESIAN_POINT('Ctrl Pts',(6.48261563787639,-28.7639919398808,
126.911627899808));
#136049=CARTESIAN_POINT('Ctrl Pts',(6.59375090871494,-30.9356754850877,
127.075222527492));
#136050=CARTESIAN_POINT('Ctrl Pts',(6.70488617955351,-32.250961617589,125.339424436586));
#136051=CARTESIAN_POINT('Ctrl Pts',(6.81602145039206,-31.5060059930522,
123.292960720756));
#136052=CARTESIAN_POINT('Ctrl Pts',(6.92715672123063,-29.3826455085853,
122.808901968433));
#136053=CARTESIAN_POINT('Ctrl Pts',(7.03829199206918,-27.8243321986736,
124.330293519274));
#136054=CARTESIAN_POINT('Ctrl Pts',(7.14942726290775,-28.2573463369091,
126.464648545692));
#136055=CARTESIAN_POINT('Ctrl Pts',(7.2605625337463,-30.2853622808052,127.258452018697));
#136056=CARTESIAN_POINT('Ctrl Pts',(7.37169780458487,-32.0521941681802,
125.985157981475));
#136057=CARTESIAN_POINT('Ctrl Pts',(7.48283307542342,-31.9407105451174,
123.810176596711));
#136058=CARTESIAN_POINT('Ctrl Pts',(7.59396834626198,-30.0529492324178,
122.724207054324));
#136059=CARTESIAN_POINT('Ctrl Pts',(7.70510361710054,-28.1167249772821,
123.72120668464));
#136060=CARTESIAN_POINT('Ctrl Pts',(7.8162388879391,-27.9042093002458,125.888649810584));
#136061=CARTESIAN_POINT('Ctrl Pts',(7.92737415877766,-29.6099118037608,
127.242736801369));
#136062=CARTESIAN_POINT('Ctrl Pts',(8.03850942961621,-31.6726510577123,
126.544109972787));
#136063=CARTESIAN_POINT('Ctrl Pts',(8.14964470045479,-32.204459891147,124.432202794999));
#136064=CARTESIAN_POINT('Ctrl Pts',(8.26077997129334,-30.7185887433181,
122.839984383425));
#136065=CARTESIAN_POINT('Ctrl Pts',(8.3719152421319,-28.575013449493,123.224767457061));
#136066=CARTESIAN_POINT('Ctrl Pts',(8.48305051297046,-27.7356884300987,
125.234370784613));
#136067=CARTESIAN_POINT('Ctrl Pts',(8.59418578380902,-28.9688235415151,
127.029461303115));
#136068=CARTESIAN_POINT('Ctrl Pts',(8.70532105464758,-31.1457663509141,
126.96704272297));
#136069=CARTESIAN_POINT('Ctrl Pts',(8.81645632548615,-32.2740196035565,
125.104246039584));
#136070=CARTESIAN_POINT('Ctrl Pts',(8.92759159632469,-31.3209306080953,
123.146034499879));
#136071=CARTESIAN_POINT('Ctrl Pts',(9.03872686716326,-29.1588232739099,
122.884708175857));
#136072=CARTESIAN_POINT('Ctrl Pts',(9.14986213800182,-27.766637026802,124.559443154956));
#136073=CARTESIAN_POINT('Ctrl Pts',(9.26099740884039,-28.4185531424342,
126.637418975915));
#136074=CARTESIAN_POINT('Ctrl Pts',(9.37213267967894,-30.5179875240813,
127.216687897858));
#136075=CARTESIAN_POINT('Ctrl Pts',(9.48326795051749,-32.1431918678755,
125.767132301983));
#136076=CARTESIAN_POINT('Ctrl Pts',(9.59440322135606,-31.8070576786659,
123.615345981355));
#136077=CARTESIAN_POINT('Ctrl Pts',(9.70553849219461,-29.8164385521741,
122.731089184406));
#136078=CARTESIAN_POINT('Ctrl Pts',(9.81667376303317,-27.9949139870427,
123.92310824152));
#136079=CARTESIAN_POINT('Ctrl Pts',(9.92780903387173,-28.0063800469214,
126.101572843314));
#136080=CARTESIAN_POINT('Ctrl Pts',(10.0389573752036,-29.8473209375447,
127.270318651986));
#136081=CARTESIAN_POINT('Ctrl Pts',(10.1130606262561,-31.1601332775016,
126.665485589114));
#136082=CARTESIAN_POINT('Ctrl Pts',(10.1501187870289,-31.5433488241895,
126.152102533069));
#136083=CARTESIAN_POINT('Ctrl Pts',(-0.150285032926765,-29.5369931863691,
123.266312951517));
#136084=CARTESIAN_POINT('Ctrl Pts',(-0.113239942647244,-28.960514585617,
123.420270103296));
#136085=CARTESIAN_POINT('Ctrl Pts',(-0.039149762088205,-27.98327873956,
124.34645513972));
#136086=CARTESIAN_POINT('Ctrl Pts',(0.0719855087503543,-28.3570192868022,
126.343260185732));
#136087=CARTESIAN_POINT('Ctrl Pts',(0.183120779588914,-30.2375095091741,
127.107237423931));
#136088=CARTESIAN_POINT('Ctrl Pts',(0.294256050427474,-31.8991603342567,
125.944153895663));
#136089=CARTESIAN_POINT('Ctrl Pts',(0.405391321266033,-31.8232801796302,
123.916110006682));
#136090=CARTESIAN_POINT('Ctrl Pts',(0.516526592104593,-30.0782490952753,
122.880516316575));
#136091=CARTESIAN_POINT('Ctrl Pts',(0.627661862943152,-28.2617735749423,
123.784630715575));
#136092=CARTESIAN_POINT('Ctrl Pts',(0.738797133781711,-28.0361614482572,
125.801234968357));
#136093=CARTESIAN_POINT('Ctrl Pts',(0.849932404620271,-29.6080380285948,
127.084443736908));
#136094=CARTESIAN_POINT('Ctrl Pts',(0.96106767545883,-31.5386453238836,
126.459843420204));
#136095=CARTESIAN_POINT('Ctrl Pts',(1.07220294629739,-32.0609842855166,
124.499077919934));
#136096=CARTESIAN_POINT('Ctrl Pts',(1.18333821713595,-30.6969572620888,
122.996798028534));
#136097=CARTESIAN_POINT('Ctrl Pts',(1.2944734879745,-28.6950274226374,123.327989635352));
#136098=CARTESIAN_POINT('Ctrl Pts',(1.40560875881306,-27.887500970821,125.189526626394));
#136099=CARTESIAN_POINT('Ctrl Pts',(1.51674402965162,-29.0134859867694,
126.877594544449));
#136100=CARTESIAN_POINT('Ctrl Pts',(1.62787930049018,-31.0423991832815,
126.847153410613));
#136101=CARTESIAN_POINT('Ctrl Pts',(1.73901457132874,-32.1172339231171,
125.126064627507));
#136102=CARTESIAN_POINT('Ctrl Pts',(1.8501498421673,-31.2542240231409,123.289592525368));
#136103=CARTESIAN_POINT('Ctrl Pts',(1.96128511300586,-29.2432582440533,
123.018608160027));
#136104=CARTESIAN_POINT('Ctrl Pts',(2.07242038384442,-27.9249168579956,
124.561135948557));
#136105=CARTESIAN_POINT('Ctrl Pts',(2.18355565468298,-28.5058406238613,
126.50534363018));
#136106=CARTESIAN_POINT('Ctrl Pts',(2.29469092552154,-30.4543263705213,
127.071752698882));
#136107=CARTESIAN_POINT('Ctrl Pts',(2.4058261963601,-31.9869799911926,125.741944882932));
#136108=CARTESIAN_POINT('Ctrl Pts',(2.51696146719866,-31.7010067998036,
123.733055818073));
#136109=CARTESIAN_POINT('Ctrl Pts',(2.62809673803722,-29.8581500039272,
122.883765071417));
#136110=CARTESIAN_POINT('Ctrl Pts',(2.73923200887578,-28.145124513156,123.971404539008));
#136111=CARTESIAN_POINT('Ctrl Pts',(2.85036727971433,-28.1298143021666,
126.000488455471));
#136112=CARTESIAN_POINT('Ctrl Pts',(2.9615025505529,-29.8262323755821,127.113853473344));
#136113=CARTESIAN_POINT('Ctrl Pts',(3.07263782139145,-31.6816950604738,
126.29246795612));
#136114=CARTESIAN_POINT('Ctrl Pts',(3.18377309223002,-31.9979496313109,
124.288122928624));
#136115=CARTESIAN_POINT('Ctrl Pts',(3.29490836306857,-30.485537188596,122.935338930354));
#136116=CARTESIAN_POINT('Ctrl Pts',(3.40604363390714,-28.5287262351604,
123.472281045836));
#136117=CARTESIAN_POINT('Ctrl Pts',(3.51717890474571,-27.9185307116224,
125.40750128289));
#136118=CARTESIAN_POINT('Ctrl Pts',(3.62831417558425,-29.2134453909351,
126.969747075382));
#136119=CARTESIAN_POINT('Ctrl Pts',(3.73944944642281,-31.2282713459977,
126.729138859265));
#136120=CARTESIAN_POINT('Ctrl Pts',(3.85058471726137,-32.1188951395408,
124.905898556608));
#136121=CARTESIAN_POINT('Ctrl Pts',(3.96171998809993,-31.0701539029816,
123.168786654169));
#136122=CARTESIAN_POINT('Ctrl Pts',(4.07285525893849,-29.0419309461898,
123.107732740296));
#136123=CARTESIAN_POINT('Ctrl Pts',(4.18399052977705,-27.8906016047118,
124.778617742416));
#136124=CARTESIAN_POINT('Ctrl Pts',(4.29512580061561,-28.6699451908533,
126.652127688372));
#136125=CARTESIAN_POINT('Ctrl Pts',(4.40626107145418,-30.6666504750058,
127.013491703035));
#136126=CARTESIAN_POINT('Ctrl Pts',(4.51739634229273,-32.0531893595093,
125.531963483724));
#136127=CARTESIAN_POINT('Ctrl Pts',(4.62853161313129,-31.5605018633842,
123.563544073634));
#136128=CARTESIAN_POINT('Ctrl Pts',(4.73966688396984,-29.6395309723986,
122.909872306734));
#136129=CARTESIAN_POINT('Ctrl Pts',(4.85080215480841,-28.0484872276504,
124.169235536765));
#136130=CARTESIAN_POINT('Ctrl Pts',(4.96193742564696,-28.2436081476214,
126.188974076638));
#136131=CARTESIAN_POINT('Ctrl Pts',(5.07307269648554,-30.0463050509881,
127.120478138598));
#136132=CARTESIAN_POINT('Ctrl Pts',(5.18420796732408,-31.806620245639,126.111168296014));
#136133=CARTESIAN_POINT('Ctrl Pts',(5.29534323816265,-31.9133868235204,
124.084837414666));
#136134=CARTESIAN_POINT('Ctrl Pts',(5.40647850900121,-30.268884343605,122.896129066749));
#136135=CARTESIAN_POINT('Ctrl Pts',(5.51761377983977,-28.3782795986937,
123.633034516162));
#136136=CARTESIAN_POINT('Ctrl Pts',(5.62874905067832,-27.9719898518237,
125.621084964325));
#136137=CARTESIAN_POINT('Ctrl Pts',(5.7398843215169,-29.4218806627693,127.040673841146));
#136138=CARTESIAN_POINT('Ctrl Pts',(5.85101959235544,-31.4009078169576,
126.592491438723));
#136139=CARTESIAN_POINT('Ctrl Pts',(5.962154863194,-32.0977235110765,124.686746484305));
#136140=CARTESIAN_POINT('Ctrl Pts',(6.07329013403256,-30.8745519702031,
123.06771364818));
#136141=CARTESIAN_POINT('Ctrl Pts',(6.18442540487112,-28.8509276478927,
123.217248075688));
#136142=CARTESIAN_POINT('Ctrl Pts',(6.29556067570968,-27.8790168790981,
124.998485117847));
#136143=CARTESIAN_POINT('Ctrl Pts',(6.40669594654826,-28.848382210926,126.781108688965));
#136144=CARTESIAN_POINT('Ctrl Pts',(6.51783121738679,-30.8717908630171,
126.933533652455));
#136145=CARTESIAN_POINT('Ctrl Pts',(6.62896648822536,-32.0972738972983,
125.316249733178));
#136146=CARTESIAN_POINT('Ctrl Pts',(6.74010175906393,-31.403181215407,123.409511342155));
#136147=CARTESIAN_POINT('Ctrl Pts',(6.85123702990247,-29.4247962959002,
122.958502414204));
#136148=CARTESIAN_POINT('Ctrl Pts',(6.96237230074105,-27.9728791227451,
124.376018715778));
#136149=CARTESIAN_POINT('Ctrl Pts',(7.0735075715796,-28.3763285828275,126.364647508688));
#136150=CARTESIAN_POINT('Ctrl Pts',(7.18464284241815,-30.2658787507214,
127.104252880237));
#136151=CARTESIAN_POINT('Ctrl Pts',(7.29577811325673,-31.9120775882985,
125.917894869072));
#136152=CARTESIAN_POINT('Ctrl Pts',(7.40691338409527,-31.8082056738248,
123.891413542278));
#136153=CARTESIAN_POINT('Ctrl Pts',(7.51804865493385,-30.049334045576,122.879590170119));
#136154=CARTESIAN_POINT('Ctrl Pts',(7.62918392577238,-28.2453083536756,
123.808518182013));
#136155=CARTESIAN_POINT('Ctrl Pts',(7.74031919661097,-28.047302497542,125.827975935714));
#136156=CARTESIAN_POINT('Ctrl Pts',(7.85145446744951,-29.6365456499907,
127.089610642521));
#136157=CARTESIAN_POINT('Ctrl Pts',(7.96258973828808,-31.5584483427957,
126.438683589794));
#136158=CARTESIAN_POINT('Ctrl Pts',(8.07372500912664,-32.0539471447299,
124.470969985582));
#136159=CARTESIAN_POINT('Ctrl Pts',(8.18486027996519,-30.6695260383283,
122.987462631525));
#136160=CARTESIAN_POINT('Ctrl Pts',(8.29599555080376,-28.6723065053501,
123.345974073992));
#136161=CARTESIAN_POINT('Ctrl Pts',(8.40713082164232,-27.8902876380491,
125.218368774047));
#136162=CARTESIAN_POINT('Ctrl Pts',(8.51826609248088,-29.0392286332251,
126.890896843083));
#136163=CARTESIAN_POINT('Ctrl Pts',(8.62940136331943,-31.0675374654984,
126.832739983445));
#136164=CARTESIAN_POINT('Ctrl Pts',(8.74053663415801,-32.1187575653075,
125.097128487668));
#136165=CARTESIAN_POINT('Ctrl Pts',(8.85167190499654,-31.2307421249892,
123.272616725442));
#136166=CARTESIAN_POINT('Ctrl Pts',(8.96280717583512,-29.2162558540056,
123.029132841148));
#136167=CARTESIAN_POINT('Ctrl Pts',(9.07394244667367,-27.9191231737227,
124.589522822528));
#136168=CARTESIAN_POINT('Ctrl Pts',(9.18507771751223,-28.5265287562346,
126.525621783282));
#136169=CARTESIAN_POINT('Ctrl Pts',(9.2962129883508,-30.4826211628368,127.065340266269));
#136170=CARTESIAN_POINT('Ctrl Pts',(9.40734825918934,-31.9968622860001,
125.714755214017));
#136171=CARTESIAN_POINT('Ctrl Pts',(9.51848353002791,-31.6836781537117,
123.709885274187));
#136172=CARTESIAN_POINT('Ctrl Pts',(9.62961880086647,-29.8289714804254,
122.886002412632));
#136173=CARTESIAN_POINT('Ctrl Pts',(9.74075407170503,-28.1318141882324,
123.99663461268));
#136174=CARTESIAN_POINT('Ctrl Pts',(9.85188934254358,-28.1424973859825,
126.026361334731));
#136175=CARTESIAN_POINT('Ctrl Pts',(9.96303768387549,-29.8577453254426,
127.115309301658));
#136176=CARTESIAN_POINT('Ctrl Pts',(10.0371409349279,-31.0809234690093,
126.551772107121));
#136177=CARTESIAN_POINT('Ctrl Pts',(10.0741990957007,-31.4379744097394,
126.073441035482));
#136178=CARTESIAN_POINT('Ctrl Pts',(-0.226204724254913,-29.570922212882,
123.393357116098));
#136179=CARTESIAN_POINT('Ctrl Pts',(-0.189159633975392,-29.0366878235607,
123.536032325299));
#136180=CARTESIAN_POINT('Ctrl Pts',(-0.115069453416353,-28.1310635822448,
124.394346747875));
#136181=CARTESIAN_POINT('Ctrl Pts',(-0.00393418257779361,-28.4774165132295,
126.244826406544));
#136182=CARTESIAN_POINT('Ctrl Pts',(0.107201088260766,-30.2201048702,126.952819578836));
#136183=CARTESIAN_POINT('Ctrl Pts',(0.218336359099326,-31.7599903276045,
125.874966528187));
#136184=CARTESIAN_POINT('Ctrl Pts',(0.329471629937885,-31.6896706522244,
123.995537201353));
#136185=CARTESIAN_POINT('Ctrl Pts',(0.440606900776445,-30.0725150206353,
123.035831564584));
#136186=CARTESIAN_POINT('Ctrl Pts',(0.551742171615005,-28.3891503839325,
123.87369268067));
#136187=CARTESIAN_POINT('Ctrl Pts',(0.662877442453563,-28.1800710589308,
125.742520665059));
#136188=CARTESIAN_POINT('Ctrl Pts',(0.774012713292123,-29.6367609063761,
126.931696207645));
#136189=CARTESIAN_POINT('Ctrl Pts',(0.885147984130682,-31.4258937693687,
126.352866449995));
#136190=CARTESIAN_POINT('Ctrl Pts',(0.996283254969241,-31.909955859137,
124.535785367934));
#136191=CARTESIAN_POINT('Ctrl Pts',(1.10741852580781,-30.6458844037042,
123.143592181016));
#136192=CARTESIAN_POINT('Ctrl Pts',(1.21855379664637,-28.7906554952107,
123.450514147566));
#136193=CARTESIAN_POINT('Ctrl Pts',(1.32968906748491,-28.042304385067,125.175638161381));
#136194=CARTESIAN_POINT('Ctrl Pts',(1.44082433832348,-29.0857774933408,
126.740004873621));
#136195=CARTESIAN_POINT('Ctrl Pts',(1.55195960916203,-30.9660124250627,
126.711794458656));
#136196=CARTESIAN_POINT('Ctrl Pts',(1.6630948800006,-31.9620835369967,125.116826642314));
#136197=CARTESIAN_POINT('Ctrl Pts',(1.77423015083916,-31.1623147922585,
123.414930768448));
#136198=CARTESIAN_POINT('Ctrl Pts',(1.88536542167772,-29.2987120955841,
123.163804071385));
#136199=CARTESIAN_POINT('Ctrl Pts',(1.99650069251628,-28.0769784451441,
124.593295799339));
#136200=CARTESIAN_POINT('Ctrl Pts',(2.10763596335484,-28.6153322589623,
126.395032415667));
#136201=CARTESIAN_POINT('Ctrl Pts',(2.21877123419339,-30.4210334447649,
126.919935165794));
#136202=CARTESIAN_POINT('Ctrl Pts',(2.32990650503196,-31.8413745814733,
125.687575342652));
#136203=CARTESIAN_POINT('Ctrl Pts',(2.44104177587052,-31.5763574358852,
123.825897179092));
#136204=CARTESIAN_POINT('Ctrl Pts',(2.55217704670908,-29.8685447370843,
123.038842251461));
#136205=CARTESIAN_POINT('Ctrl Pts',(2.66331231754763,-28.2810493369777,
124.04677976382));
#136206=CARTESIAN_POINT('Ctrl Pts',(2.77444758838619,-28.2668610545202,
125.927172905177));
#136207=CARTESIAN_POINT('Ctrl Pts',(2.88558285922476,-29.8389660247691,
126.958950805759));
#136208=CARTESIAN_POINT('Ctrl Pts',(2.99671813006331,-31.5584608561091,
126.197756219146));
#136209=CARTESIAN_POINT('Ctrl Pts',(3.10785340090188,-31.851540369036,124.340289106999));
#136210=CARTESIAN_POINT('Ctrl Pts',(3.21898867174044,-30.4499571416943,
123.086636790579));
#136211=CARTESIAN_POINT('Ctrl Pts',(3.330123942579,-28.6365408182404,123.584231918639));
#136212=CARTESIAN_POINT('Ctrl Pts',(3.44125921341756,-28.0710602740216,
125.377639688149));
#136213=CARTESIAN_POINT('Ctrl Pts',(3.55239448425611,-29.2710839210799,
126.825404489536));
#136214=CARTESIAN_POINT('Ctrl Pts',(3.66352975509468,-31.1382639209742,
126.602427984882));
#136215=CARTESIAN_POINT('Ctrl Pts',(3.77466502593323,-31.9636230198854,
124.912794287456));
#136216=CARTESIAN_POINT('Ctrl Pts',(3.8858002967718,-30.9917332856643,123.302977522061));
#136217=CARTESIAN_POINT('Ctrl Pts',(3.99693556761035,-29.112138013064,123.246397624124));
#136218=CARTESIAN_POINT('Ctrl Pts',(4.10807083844891,-28.0451778052617,
124.794840580322));
#136219=CARTESIAN_POINT('Ctrl Pts',(4.21920610928747,-28.7674112832615,
126.531060173832));
#136220=CARTESIAN_POINT('Ctrl Pts',(4.33034138012603,-30.6177984905958,
126.865943521531));
#136221=CARTESIAN_POINT('Ctrl Pts',(4.44147665096459,-31.9027321434086,
125.492981329225));
#136222=CARTESIAN_POINT('Ctrl Pts',(4.55261192180315,-31.4461486669792,
123.668807213992));
#136223=CARTESIAN_POINT('Ctrl Pts',(4.66374719264171,-29.6659460549298,
123.063036354934));
#136224=CARTESIAN_POINT('Ctrl Pts',(4.77488246348027,-28.1914936082128,
124.230113754254));
#136225=CARTESIAN_POINT('Ctrl Pts',(4.88601773431883,-28.3723161147005,
126.10184634594));
#136226=CARTESIAN_POINT('Ctrl Pts',(4.99715300515739,-30.0429118281317,
126.965090017157));
#136227=CARTESIAN_POINT('Ctrl Pts',(5.10828827599595,-31.6742315541376,
126.029742153966));
#136228=CARTESIAN_POINT('Ctrl Pts',(5.21942354683449,-31.7731743032006,
124.151900305982));
#136229=CARTESIAN_POINT('Ctrl Pts',(5.33055881767307,-30.2491805644068,
123.050300216227));
#136230=CARTESIAN_POINT('Ctrl Pts',(5.44169408851162,-28.4971188746447,
123.73320541382));
#136231=CARTESIAN_POINT('Ctrl Pts',(5.55282935935019,-28.1206019414517,
125.575572009438));
#136232=CARTESIAN_POINT('Ctrl Pts',(5.66396463018875,-29.4642451069697,
126.891133759182));
#136233=CARTESIAN_POINT('Ctrl Pts',(5.7750999010273,-31.298249633397,126.47579405403));
#136234=CARTESIAN_POINT('Ctrl Pts',(5.88623517186586,-31.9440028431976,
124.709701625626));
#136235=CARTESIAN_POINT('Ctrl Pts',(5.99737044270442,-30.8104650148705,
123.209311121329));
#136236=CARTESIAN_POINT('Ctrl Pts',(6.10850571354298,-28.9351313899371,
123.347887702416));
#136237=CARTESIAN_POINT('Ctrl Pts',(6.21964098438154,-28.0344420055189,
124.998596128041));
#136238=CARTESIAN_POINT('Ctrl Pts',(6.3307762552201,-28.9327724819712,126.650589478122));
#136239=CARTESIAN_POINT('Ctrl Pts',(6.44191152605866,-30.8079062409465,
126.791844777419));
#136240=CARTESIAN_POINT('Ctrl Pts',(6.55304679689722,-31.9435861770076,
125.29307502977));
#136241=CARTESIAN_POINT('Ctrl Pts',(6.66418206773578,-31.3003564377619,
123.526061963553));
#136242=CARTESIAN_POINT('Ctrl Pts',(6.77531733857434,-29.4669470832149,
123.108102859975));
#136243=CARTESIAN_POINT('Ctrl Pts',(6.8864526094129,-28.1214260468166,124.421743912282));
#136244=CARTESIAN_POINT('Ctrl Pts',(6.99758788025146,-28.4953108287459,
126.264646471684));
#136245=CARTESIAN_POINT('Ctrl Pts',(7.10872315109001,-30.2463952206375,
126.950053741776));
#136246=CARTESIAN_POINT('Ctrl Pts',(7.21985842192858,-31.7719610084168,
125.850631756669));
#136247=CARTESIAN_POINT('Ctrl Pts',(7.33099369276713,-31.6757008025321,
123.972650487844));
#136248=CARTESIAN_POINT('Ctrl Pts',(7.4421289636057,-30.0457188587341,123.034973285914));
#136249=CARTESIAN_POINT('Ctrl Pts',(7.55326423444425,-28.3738917300693,
123.895829679386));
#136250=CARTESIAN_POINT('Ctrl Pts',(7.66439950528281,-28.1903956948382,
125.767302060842));
#136251=CARTESIAN_POINT('Ctrl Pts',(7.77553477612138,-29.6631794962207,
126.936484483674));
#136252=CARTESIAN_POINT('Ctrl Pts',(7.88667004695993,-31.4442456278791,
126.333257206803));
#136253=CARTESIAN_POINT('Ctrl Pts',(7.9978053177985,-31.9034343983128,124.509737176165));
#136254=CARTESIAN_POINT('Ctrl Pts',(8.10894058863705,-30.6204633333385,
123.134940879626));
#136255=CARTESIAN_POINT('Ctrl Pts',(8.22007585947561,-28.7695995612073,
123.467180690923));
#136256=CARTESIAN_POINT('Ctrl Pts',(8.33121113031418,-28.0448868459996,
125.20236676348));
#136257=CARTESIAN_POINT('Ctrl Pts',(8.44234640115272,-29.109633724935,126.75233238305));
#136258=CARTESIAN_POINT('Ctrl Pts',(8.55348167199129,-30.9893085800826,
126.698437243919));
#136259=CARTESIAN_POINT('Ctrl Pts',(8.66461694282985,-31.9634955270585,
125.090010935753));
#136260=CARTESIAN_POINT('Ctrl Pts',(8.7757522136684,-31.1405536418831,123.399198951005));
#136261=CARTESIAN_POINT('Ctrl Pts',(8.88688748450698,-29.2736884341012,
123.173557506439));
#136262=CARTESIAN_POINT('Ctrl Pts',(8.99802275534552,-28.0716093206434,
124.619602490099));
#136263=CARTESIAN_POINT('Ctrl Pts',(9.10915802618409,-28.634504370035,126.41382459065));
#136264=CARTESIAN_POINT('Ctrl Pts',(9.22029329702265,-30.4472548015924,
126.913992634681));
#136265=CARTESIAN_POINT('Ctrl Pts',(9.3314285678612,-31.8505327041246,125.662378126051));
#136266=CARTESIAN_POINT('Ctrl Pts',(9.44256383869977,-31.5602986287577,
123.804424567018));
#136267=CARTESIAN_POINT('Ctrl Pts',(9.55369910953832,-29.8415044086767,
123.040915640856));
#136268=CARTESIAN_POINT('Ctrl Pts',(9.66483438037689,-28.2687143894222,
124.070160983838));
#136269=CARTESIAN_POINT('Ctrl Pts',(9.77596965121544,-28.2786147250435,
125.951149826147));
#136270=CARTESIAN_POINT('Ctrl Pts',(9.88711799254734,-29.8681697133404,
126.960299951329));
#136271=CARTESIAN_POINT('Ctrl Pts',(9.96122124359971,-31.0017136605171,
126.438058625129));
#136272=CARTESIAN_POINT('Ctrl Pts',(9.99827940437256,-31.3325999952893,
125.994779537896));
#136273=CARTESIAN_POINT('Ctrl Pts',(10.,-31.3346917155535,125.997072727755));
#136274=CARTESIAN_POINT('Ctrl Pts',(9.99999999999997,-31.3032949818861,
126.051116469759));
#136275=CARTESIAN_POINT('Ctrl Pts',(9.99999999999998,-31.2687047283496,
126.103084815638));
#136276=CARTESIAN_POINT('Ctrl Pts',(10.,-31.2312473715225,126.152891889409));
#136277=CARTESIAN_POINT('Ctrl Pts',(10.,-31.2074935522595,126.184477359623));
#136278=CARTESIAN_POINT('Ctrl Pts',(9.9999999999999,-31.1825856296951,126.215193469153));
#136279=CARTESIAN_POINT('Ctrl Pts',(9.99999999999999,-31.1565968715116,
126.24501511677));
#136280=CARTESIAN_POINT('Ctrl Pts',(10.,-31.1389352785806,126.265281487214));
#136281=CARTESIAN_POINT('Ctrl Pts',(10.0000000000001,-31.1207743588366,
126.285134707583));
#136282=CARTESIAN_POINT('Ctrl Pts',(10.,-31.1021353208467,126.304566020695));
#136283=CARTESIAN_POINT('Ctrl Pts',(9.99999999999995,-31.092131473339,126.314995093985));
#136284=CARTESIAN_POINT('Ctrl Pts',(10.0000000000001,-31.0819897769253,
126.325302541625));
#136285=CARTESIAN_POINT('Ctrl Pts',(10.,-31.0717240566778,126.335476823968));
#136286=CARTESIAN_POINT('Ctrl Pts',(9.99999999999984,-31.0248714183304,
126.381912140689));
#136287=CARTESIAN_POINT('Ctrl Pts',(9.99999999999995,-30.9753875180743,
126.425630314061));
#136288=CARTESIAN_POINT('Ctrl Pts',(9.99999999999986,-30.9236079996157,
126.466521663676));
#136289=CARTESIAN_POINT('Ctrl Pts',(9.99999999999981,-30.8862479946937,
126.496025627181));
#136290=CARTESIAN_POINT('Ctrl Pts',(9.99999999999995,-30.847691738784,126.524057613651));
#136291=CARTESIAN_POINT('Ctrl Pts',(10.,-30.8080509947417,126.550567733346));
#136292=CARTESIAN_POINT('Ctrl Pts',(10.,-30.7972669055174,126.557779694248));
#136293=CARTESIAN_POINT('Ctrl Pts',(9.99999999999982,-30.7864024946457,
126.564878974989));
#136294=CARTESIAN_POINT('Ctrl Pts',(9.9999999999999,-30.7754598842327,126.571864456785));
#136295=CARTESIAN_POINT('Ctrl Pts',(9.99999999999999,-30.7640699579655,
126.579135493548));
#136296=CARTESIAN_POINT('Ctrl Pts',(10.0000000000001,-30.7526018652892,
126.586278999636));
#136297=CARTESIAN_POINT('Ctrl Pts',(10.0000000000001,-30.7410634609561,
126.593291059087));
#136298=CARTESIAN_POINT('Ctrl Pts',(10.0000000000001,-30.6830797616217,
126.628528613187));
#136299=CARTESIAN_POINT('Ctrl Pts',(9.99999999999987,-30.623284545528,126.660474164912));
#136300=CARTESIAN_POINT('Ctrl Pts',(9.99999999999988,-30.5620183695342,
126.689017211284));
#136301=CARTESIAN_POINT('Ctrl Pts',(9.9999999999999,-30.4998607710709,126.717975558798));
#136302=CARTESIAN_POINT('Ctrl Pts',(10.,-30.4361883312143,126.74343240662));
#136303=CARTESIAN_POINT('Ctrl Pts',(9.99999999999992,-30.3713163621627,
126.765238169052));
#136304=CARTESIAN_POINT('Ctrl Pts',(9.99999999999985,-30.3311211104448,
126.778749214311));
#136305=CARTESIAN_POINT('Ctrl Pts',(10.,-30.2904645887863,126.790857837192));
#136306=CARTESIAN_POINT('Ctrl Pts',(9.99999999999999,-30.2494162442241,
126.801520088512));
#136307=CARTESIAN_POINT('Ctrl Pts',(9.99999999999994,-30.21580979325,126.810249318157));
#136308=CARTESIAN_POINT('Ctrl Pts',(9.99999999999999,-30.1819406176338,
126.81800897399));
#136309=CARTESIAN_POINT('Ctrl Pts',(9.9999999999999,-30.1478454088751,126.824771201514));
#136310=CARTESIAN_POINT('Ctrl Pts',(9.99999999999986,-30.1338751424326,
126.827541975581));
#136311=CARTESIAN_POINT('Ctrl Pts',(10.0000000000001,-30.1198643123212,
126.830145566994));
#136312=CARTESIAN_POINT('Ctrl Pts',(10.0000000000001,-30.1058393901247,
126.832576128087));
#136313=CARTESIAN_POINT('Ctrl Pts',(10.0000000000002,-30.0363859437807,
126.844612618707));
#136314=CARTESIAN_POINT('Ctrl Pts',(9.99999999999996,-29.9664681718509,
126.852434897851));
#136315=CARTESIAN_POINT('Ctrl Pts',(9.99999999999994,-29.8964212696988,
126.855902603765));
#136316=CARTESIAN_POINT('Ctrl Pts',(9.99999999999994,-29.8886375030675,
126.856287942913));
#136317=CARTESIAN_POINT('Ctrl Pts',(9.99999999999996,-29.8808521119947,
126.856619467432));
#136318=CARTESIAN_POINT('Ctrl Pts',(9.99999999999997,-29.8730655354866,
126.856896950862));
#136319=CARTESIAN_POINT('Ctrl Pts',(10.,-29.8056773383807,126.85929840522));
#136320=CARTESIAN_POINT('Ctrl Pts',(9.99999999999989,-29.7382014882899,
126.857656501328));
#136321=CARTESIAN_POINT('Ctrl Pts',(9.99999999999988,-29.6709003004103,
126.852189051701));
#136322=CARTESIAN_POINT('Ctrl Pts',(9.99999999999987,-29.5985034520534,
126.846307638102));
#136323=CARTESIAN_POINT('Ctrl Pts',(9.99999999999992,-29.5263078059746,
126.835999878972));
#136324=CARTESIAN_POINT('Ctrl Pts',(9.99999999999983,-29.4546313182209,
126.8214732487));
#136325=CARTESIAN_POINT('Ctrl Pts',(9.99999999999982,-29.4415872896375,
126.818829623343));
#136326=CARTESIAN_POINT('Ctrl Pts',(9.99999999999981,-29.4285604566208,
126.816046107482));
#136327=CARTESIAN_POINT('Ctrl Pts',(9.99999999999985,-29.4155527485577,
126.813123730597));
#136328=CARTESIAN_POINT('Ctrl Pts',(9.99999999999989,-29.4042297181811,
126.810579841844));
#136329=CARTESIAN_POINT('Ctrl Pts',(10.,-29.392930117574,126.807932726357));
#136330=CARTESIAN_POINT('Ctrl Pts',(10.,-29.3816571293467,126.805184037638));
#136331=CARTESIAN_POINT('Ctrl Pts',(10.0000000000001,-29.3126125113312,
126.78834891293));
#136332=CARTESIAN_POINT('Ctrl Pts',(9.99999999999981,-29.244543771198,126.767702608814));
#136333=CARTESIAN_POINT('Ctrl Pts',(9.99999999999989,-29.1777377507782,
126.743495272553));
#136334=CARTESIAN_POINT('Ctrl Pts',(9.99999999999997,-29.1095249755724,
126.718778195015));
#136335=CARTESIAN_POINT('Ctrl Pts',(9.99999999999996,-29.0426277353696,
126.690348379079));
#136336=CARTESIAN_POINT('Ctrl Pts',(9.99999999999993,-28.977347346887,126.658417134553));
#136337=CARTESIAN_POINT('Ctrl Pts',(9.9999999999999,-28.9116724977334,126.626292943562));
#136338=CARTESIAN_POINT('Ctrl Pts',(10.,-28.8476330737593,126.590624566029));
#136339=CARTESIAN_POINT('Ctrl Pts',(10.,-28.7855466623976,126.551575878805));
#136340=CARTESIAN_POINT('Ctrl Pts',(9.99999999999999,-28.7702070472662,
126.541928166524));
#136341=CARTESIAN_POINT('Ctrl Pts',(10.,-28.7549867432889,126.53207387934));
#136342=CARTESIAN_POINT('Ctrl Pts',(10.,-28.7398907549959,126.522015045523));
#136343=CARTESIAN_POINT('Ctrl Pts',(10.,-28.7280685454367,126.514137612195));
#136344=CARTESIAN_POINT('Ctrl Pts',(10.0000000000001,-28.7163212920593,
126.506133688814));
#136345=CARTESIAN_POINT('Ctrl Pts',(10.0000000000001,-28.7046689957787,
126.498016823557));
#136346=CARTESIAN_POINT('Ctrl Pts',(10.,-28.6428534396378,126.45495676673));
#136347=CARTESIAN_POINT('Ctrl Pts',(10.0000000000002,-28.5835957840056,
126.408648117515));
#136348=CARTESIAN_POINT('Ctrl Pts',(10.0000000000001,-28.5272089070883,
126.359324350215));
#136349=CARTESIAN_POINT('Ctrl Pts',(10.0000000000001,-28.4707612462639,
126.309947412896));
#136350=CARTESIAN_POINT('Ctrl Pts',(9.99999999999986,-28.4171895082972,
126.257548438498));
#136351=CARTESIAN_POINT('Ctrl Pts',(9.99999999999999,-28.3668234268913,
126.202312178068));
#136352=CARTESIAN_POINT('Ctrl Pts',(10.0000000000001,-28.3176028887393,
126.148332229897));
#136353=CARTESIAN_POINT('Ctrl Pts',(9.99999999999988,-28.271442962171,126.091642044011));
#136354=CARTESIAN_POINT('Ctrl Pts',(9.99999999999992,-28.2286806046144,
126.032374216658));
#136355=CARTESIAN_POINT('Ctrl Pts',(9.99999999999993,-28.2195018418537,
126.019652623235));
#136356=CARTESIAN_POINT('Ctrl Pts',(10.,-28.2104797516011,126.006812138555));
#136357=CARTESIAN_POINT('Ctrl Pts',(10.,-28.2016179073793,125.993853863974));
#136358=CARTESIAN_POINT('Ctrl Pts',(10.0000000000001,-28.1941462419212,
125.982928385015));
#136359=CARTESIAN_POINT('Ctrl Pts',(10.0000000000001,-28.1867884914522,
125.971919171957));
#136360=CARTESIAN_POINT('Ctrl Pts',(9.99999999999996,-28.1795446482253,
125.960828055739));
#136361=CARTESIAN_POINT('',(-0.000876815277413574,-28.7297206906101,126.080257502575));
#136362=CARTESIAN_POINT('Ctrl Pts',(-0.000876815277414122,-28.7308655491349,
126.07928390409));
#136363=CARTESIAN_POINT('Ctrl Pts',(-0.000584543518276265,-28.7363646204801,
126.085750285054));
#136364=CARTESIAN_POINT('Ctrl Pts',(-0.000292271759137858,-28.7419131131761,
126.092174637624));
#136365=CARTESIAN_POINT('Ctrl Pts',(0.,-28.7475103790669,126.098556211331));
#136366=CARTESIAN_POINT('Ctrl Pts',(-2.7820627745978E-16,-29.4698297828114,
123.014825674328));
#136367=CARTESIAN_POINT('Ctrl Pts',(-1.97609861837893E-13,-29.401170043366,
123.040247830321));
#136368=CARTESIAN_POINT('Ctrl Pts',(-5.5152163697422E-14,-29.334213616656,
123.069560472599));
#136369=CARTESIAN_POINT('Ctrl Pts',(-1.60201713006458E-13,-29.2691493442699,
123.102469334512));
#136370=CARTESIAN_POINT('Ctrl Pts',(-2.68200217276662E-13,-29.2022698079646,
123.136296338862));
#136371=CARTESIAN_POINT('Ctrl Pts',(-2.29820772041161E-13,-29.1373887076476,
123.17392371655));
#136372=CARTESIAN_POINT('Ctrl Pts',(-9.11840047912449E-14,-29.0747423504468,
123.215076533735));
#136373=CARTESIAN_POINT('Ctrl Pts',(2.61392724717173E-14,-29.0218080377509,
123.249849442975));
#136374=CARTESIAN_POINT('Ctrl Pts',(-9.38998899934961E-14,-28.9704696095689,
123.287140478707));
#136375=CARTESIAN_POINT('Ctrl Pts',(-7.41143257876331E-14,-28.920892369119,
123.326801793383));
#136376=CARTESIAN_POINT('Ctrl Pts',(-6.55476793573773E-14,-28.8988614666167,
123.344426303114));
#136377=CARTESIAN_POINT('Ctrl Pts',(-1.32835642465106E-13,-28.8771786481344,
123.36251904944));
#136378=CARTESIAN_POINT('Ctrl Pts',(-8.67986238439755E-14,-28.8558599729151,
123.381067782614));
#136379=CARTESIAN_POINT('Ctrl Pts',(-6.15038739588855E-14,-28.8441494340358,
123.391256767565));
#136380=CARTESIAN_POINT('Ctrl Pts',(-1.86758897242026E-13,-28.8325487895349,
123.401583348733));
#136381=CARTESIAN_POINT('Ctrl Pts',(-1.02785835398578E-13,-28.8210608353787,
123.412045537351));
#136382=CARTESIAN_POINT('Ctrl Pts',(-2.52615601302705E-14,-28.8104650682277,
123.421695202817));
#136383=CARTESIAN_POINT('Ctrl Pts',(-3.88065258281064E-14,-28.7999637294668,
123.431461749876));
#136384=CARTESIAN_POINT('Ctrl Pts',(-4.03774236268362E-14,-28.789574909979,
123.441328151629));
#136385=CARTESIAN_POINT('Ctrl Pts',(-4.90462452237839E-14,-28.7365434906851,
123.491692804601));
#136386=CARTESIAN_POINT('Ctrl Pts',(-1.84085511397076E-13,-28.6863464726686,
123.544740799507));
#136387=CARTESIAN_POINT('Ctrl Pts',(-1.0035722253221E-13,-28.6392018003405,
123.60021312434));
#136388=CARTESIAN_POINT('Ctrl Pts',(-1.71114058750102E-14,-28.5923287923977,
123.655365797888));
#136389=CARTESIAN_POINT('Ctrl Pts',(-1.31233249041967E-13,-28.5484725296676,
123.712915819897));
#136390=CARTESIAN_POINT('Ctrl Pts',(-9.71167590790856E-14,-28.507892135908,
123.772632946222));
#136391=CARTESIAN_POINT('Ctrl Pts',(-6.85507458244374E-14,-28.4742027907302,
123.822209372063));
#136392=CARTESIAN_POINT('Ctrl Pts',(-1.73770042367498E-13,-28.4427718620505,
123.873280045604));
#136393=CARTESIAN_POINT('Ctrl Pts',(-1.43815515052381E-13,-28.4137752342028,
123.925719701626));
#136394=CARTESIAN_POINT('Ctrl Pts',(-1.31281996901083E-13,-28.4016706643393,
123.947610505042));
#136395=CARTESIAN_POINT('Ctrl Pts',(-1.70300290126942E-14,-28.389990623329,
123.969739909637));
#136396=CARTESIAN_POINT('Ctrl Pts',(-9.5590202420226E-14,-28.378749346911,
123.992098885363));
#136397=CARTESIAN_POINT('Ctrl Pts',(-1.31953464075218E-13,-28.3735483020346,
124.002443799216));
#136398=CARTESIAN_POINT('Ctrl Pts',(2.40083866636569E-14,-28.3684411946227,
124.012837856646));
#136399=CARTESIAN_POINT('Ctrl Pts',(-1.70835567914196E-14,-28.3634294998546,
124.023280161284));
#136400=CARTESIAN_POINT('Ctrl Pts',(-5.97973873750489E-14,-28.3581982914169,
124.034179841862));
#136401=CARTESIAN_POINT('Ctrl Pts',(-9.27396819412998E-14,-28.3530746474019,
124.045124632974));
#136402=CARTESIAN_POINT('Ctrl Pts',(-1.00863761787195E-13,-28.348061622022,
124.056109233392));
#136403=CARTESIAN_POINT('Ctrl Pts',(-1.47355037682488E-13,-28.3195209836541,
124.118647817258));
#136404=CARTESIAN_POINT('Ctrl Pts',(-2.85071571274172E-14,-28.2945413176299,
124.182518755638));
#136405=CARTESIAN_POINT('Ctrl Pts',(-3.02674552088433E-14,-28.2733460518275,
124.247517313807));
#136406=CARTESIAN_POINT('Ctrl Pts',(-3.16869797246774E-14,-28.2541404972774,
124.306414114924));
#136407=CARTESIAN_POINT('Ctrl Pts',(-3.55485677518699E-14,-28.2380424914015,
124.366237360219));
#136408=CARTESIAN_POINT('Ctrl Pts',(-4.01484401280072E-14,-28.2252549794995,
124.42683954573));
#136409=CARTESIAN_POINT('Ctrl Pts',(-4.59179637818739E-14,-28.2101233382629,
124.498550957328));
#136410=CARTESIAN_POINT('Ctrl Pts',(-5.45851067606379E-15,-28.1996265542869,
124.57135458373));
#136411=CARTESIAN_POINT('Ctrl Pts',(-1.19071419391048E-14,-28.1936895357657,
124.644827593783));
#136412=CARTESIAN_POINT('Ctrl Pts',(-1.33052481531539E-14,-28.1923826402661,
124.661000955183));
#136413=CARTESIAN_POINT('Ctrl Pts',(9.44554714602467E-15,-28.1912969153211,
124.677206670197));
#136414=CARTESIAN_POINT('Ctrl Pts',(2.38697950294409E-15,-28.1904319294748,
124.693440064206));
#136415=CARTESIAN_POINT('Ctrl Pts',(-4.91010865300255E-15,-28.1895379671049,
124.710217267488));
#136416=CARTESIAN_POINT('Ctrl Pts',(-1.03906427062131E-14,-28.1888797709736,
124.727030207538));
#136417=CARTESIAN_POINT('Ctrl Pts',(-6.30051566474776E-15,-28.1884574247814,
124.74383953316));
#136418=CARTESIAN_POINT('Ctrl Pts',(1.08928320408804E-14,-28.1867348754449,
124.812396781292));
#136419=CARTESIAN_POINT('Ctrl Pts',(-5.5157119594787E-15,-28.1889237895494,
124.880980752938));
#136420=CARTESIAN_POINT('Ctrl Pts',(-5.52335954751015E-15,-28.1949036163297,
124.949253382792));
#136421=CARTESIAN_POINT('Ctrl Pts',(-5.57772555860731E-15,-28.2008822534432,
125.017512430031));
#136422=CARTESIAN_POINT('Ctrl Pts',(3.50880129321791E-14,-28.2106507485166,
125.085461330334));
#136423=CARTESIAN_POINT('Ctrl Pts',(1.07414077632484E-14,-28.2241382280736,
125.152747182718));
#136424=CARTESIAN_POINT('Ctrl Pts',(-6.8258769737951E-15,-28.2338995436464,
125.201444082382));
#136425=CARTESIAN_POINT('Ctrl Pts',(-2.91457997124025E-14,-28.2456098667842,
125.249793420514));
#136426=CARTESIAN_POINT('Ctrl Pts',(4.16333634234434E-16,-28.2592565463921,
125.297651761821));
#136427=CARTESIAN_POINT('Ctrl Pts',(2.27944565755811E-14,-28.2694943306151,
125.333555247918));
#136428=CARTESIAN_POINT('Ctrl Pts',(7.45391254632543E-14,-28.2808221554132,
125.369182243487));
#136429=CARTESIAN_POINT('Ctrl Pts',(4.55191440096314E-15,-28.2932385970371,
125.404468009152));
#136430=CARTESIAN_POINT('Ctrl Pts',(-1.88360276278269E-14,-28.2973646052875,
125.416193539273));
#136431=CARTESIAN_POINT('Ctrl Pts',(8.25076564039632E-14,-28.3016076190464,
125.427872169366));
#136432=CARTESIAN_POINT('Ctrl Pts',(8.58757509547559E-14,-28.3059670179929,
125.439501411337));
#136433=CARTESIAN_POINT('Ctrl Pts',(1.03680549446333E-13,-28.3290907711057,
125.501186915127));
#136434=CARTESIAN_POINT('Ctrl Pts',(-3.99986743471012E-14,-28.3554872924869,
125.561488823148));
#136435=CARTESIAN_POINT('Ctrl Pts',(3.84969833788773E-14,-28.3851066181449,
125.620073246654));
#136436=CARTESIAN_POINT('Ctrl Pts',(9.41574255422266E-14,-28.4059439023546,
125.661287563851));
#136437=CARTESIAN_POINT('Ctrl Pts',(7.40228323442486E-14,-28.428377060535,
125.70165134068));
#136438=CARTESIAN_POINT('Ctrl Pts',(-9.99200722162641E-15,-28.4523991071197,
125.741036970346));
#136439=CARTESIAN_POINT('Ctrl Pts',(-3.69244381206805E-14,-28.460111515178,
125.753681939897));
#136440=CARTESIAN_POINT('Ctrl Pts',(9.89854782698033E-14,-28.4679888668089,
125.766227705693));
#136441=CARTESIAN_POINT('Ctrl Pts',(8.2794882061421E-14,-28.4760275745915,
125.778664362048));
#136442=CARTESIAN_POINT('Ctrl Pts',(1.33122388715207E-14,-28.5102739274187,
125.831646773282));
#136443=CARTESIAN_POINT('Ctrl Pts',(9.60593437654786E-14,-28.5473763329624,
125.882545618706));
#136444=CARTESIAN_POINT('Ctrl Pts',(4.16888745746746E-14,-28.5873005880483,
125.931045842962));
#136445=CARTESIAN_POINT('Ctrl Pts',(-8.43323934842311E-15,-28.6240900287733,
125.975737875952));
#136446=CARTESIAN_POINT('Ctrl Pts',(-1.05109709785338E-13,-28.6632761651105,
126.018393268337));
#136447=CARTESIAN_POINT('Ctrl Pts',(-1.17544862732188E-13,-28.7048536785431,
126.058732609253));
#136448=CARTESIAN_POINT('Ctrl Pts',(-1.1948434771856E-13,-28.7126567769435,
126.066303332478));
#136449=CARTESIAN_POINT('Ctrl Pts',(2.25053579668865E-14,-28.7205441578753,
126.073792376282));
#136450=CARTESIAN_POINT('Ctrl Pts',(-5.02375918642883E-15,-28.7285142384905,
126.081199077946));
#136451=CARTESIAN_POINT('Origin',(10.,30.,55.));
#136452=CARTESIAN_POINT('Origin',(10.,-30.,55.));
#136453=CARTESIAN_POINT('Origin',(10.,-30.,125.));
#136454=CARTESIAN_POINT('Origin',(10.,30.,125.));
#136455=CARTESIAN_POINT('Origin',(60.,0.,90.));
#136456=CARTESIAN_POINT('',(120.,-22.,90.));
#136457=CARTESIAN_POINT('Origin',(120.,0.,90.));
#136458=CARTESIAN_POINT('',(0.,-22.,90.));
#136459=CARTESIAN_POINT('',(60.,-22.,90.));
#136460=CARTESIAN_POINT('Origin',(0.,0.,90.));
#136461=CARTESIAN_POINT('Origin',(60.,0.,40.));
#136462=CARTESIAN_POINT('',(-20.,50.,40.));
#136463=CARTESIAN_POINT('',(-20.,-50.,40.));
#136464=CARTESIAN_POINT('',(-20.,50.,40.));
#136465=CARTESIAN_POINT('',(140.,-50.,40.));
#136466=CARTESIAN_POINT('',(-20.,-50.,40.));
#136467=CARTESIAN_POINT('',(140.,50.,40.));
#136468=CARTESIAN_POINT('',(140.,-50.,40.));
#136469=CARTESIAN_POINT('',(140.,50.,40.));
#136470=CARTESIAN_POINT('',(120.,40.,40.));
#136471=CARTESIAN_POINT('',(0.,40.,40.));
#136472=CARTESIAN_POINT('',(120.,40.,40.));
#136473=CARTESIAN_POINT('',(120.,-40.,40.));
#136474=CARTESIAN_POINT('',(120.,-40.,40.));
#136475=CARTESIAN_POINT('',(0.,-40.,40.));
#136476=CARTESIAN_POINT('',(0.,-40.,40.));
#136477=CARTESIAN_POINT('',(0.,40.,40.));
#136478=CARTESIAN_POINT('Origin',(140.,50.,30.));
#136479=CARTESIAN_POINT('',(140.,50.,30.));
#136480=CARTESIAN_POINT('',(-20.,50.,30.));
#136481=CARTESIAN_POINT('',(140.,50.,30.));
#136482=CARTESIAN_POINT('',(-20.,50.,30.));
#136483=CARTESIAN_POINT('',(140.,50.,30.));
#136484=CARTESIAN_POINT('Origin',(140.,-50.,30.));
#136485=CARTESIAN_POINT('',(140.,-50.,30.));
#136486=CARTESIAN_POINT('',(140.,-50.,30.));
#136487=CARTESIAN_POINT('',(140.,-50.,30.));
#136488=CARTESIAN_POINT('Origin',(-20.,-50.,30.));
#136489=CARTESIAN_POINT('',(-20.,-50.,30.));
#136490=CARTESIAN_POINT('',(-20.,-50.,30.));
#136491=CARTESIAN_POINT('',(-20.,-50.,30.));
#136492=CARTESIAN_POINT('Origin',(-20.,50.,30.));
#136493=CARTESIAN_POINT('',(-20.,50.,30.));
#136494=CARTESIAN_POINT('Origin',(60.,0.,30.));
#136495=CARTESIAN_POINT('Origin',(120.,40.,40.));
#136496=CARTESIAN_POINT('',(0.,40.,140.));
#136497=CARTESIAN_POINT('',(0.,40.,40.));
#136498=CARTESIAN_POINT('',(120.,40.,140.));
#136499=CARTESIAN_POINT('',(120.,40.,140.));
#136500=CARTESIAN_POINT('',(120.,40.,40.));
#136501=CARTESIAN_POINT('Origin',(120.,-40.,40.));
#136502=CARTESIAN_POINT('',(120.,-40.,140.));
#136503=CARTESIAN_POINT('',(120.,-40.,140.));
#136504=CARTESIAN_POINT('',(120.,-40.,40.));
#136505=CARTESIAN_POINT('Origin',(0.,-40.,40.));
#136506=CARTESIAN_POINT('',(0.,-40.,140.));
#136507=CARTESIAN_POINT('',(0.,-40.,140.));
#136508=CARTESIAN_POINT('',(0.,-40.,40.));
#136509=CARTESIAN_POINT('Origin',(0.,40.,40.));
#136510=CARTESIAN_POINT('',(0.,40.,140.));
#136511=CARTESIAN_POINT('Origin',(60.,0.,140.));
#289352=UNCERTAINTY_MEASURE_WITH_UNIT(LENGTH_MEASURE(0.01),#289388,
'DISTANCE_ACCURACY_VALUE',
'Maximum model space distance between geometric entities at asserted c
onnectivities');
#289368=UNCERTAINTY_MEASURE_WITH_UNIT(LENGTH_MEASURE(0.01),#289388,
'DISTANCE_ACCURACY_VALUE',
'Maximum model space distance between geometric entities at asserted c
onnectivities');
#289371=(
GEOMETRIC_REPRESENTATION_CONTEXT(3)
GLOBAL_UNCERTAINTY_ASSIGNED_CONTEXT((#289352))
GLOBAL_UNIT_ASSIGNED_CONTEXT((#289388,#289390,#289391))
REPRESENTATION_CONTEXT('','3D')
);
#289387=(
GEOMETRIC_REPRESENTATION_CONTEXT(3)
GLOBAL_UNCERTAINTY_ASSIGNED_CONTEXT((#289368))
GLOBAL_UNIT_ASSIGNED_CONTEXT((#289388,#289390,#289391))
REPRESENTATION_CONTEXT('','3D')
);
#289388=(
LENGTH_UNIT()
NAMED_UNIT(*)
SI_UNIT(.MILLI.,.METRE.)
);
#289390=(
NAMED_UNIT(*)
PLANE_ANGLE_UNIT()
SI_UNIT($,.RADIAN.)
);
#289391=(
NAMED_UNIT(*)
SI_UNIT($,.STERADIAN.)
SOLID_ANGLE_UNIT()
);
#289394=SHAPE_DEFINITION_REPRESENTATION(#289412,#289455);
#289412=PRODUCT_DEFINITION_SHAPE('',$,#289474);
#289455=SHAPE_REPRESENTATION('',(#17186),#289371);
#289471=PRODUCT_DEFINITION_CONTEXT('part definition',#289527,'design');
#289474=PRODUCT_DEFINITION('Quill housing','Quill housing',#289492,#289471);
#289492=PRODUCT_DEFINITION_FORMATION('',$,#289531);
#289527=APPLICATION_CONTEXT(
'Core Data for Automotive Mechanical Design Process');
#289528=PRODUCT_CONTEXT('part definition',#289527,'mechanical');
#289531=PRODUCT('Quill housing','Quill housing',$,(#289528));
#289549=PRESENTATION_STYLE_ASSIGNMENT((#289556));
#289556=SURFACE_STYLE_USAGE(.BOTH.,#289563);
#289563=SURFACE_SIDE_STYLE('',(#289570));
#289570=SURFACE_STYLE_FILL_AREA(#289577);
#289577=FILL_AREA_STYLE('Opaque(23,69,131)',(#289584));
#289584=FILL_AREA_STYLE_COLOUR('Opaque(23,69,131)',#289591);
#289591=COLOUR_RGB('Opaque(23,69,131)',0.0901960784313725,0.270588235294118,
0.513725490196078);
ENDSEC;
END-ISO-10303-21;
